#130130=CARTESIAN_POINT ( 'NONE',  ( -14.34966873604972548, 8.224510206698743886, 63.33442372801900433 ) ) ;
#130131=CARTESIAN_POINT ( 'NONE',  ( 10.72451020669871369, 18.67979575497193778, 107.0844237280190043 ) ) ;
#130132=CARTESIAN_POINT ( 'NONE',  ( -19.05341960407611168, -5.049401038298163336, 46.45724293864768129 ) ) ;
#130133=CARTESIAN_POINT ( 'NONE',  ( -16.53943276465976808, 0.05219959533911058130, 46.24890960531435979 ) ) ;
#130134=CARTESIAN_POINT ( 'NONE',  ( 16.52544592524342804, -4.483927247898539470, 78.54057627198103830 ) ) ;
#130135=CARTESIAN_POINT ( 'NONE',  ( -16.46253265017160317, 9.564922557960807481, 80.83224293864769550 ) ) ;
#130136=CARTESIAN_POINT ( 'NONE',  ( 18.67979575497194134, -10.72451020669871369, 40.83442372801901854 ) ) ;
#130137=CARTESIAN_POINT ( 'NONE',  ( -9.474510206698964154, 16.51473224551069663, 95.41557627198102409 ) ) ;
#130138=CARTESIAN_POINT ( 'NONE',  ( 21.52544592524334988, 5.823673210054432836, 101.4594237280190185 ) ) ;
#130139=CARTESIAN_POINT ( 'NONE',  ( -14.34966873604972548, 8.224510206698743886, 63.33442372801900433 ) ) ;
#130140=CARTESIAN_POINT ( 'NONE',  ( 0.05219959533937995610, -21.53943276465977519, 30.00109039468568284 ) ) ;
#130141=CARTESIAN_POINT ( 'NONE',  ( 0.05219959533909260263, 19.03943276465977164, 114.9989096053143669 ) ) ;
#130142=CARTESIAN_POINT ( 'NONE',  ( 18.67979575497178502, 10.72451020669898547, 84.16557627198103830 ) ) ;
#130143=CARTESIAN_POINT ( 'NONE',  ( -8.314922557960811034, -14.29746914071050412, 52.08224293864768839 ) ) ;
#130144=CARTESIAN_POINT ( 'NONE',  ( 9.474510206698971260, -16.51473224551069308, 47.91557627198102409 ) ) ;
#130145=CARTESIAN_POINT ( 'NONE',  ( 14.29746914071049879, -8.314922557960816363, 63.33224293864770260 ) ) ;
#130146=CARTESIAN_POINT ( 'NONE',  ( -21.52544592524343514, 5.823673210054127303, 31.04057627198102409 ) ) ;
#130147=CARTESIAN_POINT ( 'NONE',  ( -9.564922557961040184, 16.46253265017147172, 27.91775706135232582 ) ) ;
#130148=CARTESIAN_POINT ( 'NONE',  ( 16.52544592524342804, -4.483927247898539470, 93.54057627198103830 ) ) ;
#130149=CARTESIAN_POINT ( 'NONE',  ( 9.564922557960805705, 16.46253265017160317, 114.5822429386476955 ) ) ;
#130151=CARTESIAN_POINT ( 'NONE',  ( 4.483927247898790824, -16.52544592524335698, 55.20942372801902565 ) ) ;
#130152=CARTESIAN_POINT ( 'NONE',  ( -9.564922557960796823, -16.46253265017161027, 52.08224293864768839 ) ) ;
#130154=CARTESIAN_POINT ( 'NONE',  ( -4.483927247898782831, 16.52544592524335698, 97.70942372801904696 ) ) ;
#130155=CARTESIAN_POINT ( 'NONE',  ( 16.46253265017146816, 9.564922557961045513, 106.6677570613523471 ) ) ;
#130156=CARTESIAN_POINT ( 'NONE',  ( 21.55341960407619695, -5.719274019375665929, 76.04275706135237556 ) ) ;
#130157=CARTESIAN_POINT ( 'NONE',  ( 19.03943276465977164, -0.05219959533909143690, 68.74890960531436690 ) ) ;
#130158=CARTESIAN_POINT ( 'NONE',  ( 5.823673210054125526, 21.52544592524343514, 109.7905762719810383 ) ) ;
#130159=CARTESIAN_POINT ( 'NONE',  ( 16.52544592524335698, 4.483927247898782831, 41.45942372801901143 ) ) ;
#130160=CARTESIAN_POINT ( 'NONE',  ( 8.314922557960818139, 14.29746914071049879, 114.5822429386477097 ) ) ;
#130161=CARTESIAN_POINT ( 'NONE',  ( -13.97604488694547697, 13.89961937509957934, 113.1260903946856757 ) ) ;
#130162=CARTESIAN_POINT ( 'NONE',  ( -0.05219959533936034679, 19.03943276465977164, 87.50109039468567573 ) ) ;
#130163=CARTESIAN_POINT ( 'NONE',  ( -5.719274019375978568, 21.55341960407610458, 80.20724293864769550 ) ) ;
#130164=CARTESIAN_POINT ( 'NONE',  ( 9.474510206698729675, 16.51473224551082808, 57.08442372801900433 ) ) ;
#130165=CARTESIAN_POINT ( 'NONE',  ( -16.51473224551069308, -9.474510206698971260, 111.6655762719810383 ) ) ;
#130166=CARTESIAN_POINT ( 'NONE',  ( 21.55341960407610458, 5.719274019375980345, 98.95724293864770971 ) ) ;
#130167=CARTESIAN_POINT ( 'NONE',  ( 17.50000000000001421, 3.209263204892573995, 27.73803174393734494 ) ) ;
#130168=CARTESIAN_POINT ( 'NONE',  ( 16.46253265017160672, -9.564922557960803928, 63.33224293864769550 ) ) ;
#130169=LINE ( 'NONE', #24028, #136973 ) ;
#130170=CARTESIAN_POINT ( 'NONE',  ( 0.05219959533936267826, -19.03943276465977164, 110.0010903946856757 ) ) ;
#130172=CARTESIAN_POINT ( 'NONE',  ( 5.823673210054444382, -21.52544592524334988, 55.20942372801902565 ) ) ;
#130173=CARTESIAN_POINT ( 'NONE',  ( 15.72974639402199770, -15.80617190586745480, 103.1239096053143811 ) ) ;
#130174=CARTESIAN_POINT ( 'NONE',  ( -12.14591786802309592, -12.06949235617757132, 61.87390960531436690 ) ) ;
#130175=CARTESIAN_POINT ( 'NONE',  ( 19.05341960407611168, 5.049401038298154454, 73.95724293864768129 ) ) ;
#130176=CARTESIAN_POINT ( 'NONE',  ( -10.81492255796105439, 18.62759615963255655, 67.91775706135234714 ) ) ;
#130177=CARTESIAN_POINT ( 'NONE',  ( -4.483927247898782831, 16.52544592524335698, 22.70942372801901499 ) ) ;
#130178=CARTESIAN_POINT ( 'NONE',  ( -19.05341960407617563, 5.049401038297882671, 28.54275706135232937 ) ) ;
#130180=CARTESIAN_POINT ( 'NONE',  ( -21.52544592524334988, -5.823673210054445271, 58.95942372801902565 ) ) ;
#130181=CARTESIAN_POINT ( 'NONE',  ( 18.62759615963271287, -10.81492255796078972, 108.3322429386477097 ) ) ;
#130182=CARTESIAN_POINT ( 'NONE',  ( -0.05219959533907301413, -21.53943276465977519, 57.49890960531435979 ) ) ;
#130183=CARTESIAN_POINT ( 'NONE',  ( 9.474510206698729675, 16.51473224551082808, 102.0844237280190043 ) ) ;
#130184=CARTESIAN_POINT ( 'NONE',  ( -16.46253265017146816, -9.564922557961047289, 64.16775706135233293 ) ) ;
#130185=CARTESIAN_POINT ( 'NONE',  ( 10.81492255796106328, -18.62759615963255655, 85.41775706135236135 ) ) ;
#130186=CARTESIAN_POINT ( 'NONE',  ( -13.97604488694547697, 13.89961937509957934, 53.12609039468565442 ) ) ;
#130187=CARTESIAN_POINT ( 'NONE',  ( -0.05219959533909027116, -19.03943276465977164, 42.49890960531435269 ) ) ;
#130188=CARTESIAN_POINT ( 'NONE',  ( -21.55341960407610458, -5.719274019375992779, 61.45724293864770260 ) ) ;
#130189=CARTESIAN_POINT ( 'NONE',  ( 14.29746914071049879, -8.314922557960816363, 53.33224293864769550 ) ) ;
#130191=CARTESIAN_POINT ( 'NONE',  ( 13.89961937509957401, 13.97604488694547697, 36.87609039468565442 ) ) ;
#130192=CARTESIAN_POINT ( 'NONE',  ( -16.53943276465976808, -0.05219959533934237506, 88.75109039468567573 ) ) ;
#130193=CARTESIAN_POINT ( 'NONE',  ( 16.52544592524342804, -4.483927247898539470, 53.54057627198103120 ) ) ;
#130194=CARTESIAN_POINT ( 'NONE',  ( 10.72451020669871369, 18.67979575497193778, 77.08442372801901854 ) ) ;
#130195=CARTESIAN_POINT ( 'NONE',  ( 15.72974639402176855, 15.80617190586768217, 76.87609039468567573 ) ) ;
#130196=CARTESIAN_POINT ( 'NONE',  ( -5.719274019375978568, 21.55341960407610458, 75.20724293864769550 ) ) ;
#130198=CARTESIAN_POINT ( 'NONE',  ( 5.153800228976335163, 19.02544592524342804, 39.79057627198100988 ) ) ;
#130199=CARTESIAN_POINT ( 'NONE',  ( 21.55341960407619695, -5.719274019375665929, 51.04275706135234714 ) ) ;
#130200=CARTESIAN_POINT ( 'NONE',  ( -13.97604488694527625, -13.89961937509977652, 31.87390960531435979 ) ) ;
#130201=CARTESIAN_POINT ( 'NONE',  ( 13.89961937509977652, -13.97604488694527269, 58.12390960531436690 ) ) ;
#130202=CARTESIAN_POINT ( 'NONE',  ( -8.224510206698948167, 14.34966873604960824, 100.4155762719810241 ) ) ;
#130203=CARTESIAN_POINT ( 'NONE',  ( 19.05341960407611168, 5.049401038298154454, 103.9572429386476671 ) ) ;
#130204=CARTESIAN_POINT ( 'NONE',  ( -14.34966873604960291, -8.224510206698953496, 46.66557627198102409 ) ) ;
#130205=CARTESIAN_POINT ( 'NONE',  ( 4.379528057220339221, -16.55341960407611168, 112.7072429386476955 ) ) ;
#130206=CARTESIAN_POINT ( 'NONE',  ( -0.05219959533907301413, -21.53943276465977519, 87.49890960531436690 ) ) ;
#130207=CARTESIAN_POINT ( 'NONE',  ( -5.719274019375665041, -21.55341960407619695, 19.79275706135235069 ) ) ;
#130209=CARTESIAN_POINT ( 'NONE',  ( 12.14591786802327356, -12.06949235617739191, 35.62609039468568994 ) ) ;
#130210=ORIENTED_EDGE ( 'NONE', *, *, #108344, .T. ) ;
#130211=CARTESIAN_POINT ( 'NONE',  ( -15.72974639402197994, 15.80617190586746368, 65.62390960531436690 ) ) ;
#130212=CARTESIAN_POINT ( 'NONE',  ( 10.81492255796106328, -18.62759615963255655, 95.41775706135234714 ) ) ;
#130213=CARTESIAN_POINT ( 'NONE',  ( -5.153800228976328057, -19.02544592524343514, 97.29057627198099567 ) ) ;
#130214=CARTESIAN_POINT ( 'NONE',  ( 15.80617190586769283, -15.72974639402175789, 25.62609039468567929 ) ) ;
#130216=CARTESIAN_POINT ( 'NONE',  ( -21.53943276465977519, 0.05219959533907696930, 26.24890960531435624 ) ) ;
#130217=CARTESIAN_POINT ( 'NONE',  ( 4.483927247898790824, -16.52544592524335698, 85.20942372801901854 ) ) ;
#130218=CARTESIAN_POINT ( 'NONE',  ( -5.823673210054431948, 21.52544592524334988, 87.70942372801901854 ) ) ;
#130219=CARTESIAN_POINT ( 'NONE',  ( -10.81492255796105439, 18.62759615963255655, 112.9177570613523329 ) ) ;
#130220=CARTESIAN_POINT ( 'NONE',  ( -8.224510206698735004, -14.34966873604973081, 79.58442372801903275 ) ) ;
#130221=CARTESIAN_POINT ( 'NONE',  ( -15.80617190586768217, 15.72974639402176855, 23.12609039468567573 ) ) ;
#130222=CARTESIAN_POINT ( 'NONE',  ( -13.89961937509977652, 13.97604488694528158, 30.62390960531435269 ) ) ;
#130223=CARTESIAN_POINT ( 'NONE',  ( 10.72451020669871369, 18.67979575497193778, 102.0844237280190185 ) ) ;
#130224=CARTESIAN_POINT ( 'NONE',  ( -13.97604488694527625, -13.89961937509977652, 111.8739096053143243 ) ) ;
#130225=CARTESIAN_POINT ( 'NONE',  ( -15.80617190586745835, -15.72974639402198527, 106.8739096053143811 ) ) ;
#130226=CARTESIAN_POINT ( 'NONE',  ( 19.20446147854523389, 5.500000000000087041, 81.88999695167674986 ) ) ;
#130227=CARTESIAN_POINT ( 'NONE',  ( -21.55341960407610458, -5.719274019375992779, 61.45724293864770260 ) ) ;
#130228=CARTESIAN_POINT ( 'NONE',  ( 12.14591786802327356, -12.06949235617739191, 50.62609039468568994 ) ) ;
#130229=CARTESIAN_POINT ( 'NONE',  ( -14.29746914071049879, 8.314922557960819915, 50.83224293864770971 ) ) ;
#130231=CARTESIAN_POINT ( 'NONE',  ( -13.97604488694547697, 13.89961937509957934, 78.12609039468567573 ) ) ;
#130232=CARTESIAN_POINT ( 'NONE',  ( -17.26172910966780094, 6.454744622555846689, 105.8064690864922426 ) ) ;
#130233=CARTESIAN_POINT ( 'NONE',  ( -8.224510206698735004, -14.34966873604973081, 24.58442372801901499 ) ) ;
#130234=CARTESIAN_POINT ( 'NONE',  ( 15.72974639402199770, -15.80617190586745480, 83.12390960531436690 ) ) ;
#130235=CARTESIAN_POINT ( 'NONE',  ( 16.53943276465976808, -0.05219959533910856209, 63.74890960531435979 ) ) ;
#130236=CARTESIAN_POINT ( 'NONE',  ( 0.05219959533909260263, 19.03943276465977164, 104.9989096053143669 ) ) ;
#130237=CARTESIAN_POINT ( 'NONE',  ( -4.483927247898782831, 16.52544592524335698, 47.70942372801902565 ) ) ;
#130238=CARTESIAN_POINT ( 'NONE',  ( -13.97604488694527625, -13.89961937509977652, 51.87390960531436690 ) ) ;
#130239=CARTESIAN_POINT ( 'NONE',  ( -0.05219959533937732626, 21.53943276465977519, 27.50109039468567929 ) ) ;
#130240=CARTESIAN_POINT ( 'NONE',  ( 16.46253265017146816, 9.564922557961045513, 101.6677570613523329 ) ) ;
#130241=CARTESIAN_POINT ( 'NONE',  ( -19.05341960407611168, -5.049401038298163336, 96.45724293864769550 ) ) ;
#130242=CARTESIAN_POINT ( 'NONE',  ( -13.89961937509977652, 13.97604488694528158, 85.62390960531433848 ) ) ;
#130243=CARTESIAN_POINT ( 'NONE',  ( -5.823673210054116645, -21.52544592524344225, 87.29057627198103830 ) ) ;
#130244=CARTESIAN_POINT ( 'NONE',  ( 13.97604488694527802, 13.89961937509977652, 44.37390960531435269 ) ) ;
#130245=CARTESIAN_POINT ( 'NONE',  ( -17.49999999999999645, -5.624438216177605199, 59.18329655085358354 ) ) ;
#130246=CARTESIAN_POINT ( 'NONE',  ( 0.05219959533910956823, 16.53943276465976808, 69.99890960531435269 ) ) ;
#130247=CARTESIAN_POINT ( 'NONE',  ( 5.049401038298161559, -19.05341960407611168, 107.7072429386476955 ) ) ;
#130249=CARTESIAN_POINT ( 'NONE',  ( 19.02544592524334988, 5.153800228976608722, 76.45942372801897591 ) ) ;
#130250=CARTESIAN_POINT ( 'NONE',  ( -5.719274019375978568, 21.55341960407610458, 85.20724293864770971 ) ) ;
#130251=CARTESIAN_POINT ( 'NONE',  ( -19.02544592524334988, -5.153800228976617603, 43.95942372801899012 ) ) ;
#130252=CARTESIAN_POINT ( 'NONE',  ( -13.89961937509977652, 13.97604488694528158, 100.6239096053143669 ) ) ;
#130253=( NAMED_UNIT ( * ) PLANE_ANGLE_UNIT ( ) SI_UNIT ( $, .RADIAN. ) );
#130254=CARTESIAN_POINT ( 'NONE',  ( -18.62759615963270932, 10.81492255796079327, 45.83224293864769550 ) ) ;
#130255=CARTESIAN_POINT ( 'NONE',  ( 9.564922557960805705, 16.46253265017160317, 89.58224293864769550 ) ) ;
#130256=CARTESIAN_POINT ( 'NONE',  ( 18.62759615963255655, 10.81492255796105972, 71.66775706135234714 ) ) ;
#130257=CARTESIAN_POINT ( 'NONE',  ( 19.03943276465977164, -0.05219959533909143690, 33.74890960531435979 ) ) ;
#130258=CARTESIAN_POINT ( 'NONE',  ( 14.29746914071049879, -8.314922557960816363, 73.33224293864769550 ) ) ;
#130259=CARTESIAN_POINT ( 'NONE',  ( 16.53943276465976808, 0.05219959533934440121, 21.25109039468567218 ) ) ;
#130260=CARTESIAN_POINT ( 'NONE',  ( 15.72974639402176855, 15.80617190586768217, 46.87609039468568994 ) ) ;
#130262=CARTESIAN_POINT ( 'NONE',  ( 5.153800228976335163, 19.02544592524342804, 114.7905762719810241 ) ) ;
#130263=CARTESIAN_POINT ( 'NONE',  ( -9.474510206698720793, -16.51473224551083518, 84.58442372801900433 ) ) ;
#130264=EDGE_CURVE ( 'NONE', #102413, #165180, #13310, .T. ) ;
#130266=CARTESIAN_POINT ( 'NONE',  ( -21.53943276465977519, -0.05219959533937600094, 23.75109039468567929 ) ) ;
#130267=CARTESIAN_POINT ( 'NONE',  ( -19.35543954521082100, -5.499999999999585221, 44.58901960356452321 ) ) ;
#130268=CARTESIAN_POINT ( 'NONE',  ( 15.80617190586769283, -15.72974639402175789, 110.6260903946857042 ) ) ;
#130269=CARTESIAN_POINT ( 'NONE',  ( 13.97604488694527802, 13.89961937509977652, 49.37390960531434558 ) ) ;
#130270=CARTESIAN_POINT ( 'NONE',  ( 9.564922557961047289, -16.46253265017146816, 20.41775706135233293 ) ) ;
#130271=CARTESIAN_POINT ( 'NONE',  ( -4.379528057220086978, -16.55341960407618274, 99.79275706135234714 ) ) ;
#130272=CARTESIAN_POINT ( 'NONE',  ( -16.51473224551069308, -9.474510206698971260, 106.6655762719810383 ) ) ;
#130273=CARTESIAN_POINT ( 'NONE',  ( -10.81492255796105439, 18.62759615963255655, 77.91775706135231871 ) ) ;
#130277=CARTESIAN_POINT ( 'NONE',  ( -18.67979575497193778, 10.72451020669871902, 73.33442372801901854 ) ) ;
#130278=CARTESIAN_POINT ( 'NONE',  ( -5.823673210054431948, 21.52544592524334988, 97.70942372801904696 ) ) ;
#130280=CARTESIAN_POINT ( 'NONE',  ( 17.44270441346513678, -5.991230190323081573, 41.13664920735773478 ) ) ;
#130281=CARTESIAN_POINT ( 'NONE',  ( 9.564922557960805705, 16.46253265017160317, 89.58224293864769550 ) ) ;
#130282=CARTESIAN_POINT ( 'NONE',  ( 19.03943276465977164, -0.05219959533909143690, 108.7489096053143527 ) ) ;
#130284=CARTESIAN_POINT ( 'NONE',  ( -16.51473224551069308, -9.474510206698971260, 41.66557627198103120 ) ) ;
#130285=CARTESIAN_POINT ( 'NONE',  ( 5.823673210054125526, 21.52544592524343514, 54.79057627198104541 ) ) ;
#130286=CARTESIAN_POINT ( 'NONE',  ( 12.14591786802327356, -12.06949235617739191, 100.6260903946857184 ) ) ;
#130287=CARTESIAN_POINT ( 'NONE',  ( 8.224510206698953496, -14.34966873604960469, 97.91557627198103830 ) ) ;
#130288=CARTESIAN_POINT ( 'NONE',  ( 9.474510206698971260, -16.51473224551069308, 87.91557627198102409 ) ) ;
#130289=CARTESIAN_POINT ( 'NONE',  ( -15.72974639402176322, -15.80617190586768395, 104.3760903946856899 ) ) ;
#130290=CARTESIAN_POINT ( 'NONE',  ( 13.89961937509977652, -13.97604488694527269, 38.12390960531436690 ) ) ;
#130291=CARTESIAN_POINT ( 'NONE',  ( 16.55341960407611168, 4.379528057220329451, 93.95724293864770971 ) ) ;
#130292=CARTESIAN_POINT ( 'NONE',  ( -21.53943276465977519, -0.05219959533937600094, 53.75109039468568994 ) ) ;
#130293=CARTESIAN_POINT ( 'NONE',  ( 0.05219959533907565091, 21.53943276465977519, 84.99890960531436690 ) ) ;
#130294=CARTESIAN_POINT ( 'NONE',  ( 19.03943276465977164, 0.05219959533936151252, 46.25109039468566863 ) ) ;
#130296=CARTESIAN_POINT ( 'NONE',  ( -16.51473224551069308, -9.474510206698971260, 91.66557627198103830 ) ) ;
#130297=CARTESIAN_POINT ( 'NONE',  ( -0.05219959533910754901, -16.53943276465976808, 57.49890960531435979 ) ) ;
#130298=CARTESIAN_POINT ( 'NONE',  ( 5.153800228976615827, -19.02544592524334988, 45.20942372801901143 ) ) ;
#130299=CARTESIAN_POINT ( 'NONE',  ( 13.89961937509977652, -13.97604488694527269, 53.12390960531434558 ) ) ;
#130300=CARTESIAN_POINT ( 'NONE',  ( 16.55341960407611168, 4.379528057220329451, 43.95724293864769550 ) ) ;
#130301=CARTESIAN_POINT ( 'NONE',  ( -16.51473224551082808, 9.474510206698731452, 78.33442372801900433 ) ) ;
#130302=CARTESIAN_POINT ( 'NONE',  ( -18.56453257813363678, 5.500000000000055955, 85.99000423690684158 ) ) ;
#130303=CARTESIAN_POINT ( 'NONE',  ( -21.55341960407610458, -5.719274019375992779, 41.45724293864769550 ) ) ;
#130304=CARTESIAN_POINT ( 'NONE',  ( 14.29746914071049879, -8.314922557960816363, 103.3322429386476955 ) ) ;
#130306=CARTESIAN_POINT ( 'NONE',  ( 0.05219959533909260263, 19.03943276465977164, 54.99890960531435979 ) ) ;
#130307=CARTESIAN_POINT ( 'NONE',  ( 21.53943276465977519, -0.05219959533907433946, 43.74890960531435979 ) ) ;
#130308=CARTESIAN_POINT ( 'NONE',  ( 16.51473224551069308, 9.474510206698969483, 29.16557627198103475 ) ) ;
#130309=CARTESIAN_POINT ( 'NONE',  ( 14.29746914071037800, 8.314922557961029526, 76.66775706135234714 ) ) ;
#130310=CARTESIAN_POINT ( 'NONE',  ( -0.05219959533909027116, -19.03943276465977164, 62.49890960531435979 ) ) ;
#130311=CARTESIAN_POINT ( 'NONE',  ( -19.02544592524334988, -5.153800228976617603, 38.95942372801900433 ) ) ;
#130312=CARTESIAN_POINT ( 'NONE',  ( -21.53943276465977519, -0.05219959533937600094, 73.75109039468567573 ) ) ;
#130313=CARTESIAN_POINT ( 'NONE',  ( -21.52544592524343514, 5.823673210054127303, 46.04057627198103830 ) ) ;
#130314=CARTESIAN_POINT ( 'NONE',  ( -16.51473224551069308, -9.474510206698971260, 21.66557627198102765 ) ) ;
#130315=CARTESIAN_POINT ( 'NONE',  ( -16.51473224551082808, 9.474510206698731452, 108.3344237280190043 ) ) ;
#130316=DIRECTION ( 'NONE',  ( -1.734723475976805517E-15, 0.000000000000000000, -1.000000000000000000 ) ) ;
#130318=CARTESIAN_POINT ( 'NONE',  ( -5.823673210054116645, -21.52544592524344225, 42.29057627198103120 ) ) ;
#130319=CARTESIAN_POINT ( 'NONE',  ( 16.18388926212234935, -7.379444403734663815, 67.06046848633847901 ) ) ;
#130320=CARTESIAN_POINT ( 'NONE',  ( 21.52544592524334988, 5.823673210054432836, 86.45942372801901854 ) ) ;
#130321=CARTESIAN_POINT ( 'NONE',  ( -8.314922557960811034, -14.29746914071050412, 52.08224293864768839 ) ) ;
#130322=CARTESIAN_POINT ( 'NONE',  ( 4.483927247898545687, 16.52544592524342804, 59.79057627198103120 ) ) ;
#130323=CARTESIAN_POINT ( 'NONE',  ( 18.62759615963271287, -10.81492255796078972, 83.33224293864769550 ) ) ;
#130324=CARTESIAN_POINT ( 'NONE',  ( -5.823673210054116645, -21.52544592524344225, 72.29057627198102409 ) ) ;
#130326=CARTESIAN_POINT ( 'NONE',  ( -10.72451020669898014, 18.67979575497178502, 35.41557627198102409 ) ) ;
#130327=CARTESIAN_POINT ( 'NONE',  ( 4.483927247898790824, -16.52544592524335698, 60.20942372801902565 ) ) ;
#130328=CARTESIAN_POINT ( 'NONE',  ( 8.314922557960818139, 14.29746914071049879, 79.58224293864769550 ) ) ;
#130329=CARTESIAN_POINT ( 'NONE',  ( 5.049401038298161559, -19.05341960407611168, 57.70724293864769550 ) ) ;
#130330=CARTESIAN_POINT ( 'NONE',  ( -16.51473224551069308, -9.474510206698971260, 26.66557627198103120 ) ) ;
#130333=CARTESIAN_POINT ( 'NONE',  ( -16.53943276465976808, -0.05219959533934237506, 88.75109039468567573 ) ) ;
#130334=CARTESIAN_POINT ( 'NONE',  ( 18.62759615963255655, 10.81492255796105972, 21.66775706135235069 ) ) ;
#130335=CARTESIAN_POINT ( 'NONE',  ( 19.03943276465977164, -0.05219959533909143690, 83.74890960531436690 ) ) ;
#130336=CARTESIAN_POINT ( 'NONE',  ( 15.80617190586769283, -15.72974639402175789, 50.62609039468568994 ) ) ;
#130337=CARTESIAN_POINT ( 'NONE',  ( 16.46253265017160672, -9.564922557960803928, 113.3322429386476955 ) ) ;
#130339=ORIENTED_EDGE ( 'NONE', *, *, #83608, .F. ) ;
#130340=CARTESIAN_POINT ( 'NONE',  ( 21.53943276465977519, 0.05219959533937863772, 46.25109039468567573 ) ) ;
#130341=CARTESIAN_POINT ( 'NONE',  ( -16.46253265017160317, 9.564922557960807481, 40.83224293864769550 ) ) ;
#130342=CARTESIAN_POINT ( 'NONE',  ( 5.049401038298161559, -19.05341960407611168, 102.7072429386476955 ) ) ;
#130343=CARTESIAN_POINT ( 'NONE',  ( 19.02544592524334988, 5.153800228976608722, 51.45942372801900433 ) ) ;
#130344=CARTESIAN_POINT ( 'NONE',  ( -21.55341960407619339, 5.719274019375674811, 28.54275706135234358 ) ) ;
#130345=CARTESIAN_POINT ( 'NONE',  ( -19.02544592524334988, -5.153800228976617603, 43.95942372801899012 ) ) ;
#130346=CARTESIAN_POINT ( 'NONE',  ( 9.564922557960805705, 16.46253265017160317, 29.58224293864769550 ) ) ;
#130347=CARTESIAN_POINT ( 'NONE',  ( 12.14591786802327356, -12.06949235617739191, 95.62609039468568994 ) ) ;
#130348=CARTESIAN_POINT ( 'NONE',  ( -13.97604488694547697, 13.89961937509957934, 63.12609039468566152 ) ) ;
#130349=CARTESIAN_POINT ( 'NONE',  ( -4.483927247898782831, 16.52544592524335698, 107.7094237280190328 ) ) ;
#130351=CARTESIAN_POINT ( 'NONE',  ( -5.049401038298153566, 19.05341960407611168, 85.20724293864766707 ) ) ;
#130352=CARTESIAN_POINT ( 'NONE',  ( 18.62759615963255655, 10.81492255796105972, 96.66775706135234714 ) ) ;
#130353=CARTESIAN_POINT ( 'NONE',  ( -18.62759615963255300, -10.81492255796106328, 109.1677570613523613 ) ) ;
#130355=CARTESIAN_POINT ( 'NONE',  ( 16.46253265017160672, -9.564922557960803928, 103.3322429386476955 ) ) ;
#130356=CARTESIAN_POINT ( 'NONE',  ( -21.52544592524334988, -5.823673210054445271, 73.95942372801901854 ) ) ;
#130357=CARTESIAN_POINT ( 'NONE',  ( -13.97604488694547697, 13.89961937509957934, 113.1260903946856757 ) ) ;
#130359=CARTESIAN_POINT ( 'NONE',  ( -16.46253265017160317, 9.564922557960807481, 85.83224293864769550 ) ) ;
#130360=CARTESIAN_POINT ( 'NONE',  ( 0.05219959533907565091, 21.53943276465977519, 24.99890960531435624 ) ) ;
#130362=CARTESIAN_POINT ( 'NONE',  ( 5.049401038298161559, -19.05341960407611168, 87.70724293864769550 ) ) ;
#130363=CARTESIAN_POINT ( 'NONE',  ( -16.61371651742602396, -7.165104196376147705, 91.14584930007005426 ) ) ;
#130364=CARTESIAN_POINT ( 'NONE',  ( -19.02544592524342804, 5.153800228976336051, 76.04057627198102409 ) ) ;
#130365=CARTESIAN_POINT ( 'NONE',  ( -5.049401038298153566, 19.05341960407611168, 70.20724293864769550 ) ) ;
#130366=CARTESIAN_POINT ( 'NONE',  ( -4.379528057220086978, -16.55341960407618274, 99.79275706135234714 ) ) ;
#130368=CARTESIAN_POINT ( 'NONE',  ( -13.89961937509957401, -13.97604488694547875, 64.37609039468567573 ) ) ;
#130369=CARTESIAN_POINT ( 'NONE',  ( 0.05219959533909260263, 19.03943276465977164, 89.99890960531436690 ) ) ;
#130370=CARTESIAN_POINT ( 'NONE',  ( 16.53943276465976808, -0.05219959533910856209, 83.74890960531435269 ) ) ;
#130371=CARTESIAN_POINT ( 'NONE',  ( 15.72974639402199770, -15.80617190586745480, 28.12390960531435979 ) ) ;
#130372=CARTESIAN_POINT ( 'NONE',  ( 19.05341960407611168, 5.049401038298154454, 113.9572429386477097 ) ) ;
#130373=CARTESIAN_POINT ( 'NONE',  ( 0.05219959533910956823, 16.53943276465976808, 89.99890960531438111 ) ) ;
#130375=CARTESIAN_POINT ( 'NONE',  ( 0.05219959533936267826, -19.03943276465977164, 40.00109039468566152 ) ) ;
#130376=CARTESIAN_POINT ( 'NONE',  ( -8.314922557960811034, -14.29746914071050412, 22.08224293864769194 ) ) ;
#130377=CARTESIAN_POINT ( 'NONE',  ( 19.02544592524343514, -5.153800228976328945, 103.5405762719809957 ) ) ;
#130378=CARTESIAN_POINT ( 'NONE',  ( -5.823673210054431948, 21.52544592524334988, 62.70942372801902565 ) ) ;
#130379=CARTESIAN_POINT ( 'NONE',  ( 18.62759615963271287, -10.81492255796078972, 53.33224293864769550 ) ) ;
#130380=CARTESIAN_POINT ( 'NONE',  ( 15.72974639402176855, 15.80617190586768217, 31.87609039468567929 ) ) ;
#130381=CARTESIAN_POINT ( 'NONE',  ( 5.719274019375991003, -21.55341960407610458, 87.70724293864769550 ) ) ;
#130382=CARTESIAN_POINT ( 'NONE',  ( -18.67979575497193778, 10.72451020669871902, 43.33442372801901143 ) ) ;
#130383=CARTESIAN_POINT ( 'NONE',  ( -4.483927247898539470, -16.52544592524342804, 112.2905762719810241 ) ) ;
#130385=CARTESIAN_POINT ( 'NONE',  ( -13.97604488694547697, 13.89961937509957934, 73.12609039468568994 ) ) ;
#130386=CARTESIAN_POINT ( 'NONE',  ( 19.03943276465977164, -0.05219959533909143690, 48.74890960531435979 ) ) ;
#130387=CARTESIAN_POINT ( 'NONE',  ( -14.29746914071049879, 8.314922557960819915, 85.83224293864768129 ) ) ;
#130388=CARTESIAN_POINT ( 'NONE',  ( -13.97604488694527625, -13.89961937509977652, 91.87390960531432427 ) ) ;
#130389=CARTESIAN_POINT ( 'NONE',  ( -13.89961937509977652, 13.97604488694528158, 90.62390960531432427 ) ) ;
#130390=CARTESIAN_POINT ( 'NONE',  ( 0.05219959533909260263, 19.03943276465977164, 24.99890960531435269 ) ) ;
#130391=CARTESIAN_POINT ( 'NONE',  ( -16.53943276465976808, 0.05219959533911058130, 36.24890960531435979 ) ) ;
#130392=CARTESIAN_POINT ( 'NONE',  ( -16.53943276465976808, -0.05219959533934237506, 93.75109039468567573 ) ) ;
#130393=CARTESIAN_POINT ( 'NONE',  ( 19.05341960407611168, 5.049401038298154454, 58.95724293864768129 ) ) ;
#130394=CARTESIAN_POINT ( 'NONE',  ( -19.05341960407611168, -5.049401038298163336, 21.45724293864768839 ) ) ;
#130395=CARTESIAN_POINT ( 'NONE',  ( -16.46253265017146816, -9.564922557961047289, 29.16775706135232937 ) ) ;
#130396=CARTESIAN_POINT ( 'NONE',  ( -13.89961937509977652, 13.97604488694528158, 110.6239096053143243 ) ) ;
#130397=CARTESIAN_POINT ( 'NONE',  ( 16.53943276465976808, 0.05219959533934440121, 111.2510903946856899 ) ) ;
#130398=CARTESIAN_POINT ( 'NONE',  ( -21.53943276465977519, -0.05219959533937600094, 43.75109039468568284 ) ) ;
#130399=CARTESIAN_POINT ( 'NONE',  ( 0.05219959533909260263, 19.03943276465977164, 99.99890960531436690 ) ) ;
#130400=CARTESIAN_POINT ( 'NONE',  ( 0.05219959533934541429, -16.53943276465976808, 50.00109039468568994 ) ) ;
#130401=CARTESIAN_POINT ( 'NONE',  ( 14.29746914071037800, 8.314922557961029526, 106.6677570613523756 ) ) ;
#130402=CARTESIAN_POINT ( 'NONE',  ( 13.89961937509977652, -13.97604488694527269, 48.12390960531435979 ) ) ;
#130403=CARTESIAN_POINT ( 'NONE',  ( -14.34966873604972548, 8.224510206698743886, 88.33442372801901854 ) ) ;
#130404=CARTESIAN_POINT ( 'NONE',  ( -8.314922557961024197, 14.29746914071037800, 32.91775706135234714 ) ) ;
#130405=CARTESIAN_POINT ( 'NONE',  ( -16.51473224551069308, -9.474510206698971260, 51.66557627198102409 ) ) ;
#130406=CARTESIAN_POINT ( 'NONE',  ( -8.224510206698948167, 14.34966873604960824, 110.4155762719810383 ) ) ;
#130407=CARTESIAN_POINT ( 'NONE',  ( -21.53943276465977519, 0.05219959533907696930, 111.2489096053143669 ) ) ;
#130408=CARTESIAN_POINT ( 'NONE',  ( -13.97604488694527625, -13.89961937509977652, 51.87390960531436690 ) ) ;
#130409=CARTESIAN_POINT ( 'NONE',  ( -16.51473224551069308, -9.474510206698971260, 106.6655762719810383 ) ) ;
#130410=CARTESIAN_POINT ( 'NONE',  ( 13.97604488694527802, 13.89961937509977652, 29.37390960531435979 ) ) ;
#130411=CARTESIAN_POINT ( 'NONE',  ( -19.02544592524342804, 5.153800228976336051, 111.0405762719810099 ) ) ;
#130412=CARTESIAN_POINT ( 'NONE',  ( -17.40861289039006010, -6.110651285853200498, 36.37232470827432707 ) ) ;
#130413=CARTESIAN_POINT ( 'NONE',  ( 9.474510206698971260, -16.51473224551069308, 97.91557627198102409 ) ) ;
#130414=CARTESIAN_POINT ( 'NONE',  ( -10.72451020669870658, -18.67979575497194134, 44.58442372801901854 ) ) ;
#130415=CARTESIAN_POINT ( 'NONE',  ( 4.379528057220339221, -16.55341960407611168, 102.7072429386476955 ) ) ;
#130416=CARTESIAN_POINT ( 'NONE',  ( 19.02544592524343514, -5.153800228976328945, 103.5405762719809957 ) ) ;
#130419=CARTESIAN_POINT ( 'NONE',  ( 8.314922557961029526, -14.29746914071037800, 60.41775706135235424 ) ) ;
#130420=CARTESIAN_POINT ( 'NONE',  ( -5.823673210054431948, 21.52544592524334988, 87.70942372801901854 ) ) ;
#130421=CARTESIAN_POINT ( 'NONE',  ( -16.55341960407617563, 4.379528057220093196, 38.54275706135234714 ) ) ;
#130422=CARTESIAN_POINT ( 'NONE',  ( -16.51473224551069308, -9.474510206698971260, 81.66557627198103830 ) ) ;
#130423=CARTESIAN_POINT ( 'NONE',  ( -16.55341960407617563, 4.379528057220093196, 33.54275706135234714 ) ) ;
#130424=CARTESIAN_POINT ( 'NONE',  ( 0.05219959533934541429, -16.53943276465976808, 20.00109039468568639 ) ) ;
#130425=CARTESIAN_POINT ( 'NONE',  ( 12.06949235617739724, 12.14591786802326823, 76.87609039468567573 ) ) ;
#130426=CARTESIAN_POINT ( 'NONE',  ( -5.153800228976607833, 19.02544592524334988, 92.70942372801901854 ) ) ;
#130427=CARTESIAN_POINT ( 'NONE',  ( -9.564922557960796823, -16.46253265017161027, 82.08224293864768129 ) ) ;
#130428=CARTESIAN_POINT ( 'NONE',  ( -15.72974639402197994, 15.80617190586746368, 95.62390960531436690 ) ) ;
#130429=CARTESIAN_POINT ( 'NONE',  ( 16.55341960407611168, 4.379528057220329451, 88.95724293864769550 ) ) ;
#130430=CARTESIAN_POINT ( 'NONE',  ( 13.97604488694548053, -13.89961937509957401, 90.62609039468567573 ) ) ;
#130431=CARTESIAN_POINT ( 'NONE',  ( 4.483927247898790824, -16.52544592524335698, 70.20942372801904696 ) ) ;
#130433=CARTESIAN_POINT ( 'NONE',  ( -16.51473224551082808, 9.474510206698731452, 73.33442372801900433 ) ) ;
#130434=CARTESIAN_POINT ( 'NONE',  ( -14.29746914071049879, 8.314922557960819915, 30.83224293864770260 ) ) ;
#130435=CARTESIAN_POINT ( 'NONE',  ( 8.224510206698953496, -14.34966873604960469, 97.91557627198103830 ) ) ;
#130436=CARTESIAN_POINT ( 'NONE',  ( -13.89961937509957401, -13.97604488694547875, 34.37609039468566863 ) ) ;
#130437=CARTESIAN_POINT ( 'NONE',  ( -5.049401038297874678, -19.05341960407618274, 44.79275706135232582 ) ) ;
#130438=CARTESIAN_POINT ( 'NONE',  ( -10.72451020669898014, 18.67979575497178502, 115.4155762719810241 ) ) ;
#130439=CARTESIAN_POINT ( 'NONE',  ( 13.97604488694527802, 13.89961937509977652, 109.3739096053143669 ) ) ;
#130440=CARTESIAN_POINT ( 'NONE',  ( -19.02544592524342804, 5.153800228976336051, 96.04057627198103830 ) ) ;
#130441=CARTESIAN_POINT ( 'NONE',  ( 0.05219959533937995610, -21.53943276465977519, 95.00109039468568994 ) ) ;
#130442=CARTESIAN_POINT ( 'NONE',  ( -19.02544592524342804, 5.153800228976336051, 71.04057627198099567 ) ) ;
#130444=CARTESIAN_POINT ( 'NONE',  ( -15.80617190586745835, -15.72974639402198527, 41.87390960531435979 ) ) ;
#130445=CARTESIAN_POINT ( 'NONE',  ( 16.55341960407611168, 4.379528057220329451, 93.95724293864770971 ) ) ;
#130446=CARTESIAN_POINT ( 'NONE',  ( 16.51473224551069308, 9.474510206698969483, 59.16557627198102409 ) ) ;
#130447=CARTESIAN_POINT ( 'NONE',  ( -16.52544592524342804, 4.483927247898546575, 116.0405762719810383 ) ) ;
#130449=CARTESIAN_POINT ( 'NONE',  ( -15.80617190586768217, 15.72974639402176855, 23.12609039468567573 ) ) ;
#130450=CARTESIAN_POINT ( 'NONE',  ( -18.62759615963255300, -10.81492255796106328, 64.16775706135234714 ) ) ;
#130451=CARTESIAN_POINT ( 'NONE',  ( -16.51473224551069308, -9.474510206698971260, 46.66557627198102409 ) ) ;
#130452=CARTESIAN_POINT ( 'NONE',  ( 12.14591786802327356, -12.06949235617739191, 80.62609039468567573 ) ) ;
#130453=B_SPLINE_CURVE_WITH_KNOTS ( 'NONE', 3,
 ( #66823, #128486, #175013, #51657, #191179, #36477, #98134, #99150, #160839, #22328, #83978, #115336, #64842, #177027, #38497, #100153, #150676, #166840, #12174, #39483, #54653, #73839, #193180, #11168, #57671, #70833, #103166, #84972, #72843, #134513, #41502, #165843 ),
 .UNSPECIFIED., .F., .F.,
 ( 4, 2, 2, 2, 2, 2, 2, 2, 2, 2, 2, 2, 2, 2, 2, 4 ),
 ( 1.684111863762029156E-17, 0.0003712461730036760443, 0.0007424923460073351751, 0.001113738519010994523, 0.001484984692014653654, 0.002227477038021980372, 0.002598723211025658585, 0.002969969384029335930, 0.003341215557033014143, 0.003712461730036691488, 0.004083707903040368833, 0.004454954076044045745, 0.004826200249047724392, 0.005197446422051402171, 0.005568692595055079082, 0.005939938768058757729 ),
 .UNSPECIFIED. ) ;
#130454=CARTESIAN_POINT ( 'NONE',  ( -21.52544592524343514, 5.823673210054127303, 111.0405762719810525 ) ) ;
#130456=CARTESIAN_POINT ( 'NONE',  ( -18.62759615963270932, 10.81492255796079327, 105.8322429386476955 ) ) ;
#130457=CARTESIAN_POINT ( 'NONE',  ( 19.05341960407617918, -5.049401038297876454, 56.04275706135234714 ) ) ;
#130458=CARTESIAN_POINT ( 'NONE',  ( 13.89961937509977652, -13.97604488694527269, 63.12390960531435979 ) ) ;
#130459=CARTESIAN_POINT ( 'NONE',  ( 19.05341960407617918, -5.049401038297876454, 31.04275706135232227 ) ) ;
#130460=CARTESIAN_POINT ( 'NONE',  ( 0.05219959533937995610, -21.53943276465977519, 75.00109039468568994 ) ) ;
#130461=CARTESIAN_POINT ( 'NONE',  ( 5.719274019375991003, -21.55341960407610458, 67.70724293864769550 ) ) ;
#130462=CARTESIAN_POINT ( 'NONE',  ( -4.379528057220328563, 16.55341960407611168, 50.20724293864769550 ) ) ;
#130463=CARTESIAN_POINT ( 'NONE',  ( -18.62759615963255300, -10.81492255796106328, 84.16775706135234714 ) ) ;
#130464=CARTESIAN_POINT ( 'NONE',  ( -19.02544592524334988, -5.153800228976617603, 33.95942372801897591 ) ) ;
#130465=CARTESIAN_POINT ( 'NONE',  ( 14.29746914071049879, -8.314922557960816363, 68.33224293864769550 ) ) ;
#130466=CARTESIAN_POINT ( 'NONE',  ( -0.05219959533910754901, -16.53943276465976808, 107.4989096053143669 ) ) ;
#130467=CARTESIAN_POINT ( 'NONE',  ( -19.03943276465977164, -0.05219959533935918106, 63.75109039468566863 ) ) ;
#130468=CARTESIAN_POINT ( 'NONE',  ( -16.53943276465976808, -0.05219959533934237506, 113.7510903946856757 ) ) ;
#130469=CARTESIAN_POINT ( 'NONE',  ( 18.62759615963255655, 10.81492255796105972, 66.66775706135234714 ) ) ;
#130471=CARTESIAN_POINT ( 'NONE',  ( 5.153800228976335163, 19.02544592524342804, 74.79057627198103830 ) ) ;
#130472=CARTESIAN_POINT ( 'NONE',  ( 9.564922557961047289, -16.46253265017146816, 45.41775706135232582 ) ) ;
#130473=CARTESIAN_POINT ( 'NONE',  ( -5.823673210054116645, -21.52544592524344225, 52.29057627198102409 ) ) ;
#130474=CARTESIAN_POINT ( 'NONE',  ( -18.62759615963255300, -10.81492255796106328, 44.16775706135234714 ) ) ;
#130475=CARTESIAN_POINT ( 'NONE',  ( -5.823673210054116645, -21.52544592524344225, 107.2905762719810525 ) ) ;
#130476=CARTESIAN_POINT ( 'NONE',  ( -9.564922557961040184, 16.46253265017147172, 102.9177570613523329 ) ) ;
#130477=CARTESIAN_POINT ( 'NONE',  ( -16.55341960407617563, 4.379528057220093196, 68.54275706135234714 ) ) ;
#130479=CARTESIAN_POINT ( 'NONE',  ( -21.53943276465977519, 0.05219959533907696930, 101.2489096053143669 ) ) ;
#130480=CARTESIAN_POINT ( 'NONE',  ( 4.483927247898545687, 16.52544592524342804, 94.79057627198105251 ) ) ;
#130481=CARTESIAN_POINT ( 'NONE',  ( -17.49999999999999645, -3.209263204892548238, 30.23803174393719573 ) ) ;
#130482=CARTESIAN_POINT ( 'NONE',  ( 16.55341960407618274, -4.379528057220086978, 21.04275706135234714 ) ) ;
#130483=CARTESIAN_POINT ( 'NONE',  ( -18.62759615963270932, 10.81492255796079327, 50.83224293864770971 ) ) ;
#130484=CARTESIAN_POINT ( 'NONE',  ( 14.34966873604972726, -8.224510206698740333, 90.83442372801901854 ) ) ;
#130487=CARTESIAN_POINT ( 'NONE',  ( -16.53943276465976808, -0.05219959533934237506, 68.75109039468568994 ) ) ;
#130488=CARTESIAN_POINT ( 'NONE',  ( -5.719274019375665041, -21.55341960407619695, 34.79275706135235424 ) ) ;
#130489=CARTESIAN_POINT ( 'NONE',  ( 18.62759615963271287, -10.81492255796078972, 58.33224293864768839 ) ) ;
#130490=CARTESIAN_POINT ( 'NONE',  ( 8.224510206698742110, 14.34966873604972548, 82.08442372801901854 ) ) ;
#130491=CARTESIAN_POINT ( 'NONE',  ( 5.049401038298161559, -19.05341960407611168, 92.70724293864769550 ) ) ;
#130492=CARTESIAN_POINT ( 'NONE',  ( -10.72451020669870658, -18.67979575497194134, 69.58442372801900433 ) ) ;
#130493=CARTESIAN_POINT ( 'NONE',  ( 10.72451020669898902, -18.67979575497178502, 42.91557627198103120 ) ) ;
#130494=CARTESIAN_POINT ( 'NONE',  ( -18.62759615963270932, 10.81492255796079327, 30.83224293864770260 ) ) ;
#130496=CARTESIAN_POINT ( 'NONE',  ( -13.97604488694547697, 13.89961937509957934, 58.12609039468566863 ) ) ;
#130497=CARTESIAN_POINT ( 'NONE',  ( 0.05219959533934541429, -16.53943276465976808, 65.00109039468568994 ) ) ;
#130498=CARTESIAN_POINT ( 'NONE',  ( 10.72451020669898902, -18.67979575497178502, 32.91557627198102409 ) ) ;
#130500=CARTESIAN_POINT ( 'NONE',  ( -5.049401038298153566, 19.05341960407611168, 85.20724293864766707 ) ) ;
#130501=CARTESIAN_POINT ( 'NONE',  ( 8.314922557960818139, 14.29746914071049879, 24.58224293864768839 ) ) ;
#130502=CARTESIAN_POINT ( 'NONE',  ( -18.22780087662123805, 5.499999999999981348, 86.01763182126894947 ) ) ;
#130503=CARTESIAN_POINT ( 'NONE',  ( 4.483927247898545687, 16.52544592524342804, 109.7905762719810383 ) ) ;
#130504=CARTESIAN_POINT ( 'NONE',  ( -21.52544592524343514, 5.823673210054127303, 46.04057627198103830 ) ) ;
#130505=CARTESIAN_POINT ( 'NONE',  ( 5.153800228976335163, 19.02544592524342804, 49.79057627198100988 ) ) ;
#130506=CARTESIAN_POINT ( 'NONE',  ( 4.379528057220092307, 16.55341960407617563, 87.29275706135236135 ) ) ;
#130507=CARTESIAN_POINT ( 'NONE',  ( -10.81492255796105439, 18.62759615963255655, 27.91775706135234358 ) ) ;
#130508=CARTESIAN_POINT ( 'NONE',  ( 13.97604488694548053, -13.89961937509957401, 85.62609039468568994 ) ) ;
#130509=CARTESIAN_POINT ( 'NONE',  ( 16.55341960407611168, 4.379528057220329451, 93.95724293864770971 ) ) ;
#130510=CARTESIAN_POINT ( 'NONE',  ( -13.89961937509977652, 13.97604488694528158, 50.62390960531435979 ) ) ;
#130511=CARTESIAN_POINT ( 'NONE',  ( -9.474510206698964154, 16.51473224551069663, 30.41557627198102054 ) ) ;
#130512=CARTESIAN_POINT ( 'NONE',  ( 21.52544592524334988, 5.823673210054432836, 106.4594237280190328 ) ) ;
#130513=CARTESIAN_POINT ( 'NONE',  ( -16.51473224551069308, -9.474510206698971260, 71.66557627198102409 ) ) ;
#130514=CARTESIAN_POINT ( 'NONE',  ( -8.314922557961024197, 14.29746914071037800, 62.91775706135236135 ) ) ;
#130515=CARTESIAN_POINT ( 'NONE',  ( 18.62759615963255655, 10.81492255796105972, 96.66775706135234714 ) ) ;
#130516=CARTESIAN_POINT ( 'NONE',  ( -5.823673210054116645, -21.52544592524344225, 52.29057627198102409 ) ) ;
#130517=CARTESIAN_POINT ( 'NONE',  ( -14.29746914071037622, -8.314922557961029526, 69.16775706135234714 ) ) ;
#130518=CARTESIAN_POINT ( 'NONE',  ( 16.46253265017146816, 9.564922557961045513, 51.66775706135233293 ) ) ;
#130519=CARTESIAN_POINT ( 'NONE',  ( 19.05341960407617918, -5.049401038297876454, 61.04275706135232582 ) ) ;
#130521=CARTESIAN_POINT ( 'NONE',  ( -5.823673210054431948, 21.52544592524334988, 62.70942372801902565 ) ) ;
#130522=CARTESIAN_POINT ( 'NONE',  ( -16.46253265017160317, 9.564922557960807481, 60.83224293864769550 ) ) ;
#130523=CARTESIAN_POINT ( 'NONE',  ( -13.97604488694527625, -13.89961937509977652, 31.87390960531435979 ) ) ;
#130524=CARTESIAN_POINT ( 'NONE',  ( -16.51473224551082808, 9.474510206698731452, 63.33442372801900433 ) ) ;
#130525=CARTESIAN_POINT ( 'NONE',  ( -5.049401038298153566, 19.05341960407611168, 115.2072429386477097 ) ) ;
#130526=CARTESIAN_POINT ( 'NONE',  ( -19.03943276465977164, 0.05219959533909376836, 101.2489096053143669 ) ) ;
#130527=CARTESIAN_POINT ( 'NONE',  ( -14.34966873604960291, -8.224510206698953496, 51.66557627198102409 ) ) ;
#130528=CARTESIAN_POINT ( 'NONE',  ( -21.53943276465977519, 0.05219959533907696930, 51.24890960531436690 ) ) ;
#130529=CARTESIAN_POINT ( 'NONE',  ( 18.22780087662122384, -5.500000000000022204, 91.01540105326107266 ) ) ;
#130530=CARTESIAN_POINT ( 'NONE',  ( 18.62759615963255655, 10.81492255796105972, 111.6677570613523613 ) ) ;
#130531=CARTESIAN_POINT ( 'NONE',  ( -16.21995358207303184, -7.366697692864244473, 80.06448998487843483 ) ) ;
#130532=CARTESIAN_POINT ( 'NONE',  ( 19.05341960407611168, 5.049401038298154454, 53.95724293864770260 ) ) ;
#130535=CARTESIAN_POINT ( 'NONE',  ( 0.05219959533934541429, -16.53943276465976808, 75.00109039468568994 ) ) ;
#130536=CARTESIAN_POINT ( 'NONE',  ( 15.80617190586746368, 15.72974639402197994, 99.37390960531436690 ) ) ;
#130538=CARTESIAN_POINT ( 'NONE',  ( 4.483927247898545687, 16.52544592524342804, 54.79057627198104541 ) ) ;
#130539=CARTESIAN_POINT ( 'NONE',  ( 16.46253265017160672, -9.564922557960803928, 43.33224293864769550 ) ) ;
#130541=CARTESIAN_POINT ( 'NONE',  ( -10.72451020669870658, -18.67979575497194134, 34.58442372801900433 ) ) ;
#130542=CARTESIAN_POINT ( 'NONE',  ( -5.153800228976607833, 19.02544592524334988, 42.70942372801901143 ) ) ;
#130543=CARTESIAN_POINT ( 'NONE',  ( 9.474510206698971260, -16.51473224551069308, 42.91557627198103120 ) ) ;
#130544=CARTESIAN_POINT ( 'NONE',  ( -5.719274019375665041, -21.55341960407619695, 89.79275706135236135 ) ) ;
#130545=CARTESIAN_POINT ( 'NONE',  ( -0.05219959533909027116, -19.03943276465977164, 22.49890960531436690 ) ) ;
#130546=ORIENTED_EDGE ( 'NONE', *, *, #189415, .F. ) ;
#130547=CARTESIAN_POINT ( 'NONE',  ( -14.29746914071049879, 8.314922557960819915, 40.83224293864769550 ) ) ;
#130548=CARTESIAN_POINT ( 'NONE',  ( 18.22780087662126647, 5.499999999999818812, 41.48236817873107185 ) ) ;
#130549=CARTESIAN_POINT ( 'NONE',  ( 21.55341960407610458, 5.719274019375980345, 43.95724293864769550 ) ) ;
#130551=CARTESIAN_POINT ( 'NONE',  ( 9.564922557960805705, 16.46253265017160317, 104.5822429386476955 ) ) ;
#130552=CARTESIAN_POINT ( 'NONE',  ( -16.53943276465976808, 0.05219959533911058130, 86.24890960531436690 ) ) ;
#130553=CARTESIAN_POINT ( 'NONE',  ( -4.379528057220086978, -16.55341960407618274, 19.79275706135235069 ) ) ;
#130554=CARTESIAN_POINT ( 'NONE',  ( -8.224510206698735004, -14.34966873604973081, 109.5844237280190328 ) ) ;
#130556=CARTESIAN_POINT ( 'NONE',  ( 16.46253265017160672, -9.564922557960803928, 93.33224293864769550 ) ) ;
#130557=CARTESIAN_POINT ( 'NONE',  ( -5.823673210054116645, -21.52544592524344225, 102.2905762719810383 ) ) ;
#130558=CARTESIAN_POINT ( 'NONE',  ( 16.52544592524342804, -4.483927247898539470, 28.54057627198103120 ) ) ;
#130559=CARTESIAN_POINT ( 'NONE',  ( 0.05219959533909260263, 19.03943276465977164, 99.99890960531436690 ) ) ;
#130560=CARTESIAN_POINT ( 'NONE',  ( 9.474510206698729675, 16.51473224551082808, 77.08442372801900433 ) ) ;
#130561=CARTESIAN_POINT ( 'NONE',  ( 15.72974639402176855, 15.80617190586768217, 111.8760903946856615 ) ) ;
#130562=CARTESIAN_POINT ( 'NONE',  ( -15.72974639402197994, 15.80617190586746368, 85.62390960531436690 ) ) ;
#130563=CARTESIAN_POINT ( 'NONE',  ( -15.72974639402197994, 15.80617190586746368, 50.62390960531435979 ) ) ;
#130565=CARTESIAN_POINT ( 'NONE',  ( -9.564922557960796823, -16.46253265017161027, 67.08224293864769550 ) ) ;
#130566=CARTESIAN_POINT ( 'NONE',  ( -14.34966873604960291, -8.224510206698953496, 31.66557627198102054 ) ) ;
#130567=CARTESIAN_POINT ( 'NONE',  ( 16.46253265017160672, -9.564922557960803928, 78.33224293864769550 ) ) ;
#130568=ORIENTED_EDGE ( 'NONE', *, *, #63230, .F. ) ;
#130570=CARTESIAN_POINT ( 'NONE',  ( 19.05341960407617918, -5.049401038297876454, 26.04275706135233293 ) ) ;
#130571=CARTESIAN_POINT ( 'NONE',  ( 16.55341960407611168, 4.379528057220329451, 88.95724293864769550 ) ) ;
#130573=( BOUNDED_SURFACE ( )  B_SPLINE_SURFACE ( 3, 2, ( 
 ( #71969, #85122, #147827, #7283, #116476, #129618, #191313, #178165, #39630, #24485, #130631, #68967, #52790, #86136, #54801, #21464, #131645, #176160, #117474, #102309, #175153, #84121, #114458, #192325, #8300, #145800, #69977, #100299, #36620, #37630, #190323, #148822, #98277, #132646, #38642, #99293, #159978, #161977, #9313, #179172, #160979, #23473, #193327, #25495, #163999, #101290, #162980, #70978, #194334, #115481, #22473, #53806, #55802, #40640, #146806, #177169, #87138, #10312, #51800, #113459, #83126, #144802, #6285, #67964, #165987, #166980, #119483, #58783, #15272, #42642, #41648, #56814, #137614, #152779, #184129, #28483, #92088, #59777, #90117, #133643, #73980, #122437, #26486, #72988, #198300, #104304, #164992, #75939, #105292, #88128, #199298, #195334, #181165, #45612, #151801, #27487, #106275, #135649, #149812, #118488, #153777, #136619, #60765, #11318, #44622, #134657, #43629, #13292, #12315, #74957, #121446, #183138, #89130, #180179, #196343, #30442, #150818, #167960, #107264, #29459, #168935, #14270, #91091, #103312, #57811, #197320, #120452, #182145, #46604, #154773, #112248, #156772, #3079, #142581, #169944, #173939, #31435, #17262, #50588, #65738, #62750, #35407, #126417, #34419, #80904, #63762, #97059, #94085, #187131, #158741, #171936, #16270, #78915, #140592, #157767, #2082, #125435, #95084, #48603, #170939, #110255, #49586, #76932, #172940, #123421, #186127, #108265, #33425, #111249, #18266, #188114, #64755, #4060, #79919, #32431, #127406, #138601, #96078, #141592, #19258, #189115, #155764, #93089, #83, #77922, #61753, #47606, #185114, #139589, #1075, #124430, #109260, #81193, #17564, #157068, #95382, #65049, #171246, #138906, #16572, #189406, #140894, #48899, #1379, #142874, #172235, #385, #18564, #32735, #62058, #127706, #79225, #66039, #20530, #33720, #96370, #156066, #126705, #78219, #139890, #188409, #49886, #173237, #2383, #64062, #63058, #34713, #3374, #170249, #80212, #124738, #50883, #112541, #123723, #94387, #186435, #125732, #141883, #187431, #111552, #110554, #185420, #47911, #158058, #109565, #19548, #4354, #174235, #35704, #97351, #159037, #46912, #108572, #31743, #93391, #155077, #36687, #23540, #114527, #115548, #68031, #7347, #164063, #191380, #190393, #5353, #86202, #101356, #132710, #177236, #40704, #8367, #38708, #82178, #22538, #71043, #175222, #21533, #146875, #52856, #113528, #24552, #53874, #98347, #147892, #143873, #129682, #194398, #100365, #176228, #54868, #84185, #160046, #67037, #102374, #85186, #9378, #83194, #128696, #55866, #145865, #117540, #161044, #162044, #70042, #131711, #37697, #51868, #144868, #179238, #69032, #192391, #6351, #99361, #193392, #130697, #116542, #178230, #39694, #163045, #104368, #152842, #107324, #120516, #183202, #42707, #151862, #165055, #26548, #13353, #75017, #59839, #166052, #27552, #88192, #121508, #90179, #56878, #167041, #11381, #14336, #137675, #10378, #119548, #149876, #89192, #43692, #181231, #105354, #135713, #72035, #73051, #25562, #184191, #133708, #168023, #74042, #134723, #195400, #197384, #44684, #76001, #196406, #58849, #28543, #60826, #199361, #136682, #198364, #106337, #29519, #182208, #57876, #118552, #91153, #122500, #45673, #150885, #87206, #148887, #180243, #41712, #103377, #12380, #171997, #172999, #94147, #77982, #32494, #126476, #141650, #125495, #154834, #78978, #157825, #124494, #110315, #4117, #19315, #123484, #33485, #1137, #2144, #16333, #155826, #50643, #139649, #76993, #92152, #34477, #188174, #80963, #63822, #127465, #95143, #187192, #168997, #109322, #142639, #61814, #108326, #156832, #62811, #145, #111310, #140653, #185176, #96136, #30501, #186189, #65796, #48663, #47670, #3140, #171002, #46667, #153838, #189171, #18325, #15335, #170006, #138664, #31497, #17323, #93150, #79982, #64815, #49647, #38465, #144629, #112305, #190151, #162800, #114285, #22297, #174982, #116296 ),
 ( #100121, #130447, #6112, #146624, #175988, #66791, #20287, #160809, #177986, #52623, #23299, #143625, #173995, #24309, #194160, #113291, #83948, #85958, #81933, #131462, #70801, #35464, #53627, #158798, #161804, #9135, #82951, #7108, #147646, #51626, #132469, #37457, #145628, #36446, #39453, #68790, #97115, #192146, #67794, #5110, #101114, #191149, #128455, #98101, #115302, #69795, #129450, #84943, #159799, #21294, #8117, #193149, #54621, #99117, #176995, #195155, #151631, #120282, #86961, #197149, #41470, #182967, #167789, #40460, #149640, #56637, #72812, #73808, #11137, #135480, #165812, #102133, #180002, #55624, #14095, #163817, #198131, #104130, #103134, #25319, #27309, #13125, #44450, #118310, #88957, #58615, #90919, #29288, #181974, #43456, #105125, #59599, #180990, #164815, #119306, #74788, #28311, #12144, #26311, #150647, #106104, #134481, #166811, #152605, #75762, #10135, #89951, #87951, #136450, #196166, #42467, #137440, #57640, #148646, #178992, #121273, #117297, #71796, #133465, #157590, #125262, #93916, #199119, #139419, #187944, #91908, #138432, #63588, #108084, #30264, #141417, #170769, #153601, #2905, #60586, #46426, #111076, #32258, #31262, #171766, #901, #15098, #122262, #19082, #1909, #64583, #76757, #45437, #126248, #62575, #49413, #77753, #17089, #155594, #186960, #92913, #183951, #34246, #172765, #200113, #140418, #154599, #78742, #184941, #124253, #80730, #169769, #107090, #168761, #95906, #18093, #61581, #48431, #123250, #110087, #33255, #16095, #185949, #47433, #109089, #94913, #156598, #79748, #173766, #87481, #116817, #96887, #149168, #3887, #192668, #57159, #178508, #177514, #117827, #147161, #35233, #142409, #103660, #148166, #10658, #158570, #188940, #72321, #85472, #133997, #23822, #163335, #101644, #71323, #38984, #65566, #20059, #195688, #8649, #55146, #7627, #118838, #39974, #127226, #24831, #100640, #50418, #180521, #70323, #41994, #26830, #86481, #102657, #162321, #132986, #81703, #143386, #194677, #56146, #179520, #131990, #193675, #69311, #40989, #9657, #130977, #164342, #54151, #165338, #112077, #115824, #25837, #27834, #105634, #106623, #43972, #168297, #198653, #135006, #12654, #88471, #46945, #196684, #30786, #136964, #135988, #58153, #60119, #184468, #77270, #89475, #121787, #29793, #123756, #419, #14620, #91429, #153116, #92433, #13626, #197659, #152143, #45947, #61105, #44965, #74321, #183481, #138939, #167323, #76277, #73334, #11668, #150168, #104649, #122778, #59125, #28819, #75293, #151166, #119821, #154120, #137955, #90459, #199639, #182491, #107602, #169280, #108605, #185455, #15613, #62093, #181506, #170282, #42984, #166336, #120791, #128731, #158091, #49921, #125764, #66073, #95416, #186470, #139925, #80245, #97385, #172267, #142907, #63093, #31776, #143907, #113562, #32769, #3406, #82216, #1414, #50918, #190427, #93424, #173271, #78252, #19583, #51903, #2416, #126739, #5389, #34745, #174270, #112576, #111586, #96404, #65081, #124772, #35738, #155111, #47947, #109598, #67072, #81226, #4388, #159071, #171281, #16605, #94421, #33757, #156101, #20565, #17599, #79258, #127739, #189441, #140930, #18597, #64096, #48932, #141915, #187464, #188442, #110586, #157101, #177273, #55904, #38744, #100402, #193430, #115585, #69069, #85225, #147927, #195440, #71079, #21568, #84222, #144903, #23577, #9413, #162083, #24589, #101392, #179277, #146916, #130736, #25598, #133745, #194433, #54906, #132745, #116579, #192428, #129719, #8405, #6386, #70080, #145901, #131748, #37735, #53910, #178268, #117577, #98384, #163085, #72072, #86237, #39731, #40742, #102412, #164099, #191416, #83228, #87242, #148925, #10414, #56915, #68065, #175256, #36722, #160081, #176264, #52892, #114567, #99397, #161080, #22575, #7385, #59879, #165092, #106377, #15373, #89230, #13390, #30539, #121545, #60862, #199398, #198401, #183240, #151900, #26586, #137714, #180280, #88229, #196443 ),
 ( #76039, #122537, #105393, #138701, #135750, #28581, #77029, #75054, #57913, #120553, #182246, #184228, #43731, #167079, #136720, #58887, #12417, #90217, #91189, #183, #14373, #149913, #27592, #11420, #44721, #152878, #168059, #29556, #45709, #107360, #169033, #74079, #92191, #118590, #153875, #41750, #103414, #73090, #197421, #134761, #119585, #181268, #42745, #150924, #104407, #166089, #79014, #95183, #46704, #185213, #123520, #78017, #96174, #32530, #140688, #187228, #62847, #61851, #4156, #141687, #2180, #48699, #155861, #126513, #142677, #20326, #97155, #173038, #50687, #108366, #81003, #188211, #3178, #64851, #65835, #110351, #171039, #125531, #19354, #34516, #18365, #47707, #172033, #112344, #17359, #49683, #158838, #174034, #16369, #111348, #94182, #156869, #109357, #33521, #143669, #63860, #170044, #31534, #127505, #189209, #35505, #80018, #81975, #157864, #93187, #154872, #139686, #1172, #124531, #186226, #69834, #114325, #36486, #147687, #177035, #159841, #9174, #66832, #52663, #117337, #38505, #37496, #178024, #7147, #98142, #5150, #163859, #8158, #70841, #21334, #51666, #132509, #145666, #194198, #83987, #23337, #161843, #131501, #99158, #128496, #82992, #55663, #68831, #115345, #67833, #179032, #100161, #190191, #84981, #160847, #113330, #40499, #130490, #102171, #86999, #146663, #162839, #22336, #193188, #144668, #6153, #54661, #116335, #39492, #192186, #53667, #129489, #101152, #24347, #191187, #85998, #176028, #25358, #175023, #133503, #42505, #87990, #165851, #166847, #104169, #28349, #58652, #195195, #72851, #148686, #107126, #56675, #90954, #197188, #196207, #118348, #120318, #44487, #137476, #149678, #182012, #89987, #183987, #60623, #10174, #180042, #26350, #45472, #151668, #74826, #14131, #41511, #168797, #103174, #88993, #122297, #199156, #134521, #30301, #198167, #106143, #152641, #135517, #71834, #27347, #43495, #164854, #105161, #11176, #150684, #12182, #29324, #73846, #13162, #136487, #59637, #121311, #183003, #167825, #57679, #75798, #119347, #181031, #61616, #140452, #64618, #17124, #141453, #18126, #95938, #32294, #185984, #142442, #50449, #111109, #171799, #49446, #110121, #109124, #46460, #1942, #123284, #78776, #62608, #93950, #154634, #170802, #125298, #76794, #15132, #153637, #108120, #126280, #124287, #155628, #63622, #92948, #91944, #34279, #33287, #186994, #48464, #47467, #156631, #172798, #112108, #127260, #2938, #80764, #138465, #157624, #19114, #200146, #79781, #188973, #187977, #94947, #3920, #65600, #173799, #169803, #184975, #31296, #16129, #77784, #139453, #934, #35265, #147438, #117087, #36246, #6902, #85751, #143422, #54424, #193953, #96920, #176786, #81736, #23092, #132262, #5910, #130237, #8926, #38259, #177782, #116094, #115094, #99913, #68581, #4909, #39252, #37251, #128256, #158602, #55416, #161598, #100908, #189954, #66592, #162592, #175777, #24097, #114076, #53417, #191933, #84737, #67587, #20092, #113088, #70594, #98908, #145420, #97899, #51428, #146415, #174780, #7906, #129245, #159590, #21087, #160601, #82744, #144424, #69590, #192945, #52418, #131257, #190941, #22091, #83741, #104916, #12915, #119105, #57432, #118101, #74579, #43248, #9929, #120079, #164607, #105900, #90720, #163606, #72598, #179791, #195959, #196944, #134272, #58412, #88748, #25107, #102922, #178782, #137233, #86751, #121065, #27102, #26101, #148434, #150441, #136247, #167586, #41260, #11937, #181767, #13890, #152403, #166603, #28103, #89742, #182759, #103923, #87744, #42263, #197923, #151428, #135272, #149429, #73600, #29081, #180786, #59391, #75557, #198917, #133254, #44243, #10925, #60386, #165603, #40250, #101924, #71588, #194945, #56421, #126042, #141207, #172552, #16879, #80522, #48218, #78530, #122058, #62365, #110867, #14894, #61377, #186748, #31057, #153396, #64374, #93707, #76555, #187738, #183750, #169560, #34038, #155389, #154393, #94701, #156378, #92705 ),
 ( #45236, #95695, #693, #49209, #3679, #140204, #79537, #139218, #109872, #123048, #184734, #171556, #33046, #17883, #124034, #185733, #46219, #2697, #157383, #138231, #63374, #107872, #18876, #142196, #106890, #15888, #77546, #47222, #1698, #108881, #125051, #32050, #168563, #170560, #30061, #91702, #199913, #7661, #113836, #112851, #35023, #175532, #161360, #54186, #4662, #98667, #6663, #100673, #177549, #191691, #68341, #129991, #69345, #190705, #174542, #129006, #22851, #38020, #21851, #51190, #37006, #115859, #20843, #53173, #162355, #39018, #19855, #114850, #97658, #160361, #36009, #52178, #147195, #159347, #173554, #188725, #131012, #84498, #23856, #83502, #85506, #176544, #145179, #65357, #5669, #127018, #158366, #66354, #99676, #82501, #96678, #192703, #146176, #81495, #50210, #111864, #144183, #143182, #128015, #67345, #189717, #10694, #101679, #8685, #167357, #11703, #151200, #163369, #55181, #12688, #149203, #74354, #87515, #26867, #194711, #136020, #120828, #193712, #102690, #148199, #25871, #88510, #164378, #150205, #118872, #116850, #133021, #70356, #28855, #178541, #197694, #57197, #56180, #40007, #180556, #104685, #59160, #9692, #42030, #73370, #44010, #182528, #135042, #196718, #58187, #105671, #134031, #117863, #72357, #166373, #181539, #165373, #179554, #103694, #90495, #195724, #119855, #132023, #24866, #86515, #43018, #41024, #27869, #89510, #71357, #36517, #63891, #60154, #75328, #158868, #174066, #5181, #49714, #113361, #81030, #111379, #152177, #95213, #143699, #47736, #94213, #19381, #125562, #186258, #97182, #126540, #109389, #20357, #13661, #2210, #66862, #188239, #187259, #127536, #156899, #171069, #136998, #175053, #157892, #82005, #32559, #198687, #128525, #18395, #190219, #33551, #173067, #34544, #142706, #48728, #124561, #155892, #51698, #80046, #64879, #17390, #79046, #96203, #140720, #4185, #110381, #172064, #141715, #3205, #65864, #189238, #50716, #112374, #35534, #24382, #37528, #99191, #86033, #147720, #132542, #38539, #177068, #160879, #194230, #162874, #129518, #39525, #130524, #131538, #84021, #23371, #180074, #7181, #6183, #21365, #102206, #117369, #148718, #193222, #56707, #9207, #54696, #98172, #100195, #87033, #191218, #22370, #70874, #68865, #52692, #40535, #69869, #114356, #163895, #159874, #145699, #10206, #116369, #192221, #55696, #161877, #176061, #83023, #118380, #101185, #25391, #53703, #144697, #71866, #85016, #133534, #146697, #178057, #179066, #195226, #115380, #67863, #8194, #91975, #43526, #151700, #104200, #45503, #74856, #41543, #121341, #135547, #103206, #30334, #120348, #168829, #123315, #136518, #199189, #58681, #167856, #181062, #42537, #29356, #90986, #75830, #182043, #105191, #165881, #137508, #106173, #72883, #183034, #27378, #153669, #15166, #26382, #197219, #89024, #166878, #59669, #28379, #44517, #13193, #88021, #150715, #164888, #200178, #149709, #184021, #90017, #12214, #11208, #198199, #60656, #76825, #73877, #152673, #14162, #138496, #61647, #122329, #107158, #134551, #196240, #57709, #119379, #48498, #142473, #157656, #141486, #170835, #94979, #173830, #140488, #126311, #20122, #35295, #139485, #188007, #19145, #155660, #154666, #143453, #967, #31330, #187027, #156664, #47500, #189003, #18159, #185008, #64649, #78809, #46493, #96951, #63656, #112138, #66622, #79815, #3951, #1976, #111140, #124320, #186018, #172830, #34309, #80795, #125330, #110152, #109156, #65630, #49477, #16162, #95972, #32327, #158631, #81766, #169836, #171830, #93980, #33318, #2969, #127290, #50478, #4938, #92981, #17156, #108154, #77816, #62643, #70628, #176817, #175809, #97930, #38289, #24132, #117120, #67616, #161629, #69622, #163639, #40284, #54455, #131288, #192976, #132295, #53449, #37282, #191963, #85784, #100941, #84768, #114106, #99943, #178814, #83771, #116125, #25141, #101958, #82774, #177814, #160630, #23123, #98939, #115124, #9961 ),
 ( #21118, #129277, #39284, #22121, #159623, #193987, #146446, #144455, #55449, #189984, #145451, #86783, #7939, #6933, #162625, #130268, #5940, #128286, #148468, #147470, #51458, #190972, #174810, #113120, #68612, #36275, #8960, #52449, #179824, #11968, #12950, #88780, #89777, #28137, #182794, #165635, #180817, #167620, #13924, #197957, #181801, #59426, #120111, #42296, #102955, #73633, #41294, #135304, #57465, #27133, #10957, #103956, #196976, #194977, #133287, #56456, #164639, #74615, #119137, #150473, #26134, #118135, #43280, #121100, #104949, #58443, #166635, #151462, #136281, #44277, #75591, #90755, #105935, #29116, #71621, #137270, #152438, #149462, #87777, #72631, #134306, #195992, #146109, #86449, #115792, #6596, #160294, #100607, #117796, #192636, #163301, #83435, #52113, #164311, #133965, #53105, #23789, #102626, #21784, #71292, #10626, #113770, #193643, #98600, #39942, #149136, #22785, #147130, #25804, #55115, #194643, #132955, #131958, #116784, #85439, #145112, #56113, #175466, #68274, #129925, #87450, #178475, #101612, #179489, #191625, #72287, #114783, #54119, #36938, #40953, #37952, #176476, #24800, #9625, #99610, #38951, #161290, #69280, #162290, #84432, #8618, #7593, #177481, #70290, #130946, #148134, #120757, #13591, #135955, #89440, #105599, #168262, #15579, #91393, #41962, #197625, #58119, #12621, #28783, #180490, #118803, #57128, #11635, #29758, #166303, #74285, #26798, #103628, #198617, #137920, #75258, #59091, #182458, #151129, #60084, #76242, #154085, #30751, #106585, #184433, #195657, #14585, #153082, #165304, #183445, #92399, #121752, #136929, #43938, #199604, #167286, #150134, #88439, #90422, #61070, #152107, #122742, #73302, #134973, #107566, #77237, #196649, #44929, #45913, #119788, #169244, #181472, #42950, #104614, #27799, #146694, #52689, #118378, #6180, #40532, #8191, #145696, #67860, #69866, #194227, #87030, #37525, #131535, #39522, #133532, #10203, #24379, #101182, #162871, #102203, #23368, #7178, #161874, #55693, #70871, #54693, #84018, #193219, #148715, #53700, #86030, #195224, #71863, #114353, #147717, #130521, #116366, #68862, #85013, #180072, #192217, #129515, #21362, #163892, #117366, #56705, #178054, #98169, #9205, #132539, #159870, #38536, #83020, #191215, #99188, #179063, #115377, #176057, #25388, #144694, #160876, #22367, #177065, #100192, #153667, #74854, #73875, #14160, #43524, #134549, #41541, #200176, #44515, #88019, #106171, #184019, #121339, #58679, #166876, #135544, #167854, #122327, #61645, #76823, #152671, #30332, #103204, #60654, #199186, #164885, #29354, #138494, #90983, #59667, #197217, #75828, #105189, #196238, #149707, #90015, #107156, #182041, #137506, #72881, #26380, #15163, #123313, #42535, #13190, #91973, #11206, #45501, #57707, #119377, #183032, #181059, #168826, #136516, #104198, #198197, #165879, #27376, #89022, #150713, #12212, #120346, #28377, #151699, #3949, #46490, #154664, #62641, #20120, #64647, #111138, #50476, #77814, #81764, #139483, #125328, #158629, #173828, #170833, #143451, #34307, #142471, #189001, #171829, #4936, #1973, #94977, #66620, #79811, #124317, #187025, #48496, #65628, #110150, #33316, #2967, #156662, #78807, #18157, #157653, #185006, #80793, #31327, #93978, #16160, #141484, #19143, #126309, #95969, #172828, #112136, #188005, #140486, #35292, #108152, #127288, #49475, #96949, #169834, #63654, #965, #92979, #186016, #47497, #155658, #109154, #32325, #17154, #161627, #113117, #51456, #189982, #144453, #162622, #98937, #145449, #159621, #7936, #54452, #193983, #21116, #25137, #82772, #68609, #101953, #117116, #114104, #86779, #177811, #85781, #132291, #115122, #148464, #6931, #38287, #9957, #23121, #5938, #130266, #191961, #8957, #53447, #176815, #146443, #99941, #22119, #84766, #100938, #128284, #24128, #174808, #37280, #97928, #69619, #147467, #131285, #39281, #116122, #55445, #192973, #83769, #178810, #36273 ),
 ( #70625, #67614, #129275, #190969, #52447, #40280, #160628, #163635, #175807, #118131, #74611, #13920, #151458, #88776, #196972, #165631, #136277, #152434, #30093, #106920, #182790, #60416, #71617, #90751, #29112, #194973, #59422, #168593, #197953, #89773, #27129, #105931, #135299, #26130, #179819, #120107, #137266, #11964, #44273, #102951, #133283, #183780, #153428, #72627, #43276, #122089, #41290, #75587, #91732, #56452, #12946, #149458, #167616, #166631, #164635, #28133, #45266, #121096, #198949, #87773, #10953, #134302, #104945, #195988, #57460, #119133, #180813, #42292, #103952, #58439, #150469, #73629, #181797, #114622, #109905, #92738, #16911, #78564, #98445, #140237, #1730, #33077, #155421, #108913, #125083, #190487, #37791, #113619, #61409, #124067, #184766, #63408, #51959, #186781, #67129, #143965, #21627, #48251, #170593, #68121, #176323, #36778, #94733, #175313, #156412, #31090, #123080, #171589, #99455, #17914, #185769, #82273, #77578, #32083, #5445, #199945, #138262, #76586, #154426, #160139, #47256, #93740, #46252, #107906, #128787, #83284, #144958, #6439, #129773, #191469, #52947, #14926, #169592, #15920, #139250, #726, #62398, #180336, #118644, #84278, #148981, #57969, #87297, #179335, #54962, #195497, #24645, #115640, #69124, #9472, #26641, #101450, #72131, #192483, #161135, #73149, #42802, #162137, #132801, #11478, #130791, #41804, #119640, #22631, #102467, #38800, #56971, #55960, #181323, #117636, #134819, #164155, #103471, #165150, #40798, #25652, #194488, #53966, #88284, #145959, #177329, #100457, #196499, #10470, #133805, #149972, #23633, #7440, #85281, #163142, #146973, #8461, #70134, #131806, #193485, #116634, #178323, #39786, #86293, #147983, #71135, #58943, #12474, #152930, #170097, #44777, #15428, #135806, #104464, #16424, #186282, #105451, #76092, #154926, #74135, #123576, #62906, #166147, #45765, #182306, #238, #199451, #1228, #60919, #78071, #107417, #46763, #185271, #184282, #169090, #137767, #197477, #108422, #27650, #120612, #43787, #139739, #30596, #92249, #31591, #167135, #124587, #28635, #106430, #89289, #93241, #90272, #150980, #153934, #61905, #151955, #91240, #13444, #121600, #14427, #75108, #122594, #136775, #168111, #29608, #198461, #77087, #138756, #59933, #183295, #141739, #157915, #20382, #67887, #143725, #94238, #156923, #17414, #96226, #82029, #173092, #97206, #174089, #51721, #188263, #3229, #98196, #6207, #66886, #127562, #5205, #65888, #63915, #155919, #4210, #144721, #34570, #18420, #49738, #110406, #64903, #81054, #32585, #171094, #109415, #125585, #128547, #80069, #126564, #79071, #140745, #50739, #190244, #189264, #111406, #19405, #142730, #112398, #113384, #129540, #83046, #158892, #36540, #47761, #175074, #159899, #2233, #35558, #187282, #21388, #48753, #172088, #33575, #95237, #72909, #132566, #68889, #87058, #86056, #88046, #147745, #103231, #194255, #133561, #71891, #70899, #55722, #24407, #99214, #10231, #52714, #160902, #130549, #26407, #117394, #179093, #56736, #84045, #149734, #145724, #131563, #164913, #180100, #177091, #11235, #40562, #148743, #195251, #178082, #191240, #8219, #101209, #114378, #9232, #192246, #193247, #54720, #118406, #116392, #39550, #102231, #162898, #85041, #163920, #25416, #176082, #41568, #37551, #100219, #22395, #7205, #53727, #115403, #38563, #161900, #23395, #146722, #69895, #185034, #93006, #153694, #14187, #92000, #152698, #150739, #42562, #91012, #31355, #121366, #105216, #136542, #197243, #151724, #167882, #119404, #57734, #196265, #12239, #168853, #166903, #13217, #165906, #181087, #137532, #76849, #75856, #74880, #59695, #28403, #199214, #15190, #154692, #169861, #45528, #123341, #134578, #138520, #14549, #104225, #122356, #16187, #60681, #184045, #90042, #30358, #198223, #89049, #27404, #183059, #61672, #44543, #107182, #73901, #135571, #46521, #58704, #120374, #106198, #182067, #43550, #29381, #108180 ),
 ( #64672, #97957, #95001, #188031, #174837, #172853, #155684, #79839, #141509, #158656, #2994, #126334, #95995, #18182, #171854, #49501, #50502, #159649, #173855, #124346, #187051, #47524, #111164, #112166, #34334, #127317, #3975, #81792, #157680, #33342, #128311, #36302, #96975, #19170, #35321, #80819, #94003, #186041, #142497, #77842, #65655, #48521, #189028, #140511, #156688, #20147, #62666, #992, #139509, #17179, #143479, #110175, #4963, #109180, #170859, #66649, #190011, #51485, #113147, #32350, #78833, #2000, #63679, #125354, #56485, #132325, #9991, #21145, #40312, #178845, #144482, #8991, #118163, #147500, #39313, #115154, #55480, #84797, #175835, #129303, #69651, #86814, #161657, #194017, #52475, #82800, #133318, #102984, #22149, #193007, #71651, #190999, #101989, #179853, #5966, #162657, #98967, #117150, #116154, #41324, #177845, #195007, #24163, #163670, #25172, #100972, #85814, #54484, #114134, #148500, #67644, #37308, #160657, #83799, #70659, #145479, #6960, #68640, #130296, #191990, #53477, #176847, #38318, #99973, #23153, #146476, #7968, #131317, #183811, #26165, #134336, #42325, #199977, #44307, #90784, #30125, #57496, #61442, #119165, #104979, #138296, #153461, #150503, #123114, #13954, #122123, #168625, #151491, #184799, #181832, #74646, #46285, #59457, #103986, #166666, #28167, #45300, #89809, #12982, #182825, #136312, #58474, #197987, #137300, #164669, #60448, #10988, #73663, #196020, #121131, #198981, #105966, #75620, #152468, #91766, #167651, #120141, #14958, #87806, #106952, #29147, #76618, #149492, #180848, #72661, #165665, #27163, #88811, #135335, #12000, #197008, #43311, #141271, #92772, #31124, #169628, #124104, #142260, #78599, #125118, #139284, #154462, #110930, #50273, #187803, #186816, #33111, #1765, #172616, #188790, #66418, #143245, #18941, #96740, #107941, #127082, #65421, #15954, #95761, #4728, #34104, #126107, #63442, #3744, #171623, #62432, #77613, #156449, #173617, #48286, #80586, #761, #185804, #19917, #189782, #108947, #79602, #158429, #47291, #111931, #109941, #94767, #81559, #128079, #35087, #49272, #170628, #157446, #32117, #93774, #64437, #155455, #17949, #140272, #2761, #16945, #68405, #84562, #36074, #174608, #112914, #67411, #85573, #21915, #130057, #82567, #97723, #54250, #193776, #131078, #191757, #176610, #145246, #115922, #132087, #9754, #86577, #162417, #40069, #51254, #70420, #8750, #159413, #39080, #148261, #177612, #69412, #6727, #147260, #114917, #5732, #20908, #99740, #116913, #53240, #23919, #144248, #129066, #163435, #133082, #52242, #22916, #101746, #190767, #55245, #71418, #113899, #192767, #175597, #178606, #146240, #37073, #7726, #24932, #100736, #98733, #160426, #83567, #38084, #161424, #102752, #13723, #56246, #164440, #72420, #29891, #74415, #120891, #60216, #87577, #91529, #149264, #135103, #168396, #183579, #180619, #153216, #44074, #152238, #198751, #181601, #14721, #11766, #104745, #76381, #89574, #134097, #196779, #58247, #75389, #119915, #43078, #12750, #166436, #88573, #27931, #167420, #194772, #90556, #41089, #103757, #25934, #151260, #28916, #136081, #105733, #182590, #197755, #137061, #59222, #121886, #45064, #106722, #150271, #117927, #179617, #10756, #195788, #57260, #165436, #118934, #42092, #26931, #73432, #187566, #64199, #142017, #78355, #31877, #188547, #96502, #157204, #17704, #95518, #156204, #154224, #46046, #94522, #34847, #124875, #108707, #140029, #522, #155216, #171385, #122877, #61205, #199739, #15714, #172368, #170386, #16705, #169380, #184565, #141032, #80345, #79361, #1518, #63195, #93531, #2519, #18698, #158192, #173377, #49033, #126841, #138058, #3506, #65182, #107701, #125866, #19682, #110688, #33858, #186574, #50025, #48047, #92535, #30888, #109703, #111690, #32872, #77374, #139042, #62194, #123858, #185556, #47050, #52993, #131849, #189543, #100502, #39830, #163185, #22677, #159170, #177373 ) ),
 .UNSPECIFIED., .T., .F., .F. ) 
 B_SPLINE_SURFACE_WITH_KNOTS ( ( 4, 3, 4 ),
 ( 3, 2, 2, 2, 2, 2, 2, 2, 2, 2, 2, 2, 2, 2, 2, 2, 2, 2, 2, 2, 2, 2, 2, 2, 2, 2, 2, 2, 2, 2, 2, 2, 2, 2, 2, 2, 2, 2, 2, 2, 2, 2, 2, 2, 2, 2, 2, 2, 2, 2, 2, 2, 2, 2, 2, 2, 2, 2, 2, 2, 2, 2, 2, 2, 2, 2, 2, 2, 2, 2, 2, 2, 2, 2, 2, 2, 2, 2, 2, 2, 2, 2, 2, 2, 2, 2, 2, 2, 2, 2, 2, 2, 2, 2, 2, 2, 2, 2, 2, 2, 2, 2, 2, 2, 2, 2, 2, 2, 2, 2, 2, 2, 2, 2, 2, 2, 2, 2, 2, 2, 2, 2, 2, 2, 2, 2, 2, 2, 2, 2, 2, 2, 2, 2, 2, 2, 2, 2, 2, 2, 2, 2, 2, 2, 2, 2, 2, 2, 2, 2, 2, 2, 2, 2, 2, 2, 2, 2, 2, 2, 2, 2, 2, 2, 2, 2, 2, 2, 2, 2, 2, 2, 2, 2, 2, 2, 2, 2, 2, 2, 2, 2, 2, 2, 2, 2, 2, 2, 2, 2, 2, 2, 2, 2, 2, 2, 2, 2, 2, 2, 2, 2, 2, 2, 2, 2, 2, 2, 2, 2, 2, 2, 2, 2, 2, 2, 2, 2, 2, 2, 2, 2, 2, 2, 2, 2, 2, 2, 3 ),
 ( 0.000000000000000000, 0.5000000000000000000, 1.000000000000000000 ),
 ( 0.000000000000000000, 0.004385964912280701511, 0.008771929824561403022, 0.01315789473684210453, 0.01754385964912280604, 0.02192982456140350755, 0.02631578947368420907, 0.03070175438596491058, 0.03508771929824561209, 0.03947368421052631360, 0.04385964912280701511, 0.04824561403508771662, 0.05263157894736841813, 0.05701754385964911964, 0.06140350877192982115, 0.06578947368421052266, 0.07017543859649122417, 0.07456140350877192569, 0.07894736842105262720, 0.08333333333333332871, 0.08771929824561403022, 0.09210526315789473173, 0.09649122807017543324, 0.1008771929824561348, 0.1052631578947368363, 0.1096491228070175378, 0.1140350877192982393, 0.1184210526315789408, 0.1228070175438596423, 0.1271929824561403577, 0.1315789473684210453, 0.1359649122807017607, 0.1403508771929824483, 0.1447368421052631637, 0.1491228070175438514, 0.1535087719298245668, 0.1578947368421052544, 0.1622807017543859698, 0.1666666666666666574, 0.1710526315789473728, 0.1754385964912280604, 0.1798245614035087758, 0.1842105263157894635, 0.1885964912280701788, 0.1929824561403508665, 0.1973684210526315819, 0.2017543859649122695, 0.2061403508771929849, 0.2105263157894736725, 0.2149122807017543879, 0.2192982456140350755, 0.2236842105263157909, 0.2280701754385964786, 0.2324561403508771940, 0.2368421052631578816, 0.2412280701754385970, 0.2456140350877192846, 0.2500000000000000000, 0.2543859649122807154, 0.2587719298245614308, 0.2631578947368420907, 0.2675438596491228060, 0.2719298245614035214, 0.2763157894736842368, 0.2807017543859648967, 0.2850877192982456121, 0.2894736842105263275, 0.2938596491228070429, 0.2982456140350877027, 0.3026315789473684181, 0.3070175438596491335, 0.3114035087719298489, 0.3157894736842105088, 0.3201754385964912242, 0.3245614035087719396, 0.3289473684210526550, 0.3333333333333333148, 0.3377192982456140302, 0.3421052631578947456, 0.3464912280701754610, 0.3508771929824561209, 0.3552631578947368363, 0.3596491228070175517, 0.3640350877192982670, 0.3684210526315789269, 0.3728070175438596423, 0.3771929824561403577, 0.3815789473684210731, 0.3859649122807017330, 0.3903508771929824483, 0.3947368421052631637, 0.3991228070175438791, 0.4035087719298245390, 0.4078947368421052544, 0.4122807017543859698, 0.4166666666666666852, 0.4210526315789473450, 0.4254385964912280604, 0.4298245614035087758, 0.4342105263157894912, 0.4385964912280701511, 0.4429824561403508665, 0.4473684210526315819, 0.4517543859649122973, 0.4561403508771929571, 0.4605263157894736725, 0.4649122807017543879, 0.4692982456140351033, 0.4736842105263157632, 0.4780701754385964786, 0.4824561403508771940, 0.4868421052631579093, 0.4912280701754385692, 0.4956140350877192846, 0.5000000000000000000, 0.5043859649122807154, 0.5087719298245614308, 0.5131578947368421462, 0.5175438596491228616, 0.5219298245614034659, 0.5263157894736841813, 0.5307017543859648967, 0.5350877192982456121, 0.5394736842105263275, 0.5438596491228070429, 0.5482456140350877583, 0.5526315789473684736, 0.5570175438596490780, 0.5614035087719297934, 0.5657894736842105088, 0.5701754385964912242, 0.5745614035087719396, 0.5789473684210526550, 0.5833333333333333703, 0.5877192982456140857, 0.5921052631578946901, 0.5964912280701754055, 0.6008771929824561209, 0.6052631578947368363, 0.6096491228070175517, 0.6140350877192982670, 0.6184210526315789824, 0.6228070175438596978, 0.6271929824561403022, 0.6315789473684210176, 0.6359649122807017330, 0.6403508771929824483, 0.6447368421052631637, 0.6491228070175438791, 0.6535087719298245945, 0.6578947368421053099, 0.6622807017543859143, 0.6666666666666666297, 0.6710526315789473450, 0.6754385964912280604, 0.6798245614035087758, 0.6842105263157894912, 0.6885964912280702066, 0.6929824561403509220, 0.6973684210526315264, 0.7017543859649122417, 0.7061403508771929571, 0.7105263157894736725, 0.7149122807017543879, 0.7192982456140351033, 0.7236842105263158187, 0.7280701754385965341, 0.7324561403508771384, 0.7368421052631578538, 0.7412280701754385692, 0.7456140350877192846, 0.7500000000000000000, 0.7543859649122807154, 0.7587719298245614308, 0.7631578947368421462, 0.7675438596491228616, 0.7719298245614034659, 0.7763157894736841813, 0.7807017543859648967, 0.7850877192982456121, 0.7894736842105263275, 0.7938596491228070429, 0.7982456140350877583, 0.8026315789473684736, 0.8070175438596490780, 0.8114035087719297934, 0.8157894736842105088, 0.8201754385964912242, 0.8245614035087719396, 0.8289473684210526550, 0.8333333333333333703, 0.8377192982456140857, 0.8421052631578946901, 0.8464912280701754055, 0.8508771929824561209, 0.8552631578947368363, 0.8596491228070175517, 0.8640350877192982670, 0.8684210526315789824, 0.8728070175438596978, 0.8771929824561403022, 0.8815789473684210176, 0.8859649122807017330, 0.8903508771929824483, 0.8947368421052631637, 0.8991228070175438791, 0.9035087719298245945, 0.9078947368421053099, 0.9122807017543859143, 0.9166666666666666297, 0.9210526315789473450, 0.9254385964912280604, 0.9298245614035087758, 0.9342105263157894912, 0.9385964912280702066, 0.9429824561403509220, 0.9473684210526315264, 0.9517543859649122417, 0.9561403508771929571, 0.9605263157894736725, 0.9649122807017543879, 0.9692982456140351033, 0.9736842105263158187, 0.9780701754385965341, 0.9824561403508771384, 0.9868421052631578538, 0.9912280701754385692, 0.9956140350877192846, 1.000000000000000000 ),
 .UNSPECIFIED. ) 
 GEOMETRIC_REPRESENTATION_ITEM ( )  RATIONAL_B_SPLINE_SURFACE ( (
 ( 1.000000000000000000, 0.9659258262890683122, 1.000000000000000000, 0.9659258262890683122, 1.000000000000000000, 0.9659258262890683122, 1.000000000000000000, 0.9659258262890683122, 1.000000000000000000, 0.9659258262890683122, 1.000000000000000000, 0.9659258262890683122, 1.000000000000000000, 0.9659258262890683122, 1.000000000000000000, 0.9659258262890683122, 1.000000000000000000, 0.9659258262890683122, 1.000000000000000000, 0.9659258262890683122, 1.000000000000000000, 0.9659258262890683122, 1.000000000000000000, 0.9659258262890683122, 1.000000000000000000, 0.9659258262890683122, 1.000000000000000000, 0.9659258262890683122, 1.000000000000000000, 0.9659258262890683122, 1.000000000000000000, 0.9659258262890683122, 1.000000000000000000, 0.9659258262890683122, 1.000000000000000000, 0.9659258262890683122, 1.000000000000000000, 0.9659258262890683122, 1.000000000000000000, 0.9659258262890683122, 1.000000000000000000, 0.9659258262890683122, 1.000000000000000000, 0.9659258262890683122, 1.000000000000000000, 0.9659258262890683122, 1.000000000000000000, 0.9659258262890683122, 1.000000000000000000, 0.9659258262890683122, 1.000000000000000000, 0.9659258262890683122, 1.000000000000000000, 0.9659258262890683122, 1.000000000000000000, 0.9659258262890683122, 1.000000000000000000, 0.9659258262890683122, 1.000000000000000000, 0.9659258262890683122, 1.000000000000000000, 0.9659258262890683122, 1.000000000000000000, 0.9659258262890683122, 1.000000000000000000, 0.9659258262890683122, 1.000000000000000000, 0.9659258262890683122, 1.000000000000000000, 0.9659258262890683122, 1.000000000000000000, 0.9659258262890683122, 1.000000000000000000, 0.9659258262890683122, 1.000000000000000000, 0.9659258262890683122, 1.000000000000000000, 0.9659258262890683122, 1.000000000000000000, 0.9659258262890683122, 1.000000000000000000, 0.9659258262890683122, 1.000000000000000000, 0.9659258262890683122, 1.000000000000000000, 0.9659258262890683122, 1.000000000000000000, 0.9659258262890683122, 1.000000000000000000, 0.9659258262890683122, 1.000000000000000000, 0.9659258262890683122, 1.000000000000000000, 0.9659258262890683122, 1.000000000000000000, 0.9659258262890683122, 1.000000000000000000, 0.9659258262890683122, 1.000000000000000000, 0.9659258262890683122, 1.000000000000000000, 0.9659258262890683122, 1.000000000000000000, 0.9659258262890683122, 1.000000000000000000, 0.9659258262890683122, 1.000000000000000000, 0.9659258262890683122, 1.000000000000000000, 0.9659258262890683122, 1.000000000000000000, 0.9659258262890683122, 1.000000000000000000, 0.9659258262890683122, 1.000000000000000000, 0.9659258262890683122, 1.000000000000000000, 0.9659258262890683122, 1.000000000000000000, 0.9659258262890683122, 1.000000000000000000, 0.9659258262890683122, 1.000000000000000000, 0.9659258262890683122, 1.000000000000000000, 0.9659258262890683122, 1.000000000000000000, 0.9659258262890683122, 1.000000000000000000, 0.9659258262890683122, 1.000000000000000000, 0.9659258262890683122, 1.000000000000000000, 0.9659258262890683122, 1.000000000000000000, 0.9659258262890683122, 1.000000000000000000, 0.9659258262890683122, 1.000000000000000000, 0.9659258262890683122, 1.000000000000000000, 0.9659258262890683122, 1.000000000000000000, 0.9659258262890683122, 1.000000000000000000, 0.9659258262890683122, 1.000000000000000000, 0.9659258262890683122, 1.000000000000000000, 0.9659258262890683122, 1.000000000000000000, 0.9659258262890683122, 1.000000000000000000, 0.9659258262890683122, 1.000000000000000000, 0.9659258262890683122, 1.000000000000000000, 0.9659258262890683122, 1.000000000000000000, 0.9659258262890683122, 1.000000000000000000, 0.9659258262890683122, 1.000000000000000000, 0.9659258262890683122, 1.000000000000000000, 0.9659258262890683122, 1.000000000000000000, 0.9659258262890683122, 1.000000000000000000, 0.9659258262890683122, 1.000000000000000000, 0.9659258262890683122, 1.000000000000000000, 0.9659258262890683122, 1.000000000000000000, 0.9659258262890683122, 1.000000000000000000, 0.9659258262890683122, 1.000000000000000000, 0.9659258262890683122, 1.000000000000000000, 0.9659258262890683122, 1.000000000000000000, 0.9659258262890683122, 1.000000000000000000, 0.9659258262890683122, 1.000000000000000000, 0.9659258262890683122, 1.000000000000000000, 0.9659258262890683122, 1.000000000000000000, 0.9659258262890683122, 1.000000000000000000, 0.9659258262890683122, 1.000000000000000000, 0.9659258262890683122, 1.000000000000000000, 0.9659258262890683122, 1.000000000000000000, 0.9659258262890683122, 1.000000000000000000, 0.9659258262890683122, 1.000000000000000000, 0.9659258262890683122, 1.000000000000000000, 0.9659258262890683122, 1.000000000000000000, 0.9659258262890683122, 1.000000000000000000, 0.9659258262890683122, 1.000000000000000000, 0.9659258262890683122, 1.000000000000000000, 0.9659258262890683122, 1.000000000000000000, 0.9659258262890683122, 1.000000000000000000, 0.9659258262890683122, 1.000000000000000000, 0.9659258262890683122, 1.000000000000000000, 0.9659258262890683122, 1.000000000000000000, 0.9659258262890683122, 1.000000000000000000, 0.9659258262890683122, 1.000000000000000000, 0.9659258262890683122, 1.000000000000000000, 0.9659258262890683122, 1.000000000000000000, 0.9659258262890683122, 1.000000000000000000, 0.9659258262890683122, 1.000000000000000000, 0.9659258262890683122, 1.000000000000000000, 0.9659258262890683122, 1.000000000000000000, 0.9659258262890683122, 1.000000000000000000, 0.9659258262890683122, 1.000000000000000000, 0.9659258262890683122, 1.000000000000000000, 0.9659258262890683122, 1.000000000000000000, 0.9659258262890683122, 1.000000000000000000, 0.9659258262890683122, 1.000000000000000000, 0.9659258262890683122, 1.000000000000000000, 0.9659258262890683122, 1.000000000000000000, 0.9659258262890683122, 1.000000000000000000, 0.9659258262890683122, 1.000000000000000000, 0.9659258262890683122, 1.000000000000000000, 0.9659258262890683122, 1.000000000000000000, 0.9659258262890683122, 1.000000000000000000, 0.9659258262890683122, 1.000000000000000000, 0.9659258262890683122, 1.000000000000000000, 0.9659258262890683122, 1.000000000000000000, 0.9659258262890683122, 1.000000000000000000, 0.9659258262890683122, 1.000000000000000000, 0.9659258262890683122, 1.000000000000000000, 0.9659258262890683122, 1.000000000000000000, 0.9659258262890683122, 1.000000000000000000, 0.9659258262890683122, 1.000000000000000000, 0.9659258262890683122, 1.000000000000000000, 0.9659258262890683122, 1.000000000000000000, 0.9659258262890683122, 1.000000000000000000, 0.9659258262890683122, 1.000000000000000000, 0.9659258262890683122, 1.000000000000000000, 0.9659258262890683122, 1.000000000000000000, 0.9659258262890683122, 1.000000000000000000, 0.9659258262890683122, 1.000000000000000000, 0.9659258262890683122, 1.000000000000000000, 0.9659258262890683122, 1.000000000000000000, 0.9659258262890683122, 1.000000000000000000, 0.9659258262890683122, 1.000000000000000000, 0.9659258262890683122, 1.000000000000000000, 0.9659258262890683122, 1.000000000000000000, 0.9659258262890683122, 1.000000000000000000, 0.9659258262890683122, 1.000000000000000000, 0.9659258262890683122, 1.000000000000000000, 0.9659258262890683122, 1.000000000000000000, 0.9659258262890683122, 1.000000000000000000, 0.9659258262890683122, 1.000000000000000000, 0.9659258262890683122, 1.000000000000000000, 0.9659258262890683122, 1.000000000000000000, 0.9659258262890683122, 1.000000000000000000, 0.9659258262890683122, 1.000000000000000000, 0.9659258262890683122, 1.000000000000000000, 0.9659258262890683122, 1.000000000000000000, 0.9659258262890683122, 1.000000000000000000, 0.9659258262890683122, 1.000000000000000000, 0.9659258262890683122, 1.000000000000000000, 0.9659258262890683122, 1.000000000000000000, 0.9659258262890683122, 1.000000000000000000, 0.9659258262890683122, 1.000000000000000000, 0.9659258262890683122, 1.000000000000000000, 0.9659258262890683122, 1.000000000000000000, 0.9659258262890683122, 1.000000000000000000, 0.9659258262890683122, 1.000000000000000000, 0.9659258262890683122, 1.000000000000000000, 0.9659258262890683122, 1.000000000000000000, 0.9659258262890683122, 1.000000000000000000, 0.9659258262890683122, 1.000000000000000000, 0.9659258262890683122, 1.000000000000000000, 0.9659258262890683122, 1.000000000000000000, 0.9659258262890683122, 1.000000000000000000, 0.9659258262890683122, 1.000000000000000000, 0.9659258262890683122, 1.000000000000000000, 0.9659258262890683122, 1.000000000000000000, 0.9659258262890683122, 1.000000000000000000, 0.9659258262890683122, 1.000000000000000000, 0.9659258262890683122, 1.000000000000000000, 0.9659258262890683122, 1.000000000000000000, 0.9659258262890683122, 1.000000000000000000, 0.9659258262890683122, 1.000000000000000000, 0.9659258262890683122, 1.000000000000000000, 0.9659258262890683122, 1.000000000000000000, 0.9659258262890683122, 1.000000000000000000, 0.9659258262890683122, 1.000000000000000000, 0.9659258262890683122, 1.000000000000000000, 0.9659258262890683122, 1.000000000000000000, 0.9659258262890683122, 1.000000000000000000, 0.9659258262890683122, 1.000000000000000000, 0.9659258262890683122, 1.000000000000000000, 0.9659258262890683122, 1.000000000000000000, 0.9659258262890683122, 1.000000000000000000, 0.9659258262890683122, 1.000000000000000000, 0.9659258262890683122, 1.000000000000000000, 0.9659258262890683122, 1.000000000000000000, 0.9659258262890683122, 1.000000000000000000, 0.9659258262890683122, 1.000000000000000000, 0.9659258262890683122, 1.000000000000000000, 0.9659258262890683122, 1.000000000000000000, 0.9659258262890683122, 1.000000000000000000, 0.9659258262890683122, 1.000000000000000000, 0.9659258262890683122, 1.000000000000000000, 0.9659258262890683122, 1.000000000000000000, 0.9659258262890683122, 1.000000000000000000, 0.9659258262890683122, 1.000000000000000000, 0.9659258262890683122, 1.000000000000000000, 0.9659258262890683122, 1.000000000000000000, 0.9659258262890683122, 1.000000000000000000, 0.9659258262890683122, 1.000000000000000000, 0.9659258262890683122, 1.000000000000000000, 0.9659258262890683122, 1.000000000000000000, 0.9659258262890683122, 1.000000000000000000, 0.9659258262890683122, 1.000000000000000000, 0.9659258262890683122, 1.000000000000000000, 0.9659258262890683122, 1.000000000000000000, 0.9659258262890683122, 1.000000000000000000),
 ( 0.3333333333333333703, 0.3219752754296894559, 0.3333333333333333703, 0.3219752754296894559, 0.3333333333333333703, 0.3219752754296894559, 0.3333333333333333703, 0.3219752754296894559, 0.3333333333333333703, 0.3219752754296894559, 0.3333333333333333703, 0.3219752754296894559, 0.3333333333333333703, 0.3219752754296894559, 0.3333333333333333703, 0.3219752754296894559, 0.3333333333333333703, 0.3219752754296894559, 0.3333333333333333703, 0.3219752754296894559, 0.3333333333333333703, 0.3219752754296894559, 0.3333333333333333703, 0.3219752754296894559, 0.3333333333333333703, 0.3219752754296894559, 0.3333333333333333703, 0.3219752754296894559, 0.3333333333333333703, 0.3219752754296894559, 0.3333333333333333703, 0.3219752754296894559, 0.3333333333333333703, 0.3219752754296894559, 0.3333333333333333703, 0.3219752754296894559, 0.3333333333333333703, 0.3219752754296894559, 0.3333333333333333703, 0.3219752754296894559, 0.3333333333333333703, 0.3219752754296894559, 0.3333333333333333703, 0.3219752754296894559, 0.3333333333333333703, 0.3219752754296894559, 0.3333333333333333703, 0.3219752754296894559, 0.3333333333333333703, 0.3219752754296894559, 0.3333333333333333703, 0.3219752754296894559, 0.3333333333333333703, 0.3219752754296894559, 0.3333333333333333703, 0.3219752754296894559, 0.3333333333333333703, 0.3219752754296894559, 0.3333333333333333703, 0.3219752754296894559, 0.3333333333333333703, 0.3219752754296894559, 0.3333333333333333703, 0.3219752754296894559, 0.3333333333333333703, 0.3219752754296894559, 0.3333333333333333703, 0.3219752754296894559, 0.3333333333333333703, 0.3219752754296894559, 0.3333333333333333703, 0.3219752754296894559, 0.3333333333333333703, 0.3219752754296894559, 0.3333333333333333703, 0.3219752754296894559, 0.3333333333333333703, 0.3219752754296894559, 0.3333333333333333703, 0.3219752754296894559, 0.3333333333333333703, 0.3219752754296894559, 0.3333333333333333703, 0.3219752754296894559, 0.3333333333333333703, 0.3219752754296894559, 0.3333333333333333703, 0.3219752754296894559, 0.3333333333333333703, 0.3219752754296894559, 0.3333333333333333703, 0.3219752754296894559, 0.3333333333333333703, 0.3219752754296894559, 0.3333333333333333703, 0.3219752754296894559, 0.3333333333333333703, 0.3219752754296894559, 0.3333333333333333703, 0.3219752754296894559, 0.3333333333333333703, 0.3219752754296894559, 0.3333333333333333703, 0.3219752754296894559, 0.3333333333333333703, 0.3219752754296894559, 0.3333333333333333703, 0.3219752754296894559, 0.3333333333333333703, 0.3219752754296894559, 0.3333333333333333703, 0.3219752754296894559, 0.3333333333333333703, 0.3219752754296894559, 0.3333333333333333703, 0.3219752754296894559, 0.3333333333333333703, 0.3219752754296894559, 0.3333333333333333703, 0.3219752754296894559, 0.3333333333333333703, 0.3219752754296894559, 0.3333333333333333703, 0.3219752754296894559, 0.3333333333333333703, 0.3219752754296894559, 0.3333333333333333703, 0.3219752754296894559, 0.3333333333333333703, 0.3219752754296894559, 0.3333333333333333703, 0.3219752754296894559, 0.3333333333333333703, 0.3219752754296894559, 0.3333333333333333703, 0.3219752754296894559, 0.3333333333333333703, 0.3219752754296894559, 0.3333333333333333703, 0.3219752754296894559, 0.3333333333333333703, 0.3219752754296894559, 0.3333333333333333703, 0.3219752754296894559, 0.3333333333333333703, 0.3219752754296894559, 0.3333333333333333703, 0.3219752754296894559, 0.3333333333333333703, 0.3219752754296894559, 0.3333333333333333703, 0.3219752754296894559, 0.3333333333333333703, 0.3219752754296894559, 0.3333333333333333703, 0.3219752754296894559, 0.3333333333333333703, 0.3219752754296894559, 0.3333333333333333703, 0.3219752754296894559, 0.3333333333333333703, 0.3219752754296894559, 0.3333333333333333703, 0.3219752754296894559, 0.3333333333333333703, 0.3219752754296894559, 0.3333333333333333703, 0.3219752754296894559, 0.3333333333333333703, 0.3219752754296894559, 0.3333333333333333703, 0.3219752754296894559, 0.3333333333333333703, 0.3219752754296894559, 0.3333333333333333703, 0.3219752754296894559, 0.3333333333333333703, 0.3219752754296894559, 0.3333333333333333703, 0.3219752754296894559, 0.3333333333333333703, 0.3219752754296894559, 0.3333333333333333703, 0.3219752754296894559, 0.3333333333333333703, 0.3219752754296894559, 0.3333333333333333703, 0.3219752754296894559, 0.3333333333333333703, 0.3219752754296894559, 0.3333333333333333703, 0.3219752754296894559, 0.3333333333333333703, 0.3219752754296894559, 0.3333333333333333703, 0.3219752754296894559, 0.3333333333333333703, 0.3219752754296894559, 0.3333333333333333703, 0.3219752754296894559, 0.3333333333333333703, 0.3219752754296894559, 0.3333333333333333703, 0.3219752754296894559, 0.3333333333333333703, 0.3219752754296894559, 0.3333333333333333703, 0.3219752754296894559, 0.3333333333333333703, 0.3219752754296894559, 0.3333333333333333703, 0.3219752754296894559, 0.3333333333333333703, 0.3219752754296894559, 0.3333333333333333703, 0.3219752754296894559, 0.3333333333333333703, 0.3219752754296894559, 0.3333333333333333703, 0.3219752754296894559, 0.3333333333333333703, 0.3219752754296894559, 0.3333333333333333703, 0.3219752754296894559, 0.3333333333333333703, 0.3219752754296894559, 0.3333333333333333703, 0.3219752754296894559, 0.3333333333333333703, 0.3219752754296894559, 0.3333333333333333703, 0.3219752754296894559, 0.3333333333333333703, 0.3219752754296894559, 0.3333333333333333703, 0.3219752754296894559, 0.3333333333333333703, 0.3219752754296894559, 0.3333333333333333703, 0.3219752754296894559, 0.3333333333333333703, 0.3219752754296894559, 0.3333333333333333703, 0.3219752754296894559, 0.3333333333333333703, 0.3219752754296894559, 0.3333333333333333703, 0.3219752754296894559, 0.3333333333333333703, 0.3219752754296894559, 0.3333333333333333703, 0.3219752754296894559, 0.3333333333333333703, 0.3219752754296894559, 0.3333333333333333703, 0.3219752754296894559, 0.3333333333333333703, 0.3219752754296894559, 0.3333333333333333703, 0.3219752754296894559, 0.3333333333333333703, 0.3219752754296894559, 0.3333333333333333703, 0.3219752754296894559, 0.3333333333333333703, 0.3219752754296894559, 0.3333333333333333703, 0.3219752754296894559, 0.3333333333333333703, 0.3219752754296894559, 0.3333333333333333703, 0.3219752754296894559, 0.3333333333333333703, 0.3219752754296894559, 0.3333333333333333703, 0.3219752754296894559, 0.3333333333333333703, 0.3219752754296894559, 0.3333333333333333703, 0.3219752754296894559, 0.3333333333333333703, 0.3219752754296894559, 0.3333333333333333703, 0.3219752754296894559, 0.3333333333333333703, 0.3219752754296894559, 0.3333333333333333703, 0.3219752754296894559, 0.3333333333333333703, 0.3219752754296894559, 0.3333333333333333703, 0.3219752754296894559, 0.3333333333333333703, 0.3219752754296894559, 0.3333333333333333703, 0.3219752754296894559, 0.3333333333333333703, 0.3219752754296894559, 0.3333333333333333703, 0.3219752754296894559, 0.3333333333333333703, 0.3219752754296894559, 0.3333333333333333703, 0.3219752754296894559, 0.3333333333333333703, 0.3219752754296894559, 0.3333333333333333703, 0.3219752754296894559, 0.3333333333333333703, 0.3219752754296894559, 0.3333333333333333703, 0.3219752754296894559, 0.3333333333333333703, 0.3219752754296894559, 0.3333333333333333703, 0.3219752754296894559, 0.3333333333333333703, 0.3219752754296894559, 0.3333333333333333703, 0.3219752754296894559, 0.3333333333333333703, 0.3219752754296894559, 0.3333333333333333703, 0.3219752754296894559, 0.3333333333333333703, 0.3219752754296894559, 0.3333333333333333703, 0.3219752754296894559, 0.3333333333333333703, 0.3219752754296894559, 0.3333333333333333703, 0.3219752754296894559, 0.3333333333333333703, 0.3219752754296894559, 0.3333333333333333703, 0.3219752754296894559, 0.3333333333333333703, 0.3219752754296894559, 0.3333333333333333703, 0.3219752754296894559, 0.3333333333333333703, 0.3219752754296894559, 0.3333333333333333703, 0.3219752754296894559, 0.3333333333333333703, 0.3219752754296894559, 0.3333333333333333703, 0.3219752754296894559, 0.3333333333333333703, 0.3219752754296894559, 0.3333333333333333703, 0.3219752754296894559, 0.3333333333333333703, 0.3219752754296894559, 0.3333333333333333703, 0.3219752754296894559, 0.3333333333333333703, 0.3219752754296894559, 0.3333333333333333703, 0.3219752754296894559, 0.3333333333333333703, 0.3219752754296894559, 0.3333333333333333703, 0.3219752754296894559, 0.3333333333333333703, 0.3219752754296894559, 0.3333333333333333703, 0.3219752754296894559, 0.3333333333333333703, 0.3219752754296894559, 0.3333333333333333703, 0.3219752754296894559, 0.3333333333333333703, 0.3219752754296894559, 0.3333333333333333703, 0.3219752754296894559, 0.3333333333333333703, 0.3219752754296894559, 0.3333333333333333703, 0.3219752754296894559, 0.3333333333333333703, 0.3219752754296894559, 0.3333333333333333703, 0.3219752754296894559, 0.3333333333333333703, 0.3219752754296894559, 0.3333333333333333703, 0.3219752754296894559, 0.3333333333333333703, 0.3219752754296894559, 0.3333333333333333703, 0.3219752754296894559, 0.3333333333333333703, 0.3219752754296894559, 0.3333333333333333703, 0.3219752754296894559, 0.3333333333333333703, 0.3219752754296894559, 0.3333333333333333703, 0.3219752754296894559, 0.3333333333333333703, 0.3219752754296894559, 0.3333333333333333703, 0.3219752754296894559, 0.3333333333333333703, 0.3219752754296894559, 0.3333333333333333703, 0.3219752754296894559, 0.3333333333333333703, 0.3219752754296894559, 0.3333333333333333703, 0.3219752754296894559, 0.3333333333333333703, 0.3219752754296894559, 0.3333333333333333703, 0.3219752754296894559, 0.3333333333333333703, 0.3219752754296894559, 0.3333333333333333703, 0.3219752754296894559, 0.3333333333333333703, 0.3219752754296894559, 0.3333333333333333703, 0.3219752754296894559, 0.3333333333333333703, 0.3219752754296894559, 0.3333333333333333703, 0.3219752754296894559, 0.3333333333333333703, 0.3219752754296894559, 0.3333333333333333703, 0.3219752754296894559, 0.3333333333333333703, 0.3219752754296894559, 0.3333333333333333703, 0.3219752754296894559, 0.3333333333333333703, 0.3219752754296894559, 0.3333333333333333703, 0.3219752754296894559, 0.3333333333333333703, 0.3219752754296894559, 0.3333333333333333703, 0.3219752754296894559, 0.3333333333333333703, 0.3219752754296894559, 0.3333333333333333703, 0.3219752754296894559, 0.3333333333333333703, 0.3219752754296894559, 0.3333333333333333703, 0.3219752754296894559, 0.3333333333333333703, 0.3219752754296894559, 0.3333333333333333703, 0.3219752754296894559, 0.3333333333333333703),
 ( 0.3333333333333333703, 0.3219752754296894559, 0.3333333333333333703, 0.3219752754296894559, 0.3333333333333333703, 0.3219752754296894559, 0.3333333333333333703, 0.3219752754296894559, 0.3333333333333333703, 0.3219752754296894559, 0.3333333333333333703, 0.3219752754296894559, 0.3333333333333333703, 0.3219752754296894559, 0.3333333333333333703, 0.3219752754296894559, 0.3333333333333333703, 0.3219752754296894559, 0.3333333333333333703, 0.3219752754296894559, 0.3333333333333333703, 0.3219752754296894559, 0.3333333333333333703, 0.3219752754296894559, 0.3333333333333333703, 0.3219752754296894559, 0.3333333333333333703, 0.3219752754296894559, 0.3333333333333333703, 0.3219752754296894559, 0.3333333333333333703, 0.3219752754296894559, 0.3333333333333333703, 0.3219752754296894559, 0.3333333333333333703, 0.3219752754296894559, 0.3333333333333333703, 0.3219752754296894559, 0.3333333333333333703, 0.3219752754296894559, 0.3333333333333333703, 0.3219752754296894559, 0.3333333333333333703, 0.3219752754296894559, 0.3333333333333333703, 0.3219752754296894559, 0.3333333333333333703, 0.3219752754296894559, 0.3333333333333333703, 0.3219752754296894559, 0.3333333333333333703, 0.3219752754296894559, 0.3333333333333333703, 0.3219752754296894559, 0.3333333333333333703, 0.3219752754296894559, 0.3333333333333333703, 0.3219752754296894559, 0.3333333333333333703, 0.3219752754296894559, 0.3333333333333333703, 0.3219752754296894559, 0.3333333333333333703, 0.3219752754296894559, 0.3333333333333333703, 0.3219752754296894559, 0.3333333333333333703, 0.3219752754296894559, 0.3333333333333333703, 0.3219752754296894559, 0.3333333333333333703, 0.3219752754296894559, 0.3333333333333333703, 0.3219752754296894559, 0.3333333333333333703, 0.3219752754296894559, 0.3333333333333333703, 0.3219752754296894559, 0.3333333333333333703, 0.3219752754296894559, 0.3333333333333333703, 0.3219752754296894559, 0.3333333333333333703, 0.3219752754296894559, 0.3333333333333333703, 0.3219752754296894559, 0.3333333333333333703, 0.3219752754296894559, 0.3333333333333333703, 0.3219752754296894559, 0.3333333333333333703, 0.3219752754296894559, 0.3333333333333333703, 0.3219752754296894559, 0.3333333333333333703, 0.3219752754296894559, 0.3333333333333333703, 0.3219752754296894559, 0.3333333333333333703, 0.3219752754296894559, 0.3333333333333333703, 0.3219752754296894559, 0.3333333333333333703, 0.3219752754296894559, 0.3333333333333333703, 0.3219752754296894559, 0.3333333333333333703, 0.3219752754296894559, 0.3333333333333333703, 0.3219752754296894559, 0.3333333333333333703, 0.3219752754296894559, 0.3333333333333333703, 0.3219752754296894559, 0.3333333333333333703, 0.3219752754296894559, 0.3333333333333333703, 0.3219752754296894559, 0.3333333333333333703, 0.3219752754296894559, 0.3333333333333333703, 0.3219752754296894559, 0.3333333333333333703, 0.3219752754296894559, 0.3333333333333333703, 0.3219752754296894559, 0.3333333333333333703, 0.3219752754296894559, 0.3333333333333333703, 0.3219752754296894559, 0.3333333333333333703, 0.3219752754296894559, 0.3333333333333333703, 0.3219752754296894559, 0.3333333333333333703, 0.3219752754296894559, 0.3333333333333333703, 0.3219752754296894559, 0.3333333333333333703, 0.3219752754296894559, 0.3333333333333333703, 0.3219752754296894559, 0.3333333333333333703, 0.3219752754296894559, 0.3333333333333333703, 0.3219752754296894559, 0.3333333333333333703, 0.3219752754296894559, 0.3333333333333333703, 0.3219752754296894559, 0.3333333333333333703, 0.3219752754296894559, 0.3333333333333333703, 0.3219752754296894559, 0.3333333333333333703, 0.3219752754296894559, 0.3333333333333333703, 0.3219752754296894559, 0.3333333333333333703, 0.3219752754296894559, 0.3333333333333333703, 0.3219752754296894559, 0.3333333333333333703, 0.3219752754296894559, 0.3333333333333333703, 0.3219752754296894559, 0.3333333333333333703, 0.3219752754296894559, 0.3333333333333333703, 0.3219752754296894559, 0.3333333333333333703, 0.3219752754296894559, 0.3333333333333333703, 0.3219752754296894559, 0.3333333333333333703, 0.3219752754296894559, 0.3333333333333333703, 0.3219752754296894559, 0.3333333333333333703, 0.3219752754296894559, 0.3333333333333333703, 0.3219752754296894559, 0.3333333333333333703, 0.3219752754296894559, 0.3333333333333333703, 0.3219752754296894559, 0.3333333333333333703, 0.3219752754296894559, 0.3333333333333333703, 0.3219752754296894559, 0.3333333333333333703, 0.3219752754296894559, 0.3333333333333333703, 0.3219752754296894559, 0.3333333333333333703, 0.3219752754296894559, 0.3333333333333333703, 0.3219752754296894559, 0.3333333333333333703, 0.3219752754296894559, 0.3333333333333333703, 0.3219752754296894559, 0.3333333333333333703, 0.3219752754296894559, 0.3333333333333333703, 0.3219752754296894559, 0.3333333333333333703, 0.3219752754296894559, 0.3333333333333333703, 0.3219752754296894559, 0.3333333333333333703, 0.3219752754296894559, 0.3333333333333333703, 0.3219752754296894559, 0.3333333333333333703, 0.3219752754296894559, 0.3333333333333333703, 0.3219752754296894559, 0.3333333333333333703, 0.3219752754296894559, 0.3333333333333333703, 0.3219752754296894559, 0.3333333333333333703, 0.3219752754296894559, 0.3333333333333333703, 0.3219752754296894559, 0.3333333333333333703, 0.3219752754296894559, 0.3333333333333333703, 0.3219752754296894559, 0.3333333333333333703, 0.3219752754296894559, 0.3333333333333333703, 0.3219752754296894559, 0.3333333333333333703, 0.3219752754296894559, 0.3333333333333333703, 0.3219752754296894559, 0.3333333333333333703, 0.3219752754296894559, 0.3333333333333333703, 0.3219752754296894559, 0.3333333333333333703, 0.3219752754296894559, 0.3333333333333333703, 0.3219752754296894559, 0.3333333333333333703, 0.3219752754296894559, 0.3333333333333333703, 0.3219752754296894559, 0.3333333333333333703, 0.3219752754296894559, 0.3333333333333333703, 0.3219752754296894559, 0.3333333333333333703, 0.3219752754296894559, 0.3333333333333333703, 0.3219752754296894559, 0.3333333333333333703, 0.3219752754296894559, 0.3333333333333333703, 0.3219752754296894559, 0.3333333333333333703, 0.3219752754296894559, 0.3333333333333333703, 0.3219752754296894559, 0.3333333333333333703, 0.3219752754296894559, 0.3333333333333333703, 0.3219752754296894559, 0.3333333333333333703, 0.3219752754296894559, 0.3333333333333333703, 0.3219752754296894559, 0.3333333333333333703, 0.3219752754296894559, 0.3333333333333333703, 0.3219752754296894559, 0.3333333333333333703, 0.3219752754296894559, 0.3333333333333333703, 0.3219752754296894559, 0.3333333333333333703, 0.3219752754296894559, 0.3333333333333333703, 0.3219752754296894559, 0.3333333333333333703, 0.3219752754296894559, 0.3333333333333333703, 0.3219752754296894559, 0.3333333333333333703, 0.3219752754296894559, 0.3333333333333333703, 0.3219752754296894559, 0.3333333333333333703, 0.3219752754296894559, 0.3333333333333333703, 0.3219752754296894559, 0.3333333333333333703, 0.3219752754296894559, 0.3333333333333333703, 0.3219752754296894559, 0.3333333333333333703, 0.3219752754296894559, 0.3333333333333333703, 0.3219752754296894559, 0.3333333333333333703, 0.3219752754296894559, 0.3333333333333333703, 0.3219752754296894559, 0.3333333333333333703, 0.3219752754296894559, 0.3333333333333333703, 0.3219752754296894559, 0.3333333333333333703, 0.3219752754296894559, 0.3333333333333333703, 0.3219752754296894559, 0.3333333333333333703, 0.3219752754296894559, 0.3333333333333333703, 0.3219752754296894559, 0.3333333333333333703, 0.3219752754296894559, 0.3333333333333333703, 0.3219752754296894559, 0.3333333333333333703, 0.3219752754296894559, 0.3333333333333333703, 0.3219752754296894559, 0.3333333333333333703, 0.3219752754296894559, 0.3333333333333333703, 0.3219752754296894559, 0.3333333333333333703, 0.3219752754296894559, 0.3333333333333333703, 0.3219752754296894559, 0.3333333333333333703, 0.3219752754296894559, 0.3333333333333333703, 0.3219752754296894559, 0.3333333333333333703, 0.3219752754296894559, 0.3333333333333333703, 0.3219752754296894559, 0.3333333333333333703, 0.3219752754296894559, 0.3333333333333333703, 0.3219752754296894559, 0.3333333333333333703, 0.3219752754296894559, 0.3333333333333333703, 0.3219752754296894559, 0.3333333333333333703, 0.3219752754296894559, 0.3333333333333333703, 0.3219752754296894559, 0.3333333333333333703, 0.3219752754296894559, 0.3333333333333333703, 0.3219752754296894559, 0.3333333333333333703, 0.3219752754296894559, 0.3333333333333333703, 0.3219752754296894559, 0.3333333333333333703, 0.3219752754296894559, 0.3333333333333333703, 0.3219752754296894559, 0.3333333333333333703, 0.3219752754296894559, 0.3333333333333333703, 0.3219752754296894559, 0.3333333333333333703, 0.3219752754296894559, 0.3333333333333333703, 0.3219752754296894559, 0.3333333333333333703, 0.3219752754296894559, 0.3333333333333333703, 0.3219752754296894559, 0.3333333333333333703, 0.3219752754296894559, 0.3333333333333333703, 0.3219752754296894559, 0.3333333333333333703, 0.3219752754296894559, 0.3333333333333333703, 0.3219752754296894559, 0.3333333333333333703, 0.3219752754296894559, 0.3333333333333333703, 0.3219752754296894559, 0.3333333333333333703, 0.3219752754296894559, 0.3333333333333333703, 0.3219752754296894559, 0.3333333333333333703, 0.3219752754296894559, 0.3333333333333333703, 0.3219752754296894559, 0.3333333333333333703, 0.3219752754296894559, 0.3333333333333333703, 0.3219752754296894559, 0.3333333333333333703, 0.3219752754296894559, 0.3333333333333333703, 0.3219752754296894559, 0.3333333333333333703, 0.3219752754296894559, 0.3333333333333333703, 0.3219752754296894559, 0.3333333333333333703, 0.3219752754296894559, 0.3333333333333333703, 0.3219752754296894559, 0.3333333333333333703, 0.3219752754296894559, 0.3333333333333333703, 0.3219752754296894559, 0.3333333333333333703, 0.3219752754296894559, 0.3333333333333333703, 0.3219752754296894559, 0.3333333333333333703, 0.3219752754296894559, 0.3333333333333333703, 0.3219752754296894559, 0.3333333333333333703, 0.3219752754296894559, 0.3333333333333333703, 0.3219752754296894559, 0.3333333333333333703, 0.3219752754296894559, 0.3333333333333333703, 0.3219752754296894559, 0.3333333333333333703, 0.3219752754296894559, 0.3333333333333333703, 0.3219752754296894559, 0.3333333333333333703, 0.3219752754296894559, 0.3333333333333333703, 0.3219752754296894559, 0.3333333333333333703, 0.3219752754296894559, 0.3333333333333333703, 0.3219752754296894559, 0.3333333333333333703, 0.3219752754296894559, 0.3333333333333333703, 0.3219752754296894559, 0.3333333333333333703, 0.3219752754296894559, 0.3333333333333333703),
 ( 1.000000000000000000, 0.9659258262890683122, 1.000000000000000000, 0.9659258262890683122, 1.000000000000000000, 0.9659258262890683122, 1.000000000000000000, 0.9659258262890683122, 1.000000000000000000, 0.9659258262890683122, 1.000000000000000000, 0.9659258262890683122, 1.000000000000000000, 0.9659258262890683122, 1.000000000000000000, 0.9659258262890683122, 1.000000000000000000, 0.9659258262890683122, 1.000000000000000000, 0.9659258262890683122, 1.000000000000000000, 0.9659258262890683122, 1.000000000000000000, 0.9659258262890683122, 1.000000000000000000, 0.9659258262890683122, 1.000000000000000000, 0.9659258262890683122, 1.000000000000000000, 0.9659258262890683122, 1.000000000000000000, 0.9659258262890683122, 1.000000000000000000, 0.9659258262890683122, 1.000000000000000000, 0.9659258262890683122, 1.000000000000000000, 0.9659258262890683122, 1.000000000000000000, 0.9659258262890683122, 1.000000000000000000, 0.9659258262890683122, 1.000000000000000000, 0.9659258262890683122, 1.000000000000000000, 0.9659258262890683122, 1.000000000000000000, 0.9659258262890683122, 1.000000000000000000, 0.9659258262890683122, 1.000000000000000000, 0.9659258262890683122, 1.000000000000000000, 0.9659258262890683122, 1.000000000000000000, 0.9659258262890683122, 1.000000000000000000, 0.9659258262890683122, 1.000000000000000000, 0.9659258262890683122, 1.000000000000000000, 0.9659258262890683122, 1.000000000000000000, 0.9659258262890683122, 1.000000000000000000, 0.9659258262890683122, 1.000000000000000000, 0.9659258262890683122, 1.000000000000000000, 0.9659258262890683122, 1.000000000000000000, 0.9659258262890683122, 1.000000000000000000, 0.9659258262890683122, 1.000000000000000000, 0.9659258262890683122, 1.000000000000000000, 0.9659258262890683122, 1.000000000000000000, 0.9659258262890683122, 1.000000000000000000, 0.9659258262890683122, 1.000000000000000000, 0.9659258262890683122, 1.000000000000000000, 0.9659258262890683122, 1.000000000000000000, 0.9659258262890683122, 1.000000000000000000, 0.9659258262890683122, 1.000000000000000000, 0.9659258262890683122, 1.000000000000000000, 0.9659258262890683122, 1.000000000000000000, 0.9659258262890683122, 1.000000000000000000, 0.9659258262890683122, 1.000000000000000000, 0.9659258262890683122, 1.000000000000000000, 0.9659258262890683122, 1.000000000000000000, 0.9659258262890683122, 1.000000000000000000, 0.9659258262890683122, 1.000000000000000000, 0.9659258262890683122, 1.000000000000000000, 0.9659258262890683122, 1.000000000000000000, 0.9659258262890683122, 1.000000000000000000, 0.9659258262890683122, 1.000000000000000000, 0.9659258262890683122, 1.000000000000000000, 0.9659258262890683122, 1.000000000000000000, 0.9659258262890683122, 1.000000000000000000, 0.9659258262890683122, 1.000000000000000000, 0.9659258262890683122, 1.000000000000000000, 0.9659258262890683122, 1.000000000000000000, 0.9659258262890683122, 1.000000000000000000, 0.9659258262890683122, 1.000000000000000000, 0.9659258262890683122, 1.000000000000000000, 0.9659258262890683122, 1.000000000000000000, 0.9659258262890683122, 1.000000000000000000, 0.9659258262890683122, 1.000000000000000000, 0.9659258262890683122, 1.000000000000000000, 0.9659258262890683122, 1.000000000000000000, 0.9659258262890683122, 1.000000000000000000, 0.9659258262890683122, 1.000000000000000000, 0.9659258262890683122, 1.000000000000000000, 0.9659258262890683122, 1.000000000000000000, 0.9659258262890683122, 1.000000000000000000, 0.9659258262890683122, 1.000000000000000000, 0.9659258262890683122, 1.000000000000000000, 0.9659258262890683122, 1.000000000000000000, 0.9659258262890683122, 1.000000000000000000, 0.9659258262890683122, 1.000000000000000000, 0.9659258262890683122, 1.000000000000000000, 0.9659258262890683122, 1.000000000000000000, 0.9659258262890683122, 1.000000000000000000, 0.9659258262890683122, 1.000000000000000000, 0.9659258262890683122, 1.000000000000000000, 0.9659258262890683122, 1.000000000000000000, 0.9659258262890683122, 1.000000000000000000, 0.9659258262890683122, 1.000000000000000000, 0.9659258262890683122, 1.000000000000000000, 0.9659258262890683122, 1.000000000000000000, 0.9659258262890683122, 1.000000000000000000, 0.9659258262890683122, 1.000000000000000000, 0.9659258262890683122, 1.000000000000000000, 0.9659258262890683122, 1.000000000000000000, 0.9659258262890683122, 1.000000000000000000, 0.9659258262890683122, 1.000000000000000000, 0.9659258262890683122, 1.000000000000000000, 0.9659258262890683122, 1.000000000000000000, 0.9659258262890683122, 1.000000000000000000, 0.9659258262890683122, 1.000000000000000000, 0.9659258262890683122, 1.000000000000000000, 0.9659258262890683122, 1.000000000000000000, 0.9659258262890683122, 1.000000000000000000, 0.9659258262890683122, 1.000000000000000000, 0.9659258262890683122, 1.000000000000000000, 0.9659258262890683122, 1.000000000000000000, 0.9659258262890683122, 1.000000000000000000, 0.9659258262890683122, 1.000000000000000000, 0.9659258262890683122, 1.000000000000000000, 0.9659258262890683122, 1.000000000000000000, 0.9659258262890683122, 1.000000000000000000, 0.9659258262890683122, 1.000000000000000000, 0.9659258262890683122, 1.000000000000000000, 0.9659258262890683122, 1.000000000000000000, 0.9659258262890683122, 1.000000000000000000, 0.9659258262890683122, 1.000000000000000000, 0.9659258262890683122, 1.000000000000000000, 0.9659258262890683122, 1.000000000000000000, 0.9659258262890683122, 1.000000000000000000, 0.9659258262890683122, 1.000000000000000000, 0.9659258262890683122, 1.000000000000000000, 0.9659258262890683122, 1.000000000000000000, 0.9659258262890683122, 1.000000000000000000, 0.9659258262890683122, 1.000000000000000000, 0.9659258262890683122, 1.000000000000000000, 0.9659258262890683122, 1.000000000000000000, 0.9659258262890683122, 1.000000000000000000, 0.9659258262890683122, 1.000000000000000000, 0.9659258262890683122, 1.000000000000000000, 0.9659258262890683122, 1.000000000000000000, 0.9659258262890683122, 1.000000000000000000, 0.9659258262890683122, 1.000000000000000000, 0.9659258262890683122, 1.000000000000000000, 0.9659258262890683122, 1.000000000000000000, 0.9659258262890683122, 1.000000000000000000, 0.9659258262890683122, 1.000000000000000000, 0.9659258262890683122, 1.000000000000000000, 0.9659258262890683122, 1.000000000000000000, 0.9659258262890683122, 1.000000000000000000, 0.9659258262890683122, 1.000000000000000000, 0.9659258262890683122, 1.000000000000000000, 0.9659258262890683122, 1.000000000000000000, 0.9659258262890683122, 1.000000000000000000, 0.9659258262890683122, 1.000000000000000000, 0.9659258262890683122, 1.000000000000000000, 0.9659258262890683122, 1.000000000000000000, 0.9659258262890683122, 1.000000000000000000, 0.9659258262890683122, 1.000000000000000000, 0.9659258262890683122, 1.000000000000000000, 0.9659258262890683122, 1.000000000000000000, 0.9659258262890683122, 1.000000000000000000, 0.9659258262890683122, 1.000000000000000000, 0.9659258262890683122, 1.000000000000000000, 0.9659258262890683122, 1.000000000000000000, 0.9659258262890683122, 1.000000000000000000, 0.9659258262890683122, 1.000000000000000000, 0.9659258262890683122, 1.000000000000000000, 0.9659258262890683122, 1.000000000000000000, 0.9659258262890683122, 1.000000000000000000, 0.9659258262890683122, 1.000000000000000000, 0.9659258262890683122, 1.000000000000000000, 0.9659258262890683122, 1.000000000000000000, 0.9659258262890683122, 1.000000000000000000, 0.9659258262890683122, 1.000000000000000000, 0.9659258262890683122, 1.000000000000000000, 0.9659258262890683122, 1.000000000000000000, 0.9659258262890683122, 1.000000000000000000, 0.9659258262890683122, 1.000000000000000000, 0.9659258262890683122, 1.000000000000000000, 0.9659258262890683122, 1.000000000000000000, 0.9659258262890683122, 1.000000000000000000, 0.9659258262890683122, 1.000000000000000000, 0.9659258262890683122, 1.000000000000000000, 0.9659258262890683122, 1.000000000000000000, 0.9659258262890683122, 1.000000000000000000, 0.9659258262890683122, 1.000000000000000000, 0.9659258262890683122, 1.000000000000000000, 0.9659258262890683122, 1.000000000000000000, 0.9659258262890683122, 1.000000000000000000, 0.9659258262890683122, 1.000000000000000000, 0.9659258262890683122, 1.000000000000000000, 0.9659258262890683122, 1.000000000000000000, 0.9659258262890683122, 1.000000000000000000, 0.9659258262890683122, 1.000000000000000000, 0.9659258262890683122, 1.000000000000000000, 0.9659258262890683122, 1.000000000000000000, 0.9659258262890683122, 1.000000000000000000, 0.9659258262890683122, 1.000000000000000000, 0.9659258262890683122, 1.000000000000000000, 0.9659258262890683122, 1.000000000000000000, 0.9659258262890683122, 1.000000000000000000, 0.9659258262890683122, 1.000000000000000000, 0.9659258262890683122, 1.000000000000000000, 0.9659258262890683122, 1.000000000000000000, 0.9659258262890683122, 1.000000000000000000, 0.9659258262890683122, 1.000000000000000000, 0.9659258262890683122, 1.000000000000000000, 0.9659258262890683122, 1.000000000000000000, 0.9659258262890683122, 1.000000000000000000, 0.9659258262890683122, 1.000000000000000000, 0.9659258262890683122, 1.000000000000000000, 0.9659258262890683122, 1.000000000000000000, 0.9659258262890683122, 1.000000000000000000, 0.9659258262890683122, 1.000000000000000000, 0.9659258262890683122, 1.000000000000000000, 0.9659258262890683122, 1.000000000000000000, 0.9659258262890683122, 1.000000000000000000, 0.9659258262890683122, 1.000000000000000000, 0.9659258262890683122, 1.000000000000000000, 0.9659258262890683122, 1.000000000000000000, 0.9659258262890683122, 1.000000000000000000, 0.9659258262890683122, 1.000000000000000000, 0.9659258262890683122, 1.000000000000000000, 0.9659258262890683122, 1.000000000000000000, 0.9659258262890683122, 1.000000000000000000, 0.9659258262890683122, 1.000000000000000000, 0.9659258262890683122, 1.000000000000000000, 0.9659258262890683122, 1.000000000000000000, 0.9659258262890683122, 1.000000000000000000, 0.9659258262890683122, 1.000000000000000000, 0.9659258262890683122, 1.000000000000000000, 0.9659258262890683122, 1.000000000000000000, 0.9659258262890683122, 1.000000000000000000, 0.9659258262890683122, 1.000000000000000000, 0.9659258262890683122, 1.000000000000000000, 0.9659258262890683122, 1.000000000000000000, 0.9659258262890683122, 1.000000000000000000),
 ( 0.3333333333333333703, 0.3219752754296894559, 0.3333333333333333703, 0.3219752754296894559, 0.3333333333333333703, 0.3219752754296894559, 0.3333333333333333703, 0.3219752754296894559, 0.3333333333333333703, 0.3219752754296894559, 0.3333333333333333703, 0.3219752754296894559, 0.3333333333333333703, 0.3219752754296894559, 0.3333333333333333703, 0.3219752754296894559, 0.3333333333333333703, 0.3219752754296894559, 0.3333333333333333703, 0.3219752754296894559, 0.3333333333333333703, 0.3219752754296894559, 0.3333333333333333703, 0.3219752754296894559, 0.3333333333333333703, 0.3219752754296894559, 0.3333333333333333703, 0.3219752754296894559, 0.3333333333333333703, 0.3219752754296894559, 0.3333333333333333703, 0.3219752754296894559, 0.3333333333333333703, 0.3219752754296894559, 0.3333333333333333703, 0.3219752754296894559, 0.3333333333333333703, 0.3219752754296894559, 0.3333333333333333703, 0.3219752754296894559, 0.3333333333333333703, 0.3219752754296894559, 0.3333333333333333703, 0.3219752754296894559, 0.3333333333333333703, 0.3219752754296894559, 0.3333333333333333703, 0.3219752754296894559, 0.3333333333333333703, 0.3219752754296894559, 0.3333333333333333703, 0.3219752754296894559, 0.3333333333333333703, 0.3219752754296894559, 0.3333333333333333703, 0.3219752754296894559, 0.3333333333333333703, 0.3219752754296894559, 0.3333333333333333703, 0.3219752754296894559, 0.3333333333333333703, 0.3219752754296894559, 0.3333333333333333703, 0.3219752754296894559, 0.3333333333333333703, 0.3219752754296894559, 0.3333333333333333703, 0.3219752754296894559, 0.3333333333333333703, 0.3219752754296894559, 0.3333333333333333703, 0.3219752754296894559, 0.3333333333333333703, 0.3219752754296894559, 0.3333333333333333703, 0.3219752754296894559, 0.3333333333333333703, 0.3219752754296894559, 0.3333333333333333703, 0.3219752754296894559, 0.3333333333333333703, 0.3219752754296894559, 0.3333333333333333703, 0.3219752754296894559, 0.3333333333333333703, 0.3219752754296894559, 0.3333333333333333703, 0.3219752754296894559, 0.3333333333333333703, 0.3219752754296894559, 0.3333333333333333703, 0.3219752754296894559, 0.3333333333333333703, 0.3219752754296894559, 0.3333333333333333703, 0.3219752754296894559, 0.3333333333333333703, 0.3219752754296894559, 0.3333333333333333703, 0.3219752754296894559, 0.3333333333333333703, 0.3219752754296894559, 0.3333333333333333703, 0.3219752754296894559, 0.3333333333333333703, 0.3219752754296894559, 0.3333333333333333703, 0.3219752754296894559, 0.3333333333333333703, 0.3219752754296894559, 0.3333333333333333703, 0.3219752754296894559, 0.3333333333333333703, 0.3219752754296894559, 0.3333333333333333703, 0.3219752754296894559, 0.3333333333333333703, 0.3219752754296894559, 0.3333333333333333703, 0.3219752754296894559, 0.3333333333333333703, 0.3219752754296894559, 0.3333333333333333703, 0.3219752754296894559, 0.3333333333333333703, 0.3219752754296894559, 0.3333333333333333703, 0.3219752754296894559, 0.3333333333333333703, 0.3219752754296894559, 0.3333333333333333703, 0.3219752754296894559, 0.3333333333333333703, 0.3219752754296894559, 0.3333333333333333703, 0.3219752754296894559, 0.3333333333333333703, 0.3219752754296894559, 0.3333333333333333703, 0.3219752754296894559, 0.3333333333333333703, 0.3219752754296894559, 0.3333333333333333703, 0.3219752754296894559, 0.3333333333333333703, 0.3219752754296894559, 0.3333333333333333703, 0.3219752754296894559, 0.3333333333333333703, 0.3219752754296894559, 0.3333333333333333703, 0.3219752754296894559, 0.3333333333333333703, 0.3219752754296894559, 0.3333333333333333703, 0.3219752754296894559, 0.3333333333333333703, 0.3219752754296894559, 0.3333333333333333703, 0.3219752754296894559, 0.3333333333333333703, 0.3219752754296894559, 0.3333333333333333703, 0.3219752754296894559, 0.3333333333333333703, 0.3219752754296894559, 0.3333333333333333703, 0.3219752754296894559, 0.3333333333333333703, 0.3219752754296894559, 0.3333333333333333703, 0.3219752754296894559, 0.3333333333333333703, 0.3219752754296894559, 0.3333333333333333703, 0.3219752754296894559, 0.3333333333333333703, 0.3219752754296894559, 0.3333333333333333703, 0.3219752754296894559, 0.3333333333333333703, 0.3219752754296894559, 0.3333333333333333703, 0.3219752754296894559, 0.3333333333333333703, 0.3219752754296894559, 0.3333333333333333703, 0.3219752754296894559, 0.3333333333333333703, 0.3219752754296894559, 0.3333333333333333703, 0.3219752754296894559, 0.3333333333333333703, 0.3219752754296894559, 0.3333333333333333703, 0.3219752754296894559, 0.3333333333333333703, 0.3219752754296894559, 0.3333333333333333703, 0.3219752754296894559, 0.3333333333333333703, 0.3219752754296894559, 0.3333333333333333703, 0.3219752754296894559, 0.3333333333333333703, 0.3219752754296894559, 0.3333333333333333703, 0.3219752754296894559, 0.3333333333333333703, 0.3219752754296894559, 0.3333333333333333703, 0.3219752754296894559, 0.3333333333333333703, 0.3219752754296894559, 0.3333333333333333703, 0.3219752754296894559, 0.3333333333333333703, 0.3219752754296894559, 0.3333333333333333703, 0.3219752754296894559, 0.3333333333333333703, 0.3219752754296894559, 0.3333333333333333703, 0.3219752754296894559, 0.3333333333333333703, 0.3219752754296894559, 0.3333333333333333703, 0.3219752754296894559, 0.3333333333333333703, 0.3219752754296894559, 0.3333333333333333703, 0.3219752754296894559, 0.3333333333333333703, 0.3219752754296894559, 0.3333333333333333703, 0.3219752754296894559, 0.3333333333333333703, 0.3219752754296894559, 0.3333333333333333703, 0.3219752754296894559, 0.3333333333333333703, 0.3219752754296894559, 0.3333333333333333703, 0.3219752754296894559, 0.3333333333333333703, 0.3219752754296894559, 0.3333333333333333703, 0.3219752754296894559, 0.3333333333333333703, 0.3219752754296894559, 0.3333333333333333703, 0.3219752754296894559, 0.3333333333333333703, 0.3219752754296894559, 0.3333333333333333703, 0.3219752754296894559, 0.3333333333333333703, 0.3219752754296894559, 0.3333333333333333703, 0.3219752754296894559, 0.3333333333333333703, 0.3219752754296894559, 0.3333333333333333703, 0.3219752754296894559, 0.3333333333333333703, 0.3219752754296894559, 0.3333333333333333703, 0.3219752754296894559, 0.3333333333333333703, 0.3219752754296894559, 0.3333333333333333703, 0.3219752754296894559, 0.3333333333333333703, 0.3219752754296894559, 0.3333333333333333703, 0.3219752754296894559, 0.3333333333333333703, 0.3219752754296894559, 0.3333333333333333703, 0.3219752754296894559, 0.3333333333333333703, 0.3219752754296894559, 0.3333333333333333703, 0.3219752754296894559, 0.3333333333333333703, 0.3219752754296894559, 0.3333333333333333703, 0.3219752754296894559, 0.3333333333333333703, 0.3219752754296894559, 0.3333333333333333703, 0.3219752754296894559, 0.3333333333333333703, 0.3219752754296894559, 0.3333333333333333703, 0.3219752754296894559, 0.3333333333333333703, 0.3219752754296894559, 0.3333333333333333703, 0.3219752754296894559, 0.3333333333333333703, 0.3219752754296894559, 0.3333333333333333703, 0.3219752754296894559, 0.3333333333333333703, 0.3219752754296894559, 0.3333333333333333703, 0.3219752754296894559, 0.3333333333333333703, 0.3219752754296894559, 0.3333333333333333703, 0.3219752754296894559, 0.3333333333333333703, 0.3219752754296894559, 0.3333333333333333703, 0.3219752754296894559, 0.3333333333333333703, 0.3219752754296894559, 0.3333333333333333703, 0.3219752754296894559, 0.3333333333333333703, 0.3219752754296894559, 0.3333333333333333703, 0.3219752754296894559, 0.3333333333333333703, 0.3219752754296894559, 0.3333333333333333703, 0.3219752754296894559, 0.3333333333333333703, 0.3219752754296894559, 0.3333333333333333703, 0.3219752754296894559, 0.3333333333333333703, 0.3219752754296894559, 0.3333333333333333703, 0.3219752754296894559, 0.3333333333333333703, 0.3219752754296894559, 0.3333333333333333703, 0.3219752754296894559, 0.3333333333333333703, 0.3219752754296894559, 0.3333333333333333703, 0.3219752754296894559, 0.3333333333333333703, 0.3219752754296894559, 0.3333333333333333703, 0.3219752754296894559, 0.3333333333333333703, 0.3219752754296894559, 0.3333333333333333703, 0.3219752754296894559, 0.3333333333333333703, 0.3219752754296894559, 0.3333333333333333703, 0.3219752754296894559, 0.3333333333333333703, 0.3219752754296894559, 0.3333333333333333703, 0.3219752754296894559, 0.3333333333333333703, 0.3219752754296894559, 0.3333333333333333703, 0.3219752754296894559, 0.3333333333333333703, 0.3219752754296894559, 0.3333333333333333703, 0.3219752754296894559, 0.3333333333333333703, 0.3219752754296894559, 0.3333333333333333703, 0.3219752754296894559, 0.3333333333333333703, 0.3219752754296894559, 0.3333333333333333703, 0.3219752754296894559, 0.3333333333333333703, 0.3219752754296894559, 0.3333333333333333703, 0.3219752754296894559, 0.3333333333333333703, 0.3219752754296894559, 0.3333333333333333703, 0.3219752754296894559, 0.3333333333333333703, 0.3219752754296894559, 0.3333333333333333703, 0.3219752754296894559, 0.3333333333333333703, 0.3219752754296894559, 0.3333333333333333703, 0.3219752754296894559, 0.3333333333333333703, 0.3219752754296894559, 0.3333333333333333703, 0.3219752754296894559, 0.3333333333333333703, 0.3219752754296894559, 0.3333333333333333703, 0.3219752754296894559, 0.3333333333333333703, 0.3219752754296894559, 0.3333333333333333703, 0.3219752754296894559, 0.3333333333333333703, 0.3219752754296894559, 0.3333333333333333703, 0.3219752754296894559, 0.3333333333333333703, 0.3219752754296894559, 0.3333333333333333703, 0.3219752754296894559, 0.3333333333333333703, 0.3219752754296894559, 0.3333333333333333703, 0.3219752754296894559, 0.3333333333333333703, 0.3219752754296894559, 0.3333333333333333703, 0.3219752754296894559, 0.3333333333333333703, 0.3219752754296894559, 0.3333333333333333703, 0.3219752754296894559, 0.3333333333333333703, 0.3219752754296894559, 0.3333333333333333703, 0.3219752754296894559, 0.3333333333333333703, 0.3219752754296894559, 0.3333333333333333703, 0.3219752754296894559, 0.3333333333333333703, 0.3219752754296894559, 0.3333333333333333703, 0.3219752754296894559, 0.3333333333333333703, 0.3219752754296894559, 0.3333333333333333703, 0.3219752754296894559, 0.3333333333333333703, 0.3219752754296894559, 0.3333333333333333703, 0.3219752754296894559, 0.3333333333333333703, 0.3219752754296894559, 0.3333333333333333703, 0.3219752754296894559, 0.3333333333333333703, 0.3219752754296894559, 0.3333333333333333703, 0.3219752754296894559, 0.3333333333333333703, 0.3219752754296894559, 0.3333333333333333703, 0.3219752754296894559, 0.3333333333333333703),
 ( 0.3333333333333333703, 0.3219752754296894559, 0.3333333333333333703, 0.3219752754296894559, 0.3333333333333333703, 0.3219752754296894559, 0.3333333333333333703, 0.3219752754296894559, 0.3333333333333333703, 0.3219752754296894559, 0.3333333333333333703, 0.3219752754296894559, 0.3333333333333333703, 0.3219752754296894559, 0.3333333333333333703, 0.3219752754296894559, 0.3333333333333333703, 0.3219752754296894559, 0.3333333333333333703, 0.3219752754296894559, 0.3333333333333333703, 0.3219752754296894559, 0.3333333333333333703, 0.3219752754296894559, 0.3333333333333333703, 0.3219752754296894559, 0.3333333333333333703, 0.3219752754296894559, 0.3333333333333333703, 0.3219752754296894559, 0.3333333333333333703, 0.3219752754296894559, 0.3333333333333333703, 0.3219752754296894559, 0.3333333333333333703, 0.3219752754296894559, 0.3333333333333333703, 0.3219752754296894559, 0.3333333333333333703, 0.3219752754296894559, 0.3333333333333333703, 0.3219752754296894559, 0.3333333333333333703, 0.3219752754296894559, 0.3333333333333333703, 0.3219752754296894559, 0.3333333333333333703, 0.3219752754296894559, 0.3333333333333333703, 0.3219752754296894559, 0.3333333333333333703, 0.3219752754296894559, 0.3333333333333333703, 0.3219752754296894559, 0.3333333333333333703, 0.3219752754296894559, 0.3333333333333333703, 0.3219752754296894559, 0.3333333333333333703, 0.3219752754296894559, 0.3333333333333333703, 0.3219752754296894559, 0.3333333333333333703, 0.3219752754296894559, 0.3333333333333333703, 0.3219752754296894559, 0.3333333333333333703, 0.3219752754296894559, 0.3333333333333333703, 0.3219752754296894559, 0.3333333333333333703, 0.3219752754296894559, 0.3333333333333333703, 0.3219752754296894559, 0.3333333333333333703, 0.3219752754296894559, 0.3333333333333333703, 0.3219752754296894559, 0.3333333333333333703, 0.3219752754296894559, 0.3333333333333333703, 0.3219752754296894559, 0.3333333333333333703, 0.3219752754296894559, 0.3333333333333333703, 0.3219752754296894559, 0.3333333333333333703, 0.3219752754296894559, 0.3333333333333333703, 0.3219752754296894559, 0.3333333333333333703, 0.3219752754296894559, 0.3333333333333333703, 0.3219752754296894559, 0.3333333333333333703, 0.3219752754296894559, 0.3333333333333333703, 0.3219752754296894559, 0.3333333333333333703, 0.3219752754296894559, 0.3333333333333333703, 0.3219752754296894559, 0.3333333333333333703, 0.3219752754296894559, 0.3333333333333333703, 0.3219752754296894559, 0.3333333333333333703, 0.3219752754296894559, 0.3333333333333333703, 0.3219752754296894559, 0.3333333333333333703, 0.3219752754296894559, 0.3333333333333333703, 0.3219752754296894559, 0.3333333333333333703, 0.3219752754296894559, 0.3333333333333333703, 0.3219752754296894559, 0.3333333333333333703, 0.3219752754296894559, 0.3333333333333333703, 0.3219752754296894559, 0.3333333333333333703, 0.3219752754296894559, 0.3333333333333333703, 0.3219752754296894559, 0.3333333333333333703, 0.3219752754296894559, 0.3333333333333333703, 0.3219752754296894559, 0.3333333333333333703, 0.3219752754296894559, 0.3333333333333333703, 0.3219752754296894559, 0.3333333333333333703, 0.3219752754296894559, 0.3333333333333333703, 0.3219752754296894559, 0.3333333333333333703, 0.3219752754296894559, 0.3333333333333333703, 0.3219752754296894559, 0.3333333333333333703, 0.3219752754296894559, 0.3333333333333333703, 0.3219752754296894559, 0.3333333333333333703, 0.3219752754296894559, 0.3333333333333333703, 0.3219752754296894559, 0.3333333333333333703, 0.3219752754296894559, 0.3333333333333333703, 0.3219752754296894559, 0.3333333333333333703, 0.3219752754296894559, 0.3333333333333333703, 0.3219752754296894559, 0.3333333333333333703, 0.3219752754296894559, 0.3333333333333333703, 0.3219752754296894559, 0.3333333333333333703, 0.3219752754296894559, 0.3333333333333333703, 0.3219752754296894559, 0.3333333333333333703, 0.3219752754296894559, 0.3333333333333333703, 0.3219752754296894559, 0.3333333333333333703, 0.3219752754296894559, 0.3333333333333333703, 0.3219752754296894559, 0.3333333333333333703, 0.3219752754296894559, 0.3333333333333333703, 0.3219752754296894559, 0.3333333333333333703, 0.3219752754296894559, 0.3333333333333333703, 0.3219752754296894559, 0.3333333333333333703, 0.3219752754296894559, 0.3333333333333333703, 0.3219752754296894559, 0.3333333333333333703, 0.3219752754296894559, 0.3333333333333333703, 0.3219752754296894559, 0.3333333333333333703, 0.3219752754296894559, 0.3333333333333333703, 0.3219752754296894559, 0.3333333333333333703, 0.3219752754296894559, 0.3333333333333333703, 0.3219752754296894559, 0.3333333333333333703, 0.3219752754296894559, 0.3333333333333333703, 0.3219752754296894559, 0.3333333333333333703, 0.3219752754296894559, 0.3333333333333333703, 0.3219752754296894559, 0.3333333333333333703, 0.3219752754296894559, 0.3333333333333333703, 0.3219752754296894559, 0.3333333333333333703, 0.3219752754296894559, 0.3333333333333333703, 0.3219752754296894559, 0.3333333333333333703, 0.3219752754296894559, 0.3333333333333333703, 0.3219752754296894559, 0.3333333333333333703, 0.3219752754296894559, 0.3333333333333333703, 0.3219752754296894559, 0.3333333333333333703, 0.3219752754296894559, 0.3333333333333333703, 0.3219752754296894559, 0.3333333333333333703, 0.3219752754296894559, 0.3333333333333333703, 0.3219752754296894559, 0.3333333333333333703, 0.3219752754296894559, 0.3333333333333333703, 0.3219752754296894559, 0.3333333333333333703, 0.3219752754296894559, 0.3333333333333333703, 0.3219752754296894559, 0.3333333333333333703, 0.3219752754296894559, 0.3333333333333333703, 0.3219752754296894559, 0.3333333333333333703, 0.3219752754296894559, 0.3333333333333333703, 0.3219752754296894559, 0.3333333333333333703, 0.3219752754296894559, 0.3333333333333333703, 0.3219752754296894559, 0.3333333333333333703, 0.3219752754296894559, 0.3333333333333333703, 0.3219752754296894559, 0.3333333333333333703, 0.3219752754296894559, 0.3333333333333333703, 0.3219752754296894559, 0.3333333333333333703, 0.3219752754296894559, 0.3333333333333333703, 0.3219752754296894559, 0.3333333333333333703, 0.3219752754296894559, 0.3333333333333333703, 0.3219752754296894559, 0.3333333333333333703, 0.3219752754296894559, 0.3333333333333333703, 0.3219752754296894559, 0.3333333333333333703, 0.3219752754296894559, 0.3333333333333333703, 0.3219752754296894559, 0.3333333333333333703, 0.3219752754296894559, 0.3333333333333333703, 0.3219752754296894559, 0.3333333333333333703, 0.3219752754296894559, 0.3333333333333333703, 0.3219752754296894559, 0.3333333333333333703, 0.3219752754296894559, 0.3333333333333333703, 0.3219752754296894559, 0.3333333333333333703, 0.3219752754296894559, 0.3333333333333333703, 0.3219752754296894559, 0.3333333333333333703, 0.3219752754296894559, 0.3333333333333333703, 0.3219752754296894559, 0.3333333333333333703, 0.3219752754296894559, 0.3333333333333333703, 0.3219752754296894559, 0.3333333333333333703, 0.3219752754296894559, 0.3333333333333333703, 0.3219752754296894559, 0.3333333333333333703, 0.3219752754296894559, 0.3333333333333333703, 0.3219752754296894559, 0.3333333333333333703, 0.3219752754296894559, 0.3333333333333333703, 0.3219752754296894559, 0.3333333333333333703, 0.3219752754296894559, 0.3333333333333333703, 0.3219752754296894559, 0.3333333333333333703, 0.3219752754296894559, 0.3333333333333333703, 0.3219752754296894559, 0.3333333333333333703, 0.3219752754296894559, 0.3333333333333333703, 0.3219752754296894559, 0.3333333333333333703, 0.3219752754296894559, 0.3333333333333333703, 0.3219752754296894559, 0.3333333333333333703, 0.3219752754296894559, 0.3333333333333333703, 0.3219752754296894559, 0.3333333333333333703, 0.3219752754296894559, 0.3333333333333333703, 0.3219752754296894559, 0.3333333333333333703, 0.3219752754296894559, 0.3333333333333333703, 0.3219752754296894559, 0.3333333333333333703, 0.3219752754296894559, 0.3333333333333333703, 0.3219752754296894559, 0.3333333333333333703, 0.3219752754296894559, 0.3333333333333333703, 0.3219752754296894559, 0.3333333333333333703, 0.3219752754296894559, 0.3333333333333333703, 0.3219752754296894559, 0.3333333333333333703, 0.3219752754296894559, 0.3333333333333333703, 0.3219752754296894559, 0.3333333333333333703, 0.3219752754296894559, 0.3333333333333333703, 0.3219752754296894559, 0.3333333333333333703, 0.3219752754296894559, 0.3333333333333333703, 0.3219752754296894559, 0.3333333333333333703, 0.3219752754296894559, 0.3333333333333333703, 0.3219752754296894559, 0.3333333333333333703, 0.3219752754296894559, 0.3333333333333333703, 0.3219752754296894559, 0.3333333333333333703, 0.3219752754296894559, 0.3333333333333333703, 0.3219752754296894559, 0.3333333333333333703, 0.3219752754296894559, 0.3333333333333333703, 0.3219752754296894559, 0.3333333333333333703, 0.3219752754296894559, 0.3333333333333333703, 0.3219752754296894559, 0.3333333333333333703, 0.3219752754296894559, 0.3333333333333333703, 0.3219752754296894559, 0.3333333333333333703, 0.3219752754296894559, 0.3333333333333333703, 0.3219752754296894559, 0.3333333333333333703, 0.3219752754296894559, 0.3333333333333333703, 0.3219752754296894559, 0.3333333333333333703, 0.3219752754296894559, 0.3333333333333333703, 0.3219752754296894559, 0.3333333333333333703, 0.3219752754296894559, 0.3333333333333333703, 0.3219752754296894559, 0.3333333333333333703, 0.3219752754296894559, 0.3333333333333333703, 0.3219752754296894559, 0.3333333333333333703, 0.3219752754296894559, 0.3333333333333333703, 0.3219752754296894559, 0.3333333333333333703, 0.3219752754296894559, 0.3333333333333333703, 0.3219752754296894559, 0.3333333333333333703, 0.3219752754296894559, 0.3333333333333333703, 0.3219752754296894559, 0.3333333333333333703, 0.3219752754296894559, 0.3333333333333333703, 0.3219752754296894559, 0.3333333333333333703, 0.3219752754296894559, 0.3333333333333333703, 0.3219752754296894559, 0.3333333333333333703, 0.3219752754296894559, 0.3333333333333333703, 0.3219752754296894559, 0.3333333333333333703, 0.3219752754296894559, 0.3333333333333333703, 0.3219752754296894559, 0.3333333333333333703, 0.3219752754296894559, 0.3333333333333333703, 0.3219752754296894559, 0.3333333333333333703, 0.3219752754296894559, 0.3333333333333333703, 0.3219752754296894559, 0.3333333333333333703, 0.3219752754296894559, 0.3333333333333333703, 0.3219752754296894559, 0.3333333333333333703, 0.3219752754296894559, 0.3333333333333333703, 0.3219752754296894559, 0.3333333333333333703, 0.3219752754296894559, 0.3333333333333333703, 0.3219752754296894559, 0.3333333333333333703, 0.3219752754296894559, 0.3333333333333333703),
 ( 1.000000000000000000, 0.9659258262890683122, 1.000000000000000000, 0.9659258262890683122, 1.000000000000000000, 0.9659258262890683122, 1.000000000000000000, 0.9659258262890683122, 1.000000000000000000, 0.9659258262890683122, 1.000000000000000000, 0.9659258262890683122, 1.000000000000000000, 0.9659258262890683122, 1.000000000000000000, 0.9659258262890683122, 1.000000000000000000, 0.9659258262890683122, 1.000000000000000000, 0.9659258262890683122, 1.000000000000000000, 0.9659258262890683122, 1.000000000000000000, 0.9659258262890683122, 1.000000000000000000, 0.9659258262890683122, 1.000000000000000000, 0.9659258262890683122, 1.000000000000000000, 0.9659258262890683122, 1.000000000000000000, 0.9659258262890683122, 1.000000000000000000, 0.9659258262890683122, 1.000000000000000000, 0.9659258262890683122, 1.000000000000000000, 0.9659258262890683122, 1.000000000000000000, 0.9659258262890683122, 1.000000000000000000, 0.9659258262890683122, 1.000000000000000000, 0.9659258262890683122, 1.000000000000000000, 0.9659258262890683122, 1.000000000000000000, 0.9659258262890683122, 1.000000000000000000, 0.9659258262890683122, 1.000000000000000000, 0.9659258262890683122, 1.000000000000000000, 0.9659258262890683122, 1.000000000000000000, 0.9659258262890683122, 1.000000000000000000, 0.9659258262890683122, 1.000000000000000000, 0.9659258262890683122, 1.000000000000000000, 0.9659258262890683122, 1.000000000000000000, 0.9659258262890683122, 1.000000000000000000, 0.9659258262890683122, 1.000000000000000000, 0.9659258262890683122, 1.000000000000000000, 0.9659258262890683122, 1.000000000000000000, 0.9659258262890683122, 1.000000000000000000, 0.9659258262890683122, 1.000000000000000000, 0.9659258262890683122, 1.000000000000000000, 0.9659258262890683122, 1.000000000000000000, 0.9659258262890683122, 1.000000000000000000, 0.9659258262890683122, 1.000000000000000000, 0.9659258262890683122, 1.000000000000000000, 0.9659258262890683122, 1.000000000000000000, 0.9659258262890683122, 1.000000000000000000, 0.9659258262890683122, 1.000000000000000000, 0.9659258262890683122, 1.000000000000000000, 0.9659258262890683122, 1.000000000000000000, 0.9659258262890683122, 1.000000000000000000, 0.9659258262890683122, 1.000000000000000000, 0.9659258262890683122, 1.000000000000000000, 0.9659258262890683122, 1.000000000000000000, 0.9659258262890683122, 1.000000000000000000, 0.9659258262890683122, 1.000000000000000000, 0.9659258262890683122, 1.000000000000000000, 0.9659258262890683122, 1.000000000000000000, 0.9659258262890683122, 1.000000000000000000, 0.9659258262890683122, 1.000000000000000000, 0.9659258262890683122, 1.000000000000000000, 0.9659258262890683122, 1.000000000000000000, 0.9659258262890683122, 1.000000000000000000, 0.9659258262890683122, 1.000000000000000000, 0.9659258262890683122, 1.000000000000000000, 0.9659258262890683122, 1.000000000000000000, 0.9659258262890683122, 1.000000000000000000, 0.9659258262890683122, 1.000000000000000000, 0.9659258262890683122, 1.000000000000000000, 0.9659258262890683122, 1.000000000000000000, 0.9659258262890683122, 1.000000000000000000, 0.9659258262890683122, 1.000000000000000000, 0.9659258262890683122, 1.000000000000000000, 0.9659258262890683122, 1.000000000000000000, 0.9659258262890683122, 1.000000000000000000, 0.9659258262890683122, 1.000000000000000000, 0.9659258262890683122, 1.000000000000000000, 0.9659258262890683122, 1.000000000000000000, 0.9659258262890683122, 1.000000000000000000, 0.9659258262890683122, 1.000000000000000000, 0.9659258262890683122, 1.000000000000000000, 0.9659258262890683122, 1.000000000000000000, 0.9659258262890683122, 1.000000000000000000, 0.9659258262890683122, 1.000000000000000000, 0.9659258262890683122, 1.000000000000000000, 0.9659258262890683122, 1.000000000000000000, 0.9659258262890683122, 1.000000000000000000, 0.9659258262890683122, 1.000000000000000000, 0.9659258262890683122, 1.000000000000000000, 0.9659258262890683122, 1.000000000000000000, 0.9659258262890683122, 1.000000000000000000, 0.9659258262890683122, 1.000000000000000000, 0.9659258262890683122, 1.000000000000000000, 0.9659258262890683122, 1.000000000000000000, 0.9659258262890683122, 1.000000000000000000, 0.9659258262890683122, 1.000000000000000000, 0.9659258262890683122, 1.000000000000000000, 0.9659258262890683122, 1.000000000000000000, 0.9659258262890683122, 1.000000000000000000, 0.9659258262890683122, 1.000000000000000000, 0.9659258262890683122, 1.000000000000000000, 0.9659258262890683122, 1.000000000000000000, 0.9659258262890683122, 1.000000000000000000, 0.9659258262890683122, 1.000000000000000000, 0.9659258262890683122, 1.000000000000000000, 0.9659258262890683122, 1.000000000000000000, 0.9659258262890683122, 1.000000000000000000, 0.9659258262890683122, 1.000000000000000000, 0.9659258262890683122, 1.000000000000000000, 0.9659258262890683122, 1.000000000000000000, 0.9659258262890683122, 1.000000000000000000, 0.9659258262890683122, 1.000000000000000000, 0.9659258262890683122, 1.000000000000000000, 0.9659258262890683122, 1.000000000000000000, 0.9659258262890683122, 1.000000000000000000, 0.9659258262890683122, 1.000000000000000000, 0.9659258262890683122, 1.000000000000000000, 0.9659258262890683122, 1.000000000000000000, 0.9659258262890683122, 1.000000000000000000, 0.9659258262890683122, 1.000000000000000000, 0.9659258262890683122, 1.000000000000000000, 0.9659258262890683122, 1.000000000000000000, 0.9659258262890683122, 1.000000000000000000, 0.9659258262890683122, 1.000000000000000000, 0.9659258262890683122, 1.000000000000000000, 0.9659258262890683122, 1.000000000000000000, 0.9659258262890683122, 1.000000000000000000, 0.9659258262890683122, 1.000000000000000000, 0.9659258262890683122, 1.000000000000000000, 0.9659258262890683122, 1.000000000000000000, 0.9659258262890683122, 1.000000000000000000, 0.9659258262890683122, 1.000000000000000000, 0.9659258262890683122, 1.000000000000000000, 0.9659258262890683122, 1.000000000000000000, 0.9659258262890683122, 1.000000000000000000, 0.9659258262890683122, 1.000000000000000000, 0.9659258262890683122, 1.000000000000000000, 0.9659258262890683122, 1.000000000000000000, 0.9659258262890683122, 1.000000000000000000, 0.9659258262890683122, 1.000000000000000000, 0.9659258262890683122, 1.000000000000000000, 0.9659258262890683122, 1.000000000000000000, 0.9659258262890683122, 1.000000000000000000, 0.9659258262890683122, 1.000000000000000000, 0.9659258262890683122, 1.000000000000000000, 0.9659258262890683122, 1.000000000000000000, 0.9659258262890683122, 1.000000000000000000, 0.9659258262890683122, 1.000000000000000000, 0.9659258262890683122, 1.000000000000000000, 0.9659258262890683122, 1.000000000000000000, 0.9659258262890683122, 1.000000000000000000, 0.9659258262890683122, 1.000000000000000000, 0.9659258262890683122, 1.000000000000000000, 0.9659258262890683122, 1.000000000000000000, 0.9659258262890683122, 1.000000000000000000, 0.9659258262890683122, 1.000000000000000000, 0.9659258262890683122, 1.000000000000000000, 0.9659258262890683122, 1.000000000000000000, 0.9659258262890683122, 1.000000000000000000, 0.9659258262890683122, 1.000000000000000000, 0.9659258262890683122, 1.000000000000000000, 0.9659258262890683122, 1.000000000000000000, 0.9659258262890683122, 1.000000000000000000, 0.9659258262890683122, 1.000000000000000000, 0.9659258262890683122, 1.000000000000000000, 0.9659258262890683122, 1.000000000000000000, 0.9659258262890683122, 1.000000000000000000, 0.9659258262890683122, 1.000000000000000000, 0.9659258262890683122, 1.000000000000000000, 0.9659258262890683122, 1.000000000000000000, 0.9659258262890683122, 1.000000000000000000, 0.9659258262890683122, 1.000000000000000000, 0.9659258262890683122, 1.000000000000000000, 0.9659258262890683122, 1.000000000000000000, 0.9659258262890683122, 1.000000000000000000, 0.9659258262890683122, 1.000000000000000000, 0.9659258262890683122, 1.000000000000000000, 0.9659258262890683122, 1.000000000000000000, 0.9659258262890683122, 1.000000000000000000, 0.9659258262890683122, 1.000000000000000000, 0.9659258262890683122, 1.000000000000000000, 0.9659258262890683122, 1.000000000000000000, 0.9659258262890683122, 1.000000000000000000, 0.9659258262890683122, 1.000000000000000000, 0.9659258262890683122, 1.000000000000000000, 0.9659258262890683122, 1.000000000000000000, 0.9659258262890683122, 1.000000000000000000, 0.9659258262890683122, 1.000000000000000000, 0.9659258262890683122, 1.000000000000000000, 0.9659258262890683122, 1.000000000000000000, 0.9659258262890683122, 1.000000000000000000, 0.9659258262890683122, 1.000000000000000000, 0.9659258262890683122, 1.000000000000000000, 0.9659258262890683122, 1.000000000000000000, 0.9659258262890683122, 1.000000000000000000, 0.9659258262890683122, 1.000000000000000000, 0.9659258262890683122, 1.000000000000000000, 0.9659258262890683122, 1.000000000000000000, 0.9659258262890683122, 1.000000000000000000, 0.9659258262890683122, 1.000000000000000000, 0.9659258262890683122, 1.000000000000000000, 0.9659258262890683122, 1.000000000000000000, 0.9659258262890683122, 1.000000000000000000, 0.9659258262890683122, 1.000000000000000000, 0.9659258262890683122, 1.000000000000000000, 0.9659258262890683122, 1.000000000000000000, 0.9659258262890683122, 1.000000000000000000, 0.9659258262890683122, 1.000000000000000000, 0.9659258262890683122, 1.000000000000000000, 0.9659258262890683122, 1.000000000000000000, 0.9659258262890683122, 1.000000000000000000, 0.9659258262890683122, 1.000000000000000000, 0.9659258262890683122, 1.000000000000000000, 0.9659258262890683122, 1.000000000000000000, 0.9659258262890683122, 1.000000000000000000, 0.9659258262890683122, 1.000000000000000000, 0.9659258262890683122, 1.000000000000000000, 0.9659258262890683122, 1.000000000000000000, 0.9659258262890683122, 1.000000000000000000, 0.9659258262890683122, 1.000000000000000000, 0.9659258262890683122, 1.000000000000000000, 0.9659258262890683122, 1.000000000000000000, 0.9659258262890683122, 1.000000000000000000, 0.9659258262890683122, 1.000000000000000000, 0.9659258262890683122, 1.000000000000000000, 0.9659258262890683122, 1.000000000000000000, 0.9659258262890683122, 1.000000000000000000, 0.9659258262890683122, 1.000000000000000000, 0.9659258262890683122, 1.000000000000000000, 0.9659258262890683122, 1.000000000000000000, 0.9659258262890683122, 1.000000000000000000) ) ) 
 REPRESENTATION_ITEM ( '' )  SURFACE ( )  );
#130574=CARTESIAN_POINT ( 'NONE',  ( 15.72974639402176855, 15.80617190586768217, 26.87609039468567218 ) ) ;
#130576=CARTESIAN_POINT ( 'NONE',  ( 8.224510206698742110, 14.34966873604972548, 107.0844237280190043 ) ) ;
#130577=CARTESIAN_POINT ( 'NONE',  ( 16.55341960407611168, 4.379528057220329451, 113.9572429386477239 ) ) ;
#130578=CARTESIAN_POINT ( 'NONE',  ( -19.02544592524342804, 5.153800228976336051, 76.04057627198102409 ) ) ;
#130579=CARTESIAN_POINT ( 'NONE',  ( 16.20063489777861676, -7.373262058553140541, 22.00000000000000711 ) ) ;
#130581=CARTESIAN_POINT ( 'NONE',  ( -16.52544592524342804, 4.483927247898546575, 31.04057627198102409 ) ) ;
#130582=CARTESIAN_POINT ( 'NONE',  ( 21.53943276465977519, 0.05219959533937863772, 56.25109039468568284 ) ) ;
#130584=CARTESIAN_POINT ( 'NONE',  ( -10.81492255796105439, 18.62759615963255655, 87.91775706135234714 ) ) ;
#130585=CARTESIAN_POINT ( 'NONE',  ( -5.049401038298153566, 19.05341960407611168, 50.20724293864770260 ) ) ;
#130586=CARTESIAN_POINT ( 'NONE',  ( -16.46253265017160317, 9.564922557960807481, 50.83224293864770260 ) ) ;
#130587=ORIENTED_EDGE ( 'NONE', *, *, #181371, .F. ) ;
#130588=CARTESIAN_POINT ( 'NONE',  ( 21.55341960407619695, -5.719274019375665929, 96.04275706135236135 ) ) ;
#130589=CARTESIAN_POINT ( 'NONE',  ( 14.34966873604972726, -8.224510206698740333, 60.83442372801901854 ) ) ;
#130590=CARTESIAN_POINT ( 'NONE',  ( -21.52544592524334988, -5.823673210054445271, 88.95942372801901854 ) ) ;
#130591=CARTESIAN_POINT ( 'NONE',  ( 10.81492255796078972, 18.62759615963270932, 24.58224293864768839 ) ) ;
#130592=CARTESIAN_POINT ( 'NONE',  ( 5.153800228976615827, -19.02544592524334988, 95.20942372801897591 ) ) ;
#130593=CARTESIAN_POINT ( 'NONE',  ( 21.53943276465977519, 0.05219959533937863772, 66.25109039468567573 ) ) ;
#130594=CARTESIAN_POINT ( 'NONE',  ( 4.483927247898790824, -16.52544592524335698, 35.20942372801901854 ) ) ;
#130595=CARTESIAN_POINT ( 'NONE',  ( 21.55341960407610458, 5.719274019375980345, 88.95724293864769550 ) ) ;
#130596=CARTESIAN_POINT ( 'NONE',  ( 13.97604488694548053, -13.89961937509957401, 80.62609039468567573 ) ) ;
#130597=CARTESIAN_POINT ( 'NONE',  ( 13.97604488694527802, 13.89961937509977652, 64.37390960531436690 ) ) ;
#130598=CARTESIAN_POINT ( 'NONE',  ( -9.564922557961040184, 16.46253265017147172, 97.91775706135233293 ) ) ;
#130600=CARTESIAN_POINT ( 'NONE',  ( 5.049401038297881783, 19.05341960407617563, 107.2927570613523187 ) ) ;
#130601=CARTESIAN_POINT ( 'NONE',  ( 14.29746914071049879, -8.314922557960816363, 53.33224293864769550 ) ) ;
#130603=CARTESIAN_POINT ( 'NONE',  ( 16.51473224551083163, -9.474510206698727899, 75.83442372801900433 ) ) ;
#130604=CARTESIAN_POINT ( 'NONE',  ( 4.483927247898790824, -16.52544592524335698, 65.20942372801901854 ) ) ;
#130605=CARTESIAN_POINT ( 'NONE',  ( -13.89961937509977652, 13.97604488694528158, 35.62390960531435269 ) ) ;
#130606=CARTESIAN_POINT ( 'NONE',  ( -0.05219959533909027116, -19.03943276465977164, 57.49890960531435979 ) ) ;
#130607=CARTESIAN_POINT ( 'NONE',  ( 16.55341960407618274, -4.379528057220086978, 56.04275706135235424 ) ) ;
#130609=CARTESIAN_POINT ( 'NONE',  ( -5.049401038298153566, 19.05341960407611168, 110.2072429386476671 ) ) ;
#130610=CARTESIAN_POINT ( 'NONE',  ( 19.05341960407611168, 5.049401038298154454, 23.95724293864769194 ) ) ;
#130612=CARTESIAN_POINT ( 'NONE',  ( 13.89961937509957401, 13.97604488694547697, 106.8760903946856757 ) ) ;
#130613=CARTESIAN_POINT ( 'NONE',  ( -10.81492255796078084, -18.62759615963271287, 42.08224293864769550 ) ) ;
#130614=CARTESIAN_POINT ( 'NONE',  ( 9.564922557961047289, -16.46253265017146816, 35.41775706135233293 ) ) ;
#130615=CARTESIAN_POINT ( 'NONE',  ( -14.34966873604972548, 8.224510206698743886, 28.33442372801902209 ) ) ;
#130616=CARTESIAN_POINT ( 'NONE',  ( 19.03943276465977164, -0.05219959533909143690, 23.74890960531435269 ) ) ;
#130617=CARTESIAN_POINT ( 'NONE',  ( -9.474510206698964154, 16.51473224551069663, 45.41557627198103120 ) ) ;
#130618=CARTESIAN_POINT ( 'NONE',  ( -15.72974639402197994, 15.80617190586746368, 75.62390960531439532 ) ) ;
#130619=CARTESIAN_POINT ( 'NONE',  ( -16.51473224551069308, -9.474510206698971260, 101.6655762719810241 ) ) ;
#130620=CARTESIAN_POINT ( 'NONE',  ( 19.05341960407611168, 5.049401038298154454, 53.95724293864770260 ) ) ;
#130622=CARTESIAN_POINT ( 'NONE',  ( 5.153800228976615827, -19.02544592524334988, 80.20942372801901854 ) ) ;
#130623=CARTESIAN_POINT ( 'NONE',  ( -16.52544592524342804, 4.483927247898546575, 71.04057627198103830 ) ) ;
#130624=CARTESIAN_POINT ( 'NONE',  ( 21.52544592524344225, -5.823673210054117533, 48.54057627198103120 ) ) ;
#130625=CARTESIAN_POINT ( 'NONE',  ( -18.62759615963255300, -10.81492255796106328, 109.1677570613523613 ) ) ;
#130626=CARTESIAN_POINT ( 'NONE',  ( -5.823673210054116645, -21.52544592524344225, 97.29057627198105251 ) ) ;
#130627=CARTESIAN_POINT ( 'NONE',  ( -10.72451020669870658, -18.67979575497194134, 69.58442372801900433 ) ) ;
#130628=B_SPLINE_CURVE_WITH_KNOTS ( 'NONE', 3,
 ( #73957, #130862, #29435, #105270, #91066, #182119, #59753, #122414, #137589, #38870, #90095, #131873, #199272, #12292, #167936, #70206, #152753, #54036, #121423, #14243, #106253, #197296, #75915, #151777, #115710, #74933, #193558, #177398, #58759, #183115, #120428, #136596 ),
 .UNSPECIFIED., .F., .F.,
 ( 4, 2, 2, 2, 2, 2, 2, 2, 2, 2, 2, 2, 2, 2, 2, 4 ),
 ( 2.969368287472575283E-17, 0.0003712461730036904100, 0.0007424923460073511129, 0.001113738519011011653, 0.001484984692014672519, 0.002227477038022000321, 0.002598723211025682003, 0.002969969384029364119, 0.003341215557033045368, 0.003712461730036727917, 0.004083707903040409599, 0.004454954076044090848, 0.004826200249047772964, 0.005197446422051455080, 0.005568692595055137196, 0.005939938768058818444 ),
 .UNSPECIFIED. ) ;
#130629=CARTESIAN_POINT ( 'NONE',  ( -21.52544592524334988, -5.823673210054445271, 78.95942372801901854 ) ) ;
#130631=CARTESIAN_POINT ( 'NONE',  ( 16.51473224551069308, 9.474510206698969483, 114.1655762719810241 ) ) ;
#130632=CARTESIAN_POINT ( 'NONE',  ( -0.05219959533934338120, 16.53943276465976808, 112.5010903946857042 ) ) ;
#130633=CARTESIAN_POINT ( 'NONE',  ( 15.72974639402176855, 15.80617190586768217, 71.87609039468568994 ) ) ;
#130634=CARTESIAN_POINT ( 'NONE',  ( -19.03943276465977164, 0.05219959533909376836, 66.24890960531436690 ) ) ;
#130635=CARTESIAN_POINT ( 'NONE',  ( -21.53943276465977519, -0.05219959533937600094, 28.75109039468567929 ) ) ;
#130636=CARTESIAN_POINT ( 'NONE',  ( -5.049401038298153566, 19.05341960407611168, 65.20724293864765286 ) ) ;
#130637=CARTESIAN_POINT ( 'NONE',  ( 12.14591786802309770, 12.06949235617756955, 74.37390960531436690 ) ) ;
#130638=CARTESIAN_POINT ( 'NONE',  ( 12.06949235617757843, -12.14591786802309237, 43.12390960531435269 ) ) ;
#130639=CARTESIAN_POINT ( 'NONE',  ( 15.72974639402199770, -15.80617190586745480, 53.12390960531436690 ) ) ;
#130641=CARTESIAN_POINT ( 'NONE',  ( -19.05341960407611168, -5.049401038298163336, 61.45724293864769550 ) ) ;
#130642=CARTESIAN_POINT ( 'NONE',  ( 21.55341960407610458, 5.719274019375980345, 68.95724293864769550 ) ) ;
#130643=CARTESIAN_POINT ( 'NONE',  ( 19.05341960407617918, -5.049401038297876454, 66.04275706135233293 ) ) ;
#130644=CARTESIAN_POINT ( 'NONE',  ( -16.46253265017146816, -9.564922557961047289, 19.16775706135233293 ) ) ;
#130645=CARTESIAN_POINT ( 'NONE',  ( 4.483927247898545687, 16.52544592524342804, 64.79057627198103830 ) ) ;
#130646=CARTESIAN_POINT ( 'NONE',  ( 18.62759615963271287, -10.81492255796078972, 43.33224293864769550 ) ) ;
#130648=LINE ( 'NONE', #126654, #133424 ) ;
#130649=CARTESIAN_POINT ( 'NONE',  ( 16.52544592524335698, 4.483927247898782831, 96.45942372801901854 ) ) ;
#130651=CARTESIAN_POINT ( 'NONE',  ( -13.89961937509957401, -13.97604488694547875, 84.37609039468567573 ) ) ;
#130652=CARTESIAN_POINT ( 'NONE',  ( 12.06949235617757843, -12.14591786802309237, 73.12390960531436690 ) ) ;
#130654=CARTESIAN_POINT ( 'NONE',  ( -5.049401038298153566, 19.05341960407611168, 65.20724293864765286 ) ) ;
#130655=CARTESIAN_POINT ( 'NONE',  ( -14.34966873604960291, -8.224510206698953496, 51.66557627198102409 ) ) ;
#130656=CARTESIAN_POINT ( 'NONE',  ( -5.153800228976328057, -19.02544592524343514, 82.29057627198103830 ) ) ;
#130658=CARTESIAN_POINT ( 'NONE',  ( 13.97604488694548053, -13.89961937509957401, 75.62609039468564731 ) ) ;
#130659=CARTESIAN_POINT ( 'NONE',  ( 0.05219959533909260263, 19.03943276465977164, 49.99890960531435979 ) ) ;
#130660=CARTESIAN_POINT ( 'NONE',  ( -9.474510206698964154, 16.51473224551069663, 80.41557627198103830 ) ) ;
#130661=CARTESIAN_POINT ( 'NONE',  ( -16.51473224551069308, -9.474510206698971260, 21.66557627198102765 ) ) ;
#130662=CARTESIAN_POINT ( 'NONE',  ( -19.05341960407611168, -5.049401038298163336, 66.45724293864769550 ) ) ;
#130663=CARTESIAN_POINT ( 'NONE',  ( -21.53943276465977519, 0.05219959533907696930, 56.24890960531436690 ) ) ;
#130664=CARTESIAN_POINT ( 'NONE',  ( -16.46253265017160317, 9.564922557960807481, 45.83224293864769550 ) ) ;
#130665=CARTESIAN_POINT ( 'NONE',  ( 21.52544592524344225, -5.823673210054117533, 53.54057627198103120 ) ) ;
#130666=CARTESIAN_POINT ( 'NONE',  ( 9.564922557961047289, -16.46253265017146816, 80.41775706135234714 ) ) ;
#130667=CARTESIAN_POINT ( 'NONE',  ( -8.314922557961024197, 14.29746914071037800, 102.9177570613523756 ) ) ;
#130668=CARTESIAN_POINT ( 'NONE',  ( 9.474510206698729675, 16.51473224551082808, 42.08442372801900433 ) ) ;
#130669=CARTESIAN_POINT ( 'NONE',  ( -0.05219959533934338120, 16.53943276465976808, 57.50109039468568994 ) ) ;
#130670=CARTESIAN_POINT ( 'NONE',  ( -16.53943276465976808, -0.05219959533934237506, 98.75109039468568994 ) ) ;
#130671=CARTESIAN_POINT ( 'NONE',  ( 18.39443945427631277, -5.499999999999984013, 41.01745347608650860 ) ) ;
#130672=CARTESIAN_POINT ( 'NONE',  ( 14.29746914071037800, 8.314922557961029526, 76.66775706135234714 ) ) ;
#130673=CARTESIAN_POINT ( 'NONE',  ( -5.719274019375978568, 21.55341960407610458, 30.20724293864769550 ) ) ;
#130674=CARTESIAN_POINT ( 'NONE',  ( -19.05341960407611168, -5.049401038298163336, 31.45724293864769550 ) ) ;
#130675=CARTESIAN_POINT ( 'NONE',  ( -16.53943276465976808, -0.05219959533934237506, 33.75109039468568284 ) ) ;
#130676=CARTESIAN_POINT ( 'NONE',  ( 9.564922557960805705, 16.46253265017160317, 44.58224293864769550 ) ) ;
#130677=CARTESIAN_POINT ( 'NONE',  ( -18.67979575497193778, 10.72451020669871902, 43.33442372801901143 ) ) ;
#130678=CARTESIAN_POINT ( 'NONE',  ( -16.52544592524335698, -4.483927247898792601, 43.95942372801902565 ) ) ;
#130679=CARTESIAN_POINT ( 'NONE',  ( -8.314922557960811034, -14.29746914071050412, 22.08224293864769194 ) ) ;
#130680=CARTESIAN_POINT ( 'NONE',  ( 5.153800228976335163, 19.02544592524342804, 24.79057627198102765 ) ) ;
#130681=CARTESIAN_POINT ( 'NONE',  ( 16.46253265017146816, 9.564922557961045513, 21.66775706135233648 ) ) ;
#130682=CARTESIAN_POINT ( 'NONE',  ( 13.97604488694548053, -13.89961937509957401, 110.6260903946856615 ) ) ;
#130683=CARTESIAN_POINT ( 'NONE',  ( -9.564922557961040184, 16.46253265017147172, 67.91775706135233293 ) ) ;
#130684=CARTESIAN_POINT ( 'NONE',  ( 14.34966873604960469, 8.224510206698951720, 69.16557627198102409 ) ) ;
#130685=CARTESIAN_POINT ( 'NONE',  ( 5.049401038298161559, -19.05341960407611168, 42.70724293864767418 ) ) ;
#130686=CARTESIAN_POINT ( 'NONE',  ( 13.97604488694548053, -13.89961937509957401, 80.62609039468567573 ) ) ;
#130688=CARTESIAN_POINT ( 'NONE',  ( 21.53943276465977519, 0.05219959533937863772, 66.25109039468567573 ) ) ;
#130689=CARTESIAN_POINT ( 'NONE',  ( 16.52544592524335698, 4.483927247898782831, 46.45942372801901854 ) ) ;
#130690=CARTESIAN_POINT ( 'NONE',  ( 19.52837319214028255, -5.499999999999890754, 57.10471352585541638 ) ) ;
#130691=CARTESIAN_POINT ( 'NONE',  ( -21.55341960407610458, -5.719274019375992779, 31.45724293864769550 ) ) ;
#130692=CARTESIAN_POINT ( 'NONE',  ( 16.53943276465976808, 0.05219959533934440121, 26.25109039468567573 ) ) ;
#130695=CARTESIAN_POINT ( 'NONE',  ( 19.03943276465977164, -0.05219959533909143690, 43.74890960531435979 ) ) ;
#130696=CARTESIAN_POINT ( 'NONE',  ( -0.05219959533937732626, 21.53943276465977519, 107.5010903946856899 ) ) ;
#130697=CARTESIAN_POINT ( 'NONE',  ( -13.89961937509977652, 13.97604488694528158, 50.62390960531435979 ) ) ;
#130698=CARTESIAN_POINT ( 'NONE',  ( -10.72451020669870658, -18.67979575497194134, 69.58442372801900433 ) ) ;
#130699=CARTESIAN_POINT ( 'NONE',  ( 21.52544592524334988, 5.823673210054432836, 106.4594237280190328 ) ) ;
#130700=CARTESIAN_POINT ( 'NONE',  ( -16.55341960407617563, 4.379528057220093196, 113.5427570613523756 ) ) ;
#130701=CARTESIAN_POINT ( 'NONE',  ( -13.89961937509977652, 13.97604488694528158, 35.62390960531435269 ) ) ;
#130702=CARTESIAN_POINT ( 'NONE',  ( -19.05341960407611168, -5.049401038298163336, 86.45724293864769550 ) ) ;
#130703=CARTESIAN_POINT ( 'NONE',  ( 21.52544592524334988, 5.823673210054432836, 51.45942372801901854 ) ) ;
#130704=CARTESIAN_POINT ( 'NONE',  ( -9.564922557960796823, -16.46253265017161027, 32.08224293864769550 ) ) ;
#130706=CARTESIAN_POINT ( 'NONE',  ( -18.67979575497193778, 10.72451020669871902, 48.33442372801902565 ) ) ;
#130707=CARTESIAN_POINT ( 'NONE',  ( -16.46253265017146816, -9.564922557961047289, 94.16775706135233293 ) ) ;
#130708=CARTESIAN_POINT ( 'NONE',  ( -5.153800228976328057, -19.02544592524343514, 107.2905762719810383 ) ) ;
#130709=CARTESIAN_POINT ( 'NONE',  ( 19.05341960407611168, 5.049401038298154454, 23.95724293864769194 ) ) ;
#130710=CARTESIAN_POINT ( 'NONE',  ( -21.52544592524343514, 5.823673210054127303, 111.0405762719810525 ) ) ;
#130711=CARTESIAN_POINT ( 'NONE',  ( 16.46253265017146816, 9.564922557961045513, 31.66775706135232937 ) ) ;
#130712=CARTESIAN_POINT ( 'NONE',  ( 16.52544592524342804, -4.483927247898539470, 113.5405762719810383 ) ) ;
#130713=CARTESIAN_POINT ( 'NONE',  ( -0.05219959533909027116, -19.03943276465977164, 62.49890960531435979 ) ) ;
#130714=CARTESIAN_POINT ( 'NONE',  ( 13.89961937509957401, 13.97604488694547697, 91.87609039468567573 ) ) ;
#130716=CARTESIAN_POINT ( 'NONE',  ( -4.379528057220328563, 16.55341960407611168, 65.20724293864768129 ) ) ;
#130717=CARTESIAN_POINT ( 'NONE',  ( 5.049401038297881783, 19.05341960407617563, 27.29275706135232937 ) ) ;
#130718=CARTESIAN_POINT ( 'NONE',  ( 5.049401038298161559, -19.05341960407611168, 112.7072429386476813 ) ) ;
#130719=CARTESIAN_POINT ( 'NONE',  ( -9.474510206698720793, -16.51473224551083518, 94.58442372801900433 ) ) ;
#130720=CARTESIAN_POINT ( 'NONE',  ( -21.53943276465977519, 0.05219959533907696930, 91.24890960531436690 ) ) ;
#130722=CARTESIAN_POINT ( 'NONE',  ( 15.80617190586769283, -15.72974639402175789, 45.62609039468567573 ) ) ;
#130723=CARTESIAN_POINT ( 'NONE',  ( -4.483927247898782831, 16.52544592524335698, 42.70942372801901854 ) ) ;
#130724=CARTESIAN_POINT ( 'NONE',  ( -0.05219959533934338120, 16.53943276465976808, 102.5010903946856899 ) ) ;
#130725=CARTESIAN_POINT ( 'NONE',  ( 4.483927247898790824, -16.52544592524335698, 45.20942372801901854 ) ) ;
#130726=CARTESIAN_POINT ( 'NONE',  ( -10.72451020669870658, -18.67979575497194134, 49.58442372801901143 ) ) ;
#130727=CARTESIAN_POINT ( 'NONE',  ( -21.55341960407610458, -5.719274019375992779, 51.45724293864770260 ) ) ;
#130728=CARTESIAN_POINT ( 'NONE',  ( 13.89961937509977652, -13.97604488694527269, 28.12390960531435624 ) ) ;
#130730=CARTESIAN_POINT ( 'NONE',  ( 0.05219959533934541429, -16.53943276465976808, 60.00109039468568284 ) ) ;
#130731=CARTESIAN_POINT ( 'NONE',  ( 10.72451020669898902, -18.67979575497178502, 87.91557627198103830 ) ) ;
#130732=CARTESIAN_POINT ( 'NONE',  ( 4.483927247898545687, 16.52544592524342804, 39.79057627198103830 ) ) ;
#130733=CARTESIAN_POINT ( 'NONE',  ( -8.224510206698735004, -14.34966873604973081, 59.58442372801901854 ) ) ;
#130734=CARTESIAN_POINT ( 'NONE',  ( -19.05341960407617563, 5.049401038297882671, 103.5427570613523329 ) ) ;
#130735=CARTESIAN_POINT ( 'NONE',  ( 5.719274019375991003, -21.55341960407610458, 97.70724293864772392 ) ) ;
#130736=CARTESIAN_POINT ( 'NONE',  ( 16.53943276465976808, -0.05219959533910856209, 33.74890960531436690 ) ) ;
#130738=CARTESIAN_POINT ( 'NONE',  ( -16.53943276465976808, -0.05219959533934237506, 73.75109039468567573 ) ) ;
#130740=CARTESIAN_POINT ( 'NONE',  ( -18.62759615963270932, 10.81492255796079327, 70.83224293864770971 ) ) ;
#130741=CARTESIAN_POINT ( 'NONE',  ( 16.52544592524335698, 4.483927247898782831, 101.4594237280190185 ) ) ;
#130743=CARTESIAN_POINT ( 'NONE',  ( 19.20446147854527297, 5.499999999999894307, 86.88999695167679249 ) ) ;
#130744=CARTESIAN_POINT ( 'NONE',  ( 21.55341960407610458, 5.719274019375980345, 93.95724293864770971 ) ) ;
#130745=CARTESIAN_POINT ( 'NONE',  ( -18.62759615963270932, 10.81492255796079327, 105.8322429386476955 ) ) ;
#130746=CARTESIAN_POINT ( 'NONE',  ( 12.14591786802309770, 12.06949235617756955, 39.37390960531436690 ) ) ;
#130748=CARTESIAN_POINT ( 'NONE',  ( -14.29746914071037622, -8.314922557961029526, 39.16775706135235424 ) ) ;
#130749=CARTESIAN_POINT ( 'NONE',  ( -19.05341960407611168, -5.049401038298163336, 46.45724293864768129 ) ) ;
#130750=CARTESIAN_POINT ( 'NONE',  ( 19.03943276465977164, -0.05219959533909143690, 63.74890960531435979 ) ) ;
#130751=CARTESIAN_POINT ( 'NONE',  ( 13.97604488694527802, 13.89961937509977652, 114.3739096053143669 ) ) ;
#130752=CARTESIAN_POINT ( 'NONE',  ( -9.474510206698964154, 16.51473224551069663, 115.4155762719810241 ) ) ;
#130753=CARTESIAN_POINT ( 'NONE',  ( -9.564922557961040184, 16.46253265017147172, 102.9177570613523329 ) ) ;
#130754=CARTESIAN_POINT ( 'NONE',  ( -19.02544592524334988, -5.153800228976617603, 48.95942372801900433 ) ) ;
#130755=CARTESIAN_POINT ( 'NONE',  ( 18.67979575497178502, 10.72451020669898547, 94.16557627198103830 ) ) ;
#130756=CARTESIAN_POINT ( 'NONE',  ( -12.06949235617756955, 12.14591786802309770, 25.62390960531435624 ) ) ;
#130757=CARTESIAN_POINT ( 'NONE',  ( 10.72451020669898902, -18.67979575497178502, 42.91557627198103120 ) ) ;
#130758=CARTESIAN_POINT ( 'NONE',  ( 18.67979575497178502, 10.72451020669898547, 84.16557627198103830 ) ) ;
#130759=CARTESIAN_POINT ( 'NONE',  ( -5.049401038297874678, -19.05341960407617918, 109.7927570613523187 ) ) ;
#130760=CARTESIAN_POINT ( 'NONE',  ( -5.049401038298153566, 19.05341960407611168, 105.2072429386476671 ) ) ;
#130761=CARTESIAN_POINT ( 'NONE',  ( 5.823673210054444382, -21.52544592524334988, 75.20942372801901854 ) ) ;
#130762=CARTESIAN_POINT ( 'NONE',  ( 13.89961937509977652, -13.97604488694527269, 68.12390960531436690 ) ) ;
#130764=CARTESIAN_POINT ( 'NONE',  ( -5.049401038298153566, 19.05341960407611168, 70.20724293864769550 ) ) ;
#130765=CARTESIAN_POINT ( 'NONE',  ( -8.224510206698948167, 14.34966873604960824, 85.41557627198102409 ) ) ;
#130767=CARTESIAN_POINT ( 'NONE',  ( -9.474510206698720793, -16.51473224551083518, 104.5844237280190043 ) ) ;
#130768=CARTESIAN_POINT ( 'NONE',  ( 16.18388926212238488, -7.379444403734519931, 82.06046848633847901 ) ) ;
#130769=CARTESIAN_POINT ( 'NONE',  ( 19.05341960407611168, 5.049401038298154454, 68.95724293864769550 ) ) ;
#130770=CARTESIAN_POINT ( 'NONE',  ( -5.719274019375665041, -21.55341960407619695, 84.79275706135234714 ) ) ;
#130771=CARTESIAN_POINT ( 'NONE',  ( -9.564922557960796823, -16.46253265017161027, 97.08224293864769550 ) ) ;
#130772=CARTESIAN_POINT ( 'NONE',  ( 8.224510206698742110, 14.34966873604972548, 82.08442372801901854 ) ) ;
#130774=CARTESIAN_POINT ( 'NONE',  ( -5.153800228976607833, 19.02544592524334988, 62.70942372801899722 ) ) ;
#130775=CARTESIAN_POINT ( 'NONE',  ( -15.72974639402176322, -15.80617190586768395, 94.37609039468568994 ) ) ;
#130779=CARTESIAN_POINT ( 'NONE',  ( -4.379528057220086978, -16.55341960407618274, 109.7927570613523613 ) ) ;
#130780=CARTESIAN_POINT ( 'NONE',  ( 0.05219959533936267826, -19.03943276465977164, 75.00109039468566152 ) ) ;
#130781=CARTESIAN_POINT ( 'NONE',  ( 0.05219959533934541429, -16.53943276465976808, 90.00109039468567573 ) ) ;
#130783=CARTESIAN_POINT ( 'NONE',  ( -12.14591786802326823, 12.06949235617739902, 73.12609039468567573 ) ) ;
#130784=CARTESIAN_POINT ( 'NONE',  ( 5.719274019375673035, 21.55341960407619339, 82.29275706135234714 ) ) ;
#130785=CARTESIAN_POINT ( 'NONE',  ( 19.03943276465977164, 0.05219959533936151252, 86.25109039468567573 ) ) ;
#130786=CARTESIAN_POINT ( 'NONE',  ( -19.05341960407617563, 5.049401038297882671, 33.54275706135231871 ) ) ;
#130788=CARTESIAN_POINT ( 'NONE',  ( -19.03943276465977164, 0.05219959533909376836, 66.24890960531436690 ) ) ;
#130789=CARTESIAN_POINT ( 'NONE',  ( -5.049401038298153566, 19.05341960407611168, 55.20724293864769550 ) ) ;
#130790=CARTESIAN_POINT ( 'NONE',  ( -16.51473224551069308, -9.474510206698971260, 86.66557627198102409 ) ) ;
#130791=CARTESIAN_POINT ( 'NONE',  ( 10.72451020669898902, -18.67979575497178502, 82.91557627198103830 ) ) ;
#130792=CARTESIAN_POINT ( 'NONE',  ( -18.62759615963270932, 10.81492255796079327, 50.83224293864770971 ) ) ;
#130793=CARTESIAN_POINT ( 'NONE',  ( 5.049401038298161559, -19.05341960407611168, 27.70724293864769550 ) ) ;
#130794=CARTESIAN_POINT ( 'NONE',  ( 4.483927247898790824, -16.52544592524335698, 70.20942372801904696 ) ) ;
#130797=CARTESIAN_POINT ( 'NONE',  ( 18.67979575497194134, -10.72451020669871369, 45.83442372801901854 ) ) ;
#130798=CONICAL_SURFACE ( 'NONE', #43654, 2.500000000000002220, 1.029744258676656754 ) ;
#130799=CARTESIAN_POINT ( 'NONE',  ( -8.224510206698948167, 14.34966873604960824, 60.41557627198102409 ) ) ;
#130801=CARTESIAN_POINT ( 'NONE',  ( 12.06949235617739724, 12.14591786802326823, 41.87609039468568284 ) ) ;
#130802=CARTESIAN_POINT ( 'NONE',  ( 5.049401038297881783, 19.05341960407617563, 57.29275706135231871 ) ) ;
#130803=CARTESIAN_POINT ( 'NONE',  ( 16.55341960407611168, 4.379528057220329451, 53.95724293864770260 ) ) ;
#130804=CARTESIAN_POINT ( 'NONE',  ( 18.62759615963255655, 10.81492255796105972, 36.66775706135234714 ) ) ;
#130806=CARTESIAN_POINT ( 'NONE',  ( 5.719274019375991003, -21.55341960407610458, 87.70724293864769550 ) ) ;
#130807=CARTESIAN_POINT ( 'NONE',  ( 19.02544592524343514, -5.153800228976328945, 103.5405762719809957 ) ) ;
#130808=CARTESIAN_POINT ( 'NONE',  ( 0.05219959533910956823, 16.53943276465976808, 79.99890960531435269 ) ) ;
#130811=CARTESIAN_POINT ( 'NONE',  ( 16.46253265017146816, 9.564922557961045513, 66.66775706135233293 ) ) ;
#130812=CARTESIAN_POINT ( 'NONE',  ( -21.53943276465977519, -0.05219959533937600094, 18.75109039468568639 ) ) ;
#130813=CARTESIAN_POINT ( 'NONE',  ( -0.05219959533909027116, -19.03943276465977164, 57.49890960531435979 ) ) ;
#130814=CARTESIAN_POINT ( 'NONE',  ( 19.03943276465977164, 0.05219959533936151252, 61.25109039468566863 ) ) ;
#130815=CARTESIAN_POINT ( 'NONE',  ( 9.474510206698971260, -16.51473224551069308, 27.91557627198103120 ) ) ;
#130816=CARTESIAN_POINT ( 'NONE',  ( 5.823673210054444382, -21.52544592524334988, 70.20942372801904696 ) ) ;
#130817=CARTESIAN_POINT ( 'NONE',  ( -16.21995358207302829, -7.366697692864232039, 70.06448998487846325 ) ) ;
#130818=CARTESIAN_POINT ( 'NONE',  ( -12.14591786802309592, -12.06949235617757132, 51.87390960531437401 ) ) ;
#130819=CARTESIAN_POINT ( 'NONE',  ( -5.049401038298153566, 19.05341960407611168, 60.20724293864768129 ) ) ;
#130820=CARTESIAN_POINT ( 'NONE',  ( -21.53943276465977519, 0.05219959533907696930, 91.24890960531436690 ) ) ;
#130821=CARTESIAN_POINT ( 'NONE',  ( 9.474510206698971260, -16.51473224551069308, 52.91557627198102409 ) ) ;
#130822=ORIENTED_EDGE ( 'NONE', *, *, #94296, .T. ) ;
#130823=CARTESIAN_POINT ( 'NONE',  ( 5.823673210054125526, 21.52544592524343514, 79.79057627198102409 ) ) ;
#130825=CARTESIAN_POINT ( 'NONE',  ( -18.67979575497193778, 10.72451020669871902, 103.3344237280190043 ) ) ;
#130826=CARTESIAN_POINT ( 'NONE',  ( 9.474510206698971260, -16.51473224551069308, 22.91557627198102765 ) ) ;
#130827=CARTESIAN_POINT ( 'NONE',  ( -16.52544592524335698, -4.483927247898792601, 93.95942372801903275 ) ) ;
#130828=CARTESIAN_POINT ( 'NONE',  ( 14.34966873604960469, 8.224510206698951720, 94.16557627198103830 ) ) ;
#130829=CARTESIAN_POINT ( 'NONE',  ( -9.564922557961040184, 16.46253265017147172, 97.91775706135233293 ) ) ;
#130831=CARTESIAN_POINT ( 'NONE',  ( 10.72451020669871369, 18.67979575497193778, 22.08442372801901143 ) ) ;
#130832=CARTESIAN_POINT ( 'NONE',  ( -5.153800228976607833, 19.02544592524334988, 37.70942372801899722 ) ) ;
#130833=CARTESIAN_POINT ( 'NONE',  ( -14.34966873604972548, 8.224510206698743886, 103.3344237280190043 ) ) ;
#130834=CARTESIAN_POINT ( 'NONE',  ( -16.46253265017146816, -9.564922557961047289, 29.16775706135232937 ) ) ;
#130835=CARTESIAN_POINT ( 'NONE',  ( -9.564922557960796823, -16.46253265017161027, 92.08224293864769550 ) ) ;
#130836=CARTESIAN_POINT ( 'NONE',  ( -0.05219959533907301413, -21.53943276465977519, 67.49890960531436690 ) ) ;
#130837=CARTESIAN_POINT ( 'NONE',  ( -19.01533133064921088, 5.499999999999432454, 48.76586590595736226 ) ) ;
#130838=CARTESIAN_POINT ( 'NONE',  ( -19.05341960407611168, -5.049401038298163336, 21.45724293864768839 ) ) ;
#130839=CARTESIAN_POINT ( 'NONE',  ( -16.46253265017146816, -9.564922557961047289, 19.16775706135233293 ) ) ;
#130840=CARTESIAN_POINT ( 'NONE',  ( 16.55341960407618274, -4.379528057220086978, 81.04275706135236135 ) ) ;
#130841=CARTESIAN_POINT ( 'NONE',  ( -0.05219959533937732626, 21.53943276465977519, 22.50109039468567573 ) ) ;
#130842=CARTESIAN_POINT ( 'NONE',  ( -14.29746914071037622, -8.314922557961029526, 29.16775706135234003 ) ) ;
#130843=CARTESIAN_POINT ( 'NONE',  ( 5.049401038298161559, -19.05341960407611168, 107.7072429386476955 ) ) ;
#130844=CARTESIAN_POINT ( 'NONE',  ( -13.89961937509977652, 13.97604488694528158, 40.62390960531435979 ) ) ;
#130845=CARTESIAN_POINT ( 'NONE',  ( -5.049401038298153566, 19.05341960407611168, 70.20724293864769550 ) ) ;
#130846=CARTESIAN_POINT ( 'NONE',  ( 8.314922557961029526, -14.29746914071037800, 45.41775706135234003 ) ) ;
#130847=CARTESIAN_POINT ( 'NONE',  ( -8.314922557960811034, -14.29746914071050412, 87.08224293864769550 ) ) ;
#130848=CARTESIAN_POINT ( 'NONE',  ( 16.55341960407618274, -4.379528057220086978, 96.04275706135236135 ) ) ;
#130849=CARTESIAN_POINT ( 'NONE',  ( -15.80617190586768217, 15.72974639402176855, 58.12609039468568994 ) ) ;
#130850=CARTESIAN_POINT ( 'NONE',  ( -19.03943276465977164, 0.05219959533909376836, 76.24890960531435269 ) ) ;
#130851=CARTESIAN_POINT ( 'NONE',  ( -13.89961937509977652, 13.97604488694528158, 70.62390960531432427 ) ) ;
#130852=CARTESIAN_POINT ( 'NONE',  ( -19.02544592524342804, 5.153800228976336051, 101.0405762719810241 ) ) ;
#130853=CARTESIAN_POINT ( 'NONE',  ( -16.55341960407611168, -4.379528057220339221, 46.45724293864769550 ) ) ;
#130854=CARTESIAN_POINT ( 'NONE',  ( -4.379528057220086978, -16.55341960407618274, 94.79275706135234714 ) ) ;
#130856=CARTESIAN_POINT ( 'NONE',  ( 13.89961937509957401, 13.97604488694547697, 46.87609039468565442 ) ) ;
#130857=CARTESIAN_POINT ( 'NONE',  ( 9.564922557960805705, 16.46253265017160317, 114.5822429386476955 ) ) ;
#130859=CARTESIAN_POINT ( 'NONE',  ( -9.564922557960796823, -16.46253265017161027, 62.08224293864769550 ) ) ;
#130860=CARTESIAN_POINT ( 'NONE',  ( 0.05219959533936267826, -19.03943276465977164, 45.00109039468566863 ) ) ;
#130862=CARTESIAN_POINT ( 'NONE',  ( -17.49999999999998934, -5.624438216177606087, 64.18329655085355512 ) ) ;
#130863=CARTESIAN_POINT ( 'NONE',  ( -14.29746914071037622, -8.314922557961029526, 59.16775706135234714 ) ) ;
#130865=CARTESIAN_POINT ( 'NONE',  ( 0.05219959533936267826, -19.03943276465977164, 70.00109039468566152 ) ) ;
#130866=CARTESIAN_POINT ( 'NONE',  ( 12.06949235617739724, 12.14591786802326823, 71.87609039468568994 ) ) ;
#130867=CARTESIAN_POINT ( 'NONE',  ( 17.40805194822030799, 6.112264579159338851, 91.66628727489390371 ) ) ;
#130868=CARTESIAN_POINT ( 'NONE',  ( 16.51473224551069308, 9.474510206698969483, 84.16557627198102409 ) ) ;
#130869=CARTESIAN_POINT ( 'NONE',  ( -5.823673210054431948, 21.52544592524334988, 27.70942372801901854 ) ) ;
#130870=CARTESIAN_POINT ( 'NONE',  ( -0.05219959533936034679, 19.03943276465977164, 77.50109039468566152 ) ) ;
#130871=CARTESIAN_POINT ( 'NONE',  ( -16.51473224551069308, -9.474510206698971260, 106.6655762719810383 ) ) ;
#130872=CARTESIAN_POINT ( 'NONE',  ( 16.51473224551069308, 9.474510206698969483, 39.16557627198103120 ) ) ;
#130873=CARTESIAN_POINT ( 'NONE',  ( 9.564922557960805705, 16.46253265017160317, 94.58224293864769550 ) ) ;
#130874=CARTESIAN_POINT ( 'NONE',  ( 8.224510206698953496, -14.34966873604960469, 47.91557627198102409 ) ) ;
#130875=CARTESIAN_POINT ( 'NONE',  ( -19.02544592524342804, 5.153800228976336051, 41.04057627198103120 ) ) ;
#130876=CARTESIAN_POINT ( 'NONE',  ( 9.564922557961047289, -16.46253265017146816, 45.41775706135232582 ) ) ;
#130877=CARTESIAN_POINT ( 'NONE',  ( 14.34966873604960469, 8.224510206698951720, 94.16557627198103830 ) ) ;
#130878=CARTESIAN_POINT ( 'NONE',  ( 18.67979575497194134, -10.72451020669871369, 110.8344237280190043 ) ) ;
#130879=CARTESIAN_POINT ( 'NONE',  ( 19.05341960407611168, 5.049401038298154454, 53.95724293864770260 ) ) ;
#130881=CARTESIAN_POINT ( 'NONE',  ( 21.53943276465977519, -0.05219959533907433946, 58.74890960531436690 ) ) ;
#130882=CARTESIAN_POINT ( 'NONE',  ( 14.34966873604960469, 8.224510206698951720, 49.16557627198102409 ) ) ;
#130883=CARTESIAN_POINT ( 'NONE',  ( 16.51473224551083163, -9.474510206698727899, 20.83442372801899722 ) ) ;
#130884=CARTESIAN_POINT ( 'NONE',  ( -5.049401038298153566, 19.05341960407611168, 105.2072429386476671 ) ) ;
#130885=CARTESIAN_POINT ( 'NONE',  ( -5.049401038298153566, 19.05341960407611168, 110.2072429386476671 ) ) ;
#130886=CARTESIAN_POINT ( 'NONE',  ( 5.049401038298161559, -19.05341960407611168, 52.70724293864767418 ) ) ;
#130887=CARTESIAN_POINT ( 'NONE',  ( -13.89961937509977652, 13.97604488694528158, 25.62390960531434558 ) ) ;
#130888=CARTESIAN_POINT ( 'NONE',  ( -14.34966873604960291, -8.224510206698953496, 91.66557627198103830 ) ) ;
#130889=CARTESIAN_POINT ( 'NONE',  ( -5.719274019375978568, 21.55341960407610458, 100.2072429386476955 ) ) ;
#130890=CARTESIAN_POINT ( 'NONE',  ( 13.89961937509977652, -13.97604488694527269, 98.12390960531433848 ) ) ;
#130891=CARTESIAN_POINT ( 'NONE',  ( -10.72451020669870658, -18.67979575497194134, 19.58442372801901143 ) ) ;
#130892=CARTESIAN_POINT ( 'NONE',  ( 5.153800228976335163, 19.02544592524342804, 109.7905762719810099 ) ) ;
#130893=CARTESIAN_POINT ( 'NONE',  ( 16.51473224551069308, 9.474510206698969483, 24.16557627198102765 ) ) ;
#130894=CARTESIAN_POINT ( 'NONE',  ( -10.81492255796105439, 18.62759615963255655, 77.91775706135231871 ) ) ;
#130895=CARTESIAN_POINT ( 'NONE',  ( -21.53943276465977519, 0.05219959533907696930, 91.24890960531436690 ) ) ;
#130896=CARTESIAN_POINT ( 'NONE',  ( 17.50000000000000355, -5.624438216177586547, 108.3167034491464591 ) ) ;
#130899=CARTESIAN_POINT ( 'NONE',  ( -14.34966873604972548, 8.224510206698743886, 33.33442372801900433 ) ) ;
#130900=CARTESIAN_POINT ( 'NONE',  ( 14.34966873604960469, 8.224510206698951720, 104.1655762719810241 ) ) ;
#130902=CARTESIAN_POINT ( 'NONE',  ( -9.474510206698964154, 16.51473224551069663, 55.41557627198103120 ) ) ;
#130903=CARTESIAN_POINT ( 'NONE',  ( 12.14591786802309770, 12.06949235617756955, 89.37390960531435269 ) ) ;
#130904=CARTESIAN_POINT ( 'NONE',  ( 21.55341960407610458, 5.719274019375980345, 28.95724293864769905 ) ) ;
#130905=CARTESIAN_POINT ( 'NONE',  ( 0.05219959533910956823, 16.53943276465976808, 59.99890960531436690 ) ) ;
#130906=CARTESIAN_POINT ( 'NONE',  ( 16.51473224551083163, -9.474510206698727899, 110.8344237280190043 ) ) ;
#130907=CARTESIAN_POINT ( 'NONE',  ( 15.72974639402176855, 15.80617190586768217, 66.87609039468568994 ) ) ;
#130908=CARTESIAN_POINT ( 'NONE',  ( 16.29526858892876362, -7.335722546920109721, 76.70329402199793378 ) ) ;
#130909=CARTESIAN_POINT ( 'NONE',  ( 16.46253265017160672, -9.564922557960803928, 108.3322429386476955 ) ) ;
#130910=CARTESIAN_POINT ( 'NONE',  ( 14.29746914071037800, 8.314922557961029526, 96.66775706135234714 ) ) ;
#130911=CARTESIAN_POINT ( 'NONE',  ( -19.03943276465977164, 0.05219959533909376836, 41.24890960531435269 ) ) ;
#130912=CARTESIAN_POINT ( 'NONE',  ( 9.564922557960805705, 16.46253265017160317, 84.58224293864769550 ) ) ;
#130913=CARTESIAN_POINT ( 'NONE',  ( -10.81492255796078084, -18.62759615963271287, 92.08224293864769550 ) ) ;
#130914=CARTESIAN_POINT ( 'NONE',  ( 12.14591786802327356, -12.06949235617739191, 30.62609039468567929 ) ) ;
#130915=CARTESIAN_POINT ( 'NONE',  ( 0.05219959533910956823, 16.53943276465976808, 59.99890960531436690 ) ) ;
#130916=CARTESIAN_POINT ( 'NONE',  ( 5.719274019375673035, 21.55341960407619339, 67.29275706135234714 ) ) ;
#130917=CARTESIAN_POINT ( 'NONE',  ( 16.55341960407618274, -4.379528057220086978, 101.0427570613523756 ) ) ;
#130918=CARTESIAN_POINT ( 'NONE',  ( 16.19135201231369692, 7.376712067591807198, 27.68680854052031393 ) ) ;
#130919=CARTESIAN_POINT ( 'NONE',  ( -17.49999999999999645, 5.624438216177592764, 80.81670344914644488 ) ) ;
#130920=CARTESIAN_POINT ( 'NONE',  ( -16.52544592524342804, 4.483927247898546575, 31.04057627198102409 ) ) ;
#130921=CARTESIAN_POINT ( 'NONE',  ( -4.483927247898782831, 16.52544592524335698, 67.70942372801901854 ) ) ;
#130922=CARTESIAN_POINT ( 'NONE',  ( 5.153800228976335163, 19.02544592524342804, 74.79057627198103830 ) ) ;
#130923=CARTESIAN_POINT ( 'NONE',  ( -16.51473224551069308, -9.474510206698971260, 91.66557627198103830 ) ) ;
#130924=CARTESIAN_POINT ( 'NONE',  ( 15.72974639402176855, 15.80617190586768217, 91.87609039468568994 ) ) ;
#130925=CARTESIAN_POINT ( 'NONE',  ( -16.53943276465976808, -0.05219959533934237506, 83.75109039468568994 ) ) ;
#130926=CARTESIAN_POINT ( 'NONE',  ( 16.53943276465976808, -0.05219959533910856209, 63.74890960531435979 ) ) ;
#130927=CARTESIAN_POINT ( 'NONE',  ( 9.564922557960805705, 16.46253265017160317, 74.58224293864769550 ) ) ;
#130928=ORIENTED_EDGE ( 'NONE', *, *, #183592, .T. ) ;
#130929=CARTESIAN_POINT ( 'NONE',  ( -5.153800228976607833, 19.02544592524334988, 112.7094237280190043 ) ) ;
#130930=CARTESIAN_POINT ( 'NONE',  ( 0.05219959533910956823, 16.53943276465976808, 109.9989096053143527 ) ) ;
#130931=CARTESIAN_POINT ( 'NONE',  ( -0.05219959533909027116, -19.03943276465977164, 77.49890960531435269 ) ) ;
#130932=CARTESIAN_POINT ( 'NONE',  ( -9.564922557961040184, 16.46253265017147172, 107.9177570613523471 ) ) ;
#130934=CARTESIAN_POINT ( 'NONE',  ( 13.97604488694548053, -13.89961937509957401, 20.62609039468567573 ) ) ;
#130935=CARTESIAN_POINT ( 'NONE',  ( -12.06949235617739369, -12.14591786802326823, 79.37609039468567573 ) ) ;
#130936=CARTESIAN_POINT ( 'NONE',  ( 5.049401038297881783, 19.05341960407617563, 87.29275706135234714 ) ) ;
#130937=CARTESIAN_POINT ( 'NONE',  ( 14.34966873604960469, 8.224510206698951720, 109.1655762719810383 ) ) ;
#130938=CARTESIAN_POINT ( 'NONE',  ( -16.55341960407617563, 4.379528057220093196, 68.54275706135234714 ) ) ;
#130940=CARTESIAN_POINT ( 'NONE',  ( 0.05219959533936267826, -19.03943276465977164, 60.00109039468566863 ) ) ;
#130942=CARTESIAN_POINT ( 'NONE',  ( 18.67979575497194134, -10.72451020669871369, 95.83442372801903275 ) ) ;
#130943=CARTESIAN_POINT ( 'NONE',  ( -16.51473224551069308, -9.474510206698971260, 36.66557627198102409 ) ) ;
#130944=CARTESIAN_POINT ( 'NONE',  ( -9.564922557960796823, -16.46253265017161027, 77.08224293864769550 ) ) ;
#130945=CARTESIAN_POINT ( 'NONE',  ( -16.55341960407611168, -4.379528057220339221, 76.45724293864769550 ) ) ;
#130946=CARTESIAN_POINT ( 'NONE',  ( -21.53943276465977519, -0.05219959533937600094, 83.75109039468568994 ) ) ;
#130947=CARTESIAN_POINT ( 'NONE',  ( 16.46253265017146816, 9.564922557961045513, 61.66775706135234003 ) ) ;
#130948=CARTESIAN_POINT ( 'NONE',  ( 19.03943276465977164, 0.05219959533936151252, 46.25109039468566863 ) ) ;
#130949=CARTESIAN_POINT ( 'NONE',  ( -18.62759615963270932, 10.81492255796079327, 35.83224293864768839 ) ) ;
#130950=CARTESIAN_POINT ( 'NONE',  ( 18.67979575497194134, -10.72451020669871369, 95.83442372801903275 ) ) ;
#130951=CARTESIAN_POINT ( 'NONE',  ( -5.153800228976328057, -19.02544592524343514, 82.29057627198103830 ) ) ;
#130952=CARTESIAN_POINT ( 'NONE',  ( 18.62759615963255655, 10.81492255796105972, 106.6677570613523756 ) ) ;
#130953=CARTESIAN_POINT ( 'NONE',  ( -18.62759615963270932, 10.81492255796079327, 45.83224293864769550 ) ) ;
#130954=CARTESIAN_POINT ( 'NONE',  ( -19.02544592524342804, 5.153800228976336051, 101.0405762719810241 ) ) ;
#130955=CARTESIAN_POINT ( 'NONE',  ( -16.46253265017146816, -9.564922557961047289, 69.16775706135233293 ) ) ;
#130956=CARTESIAN_POINT ( 'NONE',  ( -16.46253265017160317, 9.564922557960807481, 100.8322429386477097 ) ) ;
#130957=CARTESIAN_POINT ( 'NONE',  ( -19.02544592524334988, -5.153800228976617603, 93.95942372801900433 ) ) ;
#130958=CARTESIAN_POINT ( 'NONE',  ( 16.52544592524335698, 4.483927247898782831, 46.45942372801901854 ) ) ;
#130959=CARTESIAN_POINT ( 'NONE',  ( -14.34966873604960291, -8.224510206698953496, 96.66557627198102409 ) ) ;
#130960=CARTESIAN_POINT ( 'NONE',  ( 19.03943276465977164, -0.05219959533909143690, 83.74890960531436690 ) ) ;
#130961=CARTESIAN_POINT ( 'NONE',  ( 21.53943276465977519, -0.05219959533907433946, 58.74890960531436690 ) ) ;
#130962=CARTESIAN_POINT ( 'NONE',  ( -8.314922557961024197, 14.29746914071037800, 32.91775706135234714 ) ) ;
#130963=CARTESIAN_POINT ( 'NONE',  ( 15.80617190586769283, -15.72974639402175789, 30.62609039468567929 ) ) ;
#130964=CARTESIAN_POINT ( 'NONE',  ( -21.53943276465977519, -0.05219959533937600094, 88.75109039468567573 ) ) ;
#130965=CARTESIAN_POINT ( 'NONE',  ( 16.55341960407618274, -4.379528057220086978, 81.04275706135236135 ) ) ;
#130966=CARTESIAN_POINT ( 'NONE',  ( 19.03943276465977164, -0.05219959533909143690, 73.74890960531435269 ) ) ;
#130967=CARTESIAN_POINT ( 'NONE',  ( -16.55341960407611168, -4.379528057220339221, 81.45724293864769550 ) ) ;
#130968=CARTESIAN_POINT ( 'NONE',  ( -12.06949235617739369, -12.14591786802326823, 109.3760903946857042 ) ) ;
#130969=CARTESIAN_POINT ( 'NONE',  ( 16.46253265017146816, 9.564922557961045513, 51.66775706135233293 ) ) ;
#130970=CARTESIAN_POINT ( 'NONE',  ( -21.52544592524334988, -5.823673210054445271, 28.95942372801902209 ) ) ;
#130971=CARTESIAN_POINT ( 'NONE',  ( 12.14591786802309770, 12.06949235617756955, 84.37390960531438111 ) ) ;
#130972=CARTESIAN_POINT ( 'NONE',  ( 5.153800228976335163, 19.02544592524342804, 104.7905762719809957 ) ) ;
#130973=CARTESIAN_POINT ( 'NONE',  ( -16.52544592524335698, -4.483927247898792601, 103.9594237280190185 ) ) ;
#130974=CARTESIAN_POINT ( 'NONE',  ( 21.53943276465977519, 0.05219959533937863772, 76.25109039468568994 ) ) ;
#130975=CARTESIAN_POINT ( 'NONE',  ( 8.314922557961029526, -14.29746914071037800, 50.41775706135235424 ) ) ;
#130976=CARTESIAN_POINT ( 'NONE',  ( 10.72451020669871369, 18.67979575497193778, 47.08442372801901854 ) ) ;
#130977=CARTESIAN_POINT ( 'NONE',  ( -16.53943276465976808, 0.05219959533911058130, 66.24890960531436690 ) ) ;
#130979=CARTESIAN_POINT ( 'NONE',  ( 15.80617190586746368, 15.72974639402197994, 114.3739096053143527 ) ) ;
#130980=CARTESIAN_POINT ( 'NONE',  ( -14.34966873604960291, -8.224510206698953496, 91.66557627198103830 ) ) ;
#130981=CARTESIAN_POINT ( 'NONE',  ( 17.50000000000001776, -3.565345528327878100, 26.92494486806473120 ) ) ;
#130982=CARTESIAN_POINT ( 'NONE',  ( 14.34966873604960469, 8.224510206698951720, 59.16557627198103120 ) ) ;
#130983=CARTESIAN_POINT ( 'NONE',  ( -9.474510206698964154, 16.51473224551069663, 25.41557627198103120 ) ) ;
#130984=CARTESIAN_POINT ( 'NONE',  ( -21.53943276465977519, 0.05219959533907696930, 41.24890960531435269 ) ) ;
#130985=CARTESIAN_POINT ( 'NONE',  ( -12.14591786802309592, -12.06949235617757132, 81.87390960531435269 ) ) ;
#130986=CARTESIAN_POINT ( 'NONE',  ( 18.62759615963271287, -10.81492255796078972, 78.33224293864770971 ) ) ;
#130987=CARTESIAN_POINT ( 'NONE',  ( 16.51473224551069308, 9.474510206698969483, 84.16557627198102409 ) ) ;
#130988=CARTESIAN_POINT ( 'NONE',  ( 5.049401038298161559, -19.05341960407611168, 37.70724293864768839 ) ) ;
#130989=CARTESIAN_POINT ( 'NONE',  ( 5.153800228976615827, -19.02544592524334988, 85.20942372801900433 ) ) ;
#130990=CARTESIAN_POINT ( 'NONE',  ( 0.05219959533937995610, -21.53943276465977519, 55.00109039468568284 ) ) ;
#130991=CARTESIAN_POINT ( 'NONE',  ( 5.719274019375991003, -21.55341960407610458, 67.70724293864769550 ) ) ;
#130992=CARTESIAN_POINT ( 'NONE',  ( -9.474510206698964154, 16.51473224551069663, 35.41557627198102409 ) ) ;
#130993=CARTESIAN_POINT ( 'NONE',  ( -0.05219959533909027116, -19.03943276465977164, 77.49890960531435269 ) ) ;
#130995=CARTESIAN_POINT ( 'NONE',  ( 16.55341960407618274, -4.379528057220086978, 46.04275706135234714 ) ) ;
#130996=CARTESIAN_POINT ( 'NONE',  ( 15.72974639402176855, 15.80617190586768217, 31.87609039468567929 ) ) ;
#130997=CARTESIAN_POINT ( 'NONE',  ( 21.52544592524334988, 5.823673210054432836, 76.45942372801901854 ) ) ;
#130998=CARTESIAN_POINT ( 'NONE',  ( 15.80617190586746368, 15.72974639402197994, 24.37390960531435979 ) ) ;
#130999=CARTESIAN_POINT ( 'NONE',  ( -15.72974639402197994, 15.80617190586746368, 90.62390960531436690 ) ) ;
#131000=CARTESIAN_POINT ( 'NONE',  ( -21.53943276465977519, -0.05219959533937600094, 18.75109039468568639 ) ) ;
#131001=CARTESIAN_POINT ( 'NONE',  ( -16.55341960407617563, 4.379528057220093196, 48.54275706135234714 ) ) ;
#131002=CARTESIAN_POINT ( 'NONE',  ( -15.80617190586745835, -15.72974639402198527, 51.87390960531437401 ) ) ;
#131003=CARTESIAN_POINT ( 'NONE',  ( -19.03943276465977164, -0.05219959533935918106, 23.75109039468566152 ) ) ;
#131004=CARTESIAN_POINT ( 'NONE',  ( 19.03943276465977164, -0.05219959533909143690, 58.74890960531435979 ) ) ;
#131005=CARTESIAN_POINT ( 'NONE',  ( -0.05219959533909027116, -19.03943276465977164, 112.4989096053143669 ) ) ;
#131006=CARTESIAN_POINT ( 'NONE',  ( 16.51473224551069308, 9.474510206698969483, 89.16557627198103830 ) ) ;
#131007=CARTESIAN_POINT ( 'NONE',  ( 9.474510206698729675, 16.51473224551082808, 52.08442372801900433 ) ) ;
#131008=EDGE_CURVE ( 'NONE', #165007, #21338, #188507, .T. ) ;
#131009=CARTESIAN_POINT ( 'NONE',  ( -9.564922557961040184, 16.46253265017147172, 62.91775706135233293 ) ) ;
#131010=CARTESIAN_POINT ( 'NONE',  ( -5.823673210054116645, -21.52544592524344225, 42.29057627198103120 ) ) ;
#131011=CARTESIAN_POINT ( 'NONE',  ( 14.34966873604960469, 8.224510206698951720, 29.16557627198103120 ) ) ;
#131012=CARTESIAN_POINT ( 'NONE',  ( -9.564922557961040184, 16.46253265017147172, 97.91775706135233293 ) ) ;
#131013=EDGE_CURVE ( 'NONE', #127046, #164406, #155783, .T. ) ;
#131015=CARTESIAN_POINT ( 'NONE',  ( 19.03943276465977164, 0.05219959533936151252, 21.25109039468565797 ) ) ;
#131016=CARTESIAN_POINT ( 'NONE',  ( 16.51473224551083163, -9.474510206698727899, 100.8344237280190043 ) ) ;
#131017=CARTESIAN_POINT ( 'NONE',  ( -21.55341960407610458, -5.719274019375992779, 86.45724293864770971 ) ) ;
#131018=CARTESIAN_POINT ( 'NONE',  ( -16.51473224551082808, 9.474510206698731452, 53.33442372801900433 ) ) ;
#131021=CARTESIAN_POINT ( 'NONE',  ( -16.51473224551069308, -9.474510206698971260, 56.66557627198103120 ) ) ;
#131022=CARTESIAN_POINT ( 'NONE',  ( -12.14591786802309592, -12.06949235617757132, 66.87390960531436690 ) ) ;
#131023=CARTESIAN_POINT ( 'NONE',  ( -5.153800228976328057, -19.02544592524343514, 37.29057627198102409 ) ) ;
#131024=CARTESIAN_POINT ( 'NONE',  ( -12.14591786802309592, -12.06949235617757132, 36.87390960531435979 ) ) ;
#131025=FACE_OUTER_BOUND ( 'NONE', #7505, .T. ) ;
#131026=CARTESIAN_POINT ( 'NONE',  ( -16.53943276465976808, -0.05219959533934237506, 103.7510903946857042 ) ) ;
#131027=CARTESIAN_POINT ( 'NONE',  ( -13.89961937509977652, 13.97604488694528158, 65.62390960531436690 ) ) ;
#131028=CARTESIAN_POINT ( 'NONE',  ( -13.97604488694547697, 13.89961937509957934, 23.12609039468565442 ) ) ;
#131029=CARTESIAN_POINT ( 'NONE',  ( -4.379528057220086978, -16.55341960407618274, 39.79275706135235424 ) ) ;
#131030=CARTESIAN_POINT ( 'NONE',  ( -5.719274019375978568, 21.55341960407610458, 55.20724293864770260 ) ) ;
#131031=CARTESIAN_POINT ( 'NONE',  ( -15.72974639402176322, -15.80617190586768395, 109.3760903946857042 ) ) ;
#131032=EDGE_LOOP ( 'NONE', ( #123245, #160459, #5632, #18952 ) ) ;
#131033=CARTESIAN_POINT ( 'NONE',  ( -19.02544592524342804, 5.153800228976336051, 61.04057627198103120 ) ) ;
#131034=CARTESIAN_POINT ( 'NONE',  ( 16.51473224551069308, 9.474510206698969483, 114.1655762719810241 ) ) ;
#131035=CARTESIAN_POINT ( 'NONE',  ( -9.564922557960796823, -16.46253265017161027, 97.08224293864769550 ) ) ;
#131037=CARTESIAN_POINT ( 'NONE',  ( 21.55341960407619695, -5.719274019375665929, 21.04275706135234714 ) ) ;
#131039=CARTESIAN_POINT ( 'NONE',  ( 14.34966873604960469, 8.224510206698951720, 94.16557627198103830 ) ) ;
#131040=CARTESIAN_POINT ( 'NONE',  ( 10.81492255796078972, 18.62759615963270932, 94.58224293864769550 ) ) ;
#131041=CARTESIAN_POINT ( 'NONE',  ( 9.564922557960805705, 16.46253265017160317, 64.58224293864769550 ) ) ;
#131042=CARTESIAN_POINT ( 'NONE',  ( 16.46253265017160672, -9.564922557960803928, 68.33224293864770971 ) ) ;
#131043=CARTESIAN_POINT ( 'NONE',  ( 15.80617190586746368, 15.72974639402197994, 104.3739096053143669 ) ) ;
#131045=CARTESIAN_POINT ( 'NONE',  ( -0.05219959533909027116, -19.03943276465977164, 72.49890960531435269 ) ) ;
#131046=CARTESIAN_POINT ( 'NONE',  ( 18.22780087662123805, -5.499999999999976019, 98.51763182126896368 ) ) ;
#131047=CARTESIAN_POINT ( 'NONE',  ( -16.55341960407611168, -4.379528057220339221, 101.4572429386476955 ) ) ;
#131049=CARTESIAN_POINT ( 'NONE',  ( 9.564922557961047289, -16.46253265017146816, 90.41775706135234714 ) ) ;
#131050=CARTESIAN_POINT ( 'NONE',  ( -14.29746914071049879, 8.314922557960819915, 100.8322429386477097 ) ) ;
#131051=CARTESIAN_POINT ( 'NONE',  ( 5.719274019375673035, 21.55341960407619339, 77.29275706135234714 ) ) ;
#131052=CARTESIAN_POINT ( 'NONE',  ( 19.05341960407611168, 5.049401038298154454, 58.95724293864768129 ) ) ;
#131053=CARTESIAN_POINT ( 'NONE',  ( 18.62759615963255655, 10.81492255796105972, 31.66775706135234358 ) ) ;
#131054=CARTESIAN_POINT ( 'NONE',  ( 0.05219959533907565091, 21.53943276465977519, 109.9989096053143527 ) ) ;
#131056=CARTESIAN_POINT ( 'NONE',  ( 5.049401038298161559, -19.05341960407611168, 72.70724293864768129 ) ) ;
#131058=CARTESIAN_POINT ( 'NONE',  ( -16.53943276465976808, -0.05219959533934237506, 23.75109039468567929 ) ) ;
#131059=CARTESIAN_POINT ( 'NONE',  ( 0.05219959533907565091, 21.53943276465977519, 24.99890960531435624 ) ) ;
#131060=CARTESIAN_POINT ( 'NONE',  ( -18.62759615963255300, -10.81492255796106328, 69.16775706135234714 ) ) ;
#131061=CARTESIAN_POINT ( 'NONE',  ( 9.564922557960805705, 16.46253265017160317, 104.5822429386476955 ) ) ;
#131062=CARTESIAN_POINT ( 'NONE',  ( -13.97604488694547697, 13.89961937509957934, 98.12609039468566152 ) ) ;
#131063=CARTESIAN_POINT ( 'NONE',  ( 0.05219959533909260263, 19.03943276465977164, 44.99890960531435979 ) ) ;
#131064=CARTESIAN_POINT ( 'NONE',  ( -19.03943276465977164, 0.05219959533909376836, 76.24890960531435269 ) ) ;
#131065=CARTESIAN_POINT ( 'NONE',  ( 8.314922557960818139, 14.29746914071049879, 94.58224293864769550 ) ) ;
#131066=CARTESIAN_POINT ( 'NONE',  ( -9.474510206698964154, 16.51473224551069663, 100.4155762719810241 ) ) ;
#131067=CARTESIAN_POINT ( 'NONE',  ( 16.53943276465976808, -0.05219959533910856209, 88.74890960531436690 ) ) ;
#131068=CARTESIAN_POINT ( 'NONE',  ( 13.97604488694527802, 13.89961937509977652, 104.3739096053143385 ) ) ;
#131069=CARTESIAN_POINT ( 'NONE',  ( 14.34966873604960469, 8.224510206698951720, 49.16557627198102409 ) ) ;
#131070=CARTESIAN_POINT ( 'NONE',  ( -0.05219959533909027116, -19.03943276465977164, 42.49890960531435269 ) ) ;
#131071=CARTESIAN_POINT ( 'NONE',  ( -21.52544592524334988, -5.823673210054445271, 58.95942372801902565 ) ) ;
#131072=CARTESIAN_POINT ( 'NONE',  ( -0.05219959533936034679, 19.03943276465977164, 92.50109039468566152 ) ) ;
#131073=CARTESIAN_POINT ( 'NONE',  ( 12.14591786802309770, 12.06949235617756955, 49.37390960531436690 ) ) ;
#131074=CARTESIAN_POINT ( 'NONE',  ( -10.81492255796078084, -18.62759615963271287, 102.0822429386476955 ) ) ;
#131075=CARTESIAN_POINT ( 'NONE',  ( 10.72451020669898902, -18.67979575497178502, 42.91557627198103120 ) ) ;
#131076=CARTESIAN_POINT ( 'NONE',  ( 9.474510206698971260, -16.51473224551069308, 107.9155762719810383 ) ) ;
#131077=CARTESIAN_POINT ( 'NONE',  ( 8.224510206698953496, -14.34966873604960469, 82.91557627198103830 ) ) ;
#131078=CARTESIAN_POINT ( 'NONE',  ( -5.049401038298153566, 19.05341960407611168, 60.20724293864768129 ) ) ;
#131079=CARTESIAN_POINT ( 'NONE',  ( 4.483927247898545687, 16.52544592524342804, 29.79057627198102409 ) ) ;
#131080=CARTESIAN_POINT ( 'NONE',  ( -0.05219959533934338120, 16.53943276465976808, 102.5010903946856899 ) ) ;
#131081=CARTESIAN_POINT ( 'NONE',  ( -8.314922557961024197, 14.29746914071037800, 87.91775706135234714 ) ) ;
#131082=CARTESIAN_POINT ( 'NONE',  ( 0.05219959533936267826, -19.03943276465977164, 35.00109039468566863 ) ) ;
#131084=CARTESIAN_POINT ( 'NONE',  ( 19.05341960407611168, 5.049401038298154454, 103.9572429386476671 ) ) ;
#131085=CARTESIAN_POINT ( 'NONE',  ( 16.46253265017160672, -9.564922557960803928, 73.33224293864769550 ) ) ;
#131086=CARTESIAN_POINT ( 'NONE',  ( -5.153800228976328057, -19.02544592524343514, 32.29057627198102409 ) ) ;
#131087=EDGE_CURVE ( 'NONE', #179813, #123998, #60648, .T. ) ;
#131088=CARTESIAN_POINT ( 'NONE',  ( 16.55341960407611168, 4.379528057220329451, 53.95724293864770260 ) ) ;
#131089=CARTESIAN_POINT ( 'NONE',  ( 16.46253265017160672, -9.564922557960803928, 113.3322429386476955 ) ) ;
#131090=CARTESIAN_POINT ( 'NONE',  ( 19.05341960407611168, 5.049401038298154454, 108.9572429386477097 ) ) ;
#131091=CARTESIAN_POINT ( 'NONE',  ( 15.80617190586746368, 15.72974639402197994, 44.37390960531435979 ) ) ;
#131092=CARTESIAN_POINT ( 'NONE',  ( 12.06949235617757843, -12.14591786802309237, 88.12390960531436690 ) ) ;
#131093=CARTESIAN_POINT ( 'NONE',  ( -4.379528057220086978, -16.55341960407618274, 34.79275706135235424 ) ) ;
#131094=CARTESIAN_POINT ( 'NONE',  ( 14.34966873604960469, 8.224510206698951720, 59.16557627198103120 ) ) ;
#131096=CARTESIAN_POINT ( 'NONE',  ( 16.51473224551083163, -9.474510206698727899, 70.83442372801900433 ) ) ;
#131097=CARTESIAN_POINT ( 'NONE',  ( 19.02544592524343514, -5.153800228976328945, 108.5405762719810383 ) ) ;
#131098=CARTESIAN_POINT ( 'NONE',  ( 5.153800228976615827, -19.02544592524334988, 80.20942372801901854 ) ) ;
#131099=ADVANCED_FACE ( 'NONE', ( #93106 ), #185404, .F. ) ;
#131101=CARTESIAN_POINT ( 'NONE',  ( -14.29746914071037622, -8.314922557961029526, 29.16775706135234003 ) ) ;
#131102=CARTESIAN_POINT ( 'NONE',  ( -4.483927247898782831, 16.52544592524335698, 102.7094237280190185 ) ) ;
#131103=CARTESIAN_POINT ( 'NONE',  ( -5.049401038297874678, -19.05341960407617918, 69.79275706135233293 ) ) ;
#131104=CARTESIAN_POINT ( 'NONE',  ( -5.719274019375978568, 21.55341960407610458, 30.20724293864769550 ) ) ;
#131105=CARTESIAN_POINT ( 'NONE',  ( -0.05219959533937732626, 21.53943276465977519, 67.50109039468568994 ) ) ;
#131107=CARTESIAN_POINT ( 'NONE',  ( 16.51473224551083163, -9.474510206698727899, 110.8344237280190043 ) ) ;
#131108=LINE ( 'NONE', #192796, #60450 ) ;
#131109=CARTESIAN_POINT ( 'NONE',  ( -19.02544592524342804, 5.153800228976336051, 71.04057627198099567 ) ) ;
#131110=CARTESIAN_POINT ( 'NONE',  ( -5.049401038298153566, 19.05341960407611168, 25.20724293864768484 ) ) ;
#131111=CARTESIAN_POINT ( 'NONE',  ( -12.14591786802309592, -12.06949235617757132, 81.87390960531435269 ) ) ;
#131112=CARTESIAN_POINT ( 'NONE',  ( -16.51473224551069308, -9.474510206698971260, 71.66557627198102409 ) ) ;
#131113=CARTESIAN_POINT ( 'NONE',  ( 0.05219959533909260263, 19.03943276465977164, 89.99890960531436690 ) ) ;
#131115=CARTESIAN_POINT ( 'NONE',  ( 13.89961937509957401, 13.97604488694547697, 86.87609039468567573 ) ) ;
#131116=CARTESIAN_POINT ( 'NONE',  ( -18.62759615963270932, 10.81492255796079327, 75.83224293864769550 ) ) ;
#131117=CARTESIAN_POINT ( 'NONE',  ( 19.02544592524343514, -5.153800228976328945, 28.54057627198102409 ) ) ;
#131118=CARTESIAN_POINT ( 'NONE',  ( 19.05341960407617918, -5.049401038297876454, 66.04275706135233293 ) ) ;
#131119=CARTESIAN_POINT ( 'NONE',  ( 21.55341960407610458, 5.719274019375980345, 108.9572429386476955 ) ) ;
#131120=CARTESIAN_POINT ( 'NONE',  ( -5.153800228976328057, -19.02544592524343514, 67.29057627198102409 ) ) ;
#131121=CARTESIAN_POINT ( 'NONE',  ( -9.474510206698964154, 16.51473224551069663, 105.4155762719810383 ) ) ;
#131123=CARTESIAN_POINT ( 'NONE',  ( 21.53943276465977519, -0.05219959533907433946, 98.74890960531438111 ) ) ;
#131124=CARTESIAN_POINT ( 'NONE',  ( 16.53943276465976808, -0.05219959533910856209, 98.74890960531438111 ) ) ;
#131125=CARTESIAN_POINT ( 'NONE',  ( 5.153800228976335163, 19.02544592524342804, 84.79057627198099567 ) ) ;
#131126=CARTESIAN_POINT ( 'NONE',  ( 13.89961937509957401, 13.97604488694547697, 66.87609039468567573 ) ) ;
#131127=CARTESIAN_POINT ( 'NONE',  ( 18.62759615963271287, -10.81492255796078972, 83.33224293864769550 ) ) ;
#131128=CARTESIAN_POINT ( 'NONE',  ( 15.80617190586746368, 15.72974639402197994, 69.37390960531436690 ) ) ;
#131129=CARTESIAN_POINT ( 'NONE',  ( -14.29746914071049879, 8.314922557960819915, 40.83224293864769550 ) ) ;
#131130=CARTESIAN_POINT ( 'NONE',  ( 10.72451020669871369, 18.67979575497193778, 107.0844237280190043 ) ) ;
#131131=CARTESIAN_POINT ( 'NONE',  ( 16.53943276465976808, 0.05219959533934440121, 66.25109039468567573 ) ) ;
#131133=CARTESIAN_POINT ( 'NONE',  ( -19.02544592524342804, 5.153800228976336051, 96.04057627198103830 ) ) ;
#131134=CARTESIAN_POINT ( 'NONE',  ( 19.02544592524343514, -5.153800228976328945, 33.54057627198102409 ) ) ;
#131135=CARTESIAN_POINT ( 'NONE',  ( 21.53943276465977519, 0.05219959533937863772, 36.25109039468567573 ) ) ;
#131136=CARTESIAN_POINT ( 'NONE',  ( 18.67979575497194134, -10.72451020669871369, 55.83442372801901854 ) ) ;
#131137=CARTESIAN_POINT ( 'NONE',  ( -19.03943276465977164, 0.05219959533909376836, 61.24890960531436690 ) ) ;
#131138=CARTESIAN_POINT ( 'NONE',  ( -18.67979575497193778, 10.72451020669871902, 33.33442372801900433 ) ) ;
#131139=CARTESIAN_POINT ( 'NONE',  ( -9.474510206698720793, -16.51473224551083518, 79.58442372801899012 ) ) ;
#131140=CARTESIAN_POINT ( 'NONE',  ( -19.02544592524334988, -5.153800228976617603, 73.95942372801900433 ) ) ;
#131141=CARTESIAN_POINT ( 'NONE',  ( 16.46253265017160672, -9.564922557960803928, 43.33224293864769550 ) ) ;
#131142=CARTESIAN_POINT ( 'NONE',  ( 12.14591786802327356, -12.06949235617739191, 90.62609039468567573 ) ) ;
#131143=CARTESIAN_POINT ( 'NONE',  ( -19.05341960407611168, -5.049401038298163336, 51.45724293864770260 ) ) ;
#131144=DIRECTION ( 'NONE',  ( 0.5150380749100522682, 1.049727191138620051E-16, 0.8571673007021134438 ) ) ;
#131145=CARTESIAN_POINT ( 'NONE',  ( -16.46253265017160317, 9.564922557960807481, 95.83224293864769550 ) ) ;
#131146=CARTESIAN_POINT ( 'NONE',  ( 16.51473224551069308, 9.474510206698969483, 44.16557627198103120 ) ) ;
#131147=CARTESIAN_POINT ( 'NONE',  ( -5.719274019375978568, 21.55341960407610458, 70.20724293864769550 ) ) ;
#131148=CARTESIAN_POINT ( 'NONE',  ( 12.14591786802327356, -12.06949235617739191, 60.62609039468567573 ) ) ;
#131149=CARTESIAN_POINT ( 'NONE',  ( -15.80617190586768217, 15.72974639402176855, 113.1260903946856899 ) ) ;
#131150=CARTESIAN_POINT ( 'NONE',  ( -16.51473224551069308, -9.474510206698971260, 56.66557627198103120 ) ) ;
#131151=CARTESIAN_POINT ( 'NONE',  ( -4.379528057220328563, 16.55341960407611168, 40.20724293864769550 ) ) ;
#131152=CARTESIAN_POINT ( 'NONE',  ( -0.05219959533910754901, -16.53943276465976808, 77.49890960531433848 ) ) ;
#131153=CARTESIAN_POINT ( 'NONE',  ( 0.05219959533909260263, 19.03943276465977164, 79.99890960531436690 ) ) ;
#131154=CARTESIAN_POINT ( 'NONE',  ( -5.823673210054431948, 21.52544592524334988, 37.70942372801900433 ) ) ;
#131155=CARTESIAN_POINT ( 'NONE',  ( -9.564922557960796823, -16.46253265017161027, 92.08224293864769550 ) ) ;
#131156=CARTESIAN_POINT ( 'NONE',  ( -18.67979575497193778, 10.72451020669871902, 103.3344237280190043 ) ) ;
#131157=CARTESIAN_POINT ( 'NONE',  ( -4.483927247898782831, 16.52544592524335698, 62.70942372801902565 ) ) ;
#131158=CARTESIAN_POINT ( 'NONE',  ( 5.719274019375673035, 21.55341960407619339, 32.29275706135235424 ) ) ;
#131159=CARTESIAN_POINT ( 'NONE',  ( -5.153800228976328057, -19.02544592524343514, 102.2905762719810383 ) ) ;
#131160=CARTESIAN_POINT ( 'NONE',  ( 21.53943276465977519, -0.05219959533907433946, 83.74890960531435269 ) ) ;
#131161=CARTESIAN_POINT ( 'NONE',  ( -4.483927247898539470, -16.52544592524342804, 52.29057627198102409 ) ) ;
#131162=CARTESIAN_POINT ( 'NONE',  ( -13.89961937509977652, 13.97604488694528158, 45.62390960531433848 ) ) ;
#131163=CARTESIAN_POINT ( 'NONE',  ( 4.379528057220339221, -16.55341960407611168, 62.70724293864769550 ) ) ;
#131164=CARTESIAN_POINT ( 'NONE',  ( 5.719274019375991003, -21.55341960407610458, 32.70724293864770260 ) ) ;
#131165=CARTESIAN_POINT ( 'NONE',  ( 10.72451020669898902, -18.67979575497178502, 27.91557627198103830 ) ) ;
#131166=CARTESIAN_POINT ( 'NONE',  ( 19.03943276465977164, 0.05219959533936151252, 26.25109039468566507 ) ) ;
#131167=CARTESIAN_POINT ( 'NONE',  ( -12.06949235617756955, 12.14591786802309770, 95.62390960531436690 ) ) ;
#131168=CARTESIAN_POINT ( 'NONE',  ( -13.89961937509977652, 13.97604488694528158, 105.6239096053143527 ) ) ;
#131169=ORIENTED_EDGE ( 'NONE', *, *, #137592, .T. ) ;
#131170=CARTESIAN_POINT ( 'NONE',  ( -12.14591786802326823, 12.06949235617739902, 53.12609039468568284 ) ) ;
#131171=CARTESIAN_POINT ( 'NONE',  ( 19.03943276465977164, -0.05219959533909143690, 48.74890960531435979 ) ) ;
#131172=CARTESIAN_POINT ( 'NONE',  ( -16.75229466661211930, -6.775384016297254952, 21.10007927763472679 ) ) ;
#131173=CARTESIAN_POINT ( 'NONE',  ( 13.97604488694548053, -13.89961937509957401, 60.62609039468564731 ) ) ;
#131174=CARTESIAN_POINT ( 'NONE',  ( 4.483927247898790824, -16.52544592524335698, 100.2094237280190043 ) ) ;
#131175=CARTESIAN_POINT ( 'NONE',  ( 0.05219959533936267826, -19.03943276465977164, 95.00109039468567573 ) ) ;
#131176=CARTESIAN_POINT ( 'NONE',  ( 0.05219959533937995610, -21.53943276465977519, 65.00109039468568994 ) ) ;
#131177=CARTESIAN_POINT ( 'NONE',  ( -16.51473224551069308, -9.474510206698971260, 71.66557627198102409 ) ) ;
#131178=CARTESIAN_POINT ( 'NONE',  ( 0.05219959533907565091, 21.53943276465977519, 89.99890960531438111 ) ) ;
#131179=CARTESIAN_POINT ( 'NONE',  ( -4.483927247898782831, 16.52544592524335698, 47.70942372801902565 ) ) ;
#131180=CARTESIAN_POINT ( 'NONE',  ( -8.314922557960811034, -14.29746914071050412, 112.0822429386477097 ) ) ;
#131181=CARTESIAN_POINT ( 'NONE',  ( -13.97604488694547697, 13.89961937509957934, 78.12609039468567573 ) ) ;
#131182=CARTESIAN_POINT ( 'NONE',  ( -5.823673210054116645, -21.52544592524344225, 72.29057627198102409 ) ) ;
#131183=CARTESIAN_POINT ( 'NONE',  ( 5.153800228976615827, -19.02544592524334988, 45.20942372801901143 ) ) ;
#131184=CARTESIAN_POINT ( 'NONE',  ( 13.97604488694527802, 13.89961937509977652, 114.3739096053143669 ) ) ;
#131185=CARTESIAN_POINT ( 'NONE',  ( 21.55341960407610458, 5.719274019375980345, 88.95724293864769550 ) ) ;
#131186=CARTESIAN_POINT ( 'NONE',  ( 17.50000000000001421, 3.189878218039106983, 27.62948562571252964 ) ) ;
#131187=CARTESIAN_POINT ( 'NONE',  ( -13.89961937509977652, 13.97604488694528158, 70.62390960531432427 ) ) ;
#131189=CARTESIAN_POINT ( 'NONE',  ( -19.05341960407617563, 5.049401038297882671, 113.5427570613523471 ) ) ;
#131191=CARTESIAN_POINT ( 'NONE',  ( -9.474510206698964154, 16.51473224551069663, 50.41557627198102409 ) ) ;
#131192=CARTESIAN_POINT ( 'NONE',  ( 5.823673210054125526, 21.52544592524343514, 104.7905762719810241 ) ) ;
#131193=CARTESIAN_POINT ( 'NONE',  ( 12.14591786802309770, 12.06949235617756955, 54.37390960531435979 ) ) ;
#131194=CARTESIAN_POINT ( 'NONE',  ( 5.049401038298161559, -19.05341960407611168, 52.70724293864767418 ) ) ;
#131195=CARTESIAN_POINT ( 'NONE',  ( -10.81492255796105439, 18.62759615963255655, 72.91775706135234714 ) ) ;
#131196=CARTESIAN_POINT ( 'NONE',  ( -16.51473224551082808, 9.474510206698731452, 113.3344237280190043 ) ) ;
#131197=CARTESIAN_POINT ( 'NONE',  ( 0.05219959533936267826, -19.03943276465977164, 25.00109039468566152 ) ) ;
#131198=CARTESIAN_POINT ( 'NONE',  ( -8.224510206698948167, 14.34966873604960824, 25.41557627198103120 ) ) ;
#131199=CARTESIAN_POINT ( 'NONE',  ( -10.72451020669870658, -18.67979575497194134, 44.58442372801901854 ) ) ;
#131200=CARTESIAN_POINT ( 'NONE',  ( -5.823673210054431948, 21.52544592524334988, 22.70942372801901499 ) ) ;
#131201=CARTESIAN_POINT ( 'NONE',  ( 5.823673210054125526, 21.52544592524343514, 59.79057627198103120 ) ) ;
#131202=CARTESIAN_POINT ( 'NONE',  ( -16.46253265017146816, -9.564922557961047289, 94.16775706135233293 ) ) ;
#131203=CARTESIAN_POINT ( 'NONE',  ( 5.049401038297881783, 19.05341960407617563, 62.29275706135234003 ) ) ;
#131204=CARTESIAN_POINT ( 'NONE',  ( 18.62759615963255655, 10.81492255796105972, 66.66775706135234714 ) ) ;
#131205=CARTESIAN_POINT ( 'NONE',  ( -5.153800228976607833, 19.02544592524334988, 52.70942372801900433 ) ) ;
#131206=CARTESIAN_POINT ( 'NONE',  ( -16.52544592524342804, 4.483927247898546575, 116.0405762719810383 ) ) ;
#131207=CARTESIAN_POINT ( 'NONE',  ( -0.05219959533907301413, -21.53943276465977519, 52.49890960531435979 ) ) ;
#131208=CARTESIAN_POINT ( 'NONE',  ( -8.224510206698948167, 14.34966873604960824, 45.41557627198103830 ) ) ;
#131210=CARTESIAN_POINT ( 'NONE',  ( -10.72451020669870658, -18.67979575497194134, 109.5844237280190328 ) ) ;
#131211=CARTESIAN_POINT ( 'NONE',  ( 12.14591786802327356, -12.06949235617739191, 85.62609039468568994 ) ) ;
#131212=CARTESIAN_POINT ( 'NONE',  ( 12.06949235617757843, -12.14591786802309237, 38.12390960531436690 ) ) ;
#131213=CARTESIAN_POINT ( 'NONE',  ( 15.80617190586769283, -15.72974639402175789, 75.62609039468567573 ) ) ;
#131214=CARTESIAN_POINT ( 'NONE',  ( 5.823673210054444382, -21.52544592524334988, 75.20942372801901854 ) ) ;
#131215=CARTESIAN_POINT ( 'NONE',  ( 21.55341960407610458, 5.719274019375980345, 83.95724293864770971 ) ) ;
#131216=CARTESIAN_POINT ( 'NONE',  ( 13.97604488694527802, 13.89961937509977652, 34.37390960531436690 ) ) ;
#131217=CARTESIAN_POINT ( 'NONE',  ( -10.72451020669870658, -18.67979575497194134, 59.58442372801901854 ) ) ;
#131218=CARTESIAN_POINT ( 'NONE',  ( 5.049401038298161559, -19.05341960407611168, 42.70724293864767418 ) ) ;
#131219=CARTESIAN_POINT ( 'NONE',  ( 13.97604488694527802, 13.89961937509977652, 54.37390960531435979 ) ) ;
#131220=CARTESIAN_POINT ( 'NONE',  ( 16.55341960407611168, 4.379528057220329451, 98.95724293864770971 ) ) ;
#131221=CARTESIAN_POINT ( 'NONE',  ( 9.474510206698971260, -16.51473224551069308, 97.91557627198102409 ) ) ;
#131223=CARTESIAN_POINT ( 'NONE',  ( 12.14591786802309770, 12.06949235617756955, 34.37390960531435979 ) ) ;
#131224=CARTESIAN_POINT ( 'NONE',  ( 8.224510206698953496, -14.34966873604960469, 107.9155762719810241 ) ) ;
#131225=CARTESIAN_POINT ( 'NONE',  ( 21.52544592524344225, -5.823673210054117533, 78.54057627198103830 ) ) ;
#131227=CARTESIAN_POINT ( 'NONE',  ( -21.55341960407619339, 5.719274019375674811, 23.54275706135235424 ) ) ;
#131229=CARTESIAN_POINT ( 'NONE',  ( 8.314922557961029526, -14.29746914071037800, 25.41775706135235779 ) ) ;
#131230=CARTESIAN_POINT ( 'NONE',  ( 18.67979575497178502, 10.72451020669898547, 74.16557627198102409 ) ) ;
#131231=CARTESIAN_POINT ( 'NONE',  ( -21.53943276465977519, -0.05219959533937600094, 93.75109039468567573 ) ) ;
#131232=B_SPLINE_CURVE_WITH_KNOTS ( 'NONE', 3,
 ( #54595, #115274, #85930, #129421, #71767, #131435 ),
 .UNSPECIFIED., .F., .F.,
 ( 4, 2, 4 ),
 ( 0.003239945802372248222, 0.003620412082092099547, 0.004000878361811951306 ),
 .UNSPECIFIED. ) ;
#131233=CARTESIAN_POINT ( 'NONE',  ( -9.474510206698964154, 16.51473224551069663, 85.41557627198102409 ) ) ;
#131234=CARTESIAN_POINT ( 'NONE',  ( -18.62759615963255300, -10.81492255796106328, 24.16775706135235424 ) ) ;
#131235=CARTESIAN_POINT ( 'NONE',  ( 5.049401038298161559, -19.05341960407611168, 112.7072429386476813 ) ) ;
#131236=CARTESIAN_POINT ( 'NONE',  ( -8.224510206698735004, -14.34966873604973081, 94.58442372801901854 ) ) ;
#131237=CARTESIAN_POINT ( 'NONE',  ( 18.62759615963255655, 10.81492255796105972, 76.66775706135234714 ) ) ;
#131238=CARTESIAN_POINT ( 'NONE',  ( 19.02544592524334988, 5.153800228976608722, 21.45942372801899012 ) ) ;
#131239=CARTESIAN_POINT ( 'NONE',  ( 4.483927247898790824, -16.52544592524335698, 70.20942372801904696 ) ) ;
#131240=CARTESIAN_POINT ( 'NONE',  ( 15.72974639402176855, 15.80617190586768217, 31.87609039468567929 ) ) ;
#131241=CARTESIAN_POINT ( 'NONE',  ( 16.46253265017160672, -9.564922557960803928, 33.33224293864770260 ) ) ;
#131242=CARTESIAN_POINT ( 'NONE',  ( -21.53943276465977519, -0.05219959533937600094, 88.75109039468567573 ) ) ;
#131243=CARTESIAN_POINT ( 'NONE',  ( -19.05341960407611168, -5.049401038298163336, 91.45724293864766707 ) ) ;
#131244=CARTESIAN_POINT ( 'NONE',  ( 0.05219959533907565091, 21.53943276465977519, 104.9989096053143669 ) ) ;
#131245=CARTESIAN_POINT ( 'NONE',  ( 19.34837522270368027, 5.499999999999741540, 83.36337684832578532 ) ) ;
#131246=CARTESIAN_POINT ( 'NONE',  ( 21.55341960407610458, 5.719274019375980345, 58.95724293864770971 ) ) ;
#131247=CARTESIAN_POINT ( 'NONE',  ( 13.89961937509977652, -13.97604488694527269, 93.12390960531436690 ) ) ;
#131248=CARTESIAN_POINT ( 'NONE',  ( 4.379528057220339221, -16.55341960407611168, 47.70724293864770260 ) ) ;
#131250=CARTESIAN_POINT ( 'NONE',  ( -0.05219959533936034679, 19.03943276465977164, 82.50109039468567573 ) ) ;
#131251=CARTESIAN_POINT ( 'NONE',  ( -16.18388926212237777, 7.379444403734522595, 104.5604684863385216 ) ) ;
#131252=EDGE_CURVE ( 'NONE', #22005, #114833, #18284, .T. ) ;
#131253=CARTESIAN_POINT ( 'NONE',  ( 9.564922557961047289, -16.46253265017146816, 105.4177570613523471 ) ) ;
#131254=CARTESIAN_POINT ( 'NONE',  ( -10.72451020669898014, 18.67979575497178502, 80.41557627198103830 ) ) ;
#131255=CARTESIAN_POINT ( 'NONE',  ( -8.224510206698948167, 14.34966873604960824, 65.41557627198102409 ) ) ;
#131256=CARTESIAN_POINT ( 'NONE',  ( -13.89961937509977652, 13.97604488694528158, 100.6239096053143669 ) ) ;
#131257=CARTESIAN_POINT ( 'NONE',  ( -14.34966873604972548, 8.224510206698743886, 38.33442372801900433 ) ) ;
#131258=CARTESIAN_POINT ( 'NONE',  ( 19.05341960407611168, 5.049401038298154454, 63.95724293864769550 ) ) ;
#131259=CARTESIAN_POINT ( 'NONE',  ( 21.52544592524334988, 5.823673210054432836, 26.45942372801901854 ) ) ;
#131260=CARTESIAN_POINT ( 'NONE',  ( -0.05219959533936034679, 19.03943276465977164, 97.50109039468567573 ) ) ;
#131261=CARTESIAN_POINT ( 'NONE',  ( -19.02544592524342804, 5.153800228976336051, 101.0405762719810241 ) ) ;
#131262=CARTESIAN_POINT ( 'NONE',  ( -19.03943276465977164, 0.05219959533909376836, 86.24890960531436690 ) ) ;
#131263=CARTESIAN_POINT ( 'NONE',  ( -5.719274019375978568, 21.55341960407610458, 90.20724293864770971 ) ) ;
#131264=CARTESIAN_POINT ( 'NONE',  ( -9.474510206698964154, 16.51473224551069663, 40.41557627198103120 ) ) ;
#131265=CARTESIAN_POINT ( 'NONE',  ( -16.29526858892878494, -7.335722546920003140, 60.79670597800208753 ) ) ;
#131266=CARTESIAN_POINT ( 'NONE',  ( -16.52544592524342804, 4.483927247898546575, 71.04057627198103830 ) ) ;
#131267=CARTESIAN_POINT ( 'NONE',  ( 5.049401038298161559, -19.05341960407611168, 102.7072429386476955 ) ) ;
#131268=CARTESIAN_POINT ( 'NONE',  ( -18.09805431107247031, 5.500000000000101252, 61.01606229291886763 ) ) ;
#131269=CARTESIAN_POINT ( 'NONE',  ( -9.474510206698720793, -16.51473224551083518, 59.58442372801900433 ) ) ;
#131270=CARTESIAN_POINT ( 'NONE',  ( 15.72974639402199770, -15.80617190586745480, 93.12390960531436690 ) ) ;
#131271=CARTESIAN_POINT ( 'NONE',  ( 5.049401038297881783, 19.05341960407617563, 52.29275706135234003 ) ) ;
#131272=CARTESIAN_POINT ( 'NONE',  ( -0.05219959533909027116, -19.03943276465977164, 97.49890960531436690 ) ) ;
#131273=CARTESIAN_POINT ( 'NONE',  ( 5.719274019375991003, -21.55341960407610458, 47.70724293864770260 ) ) ;
#131274=CARTESIAN_POINT ( 'NONE',  ( -13.97604488694527625, -13.89961937509977652, 91.87390960531432427 ) ) ;
#131275=CARTESIAN_POINT ( 'NONE',  ( -10.72451020669870658, -18.67979575497194134, 69.58442372801900433 ) ) ;
#131276=CARTESIAN_POINT ( 'NONE',  ( -19.03943276465977164, 0.05219959533909376836, 41.24890960531435269 ) ) ;
#131278=CARTESIAN_POINT ( 'NONE',  ( -8.224510206698948167, 14.34966873604960824, 75.41557627198102409 ) ) ;
#131279=CARTESIAN_POINT ( 'NONE',  ( -8.224510206698735004, -14.34966873604973081, 24.58442372801901499 ) ) ;
#131280=CARTESIAN_POINT ( 'NONE',  ( 5.823673210054444382, -21.52544592524334988, 50.20942372801901854 ) ) ;
#131282=CARTESIAN_POINT ( 'NONE',  ( 19.02544592524343514, -5.153800228976328945, 113.5405762719810241 ) ) ;
#131283=CARTESIAN_POINT ( 'NONE',  ( 9.564922557961047289, -16.46253265017146816, 65.41775706135233293 ) ) ;
#131285=CARTESIAN_POINT ( 'NONE',  ( 5.823673210054444382, -21.52544592524334988, 20.20942372801900788 ) ) ;
#131286=CARTESIAN_POINT ( 'NONE',  ( -19.03943276465977164, 0.05219959533909376836, 56.24890960531435979 ) ) ;
#131288=CARTESIAN_POINT ( 'NONE',  ( -16.51473224551082808, 9.474510206698731452, 23.33442372801900078 ) ) ;
#131289=CARTESIAN_POINT ( 'NONE',  ( -5.049401038298153566, 19.05341960407611168, 55.20724293864769550 ) ) ;
#131290=CARTESIAN_POINT ( 'NONE',  ( -18.67979575497193778, 10.72451020669871902, 108.3344237280190185 ) ) ;
#131291=CARTESIAN_POINT ( 'NONE',  ( 0.05219959533934541429, -16.53943276465976808, 100.0010903946857042 ) ) ;
#131292=CARTESIAN_POINT ( 'NONE',  ( -9.564922557960796823, -16.46253265017161027, 102.0822429386477097 ) ) ;
#131293=CARTESIAN_POINT ( 'NONE',  ( 5.719274019375673035, 21.55341960407619339, 72.29275706135236135 ) ) ;
#131295=CARTESIAN_POINT ( 'NONE',  ( 16.51473224551069308, 9.474510206698969483, 114.1655762719810241 ) ) ;
#131296=CARTESIAN_POINT ( 'NONE',  ( -17.49999999999999645, -5.499999999999992895, 94.20309617465827046 ) ) ;
#131297=CARTESIAN_POINT ( 'NONE',  ( -4.379528057220086978, -16.55341960407618274, 59.79275706135234714 ) ) ;
#131298=CARTESIAN_POINT ( 'NONE',  ( 10.81492255796106328, -18.62759615963255655, 75.41775706135233293 ) ) ;
#131299=CARTESIAN_POINT ( 'NONE',  ( -15.80617190586768217, 15.72974639402176855, 103.1260903946856757 ) ) ;
#131301=CARTESIAN_POINT ( 'NONE',  ( -19.02544592524342804, 5.153800228976336051, 81.04057627198103830 ) ) ;
#131302=CARTESIAN_POINT ( 'NONE',  ( -5.049401038298153566, 19.05341960407611168, 105.2072429386476671 ) ) ;
#131304=CARTESIAN_POINT ( 'NONE',  ( 16.52216118717209170, 7.221426719304526287, 43.57599021046996057 ) ) ;
#131305=CARTESIAN_POINT ( 'NONE',  ( -5.049401038298153566, 19.05341960407611168, 45.20724293864769550 ) ) ;
#131306=CARTESIAN_POINT ( 'NONE',  ( 5.719274019375991003, -21.55341960407610458, 47.70724293864770260 ) ) ;
#131307=CARTESIAN_POINT ( 'NONE',  ( 14.29746914071037800, 8.314922557961029526, 111.6677570613523613 ) ) ;
#131308=CARTESIAN_POINT ( 'NONE',  ( 16.55341960407611168, 4.379528057220329451, 83.95724293864770971 ) ) ;
#131309=CARTESIAN_POINT ( 'NONE',  ( 5.153800228976335163, 19.02544592524342804, 84.79057627198099567 ) ) ;
#131310=CARTESIAN_POINT ( 'NONE',  ( 21.53943276465977519, 0.05219959533937863772, 101.2510903946856757 ) ) ;
#131311=CARTESIAN_POINT ( 'NONE',  ( -5.153800228976328057, -19.02544592524343514, 32.29057627198102409 ) ) ;
#131312=CARTESIAN_POINT ( 'NONE',  ( -16.52544592524342804, 4.483927247898546575, 86.04057627198102409 ) ) ;
#131313=CARTESIAN_POINT ( 'NONE',  ( -21.52544592524334988, -5.823673210054445271, 43.95942372801902565 ) ) ;
#131314=CARTESIAN_POINT ( 'NONE',  ( 18.67979575497178502, 10.72451020669898547, 89.16557627198102409 ) ) ;
#131315=CARTESIAN_POINT ( 'NONE',  ( 0.05219959533936267826, -19.03943276465977164, 45.00109039468566863 ) ) ;
#131317=CARTESIAN_POINT ( 'NONE',  ( 5.153800228976335163, 19.02544592524342804, 89.79057627198102409 ) ) ;
#131318=CARTESIAN_POINT ( 'NONE',  ( 14.34966873604960469, 8.224510206698951720, 64.16557627198102409 ) ) ;
#131320=CARTESIAN_POINT ( 'NONE',  ( -16.53943276465976808, 0.05219959533911058130, 51.24890960531436690 ) ) ;
#131321=CARTESIAN_POINT ( 'NONE',  ( -16.46253265017146816, -9.564922557961047289, 84.16775706135233293 ) ) ;
#131323=CARTESIAN_POINT ( 'NONE',  ( -5.719274019375978568, 21.55341960407610458, 25.20724293864769550 ) ) ;
#131325=CARTESIAN_POINT ( 'NONE',  ( -4.483927247898539470, -16.52544592524342804, 92.29057627198103830 ) ) ;
#131327=CARTESIAN_POINT ( 'NONE',  ( 9.564922557960805705, 16.46253265017160317, 49.58224293864770260 ) ) ;
#131328=CARTESIAN_POINT ( 'NONE',  ( -21.55341960407610458, -5.719274019375992779, 51.45724293864770260 ) ) ;
#131329=CARTESIAN_POINT ( 'NONE',  ( -5.049401038298153566, 19.05341960407611168, 30.20724293864768839 ) ) ;
#131330=CARTESIAN_POINT ( 'NONE',  ( -14.34966873604972548, 8.224510206698743886, 73.33442372801901854 ) ) ;
#131331=CARTESIAN_POINT ( 'NONE',  ( -16.51473224551069308, -9.474510206698971260, 61.66557627198103120 ) ) ;
#131332=CARTESIAN_POINT ( 'NONE',  ( -13.89961937509957401, -13.97604488694547875, 34.37609039468566863 ) ) ;
#131333=CARTESIAN_POINT ( 'NONE',  ( 18.67979575497194134, -10.72451020669871369, 70.83442372801901854 ) ) ;
#131334=CARTESIAN_POINT ( 'NONE',  ( 18.62759615963271287, -10.81492255796078972, 38.33224293864768839 ) ) ;
#131335=CARTESIAN_POINT ( 'NONE',  ( 16.46253265017160672, -9.564922557960803928, 23.33224293864769194 ) ) ;
#131336=CARTESIAN_POINT ( 'NONE',  ( 13.89961937509957401, 13.97604488694547697, 96.87609039468566152 ) ) ;
#131339=CARTESIAN_POINT ( 'NONE',  ( -0.05219959533907301413, -21.53943276465977519, 42.49890960531435979 ) ) ;
#131340=CARTESIAN_POINT ( 'NONE',  ( 16.51473224551069308, 9.474510206698969483, 24.16557627198102765 ) ) ;
#131341=CARTESIAN_POINT ( 'NONE',  ( -15.80617190586768217, 15.72974639402176855, 78.12609039468570415 ) ) ;
#131342=CARTESIAN_POINT ( 'NONE',  ( -14.34966873604960291, -8.224510206698953496, 46.66557627198102409 ) ) ;
#131343=CARTESIAN_POINT ( 'NONE',  ( -4.379528057220086978, -16.55341960407618274, 74.79275706135234714 ) ) ;
#131344=CARTESIAN_POINT ( 'NONE',  ( 16.52544592524342804, -4.483927247898539470, 53.54057627198103120 ) ) ;
#131345=CARTESIAN_POINT ( 'NONE',  ( 21.52544592524344225, -5.823673210054117533, 78.54057627198103830 ) ) ;
#131346=CARTESIAN_POINT ( 'NONE',  ( 0.05219959533907565091, 21.53943276465977519, 74.99890960531435269 ) ) ;
#131348=CARTESIAN_POINT ( 'NONE',  ( -10.81492255796078084, -18.62759615963271287, 37.08224293864768129 ) ) ;
#131349=CARTESIAN_POINT ( 'NONE',  ( -0.05219959533934338120, 16.53943276465976808, 47.50109039468568994 ) ) ;
#131350=CARTESIAN_POINT ( 'NONE',  ( 16.52544592524342804, -4.483927247898539470, 78.54057627198103830 ) ) ;
#131351=CARTESIAN_POINT ( 'NONE',  ( 16.46253265017160672, -9.564922557960803928, 68.33224293864770971 ) ) ;
#131352=CARTESIAN_POINT ( 'NONE',  ( -16.51473224551069308, -9.474510206698971260, 31.66557627198102054 ) ) ;
#131353=CARTESIAN_POINT ( 'NONE',  ( -17.72517630440434289, 5.499999999999977796, 75.92175719257211597 ) ) ;
#131354=CARTESIAN_POINT ( 'NONE',  ( 12.06949235617739724, 12.14591786802326823, 76.87609039468567573 ) ) ;
#131355=CARTESIAN_POINT ( 'NONE',  ( 15.80617190586746368, 15.72974639402197994, 114.3739096053143527 ) ) ;
#131356=CARTESIAN_POINT ( 'NONE',  ( -16.51473224551069308, -9.474510206698971260, 66.66557627198102409 ) ) ;
#131357=CARTESIAN_POINT ( 'NONE',  ( -5.823673210054431948, 21.52544592524334988, 52.70942372801902565 ) ) ;
#131358=CARTESIAN_POINT ( 'NONE',  ( -0.05219959533909027116, -19.03943276465977164, 112.4989096053143669 ) ) ;
#131361=CARTESIAN_POINT ( 'NONE',  ( 0.05219959533937995610, -21.53943276465977519, 50.00109039468568994 ) ) ;
#131362=CARTESIAN_POINT ( 'NONE',  ( -9.474510206698964154, 16.51473224551069663, 115.4155762719810241 ) ) ;
#131363=CARTESIAN_POINT ( 'NONE',  ( 16.46253265017160672, -9.564922557960803928, 103.3322429386476955 ) ) ;
#131364=CARTESIAN_POINT ( 'NONE',  ( 0.05219959533936267826, -19.03943276465977164, 55.00109039468566863 ) ) ;
#131365=CARTESIAN_POINT ( 'NONE',  ( -21.52544592524343514, 5.823673210054127303, 111.0405762719810525 ) ) ;
#131366=CARTESIAN_POINT ( 'NONE',  ( -9.564922557961040184, 16.46253265017147172, 42.91775706135234003 ) ) ;
#131367=CARTESIAN_POINT ( 'NONE',  ( -19.03943276465977164, -0.05219959533935918106, 68.75109039468566152 ) ) ;
#131368=CARTESIAN_POINT ( 'NONE',  ( 12.14591786802327356, -12.06949235617739191, 100.6260903946857184 ) ) ;
#131369=CARTESIAN_POINT ( 'NONE',  ( 30.00000000000000000, -5.510910596163089556E-15, 42.49999999999999289 ) ) ;
#131371=CARTESIAN_POINT ( 'NONE',  ( 16.51473224551069308, 9.474510206698969483, 84.16557627198102409 ) ) ;
#131373=CARTESIAN_POINT ( 'NONE',  ( 18.62759615963255655, 10.81492255796105972, 91.66775706135234714 ) ) ;
#131374=CARTESIAN_POINT ( 'NONE',  ( 10.81492255796106328, -18.62759615963255655, 90.41775706135236135 ) ) ;
#131376=CARTESIAN_POINT ( 'NONE',  ( -5.153800228976328057, -19.02544592524343514, 107.2905762719810383 ) ) ;
#131377=CARTESIAN_POINT ( 'NONE',  ( 5.823673210054444382, -21.52544592524334988, 75.20942372801901854 ) ) ;
#131378=CARTESIAN_POINT ( 'NONE',  ( -19.03943276465977164, -0.05219959533935918106, 108.7510903946856615 ) ) ;
#131379=CARTESIAN_POINT ( 'NONE',  ( -19.05341960407611168, -5.049401038298163336, 81.45724293864769550 ) ) ;
#131380=CARTESIAN_POINT ( 'NONE',  ( -5.823673210054116645, -21.52544592524344225, 27.29057627198103120 ) ) ;
#131381=CARTESIAN_POINT ( 'NONE',  ( 19.02544592524343514, -5.153800228976328945, 98.54057627198100988 ) ) ;
#131382=CARTESIAN_POINT ( 'NONE',  ( -17.05116617787826527, -6.768360034955815507, 91.34324446740806991 ) ) ;
#131383=CARTESIAN_POINT ( 'NONE',  ( 13.97604488694527802, 13.89961937509977652, 79.37390960531435269 ) ) ;
#131384=CARTESIAN_POINT ( 'NONE',  ( -19.05341960407611168, -5.049401038298163336, 66.45724293864769550 ) ) ;
#131385=CARTESIAN_POINT ( 'NONE',  ( 0.05219959533907565091, 21.53943276465977519, 109.9989096053143527 ) ) ;
#131386=CARTESIAN_POINT ( 'NONE',  ( -8.314922557961024197, 14.29746914071037800, 97.91775706135236135 ) ) ;
#131388=CARTESIAN_POINT ( 'NONE',  ( -5.153800228976607833, 19.02544592524334988, 52.70942372801900433 ) ) ;
#131389=CARTESIAN_POINT ( 'NONE',  ( -13.97604488694527625, -13.89961937509977652, 96.87390960531433848 ) ) ;
#131390=CARTESIAN_POINT ( 'NONE',  ( -8.314922557960811034, -14.29746914071050412, 87.08224293864769550 ) ) ;
#131391=B_SPLINE_CURVE_WITH_KNOTS ( 'NONE', 3,
 ( #44873, #27741, #89383, #182402, #169187, #12563, #14526, #74229, #75202, #106529, #168206, #76187, #199546, #61016, #144814, #156010, #17507, #173182, #159991, #79165 ),
 .UNSPECIFIED., .F., .F.,
 ( 4, 2, 2, 2, 2, 2, 2, 2, 2, 4 ),
 ( 0.000000000000000000, 0.0004987090165372591501, 0.0009974180330745183003, 0.001246772541343151670, 0.001496127049611785040, 0.001994836066149047443, 0.002493545082686309412, 0.002742899590954942565, 0.002992254099223575717, 0.003989672132298185958 ),
 .UNSPECIFIED. ) ;
#131392=CARTESIAN_POINT ( 'NONE',  ( 21.53943276465977519, -0.05219959533907433946, 28.74890960531435624 ) ) ;
#131393=CARTESIAN_POINT ( 'NONE',  ( -9.564922557960796823, -16.46253265017161027, 112.0822429386476955 ) ) ;
#131394=CARTESIAN_POINT ( 'NONE',  ( -16.55341960407611168, -4.379528057220339221, 96.45724293864770971 ) ) ;
#131395=CARTESIAN_POINT ( 'NONE',  ( -16.61371651742604172, 7.165104196376022472, 53.85415069992998127 ) ) ;
#131396=CARTESIAN_POINT ( 'NONE',  ( 19.05341960407617918, -5.049401038297876454, 41.04275706135233293 ) ) ;
#131397=CARTESIAN_POINT ( 'NONE',  ( -16.53943276465976808, -0.05219959533934237506, 108.7510903946857042 ) ) ;
#131398=CARTESIAN_POINT ( 'NONE',  ( 9.564922557960805705, 16.46253265017160317, 84.58224293864769550 ) ) ;
#131399=CARTESIAN_POINT ( 'NONE',  ( 21.53943276465977519, 0.05219959533937863772, 71.25109039468568994 ) ) ;
#131400=CARTESIAN_POINT ( 'NONE',  ( -21.53943276465977519, 0.05219959533907696930, 51.24890960531436690 ) ) ;
#131401=CARTESIAN_POINT ( 'NONE',  ( -15.72974639402176322, -15.80617190586768395, 34.37609039468568284 ) ) ;
#131402=CARTESIAN_POINT ( 'NONE',  ( 21.53943276465977519, -0.05219959533907433946, 88.74890960531436690 ) ) ;
#131403=CARTESIAN_POINT ( 'NONE',  ( 8.314922557960818139, 14.29746914071049879, 114.5822429386477097 ) ) ;
#131404=CARTESIAN_POINT ( 'NONE',  ( -19.05341960407617563, 5.049401038297882671, 68.54275706135230450 ) ) ;
#131405=CARTESIAN_POINT ( 'NONE',  ( 13.97604488694527802, 13.89961937509977652, 44.37390960531435269 ) ) ;
#131406=( BOUNDED_SURFACE ( )  B_SPLINE_SURFACE ( 3, 2, ( 
 ( #39061, #142242, #20892, #96724, #173600, #129050, #18922, #53221, #130039, #127065, #191738, #190751, #21898, #6709, #38066, #143229, #189765, #114898, #82550, #83548, #176592, #80567, #36057, #99722, #144232, #37056, #51237, #97706, #5716, #175579, #4712, #65404, #84544, #3727, #174592, #145227, #66401, #67393, #128063, #52225, #35069, #146221, #161406, #22898, #188773, #112898, #50256, #68387, #98715, #111912, #54233, #158412, #7709, #69393, #115904, #160409, #131061, #192750, #177594, #157428, #19901, #81542, #193759, #133066, #102734, #164423, #178588, #59202, #23902, #179599, #89555, #150253, #40052, #120871, #25916, #58228, #57242, #55227, #181582, #182571, #103738, #117910, #104726, #74396, #101729, #88554, #165418, #9738, #27912, #26911, #135085, #163417, #11747, #196761, #119897, #87560, #24913, #132070, #162399, #134079, #10738, #73414, #43060, #194756, #116896, #166418, #149247, #151241, #195768, #86560, #118916, #180600, #12730, #41071, #42074, #136061, #85556, #100719, #147241, #8733, #72402, #197736, #70402, #148244, #71402, #56228, #183559, #155196, #47029, #106703, #125844, #185536, #44054, #105714, #502, #170365, #138039, #121867, #108687, #31857, #141011, #93510, #154204, #167401, #153196, #107682, #123838, #79341, #61186, #28897, #13703, #124854, #60197, #90537, #122858, #16685, #75370, #17683, #186554, #30869, #156184, #152219, #199720, #168376, #184546, #137040, #29872, #91509, #2498, #1497, #109683, #78335, #45045, #171364, #198731, #32852, #62174, #46026, #14700, #140008, #48026, #76362, #169359, #63175, #92515, #94502, #64179, #15694, #77355, #139022, #112655, #67151, #81302, #127816, #174346, #143988, #34826, #95497, #114646, #110668, #4464, #51982, #173355, #97462, #96481, #159148, #65161, #176344, #68143, #21652, #172348, #158169, #18677, #113640, #20644, #80323, #84301, #128809, #188526, #35816, #142986, #50003, #37816, #33837, #157183, #141996, #82297, #83305, #3484, #190508, #126820, #19661, #144982, #111668, #99477, #36802, #66153, #189521, #49013, #6462, #50994, #5469, #175335, #98467, #160161, #129794, #161158, #69146, #191491, #187546, #52969, #22654, #145980, #7462, #8481, #133827, #72151, #27670, #118665, #40818, #53988, #39806, #194508, #10491, #166169, #148003, #192504, #100479, #11499, #146994, #115661, #9493, #195518, #162158, #104485, #73170, #117658, #42822, #12494, #24665, #54984, #86314, #130813, #193507, #116653, #89310, #88305, #196519, #56991, #70156, #57990, #23654, #119661, #87318, #132822, #178344, #177351, #180356, #181343, #151003, #71156, #179355, #149002, #41825, #163162, #38821, #103492, #85302, #134840, #165170, #131826, #101472, #55981, #26663, #102488, #164175, #25673, #149993, #75128, #60941, #168132, #136796, #65667, #120632, #58964, #182329, #122616, #111176, #90292, #77109, #13464, #121621, #172866, #105471, #127329, #126346, #151976, #198482, #135827, #34347, #76113, #92271, #183316, #64684, #96008, #197497, #138779, #260, #184306, #45787, #59954, #44798, #107439, #43808, #152951, #169111, #49513, #3987, #189041, #153955, #50516, #188043, #157692, #167157, #30618, #106453, #19183, #28657, #137790, #29628, #15451, #80832, #142509, #74156, #112179, #35335, #91260, #173867, #96988, #158670, #14450, #199474, #159661, #193017, #145492, #6972, #55492, #161669, #81805, #146487, #117162, #143492, #176859, #84808, #102000, #4977, #22161, #21158, #36315, #192003, #66663, #116166, #54494, #190025, #177856, #53489, #7978, #69662, #100984, #5978, #52487, #39325, #68652, #131329, #162668, #128326, #98979, #24174, #130308, #99984, #114147, #160669, #115166, #38328, #67658, #51499, #147513, #113159, #37321, #85825, #129315, #23165, #191011, #9003, #97969, #83812, #70670, #132337, #175848, #174849, #194029, #82813, #178858, #40324, #20160, #144495, #149504, #73675, #41336, #90796, #44319, #198000, #148513, #72673, #195021, #28180, #135347 ),
 ( #197021, #58487, #59470, #42338, #43324, #13967, #10003, #183823, #122136, #71663, #120154, #12014, #25185, #118175, #136325, #181844, #86827, #11001, #182837, #121143, #45313, #104991, #163682, #133330, #166679, #89822, #57508, #102997, #151503, #12995, #60461, #74658, #105978, #56497, #134350, #27176, #167663, #198993, #180862, #179866, #164683, #29159, #26177, #87818, #103999, #152480, #196032, #137312, #75634, #150516, #119177, #165677, #88823, #31138, #62444, #188803, #169642, #92786, #65433, #64450, #172627, #186830, #123127, #34115, #76630, #95773, #63456, #108961, #154474, #168637, #33123, #157459, #3756, #774, #155467, #125132, #48298, #139296, #106963, #109955, #199989, #124118, #170641, #32129, #184812, #127094, #30137, #185818, #18953, #156461, #46298, #91780, #93787, #94780, #153474, #16958, #15967, #78612, #140286, #171634, #14970, #17960, #138308, #61456, #1777, #79615, #141284, #142274, #107955, #77627, #2774, #126120, #187815, #47305, #49284, #110942, #80598, #85586, #111943, #6739, #114930, #132098, #35100, #52254, #189795, #66430, #21928, #173630, #146253, #22929, #19930, #84575, #83579, #176623, #99753, #131092, #36086, #82579, #7739, #175610, #38098, #69425, #96752, #129078, #192780, #37086, #130070, #144260, #190779, #98745, #68417, #97736, #158442, #177625, #81571, #67423, #161437, #159425, #160438, #20921, #145258, #128091, #39093, #54263, #115935, #143257, #5747, #4741, #100749, #191769, #51266, #147272, #53252, #112926, #162430, #113911, #174621, #23931, #8763, #70432, #50286, #42105, #27945, #9767, #196791, #133095, #41101, #89586, #24944, #182603, #43091, #71431, #194785, #55257, #151272, #195800, #11780, #102766, #181613, #12762, #116925, #58259, #119928, #103769, #165448, #56258, #117941, #180632, #178618, #72435, #26943, #166448, #120904, #44088, #73444, #105747, #104759, #74427, #40081, #88585, #25947, #136093, #75403, #135115, #193788, #101759, #150284, #197768, #87590, #179630, #59234, #167433, #90569, #28929, #152251, #163447, #164453, #57272, #13736, #86592, #10769, #148275, #149276, #134111, #118947, #60230, #15728, #16721, #106735, #110706, #17721, #123872, #49051, #18716, #30902, #61219, #92549, #137075, #199752, #122890, #95536, #94540, #2536, #78370, #153231, #64217, #168409, #125883, #93546, #139057, #184578, #198764, #63212, #187583, #33877, #154238, #185571, #155231, #140044, #169394, #121899, #1534, #29904, #77388, #536, #62208, #14734, #157223, #183593, #47064, #172387, #186591, #76395, #45077, #108724, #156221, #124892, #91542, #79379, #138071, #48063, #170401, #141050, #46059, #107714, #109719, #171402, #31892, #32889, #145021, #114689, #158209, #6502, #176384, #37858, #144027, #4502, #111708, #142036, #113679, #190546, #53010, #161199, #112693, #173394, #99517, #5509, #68182, #175373, #143024, #36841, #98506, #22694, #159187, #160201, #130853, #65200, #100518, #38862, #126859, #52020, #128847, #3524, #34864, #84341, #21691, #188565, #127856, #146020, #69187, #50045, #96519, #19699, #83345, #7503, #81341, #129834, #66193, #189560, #192545, #51032, #54028, #191533, #174385, #35855, #97501, #115701, #82337, #177390, #20682, #162197, #80363, #67190, #57032, #118705, #164214, #25711, #39846, #116693, #87356, #147036, #56019, #149042, #165208, #196556, #119697, #133867, #181380, #41867, #180396, #85343, #102531, #71196, #103533, #8520, #117697, #148041, #10530, #72194, #195558, #23695, #26703, #70198, #163202, #88343, #150035, #11541, #131865, #193549, #132860, #58027, #73209, #134880, #55022, #42858, #101512, #104523, #178382, #86355, #166204, #27706, #24706, #194549, #89348, #9530, #179394, #40857, #65843, #100172, #177046, #174045, #38516, #176037, #68842, #53679, #84993, #190199, #36496, #161854, #129497, #130501, #23348, #127513, #83001, #146674, #191196, #83998, #98150, #144676, #52671, #160857, #51677, #112354, #131513, #189217, #21343, #192197 ),
 ( #35514, #101163, #145677, #5158, #114334, #159850, #66841, #37505, #7159, #4165, #115356, #162851, #97162, #99167, #22347, #8169, #39503, #24358, #143677, #69845, #193199, #54672, #86009, #116346, #50696, #178035, #158847, #20335, #81984, #128504, #113339, #175031, #6161, #67841, #163871, #119358, #9186, #43505, #120327, #117348, #182022, #181042, #12193, #197198, #28359, #133515, #180054, #105171, #72863, #73858, #166857, #70851, #26362, #89997, #134533, #27358, #41523, #88002, #196220, #104180, #195207, #55674, #74835, #132520, #164867, #135527, #56687, #57690, #118361, #42517, #25370, #136497, #151679, #13172, #194209, #103186, #179044, #58661, #165862, #40512, #44497, #89004, #148698, #150695, #149690, #10186, #198177, #102183, #87012, #71846, #59647, #121321, #11188, #183013, #106153, #167835, #29336, #147698, #99803, #7793, #34162, #159475, #97786, #110992, #3804, #21978, #20969, #172677, #96805, #68469, #6790, #131142, #190828, #49331, #95823, #5798, #175660, #143304, #127144, #52304, #113961, #146304, #37134, #82626, #157508, #158491, #112976, #129130, #84626, #66480, #19002, #80648, #130124, #65482, #142324, #67471, #81621, #188851, #98794, #50335, #4790, #51315, #174669, #111992, #69476, #173682, #128142, #38149, #160488, #35149, #19978, #36134, #191821, #83630, #189842, #53301, #144308, #145307, #114980, #176673, #22977, #161489, #180677, #195845, #101808, #119971, #57318, #26989, #70480, #118994, #88634, #150330, #56306, #116975, #23980, #54311, #25991, #102813, #165493, #73490, #24994, #85636, #11825, #117988, #42153, #87634, #55303, #149320, #10814, #135163, #71477, #134157, #133142, #72484, #43136, #151319, #177672, #164498, #41150, #115983, #147323, #196836, #103813, #39140, #40130, #58304, #181657, #74475, #104805, #192830, #100795, #166494, #27992, #86638, #132146, #89631, #12808, #162478, #8811, #193839, #178667, #163496, #179678, #148321, #9816, #194833, #197816, #105793, #16765, #152298, #59281, #14782, #15774, #167479, #109760, #78413, #122937, #48104, #17766, #29953, #60275, #91591, #136140, #198810, #121948, #94586, #93590, #1581, #77433, #13782, #63256, #28974, #124936, #92594, #138119, #183641, #120951, #62250, #186633, #32931, #153281, #184624, #154284, #168456, #123919, #182650, #199800, #45123, #46106, #169445, #139105, #44134, #185618, #156265, #90616, #30947, #579, #47108, #171444, #75449, #137123, #108767, #61267, #107760, #106781, #170445, #76442, #31936, #155276, #140089, #35898, #144071, #161243, #64260, #81382, #18760, #95579, #51074, #141093, #175418, #52065, #49095, #113722, #112735, #5552, #128889, #160246, #65243, #111750, #36886, #4545, #67231, #98552, #2580, #158251, #21735, #66239, #159231, #173438, #19741, #127899, #97544, #126903, #187625, #6546, #125926, #96563, #190589, #188609, #189601, #50090, #174428, #157264, #68225, #83388, #145065, #110752, #34907, #172433, #129878, #20726, #33922, #176429, #82383, #80407, #191577, #143067, #142079, #53055, #3565, #114735, #37903, #99561, #79422, #56063, #57077, #101558, #164260, #163250, #102576, #73251, #181422, #7546, #132904, #71241, #84385, #177433, #195604, #194592, #146062, #70243, #41912, #180440, #104565, #25755, #22737, #69232, #179437, #149086, #116737, #100561, #87401, #10574, #119739, #72237, #117742, #130899, #131911, #86399, #133913, #118751, #178427, #24752, #148084, #40903, #193595, #192589, #150079, #54072, #39891, #103578, #8568, #165253, #55066, #26747, #162241, #11584, #88385, #134921, #115746, #9575, #38904, #196598, #58069, #23741, #42900, #85390, #147084, #153033, #60036, #167238, #155028, #12570, #93343, #75209, #46861, #91342, #182409, #169194, #105552, #13543, #108522, #170201, #16524, #76194, #43888, #28736, #27748, #339, #168213, #184384, #136880, #154037, #123672, #89391, #30701, #92351, #14533, #137873, #90373, #152058, #199553, #151079, #44880, #61023, #138859, #78171 ),
 ( #74236, #106536, #45865, #135905, #139840, #31694, #122695, #1329, #47862, #121703, #198566, #183397, #166247, #29710, #107518, #124688, #185370, #63009, #15532, #77189, #186384, #197576, #59043, #62007, #120709, #172185, #171197, #35654, #36638, #6304, #3326, #158009, #65988, #127658, #141834, #191332, #189358, #2332, #64999, #111502, #173188, #187380, #67982, #32686, #188360, #98295, #158988, #48849, #129636, #110503, #159997, #190342, #143823, #94338, #18515, #140843, #174186, #19500, #64013, #109515, #50835, #33670, #96322, #126657, #95332, #21484, #156017, #83146, #80162, #51818, #34664, #125682, #112492, #157017, #49838, #113478, #175172, #144820, #81145, #142826, #4306, #17514, #5304, #97302, #20480, #82130, #66988, #128647, #79172, #55822, #117495, #101311, #163000, #192345, #68987, #39650, #37650, #131665, #24506, #25515, #180198, #103331, #132666, #165010, #102329, #40660, #114477, #86157, #85142, #164019, #176180, #54822, #161997, #147847, #9333, #194355, #52810, #179192, #11336, #145819, #70999, #87160, #148842, #88146, #73007, #53827, #10332, #178185, #71989, #149832, #133663, #99314, #195353, #134676, #160999, #56833, #118508, #22493, #84140, #116497, #115502, #130651, #41667, #7302, #26504, #177189, #38663, #100318, #23493, #146827, #8321, #69997, #193347, #28500, #153793, #121464, #60783, #15288, #119503, #74974, #76947, #183157, #75957, #90134, #136636, #44641, #152797, #43647, #104323, #123436, #181184, #13308, #122454, #182163, #106293, #105311, #167979, #151819, #120471, #198318, #77937, #58803, #166998, #154788, #138617, #61768, #137631, #12334, #185129, #166007, #46620, #14289, #59795, #29477, #57830, #184147, #108281, #93104, #91108, #199316, #45628, #107280, #168951, #196362, #30457, #89149, #92105, #99, #169959, #73998, #16287, #42661, #31451, #27508, #150838, #135668, #197340, #141607, #97074, #96094, #32448, #20244, #162511, #142596, #156789, #143585, #116013, #17278, #127423, #4076, #48620, #69507, #65753, #173954, #78932, #189131, #35421, #158755, #3094, #63779, #170955, #1090, #172956, #49602, #112262, #81892, #171953, #94102, #5068, #110271, #19273, #155781, #111265, #34434, #157783, #131173, #18282, #80920, #79937, #50603, #192863, #100828, #124447, #54342, #188130, #62766, #140608, #177703, #39170, #186143, #187147, #24012, #139604, #47622, #109276, #2098, #125451, #33441, #95100, #64771, #126433, #88670, #27025, #182685, #73527, #195881, #8843, #194865, #149352, #165529, #120987, #102844, #147355, #55336, #166530, #101838, #70511, #164529, #150366, #117006, #59318, #28027, #72518, #197851, #167516, #87667, #103848, #133175, #135198, #43172, #132179, #11862, #196871, #134193, #57354, #25025, #163525, #119029, #193870, #26022, #180712, #58338, #12844, #136176, #120006, #44170, #181691, #104839, #178701, #42188, #118020, #89668, #40163, #10849, #56338, #151355, #74510, #105829, #85668, #86669, #148352, #9848, #71507, #179709, #41181, #64296, #187661, #168492, #1617, #154320, #15809, #125963, #170482, #90651, #155313, #49132, #152333, #185653, #93628, #110790, #13819, #30981, #29990, #45162, #617, #75485, #124973, #63293, #198847, #186670, #62287, #16802, #78452, #109797, #14818, #61304, #48140, #77470, #140126, #171480, #137158, #107797, #32969, #139140, #108803, #122974, #169481, #123955, #47145, #76479, #60311, #156302, #121987, #46143, #94623, #138156, #31972, #199837, #17803, #106818, #79460, #141129, #2619, #183677, #184661, #91629, #29011, #153317, #92629, #69268, #52101, #173474, #159267, #66276, #34947, #161278, #18798, #99598, #81418, #53092, #97579, #188647, #175454, #111786, #19777, #114770, #176464, #22773, #82418, #50126, #96599, #33958, #6583, #20763, #127935, #158288, #84421, #80443, #146098, #143104, #37937, #144107, #4583, #36925, #189637, #51112, #7582, #130934, #192625, #5587, #112771, #174464, #95616, #68262, #35933, #190626, #67267 ),
 ( #145100, #54107, #172471, #113758, #157301, #21772, #160281, #142116, #128925, #98587, #83423, #3601, #129913, #191613, #65280, #126939, #57117, #115781, #41951, #74275, #8606, #10615, #72276, #133953, #151119, #135945, #55103, #88428, #40942, #102614, #12611, #118791, #177470, #103617, #197615, #38939, #195644, #180480, #100596, #162278, #117783, #116773, #131947, #87439, #23778, #11623, #150122, #85428, #73291, #149124, #165293, #26786, #196639, #101600, #148123, #134961, #164300, #58108, #119778, #147119, #194632, #181462, #25793, #42940, #9614, #56102, #104604, #166292, #163288, #70279, #27788, #193631, #132944, #89430, #24789, #178464, #86437, #39931, #71279, #179477, #139879, #93381, #43926, #168251, #90411, #123713, #169234, #152096, #156056, #138896, #60073, #185410, #153071, #136918, #62048, #376, #17553, #46901, #30740, #182446, #29747, #122732, #108561, #94376, #76231, #120747, #28773, #1368, #75247, #105588, #137911, #170239, #13580, #32724, #63047, #45903, #171235, #140882, #14573, #183433, #199593, #59080, #121741, #44918, #79213, #16562, #124726, #31733, #198605, #186424, #106574, #47900, #15569, #61060, #91382, #167274, #155067, #109554, #184423, #107556, #92388, #77227, #78209, #154075, #84176, #20520, #95372, #34703, #4344, #66029, #80202, #161035, #125722, #81183, #191370, #51858, #141873, #22529, #127696, #160036, #159027, #157057, #83184, #2372, #5343, #19538, #6341, #176218, #3364, #190383, #67027, #111542, #129672, #128686, #36677, #65039, #113518, #98337, #21523, #189396, #126695, #33710, #64052, #35694, #112531, #175212, #144858, #96360, #18554, #68021, #173227, #82168, #188399, #174225, #97341, #143864, #52846, #142865, #114517, #50873, #37687, #99352, #187421, #48889, #110544, #172225, #49877, #158048, #118544, #194390, #7338, #193383, #165046, #103368, #27542, #87197, #145856, #69023, #102365, #10369, #180234, #23531, #72026, #41703, #26539, #9369, #70033, #177227, #130688, #179229, #55857, #88183, #149867, #178221, #38699, #11372, #116533, #25553, #100356, #117531, #40695, #164054, #73042, #24543, #148878, #86193, #133699, #196397, #104358, #192382, #195391, #56869, #53865, #162035, #134714, #57866, #115539, #54859, #119538, #181221, #85177, #42697, #146866, #8358, #166042, #131702, #39685, #101347, #163036, #147883, #71034, #132701, #199351, #12369, #198354, #152832, #168987, #124483, #106327, #150875, #58839, #169996, #105344, #74032, #168013, #30491, #120506, #62801, #31487, #75991, #1127, #170991, #183192, #13343, #44674, #89183, #151852, #75007, #47661, #46657, #154824, #92142, #167031, #16322, #182197, #77972, #45663, #91143, #136672, #135703, #15324, #139639, #186179, #29509, #137664, #107314, #153829, #121498, #197374, #76983, #43682, #14326, #60816, #122490, #28533, #109312, #90169, #184181, #59828, #138654, #135, #61804, #123474, #108316, #185166, #93139, #113282, #52613, #35456, #49639, #36437, #6103, #110307, #20279, #97107, #141642, #159790, #34469, #171989, #48655, #4109, #94137, #128445, #5101, #2134, #66783, #65788, #158790, #81925, #174973, #18317, #64807, #190141, #157817, #143617, #51617, #155816, #111302, #98092, #19307, #112297, #126468, #172991, #80955, #189163, #79974, #140644, #21285, #17314, #96128, #82942, #3132, #142630, #188166, #127457, #33477, #144620, #67784, #129441, #78969, #50635, #63814, #191140, #173987, #125487, #114275, #32484, #95135, #187184, #156824, #176987, #164807, #22288, #103126, #84935, #56628, #101106, #192137, #178984, #115294, #23291, #118302, #179994, #26302, #85949, #53618, #38457, #37447, #10127, #177978, #194152, #146616, #163809, #133457, #99108, #40451, #102125, #24301, #147638, #100112, #161796, #162792, #160800, #54613, #9127, #148637, #87942, #149630, #55616, #11128, #25311, #86953, #83939, #70793, #8108, #71787, #145620, #39446, #69786, #132461, #117290, #195147, #175979, #131454, #41461, #72803, #134473 ),
 ( #7099, #196158, #57631, #68781, #130438, #193141, #116288, #197139, #45428, #15088, #153590, #182958, #43446, #150638, #180981, #152596, #29279, #91899, #200104, #151623, #12134, #76749, #89942, #199110, #73798, #90911, #14087, #75753, #138424, #198123, #60577, #59590, #122253, #169759, #77744, #104121, #137430, #167781, #42457, #135471, #61572, #183943, #165803, #166801, #123241, #184932, #892, #107081, #119298, #27300, #168753, #30256, #13116, #58606, #46417, #108075, #16086, #31254, #92904, #88947, #28302, #44441, #154590, #139410, #136442, #120272, #181964, #105115, #74780, #121264, #106095, #111066, #156588, #110077, #143375, #49403, #174741, #144382, #18083, #186950, #79738, #62567, #125252, #48421, #21045, #20050, #128216, #142399, #78733, #189913, #32248, #51388, #19073, #64574, #171757, #124244, #188930, #113049, #159547, #141407, #172754, #80721, #3878, #94904, #185939, #65557, #155584, #2895, #126239, #187934, #140409, #82698, #47424, #34235, #36204, #112068, #1898, #109080, #95897, #81693, #127216, #17079, #4867, #170759, #50408, #157580, #66552, #97858, #63578, #173756, #35224, #33246, #93906, #96877, #158560, #192906, #38219, #193912, #67545, #7864, #115054, #116055, #39213, #40204, #114034, #99875, #84697, #98866, #100869, #162551, #24055, #41222, #164568, #145380, #178741, #131215, #54383, #102883, #147397, #129203, #132220, #26062, #190901, #85711, #70553, #87705, #52377, #69551, #6862, #22051, #177744, #175731, #101884, #163566, #37210, #25066, #8885, #55376, #117046, #86709, #191892, #161559, #148394, #9888, #71548, #133214, #160561, #146377, #194905, #56379, #118062, #23052, #179752, #5869, #83702, #53376, #68541, #130196, #176746, #166567, #13856, #135237, #59357, #196909, #121026, #27063, #79249, #32760, #186459, #134234, #58376, #180749, #75523, #182723, #42225, #48923, #29049, #150405, #136213, #43211, #11901, #140920, #195919, #2407, #120043, #94411, #74548, #165566, #152371, #88709, #181730, #156092, #17589, #64086, #44208, #73564, #104878, #10886, #47935, #151393, #167554, #28067, #137198, #109589, #72557, #198884, #60351, #197888, #105867, #89707, #12883, #90689, #57394, #122025, #171272, #125755, #187455, #110577, #172258, #33746, #149390, #103886, #119067, #128721, #5379, #68056, #176255, #127730, #126730, #129710, #66063, #175247, #188433, #67063, #190418, #51894, #191406, #174261, #36712, #35729, #98374, #145892, #53901, #80235, #113553, #143898, #157092, #49911, #52883, #160072, #18588, #142897, #114557, #37726, #177263, #21559, #95406, #141906, #83219, #144894, #189432, #173261, #6376, #99388, #192419, #161071, #22566, #3397, #4379, #159062, #84212, #130727, #112566, #65072, #111577, #7375, #34736, #96394, #69060, #115576, #50908, #97376, #158081, #82206, #19572, #81216, #20556, #39719, #147917, #104395, #178258, #101382, #42733, #103402, #149901, #148913, #131738, #11408, #146905, #73077, #25587, #194423, #116569, #38735, #56904, #134749, #100393, #71069, #102401, #10403, #72060, #9403, #162071, #133734, #193420, #132735, #117566, #179266, #163073, #23567, #8395, #40731, #181256, #165080, #24578, #85215, #164088, #196431, #118578, #86227, #57901, #70070, #26574, #87231, #54895, #55893, #119573, #195427, #180268, #41738, #88217, #83862, #53540, #97038, #145544, #115217, #176910, #82868, #143544, #38381, #142560, #98018, #100037, #144546, #99031, #113212, #159713, #6031, #175902, #66715, #127383, #146538, #4038, #36366, #7022, #5030, #129368, #128376, #191064, #158718, #8032, #161723, #23218, #65716, #190072, #50567, #68704, #52537, #112227, #116217, #160721, #20208, #67710, #174901, #81854, #69713, #189094, #131380, #51548, #84861, #114197, #35386, #22213, #21211, #37373, #193068, #54544, #177908, #130360, #192058, #39376, #80883, #101035, #19235, #173917, #10052, #150564, #120202, #85877, #165727, #27223, #11049, #72725, #102051, #178909, #149554, #147565 ),
 ( #24226, #164732, #71712, #134398, #196085, #197069, #70720, #195070, #41385, #55544, #57555, #119225, #180909, #198049, #121192, #163736, #135398, #87866, #42384, #59515, #104047, #9050, #88871, #182885, #132388, #12063, #73725, #44368, #194081, #26226, #25236, #40377, #58536, #117216, #181892, #43370, #86877, #105042, #166726, #28230, #89870, #151552, #148561, #56550, #13042, #74709, #136372, #162720, #133380, #179918, #118227, #103050, #183875, #93833, #109009, #15018, #33172, #170688, #140335, #45360, #32177, #1825, #63507, #169688, #30186, #137359, #167712, #139342, #16016, #78660, #186878, #138355, #199038, #125182, #76679, #185868, #60508, #77673, #821, #62495, #48348, #184862, #47354, #46345, #155513, #156509, #64500, #90842, #124166, #154519, #29208, #122183, #110002, #17008, #152527, #153521, #171683, #94831, #187862, #18010, #106025, #14014, #79664, #141335, #200037, #107012, #2822, #126167, #75680, #168685, #91828, #61505, #123174, #31183, #108002, #92834, #189366, #4314, #20489, #127666, #128655, #51826, #52818, #126665, #50843, #97310, #111510, #113486, #175180, #36646, #53837, #177199, #158017, #191340, #143832, #5312, #115511, #160005, #80171, #144828, #38672, #141843, #98305, #83154, #100327, #3334, #82138, #19508, #34672, #190350, #65008, #114486, #176189, #188369, #37658, #21493, #6312, #67990, #99323, #65997, #112500, #161007, #66996, #129644, #22501, #49846, #158996, #84148, #145827, #7310, #174194, #68995, #130660, #192353, #173196, #18524, #96330, #35662, #81153, #142835, #71997, #147855, #133671, #39658, #89157, #42671, #196371, #146836, #71007, #193355, #26512, #195362, #54831, #58811, #41675, #163008, #148850, #55830, #24515, #150846, #8329, #12342, #132675, #104332, #87169, #178193, #165019, #101319, #9342, #166016, #27516, #74006, #56841, #86165, #194363, #23502, #57839, #164027, #180206, #117503, #149841, #119512, #85150, #88156, #11345, #10341, #118516, #179200, #40668, #103339, #70004, #102337, #73016, #134685, #135676, #197348, #181193, #120480, #182171, #43657, #131674, #162006, #116505, #25523, #91116, #107288, #14298, #15296, #138626, #139612, #13316, #137639, #184155, #198327, #107, #61777, #123445, #140616, #63787, #44649, #77945, #30465, #92113, #2106, #46629, #167006, #31460, #125459, #28508, #185138, #169967, #187156, #90142, #168959, #106301, #121473, #76956, #151827, #1098, #62774, #74982, #124455, #108289, #93112, #154797, #186151, #152806, #199326, #47630, #153802, #16295, #109285, #136644, #45636, #170963, #32457, #94110, #60791, #155789, #17286, #78940, #75966, #105319, #59803, #122462, #183165, #167987, #29485, #160769, #130408, #142604, #172964, #4083, #48628, #111273, #34442, #7069, #6076, #114243, #128419, #64780, #175950, #18290, #37419, #5075, #50610, #96101, #110280, #174946, #99079, #145591, #65761, #97081, #66758, #190115, #80927, #171961, #51590, #141615, #127430, #112269, #173961, #126441, #68751, #33449, #189138, #22259, #98063, #188139, #95108, #35428, #67754, #113255, #3102, #129412, #156797, #36408, #158762, #52584, #83908, #49610, #159762, #21257, #157790, #79945, #82912, #144590, #19280, #191109, #20253, #81899, #143592, #116259, #23263, #53589, #25280, #102094, #164777, #72773, #24271, #84907, #26271, #162762, #71757, #146586, #163779, #86923, #148605, #87913, #70763, #133427, #132431, #195115, #42429, #150609, #176958, #10097, #40423, #115265, #8080, #149600, #56598, #38427, #39418, #11097, #134443, #73768, #118272, #192106, #100083, #179962, #41429, #85920, #69756, #103095, #196128, #88917, #57599, #119268, #161768, #101077, #55586, #147608, #12105, #180951, #131426, #193112, #104091, #54586, #177950, #9096, #194123, #117261, #165774, #27268, #178953, #93877, #137400, #92874, #91869, #28273, #16057, #155555, #138395, #152568, #139381, #109051, #13085, #123213, #200076, #44412, #62538, #61544, #169730, #74750, #184903, #31225 ) ),
 .UNSPECIFIED., .T., .F., .T. ) 
 B_SPLINE_SURFACE_WITH_KNOTS ( ( 4, 3, 4 ),
 ( 3, 2, 2, 2, 2, 2, 2, 2, 2, 2, 2, 2, 2, 2, 2, 2, 2, 2, 2, 2, 2, 2, 2, 2, 2, 2, 2, 2, 2, 2, 2, 2, 2, 2, 2, 2, 2, 2, 2, 2, 2, 2, 2, 2, 2, 2, 2, 2, 2, 2, 2, 2, 2, 2, 2, 2, 2, 2, 2, 2, 2, 2, 2, 2, 2, 2, 2, 2, 2, 2, 2, 2, 2, 2, 2, 2, 2, 2, 2, 2, 2, 2, 2, 2, 2, 2, 2, 2, 2, 2, 2, 2, 2, 2, 2, 2, 2, 2, 2, 2, 2, 2, 2, 2, 2, 2, 2, 2, 2, 2, 2, 2, 2, 2, 2, 2, 2, 2, 2, 2, 2, 2, 2, 2, 2, 2, 2, 2, 2, 2, 2, 2, 2, 2, 2, 2, 2, 2, 2, 2, 2, 2, 2, 2, 2, 2, 2, 2, 2, 2, 2, 2, 2, 2, 2, 2, 2, 2, 2, 2, 2, 2, 2, 2, 2, 2, 2, 2, 2, 2, 2, 2, 2, 2, 2, 2, 2, 2, 2, 2, 2, 2, 2, 2, 2, 2, 2, 2, 2, 2, 2, 2, 2, 2, 2, 2, 2, 2, 2, 2, 2, 2, 2, 2, 2, 2, 2, 2, 2, 2, 2, 2, 2, 2, 2, 2, 2, 2, 2, 2, 2, 2, 2, 2, 2, 2, 2, 2, 3 ),
 ( 0.000000000000000000, 0.5000000000000000000, 1.000000000000000000 ),
 ( 0.000000000000000000, 0.004385964912280701511, 0.008771929824561403022, 0.01315789473684210453, 0.01754385964912280604, 0.02192982456140350755, 0.02631578947368420907, 0.03070175438596491058, 0.03508771929824561209, 0.03947368421052631360, 0.04385964912280701511, 0.04824561403508771662, 0.05263157894736841813, 0.05701754385964911964, 0.06140350877192982115, 0.06578947368421052266, 0.07017543859649122417, 0.07456140350877192569, 0.07894736842105262720, 0.08333333333333332871, 0.08771929824561403022, 0.09210526315789473173, 0.09649122807017543324, 0.1008771929824561348, 0.1052631578947368363, 0.1096491228070175378, 0.1140350877192982393, 0.1184210526315789408, 0.1228070175438596423, 0.1271929824561403577, 0.1315789473684210453, 0.1359649122807017607, 0.1403508771929824483, 0.1447368421052631637, 0.1491228070175438514, 0.1535087719298245668, 0.1578947368421052544, 0.1622807017543859698, 0.1666666666666666574, 0.1710526315789473728, 0.1754385964912280604, 0.1798245614035087758, 0.1842105263157894635, 0.1885964912280701788, 0.1929824561403508665, 0.1973684210526315819, 0.2017543859649122695, 0.2061403508771929849, 0.2105263157894736725, 0.2149122807017543879, 0.2192982456140350755, 0.2236842105263157909, 0.2280701754385964786, 0.2324561403508771940, 0.2368421052631578816, 0.2412280701754385970, 0.2456140350877192846, 0.2500000000000000000, 0.2543859649122807154, 0.2587719298245614308, 0.2631578947368420907, 0.2675438596491228060, 0.2719298245614035214, 0.2763157894736842368, 0.2807017543859648967, 0.2850877192982456121, 0.2894736842105263275, 0.2938596491228070429, 0.2982456140350877027, 0.3026315789473684181, 0.3070175438596491335, 0.3114035087719298489, 0.3157894736842105088, 0.3201754385964912242, 0.3245614035087719396, 0.3289473684210526550, 0.3333333333333333148, 0.3377192982456140302, 0.3421052631578947456, 0.3464912280701754610, 0.3508771929824561209, 0.3552631578947368363, 0.3596491228070175517, 0.3640350877192982670, 0.3684210526315789269, 0.3728070175438596423, 0.3771929824561403577, 0.3815789473684210731, 0.3859649122807017330, 0.3903508771929824483, 0.3947368421052631637, 0.3991228070175438791, 0.4035087719298245390, 0.4078947368421052544, 0.4122807017543859698, 0.4166666666666666852, 0.4210526315789473450, 0.4254385964912280604, 0.4298245614035087758, 0.4342105263157894912, 0.4385964912280701511, 0.4429824561403508665, 0.4473684210526315819, 0.4517543859649122973, 0.4561403508771929571, 0.4605263157894736725, 0.4649122807017543879, 0.4692982456140351033, 0.4736842105263157632, 0.4780701754385964786, 0.4824561403508771940, 0.4868421052631579093, 0.4912280701754385692, 0.4956140350877192846, 0.5000000000000000000, 0.5043859649122807154, 0.5087719298245614308, 0.5131578947368421462, 0.5175438596491228616, 0.5219298245614034659, 0.5263157894736841813, 0.5307017543859648967, 0.5350877192982456121, 0.5394736842105263275, 0.5438596491228070429, 0.5482456140350877583, 0.5526315789473684736, 0.5570175438596490780, 0.5614035087719297934, 0.5657894736842105088, 0.5701754385964912242, 0.5745614035087719396, 0.5789473684210526550, 0.5833333333333333703, 0.5877192982456140857, 0.5921052631578946901, 0.5964912280701754055, 0.6008771929824561209, 0.6052631578947368363, 0.6096491228070175517, 0.6140350877192982670, 0.6184210526315789824, 0.6228070175438596978, 0.6271929824561403022, 0.6315789473684210176, 0.6359649122807017330, 0.6403508771929824483, 0.6447368421052631637, 0.6491228070175438791, 0.6535087719298245945, 0.6578947368421053099, 0.6622807017543859143, 0.6666666666666666297, 0.6710526315789473450, 0.6754385964912280604, 0.6798245614035087758, 0.6842105263157894912, 0.6885964912280702066, 0.6929824561403509220, 0.6973684210526315264, 0.7017543859649122417, 0.7061403508771929571, 0.7105263157894736725, 0.7149122807017543879, 0.7192982456140351033, 0.7236842105263158187, 0.7280701754385965341, 0.7324561403508771384, 0.7368421052631578538, 0.7412280701754385692, 0.7456140350877192846, 0.7500000000000000000, 0.7543859649122807154, 0.7587719298245614308, 0.7631578947368421462, 0.7675438596491228616, 0.7719298245614034659, 0.7763157894736841813, 0.7807017543859648967, 0.7850877192982456121, 0.7894736842105263275, 0.7938596491228070429, 0.7982456140350877583, 0.8026315789473684736, 0.8070175438596490780, 0.8114035087719297934, 0.8157894736842105088, 0.8201754385964912242, 0.8245614035087719396, 0.8289473684210526550, 0.8333333333333333703, 0.8377192982456140857, 0.8421052631578946901, 0.8464912280701754055, 0.8508771929824561209, 0.8552631578947368363, 0.8596491228070175517, 0.8640350877192982670, 0.8684210526315789824, 0.8728070175438596978, 0.8771929824561403022, 0.8815789473684210176, 0.8859649122807017330, 0.8903508771929824483, 0.8947368421052631637, 0.8991228070175438791, 0.9035087719298245945, 0.9078947368421053099, 0.9122807017543859143, 0.9166666666666666297, 0.9210526315789473450, 0.9254385964912280604, 0.9298245614035087758, 0.9342105263157894912, 0.9385964912280702066, 0.9429824561403509220, 0.9473684210526315264, 0.9517543859649122417, 0.9561403508771929571, 0.9605263157894736725, 0.9649122807017543879, 0.9692982456140351033, 0.9736842105263158187, 0.9780701754385965341, 0.9824561403508771384, 0.9868421052631578538, 0.9912280701754385692, 0.9956140350877192846, 1.000000000000000000 ),
 .UNSPECIFIED. ) 
 GEOMETRIC_REPRESENTATION_ITEM ( )  RATIONAL_B_SPLINE_SURFACE ( (
 ( 1.000000000000000000, 0.9659258262890683122, 1.000000000000000000, 0.9659258262890683122, 1.000000000000000000, 0.9659258262890683122, 1.000000000000000000, 0.9659258262890683122, 1.000000000000000000, 0.9659258262890683122, 1.000000000000000000, 0.9659258262890683122, 1.000000000000000000, 0.9659258262890683122, 1.000000000000000000, 0.9659258262890683122, 1.000000000000000000, 0.9659258262890683122, 1.000000000000000000, 0.9659258262890683122, 1.000000000000000000, 0.9659258262890683122, 1.000000000000000000, 0.9659258262890683122, 1.000000000000000000, 0.9659258262890683122, 1.000000000000000000, 0.9659258262890683122, 1.000000000000000000, 0.9659258262890683122, 1.000000000000000000, 0.9659258262890683122, 1.000000000000000000, 0.9659258262890683122, 1.000000000000000000, 0.9659258262890683122, 1.000000000000000000, 0.9659258262890683122, 1.000000000000000000, 0.9659258262890683122, 1.000000000000000000, 0.9659258262890683122, 1.000000000000000000, 0.9659258262890683122, 1.000000000000000000, 0.9659258262890683122, 1.000000000000000000, 0.9659258262890683122, 1.000000000000000000, 0.9659258262890683122, 1.000000000000000000, 0.9659258262890683122, 1.000000000000000000, 0.9659258262890683122, 1.000000000000000000, 0.9659258262890683122, 1.000000000000000000, 0.9659258262890683122, 1.000000000000000000, 0.9659258262890683122, 1.000000000000000000, 0.9659258262890683122, 1.000000000000000000, 0.9659258262890683122, 1.000000000000000000, 0.9659258262890683122, 1.000000000000000000, 0.9659258262890683122, 1.000000000000000000, 0.9659258262890683122, 1.000000000000000000, 0.9659258262890683122, 1.000000000000000000, 0.9659258262890683122, 1.000000000000000000, 0.9659258262890683122, 1.000000000000000000, 0.9659258262890683122, 1.000000000000000000, 0.9659258262890683122, 1.000000000000000000, 0.9659258262890683122, 1.000000000000000000, 0.9659258262890683122, 1.000000000000000000, 0.9659258262890683122, 1.000000000000000000, 0.9659258262890683122, 1.000000000000000000, 0.9659258262890683122, 1.000000000000000000, 0.9659258262890683122, 1.000000000000000000, 0.9659258262890683122, 1.000000000000000000, 0.9659258262890683122, 1.000000000000000000, 0.9659258262890683122, 1.000000000000000000, 0.9659258262890683122, 1.000000000000000000, 0.9659258262890683122, 1.000000000000000000, 0.9659258262890683122, 1.000000000000000000, 0.9659258262890683122, 1.000000000000000000, 0.9659258262890683122, 1.000000000000000000, 0.9659258262890683122, 1.000000000000000000, 0.9659258262890683122, 1.000000000000000000, 0.9659258262890683122, 1.000000000000000000, 0.9659258262890683122, 1.000000000000000000, 0.9659258262890683122, 1.000000000000000000, 0.9659258262890683122, 1.000000000000000000, 0.9659258262890683122, 1.000000000000000000, 0.9659258262890683122, 1.000000000000000000, 0.9659258262890683122, 1.000000000000000000, 0.9659258262890683122, 1.000000000000000000, 0.9659258262890683122, 1.000000000000000000, 0.9659258262890683122, 1.000000000000000000, 0.9659258262890683122, 1.000000000000000000, 0.9659258262890683122, 1.000000000000000000, 0.9659258262890683122, 1.000000000000000000, 0.9659258262890683122, 1.000000000000000000, 0.9659258262890683122, 1.000000000000000000, 0.9659258262890683122, 1.000000000000000000, 0.9659258262890683122, 1.000000000000000000, 0.9659258262890683122, 1.000000000000000000, 0.9659258262890683122, 1.000000000000000000, 0.9659258262890683122, 1.000000000000000000, 0.9659258262890683122, 1.000000000000000000, 0.9659258262890683122, 1.000000000000000000, 0.9659258262890683122, 1.000000000000000000, 0.9659258262890683122, 1.000000000000000000, 0.9659258262890683122, 1.000000000000000000, 0.9659258262890683122, 1.000000000000000000, 0.9659258262890683122, 1.000000000000000000, 0.9659258262890683122, 1.000000000000000000, 0.9659258262890683122, 1.000000000000000000, 0.9659258262890683122, 1.000000000000000000, 0.9659258262890683122, 1.000000000000000000, 0.9659258262890683122, 1.000000000000000000, 0.9659258262890683122, 1.000000000000000000, 0.9659258262890683122, 1.000000000000000000, 0.9659258262890683122, 1.000000000000000000, 0.9659258262890683122, 1.000000000000000000, 0.9659258262890683122, 1.000000000000000000, 0.9659258262890683122, 1.000000000000000000, 0.9659258262890683122, 1.000000000000000000, 0.9659258262890683122, 1.000000000000000000, 0.9659258262890683122, 1.000000000000000000, 0.9659258262890683122, 1.000000000000000000, 0.9659258262890683122, 1.000000000000000000, 0.9659258262890683122, 1.000000000000000000, 0.9659258262890683122, 1.000000000000000000, 0.9659258262890683122, 1.000000000000000000, 0.9659258262890683122, 1.000000000000000000, 0.9659258262890683122, 1.000000000000000000, 0.9659258262890683122, 1.000000000000000000, 0.9659258262890683122, 1.000000000000000000, 0.9659258262890683122, 1.000000000000000000, 0.9659258262890683122, 1.000000000000000000, 0.9659258262890683122, 1.000000000000000000, 0.9659258262890683122, 1.000000000000000000, 0.9659258262890683122, 1.000000000000000000, 0.9659258262890683122, 1.000000000000000000, 0.9659258262890683122, 1.000000000000000000, 0.9659258262890683122, 1.000000000000000000, 0.9659258262890683122, 1.000000000000000000, 0.9659258262890683122, 1.000000000000000000, 0.9659258262890683122, 1.000000000000000000, 0.9659258262890683122, 1.000000000000000000, 0.9659258262890683122, 1.000000000000000000, 0.9659258262890683122, 1.000000000000000000, 0.9659258262890683122, 1.000000000000000000, 0.9659258262890683122, 1.000000000000000000, 0.9659258262890683122, 1.000000000000000000, 0.9659258262890683122, 1.000000000000000000, 0.9659258262890683122, 1.000000000000000000, 0.9659258262890683122, 1.000000000000000000, 0.9659258262890683122, 1.000000000000000000, 0.9659258262890683122, 1.000000000000000000, 0.9659258262890683122, 1.000000000000000000, 0.9659258262890683122, 1.000000000000000000, 0.9659258262890683122, 1.000000000000000000, 0.9659258262890683122, 1.000000000000000000, 0.9659258262890683122, 1.000000000000000000, 0.9659258262890683122, 1.000000000000000000, 0.9659258262890683122, 1.000000000000000000, 0.9659258262890683122, 1.000000000000000000, 0.9659258262890683122, 1.000000000000000000, 0.9659258262890683122, 1.000000000000000000, 0.9659258262890683122, 1.000000000000000000, 0.9659258262890683122, 1.000000000000000000, 0.9659258262890683122, 1.000000000000000000, 0.9659258262890683122, 1.000000000000000000, 0.9659258262890683122, 1.000000000000000000, 0.9659258262890683122, 1.000000000000000000, 0.9659258262890683122, 1.000000000000000000, 0.9659258262890683122, 1.000000000000000000, 0.9659258262890683122, 1.000000000000000000, 0.9659258262890683122, 1.000000000000000000, 0.9659258262890683122, 1.000000000000000000, 0.9659258262890683122, 1.000000000000000000, 0.9659258262890683122, 1.000000000000000000, 0.9659258262890683122, 1.000000000000000000, 0.9659258262890683122, 1.000000000000000000, 0.9659258262890683122, 1.000000000000000000, 0.9659258262890683122, 1.000000000000000000, 0.9659258262890683122, 1.000000000000000000, 0.9659258262890683122, 1.000000000000000000, 0.9659258262890683122, 1.000000000000000000, 0.9659258262890683122, 1.000000000000000000, 0.9659258262890683122, 1.000000000000000000, 0.9659258262890683122, 1.000000000000000000, 0.9659258262890683122, 1.000000000000000000, 0.9659258262890683122, 1.000000000000000000, 0.9659258262890683122, 1.000000000000000000, 0.9659258262890683122, 1.000000000000000000, 0.9659258262890683122, 1.000000000000000000, 0.9659258262890683122, 1.000000000000000000, 0.9659258262890683122, 1.000000000000000000, 0.9659258262890683122, 1.000000000000000000, 0.9659258262890683122, 1.000000000000000000, 0.9659258262890683122, 1.000000000000000000, 0.9659258262890683122, 1.000000000000000000, 0.9659258262890683122, 1.000000000000000000, 0.9659258262890683122, 1.000000000000000000, 0.9659258262890683122, 1.000000000000000000, 0.9659258262890683122, 1.000000000000000000, 0.9659258262890683122, 1.000000000000000000, 0.9659258262890683122, 1.000000000000000000, 0.9659258262890683122, 1.000000000000000000, 0.9659258262890683122, 1.000000000000000000, 0.9659258262890683122, 1.000000000000000000, 0.9659258262890683122, 1.000000000000000000, 0.9659258262890683122, 1.000000000000000000, 0.9659258262890683122, 1.000000000000000000, 0.9659258262890683122, 1.000000000000000000, 0.9659258262890683122, 1.000000000000000000, 0.9659258262890683122, 1.000000000000000000, 0.9659258262890683122, 1.000000000000000000, 0.9659258262890683122, 1.000000000000000000, 0.9659258262890683122, 1.000000000000000000, 0.9659258262890683122, 1.000000000000000000, 0.9659258262890683122, 1.000000000000000000, 0.9659258262890683122, 1.000000000000000000, 0.9659258262890683122, 1.000000000000000000, 0.9659258262890683122, 1.000000000000000000, 0.9659258262890683122, 1.000000000000000000, 0.9659258262890683122, 1.000000000000000000, 0.9659258262890683122, 1.000000000000000000, 0.9659258262890683122, 1.000000000000000000, 0.9659258262890683122, 1.000000000000000000, 0.9659258262890683122, 1.000000000000000000, 0.9659258262890683122, 1.000000000000000000, 0.9659258262890683122, 1.000000000000000000, 0.9659258262890683122, 1.000000000000000000, 0.9659258262890683122, 1.000000000000000000, 0.9659258262890683122, 1.000000000000000000, 0.9659258262890683122, 1.000000000000000000, 0.9659258262890683122, 1.000000000000000000, 0.9659258262890683122, 1.000000000000000000, 0.9659258262890683122, 1.000000000000000000, 0.9659258262890683122, 1.000000000000000000, 0.9659258262890683122, 1.000000000000000000, 0.9659258262890683122, 1.000000000000000000, 0.9659258262890683122, 1.000000000000000000, 0.9659258262890683122, 1.000000000000000000, 0.9659258262890683122, 1.000000000000000000, 0.9659258262890683122, 1.000000000000000000, 0.9659258262890683122, 1.000000000000000000, 0.9659258262890683122, 1.000000000000000000, 0.9659258262890683122, 1.000000000000000000, 0.9659258262890683122, 1.000000000000000000, 0.9659258262890683122, 1.000000000000000000, 0.9659258262890683122, 1.000000000000000000, 0.9659258262890683122, 1.000000000000000000, 0.9659258262890683122, 1.000000000000000000, 0.9659258262890683122, 1.000000000000000000, 0.9659258262890683122, 1.000000000000000000, 0.9659258262890683122, 1.000000000000000000),
 ( 0.3333333333333333703, 0.3219752754296894559, 0.3333333333333333703, 0.3219752754296894559, 0.3333333333333333703, 0.3219752754296894559, 0.3333333333333333703, 0.3219752754296894559, 0.3333333333333333703, 0.3219752754296894559, 0.3333333333333333703, 0.3219752754296894559, 0.3333333333333333703, 0.3219752754296894559, 0.3333333333333333703, 0.3219752754296894559, 0.3333333333333333703, 0.3219752754296894559, 0.3333333333333333703, 0.3219752754296894559, 0.3333333333333333703, 0.3219752754296894559, 0.3333333333333333703, 0.3219752754296894559, 0.3333333333333333703, 0.3219752754296894559, 0.3333333333333333703, 0.3219752754296894559, 0.3333333333333333703, 0.3219752754296894559, 0.3333333333333333703, 0.3219752754296894559, 0.3333333333333333703, 0.3219752754296894559, 0.3333333333333333703, 0.3219752754296894559, 0.3333333333333333703, 0.3219752754296894559, 0.3333333333333333703, 0.3219752754296894559, 0.3333333333333333703, 0.3219752754296894559, 0.3333333333333333703, 0.3219752754296894559, 0.3333333333333333703, 0.3219752754296894559, 0.3333333333333333703, 0.3219752754296894559, 0.3333333333333333703, 0.3219752754296894559, 0.3333333333333333703, 0.3219752754296894559, 0.3333333333333333703, 0.3219752754296894559, 0.3333333333333333703, 0.3219752754296894559, 0.3333333333333333703, 0.3219752754296894559, 0.3333333333333333703, 0.3219752754296894559, 0.3333333333333333703, 0.3219752754296894559, 0.3333333333333333703, 0.3219752754296894559, 0.3333333333333333703, 0.3219752754296894559, 0.3333333333333333703, 0.3219752754296894559, 0.3333333333333333703, 0.3219752754296894559, 0.3333333333333333703, 0.3219752754296894559, 0.3333333333333333703, 0.3219752754296894559, 0.3333333333333333703, 0.3219752754296894559, 0.3333333333333333703, 0.3219752754296894559, 0.3333333333333333703, 0.3219752754296894559, 0.3333333333333333703, 0.3219752754296894559, 0.3333333333333333703, 0.3219752754296894559, 0.3333333333333333703, 0.3219752754296894559, 0.3333333333333333703, 0.3219752754296894559, 0.3333333333333333703, 0.3219752754296894559, 0.3333333333333333703, 0.3219752754296894559, 0.3333333333333333703, 0.3219752754296894559, 0.3333333333333333703, 0.3219752754296894559, 0.3333333333333333703, 0.3219752754296894559, 0.3333333333333333703, 0.3219752754296894559, 0.3333333333333333703, 0.3219752754296894559, 0.3333333333333333703, 0.3219752754296894559, 0.3333333333333333703, 0.3219752754296894559, 0.3333333333333333703, 0.3219752754296894559, 0.3333333333333333703, 0.3219752754296894559, 0.3333333333333333703, 0.3219752754296894559, 0.3333333333333333703, 0.3219752754296894559, 0.3333333333333333703, 0.3219752754296894559, 0.3333333333333333703, 0.3219752754296894559, 0.3333333333333333703, 0.3219752754296894559, 0.3333333333333333703, 0.3219752754296894559, 0.3333333333333333703, 0.3219752754296894559, 0.3333333333333333703, 0.3219752754296894559, 0.3333333333333333703, 0.3219752754296894559, 0.3333333333333333703, 0.3219752754296894559, 0.3333333333333333703, 0.3219752754296894559, 0.3333333333333333703, 0.3219752754296894559, 0.3333333333333333703, 0.3219752754296894559, 0.3333333333333333703, 0.3219752754296894559, 0.3333333333333333703, 0.3219752754296894559, 0.3333333333333333703, 0.3219752754296894559, 0.3333333333333333703, 0.3219752754296894559, 0.3333333333333333703, 0.3219752754296894559, 0.3333333333333333703, 0.3219752754296894559, 0.3333333333333333703, 0.3219752754296894559, 0.3333333333333333703, 0.3219752754296894559, 0.3333333333333333703, 0.3219752754296894559, 0.3333333333333333703, 0.3219752754296894559, 0.3333333333333333703, 0.3219752754296894559, 0.3333333333333333703, 0.3219752754296894559, 0.3333333333333333703, 0.3219752754296894559, 0.3333333333333333703, 0.3219752754296894559, 0.3333333333333333703, 0.3219752754296894559, 0.3333333333333333703, 0.3219752754296894559, 0.3333333333333333703, 0.3219752754296894559, 0.3333333333333333703, 0.3219752754296894559, 0.3333333333333333703, 0.3219752754296894559, 0.3333333333333333703, 0.3219752754296894559, 0.3333333333333333703, 0.3219752754296894559, 0.3333333333333333703, 0.3219752754296894559, 0.3333333333333333703, 0.3219752754296894559, 0.3333333333333333703, 0.3219752754296894559, 0.3333333333333333703, 0.3219752754296894559, 0.3333333333333333703, 0.3219752754296894559, 0.3333333333333333703, 0.3219752754296894559, 0.3333333333333333703, 0.3219752754296894559, 0.3333333333333333703, 0.3219752754296894559, 0.3333333333333333703, 0.3219752754296894559, 0.3333333333333333703, 0.3219752754296894559, 0.3333333333333333703, 0.3219752754296894559, 0.3333333333333333703, 0.3219752754296894559, 0.3333333333333333703, 0.3219752754296894559, 0.3333333333333333703, 0.3219752754296894559, 0.3333333333333333703, 0.3219752754296894559, 0.3333333333333333703, 0.3219752754296894559, 0.3333333333333333703, 0.3219752754296894559, 0.3333333333333333703, 0.3219752754296894559, 0.3333333333333333703, 0.3219752754296894559, 0.3333333333333333703, 0.3219752754296894559, 0.3333333333333333703, 0.3219752754296894559, 0.3333333333333333703, 0.3219752754296894559, 0.3333333333333333703, 0.3219752754296894559, 0.3333333333333333703, 0.3219752754296894559, 0.3333333333333333703, 0.3219752754296894559, 0.3333333333333333703, 0.3219752754296894559, 0.3333333333333333703, 0.3219752754296894559, 0.3333333333333333703, 0.3219752754296894559, 0.3333333333333333703, 0.3219752754296894559, 0.3333333333333333703, 0.3219752754296894559, 0.3333333333333333703, 0.3219752754296894559, 0.3333333333333333703, 0.3219752754296894559, 0.3333333333333333703, 0.3219752754296894559, 0.3333333333333333703, 0.3219752754296894559, 0.3333333333333333703, 0.3219752754296894559, 0.3333333333333333703, 0.3219752754296894559, 0.3333333333333333703, 0.3219752754296894559, 0.3333333333333333703, 0.3219752754296894559, 0.3333333333333333703, 0.3219752754296894559, 0.3333333333333333703, 0.3219752754296894559, 0.3333333333333333703, 0.3219752754296894559, 0.3333333333333333703, 0.3219752754296894559, 0.3333333333333333703, 0.3219752754296894559, 0.3333333333333333703, 0.3219752754296894559, 0.3333333333333333703, 0.3219752754296894559, 0.3333333333333333703, 0.3219752754296894559, 0.3333333333333333703, 0.3219752754296894559, 0.3333333333333333703, 0.3219752754296894559, 0.3333333333333333703, 0.3219752754296894559, 0.3333333333333333703, 0.3219752754296894559, 0.3333333333333333703, 0.3219752754296894559, 0.3333333333333333703, 0.3219752754296894559, 0.3333333333333333703, 0.3219752754296894559, 0.3333333333333333703, 0.3219752754296894559, 0.3333333333333333703, 0.3219752754296894559, 0.3333333333333333703, 0.3219752754296894559, 0.3333333333333333703, 0.3219752754296894559, 0.3333333333333333703, 0.3219752754296894559, 0.3333333333333333703, 0.3219752754296894559, 0.3333333333333333703, 0.3219752754296894559, 0.3333333333333333703, 0.3219752754296894559, 0.3333333333333333703, 0.3219752754296894559, 0.3333333333333333703, 0.3219752754296894559, 0.3333333333333333703, 0.3219752754296894559, 0.3333333333333333703, 0.3219752754296894559, 0.3333333333333333703, 0.3219752754296894559, 0.3333333333333333703, 0.3219752754296894559, 0.3333333333333333703, 0.3219752754296894559, 0.3333333333333333703, 0.3219752754296894559, 0.3333333333333333703, 0.3219752754296894559, 0.3333333333333333703, 0.3219752754296894559, 0.3333333333333333703, 0.3219752754296894559, 0.3333333333333333703, 0.3219752754296894559, 0.3333333333333333703, 0.3219752754296894559, 0.3333333333333333703, 0.3219752754296894559, 0.3333333333333333703, 0.3219752754296894559, 0.3333333333333333703, 0.3219752754296894559, 0.3333333333333333703, 0.3219752754296894559, 0.3333333333333333703, 0.3219752754296894559, 0.3333333333333333703, 0.3219752754296894559, 0.3333333333333333703, 0.3219752754296894559, 0.3333333333333333703, 0.3219752754296894559, 0.3333333333333333703, 0.3219752754296894559, 0.3333333333333333703, 0.3219752754296894559, 0.3333333333333333703, 0.3219752754296894559, 0.3333333333333333703, 0.3219752754296894559, 0.3333333333333333703, 0.3219752754296894559, 0.3333333333333333703, 0.3219752754296894559, 0.3333333333333333703, 0.3219752754296894559, 0.3333333333333333703, 0.3219752754296894559, 0.3333333333333333703, 0.3219752754296894559, 0.3333333333333333703, 0.3219752754296894559, 0.3333333333333333703, 0.3219752754296894559, 0.3333333333333333703, 0.3219752754296894559, 0.3333333333333333703, 0.3219752754296894559, 0.3333333333333333703, 0.3219752754296894559, 0.3333333333333333703, 0.3219752754296894559, 0.3333333333333333703, 0.3219752754296894559, 0.3333333333333333703, 0.3219752754296894559, 0.3333333333333333703, 0.3219752754296894559, 0.3333333333333333703, 0.3219752754296894559, 0.3333333333333333703, 0.3219752754296894559, 0.3333333333333333703, 0.3219752754296894559, 0.3333333333333333703, 0.3219752754296894559, 0.3333333333333333703, 0.3219752754296894559, 0.3333333333333333703, 0.3219752754296894559, 0.3333333333333333703, 0.3219752754296894559, 0.3333333333333333703, 0.3219752754296894559, 0.3333333333333333703, 0.3219752754296894559, 0.3333333333333333703, 0.3219752754296894559, 0.3333333333333333703, 0.3219752754296894559, 0.3333333333333333703, 0.3219752754296894559, 0.3333333333333333703, 0.3219752754296894559, 0.3333333333333333703, 0.3219752754296894559, 0.3333333333333333703, 0.3219752754296894559, 0.3333333333333333703, 0.3219752754296894559, 0.3333333333333333703, 0.3219752754296894559, 0.3333333333333333703, 0.3219752754296894559, 0.3333333333333333703, 0.3219752754296894559, 0.3333333333333333703, 0.3219752754296894559, 0.3333333333333333703, 0.3219752754296894559, 0.3333333333333333703, 0.3219752754296894559, 0.3333333333333333703, 0.3219752754296894559, 0.3333333333333333703, 0.3219752754296894559, 0.3333333333333333703, 0.3219752754296894559, 0.3333333333333333703, 0.3219752754296894559, 0.3333333333333333703, 0.3219752754296894559, 0.3333333333333333703, 0.3219752754296894559, 0.3333333333333333703, 0.3219752754296894559, 0.3333333333333333703, 0.3219752754296894559, 0.3333333333333333703, 0.3219752754296894559, 0.3333333333333333703, 0.3219752754296894559, 0.3333333333333333703, 0.3219752754296894559, 0.3333333333333333703, 0.3219752754296894559, 0.3333333333333333703, 0.3219752754296894559, 0.3333333333333333703, 0.3219752754296894559, 0.3333333333333333703, 0.3219752754296894559, 0.3333333333333333703, 0.3219752754296894559, 0.3333333333333333703, 0.3219752754296894559, 0.3333333333333333703),
 ( 0.3333333333333333703, 0.3219752754296894559, 0.3333333333333333703, 0.3219752754296894559, 0.3333333333333333703, 0.3219752754296894559, 0.3333333333333333703, 0.3219752754296894559, 0.3333333333333333703, 0.3219752754296894559, 0.3333333333333333703, 0.3219752754296894559, 0.3333333333333333703, 0.3219752754296894559, 0.3333333333333333703, 0.3219752754296894559, 0.3333333333333333703, 0.3219752754296894559, 0.3333333333333333703, 0.3219752754296894559, 0.3333333333333333703, 0.3219752754296894559, 0.3333333333333333703, 0.3219752754296894559, 0.3333333333333333703, 0.3219752754296894559, 0.3333333333333333703, 0.3219752754296894559, 0.3333333333333333703, 0.3219752754296894559, 0.3333333333333333703, 0.3219752754296894559, 0.3333333333333333703, 0.3219752754296894559, 0.3333333333333333703, 0.3219752754296894559, 0.3333333333333333703, 0.3219752754296894559, 0.3333333333333333703, 0.3219752754296894559, 0.3333333333333333703, 0.3219752754296894559, 0.3333333333333333703, 0.3219752754296894559, 0.3333333333333333703, 0.3219752754296894559, 0.3333333333333333703, 0.3219752754296894559, 0.3333333333333333703, 0.3219752754296894559, 0.3333333333333333703, 0.3219752754296894559, 0.3333333333333333703, 0.3219752754296894559, 0.3333333333333333703, 0.3219752754296894559, 0.3333333333333333703, 0.3219752754296894559, 0.3333333333333333703, 0.3219752754296894559, 0.3333333333333333703, 0.3219752754296894559, 0.3333333333333333703, 0.3219752754296894559, 0.3333333333333333703, 0.3219752754296894559, 0.3333333333333333703, 0.3219752754296894559, 0.3333333333333333703, 0.3219752754296894559, 0.3333333333333333703, 0.3219752754296894559, 0.3333333333333333703, 0.3219752754296894559, 0.3333333333333333703, 0.3219752754296894559, 0.3333333333333333703, 0.3219752754296894559, 0.3333333333333333703, 0.3219752754296894559, 0.3333333333333333703, 0.3219752754296894559, 0.3333333333333333703, 0.3219752754296894559, 0.3333333333333333703, 0.3219752754296894559, 0.3333333333333333703, 0.3219752754296894559, 0.3333333333333333703, 0.3219752754296894559, 0.3333333333333333703, 0.3219752754296894559, 0.3333333333333333703, 0.3219752754296894559, 0.3333333333333333703, 0.3219752754296894559, 0.3333333333333333703, 0.3219752754296894559, 0.3333333333333333703, 0.3219752754296894559, 0.3333333333333333703, 0.3219752754296894559, 0.3333333333333333703, 0.3219752754296894559, 0.3333333333333333703, 0.3219752754296894559, 0.3333333333333333703, 0.3219752754296894559, 0.3333333333333333703, 0.3219752754296894559, 0.3333333333333333703, 0.3219752754296894559, 0.3333333333333333703, 0.3219752754296894559, 0.3333333333333333703, 0.3219752754296894559, 0.3333333333333333703, 0.3219752754296894559, 0.3333333333333333703, 0.3219752754296894559, 0.3333333333333333703, 0.3219752754296894559, 0.3333333333333333703, 0.3219752754296894559, 0.3333333333333333703, 0.3219752754296894559, 0.3333333333333333703, 0.3219752754296894559, 0.3333333333333333703, 0.3219752754296894559, 0.3333333333333333703, 0.3219752754296894559, 0.3333333333333333703, 0.3219752754296894559, 0.3333333333333333703, 0.3219752754296894559, 0.3333333333333333703, 0.3219752754296894559, 0.3333333333333333703, 0.3219752754296894559, 0.3333333333333333703, 0.3219752754296894559, 0.3333333333333333703, 0.3219752754296894559, 0.3333333333333333703, 0.3219752754296894559, 0.3333333333333333703, 0.3219752754296894559, 0.3333333333333333703, 0.3219752754296894559, 0.3333333333333333703, 0.3219752754296894559, 0.3333333333333333703, 0.3219752754296894559, 0.3333333333333333703, 0.3219752754296894559, 0.3333333333333333703, 0.3219752754296894559, 0.3333333333333333703, 0.3219752754296894559, 0.3333333333333333703, 0.3219752754296894559, 0.3333333333333333703, 0.3219752754296894559, 0.3333333333333333703, 0.3219752754296894559, 0.3333333333333333703, 0.3219752754296894559, 0.3333333333333333703, 0.3219752754296894559, 0.3333333333333333703, 0.3219752754296894559, 0.3333333333333333703, 0.3219752754296894559, 0.3333333333333333703, 0.3219752754296894559, 0.3333333333333333703, 0.3219752754296894559, 0.3333333333333333703, 0.3219752754296894559, 0.3333333333333333703, 0.3219752754296894559, 0.3333333333333333703, 0.3219752754296894559, 0.3333333333333333703, 0.3219752754296894559, 0.3333333333333333703, 0.3219752754296894559, 0.3333333333333333703, 0.3219752754296894559, 0.3333333333333333703, 0.3219752754296894559, 0.3333333333333333703, 0.3219752754296894559, 0.3333333333333333703, 0.3219752754296894559, 0.3333333333333333703, 0.3219752754296894559, 0.3333333333333333703, 0.3219752754296894559, 0.3333333333333333703, 0.3219752754296894559, 0.3333333333333333703, 0.3219752754296894559, 0.3333333333333333703, 0.3219752754296894559, 0.3333333333333333703, 0.3219752754296894559, 0.3333333333333333703, 0.3219752754296894559, 0.3333333333333333703, 0.3219752754296894559, 0.3333333333333333703, 0.3219752754296894559, 0.3333333333333333703, 0.3219752754296894559, 0.3333333333333333703, 0.3219752754296894559, 0.3333333333333333703, 0.3219752754296894559, 0.3333333333333333703, 0.3219752754296894559, 0.3333333333333333703, 0.3219752754296894559, 0.3333333333333333703, 0.3219752754296894559, 0.3333333333333333703, 0.3219752754296894559, 0.3333333333333333703, 0.3219752754296894559, 0.3333333333333333703, 0.3219752754296894559, 0.3333333333333333703, 0.3219752754296894559, 0.3333333333333333703, 0.3219752754296894559, 0.3333333333333333703, 0.3219752754296894559, 0.3333333333333333703, 0.3219752754296894559, 0.3333333333333333703, 0.3219752754296894559, 0.3333333333333333703, 0.3219752754296894559, 0.3333333333333333703, 0.3219752754296894559, 0.3333333333333333703, 0.3219752754296894559, 0.3333333333333333703, 0.3219752754296894559, 0.3333333333333333703, 0.3219752754296894559, 0.3333333333333333703, 0.3219752754296894559, 0.3333333333333333703, 0.3219752754296894559, 0.3333333333333333703, 0.3219752754296894559, 0.3333333333333333703, 0.3219752754296894559, 0.3333333333333333703, 0.3219752754296894559, 0.3333333333333333703, 0.3219752754296894559, 0.3333333333333333703, 0.3219752754296894559, 0.3333333333333333703, 0.3219752754296894559, 0.3333333333333333703, 0.3219752754296894559, 0.3333333333333333703, 0.3219752754296894559, 0.3333333333333333703, 0.3219752754296894559, 0.3333333333333333703, 0.3219752754296894559, 0.3333333333333333703, 0.3219752754296894559, 0.3333333333333333703, 0.3219752754296894559, 0.3333333333333333703, 0.3219752754296894559, 0.3333333333333333703, 0.3219752754296894559, 0.3333333333333333703, 0.3219752754296894559, 0.3333333333333333703, 0.3219752754296894559, 0.3333333333333333703, 0.3219752754296894559, 0.3333333333333333703, 0.3219752754296894559, 0.3333333333333333703, 0.3219752754296894559, 0.3333333333333333703, 0.3219752754296894559, 0.3333333333333333703, 0.3219752754296894559, 0.3333333333333333703, 0.3219752754296894559, 0.3333333333333333703, 0.3219752754296894559, 0.3333333333333333703, 0.3219752754296894559, 0.3333333333333333703, 0.3219752754296894559, 0.3333333333333333703, 0.3219752754296894559, 0.3333333333333333703, 0.3219752754296894559, 0.3333333333333333703, 0.3219752754296894559, 0.3333333333333333703, 0.3219752754296894559, 0.3333333333333333703, 0.3219752754296894559, 0.3333333333333333703, 0.3219752754296894559, 0.3333333333333333703, 0.3219752754296894559, 0.3333333333333333703, 0.3219752754296894559, 0.3333333333333333703, 0.3219752754296894559, 0.3333333333333333703, 0.3219752754296894559, 0.3333333333333333703, 0.3219752754296894559, 0.3333333333333333703, 0.3219752754296894559, 0.3333333333333333703, 0.3219752754296894559, 0.3333333333333333703, 0.3219752754296894559, 0.3333333333333333703, 0.3219752754296894559, 0.3333333333333333703, 0.3219752754296894559, 0.3333333333333333703, 0.3219752754296894559, 0.3333333333333333703, 0.3219752754296894559, 0.3333333333333333703, 0.3219752754296894559, 0.3333333333333333703, 0.3219752754296894559, 0.3333333333333333703, 0.3219752754296894559, 0.3333333333333333703, 0.3219752754296894559, 0.3333333333333333703, 0.3219752754296894559, 0.3333333333333333703, 0.3219752754296894559, 0.3333333333333333703, 0.3219752754296894559, 0.3333333333333333703, 0.3219752754296894559, 0.3333333333333333703, 0.3219752754296894559, 0.3333333333333333703, 0.3219752754296894559, 0.3333333333333333703, 0.3219752754296894559, 0.3333333333333333703, 0.3219752754296894559, 0.3333333333333333703, 0.3219752754296894559, 0.3333333333333333703, 0.3219752754296894559, 0.3333333333333333703, 0.3219752754296894559, 0.3333333333333333703, 0.3219752754296894559, 0.3333333333333333703, 0.3219752754296894559, 0.3333333333333333703, 0.3219752754296894559, 0.3333333333333333703, 0.3219752754296894559, 0.3333333333333333703, 0.3219752754296894559, 0.3333333333333333703, 0.3219752754296894559, 0.3333333333333333703, 0.3219752754296894559, 0.3333333333333333703, 0.3219752754296894559, 0.3333333333333333703, 0.3219752754296894559, 0.3333333333333333703, 0.3219752754296894559, 0.3333333333333333703, 0.3219752754296894559, 0.3333333333333333703, 0.3219752754296894559, 0.3333333333333333703, 0.3219752754296894559, 0.3333333333333333703, 0.3219752754296894559, 0.3333333333333333703, 0.3219752754296894559, 0.3333333333333333703, 0.3219752754296894559, 0.3333333333333333703, 0.3219752754296894559, 0.3333333333333333703, 0.3219752754296894559, 0.3333333333333333703, 0.3219752754296894559, 0.3333333333333333703, 0.3219752754296894559, 0.3333333333333333703, 0.3219752754296894559, 0.3333333333333333703, 0.3219752754296894559, 0.3333333333333333703, 0.3219752754296894559, 0.3333333333333333703, 0.3219752754296894559, 0.3333333333333333703, 0.3219752754296894559, 0.3333333333333333703, 0.3219752754296894559, 0.3333333333333333703, 0.3219752754296894559, 0.3333333333333333703, 0.3219752754296894559, 0.3333333333333333703, 0.3219752754296894559, 0.3333333333333333703, 0.3219752754296894559, 0.3333333333333333703, 0.3219752754296894559, 0.3333333333333333703, 0.3219752754296894559, 0.3333333333333333703, 0.3219752754296894559, 0.3333333333333333703, 0.3219752754296894559, 0.3333333333333333703, 0.3219752754296894559, 0.3333333333333333703, 0.3219752754296894559, 0.3333333333333333703, 0.3219752754296894559, 0.3333333333333333703, 0.3219752754296894559, 0.3333333333333333703, 0.3219752754296894559, 0.3333333333333333703, 0.3219752754296894559, 0.3333333333333333703, 0.3219752754296894559, 0.3333333333333333703, 0.3219752754296894559, 0.3333333333333333703),
 ( 1.000000000000000000, 0.9659258262890683122, 1.000000000000000000, 0.9659258262890683122, 1.000000000000000000, 0.9659258262890683122, 1.000000000000000000, 0.9659258262890683122, 1.000000000000000000, 0.9659258262890683122, 1.000000000000000000, 0.9659258262890683122, 1.000000000000000000, 0.9659258262890683122, 1.000000000000000000, 0.9659258262890683122, 1.000000000000000000, 0.9659258262890683122, 1.000000000000000000, 0.9659258262890683122, 1.000000000000000000, 0.9659258262890683122, 1.000000000000000000, 0.9659258262890683122, 1.000000000000000000, 0.9659258262890683122, 1.000000000000000000, 0.9659258262890683122, 1.000000000000000000, 0.9659258262890683122, 1.000000000000000000, 0.9659258262890683122, 1.000000000000000000, 0.9659258262890683122, 1.000000000000000000, 0.9659258262890683122, 1.000000000000000000, 0.9659258262890683122, 1.000000000000000000, 0.9659258262890683122, 1.000000000000000000, 0.9659258262890683122, 1.000000000000000000, 0.9659258262890683122, 1.000000000000000000, 0.9659258262890683122, 1.000000000000000000, 0.9659258262890683122, 1.000000000000000000, 0.9659258262890683122, 1.000000000000000000, 0.9659258262890683122, 1.000000000000000000, 0.9659258262890683122, 1.000000000000000000, 0.9659258262890683122, 1.000000000000000000, 0.9659258262890683122, 1.000000000000000000, 0.9659258262890683122, 1.000000000000000000, 0.9659258262890683122, 1.000000000000000000, 0.9659258262890683122, 1.000000000000000000, 0.9659258262890683122, 1.000000000000000000, 0.9659258262890683122, 1.000000000000000000, 0.9659258262890683122, 1.000000000000000000, 0.9659258262890683122, 1.000000000000000000, 0.9659258262890683122, 1.000000000000000000, 0.9659258262890683122, 1.000000000000000000, 0.9659258262890683122, 1.000000000000000000, 0.9659258262890683122, 1.000000000000000000, 0.9659258262890683122, 1.000000000000000000, 0.9659258262890683122, 1.000000000000000000, 0.9659258262890683122, 1.000000000000000000, 0.9659258262890683122, 1.000000000000000000, 0.9659258262890683122, 1.000000000000000000, 0.9659258262890683122, 1.000000000000000000, 0.9659258262890683122, 1.000000000000000000, 0.9659258262890683122, 1.000000000000000000, 0.9659258262890683122, 1.000000000000000000, 0.9659258262890683122, 1.000000000000000000, 0.9659258262890683122, 1.000000000000000000, 0.9659258262890683122, 1.000000000000000000, 0.9659258262890683122, 1.000000000000000000, 0.9659258262890683122, 1.000000000000000000, 0.9659258262890683122, 1.000000000000000000, 0.9659258262890683122, 1.000000000000000000, 0.9659258262890683122, 1.000000000000000000, 0.9659258262890683122, 1.000000000000000000, 0.9659258262890683122, 1.000000000000000000, 0.9659258262890683122, 1.000000000000000000, 0.9659258262890683122, 1.000000000000000000, 0.9659258262890683122, 1.000000000000000000, 0.9659258262890683122, 1.000000000000000000, 0.9659258262890683122, 1.000000000000000000, 0.9659258262890683122, 1.000000000000000000, 0.9659258262890683122, 1.000000000000000000, 0.9659258262890683122, 1.000000000000000000, 0.9659258262890683122, 1.000000000000000000, 0.9659258262890683122, 1.000000000000000000, 0.9659258262890683122, 1.000000000000000000, 0.9659258262890683122, 1.000000000000000000, 0.9659258262890683122, 1.000000000000000000, 0.9659258262890683122, 1.000000000000000000, 0.9659258262890683122, 1.000000000000000000, 0.9659258262890683122, 1.000000000000000000, 0.9659258262890683122, 1.000000000000000000, 0.9659258262890683122, 1.000000000000000000, 0.9659258262890683122, 1.000000000000000000, 0.9659258262890683122, 1.000000000000000000, 0.9659258262890683122, 1.000000000000000000, 0.9659258262890683122, 1.000000000000000000, 0.9659258262890683122, 1.000000000000000000, 0.9659258262890683122, 1.000000000000000000, 0.9659258262890683122, 1.000000000000000000, 0.9659258262890683122, 1.000000000000000000, 0.9659258262890683122, 1.000000000000000000, 0.9659258262890683122, 1.000000000000000000, 0.9659258262890683122, 1.000000000000000000, 0.9659258262890683122, 1.000000000000000000, 0.9659258262890683122, 1.000000000000000000, 0.9659258262890683122, 1.000000000000000000, 0.9659258262890683122, 1.000000000000000000, 0.9659258262890683122, 1.000000000000000000, 0.9659258262890683122, 1.000000000000000000, 0.9659258262890683122, 1.000000000000000000, 0.9659258262890683122, 1.000000000000000000, 0.9659258262890683122, 1.000000000000000000, 0.9659258262890683122, 1.000000000000000000, 0.9659258262890683122, 1.000000000000000000, 0.9659258262890683122, 1.000000000000000000, 0.9659258262890683122, 1.000000000000000000, 0.9659258262890683122, 1.000000000000000000, 0.9659258262890683122, 1.000000000000000000, 0.9659258262890683122, 1.000000000000000000, 0.9659258262890683122, 1.000000000000000000, 0.9659258262890683122, 1.000000000000000000, 0.9659258262890683122, 1.000000000000000000, 0.9659258262890683122, 1.000000000000000000, 0.9659258262890683122, 1.000000000000000000, 0.9659258262890683122, 1.000000000000000000, 0.9659258262890683122, 1.000000000000000000, 0.9659258262890683122, 1.000000000000000000, 0.9659258262890683122, 1.000000000000000000, 0.9659258262890683122, 1.000000000000000000, 0.9659258262890683122, 1.000000000000000000, 0.9659258262890683122, 1.000000000000000000, 0.9659258262890683122, 1.000000000000000000, 0.9659258262890683122, 1.000000000000000000, 0.9659258262890683122, 1.000000000000000000, 0.9659258262890683122, 1.000000000000000000, 0.9659258262890683122, 1.000000000000000000, 0.9659258262890683122, 1.000000000000000000, 0.9659258262890683122, 1.000000000000000000, 0.9659258262890683122, 1.000000000000000000, 0.9659258262890683122, 1.000000000000000000, 0.9659258262890683122, 1.000000000000000000, 0.9659258262890683122, 1.000000000000000000, 0.9659258262890683122, 1.000000000000000000, 0.9659258262890683122, 1.000000000000000000, 0.9659258262890683122, 1.000000000000000000, 0.9659258262890683122, 1.000000000000000000, 0.9659258262890683122, 1.000000000000000000, 0.9659258262890683122, 1.000000000000000000, 0.9659258262890683122, 1.000000000000000000, 0.9659258262890683122, 1.000000000000000000, 0.9659258262890683122, 1.000000000000000000, 0.9659258262890683122, 1.000000000000000000, 0.9659258262890683122, 1.000000000000000000, 0.9659258262890683122, 1.000000000000000000, 0.9659258262890683122, 1.000000000000000000, 0.9659258262890683122, 1.000000000000000000, 0.9659258262890683122, 1.000000000000000000, 0.9659258262890683122, 1.000000000000000000, 0.9659258262890683122, 1.000000000000000000, 0.9659258262890683122, 1.000000000000000000, 0.9659258262890683122, 1.000000000000000000, 0.9659258262890683122, 1.000000000000000000, 0.9659258262890683122, 1.000000000000000000, 0.9659258262890683122, 1.000000000000000000, 0.9659258262890683122, 1.000000000000000000, 0.9659258262890683122, 1.000000000000000000, 0.9659258262890683122, 1.000000000000000000, 0.9659258262890683122, 1.000000000000000000, 0.9659258262890683122, 1.000000000000000000, 0.9659258262890683122, 1.000000000000000000, 0.9659258262890683122, 1.000000000000000000, 0.9659258262890683122, 1.000000000000000000, 0.9659258262890683122, 1.000000000000000000, 0.9659258262890683122, 1.000000000000000000, 0.9659258262890683122, 1.000000000000000000, 0.9659258262890683122, 1.000000000000000000, 0.9659258262890683122, 1.000000000000000000, 0.9659258262890683122, 1.000000000000000000, 0.9659258262890683122, 1.000000000000000000, 0.9659258262890683122, 1.000000000000000000, 0.9659258262890683122, 1.000000000000000000, 0.9659258262890683122, 1.000000000000000000, 0.9659258262890683122, 1.000000000000000000, 0.9659258262890683122, 1.000000000000000000, 0.9659258262890683122, 1.000000000000000000, 0.9659258262890683122, 1.000000000000000000, 0.9659258262890683122, 1.000000000000000000, 0.9659258262890683122, 1.000000000000000000, 0.9659258262890683122, 1.000000000000000000, 0.9659258262890683122, 1.000000000000000000, 0.9659258262890683122, 1.000000000000000000, 0.9659258262890683122, 1.000000000000000000, 0.9659258262890683122, 1.000000000000000000, 0.9659258262890683122, 1.000000000000000000, 0.9659258262890683122, 1.000000000000000000, 0.9659258262890683122, 1.000000000000000000, 0.9659258262890683122, 1.000000000000000000, 0.9659258262890683122, 1.000000000000000000, 0.9659258262890683122, 1.000000000000000000, 0.9659258262890683122, 1.000000000000000000, 0.9659258262890683122, 1.000000000000000000, 0.9659258262890683122, 1.000000000000000000, 0.9659258262890683122, 1.000000000000000000, 0.9659258262890683122, 1.000000000000000000, 0.9659258262890683122, 1.000000000000000000, 0.9659258262890683122, 1.000000000000000000, 0.9659258262890683122, 1.000000000000000000, 0.9659258262890683122, 1.000000000000000000, 0.9659258262890683122, 1.000000000000000000, 0.9659258262890683122, 1.000000000000000000, 0.9659258262890683122, 1.000000000000000000, 0.9659258262890683122, 1.000000000000000000, 0.9659258262890683122, 1.000000000000000000, 0.9659258262890683122, 1.000000000000000000, 0.9659258262890683122, 1.000000000000000000, 0.9659258262890683122, 1.000000000000000000, 0.9659258262890683122, 1.000000000000000000, 0.9659258262890683122, 1.000000000000000000, 0.9659258262890683122, 1.000000000000000000, 0.9659258262890683122, 1.000000000000000000, 0.9659258262890683122, 1.000000000000000000, 0.9659258262890683122, 1.000000000000000000, 0.9659258262890683122, 1.000000000000000000, 0.9659258262890683122, 1.000000000000000000, 0.9659258262890683122, 1.000000000000000000, 0.9659258262890683122, 1.000000000000000000, 0.9659258262890683122, 1.000000000000000000, 0.9659258262890683122, 1.000000000000000000, 0.9659258262890683122, 1.000000000000000000, 0.9659258262890683122, 1.000000000000000000, 0.9659258262890683122, 1.000000000000000000, 0.9659258262890683122, 1.000000000000000000, 0.9659258262890683122, 1.000000000000000000, 0.9659258262890683122, 1.000000000000000000, 0.9659258262890683122, 1.000000000000000000, 0.9659258262890683122, 1.000000000000000000, 0.9659258262890683122, 1.000000000000000000, 0.9659258262890683122, 1.000000000000000000, 0.9659258262890683122, 1.000000000000000000, 0.9659258262890683122, 1.000000000000000000, 0.9659258262890683122, 1.000000000000000000, 0.9659258262890683122, 1.000000000000000000, 0.9659258262890683122, 1.000000000000000000),
 ( 0.3333333333333333703, 0.3219752754296894559, 0.3333333333333333703, 0.3219752754296894559, 0.3333333333333333703, 0.3219752754296894559, 0.3333333333333333703, 0.3219752754296894559, 0.3333333333333333703, 0.3219752754296894559, 0.3333333333333333703, 0.3219752754296894559, 0.3333333333333333703, 0.3219752754296894559, 0.3333333333333333703, 0.3219752754296894559, 0.3333333333333333703, 0.3219752754296894559, 0.3333333333333333703, 0.3219752754296894559, 0.3333333333333333703, 0.3219752754296894559, 0.3333333333333333703, 0.3219752754296894559, 0.3333333333333333703, 0.3219752754296894559, 0.3333333333333333703, 0.3219752754296894559, 0.3333333333333333703, 0.3219752754296894559, 0.3333333333333333703, 0.3219752754296894559, 0.3333333333333333703, 0.3219752754296894559, 0.3333333333333333703, 0.3219752754296894559, 0.3333333333333333703, 0.3219752754296894559, 0.3333333333333333703, 0.3219752754296894559, 0.3333333333333333703, 0.3219752754296894559, 0.3333333333333333703, 0.3219752754296894559, 0.3333333333333333703, 0.3219752754296894559, 0.3333333333333333703, 0.3219752754296894559, 0.3333333333333333703, 0.3219752754296894559, 0.3333333333333333703, 0.3219752754296894559, 0.3333333333333333703, 0.3219752754296894559, 0.3333333333333333703, 0.3219752754296894559, 0.3333333333333333703, 0.3219752754296894559, 0.3333333333333333703, 0.3219752754296894559, 0.3333333333333333703, 0.3219752754296894559, 0.3333333333333333703, 0.3219752754296894559, 0.3333333333333333703, 0.3219752754296894559, 0.3333333333333333703, 0.3219752754296894559, 0.3333333333333333703, 0.3219752754296894559, 0.3333333333333333703, 0.3219752754296894559, 0.3333333333333333703, 0.3219752754296894559, 0.3333333333333333703, 0.3219752754296894559, 0.3333333333333333703, 0.3219752754296894559, 0.3333333333333333703, 0.3219752754296894559, 0.3333333333333333703, 0.3219752754296894559, 0.3333333333333333703, 0.3219752754296894559, 0.3333333333333333703, 0.3219752754296894559, 0.3333333333333333703, 0.3219752754296894559, 0.3333333333333333703, 0.3219752754296894559, 0.3333333333333333703, 0.3219752754296894559, 0.3333333333333333703, 0.3219752754296894559, 0.3333333333333333703, 0.3219752754296894559, 0.3333333333333333703, 0.3219752754296894559, 0.3333333333333333703, 0.3219752754296894559, 0.3333333333333333703, 0.3219752754296894559, 0.3333333333333333703, 0.3219752754296894559, 0.3333333333333333703, 0.3219752754296894559, 0.3333333333333333703, 0.3219752754296894559, 0.3333333333333333703, 0.3219752754296894559, 0.3333333333333333703, 0.3219752754296894559, 0.3333333333333333703, 0.3219752754296894559, 0.3333333333333333703, 0.3219752754296894559, 0.3333333333333333703, 0.3219752754296894559, 0.3333333333333333703, 0.3219752754296894559, 0.3333333333333333703, 0.3219752754296894559, 0.3333333333333333703, 0.3219752754296894559, 0.3333333333333333703, 0.3219752754296894559, 0.3333333333333333703, 0.3219752754296894559, 0.3333333333333333703, 0.3219752754296894559, 0.3333333333333333703, 0.3219752754296894559, 0.3333333333333333703, 0.3219752754296894559, 0.3333333333333333703, 0.3219752754296894559, 0.3333333333333333703, 0.3219752754296894559, 0.3333333333333333703, 0.3219752754296894559, 0.3333333333333333703, 0.3219752754296894559, 0.3333333333333333703, 0.3219752754296894559, 0.3333333333333333703, 0.3219752754296894559, 0.3333333333333333703, 0.3219752754296894559, 0.3333333333333333703, 0.3219752754296894559, 0.3333333333333333703, 0.3219752754296894559, 0.3333333333333333703, 0.3219752754296894559, 0.3333333333333333703, 0.3219752754296894559, 0.3333333333333333703, 0.3219752754296894559, 0.3333333333333333703, 0.3219752754296894559, 0.3333333333333333703, 0.3219752754296894559, 0.3333333333333333703, 0.3219752754296894559, 0.3333333333333333703, 0.3219752754296894559, 0.3333333333333333703, 0.3219752754296894559, 0.3333333333333333703, 0.3219752754296894559, 0.3333333333333333703, 0.3219752754296894559, 0.3333333333333333703, 0.3219752754296894559, 0.3333333333333333703, 0.3219752754296894559, 0.3333333333333333703, 0.3219752754296894559, 0.3333333333333333703, 0.3219752754296894559, 0.3333333333333333703, 0.3219752754296894559, 0.3333333333333333703, 0.3219752754296894559, 0.3333333333333333703, 0.3219752754296894559, 0.3333333333333333703, 0.3219752754296894559, 0.3333333333333333703, 0.3219752754296894559, 0.3333333333333333703, 0.3219752754296894559, 0.3333333333333333703, 0.3219752754296894559, 0.3333333333333333703, 0.3219752754296894559, 0.3333333333333333703, 0.3219752754296894559, 0.3333333333333333703, 0.3219752754296894559, 0.3333333333333333703, 0.3219752754296894559, 0.3333333333333333703, 0.3219752754296894559, 0.3333333333333333703, 0.3219752754296894559, 0.3333333333333333703, 0.3219752754296894559, 0.3333333333333333703, 0.3219752754296894559, 0.3333333333333333703, 0.3219752754296894559, 0.3333333333333333703, 0.3219752754296894559, 0.3333333333333333703, 0.3219752754296894559, 0.3333333333333333703, 0.3219752754296894559, 0.3333333333333333703, 0.3219752754296894559, 0.3333333333333333703, 0.3219752754296894559, 0.3333333333333333703, 0.3219752754296894559, 0.3333333333333333703, 0.3219752754296894559, 0.3333333333333333703, 0.3219752754296894559, 0.3333333333333333703, 0.3219752754296894559, 0.3333333333333333703, 0.3219752754296894559, 0.3333333333333333703, 0.3219752754296894559, 0.3333333333333333703, 0.3219752754296894559, 0.3333333333333333703, 0.3219752754296894559, 0.3333333333333333703, 0.3219752754296894559, 0.3333333333333333703, 0.3219752754296894559, 0.3333333333333333703, 0.3219752754296894559, 0.3333333333333333703, 0.3219752754296894559, 0.3333333333333333703, 0.3219752754296894559, 0.3333333333333333703, 0.3219752754296894559, 0.3333333333333333703, 0.3219752754296894559, 0.3333333333333333703, 0.3219752754296894559, 0.3333333333333333703, 0.3219752754296894559, 0.3333333333333333703, 0.3219752754296894559, 0.3333333333333333703, 0.3219752754296894559, 0.3333333333333333703, 0.3219752754296894559, 0.3333333333333333703, 0.3219752754296894559, 0.3333333333333333703, 0.3219752754296894559, 0.3333333333333333703, 0.3219752754296894559, 0.3333333333333333703, 0.3219752754296894559, 0.3333333333333333703, 0.3219752754296894559, 0.3333333333333333703, 0.3219752754296894559, 0.3333333333333333703, 0.3219752754296894559, 0.3333333333333333703, 0.3219752754296894559, 0.3333333333333333703, 0.3219752754296894559, 0.3333333333333333703, 0.3219752754296894559, 0.3333333333333333703, 0.3219752754296894559, 0.3333333333333333703, 0.3219752754296894559, 0.3333333333333333703, 0.3219752754296894559, 0.3333333333333333703, 0.3219752754296894559, 0.3333333333333333703, 0.3219752754296894559, 0.3333333333333333703, 0.3219752754296894559, 0.3333333333333333703, 0.3219752754296894559, 0.3333333333333333703, 0.3219752754296894559, 0.3333333333333333703, 0.3219752754296894559, 0.3333333333333333703, 0.3219752754296894559, 0.3333333333333333703, 0.3219752754296894559, 0.3333333333333333703, 0.3219752754296894559, 0.3333333333333333703, 0.3219752754296894559, 0.3333333333333333703, 0.3219752754296894559, 0.3333333333333333703, 0.3219752754296894559, 0.3333333333333333703, 0.3219752754296894559, 0.3333333333333333703, 0.3219752754296894559, 0.3333333333333333703, 0.3219752754296894559, 0.3333333333333333703, 0.3219752754296894559, 0.3333333333333333703, 0.3219752754296894559, 0.3333333333333333703, 0.3219752754296894559, 0.3333333333333333703, 0.3219752754296894559, 0.3333333333333333703, 0.3219752754296894559, 0.3333333333333333703, 0.3219752754296894559, 0.3333333333333333703, 0.3219752754296894559, 0.3333333333333333703, 0.3219752754296894559, 0.3333333333333333703, 0.3219752754296894559, 0.3333333333333333703, 0.3219752754296894559, 0.3333333333333333703, 0.3219752754296894559, 0.3333333333333333703, 0.3219752754296894559, 0.3333333333333333703, 0.3219752754296894559, 0.3333333333333333703, 0.3219752754296894559, 0.3333333333333333703, 0.3219752754296894559, 0.3333333333333333703, 0.3219752754296894559, 0.3333333333333333703, 0.3219752754296894559, 0.3333333333333333703, 0.3219752754296894559, 0.3333333333333333703, 0.3219752754296894559, 0.3333333333333333703, 0.3219752754296894559, 0.3333333333333333703, 0.3219752754296894559, 0.3333333333333333703, 0.3219752754296894559, 0.3333333333333333703, 0.3219752754296894559, 0.3333333333333333703, 0.3219752754296894559, 0.3333333333333333703, 0.3219752754296894559, 0.3333333333333333703, 0.3219752754296894559, 0.3333333333333333703, 0.3219752754296894559, 0.3333333333333333703, 0.3219752754296894559, 0.3333333333333333703, 0.3219752754296894559, 0.3333333333333333703, 0.3219752754296894559, 0.3333333333333333703, 0.3219752754296894559, 0.3333333333333333703, 0.3219752754296894559, 0.3333333333333333703, 0.3219752754296894559, 0.3333333333333333703, 0.3219752754296894559, 0.3333333333333333703, 0.3219752754296894559, 0.3333333333333333703, 0.3219752754296894559, 0.3333333333333333703, 0.3219752754296894559, 0.3333333333333333703, 0.3219752754296894559, 0.3333333333333333703, 0.3219752754296894559, 0.3333333333333333703, 0.3219752754296894559, 0.3333333333333333703, 0.3219752754296894559, 0.3333333333333333703, 0.3219752754296894559, 0.3333333333333333703, 0.3219752754296894559, 0.3333333333333333703, 0.3219752754296894559, 0.3333333333333333703, 0.3219752754296894559, 0.3333333333333333703, 0.3219752754296894559, 0.3333333333333333703, 0.3219752754296894559, 0.3333333333333333703, 0.3219752754296894559, 0.3333333333333333703, 0.3219752754296894559, 0.3333333333333333703, 0.3219752754296894559, 0.3333333333333333703, 0.3219752754296894559, 0.3333333333333333703, 0.3219752754296894559, 0.3333333333333333703, 0.3219752754296894559, 0.3333333333333333703, 0.3219752754296894559, 0.3333333333333333703, 0.3219752754296894559, 0.3333333333333333703, 0.3219752754296894559, 0.3333333333333333703, 0.3219752754296894559, 0.3333333333333333703, 0.3219752754296894559, 0.3333333333333333703, 0.3219752754296894559, 0.3333333333333333703, 0.3219752754296894559, 0.3333333333333333703, 0.3219752754296894559, 0.3333333333333333703, 0.3219752754296894559, 0.3333333333333333703, 0.3219752754296894559, 0.3333333333333333703, 0.3219752754296894559, 0.3333333333333333703, 0.3219752754296894559, 0.3333333333333333703, 0.3219752754296894559, 0.3333333333333333703, 0.3219752754296894559, 0.3333333333333333703, 0.3219752754296894559, 0.3333333333333333703, 0.3219752754296894559, 0.3333333333333333703),
 ( 0.3333333333333333703, 0.3219752754296894559, 0.3333333333333333703, 0.3219752754296894559, 0.3333333333333333703, 0.3219752754296894559, 0.3333333333333333703, 0.3219752754296894559, 0.3333333333333333703, 0.3219752754296894559, 0.3333333333333333703, 0.3219752754296894559, 0.3333333333333333703, 0.3219752754296894559, 0.3333333333333333703, 0.3219752754296894559, 0.3333333333333333703, 0.3219752754296894559, 0.3333333333333333703, 0.3219752754296894559, 0.3333333333333333703, 0.3219752754296894559, 0.3333333333333333703, 0.3219752754296894559, 0.3333333333333333703, 0.3219752754296894559, 0.3333333333333333703, 0.3219752754296894559, 0.3333333333333333703, 0.3219752754296894559, 0.3333333333333333703, 0.3219752754296894559, 0.3333333333333333703, 0.3219752754296894559, 0.3333333333333333703, 0.3219752754296894559, 0.3333333333333333703, 0.3219752754296894559, 0.3333333333333333703, 0.3219752754296894559, 0.3333333333333333703, 0.3219752754296894559, 0.3333333333333333703, 0.3219752754296894559, 0.3333333333333333703, 0.3219752754296894559, 0.3333333333333333703, 0.3219752754296894559, 0.3333333333333333703, 0.3219752754296894559, 0.3333333333333333703, 0.3219752754296894559, 0.3333333333333333703, 0.3219752754296894559, 0.3333333333333333703, 0.3219752754296894559, 0.3333333333333333703, 0.3219752754296894559, 0.3333333333333333703, 0.3219752754296894559, 0.3333333333333333703, 0.3219752754296894559, 0.3333333333333333703, 0.3219752754296894559, 0.3333333333333333703, 0.3219752754296894559, 0.3333333333333333703, 0.3219752754296894559, 0.3333333333333333703, 0.3219752754296894559, 0.3333333333333333703, 0.3219752754296894559, 0.3333333333333333703, 0.3219752754296894559, 0.3333333333333333703, 0.3219752754296894559, 0.3333333333333333703, 0.3219752754296894559, 0.3333333333333333703, 0.3219752754296894559, 0.3333333333333333703, 0.3219752754296894559, 0.3333333333333333703, 0.3219752754296894559, 0.3333333333333333703, 0.3219752754296894559, 0.3333333333333333703, 0.3219752754296894559, 0.3333333333333333703, 0.3219752754296894559, 0.3333333333333333703, 0.3219752754296894559, 0.3333333333333333703, 0.3219752754296894559, 0.3333333333333333703, 0.3219752754296894559, 0.3333333333333333703, 0.3219752754296894559, 0.3333333333333333703, 0.3219752754296894559, 0.3333333333333333703, 0.3219752754296894559, 0.3333333333333333703, 0.3219752754296894559, 0.3333333333333333703, 0.3219752754296894559, 0.3333333333333333703, 0.3219752754296894559, 0.3333333333333333703, 0.3219752754296894559, 0.3333333333333333703, 0.3219752754296894559, 0.3333333333333333703, 0.3219752754296894559, 0.3333333333333333703, 0.3219752754296894559, 0.3333333333333333703, 0.3219752754296894559, 0.3333333333333333703, 0.3219752754296894559, 0.3333333333333333703, 0.3219752754296894559, 0.3333333333333333703, 0.3219752754296894559, 0.3333333333333333703, 0.3219752754296894559, 0.3333333333333333703, 0.3219752754296894559, 0.3333333333333333703, 0.3219752754296894559, 0.3333333333333333703, 0.3219752754296894559, 0.3333333333333333703, 0.3219752754296894559, 0.3333333333333333703, 0.3219752754296894559, 0.3333333333333333703, 0.3219752754296894559, 0.3333333333333333703, 0.3219752754296894559, 0.3333333333333333703, 0.3219752754296894559, 0.3333333333333333703, 0.3219752754296894559, 0.3333333333333333703, 0.3219752754296894559, 0.3333333333333333703, 0.3219752754296894559, 0.3333333333333333703, 0.3219752754296894559, 0.3333333333333333703, 0.3219752754296894559, 0.3333333333333333703, 0.3219752754296894559, 0.3333333333333333703, 0.3219752754296894559, 0.3333333333333333703, 0.3219752754296894559, 0.3333333333333333703, 0.3219752754296894559, 0.3333333333333333703, 0.3219752754296894559, 0.3333333333333333703, 0.3219752754296894559, 0.3333333333333333703, 0.3219752754296894559, 0.3333333333333333703, 0.3219752754296894559, 0.3333333333333333703, 0.3219752754296894559, 0.3333333333333333703, 0.3219752754296894559, 0.3333333333333333703, 0.3219752754296894559, 0.3333333333333333703, 0.3219752754296894559, 0.3333333333333333703, 0.3219752754296894559, 0.3333333333333333703, 0.3219752754296894559, 0.3333333333333333703, 0.3219752754296894559, 0.3333333333333333703, 0.3219752754296894559, 0.3333333333333333703, 0.3219752754296894559, 0.3333333333333333703, 0.3219752754296894559, 0.3333333333333333703, 0.3219752754296894559, 0.3333333333333333703, 0.3219752754296894559, 0.3333333333333333703, 0.3219752754296894559, 0.3333333333333333703, 0.3219752754296894559, 0.3333333333333333703, 0.3219752754296894559, 0.3333333333333333703, 0.3219752754296894559, 0.3333333333333333703, 0.3219752754296894559, 0.3333333333333333703, 0.3219752754296894559, 0.3333333333333333703, 0.3219752754296894559, 0.3333333333333333703, 0.3219752754296894559, 0.3333333333333333703, 0.3219752754296894559, 0.3333333333333333703, 0.3219752754296894559, 0.3333333333333333703, 0.3219752754296894559, 0.3333333333333333703, 0.3219752754296894559, 0.3333333333333333703, 0.3219752754296894559, 0.3333333333333333703, 0.3219752754296894559, 0.3333333333333333703, 0.3219752754296894559, 0.3333333333333333703, 0.3219752754296894559, 0.3333333333333333703, 0.3219752754296894559, 0.3333333333333333703, 0.3219752754296894559, 0.3333333333333333703, 0.3219752754296894559, 0.3333333333333333703, 0.3219752754296894559, 0.3333333333333333703, 0.3219752754296894559, 0.3333333333333333703, 0.3219752754296894559, 0.3333333333333333703, 0.3219752754296894559, 0.3333333333333333703, 0.3219752754296894559, 0.3333333333333333703, 0.3219752754296894559, 0.3333333333333333703, 0.3219752754296894559, 0.3333333333333333703, 0.3219752754296894559, 0.3333333333333333703, 0.3219752754296894559, 0.3333333333333333703, 0.3219752754296894559, 0.3333333333333333703, 0.3219752754296894559, 0.3333333333333333703, 0.3219752754296894559, 0.3333333333333333703, 0.3219752754296894559, 0.3333333333333333703, 0.3219752754296894559, 0.3333333333333333703, 0.3219752754296894559, 0.3333333333333333703, 0.3219752754296894559, 0.3333333333333333703, 0.3219752754296894559, 0.3333333333333333703, 0.3219752754296894559, 0.3333333333333333703, 0.3219752754296894559, 0.3333333333333333703, 0.3219752754296894559, 0.3333333333333333703, 0.3219752754296894559, 0.3333333333333333703, 0.3219752754296894559, 0.3333333333333333703, 0.3219752754296894559, 0.3333333333333333703, 0.3219752754296894559, 0.3333333333333333703, 0.3219752754296894559, 0.3333333333333333703, 0.3219752754296894559, 0.3333333333333333703, 0.3219752754296894559, 0.3333333333333333703, 0.3219752754296894559, 0.3333333333333333703, 0.3219752754296894559, 0.3333333333333333703, 0.3219752754296894559, 0.3333333333333333703, 0.3219752754296894559, 0.3333333333333333703, 0.3219752754296894559, 0.3333333333333333703, 0.3219752754296894559, 0.3333333333333333703, 0.3219752754296894559, 0.3333333333333333703, 0.3219752754296894559, 0.3333333333333333703, 0.3219752754296894559, 0.3333333333333333703, 0.3219752754296894559, 0.3333333333333333703, 0.3219752754296894559, 0.3333333333333333703, 0.3219752754296894559, 0.3333333333333333703, 0.3219752754296894559, 0.3333333333333333703, 0.3219752754296894559, 0.3333333333333333703, 0.3219752754296894559, 0.3333333333333333703, 0.3219752754296894559, 0.3333333333333333703, 0.3219752754296894559, 0.3333333333333333703, 0.3219752754296894559, 0.3333333333333333703, 0.3219752754296894559, 0.3333333333333333703, 0.3219752754296894559, 0.3333333333333333703, 0.3219752754296894559, 0.3333333333333333703, 0.3219752754296894559, 0.3333333333333333703, 0.3219752754296894559, 0.3333333333333333703, 0.3219752754296894559, 0.3333333333333333703, 0.3219752754296894559, 0.3333333333333333703, 0.3219752754296894559, 0.3333333333333333703, 0.3219752754296894559, 0.3333333333333333703, 0.3219752754296894559, 0.3333333333333333703, 0.3219752754296894559, 0.3333333333333333703, 0.3219752754296894559, 0.3333333333333333703, 0.3219752754296894559, 0.3333333333333333703, 0.3219752754296894559, 0.3333333333333333703, 0.3219752754296894559, 0.3333333333333333703, 0.3219752754296894559, 0.3333333333333333703, 0.3219752754296894559, 0.3333333333333333703, 0.3219752754296894559, 0.3333333333333333703, 0.3219752754296894559, 0.3333333333333333703, 0.3219752754296894559, 0.3333333333333333703, 0.3219752754296894559, 0.3333333333333333703, 0.3219752754296894559, 0.3333333333333333703, 0.3219752754296894559, 0.3333333333333333703, 0.3219752754296894559, 0.3333333333333333703, 0.3219752754296894559, 0.3333333333333333703, 0.3219752754296894559, 0.3333333333333333703, 0.3219752754296894559, 0.3333333333333333703, 0.3219752754296894559, 0.3333333333333333703, 0.3219752754296894559, 0.3333333333333333703, 0.3219752754296894559, 0.3333333333333333703, 0.3219752754296894559, 0.3333333333333333703, 0.3219752754296894559, 0.3333333333333333703, 0.3219752754296894559, 0.3333333333333333703, 0.3219752754296894559, 0.3333333333333333703, 0.3219752754296894559, 0.3333333333333333703, 0.3219752754296894559, 0.3333333333333333703, 0.3219752754296894559, 0.3333333333333333703, 0.3219752754296894559, 0.3333333333333333703, 0.3219752754296894559, 0.3333333333333333703, 0.3219752754296894559, 0.3333333333333333703, 0.3219752754296894559, 0.3333333333333333703, 0.3219752754296894559, 0.3333333333333333703, 0.3219752754296894559, 0.3333333333333333703, 0.3219752754296894559, 0.3333333333333333703, 0.3219752754296894559, 0.3333333333333333703, 0.3219752754296894559, 0.3333333333333333703, 0.3219752754296894559, 0.3333333333333333703, 0.3219752754296894559, 0.3333333333333333703, 0.3219752754296894559, 0.3333333333333333703, 0.3219752754296894559, 0.3333333333333333703, 0.3219752754296894559, 0.3333333333333333703, 0.3219752754296894559, 0.3333333333333333703, 0.3219752754296894559, 0.3333333333333333703, 0.3219752754296894559, 0.3333333333333333703, 0.3219752754296894559, 0.3333333333333333703, 0.3219752754296894559, 0.3333333333333333703, 0.3219752754296894559, 0.3333333333333333703, 0.3219752754296894559, 0.3333333333333333703, 0.3219752754296894559, 0.3333333333333333703, 0.3219752754296894559, 0.3333333333333333703, 0.3219752754296894559, 0.3333333333333333703, 0.3219752754296894559, 0.3333333333333333703, 0.3219752754296894559, 0.3333333333333333703, 0.3219752754296894559, 0.3333333333333333703, 0.3219752754296894559, 0.3333333333333333703, 0.3219752754296894559, 0.3333333333333333703, 0.3219752754296894559, 0.3333333333333333703, 0.3219752754296894559, 0.3333333333333333703),
 ( 1.000000000000000000, 0.9659258262890683122, 1.000000000000000000, 0.9659258262890683122, 1.000000000000000000, 0.9659258262890683122, 1.000000000000000000, 0.9659258262890683122, 1.000000000000000000, 0.9659258262890683122, 1.000000000000000000, 0.9659258262890683122, 1.000000000000000000, 0.9659258262890683122, 1.000000000000000000, 0.9659258262890683122, 1.000000000000000000, 0.9659258262890683122, 1.000000000000000000, 0.9659258262890683122, 1.000000000000000000, 0.9659258262890683122, 1.000000000000000000, 0.9659258262890683122, 1.000000000000000000, 0.9659258262890683122, 1.000000000000000000, 0.9659258262890683122, 1.000000000000000000, 0.9659258262890683122, 1.000000000000000000, 0.9659258262890683122, 1.000000000000000000, 0.9659258262890683122, 1.000000000000000000, 0.9659258262890683122, 1.000000000000000000, 0.9659258262890683122, 1.000000000000000000, 0.9659258262890683122, 1.000000000000000000, 0.9659258262890683122, 1.000000000000000000, 0.9659258262890683122, 1.000000000000000000, 0.9659258262890683122, 1.000000000000000000, 0.9659258262890683122, 1.000000000000000000, 0.9659258262890683122, 1.000000000000000000, 0.9659258262890683122, 1.000000000000000000, 0.9659258262890683122, 1.000000000000000000, 0.9659258262890683122, 1.000000000000000000, 0.9659258262890683122, 1.000000000000000000, 0.9659258262890683122, 1.000000000000000000, 0.9659258262890683122, 1.000000000000000000, 0.9659258262890683122, 1.000000000000000000, 0.9659258262890683122, 1.000000000000000000, 0.9659258262890683122, 1.000000000000000000, 0.9659258262890683122, 1.000000000000000000, 0.9659258262890683122, 1.000000000000000000, 0.9659258262890683122, 1.000000000000000000, 0.9659258262890683122, 1.000000000000000000, 0.9659258262890683122, 1.000000000000000000, 0.9659258262890683122, 1.000000000000000000, 0.9659258262890683122, 1.000000000000000000, 0.9659258262890683122, 1.000000000000000000, 0.9659258262890683122, 1.000000000000000000, 0.9659258262890683122, 1.000000000000000000, 0.9659258262890683122, 1.000000000000000000, 0.9659258262890683122, 1.000000000000000000, 0.9659258262890683122, 1.000000000000000000, 0.9659258262890683122, 1.000000000000000000, 0.9659258262890683122, 1.000000000000000000, 0.9659258262890683122, 1.000000000000000000, 0.9659258262890683122, 1.000000000000000000, 0.9659258262890683122, 1.000000000000000000, 0.9659258262890683122, 1.000000000000000000, 0.9659258262890683122, 1.000000000000000000, 0.9659258262890683122, 1.000000000000000000, 0.9659258262890683122, 1.000000000000000000, 0.9659258262890683122, 1.000000000000000000, 0.9659258262890683122, 1.000000000000000000, 0.9659258262890683122, 1.000000000000000000, 0.9659258262890683122, 1.000000000000000000, 0.9659258262890683122, 1.000000000000000000, 0.9659258262890683122, 1.000000000000000000, 0.9659258262890683122, 1.000000000000000000, 0.9659258262890683122, 1.000000000000000000, 0.9659258262890683122, 1.000000000000000000, 0.9659258262890683122, 1.000000000000000000, 0.9659258262890683122, 1.000000000000000000, 0.9659258262890683122, 1.000000000000000000, 0.9659258262890683122, 1.000000000000000000, 0.9659258262890683122, 1.000000000000000000, 0.9659258262890683122, 1.000000000000000000, 0.9659258262890683122, 1.000000000000000000, 0.9659258262890683122, 1.000000000000000000, 0.9659258262890683122, 1.000000000000000000, 0.9659258262890683122, 1.000000000000000000, 0.9659258262890683122, 1.000000000000000000, 0.9659258262890683122, 1.000000000000000000, 0.9659258262890683122, 1.000000000000000000, 0.9659258262890683122, 1.000000000000000000, 0.9659258262890683122, 1.000000000000000000, 0.9659258262890683122, 1.000000000000000000, 0.9659258262890683122, 1.000000000000000000, 0.9659258262890683122, 1.000000000000000000, 0.9659258262890683122, 1.000000000000000000, 0.9659258262890683122, 1.000000000000000000, 0.9659258262890683122, 1.000000000000000000, 0.9659258262890683122, 1.000000000000000000, 0.9659258262890683122, 1.000000000000000000, 0.9659258262890683122, 1.000000000000000000, 0.9659258262890683122, 1.000000000000000000, 0.9659258262890683122, 1.000000000000000000, 0.9659258262890683122, 1.000000000000000000, 0.9659258262890683122, 1.000000000000000000, 0.9659258262890683122, 1.000000000000000000, 0.9659258262890683122, 1.000000000000000000, 0.9659258262890683122, 1.000000000000000000, 0.9659258262890683122, 1.000000000000000000, 0.9659258262890683122, 1.000000000000000000, 0.9659258262890683122, 1.000000000000000000, 0.9659258262890683122, 1.000000000000000000, 0.9659258262890683122, 1.000000000000000000, 0.9659258262890683122, 1.000000000000000000, 0.9659258262890683122, 1.000000000000000000, 0.9659258262890683122, 1.000000000000000000, 0.9659258262890683122, 1.000000000000000000, 0.9659258262890683122, 1.000000000000000000, 0.9659258262890683122, 1.000000000000000000, 0.9659258262890683122, 1.000000000000000000, 0.9659258262890683122, 1.000000000000000000, 0.9659258262890683122, 1.000000000000000000, 0.9659258262890683122, 1.000000000000000000, 0.9659258262890683122, 1.000000000000000000, 0.9659258262890683122, 1.000000000000000000, 0.9659258262890683122, 1.000000000000000000, 0.9659258262890683122, 1.000000000000000000, 0.9659258262890683122, 1.000000000000000000, 0.9659258262890683122, 1.000000000000000000, 0.9659258262890683122, 1.000000000000000000, 0.9659258262890683122, 1.000000000000000000, 0.9659258262890683122, 1.000000000000000000, 0.9659258262890683122, 1.000000000000000000, 0.9659258262890683122, 1.000000000000000000, 0.9659258262890683122, 1.000000000000000000, 0.9659258262890683122, 1.000000000000000000, 0.9659258262890683122, 1.000000000000000000, 0.9659258262890683122, 1.000000000000000000, 0.9659258262890683122, 1.000000000000000000, 0.9659258262890683122, 1.000000000000000000, 0.9659258262890683122, 1.000000000000000000, 0.9659258262890683122, 1.000000000000000000, 0.9659258262890683122, 1.000000000000000000, 0.9659258262890683122, 1.000000000000000000, 0.9659258262890683122, 1.000000000000000000, 0.9659258262890683122, 1.000000000000000000, 0.9659258262890683122, 1.000000000000000000, 0.9659258262890683122, 1.000000000000000000, 0.9659258262890683122, 1.000000000000000000, 0.9659258262890683122, 1.000000000000000000, 0.9659258262890683122, 1.000000000000000000, 0.9659258262890683122, 1.000000000000000000, 0.9659258262890683122, 1.000000000000000000, 0.9659258262890683122, 1.000000000000000000, 0.9659258262890683122, 1.000000000000000000, 0.9659258262890683122, 1.000000000000000000, 0.9659258262890683122, 1.000000000000000000, 0.9659258262890683122, 1.000000000000000000, 0.9659258262890683122, 1.000000000000000000, 0.9659258262890683122, 1.000000000000000000, 0.9659258262890683122, 1.000000000000000000, 0.9659258262890683122, 1.000000000000000000, 0.9659258262890683122, 1.000000000000000000, 0.9659258262890683122, 1.000000000000000000, 0.9659258262890683122, 1.000000000000000000, 0.9659258262890683122, 1.000000000000000000, 0.9659258262890683122, 1.000000000000000000, 0.9659258262890683122, 1.000000000000000000, 0.9659258262890683122, 1.000000000000000000, 0.9659258262890683122, 1.000000000000000000, 0.9659258262890683122, 1.000000000000000000, 0.9659258262890683122, 1.000000000000000000, 0.9659258262890683122, 1.000000000000000000, 0.9659258262890683122, 1.000000000000000000, 0.9659258262890683122, 1.000000000000000000, 0.9659258262890683122, 1.000000000000000000, 0.9659258262890683122, 1.000000000000000000, 0.9659258262890683122, 1.000000000000000000, 0.9659258262890683122, 1.000000000000000000, 0.9659258262890683122, 1.000000000000000000, 0.9659258262890683122, 1.000000000000000000, 0.9659258262890683122, 1.000000000000000000, 0.9659258262890683122, 1.000000000000000000, 0.9659258262890683122, 1.000000000000000000, 0.9659258262890683122, 1.000000000000000000, 0.9659258262890683122, 1.000000000000000000, 0.9659258262890683122, 1.000000000000000000, 0.9659258262890683122, 1.000000000000000000, 0.9659258262890683122, 1.000000000000000000, 0.9659258262890683122, 1.000000000000000000, 0.9659258262890683122, 1.000000000000000000, 0.9659258262890683122, 1.000000000000000000, 0.9659258262890683122, 1.000000000000000000, 0.9659258262890683122, 1.000000000000000000, 0.9659258262890683122, 1.000000000000000000, 0.9659258262890683122, 1.000000000000000000, 0.9659258262890683122, 1.000000000000000000, 0.9659258262890683122, 1.000000000000000000, 0.9659258262890683122, 1.000000000000000000, 0.9659258262890683122, 1.000000000000000000, 0.9659258262890683122, 1.000000000000000000, 0.9659258262890683122, 1.000000000000000000, 0.9659258262890683122, 1.000000000000000000, 0.9659258262890683122, 1.000000000000000000, 0.9659258262890683122, 1.000000000000000000, 0.9659258262890683122, 1.000000000000000000, 0.9659258262890683122, 1.000000000000000000, 0.9659258262890683122, 1.000000000000000000, 0.9659258262890683122, 1.000000000000000000, 0.9659258262890683122, 1.000000000000000000, 0.9659258262890683122, 1.000000000000000000, 0.9659258262890683122, 1.000000000000000000, 0.9659258262890683122, 1.000000000000000000, 0.9659258262890683122, 1.000000000000000000, 0.9659258262890683122, 1.000000000000000000, 0.9659258262890683122, 1.000000000000000000, 0.9659258262890683122, 1.000000000000000000, 0.9659258262890683122, 1.000000000000000000, 0.9659258262890683122, 1.000000000000000000, 0.9659258262890683122, 1.000000000000000000, 0.9659258262890683122, 1.000000000000000000, 0.9659258262890683122, 1.000000000000000000, 0.9659258262890683122, 1.000000000000000000, 0.9659258262890683122, 1.000000000000000000, 0.9659258262890683122, 1.000000000000000000, 0.9659258262890683122, 1.000000000000000000, 0.9659258262890683122, 1.000000000000000000, 0.9659258262890683122, 1.000000000000000000, 0.9659258262890683122, 1.000000000000000000, 0.9659258262890683122, 1.000000000000000000, 0.9659258262890683122, 1.000000000000000000, 0.9659258262890683122, 1.000000000000000000, 0.9659258262890683122, 1.000000000000000000, 0.9659258262890683122, 1.000000000000000000, 0.9659258262890683122, 1.000000000000000000, 0.9659258262890683122, 1.000000000000000000, 0.9659258262890683122, 1.000000000000000000, 0.9659258262890683122, 1.000000000000000000, 0.9659258262890683122, 1.000000000000000000, 0.9659258262890683122, 1.000000000000000000) ) ) 
 REPRESENTATION_ITEM ( '' )  SURFACE ( )  );
#131407=CARTESIAN_POINT ( 'NONE',  ( -9.474510206698964154, 16.51473224551069663, 100.4155762719810241 ) ) ;
#131408=CARTESIAN_POINT ( 'NONE',  ( -19.03943276465977164, 0.05219959533909376836, 96.24890960531436690 ) ) ;
#131409=CARTESIAN_POINT ( 'NONE',  ( 16.53943276465976808, -0.05219959533910856209, 108.7489096053143669 ) ) ;
#131410=CARTESIAN_POINT ( 'NONE',  ( -12.06949235617756955, 12.14591786802309770, 45.62390960531436690 ) ) ;
#131411=CARTESIAN_POINT ( 'NONE',  ( 14.29746914071037800, 8.314922557961029526, 46.66775706135234714 ) ) ;
#131412=CARTESIAN_POINT ( 'NONE',  ( 5.049401038298161559, -19.05341960407611168, 22.70724293864769194 ) ) ;
#131413=CARTESIAN_POINT ( 'NONE',  ( 5.823673210054444382, -21.52544592524334988, 100.2094237280190043 ) ) ;
#131414=CARTESIAN_POINT ( 'NONE',  ( 19.02544592524343514, -5.153800228976328945, 108.5405762719810383 ) ) ;
#131415=CARTESIAN_POINT ( 'NONE',  ( -8.224510206698735004, -14.34966873604973081, 109.5844237280190328 ) ) ;
#131416=CARTESIAN_POINT ( 'NONE',  ( -0.05219959533937732626, 21.53943276465977519, 32.50109039468568284 ) ) ;
#131417=CARTESIAN_POINT ( 'NONE',  ( -9.564922557960796823, -16.46253265017161027, 107.0822429386476955 ) ) ;
#131418=CARTESIAN_POINT ( 'NONE',  ( 8.314922557961029526, -14.29746914071037800, 40.41775706135234714 ) ) ;
#131419=CARTESIAN_POINT ( 'NONE',  ( 8.314922557961029526, -14.29746914071037800, 110.4177570613523756 ) ) ;
#131420=CARTESIAN_POINT ( 'NONE',  ( 12.06949235617739724, 12.14591786802326823, 86.87609039468568994 ) ) ;
#131421=CARTESIAN_POINT ( 'NONE',  ( 8.314922557961029526, -14.29746914071037800, 30.41775706135234358 ) ) ;
#131423=CARTESIAN_POINT ( 'NONE',  ( 16.46253265017160672, -9.564922557960803928, 53.33224293864768839 ) ) ;
#131424=CARTESIAN_POINT ( 'NONE',  ( 0.05219959533910956823, 16.53943276465976808, 109.9989096053143527 ) ) ;
#131425=CARTESIAN_POINT ( 'NONE',  ( -18.67979575497178146, -10.72451020669898902, 111.6655762719810525 ) ) ;
#131426=CARTESIAN_POINT ( 'NONE',  ( 5.049401038298161559, -19.05341960407611168, 27.70724293864769550 ) ) ;
#131427=CARTESIAN_POINT ( 'NONE',  ( -19.05341960407611168, -5.049401038298163336, 101.4572429386476955 ) ) ;
#131428=CARTESIAN_POINT ( 'NONE',  ( 16.46253265017160672, -9.564922557960803928, 38.33224293864768839 ) ) ;
#131429=CARTESIAN_POINT ( 'NONE',  ( -16.46253265017160317, 9.564922557960807481, 105.8322429386476955 ) ) ;
#131430=CARTESIAN_POINT ( 'NONE',  ( -17.50000000000000711, -5.624438216177558125, 34.18329655085356933 ) ) ;
#131431=CARTESIAN_POINT ( 'NONE',  ( -19.02544592524342804, 5.153800228976336051, 96.04057627198103830 ) ) ;
#131432=CARTESIAN_POINT ( 'NONE',  ( -0.05219959533937732626, 21.53943276465977519, 42.50109039468567573 ) ) ;
#131433=CARTESIAN_POINT ( 'NONE',  ( 12.14591786802309770, 12.06949235617756955, 94.37390960531436690 ) ) ;
#131434=CARTESIAN_POINT ( 'NONE',  ( -16.46253265017160317, 9.564922557960807481, 110.8322429386476955 ) ) ;
#131435=CARTESIAN_POINT ( 'NONE',  ( 18.22780087662122384, -5.500000000000022204, 96.01540105326108687 ) ) ;
#131436=CARTESIAN_POINT ( 'NONE',  ( 14.34966873604972726, -8.224510206698740333, 60.83442372801901854 ) ) ;
#131437=CARTESIAN_POINT ( 'NONE',  ( -0.05219959533937732626, 21.53943276465977519, 72.50109039468568994 ) ) ;
#131438=CARTESIAN_POINT ( 'NONE',  ( 16.55341960407618274, -4.379528057220086978, 41.04275706135236135 ) ) ;
#131439=CARTESIAN_POINT ( 'NONE',  ( -16.46253265017160317, 9.564922557960807481, 75.83224293864769550 ) ) ;
#131440=CARTESIAN_POINT ( 'NONE',  ( -19.02544592524334988, -5.153800228976617603, 108.9594237280189759 ) ) ;
#131441=CARTESIAN_POINT ( 'NONE',  ( -12.06949235617739369, -12.14591786802326823, 89.37609039468568994 ) ) ;
#131442=CARTESIAN_POINT ( 'NONE',  ( -13.89961937509957401, -13.97604488694547875, 89.37609039468563310 ) ) ;
#131443=CARTESIAN_POINT ( 'NONE',  ( 16.46253265017160672, -9.564922557960803928, 58.33224293864769550 ) ) ;
#131444=CARTESIAN_POINT ( 'NONE',  ( 10.81492255796078972, 18.62759615963270932, 94.58224293864769550 ) ) ;
#131445=CARTESIAN_POINT ( 'NONE',  ( 8.314922557960818139, 14.29746914071049879, 94.58224293864769550 ) ) ;
#131446=CARTESIAN_POINT ( 'NONE',  ( 16.46253265017146816, 9.564922557961045513, 91.66775706135234714 ) ) ;
#131447=CARTESIAN_POINT ( 'NONE',  ( 0.05219959533934541429, -16.53943276465976808, 60.00109039468568284 ) ) ;
#131449=CARTESIAN_POINT ( 'NONE',  ( -19.05341960407617563, 5.049401038297882671, 73.54275706135233293 ) ) ;
#131450=CARTESIAN_POINT ( 'NONE',  ( -16.55341960407611168, -4.379528057220339221, 36.45724293864768839 ) ) ;
#131451=CARTESIAN_POINT ( 'NONE',  ( 14.29746914071049879, -8.314922557960816363, 78.33224293864770971 ) ) ;
#131452=CARTESIAN_POINT ( 'NONE',  ( -13.97604488694547697, 13.89961937509957934, 23.12609039468565442 ) ) ;
#131453=CARTESIAN_POINT ( 'NONE',  ( -17.44270441346522560, 5.991230190322816895, 38.63664920735773478 ) ) ;
#131454=CARTESIAN_POINT ( 'NONE',  ( -15.72974639402176322, -15.80617190586768395, 19.37609039468568639 ) ) ;
#131455=CARTESIAN_POINT ( 'NONE',  ( 5.153800228976335163, 19.02544592524342804, 114.7905762719810241 ) ) ;
#131456=CARTESIAN_POINT ( 'NONE',  ( -16.51473224551069308, -9.474510206698971260, 81.66557627198103830 ) ) ;
#131457=CARTESIAN_POINT ( 'NONE',  ( -10.81492255796105439, 18.62759615963255655, 97.91775706135236135 ) ) ;
#131458=CARTESIAN_POINT ( 'NONE',  ( -19.02544592524342804, 5.153800228976336051, 81.04057627198103830 ) ) ;
#131459=CARTESIAN_POINT ( 'NONE',  ( 0.05219959533907565091, 21.53943276465977519, 39.99890960531436690 ) ) ;
#131460=CARTESIAN_POINT ( 'NONE',  ( 14.34966873604960469, 8.224510206698951720, 79.16557627198103830 ) ) ;
#131461=CARTESIAN_POINT ( 'NONE',  ( 0.05219959533909260263, 19.03943276465977164, 54.99890960531435979 ) ) ;
#131462=CARTESIAN_POINT ( 'NONE',  ( -4.483927247898539470, -16.52544592524342804, 112.2905762719810241 ) ) ;
#131464=CARTESIAN_POINT ( 'NONE',  ( -5.823673210054431948, 21.52544592524334988, 27.70942372801901854 ) ) ;
#131465=CARTESIAN_POINT ( 'NONE',  ( -0.05219959533937732626, 21.53943276465977519, 67.50109039468568994 ) ) ;
#131466=CARTESIAN_POINT ( 'NONE',  ( -19.02544592524342804, 5.153800228976336051, 46.04057627198101699 ) ) ;
#131467=CARTESIAN_POINT ( 'NONE',  ( 16.53943276465976808, 0.05219959533934440121, 71.25109039468568994 ) ) ;
#131468=CARTESIAN_POINT ( 'NONE',  ( -18.62759615963270932, 10.81492255796079327, 110.8322429386476955 ) ) ;
#131469=CARTESIAN_POINT ( 'NONE',  ( 5.719274019375991003, -21.55341960407610458, 112.7072429386476955 ) ) ;
#131470=CARTESIAN_POINT ( 'NONE',  ( -16.46253265017146816, -9.564922557961047289, 44.16775706135232582 ) ) ;
#131471=CARTESIAN_POINT ( 'NONE',  ( 0.05219959533909260263, 19.03943276465977164, 59.99890960531436690 ) ) ;
#131472=CARTESIAN_POINT ( 'NONE',  ( 19.03943276465977164, 0.05219959533936151252, 31.25109039468566863 ) ) ;
#131473=CARTESIAN_POINT ( 'NONE',  ( -18.67979575497193778, 10.72451020669871902, 68.33442372801900433 ) ) ;
#131474=CARTESIAN_POINT ( 'NONE',  ( 15.72974639402199770, -15.80617190586745480, 68.12390960531436690 ) ) ;
#131475=CARTESIAN_POINT ( 'NONE',  ( 4.379528057220339221, -16.55341960407611168, 32.70724293864770260 ) ) ;
#131476=CARTESIAN_POINT ( 'NONE',  ( 0.05219959533937995610, -21.53943276465977519, 85.00109039468568994 ) ) ;
#131477=CARTESIAN_POINT ( 'NONE',  ( -10.81492255796105439, 18.62759615963255655, 107.9177570613523471 ) ) ;
#131478=CARTESIAN_POINT ( 'NONE',  ( 4.483927247898545687, 16.52544592524342804, 54.79057627198104541 ) ) ;
#131479=CARTESIAN_POINT ( 'NONE',  ( -0.05219959533910754901, -16.53943276465976808, 102.4989096053143811 ) ) ;
#131480=CARTESIAN_POINT ( 'NONE',  ( -5.049401038297874678, -19.05341960407617918, 54.79275706135234003 ) ) ;
#131481=CARTESIAN_POINT ( 'NONE',  ( 8.224510206698953496, -14.34966873604960469, 22.91557627198102765 ) ) ;
#131482=CARTESIAN_POINT ( 'NONE',  ( -10.81492255796105439, 18.62759615963255655, 62.91775706135236135 ) ) ;
#131483=CARTESIAN_POINT ( 'NONE',  ( 16.46253265017160672, -9.564922557960803928, 73.33224293864769550 ) ) ;
#131484=CARTESIAN_POINT ( 'NONE',  ( -19.03943276465977164, -0.05219959533935918106, 33.75109039468566863 ) ) ;
#131485=CARTESIAN_POINT ( 'NONE',  ( 21.52544592524344225, -5.823673210054117533, 53.54057627198103120 ) ) ;
#131486=CARTESIAN_POINT ( 'NONE',  ( 10.81492255796106328, -18.62759615963255655, 40.41775706135234714 ) ) ;
#131487=CARTESIAN_POINT ( 'NONE',  ( 21.52544592524344225, -5.823673210054117533, 98.54057627198105251 ) ) ;
#131488=CARTESIAN_POINT ( 'NONE',  ( 0.05219959533936267826, -19.03943276465977164, 95.00109039468567573 ) ) ;
#131489=CARTESIAN_POINT ( 'NONE',  ( -14.29746914071037622, -8.314922557961029526, 69.16775706135234714 ) ) ;
#131491=CARTESIAN_POINT ( 'NONE',  ( 5.823673210054125526, 21.52544592524343514, 99.79057627198103830 ) ) ;
#131492=CARTESIAN_POINT ( 'NONE',  ( -14.34966873604960291, -8.224510206698953496, 86.66557627198102409 ) ) ;
#131494=CARTESIAN_POINT ( 'NONE',  ( -16.55341960407617563, 4.379528057220093196, 28.54275706135234358 ) ) ;
#131495=CARTESIAN_POINT ( 'NONE',  ( 18.62759615963271287, -10.81492255796078972, 48.33224293864770260 ) ) ;
#131496=CARTESIAN_POINT ( 'NONE',  ( -14.29746914071037622, -8.314922557961029526, 94.16775706135237556 ) ) ;
#131497=CARTESIAN_POINT ( 'NONE',  ( -16.51473224551069308, -9.474510206698971260, 21.66557627198102765 ) ) ;
#131498=CARTESIAN_POINT ( 'NONE',  ( 12.06949235617739724, 12.14591786802326823, 56.87609039468568994 ) ) ;
#131499=CARTESIAN_POINT ( 'NONE',  ( -15.80617190586768217, 15.72974639402176855, 28.12609039468568284 ) ) ;
#131500=CARTESIAN_POINT ( 'NONE',  ( 5.719274019375991003, -21.55341960407610458, 47.70724293864770260 ) ) ;
#131501=CARTESIAN_POINT ( 'NONE',  ( 4.483927247898790824, -16.52544592524335698, 85.20942372801901854 ) ) ;
#131502=CARTESIAN_POINT ( 'NONE',  ( 13.89961937509977652, -13.97604488694527269, 98.12390960531433848 ) ) ;
#131503=CARTESIAN_POINT ( 'NONE',  ( -10.81492255796105439, 18.62759615963255655, 72.91775706135234714 ) ) ;
#131504=CARTESIAN_POINT ( 'NONE',  ( 5.823673210054125526, 21.52544592524343514, 44.79057627198103120 ) ) ;
#131505=CARTESIAN_POINT ( 'NONE',  ( -15.72974639402197994, 15.80617190586746368, 25.62390960531435624 ) ) ;
#131507=CARTESIAN_POINT ( 'NONE',  ( 13.89961937509957401, 13.97604488694547697, 56.87609039468564731 ) ) ;
#131508=CARTESIAN_POINT ( 'NONE',  ( -16.52544592524335698, -4.483927247898792601, 63.95942372801901854 ) ) ;
#131509=CARTESIAN_POINT ( 'NONE',  ( -5.719274019375978568, 21.55341960407610458, 35.20724293864768839 ) ) ;
#131511=EDGE_CURVE ( 'NONE', #159561, #168063, #106491, .T. ) ;
#131512=CARTESIAN_POINT ( 'NONE',  ( -19.02544592524342804, 5.153800228976336051, 86.04057627198103830 ) ) ;
#131513=CARTESIAN_POINT ( 'NONE',  ( -12.14591786802309592, -12.06949235617757132, 21.87390960531436690 ) ) ;
#131514=CARTESIAN_POINT ( 'NONE',  ( -17.72560187377287022, -5.499999999999976019, 79.07814504131323474 ) ) ;
#131515=CARTESIAN_POINT ( 'NONE',  ( 0.05219959533910956823, 16.53943276465976808, 104.9989096053143669 ) ) ;
#131516=CARTESIAN_POINT ( 'NONE',  ( -10.81492255796078084, -18.62759615963271287, 42.08224293864769550 ) ) ;
#131517=CARTESIAN_POINT ( 'NONE',  ( -13.89961937509977652, 13.97604488694528158, 50.62390960531435979 ) ) ;
#131518=CARTESIAN_POINT ( 'NONE',  ( -12.14591786802326823, 12.06949235617739902, 78.12609039468570415 ) ) ;
#131519=CARTESIAN_POINT ( 'NONE',  ( -0.05219959533937732626, 21.53943276465977519, 27.50109039468567929 ) ) ;
#131520=CARTESIAN_POINT ( 'NONE',  ( 16.46253265017146816, 9.564922557961045513, 86.66775706135233293 ) ) ;
#131521=CARTESIAN_POINT ( 'NONE',  ( 8.224510206698953496, -14.34966873604960469, 87.91557627198103830 ) ) ;
#131522=CARTESIAN_POINT ( 'NONE',  ( 19.03943276465977164, -0.05219959533909143690, 58.74890960531435979 ) ) ;
#131524=CARTESIAN_POINT ( 'NONE',  ( 5.049401038298161559, -19.05341960407611168, 27.70724293864769550 ) ) ;
#131525=CARTESIAN_POINT ( 'NONE',  ( 21.52544592524334988, 5.823673210054432836, 101.4594237280190185 ) ) ;
#131526=CARTESIAN_POINT ( 'NONE',  ( 16.46253265017160672, -9.564922557960803928, 83.33224293864768129 ) ) ;
#131528=CARTESIAN_POINT ( 'NONE',  ( -14.29746914071037622, -8.314922557961029526, 69.16775706135234714 ) ) ;
#131529=CARTESIAN_POINT ( 'NONE',  ( -21.52544592524334988, -5.823673210054445271, 93.95942372801903275 ) ) ;
#131530=CARTESIAN_POINT ( 'NONE',  ( -10.72451020669898014, 18.67979575497178502, 45.41557627198103830 ) ) ;
#131531=CARTESIAN_POINT ( 'NONE',  ( -8.224510206698735004, -14.34966873604973081, 79.58442372801903275 ) ) ;
#131532=CARTESIAN_POINT ( 'NONE',  ( 5.049401038297881783, 19.05341960407617563, 47.29275706135231161 ) ) ;
#131533=CARTESIAN_POINT ( 'NONE',  ( 13.97604488694548053, -13.89961937509957401, 60.62609039468564731 ) ) ;
#131534=ORIENTED_EDGE ( 'NONE', *, *, #27507, .F. ) ;
#131535=CARTESIAN_POINT ( 'NONE',  ( -0.05219959533937732626, 21.53943276465977519, 67.50109039468568994 ) ) ;
#131536=CARTESIAN_POINT ( 'NONE',  ( -9.564922557960796823, -16.46253265017161027, 62.08224293864769550 ) ) ;
#131537=CARTESIAN_POINT ( 'NONE',  ( -18.22780087662123805, 5.499999999999981348, 91.01763182126894947 ) ) ;
#131538=CARTESIAN_POINT ( 'NONE',  ( -13.97604488694547697, 13.89961937509957934, 63.12609039468566152 ) ) ;
#131539=DIRECTION ( 'NONE',  ( 0.000000000000000000, 0.000000000000000000, -1.000000000000000000 ) ) ;
#131540=CARTESIAN_POINT ( 'NONE',  ( -16.46253265017160317, 9.564922557960807481, 90.83224293864769550 ) ) ;
#131541=CARTESIAN_POINT ( 'NONE',  ( -12.14591786802309592, -12.06949235617757132, 46.87390960531435979 ) ) ;
#131542=CARTESIAN_POINT ( 'NONE',  ( 21.55341960407610458, 5.719274019375980345, 48.95724293864770971 ) ) ;
#131544=CARTESIAN_POINT ( 'NONE',  ( 21.53943276465977519, 0.05219959533937863772, 111.2510903946856899 ) ) ;
#131545=CARTESIAN_POINT ( 'NONE',  ( -17.50000000000001421, -5.622605283950846911, 81.31207310596113302 ) ) ;
#131546=CARTESIAN_POINT ( 'NONE',  ( -9.474510206698964154, 16.51473224551069663, 55.41557627198103120 ) ) ;
#131547=CARTESIAN_POINT ( 'NONE',  ( 16.46253265017160672, -9.564922557960803928, 28.33224293864769550 ) ) ;
#131550=CARTESIAN_POINT ( 'NONE',  ( -12.14591786802326823, 12.06949235617739902, 68.12609039468567573 ) ) ;
#131551=CARTESIAN_POINT ( 'NONE',  ( -21.53943276465977519, 0.05219959533907696930, 86.24890960531436690 ) ) ;
#131552=CARTESIAN_POINT ( 'NONE',  ( 4.483927247898545687, 16.52544592524342804, 59.79057627198103120 ) ) ;
#131553=CARTESIAN_POINT ( 'NONE',  ( -13.89961937509977652, 13.97604488694528158, 45.62390960531433848 ) ) ;
#131554=CARTESIAN_POINT ( 'NONE',  ( -19.02544592524342804, 5.153800228976336051, 116.0405762719810383 ) ) ;
#131555=CARTESIAN_POINT ( 'NONE',  ( -5.719274019375665041, -21.55341960407619695, 34.79275706135235424 ) ) ;
#131556=CARTESIAN_POINT ( 'NONE',  ( -9.474510206698720793, -16.51473224551083518, 54.58442372801899722 ) ) ;
#131557=CARTESIAN_POINT ( 'NONE',  ( -0.05219959533909027116, -19.03943276465977164, 37.49890960531436690 ) ) ;
#131558=CARTESIAN_POINT ( 'NONE',  ( -21.55341960407619339, 5.719274019375674811, 93.54275706135234714 ) ) ;
#131561=CARTESIAN_POINT ( 'NONE',  ( 12.14591786802309770, 12.06949235617756955, 44.37390960531435979 ) ) ;
#131563=CARTESIAN_POINT ( 'NONE',  ( -5.823673210054116645, -21.52544592524344225, 42.29057627198103120 ) ) ;
#131565=CARTESIAN_POINT ( 'NONE',  ( -19.02544592524342804, 5.153800228976336051, 91.04057627198100988 ) ) ;
#131566=CARTESIAN_POINT ( 'NONE',  ( -4.379528057220328563, 16.55341960407611168, 85.20724293864770971 ) ) ;
#131567=CARTESIAN_POINT ( 'NONE',  ( 14.29746914071037800, 8.314922557961029526, 21.66775706135235069 ) ) ;
#131568=CARTESIAN_POINT ( 'NONE',  ( 14.29746914071037800, 8.314922557961029526, 111.6677570613523613 ) ) ;
#131570=CARTESIAN_POINT ( 'NONE',  ( 16.51473224551069308, 9.474510206698969483, 44.16557627198103120 ) ) ;
#131571=CARTESIAN_POINT ( 'NONE',  ( -19.03943276465977164, 0.05219959533909376836, 91.24890960531436690 ) ) ;
#131572=CARTESIAN_POINT ( 'NONE',  ( -10.72451020669898014, 18.67979575497178502, 85.41557627198102409 ) ) ;
#131573=CARTESIAN_POINT ( 'NONE',  ( -12.14591786802309592, -12.06949235617757132, 31.87390960531435979 ) ) ;
#131574=CARTESIAN_POINT ( 'NONE',  ( 9.564922557960805705, 16.46253265017160317, 99.58224293864770971 ) ) ;
#131575=CARTESIAN_POINT ( 'NONE',  ( -5.049401038297874678, -19.05341960407617918, 74.79275706135231871 ) ) ;
#131576=CARTESIAN_POINT ( 'NONE',  ( -21.53943276465977519, -0.05219959533937600094, 103.7510903946857042 ) ) ;
#131577=CARTESIAN_POINT ( 'NONE',  ( -15.72974639402197994, 15.80617190586746368, 95.62390960531436690 ) ) ;
#131578=CARTESIAN_POINT ( 'NONE',  ( -0.05219959533907301413, -21.53943276465977519, 37.49890960531436690 ) ) ;
#131579=CARTESIAN_POINT ( 'NONE',  ( -5.153800228976328057, -19.02544592524343514, 67.29057627198102409 ) ) ;
#131580=CARTESIAN_POINT ( 'NONE',  ( -14.29746914071037622, -8.314922557961029526, 109.1677570613523613 ) ) ;
#131581=CARTESIAN_POINT ( 'NONE',  ( -16.51473224551069308, -9.474510206698971260, 71.66557627198102409 ) ) ;
#131584=CARTESIAN_POINT ( 'NONE',  ( -9.564922557961040184, 16.46253265017147172, 22.91775706135233648 ) ) ;
#131585=CARTESIAN_POINT ( 'NONE',  ( -14.29746914071049879, 8.314922557960819915, 85.83224293864768129 ) ) ;
#131586=CARTESIAN_POINT ( 'NONE',  ( 10.72451020669871369, 18.67979575497193778, 22.08442372801901143 ) ) ;
#131588=CARTESIAN_POINT ( 'NONE',  ( 21.53943276465977519, -0.05219959533907433946, 68.74890960531435269 ) ) ;
#131589=CARTESIAN_POINT ( 'NONE',  ( 4.379528057220092307, 16.55341960407617563, 97.29275706135234714 ) ) ;
#131590=CARTESIAN_POINT ( 'NONE',  ( 19.02544592524343514, -5.153800228976328945, 23.54057627198102054 ) ) ;
#131591=CARTESIAN_POINT ( 'NONE',  ( -0.05219959533909027116, -19.03943276465977164, 72.49890960531435269 ) ) ;
#131593=CARTESIAN_POINT ( 'NONE',  ( -16.55341960407611168, -4.379528057220339221, 36.45724293864768839 ) ) ;
#131594=CARTESIAN_POINT ( 'NONE',  ( 18.62759615963255655, 10.81492255796105972, 66.66775706135234714 ) ) ;
#131595=CARTESIAN_POINT ( 'NONE',  ( -13.97604488694527625, -13.89961937509977652, 106.8739096053143669 ) ) ;
#131596=CARTESIAN_POINT ( 'NONE',  ( 10.81492255796106328, -18.62759615963255655, 90.41775706135236135 ) ) ;
#131597=CARTESIAN_POINT ( 'NONE',  ( -19.02544592524342804, 5.153800228976336051, 41.04057627198103120 ) ) ;
#131598=CARTESIAN_POINT ( 'NONE',  ( 16.46253265017160672, -9.564922557960803928, 48.33224293864769550 ) ) ;
#131599=ORIENTED_EDGE ( 'NONE', *, *, #137500, .T. ) ;
#131600=CARTESIAN_POINT ( 'NONE',  ( -21.52544592524334988, -5.823673210054445271, 98.95942372801903275 ) ) ;
#131601=CARTESIAN_POINT ( 'NONE',  ( -0.05219959533934338120, 16.53943276465976808, 62.50109039468568284 ) ) ;
#131602=CARTESIAN_POINT ( 'NONE',  ( -15.80617190586768217, 15.72974639402176855, 88.12609039468570415 ) ) ;
#131603=CARTESIAN_POINT ( 'NONE',  ( -5.049401038298153566, 19.05341960407611168, 115.2072429386477097 ) ) ;
#131604=CARTESIAN_POINT ( 'NONE',  ( 19.03943276465977164, 0.05219959533936151252, 91.25109039468566152 ) ) ;
#131605=CARTESIAN_POINT ( 'NONE',  ( -21.52544592524334988, -5.823673210054445271, 58.95942372801902565 ) ) ;
#131606=CARTESIAN_POINT ( 'NONE',  ( 0.05219959533934541429, -16.53943276465976808, 40.00109039468567573 ) ) ;
#131607=CARTESIAN_POINT ( 'NONE',  ( -21.55341960407610458, -5.719274019375992779, 91.45724293864769550 ) ) ;
#131608=CARTESIAN_POINT ( 'NONE',  ( 19.03943276465977164, 0.05219959533936151252, 86.25109039468567573 ) ) ;
#131609=CARTESIAN_POINT ( 'NONE',  ( 0.05219959533909260263, 19.03943276465977164, 59.99890960531436690 ) ) ;
#131610=CARTESIAN_POINT ( 'NONE',  ( -13.89961937509957401, -13.97604488694547875, 94.37609039468566152 ) ) ;
#131612=CARTESIAN_POINT ( 'NONE',  ( -13.97604488694547697, 13.89961937509957934, 103.1260903946856473 ) ) ;
#131613=CARTESIAN_POINT ( 'NONE',  ( -12.14591786802309592, -12.06949235617757132, 51.87390960531437401 ) ) ;
#131614=CARTESIAN_POINT ( 'NONE',  ( -16.46253265017146816, -9.564922557961047289, 79.16775706135234714 ) ) ;
#131615=CARTESIAN_POINT ( 'NONE',  ( 8.224510206698742110, 14.34966873604972548, 67.08442372801901854 ) ) ;
#131616=CARTESIAN_POINT ( 'NONE',  ( -16.46253265017146816, -9.564922557961047289, 44.16775706135232582 ) ) ;
#131617=CARTESIAN_POINT ( 'NONE',  ( -9.564922557960796823, -16.46253265017161027, 42.08224293864769550 ) ) ;
#131618=CARTESIAN_POINT ( 'NONE',  ( -19.05341960407611168, -5.049401038298163336, 51.45724293864770260 ) ) ;
#131619=CARTESIAN_POINT ( 'NONE',  ( 16.52544592524335698, 4.483927247898782831, 61.45942372801901854 ) ) ;
#131622=CARTESIAN_POINT ( 'NONE',  ( -5.049401038298153566, 19.05341960407611168, 105.2072429386476671 ) ) ;
#131624=CARTESIAN_POINT ( 'NONE',  ( -9.564922557960796823, -16.46253265017161027, 22.08224293864768839 ) ) ;
#131626=CARTESIAN_POINT ( 'NONE',  ( -19.05341960407617563, 5.049401038297882671, 98.54275706135233293 ) ) ;
#131627=CARTESIAN_POINT ( 'NONE',  ( -18.67979575497178146, -10.72451020669898902, 36.66557627198103120 ) ) ;
#131628=CARTESIAN_POINT ( 'NONE',  ( -13.97604488694547697, 13.89961937509957934, 28.12609039468565797 ) ) ;
#131629=CARTESIAN_POINT ( 'NONE',  ( 8.224510206698742110, 14.34966873604972548, 22.08442372801901143 ) ) ;
#131630=CARTESIAN_POINT ( 'NONE',  ( 19.02544592524343514, -5.153800228976328945, 33.54057627198102409 ) ) ;
#131631=CARTESIAN_POINT ( 'NONE',  ( 5.153800228976335163, 19.02544592524342804, 44.79057627198103830 ) ) ;
#131632=CARTESIAN_POINT ( 'NONE',  ( 5.823673210054125526, 21.52544592524343514, 69.79057627198102409 ) ) ;
#131633=CARTESIAN_POINT ( 'NONE',  ( -19.05341960407611168, -5.049401038298163336, 101.4572429386476955 ) ) ;
#131634=CARTESIAN_POINT ( 'NONE',  ( 16.51473224551069308, 9.474510206698969483, 34.16557627198102409 ) ) ;
#131636=CARTESIAN_POINT ( 'NONE',  ( 0.05219959533936267826, -19.03943276465977164, 90.00109039468567573 ) ) ;
#131637=CARTESIAN_POINT ( 'NONE',  ( 4.379528057220339221, -16.55341960407611168, 52.70724293864769550 ) ) ;
#131639=CARTESIAN_POINT ( 'NONE',  ( 10.72451020669898902, -18.67979575497178502, 42.91557627198103120 ) ) ;
#131640=CARTESIAN_POINT ( 'NONE',  ( -5.823673210054431948, 21.52544592524334988, 107.7094237280190328 ) ) ;
#131642=CARTESIAN_POINT ( 'NONE',  ( -18.62759615963270932, 10.81492255796079327, 95.83224293864770971 ) ) ;
#131643=CARTESIAN_POINT ( 'NONE',  ( 21.53943276465977519, 0.05219959533937863772, 66.25109039468567573 ) ) ;
#131644=CARTESIAN_POINT ( 'NONE',  ( -0.05219959533937732626, 21.53943276465977519, 72.50109039468568994 ) ) ;
#131645=CARTESIAN_POINT ( 'NONE',  ( 9.474510206698971260, -16.51473224551069308, 112.9155762719810383 ) ) ;
#131646=CARTESIAN_POINT ( 'NONE',  ( -16.55341960407617563, 4.379528057220093196, 108.5427570613523756 ) ) ;
#131647=CARTESIAN_POINT ( 'NONE',  ( 21.52544592524334988, 5.823673210054432836, 66.45942372801903275 ) ) ;
#131648=CARTESIAN_POINT ( 'NONE',  ( 9.474510206698971260, -16.51473224551069308, 62.91557627198102409 ) ) ;
#131649=CARTESIAN_POINT ( 'NONE',  ( 13.89961937509957401, 13.97604488694547697, 31.87609039468566863 ) ) ;
#131650=CARTESIAN_POINT ( 'NONE',  ( -15.72974639402176322, -15.80617190586768395, 29.37609039468568284 ) ) ;
#131651=CARTESIAN_POINT ( 'NONE',  ( 19.05341960407611168, 5.049401038298154454, 68.95724293864769550 ) ) ;
#131652=CARTESIAN_POINT ( 'NONE',  ( -4.379528057220328563, 16.55341960407611168, 85.20724293864770971 ) ) ;
#131653=CARTESIAN_POINT ( 'NONE',  ( -14.34966873604960291, -8.224510206698953496, 41.66557627198103120 ) ) ;
#131654=CARTESIAN_POINT ( 'NONE',  ( -18.67979575497178146, -10.72451020669898902, 56.66557627198103830 ) ) ;
#131655=CARTESIAN_POINT ( 'NONE',  ( -0.05219959533909027116, -19.03943276465977164, 62.49890960531435979 ) ) ;
#131656=CARTESIAN_POINT ( 'NONE',  ( -5.823673210054116645, -21.52544592524344225, 67.29057627198103830 ) ) ;
#131657=CARTESIAN_POINT ( 'NONE',  ( 19.03943276465977164, 0.05219959533936151252, 66.25109039468567573 ) ) ;
#131658=CARTESIAN_POINT ( 'NONE',  ( 13.89961937509957579, 13.97604488694547520, 26.87609039468566507 ) ) ;
#131659=CARTESIAN_POINT ( 'NONE',  ( -0.05219959533910754901, -16.53943276465976808, 57.49890960531435979 ) ) ;
#131660=CARTESIAN_POINT ( 'NONE',  ( -21.53943276465977519, 0.05219959533907696930, 36.24890960531435979 ) ) ;
#131663=CARTESIAN_POINT ( 'NONE',  ( 12.06949235617739724, 12.14591786802326823, 81.87609039468568994 ) ) ;
#131665=CARTESIAN_POINT ( 'NONE',  ( -19.05341960407617563, 5.049401038297882671, 93.54275706135234714 ) ) ;
#131666=CARTESIAN_POINT ( 'NONE',  ( -16.52544592524342804, 4.483927247898546575, 61.04057627198103120 ) ) ;
#131668=CARTESIAN_POINT ( 'NONE',  ( -5.153800228976328057, -19.02544592524343514, 52.29057627198100988 ) ) ;
#131669=CARTESIAN_POINT ( 'NONE',  ( 16.53943276465976808, -0.05219959533910856209, 43.74890960531435979 ) ) ;
#131671=CARTESIAN_POINT ( 'NONE',  ( -9.564922557960796823, -16.46253265017161027, 87.08224293864769550 ) ) ;
#131672=CARTESIAN_POINT ( 'NONE',  ( -13.97604488694527625, -13.89961937509977652, 46.87390960531435979 ) ) ;
#131673=CARTESIAN_POINT ( 'NONE',  ( 10.72451020669871369, 18.67979575497193778, 62.08442372801901143 ) ) ;
#131674=CARTESIAN_POINT ( 'NONE',  ( -19.03943276465977164, 0.05219959533909376836, 66.24890960531436690 ) ) ;
#131675=CARTESIAN_POINT ( 'NONE',  ( -19.03943276465977164, 0.05219959533909376836, 21.24890960531436335 ) ) ;
#131676=CARTESIAN_POINT ( 'NONE',  ( 19.02544592524343514, -5.153800228976328945, 78.54057627198099567 ) ) ;
#131677=CARTESIAN_POINT ( 'NONE',  ( -5.823673210054116645, -21.52544592524344225, 47.29057627198103120 ) ) ;
#131678=CARTESIAN_POINT ( 'NONE',  ( -13.97604488694527625, -13.89961937509977652, 51.87390960531436690 ) ) ;
#131679=CARTESIAN_POINT ( 'NONE',  ( 21.55341960407610458, 5.719274019375980345, 58.95724293864770971 ) ) ;
#131680=CARTESIAN_POINT ( 'NONE',  ( -19.05341960407617563, 5.049401038297882671, 78.54275706135233293 ) ) ;
#131681=CARTESIAN_POINT ( 'NONE',  ( -16.52544592524335698, -4.483927247898792601, 103.9594237280190185 ) ) ;
#131682=CARTESIAN_POINT ( 'NONE',  ( -5.153800228976607833, 19.02544592524334988, 27.70942372801899722 ) ) ;
#131683=CARTESIAN_POINT ( 'NONE',  ( 4.483927247898790824, -16.52544592524335698, 65.20942372801901854 ) ) ;
#131684=CARTESIAN_POINT ( 'NONE',  ( 14.34966873604972726, -8.224510206698740333, 85.83442372801901854 ) ) ;
#131685=CARTESIAN_POINT ( 'NONE',  ( -17.97182807773871716, 5.500000000000050626, 68.53038844047289047 ) ) ;
#131686=CARTESIAN_POINT ( 'NONE',  ( 0.05219959533934541429, -16.53943276465976808, 65.00109039468568994 ) ) ;
#131687=CARTESIAN_POINT ( 'NONE',  ( -15.72974639402197994, 15.80617190586746368, 30.62390960531436335 ) ) ;
#131688=CARTESIAN_POINT ( 'NONE',  ( 19.02544592524343514, -5.153800228976328945, 38.54057627198103120 ) ) ;
#131689=CARTESIAN_POINT ( 'NONE',  ( -16.55341960407617563, 4.379528057220093196, 38.54275706135234714 ) ) ;
#131690=CARTESIAN_POINT ( 'NONE',  ( 19.03943276465977164, -0.05219959533909143690, 48.74890960531435979 ) ) ;
#131691=CARTESIAN_POINT ( 'NONE',  ( 15.80617190586769283, -15.72974639402175789, 40.62609039468567573 ) ) ;
#131692=CARTESIAN_POINT ( 'NONE',  ( 4.379528057220092307, 16.55341960407617563, 32.29275706135235424 ) ) ;
#131693=CARTESIAN_POINT ( 'NONE',  ( 12.14591786802327356, -12.06949235617739191, 100.6260903946857184 ) ) ;
#131695=CARTESIAN_POINT ( 'NONE',  ( -0.05219959533936034679, 19.03943276465977164, 22.50109039468566152 ) ) ;
#131696=CARTESIAN_POINT ( 'NONE',  ( 19.02544592524334988, 5.153800228976608722, 106.4594237280190185 ) ) ;
#131697=CARTESIAN_POINT ( 'NONE',  ( -9.474510206698720793, -16.51473224551083518, 64.58442372801900433 ) ) ;
#131698=CARTESIAN_POINT ( 'NONE',  ( -4.483927247898539470, -16.52544592524342804, 72.29057627198102409 ) ) ;
#131699=CARTESIAN_POINT ( 'NONE',  ( -9.564922557960796823, -16.46253265017161027, 22.08224293864768839 ) ) ;
#131700=CARTESIAN_POINT ( 'NONE',  ( 16.46253265017146816, 9.564922557961045513, 61.66775706135234003 ) ) ;
#131701=DIRECTION ( 'NONE',  ( 0.000000000000000000, 1.000000000000000000, -4.336808689942013299E-16 ) ) ;
#131702=CARTESIAN_POINT ( 'NONE',  ( -21.55341960407619339, 5.719274019375674811, 58.54275706135235424 ) ) ;
#131703=CARTESIAN_POINT ( 'NONE',  ( 0.05219959533934541429, -16.53943276465976808, 40.00109039468567573 ) ) ;
#131705=CARTESIAN_POINT ( 'NONE',  ( -10.81492255796078084, -18.62759615963271287, 27.08224293864769550 ) ) ;
#131706=CARTESIAN_POINT ( 'NONE',  ( -9.564922557961040184, 16.46253265017147172, 102.9177570613523329 ) ) ;
#131709=CARTESIAN_POINT ( 'NONE',  ( -9.564922557960796823, -16.46253265017161027, 27.08224293864769550 ) ) ;
#131710=CARTESIAN_POINT ( 'NONE',  ( -21.52544592524334988, -5.823673210054445271, 103.9594237280190185 ) ) ;
#131711=CARTESIAN_POINT ( 'NONE',  ( 5.049401038298161559, -19.05341960407611168, 52.70724293864767418 ) ) ;
#131712=CARTESIAN_POINT ( 'NONE',  ( -21.53943276465977519, -0.05219959533937600094, 58.75109039468568994 ) ) ;
#131713=CARTESIAN_POINT ( 'NONE',  ( 21.53943276465977519, 0.05219959533937863772, 96.25109039468568994 ) ) ;
#131714=CARTESIAN_POINT ( 'NONE',  ( 12.06949235617757843, -12.14591786802309237, 23.12390960531436335 ) ) ;
#131715=CARTESIAN_POINT ( 'NONE',  ( -9.474510206698964154, 16.51473224551069663, 35.41557627198102409 ) ) ;
#131716=CARTESIAN_POINT ( 'NONE',  ( -19.02544592524342804, 5.153800228976336051, 76.04057627198102409 ) ) ;
#131717=CARTESIAN_POINT ( 'NONE',  ( -10.81492255796105439, 18.62759615963255655, 57.91775706135234714 ) ) ;
#131718=CARTESIAN_POINT ( 'NONE',  ( 13.89961937509977652, -13.97604488694527269, 43.12390960531434558 ) ) ;
#131719=CARTESIAN_POINT ( 'NONE',  ( 10.72451020669871369, 18.67979575497193778, 57.08442372801901854 ) ) ;
#131720=CARTESIAN_POINT ( 'NONE',  ( -19.05341960407617563, 5.049401038297882671, 78.54275706135233293 ) ) ;
#131721=CARTESIAN_POINT ( 'NONE',  ( 19.02544592524343514, -5.153800228976328945, 108.5405762719810383 ) ) ;
#131722=CARTESIAN_POINT ( 'NONE',  ( -19.02544592524342804, 5.153800228976336051, 26.04057627198103120 ) ) ;
#131723=CARTESIAN_POINT ( 'NONE',  ( -18.67979575497178146, -10.72451020669898902, 111.6655762719810525 ) ) ;
#131724=CARTESIAN_POINT ( 'NONE',  ( 16.51473224551083163, -9.474510206698727899, 40.83442372801900433 ) ) ;
#131725=CARTESIAN_POINT ( 'NONE',  ( -12.14591786802309592, -12.06949235617757132, 96.87390960531436690 ) ) ;
#131726=CARTESIAN_POINT ( 'NONE',  ( 9.564922557960805705, 16.46253265017160317, 54.58224293864769550 ) ) ;
#131727=CARTESIAN_POINT ( 'NONE',  ( 0.05219959533936267826, -19.03943276465977164, 100.0010903946856757 ) ) ;
#131728=CARTESIAN_POINT ( 'NONE',  ( -8.314922557960811034, -14.29746914071050412, 62.08224293864769550 ) ) ;
#131729=CARTESIAN_POINT ( 'NONE',  ( -5.823673210054431948, 21.52544592524334988, 112.7094237280190328 ) ) ;
#131730=CARTESIAN_POINT ( 'NONE',  ( -5.049401038298153566, 19.05341960407611168, 100.2072429386476955 ) ) ;
#131731=CARTESIAN_POINT ( 'NONE',  ( 9.474510206698729675, 16.51473224551082808, 92.08442372801900433 ) ) ;
#131732=CARTESIAN_POINT ( 'NONE',  ( -5.719274019375978568, 21.55341960407610458, 90.20724293864770971 ) ) ;
#131733=CARTESIAN_POINT ( 'NONE',  ( -5.823673210054431948, 21.52544592524334988, 42.70942372801901854 ) ) ;
#131734=CARTESIAN_POINT ( 'NONE',  ( -16.55341960407617563, 4.379528057220093196, 43.54275706135235424 ) ) ;
#131735=CARTESIAN_POINT ( 'NONE',  ( -12.14591786802326823, 12.06949235617739902, 108.1260903946856757 ) ) ;
#131736=CARTESIAN_POINT ( 'NONE',  ( 0.05219959533934541429, -16.53943276465976808, 40.00109039468567573 ) ) ;
#131737=CARTESIAN_POINT ( 'NONE',  ( -5.823673210054431948, 21.52544592524334988, 42.70942372801901854 ) ) ;
#131738=CARTESIAN_POINT ( 'NONE',  ( -21.53943276465977519, 0.05219959533907696930, 46.24890960531435979 ) ) ;
#131739=CARTESIAN_POINT ( 'NONE',  ( -0.05219959533909027116, -19.03943276465977164, 32.49890960531435979 ) ) ;
#131741=CARTESIAN_POINT ( 'NONE',  ( -12.14591786802326823, 12.06949235617739902, 68.12609039468567573 ) ) ;
#131742=CARTESIAN_POINT ( 'NONE',  ( -5.823673210054116645, -21.52544592524344225, 92.29057627198103830 ) ) ;
#131743=CARTESIAN_POINT ( 'NONE',  ( 16.52544592524342804, -4.483927247898539470, 43.54057627198103830 ) ) ;
#131744=CARTESIAN_POINT ( 'NONE',  ( 12.06949235617739724, 12.14591786802326823, 56.87609039468568994 ) ) ;
#131745=CARTESIAN_POINT ( 'NONE',  ( -5.153800228976328057, -19.02544592524343514, 62.29057627198100988 ) ) ;
#131746=CARTESIAN_POINT ( 'NONE',  ( 9.564922557961047289, -16.46253265017146816, 95.41775706135233293 ) ) ;
#131747=CARTESIAN_POINT ( 'NONE',  ( -10.72451020669898014, 18.67979575497178502, 90.41557627198103830 ) ) ;
#131748=CARTESIAN_POINT ( 'NONE',  ( -16.52544592524342804, 4.483927247898546575, 31.04057627198102409 ) ) ;
#131749=ORIENTED_EDGE ( 'NONE', *, *, #6444, .F. ) ;
#131751=CARTESIAN_POINT ( 'NONE',  ( 21.53943276465977519, -0.05219959533907433946, 68.74890960531435269 ) ) ;
#131753=CARTESIAN_POINT ( 'NONE',  ( -16.53943276465976808, -0.05219959533934237506, 108.7510903946857042 ) ) ;
#131755=CARTESIAN_POINT ( 'NONE',  ( 17.50000000000000711, -4.703611302593163401, 103.1505057453771030 ) ) ;
#131756=CARTESIAN_POINT ( 'NONE',  ( 15.80617190586746368, 15.72974639402197994, 89.37390960531435269 ) ) ;
#131757=CARTESIAN_POINT ( 'NONE',  ( 15.80617190586746368, 15.72974639402197994, 114.3739096053143527 ) ) ;
#131758=CARTESIAN_POINT ( 'NONE',  ( 4.483927247898545687, 16.52544592524342804, 24.79057627198103120 ) ) ;
#131759=CARTESIAN_POINT ( 'NONE',  ( -14.34966873604972548, 8.224510206698743886, 28.33442372801902209 ) ) ;
#131760=CARTESIAN_POINT ( 'NONE',  ( 19.03943276465977164, -0.05219959533909143690, 38.74890960531436690 ) ) ;
#131761=CARTESIAN_POINT ( 'NONE',  ( 19.05341960407611168, 5.049401038298154454, 68.95724293864769550 ) ) ;
#131763=CARTESIAN_POINT ( 'NONE',  ( 15.72974639402199770, -15.80617190586745480, 28.12390960531435979 ) ) ;
#131765=CARTESIAN_POINT ( 'NONE',  ( 5.049401038297881783, 19.05341960407617563, 102.2927570613523045 ) ) ;
#131766=CARTESIAN_POINT ( 'NONE',  ( -13.97604488694547697, 13.89961937509957934, 43.12609039468566152 ) ) ;
#131767=CARTESIAN_POINT ( 'NONE',  ( -10.72451020669898014, 18.67979575497178502, 85.41557627198102409 ) ) ;
#131768=CARTESIAN_POINT ( 'NONE',  ( -12.06949235617739369, -12.14591786802326823, 109.3760903946857042 ) ) ;
#131769=CARTESIAN_POINT ( 'NONE',  ( -18.67979575497178146, -10.72451020669898902, 51.66557627198102409 ) ) ;
#131770=CARTESIAN_POINT ( 'NONE',  ( -5.719274019375978568, 21.55341960407610458, 80.20724293864769550 ) ) ;
#131771=CARTESIAN_POINT ( 'NONE',  ( 19.02544592524334988, 5.153800228976608722, 101.4594237280189759 ) ) ;
#131772=CARTESIAN_POINT ( 'NONE',  ( 19.03943276465977164, -0.05219959533909143690, 98.74890960531436690 ) ) ;
#131773=CARTESIAN_POINT ( 'NONE',  ( -18.62759615963255300, -10.81492255796106328, 74.16775706135231871 ) ) ;
#131774=CARTESIAN_POINT ( 'NONE',  ( 5.153800228976335163, 19.02544592524342804, 79.79057627198102409 ) ) ;
#131775=CARTESIAN_POINT ( 'NONE',  ( -0.05219959533910754901, -16.53943276465976808, 97.49890960531436690 ) ) ;
#131777=CARTESIAN_POINT ( 'NONE',  ( 19.03943276465977164, -0.05219959533909143690, 68.74890960531436690 ) ) ;
#131778=CARTESIAN_POINT ( 'NONE',  ( 4.379528057220339221, -16.55341960407611168, 97.70724293864772392 ) ) ;
#131779=ORIENTED_EDGE ( 'NONE', *, *, #27507, .T. ) ;
#131780=CARTESIAN_POINT ( 'NONE',  ( 5.153800228976615827, -19.02544592524334988, 90.20942372801900433 ) ) ;
#131783=CARTESIAN_POINT ( 'NONE',  ( 19.05341960407611168, 5.049401038298154454, 63.95724293864769550 ) ) ;
#131785=CARTESIAN_POINT ( 'NONE',  ( -21.53943276465977519, -0.05219959533937600094, 83.75109039468568994 ) ) ;
#131786=CARTESIAN_POINT ( 'NONE',  ( 16.51473224551069308, 9.474510206698969483, 104.1655762719810241 ) ) ;
#131787=CARTESIAN_POINT ( 'NONE',  ( -12.14591786802326823, 12.06949235617739902, 83.12609039468568994 ) ) ;
#131789=CARTESIAN_POINT ( 'NONE',  ( 19.03943276465977164, 0.05219959533936151252, 56.25109039468566863 ) ) ;
#131790=CARTESIAN_POINT ( 'NONE',  ( -10.72451020669870658, -18.67979575497194134, 99.58442372801900433 ) ) ;
#131793=CARTESIAN_POINT ( 'NONE',  ( 14.34966873604972726, -8.224510206698740333, 105.8344237280190328 ) ) ;
#131794=ADVANCED_FACE ( 'NONE', ( #74639 ), #82738, .T. ) ;
#131796=CARTESIAN_POINT ( 'NONE',  ( -4.379528057220086978, -16.55341960407618274, 94.79275706135234714 ) ) ;
#131798=CARTESIAN_POINT ( 'NONE',  ( -16.52544592524335698, -4.483927247898792601, 73.95942372801901854 ) ) ;
#131800=CARTESIAN_POINT ( 'NONE',  ( 21.55341960407619695, -5.719274019375665929, 81.04275706135236135 ) ) ;
#131801=CARTESIAN_POINT ( 'NONE',  ( 0.05219959533936267826, -19.03943276465977164, 85.00109039468567573 ) ) ;
#131802=CARTESIAN_POINT ( 'NONE',  ( 16.51473224551083163, -9.474510206698727899, 45.83442372801900433 ) ) ;
#131803=CARTESIAN_POINT ( 'NONE',  ( 9.474510206698971260, -16.51473224551069308, 67.91557627198102409 ) ) ;
#131804=CARTESIAN_POINT ( 'NONE',  ( -13.97604488694527625, -13.89961937509977652, 61.87390960531435979 ) ) ;
#131806=CARTESIAN_POINT ( 'NONE',  ( -21.52544592524343514, 5.823673210054127303, 76.04057627198102409 ) ) ;
#131807=CARTESIAN_POINT ( 'NONE',  ( -21.52544592524343514, 5.823673210054127303, 41.04057627198103120 ) ) ;
#131808=CARTESIAN_POINT ( 'NONE',  ( 9.474510206698971260, -16.51473224551069308, 27.91557627198103120 ) ) ;
#131809=CARTESIAN_POINT ( 'NONE',  ( -4.379528057220086978, -16.55341960407618274, 64.79275706135234714 ) ) ;
#131811=CARTESIAN_POINT ( 'NONE',  ( 5.823673210054444382, -21.52544592524334988, 30.20942372801902565 ) ) ;
#131812=CARTESIAN_POINT ( 'NONE',  ( -14.29746914071049879, 8.314922557960819915, 70.83224293864770971 ) ) ;
#131814=CARTESIAN_POINT ( 'NONE',  ( -8.314922557961024197, 14.29746914071037800, 22.91775706135235069 ) ) ;
#131815=CARTESIAN_POINT ( 'NONE',  ( 5.153800228976615827, -19.02544592524334988, 55.20942372801899722 ) ) ;
#131816=CARTESIAN_POINT ( 'NONE',  ( 4.483927247898545687, 16.52544592524342804, 54.79057627198104541 ) ) ;
#131817=CARTESIAN_POINT ( 'NONE',  ( 21.55341960407619695, -5.719274019375665929, 26.04275706135235779 ) ) ;
#131819=CARTESIAN_POINT ( 'NONE',  ( -21.53943276465977519, 0.05219959533907696930, 71.24890960531435269 ) ) ;
#131820=CARTESIAN_POINT ( 'NONE',  ( 5.153800228976335163, 19.02544592524342804, 99.79057627198102409 ) ) ;
#131821=CARTESIAN_POINT ( 'NONE',  ( -16.52544592524342804, 4.483927247898546575, 81.04057627198102409 ) ) ;
#131824=CARTESIAN_POINT ( 'NONE',  ( 16.51473224551083163, -9.474510206698727899, 65.83442372801900433 ) ) ;
#131825=CARTESIAN_POINT ( 'NONE',  ( 10.81492255796106328, -18.62759615963255655, 25.41775706135235779 ) ) ;
#131826=CARTESIAN_POINT ( 'NONE',  ( -16.51473224551069308, -9.474510206698971260, 51.66557627198102409 ) ) ;
#131827=CARTESIAN_POINT ( 'NONE',  ( 19.02544592524334988, 5.153800228976608722, 41.45942372801900433 ) ) ;
#131828=CARTESIAN_POINT ( 'NONE',  ( -16.46253265017160317, 9.564922557960807481, 25.83224293864769194 ) ) ;
#131829=CARTESIAN_POINT ( 'NONE',  ( -15.80617190586768217, 15.72974639402176855, 58.12609039468568994 ) ) ;
#131831=CARTESIAN_POINT ( 'NONE',  ( 16.53943276465976808, -0.05219959533910856209, 43.74890960531435979 ) ) ;
#131832=CARTESIAN_POINT ( 'NONE',  ( 16.51473224551069308, 9.474510206698969483, 64.16557627198102409 ) ) ;
#131833=CARTESIAN_POINT ( 'NONE',  ( 0.05219959533907565091, 21.53943276465977519, 84.99890960531436690 ) ) ;
#131834=CARTESIAN_POINT ( 'NONE',  ( -19.02544592524342804, 5.153800228976336051, 61.04057627198103120 ) ) ;
#131836=CARTESIAN_POINT ( 'NONE',  ( 10.81492255796078972, 18.62759615963270932, 69.58224293864769550 ) ) ;
#131837=CARTESIAN_POINT ( 'NONE',  ( -21.53943276465977519, -0.05219959533937600094, 103.7510903946857042 ) ) ;
#131838=CARTESIAN_POINT ( 'NONE',  ( -9.474510206698964154, 16.51473224551069663, 25.41557627198103120 ) ) ;
#131839=CARTESIAN_POINT ( 'NONE',  ( 16.55341960407618274, -4.379528057220086978, 91.04275706135236135 ) ) ;
#131840=CARTESIAN_POINT ( 'NONE',  ( 14.29746914071049879, -8.314922557960816363, 88.33224293864769550 ) ) ;
#131841=CARTESIAN_POINT ( 'NONE',  ( 16.51473224551083163, -9.474510206698727899, 90.83442372801900433 ) ) ;
#131843=CARTESIAN_POINT ( 'NONE',  ( 15.80617190586746368, 15.72974639402197994, 114.3739096053143527 ) ) ;
#131844=CARTESIAN_POINT ( 'NONE',  ( 5.049401038297881783, 19.05341960407617563, 42.29275706135234003 ) ) ;
#131845=CARTESIAN_POINT ( 'NONE',  ( 16.52544592524335698, 4.483927247898782831, 96.45942372801901854 ) ) ;
#131846=CARTESIAN_POINT ( 'NONE',  ( -13.97604488694547697, 13.89961937509957934, 33.12609039468566863 ) ) ;
#131847=CARTESIAN_POINT ( 'NONE',  ( -0.05219959533909027116, -19.03943276465977164, 87.49890960531436690 ) ) ;
#131848=CARTESIAN_POINT ( 'NONE',  ( -15.80617190586745835, -15.72974639402198527, 61.87390960531436690 ) ) ;
#131849=CARTESIAN_POINT ( 'NONE',  ( 5.049401038298161559, -19.05341960407611168, 22.70724293864769194 ) ) ;
#131850=CARTESIAN_POINT ( 'NONE',  ( -0.05219959533910754901, -16.53943276465976808, 112.4989096053143669 ) ) ;
#131851=CARTESIAN_POINT ( 'NONE',  ( 18.67979575497194134, -10.72451020669871369, 100.8344237280190185 ) ) ;
#131852=CARTESIAN_POINT ( 'NONE',  ( 0.05219959533934541429, -16.53943276465976808, 75.00109039468568994 ) ) ;
#131853=CARTESIAN_POINT ( 'NONE',  ( -10.72451020669870658, -18.67979575497194134, 34.58442372801900433 ) ) ;
#131854=CARTESIAN_POINT ( 'NONE',  ( 8.224510206698742110, 14.34966873604972548, 32.08442372801901854 ) ) ;
#131855=CARTESIAN_POINT ( 'NONE',  ( 9.474510206698971260, -16.51473224551069308, 102.9155762719810241 ) ) ;
#131856=CARTESIAN_POINT ( 'NONE',  ( -13.89961937509977652, 13.97604488694528158, 35.62390960531435269 ) ) ;
#131857=CARTESIAN_POINT ( 'NONE',  ( -19.02544592524342804, 5.153800228976336051, 61.04057627198103120 ) ) ;
#131858=CARTESIAN_POINT ( 'NONE',  ( -4.483927247898782831, 16.52544592524335698, 52.70942372801902565 ) ) ;
#131859=CARTESIAN_POINT ( 'NONE',  ( 4.379528057220339221, -16.55341960407611168, 97.70724293864772392 ) ) ;
#131860=CARTESIAN_POINT ( 'NONE',  ( -4.379528057220086978, -16.55341960407618274, 94.79275706135234714 ) ) ;
#131861=CARTESIAN_POINT ( 'NONE',  ( -18.62759615963255300, -10.81492255796106328, 44.16775706135234714 ) ) ;
#131862=CARTESIAN_POINT ( 'NONE',  ( -5.049401038298153566, 19.05341960407611168, 80.20724293864769550 ) ) ;
#131863=CARTESIAN_POINT ( 'NONE',  ( -16.51473224551069308, -9.474510206698971260, 66.66557627198102409 ) ) ;
#131864=CARTESIAN_POINT ( 'NONE',  ( -16.46253265017160317, 9.564922557960807481, 100.8322429386477097 ) ) ;
#131865=CARTESIAN_POINT ( 'NONE',  ( -16.55341960407611168, -4.379528057220339221, 31.45724293864769550 ) ) ;
#131866=CARTESIAN_POINT ( 'NONE',  ( -0.05219959533934338120, 16.53943276465976808, 97.50109039468567573 ) ) ;
#131867=ORIENTED_EDGE ( 'NONE', *, *, #181095, .T. ) ;
#131868=CARTESIAN_POINT ( 'NONE',  ( -16.51473224551082808, 9.474510206698731452, 43.33442372801900433 ) ) ;
#131869=CARTESIAN_POINT ( 'NONE',  ( 16.46253265017160672, -9.564922557960803928, 108.3322429386476955 ) ) ;
#131870=CARTESIAN_POINT ( 'NONE',  ( 9.474510206698971260, -16.51473224551069308, 62.91557627198102409 ) ) ;
#131871=CARTESIAN_POINT ( 'NONE',  ( -13.89961937509957401, -13.97604488694547875, 44.37609039468566863 ) ) ;
#131873=CARTESIAN_POINT ( 'NONE',  ( -16.38665767535052353, -7.295008042176046814, 64.73599135785458714 ) ) ;
#131874=CARTESIAN_POINT ( 'NONE',  ( -0.05219959533934338120, 16.53943276465976808, 42.50109039468567573 ) ) ;
#131875=CARTESIAN_POINT ( 'NONE',  ( 0.05219959533936267826, -19.03943276465977164, 65.00109039468567573 ) ) ;
#131876=CARTESIAN_POINT ( 'NONE',  ( -8.314922557961024197, 14.29746914071037800, 52.91775706135235424 ) ) ;
#131877=CARTESIAN_POINT ( 'NONE',  ( -5.049401038298153566, 19.05341960407611168, 115.2072429386477097 ) ) ;
#131878=CARTESIAN_POINT ( 'NONE',  ( -19.02544592524342804, 5.153800228976336051, 96.04057627198103830 ) ) ;
#131879=CARTESIAN_POINT ( 'NONE',  ( 15.80617190586746368, 15.72974639402197994, 109.3739096053143811 ) ) ;
#131880=CARTESIAN_POINT ( 'NONE',  ( 13.97604488694548053, -13.89961937509957401, 75.62609039468564731 ) ) ;
#131881=CARTESIAN_POINT ( 'NONE',  ( -5.153800228976328057, -19.02544592524343514, 102.2905762719810383 ) ) ;
#131882=CARTESIAN_POINT ( 'NONE',  ( 19.03943276465977164, -0.05219959533909143690, 28.74890960531435624 ) ) ;
#131883=CARTESIAN_POINT ( 'NONE',  ( 19.02544592524343514, -5.153800228976328945, 78.54057627198099567 ) ) ;
#131884=CARTESIAN_POINT ( 'NONE',  ( -0.05219959533910754901, -16.53943276465976808, 52.49890960531435979 ) ) ;
#131885=CARTESIAN_POINT ( 'NONE',  ( 5.049401038298161559, -19.05341960407611168, 42.70724293864767418 ) ) ;
#131886=CARTESIAN_POINT ( 'NONE',  ( 19.02544592524334988, 5.153800228976608722, 51.45942372801900433 ) ) ;
#131887=B_SPLINE_CURVE_WITH_KNOTS ( 'NONE', 3,
 ( #183120, #88110, #148804, #26468, #11299, #72970, #15253, #139571 ),
 .UNSPECIFIED., .F., .F.,
 ( 4, 2, 2, 4 ),
 ( 0.002324770996991016962, 0.005594641632892926458, 0.007229576950843881640, 0.008864512268794836822 ),
 .UNSPECIFIED. ) ;
#131888=CARTESIAN_POINT ( 'NONE',  ( 8.224510206698953496, -14.34966873604960469, 87.91557627198103830 ) ) ;
#131889=CARTESIAN_POINT ( 'NONE',  ( 15.72974639402176855, 15.80617190586768217, 106.8760903946856899 ) ) ;
#131890=CARTESIAN_POINT ( 'NONE',  ( -5.049401038298153566, 19.05341960407611168, 55.20724293864769550 ) ) ;
#131891=CARTESIAN_POINT ( 'NONE',  ( -10.72451020669898014, 18.67979575497178502, 55.41557627198102409 ) ) ;
#131892=CARTESIAN_POINT ( 'NONE',  ( -4.483927247898539470, -16.52544592524342804, 47.29057627198103120 ) ) ;
#131893=CARTESIAN_POINT ( 'NONE',  ( -13.97604488694547697, 13.89961937509957934, 23.12609039468565442 ) ) ;
#131894=CARTESIAN_POINT ( 'NONE',  ( 9.564922557960805705, 16.46253265017160317, 104.5822429386476955 ) ) ;
#131895=CARTESIAN_POINT ( 'NONE',  ( 16.46253265017160672, -9.564922557960803928, 103.3322429386476955 ) ) ;
#131896=CARTESIAN_POINT ( 'NONE',  ( -9.474510206698964154, 16.51473224551069663, 35.41557627198102409 ) ) ;
#131897=CARTESIAN_POINT ( 'NONE',  ( -13.97604488694527625, -13.89961937509977652, 31.87390960531435979 ) ) ;
#131898=CARTESIAN_POINT ( 'NONE',  ( 8.224510206698953496, -14.34966873604960469, 87.91557627198103830 ) ) ;
#131899=CARTESIAN_POINT ( 'NONE',  ( -18.67979575497178146, -10.72451020669898902, 91.66557627198103830 ) ) ;
#131900=CARTESIAN_POINT ( 'NONE',  ( -16.46253265017160317, 9.564922557960807481, 105.8322429386476955 ) ) ;
#131901=CARTESIAN_POINT ( 'NONE',  ( -18.67979575497178146, -10.72451020669898902, 106.6655762719810383 ) ) ;
#131902=CARTESIAN_POINT ( 'NONE',  ( 13.89961937509977652, -13.97604488694527269, 98.12390960531433848 ) ) ;
#131904=CARTESIAN_POINT ( 'NONE',  ( 4.483927247898545687, 16.52544592524342804, 104.7905762719810241 ) ) ;
#131905=CARTESIAN_POINT ( 'NONE',  ( 13.97604488694527802, 13.89961937509977652, 74.37390960531436690 ) ) ;
#131906=CARTESIAN_POINT ( 'NONE',  ( -21.53943276465977519, 0.05219959533907696930, 86.24890960531436690 ) ) ;
#131907=CARTESIAN_POINT ( 'NONE',  ( 17.50000000000001066, -5.622605283950885990, 106.1879268940388954 ) ) ;
#131909=CARTESIAN_POINT ( 'NONE',  ( -15.72974639402197994, 15.80617190586746368, 25.62390960531435624 ) ) ;
#131910=CARTESIAN_POINT ( 'NONE',  ( 19.49149378614658090, -5.499999999999772626, 66.93757513605362419 ) ) ;
#131911=CARTESIAN_POINT ( 'NONE',  ( -12.14591786802326823, 12.06949235617739902, 33.12609039468569705 ) ) ;
#131912=CARTESIAN_POINT ( 'NONE',  ( -16.53943276465976808, 0.05219959533911058130, 101.2489096053143669 ) ) ;
#131913=CARTESIAN_POINT ( 'NONE',  ( 18.39443945427642291, -5.499999999999867661, 51.01745347608655123 ) ) ;
#131914=CARTESIAN_POINT ( 'NONE',  ( -0.05219959533909027116, -19.03943276465977164, 52.49890960531436690 ) ) ;
#131915=CARTESIAN_POINT ( 'NONE',  ( -4.379528057220328563, 16.55341960407611168, 75.20724293864769550 ) ) ;
#131916=CARTESIAN_POINT ( 'NONE',  ( -18.67979575497178146, -10.72451020669898902, 26.66557627198103475 ) ) ;
#131917=CARTESIAN_POINT ( 'NONE',  ( -16.52544592524342804, 4.483927247898546575, 66.04057627198103830 ) ) ;
#131918=CARTESIAN_POINT ( 'NONE',  ( -16.53943276465976808, -0.05219959533934237506, 23.75109039468567929 ) ) ;
#131919=CARTESIAN_POINT ( 'NONE',  ( -21.55341960407619339, 5.719274019375674811, 78.54275706135236135 ) ) ;
#131920=CARTESIAN_POINT ( 'NONE',  ( 17.26058549869092573, -6.457015423128476428, 76.12254162523932166 ) ) ;
#131921=CARTESIAN_POINT ( 'NONE',  ( 5.719274019375991003, -21.55341960407610458, 22.70724293864769194 ) ) ;
#131922=CARTESIAN_POINT ( 'NONE',  ( 8.314922557961029526, -14.29746914071037800, 80.41775706135234714 ) ) ;
#131923=CARTESIAN_POINT ( 'NONE',  ( 16.46253265017160672, -9.564922557960803928, 43.33224293864769550 ) ) ;
#131924=CARTESIAN_POINT ( 'NONE',  ( -0.05219959533909027116, -19.03943276465977164, 92.49890960531436690 ) ) ;
#131925=CARTESIAN_POINT ( 'NONE',  ( -18.67979575497178146, -10.72451020669898902, 96.66557627198102409 ) ) ;
#131926=CARTESIAN_POINT ( 'NONE',  ( 16.52544592524335698, 4.483927247898782831, 21.45942372801901499 ) ) ;
#131927=CARTESIAN_POINT ( 'NONE',  ( -8.314922557960811034, -14.29746914071050412, 57.08224293864769550 ) ) ;
#131928=CARTESIAN_POINT ( 'NONE',  ( 18.67979575497194134, -10.72451020669871369, 70.83442372801901854 ) ) ;
#131930=CARTESIAN_POINT ( 'NONE',  ( 4.379528057220092307, 16.55341960407617563, 102.2927570613523613 ) ) ;
#131933=CARTESIAN_POINT ( 'NONE',  ( -16.55341960407611168, -4.379528057220339221, 21.45724293864769550 ) ) ;
#131934=CARTESIAN_POINT ( 'NONE',  ( -14.34966873604972548, 8.224510206698743886, 63.33442372801900433 ) ) ;
#131935=CARTESIAN_POINT ( 'NONE',  ( -9.474510206698964154, 16.51473224551069663, 75.41557627198103830 ) ) ;
#131936=CARTESIAN_POINT ( 'NONE',  ( -13.97604488694527625, -13.89961937509977652, 81.87390960531436690 ) ) ;
#131937=CARTESIAN_POINT ( 'NONE',  ( 21.53943276465977519, 0.05219959533937863772, 66.25109039468567573 ) ) ;
#131938=CARTESIAN_POINT ( 'NONE',  ( 16.53943276465976808, 0.05219959533934440121, 71.25109039468568994 ) ) ;
#131939=CARTESIAN_POINT ( 'NONE',  ( -16.55341960407611168, -4.379528057220339221, 56.45724293864768839 ) ) ;
#131940=CARTESIAN_POINT ( 'NONE',  ( 0.05219959533909260263, 19.03943276465977164, 49.99890960531435979 ) ) ;
#131942=CARTESIAN_POINT ( 'NONE',  ( -0.05219959533936034679, 19.03943276465977164, 102.5010903946856757 ) ) ;
#131943=CARTESIAN_POINT ( 'NONE',  ( -16.52544592524342804, 4.483927247898546575, 106.0405762719810525 ) ) ;
#131944=CARTESIAN_POINT ( 'NONE',  ( 9.564922557960805705, 16.46253265017160317, 84.58224293864769550 ) ) ;
#131945=CARTESIAN_POINT ( 'NONE',  ( 8.314922557961029526, -14.29746914071037800, 20.41775706135234714 ) ) ;
#131947=CARTESIAN_POINT ( 'NONE',  ( 0.05219959533937995610, -21.53943276465977519, 105.0010903946856757 ) ) ;
#131948=CARTESIAN_POINT ( 'NONE',  ( 4.483927247898790824, -16.52544592524335698, 75.20942372801901854 ) ) ;
#131949=CARTESIAN_POINT ( 'NONE',  ( -0.05219959533936034679, 19.03943276465977164, 92.50109039468566152 ) ) ;
#131950=CARTESIAN_POINT ( 'NONE',  ( 10.72451020669898902, -18.67979575497178502, 57.91557627198103120 ) ) ;
#131951=CARTESIAN_POINT ( 'NONE',  ( -16.52544592524335698, -4.483927247898792601, 68.95942372801901854 ) ) ;
#131953=CARTESIAN_POINT ( 'NONE',  ( 5.153800228976615827, -19.02544592524334988, 50.20942372801897591 ) ) ;
#131954=CARTESIAN_POINT ( 'NONE',  ( -18.67979575497193778, 10.72451020669871902, 93.33442372801901854 ) ) ;
#131955=CARTESIAN_POINT ( 'NONE',  ( 13.97604488694527802, 13.89961937509977652, 39.37390960531435269 ) ) ;
#131956=CARTESIAN_POINT ( 'NONE',  ( 9.474510206698971260, -16.51473224551069308, 77.91557627198103830 ) ) ;
#131957=CARTESIAN_POINT ( 'NONE',  ( -12.06949235617756955, 12.14591786802309770, 70.62390960531436690 ) ) ;
#131958=CARTESIAN_POINT ( 'NONE',  ( 10.81492255796106328, -18.62759615963255655, 90.41775706135236135 ) ) ;
#131959=CARTESIAN_POINT ( 'NONE',  ( 13.89961937509957401, 13.97604488694547697, 51.87609039468566863 ) ) ;
#131960=CARTESIAN_POINT ( 'NONE',  ( 19.02544592524334988, 5.153800228976608722, 36.45942372801900433 ) ) ;
#131961=CARTESIAN_POINT ( 'NONE',  ( 21.53943276465977519, -0.05219959533907433946, 38.74890960531435979 ) ) ;
#131962=CARTESIAN_POINT ( 'NONE',  ( -18.67979575497193778, 10.72451020669871902, 98.33442372801901854 ) ) ;
#131963=CARTESIAN_POINT ( 'NONE',  ( 19.03943276465977164, -0.05219959533909143690, 78.74890960531436690 ) ) ;
#131964=CARTESIAN_POINT ( 'NONE',  ( 10.72451020669871369, 18.67979575497193778, 97.08442372801904696 ) ) ;
#131965=CARTESIAN_POINT ( 'NONE',  ( -0.05219959533907301413, -21.53943276465977519, 52.49890960531435979 ) ) ;
#131966=CARTESIAN_POINT ( 'NONE',  ( 5.153800228976335163, 19.02544592524342804, 89.79057627198102409 ) ) ;
#131967=B_SPLINE_CURVE_WITH_KNOTS ( 'NONE', 3,
 ( #128697, #51869, #173239, #113529, #66040, #127707, #16573, #172236, #157070, #18565, #34714, #175223, #50884, #174236, #35705, #159038, #196523, #102494, #195522, #101476 ),
 .UNSPECIFIED., .F., .F.,
 ( 4, 2, 2, 2, 2, 2, 2, 2, 2, 4 ),
 ( 0.004000878361811991205, 0.004499404418915995893, 0.004997930476019999714, 0.005496456533124003535, 0.005994982590228008223, 0.006244245618780010568, 0.006493508647332012912, 0.006992034704436012396, 0.007490560761540013615, 0.007989086818644013099 ),
 .UNSPECIFIED. ) ;
#131968=CARTESIAN_POINT ( 'NONE',  ( -9.474510206698720793, -16.51473224551083518, 79.58442372801899012 ) ) ;
#131969=CARTESIAN_POINT ( 'NONE',  ( 16.46253265017160672, -9.564922557960803928, 93.33224293864769550 ) ) ;
#131970=CARTESIAN_POINT ( 'NONE',  ( 13.97604488694548053, -13.89961937509957401, 90.62609039468567573 ) ) ;
#131971=CARTESIAN_POINT ( 'NONE',  ( 16.53943276465976808, 0.05219959533934440121, 36.25109039468567573 ) ) ;
#131972=CARTESIAN_POINT ( 'NONE',  ( -14.29746914071049879, 8.314922557960819915, 95.83224293864770971 ) ) ;
#131973=CARTESIAN_POINT ( 'NONE',  ( 9.564922557960805705, 16.46253265017160317, 69.58224293864770971 ) ) ;
#131974=CARTESIAN_POINT ( 'NONE',  ( -21.52544592524343514, 5.823673210054127303, 66.04057627198103830 ) ) ;
#131975=CARTESIAN_POINT ( 'NONE',  ( 0.05219959533934541429, -16.53943276465976808, 30.00109039468568284 ) ) ;
#131976=CARTESIAN_POINT ( 'NONE',  ( 15.72974639402176855, 15.80617190586768217, 36.87609039468568994 ) ) ;
#131977=CARTESIAN_POINT ( 'NONE',  ( -15.80617190586768217, 15.72974639402176855, 88.12609039468570415 ) ) ;
#131978=CARTESIAN_POINT ( 'NONE',  ( -8.314922557961024197, 14.29746914071037800, 82.91775706135234714 ) ) ;
#131979=CARTESIAN_POINT ( 'NONE',  ( 13.89961937509977652, -13.97604488694527269, 68.12390960531436690 ) ) ;
#131980=CARTESIAN_POINT ( 'NONE',  ( 16.53943276465976808, -0.05219959533910856209, 78.74890960531436690 ) ) ;
#131981=CARTESIAN_POINT ( 'NONE',  ( 16.52544592524335698, 4.483927247898782831, 96.45942372801901854 ) ) ;
#131982=CARTESIAN_POINT ( 'NONE',  ( -5.049401038297874678, -19.05341960407617918, 59.79275706135231871 ) ) ;
#131983=CARTESIAN_POINT ( 'NONE',  ( 21.53943276465977519, 0.05219959533937863772, 26.25109039468567573 ) ) ;
#131984=CARTESIAN_POINT ( 'NONE',  ( 16.55341960407611168, 4.379528057220329451, 78.95724293864769550 ) ) ;
#131985=CARTESIAN_POINT ( 'NONE',  ( -5.049401038298153566, 19.05341960407611168, 95.20724293864770971 ) ) ;
#131986=CARTESIAN_POINT ( 'NONE',  ( 12.14591786802327356, -12.06949235617739191, 100.6260903946857184 ) ) ;
#131987=CARTESIAN_POINT ( 'NONE',  ( 15.80617190586769283, -15.72974639402175789, 75.62609039468567573 ) ) ;
#131988=CARTESIAN_POINT ( 'NONE',  ( 8.314922557961029526, -14.29746914071037800, 45.41775706135234003 ) ) ;
#131989=CARTESIAN_POINT ( 'NONE',  ( -5.823673210054431948, 21.52544592524334988, 27.70942372801901854 ) ) ;
#131990=CARTESIAN_POINT ( 'NONE',  ( -4.483927247898539470, -16.52544592524342804, 67.29057627198103830 ) ) ;
#131992=CARTESIAN_POINT ( 'NONE',  ( 5.719274019375991003, -21.55341960407610458, 112.7072429386476955 ) ) ;
#131994=CARTESIAN_POINT ( 'NONE',  ( -12.06949235617756955, 12.14591786802309770, 55.62390960531436690 ) ) ;
#131995=CARTESIAN_POINT ( 'NONE',  ( -13.97604488694527625, -13.89961937509977652, 21.87390960531435979 ) ) ;
#131996=CARTESIAN_POINT ( 'NONE',  ( -21.52544592524343514, 5.823673210054127303, 36.04057627198102409 ) ) ;
#131997=CARTESIAN_POINT ( 'NONE',  ( 8.224510206698953496, -14.34966873604960469, 77.91557627198102409 ) ) ;
#131998=CARTESIAN_POINT ( 'NONE',  ( 18.67979575497178502, 10.72451020669898547, 79.16557627198103830 ) ) ;
#131999=CARTESIAN_POINT ( 'NONE',  ( 16.46253265017160672, -9.564922557960803928, 73.33224293864769550 ) ) ;
#132000=CARTESIAN_POINT ( 'NONE',  ( -19.02544592524342804, 5.153800228976336051, 36.04057627198100988 ) ) ;
#132001=CARTESIAN_POINT ( 'NONE',  ( 13.89961937509957401, 13.97604488694547697, 81.87609039468564731 ) ) ;
#132002=CARTESIAN_POINT ( 'NONE',  ( -21.55341960407619339, 5.719274019375674811, 53.54275706135234714 ) ) ;
#132003=CARTESIAN_POINT ( 'NONE',  ( 18.67979575497178502, 10.72451020669898547, 59.16557627198103120 ) ) ;
#132004=CARTESIAN_POINT ( 'NONE',  ( 9.564922557960805705, 16.46253265017160317, 44.58224293864769550 ) ) ;
#132005=CARTESIAN_POINT ( 'NONE',  ( 16.46253265017160672, -9.564922557960803928, 78.33224293864769550 ) ) ;
#132007=CARTESIAN_POINT ( 'NONE',  ( -8.224510206698735004, -14.34966873604973081, 49.58442372801901143 ) ) ;
#132008=CARTESIAN_POINT ( 'NONE',  ( 5.823673210054444382, -21.52544592524334988, 25.20942372801901854 ) ) ;
#132009=CARTESIAN_POINT ( 'NONE',  ( -21.53943276465977519, -0.05219959533937600094, 58.75109039468568994 ) ) ;
#132010=CARTESIAN_POINT ( 'NONE',  ( 0.05219959533909260263, 19.03943276465977164, 109.9989096053143669 ) ) ;
#132011=CARTESIAN_POINT ( 'NONE',  ( 10.72451020669898902, -18.67979575497178502, 87.91557627198103830 ) ) ;
#132012=CARTESIAN_POINT ( 'NONE',  ( 18.62759615963255655, 10.81492255796105972, 21.66775706135235069 ) ) ;
#132013=CARTESIAN_POINT ( 'NONE',  ( 8.314922557961029526, -14.29746914071037800, 55.41775706135234714 ) ) ;
#132014=CARTESIAN_POINT ( 'NONE',  ( 21.53943276465977519, -0.05219959533907433946, 48.74890960531435979 ) ) ;
#132015=CARTESIAN_POINT ( 'NONE',  ( -21.55341960407619339, 5.719274019375674811, 113.5427570613523756 ) ) ;
#132016=CARTESIAN_POINT ( 'NONE',  ( 13.97604488694527802, 13.89961937509977652, 59.37390960531434558 ) ) ;
#132017=CARTESIAN_POINT ( 'NONE',  ( 19.05341960407611168, 5.049401038298154454, 108.9572429386477097 ) ) ;
#132018=CARTESIAN_POINT ( 'NONE',  ( -19.05341960407611168, -5.049401038298163336, 86.45724293864769550 ) ) ;
#132019=CARTESIAN_POINT ( 'NONE',  ( 16.46253265017146816, 9.564922557961045513, 51.66775706135233293 ) ) ;
#132020=CARTESIAN_POINT ( 'NONE',  ( -5.049401038297874678, -19.05341960407617918, 69.79275706135233293 ) ) ;
#132021=CARTESIAN_POINT ( 'NONE',  ( -10.72451020669898014, 18.67979575497178502, 45.41557627198103830 ) ) ;
#132022=CARTESIAN_POINT ( 'NONE',  ( -8.224510206698948167, 14.34966873604960824, 30.41557627198101699 ) ) ;
#132023=CARTESIAN_POINT ( 'NONE',  ( 19.05341960407617918, -5.049401038297876454, 81.04275706135231871 ) ) ;
#132025=CARTESIAN_POINT ( 'NONE',  ( 21.55341960407619695, -5.719274019375665929, 111.0427570613523613 ) ) ;
#132026=CARTESIAN_POINT ( 'NONE',  ( 5.153800228976615827, -19.02544592524334988, 95.20942372801897591 ) ) ;
#132027=CARTESIAN_POINT ( 'NONE',  ( -5.153800228976607833, 19.02544592524334988, 47.70942372801900433 ) ) ;
#132029=CARTESIAN_POINT ( 'NONE',  ( -19.05341960407611168, -5.049401038298163336, 51.45724293864770260 ) ) ;
#132030=CARTESIAN_POINT ( 'NONE',  ( 16.53943276465976808, -0.05219959533910856209, 68.74890960531435269 ) ) ;
#132032=CARTESIAN_POINT ( 'NONE',  ( -19.02544592524342804, 5.153800228976336051, 31.04057627198102409 ) ) ;
#132033=CARTESIAN_POINT ( 'NONE',  ( -4.483927247898539470, -16.52544592524342804, 37.29057627198102409 ) ) ;
#132035=CARTESIAN_POINT ( 'NONE',  ( -0.05219959533934338120, 16.53943276465976808, 102.5010903946856899 ) ) ;
#132036=CARTESIAN_POINT ( 'NONE',  ( 0.05219959533909260263, 19.03943276465977164, 64.99890960531436690 ) ) ;
#132037=CARTESIAN_POINT ( 'NONE',  ( 5.153800228976615827, -19.02544592524334988, 20.20942372801899722 ) ) ;
#132038=CARTESIAN_POINT ( 'NONE',  ( -0.05219959533934338120, 16.53943276465976808, 27.50109039468567929 ) ) ;
#132039=CARTESIAN_POINT ( 'NONE',  ( 21.53943276465977519, -0.05219959533907433946, 48.74890960531435979 ) ) ;
#132040=CARTESIAN_POINT ( 'NONE',  ( -21.52544592524334988, -5.823673210054445271, 103.9594237280190185 ) ) ;
#132042=CARTESIAN_POINT ( 'NONE',  ( 5.153800228976335163, 19.02544592524342804, 59.79057627198100988 ) ) ;
#132043=CARTESIAN_POINT ( 'NONE',  ( 0.05219959533909260263, 19.03943276465977164, 109.9989096053143669 ) ) ;
#132044=CARTESIAN_POINT ( 'NONE',  ( 9.564922557960805705, 16.46253265017160317, 99.58224293864770971 ) ) ;
#132046=CARTESIAN_POINT ( 'NONE',  ( 10.81492255796106328, -18.62759615963255655, 20.41775706135234714 ) ) ;
#132047=CARTESIAN_POINT ( 'NONE',  ( -8.224510206698948167, 14.34966873604960824, 90.41557627198103830 ) ) ;
#132048=CARTESIAN_POINT ( 'NONE',  ( 5.719274019375991003, -21.55341960407610458, 82.70724293864770971 ) ) ;
#132049=CARTESIAN_POINT ( 'NONE',  ( -9.564922557960796823, -16.46253265017161027, 62.08224293864769550 ) ) ;
#132050=CARTESIAN_POINT ( 'NONE',  ( -5.153800228976328057, -19.02544592524343514, 67.29057627198102409 ) ) ;
#132051=CARTESIAN_POINT ( 'NONE',  ( -21.52544592524334988, -5.823673210054445271, 18.95942372801901143 ) ) ;
#132053=CARTESIAN_POINT ( 'NONE',  ( 16.46253265017160672, -9.564922557960803928, 68.33224293864770971 ) ) ;
#132055=CARTESIAN_POINT ( 'NONE',  ( -0.05219959533910754901, -16.53943276465976808, 107.4989096053143669 ) ) ;
#132057=CARTESIAN_POINT ( 'NONE',  ( 9.564922557960805705, 16.46253265017160317, 64.58224293864769550 ) ) ;
#132058=CARTESIAN_POINT ( 'NONE',  ( -5.049401038297874678, -19.05341960407617918, 94.79275706135230450 ) ) ;
#132059=CARTESIAN_POINT ( 'NONE',  ( 16.53943276465976808, -0.05219959533910856209, 98.74890960531438111 ) ) ;
#132060=CARTESIAN_POINT ( 'NONE',  ( -18.67979575497193778, 10.72451020669871902, 78.33442372801901854 ) ) ;
#132061=CARTESIAN_POINT ( 'NONE',  ( 16.51473224551069308, 9.474510206698969483, 54.16557627198103120 ) ) ;
#132062=CARTESIAN_POINT ( 'NONE',  ( -10.72451020669870658, -18.67979575497194134, 29.58442372801901854 ) ) ;
#132063=CARTESIAN_POINT ( 'NONE',  ( -5.823673210054116645, -21.52544592524344225, 107.2905762719810525 ) ) ;
#132065=CARTESIAN_POINT ( 'NONE',  ( -16.51473224551069308, -9.474510206698971260, 66.66557627198102409 ) ) ;
#132067=CARTESIAN_POINT ( 'NONE',  ( -19.02544592524334988, -5.153800228976617603, 103.9594237280190043 ) ) ;
#132068=CARTESIAN_POINT ( 'NONE',  ( -21.52544592524343514, 5.823673210054127303, 31.04057627198102409 ) ) ;
#132069=CARTESIAN_POINT ( 'NONE',  ( 5.823673210054444382, -21.52544592524334988, 65.20942372801901854 ) ) ;
#132070=CARTESIAN_POINT ( 'NONE',  ( -19.02544592524342804, 5.153800228976336051, 96.04057627198103830 ) ) ;
#132071=CARTESIAN_POINT ( 'NONE',  ( 19.03943276465977164, 0.05219959533936151252, 86.25109039468567573 ) ) ;
#132072=CARTESIAN_POINT ( 'NONE',  ( 16.46253265017160672, -9.564922557960803928, 48.33224293864769550 ) ) ;
#132073=CARTESIAN_POINT ( 'NONE',  ( 9.474510206698971260, -16.51473224551069308, 77.91557627198103830 ) ) ;
#132074=CARTESIAN_POINT ( 'NONE',  ( 8.224510206698953496, -14.34966873604960469, 82.91557627198103830 ) ) ;
#132075=CARTESIAN_POINT ( 'NONE',  ( 9.564922557960805705, 16.46253265017160317, 99.58224293864770971 ) ) ;
#132076=CARTESIAN_POINT ( 'NONE',  ( 14.29746914071049879, -8.314922557960816363, 93.33224293864769550 ) ) ;
#132077=CARTESIAN_POINT ( 'NONE',  ( -16.46253265017160317, 9.564922557960807481, 95.83224293864769550 ) ) ;
#132078=CARTESIAN_POINT ( 'NONE',  ( -0.05219959533910754901, -16.53943276465976808, 37.49890960531436690 ) ) ;
#132079=CARTESIAN_POINT ( 'NONE',  ( -13.89961937509977652, 13.97604488694528158, 25.62390960531434558 ) ) ;
#132081=CARTESIAN_POINT ( 'NONE',  ( 18.67979575497194134, -10.72451020669871369, 55.83442372801901854 ) ) ;
#132082=CARTESIAN_POINT ( 'NONE',  ( -13.97604488694547697, 13.89961937509957934, 83.12609039468564731 ) ) ;
#132083=CARTESIAN_POINT ( 'NONE',  ( 16.53943276465976808, -0.05219959533910856209, 43.74890960531435979 ) ) ;
#132084=CARTESIAN_POINT ( 'NONE',  ( 5.823673210054125526, 21.52544592524343514, 94.79057627198105251 ) ) ;
#132085=CARTESIAN_POINT ( 'NONE',  ( -0.05219959533907301413, -21.53943276465977519, 32.49890960531435979 ) ) ;
#132086=CARTESIAN_POINT ( 'NONE',  ( 12.14591786802309770, 12.06949235617756955, 89.37390960531435269 ) ) ;
#132087=CARTESIAN_POINT ( 'NONE',  ( 16.51473224551069308, 9.474510206698969483, 59.16557627198102409 ) ) ;
#132088=CARTESIAN_POINT ( 'NONE',  ( -14.29746914071049879, 8.314922557960819915, 25.83224293864769194 ) ) ;
#132089=CARTESIAN_POINT ( 'NONE',  ( -0.05219959533934338120, 16.53943276465976808, 97.50109039468567573 ) ) ;
#132090=CARTESIAN_POINT ( 'NONE',  ( 12.06949235617739724, 12.14591786802326823, 71.87609039468568994 ) ) ;
#132091=CARTESIAN_POINT ( 'NONE',  ( 0.05219959533936267826, -19.03943276465977164, 25.00109039468566152 ) ) ;
#132092=CARTESIAN_POINT ( 'NONE',  ( -13.97604488694527625, -13.89961937509977652, 101.8739096053143811 ) ) ;
#132093=CARTESIAN_POINT ( 'NONE',  ( -13.97604488694527625, -13.89961937509977652, 71.87390960531433848 ) ) ;
#132094=CARTESIAN_POINT ( 'NONE',  ( -19.02544592524342804, 5.153800228976336051, 36.04057627198100988 ) ) ;
#132095=CARTESIAN_POINT ( 'NONE',  ( -4.483927247898539470, -16.52544592524342804, 47.29057627198103120 ) ) ;
#132096=CARTESIAN_POINT ( 'NONE',  ( 16.51473224551069308, 9.474510206698969483, 109.1655762719810383 ) ) ;
#132097=CARTESIAN_POINT ( 'NONE',  ( 15.72974639402199770, -15.80617190586745480, 38.12390960531436690 ) ) ;
#132098=CARTESIAN_POINT ( 'NONE',  ( -16.52544592524342804, 4.483927247898546575, 91.04057627198103830 ) ) ;
#132099=CARTESIAN_POINT ( 'NONE',  ( -8.224510206698735004, -14.34966873604973081, 24.58442372801901499 ) ) ;
#132100=CARTESIAN_POINT ( 'NONE',  ( -16.53943276465976808, 0.05219959533911058130, 66.24890960531436690 ) ) ;
#132102=CARTESIAN_POINT ( 'NONE',  ( 9.474510206698729675, 16.51473224551082808, 67.08442372801900433 ) ) ;
#132103=CARTESIAN_POINT ( 'NONE',  ( 19.03943276465977164, -0.05219959533909143690, 108.7489096053143527 ) ) ;
#132104=CARTESIAN_POINT ( 'NONE',  ( -9.474510206698720793, -16.51473224551083518, 84.58442372801900433 ) ) ;
#132106=CARTESIAN_POINT ( 'NONE',  ( -19.02544592524334988, -5.153800228976617603, 108.9594237280189759 ) ) ;
#132107=CARTESIAN_POINT ( 'NONE',  ( 12.14591786802327356, -12.06949235617739191, 110.6260903946857042 ) ) ;
#132108=CARTESIAN_POINT ( 'NONE',  ( -9.474510206698964154, 16.51473224551069663, 45.41557627198103120 ) ) ;
#132109=CARTESIAN_POINT ( 'NONE',  ( 21.53943276465977519, -0.05219959533907433946, 33.74890960531436690 ) ) ;
#132110=CARTESIAN_POINT ( 'NONE',  ( -21.53943276465977519, -0.05219959533937600094, 53.75109039468568994 ) ) ;
#132111=CARTESIAN_POINT ( 'NONE',  ( 19.15291303114474886, 5.500000000000047962, 38.60837706366875466 ) ) ;
#132112=CARTESIAN_POINT ( 'NONE',  ( 8.314922557961029526, -14.29746914071037800, 25.41775706135235779 ) ) ;
#132113=CARTESIAN_POINT ( 'NONE',  ( 17.50000000000000355, 3.201899417648170321, 22.70706107622752512 ) ) ;
#132114=CARTESIAN_POINT ( 'NONE',  ( 5.153800228976335163, 19.02544592524342804, 69.79057627198103830 ) ) ;
#132116=CARTESIAN_POINT ( 'NONE',  ( 16.55341960407611168, 4.379528057220329451, 83.95724293864770971 ) ) ;
#132117=CARTESIAN_POINT ( 'NONE',  ( -13.97604488694527625, -13.89961937509977652, 76.87390960531433848 ) ) ;
#132118=CARTESIAN_POINT ( 'NONE',  ( 9.474510206698971260, -16.51473224551069308, 87.91557627198102409 ) ) ;
#132119=ORIENTED_EDGE ( 'NONE', *, *, #109656, .F. ) ;
#132120=CARTESIAN_POINT ( 'NONE',  ( -13.89961937509957401, -13.97604488694547875, 94.37609039468566152 ) ) ;
#132121=CARTESIAN_POINT ( 'NONE',  ( 0.05219959533907565091, 21.53943276465977519, 64.99890960531435269 ) ) ;
#132122=CARTESIAN_POINT ( 'NONE',  ( 19.05341960407611168, 5.049401038298154454, 23.95724293864769194 ) ) ;
#132123=CARTESIAN_POINT ( 'NONE',  ( -5.153800228976607833, 19.02544592524334988, 62.70942372801899722 ) ) ;
#132124=CARTESIAN_POINT ( 'NONE',  ( -13.89961937509977652, 13.97604488694528158, 50.62390960531435979 ) ) ;
#132125=CARTESIAN_POINT ( 'NONE',  ( -9.564922557960796823, -16.46253265017161027, 97.08224293864769550 ) ) ;
#132127=CARTESIAN_POINT ( 'NONE',  ( -18.62759615963270932, 10.81492255796079327, 85.83224293864768129 ) ) ;
#132128=CARTESIAN_POINT ( 'NONE',  ( -8.314922557960811034, -14.29746914071050412, 87.08224293864769550 ) ) ;
#132129=CARTESIAN_POINT ( 'NONE',  ( -19.03943276465977164, 0.05219959533909376836, 86.24890960531436690 ) ) ;
#132130=CARTESIAN_POINT ( 'NONE',  ( -16.51473224551082808, 9.474510206698731452, 58.33442372801900433 ) ) ;
#132131=CARTESIAN_POINT ( 'NONE',  ( -18.62759615963270932, 10.81492255796079327, 90.83224293864769550 ) ) ;
#132132=B_SPLINE_CURVE_WITH_KNOTS ( 'NONE', 3,
 ( #140050, #44092, #167436, #12766, #47068, #43095 ),
 .UNSPECIFIED., .F., .F.,
 ( 4, 2, 4 ),
 ( 0.007228050697041446017, 0.007608510107494925040, 0.007988969517948404930 ),
 .UNSPECIFIED. ) ;
#132133=CARTESIAN_POINT ( 'NONE',  ( 10.72451020669898902, -18.67979575497178502, 72.91557627198103830 ) ) ;
#132134=CARTESIAN_POINT ( 'NONE',  ( 16.55341960407611168, 4.379528057220329451, 38.95724293864768839 ) ) ;
#132135=CARTESIAN_POINT ( 'NONE',  ( -10.81492255796105439, 18.62759615963255655, 97.91775706135236135 ) ) ;
#132136=CARTESIAN_POINT ( 'NONE',  ( 0.05219959533934541429, -16.53943276465976808, 70.00109039468568994 ) ) ;
#132137=CARTESIAN_POINT ( 'NONE',  ( -19.05341960407611168, -5.049401038298163336, 76.45724293864769550 ) ) ;
#132138=CARTESIAN_POINT ( 'NONE',  ( 9.474510206698971260, -16.51473224551069308, 27.91557627198103120 ) ) ;
#132139=CARTESIAN_POINT ( 'NONE',  ( -21.55341960407619339, 5.719274019375674811, 33.54275706135234714 ) ) ;
#132140=CARTESIAN_POINT ( 'NONE',  ( -21.55341960407619339, 5.719274019375674811, 58.54275706135235424 ) ) ;
#132141=CARTESIAN_POINT ( 'NONE',  ( 5.153800228976335163, 19.02544592524342804, 44.79057627198103830 ) ) ;
#132142=CARTESIAN_POINT ( 'NONE',  ( -18.62759615963255300, -10.81492255796106328, 24.16775706135235424 ) ) ;
#132143=CARTESIAN_POINT ( 'NONE',  ( -19.02544592524334988, -5.153800228976617603, 73.95942372801900433 ) ) ;
#132144=CARTESIAN_POINT ( 'NONE',  ( 5.049401038297881783, 19.05341960407617563, 72.29275706135234714 ) ) ;
#132145=CARTESIAN_POINT ( 'NONE',  ( -5.049401038298153566, 19.05341960407611168, 25.20724293864768484 ) ) ;
#132146=CARTESIAN_POINT ( 'NONE',  ( -14.29746914071037622, -8.314922557961029526, 69.16775706135234714 ) ) ;
#132147=CARTESIAN_POINT ( 'NONE',  ( -0.05219959533909027116, -19.03943276465977164, 47.49890960531435979 ) ) ;
#132149=CARTESIAN_POINT ( 'NONE',  ( -19.03943276465977164, 0.05219959533909376836, 96.24890960531436690 ) ) ;
#132150=CARTESIAN_POINT ( 'NONE',  ( 16.46253265017160672, -9.564922557960803928, 38.33224293864768839 ) ) ;
#132151=CARTESIAN_POINT ( 'NONE',  ( -10.81492255796078084, -18.62759615963271287, 67.08224293864770971 ) ) ;
#132152=CARTESIAN_POINT ( 'NONE',  ( 16.55341960407618274, -4.379528057220086978, 56.04275706135235424 ) ) ;
#132153=CARTESIAN_POINT ( 'NONE',  ( -21.55341960407619339, 5.719274019375674811, 108.5427570613523756 ) ) ;
#132154=CARTESIAN_POINT ( 'NONE',  ( -19.03943276465977164, 0.05219959533909376836, 51.24890960531436690 ) ) ;
#132155=CARTESIAN_POINT ( 'NONE',  ( -16.52544592524342804, 4.483927247898546575, 26.04057627198103475 ) ) ;
#132156=CARTESIAN_POINT ( 'NONE',  ( -8.224510206698948167, 14.34966873604960824, 70.41557627198102409 ) ) ;
#132158=CARTESIAN_POINT ( 'NONE',  ( -5.049401038298153566, 19.05341960407611168, 75.20724293864769550 ) ) ;
#132159=CARTESIAN_POINT ( 'NONE',  ( -21.53943276465977519, -0.05219959533937600094, 33.75109039468568284 ) ) ;
#132160=CARTESIAN_POINT ( 'NONE',  ( -9.564922557960796823, -16.46253265017161027, 97.08224293864769550 ) ) ;
#132161=CARTESIAN_POINT ( 'NONE',  ( 18.62759615963255655, 10.81492255796105972, 96.66775706135234714 ) ) ;
#132162=CARTESIAN_POINT ( 'NONE',  ( 8.224510206698742110, 14.34966873604972548, 67.08442372801901854 ) ) ;
#132164=CARTESIAN_POINT ( 'NONE',  ( 13.97604488694527802, 13.89961937509977652, 109.3739096053143669 ) ) ;
#132165=CARTESIAN_POINT ( 'NONE',  ( 18.62759615963271287, -10.81492255796078972, 93.33224293864769550 ) ) ;
#132166=CARTESIAN_POINT ( 'NONE',  ( -16.53943276465976808, 0.05219959533911058130, 51.24890960531436690 ) ) ;
#132167=CARTESIAN_POINT ( 'NONE',  ( 5.153800228976335163, 19.02544592524342804, 29.79057627198102409 ) ) ;
#132168=CARTESIAN_POINT ( 'NONE',  ( 4.379528057220092307, 16.55341960407617563, 57.29275706135234714 ) ) ;
#132169=CARTESIAN_POINT ( 'NONE',  ( -12.14591786802309592, -12.06949235617757132, 61.87390960531436690 ) ) ;
#132170=CARTESIAN_POINT ( 'NONE',  ( -16.51473224551069308, -9.474510206698971260, 111.6655762719810383 ) ) ;
#132171=CARTESIAN_POINT ( 'NONE',  ( -5.823673210054116645, -21.52544592524344225, 37.29057627198102409 ) ) ;
#132172=CARTESIAN_POINT ( 'NONE',  ( 19.02544592524334988, 5.153800228976608722, 26.45942372801899722 ) ) ;
#132173=CARTESIAN_POINT ( 'NONE',  ( 16.53943276465976808, -0.05219959533910856209, 98.74890960531438111 ) ) ;
#132174=CARTESIAN_POINT ( 'NONE',  ( 13.89961937509977652, -13.97604488694527269, 108.1239096053143669 ) ) ;
#132175=ORIENTED_EDGE ( 'NONE', *, *, #56209, .F. ) ;
#132176=CARTESIAN_POINT ( 'NONE',  ( -0.05219959533934338120, 16.53943276465976808, 57.50109039468568994 ) ) ;
#132177=CARTESIAN_POINT ( 'NONE',  ( -0.05219959533909027116, -19.03943276465977164, 57.49890960531435979 ) ) ;
#132179=CARTESIAN_POINT ( 'NONE',  ( -16.46253265017146816, -9.564922557961047289, 49.16775706135233293 ) ) ;
#132180=CARTESIAN_POINT ( 'NONE',  ( -16.52544592524335698, -4.483927247898792601, 98.95942372801903275 ) ) ;
#132181=CARTESIAN_POINT ( 'NONE',  ( 16.51473224551083163, -9.474510206698727899, 90.83442372801900433 ) ) ;
#132182=CARTESIAN_POINT ( 'NONE',  ( 18.62759615963255655, 10.81492255796105972, 61.66775706135235424 ) ) ;
#132183=CARTESIAN_POINT ( 'NONE',  ( 5.153800228976335163, 19.02544592524342804, 69.79057627198103830 ) ) ;
#132184=CARTESIAN_POINT ( 'NONE',  ( -10.72451020669898014, 18.67979575497178502, 90.41557627198103830 ) ) ;
#132185=CARTESIAN_POINT ( 'NONE',  ( 8.314922557960818139, 14.29746914071049879, 109.5822429386476955 ) ) ;
#132187=CARTESIAN_POINT ( 'NONE',  ( 16.51473224551083163, -9.474510206698727899, 85.83442372801900433 ) ) ;
#132188=CARTESIAN_POINT ( 'NONE',  ( 18.62759615963271287, -10.81492255796078972, 83.33224293864769550 ) ) ;
#132189=CARTESIAN_POINT ( 'NONE',  ( -9.564922557961040184, 16.46253265017147172, 37.91775706135233293 ) ) ;
#132191=CARTESIAN_POINT ( 'NONE',  ( -18.67979575497178146, -10.72451020669898902, 86.66557627198102409 ) ) ;
#132192=CARTESIAN_POINT ( 'NONE',  ( -19.35633801406906684, 5.499999999999777955, 54.13373818172763663 ) ) ;
#132193=CARTESIAN_POINT ( 'NONE',  ( -16.46253265017160317, 9.564922557960807481, 70.83224293864770971 ) ) ;
#132195=CARTESIAN_POINT ( 'NONE',  ( 16.55341960407618274, -4.379528057220086978, 26.04275706135235779 ) ) ;
#132197=CARTESIAN_POINT ( 'NONE',  ( 13.89961937509977652, -13.97604488694527269, 48.12390960531435979 ) ) ;
#132198=CARTESIAN_POINT ( 'NONE',  ( 5.049401038298161559, -19.05341960407611168, 107.7072429386476955 ) ) ;
#132199=CARTESIAN_POINT ( 'NONE',  ( 21.55341960407610458, 5.719274019375980345, 108.9572429386476955 ) ) ;
#132200=CARTESIAN_POINT ( 'NONE',  ( -12.06949235617756955, 12.14591786802309770, 45.62390960531436690 ) ) ;
#132201=CARTESIAN_POINT ( 'NONE',  ( 10.72451020669871369, 18.67979575497193778, 77.08442372801901854 ) ) ;
#132202=CARTESIAN_POINT ( 'NONE',  ( -12.06949235617739369, -12.14591786802326823, 29.37609039468568284 ) ) ;
#132203=CARTESIAN_POINT ( 'NONE',  ( -19.03943276465977164, -0.05219959533935918106, 23.75109039468566152 ) ) ;
#132204=CARTESIAN_POINT ( 'NONE',  ( 8.224510206698953496, -14.34966873604960469, 32.91557627198102409 ) ) ;
#132205=CARTESIAN_POINT ( 'NONE',  ( -10.81492255796105439, 18.62759615963255655, 32.91775706135234714 ) ) ;
#132206=CARTESIAN_POINT ( 'NONE',  ( -21.53943276465977519, 0.05219959533907696930, 116.2489096053143669 ) ) ;
#132207=CARTESIAN_POINT ( 'NONE',  ( 14.34966873604960469, 8.224510206698951720, 44.16557627198103120 ) ) ;
#132208=CARTESIAN_POINT ( 'NONE',  ( -19.03943276465977164, -0.05219959533935918106, 98.75109039468567573 ) ) ;
#132209=CARTESIAN_POINT ( 'NONE',  ( 13.89961937509957401, 13.97604488694547697, 71.87609039468567573 ) ) ;
#132210=CARTESIAN_POINT ( 'NONE',  ( -18.67979575497193778, 10.72451020669871902, 73.33442372801901854 ) ) ;
#132211=CARTESIAN_POINT ( 'NONE',  ( 9.564922557961047289, -16.46253265017146816, 55.41775706135234003 ) ) ;
#132212=CARTESIAN_POINT ( 'NONE',  ( -19.03943276465977164, 0.05219959533909376836, 26.24890960531435624 ) ) ;
#132213=CARTESIAN_POINT ( 'NONE',  ( 15.72974639402199770, -15.80617190586745480, 48.12390960531436690 ) ) ;
#132214=CARTESIAN_POINT ( 'NONE',  ( 14.29746914071049879, -8.314922557960816363, 48.33224293864770260 ) ) ;
#132215=CARTESIAN_POINT ( 'NONE',  ( 5.049401038297881783, 19.05341960407617563, 22.29275706135233648 ) ) ;
#132216=CARTESIAN_POINT ( 'NONE',  ( 16.53943276465976808, 0.05219959533934440121, 81.25109039468568994 ) ) ;
#132217=CARTESIAN_POINT ( 'NONE',  ( 12.14591786802309770, 12.06949235617756955, 34.37390960531435979 ) ) ;
#132218=CARTESIAN_POINT ( 'NONE',  ( 5.719274019375673035, 21.55341960407619339, 82.29275706135234714 ) ) ;
#132219=CARTESIAN_POINT ( 'NONE',  ( -5.823673210054431948, 21.52544592524334988, 77.70942372801900433 ) ) ;
#132220=CARTESIAN_POINT ( 'NONE',  ( 10.72451020669898902, -18.67979575497178502, 82.91557627198103830 ) ) ;
#132221=CARTESIAN_POINT ( 'NONE',  ( -5.153800228976328057, -19.02544592524343514, 32.29057627198102409 ) ) ;
#132222=CARTESIAN_POINT ( 'NONE',  ( -10.81492255796105439, 18.62759615963255655, 62.91775706135236135 ) ) ;
#132223=CARTESIAN_POINT ( 'NONE',  ( 9.474510206698971260, -16.51473224551069308, 42.91557627198103120 ) ) ;
#132224=CARTESIAN_POINT ( 'NONE',  ( -19.05341960407611168, -5.049401038298163336, 56.45724293864768129 ) ) ;
#132225=CARTESIAN_POINT ( 'NONE',  ( -16.53943276465976808, 0.05219959533911058130, 86.24890960531436690 ) ) ;
#132226=CARTESIAN_POINT ( 'NONE',  ( 16.46253265017160672, -9.564922557960803928, 98.33224293864769550 ) ) ;
#132227=CARTESIAN_POINT ( 'NONE',  ( -8.314922557960811034, -14.29746914071050412, 37.08224293864768129 ) ) ;
#132228=CARTESIAN_POINT ( 'NONE',  ( -16.53943276465976808, 0.05219959533911058130, 111.2489096053143669 ) ) ;
#132229=CARTESIAN_POINT ( 'NONE',  ( -21.55341960407610458, -5.719274019375992779, 76.45724293864769550 ) ) ;
#132230=CARTESIAN_POINT ( 'NONE',  ( -21.53943276465977519, -0.05219959533937600094, 28.75109039468567929 ) ) ;
#132231=DIRECTION ( 'NONE',  ( 0.000000000000000000, 0.000000000000000000, -1.000000000000000000 ) ) ;
#132233=CARTESIAN_POINT ( 'NONE',  ( -13.89961937509977652, 13.97604488694528158, 75.62390960531438111 ) ) ;
#132234=CARTESIAN_POINT ( 'NONE',  ( 16.55341960407618274, -4.379528057220086978, 26.04275706135235779 ) ) ;
#132235=CARTESIAN_POINT ( 'NONE',  ( 10.72451020669898902, -18.67979575497178502, 72.91557627198103830 ) ) ;
#132236=CARTESIAN_POINT ( 'NONE',  ( 21.52544592524334988, 5.823673210054432836, 96.45942372801901854 ) ) ;
#132237=CARTESIAN_POINT ( 'NONE',  ( -9.474510206698964154, 16.51473224551069663, 80.41557627198103830 ) ) ;
#132238=CARTESIAN_POINT ( 'NONE',  ( 5.823673210054444382, -21.52544592524334988, 35.20942372801901854 ) ) ;
#132239=CARTESIAN_POINT ( 'NONE',  ( 15.72974639402199770, -15.80617190586745480, 23.12390960531436335 ) ) ;
#132240=CARTESIAN_POINT ( 'NONE',  ( -12.06949235617739369, -12.14591786802326823, 84.37609039468570415 ) ) ;
#132241=CARTESIAN_POINT ( 'NONE',  ( -10.72451020669870658, -18.67979575497194134, 69.58442372801900433 ) ) ;
#132242=CARTESIAN_POINT ( 'NONE',  ( -21.52544592524334988, -5.823673210054445271, 103.9594237280190185 ) ) ;
#132243=CARTESIAN_POINT ( 'NONE',  ( 4.379528057220092307, 16.55341960407617563, 77.29275706135234714 ) ) ;
#132244=CARTESIAN_POINT ( 'NONE',  ( -10.81492255796105439, 18.62759615963255655, 22.91775706135235069 ) ) ;
#132245=CARTESIAN_POINT ( 'NONE',  ( -13.89961937509977652, 13.97604488694528158, 25.62390960531434558 ) ) ;
#132246=CARTESIAN_POINT ( 'NONE',  ( -21.53943276465977519, -0.05219959533937600094, 93.75109039468567573 ) ) ;
#132247=CARTESIAN_POINT ( 'NONE',  ( -0.05219959533909027116, -19.03943276465977164, 87.49890960531436690 ) ) ;
#132249=CARTESIAN_POINT ( 'NONE',  ( 21.55341960407610458, 5.719274019375980345, 93.95724293864770971 ) ) ;
#132250=CARTESIAN_POINT ( 'NONE',  ( 19.05341960407617918, -5.049401038297876454, 61.04275706135232582 ) ) ;
#132251=CARTESIAN_POINT ( 'NONE',  ( 18.39639308325437028, 5.500000000000035527, 83.98252246182197212 ) ) ;
#132252=CARTESIAN_POINT ( 'NONE',  ( -15.80617190586745835, -15.72974639402198527, 51.87390960531437401 ) ) ;
#132253=CARTESIAN_POINT ( 'NONE',  ( -0.05219959533909027116, -19.03943276465977164, 92.49890960531436690 ) ) ;
#132254=CARTESIAN_POINT ( 'NONE',  ( 8.314922557960818139, 14.29746914071049879, 54.58224293864769550 ) ) ;
#132256=CARTESIAN_POINT ( 'NONE',  ( 19.05341960407617918, -5.049401038297876454, 81.04275706135231871 ) ) ;
#132258=CARTESIAN_POINT ( 'NONE',  ( 13.89961937509957401, 13.97604488694547697, 101.8760903946856331 ) ) ;
#132259=CARTESIAN_POINT ( 'NONE',  ( -21.55341960407610458, -5.719274019375992779, 86.45724293864770971 ) ) ;
#132260=CARTESIAN_POINT ( 'NONE',  ( -16.52544592524342804, 4.483927247898546575, 71.04057627198103830 ) ) ;
#132261=CARTESIAN_POINT ( 'NONE',  ( 16.46253265017160672, -9.564922557960803928, 103.3322429386476955 ) ) ;
#132262=CARTESIAN_POINT ( 'NONE',  ( -12.14591786802326823, 12.06949235617739902, 48.12609039468568284 ) ) ;
#132263=CARTESIAN_POINT ( 'NONE',  ( 5.049401038298161559, -19.05341960407611168, 52.70724293864767418 ) ) ;
#132264=CARTESIAN_POINT ( 'NONE',  ( -5.823673210054431948, 21.52544592524334988, 22.70942372801901499 ) ) ;
#132265=CARTESIAN_POINT ( 'NONE',  ( -13.97604488694547697, 13.89961937509957934, 83.12609039468564731 ) ) ;
#132266=CARTESIAN_POINT ( 'NONE',  ( 16.46253265017160672, -9.564922557960803928, 93.33224293864769550 ) ) ;
#132267=CARTESIAN_POINT ( 'NONE',  ( 9.474510206698971260, -16.51473224551069308, 72.91557627198102409 ) ) ;
#132268=CARTESIAN_POINT ( 'NONE',  ( -15.72974639402197994, 15.80617190586746368, 80.62390960531438111 ) ) ;
#132269=CARTESIAN_POINT ( 'NONE',  ( 19.02544592524343514, -5.153800228976328945, 43.54057627198103120 ) ) ;
#132271=CARTESIAN_POINT ( 'NONE',  ( 16.52544592524342804, -4.483927247898539470, 53.54057627198103120 ) ) ;
#132272=CARTESIAN_POINT ( 'NONE',  ( -19.03943276465977164, 0.05219959533909376836, 106.2489096053143669 ) ) ;
#132274=CARTESIAN_POINT ( 'NONE',  ( 13.97604488694548053, -13.89961937509957401, 70.62609039468567573 ) ) ;
#132275=CARTESIAN_POINT ( 'NONE',  ( 0.05219959533907565091, 21.53943276465977519, 89.99890960531438111 ) ) ;
#132276=CARTESIAN_POINT ( 'NONE',  ( -19.02544592524334988, -5.153800228976617603, 48.95942372801900433 ) ) ;
#132277=CARTESIAN_POINT ( 'NONE',  ( 5.153800228976335163, 19.02544592524342804, 94.79057627198103830 ) ) ;
#132279=CARTESIAN_POINT ( 'NONE',  ( -15.80617190586745835, -15.72974639402198527, 41.87390960531435979 ) ) ;
#132280=CARTESIAN_POINT ( 'NONE',  ( 19.03943276465977164, -0.05219959533909143690, 78.74890960531436690 ) ) ;
#132281=CARTESIAN_POINT ( 'NONE',  ( 21.53943276465977519, 0.05219959533937863772, 71.25109039468568994 ) ) ;
#132282=CARTESIAN_POINT ( 'NONE',  ( 9.564922557960805705, 16.46253265017160317, 39.58224293864768839 ) ) ;
#132283=CARTESIAN_POINT ( 'NONE',  ( 16.52544592524342804, -4.483927247898539470, 73.54057627198102409 ) ) ;
#132285=CARTESIAN_POINT ( 'NONE',  ( 12.06949235617739724, 12.14591786802326823, 26.87609039468567218 ) ) ;
#132286=CARTESIAN_POINT ( 'NONE',  ( -10.81492255796105439, 18.62759615963255655, 57.91775706135234714 ) ) ;
#132287=ORIENTED_EDGE ( 'NONE', *, *, #70955, .F. ) ;
#132289=CARTESIAN_POINT ( 'NONE',  ( 13.97604488694548053, -13.89961937509957401, 70.62609039468567573 ) ) ;
#132291=CARTESIAN_POINT ( 'NONE',  ( 10.81492255796106328, -18.62759615963255655, 25.41775706135235779 ) ) ;
#132292=CARTESIAN_POINT ( 'NONE',  ( 5.153800228976335163, 19.02544592524342804, 59.79057627198100988 ) ) ;
#132293=CARTESIAN_POINT ( 'NONE',  ( -0.05219959533934338120, 16.53943276465976808, 42.50109039468567573 ) ) ;
#132295=CARTESIAN_POINT ( 'NONE',  ( -9.564922557961040184, 16.46253265017147172, 22.91775706135233648 ) ) ;
#132296=CARTESIAN_POINT ( 'NONE',  ( -13.97604488694527625, -13.89961937509977652, 41.87390960531435979 ) ) ;
#132297=CARTESIAN_POINT ( 'NONE',  ( 5.823673210054444382, -21.52544592524334988, 110.2094237280190185 ) ) ;
#132298=CARTESIAN_POINT ( 'NONE',  ( 16.52544592524335698, 4.483927247898782831, 96.45942372801901854 ) ) ;
#132299=CARTESIAN_POINT ( 'NONE',  ( -16.46253265017160317, 9.564922557960807481, 105.8322429386476955 ) ) ;
#132300=CARTESIAN_POINT ( 'NONE',  ( -21.55341960407619339, 5.719274019375674811, 68.54275706135234714 ) ) ;
#132302=CARTESIAN_POINT ( 'NONE',  ( -19.03943276465977164, 0.05219959533909376836, 111.2489096053143669 ) ) ;
#132303=DIRECTION ( 'NONE',  ( 0.000000000000000000, 0.000000000000000000, -1.000000000000000000 ) ) ;
#132304=CARTESIAN_POINT ( 'NONE',  ( -8.224510206698735004, -14.34966873604973081, 54.58442372801901143 ) ) ;
#132305=CARTESIAN_POINT ( 'NONE',  ( 5.823673210054444382, -21.52544592524334988, 70.20942372801904696 ) ) ;
#132306=CARTESIAN_POINT ( 'NONE',  ( -15.72974639402176322, -15.80617190586768395, 99.37609039468568994 ) ) ;
#132308=CARTESIAN_POINT ( 'NONE',  ( 16.52544592524335698, 4.483927247898782831, 31.45942372801901854 ) ) ;
#132309=CARTESIAN_POINT ( 'NONE',  ( 19.03943276465977164, -0.05219959533909143690, 83.74890960531436690 ) ) ;
#132310=CARTESIAN_POINT ( 'NONE',  ( 19.05341960407611168, 5.049401038298154454, 108.9572429386477097 ) ) ;
#132312=CARTESIAN_POINT ( 'NONE',  ( 16.21995358207306026, 7.366697692864113911, 42.56448998487845614 ) ) ;
#132313=CARTESIAN_POINT ( 'NONE',  ( 19.05341960407611168, 5.049401038298154454, 33.95724293864769550 ) ) ;
#132314=CARTESIAN_POINT ( 'NONE',  ( 18.62759615963271287, -10.81492255796078972, 48.33224293864770260 ) ) ;
#132315=CARTESIAN_POINT ( 'NONE',  ( -16.55341960407617563, 4.379528057220093196, 108.5427570613523756 ) ) ;
#132316=CARTESIAN_POINT ( 'NONE',  ( 14.34966873604960469, 8.224510206698951720, 89.16557627198102409 ) ) ;
#132317=CARTESIAN_POINT ( 'NONE',  ( -19.02544592524342804, 5.153800228976336051, 66.04057627198103830 ) ) ;
#132318=CARTESIAN_POINT ( 'NONE',  ( 5.823673210054444382, -21.52544592524334988, 100.2094237280190043 ) ) ;
#132319=CARTESIAN_POINT ( 'NONE',  ( 12.06949235617739724, 12.14591786802326823, 26.87609039468567218 ) ) ;
#132320=CARTESIAN_POINT ( 'NONE',  ( -12.06949235617756955, 12.14591786802309770, 85.62390960531436690 ) ) ;
#132321=CARTESIAN_POINT ( 'NONE',  ( 5.823673210054444382, -21.52544592524334988, 35.20942372801901854 ) ) ;
#132322=CARTESIAN_POINT ( 'NONE',  ( 15.80617190586746368, 15.72974639402197994, 69.37390960531436690 ) ) ;
#132323=CARTESIAN_POINT ( 'NONE',  ( 19.02544592524334988, 5.153800228976608722, 56.45942372801898301 ) ) ;
#132325=CARTESIAN_POINT ( 'NONE',  ( 5.049401038298161559, -19.05341960407611168, 102.7072429386476955 ) ) ;
#132326=CARTESIAN_POINT ( 'NONE',  ( 4.483927247898545687, 16.52544592524342804, 69.79057627198102409 ) ) ;
#132328=CARTESIAN_POINT ( 'NONE',  ( 14.29746914071049879, -8.314922557960816363, 48.33224293864770260 ) ) ;
#132329=CARTESIAN_POINT ( 'NONE',  ( -4.483927247898782831, 16.52544592524335698, 112.7094237280190328 ) ) ;
#132330=CARTESIAN_POINT ( 'NONE',  ( 9.474510206698729675, 16.51473224551082808, 72.08442372801900433 ) ) ;
#132331=CARTESIAN_POINT ( 'NONE',  ( -19.26498983726237313, 5.499999999999802824, 85.55319577422001487 ) ) ;
#132332=CARTESIAN_POINT ( 'NONE',  ( 21.55341960407610458, 5.719274019375980345, 23.95724293864769550 ) ) ;
#132333=CARTESIAN_POINT ( 'NONE',  ( -14.34966873604960291, -8.224510206698953496, 86.66557627198102409 ) ) ;
#132335=CARTESIAN_POINT ( 'NONE',  ( -19.03943276465977164, 0.05219959533909376836, 51.24890960531436690 ) ) ;
#132336=CARTESIAN_POINT ( 'NONE',  ( -15.80617190586745835, -15.72974639402198527, 51.87390960531437401 ) ) ;
#132337=CARTESIAN_POINT ( 'NONE',  ( -5.049401038298153566, 19.05341960407611168, 25.20724293864768484 ) ) ;
#132338=CARTESIAN_POINT ( 'NONE',  ( -0.05219959533934338120, 16.53943276465976808, 67.50109039468568994 ) ) ;
#132339=CARTESIAN_POINT ( 'NONE',  ( 19.05341960407611168, 5.049401038298154454, 58.95724293864768129 ) ) ;
#132340=CARTESIAN_POINT ( 'NONE',  ( 5.153800228976615827, -19.02544592524334988, 35.20942372801899722 ) ) ;
#132341=CARTESIAN_POINT ( 'NONE',  ( -10.72451020669870658, -18.67979575497194134, 49.58442372801901143 ) ) ;
#132342=CARTESIAN_POINT ( 'NONE',  ( 5.719274019375991003, -21.55341960407610458, 42.70724293864770260 ) ) ;
#132343=CARTESIAN_POINT ( 'NONE',  ( 14.34966873604960469, 8.224510206698951720, 99.16557627198100988 ) ) ;
#132344=CARTESIAN_POINT ( 'NONE',  ( -19.02544592524334988, -5.153800228976617603, 93.95942372801900433 ) ) ;
#132347=CARTESIAN_POINT ( 'NONE',  ( -15.80617190586745835, -15.72974639402198527, 46.87390960531435979 ) ) ;
#132348=CARTESIAN_POINT ( 'NONE',  ( -13.89961937509977652, 13.97604488694528158, 25.62390960531434558 ) ) ;
#132349=CARTESIAN_POINT ( 'NONE',  ( -15.80617190586768217, 15.72974639402176855, 88.12609039468570415 ) ) ;
#132350=CARTESIAN_POINT ( 'NONE',  ( 16.52544592524342804, -4.483927247898539470, 48.54057627198103120 ) ) ;
#132351=CARTESIAN_POINT ( 'NONE',  ( -14.29746914071037622, -8.314922557961029526, 59.16775706135234714 ) ) ;
#132352=CARTESIAN_POINT ( 'NONE',  ( 16.55341960407611168, 4.379528057220329451, 53.95724293864770260 ) ) ;
#132353=CARTESIAN_POINT ( 'NONE',  ( 15.72974639402199770, -15.80617190586745480, 83.12390960531436690 ) ) ;
#132354=CARTESIAN_POINT ( 'NONE',  ( -10.72451020669898014, 18.67979575497178502, 70.41557627198102409 ) ) ;
#132356=CARTESIAN_POINT ( 'NONE',  ( 13.89961937509957401, 13.97604488694547697, 86.87609039468567573 ) ) ;
#132357=CARTESIAN_POINT ( 'NONE',  ( -15.80617190586745835, -15.72974639402198527, 21.87390960531436690 ) ) ;
#132359=CARTESIAN_POINT ( 'NONE',  ( 19.02544592524343514, -5.153800228976328945, 63.54057627198103830 ) ) ;
#132360=CARTESIAN_POINT ( 'NONE',  ( 19.05341960407611168, 5.049401038298154454, 28.95724293864769550 ) ) ;
#132361=CARTESIAN_POINT ( 'NONE',  ( 17.49999999999999289, 5.500000000000006217, 48.78230962303565121 ) ) ;
#132362=ORIENTED_EDGE ( 'NONE', *, *, #98398, .T. ) ;
#132363=CARTESIAN_POINT ( 'NONE',  ( -16.55341960407617563, 4.379528057220093196, 88.54275706135236135 ) ) ;
#132364=CARTESIAN_POINT ( 'NONE',  ( -15.80617190586768217, 15.72974639402176855, 23.12609039468567573 ) ) ;
#132365=CARTESIAN_POINT ( 'NONE',  ( 16.46253265017160672, -9.564922557960803928, 63.33224293864769550 ) ) ;
#132366=CARTESIAN_POINT ( 'NONE',  ( 5.823673210054444382, -21.52544592524334988, 50.20942372801901854 ) ) ;
#132367=CARTESIAN_POINT ( 'NONE',  ( -5.153800228976328057, -19.02544592524343514, 102.2905762719810383 ) ) ;
#132370=CARTESIAN_POINT ( 'NONE',  ( -5.823673210054431948, 21.52544592524334988, 42.70942372801901854 ) ) ;
#132371=CARTESIAN_POINT ( 'NONE',  ( -19.05341960407611168, -5.049401038298163336, 21.45724293864768839 ) ) ;
#132372=CARTESIAN_POINT ( 'NONE',  ( 19.02544592524343514, -5.153800228976328945, 108.5405762719810383 ) ) ;
#132373=CARTESIAN_POINT ( 'NONE',  ( -16.46253265017146816, -9.564922557961047289, 54.16775706135234003 ) ) ;
#132374=CARTESIAN_POINT ( 'NONE',  ( 21.55341960407610458, 5.719274019375980345, 113.9572429386477239 ) ) ;
#132375=CARTESIAN_POINT ( 'NONE',  ( -19.03943276465977164, -0.05219959533935918106, 43.75109039468566863 ) ) ;
#132376=CARTESIAN_POINT ( 'NONE',  ( 13.97604488694548053, -13.89961937509957401, 45.62609039468566863 ) ) ;
#132377=CARTESIAN_POINT ( 'NONE',  ( -14.34966873604972548, 8.224510206698743886, 108.3344237280190185 ) ) ;
#132379=VERTEX_POINT ( 'NONE', #161718 ) ;
#132380=CARTESIAN_POINT ( 'NONE',  ( 9.474510206698971260, -16.51473224551069308, 72.91557627198102409 ) ) ;
#132381=CARTESIAN_POINT ( 'NONE',  ( -5.823673210054431948, 21.52544592524334988, 77.70942372801900433 ) ) ;
#132382=CARTESIAN_POINT ( 'NONE',  ( 21.53943276465977519, 0.05219959533937863772, 91.25109039468568994 ) ) ;
#132384=CARTESIAN_POINT ( 'NONE',  ( -5.049401038298153566, 19.05341960407611168, 85.20724293864766707 ) ) ;
#132385=CARTESIAN_POINT ( 'NONE',  ( 10.72451020669871369, 18.67979575497193778, 82.08442372801901854 ) ) ;
#132386=CARTESIAN_POINT ( 'NONE',  ( -0.05219959533936034679, 19.03943276465977164, 112.5010903946856757 ) ) ;
#132387=CARTESIAN_POINT ( 'NONE',  ( 0.05219959533909260263, 19.03943276465977164, 74.99890960531435269 ) ) ;
#132388=CARTESIAN_POINT ( 'NONE',  ( -19.03943276465977164, 0.05219959533909376836, 111.2489096053143669 ) ) ;
#132389=CARTESIAN_POINT ( 'NONE',  ( 16.51473224551069308, 9.474510206698969483, 89.16557627198103830 ) ) ;
#132391=CARTESIAN_POINT ( 'NONE',  ( -5.153800228976328057, -19.02544592524343514, 82.29057627198103830 ) ) ;
#132392=CARTESIAN_POINT ( 'NONE',  ( 19.02544592524343514, -5.153800228976328945, 63.54057627198103830 ) ) ;
#132393=CARTESIAN_POINT ( 'NONE',  ( -15.80617190586745835, -15.72974639402198527, 106.8739096053143811 ) ) ;
#132394=CARTESIAN_POINT ( 'NONE',  ( -14.34966873604972548, 8.224510206698743886, 98.33442372801901854 ) ) ;
#132396=CARTESIAN_POINT ( 'NONE',  ( 19.02544592524334988, 5.153800228976608722, 51.45942372801900433 ) ) ;
#132397=CARTESIAN_POINT ( 'NONE',  ( 19.02544592524343514, -5.153800228976328945, 93.54057627198102409 ) ) ;
#132398=CARTESIAN_POINT ( 'NONE',  ( -8.224510206698948167, 14.34966873604960824, 85.41557627198102409 ) ) ;
#132399=CARTESIAN_POINT ( 'NONE',  ( 13.97604488694527802, 13.89961937509977652, 24.37390960531435624 ) ) ;
#132400=CARTESIAN_POINT ( 'NONE',  ( 5.719274019375991003, -21.55341960407610458, 27.70724293864769905 ) ) ;
#132401=CARTESIAN_POINT ( 'NONE',  ( 18.62759615963271287, -10.81492255796078972, 23.33224293864769194 ) ) ;
#132402=CARTESIAN_POINT ( 'NONE',  ( -4.379528057220328563, 16.55341960407611168, 95.20724293864769550 ) ) ;
#132404=CARTESIAN_POINT ( 'NONE',  ( -19.03943276465977164, -0.05219959533935918106, 48.75109039468566863 ) ) ;
#132405=CARTESIAN_POINT ( 'NONE',  ( 4.379528057220092307, 16.55341960407617563, 102.2927570613523613 ) ) ;
#132406=CARTESIAN_POINT ( 'NONE',  ( -5.153800228976328057, -19.02544592524343514, 82.29057627198103830 ) ) ;
#132408=CARTESIAN_POINT ( 'NONE',  ( -18.67979575497193778, 10.72451020669871902, 63.33442372801900433 ) ) ;
#132409=CARTESIAN_POINT ( 'NONE',  ( 0.05219959533907565091, 21.53943276465977519, 44.99890960531435979 ) ) ;
#132410=CARTESIAN_POINT ( 'NONE',  ( 18.62759615963255655, 10.81492255796105972, 36.66775706135234714 ) ) ;
#132411=CARTESIAN_POINT ( 'NONE',  ( 0.05219959533907565091, 21.53943276465977519, 79.99890960531435269 ) ) ;
#132412=CARTESIAN_POINT ( 'NONE',  ( 16.55341960407611168, 4.379528057220329451, 103.9572429386476813 ) ) ;
#132413=CARTESIAN_POINT ( 'NONE',  ( 13.89961937509957401, 13.97604488694547697, 71.87609039468567573 ) ) ;
#132414=CARTESIAN_POINT ( 'NONE',  ( -13.97604488694527625, -13.89961937509977652, 41.87390960531435979 ) ) ;
#132415=CARTESIAN_POINT ( 'NONE',  ( 5.049401038298161559, -19.05341960407611168, 92.70724293864769550 ) ) ;
#132416=CARTESIAN_POINT ( 'NONE',  ( -19.03943276465977164, 0.05219959533909376836, 101.2489096053143669 ) ) ;
#132417=CARTESIAN_POINT ( 'NONE',  ( -9.564922557960796823, -16.46253265017161027, 22.08224293864768839 ) ) ;
#132418=CARTESIAN_POINT ( 'NONE',  ( 4.379528057220339221, -16.55341960407611168, 42.70724293864770260 ) ) ;
#132419=CARTESIAN_POINT ( 'NONE',  ( 12.06949235617739724, 12.14591786802326823, 36.87609039468568994 ) ) ;
#132420=CARTESIAN_POINT ( 'NONE',  ( -10.81492255796105439, 18.62759615963255655, 112.9177570613523329 ) ) ;
#132421=DIRECTION ( 'NONE',  ( 0.000000000000000000, 1.000000000000000000, 0.000000000000000000 ) ) ;
#132422=CARTESIAN_POINT ( 'NONE',  ( -16.55341960407611168, -4.379528057220339221, 21.45724293864769550 ) ) ;
#132423=CARTESIAN_POINT ( 'NONE',  ( -18.62759615963255300, -10.81492255796106328, 34.16775706135234714 ) ) ;
#132424=CARTESIAN_POINT ( 'NONE',  ( 5.049401038298161559, -19.05341960407611168, 102.7072429386476955 ) ) ;
#132425=CARTESIAN_POINT ( 'NONE',  ( -12.14591786802326823, 12.06949235617739902, 108.1260903946856757 ) ) ;
#132426=CARTESIAN_POINT ( 'NONE',  ( 4.379528057220092307, 16.55341960407617563, 97.29275706135234714 ) ) ;
#132427=CARTESIAN_POINT ( 'NONE',  ( 4.483927247898790824, -16.52544592524335698, 25.20942372801901854 ) ) ;
#132428=CARTESIAN_POINT ( 'NONE',  ( 19.05341960407611168, 5.049401038298154454, 53.95724293864770260 ) ) ;
#132429=CARTESIAN_POINT ( 'NONE',  ( -4.379528057220328563, 16.55341960407611168, 105.2072429386477097 ) ) ;
#132430=CARTESIAN_POINT ( 'NONE',  ( 18.62759615963255655, 10.81492255796105972, 21.66775706135235069 ) ) ;
#132431=CARTESIAN_POINT ( 'NONE',  ( 5.153800228976335163, 19.02544592524342804, 34.79057627198102409 ) ) ;
#132432=CARTESIAN_POINT ( 'NONE',  ( 19.03943276465977164, -0.05219959533909143690, 108.7489096053143527 ) ) ;
#132433=CARTESIAN_POINT ( 'NONE',  ( -18.67979575497193778, 10.72451020669871902, 38.33442372801900433 ) ) ;
#132434=CARTESIAN_POINT ( 'NONE',  ( 19.03943276465977164, -0.05219959533909143690, 28.74890960531435624 ) ) ;
#132435=CARTESIAN_POINT ( 'NONE',  ( -13.97604488694527625, -13.89961937509977652, 106.8739096053143669 ) ) ;
#132436=CARTESIAN_POINT ( 'NONE',  ( -16.36317988757060604, -7.306389748694898323, 35.90210391636776421 ) ) ;
#132438=CARTESIAN_POINT ( 'NONE',  ( -0.05219959533909027116, -19.03943276465977164, 97.49890960531436690 ) ) ;
#132439=CARTESIAN_POINT ( 'NONE',  ( -21.52544592524334988, -5.823673210054445271, 48.95942372801902565 ) ) ;
#132440=CARTESIAN_POINT ( 'NONE',  ( 12.06949235617757843, -12.14591786802309237, 88.12390960531436690 ) ) ;
#132441=CARTESIAN_POINT ( 'NONE',  ( 19.05341960407611168, 5.049401038298154454, 98.95724293864766707 ) ) ;
#132443=CARTESIAN_POINT ( 'NONE',  ( 12.06949235617739724, 12.14591786802326823, 66.87609039468568994 ) ) ;
#132444=CARTESIAN_POINT ( 'NONE',  ( -21.52544592524334988, -5.823673210054445271, 78.95942372801901854 ) ) ;
#132445=CARTESIAN_POINT ( 'NONE',  ( 14.34966873604972726, -8.224510206698740333, 35.83442372801901143 ) ) ;
#132446=CARTESIAN_POINT ( 'NONE',  ( -13.97604488694527625, -13.89961937509977652, 76.87390960531433848 ) ) ;
#132447=CARTESIAN_POINT ( 'NONE',  ( -12.06949235617739369, -12.14591786802326823, 19.37609039468568639 ) ) ;
#132448=CARTESIAN_POINT ( 'NONE',  ( 12.06949235617739724, 12.14591786802326823, 71.87609039468568994 ) ) ;
#132449=CARTESIAN_POINT ( 'NONE',  ( -19.05341960407617563, 5.049401038297882671, 88.54275706135230450 ) ) ;
#132450=CARTESIAN_POINT ( 'NONE',  ( 5.153800228976335163, 19.02544592524342804, 64.79057627198100988 ) ) ;
#132451=CARTESIAN_POINT ( 'NONE',  ( -18.62759615963270932, 10.81492255796079327, 90.83224293864769550 ) ) ;
#132452=CARTESIAN_POINT ( 'NONE',  ( 12.06949235617757843, -12.14591786802309237, 93.12390960531436690 ) ) ;
#132453=CARTESIAN_POINT ( 'NONE',  ( -16.46253265017146816, -9.564922557961047289, 94.16775706135233293 ) ) ;
#132454=CARTESIAN_POINT ( 'NONE',  ( -14.34966873604972548, 8.224510206698743886, 53.33442372801901854 ) ) ;
#132455=CARTESIAN_POINT ( 'NONE',  ( -19.48894818550246200, 5.499999999999919176, 80.10307310435239003 ) ) ;
#132456=CARTESIAN_POINT ( 'NONE',  ( -5.153800228976607833, 19.02544592524334988, 62.70942372801899722 ) ) ;
#132457=CARTESIAN_POINT ( 'NONE',  ( -12.06949235617756955, 12.14591786802309770, 35.62390960531437401 ) ) ;
#132458=CARTESIAN_POINT ( 'NONE',  ( 16.53943276465976808, -0.05219959533910856209, 73.74890960531433848 ) ) ;
#132459=CARTESIAN_POINT ( 'NONE',  ( 19.02544592524334988, 5.153800228976608722, 21.45942372801899012 ) ) ;
#132460=CARTESIAN_POINT ( 'NONE',  ( -17.05116617787847844, 6.768360034955528626, 38.65675553259191588 ) ) ;
#132461=CARTESIAN_POINT ( 'NONE',  ( 5.823673210054444382, -21.52544592524334988, 20.20942372801900788 ) ) ;
#132463=CARTESIAN_POINT ( 'NONE',  ( -19.03943276465977164, 0.05219959533909376836, 76.24890960531435269 ) ) ;
#132464=CARTESIAN_POINT ( 'NONE',  ( 5.823673210054444382, -21.52544592524334988, 100.2094237280190043 ) ) ;
#132465=CARTESIAN_POINT ( 'NONE',  ( -9.474510206698964154, 16.51473224551069663, 80.41557627198103830 ) ) ;
#132466=CARTESIAN_POINT ( 'NONE',  ( 15.72974639402199770, -15.80617190586745480, 43.12390960531435269 ) ) ;
#132467=CARTESIAN_POINT ( 'NONE',  ( -14.34966873604960291, -8.224510206698953496, 76.66557627198103830 ) ) ;
#132468=CARTESIAN_POINT ( 'NONE',  ( 19.02544592524343514, -5.153800228976328945, 53.54057627198102409 ) ) ;
#132469=CARTESIAN_POINT ( 'NONE',  ( 0.05219959533910956823, 16.53943276465976808, 109.9989096053143527 ) ) ;
#132470=CARTESIAN_POINT ( 'NONE',  ( -18.62759615963255300, -10.81492255796106328, 19.16775706135234714 ) ) ;
#132471=AXIS2_PLACEMENT_3D ( 'NONE', #77211, #185393, #78193 ) ;
#132472=CARTESIAN_POINT ( 'NONE',  ( 21.52544592524334988, 5.823673210054432836, 66.45942372801903275 ) ) ;
#132473=CARTESIAN_POINT ( 'NONE',  ( -19.05341960407611168, -5.049401038298163336, 46.45724293864768129 ) ) ;
#132474=EDGE_CURVE ( 'NONE', #106381, #23056, #27032, .T. ) ;
#132475=CARTESIAN_POINT ( 'NONE',  ( -16.55341960407617563, 4.379528057220093196, 63.54275706135234003 ) ) ;
#132476=CARTESIAN_POINT ( 'NONE',  ( -5.823673210054431948, 21.52544592524334988, 22.70942372801901499 ) ) ;
#132477=CARTESIAN_POINT ( 'NONE',  ( -18.62759615963255300, -10.81492255796106328, 19.16775706135234714 ) ) ;
#132478=CARTESIAN_POINT ( 'NONE',  ( -5.049401038297874678, -19.05341960407617918, 44.79275706135232582 ) ) ;
#132479=CARTESIAN_POINT ( 'NONE',  ( 16.51473224551069308, 9.474510206698969483, 69.16557627198102409 ) ) ;
#132480=CARTESIAN_POINT ( 'NONE',  ( -18.22780087662119541, 5.500000000000102141, 41.01763182126894236 ) ) ;
#132481=CARTESIAN_POINT ( 'NONE',  ( 0.05219959533937995610, -21.53943276465977519, 65.00109039468568994 ) ) ;
#132482=CARTESIAN_POINT ( 'NONE',  ( -10.81492255796078084, -18.62759615963271287, 57.08224293864769550 ) ) ;
#132483=CARTESIAN_POINT ( 'NONE',  ( -14.29746914071049879, 8.314922557960819915, 35.83224293864768839 ) ) ;
#132484=CARTESIAN_POINT ( 'NONE',  ( -10.81492255796105439, 18.62759615963255655, 72.91775706135234714 ) ) ;
#132485=CARTESIAN_POINT ( 'NONE',  ( 13.89961937509957401, 13.97604488694547697, 21.87609039468566152 ) ) ;
#132486=CARTESIAN_POINT ( 'NONE',  ( 14.29746914071049879, -8.314922557960816363, 63.33224293864770260 ) ) ;
#132487=CARTESIAN_POINT ( 'NONE',  ( -12.06949235617756955, 12.14591786802309770, 110.6239096053143669 ) ) ;
#132488=CARTESIAN_POINT ( 'NONE',  ( -16.51473224551082808, 9.474510206698731452, 63.33442372801900433 ) ) ;
#132489=CARTESIAN_POINT ( 'NONE',  ( 14.29746914071049879, -8.314922557960816363, 28.33224293864769550 ) ) ;
#132490=CARTESIAN_POINT ( 'NONE',  ( 5.719274019375673035, 21.55341960407619339, 72.29275706135236135 ) ) ;
#132491=CARTESIAN_POINT ( 'NONE',  ( -13.97604488694527625, -13.89961937509977652, 76.87390960531433848 ) ) ;
#132492=CARTESIAN_POINT ( 'NONE',  ( 0.05219959533936267826, -19.03943276465977164, 30.00109039468566863 ) ) ;
#132493=CARTESIAN_POINT ( 'NONE',  ( -18.67979575497178146, -10.72451020669898902, 41.66557627198103120 ) ) ;
#132494=CARTESIAN_POINT ( 'NONE',  ( 18.67979575497194134, -10.72451020669871369, 30.83442372801902209 ) ) ;
#132495=CARTESIAN_POINT ( 'NONE',  ( 15.72974639402199770, -15.80617190586745480, 93.12390960531436690 ) ) ;
#132496=CARTESIAN_POINT ( 'NONE',  ( -5.153800228976607833, 19.02544592524334988, 102.7094237280189759 ) ) ;
#132497=CARTESIAN_POINT ( 'NONE',  ( 16.52544592524335698, 4.483927247898782831, 51.45942372801901854 ) ) ;
#132499=CARTESIAN_POINT ( 'NONE',  ( 15.72974639402199770, -15.80617190586745480, 93.12390960531436690 ) ) ;
#132500=CARTESIAN_POINT ( 'NONE',  ( 14.29746914071049879, -8.314922557960816363, 93.33224293864769550 ) ) ;
#132502=CARTESIAN_POINT ( 'NONE',  ( 16.46253265017146816, 9.564922557961045513, 111.6677570613523329 ) ) ;
#132503=CARTESIAN_POINT ( 'NONE',  ( -10.81492255796078084, -18.62759615963271287, 52.08224293864768839 ) ) ;
#132504=CARTESIAN_POINT ( 'NONE',  ( 16.52544592524335698, 4.483927247898782831, 96.45942372801901854 ) ) ;
#132505=CARTESIAN_POINT ( 'NONE',  ( 13.89961937509977652, -13.97604488694527269, 23.12390960531436335 ) ) ;
#132506=CARTESIAN_POINT ( 'NONE',  ( 4.379528057220092307, 16.55341960407617563, 47.29275706135234003 ) ) ;
#132507=CARTESIAN_POINT ( 'NONE',  ( -0.05219959533937732626, 21.53943276465977519, 27.50109039468567929 ) ) ;
#132508=CARTESIAN_POINT ( 'NONE',  ( 18.62759615963271287, -10.81492255796078972, 48.33224293864770260 ) ) ;
#132509=CARTESIAN_POINT ( 'NONE',  ( 16.52544592524335698, 4.483927247898782831, 86.45942372801901854 ) ) ;
#132510=CARTESIAN_POINT ( 'NONE',  ( -9.564922557960796823, -16.46253265017161027, 97.08224293864769550 ) ) ;
#132511=CARTESIAN_POINT ( 'NONE',  ( -15.80617190586768217, 15.72974639402176855, 68.12609039468567573 ) ) ;
#132512=CARTESIAN_POINT ( 'NONE',  ( 15.72974639402199770, -15.80617190586745480, 43.12390960531435269 ) ) ;
#132513=CARTESIAN_POINT ( 'NONE',  ( 13.89961937509977652, -13.97604488694527269, 113.1239096053143527 ) ) ;
#132514=VERTEX_POINT ( 'NONE', #81850 ) ;
#132515=CARTESIAN_POINT ( 'NONE',  ( -5.153800228976607833, 19.02544592524334988, 52.70942372801900433 ) ) ;
#132516=CARTESIAN_POINT ( 'NONE',  ( -14.29746914071037622, -8.314922557961029526, 69.16775706135234714 ) ) ;
#132517=CARTESIAN_POINT ( 'NONE',  ( -19.02544592524342804, 5.153800228976336051, 116.0405762719810383 ) ) ;
#132519=CARTESIAN_POINT ( 'NONE',  ( 16.51473224551069308, 9.474510206698969483, 89.16557627198103830 ) ) ;
#132520=CARTESIAN_POINT ( 'NONE',  ( 12.14591786802327356, -12.06949235617739191, 100.6260903946857184 ) ) ;
#132522=CARTESIAN_POINT ( 'NONE',  ( 16.52544592524342804, -4.483927247898539470, 98.54057627198105251 ) ) ;
#132523=CARTESIAN_POINT ( 'NONE',  ( -18.62759615963270932, 10.81492255796079327, 50.83224293864770971 ) ) ;
#132524=CARTESIAN_POINT ( 'NONE',  ( 13.97604488694527802, 13.89961937509977652, 34.37390960531436690 ) ) ;
#132525=CARTESIAN_POINT ( 'NONE',  ( 16.53943276465976808, 0.05219959533934440121, 71.25109039468568994 ) ) ;
#132526=CARTESIAN_POINT ( 'NONE',  ( -15.72974639402176322, -15.80617190586768395, 34.37609039468568284 ) ) ;
#132527=CARTESIAN_POINT ( 'NONE',  ( 19.02544592524334988, 5.153800228976608722, 86.45942372801900433 ) ) ;
#132528=CARTESIAN_POINT ( 'NONE',  ( -14.34966873604960291, -8.224510206698953496, 91.66557627198103830 ) ) ;
#132529=CARTESIAN_POINT ( 'NONE',  ( -16.46253265017160317, 9.564922557960807481, 55.83224293864769550 ) ) ;
#132530=CARTESIAN_POINT ( 'NONE',  ( 0.05219959533909260263, 19.03943276465977164, 114.9989096053143669 ) ) ;
#132531=CARTESIAN_POINT ( 'NONE',  ( -21.52544592524334988, -5.823673210054445271, 108.9594237280190185 ) ) ;
#132532=CARTESIAN_POINT ( 'NONE',  ( -0.05219959533909027116, -19.03943276465977164, 77.49890960531435269 ) ) ;
#132533=CARTESIAN_POINT ( 'NONE',  ( -16.53943276465976808, -0.05219959533934237506, 58.75109039468568994 ) ) ;
#132534=CARTESIAN_POINT ( 'NONE',  ( -21.53943276465977519, -0.05219959533937600094, 98.75109039468568994 ) ) ;
#132535=CARTESIAN_POINT ( 'NONE',  ( 8.314922557961029526, -14.29746914071037800, 75.41775706135233293 ) ) ;
#132536=CARTESIAN_POINT ( 'NONE',  ( 0.05219959533936267826, -19.03943276465977164, 55.00109039468566863 ) ) ;
#132537=CARTESIAN_POINT ( 'NONE',  ( -5.153800228976607833, 19.02544592524334988, 72.70942372801900433 ) ) ;
#132539=CARTESIAN_POINT ( 'NONE',  ( -5.719274019375665041, -21.55341960407619695, 59.79275706135234714 ) ) ;
#132540=CARTESIAN_POINT ( 'NONE',  ( 16.46253265017160672, -9.564922557960803928, 68.33224293864770971 ) ) ;
#132542=CARTESIAN_POINT ( 'NONE',  ( 0.05219959533936267826, -19.03943276465977164, 65.00109039468567573 ) ) ;
#132543=CARTESIAN_POINT ( 'NONE',  ( 19.05341960407611168, 5.049401038298154454, 88.95724293864769550 ) ) ;
#132544=CARTESIAN_POINT ( 'NONE',  ( -4.483927247898539470, -16.52544592524342804, 42.29057627198103120 ) ) ;
#132545=CARTESIAN_POINT ( 'NONE',  ( 21.55341960407610458, 5.719274019375980345, 53.95724293864770260 ) ) ;
#132548=CARTESIAN_POINT ( 'NONE',  ( 19.02544592524334988, 5.153800228976608722, 21.45942372801899012 ) ) ;
#132549=CARTESIAN_POINT ( 'NONE',  ( -17.44270441346519007, -5.991230190322953675, 81.36335079264232206 ) ) ;
#132550=CARTESIAN_POINT ( 'NONE',  ( -19.03943276465977164, 0.05219959533909376836, 36.24890960531436690 ) ) ;
#132551=CARTESIAN_POINT ( 'NONE',  ( 13.89961937509977652, -13.97604488694527269, 28.12390960531435624 ) ) ;
#132552=CARTESIAN_POINT ( 'NONE',  ( -18.09805431107249518, 5.499999999999980460, 81.01606229291886052 ) ) ;
#132553=CARTESIAN_POINT ( 'NONE',  ( 21.53943276465977519, 0.05219959533937863772, 66.25109039468567573 ) ) ;
#132555=CARTESIAN_POINT ( 'NONE',  ( -4.483927247898782831, 16.52544592524335698, 62.70942372801902565 ) ) ;
#132556=CARTESIAN_POINT ( 'NONE',  ( 15.80617190586746368, 15.72974639402197994, 84.37390960531438111 ) ) ;
#132557=CARTESIAN_POINT ( 'NONE',  ( -8.314922557960811034, -14.29746914071050412, 57.08224293864769550 ) ) ;
#132558=CARTESIAN_POINT ( 'NONE',  ( 19.02544592524343514, -5.153800228976328945, 33.54057627198102409 ) ) ;
#132559=CARTESIAN_POINT ( 'NONE',  ( -5.719274019375665041, -21.55341960407619695, 44.79275706135234714 ) ) ;
#132560=CARTESIAN_POINT ( 'NONE',  ( -9.474510206698720793, -16.51473224551083518, 44.58442372801900433 ) ) ;
#132561=CARTESIAN_POINT ( 'NONE',  ( 9.474510206698971260, -16.51473224551069308, 27.91557627198103120 ) ) ;
#132562=CARTESIAN_POINT ( 'NONE',  ( 5.823673210054444382, -21.52544592524334988, 85.20942372801901854 ) ) ;
#132563=CARTESIAN_POINT ( 'NONE',  ( 16.18388926212238488, 7.379444403734537694, 97.93953151366152099 ) ) ;
#132564=CARTESIAN_POINT ( 'NONE',  ( -8.314922557960811034, -14.29746914071050412, 37.08224293864768129 ) ) ;
#132565=CARTESIAN_POINT ( 'NONE',  ( 17.50000000000000711, 3.237210098469639696, 112.7876301262046894 ) ) ;
#132566=CARTESIAN_POINT ( 'NONE',  ( -0.05219959533907301413, -21.53943276465977519, 47.49890960531435979 ) ) ;
#132568=CARTESIAN_POINT ( 'NONE',  ( 9.564922557960805705, 16.46253265017160317, 89.58224293864769550 ) ) ;
#132569=CARTESIAN_POINT ( 'NONE',  ( -14.34966873604960291, -8.224510206698953496, 91.66557627198103830 ) ) ;
#132570=CARTESIAN_POINT ( 'NONE',  ( 4.483927247898790824, -16.52544592524335698, 30.20942372801902565 ) ) ;
#132571=CARTESIAN_POINT ( 'NONE',  ( -5.719274019375978568, 21.55341960407610458, 60.20724293864768839 ) ) ;
#132573=CARTESIAN_POINT ( 'NONE',  ( -13.97604488694527625, -13.89961937509977652, 31.87390960531435979 ) ) ;
#132575=CARTESIAN_POINT ( 'NONE',  ( 13.97604488694527802, 13.89961937509977652, 79.37390960531435269 ) ) ;
#132576=CARTESIAN_POINT ( 'NONE',  ( 21.52544592524344225, -5.823673210054117533, 83.54057627198102409 ) ) ;
#132577=CARTESIAN_POINT ( 'NONE',  ( -8.314922557960811034, -14.29746914071050412, 32.08224293864769550 ) ) ;
#132578=CARTESIAN_POINT ( 'NONE',  ( -13.89961937509977652, 13.97604488694528158, 95.62390960531436690 ) ) ;
#132579=CARTESIAN_POINT ( 'NONE',  ( 13.89961937509957401, 13.97604488694547697, 76.87609039468566152 ) ) ;
#132580=CARTESIAN_POINT ( 'NONE',  ( -16.46253265017146816, -9.564922557961047289, 19.16775706135233293 ) ) ;
#132581=CARTESIAN_POINT ( 'NONE',  ( -0.05219959533907301413, -21.53943276465977519, 82.49890960531436690 ) ) ;
#132582=CARTESIAN_POINT ( 'NONE',  ( -0.05219959533907301413, -21.53943276465977519, 42.49890960531435979 ) ) ;
#132583=CARTESIAN_POINT ( 'NONE',  ( -13.97604488694527625, -13.89961937509977652, 51.87390960531436690 ) ) ;
#132584=CARTESIAN_POINT ( 'NONE',  ( -14.34966873604972548, 8.224510206698743886, 113.3344237280190328 ) ) ;
#132585=CARTESIAN_POINT ( 'NONE',  ( 16.51473224551069308, 9.474510206698969483, 79.16557627198103830 ) ) ;
#132587=CARTESIAN_POINT ( 'NONE',  ( -19.02544592524334988, -5.153800228976617603, 28.95942372801900433 ) ) ;
#132588=CARTESIAN_POINT ( 'NONE',  ( 12.06949235617757843, -12.14591786802309237, 83.12390960531436690 ) ) ;
#132589=CARTESIAN_POINT ( 'NONE',  ( 10.81492255796106328, -18.62759615963255655, 30.41775706135234358 ) ) ;
#132591=CARTESIAN_POINT ( 'NONE',  ( 10.81492255796078972, 18.62759615963270932, 64.58224293864769550 ) ) ;
#132592=CARTESIAN_POINT ( 'NONE',  ( 4.379528057220092307, 16.55341960407617563, 87.29275706135236135 ) ) ;
#132593=CARTESIAN_POINT ( 'NONE',  ( 0.05219959533909260263, 19.03943276465977164, 24.99890960531435269 ) ) ;
#132594=CARTESIAN_POINT ( 'NONE',  ( -19.03943276465977164, 0.05219959533909376836, 76.24890960531435269 ) ) ;
#132595=CARTESIAN_POINT ( 'NONE',  ( -19.03943276465977164, 0.05219959533909376836, 21.24890960531436335 ) ) ;
#132596=CARTESIAN_POINT ( 'NONE',  ( 12.06949235617757843, -12.14591786802309237, 28.12390960531435979 ) ) ;
#132597=CARTESIAN_POINT ( 'NONE',  ( 21.53943276465977519, 0.05219959533937863772, 61.25109039468567573 ) ) ;
#132598=CARTESIAN_POINT ( 'NONE',  ( -19.02544592524342804, 5.153800228976336051, 111.0405762719810099 ) ) ;
#132599=CARTESIAN_POINT ( 'NONE',  ( 5.823673210054444382, -21.52544592524334988, 95.20942372801903275 ) ) ;
#132600=CARTESIAN_POINT ( 'NONE',  ( 16.51473224551069308, 9.474510206698969483, 39.16557627198103120 ) ) ;
#132601=CARTESIAN_POINT ( 'NONE',  ( 9.474510206698971260, -16.51473224551069308, 42.91557627198103120 ) ) ;
#132603=VERTEX_POINT ( 'NONE', #20204 ) ;
#132604=CARTESIAN_POINT ( 'NONE',  ( -10.72451020669870658, -18.67979575497194134, 94.58442372801901854 ) ) ;
#132605=CARTESIAN_POINT ( 'NONE',  ( 12.14591786802327356, -12.06949235617739191, 60.62609039468567573 ) ) ;
#132606=CARTESIAN_POINT ( 'NONE',  ( 21.55341960407619695, -5.719274019375665929, 81.04275706135236135 ) ) ;
#132607=CARTESIAN_POINT ( 'NONE',  ( 15.72974639402199770, -15.80617190586745480, 23.12390960531436335 ) ) ;
#132608=CARTESIAN_POINT ( 'NONE',  ( -19.05341960407617563, 5.049401038297882671, 93.54275706135234714 ) ) ;
#132609=CARTESIAN_POINT ( 'NONE',  ( -10.72451020669870658, -18.67979575497194134, 59.58442372801901854 ) ) ;
#132610=CARTESIAN_POINT ( 'NONE',  ( 16.55341960407618274, -4.379528057220086978, 36.04275706135234714 ) ) ;
#132611=CARTESIAN_POINT ( 'NONE',  ( -0.05219959533936034679, 19.03943276465977164, 87.50109039468567573 ) ) ;
#132612=CARTESIAN_POINT ( 'NONE',  ( -19.05341960407611168, -5.049401038298163336, 56.45724293864768129 ) ) ;
#132613=CARTESIAN_POINT ( 'NONE',  ( 19.03943276465977164, 0.05219959533936151252, 96.25109039468567573 ) ) ;
#132616=CARTESIAN_POINT ( 'NONE',  ( -5.153800228976607833, 19.02544592524334988, 87.70942372801897591 ) ) ;
#132617=CARTESIAN_POINT ( 'NONE',  ( 12.14591786802309770, 12.06949235617756955, 54.37390960531435979 ) ) ;
#132618=CARTESIAN_POINT ( 'NONE',  ( -16.51473224551082808, 9.474510206698731452, 73.33442372801900433 ) ) ;
#132619=CARTESIAN_POINT ( 'NONE',  ( -12.06949235617739369, -12.14591786802326823, 54.37609039468568994 ) ) ;
#132620=CARTESIAN_POINT ( 'NONE',  ( 19.05341960407617918, -5.049401038297876454, 21.04275706135232582 ) ) ;
#132621=CARTESIAN_POINT ( 'NONE',  ( 19.05341960407611168, 5.049401038298154454, 33.95724293864769550 ) ) ;
#132622=CARTESIAN_POINT ( 'NONE',  ( 19.05341960407611168, 5.049401038298154454, 43.95724293864769550 ) ) ;
#132623=CARTESIAN_POINT ( 'NONE',  ( 4.379528057220092307, 16.55341960407617563, 57.29275706135234714 ) ) ;
#132626=CARTESIAN_POINT ( 'NONE',  ( -0.05219959533909027116, -19.03943276465977164, 102.4989096053143669 ) ) ;
#132629=CARTESIAN_POINT ( 'NONE',  ( 19.03943276465977164, 0.05219959533936151252, 101.2510903946856757 ) ) ;
#132630=CARTESIAN_POINT ( 'NONE',  ( 5.719274019375991003, -21.55341960407610458, 32.70724293864770260 ) ) ;
#132631=CARTESIAN_POINT ( 'NONE',  ( 19.05341960407617918, -5.049401038297876454, 31.04275706135232227 ) ) ;
#132632=CARTESIAN_POINT ( 'NONE',  ( 16.46253265017146816, 9.564922557961045513, 111.6677570613523329 ) ) ;
#132633=CARTESIAN_POINT ( 'NONE',  ( -19.02544592524342804, 5.153800228976336051, 36.04057627198100988 ) ) ;
#132634=CARTESIAN_POINT ( 'NONE',  ( -0.05219959533909027116, -19.03943276465977164, 37.49890960531436690 ) ) ;
#132635=CARTESIAN_POINT ( 'NONE',  ( -15.80617190586745835, -15.72974639402198527, 71.87390960531438111 ) ) ;
#132636=CARTESIAN_POINT ( 'NONE',  ( -0.05219959533909027116, -19.03943276465977164, 102.4989096053143669 ) ) ;
#132637=CARTESIAN_POINT ( 'NONE',  ( -9.564922557960796823, -16.46253265017161027, 32.08224293864769550 ) ) ;
#132639=CARTESIAN_POINT ( 'NONE',  ( 5.049401038297881783, 19.05341960407617563, 87.29275706135234714 ) ) ;
#132640=CARTESIAN_POINT ( 'NONE',  ( 14.29746914071049879, -8.314922557960816363, 48.33224293864770260 ) ) ;
#132641=CARTESIAN_POINT ( 'NONE',  ( 0.05219959533907565091, 21.53943276465977519, 39.99890960531436690 ) ) ;
#132642=CARTESIAN_POINT ( 'NONE',  ( -10.81492255796105439, 18.62759615963255655, 102.9177570613523756 ) ) ;
#132643=CARTESIAN_POINT ( 'NONE',  ( 18.67979575497178502, 10.72451020669898547, 99.16557627198100988 ) ) ;
#132644=CARTESIAN_POINT ( 'NONE',  ( 15.72974639402176855, 15.80617190586768217, 76.87609039468567573 ) ) ;
#132645=CARTESIAN_POINT ( 'NONE',  ( -5.719274019375665041, -21.55341960407619695, 74.79275706135234714 ) ) ;
#132646=CARTESIAN_POINT ( 'NONE',  ( 13.97604488694527802, 13.89961937509977652, 109.3739096053143669 ) ) ;
#132647=CARTESIAN_POINT ( 'NONE',  ( 16.55341960407618274, -4.379528057220086978, 111.0427570613523613 ) ) ;
#132648=CARTESIAN_POINT ( 'NONE',  ( 5.823673210054444382, -21.52544592524334988, 65.20942372801901854 ) ) ;
#132649=CARTESIAN_POINT ( 'NONE',  ( 19.03943276465977164, -0.05219959533909143690, 58.74890960531435979 ) ) ;
#132650=CARTESIAN_POINT ( 'NONE',  ( 5.049401038297881783, 19.05341960407617563, 37.29275706135232582 ) ) ;
#132651=CARTESIAN_POINT ( 'NONE',  ( -0.05219959533937732626, 21.53943276465977519, 32.50109039468568284 ) ) ;
#132652=CARTESIAN_POINT ( 'NONE',  ( -9.564922557960796823, -16.46253265017161027, 67.08224293864769550 ) ) ;
#132653=CARTESIAN_POINT ( 'NONE',  ( -12.06949235617756955, 12.14591786802309770, 85.62390960531436690 ) ) ;
#132654=CARTESIAN_POINT ( 'NONE',  ( -8.314922557960811034, -14.29746914071050412, 52.08224293864768839 ) ) ;
#132655=CARTESIAN_POINT ( 'NONE',  ( -21.55341960407610458, -5.719274019375992779, 61.45724293864770260 ) ) ;
#132656=CARTESIAN_POINT ( 'NONE',  ( 9.564922557960805705, 16.46253265017160317, 64.58224293864769550 ) ) ;
#132657=CARTESIAN_POINT ( 'NONE',  ( 10.72451020669898902, -18.67979575497178502, 77.91557627198102409 ) ) ;
#132658=CARTESIAN_POINT ( 'NONE',  ( 19.02544592524334988, 5.153800228976608722, 56.45942372801898301 ) ) ;
#132660=CARTESIAN_POINT ( 'NONE',  ( 16.52544592524342804, -4.483927247898539470, 58.54057627198103120 ) ) ;
#132661=CARTESIAN_POINT ( 'NONE',  ( -15.72974639402197994, 15.80617190586746368, 35.62390960531437401 ) ) ;
#132663=CARTESIAN_POINT ( 'NONE',  ( 16.21995358207305316, 7.366697692864181413, 102.5644899848784348 ) ) ;
#132664=CARTESIAN_POINT ( 'NONE',  ( 0.05219959533934541429, -16.53943276465976808, 85.00109039468568994 ) ) ;
#132666=CARTESIAN_POINT ( 'NONE',  ( -0.05219959533936034679, 19.03943276465977164, 92.50109039468566152 ) ) ;
#132668=CARTESIAN_POINT ( 'NONE',  ( -14.34966873604960291, -8.224510206698953496, 56.66557627198103830 ) ) ;
#132670=CARTESIAN_POINT ( 'NONE',  ( 16.51473224551069308, 9.474510206698969483, 44.16557627198103120 ) ) ;
#132671=CARTESIAN_POINT ( 'NONE',  ( 0.05219959533910956823, 16.53943276465976808, 44.99890960531435979 ) ) ;
#132672=CARTESIAN_POINT ( 'NONE',  ( 13.97604488694527802, 13.89961937509977652, 84.37390960531433848 ) ) ;
#132673=CARTESIAN_POINT ( 'NONE',  ( -16.46253265017160317, 9.564922557960807481, 50.83224293864770260 ) ) ;
#132674=CARTESIAN_POINT ( 'NONE',  ( 15.80617190586769283, -15.72974639402175789, 55.62609039468568284 ) ) ;
#132675=CARTESIAN_POINT ( 'NONE',  ( 16.51473224551069308, 9.474510206698969483, 74.16557627198103830 ) ) ;
#132676=CARTESIAN_POINT ( 'NONE',  ( 13.97604488694527802, 13.89961937509977652, 24.37390960531435624 ) ) ;
#132677=CARTESIAN_POINT ( 'NONE',  ( -19.05341960407611168, -5.049401038298163336, 71.45724293864766707 ) ) ;
#132678=CARTESIAN_POINT ( 'NONE',  ( 18.67979575497178502, 10.72451020669898547, 44.16557627198103120 ) ) ;
#132679=CARTESIAN_POINT ( 'NONE',  ( -13.89961937509977652, 13.97604488694528158, 40.62390960531435979 ) ) ;
#132680=CARTESIAN_POINT ( 'NONE',  ( 18.62759615963271287, -10.81492255796078972, 38.33224293864768839 ) ) ;
#132681=CARTESIAN_POINT ( 'NONE',  ( 8.224510206698742110, 14.34966873604972548, 107.0844237280190043 ) ) ;
#132682=CARTESIAN_POINT ( 'NONE',  ( -13.89961937509957401, -13.97604488694547875, 29.37609039468565797 ) ) ;
#132683=CARTESIAN_POINT ( 'NONE',  ( 8.314922557961029526, -14.29746914071037800, 45.41775706135234003 ) ) ;
#132684=CARTESIAN_POINT ( 'NONE',  ( 14.34966873604972726, -8.224510206698740333, 80.83442372801901854 ) ) ;
#132685=CARTESIAN_POINT ( 'NONE',  ( -19.02544592524342804, 5.153800228976336051, 116.0405762719810383 ) ) ;
#132686=CARTESIAN_POINT ( 'NONE',  ( -8.314922557961024197, 14.29746914071037800, 62.91775706135236135 ) ) ;
#132687=CARTESIAN_POINT ( 'NONE',  ( 21.55341960407610458, 5.719274019375980345, 28.95724293864769905 ) ) ;
#132688=CARTESIAN_POINT ( 'NONE',  ( -5.049401038298153566, 19.05341960407611168, 30.20724293864768839 ) ) ;
#132689=CARTESIAN_POINT ( 'NONE',  ( 16.55341960407618274, -4.379528057220086978, 36.04275706135234714 ) ) ;
#132690=CARTESIAN_POINT ( 'NONE',  ( -9.474510206698964154, 16.51473224551069663, 45.41557627198103120 ) ) ;
#132691=CARTESIAN_POINT ( 'NONE',  ( 10.81492255796106328, -18.62759615963255655, 20.41775706135234714 ) ) ;
#132692=CARTESIAN_POINT ( 'NONE',  ( -12.14591786802326823, 12.06949235617739902, 33.12609039468569705 ) ) ;
#132693=CARTESIAN_POINT ( 'NONE',  ( 14.34966873604972726, -8.224510206698740333, 105.8344237280190328 ) ) ;
#132694=CARTESIAN_POINT ( 'NONE',  ( 5.719274019375673035, 21.55341960407619339, 107.2927570613523471 ) ) ;
#132695=CARTESIAN_POINT ( 'NONE',  ( 5.049401038297881783, 19.05341960407617563, 102.2927570613523045 ) ) ;
#132696=CARTESIAN_POINT ( 'NONE',  ( 9.474510206698729675, 16.51473224551082808, 52.08442372801900433 ) ) ;
#132697=CARTESIAN_POINT ( 'NONE',  ( 16.55341960407611168, 4.379528057220329451, 73.95724293864769550 ) ) ;
#132698=CARTESIAN_POINT ( 'NONE',  ( -8.224510206698948167, 14.34966873604960824, 115.4155762719810241 ) ) ;
#132699=CARTESIAN_POINT ( 'NONE',  ( 5.153800228976615827, -19.02544592524334988, 55.20942372801899722 ) ) ;
#132701=CARTESIAN_POINT ( 'NONE',  ( 5.719274019375673035, 21.55341960407619339, 57.29275706135234714 ) ) ;
#132702=CARTESIAN_POINT ( 'NONE',  ( 14.34966873604972726, -8.224510206698740333, 30.83442372801902209 ) ) ;
#132703=CARTESIAN_POINT ( 'NONE',  ( 19.49149378614658090, -5.499999999999769074, 56.93757513605362419 ) ) ;
#132704=CARTESIAN_POINT ( 'NONE',  ( 15.72974639402199770, -15.80617190586745480, 28.12390960531435979 ) ) ;
#132705=CARTESIAN_POINT ( 'NONE',  ( -5.049401038297874678, -19.05341960407617918, 109.7927570613523187 ) ) ;
#132708=CARTESIAN_POINT ( 'NONE',  ( 4.483927247898545687, 16.52544592524342804, 114.7905762719810383 ) ) ;
#132709=CARTESIAN_POINT ( 'NONE',  ( 18.67979575497194134, -10.72451020669871369, 110.8344237280190043 ) ) ;
#132710=CARTESIAN_POINT ( 'NONE',  ( -9.474510206698964154, 16.51473224551069663, 60.41557627198102409 ) ) ;
#132711=CARTESIAN_POINT ( 'NONE',  ( 18.67979575497194134, -10.72451020669871369, 65.83442372801900433 ) ) ;
#132712=CARTESIAN_POINT ( 'NONE',  ( 0.05219959533937995610, -21.53943276465977519, 100.0010903946857042 ) ) ;
#132713=CARTESIAN_POINT ( 'NONE',  ( -14.34966873604972548, 8.224510206698743886, 98.33442372801901854 ) ) ;
#132714=CARTESIAN_POINT ( 'NONE',  ( 19.02544592524343514, -5.153800228976328945, 73.54057627198103830 ) ) ;
#132715=CARTESIAN_POINT ( 'NONE',  ( -5.823673210054431948, 21.52544592524334988, 52.70942372801902565 ) ) ;
#132716=CARTESIAN_POINT ( 'NONE',  ( -18.67979575497193778, 10.72451020669871902, 53.33442372801901854 ) ) ;
#132717=CARTESIAN_POINT ( 'NONE',  ( -13.89961937509957401, -13.97604488694547875, 84.37609039468567573 ) ) ;
#132718=CARTESIAN_POINT ( 'NONE',  ( 16.51473224551069308, 9.474510206698969483, 109.1655762719810383 ) ) ;
#132719=CARTESIAN_POINT ( 'NONE',  ( -19.03943276465977164, 0.05219959533909376836, 21.24890960531436335 ) ) ;
#132720=CARTESIAN_POINT ( 'NONE',  ( 10.81492255796078972, 18.62759615963270932, 99.58224293864770971 ) ) ;
#132721=CARTESIAN_POINT ( 'NONE',  ( -0.05219959533936034679, 19.03943276465977164, 27.50109039468566507 ) ) ;
#132722=CARTESIAN_POINT ( 'NONE',  ( 14.34966873604960469, 8.224510206698951720, 99.16557627198100988 ) ) ;
#132723=CARTESIAN_POINT ( 'NONE',  ( 5.049401038298161559, -19.05341960407611168, 47.70724293864770260 ) ) ;
#132724=CARTESIAN_POINT ( 'NONE',  ( -0.05219959533936034679, 19.03943276465977164, 102.5010903946856757 ) ) ;
#132725=CARTESIAN_POINT ( 'NONE',  ( 16.55341960407611168, 4.379528057220329451, 63.95724293864770260 ) ) ;
#132726=CARTESIAN_POINT ( 'NONE',  ( -21.52544592524334988, -5.823673210054445271, 103.9594237280190185 ) ) ;
#132727=CARTESIAN_POINT ( 'NONE',  ( 19.05341960407611168, 5.049401038298154454, 108.9572429386477097 ) ) ;
#132728=CARTESIAN_POINT ( 'NONE',  ( -19.05341960407617563, 5.049401038297882671, 68.54275706135230450 ) ) ;
#132729=CARTESIAN_POINT ( 'NONE',  ( -5.719274019375978568, 21.55341960407610458, 80.20724293864769550 ) ) ;
#132730=CARTESIAN_POINT ( 'NONE',  ( -15.72974639402176322, -15.80617190586768395, 39.37609039468567573 ) ) ;
#132731=CARTESIAN_POINT ( 'NONE',  ( 8.224510206698742110, 14.34966873604972548, 42.08442372801901854 ) ) ;
#132732=CARTESIAN_POINT ( 'NONE',  ( -12.14591786802326823, 12.06949235617739902, 93.12609039468568994 ) ) ;
#132733=CARTESIAN_POINT ( 'NONE',  ( 4.379528057220092307, 16.55341960407617563, 37.29275706135235424 ) ) ;
#132734=CARTESIAN_POINT ( 'NONE',  ( 18.62759615963255655, 10.81492255796105972, 31.66775706135234358 ) ) ;
#132735=CARTESIAN_POINT ( 'NONE',  ( -5.823673210054116645, -21.52544592524344225, 42.29057627198103120 ) ) ;
#132736=CARTESIAN_POINT ( 'NONE',  ( 5.049401038298161559, -19.05341960407611168, 37.70724293864768839 ) ) ;
#132738=CARTESIAN_POINT ( 'NONE',  ( 14.34966873604972726, -8.224510206698740333, 55.83442372801901854 ) ) ;
#132739=CARTESIAN_POINT ( 'NONE',  ( 21.55341960407610458, 5.719274019375980345, 88.95724293864769550 ) ) ;
#132740=CARTESIAN_POINT ( 'NONE',  ( -16.53943276465976808, 0.05219959533911058130, 36.24890960531435979 ) ) ;
#132741=CARTESIAN_POINT ( 'NONE',  ( -4.379528057220086978, -16.55341960407618274, 44.79275706135234714 ) ) ;
#132742=CARTESIAN_POINT ( 'NONE',  ( 5.153800228976335163, 19.02544592524342804, 59.79057627198100988 ) ) ;
#132743=CARTESIAN_POINT ( 'NONE',  ( -16.46253265017146816, -9.564922557961047289, 89.16775706135234714 ) ) ;
#132744=CARTESIAN_POINT ( 'NONE',  ( -18.62759615963270932, 10.81492255796079327, 80.83224293864769550 ) ) ;
#132745=CARTESIAN_POINT ( 'NONE',  ( 4.379528057220339221, -16.55341960407611168, 32.70724293864770260 ) ) ;
#132748=CARTESIAN_POINT ( 'NONE',  ( -18.67979575497178146, -10.72451020669898902, 56.66557627198103830 ) ) ;
#132750=CARTESIAN_POINT ( 'NONE',  ( 16.55341960407618274, -4.379528057220086978, 106.0427570613523471 ) ) ;
#132752=CARTESIAN_POINT ( 'NONE',  ( 19.49671883438228193, 5.499999999999968026, 87.39279849105679432 ) ) ;
#132753=CARTESIAN_POINT ( 'NONE',  ( -10.72451020669898014, 18.67979575497178502, 85.41557627198102409 ) ) ;
#132754=CARTESIAN_POINT ( 'NONE',  ( 16.52544592524342804, -4.483927247898539470, 28.54057627198103120 ) ) ;
#132755=CARTESIAN_POINT ( 'NONE',  ( -14.34966873604972548, 8.224510206698743886, 38.33442372801900433 ) ) ;
#132756=CARTESIAN_POINT ( 'NONE',  ( 13.97604488694527802, 13.89961937509977652, 39.37390960531435269 ) ) ;
#132757=CARTESIAN_POINT ( 'NONE',  ( 13.97604488694527802, 13.89961937509977652, 64.37390960531436690 ) ) ;
#132759=CARTESIAN_POINT ( 'NONE',  ( -16.46253265017160317, 9.564922557960807481, 115.8322429386477097 ) ) ;
#132761=CARTESIAN_POINT ( 'NONE',  ( -12.06949235617739369, -12.14591786802326823, 99.37609039468568994 ) ) ;
#132762=CARTESIAN_POINT ( 'NONE',  ( 19.02544592524334988, 5.153800228976608722, 106.4594237280190185 ) ) ;
#132763=CARTESIAN_POINT ( 'NONE',  ( 9.474510206698729675, 16.51473224551082808, 32.08442372801900433 ) ) ;
#132764=CARTESIAN_POINT ( 'NONE',  ( 10.72451020669898902, -18.67979575497178502, 82.91557627198103830 ) ) ;
#132765=CARTESIAN_POINT ( 'NONE',  ( 8.224510206698953496, -14.34966873604960469, 22.91557627198102765 ) ) ;
#132766=CARTESIAN_POINT ( 'NONE',  ( 10.81492255796078972, 18.62759615963270932, 44.58224293864769550 ) ) ;
#132767=CARTESIAN_POINT ( 'NONE',  ( 15.80617190586746368, 15.72974639402197994, 69.37390960531436690 ) ) ;
#132768=CARTESIAN_POINT ( 'NONE',  ( 16.51473224551083163, -9.474510206698727899, 110.8344237280190043 ) ) ;
#132769=CARTESIAN_POINT ( 'NONE',  ( -5.049401038298153566, 19.05341960407611168, 110.2072429386476671 ) ) ;
#132770=CARTESIAN_POINT ( 'NONE',  ( -18.67979575497193778, 10.72451020669871902, 63.33442372801900433 ) ) ;
#132771=CARTESIAN_POINT ( 'NONE',  ( 13.97604488694527802, 13.89961937509977652, 54.37390960531435979 ) ) ;
#132772=CARTESIAN_POINT ( 'NONE',  ( -16.53943276465976808, 0.05219959533911058130, 96.24890960531435269 ) ) ;
#132774=CARTESIAN_POINT ( 'NONE',  ( 16.51473224551069308, 9.474510206698969483, 69.16557627198102409 ) ) ;
#132775=CARTESIAN_POINT ( 'NONE',  ( 12.14591786802309770, 12.06949235617756955, 79.37390960531436690 ) ) ;
#132776=ORIENTED_EDGE ( 'NONE', *, *, #118723, .T. ) ;
#132777=CARTESIAN_POINT ( 'NONE',  ( -19.05341960407617563, 5.049401038297882671, 93.54275706135234714 ) ) ;
#132779=CARTESIAN_POINT ( 'NONE',  ( 16.51473224551069308, 9.474510206698969483, 54.16557627198103120 ) ) ;
#132781=CARTESIAN_POINT ( 'NONE',  ( 21.52544592524334988, 5.823673210054432836, 86.45942372801901854 ) ) ;
#132782=CARTESIAN_POINT ( 'NONE',  ( 5.153800228976335163, 19.02544592524342804, 104.7905762719809957 ) ) ;
#132783=CARTESIAN_POINT ( 'NONE',  ( 8.314922557961029526, -14.29746914071037800, 70.41775706135236135 ) ) ;
#132785=CARTESIAN_POINT ( 'NONE',  ( 5.049401038297881783, 19.05341960407617563, 47.29275706135231161 ) ) ;
#132786=CARTESIAN_POINT ( 'NONE',  ( -10.72451020669870658, -18.67979575497194134, 104.5844237280190185 ) ) ;
#132788=CARTESIAN_POINT ( 'NONE',  ( -19.05341960407611168, -5.049401038298163336, 21.45724293864768839 ) ) ;
#132789=CARTESIAN_POINT ( 'NONE',  ( -8.314922557961024197, 14.29746914071037800, 102.9177570613523756 ) ) ;
#132791=CARTESIAN_POINT ( 'NONE',  ( -8.314922557961024197, 14.29746914071037800, 97.91775706135236135 ) ) ;
#132793=CARTESIAN_POINT ( 'NONE',  ( -14.29746914071037622, -8.314922557961029526, 74.16775706135231871 ) ) ;
#132794=CARTESIAN_POINT ( 'NONE',  ( 17.60728821186566506, -5.500000000000022204, 68.36690927743006796 ) ) ;
#132795=CARTESIAN_POINT ( 'NONE',  ( 15.80617190586769283, -15.72974639402175789, 75.62609039468567573 ) ) ;
#132796=CARTESIAN_POINT ( 'NONE',  ( -9.474510206698720793, -16.51473224551083518, 94.58442372801900433 ) ) ;
#132797=CARTESIAN_POINT ( 'NONE',  ( 19.02544592524334988, 5.153800228976608722, 21.45942372801899012 ) ) ;
#132798=CARTESIAN_POINT ( 'NONE',  ( -9.474510206698964154, 16.51473224551069663, 65.41557627198102409 ) ) ;
#132799=CARTESIAN_POINT ( 'NONE',  ( 5.049401038298161559, -19.05341960407611168, 62.70724293864769550 ) ) ;
#132801=CARTESIAN_POINT ( 'NONE',  ( 18.62759615963271287, -10.81492255796078972, 83.33224293864769550 ) ) ;
#132802=CARTESIAN_POINT ( 'NONE',  ( -21.52544592524343514, 5.823673210054127303, 31.04057627198102409 ) ) ;
#132803=CARTESIAN_POINT ( 'NONE',  ( -16.46253265017160317, 9.564922557960807481, 35.83224293864768839 ) ) ;
#132804=CARTESIAN_POINT ( 'NONE',  ( 12.14591786802327356, -12.06949235617739191, 65.62609039468568994 ) ) ;
#132807=CARTESIAN_POINT ( 'NONE',  ( -18.67979575497193778, 10.72451020669871902, 33.33442372801900433 ) ) ;
#132808=CARTESIAN_POINT ( 'NONE',  ( 14.29746914071049879, -8.314922557960816363, 63.33224293864770260 ) ) ;
#132810=CARTESIAN_POINT ( 'NONE',  ( -4.379528057220086978, -16.55341960407618274, 29.79275706135234358 ) ) ;
#132811=CARTESIAN_POINT ( 'NONE',  ( -5.153800228976607833, 19.02544592524334988, 52.70942372801900433 ) ) ;
#132812=CARTESIAN_POINT ( 'NONE',  ( -14.34966873604960291, -8.224510206698953496, 61.66557627198103120 ) ) ;
#132813=CARTESIAN_POINT ( 'NONE',  ( 10.81492255796078972, 18.62759615963270932, 114.5822429386477097 ) ) ;
#132814=CARTESIAN_POINT ( 'NONE',  ( -18.22780087662123805, 5.499999999999981348, 101.0176318212689495 ) ) ;
#132815=CARTESIAN_POINT ( 'NONE',  ( -10.81492255796078084, -18.62759615963271287, 72.08224293864769550 ) ) ;
#132816=CARTESIAN_POINT ( 'NONE',  ( 19.05341960407611168, 5.049401038298154454, 93.95724293864769550 ) ) ;
#132817=CARTESIAN_POINT ( 'NONE',  ( 4.483927247898545687, 16.52544592524342804, 64.79057627198103830 ) ) ;
#132818=CARTESIAN_POINT ( 'NONE',  ( -5.049401038298153566, 19.05341960407611168, 115.2072429386477097 ) ) ;
#132820=CARTESIAN_POINT ( 'NONE',  ( -5.153800228976607833, 19.02544592524334988, 62.70942372801899722 ) ) ;
#132821=CARTESIAN_POINT ( 'NONE',  ( 21.52544592524344225, -5.823673210054117533, 113.5405762719810383 ) ) ;
#132822=CARTESIAN_POINT ( 'NONE',  ( 0.05219959533909260263, 19.03943276465977164, 54.99890960531435979 ) ) ;
#132823=CARTESIAN_POINT ( 'NONE',  ( -16.51473224551082808, 9.474510206698731452, 43.33442372801900433 ) ) ;
#132824=CARTESIAN_POINT ( 'NONE',  ( -5.049401038298153566, 19.05341960407611168, 35.20724293864768839 ) ) ;
#132825=CARTESIAN_POINT ( 'NONE',  ( -21.55341960407619339, 5.719274019375674811, 63.54275706135234003 ) ) ;
#132826=CARTESIAN_POINT ( 'NONE',  ( -17.49999999999999645, -5.499999999999992895, 69.20309617465828467 ) ) ;
#132827=CARTESIAN_POINT ( 'NONE',  ( -14.34966873604960291, -8.224510206698953496, 36.66557627198103120 ) ) ;
#132828=CARTESIAN_POINT ( 'NONE',  ( -9.564922557960796823, -16.46253265017161027, 57.08224293864769550 ) ) ;
#132829=CARTESIAN_POINT ( 'NONE',  ( -15.80617190586745835, -15.72974639402198527, 71.87390960531438111 ) ) ;
#132830=CARTESIAN_POINT ( 'NONE',  ( 9.564922557960805705, 16.46253265017160317, 59.58224293864769550 ) ) ;
#132832=CARTESIAN_POINT ( 'NONE',  ( 10.72451020669898902, -18.67979575497178502, 67.91557627198102409 ) ) ;
#132833=CARTESIAN_POINT ( 'NONE',  ( 15.72974639402176855, 15.80617190586768217, 101.8760903946857042 ) ) ;
#132835=CARTESIAN_POINT ( 'NONE',  ( -4.379528057220086978, -16.55341960407618274, 99.79275706135234714 ) ) ;
#132836=CARTESIAN_POINT ( 'NONE',  ( 12.14591786802309770, 12.06949235617756955, 89.37390960531435269 ) ) ;
#132837=CARTESIAN_POINT ( 'NONE',  ( -9.474510206698720793, -16.51473224551083518, 89.58442372801900433 ) ) ;
#132839=CARTESIAN_POINT ( 'NONE',  ( 9.564922557961047289, -16.46253265017146816, 40.41775706135234003 ) ) ;
#132840=CARTESIAN_POINT ( 'NONE',  ( -4.483927247898782831, 16.52544592524335698, 107.7094237280190328 ) ) ;
#132841=CARTESIAN_POINT ( 'NONE',  ( -19.05341960407617563, 5.049401038297882671, 28.54275706135232937 ) ) ;
#132842=CARTESIAN_POINT ( 'NONE',  ( 9.564922557960805705, 16.46253265017160317, 94.58224293864769550 ) ) ;
#132843=CARTESIAN_POINT ( 'NONE',  ( -5.823673210054116645, -21.52544592524344225, 62.29057627198102409 ) ) ;
#132844=CARTESIAN_POINT ( 'NONE',  ( -18.22780087662119541, 5.500000000000102141, 51.01763182126894947 ) ) ;
#132845=CARTESIAN_POINT ( 'NONE',  ( -19.03943276465977164, 0.05219959533909376836, 21.24890960531436335 ) ) ;
#132846=CARTESIAN_POINT ( 'NONE',  ( 21.53943276465977519, 0.05219959533937863772, 91.25109039468568994 ) ) ;
#132847=CARTESIAN_POINT ( 'NONE',  ( 8.224510206698742110, 14.34966873604972548, 82.08442372801901854 ) ) ;
#132848=CARTESIAN_POINT ( 'NONE',  ( -15.80617190586768217, 15.72974639402176855, 23.12609039468567573 ) ) ;
#132849=CARTESIAN_POINT ( 'NONE',  ( 0.05219959533934541429, -16.53943276465976808, 35.00109039468568284 ) ) ;
#132850=CARTESIAN_POINT ( 'NONE',  ( 9.564922557960805705, 16.46253265017160317, 109.5822429386476955 ) ) ;
#132851=CARTESIAN_POINT ( 'NONE',  ( 16.51473224551069308, 9.474510206698969483, 34.16557627198102409 ) ) ;
#132852=CARTESIAN_POINT ( 'NONE',  ( 19.02544592524343514, -5.153800228976328945, 58.54057627198102409 ) ) ;
#132853=CARTESIAN_POINT ( 'NONE',  ( -16.55341960407617563, 4.379528057220093196, 33.54275706135234714 ) ) ;
#132854=CARTESIAN_POINT ( 'NONE',  ( 14.29746914071049879, -8.314922557960816363, 98.33224293864769550 ) ) ;
#132855=CARTESIAN_POINT ( 'NONE',  ( -12.14591786802326823, 12.06949235617739902, 103.1260903946856757 ) ) ;
#132856=CARTESIAN_POINT ( 'NONE',  ( 0.05219959533937995610, -21.53943276465977519, 45.00109039468568284 ) ) ;
#132857=CARTESIAN_POINT ( 'NONE',  ( -9.564922557960796823, -16.46253265017161027, 82.08224293864768129 ) ) ;
#132858=CARTESIAN_POINT ( 'NONE',  ( 0.05219959533909260263, 19.03943276465977164, 69.99890960531435269 ) ) ;
#132859=CARTESIAN_POINT ( 'NONE',  ( -16.51473224551069308, -9.474510206698971260, 86.66557627198102409 ) ) ;
#132860=CARTESIAN_POINT ( 'NONE',  ( -16.52544592524342804, 4.483927247898546575, 31.04057627198102409 ) ) ;
#132861=CARTESIAN_POINT ( 'NONE',  ( 16.55341960407618274, -4.379528057220086978, 96.04275706135236135 ) ) ;
#132863=CARTESIAN_POINT ( 'NONE',  ( -19.02544592524334988, -5.153800228976617603, 38.95942372801900433 ) ) ;
#132864=CARTESIAN_POINT ( 'NONE',  ( -9.564922557960796823, -16.46253265017161027, 107.0822429386476955 ) ) ;
#132865=CARTESIAN_POINT ( 'NONE',  ( -19.05341960407611168, -5.049401038298163336, 56.45724293864768129 ) ) ;
#132866=CARTESIAN_POINT ( 'NONE',  ( -19.05341960407617563, 5.049401038297882671, 43.54275706135232582 ) ) ;
#132868=CARTESIAN_POINT ( 'NONE',  ( 4.483927247898790824, -16.52544592524335698, 40.20942372801901854 ) ) ;
#132869=CARTESIAN_POINT ( 'NONE',  ( 19.05341960407617918, -5.049401038297876454, 76.04275706135230450 ) ) ;
#132870=CARTESIAN_POINT ( 'NONE',  ( 14.29746914071037800, 8.314922557961029526, 51.66775706135234714 ) ) ;
#132871=CARTESIAN_POINT ( 'NONE',  ( 16.51473224551069308, 9.474510206698969483, 114.1655762719810241 ) ) ;
#132872=CARTESIAN_POINT ( 'NONE',  ( -19.05341960407611168, -5.049401038298163336, 86.45724293864769550 ) ) ;
#132873=CARTESIAN_POINT ( 'NONE',  ( -18.67979575497178146, -10.72451020669898902, 106.6655762719810383 ) ) ;
#132874=CARTESIAN_POINT ( 'NONE',  ( 19.03943276465977164, 0.05219959533936151252, 81.25109039468567573 ) ) ;
#132875=CARTESIAN_POINT ( 'NONE',  ( -19.02544592524342804, 5.153800228976336051, 106.0405762719810241 ) ) ;
#132876=CARTESIAN_POINT ( 'NONE',  ( -5.153800228976328057, -19.02544592524343514, 37.29057627198102409 ) ) ;
#132877=CARTESIAN_POINT ( 'NONE',  ( 19.02544592524343514, -5.153800228976328945, 83.54057627198100988 ) ) ;
#132878=CARTESIAN_POINT ( 'NONE',  ( -12.14591786802309592, -12.06949235617757132, 31.87390960531435979 ) ) ;
#132879=CARTESIAN_POINT ( 'NONE',  ( 13.97604488694527802, 13.89961937509977652, 39.37390960531435269 ) ) ;
#132880=CARTESIAN_POINT ( 'NONE',  ( 16.46253265017146816, 9.564922557961045513, 56.66775706135233293 ) ) ;
#132881=CARTESIAN_POINT ( 'NONE',  ( 16.52544592524342804, -4.483927247898539470, 93.54057627198103830 ) ) ;
#132882=CARTESIAN_POINT ( 'NONE',  ( 10.81492255796106328, -18.62759615963255655, 105.4177570613523613 ) ) ;
#132883=CARTESIAN_POINT ( 'NONE',  ( -13.97604488694527625, -13.89961937509977652, 46.87390960531435979 ) ) ;
#132884=CARTESIAN_POINT ( 'NONE',  ( -5.719274019375978568, 21.55341960407610458, 45.20724293864769550 ) ) ;
#132885=CARTESIAN_POINT ( 'NONE',  ( 16.55341960407611168, 4.379528057220329451, 53.95724293864770260 ) ) ;
#132886=CARTESIAN_POINT ( 'NONE',  ( -18.62759615963255300, -10.81492255796106328, 99.16775706135234714 ) ) ;
#132887=CARTESIAN_POINT ( 'NONE',  ( -13.89961937509977652, 13.97604488694528158, 110.6239096053143243 ) ) ;
#132888=CARTESIAN_POINT ( 'NONE',  ( 16.51473224551069308, 9.474510206698969483, 104.1655762719810241 ) ) ;
#132889=CARTESIAN_POINT ( 'NONE',  ( 16.51473224551069308, 9.474510206698969483, 34.16557627198102409 ) ) ;
#132890=CARTESIAN_POINT ( 'NONE',  ( 9.564922557960805705, 16.46253265017160317, 29.58224293864769550 ) ) ;
#132891=CARTESIAN_POINT ( 'NONE',  ( -14.34966873604960291, -8.224510206698953496, 81.66557627198103830 ) ) ;
#132892=CARTESIAN_POINT ( 'NONE',  ( -21.52544592524343514, 5.823673210054127303, 96.04057627198102409 ) ) ;
#132893=CARTESIAN_POINT ( 'NONE',  ( 9.564922557960805705, 16.46253265017160317, 99.58224293864770971 ) ) ;
#132894=CARTESIAN_POINT ( 'NONE',  ( -5.823673210054116645, -21.52544592524344225, 112.2905762719810241 ) ) ;
#132895=CARTESIAN_POINT ( 'NONE',  ( 5.049401038298161559, -19.05341960407611168, 87.70724293864769550 ) ) ;
#132896=CARTESIAN_POINT ( 'NONE',  ( 17.50000000000000000, 5.499999999999997335, 120.0000000000000142 ) ) ;
#132897=CARTESIAN_POINT ( 'NONE',  ( -4.483927247898539470, -16.52544592524342804, 97.29057627198105251 ) ) ;
#132898=CARTESIAN_POINT ( 'NONE',  ( -9.474510206698964154, 16.51473224551069663, 70.41557627198102409 ) ) ;
#132899=CARTESIAN_POINT ( 'NONE',  ( -10.72451020669898014, 18.67979575497178502, 75.41557627198102409 ) ) ;
#132902=CARTESIAN_POINT ( 'NONE',  ( 21.52544592524344225, -5.823673210054117533, 33.54057627198102409 ) ) ;
#132904=CARTESIAN_POINT ( 'NONE',  ( -12.14591786802326823, 12.06949235617739902, 38.12609039468567573 ) ) ;
#132905=EDGE_CURVE ( 'NONE', #94779, #138821, #159548, .T. ) ;
#132906=CARTESIAN_POINT ( 'NONE',  ( 4.483927247898545687, 16.52544592524342804, 94.79057627198105251 ) ) ;
#132907=CARTESIAN_POINT ( 'NONE',  ( -17.50000000000000355, -3.189878218039142954, 110.1294856257124337 ) ) ;
#132908=CARTESIAN_POINT ( 'NONE',  ( 19.02544592524343514, -5.153800228976328945, 93.54057627198102409 ) ) ;
#132909=CARTESIAN_POINT ( 'NONE',  ( -19.02544592524342804, 5.153800228976336051, 51.04057627198103120 ) ) ;
#132910=CARTESIAN_POINT ( 'NONE',  ( 16.52544592524342804, -4.483927247898539470, 83.54057627198102409 ) ) ;
#132911=CARTESIAN_POINT ( 'NONE',  ( 15.80617190586746368, 15.72974639402197994, 34.37390960531435979 ) ) ;
#132912=CARTESIAN_POINT ( 'NONE',  ( -16.55341960407611168, -4.379528057220339221, 51.45724293864770260 ) ) ;
#132913=CARTESIAN_POINT ( 'NONE',  ( 8.314922557961029526, -14.29746914071037800, 25.41775706135235779 ) ) ;
#132914=CARTESIAN_POINT ( 'NONE',  ( -21.53943276465977519, -0.05219959533937600094, 73.75109039468567573 ) ) ;
#132916=CARTESIAN_POINT ( 'NONE',  ( -0.05219959533909027116, -19.03943276465977164, 112.4989096053143669 ) ) ;
#132917=CARTESIAN_POINT ( 'NONE',  ( -16.55341960407617563, 4.379528057220093196, 83.54275706135234714 ) ) ;
#132918=CARTESIAN_POINT ( 'NONE',  ( -16.46253265017160317, 9.564922557960807481, 25.83224293864769194 ) ) ;
#132919=CARTESIAN_POINT ( 'NONE',  ( 19.05341960407611168, 5.049401038298154454, 78.95724293864769550 ) ) ;
#132920=CARTESIAN_POINT ( 'NONE',  ( -15.80617190586745835, -15.72974639402198527, 81.87390960531435269 ) ) ;
#132921=CARTESIAN_POINT ( 'NONE',  ( 8.224510206698742110, 14.34966873604972548, 32.08442372801901854 ) ) ;
#132922=CARTESIAN_POINT ( 'NONE',  ( -8.224510206698948167, 14.34966873604960824, 55.41557627198102409 ) ) ;
#132923=CARTESIAN_POINT ( 'NONE',  ( -10.81492255796105439, 18.62759615963255655, 72.91775706135234714 ) ) ;
#132924=CARTESIAN_POINT ( 'NONE',  ( -8.314922557961024197, 14.29746914071037800, 92.91775706135236135 ) ) ;
#132925=CARTESIAN_POINT ( 'NONE',  ( 16.46253265017160672, -9.564922557960803928, 113.3322429386476955 ) ) ;
#132926=CARTESIAN_POINT ( 'NONE',  ( 17.05116617787826172, 6.768360034955700044, 28.84324446740803083 ) ) ;
#132928=CARTESIAN_POINT ( 'NONE',  ( 8.224510206698742110, 14.34966873604972548, 102.0844237280190185 ) ) ;
#132929=CARTESIAN_POINT ( 'NONE',  ( -4.379528057220086978, -16.55341960407618274, 59.79275706135234714 ) ) ;
#132930=CARTESIAN_POINT ( 'NONE',  ( -19.03943276465977164, 0.05219959533909376836, 66.24890960531436690 ) ) ;
#132931=CARTESIAN_POINT ( 'NONE',  ( -16.46253265017160317, 9.564922557960807481, 90.83224293864769550 ) ) ;
#132932=CARTESIAN_POINT ( 'NONE',  ( -21.53943276465977519, -0.05219959533937600094, 73.75109039468567573 ) ) ;
#132934=CARTESIAN_POINT ( 'NONE',  ( -14.34966873604972548, 8.224510206698743886, 78.33442372801901854 ) ) ;
#132935=CARTESIAN_POINT ( 'NONE',  ( -16.55341960407611168, -4.379528057220339221, 41.45724293864769550 ) ) ;
#132936=CARTESIAN_POINT ( 'NONE',  ( -16.46253265017160317, 9.564922557960807481, 50.83224293864770260 ) ) ;
#132937=CARTESIAN_POINT ( 'NONE',  ( 16.46253265017160672, -9.564922557960803928, 48.33224293864769550 ) ) ;
#132939=CARTESIAN_POINT ( 'NONE',  ( 5.049401038297881783, 19.05341960407617563, 112.2927570613523471 ) ) ;
#132940=CARTESIAN_POINT ( 'NONE',  ( -16.52544592524342804, 4.483927247898546575, 111.0405762719810525 ) ) ;
#132941=CARTESIAN_POINT ( 'NONE',  ( -16.51473224551069308, -9.474510206698971260, 66.66557627198102409 ) ) ;
#132942=CARTESIAN_POINT ( 'NONE',  ( 9.474510206698729675, 16.51473224551082808, 97.08442372801900433 ) ) ;
#132944=CARTESIAN_POINT ( 'NONE',  ( -21.53943276465977519, -0.05219959533937600094, 98.75109039468568994 ) ) ;
#132945=CARTESIAN_POINT ( 'NONE',  ( 0.05219959533934541429, -16.53943276465976808, 70.00109039468568994 ) ) ;
#132946=CARTESIAN_POINT ( 'NONE',  ( -9.474510206698720793, -16.51473224551083518, 94.58442372801900433 ) ) ;
#132947=CARTESIAN_POINT ( 'NONE',  ( -15.72974639402197994, 15.80617190586746368, 60.62390960531437401 ) ) ;
#132948=CARTESIAN_POINT ( 'NONE',  ( -8.314922557961024197, 14.29746914071037800, 57.91775706135234714 ) ) ;
#132950=CARTESIAN_POINT ( 'NONE',  ( 16.51473224551083163, -9.474510206698727899, 60.83442372801900433 ) ) ;
#132951=CARTESIAN_POINT ( 'NONE',  ( -18.67979575497193778, 10.72451020669871902, 103.3344237280190043 ) ) ;
#132952=CARTESIAN_POINT ( 'NONE',  ( -8.224510206698948167, 14.34966873604960824, 115.4155762719810241 ) ) ;
#132953=CARTESIAN_POINT ( 'NONE',  ( -9.474510206698964154, 16.51473224551069663, 65.41557627198102409 ) ) ;
#132954=CARTESIAN_POINT ( 'NONE',  ( 8.314922557960818139, 14.29746914071049879, 59.58224293864770260 ) ) ;
#132955=CARTESIAN_POINT ( 'NONE',  ( 15.80617190586769283, -15.72974639402175789, 90.62609039468567573 ) ) ;
#132956=CARTESIAN_POINT ( 'NONE',  ( -0.05219959533936034679, 19.03943276465977164, 42.50109039468566152 ) ) ;
#132957=CARTESIAN_POINT ( 'NONE',  ( 16.46253265017146816, 9.564922557961045513, 21.66775706135233648 ) ) ;
#132958=CARTESIAN_POINT ( 'NONE',  ( 18.62759615963271287, -10.81492255796078972, 23.33224293864769194 ) ) ;
#132959=CARTESIAN_POINT ( 'NONE',  ( 10.81492255796106328, -18.62759615963255655, 95.41775706135234714 ) ) ;
#132960=CARTESIAN_POINT ( 'NONE',  ( -9.474510206698964154, 16.51473224551069663, 75.41557627198103830 ) ) ;
#132961=CARTESIAN_POINT ( 'NONE',  ( 0.05219959533937995610, -21.53943276465977519, 90.00109039468567573 ) ) ;
#132962=CARTESIAN_POINT ( 'NONE',  ( -15.72974639402197994, 15.80617190586746368, 50.62390960531435979 ) ) ;
#132963=CARTESIAN_POINT ( 'NONE',  ( 19.02544592524343514, -5.153800228976328945, 83.54057627198100988 ) ) ;
#132964=CARTESIAN_POINT ( 'NONE',  ( 16.46253265017146816, 9.564922557961045513, 76.66775706135234714 ) ) ;
#132965=CARTESIAN_POINT ( 'NONE',  ( 13.97604488694527802, 13.89961937509977652, 39.37390960531435269 ) ) ;
#132966=CARTESIAN_POINT ( 'NONE',  ( 13.97604488694527802, 13.89961937509977652, 94.37390960531436690 ) ) ;
#132967=CARTESIAN_POINT ( 'NONE',  ( 16.46253265017146816, 9.564922557961045513, 86.66775706135233293 ) ) ;
#132968=CARTESIAN_POINT ( 'NONE',  ( -12.14591786802326823, 12.06949235617739902, 43.12609039468568284 ) ) ;
#132969=CARTESIAN_POINT ( 'NONE',  ( 16.53943276465976808, -0.05219959533910856209, 108.7489096053143669 ) ) ;
#132970=CARTESIAN_POINT ( 'NONE',  ( 9.474510206698971260, -16.51473224551069308, 67.91557627198102409 ) ) ;
#132971=CARTESIAN_POINT ( 'NONE',  ( 15.80617190586746368, 15.72974639402197994, 44.37390960531435979 ) ) ;
#132972=CARTESIAN_POINT ( 'NONE',  ( -8.314922557961024197, 14.29746914071037800, 22.91775706135235069 ) ) ;
#132973=CARTESIAN_POINT ( 'NONE',  ( -10.81492255796105439, 18.62759615963255655, 32.91775706135234714 ) ) ;
#132974=CARTESIAN_POINT ( 'NONE',  ( 5.719274019375673035, 21.55341960407619339, 87.29275706135236135 ) ) ;
#132975=CARTESIAN_POINT ( 'NONE',  ( -0.05219959533934338120, 16.53943276465976808, 82.50109039468568994 ) ) ;
#132976=CARTESIAN_POINT ( 'NONE',  ( -5.049401038298153566, 19.05341960407611168, 75.20724293864769550 ) ) ;
#132977=CARTESIAN_POINT ( 'NONE',  ( 16.52544592524335698, 4.483927247898782831, 106.4594237280190328 ) ) ;
#132978=CARTESIAN_POINT ( 'NONE',  ( 13.89961937509957401, 13.97604488694547697, 51.87609039468566863 ) ) ;
#132979=CARTESIAN_POINT ( 'NONE',  ( -18.62759615963255300, -10.81492255796106328, 29.16775706135234003 ) ) ;
#132980=CARTESIAN_POINT ( 'NONE',  ( -0.05219959533910754901, -16.53943276465976808, 77.49890960531433848 ) ) ;
#132981=CARTESIAN_POINT ( 'NONE',  ( 16.51473224551069308, 9.474510206698969483, 94.16557627198103830 ) ) ;
#132982=CARTESIAN_POINT ( 'NONE',  ( -4.379528057220086978, -16.55341960407618274, 104.7927570613523898 ) ) ;
#132983=CARTESIAN_POINT ( 'NONE',  ( 5.719274019375673035, 21.55341960407619339, 77.29275706135234714 ) ) ;
#132984=CARTESIAN_POINT ( 'NONE',  ( 16.55341960407618274, -4.379528057220086978, 36.04275706135234714 ) ) ;
#132985=CARTESIAN_POINT ( 'NONE',  ( -18.67979575497193778, 10.72451020669871902, 28.33442372801902209 ) ) ;
#132986=CARTESIAN_POINT ( 'NONE',  ( 16.52544592524342804, -4.483927247898539470, 68.54057627198103830 ) ) ;
#132988=CARTESIAN_POINT ( 'NONE',  ( 5.719274019375991003, -21.55341960407610458, 102.7072429386476955 ) ) ;
#132989=CARTESIAN_POINT ( 'NONE',  ( 16.53943276465976808, -0.05219959533910856209, 53.74890960531437401 ) ) ;
#132990=CARTESIAN_POINT ( 'NONE',  ( 13.89961937509977652, -13.97604488694527269, 23.12390960531436335 ) ) ;
#132991=CARTESIAN_POINT ( 'NONE',  ( 5.719274019375991003, -21.55341960407610458, 27.70724293864769905 ) ) ;
#132992=CARTESIAN_POINT ( 'NONE',  ( 18.62759615963255655, 10.81492255796105972, 51.66775706135234714 ) ) ;
#132993=CARTESIAN_POINT ( 'NONE',  ( 8.224510206698953496, -14.34966873604960469, 67.91557627198102409 ) ) ;
#132994=CARTESIAN_POINT ( 'NONE',  ( 21.53943276465977519, -0.05219959533907433946, 73.74890960531433848 ) ) ;
#132995=CARTESIAN_POINT ( 'NONE',  ( -5.153800228976328057, -19.02544592524343514, 72.29057627198102409 ) ) ;
#132996=CARTESIAN_POINT ( 'NONE',  ( -19.05341960407611168, -5.049401038298163336, 26.45724293864769550 ) ) ;
#132997=CARTESIAN_POINT ( 'NONE',  ( -5.049401038297874678, -19.05341960407617918, 74.79275706135231871 ) ) ;
#132998=CARTESIAN_POINT ( 'NONE',  ( -5.719274019375665041, -21.55341960407619695, 59.79275706135234714 ) ) ;
#132999=CARTESIAN_POINT ( 'NONE',  ( -0.05219959533907301413, -21.53943276465977519, 62.49890960531436690 ) ) ;
#133000=B_SPLINE_CURVE_WITH_KNOTS ( 'NONE', 3,
 ( #106020, #123169, #158235, #89865, #66222, #167707 ),
 .UNSPECIFIED., .F., .F.,
 ( 4, 2, 4 ),
 ( 0.003989672132298083609, 0.004372778065220518998, 0.004755883998142954386 ),
 .UNSPECIFIED. ) ;
#133001=CARTESIAN_POINT ( 'NONE',  ( -5.049401038298153566, 19.05341960407611168, 40.20724293864768839 ) ) ;
#133002=CARTESIAN_POINT ( 'NONE',  ( -13.89961937509977652, 13.97604488694528158, 70.62390960531432427 ) ) ;
#133003=VERTEX_POINT ( 'NONE', #165722 ) ;
#133004=CARTESIAN_POINT ( 'NONE',  ( 4.483927247898790824, -16.52544592524335698, 45.20942372801901854 ) ) ;
#133005=CARTESIAN_POINT ( 'NONE',  ( -18.62759615963255300, -10.81492255796106328, 34.16775706135234714 ) ) ;
#133006=CARTESIAN_POINT ( 'NONE',  ( -15.72974639402176322, -15.80617190586768395, 59.37609039468568284 ) ) ;
#133007=CARTESIAN_POINT ( 'NONE',  ( 16.51473224551069308, 9.474510206698969483, 99.16557627198102409 ) ) ;
#133008=CARTESIAN_POINT ( 'NONE',  ( -5.823673210054116645, -21.52544592524344225, 82.29057627198103830 ) ) ;
#133009=CARTESIAN_POINT ( 'NONE',  ( -0.05219959533937732626, 21.53943276465977519, 22.50109039468567573 ) ) ;
#133010=CARTESIAN_POINT ( 'NONE',  ( 14.29746914071037800, 8.314922557961029526, 46.66775706135234714 ) ) ;
#133012=CARTESIAN_POINT ( 'NONE',  ( 0.05219959533907565091, 21.53943276465977519, 49.99890960531437401 ) ) ;
#133013=CARTESIAN_POINT ( 'NONE',  ( 18.67979575497194134, -10.72451020669871369, 110.8344237280190043 ) ) ;
#133014=CARTESIAN_POINT ( 'NONE',  ( 13.89961937509977652, -13.97604488694527269, 53.12390960531434558 ) ) ;
#133015=CARTESIAN_POINT ( 'NONE',  ( -9.474510206698964154, 16.51473224551069663, 110.4155762719810383 ) ) ;
#133016=CARTESIAN_POINT ( 'NONE',  ( 16.51473224551069308, 9.474510206698969483, 84.16557627198102409 ) ) ;
#133018=CARTESIAN_POINT ( 'NONE',  ( 16.46253265017146816, 9.564922557961045513, 71.66775706135233293 ) ) ;
#133019=CARTESIAN_POINT ( 'NONE',  ( 10.81492255796078972, 18.62759615963270932, 44.58224293864769550 ) ) ;
#133020=CARTESIAN_POINT ( 'NONE',  ( -12.14591786802309592, -12.06949235617757132, 31.87390960531435979 ) ) ;
#133021=CARTESIAN_POINT ( 'NONE',  ( -0.05219959533936034679, 19.03943276465977164, 87.50109039468567573 ) ) ;
#133022=CARTESIAN_POINT ( 'NONE',  ( -17.44279575226822843, 5.990770900252466724, 60.83557567514318265 ) ) ;
#133023=CARTESIAN_POINT ( 'NONE',  ( 5.719274019375673035, 21.55341960407619339, 112.2927570613523471 ) ) ;
#133024=CARTESIAN_POINT ( 'NONE',  ( 16.46253265017146816, 9.564922557961045513, 81.66775706135233293 ) ) ;
#133025=CARTESIAN_POINT ( 'NONE',  ( -5.049401038297874678, -19.05341960407617918, 49.79275706135231871 ) ) ;
#133027=CARTESIAN_POINT ( 'NONE',  ( 5.049401038298161559, -19.05341960407611168, 57.70724293864769550 ) ) ;
#133028=CARTESIAN_POINT ( 'NONE',  ( 14.29746914071049879, -8.314922557960816363, 48.33224293864770260 ) ) ;
#133029=CARTESIAN_POINT ( 'NONE',  ( 5.153800228976335163, 19.02544592524342804, 34.79057627198102409 ) ) ;
#133030=CARTESIAN_POINT ( 'NONE',  ( -8.314922557960811034, -14.29746914071050412, 42.08224293864769550 ) ) ;
#133032=CARTESIAN_POINT ( 'NONE',  ( 16.52544592524335698, 4.483927247898782831, 111.4594237280190328 ) ) ;
#133033=CARTESIAN_POINT ( 'NONE',  ( 9.564922557960805705, 16.46253265017160317, 44.58224293864769550 ) ) ;
#133034=CARTESIAN_POINT ( 'NONE',  ( -19.03943276465977164, -0.05219959533935918106, 23.75109039468566152 ) ) ;
#133035=CARTESIAN_POINT ( 'NONE',  ( -12.06949235617739369, -12.14591786802326823, 39.37609039468567573 ) ) ;
#133036=CARTESIAN_POINT ( 'NONE',  ( 15.72974639402199770, -15.80617190586745480, 33.12390960531435979 ) ) ;
#133037=CARTESIAN_POINT ( 'NONE',  ( 0.05219959533937995610, -21.53943276465977519, 90.00109039468567573 ) ) ;
#133039=CARTESIAN_POINT ( 'NONE',  ( 0.05219959533909260263, 19.03943276465977164, 59.99890960531436690 ) ) ;
#133040=CARTESIAN_POINT ( 'NONE',  ( -9.564922557960796823, -16.46253265017161027, 107.0822429386476955 ) ) ;
#133041=CARTESIAN_POINT ( 'NONE',  ( 19.02544592524343514, -5.153800228976328945, 98.54057627198100988 ) ) ;
#133043=CARTESIAN_POINT ( 'NONE',  ( 21.53943276465977519, 0.05219959533937863772, 26.25109039468567573 ) ) ;
#133044=CARTESIAN_POINT ( 'NONE',  ( 8.224510206698953496, -14.34966873604960469, 82.91557627198103830 ) ) ;
#133045=CARTESIAN_POINT ( 'NONE',  ( 10.72451020669898902, -18.67979575497178502, 72.91557627198103830 ) ) ;
#133046=CARTESIAN_POINT ( 'NONE',  ( -9.474510206698964154, 16.51473224551069663, 70.41557627198102409 ) ) ;
#133047=CARTESIAN_POINT ( 'NONE',  ( -5.049401038298153566, 19.05341960407611168, 70.20724293864769550 ) ) ;
#133048=CARTESIAN_POINT ( 'NONE',  ( 5.823673210054125526, 21.52544592524343514, 109.7905762719810383 ) ) ;
#133050=CARTESIAN_POINT ( 'NONE',  ( 13.97604488694527802, 13.89961937509977652, 69.37390960531436690 ) ) ;
#133051=CARTESIAN_POINT ( 'NONE',  ( 12.06949235617757843, -12.14591786802309237, 103.1239096053143811 ) ) ;
#133053=CARTESIAN_POINT ( 'NONE',  ( 9.564922557960805705, 16.46253265017160317, 59.58224293864769550 ) ) ;
#133054=CARTESIAN_POINT ( 'NONE',  ( 19.02544592524334988, 5.153800228976608722, 96.45942372801897591 ) ) ;
#133055=CARTESIAN_POINT ( 'NONE',  ( 12.06949235617757843, -12.14591786802309237, 103.1239096053143811 ) ) ;
#133056=CARTESIAN_POINT ( 'NONE',  ( -5.719274019375665041, -21.55341960407619695, 74.79275706135234714 ) ) ;
#133057=CARTESIAN_POINT ( 'NONE',  ( -19.03943276465977164, 0.05219959533909376836, 46.24890960531435979 ) ) ;
#133058=CARTESIAN_POINT ( 'NONE',  ( -15.72974639402176322, -15.80617190586768395, 24.37609039468567573 ) ) ;
#133059=CARTESIAN_POINT ( 'NONE',  ( -16.52544592524342804, 4.483927247898546575, 96.04057627198102409 ) ) ;
#133061=CARTESIAN_POINT ( 'NONE',  ( 16.46253265017160672, -9.564922557960803928, 78.33224293864769550 ) ) ;
#133062=CARTESIAN_POINT ( 'NONE',  ( 16.20579543436677739, 7.371946100355099674, 113.0652083417187441 ) ) ;
#133063=CARTESIAN_POINT ( 'NONE',  ( -12.06949235617739369, -12.14591786802326823, 19.37609039468568639 ) ) ;
#133064=CARTESIAN_POINT ( 'NONE',  ( 21.55341960407610458, 5.719274019375980345, 33.95724293864769550 ) ) ;
#133065=CARTESIAN_POINT ( 'NONE',  ( 15.80617190586769283, -15.72974639402175789, 50.62609039468568994 ) ) ;
#133066=CARTESIAN_POINT ( 'NONE',  ( 13.89961937509977652, -13.97604488694527269, 103.1239096053143527 ) ) ;
#133067=CARTESIAN_POINT ( 'NONE',  ( -13.89961937509957401, -13.97604488694547875, 79.37609039468567573 ) ) ;
#133068=CARTESIAN_POINT ( 'NONE',  ( -16.51473224551069308, -9.474510206698971260, 71.66557627198102409 ) ) ;
#133069=CARTESIAN_POINT ( 'NONE',  ( -4.483927247898539470, -16.52544592524342804, 82.29057627198103830 ) ) ;
#133070=CARTESIAN_POINT ( 'NONE',  ( -16.46253265017160317, 9.564922557960807481, 100.8322429386477097 ) ) ;
#133071=CARTESIAN_POINT ( 'NONE',  ( -16.53943276465976808, 0.05219959533911058130, 91.24890960531436690 ) ) ;
#133072=CARTESIAN_POINT ( 'NONE',  ( 5.049401038298161559, -19.05341960407611168, 92.70724293864769550 ) ) ;
#133073=CARTESIAN_POINT ( 'NONE',  ( 16.52544592524342804, -4.483927247898539470, 43.54057627198103830 ) ) ;
#133074=CARTESIAN_POINT ( 'NONE',  ( -19.05341960407611168, -5.049401038298163336, 31.45724293864769550 ) ) ;
#133076=CARTESIAN_POINT ( 'NONE',  ( -10.81492255796105439, 18.62759615963255655, 57.91775706135234714 ) ) ;
#133077=CARTESIAN_POINT ( 'NONE',  ( -9.564922557961040184, 16.46253265017147172, 82.91775706135233293 ) ) ;
#133078=CARTESIAN_POINT ( 'NONE',  ( 16.52544592524342804, -4.483927247898539470, 43.54057627198103830 ) ) ;
#133079=CARTESIAN_POINT ( 'NONE',  ( 21.52544592524344225, -5.823673210054117533, 98.54057627198105251 ) ) ;
#133080=CARTESIAN_POINT ( 'NONE',  ( 18.62759615963271287, -10.81492255796078972, 33.33224293864769550 ) ) ;
#133081=CARTESIAN_POINT ( 'NONE',  ( -8.314922557960811034, -14.29746914071050412, 87.08224293864769550 ) ) ;
#133082=CARTESIAN_POINT ( 'NONE',  ( 19.05341960407611168, 5.049401038298154454, 53.95724293864770260 ) ) ;
#133083=CARTESIAN_POINT ( 'NONE',  ( -12.14591786802309592, -12.06949235617757132, 21.87390960531436690 ) ) ;
#133084=CARTESIAN_POINT ( 'NONE',  ( -14.34966873604972548, 8.224510206698743886, 88.33442372801901854 ) ) ;
#133085=CARTESIAN_POINT ( 'NONE',  ( -16.52544592524335698, -4.483927247898792601, 73.95942372801901854 ) ) ;
#133086=CARTESIAN_POINT ( 'NONE',  ( -9.474510206698720793, -16.51473224551083518, 19.58442372801899722 ) ) ;
#133087=CARTESIAN_POINT ( 'NONE',  ( 19.02544592524343514, -5.153800228976328945, 88.54057627198102409 ) ) ;
#133088=CARTESIAN_POINT ( 'NONE',  ( -9.564922557960796823, -16.46253265017161027, 82.08224293864768129 ) ) ;
#133089=CARTESIAN_POINT ( 'NONE',  ( 16.52544592524335698, 4.483927247898782831, 91.45942372801901854 ) ) ;
#133090=CARTESIAN_POINT ( 'NONE',  ( -19.03943276465977164, 0.05219959533909376836, 41.24890960531435269 ) ) ;
#133091=CARTESIAN_POINT ( 'NONE',  ( 12.14591786802309770, 12.06949235617756955, 54.37390960531435979 ) ) ;
#133093=CARTESIAN_POINT ( 'NONE',  ( 16.46253265017160672, -9.564922557960803928, 103.3322429386476955 ) ) ;
#133094=CARTESIAN_POINT ( 'NONE',  ( -15.72974639402197994, 15.80617190586746368, 35.62390960531437401 ) ) ;
#133095=CARTESIAN_POINT ( 'NONE',  ( 4.379528057220339221, -16.55341960407611168, 77.70724293864770971 ) ) ;
#133096=CARTESIAN_POINT ( 'NONE',  ( 16.55341960407618274, -4.379528057220086978, 31.04275706135234714 ) ) ;
#133098=CARTESIAN_POINT ( 'NONE',  ( 8.314922557960818139, 14.29746914071049879, 59.58224293864770260 ) ) ;
#133100=CARTESIAN_POINT ( 'NONE',  ( -5.153800228976607833, 19.02544592524334988, 57.70942372801899012 ) ) ;
#133101=CARTESIAN_POINT ( 'NONE',  ( -5.049401038298153566, 19.05341960407611168, 100.2072429386476955 ) ) ;
#133102=CARTESIAN_POINT ( 'NONE',  ( -5.049401038297874678, -19.05341960407617918, 74.79275706135231871 ) ) ;
#133104=CARTESIAN_POINT ( 'NONE',  ( 19.02544592524334988, 5.153800228976608722, 106.4594237280190185 ) ) ;
#133105=CARTESIAN_POINT ( 'NONE',  ( 16.53943276465976808, 0.05219959533934440121, 101.2510903946856757 ) ) ;
#133106=CARTESIAN_POINT ( 'NONE',  ( 9.564922557960805705, 16.46253265017160317, 34.58224293864770260 ) ) ;
#133107=CARTESIAN_POINT ( 'NONE',  ( 18.67979575497178502, 10.72451020669898547, 29.16557627198103120 ) ) ;
#133108=CARTESIAN_POINT ( 'NONE',  ( 21.55341960407619695, -5.719274019375665929, 56.04275706135235424 ) ) ;
#133109=CARTESIAN_POINT ( 'NONE',  ( -19.05341960407617563, 5.049401038297882671, 113.5427570613523471 ) ) ;
#133111=CARTESIAN_POINT ( 'NONE',  ( -16.51473224551069308, -9.474510206698971260, 76.66557627198103830 ) ) ;
#133113=CARTESIAN_POINT ( 'NONE',  ( 16.53943276465976808, -0.05219959533910856209, 68.74890960531435269 ) ) ;
#133114=CARTESIAN_POINT ( 'NONE',  ( -13.97604488694527625, -13.89961937509977652, 71.87390960531433848 ) ) ;
#133115=CARTESIAN_POINT ( 'NONE',  ( -9.564922557960796823, -16.46253265017161027, 92.08224293864769550 ) ) ;
#133116=ORIENTED_EDGE ( 'NONE', *, *, #93518, .F. ) ;
#133117=CARTESIAN_POINT ( 'NONE',  ( 19.05341960407617918, -5.049401038297876454, 96.04275706135231871 ) ) ;
#133118=CARTESIAN_POINT ( 'NONE',  ( 21.55341960407610458, 5.719274019375980345, 63.95724293864770260 ) ) ;
#133119=CARTESIAN_POINT ( 'NONE',  ( -9.474510206698964154, 16.51473224551069663, 35.41557627198102409 ) ) ;
#133120=CARTESIAN_POINT ( 'NONE',  ( -13.97604488694547697, 13.89961937509957934, 63.12609039468566152 ) ) ;
#133121=CARTESIAN_POINT ( 'NONE',  ( -16.46253265017160317, 9.564922557960807481, 60.83224293864769550 ) ) ;
#133122=CARTESIAN_POINT ( 'NONE',  ( 19.03943276465977164, -0.05219959533909143690, 88.74890960531436690 ) ) ;
#133123=VERTEX_POINT ( 'NONE', #73720 ) ;
#133124=CARTESIAN_POINT ( 'NONE',  ( -21.53943276465977519, 0.05219959533907696930, 96.24890960531435269 ) ) ;
#133125=CARTESIAN_POINT ( 'NONE',  ( 16.55341960407611168, 4.379528057220329451, 93.95724293864770971 ) ) ;
#133126=CARTESIAN_POINT ( 'NONE',  ( -19.05341960407617563, 5.049401038297882671, 53.54275706135231871 ) ) ;
#133127=CARTESIAN_POINT ( 'NONE',  ( 0.05219959533907565091, 21.53943276465977519, 94.99890960531436690 ) ) ;
#133128=CARTESIAN_POINT ( 'NONE',  ( -21.53943276465977519, 0.05219959533907696930, 76.24890960531435269 ) ) ;
#133129=CARTESIAN_POINT ( 'NONE',  ( -12.14591786802309592, -12.06949235617757132, 31.87390960531435979 ) ) ;
#133130=CARTESIAN_POINT ( 'NONE',  ( 18.67979575497194134, -10.72451020669871369, 105.8344237280190328 ) ) ;
#133131=CARTESIAN_POINT ( 'NONE',  ( -12.06949235617739369, -12.14591786802326823, 49.37609039468569705 ) ) ;
#133132=CARTESIAN_POINT ( 'NONE',  ( -13.97604488694527625, -13.89961937509977652, 81.87390960531436690 ) ) ;
#133133=CARTESIAN_POINT ( 'NONE',  ( -19.02544592524342804, 5.153800228976336051, 26.04057627198103120 ) ) ;
#133134=CARTESIAN_POINT ( 'NONE',  ( -10.81492255796105439, 18.62759615963255655, 37.91775706135235424 ) ) ;
#133135=CARTESIAN_POINT ( 'NONE',  ( 10.81492255796106328, -18.62759615963255655, 60.41775706135235424 ) ) ;
#133136=CARTESIAN_POINT ( 'NONE',  ( 0.05219959533909260263, 19.03943276465977164, 44.99890960531435979 ) ) ;
#133137=CARTESIAN_POINT ( 'NONE',  ( -18.62759615963255300, -10.81492255796106328, 19.16775706135234714 ) ) ;
#133138=CARTESIAN_POINT ( 'NONE',  ( -5.153800228976607833, 19.02544592524334988, 67.70942372801900433 ) ) ;
#133139=CARTESIAN_POINT ( 'NONE',  ( 5.049401038297881783, 19.05341960407617563, 77.29275706135231871 ) ) ;
#133140=CARTESIAN_POINT ( 'NONE',  ( -14.34966873604972548, 8.224510206698743886, 28.33442372801902209 ) ) ;
#133141=CARTESIAN_POINT ( 'NONE',  ( -5.049401038298153566, 19.05341960407611168, 30.20724293864768839 ) ) ;
#133142=CARTESIAN_POINT ( 'NONE',  ( -16.53943276465976808, -0.05219959533934237506, 73.75109039468567573 ) ) ;
#133143=CARTESIAN_POINT ( 'NONE',  ( 13.97604488694527802, 13.89961937509977652, 44.37390960531435269 ) ) ;
#133145=CARTESIAN_POINT ( 'NONE',  ( 5.153800228976335163, 19.02544592524342804, 104.7905762719809957 ) ) ;
#133146=CARTESIAN_POINT ( 'NONE',  ( -19.05341960407611168, -5.049401038298163336, 31.45724293864769550 ) ) ;
#133147=CARTESIAN_POINT ( 'NONE',  ( -21.52544592524343514, 5.823673210054127303, 71.04057627198103830 ) ) ;
#133148=CARTESIAN_POINT ( 'NONE',  ( -12.06949235617739369, -12.14591786802326823, 59.37609039468568284 ) ) ;
#133149=CARTESIAN_POINT ( 'NONE',  ( -21.53943276465977519, -0.05219959533937600094, 108.7510903946857042 ) ) ;
#133151=CARTESIAN_POINT ( 'NONE',  ( -0.05219959533909027116, -19.03943276465977164, 42.49890960531435269 ) ) ;
#133152=CARTESIAN_POINT ( 'NONE',  ( -12.06949235617756955, 12.14591786802309770, 25.62390960531435624 ) ) ;
#133153=CARTESIAN_POINT ( 'NONE',  ( -8.314922557960811034, -14.29746914071050412, 62.08224293864769550 ) ) ;
#133154=CARTESIAN_POINT ( 'NONE',  ( 19.02544592524343514, -5.153800228976328945, 68.54057627198103830 ) ) ;
#133155=CARTESIAN_POINT ( 'NONE',  ( 18.62759615963255655, 10.81492255796105972, 41.66775706135235424 ) ) ;
#133156=CARTESIAN_POINT ( 'NONE',  ( -13.97604488694527625, -13.89961937509977652, 81.87390960531436690 ) ) ;
#133157=CARTESIAN_POINT ( 'NONE',  ( 15.80617190586769283, -15.72974639402175789, 85.62609039468568994 ) ) ;
#133158=CARTESIAN_POINT ( 'NONE',  ( -14.29746914071037622, -8.314922557961029526, 69.16775706135234714 ) ) ;
#133159=CARTESIAN_POINT ( 'NONE',  ( -5.049401038298153566, 19.05341960407611168, 105.2072429386476671 ) ) ;
#133160=CARTESIAN_POINT ( 'NONE',  ( -16.52544592524342804, 4.483927247898546575, 46.04057627198103830 ) ) ;
#133161=CARTESIAN_POINT ( 'NONE',  ( -16.51473224551069308, -9.474510206698971260, 21.66557627198102765 ) ) ;
#133162=CARTESIAN_POINT ( 'NONE',  ( -14.29746914071037622, -8.314922557961029526, 49.16775706135234003 ) ) ;
#133163=CARTESIAN_POINT ( 'NONE',  ( -8.224510206698948167, 14.34966873604960824, 60.41557627198102409 ) ) ;
#133165=CARTESIAN_POINT ( 'NONE',  ( -5.823673210054116645, -21.52544592524344225, 22.29057627198102765 ) ) ;
#133166=CARTESIAN_POINT ( 'NONE',  ( -10.81492255796078084, -18.62759615963271287, 27.08224293864769550 ) ) ;
#133167=CARTESIAN_POINT ( 'NONE',  ( 21.55341960407619695, -5.719274019375665929, 111.0427570613523613 ) ) ;
#133169=CARTESIAN_POINT ( 'NONE',  ( -14.29746914071049879, 8.314922557960819915, 90.83224293864769550 ) ) ;
#133170=CARTESIAN_POINT ( 'NONE',  ( -19.02544592524342804, 5.153800228976336051, 101.0405762719810241 ) ) ;
#133171=VERTEX_POINT ( 'NONE', #87861 ) ;
#133172=CARTESIAN_POINT ( 'NONE',  ( 4.483927247898790824, -16.52544592524335698, 60.20942372801902565 ) ) ;
#133173=CARTESIAN_POINT ( 'NONE',  ( -5.049401038298153566, 19.05341960407611168, 55.20724293864769550 ) ) ;
#133175=CARTESIAN_POINT ( 'NONE',  ( -5.049401038297874678, -19.05341960407617918, 49.79275706135231871 ) ) ;
#133176=CARTESIAN_POINT ( 'NONE',  ( 14.34966873604972726, -8.224510206698740333, 80.83442372801901854 ) ) ;
#133177=CARTESIAN_POINT ( 'NONE',  ( 5.049401038297881783, 19.05341960407617563, 102.2927570613523045 ) ) ;
#133178=CARTESIAN_POINT ( 'NONE',  ( -21.53943276465977519, -0.05219959533937600094, 63.75109039468568284 ) ) ;
#133179=CARTESIAN_POINT ( 'NONE',  ( 5.049401038298161559, -19.05341960407611168, 72.70724293864768129 ) ) ;
#133180=CARTESIAN_POINT ( 'NONE',  ( 15.80617190586746368, 15.72974639402197994, 89.37390960531435269 ) ) ;
#133181=CARTESIAN_POINT ( 'NONE',  ( 16.52544592524342804, -4.483927247898539470, 103.5405762719810383 ) ) ;
#133182=CARTESIAN_POINT ( 'NONE',  ( -13.97604488694547697, 13.89961937509957934, 73.12609039468568994 ) ) ;
#133183=CARTESIAN_POINT ( 'NONE',  ( 15.80617190586746368, 15.72974639402197994, 69.37390960531436690 ) ) ;
#133184=CARTESIAN_POINT ( 'NONE',  ( 16.51473224551083163, -9.474510206698727899, 35.83442372801899722 ) ) ;
#133185=CARTESIAN_POINT ( 'NONE',  ( -5.823673210054116645, -21.52544592524344225, 92.29057627198103830 ) ) ;
#133186=CARTESIAN_POINT ( 'NONE',  ( 18.22780087662125226, -5.499999999999864997, 51.01540105326108687 ) ) ;
#133187=CARTESIAN_POINT ( 'NONE',  ( -13.89961937509977652, 13.97604488694528158, 60.62390960531436690 ) ) ;
#133188=LINE ( 'NONE', #76243, #195009 ) ;
#133189=CARTESIAN_POINT ( 'NONE',  ( 5.153800228976615827, -19.02544592524334988, 110.2094237280189901 ) ) ;
#133191=CARTESIAN_POINT ( 'NONE',  ( 19.02544592524343514, -5.153800228976328945, 53.54057627198102409 ) ) ;
#133192=CARTESIAN_POINT ( 'NONE',  ( -13.89961937509977652, 13.97604488694528158, 105.6239096053143527 ) ) ;
#133193=CARTESIAN_POINT ( 'NONE',  ( 5.823673210054125526, 21.52544592524343514, 84.79057627198102409 ) ) ;
#133194=CARTESIAN_POINT ( 'NONE',  ( -4.379528057220328563, 16.55341960407611168, 45.20724293864769550 ) ) ;
#133195=CARTESIAN_POINT ( 'NONE',  ( 21.55341960407619695, -5.719274019375665929, 76.04275706135237556 ) ) ;
#133196=CARTESIAN_POINT ( 'NONE',  ( 8.314922557961029526, -14.29746914071037800, 25.41775706135235779 ) ) ;
#133197=CARTESIAN_POINT ( 'NONE',  ( -9.474510206698720793, -16.51473224551083518, 24.58442372801900078 ) ) ;
#133198=CARTESIAN_POINT ( 'NONE',  ( 16.52544592524342804, -4.483927247898539470, 28.54057627198103120 ) ) ;
#133199=CARTESIAN_POINT ( 'NONE',  ( 10.81492255796078972, 18.62759615963270932, 109.5822429386476955 ) ) ;
#133200=CARTESIAN_POINT ( 'NONE',  ( 14.29746914071049879, -8.314922557960816363, 48.33224293864770260 ) ) ;
#133201=CARTESIAN_POINT ( 'NONE',  ( -19.02544592524334988, -5.153800228976617603, 98.95942372801900433 ) ) ;
#133202=CARTESIAN_POINT ( 'NONE',  ( -5.153800228976607833, 19.02544592524334988, 72.70942372801900433 ) ) ;
#133203=CARTESIAN_POINT ( 'NONE',  ( 10.72451020669871369, 18.67979575497193778, 67.08442372801901854 ) ) ;
#133204=CARTESIAN_POINT ( 'NONE',  ( 5.049401038297881783, 19.05341960407617563, 57.29275706135231871 ) ) ;
#133205=CARTESIAN_POINT ( 'NONE',  ( 9.564922557960805705, 16.46253265017160317, 29.58224293864769550 ) ) ;
#133206=CARTESIAN_POINT ( 'NONE',  ( -5.719274019375978568, 21.55341960407610458, 45.20724293864769550 ) ) ;
#133207=CARTESIAN_POINT ( 'NONE',  ( 16.53943276465976808, -0.05219959533910856209, 48.74890960531435979 ) ) ;
#133208=CARTESIAN_POINT ( 'NONE',  ( -18.39635199886970440, 5.499999999999980460, 96.01967076360006104 ) ) ;
#133209=CARTESIAN_POINT ( 'NONE',  ( 0.05219959533936267826, -19.03943276465977164, 20.00109039468567218 ) ) ;
#133210=CARTESIAN_POINT ( 'NONE',  ( 16.55341960407618274, -4.379528057220086978, 86.04275706135236135 ) ) ;
#133211=CARTESIAN_POINT ( 'NONE',  ( 4.483927247898545687, 16.52544592524342804, 44.79057627198103120 ) ) ;
#133212=CARTESIAN_POINT ( 'NONE',  ( -5.719274019375665041, -21.55341960407619695, 74.79275706135234714 ) ) ;
#133213=CARTESIAN_POINT ( 'NONE',  ( -21.55341960407619339, 5.719274019375674811, 73.54275706135234714 ) ) ;
#133214=CARTESIAN_POINT ( 'NONE',  ( 5.719274019375991003, -21.55341960407610458, 77.70724293864770971 ) ) ;
#133215=CARTESIAN_POINT ( 'NONE',  ( -19.03943276465977164, 0.05219959533909376836, 41.24890960531435269 ) ) ;
#133216=CARTESIAN_POINT ( 'NONE',  ( -0.05219959533937732626, 21.53943276465977519, 52.50109039468567573 ) ) ;
#133217=CARTESIAN_POINT ( 'NONE',  ( 16.46253265017160672, -9.564922557960803928, 33.33224293864770260 ) ) ;
#133218=CARTESIAN_POINT ( 'NONE',  ( -9.564922557960796823, -16.46253265017161027, 47.08224293864769550 ) ) ;
#133219=CARTESIAN_POINT ( 'NONE',  ( 14.29746914071049879, -8.314922557960816363, 93.33224293864769550 ) ) ;
#133220=CARTESIAN_POINT ( 'NONE',  ( -19.05341960407611168, -5.049401038298163336, 81.45724293864769550 ) ) ;
#133221=CARTESIAN_POINT ( 'NONE',  ( 0.05219959533910956823, 16.53943276465976808, 39.99890960531436690 ) ) ;
#133222=CARTESIAN_POINT ( 'NONE',  ( 16.52544592524342804, -4.483927247898539470, 98.54057627198105251 ) ) ;
#133223=CARTESIAN_POINT ( 'NONE',  ( -18.62759615963270932, 10.81492255796079327, 70.83224293864770971 ) ) ;
#133224=CARTESIAN_POINT ( 'NONE',  ( -15.72974639402176322, -15.80617190586768395, 24.37609039468567573 ) ) ;
#133226=CARTESIAN_POINT ( 'NONE',  ( 5.049401038298161559, -19.05341960407611168, 82.70724293864770971 ) ) ;
#133227=CARTESIAN_POINT ( 'NONE',  ( 8.314922557961029526, -14.29746914071037800, 30.41775706135234358 ) ) ;
#133228=CARTESIAN_POINT ( 'NONE',  ( -10.72451020669898014, 18.67979575497178502, 75.41557627198102409 ) ) ;
#133229=CARTESIAN_POINT ( 'NONE',  ( -5.823673210054431948, 21.52544592524334988, 92.70942372801901854 ) ) ;
#133230=CARTESIAN_POINT ( 'NONE',  ( 19.02544592524343514, -5.153800228976328945, 83.54057627198100988 ) ) ;
#133231=CARTESIAN_POINT ( 'NONE',  ( -18.62759615963270932, 10.81492255796079327, 110.8322429386476955 ) ) ;
#133232=CARTESIAN_POINT ( 'NONE',  ( 13.97604488694527802, 13.89961937509977652, 109.3739096053143669 ) ) ;
#133233=CARTESIAN_POINT ( 'NONE',  ( -12.06949235617739369, -12.14591786802326823, 94.37609039468568994 ) ) ;
#133234=CARTESIAN_POINT ( 'NONE',  ( 21.55341960407619695, -5.719274019375665929, 76.04275706135237556 ) ) ;
#133235=CARTESIAN_POINT ( 'NONE',  ( -21.53943276465977519, -0.05219959533937600094, 93.75109039468567573 ) ) ;
#133236=CARTESIAN_POINT ( 'NONE',  ( -8.314922557961024197, 14.29746914071037800, 62.91775706135236135 ) ) ;
#133237=CARTESIAN_POINT ( 'NONE',  ( 21.52544592524334988, 5.823673210054432836, 26.45942372801901854 ) ) ;
#133238=CARTESIAN_POINT ( 'NONE',  ( 13.97604488694527802, 13.89961937509977652, 114.3739096053143669 ) ) ;
#133239=CARTESIAN_POINT ( 'NONE',  ( -18.67979575497193778, 10.72451020669871902, 88.33442372801901854 ) ) ;
#133240=CARTESIAN_POINT ( 'NONE',  ( -0.05219959533909027116, -19.03943276465977164, 97.49890960531436690 ) ) ;
#133241=CARTESIAN_POINT ( 'NONE',  ( -15.72974639402197994, 15.80617190586746368, 95.62390960531436690 ) ) ;
#133242=CARTESIAN_POINT ( 'NONE',  ( -19.05341960407617563, 5.049401038297882671, 58.54275706135234003 ) ) ;
#133244=CARTESIAN_POINT ( 'NONE',  ( 21.53943276465977519, -0.05219959533907433946, 58.74890960531436690 ) ) ;
#133245=CARTESIAN_POINT ( 'NONE',  ( 16.46253265017160672, -9.564922557960803928, 88.33224293864769550 ) ) ;
#133246=CARTESIAN_POINT ( 'NONE',  ( 8.314922557960818139, 14.29746914071049879, 34.58224293864770260 ) ) ;
#133248=CARTESIAN_POINT ( 'NONE',  ( 5.049401038297881783, 19.05341960407617563, 77.29275706135231871 ) ) ;
#133250=CARTESIAN_POINT ( 'NONE',  ( -13.97604488694547697, 13.89961937509957934, 113.1260903946856757 ) ) ;
#133251=CARTESIAN_POINT ( 'NONE',  ( -15.80617190586745835, -15.72974639402198527, 86.87390960531438111 ) ) ;
#133252=CARTESIAN_POINT ( 'NONE',  ( 16.55341960407611168, 4.379528057220329451, 63.95724293864770260 ) ) ;
#133253=CARTESIAN_POINT ( 'NONE',  ( -5.049401038298153566, 19.05341960407611168, 95.20724293864770971 ) ) ;
#133254=CARTESIAN_POINT ( 'NONE',  ( 16.53943276465976808, 0.05219959533934440121, 26.25109039468567573 ) ) ;
#133255=CARTESIAN_POINT ( 'NONE',  ( 5.049401038298161559, -19.05341960407611168, 47.70724293864770260 ) ) ;
#133256=CARTESIAN_POINT ( 'NONE',  ( -21.55341960407610458, -5.719274019375992779, 111.4572429386476813 ) ) ;
#133257=CARTESIAN_POINT ( 'NONE',  ( 16.51473224551083163, -9.474510206698727899, 85.83442372801900433 ) ) ;
#133258=CARTESIAN_POINT ( 'NONE',  ( -16.51473224551069308, -9.474510206698971260, 96.66557627198102409 ) ) ;
#133259=CARTESIAN_POINT ( 'NONE',  ( -5.049401038298153566, 19.05341960407611168, 75.20724293864769550 ) ) ;
#133260=CARTESIAN_POINT ( 'NONE',  ( -18.62759615963270932, 10.81492255796079327, 70.83224293864770971 ) ) ;
#133261=CARTESIAN_POINT ( 'NONE',  ( 0.05219959533909260263, 19.03943276465977164, 49.99890960531435979 ) ) ;
#133263=CARTESIAN_POINT ( 'NONE',  ( 4.483927247898545687, 16.52544592524342804, 49.79057627198102409 ) ) ;
#133264=CARTESIAN_POINT ( 'NONE',  ( 19.05341960407611168, 5.049401038298154454, 98.95724293864766707 ) ) ;
#133266=CARTESIAN_POINT ( 'NONE',  ( -16.51473224551082808, 9.474510206698731452, 68.33442372801900433 ) ) ;
#133267=CARTESIAN_POINT ( 'NONE',  ( 21.52544592524344225, -5.823673210054117533, 83.54057627198102409 ) ) ;
#133268=CARTESIAN_POINT ( 'NONE',  ( -16.46253265017146816, -9.564922557961047289, 54.16775706135234003 ) ) ;
#133269=CARTESIAN_POINT ( 'NONE',  ( -0.05219959533909027116, -19.03943276465977164, 102.4989096053143669 ) ) ;
#133271=CARTESIAN_POINT ( 'NONE',  ( 21.52544592524344225, -5.823673210054117533, 43.54057627198103830 ) ) ;
#133272=CARTESIAN_POINT ( 'NONE',  ( -0.05219959533909027116, -19.03943276465977164, 67.49890960531436690 ) ) ;
#133273=CARTESIAN_POINT ( 'NONE',  ( 15.72974639402176855, 15.80617190586768217, 71.87609039468568994 ) ) ;
#133274=CARTESIAN_POINT ( 'NONE',  ( 16.52544592524342804, -4.483927247898539470, 113.5405762719810383 ) ) ;
#133275=CARTESIAN_POINT ( 'NONE',  ( 5.719274019375673035, 21.55341960407619339, 22.29275706135235069 ) ) ;
#133277=CARTESIAN_POINT ( 'NONE',  ( 18.67979575497194134, -10.72451020669871369, 50.83442372801901143 ) ) ;
#133278=ORIENTED_EDGE ( 'NONE', *, *, #11460, .T. ) ;
#133279=CARTESIAN_POINT ( 'NONE',  ( -16.46253265017160317, 9.564922557960807481, 110.8322429386476955 ) ) ;
#133280=CARTESIAN_POINT ( 'NONE',  ( 16.51473224551083163, -9.474510206698727899, 65.83442372801900433 ) ) ;
#133283=CARTESIAN_POINT ( 'NONE',  ( 10.72451020669898902, -18.67979575497178502, 107.9155762719810241 ) ) ;
#133284=CARTESIAN_POINT ( 'NONE',  ( -19.02544592524342804, 5.153800228976336051, 66.04057627198103830 ) ) ;
#133285=CARTESIAN_POINT ( 'NONE',  ( -4.483927247898782831, 16.52544592524335698, 42.70942372801901854 ) ) ;
#133287=CARTESIAN_POINT ( 'NONE',  ( -0.05219959533937732626, 21.53943276465977519, 102.5010903946856899 ) ) ;
#133288=CARTESIAN_POINT ( 'NONE',  ( -9.564922557960796823, -16.46253265017161027, 37.08224293864768839 ) ) ;
#133289=CARTESIAN_POINT ( 'NONE',  ( 13.97604488694548053, -13.89961937509957401, 20.62609039468567573 ) ) ;
#133290=CARTESIAN_POINT ( 'NONE',  ( 4.483927247898790824, -16.52544592524335698, 85.20942372801901854 ) ) ;
#133291=CARTESIAN_POINT ( 'NONE',  ( -5.049401038298153566, 19.05341960407611168, 95.20724293864770971 ) ) ;
#133292=CARTESIAN_POINT ( 'NONE',  ( -21.52544592524334988, -5.823673210054445271, 53.95942372801900433 ) ) ;
#133294=CARTESIAN_POINT ( 'NONE',  ( -16.46253265017160317, 9.564922557960807481, 115.8322429386477097 ) ) ;
#133295=CARTESIAN_POINT ( 'NONE',  ( 17.72560187377285601, 5.500000000000048850, 46.57814504131322053 ) ) ;
#133296=CARTESIAN_POINT ( 'NONE',  ( -16.53943276465976808, -0.05219959533934237506, 48.75109039468568284 ) ) ;
#133297=CARTESIAN_POINT ( 'NONE',  ( 0.05219959533937995610, -21.53943276465977519, 70.00109039468568994 ) ) ;
#133298=CARTESIAN_POINT ( 'NONE',  ( -21.52544592524334988, -5.823673210054445271, 93.95942372801903275 ) ) ;
#133300=CARTESIAN_POINT ( 'NONE',  ( 8.314922557961029526, -14.29746914071037800, 25.41775706135235779 ) ) ;
#133301=CARTESIAN_POINT ( 'NONE',  ( -19.02544592524342804, 5.153800228976336051, 91.04057627198100988 ) ) ;
#133303=CARTESIAN_POINT ( 'NONE',  ( 16.51473224551069308, 9.474510206698969483, 109.1655762719810383 ) ) ;
#133305=CARTESIAN_POINT ( 'NONE',  ( 17.50000000000000355, 5.622605283950885990, 43.81207310596114013 ) ) ;
#133306=CARTESIAN_POINT ( 'NONE',  ( -4.379528057220328563, 16.55341960407611168, 115.2072429386476955 ) ) ;
#133307=CARTESIAN_POINT ( 'NONE',  ( 10.72451020669898902, -18.67979575497178502, 42.91557627198103120 ) ) ;
#133308=CARTESIAN_POINT ( 'NONE',  ( -12.06949235617739369, -12.14591786802326823, 109.3760903946857042 ) ) ;
#133309=CARTESIAN_POINT ( 'NONE',  ( -14.29746914071049879, 8.314922557960819915, 85.83224293864768129 ) ) ;
#133310=CARTESIAN_POINT ( 'NONE',  ( 9.564922557960805705, 16.46253265017160317, 64.58224293864769550 ) ) ;
#133311=CARTESIAN_POINT ( 'NONE',  ( 21.53943276465977519, 0.05219959533937863772, 86.25109039468568994 ) ) ;
#133312=CARTESIAN_POINT ( 'NONE',  ( -4.379528057220086978, -16.55341960407618274, 29.79275706135234358 ) ) ;
#133313=CARTESIAN_POINT ( 'NONE',  ( 12.14591786802309770, 12.06949235617756955, 84.37390960531438111 ) ) ;
#133314=CARTESIAN_POINT ( 'NONE',  ( -21.55341960407619339, 5.719274019375674811, 38.54275706135234714 ) ) ;
#133315=CARTESIAN_POINT ( 'NONE',  ( 21.52544592524344225, -5.823673210054117533, 73.54057627198102409 ) ) ;
#133316=CARTESIAN_POINT ( 'NONE',  ( 13.89961937509957401, 13.97604488694547697, 31.87609039468566863 ) ) ;
#133318=CARTESIAN_POINT ( 'NONE',  ( 16.46253265017160672, -9.564922557960803928, 98.33224293864769550 ) ) ;
#133319=CARTESIAN_POINT ( 'NONE',  ( 12.14591786802309770, 12.06949235617756955, 64.37390960531435269 ) ) ;
#133320=CARTESIAN_POINT ( 'NONE',  ( -4.379528057220328563, 16.55341960407611168, 55.20724293864770260 ) ) ;
#133321=CARTESIAN_POINT ( 'NONE',  ( 16.52544592524335698, 4.483927247898782831, 111.4594237280190328 ) ) ;
#133322=CARTESIAN_POINT ( 'NONE',  ( -19.02544592524334988, -5.153800228976617603, 63.95942372801899012 ) ) ;
#133323=CARTESIAN_POINT ( 'NONE',  ( 18.22780087662126647, 5.499999999999818812, 51.48236817873107896 ) ) ;
#133324=CARTESIAN_POINT ( 'NONE',  ( -5.153800228976328057, -19.02544592524343514, 112.2905762719810099 ) ) ;
#133325=CARTESIAN_POINT ( 'NONE',  ( -0.05219959533910754901, -16.53943276465976808, 82.49890960531436690 ) ) ;
#133326=CARTESIAN_POINT ( 'NONE',  ( 19.48255537605750831, -5.500000000000005329, 37.64712184717532750 ) ) ;
#133327=CARTESIAN_POINT ( 'NONE',  ( 19.03943276465977164, -0.05219959533909143690, 48.74890960531435979 ) ) ;
#133328=CARTESIAN_POINT ( 'NONE',  ( 21.52544592524344225, -5.823673210054117533, 48.54057627198103120 ) ) ;
#133329=CARTESIAN_POINT ( 'NONE',  ( 0.05219959533907565091, 21.53943276465977519, 84.99890960531436690 ) ) ;
#133330=CARTESIAN_POINT ( 'NONE',  ( -16.55341960407611168, -4.379528057220339221, 111.4572429386476813 ) ) ;
#133331=CARTESIAN_POINT ( 'NONE',  ( 16.53943276465976808, 0.05219959533934440121, 71.25109039468568994 ) ) ;
#133332=CARTESIAN_POINT ( 'NONE',  ( -13.97604488694527625, -13.89961937509977652, 51.87390960531436690 ) ) ;
#133333=CARTESIAN_POINT ( 'NONE',  ( -19.05341960407617563, 5.049401038297882671, 38.54275706135233293 ) ) ;
#133334=CARTESIAN_POINT ( 'NONE',  ( 18.67979575497194134, -10.72451020669871369, 55.83442372801901854 ) ) ;
#133335=CARTESIAN_POINT ( 'NONE',  ( -14.29746914071049879, 8.314922557960819915, 105.8322429386476955 ) ) ;
#133336=CARTESIAN_POINT ( 'NONE',  ( 9.474510206698729675, 16.51473224551082808, 97.08442372801900433 ) ) ;
#133338=CARTESIAN_POINT ( 'NONE',  ( -18.22780087662123094, -5.499999999999984901, 91.48459894673894155 ) ) ;
#133339=CARTESIAN_POINT ( 'NONE',  ( -21.52544592524343514, 5.823673210054127303, 46.04057627198103830 ) ) ;
#133340=CARTESIAN_POINT ( 'NONE',  ( 19.05341960407611168, 5.049401038298154454, 23.95724293864769194 ) ) ;
#133341=CARTESIAN_POINT ( 'NONE',  ( -18.67979575497193778, 10.72451020669871902, 83.33442372801903275 ) ) ;
#133342=CARTESIAN_POINT ( 'NONE',  ( -8.314922557960811034, -14.29746914071050412, 37.08224293864768129 ) ) ;
#133343=CARTESIAN_POINT ( 'NONE',  ( 4.379528057220092307, 16.55341960407617563, 52.29275706135236135 ) ) ;
#133344=CARTESIAN_POINT ( 'NONE',  ( -0.05219959533910754901, -16.53943276465976808, 37.49890960531436690 ) ) ;
#133345=CARTESIAN_POINT ( 'NONE',  ( -5.719274019375978568, 21.55341960407610458, 75.20724293864769550 ) ) ;
#133346=CARTESIAN_POINT ( 'NONE',  ( -10.81492255796078084, -18.62759615963271287, 82.08224293864768129 ) ) ;
#133348=CARTESIAN_POINT ( 'NONE',  ( -13.97604488694547697, 13.89961937509957934, 88.12609039468563310 ) ) ;
#133349=CARTESIAN_POINT ( 'NONE',  ( 16.51473224551069308, 9.474510206698969483, 109.1655762719810383 ) ) ;
#133350=CARTESIAN_POINT ( 'NONE',  ( 13.89961937509977652, -13.97604488694527269, 43.12390960531434558 ) ) ;
#133351=CARTESIAN_POINT ( 'NONE',  ( 19.05341960407611168, 5.049401038298154454, 33.95724293864769550 ) ) ;
#133354=ORIENTED_EDGE ( 'NONE', *, *, #112928, .F. ) ;
#133355=CARTESIAN_POINT ( 'NONE',  ( 8.314922557961029526, -14.29746914071037800, 85.41775706135236135 ) ) ;
#133356=CARTESIAN_POINT ( 'NONE',  ( 0.05219959533907565091, 21.53943276465977519, 109.9989096053143527 ) ) ;
#133357=CARTESIAN_POINT ( 'NONE',  ( -13.89961937509977652, 13.97604488694528158, 75.62390960531438111 ) ) ;
#133358=CARTESIAN_POINT ( 'NONE',  ( -10.72451020669870658, -18.67979575497194134, 44.58442372801901854 ) ) ;
#133359=CARTESIAN_POINT ( 'NONE',  ( 13.89961937509977652, -13.97604488694527269, 98.12390960531433848 ) ) ;
#133362=CARTESIAN_POINT ( 'NONE',  ( 18.62759615963255655, 10.81492255796105972, 31.66775706135234358 ) ) ;
#133363=CARTESIAN_POINT ( 'NONE',  ( 19.03943276465977164, -0.05219959533909143690, 113.7489096053143669 ) ) ;
#133364=CARTESIAN_POINT ( 'NONE',  ( -19.03943276465977164, 0.05219959533909376836, 101.2489096053143669 ) ) ;
#133365=CARTESIAN_POINT ( 'NONE',  ( 0.05219959533936267826, -19.03943276465977164, 35.00109039468566863 ) ) ;
#133366=CARTESIAN_POINT ( 'NONE',  ( -21.52544592524334988, -5.823673210054445271, 18.95942372801901143 ) ) ;
#133367=CARTESIAN_POINT ( 'NONE',  ( 19.03943276465977164, 0.05219959533936151252, 41.25109039468566152 ) ) ;
#133368=CARTESIAN_POINT ( 'NONE',  ( 19.05341960407617918, -5.049401038297876454, 46.04275706135233293 ) ) ;
#133369=CARTESIAN_POINT ( 'NONE',  ( 4.379528057220092307, 16.55341960407617563, 97.29275706135234714 ) ) ;
#133372=CARTESIAN_POINT ( 'NONE',  ( -19.03943276465977164, 0.05219959533909376836, 71.24890960531435269 ) ) ;
#133373=CARTESIAN_POINT ( 'NONE',  ( -18.62759615963255300, -10.81492255796106328, 74.16775706135231871 ) ) ;
#133374=CARTESIAN_POINT ( 'NONE',  ( -18.62759615963255300, -10.81492255796106328, 89.16775706135236135 ) ) ;
#133376=CARTESIAN_POINT ( 'NONE',  ( 9.474510206698971260, -16.51473224551069308, 82.91557627198103830 ) ) ;
#133377=CARTESIAN_POINT ( 'NONE',  ( -21.53943276465977519, -0.05219959533937600094, 68.75109039468568994 ) ) ;
#133378=CARTESIAN_POINT ( 'NONE',  ( -13.97604488694547697, 13.89961937509957934, 98.12609039468566152 ) ) ;
#133379=CARTESIAN_POINT ( 'NONE',  ( -19.05341960407611168, -5.049401038298163336, 66.45724293864769550 ) ) ;
#133380=CARTESIAN_POINT ( 'NONE',  ( -19.03943276465977164, 0.05219959533909376836, 106.2489096053143669 ) ) ;
#133381=CARTESIAN_POINT ( 'NONE',  ( 0.05219959533909260263, 19.03943276465977164, 84.99890960531436690 ) ) ;
#133382=CARTESIAN_POINT ( 'NONE',  ( -17.49999999999999645, -5.499999999999992895, 89.20309617465829888 ) ) ;
#133383=CARTESIAN_POINT ( 'NONE',  ( -0.05219959533909027116, -19.03943276465977164, 67.49890960531436690 ) ) ;
#133384=CARTESIAN_POINT ( 'NONE',  ( 19.03943276465977164, -0.05219959533909143690, 53.74890960531436690 ) ) ;
#133385=CARTESIAN_POINT ( 'NONE',  ( -21.52544592524343514, 5.823673210054127303, 116.0405762719810383 ) ) ;
#133386=CARTESIAN_POINT ( 'NONE',  ( -14.29746914071037622, -8.314922557961029526, 99.16775706135234714 ) ) ;
#133389=CARTESIAN_POINT ( 'NONE',  ( 16.46253265017146816, 9.564922557961045513, 56.66775706135233293 ) ) ;
#133390=CARTESIAN_POINT ( 'NONE',  ( -13.89961937509977652, 13.97604488694528158, 85.62390960531433848 ) ) ;
#133391=CARTESIAN_POINT ( 'NONE',  ( -14.34966873604960291, -8.224510206698953496, 66.66557627198102409 ) ) ;
#133392=CARTESIAN_POINT ( 'NONE',  ( -0.05219959533910754901, -16.53943276465976808, 102.4989096053143811 ) ) ;
#133393=CARTESIAN_POINT ( 'NONE',  ( 10.72451020669898902, -18.67979575497178502, 37.91557627198102409 ) ) ;
#133394=CARTESIAN_POINT ( 'NONE',  ( 15.80617190586746368, 15.72974639402197994, 29.37390960531435269 ) ) ;
#133396=CARTESIAN_POINT ( 'NONE',  ( 16.52544592524342804, -4.483927247898539470, 98.54057627198105251 ) ) ;
#133398=CARTESIAN_POINT ( 'NONE',  ( -5.049401038297874678, -19.05341960407617918, 24.79275706135233648 ) ) ;
#133399=CARTESIAN_POINT ( 'NONE',  ( 12.14591786802327356, -12.06949235617739191, 110.6260903946857042 ) ) ;
#133400=CARTESIAN_POINT ( 'NONE',  ( 0.05219959533909260263, 19.03943276465977164, 89.99890960531436690 ) ) ;
#133401=CARTESIAN_POINT ( 'NONE',  ( -18.67979575497193778, 10.72451020669871902, 58.33442372801901143 ) ) ;
#133402=CARTESIAN_POINT ( 'NONE',  ( 5.823673210054125526, 21.52544592524343514, 49.79057627198102409 ) ) ;
#133403=CARTESIAN_POINT ( 'NONE',  ( 5.719274019375673035, 21.55341960407619339, 27.29275706135234358 ) ) ;
#133404=CARTESIAN_POINT ( 'NONE',  ( 18.62759615963271287, -10.81492255796078972, 78.33224293864770971 ) ) ;
#133405=CARTESIAN_POINT ( 'NONE',  ( 8.224510206698953496, -14.34966873604960469, 97.91557627198103830 ) ) ;
#133406=CARTESIAN_POINT ( 'NONE',  ( 9.474510206698729675, 16.51473224551082808, 62.08442372801899722 ) ) ;
#133408=CARTESIAN_POINT ( 'NONE',  ( -9.474510206698964154, 16.51473224551069663, 40.41557627198103120 ) ) ;
#133409=CARTESIAN_POINT ( 'NONE',  ( -0.05219959533909027116, -19.03943276465977164, 92.49890960531436690 ) ) ;
#133410=CARTESIAN_POINT ( 'NONE',  ( -19.05341960407611168, -5.049401038298163336, 101.4572429386476955 ) ) ;
#133411=CARTESIAN_POINT ( 'NONE',  ( -14.34966873604960291, -8.224510206698953496, 111.6655762719810525 ) ) ;
#133412=CARTESIAN_POINT ( 'NONE',  ( -16.53943276465976808, 0.05219959533911058130, 41.24890960531435269 ) ) ;
#133413=CARTESIAN_POINT ( 'NONE',  ( 16.53943276465976808, 0.05219959533934440121, 36.25109039468567573 ) ) ;
#133414=CARTESIAN_POINT ( 'NONE',  ( -18.67979575497193778, 10.72451020669871902, 103.3344237280190043 ) ) ;
#133415=CARTESIAN_POINT ( 'NONE',  ( -19.02544592524342804, 5.153800228976336051, 116.0405762719810383 ) ) ;
#133416=CARTESIAN_POINT ( 'NONE',  ( -8.314922557961024197, 14.29746914071037800, 112.9177570613523329 ) ) ;
#133417=CARTESIAN_POINT ( 'NONE',  ( -15.72974639402176322, -15.80617190586768395, 39.37609039468567573 ) ) ;
#133418=CARTESIAN_POINT ( 'NONE',  ( -13.97604488694527625, -13.89961937509977652, 106.8739096053143669 ) ) ;
#133419=CARTESIAN_POINT ( 'NONE',  ( -14.29746914071037622, -8.314922557961029526, 39.16775706135235424 ) ) ;
#133420=CARTESIAN_POINT ( 'NONE',  ( -16.55341960407617563, 4.379528057220093196, 113.5427570613523756 ) ) ;
#133421=CARTESIAN_POINT ( 'NONE',  ( 14.29746914071037800, 8.314922557961029526, 96.66775706135234714 ) ) ;
#133422=CARTESIAN_POINT ( 'NONE',  ( 4.483927247898790824, -16.52544592524335698, 30.20942372801902565 ) ) ;
#133423=CARTESIAN_POINT ( 'NONE',  ( -13.89961937509977652, 13.97604488694528158, 35.62390960531435269 ) ) ;
#133424=VECTOR ( 'NONE', #114474, 1000.000000000000000 ) ;
#133425=CARTESIAN_POINT ( 'NONE',  ( 4.379528057220339221, -16.55341960407611168, 107.7072429386476955 ) ) ;
#133426=CARTESIAN_POINT ( 'NONE',  ( -0.05219959533907301413, -21.53943276465977519, 112.4989096053143669 ) ) ;
#133427=CARTESIAN_POINT ( 'NONE',  ( 0.05219959533909260263, 19.03943276465977164, 34.99890960531435979 ) ) ;
#133428=CARTESIAN_POINT ( 'NONE',  ( 5.153800228976335163, 19.02544592524342804, 104.7905762719809957 ) ) ;
#133429=CARTESIAN_POINT ( 'NONE',  ( 5.719274019375673035, 21.55341960407619339, 32.29275706135235424 ) ) ;
#133430=CARTESIAN_POINT ( 'NONE',  ( -16.46253265017160317, 9.564922557960807481, 25.83224293864769194 ) ) ;
#133431=CARTESIAN_POINT ( 'NONE',  ( -0.05219959533909027116, -19.03943276465977164, 102.4989096053143669 ) ) ;
#133432=CARTESIAN_POINT ( 'NONE',  ( 17.05587630539789146, -6.762274262135674618, 113.2418030903731534 ) ) ;
#133433=CARTESIAN_POINT ( 'NONE',  ( 19.02544592524343514, -5.153800228976328945, 98.54057627198100988 ) ) ;
#133434=CARTESIAN_POINT ( 'NONE',  ( 10.72451020669871369, 18.67979575497193778, 47.08442372801901854 ) ) ;
#133435=CARTESIAN_POINT ( 'NONE',  ( -0.05219959533910754901, -16.53943276465976808, 92.49890960531436690 ) ) ;
#133436=CARTESIAN_POINT ( 'NONE',  ( 9.474510206698971260, -16.51473224551069308, 102.9155762719810241 ) ) ;
#133438=CARTESIAN_POINT ( 'NONE',  ( 8.224510206698742110, 14.34966873604972548, 62.08442372801901143 ) ) ;
#133439=CARTESIAN_POINT ( 'NONE',  ( -5.719274019375665041, -21.55341960407619695, 84.79275706135234714 ) ) ;
#133440=CARTESIAN_POINT ( 'NONE',  ( 12.06949235617739724, 12.14591786802326823, 46.87609039468568994 ) ) ;
#133441=CARTESIAN_POINT ( 'NONE',  ( 19.03943276465977164, -0.05219959533909143690, 78.74890960531436690 ) ) ;
#133442=CARTESIAN_POINT ( 'NONE',  ( -14.29746914071037622, -8.314922557961029526, 19.16775706135234714 ) ) ;
#133443=CARTESIAN_POINT ( 'NONE',  ( -12.06949235617739369, -12.14591786802326823, 64.37609039468568994 ) ) ;
#133444=CARTESIAN_POINT ( 'NONE',  ( -0.05219959533937732626, 21.53943276465977519, 112.5010903946857042 ) ) ;
#133445=CARTESIAN_POINT ( 'NONE',  ( 5.049401038297881783, 19.05341960407617563, 87.29275706135234714 ) ) ;
#133446=CARTESIAN_POINT ( 'NONE',  ( -5.153800228976328057, -19.02544592524343514, 57.29057627198103120 ) ) ;
#133447=CARTESIAN_POINT ( 'NONE',  ( 5.823673210054125526, 21.52544592524343514, 79.79057627198102409 ) ) ;
#133448=CARTESIAN_POINT ( 'NONE',  ( 12.06949235617757843, -12.14591786802309237, 88.12390960531436690 ) ) ;
#133449=CARTESIAN_POINT ( 'NONE',  ( 5.153800228976615827, -19.02544592524334988, 95.20942372801897591 ) ) ;
#133450=CARTESIAN_POINT ( 'NONE',  ( 12.14591786802327356, -12.06949235617739191, 60.62609039468567573 ) ) ;
#133452=CARTESIAN_POINT ( 'NONE',  ( -16.51473224551082808, 9.474510206698731452, 63.33442372801900433 ) ) ;
#133453=CARTESIAN_POINT ( 'NONE',  ( -16.52544592524342804, 4.483927247898546575, 36.04057627198102409 ) ) ;
#133454=CARTESIAN_POINT ( 'NONE',  ( -16.52544592524342804, 4.483927247898546575, 76.04057627198102409 ) ) ;
#133455=CARTESIAN_POINT ( 'NONE',  ( -13.89961937509957401, -13.97604488694547875, 19.37609039468566507 ) ) ;
#133456=CARTESIAN_POINT ( 'NONE',  ( -17.48853670773248226, 5.747243402302952830, 38.66671299749993551 ) ) ;
#133457=CARTESIAN_POINT ( 'NONE',  ( 15.80617190586769283, -15.72974639402175789, 25.62609039468567929 ) ) ;
#133458=CARTESIAN_POINT ( 'NONE',  ( 9.564922557960805705, 16.46253265017160317, 104.5822429386476955 ) ) ;
#133459=CARTESIAN_POINT ( 'NONE',  ( -19.05341960407611168, -5.049401038298163336, 76.45724293864769550 ) ) ;
#133460=CARTESIAN_POINT ( 'NONE',  ( -5.823673210054431948, 21.52544592524334988, 92.70942372801901854 ) ) ;
#133461=CARTESIAN_POINT ( 'NONE',  ( -16.46253265017160317, 9.564922557960807481, 75.83224293864769550 ) ) ;
#133462=CARTESIAN_POINT ( 'NONE',  ( 10.72451020669898902, -18.67979575497178502, 37.91557627198102409 ) ) ;
#133463=CARTESIAN_POINT ( 'NONE',  ( 8.314922557960818139, 14.29746914071049879, 74.58224293864768129 ) ) ;
#133464=CARTESIAN_POINT ( 'NONE',  ( 19.02544592524343514, -5.153800228976328945, 38.54057627198103120 ) ) ;
#133465=CARTESIAN_POINT ( 'NONE',  ( -14.34966873604960291, -8.224510206698953496, 91.66557627198103830 ) ) ;
#133466=CARTESIAN_POINT ( 'NONE',  ( 18.62759615963271287, -10.81492255796078972, 108.3322429386477097 ) ) ;
#133467=CARTESIAN_POINT ( 'NONE',  ( 15.72974639402176855, 15.80617190586768217, 61.87609039468568284 ) ) ;
#133468=CARTESIAN_POINT ( 'NONE',  ( -0.05219959533909027116, -19.03943276465977164, 27.49890960531435624 ) ) ;
#133469=CARTESIAN_POINT ( 'NONE',  ( 12.14591786802327356, -12.06949235617739191, 65.62609039468568994 ) ) ;
#133470=CARTESIAN_POINT ( 'NONE',  ( 5.823673210054444382, -21.52544592524334988, 20.20942372801900788 ) ) ;
#133471=CARTESIAN_POINT ( 'NONE',  ( -15.80617190586745835, -15.72974639402198527, 106.8739096053143811 ) ) ;
#133472=CARTESIAN_POINT ( 'NONE',  ( -16.46253265017146816, -9.564922557961047289, 39.16775706135234003 ) ) ;
#133473=CARTESIAN_POINT ( 'NONE',  ( 16.46253265017160672, -9.564922557960803928, 48.33224293864769550 ) ) ;
#133474=CARTESIAN_POINT ( 'NONE',  ( -18.62759615963255300, -10.81492255796106328, 74.16775706135231871 ) ) ;
#133475=CARTESIAN_POINT ( 'NONE',  ( -18.62759615963270932, 10.81492255796079327, 60.83224293864769550 ) ) ;
#133476=CARTESIAN_POINT ( 'NONE',  ( -12.14591786802309592, -12.06949235617757132, 31.87390960531435979 ) ) ;
#133477=CARTESIAN_POINT ( 'NONE',  ( 18.62759615963255655, 10.81492255796105972, 81.66775706135236135 ) ) ;
#133478=CARTESIAN_POINT ( 'NONE',  ( 16.46253265017146816, 9.564922557961045513, 21.66775706135233648 ) ) ;
#133479=CARTESIAN_POINT ( 'NONE',  ( 14.29746914071049879, -8.314922557960816363, 53.33224293864769550 ) ) ;
#133480=CARTESIAN_POINT ( 'NONE',  ( -16.53943276465976808, 0.05219959533911058130, 106.2489096053143811 ) ) ;
#133481=CARTESIAN_POINT ( 'NONE',  ( 19.03943276465977164, 0.05219959533936151252, 46.25109039468566863 ) ) ;
#133482=CARTESIAN_POINT ( 'NONE',  ( 14.34966873604972726, -8.224510206698740333, 95.83442372801903275 ) ) ;
#133483=CARTESIAN_POINT ( 'NONE',  ( 15.80617190586769283, -15.72974639402175789, 65.62609039468568994 ) ) ;
#133484=CARTESIAN_POINT ( 'NONE',  ( -13.89961937509977652, 13.97604488694528158, 65.62390960531436690 ) ) ;
#133485=CARTESIAN_POINT ( 'NONE',  ( 9.564922557961047289, -16.46253265017146816, 40.41775706135234003 ) ) ;
#133486=CARTESIAN_POINT ( 'NONE',  ( 15.72974639402199770, -15.80617190586745480, 33.12390960531435979 ) ) ;
#133487=CARTESIAN_POINT ( 'NONE',  ( 10.72451020669871369, 18.67979575497193778, 37.08442372801901143 ) ) ;
#133488=CARTESIAN_POINT ( 'NONE',  ( 18.62759615963271287, -10.81492255796078972, 93.33224293864769550 ) ) ;
#133489=CARTESIAN_POINT ( 'NONE',  ( -5.049401038297874678, -19.05341960407617918, 84.79275706135233293 ) ) ;
#133490=CARTESIAN_POINT ( 'NONE',  ( -12.14591786802326823, 12.06949235617739902, 48.12609039468568284 ) ) ;
#133492=CARTESIAN_POINT ( 'NONE',  ( -15.80617190586745835, -15.72974639402198527, 96.87390960531436690 ) ) ;
#133493=CARTESIAN_POINT ( 'NONE',  ( -8.224510206698948167, 14.34966873604960824, 70.41557627198102409 ) ) ;
#133495=CARTESIAN_POINT ( 'NONE',  ( 4.379528057220092307, 16.55341960407617563, 27.29275706135234358 ) ) ;
#133497=CARTESIAN_POINT ( 'NONE',  ( -0.05219959533907301413, -21.53943276465977519, 47.49890960531435979 ) ) ;
#133498=CARTESIAN_POINT ( 'NONE',  ( 14.29746914071037800, 8.314922557961029526, 76.66775706135234714 ) ) ;
#133500=CARTESIAN_POINT ( 'NONE',  ( -8.314922557961024197, 14.29746914071037800, 57.91775706135234714 ) ) ;
#133501=CARTESIAN_POINT ( 'NONE',  ( 15.72974639402176855, 15.80617190586768217, 26.87609039468567218 ) ) ;
#133502=CARTESIAN_POINT ( 'NONE',  ( 15.80617190586746368, 15.72974639402197994, 44.37390960531435979 ) ) ;
#133503=CARTESIAN_POINT ( 'NONE',  ( -0.05219959533934338120, 16.53943276465976808, 77.50109039468567573 ) ) ;
#133504=CARTESIAN_POINT ( 'NONE',  ( 16.51473224551069308, 9.474510206698969483, 99.16557627198102409 ) ) ;
#133505=CARTESIAN_POINT ( 'NONE',  ( -18.62759615963255300, -10.81492255796106328, 59.16775706135234714 ) ) ;
#133506=CARTESIAN_POINT ( 'NONE',  ( 13.97604488694527802, 13.89961937509977652, 29.37390960531435979 ) ) ;
#133507=CARTESIAN_POINT ( 'NONE',  ( -21.52544592524343514, 5.823673210054127303, 36.04057627198102409 ) ) ;
#133508=CARTESIAN_POINT ( 'NONE',  ( -13.89961937509977652, 13.97604488694528158, 110.6239096053143243 ) ) ;
#133510=CARTESIAN_POINT ( 'NONE',  ( 19.02544592524334988, 5.153800228976608722, 36.45942372801900433 ) ) ;
#133511=CARTESIAN_POINT ( 'NONE',  ( -16.53943276465976808, -0.05219959533934237506, 53.75109039468568994 ) ) ;
#133512=CARTESIAN_POINT ( 'NONE',  ( 0.05219959533909260263, 19.03943276465977164, 109.9989096053143669 ) ) ;
#133513=EDGE_LOOP ( 'NONE', ( #53390, #122661, #36845, #161378 ) ) ;
#133514=CARTESIAN_POINT ( 'NONE',  ( -19.05341960407611168, -5.049401038298163336, 86.45724293864769550 ) ) ;
#133515=CARTESIAN_POINT ( 'NONE',  ( -12.06949235617739369, -12.14591786802326823, 104.3760903946856899 ) ) ;
#133517=CARTESIAN_POINT ( 'NONE',  ( -4.379528057220328563, 16.55341960407611168, 90.20724293864770971 ) ) ;
#133518=CARTESIAN_POINT ( 'NONE',  ( 15.80617190586746368, 15.72974639402197994, 49.37390960531436690 ) ) ;
#133519=CARTESIAN_POINT ( 'NONE',  ( -19.05341960407611168, -5.049401038298163336, 31.45724293864769550 ) ) ;
#133520=CARTESIAN_POINT ( 'NONE',  ( -12.14591786802326823, 12.06949235617739902, 73.12609039468567573 ) ) ;
#133521=CARTESIAN_POINT ( 'NONE',  ( 21.55341960407619695, -5.719274019375665929, 26.04275706135235779 ) ) ;
#133522=CARTESIAN_POINT ( 'NONE',  ( 19.05341960407617918, -5.049401038297876454, 96.04275706135231871 ) ) ;
#133523=CARTESIAN_POINT ( 'NONE',  ( -16.51473224551069308, -9.474510206698971260, 46.66557627198102409 ) ) ;
#133524=CARTESIAN_POINT ( 'NONE',  ( -9.564922557960796823, -16.46253265017161027, 107.0822429386476955 ) ) ;
#133525=CARTESIAN_POINT ( 'NONE',  ( 15.80617190586769283, -15.72974639402175789, 105.6260903946856899 ) ) ;
#133526=CARTESIAN_POINT ( 'NONE',  ( 5.153800228976335163, 19.02544592524342804, 84.79057627198099567 ) ) ;
#133527=CARTESIAN_POINT ( 'NONE',  ( 12.06949235617739724, 12.14591786802326823, 56.87609039468568994 ) ) ;
#133528=CARTESIAN_POINT ( 'NONE',  ( -10.81492255796105439, 18.62759615963255655, 97.91775706135236135 ) ) ;
#133529=CARTESIAN_POINT ( 'NONE',  ( -13.89961937509957401, -13.97604488694547875, 49.37609039468567573 ) ) ;
#133530=CARTESIAN_POINT ( 'NONE',  ( -9.474510206698720793, -16.51473224551083518, 69.58442372801901854 ) ) ;
#133531=ORIENTED_EDGE ( 'NONE', *, *, #160688, .T. ) ;
#133532=CARTESIAN_POINT ( 'NONE',  ( 10.72451020669871369, 18.67979575497193778, 67.08442372801901854 ) ) ;
#133533=DIRECTION ( 'NONE',  ( 0.000000000000000000, 0.000000000000000000, -1.000000000000000000 ) ) ;
#133534=CARTESIAN_POINT ( 'NONE',  ( -13.89961937509957401, -13.97604488694547875, 54.37609039468565442 ) ) ;
#133536=CARTESIAN_POINT ( 'NONE',  ( 19.05341960407611168, 5.049401038298154454, 83.95724293864766707 ) ) ;
#133537=CARTESIAN_POINT ( 'NONE',  ( 16.55341960407611168, 4.379528057220329451, 43.95724293864769550 ) ) ;
#133538=CARTESIAN_POINT ( 'NONE',  ( 21.52544592524344225, -5.823673210054117533, 33.54057627198102409 ) ) ;
#133539=CARTESIAN_POINT ( 'NONE',  ( 17.49999999999999645, 5.624438216177602534, 56.68329655085356933 ) ) ;
#133540=( BOUNDED_CURVE ( )  B_SPLINE_CURVE ( 2, ( #173236, #33719, #159036, #68030, #99360, #7346, #161043, #112540, #176227, #5352, #114526, #81192, #67036 ),
 .UNSPECIFIED., .F., .T. ) 
 B_SPLINE_CURVE_WITH_KNOTS ( ( 3, 2, 2, 2, 2, 2, 3 ),
 ( 0.5814234846701880066, 0.5833333333333333703, 0.5877192982456140857, 0.5921052631578946901, 0.5964912280701754055, 0.6008771929824561209, 0.6028327214676918455 ),
 .UNSPECIFIED. ) 
 CURVE ( )  GEOMETRIC_REPRESENTATION_ITEM ( )  RATIONAL_B_SPLINE_CURVE ( ( 0.9832469066685285419, 0.9851625545550100060, 1.000000000000000000, 0.9659258262890683122, 1.000000000000000000, 0.9659258262890683122, 1.000000000000000000, 0.9659258262890683122, 1.000000000000000000, 0.9659258262890683122, 1.000000000000000000, 0.9848076720550078544, 0.9831626618144001517 ) ) 
 REPRESENTATION_ITEM ( '' )  );
#133541=CARTESIAN_POINT ( 'NONE',  ( -21.53943276465977519, -0.05219959533937600094, 113.7510903946856757 ) ) ;
#133543=CARTESIAN_POINT ( 'NONE',  ( -16.46253265017160317, 9.564922557960807481, 40.83224293864769550 ) ) ;
#133544=CARTESIAN_POINT ( 'NONE',  ( -17.58332526062529411, 7.635886036038502134, 85.92334959558466778 ) ) ;
#133546=CARTESIAN_POINT ( 'NONE',  ( -18.22780087662123805, 5.499999999999981348, 81.01763182126896368 ) ) ;
#133547=CARTESIAN_POINT ( 'NONE',  ( 21.52544592524334988, 5.823673210054432836, 66.45942372801903275 ) ) ;
#133549=CARTESIAN_POINT ( 'NONE',  ( -14.34966873604972548, 8.224510206698743886, 63.33442372801900433 ) ) ;
#133550=CARTESIAN_POINT ( 'NONE',  ( 18.67979575497178502, 10.72451020669898547, 84.16557627198103830 ) ) ;
#133551=CARTESIAN_POINT ( 'NONE',  ( 16.52544592524342804, -4.483927247898539470, 53.54057627198103120 ) ) ;
#133552=CARTESIAN_POINT ( 'NONE',  ( 16.46253265017160672, -9.564922557960803928, 23.33224293864769194 ) ) ;
#133553=CARTESIAN_POINT ( 'NONE',  ( -13.97604488694527625, -13.89961937509977652, 106.8739096053143669 ) ) ;
#133554=CARTESIAN_POINT ( 'NONE',  ( 18.62759615963255655, 10.81492255796105972, 31.66775706135234358 ) ) ;
#133555=CARTESIAN_POINT ( 'NONE',  ( -19.02544592524334988, -5.153800228976617603, 53.95942372801898301 ) ) ;
#133556=CARTESIAN_POINT ( 'NONE',  ( 16.51473224551069308, 9.474510206698969483, 39.16557627198103120 ) ) ;
#133557=CARTESIAN_POINT ( 'NONE',  ( 15.72974639402176855, 15.80617190586768217, 81.87609039468568994 ) ) ;
#133558=CARTESIAN_POINT ( 'NONE',  ( 16.18388926212234580, -7.379444403734662927, 32.06046848633847901 ) ) ;
#133559=CARTESIAN_POINT ( 'NONE',  ( 16.53943276465976808, -0.05219959533910856209, 28.74890960531435624 ) ) ;
#133560=CARTESIAN_POINT ( 'NONE',  ( 17.50000000000148148, 3.254303733634527074, 112.4760410692860830 ) ) ;
#133561=CARTESIAN_POINT ( 'NONE',  ( -18.62759615963270932, 10.81492255796079327, 45.83224293864769550 ) ) ;
#133562=CARTESIAN_POINT ( 'NONE',  ( 16.52544592524342804, -4.483927247898539470, 103.5405762719810383 ) ) ;
#133564=CARTESIAN_POINT ( 'NONE',  ( 9.474510206698971260, -16.51473224551069308, 87.91557627198102409 ) ) ;
#133565=CARTESIAN_POINT ( 'NONE',  ( 0.05219959533910956823, 16.53943276465976808, 94.99890960531436690 ) ) ;
#133566=CARTESIAN_POINT ( 'NONE',  ( 16.51473224551083163, -9.474510206698727899, 105.8344237280190043 ) ) ;
#133567=CARTESIAN_POINT ( 'NONE',  ( -5.719274019375978568, 21.55341960407610458, 65.20724293864768129 ) ) ;
#133569=CARTESIAN_POINT ( 'NONE',  ( 19.03943276465977164, -0.05219959533909143690, 28.74890960531435624 ) ) ;
#133570=CARTESIAN_POINT ( 'NONE',  ( -0.05219959533909027116, -19.03943276465977164, 87.49890960531436690 ) ) ;
#133571=CARTESIAN_POINT ( 'NONE',  ( 21.53943276465977519, -0.05219959533907433946, 93.74890960531436690 ) ) ;
#133573=CARTESIAN_POINT ( 'NONE',  ( 12.06949235617739724, 12.14591786802326823, 106.8760903946856899 ) ) ;
#133574=CARTESIAN_POINT ( 'NONE',  ( 9.474510206698971260, -16.51473224551069308, 102.9155762719810241 ) ) ;
#133575=CARTESIAN_POINT ( 'NONE',  ( 19.05341960407617918, -5.049401038297876454, 76.04275706135230450 ) ) ;
#133576=CARTESIAN_POINT ( 'NONE',  ( -21.53943276465977519, -0.05219959533937600094, 98.75109039468568994 ) ) ;
#133577=CARTESIAN_POINT ( 'NONE',  ( 18.67979575497178502, 10.72451020669898547, 74.16557627198102409 ) ) ;
#133578=CARTESIAN_POINT ( 'NONE',  ( 21.53943276465977519, -0.05219959533907433946, 43.74890960531435979 ) ) ;
#133579=CARTESIAN_POINT ( 'NONE',  ( -19.03943276465977164, 0.05219959533909376836, 56.24890960531435979 ) ) ;
#133580=CARTESIAN_POINT ( 'NONE',  ( -8.224510206698735004, -14.34966873604973081, 109.5844237280190328 ) ) ;
#133581=CARTESIAN_POINT ( 'NONE',  ( -19.05341960407611168, -5.049401038298163336, 66.45724293864769550 ) ) ;
#133584=CARTESIAN_POINT ( 'NONE',  ( 16.51473224551083163, -9.474510206698727899, 25.83442372801900078 ) ) ;
#133585=CARTESIAN_POINT ( 'NONE',  ( 16.52544592524342804, -4.483927247898539470, 78.54057627198103830 ) ) ;
#133586=CARTESIAN_POINT ( 'NONE',  ( -21.52544592524343514, 5.823673210054127303, 116.0405762719810383 ) ) ;
#133588=CARTESIAN_POINT ( 'NONE',  ( -18.67979575497178146, -10.72451020669898902, 56.66557627198103830 ) ) ;
#133589=CARTESIAN_POINT ( 'NONE',  ( -8.224510206698735004, -14.34966873604973081, 94.58442372801901854 ) ) ;
#133590=CARTESIAN_POINT ( 'NONE',  ( 4.483927247898545687, 16.52544592524342804, 109.7905762719810383 ) ) ;
#133591=CARTESIAN_POINT ( 'NONE',  ( 13.89961937509977652, -13.97604488694527269, 73.12390960531436690 ) ) ;
#133592=CARTESIAN_POINT ( 'NONE',  ( -14.34966873604960291, -8.224510206698953496, 31.66557627198102054 ) ) ;
#133593=CARTESIAN_POINT ( 'NONE',  ( -0.05219959533937732626, 21.53943276465977519, 42.50109039468567573 ) ) ;
#133594=CARTESIAN_POINT ( 'NONE',  ( -19.02544592524342804, 5.153800228976336051, 106.0405762719810241 ) ) ;
#133595=CARTESIAN_POINT ( 'NONE',  ( 5.823673210054444382, -21.52544592524334988, 80.20942372801901854 ) ) ;
#133596=CARTESIAN_POINT ( 'NONE',  ( 5.049401038298161559, -19.05341960407611168, 27.70724293864769550 ) ) ;
#133597=CARTESIAN_POINT ( 'NONE',  ( -0.05219959533909027116, -19.03943276465977164, 32.49890960531435979 ) ) ;
#133599=CARTESIAN_POINT ( 'NONE',  ( 18.62759615963255655, 10.81492255796105972, 101.6677570613523613 ) ) ;
#133600=CARTESIAN_POINT ( 'NONE',  ( 14.34966873604972726, -8.224510206698740333, 45.83442372801901854 ) ) ;
#133601=CARTESIAN_POINT ( 'NONE',  ( -15.72974639402176322, -15.80617190586768395, 74.37609039468568994 ) ) ;
#133602=CARTESIAN_POINT ( 'NONE',  ( -16.51473224551069308, -9.474510206698971260, 106.6655762719810383 ) ) ;
#133603=CARTESIAN_POINT ( 'NONE',  ( 19.05341960407617918, -5.049401038297876454, 76.04275706135230450 ) ) ;
#133604=CARTESIAN_POINT ( 'NONE',  ( 10.72451020669871369, 18.67979575497193778, 52.08442372801901854 ) ) ;
#133605=CARTESIAN_POINT ( 'NONE',  ( 4.483927247898790824, -16.52544592524335698, 25.20942372801901854 ) ) ;
#133606=CARTESIAN_POINT ( 'NONE',  ( -9.474510206698720793, -16.51473224551083518, 79.58442372801899012 ) ) ;
#133607=CARTESIAN_POINT ( 'NONE',  ( -13.97604488694527625, -13.89961937509977652, 46.87390960531435979 ) ) ;
#133608=CARTESIAN_POINT ( 'NONE',  ( 9.564922557961047289, -16.46253265017146816, 100.4177570613523329 ) ) ;
#133609=CARTESIAN_POINT ( 'NONE',  ( -16.55341960407617563, 4.379528057220093196, 113.5427570613523756 ) ) ;
#133610=CARTESIAN_POINT ( 'NONE',  ( 16.51473224551083163, -9.474510206698727899, 90.83442372801900433 ) ) ;
#133611=CARTESIAN_POINT ( 'NONE',  ( -4.379528057220328563, 16.55341960407611168, 50.20724293864769550 ) ) ;
#133612=CARTESIAN_POINT ( 'NONE',  ( 13.97604488694548053, -13.89961937509957401, 60.62609039468564731 ) ) ;
#133613=CARTESIAN_POINT ( 'NONE',  ( -14.29746914071037622, -8.314922557961029526, 64.16775706135234714 ) ) ;
#133614=CARTESIAN_POINT ( 'NONE',  ( -18.67979575497193778, 10.72451020669871902, 113.3344237280190328 ) ) ;
#133616=CARTESIAN_POINT ( 'NONE',  ( -19.03943276465977164, 0.05219959533909376836, 21.24890960531436335 ) ) ;
#133617=CARTESIAN_POINT ( 'NONE',  ( -9.564922557960796823, -16.46253265017161027, 47.08224293864769550 ) ) ;
#133618=CARTESIAN_POINT ( 'NONE',  ( 0.05219959533934541429, -16.53943276465976808, 55.00109039468568284 ) ) ;
#133621=CARTESIAN_POINT ( 'NONE',  ( -5.153800228976328057, -19.02544592524343514, 87.29057627198103830 ) ) ;
#133622=CARTESIAN_POINT ( 'NONE',  ( 17.50000000000000000, 5.499999999999997335, 120.0000000000000142 ) ) ;
#133624=ORIENTED_EDGE ( 'NONE', *, *, #56474, .T. ) ;
#133625=CARTESIAN_POINT ( 'NONE',  ( 19.05341960407617918, -5.049401038297876454, 101.0427570613523045 ) ) ;
#133627=CARTESIAN_POINT ( 'NONE',  ( -21.55341960407610458, -5.719274019375992779, 36.45724293864768839 ) ) ;
#133628=CARTESIAN_POINT ( 'NONE',  ( 16.46253265017146816, 9.564922557961045513, 36.66775706135233293 ) ) ;
#133629=CARTESIAN_POINT ( 'NONE',  ( 16.51473224551083163, -9.474510206698727899, 110.8344237280190043 ) ) ;
#133630=CARTESIAN_POINT ( 'NONE',  ( -16.55341960407611168, -4.379528057220339221, 111.4572429386476813 ) ) ;
#133631=CARTESIAN_POINT ( 'NONE',  ( -5.153800228976328057, -19.02544592524343514, 42.29057627198101699 ) ) ;
#133632=CARTESIAN_POINT ( 'NONE',  ( 21.53943276465977519, -0.05219959533907433946, 78.74890960531436690 ) ) ;
#133634=CARTESIAN_POINT ( 'NONE',  ( -9.474510206698964154, 16.51473224551069663, 30.41557627198102054 ) ) ;
#133636=CARTESIAN_POINT ( 'NONE',  ( 19.02544592524334988, 5.153800228976608722, 86.45942372801900433 ) ) ;
#133637=CARTESIAN_POINT ( 'NONE',  ( 12.06949235617757843, -12.14591786802309237, 53.12390960531436690 ) ) ;
#133638=CARTESIAN_POINT ( 'NONE',  ( -15.80617190586745835, -15.72974639402198527, 26.87390960531435979 ) ) ;
#133639=CARTESIAN_POINT ( 'NONE',  ( -15.72974639402176322, -15.80617190586768395, 94.37609039468568994 ) ) ;
#133640=CARTESIAN_POINT ( 'NONE',  ( 10.72451020669898902, -18.67979575497178502, 82.91557627198103830 ) ) ;
#133641=CARTESIAN_POINT ( 'NONE',  ( 10.72451020669871369, 18.67979575497193778, 77.08442372801901854 ) ) ;
#133642=CARTESIAN_POINT ( 'NONE',  ( 0.05219959533937995610, -21.53943276465977519, 60.00109039468568284 ) ) ;
#133643=CARTESIAN_POINT ( 'NONE',  ( 5.153800228976335163, 19.02544592524342804, 99.79057627198102409 ) ) ;
#133644=CARTESIAN_POINT ( 'NONE',  ( -4.483927247898782831, 16.52544592524335698, 112.7094237280190328 ) ) ;
#133645=CARTESIAN_POINT ( 'NONE',  ( -21.52544592524334988, -5.823673210054445271, 63.95942372801901854 ) ) ;
#133646=CARTESIAN_POINT ( 'NONE',  ( 19.05341960407611168, 5.049401038298154454, 53.95724293864770260 ) ) ;
#133647=CARTESIAN_POINT ( 'NONE',  ( -18.67979575497193778, 10.72451020669871902, 33.33442372801900433 ) ) ;
#133648=CARTESIAN_POINT ( 'NONE',  ( 19.05341960407611168, 5.049401038298154454, 63.95724293864769550 ) ) ;
#133649=CARTESIAN_POINT ( 'NONE',  ( 16.52544592524342804, -4.483927247898539470, 83.54057627198102409 ) ) ;
#133650=CARTESIAN_POINT ( 'NONE',  ( -14.29746914071049879, 8.314922557960819915, 45.83224293864769550 ) ) ;
#133651=CARTESIAN_POINT ( 'NONE',  ( 10.72451020669898902, -18.67979575497178502, 62.91557627198102409 ) ) ;
#133652=CARTESIAN_POINT ( 'NONE',  ( 19.05341960407611168, 5.049401038298154454, 43.95724293864769550 ) ) ;
#133653=CARTESIAN_POINT ( 'NONE',  ( -5.719274019375978568, 21.55341960407610458, 65.20724293864768129 ) ) ;
#133654=CARTESIAN_POINT ( 'NONE',  ( -19.05341960407617563, 5.049401038297882671, 48.54275706135233293 ) ) ;
#133656=CARTESIAN_POINT ( 'NONE',  ( 9.564922557961047289, -16.46253265017146816, 20.41775706135233293 ) ) ;
#133657=CARTESIAN_POINT ( 'NONE',  ( -0.05219959533910754901, -16.53943276465976808, 62.49890960531436690 ) ) ;
#133658=CARTESIAN_POINT ( 'NONE',  ( -10.72451020669898014, 18.67979575497178502, 40.41557627198103120 ) ) ;
#133661=CARTESIAN_POINT ( 'NONE',  ( -8.224510206698735004, -14.34966873604973081, 84.58442372801903275 ) ) ;
#133663=CARTESIAN_POINT ( 'NONE',  ( 16.46253265017146816, 9.564922557961045513, 86.66775706135233293 ) ) ;
#133664=CARTESIAN_POINT ( 'NONE',  ( 14.29746914071049879, -8.314922557960816363, 58.33224293864768839 ) ) ;
#133665=CARTESIAN_POINT ( 'NONE',  ( -19.20446147854528718, -5.499999999999910294, 59.38999695167679960 ) ) ;
#133666=CARTESIAN_POINT ( 'NONE',  ( -5.153800228976328057, -19.02544592524343514, 47.29057627198102409 ) ) ;
#133667=CARTESIAN_POINT ( 'NONE',  ( 8.314922557960818139, 14.29746914071049879, 44.58224293864769550 ) ) ;
#133668=CARTESIAN_POINT ( 'NONE',  ( -16.46253265017160317, 9.564922557960807481, 85.83224293864769550 ) ) ;
#133669=CARTESIAN_POINT ( 'NONE',  ( 9.564922557960805705, 16.46253265017160317, 54.58224293864769550 ) ) ;
#133670=CARTESIAN_POINT ( 'NONE',  ( -0.05219959533937732626, 21.53943276465977519, 62.50109039468568284 ) ) ;
#133671=CARTESIAN_POINT ( 'NONE',  ( 16.46253265017160672, -9.564922557960803928, 78.33224293864769550 ) ) ;
#133672=CARTESIAN_POINT ( 'NONE',  ( 16.51473224551069308, 9.474510206698969483, 24.16557627198102765 ) ) ;
#133673=CARTESIAN_POINT ( 'NONE',  ( -13.89961937509977652, 13.97604488694528158, 65.62390960531436690 ) ) ;
#133674=CARTESIAN_POINT ( 'NONE',  ( 15.72974639402199770, -15.80617190586745480, 43.12390960531435269 ) ) ;
#133675=CARTESIAN_POINT ( 'NONE',  ( -5.049401038298153566, 19.05341960407611168, 30.20724293864768839 ) ) ;
#133676=CARTESIAN_POINT ( 'NONE',  ( 5.823673210054125526, 21.52544592524343514, 39.79057627198103830 ) ) ;
#133677=CARTESIAN_POINT ( 'NONE',  ( 4.379528057220092307, 16.55341960407617563, 102.2927570613523613 ) ) ;
#133678=CARTESIAN_POINT ( 'NONE',  ( -13.89961937509957401, -13.97604488694547875, 24.37609039468565442 ) ) ;
#133679=CARTESIAN_POINT ( 'NONE',  ( 16.52544592524335698, 4.483927247898782831, 41.45942372801901143 ) ) ;
#133680=CARTESIAN_POINT ( 'NONE',  ( -12.14591786802326823, 12.06949235617739902, 78.12609039468570415 ) ) ;
#133682=CARTESIAN_POINT ( 'NONE',  ( 8.314922557961029526, -14.29746914071037800, 70.41775706135236135 ) ) ;
#133683=CARTESIAN_POINT ( 'NONE',  ( -16.52544592524335698, -4.483927247898792601, 53.95942372801900433 ) ) ;
#133684=CARTESIAN_POINT ( 'NONE',  ( 19.05341960407611168, 5.049401038298154454, 103.9572429386476671 ) ) ;
#133685=CARTESIAN_POINT ( 'NONE',  ( -16.46253265017160317, 9.564922557960807481, 30.83224293864769550 ) ) ;
#133686=CARTESIAN_POINT ( 'NONE',  ( -0.05219959533934338120, 16.53943276465976808, 32.50109039468568284 ) ) ;
#133687=CARTESIAN_POINT ( 'NONE',  ( 13.97604488694527802, 13.89961937509977652, 49.37390960531434558 ) ) ;
#133688=CARTESIAN_POINT ( 'NONE',  ( 5.719274019375673035, 21.55341960407619339, 27.29275706135234358 ) ) ;
#133689=CARTESIAN_POINT ( 'NONE',  ( -14.34966873604972548, 8.224510206698743886, 38.33442372801900433 ) ) ;
#133690=CARTESIAN_POINT ( 'NONE',  ( -16.53943276465976808, -0.05219959533934237506, 103.7510903946857042 ) ) ;
#133692=CARTESIAN_POINT ( 'NONE',  ( 10.81492255796106328, -18.62759615963255655, 105.4177570613523613 ) ) ;
#133693=CARTESIAN_POINT ( 'NONE',  ( 9.474510206698729675, 16.51473224551082808, 92.08442372801900433 ) ) ;
#133694=CARTESIAN_POINT ( 'NONE',  ( -16.46253265017146816, -9.564922557961047289, 59.16775706135233293 ) ) ;
#133695=CARTESIAN_POINT ( 'NONE',  ( -4.379528057220328563, 16.55341960407611168, 60.20724293864768839 ) ) ;
#133696=CARTESIAN_POINT ( 'NONE',  ( -9.474510206698964154, 16.51473224551069663, 30.41557627198102054 ) ) ;
#133697=CARTESIAN_POINT ( 'NONE',  ( 5.049401038297881783, 19.05341960407617563, 67.29275706135234714 ) ) ;
#133699=CARTESIAN_POINT ( 'NONE',  ( -0.05219959533937732626, 21.53943276465977519, 62.50109039468568284 ) ) ;
#133700=CARTESIAN_POINT ( 'NONE',  ( 16.53943276465976808, 0.05219959533934440121, 31.25109039468568639 ) ) ;
#133701=CARTESIAN_POINT ( 'NONE',  ( 17.50000000000000000, 5.499999999999992895, 81.70309617465829888 ) ) ;
#133702=CARTESIAN_POINT ( 'NONE',  ( -5.049401038298153566, 19.05341960407611168, 115.2072429386477097 ) ) ;
#133703=CARTESIAN_POINT ( 'NONE',  ( 19.05341960407617918, -5.049401038297876454, 111.0427570613523329 ) ) ;
#133706=CARTESIAN_POINT ( 'NONE',  ( 13.97604488694527802, 13.89961937509977652, 24.37390960531435624 ) ) ;
#133707=CARTESIAN_POINT ( 'NONE',  ( 10.72451020669871369, 18.67979575497193778, 107.0844237280190043 ) ) ;
#133708=CARTESIAN_POINT ( 'NONE',  ( -0.05219959533909027116, -19.03943276465977164, 42.49890960531435269 ) ) ;
#133709=CARTESIAN_POINT ( 'NONE',  ( -21.53943276465977519, -0.05219959533937600094, 68.75109039468568994 ) ) ;
#133710=CARTESIAN_POINT ( 'NONE',  ( 21.55341960407619695, -5.719274019375665929, 106.0427570613523471 ) ) ;
#133711=CARTESIAN_POINT ( 'NONE',  ( -16.53943276465976808, -0.05219959533934237506, 103.7510903946857042 ) ) ;
#133712=CARTESIAN_POINT ( 'NONE',  ( 19.05341960407611168, 5.049401038298154454, 78.95724293864769550 ) ) ;
#133713=CARTESIAN_POINT ( 'NONE',  ( -21.55341960407619339, 5.719274019375674811, 53.54275706135234714 ) ) ;
#133715=CARTESIAN_POINT ( 'NONE',  ( -21.52544592524334988, -5.823673210054445271, 53.95942372801900433 ) ) ;
#133716=CARTESIAN_POINT ( 'NONE',  ( 19.02544592524334988, 5.153800228976608722, 76.45942372801897591 ) ) ;
#133717=CARTESIAN_POINT ( 'NONE',  ( 5.049401038298161559, -19.05341960407611168, 107.7072429386476955 ) ) ;
#133718=CARTESIAN_POINT ( 'NONE',  ( 13.89961937509977652, -13.97604488694527269, 28.12390960531435624 ) ) ;
#133719=CARTESIAN_POINT ( 'NONE',  ( -5.719274019375978568, 21.55341960407610458, 95.20724293864769550 ) ) ;
#133720=CARTESIAN_POINT ( 'NONE',  ( -21.53943276465977519, -0.05219959533937600094, 113.7510903946856757 ) ) ;
#133721=CARTESIAN_POINT ( 'NONE',  ( -8.314922557960811034, -14.29746914071050412, 97.08224293864770971 ) ) ;
#133722=CARTESIAN_POINT ( 'NONE',  ( 19.03943276465977164, -0.05219959533909143690, 48.74890960531435979 ) ) ;
#133723=CARTESIAN_POINT ( 'NONE',  ( 9.564922557961047289, -16.46253265017146816, 80.41775706135234714 ) ) ;
#133724=CARTESIAN_POINT ( 'NONE',  ( -8.224510206698948167, 14.34966873604960824, 65.41557627198102409 ) ) ;
#133725=CARTESIAN_POINT ( 'NONE',  ( -19.03943276465977164, -0.05219959533935918106, 18.75109039468567218 ) ) ;
#133726=CARTESIAN_POINT ( 'NONE',  ( -19.05341960407611168, -5.049401038298163336, 106.4572429386476955 ) ) ;
#133727=CARTESIAN_POINT ( 'NONE',  ( 16.46253265017146816, 9.564922557961045513, 76.66775706135234714 ) ) ;
#133728=CARTESIAN_POINT ( 'NONE',  ( 10.81492255796078972, 18.62759615963270932, 74.58224293864768129 ) ) ;
#133729=CARTESIAN_POINT ( 'NONE',  ( -10.81492255796105439, 18.62759615963255655, 32.91775706135234714 ) ) ;
#133730=CARTESIAN_POINT ( 'NONE',  ( 8.314922557961029526, -14.29746914071037800, 30.41775706135234358 ) ) ;
#133731=CARTESIAN_POINT ( 'NONE',  ( 4.379528057220092307, 16.55341960407617563, 87.29275706135236135 ) ) ;
#133732=CARTESIAN_POINT ( 'NONE',  ( -4.379528057220086978, -16.55341960407618274, 44.79275706135234714 ) ) ;
#133733=CARTESIAN_POINT ( 'NONE',  ( -10.72451020669870658, -18.67979575497194134, 34.58442372801900433 ) ) ;
#133734=CARTESIAN_POINT ( 'NONE',  ( 5.719274019375991003, -21.55341960407610458, 42.70724293864770260 ) ) ;
#133735=CARTESIAN_POINT ( 'NONE',  ( -9.474510206698964154, 16.51473224551069663, 30.41557627198102054 ) ) ;
#133737=CARTESIAN_POINT ( 'NONE',  ( -16.53943276465976808, -0.05219959533934237506, 58.75109039468568994 ) ) ;
#133738=CARTESIAN_POINT ( 'NONE',  ( 15.72974639402199770, -15.80617190586745480, 88.12390960531436690 ) ) ;
#133739=CARTESIAN_POINT ( 'NONE',  ( 4.379528057220339221, -16.55341960407611168, 42.70724293864770260 ) ) ;
#133740=CARTESIAN_POINT ( 'NONE',  ( 16.52544592524335698, 4.483927247898782831, 46.45942372801901854 ) ) ;
#133741=CARTESIAN_POINT ( 'NONE',  ( 0.05219959533909260263, 19.03943276465977164, 64.99890960531436690 ) ) ;
#133742=CARTESIAN_POINT ( 'NONE',  ( -16.52544592524335698, -4.483927247898792601, 98.95942372801903275 ) ) ;
#133743=CARTESIAN_POINT ( 'NONE',  ( 9.564922557961047289, -16.46253265017146816, 90.41775706135234714 ) ) ;
#133744=CARTESIAN_POINT ( 'NONE',  ( -5.823673210054116645, -21.52544592524344225, 87.29057627198103830 ) ) ;
#133745=CARTESIAN_POINT ( 'NONE',  ( 14.29746914071049879, -8.314922557960816363, 33.33224293864769550 ) ) ;
#133748=VECTOR ( 'NONE', #92107, 1000.000000000000000 ) ;
#133749=CARTESIAN_POINT ( 'NONE',  ( 18.62759615963271287, -10.81492255796078972, 58.33224293864768839 ) ) ;
#133750=ORIENTED_EDGE ( 'NONE', *, *, #6380, .T. ) ;
#133751=CARTESIAN_POINT ( 'NONE',  ( 4.379528057220092307, 16.55341960407617563, 107.2927570613523471 ) ) ;
#133753=CARTESIAN_POINT ( 'NONE',  ( -5.719274019375978568, 21.55341960407610458, 30.20724293864769550 ) ) ;
#133755=CARTESIAN_POINT ( 'NONE',  ( 5.719274019375991003, -21.55341960407610458, 92.70724293864770971 ) ) ;
#133756=CARTESIAN_POINT ( 'NONE',  ( 12.06949235617739724, 12.14591786802326823, 111.8760903946856615 ) ) ;
#133757=CARTESIAN_POINT ( 'NONE',  ( -16.55341960407617563, 4.379528057220093196, 38.54275706135234714 ) ) ;
#133758=CARTESIAN_POINT ( 'NONE',  ( 19.02544592524343514, -5.153800228976328945, 28.54057627198102409 ) ) ;
#133759=CARTESIAN_POINT ( 'NONE',  ( 16.52544592524335698, 4.483927247898782831, 31.45942372801901854 ) ) ;
#133760=CARTESIAN_POINT ( 'NONE',  ( 19.03943276465977164, -0.05219959533909143690, 53.74890960531436690 ) ) ;
#133762=CARTESIAN_POINT ( 'NONE',  ( 13.97604488694527802, 13.89961937509977652, 109.3739096053143669 ) ) ;
#133763=CARTESIAN_POINT ( 'NONE',  ( 19.03943276465977164, -0.05219959533909143690, 113.7489096053143669 ) ) ;
#133764=CARTESIAN_POINT ( 'NONE',  ( 12.14591786802327356, -12.06949235617739191, 100.6260903946857184 ) ) ;
#133765=CARTESIAN_POINT ( 'NONE',  ( 5.049401038297881783, 19.05341960407617563, 87.29275706135234714 ) ) ;
#133766=CARTESIAN_POINT ( 'NONE',  ( 13.89961937509957401, 13.97604488694547697, 36.87609039468565442 ) ) ;
#133767=CARTESIAN_POINT ( 'NONE',  ( 21.53943276465977519, -0.05219959533907433946, 88.74890960531436690 ) ) ;
#133768=CARTESIAN_POINT ( 'NONE',  ( 0.05219959533934541429, -16.53943276465976808, 100.0010903946857042 ) ) ;
#133769=CARTESIAN_POINT ( 'NONE',  ( -18.67979575497178146, -10.72451020669898902, 31.66557627198102054 ) ) ;
#133770=CARTESIAN_POINT ( 'NONE',  ( -0.05219959533936034679, 19.03943276465977164, 102.5010903946856757 ) ) ;
#133771=CARTESIAN_POINT ( 'NONE',  ( -13.97604488694527625, -13.89961937509977652, 106.8739096053143669 ) ) ;
#133773=CARTESIAN_POINT ( 'NONE',  ( -18.62759615963255300, -10.81492255796106328, 59.16775706135234714 ) ) ;
#133774=CARTESIAN_POINT ( 'NONE',  ( -5.153800228976328057, -19.02544592524343514, 57.29057627198103120 ) ) ;
#133775=CARTESIAN_POINT ( 'NONE',  ( -4.379528057220328563, 16.55341960407611168, 95.20724293864769550 ) ) ;
#133777=CARTESIAN_POINT ( 'NONE',  ( -14.34966873604960291, -8.224510206698953496, 71.66557627198100988 ) ) ;
#133779=CARTESIAN_POINT ( 'NONE',  ( -0.05219959533936034679, 19.03943276465977164, 87.50109039468567573 ) ) ;
#133781=CARTESIAN_POINT ( 'NONE',  ( -5.049401038298153566, 19.05341960407611168, 65.20724293864765286 ) ) ;
#133783=CARTESIAN_POINT ( 'NONE',  ( 16.51473224551069308, 9.474510206698969483, 79.16557627198103830 ) ) ;
#133784=CARTESIAN_POINT ( 'NONE',  ( 19.05341960407611168, 5.049401038298154454, 88.95724293864769550 ) ) ;
#133786=CARTESIAN_POINT ( 'NONE',  ( 8.314922557961029526, -14.29746914071037800, 65.41775706135234714 ) ) ;
#133787=CARTESIAN_POINT ( 'NONE',  ( -16.21995358207306381, -7.366697692864125457, 50.06448998487844904 ) ) ;
#133788=CARTESIAN_POINT ( 'NONE',  ( -9.474510206698720793, -16.51473224551083518, 44.58442372801900433 ) ) ;
#133789=CARTESIAN_POINT ( 'NONE',  ( 21.53943276465977519, 0.05219959533937863772, 101.2510903946856757 ) ) ;
#133791=CARTESIAN_POINT ( 'NONE',  ( -16.46253265017160317, 9.564922557960807481, 115.8322429386477097 ) ) ;
#133792=CARTESIAN_POINT ( 'NONE',  ( 16.55341960407618274, -4.379528057220086978, 96.04275706135236135 ) ) ;
#133794=CARTESIAN_POINT ( 'NONE',  ( 12.06949235617739724, 12.14591786802326823, 91.87609039468568994 ) ) ;
#133795=CARTESIAN_POINT ( 'NONE',  ( -17.44279575226823198, 5.990770900252466724, 30.83557567514319331 ) ) ;
#133796=( BOUNDED_CURVE ( )  B_SPLINE_CURVE ( 2, ( #164806, #134472, #163808, #179993, #100111, #68780, #42456, #130437, #192136, #53617, #176986, #41460, #117289 ),
 .UNSPECIFIED., .F., .T. ) 
 B_SPLINE_CURVE_WITH_KNOTS ( ( 3, 2, 2, 2, 2, 2, 3 ),
 ( 0.7130024320386090242, 0.7149122807017543879, 0.7192982456140351033, 0.7236842105263158187, 0.7280701754385965341, 0.7324561403508771384, 0.7344116688361128631 ),
 .UNSPECIFIED. ) 
 CURVE ( )  GEOMETRIC_REPRESENTATION_ITEM ( )  RATIONAL_B_SPLINE_CURVE ( ( 0.9832469066685285419, 0.9851625545550100060, 1.000000000000000000, 0.9659258262890683122, 1.000000000000000000, 0.9659258262890683122, 1.000000000000000000, 0.9659258262890683122, 1.000000000000000000, 0.9659258262890683122, 1.000000000000000000, 0.9848076720550078544, 0.9831626618144001517 ) ) 
 REPRESENTATION_ITEM ( '' )  );
#133797=CARTESIAN_POINT ( 'NONE',  ( 16.52544592524335698, 4.483927247898782831, 66.45942372801903275 ) ) ;
#133798=CARTESIAN_POINT ( 'NONE',  ( -17.60691670004651499, -5.500000000000069278, 59.13333313366439370 ) ) ;
#133799=CARTESIAN_POINT ( 'NONE',  ( 5.719274019375673035, 21.55341960407619339, 87.29275706135236135 ) ) ;
#133800=CARTESIAN_POINT ( 'NONE',  ( -19.05341960407617563, 5.049401038297882671, 93.54275706135234714 ) ) ;
#133801=CARTESIAN_POINT ( 'NONE',  ( 13.97604488694548053, -13.89961937509957401, 30.62609039468566863 ) ) ;
#133802=CARTESIAN_POINT ( 'NONE',  ( 13.97604488694527802, 13.89961937509977652, 64.37390960531436690 ) ) ;
#133803=CARTESIAN_POINT ( 'NONE',  ( -9.474510206698964154, 16.51473224551069663, 45.41557627198103120 ) ) ;
#133805=CARTESIAN_POINT ( 'NONE',  ( 10.72451020669898902, -18.67979575497178502, 77.91557627198102409 ) ) ;
#133806=AXIS2_PLACEMENT_3D ( 'NONE', #33632, #97261, #191293 ) ;
#133807=CARTESIAN_POINT ( 'NONE',  ( 21.55341960407610458, 5.719274019375980345, 33.95724293864769550 ) ) ;
#133808=CARTESIAN_POINT ( 'NONE',  ( 5.153800228976335163, 19.02544592524342804, 29.79057627198102409 ) ) ;
#133809=CARTESIAN_POINT ( 'NONE',  ( 16.55341960407618274, -4.379528057220086978, 56.04275706135235424 ) ) ;
#133810=EDGE_CURVE ( 'NONE', #46248, #10418, #133000, .T. ) ;
#133811=VERTEX_POINT ( 'NONE', #50074 ) ;
#133812=CARTESIAN_POINT ( 'NONE',  ( 0.05219959533937995610, -21.53943276465977519, 30.00109039468568284 ) ) ;
#133813=CARTESIAN_POINT ( 'NONE',  ( -8.314922557960811034, -14.29746914071050412, 57.08224293864769550 ) ) ;
#133815=CARTESIAN_POINT ( 'NONE',  ( -8.224510206698735004, -14.34966873604973081, 24.58442372801901499 ) ) ;
#133816=CARTESIAN_POINT ( 'NONE',  ( 5.153800228976615827, -19.02544592524334988, 40.20942372801898301 ) ) ;
#133817=CARTESIAN_POINT ( 'NONE',  ( 16.53943276465976808, -0.05219959533910856209, 58.74890960531436690 ) ) ;
#133818=CARTESIAN_POINT ( 'NONE',  ( 21.53943276465977519, -0.05219959533907433946, 113.7489096053143527 ) ) ;
#133820=CARTESIAN_POINT ( 'NONE',  ( -21.53943276465977519, 0.05219959533907696930, 76.24890960531435269 ) ) ;
#133821=CARTESIAN_POINT ( 'NONE',  ( -5.049401038298153566, 19.05341960407611168, 90.20724293864766707 ) ) ;
#133822=CARTESIAN_POINT ( 'NONE',  ( -8.314922557960811034, -14.29746914071050412, 67.08224293864770971 ) ) ;
#133823=CARTESIAN_POINT ( 'NONE',  ( 13.89961937509977652, -13.97604488694527269, 98.12390960531433848 ) ) ;
#133825=CARTESIAN_POINT ( 'NONE',  ( 0.05219959533936267826, -19.03943276465977164, 70.00109039468566152 ) ) ;
#133826=CARTESIAN_POINT ( 'NONE',  ( -0.05219959533907301413, -21.53943276465977519, 107.4989096053143669 ) ) ;
#133827=CARTESIAN_POINT ( 'NONE',  ( 13.89961937509977652, -13.97604488694527269, 63.12390960531435979 ) ) ;
#133828=CARTESIAN_POINT ( 'NONE',  ( -19.02544592524334988, -5.153800228976617603, 48.95942372801900433 ) ) ;
#133829=CARTESIAN_POINT ( 'NONE',  ( 16.52544592524342804, -4.483927247898539470, 108.5405762719810241 ) ) ;
#133830=CARTESIAN_POINT ( 'NONE',  ( 15.80617190586769283, -15.72974639402175789, 65.62609039468568994 ) ) ;
#133831=CARTESIAN_POINT ( 'NONE',  ( -17.05116617787826172, -6.768360034955815507, 71.34324446740799885 ) ) ;
#133832=CARTESIAN_POINT ( 'NONE',  ( 16.55341960407611168, 4.379528057220329451, 43.95724293864769550 ) ) ;
#133833=CARTESIAN_POINT ( 'NONE',  ( -9.564922557960796823, -16.46253265017161027, 62.08224293864769550 ) ) ;
#133834=CARTESIAN_POINT ( 'NONE',  ( -21.55341960407610458, -5.719274019375992779, 76.45724293864769550 ) ) ;
#133836=CARTESIAN_POINT ( 'NONE',  ( -5.049401038298153566, 19.05341960407611168, 55.20724293864769550 ) ) ;
#133838=CARTESIAN_POINT ( 'NONE',  ( -10.81492255796078084, -18.62759615963271287, 67.08224293864770971 ) ) ;
#133840=CARTESIAN_POINT ( 'NONE',  ( -10.81492255796105439, 18.62759615963255655, 102.9177570613523756 ) ) ;
#133841=CARTESIAN_POINT ( 'NONE',  ( 17.60779699588839975, 5.500000000000012434, 53.84981316670104690 ) ) ;
#133842=CARTESIAN_POINT ( 'NONE',  ( 12.14591786802327356, -12.06949235617739191, 95.62609039468568994 ) ) ;
#133843=CARTESIAN_POINT ( 'NONE',  ( 4.379528057220339221, -16.55341960407611168, 87.70724293864769550 ) ) ;
#133844=CARTESIAN_POINT ( 'NONE',  ( 0.05219959533909260263, 19.03943276465977164, 64.99890960531436690 ) ) ;
#133846=CARTESIAN_POINT ( 'NONE',  ( -19.03943276465977164, -0.05219959533935918106, 33.75109039468566863 ) ) ;
#133847=CARTESIAN_POINT ( 'NONE',  ( -8.224510206698735004, -14.34966873604973081, 84.58442372801903275 ) ) ;
#133848=CARTESIAN_POINT ( 'NONE',  ( -16.51473224551082808, 9.474510206698731452, 33.33442372801899722 ) ) ;
#133849=CARTESIAN_POINT ( 'NONE',  ( 16.51473224551069308, 9.474510206698969483, 94.16557627198103830 ) ) ;
#133850=CARTESIAN_POINT ( 'NONE',  ( 18.67979575497178502, 10.72451020669898547, 64.16557627198102409 ) ) ;
#133851=DIRECTION ( 'NONE',  ( -1.000000000000000000, 0.000000000000000000, 0.000000000000000000 ) ) ;
#133852=CARTESIAN_POINT ( 'NONE',  ( -5.153800228976328057, -19.02544592524343514, 22.29057627198102765 ) ) ;
#133853=CARTESIAN_POINT ( 'NONE',  ( 5.823673210054444382, -21.52544592524334988, 100.2094237280190043 ) ) ;
#133854=CARTESIAN_POINT ( 'NONE',  ( 16.52544592524335698, 4.483927247898782831, 61.45942372801901854 ) ) ;
#133855=CARTESIAN_POINT ( 'NONE',  ( -18.67979575497193778, 10.72451020669871902, 28.33442372801902209 ) ) ;
#133856=CARTESIAN_POINT ( 'NONE',  ( -0.05219959533934338120, 16.53943276465976808, 32.50109039468568284 ) ) ;
#133857=CARTESIAN_POINT ( 'NONE',  ( -9.474510206698964154, 16.51473224551069663, 95.41557627198102409 ) ) ;
#133858=CARTESIAN_POINT ( 'NONE',  ( -9.474510206698964154, 16.51473224551069663, 40.41557627198103120 ) ) ;
#133859=CARTESIAN_POINT ( 'NONE',  ( 5.049401038298161559, -19.05341960407611168, 52.70724293864767418 ) ) ;
#133860=CARTESIAN_POINT ( 'NONE',  ( -14.29746914071037622, -8.314922557961029526, 34.16775706135234714 ) ) ;
#133861=CARTESIAN_POINT ( 'NONE',  ( 0.05219959533910956823, 16.53943276465976808, 94.99890960531436690 ) ) ;
#133862=CARTESIAN_POINT ( 'NONE',  ( 4.379528057220092307, 16.55341960407617563, 107.2927570613523471 ) ) ;
#133863=CARTESIAN_POINT ( 'NONE',  ( -5.719274019375665041, -21.55341960407619695, 49.79275706135234714 ) ) ;
#133864=CARTESIAN_POINT ( 'NONE',  ( 13.89961937509977652, -13.97604488694527269, 78.12390960531433848 ) ) ;
#133865=CARTESIAN_POINT ( 'NONE',  ( 13.97604488694527802, 13.89961937509977652, 49.37390960531434558 ) ) ;
#133866=CARTESIAN_POINT ( 'NONE',  ( 5.153800228976335163, 19.02544592524342804, 84.79057627198099567 ) ) ;
#133867=CARTESIAN_POINT ( 'NONE',  ( -14.29746914071049879, 8.314922557960819915, 35.83224293864768839 ) ) ;
#133868=CARTESIAN_POINT ( 'NONE',  ( 8.314922557961029526, -14.29746914071037800, 95.41775706135234714 ) ) ;
#133871=CARTESIAN_POINT ( 'NONE',  ( 16.46253265017146816, 9.564922557961045513, 41.66775706135234003 ) ) ;
#133872=CARTESIAN_POINT ( 'NONE',  ( 19.03943276465977164, -0.05219959533909143690, 113.7489096053143669 ) ) ;
#133873=CARTESIAN_POINT ( 'NONE',  ( -5.049401038298153566, 19.05341960407611168, 50.20724293864770260 ) ) ;
#133874=CARTESIAN_POINT ( 'NONE',  ( -9.474510206698720793, -16.51473224551083518, 19.58442372801899722 ) ) ;
#133876=CARTESIAN_POINT ( 'NONE',  ( 8.224510206698742110, 14.34966873604972548, 37.08442372801901143 ) ) ;
#133877=CARTESIAN_POINT ( 'NONE',  ( -9.564922557961040184, 16.46253265017147172, 72.91775706135233293 ) ) ;
#133878=CARTESIAN_POINT ( 'NONE',  ( 16.55341960407618274, -4.379528057220086978, 61.04275706135234714 ) ) ;
#133879=CARTESIAN_POINT ( 'NONE',  ( 5.153800228976335163, 19.02544592524342804, 114.7905762719810241 ) ) ;
#133880=CARTESIAN_POINT ( 'NONE',  ( -13.97604488694527625, -13.89961937509977652, 76.87390960531433848 ) ) ;
#133881=CARTESIAN_POINT ( 'NONE',  ( 18.67979575497194134, -10.72451020669871369, 20.83442372801901143 ) ) ;
#133882=CARTESIAN_POINT ( 'NONE',  ( 19.05341960407617918, -5.049401038297876454, 81.04275706135231871 ) ) ;
#133883=CARTESIAN_POINT ( 'NONE',  ( 16.51473224551069308, 9.474510206698969483, 109.1655762719810383 ) ) ;
#133884=CARTESIAN_POINT ( 'NONE',  ( 9.564922557960805705, 16.46253265017160317, 29.58224293864769550 ) ) ;
#133885=CARTESIAN_POINT ( 'NONE',  ( 9.564922557960805705, 16.46253265017160317, 74.58224293864769550 ) ) ;
#133886=CARTESIAN_POINT ( 'NONE',  ( 16.52544592524342804, -4.483927247898539470, 28.54057627198103120 ) ) ;
#133887=CARTESIAN_POINT ( 'NONE',  ( 13.89961937509977652, -13.97604488694527269, 33.12390960531434558 ) ) ;
#133888=CARTESIAN_POINT ( 'NONE',  ( -5.153800228976607833, 19.02544592524334988, 52.70942372801900433 ) ) ;
#133889=CARTESIAN_POINT ( 'NONE',  ( 14.29746914071049879, -8.314922557960816363, 78.33224293864770971 ) ) ;
#133890=CARTESIAN_POINT ( 'NONE',  ( -9.474510206698720793, -16.51473224551083518, 19.58442372801899722 ) ) ;
#133891=CARTESIAN_POINT ( 'NONE',  ( -13.97604488694527625, -13.89961937509977652, 56.87390960531434558 ) ) ;
#133893=CARTESIAN_POINT ( 'NONE',  ( -0.05219959533907301413, -21.53943276465977519, 47.49890960531435979 ) ) ;
#133894=CARTESIAN_POINT ( 'NONE',  ( -16.52544592524342804, 4.483927247898546575, 51.04057627198103120 ) ) ;
#133895=CARTESIAN_POINT ( 'NONE',  ( 10.81492255796106328, -18.62759615963255655, 100.4177570613523471 ) ) ;
#133896=CARTESIAN_POINT ( 'NONE',  ( -19.05341960407611168, -5.049401038298163336, 96.45724293864769550 ) ) ;
#133897=CARTESIAN_POINT ( 'NONE',  ( 9.564922557960805705, 16.46253265017160317, 109.5822429386476955 ) ) ;
#133898=CARTESIAN_POINT ( 'NONE',  ( 16.46253265017160672, -9.564922557960803928, 38.33224293864768839 ) ) ;
#133899=CARTESIAN_POINT ( 'NONE',  ( 4.483927247898545687, 16.52544592524342804, 114.7905762719810383 ) ) ;
#133900=CARTESIAN_POINT ( 'NONE',  ( 16.55341960407611168, 4.379528057220329451, 93.95724293864770971 ) ) ;
#133901=CARTESIAN_POINT ( 'NONE',  ( -15.72974639402197994, 15.80617190586746368, 100.6239096053143811 ) ) ;
#133902=CARTESIAN_POINT ( 'NONE',  ( 19.05341960407611168, 5.049401038298154454, 83.95724293864766707 ) ) ;
#133903=CARTESIAN_POINT ( 'NONE',  ( -21.53943276465977519, -0.05219959533937600094, 18.75109039468568639 ) ) ;
#133904=CARTESIAN_POINT ( 'NONE',  ( -19.03943276465977164, 0.05219959533909376836, 91.24890960531436690 ) ) ;
#133906=CARTESIAN_POINT ( 'NONE',  ( 16.55341960407611168, 4.379528057220329451, 103.9572429386476813 ) ) ;
#133907=CARTESIAN_POINT ( 'NONE',  ( 19.03943276465977164, -0.05219959533909143690, 73.74890960531435269 ) ) ;
#133908=CARTESIAN_POINT ( 'NONE',  ( -21.53943276465977519, 0.05219959533907696930, 76.24890960531435269 ) ) ;
#133909=CARTESIAN_POINT ( 'NONE',  ( -13.89961937509977652, 13.97604488694528158, 115.6239096053143669 ) ) ;
#133911=CARTESIAN_POINT ( 'NONE',  ( 18.62759615963271287, -10.81492255796078972, 33.33224293864769550 ) ) ;
#133912=CARTESIAN_POINT ( 'NONE',  ( 18.22780087662119897, -5.500000000000096811, 68.51763182126893525 ) ) ;
#133913=CARTESIAN_POINT ( 'NONE',  ( -4.483927247898782831, 16.52544592524335698, 32.70942372801900433 ) ) ;
#133914=CARTESIAN_POINT ( 'NONE',  ( -12.14591786802309592, -12.06949235617757132, 91.87390960531436690 ) ) ;
#133916=CARTESIAN_POINT ( 'NONE',  ( -17.50000000000001066, -3.471454075611646317, 110.5166741885564505 ) ) ;
#133917=CARTESIAN_POINT ( 'NONE',  ( -0.05219959533909027116, -19.03943276465977164, 82.49890960531436690 ) ) ;
#133918=CARTESIAN_POINT ( 'NONE',  ( 5.049401038298161559, -19.05341960407611168, 42.70724293864767418 ) ) ;
#133919=CARTESIAN_POINT ( 'NONE',  ( 16.52544592524342804, -4.483927247898539470, 78.54057627198103830 ) ) ;
#133920=CARTESIAN_POINT ( 'NONE',  ( -0.05219959533907301413, -21.53943276465977519, 37.49890960531436690 ) ) ;
#133921=CARTESIAN_POINT ( 'NONE',  ( -0.05219959533910754901, -16.53943276465976808, 57.49890960531435979 ) ) ;
#133922=CARTESIAN_POINT ( 'NONE',  ( 13.97604488694548053, -13.89961937509957401, 105.6260903946856757 ) ) ;
#133923=CARTESIAN_POINT ( 'NONE',  ( 15.80617190586769283, -15.72974639402175789, 65.62609039468568994 ) ) ;
#133926=CARTESIAN_POINT ( 'NONE',  ( -5.049401038298153566, 19.05341960407611168, 115.2072429386477097 ) ) ;
#133927=CARTESIAN_POINT ( 'NONE',  ( 12.14591786802327356, -12.06949235617739191, 85.62609039468568994 ) ) ;
#133928=CARTESIAN_POINT ( 'NONE',  ( -17.31728774477212340, 6.344390552233681646, 95.81906651689308774 ) ) ;
#133929=CARTESIAN_POINT ( 'NONE',  ( -0.05219959533909027116, -19.03943276465977164, 72.49890960531435269 ) ) ;
#133930=CARTESIAN_POINT ( 'NONE',  ( 5.719274019375991003, -21.55341960407610458, 77.70724293864770971 ) ) ;
#133931=CARTESIAN_POINT ( 'NONE',  ( -4.483927247898782831, 16.52544592524335698, 22.70942372801901499 ) ) ;
#133932=CARTESIAN_POINT ( 'NONE',  ( -16.53943276465976808, 0.05219959533911058130, 51.24890960531436690 ) ) ;
#133933=CARTESIAN_POINT ( 'NONE',  ( -21.52544592524334988, -5.823673210054445271, 58.95942372801902565 ) ) ;
#133934=CARTESIAN_POINT ( 'NONE',  ( -16.52544592524335698, -4.483927247898792601, 83.95942372801900433 ) ) ;
#133935=CARTESIAN_POINT ( 'NONE',  ( 18.67979575497178502, 10.72451020669898547, 24.16557627198103120 ) ) ;
#133936=CARTESIAN_POINT ( 'NONE',  ( -13.89961937509977830, 13.97604488694528158, 115.6239096053143669 ) ) ;
#133937=CARTESIAN_POINT ( 'NONE',  ( -17.48847506799967633, 5.747544572773789717, 80.82697437843280852 ) ) ;
#133938=CARTESIAN_POINT ( 'NONE',  ( 16.55341960407618274, -4.379528057220086978, 101.0427570613523756 ) ) ;
#133939=CARTESIAN_POINT ( 'NONE',  ( -8.224510206698735004, -14.34966873604973081, 54.58442372801901143 ) ) ;
#133940=CARTESIAN_POINT ( 'NONE',  ( 16.46253265017160672, -9.564922557960803928, 78.33224293864769550 ) ) ;
#133941=CARTESIAN_POINT ( 'NONE',  ( -19.02544592524342804, 5.153800228976336051, 91.04057627198100988 ) ) ;
#133942=CARTESIAN_POINT ( 'NONE',  ( 5.719274019375673035, 21.55341960407619339, 77.29275706135234714 ) ) ;
#133943=CARTESIAN_POINT ( 'NONE',  ( 16.52544592524335698, 4.483927247898782831, 71.45942372801901854 ) ) ;
#133944=CARTESIAN_POINT ( 'NONE',  ( -4.483927247898539470, -16.52544592524342804, 47.29057627198103120 ) ) ;
#133945=CARTESIAN_POINT ( 'NONE',  ( 19.02544592524343514, -5.153800228976328945, 48.54057627198103120 ) ) ;
#133946=CARTESIAN_POINT ( 'NONE',  ( -13.97604488694527625, -13.89961937509977652, 41.87390960531435979 ) ) ;
#133948=CARTESIAN_POINT ( 'NONE',  ( 5.153800228976615827, -19.02544592524334988, 90.20942372801900433 ) ) ;
#133949=CARTESIAN_POINT ( 'NONE',  ( 12.06949235617757843, -12.14591786802309237, 103.1239096053143811 ) ) ;
#133950=CARTESIAN_POINT ( 'NONE',  ( -19.03943276465977164, 0.05219959533909376836, 61.24890960531436690 ) ) ;
#133951=CARTESIAN_POINT ( 'NONE',  ( 5.049401038297881783, 19.05341960407617563, 107.2927570613523187 ) ) ;
#133953=CARTESIAN_POINT ( 'NONE',  ( -21.52544592524334988, -5.823673210054445271, 108.9594237280190185 ) ) ;
#133954=CARTESIAN_POINT ( 'NONE',  ( -4.379528057220086978, -16.55341960407618274, 69.79275706135234714 ) ) ;
#133955=CARTESIAN_POINT ( 'NONE',  ( -19.05341960407617563, 5.049401038297882671, 93.54275706135234714 ) ) ;
#133956=CARTESIAN_POINT ( 'NONE',  ( 15.80617190586746368, 15.72974639402197994, 59.37390960531436690 ) ) ;
#133957=CARTESIAN_POINT ( 'NONE',  ( 16.55341960407618274, -4.379528057220086978, 56.04275706135235424 ) ) ;
#133959=CARTESIAN_POINT ( 'NONE',  ( -5.153800228976607833, 19.02544592524334988, 52.70942372801900433 ) ) ;
#133960=CARTESIAN_POINT ( 'NONE',  ( 0.05219959533909260263, 19.03943276465977164, 84.99890960531436690 ) ) ;
#133961=CARTESIAN_POINT ( 'NONE',  ( -16.52544592524342804, 4.483927247898546575, 111.0405762719810525 ) ) ;
#133962=CARTESIAN_POINT ( 'NONE',  ( -9.564922557960796823, -16.46253265017161027, 62.08224293864769550 ) ) ;
#133963=CARTESIAN_POINT ( 'NONE',  ( -14.34966873604960291, -8.224510206698953496, 56.66557627198103830 ) ) ;
#133965=CARTESIAN_POINT ( 'NONE',  ( -18.62759615963255300, -10.81492255796106328, 94.16775706135237556 ) ) ;
#133966=CARTESIAN_POINT ( 'NONE',  ( -16.51473224551082808, 9.474510206698731452, 48.33442372801900433 ) ) ;
#133967=CARTESIAN_POINT ( 'NONE',  ( -0.05219959533936034679, 19.03943276465977164, 27.50109039468566507 ) ) ;
#133968=CARTESIAN_POINT ( 'NONE',  ( 21.52544592524344225, -5.823673210054117533, 23.54057627198102765 ) ) ;
#133969=CARTESIAN_POINT ( 'NONE',  ( -21.55341960407619339, 5.719274019375674811, 93.54275706135234714 ) ) ;
#133970=CARTESIAN_POINT ( 'NONE',  ( 16.46253265017160672, -9.564922557960803928, 78.33224293864769550 ) ) ;
#133972=CARTESIAN_POINT ( 'NONE',  ( -5.719274019375665041, -21.55341960407619695, 99.79275706135234714 ) ) ;
#133973=CARTESIAN_POINT ( 'NONE',  ( -21.53943276465977519, 0.05219959533907696930, 46.24890960531435979 ) ) ;
#133974=CARTESIAN_POINT ( 'NONE',  ( 5.153800228976335163, 19.02544592524342804, 84.79057627198099567 ) ) ;
#133975=CARTESIAN_POINT ( 'NONE',  ( -0.05219959533936034679, 19.03943276465977164, 67.50109039468566152 ) ) ;
#133976=CARTESIAN_POINT ( 'NONE',  ( -9.564922557960796823, -16.46253265017161027, 37.08224293864768839 ) ) ;
#133977=CARTESIAN_POINT ( 'NONE',  ( 19.03943276465977164, -0.05219959533909143690, 93.74890960531435269 ) ) ;
#133978=CARTESIAN_POINT ( 'NONE',  ( -9.564922557961040184, 16.46253265017147172, 87.91775706135233293 ) ) ;
#133979=CARTESIAN_POINT ( 'NONE',  ( -16.52544592524335698, -4.483927247898792601, 43.95942372801902565 ) ) ;
#133980=CARTESIAN_POINT ( 'NONE',  ( 14.34966873604960469, 8.224510206698951720, 99.16557627198100988 ) ) ;
#133981=CARTESIAN_POINT ( 'NONE',  ( 19.02544592524343514, -5.153800228976328945, 68.54057627198103830 ) ) ;
#133982=CARTESIAN_POINT ( 'NONE',  ( 10.81492255796078972, 18.62759615963270932, 54.58224293864769550 ) ) ;
#133983=CARTESIAN_POINT ( 'NONE',  ( 5.153800228976615827, -19.02544592524334988, 110.2094237280189901 ) ) ;
#133984=CARTESIAN_POINT ( 'NONE',  ( 5.823673210054125526, 21.52544592524343514, 114.7905762719810383 ) ) ;
#133985=CARTESIAN_POINT ( 'NONE',  ( 18.62759615963255655, 10.81492255796105972, 71.66775706135234714 ) ) ;
#133986=CARTESIAN_POINT ( 'NONE',  ( -8.314922557961024197, 14.29746914071037800, 77.91775706135231871 ) ) ;
#133987=CARTESIAN_POINT ( 'NONE',  ( -9.564922557960796823, -16.46253265017161027, 72.08224293864770971 ) ) ;
#133988=CARTESIAN_POINT ( 'NONE',  ( -0.05219959533934338120, 16.53943276465976808, 107.5010903946856899 ) ) ;
#133989=CARTESIAN_POINT ( 'NONE',  ( -13.89961937509957401, -13.97604488694547875, 39.37609039468566152 ) ) ;
#133990=CARTESIAN_POINT ( 'NONE',  ( 18.62759615963255655, 10.81492255796105972, 36.66775706135234714 ) ) ;
#133991=CARTESIAN_POINT ( 'NONE',  ( -0.05219959533910754901, -16.53943276465976808, 82.49890960531436690 ) ) ;
#133992=CARTESIAN_POINT ( 'NONE',  ( -19.03943276465977164, 0.05219959533909376836, 101.2489096053143669 ) ) ;
#133993=CARTESIAN_POINT ( 'NONE',  ( -16.55341960407617563, 4.379528057220093196, 83.54275706135234714 ) ) ;
#133994=CARTESIAN_POINT ( 'NONE',  ( 21.55341960407619695, -5.719274019375665929, 76.04275706135237556 ) ) ;
#133995=CARTESIAN_POINT ( 'NONE',  ( -16.52544592524335698, -4.483927247898792601, 28.95942372801902209 ) ) ;
#133996=CARTESIAN_POINT ( 'NONE',  ( 21.52544592524334988, 5.823673210054432836, 26.45942372801901854 ) ) ;
#133997=CARTESIAN_POINT ( 'NONE',  ( 16.53943276465976808, -0.05219959533910856209, 73.74890960531433848 ) ) ;
#133999=CARTESIAN_POINT ( 'NONE',  ( 5.823673210054125526, 21.52544592524343514, 94.79057627198105251 ) ) ;
#134000=CARTESIAN_POINT ( 'NONE',  ( 0.05219959533910956823, 16.53943276465976808, 54.99890960531435269 ) ) ;
#134001=ORIENTED_EDGE ( 'NONE', *, *, #195051, .T. ) ;
#134002=CARTESIAN_POINT ( 'NONE',  ( -13.97604488694527625, -13.89961937509977652, 31.87390960531435979 ) ) ;
#134003=CARTESIAN_POINT ( 'NONE',  ( 15.80617190586746368, 15.72974639402197994, 24.37390960531435979 ) ) ;
#134004=CARTESIAN_POINT ( 'NONE',  ( 10.81492255796106328, -18.62759615963255655, 40.41775706135234714 ) ) ;
#134005=CARTESIAN_POINT ( 'NONE',  ( 12.14591786802309770, 12.06949235617756955, 69.37390960531436690 ) ) ;
#134006=CARTESIAN_POINT ( 'NONE',  ( -10.81492255796078084, -18.62759615963271287, 72.08224293864769550 ) ) ;
#134007=CARTESIAN_POINT ( 'NONE',  ( 5.049401038298161559, -19.05341960407611168, 77.70724293864765286 ) ) ;
#134008=CARTESIAN_POINT ( 'NONE',  ( 9.564922557960805705, 16.46253265017160317, 24.58224293864769194 ) ) ;
#134009=CARTESIAN_POINT ( 'NONE',  ( 19.03943276465977164, 0.05219959533936151252, 76.25109039468566152 ) ) ;
#134010=CARTESIAN_POINT ( 'NONE',  ( -18.62759615963270932, 10.81492255796079327, 60.83224293864769550 ) ) ;
#134011=CARTESIAN_POINT ( 'NONE',  ( 9.474510206698971260, -16.51473224551069308, 37.91557627198102409 ) ) ;
#134012=CARTESIAN_POINT ( 'NONE',  ( -13.97604488694527625, -13.89961937509977652, 66.87390960531436690 ) ) ;
#134013=ORIENTED_EDGE ( 'NONE', *, *, #193512, .F. ) ;
#134014=CARTESIAN_POINT ( 'NONE',  ( 12.14591786802327356, -12.06949235617739191, 50.62609039468568994 ) ) ;
#134015=CARTESIAN_POINT ( 'NONE',  ( 18.67979575497194134, -10.72451020669871369, 25.83442372801901499 ) ) ;
#134016=CARTESIAN_POINT ( 'NONE',  ( -21.52544592524334988, -5.823673210054445271, 53.95942372801900433 ) ) ;
#134017=CARTESIAN_POINT ( 'NONE',  ( 13.97604488694527802, 13.89961937509977652, 104.3739096053143385 ) ) ;
#134018=CARTESIAN_POINT ( 'NONE',  ( 15.80617190586746368, 15.72974639402197994, 69.37390960531436690 ) ) ;
#134019=CARTESIAN_POINT ( 'NONE',  ( 21.52544592524344225, -5.823673210054117533, 113.5405762719810383 ) ) ;
#134020=CARTESIAN_POINT ( 'NONE',  ( -16.53943276465976808, -0.05219959533934237506, 48.75109039468568284 ) ) ;
#134021=CARTESIAN_POINT ( 'NONE',  ( 15.72974639402199770, -15.80617190586745480, 48.12390960531436690 ) ) ;
#134022=CARTESIAN_POINT ( 'NONE',  ( 18.67979575497194134, -10.72451020669871369, 105.8344237280190328 ) ) ;
#134023=CARTESIAN_POINT ( 'NONE',  ( 9.474510206698971260, -16.51473224551069308, 57.91557627198103120 ) ) ;
#134025=CARTESIAN_POINT ( 'NONE',  ( 13.97604488694527802, 13.89961937509977652, 74.37390960531436690 ) ) ;
#134027=CARTESIAN_POINT ( 'NONE',  ( -5.049401038297874678, -19.05341960407617918, 64.79275706135233293 ) ) ;
#134028=CARTESIAN_POINT ( 'NONE',  ( 16.51473224551083163, -9.474510206698727899, 20.83442372801899722 ) ) ;
#134029=CARTESIAN_POINT ( 'NONE',  ( -5.719274019375978568, 21.55341960407610458, 40.20724293864769550 ) ) ;
#134030=CARTESIAN_POINT ( 'NONE',  ( -14.29746914071037622, -8.314922557961029526, 109.1677570613523613 ) ) ;
#134031=CARTESIAN_POINT ( 'NONE',  ( -16.51473224551082808, 9.474510206698731452, 83.33442372801899012 ) ) ;
#134032=CARTESIAN_POINT ( 'NONE',  ( -17.31728774477273802, 6.344390552232390235, 60.81906651689319432 ) ) ;
#134033=CARTESIAN_POINT ( 'NONE',  ( 19.02544592524334988, 5.153800228976608722, 26.45942372801899722 ) ) ;
#134034=CARTESIAN_POINT ( 'NONE',  ( -19.03943276465977164, -0.05219959533935918106, 78.75109039468567573 ) ) ;
#134035=CARTESIAN_POINT ( 'NONE',  ( 5.049401038297881783, 19.05341960407617563, 47.29275706135231161 ) ) ;
#134036=CARTESIAN_POINT ( 'NONE',  ( -17.44279575226823198, -5.990770900252489817, 44.16442432485681735 ) ) ;
#134037=CARTESIAN_POINT ( 'NONE',  ( 5.153800228976335163, 19.02544592524342804, 39.79057627198100988 ) ) ;
#134038=CARTESIAN_POINT ( 'NONE',  ( -8.314922557960811034, -14.29746914071050412, 52.08224293864768839 ) ) ;
#134039=CARTESIAN_POINT ( 'NONE',  ( -19.02544592524342804, 5.153800228976336051, 36.04057627198100988 ) ) ;
#134040=CARTESIAN_POINT ( 'NONE',  ( 4.483927247898545687, 16.52544592524342804, 44.79057627198103120 ) ) ;
#134042=CARTESIAN_POINT ( 'NONE',  ( -14.34966873604972548, 8.224510206698743886, 108.3344237280190185 ) ) ;
#134043=CARTESIAN_POINT ( 'NONE',  ( 19.02544592524343514, -5.153800228976328945, 48.54057627198103120 ) ) ;
#134044=CARTESIAN_POINT ( 'NONE',  ( -5.153800228976607833, 19.02544592524334988, 27.70942372801899722 ) ) ;
#134045=CARTESIAN_POINT ( 'NONE',  ( 12.14591786802327356, -12.06949235617739191, 30.62609039468567929 ) ) ;
#134046=CARTESIAN_POINT ( 'NONE',  ( 15.80617190586746368, 15.72974639402197994, 39.37390960531436690 ) ) ;
#134047=CARTESIAN_POINT ( 'NONE',  ( -10.72451020669870658, -18.67979575497194134, 94.58442372801901854 ) ) ;
#134048=VERTEX_POINT ( 'NONE', #3549 ) ;
#134049=CARTESIAN_POINT ( 'NONE',  ( -16.46253265017160317, 9.564922557960807481, 110.8322429386476955 ) ) ;
#134050=CARTESIAN_POINT ( 'NONE',  ( 9.564922557960805705, 16.46253265017160317, 94.58224293864769550 ) ) ;
#134052=CARTESIAN_POINT ( 'NONE',  ( 15.72974639402199770, -15.80617190586745480, 103.1239096053143811 ) ) ;
#134054=CARTESIAN_POINT ( 'NONE',  ( 16.52544592524342804, -4.483927247898539470, 73.54057627198102409 ) ) ;
#134055=CARTESIAN_POINT ( 'NONE',  ( 18.62759615963271287, -10.81492255796078972, 78.33224293864770971 ) ) ;
#134056=CARTESIAN_POINT ( 'NONE',  ( -16.46253265017160317, 9.564922557960807481, 65.83224293864769550 ) ) ;
#134057=CARTESIAN_POINT ( 'NONE',  ( -5.153800228976328057, -19.02544592524343514, 72.29057627198102409 ) ) ;
#134058=CARTESIAN_POINT ( 'NONE',  ( 21.55341960407610458, 5.719274019375980345, 98.95724293864770971 ) ) ;
#134061=CARTESIAN_POINT ( 'NONE',  ( -9.564922557960796823, -16.46253265017161027, 62.08224293864769550 ) ) ;
#134062=CARTESIAN_POINT ( 'NONE',  ( -8.314922557960811034, -14.29746914071050412, 112.0822429386477097 ) ) ;
#134063=CARTESIAN_POINT ( 'NONE',  ( -19.05341960407611168, -5.049401038298163336, 26.45724293864769550 ) ) ;
#134064=CARTESIAN_POINT ( 'NONE',  ( 9.474510206698971260, -16.51473224551069308, 57.91557627198103120 ) ) ;
#134065=CARTESIAN_POINT ( 'NONE',  ( 19.03943276465977164, 0.05219959533936151252, 86.25109039468567573 ) ) ;
#134067=CARTESIAN_POINT ( 'NONE',  ( -12.06949235617756955, 12.14591786802309770, 100.6239096053143811 ) ) ;
#134068=CARTESIAN_POINT ( 'NONE',  ( -18.67979575497193778, 10.72451020669871902, 53.33442372801901854 ) ) ;
#134069=CARTESIAN_POINT ( 'NONE',  ( 13.89961937509977652, -13.97604488694527269, 48.12390960531435979 ) ) ;
#134070=CARTESIAN_POINT ( 'NONE',  ( 10.72451020669898902, -18.67979575497178502, 112.9155762719810383 ) ) ;
#134071=CARTESIAN_POINT ( 'NONE',  ( -8.224510206698948167, 14.34966873604960824, 95.41557627198102409 ) ) ;
#134073=CARTESIAN_POINT ( 'NONE',  ( -9.564922557960796823, -16.46253265017161027, 77.08224293864769550 ) ) ;
#134075=CARTESIAN_POINT ( 'NONE',  ( -8.224510206698735004, -14.34966873604973081, 19.58442372801901143 ) ) ;
#134076=CARTESIAN_POINT ( 'NONE',  ( 0.05219959533907565091, 21.53943276465977519, 29.99890960531435979 ) ) ;
#134077=CARTESIAN_POINT ( 'NONE',  ( 10.72451020669871369, 18.67979575497193778, 52.08442372801901854 ) ) ;
#134079=CARTESIAN_POINT ( 'NONE',  ( -13.89961937509977652, 13.97604488694528158, 95.62390960531436690 ) ) ;
#134080=CARTESIAN_POINT ( 'NONE',  ( 13.89961937509957401, 13.97604488694547697, 86.87609039468567573 ) ) ;
#134081=CARTESIAN_POINT ( 'NONE',  ( -16.46253265017160317, 9.564922557960807481, 65.83224293864769550 ) ) ;
#134082=CARTESIAN_POINT ( 'NONE',  ( 0.05219959533910956823, 16.53943276465976808, 84.99890960531436690 ) ) ;
#134083=CARTESIAN_POINT ( 'NONE',  ( 19.03943276465977164, -0.05219959533909143690, 108.7489096053143527 ) ) ;
#134084=CARTESIAN_POINT ( 'NONE',  ( 4.483927247898545687, 16.52544592524342804, 79.79057627198102409 ) ) ;
#134085=CARTESIAN_POINT ( 'NONE',  ( 9.474510206698971260, -16.51473224551069308, 92.91557627198103830 ) ) ;
#134086=CARTESIAN_POINT ( 'NONE',  ( 16.51473224551083163, -9.474510206698727899, 40.83442372801900433 ) ) ;
#134087=CARTESIAN_POINT ( 'NONE',  ( -19.03943276465977164, 0.05219959533909376836, 46.24890960531435979 ) ) ;
#134088=CARTESIAN_POINT ( 'NONE',  ( 12.14591786802309770, 12.06949235617756955, 39.37390960531436690 ) ) ;
#134089=CARTESIAN_POINT ( 'NONE',  ( -19.03943276465977164, 0.05219959533909376836, 31.24890960531435979 ) ) ;
#134091=CARTESIAN_POINT ( 'NONE',  ( -5.719274019375665041, -21.55341960407619695, 39.79275706135235424 ) ) ;
#134092=CARTESIAN_POINT ( 'NONE',  ( 13.97604488694548053, -13.89961937509957401, 85.62609039468568994 ) ) ;
#134093=CARTESIAN_POINT ( 'NONE',  ( 16.53943276465976808, -0.05219959533910856209, 53.74890960531437401 ) ) ;
#134094=CARTESIAN_POINT ( 'NONE',  ( -21.52544592524343514, 5.823673210054127303, 106.0405762719810525 ) ) ;
#134095=CARTESIAN_POINT ( 'NONE',  ( -21.53943276465977519, 0.05219959533907696930, 36.24890960531435979 ) ) ;
#134096=CARTESIAN_POINT ( 'NONE',  ( 4.483927247898545687, 16.52544592524342804, 79.79057627198102409 ) ) ;
#134097=CARTESIAN_POINT ( 'NONE',  ( 16.51473224551069308, 9.474510206698969483, 44.16557627198103120 ) ) ;
#134098=CARTESIAN_POINT ( 'NONE',  ( -12.14591786802326823, 12.06949235617739902, 113.1260903946856899 ) ) ;
#134100=CARTESIAN_POINT ( 'NONE',  ( 12.14591786802327356, -12.06949235617739191, 90.62609039468567573 ) ) ;
#134101=CARTESIAN_POINT ( 'NONE',  ( 16.52544592524335698, 4.483927247898782831, 76.45942372801901854 ) ) ;
#134102=CARTESIAN_POINT ( 'NONE',  ( 5.153800228976615827, -19.02544592524334988, 30.20942372801900433 ) ) ;
#134103=CARTESIAN_POINT ( 'NONE',  ( 19.05341960407611168, 5.049401038298154454, 88.95724293864769550 ) ) ;
#134104=CARTESIAN_POINT ( 'NONE',  ( -13.89961937509977652, 13.97604488694528158, 75.62390960531438111 ) ) ;
#134105=CARTESIAN_POINT ( 'NONE',  ( 8.224510206698742110, 14.34966873604972548, 72.08442372801899012 ) ) ;
#134106=CARTESIAN_POINT ( 'NONE',  ( -0.05219959533909027116, -19.03943276465977164, 37.49890960531436690 ) ) ;
#134107=CARTESIAN_POINT ( 'NONE',  ( 0.05219959533910956823, 16.53943276465976808, 49.99890960531437401 ) ) ;
#134109=CARTESIAN_POINT ( 'NONE',  ( 19.02544592524343514, -5.153800228976328945, 98.54057627198100988 ) ) ;
#134110=CARTESIAN_POINT ( 'NONE',  ( -10.72451020669898014, 18.67979575497178502, 30.41557627198101699 ) ) ;
#134111=CARTESIAN_POINT ( 'NONE',  ( -12.06949235617756955, 12.14591786802309770, 65.62390960531436690 ) ) ;
#134112=ORIENTED_EDGE ( 'NONE', *, *, #66266, .F. ) ;
#134113=CARTESIAN_POINT ( 'NONE',  ( -16.52544592524342804, 4.483927247898546575, 66.04057627198103830 ) ) ;
#134115=CARTESIAN_POINT ( 'NONE',  ( -9.564922557961040184, 16.46253265017147172, 67.91775706135233293 ) ) ;
#134116=CARTESIAN_POINT ( 'NONE',  ( 5.049401038298161559, -19.05341960407611168, 87.70724293864769550 ) ) ;
#134117=CARTESIAN_POINT ( 'NONE',  ( -9.474510206698720793, -16.51473224551083518, 74.58442372801900433 ) ) ;
#134118=CARTESIAN_POINT ( 'NONE',  ( -18.22780087662123805, -5.499999999999968026, 93.98236817873105053 ) ) ;
#134119=CARTESIAN_POINT ( 'NONE',  ( -4.379528057220086978, -16.55341960407618274, 19.79275706135235069 ) ) ;
#134120=CARTESIAN_POINT ( 'NONE',  ( 0.05219959533934541429, -16.53943276465976808, 100.0010903946857042 ) ) ;
#134121=CARTESIAN_POINT ( 'NONE',  ( 9.564922557960805705, 16.46253265017160317, 44.58224293864769550 ) ) ;
#134122=CARTESIAN_POINT ( 'NONE',  ( 21.52544592524344225, -5.823673210054117533, 28.54057627198103120 ) ) ;
#134123=CARTESIAN_POINT ( 'NONE',  ( -18.62759615963255300, -10.81492255796106328, 54.16775706135235424 ) ) ;
#134124=CARTESIAN_POINT ( 'NONE',  ( -4.483927247898782831, 16.52544592524335698, 22.70942372801901499 ) ) ;
#134125=CARTESIAN_POINT ( 'NONE',  ( -18.22780087662126647, -5.499999999999827693, 53.98236817873107185 ) ) ;
#134126=CARTESIAN_POINT ( 'NONE',  ( 0.05219959533909260263, 19.03943276465977164, 74.99890960531435269 ) ) ;
#134127=CARTESIAN_POINT ( 'NONE',  ( -5.153800228976328057, -19.02544592524343514, 112.2905762719810099 ) ) ;
#134128=CARTESIAN_POINT ( 'NONE',  ( -16.53943276465976808, 0.05219959533911058130, 76.24890960531435269 ) ) ;
#134129=CARTESIAN_POINT ( 'NONE',  ( -5.049401038298153566, 19.05341960407611168, 75.20724293864769550 ) ) ;
#134130=CARTESIAN_POINT ( 'NONE',  ( 0.05219959533909260263, 19.03943276465977164, 79.99890960531436690 ) ) ;
#134132=CARTESIAN_POINT ( 'NONE',  ( 13.97604488694548053, -13.89961937509957401, 85.62609039468568994 ) ) ;
#134133=CARTESIAN_POINT ( 'NONE',  ( -10.72451020669898014, 18.67979575497178502, 65.41557627198102409 ) ) ;
#134134=CARTESIAN_POINT ( 'NONE',  ( 5.049401038298161559, -19.05341960407611168, 27.70724293864769550 ) ) ;
#134135=CARTESIAN_POINT ( 'NONE',  ( 16.51473224551083163, -9.474510206698727899, 60.83442372801900433 ) ) ;
#134136=CARTESIAN_POINT ( 'NONE',  ( 9.564922557960805705, 16.46253265017160317, 59.58224293864769550 ) ) ;
#134137=CARTESIAN_POINT ( 'NONE',  ( -16.51473224551069308, -9.474510206698971260, 96.66557627198102409 ) ) ;
#134139=CARTESIAN_POINT ( 'NONE',  ( -15.72974639402197994, 15.80617190586746368, 85.62390960531436690 ) ) ;
#134140=CARTESIAN_POINT ( 'NONE',  ( -8.314922557960811034, -14.29746914071050412, 97.08224293864770971 ) ) ;
#134141=CARTESIAN_POINT ( 'NONE',  ( 16.46253265017146816, 9.564922557961045513, 51.66775706135233293 ) ) ;
#134142=CARTESIAN_POINT ( 'NONE',  ( -5.719274019375978568, 21.55341960407610458, 85.20724293864770971 ) ) ;
#134143=CARTESIAN_POINT ( 'NONE',  ( 18.67979575497178502, 10.72451020669898547, 79.16557627198103830 ) ) ;
#134145=CARTESIAN_POINT ( 'NONE',  ( 16.53943276465976808, -0.05219959533910856209, 38.74890960531435979 ) ) ;
#134146=CARTESIAN_POINT ( 'NONE',  ( -15.80617190586768217, 15.72974639402176855, 108.1260903946856757 ) ) ;
#134147=CARTESIAN_POINT ( 'NONE',  ( 19.05341960407611168, 5.049401038298154454, 73.95724293864768129 ) ) ;
#134148=CARTESIAN_POINT ( 'NONE',  ( -19.02544592524342804, 5.153800228976336051, 36.04057627198100988 ) ) ;
#134149=CARTESIAN_POINT ( 'NONE',  ( 15.80617190586769283, -15.72974639402175789, 45.62609039468567573 ) ) ;
#134150=CARTESIAN_POINT ( 'NONE',  ( 18.67979575497194134, -10.72451020669871369, 50.83442372801901143 ) ) ;
#134151=CARTESIAN_POINT ( 'NONE',  ( 0.05219959533909260263, 19.03943276465977164, 49.99890960531435979 ) ) ;
#134152=CARTESIAN_POINT ( 'NONE',  ( 5.719274019375673035, 21.55341960407619339, 22.29275706135235069 ) ) ;
#134153=CARTESIAN_POINT ( 'NONE',  ( -9.474510206698720793, -16.51473224551083518, 54.58442372801899722 ) ) ;
#134154=CARTESIAN_POINT ( 'NONE',  ( -9.564922557960796823, -16.46253265017161027, 42.08224293864769550 ) ) ;
#134155=CARTESIAN_POINT ( 'NONE',  ( -14.34966873604972548, 8.224510206698743886, 23.33442372801901499 ) ) ;
#134156=CARTESIAN_POINT ( 'NONE',  ( -0.05219959533909027116, -19.03943276465977164, 22.49890960531436690 ) ) ;
#134157=CARTESIAN_POINT ( 'NONE',  ( -16.52544592524335698, -4.483927247898792601, 73.95942372801901854 ) ) ;
#134158=CARTESIAN_POINT ( 'NONE',  ( -13.89961937509977652, 13.97604488694528158, 40.62390960531435979 ) ) ;
#134160=CARTESIAN_POINT ( 'NONE',  ( -5.049401038298153566, 19.05341960407611168, 80.20724293864769550 ) ) ;
#134161=CARTESIAN_POINT ( 'NONE',  ( -13.97604488694527625, -13.89961937509977652, 31.87390960531435979 ) ) ;
#134162=CARTESIAN_POINT ( 'NONE',  ( 10.81492255796078972, 18.62759615963270932, 74.58224293864768129 ) ) ;
#134163=CARTESIAN_POINT ( 'NONE',  ( -12.14591786802326823, 12.06949235617739902, 43.12609039468568284 ) ) ;
#134164=CARTESIAN_POINT ( 'NONE',  ( -21.53943276465977519, -0.05219959533937600094, 113.7510903946856757 ) ) ;
#134166=CARTESIAN_POINT ( 'NONE',  ( 19.02544592524343514, -5.153800228976328945, 33.54057627198102409 ) ) ;
#134167=CARTESIAN_POINT ( 'NONE',  ( -8.224510206698948167, 14.34966873604960824, 25.41557627198103120 ) ) ;
#134168=CARTESIAN_POINT ( 'NONE',  ( 4.483927247898545687, 16.52544592524342804, 69.79057627198102409 ) ) ;
#134169=CARTESIAN_POINT ( 'NONE',  ( 9.564922557960805705, 16.46253265017160317, 69.58224293864770971 ) ) ;
#134170=CARTESIAN_POINT ( 'NONE',  ( -21.55341960407619339, 5.719274019375674811, 108.5427570613523756 ) ) ;
#134171=CARTESIAN_POINT ( 'NONE',  ( -10.81492255796105439, 18.62759615963255655, 27.91775706135234358 ) ) ;
#134172=CARTESIAN_POINT ( 'NONE',  ( -5.049401038298153566, 19.05341960407611168, 75.20724293864769550 ) ) ;
#134173=CARTESIAN_POINT ( 'NONE',  ( -21.52544592524334988, -5.823673210054445271, 88.95942372801901854 ) ) ;
#134174=CARTESIAN_POINT ( 'NONE',  ( 14.29746914071037800, 8.314922557961029526, 66.66775706135234714 ) ) ;
#134175=CARTESIAN_POINT ( 'NONE',  ( 0.05219959533934541429, -16.53943276465976808, 35.00109039468568284 ) ) ;
#134176=CARTESIAN_POINT ( 'NONE',  ( -14.34966873604960291, -8.224510206698953496, 91.66557627198103830 ) ) ;
#134177=CARTESIAN_POINT ( 'NONE',  ( 9.474510206698971260, -16.51473224551069308, 102.9155762719810241 ) ) ;
#134178=ADVANCED_FACE ( 'NONE', ( #90837 ), #47937, .T. ) ;
#134179=CARTESIAN_POINT ( 'NONE',  ( 14.34966873604960469, 8.224510206698951720, 34.16557627198102409 ) ) ;
#134180=CARTESIAN_POINT ( 'NONE',  ( -13.89961937509977652, 13.97604488694528158, 25.62390960531434558 ) ) ;
#134181=CARTESIAN_POINT ( 'NONE',  ( -16.53943276465976808, -0.05219959533934237506, 48.75109039468568284 ) ) ;
#134182=CARTESIAN_POINT ( 'NONE',  ( 0.05219959533910956823, 16.53943276465976808, 49.99890960531437401 ) ) ;
#134183=CARTESIAN_POINT ( 'NONE',  ( -12.14591786802326823, 12.06949235617739902, 98.12609039468570415 ) ) ;
#134184=CARTESIAN_POINT ( 'NONE',  ( -16.46253265017160317, 9.564922557960807481, 115.8322429386477097 ) ) ;
#134185=CARTESIAN_POINT ( 'NONE',  ( -5.719274019375978568, 21.55341960407610458, 30.20724293864769550 ) ) ;
#134186=CARTESIAN_POINT ( 'NONE',  ( 5.823673210054444382, -21.52544592524334988, 110.2094237280190185 ) ) ;
#134187=CARTESIAN_POINT ( 'NONE',  ( -8.314922557960811034, -14.29746914071050412, 82.08224293864768129 ) ) ;
#134188=CARTESIAN_POINT ( 'NONE',  ( 0.05219959533909260263, 19.03943276465977164, 89.99890960531436690 ) ) ;
#134190=CARTESIAN_POINT ( 'NONE',  ( -8.224510206698735004, -14.34966873604973081, 39.58442372801901143 ) ) ;
#134191=CARTESIAN_POINT ( 'NONE',  ( 0.05219959533909260263, 19.03943276465977164, 39.99890960531436690 ) ) ;
#134192=CARTESIAN_POINT ( 'NONE',  ( -17.33423593373957772, -5.611347464745015223, 21.19882084351016971 ) ) ;
#134193=CARTESIAN_POINT ( 'NONE',  ( -19.05341960407617563, 5.049401038297882671, 48.54275706135233293 ) ) ;
#134194=CARTESIAN_POINT ( 'NONE',  ( 5.049401038298161559, -19.05341960407611168, 42.70724293864767418 ) ) ;
#134195=CARTESIAN_POINT ( 'NONE',  ( -14.29746914071037622, -8.314922557961029526, 74.16775706135231871 ) ) ;
#134196=CARTESIAN_POINT ( 'NONE',  ( 16.46253265017146816, 9.564922557961045513, 91.66775706135234714 ) ) ;
#134197=CARTESIAN_POINT ( 'NONE',  ( 9.474510206698971260, -16.51473224551069308, 57.91557627198103120 ) ) ;
#134198=CARTESIAN_POINT ( 'NONE',  ( 10.72451020669898902, -18.67979575497178502, 87.91557627198103830 ) ) ;
#134199=CARTESIAN_POINT ( 'NONE',  ( -16.55341960407611168, -4.379528057220339221, 96.45724293864770971 ) ) ;
#134201=CARTESIAN_POINT ( 'NONE',  ( -9.564922557961040184, 16.46253265017147172, 67.91775706135233293 ) ) ;
#134202=CARTESIAN_POINT ( 'NONE',  ( 0.05219959533907565091, 21.53943276465977519, 59.99890960531436690 ) ) ;
#134203=CARTESIAN_POINT ( 'NONE',  ( 16.46253265017146816, 9.564922557961045513, 46.66775706135233293 ) ) ;
#134204=CARTESIAN_POINT ( 'NONE',  ( 5.049401038298161559, -19.05341960407611168, 112.7072429386476813 ) ) ;
#134206=CARTESIAN_POINT ( 'NONE',  ( -10.81492255796078084, -18.62759615963271287, 92.08224293864769550 ) ) ;
#134207=CARTESIAN_POINT ( 'NONE',  ( -18.56453257813361191, 5.500000000000043521, 55.99000423690686290 ) ) ;
#134208=CARTESIAN_POINT ( 'NONE',  ( -9.474510206698720793, -16.51473224551083518, 104.5844237280190043 ) ) ;
#134209=CARTESIAN_POINT ( 'NONE',  ( -18.39443945427639449, 5.500000000000033751, 58.51745347608655123 ) ) ;
#134210=CARTESIAN_POINT ( 'NONE',  ( -14.29746914071037622, -8.314922557961029526, 29.16775706135234003 ) ) ;
#134211=CARTESIAN_POINT ( 'NONE',  ( -16.46253265017160317, 9.564922557960807481, 45.83224293864769550 ) ) ;
#134212=CARTESIAN_POINT ( 'NONE',  ( 13.89961937509977652, -13.97604488694527269, 113.1239096053143527 ) ) ;
#134213=CARTESIAN_POINT ( 'NONE',  ( 21.53943276465977519, -0.05219959533907433946, 83.74890960531435269 ) ) ;
#134215=CARTESIAN_POINT ( 'NONE',  ( -15.72974639402176322, -15.80617190586768395, 64.37609039468568994 ) ) ;
#134216=CARTESIAN_POINT ( 'NONE',  ( 9.564922557961047289, -16.46253265017146816, 110.4177570613523471 ) ) ;
#134217=CARTESIAN_POINT ( 'NONE',  ( -13.97604488694547697, 13.89961937509957934, 33.12609039468566863 ) ) ;
#134218=CARTESIAN_POINT ( 'NONE',  ( -14.29746914071049879, 8.314922557960819915, 35.83224293864768839 ) ) ;
#134219=CARTESIAN_POINT ( 'NONE',  ( 10.72451020669898902, -18.67979575497178502, 97.91557627198103830 ) ) ;
#134220=CARTESIAN_POINT ( 'NONE',  ( -16.53943276465976808, 0.05219959533911058130, 51.24890960531436690 ) ) ;
#134221=CARTESIAN_POINT ( 'NONE',  ( 0.05219959533936267826, -19.03943276465977164, 100.0010903946856757 ) ) ;
#134222=CARTESIAN_POINT ( 'NONE',  ( 16.51473224551083163, -9.474510206698727899, 55.83442372801899722 ) ) ;
#134224=CARTESIAN_POINT ( 'NONE',  ( -0.05219959533937732626, 21.53943276465977519, 77.50109039468567573 ) ) ;
#134225=CARTESIAN_POINT ( 'NONE',  ( 0.05219959533936267826, -19.03943276465977164, 45.00109039468566863 ) ) ;
#134226=CARTESIAN_POINT ( 'NONE',  ( -19.05341960407611168, -5.049401038298163336, 21.45724293864768839 ) ) ;
#134227=CARTESIAN_POINT ( 'NONE',  ( 21.52544592524344225, -5.823673210054117533, 43.54057627198103830 ) ) ;
#134228=CARTESIAN_POINT ( 'NONE',  ( -12.14591786802309592, -12.06949235617757132, 36.87390960531435979 ) ) ;
#134229=CARTESIAN_POINT ( 'NONE',  ( -21.55341960407619339, 5.719274019375674811, 113.5427570613523756 ) ) ;
#134230=CARTESIAN_POINT ( 'NONE',  ( 8.314922557961029526, -14.29746914071037800, 70.41775706135236135 ) ) ;
#134231=CARTESIAN_POINT ( 'NONE',  ( -14.29746914071049879, 8.314922557960819915, 40.83224293864769550 ) ) ;
#134232=CARTESIAN_POINT ( 'NONE',  ( 21.52544592524334988, 5.823673210054432836, 71.45942372801901854 ) ) ;
#134233=CARTESIAN_POINT ( 'NONE',  ( -18.62759615963255300, -10.81492255796106328, 64.16775706135234714 ) ) ;
#134234=CARTESIAN_POINT ( 'NONE',  ( 5.719274019375991003, -21.55341960407610458, 72.70724293864769550 ) ) ;
#134235=CARTESIAN_POINT ( 'NONE',  ( 13.89961937509977652, -13.97604488694527269, 43.12390960531434558 ) ) ;
#134236=CARTESIAN_POINT ( 'NONE',  ( -0.05219959533937732626, 21.53943276465977519, 47.50109039468568994 ) ) ;
#134237=CARTESIAN_POINT ( 'NONE',  ( -16.52544592524342804, 4.483927247898546575, 116.0405762719810383 ) ) ;
#134238=CARTESIAN_POINT ( 'NONE',  ( -9.474510206698964154, 16.51473224551069663, 40.41557627198103120 ) ) ;
#134239=CARTESIAN_POINT ( 'NONE',  ( 16.55341960407611168, 4.379528057220329451, 88.95724293864769550 ) ) ;
#134240=CARTESIAN_POINT ( 'NONE',  ( 19.03943276465977164, -0.05219959533909143690, 78.74890960531436690 ) ) ;
#134241=CARTESIAN_POINT ( 'NONE',  ( -12.14591786802309592, -12.06949235617757132, 46.87390960531435979 ) ) ;
#134242=CARTESIAN_POINT ( 'NONE',  ( 0.05219959533910956823, 16.53943276465976808, 94.99890960531436690 ) ) ;
#134243=CARTESIAN_POINT ( 'NONE',  ( 21.53943276465977519, -0.05219959533907433946, 63.74890960531435979 ) ) ;
#134244=CARTESIAN_POINT ( 'NONE',  ( -5.719274019375978568, 21.55341960407610458, 110.2072429386477239 ) ) ;
#134245=CARTESIAN_POINT ( 'NONE',  ( -9.564922557960796823, -16.46253265017161027, 112.0822429386476955 ) ) ;
#134246=CARTESIAN_POINT ( 'NONE',  ( 9.564922557960805705, 16.46253265017160317, 59.58224293864769550 ) ) ;
#134247=CARTESIAN_POINT ( 'NONE',  ( -4.379528057220086978, -16.55341960407618274, 24.79275706135235779 ) ) ;
#134248=CARTESIAN_POINT ( 'NONE',  ( -18.67979575497178146, -10.72451020669898902, 61.66557627198103120 ) ) ;
#134249=CARTESIAN_POINT ( 'NONE',  ( -15.80617190586768217, 15.72974639402176855, 98.12609039468570415 ) ) ;
#134250=CARTESIAN_POINT ( 'NONE',  ( 0.05219959533909260263, 19.03943276465977164, 74.99890960531435269 ) ) ;
#134251=CARTESIAN_POINT ( 'NONE',  ( 18.62759615963255655, 10.81492255796105972, 21.66775706135235069 ) ) ;
#134252=CARTESIAN_POINT ( 'NONE',  ( 19.03943276465977164, -0.05219959533909143690, 108.7489096053143527 ) ) ;
#134253=CARTESIAN_POINT ( 'NONE',  ( -8.224510206698735004, -14.34966873604973081, 89.58442372801901854 ) ) ;
#134254=CARTESIAN_POINT ( 'NONE',  ( 18.62759615963255655, 10.81492255796105972, 66.66775706135234714 ) ) ;
#134255=CARTESIAN_POINT ( 'NONE',  ( 5.823673210054444382, -21.52544592524334988, 105.2094237280190328 ) ) ;
#134256=CARTESIAN_POINT ( 'NONE',  ( 12.14591786802327356, -12.06949235617739191, 60.62609039468567573 ) ) ;
#134257=CARTESIAN_POINT ( 'NONE',  ( 18.62759615963255655, 10.81492255796105972, 26.66775706135235424 ) ) ;
#134258=CARTESIAN_POINT ( 'NONE',  ( -19.03943276465977164, 0.05219959533909376836, 111.2489096053143669 ) ) ;
#134259=CARTESIAN_POINT ( 'NONE',  ( 21.55341960407619695, -5.719274019375665929, 86.04275706135236135 ) ) ;
#134260=CARTESIAN_POINT ( 'NONE',  ( 9.474510206698971260, -16.51473224551069308, 92.91557627198103830 ) ) ;
#134261=CARTESIAN_POINT ( 'NONE',  ( 10.72451020669898902, -18.67979575497178502, 87.91557627198103830 ) ) ;
#134262=CARTESIAN_POINT ( 'NONE',  ( -0.05219959533936034679, 19.03943276465977164, 52.50109039468566863 ) ) ;
#134263=CARTESIAN_POINT ( 'NONE',  ( -15.72974639402197994, 15.80617190586746368, 55.62390960531436690 ) ) ;
#134264=CARTESIAN_POINT ( 'NONE',  ( 16.51473224551069308, 9.474510206698969483, 94.16557627198103830 ) ) ;
#134265=CARTESIAN_POINT ( 'NONE',  ( -8.314922557960811034, -14.29746914071050412, 42.08224293864769550 ) ) ;
#134267=CARTESIAN_POINT ( 'NONE',  ( 13.89961937509957401, 13.97604488694547697, 61.87609039468566863 ) ) ;
#134269=CARTESIAN_POINT ( 'NONE',  ( 0.05219959533936267826, -19.03943276465977164, 105.0010903946856615 ) ) ;
#134270=CARTESIAN_POINT ( 'NONE',  ( 18.67979575497178502, 10.72451020669898547, 89.16557627198102409 ) ) ;
#134271=CARTESIAN_POINT ( 'NONE',  ( -16.53943276465976808, 0.05219959533911058130, 56.24890960531436690 ) ) ;
#134272=CARTESIAN_POINT ( 'NONE',  ( -16.52544592524335698, -4.483927247898792601, 33.95942372801901143 ) ) ;
#134273=CARTESIAN_POINT ( 'NONE',  ( 19.02544592524343514, -5.153800228976328945, 48.54057627198103120 ) ) ;
#134274=CARTESIAN_POINT ( 'NONE',  ( -15.72974639402176322, -15.80617190586768395, 19.37609039468568639 ) ) ;
#134275=CARTESIAN_POINT ( 'NONE',  ( 5.153800228976615827, -19.02544592524334988, 90.20942372801900433 ) ) ;
#134276=CARTESIAN_POINT ( 'NONE',  ( -19.02544592524342804, 5.153800228976336051, 91.04057627198100988 ) ) ;
#134277=CARTESIAN_POINT ( 'NONE',  ( -19.02544592524342804, 5.153800228976336051, 81.04057627198103830 ) ) ;
#134278=CARTESIAN_POINT ( 'NONE',  ( 10.72451020669898902, -18.67979575497178502, 82.91557627198103830 ) ) ;
#134279=CARTESIAN_POINT ( 'NONE',  ( -13.97604488694527625, -13.89961937509977652, 46.87390960531435979 ) ) ;
#134281=CARTESIAN_POINT ( 'NONE',  ( 4.483927247898545687, 16.52544592524342804, 59.79057627198103120 ) ) ;
#134282=CARTESIAN_POINT ( 'NONE',  ( 9.474510206698971260, -16.51473224551069308, 92.91557627198103830 ) ) ;
#134284=CARTESIAN_POINT ( 'NONE',  ( -5.153800228976607833, 19.02544592524334988, 62.70942372801899722 ) ) ;
#134286=CARTESIAN_POINT ( 'NONE',  ( -10.81492255796078084, -18.62759615963271287, 72.08224293864769550 ) ) ;
#134287=CARTESIAN_POINT ( 'NONE',  ( -19.03943276465977164, -0.05219959533935918106, 33.75109039468566863 ) ) ;
#134288=CARTESIAN_POINT ( 'NONE',  ( 9.564922557960805705, 16.46253265017160317, 99.58224293864770971 ) ) ;
#134290=CARTESIAN_POINT ( 'NONE',  ( 18.62759615963271287, -10.81492255796078972, 38.33224293864768839 ) ) ;
#134291=CARTESIAN_POINT ( 'NONE',  ( 19.02544592524343514, -5.153800228976328945, 73.54057627198103830 ) ) ;
#134293=CARTESIAN_POINT ( 'NONE',  ( -15.72974639402176322, -15.80617190586768395, 59.37609039468568284 ) ) ;
#134294=CARTESIAN_POINT ( 'NONE',  ( -5.049401038298153566, 19.05341960407611168, 30.20724293864768839 ) ) ;
#134295=CARTESIAN_POINT ( 'NONE',  ( -5.823673210054116645, -21.52544592524344225, 112.2905762719810241 ) ) ;
#134297=CARTESIAN_POINT ( 'NONE',  ( -18.67979575497193778, 10.72451020669871902, 48.33442372801902565 ) ) ;
#134299=CARTESIAN_POINT ( 'NONE',  ( -19.02544592524342804, 5.153800228976336051, 96.04057627198103830 ) ) ;
#134300=CARTESIAN_POINT ( 'NONE',  ( 9.474510206698729675, 16.51473224551082808, 72.08442372801900433 ) ) ;
#134302=CARTESIAN_POINT ( 'NONE',  ( 21.52544592524344225, -5.823673210054117533, 103.5405762719810383 ) ) ;
#134303=CARTESIAN_POINT ( 'NONE',  ( -19.05341960407611168, -5.049401038298163336, 56.45724293864768129 ) ) ;
#134304=CARTESIAN_POINT ( 'NONE',  ( -4.379528057220086978, -16.55341960407618274, 34.79275706135235424 ) ) ;
#134306=CARTESIAN_POINT ( 'NONE',  ( 10.72451020669871369, 18.67979575497193778, 97.08442372801904696 ) ) ;
#134307=CARTESIAN_POINT ( 'NONE',  ( 19.02544592524343514, -5.153800228976328945, 48.54057627198103120 ) ) ;
#134308=CARTESIAN_POINT ( 'NONE',  ( -5.719274019375665041, -21.55341960407619695, 104.7927570613523898 ) ) ;
#134309=CARTESIAN_POINT ( 'NONE',  ( 9.564922557960805705, 16.46253265017160317, 94.58224293864769550 ) ) ;
#134310=CARTESIAN_POINT ( 'NONE',  ( 21.55341960407619695, -5.719274019375665929, 61.04275706135234714 ) ) ;
#134312=CARTESIAN_POINT ( 'NONE',  ( -9.474510206698964154, 16.51473224551069663, 110.4155762719810383 ) ) ;
#134314=CARTESIAN_POINT ( 'NONE',  ( -16.55341960407617563, 4.379528057220093196, 48.54275706135234714 ) ) ;
#134315=CARTESIAN_POINT ( 'NONE',  ( 15.72974639402176855, 15.80617190586768217, 66.87609039468568994 ) ) ;
#134316=CARTESIAN_POINT ( 'NONE',  ( -0.05219959533937732626, 21.53943276465977519, 92.50109039468567573 ) ) ;
#134318=CARTESIAN_POINT ( 'NONE',  ( 16.52544592524335698, 4.483927247898782831, 21.45942372801901499 ) ) ;
#134319=CARTESIAN_POINT ( 'NONE',  ( 9.564922557960805705, 16.46253265017160317, 69.58224293864770971 ) ) ;
#134320=CARTESIAN_POINT ( 'NONE',  ( -13.97604488694527625, -13.89961937509977652, 106.8739096053143669 ) ) ;
#134322=CARTESIAN_POINT ( 'NONE',  ( 5.153800228976335163, 19.02544592524342804, 24.79057627198102765 ) ) ;
#134323=CARTESIAN_POINT ( 'NONE',  ( 21.55341960407610458, 5.719274019375980345, 48.95724293864770971 ) ) ;
#134324=EDGE_CURVE ( 'NONE', #135096, #59793, #169152, .T. ) ;
#134325=CARTESIAN_POINT ( 'NONE',  ( -16.52544592524335698, -4.483927247898792601, 98.95942372801903275 ) ) ;
#134326=CARTESIAN_POINT ( 'NONE',  ( -16.55341960407611168, -4.379528057220339221, 81.45724293864769550 ) ) ;
#134327=CARTESIAN_POINT ( 'NONE',  ( 19.02544592524343514, -5.153800228976328945, 63.54057627198103830 ) ) ;
#134328=CARTESIAN_POINT ( 'NONE',  ( 0.05219959533937995610, -21.53943276465977519, 85.00109039468568994 ) ) ;
#134330=CARTESIAN_POINT ( 'NONE',  ( -16.51473224551082808, 9.474510206698731452, 113.3344237280190043 ) ) ;
#134331=CARTESIAN_POINT ( 'NONE',  ( 14.29746914071049879, -8.314922557960816363, 93.33224293864769550 ) ) ;
#134332=CARTESIAN_POINT ( 'NONE',  ( -15.80617190586768217, 15.72974639402176855, 38.12609039468567573 ) ) ;
#134333=CARTESIAN_POINT ( 'NONE',  ( -5.823673210054116645, -21.52544592524344225, 72.29057627198102409 ) ) ;
#134334=CARTESIAN_POINT ( 'NONE',  ( 13.97604488694548053, -13.89961937509957401, 40.62609039468564731 ) ) ;
#134336=CARTESIAN_POINT ( 'NONE',  ( 16.51473224551069308, 9.474510206698969483, 89.16557627198103830 ) ) ;
#134337=CARTESIAN_POINT ( 'NONE',  ( -16.55341960407611168, -4.379528057220339221, 66.45724293864768129 ) ) ;
#134338=EDGE_CURVE ( 'NONE', #184472, #70081, #144778, .T. ) ;
#134339=CARTESIAN_POINT ( 'NONE',  ( -0.05219959533910754901, -16.53943276465976808, 32.49890960531435979 ) ) ;
#134340=CARTESIAN_POINT ( 'NONE',  ( 14.34966873604972726, -8.224510206698740333, 105.8344237280190328 ) ) ;
#134341=CARTESIAN_POINT ( 'NONE',  ( -5.049401038297874678, -19.05341960407617918, 69.79275706135233293 ) ) ;
#134344=CARTESIAN_POINT ( 'NONE',  ( -18.67979575497178146, -10.72451020669898902, 26.66557627198103475 ) ) ;
#134345=CARTESIAN_POINT ( 'NONE',  ( 4.483927247898545687, 16.52544592524342804, 89.79057627198103830 ) ) ;
#134347=CARTESIAN_POINT ( 'NONE',  ( 5.049401038298161559, -19.05341960407611168, 47.70724293864770260 ) ) ;
#134348=CARTESIAN_POINT ( 'NONE',  ( -15.80617190586745835, -15.72974639402198527, 46.87390960531435979 ) ) ;
#134349=CARTESIAN_POINT ( 'NONE',  ( 0.05219959533907565091, 21.53943276465977519, 69.99890960531435269 ) ) ;
#134350=CARTESIAN_POINT ( 'NONE',  ( 14.34966873604960469, 8.224510206698951720, 109.1655762719810383 ) ) ;
#134351=CARTESIAN_POINT ( 'NONE',  ( -8.224510206698735004, -14.34966873604973081, 59.58442372801901854 ) ) ;
#134352=CARTESIAN_POINT ( 'NONE',  ( -19.05341960407611168, -5.049401038298163336, 41.45724293864769550 ) ) ;
#134353=CARTESIAN_POINT ( 'NONE',  ( -15.80617190586768217, 15.72974639402176855, 53.12609039468568284 ) ) ;
#134354=CARTESIAN_POINT ( 'NONE',  ( -12.06949235617756955, 12.14591786802309770, 105.6239096053143669 ) ) ;
#134355=CARTESIAN_POINT ( 'NONE',  ( 16.46253265017146816, 9.564922557961045513, 91.66775706135234714 ) ) ;
#134358=CARTESIAN_POINT ( 'NONE',  ( 18.67979575497178502, 10.72451020669898547, 49.16557627198102409 ) ) ;
#134359=CARTESIAN_POINT ( 'NONE',  ( 16.19135201231363297, -7.376712067592068323, 67.31319145947966831 ) ) ;
#134360=CARTESIAN_POINT ( 'NONE',  ( 21.53943276465977519, 0.05219959533937863772, 71.25109039468568994 ) ) ;
#134361=CARTESIAN_POINT ( 'NONE',  ( -14.34966873604972548, 8.224510206698743886, 53.33442372801901854 ) ) ;
#134362=CARTESIAN_POINT ( 'NONE',  ( -14.34966873604960291, -8.224510206698953496, 36.66557627198103120 ) ) ;
#134363=CARTESIAN_POINT ( 'NONE',  ( 15.80617190586746368, 15.72974639402197994, 74.37390960531436690 ) ) ;
#134364=CARTESIAN_POINT ( 'NONE',  ( 15.80617190586746368, 15.72974639402197994, 69.37390960531436690 ) ) ;
#134366=CARTESIAN_POINT ( 'NONE',  ( 9.564922557961047289, -16.46253265017146816, 85.41775706135233293 ) ) ;
#134367=CARTESIAN_POINT ( 'NONE',  ( -13.97604488694527625, -13.89961937509977652, 111.8739096053143243 ) ) ;
#134368=CARTESIAN_POINT ( 'NONE',  ( 16.51473224551069308, 9.474510206698969483, 54.16557627198103120 ) ) ;
#134369=CARTESIAN_POINT ( 'NONE',  ( -19.03943276465977164, 0.05219959533909376836, 21.24890960531436335 ) ) ;
#134372=CARTESIAN_POINT ( 'NONE',  ( 14.29746914071037800, 8.314922557961029526, 86.66775706135234714 ) ) ;
#134373=CARTESIAN_POINT ( 'NONE',  ( 15.80617190586746368, 15.72974639402197994, 104.3739096053143669 ) ) ;
#134374=CARTESIAN_POINT ( 'NONE',  ( -9.564922557960796823, -16.46253265017161027, 72.08224293864770971 ) ) ;
#134375=CARTESIAN_POINT ( 'NONE',  ( -5.823673210054431948, 21.52544592524334988, 42.70942372801901854 ) ) ;
#134376=CARTESIAN_POINT ( 'NONE',  ( 9.564922557960805705, 16.46253265017160317, 99.58224293864770971 ) ) ;
#134379=CARTESIAN_POINT ( 'NONE',  ( 18.67979575497194134, -10.72451020669871369, 25.83442372801901499 ) ) ;
#134380=CARTESIAN_POINT ( 'NONE',  ( -16.51473224551069308, -9.474510206698971260, 21.66557627198102765 ) ) ;
#134381=CARTESIAN_POINT ( 'NONE',  ( 13.89961937509957401, 13.97604488694547697, 86.87609039468567573 ) ) ;
#134382=CARTESIAN_POINT ( 'NONE',  ( -9.564922557961040184, 16.46253265017147172, 37.91775706135233293 ) ) ;
#134383=CARTESIAN_POINT ( 'NONE',  ( -21.53943276465977519, 0.05219959533907696930, 116.2489096053143669 ) ) ;
#134384=CARTESIAN_POINT ( 'NONE',  ( 19.02544592524334988, 5.153800228976608722, 36.45942372801900433 ) ) ;
#134385=CARTESIAN_POINT ( 'NONE',  ( -19.02544592524334988, -5.153800228976617603, 43.95942372801899012 ) ) ;
#134386=CARTESIAN_POINT ( 'NONE',  ( 14.34966873604972726, -8.224510206698740333, 95.83442372801903275 ) ) ;
#134387=CARTESIAN_POINT ( 'NONE',  ( 19.05341960407611168, 5.049401038298154454, 113.9572429386477097 ) ) ;
#134389=CARTESIAN_POINT ( 'NONE',  ( 13.89961937509977652, -13.97604488694527269, 68.12390960531436690 ) ) ;
#134391=CARTESIAN_POINT ( 'NONE',  ( 0.05219959533937995610, -21.53943276465977519, 75.00109039468568994 ) ) ;
#134392=CARTESIAN_POINT ( 'NONE',  ( -21.53943276465977519, -0.05219959533937600094, 98.75109039468568994 ) ) ;
#134394=CARTESIAN_POINT ( 'NONE',  ( 16.51473224551069308, 9.474510206698969483, 84.16557627198102409 ) ) ;
#134395=CARTESIAN_POINT ( 'NONE',  ( -18.67979575497193778, 10.72451020669871902, 58.33442372801901143 ) ) ;
#134396=CARTESIAN_POINT ( 'NONE',  ( 0.05219959533936267826, -19.03943276465977164, 95.00109039468567573 ) ) ;
#134397=CARTESIAN_POINT ( 'NONE',  ( 13.97604488694527802, 13.89961937509977652, 64.37390960531436690 ) ) ;
#134398=CARTESIAN_POINT ( 'NONE',  ( -13.89961937509977652, 13.97604488694528158, 115.6239096053143669 ) ) ;
#134399=CARTESIAN_POINT ( 'NONE',  ( 13.97604488694527802, 13.89961937509977652, 74.37390960531436690 ) ) ;
#134401=CARTESIAN_POINT ( 'NONE',  ( 13.89961937509977652, -13.97604488694527269, 68.12390960531436690 ) ) ;
#134402=CARTESIAN_POINT ( 'NONE',  ( -5.049401038298153566, 19.05341960407611168, 55.20724293864769550 ) ) ;
#134403=CARTESIAN_POINT ( 'NONE',  ( 5.823673210054125526, 21.52544592524343514, 114.7905762719810383 ) ) ;
#134404=CARTESIAN_POINT ( 'NONE',  ( -16.53943276465976808, -0.05219959533934237506, 83.75109039468568994 ) ) ;
#134407=CARTESIAN_POINT ( 'NONE',  ( 9.474510206698729675, 16.51473224551082808, 57.08442372801900433 ) ) ;
#134409=CARTESIAN_POINT ( 'NONE',  ( -16.51473224551069308, -9.474510206698971260, 76.66557627198103830 ) ) ;
#134410=CARTESIAN_POINT ( 'NONE',  ( -0.05219959533910754901, -16.53943276465976808, 67.49890960531436690 ) ) ;
#134411=CARTESIAN_POINT ( 'NONE',  ( 14.29746914071049879, -8.314922557960816363, 103.3322429386476955 ) ) ;
#134412=CARTESIAN_POINT ( 'NONE',  ( -21.53943276465977519, 0.05219959533907696930, 31.24890960531435979 ) ) ;
#134413=CARTESIAN_POINT ( 'NONE',  ( -9.564922557960796823, -16.46253265017161027, 107.0822429386476955 ) ) ;
#134414=CARTESIAN_POINT ( 'NONE',  ( 8.314922557960818139, 14.29746914071049879, 94.58224293864769550 ) ) ;
#134416=CARTESIAN_POINT ( 'NONE',  ( 13.89961937509957401, 13.97604488694547697, 36.87609039468565442 ) ) ;
#134417=CARTESIAN_POINT ( 'NONE',  ( -12.14591786802326823, 12.06949235617739902, 103.1260903946856757 ) ) ;
#134418=CARTESIAN_POINT ( 'NONE',  ( 0.05219959533909260263, 19.03943276465977164, 84.99890960531436690 ) ) ;
#134419=CARTESIAN_POINT ( 'NONE',  ( 18.62759615963255655, 10.81492255796105972, 56.66775706135235424 ) ) ;
#134420=CARTESIAN_POINT ( 'NONE',  ( 21.55341960407610458, 5.719274019375980345, 43.95724293864769550 ) ) ;
#134421=CARTESIAN_POINT ( 'NONE',  ( -21.55341960407610458, -5.719274019375992779, 111.4572429386476813 ) ) ;
#134422=CARTESIAN_POINT ( 'NONE',  ( 10.72451020669898902, -18.67979575497178502, 72.91557627198103830 ) ) ;
#134423=CARTESIAN_POINT ( 'NONE',  ( -4.379528057220328563, 16.55341960407611168, 90.20724293864770971 ) ) ;
#134424=CARTESIAN_POINT ( 'NONE',  ( -13.97604488694547697, 13.89961937509957934, 63.12609039468566152 ) ) ;
#134425=CARTESIAN_POINT ( 'NONE',  ( -9.474510206698964154, 16.51473224551069663, 30.41557627198102054 ) ) ;
#134426=CARTESIAN_POINT ( 'NONE',  ( 0.05219959533909260263, 19.03943276465977164, 99.99890960531436690 ) ) ;
#134427=CARTESIAN_POINT ( 'NONE',  ( -19.03943276465977164, 0.05219959533909376836, 91.24890960531436690 ) ) ;
#134428=CARTESIAN_POINT ( 'NONE',  ( 12.06949235617757843, -12.14591786802309237, 108.1239096053143811 ) ) ;
#134429=CARTESIAN_POINT ( 'NONE',  ( 14.34966873604960469, 8.224510206698951720, 24.16557627198103120 ) ) ;
#134430=CARTESIAN_POINT ( 'NONE',  ( 4.483927247898790824, -16.52544592524335698, 40.20942372801901854 ) ) ;
#134431=CARTESIAN_POINT ( 'NONE',  ( -15.80617190586768217, 15.72974639402176855, 113.1260903946856899 ) ) ;
#134432=CARTESIAN_POINT ( 'NONE',  ( 0.05219959533909260263, 19.03943276465977164, 104.9989096053143669 ) ) ;
#134433=CARTESIAN_POINT ( 'NONE',  ( 16.52544592524342804, -4.483927247898539470, 28.54057627198103120 ) ) ;
#134434=CARTESIAN_POINT ( 'NONE',  ( -18.67979575497193778, 10.72451020669871902, 33.33442372801900433 ) ) ;
#134435=CARTESIAN_POINT ( 'NONE',  ( 16.51473224551069308, 9.474510206698969483, 44.16557627198103120 ) ) ;
#134436=CARTESIAN_POINT ( 'NONE',  ( -4.379528057220086978, -16.55341960407618274, 44.79275706135234714 ) ) ;
#134437=CARTESIAN_POINT ( 'NONE',  ( 4.483927247898790824, -16.52544592524335698, 110.2094237280190185 ) ) ;
#134438=CARTESIAN_POINT ( 'NONE',  ( 12.14591786802327356, -12.06949235617739191, 95.62609039468568994 ) ) ;
#134439=CARTESIAN_POINT ( 'NONE',  ( -16.52544592524335698, -4.483927247898792601, 18.95942372801901143 ) ) ;
#134440=CARTESIAN_POINT ( 'NONE',  ( 19.05341960407611168, 5.049401038298154454, 28.95724293864769550 ) ) ;
#134441=CARTESIAN_POINT ( 'NONE',  ( -8.224510206698948167, 14.34966873604960824, 90.41557627198103830 ) ) ;
#134442=CARTESIAN_POINT ( 'NONE',  ( 5.719274019375991003, -21.55341960407610458, 107.7072429386476955 ) ) ;
#134443=CARTESIAN_POINT ( 'NONE',  ( -13.97604488694527625, -13.89961937509977652, 31.87390960531435979 ) ) ;
#134444=CARTESIAN_POINT ( 'NONE',  ( -19.03943276465977164, 0.05219959533909376836, 101.2489096053143669 ) ) ;
#134445=CARTESIAN_POINT ( 'NONE',  ( -5.823673210054431948, 21.52544592524334988, 37.70942372801900433 ) ) ;
#134447=CARTESIAN_POINT ( 'NONE',  ( -13.89961937509977652, 13.97604488694528158, 105.6239096053143527 ) ) ;
#134448=CARTESIAN_POINT ( 'NONE',  ( 16.38665767535056261, -7.295008042176093888, 112.7640086421455123 ) ) ;
#134449=CARTESIAN_POINT ( 'NONE',  ( -16.51473224551069308, -9.474510206698971260, 86.66557627198102409 ) ) ;
#134450=CARTESIAN_POINT ( 'NONE',  ( -21.53943276465977519, -0.05219959533937600094, 28.75109039468567929 ) ) ;
#134451=CARTESIAN_POINT ( 'NONE',  ( 16.55341960407611168, 4.379528057220329451, 93.95724293864770971 ) ) ;
#134452=CARTESIAN_POINT ( 'NONE',  ( -5.153800228976328057, -19.02544592524343514, 92.29057627198099567 ) ) ;
#134453=CARTESIAN_POINT ( 'NONE',  ( -16.51473224551082808, 9.474510206698731452, 28.33442372801900433 ) ) ;
#134454=CARTESIAN_POINT ( 'NONE',  ( -14.29746914071037622, -8.314922557961029526, 59.16775706135234714 ) ) ;
#134455=CARTESIAN_POINT ( 'NONE',  ( -21.55341960407619339, 5.719274019375674811, 73.54275706135234714 ) ) ;
#134456=CARTESIAN_POINT ( 'NONE',  ( -14.34966873604972548, 8.224510206698743886, 38.33442372801900433 ) ) ;
#134457=CARTESIAN_POINT ( 'NONE',  ( -16.51473224551069308, -9.474510206698971260, 76.66557627198103830 ) ) ;
#134458=CARTESIAN_POINT ( 'NONE',  ( 13.97604488694548053, -13.89961937509957401, 100.6260903946856615 ) ) ;
#134459=CARTESIAN_POINT ( 'NONE',  ( -8.314922557961024197, 14.29746914071037800, 62.91775706135236135 ) ) ;
#134460=CARTESIAN_POINT ( 'NONE',  ( 21.53943276465977519, 0.05219959533937863772, 106.2510903946856757 ) ) ;
#134461=CARTESIAN_POINT ( 'NONE',  ( 16.46253265017146816, 9.564922557961045513, 86.66775706135233293 ) ) ;
#134462=CARTESIAN_POINT ( 'NONE',  ( -9.564922557960796823, -16.46253265017161027, 67.08224293864769550 ) ) ;
#134463=CARTESIAN_POINT ( 'NONE',  ( 5.719274019375991003, -21.55341960407610458, 87.70724293864769550 ) ) ;
#134464=CARTESIAN_POINT ( 'NONE',  ( -4.379528057220328563, 16.55341960407611168, 85.20724293864770971 ) ) ;
#134465=CARTESIAN_POINT ( 'NONE',  ( 13.89961937509957401, 13.97604488694547697, 86.87609039468567573 ) ) ;
#134466=CARTESIAN_POINT ( 'NONE',  ( 14.29746914071037800, 8.314922557961029526, 61.66775706135235424 ) ) ;
#134467=CARTESIAN_POINT ( 'NONE',  ( -18.22780087662122028, 5.500000000000031086, 78.51540105326107266 ) ) ;
#134468=CARTESIAN_POINT ( 'NONE',  ( -19.03943276465977164, -0.05219959533935918106, 53.75109039468566863 ) ) ;
#134469=CARTESIAN_POINT ( 'NONE',  ( -16.55341960407611168, -4.379528057220339221, 21.45724293864769550 ) ) ;
#134470=CARTESIAN_POINT ( 'NONE',  ( -0.05219959533910754901, -16.53943276465976808, 82.49890960531436690 ) ) ;
#134471=CARTESIAN_POINT ( 'NONE',  ( 9.564922557961047289, -16.46253265017146816, 20.41775706135233293 ) ) ;
#134472=CARTESIAN_POINT ( 'NONE',  ( 17.59860650958994555, -7.585241751806880650, 45.92337014262493966 ) ) ;
#134473=CARTESIAN_POINT ( 'NONE',  ( -21.53943276465977519, -0.05219959533937600094, 18.75109039468568639 ) ) ;
#134474=CARTESIAN_POINT ( 'NONE',  ( -16.51473224551069308, -9.474510206698971260, 101.6655762719810241 ) ) ;
#134475=CARTESIAN_POINT ( 'NONE',  ( 0.05219959533909260263, 19.03943276465977164, 74.99890960531435269 ) ) ;
#134476=CARTESIAN_POINT ( 'NONE',  ( -21.55341960407619339, 5.719274019375674811, 88.54275706135236135 ) ) ;
#134477=CARTESIAN_POINT ( 'NONE',  ( 19.03943276465977164, -0.05219959533909143690, 58.74890960531435979 ) ) ;
#134478=CARTESIAN_POINT ( 'NONE',  ( 15.80617190586746368, 15.72974639402197994, 29.37390960531435269 ) ) ;
#134479=CARTESIAN_POINT ( 'NONE',  ( -12.06949235617756955, 12.14591786802309770, 80.62390960531438111 ) ) ;
#134480=CARTESIAN_POINT ( 'NONE',  ( 19.05341960407611168, 5.049401038298154454, 38.95724293864767418 ) ) ;
#134481=CARTESIAN_POINT ( 'NONE',  ( -4.379528057220328563, 16.55341960407611168, 95.20724293864769550 ) ) ;
#134482=CARTESIAN_POINT ( 'NONE',  ( 10.81492255796078972, 18.62759615963270932, 104.5822429386477097 ) ) ;
#134483=CARTESIAN_POINT ( 'NONE',  ( 0.05219959533937995610, -21.53943276465977519, 65.00109039468568994 ) ) ;
#134484=CARTESIAN_POINT ( 'NONE',  ( -19.05341960407611168, -5.049401038298163336, 26.45724293864769550 ) ) ;
#134485=CARTESIAN_POINT ( 'NONE',  ( 8.224510206698742110, 14.34966873604972548, 62.08442372801901143 ) ) ;
#134486=CARTESIAN_POINT ( 'NONE',  ( -21.53943276465977519, 0.05219959533907696930, 101.2489096053143669 ) ) ;
#134487=CARTESIAN_POINT ( 'NONE',  ( -18.67979575497178146, -10.72451020669898902, 111.6655762719810525 ) ) ;
#134488=CARTESIAN_POINT ( 'NONE',  ( 9.564922557961047289, -16.46253265017146816, 40.41775706135234003 ) ) ;
#134489=CARTESIAN_POINT ( 'NONE',  ( -0.05219959533909027116, -19.03943276465977164, 47.49890960531435979 ) ) ;
#134491=CARTESIAN_POINT ( 'NONE',  ( -21.52544592524334988, -5.823673210054445271, 53.95942372801900433 ) ) ;
#134492=CARTESIAN_POINT ( 'NONE',  ( -5.719274019375978568, 21.55341960407610458, 60.20724293864768839 ) ) ;
#134493=CARTESIAN_POINT ( 'NONE',  ( 14.29746914071049879, -8.314922557960816363, 38.33224293864768839 ) ) ;
#134494=CARTESIAN_POINT ( 'NONE',  ( 10.72451020669871369, 18.67979575497193778, 72.08442372801899012 ) ) ;
#134495=CARTESIAN_POINT ( 'NONE',  ( 21.52544592524334988, 5.823673210054432836, 111.4594237280190328 ) ) ;
#134496=CARTESIAN_POINT ( 'NONE',  ( 16.52544592524342804, -4.483927247898539470, 63.54057627198103830 ) ) ;
#134497=CARTESIAN_POINT ( 'NONE',  ( 8.314922557960818139, 14.29746914071049879, 104.5822429386477097 ) ) ;
#134498=B_SPLINE_CURVE_WITH_KNOTS ( 'NONE', 3,
 ( #158059, #124740, #189408, #95383, #97352, #17565 ),
 .UNSPECIFIED., .F., .F.,
 ( 4, 2, 4 ),
 ( 3.469446951953614189E-18, 0.0003837532665635036075, 0.0007675065331270037455 ),
 .UNSPECIFIED. ) ;
#134499=CARTESIAN_POINT ( 'NONE',  ( 19.05341960407617918, -5.049401038297876454, 41.04275706135233293 ) ) ;
#134500=CARTESIAN_POINT ( 'NONE',  ( 14.29746914071037800, 8.314922557961029526, 96.66775706135234714 ) ) ;
#134501=CARTESIAN_POINT ( 'NONE',  ( 10.72451020669871369, 18.67979575497193778, 67.08442372801901854 ) ) ;
#134502=CARTESIAN_POINT ( 'NONE',  ( 9.564922557960805705, 16.46253265017160317, 54.58224293864769550 ) ) ;
#134503=CARTESIAN_POINT ( 'NONE',  ( 19.05341960407617918, -5.049401038297876454, 41.04275706135233293 ) ) ;
#134504=CARTESIAN_POINT ( 'NONE',  ( 15.72974639402199770, -15.80617190586745480, 43.12390960531435269 ) ) ;
#134505=CARTESIAN_POINT ( 'NONE',  ( 21.53943276465977519, 0.05219959533937863772, 31.25109039468568639 ) ) ;
#134506=CARTESIAN_POINT ( 'NONE',  ( -15.80617190586745835, -15.72974639402198527, 81.87390960531435269 ) ) ;
#134507=CARTESIAN_POINT ( 'NONE',  ( 9.564922557961047289, -16.46253265017146816, 85.41775706135233293 ) ) ;
#134508=CARTESIAN_POINT ( 'NONE',  ( 16.55341960407618274, -4.379528057220086978, 51.04275706135234714 ) ) ;
#134510=CARTESIAN_POINT ( 'NONE',  ( -21.52544592524343514, 5.823673210054127303, 91.04057627198103830 ) ) ;
#134511=CARTESIAN_POINT ( 'NONE',  ( -12.14591786802326823, 12.06949235617739902, 83.12609039468568994 ) ) ;
#134512=CARTESIAN_POINT ( 'NONE',  ( 12.14591786802309770, 12.06949235617756955, 74.37390960531436690 ) ) ;
#134513=CARTESIAN_POINT ( 'NONE',  ( -17.48853670773243607, -5.747243402303094051, 101.3332870025000574 ) ) ;
#134514=CARTESIAN_POINT ( 'NONE',  ( -0.05219959533934338120, 16.53943276465976808, 22.50109039468567573 ) ) ;
#134515=CARTESIAN_POINT ( 'NONE',  ( 18.62759615963271287, -10.81492255796078972, 33.33224293864769550 ) ) ;
#134516=CARTESIAN_POINT ( 'NONE',  ( 8.224510206698742110, 14.34966873604972548, 82.08442372801901854 ) ) ;
#134518=CARTESIAN_POINT ( 'NONE',  ( 4.379528057220092307, 16.55341960407617563, 52.29275706135236135 ) ) ;
#134519=CARTESIAN_POINT ( 'NONE',  ( -18.67979575497193778, 10.72451020669871902, 33.33442372801900433 ) ) ;
#134520=CARTESIAN_POINT ( 'NONE',  ( 5.719274019375991003, -21.55341960407610458, 42.70724293864770260 ) ) ;
#134521=CARTESIAN_POINT ( 'NONE',  ( -8.224510206698735004, -14.34966873604973081, 69.58442372801900433 ) ) ;
#134522=CARTESIAN_POINT ( 'NONE',  ( 16.51473224551069308, 9.474510206698969483, 89.16557627198103830 ) ) ;
#134523=CARTESIAN_POINT ( 'NONE',  ( -10.72451020669870658, -18.67979575497194134, 54.58442372801901143 ) ) ;
#134524=CARTESIAN_POINT ( 'NONE',  ( 9.564922557960805705, 16.46253265017160317, 29.58224293864769550 ) ) ;
#134525=CARTESIAN_POINT ( 'NONE',  ( -5.719274019375978568, 21.55341960407610458, 35.20724293864768839 ) ) ;
#134526=CARTESIAN_POINT ( 'NONE',  ( -19.03943276465977164, 0.05219959533909376836, 116.2489096053143669 ) ) ;
#134528=CARTESIAN_POINT ( 'NONE',  ( -19.03943276465977164, -0.05219959533935918106, 38.75109039468566152 ) ) ;
#134529=CARTESIAN_POINT ( 'NONE',  ( 8.314922557961029526, -14.29746914071037800, 55.41775706135234714 ) ) ;
#134530=CARTESIAN_POINT ( 'NONE',  ( 9.474510206698971260, -16.51473224551069308, 107.9155762719810383 ) ) ;
#134532=CARTESIAN_POINT ( 'NONE',  ( -9.564922557960796823, -16.46253265017161027, 82.08224293864768129 ) ) ;
#134533=CARTESIAN_POINT ( 'NONE',  ( -0.05219959533934338120, 16.53943276465976808, 102.5010903946856899 ) ) ;
#134534=CARTESIAN_POINT ( 'NONE',  ( -14.29746914071049879, 8.314922557960819915, 95.83224293864770971 ) ) ;
#134535=CARTESIAN_POINT ( 'NONE',  ( 5.719274019375991003, -21.55341960407610458, 32.70724293864770260 ) ) ;
#134536=CARTESIAN_POINT ( 'NONE',  ( 13.89961937509977652, -13.97604488694527269, 33.12390960531434558 ) ) ;
#134537=CARTESIAN_POINT ( 'NONE',  ( -8.224510206698735004, -14.34966873604973081, 79.58442372801903275 ) ) ;
#134538=CARTESIAN_POINT ( 'NONE',  ( 21.52544592524334988, 5.823673210054432836, 21.45942372801901499 ) ) ;
#134539=CARTESIAN_POINT ( 'NONE',  ( 9.564922557961047289, -16.46253265017146816, 80.41775706135234714 ) ) ;
#134540=CARTESIAN_POINT ( 'NONE',  ( 13.97604488694527802, 13.89961937509977652, 34.37390960531436690 ) ) ;
#134542=CARTESIAN_POINT ( 'NONE',  ( 5.823673210054444382, -21.52544592524334988, 105.2094237280190328 ) ) ;
#134543=CARTESIAN_POINT ( 'NONE',  ( -13.97604488694527625, -13.89961937509977652, 61.87390960531435979 ) ) ;
#134544=CARTESIAN_POINT ( 'NONE',  ( 16.52544592524335698, 4.483927247898782831, 51.45942372801901854 ) ) ;
#134545=CARTESIAN_POINT ( 'NONE',  ( 21.53943276465977519, 0.05219959533937863772, 86.25109039468568994 ) ) ;
#134546=CARTESIAN_POINT ( 'NONE',  ( 9.474510206698729675, 16.51473224551082808, 47.08442372801900433 ) ) ;
#134547=CARTESIAN_POINT ( 'NONE',  ( -19.05341960407617563, 5.049401038297882671, 58.54275706135234003 ) ) ;
#134549=CARTESIAN_POINT ( 'NONE',  ( 15.80617190586769283, -15.72974639402175789, 55.62609039468568284 ) ) ;
#134551=CARTESIAN_POINT ( 'NONE',  ( 5.153800228976615827, -19.02544592524334988, 40.20942372801898301 ) ) ;
#134552=B_SPLINE_CURVE_WITH_KNOTS ( 'NONE', 3,
 ( #172578, #54955, #126069, #174570, #132794, #20871 ),
 .UNSPECIFIED., .F., .F.,
 ( 4, 2, 4 ),
 ( 0.000000000000000000, 0.0003837532665635039327, 0.0007675065331270078655 ),
 .UNSPECIFIED. ) ;
#134553=CARTESIAN_POINT ( 'NONE',  ( -13.89961937509977652, 13.97604488694528158, 95.62390960531436690 ) ) ;
#134554=CARTESIAN_POINT ( 'NONE',  ( -0.05219959533909027116, -19.03943276465977164, 77.49890960531435269 ) ) ;
#134555=CARTESIAN_POINT ( 'NONE',  ( -12.14591786802309592, -12.06949235617757132, 31.87390960531435979 ) ) ;
#134556=CARTESIAN_POINT ( 'NONE',  ( 21.53943276465977519, -0.05219959533907433946, 28.74890960531435624 ) ) ;
#134559=CARTESIAN_POINT ( 'NONE',  ( -0.05219959533937732626, 21.53943276465977519, 112.5010903946857042 ) ) ;
#134561=CARTESIAN_POINT ( 'NONE',  ( -19.02544592524342804, 5.153800228976336051, 41.04057627198103120 ) ) ;
#134562=CARTESIAN_POINT ( 'NONE',  ( 19.02544592524343514, -5.153800228976328945, 28.54057627198102409 ) ) ;
#134565=CARTESIAN_POINT ( 'NONE',  ( 12.06949235617739724, 12.14591786802326823, 61.87609039468568284 ) ) ;
#134566=CARTESIAN_POINT ( 'NONE',  ( 18.62759615963271287, -10.81492255796078972, 83.33224293864769550 ) ) ;
#134567=EDGE_CURVE ( 'NONE', #141307, #46822, #120371, .T. ) ;
#134568=CARTESIAN_POINT ( 'NONE',  ( -4.483927247898539470, -16.52544592524342804, 57.29057627198103120 ) ) ;
#134569=CARTESIAN_POINT ( 'NONE',  ( 19.02544592524343514, -5.153800228976328945, 28.54057627198102409 ) ) ;
#134570=CARTESIAN_POINT ( 'NONE',  ( -19.03943276465977164, 0.05219959533909376836, 111.2489096053143669 ) ) ;
#134571=CARTESIAN_POINT ( 'NONE',  ( -15.72974639402176322, -15.80617190586768395, 29.37609039468568284 ) ) ;
#134572=CARTESIAN_POINT ( 'NONE',  ( 13.97604488694548053, -13.89961937509957401, 40.62609039468564731 ) ) ;
#134573=CARTESIAN_POINT ( 'NONE',  ( 9.474510206698971260, -16.51473224551069308, 37.91557627198102409 ) ) ;
#134574=CARTESIAN_POINT ( 'NONE',  ( -10.81492255796105439, 18.62759615963255655, 87.91775706135234714 ) ) ;
#134575=CARTESIAN_POINT ( 'NONE',  ( 16.61371651742598132, -7.165104196376269385, 31.35415069992996706 ) ) ;
#134576=CARTESIAN_POINT ( 'NONE',  ( -4.483927247898539470, -16.52544592524342804, 22.29057627198102765 ) ) ;
#134578=CARTESIAN_POINT ( 'NONE',  ( -18.67979575497178146, -10.72451020669898902, 26.66557627198103475 ) ) ;
#134579=CARTESIAN_POINT ( 'NONE',  ( 12.14591786802309770, 12.06949235617756955, 104.3739096053143669 ) ) ;
#134582=CARTESIAN_POINT ( 'NONE',  ( 19.02544592524343514, -5.153800228976328945, 93.54057627198102409 ) ) ;
#134583=CARTESIAN_POINT ( 'NONE',  ( -16.53943276465976808, 0.05219959533911058130, 81.24890960531436690 ) ) ;
#134584=CARTESIAN_POINT ( 'NONE',  ( 19.05341960407617918, -5.049401038297876454, 101.0427570613523045 ) ) ;
#134585=CARTESIAN_POINT ( 'NONE',  ( 18.62759615963271287, -10.81492255796078972, 68.33224293864769550 ) ) ;
#134587=CARTESIAN_POINT ( 'NONE',  ( -5.153800228976328057, -19.02544592524343514, 27.29057627198103120 ) ) ;
#134588=CARTESIAN_POINT ( 'NONE',  ( -16.46253265017160317, 9.564922557960807481, 90.83224293864769550 ) ) ;
#134589=CARTESIAN_POINT ( 'NONE',  ( 15.72974639402199770, -15.80617190586745480, 93.12390960531436690 ) ) ;
#134590=CARTESIAN_POINT ( 'NONE',  ( 12.06949235617739724, 12.14591786802326823, 111.8760903946856615 ) ) ;
#134591=CARTESIAN_POINT ( 'NONE',  ( -0.05219959533909027116, -19.03943276465977164, 87.49890960531436690 ) ) ;
#134592=CARTESIAN_POINT ( 'NONE',  ( 5.153800228976615827, -19.02544592524334988, 80.20942372801901854 ) ) ;
#134593=CARTESIAN_POINT ( 'NONE',  ( 18.67979575497194134, -10.72451020669871369, 90.83442372801901854 ) ) ;
#134594=CARTESIAN_POINT ( 'NONE',  ( -5.823673210054116645, -21.52544592524344225, 82.29057627198103830 ) ) ;
#134595=CARTESIAN_POINT ( 'NONE',  ( 10.81492255796078972, 18.62759615963270932, 34.58224293864770260 ) ) ;
#134596=CARTESIAN_POINT ( 'NONE',  ( 0.05219959533909260263, 19.03943276465977164, 49.99890960531435979 ) ) ;
#134597=CARTESIAN_POINT ( 'NONE',  ( -16.52544592524342804, 4.483927247898546575, 26.04057627198103475 ) ) ;
#134598=CARTESIAN_POINT ( 'NONE',  ( -19.02544592524342804, 5.153800228976336051, 61.04057627198103120 ) ) ;
#134600=CARTESIAN_POINT ( 'NONE',  ( 5.153800228976615827, -19.02544592524334988, 25.20942372801900433 ) ) ;
#134601=CARTESIAN_POINT ( 'NONE',  ( -4.483927247898539470, -16.52544592524342804, 67.29057627198103830 ) ) ;
#134602=CARTESIAN_POINT ( 'NONE',  ( 21.52544592524344225, -5.823673210054117533, 113.5405762719810383 ) ) ;
#134604=CARTESIAN_POINT ( 'NONE',  ( -5.719274019375978568, 21.55341960407610458, 55.20724293864770260 ) ) ;
#134605=CARTESIAN_POINT ( 'NONE',  ( -12.14591786802326823, 12.06949235617739902, 93.12609039468568994 ) ) ;
#134606=CARTESIAN_POINT ( 'NONE',  ( -12.14591786802309592, -12.06949235617757132, 106.8739096053143811 ) ) ;
#134607=CARTESIAN_POINT ( 'NONE',  ( -16.46253265017160317, 9.564922557960807481, 65.83224293864769550 ) ) ;
#134609=CARTESIAN_POINT ( 'NONE',  ( -4.379528057220328563, 16.55341960407611168, 35.20724293864768839 ) ) ;
#134610=ORIENTED_EDGE ( 'NONE', *, *, #43224, .F. ) ;
#134611=CARTESIAN_POINT ( 'NONE',  ( 21.52544592524334988, 5.823673210054432836, 46.45942372801901854 ) ) ;
#134612=CARTESIAN_POINT ( 'NONE',  ( 5.153800228976335163, 19.02544592524342804, 109.7905762719810099 ) ) ;
#134613=CARTESIAN_POINT ( 'NONE',  ( -5.719274019375665041, -21.55341960407619695, 79.79275706135236135 ) ) ;
#134614=CARTESIAN_POINT ( 'NONE',  ( -0.05219959533909027116, -19.03943276465977164, 27.49890960531435624 ) ) ;
#134615=CARTESIAN_POINT ( 'NONE',  ( 19.03943276465977164, -0.05219959533909143690, 38.74890960531436690 ) ) ;
#134616=ORIENTED_EDGE ( 'NONE', *, *, #145209, .T. ) ;
#134617=CARTESIAN_POINT ( 'NONE',  ( 10.81492255796106328, -18.62759615963255655, 90.41775706135236135 ) ) ;
#134618=CARTESIAN_POINT ( 'NONE',  ( -12.06949235617739369, -12.14591786802326823, 44.37609039468567573 ) ) ;
#134619=CARTESIAN_POINT ( 'NONE',  ( 18.67979575497194134, -10.72451020669871369, 70.83442372801901854 ) ) ;
#134620=CARTESIAN_POINT ( 'NONE',  ( -13.97604488694527625, -13.89961937509977652, 96.87390960531433848 ) ) ;
#134621=CARTESIAN_POINT ( 'NONE',  ( 13.89961937509957401, 13.97604488694547697, 86.87609039468567573 ) ) ;
#134622=CARTESIAN_POINT ( 'NONE',  ( 18.67979575497194134, -10.72451020669871369, 50.83442372801901143 ) ) ;
#134623=CARTESIAN_POINT ( 'NONE',  ( -14.34966873604972548, 8.224510206698743886, 23.33442372801901499 ) ) ;
#134624=CARTESIAN_POINT ( 'NONE',  ( 9.564922557961047289, -16.46253265017146816, 85.41775706135233293 ) ) ;
#134625=CARTESIAN_POINT ( 'NONE',  ( 9.474510206698971260, -16.51473224551069308, 52.91557627198102409 ) ) ;
#134626=CARTESIAN_POINT ( 'NONE',  ( -16.51473224551082808, 9.474510206698731452, 83.33442372801899012 ) ) ;
#134627=CARTESIAN_POINT ( 'NONE',  ( -16.53943276465976808, 0.05219959533911058130, 21.24890960531436690 ) ) ;
#134628=CARTESIAN_POINT ( 'NONE',  ( 0.05219959533936267826, -19.03943276465977164, 90.00109039468567573 ) ) ;
#134629=CARTESIAN_POINT ( 'NONE',  ( -16.53943276465976808, 0.05219959533911058130, 36.24890960531435979 ) ) ;
#134630=CARTESIAN_POINT ( 'NONE',  ( 13.97604488694548053, -13.89961937509957401, 65.62609039468567573 ) ) ;
#134631=CARTESIAN_POINT ( 'NONE',  ( 12.14591786802327356, -12.06949235617739191, 45.62609039468567573 ) ) ;
#134632=CARTESIAN_POINT ( 'NONE',  ( 13.97604488694548053, -13.89961937509957401, 25.62609039468566507 ) ) ;
#134633=CARTESIAN_POINT ( 'NONE',  ( 8.314922557960818139, 14.29746914071049879, 114.5822429386477097 ) ) ;
#134634=CARTESIAN_POINT ( 'NONE',  ( 5.153800228976335163, 19.02544592524342804, 39.79057627198100988 ) ) ;
#134635=CARTESIAN_POINT ( 'NONE',  ( 8.224510206698742110, 14.34966873604972548, 52.08442372801901854 ) ) ;
#134638=CARTESIAN_POINT ( 'NONE',  ( -19.03943276465977164, 0.05219959533909376836, 86.24890960531436690 ) ) ;
#134640=ORIENTED_EDGE ( 'NONE', *, *, #59992, .F. ) ;
#134641=CARTESIAN_POINT ( 'NONE',  ( -13.97604488694547697, 13.89961937509957934, 93.12609039468566152 ) ) ;
#134642=CARTESIAN_POINT ( 'NONE',  ( -15.72974639402197994, 15.80617190586746368, 25.62390960531435624 ) ) ;
#134643=CARTESIAN_POINT ( 'NONE',  ( 19.05341960407617918, -5.049401038297876454, 36.04275706135234003 ) ) ;
#134644=CARTESIAN_POINT ( 'NONE',  ( -9.474510206698720793, -16.51473224551083518, 104.5844237280190043 ) ) ;
#134645=CARTESIAN_POINT ( 'NONE',  ( -12.14591786802309592, -12.06949235617757132, 106.8739096053143811 ) ) ;
#134646=CARTESIAN_POINT ( 'NONE',  ( 19.02544592524343514, -5.153800228976328945, 33.54057627198102409 ) ) ;
#134647=CARTESIAN_POINT ( 'NONE',  ( -15.80617190586745835, -15.72974639402198527, 76.87390960531439532 ) ) ;
#134648=CARTESIAN_POINT ( 'NONE',  ( -19.03943276465977164, 0.05219959533909376836, 36.24890960531436690 ) ) ;
#134649=DIRECTION ( 'NONE',  ( 1.000000000000000000, -0.000000000000000000, -0.000000000000000000 ) ) ;
#134650=CARTESIAN_POINT ( 'NONE',  ( 9.564922557961047289, -16.46253265017146816, 70.41775706135233293 ) ) ;
#134651=CARTESIAN_POINT ( 'NONE',  ( 8.224510206698953496, -14.34966873604960469, 57.91557627198103120 ) ) ;
#134652=CARTESIAN_POINT ( 'NONE',  ( 18.62759615963271287, -10.81492255796078972, 38.33224293864768839 ) ) ;
#134653=CARTESIAN_POINT ( 'NONE',  ( -15.72974639402176322, -15.80617190586768395, 89.37609039468568994 ) ) ;
#134654=CARTESIAN_POINT ( 'NONE',  ( 21.53943276465977519, -0.05219959533907433946, 78.74890960531436690 ) ) ;
#134655=CARTESIAN_POINT ( 'NONE',  ( -18.67979575497193778, 10.72451020669871902, 73.33442372801901854 ) ) ;
#134656=CARTESIAN_POINT ( 'NONE',  ( 18.67979575497194134, -10.72451020669871369, 60.83442372801901854 ) ) ;
#134657=CARTESIAN_POINT ( 'NONE',  ( 13.97604488694527802, 13.89961937509977652, 94.37390960531436690 ) ) ;
#134658=CARTESIAN_POINT ( 'NONE',  ( -12.06949235617739369, -12.14591786802326823, 99.37609039468568994 ) ) ;
#134659=CARTESIAN_POINT ( 'NONE',  ( -18.62759615963255300, -10.81492255796106328, 59.16775706135234714 ) ) ;
#134660=CARTESIAN_POINT ( 'NONE',  ( -13.89961937509977652, 13.97604488694528158, 55.62390960531434558 ) ) ;
#134661=CARTESIAN_POINT ( 'NONE',  ( -21.52544592524334988, -5.823673210054445271, 33.95942372801901143 ) ) ;
#134662=CARTESIAN_POINT ( 'NONE',  ( 13.97604488694527802, 13.89961937509977652, 69.37390960531436690 ) ) ;
#134663=CARTESIAN_POINT ( 'NONE',  ( 0.05219959533910956823, 16.53943276465976808, 69.99890960531435269 ) ) ;
#134664=CARTESIAN_POINT ( 'NONE',  ( -4.379528057220328563, 16.55341960407611168, 40.20724293864769550 ) ) ;
#134665=CARTESIAN_POINT ( 'NONE',  ( 5.823673210054125526, 21.52544592524343514, 49.79057627198102409 ) ) ;
#134666=CARTESIAN_POINT ( 'NONE',  ( -5.049401038298153566, 19.05341960407611168, 45.20724293864769550 ) ) ;
#134667=CARTESIAN_POINT ( 'NONE',  ( 21.55341960407610458, 5.719274019375980345, 63.95724293864770260 ) ) ;
#134668=CARTESIAN_POINT ( 'NONE',  ( 0.05219959533936267826, -19.03943276465977164, 55.00109039468566863 ) ) ;
#134671=CARTESIAN_POINT ( 'NONE',  ( 8.224510206698953496, -14.34966873604960469, 67.91557627198102409 ) ) ;
#134672=CARTESIAN_POINT ( 'NONE',  ( -15.80617190586745835, -15.72974639402198527, 36.87390960531435979 ) ) ;
#134675=CARTESIAN_POINT ( 'NONE',  ( 0.05219959533934541429, -16.53943276465976808, 90.00109039468567573 ) ) ;
#134676=CARTESIAN_POINT ( 'NONE',  ( 19.05341960407617918, -5.049401038297876454, 86.04275706135233293 ) ) ;
#134677=CARTESIAN_POINT ( 'NONE',  ( 8.224510206698953496, -14.34966873604960469, 57.91557627198103120 ) ) ;
#134678=CARTESIAN_POINT ( 'NONE',  ( 17.50000000000002132, -5.624438216177543026, 53.31670344914648041 ) ) ;
#134679=CARTESIAN_POINT ( 'NONE',  ( -19.03943276465977164, 0.05219959533909376836, 51.24890960531436690 ) ) ;
#134680=CARTESIAN_POINT ( 'NONE',  ( -14.29746914071049879, 8.314922557960819915, 35.83224293864768839 ) ) ;
#134681=CARTESIAN_POINT ( 'NONE',  ( -13.89961937509977652, 13.97604488694528158, 50.62390960531435979 ) ) ;
#134682=CARTESIAN_POINT ( 'NONE',  ( -9.474510206698964154, 16.51473224551069663, 70.41557627198102409 ) ) ;
#134683=CARTESIAN_POINT ( 'NONE',  ( 19.03943276465977164, -0.05219959533909143690, 38.74890960531436690 ) ) ;
#134684=CARTESIAN_POINT ( 'NONE',  ( 0.05219959533937995610, -21.53943276465977519, 50.00109039468568994 ) ) ;
#134685=CARTESIAN_POINT ( 'NONE',  ( 5.049401038298161559, -19.05341960407611168, 67.70724293864769550 ) ) ;
#134686=CARTESIAN_POINT ( 'NONE',  ( 5.153800228976335163, 19.02544592524342804, 24.79057627198102765 ) ) ;
#134688=CARTESIAN_POINT ( 'NONE',  ( -19.02544592524342804, 5.153800228976336051, 56.04057627198100988 ) ) ;
#134689=CARTESIAN_POINT ( 'NONE',  ( -15.72974639402197994, 15.80617190586746368, 45.62390960531436690 ) ) ;
#134690=CARTESIAN_POINT ( 'NONE',  ( -19.02544592524342804, 5.153800228976336051, 41.04057627198103120 ) ) ;
#134691=CARTESIAN_POINT ( 'NONE',  ( -15.72974639402197994, 15.80617190586746368, 45.62390960531436690 ) ) ;
#134693=CARTESIAN_POINT ( 'NONE',  ( -8.224510206698735004, -14.34966873604973081, 99.58442372801900433 ) ) ;
#134695=CARTESIAN_POINT ( 'NONE',  ( 19.03943276465977164, 0.05219959533936151252, 21.25109039468565797 ) ) ;
#134696=CARTESIAN_POINT ( 'NONE',  ( -16.55341960407617563, 4.379528057220093196, 43.54275706135235424 ) ) ;
#134697=CARTESIAN_POINT ( 'NONE',  ( -14.29746914071037622, -8.314922557961029526, 79.16775706135234714 ) ) ;
#134699=CARTESIAN_POINT ( 'NONE',  ( -0.05219959533934338120, 16.53943276465976808, 67.50109039468568994 ) ) ;
#134700=CARTESIAN_POINT ( 'NONE',  ( 16.53943276465976808, 0.05219959533934440121, 51.25109039468568994 ) ) ;
#134701=CARTESIAN_POINT ( 'NONE',  ( 0.05219959533909260263, 19.03943276465977164, 104.9989096053143669 ) ) ;
#134702=CARTESIAN_POINT ( 'NONE',  ( 14.29746914071037800, 8.314922557961029526, 41.66775706135235424 ) ) ;
#134703=CARTESIAN_POINT ( 'NONE',  ( -5.049401038298153566, 19.05341960407611168, 35.20724293864768839 ) ) ;
#134704=CARTESIAN_POINT ( 'NONE',  ( 21.52544592524334988, 5.823673210054432836, 31.45942372801901854 ) ) ;
#134705=CARTESIAN_POINT ( 'NONE',  ( -8.224510206698735004, -14.34966873604973081, 34.58442372801900433 ) ) ;
#134706=CARTESIAN_POINT ( 'NONE',  ( 14.29746914071037800, 8.314922557961029526, 101.6677570613523613 ) ) ;
#134707=CARTESIAN_POINT ( 'NONE',  ( -17.97214573761834799, -5.500000000000021316, 71.46970049038654338 ) ) ;
#134708=CARTESIAN_POINT ( 'NONE',  ( 21.52544592524334988, 5.823673210054432836, 106.4594237280190328 ) ) ;
#134709=CARTESIAN_POINT ( 'NONE',  ( 9.564922557961047289, -16.46253265017146816, 100.4177570613523329 ) ) ;
#134710=CARTESIAN_POINT ( 'NONE',  ( 8.224510206698953496, -14.34966873604960469, 62.91557627198102409 ) ) ;
#134711=CARTESIAN_POINT ( 'NONE',  ( 9.474510206698971260, -16.51473224551069308, 22.91557627198102765 ) ) ;
#134712=CARTESIAN_POINT ( 'NONE',  ( 19.03943276465977164, 0.05219959533936151252, 56.25109039468566863 ) ) ;
#134713=CARTESIAN_POINT ( 'NONE',  ( 17.50000000000001066, 5.622605283950888655, 78.81207310596111881 ) ) ;
#134714=CARTESIAN_POINT ( 'NONE',  ( 18.67979575497194134, -10.72451020669871369, 60.83442372801901854 ) ) ;
#134715=CARTESIAN_POINT ( 'NONE',  ( -14.29746914071037622, -8.314922557961029526, 29.16775706135234003 ) ) ;
#134716=CARTESIAN_POINT ( 'NONE',  ( 17.50000000000000000, 5.500000000000013323, 63.78230962303565832 ) ) ;
#134717=CARTESIAN_POINT ( 'NONE',  ( 5.719274019375991003, -21.55341960407610458, 27.70724293864769905 ) ) ;
#134718=CARTESIAN_POINT ( 'NONE',  ( 13.97604488694548053, -13.89961937509957401, 105.6260903946856757 ) ) ;
#134721=CARTESIAN_POINT ( 'NONE',  ( -5.049401038298153566, 19.05341960407611168, 25.20724293864768484 ) ) ;
#134722=CARTESIAN_POINT ( 'NONE',  ( 10.72451020669871369, 18.67979575497193778, 102.0844237280190185 ) ) ;
#134723=CARTESIAN_POINT ( 'NONE',  ( -13.97604488694527625, -13.89961937509977652, 41.87390960531435979 ) ) ;
#134724=CIRCLE ( 'NONE', #166906, 2.000000000000001776 ) ;
#134725=CARTESIAN_POINT ( 'NONE',  ( 15.80617190586769283, -15.72974639402175789, 50.62609039468568994 ) ) ;
#134726=CARTESIAN_POINT ( 'NONE',  ( 5.719274019375673035, 21.55341960407619339, 97.29275706135234714 ) ) ;
#134727=CARTESIAN_POINT ( 'NONE',  ( -14.29746914071037622, -8.314922557961029526, 99.16775706135234714 ) ) ;
#134728=CARTESIAN_POINT ( 'NONE',  ( 19.05341960407611168, 5.049401038298154454, 83.95724293864766707 ) ) ;
#134729=CARTESIAN_POINT ( 'NONE',  ( -15.80617190586768217, 15.72974639402176855, 48.12609039468568284 ) ) ;
#134730=CARTESIAN_POINT ( 'NONE',  ( -18.62759615963255300, -10.81492255796106328, 49.16775706135234003 ) ) ;
#134731=CARTESIAN_POINT ( 'NONE',  ( -9.564922557961040184, 16.46253265017147172, 77.91775706135234714 ) ) ;
#134732=CARTESIAN_POINT ( 'NONE',  ( -13.89961937509977652, 13.97604488694528158, 90.62390960531432427 ) ) ;
#134733=CARTESIAN_POINT ( 'NONE',  ( -12.06949235617756955, 12.14591786802309770, 100.6239096053143811 ) ) ;
#134734=CARTESIAN_POINT ( 'NONE',  ( -5.719274019375978568, 21.55341960407610458, 100.2072429386476955 ) ) ;
#134735=CARTESIAN_POINT ( 'NONE',  ( 19.05341960407617918, -5.049401038297876454, 21.04275706135232582 ) ) ;
#134736=CARTESIAN_POINT ( 'NONE',  ( 14.34966873604960469, 8.224510206698951720, 94.16557627198103830 ) ) ;
#134737=CARTESIAN_POINT ( 'NONE',  ( -9.564922557960796823, -16.46253265017161027, 47.08224293864769550 ) ) ;
#134738=CARTESIAN_POINT ( 'NONE',  ( 0.05219959533936267826, -19.03943276465977164, 80.00109039468567573 ) ) ;
#134739=CARTESIAN_POINT ( 'NONE',  ( 16.52544592524342804, -4.483927247898539470, 43.54057627198103830 ) ) ;
#134740=CARTESIAN_POINT ( 'NONE',  ( -5.049401038297874678, -19.05341960407617918, 19.79275706135233293 ) ) ;
#134741=CARTESIAN_POINT ( 'NONE',  ( 13.89961937509977652, -13.97604488694527269, 108.1239096053143669 ) ) ;
#134742=CARTESIAN_POINT ( 'NONE',  ( -0.05219959533936034679, 19.03943276465977164, 77.50109039468566152 ) ) ;
#134743=CARTESIAN_POINT ( 'NONE',  ( -21.55341960407610458, -5.719274019375992779, 81.45724293864769550 ) ) ;
#134744=CARTESIAN_POINT ( 'NONE',  ( 21.52544592524334988, 5.823673210054432836, 36.45942372801901143 ) ) ;
#134745=CARTESIAN_POINT ( 'NONE',  ( -4.379528057220086978, -16.55341960407618274, 29.79275706135234358 ) ) ;
#134746=CARTESIAN_POINT ( 'NONE',  ( 12.06949235617739724, 12.14591786802326823, 86.87609039468568994 ) ) ;
#134747=CARTESIAN_POINT ( 'NONE',  ( 17.50000000000000000, 5.499999999999992895, 61.70309617465829177 ) ) ;
#134748=CARTESIAN_POINT ( 'NONE',  ( 5.823673210054444382, -21.52544592524334988, 30.20942372801902565 ) ) ;
#134749=CARTESIAN_POINT ( 'NONE',  ( 15.80617190586746368, 15.72974639402197994, 44.37390960531435979 ) ) ;
#134750=CARTESIAN_POINT ( 'NONE',  ( 9.474510206698971260, -16.51473224551069308, 27.91557627198103120 ) ) ;
#134752=CARTESIAN_POINT ( 'NONE',  ( 8.224510206698742110, 14.34966873604972548, 57.08442372801901854 ) ) ;
#134753=CARTESIAN_POINT ( 'NONE',  ( 4.379528057220339221, -16.55341960407611168, 92.70724293864770971 ) ) ;
#134754=CARTESIAN_POINT ( 'NONE',  ( 0.05219959533907565091, 21.53943276465977519, 79.99890960531435269 ) ) ;
#134755=CARTESIAN_POINT ( 'NONE',  ( 14.29746914071037800, 8.314922557961029526, 111.6677570613523613 ) ) ;
#134756=CARTESIAN_POINT ( 'NONE',  ( 0.05219959533934541429, -16.53943276465976808, 45.00109039468568284 ) ) ;
#134757=CARTESIAN_POINT ( 'NONE',  ( -13.89961937509977652, 13.97604488694528158, 55.62390960531434558 ) ) ;
#134758=CARTESIAN_POINT ( 'NONE',  ( 12.06949235617739724, 12.14591786802326823, 86.87609039468568994 ) ) ;
#134759=CARTESIAN_POINT ( 'NONE',  ( -19.02544592524334988, -5.153800228976617603, 83.95942372801901854 ) ) ;
#134760=CARTESIAN_POINT ( 'NONE',  ( 10.81492255796078972, 18.62759615963270932, 84.58224293864769550 ) ) ;
#134761=CARTESIAN_POINT ( 'NONE',  ( 12.14591786802327356, -12.06949235617739191, 105.6260903946856899 ) ) ;
#134764=CARTESIAN_POINT ( 'NONE',  ( 5.823673210054125526, 21.52544592524343514, 59.79057627198103120 ) ) ;
#134765=CARTESIAN_POINT ( 'NONE',  ( 16.53943276465976808, 0.05219959533934440121, 96.25109039468568994 ) ) ;
#134767=CARTESIAN_POINT ( 'NONE',  ( -21.53943276465977519, 0.05219959533907696930, 31.24890960531435979 ) ) ;
#134768=CARTESIAN_POINT ( 'NONE',  ( -19.48894818550246200, 5.499999999999919176, 75.10307310435239003 ) ) ;
#134769=CARTESIAN_POINT ( 'NONE',  ( 21.53943276465977519, -0.05219959533907433946, 83.74890960531435269 ) ) ;
#134770=CARTESIAN_POINT ( 'NONE',  ( -0.05219959533910754901, -16.53943276465976808, 27.49890960531435269 ) ) ;
#134771=CARTESIAN_POINT ( 'NONE',  ( 8.314922557961029526, -14.29746914071037800, 20.41775706135234714 ) ) ;
#134772=CARTESIAN_POINT ( 'NONE',  ( -5.153800228976328057, -19.02544592524343514, 32.29057627198102409 ) ) ;
#134773=CARTESIAN_POINT ( 'NONE',  ( -16.53943276465976808, -0.05219959533934237506, 23.75109039468567929 ) ) ;
#134774=CARTESIAN_POINT ( 'NONE',  ( -13.97604488694527625, -13.89961937509977652, 51.87390960531436690 ) ) ;
#134777=CARTESIAN_POINT ( 'NONE',  ( -5.049401038298153566, 19.05341960407611168, 105.2072429386476671 ) ) ;
#134778=CARTESIAN_POINT ( 'NONE',  ( 9.564922557960805705, 16.46253265017160317, 109.5822429386476955 ) ) ;
#134779=CARTESIAN_POINT ( 'NONE',  ( 16.52544592524335698, 4.483927247898782831, 86.45942372801901854 ) ) ;
#134780=CARTESIAN_POINT ( 'NONE',  ( 9.474510206698729675, 16.51473224551082808, 97.08442372801900433 ) ) ;
#134781=CARTESIAN_POINT ( 'NONE',  ( -19.05341960407617563, 5.049401038297882671, 33.54275706135231871 ) ) ;
#134782=CARTESIAN_POINT ( 'NONE',  ( -15.72974639402197994, 15.80617190586746368, 75.62390960531439532 ) ) ;
#134783=CARTESIAN_POINT ( 'NONE',  ( 16.53943276465976808, 0.05219959533934440121, 106.2510903946856757 ) ) ;
#134784=CARTESIAN_POINT ( 'NONE',  ( -18.67979575497178146, -10.72451020669898902, 36.66557627198103120 ) ) ;
#134785=CARTESIAN_POINT ( 'NONE',  ( -13.97604488694547697, 13.89961937509957934, 93.12609039468566152 ) ) ;
#134786=CARTESIAN_POINT ( 'NONE',  ( 13.89961937509977652, -13.97604488694527269, 53.12390960531434558 ) ) ;
#134787=CARTESIAN_POINT ( 'NONE',  ( -19.05341960407611168, -5.049401038298163336, 101.4572429386476955 ) ) ;
#134788=CARTESIAN_POINT ( 'NONE',  ( 15.80617190586769283, -15.72974639402175789, 65.62609039468568994 ) ) ;
#134789=CARTESIAN_POINT ( 'NONE',  ( -16.51473224551069308, -9.474510206698971260, 66.66557627198102409 ) ) ;
#134790=CARTESIAN_POINT ( 'NONE',  ( 16.55341960407611168, 4.379528057220329451, 93.95724293864770971 ) ) ;
#134792=CARTESIAN_POINT ( 'NONE',  ( -12.06949235617756955, 12.14591786802309770, 75.62390960531439532 ) ) ;
#134793=CARTESIAN_POINT ( 'NONE',  ( -5.719274019375978568, 21.55341960407610458, 80.20724293864769550 ) ) ;
#134795=CARTESIAN_POINT ( 'NONE',  ( 16.51473224551083163, -9.474510206698727899, 85.83442372801900433 ) ) ;
#134796=CARTESIAN_POINT ( 'NONE',  ( 16.52216118717209881, -7.221426719304498754, 81.42400978953010338 ) ) ;
#134797=CARTESIAN_POINT ( 'NONE',  ( 0.05219959533909260263, 19.03943276465977164, 64.99890960531436690 ) ) ;
#134798=CARTESIAN_POINT ( 'NONE',  ( 17.31728774477215183, -6.344390552233685199, 73.31906651689308774 ) ) ;
#134799=CARTESIAN_POINT ( 'NONE',  ( -19.05341960407611168, -5.049401038298163336, 81.45724293864769550 ) ) ;
#134800=CARTESIAN_POINT ( 'NONE',  ( 9.474510206698971260, -16.51473224551069308, 82.91557627198103830 ) ) ;
#134801=CARTESIAN_POINT ( 'NONE',  ( -12.14591786802326823, 12.06949235617739902, 58.12609039468568994 ) ) ;
#134802=EDGE_CURVE ( 'NONE', #38745, #146788, #79610, .T. ) ;
#134803=CARTESIAN_POINT ( 'NONE',  ( -16.18388926212241330, -7.379444403734411573, 50.43953151366153520 ) ) ;
#134804=CARTESIAN_POINT ( 'NONE',  ( -5.049401038297874678, -19.05341960407617918, 39.79275706135232582 ) ) ;
#134805=CARTESIAN_POINT ( 'NONE',  ( 17.31245056299218632, 6.303547735381235917, 21.68954763021610432 ) ) ;
#134806=CARTESIAN_POINT ( 'NONE',  ( 19.03943276465977164, -0.05219959533909143690, 108.7489096053143527 ) ) ;
#134807=CARTESIAN_POINT ( 'NONE',  ( -14.34966873604972548, 8.224510206698743886, 103.3344237280190043 ) ) ;
#134809=CARTESIAN_POINT ( 'NONE',  ( -16.52544592524335698, -4.483927247898792601, 93.95942372801903275 ) ) ;
#134810=CARTESIAN_POINT ( 'NONE',  ( -17.49999999999999645, 5.499999999999992006, 28.71769037696435234 ) ) ;
#134811=CARTESIAN_POINT ( 'NONE',  ( 16.52544592524335698, 4.483927247898782831, 71.45942372801901854 ) ) ;
#134812=CARTESIAN_POINT ( 'NONE',  ( 13.97604488694527802, 13.89961937509977830, 74.37390960531436690 ) ) ;
#134813=CARTESIAN_POINT ( 'NONE',  ( -18.62759615963255300, -10.81492255796106328, 64.16775706135234714 ) ) ;
#134814=CARTESIAN_POINT ( 'NONE',  ( 19.05341960407617918, -5.049401038297876454, 76.04275706135230450 ) ) ;
#134815=CARTESIAN_POINT ( 'NONE',  ( -9.564922557961040184, 16.46253265017147172, 32.91775706135233293 ) ) ;
#134816=CARTESIAN_POINT ( 'NONE',  ( -19.05341960407611168, -5.049401038298163336, 66.45724293864769550 ) ) ;
#134817=CARTESIAN_POINT ( 'NONE',  ( 13.89961937509977652, -13.97604488694527269, 48.12390960531435979 ) ) ;
#134819=CARTESIAN_POINT ( 'NONE',  ( -18.62759615963270932, 10.81492255796079327, 80.83224293864769550 ) ) ;
#134820=AXIS2_PLACEMENT_3D ( 'NONE', #27960, #59252, #182620 ) ;
#134821=CARTESIAN_POINT ( 'NONE',  ( -18.62759615963270932, 10.81492255796079327, 35.83224293864768839 ) ) ;
#134822=CARTESIAN_POINT ( 'NONE',  ( 13.97604488694527802, 13.89961937509977652, 34.37390960531436690 ) ) ;
#134823=CARTESIAN_POINT ( 'NONE',  ( -16.55341960407617563, 4.379528057220093196, 48.54275706135234714 ) ) ;
#134824=VERTEX_POINT ( 'NONE', #117391 ) ;
#134825=CARTESIAN_POINT ( 'NONE',  ( 15.80617190586769283, -15.72974639402175789, 35.62609039468568994 ) ) ;
#134826=CARTESIAN_POINT ( 'NONE',  ( -12.06949235617756955, 12.14591786802309770, 50.62390960531435979 ) ) ;
#134828=CARTESIAN_POINT ( 'NONE',  ( -14.34966873604972548, 8.224510206698743886, 23.33442372801901499 ) ) ;
#134829=CARTESIAN_POINT ( 'NONE',  ( -0.05219959533936034679, 19.03943276465977164, 42.50109039468566152 ) ) ;
#134830=CARTESIAN_POINT ( 'NONE',  ( -16.53943276465976808, 0.05219959533911058130, 61.24890960531435979 ) ) ;
#134831=CARTESIAN_POINT ( 'NONE',  ( -18.67979575497193778, 10.72451020669871902, 23.33442372801901499 ) ) ;
#134833=CARTESIAN_POINT ( 'NONE',  ( 18.62759615963271287, -10.81492255796078972, 73.33224293864769550 ) ) ;
#134834=CARTESIAN_POINT ( 'NONE',  ( -0.05219959533909027116, -19.03943276465977164, 87.49890960531436690 ) ) ;
#134835=CARTESIAN_POINT ( 'NONE',  ( -12.06949235617756955, 12.14591786802309770, 65.62390960531436690 ) ) ;
#134836=CARTESIAN_POINT ( 'NONE',  ( 9.474510206698971260, -16.51473224551069308, 107.9155762719810383 ) ) ;
#134838=CARTESIAN_POINT ( 'NONE',  ( -13.97604488694547697, 13.89961937509957934, 73.12609039468568994 ) ) ;
#134839=CARTESIAN_POINT ( 'NONE',  ( -21.52544592524343514, 5.823673210054127303, 111.0405762719810525 ) ) ;
#134840=CARTESIAN_POINT ( 'NONE',  ( -9.564922557960796823, -16.46253265017161027, 52.08224293864768839 ) ) ;
#134841=CARTESIAN_POINT ( 'NONE',  ( -19.05341960407617563, 5.049401038297882671, 43.54275706135232582 ) ) ;
#134842=CARTESIAN_POINT ( 'NONE',  ( 4.483927247898545687, 16.52544592524342804, 114.7905762719810383 ) ) ;
#134843=CARTESIAN_POINT ( 'NONE',  ( -10.72451020669870658, -18.67979575497194134, 64.58442372801900433 ) ) ;
#134845=CARTESIAN_POINT ( 'NONE',  ( -16.52216118717210591, -7.221426719304506747, 71.07599021046993926 ) ) ;
#134846=CARTESIAN_POINT ( 'NONE',  ( -8.314922557960811034, -14.29746914071050412, 42.08224293864769550 ) ) ;
#134847=CARTESIAN_POINT ( 'NONE',  ( -16.46253265017160317, 9.564922557960807481, 50.83224293864770260 ) ) ;
#134848=CARTESIAN_POINT ( 'NONE',  ( 19.20446147854523389, 5.500000000000086153, 71.88999695167674986 ) ) ;
#134849=CARTESIAN_POINT ( 'NONE',  ( -5.719274019375978568, 21.55341960407610458, 80.20724293864769550 ) ) ;
#134851=CARTESIAN_POINT ( 'NONE',  ( 0.05219959533909260263, 19.03943276465977164, 44.99890960531435979 ) ) ;
#134852=CARTESIAN_POINT ( 'NONE',  ( -0.05219959533907301413, -21.53943276465977519, 62.49890960531436690 ) ) ;
#134854=CARTESIAN_POINT ( 'NONE',  ( 18.67979575497194134, -10.72451020669871369, 80.83442372801901854 ) ) ;
#134856=CARTESIAN_POINT ( 'NONE',  ( 16.53943276465976808, 0.05219959533934440121, 86.25109039468568994 ) ) ;
#134857=CARTESIAN_POINT ( 'NONE',  ( 12.14591786802309770, 12.06949235617756955, 84.37390960531438111 ) ) ;
#134858=CARTESIAN_POINT ( 'NONE',  ( 16.46253265017160672, -9.564922557960803928, 73.33224293864769550 ) ) ;
#134860=CARTESIAN_POINT ( 'NONE',  ( -19.03943276465977164, -0.05219959533935918106, 38.75109039468566152 ) ) ;
#134861=CARTESIAN_POINT ( 'NONE',  ( 12.06949235617739724, 12.14591786802326823, 81.87609039468568994 ) ) ;
#134862=CARTESIAN_POINT ( 'NONE',  ( -13.97604488694547697, 13.89961937509957934, 23.12609039468565442 ) ) ;
#134863=CARTESIAN_POINT ( 'NONE',  ( 9.474510206698971260, -16.51473224551069308, 82.91557627198103830 ) ) ;
#134864=CARTESIAN_POINT ( 'NONE',  ( 21.53943276465977519, -0.05219959533907433946, 43.74890960531435979 ) ) ;
#134865=CARTESIAN_POINT ( 'NONE',  ( 21.53943276465977519, 0.05219959533937863772, 96.25109039468568994 ) ) ;
#134866=CARTESIAN_POINT ( 'NONE',  ( -12.14591786802326823, 12.06949235617739902, 58.12609039468568994 ) ) ;
#134867=CARTESIAN_POINT ( 'NONE',  ( -15.80617190586745835, -15.72974639402198527, 106.8739096053143811 ) ) ;
#134868=CARTESIAN_POINT ( 'NONE',  ( -16.53943276465976808, -0.05219959533934237506, 33.75109039468568284 ) ) ;
#134869=CARTESIAN_POINT ( 'NONE',  ( 19.05341960407611168, 5.049401038298154454, 88.95724293864769550 ) ) ;
#134870=CARTESIAN_POINT ( 'NONE',  ( 16.46253265017160672, -9.564922557960803928, 43.33224293864769550 ) ) ;
#134871=CARTESIAN_POINT ( 'NONE',  ( -19.02544592524342804, 5.153800228976336051, 51.04057627198103120 ) ) ;
#134873=CARTESIAN_POINT ( 'NONE',  ( -14.34966873604972548, 8.224510206698743886, 28.33442372801902209 ) ) ;
#134874=CARTESIAN_POINT ( 'NONE',  ( 8.314922557960818139, 14.29746914071049879, 84.58224293864769550 ) ) ;
#134875=CARTESIAN_POINT ( 'NONE',  ( 0.05219959533934541429, -16.53943276465976808, 90.00109039468567573 ) ) ;
#134876=CARTESIAN_POINT ( 'NONE',  ( -10.81492255796105439, 18.62759615963255655, 47.91775706135234714 ) ) ;
#134877=CARTESIAN_POINT ( 'NONE',  ( -5.049401038298153566, 19.05341960407611168, 70.20724293864769550 ) ) ;
#134878=CARTESIAN_POINT ( 'NONE',  ( -9.474510206698964154, 16.51473224551069663, 55.41557627198103120 ) ) ;
#134879=CARTESIAN_POINT ( 'NONE',  ( -19.03943276465977164, 0.05219959533909376836, 76.24890960531435269 ) ) ;
#134880=CARTESIAN_POINT ( 'NONE',  ( -8.224510206698948167, 14.34966873604960824, 30.41557627198101699 ) ) ;
#134881=CARTESIAN_POINT ( 'NONE',  ( 0.05219959533934541429, -16.53943276465976808, 90.00109039468567573 ) ) ;
#134883=CARTESIAN_POINT ( 'NONE',  ( -5.049401038297874678, -19.05341960407617918, 29.79275706135232227 ) ) ;
#134884=CARTESIAN_POINT ( 'NONE',  ( 13.97604488694527802, 13.89961937509977652, 104.3739096053143385 ) ) ;
#134885=CARTESIAN_POINT ( 'NONE',  ( 19.03943276465977164, -0.05219959533909143690, 43.74890960531435979 ) ) ;
#134887=CARTESIAN_POINT ( 'NONE',  ( 16.55341960407618274, -4.379528057220086978, 41.04275706135236135 ) ) ;
#134888=CARTESIAN_POINT ( 'NONE',  ( 5.049401038297881783, 19.05341960407617563, 72.29275706135234714 ) ) ;
#134889=CARTESIAN_POINT ( 'NONE',  ( -16.52544592524335698, -4.483927247898792601, 58.95942372801902565 ) ) ;
#134891=CARTESIAN_POINT ( 'NONE',  ( 16.46253265017160672, -9.564922557960803928, 83.33224293864768129 ) ) ;
#134892=CARTESIAN_POINT ( 'NONE',  ( -18.62759615963255300, -10.81492255796106328, 19.16775706135234714 ) ) ;
#134893=CARTESIAN_POINT ( 'NONE',  ( -9.564922557961040184, 16.46253265017147172, 62.91775706135233293 ) ) ;
#134894=CARTESIAN_POINT ( 'NONE',  ( -19.05341960407611168, -5.049401038298163336, 111.4572429386476671 ) ) ;
#134895=CARTESIAN_POINT ( 'NONE',  ( -13.97604488694527625, -13.89961937509977652, 36.87390960531436690 ) ) ;
#134896=CARTESIAN_POINT ( 'NONE',  ( -19.02544592524342804, 5.153800228976336051, 81.04057627198103830 ) ) ;
#134897=CARTESIAN_POINT ( 'NONE',  ( -0.05219959533910754901, -16.53943276465976808, 37.49890960531436690 ) ) ;
#134898=CARTESIAN_POINT ( 'NONE',  ( -13.89961937509977830, 13.97604488694528158, 70.62390960531435269 ) ) ;
#134899=CARTESIAN_POINT ( 'NONE',  ( -16.46253265017146816, -9.564922557961047289, 34.16775706135233293 ) ) ;
#134900=CARTESIAN_POINT ( 'NONE',  ( -16.55341960407611168, -4.379528057220339221, 71.45724293864769550 ) ) ;
#134901=CARTESIAN_POINT ( 'NONE',  ( -5.719274019375665041, -21.55341960407619695, 109.7927570613523613 ) ) ;
#134902=CARTESIAN_POINT ( 'NONE',  ( 19.03943276465977164, -0.05219959533909143690, 53.74890960531436690 ) ) ;
#134903=CARTESIAN_POINT ( 'NONE',  ( -12.06949235617756955, 12.14591786802309770, 35.62390960531437401 ) ) ;
#134904=CARTESIAN_POINT ( 'NONE',  ( -10.72451020669870658, -18.67979575497194134, 104.5844237280190185 ) ) ;
#134905=CARTESIAN_POINT ( 'NONE',  ( 13.89961937509977652, -13.97604488694527269, 93.12390960531436690 ) ) ;
#134906=CARTESIAN_POINT ( 'NONE',  ( -13.89961937509977652, 13.97604488694528158, 105.6239096053143527 ) ) ;
#134907=CARTESIAN_POINT ( 'NONE',  ( -9.564922557960796823, -16.46253265017161027, 42.08224293864769550 ) ) ;
#134908=CARTESIAN_POINT ( 'NONE',  ( -12.06949235617756955, 12.14591786802309770, 110.6239096053143669 ) ) ;
#134909=CARTESIAN_POINT ( 'NONE',  ( 8.224510206698953496, -14.34966873604960469, 92.91557627198103830 ) ) ;
#134910=CARTESIAN_POINT ( 'NONE',  ( -21.55341960407610458, -5.719274019375992779, 101.4572429386476955 ) ) ;
#134911=CARTESIAN_POINT ( 'NONE',  ( 19.02544592524343514, -5.153800228976328945, 93.54057627198102409 ) ) ;
#134912=CARTESIAN_POINT ( 'NONE',  ( -18.67979575497178146, -10.72451020669898902, 96.66557627198102409 ) ) ;
#134913=CARTESIAN_POINT ( 'NONE',  ( -13.97604488694527625, -13.89961937509977652, 91.87390960531432427 ) ) ;
#134914=DIRECTION ( 'NONE',  ( 1.000000000000000000, 0.000000000000000000, 0.000000000000000000 ) ) ;
#134915=CARTESIAN_POINT ( 'NONE',  ( 14.34966873604960469, 8.224510206698951720, 104.1655762719810241 ) ) ;
#134916=CARTESIAN_POINT ( 'NONE',  ( -16.51473224551069308, -9.474510206698971260, 66.66557627198102409 ) ) ;
#134917=CARTESIAN_POINT ( 'NONE',  ( 21.55341960407610458, 5.719274019375980345, 83.95724293864770971 ) ) ;
#134919=CARTESIAN_POINT ( 'NONE',  ( 10.72451020669898902, -18.67979575497178502, 32.91557627198102409 ) ) ;
#134920=CARTESIAN_POINT ( 'NONE',  ( 17.50000000000000000, 5.499999999999997335, 120.0000000000000142 ) ) ;
#134921=CARTESIAN_POINT ( 'NONE',  ( -16.53943276465976808, -0.05219959533934237506, 28.75109039468567929 ) ) ;
#134922=CARTESIAN_POINT ( 'NONE',  ( 12.14591786802309770, 12.06949235617756955, 99.37390960531436690 ) ) ;
#134924=CARTESIAN_POINT ( 'NONE',  ( -16.46253265017160317, 9.564922557960807481, 85.83224293864769550 ) ) ;
#134925=CARTESIAN_POINT ( 'NONE',  ( 0.05219959533909260263, 19.03943276465977164, 44.99890960531435979 ) ) ;
#134926=CARTESIAN_POINT ( 'NONE',  ( 16.55341960407611168, 4.379528057220329451, 78.95724293864769550 ) ) ;
#134927=CARTESIAN_POINT ( 'NONE',  ( -5.719274019375978568, 21.55341960407610458, 25.20724293864769550 ) ) ;
#134928=CARTESIAN_POINT ( 'NONE',  ( -16.52544592524342804, 4.483927247898546575, 56.04057627198102409 ) ) ;
#134929=CARTESIAN_POINT ( 'NONE',  ( 9.564922557961047289, -16.46253265017146816, 105.4177570613523471 ) ) ;
#134930=CARTESIAN_POINT ( 'NONE',  ( -0.05219959533937732626, 21.53943276465977519, 57.50109039468568994 ) ) ;
#134932=CARTESIAN_POINT ( 'NONE',  ( 0.05219959533909260263, 19.03943276465977164, 99.99890960531436690 ) ) ;
#134933=CARTESIAN_POINT ( 'NONE',  ( 16.53943276465976808, 0.05219959533934440121, 81.25109039468568994 ) ) ;
#134934=CARTESIAN_POINT ( 'NONE',  ( -17.13100169013222640, 6.664070546374242454, 95.76789835699824494 ) ) ;
#134935=CARTESIAN_POINT ( 'NONE',  ( -16.51473224551069308, -9.474510206698971260, 76.66557627198103830 ) ) ;
#134936=CARTESIAN_POINT ( 'NONE',  ( -5.823673210054116645, -21.52544592524344225, 87.29057627198103830 ) ) ;
#134937=CARTESIAN_POINT ( 'NONE',  ( 16.51473224551083163, -9.474510206698727899, 105.8344237280190043 ) ) ;
#134938=CARTESIAN_POINT ( 'NONE',  ( -12.14591786802309592, -12.06949235617757132, 51.87390960531437401 ) ) ;
#134939=CARTESIAN_POINT ( 'NONE',  ( 21.55341960407619695, -5.719274019375665929, 61.04275706135234714 ) ) ;
#134941=CARTESIAN_POINT ( 'NONE',  ( 8.224510206698742110, 14.34966873604972548, 82.08442372801901854 ) ) ;
#134942=CARTESIAN_POINT ( 'NONE',  ( -9.474510206698964154, 16.51473224551069663, 115.4155762719810241 ) ) ;
#134943=CARTESIAN_POINT ( 'NONE',  ( 16.46253265017160672, -9.564922557960803928, 113.3322429386476955 ) ) ;
#134945=CARTESIAN_POINT ( 'NONE',  ( 12.14591786802327356, -12.06949235617739191, 110.6260903946857042 ) ) ;
#134946=CARTESIAN_POINT ( 'NONE',  ( -8.224510206698735004, -14.34966873604973081, 64.58442372801900433 ) ) ;
#134947=CARTESIAN_POINT ( 'NONE',  ( 19.05341960407611168, 5.049401038298154454, 68.95724293864769550 ) ) ;
#134948=CARTESIAN_POINT ( 'NONE',  ( -13.89961937509977652, 13.97604488694528158, 70.62390960531432427 ) ) ;
#134949=CARTESIAN_POINT ( 'NONE',  ( -5.823673210054431948, 21.52544592524334988, 72.70942372801901854 ) ) ;
#134950=CARTESIAN_POINT ( 'NONE',  ( -8.224510206698735004, -14.34966873604973081, 79.58442372801903275 ) ) ;
#134951=CARTESIAN_POINT ( 'NONE',  ( 4.379528057220339221, -16.55341960407611168, 47.70724293864770260 ) ) ;
#134952=CARTESIAN_POINT ( 'NONE',  ( -9.474510206698964154, 16.51473224551069663, 60.41557627198102409 ) ) ;
#134953=CARTESIAN_POINT ( 'NONE',  ( 0.05219959533909260263, 19.03943276465977164, 49.99890960531435979 ) ) ;
#134954=CARTESIAN_POINT ( 'NONE',  ( -14.34966873604972548, 8.224510206698743886, 48.33442372801902565 ) ) ;
#134956=CARTESIAN_POINT ( 'NONE',  ( -13.89961937509957401, -13.97604488694547875, 99.37609039468567573 ) ) ;
#134957=CARTESIAN_POINT ( 'NONE',  ( -16.52544592524342804, 4.483927247898546575, 101.0405762719810383 ) ) ;
#134958=CARTESIAN_POINT ( 'NONE',  ( -13.89961937509977652, 13.97604488694528158, 70.62390960531432427 ) ) ;
#134959=CARTESIAN_POINT ( 'NONE',  ( -19.03943276465977164, -0.05219959533935918106, 103.7510903946856757 ) ) ;
#134961=CARTESIAN_POINT ( 'NONE',  ( 5.719274019375673035, 21.55341960407619339, 102.2927570613523613 ) ) ;
#134962=CARTESIAN_POINT ( 'NONE',  ( -16.55341960407617563, 4.379528057220093196, 73.54275706135234714 ) ) ;
#134964=CARTESIAN_POINT ( 'NONE',  ( 15.72974639402199770, -15.80617190586745480, 68.12390960531436690 ) ) ;
#134965=CARTESIAN_POINT ( 'NONE',  ( -14.34966873604972548, 8.224510206698743886, 58.33442372801901143 ) ) ;
#134967=CARTESIAN_POINT ( 'NONE',  ( -16.51473224551082808, 9.474510206698731452, 48.33442372801900433 ) ) ;
#134968=CARTESIAN_POINT ( 'NONE',  ( -19.02544592524342804, 5.153800228976336051, 86.04057627198103830 ) ) ;
#134969=CARTESIAN_POINT ( 'NONE',  ( -9.564922557960796823, -16.46253265017161027, 27.08224293864769550 ) ) ;
#134970=CARTESIAN_POINT ( 'NONE',  ( -0.05219959533909027116, -19.03943276465977164, 67.49890960531436690 ) ) ;
#134971=CARTESIAN_POINT ( 'NONE',  ( 0.05219959533910956823, 16.53943276465976808, 59.99890960531436690 ) ) ;
#134973=CARTESIAN_POINT ( 'NONE',  ( -0.05219959533937732626, 21.53943276465977519, 72.50109039468568994 ) ) ;
#134974=CARTESIAN_POINT ( 'NONE',  ( 19.05341960407617918, -5.049401038297876454, 41.04275706135233293 ) ) ;
#134975=CARTESIAN_POINT ( 'NONE',  ( 9.474510206698729675, 16.51473224551082808, 32.08442372801900433 ) ) ;
#134976=CARTESIAN_POINT ( 'NONE',  ( -13.89961937509977652, 13.97604488694528158, 50.62390960531435979 ) ) ;
#134977=CARTESIAN_POINT ( 'NONE',  ( 18.62759615963271287, -10.81492255796078972, 28.33224293864769550 ) ) ;
#134978=CARTESIAN_POINT ( 'NONE',  ( 18.62759615963255655, 10.81492255796105972, 101.6677570613523613 ) ) ;
#134979=CARTESIAN_POINT ( 'NONE',  ( 0.05219959533909260263, 19.03943276465977164, 64.99890960531436690 ) ) ;
#134980=CARTESIAN_POINT ( 'NONE',  ( -18.62759615963255300, -10.81492255796106328, 94.16775706135237556 ) ) ;
#134981=CARTESIAN_POINT ( 'NONE',  ( 15.72974639402199770, -15.80617190586745480, 33.12390960531435979 ) ) ;
#134982=CARTESIAN_POINT ( 'NONE',  ( -9.474510206698964154, 16.51473224551069663, 80.41557627198103830 ) ) ;
#134983=CARTESIAN_POINT ( 'NONE',  ( -5.153800228976607833, 19.02544592524334988, 62.70942372801899722 ) ) ;
#134984=CARTESIAN_POINT ( 'NONE',  ( 19.02544592524343514, -5.153800228976328945, 43.54057627198103120 ) ) ;
#134985=CARTESIAN_POINT ( 'NONE',  ( 0.05219959533909260263, 19.03943276465977164, 89.99890960531436690 ) ) ;
#134986=CARTESIAN_POINT ( 'NONE',  ( 8.314922557961029526, -14.29746914071037800, 30.41775706135234358 ) ) ;
#134987=CARTESIAN_POINT ( 'NONE',  ( -14.34966873604960291, -8.224510206698953496, 91.66557627198103830 ) ) ;
#134988=CARTESIAN_POINT ( 'NONE',  ( -19.05341960407611168, -5.049401038298163336, 76.45724293864769550 ) ) ;
#134989=CARTESIAN_POINT ( 'NONE',  ( -5.719274019375978568, 21.55341960407610458, 50.20724293864769550 ) ) ;
#134990=CARTESIAN_POINT ( 'NONE',  ( -16.51473224551082808, 9.474510206698731452, 108.3344237280190043 ) ) ;
#134991=CARTESIAN_POINT ( 'NONE',  ( 15.72974639402199770, -15.80617190586745480, 113.1239096053143953 ) ) ;
#134992=CARTESIAN_POINT ( 'NONE',  ( -15.72974639402176322, -15.80617190586768395, 64.37609039468568994 ) ) ;
#134993=CARTESIAN_POINT ( 'NONE',  ( -8.224510206698735004, -14.34966873604973081, 69.58442372801900433 ) ) ;
#134994=CARTESIAN_POINT ( 'NONE',  ( 4.483927247898790824, -16.52544592524335698, 65.20942372801901854 ) ) ;
#134995=CARTESIAN_POINT ( 'NONE',  ( -19.02544592524342804, 5.153800228976336051, 56.04057627198100988 ) ) ;
#134996=CARTESIAN_POINT ( 'NONE',  ( -4.483927247898782831, 16.52544592524335698, 97.70942372801904696 ) ) ;
#134997=CARTESIAN_POINT ( 'NONE',  ( -16.46253265017146816, -9.564922557961047289, 44.16775706135232582 ) ) ;
#134999=CARTESIAN_POINT ( 'NONE',  ( -18.67979575497193778, 10.72451020669871902, 28.33442372801902209 ) ) ;
#135000=CARTESIAN_POINT ( 'NONE',  ( -12.14591786802309592, -12.06949235617757132, 61.87390960531436690 ) ) ;
#135001=CARTESIAN_POINT ( 'NONE',  ( 9.564922557960805705, 16.46253265017160317, 104.5822429386476955 ) ) ;
#135002=CARTESIAN_POINT ( 'NONE',  ( -14.29746914071037622, -8.314922557961029526, 89.16775706135236135 ) ) ;
#135003=CARTESIAN_POINT ( 'NONE',  ( -5.823673210054431948, 21.52544592524334988, 72.70942372801901854 ) ) ;
#135004=CARTESIAN_POINT ( 'NONE',  ( 12.14591786802327356, -12.06949235617739191, 30.62609039468567929 ) ) ;
#135005=CARTESIAN_POINT ( 'NONE',  ( -18.62759615963255300, -10.81492255796106328, 29.16775706135234003 ) ) ;
#135006=CARTESIAN_POINT ( 'NONE',  ( 16.52544592524342804, -4.483927247898539470, 63.54057627198103830 ) ) ;
#135009=CARTESIAN_POINT ( 'NONE',  ( -10.72451020669898014, 18.67979575497178502, 105.4155762719810383 ) ) ;
#135010=CARTESIAN_POINT ( 'NONE',  ( -12.14591786802309592, -12.06949235617757132, 41.87390960531435979 ) ) ;
#135012=CARTESIAN_POINT ( 'NONE',  ( 5.049401038298161559, -19.05341960407611168, 22.70724293864769194 ) ) ;
#135013=CARTESIAN_POINT ( 'NONE',  ( 15.72974639402199770, -15.80617190586745480, 33.12390960531435979 ) ) ;
#135014=CARTESIAN_POINT ( 'NONE',  ( -10.72451020669870658, -18.67979575497194134, 39.58442372801901143 ) ) ;
#135015=CARTESIAN_POINT ( 'NONE',  ( -4.379528057220328563, 16.55341960407611168, 65.20724293864768129 ) ) ;
#135016=CARTESIAN_POINT ( 'NONE',  ( 18.62759615963271287, -10.81492255796078972, 68.33224293864769550 ) ) ;
#135017=CARTESIAN_POINT ( 'NONE',  ( 0.05219959533909260263, 19.03943276465977164, 69.99890960531435269 ) ) ;
#135018=CARTESIAN_POINT ( 'NONE',  ( -9.474510206698964154, 16.51473224551069663, 30.41557627198102054 ) ) ;
#135019=CARTESIAN_POINT ( 'NONE',  ( 19.05341960407617918, -5.049401038297876454, 81.04275706135231871 ) ) ;
#135021=CARTESIAN_POINT ( 'NONE',  ( 18.67979575497178502, 10.72451020669898547, 44.16557627198103120 ) ) ;
#135022=CARTESIAN_POINT ( 'NONE',  ( 13.97604488694527802, 13.89961937509977652, 39.37390960531435269 ) ) ;
#135023=CARTESIAN_POINT ( 'NONE',  ( 19.02544592524343514, -5.153800228976328945, 68.54057627198103830 ) ) ;
#135025=CARTESIAN_POINT ( 'NONE',  ( 14.34966873604972726, -8.224510206698740333, 40.83442372801901854 ) ) ;
#135026=CARTESIAN_POINT ( 'NONE',  ( 5.719274019375673035, 21.55341960407619339, 22.29275706135235069 ) ) ;
#135027=CARTESIAN_POINT ( 'NONE',  ( -14.34966873604960291, -8.224510206698953496, 41.66557627198103120 ) ) ;
#135028=CARTESIAN_POINT ( 'NONE',  ( 19.02544592524343514, -5.153800228976328945, 108.5405762719810383 ) ) ;
#135029=CARTESIAN_POINT ( 'NONE',  ( -21.52544592524343514, 5.823673210054127303, 76.04057627198102409 ) ) ;
#135030=CARTESIAN_POINT ( 'NONE',  ( 18.67979575497178502, 10.72451020669898547, 104.1655762719810241 ) ) ;
#135031=CARTESIAN_POINT ( 'NONE',  ( 4.379528057220092307, 16.55341960407617563, 52.29275706135236135 ) ) ;
#135032=CARTESIAN_POINT ( 'NONE',  ( -5.823673210054116645, -21.52544592524344225, 47.29057627198103120 ) ) ;
#135033=CARTESIAN_POINT ( 'NONE',  ( -10.81492255796105439, 18.62759615963255655, 97.91775706135236135 ) ) ;
#135034=CARTESIAN_POINT ( 'NONE',  ( 13.89961937509977652, -13.97604488694527269, 43.12390960531434558 ) ) ;
#135035=CARTESIAN_POINT ( 'NONE',  ( 13.89961937509977652, -13.97604488694527269, 103.1239096053143527 ) ) ;
#135036=CARTESIAN_POINT ( 'NONE',  ( 0.05219959533909260263, 19.03943276465977164, 69.99890960531435269 ) ) ;
#135038=CARTESIAN_POINT ( 'NONE',  ( -5.049401038297874678, -19.05341960407617918, 59.79275706135231871 ) ) ;
#135039=CARTESIAN_POINT ( 'NONE',  ( -15.72974639402176322, -15.80617190586768395, 109.3760903946857042 ) ) ;
#135040=CARTESIAN_POINT ( 'NONE',  ( 21.53943276465977519, -0.05219959533907433946, 33.74890960531436690 ) ) ;
#135041=CARTESIAN_POINT ( 'NONE',  ( -16.52544592524335698, -4.483927247898792601, 98.95942372801903275 ) ) ;
#135042=CARTESIAN_POINT ( 'NONE',  ( -16.46253265017146816, -9.564922557961047289, 84.16775706135233293 ) ) ;
#135044=CARTESIAN_POINT ( 'NONE',  ( 13.89961937509977652, -13.97604488694527269, 103.1239096053143527 ) ) ;
#135045=CARTESIAN_POINT ( 'NONE',  ( -9.564922557961040184, 16.46253265017147172, 82.91775706135233293 ) ) ;
#135046=CARTESIAN_POINT ( 'NONE',  ( -16.46253265017146816, -9.564922557961047289, 49.16775706135233293 ) ) ;
#135047=CARTESIAN_POINT ( 'NONE',  ( -17.13100169013299023, -6.664070546373169535, 44.23210164300152059 ) ) ;
#135048=CARTESIAN_POINT ( 'NONE',  ( 5.049401038298161559, -19.05341960407611168, 47.70724293864770260 ) ) ;
#135049=CARTESIAN_POINT ( 'NONE',  ( -16.55341960407611168, -4.379528057220339221, 51.45724293864770260 ) ) ;
#135050=CARTESIAN_POINT ( 'NONE',  ( 13.97604488694527802, 13.89961937509977652, 39.37390960531435269 ) ) ;
#135051=CARTESIAN_POINT ( 'NONE',  ( -4.379528057220328563, 16.55341960407611168, 45.20724293864769550 ) ) ;
#135053=CARTESIAN_POINT ( 'NONE',  ( 0.05219959533934541429, -16.53943276465976808, 105.0010903946856757 ) ) ;
#135054=CARTESIAN_POINT ( 'NONE',  ( -19.02544592524342804, 5.153800228976336051, 51.04057627198103120 ) ) ;
#135055=CARTESIAN_POINT ( 'NONE',  ( 10.72451020669871369, 18.67979575497193778, 107.0844237280190043 ) ) ;
#135056=CARTESIAN_POINT ( 'NONE',  ( -14.34966873604972548, 8.224510206698743886, 38.33442372801900433 ) ) ;
#135057=CARTESIAN_POINT ( 'NONE',  ( 0.05219959533907565091, 21.53943276465977519, 39.99890960531436690 ) ) ;
#135058=CARTESIAN_POINT ( 'NONE',  ( -5.823673210054431948, 21.52544592524334988, 97.70942372801904696 ) ) ;
#135059=ORIENTED_EDGE ( 'NONE', *, *, #124207, .F. ) ;
#135060=CARTESIAN_POINT ( 'NONE',  ( -19.03943276465977164, 0.05219959533909376836, 111.2489096053143669 ) ) ;
#135061=CARTESIAN_POINT ( 'NONE',  ( 19.05341960407611168, 5.049401038298154454, 83.95724293864766707 ) ) ;
#135063=CARTESIAN_POINT ( 'NONE',  ( 5.719274019375991003, -21.55341960407610458, 107.7072429386476955 ) ) ;
#135064=CARTESIAN_POINT ( 'NONE',  ( 0.05219959533910956823, 16.53943276465976808, 74.99890960531435269 ) ) ;
#135065=CARTESIAN_POINT ( 'NONE',  ( -10.81492255796078084, -18.62759615963271287, 72.08224293864769550 ) ) ;
#135066=CARTESIAN_POINT ( 'NONE',  ( -16.46253265017160317, 9.564922557960807481, 75.83224293864769550 ) ) ;
#135067=CARTESIAN_POINT ( 'NONE',  ( 5.719274019375991003, -21.55341960407610458, 92.70724293864770971 ) ) ;
#135069=CARTESIAN_POINT ( 'NONE',  ( -16.51473224551069308, -9.474510206698971260, 66.66557627198102409 ) ) ;
#135070=CARTESIAN_POINT ( 'NONE',  ( 4.379528057220339221, -16.55341960407611168, 92.70724293864770971 ) ) ;
#135071=CARTESIAN_POINT ( 'NONE',  ( 13.97604488694527802, 13.89961937509977652, 24.37390960531435624 ) ) ;
#135072=CARTESIAN_POINT ( 'NONE',  ( -9.474510206698964154, 16.51473224551069663, 65.41557627198102409 ) ) ;
#135073=CARTESIAN_POINT ( 'NONE',  ( -13.89961937509957401, -13.97604488694547875, 74.37609039468566152 ) ) ;
#135074=CARTESIAN_POINT ( 'NONE',  ( -14.34966873604960291, -8.224510206698953496, 96.66557627198102409 ) ) ;
#135075=CARTESIAN_POINT ( 'NONE',  ( 18.67979575497194134, -10.72451020669871369, 60.83442372801901854 ) ) ;
#135076=CARTESIAN_POINT ( 'NONE',  ( 5.049401038298161559, -19.05341960407611168, 52.70724293864767418 ) ) ;
#135077=CARTESIAN_POINT ( 'NONE',  ( 21.55341960407610458, 5.719274019375980345, 113.9572429386477239 ) ) ;
#135078=CARTESIAN_POINT ( 'NONE',  ( -4.483927247898539470, -16.52544592524342804, 97.29057627198105251 ) ) ;
#135080=CARTESIAN_POINT ( 'NONE',  ( 19.05341960407611168, 5.049401038298154454, 58.95724293864768129 ) ) ;
#135082=CARTESIAN_POINT ( 'NONE',  ( -19.05341960407617563, 5.049401038297882671, 108.5427570613523187 ) ) ;
#135083=CARTESIAN_POINT ( 'NONE',  ( -13.97604488694527625, -13.89961937509977652, 111.8739096053143243 ) ) ;
#135084=CARTESIAN_POINT ( 'NONE',  ( -18.67979575497193778, 10.72451020669871902, 43.33442372801901143 ) ) ;
#135085=CARTESIAN_POINT ( 'NONE',  ( -0.05219959533909027116, -19.03943276465977164, 97.49890960531436690 ) ) ;
#135086=CARTESIAN_POINT ( 'NONE',  ( 5.153800228976615827, -19.02544592524334988, 85.20942372801900433 ) ) ;
#135087=CARTESIAN_POINT ( 'NONE',  ( 16.51473224551069308, 9.474510206698969483, 59.16557627198102409 ) ) ;
#135088=CARTESIAN_POINT ( 'NONE',  ( -4.379528057220328563, 16.55341960407611168, 75.20724293864769550 ) ) ;
#135089=CARTESIAN_POINT ( 'NONE',  ( 5.049401038298161559, -19.05341960407611168, 92.70724293864769550 ) ) ;
#135090=CARTESIAN_POINT ( 'NONE',  ( -0.05219959533910754901, -16.53943276465976808, 72.49890960531435269 ) ) ;
#135091=CARTESIAN_POINT ( 'NONE',  ( 16.46253265017160672, -9.564922557960803928, 78.33224293864769550 ) ) ;
#135092=CARTESIAN_POINT ( 'NONE',  ( 16.46253265017146816, 9.564922557961045513, 31.66775706135232937 ) ) ;
#135093=CARTESIAN_POINT ( 'NONE',  ( -9.474510206698964154, 16.51473224551069663, 55.41557627198103120 ) ) ;
#135094=CARTESIAN_POINT ( 'NONE',  ( -4.483927247898539470, -16.52544592524342804, 42.29057627198103120 ) ) ;
#135095=CARTESIAN_POINT ( 'NONE',  ( 13.89961937509977652, -13.97604488694527269, 23.12390960531436335 ) ) ;
#135096=VERTEX_POINT ( 'NONE', #103228 ) ;
#135097=CARTESIAN_POINT ( 'NONE',  ( 21.52544592524334988, 5.823673210054432836, 41.45942372801901143 ) ) ;
#135098=CARTESIAN_POINT ( 'NONE',  ( 13.97604488694548053, -13.89961937509957401, 75.62609039468564731 ) ) ;
#135099=CARTESIAN_POINT ( 'NONE',  ( 0.05219959533910956823, 16.53943276465976808, 29.99890960531435979 ) ) ;
#135100=CARTESIAN_POINT ( 'NONE',  ( -5.719274019375978568, 21.55341960407610458, 105.2072429386477097 ) ) ;
#135101=CARTESIAN_POINT ( 'NONE',  ( 15.80617190586746368, 15.72974639402197994, 39.37390960531436690 ) ) ;
#135102=CARTESIAN_POINT ( 'NONE',  ( 14.34966873604960469, 8.224510206698951720, 69.16557627198102409 ) ) ;
#135103=CARTESIAN_POINT ( 'NONE',  ( -9.564922557960796823, -16.46253265017161027, 47.08224293864769550 ) ) ;
#135104=CARTESIAN_POINT ( 'NONE',  ( 14.34966873604972726, -8.224510206698740333, 100.8344237280190185 ) ) ;
#135105=CARTESIAN_POINT ( 'NONE',  ( -12.06949235617739369, -12.14591786802326823, 64.37609039468568994 ) ) ;
#135106=CARTESIAN_POINT ( 'NONE',  ( -19.03943276465977164, -0.05219959533935918106, 23.75109039468566152 ) ) ;
#135107=CARTESIAN_POINT ( 'NONE',  ( 19.03943276465977164, -0.05219959533909143690, 98.74890960531436690 ) ) ;
#135108=CARTESIAN_POINT ( 'NONE',  ( -16.51473224551069308, -9.474510206698971260, 81.66557627198103830 ) ) ;
#135109=CARTESIAN_POINT ( 'NONE',  ( -16.55341960407617563, 4.379528057220093196, 68.54275706135234714 ) ) ;
#135110=CARTESIAN_POINT ( 'NONE',  ( 19.03943276465977164, -0.05219959533909143690, 23.74890960531435269 ) ) ;
#135111=CARTESIAN_POINT ( 'NONE',  ( -12.14591786802309592, -12.06949235617757132, 46.87390960531435979 ) ) ;
#135112=CARTESIAN_POINT ( 'NONE',  ( -16.51473224551069308, -9.474510206698971260, 101.6655762719810241 ) ) ;
#135113=CARTESIAN_POINT ( 'NONE',  ( -9.564922557960796823, -16.46253265017161027, 87.08224293864769550 ) ) ;
#135114=CARTESIAN_POINT ( 'NONE',  ( 0.05219959533907565091, 21.53943276465977519, 24.99890960531435624 ) ) ;
#135115=CARTESIAN_POINT ( 'NONE',  ( 4.483927247898545687, 16.52544592524342804, 69.79057627198102409 ) ) ;
#135118=CARTESIAN_POINT ( 'NONE',  ( 14.34966873604960469, 8.224510206698951720, 69.16557627198102409 ) ) ;
#135119=CARTESIAN_POINT ( 'NONE',  ( 16.55341960407618274, -4.379528057220086978, 56.04275706135235424 ) ) ;
#135121=CARTESIAN_POINT ( 'NONE',  ( 16.46253265017146816, 9.564922557961045513, 61.66775706135234003 ) ) ;
#135122=CARTESIAN_POINT ( 'NONE',  ( 19.02544592524343514, -5.153800228976328945, 83.54057627198100988 ) ) ;
#135123=CARTESIAN_POINT ( 'NONE',  ( 0.05219959533936267826, -19.03943276465977164, 60.00109039468566863 ) ) ;
#135125=CARTESIAN_POINT ( 'NONE',  ( 16.46253265017146816, 9.564922557961045513, 111.6677570613523329 ) ) ;
#135126=CARTESIAN_POINT ( 'NONE',  ( -14.29746914071037622, -8.314922557961029526, 94.16775706135237556 ) ) ;
#135127=CARTESIAN_POINT ( 'NONE',  ( 19.02544592524343514, -5.153800228976328945, 38.54057627198103120 ) ) ;
#135128=CARTESIAN_POINT ( 'NONE',  ( 21.55341960407610458, 5.719274019375980345, 23.95724293864769550 ) ) ;
#135129=CARTESIAN_POINT ( 'NONE',  ( -5.719274019375665041, -21.55341960407619695, 49.79275706135234714 ) ) ;
#135130=CARTESIAN_POINT ( 'NONE',  ( -16.46253265017146816, -9.564922557961047289, 109.1677570613523471 ) ) ;
#135132=CARTESIAN_POINT ( 'NONE',  ( -13.89961937509977652, 13.97604488694528158, 80.62390960531436690 ) ) ;
#135135=CARTESIAN_POINT ( 'NONE',  ( 4.483927247898545687, 16.52544592524342804, 74.79057627198105251 ) ) ;
#135136=CARTESIAN_POINT ( 'NONE',  ( 5.049401038298161559, -19.05341960407611168, 77.70724293864765286 ) ) ;
#135137=CARTESIAN_POINT ( 'NONE',  ( 5.049401038298161559, -19.05341960407611168, 72.70724293864768129 ) ) ;
#135138=CARTESIAN_POINT ( 'NONE',  ( -5.049401038297874678, -19.05341960407617918, 74.79275706135231871 ) ) ;
#135139=CARTESIAN_POINT ( 'NONE',  ( 10.72451020669898902, -18.67979575497178502, 62.91557627198102409 ) ) ;
#135140=CARTESIAN_POINT ( 'NONE',  ( -16.55341960407611168, -4.379528057220339221, 111.4572429386476813 ) ) ;
#135141=CARTESIAN_POINT ( 'NONE',  ( -5.049401038297874678, -19.05341960407617918, 54.79275706135234003 ) ) ;
#135142=CARTESIAN_POINT ( 'NONE',  ( -19.03943276465977164, 0.05219959533909376836, 51.24890960531436690 ) ) ;
#135143=CARTESIAN_POINT ( 'NONE',  ( -5.049401038298153566, 19.05341960407611168, 90.20724293864766707 ) ) ;
#135145=CARTESIAN_POINT ( 'NONE',  ( 21.52544592524344225, -5.823673210054117533, 83.54057627198102409 ) ) ;
#135146=CARTESIAN_POINT ( 'NONE',  ( 0.05219959533910956823, 16.53943276465976808, 89.99890960531438111 ) ) ;
#135147=CARTESIAN_POINT ( 'NONE',  ( 13.89961937509957401, 13.97604488694547697, 41.87609039468566152 ) ) ;
#135148=CARTESIAN_POINT ( 'NONE',  ( -5.719274019375978568, 21.55341960407610458, 80.20724293864769550 ) ) ;
#135149=CARTESIAN_POINT ( 'NONE',  ( -10.81492255796078084, -18.62759615963271287, 57.08224293864769550 ) ) ;
#135150=CARTESIAN_POINT ( 'NONE',  ( -12.06949235617756955, 12.14591786802309770, 35.62390960531437401 ) ) ;
#135151=CARTESIAN_POINT ( 'NONE',  ( 21.55341960407619695, -5.719274019375665929, 101.0427570613523756 ) ) ;
#135152=CARTESIAN_POINT ( 'NONE',  ( 9.474510206698971260, -16.51473224551069308, 77.91557627198103830 ) ) ;
#135153=CARTESIAN_POINT ( 'NONE',  ( -0.05219959533909027116, -19.03943276465977164, 37.49890960531436690 ) ) ;
#135154=CARTESIAN_POINT ( 'NONE',  ( 5.719274019375673035, 21.55341960407619339, 42.29275706135235424 ) ) ;
#135155=CARTESIAN_POINT ( 'NONE',  ( 18.67979575497194134, -10.72451020669871369, 35.83442372801901143 ) ) ;
#135156=CARTESIAN_POINT ( 'NONE',  ( -5.049401038298153566, 19.05341960407611168, 50.20724293864770260 ) ) ;
#135157=CARTESIAN_POINT ( 'NONE',  ( -5.823673210054431948, 21.52544592524334988, 22.70942372801901499 ) ) ;
#135158=CARTESIAN_POINT ( 'NONE',  ( 0.05219959533936267826, -19.03943276465977164, 65.00109039468567573 ) ) ;
#135159=B_SPLINE_CURVE_WITH_KNOTS ( 'NONE', 3,
 ( #65593, #4902, #98900, #145413, #50442, #96912, #6895, #68573, #20084, #173791, #158595, #143414 ),
 .UNSPECIFIED., .F., .F.,
 ( 4, 2, 2, 2, 2, 4 ),
 ( 0.002244533994399153676, 0.002800305961463194111, 0.003078191944995206306, 0.003356077928527217633, 0.003911849895591248093, 0.004467621862655278553 ),
 .UNSPECIFIED. ) ;
#135160=CARTESIAN_POINT ( 'NONE',  ( 16.46253265017160672, -9.564922557960803928, 33.33224293864770260 ) ) ;
#135161=CARTESIAN_POINT ( 'NONE',  ( 16.53943276465976808, 0.05219959533934440121, 31.25109039468568639 ) ) ;
#135162=CARTESIAN_POINT ( 'NONE',  ( 19.05341960407611168, 5.049401038298154454, 28.95724293864769550 ) ) ;
#135163=CARTESIAN_POINT ( 'NONE',  ( -12.06949235617739369, -12.14591786802326823, 74.37609039468568994 ) ) ;
#135164=CARTESIAN_POINT ( 'NONE',  ( 0.05219959533909260263, 19.03943276465977164, 39.99890960531436690 ) ) ;
#135166=CARTESIAN_POINT ( 'NONE',  ( -16.46253265017160317, 9.564922557960807481, 90.83224293864769550 ) ) ;
#135167=CARTESIAN_POINT ( 'NONE',  ( -13.89961937509977652, 13.97604488694528158, 30.62390960531435269 ) ) ;
#135168=CARTESIAN_POINT ( 'NONE',  ( -21.55341960407610458, -5.719274019375992779, 71.45724293864769550 ) ) ;
#135169=CARTESIAN_POINT ( 'NONE',  ( -16.53943276465976808, -0.05219959533934237506, 53.75109039468568994 ) ) ;
#135170=CARTESIAN_POINT ( 'NONE',  ( 21.52544592524334988, 5.823673210054432836, 96.45942372801901854 ) ) ;
#135171=CARTESIAN_POINT ( 'NONE',  ( 9.474510206698971260, -16.51473224551069308, 42.91557627198103120 ) ) ;
#135172=CARTESIAN_POINT ( 'NONE',  ( -4.379528057220328563, 16.55341960407611168, 35.20724293864768839 ) ) ;
#135173=CARTESIAN_POINT ( 'NONE',  ( 8.314922557960818139, 14.29746914071049879, 74.58224293864768129 ) ) ;
#135174=CARTESIAN_POINT ( 'NONE',  ( 19.05341960407611168, 5.049401038298154454, 68.95724293864769550 ) ) ;
#135175=CARTESIAN_POINT ( 'NONE',  ( 5.153800228976615827, -19.02544592524334988, 20.20942372801899722 ) ) ;
#135176=CARTESIAN_POINT ( 'NONE',  ( 10.72451020669871369, 18.67979575497193778, 22.08442372801901143 ) ) ;
#135177=CARTESIAN_POINT ( 'NONE',  ( 19.02544592524343514, -5.153800228976328945, 83.54057627198100988 ) ) ;
#135178=CARTESIAN_POINT ( 'NONE',  ( -10.72451020669870658, -18.67979575497194134, 89.58442372801901854 ) ) ;
#135179=CARTESIAN_POINT ( 'NONE',  ( 4.379528057220092307, 16.55341960407617563, 47.29275706135234003 ) ) ;
#135180=CARTESIAN_POINT ( 'NONE',  ( -4.379528057220086978, -16.55341960407618274, 24.79275706135235779 ) ) ;
#135181=CARTESIAN_POINT ( 'NONE',  ( -0.05219959533910754901, -16.53943276465976808, 92.49890960531436690 ) ) ;
#135182=CARTESIAN_POINT ( 'NONE',  ( 10.72451020669871369, 18.67979575497193778, 97.08442372801904696 ) ) ;
#135183=CARTESIAN_POINT ( 'NONE',  ( 4.483927247898545687, 16.52544592524342804, 34.79057627198103120 ) ) ;
#135184=CARTESIAN_POINT ( 'NONE',  ( -16.46253265017160317, 9.564922557960807481, 25.83224293864769194 ) ) ;
#135185=CARTESIAN_POINT ( 'NONE',  ( -8.314922557961024197, 14.29746914071037800, 57.91775706135234714 ) ) ;
#135186=CARTESIAN_POINT ( 'NONE',  ( -4.483927247898539470, -16.52544592524342804, 52.29057627198102409 ) ) ;
#135187=CARTESIAN_POINT ( 'NONE',  ( 16.55341960407618274, -4.379528057220086978, 96.04275706135236135 ) ) ;
#135188=CARTESIAN_POINT ( 'NONE',  ( -10.81492255796078084, -18.62759615963271287, 22.08224293864769194 ) ) ;
#135189=CARTESIAN_POINT ( 'NONE',  ( 5.719274019375991003, -21.55341960407610458, 37.70724293864769550 ) ) ;
#135190=CARTESIAN_POINT ( 'NONE',  ( 15.72974639402176855, 15.80617190586768217, 111.8760903946856615 ) ) ;
#135191=CARTESIAN_POINT ( 'NONE',  ( 8.224510206698953496, -14.34966873604960469, 92.91557627198103830 ) ) ;
#135192=CARTESIAN_POINT ( 'NONE',  ( 5.049401038298161559, -19.05341960407611168, 92.70724293864769550 ) ) ;
#135194=CARTESIAN_POINT ( 'NONE',  ( -8.314922557961024197, 14.29746914071037800, 37.91775706135235424 ) ) ;
#135195=CARTESIAN_POINT ( 'NONE',  ( -16.46253265017160317, 9.564922557960807481, 35.83224293864768839 ) ) ;
#135196=CARTESIAN_POINT ( 'NONE',  ( 16.55341960407618274, -4.379528057220086978, 46.04275706135234714 ) ) ;
#135197=DIRECTION ( 'NONE',  ( -1.000000000000000000, -0.000000000000000000, -0.000000000000000000 ) ) ;
#135198=CARTESIAN_POINT ( 'NONE',  ( -9.474510206698720793, -16.51473224551083518, 49.58442372801899722 ) ) ;
#135200=CARTESIAN_POINT ( 'NONE',  ( -13.89961937509977652, 13.97604488694528158, 40.62390960531435979 ) ) ;
#135201=CARTESIAN_POINT ( 'NONE',  ( 4.483927247898790824, -16.52544592524335698, 85.20942372801901854 ) ) ;
#135202=CARTESIAN_POINT ( 'NONE',  ( 19.05341960407617918, -5.049401038297876454, 96.04275706135231871 ) ) ;
#135203=CARTESIAN_POINT ( 'NONE',  ( 19.02544592524334988, 5.153800228976608722, 31.45942372801900433 ) ) ;
#135204=CARTESIAN_POINT ( 'NONE',  ( 13.97604488694527802, 13.89961937509977652, 59.37390960531434558 ) ) ;
#135205=CARTESIAN_POINT ( 'NONE',  ( 14.29746914071049879, -8.314922557960816363, 93.33224293864769550 ) ) ;
#135207=CARTESIAN_POINT ( 'NONE',  ( -5.049401038297874678, -19.05341960407617918, 64.79275706135233293 ) ) ;
#135208=CARTESIAN_POINT ( 'NONE',  ( 10.81492255796078972, 18.62759615963270932, 64.58224293864769550 ) ) ;
#135209=CARTESIAN_POINT ( 'NONE',  ( -5.049401038297874678, -19.05341960407617918, 34.79275706135233293 ) ) ;
#135210=CARTESIAN_POINT ( 'NONE',  ( -13.89961937509977652, 13.97604488694528158, 100.6239096053143669 ) ) ;
#135211=CARTESIAN_POINT ( 'NONE',  ( -15.80617190586745835, -15.72974639402198527, 86.87390960531438111 ) ) ;
#135212=CARTESIAN_POINT ( 'NONE',  ( -16.18388926212237777, 7.379444403734523483, 84.56046848633847901 ) ) ;
#135213=CARTESIAN_POINT ( 'NONE',  ( -0.05219959533936034679, 19.03943276465977164, 97.50109039468567573 ) ) ;
#135214=CARTESIAN_POINT ( 'NONE',  ( -18.22780087662122028, 5.500000000000031086, 98.51540105326105845 ) ) ;
#135215=CARTESIAN_POINT ( 'NONE',  ( -14.29746914071037622, -8.314922557961029526, 24.16775706135235424 ) ) ;
#135216=CARTESIAN_POINT ( 'NONE',  ( -9.474510206698964154, 16.51473224551069663, 45.41557627198103120 ) ) ;
#135217=CARTESIAN_POINT ( 'NONE',  ( 19.03943276465977164, -0.05219959533909143690, 113.7489096053143669 ) ) ;
#135218=CARTESIAN_POINT ( 'NONE',  ( 21.52544592524344225, -5.823673210054117533, 93.54057627198103830 ) ) ;
#135219=CARTESIAN_POINT ( 'NONE',  ( -15.72974639402176322, -15.80617190586768395, 59.37609039468568284 ) ) ;
#135220=CARTESIAN_POINT ( 'NONE',  ( 16.46253265017146816, 9.564922557961045513, 111.6677570613523329 ) ) ;
#135221=CARTESIAN_POINT ( 'NONE',  ( -10.81492255796105439, 18.62759615963255655, 112.9177570613523329 ) ) ;
#135222=CARTESIAN_POINT ( 'NONE',  ( -4.483927247898539470, -16.52544592524342804, 22.29057627198102765 ) ) ;
#135223=CARTESIAN_POINT ( 'NONE',  ( 21.53943276465977519, -0.05219959533907433946, 103.7489096053143669 ) ) ;
#135224=CARTESIAN_POINT ( 'NONE',  ( 0.05219959533910956823, 16.53943276465976808, 49.99890960531437401 ) ) ;
#135225=CARTESIAN_POINT ( 'NONE',  ( -0.05219959533936034679, 19.03943276465977164, 82.50109039468567573 ) ) ;
#135226=CARTESIAN_POINT ( 'NONE',  ( 19.03943276465977164, 0.05219959533936151252, 51.25109039468567573 ) ) ;
#135227=CARTESIAN_POINT ( 'NONE',  ( 10.72451020669871369, 18.67979575497193778, 72.08442372801899012 ) ) ;
#135228=CARTESIAN_POINT ( 'NONE',  ( -16.51473224551082808, 9.474510206698731452, 33.33442372801899722 ) ) ;
#135229=CARTESIAN_POINT ( 'NONE',  ( 5.153800228976335163, 19.02544592524342804, 24.79057627198102765 ) ) ;
#135230=CARTESIAN_POINT ( 'NONE',  ( -15.72974639402197994, 15.80617190586746368, 40.62390960531435269 ) ) ;
#135231=CARTESIAN_POINT ( 'NONE',  ( 16.55341960407611168, 4.379528057220329451, 38.95724293864768839 ) ) ;
#135232=CARTESIAN_POINT ( 'NONE',  ( 21.53943276465977519, 0.05219959533937863772, 106.2510903946856757 ) ) ;
#135233=CARTESIAN_POINT ( 'NONE',  ( 4.379528057220092307, 16.55341960407617563, 77.29275706135234714 ) ) ;
#135234=CARTESIAN_POINT ( 'NONE',  ( 8.314922557960818139, 14.29746914071049879, 24.58224293864768839 ) ) ;
#135235=CARTESIAN_POINT ( 'NONE',  ( -21.52544592524334988, -5.823673210054445271, 63.95942372801901854 ) ) ;
#135236=CARTESIAN_POINT ( 'NONE',  ( 5.719274019375673035, 21.55341960407619339, 72.29275706135236135 ) ) ;
#135237=CARTESIAN_POINT ( 'NONE',  ( 15.80617190586746368, 15.72974639402197994, 74.37390960531436690 ) ) ;
#135239=CARTESIAN_POINT ( 'NONE',  ( -0.05219959533909027116, -19.03943276465977164, 22.49890960531436690 ) ) ;
#135240=CARTESIAN_POINT ( 'NONE',  ( -10.72451020669870658, -18.67979575497194134, 49.58442372801901143 ) ) ;
#135241=CARTESIAN_POINT ( 'NONE',  ( -0.05219959533909027116, -19.03943276465977164, 27.49890960531435624 ) ) ;
#135242=CARTESIAN_POINT ( 'NONE',  ( 5.049401038298161559, -19.05341960407611168, 42.70724293864767418 ) ) ;
#135243=CARTESIAN_POINT ( 'NONE',  ( -14.29746914071049879, 8.314922557960819915, 90.83224293864769550 ) ) ;
#135244=CARTESIAN_POINT ( 'NONE',  ( 5.049401038298161559, -19.05341960407611168, 87.70724293864769550 ) ) ;
#135245=CARTESIAN_POINT ( 'NONE',  ( 4.483927247898545687, 16.52544592524342804, 29.79057627198102409 ) ) ;
#135246=CARTESIAN_POINT ( 'NONE',  ( -8.224510206698948167, 14.34966873604960824, 100.4155762719810241 ) ) ;
#135247=CARTESIAN_POINT ( 'NONE',  ( -15.72974639402197994, 15.80617190586746368, 70.62390960531436690 ) ) ;
#135248=CARTESIAN_POINT ( 'NONE',  ( -5.823673210054116645, -21.52544592524344225, 102.2905762719810383 ) ) ;
#135249=CARTESIAN_POINT ( 'NONE',  ( -13.97604488694527625, -13.89961937509977652, 111.8739096053143243 ) ) ;
#135250=CARTESIAN_POINT ( 'NONE',  ( 0.05219959533909260263, 19.03943276465977164, 64.99890960531436690 ) ) ;
#135251=CARTESIAN_POINT ( 'NONE',  ( -16.52544592524335698, -4.483927247898792601, 23.95942372801901143 ) ) ;
#135252=CARTESIAN_POINT ( 'NONE',  ( 10.72451020669898902, -18.67979575497178502, 57.91557627198103120 ) ) ;
#135253=CARTESIAN_POINT ( 'NONE',  ( 21.53943276465977519, 0.05219959533937863772, 86.25109039468568994 ) ) ;
#135254=CARTESIAN_POINT ( 'NONE',  ( 5.049401038298161559, -19.05341960407611168, 77.70724293864765286 ) ) ;
#135255=CARTESIAN_POINT ( 'NONE',  ( -5.049401038298153566, 19.05341960407611168, 115.2072429386477097 ) ) ;
#135256=CARTESIAN_POINT ( 'NONE',  ( 14.29746914071037800, 8.314922557961029526, 81.66775706135236135 ) ) ;
#135257=CARTESIAN_POINT ( 'NONE',  ( 5.823673210054444382, -21.52544592524334988, 60.20942372801902565 ) ) ;
#135258=CARTESIAN_POINT ( 'NONE',  ( 10.81492255796106328, -18.62759615963255655, 95.41775706135234714 ) ) ;
#135259=CARTESIAN_POINT ( 'NONE',  ( 14.29746914071037800, 8.314922557961029526, 61.66775706135235424 ) ) ;
#135260=CARTESIAN_POINT ( 'NONE',  ( 21.55341960407610458, 5.719274019375980345, 108.9572429386476955 ) ) ;
#135261=CARTESIAN_POINT ( 'NONE',  ( -0.05219959533909027116, -19.03943276465977164, 22.49890960531436690 ) ) ;
#135263=CARTESIAN_POINT ( 'NONE',  ( 21.53943276465977519, -0.05219959533907433946, 93.74890960531436690 ) ) ;
#135264=CARTESIAN_POINT ( 'NONE',  ( 9.474510206698729675, 16.51473224551082808, 52.08442372801900433 ) ) ;
#135265=CARTESIAN_POINT ( 'NONE',  ( -15.80617190586745835, -15.72974639402198527, 56.87390960531436690 ) ) ;
#135266=CARTESIAN_POINT ( 'NONE',  ( -5.049401038298153566, 19.05341960407611168, 95.20724293864770971 ) ) ;
#135267=CARTESIAN_POINT ( 'NONE',  ( -4.483927247898539470, -16.52544592524342804, 32.29057627198102409 ) ) ;
#135269=CARTESIAN_POINT ( 'NONE',  ( 9.564922557961047289, -16.46253265017146816, 110.4177570613523471 ) ) ;
#135270=CARTESIAN_POINT ( 'NONE',  ( 10.81492255796078972, 18.62759615963270932, 74.58224293864768129 ) ) ;
#135271=CARTESIAN_POINT ( 'NONE',  ( -8.314922557960811034, -14.29746914071050412, 57.08224293864769550 ) ) ;
#135272=CARTESIAN_POINT ( 'NONE',  ( -8.314922557961024197, 14.29746914071037800, 27.91775706135234358 ) ) ;
#135273=CARTESIAN_POINT ( 'NONE',  ( -9.474510206698964154, 16.51473224551069663, 45.41557627198103120 ) ) ;
#135274=CARTESIAN_POINT ( 'NONE',  ( -15.72974639402197994, 15.80617190586746368, 115.6239096053143669 ) ) ;
#135275=CARTESIAN_POINT ( 'NONE',  ( 16.46253265017146816, 9.564922557961045513, 81.66775706135233293 ) ) ;
#135276=CARTESIAN_POINT ( 'NONE',  ( 9.564922557960805705, 16.46253265017160317, 79.58224293864769550 ) ) ;
#135277=CARTESIAN_POINT ( 'NONE',  ( 16.51473224551069308, 9.474510206698969483, 79.16557627198103830 ) ) ;
#135278=CARTESIAN_POINT ( 'NONE',  ( 18.67979575497178502, 10.72451020669898547, 79.16557627198103830 ) ) ;
#135279=CARTESIAN_POINT ( 'NONE',  ( -19.02544592524342804, 5.153800228976336051, 36.04057627198100988 ) ) ;
#135281=CARTESIAN_POINT ( 'NONE',  ( 12.06949235617757843, -12.14591786802309237, 53.12390960531436690 ) ) ;
#135282=CARTESIAN_POINT ( 'NONE',  ( 19.03943276465977164, -0.05219959533909143690, 83.74890960531436690 ) ) ;
#135284=CARTESIAN_POINT ( 'NONE',  ( 19.03943276465977164, 0.05219959533936151252, 71.25109039468566152 ) ) ;
#135285=CARTESIAN_POINT ( 'NONE',  ( -15.80617190586745835, -15.72974639402198527, 76.87390960531439532 ) ) ;
#135286=CARTESIAN_POINT ( 'NONE',  ( 9.564922557961047289, -16.46253265017146816, 40.41775706135234003 ) ) ;
#135287=CARTESIAN_POINT ( 'NONE',  ( 13.97604488694527802, 13.89961937509977652, 84.37390960531433848 ) ) ;
#135289=CARTESIAN_POINT ( 'NONE',  ( 5.719274019375991003, -21.55341960407610458, 32.70724293864770260 ) ) ;
#135290=CARTESIAN_POINT ( 'NONE',  ( 16.46253265017160672, -9.564922557960803928, 78.33224293864769550 ) ) ;
#135291=CARTESIAN_POINT ( 'NONE',  ( 10.81492255796106328, -18.62759615963255655, 50.41775706135235424 ) ) ;
#135292=CARTESIAN_POINT ( 'NONE',  ( -19.05341960407611168, -5.049401038298163336, 26.45724293864769550 ) ) ;
#135293=CARTESIAN_POINT ( 'NONE',  ( 21.52544592524344225, -5.823673210054117533, 113.5405762719810383 ) ) ;
#135294=ORIENTED_EDGE ( 'NONE', *, *, #40745, .T. ) ;
#135295=CARTESIAN_POINT ( 'NONE',  ( -21.52544592524334988, -5.823673210054445271, 43.95942372801902565 ) ) ;
#135296=ORIENTED_EDGE ( 'NONE', *, *, #102991, .T. ) ;
#135297=CARTESIAN_POINT ( 'NONE',  ( -19.02544592524342804, 5.153800228976336051, 106.0405762719810241 ) ) ;
#135299=CARTESIAN_POINT ( 'NONE',  ( 10.81492255796078972, 18.62759615963270932, 109.5822429386476955 ) ) ;
#135300=CARTESIAN_POINT ( 'NONE',  ( -13.97604488694527625, -13.89961937509977652, 61.87390960531435979 ) ) ;
#135301=CARTESIAN_POINT ( 'NONE',  ( -16.52544592524335698, -4.483927247898792601, 18.95942372801901143 ) ) ;
#135302=EDGE_CURVE ( 'NONE', #132379, #88260, #144383, .T. ) ;
#135304=CARTESIAN_POINT ( 'NONE',  ( -21.52544592524334988, -5.823673210054445271, 103.9594237280190185 ) ) ;
#135305=CARTESIAN_POINT ( 'NONE',  ( 9.564922557960805705, 16.46253265017160317, 44.58224293864769550 ) ) ;
#135306=CARTESIAN_POINT ( 'NONE',  ( 10.72451020669871369, 18.67979575497193778, 97.08442372801904696 ) ) ;
#135307=CARTESIAN_POINT ( 'NONE',  ( -5.049401038298153566, 19.05341960407611168, 90.20724293864766707 ) ) ;
#135308=CARTESIAN_POINT ( 'NONE',  ( 10.81492255796106328, -18.62759615963255655, 60.41775706135235424 ) ) ;
#135310=CARTESIAN_POINT ( 'NONE',  ( -5.153800228976328057, -19.02544592524343514, 97.29057627198099567 ) ) ;
#135312=CARTESIAN_POINT ( 'NONE',  ( 16.55341960407618274, -4.379528057220086978, 56.04275706135235424 ) ) ;
#135313=CARTESIAN_POINT ( 'NONE',  ( -16.52544592524335698, -4.483927247898792601, 63.95942372801901854 ) ) ;
#135314=CARTESIAN_POINT ( 'NONE',  ( 21.53943276465977519, 0.05219959533937863772, 61.25109039468567573 ) ) ;
#135315=CARTESIAN_POINT ( 'NONE',  ( -21.53943276465977519, -0.05219959533937600094, 83.75109039468568994 ) ) ;
#135317=CARTESIAN_POINT ( 'NONE',  ( 8.224510206698742110, 14.34966873604972548, 27.08442372801901854 ) ) ;
#135318=CARTESIAN_POINT ( 'NONE',  ( 16.51473224551069308, 9.474510206698969483, 74.16557627198103830 ) ) ;
#135319=CARTESIAN_POINT ( 'NONE',  ( -16.46253265017160317, 9.564922557960807481, 100.8322429386477097 ) ) ;
#135321=CARTESIAN_POINT ( 'NONE',  ( 16.79531203550650176, 7.028104445595485750, 43.75244988220443787 ) ) ;
#135322=CARTESIAN_POINT ( 'NONE',  ( 5.153800228976335163, 19.02544592524342804, 29.79057627198102409 ) ) ;
#135323=CARTESIAN_POINT ( 'NONE',  ( -15.72974639402197994, 15.80617190586746368, 40.62390960531435269 ) ) ;
#135324=CARTESIAN_POINT ( 'NONE',  ( -16.53943276465976808, -0.05219959533934237506, 88.75109039468567573 ) ) ;
#135325=CARTESIAN_POINT ( 'NONE',  ( 8.314922557960818139, 14.29746914071049879, 89.58224293864768129 ) ) ;
#135326=CARTESIAN_POINT ( 'NONE',  ( -16.51473224551069308, -9.474510206698971260, 61.66557627198103120 ) ) ;
#135327=CARTESIAN_POINT ( 'NONE',  ( -15.80617190586768217, 15.72974639402176855, 88.12609039468570415 ) ) ;
#135329=CARTESIAN_POINT ( 'NONE',  ( 8.224510206698742110, 14.34966873604972548, 22.08442372801901143 ) ) ;
#135330=CARTESIAN_POINT ( 'NONE',  ( 12.14591786802309770, 12.06949235617756955, 79.37390960531436690 ) ) ;
#135331=CARTESIAN_POINT ( 'NONE',  ( -10.81492255796105439, 18.62759615963255655, 47.91775706135234714 ) ) ;
#135332=CARTESIAN_POINT ( 'NONE',  ( -15.80617190586745835, -15.72974639402198527, 71.87390960531438111 ) ) ;
#135333=CARTESIAN_POINT ( 'NONE',  ( -13.89961937509957401, -13.97604488694547875, 34.37609039468566863 ) ) ;
#135334=CARTESIAN_POINT ( 'NONE',  ( 18.22780087662121673, 5.500000000000056843, 43.98459894673892734 ) ) ;
#135335=CARTESIAN_POINT ( 'NONE',  ( -9.564922557960796823, -16.46253265017161027, 77.08224293864769550 ) ) ;
#135336=CARTESIAN_POINT ( 'NONE',  ( -8.224510206698948167, 14.34966873604960824, 45.41557627198103830 ) ) ;
#135337=CARTESIAN_POINT ( 'NONE',  ( 16.55341960407611168, 4.379528057220329451, 33.95724293864769550 ) ) ;
#135338=CARTESIAN_POINT ( 'NONE',  ( -16.53943276465976808, 0.05219959533911058130, 21.24890960531436690 ) ) ;
#135339=CARTESIAN_POINT ( 'NONE',  ( 19.02544592524334988, 5.153800228976608722, 66.45942372801899012 ) ) ;
#135340=CARTESIAN_POINT ( 'NONE',  ( 18.87255363501902394, 5.499999999999941380, 53.82513748171829349 ) ) ;
#135341=CARTESIAN_POINT ( 'NONE',  ( 15.80617190586746368, 15.72974639402197994, 29.37390960531435269 ) ) ;
#135342=CARTESIAN_POINT ( 'NONE',  ( 16.55341960407611168, 4.379528057220329451, 93.95724293864770971 ) ) ;
#135344=CARTESIAN_POINT ( 'NONE',  ( 13.97604488694527802, 13.89961937509977652, 39.37390960531435269 ) ) ;
#135345=CARTESIAN_POINT ( 'NONE',  ( -18.62759615963270932, 10.81492255796079327, 30.83224293864770260 ) ) ;
#135346=CARTESIAN_POINT ( 'NONE',  ( 5.719274019375991003, -21.55341960407610458, 62.70724293864769550 ) ) ;
#135347=CARTESIAN_POINT ( 'NONE',  ( -19.03943276465977164, 0.05219959533909376836, 21.24890960531436335 ) ) ;
#135348=CARTESIAN_POINT ( 'NONE',  ( -14.29746914071037622, -8.314922557961029526, 69.16775706135234714 ) ) ;
#135349=CARTESIAN_POINT ( 'NONE',  ( 5.049401038298161559, -19.05341960407611168, 52.70724293864767418 ) ) ;
#135351=CARTESIAN_POINT ( 'NONE',  ( 10.72451020669871369, 18.67979575497193778, 52.08442372801901854 ) ) ;
#135352=VERTEX_POINT ( 'NONE', #184042 ) ;
#135353=CARTESIAN_POINT ( 'NONE',  ( -12.14591786802309592, -12.06949235617757132, 101.8739096053143811 ) ) ;
#135354=CARTESIAN_POINT ( 'NONE',  ( 9.564922557961047289, -16.46253265017146816, 90.41775706135234714 ) ) ;
#135356=LINE ( 'NONE', #124887, #170195 ) ;
#135357=CARTESIAN_POINT ( 'NONE',  ( -15.80617190586745835, -15.72974639402198527, 36.87390960531435979 ) ) ;
#135358=CARTESIAN_POINT ( 'NONE',  ( 17.49999999999998934, -5.500000000000023981, 78.29690382534170112 ) ) ;
#135359=CARTESIAN_POINT ( 'NONE',  ( -21.55341960407619339, 5.719274019375674811, 73.54275706135234714 ) ) ;
#135361=CARTESIAN_POINT ( 'NONE',  ( 4.483927247898790824, -16.52544592524335698, 50.20942372801901854 ) ) ;
#135362=CARTESIAN_POINT ( 'NONE',  ( -0.05219959533910754901, -16.53943276465976808, 42.49890960531435979 ) ) ;
#135363=CARTESIAN_POINT ( 'NONE',  ( 21.53943276465977519, -0.05219959533907433946, 68.74890960531435269 ) ) ;
#135364=CARTESIAN_POINT ( 'NONE',  ( -15.80617190586745835, -15.72974639402198527, 66.87390960531436690 ) ) ;
#135366=CARTESIAN_POINT ( 'NONE',  ( -13.97604488694547697, 13.89961937509957934, 83.12609039468564731 ) ) ;
#135367=CARTESIAN_POINT ( 'NONE',  ( -18.62759615963270932, 10.81492255796079327, 25.83224293864769194 ) ) ;
#135368=CARTESIAN_POINT ( 'NONE',  ( 9.474510206698971260, -16.51473224551069308, 47.91557627198102409 ) ) ;
#135369=CARTESIAN_POINT ( 'NONE',  ( 8.314922557960818139, 14.29746914071049879, 109.5822429386476955 ) ) ;
#135371=CARTESIAN_POINT ( 'NONE',  ( -19.02544592524342804, 5.153800228976336051, 116.0405762719810383 ) ) ;
#135373=CARTESIAN_POINT ( 'NONE',  ( 12.06949235617739724, 12.14591786802326823, 71.87609039468568994 ) ) ;
#135374=CARTESIAN_POINT ( 'NONE',  ( 10.72451020669898902, -18.67979575497178502, 102.9155762719810383 ) ) ;
#135375=CARTESIAN_POINT ( 'NONE',  ( -13.97604488694527625, -13.89961937509977652, 66.87390960531436690 ) ) ;
#135376=CARTESIAN_POINT ( 'NONE',  ( -15.72974639402176322, -15.80617190586768395, 39.37609039468567573 ) ) ;
#135377=CARTESIAN_POINT ( 'NONE',  ( -13.97604488694527625, -13.89961937509977652, 101.8739096053143811 ) ) ;
#135380=CARTESIAN_POINT ( 'NONE',  ( 5.719274019375673035, 21.55341960407619339, 32.29275706135235424 ) ) ;
#135381=CARTESIAN_POINT ( 'NONE',  ( 5.153800228976335163, 19.02544592524342804, 24.79057627198102765 ) ) ;
#135382=CARTESIAN_POINT ( 'NONE',  ( -19.05341960407617563, 5.049401038297882671, 93.54275706135234714 ) ) ;
#135383=CARTESIAN_POINT ( 'NONE',  ( 9.474510206698729675, 16.51473224551082808, 47.08442372801900433 ) ) ;
#135384=CARTESIAN_POINT ( 'NONE',  ( -18.62759615963270932, 10.81492255796079327, 100.8322429386477097 ) ) ;
#135385=CARTESIAN_POINT ( 'NONE',  ( 5.049401038297881783, 19.05341960407617563, 37.29275706135232582 ) ) ;
#135386=CARTESIAN_POINT ( 'NONE',  ( 19.03943276465977164, 0.05219959533936151252, 46.25109039468566863 ) ) ;
#135387=CARTESIAN_POINT ( 'NONE',  ( 4.483927247898790824, -16.52544592524335698, 95.20942372801903275 ) ) ;
#135388=CARTESIAN_POINT ( 'NONE',  ( -16.46253265017160317, 9.564922557960807481, 115.8322429386477097 ) ) ;
#135390=CARTESIAN_POINT ( 'NONE',  ( -5.153800228976328057, -19.02544592524343514, 67.29057627198102409 ) ) ;
#135391=CARTESIAN_POINT ( 'NONE',  ( -0.05219959533937732626, 21.53943276465977519, 82.50109039468568994 ) ) ;
#135392=CARTESIAN_POINT ( 'NONE',  ( 15.80617190586769283, -15.72974639402175789, 90.62609039468567573 ) ) ;
#135394=CARTESIAN_POINT ( 'NONE',  ( 9.564922557960805705, 16.46253265017160317, 89.58224293864769550 ) ) ;
#135395=CARTESIAN_POINT ( 'NONE',  ( 5.823673210054444382, -21.52544592524334988, 60.20942372801902565 ) ) ;
#135396=CARTESIAN_POINT ( 'NONE',  ( 9.474510206698729675, 16.51473224551082808, 107.0844237280190043 ) ) ;
#135397=CARTESIAN_POINT ( 'NONE',  ( -13.97604488694527625, -13.89961937509977652, 61.87390960531435979 ) ) ;
#135398=CARTESIAN_POINT ( 'NONE',  ( 9.474510206698971260, -16.51473224551069308, 112.9155762719810383 ) ) ;
#135399=CARTESIAN_POINT ( 'NONE',  ( 13.97604488694527802, 13.89961937509977652, 84.37390960531433848 ) ) ;
#135400=CARTESIAN_POINT ( 'NONE',  ( -17.44270441346520073, -5.991230190322948346, 91.36335079264229364 ) ) ;
#135401=CARTESIAN_POINT ( 'NONE',  ( 13.97604488694527802, 13.89961937509977652, 64.37390960531436690 ) ) ;
#135402=CARTESIAN_POINT ( 'NONE',  ( -19.02544592524342804, 5.153800228976336051, 46.04057627198101699 ) ) ;
#135403=CARTESIAN_POINT ( 'NONE',  ( -10.72451020669898014, 18.67979575497178502, 110.4155762719810383 ) ) ;
#135404=CARTESIAN_POINT ( 'NONE',  ( -12.14591786802326823, 12.06949235617739902, 88.12609039468570415 ) ) ;
#135406=CARTESIAN_POINT ( 'NONE',  ( -16.46253265017146816, -9.564922557961047289, 49.16775706135233293 ) ) ;
#135407=CARTESIAN_POINT ( 'NONE',  ( 13.89961937509977652, -13.97604488694527269, 73.12390960531436690 ) ) ;
#135408=CARTESIAN_POINT ( 'NONE',  ( -12.06949235617756955, 12.14591786802309770, 65.62390960531436690 ) ) ;
#135409=CARTESIAN_POINT ( 'NONE',  ( -14.34966873604960291, -8.224510206698953496, 106.6655762719810383 ) ) ;
#135410=CARTESIAN_POINT ( 'NONE',  ( -16.46253265017160317, 9.564922557960807481, 110.8322429386476955 ) ) ;
#135411=CARTESIAN_POINT ( 'NONE',  ( -13.97604488694527625, -13.89961937509977652, 111.8739096053143243 ) ) ;
#135412=CARTESIAN_POINT ( 'NONE',  ( -14.29746914071049879, 8.314922557960819915, 75.83224293864769550 ) ) ;
#135414=CARTESIAN_POINT ( 'NONE',  ( -16.46253265017146816, -9.564922557961047289, 29.16775706135232937 ) ) ;
#135415=CARTESIAN_POINT ( 'NONE',  ( 12.14591786802327356, -12.06949235617739191, 100.6260903946857184 ) ) ;
#135416=CARTESIAN_POINT ( 'NONE',  ( -9.474510206698964154, 16.51473224551069663, 85.41557627198102409 ) ) ;
#135417=CARTESIAN_POINT ( 'NONE',  ( 10.81492255796106328, -18.62759615963255655, 55.41775706135234714 ) ) ;
#135418=CARTESIAN_POINT ( 'NONE',  ( -21.55341960407610458, -5.719274019375992779, 46.45724293864769550 ) ) ;
#135419=CARTESIAN_POINT ( 'NONE',  ( -21.53943276465977519, 0.05219959533907696930, 111.2489096053143669 ) ) ;
#135420=CARTESIAN_POINT ( 'NONE',  ( 21.52544592524344225, -5.823673210054117533, 63.54057627198103830 ) ) ;
#135421=CARTESIAN_POINT ( 'NONE',  ( 8.314922557960818139, 14.29746914071049879, 94.58224293864769550 ) ) ;
#135422=CARTESIAN_POINT ( 'NONE',  ( -16.51473224551082808, 9.474510206698731452, 58.33442372801900433 ) ) ;
#135423=CARTESIAN_POINT ( 'NONE',  ( -9.474510206698964154, 16.51473224551069663, 25.41557627198103120 ) ) ;
#135424=CARTESIAN_POINT ( 'NONE',  ( 9.564922557960805705, 16.46253265017160317, 84.58224293864769550 ) ) ;
#135425=CARTESIAN_POINT ( 'NONE',  ( 19.03943276465977164, -0.05219959533909143690, 83.74890960531436690 ) ) ;
#135426=CARTESIAN_POINT ( 'NONE',  ( -8.314922557960811034, -14.29746914071050412, 107.0822429386476955 ) ) ;
#135427=ORIENTED_EDGE ( 'NONE', *, *, #172537, .F. ) ;
#135428=CARTESIAN_POINT ( 'NONE',  ( -8.224510206698948167, 14.34966873604960824, 30.41557627198101699 ) ) ;
#135429=CARTESIAN_POINT ( 'NONE',  ( -16.52544592524335698, -4.483927247898792601, 38.95942372801901854 ) ) ;
#135430=CARTESIAN_POINT ( 'NONE',  ( 0.05219959533937995610, -21.53943276465977519, 105.0010903946856757 ) ) ;
#135431=CARTESIAN_POINT ( 'NONE',  ( -16.46253265017160317, 9.564922557960807481, 95.83224293864769550 ) ) ;
#135432=CARTESIAN_POINT ( 'NONE',  ( -5.719274019375665041, -21.55341960407619695, 34.79275706135235424 ) ) ;
#135433=CARTESIAN_POINT ( 'NONE',  ( 9.564922557960805705, 16.46253265017160317, 49.58224293864770260 ) ) ;
#135434=CARTESIAN_POINT ( 'NONE',  ( 8.314922557961029526, -14.29746914071037800, 45.41775706135234003 ) ) ;
#135436=CARTESIAN_POINT ( 'NONE',  ( -13.97604488694547697, 13.89961937509957934, 108.1260903946856331 ) ) ;
#135437=CARTESIAN_POINT ( 'NONE',  ( 0.05219959533909260263, 19.03943276465977164, 39.99890960531436690 ) ) ;
#135438=CARTESIAN_POINT ( 'NONE',  ( 4.379528057220339221, -16.55341960407611168, 97.70724293864772392 ) ) ;
#135439=CARTESIAN_POINT ( 'NONE',  ( 18.67979575497178502, 10.72451020669898547, 99.16557627198100988 ) ) ;
#135440=CARTESIAN_POINT ( 'NONE',  ( -5.153800228976607833, 19.02544592524334988, 77.70942372801900433 ) ) ;
#135442=CARTESIAN_POINT ( 'NONE',  ( 16.51473224551069308, 9.474510206698969483, 89.16557627198103830 ) ) ;
#135443=CARTESIAN_POINT ( 'NONE',  ( 18.67979575497194134, -10.72451020669871369, 35.83442372801901143 ) ) ;
#135444=CARTESIAN_POINT ( 'NONE',  ( -19.03943276465977164, 0.05219959533909376836, 21.24890960531436335 ) ) ;
#135445=CARTESIAN_POINT ( 'NONE',  ( -16.51473224551069308, -9.474510206698971260, 91.66557627198103830 ) ) ;
#135446=CARTESIAN_POINT ( 'NONE',  ( 17.31728774477275223, -6.344390552232368030, 113.3190665168932014 ) ) ;
#135447=CARTESIAN_POINT ( 'NONE',  ( -13.89961937509977652, 13.97604488694528158, 85.62390960531433848 ) ) ;
#135448=CARTESIAN_POINT ( 'NONE',  ( -18.62759615963255300, -10.81492255796106328, 34.16775706135234714 ) ) ;
#135449=CARTESIAN_POINT ( 'NONE',  ( -4.379528057220328563, 16.55341960407611168, 85.20724293864770971 ) ) ;
#135450=CARTESIAN_POINT ( 'NONE',  ( -13.97604488694527625, -13.89961937509977652, 96.87390960531433848 ) ) ;
#135451=CARTESIAN_POINT ( 'NONE',  ( -21.55341960407619339, 5.719274019375674811, 113.5427570613523756 ) ) ;
#135452=CARTESIAN_POINT ( 'NONE',  ( 12.06949235617739724, 12.14591786802326823, 51.87609039468568284 ) ) ;
#135453=CARTESIAN_POINT ( 'NONE',  ( -18.62759615963255300, -10.81492255796106328, 74.16775706135231871 ) ) ;
#135454=CARTESIAN_POINT ( 'NONE',  ( -16.55341960407617563, 4.379528057220093196, 28.54275706135234358 ) ) ;
#135455=CARTESIAN_POINT ( 'NONE',  ( -19.03943276465977164, 0.05219959533909376836, 66.24890960531436690 ) ) ;
#135456=CARTESIAN_POINT ( 'NONE',  ( 13.97604488694548053, -13.89961937509957401, 90.62609039468567573 ) ) ;
#135457=CARTESIAN_POINT ( 'NONE',  ( -16.52544592524335698, -4.483927247898792601, 68.95942372801901854 ) ) ;
#135458=CARTESIAN_POINT ( 'NONE',  ( 16.46253265017146816, 9.564922557961045513, 21.66775706135233648 ) ) ;
#135459=CARTESIAN_POINT ( 'NONE',  ( 9.474510206698729675, 16.51473224551082808, 82.08442372801899012 ) ) ;
#135460=CARTESIAN_POINT ( 'NONE',  ( 19.05341960407611168, 5.049401038298154454, 58.95724293864768129 ) ) ;
#135461=CARTESIAN_POINT ( 'NONE',  ( 15.80617190586746368, 15.72974639402197994, 89.37390960531435269 ) ) ;
#135462=CARTESIAN_POINT ( 'NONE',  ( -8.224510206698948167, 14.34966873604960824, 75.41557627198102409 ) ) ;
#135463=CARTESIAN_POINT ( 'NONE',  ( -19.03943276465977164, -0.05219959533935918106, 78.75109039468567573 ) ) ;
#135464=CARTESIAN_POINT ( 'NONE',  ( -17.49999999999999645, -5.499999999999992895, 74.20309617465828467 ) ) ;
#135465=CARTESIAN_POINT ( 'NONE',  ( 19.03943276465977164, 0.05219959533936151252, 51.25109039468567573 ) ) ;
#135466=ADVANCED_FACE ( 'NONE', ( #16183 ), #28473, .T. ) ;
#135467=CARTESIAN_POINT ( 'NONE',  ( 8.314922557960818139, 14.29746914071049879, 24.58224293864768839 ) ) ;
#135468=CARTESIAN_POINT ( 'NONE',  ( -14.34966873604960291, -8.224510206698953496, 81.66557627198103830 ) ) ;
#135469=CARTESIAN_POINT ( 'NONE',  ( -15.80617190586768217, 15.72974639402176855, 113.1260903946856899 ) ) ;
#135471=CARTESIAN_POINT ( 'NONE',  ( 15.72974639402199770, -15.80617190586745480, 108.1239096053143811 ) ) ;
#135472=CARTESIAN_POINT ( 'NONE',  ( -9.474510206698964154, 16.51473224551069663, 100.4155762719810241 ) ) ;
#135473=CARTESIAN_POINT ( 'NONE',  ( 13.89961937509977652, -13.97604488694527269, 68.12390960531436690 ) ) ;
#135474=CARTESIAN_POINT ( 'NONE',  ( -15.72974639402176322, -15.80617190586768395, 79.37609039468567573 ) ) ;
#135475=CARTESIAN_POINT ( 'NONE',  ( -19.05341960407611168, -5.049401038298163336, 66.45724293864769550 ) ) ;
#135476=CARTESIAN_POINT ( 'NONE',  ( -16.46253265017160317, 9.564922557960807481, 35.83224293864768839 ) ) ;
#135477=CARTESIAN_POINT ( 'NONE',  ( -5.719274019375978568, 21.55341960407610458, 25.20724293864769550 ) ) ;
#135478=CARTESIAN_POINT ( 'NONE',  ( -14.29746914071049879, 8.314922557960819915, 85.83224293864768129 ) ) ;
#135479=CARTESIAN_POINT ( 'NONE',  ( 5.153800228976335163, 19.02544592524342804, 44.79057627198103830 ) ) ;
#135480=CARTESIAN_POINT ( 'NONE',  ( -12.14591786802309592, -12.06949235617757132, 101.8739096053143811 ) ) ;
#135481=CARTESIAN_POINT ( 'NONE',  ( 18.67979575497178502, 10.72451020669898547, 109.1655762719810383 ) ) ;
#135482=CARTESIAN_POINT ( 'NONE',  ( -10.72451020669870658, -18.67979575497194134, 44.58442372801901854 ) ) ;
#135483=CARTESIAN_POINT ( 'NONE',  ( 16.51473224551069308, 9.474510206698969483, 34.16557627198102409 ) ) ;
#135484=CARTESIAN_POINT ( 'NONE',  ( 4.483927247898790824, -16.52544592524335698, 70.20942372801904696 ) ) ;
#135485=CARTESIAN_POINT ( 'NONE',  ( -15.80617190586745835, -15.72974639402198527, 96.87390960531436690 ) ) ;
#135486=CARTESIAN_POINT ( 'NONE',  ( -21.52544592524343514, 5.823673210054127303, 96.04057627198102409 ) ) ;
#135487=CARTESIAN_POINT ( 'NONE',  ( -19.02544592524334988, -5.153800228976617603, 23.95942372801900078 ) ) ;
#135488=CARTESIAN_POINT ( 'NONE',  ( 19.02544592524343514, -5.153800228976328945, 58.54057627198102409 ) ) ;
#135489=CARTESIAN_POINT ( 'NONE',  ( -17.97161686094258215, 5.499999999999976019, 40.99637206859248550 ) ) ;
#135490=CARTESIAN_POINT ( 'NONE',  ( -10.72451020669870658, -18.67979575497194134, 59.58442372801901854 ) ) ;
#135491=CARTESIAN_POINT ( 'NONE',  ( -15.72974639402197994, 15.80617190586746368, 60.62390960531437401 ) ) ;
#135492=CARTESIAN_POINT ( 'NONE',  ( 0.05219959533910956823, 16.53943276465976808, 24.99890960531435624 ) ) ;
#135493=CARTESIAN_POINT ( 'NONE',  ( -21.55341960407619339, 5.719274019375674811, 73.54275706135234714 ) ) ;
#135494=CARTESIAN_POINT ( 'NONE',  ( 9.474510206698729675, 16.51473224551082808, 22.08442372801899722 ) ) ;
#135495=CARTESIAN_POINT ( 'NONE',  ( 5.049401038297881783, 19.05341960407617563, 47.29275706135231161 ) ) ;
#135496=CARTESIAN_POINT ( 'NONE',  ( 16.53943276465976808, 0.05219959533934440121, 96.25109039468568994 ) ) ;
#135497=CARTESIAN_POINT ( 'NONE',  ( -10.81492255796105439, 18.62759615963255655, 52.91775706135235424 ) ) ;
#135498=CARTESIAN_POINT ( 'NONE',  ( 9.474510206698971260, -16.51473224551069308, 52.91557627198102409 ) ) ;
#135499=CARTESIAN_POINT ( 'NONE',  ( 5.153800228976615827, -19.02544592524334988, 40.20942372801898301 ) ) ;
#135500=CARTESIAN_POINT ( 'NONE',  ( -5.719274019375978568, 21.55341960407610458, 35.20724293864768839 ) ) ;
#135501=CARTESIAN_POINT ( 'NONE',  ( -21.53943276465977519, -0.05219959533937600094, 33.75109039468568284 ) ) ;
#135503=CARTESIAN_POINT ( 'NONE',  ( -21.52544592524343514, 5.823673210054127303, 86.04057627198102409 ) ) ;
#135504=CARTESIAN_POINT ( 'NONE',  ( -5.153800228976607833, 19.02544592524334988, 82.70942372801897591 ) ) ;
#135505=CARTESIAN_POINT ( 'NONE',  ( 14.34966873604972726, -8.224510206698740333, 50.83442372801901143 ) ) ;
#135507=CARTESIAN_POINT ( 'NONE',  ( 0.05219959533907565091, 21.53943276465977519, 94.99890960531436690 ) ) ;
#135508=CARTESIAN_POINT ( 'NONE',  ( 12.06949235617739724, 12.14591786802326823, 81.87609039468568994 ) ) ;
#135509=CARTESIAN_POINT ( 'NONE',  ( -8.224510206698948167, 14.34966873604960824, 80.41557627198103830 ) ) ;
#135511=CARTESIAN_POINT ( 'NONE',  ( 13.89961937509957401, 13.97604488694547697, 101.8760903946856331 ) ) ;
#135512=CARTESIAN_POINT ( 'NONE',  ( 15.80617190586746368, 15.72974639402197994, 34.37390960531435979 ) ) ;
#135513=CARTESIAN_POINT ( 'NONE',  ( -18.22780087662123805, 5.499999999999981348, 96.01763182126897789 ) ) ;
#135514=CARTESIAN_POINT ( 'NONE',  ( -8.224510206698735004, -14.34966873604973081, 49.58442372801901143 ) ) ;
#135515=CARTESIAN_POINT ( 'NONE',  ( -15.80617190586768217, 15.72974639402176855, 33.12609039468569705 ) ) ;
#135516=CARTESIAN_POINT ( 'NONE',  ( 21.52544592524344225, -5.823673210054117533, 33.54057627198102409 ) ) ;
#135517=CARTESIAN_POINT ( 'NONE',  ( -16.55341960407617563, 4.379528057220093196, 68.54275706135234714 ) ) ;
#135518=CARTESIAN_POINT ( 'NONE',  ( -0.05219959533909027116, -19.03943276465977164, 87.49890960531436690 ) ) ;
#135519=CARTESIAN_POINT ( 'NONE',  ( -15.80617190586768217, 15.72974639402176855, 58.12609039468568994 ) ) ;
#135520=CARTESIAN_POINT ( 'NONE',  ( 13.89961937509977652, -13.97604488694527269, 28.12390960531435624 ) ) ;
#135521=CARTESIAN_POINT ( 'NONE',  ( 5.719274019375991003, -21.55341960407610458, 27.70724293864769905 ) ) ;
#135523=CARTESIAN_POINT ( 'NONE',  ( 13.89961937509957401, 13.97604488694547697, 36.87609039468565442 ) ) ;
#135524=CARTESIAN_POINT ( 'NONE',  ( 8.224510206698742110, 14.34966873604972548, 57.08442372801901854 ) ) ;
#135525=CARTESIAN_POINT ( 'NONE',  ( 5.823673210054125526, 21.52544592524343514, 24.79057627198103120 ) ) ;
#135526=CARTESIAN_POINT ( 'NONE',  ( 19.05341960407611168, 5.049401038298154454, 68.95724293864769550 ) ) ;
#135527=CARTESIAN_POINT ( 'NONE',  ( 4.483927247898790824, -16.52544592524335698, 100.2094237280190043 ) ) ;
#135529=CARTESIAN_POINT ( 'NONE',  ( -14.34966873604960291, -8.224510206698953496, 96.66557627198102409 ) ) ;
#135530=CARTESIAN_POINT ( 'NONE',  ( 0.05219959533907565091, 21.53943276465977519, 34.99890960531435979 ) ) ;
#135531=CARTESIAN_POINT ( 'NONE',  ( -13.97604488694527625, -13.89961937509977652, 36.87390960531436690 ) ) ;
#135532=CARTESIAN_POINT ( 'NONE',  ( -8.224510206698735004, -14.34966873604973081, 74.58442372801901854 ) ) ;
#135533=CARTESIAN_POINT ( 'NONE',  ( -5.719274019375665041, -21.55341960407619695, 19.79275706135235069 ) ) ;
#135534=CARTESIAN_POINT ( 'NONE',  ( -16.46253265017146816, -9.564922557961047289, 74.16775706135234714 ) ) ;
#135535=CARTESIAN_POINT ( 'NONE',  ( 13.89961937509977652, -13.97604488694527269, 43.12390960531434558 ) ) ;
#135536=VECTOR ( 'NONE', #65589, 1000.000000000000000 ) ;
#135537=CARTESIAN_POINT ( 'NONE',  ( -13.89961937509977652, 13.97604488694528158, 110.6239096053143243 ) ) ;
#135538=CARTESIAN_POINT ( 'NONE',  ( 5.719274019375673035, 21.55341960407619339, 97.29275706135234714 ) ) ;
#135539=CARTESIAN_POINT ( 'NONE',  ( 19.02544592524343514, -5.153800228976328945, 58.54057627198102409 ) ) ;
#135540=CARTESIAN_POINT ( 'NONE',  ( -12.14591786802326823, 12.06949235617739902, 53.12609039468568284 ) ) ;
#135541=CARTESIAN_POINT ( 'NONE',  ( -21.52544592524334988, -5.823673210054445271, 83.95942372801900433 ) ) ;
#135542=CARTESIAN_POINT ( 'NONE',  ( 19.05341960407617918, -5.049401038297876454, 36.04275706135234003 ) ) ;
#135543=CARTESIAN_POINT ( 'NONE',  ( 0.05219959533936267826, -19.03943276465977164, 55.00109039468566863 ) ) ;
#135544=CARTESIAN_POINT ( 'NONE',  ( -21.55341960407619339, 5.719274019375674811, 53.54275706135234714 ) ) ;
#135545=EDGE_CURVE ( 'NONE', #91305, #199831, #49110, .T. ) ;
#135546=CARTESIAN_POINT ( 'NONE',  ( -5.049401038298153566, 19.05341960407611168, 25.20724293864768484 ) ) ;
#135547=CARTESIAN_POINT ( 'NONE',  ( 19.05341960407617918, -5.049401038297876454, 51.04275706135231871 ) ) ;
#135548=CARTESIAN_POINT ( 'NONE',  ( 13.89961937509977652, -13.97604488694527269, 98.12390960531433848 ) ) ;
#135549=CARTESIAN_POINT ( 'NONE',  ( 16.51473224551069308, 9.474510206698969483, 79.16557627198103830 ) ) ;
#135550=CARTESIAN_POINT ( 'NONE',  ( 14.29746914071049879, -8.314922557960816363, 38.33224293864768839 ) ) ;
#135551=CARTESIAN_POINT ( 'NONE',  ( -21.55341960407610458, -5.719274019375992779, 36.45724293864768839 ) ) ;
#135554=CARTESIAN_POINT ( 'NONE',  ( 10.81492255796106328, -18.62759615963255655, 95.41775706135234714 ) ) ;
#135556=CARTESIAN_POINT ( 'NONE',  ( 19.03943276465977164, -0.05219959533909143690, 38.74890960531436690 ) ) ;
#135558=CARTESIAN_POINT ( 'NONE',  ( 0.05219959533934541429, -16.53943276465976808, 65.00109039468568994 ) ) ;
#135560=CARTESIAN_POINT ( 'NONE',  ( -5.823673210054116645, -21.52544592524344225, 77.29057627198102409 ) ) ;
#135561=CARTESIAN_POINT ( 'NONE',  ( 12.06949235617757843, -12.14591786802309237, 38.12390960531436690 ) ) ;
#135562=CARTESIAN_POINT ( 'NONE',  ( -9.474510206698964154, 16.51473224551069663, 30.41557627198102054 ) ) ;
#135563=CARTESIAN_POINT ( 'NONE',  ( 13.89961937509977652, -13.97604488694527269, 108.1239096053143669 ) ) ;
#135564=CARTESIAN_POINT ( 'NONE',  ( -21.53943276465977519, -0.05219959533937600094, 23.75109039468567929 ) ) ;
#135565=CARTESIAN_POINT ( 'NONE',  ( -9.474510206698720793, -16.51473224551083518, 29.58442372801900433 ) ) ;
#135566=CARTESIAN_POINT ( 'NONE',  ( -19.03943276465977164, 0.05219959533909376836, 21.24890960531436335 ) ) ;
#135567=CARTESIAN_POINT ( 'NONE',  ( 21.53943276465977519, 0.05219959533937863772, 81.25109039468568994 ) ) ;
#135569=CARTESIAN_POINT ( 'NONE',  ( -14.34966873604960291, -8.224510206698953496, 21.66557627198102409 ) ) ;
#135571=CARTESIAN_POINT ( 'NONE',  ( 10.72451020669898902, -18.67979575497178502, 22.91557627198102765 ) ) ;
#135572=CARTESIAN_POINT ( 'NONE',  ( -0.05219959533910754901, -16.53943276465976808, 102.4989096053143811 ) ) ;
#135574=CARTESIAN_POINT ( 'NONE',  ( 0.05219959533909260263, 19.03943276465977164, 84.99890960531436690 ) ) ;
#135575=CARTESIAN_POINT ( 'NONE',  ( -12.06949235617756955, 12.14591786802309770, 70.62390960531436690 ) ) ;
#135576=CARTESIAN_POINT ( 'NONE',  ( -9.474510206698720793, -16.51473224551083518, 99.58442372801900433 ) ) ;
#135577=CARTESIAN_POINT ( 'NONE',  ( -5.823673210054116645, -21.52544592524344225, 62.29057627198102409 ) ) ;
#135579=CARTESIAN_POINT ( 'NONE',  ( 19.02544592524343514, -5.153800228976328945, 33.54057627198102409 ) ) ;
#135580=CARTESIAN_POINT ( 'NONE',  ( -16.51473224551069308, -9.474510206698971260, 91.66557627198103830 ) ) ;
#135581=CARTESIAN_POINT ( 'NONE',  ( -18.67979575497178146, -10.72451020669898902, 86.66557627198102409 ) ) ;
#135582=CARTESIAN_POINT ( 'NONE',  ( -16.52544592524335698, -4.483927247898792601, 98.95942372801903275 ) ) ;
#135583=CARTESIAN_POINT ( 'NONE',  ( -19.02544592524342804, 5.153800228976336051, 81.04057627198103830 ) ) ;
#135584=CARTESIAN_POINT ( 'NONE',  ( -5.153800228976607833, 19.02544592524334988, 67.70942372801900433 ) ) ;
#135585=CARTESIAN_POINT ( 'NONE',  ( 10.72451020669871369, 18.67979575497193778, 92.08442372801901854 ) ) ;
#135586=CARTESIAN_POINT ( 'NONE',  ( -18.62759615963270932, 10.81492255796079327, 70.83224293864770971 ) ) ;
#135587=CARTESIAN_POINT ( 'NONE',  ( 21.55341960407610458, 5.719274019375980345, 38.95724293864768839 ) ) ;
#135588=CARTESIAN_POINT ( 'NONE',  ( -16.51473224551069308, -9.474510206698971260, 56.66557627198103120 ) ) ;
#135589=CARTESIAN_POINT ( 'NONE',  ( -14.34966873604960291, -8.224510206698953496, 21.66557627198102409 ) ) ;
#135590=CARTESIAN_POINT ( 'NONE',  ( 9.474510206698971260, -16.51473224551069308, 62.91557627198102409 ) ) ;
#135591=CARTESIAN_POINT ( 'NONE',  ( 17.50000000000000000, 5.624438216177601646, 51.68329655085358354 ) ) ;
#135592=CARTESIAN_POINT ( 'NONE',  ( 18.67979575497194134, -10.72451020669871369, 105.8344237280190328 ) ) ;
#135593=CARTESIAN_POINT ( 'NONE',  ( -14.29746914071049879, 8.314922557960819915, 75.83224293864769550 ) ) ;
#135594=CARTESIAN_POINT ( 'NONE',  ( 15.72974639402199770, -15.80617190586745480, 108.1239096053143811 ) ) ;
#135595=CARTESIAN_POINT ( 'NONE',  ( -15.72974639402197994, 15.80617190586746368, 105.6239096053143669 ) ) ;
#135597=CARTESIAN_POINT ( 'NONE',  ( 15.80617190586746368, 15.72974639402197994, 64.37390960531435269 ) ) ;
#135598=CARTESIAN_POINT ( 'NONE',  ( 8.314922557961029526, -14.29746914071037800, 85.41775706135236135 ) ) ;
#135599=CARTESIAN_POINT ( 'NONE',  ( -16.52544592524342804, 4.483927247898546575, 106.0405762719810525 ) ) ;
#135600=CARTESIAN_POINT ( 'NONE',  ( -9.474510206698964154, 16.51473224551069663, 65.41557627198102409 ) ) ;
#135602=CARTESIAN_POINT ( 'NONE',  ( -4.379528057220086978, -16.55341960407618274, 104.7927570613523898 ) ) ;
#135603=CARTESIAN_POINT ( 'NONE',  ( -21.53943276465977519, -0.05219959533937600094, 48.75109039468568284 ) ) ;
#135604=CARTESIAN_POINT ( 'NONE',  ( 16.46253265017160672, -9.564922557960803928, 103.3322429386476955 ) ) ;
#135605=CARTESIAN_POINT ( 'NONE',  ( 18.67979575497194134, -10.72451020669871369, 85.83442372801901854 ) ) ;
#135606=CARTESIAN_POINT ( 'NONE',  ( -9.474510206698964154, 16.51473224551069663, 25.41557627198103120 ) ) ;
#135607=CARTESIAN_POINT ( 'NONE',  ( -13.97604488694527625, -13.89961937509977652, 36.87390960531436690 ) ) ;
#135609=CARTESIAN_POINT ( 'NONE',  ( 10.81492255796106328, -18.62759615963255655, 80.41775706135234714 ) ) ;
#135610=CARTESIAN_POINT ( 'NONE',  ( -15.80617190586768217, 15.72974639402176855, 73.12609039468567573 ) ) ;
#135611=CARTESIAN_POINT ( 'NONE',  ( 9.564922557960805705, 16.46253265017160317, 104.5822429386476955 ) ) ;
#135612=CARTESIAN_POINT ( 'NONE',  ( 9.474510206698729675, 16.51473224551082808, 77.08442372801900433 ) ) ;
#135613=CARTESIAN_POINT ( 'NONE',  ( 5.823673210054444382, -21.52544592524334988, 50.20942372801901854 ) ) ;
#135614=CARTESIAN_POINT ( 'NONE',  ( -12.06949235617739369, -12.14591786802326823, 24.37609039468567573 ) ) ;
#135615=CARTESIAN_POINT ( 'NONE',  ( -13.89961937509957401, -13.97604488694547875, 74.37609039468566152 ) ) ;
#135616=CARTESIAN_POINT ( 'NONE',  ( 16.46253265017160672, -9.564922557960803928, 48.33224293864769550 ) ) ;
#135617=CARTESIAN_POINT ( 'NONE',  ( -0.05219959533936034679, 19.03943276465977164, 77.50109039468566152 ) ) ;
#135618=CARTESIAN_POINT ( 'NONE',  ( 0.05219959533910956823, 16.53943276465976808, 24.99890960531435624 ) ) ;
#135619=CARTESIAN_POINT ( 'NONE',  ( 0.05219959533936267826, -19.03943276465977164, 95.00109039468567573 ) ) ;
#135620=CARTESIAN_POINT ( 'NONE',  ( 0.05219959533910956823, 16.53943276465976808, 39.99890960531436690 ) ) ;
#135621=CARTESIAN_POINT ( 'NONE',  ( -13.89961937509957401, -13.97604488694547875, 64.37609039468567573 ) ) ;
#135622=CARTESIAN_POINT ( 'NONE',  ( -8.314922557961024197, 14.29746914071037800, 42.91775706135235424 ) ) ;
#135623=CARTESIAN_POINT ( 'NONE',  ( 5.049401038297881783, 19.05341960407617563, 27.29275706135232937 ) ) ;
#135624=CARTESIAN_POINT ( 'NONE',  ( -9.564922557960796823, -16.46253265017161027, 37.08224293864768839 ) ) ;
#135625=CARTESIAN_POINT ( 'NONE',  ( -17.59860650958989936, -7.585241751807033417, 66.57662985737508166 ) ) ;
#135626=CARTESIAN_POINT ( 'NONE',  ( 16.55341960407618274, -4.379528057220086978, 46.04275706135234714 ) ) ;
#135629=CARTESIAN_POINT ( 'NONE',  ( -16.46253265017160317, 9.564922557960807481, 95.83224293864769550 ) ) ;
#135630=CARTESIAN_POINT ( 'NONE',  ( -17.58332526062526213, -7.635886036038624702, 84.07665040441537485 ) ) ;
#135632=CARTESIAN_POINT ( 'NONE',  ( 0.05219959533936267826, -19.03943276465977164, 95.00109039468567573 ) ) ;
#135634=CARTESIAN_POINT ( 'NONE',  ( -15.80617190586745835, -15.72974639402198527, 21.87390960531436690 ) ) ;
#135635=CARTESIAN_POINT ( 'NONE',  ( 21.53943276465977519, 0.05219959533937863772, 111.2510903946856899 ) ) ;
#135636=CARTESIAN_POINT ( 'NONE',  ( 13.89961937509957401, 13.97604488694547697, 106.8760903946856757 ) ) ;
#135637=CARTESIAN_POINT ( 'NONE',  ( -16.51473224551069308, -9.474510206698971260, 21.66557627198102765 ) ) ;
#135638=CARTESIAN_POINT ( 'NONE',  ( -5.153800228976328057, -19.02544592524343514, 37.29057627198102409 ) ) ;
#135639=CARTESIAN_POINT ( 'NONE',  ( -21.52544592524343514, 5.823673210054127303, 56.04057627198102409 ) ) ;
#135640=CARTESIAN_POINT ( 'NONE',  ( -13.89961937509977652, 13.97604488694528158, 35.62390960531435269 ) ) ;
#135642=CARTESIAN_POINT ( 'NONE',  ( -19.05341960407617563, 5.049401038297882671, 68.54275706135230450 ) ) ;
#135643=CARTESIAN_POINT ( 'NONE',  ( -16.53943276465976808, 0.05219959533911058130, 56.24890960531436690 ) ) ;
#135644=CARTESIAN_POINT ( 'NONE',  ( 21.52544592524344225, -5.823673210054117533, 28.54057627198103120 ) ) ;
#135645=CARTESIAN_POINT ( 'NONE',  ( -21.55341960407619339, 5.719274019375674811, 93.54275706135234714 ) ) ;
#135646=CARTESIAN_POINT ( 'NONE',  ( 21.53943276465977519, -0.05219959533907433946, 83.74890960531435269 ) ) ;
#135647=CARTESIAN_POINT ( 'NONE',  ( 21.55341960407619695, -5.719274019375665929, 61.04275706135234714 ) ) ;
#135648=CARTESIAN_POINT ( 'NONE',  ( 0.05219959533937995610, -21.53943276465977519, 70.00109039468568994 ) ) ;
#135649=CARTESIAN_POINT ( 'NONE',  ( -19.02544592524342804, 5.153800228976336051, 96.04057627198103830 ) ) ;
#135650=CARTESIAN_POINT ( 'NONE',  ( -16.52544592524335698, -4.483927247898792601, 88.95942372801901854 ) ) ;
#135651=CARTESIAN_POINT ( 'NONE',  ( -10.72451020669870658, -18.67979575497194134, 64.58442372801900433 ) ) ;
#135652=CARTESIAN_POINT ( 'NONE',  ( 19.03943276465977164, -0.05219959533909143690, 53.74890960531436690 ) ) ;
#135653=CARTESIAN_POINT ( 'NONE',  ( -9.564922557960796823, -16.46253265017161027, 22.08224293864768839 ) ) ;
#135654=CARTESIAN_POINT ( 'NONE',  ( 16.51473224551069308, 9.474510206698969483, 49.16557627198102409 ) ) ;
#135655=CARTESIAN_POINT ( 'NONE',  ( 16.52544592524342804, -4.483927247898539470, 68.54057627198103830 ) ) ;
#135656=CARTESIAN_POINT ( 'NONE',  ( 16.53943276465976808, -0.05219959533910856209, 33.74890960531436690 ) ) ;
#135657=CARTESIAN_POINT ( 'NONE',  ( 21.53943276465977519, -0.05219959533907433946, 48.74890960531435979 ) ) ;
#135658=CARTESIAN_POINT ( 'NONE',  ( 19.05341960407611168, 5.049401038298154454, 53.95724293864770260 ) ) ;
#135659=CARTESIAN_POINT ( 'NONE',  ( 10.81492255796078972, 18.62759615963270932, 59.58224293864770260 ) ) ;
#135660=CARTESIAN_POINT ( 'NONE',  ( -9.564922557961040184, 16.46253265017147172, 47.91775706135233293 ) ) ;
#135662=CARTESIAN_POINT ( 'NONE',  ( 16.55341960407611168, 4.379528057220329451, 53.95724293864770260 ) ) ;
#135663=CARTESIAN_POINT ( 'NONE',  ( -0.05219959533907301413, -21.53943276465977519, 27.49890960531435269 ) ) ;
#135666=CARTESIAN_POINT ( 'NONE',  ( 17.26058549869091152, 6.457015423128542153, 103.8774583747606783 ) ) ;
#135667=CARTESIAN_POINT ( 'NONE',  ( 12.14591786802327356, -12.06949235617739191, 65.62609039468568994 ) ) ;
#135668=CARTESIAN_POINT ( 'NONE',  ( -19.02544592524334988, -5.153800228976617603, 68.95942372801896170 ) ) ;
#135669=CARTESIAN_POINT ( 'NONE',  ( -8.224510206698948167, 14.34966873604960824, 55.41557627198102409 ) ) ;
#135671=CARTESIAN_POINT ( 'NONE',  ( -14.29746914071049879, 8.314922557960819915, 40.83224293864769550 ) ) ;
#135672=CARTESIAN_POINT ( 'NONE',  ( 5.049401038298161559, -19.05341960407611168, 47.70724293864770260 ) ) ;
#135673=CARTESIAN_POINT ( 'NONE',  ( 9.564922557960805705, 16.46253265017160317, 69.58224293864770971 ) ) ;
#135674=CARTESIAN_POINT ( 'NONE',  ( -19.02544592524342804, 5.153800228976336051, 41.04057627198103120 ) ) ;
#135675=CARTESIAN_POINT ( 'NONE',  ( 15.72974639402176855, 15.80617190586768217, 41.87609039468568284 ) ) ;
#135676=CARTESIAN_POINT ( 'NONE',  ( -0.05219959533909027116, -19.03943276465977164, 67.49890960531436690 ) ) ;
#135677=CARTESIAN_POINT ( 'NONE',  ( 17.97182807773871005, -5.500000000000040856, 81.03038844047284783 ) ) ;
#135678=CARTESIAN_POINT ( 'NONE',  ( -5.153800228976328057, -19.02544592524343514, 57.29057627198103120 ) ) ;
#135679=CARTESIAN_POINT ( 'NONE',  ( 15.80617190586746368, 15.72974639402197994, 39.37390960531436690 ) ) ;
#135680=CARTESIAN_POINT ( 'NONE',  ( 16.46253265017160672, -9.564922557960803928, 33.33224293864770260 ) ) ;
#135681=CARTESIAN_POINT ( 'NONE',  ( 15.72974639402199770, -15.80617190586745480, 43.12390960531435269 ) ) ;
#135682=CARTESIAN_POINT ( 'NONE',  ( 12.14591786802327356, -12.06949235617739191, 95.62609039468568994 ) ) ;
#135683=CARTESIAN_POINT ( 'NONE',  ( 19.05341960407617918, -5.049401038297876454, 21.04275706135232582 ) ) ;
#135684=CARTESIAN_POINT ( 'NONE',  ( -0.05219959533934338120, 16.53943276465976808, 52.50109039468567573 ) ) ;
#135685=CARTESIAN_POINT ( 'NONE',  ( 12.14591786802327356, -12.06949235617739191, 75.62609039468567573 ) ) ;
#135686=CARTESIAN_POINT ( 'NONE',  ( 5.153800228976335163, 19.02544592524342804, 104.7905762719809957 ) ) ;
#135687=CARTESIAN_POINT ( 'NONE',  ( -12.14591786802326823, 12.06949235617739902, 68.12609039468567573 ) ) ;
#135688=CARTESIAN_POINT ( 'NONE',  ( -4.379528057220086978, -16.55341960407618274, 44.79275706135234714 ) ) ;
#135689=CARTESIAN_POINT ( 'NONE',  ( 5.153800228976335163, 19.02544592524342804, 109.7905762719810099 ) ) ;
#135690=CARTESIAN_POINT ( 'NONE',  ( 12.14591786802327356, -12.06949235617739191, 20.62609039468568639 ) ) ;
#135691=CARTESIAN_POINT ( 'NONE',  ( 5.153800228976335163, 19.02544592524342804, 34.79057627198102409 ) ) ;
#135692=CARTESIAN_POINT ( 'NONE',  ( 15.80617190586769283, -15.72974639402175789, 30.62609039468567929 ) ) ;
#135693=CARTESIAN_POINT ( 'NONE',  ( -8.314922557961024197, 14.29746914071037800, 32.91775706135234714 ) ) ;
#135694=CARTESIAN_POINT ( 'NONE',  ( 12.06949235617739724, 12.14591786802326823, 101.8760903946857042 ) ) ;
#135696=CARTESIAN_POINT ( 'NONE',  ( -10.81492255796105439, 18.62759615963255655, 97.91775706135236135 ) ) ;
#135697=CARTESIAN_POINT ( 'NONE',  ( -9.474510206698720793, -16.51473224551083518, 94.58442372801900433 ) ) ;
#135699=CARTESIAN_POINT ( 'NONE',  ( 4.379528057220339221, -16.55341960407611168, 62.70724293864769550 ) ) ;
#135700=CARTESIAN_POINT ( 'NONE',  ( -16.46253265017160317, 9.564922557960807481, 30.83224293864769550 ) ) ;
#135701=CARTESIAN_POINT ( 'NONE',  ( 9.564922557961047289, -16.46253265017146816, 55.41775706135234003 ) ) ;
#135702=CARTESIAN_POINT ( 'NONE',  ( 17.50000000001358202, -5.500000000000038192, 58.29690382535058291 ) ) ;
#135703=CARTESIAN_POINT ( 'NONE',  ( -15.72974639402176322, -15.80617190586768395, 49.37609039468569705 ) ) ;
#135704=CARTESIAN_POINT ( 'NONE',  ( 14.29746914071037800, 8.314922557961029526, 31.66775706135234358 ) ) ;
#135705=CARTESIAN_POINT ( 'NONE',  ( 17.13100169013299734, 6.664070546373167758, 81.73210164300149927 ) ) ;
#135706=CARTESIAN_POINT ( 'NONE',  ( 13.89961937509977652, -13.97604488694527269, 113.1239096053143527 ) ) ;
#135707=CARTESIAN_POINT ( 'NONE',  ( -15.72974639402197994, 15.80617190586746368, 75.62390960531439532 ) ) ;
#135708=CARTESIAN_POINT ( 'NONE',  ( -13.97604488694547697, 13.89961937509957934, 113.1260903946856757 ) ) ;
#135709=CARTESIAN_POINT ( 'NONE',  ( -19.05341960407611168, -5.049401038298163336, 106.4572429386476955 ) ) ;
#135711=CARTESIAN_POINT ( 'NONE',  ( 9.474510206698971260, -16.51473224551069308, 22.91557627198102765 ) ) ;
#135712=CARTESIAN_POINT ( 'NONE',  ( -10.81492255796105439, 18.62759615963255655, 87.91775706135234714 ) ) ;
#135713=CARTESIAN_POINT ( 'NONE',  ( 19.02544592524343514, -5.153800228976328945, 43.54057627198103120 ) ) ;
#135714=CARTESIAN_POINT ( 'NONE',  ( -21.55341960407619339, 5.719274019375674811, 48.54275706135234714 ) ) ;
#135715=CARTESIAN_POINT ( 'NONE',  ( -18.67979575497193778, 10.72451020669871902, 88.33442372801901854 ) ) ;
#135716=CARTESIAN_POINT ( 'NONE',  ( 8.314922557961029526, -14.29746914071037800, 100.4177570613523471 ) ) ;
#135717=CARTESIAN_POINT ( 'NONE',  ( -19.03943276465977164, 0.05219959533909376836, 81.24890960531436690 ) ) ;
#135718=CARTESIAN_POINT ( 'NONE',  ( 21.53943276465977519, 0.05219959533937863772, 46.25109039468567573 ) ) ;
#135719=CARTESIAN_POINT ( 'NONE',  ( 10.72451020669871369, 18.67979575497193778, 37.08442372801901143 ) ) ;
#135720=CARTESIAN_POINT ( 'NONE',  ( -19.02544592524334988, -5.153800228976617603, 73.95942372801900433 ) ) ;
#135721=CARTESIAN_POINT ( 'NONE',  ( -5.049401038298153566, 19.05341960407611168, 90.20724293864766707 ) ) ;
#135722=CARTESIAN_POINT ( 'NONE',  ( -8.224510206698948167, 14.34966873604960824, 110.4155762719810383 ) ) ;
#135723=CARTESIAN_POINT ( 'NONE',  ( 18.62759615963271287, -10.81492255796078972, 93.33224293864769550 ) ) ;
#135724=CARTESIAN_POINT ( 'NONE',  ( 12.14591786802309770, 12.06949235617756955, 79.37390960531436690 ) ) ;
#135725=CARTESIAN_POINT ( 'NONE',  ( 5.049401038297881783, 19.05341960407617563, 22.29275706135233648 ) ) ;
#135726=CARTESIAN_POINT ( 'NONE',  ( -14.29746914071049879, 8.314922557960819915, 95.83224293864770971 ) ) ;
#135727=CARTESIAN_POINT ( 'NONE',  ( -9.564922557960796823, -16.46253265017161027, 52.08224293864768839 ) ) ;
#135728=CARTESIAN_POINT ( 'NONE',  ( 19.03943276465977164, 0.05219959533936151252, 86.25109039468567573 ) ) ;
#135729=CARTESIAN_POINT ( 'NONE',  ( -16.52544592524342804, 4.483927247898546575, 46.04057627198103830 ) ) ;
#135730=CARTESIAN_POINT ( 'NONE',  ( 5.719274019375673035, 21.55341960407619339, 112.2927570613523471 ) ) ;
#135731=CARTESIAN_POINT ( 'NONE',  ( 19.02544592524343514, -5.153800228976328945, 108.5405762719810383 ) ) ;
#135732=CARTESIAN_POINT ( 'NONE',  ( -19.02544592524334988, -5.153800228976617603, 73.95942372801900433 ) ) ;
#135733=CARTESIAN_POINT ( 'NONE',  ( -0.05219959533907301413, -21.53943276465977519, 77.49890960531433848 ) ) ;
#135734=CARTESIAN_POINT ( 'NONE',  ( 5.823673210054444382, -21.52544592524334988, 35.20942372801901854 ) ) ;
#135735=CARTESIAN_POINT ( 'NONE',  ( -16.55341960407617563, 4.379528057220093196, 33.54275706135234714 ) ) ;
#135736=CARTESIAN_POINT ( 'NONE',  ( -8.314922557961024197, 14.29746914071037800, 97.91775706135236135 ) ) ;
#135737=CARTESIAN_POINT ( 'NONE',  ( -9.564922557960796823, -16.46253265017161027, 22.08224293864768839 ) ) ;
#135738=CARTESIAN_POINT ( 'NONE',  ( -21.53943276465977519, -0.05219959533937600094, 38.75109039468567573 ) ) ;
#135739=CARTESIAN_POINT ( 'NONE',  ( -19.02544592524342804, 5.153800228976336051, 26.04057627198103120 ) ) ;
#135741=CARTESIAN_POINT ( 'NONE',  ( 0.05219959533934541429, -16.53943276465976808, 50.00109039468568994 ) ) ;
#135742=CARTESIAN_POINT ( 'NONE',  ( 16.55341960407611168, 4.379528057220329451, 83.95724293864770971 ) ) ;
#135743=CARTESIAN_POINT ( 'NONE',  ( 21.55341960407610458, 5.719274019375980345, 78.95724293864769550 ) ) ;
#135744=CARTESIAN_POINT ( 'NONE',  ( -4.483927247898539470, -16.52544592524342804, 22.29057627198102765 ) ) ;
#135745=CARTESIAN_POINT ( 'NONE',  ( -4.483927247898782831, 16.52544592524335698, 52.70942372801902565 ) ) ;
#135746=CARTESIAN_POINT ( 'NONE',  ( 16.51473224551069308, 9.474510206698969483, 44.16557627198103120 ) ) ;
#135747=CARTESIAN_POINT ( 'NONE',  ( -14.34966873604972548, 8.224510206698743886, 93.33442372801901854 ) ) ;
#135748=CARTESIAN_POINT ( 'NONE',  ( 13.89961937509957401, 13.97604488694547697, 86.87609039468567573 ) ) ;
#135749=CARTESIAN_POINT ( 'NONE',  ( -21.55341960407610458, -5.719274019375992779, 81.45724293864769550 ) ) ;
#135750=CARTESIAN_POINT ( 'NONE',  ( -8.314922557961024197, 14.29746914071037800, 112.9177570613523329 ) ) ;
#135752=CARTESIAN_POINT ( 'NONE',  ( 9.474510206698971260, -16.51473224551069308, 112.9155762719810383 ) ) ;
#135753=CARTESIAN_POINT ( 'NONE',  ( -5.823673210054116645, -21.52544592524344225, 67.29057627198103830 ) ) ;
#135755=CARTESIAN_POINT ( 'NONE',  ( 8.314922557961029526, -14.29746914071037800, 95.41775706135234714 ) ) ;
#135756=ORIENTED_EDGE ( 'NONE', *, *, #109880, .T. ) ;
#135757=CARTESIAN_POINT ( 'NONE',  ( 21.53943276465977519, -0.05219959533907433946, 33.74890960531436690 ) ) ;
#135758=CARTESIAN_POINT ( 'NONE',  ( 17.50000000000014566, 3.417042746626903771, 107.3261960376752455 ) ) ;
#135759=CARTESIAN_POINT ( 'NONE',  ( 21.55341960407610458, 5.719274019375980345, 78.95724293864769550 ) ) ;
#135760=CARTESIAN_POINT ( 'NONE',  ( 8.224510206698953496, -14.34966873604960469, 22.91557627198102765 ) ) ;
#135761=CARTESIAN_POINT ( 'NONE',  ( 9.474510206698729675, 16.51473224551082808, 112.0844237280190043 ) ) ;
#135762=CARTESIAN_POINT ( 'NONE',  ( -19.02544592524342804, 5.153800228976336051, 31.04057627198102409 ) ) ;
#135763=CARTESIAN_POINT ( 'NONE',  ( -4.379528057220086978, -16.55341960407618274, 29.79275706135234358 ) ) ;
#135764=CARTESIAN_POINT ( 'NONE',  ( -9.564922557960796823, -16.46253265017161027, 52.08224293864768839 ) ) ;
#135766=CARTESIAN_POINT ( 'NONE',  ( -13.97604488694527625, -13.89961937509977652, 106.8739096053143669 ) ) ;
#135767=CARTESIAN_POINT ( 'NONE',  ( -16.51473224551069308, -9.474510206698971260, 101.6655762719810241 ) ) ;
#135768=CARTESIAN_POINT ( 'NONE',  ( 4.379528057220092307, 16.55341960407617563, 87.29275706135236135 ) ) ;
#135769=CARTESIAN_POINT ( 'NONE',  ( 19.03943276465977164, 0.05219959533936151252, 86.25109039468567573 ) ) ;
#135770=CARTESIAN_POINT ( 'NONE',  ( 19.05341960407617918, -5.049401038297876454, 31.04275706135232227 ) ) ;
#135771=CARTESIAN_POINT ( 'NONE',  ( -18.62759615963270932, 10.81492255796079327, 80.83224293864769550 ) ) ;
#135772=CARTESIAN_POINT ( 'NONE',  ( 14.29746914071037800, 8.314922557961029526, 96.66775706135234714 ) ) ;
#135773=CARTESIAN_POINT ( 'NONE',  ( -10.81492255796078084, -18.62759615963271287, 32.08224293864769550 ) ) ;
#135774=CARTESIAN_POINT ( 'NONE',  ( -19.02544592524334988, -5.153800228976617603, 98.95942372801900433 ) ) ;
#135775=CARTESIAN_POINT ( 'NONE',  ( -5.049401038298153566, 19.05341960407611168, 45.20724293864769550 ) ) ;
#135776=CARTESIAN_POINT ( 'NONE',  ( 13.89961937509977652, -13.97604488694527269, 93.12390960531436690 ) ) ;
#135777=CARTESIAN_POINT ( 'NONE',  ( 21.55341960407619695, -5.719274019375665929, 66.04275706135236135 ) ) ;
#135778=CARTESIAN_POINT ( 'NONE',  ( 9.564922557960805705, 16.46253265017160317, 54.58224293864769550 ) ) ;
#135779=CARTESIAN_POINT ( 'NONE',  ( -16.52544592524342804, 4.483927247898546575, 106.0405762719810525 ) ) ;
#135781=CARTESIAN_POINT ( 'NONE',  ( 4.379528057220339221, -16.55341960407611168, 82.70724293864770971 ) ) ;
#135782=CARTESIAN_POINT ( 'NONE',  ( 0.05219959533907565091, 21.53943276465977519, 79.99890960531435269 ) ) ;
#135783=CARTESIAN_POINT ( 'NONE',  ( 13.97604488694548053, -13.89961937509957401, 90.62609039468567573 ) ) ;
#135784=CARTESIAN_POINT ( 'NONE',  ( 16.36317988757059894, -7.306389748694929409, 81.59789608363225000 ) ) ;
#135785=CARTESIAN_POINT ( 'NONE',  ( 13.97604488694548053, -13.89961937509957401, 40.62609039468564731 ) ) ;
#135786=CARTESIAN_POINT ( 'NONE',  ( 17.48847506799950224, -5.747544572775296068, 73.32697437843290800 ) ) ;
#135787=CARTESIAN_POINT ( 'NONE',  ( -19.05341960407611168, -5.049401038298163336, 76.45724293864769550 ) ) ;
#135788=CARTESIAN_POINT ( 'NONE',  ( -13.89961937509977652, 13.97604488694528158, 85.62390960531433848 ) ) ;
#135789=CARTESIAN_POINT ( 'NONE',  ( -14.34966873604972548, 8.224510206698743886, 68.33442372801900433 ) ) ;
#135791=CARTESIAN_POINT ( 'NONE',  ( 13.89961937509957401, 13.97604488694547697, 46.87609039468565442 ) ) ;
#135793=CARTESIAN_POINT ( 'NONE',  ( 13.97604488694527802, 13.89961937509977652, 109.3739096053143669 ) ) ;
#135794=CARTESIAN_POINT ( 'NONE',  ( -12.06949235617739369, -12.14591786802326823, 99.37609039468568994 ) ) ;
#135796=CARTESIAN_POINT ( 'NONE',  ( 16.55341960407618274, -4.379528057220086978, 76.04275706135237556 ) ) ;
#135798=CARTESIAN_POINT ( 'NONE',  ( -4.379528057220086978, -16.55341960407618274, 59.79275706135234714 ) ) ;
#135799=CARTESIAN_POINT ( 'NONE',  ( -18.22780087662124160, -5.499999999999927169, 78.98236817873106475 ) ) ;
#135800=CARTESIAN_POINT ( 'NONE',  ( -21.53943276465977519, -0.05219959533937600094, 68.75109039468568994 ) ) ;
#135801=CARTESIAN_POINT ( 'NONE',  ( 9.564922557961047289, -16.46253265017146816, 70.41775706135233293 ) ) ;
#135802=CARTESIAN_POINT ( 'NONE',  ( 5.049401038297881783, 19.05341960407617563, 22.29275706135233648 ) ) ;
#135803=CARTESIAN_POINT ( 'NONE',  ( 19.02544592524343514, -5.153800228976328945, 53.54057627198102409 ) ) ;
#135804=CARTESIAN_POINT ( 'NONE',  ( -9.474510206698964154, 16.51473224551069663, 40.41557627198103120 ) ) ;
#135806=CARTESIAN_POINT ( 'NONE',  ( 15.72974639402199770, -15.80617190586745480, 73.12390960531436690 ) ) ;
#135808=CARTESIAN_POINT ( 'NONE',  ( -15.80617190586745835, -15.72974639402198527, 36.87390960531435979 ) ) ;
#135809=CARTESIAN_POINT ( 'NONE',  ( -16.52544592524342804, 4.483927247898546575, 116.0405762719810383 ) ) ;
#135810=CARTESIAN_POINT ( 'NONE',  ( -16.53943276465976808, -0.05219959533934237506, 48.75109039468568284 ) ) ;
#135811=VERTEX_POINT ( 'NONE', #111338 ) ;
#135812=CARTESIAN_POINT ( 'NONE',  ( -5.823673210054431948, 21.52544592524334988, 32.70942372801900433 ) ) ;
#135813=CARTESIAN_POINT ( 'NONE',  ( 12.06949235617757843, -12.14591786802309237, 48.12390960531436690 ) ) ;
#135815=CARTESIAN_POINT ( 'NONE',  ( 8.314922557961029526, -14.29746914071037800, 30.41775706135234358 ) ) ;
#135816=CARTESIAN_POINT ( 'NONE',  ( 9.474510206698729675, 16.51473224551082808, 42.08442372801900433 ) ) ;
#135817=CARTESIAN_POINT ( 'NONE',  ( 16.55341960407611168, 4.379528057220329451, 43.95724293864769550 ) ) ;
#135818=CARTESIAN_POINT ( 'NONE',  ( -21.52544592524334988, -5.823673210054445271, 18.95942372801901143 ) ) ;
#135819=CARTESIAN_POINT ( 'NONE',  ( -9.474510206698964154, 16.51473224551069663, 100.4155762719810241 ) ) ;
#135820=CARTESIAN_POINT ( 'NONE',  ( 21.53943276465977519, -0.05219959533907433946, 73.74890960531433848 ) ) ;
#135821=CARTESIAN_POINT ( 'NONE',  ( 0.05219959533909260263, 19.03943276465977164, 89.99890960531436690 ) ) ;
#135822=CARTESIAN_POINT ( 'NONE',  ( -16.52544592524342804, 4.483927247898546575, 66.04057627198103830 ) ) ;
#135823=CARTESIAN_POINT ( 'NONE',  ( 19.02544592524343514, -5.153800228976328945, 103.5405762719809957 ) ) ;
#135825=CARTESIAN_POINT ( 'NONE',  ( -9.564922557961040184, 16.46253265017147172, 57.91775706135233293 ) ) ;
#135826=CARTESIAN_POINT ( 'NONE',  ( -18.62759615963270932, 10.81492255796079327, 100.8322429386477097 ) ) ;
#135827=CARTESIAN_POINT ( 'NONE',  ( -16.46253265017160317, 9.564922557960807481, 45.83224293864769550 ) ) ;
#135828=CARTESIAN_POINT ( 'NONE',  ( -0.05219959533909027116, -19.03943276465977164, 22.49890960531436690 ) ) ;
#135830=CARTESIAN_POINT ( 'NONE',  ( 15.72974639402176855, 15.80617190586768217, 51.87609039468568284 ) ) ;
#135832=CARTESIAN_POINT ( 'NONE',  ( -8.224510206698948167, 14.34966873604960824, 35.41557627198102409 ) ) ;
#135833=CARTESIAN_POINT ( 'NONE',  ( 9.564922557960805705, 16.46253265017160317, 44.58224293864769550 ) ) ;
#135834=CARTESIAN_POINT ( 'NONE',  ( 9.474510206698971260, -16.51473224551069308, 97.91557627198102409 ) ) ;
#135835=CARTESIAN_POINT ( 'NONE',  ( -15.72974639402197994, 15.80617190586746368, 75.62390960531439532 ) ) ;
#135837=CARTESIAN_POINT ( 'NONE',  ( 19.03943276465977164, -0.05219959533909143690, 48.74890960531435979 ) ) ;
#135838=CARTESIAN_POINT ( 'NONE',  ( 5.719274019375991003, -21.55341960407610458, 72.70724293864769550 ) ) ;
#135839=CARTESIAN_POINT ( 'NONE',  ( 10.81492255796106328, -18.62759615963255655, 90.41775706135236135 ) ) ;
#135841=CARTESIAN_POINT ( 'NONE',  ( 12.14591786802327356, -12.06949235617739191, 80.62609039468567573 ) ) ;
#135842=CARTESIAN_POINT ( 'NONE',  ( -0.05219959533910754901, -16.53943276465976808, 67.49890960531436690 ) ) ;
#135843=CARTESIAN_POINT ( 'NONE',  ( -9.564922557960796823, -16.46253265017161027, 67.08224293864769550 ) ) ;
#135845=CARTESIAN_POINT ( 'NONE',  ( 13.89961937509957401, 13.97604488694547697, 31.87609039468566863 ) ) ;
#135846=CARTESIAN_POINT ( 'NONE',  ( 14.34966873604972726, -8.224510206698740333, 90.83442372801901854 ) ) ;
#135847=CARTESIAN_POINT ( 'NONE',  ( -10.72451020669870658, -18.67979575497194134, 109.5844237280190328 ) ) ;
#135848=CARTESIAN_POINT ( 'NONE',  ( -9.564922557960796823, -16.46253265017161027, 82.08224293864768129 ) ) ;
#135849=CARTESIAN_POINT ( 'NONE',  ( 5.823673210054125526, 21.52544592524343514, 44.79057627198103120 ) ) ;
#135850=CARTESIAN_POINT ( 'NONE',  ( -10.72451020669870658, -18.67979575497194134, 99.58442372801900433 ) ) ;
#135851=CARTESIAN_POINT ( 'NONE',  ( 0.05219959533934541429, -16.53943276465976808, 65.00109039468568994 ) ) ;
#135852=CARTESIAN_POINT ( 'NONE',  ( 18.62759615963271287, -10.81492255796078972, 108.3322429386477097 ) ) ;
#135853=CARTESIAN_POINT ( 'NONE',  ( 13.97604488694548053, -13.89961937509957401, 110.6260903946856615 ) ) ;
#135854=CARTESIAN_POINT ( 'NONE',  ( 19.03943276465977164, -0.05219959533909143690, 88.74890960531436690 ) ) ;
#135855=CARTESIAN_POINT ( 'NONE',  ( 16.52544592524335698, 4.483927247898782831, 31.45942372801901854 ) ) ;
#135856=CARTESIAN_POINT ( 'NONE',  ( -16.46253265017160317, 9.564922557960807481, 50.83224293864770260 ) ) ;
#135857=CARTESIAN_POINT ( 'NONE',  ( 16.55341960407618274, -4.379528057220086978, 36.04275706135234714 ) ) ;
#135858=CARTESIAN_POINT ( 'NONE',  ( -12.14591786802309592, -12.06949235617757132, 81.87390960531435269 ) ) ;
#135859=CARTESIAN_POINT ( 'NONE',  ( -14.29746914071037622, -8.314922557961029526, 89.16775706135236135 ) ) ;
#135860=CARTESIAN_POINT ( 'NONE',  ( -10.72451020669870658, -18.67979575497194134, 39.58442372801901143 ) ) ;
#135861=CARTESIAN_POINT ( 'NONE',  ( 16.51473224551069308, 9.474510206698969483, 59.16557627198102409 ) ) ;
#135862=CARTESIAN_POINT ( 'NONE',  ( 19.05341960407611168, 5.049401038298154454, 78.95724293864769550 ) ) ;
#135863=CARTESIAN_POINT ( 'NONE',  ( -16.55341960407617563, 4.379528057220093196, 88.54275706135236135 ) ) ;
#135866=CARTESIAN_POINT ( 'NONE',  ( 5.049401038297881783, 19.05341960407617563, 37.29275706135232582 ) ) ;
#135867=CARTESIAN_POINT ( 'NONE',  ( -19.05341960407611168, -5.049401038298163336, 101.4572429386476955 ) ) ;
#135868=CARTESIAN_POINT ( 'NONE',  ( -19.03943276465977164, 0.05219959533909376836, 51.24890960531436690 ) ) ;
#135869=CARTESIAN_POINT ( 'NONE',  ( 5.153800228976335163, 19.02544592524342804, 109.7905762719810099 ) ) ;
#135870=CARTESIAN_POINT ( 'NONE',  ( -16.53943276465976808, -0.05219959533934237506, 48.75109039468568284 ) ) ;
#135871=CARTESIAN_POINT ( 'NONE',  ( -9.474510206698720793, -16.51473224551083518, 59.58442372801900433 ) ) ;
#135872=CARTESIAN_POINT ( 'NONE',  ( -12.06949235617739369, -12.14591786802326823, 59.37609039468568284 ) ) ;
#135874=CARTESIAN_POINT ( 'NONE',  ( -16.46253265017160317, 9.564922557960807481, 80.83224293864769550 ) ) ;
#135875=CARTESIAN_POINT ( 'NONE',  ( -5.719274019375665041, -21.55341960407619695, 19.79275706135235069 ) ) ;
#135876=CARTESIAN_POINT ( 'NONE',  ( -19.02544592524334988, -5.153800228976617603, 68.95942372801896170 ) ) ;
#135877=CARTESIAN_POINT ( 'NONE',  ( 13.97604488694527802, 13.89961937509977652, 89.37390960531436690 ) ) ;
#135878=CARTESIAN_POINT ( 'NONE',  ( -13.97604488694527625, -13.89961937509977652, 26.87390960531434558 ) ) ;
#135879=CARTESIAN_POINT ( 'NONE',  ( 9.474510206698971260, -16.51473224551069308, 72.91557627198102409 ) ) ;
#135880=CARTESIAN_POINT ( 'NONE',  ( -14.29746914071049879, 8.314922557960819915, 30.83224293864770260 ) ) ;
#135881=CARTESIAN_POINT ( 'NONE',  ( 19.03943276465977164, -0.05219959533909143690, 28.74890960531435624 ) ) ;
#135882=CARTESIAN_POINT ( 'NONE',  ( 16.51473224551083163, -9.474510206698727899, 40.83442372801900433 ) ) ;
#135883=CARTESIAN_POINT ( 'NONE',  ( 12.14591786802309770, 12.06949235617756955, 69.37390960531436690 ) ) ;
#135884=CARTESIAN_POINT ( 'NONE',  ( -15.72974639402176322, -15.80617190586768395, 99.37609039468568994 ) ) ;
#135885=CARTESIAN_POINT ( 'NONE',  ( 13.97604488694527802, 13.89961937509977652, 39.37390960531435269 ) ) ;
#135886=CARTESIAN_POINT ( 'NONE',  ( 4.483927247898545687, 16.52544592524342804, 44.79057627198103120 ) ) ;
#135887=CARTESIAN_POINT ( 'NONE',  ( -21.55341960407619339, 5.719274019375674811, 98.54275706135234714 ) ) ;
#135888=CARTESIAN_POINT ( 'NONE',  ( -9.564922557960796823, -16.46253265017161027, 97.08224293864769550 ) ) ;
#135889=CARTESIAN_POINT ( 'NONE',  ( -5.049401038298153566, 19.05341960407611168, 90.20724293864766707 ) ) ;
#135890=CARTESIAN_POINT ( 'NONE',  ( 5.153800228976335163, 19.02544592524342804, 39.79057627198100988 ) ) ;
#135891=CARTESIAN_POINT ( 'NONE',  ( -16.52544592524342804, 4.483927247898546575, 106.0405762719810525 ) ) ;
#135892=CARTESIAN_POINT ( 'NONE',  ( -8.314922557960811034, -14.29746914071050412, 72.08224293864769550 ) ) ;
#135893=CARTESIAN_POINT ( 'NONE',  ( 21.55341960407610458, 5.719274019375980345, 83.95724293864770971 ) ) ;
#135894=CARTESIAN_POINT ( 'NONE',  ( 13.97604488694527802, 13.89961937509977652, 84.37390960531433848 ) ) ;
#135895=CARTESIAN_POINT ( 'NONE',  ( 18.62759615963271287, -10.81492255796078972, 93.33224293864769550 ) ) ;
#135896=CARTESIAN_POINT ( 'NONE',  ( 13.97604488694527802, 13.89961937509977652, 89.37390960531436690 ) ) ;
#135897=CARTESIAN_POINT ( 'NONE',  ( 17.50000000001358202, -5.500000000000038192, 88.29690382535061133 ) ) ;
#135898=CARTESIAN_POINT ( 'NONE',  ( 4.483927247898545687, 16.52544592524342804, 89.79057627198103830 ) ) ;
#135899=CARTESIAN_POINT ( 'NONE',  ( 9.564922557960805705, 16.46253265017160317, 69.58224293864770971 ) ) ;
#135900=CARTESIAN_POINT ( 'NONE',  ( 18.67979575497178502, 10.72451020669898547, 79.16557627198103830 ) ) ;
#135901=EDGE_CURVE ( 'NONE', #167324, #197337, #26645, .T. ) ;
#135903=CARTESIAN_POINT ( 'NONE',  ( 21.53943276465977519, -0.05219959533907433946, 33.74890960531436690 ) ) ;
#135904=CARTESIAN_POINT ( 'NONE',  ( 19.35633801406907750, -5.499999999999773515, 66.63373818172765084 ) ) ;
#135905=CARTESIAN_POINT ( 'NONE',  ( -13.97604488694547697, 13.89961937509957934, 113.1260903946856757 ) ) ;
#135906=CARTESIAN_POINT ( 'NONE',  ( 16.55341960407611168, 4.379528057220329451, 93.95724293864770971 ) ) ;
#135907=CARTESIAN_POINT ( 'NONE',  ( -17.05116617787827238, -6.768360034955764881, 96.34324446740805570 ) ) ;
#135908=CARTESIAN_POINT ( 'NONE',  ( 16.51473224551069308, 9.474510206698969483, 89.16557627198103830 ) ) ;
#135909=CARTESIAN_POINT ( 'NONE',  ( -5.153800228976328057, -19.02544592524343514, 52.29057627198100988 ) ) ;
#135910=CARTESIAN_POINT ( 'NONE',  ( -12.14591786802309592, -12.06949235617757132, 81.87390960531435269 ) ) ;
#135911=CARTESIAN_POINT ( 'NONE',  ( -19.02544592524342804, 5.153800228976336051, 111.0405762719810099 ) ) ;
#135912=CARTESIAN_POINT ( 'NONE',  ( -8.224510206698948167, 14.34966873604960824, 55.41557627198102409 ) ) ;
#135913=CARTESIAN_POINT ( 'NONE',  ( -13.97604488694547697, 13.89961937509957934, 108.1260903946856331 ) ) ;
#135914=CARTESIAN_POINT ( 'NONE',  ( 0.05219959533937995610, -21.53943276465977519, 55.00109039468568284 ) ) ;
#135916=CARTESIAN_POINT ( 'NONE',  ( 19.03943276465977164, -0.05219959533909143690, 93.74890960531435269 ) ) ;
#135917=CARTESIAN_POINT ( 'NONE',  ( -0.05219959533907301413, -21.53943276465977519, 92.49890960531436690 ) ) ;
#135918=CARTESIAN_POINT ( 'NONE',  ( -16.52544592524335698, -4.483927247898792601, 83.95942372801900433 ) ) ;
#135919=CARTESIAN_POINT ( 'NONE',  ( 9.564922557960805705, 16.46253265017160317, 24.58224293864769194 ) ) ;
#135920=CARTESIAN_POINT ( 'NONE',  ( -13.89961937509977652, 13.97604488694528158, 80.62390960531436690 ) ) ;
#135921=CARTESIAN_POINT ( 'NONE',  ( 5.823673210054125526, 21.52544592524343514, 84.79057627198102409 ) ) ;
#135923=CARTESIAN_POINT ( 'NONE',  ( -19.02544592524334988, -5.153800228976617603, 103.9594237280190043 ) ) ;
#135924=CARTESIAN_POINT ( 'NONE',  ( -4.483927247898539470, -16.52544592524342804, 47.29057627198103120 ) ) ;
#135925=CARTESIAN_POINT ( 'NONE',  ( 10.81492255796106328, -18.62759615963255655, 65.41775706135234714 ) ) ;
#135926=CARTESIAN_POINT ( 'NONE',  ( 4.379528057220092307, 16.55341960407617563, 92.29275706135236135 ) ) ;
#135927=CARTESIAN_POINT ( 'NONE',  ( 19.05341960407611168, 5.049401038298154454, 113.9572429386477097 ) ) ;
#135928=CARTESIAN_POINT ( 'NONE',  ( 16.51473224551069308, 9.474510206698969483, 109.1655762719810383 ) ) ;
#135929=CARTESIAN_POINT ( 'NONE',  ( -16.29526858892876717, 7.335722546920118603, 79.20329402199793378 ) ) ;
#135930=CARTESIAN_POINT ( 'NONE',  ( -4.483927247898782831, 16.52544592524335698, 102.7094237280190185 ) ) ;
#135931=CARTESIAN_POINT ( 'NONE',  ( -14.34966873604972548, 8.224510206698743886, 53.33442372801901854 ) ) ;
#135932=CARTESIAN_POINT ( 'NONE',  ( -19.03943276465977164, 0.05219959533909376836, 61.24890960531436690 ) ) ;
#135933=CARTESIAN_POINT ( 'NONE',  ( 19.02544592524343514, -5.153800228976328945, 73.54057627198103830 ) ) ;
#135934=CARTESIAN_POINT ( 'NONE',  ( 0.05219959533934541429, -16.53943276465976808, 80.00109039468568994 ) ) ;
#135935=CARTESIAN_POINT ( 'NONE',  ( 16.52544592524342804, -4.483927247898539470, 43.54057627198103830 ) ) ;
#135936=CARTESIAN_POINT ( 'NONE',  ( 13.97604488694527802, 13.89961937509977652, 54.37390960531435979 ) ) ;
#135937=CARTESIAN_POINT ( 'NONE',  ( -9.564922557960796823, -16.46253265017161027, 47.08224293864769550 ) ) ;
#135938=CARTESIAN_POINT ( 'NONE',  ( -8.314922557961024197, 14.29746914071037800, 47.91775706135234714 ) ) ;
#135940=CARTESIAN_POINT ( 'NONE',  ( 19.02544592524334988, 5.153800228976608722, 91.45942372801900433 ) ) ;
#135941=CARTESIAN_POINT ( 'NONE',  ( 14.29746914071049879, -8.314922557960816363, 93.33224293864769550 ) ) ;
#135942=CARTESIAN_POINT ( 'NONE',  ( 9.474510206698971260, -16.51473224551069308, 67.91557627198102409 ) ) ;
#135943=CARTESIAN_POINT ( 'NONE',  ( -9.474510206698720793, -16.51473224551083518, 104.5844237280190043 ) ) ;
#135945=CARTESIAN_POINT ( 'NONE',  ( -21.55341960407619339, 5.719274019375674811, 108.5427570613523756 ) ) ;
#135946=CARTESIAN_POINT ( 'NONE',  ( 16.55341960407618274, -4.379528057220086978, 71.04275706135234714 ) ) ;
#135947=CARTESIAN_POINT ( 'NONE',  ( 30.00000000000000000, -5.499999999999992895, 102.5000000000000142 ) ) ;
#135948=CARTESIAN_POINT ( 'NONE',  ( 0.05219959533907565091, 21.53943276465977519, 59.99890960531436690 ) ) ;
#135949=CARTESIAN_POINT ( 'NONE',  ( -16.55341960407617563, 4.379528057220093196, 58.54275706135235424 ) ) ;
#135950=CARTESIAN_POINT ( 'NONE',  ( -19.05341960407611168, -5.049401038298164224, 31.45724293864769905 ) ) ;
#135951=CARTESIAN_POINT ( 'NONE',  ( -5.153800228976607833, 19.02544592524334988, 37.70942372801899722 ) ) ;
#135952=CARTESIAN_POINT ( 'NONE',  ( -0.05219959533909027116, -19.03943276465977164, 92.49890960531436690 ) ) ;
#135953=CARTESIAN_POINT ( 'NONE',  ( 16.52544592524342804, -4.483927247898539470, 113.5405762719810383 ) ) ;
#135954=CARTESIAN_POINT ( 'NONE',  ( -16.51473224551069308, -9.474510206698971260, 61.66557627198103120 ) ) ;
#135955=CARTESIAN_POINT ( 'NONE',  ( -10.81492255796105439, 18.62759615963255655, 82.91775706135234714 ) ) ;
#135956=CARTESIAN_POINT ( 'NONE',  ( -16.51473224551082808, 9.474510206698731452, 38.33442372801899722 ) ) ;
#135957=CARTESIAN_POINT ( 'NONE',  ( -0.05219959533936034679, 19.03943276465977164, 32.50109039468566863 ) ) ;
#135958=CARTESIAN_POINT ( 'NONE',  ( -16.46253265017160317, 9.564922557960807481, 55.83224293864769550 ) ) ;
#135959=CARTESIAN_POINT ( 'NONE',  ( 5.823673210054125526, 21.52544592524343514, 29.79057627198102409 ) ) ;
#135960=CARTESIAN_POINT ( 'NONE',  ( 10.72451020669871369, 18.67979575497193778, 82.08442372801901854 ) ) ;
#135961=CARTESIAN_POINT ( 'NONE',  ( -13.89961937509977652, 13.97604488694528158, 60.62390960531436690 ) ) ;
#135962=CARTESIAN_POINT ( 'NONE',  ( -5.823673210054431948, 21.52544592524334988, 92.70942372801901854 ) ) ;
#135963=CARTESIAN_POINT ( 'NONE',  ( -15.80617190586745835, -15.72974639402198527, 41.87390960531435979 ) ) ;
#135964=CARTESIAN_POINT ( 'NONE',  ( -13.97604488694527625, -13.89961937509977652, 81.87390960531436690 ) ) ;
#135965=CARTESIAN_POINT ( 'NONE',  ( 0.05219959533937995610, -21.53943276465977519, 40.00109039468567573 ) ) ;
#135966=CARTESIAN_POINT ( 'NONE',  ( 16.51473224551083163, -9.474510206698727899, 55.83442372801899722 ) ) ;
#135967=CARTESIAN_POINT ( 'NONE',  ( -16.46253265017160317, 9.564922557960807481, 35.83224293864768839 ) ) ;
#135968=CARTESIAN_POINT ( 'NONE',  ( -16.46253265017160317, 9.564922557960807481, 85.83224293864769550 ) ) ;
#135969=CARTESIAN_POINT ( 'NONE',  ( -12.14591786802326823, 12.06949235617739902, 23.12609039468567573 ) ) ;
#135970=CARTESIAN_POINT ( 'NONE',  ( 14.34966873604960469, 8.224510206698951720, 94.16557627198103830 ) ) ;
#135971=CARTESIAN_POINT ( 'NONE',  ( -19.02544592524342804, 5.153800228976336051, 71.04057627198099567 ) ) ;
#135972=CARTESIAN_POINT ( 'NONE',  ( -5.823673210054116645, -21.52544592524344225, 47.29057627198103120 ) ) ;
#135973=CARTESIAN_POINT ( 'NONE',  ( 14.34966873604972726, -8.224510206698740333, 25.83442372801901499 ) ) ;
#135974=CARTESIAN_POINT ( 'NONE',  ( 5.719274019375991003, -21.55341960407610458, 112.7072429386476955 ) ) ;
#135975=CARTESIAN_POINT ( 'NONE',  ( 21.55341960407619695, -5.719274019375665929, 76.04275706135237556 ) ) ;
#135976=CARTESIAN_POINT ( 'NONE',  ( -8.314922557961024197, 14.29746914071037800, 72.91775706135234714 ) ) ;
#135977=CARTESIAN_POINT ( 'NONE',  ( 4.379528057220092307, 16.55341960407617563, 62.29275706135236845 ) ) ;
#135978=CARTESIAN_POINT ( 'NONE',  ( -19.05341960407611168, -5.049401038298163336, 66.45724293864769550 ) ) ;
#135979=CARTESIAN_POINT ( 'NONE',  ( -12.06949235617739369, -12.14591786802326823, 99.37609039468568994 ) ) ;
#135980=CARTESIAN_POINT ( 'NONE',  ( 5.049401038297881783, 19.05341960407617563, 47.29275706135231161 ) ) ;
#135981=CARTESIAN_POINT ( 'NONE',  ( 15.72974639402199770, -15.80617190586745480, 113.1239096053143953 ) ) ;
#135982=CARTESIAN_POINT ( 'NONE',  ( -4.379528057220328563, 16.55341960407611168, 60.20724293864768839 ) ) ;
#135983=CARTESIAN_POINT ( 'NONE',  ( 5.049401038298161559, -19.05341960407611168, 92.70724293864769550 ) ) ;
#135984=CARTESIAN_POINT ( 'NONE',  ( -12.06949235617739369, -12.14591786802326823, 94.37609039468568994 ) ) ;
#135985=CARTESIAN_POINT ( 'NONE',  ( 21.52544592524334988, 5.823673210054432836, 56.45942372801902565 ) ) ;
#135986=CARTESIAN_POINT ( 'NONE',  ( -4.379528057220086978, -16.55341960407618274, 29.79275706135234358 ) ) ;
#135987=CARTESIAN_POINT ( 'NONE',  ( -21.55341960407619339, 5.719274019375674811, 33.54275706135234714 ) ) ;
#135988=CARTESIAN_POINT ( 'NONE',  ( -8.314922557960811034, -14.29746914071050412, 62.08224293864769550 ) ) ;
#135989=VERTEX_POINT ( 'NONE', #50675 ) ;
#135990=CARTESIAN_POINT ( 'NONE',  ( -21.52544592524343514, 5.823673210054127303, 101.0405762719810383 ) ) ;
#135991=CARTESIAN_POINT ( 'NONE',  ( -12.14591786802309592, -12.06949235617757132, 36.87390960531435979 ) ) ;
#135994=CARTESIAN_POINT ( 'NONE',  ( 0.05219959533907565091, 21.53943276465977519, 34.99890960531435979 ) ) ;
#135995=CARTESIAN_POINT ( 'NONE',  ( -10.81492255796105439, 18.62759615963255655, 37.91775706135235424 ) ) ;
#135996=CARTESIAN_POINT ( 'NONE',  ( -16.52544592524342804, 4.483927247898546575, 61.04057627198103120 ) ) ;
#135997=CARTESIAN_POINT ( 'NONE',  ( -5.823673210054116645, -21.52544592524344225, 67.29057627198103830 ) ) ;
#135998=CARTESIAN_POINT ( 'NONE',  ( -9.474510206698964154, 16.51473224551069663, 70.41557627198102409 ) ) ;
#135999=CARTESIAN_POINT ( 'NONE',  ( -5.049401038298153566, 19.05341960407611168, 30.20724293864768839 ) ) ;
#136000=CARTESIAN_POINT ( 'NONE',  ( -16.46253265017146816, -9.564922557961047289, 69.16775706135233293 ) ) ;
#136001=CARTESIAN_POINT ( 'NONE',  ( -18.67979575497178146, -10.72451020669898902, 46.66557627198102409 ) ) ;
#136002=CARTESIAN_POINT ( 'NONE',  ( 5.153800228976335163, 19.02544592524342804, 59.79057627198100988 ) ) ;
#136003=CARTESIAN_POINT ( 'NONE',  ( 12.06949235617739724, 12.14591786802326823, 41.87609039468568284 ) ) ;
#136004=CARTESIAN_POINT ( 'NONE',  ( 18.67979575497194134, -10.72451020669871369, 20.83442372801901143 ) ) ;
#136005=CARTESIAN_POINT ( 'NONE',  ( 16.55341960407611168, 4.379528057220329451, 53.95724293864770260 ) ) ;
#136006=CARTESIAN_POINT ( 'NONE',  ( -16.46253265017160317, 9.564922557960807481, 85.83224293864769550 ) ) ;
#136007=CARTESIAN_POINT ( 'NONE',  ( -10.81492255796078084, -18.62759615963271287, 77.08224293864769550 ) ) ;
#136008=CARTESIAN_POINT ( 'NONE',  ( -18.62759615963270932, 10.81492255796079327, 110.8322429386476955 ) ) ;
#136009=CARTESIAN_POINT ( 'NONE',  ( -12.14591786802326823, 12.06949235617739902, 38.12609039468567573 ) ) ;
#136010=CARTESIAN_POINT ( 'NONE',  ( -10.81492255796078084, -18.62759615963271287, 37.08224293864768129 ) ) ;
#136011=CARTESIAN_POINT ( 'NONE',  ( -18.67979575497193778, 10.72451020669871902, 98.33442372801901854 ) ) ;
#136012=CARTESIAN_POINT ( 'NONE',  ( 13.89961937509977652, -13.97604488694527269, 48.12390960531435979 ) ) ;
#136013=CARTESIAN_POINT ( 'NONE',  ( -9.564922557960796823, -16.46253265017161027, 102.0822429386477097 ) ) ;
#136014=CARTESIAN_POINT ( 'NONE',  ( -19.02544592524342804, 5.153800228976336051, 76.04057627198102409 ) ) ;
#136016=CARTESIAN_POINT ( 'NONE',  ( 19.02544592524334988, 5.153800228976608722, 51.45942372801900433 ) ) ;
#136017=CARTESIAN_POINT ( 'NONE',  ( 21.53943276465977519, 0.05219959533937863772, 106.2510903946856757 ) ) ;
#136018=CARTESIAN_POINT ( 'NONE',  ( 10.81492255796078972, 18.62759615963270932, 29.58224293864769905 ) ) ;
#136019=CARTESIAN_POINT ( 'NONE',  ( 8.224510206698742110, 14.34966873604972548, 102.0844237280190185 ) ) ;
#136020=CARTESIAN_POINT ( 'NONE',  ( -5.049401038297874678, -19.05341960407617918, 89.79275706135230450 ) ) ;
#136021=CARTESIAN_POINT ( 'NONE',  ( -16.81555441253552274, 7.025013491695479395, 60.63685445334257906 ) ) ;
#136022=CARTESIAN_POINT ( 'NONE',  ( 5.153800228976615827, -19.02544592524334988, 90.20942372801900433 ) ) ;
#136023=CARTESIAN_POINT ( 'NONE',  ( 0.05219959533936267826, -19.03943276465977164, 50.00109039468566863 ) ) ;
#136024=CARTESIAN_POINT ( 'NONE',  ( -16.21995358207306026, -7.366697692864121016, 45.06448998487843483 ) ) ;
#136025=CARTESIAN_POINT ( 'NONE',  ( 19.03943276465977164, -0.05219959533909143690, 38.74890960531436690 ) ) ;
#136026=CARTESIAN_POINT ( 'NONE',  ( 0.05219959533910956823, 16.53943276465976808, 54.99890960531435269 ) ) ;
#136027=CARTESIAN_POINT ( 'NONE',  ( 5.153800228976335163, 19.02544592524342804, 24.79057627198102765 ) ) ;
#136028=CARTESIAN_POINT ( 'NONE',  ( 14.29746914071049879, -8.314922557960816363, 23.33224293864769194 ) ) ;
#136029=DIRECTION ( 'NONE',  ( -1.000000000000000000, -0.000000000000000000, -0.000000000000000000 ) ) ;
#136030=CARTESIAN_POINT ( 'NONE',  ( 8.314922557961029526, -14.29746914071037800, 90.41775706135236135 ) ) ;
#136031=CARTESIAN_POINT ( 'NONE',  ( -13.89961937509977652, 13.97604488694528158, 50.62390960531435979 ) ) ;
#136032=CARTESIAN_POINT ( 'NONE',  ( -10.81492255796105439, 18.62759615963255655, 102.9177570613523756 ) ) ;
#136033=CARTESIAN_POINT ( 'NONE',  ( 14.29746914071037800, 8.314922557961029526, 21.66775706135235069 ) ) ;
#136034=CARTESIAN_POINT ( 'NONE',  ( 15.80617190586746368, 15.72974639402197994, 34.37390960531435979 ) ) ;
#136035=CARTESIAN_POINT ( 'NONE',  ( -21.53943276465977519, -0.05219959533937600094, 93.75109039468567573 ) ) ;
#136036=CARTESIAN_POINT ( 'NONE',  ( 16.46253265017160672, -9.564922557960803928, 103.3322429386476955 ) ) ;
#136037=CARTESIAN_POINT ( 'NONE',  ( 19.05341960407611168, 5.049401038298154454, 88.95724293864769550 ) ) ;
#136039=CARTESIAN_POINT ( 'NONE',  ( 21.53943276465977519, -0.05219959533907433946, 103.7489096053143669 ) ) ;
#136040=CARTESIAN_POINT ( 'NONE',  ( 16.53943276465976808, -0.05219959533910856209, 78.74890960531436690 ) ) ;
#136041=CARTESIAN_POINT ( 'NONE',  ( 5.823673210054125526, 21.52544592524343514, 79.79057627198102409 ) ) ;
#136042=CARTESIAN_POINT ( 'NONE',  ( -19.05341960407611168, -5.049401038298163336, 66.45724293864769550 ) ) ;
#136043=CARTESIAN_POINT ( 'NONE',  ( 21.52544592524344225, -5.823673210054117533, 103.5405762719810383 ) ) ;
#136045=CARTESIAN_POINT ( 'NONE',  ( 19.03943276465977164, -0.05219959533909143690, 63.74890960531435979 ) ) ;
#136046=CARTESIAN_POINT ( 'NONE',  ( 16.55341960407611168, 4.379528057220329451, 88.95724293864769550 ) ) ;
#136048=CARTESIAN_POINT ( 'NONE',  ( 16.51473224551069308, 9.474510206698969483, 64.16557627198102409 ) ) ;
#136049=CARTESIAN_POINT ( 'NONE',  ( 19.03943276465977164, 0.05219959533936151252, 81.25109039468567573 ) ) ;
#136050=CARTESIAN_POINT ( 'NONE',  ( -8.224510206698948167, 14.34966873604960824, 90.41557627198103830 ) ) ;
#136051=CARTESIAN_POINT ( 'NONE',  ( -18.67979575497193778, 10.72451020669871902, 58.33442372801901143 ) ) ;
#136052=CARTESIAN_POINT ( 'NONE',  ( -19.05341960407611168, -5.049401038298163336, 51.45724293864770260 ) ) ;
#136053=CARTESIAN_POINT ( 'NONE',  ( 5.823673210054444382, -21.52544592524334988, 25.20942372801901854 ) ) ;
#136054=CARTESIAN_POINT ( 'NONE',  ( 14.34966873604960469, 8.224510206698951720, 99.16557627198100988 ) ) ;
#136055=CARTESIAN_POINT ( 'NONE',  ( 0.000000000000000000, -5.500000000000000888, 118.0000000000000142 ) ) ;
#136056=CARTESIAN_POINT ( 'NONE',  ( -16.51473224551069308, -9.474510206698971260, 61.66557627198103120 ) ) ;
#136058=CARTESIAN_POINT ( 'NONE',  ( 13.97604488694548053, -13.89961937509957401, 110.6260903946856615 ) ) ;
#136059=CARTESIAN_POINT ( 'NONE',  ( 19.05341960407611168, 5.049401038298154454, 113.9572429386477097 ) ) ;
#136060=CARTESIAN_POINT ( 'NONE',  ( -21.55341960407619339, 5.719274019375674811, 53.54275706135234714 ) ) ;
#136061=CARTESIAN_POINT ( 'NONE',  ( -5.153800228976328057, -19.02544592524343514, 92.29057627198099567 ) ) ;
#136062=CARTESIAN_POINT ( 'NONE',  ( 5.049401038297881783, 19.05341960407617563, 82.29275706135229029 ) ) ;
#136063=CARTESIAN_POINT ( 'NONE',  ( 9.474510206698971260, -16.51473224551069308, 62.91557627198102409 ) ) ;
#136064=EDGE_CURVE ( 'NONE', #129907, #115190, #6143, .T. ) ;
#136065=CARTESIAN_POINT ( 'NONE',  ( -16.55341960407611168, -4.379528057220339221, 76.45724293864769550 ) ) ;
#136066=CARTESIAN_POINT ( 'NONE',  ( -16.53943276465976808, 0.05219959533911058130, 86.24890960531436690 ) ) ;
#136067=CARTESIAN_POINT ( 'NONE',  ( -13.97604488694527625, -13.89961937509977652, 86.87390960531436690 ) ) ;
#136068=CARTESIAN_POINT ( 'NONE',  ( 4.379528057220339221, -16.55341960407611168, 82.70724293864770971 ) ) ;
#136069=CARTESIAN_POINT ( 'NONE',  ( 5.049401038298161559, -19.05341960407611168, 82.70724293864770971 ) ) ;
#136070=CARTESIAN_POINT ( 'NONE',  ( 13.97604488694548053, -13.89961937509957401, 25.62609039468566507 ) ) ;
#136071=CARTESIAN_POINT ( 'NONE',  ( -0.05219959533909027116, -19.03943276465977164, 52.49890960531436690 ) ) ;
#136072=CARTESIAN_POINT ( 'NONE',  ( 12.14591786802309770, 12.06949235617756955, 24.37390960531435979 ) ) ;
#136073=CARTESIAN_POINT ( 'NONE',  ( -16.51473224551069308, -9.474510206698971260, 31.66557627198102054 ) ) ;
#136075=CARTESIAN_POINT ( 'NONE',  ( 21.53943276465977519, 0.05219959533937863772, 46.25109039468567573 ) ) ;
#136076=CARTESIAN_POINT ( 'NONE',  ( 5.153800228976615827, -19.02544592524334988, 60.20942372801899012 ) ) ;
#136077=CARTESIAN_POINT ( 'NONE',  ( 16.53943276465976808, -0.05219959533910856209, 38.74890960531435979 ) ) ;
#136078=CARTESIAN_POINT ( 'NONE',  ( -15.72974639402197994, 15.80617190586746368, 90.62390960531436690 ) ) ;
#136079=CARTESIAN_POINT ( 'NONE',  ( -18.62759615963270932, 10.81492255796079327, 30.83224293864770260 ) ) ;
#136080=CARTESIAN_POINT ( 'NONE',  ( -14.29746914071049879, 8.314922557960819915, 70.83224293864770971 ) ) ;
#136081=CARTESIAN_POINT ( 'NONE',  ( -9.474510206698964154, 16.51473224551069663, 40.41557627198103120 ) ) ;
#136082=CARTESIAN_POINT ( 'NONE',  ( 16.53943276465976808, 0.05219959533934440121, 96.25109039468568994 ) ) ;
#136083=CARTESIAN_POINT ( 'NONE',  ( -12.14591786802326823, 12.06949235617739902, 73.12609039468567573 ) ) ;
#136084=CARTESIAN_POINT ( 'NONE',  ( -15.80617190586745835, -15.72974639402198527, 31.87390960531435979 ) ) ;
#136085=CARTESIAN_POINT ( 'NONE',  ( -0.05219959533936034679, 19.03943276465977164, 32.50109039468566863 ) ) ;
#136086=CARTESIAN_POINT ( 'NONE',  ( -19.03943276465977164, 0.05219959533909376836, 91.24890960531436690 ) ) ;
#136087=CARTESIAN_POINT ( 'NONE',  ( -12.06949235617739369, -12.14591786802326823, 74.37609039468568994 ) ) ;
#136088=CARTESIAN_POINT ( 'NONE',  ( -14.29746914071049879, 8.314922557960819915, 115.8322429386477097 ) ) ;
#136089=CARTESIAN_POINT ( 'NONE',  ( 16.55341960407611168, 4.379528057220329451, 33.95724293864769550 ) ) ;
#136090=CARTESIAN_POINT ( 'NONE',  ( -9.474510206698964154, 16.51473224551069663, 100.4155762719810241 ) ) ;
#136091=CARTESIAN_POINT ( 'NONE',  ( -16.51473224551069308, -9.474510206698971260, 86.66557627198102409 ) ) ;
#136092=CARTESIAN_POINT ( 'NONE',  ( -15.80617190586745835, -15.72974639402198527, 26.87390960531435979 ) ) ;
#136093=CARTESIAN_POINT ( 'NONE',  ( -4.379528057220328563, 16.55341960407611168, 70.20724293864769550 ) ) ;
#136094=EDGE_LOOP ( 'NONE', ( #109478, #49470, #157584, #175686, #35349, #184558, #114952, #23873, #3836, #65623, #93046, #19137, #160113, #130210, #136780, #23823, #94303, #188215, #12940, #28354, #168177, #186232, #165856, #181507, #68982, #185332, #103476, #25898, #60413, #157197, #25599, #71922, #41540, #108371, #181180, #804, #132287, #143522, #134112, #197042, #14921, #126620, #119677, #193519, #199020, #151527, #132175, #113184, #147059, #185460, #147486, #176387, #175513, #194967, #166096, #5581 ) ) ;
#136095=CARTESIAN_POINT ( 'NONE',  ( 16.53943276465976808, -0.05219959533910856209, 53.74890960531437401 ) ) ;
#136096=CARTESIAN_POINT ( 'NONE',  ( -8.314922557961024197, 14.29746914071037800, 52.91775706135235424 ) ) ;
#136098=CARTESIAN_POINT ( 'NONE',  ( 5.153800228976615827, -19.02544592524334988, 50.20942372801897591 ) ) ;
#136099=CARTESIAN_POINT ( 'NONE',  ( -19.02544592524342804, 5.153800228976336051, 86.04057627198103830 ) ) ;
#136100=CARTESIAN_POINT ( 'NONE',  ( -16.51473224551082808, 9.474510206698731452, 68.33442372801900433 ) ) ;
#136102=CARTESIAN_POINT ( 'NONE',  ( 5.153800228976615827, -19.02544592524334988, 60.20942372801899012 ) ) ;
#136103=CARTESIAN_POINT ( 'NONE',  ( 5.049401038297881783, 19.05341960407617563, 112.2927570613523471 ) ) ;
#136104=CARTESIAN_POINT ( 'NONE',  ( -4.379528057220086978, -16.55341960407618274, 89.79275706135236135 ) ) ;
#136106=CARTESIAN_POINT ( 'NONE',  ( -9.564922557960796823, -16.46253265017161027, 37.08224293864768839 ) ) ;
#136107=CARTESIAN_POINT ( 'NONE',  ( -15.80617190586745835, -15.72974639402198527, 21.87390960531436690 ) ) ;
#136108=CARTESIAN_POINT ( 'NONE',  ( -21.53943276465977519, -0.05219959533937600094, 58.75109039468568994 ) ) ;
#136109=CARTESIAN_POINT ( 'NONE',  ( -5.153800228976607833, 19.02544592524334988, 97.70942372801900433 ) ) ;
#136111=CARTESIAN_POINT ( 'NONE',  ( 19.02544592524343514, -5.153800228976328945, 63.54057627198103830 ) ) ;
#136112=CARTESIAN_POINT ( 'NONE',  ( 5.153800228976335163, 19.02544592524342804, 114.7905762719810241 ) ) ;
#136113=CARTESIAN_POINT ( 'NONE',  ( -16.52544592524342804, 4.483927247898546575, 76.04057627198102409 ) ) ;
#136114=CARTESIAN_POINT ( 'NONE',  ( 9.564922557960805705, 16.46253265017160317, 69.58224293864770971 ) ) ;
#136115=CARTESIAN_POINT ( 'NONE',  ( -19.03943276465977164, 0.05219959533909376836, 71.24890960531435269 ) ) ;
#136116=CARTESIAN_POINT ( 'NONE',  ( -13.97604488694547697, 13.89961937509957934, 78.12609039468567573 ) ) ;
#136117=CARTESIAN_POINT ( 'NONE',  ( -10.72451020669898014, 18.67979575497178502, 70.41557627198102409 ) ) ;
#136118=CARTESIAN_POINT ( 'NONE',  ( 8.314922557960818139, 14.29746914071049879, 109.5822429386476955 ) ) ;
#136119=CARTESIAN_POINT ( 'NONE',  ( 13.97604488694548053, -13.89961937509957401, 60.62609039468564731 ) ) ;
#136120=CARTESIAN_POINT ( 'NONE',  ( -19.02544592524342804, 5.153800228976336051, 51.04057627198103120 ) ) ;
#136121=CARTESIAN_POINT ( 'NONE',  ( -13.97604488694527625, -13.89961937509977652, 81.87390960531436690 ) ) ;
#136122=CARTESIAN_POINT ( 'NONE',  ( -10.81492255796078084, -18.62759615963271287, 92.08224293864769550 ) ) ;
#136123=CARTESIAN_POINT ( 'NONE',  ( 14.29746914071049879, -8.314922557960816363, 83.33224293864769550 ) ) ;
#136124=CARTESIAN_POINT ( 'NONE',  ( 13.89961937509957401, 13.97604488694547697, 46.87609039468565442 ) ) ;
#136125=CARTESIAN_POINT ( 'NONE',  ( -5.823673210054116645, -21.52544592524344225, 82.29057627198103830 ) ) ;
#136126=CARTESIAN_POINT ( 'NONE',  ( -10.72451020669898014, 18.67979575497178502, 55.41557627198102409 ) ) ;
#136127=CARTESIAN_POINT ( 'NONE',  ( -12.14591786802309592, -12.06949235617757132, 36.87390960531435979 ) ) ;
#136128=CARTESIAN_POINT ( 'NONE',  ( 5.823673210054444382, -21.52544592524334988, 90.20942372801903275 ) ) ;
#136129=CARTESIAN_POINT ( 'NONE',  ( 9.564922557960805705, 16.46253265017160317, 84.58224293864769550 ) ) ;
#136130=CARTESIAN_POINT ( 'NONE',  ( 12.06949235617757843, -12.14591786802309237, 113.1239096053143953 ) ) ;
#136131=CARTESIAN_POINT ( 'NONE',  ( 15.72974639402176855, 15.80617190586768217, 26.87609039468567218 ) ) ;
#136132=CARTESIAN_POINT ( 'NONE',  ( 21.55341960407619695, -5.719274019375665929, 41.04275706135236135 ) ) ;
#136133=CARTESIAN_POINT ( 'NONE',  ( -16.46253265017160317, 9.564922557960807481, 45.83224293864769550 ) ) ;
#136134=CARTESIAN_POINT ( 'NONE',  ( 21.55341960407619695, -5.719274019375665929, 26.04275706135235779 ) ) ;
#136135=EDGE_CURVE ( 'NONE', #99274, #91848, #130453, .T. ) ;
#136136=CARTESIAN_POINT ( 'NONE',  ( 16.51473224551083163, -9.474510206698727899, 60.83442372801900433 ) ) ;
#136137=CARTESIAN_POINT ( 'NONE',  ( -13.97604488694527625, -13.89961937509977652, 41.87390960531435979 ) ) ;
#136138=CARTESIAN_POINT ( 'NONE',  ( 4.379528057220092307, 16.55341960407617563, 32.29275706135235424 ) ) ;
#136139=CARTESIAN_POINT ( 'NONE',  ( -13.89961937509977652, 13.97604488694528158, 30.62390960531435269 ) ) ;
#136140=CARTESIAN_POINT ( 'NONE',  ( -14.34966873604972548, 8.224510206698743886, 63.33442372801900433 ) ) ;
#136141=CARTESIAN_POINT ( 'NONE',  ( 19.05341960407611168, 5.049401038298154454, 38.95724293864767418 ) ) ;
#136143=CARTESIAN_POINT ( 'NONE',  ( -5.049401038298153566, 19.05341960407611168, 85.20724293864766707 ) ) ;
#136144=CARTESIAN_POINT ( 'NONE',  ( -9.564922557960796823, -16.46253265017161027, 27.08224293864769550 ) ) ;
#136145=CARTESIAN_POINT ( 'NONE',  ( 18.62759615963271287, -10.81492255796078972, 58.33224293864768839 ) ) ;
#136146=CARTESIAN_POINT ( 'NONE',  ( 14.34966873604972726, -8.224510206698740333, 45.83442372801901854 ) ) ;
#136147=CARTESIAN_POINT ( 'NONE',  ( 18.67979575497194134, -10.72451020669871369, 95.83442372801903275 ) ) ;
#136148=CARTESIAN_POINT ( 'NONE',  ( 13.89961937509977652, -13.97604488694527269, 43.12390960531434558 ) ) ;
#136149=EDGE_CURVE ( 'NONE', #13391, #20566, #19460, .T. ) ;
#136150=CARTESIAN_POINT ( 'NONE',  ( 0.05219959533910956823, 16.53943276465976808, 29.99890960531435979 ) ) ;
#136151=CARTESIAN_POINT ( 'NONE',  ( -12.06949235617756955, 12.14591786802309770, 65.62390960531436690 ) ) ;
#136152=CARTESIAN_POINT ( 'NONE',  ( 5.049401038298161559, -19.05341960407611168, 62.70724293864769550 ) ) ;
#136153=CARTESIAN_POINT ( 'NONE',  ( 13.97604488694548053, -13.89961937509957401, 20.62609039468567573 ) ) ;
#136154=CARTESIAN_POINT ( 'NONE',  ( -15.72974639402176322, -15.80617190586768395, 24.37609039468567573 ) ) ;
#136155=CARTESIAN_POINT ( 'NONE',  ( 19.02544592524343514, -5.153800228976328945, 78.54057627198099567 ) ) ;
#136156=CARTESIAN_POINT ( 'NONE',  ( 18.62759615963255655, 10.81492255796105972, 86.66775706135234714 ) ) ;
#136157=CARTESIAN_POINT ( 'NONE',  ( -12.06949235617739369, -12.14591786802326823, 49.37609039468569705 ) ) ;
#136158=CARTESIAN_POINT ( 'NONE',  ( 0.05219959533934541429, -16.53943276465976808, 25.00109039468567218 ) ) ;
#136159=CARTESIAN_POINT ( 'NONE',  ( 12.06949235617757843, -12.14591786802309237, 98.12390960531436690 ) ) ;
#136160=CARTESIAN_POINT ( 'NONE',  ( 15.80617190586769283, -15.72974639402175789, 95.62609039468568994 ) ) ;
#136161=CARTESIAN_POINT ( 'NONE',  ( -0.05219959533910754901, -16.53943276465976808, 32.49890960531435979 ) ) ;
#136162=CARTESIAN_POINT ( 'NONE',  ( 16.46253265017160672, -9.564922557960803928, 33.33224293864770260 ) ) ;
#136163=CARTESIAN_POINT ( 'NONE',  ( -8.314922557961024197, 14.29746914071037800, 47.91775706135234714 ) ) ;
#136164=CARTESIAN_POINT ( 'NONE',  ( -8.314922557960811034, -14.29746914071050412, 57.08224293864769550 ) ) ;
#136165=CARTESIAN_POINT ( 'NONE',  ( 12.14591786802327356, -12.06949235617739191, 100.6260903946857184 ) ) ;
#136166=CARTESIAN_POINT ( 'NONE',  ( -19.02544592524342804, 5.153800228976336051, 111.0405762719810099 ) ) ;
#136167=CARTESIAN_POINT ( 'NONE',  ( 9.474510206698971260, -16.51473224551069308, 107.9155762719810383 ) ) ;
#136168=CARTESIAN_POINT ( 'NONE',  ( -19.03943276465977164, -0.05219959533935918106, 23.75109039468566152 ) ) ;
#136169=CARTESIAN_POINT ( 'NONE',  ( -14.34966873604960291, -8.224510206698953496, 86.66557627198102409 ) ) ;
#136170=CARTESIAN_POINT ( 'NONE',  ( -16.51473224551069308, -9.474510206698971260, 101.6655762719810241 ) ) ;
#136171=ORIENTED_EDGE ( 'NONE', *, *, #63061, .F. ) ;
#136172=CARTESIAN_POINT ( 'NONE',  ( -14.29746914071037622, -8.314922557961029526, 39.16775706135235424 ) ) ;
#136173=CARTESIAN_POINT ( 'NONE',  ( -9.474510206698964154, 16.51473224551069663, 35.41557627198102409 ) ) ;
#136174=CARTESIAN_POINT ( 'NONE',  ( -16.55341960407617563, 4.379528057220093196, 48.54275706135234714 ) ) ;
#136176=CARTESIAN_POINT ( 'NONE',  ( 19.02544592524334988, 5.153800228976608722, 46.45942372801899012 ) ) ;
#136177=CARTESIAN_POINT ( 'NONE',  ( -13.89961937509977652, 13.97604488694528158, 50.62390960531435979 ) ) ;
#136178=CARTESIAN_POINT ( 'NONE',  ( 16.55341960407618274, -4.379528057220086978, 81.04275706135236135 ) ) ;
#136179=CARTESIAN_POINT ( 'NONE',  ( 13.89961937509957401, 13.97604488694547697, 81.87609039468564731 ) ) ;
#136180=CARTESIAN_POINT ( 'NONE',  ( -9.474510206698720793, -16.51473224551083518, 29.58442372801900433 ) ) ;
#136181=CARTESIAN_POINT ( 'NONE',  ( -13.97604488694527625, -13.89961937509977652, 61.87390960531435979 ) ) ;
#136182=CARTESIAN_POINT ( 'NONE',  ( -12.14591786802309592, -12.06949235617757132, 101.8739096053143811 ) ) ;
#136183=CARTESIAN_POINT ( 'NONE',  ( 19.03943276465977164, 0.05219959533936151252, 66.25109039468567573 ) ) ;
#136184=CARTESIAN_POINT ( 'NONE',  ( 21.52544592524344225, -5.823673210054117533, 63.54057627198103830 ) ) ;
#136185=CARTESIAN_POINT ( 'NONE',  ( -9.474510206698720793, -16.51473224551083518, 24.58442372801900078 ) ) ;
#136186=CARTESIAN_POINT ( 'NONE',  ( -16.46253265017160317, 9.564922557960807481, 105.8322429386476955 ) ) ;
#136187=CARTESIAN_POINT ( 'NONE',  ( -18.67979575497178146, -10.72451020669898902, 81.66557627198103830 ) ) ;
#136188=CARTESIAN_POINT ( 'NONE',  ( -17.05587630539787014, 6.762274262135701264, 85.74180309037315340 ) ) ;
#136189=CARTESIAN_POINT ( 'NONE',  ( -5.049401038297874678, -19.05341960407617918, 99.79275706135234714 ) ) ;
#136190=CARTESIAN_POINT ( 'NONE',  ( -17.59860650958993844, 7.585241751806885979, 98.42337014262494677 ) ) ;
#136191=CARTESIAN_POINT ( 'NONE',  ( 4.379528057220092307, 16.55341960407617563, 32.29275706135235424 ) ) ;
#136192=CARTESIAN_POINT ( 'NONE',  ( 5.049401038298161559, -19.05341960407611168, 32.70724293864768129 ) ) ;
#136193=CARTESIAN_POINT ( 'NONE',  ( -5.153800228976328057, -19.02544592524343514, 107.2905762719810383 ) ) ;
#136194=CARTESIAN_POINT ( 'NONE',  ( -21.53943276465977519, 0.05219959533907696930, 96.24890960531435269 ) ) ;
#136195=CARTESIAN_POINT ( 'NONE',  ( -0.05219959533937732626, 21.53943276465977519, 62.50109039468568284 ) ) ;
#136196=CARTESIAN_POINT ( 'NONE',  ( 5.049401038297881783, 19.05341960407617563, 107.2927570613523187 ) ) ;
#136197=CARTESIAN_POINT ( 'NONE',  ( -15.80617190586768217, 15.72974639402176855, 113.1260903946856899 ) ) ;
#136198=CARTESIAN_POINT ( 'NONE',  ( -14.34966873604972548, 8.224510206698743886, 103.3344237280190043 ) ) ;
#136199=CARTESIAN_POINT ( 'NONE',  ( -21.55341960407610458, -5.719274019375992779, 106.4572429386477097 ) ) ;
#136200=CARTESIAN_POINT ( 'NONE',  ( 4.379528057220339221, -16.55341960407611168, 47.70724293864770260 ) ) ;
#136201=CARTESIAN_POINT ( 'NONE',  ( 5.049401038297881783, 19.05341960407617563, 87.29275706135234714 ) ) ;
#136202=CARTESIAN_POINT ( 'NONE',  ( -9.474510206698720793, -16.51473224551083518, 54.58442372801899722 ) ) ;
#136203=CARTESIAN_POINT ( 'NONE',  ( -18.67979575497193778, 10.72451020669871902, 53.33442372801901854 ) ) ;
#136204=CARTESIAN_POINT ( 'NONE',  ( 19.03943276465977164, 0.05219959533936151252, 46.25109039468566863 ) ) ;
#136205=CARTESIAN_POINT ( 'NONE',  ( 8.314922557960818139, 14.29746914071049879, 104.5822429386477097 ) ) ;
#136206=CARTESIAN_POINT ( 'NONE',  ( 10.81492255796078972, 18.62759615963270932, 24.58224293864768839 ) ) ;
#136207=CARTESIAN_POINT ( 'NONE',  ( -14.34966873604960291, -8.224510206698953496, 36.66557627198103120 ) ) ;
#136208=CARTESIAN_POINT ( 'NONE',  ( 21.52544592524334988, 5.823673210054432836, 101.4594237280190185 ) ) ;
#136209=CARTESIAN_POINT ( 'NONE',  ( 8.314922557961029526, -14.29746914071037800, 75.41775706135233293 ) ) ;
#136210=CARTESIAN_POINT ( 'NONE',  ( -0.05219959533910754901, -16.53943276465976808, 22.49890960531436335 ) ) ;
#136211=CARTESIAN_POINT ( 'NONE',  ( 18.62759615963255655, 10.81492255796105972, 56.66775706135235424 ) ) ;
#136212=CARTESIAN_POINT ( 'NONE',  ( -5.823673210054431948, 21.52544592524334988, 62.70942372801902565 ) ) ;
#136213=CARTESIAN_POINT ( 'NONE',  ( -18.62759615963270932, 10.81492255796079327, 70.83224293864770971 ) ) ;
#136215=CARTESIAN_POINT ( 'NONE',  ( 5.153800228976335163, 19.02544592524342804, 29.79057627198102409 ) ) ;
#136216=CARTESIAN_POINT ( 'NONE',  ( -18.62759615963255300, -10.81492255796106328, 44.16775706135234714 ) ) ;
#136217=CARTESIAN_POINT ( 'NONE',  ( -8.224510206698948167, 14.34966873604960824, 115.4155762719810241 ) ) ;
#136218=CARTESIAN_POINT ( 'NONE',  ( -5.049401038298153566, 19.05341960407611168, 45.20724293864769550 ) ) ;
#136219=CARTESIAN_POINT ( 'NONE',  ( 16.53943276465976808, -0.05219959533910856209, 78.74890960531436690 ) ) ;
#136220=CARTESIAN_POINT ( 'NONE',  ( -19.02544592524342804, 5.153800228976336051, 86.04057627198103830 ) ) ;
#136221=CARTESIAN_POINT ( 'NONE',  ( -14.34966873604972548, 8.224510206698743886, 113.3344237280190328 ) ) ;
#136222=CARTESIAN_POINT ( 'NONE',  ( -12.14591786802309592, -12.06949235617757132, 96.87390960531436690 ) ) ;
#136223=CARTESIAN_POINT ( 'NONE',  ( -21.53943276465977519, 0.05219959533907696930, 71.24890960531435269 ) ) ;
#136224=CARTESIAN_POINT ( 'NONE',  ( -15.80617190586745835, -15.72974639402198527, 111.8739096053143669 ) ) ;
#136225=CARTESIAN_POINT ( 'NONE',  ( 9.474510206698971260, -16.51473224551069308, 112.9155762719810383 ) ) ;
#136226=CARTESIAN_POINT ( 'NONE',  ( -19.02544592524342804, 5.153800228976336051, 66.04057627198103830 ) ) ;
#136227=CARTESIAN_POINT ( 'NONE',  ( 19.05341960407617918, -5.049401038297876454, 101.0427570613523045 ) ) ;
#136228=CARTESIAN_POINT ( 'NONE',  ( -21.52544592524343514, 5.823673210054127303, 61.04057627198103120 ) ) ;
#136229=CARTESIAN_POINT ( 'NONE',  ( -21.52544592524334988, -5.823673210054445271, 83.95942372801900433 ) ) ;
#136230=CARTESIAN_POINT ( 'NONE',  ( 5.049401038298161559, -19.05341960407611168, 62.70724293864769550 ) ) ;
#136232=CARTESIAN_POINT ( 'NONE',  ( -19.05341960407611168, -5.049401038298163336, 96.45724293864769550 ) ) ;
#136233=CARTESIAN_POINT ( 'NONE',  ( 4.483927247898790824, -16.52544592524335698, 80.20942372801901854 ) ) ;
#136234=CARTESIAN_POINT ( 'NONE',  ( -10.81492255796105439, 18.62759615963255655, 57.91775706135234714 ) ) ;
#136235=CARTESIAN_POINT ( 'NONE',  ( -10.81492255796105439, 18.62759615963255655, 102.9177570613523756 ) ) ;
#136236=CARTESIAN_POINT ( 'NONE',  ( 18.62759615963271287, -10.81492255796078972, 113.3322429386476955 ) ) ;
#136237=CARTESIAN_POINT ( 'NONE',  ( -21.53943276465977519, 0.05219959533907696930, 86.24890960531436690 ) ) ;
#136238=CARTESIAN_POINT ( 'NONE',  ( 16.46253265017146816, 9.564922557961045513, 51.66775706135233293 ) ) ;
#136239=CARTESIAN_POINT ( 'NONE',  ( -21.55341960407610458, -5.719274019375992779, 46.45724293864769550 ) ) ;
#136240=CARTESIAN_POINT ( 'NONE',  ( -5.049401038298153566, 19.05341960407611168, 80.20724293864769550 ) ) ;
#136241=CARTESIAN_POINT ( 'NONE',  ( -16.52544592524342804, 4.483927247898546575, 31.04057627198102409 ) ) ;
#136243=CARTESIAN_POINT ( 'NONE',  ( -18.56101223717333326, -5.500000000000065725, 81.44978406935680937 ) ) ;
#136244=CARTESIAN_POINT ( 'NONE',  ( 16.51473224551083163, -9.474510206698727899, 95.83442372801900433 ) ) ;
#136245=CARTESIAN_POINT ( 'NONE',  ( -21.52544592524343514, 5.823673210054127303, 66.04057627198103830 ) ) ;
#136246=CARTESIAN_POINT ( 'NONE',  ( 4.483927247898545687, 16.52544592524342804, 49.79057627198102409 ) ) ;
#136247=CARTESIAN_POINT ( 'NONE',  ( 16.53943276465976808, 0.05219959533934440121, 31.25109039468568639 ) ) ;
#136248=CARTESIAN_POINT ( 'NONE',  ( -16.51473224551069308, -9.474510206698971260, 46.66557627198102409 ) ) ;
#136249=CARTESIAN_POINT ( 'NONE',  ( 10.72451020669898902, -18.67979575497178502, 107.9155762719810241 ) ) ;
#136250=CARTESIAN_POINT ( 'NONE',  ( 0.05219959533936267826, -19.03943276465977164, 85.00109039468567573 ) ) ;
#136251=CARTESIAN_POINT ( 'NONE',  ( -9.474510206698964154, 16.51473224551069663, 75.41557627198103830 ) ) ;
#136252=CARTESIAN_POINT ( 'NONE',  ( -16.52544592524342804, 4.483927247898546575, 86.04057627198102409 ) ) ;
#136253=CARTESIAN_POINT ( 'NONE',  ( -13.89961937509977652, 13.97604488694528158, 80.62390960531436690 ) ) ;
#136254=CARTESIAN_POINT ( 'NONE',  ( -0.05219959533907301413, -21.53943276465977519, 77.49890960531433848 ) ) ;
#136255=CARTESIAN_POINT ( 'NONE',  ( 9.474510206698971260, -16.51473224551069308, 27.91557627198103120 ) ) ;
#136257=CARTESIAN_POINT ( 'NONE',  ( 14.34966873604960469, 8.224510206698951720, 54.16557627198103120 ) ) ;
#136258=CARTESIAN_POINT ( 'NONE',  ( -13.97604488694527625, -13.89961937509977652, 91.87390960531432427 ) ) ;
#136260=CARTESIAN_POINT ( 'NONE',  ( -16.46253265017146816, -9.564922557961047289, 49.16775706135233293 ) ) ;
#136261=CARTESIAN_POINT ( 'NONE',  ( -8.224510206698735004, -14.34966873604973081, 54.58442372801901143 ) ) ;
#136262=CARTESIAN_POINT ( 'NONE',  ( -18.67979575497178146, -10.72451020669898902, 76.66557627198103830 ) ) ;
#136263=CARTESIAN_POINT ( 'NONE',  ( -9.564922557961040184, 16.46253265017147172, 37.91775706135233293 ) ) ;
#136264=CARTESIAN_POINT ( 'NONE',  ( 9.564922557960805705, 16.46253265017160317, 84.58224293864769550 ) ) ;
#136265=CARTESIAN_POINT ( 'NONE',  ( -17.49999999999999645, 3.209263204892610410, 114.7619682560627297 ) ) ;
#136266=CARTESIAN_POINT ( 'NONE',  ( 21.52544592524344225, -5.823673210054117533, 23.54057627198102765 ) ) ;
#136267=CARTESIAN_POINT ( 'NONE',  ( -9.564922557960796823, -16.46253265017161027, 72.08224293864770971 ) ) ;
#136268=CARTESIAN_POINT ( 'NONE',  ( -18.62759615963255300, -10.81492255796106328, 49.16775706135234003 ) ) ;
#136269=CARTESIAN_POINT ( 'NONE',  ( 16.51473224551069308, 9.474510206698969483, 24.16557627198102765 ) ) ;
#136270=CARTESIAN_POINT ( 'NONE',  ( -18.62759615963270932, 10.81492255796079327, 110.8322429386476955 ) ) ;
#136271=CARTESIAN_POINT ( 'NONE',  ( 16.46253265017160672, -9.564922557960803928, 93.33224293864769550 ) ) ;
#136273=CARTESIAN_POINT ( 'NONE',  ( -5.823673210054431948, 21.52544592524334988, 42.70942372801901854 ) ) ;
#136275=CARTESIAN_POINT ( 'NONE',  ( 13.97604488694527802, 13.89961937509977652, 99.37390960531436690 ) ) ;
#136276=CARTESIAN_POINT ( 'NONE',  ( 16.51473224551069308, 9.474510206698969483, 89.16557627198103830 ) ) ;
#136277=CARTESIAN_POINT ( 'NONE',  ( 10.72451020669898902, -18.67979575497178502, 112.9155762719810383 ) ) ;
#136278=CARTESIAN_POINT ( 'NONE',  ( 13.89961937509977652, -13.97604488694527269, 48.12390960531435979 ) ) ;
#136279=CARTESIAN_POINT ( 'NONE',  ( -16.53943276465976808, -0.05219959533934237506, 28.75109039468567929 ) ) ;
#136281=CARTESIAN_POINT ( 'NONE',  ( -10.72451020669870658, -18.67979575497194134, 99.58442372801900433 ) ) ;
#136282=CARTESIAN_POINT ( 'NONE',  ( -9.564922557960796823, -16.46253265017161027, 32.08224293864769550 ) ) ;
#136283=CARTESIAN_POINT ( 'NONE',  ( -5.823673210054431948, 21.52544592524334988, 92.70942372801901854 ) ) ;
#136284=CARTESIAN_POINT ( 'NONE',  ( 16.51473224551069308, 9.474510206698969483, 89.16557627198103830 ) ) ;
#136285=CARTESIAN_POINT ( 'NONE',  ( 10.72451020669871369, 18.67979575497193778, 62.08442372801901143 ) ) ;
#136287=CARTESIAN_POINT ( 'NONE',  ( -9.474510206698964154, 16.51473224551069663, 105.4155762719810383 ) ) ;
#136288=CARTESIAN_POINT ( 'NONE',  ( 15.50000000000000178, -5.500000000000000888, 22.00000000000000711 ) ) ;
#136289=CARTESIAN_POINT ( 'NONE',  ( 14.29746914071037800, 8.314922557961029526, 51.66775706135234714 ) ) ;
#136290=CARTESIAN_POINT ( 'NONE',  ( 16.52544592524335698, 4.483927247898782831, 71.45942372801901854 ) ) ;
#136291=CARTESIAN_POINT ( 'NONE',  ( 21.55341960407619695, -5.719274019375665929, 56.04275706135235424 ) ) ;
#136292=CARTESIAN_POINT ( 'NONE',  ( 5.719274019375673035, 21.55341960407619339, 92.29275706135236135 ) ) ;
#136293=CARTESIAN_POINT ( 'NONE',  ( -18.22780087662124160, -5.499999999999927169, 68.98236817873106475 ) ) ;
#136294=CARTESIAN_POINT ( 'NONE',  ( -16.53943276465976808, -0.05219959533934237506, 28.75109039468567929 ) ) ;
#136295=CARTESIAN_POINT ( 'NONE',  ( 5.049401038298161559, -19.05341960407611168, 72.70724293864768129 ) ) ;
#136296=CARTESIAN_POINT ( 'NONE',  ( -19.02544592524342804, 5.153800228976336051, 96.04057627198103830 ) ) ;
#136299=CARTESIAN_POINT ( 'NONE',  ( -9.564922557960796823, -16.46253265017161027, 22.08224293864768839 ) ) ;
#136300=CARTESIAN_POINT ( 'NONE',  ( 15.80617190586746368, 15.72974639402197994, 24.37390960531435979 ) ) ;
#136301=CARTESIAN_POINT ( 'NONE',  ( -12.06949235617739369, -12.14591786802326823, 89.37609039468568994 ) ) ;
#136302=CARTESIAN_POINT ( 'NONE',  ( -14.34966873604960291, -8.224510206698953496, 76.66557627198103830 ) ) ;
#136303=CARTESIAN_POINT ( 'NONE',  ( 16.46253265017160672, -9.564922557960803928, 68.33224293864770971 ) ) ;
#136304=CARTESIAN_POINT ( 'NONE',  ( 5.719274019375673035, 21.55341960407619339, 97.29275706135234714 ) ) ;
#136306=CARTESIAN_POINT ( 'NONE',  ( 14.34966873604972726, -8.224510206698740333, 25.83442372801901499 ) ) ;
#136307=CARTESIAN_POINT ( 'NONE',  ( 12.14591786802309770, 12.06949235617756955, 69.37390960531436690 ) ) ;
#136308=CARTESIAN_POINT ( 'NONE',  ( 0.05219959533937995610, -21.53943276465977519, 25.00109039468567218 ) ) ;
#136309=CARTESIAN_POINT ( 'NONE',  ( 0.05219959533907565091, 21.53943276465977519, 79.99890960531435269 ) ) ;
#136310=CARTESIAN_POINT ( 'NONE',  ( -19.05341960407617563, 5.049401038297882671, 38.54275706135233293 ) ) ;
#136312=CARTESIAN_POINT ( 'NONE',  ( 9.474510206698971260, -16.51473224551069308, 82.91557627198103830 ) ) ;
#136313=CARTESIAN_POINT ( 'NONE',  ( -16.53943276465976808, 0.05219959533911058130, 46.24890960531435979 ) ) ;
#136314=CARTESIAN_POINT ( 'NONE',  ( 14.29746914071049879, -8.314922557960816363, 33.33224293864769550 ) ) ;
#136315=CARTESIAN_POINT ( 'NONE',  ( -12.14591786802326823, 12.06949235617739902, 113.1260903946856899 ) ) ;
#136316=CARTESIAN_POINT ( 'NONE',  ( 16.51473224551083163, -9.474510206698727899, 60.83442372801900433 ) ) ;
#136317=CARTESIAN_POINT ( 'NONE',  ( 19.35543954521082455, 5.499999999999579892, 52.08901960356453742 ) ) ;
#136318=CARTESIAN_POINT ( 'NONE',  ( -13.89961937509977652, 13.97604488694528158, 110.6239096053143243 ) ) ;
#136320=CARTESIAN_POINT ( 'NONE',  ( -4.379528057220328563, 16.55341960407611168, 75.20724293864769550 ) ) ;
#136322=CARTESIAN_POINT ( 'NONE',  ( -19.03943276465977164, 0.05219959533909376836, 31.24890960531435979 ) ) ;
#136323=CARTESIAN_POINT ( 'NONE',  ( -21.55341960407610458, -5.719274019375992779, 41.45724293864769550 ) ) ;
#136324=CARTESIAN_POINT ( 'NONE',  ( -0.05219959533907301413, -21.53943276465977519, 67.49890960531436690 ) ) ;
#136325=CARTESIAN_POINT ( 'NONE',  ( 14.29746914071049879, -8.314922557960816363, 113.3322429386476955 ) ) ;
#136326=CARTESIAN_POINT ( 'NONE',  ( 14.29746914071037800, 8.314922557961029526, 61.66775706135235424 ) ) ;
#136327=CARTESIAN_POINT ( 'NONE',  ( 19.02544592524343514, -5.153800228976328945, 53.54057627198102409 ) ) ;
#136328=CARTESIAN_POINT ( 'NONE',  ( 15.80617190586769283, -15.72974639402175789, 50.62609039468568994 ) ) ;
#136329=ORIENTED_EDGE ( 'NONE', *, *, #70955, .T. ) ;
#136330=CARTESIAN_POINT ( 'NONE',  ( -8.224510206698948167, 14.34966873604960824, 95.41557627198102409 ) ) ;
#136331=CARTESIAN_POINT ( 'NONE',  ( -17.50000000001356781, 5.500000000000039968, 40.79690382535057580 ) ) ;
#136332=CARTESIAN_POINT ( 'NONE',  ( -17.49999999999999645, 5.624438216177593652, 50.81670344914645909 ) ) ;
#136333=CARTESIAN_POINT ( 'NONE',  ( 21.55341960407610458, 5.719274019375980345, 38.95724293864768839 ) ) ;
#136335=CARTESIAN_POINT ( 'NONE',  ( -21.52544592524334988, -5.823673210054445271, 73.95942372801901854 ) ) ;
#136336=DIRECTION ( 'NONE',  ( 0.000000000000000000, 0.000000000000000000, -1.000000000000000000 ) ) ;
#136337=CARTESIAN_POINT ( 'NONE',  ( 14.29746914071037800, 8.314922557961029526, 61.66775706135235424 ) ) ;
#136338=CARTESIAN_POINT ( 'NONE',  ( 8.224510206698953496, -14.34966873604960469, 37.91557627198102409 ) ) ;
#136339=CARTESIAN_POINT ( 'NONE',  ( 5.823673210054125526, 21.52544592524343514, 74.79057627198105251 ) ) ;
#136340=CARTESIAN_POINT ( 'NONE',  ( 15.72974639402199770, -15.80617190586745480, 58.12390960531435979 ) ) ;
#136342=CARTESIAN_POINT ( 'NONE',  ( -19.02544592524334988, -5.153800228976617603, 78.95942372801900433 ) ) ;
#136343=CARTESIAN_POINT ( 'NONE',  ( 19.02544592524343514, -5.153800228976328945, 113.5405762719810241 ) ) ;
#136344=CARTESIAN_POINT ( 'NONE',  ( 9.564922557960805705, 16.46253265017160317, 54.58224293864769550 ) ) ;
#136345=CARTESIAN_POINT ( 'NONE',  ( -9.564922557960796823, -16.46253265017161027, 22.08224293864768839 ) ) ;
#136348=CARTESIAN_POINT ( 'NONE',  ( -16.53943276465976808, -0.05219959533934237506, 63.75109039468568284 ) ) ;
#136349=CARTESIAN_POINT ( 'NONE',  ( -15.80617190586745835, -15.72974639402198527, 101.8739096053143811 ) ) ;
#136350=CARTESIAN_POINT ( 'NONE',  ( -19.02544592524342804, 5.153800228976336051, 51.04057627198103120 ) ) ;
#136351=CARTESIAN_POINT ( 'NONE',  ( 21.55341960407619695, -5.719274019375665929, 41.04275706135236135 ) ) ;
#136352=CARTESIAN_POINT ( 'NONE',  ( -16.46253265017160317, 9.564922557960807481, 95.83224293864769550 ) ) ;
#136354=ORIENTED_EDGE ( 'NONE', *, *, #26797, .F. ) ;
#136355=CARTESIAN_POINT ( 'NONE',  ( -10.72451020669870658, -18.67979575497194134, 29.58442372801901854 ) ) ;
#136356=CARTESIAN_POINT ( 'NONE',  ( -19.03943276465977164, 0.05219959533909376836, 106.2489096053143669 ) ) ;
#136357=CARTESIAN_POINT ( 'NONE',  ( -16.46253265017146816, -9.564922557961047289, 84.16775706135233293 ) ) ;
#136358=CARTESIAN_POINT ( 'NONE',  ( 16.46253265017146816, 9.564922557961045513, 41.66775706135234003 ) ) ;
#136359=CARTESIAN_POINT ( 'NONE',  ( 15.80617190586746368, 15.72974639402197994, 104.3739096053143669 ) ) ;
#136360=CARTESIAN_POINT ( 'NONE',  ( 16.51473224551083163, -9.474510206698727899, 35.83442372801899722 ) ) ;
#136361=CARTESIAN_POINT ( 'NONE',  ( 5.153800228976615827, -19.02544592524334988, 40.20942372801898301 ) ) ;
#136362=CARTESIAN_POINT ( 'NONE',  ( -16.52544592524335698, -4.483927247898792601, 88.95942372801901854 ) ) ;
#136363=FACE_OUTER_BOUND ( 'NONE', #102840, .T. ) ;
#136364=CARTESIAN_POINT ( 'NONE',  ( -19.03943276465977164, 0.05219959533909376836, 66.24890960531436690 ) ) ;
#136365=CARTESIAN_POINT ( 'NONE',  ( -18.67979575497193778, 10.72451020669871902, 78.33442372801901854 ) ) ;
#136366=CARTESIAN_POINT ( 'NONE',  ( 5.823673210054444382, -21.52544592524334988, 75.20942372801901854 ) ) ;
#136368=CARTESIAN_POINT ( 'NONE',  ( 5.049401038298161559, -19.05341960407611168, 87.70724293864769550 ) ) ;
#136369=CARTESIAN_POINT ( 'NONE',  ( 18.67979575497194134, -10.72451020669871369, 65.83442372801900433 ) ) ;
#136370=CARTESIAN_POINT ( 'NONE',  ( -19.05341960407617563, 5.049401038297882671, 98.54275706135233293 ) ) ;
#136371=CARTESIAN_POINT ( 'NONE',  ( -9.564922557960796823, -16.46253265017161027, 67.08224293864769550 ) ) ;
#136372=CARTESIAN_POINT ( 'NONE',  ( -16.51473224551069308, -9.474510206698971260, 106.6655762719810383 ) ) ;
#136373=CARTESIAN_POINT ( 'NONE',  ( -16.46253265017160317, 9.564922557960807481, 75.83224293864769550 ) ) ;
#136375=CARTESIAN_POINT ( 'NONE',  ( -13.97604488694527625, -13.89961937509977652, 71.87390960531433848 ) ) ;
#136376=CARTESIAN_POINT ( 'NONE',  ( -19.05341960407611168, -5.049401038298163336, 51.45724293864770260 ) ) ;
#136377=CARTESIAN_POINT ( 'NONE',  ( -21.52544592524343514, 5.823673210054127303, 101.0405762719810383 ) ) ;
#136378=CARTESIAN_POINT ( 'NONE',  ( 14.34966873604972726, -8.224510206698740333, 80.83442372801901854 ) ) ;
#136379=CARTESIAN_POINT ( 'NONE',  ( -15.49999999999999822, 5.499999999999998224, 22.00000000000000000 ) ) ;
#136380=CARTESIAN_POINT ( 'NONE',  ( 19.02544592524334988, 5.153800228976608722, 41.45942372801900433 ) ) ;
#136381=CARTESIAN_POINT ( 'NONE',  ( 16.51473224551069308, 9.474510206698969483, 79.16557627198103830 ) ) ;
#136382=CARTESIAN_POINT ( 'NONE',  ( 0.05219959533910956823, 16.53943276465976808, 74.99890960531435269 ) ) ;
#136383=CARTESIAN_POINT ( 'NONE',  ( 12.14591786802309770, 12.06949235617756955, 114.3739096053143527 ) ) ;
#136384=CARTESIAN_POINT ( 'NONE',  ( 5.823673210054125526, 21.52544592524343514, 24.79057627198103120 ) ) ;
#136385=CARTESIAN_POINT ( 'NONE',  ( -19.02544592524342804, 5.153800228976336051, 101.0405762719810241 ) ) ;
#136386=CARTESIAN_POINT ( 'NONE',  ( -14.29746914071049879, 8.314922557960819915, 80.83224293864769550 ) ) ;
#136388=CARTESIAN_POINT ( 'NONE',  ( 13.97604488694548053, -13.89961937509957401, 25.62609039468566507 ) ) ;
#136389=CARTESIAN_POINT ( 'NONE',  ( -8.314922557961024197, 14.29746914071037800, 97.91775706135236135 ) ) ;
#136390=CARTESIAN_POINT ( 'NONE',  ( 16.46253265017160672, -9.564922557960803928, 78.33224293864769550 ) ) ;
#136391=CARTESIAN_POINT ( 'NONE',  ( 15.80617190586769283, -15.72974639402175789, 50.62609039468568994 ) ) ;
#136392=CARTESIAN_POINT ( 'NONE',  ( 15.80617190586746368, 15.72974639402197994, 39.37390960531436690 ) ) ;
#136393=CARTESIAN_POINT ( 'NONE',  ( 18.62759615963271287, -10.81492255796078972, 113.3322429386476955 ) ) ;
#136394=CARTESIAN_POINT ( 'NONE',  ( 18.62759615963271287, -10.81492255796078972, 73.33224293864769550 ) ) ;
#136395=CARTESIAN_POINT ( 'NONE',  ( 16.52544592524342804, -4.483927247898539470, 93.54057627198103830 ) ) ;
#136396=CARTESIAN_POINT ( 'NONE',  ( 13.89961937509957401, 13.97604488694547697, 61.87609039468566863 ) ) ;
#136397=CARTESIAN_POINT ( 'NONE',  ( -9.474510206698964154, 16.51473224551069663, 35.41557627198102409 ) ) ;
#136398=CARTESIAN_POINT ( 'NONE',  ( 13.97604488694527802, 13.89961937509977652, 79.37390960531435269 ) ) ;
#136399=CARTESIAN_POINT ( 'NONE',  ( 5.049401038298161559, -19.05341960407611168, 82.70724293864770971 ) ) ;
#136400=CARTESIAN_POINT ( 'NONE',  ( 14.29746914071049879, -8.314922557960816363, 98.33224293864769550 ) ) ;
#136401=CARTESIAN_POINT ( 'NONE',  ( 8.224510206698953496, -14.34966873604960469, 27.91557627198103830 ) ) ;
#136402=CARTESIAN_POINT ( 'NONE',  ( 16.52544592524335698, 4.483927247898782831, 21.45942372801901499 ) ) ;
#136403=CARTESIAN_POINT ( 'NONE',  ( -10.81492255796105439, 18.62759615963255655, 97.91775706135236135 ) ) ;
#136404=CARTESIAN_POINT ( 'NONE',  ( -19.02544592524342804, 5.153800228976336051, 101.0405762719810241 ) ) ;
#136405=CARTESIAN_POINT ( 'NONE',  ( 21.52544592524344225, -5.823673210054117533, 113.5405762719810383 ) ) ;
#136406=CARTESIAN_POINT ( 'NONE',  ( -16.51473224551069308, -9.474510206698971260, 41.66557627198103120 ) ) ;
#136407=CARTESIAN_POINT ( 'NONE',  ( -16.52544592524335698, -4.483927247898792601, 43.95942372801902565 ) ) ;
#136408=CARTESIAN_POINT ( 'NONE',  ( -19.05341960407617563, 5.049401038297882671, 103.5427570613523329 ) ) ;
#136409=CARTESIAN_POINT ( 'NONE',  ( -5.153800228976328057, -19.02544592524343514, 37.29057627198102409 ) ) ;
#136410=CARTESIAN_POINT ( 'NONE',  ( 16.53943276465976808, -0.05219959533910856209, 98.74890960531438111 ) ) ;
#136411=CARTESIAN_POINT ( 'NONE',  ( 15.72974639402199770, -15.80617190586745480, 103.1239096053143811 ) ) ;
#136412=CARTESIAN_POINT ( 'NONE',  ( 19.02544592524334988, 5.153800228976608722, 66.45942372801899012 ) ) ;
#136413=CARTESIAN_POINT ( 'NONE',  ( -17.60691670004651499, -5.500000000000069278, 64.13333313366436528 ) ) ;
#136414=CARTESIAN_POINT ( 'NONE',  ( 5.153800228976335163, 19.02544592524342804, 94.79057627198103830 ) ) ;
#136415=CARTESIAN_POINT ( 'NONE',  ( 18.62759615963255655, 10.81492255796105972, 21.66775706135235069 ) ) ;
#136417=CARTESIAN_POINT ( 'NONE',  ( -19.05341960407611168, -5.049401038298163336, 86.45724293864769550 ) ) ;
#136418=CARTESIAN_POINT ( 'NONE',  ( 17.05116617787824396, -6.768360034955819060, 111.1567555325920011 ) ) ;
#136419=CARTESIAN_POINT ( 'NONE',  ( 13.89961937509977652, -13.97604488694527269, 83.12390960531436690 ) ) ;
#136420=CARTESIAN_POINT ( 'NONE',  ( -15.80617190586768217, 15.72974639402176855, 38.12609039468567573 ) ) ;
#136421=CARTESIAN_POINT ( 'NONE',  ( 16.53943276465976808, -0.05219959533910856209, 78.74890960531436690 ) ) ;
#136422=CARTESIAN_POINT ( 'NONE',  ( -19.02544592524342804, 5.153800228976336051, 86.04057627198103830 ) ) ;
#136423=CARTESIAN_POINT ( 'NONE',  ( 9.564922557961047289, -16.46253265017146816, 25.41775706135234003 ) ) ;
#136424=CARTESIAN_POINT ( 'NONE',  ( 14.34966873604972726, -8.224510206698740333, 55.83442372801901854 ) ) ;
#136425=CARTESIAN_POINT ( 'NONE',  ( 21.53943276465977519, 0.05219959533937863772, 71.25109039468568994 ) ) ;
#136426=CARTESIAN_POINT ( 'NONE',  ( 16.52544592524335698, 4.483927247898782831, 21.45942372801901499 ) ) ;
#136427=CARTESIAN_POINT ( 'NONE',  ( 9.564922557960805705, 16.46253265017160317, 64.58224293864769550 ) ) ;
#136428=CARTESIAN_POINT ( 'NONE',  ( -5.049401038297874678, -19.05341960407617918, 94.79275706135230450 ) ) ;
#136429=CARTESIAN_POINT ( 'NONE',  ( 14.34966873604972726, -8.224510206698740333, 65.83442372801900433 ) ) ;
#136430=CARTESIAN_POINT ( 'NONE',  ( -10.81492255796105439, 18.62759615963255655, 107.9177570613523471 ) ) ;
#136431=CARTESIAN_POINT ( 'NONE',  ( -19.03943276465977164, -0.05219959533935918106, 73.75109039468566152 ) ) ;
#136432=CARTESIAN_POINT ( 'NONE',  ( 13.89961937509977652, -13.97604488694527269, 53.12390960531434558 ) ) ;
#136433=CARTESIAN_POINT ( 'NONE',  ( 0.05219959533907565091, 21.53943276465977519, 79.99890960531435269 ) ) ;
#136434=CARTESIAN_POINT ( 'NONE',  ( 16.53943276465976808, -0.05219959533910856209, 73.74890960531433848 ) ) ;
#136435=CARTESIAN_POINT ( 'NONE',  ( 13.89961937509957401, 13.97604488694547697, 81.87609039468564731 ) ) ;
#136437=CARTESIAN_POINT ( 'NONE',  ( -9.474510206698720793, -16.51473224551083518, 44.58442372801900433 ) ) ;
#136438=CARTESIAN_POINT ( 'NONE',  ( 16.53943276465976808, 0.05219959533934440121, 106.2510903946856757 ) ) ;
#136439=CARTESIAN_POINT ( 'NONE',  ( 14.29746914071049879, -8.314922557960816363, 63.33224293864770260 ) ) ;
#136440=CARTESIAN_POINT ( 'NONE',  ( -0.05219959533937732626, 21.53943276465977519, 97.50109039468567573 ) ) ;
#136442=CARTESIAN_POINT ( 'NONE',  ( 10.72451020669898902, -18.67979575497178502, 102.9155762719810383 ) ) ;
#136443=CARTESIAN_POINT ( 'NONE',  ( -13.89961937509977652, 13.97604488694528158, 60.62390960531436690 ) ) ;
#136444=CARTESIAN_POINT ( 'NONE',  ( -10.81492255796105439, 18.62759615963255655, 77.91775706135231871 ) ) ;
#136445=CARTESIAN_POINT ( 'NONE',  ( -0.05219959533909027116, -19.03943276465977164, 67.49890960531436690 ) ) ;
#136446=CARTESIAN_POINT ( 'NONE',  ( -5.049401038298153566, 19.05341960407611168, 25.20724293864768484 ) ) ;
#136447=CARTESIAN_POINT ( 'NONE',  ( -15.72974639402197994, 15.80617190586746368, 25.62390960531435624 ) ) ;
#136448=CARTESIAN_POINT ( 'NONE',  ( 4.483927247898545687, 16.52544592524342804, 64.79057627198103830 ) ) ;
#136449=CARTESIAN_POINT ( 'NONE',  ( 19.03943276465977164, -0.05219959533909143690, 38.74890960531436690 ) ) ;
#136450=CARTESIAN_POINT ( 'NONE',  ( 16.53943276465976808, -0.05219959533910856209, 93.74890960531436690 ) ) ;
#136451=CARTESIAN_POINT ( 'NONE',  ( 15.72974639402199770, -15.80617190586745480, 108.1239096053143811 ) ) ;
#136452=CARTESIAN_POINT ( 'NONE',  ( -18.67979575497193778, 10.72451020669871902, 53.33442372801901854 ) ) ;
#136453=CARTESIAN_POINT ( 'NONE',  ( 16.46253265017160672, -9.564922557960803928, 28.33224293864769550 ) ) ;
#136454=CARTESIAN_POINT ( 'NONE',  ( -14.29746914071037622, -8.314922557961029526, 69.16775706135234714 ) ) ;
#136455=CARTESIAN_POINT ( 'NONE',  ( -21.53943276465977519, 0.05219959533907696930, 106.2489096053143811 ) ) ;
#136456=CARTESIAN_POINT ( 'NONE',  ( -18.67979575497178146, -10.72451020669898902, 101.6655762719810383 ) ) ;
#136457=CARTESIAN_POINT ( 'NONE',  ( -9.474510206698720793, -16.51473224551083518, 24.58442372801900078 ) ) ;
#136458=CARTESIAN_POINT ( 'NONE',  ( -13.89961937509977652, 13.97604488694528158, 55.62390960531434558 ) ) ;
#136459=CARTESIAN_POINT ( 'NONE',  ( -18.10062525802553424, 5.500000000000031086, 83.51383468041922242 ) ) ;
#136460=CARTESIAN_POINT ( 'NONE',  ( -15.72974639402176322, -15.80617190586768395, 54.37609039468568994 ) ) ;
#136462=CARTESIAN_POINT ( 'NONE',  ( -15.72974639402197994, 15.80617190586746368, 50.62390960531435979 ) ) ;
#136463=CARTESIAN_POINT ( 'NONE',  ( 4.379528057220339221, -16.55341960407611168, 22.70724293864769194 ) ) ;
#136464=CARTESIAN_POINT ( 'NONE',  ( 21.53943276465977519, 0.05219959533937863772, 76.25109039468568994 ) ) ;
#136465=CARTESIAN_POINT ( 'NONE',  ( 18.62759615963255655, 10.81492255796105972, 101.6677570613523613 ) ) ;
#136466=CARTESIAN_POINT ( 'NONE',  ( 16.46253265017146816, 9.564922557961045513, 46.66775706135233293 ) ) ;
#136467=CARTESIAN_POINT ( 'NONE',  ( 0.05219959533934541429, -16.53943276465976808, 105.0010903946856757 ) ) ;
#136468=CARTESIAN_POINT ( 'NONE',  ( -5.719274019375665041, -21.55341960407619695, 59.79275706135234714 ) ) ;
#136469=CARTESIAN_POINT ( 'NONE',  ( 0.05219959533909260263, 19.03943276465977164, 64.99890960531436690 ) ) ;
#136470=CARTESIAN_POINT ( 'NONE',  ( 19.03943276465977164, 0.05219959533936151252, 26.25109039468566507 ) ) ;
#136471=CARTESIAN_POINT ( 'NONE',  ( -10.72451020669898014, 18.67979575497178502, 40.41557627198103120 ) ) ;
#136472=CARTESIAN_POINT ( 'NONE',  ( 15.72974639402176855, 15.80617190586768217, 26.87609039468567218 ) ) ;
#136473=CARTESIAN_POINT ( 'NONE',  ( 21.52544592524344225, -5.823673210054117533, 83.54057627198102409 ) ) ;
#136474=CARTESIAN_POINT ( 'NONE',  ( -19.02544592524334988, -5.153800228976617603, 88.95942372801897591 ) ) ;
#136475=CARTESIAN_POINT ( 'NONE',  ( -16.52544592524335698, -4.483927247898792601, 53.95942372801900433 ) ) ;
#136476=CARTESIAN_POINT ( 'NONE',  ( 18.22780087662121673, 5.500000000000056843, 63.98459894673894155 ) ) ;
#136477=CARTESIAN_POINT ( 'NONE',  ( 5.719274019375991003, -21.55341960407610458, 82.70724293864770971 ) ) ;
#136478=CARTESIAN_POINT ( 'NONE',  ( 8.314922557961029526, -14.29746914071037800, 70.41775706135236135 ) ) ;
#136479=CARTESIAN_POINT ( 'NONE',  ( 4.379528057220339221, -16.55341960407611168, 77.70724293864770971 ) ) ;
#136481=CARTESIAN_POINT ( 'NONE',  ( -13.97604488694547697, 13.89961937509957934, 98.12609039468566152 ) ) ;
#136482=CARTESIAN_POINT ( 'NONE',  ( 5.719274019375991003, -21.55341960407610458, 37.70724293864769550 ) ) ;
#136483=CARTESIAN_POINT ( 'NONE',  ( -17.58332526062529411, 7.635886036038502134, 95.92334959558468199 ) ) ;
#136484=CARTESIAN_POINT ( 'NONE',  ( 14.29746914071037800, 8.314922557961029526, 41.66775706135235424 ) ) ;
#136485=CARTESIAN_POINT ( 'NONE',  ( 5.719274019375991003, -21.55341960407610458, 107.7072429386476955 ) ) ;
#136486=CARTESIAN_POINT ( 'NONE',  ( 21.52544592524344225, -5.823673210054117533, 38.54057627198103120 ) ) ;
#136487=CARTESIAN_POINT ( 'NONE',  ( 16.55341960407618274, -4.379528057220086978, 66.04275706135236135 ) ) ;
#136488=CARTESIAN_POINT ( 'NONE',  ( 19.03943276465977164, -0.05219959533909143690, 83.74890960531436690 ) ) ;
#136489=CARTESIAN_POINT ( 'NONE',  ( 15.80617190586769283, -15.72974639402175789, 50.62609039468568994 ) ) ;
#136490=CARTESIAN_POINT ( 'NONE',  ( -16.51473224551069308, -9.474510206698971260, 31.66557627198102054 ) ) ;
#136491=CARTESIAN_POINT ( 'NONE',  ( -18.67979575497178146, -10.72451020669898902, 21.66557627198102409 ) ) ;
#136493=CARTESIAN_POINT ( 'NONE',  ( 5.153800228976615827, -19.02544592524334988, 40.20942372801898301 ) ) ;
#136494=CARTESIAN_POINT ( 'NONE',  ( 4.379528057220092307, 16.55341960407617563, 47.29275706135234003 ) ) ;
#136495=CARTESIAN_POINT ( 'NONE',  ( -16.46253265017160317, 9.564922557960807481, 110.8322429386476955 ) ) ;
#136496=CARTESIAN_POINT ( 'NONE',  ( 9.474510206698971260, -16.51473224551069308, 72.91557627198102409 ) ) ;
#136497=CARTESIAN_POINT ( 'NONE',  ( -16.52544592524335698, -4.483927247898792601, 98.95942372801903275 ) ) ;
#136499=CARTESIAN_POINT ( 'NONE',  ( 4.483927247898545687, 16.52544592524342804, 99.79057627198103830 ) ) ;
#136500=CARTESIAN_POINT ( 'NONE',  ( 18.67979575497178502, 10.72451020669898547, 29.16557627198103120 ) ) ;
#136501=CARTESIAN_POINT ( 'NONE',  ( 5.153800228976335163, 19.02544592524342804, 29.79057627198102409 ) ) ;
#136502=CARTESIAN_POINT ( 'NONE',  ( -16.55341960407617563, 4.379528057220093196, 63.54275706135234003 ) ) ;
#136503=CARTESIAN_POINT ( 'NONE',  ( 10.81492255796078972, 18.62759615963270932, 114.5822429386477097 ) ) ;
#136504=CARTESIAN_POINT ( 'NONE',  ( 13.89961937509957401, 13.97604488694547697, 81.87609039468564731 ) ) ;
#136505=CARTESIAN_POINT ( 'NONE',  ( -5.049401038298153566, 19.05341960407611168, 45.20724293864769550 ) ) ;
#136506=CARTESIAN_POINT ( 'NONE',  ( -0.05219959533907301413, -21.53943276465977519, 67.49890960531436690 ) ) ;
#136507=CARTESIAN_POINT ( 'NONE',  ( 19.05341960407611168, 5.049401038298154454, 108.9572429386477097 ) ) ;
#136508=CARTESIAN_POINT ( 'NONE',  ( 5.719274019375673035, 21.55341960407619339, 87.29275706135236135 ) ) ;
#136509=CARTESIAN_POINT ( 'NONE',  ( 0.05219959533909260263, 19.03943276465977164, 69.99890960531435269 ) ) ;
#136510=CARTESIAN_POINT ( 'NONE',  ( 8.314922557961029526, -14.29746914071037800, 50.41775706135235424 ) ) ;
#136511=CARTESIAN_POINT ( 'NONE',  ( -19.03943276465977164, 0.05219959533909376836, 66.24890960531436690 ) ) ;
#136512=CARTESIAN_POINT ( 'NONE',  ( 21.52544592524334988, 5.823673210054432836, 81.45942372801900433 ) ) ;
#136513=CARTESIAN_POINT ( 'NONE',  ( 0.05219959533936267826, -19.03943276465977164, 35.00109039468566863 ) ) ;
#136514=CARTESIAN_POINT ( 'NONE',  ( -19.03943276465977164, -0.05219959533935918106, 53.75109039468566863 ) ) ;
#136516=CARTESIAN_POINT ( 'NONE',  ( 15.80617190586769283, -15.72974639402175789, 45.62609039468567573 ) ) ;
#136518=CARTESIAN_POINT ( 'NONE',  ( -5.049401038297874678, -19.05341960407617918, 49.79275706135231871 ) ) ;
#136519=CARTESIAN_POINT ( 'NONE',  ( 5.153800228976335163, 19.02544592524342804, 99.79057627198102409 ) ) ;
#136520=CARTESIAN_POINT ( 'NONE',  ( 16.46253265017160672, -9.564922557960803928, 83.33224293864768129 ) ) ;
#136521=CARTESIAN_POINT ( 'NONE',  ( 12.14591786802309770, 12.06949235617756955, 34.37390960531435979 ) ) ;
#136522=CARTESIAN_POINT ( 'NONE',  ( -10.81492255796078084, -18.62759615963271287, 32.08224293864769550 ) ) ;
#136525=CARTESIAN_POINT ( 'NONE',  ( -10.72451020669870658, -18.67979575497194134, 94.58442372801901854 ) ) ;
#136527=CARTESIAN_POINT ( 'NONE',  ( 5.049401038298161559, -19.05341960407611168, 32.70724293864768129 ) ) ;
#136528=CARTESIAN_POINT ( 'NONE',  ( 0.05219959533909260263, 19.03943276465977164, 109.9989096053143669 ) ) ;
#136529=DIRECTION ( 'NONE',  ( 1.000000000000000000, -0.000000000000000000, -0.000000000000000000 ) ) ;
#136530=CARTESIAN_POINT ( 'NONE',  ( -14.34966873604972548, 8.224510206698743886, 48.33442372801902565 ) ) ;
#136531=CARTESIAN_POINT ( 'NONE',  ( -18.62759615963270932, 10.81492255796079327, 75.83224293864769550 ) ) ;
#136532=CARTESIAN_POINT ( 'NONE',  ( 16.53943276465976808, -0.05219959533910856209, 33.74890960531436690 ) ) ;
#136533=CARTESIAN_POINT ( 'NONE',  ( -19.02544592524342804, 5.153800228976336051, 26.04057627198103120 ) ) ;
#136534=CARTESIAN_POINT ( 'NONE',  ( 5.049401038298161559, -19.05341960407611168, 107.7072429386476955 ) ) ;
#136535=CARTESIAN_POINT ( 'NONE',  ( 15.72974639402176855, 15.80617190586768217, 26.87609039468567218 ) ) ;
#136536=CARTESIAN_POINT ( 'NONE',  ( 19.05341960407617918, -5.049401038297876454, 41.04275706135233293 ) ) ;
#136537=CARTESIAN_POINT ( 'NONE',  ( -8.224510206698948167, 14.34966873604960824, 110.4155762719810383 ) ) ;
#136538=CARTESIAN_POINT ( 'NONE',  ( -0.05219959533937732626, 21.53943276465977519, 87.50109039468568994 ) ) ;
#136539=CARTESIAN_POINT ( 'NONE',  ( 17.31747979337950483, -6.344076630960993946, 31.12055131934817354 ) ) ;
#136540=CARTESIAN_POINT ( 'NONE',  ( -12.14591786802309592, -12.06949235617757132, 26.87390960531435979 ) ) ;
#136542=CARTESIAN_POINT ( 'NONE',  ( -15.80617190586745835, -15.72974639402198527, 31.87390960531435979 ) ) ;
#136543=CARTESIAN_POINT ( 'NONE',  ( -16.53943276465976808, 0.05219959533911058130, 91.24890960531436690 ) ) ;
#136545=CARTESIAN_POINT ( 'NONE',  ( -19.02544592524342804, 5.153800228976336051, 76.04057627198102409 ) ) ;
#136546=CARTESIAN_POINT ( 'NONE',  ( -12.06949235617756955, 12.14591786802309770, 80.62390960531438111 ) ) ;
#136547=CARTESIAN_POINT ( 'NONE',  ( 5.049401038297881783, 19.05341960407617563, 112.2927570613523471 ) ) ;
#136548=CARTESIAN_POINT ( 'NONE',  ( -10.72451020669898014, 18.67979575497178502, 60.41557627198102409 ) ) ;
#136549=ORIENTED_EDGE ( 'NONE', *, *, #181095, .F. ) ;
#136551=CARTESIAN_POINT ( 'NONE',  ( -5.049401038298153566, 19.05341960407611168, 35.20724293864768839 ) ) ;
#136552=CARTESIAN_POINT ( 'NONE',  ( -5.049401038298153566, 19.05341960407611168, 70.20724293864769550 ) ) ;
#136553=CARTESIAN_POINT ( 'NONE',  ( 10.81492255796078972, 18.62759615963270932, 69.58224293864769550 ) ) ;
#136554=CARTESIAN_POINT ( 'NONE',  ( 14.34966873604972726, -8.224510206698740333, 105.8344237280190328 ) ) ;
#136555=CARTESIAN_POINT ( 'NONE',  ( 5.049401038298161559, -19.05341960407611168, 82.70724293864770971 ) ) ;
#136556=CARTESIAN_POINT ( 'NONE',  ( -13.89961937509957401, -13.97604488694547875, 64.37609039468567573 ) ) ;
#136557=CARTESIAN_POINT ( 'NONE',  ( -15.72974639402176322, -15.80617190586768395, 99.37609039468568994 ) ) ;
#136558=CARTESIAN_POINT ( 'NONE',  ( -10.81492255796078084, -18.62759615963271287, 77.08224293864769550 ) ) ;
#136559=CARTESIAN_POINT ( 'NONE',  ( -15.80617190586745835, -15.72974639402198527, 21.87390960531436690 ) ) ;
#136560=CARTESIAN_POINT ( 'NONE',  ( 9.564922557960805705, 16.46253265017160317, 49.58224293864770260 ) ) ;
#136561=CARTESIAN_POINT ( 'NONE',  ( 8.224510206698742110, 14.34966873604972548, 97.08442372801904696 ) ) ;
#136562=CARTESIAN_POINT ( 'NONE',  ( 13.97604488694527802, 13.89961937509977652, 64.37390960531436690 ) ) ;
#136564=CARTESIAN_POINT ( 'NONE',  ( -21.55341960407619339, 5.719274019375674811, 103.5427570613523613 ) ) ;
#136565=CARTESIAN_POINT ( 'NONE',  ( -12.14591786802309592, -12.06949235617757132, 66.87390960531436690 ) ) ;
#136567=CARTESIAN_POINT ( 'NONE',  ( -21.55341960407610458, -5.719274019375992779, 111.4572429386476813 ) ) ;
#136568=CARTESIAN_POINT ( 'NONE',  ( 15.72974639402199770, -15.80617190586745480, 98.12390960531436690 ) ) ;
#136569=LINE ( 'NONE', #150766, #62630 ) ;
#136570=CARTESIAN_POINT ( 'NONE',  ( -15.80617190586745835, -15.72974639402198527, 61.87390960531436690 ) ) ;
#136571=CARTESIAN_POINT ( 'NONE',  ( -4.379528057220086978, -16.55341960407618274, 79.79275706135236135 ) ) ;
#136572=CARTESIAN_POINT ( 'NONE',  ( -4.379528057220328563, 16.55341960407611168, 100.2072429386476955 ) ) ;
#136573=CARTESIAN_POINT ( 'NONE',  ( 13.89961937509977652, -13.97604488694527269, 58.12390960531436690 ) ) ;
#136574=CARTESIAN_POINT ( 'NONE',  ( 16.52544592524335698, 4.483927247898782831, 111.4594237280190328 ) ) ;
#136575=CARTESIAN_POINT ( 'NONE',  ( 5.719274019375673035, 21.55341960407619339, 47.29275706135234003 ) ) ;
#136576=CARTESIAN_POINT ( 'NONE',  ( -19.05341960407611168, -5.049401038298163336, 96.45724293864769550 ) ) ;
#136577=CARTESIAN_POINT ( 'NONE',  ( -0.05219959533937732626, 21.53943276465977519, 77.50109039468567573 ) ) ;
#136578=CARTESIAN_POINT ( 'NONE',  ( 13.97604488694527802, 13.89961937509977652, 24.37390960531435624 ) ) ;
#136579=CARTESIAN_POINT ( 'NONE',  ( 13.97604488694527802, 13.89961937509977652, 34.37390960531436690 ) ) ;
#136580=ORIENTED_EDGE ( 'NONE', *, *, #117330, .T. ) ;
#136581=CARTESIAN_POINT ( 'NONE',  ( -10.81492255796105439, 18.62759615963255655, 77.91775706135231871 ) ) ;
#136582=CARTESIAN_POINT ( 'NONE',  ( -16.46253265017160317, 9.564922557960807481, 105.8322429386476955 ) ) ;
#136583=CARTESIAN_POINT ( 'NONE',  ( 13.97604488694548053, -13.89961937509957401, 85.62609039468568994 ) ) ;
#136584=CARTESIAN_POINT ( 'NONE',  ( 10.81492255796106328, -18.62759615963255655, 40.41775706135234714 ) ) ;
#136585=CARTESIAN_POINT ( 'NONE',  ( 0.05219959533934541429, -16.53943276465976808, 20.00109039468568639 ) ) ;
#136586=CARTESIAN_POINT ( 'NONE',  ( -16.51473224551082808, 9.474510206698731452, 68.33442372801900433 ) ) ;
#136587=CARTESIAN_POINT ( 'NONE',  ( 16.46253265017160672, -9.564922557960803928, 53.33224293864768839 ) ) ;
#136588=CARTESIAN_POINT ( 'NONE',  ( -19.05341960407617563, 5.049401038297882671, 83.54275706135233293 ) ) ;
#136589=CARTESIAN_POINT ( 'NONE',  ( 0.05219959533910956823, 16.53943276465976808, 29.99890960531435979 ) ) ;
#136590=CARTESIAN_POINT ( 'NONE',  ( 9.564922557961047289, -16.46253265017146816, 85.41775706135233293 ) ) ;
#136591=CARTESIAN_POINT ( 'NONE',  ( 8.314922557960818139, 14.29746914071049879, 39.58224293864769550 ) ) ;
#136592=CARTESIAN_POINT ( 'NONE',  ( 0.05219959533936267826, -19.03943276465977164, 60.00109039468566863 ) ) ;
#136593=CARTESIAN_POINT ( 'NONE',  ( 12.06949235617739724, 12.14591786802326823, 46.87609039468568994 ) ) ;
#136594=CARTESIAN_POINT ( 'NONE',  ( 9.474510206698729675, 16.51473224551082808, 27.08442372801900433 ) ) ;
#136595=CARTESIAN_POINT ( 'NONE',  ( 19.03943276465977164, -0.05219959533909143690, 38.74890960531436690 ) ) ;
#136596=CARTESIAN_POINT ( 'NONE',  ( -17.50000000000000355, -5.500000000000022204, 66.28230962303567253 ) ) ;
#136597=CARTESIAN_POINT ( 'NONE',  ( 4.379528057220092307, 16.55341960407617563, 47.29275706135234003 ) ) ;
#136600=CARTESIAN_POINT ( 'NONE',  ( 13.89961937509977652, -13.97604488694527269, 93.12390960531436690 ) ) ;
#136601=CARTESIAN_POINT ( 'NONE',  ( -18.22780087662124160, -5.499999999999927169, 68.98236817873106475 ) ) ;
#136602=ORIENTED_EDGE ( 'NONE', *, *, #85875, .F. ) ;
#136603=CARTESIAN_POINT ( 'NONE',  ( -16.51473224551082808, 9.474510206698731452, 88.33442372801900433 ) ) ;
#136604=CARTESIAN_POINT ( 'NONE',  ( 18.62759615963271287, -10.81492255796078972, 23.33224293864769194 ) ) ;
#136605=CARTESIAN_POINT ( 'NONE',  ( -13.97604488694547697, 13.89961937509957934, 23.12609039468565442 ) ) ;
#136606=CARTESIAN_POINT ( 'NONE',  ( -5.153800228976607833, 19.02544592524334988, 102.7094237280189759 ) ) ;
#136607=CARTESIAN_POINT ( 'NONE',  ( -19.05341960407611168, -5.049401038298163336, 21.45724293864768839 ) ) ;
#136608=CARTESIAN_POINT ( 'NONE',  ( -19.05341960407611168, -5.049401038298163336, 36.45724293864766707 ) ) ;
#136609=CARTESIAN_POINT ( 'NONE',  ( 18.62759615963271287, -10.81492255796078972, 58.33224293864768839 ) ) ;
#136610=CARTESIAN_POINT ( 'NONE',  ( -5.153800228976328057, -19.02544592524343514, 22.29057627198102765 ) ) ;
#136611=CARTESIAN_POINT ( 'NONE',  ( 18.22780087662121673, 5.500000000000056843, 78.98459894673892734 ) ) ;
#136612=CARTESIAN_POINT ( 'NONE',  ( 5.049401038297881783, 19.05341960407617563, 72.29275706135234714 ) ) ;
#136613=CARTESIAN_POINT ( 'NONE',  ( 0.05219959533910956823, 16.53943276465976808, 34.99890960531435979 ) ) ;
#136614=CARTESIAN_POINT ( 'NONE',  ( 18.62759615963271287, -10.81492255796078972, 28.33224293864769550 ) ) ;
#136615=CARTESIAN_POINT ( 'NONE',  ( -18.67979575497193778, 10.72451020669871902, 98.33442372801901854 ) ) ;
#136616=CARTESIAN_POINT ( 'NONE',  ( -10.81492255796078084, -18.62759615963271287, 87.08224293864769550 ) ) ;
#136617=CARTESIAN_POINT ( 'NONE',  ( 5.719274019375673035, 21.55341960407619339, 52.29275706135236135 ) ) ;
#136618=CARTESIAN_POINT ( 'NONE',  ( 10.72451020669871369, 18.67979575497193778, 67.08442372801901854 ) ) ;
#136619=CARTESIAN_POINT ( 'NONE',  ( -5.049401038298153566, 19.05341960407611168, 95.20724293864770971 ) ) ;
#136620=CARTESIAN_POINT ( 'NONE',  ( 16.52544592524335698, 4.483927247898782831, 91.45942372801901854 ) ) ;
#136621=CARTESIAN_POINT ( 'NONE',  ( 5.823673210054444382, -21.52544592524334988, 55.20942372801902565 ) ) ;
#136622=CARTESIAN_POINT ( 'NONE',  ( 16.55341960407611168, 4.379528057220329451, 113.9572429386477239 ) ) ;
#136623=CARTESIAN_POINT ( 'NONE',  ( -16.53943276465976808, 0.05219959533911058130, 61.24890960531435979 ) ) ;
#136624=CARTESIAN_POINT ( 'NONE',  ( -16.55341960407611168, -4.379528057220339221, 36.45724293864768839 ) ) ;
#136625=CARTESIAN_POINT ( 'NONE',  ( 5.719274019375991003, -21.55341960407610458, 37.70724293864769550 ) ) ;
#136626=CARTESIAN_POINT ( 'NONE',  ( 19.05341960407611168, 5.049401038298154454, 48.95724293864768129 ) ) ;
#136627=CARTESIAN_POINT ( 'NONE',  ( 21.53943276465977519, -0.05219959533907433946, 53.74890960531437401 ) ) ;
#136628=CARTESIAN_POINT ( 'NONE',  ( 5.153800228976615827, -19.02544592524334988, 45.20942372801901143 ) ) ;
#136630=CARTESIAN_POINT ( 'NONE',  ( -16.53943276465976808, 0.05219959533911058130, 51.24890960531436690 ) ) ;
#136631=CARTESIAN_POINT ( 'NONE',  ( 15.72974639402199770, -15.80617190586745480, 33.12390960531435979 ) ) ;
#136633=ORIENTED_EDGE ( 'NONE', *, *, #185965, .F. ) ;
#136634=CARTESIAN_POINT ( 'NONE',  ( -22.00000000000000000, -5.510910596163089556E-15, 45.00000000000000000 ) ) ;
#136635=CARTESIAN_POINT ( 'NONE',  ( 4.379528057220092307, 16.55341960407617563, 72.29275706135236135 ) ) ;
#136636=CARTESIAN_POINT ( 'NONE',  ( -9.474510206698720793, -16.51473224551083518, 79.58442372801899012 ) ) ;
#136637=CARTESIAN_POINT ( 'NONE',  ( 12.14591786802309770, 12.06949235617756955, 44.37390960531435979 ) ) ;
#136639=CARTESIAN_POINT ( 'NONE',  ( -0.05219959533910754901, -16.53943276465976808, 32.49890960531435979 ) ) ;
#136640=CARTESIAN_POINT ( 'NONE',  ( 13.89961937509977652, -13.97604488694527269, 53.12390960531434558 ) ) ;
#136641=CARTESIAN_POINT ( 'NONE',  ( 13.97604488694527802, 13.89961937509977652, 79.37390960531435269 ) ) ;
#136642=CARTESIAN_POINT ( 'NONE',  ( -0.05219959533909027116, -19.03943276465977164, 42.49890960531435269 ) ) ;
#136643=CARTESIAN_POINT ( 'NONE',  ( 18.62759615963255655, 10.81492255796105972, 46.66775706135234714 ) ) ;
#136644=CARTESIAN_POINT ( 'NONE',  ( -9.474510206698964154, 16.51473224551069663, 55.41557627198103120 ) ) ;
#136646=CARTESIAN_POINT ( 'NONE',  ( 19.03943276465977164, -0.05219959533909143690, 58.74890960531435979 ) ) ;
#136648=CARTESIAN_POINT ( 'NONE',  ( 15.80617190586746368, 15.72974639402197994, 34.37390960531435979 ) ) ;
#136649=CARTESIAN_POINT ( 'NONE',  ( -9.564922557960796823, -16.46253265017161027, 42.08224293864769550 ) ) ;
#136650=CARTESIAN_POINT ( 'NONE',  ( -21.53943276465977519, 0.05219959533907696930, 46.24890960531435979 ) ) ;
#136652=CARTESIAN_POINT ( 'NONE',  ( 8.224510206698742110, 14.34966873604972548, 87.08442372801901854 ) ) ;
#136653=CARTESIAN_POINT ( 'NONE',  ( 10.72451020669871369, 18.67979575497193778, 112.0844237280190185 ) ) ;
#136654=CARTESIAN_POINT ( 'NONE',  ( -4.483927247898782831, 16.52544592524335698, 62.70942372801902565 ) ) ;
#136655=CARTESIAN_POINT ( 'NONE',  ( -5.153800228976328057, -19.02544592524343514, 102.2905762719810383 ) ) ;
#136657=CARTESIAN_POINT ( 'NONE',  ( 0.05219959533934541429, -16.53943276465976808, 55.00109039468568284 ) ) ;
#136658=CARTESIAN_POINT ( 'NONE',  ( -12.14591786802326823, 12.06949235617739902, 43.12609039468568284 ) ) ;
#136659=CARTESIAN_POINT ( 'NONE',  ( 19.03943276465977164, -0.05219959533909143690, 113.7489096053143669 ) ) ;
#136660=CARTESIAN_POINT ( 'NONE',  ( -14.29746914071037622, -8.314922557961029526, 29.16775706135234003 ) ) ;
#136661=CARTESIAN_POINT ( 'NONE',  ( -5.049401038298153566, 19.05341960407611168, 40.20724293864768839 ) ) ;
#136662=CARTESIAN_POINT ( 'NONE',  ( 15.72974639402176855, 15.80617190586768217, 26.87609039468567218 ) ) ;
#136663=CARTESIAN_POINT ( 'NONE',  ( 19.03943276465977164, 0.05219959533936151252, 111.2510903946856757 ) ) ;
#136664=CARTESIAN_POINT ( 'NONE',  ( -8.224510206698735004, -14.34966873604973081, 89.58442372801901854 ) ) ;
#136666=CARTESIAN_POINT ( 'NONE',  ( -15.80617190586768217, 15.72974639402176855, 98.12609039468570415 ) ) ;
#136667=CARTESIAN_POINT ( 'NONE',  ( -13.89961937509957401, -13.97604488694547875, 94.37609039468566152 ) ) ;
#136668=CARTESIAN_POINT ( 'NONE',  ( -16.53943276465976808, 0.05219959533911058130, 51.24890960531436690 ) ) ;
#136669=CARTESIAN_POINT ( 'NONE',  ( 4.379528057220339221, -16.55341960407611168, 102.7072429386476955 ) ) ;
#136670=CARTESIAN_POINT ( 'NONE',  ( 5.153800228976615827, -19.02544592524334988, 45.20942372801901143 ) ) ;
#136672=CARTESIAN_POINT ( 'NONE',  ( -10.72451020669870658, -18.67979575497194134, 49.58442372801901143 ) ) ;
#136673=CARTESIAN_POINT ( 'NONE',  ( -0.05219959533936034679, 19.03943276465977164, 107.5010903946856615 ) ) ;
#136674=CARTESIAN_POINT ( 'NONE',  ( -17.49999999999999645, 5.499999999999992895, 63.71769037696435589 ) ) ;
#136675=CARTESIAN_POINT ( 'NONE',  ( 16.51473224551069308, 9.474510206698969483, 104.1655762719810241 ) ) ;
#136676=CARTESIAN_POINT ( 'NONE',  ( -15.80617190586745835, -15.72974639402198527, 71.87390960531438111 ) ) ;
#136677=CARTESIAN_POINT ( 'NONE',  ( 9.564922557961047289, -16.46253265017146816, 95.41775706135233293 ) ) ;
#136678=CARTESIAN_POINT ( 'NONE',  ( 9.564922557960805705, 16.46253265017160317, 109.5822429386476955 ) ) ;
#136680=CARTESIAN_POINT ( 'NONE',  ( 4.379528057220339221, -16.55341960407611168, 102.7072429386476955 ) ) ;
#136681=CARTESIAN_POINT ( 'NONE',  ( -18.62759615963255300, -10.81492255796106328, 94.16775706135237556 ) ) ;
#136682=CARTESIAN_POINT ( 'NONE',  ( 5.153800228976335163, 19.02544592524342804, 39.79057627198100988 ) ) ;
#136683=CARTESIAN_POINT ( 'NONE',  ( -21.53943276465977519, -0.05219959533937600094, 53.75109039468568994 ) ) ;
#136684=CARTESIAN_POINT ( 'NONE',  ( 10.72451020669871369, 18.67979575497193778, 92.08442372801901854 ) ) ;
#136685=CARTESIAN_POINT ( 'NONE',  ( -8.224510206698735004, -14.34966873604973081, 109.5844237280190328 ) ) ;
#136686=CARTESIAN_POINT ( 'NONE',  ( -16.51473224551069308, -9.474510206698971260, 61.66557627198103120 ) ) ;
#136687=CARTESIAN_POINT ( 'NONE',  ( -10.81492255796105439, 18.62759615963255655, 37.91775706135235424 ) ) ;
#136688=CARTESIAN_POINT ( 'NONE',  ( -10.72451020669870658, -18.67979575497194134, 44.58442372801901854 ) ) ;
#136689=CARTESIAN_POINT ( 'NONE',  ( 0.05219959533936267826, -19.03943276465977164, 70.00109039468566152 ) ) ;
#136690=CARTESIAN_POINT ( 'NONE',  ( 5.153800228976335163, 19.02544592524342804, 94.79057627198103830 ) ) ;
#136691=CARTESIAN_POINT ( 'NONE',  ( 0.05219959533910956823, 16.53943276465976808, 104.9989096053143669 ) ) ;
#136693=CARTESIAN_POINT ( 'NONE',  ( 10.81492255796078972, 18.62759615963270932, 94.58224293864769550 ) ) ;
#136694=CARTESIAN_POINT ( 'NONE',  ( 14.34966873604960469, 8.224510206698951720, 69.16557627198102409 ) ) ;
#136695=CARTESIAN_POINT ( 'NONE',  ( -16.51473224551082808, 9.474510206698731452, 23.33442372801900078 ) ) ;
#136696=CARTESIAN_POINT ( 'NONE',  ( -12.14591786802309592, -12.06949235617757132, 86.87390960531438111 ) ) ;
#136697=CARTESIAN_POINT ( 'NONE',  ( 19.03943276465977164, -0.05219959533909143690, 38.74890960531436690 ) ) ;
#136698=CARTESIAN_POINT ( 'NONE',  ( 0.05219959533936267826, -19.03943276465977164, 90.00109039468567573 ) ) ;
#136699=CARTESIAN_POINT ( 'NONE',  ( -12.14591786802309592, -12.06949235617757132, 51.87390960531437401 ) ) ;
#136700=CARTESIAN_POINT ( 'NONE',  ( -18.67979575497193778, 10.72451020669871902, 93.33442372801901854 ) ) ;
#136701=CARTESIAN_POINT ( 'NONE',  ( 5.049401038298161559, -19.05341960407611168, 87.70724293864769550 ) ) ;
#136702=CARTESIAN_POINT ( 'NONE',  ( -19.02544592524334988, -5.153800228976617603, 78.95942372801900433 ) ) ;
#136703=CARTESIAN_POINT ( 'NONE',  ( -5.719274019375978568, 21.55341960407610458, 75.20724293864769550 ) ) ;
#136704=CARTESIAN_POINT ( 'NONE',  ( 21.53943276465977519, 0.05219959533937863772, 26.25109039468567573 ) ) ;
#136705=CARTESIAN_POINT ( 'NONE',  ( -4.379528057220086978, -16.55341960407618274, 34.79275706135235424 ) ) ;
#136706=CARTESIAN_POINT ( 'NONE',  ( -16.52544592524335698, -4.483927247898792601, 88.95942372801901854 ) ) ;
#136707=CARTESIAN_POINT ( 'NONE',  ( -16.51473224551069308, -9.474510206698971260, 26.66557627198103120 ) ) ;
#136708=CARTESIAN_POINT ( 'NONE',  ( -21.52544592524334988, -5.823673210054445271, 38.95942372801901854 ) ) ;
#136709=CARTESIAN_POINT ( 'NONE',  ( 19.03943276465977164, -0.05219959533909143690, 23.74890960531435269 ) ) ;
#136711=CARTESIAN_POINT ( 'NONE',  ( 0.05219959533934541429, -16.53943276465976808, 55.00109039468568284 ) ) ;
#136712=CARTESIAN_POINT ( 'NONE',  ( 8.314922557960818139, 14.29746914071049879, 74.58224293864768129 ) ) ;
#136713=CARTESIAN_POINT ( 'NONE',  ( -10.72451020669898014, 18.67979575497178502, 80.41557627198103830 ) ) ;
#136714=CARTESIAN_POINT ( 'NONE',  ( 12.06949235617757843, -12.14591786802309237, 28.12390960531435979 ) ) ;
#136715=CARTESIAN_POINT ( 'NONE',  ( -0.05219959533934338120, 16.53943276465976808, 52.50109039468567573 ) ) ;
#136716=CARTESIAN_POINT ( 'NONE',  ( -13.97604488694527625, -13.89961937509977652, 41.87390960531435979 ) ) ;
#136717=CARTESIAN_POINT ( 'NONE',  ( -14.34966873604972548, 8.224510206698743886, 98.33442372801901854 ) ) ;
#136718=CARTESIAN_POINT ( 'NONE',  ( 13.97604488694548053, -13.89961937509957401, 80.62609039468567573 ) ) ;
#136719=CARTESIAN_POINT ( 'NONE',  ( 18.62759615963271287, -10.81492255796078972, 78.33224293864770971 ) ) ;
#136720=CARTESIAN_POINT ( 'NONE',  ( 14.34966873604972726, -8.224510206698740333, 110.8344237280190043 ) ) ;
#136723=CARTESIAN_POINT ( 'NONE',  ( 18.67979575497178502, 10.72451020669898547, 59.16557627198103120 ) ) ;
#136725=CARTESIAN_POINT ( 'NONE',  ( 16.53943276465976808, 0.05219959533934440121, 86.25109039468568994 ) ) ;
#136727=CARTESIAN_POINT ( 'NONE',  ( -5.153800228976328057, -19.02544592524343514, 107.2905762719810383 ) ) ;
#136728=CARTESIAN_POINT ( 'NONE',  ( 17.49999999999999289, 4.640572885337564735, 106.8621183545116082 ) ) ;
#136729=CARTESIAN_POINT ( 'NONE',  ( 18.67979575497178502, 10.72451020669898547, 79.16557627198103830 ) ) ;
#136730=CARTESIAN_POINT ( 'NONE',  ( -8.224510206698735004, -14.34966873604973081, 109.5844237280190328 ) ) ;
#136731=CARTESIAN_POINT ( 'NONE',  ( -19.05341960407617563, 5.049401038297882671, 113.5427570613523471 ) ) ;
#136732=CARTESIAN_POINT ( 'NONE',  ( 0.05219959533909260263, 19.03943276465977164, 24.99890960531435269 ) ) ;
#136733=CARTESIAN_POINT ( 'NONE',  ( 16.53943276465976808, 0.05219959533934440121, 26.25109039468567573 ) ) ;
#136734=CARTESIAN_POINT ( 'NONE',  ( -13.97604488694527625, -13.89961937509977652, 56.87390960531434558 ) ) ;
#136736=CARTESIAN_POINT ( 'NONE',  ( 19.02544592524343514, -5.153800228976328945, 103.5405762719809957 ) ) ;
#136737=CARTESIAN_POINT ( 'NONE',  ( -14.34966873604972548, 8.224510206698743886, 93.33442372801901854 ) ) ;
#136738=CARTESIAN_POINT ( 'NONE',  ( 13.89961937509957401, 13.97604488694547697, 96.87609039468566152 ) ) ;
#136739=CARTESIAN_POINT ( 'NONE',  ( -16.51473224551082808, 9.474510206698731452, 23.33442372801900078 ) ) ;
#136740=CARTESIAN_POINT ( 'NONE',  ( 15.80617190586746368, 15.72974639402197994, 79.37390960531436690 ) ) ;
#136741=CARTESIAN_POINT ( 'NONE',  ( 16.52544592524335698, 4.483927247898782831, 106.4594237280190328 ) ) ;
#136743=CARTESIAN_POINT ( 'NONE',  ( -19.02544592524334988, -5.153800228976617603, 93.95942372801900433 ) ) ;
#136744=CARTESIAN_POINT ( 'NONE',  ( -9.474510206698964154, 16.51473224551069663, 55.41557627198103120 ) ) ;
#136745=CARTESIAN_POINT ( 'NONE',  ( -0.05219959533909027116, -19.03943276465977164, 92.49890960531436690 ) ) ;
#136746=CARTESIAN_POINT ( 'NONE',  ( 21.52544592524334988, 5.823673210054432836, 56.45942372801902565 ) ) ;
#136747=CARTESIAN_POINT ( 'NONE',  ( 19.05341960407611168, 5.049401038298154454, 63.95724293864769550 ) ) ;
#136748=CARTESIAN_POINT ( 'NONE',  ( -0.05219959533910754901, -16.53943276465976808, 92.49890960531436690 ) ) ;
#136750=CARTESIAN_POINT ( 'NONE',  ( -16.55341960407611168, -4.379528057220339221, 76.45724293864769550 ) ) ;
#136751=CARTESIAN_POINT ( 'NONE',  ( -15.72974639402197994, 15.80617190586746368, 80.62390960531438111 ) ) ;
#136753=CARTESIAN_POINT ( 'NONE',  ( 16.61371651742602396, -7.165104196376141488, 81.35415069992998838 ) ) ;
#136754=CARTESIAN_POINT ( 'NONE',  ( 19.05341960407617918, -5.049401038297876454, 46.04275706135233293 ) ) ;
#136755=CARTESIAN_POINT ( 'NONE',  ( 17.26172910966714724, -6.454744622557085698, 73.30646908649207205 ) ) ;
#136756=CARTESIAN_POINT ( 'NONE',  ( 16.51473224551069308, 9.474510206698969483, 74.16557627198103830 ) ) ;
#136757=CARTESIAN_POINT ( 'NONE',  ( -19.02544592524342804, 5.153800228976336051, 86.04057627198103830 ) ) ;
#136758=CARTESIAN_POINT ( 'NONE',  ( 8.224510206698742110, 14.34966873604972548, 62.08442372801901143 ) ) ;
#136760=CARTESIAN_POINT ( 'NONE',  ( -16.46253265017146816, -9.564922557961047289, 49.16775706135233293 ) ) ;
#136762=CARTESIAN_POINT ( 'NONE',  ( 19.02544592524343514, -5.153800228976328945, 108.5405762719810383 ) ) ;
#136763=CARTESIAN_POINT ( 'NONE',  ( 14.29746914071037800, 8.314922557961029526, 86.66775706135234714 ) ) ;
#136765=CARTESIAN_POINT ( 'NONE',  ( -14.29746914071037622, -8.314922557961029526, 74.16775706135231871 ) ) ;
#136766=DIRECTION ( 'NONE',  ( 0.000000000000000000, -1.000000000000000000, 0.000000000000000000 ) ) ;
#136767=CARTESIAN_POINT ( 'NONE',  ( 12.14591786802327356, -12.06949235617739191, 55.62609039468568284 ) ) ;
#136768=CARTESIAN_POINT ( 'NONE',  ( -16.46253265017160317, 9.564922557960807481, 75.83224293864769550 ) ) ;
#136769=CARTESIAN_POINT ( 'NONE',  ( 21.53943276465977519, 0.05219959533937863772, 61.25109039468567573 ) ) ;
#136770=CARTESIAN_POINT ( 'NONE',  ( -9.474510206698720793, -16.51473224551083518, 79.58442372801899012 ) ) ;
#136771=CARTESIAN_POINT ( 'NONE',  ( 5.153800228976615827, -19.02544592524334988, 20.20942372801899722 ) ) ;
#136772=CARTESIAN_POINT ( 'NONE',  ( -5.049401038298153566, 19.05341960407611168, 50.20724293864770260 ) ) ;
#136773=CARTESIAN_POINT ( 'NONE',  ( 5.153800228976335163, 19.02544592524342804, 44.79057627198103830 ) ) ;
#136774=CARTESIAN_POINT ( 'NONE',  ( 16.62544781628812274, 7.153289815129877383, 22.00000000000000000 ) ) ;
#136775=CARTESIAN_POINT ( 'NONE',  ( 5.719274019375991003, -21.55341960407610458, 62.70724293864769550 ) ) ;
#136777=CARTESIAN_POINT ( 'NONE',  ( 19.05341960407611168, 5.049401038298154454, 113.9572429386477097 ) ) ;
#136778=CARTESIAN_POINT ( 'NONE',  ( 4.379528057220339221, -16.55341960407611168, 112.7072429386476955 ) ) ;
#136779=CARTESIAN_POINT ( 'NONE',  ( -14.29746914071037622, -8.314922557961029526, 54.16775706135235424 ) ) ;
#136780=ORIENTED_EDGE ( 'NONE', *, *, #87285, .F. ) ;
#136781=CARTESIAN_POINT ( 'NONE',  ( -21.53943276465977519, -0.05219959533937600094, 23.75109039468567929 ) ) ;
#136782=CARTESIAN_POINT ( 'NONE',  ( -16.53943276465976808, 0.05219959533911058130, 51.24890960531436690 ) ) ;
#136784=CARTESIAN_POINT ( 'NONE',  ( -0.05219959533936034679, 19.03943276465977164, 107.5010903946856615 ) ) ;
#136785=CARTESIAN_POINT ( 'NONE',  ( 5.049401038297881783, 19.05341960407617563, 37.29275706135232582 ) ) ;
#136786=CARTESIAN_POINT ( 'NONE',  ( 12.14591786802309770, 12.06949235617756955, 39.37390960531436690 ) ) ;
#136787=CARTESIAN_POINT ( 'NONE',  ( -10.81492255796105439, 18.62759615963255655, 22.91775706135235069 ) ) ;
#136788=CARTESIAN_POINT ( 'NONE',  ( 17.12812012977024878, 6.668231424566067211, 33.85948759323144941 ) ) ;
#136789=CARTESIAN_POINT ( 'NONE',  ( 10.72451020669898902, -18.67979575497178502, 57.91557627198103120 ) ) ;
#136790=CARTESIAN_POINT ( 'NONE',  ( 19.02544592524343514, -5.153800228976328945, 93.54057627198102409 ) ) ;
#136791=CARTESIAN_POINT ( 'NONE',  ( -16.53943276465976808, 0.05219959533911058130, 56.24890960531436690 ) ) ;
#136792=CARTESIAN_POINT ( 'NONE',  ( 5.049401038298161559, -19.05341960407611168, 107.7072429386476955 ) ) ;
#136794=CARTESIAN_POINT ( 'NONE',  ( -19.03943276465977164, -0.05219959533935918106, 48.75109039468566863 ) ) ;
#136795=CARTESIAN_POINT ( 'NONE',  ( -18.67979575497178146, -10.72451020669898902, 91.66557627198103830 ) ) ;
#136796=CARTESIAN_POINT ( 'NONE',  ( 13.97604488694527802, 13.89961937509977652, 49.37390960531434558 ) ) ;
#136797=B_SPLINE_CURVE_WITH_KNOTS ( 'NONE', 3,
 ( #81462, #92675, #32019, #66319, #187706, #49178, #46188, #154363 ),
 .UNSPECIFIED., .F., .F.,
 ( 4, 2, 2, 4 ),
 ( 2.110382192020081086E-17, 0.002784256700436093385, 0.005568513400872164218, 0.01113702680174430762 ),
 .UNSPECIFIED. ) ;
#136798=CARTESIAN_POINT ( 'NONE',  ( -4.379528057220328563, 16.55341960407611168, 110.2072429386477239 ) ) ;
#136800=CARTESIAN_POINT ( 'NONE',  ( 5.823673210054444382, -21.52544592524334988, 45.20942372801901854 ) ) ;
#136802=CARTESIAN_POINT ( 'NONE',  ( 14.34966873604960469, 8.224510206698951720, 24.16557627198103120 ) ) ;
#136803=CARTESIAN_POINT ( 'NONE',  ( -16.46253265017160317, 9.564922557960807481, 55.83224293864769550 ) ) ;
#136804=CARTESIAN_POINT ( 'NONE',  ( 19.05341960407611168, 5.049401038298154454, 93.95724293864769550 ) ) ;
#136805=CARTESIAN_POINT ( 'NONE',  ( 5.719274019375991003, -21.55341960407610458, 72.70724293864769550 ) ) ;
#136807=CARTESIAN_POINT ( 'NONE',  ( 5.153800228976335163, 19.02544592524342804, 49.79057627198100988 ) ) ;
#136808=CARTESIAN_POINT ( 'NONE',  ( 21.52544592524344225, -5.823673210054117533, 48.54057627198103120 ) ) ;
#136811=CARTESIAN_POINT ( 'NONE',  ( -15.72974639402176322, -15.80617190586768395, 89.37609039468568994 ) ) ;
#136813=CARTESIAN_POINT ( 'NONE',  ( 14.29746914071037800, 8.314922557961029526, 76.66775706135234714 ) ) ;
#136814=CARTESIAN_POINT ( 'NONE',  ( 12.14591786802309770, 12.06949235617756955, 64.37390960531435269 ) ) ;
#136815=CARTESIAN_POINT ( 'NONE',  ( 9.564922557960805705, 16.46253265017160317, 74.58224293864769550 ) ) ;
#136817=CARTESIAN_POINT ( 'NONE',  ( -13.89961937509957401, -13.97604488694547875, 29.37609039468565797 ) ) ;
#136818=CARTESIAN_POINT ( 'NONE',  ( -14.29746914071037622, -8.314922557961029526, 89.16775706135236135 ) ) ;
#136819=CARTESIAN_POINT ( 'NONE',  ( 10.81492255796106328, -18.62759615963255655, 110.4177570613523756 ) ) ;
#136820=CARTESIAN_POINT ( 'NONE',  ( -5.049401038298153566, 19.05341960407611168, 75.20724293864769550 ) ) ;
#136821=CARTESIAN_POINT ( 'NONE',  ( -5.823673210054116645, -21.52544592524344225, 47.29057627198103120 ) ) ;
#136822=CARTESIAN_POINT ( 'NONE',  ( -16.55341960407617563, 4.379528057220093196, 28.54275706135234358 ) ) ;
#136823=CARTESIAN_POINT ( 'NONE',  ( -21.53943276465977519, -0.05219959533937600094, 88.75109039468567573 ) ) ;
#136824=CARTESIAN_POINT ( 'NONE',  ( -16.55341960407617563, 4.379528057220093196, 68.54275706135234714 ) ) ;
#136825=CARTESIAN_POINT ( 'NONE',  ( -18.62759615963270932, 10.81492255796079327, 110.8322429386476955 ) ) ;
#136826=CARTESIAN_POINT ( 'NONE',  ( 19.03943276465977164, 0.05219959533936151252, 111.2510903946856757 ) ) ;
#136827=CARTESIAN_POINT ( 'NONE',  ( -9.474510206698964154, 16.51473224551069663, 85.41557627198102409 ) ) ;
#136829=CARTESIAN_POINT ( 'NONE',  ( -14.34966873604972548, 8.224510206698743886, 33.33442372801900433 ) ) ;
#136830=CARTESIAN_POINT ( 'NONE',  ( 16.51473224551069308, 9.474510206698969483, 59.16557627198102409 ) ) ;
#136831=CARTESIAN_POINT ( 'NONE',  ( 12.14591786802327356, -12.06949235617739191, 30.62609039468567929 ) ) ;
#136832=CARTESIAN_POINT ( 'NONE',  ( -12.06949235617756955, 12.14591786802309770, 85.62390960531436690 ) ) ;
#136833=CARTESIAN_POINT ( 'NONE',  ( -8.224510206698735004, -14.34966873604973081, 89.58442372801901854 ) ) ;
#136834=CARTESIAN_POINT ( 'NONE',  ( -5.719274019375665041, -21.55341960407619695, 24.79275706135235779 ) ) ;
#136835=CARTESIAN_POINT ( 'NONE',  ( 13.97604488694527802, 13.89961937509977652, 69.37390960531436690 ) ) ;
#136836=CARTESIAN_POINT ( 'NONE',  ( 19.03943276465977164, -0.05219959533909143690, 78.74890960531436690 ) ) ;
#136837=CARTESIAN_POINT ( 'NONE',  ( -0.05219959533934338120, 16.53943276465976808, 87.50109039468568994 ) ) ;
#136839=ORIENTED_EDGE ( 'NONE', *, *, #95776, .F. ) ;
#136841=CARTESIAN_POINT ( 'NONE',  ( 5.153800228976615827, -19.02544592524334988, 30.20942372801900433 ) ) ;
#136842=CARTESIAN_POINT ( 'NONE',  ( 9.564922557960805705, 16.46253265017160317, 104.5822429386476955 ) ) ;
#136843=CARTESIAN_POINT ( 'NONE',  ( -19.03943276465977164, 0.05219959533909376836, 46.24890960531435979 ) ) ;
#136844=CARTESIAN_POINT ( 'NONE',  ( 16.51473224551069308, 9.474510206698969483, 114.1655762719810241 ) ) ;
#136845=CARTESIAN_POINT ( 'NONE',  ( 12.06949235617739724, 12.14591786802326823, 31.87609039468567929 ) ) ;
#136846=CARTESIAN_POINT ( 'NONE',  ( -16.46253265017146816, -9.564922557961047289, 54.16775706135234003 ) ) ;
#136847=CARTESIAN_POINT ( 'NONE',  ( -14.29746914071037622, -8.314922557961029526, 39.16775706135235424 ) ) ;
#136848=CARTESIAN_POINT ( 'NONE',  ( -16.51473224551069308, -9.474510206698971260, 111.6655762719810383 ) ) ;
#136849=CARTESIAN_POINT ( 'NONE',  ( 19.02544592524343514, -5.153800228976328945, 78.54057627198099567 ) ) ;
#136850=CARTESIAN_POINT ( 'NONE',  ( 18.67979575497178502, 10.72451020669898547, 99.16557627198100988 ) ) ;
#136851=CARTESIAN_POINT ( 'NONE',  ( -5.049401038297874678, -19.05341960407617918, 69.79275706135233293 ) ) ;
#136852=CARTESIAN_POINT ( 'NONE',  ( -19.05341960407611168, -5.049401038298163336, 86.45724293864769550 ) ) ;
#136853=CARTESIAN_POINT ( 'NONE',  ( 17.49809244619821413, -3.610541912967066835, 21.90429107297349987 ) ) ;
#136854=CARTESIAN_POINT ( 'NONE',  ( 5.049401038298161559, -19.05341960407611168, 67.70724293864769550 ) ) ;
#136855=CARTESIAN_POINT ( 'NONE',  ( -8.224510206698948167, 14.34966873604960824, 35.41557627198102409 ) ) ;
#136856=CARTESIAN_POINT ( 'NONE',  ( 0.05219959533909260263, 19.03943276465977164, 24.99890960531435269 ) ) ;
#136857=CARTESIAN_POINT ( 'NONE',  ( -0.05219959533936034679, 19.03943276465977164, 37.50109039468567573 ) ) ;
#136858=CARTESIAN_POINT ( 'NONE',  ( 12.06949235617757843, -12.14591786802309237, 78.12390960531436690 ) ) ;
#136859=CARTESIAN_POINT ( 'NONE',  ( 15.80617190586769283, -15.72974639402175789, 95.62609039468568994 ) ) ;
#136860=CARTESIAN_POINT ( 'NONE',  ( 19.02544592524343514, -5.153800228976328945, 33.54057627198102409 ) ) ;
#136861=CARTESIAN_POINT ( 'NONE',  ( -0.05219959533934338120, 16.53943276465976808, 57.50109039468568994 ) ) ;
#136862=CARTESIAN_POINT ( 'NONE',  ( -4.483927247898539470, -16.52544592524342804, 42.29057627198103120 ) ) ;
#136863=CARTESIAN_POINT ( 'NONE',  ( 18.67979575497194134, -10.72451020669871369, 100.8344237280190185 ) ) ;
#136864=CARTESIAN_POINT ( 'NONE',  ( -19.05341960407611168, -5.049401038298163336, 91.45724293864766707 ) ) ;
#136865=CARTESIAN_POINT ( 'NONE',  ( -19.02544592524342804, 5.153800228976336051, 96.04057627198103830 ) ) ;
#136866=CARTESIAN_POINT ( 'NONE',  ( 0.05219959533909260263, 19.03943276465977164, 24.99890960531435269 ) ) ;
#136867=CARTESIAN_POINT ( 'NONE',  ( 14.29746914071049879, -8.314922557960816363, 103.3322429386476955 ) ) ;
#136868=CARTESIAN_POINT ( 'NONE',  ( 0.05219959533910956823, 16.53943276465976808, 79.99890960531435269 ) ) ;
#136869=CARTESIAN_POINT ( 'NONE',  ( 21.55341960407610458, 5.719274019375980345, 78.95724293864769550 ) ) ;
#136870=CARTESIAN_POINT ( 'NONE',  ( -16.46253265017160317, 9.564922557960807481, 85.83224293864769550 ) ) ;
#136871=CARTESIAN_POINT ( 'NONE',  ( 5.823673210054125526, 21.52544592524343514, 99.79057627198103830 ) ) ;
#136872=CARTESIAN_POINT ( 'NONE',  ( -13.97604488694527625, -13.89961937509977652, 86.87390960531436690 ) ) ;
#136874=CARTESIAN_POINT ( 'NONE',  ( -12.14591786802309592, -12.06949235617757132, 86.87390960531438111 ) ) ;
#136875=CARTESIAN_POINT ( 'NONE',  ( -5.153800228976328057, -19.02544592524343514, 57.29057627198103120 ) ) ;
#136876=CARTESIAN_POINT ( 'NONE',  ( -21.55341960407610458, -5.719274019375992779, 71.45724293864769550 ) ) ;
#136878=CARTESIAN_POINT ( 'NONE',  ( 8.314922557960818139, 14.29746914071049879, 24.58224293864768839 ) ) ;
#136880=CARTESIAN_POINT ( 'NONE',  ( 12.06949235617739724, 12.14591786802326823, 21.87609039468567573 ) ) ;
#136881=CARTESIAN_POINT ( 'NONE',  ( 4.379528057220339221, -16.55341960407611168, 77.70724293864770971 ) ) ;
#136882=CARTESIAN_POINT ( 'NONE',  ( -17.44270441346516165, -5.991230190323025617, 96.36335079264230785 ) ) ;
#136883=CARTESIAN_POINT ( 'NONE',  ( -16.46253265017160317, 9.564922557960807481, 80.83224293864769550 ) ) ;
#136884=CARTESIAN_POINT ( 'NONE',  ( 0.05219959533909260263, 19.03943276465977164, 49.99890960531435979 ) ) ;
#136885=CARTESIAN_POINT ( 'NONE',  ( -16.55341960407611168, -4.379528057220339221, 66.45724293864768129 ) ) ;
#136887=CARTESIAN_POINT ( 'NONE',  ( -19.03943276465977164, 0.05219959533909376836, 111.2489096053143669 ) ) ;
#136888=CARTESIAN_POINT ( 'NONE',  ( -19.03943276465977164, -0.05219959533935918106, 98.75109039468567573 ) ) ;
#136889=CARTESIAN_POINT ( 'NONE',  ( 5.719274019375673035, 21.55341960407619339, 57.29275706135234714 ) ) ;
#136890=CARTESIAN_POINT ( 'NONE',  ( -5.049401038298153566, 19.05341960407611168, 105.2072429386476671 ) ) ;
#136891=CARTESIAN_POINT ( 'NONE',  ( 21.55341960407610458, 5.719274019375980345, 78.95724293864769550 ) ) ;
#136892=CARTESIAN_POINT ( 'NONE',  ( 8.224510206698742110, 14.34966873604972548, 67.08442372801901854 ) ) ;
#136893=CARTESIAN_POINT ( 'NONE',  ( 5.153800228976335163, 19.02544592524342804, 29.79057627198102409 ) ) ;
#136894=CARTESIAN_POINT ( 'NONE',  ( -16.46253265017160317, 9.564922557960807481, 75.83224293864769550 ) ) ;
#136895=CARTESIAN_POINT ( 'NONE',  ( 21.53943276465977519, -0.05219959533907433946, 83.74890960531435269 ) ) ;
#136896=CARTESIAN_POINT ( 'NONE',  ( -13.97604488694547697, 13.89961937509957934, 113.1260903946856757 ) ) ;
#136897=CARTESIAN_POINT ( 'NONE',  ( -16.53943276465976808, 0.05219959533911058130, 41.24890960531435269 ) ) ;
#136898=CARTESIAN_POINT ( 'NONE',  ( 0.05219959533937995610, -21.53943276465977519, 60.00109039468568284 ) ) ;
#136899=CARTESIAN_POINT ( 'NONE',  ( 16.52544592524335698, 4.483927247898782831, 91.45942372801901854 ) ) ;
#136900=CARTESIAN_POINT ( 'NONE',  ( -9.564922557960796823, -16.46253265017161027, 102.0822429386477097 ) ) ;
#136901=CARTESIAN_POINT ( 'NONE',  ( -16.51473224551069308, -9.474510206698971260, 106.6655762719810383 ) ) ;
#136903=CARTESIAN_POINT ( 'NONE',  ( 16.52544592524335698, 4.483927247898782831, 91.45942372801901854 ) ) ;
#136904=CARTESIAN_POINT ( 'NONE',  ( -14.29746914071037622, -8.314922557961029526, 49.16775706135234003 ) ) ;
#136905=CARTESIAN_POINT ( 'NONE',  ( -13.89961937509977652, 13.97604488694528158, 55.62390960531434558 ) ) ;
#136906=CARTESIAN_POINT ( 'NONE',  ( 16.46253265017160672, -9.564922557960803928, 68.33224293864770971 ) ) ;
#136907=CARTESIAN_POINT ( 'NONE',  ( 10.81492255796106328, -18.62759615963255655, 65.41775706135234714 ) ) ;
#136908=CARTESIAN_POINT ( 'NONE',  ( 8.314922557961029526, -14.29746914071037800, 65.41775706135234714 ) ) ;
#136909=CARTESIAN_POINT ( 'NONE',  ( -16.52544592524342804, 4.483927247898546575, 51.04057627198103120 ) ) ;
#136910=CARTESIAN_POINT ( 'NONE',  ( -9.474510206698964154, 16.51473224551069663, 45.41557627198103120 ) ) ;
#136911=CARTESIAN_POINT ( 'NONE',  ( -9.564922557960796823, -16.46253265017161027, 52.08224293864768839 ) ) ;
#136912=CARTESIAN_POINT ( 'NONE',  ( 12.06949235617739724, 12.14591786802326823, 46.87609039468568994 ) ) ;
#136913=CARTESIAN_POINT ( 'NONE',  ( -16.51473224551082808, 9.474510206698731452, 93.33442372801900433 ) ) ;
#136914=CARTESIAN_POINT ( 'NONE',  ( -14.29746914071049879, 8.314922557960819915, 90.83224293864769550 ) ) ;
#136915=CARTESIAN_POINT ( 'NONE',  ( -19.02544592524342804, 5.153800228976336051, 66.04057627198103830 ) ) ;
#136916=CARTESIAN_POINT ( 'NONE',  ( -19.02544592524334988, -5.153800228976617603, 103.9594237280190043 ) ) ;
#136917=CARTESIAN_POINT ( 'NONE',  ( 30.00000000000000000, 5.499999999999992895, 102.5000000000000142 ) ) ;
#136918=CARTESIAN_POINT ( 'NONE',  ( -15.72974639402176322, -15.80617190586768395, 94.37609039468568994 ) ) ;
#136919=CARTESIAN_POINT ( 'NONE',  ( 8.224510206698742110, 14.34966873604972548, 67.08442372801901854 ) ) ;
#136921=CARTESIAN_POINT ( 'NONE',  ( 5.719274019375991003, -21.55341960407610458, 52.70724293864769550 ) ) ;
#136922=CARTESIAN_POINT ( 'NONE',  ( -16.53943276465976808, -0.05219959533934237506, 48.75109039468568284 ) ) ;
#136923=CARTESIAN_POINT ( 'NONE',  ( -19.53037848336980886, 5.499999999999899636, 69.85532783611442653 ) ) ;
#136924=CARTESIAN_POINT ( 'NONE',  ( 0.05219959533936267826, -19.03943276465977164, 45.00109039468566863 ) ) ;
#136925=CARTESIAN_POINT ( 'NONE',  ( -19.03943276465977164, 0.05219959533909376836, 96.24890960531436690 ) ) ;
#136926=CARTESIAN_POINT ( 'NONE',  ( 5.153800228976335163, 19.02544592524342804, 24.79057627198102765 ) ) ;
#136927=CARTESIAN_POINT ( 'NONE',  ( -19.02544592524342804, 5.153800228976336051, 46.04057627198101699 ) ) ;
#136928=DIRECTION ( 'NONE',  ( 1.000000000000000000, -0.000000000000000000, -0.000000000000000000 ) ) ;
#136929=CARTESIAN_POINT ( 'NONE',  ( -5.719274019375665041, -21.55341960407619695, 74.79275706135234714 ) ) ;
#136931=CARTESIAN_POINT ( 'NONE',  ( -19.02544592524334988, -5.153800228976617603, 28.95942372801900433 ) ) ;
#136932=CARTESIAN_POINT ( 'NONE',  ( -0.05219959533936034679, 19.03943276465977164, 22.50109039468566152 ) ) ;
#136933=CARTESIAN_POINT ( 'NONE',  ( 0.05219959533910956823, 16.53943276465976808, 54.99890960531435269 ) ) ;
#136934=CARTESIAN_POINT ( 'NONE',  ( -13.89961937509977652, 13.97604488694528158, 55.62390960531434558 ) ) ;
#136935=CARTESIAN_POINT ( 'NONE',  ( 10.72451020669898902, -18.67979575497178502, 22.91557627198102765 ) ) ;
#136936=CARTESIAN_POINT ( 'NONE',  ( 18.67979575497194134, -10.72451020669871369, 80.83442372801901854 ) ) ;
#136937=CARTESIAN_POINT ( 'NONE',  ( -5.153800228976328057, -19.02544592524343514, 62.29057627198100988 ) ) ;
#136938=CARTESIAN_POINT ( 'NONE',  ( 10.81492255796106328, -18.62759615963255655, 75.41775706135233293 ) ) ;
#136939=CARTESIAN_POINT ( 'NONE',  ( -18.62759615963270932, 10.81492255796079327, 30.83224293864770260 ) ) ;
#136940=CARTESIAN_POINT ( 'NONE',  ( 18.62759615963255655, 10.81492255796105972, 36.66775706135234714 ) ) ;
#136941=CARTESIAN_POINT ( 'NONE',  ( -5.153800228976607833, 19.02544592524334988, 67.70942372801900433 ) ) ;
#136942=CARTESIAN_POINT ( 'NONE',  ( 13.97604488694527802, 13.89961937509977652, 44.37390960531435269 ) ) ;
#136943=CARTESIAN_POINT ( 'NONE',  ( -9.564922557960796823, -16.46253265017161027, 82.08224293864768129 ) ) ;
#136944=CARTESIAN_POINT ( 'NONE',  ( -12.06949235617739369, -12.14591786802326823, 34.37609039468568284 ) ) ;
#136945=CARTESIAN_POINT ( 'NONE',  ( 16.53943276465976808, -0.05219959533910856209, 88.74890960531436690 ) ) ;
#136946=CARTESIAN_POINT ( 'NONE',  ( 13.97604488694527802, 13.89961937509977652, 54.37390960531435979 ) ) ;
#136947=CARTESIAN_POINT ( 'NONE',  ( -10.72451020669898014, 18.67979575497178502, 45.41557627198103830 ) ) ;
#136948=CARTESIAN_POINT ( 'NONE',  ( -8.224510206698735004, -14.34966873604973081, 19.58442372801901143 ) ) ;
#136949=CARTESIAN_POINT ( 'NONE',  ( 5.719274019375673035, 21.55341960407619339, 22.29275706135235069 ) ) ;
#136950=CARTESIAN_POINT ( 'NONE',  ( 10.72451020669871369, 18.67979575497193778, 72.08442372801899012 ) ) ;
#136951=CARTESIAN_POINT ( 'NONE',  ( -12.14591786802326823, 12.06949235617739902, 73.12609039468567573 ) ) ;
#136952=CARTESIAN_POINT ( 'NONE',  ( -8.224510206698735004, -14.34966873604973081, 74.58442372801901854 ) ) ;
#136954=CARTESIAN_POINT ( 'NONE',  ( 0.05219959533909260263, 19.03943276465977164, 54.99890960531435979 ) ) ;
#136955=CARTESIAN_POINT ( 'NONE',  ( -12.14591786802326823, 12.06949235617739902, 88.12609039468570415 ) ) ;
#136956=CARTESIAN_POINT ( 'NONE',  ( 16.51473224551083163, -9.474510206698727899, 40.83442372801900433 ) ) ;
#136957=CARTESIAN_POINT ( 'NONE',  ( -5.719274019375665041, -21.55341960407619695, 19.79275706135235069 ) ) ;
#136958=CARTESIAN_POINT ( 'NONE',  ( 14.34966873604960469, 8.224510206698951720, 59.16557627198103120 ) ) ;
#136959=CARTESIAN_POINT ( 'NONE',  ( -16.51473224551069308, -9.474510206698971260, 81.66557627198103830 ) ) ;
#136960=CARTESIAN_POINT ( 'NONE',  ( -16.55341960407617563, 4.379528057220093196, 93.54275706135234714 ) ) ;
#136961=CARTESIAN_POINT ( 'NONE',  ( 18.62759615963255655, 10.81492255796105972, 61.66775706135235424 ) ) ;
#136962=CARTESIAN_POINT ( 'NONE',  ( -12.14591786802326823, 12.06949235617739902, 38.12609039468567573 ) ) ;
#136963=CARTESIAN_POINT ( 'NONE',  ( -10.72451020669898014, 18.67979575497178502, 105.4155762719810383 ) ) ;
#136964=CARTESIAN_POINT ( 'NONE',  ( -4.483927247898539470, -16.52544592524342804, 62.29057627198102409 ) ) ;
#136966=CARTESIAN_POINT ( 'NONE',  ( 21.53943276465977519, -0.05219959533907433946, 103.7489096053143669 ) ) ;
#136967=CARTESIAN_POINT ( 'NONE',  ( 12.06949235617757843, -12.14591786802309237, 38.12390960531436690 ) ) ;
#136970=CARTESIAN_POINT ( 'NONE',  ( 16.46253265017160672, -9.564922557960803928, 108.3322429386476955 ) ) ;
#136971=CARTESIAN_POINT ( 'NONE',  ( -21.53943276465977519, -0.05219959533937600094, 38.75109039468567573 ) ) ;
#136972=CARTESIAN_POINT ( 'NONE',  ( -16.55341960407611168, -4.379528057220339221, 71.45724293864769550 ) ) ;
#136973=VECTOR ( 'NONE', #191866, 1000.000000000000000 ) ;
#136974=CARTESIAN_POINT ( 'NONE',  ( 19.02544592524343514, -5.153800228976328945, 63.54057627198103830 ) ) ;
#136975=CARTESIAN_POINT ( 'NONE',  ( 16.46253265017146816, 9.564922557961045513, 61.66775706135234003 ) ) ;
#136976=CARTESIAN_POINT ( 'NONE',  ( 21.52544592524344225, -5.823673210054117533, 53.54057627198103120 ) ) ;
#136978=CARTESIAN_POINT ( 'NONE',  ( -0.05219959533909027116, -19.03943276465977164, 57.49890960531435979 ) ) ;
#136979=CARTESIAN_POINT ( 'NONE',  ( 4.483927247898790824, -16.52544592524335698, 40.20942372801901854 ) ) ;
#136980=CARTESIAN_POINT ( 'NONE',  ( -18.67979575497193778, 10.72451020669871902, 23.33442372801901499 ) ) ;
#136981=CARTESIAN_POINT ( 'NONE',  ( -16.55341960407611168, -4.379528057220339221, 51.45724293864770260 ) ) ;
#136983=CARTESIAN_POINT ( 'NONE',  ( -13.97604488694527625, -13.89961937509977652, 86.87390960531436690 ) ) ;
#136984=CARTESIAN_POINT ( 'NONE',  ( 21.53943276465977519, -0.05219959533907433946, 68.74890960531435269 ) ) ;
#136985=CARTESIAN_POINT ( 'NONE',  ( -21.53943276465977519, 0.05219959533907696930, 111.2489096053143669 ) ) ;
#136986=CARTESIAN_POINT ( 'NONE',  ( -16.53943276465976808, -0.05219959533934237506, 38.75109039468567573 ) ) ;
#136987=CARTESIAN_POINT ( 'NONE',  ( -10.81492255796078084, -18.62759615963271287, 32.08224293864769550 ) ) ;
#136988=CARTESIAN_POINT ( 'NONE',  ( -21.53943276465977519, -0.05219959533937600094, 103.7510903946857042 ) ) ;
#136989=CARTESIAN_POINT ( 'NONE',  ( -5.153800228976328057, -19.02544592524343514, 102.2905762719810383 ) ) ;
#136990=CARTESIAN_POINT ( 'NONE',  ( -19.05341960407611168, -5.049401038298163336, 46.45724293864768129 ) ) ;
#136991=CARTESIAN_POINT ( 'NONE',  ( 5.049401038298161559, -19.05341960407611168, 92.70724293864769550 ) ) ;
#136992=CARTESIAN_POINT ( 'NONE',  ( -9.474510206698964154, 16.51473224551069663, 75.41557627198103830 ) ) ;
#136994=CARTESIAN_POINT ( 'NONE',  ( -19.02544592524334988, -5.153800228976617603, 53.95942372801898301 ) ) ;
#136995=CARTESIAN_POINT ( 'NONE',  ( -21.55341960407619339, 5.719274019375674811, 108.5427570613523756 ) ) ;
#136996=CARTESIAN_POINT ( 'NONE',  ( 18.67979575497178502, 10.72451020669898547, 29.16557627198103120 ) ) ;
#136997=CARTESIAN_POINT ( 'NONE',  ( 12.06949235617739724, 12.14591786802326823, 101.8760903946857042 ) ) ;
#136998=CARTESIAN_POINT ( 'NONE',  ( -9.564922557961040184, 16.46253265017147172, 72.91775706135233293 ) ) ;
#137000=CARTESIAN_POINT ( 'NONE',  ( 17.59860650958989936, 7.585241751807028088, 39.07662985737508166 ) ) ;
#137001=CARTESIAN_POINT ( 'NONE',  ( -0.05219959533936034679, 19.03943276465977164, 82.50109039468567573 ) ) ;
#137002=CARTESIAN_POINT ( 'NONE',  ( -13.89961937509957401, -13.97604488694547875, 34.37609039468566863 ) ) ;
#137003=CARTESIAN_POINT ( 'NONE',  ( 13.97604488694527802, 13.89961937509977652, 39.37390960531435269 ) ) ;
#137004=CARTESIAN_POINT ( 'NONE',  ( 12.14591786802309770, 12.06949235617756955, 44.37390960531435979 ) ) ;
#137005=CARTESIAN_POINT ( 'NONE',  ( -17.44279575226825685, -5.990770900252416098, 109.1644243248568387 ) ) ;
#137006=CARTESIAN_POINT ( 'NONE',  ( 8.314922557960818139, 14.29746914071049879, 29.58224293864769905 ) ) ;
#137008=CARTESIAN_POINT ( 'NONE',  ( -14.34966873604972548, 8.224510206698743886, 88.33442372801901854 ) ) ;
#137009=CARTESIAN_POINT ( 'NONE',  ( 5.153800228976335163, 19.02544592524342804, 54.79057627198103120 ) ) ;
#137010=CARTESIAN_POINT ( 'NONE',  ( 15.72974639402176855, 15.80617190586768217, 106.8760903946856899 ) ) ;
#137011=CARTESIAN_POINT ( 'NONE',  ( -8.314922557961024197, 14.29746914071037800, 22.91775706135235069 ) ) ;
#137012=CARTESIAN_POINT ( 'NONE',  ( 18.67979575497194134, -10.72451020669871369, 90.83442372801901854 ) ) ;
#137013=CARTESIAN_POINT ( 'NONE',  ( -19.02544592524342804, 5.153800228976336051, 91.04057627198100988 ) ) ;
#137014=CARTESIAN_POINT ( 'NONE',  ( -19.05341960407611168, -5.049401038298163336, 86.45724293864769550 ) ) ;
#137016=CARTESIAN_POINT ( 'NONE',  ( -10.72451020669898014, 18.67979575497178502, 105.4155762719810383 ) ) ;
#137017=CARTESIAN_POINT ( 'NONE',  ( -16.55341960407611168, -4.379528057220339221, 81.45724293864769550 ) ) ;
#137019=CARTESIAN_POINT ( 'NONE',  ( -0.05219959533907301413, -21.53943276465977519, 72.49890960531435269 ) ) ;
#137020=CARTESIAN_POINT ( 'NONE',  ( 5.049401038298161559, -19.05341960407611168, 62.70724293864769550 ) ) ;
#137021=CARTESIAN_POINT ( 'NONE',  ( -10.81492255796078084, -18.62759615963271287, 97.08224293864770971 ) ) ;
#137022=CARTESIAN_POINT ( 'NONE',  ( 12.14591786802327356, -12.06949235617739191, 85.62609039468568994 ) ) ;
#137024=CARTESIAN_POINT ( 'NONE',  ( 16.46253265017160672, -9.564922557960803928, 58.33224293864769550 ) ) ;
#137025=CARTESIAN_POINT ( 'NONE',  ( -16.52544592524342804, 4.483927247898546575, 86.04057627198102409 ) ) ;
#137027=CARTESIAN_POINT ( 'NONE',  ( 5.049401038298161559, -19.05341960407611168, 47.70724293864770260 ) ) ;
#137028=CARTESIAN_POINT ( 'NONE',  ( 0.05219959533936267826, -19.03943276465977164, 85.00109039468567573 ) ) ;
#137029=CARTESIAN_POINT ( 'NONE',  ( -16.53943276465976808, 0.05219959533911058130, 86.24890960531436690 ) ) ;
#137030=CARTESIAN_POINT ( 'NONE',  ( 15.72974639402176855, 15.80617190586768217, 61.87609039468568284 ) ) ;
#137031=CARTESIAN_POINT ( 'NONE',  ( -0.05219959533909027116, -19.03943276465977164, 32.49890960531435979 ) ) ;
#137032=CARTESIAN_POINT ( 'NONE',  ( 18.67979575497178502, 10.72451020669898547, 99.16557627198100988 ) ) ;
#137033=CARTESIAN_POINT ( 'NONE',  ( -4.483927247898539470, -16.52544592524342804, 102.2905762719810383 ) ) ;
#137035=CARTESIAN_POINT ( 'NONE',  ( 19.03943276465977164, -0.05219959533909143690, 63.74890960531435979 ) ) ;
#137036=CARTESIAN_POINT ( 'NONE',  ( 17.40861289039003879, 6.110651285853319514, 113.8723247082744052 ) ) ;
#137037=CARTESIAN_POINT ( 'NONE',  ( 19.02544592524334988, 5.153800228976608722, 101.4594237280189759 ) ) ;
#137038=CARTESIAN_POINT ( 'NONE',  ( -13.97604488694527625, -13.89961937509977652, 106.8739096053143669 ) ) ;
#137039=CARTESIAN_POINT ( 'NONE',  ( -21.52544592524334988, -5.823673210054445271, 43.95942372801902565 ) ) ;
#137040=CARTESIAN_POINT ( 'NONE',  ( -13.97604488694527625, -13.89961937509977652, 81.87390960531436690 ) ) ;
#137041=CARTESIAN_POINT ( 'NONE',  ( -0.05219959533936034679, 19.03943276465977164, 72.50109039468566152 ) ) ;
#137042=CARTESIAN_POINT ( 'NONE',  ( 19.02544592524343514, -5.153800228976328945, 63.54057627198103830 ) ) ;
#137043=CARTESIAN_POINT ( 'NONE',  ( 14.29746914071049879, -8.314922557960816363, 73.33224293864769550 ) ) ;
#137044=CARTESIAN_POINT ( 'NONE',  ( -8.314922557960811034, -14.29746914071050412, 67.08224293864770971 ) ) ;
#137045=CARTESIAN_POINT ( 'NONE',  ( 13.97604488694527802, 13.89961937509977652, 84.37390960531433848 ) ) ;
#137046=CARTESIAN_POINT ( 'NONE',  ( -8.224510206698948167, 14.34966873604960824, 80.41557627198103830 ) ) ;
#137047=CARTESIAN_POINT ( 'NONE',  ( -16.51473224551069308, -9.474510206698971260, 86.66557627198102409 ) ) ;
#137050=CARTESIAN_POINT ( 'NONE',  ( -13.89961937509957401, -13.97604488694547875, 29.37609039468565797 ) ) ;
#137051=CARTESIAN_POINT ( 'NONE',  ( -16.51473224551069308, -9.474510206698971260, 46.66557627198102409 ) ) ;
#137052=CARTESIAN_POINT ( 'NONE',  ( -14.34966873604960291, -8.224510206698953496, 26.66557627198103475 ) ) ;
#137053=CARTESIAN_POINT ( 'NONE',  ( 8.224510206698953496, -14.34966873604960469, 112.9155762719810383 ) ) ;
#137055=CARTESIAN_POINT ( 'NONE',  ( -15.72974639402176322, -15.80617190586768395, 39.37609039468567573 ) ) ;
#137056=CARTESIAN_POINT ( 'NONE',  ( 19.05341960407617918, -5.049401038297876454, 71.04275706135234714 ) ) ;
#137057=CARTESIAN_POINT ( 'NONE',  ( 14.29746914071049879, -8.314922557960816363, 38.33224293864768839 ) ) ;
#137058=CARTESIAN_POINT ( 'NONE',  ( 0.05219959533907565091, 21.53943276465977519, 79.99890960531435269 ) ) ;
#137059=CARTESIAN_POINT ( 'NONE',  ( -5.823673210054116645, -21.52544592524344225, 22.29057627198102765 ) ) ;
#137060=CARTESIAN_POINT ( 'NONE',  ( 8.314922557960818139, 14.29746914071049879, 74.58224293864768129 ) ) ;
#137061=CARTESIAN_POINT ( 'NONE',  ( 9.564922557960805705, 16.46253265017160317, 39.58224293864768839 ) ) ;
#137062=CARTESIAN_POINT ( 'NONE',  ( -0.05219959533936034679, 19.03943276465977164, 37.50109039468567573 ) ) ;
#137063=CARTESIAN_POINT ( 'NONE',  ( 14.29746914071037800, 8.314922557961029526, 101.6677570613523613 ) ) ;
#137064=CARTESIAN_POINT ( 'NONE',  ( 14.34966873604972726, -8.224510206698740333, 60.83442372801901854 ) ) ;
#137065=CARTESIAN_POINT ( 'NONE',  ( -10.72451020669898014, 18.67979575497178502, 35.41557627198102409 ) ) ;
#137066=CARTESIAN_POINT ( 'NONE',  ( 5.719274019375673035, 21.55341960407619339, 102.2927570613523613 ) ) ;
#137067=CARTESIAN_POINT ( 'NONE',  ( -19.05341960407611168, -5.049401038298163336, 91.45724293864766707 ) ) ;
#137068=CARTESIAN_POINT ( 'NONE',  ( 16.55341960407618274, -4.379528057220086978, 76.04275706135237556 ) ) ;
#137069=CARTESIAN_POINT ( 'NONE',  ( 12.06949235617757843, -12.14591786802309237, 113.1239096053143953 ) ) ;
#137070=CARTESIAN_POINT ( 'NONE',  ( 14.34966873604960469, 8.224510206698951720, 29.16557627198103120 ) ) ;
#137071=CARTESIAN_POINT ( 'NONE',  ( -16.46253265017160317, 9.564922557960807481, 110.8322429386476955 ) ) ;
#137072=CARTESIAN_POINT ( 'NONE',  ( -16.46253265017160317, 9.564922557960807481, 85.83224293864769550 ) ) ;
#137073=CARTESIAN_POINT ( 'NONE',  ( -19.02544592524342804, 5.153800228976336051, 116.0405762719810383 ) ) ;
#137075=CARTESIAN_POINT ( 'NONE',  ( 4.379528057220339221, -16.55341960407611168, 62.70724293864769550 ) ) ;
#137076=CARTESIAN_POINT ( 'NONE',  ( -16.53943276465976808, 0.05219959533911058130, 36.24890960531435979 ) ) ;
#137077=CARTESIAN_POINT ( 'NONE',  ( 4.483927247898545687, 16.52544592524342804, 54.79057627198104541 ) ) ;
#137078=CARTESIAN_POINT ( 'NONE',  ( -12.14591786802326823, 12.06949235617739902, 53.12609039468568284 ) ) ;
#137079=CARTESIAN_POINT ( 'NONE',  ( -13.89961937509957401, -13.97604488694547697, 59.37609039468566863 ) ) ;
#137081=CARTESIAN_POINT ( 'NONE',  ( 9.564922557961047289, -16.46253265017146816, 50.41775706135233293 ) ) ;
#137082=CARTESIAN_POINT ( 'NONE',  ( 9.564922557960805705, 16.46253265017160317, 94.58224293864769550 ) ) ;
#137083=CARTESIAN_POINT ( 'NONE',  ( 16.46253265017146816, 9.564922557961045513, 71.66775706135233293 ) ) ;
#137085=CARTESIAN_POINT ( 'NONE',  ( 13.97604488694548053, -13.89961937509957401, 50.62609039468566152 ) ) ;
#137086=CARTESIAN_POINT ( 'NONE',  ( -19.02544592524334988, -5.153800228976617603, 93.95942372801900433 ) ) ;
#137087=CARTESIAN_POINT ( 'NONE',  ( -0.05219959533934338120, 16.53943276465976808, 97.50109039468567573 ) ) ;
#137090=CARTESIAN_POINT ( 'NONE',  ( -16.51473224551069308, -9.474510206698971260, 21.66557627198102765 ) ) ;
#137092=CARTESIAN_POINT ( 'NONE',  ( 13.89961937509977652, -13.97604488694527269, 113.1239096053143527 ) ) ;
#137093=CARTESIAN_POINT ( 'NONE',  ( 10.81492255796106328, -18.62759615963255655, 40.41775706135234714 ) ) ;
#137094=CARTESIAN_POINT ( 'NONE',  ( 13.97604488694548053, -13.89961937509957401, 105.6260903946856757 ) ) ;
#137095=CARTESIAN_POINT ( 'NONE',  ( 17.50000000000147793, -3.254303733634592799, 107.5239589307140591 ) ) ;
#137096=CARTESIAN_POINT ( 'NONE',  ( 0.05219959533909260263, 19.03943276465977164, 54.99890960531435979 ) ) ;
#137097=CARTESIAN_POINT ( 'NONE',  ( 0.05219959533909260263, 19.03943276465977164, 99.99890960531436690 ) ) ;
#137098=CARTESIAN_POINT ( 'NONE',  ( -4.379528057220328563, 16.55341960407611168, 75.20724293864769550 ) ) ;
#137099=CARTESIAN_POINT ( 'NONE',  ( 5.153800228976335163, 19.02544592524342804, 59.79057627198100988 ) ) ;
#137100=CARTESIAN_POINT ( 'NONE',  ( -16.46253265017160317, 9.564922557960807481, 75.83224293864769550 ) ) ;
#137101=CARTESIAN_POINT ( 'NONE',  ( 5.153800228976615827, -19.02544592524334988, 80.20942372801901854 ) ) ;
#137102=CARTESIAN_POINT ( 'NONE',  ( -21.52544592524343514, 5.823673210054127303, 51.04057627198103120 ) ) ;
#137103=CARTESIAN_POINT ( 'NONE',  ( 12.06949235617757843, -12.14591786802309237, 108.1239096053143811 ) ) ;
#137104=CARTESIAN_POINT ( 'NONE',  ( -13.89961937509957401, -13.97604488694547875, 49.37609039468567573 ) ) ;
#137105=CARTESIAN_POINT ( 'NONE',  ( 13.89961937509977652, -13.97604488694527269, 73.12390960531436690 ) ) ;
#137106=CARTESIAN_POINT ( 'NONE',  ( -10.81492255796078084, -18.62759615963271287, 72.08224293864769550 ) ) ;
#137107=CARTESIAN_POINT ( 'NONE',  ( -8.224510206698948167, 14.34966873604960824, 80.41557627198103830 ) ) ;
#137108=CARTESIAN_POINT ( 'NONE',  ( -5.049401038297874678, -19.05341960407617918, 54.79275706135234003 ) ) ;
#137109=CARTESIAN_POINT ( 'NONE',  ( 15.80617190586746368, 15.72974639402197994, 74.37390960531436690 ) ) ;
#137110=CARTESIAN_POINT ( 'NONE',  ( 15.72974639402199770, -15.80617190586745480, 58.12390960531435979 ) ) ;
#137111=CARTESIAN_POINT ( 'NONE',  ( -21.52544592524343514, 5.823673210054127303, 46.04057627198103830 ) ) ;
#137112=CARTESIAN_POINT ( 'NONE',  ( 10.81492255796106328, -18.62759615963255655, 90.41775706135236135 ) ) ;
#137113=CARTESIAN_POINT ( 'NONE',  ( 16.51473224551069308, 9.474510206698969483, 69.16557627198102409 ) ) ;
#137114=CARTESIAN_POINT ( 'NONE',  ( 16.51473224551069308, 9.474510206698969483, 24.16557627198102765 ) ) ;
#137116=CARTESIAN_POINT ( 'NONE',  ( 21.55341960407619695, -5.719274019375665929, 21.04275706135234714 ) ) ;
#137117=CARTESIAN_POINT ( 'NONE',  ( -21.53943276465977519, -0.05219959533937600094, 38.75109039468567573 ) ) ;
#137118=CARTESIAN_POINT ( 'NONE',  ( 9.564922557960805705, 16.46253265017160317, 29.58224293864769550 ) ) ;
#137119=CARTESIAN_POINT ( 'NONE',  ( -15.80617190586745835, -15.72974639402198527, 106.8739096053143811 ) ) ;
#137120=CARTESIAN_POINT ( 'NONE',  ( 16.51473224551083163, -9.474510206698727899, 55.83442372801899722 ) ) ;
#137121=CARTESIAN_POINT ( 'NONE',  ( 9.564922557960805705, 16.46253265017160317, 34.58224293864770260 ) ) ;
#137122=CARTESIAN_POINT ( 'NONE',  ( 14.34966873604972726, -8.224510206698740333, 25.83442372801901499 ) ) ;
#137123=CARTESIAN_POINT ( 'NONE',  ( 8.314922557961029526, -14.29746914071037800, 55.41775706135234714 ) ) ;
#137124=CARTESIAN_POINT ( 'NONE',  ( 16.51473224551069308, 9.474510206698969483, 34.16557627198102409 ) ) ;
#137126=CARTESIAN_POINT ( 'NONE',  ( 16.51473224551069308, 9.474510206698969483, 89.16557627198103830 ) ) ;
#137127=CARTESIAN_POINT ( 'NONE',  ( 12.14591786802309770, 12.06949235617756955, 104.3739096053143669 ) ) ;
#137128=CARTESIAN_POINT ( 'NONE',  ( -18.62759615963270932, 10.81492255796079327, 60.83224293864769550 ) ) ;
#137129=CARTESIAN_POINT ( 'NONE',  ( 16.55341960407618274, -4.379528057220086978, 46.04275706135234714 ) ) ;
#137130=CARTESIAN_POINT ( 'NONE',  ( -15.72974639402176322, -15.80617190586768395, 99.37609039468568994 ) ) ;
#137131=CARTESIAN_POINT ( 'NONE',  ( -16.51473224551069308, -9.474510206698971260, 41.66557627198103120 ) ) ;
#137132=CARTESIAN_POINT ( 'NONE',  ( 4.483927247898790824, -16.52544592524335698, 105.2094237280190328 ) ) ;
#137133=CARTESIAN_POINT ( 'NONE',  ( 8.224510206698953496, -14.34966873604960469, 57.91557627198103120 ) ) ;
#137134=CARTESIAN_POINT ( 'NONE',  ( 0.05219959533909260263, 19.03943276465977164, 64.99890960531436690 ) ) ;
#137135=CARTESIAN_POINT ( 'NONE',  ( 15.72974639402176855, 15.80617190586768217, 106.8760903946856899 ) ) ;
#137136=CARTESIAN_POINT ( 'NONE',  ( 18.62759615963255655, 10.81492255796105972, 21.66775706135235069 ) ) ;
#137137=CARTESIAN_POINT ( 'NONE',  ( 5.823673210054444382, -21.52544592524334988, 80.20942372801901854 ) ) ;
#137138=CARTESIAN_POINT ( 'NONE',  ( 16.53943276465976808, 0.05219959533934440121, 46.25109039468567573 ) ) ;
#137139=CARTESIAN_POINT ( 'NONE',  ( -16.53943276465976808, -0.05219959533934237506, 33.75109039468568284 ) ) ;
#137140=CARTESIAN_POINT ( 'NONE',  ( 14.34966873604960469, 8.224510206698951720, 74.16557627198102409 ) ) ;
#137141=CARTESIAN_POINT ( 'NONE',  ( 21.55341960407619695, -5.719274019375665929, 106.0427570613523471 ) ) ;
#137142=CARTESIAN_POINT ( 'NONE',  ( -8.224510206698948167, 14.34966873604960824, 30.41557627198101699 ) ) ;
#137143=CARTESIAN_POINT ( 'NONE',  ( -16.18388926212238133, 7.379444403734517266, 114.5604684863385359 ) ) ;
#137144=CARTESIAN_POINT ( 'NONE',  ( 14.34966873604972726, -8.224510206698740333, 40.83442372801901854 ) ) ;
#137145=CARTESIAN_POINT ( 'NONE',  ( 8.224510206698953496, -14.34966873604960469, 52.91557627198103830 ) ) ;
#137146=CARTESIAN_POINT ( 'NONE',  ( 12.06949235617739724, 12.14591786802326823, 91.87609039468568994 ) ) ;
#137147=CARTESIAN_POINT ( 'NONE',  ( -0.05219959533909027116, -19.03943276465977164, 97.49890960531436690 ) ) ;
#137148=CARTESIAN_POINT ( 'NONE',  ( 0.05219959533907565091, 21.53943276465977519, 24.99890960531435624 ) ) ;
#137149=CARTESIAN_POINT ( 'NONE',  ( -21.52544592524334988, -5.823673210054445271, 98.95942372801903275 ) ) ;
#137150=CARTESIAN_POINT ( 'NONE',  ( -4.483927247898539470, -16.52544592524342804, 82.29057627198103830 ) ) ;
#137151=CARTESIAN_POINT ( 'NONE',  ( 19.02544592524343514, -5.153800228976328945, 98.54057627198100988 ) ) ;
#137153=CARTESIAN_POINT ( 'NONE',  ( 8.314922557961029526, -14.29746914071037800, 35.41775706135234003 ) ) ;
#137154=CARTESIAN_POINT ( 'NONE',  ( 19.03943276465977164, -0.05219959533909143690, 38.74890960531436690 ) ) ;
#137155=CARTESIAN_POINT ( 'NONE',  ( -19.05341960407611168, -5.049401038298163336, 106.4572429386476955 ) ) ;
#137156=CARTESIAN_POINT ( 'NONE',  ( 12.14591786802327356, -12.06949235617739191, 40.62609039468567573 ) ) ;
#137157=CARTESIAN_POINT ( 'NONE',  ( 18.09873248133752810, 5.499999999999960032, 101.4839295033382882 ) ) ;
#137158=CARTESIAN_POINT ( 'NONE',  ( -9.474510206698720793, -16.51473224551083518, 34.58442372801899722 ) ) ;
#137159=CARTESIAN_POINT ( 'NONE',  ( -5.049401038298153566, 19.05341960407611168, 45.20724293864769550 ) ) ;
#137160=CARTESIAN_POINT ( 'NONE',  ( -16.55341960407617563, 4.379528057220093196, 78.54275706135236135 ) ) ;
#137161=CARTESIAN_POINT ( 'NONE',  ( -5.153800228976607833, 19.02544592524334988, 77.70942372801900433 ) ) ;
#137162=CARTESIAN_POINT ( 'NONE',  ( 9.564922557961047289, -16.46253265017146816, 25.41775706135234003 ) ) ;
#137163=CARTESIAN_POINT ( 'NONE',  ( -13.97604488694527625, -13.89961937509977652, 66.87390960531436690 ) ) ;
#137164=CARTESIAN_POINT ( 'NONE',  ( -4.483927247898539470, -16.52544592524342804, 102.2905762719810383 ) ) ;
#137165=CARTESIAN_POINT ( 'NONE',  ( 0.05219959533936267826, -19.03943276465977164, 65.00109039468567573 ) ) ;
#137166=CARTESIAN_POINT ( 'NONE',  ( 21.52544592524344225, -5.823673210054117533, 58.54057627198103120 ) ) ;
#137167=CARTESIAN_POINT ( 'NONE',  ( -0.05219959533936034679, 19.03943276465977164, 32.50109039468566863 ) ) ;
#137168=CARTESIAN_POINT ( 'NONE',  ( 13.89961937509977652, -13.97604488694527269, 108.1239096053143669 ) ) ;
#137169=CONICAL_SURFACE ( 'NONE', #20826, 2.500000000000002220, 1.029744260000000189 ) ;
#137170=CARTESIAN_POINT ( 'NONE',  ( -10.81492255796078084, -18.62759615963271287, 72.08224293864769550 ) ) ;
#137171=CARTESIAN_POINT ( 'NONE',  ( -16.51473224551069308, -9.474510206698971260, 106.6655762719810383 ) ) ;
#137172=CARTESIAN_POINT ( 'NONE',  ( 16.51473224551083163, -9.474510206698727899, 95.83442372801900433 ) ) ;
#137173=CARTESIAN_POINT ( 'NONE',  ( -9.474510206698964154, 16.51473224551069663, 110.4155762719810383 ) ) ;
#137174=CARTESIAN_POINT ( 'NONE',  ( 16.52544592524335698, 4.483927247898782831, 21.45942372801901499 ) ) ;
#137175=CARTESIAN_POINT ( 'NONE',  ( 19.02544592524343514, -5.153800228976328945, 33.54057627198102409 ) ) ;
#137176=CARTESIAN_POINT ( 'NONE',  ( 16.46253265017160672, -9.564922557960803928, 93.33224293864769550 ) ) ;
#137177=CARTESIAN_POINT ( 'NONE',  ( -5.719274019375978568, 21.55341960407610458, 95.20724293864769550 ) ) ;
#137178=CARTESIAN_POINT ( 'NONE',  ( 10.81492255796106328, -18.62759615963255655, 60.41775706135235424 ) ) ;
#137179=CARTESIAN_POINT ( 'NONE',  ( -0.05219959533936034679, 19.03943276465977164, 102.5010903946856757 ) ) ;
#137180=CARTESIAN_POINT ( 'NONE',  ( -5.823673210054431948, 21.52544592524334988, 112.7094237280190328 ) ) ;
#137181=CARTESIAN_POINT ( 'NONE',  ( 12.06949235617739724, 12.14591786802326823, 111.8760903946856615 ) ) ;
#137182=CARTESIAN_POINT ( 'NONE',  ( -10.72451020669898014, 18.67979575497178502, 100.4155762719810241 ) ) ;
#137183=CARTESIAN_POINT ( 'NONE',  ( -16.52544592524342804, 4.483927247898546575, 36.04057627198102409 ) ) ;
#137184=CARTESIAN_POINT ( 'NONE',  ( 19.03943276465977164, 0.05219959533936151252, 86.25109039468567573 ) ) ;
#137186=CARTESIAN_POINT ( 'NONE',  ( 5.049401038297881783, 19.05341960407617563, 57.29275706135231871 ) ) ;
#137187=CARTESIAN_POINT ( 'NONE',  ( 21.53943276465977519, 0.05219959533937863772, 56.25109039468568284 ) ) ;
#137188=CARTESIAN_POINT ( 'NONE',  ( 9.564922557961047289, -16.46253265017146816, 40.41775706135234003 ) ) ;
#137189=CARTESIAN_POINT ( 'NONE',  ( 16.55341960407611168, 4.379528057220329451, 103.9572429386476813 ) ) ;
#137190=CARTESIAN_POINT ( 'NONE',  ( 18.62759615963271287, -10.81492255796078972, 33.33224293864769550 ) ) ;
#137191=CARTESIAN_POINT ( 'NONE',  ( 8.224510206698953496, -14.34966873604960469, 37.91557627198102409 ) ) ;
#137193=CARTESIAN_POINT ( 'NONE',  ( 15.72974639402176855, 15.80617190586768217, 96.87609039468568994 ) ) ;
#137194=CARTESIAN_POINT ( 'NONE',  ( -16.52544592524335698, -4.483927247898792601, 68.95942372801901854 ) ) ;
#137195=CARTESIAN_POINT ( 'NONE',  ( 16.52544592524342804, -4.483927247898539470, 28.54057627198103120 ) ) ;
#137196=CARTESIAN_POINT ( 'NONE',  ( 15.72974639402176855, 15.80617190586768217, 61.87609039468568284 ) ) ;
#137197=CARTESIAN_POINT ( 'NONE',  ( -21.53943276465977519, -0.05219959533937600094, 68.75109039468568994 ) ) ;
#137198=CARTESIAN_POINT ( 'NONE',  ( -18.62759615963270932, 10.81492255796079327, 65.83224293864769550 ) ) ;
#137200=CARTESIAN_POINT ( 'NONE',  ( 5.049401038298161559, -19.05341960407611168, 22.70724293864769194 ) ) ;
#137201=CARTESIAN_POINT ( 'NONE',  ( -15.80617190586768217, 15.72974639402176855, 43.12609039468568284 ) ) ;
#137202=CARTESIAN_POINT ( 'NONE',  ( 4.483927247898545687, 16.52544592524342804, 114.7905762719810383 ) ) ;
#137203=CARTESIAN_POINT ( 'NONE',  ( 16.46253265017160672, -9.564922557960803928, 33.33224293864770260 ) ) ;
#137204=CARTESIAN_POINT ( 'NONE',  ( -8.224510206698948167, 14.34966873604960824, 85.41557627198102409 ) ) ;
#137205=CARTESIAN_POINT ( 'NONE',  ( -19.02544592524342804, 5.153800228976336051, 81.04057627198103830 ) ) ;
#137206=CARTESIAN_POINT ( 'NONE',  ( 16.53943276465976808, -0.05219959533910856209, 28.74890960531435624 ) ) ;
#137207=CARTESIAN_POINT ( 'NONE',  ( -21.52544592524343514, 5.823673210054127303, 71.04057627198103830 ) ) ;
#137208=CARTESIAN_POINT ( 'NONE',  ( -0.05219959533907301413, -21.53943276465977519, 107.4989096053143669 ) ) ;
#137209=CARTESIAN_POINT ( 'NONE',  ( -5.153800228976328057, -19.02544592524343514, 112.2905762719810099 ) ) ;
#137210=CARTESIAN_POINT ( 'NONE',  ( -19.05341960407611168, -5.049401038298163336, 71.45724293864766707 ) ) ;
#137211=CARTESIAN_POINT ( 'NONE',  ( 5.153800228976615827, -19.02544592524334988, 105.2094237280190185 ) ) ;
#137212=CARTESIAN_POINT ( 'NONE',  ( 21.55341960407610458, 5.719274019375980345, 63.95724293864770260 ) ) ;
#137213=CARTESIAN_POINT ( 'NONE',  ( 21.55341960407619695, -5.719274019375665929, 76.04275706135237556 ) ) ;
#137214=CARTESIAN_POINT ( 'NONE',  ( -13.89961937509977652, 13.97604488694528158, 60.62390960531436690 ) ) ;
#137215=CARTESIAN_POINT ( 'NONE',  ( -9.474510206698964154, 16.51473224551069663, 100.4155762719810241 ) ) ;
#137216=CARTESIAN_POINT ( 'NONE',  ( 8.224510206698742110, 14.34966873604972548, 77.08442372801901854 ) ) ;
#137217=CARTESIAN_POINT ( 'NONE',  ( 15.72974639402176855, 15.80617190586768217, 51.87609039468568284 ) ) ;
#137218=CARTESIAN_POINT ( 'NONE',  ( -0.05219959533937732626, 21.53943276465977519, 82.50109039468568994 ) ) ;
#137219=CARTESIAN_POINT ( 'NONE',  ( -5.719274019375978568, 21.55341960407610458, 115.2072429386476955 ) ) ;
#137221=CARTESIAN_POINT ( 'NONE',  ( -5.823673210054116645, -21.52544592524344225, 72.29057627198102409 ) ) ;
#137222=CARTESIAN_POINT ( 'NONE',  ( -13.89961937509957401, -13.97604488694547875, 49.37609039468567573 ) ) ;
#137223=CARTESIAN_POINT ( 'NONE',  ( -18.62759615963270932, 10.81492255796079327, 35.83224293864768839 ) ) ;
#137224=VECTOR ( 'NONE', #111630, 1000.000000000000000 ) ;
#137225=CARTESIAN_POINT ( 'NONE',  ( 5.153800228976335163, 19.02544592524342804, 84.79057627198099567 ) ) ;
#137226=CARTESIAN_POINT ( 'NONE',  ( -0.05219959533910754901, -16.53943276465976808, 32.49890960531435979 ) ) ;
#137230=CARTESIAN_POINT ( 'NONE',  ( 19.05341960407617918, -5.049401038297876454, 91.04275706135234714 ) ) ;
#137231=CARTESIAN_POINT ( 'NONE',  ( -5.719274019375978568, 21.55341960407610458, 65.20724293864768129 ) ) ;
#137232=CARTESIAN_POINT ( 'NONE',  ( -12.14591786802309592, -12.06949235617757132, 56.87390960531436690 ) ) ;
#137233=CARTESIAN_POINT ( 'NONE',  ( -4.483927247898782831, 16.52544592524335698, 32.70942372801900433 ) ) ;
#137234=CARTESIAN_POINT ( 'NONE',  ( 5.153800228976335163, 19.02544592524342804, 44.79057627198103830 ) ) ;
#137235=CARTESIAN_POINT ( 'NONE',  ( -18.62759615963270932, 10.81492255796079327, 100.8322429386477097 ) ) ;
#137236=CARTESIAN_POINT ( 'NONE',  ( -16.51473224551082808, 9.474510206698731452, 68.33442372801900433 ) ) ;
#137237=CARTESIAN_POINT ( 'NONE',  ( -9.564922557960796823, -16.46253265017161027, 87.08224293864769550 ) ) ;
#137238=CARTESIAN_POINT ( 'NONE',  ( 4.483927247898545687, 16.52544592524342804, 89.79057627198103830 ) ) ;
#137239=CARTESIAN_POINT ( 'NONE',  ( -19.03943276465977164, 0.05219959533909376836, 61.24890960531436690 ) ) ;
#137240=CARTESIAN_POINT ( 'NONE',  ( -8.224510206698948167, 14.34966873604960824, 70.41557627198102409 ) ) ;
#137241=CARTESIAN_POINT ( 'NONE',  ( 19.05341960407611168, 5.049401038298154454, 38.95724293864767418 ) ) ;
#137242=CARTESIAN_POINT ( 'NONE',  ( -17.10208260729133301, -5.355177916403385474, 20.80190055885774569 ) ) ;
#137243=CARTESIAN_POINT ( 'NONE',  ( 14.34966873604960469, 8.224510206698951720, 44.16557627198103120 ) ) ;
#137244=CARTESIAN_POINT ( 'NONE',  ( -19.03943276465977164, 0.05219959533909376836, 86.24890960531436690 ) ) ;
#137246=CARTESIAN_POINT ( 'NONE',  ( -16.51473224551082808, 9.474510206698731452, 53.33442372801900433 ) ) ;
#137247=CARTESIAN_POINT ( 'NONE',  ( -12.06949235617739369, -12.14591786802326823, 59.37609039468568284 ) ) ;
#137248=CARTESIAN_POINT ( 'NONE',  ( -21.55341960407610458, -5.719274019375992779, 81.45724293864769550 ) ) ;
#137249=CARTESIAN_POINT ( 'NONE',  ( 19.05341960407617918, -5.049401038297876454, 41.04275706135233293 ) ) ;
#137250=CARTESIAN_POINT ( 'NONE',  ( -19.05341960407611168, -5.049401038298163336, 91.45724293864766707 ) ) ;
#137252=CARTESIAN_POINT ( 'NONE',  ( 15.72974639402199770, -15.80617190586745480, 33.12390960531435979 ) ) ;
#137254=CARTESIAN_POINT ( 'NONE',  ( 19.05341960407611168, 5.049401038298154454, 58.95724293864768129 ) ) ;
#137255=CARTESIAN_POINT ( 'NONE',  ( 15.72974639402176855, 15.80617190586768217, 51.87609039468568284 ) ) ;
#137257=CARTESIAN_POINT ( 'NONE',  ( 12.14591786802309770, 12.06949235617756955, 114.3739096053143527 ) ) ;
#137259=CARTESIAN_POINT ( 'NONE',  ( -21.55341960407610458, -5.719274019375992779, 111.4572429386476813 ) ) ;
#137260=CARTESIAN_POINT ( 'NONE',  ( -13.97604488694527625, -13.89961937509977652, 96.87390960531433848 ) ) ;
#137262=CARTESIAN_POINT ( 'NONE',  ( -21.55341960407619339, 5.719274019375674811, 43.54275706135235424 ) ) ;
#137264=CARTESIAN_POINT ( 'NONE',  ( -5.153800228976328057, -19.02544592524343514, 102.2905762719810383 ) ) ;
#137266=CARTESIAN_POINT ( 'NONE',  ( 21.53943276465977519, -0.05219959533907433946, 108.7489096053143669 ) ) ;
#137267=CARTESIAN_POINT ( 'NONE',  ( -9.474510206698964154, 16.51473224551069663, 50.41557627198102409 ) ) ;
#137268=CARTESIAN_POINT ( 'NONE',  ( -8.314922557961024197, 14.29746914071037800, 22.91775706135235069 ) ) ;
#137270=CARTESIAN_POINT ( 'NONE',  ( -15.80617190586768217, 15.72974639402176855, 98.12609039468570415 ) ) ;
#137271=CARTESIAN_POINT ( 'NONE',  ( -13.89961937509977652, 13.97604488694528158, 30.62390960531435269 ) ) ;
#137272=CARTESIAN_POINT ( 'NONE',  ( -15.72974639402176322, -15.80617190586768395, 94.37609039468568994 ) ) ;
#137273=CARTESIAN_POINT ( 'NONE',  ( 19.05341960407611168, 5.049401038298154454, 93.95724293864769550 ) ) ;
#137274=CARTESIAN_POINT ( 'NONE',  ( 18.67979575497194134, -10.72451020669871369, 65.83442372801900433 ) ) ;
#137276=CARTESIAN_POINT ( 'NONE',  ( 19.05341960407611168, 5.049401038298154454, 93.95724293864769550 ) ) ;
#137277=CARTESIAN_POINT ( 'NONE',  ( 18.87255363501903105, 5.499999999999943157, 63.82513748171827928 ) ) ;
#137278=CARTESIAN_POINT ( 'NONE',  ( 14.34966873604972726, -8.224510206698740333, 40.83442372801901854 ) ) ;
#137279=CARTESIAN_POINT ( 'NONE',  ( 16.53943276465976808, 0.05219959533934440121, 66.25109039468567573 ) ) ;
#137280=CARTESIAN_POINT ( 'NONE',  ( -15.80617190586768217, 15.72974639402176855, 53.12609039468568284 ) ) ;
#137281=CARTESIAN_POINT ( 'NONE',  ( -18.67979575497193778, 10.72451020669871902, 93.33442372801901854 ) ) ;
#137282=CARTESIAN_POINT ( 'NONE',  ( -17.49999999999999645, -5.500000000000000888, 39.20309617465829177 ) ) ;
#137283=CARTESIAN_POINT ( 'NONE',  ( -0.05219959533936034679, 19.03943276465977164, 112.5010903946856757 ) ) ;
#137284=CARTESIAN_POINT ( 'NONE',  ( 9.564922557960805705, 16.46253265017160317, 74.58224293864769550 ) ) ;
#137285=CARTESIAN_POINT ( 'NONE',  ( -19.05341960407611168, -5.049401038298163336, 101.4572429386476955 ) ) ;
#137286=CARTESIAN_POINT ( 'NONE',  ( 13.97604488694527802, 13.89961937509977652, 24.37390960531435624 ) ) ;
#137287=CARTESIAN_POINT ( 'NONE',  ( 21.52544592524344225, -5.823673210054117533, 23.54057627198102765 ) ) ;
#137288=CARTESIAN_POINT ( 'NONE',  ( -0.05219959533934338120, 16.53943276465976808, 92.50109039468567573 ) ) ;
#137289=CARTESIAN_POINT ( 'NONE',  ( 14.34966873604960469, 8.224510206698951720, 64.16557627198102409 ) ) ;
#137290=CARTESIAN_POINT ( 'NONE',  ( 5.153800228976335163, 19.02544592524342804, 54.79057627198103120 ) ) ;
#137291=CARTESIAN_POINT ( 'NONE',  ( -15.72974639402176322, -15.80617190586768395, 89.37609039468568994 ) ) ;
#137292=CARTESIAN_POINT ( 'NONE',  ( 17.50000000000000000, 4.189786006557876696, 22.00000000000000711 ) ) ;
#137293=CARTESIAN_POINT ( 'NONE',  ( -16.46253265017146816, -9.564922557961047289, 104.1677570613523329 ) ) ;
#137294=CARTESIAN_POINT ( 'NONE',  ( 14.34966873604960469, 8.224510206698951720, 79.16557627198103830 ) ) ;
#137295=CARTESIAN_POINT ( 'NONE',  ( -10.72451020669870658, -18.67979575497194134, 29.58442372801901854 ) ) ;
#137296=CARTESIAN_POINT ( 'NONE',  ( -15.72974639402197994, 15.80617190586746368, 65.62390960531436690 ) ) ;
#137298=CARTESIAN_POINT ( 'NONE',  ( 5.153800228976615827, -19.02544592524334988, 40.20942372801898301 ) ) ;
#137300=CARTESIAN_POINT ( 'NONE',  ( -5.153800228976328057, -19.02544592524343514, 82.29057627198103830 ) ) ;
#137301=CARTESIAN_POINT ( 'NONE',  ( -16.55341960407611168, -4.379528057220339221, 51.45724293864770260 ) ) ;
#137302=CARTESIAN_POINT ( 'NONE',  ( -12.14591786802309592, -12.06949235617757132, 41.87390960531435979 ) ) ;
#137303=CARTESIAN_POINT ( 'NONE',  ( -16.55341960407617563, 4.379528057220093196, 98.54275706135234714 ) ) ;
#137304=CARTESIAN_POINT ( 'NONE',  ( -19.03943276465977164, -0.05219959533935918106, 48.75109039468566863 ) ) ;
#137305=CARTESIAN_POINT ( 'NONE',  ( 18.56399227203345959, 5.499999999999819700, 51.47830131249905605 ) ) ;
#137306=CARTESIAN_POINT ( 'NONE',  ( 13.97604488694527802, 13.89961937509977652, 99.37390960531436690 ) ) ;
#137307=CARTESIAN_POINT ( 'NONE',  ( 4.483927247898545687, 16.52544592524342804, 74.79057627198105251 ) ) ;
#137308=CARTESIAN_POINT ( 'NONE',  ( 16.51473224551083163, -9.474510206698727899, 45.83442372801900433 ) ) ;
#137309=CARTESIAN_POINT ( 'NONE',  ( -9.474510206698964154, 16.51473224551069663, 30.41557627198102054 ) ) ;
#137310=CARTESIAN_POINT ( 'NONE',  ( -18.62759615963270932, 10.81492255796079327, 35.83224293864768839 ) ) ;
#137311=CARTESIAN_POINT ( 'NONE',  ( 15.80617190586746368, 15.72974639402197994, 69.37390960531436690 ) ) ;
#137312=CARTESIAN_POINT ( 'NONE',  ( -16.55341960407611168, -4.379528057220339221, 106.4572429386477097 ) ) ;
#137313=CARTESIAN_POINT ( 'NONE',  ( -16.53943276465976808, -0.05219959533934237506, 53.75109039468568994 ) ) ;
#137314=CARTESIAN_POINT ( 'NONE',  ( 19.03943276465977164, -0.05219959533909143690, 53.74890960531436690 ) ) ;
#137315=CARTESIAN_POINT ( 'NONE',  ( 21.53943276465977519, 0.05219959533937863772, 41.25109039468568284 ) ) ;
#137316=CARTESIAN_POINT ( 'NONE',  ( 16.55341960407611168, 4.379528057220329451, 93.95724293864770971 ) ) ;
#137319=CARTESIAN_POINT ( 'NONE',  ( 21.52544592524344225, -5.823673210054117533, 28.54057627198103120 ) ) ;
#137320=CARTESIAN_POINT ( 'NONE',  ( 17.40861289039004944, -6.110651285853255565, 66.12767529172569425 ) ) ;
#137322=CARTESIAN_POINT ( 'NONE',  ( 14.29746914071037800, 8.314922557961029526, 46.66775706135234714 ) ) ;
#137323=CARTESIAN_POINT ( 'NONE',  ( -14.29746914071049879, 8.314922557960819915, 45.83224293864769550 ) ) ;
#137324=CARTESIAN_POINT ( 'NONE',  ( -10.81492255796078084, -18.62759615963271287, 67.08224293864770971 ) ) ;
#137325=CARTESIAN_POINT ( 'NONE',  ( -21.52544592524343514, 5.823673210054127303, 56.04057627198102409 ) ) ;
#137327=CARTESIAN_POINT ( 'NONE',  ( 16.46253265017160672, -9.564922557960803928, 38.33224293864768839 ) ) ;
#137328=CARTESIAN_POINT ( 'NONE',  ( -5.049401038298153566, 19.05341960407611168, 105.2072429386476671 ) ) ;
#137329=CARTESIAN_POINT ( 'NONE',  ( -5.049401038298153566, 19.05341960407611168, 50.20724293864770260 ) ) ;
#137330=CARTESIAN_POINT ( 'NONE',  ( -19.05341960407611168, -5.049401038298163336, 21.45724293864768839 ) ) ;
#137332=CARTESIAN_POINT ( 'NONE',  ( 16.51473224551069308, 9.474510206698969483, 114.1655762719810241 ) ) ;
#137334=CARTESIAN_POINT ( 'NONE',  ( -12.14591786802326823, 12.06949235617739902, 68.12609039468567573 ) ) ;
#137335=CARTESIAN_POINT ( 'NONE',  ( 5.823673210054125526, 21.52544592524343514, 99.79057627198103830 ) ) ;
#137336=CARTESIAN_POINT ( 'NONE',  ( -5.153800228976328057, -19.02544592524343514, 57.29057627198103120 ) ) ;
#137337=CARTESIAN_POINT ( 'NONE',  ( 18.67979575497194134, -10.72451020669871369, 45.83442372801901854 ) ) ;
#137338=CARTESIAN_POINT ( 'NONE',  ( -5.153800228976328057, -19.02544592524343514, 87.29057627198103830 ) ) ;
#137339=CARTESIAN_POINT ( 'NONE',  ( 13.97604488694527802, 13.89961937509977652, 114.3739096053143669 ) ) ;
#137341=CARTESIAN_POINT ( 'NONE',  ( -21.53943276465977519, -0.05219959533937600094, 28.75109039468567929 ) ) ;
#137342=CARTESIAN_POINT ( 'NONE',  ( -19.05341960407611168, -5.049401038298163336, 111.4572429386476671 ) ) ;
#137343=CARTESIAN_POINT ( 'NONE',  ( 19.03943276465977164, 0.05219959533936151252, 86.25109039468567573 ) ) ;
#137344=CARTESIAN_POINT ( 'NONE',  ( 16.51473224551083163, -9.474510206698727899, 40.83442372801900433 ) ) ;
#137345=CARTESIAN_POINT ( 'NONE',  ( 21.52544592524344225, -5.823673210054117533, 103.5405762719810383 ) ) ;
#137346=CARTESIAN_POINT ( 'NONE',  ( -13.97604488694547697, 13.89961937509957934, 38.12609039468566152 ) ) ;
#137347=CARTESIAN_POINT ( 'NONE',  ( 0.05219959533936267826, -19.03943276465977164, 35.00109039468566863 ) ) ;
#137348=CARTESIAN_POINT ( 'NONE',  ( 0.05219959533934541429, -16.53943276465976808, 90.00109039468567573 ) ) ;
#137350=CARTESIAN_POINT ( 'NONE',  ( 0.05219959533909260263, 19.03943276465977164, 54.99890960531435979 ) ) ;
#137352=CARTESIAN_POINT ( 'NONE',  ( -15.80617190586768217, 15.72974639402176855, 63.12609039468568994 ) ) ;
#137353=CARTESIAN_POINT ( 'NONE',  ( 18.62759615963255655, 10.81492255796105972, 81.66775706135236135 ) ) ;
#137355=CARTESIAN_POINT ( 'NONE',  ( -0.05219959533909027116, -19.03943276465977164, 72.49890960531435269 ) ) ;
#137356=CARTESIAN_POINT ( 'NONE',  ( 5.823673210054444382, -21.52544592524334988, 65.20942372801901854 ) ) ;
#137357=CARTESIAN_POINT ( 'NONE',  ( 0.05219959533936267826, -19.03943276465977164, 105.0010903946856615 ) ) ;
#137358=CARTESIAN_POINT ( 'NONE',  ( 19.02544592524343514, -5.153800228976328945, 58.54057627198102409 ) ) ;
#137359=CARTESIAN_POINT ( 'NONE',  ( 5.049401038298161559, -19.05341960407611168, 102.7072429386476955 ) ) ;
#137360=CARTESIAN_POINT ( 'NONE',  ( -0.05219959533909027116, -19.03943276465977164, 77.49890960531435269 ) ) ;
#137362=CARTESIAN_POINT ( 'NONE',  ( -9.474510206698964154, 16.51473224551069663, 60.41557627198102409 ) ) ;
#137363=CARTESIAN_POINT ( 'NONE',  ( 21.53943276465977519, -0.05219959533907433946, 93.74890960531436690 ) ) ;
#137364=CARTESIAN_POINT ( 'NONE',  ( -8.314922557961024197, 14.29746914071037800, 92.91775706135236135 ) ) ;
#137366=CARTESIAN_POINT ( 'NONE',  ( 13.89961937509957401, 13.97604488694547697, 41.87609039468566152 ) ) ;
#137367=CARTESIAN_POINT ( 'NONE',  ( 16.51473224551069308, 9.474510206698969483, 84.16557627198102409 ) ) ;
#137368=CARTESIAN_POINT ( 'NONE',  ( 12.14591786802309770, 12.06949235617756955, 69.37390960531436690 ) ) ;
#137369=CARTESIAN_POINT ( 'NONE',  ( 8.224510206698953496, -14.34966873604960469, 107.9155762719810241 ) ) ;
#137371=CARTESIAN_POINT ( 'NONE',  ( 5.719274019375991003, -21.55341960407610458, 22.70724293864769194 ) ) ;
#137372=CARTESIAN_POINT ( 'NONE',  ( -0.05219959533909027116, -19.03943276465977164, 102.4989096053143669 ) ) ;
#137374=CARTESIAN_POINT ( 'NONE',  ( 0.05219959533936267826, -19.03943276465977164, 25.00109039468566152 ) ) ;
#137375=CARTESIAN_POINT ( 'NONE',  ( 8.224510206698742110, 14.34966873604972548, 92.08442372801901854 ) ) ;
#137376=CARTESIAN_POINT ( 'NONE',  ( -19.05341960407611168, -5.049401038298163336, 81.45724293864769550 ) ) ;
#137377=CARTESIAN_POINT ( 'NONE',  ( 15.72974639402176855, 15.80617190586768217, 51.87609039468568284 ) ) ;
#137378=CARTESIAN_POINT ( 'NONE',  ( 18.62759615963271287, -10.81492255796078972, 33.33224293864769550 ) ) ;
#137379=CARTESIAN_POINT ( 'NONE',  ( 5.823673210054444382, -21.52544592524334988, 25.20942372801901854 ) ) ;
#137380=CARTESIAN_POINT ( 'NONE',  ( -18.67979575497178146, -10.72451020669898902, 66.66557627198102409 ) ) ;
#137381=CARTESIAN_POINT ( 'NONE',  ( -4.379528057220328563, 16.55341960407611168, 100.2072429386476955 ) ) ;
#137382=CARTESIAN_POINT ( 'NONE',  ( -5.153800228976607833, 19.02544592524334988, 52.70942372801900433 ) ) ;
#137383=CARTESIAN_POINT ( 'NONE',  ( 16.46253265017160672, -9.564922557960803928, 28.33224293864769550 ) ) ;
#137384=CARTESIAN_POINT ( 'NONE',  ( -13.97604488694527625, -13.89961937509977652, 86.87390960531436690 ) ) ;
#137385=CARTESIAN_POINT ( 'NONE',  ( -0.05219959533909027116, -19.03943276465977164, 82.49890960531436690 ) ) ;
#137386=CARTESIAN_POINT ( 'NONE',  ( 16.53943276465976808, -0.05219959533910856209, 98.74890960531438111 ) ) ;
#137387=ORIENTED_EDGE ( 'NONE', *, *, #21229, .T. ) ;
#137388=CARTESIAN_POINT ( 'NONE',  ( -12.14591786802309592, -12.06949235617757132, 31.87390960531435979 ) ) ;
#137389=CARTESIAN_POINT ( 'NONE',  ( -4.483927247898782831, 16.52544592524335698, 22.70942372801901499 ) ) ;
#137390=CARTESIAN_POINT ( 'NONE',  ( -21.53943276465977519, -0.05219959533937600094, 88.75109039468567573 ) ) ;
#137391=CARTESIAN_POINT ( 'NONE',  ( 9.564922557960805705, 16.46253265017160317, 99.58224293864770971 ) ) ;
#137392=CARTESIAN_POINT ( 'NONE',  ( -18.62759615963255300, -10.81492255796106328, 24.16775706135235424 ) ) ;
#137393=CARTESIAN_POINT ( 'NONE',  ( 13.89961937509977652, -13.97604488694527269, 48.12390960531435979 ) ) ;
#137394=CARTESIAN_POINT ( 'NONE',  ( -16.53943276465976808, -0.05219959533934237506, 38.75109039468567573 ) ) ;
#137395=CARTESIAN_POINT ( 'NONE',  ( -19.02544592524334988, -5.153800228976617603, 103.9594237280190043 ) ) ;
#137396=CARTESIAN_POINT ( 'NONE',  ( -19.02544592524342804, 5.153800228976336051, 31.04057627198102409 ) ) ;
#137397=CARTESIAN_POINT ( 'NONE',  ( 0.05219959533910956823, 16.53943276465976808, 99.99890960531436690 ) ) ;
#137398=CARTESIAN_POINT ( 'NONE',  ( 18.62759615963271287, -10.81492255796078972, 108.3322429386477097 ) ) ;
#137399=CARTESIAN_POINT ( 'NONE',  ( 9.474510206698729675, 16.51473224551082808, 62.08442372801899722 ) ) ;
#137400=CARTESIAN_POINT ( 'NONE',  ( -5.049401038298153566, 19.05341960407611168, 25.20724293864768484 ) ) ;
#137401=CARTESIAN_POINT ( 'NONE',  ( 5.823673210054444382, -21.52544592524334988, 20.20942372801900788 ) ) ;
#137403=CARTESIAN_POINT ( 'NONE',  ( -13.89961937509977652, 13.97604488694528158, 85.62390960531433848 ) ) ;
#137404=CARTESIAN_POINT ( 'NONE',  ( 16.88567814943161594, -6.947325034625701612, 111.2099887734741799 ) ) ;
#137405=B_SPLINE_CURVE_WITH_KNOTS ( 'NONE', 3,
 ( #198691, #105675, #9697, #183521, #41029, #73375 ),
 .UNSPECIFIED., .F., .F.,
 ( 4, 2, 4 ),
 ( 0.003989672132298154733, 0.004372778065220565835, 0.004755883998142976937 ),
 .UNSPECIFIED. ) ;
#137406=CARTESIAN_POINT ( 'NONE',  ( 5.153800228976335163, 19.02544592524342804, 79.79057627198102409 ) ) ;
#137407=CARTESIAN_POINT ( 'NONE',  ( 10.81492255796106328, -18.62759615963255655, 35.41775706135234003 ) ) ;
#137408=CARTESIAN_POINT ( 'NONE',  ( -16.52544592524342804, 4.483927247898546575, 76.04057627198102409 ) ) ;
#137409=CARTESIAN_POINT ( 'NONE',  ( 13.97604488694527802, 13.89961937509977652, 89.37390960531436690 ) ) ;
#137410=CARTESIAN_POINT ( 'NONE',  ( 16.55341960407618274, -4.379528057220086978, 51.04275706135234714 ) ) ;
#137411=CARTESIAN_POINT ( 'NONE',  ( 13.97604488694548053, -13.89961937509957401, 50.62609039468566152 ) ) ;
#137412=CARTESIAN_POINT ( 'NONE',  ( 0.05219959533937995610, -21.53943276465977519, 70.00109039468568994 ) ) ;
#137413=CARTESIAN_POINT ( 'NONE',  ( 16.53943276465976808, 0.05219959533934440121, 26.25109039468567573 ) ) ;
#137414=CARTESIAN_POINT ( 'NONE',  ( -16.46253265017160317, 9.564922557960807481, 70.83224293864770971 ) ) ;
#137416=CARTESIAN_POINT ( 'NONE',  ( -9.564922557961040184, 16.46253265017147172, 92.91775706135233293 ) ) ;
#137417=CARTESIAN_POINT ( 'NONE',  ( 0.05219959533934541429, -16.53943276465976808, 55.00109039468568284 ) ) ;
#137418=CARTESIAN_POINT ( 'NONE',  ( -21.53943276465977519, -0.05219959533937600094, 98.75109039468568994 ) ) ;
#137419=CARTESIAN_POINT ( 'NONE',  ( 19.02544592524334988, 5.153800228976608722, 86.45942372801900433 ) ) ;
#137420=CARTESIAN_POINT ( 'NONE',  ( 16.51473224551069308, 9.474510206698969483, 49.16557627198102409 ) ) ;
#137421=CARTESIAN_POINT ( 'NONE',  ( 18.62759615963271287, -10.81492255796078972, 73.33224293864769550 ) ) ;
#137422=CARTESIAN_POINT ( 'NONE',  ( -8.314922557960811034, -14.29746914071050412, 72.08224293864769550 ) ) ;
#137423=CARTESIAN_POINT ( 'NONE',  ( 19.02544592524334988, 5.153800228976608722, 71.45942372801900433 ) ) ;
#137424=CARTESIAN_POINT ( 'NONE',  ( 17.48853670773246805, -5.747243402303059412, 61.16671299749989288 ) ) ;
#137425=CARTESIAN_POINT ( 'NONE',  ( -16.46253265017146816, -9.564922557961047289, 44.16775706135232582 ) ) ;
#137426=CARTESIAN_POINT ( 'NONE',  ( 16.55341960407611168, 4.379528057220329451, 23.95724293864769550 ) ) ;
#137427=CARTESIAN_POINT ( 'NONE',  ( -8.224510206698948167, 14.34966873604960824, 70.41557627198102409 ) ) ;
#137428=CARTESIAN_POINT ( 'NONE',  ( 21.52544592524334988, 5.823673210054432836, 96.45942372801901854 ) ) ;
#137430=CARTESIAN_POINT ( 'NONE',  ( 21.53943276465977519, -0.05219959533907433946, 108.7489096053143669 ) ) ;
#137431=CARTESIAN_POINT ( 'NONE',  ( -19.03943276465977164, 0.05219959533909376836, 71.24890960531435269 ) ) ;
#137432=CARTESIAN_POINT ( 'NONE',  ( 10.81492255796106328, -18.62759615963255655, 85.41775706135236135 ) ) ;
#137433=CARTESIAN_POINT ( 'NONE',  ( 13.89961937509977652, -13.97604488694527269, 63.12390960531435979 ) ) ;
#137435=CARTESIAN_POINT ( 'NONE',  ( -19.02544592524342804, 5.153800228976336051, 26.04057627198103120 ) ) ;
#137436=CARTESIAN_POINT ( 'NONE',  ( -21.55341960407610458, -5.719274019375992779, 36.45724293864768839 ) ) ;
#137437=VECTOR ( 'NONE', #137, 1000.000000000000000 ) ;
#137438=CARTESIAN_POINT ( 'NONE',  ( -0.05219959533910754901, -16.53943276465976808, 72.49890960531435269 ) ) ;
#137439=CARTESIAN_POINT ( 'NONE',  ( 5.049401038298161559, -19.05341960407611168, 42.70724293864767418 ) ) ;
#137440=CARTESIAN_POINT ( 'NONE',  ( 12.06949235617757843, -12.14591786802309237, 93.12390960531436690 ) ) ;
#137441=CARTESIAN_POINT ( 'NONE',  ( 5.823673210054125526, 21.52544592524343514, 114.7905762719810383 ) ) ;
#137442=CARTESIAN_POINT ( 'NONE',  ( -10.81492255796105439, 18.62759615963255655, 52.91775706135235424 ) ) ;
#137443=CARTESIAN_POINT ( 'NONE',  ( -5.049401038298153566, 19.05341960407611168, 35.20724293864768839 ) ) ;
#137444=CARTESIAN_POINT ( 'NONE',  ( -4.483927247898782831, 16.52544592524335698, 47.70942372801902565 ) ) ;
#137446=CARTESIAN_POINT ( 'NONE',  ( 15.72974639402199770, -15.80617190586745480, 98.12390960531436690 ) ) ;
#137447=CARTESIAN_POINT ( 'NONE',  ( 21.55341960407610458, 5.719274019375980345, 103.9572429386476813 ) ) ;
#137448=CARTESIAN_POINT ( 'NONE',  ( 19.02544592524334988, 5.153800228976608722, 26.45942372801899722 ) ) ;
#137449=CARTESIAN_POINT ( 'NONE',  ( 5.153800228976335163, 19.02544592524342804, 49.79057627198100988 ) ) ;
#137450=CARTESIAN_POINT ( 'NONE',  ( 0.05219959533909260263, 19.03943276465977164, 104.9989096053143669 ) ) ;
#137451=CARTESIAN_POINT ( 'NONE',  ( 21.55341960407619695, -5.719274019375665929, 56.04275706135235424 ) ) ;
#137452=CARTESIAN_POINT ( 'NONE',  ( 0.05219959533907565091, 21.53943276465977519, 49.99890960531437401 ) ) ;
#137453=CARTESIAN_POINT ( 'NONE',  ( 16.53943276465976808, 0.05219959533934440121, 111.2510903946856899 ) ) ;
#137454=CARTESIAN_POINT ( 'NONE',  ( 15.80617190586769283, -15.72974639402175789, 65.62609039468568994 ) ) ;
#137455=CARTESIAN_POINT ( 'NONE',  ( 10.81492255796106328, -18.62759615963255655, 95.41775706135234714 ) ) ;
#137456=CARTESIAN_POINT ( 'NONE',  ( 5.153800228976615827, -19.02544592524334988, 50.20942372801897591 ) ) ;
#137457=CARTESIAN_POINT ( 'NONE',  ( 14.29746914071037800, 8.314922557961029526, 106.6677570613523756 ) ) ;
#137458=CARTESIAN_POINT ( 'NONE',  ( 18.62759615963255655, 10.81492255796105972, 61.66775706135235424 ) ) ;
#137459=CARTESIAN_POINT ( 'NONE',  ( -19.02544592524342804, 5.153800228976336051, 56.04057627198100988 ) ) ;
#137460=CARTESIAN_POINT ( 'NONE',  ( -16.51473224551082808, 9.474510206698731452, 23.33442372801900078 ) ) ;
#137461=CARTESIAN_POINT ( 'NONE',  ( 5.719274019375991003, -21.55341960407610458, 22.70724293864769194 ) ) ;
#137462=CARTESIAN_POINT ( 'NONE',  ( 15.80617190586769283, -15.72974639402175789, 20.62609039468568639 ) ) ;
#137463=CARTESIAN_POINT ( 'NONE',  ( -0.05219959533907301413, -21.53943276465977519, 72.49890960531435269 ) ) ;
#137464=CARTESIAN_POINT ( 'NONE',  ( 16.53943276465976808, 0.05219959533934440121, 46.25109039468567573 ) ) ;
#137466=CARTESIAN_POINT ( 'NONE',  ( 21.55341960407610458, 5.719274019375980345, 83.95724293864770971 ) ) ;
#137467=CARTESIAN_POINT ( 'NONE',  ( 14.29746914071037800, 8.314922557961029526, 71.66775706135234714 ) ) ;
#137468=CARTESIAN_POINT ( 'NONE',  ( 16.55341960407611168, 4.379528057220329451, 73.95724293864769550 ) ) ;
#137470=CARTESIAN_POINT ( 'NONE',  ( -9.564922557961040184, 16.46253265017147172, 102.9177570613523329 ) ) ;
#137471=CARTESIAN_POINT ( 'NONE',  ( -15.80617190586745835, -15.72974639402198527, 36.87390960531435979 ) ) ;
#137472=CARTESIAN_POINT ( 'NONE',  ( 16.51473224551069308, 9.474510206698969483, 94.16557627198103830 ) ) ;
#137473=CARTESIAN_POINT ( 'NONE',  ( -4.379528057220086978, -16.55341960407618274, 34.79275706135235424 ) ) ;
#137474=CARTESIAN_POINT ( 'NONE',  ( -5.719274019375978568, 21.55341960407610458, 105.2072429386477097 ) ) ;
#137475=CARTESIAN_POINT ( 'NONE',  ( 10.72451020669898902, -18.67979575497178502, 37.91557627198102409 ) ) ;
#137476=CARTESIAN_POINT ( 'NONE',  ( -16.55341960407617563, 4.379528057220093196, 73.54275706135234714 ) ) ;
#137477=CARTESIAN_POINT ( 'NONE',  ( -9.564922557960796823, -16.46253265017161027, 87.08224293864769550 ) ) ;
#137478=CARTESIAN_POINT ( 'NONE',  ( -0.05219959533937732626, 21.53943276465977519, 37.50109039468568284 ) ) ;
#137479=CARTESIAN_POINT ( 'NONE',  ( 9.474510206698971260, -16.51473224551069308, 22.91557627198102765 ) ) ;
#137480=CARTESIAN_POINT ( 'NONE',  ( 0.05219959533907565091, 21.53943276465977519, 24.99890960531435624 ) ) ;
#137482=CARTESIAN_POINT ( 'NONE',  ( 16.51473224551083163, -9.474510206698727899, 25.83442372801900078 ) ) ;
#137483=CARTESIAN_POINT ( 'NONE',  ( -14.29746914071037622, -8.314922557961029526, 54.16775706135235424 ) ) ;
#137484=CARTESIAN_POINT ( 'NONE',  ( -19.02544592524342804, 5.153800228976336051, 106.0405762719810241 ) ) ;
#137485=CARTESIAN_POINT ( 'NONE',  ( -5.823673210054116645, -21.52544592524344225, 97.29057627198105251 ) ) ;
#137486=CARTESIAN_POINT ( 'NONE',  ( 19.02544592524343514, -5.153800228976328945, 73.54057627198103830 ) ) ;
#137489=CARTESIAN_POINT ( 'NONE',  ( 8.224510206698953496, -14.34966873604960469, 87.91557627198103830 ) ) ;
#137490=CARTESIAN_POINT ( 'NONE',  ( -15.72974639402197994, 15.80617190586746368, 30.62390960531436335 ) ) ;
#137491=CARTESIAN_POINT ( 'NONE',  ( -17.31747979337949417, 6.344076630960994834, 33.62055131934815932 ) ) ;
#137492=CARTESIAN_POINT ( 'NONE',  ( 14.34966873604972726, -8.224510206698740333, 65.83442372801900433 ) ) ;
#137493=CARTESIAN_POINT ( 'NONE',  ( 15.72974639402199770, -15.80617190586745480, 113.1239096053143953 ) ) ;
#137494=CARTESIAN_POINT ( 'NONE',  ( -9.564922557961040184, 16.46253265017147172, 72.91775706135233293 ) ) ;
#137495=CARTESIAN_POINT ( 'NONE',  ( 16.51473224551069308, 9.474510206698969483, 44.16557627198103120 ) ) ;
#137496=CARTESIAN_POINT ( 'NONE',  ( 21.53943276465977519, -0.05219959533907433946, 63.74890960531435979 ) ) ;
#137497=CARTESIAN_POINT ( 'NONE',  ( 5.153800228976335163, 19.02544592524342804, 99.79057627198102409 ) ) ;
#137498=CARTESIAN_POINT ( 'NONE',  ( 21.55341960407619695, -5.719274019375665929, 91.04275706135236135 ) ) ;
#137499=CARTESIAN_POINT ( 'NONE',  ( 9.564922557960805705, 16.46253265017160317, 69.58224293864770971 ) ) ;
#137500=EDGE_CURVE ( 'NONE', #62281, #123348, #135159, .T. ) ;
#137501=CARTESIAN_POINT ( 'NONE',  ( -16.52544592524335698, -4.483927247898792601, 43.95942372801902565 ) ) ;
#137502=CARTESIAN_POINT ( 'NONE',  ( -19.02544592524342804, 5.153800228976336051, 61.04057627198103120 ) ) ;
#137503=CARTESIAN_POINT ( 'NONE',  ( -15.72974639402176322, -15.80617190586768395, 74.37609039468568994 ) ) ;
#137504=CARTESIAN_POINT ( 'NONE',  ( 19.03943276465977164, 0.05219959533936151252, 41.25109039468566152 ) ) ;
#137505=CARTESIAN_POINT ( 'NONE',  ( -16.51473224551082808, 9.474510206698731452, 48.33442372801900433 ) ) ;
#137506=CARTESIAN_POINT ( 'NONE',  ( -21.53943276465977519, -0.05219959533937600094, 48.75109039468568284 ) ) ;
#137507=CARTESIAN_POINT ( 'NONE',  ( -18.56101223717332971, -5.499999999999953815, 46.44978406935678805 ) ) ;
#137508=CARTESIAN_POINT ( 'NONE',  ( 5.049401038297881783, 19.05341960407617563, 47.29275706135231161 ) ) ;
#137509=CARTESIAN_POINT ( 'NONE',  ( 19.02544592524343514, -5.153800228976328945, 103.5405762719809957 ) ) ;
#137510=CARTESIAN_POINT ( 'NONE',  ( 16.51473224551069308, 9.474510206698969483, 69.16557627198102409 ) ) ;
#137511=CARTESIAN_POINT ( 'NONE',  ( -16.53943276465976808, -0.05219959533934237506, 113.7510903946856757 ) ) ;
#137512=CARTESIAN_POINT ( 'NONE',  ( 21.52544592524344225, -5.823673210054117533, 28.54057627198103120 ) ) ;
#137513=CARTESIAN_POINT ( 'NONE',  ( 18.67979575497194134, -10.72451020669871369, 100.8344237280190185 ) ) ;
#137515=CARTESIAN_POINT ( 'NONE',  ( 16.21995358207306026, 7.366697692864117464, 57.56448998487844904 ) ) ;
#137516=CARTESIAN_POINT ( 'NONE',  ( -18.62759615963255300, -10.81492255796106328, 99.16775706135234714 ) ) ;
#137518=CARTESIAN_POINT ( 'NONE',  ( 5.153800228976335163, 19.02544592524342804, 24.79057627198102765 ) ) ;
#137519=CARTESIAN_POINT ( 'NONE',  ( 19.05341960407611168, 5.049401038298154454, 108.9572429386477097 ) ) ;
#137521=CARTESIAN_POINT ( 'NONE',  ( 4.379528057220092307, 16.55341960407617563, 52.29275706135236135 ) ) ;
#137522=CARTESIAN_POINT ( 'NONE',  ( 21.53943276465977519, -0.05219959533907433946, 73.74890960531433848 ) ) ;
#137523=CARTESIAN_POINT ( 'NONE',  ( 14.29746914071049879, -8.314922557960816363, 43.33224293864769550 ) ) ;
#137524=CARTESIAN_POINT ( 'NONE',  ( -16.52544592524342804, 4.483927247898546575, 111.0405762719810525 ) ) ;
#137525=CARTESIAN_POINT ( 'NONE',  ( 5.153800228976335163, 19.02544592524342804, 104.7905762719809957 ) ) ;
#137526=CARTESIAN_POINT ( 'NONE',  ( 9.474510206698729675, 16.51473224551082808, 37.08442372801899722 ) ) ;
#137527=CARTESIAN_POINT ( 'NONE',  ( -16.53943276465976808, 0.05219959533911058130, 111.2489096053143669 ) ) ;
#137528=CARTESIAN_POINT ( 'NONE',  ( -18.62759615963255300, -10.81492255796106328, 74.16775706135231871 ) ) ;
#137530=CARTESIAN_POINT ( 'NONE',  ( -16.55341960407611168, -4.379528057220339221, 31.45724293864769550 ) ) ;
#137531=CARTESIAN_POINT ( 'NONE',  ( -17.59860650958993844, 7.585241751806885979, 68.42337014262493256 ) ) ;
#137532=CARTESIAN_POINT ( 'NONE',  ( 18.67979575497178502, 10.72451020669898547, 29.16557627198103120 ) ) ;
#137533=CARTESIAN_POINT ( 'NONE',  ( 16.53943276465976808, -0.05219959533910856209, 83.74890960531435269 ) ) ;
#137536=CARTESIAN_POINT ( 'NONE',  ( 16.51473224551069308, 9.474510206698969483, 74.16557627198103830 ) ) ;
#137537=CARTESIAN_POINT ( 'NONE',  ( 0.05219959533910956823, 16.53943276465976808, 79.99890960531435269 ) ) ;
#137538=CARTESIAN_POINT ( 'NONE',  ( 5.153800228976615827, -19.02544592524334988, 110.2094237280189901 ) ) ;
#137539=CARTESIAN_POINT ( 'NONE',  ( -18.62759615963270932, 10.81492255796079327, 50.83224293864770971 ) ) ;
#137540=ORIENTED_EDGE ( 'NONE', *, *, #103145, .F. ) ;
#137541=CARTESIAN_POINT ( 'NONE',  ( -9.474510206698964154, 16.51473224551069663, 25.41557627198103120 ) ) ;
#137542=CARTESIAN_POINT ( 'NONE',  ( -9.474510206698964154, 16.51473224551069663, 75.41557627198103830 ) ) ;
#137543=CARTESIAN_POINT ( 'NONE',  ( -18.67979575497178146, -10.72451020669898902, 71.66557627198100988 ) ) ;
#137544=CARTESIAN_POINT ( 'NONE',  ( 8.314922557961029526, -14.29746914071037800, 100.4177570613523471 ) ) ;
#137545=CARTESIAN_POINT ( 'NONE',  ( -19.02544592524342804, 5.153800228976336051, 91.04057627198100988 ) ) ;
#137546=CARTESIAN_POINT ( 'NONE',  ( -5.049401038297874678, -19.05341960407617918, 64.79275706135233293 ) ) ;
#137547=CARTESIAN_POINT ( 'NONE',  ( -18.67979575497193778, 10.72451020669871902, 83.33442372801903275 ) ) ;
#137548=CARTESIAN_POINT ( 'NONE',  ( 5.719274019375991003, -21.55341960407610458, 62.70724293864769550 ) ) ;
#137549=CARTESIAN_POINT ( 'NONE',  ( -10.72451020669898014, 18.67979575497178502, 25.41557627198103120 ) ) ;
#137550=CARTESIAN_POINT ( 'NONE',  ( 16.46253265017160672, -9.564922557960803928, 43.33224293864769550 ) ) ;
#137551=CARTESIAN_POINT ( 'NONE',  ( 14.29746914071037800, 8.314922557961029526, 96.66775706135234714 ) ) ;
#137552=CARTESIAN_POINT ( 'NONE',  ( 19.02544592524343514, -5.153800228976328945, 58.54057627198102409 ) ) ;
#137553=CARTESIAN_POINT ( 'NONE',  ( -16.53943276465976808, -0.05219959533934237506, 28.75109039468567929 ) ) ;
#137554=CARTESIAN_POINT ( 'NONE',  ( 18.22780087662122739, 5.500000000000000888, 81.48236817873103632 ) ) ;
#137555=CARTESIAN_POINT ( 'NONE',  ( 16.51473224551083163, -9.474510206698727899, 20.83442372801899722 ) ) ;
#137556=CARTESIAN_POINT ( 'NONE',  ( 16.53943276465976808, -0.05219959533910856209, 68.74890960531435269 ) ) ;
#137557=CARTESIAN_POINT ( 'NONE',  ( 21.55341960407610458, 5.719274019375980345, 108.9572429386476955 ) ) ;
#137558=CARTESIAN_POINT ( 'NONE',  ( -18.67979575497178146, -10.72451020669898902, 101.6655762719810383 ) ) ;
#137560=CARTESIAN_POINT ( 'NONE',  ( 10.81492255796078972, 18.62759615963270932, 39.58224293864769550 ) ) ;
#137561=CARTESIAN_POINT ( 'NONE',  ( 8.224510206698742110, 14.34966873604972548, 82.08442372801901854 ) ) ;
#137562=CARTESIAN_POINT ( 'NONE',  ( 12.14591786802309770, 12.06949235617756955, 99.37390960531436690 ) ) ;
#137563=CARTESIAN_POINT ( 'NONE',  ( -19.03943276465977164, 0.05219959533909376836, 56.24890960531435979 ) ) ;
#137565=CARTESIAN_POINT ( 'NONE',  ( 12.06949235617739724, 12.14591786802326823, 111.8760903946856615 ) ) ;
#137567=CARTESIAN_POINT ( 'NONE',  ( 21.52544592524334988, 5.823673210054432836, 41.45942372801901143 ) ) ;
#137568=CARTESIAN_POINT ( 'NONE',  ( 16.51473224551069308, 9.474510206698969483, 94.16557627198103830 ) ) ;
#137569=CARTESIAN_POINT ( 'NONE',  ( -21.53943276465977519, -0.05219959533937600094, 83.75109039468568994 ) ) ;
#137570=CARTESIAN_POINT ( 'NONE',  ( -9.564922557960796823, -16.46253265017161027, 32.08224293864769550 ) ) ;
#137571=CARTESIAN_POINT ( 'NONE',  ( 13.89961937509977652, -13.97604488694527269, 23.12390960531436335 ) ) ;
#137573=CARTESIAN_POINT ( 'NONE',  ( 5.823673210054444382, -21.52544592524334988, 75.20942372801901854 ) ) ;
#137574=CARTESIAN_POINT ( 'NONE',  ( -9.474510206698964154, 16.51473224551069663, 100.4155762719810241 ) ) ;
#137575=CARTESIAN_POINT ( 'NONE',  ( 16.46253265017146816, 9.564922557961045513, 86.66775706135233293 ) ) ;
#137576=CARTESIAN_POINT ( 'NONE',  ( 15.72974639402176855, 15.80617190586768217, 36.87609039468568994 ) ) ;
#137577=CARTESIAN_POINT ( 'NONE',  ( -16.51473224551082808, 9.474510206698731452, 113.3344237280190043 ) ) ;
#137579=CARTESIAN_POINT ( 'NONE',  ( -19.03943276465977164, -0.05219959533935918106, 73.75109039468566152 ) ) ;
#137580=CARTESIAN_POINT ( 'NONE',  ( -5.153800228976328057, -19.02544592524343514, 42.29057627198101699 ) ) ;
#137581=CARTESIAN_POINT ( 'NONE',  ( 5.049401038297881783, 19.05341960407617563, 77.29275706135231871 ) ) ;
#137582=CARTESIAN_POINT ( 'NONE',  ( 8.224510206698953496, -14.34966873604960469, 22.91557627198102765 ) ) ;
#137583=CARTESIAN_POINT ( 'NONE',  ( -16.46253265017146816, -9.564922557961047289, 79.16775706135234714 ) ) ;
#137584=CARTESIAN_POINT ( 'NONE',  ( 16.53943276465976808, -0.05219959533910856209, 33.74890960531436690 ) ) ;
#137585=CARTESIAN_POINT ( 'NONE',  ( 0.05219959533936267826, -19.03943276465977164, 65.00109039468567573 ) ) ;
#137586=CARTESIAN_POINT ( 'NONE',  ( -21.55341960407619339, 5.719274019375674811, 108.5427570613523756 ) ) ;
#137587=CARTESIAN_POINT ( 'NONE',  ( -5.049401038297874678, -19.05341960407617918, 29.79275706135232227 ) ) ;
#137588=CARTESIAN_POINT ( 'NONE',  ( 13.89961937509977652, -13.97604488694527269, 28.12390960531435624 ) ) ;
#137589=CARTESIAN_POINT ( 'NONE',  ( -17.05587630539784527, -6.762274262135712810, 64.25819690962687503 ) ) ;
#137590=CARTESIAN_POINT ( 'NONE',  ( -14.34966873604972548, 8.224510206698743886, 48.33442372801902565 ) ) ;
#137591=CARTESIAN_POINT ( 'NONE',  ( -17.49999999999999645, 5.499999999999992895, 120.0000000000000142 ) ) ;
#137592=EDGE_CURVE ( 'NONE', #92102, #170830, #191925, .T. ) ;
#137594=CARTESIAN_POINT ( 'NONE',  ( 5.049401038298161559, -19.05341960407611168, 87.70724293864769550 ) ) ;
#137597=CARTESIAN_POINT ( 'NONE',  ( 16.51473224551083163, -9.474510206698727899, 90.83442372801900433 ) ) ;
#137598=CARTESIAN_POINT ( 'NONE',  ( -13.89961937509977652, 13.97604488694528158, 115.6239096053143669 ) ) ;
#137599=CARTESIAN_POINT ( 'NONE',  ( 5.153800228976615827, -19.02544592524334988, 20.20942372801899722 ) ) ;
#137600=CARTESIAN_POINT ( 'NONE',  ( 9.474510206698729675, 16.51473224551082808, 97.08442372801900433 ) ) ;
#137601=CARTESIAN_POINT ( 'NONE',  ( -8.314922557960811034, -14.29746914071050412, 107.0822429386476955 ) ) ;
#137602=CARTESIAN_POINT ( 'NONE',  ( 16.46253265017160672, -9.564922557960803928, 28.33224293864769550 ) ) ;
#137603=CARTESIAN_POINT ( 'NONE',  ( -21.55341960407610458, -5.719274019375992779, 56.45724293864768839 ) ) ;
#137604=CARTESIAN_POINT ( 'NONE',  ( 18.67979575497178502, 10.72451020669898547, 49.16557627198102409 ) ) ;
#137605=CARTESIAN_POINT ( 'NONE',  ( -9.474510206698964154, 16.51473224551069663, 25.41557627198103120 ) ) ;
#137607=CARTESIAN_POINT ( 'NONE',  ( -19.05341960407617563, 5.049401038297882671, 73.54275706135233293 ) ) ;
#137608=CARTESIAN_POINT ( 'NONE',  ( 12.14591786802309770, 12.06949235617756955, 34.37390960531435979 ) ) ;
#137609=CARTESIAN_POINT ( 'NONE',  ( -21.55341960407610458, -5.719274019375992779, 26.45724293864768839 ) ) ;
#137610=CARTESIAN_POINT ( 'NONE',  ( -5.823673210054431948, 21.52544592524334988, 87.70942372801901854 ) ) ;
#137611=CARTESIAN_POINT ( 'NONE',  ( -5.823673210054116645, -21.52544592524344225, 82.29057627198103830 ) ) ;
#137612=CARTESIAN_POINT ( 'NONE',  ( -10.72451020669870658, -18.67979575497194134, 54.58442372801901143 ) ) ;
#137613=CARTESIAN_POINT ( 'NONE',  ( -10.72451020669870658, -18.67979575497194134, 69.58442372801900433 ) ) ;
#137614=CARTESIAN_POINT ( 'NONE',  ( -19.03943276465977164, 0.05219959533909376836, 101.2489096053143669 ) ) ;
#137615=CARTESIAN_POINT ( 'NONE',  ( -4.483927247898782831, 16.52544592524335698, 92.70942372801901854 ) ) ;
#137616=CARTESIAN_POINT ( 'NONE',  ( -18.67979575497193778, 10.72451020669871902, 53.33442372801901854 ) ) ;
#137617=CARTESIAN_POINT ( 'NONE',  ( 4.483927247898545687, 16.52544592524342804, 114.7905762719810383 ) ) ;
#137619=CARTESIAN_POINT ( 'NONE',  ( -0.05219959533910754901, -16.53943276465976808, 72.49890960531435269 ) ) ;
#137620=CARTESIAN_POINT ( 'NONE',  ( 16.53943276465976808, -0.05219959533910856209, 38.74890960531435979 ) ) ;
#137621=CARTESIAN_POINT ( 'NONE',  ( 9.564922557960805705, 16.46253265017160317, 64.58224293864769550 ) ) ;
#137622=CARTESIAN_POINT ( 'NONE',  ( -0.05219959533909027116, -19.03943276465977164, 52.49890960531436690 ) ) ;
#137623=CARTESIAN_POINT ( 'NONE',  ( 18.62759615963271287, -10.81492255796078972, 63.33224293864770260 ) ) ;
#137624=CARTESIAN_POINT ( 'NONE',  ( -5.049401038297874678, -19.05341960407617918, 39.79275706135232582 ) ) ;
#137626=CARTESIAN_POINT ( 'NONE',  ( -8.224510206698948167, 14.34966873604960824, 55.41557627198102409 ) ) ;
#137627=CARTESIAN_POINT ( 'NONE',  ( 21.55341960407610458, 5.719274019375980345, 23.95724293864769550 ) ) ;
#137630=CARTESIAN_POINT ( 'NONE',  ( -16.55341960407617563, 4.379528057220093196, 68.54275706135234714 ) ) ;
#137631=CARTESIAN_POINT ( 'NONE',  ( 0.05219959533936267826, -19.03943276465977164, 75.00109039468566152 ) ) ;
#137632=CARTESIAN_POINT ( 'NONE',  ( -14.34966873604960291, -8.224510206698953496, 46.66557627198102409 ) ) ;
#137634=CARTESIAN_POINT ( 'NONE',  ( -14.34966873604960291, -8.224510206698953496, 26.66557627198103475 ) ) ;
#137635=CARTESIAN_POINT ( 'NONE',  ( 19.03943276465977164, -0.05219959533909143690, 53.74890960531436690 ) ) ;
#137636=CARTESIAN_POINT ( 'NONE',  ( -5.153800228976328057, -19.02544592524343514, 77.29057627198099567 ) ) ;
#137637=CARTESIAN_POINT ( 'NONE',  ( -13.89961937509977652, 13.97604488694528158, 45.62390960531433848 ) ) ;
#137638=CARTESIAN_POINT ( 'NONE',  ( -18.62759615963255300, -10.81492255796106328, 44.16775706135234714 ) ) ;
#137639=CARTESIAN_POINT ( 'NONE',  ( 19.05341960407611168, 5.049401038298154454, 63.95724293864769550 ) ) ;
#137641=CARTESIAN_POINT ( 'NONE',  ( 13.97604488694527802, 13.89961937509977652, 64.37390960531436690 ) ) ;
#137642=CARTESIAN_POINT ( 'NONE',  ( -5.823673210054116645, -21.52544592524344225, 42.29057627198103120 ) ) ;
#137643=CARTESIAN_POINT ( 'NONE',  ( 16.51473224551069308, 9.474510206698969483, 24.16557627198102765 ) ) ;
#137644=CARTESIAN_POINT ( 'NONE',  ( -10.81492255796078084, -18.62759615963271287, 32.08224293864769550 ) ) ;
#137645=CARTESIAN_POINT ( 'NONE',  ( -16.55341960407617563, 4.379528057220093196, 93.54275706135234714 ) ) ;
#137646=CARTESIAN_POINT ( 'NONE',  ( -5.719274019375665041, -21.55341960407619695, 109.7927570613523613 ) ) ;
#137647=CARTESIAN_POINT ( 'NONE',  ( 12.06949235617739724, 12.14591786802326823, 71.87609039468568994 ) ) ;
#137648=CARTESIAN_POINT ( 'NONE',  ( -5.153800228976328057, -19.02544592524343514, 112.2905762719810099 ) ) ;
#137649=CARTESIAN_POINT ( 'NONE',  ( -4.379528057220086978, -16.55341960407618274, 59.79275706135234714 ) ) ;
#137650=CARTESIAN_POINT ( 'NONE',  ( 8.314922557961029526, -14.29746914071037800, 45.41775706135234003 ) ) ;
#137651=CARTESIAN_POINT ( 'NONE',  ( -5.153800228976328057, -19.02544592524343514, 107.2905762719810383 ) ) ;
#137652=CARTESIAN_POINT ( 'NONE',  ( -12.14591786802326823, 12.06949235617739902, 23.12609039468567573 ) ) ;
#137653=CARTESIAN_POINT ( 'NONE',  ( 5.153800228976335163, 19.02544592524342804, 39.79057627198100988 ) ) ;
#137654=CARTESIAN_POINT ( 'NONE',  ( 18.67979575497178502, 10.72451020669898547, 109.1655762719810383 ) ) ;
#137655=CARTESIAN_POINT ( 'NONE',  ( -16.53943276465976808, -0.05219959533934237506, 18.75109039468568639 ) ) ;
#137656=CARTESIAN_POINT ( 'NONE',  ( 8.314922557961029526, -14.29746914071037800, 85.41775706135236135 ) ) ;
#137657=CARTESIAN_POINT ( 'NONE',  ( -17.31728774477213051, 6.344390552233684311, 45.81906651689308063 ) ) ;
#137658=CARTESIAN_POINT ( 'NONE',  ( 10.81492255796106328, -18.62759615963255655, 85.41775706135236135 ) ) ;
#137659=CARTESIAN_POINT ( 'NONE',  ( -13.97604488694547697, 13.89961937509957934, 88.12609039468563310 ) ) ;
#137660=CARTESIAN_POINT ( 'NONE',  ( 16.53943276465976808, -0.05219959533910856209, 48.74890960531435979 ) ) ;
#137661=CARTESIAN_POINT ( 'NONE',  ( 12.14591786802309770, 12.06949235617756955, 104.3739096053143669 ) ) ;
#137662=CARTESIAN_POINT ( 'NONE',  ( -9.564922557961040184, 16.46253265017147172, 42.91775706135234003 ) ) ;
#137664=CARTESIAN_POINT ( 'NONE',  ( -18.67979575497193778, 10.72451020669871902, 48.33442372801902565 ) ) ;
#137665=CARTESIAN_POINT ( 'NONE',  ( -19.02544592524334988, -5.153800228976617603, 103.9594237280190043 ) ) ;
#137666=CARTESIAN_POINT ( 'NONE',  ( 16.19135201231366494, 7.376712067591956412, 82.68680854052030327 ) ) ;
#137667=CARTESIAN_POINT ( 'NONE',  ( -19.03943276465977164, 0.05219959533909376836, 101.2489096053143669 ) ) ;
#137668=CARTESIAN_POINT ( 'NONE',  ( 10.81492255796078972, 18.62759615963270932, 74.58224293864768129 ) ) ;
#137669=CARTESIAN_POINT ( 'NONE',  ( 19.02544592524334988, 5.153800228976608722, 101.4594237280189759 ) ) ;
#137671=CARTESIAN_POINT ( 'NONE',  ( 13.97604488694527802, 13.89961937509977652, 104.3739096053143385 ) ) ;
#137672=CARTESIAN_POINT ( 'NONE',  ( 9.564922557961047289, -16.46253265017146816, 50.41775706135233293 ) ) ;
#137673=CARTESIAN_POINT ( 'NONE',  ( -14.29746914071049879, 8.314922557960819915, 100.8322429386477097 ) ) ;
#137674=CARTESIAN_POINT ( 'NONE',  ( -21.53943276465977519, -0.05219959533937600094, 88.75109039468567573 ) ) ;
#137675=CARTESIAN_POINT ( 'NONE',  ( -5.049401038298153566, 19.05341960407611168, 45.20724293864769550 ) ) ;
#137677=CARTESIAN_POINT ( 'NONE',  ( 18.67979575497194134, -10.72451020669871369, 50.83442372801901143 ) ) ;
#137678=CARTESIAN_POINT ( 'NONE',  ( -18.62759615963255300, -10.81492255796106328, 89.16775706135236135 ) ) ;
#137679=CARTESIAN_POINT ( 'NONE',  ( 0.05219959533934541429, -16.53943276465976808, 85.00109039468568994 ) ) ;
#137681=CARTESIAN_POINT ( 'NONE',  ( 5.823673210054444382, -21.52544592524334988, 40.20942372801901854 ) ) ;
#137682=CARTESIAN_POINT ( 'NONE',  ( -0.05219959533937732626, 21.53943276465977519, 42.50109039468567573 ) ) ;
#137683=CARTESIAN_POINT ( 'NONE',  ( -19.05341960407617563, 5.049401038297882671, 63.54275706135234003 ) ) ;
#137684=CARTESIAN_POINT ( 'NONE',  ( -16.51473224551069308, -9.474510206698971260, 96.66557627198102409 ) ) ;
#137685=CARTESIAN_POINT ( 'NONE',  ( 16.52544592524342804, -4.483927247898539470, 103.5405762719810383 ) ) ;
#137686=CARTESIAN_POINT ( 'NONE',  ( -15.80617190586745835, -15.72974639402198527, 81.87390960531435269 ) ) ;
#137687=CARTESIAN_POINT ( 'NONE',  ( 14.29746914071049879, -8.314922557960816363, 68.33224293864769550 ) ) ;
#137688=CARTESIAN_POINT ( 'NONE',  ( -10.72451020669870658, -18.67979575497194134, 109.5844237280190328 ) ) ;
#137689=CARTESIAN_POINT ( 'NONE',  ( 14.29746914071049879, -8.314922557960816363, 78.33224293864770971 ) ) ;
#137690=CARTESIAN_POINT ( 'NONE',  ( -16.51473224551069308, -9.474510206698971260, 36.66557627198102409 ) ) ;
#137691=CARTESIAN_POINT ( 'NONE',  ( 19.05341960407617918, -5.049401038297876454, 91.04275706135234714 ) ) ;
#137692=CARTESIAN_POINT ( 'NONE',  ( 14.34966873604960469, 8.224510206698951720, 49.16557627198102409 ) ) ;
#137693=CARTESIAN_POINT ( 'NONE',  ( -15.72974639402176322, -15.80617190586768395, 89.37609039468568994 ) ) ;
#137694=CARTESIAN_POINT ( 'NONE',  ( -13.89961937509977652, 13.97604488694528158, 85.62390960531433848 ) ) ;
#137695=CARTESIAN_POINT ( 'NONE',  ( 16.51473224551083163, -9.474510206698727899, 65.83442372801900433 ) ) ;
#137696=CARTESIAN_POINT ( 'NONE',  ( -5.719274019375978568, 21.55341960407610458, 60.20724293864768839 ) ) ;
#137697=CARTESIAN_POINT ( 'NONE',  ( -15.80617190586768217, 15.72974639402176855, 28.12609039468568284 ) ) ;
#137698=CARTESIAN_POINT ( 'NONE',  ( 12.06949235617739724, 12.14591786802326823, 26.87609039468567218 ) ) ;
#137699=CARTESIAN_POINT ( 'NONE',  ( 16.53943276465976808, 0.05219959533934440121, 81.25109039468568994 ) ) ;
#137700=CARTESIAN_POINT ( 'NONE',  ( 16.51473224551069308, 9.474510206698969483, 29.16557627198103475 ) ) ;
#137701=CARTESIAN_POINT ( 'NONE',  ( -21.52544592524334988, -5.823673210054445271, 18.95942372801901143 ) ) ;
#137702=CARTESIAN_POINT ( 'NONE',  ( -16.55341960407611168, -4.379528057220339221, 111.4572429386476813 ) ) ;
#137704=CARTESIAN_POINT ( 'NONE',  ( -14.29746914071037622, -8.314922557961029526, 54.16775706135235424 ) ) ;
#137705=B_SPLINE_CURVE_WITH_KNOTS ( 'NONE', 3,
 ( #162881, #51705, #129525, #160886, #145706, #36525, #55703, #143708, #68872, #147727, #146704, #98179, #117376, #130531, #9214, #115387, #113368, #70881, #179073, #100202, #192229, #177075, #23378, #83030, #38546, #144704, #85024, #159883, #132549, #194237, #131545, #5188 ),
 .UNSPECIFIED., .F., .F.,
 ( 4, 2, 2, 2, 2, 2, 2, 2, 2, 2, 2, 2, 2, 2, 2, 4 ),
 ( 4.336808689942017736E-18, 0.0003712461730036830374, 0.0007424923460073617381, 0.001113738519011040493, 0.001484984692014719139, 0.002227477038022076649, 0.002598723211025741418, 0.002969969384029406186, 0.003341215557033070955, 0.003712461730036735724, 0.004083707903040400058, 0.004454954076044064827, 0.004826200249047730463, 0.005197446422051395232, 0.005568692595055060000, 0.005939938768058724769 ),
 .UNSPECIFIED. ) ;
#137706=CARTESIAN_POINT ( 'NONE',  ( 12.14591786802309770, 12.06949235617756955, 79.37390960531436690 ) ) ;
#137707=CARTESIAN_POINT ( 'NONE',  ( 15.72974639402199770, -15.80617190586745480, 78.12390960531436690 ) ) ;
#137708=CARTESIAN_POINT ( 'NONE',  ( 16.53943276465976808, -0.05219959533910856209, 23.74890960531435269 ) ) ;
#137709=CARTESIAN_POINT ( 'NONE',  ( 0.05219959533934541429, -16.53943276465976808, 35.00109039468568284 ) ) ;
#137710=CARTESIAN_POINT ( 'NONE',  ( -13.89961937509977652, 13.97604488694528158, 40.62390960531435979 ) ) ;
#137711=CARTESIAN_POINT ( 'NONE',  ( -16.55341960407617563, 4.379528057220093196, 78.54275706135236135 ) ) ;
#137712=CARTESIAN_POINT ( 'NONE',  ( 16.46253265017146816, 9.564922557961045513, 71.66775706135233293 ) ) ;
#137713=CARTESIAN_POINT ( 'NONE',  ( -18.62759615963270932, 10.81492255796079327, 65.83224293864769550 ) ) ;
#137714=CARTESIAN_POINT ( 'NONE',  ( -12.14591786802309592, -12.06949235617757132, 21.87390960531436690 ) ) ;
#137717=CARTESIAN_POINT ( 'NONE',  ( 21.52544592524344225, -5.823673210054117533, 43.54057627198103830 ) ) ;
#137719=ORIENTED_EDGE ( 'NONE', *, *, #55537, .F. ) ;
#137720=CARTESIAN_POINT ( 'NONE',  ( -14.29746914071037622, -8.314922557961029526, 89.16775706135236135 ) ) ;
#137722=CARTESIAN_POINT ( 'NONE',  ( 16.46253265017160672, -9.564922557960803928, 113.3322429386476955 ) ) ;
#137724=CARTESIAN_POINT ( 'NONE',  ( 21.53943276465977519, -0.05219959533907433946, 78.74890960531436690 ) ) ;
#137725=CARTESIAN_POINT ( 'NONE',  ( -16.53943276465976808, -0.05219959533934237506, 108.7510903946857042 ) ) ;
#137726=CARTESIAN_POINT ( 'NONE',  ( 18.67979575497194134, -10.72451020669871369, 65.83442372801900433 ) ) ;
#137727=CARTESIAN_POINT ( 'NONE',  ( -4.379528057220086978, -16.55341960407618274, 24.79275706135235779 ) ) ;
#137728=CARTESIAN_POINT ( 'NONE',  ( -12.06949235617756955, 12.14591786802309770, 110.6239096053143669 ) ) ;
#137729=CARTESIAN_POINT ( 'NONE',  ( -12.14591786802326823, 12.06949235617739902, 23.12609039468567573 ) ) ;
#137730=CARTESIAN_POINT ( 'NONE',  ( 16.51473224551069308, 9.474510206698969483, 59.16557627198102409 ) ) ;
#137732=CARTESIAN_POINT ( 'NONE',  ( 16.46253265017160672, -9.564922557960803928, 108.3322429386476955 ) ) ;
#137733=CARTESIAN_POINT ( 'NONE',  ( -14.29746914071037622, -8.314922557961029526, 94.16775706135237556 ) ) ;
#137734=CARTESIAN_POINT ( 'NONE',  ( 0.05219959533936267826, -19.03943276465977164, 90.00109039468567573 ) ) ;
#137735=CARTESIAN_POINT ( 'NONE',  ( -21.55341960407619339, 5.719274019375674811, 113.5427570613523756 ) ) ;
#137736=CARTESIAN_POINT ( 'NONE',  ( 18.67979575497178502, 10.72451020669898547, 69.16557627198102409 ) ) ;
#137737=CARTESIAN_POINT ( 'NONE',  ( 8.314922557961029526, -14.29746914071037800, 105.4177570613523613 ) ) ;
#137738=CARTESIAN_POINT ( 'NONE',  ( -9.474510206698720793, -16.51473224551083518, 94.58442372801900433 ) ) ;
#137739=CARTESIAN_POINT ( 'NONE',  ( -0.05219959533909027116, -19.03943276465977164, 52.49890960531436690 ) ) ;
#137740=CARTESIAN_POINT ( 'NONE',  ( -0.05219959533909027116, -19.03943276465977164, 97.49890960531436690 ) ) ;
#137741=CARTESIAN_POINT ( 'NONE',  ( 18.62759615963255655, 10.81492255796105972, 46.66775706135234714 ) ) ;
#137742=CARTESIAN_POINT ( 'NONE',  ( 0.05219959533909260263, 19.03943276465977164, 44.99890960531435979 ) ) ;
#137744=CARTESIAN_POINT ( 'NONE',  ( 16.52544592524342804, -4.483927247898539470, 58.54057627198103120 ) ) ;
#137745=CARTESIAN_POINT ( 'NONE',  ( 10.72451020669898902, -18.67979575497178502, 72.91557627198103830 ) ) ;
#137747=CARTESIAN_POINT ( 'NONE',  ( 5.049401038297881783, 19.05341960407617563, 37.29275706135232582 ) ) ;
#137749=CARTESIAN_POINT ( 'NONE',  ( 19.02544592524343514, -5.153800228976328945, 73.54057627198103830 ) ) ;
#137750=CARTESIAN_POINT ( 'NONE',  ( 16.46253265017160672, -9.564922557960803928, 88.33224293864769550 ) ) ;
#137751=CARTESIAN_POINT ( 'NONE',  ( 16.55341960407618274, -4.379528057220086978, 56.04275706135235424 ) ) ;
#137753=CARTESIAN_POINT ( 'NONE',  ( 19.02544592524334988, 5.153800228976608722, 31.45942372801900433 ) ) ;
#137755=CARTESIAN_POINT ( 'NONE',  ( 16.53943276465976808, 0.05219959533934440121, 91.25109039468568994 ) ) ;
#137757=CARTESIAN_POINT ( 'NONE',  ( 16.53943276465976808, 0.05219959533934440121, 86.25109039468568994 ) ) ;
#137758=CARTESIAN_POINT ( 'NONE',  ( -12.06949235617739369, -12.14591786802326823, 54.37609039468568994 ) ) ;
#137759=CARTESIAN_POINT ( 'NONE',  ( -19.05341960407611168, -5.049401038298163336, 61.45724293864769550 ) ) ;
#137761=CARTESIAN_POINT ( 'NONE',  ( -5.823673210054431948, 21.52544592524334988, 62.70942372801902565 ) ) ;
#137762=CARTESIAN_POINT ( 'NONE',  ( 16.51473224551083163, -9.474510206698727899, 75.83442372801900433 ) ) ;
#137763=CARTESIAN_POINT ( 'NONE',  ( -16.46253265017146816, -9.564922557961047289, 19.16775706135233293 ) ) ;
#137764=CARTESIAN_POINT ( 'NONE',  ( 0.05219959533909260263, 19.03943276465977164, 49.99890960531435979 ) ) ;
#137765=CARTESIAN_POINT ( 'NONE',  ( -5.153800228976328057, -19.02544592524343514, 37.29057627198102409 ) ) ;
#137767=CARTESIAN_POINT ( 'NONE',  ( 18.62759615963271287, -10.81492255796078972, 68.33224293864769550 ) ) ;
#137768=CARTESIAN_POINT ( 'NONE',  ( -9.474510206698964154, 16.51473224551069663, 110.4155762719810383 ) ) ;
#137769=CARTESIAN_POINT ( 'NONE',  ( -14.29746914071049879, 8.314922557960819915, 110.8322429386476955 ) ) ;
#137770=CARTESIAN_POINT ( 'NONE',  ( -4.379528057220086978, -16.55341960407618274, 44.79275706135234714 ) ) ;
#137771=CARTESIAN_POINT ( 'NONE',  ( -12.06949235617756955, 12.14591786802309770, 30.62390960531436335 ) ) ;
#137773=CARTESIAN_POINT ( 'NONE',  ( 15.80617190586746368, 15.72974639402197994, 109.3739096053143811 ) ) ;
#137774=CARTESIAN_POINT ( 'NONE',  ( 16.55341960407611168, 4.379528057220329451, 58.95724293864770971 ) ) ;
#137776=CARTESIAN_POINT ( 'NONE',  ( -19.02544592524334988, -5.153800228976617603, 103.9594237280190043 ) ) ;
#137777=CARTESIAN_POINT ( 'NONE',  ( -5.049401038297874678, -19.05341960407617918, 39.79275706135232582 ) ) ;
#137778=CARTESIAN_POINT ( 'NONE',  ( -12.06949235617756955, 12.14591786802309770, 50.62390960531435979 ) ) ;
#137779=CARTESIAN_POINT ( 'NONE',  ( -5.719274019375978568, 21.55341960407610458, 105.2072429386477097 ) ) ;
#137781=CARTESIAN_POINT ( 'NONE',  ( 17.40861289039003879, 6.110651285853275994, 33.87232470827431996 ) ) ;
#137782=CARTESIAN_POINT ( 'NONE',  ( 18.67979575497178502, 10.72451020669898547, 59.16557627198103120 ) ) ;
#137783=CARTESIAN_POINT ( 'NONE',  ( 9.474510206698971260, -16.51473224551069308, 72.91557627198102409 ) ) ;
#137784=CARTESIAN_POINT ( 'NONE',  ( 14.29746914071049879, -8.314922557960816363, 48.33224293864770260 ) ) ;
#137785=CARTESIAN_POINT ( 'NONE',  ( -5.153800228976328057, -19.02544592524343514, 107.2905762719810383 ) ) ;
#137788=CARTESIAN_POINT ( 'NONE',  ( 5.153800228976615827, -19.02544592524334988, 55.20942372801899722 ) ) ;
#137789=CARTESIAN_POINT ( 'NONE',  ( 5.719274019375991003, -21.55341960407610458, 92.70724293864770971 ) ) ;
#137790=CARTESIAN_POINT ( 'NONE',  ( 9.564922557960805705, 16.46253265017160317, 39.58224293864768839 ) ) ;
#137791=CARTESIAN_POINT ( 'NONE',  ( -16.52544592524342804, 4.483927247898546575, 116.0405762719810383 ) ) ;
#137792=CARTESIAN_POINT ( 'NONE',  ( 10.81492255796106328, -18.62759615963255655, 50.41775706135235424 ) ) ;
#137795=CARTESIAN_POINT ( 'NONE',  ( 14.29746914071049879, -8.314922557960816363, 33.33224293864769550 ) ) ;
#137796=CARTESIAN_POINT ( 'NONE',  ( 9.474510206698971260, -16.51473224551069308, 47.91557627198102409 ) ) ;
#137797=CARTESIAN_POINT ( 'NONE',  ( 5.153800228976335163, 19.02544592524342804, 104.7905762719809957 ) ) ;
#137798=CARTESIAN_POINT ( 'NONE',  ( -15.72974639402197994, 15.80617190586746368, 65.62390960531436690 ) ) ;
#137800=CARTESIAN_POINT ( 'NONE',  ( -19.03943276465977164, 0.05219959533909376836, 46.24890960531435979 ) ) ;
#137801=CARTESIAN_POINT ( 'NONE',  ( -10.72451020669898014, 18.67979575497178502, 50.41557627198103120 ) ) ;
#137802=CARTESIAN_POINT ( 'NONE',  ( 18.62759615963255655, 10.81492255796105972, 81.66775706135236135 ) ) ;
#137804=CARTESIAN_POINT ( 'NONE',  ( -14.29746914071037622, -8.314922557961029526, 84.16775706135234714 ) ) ;
#137805=CARTESIAN_POINT ( 'NONE',  ( -14.29746914071049879, 8.314922557960819915, 70.83224293864770971 ) ) ;
#137806=CARTESIAN_POINT ( 'NONE',  ( 12.14591786802327356, -12.06949235617739191, 85.62609039468568994 ) ) ;
#137807=CARTESIAN_POINT ( 'NONE',  ( 0.05219959533909260263, 19.03943276465977164, 74.99890960531435269 ) ) ;
#137808=VERTEX_POINT ( 'NONE', #73595 ) ;
#137809=CARTESIAN_POINT ( 'NONE',  ( 13.97604488694548053, -13.89961937509957401, 25.62609039468566507 ) ) ;
#137810=CARTESIAN_POINT ( 'NONE',  ( -0.05219959533934338120, 16.53943276465976808, 92.50109039468567573 ) ) ;
#137811=CARTESIAN_POINT ( 'NONE',  ( -21.53943276465977519, -0.05219959533937600094, 113.7510903946856757 ) ) ;
#137812=CARTESIAN_POINT ( 'NONE',  ( 16.46253265017160672, -9.564922557960803928, 78.33224293864769550 ) ) ;
#137813=CARTESIAN_POINT ( 'NONE',  ( 21.52544592524344225, -5.823673210054117533, 53.54057627198103120 ) ) ;
#137814=CARTESIAN_POINT ( 'NONE',  ( 16.53943276465976808, 0.05219959533934440121, 26.25109039468567573 ) ) ;
#137815=CARTESIAN_POINT ( 'NONE',  ( 5.719274019375673035, 21.55341960407619339, 77.29275706135234714 ) ) ;
#137816=CARTESIAN_POINT ( 'NONE',  ( 4.379528057220092307, 16.55341960407617563, 67.29275706135234714 ) ) ;
#137817=CARTESIAN_POINT ( 'NONE',  ( -15.72974639402176322, -15.80617190586768395, 19.37609039468568639 ) ) ;
#137818=CARTESIAN_POINT ( 'NONE',  ( 16.46253265017146816, 9.564922557961045513, 111.6677570613523329 ) ) ;
#137819=CARTESIAN_POINT ( 'NONE',  ( -19.05341960407611168, -5.049401038298163336, 96.45724293864769550 ) ) ;
#137820=CARTESIAN_POINT ( 'NONE',  ( 14.29746914071037800, 8.314922557961029526, 26.66775706135235424 ) ) ;
#137821=CARTESIAN_POINT ( 'NONE',  ( -0.05219959533909027116, -19.03943276465977164, 37.49890960531436690 ) ) ;
#137823=CARTESIAN_POINT ( 'NONE',  ( 16.52544592524335698, 4.483927247898782831, 21.45942372801901499 ) ) ;
#137824=CARTESIAN_POINT ( 'NONE',  ( -14.29746914071049879, 8.314922557960819915, 85.83224293864768129 ) ) ;
#137825=CARTESIAN_POINT ( 'NONE',  ( 16.53943276465976808, 0.05219959533934440121, 91.25109039468568994 ) ) ;
#137826=CARTESIAN_POINT ( 'NONE',  ( 5.719274019375673035, 21.55341960407619339, 27.29275706135234358 ) ) ;
#137827=CARTESIAN_POINT ( 'NONE',  ( 16.46253265017160672, -9.564922557960803928, 68.33224293864770971 ) ) ;
#137828=CARTESIAN_POINT ( 'NONE',  ( -13.97604488694527625, -13.89961937509977652, 71.87390960531433848 ) ) ;
#137829=CARTESIAN_POINT ( 'NONE',  ( -4.379528057220086978, -16.55341960407618274, 84.79275706135234714 ) ) ;
#137834=CARTESIAN_POINT ( 'NONE',  ( 9.564922557961047289, -16.46253265017146816, 30.41775706135232937 ) ) ;
#137836=CARTESIAN_POINT ( 'NONE',  ( 13.89961937509977652, -13.97604488694527269, 48.12390960531435979 ) ) ;
#137837=CARTESIAN_POINT ( 'NONE',  ( -5.049401038298153566, 19.05341960407611168, 110.2072429386476671 ) ) ;
#137838=ORIENTED_EDGE ( 'NONE', *, *, #143824, .F. ) ;
#137839=CARTESIAN_POINT ( 'NONE',  ( -8.224510206698735004, -14.34966873604973081, 24.58442372801901499 ) ) ;
#137840=CARTESIAN_POINT ( 'NONE',  ( 13.89961937509957401, 13.97604488694547697, 56.87609039468564731 ) ) ;
#137841=CARTESIAN_POINT ( 'NONE',  ( -8.224510206698735004, -14.34966873604973081, 44.58442372801901854 ) ) ;
#137842=CARTESIAN_POINT ( 'NONE',  ( 5.153800228976335163, 19.02544592524342804, 99.79057627198102409 ) ) ;
#137843=CARTESIAN_POINT ( 'NONE',  ( 19.03943276465977164, -0.05219959533909143690, 78.74890960531436690 ) ) ;
#137844=CARTESIAN_POINT ( 'NONE',  ( 18.67979575497178502, 10.72451020669898547, 104.1655762719810241 ) ) ;
#137845=CARTESIAN_POINT ( 'NONE',  ( 9.474510206698729675, 16.51473224551082808, 67.08442372801900433 ) ) ;
#137846=CARTESIAN_POINT ( 'NONE',  ( 9.474510206698971260, -16.51473224551069308, 92.91557627198103830 ) ) ;
#137847=CARTESIAN_POINT ( 'NONE',  ( -9.564922557960796823, -16.46253265017161027, 22.08224293864768839 ) ) ;
#137848=CARTESIAN_POINT ( 'NONE',  ( 0.05219959533909260263, 19.03943276465977164, 64.99890960531436690 ) ) ;
#137849=CARTESIAN_POINT ( 'NONE',  ( 4.379528057220339221, -16.55341960407611168, 22.70724293864769194 ) ) ;
#137850=CARTESIAN_POINT ( 'NONE',  ( -0.05219959533909027116, -19.03943276465977164, 22.49890960531436690 ) ) ;
#137851=CARTESIAN_POINT ( 'NONE',  ( -13.97604488694547697, 13.89961937509957934, 43.12609039468566152 ) ) ;
#137852=CARTESIAN_POINT ( 'NONE',  ( 12.14591786802309770, 12.06949235617756955, 74.37390960531436690 ) ) ;
#137853=CARTESIAN_POINT ( 'NONE',  ( -10.81492255796105439, 18.62759615963255655, 92.91775706135236135 ) ) ;
#137854=CARTESIAN_POINT ( 'NONE',  ( -13.89961937509977652, 13.97604488694528158, 40.62390960531435979 ) ) ;
#137855=CARTESIAN_POINT ( 'NONE',  ( 16.55341960407618274, -4.379528057220086978, 56.04275706135235424 ) ) ;
#137856=CARTESIAN_POINT ( 'NONE',  ( 8.314922557960818139, 14.29746914071049879, 44.58224293864769550 ) ) ;
#137857=CARTESIAN_POINT ( 'NONE',  ( -0.05219959533937732626, 21.53943276465977519, 87.50109039468568994 ) ) ;
#137858=CARTESIAN_POINT ( 'NONE',  ( -5.153800228976328057, -19.02544592524343514, 97.29057627198099567 ) ) ;
#137859=CARTESIAN_POINT ( 'NONE',  ( 16.46253265017160672, -9.564922557960803928, 93.33224293864769550 ) ) ;
#137860=CARTESIAN_POINT ( 'NONE',  ( -4.483927247898539470, -16.52544592524342804, 107.2905762719810525 ) ) ;
#137861=CARTESIAN_POINT ( 'NONE',  ( 12.06949235617757843, -12.14591786802309237, 68.12390960531436690 ) ) ;
#137862=CARTESIAN_POINT ( 'NONE',  ( 5.823673210054125526, 21.52544592524343514, 89.79057627198103830 ) ) ;
#137863=CARTESIAN_POINT ( 'NONE',  ( -16.51473224551069308, -9.474510206698971260, 91.66557627198103830 ) ) ;
#137864=CARTESIAN_POINT ( 'NONE',  ( -15.80617190586745835, -15.72974639402198527, 96.87390960531436690 ) ) ;
#137865=CARTESIAN_POINT ( 'NONE',  ( -16.51473224551082808, 9.474510206698731452, 73.33442372801900433 ) ) ;
#137867=CARTESIAN_POINT ( 'NONE',  ( 0.05219959533910956823, 16.53943276465976808, 84.99890960531436690 ) ) ;
#137869=CARTESIAN_POINT ( 'NONE',  ( 16.46253265017160672, -9.564922557960803928, 53.33224293864768839 ) ) ;
#137870=CARTESIAN_POINT ( 'NONE',  ( 0.05219959533907565091, 21.53943276465977519, 69.99890960531435269 ) ) ;
#137871=CARTESIAN_POINT ( 'NONE',  ( 17.31728774477274158, -6.344390552232384906, 28.31906651689320142 ) ) ;
#137872=CARTESIAN_POINT ( 'NONE',  ( 4.483927247898545687, 16.52544592524342804, 24.79057627198103120 ) ) ;
#137873=CARTESIAN_POINT ( 'NONE',  ( 8.314922557961029526, -14.29746914071037800, 20.41775706135234714 ) ) ;
#137874=CARTESIAN_POINT ( 'NONE',  ( -4.483927247898539470, -16.52544592524342804, 87.29057627198103830 ) ) ;
#137875=CARTESIAN_POINT ( 'NONE',  ( -17.31747979337947285, -6.344076630961057006, 96.37944868065184778 ) ) ;
#137876=CARTESIAN_POINT ( 'NONE',  ( 5.153800228976335163, 19.02544592524342804, 69.79057627198103830 ) ) ;
#137877=CARTESIAN_POINT ( 'NONE',  ( -19.02544592524342804, 5.153800228976336051, 36.04057627198100988 ) ) ;
#137878=CARTESIAN_POINT ( 'NONE',  ( -12.06949235617756955, 12.14591786802309770, 65.62390960531436690 ) ) ;
#137879=CARTESIAN_POINT ( 'NONE',  ( -18.62759615963270932, 10.81492255796079327, 25.83224293864769194 ) ) ;
#137880=CARTESIAN_POINT ( 'NONE',  ( 5.153800228976615827, -19.02544592524334988, 90.20942372801900433 ) ) ;
#137881=CARTESIAN_POINT ( 'NONE',  ( 5.049401038298161559, -19.05341960407611168, 102.7072429386476955 ) ) ;
#137882=CARTESIAN_POINT ( 'NONE',  ( -15.80617190586745835, -15.72974639402198527, 71.87390960531438111 ) ) ;
#137883=CARTESIAN_POINT ( 'NONE',  ( -14.34966873604972548, 8.224510206698743886, 68.33442372801900433 ) ) ;
#137884=CARTESIAN_POINT ( 'NONE',  ( 13.89961937509957579, 13.97604488694547520, 106.8760903946856615 ) ) ;
#137885=CARTESIAN_POINT ( 'NONE',  ( -9.474510206698964154, 16.51473224551069663, 65.41557627198102409 ) ) ;
#137886=CARTESIAN_POINT ( 'NONE',  ( -15.80617190586745835, -15.72974639402198527, 71.87390960531438111 ) ) ;
#137887=CARTESIAN_POINT ( 'NONE',  ( -5.153800228976607833, 19.02544592524334988, 107.7094237280189759 ) ) ;
#137888=CARTESIAN_POINT ( 'NONE',  ( 8.314922557960818139, 14.29746914071049879, 39.58224293864769550 ) ) ;
#137889=CARTESIAN_POINT ( 'NONE',  ( -21.55341960407619339, 5.719274019375674811, 58.54275706135235424 ) ) ;
#137891=CARTESIAN_POINT ( 'NONE',  ( -14.34966873604972548, 8.224510206698743886, 78.33442372801901854 ) ) ;
#137892=CARTESIAN_POINT ( 'NONE',  ( -13.89961937509977652, 13.97604488694528158, 100.6239096053143669 ) ) ;
#137893=CARTESIAN_POINT ( 'NONE',  ( -13.89961937509977830, 13.97604488694528158, 105.6239096053143527 ) ) ;
#137894=CARTESIAN_POINT ( 'NONE',  ( -16.61371651742601685, 7.165104196376145040, 78.85415069992998838 ) ) ;
#137895=CARTESIAN_POINT ( 'NONE',  ( -12.14591786802326823, 12.06949235617739902, 98.12609039468570415 ) ) ;
#137896=CARTESIAN_POINT ( 'NONE',  ( 12.14591786802327356, -12.06949235617739191, 40.62609039468567573 ) ) ;
#137897=CARTESIAN_POINT ( 'NONE',  ( 0.05219959533909260263, 19.03943276465977164, 59.99890960531436690 ) ) ;
#137898=CARTESIAN_POINT ( 'NONE',  ( -5.153800228976328057, -19.02544592524343514, 72.29057627198102409 ) ) ;
#137899=CARTESIAN_POINT ( 'NONE',  ( 21.53943276465977519, 0.05219959533937863772, 66.25109039468567573 ) ) ;
#137900=CARTESIAN_POINT ( 'NONE',  ( -4.379528057220086978, -16.55341960407618274, 59.79275706135234714 ) ) ;
#137901=CARTESIAN_POINT ( 'NONE',  ( 12.06949235617757843, -12.14591786802309237, 33.12390960531435979 ) ) ;
#137902=CARTESIAN_POINT ( 'NONE',  ( 19.03943276465977164, -0.05219959533909143690, 38.74890960531436690 ) ) ;
#137903=CARTESIAN_POINT ( 'NONE',  ( -16.46253265017160317, 9.564922557960807481, 35.83224293864768839 ) ) ;
#137904=CARTESIAN_POINT ( 'NONE',  ( 12.06949235617739724, 12.14591786802326823, 31.87609039468567929 ) ) ;
#137906=CARTESIAN_POINT ( 'NONE',  ( -16.46253265017146816, -9.564922557961047289, 99.16775706135233293 ) ) ;
#137907=CARTESIAN_POINT ( 'NONE',  ( -16.53943276465976808, 0.05219959533911058130, 96.24890960531435269 ) ) ;
#137908=CARTESIAN_POINT ( 'NONE',  ( 13.97604488694527802, 13.89961937509977652, 54.37390960531435979 ) ) ;
#137909=CARTESIAN_POINT ( 'NONE',  ( -19.03943276465977164, -0.05219959533935918106, 83.75109039468567573 ) ) ;
#137911=CARTESIAN_POINT ( 'NONE',  ( 18.67979575497194134, -10.72451020669871369, 90.83442372801901854 ) ) ;
#137912=CARTESIAN_POINT ( 'NONE',  ( 0.05219959533934541429, -16.53943276465976808, 60.00109039468568284 ) ) ;
#137914=CARTESIAN_POINT ( 'NONE',  ( -5.719274019375978568, 21.55341960407610458, 45.20724293864769550 ) ) ;
#137915=CARTESIAN_POINT ( 'NONE',  ( -4.379528057220086978, -16.55341960407618274, 34.79275706135235424 ) ) ;
#137916=CARTESIAN_POINT ( 'NONE',  ( -19.02544592524334988, -5.153800228976617603, 38.95942372801900433 ) ) ;
#137917=CARTESIAN_POINT ( 'NONE',  ( -13.89961937509977652, 13.97604488694528158, 95.62390960531436690 ) ) ;
#137918=CARTESIAN_POINT ( 'NONE',  ( -13.89961937509977652, 13.97604488694528158, 50.62390960531435979 ) ) ;
#137920=CARTESIAN_POINT ( 'NONE',  ( -21.55341960407619339, 5.719274019375674811, 78.54275706135236135 ) ) ;
#137922=CARTESIAN_POINT ( 'NONE',  ( 5.049401038297881783, 19.05341960407617563, 27.29275706135232937 ) ) ;
#137923=CARTESIAN_POINT ( 'NONE',  ( -15.80617190586768217, 15.72974639402176855, 108.1260903946856757 ) ) ;
#137924=CARTESIAN_POINT ( 'NONE',  ( -4.483927247898539470, -16.52544592524342804, 47.29057627198103120 ) ) ;
#137925=CARTESIAN_POINT ( 'NONE',  ( -19.02544592524342804, 5.153800228976336051, 61.04057627198103120 ) ) ;
#137926=CARTESIAN_POINT ( 'NONE',  ( -5.049401038298153566, 19.05341960407611168, 110.2072429386476671 ) ) ;
#137927=CARTESIAN_POINT ( 'NONE',  ( -18.67979575497193778, 10.72451020669871902, 78.33442372801901854 ) ) ;
#137928=CARTESIAN_POINT ( 'NONE',  ( 5.153800228976335163, 19.02544592524342804, 69.79057627198103830 ) ) ;
#137929=CARTESIAN_POINT ( 'NONE',  ( -18.67979575497193778, 10.72451020669871902, 73.33442372801901854 ) ) ;
#137930=CARTESIAN_POINT ( 'NONE',  ( 21.52544592524344225, -5.823673210054117533, 43.54057627198103830 ) ) ;
#137931=CARTESIAN_POINT ( 'NONE',  ( -18.62759615963255300, -10.81492255796106328, 24.16775706135235424 ) ) ;
#137932=CARTESIAN_POINT ( 'NONE',  ( -9.564922557961040184, 16.46253265017147172, 62.91775706135233293 ) ) ;
#137933=CARTESIAN_POINT ( 'NONE',  ( 16.46253265017160672, -9.564922557960803928, 33.33224293864770260 ) ) ;
#137934=CARTESIAN_POINT ( 'NONE',  ( -0.05219959533909027116, -19.03943276465977164, 72.49890960531435269 ) ) ;
#137935=CARTESIAN_POINT ( 'NONE',  ( -4.379528057220086978, -16.55341960407618274, 24.79275706135235779 ) ) ;
#137936=CARTESIAN_POINT ( 'NONE',  ( 12.06949235617757843, -12.14591786802309237, 88.12390960531436690 ) ) ;
#137937=CARTESIAN_POINT ( 'NONE',  ( 9.564922557960805705, 16.46253265017160317, 54.58224293864769550 ) ) ;
#137938=CARTESIAN_POINT ( 'NONE',  ( 15.80617190586746368, 15.72974639402197994, 39.37390960531436690 ) ) ;
#137939=CARTESIAN_POINT ( 'NONE',  ( -13.89961937509957401, -13.97604488694547875, 99.37609039468567573 ) ) ;
#137940=CARTESIAN_POINT ( 'NONE',  ( -15.80617190586768217, 15.72974639402176855, 23.12609039468567573 ) ) ;
#137941=CARTESIAN_POINT ( 'NONE',  ( -18.62759615963255300, -10.81492255796106328, 74.16775706135231871 ) ) ;
#137942=CARTESIAN_POINT ( 'NONE',  ( -8.224510206698735004, -14.34966873604973081, 74.58442372801901854 ) ) ;
#137943=CARTESIAN_POINT ( 'NONE',  ( 4.379528057220092307, 16.55341960407617563, 67.29275706135234714 ) ) ;
#137945=CARTESIAN_POINT ( 'NONE',  ( 5.049401038298161559, -19.05341960407611168, 62.70724293864769550 ) ) ;
#137946=CARTESIAN_POINT ( 'NONE',  ( -12.06949235617739369, -12.14591786802326823, 84.37609039468570415 ) ) ;
#137947=CARTESIAN_POINT ( 'NONE',  ( -16.51473224551082808, 9.474510206698731452, 43.33442372801900433 ) ) ;
#137948=CARTESIAN_POINT ( 'NONE',  ( -21.55341960407610458, -5.719274019375992779, 111.4572429386476813 ) ) ;
#137949=CARTESIAN_POINT ( 'NONE',  ( 8.314922557960818139, 14.29746914071049879, 69.58224293864769550 ) ) ;
#137950=CARTESIAN_POINT ( 'NONE',  ( 9.564922557960805705, 16.46253265017160317, 89.58224293864769550 ) ) ;
#137951=CARTESIAN_POINT ( 'NONE',  ( 0.05219959533934541429, -16.53943276465976808, 85.00109039468568994 ) ) ;
#137952=CARTESIAN_POINT ( 'NONE',  ( -18.62759615963255300, -10.81492255796106328, 59.16775706135234714 ) ) ;
#137953=CARTESIAN_POINT ( 'NONE',  ( 5.049401038297881783, 19.05341960407617563, 112.2927570613523471 ) ) ;
#137954=CARTESIAN_POINT ( 'NONE',  ( -5.719274019375978568, 21.55341960407610458, 115.2072429386476955 ) ) ;
#137955=CARTESIAN_POINT ( 'NONE',  ( 8.314922557960818139, 14.29746914071049879, 54.58224293864769550 ) ) ;
#137958=CARTESIAN_POINT ( 'NONE',  ( -5.823673210054116645, -21.52544592524344225, 92.29057627198103830 ) ) ;
#137959=CARTESIAN_POINT ( 'NONE',  ( -8.224510206698948167, 14.34966873604960824, 40.41557627198103120 ) ) ;
#137960=VERTEX_POINT ( 'NONE', #195953 ) ;
#137962=CARTESIAN_POINT ( 'NONE',  ( -21.53943276465977519, -0.05219959533937600094, 23.75109039468567929 ) ) ;
#137963=CARTESIAN_POINT ( 'NONE',  ( 19.03943276465977164, -0.05219959533909143690, 108.7489096053143527 ) ) ;
#137964=CARTESIAN_POINT ( 'NONE',  ( 15.80617190586769283, -15.72974639402175789, 30.62609039468567929 ) ) ;
#137965=CARTESIAN_POINT ( 'NONE',  ( 12.06949235617757843, -12.14591786802309237, 58.12390960531435979 ) ) ;
#137967=CARTESIAN_POINT ( 'NONE',  ( -19.03943276465977164, 0.05219959533909376836, 56.24890960531435979 ) ) ;
#137968=CARTESIAN_POINT ( 'NONE',  ( -9.564922557961040184, 16.46253265017147172, 62.91775706135233293 ) ) ;
#137969=CARTESIAN_POINT ( 'NONE',  ( 13.97604488694527802, 13.89961937509977652, 89.37390960531436690 ) ) ;
#137970=CARTESIAN_POINT ( 'NONE',  ( 0.05219959533907565091, 21.53943276465977519, 44.99890960531435979 ) ) ;
#137972=CARTESIAN_POINT ( 'NONE',  ( -5.049401038298153566, 19.05341960407611168, 65.20724293864765286 ) ) ;
#137973=CARTESIAN_POINT ( 'NONE',  ( -12.14591786802326823, 12.06949235617739902, 43.12609039468568284 ) ) ;
#137974=CARTESIAN_POINT ( 'NONE',  ( 19.05341960407617918, -5.049401038297876454, 66.04275706135233293 ) ) ;
#137975=CARTESIAN_POINT ( 'NONE',  ( -5.719274019375978568, 21.55341960407610458, 110.2072429386477239 ) ) ;
#137976=CARTESIAN_POINT ( 'NONE',  ( 16.55341960407611168, 4.379528057220329451, 48.95724293864770971 ) ) ;
#137978=CARTESIAN_POINT ( 'NONE',  ( -5.153800228976328057, -19.02544592524343514, 97.29057627198099567 ) ) ;
#137979=CARTESIAN_POINT ( 'NONE',  ( 21.53943276465977519, -0.05219959533907433946, 73.74890960531433848 ) ) ;
#137980=CARTESIAN_POINT ( 'NONE',  ( 21.53943276465977519, -0.05219959533907433946, 103.7489096053143669 ) ) ;
#137981=CARTESIAN_POINT ( 'NONE',  ( 12.14591786802327356, -12.06949235617739191, 35.62609039468568994 ) ) ;
#137982=CARTESIAN_POINT ( 'NONE',  ( -21.55341960407610458, -5.719274019375992779, 31.45724293864769550 ) ) ;
#137983=CARTESIAN_POINT ( 'NONE',  ( -21.55341960407619339, 5.719274019375674811, 98.54275706135234714 ) ) ;
#137984=CARTESIAN_POINT ( 'NONE',  ( -16.51473224551069308, -9.474510206698971260, 91.66557627198103830 ) ) ;
#137985=CARTESIAN_POINT ( 'NONE',  ( -13.89961937509977652, 13.97604488694528158, 40.62390960531435979 ) ) ;
#137986=CARTESIAN_POINT ( 'NONE',  ( 13.97604488694527802, 13.89961937509977652, 99.37390960531436690 ) ) ;
#137987=CARTESIAN_POINT ( 'NONE',  ( -16.51473224551069308, -9.474510206698971260, 71.66557627198102409 ) ) ;
#137988=CARTESIAN_POINT ( 'NONE',  ( 4.483927247898790824, -16.52544592524335698, 20.20942372801900788 ) ) ;
#137989=CARTESIAN_POINT ( 'NONE',  ( 0.05219959533936267826, -19.03943276465977164, 55.00109039468566863 ) ) ;
#137991=CARTESIAN_POINT ( 'NONE',  ( -21.52544592524334988, -5.823673210054445271, 108.9594237280190185 ) ) ;
#137992=CARTESIAN_POINT ( 'NONE',  ( -21.53943276465977519, 0.05219959533907696930, 31.24890960531435979 ) ) ;
#137993=CARTESIAN_POINT ( 'NONE',  ( -16.55341960407617563, 4.379528057220093196, 103.5427570613523613 ) ) ;
#137995=CARTESIAN_POINT ( 'NONE',  ( -19.02544592524334988, -5.153800228976617603, 73.95942372801900433 ) ) ;
#137996=CARTESIAN_POINT ( 'NONE',  ( 9.564922557961047289, -16.46253265017146816, 35.41775706135233293 ) ) ;
#137998=CARTESIAN_POINT ( 'NONE',  ( -9.474510206698964154, 16.51473224551069663, 45.41557627198103120 ) ) ;
#137999=CARTESIAN_POINT ( 'NONE',  ( -16.53943276465976808, 0.05219959533911058130, 41.24890960531435269 ) ) ;
#138000=CARTESIAN_POINT ( 'NONE',  ( -0.05219959533909027116, -19.03943276465977164, 22.49890960531436690 ) ) ;
#138001=CARTESIAN_POINT ( 'NONE',  ( -0.05219959533910754901, -16.53943276465976808, 32.49890960531435979 ) ) ;
#138002=LINE ( 'NONE', #153163, #145266 ) ;
#138003=CARTESIAN_POINT ( 'NONE',  ( 0.05219959533934541429, -16.53943276465976808, 100.0010903946857042 ) ) ;
#138004=CARTESIAN_POINT ( 'NONE',  ( -19.05341960407611168, -5.049401038298163336, 36.45724293864766707 ) ) ;
#138005=CARTESIAN_POINT ( 'NONE',  ( 5.719274019375673035, 21.55341960407619339, 107.2927570613523471 ) ) ;
#138006=CARTESIAN_POINT ( 'NONE',  ( -19.03943276465977164, -0.05219959533935918106, 113.7510903946856757 ) ) ;
#138007=CARTESIAN_POINT ( 'NONE',  ( -21.53943276465977519, -0.05219959533937600094, 83.75109039468568994 ) ) ;
#138009=CARTESIAN_POINT ( 'NONE',  ( 19.02544592524334988, 5.153800228976608722, 56.45942372801898301 ) ) ;
#138010=CARTESIAN_POINT ( 'NONE',  ( 13.97604488694527802, 13.89961937509977652, 94.37390960531436690 ) ) ;
#138011=CARTESIAN_POINT ( 'NONE',  ( -0.05219959533909027116, -19.03943276465977164, 82.49890960531436690 ) ) ;
#138013=CARTESIAN_POINT ( 'NONE',  ( 21.53943276465977519, -0.05219959533907433946, 108.7489096053143669 ) ) ;
#138015=CARTESIAN_POINT ( 'NONE',  ( -16.52544592524342804, 4.483927247898546575, 66.04057627198103830 ) ) ;
#138016=CARTESIAN_POINT ( 'NONE',  ( -0.05219959533907301413, -21.53943276465977519, 67.49890960531436690 ) ) ;
#138017=CARTESIAN_POINT ( 'NONE',  ( -9.474510206698964154, 16.51473224551069663, 65.41557627198102409 ) ) ;
#138018=CARTESIAN_POINT ( 'NONE',  ( -5.823673210054116645, -21.52544592524344225, 92.29057627198103830 ) ) ;
#138019=CARTESIAN_POINT ( 'NONE',  ( 16.53943276465976808, 0.05219959533934440121, 96.25109039468568994 ) ) ;
#138020=B_SPLINE_CURVE_WITH_KNOTS ( 'NONE', 3,
 ( #86159, #40662, #37652, #22495, #145821, #53829, #38665, #100320, #161999, #89151, #195355, #44643, #56835, #90136, #10335, #150840, #133665, #183159, #165012, #12336 ),
 .UNSPECIFIED., .F., .F.,
 ( 4, 2, 2, 2, 2, 2, 2, 2, 2, 4 ),
 ( 0.000000000000000000, 0.0004987090165372568733, 0.0009974180330745137466, 0.001246772541343134973, 0.001496127049611756417, 0.001994836066149022289, 0.002493545082686287728, 0.002742899590954930421, 0.002992254099223572682, 0.003989672132298142590 ),
 .UNSPECIFIED. ) ;
#138021=VERTEX_POINT ( 'NONE', #165598 ) ;
#138022=CARTESIAN_POINT ( 'NONE',  ( -16.51473224551069308, -9.474510206698971260, 56.66557627198103120 ) ) ;
#138023=CARTESIAN_POINT ( 'NONE',  ( 8.224510206698953496, -14.34966873604960469, 97.91557627198103830 ) ) ;
#138025=CARTESIAN_POINT ( 'NONE',  ( 13.97604488694527802, 13.89961937509977652, 44.37390960531435269 ) ) ;
#138026=CARTESIAN_POINT ( 'NONE',  ( -16.51473224551082808, 9.474510206698731452, 83.33442372801899012 ) ) ;
#138027=CARTESIAN_POINT ( 'NONE',  ( 14.29746914071049879, -8.314922557960816363, 78.33224293864770971 ) ) ;
#138028=CARTESIAN_POINT ( 'NONE',  ( -0.05219959533937732626, 21.53943276465977519, 62.50109039468568284 ) ) ;
#138029=CARTESIAN_POINT ( 'NONE',  ( -9.474510206698964154, 16.51473224551069663, 30.41557627198102054 ) ) ;
#138030=CARTESIAN_POINT ( 'NONE',  ( 10.81492255796078972, 18.62759615963270932, 104.5822429386477097 ) ) ;
#138031=CARTESIAN_POINT ( 'NONE',  ( -14.34966873604960291, -8.224510206698953496, 86.66557627198102409 ) ) ;
#138034=CARTESIAN_POINT ( 'NONE',  ( 13.97604488694527802, 13.89961937509977652, 59.37390960531434558 ) ) ;
#138035=CARTESIAN_POINT ( 'NONE',  ( 19.52851543214741881, 5.500000000000026645, 47.89357721762581122 ) ) ;
#138036=CARTESIAN_POINT ( 'NONE',  ( 5.153800228976615827, -19.02544592524334988, 95.20942372801897591 ) ) ;
#138037=CARTESIAN_POINT ( 'NONE',  ( -19.03943276465977164, 0.05219959533909376836, 111.2489096053143669 ) ) ;
#138038=CARTESIAN_POINT ( 'NONE',  ( -15.72974639402176322, -15.80617190586768395, 34.37609039468568284 ) ) ;
#138039=CARTESIAN_POINT ( 'NONE',  ( 9.474510206698971260, -16.51473224551069308, 87.91557627198102409 ) ) ;
#138040=CARTESIAN_POINT ( 'NONE',  ( -13.97604488694547697, 13.89961937509957934, 73.12609039468568994 ) ) ;
#138041=CARTESIAN_POINT ( 'NONE',  ( 16.46253265017160672, -9.564922557960803928, 63.33224293864769550 ) ) ;
#138042=CARTESIAN_POINT ( 'NONE',  ( -16.53943276465976808, 0.05219959533911058130, 76.24890960531435269 ) ) ;
#138043=CARTESIAN_POINT ( 'NONE',  ( 16.52544592524342804, -4.483927247898539470, 63.54057627198103830 ) ) ;
#138044=CARTESIAN_POINT ( 'NONE',  ( -0.05219959533909027116, -19.03943276465977164, 92.49890960531436690 ) ) ;
#138045=CARTESIAN_POINT ( 'NONE',  ( 10.72451020669898902, -18.67979575497178502, 102.9155762719810383 ) ) ;
#138046=CARTESIAN_POINT ( 'NONE',  ( 16.46253265017160672, -9.564922557960803928, 88.33224293864769550 ) ) ;
#138047=CARTESIAN_POINT ( 'NONE',  ( -19.05341960407617563, 5.049401038297882671, 33.54275706135231871 ) ) ;
#138048=CARTESIAN_POINT ( 'NONE',  ( -16.46253265017160317, 9.564922557960807481, 30.83224293864769550 ) ) ;
#138049=CARTESIAN_POINT ( 'NONE',  ( 4.483927247898545687, 16.52544592524342804, 34.79057627198103120 ) ) ;
#138050=CARTESIAN_POINT ( 'NONE',  ( 12.14591786802309770, 12.06949235617756955, 104.3739096053143669 ) ) ;
#138052=CARTESIAN_POINT ( 'NONE',  ( -10.81492255796105439, 18.62759615963255655, 37.91775706135235424 ) ) ;
#138053=CARTESIAN_POINT ( 'NONE',  ( 19.02544592524334988, 5.153800228976608722, 66.45942372801899012 ) ) ;
#138054=CARTESIAN_POINT ( 'NONE',  ( 4.483927247898545687, 16.52544592524342804, 34.79057627198103120 ) ) ;
#138055=CARTESIAN_POINT ( 'NONE',  ( 21.55341960407610458, 5.719274019375980345, 88.95724293864769550 ) ) ;
#138056=CARTESIAN_POINT ( 'NONE',  ( -9.474510206698964154, 16.51473224551069663, 110.4155762719810383 ) ) ;
#138057=CARTESIAN_POINT ( 'NONE',  ( 0.05219959533910956823, 16.53943276465976808, 69.99890960531435269 ) ) ;
#138058=CARTESIAN_POINT ( 'NONE',  ( -0.05219959533909027116, -19.03943276465977164, 27.49890960531435624 ) ) ;
#138059=CARTESIAN_POINT ( 'NONE',  ( -13.97604488694547697, 13.89961937509957934, 23.12609039468565442 ) ) ;
#138060=CARTESIAN_POINT ( 'NONE',  ( 12.06949235617739724, 12.14591786802326823, 96.87609039468568994 ) ) ;
#138061=CARTESIAN_POINT ( 'NONE',  ( -16.53943276465976808, -0.05219959533934237506, 58.75109039468568994 ) ) ;
#138062=CARTESIAN_POINT ( 'NONE',  ( 10.72451020669898902, -18.67979575497178502, 37.91557627198102409 ) ) ;
#138063=CARTESIAN_POINT ( 'NONE',  ( 21.52544592524334988, 5.823673210054432836, 101.4594237280190185 ) ) ;
#138064=CARTESIAN_POINT ( 'NONE',  ( 13.89961937509977652, -13.97604488694527269, 78.12390960531433848 ) ) ;
#138065=CARTESIAN_POINT ( 'NONE',  ( -12.06949235617739369, -12.14591786802326823, 79.37609039468567573 ) ) ;
#138066=CARTESIAN_POINT ( 'NONE',  ( 16.51473224551069308, 9.474510206698969483, 24.16557627198102765 ) ) ;
#138067=CARTESIAN_POINT ( 'NONE',  ( 14.34966873604960469, 8.224510206698951720, 34.16557627198102409 ) ) ;
#138068=CARTESIAN_POINT ( 'NONE',  ( 19.03943276465977164, -0.05219959533909143690, 103.7489096053143669 ) ) ;
#138069=CARTESIAN_POINT ( 'NONE',  ( -13.89961937509977652, 13.97604488694528158, 90.62390960531432427 ) ) ;
#138070=CARTESIAN_POINT ( 'NONE',  ( 21.53943276465977519, -0.05219959533907433946, 28.74890960531435624 ) ) ;
#138071=CARTESIAN_POINT ( 'NONE',  ( 16.55341960407611168, 4.379528057220329451, 53.95724293864770260 ) ) ;
#138072=CARTESIAN_POINT ( 'NONE',  ( -4.379528057220328563, 16.55341960407611168, 35.20724293864768839 ) ) ;
#138074=CARTESIAN_POINT ( 'NONE',  ( -4.379528057220328563, 16.55341960407611168, 50.20724293864769550 ) ) ;
#138075=CARTESIAN_POINT ( 'NONE',  ( -16.52544592524335698, -4.483927247898792601, 43.95942372801902565 ) ) ;
#138077=CARTESIAN_POINT ( 'NONE',  ( -9.474510206698720793, -16.51473224551083518, 54.58442372801899722 ) ) ;
#138078=CARTESIAN_POINT ( 'NONE',  ( 19.05341960407611168, 5.049401038298154454, 88.95724293864769550 ) ) ;
#138079=CARTESIAN_POINT ( 'NONE',  ( 13.97604488694548053, -13.89961937509957401, 60.62609039468564731 ) ) ;
#138081=CARTESIAN_POINT ( 'NONE',  ( 19.02544592524334988, 5.153800228976608722, 61.45942372801900433 ) ) ;
#138082=CARTESIAN_POINT ( 'NONE',  ( 5.153800228976615827, -19.02544592524334988, 95.20942372801897591 ) ) ;
#138083=CARTESIAN_POINT ( 'NONE',  ( -14.29746914071037622, -8.314922557961029526, 84.16775706135234714 ) ) ;
#138085=CARTESIAN_POINT ( 'NONE',  ( 9.474510206698971260, -16.51473224551069308, 27.91557627198103120 ) ) ;
#138086=CARTESIAN_POINT ( 'NONE',  ( 18.62759615963271287, -10.81492255796078972, 23.33224293864769194 ) ) ;
#138087=CARTESIAN_POINT ( 'NONE',  ( 5.719274019375673035, 21.55341960407619339, 37.29275706135235424 ) ) ;
#138088=CARTESIAN_POINT ( 'NONE',  ( 5.153800228976615827, -19.02544592524334988, 110.2094237280189901 ) ) ;
#138089=CARTESIAN_POINT ( 'NONE',  ( 17.50000000000001066, 3.604700896430133472, 23.09746379124990767 ) ) ;
#138090=CARTESIAN_POINT ( 'NONE',  ( 16.46253265017160672, -9.564922557960803928, 63.33224293864769550 ) ) ;
#138091=CARTESIAN_POINT ( 'NONE',  ( -13.97604488694527625, -13.89961937509977652, 106.8739096053143669 ) ) ;
#138092=CARTESIAN_POINT ( 'NONE',  ( -14.29746914071049879, 8.314922557960819915, 55.83224293864770260 ) ) ;
#138093=CARTESIAN_POINT ( 'NONE',  ( 9.564922557960805705, 16.46253265017160317, 59.58224293864769550 ) ) ;
#138094=CARTESIAN_POINT ( 'NONE',  ( 19.02544592524343514, -5.153800228976328945, 73.54057627198103830 ) ) ;
#138095=CARTESIAN_POINT ( 'NONE',  ( -0.05219959533936034679, 19.03943276465977164, 77.50109039468566152 ) ) ;
#138096=CARTESIAN_POINT ( 'NONE',  ( 10.81492255796078972, 18.62759615963270932, 54.58224293864769550 ) ) ;
#138097=CARTESIAN_POINT ( 'NONE',  ( -14.29746914071049879, 8.314922557960819915, 110.8322429386476955 ) ) ;
#138098=CARTESIAN_POINT ( 'NONE',  ( -16.51473224551082808, 9.474510206698731452, 48.33442372801900433 ) ) ;
#138099=CARTESIAN_POINT ( 'NONE',  ( -5.049401038298153566, 19.05341960407611168, 85.20724293864766707 ) ) ;
#138100=CARTESIAN_POINT ( 'NONE',  ( -21.52544592524343514, 5.823673210054127303, 71.04057627198103830 ) ) ;
#138101=CARTESIAN_POINT ( 'NONE',  ( 14.34966873604960469, 8.224510206698951720, 79.16557627198103830 ) ) ;
#138102=CARTESIAN_POINT ( 'NONE',  ( 5.153800228976615827, -19.02544592524334988, 30.20942372801900433 ) ) ;
#138103=CARTESIAN_POINT ( 'NONE',  ( -15.80617190586745835, -15.72974639402198527, 71.87390960531438111 ) ) ;
#138104=CARTESIAN_POINT ( 'NONE',  ( 21.55341960407610458, 5.719274019375980345, 58.95724293864770971 ) ) ;
#138105=CARTESIAN_POINT ( 'NONE',  ( 5.719274019375991003, -21.55341960407610458, 42.70724293864770260 ) ) ;
#138106=CARTESIAN_POINT ( 'NONE',  ( 5.823673210054444382, -21.52544592524334988, 85.20942372801901854 ) ) ;
#138107=CARTESIAN_POINT ( 'NONE',  ( -9.564922557960796823, -16.46253265017161027, 62.08224293864769550 ) ) ;
#138108=CARTESIAN_POINT ( 'NONE',  ( 0.05219959533910956823, 16.53943276465976808, 114.9989096053143669 ) ) ;
#138110=CARTESIAN_POINT ( 'NONE',  ( -10.81492255796105439, 18.62759615963255655, 27.91775706135234358 ) ) ;
#138112=CARTESIAN_POINT ( 'NONE',  ( 15.72974639402176855, 15.80617190586768217, 36.87609039468568994 ) ) ;
#138113=CARTESIAN_POINT ( 'NONE',  ( 5.153800228976335163, 19.02544592524342804, 34.79057627198102409 ) ) ;
#138114=CARTESIAN_POINT ( 'NONE',  ( 15.72974639402199770, -15.80617190586745480, 103.1239096053143811 ) ) ;
#138115=CARTESIAN_POINT ( 'NONE',  ( -13.89961937509957401, -13.97604488694547875, 44.37609039468566863 ) ) ;
#138116=CARTESIAN_POINT ( 'NONE',  ( 0.05219959533909260263, 19.03943276465977164, 39.99890960531436690 ) ) ;
#138117=CARTESIAN_POINT ( 'NONE',  ( -9.474510206698964154, 16.51473224551069663, 25.41557627198103120 ) ) ;
#138119=CARTESIAN_POINT ( 'NONE',  ( 14.34966873604972726, -8.224510206698740333, 60.83442372801901854 ) ) ;
#138120=CARTESIAN_POINT ( 'NONE',  ( -5.153800228976328057, -19.02544592524343514, 27.29057627198103120 ) ) ;
#138122=CARTESIAN_POINT ( 'NONE',  ( -19.02544592524342804, 5.153800228976336051, 91.04057627198100988 ) ) ;
#138123=CARTESIAN_POINT ( 'NONE',  ( 14.34966873604960469, 8.224510206698951720, 104.1655762719810241 ) ) ;
#138124=CARTESIAN_POINT ( 'NONE',  ( 21.52544592524344225, -5.823673210054117533, 58.54057627198103120 ) ) ;
#138125=CARTESIAN_POINT ( 'NONE',  ( 12.14591786802327356, -12.06949235617739191, 45.62609039468567573 ) ) ;
#138126=CARTESIAN_POINT ( 'NONE',  ( 0.05219959533937995610, -21.53943276465977519, 95.00109039468568994 ) ) ;
#138127=CARTESIAN_POINT ( 'NONE',  ( -9.564922557960796823, -16.46253265017161027, 27.08224293864769550 ) ) ;
#138128=CARTESIAN_POINT ( 'NONE',  ( 12.06949235617757843, -12.14591786802309237, 23.12390960531436335 ) ) ;
#138129=CARTESIAN_POINT ( 'NONE',  ( 14.34966873604960469, 8.224510206698951720, 59.16557627198103120 ) ) ;
#138130=CARTESIAN_POINT ( 'NONE',  ( -9.474510206698964154, 16.51473224551069663, 55.41557627198103120 ) ) ;
#138131=CARTESIAN_POINT ( 'NONE',  ( -19.02544592524334988, -5.153800228976617603, 18.95942372801899722 ) ) ;
#138132=CARTESIAN_POINT ( 'NONE',  ( 10.72451020669871369, 18.67979575497193778, 27.08442372801901854 ) ) ;
#138133=CARTESIAN_POINT ( 'NONE',  ( 0.05219959533937995610, -21.53943276465977519, 75.00109039468568994 ) ) ;
#138134=CARTESIAN_POINT ( 'NONE',  ( -0.05219959533934338120, 16.53943276465976808, 57.50109039468568994 ) ) ;
#138135=CARTESIAN_POINT ( 'NONE',  ( -14.34966873604972548, 8.224510206698743886, 28.33442372801902209 ) ) ;
#138136=CARTESIAN_POINT ( 'NONE',  ( 4.379528057220339221, -16.55341960407611168, 82.70724293864770971 ) ) ;
#138137=CARTESIAN_POINT ( 'NONE',  ( -15.80617190586768217, 15.72974639402176855, 93.12609039468568994 ) ) ;
#138139=CARTESIAN_POINT ( 'NONE',  ( -8.224510206698948167, 14.34966873604960824, 25.41557627198103120 ) ) ;
#138140=CARTESIAN_POINT ( 'NONE',  ( -17.49999999999999645, 5.499999999999996447, 113.7176903769643417 ) ) ;
#138141=CARTESIAN_POINT ( 'NONE',  ( 12.06949235617739724, 12.14591786802326823, 36.87609039468568994 ) ) ;
#138142=CARTESIAN_POINT ( 'NONE',  ( 16.52544592524342804, -4.483927247898539470, 38.54057627198103120 ) ) ;
#138143=CARTESIAN_POINT ( 'NONE',  ( -12.14591786802326823, 12.06949235617739902, 88.12609039468570415 ) ) ;
#138144=CARTESIAN_POINT ( 'NONE',  ( 5.049401038298161559, -19.05341960407611168, 97.70724293864766707 ) ) ;
#138145=CARTESIAN_POINT ( 'NONE',  ( 13.97604488694527802, 13.89961937509977652, 114.3739096053143669 ) ) ;
#138146=CARTESIAN_POINT ( 'NONE',  ( 18.67979575497194134, -10.72451020669871369, 95.83442372801903275 ) ) ;
#138147=CARTESIAN_POINT ( 'NONE',  ( -4.483927247898782831, 16.52544592524335698, 97.70942372801904696 ) ) ;
#138148=CARTESIAN_POINT ( 'NONE',  ( -16.53943276465976808, 0.05219959533911058130, 71.24890960531435269 ) ) ;
#138149=CARTESIAN_POINT ( 'NONE',  ( -16.46253265017160317, 9.564922557960807481, 85.83224293864769550 ) ) ;
#138150=ORIENTED_EDGE ( 'NONE', *, *, #85603, .F. ) ;
#138151=CARTESIAN_POINT ( 'NONE',  ( 4.483927247898790824, -16.52544592524335698, 40.20942372801901854 ) ) ;
#138152=CARTESIAN_POINT ( 'NONE',  ( 16.51473224551069308, 9.474510206698969483, 44.16557627198103120 ) ) ;
#138153=CARTESIAN_POINT ( 'NONE',  ( -0.05219959533909027116, -19.03943276465977164, 97.49890960531436690 ) ) ;
#138154=CARTESIAN_POINT ( 'NONE',  ( -14.29746914071037622, -8.314922557961029526, 34.16775706135234714 ) ) ;
#138156=CARTESIAN_POINT ( 'NONE',  ( 19.02544592524334988, 5.153800228976608722, 31.45942372801900433 ) ) ;
#138157=CARTESIAN_POINT ( 'NONE',  ( -0.05219959533934338120, 16.53943276465976808, 92.50109039468567573 ) ) ;
#138158=CARTESIAN_POINT ( 'NONE',  ( 13.89961937509977652, -13.97604488694527269, 38.12390960531436690 ) ) ;
#138159=CARTESIAN_POINT ( 'NONE',  ( 8.314922557961029526, -14.29746914071037800, 85.41775706135236135 ) ) ;
#138160=CARTESIAN_POINT ( 'NONE',  ( 16.55341960407618274, -4.379528057220086978, 66.04275706135236135 ) ) ;
#138161=CARTESIAN_POINT ( 'NONE',  ( -13.97604488694547697, 13.89961937509957934, 88.12609039468563310 ) ) ;
#138162=CARTESIAN_POINT ( 'NONE',  ( -16.46253265017146816, -9.564922557961047289, 29.16775706135232937 ) ) ;
#138163=CARTESIAN_POINT ( 'NONE',  ( 13.89961937509977652, -13.97604488694527269, 63.12390960531435979 ) ) ;
#138164=CARTESIAN_POINT ( 'NONE',  ( -14.34966873604960291, -8.224510206698953496, 86.66557627198102409 ) ) ;
#138165=EDGE_CURVE ( 'NONE', #115190, #22576, #103994, .T. ) ;
#138166=CARTESIAN_POINT ( 'NONE',  ( 19.03943276465977164, 0.05219959533936151252, 56.25109039468566863 ) ) ;
#138167=CARTESIAN_POINT ( 'NONE',  ( -21.55341960407610458, -5.719274019375992779, 56.45724293864768839 ) ) ;
#138168=CARTESIAN_POINT ( 'NONE',  ( 16.46253265017146816, 9.564922557961045513, 21.66775706135233648 ) ) ;
#138169=CARTESIAN_POINT ( 'NONE',  ( 9.474510206698971260, -16.51473224551069308, 107.9155762719810383 ) ) ;
#138170=CARTESIAN_POINT ( 'NONE',  ( 21.52544592524344225, -5.823673210054117533, 83.54057627198102409 ) ) ;
#138171=CARTESIAN_POINT ( 'NONE',  ( 19.05341960407611168, 5.049401038298154454, 103.9572429386476671 ) ) ;
#138172=CARTESIAN_POINT ( 'NONE',  ( 9.474510206698729675, 16.51473224551082808, 97.08442372801900433 ) ) ;
#138173=CARTESIAN_POINT ( 'NONE',  ( -9.564922557960796823, -16.46253265017161027, 112.0822429386476955 ) ) ;
#138174=CARTESIAN_POINT ( 'NONE',  ( -13.97604488694547697, 13.89961937509957934, 108.1260903946856331 ) ) ;
#138175=CARTESIAN_POINT ( 'NONE',  ( 19.03943276465977164, -0.05219959533909143690, 33.74890960531435979 ) ) ;
#138176=CARTESIAN_POINT ( 'NONE',  ( -5.153800228976328057, -19.02544592524343514, 102.2905762719810383 ) ) ;
#138177=CARTESIAN_POINT ( 'NONE',  ( -0.05219959533907301413, -21.53943276465977519, 82.49890960531436690 ) ) ;
#138178=CARTESIAN_POINT ( 'NONE',  ( -16.52544592524335698, -4.483927247898792601, 63.95942372801901854 ) ) ;
#138179=CARTESIAN_POINT ( 'NONE',  ( 21.53943276465977519, 0.05219959533937863772, 66.25109039468567573 ) ) ;
#138180=CARTESIAN_POINT ( 'NONE',  ( 0.05219959533936267826, -19.03943276465977164, 100.0010903946856757 ) ) ;
#138181=CARTESIAN_POINT ( 'NONE',  ( 10.72451020669871369, 18.67979575497193778, 112.0844237280190185 ) ) ;
#138182=CARTESIAN_POINT ( 'NONE',  ( -12.14591786802309592, -12.06949235617757132, 21.87390960531436690 ) ) ;
#138183=CARTESIAN_POINT ( 'NONE',  ( 10.72451020669898902, -18.67979575497178502, 102.9155762719810383 ) ) ;
#138184=CARTESIAN_POINT ( 'NONE',  ( -12.06949235617756955, 12.14591786802309770, 35.62390960531437401 ) ) ;
#138185=CARTESIAN_POINT ( 'NONE',  ( 13.89961937509957401, 13.97604488694547697, 76.87609039468566152 ) ) ;
#138186=CARTESIAN_POINT ( 'NONE',  ( -21.52544592524334988, -5.823673210054445271, 58.95942372801902565 ) ) ;
#138187=CARTESIAN_POINT ( 'NONE',  ( 5.153800228976615827, -19.02544592524334988, 35.20942372801899722 ) ) ;
#138188=CARTESIAN_POINT ( 'NONE',  ( -16.55341960407611168, -4.379528057220339221, 101.4572429386476955 ) ) ;
#138189=CARTESIAN_POINT ( 'NONE',  ( -21.52544592524343514, 5.823673210054127303, 26.04057627198103475 ) ) ;
#138190=CARTESIAN_POINT ( 'NONE',  ( 12.06949235617757843, -12.14591786802309237, 38.12390960531436690 ) ) ;
#138191=CARTESIAN_POINT ( 'NONE',  ( 5.719274019375673035, 21.55341960407619339, 97.29275706135234714 ) ) ;
#138192=CARTESIAN_POINT ( 'NONE',  ( -0.05219959533934338120, 16.53943276465976808, 72.50109039468568994 ) ) ;
#138193=CARTESIAN_POINT ( 'NONE',  ( 4.379528057220339221, -16.55341960407611168, 32.70724293864770260 ) ) ;
#138194=CARTESIAN_POINT ( 'NONE',  ( -18.67979575497193778, 10.72451020669871902, 58.33442372801901143 ) ) ;
#138195=CARTESIAN_POINT ( 'NONE',  ( 10.72451020669871369, 18.67979575497193778, 52.08442372801901854 ) ) ;
#138198=CARTESIAN_POINT ( 'NONE',  ( 19.05341960407611168, 5.049401038298154454, 23.95724293864769194 ) ) ;
#138199=CARTESIAN_POINT ( 'NONE',  ( -18.62759615963255300, -10.81492255796106328, 49.16775706135234003 ) ) ;
#138200=CARTESIAN_POINT ( 'NONE',  ( 19.03943276465977164, -0.05219959533909143690, 23.74890960531435269 ) ) ;
#138201=CARTESIAN_POINT ( 'NONE',  ( 16.46253265017160672, -9.564922557960803928, 38.33224293864768839 ) ) ;
#138202=CARTESIAN_POINT ( 'NONE',  ( 4.483927247898545687, 16.52544592524342804, 84.79057627198102409 ) ) ;
#138203=CARTESIAN_POINT ( 'NONE',  ( 5.153800228976335163, 19.02544592524342804, 74.79057627198103830 ) ) ;
#138204=CARTESIAN_POINT ( 'NONE',  ( 8.224510206698953496, -14.34966873604960469, 27.91557627198103830 ) ) ;
#138205=CARTESIAN_POINT ( 'NONE',  ( -21.55341960407610458, -5.719274019375992779, 61.45724293864770260 ) ) ;
#138206=CARTESIAN_POINT ( 'NONE',  ( 16.52544592524342804, -4.483927247898539470, 93.54057627198103830 ) ) ;
#138207=CARTESIAN_POINT ( 'NONE',  ( -18.62759615963270932, 10.81492255796079327, 105.8322429386476955 ) ) ;
#138208=CARTESIAN_POINT ( 'NONE',  ( 16.46253265017160672, -9.564922557960803928, 103.3322429386476955 ) ) ;
#138209=CARTESIAN_POINT ( 'NONE',  ( -13.97604488694527625, -13.89961937509977652, 71.87390960531433848 ) ) ;
#138210=CARTESIAN_POINT ( 'NONE',  ( -9.474510206698720793, -16.51473224551083518, 99.58442372801900433 ) ) ;
#138211=CARTESIAN_POINT ( 'NONE',  ( -10.72451020669898014, 18.67979575497178502, 55.41557627198102409 ) ) ;
#138212=CARTESIAN_POINT ( 'NONE',  ( -0.05219959533937732626, 21.53943276465977519, 77.50109039468567573 ) ) ;
#138213=CARTESIAN_POINT ( 'NONE',  ( 0.05219959533909260263, 19.03943276465977164, 69.99890960531435269 ) ) ;
#138214=CARTESIAN_POINT ( 'NONE',  ( 9.564922557960805705, 16.46253265017160317, 104.5822429386476955 ) ) ;
#138215=CARTESIAN_POINT ( 'NONE',  ( -0.05219959533934338120, 16.53943276465976808, 72.50109039468568994 ) ) ;
#138216=CARTESIAN_POINT ( 'NONE',  ( -5.719274019375665041, -21.55341960407619695, 54.79275706135235424 ) ) ;
#138217=CARTESIAN_POINT ( 'NONE',  ( 21.52544592524334988, 5.823673210054432836, 81.45942372801900433 ) ) ;
#138218=CARTESIAN_POINT ( 'NONE',  ( 5.719274019375991003, -21.55341960407610458, 107.7072429386476955 ) ) ;
#138219=CARTESIAN_POINT ( 'NONE',  ( -4.483927247898782831, 16.52544592524335698, 72.70942372801901854 ) ) ;
#138220=CARTESIAN_POINT ( 'NONE',  ( 0.05219959533907565091, 21.53943276465977519, 69.99890960531435269 ) ) ;
#138221=CARTESIAN_POINT ( 'NONE',  ( -5.049401038297874678, -19.05341960407617918, 44.79275706135232582 ) ) ;
#138222=CARTESIAN_POINT ( 'NONE',  ( 10.72451020669898902, -18.67979575497178502, 37.91557627198102409 ) ) ;
#138223=CARTESIAN_POINT ( 'NONE',  ( -19.02544592524342804, 5.153800228976336051, 86.04057627198103830 ) ) ;
#138224=CARTESIAN_POINT ( 'NONE',  ( -14.34966873604972548, 8.224510206698743886, 113.3344237280190328 ) ) ;
#138225=CARTESIAN_POINT ( 'NONE',  ( -17.40861289039003168, 6.110651285853254677, 63.62767529172569425 ) ) ;
#138226=CARTESIAN_POINT ( 'NONE',  ( 19.02544592524343514, -5.153800228976328945, 113.5405762719810241 ) ) ;
#138228=CARTESIAN_POINT ( 'NONE',  ( -16.46253265017146816, -9.564922557961047289, 89.16775706135234714 ) ) ;
#138229=CARTESIAN_POINT ( 'NONE',  ( -15.80617190586745835, -15.72974639402198527, 71.87390960531438111 ) ) ;
#138230=CARTESIAN_POINT ( 'NONE',  ( -16.52544592524342804, 4.483927247898546575, 56.04057627198102409 ) ) ;
#138231=CARTESIAN_POINT ( 'NONE',  ( -5.049401038297874678, -19.05341960407617918, 109.7927570613523187 ) ) ;
#138232=CARTESIAN_POINT ( 'NONE',  ( 5.049401038298161559, -19.05341960407611168, 32.70724293864768129 ) ) ;
#138233=CARTESIAN_POINT ( 'NONE',  ( -21.52544592524343514, 5.823673210054127303, 96.04057627198102409 ) ) ;
#138234=CARTESIAN_POINT ( 'NONE',  ( -19.03943276465977164, -0.05219959533935918106, 73.75109039468566152 ) ) ;
#138235=CARTESIAN_POINT ( 'NONE',  ( 9.474510206698971260, -16.51473224551069308, 77.91557627198103830 ) ) ;
#138236=CARTESIAN_POINT ( 'NONE',  ( -16.55341960407611168, -4.379528057220339221, 81.45724293864769550 ) ) ;
#138237=CARTESIAN_POINT ( 'NONE',  ( -0.05219959533909027116, -19.03943276465977164, 57.49890960531435979 ) ) ;
#138238=CARTESIAN_POINT ( 'NONE',  ( -12.06949235617756955, 12.14591786802309770, 60.62390960531437401 ) ) ;
#138239=CARTESIAN_POINT ( 'NONE',  ( 5.049401038298161559, -19.05341960407611168, 27.70724293864769550 ) ) ;
#138241=CARTESIAN_POINT ( 'NONE',  ( 4.483927247898545687, 16.52544592524342804, 44.79057627198103120 ) ) ;
#138242=CARTESIAN_POINT ( 'NONE',  ( 16.51473224551069308, 9.474510206698969483, 89.16557627198103830 ) ) ;
#138244=CARTESIAN_POINT ( 'NONE',  ( -5.153800228976607833, 19.02544592524334988, 47.70942372801900433 ) ) ;
#138245=CARTESIAN_POINT ( 'NONE',  ( -4.483927247898782831, 16.52544592524335698, 57.70942372801901143 ) ) ;
#138246=CARTESIAN_POINT ( 'NONE',  ( -10.72451020669898014, 18.67979575497178502, 60.41557627198102409 ) ) ;
#138247=CARTESIAN_POINT ( 'NONE',  ( -0.05219959533937732626, 21.53943276465977519, 112.5010903946857042 ) ) ;
#138248=CARTESIAN_POINT ( 'NONE',  ( -13.89961937509977652, 13.97604488694528158, 90.62390960531432427 ) ) ;
#138250=CARTESIAN_POINT ( 'NONE',  ( -0.05219959533907301413, -21.53943276465977519, 27.49890960531435269 ) ) ;
#138252=CARTESIAN_POINT ( 'NONE',  ( -16.46253265017160317, 9.564922557960807481, 55.83224293864769550 ) ) ;
#138253=CARTESIAN_POINT ( 'NONE',  ( 10.81492255796106328, -18.62759615963255655, 45.41775706135234003 ) ) ;
#138254=CARTESIAN_POINT ( 'NONE',  ( 0.05219959533910956823, 16.53943276465976808, 104.9989096053143669 ) ) ;
#138255=CARTESIAN_POINT ( 'NONE',  ( 15.72974639402199770, -15.80617190586745480, 98.12390960531436690 ) ) ;
#138256=CARTESIAN_POINT ( 'NONE',  ( -5.049401038298153566, 19.05341960407611168, 100.2072429386476955 ) ) ;
#138258=CARTESIAN_POINT ( 'NONE',  ( -10.72451020669870658, -18.67979575497194134, 44.58442372801901854 ) ) ;
#138260=CARTESIAN_POINT ( 'NONE',  ( -16.46253265017160317, 9.564922557960807481, 95.83224293864769550 ) ) ;
#138262=CARTESIAN_POINT ( 'NONE',  ( -10.81492255796078084, -18.62759615963271287, 92.08224293864769550 ) ) ;
#138263=CARTESIAN_POINT ( 'NONE',  ( 16.51473224551069308, 9.474510206698969483, 44.16557627198103120 ) ) ;
#138264=CARTESIAN_POINT ( 'NONE',  ( 14.34966873604972726, -8.224510206698740333, 20.83442372801901143 ) ) ;
#138266=CARTESIAN_POINT ( 'NONE',  ( 9.474510206698971260, -16.51473224551069308, 22.91557627198102765 ) ) ;
#138267=CARTESIAN_POINT ( 'NONE',  ( -21.55341960407619339, 5.719274019375674811, 103.5427570613523613 ) ) ;
#138268=CARTESIAN_POINT ( 'NONE',  ( -13.89961937509977652, 13.97604488694528158, 75.62390960531438111 ) ) ;
#138269=CARTESIAN_POINT ( 'NONE',  ( 18.67979575497194134, -10.72451020669871369, 50.83442372801901143 ) ) ;
#138271=CARTESIAN_POINT ( 'NONE',  ( 13.89961937509977652, -13.97604488694527269, 93.12390960531436690 ) ) ;
#138272=CARTESIAN_POINT ( 'NONE',  ( 19.35543954521082455, 5.499999999999579892, 62.08901960356454452 ) ) ;
#138273=CARTESIAN_POINT ( 'NONE',  ( 14.34966873604972726, -8.224510206698740333, 35.83442372801901143 ) ) ;
#138274=CARTESIAN_POINT ( 'NONE',  ( -4.483927247898782831, 16.52544592524335698, 67.70942372801901854 ) ) ;
#138275=CARTESIAN_POINT ( 'NONE',  ( -18.67979575497193778, 10.72451020669871902, 63.33442372801900433 ) ) ;
#138276=CARTESIAN_POINT ( 'NONE',  ( 21.53943276465977519, 0.05219959533937863772, 81.25109039468568994 ) ) ;
#138278=( BOUNDED_SURFACE ( )  B_SPLINE_SURFACE ( 3, 2, ( 
 ( #41765, #22591, #115601, #69085, #130752, #99414, #25612, #24605, #148941, #177290, #10431, #72089, #133763, #161096, #56933, #103430, #165109, #149930, #84239, #129734, #192444, #53926, #100418, #45729, #201, #123540, #152894, #183257, #92211, #170064, #184247, #14390, #134778, #30559, #196460, #31554, #90234, #107381, #137732, #93206, #154891, #27609, #76056, #181284, #199416, #60880, #150941, #42761, #169053, #122557, #15392, #138720, #121562, #104424, #153896, #57930, #77049, #108387, #119601, #166107, #43748, #136736, #73108, #61870, #89249, #12435, #105411, #74097, #185233, #46724, #135767, #197438, #44738, #58904, #120570, #182264, #167095, #28596, #151917, #13406, #106394, #75070, #198418, #59895, #168076, #29573, #91204, #140709, #109376, #126531, #187247, #63880, #124550, #143688, #139705, #17378, #66853, #175043, #33539, #142696, #172052, #173058, #36508, #1192, #188230, #64869, #78036, #171058, #189229, #49703, #34535, #157883, #158858, #62868, #186247, #97173, #3196, #18385, #96194, #4176, #110370, #94201, #19372, #81021, #113351, #65854, #98162, #5170, #47725, #111369, #127525, #32548, #80036, #155881, #50707, #112365, #79034, #2199, #174056, #48717, #190210, #35525, #20346, #81995, #125551, #128515, #51689, #16389, #95202, #156889, #141705, #133526, #146686, #10197, #25381, #39515, #176050, #87023, #131526, #70864, #38528, #177058, #193211, #101175, #53691, #148709, #56699, #115369, #8182, #116358, #178047, #192209, #41534, #162863, #69858, #195218, #6173, #67853, #23360, #71857, #129508, #147711, #118372, #9198, #37518, #180066, #132532, #159863, #21356, #54685, #40525, #83013, #24371, #100184, #85005, #84011, #144688, #191208, #52683, #99180, #161866, #194221, #55686, #160869, #86022, #117360, #179056, #102196, #145689, #114346, #68854, #22359, #163884, #7171, #130513, #103198, #26373, #58673, #120339, #88013, #57701, #153659, #136509, #198189, #137499, #182034, #90009, #14154, #199180, #60646, #59659, #149701, #107149, #43517, #122320, #105183, #119370, #151693, #11199, #166870, #13183, #75821, #30324, #15155, #183026, #74846, #184012, #200169, #45494, #44509, #164878, #168819, #72875, #61638, #28371, #91966, #167848, #123306, #184999, #181053, #106165, #134543, #29348, #90977, #42528, #196232, #76816, #152664, #138487, #104191, #121333, #165873, #27369, #89016, #150707, #12206, #73869, #135539, #197210, #110141, #66612, #19133, #46483, #128276, #78798, #108143, #142461, #80784, #16153, #3939, #18148, #111129, #95960, #139476, #20111, #77807, #169827, #157644, #79802, #172818, #109145, #125319, #127279, #171820, #126299, #170824, #957, #156652, #17145, #93970, #154657, #173819, #31319, #47489, #96940, #4929, #63644, #34298, #1964, #143443, #140476, #188992, #65619, #92971, #155650, #62633, #50468, #141474, #124309, #186007, #35284, #48486, #112128, #2958, #187015, #64637, #158621, #33308, #32317, #94968, #187996, #49466, #81755, #129267, #37271, #162613, #40272, #82764, #175798, #67606, #190961, #51448, #24118, #191953, #7927, #98929, #177803, #9949, #71608, #144445, #131276, #97919, #192964, #39272, #52438, #159612, #85771, #54444, #132282, #55436, #38279, #21109, #147458, #113109, #116114, #25129, #174799, #5930, #160620, #53438, #189973, #8947, #36265, #114096, #22111, #83761, #70615, #193974, #145441, #117107, #161619, #100929, #178802, #6923, #163626, #68601, #130257, #101945, #23113, #86771, #115113, #176807, #148454, #99933, #69611, #84758, #146436, #43268, #103943, #180806, #41281, #60408, #56444, #134294, #183772, #91724, #150462, #59413, #88769, #30083, #165623, #13913, #167608, #118123, #42285, #164627, #197944, #104937, #26121, #102943, #122081, #135292, #152425, #89765, #27122, #151450, #90742, #196964, #87764, #11957, #73622, #149449, #136269, #72619, #58432, #105923, #45258, #10945, #119125, #195980, #57453, #194965, #29104, #120099, #12937, #181787, #121088 ),
 ( #106912, #168585, #74602, #166623, #75579, #153420, #44265, #182782, #179811, #137257, #28125, #14917, #198941, #133274, #141229, #48242, #2720, #126065, #169584, #50233, #46243, #158389, #187762, #109897, #64397, #139242, #155413, #157406, #1722, #156402, #717, #31082, #186772, #47248, #124059, #184758, #3702, #199937, #77570, #127041, #35046, #93732, #49232, #32075, #173577, #110890, #154418, #172575, #34061, #95720, #140229, #62389, #107897, #185760, #138254, #18899, #16903, #17906, #76578, #61401, #78554, #63398, #123072, #92729, #188748, #171581, #33069, #80545, #125075, #94724, #142219, #65381, #79562, #96700, #15912, #111888, #108905, #170584, #174567, #192728, #68365, #38044, #161384, #162377, #81518, #189740, #100696, #6687, #21876, #176570, #146199, #113860, #97682, #22875, #84522, #116873, #7685, #178564, #8710, #128039, #130016, #69369, #4686, #83526, #51213, #191715, #131039, #159371, #112874, #53199, #190729, #193736, #115882, #54211, #177572, #66378, #99700, #114875, #39039, #36033, #37031, #70379, #55204, #23879, #132047, #85531, #147219, #20868, #40029, #101703, #19878, #98693, #160387, #143205, #82526, #175556, #144208, #5693, #145204, #67369, #129028, #52202, #195746, #104705, #57220, #28875, #60175, #118893, #11725, #119876, #181561, #180578, #45022, #43039, #150229, #198708, #9716, #71380, #26889, #13681, #133044, #151220, #152197, #12709, #41048, #121844, #74375, #137017, #183537, #196740, #44031, #163393, #166395, #42052, #88532, #87538, #24890, #86538, #75348, #105692, #136040, #167378, #197715, #102712, #89533, #59180, #120849, #73393, #149225, #194734, #72379, #148222, #182549, #103716, #27891, #56204, #117887, #165396, #135064, #179577, #164401, #25893, #58207, #90515, #10716, #134054, #93485, #17657, #140987, #63151, #65139, #91487, #16662, #155171, #168354, #61164, #79317, #78310, #124830, #48003, #48989, #29850, #76339, #187524, #139983, #108664, #186530, #32827, #477, #184524, #109659, #171339, #3462, #94478, #126796, #95474, #14677, #1472, #156159, #153174, #170342, #138015, #2475, #64156, #46004, #199698, #125820, #77331, #80301, #110644, #172325, #33814, #122835, #157161, #18655, #141974, #107659, #123815, #188502, #106681, #169336, #30845, #92492, #154181, #15671, #138998, #62151, #185513, #47005, #31834, #24397, #131552, #69883, #86046, #194245, #146712, #118396, #149724, #8208, #101198, #9222, #70889, #85031, #134568, #132557, #39539, #88036, #99204, #160892, #116382, #103221, #22384, #40552, #41558, #102221, #130538, #11225, #163910, #26397, #72899, #147735, #133551, #49981, #55712, #193237, #178072, #177081, #111645, #173331, #164903, #195242, #25406, #56726, #87048, #192236, #179083, #148733, #10221, #162888, #38552, #84034, #161889, #37540, #71881, #54710, #117384, #145713, #7194, #180090, #68878, #53716, #115393, #100209, #23385, #29371, #30349, #74870, #183049, #107173, #91991, #152688, #154682, #181077, #106188, #44533, #57724, #150729, #168844, #167872, #14177, #137523, #138511, #119394, #165896, #76840, #91002, #198213, #75847, #122347, #90032, #73891, #199205, #60672, #92996, #184036, #16177, #185024, #104215, #45519, #153685, #42552, #59685, #27394, #15181, #153389, #135561, #89039, #61662, #166893, #169851, #123331, #46511, #108170, #12229, #31345, #77832, #196255, #197233, #13207, #58694, #120364, #182057, #43540, #105206, #28393, #151714, #136532, #121356, #50492, #187041, #157671, #96965, #2983, #109170, #33332, #18172, #155674, #142487, #78823, #48511, #112156, #190001, #32340, #125343, #17169, #140501, #982, #173845, #141499, #19160, #110165, #127307, #35311, #34325, #62657, #143469, #79829, #158645, #156678, #93993, #126324, #124336, #64662, #49493, #20137, #66638, #51475, #80808, #111155, #81782, #36291, #4953, #3965, #186032, #128301, #47514, #97947, #188021, #113137, #65645, #159639, #21135, #1990, #189018, #170849, #174827, #139499 ),
 ( #172844, #63669, #95986, #171844, #94992, #24153, #176837, #148490, #179843, #38308, #131307, #39303, #100962, #115144, #164659, #162647, #69641, #118153, #129293, #190989, #146466, #133308, #52465, #70649, #71641, #132315, #160647, #41314, #194007, #56475, #102974, #116144, #163659, #82790, #85804, #99963, #7958, #6950, #144472, #5956, #194997, #25162, #55470, #86804, #117140, #22139, #8981, #178835, #40303, #192997, #68630, #114123, #191980, #67634, #101979, #23143, #147490, #175825, #9981, #37298, #98957, #83789, #145469, #130286, #161647, #53467, #84787, #54474, #177835, #180837, #167640, #134325, #29136, #13943, #103975, #196010, #60437, #90773, #168614, #91755, #74635, #57485, #198970, #87796, #152457, #61431, #149481, #119155, #196996, #89798, #46274, #122112, #26154, #107930, #58463, #10977, #183801, #45289, #42314, #106941, #197976, #75609, #137288, #165654, #199966, #27152, #72650, #30114, #59446, #153449, #88799, #104968, #14947, #151480, #105955, #150492, #11989, #136301, #120130, #73652, #135324, #76607, #181821, #43300, #138285, #184788, #166655, #123103, #28156, #12971, #121119, #182813, #44296, #154450, #93763, #77602, #64426, #171612, #139273, #15943, #142249, #63431, #95750, #156438, #32106, #17937, #34092, #125107, #750, #16934, #1753, #62421, #141260, #185792, #155444, #110919, #65411, #124093, #170617, #47280, #108936, #31113, #172605, #186805, #79591, #78588, #126095, #157435, #94756, #92761, #18930, #48275, #80575, #140261, #109930, #33100, #2750, #187792, #49261, #3734, #127072, #188780, #50263, #111920, #173607, #35077, #169616, #106610, #136952, #198641, #58142, #167311, #409, #123746, #60107, #62081, #15602, #29782, #166325, #77260, #121775, #61094, #28807, #90447, #183468, #91418, #43961, #138929, #46935, #105623, #44954, #168285, #153105, #182480, #31765, #14609, #76265, #185445, #196673, #119810, #13615, #108594, #181495, #137943, #170271, #199627, #27822, #150156, #122767, #11657, #73323, #184456, #30775, #134994, #45936, #152132, #75282, #74310, #42973, #104636, #89464, #92422, #107591, #154108, #169269, #151153, #12643, #135977, #197648, #59114, #120779, #124762, #2406, #155100, #81215, #33745, #34735, #93414, #16594, #48922, #110576, #78242, #47934, #143896, #126729, #188432, #127729, #172257, #80234, #4378, #189431, #49910, #51892, #139913, #3396, #141905, #1404, #109588, #66062, #65071, #111576, #96393, #35727, #63083, #186458, #174259, #173260, #95405, #158080, #19571, #187454, #171271, #142896, #50906, #190416, #112564, #113551, #82204, #32759, #97374, #159060, #94410, #157091, #156091, #20554, #5377, #17588, #79248, #67061, #64085, #128719, #175245, #140919, #125754, #18587, #87229, #10401, #23565, #148911, #102399, #116567, #52881, #164086, #8393, #147915, #115574, #53899, #70068, #178256, #130725, #25585, #133732, #192417, #85213, #193418, #54893, #69058, #118576, #39717, #146903, #72058, #83217, #144892, #100391, #195425, #6374, #24576, #56902, #86225, #114555, #36710, #9401, #98372, #160070, #131736, #117564, #21557, #101380, #177261, #162069, #161069, #68054, #129708, #191404, #179264, #71067, #40729, #132733, #176253, #163071, #194421, #55891, #37724, #22564, #99386, #145890, #84210, #7373, #38733, #199504, #27697, #60970, #46811, #121650, #89338, #152006, #136829, #74185, #122644, #197525, #105500, #30648, #108470, #151030, #43836, #135855, #58994, #119688, #92302, #59983, #76142, #167186, #45816, #153985, #152981, #181372, #61958, #198512, #15482, #75157, #12521, #44827, #42850, #183345, #168161, #77139, #185320, #170148, #137820, #29658, #138808, #154976, #169143, #184334, #104515, #289, #166196, #16472, #106482, #123625, #107467, #78121, #139790, #120660, #31642, #182358, #93291, #58018, #28685, #90320, #13492, #91290, #14480, #111455, #20429, #98243, #112446, #142778, #62955, #158940, #124636, #159946, #18466, #174135, #65938, #21433, #83093 ),
 ( #35606, #186330, #127610, #36588, #47813, #171145, #172137, #64951, #1278, #97252, #109462, #32634, #33623, #94288, #82079, #143772, #155966, #5253, #173141, #189309, #50786, #17463, #175120, #79120, #140793, #66934, #34616, #128597, #63964, #80117, #190291, #126610, #81100, #125634, #2281, #96275, #95286, #48802, #187331, #51767, #110456, #156970, #113428, #141785, #3279, #188312, #49789, #157961, #19452, #4259, #179140, #129587, #53774, #176129, #9280, #54769, #37599, #52758, #71938, #146773, #163967, #86103, #114427, #147794, #133608, #8267, #99261, #38610, #23442, #160948, #70945, #84090, #192295, #117442, #195301, #22441, #130598, #145769, #7251, #6254, #40609, #69946, #162947, #115448, #132613, #102279, #39599, #67933, #148790, #85089, #25465, #161947, #68936, #131610, #191283, #193295, #116443, #87105, #56783, #118455, #180146, #178132, #10279, #164960, #194302, #101258, #24454, #177139, #26453, #41615, #103280, #144769, #55768, #100266, #122405, #165955, #14235, #184095, #45578, #151769, #12283, #119450, #197288, #149781, #75906, #28451, #61722, #138569, #104273, #182111, #43596, #11283, #42609, #47, #121414, #183107, #107231, #166948, #74925, #199264, #168902, #44588, #46571, #72957, #198268, #136588, #134626, #27455, #196310, #123390, #30408, #106245, #57780, #92054, #90087, #153744, #105262, #89097, #59744, #181135, #13262, #167927, #60731, #15239, #185082, #29427, #91058, #76898, #110969, #172653, #152745, #150788, #88095, #73948, #135617, #137581, #58751, #120420, #54289, #115961, #188828, #175636, #142302, #37110, #21954, #111968, #3782, #68445, #98769, #176649, #99779, #82603, #65459, #6766, #95800, #160463, #69451, #157486, #127122, #4768, #97763, #34141, #130099, #18979, #80625, #66455, #50312, #191796, #53277, #173660, #114956, #5773, #83604, #145283, #35127, #7768, #96779, #158468, #38125, #67448, #161464, #19956, #112953, #22954, #159450, #113937, #84602, #146281, #81598, #131118, #192807, #143282, #20946, #128117, #189820, #51292, #174646, #36111, #144284, #129106, #190805, #52279, #71455, #133120, #100773, #132123, #27970, #10793, #72461, #11804, #56283, #164476, #88611, #73468, #134135, #136119, #162456, #87613, #25970, #40107, #42131, #194809, #43116, #195824, #118972, #119951, #39117, #147299, #58282, #149299, #179656, #57295, #103792, #117965, #55281, #180655, #165472, #74453, #26968, #197795, #166472, #85612, #150307, #135141, #23957, #41126, #8788, #196815, #181636, #116952, #70458, #104784, #148299, #151299, #89610, #12788, #59261, #193816, #177649, #178644, #101785, #163473, #102790, #24970, #86616, #9793, #171425, #186613, #561, #137104, #48085, #92576, #31917, #199779, #138098, #154264, #62232, #14761, #109741, #17747, #76422, #169423, #77414, #139084, #153259, #2559, #123900, #107742, #156245, #167459, #28955, #184606, #32912, #90596, #108749, #94566, #170425, #198790, #79403, #93571, #141074, #120930, #15755, #1561, #182629, #185599, #61246, #46087, #45104, #44114, #105772, #152278, #63236, #155256, #122918, #13762, #75430, #30928, #60256, #121927, #47088, #183621, #106761, #16745, #78394, #140070, #124915, #168436, #29932, #91571, #129858, #161223, #158230, #112715, #20705, #82361, #96542, #146042, #144050, #51053, #99541, #110731, #172413, #127877, #114715, #33901, #52045, #53033, #113701, #142058, #22717, #175397, #37883, #84365, #97523, #145045, #64241, #67211, #81362, #189581, #188588, #125908, #187606, #176407, #6526, #36865, #68205, #98531, #3544, #190569, #160224, #21715, #174408, #50069, #95558, #173417, #49075, #83368, #4524, #157245, #18739, #80386, #19720, #143046, #65222, #126882, #111730, #159211, #5532, #191556, #66217, #35877, #34887, #128869, #164237, #166226, #192568, #117719, #56041, #70221, #72216, #24728, #73230, #25733, #149064, #150058, #69210, #177413, #88365, #194571, #9553, #87379, #133890, #101535, #85367, #10552, #195582 ),
 ( #180417, #57054, #27727, #89370, #162220, #118729, #115726, #41889, #103556, #147061, #38884, #165231, #26726, #196578, #130878, #42880, #11564, #102553, #54051, #134901, #86377, #58048, #148062, #23719, #179415, #100541, #71219, #40880, #119718, #181402, #104545, #7526, #8543, #131889, #193573, #55045, #116716, #178405, #39869, #163228, #132882, #168193, #123653, #15512, #171178, #32666, #105532, #92331, #59023, #154017, #138839, #28715, #120690, #185351, #77169, #93324, #16505, #199533, #182389, #46842, #12550, #319, #186363, #74216, #43867, #121682, #14512, #151059, #108501, #135884, #197555, #183378, #167218, #170181, #31675, #90352, #155008, #122675, #61987, #78153, #152037, #124667, #13522, #75187, #139821, #184364, #1310, #136859, #29690, #62989, #76173, #30679, #198545, #60015, #61003, #44860, #106515, #91321, #47843, #153012, #137853, #109496, #45845, #107498, #169174, #3306, #63992, #21462, #175149, #128627, #79151, #64979, #125663, #158968, #4286, #187361, #2311, #83124, #96302, #113456, #35635, #48830, #97280, #144800, #157988, #110483, #188339, #173167, #172166, #20460, #33651, #141813, #66967, #6283, #95312, #80143, #156997, #18495, #155997, #190320, #142806, #51797, #140822, #126637, #49818, #82110, #65967, #111482, #34643, #67961, #19479, #36617, #143801, #81125, #5284, #129616, #127637, #189337, #50815, #112472, #174165, #98274, #159975, #191311, #52787, #114456, #176158, #94319, #17493, #115479, #99291, #71967, #86133, #26484, #160977, #72986, #133641, #132644, #22471, #41645, #116474, #195332, #54799, #192323, #24483, #84119, #178163, #147825, #10310, #164990, #88126, #117472, #9311, #56812, #134655, #148820, #179170, #145798, #118486, #7281, #196341, #39628, #180177, #102307, #57809, #119480, #53804, #40638, #68965, #163996, #25493, #177167, #130627, #103310, #87136, #149810, #11316, #70976, #38640, #37628, #100297, #161975, #23471, #85120, #146804, #8297, #101288, #69975, #131643, #193325, #162978, #194332, #55800, #76930, #153775, #150816, #15270, #152776, #45610, #30439, #73978, #154771, #12313, #62746, #92086, #14268, #107262, #43627, #59775, #61751, #106273, #60763, #105290, #135647, #91089, #151799, #28481, #89128, #108262, #104302, #182143, #31433, #139586, #198298, #16268, #90115, #197317, #169942, #123419, #29457, #93087, #165985, #77919, #138599, #75937, #27485, #185112, #121444, #81, #183136, #58781, #167958, #120450, #44620, #137612, #46602, #1071, #181163, #122435, #199296, #42640, #166978, #13290, #184127, #74954, #136617, #168933, #82887, #141587, #97054, #189111, #144565, #6051, #78911, #65734, #32427, #127402, #112244, #2078, #94081, #158737, #50584, #66734, #190091, #172936, #155760, #20226, #186122, #173935, #159735, #47602, #17258, #95080, #188110, #124426, #81874, #109256, #170935, #156768, #140588, #143566, #5048, #63757, #128394, #96074, #35403, #51566, #125431, #98038, #187127, #48599, #113230, #157763, #174920, #110251, #3075, #36384, #49582, #4056, #171932, #33421, #34415, #18262, #79915, #64751, #21232, #126413, #111245, #19253, #80900, #142577, #41407, #176930, #37393, #195092, #148583, #102072, #52556, #38400, #99051, #132410, #177928, #160740, #175922, #56575, #69733, #86899, #9072, #22232, #70742, #118249, #131401, #83881, #161742, #146559, #145563, #194102, #7041, #115238, #40401, #179940, #68723, #53560, #130380, #192078, #129387, #163757, #191083, #100056, #103072, #101056, #162741, #25257, #8054, #54565, #178931, #10074, #24249, #26249, #114217, #39396, #116237, #23237, #55564, #84881, #133403, #85898, #117238, #71733, #193089, #147586, #164754, #87889, #149576, #67729, #137379, #105064, #88893, #14034, #152546, #108022, #199058, #169709, #200055, #119247, #121215, #75699, #196107, #74729, #180931, #182905, #60527, #150585, #42406, #59536, #181913, #184882, #107032, #122202, #168704, #57577, #167730, #198070, #44389, #104069, #28251, #61524 ),
 ( #166748, #76699, #31202, #89891, #106044, #29228, #90861, #43393, #92853, #183894, #45379, #46364, #165751, #27244, #136393, #123193, #12084, #30206, #11072, #91847, #73747, #72750, #153541, #134421, #135419, #15038, #138375, #197090, #58557, #151574, #120223, #13063, #36153, #128161, #4810, #96825, #3823, #35170, #188871, #32197, #80667, #50354, #112013, #18030, #78679, #185888, #63525, #16035, #142343, #94850, #189861, #66498, #170707, #48367, #110023, #65502, #126186, #19021, #17026, #33191, #158509, #79684, #34182, #140355, #47373, #64519, #125200, #1843, #62515, #81640, #77693, #155531, #51335, #112995, #171702, #174689, #186896, #124187, #143323, #19996, #173702, #139361, #156531, #109028, #127163, #187882, #93854, #141354, #154539, #2841, #842, #95843, #49349, #157527, #111011, #172697, #67492, #191839, #176693, #113980, #100814, #37152, #145327, #70497, #151092, #190846, #83649, #175678, #98812, #159494, #132165, #146322, #89403, #20989, #135917, #193856, #192850, #82644, #101825, #38167, #55321, #114999, #52323, #84645, #144327, #99822, #7811, #116992, #27760, #12583, #177689, #69495, #178687, #197588, #8829, #39157, #5816, #40148, #129149, #59054, #161507, #166261, #162497, #120721, #182420, #160506, #23997, #21996, #85654, #147341, #6809, #68487, #74248, #97805, #130142, #53320, #131160, #22999, #54329, #116000, #170211, #79183, #105562, #13553, #14543, #107527, #64023, #16534, #43899, #125693, #76203, #167248, #139850, #78181, #75219, #1339, #15541, #108532, #93353, #136891, #17524, #198577, #28747, #155039, #140853, #2342, #77199, #124698, #90383, #46872, #61032, #169204, #168222, #152068, #60046, #94348, #186395, #63019, #47872, #109525, #121713, #31704, #171207, #32697, #30711, #29719, #183406, #153043, #44889, #156027, #184394, #106546, #91351, #137882, #199563, #122704, #45874, #92360, #154046, #138868, #348, #62018, #123682, #185381, #98307, #21495, #143834, #145829, #172196, #97312, #35664, #49848, #51829, #4316, #52820, #5314, #128657, #129646, #48860, #157028, #67993, #174196, #189368, #66998, #113488, #81155, #65010, #190352, #175182, #84150, #36649, #37660, #160007, #80173, #50845, #83156, #110515, #144830, #33681, #7312, #65999, #6314, #191342, #68997, #187392, #141845, #114489, #95343, #176191, #99325, #126667, #18526, #161009, #22503, #3336, #188371, #158998, #111512, #173198, #34674, #96332, #158019, #19510, #142837, #127668, #112502, #20491, #82140, #130663, #150850, #163011, #192357, #26515, #103343, #100330, #165022, #102341, #195365, #180209, #23505, #104335, #162009, #12345, #41678, #164030, #56844, #193358, #9345, #11348, #55833, #88159, #85153, #166019, #146839, #53840, #149844, #25527, #118520, #54834, #71010, #73019, #117506, #10344, #116508, #8332, #40671, #101322, #178196, #38675, #57842, #115514, #131677, #181197, #89160, #147859, #27519, #39661, #70008, #119515, #134689, #196374, #177202, #24518, #86169, #42674, #87172, #132678, #194366, #179203, #148853, #72000, #133674, #43660, #15299, #62777, #137642, #105322, #167990, #152809, #90145, #76959, #13319, #121476, #46632, #124458, #167010, #59806, #151830, #74985, #135679, #108292, #122465, #186154, #197351, #109288, #169971, #168962, #58815, #77948, #14302, #31463, #91120, #28511, #60794, #120483, #75969, #184158, #93115, #1101, #47634, #153805, #170966, #61780, #136648, #199329, #138629, #182174, #154800, #198330, #32460, #45639, #16298, #110, #94113, #155792, #183169, #123448, #44652, #185141, #139615, #106304, #29487, #74008, #107291, #30468, #92117, #65764, #187159, #190118, #78943, #143595, #52587, #140619, #48631, #188142, #80931, #37422, #51593, #17289, #99082, #49613, #2109, #113258, #174950, #110283, #36412, #189140, #81902, #97084, #141618, #171964, #127433, #111276, #64783, #125463, #144593, #63790, #18293, #67757, #175953, #34445, #191113, #126444, #33452, #6079, #98066, #159765 ),
 ( #172967, #96104, #95111, #156800, #129415, #50613, #112272, #21260, #157793, #4086, #128422, #82915, #173964, #79948, #3106, #35431, #158767, #19283, #5078, #142607, #114247, #20256, #66761, #103100, #22262, #130411, #41433, #147613, #162765, #117265, #86927, #54589, #38430, #163783, #102098, #57603, #148609, #164781, #24275, #85924, #83911, #25284, #145594, #9100, #68754, #132435, #10101, #100086, #192110, #70767, #131429, #134447, #56602, #71761, #118276, #7073, #178957, #194127, #55590, #53592, #177953, #11101, #196132, #40427, #72777, #26275, #133431, #176961, #87917, #195119, #179967, #39421, #101080, #149604, #119272, #116262, #180955, #42432, #160772, #115268, #161771, #23266, #193115, #84910, #146589, #8083, #69760, #150613, #12109, #167755, #154564, #73772, #91872, #92877, #153565, #181938, #62541, #27272, #108048, #182932, #138398, #121238, #58581, #90885, #88921, #44415, #14060, #76722, #31228, #16060, #183918, #77718, #15062, #197114, #29253, #45403, #165778, #61547, #135445, #124215, #106069, #200079, #168727, #185913, #104095, #120247, #107056, #43420, #30231, #123216, #105090, #166776, #184906, #46390, #169733, #139384, #152571, #28277, #866, #89916, #151598, #13089, #74754, #136417, #198097, #75727, #59562, #137403, #199084, #60552, #122227, #109054, #143351, #20026, #17052, #81668, #19048, #112042, #96852, #140383, #21016, #78707, #129176, #158536, #80695, #173730, #110051, #126213, #128189, #172727, #127190, #171731, #1871, #157555, #18058, #94879, #155558, #174715, #170731, #48394, #97832, #5843, #64548, #82672, #156559, #63552, #36179, #189887, #4839, #32222, #79713, #125226, #35199, #142372, #186924, #33219, #159520, #49378, #66526, #188901, #141382, #50382, #144356, #111041, #2870, #187909, #34209, #95872, #51362, #3851, #65530, #113023, #67519, #47398, #93880, #145353, #6835, #52350, #132193, #131187, #86682, #114006, #71520, #55349, #116027, #194878, #38192, #175704, #193884, #117019, #98839, #178714, #54355, #24027, #8857, #22023, #9861, #160534, #56352, #70524, #177716, #85681, #68514, #23025, #40176, #69522, #100842, #191865, #83675, #192877, #176719, #53347, #37180, #163539, #130168, #115026, #148366, #190874, #101855, #99848, #147368, #39184, #161532, #84670, #146349, #162524, #25039, #133187, #7836, #81331, #2525, #79367, #98497, #173384, #190536, #112683, #141038, #174375, #160190, #34854, #64205, #65189, #50032, #187572, #35845, #110695, #18705, #144016, #21680, #125872, #157211, #49040, #172375, #32878, #5497, #19689, #83334, #94528, #6492, #67180, #66182, #156210, #175363, #111697, #128837, #188554, #33865, #158199, #17710, #96509, #143014, #52010, #145011, #68172, #51022, #129824, #159177, #95525, #4492, #97491, #80352, #113669, #142024, #191523, #127844, #36831, #20672, #53000, #171391, #3513, #82326, #126848, #189550, #102521, #192535, #84331, #149033, #179385, #57022, #180387, #163192, #146010, #87347, #176374, #40847, #150025, #37847, #7493, #85334, #178373, #134870, #10521, #114678, #11530, #99507, #69178, #147026, #39837, #196548, #72184, #161188, #22684, #8510, #130844, #133858, #195548, #54018, #118695, #86345, #164204, #25702, #115692, #88334, #177380, #38852, #41857, #148032, #103524, #100509, #193539, #165199, #101503, #194539, #162188, #23686, #24696, #70188, #131856, #55013, #26694, #116683, #9521, #73200, #71187, #132851, #56010, #117688, #25524, #165020, #8330, #56842, #26513, #88157, #194364, #54832, #162007, #39659, #192354, #118517, #71008, #104333, #181194, #146837, #24516, #86166, #53838, #85151, #42672, #164028, #87170, #149842, #9343, #117504, #41676, #11346, #148851, #89158, #115512, #40669, #179201, #193356, #195363, #147856, #196372, #10342, #71998, #73017, #177200, #100328, #134686, #102338, #132676, #133672, #180207, #55831, #70005, #103340, #57840, #27517, #119513, #166017, #150847, #12343, #38673, #130661, #23503, #131675 ) ),
 .UNSPECIFIED., .T., .F., .F. ) 
 B_SPLINE_SURFACE_WITH_KNOTS ( ( 4, 3, 4 ),
 ( 3, 2, 2, 2, 2, 2, 2, 2, 2, 2, 2, 2, 2, 2, 2, 2, 2, 2, 2, 2, 2, 2, 2, 2, 2, 2, 2, 2, 2, 2, 2, 2, 2, 2, 2, 2, 2, 2, 2, 2, 2, 2, 2, 2, 2, 2, 2, 2, 2, 2, 2, 2, 2, 2, 2, 2, 2, 2, 2, 2, 2, 2, 2, 2, 2, 2, 2, 2, 2, 2, 2, 2, 2, 2, 2, 2, 2, 2, 2, 2, 2, 2, 2, 2, 2, 2, 2, 2, 2, 2, 2, 2, 2, 2, 2, 2, 2, 2, 2, 2, 2, 2, 2, 2, 2, 2, 2, 2, 2, 2, 2, 2, 2, 2, 2, 2, 2, 2, 2, 2, 2, 2, 2, 2, 2, 2, 2, 2, 2, 2, 2, 2, 2, 2, 2, 2, 2, 2, 2, 2, 2, 2, 2, 2, 2, 2, 2, 2, 2, 2, 2, 2, 2, 2, 2, 2, 2, 2, 2, 2, 2, 2, 2, 2, 2, 2, 2, 2, 2, 2, 2, 2, 2, 2, 2, 2, 2, 2, 2, 2, 2, 2, 2, 2, 2, 2, 2, 2, 2, 2, 2, 2, 2, 2, 2, 2, 2, 2, 2, 2, 2, 2, 2, 2, 2, 2, 2, 2, 2, 2, 2, 2, 2, 2, 2, 2, 2, 2, 2, 2, 2, 2, 2, 2, 2, 2, 2, 2, 3 ),
 ( 0.000000000000000000, 0.5000000000000000000, 1.000000000000000000 ),
 ( 0.000000000000000000, 0.004385964912280701511, 0.008771929824561403022, 0.01315789473684210453, 0.01754385964912280604, 0.02192982456140350755, 0.02631578947368420907, 0.03070175438596491058, 0.03508771929824561209, 0.03947368421052631360, 0.04385964912280701511, 0.04824561403508771662, 0.05263157894736841813, 0.05701754385964911964, 0.06140350877192982115, 0.06578947368421052266, 0.07017543859649122417, 0.07456140350877192569, 0.07894736842105262720, 0.08333333333333332871, 0.08771929824561403022, 0.09210526315789473173, 0.09649122807017543324, 0.1008771929824561348, 0.1052631578947368363, 0.1096491228070175378, 0.1140350877192982393, 0.1184210526315789408, 0.1228070175438596423, 0.1271929824561403577, 0.1315789473684210453, 0.1359649122807017607, 0.1403508771929824483, 0.1447368421052631637, 0.1491228070175438514, 0.1535087719298245668, 0.1578947368421052544, 0.1622807017543859698, 0.1666666666666666574, 0.1710526315789473728, 0.1754385964912280604, 0.1798245614035087758, 0.1842105263157894635, 0.1885964912280701788, 0.1929824561403508665, 0.1973684210526315819, 0.2017543859649122695, 0.2061403508771929849, 0.2105263157894736725, 0.2149122807017543879, 0.2192982456140350755, 0.2236842105263157909, 0.2280701754385964786, 0.2324561403508771940, 0.2368421052631578816, 0.2412280701754385970, 0.2456140350877192846, 0.2500000000000000000, 0.2543859649122807154, 0.2587719298245614308, 0.2631578947368420907, 0.2675438596491228060, 0.2719298245614035214, 0.2763157894736842368, 0.2807017543859648967, 0.2850877192982456121, 0.2894736842105263275, 0.2938596491228070429, 0.2982456140350877027, 0.3026315789473684181, 0.3070175438596491335, 0.3114035087719298489, 0.3157894736842105088, 0.3201754385964912242, 0.3245614035087719396, 0.3289473684210526550, 0.3333333333333333148, 0.3377192982456140302, 0.3421052631578947456, 0.3464912280701754610, 0.3508771929824561209, 0.3552631578947368363, 0.3596491228070175517, 0.3640350877192982670, 0.3684210526315789269, 0.3728070175438596423, 0.3771929824561403577, 0.3815789473684210731, 0.3859649122807017330, 0.3903508771929824483, 0.3947368421052631637, 0.3991228070175438791, 0.4035087719298245390, 0.4078947368421052544, 0.4122807017543859698, 0.4166666666666666852, 0.4210526315789473450, 0.4254385964912280604, 0.4298245614035087758, 0.4342105263157894912, 0.4385964912280701511, 0.4429824561403508665, 0.4473684210526315819, 0.4517543859649122973, 0.4561403508771929571, 0.4605263157894736725, 0.4649122807017543879, 0.4692982456140351033, 0.4736842105263157632, 0.4780701754385964786, 0.4824561403508771940, 0.4868421052631579093, 0.4912280701754385692, 0.4956140350877192846, 0.5000000000000000000, 0.5043859649122807154, 0.5087719298245614308, 0.5131578947368421462, 0.5175438596491228616, 0.5219298245614034659, 0.5263157894736841813, 0.5307017543859648967, 0.5350877192982456121, 0.5394736842105263275, 0.5438596491228070429, 0.5482456140350877583, 0.5526315789473684736, 0.5570175438596490780, 0.5614035087719297934, 0.5657894736842105088, 0.5701754385964912242, 0.5745614035087719396, 0.5789473684210526550, 0.5833333333333333703, 0.5877192982456140857, 0.5921052631578946901, 0.5964912280701754055, 0.6008771929824561209, 0.6052631578947368363, 0.6096491228070175517, 0.6140350877192982670, 0.6184210526315789824, 0.6228070175438596978, 0.6271929824561403022, 0.6315789473684210176, 0.6359649122807017330, 0.6403508771929824483, 0.6447368421052631637, 0.6491228070175438791, 0.6535087719298245945, 0.6578947368421053099, 0.6622807017543859143, 0.6666666666666666297, 0.6710526315789473450, 0.6754385964912280604, 0.6798245614035087758, 0.6842105263157894912, 0.6885964912280702066, 0.6929824561403509220, 0.6973684210526315264, 0.7017543859649122417, 0.7061403508771929571, 0.7105263157894736725, 0.7149122807017543879, 0.7192982456140351033, 0.7236842105263158187, 0.7280701754385965341, 0.7324561403508771384, 0.7368421052631578538, 0.7412280701754385692, 0.7456140350877192846, 0.7500000000000000000, 0.7543859649122807154, 0.7587719298245614308, 0.7631578947368421462, 0.7675438596491228616, 0.7719298245614034659, 0.7763157894736841813, 0.7807017543859648967, 0.7850877192982456121, 0.7894736842105263275, 0.7938596491228070429, 0.7982456140350877583, 0.8026315789473684736, 0.8070175438596490780, 0.8114035087719297934, 0.8157894736842105088, 0.8201754385964912242, 0.8245614035087719396, 0.8289473684210526550, 0.8333333333333333703, 0.8377192982456140857, 0.8421052631578946901, 0.8464912280701754055, 0.8508771929824561209, 0.8552631578947368363, 0.8596491228070175517, 0.8640350877192982670, 0.8684210526315789824, 0.8728070175438596978, 0.8771929824561403022, 0.8815789473684210176, 0.8859649122807017330, 0.8903508771929824483, 0.8947368421052631637, 0.8991228070175438791, 0.9035087719298245945, 0.9078947368421053099, 0.9122807017543859143, 0.9166666666666666297, 0.9210526315789473450, 0.9254385964912280604, 0.9298245614035087758, 0.9342105263157894912, 0.9385964912280702066, 0.9429824561403509220, 0.9473684210526315264, 0.9517543859649122417, 0.9561403508771929571, 0.9605263157894736725, 0.9649122807017543879, 0.9692982456140351033, 0.9736842105263158187, 0.9780701754385965341, 0.9824561403508771384, 0.9868421052631578538, 0.9912280701754385692, 0.9956140350877192846, 1.000000000000000000 ),
 .UNSPECIFIED. ) 
 GEOMETRIC_REPRESENTATION_ITEM ( )  RATIONAL_B_SPLINE_SURFACE ( (
 ( 1.000000000000000000, 0.9659258262890683122, 1.000000000000000000, 0.9659258262890683122, 1.000000000000000000, 0.9659258262890683122, 1.000000000000000000, 0.9659258262890683122, 1.000000000000000000, 0.9659258262890683122, 1.000000000000000000, 0.9659258262890683122, 1.000000000000000000, 0.9659258262890683122, 1.000000000000000000, 0.9659258262890683122, 1.000000000000000000, 0.9659258262890683122, 1.000000000000000000, 0.9659258262890683122, 1.000000000000000000, 0.9659258262890683122, 1.000000000000000000, 0.9659258262890683122, 1.000000000000000000, 0.9659258262890683122, 1.000000000000000000, 0.9659258262890683122, 1.000000000000000000, 0.9659258262890683122, 1.000000000000000000, 0.9659258262890683122, 1.000000000000000000, 0.9659258262890683122, 1.000000000000000000, 0.9659258262890683122, 1.000000000000000000, 0.9659258262890683122, 1.000000000000000000, 0.9659258262890683122, 1.000000000000000000, 0.9659258262890683122, 1.000000000000000000, 0.9659258262890683122, 1.000000000000000000, 0.9659258262890683122, 1.000000000000000000, 0.9659258262890683122, 1.000000000000000000, 0.9659258262890683122, 1.000000000000000000, 0.9659258262890683122, 1.000000000000000000, 0.9659258262890683122, 1.000000000000000000, 0.9659258262890683122, 1.000000000000000000, 0.9659258262890683122, 1.000000000000000000, 0.9659258262890683122, 1.000000000000000000, 0.9659258262890683122, 1.000000000000000000, 0.9659258262890683122, 1.000000000000000000, 0.9659258262890683122, 1.000000000000000000, 0.9659258262890683122, 1.000000000000000000, 0.9659258262890683122, 1.000000000000000000, 0.9659258262890683122, 1.000000000000000000, 0.9659258262890683122, 1.000000000000000000, 0.9659258262890683122, 1.000000000000000000, 0.9659258262890683122, 1.000000000000000000, 0.9659258262890683122, 1.000000000000000000, 0.9659258262890683122, 1.000000000000000000, 0.9659258262890683122, 1.000000000000000000, 0.9659258262890683122, 1.000000000000000000, 0.9659258262890683122, 1.000000000000000000, 0.9659258262890683122, 1.000000000000000000, 0.9659258262890683122, 1.000000000000000000, 0.9659258262890683122, 1.000000000000000000, 0.9659258262890683122, 1.000000000000000000, 0.9659258262890683122, 1.000000000000000000, 0.9659258262890683122, 1.000000000000000000, 0.9659258262890683122, 1.000000000000000000, 0.9659258262890683122, 1.000000000000000000, 0.9659258262890683122, 1.000000000000000000, 0.9659258262890683122, 1.000000000000000000, 0.9659258262890683122, 1.000000000000000000, 0.9659258262890683122, 1.000000000000000000, 0.9659258262890683122, 1.000000000000000000, 0.9659258262890683122, 1.000000000000000000, 0.9659258262890683122, 1.000000000000000000, 0.9659258262890683122, 1.000000000000000000, 0.9659258262890683122, 1.000000000000000000, 0.9659258262890683122, 1.000000000000000000, 0.9659258262890683122, 1.000000000000000000, 0.9659258262890683122, 1.000000000000000000, 0.9659258262890683122, 1.000000000000000000, 0.9659258262890683122, 1.000000000000000000, 0.9659258262890683122, 1.000000000000000000, 0.9659258262890683122, 1.000000000000000000, 0.9659258262890683122, 1.000000000000000000, 0.9659258262890683122, 1.000000000000000000, 0.9659258262890683122, 1.000000000000000000, 0.9659258262890683122, 1.000000000000000000, 0.9659258262890683122, 1.000000000000000000, 0.9659258262890683122, 1.000000000000000000, 0.9659258262890683122, 1.000000000000000000, 0.9659258262890683122, 1.000000000000000000, 0.9659258262890683122, 1.000000000000000000, 0.9659258262890683122, 1.000000000000000000, 0.9659258262890683122, 1.000000000000000000, 0.9659258262890683122, 1.000000000000000000, 0.9659258262890683122, 1.000000000000000000, 0.9659258262890683122, 1.000000000000000000, 0.9659258262890683122, 1.000000000000000000, 0.9659258262890683122, 1.000000000000000000, 0.9659258262890683122, 1.000000000000000000, 0.9659258262890683122, 1.000000000000000000, 0.9659258262890683122, 1.000000000000000000, 0.9659258262890683122, 1.000000000000000000, 0.9659258262890683122, 1.000000000000000000, 0.9659258262890683122, 1.000000000000000000, 0.9659258262890683122, 1.000000000000000000, 0.9659258262890683122, 1.000000000000000000, 0.9659258262890683122, 1.000000000000000000, 0.9659258262890683122, 1.000000000000000000, 0.9659258262890683122, 1.000000000000000000, 0.9659258262890683122, 1.000000000000000000, 0.9659258262890683122, 1.000000000000000000, 0.9659258262890683122, 1.000000000000000000, 0.9659258262890683122, 1.000000000000000000, 0.9659258262890683122, 1.000000000000000000, 0.9659258262890683122, 1.000000000000000000, 0.9659258262890683122, 1.000000000000000000, 0.9659258262890683122, 1.000000000000000000, 0.9659258262890683122, 1.000000000000000000, 0.9659258262890683122, 1.000000000000000000, 0.9659258262890683122, 1.000000000000000000, 0.9659258262890683122, 1.000000000000000000, 0.9659258262890683122, 1.000000000000000000, 0.9659258262890683122, 1.000000000000000000, 0.9659258262890683122, 1.000000000000000000, 0.9659258262890683122, 1.000000000000000000, 0.9659258262890683122, 1.000000000000000000, 0.9659258262890683122, 1.000000000000000000, 0.9659258262890683122, 1.000000000000000000, 0.9659258262890683122, 1.000000000000000000, 0.9659258262890683122, 1.000000000000000000, 0.9659258262890683122, 1.000000000000000000, 0.9659258262890683122, 1.000000000000000000, 0.9659258262890683122, 1.000000000000000000, 0.9659258262890683122, 1.000000000000000000, 0.9659258262890683122, 1.000000000000000000, 0.9659258262890683122, 1.000000000000000000, 0.9659258262890683122, 1.000000000000000000, 0.9659258262890683122, 1.000000000000000000, 0.9659258262890683122, 1.000000000000000000, 0.9659258262890683122, 1.000000000000000000, 0.9659258262890683122, 1.000000000000000000, 0.9659258262890683122, 1.000000000000000000, 0.9659258262890683122, 1.000000000000000000, 0.9659258262890683122, 1.000000000000000000, 0.9659258262890683122, 1.000000000000000000, 0.9659258262890683122, 1.000000000000000000, 0.9659258262890683122, 1.000000000000000000, 0.9659258262890683122, 1.000000000000000000, 0.9659258262890683122, 1.000000000000000000, 0.9659258262890683122, 1.000000000000000000, 0.9659258262890683122, 1.000000000000000000, 0.9659258262890683122, 1.000000000000000000, 0.9659258262890683122, 1.000000000000000000, 0.9659258262890683122, 1.000000000000000000, 0.9659258262890683122, 1.000000000000000000, 0.9659258262890683122, 1.000000000000000000, 0.9659258262890683122, 1.000000000000000000, 0.9659258262890683122, 1.000000000000000000, 0.9659258262890683122, 1.000000000000000000, 0.9659258262890683122, 1.000000000000000000, 0.9659258262890683122, 1.000000000000000000, 0.9659258262890683122, 1.000000000000000000, 0.9659258262890683122, 1.000000000000000000, 0.9659258262890683122, 1.000000000000000000, 0.9659258262890683122, 1.000000000000000000, 0.9659258262890683122, 1.000000000000000000, 0.9659258262890683122, 1.000000000000000000, 0.9659258262890683122, 1.000000000000000000, 0.9659258262890683122, 1.000000000000000000, 0.9659258262890683122, 1.000000000000000000, 0.9659258262890683122, 1.000000000000000000, 0.9659258262890683122, 1.000000000000000000, 0.9659258262890683122, 1.000000000000000000, 0.9659258262890683122, 1.000000000000000000, 0.9659258262890683122, 1.000000000000000000, 0.9659258262890683122, 1.000000000000000000, 0.9659258262890683122, 1.000000000000000000, 0.9659258262890683122, 1.000000000000000000, 0.9659258262890683122, 1.000000000000000000, 0.9659258262890683122, 1.000000000000000000, 0.9659258262890683122, 1.000000000000000000, 0.9659258262890683122, 1.000000000000000000, 0.9659258262890683122, 1.000000000000000000, 0.9659258262890683122, 1.000000000000000000, 0.9659258262890683122, 1.000000000000000000, 0.9659258262890683122, 1.000000000000000000, 0.9659258262890683122, 1.000000000000000000, 0.9659258262890683122, 1.000000000000000000, 0.9659258262890683122, 1.000000000000000000, 0.9659258262890683122, 1.000000000000000000, 0.9659258262890683122, 1.000000000000000000, 0.9659258262890683122, 1.000000000000000000, 0.9659258262890683122, 1.000000000000000000, 0.9659258262890683122, 1.000000000000000000, 0.9659258262890683122, 1.000000000000000000, 0.9659258262890683122, 1.000000000000000000, 0.9659258262890683122, 1.000000000000000000, 0.9659258262890683122, 1.000000000000000000, 0.9659258262890683122, 1.000000000000000000, 0.9659258262890683122, 1.000000000000000000, 0.9659258262890683122, 1.000000000000000000, 0.9659258262890683122, 1.000000000000000000, 0.9659258262890683122, 1.000000000000000000, 0.9659258262890683122, 1.000000000000000000, 0.9659258262890683122, 1.000000000000000000, 0.9659258262890683122, 1.000000000000000000, 0.9659258262890683122, 1.000000000000000000, 0.9659258262890683122, 1.000000000000000000, 0.9659258262890683122, 1.000000000000000000, 0.9659258262890683122, 1.000000000000000000, 0.9659258262890683122, 1.000000000000000000, 0.9659258262890683122, 1.000000000000000000, 0.9659258262890683122, 1.000000000000000000, 0.9659258262890683122, 1.000000000000000000, 0.9659258262890683122, 1.000000000000000000, 0.9659258262890683122, 1.000000000000000000, 0.9659258262890683122, 1.000000000000000000, 0.9659258262890683122, 1.000000000000000000, 0.9659258262890683122, 1.000000000000000000, 0.9659258262890683122, 1.000000000000000000, 0.9659258262890683122, 1.000000000000000000, 0.9659258262890683122, 1.000000000000000000, 0.9659258262890683122, 1.000000000000000000, 0.9659258262890683122, 1.000000000000000000, 0.9659258262890683122, 1.000000000000000000, 0.9659258262890683122, 1.000000000000000000, 0.9659258262890683122, 1.000000000000000000, 0.9659258262890683122, 1.000000000000000000, 0.9659258262890683122, 1.000000000000000000, 0.9659258262890683122, 1.000000000000000000, 0.9659258262890683122, 1.000000000000000000, 0.9659258262890683122, 1.000000000000000000, 0.9659258262890683122, 1.000000000000000000, 0.9659258262890683122, 1.000000000000000000, 0.9659258262890683122, 1.000000000000000000, 0.9659258262890683122, 1.000000000000000000, 0.9659258262890683122, 1.000000000000000000, 0.9659258262890683122, 1.000000000000000000, 0.9659258262890683122, 1.000000000000000000, 0.9659258262890683122, 1.000000000000000000, 0.9659258262890683122, 1.000000000000000000, 0.9659258262890683122, 1.000000000000000000),
 ( 0.3333333333333333703, 0.3219752754296894559, 0.3333333333333333703, 0.3219752754296894559, 0.3333333333333333703, 0.3219752754296894559, 0.3333333333333333703, 0.3219752754296894559, 0.3333333333333333703, 0.3219752754296894559, 0.3333333333333333703, 0.3219752754296894559, 0.3333333333333333703, 0.3219752754296894559, 0.3333333333333333703, 0.3219752754296894559, 0.3333333333333333703, 0.3219752754296894559, 0.3333333333333333703, 0.3219752754296894559, 0.3333333333333333703, 0.3219752754296894559, 0.3333333333333333703, 0.3219752754296894559, 0.3333333333333333703, 0.3219752754296894559, 0.3333333333333333703, 0.3219752754296894559, 0.3333333333333333703, 0.3219752754296894559, 0.3333333333333333703, 0.3219752754296894559, 0.3333333333333333703, 0.3219752754296894559, 0.3333333333333333703, 0.3219752754296894559, 0.3333333333333333703, 0.3219752754296894559, 0.3333333333333333703, 0.3219752754296894559, 0.3333333333333333703, 0.3219752754296894559, 0.3333333333333333703, 0.3219752754296894559, 0.3333333333333333703, 0.3219752754296894559, 0.3333333333333333703, 0.3219752754296894559, 0.3333333333333333703, 0.3219752754296894559, 0.3333333333333333703, 0.3219752754296894559, 0.3333333333333333703, 0.3219752754296894559, 0.3333333333333333703, 0.3219752754296894559, 0.3333333333333333703, 0.3219752754296894559, 0.3333333333333333703, 0.3219752754296894559, 0.3333333333333333703, 0.3219752754296894559, 0.3333333333333333703, 0.3219752754296894559, 0.3333333333333333703, 0.3219752754296894559, 0.3333333333333333703, 0.3219752754296894559, 0.3333333333333333703, 0.3219752754296894559, 0.3333333333333333703, 0.3219752754296894559, 0.3333333333333333703, 0.3219752754296894559, 0.3333333333333333703, 0.3219752754296894559, 0.3333333333333333703, 0.3219752754296894559, 0.3333333333333333703, 0.3219752754296894559, 0.3333333333333333703, 0.3219752754296894559, 0.3333333333333333703, 0.3219752754296894559, 0.3333333333333333703, 0.3219752754296894559, 0.3333333333333333703, 0.3219752754296894559, 0.3333333333333333703, 0.3219752754296894559, 0.3333333333333333703, 0.3219752754296894559, 0.3333333333333333703, 0.3219752754296894559, 0.3333333333333333703, 0.3219752754296894559, 0.3333333333333333703, 0.3219752754296894559, 0.3333333333333333703, 0.3219752754296894559, 0.3333333333333333703, 0.3219752754296894559, 0.3333333333333333703, 0.3219752754296894559, 0.3333333333333333703, 0.3219752754296894559, 0.3333333333333333703, 0.3219752754296894559, 0.3333333333333333703, 0.3219752754296894559, 0.3333333333333333703, 0.3219752754296894559, 0.3333333333333333703, 0.3219752754296894559, 0.3333333333333333703, 0.3219752754296894559, 0.3333333333333333703, 0.3219752754296894559, 0.3333333333333333703, 0.3219752754296894559, 0.3333333333333333703, 0.3219752754296894559, 0.3333333333333333703, 0.3219752754296894559, 0.3333333333333333703, 0.3219752754296894559, 0.3333333333333333703, 0.3219752754296894559, 0.3333333333333333703, 0.3219752754296894559, 0.3333333333333333703, 0.3219752754296894559, 0.3333333333333333703, 0.3219752754296894559, 0.3333333333333333703, 0.3219752754296894559, 0.3333333333333333703, 0.3219752754296894559, 0.3333333333333333703, 0.3219752754296894559, 0.3333333333333333703, 0.3219752754296894559, 0.3333333333333333703, 0.3219752754296894559, 0.3333333333333333703, 0.3219752754296894559, 0.3333333333333333703, 0.3219752754296894559, 0.3333333333333333703, 0.3219752754296894559, 0.3333333333333333703, 0.3219752754296894559, 0.3333333333333333703, 0.3219752754296894559, 0.3333333333333333703, 0.3219752754296894559, 0.3333333333333333703, 0.3219752754296894559, 0.3333333333333333703, 0.3219752754296894559, 0.3333333333333333703, 0.3219752754296894559, 0.3333333333333333703, 0.3219752754296894559, 0.3333333333333333703, 0.3219752754296894559, 0.3333333333333333703, 0.3219752754296894559, 0.3333333333333333703, 0.3219752754296894559, 0.3333333333333333703, 0.3219752754296894559, 0.3333333333333333703, 0.3219752754296894559, 0.3333333333333333703, 0.3219752754296894559, 0.3333333333333333703, 0.3219752754296894559, 0.3333333333333333703, 0.3219752754296894559, 0.3333333333333333703, 0.3219752754296894559, 0.3333333333333333703, 0.3219752754296894559, 0.3333333333333333703, 0.3219752754296894559, 0.3333333333333333703, 0.3219752754296894559, 0.3333333333333333703, 0.3219752754296894559, 0.3333333333333333703, 0.3219752754296894559, 0.3333333333333333703, 0.3219752754296894559, 0.3333333333333333703, 0.3219752754296894559, 0.3333333333333333703, 0.3219752754296894559, 0.3333333333333333703, 0.3219752754296894559, 0.3333333333333333703, 0.3219752754296894559, 0.3333333333333333703, 0.3219752754296894559, 0.3333333333333333703, 0.3219752754296894559, 0.3333333333333333703, 0.3219752754296894559, 0.3333333333333333703, 0.3219752754296894559, 0.3333333333333333703, 0.3219752754296894559, 0.3333333333333333703, 0.3219752754296894559, 0.3333333333333333703, 0.3219752754296894559, 0.3333333333333333703, 0.3219752754296894559, 0.3333333333333333703, 0.3219752754296894559, 0.3333333333333333703, 0.3219752754296894559, 0.3333333333333333703, 0.3219752754296894559, 0.3333333333333333703, 0.3219752754296894559, 0.3333333333333333703, 0.3219752754296894559, 0.3333333333333333703, 0.3219752754296894559, 0.3333333333333333703, 0.3219752754296894559, 0.3333333333333333703, 0.3219752754296894559, 0.3333333333333333703, 0.3219752754296894559, 0.3333333333333333703, 0.3219752754296894559, 0.3333333333333333703, 0.3219752754296894559, 0.3333333333333333703, 0.3219752754296894559, 0.3333333333333333703, 0.3219752754296894559, 0.3333333333333333703, 0.3219752754296894559, 0.3333333333333333703, 0.3219752754296894559, 0.3333333333333333703, 0.3219752754296894559, 0.3333333333333333703, 0.3219752754296894559, 0.3333333333333333703, 0.3219752754296894559, 0.3333333333333333703, 0.3219752754296894559, 0.3333333333333333703, 0.3219752754296894559, 0.3333333333333333703, 0.3219752754296894559, 0.3333333333333333703, 0.3219752754296894559, 0.3333333333333333703, 0.3219752754296894559, 0.3333333333333333703, 0.3219752754296894559, 0.3333333333333333703, 0.3219752754296894559, 0.3333333333333333703, 0.3219752754296894559, 0.3333333333333333703, 0.3219752754296894559, 0.3333333333333333703, 0.3219752754296894559, 0.3333333333333333703, 0.3219752754296894559, 0.3333333333333333703, 0.3219752754296894559, 0.3333333333333333703, 0.3219752754296894559, 0.3333333333333333703, 0.3219752754296894559, 0.3333333333333333703, 0.3219752754296894559, 0.3333333333333333703, 0.3219752754296894559, 0.3333333333333333703, 0.3219752754296894559, 0.3333333333333333703, 0.3219752754296894559, 0.3333333333333333703, 0.3219752754296894559, 0.3333333333333333703, 0.3219752754296894559, 0.3333333333333333703, 0.3219752754296894559, 0.3333333333333333703, 0.3219752754296894559, 0.3333333333333333703, 0.3219752754296894559, 0.3333333333333333703, 0.3219752754296894559, 0.3333333333333333703, 0.3219752754296894559, 0.3333333333333333703, 0.3219752754296894559, 0.3333333333333333703, 0.3219752754296894559, 0.3333333333333333703, 0.3219752754296894559, 0.3333333333333333703, 0.3219752754296894559, 0.3333333333333333703, 0.3219752754296894559, 0.3333333333333333703, 0.3219752754296894559, 0.3333333333333333703, 0.3219752754296894559, 0.3333333333333333703, 0.3219752754296894559, 0.3333333333333333703, 0.3219752754296894559, 0.3333333333333333703, 0.3219752754296894559, 0.3333333333333333703, 0.3219752754296894559, 0.3333333333333333703, 0.3219752754296894559, 0.3333333333333333703, 0.3219752754296894559, 0.3333333333333333703, 0.3219752754296894559, 0.3333333333333333703, 0.3219752754296894559, 0.3333333333333333703, 0.3219752754296894559, 0.3333333333333333703, 0.3219752754296894559, 0.3333333333333333703, 0.3219752754296894559, 0.3333333333333333703, 0.3219752754296894559, 0.3333333333333333703, 0.3219752754296894559, 0.3333333333333333703, 0.3219752754296894559, 0.3333333333333333703, 0.3219752754296894559, 0.3333333333333333703, 0.3219752754296894559, 0.3333333333333333703, 0.3219752754296894559, 0.3333333333333333703, 0.3219752754296894559, 0.3333333333333333703, 0.3219752754296894559, 0.3333333333333333703, 0.3219752754296894559, 0.3333333333333333703, 0.3219752754296894559, 0.3333333333333333703, 0.3219752754296894559, 0.3333333333333333703, 0.3219752754296894559, 0.3333333333333333703, 0.3219752754296894559, 0.3333333333333333703, 0.3219752754296894559, 0.3333333333333333703, 0.3219752754296894559, 0.3333333333333333703, 0.3219752754296894559, 0.3333333333333333703, 0.3219752754296894559, 0.3333333333333333703, 0.3219752754296894559, 0.3333333333333333703, 0.3219752754296894559, 0.3333333333333333703, 0.3219752754296894559, 0.3333333333333333703, 0.3219752754296894559, 0.3333333333333333703, 0.3219752754296894559, 0.3333333333333333703, 0.3219752754296894559, 0.3333333333333333703, 0.3219752754296894559, 0.3333333333333333703, 0.3219752754296894559, 0.3333333333333333703, 0.3219752754296894559, 0.3333333333333333703, 0.3219752754296894559, 0.3333333333333333703, 0.3219752754296894559, 0.3333333333333333703, 0.3219752754296894559, 0.3333333333333333703, 0.3219752754296894559, 0.3333333333333333703, 0.3219752754296894559, 0.3333333333333333703, 0.3219752754296894559, 0.3333333333333333703, 0.3219752754296894559, 0.3333333333333333703, 0.3219752754296894559, 0.3333333333333333703, 0.3219752754296894559, 0.3333333333333333703, 0.3219752754296894559, 0.3333333333333333703, 0.3219752754296894559, 0.3333333333333333703, 0.3219752754296894559, 0.3333333333333333703, 0.3219752754296894559, 0.3333333333333333703, 0.3219752754296894559, 0.3333333333333333703, 0.3219752754296894559, 0.3333333333333333703, 0.3219752754296894559, 0.3333333333333333703, 0.3219752754296894559, 0.3333333333333333703, 0.3219752754296894559, 0.3333333333333333703, 0.3219752754296894559, 0.3333333333333333703, 0.3219752754296894559, 0.3333333333333333703, 0.3219752754296894559, 0.3333333333333333703, 0.3219752754296894559, 0.3333333333333333703, 0.3219752754296894559, 0.3333333333333333703, 0.3219752754296894559, 0.3333333333333333703, 0.3219752754296894559, 0.3333333333333333703, 0.3219752754296894559, 0.3333333333333333703, 0.3219752754296894559, 0.3333333333333333703, 0.3219752754296894559, 0.3333333333333333703, 0.3219752754296894559, 0.3333333333333333703, 0.3219752754296894559, 0.3333333333333333703, 0.3219752754296894559, 0.3333333333333333703, 0.3219752754296894559, 0.3333333333333333703),
 ( 0.3333333333333333703, 0.3219752754296894559, 0.3333333333333333703, 0.3219752754296894559, 0.3333333333333333703, 0.3219752754296894559, 0.3333333333333333703, 0.3219752754296894559, 0.3333333333333333703, 0.3219752754296894559, 0.3333333333333333703, 0.3219752754296894559, 0.3333333333333333703, 0.3219752754296894559, 0.3333333333333333703, 0.3219752754296894559, 0.3333333333333333703, 0.3219752754296894559, 0.3333333333333333703, 0.3219752754296894559, 0.3333333333333333703, 0.3219752754296894559, 0.3333333333333333703, 0.3219752754296894559, 0.3333333333333333703, 0.3219752754296894559, 0.3333333333333333703, 0.3219752754296894559, 0.3333333333333333703, 0.3219752754296894559, 0.3333333333333333703, 0.3219752754296894559, 0.3333333333333333703, 0.3219752754296894559, 0.3333333333333333703, 0.3219752754296894559, 0.3333333333333333703, 0.3219752754296894559, 0.3333333333333333703, 0.3219752754296894559, 0.3333333333333333703, 0.3219752754296894559, 0.3333333333333333703, 0.3219752754296894559, 0.3333333333333333703, 0.3219752754296894559, 0.3333333333333333703, 0.3219752754296894559, 0.3333333333333333703, 0.3219752754296894559, 0.3333333333333333703, 0.3219752754296894559, 0.3333333333333333703, 0.3219752754296894559, 0.3333333333333333703, 0.3219752754296894559, 0.3333333333333333703, 0.3219752754296894559, 0.3333333333333333703, 0.3219752754296894559, 0.3333333333333333703, 0.3219752754296894559, 0.3333333333333333703, 0.3219752754296894559, 0.3333333333333333703, 0.3219752754296894559, 0.3333333333333333703, 0.3219752754296894559, 0.3333333333333333703, 0.3219752754296894559, 0.3333333333333333703, 0.3219752754296894559, 0.3333333333333333703, 0.3219752754296894559, 0.3333333333333333703, 0.3219752754296894559, 0.3333333333333333703, 0.3219752754296894559, 0.3333333333333333703, 0.3219752754296894559, 0.3333333333333333703, 0.3219752754296894559, 0.3333333333333333703, 0.3219752754296894559, 0.3333333333333333703, 0.3219752754296894559, 0.3333333333333333703, 0.3219752754296894559, 0.3333333333333333703, 0.3219752754296894559, 0.3333333333333333703, 0.3219752754296894559, 0.3333333333333333703, 0.3219752754296894559, 0.3333333333333333703, 0.3219752754296894559, 0.3333333333333333703, 0.3219752754296894559, 0.3333333333333333703, 0.3219752754296894559, 0.3333333333333333703, 0.3219752754296894559, 0.3333333333333333703, 0.3219752754296894559, 0.3333333333333333703, 0.3219752754296894559, 0.3333333333333333703, 0.3219752754296894559, 0.3333333333333333703, 0.3219752754296894559, 0.3333333333333333703, 0.3219752754296894559, 0.3333333333333333703, 0.3219752754296894559, 0.3333333333333333703, 0.3219752754296894559, 0.3333333333333333703, 0.3219752754296894559, 0.3333333333333333703, 0.3219752754296894559, 0.3333333333333333703, 0.3219752754296894559, 0.3333333333333333703, 0.3219752754296894559, 0.3333333333333333703, 0.3219752754296894559, 0.3333333333333333703, 0.3219752754296894559, 0.3333333333333333703, 0.3219752754296894559, 0.3333333333333333703, 0.3219752754296894559, 0.3333333333333333703, 0.3219752754296894559, 0.3333333333333333703, 0.3219752754296894559, 0.3333333333333333703, 0.3219752754296894559, 0.3333333333333333703, 0.3219752754296894559, 0.3333333333333333703, 0.3219752754296894559, 0.3333333333333333703, 0.3219752754296894559, 0.3333333333333333703, 0.3219752754296894559, 0.3333333333333333703, 0.3219752754296894559, 0.3333333333333333703, 0.3219752754296894559, 0.3333333333333333703, 0.3219752754296894559, 0.3333333333333333703, 0.3219752754296894559, 0.3333333333333333703, 0.3219752754296894559, 0.3333333333333333703, 0.3219752754296894559, 0.3333333333333333703, 0.3219752754296894559, 0.3333333333333333703, 0.3219752754296894559, 0.3333333333333333703, 0.3219752754296894559, 0.3333333333333333703, 0.3219752754296894559, 0.3333333333333333703, 0.3219752754296894559, 0.3333333333333333703, 0.3219752754296894559, 0.3333333333333333703, 0.3219752754296894559, 0.3333333333333333703, 0.3219752754296894559, 0.3333333333333333703, 0.3219752754296894559, 0.3333333333333333703, 0.3219752754296894559, 0.3333333333333333703, 0.3219752754296894559, 0.3333333333333333703, 0.3219752754296894559, 0.3333333333333333703, 0.3219752754296894559, 0.3333333333333333703, 0.3219752754296894559, 0.3333333333333333703, 0.3219752754296894559, 0.3333333333333333703, 0.3219752754296894559, 0.3333333333333333703, 0.3219752754296894559, 0.3333333333333333703, 0.3219752754296894559, 0.3333333333333333703, 0.3219752754296894559, 0.3333333333333333703, 0.3219752754296894559, 0.3333333333333333703, 0.3219752754296894559, 0.3333333333333333703, 0.3219752754296894559, 0.3333333333333333703, 0.3219752754296894559, 0.3333333333333333703, 0.3219752754296894559, 0.3333333333333333703, 0.3219752754296894559, 0.3333333333333333703, 0.3219752754296894559, 0.3333333333333333703, 0.3219752754296894559, 0.3333333333333333703, 0.3219752754296894559, 0.3333333333333333703, 0.3219752754296894559, 0.3333333333333333703, 0.3219752754296894559, 0.3333333333333333703, 0.3219752754296894559, 0.3333333333333333703, 0.3219752754296894559, 0.3333333333333333703, 0.3219752754296894559, 0.3333333333333333703, 0.3219752754296894559, 0.3333333333333333703, 0.3219752754296894559, 0.3333333333333333703, 0.3219752754296894559, 0.3333333333333333703, 0.3219752754296894559, 0.3333333333333333703, 0.3219752754296894559, 0.3333333333333333703, 0.3219752754296894559, 0.3333333333333333703, 0.3219752754296894559, 0.3333333333333333703, 0.3219752754296894559, 0.3333333333333333703, 0.3219752754296894559, 0.3333333333333333703, 0.3219752754296894559, 0.3333333333333333703, 0.3219752754296894559, 0.3333333333333333703, 0.3219752754296894559, 0.3333333333333333703, 0.3219752754296894559, 0.3333333333333333703, 0.3219752754296894559, 0.3333333333333333703, 0.3219752754296894559, 0.3333333333333333703, 0.3219752754296894559, 0.3333333333333333703, 0.3219752754296894559, 0.3333333333333333703, 0.3219752754296894559, 0.3333333333333333703, 0.3219752754296894559, 0.3333333333333333703, 0.3219752754296894559, 0.3333333333333333703, 0.3219752754296894559, 0.3333333333333333703, 0.3219752754296894559, 0.3333333333333333703, 0.3219752754296894559, 0.3333333333333333703, 0.3219752754296894559, 0.3333333333333333703, 0.3219752754296894559, 0.3333333333333333703, 0.3219752754296894559, 0.3333333333333333703, 0.3219752754296894559, 0.3333333333333333703, 0.3219752754296894559, 0.3333333333333333703, 0.3219752754296894559, 0.3333333333333333703, 0.3219752754296894559, 0.3333333333333333703, 0.3219752754296894559, 0.3333333333333333703, 0.3219752754296894559, 0.3333333333333333703, 0.3219752754296894559, 0.3333333333333333703, 0.3219752754296894559, 0.3333333333333333703, 0.3219752754296894559, 0.3333333333333333703, 0.3219752754296894559, 0.3333333333333333703, 0.3219752754296894559, 0.3333333333333333703, 0.3219752754296894559, 0.3333333333333333703, 0.3219752754296894559, 0.3333333333333333703, 0.3219752754296894559, 0.3333333333333333703, 0.3219752754296894559, 0.3333333333333333703, 0.3219752754296894559, 0.3333333333333333703, 0.3219752754296894559, 0.3333333333333333703, 0.3219752754296894559, 0.3333333333333333703, 0.3219752754296894559, 0.3333333333333333703, 0.3219752754296894559, 0.3333333333333333703, 0.3219752754296894559, 0.3333333333333333703, 0.3219752754296894559, 0.3333333333333333703, 0.3219752754296894559, 0.3333333333333333703, 0.3219752754296894559, 0.3333333333333333703, 0.3219752754296894559, 0.3333333333333333703, 0.3219752754296894559, 0.3333333333333333703, 0.3219752754296894559, 0.3333333333333333703, 0.3219752754296894559, 0.3333333333333333703, 0.3219752754296894559, 0.3333333333333333703, 0.3219752754296894559, 0.3333333333333333703, 0.3219752754296894559, 0.3333333333333333703, 0.3219752754296894559, 0.3333333333333333703, 0.3219752754296894559, 0.3333333333333333703, 0.3219752754296894559, 0.3333333333333333703, 0.3219752754296894559, 0.3333333333333333703, 0.3219752754296894559, 0.3333333333333333703, 0.3219752754296894559, 0.3333333333333333703, 0.3219752754296894559, 0.3333333333333333703, 0.3219752754296894559, 0.3333333333333333703, 0.3219752754296894559, 0.3333333333333333703, 0.3219752754296894559, 0.3333333333333333703, 0.3219752754296894559, 0.3333333333333333703, 0.3219752754296894559, 0.3333333333333333703, 0.3219752754296894559, 0.3333333333333333703, 0.3219752754296894559, 0.3333333333333333703, 0.3219752754296894559, 0.3333333333333333703, 0.3219752754296894559, 0.3333333333333333703, 0.3219752754296894559, 0.3333333333333333703, 0.3219752754296894559, 0.3333333333333333703, 0.3219752754296894559, 0.3333333333333333703, 0.3219752754296894559, 0.3333333333333333703, 0.3219752754296894559, 0.3333333333333333703, 0.3219752754296894559, 0.3333333333333333703, 0.3219752754296894559, 0.3333333333333333703, 0.3219752754296894559, 0.3333333333333333703, 0.3219752754296894559, 0.3333333333333333703, 0.3219752754296894559, 0.3333333333333333703, 0.3219752754296894559, 0.3333333333333333703, 0.3219752754296894559, 0.3333333333333333703, 0.3219752754296894559, 0.3333333333333333703, 0.3219752754296894559, 0.3333333333333333703, 0.3219752754296894559, 0.3333333333333333703, 0.3219752754296894559, 0.3333333333333333703, 0.3219752754296894559, 0.3333333333333333703, 0.3219752754296894559, 0.3333333333333333703, 0.3219752754296894559, 0.3333333333333333703, 0.3219752754296894559, 0.3333333333333333703, 0.3219752754296894559, 0.3333333333333333703, 0.3219752754296894559, 0.3333333333333333703, 0.3219752754296894559, 0.3333333333333333703, 0.3219752754296894559, 0.3333333333333333703, 0.3219752754296894559, 0.3333333333333333703, 0.3219752754296894559, 0.3333333333333333703, 0.3219752754296894559, 0.3333333333333333703, 0.3219752754296894559, 0.3333333333333333703, 0.3219752754296894559, 0.3333333333333333703, 0.3219752754296894559, 0.3333333333333333703, 0.3219752754296894559, 0.3333333333333333703, 0.3219752754296894559, 0.3333333333333333703, 0.3219752754296894559, 0.3333333333333333703, 0.3219752754296894559, 0.3333333333333333703, 0.3219752754296894559, 0.3333333333333333703, 0.3219752754296894559, 0.3333333333333333703, 0.3219752754296894559, 0.3333333333333333703, 0.3219752754296894559, 0.3333333333333333703, 0.3219752754296894559, 0.3333333333333333703, 0.3219752754296894559, 0.3333333333333333703, 0.3219752754296894559, 0.3333333333333333703, 0.3219752754296894559, 0.3333333333333333703, 0.3219752754296894559, 0.3333333333333333703),
 ( 1.000000000000000000, 0.9659258262890683122, 1.000000000000000000, 0.9659258262890683122, 1.000000000000000000, 0.9659258262890683122, 1.000000000000000000, 0.9659258262890683122, 1.000000000000000000, 0.9659258262890683122, 1.000000000000000000, 0.9659258262890683122, 1.000000000000000000, 0.9659258262890683122, 1.000000000000000000, 0.9659258262890683122, 1.000000000000000000, 0.9659258262890683122, 1.000000000000000000, 0.9659258262890683122, 1.000000000000000000, 0.9659258262890683122, 1.000000000000000000, 0.9659258262890683122, 1.000000000000000000, 0.9659258262890683122, 1.000000000000000000, 0.9659258262890683122, 1.000000000000000000, 0.9659258262890683122, 1.000000000000000000, 0.9659258262890683122, 1.000000000000000000, 0.9659258262890683122, 1.000000000000000000, 0.9659258262890683122, 1.000000000000000000, 0.9659258262890683122, 1.000000000000000000, 0.9659258262890683122, 1.000000000000000000, 0.9659258262890683122, 1.000000000000000000, 0.9659258262890683122, 1.000000000000000000, 0.9659258262890683122, 1.000000000000000000, 0.9659258262890683122, 1.000000000000000000, 0.9659258262890683122, 1.000000000000000000, 0.9659258262890683122, 1.000000000000000000, 0.9659258262890683122, 1.000000000000000000, 0.9659258262890683122, 1.000000000000000000, 0.9659258262890683122, 1.000000000000000000, 0.9659258262890683122, 1.000000000000000000, 0.9659258262890683122, 1.000000000000000000, 0.9659258262890683122, 1.000000000000000000, 0.9659258262890683122, 1.000000000000000000, 0.9659258262890683122, 1.000000000000000000, 0.9659258262890683122, 1.000000000000000000, 0.9659258262890683122, 1.000000000000000000, 0.9659258262890683122, 1.000000000000000000, 0.9659258262890683122, 1.000000000000000000, 0.9659258262890683122, 1.000000000000000000, 0.9659258262890683122, 1.000000000000000000, 0.9659258262890683122, 1.000000000000000000, 0.9659258262890683122, 1.000000000000000000, 0.9659258262890683122, 1.000000000000000000, 0.9659258262890683122, 1.000000000000000000, 0.9659258262890683122, 1.000000000000000000, 0.9659258262890683122, 1.000000000000000000, 0.9659258262890683122, 1.000000000000000000, 0.9659258262890683122, 1.000000000000000000, 0.9659258262890683122, 1.000000000000000000, 0.9659258262890683122, 1.000000000000000000, 0.9659258262890683122, 1.000000000000000000, 0.9659258262890683122, 1.000000000000000000, 0.9659258262890683122, 1.000000000000000000, 0.9659258262890683122, 1.000000000000000000, 0.9659258262890683122, 1.000000000000000000, 0.9659258262890683122, 1.000000000000000000, 0.9659258262890683122, 1.000000000000000000, 0.9659258262890683122, 1.000000000000000000, 0.9659258262890683122, 1.000000000000000000, 0.9659258262890683122, 1.000000000000000000, 0.9659258262890683122, 1.000000000000000000, 0.9659258262890683122, 1.000000000000000000, 0.9659258262890683122, 1.000000000000000000, 0.9659258262890683122, 1.000000000000000000, 0.9659258262890683122, 1.000000000000000000, 0.9659258262890683122, 1.000000000000000000, 0.9659258262890683122, 1.000000000000000000, 0.9659258262890683122, 1.000000000000000000, 0.9659258262890683122, 1.000000000000000000, 0.9659258262890683122, 1.000000000000000000, 0.9659258262890683122, 1.000000000000000000, 0.9659258262890683122, 1.000000000000000000, 0.9659258262890683122, 1.000000000000000000, 0.9659258262890683122, 1.000000000000000000, 0.9659258262890683122, 1.000000000000000000, 0.9659258262890683122, 1.000000000000000000, 0.9659258262890683122, 1.000000000000000000, 0.9659258262890683122, 1.000000000000000000, 0.9659258262890683122, 1.000000000000000000, 0.9659258262890683122, 1.000000000000000000, 0.9659258262890683122, 1.000000000000000000, 0.9659258262890683122, 1.000000000000000000, 0.9659258262890683122, 1.000000000000000000, 0.9659258262890683122, 1.000000000000000000, 0.9659258262890683122, 1.000000000000000000, 0.9659258262890683122, 1.000000000000000000, 0.9659258262890683122, 1.000000000000000000, 0.9659258262890683122, 1.000000000000000000, 0.9659258262890683122, 1.000000000000000000, 0.9659258262890683122, 1.000000000000000000, 0.9659258262890683122, 1.000000000000000000, 0.9659258262890683122, 1.000000000000000000, 0.9659258262890683122, 1.000000000000000000, 0.9659258262890683122, 1.000000000000000000, 0.9659258262890683122, 1.000000000000000000, 0.9659258262890683122, 1.000000000000000000, 0.9659258262890683122, 1.000000000000000000, 0.9659258262890683122, 1.000000000000000000, 0.9659258262890683122, 1.000000000000000000, 0.9659258262890683122, 1.000000000000000000, 0.9659258262890683122, 1.000000000000000000, 0.9659258262890683122, 1.000000000000000000, 0.9659258262890683122, 1.000000000000000000, 0.9659258262890683122, 1.000000000000000000, 0.9659258262890683122, 1.000000000000000000, 0.9659258262890683122, 1.000000000000000000, 0.9659258262890683122, 1.000000000000000000, 0.9659258262890683122, 1.000000000000000000, 0.9659258262890683122, 1.000000000000000000, 0.9659258262890683122, 1.000000000000000000, 0.9659258262890683122, 1.000000000000000000, 0.9659258262890683122, 1.000000000000000000, 0.9659258262890683122, 1.000000000000000000, 0.9659258262890683122, 1.000000000000000000, 0.9659258262890683122, 1.000000000000000000, 0.9659258262890683122, 1.000000000000000000, 0.9659258262890683122, 1.000000000000000000, 0.9659258262890683122, 1.000000000000000000, 0.9659258262890683122, 1.000000000000000000, 0.9659258262890683122, 1.000000000000000000, 0.9659258262890683122, 1.000000000000000000, 0.9659258262890683122, 1.000000000000000000, 0.9659258262890683122, 1.000000000000000000, 0.9659258262890683122, 1.000000000000000000, 0.9659258262890683122, 1.000000000000000000, 0.9659258262890683122, 1.000000000000000000, 0.9659258262890683122, 1.000000000000000000, 0.9659258262890683122, 1.000000000000000000, 0.9659258262890683122, 1.000000000000000000, 0.9659258262890683122, 1.000000000000000000, 0.9659258262890683122, 1.000000000000000000, 0.9659258262890683122, 1.000000000000000000, 0.9659258262890683122, 1.000000000000000000, 0.9659258262890683122, 1.000000000000000000, 0.9659258262890683122, 1.000000000000000000, 0.9659258262890683122, 1.000000000000000000, 0.9659258262890683122, 1.000000000000000000, 0.9659258262890683122, 1.000000000000000000, 0.9659258262890683122, 1.000000000000000000, 0.9659258262890683122, 1.000000000000000000, 0.9659258262890683122, 1.000000000000000000, 0.9659258262890683122, 1.000000000000000000, 0.9659258262890683122, 1.000000000000000000, 0.9659258262890683122, 1.000000000000000000, 0.9659258262890683122, 1.000000000000000000, 0.9659258262890683122, 1.000000000000000000, 0.9659258262890683122, 1.000000000000000000, 0.9659258262890683122, 1.000000000000000000, 0.9659258262890683122, 1.000000000000000000, 0.9659258262890683122, 1.000000000000000000, 0.9659258262890683122, 1.000000000000000000, 0.9659258262890683122, 1.000000000000000000, 0.9659258262890683122, 1.000000000000000000, 0.9659258262890683122, 1.000000000000000000, 0.9659258262890683122, 1.000000000000000000, 0.9659258262890683122, 1.000000000000000000, 0.9659258262890683122, 1.000000000000000000, 0.9659258262890683122, 1.000000000000000000, 0.9659258262890683122, 1.000000000000000000, 0.9659258262890683122, 1.000000000000000000, 0.9659258262890683122, 1.000000000000000000, 0.9659258262890683122, 1.000000000000000000, 0.9659258262890683122, 1.000000000000000000, 0.9659258262890683122, 1.000000000000000000, 0.9659258262890683122, 1.000000000000000000, 0.9659258262890683122, 1.000000000000000000, 0.9659258262890683122, 1.000000000000000000, 0.9659258262890683122, 1.000000000000000000, 0.9659258262890683122, 1.000000000000000000, 0.9659258262890683122, 1.000000000000000000, 0.9659258262890683122, 1.000000000000000000, 0.9659258262890683122, 1.000000000000000000, 0.9659258262890683122, 1.000000000000000000, 0.9659258262890683122, 1.000000000000000000, 0.9659258262890683122, 1.000000000000000000, 0.9659258262890683122, 1.000000000000000000, 0.9659258262890683122, 1.000000000000000000, 0.9659258262890683122, 1.000000000000000000, 0.9659258262890683122, 1.000000000000000000, 0.9659258262890683122, 1.000000000000000000, 0.9659258262890683122, 1.000000000000000000, 0.9659258262890683122, 1.000000000000000000, 0.9659258262890683122, 1.000000000000000000, 0.9659258262890683122, 1.000000000000000000, 0.9659258262890683122, 1.000000000000000000, 0.9659258262890683122, 1.000000000000000000, 0.9659258262890683122, 1.000000000000000000, 0.9659258262890683122, 1.000000000000000000, 0.9659258262890683122, 1.000000000000000000, 0.9659258262890683122, 1.000000000000000000, 0.9659258262890683122, 1.000000000000000000, 0.9659258262890683122, 1.000000000000000000, 0.9659258262890683122, 1.000000000000000000, 0.9659258262890683122, 1.000000000000000000, 0.9659258262890683122, 1.000000000000000000, 0.9659258262890683122, 1.000000000000000000, 0.9659258262890683122, 1.000000000000000000, 0.9659258262890683122, 1.000000000000000000, 0.9659258262890683122, 1.000000000000000000, 0.9659258262890683122, 1.000000000000000000, 0.9659258262890683122, 1.000000000000000000, 0.9659258262890683122, 1.000000000000000000, 0.9659258262890683122, 1.000000000000000000, 0.9659258262890683122, 1.000000000000000000, 0.9659258262890683122, 1.000000000000000000, 0.9659258262890683122, 1.000000000000000000, 0.9659258262890683122, 1.000000000000000000, 0.9659258262890683122, 1.000000000000000000, 0.9659258262890683122, 1.000000000000000000, 0.9659258262890683122, 1.000000000000000000, 0.9659258262890683122, 1.000000000000000000, 0.9659258262890683122, 1.000000000000000000, 0.9659258262890683122, 1.000000000000000000, 0.9659258262890683122, 1.000000000000000000, 0.9659258262890683122, 1.000000000000000000, 0.9659258262890683122, 1.000000000000000000, 0.9659258262890683122, 1.000000000000000000, 0.9659258262890683122, 1.000000000000000000, 0.9659258262890683122, 1.000000000000000000, 0.9659258262890683122, 1.000000000000000000, 0.9659258262890683122, 1.000000000000000000, 0.9659258262890683122, 1.000000000000000000, 0.9659258262890683122, 1.000000000000000000, 0.9659258262890683122, 1.000000000000000000, 0.9659258262890683122, 1.000000000000000000, 0.9659258262890683122, 1.000000000000000000, 0.9659258262890683122, 1.000000000000000000, 0.9659258262890683122, 1.000000000000000000),
 ( 0.3333333333333333703, 0.3219752754296894559, 0.3333333333333333703, 0.3219752754296894559, 0.3333333333333333703, 0.3219752754296894559, 0.3333333333333333703, 0.3219752754296894559, 0.3333333333333333703, 0.3219752754296894559, 0.3333333333333333703, 0.3219752754296894559, 0.3333333333333333703, 0.3219752754296894559, 0.3333333333333333703, 0.3219752754296894559, 0.3333333333333333703, 0.3219752754296894559, 0.3333333333333333703, 0.3219752754296894559, 0.3333333333333333703, 0.3219752754296894559, 0.3333333333333333703, 0.3219752754296894559, 0.3333333333333333703, 0.3219752754296894559, 0.3333333333333333703, 0.3219752754296894559, 0.3333333333333333703, 0.3219752754296894559, 0.3333333333333333703, 0.3219752754296894559, 0.3333333333333333703, 0.3219752754296894559, 0.3333333333333333703, 0.3219752754296894559, 0.3333333333333333703, 0.3219752754296894559, 0.3333333333333333703, 0.3219752754296894559, 0.3333333333333333703, 0.3219752754296894559, 0.3333333333333333703, 0.3219752754296894559, 0.3333333333333333703, 0.3219752754296894559, 0.3333333333333333703, 0.3219752754296894559, 0.3333333333333333703, 0.3219752754296894559, 0.3333333333333333703, 0.3219752754296894559, 0.3333333333333333703, 0.3219752754296894559, 0.3333333333333333703, 0.3219752754296894559, 0.3333333333333333703, 0.3219752754296894559, 0.3333333333333333703, 0.3219752754296894559, 0.3333333333333333703, 0.3219752754296894559, 0.3333333333333333703, 0.3219752754296894559, 0.3333333333333333703, 0.3219752754296894559, 0.3333333333333333703, 0.3219752754296894559, 0.3333333333333333703, 0.3219752754296894559, 0.3333333333333333703, 0.3219752754296894559, 0.3333333333333333703, 0.3219752754296894559, 0.3333333333333333703, 0.3219752754296894559, 0.3333333333333333703, 0.3219752754296894559, 0.3333333333333333703, 0.3219752754296894559, 0.3333333333333333703, 0.3219752754296894559, 0.3333333333333333703, 0.3219752754296894559, 0.3333333333333333703, 0.3219752754296894559, 0.3333333333333333703, 0.3219752754296894559, 0.3333333333333333703, 0.3219752754296894559, 0.3333333333333333703, 0.3219752754296894559, 0.3333333333333333703, 0.3219752754296894559, 0.3333333333333333703, 0.3219752754296894559, 0.3333333333333333703, 0.3219752754296894559, 0.3333333333333333703, 0.3219752754296894559, 0.3333333333333333703, 0.3219752754296894559, 0.3333333333333333703, 0.3219752754296894559, 0.3333333333333333703, 0.3219752754296894559, 0.3333333333333333703, 0.3219752754296894559, 0.3333333333333333703, 0.3219752754296894559, 0.3333333333333333703, 0.3219752754296894559, 0.3333333333333333703, 0.3219752754296894559, 0.3333333333333333703, 0.3219752754296894559, 0.3333333333333333703, 0.3219752754296894559, 0.3333333333333333703, 0.3219752754296894559, 0.3333333333333333703, 0.3219752754296894559, 0.3333333333333333703, 0.3219752754296894559, 0.3333333333333333703, 0.3219752754296894559, 0.3333333333333333703, 0.3219752754296894559, 0.3333333333333333703, 0.3219752754296894559, 0.3333333333333333703, 0.3219752754296894559, 0.3333333333333333703, 0.3219752754296894559, 0.3333333333333333703, 0.3219752754296894559, 0.3333333333333333703, 0.3219752754296894559, 0.3333333333333333703, 0.3219752754296894559, 0.3333333333333333703, 0.3219752754296894559, 0.3333333333333333703, 0.3219752754296894559, 0.3333333333333333703, 0.3219752754296894559, 0.3333333333333333703, 0.3219752754296894559, 0.3333333333333333703, 0.3219752754296894559, 0.3333333333333333703, 0.3219752754296894559, 0.3333333333333333703, 0.3219752754296894559, 0.3333333333333333703, 0.3219752754296894559, 0.3333333333333333703, 0.3219752754296894559, 0.3333333333333333703, 0.3219752754296894559, 0.3333333333333333703, 0.3219752754296894559, 0.3333333333333333703, 0.3219752754296894559, 0.3333333333333333703, 0.3219752754296894559, 0.3333333333333333703, 0.3219752754296894559, 0.3333333333333333703, 0.3219752754296894559, 0.3333333333333333703, 0.3219752754296894559, 0.3333333333333333703, 0.3219752754296894559, 0.3333333333333333703, 0.3219752754296894559, 0.3333333333333333703, 0.3219752754296894559, 0.3333333333333333703, 0.3219752754296894559, 0.3333333333333333703, 0.3219752754296894559, 0.3333333333333333703, 0.3219752754296894559, 0.3333333333333333703, 0.3219752754296894559, 0.3333333333333333703, 0.3219752754296894559, 0.3333333333333333703, 0.3219752754296894559, 0.3333333333333333703, 0.3219752754296894559, 0.3333333333333333703, 0.3219752754296894559, 0.3333333333333333703, 0.3219752754296894559, 0.3333333333333333703, 0.3219752754296894559, 0.3333333333333333703, 0.3219752754296894559, 0.3333333333333333703, 0.3219752754296894559, 0.3333333333333333703, 0.3219752754296894559, 0.3333333333333333703, 0.3219752754296894559, 0.3333333333333333703, 0.3219752754296894559, 0.3333333333333333703, 0.3219752754296894559, 0.3333333333333333703, 0.3219752754296894559, 0.3333333333333333703, 0.3219752754296894559, 0.3333333333333333703, 0.3219752754296894559, 0.3333333333333333703, 0.3219752754296894559, 0.3333333333333333703, 0.3219752754296894559, 0.3333333333333333703, 0.3219752754296894559, 0.3333333333333333703, 0.3219752754296894559, 0.3333333333333333703, 0.3219752754296894559, 0.3333333333333333703, 0.3219752754296894559, 0.3333333333333333703, 0.3219752754296894559, 0.3333333333333333703, 0.3219752754296894559, 0.3333333333333333703, 0.3219752754296894559, 0.3333333333333333703, 0.3219752754296894559, 0.3333333333333333703, 0.3219752754296894559, 0.3333333333333333703, 0.3219752754296894559, 0.3333333333333333703, 0.3219752754296894559, 0.3333333333333333703, 0.3219752754296894559, 0.3333333333333333703, 0.3219752754296894559, 0.3333333333333333703, 0.3219752754296894559, 0.3333333333333333703, 0.3219752754296894559, 0.3333333333333333703, 0.3219752754296894559, 0.3333333333333333703, 0.3219752754296894559, 0.3333333333333333703, 0.3219752754296894559, 0.3333333333333333703, 0.3219752754296894559, 0.3333333333333333703, 0.3219752754296894559, 0.3333333333333333703, 0.3219752754296894559, 0.3333333333333333703, 0.3219752754296894559, 0.3333333333333333703, 0.3219752754296894559, 0.3333333333333333703, 0.3219752754296894559, 0.3333333333333333703, 0.3219752754296894559, 0.3333333333333333703, 0.3219752754296894559, 0.3333333333333333703, 0.3219752754296894559, 0.3333333333333333703, 0.3219752754296894559, 0.3333333333333333703, 0.3219752754296894559, 0.3333333333333333703, 0.3219752754296894559, 0.3333333333333333703, 0.3219752754296894559, 0.3333333333333333703, 0.3219752754296894559, 0.3333333333333333703, 0.3219752754296894559, 0.3333333333333333703, 0.3219752754296894559, 0.3333333333333333703, 0.3219752754296894559, 0.3333333333333333703, 0.3219752754296894559, 0.3333333333333333703, 0.3219752754296894559, 0.3333333333333333703, 0.3219752754296894559, 0.3333333333333333703, 0.3219752754296894559, 0.3333333333333333703, 0.3219752754296894559, 0.3333333333333333703, 0.3219752754296894559, 0.3333333333333333703, 0.3219752754296894559, 0.3333333333333333703, 0.3219752754296894559, 0.3333333333333333703, 0.3219752754296894559, 0.3333333333333333703, 0.3219752754296894559, 0.3333333333333333703, 0.3219752754296894559, 0.3333333333333333703, 0.3219752754296894559, 0.3333333333333333703, 0.3219752754296894559, 0.3333333333333333703, 0.3219752754296894559, 0.3333333333333333703, 0.3219752754296894559, 0.3333333333333333703, 0.3219752754296894559, 0.3333333333333333703, 0.3219752754296894559, 0.3333333333333333703, 0.3219752754296894559, 0.3333333333333333703, 0.3219752754296894559, 0.3333333333333333703, 0.3219752754296894559, 0.3333333333333333703, 0.3219752754296894559, 0.3333333333333333703, 0.3219752754296894559, 0.3333333333333333703, 0.3219752754296894559, 0.3333333333333333703, 0.3219752754296894559, 0.3333333333333333703, 0.3219752754296894559, 0.3333333333333333703, 0.3219752754296894559, 0.3333333333333333703, 0.3219752754296894559, 0.3333333333333333703, 0.3219752754296894559, 0.3333333333333333703, 0.3219752754296894559, 0.3333333333333333703, 0.3219752754296894559, 0.3333333333333333703, 0.3219752754296894559, 0.3333333333333333703, 0.3219752754296894559, 0.3333333333333333703, 0.3219752754296894559, 0.3333333333333333703, 0.3219752754296894559, 0.3333333333333333703, 0.3219752754296894559, 0.3333333333333333703, 0.3219752754296894559, 0.3333333333333333703, 0.3219752754296894559, 0.3333333333333333703, 0.3219752754296894559, 0.3333333333333333703, 0.3219752754296894559, 0.3333333333333333703, 0.3219752754296894559, 0.3333333333333333703, 0.3219752754296894559, 0.3333333333333333703, 0.3219752754296894559, 0.3333333333333333703, 0.3219752754296894559, 0.3333333333333333703, 0.3219752754296894559, 0.3333333333333333703, 0.3219752754296894559, 0.3333333333333333703, 0.3219752754296894559, 0.3333333333333333703, 0.3219752754296894559, 0.3333333333333333703, 0.3219752754296894559, 0.3333333333333333703, 0.3219752754296894559, 0.3333333333333333703, 0.3219752754296894559, 0.3333333333333333703, 0.3219752754296894559, 0.3333333333333333703, 0.3219752754296894559, 0.3333333333333333703, 0.3219752754296894559, 0.3333333333333333703, 0.3219752754296894559, 0.3333333333333333703, 0.3219752754296894559, 0.3333333333333333703, 0.3219752754296894559, 0.3333333333333333703, 0.3219752754296894559, 0.3333333333333333703, 0.3219752754296894559, 0.3333333333333333703, 0.3219752754296894559, 0.3333333333333333703, 0.3219752754296894559, 0.3333333333333333703, 0.3219752754296894559, 0.3333333333333333703, 0.3219752754296894559, 0.3333333333333333703, 0.3219752754296894559, 0.3333333333333333703, 0.3219752754296894559, 0.3333333333333333703, 0.3219752754296894559, 0.3333333333333333703, 0.3219752754296894559, 0.3333333333333333703, 0.3219752754296894559, 0.3333333333333333703, 0.3219752754296894559, 0.3333333333333333703, 0.3219752754296894559, 0.3333333333333333703, 0.3219752754296894559, 0.3333333333333333703, 0.3219752754296894559, 0.3333333333333333703, 0.3219752754296894559, 0.3333333333333333703, 0.3219752754296894559, 0.3333333333333333703, 0.3219752754296894559, 0.3333333333333333703, 0.3219752754296894559, 0.3333333333333333703, 0.3219752754296894559, 0.3333333333333333703, 0.3219752754296894559, 0.3333333333333333703, 0.3219752754296894559, 0.3333333333333333703, 0.3219752754296894559, 0.3333333333333333703, 0.3219752754296894559, 0.3333333333333333703, 0.3219752754296894559, 0.3333333333333333703, 0.3219752754296894559, 0.3333333333333333703, 0.3219752754296894559, 0.3333333333333333703),
 ( 0.3333333333333333703, 0.3219752754296894559, 0.3333333333333333703, 0.3219752754296894559, 0.3333333333333333703, 0.3219752754296894559, 0.3333333333333333703, 0.3219752754296894559, 0.3333333333333333703, 0.3219752754296894559, 0.3333333333333333703, 0.3219752754296894559, 0.3333333333333333703, 0.3219752754296894559, 0.3333333333333333703, 0.3219752754296894559, 0.3333333333333333703, 0.3219752754296894559, 0.3333333333333333703, 0.3219752754296894559, 0.3333333333333333703, 0.3219752754296894559, 0.3333333333333333703, 0.3219752754296894559, 0.3333333333333333703, 0.3219752754296894559, 0.3333333333333333703, 0.3219752754296894559, 0.3333333333333333703, 0.3219752754296894559, 0.3333333333333333703, 0.3219752754296894559, 0.3333333333333333703, 0.3219752754296894559, 0.3333333333333333703, 0.3219752754296894559, 0.3333333333333333703, 0.3219752754296894559, 0.3333333333333333703, 0.3219752754296894559, 0.3333333333333333703, 0.3219752754296894559, 0.3333333333333333703, 0.3219752754296894559, 0.3333333333333333703, 0.3219752754296894559, 0.3333333333333333703, 0.3219752754296894559, 0.3333333333333333703, 0.3219752754296894559, 0.3333333333333333703, 0.3219752754296894559, 0.3333333333333333703, 0.3219752754296894559, 0.3333333333333333703, 0.3219752754296894559, 0.3333333333333333703, 0.3219752754296894559, 0.3333333333333333703, 0.3219752754296894559, 0.3333333333333333703, 0.3219752754296894559, 0.3333333333333333703, 0.3219752754296894559, 0.3333333333333333703, 0.3219752754296894559, 0.3333333333333333703, 0.3219752754296894559, 0.3333333333333333703, 0.3219752754296894559, 0.3333333333333333703, 0.3219752754296894559, 0.3333333333333333703, 0.3219752754296894559, 0.3333333333333333703, 0.3219752754296894559, 0.3333333333333333703, 0.3219752754296894559, 0.3333333333333333703, 0.3219752754296894559, 0.3333333333333333703, 0.3219752754296894559, 0.3333333333333333703, 0.3219752754296894559, 0.3333333333333333703, 0.3219752754296894559, 0.3333333333333333703, 0.3219752754296894559, 0.3333333333333333703, 0.3219752754296894559, 0.3333333333333333703, 0.3219752754296894559, 0.3333333333333333703, 0.3219752754296894559, 0.3333333333333333703, 0.3219752754296894559, 0.3333333333333333703, 0.3219752754296894559, 0.3333333333333333703, 0.3219752754296894559, 0.3333333333333333703, 0.3219752754296894559, 0.3333333333333333703, 0.3219752754296894559, 0.3333333333333333703, 0.3219752754296894559, 0.3333333333333333703, 0.3219752754296894559, 0.3333333333333333703, 0.3219752754296894559, 0.3333333333333333703, 0.3219752754296894559, 0.3333333333333333703, 0.3219752754296894559, 0.3333333333333333703, 0.3219752754296894559, 0.3333333333333333703, 0.3219752754296894559, 0.3333333333333333703, 0.3219752754296894559, 0.3333333333333333703, 0.3219752754296894559, 0.3333333333333333703, 0.3219752754296894559, 0.3333333333333333703, 0.3219752754296894559, 0.3333333333333333703, 0.3219752754296894559, 0.3333333333333333703, 0.3219752754296894559, 0.3333333333333333703, 0.3219752754296894559, 0.3333333333333333703, 0.3219752754296894559, 0.3333333333333333703, 0.3219752754296894559, 0.3333333333333333703, 0.3219752754296894559, 0.3333333333333333703, 0.3219752754296894559, 0.3333333333333333703, 0.3219752754296894559, 0.3333333333333333703, 0.3219752754296894559, 0.3333333333333333703, 0.3219752754296894559, 0.3333333333333333703, 0.3219752754296894559, 0.3333333333333333703, 0.3219752754296894559, 0.3333333333333333703, 0.3219752754296894559, 0.3333333333333333703, 0.3219752754296894559, 0.3333333333333333703, 0.3219752754296894559, 0.3333333333333333703, 0.3219752754296894559, 0.3333333333333333703, 0.3219752754296894559, 0.3333333333333333703, 0.3219752754296894559, 0.3333333333333333703, 0.3219752754296894559, 0.3333333333333333703, 0.3219752754296894559, 0.3333333333333333703, 0.3219752754296894559, 0.3333333333333333703, 0.3219752754296894559, 0.3333333333333333703, 0.3219752754296894559, 0.3333333333333333703, 0.3219752754296894559, 0.3333333333333333703, 0.3219752754296894559, 0.3333333333333333703, 0.3219752754296894559, 0.3333333333333333703, 0.3219752754296894559, 0.3333333333333333703, 0.3219752754296894559, 0.3333333333333333703, 0.3219752754296894559, 0.3333333333333333703, 0.3219752754296894559, 0.3333333333333333703, 0.3219752754296894559, 0.3333333333333333703, 0.3219752754296894559, 0.3333333333333333703, 0.3219752754296894559, 0.3333333333333333703, 0.3219752754296894559, 0.3333333333333333703, 0.3219752754296894559, 0.3333333333333333703, 0.3219752754296894559, 0.3333333333333333703, 0.3219752754296894559, 0.3333333333333333703, 0.3219752754296894559, 0.3333333333333333703, 0.3219752754296894559, 0.3333333333333333703, 0.3219752754296894559, 0.3333333333333333703, 0.3219752754296894559, 0.3333333333333333703, 0.3219752754296894559, 0.3333333333333333703, 0.3219752754296894559, 0.3333333333333333703, 0.3219752754296894559, 0.3333333333333333703, 0.3219752754296894559, 0.3333333333333333703, 0.3219752754296894559, 0.3333333333333333703, 0.3219752754296894559, 0.3333333333333333703, 0.3219752754296894559, 0.3333333333333333703, 0.3219752754296894559, 0.3333333333333333703, 0.3219752754296894559, 0.3333333333333333703, 0.3219752754296894559, 0.3333333333333333703, 0.3219752754296894559, 0.3333333333333333703, 0.3219752754296894559, 0.3333333333333333703, 0.3219752754296894559, 0.3333333333333333703, 0.3219752754296894559, 0.3333333333333333703, 0.3219752754296894559, 0.3333333333333333703, 0.3219752754296894559, 0.3333333333333333703, 0.3219752754296894559, 0.3333333333333333703, 0.3219752754296894559, 0.3333333333333333703, 0.3219752754296894559, 0.3333333333333333703, 0.3219752754296894559, 0.3333333333333333703, 0.3219752754296894559, 0.3333333333333333703, 0.3219752754296894559, 0.3333333333333333703, 0.3219752754296894559, 0.3333333333333333703, 0.3219752754296894559, 0.3333333333333333703, 0.3219752754296894559, 0.3333333333333333703, 0.3219752754296894559, 0.3333333333333333703, 0.3219752754296894559, 0.3333333333333333703, 0.3219752754296894559, 0.3333333333333333703, 0.3219752754296894559, 0.3333333333333333703, 0.3219752754296894559, 0.3333333333333333703, 0.3219752754296894559, 0.3333333333333333703, 0.3219752754296894559, 0.3333333333333333703, 0.3219752754296894559, 0.3333333333333333703, 0.3219752754296894559, 0.3333333333333333703, 0.3219752754296894559, 0.3333333333333333703, 0.3219752754296894559, 0.3333333333333333703, 0.3219752754296894559, 0.3333333333333333703, 0.3219752754296894559, 0.3333333333333333703, 0.3219752754296894559, 0.3333333333333333703, 0.3219752754296894559, 0.3333333333333333703, 0.3219752754296894559, 0.3333333333333333703, 0.3219752754296894559, 0.3333333333333333703, 0.3219752754296894559, 0.3333333333333333703, 0.3219752754296894559, 0.3333333333333333703, 0.3219752754296894559, 0.3333333333333333703, 0.3219752754296894559, 0.3333333333333333703, 0.3219752754296894559, 0.3333333333333333703, 0.3219752754296894559, 0.3333333333333333703, 0.3219752754296894559, 0.3333333333333333703, 0.3219752754296894559, 0.3333333333333333703, 0.3219752754296894559, 0.3333333333333333703, 0.3219752754296894559, 0.3333333333333333703, 0.3219752754296894559, 0.3333333333333333703, 0.3219752754296894559, 0.3333333333333333703, 0.3219752754296894559, 0.3333333333333333703, 0.3219752754296894559, 0.3333333333333333703, 0.3219752754296894559, 0.3333333333333333703, 0.3219752754296894559, 0.3333333333333333703, 0.3219752754296894559, 0.3333333333333333703, 0.3219752754296894559, 0.3333333333333333703, 0.3219752754296894559, 0.3333333333333333703, 0.3219752754296894559, 0.3333333333333333703, 0.3219752754296894559, 0.3333333333333333703, 0.3219752754296894559, 0.3333333333333333703, 0.3219752754296894559, 0.3333333333333333703, 0.3219752754296894559, 0.3333333333333333703, 0.3219752754296894559, 0.3333333333333333703, 0.3219752754296894559, 0.3333333333333333703, 0.3219752754296894559, 0.3333333333333333703, 0.3219752754296894559, 0.3333333333333333703, 0.3219752754296894559, 0.3333333333333333703, 0.3219752754296894559, 0.3333333333333333703, 0.3219752754296894559, 0.3333333333333333703, 0.3219752754296894559, 0.3333333333333333703, 0.3219752754296894559, 0.3333333333333333703, 0.3219752754296894559, 0.3333333333333333703, 0.3219752754296894559, 0.3333333333333333703, 0.3219752754296894559, 0.3333333333333333703, 0.3219752754296894559, 0.3333333333333333703, 0.3219752754296894559, 0.3333333333333333703, 0.3219752754296894559, 0.3333333333333333703, 0.3219752754296894559, 0.3333333333333333703, 0.3219752754296894559, 0.3333333333333333703, 0.3219752754296894559, 0.3333333333333333703, 0.3219752754296894559, 0.3333333333333333703, 0.3219752754296894559, 0.3333333333333333703, 0.3219752754296894559, 0.3333333333333333703, 0.3219752754296894559, 0.3333333333333333703, 0.3219752754296894559, 0.3333333333333333703, 0.3219752754296894559, 0.3333333333333333703, 0.3219752754296894559, 0.3333333333333333703, 0.3219752754296894559, 0.3333333333333333703, 0.3219752754296894559, 0.3333333333333333703, 0.3219752754296894559, 0.3333333333333333703, 0.3219752754296894559, 0.3333333333333333703, 0.3219752754296894559, 0.3333333333333333703, 0.3219752754296894559, 0.3333333333333333703, 0.3219752754296894559, 0.3333333333333333703, 0.3219752754296894559, 0.3333333333333333703, 0.3219752754296894559, 0.3333333333333333703, 0.3219752754296894559, 0.3333333333333333703, 0.3219752754296894559, 0.3333333333333333703, 0.3219752754296894559, 0.3333333333333333703, 0.3219752754296894559, 0.3333333333333333703, 0.3219752754296894559, 0.3333333333333333703, 0.3219752754296894559, 0.3333333333333333703, 0.3219752754296894559, 0.3333333333333333703, 0.3219752754296894559, 0.3333333333333333703, 0.3219752754296894559, 0.3333333333333333703, 0.3219752754296894559, 0.3333333333333333703, 0.3219752754296894559, 0.3333333333333333703, 0.3219752754296894559, 0.3333333333333333703, 0.3219752754296894559, 0.3333333333333333703, 0.3219752754296894559, 0.3333333333333333703, 0.3219752754296894559, 0.3333333333333333703, 0.3219752754296894559, 0.3333333333333333703, 0.3219752754296894559, 0.3333333333333333703, 0.3219752754296894559, 0.3333333333333333703, 0.3219752754296894559, 0.3333333333333333703, 0.3219752754296894559, 0.3333333333333333703, 0.3219752754296894559, 0.3333333333333333703, 0.3219752754296894559, 0.3333333333333333703, 0.3219752754296894559, 0.3333333333333333703, 0.3219752754296894559, 0.3333333333333333703),
 ( 1.000000000000000000, 0.9659258262890683122, 1.000000000000000000, 0.9659258262890683122, 1.000000000000000000, 0.9659258262890683122, 1.000000000000000000, 0.9659258262890683122, 1.000000000000000000, 0.9659258262890683122, 1.000000000000000000, 0.9659258262890683122, 1.000000000000000000, 0.9659258262890683122, 1.000000000000000000, 0.9659258262890683122, 1.000000000000000000, 0.9659258262890683122, 1.000000000000000000, 0.9659258262890683122, 1.000000000000000000, 0.9659258262890683122, 1.000000000000000000, 0.9659258262890683122, 1.000000000000000000, 0.9659258262890683122, 1.000000000000000000, 0.9659258262890683122, 1.000000000000000000, 0.9659258262890683122, 1.000000000000000000, 0.9659258262890683122, 1.000000000000000000, 0.9659258262890683122, 1.000000000000000000, 0.9659258262890683122, 1.000000000000000000, 0.9659258262890683122, 1.000000000000000000, 0.9659258262890683122, 1.000000000000000000, 0.9659258262890683122, 1.000000000000000000, 0.9659258262890683122, 1.000000000000000000, 0.9659258262890683122, 1.000000000000000000, 0.9659258262890683122, 1.000000000000000000, 0.9659258262890683122, 1.000000000000000000, 0.9659258262890683122, 1.000000000000000000, 0.9659258262890683122, 1.000000000000000000, 0.9659258262890683122, 1.000000000000000000, 0.9659258262890683122, 1.000000000000000000, 0.9659258262890683122, 1.000000000000000000, 0.9659258262890683122, 1.000000000000000000, 0.9659258262890683122, 1.000000000000000000, 0.9659258262890683122, 1.000000000000000000, 0.9659258262890683122, 1.000000000000000000, 0.9659258262890683122, 1.000000000000000000, 0.9659258262890683122, 1.000000000000000000, 0.9659258262890683122, 1.000000000000000000, 0.9659258262890683122, 1.000000000000000000, 0.9659258262890683122, 1.000000000000000000, 0.9659258262890683122, 1.000000000000000000, 0.9659258262890683122, 1.000000000000000000, 0.9659258262890683122, 1.000000000000000000, 0.9659258262890683122, 1.000000000000000000, 0.9659258262890683122, 1.000000000000000000, 0.9659258262890683122, 1.000000000000000000, 0.9659258262890683122, 1.000000000000000000, 0.9659258262890683122, 1.000000000000000000, 0.9659258262890683122, 1.000000000000000000, 0.9659258262890683122, 1.000000000000000000, 0.9659258262890683122, 1.000000000000000000, 0.9659258262890683122, 1.000000000000000000, 0.9659258262890683122, 1.000000000000000000, 0.9659258262890683122, 1.000000000000000000, 0.9659258262890683122, 1.000000000000000000, 0.9659258262890683122, 1.000000000000000000, 0.9659258262890683122, 1.000000000000000000, 0.9659258262890683122, 1.000000000000000000, 0.9659258262890683122, 1.000000000000000000, 0.9659258262890683122, 1.000000000000000000, 0.9659258262890683122, 1.000000000000000000, 0.9659258262890683122, 1.000000000000000000, 0.9659258262890683122, 1.000000000000000000, 0.9659258262890683122, 1.000000000000000000, 0.9659258262890683122, 1.000000000000000000, 0.9659258262890683122, 1.000000000000000000, 0.9659258262890683122, 1.000000000000000000, 0.9659258262890683122, 1.000000000000000000, 0.9659258262890683122, 1.000000000000000000, 0.9659258262890683122, 1.000000000000000000, 0.9659258262890683122, 1.000000000000000000, 0.9659258262890683122, 1.000000000000000000, 0.9659258262890683122, 1.000000000000000000, 0.9659258262890683122, 1.000000000000000000, 0.9659258262890683122, 1.000000000000000000, 0.9659258262890683122, 1.000000000000000000, 0.9659258262890683122, 1.000000000000000000, 0.9659258262890683122, 1.000000000000000000, 0.9659258262890683122, 1.000000000000000000, 0.9659258262890683122, 1.000000000000000000, 0.9659258262890683122, 1.000000000000000000, 0.9659258262890683122, 1.000000000000000000, 0.9659258262890683122, 1.000000000000000000, 0.9659258262890683122, 1.000000000000000000, 0.9659258262890683122, 1.000000000000000000, 0.9659258262890683122, 1.000000000000000000, 0.9659258262890683122, 1.000000000000000000, 0.9659258262890683122, 1.000000000000000000, 0.9659258262890683122, 1.000000000000000000, 0.9659258262890683122, 1.000000000000000000, 0.9659258262890683122, 1.000000000000000000, 0.9659258262890683122, 1.000000000000000000, 0.9659258262890683122, 1.000000000000000000, 0.9659258262890683122, 1.000000000000000000, 0.9659258262890683122, 1.000000000000000000, 0.9659258262890683122, 1.000000000000000000, 0.9659258262890683122, 1.000000000000000000, 0.9659258262890683122, 1.000000000000000000, 0.9659258262890683122, 1.000000000000000000, 0.9659258262890683122, 1.000000000000000000, 0.9659258262890683122, 1.000000000000000000, 0.9659258262890683122, 1.000000000000000000, 0.9659258262890683122, 1.000000000000000000, 0.9659258262890683122, 1.000000000000000000, 0.9659258262890683122, 1.000000000000000000, 0.9659258262890683122, 1.000000000000000000, 0.9659258262890683122, 1.000000000000000000, 0.9659258262890683122, 1.000000000000000000, 0.9659258262890683122, 1.000000000000000000, 0.9659258262890683122, 1.000000000000000000, 0.9659258262890683122, 1.000000000000000000, 0.9659258262890683122, 1.000000000000000000, 0.9659258262890683122, 1.000000000000000000, 0.9659258262890683122, 1.000000000000000000, 0.9659258262890683122, 1.000000000000000000, 0.9659258262890683122, 1.000000000000000000, 0.9659258262890683122, 1.000000000000000000, 0.9659258262890683122, 1.000000000000000000, 0.9659258262890683122, 1.000000000000000000, 0.9659258262890683122, 1.000000000000000000, 0.9659258262890683122, 1.000000000000000000, 0.9659258262890683122, 1.000000000000000000, 0.9659258262890683122, 1.000000000000000000, 0.9659258262890683122, 1.000000000000000000, 0.9659258262890683122, 1.000000000000000000, 0.9659258262890683122, 1.000000000000000000, 0.9659258262890683122, 1.000000000000000000, 0.9659258262890683122, 1.000000000000000000, 0.9659258262890683122, 1.000000000000000000, 0.9659258262890683122, 1.000000000000000000, 0.9659258262890683122, 1.000000000000000000, 0.9659258262890683122, 1.000000000000000000, 0.9659258262890683122, 1.000000000000000000, 0.9659258262890683122, 1.000000000000000000, 0.9659258262890683122, 1.000000000000000000, 0.9659258262890683122, 1.000000000000000000, 0.9659258262890683122, 1.000000000000000000, 0.9659258262890683122, 1.000000000000000000, 0.9659258262890683122, 1.000000000000000000, 0.9659258262890683122, 1.000000000000000000, 0.9659258262890683122, 1.000000000000000000, 0.9659258262890683122, 1.000000000000000000, 0.9659258262890683122, 1.000000000000000000, 0.9659258262890683122, 1.000000000000000000, 0.9659258262890683122, 1.000000000000000000, 0.9659258262890683122, 1.000000000000000000, 0.9659258262890683122, 1.000000000000000000, 0.9659258262890683122, 1.000000000000000000, 0.9659258262890683122, 1.000000000000000000, 0.9659258262890683122, 1.000000000000000000, 0.9659258262890683122, 1.000000000000000000, 0.9659258262890683122, 1.000000000000000000, 0.9659258262890683122, 1.000000000000000000, 0.9659258262890683122, 1.000000000000000000, 0.9659258262890683122, 1.000000000000000000, 0.9659258262890683122, 1.000000000000000000, 0.9659258262890683122, 1.000000000000000000, 0.9659258262890683122, 1.000000000000000000, 0.9659258262890683122, 1.000000000000000000, 0.9659258262890683122, 1.000000000000000000, 0.9659258262890683122, 1.000000000000000000, 0.9659258262890683122, 1.000000000000000000, 0.9659258262890683122, 1.000000000000000000, 0.9659258262890683122, 1.000000000000000000, 0.9659258262890683122, 1.000000000000000000, 0.9659258262890683122, 1.000000000000000000, 0.9659258262890683122, 1.000000000000000000, 0.9659258262890683122, 1.000000000000000000, 0.9659258262890683122, 1.000000000000000000, 0.9659258262890683122, 1.000000000000000000, 0.9659258262890683122, 1.000000000000000000, 0.9659258262890683122, 1.000000000000000000, 0.9659258262890683122, 1.000000000000000000, 0.9659258262890683122, 1.000000000000000000, 0.9659258262890683122, 1.000000000000000000, 0.9659258262890683122, 1.000000000000000000, 0.9659258262890683122, 1.000000000000000000, 0.9659258262890683122, 1.000000000000000000, 0.9659258262890683122, 1.000000000000000000, 0.9659258262890683122, 1.000000000000000000, 0.9659258262890683122, 1.000000000000000000, 0.9659258262890683122, 1.000000000000000000, 0.9659258262890683122, 1.000000000000000000, 0.9659258262890683122, 1.000000000000000000, 0.9659258262890683122, 1.000000000000000000, 0.9659258262890683122, 1.000000000000000000, 0.9659258262890683122, 1.000000000000000000, 0.9659258262890683122, 1.000000000000000000, 0.9659258262890683122, 1.000000000000000000, 0.9659258262890683122, 1.000000000000000000, 0.9659258262890683122, 1.000000000000000000, 0.9659258262890683122, 1.000000000000000000, 0.9659258262890683122, 1.000000000000000000, 0.9659258262890683122, 1.000000000000000000, 0.9659258262890683122, 1.000000000000000000, 0.9659258262890683122, 1.000000000000000000, 0.9659258262890683122, 1.000000000000000000, 0.9659258262890683122, 1.000000000000000000, 0.9659258262890683122, 1.000000000000000000, 0.9659258262890683122, 1.000000000000000000, 0.9659258262890683122, 1.000000000000000000, 0.9659258262890683122, 1.000000000000000000, 0.9659258262890683122, 1.000000000000000000, 0.9659258262890683122, 1.000000000000000000, 0.9659258262890683122, 1.000000000000000000, 0.9659258262890683122, 1.000000000000000000, 0.9659258262890683122, 1.000000000000000000, 0.9659258262890683122, 1.000000000000000000, 0.9659258262890683122, 1.000000000000000000, 0.9659258262890683122, 1.000000000000000000, 0.9659258262890683122, 1.000000000000000000, 0.9659258262890683122, 1.000000000000000000, 0.9659258262890683122, 1.000000000000000000, 0.9659258262890683122, 1.000000000000000000, 0.9659258262890683122, 1.000000000000000000, 0.9659258262890683122, 1.000000000000000000, 0.9659258262890683122, 1.000000000000000000, 0.9659258262890683122, 1.000000000000000000, 0.9659258262890683122, 1.000000000000000000, 0.9659258262890683122, 1.000000000000000000, 0.9659258262890683122, 1.000000000000000000, 0.9659258262890683122, 1.000000000000000000, 0.9659258262890683122, 1.000000000000000000, 0.9659258262890683122, 1.000000000000000000, 0.9659258262890683122, 1.000000000000000000, 0.9659258262890683122, 1.000000000000000000, 0.9659258262890683122, 1.000000000000000000, 0.9659258262890683122, 1.000000000000000000, 0.9659258262890683122, 1.000000000000000000) ) ) 
 REPRESENTATION_ITEM ( '' )  SURFACE ( )  );
#138279=CARTESIAN_POINT ( 'NONE',  ( -16.46253265017146816, -9.564922557961047289, 104.1677570613523329 ) ) ;
#138280=CARTESIAN_POINT ( 'NONE',  ( 5.153800228976335163, 19.02544592524342804, 69.79057627198103830 ) ) ;
#138281=CARTESIAN_POINT ( 'NONE',  ( -9.564922557960796823, -16.46253265017161027, 97.08224293864769550 ) ) ;
#138283=CARTESIAN_POINT ( 'NONE',  ( -14.34966873604960291, -8.224510206698953496, 106.6655762719810383 ) ) ;
#138284=CARTESIAN_POINT ( 'NONE',  ( -21.53943276465977519, 0.05219959533907696930, 36.24890960531435979 ) ) ;
#138285=CARTESIAN_POINT ( 'NONE',  ( -8.314922557961024197, 14.29746914071037800, 87.91775706135234714 ) ) ;
#138286=CARTESIAN_POINT ( 'NONE',  ( 16.53943276465976808, -0.05219959533910856209, 73.74890960531433848 ) ) ;
#138287=CARTESIAN_POINT ( 'NONE',  ( -9.474510206698964154, 16.51473224551069663, 55.41557627198103120 ) ) ;
#138288=CARTESIAN_POINT ( 'NONE',  ( -0.05219959533937732626, 21.53943276465977519, 77.50109039468567573 ) ) ;
#138290=CARTESIAN_POINT ( 'NONE',  ( 9.564922557961047289, -16.46253265017146816, 100.4177570613523329 ) ) ;
#138291=CARTESIAN_POINT ( 'NONE',  ( 16.55341960407611168, 4.379528057220329451, 78.95724293864769550 ) ) ;
#138292=CARTESIAN_POINT ( 'NONE',  ( 15.80617190586769283, -15.72974639402175789, 30.62609039468567929 ) ) ;
#138293=CARTESIAN_POINT ( 'NONE',  ( -15.72974639402197994, 15.80617190586746368, 55.62390960531436690 ) ) ;
#138294=CARTESIAN_POINT ( 'NONE',  ( -17.26172910966779739, -6.454744622555836919, 104.1935309135077574 ) ) ;
#138296=CARTESIAN_POINT ( 'NONE',  ( -9.564922557960796823, -16.46253265017161027, 87.08224293864769550 ) ) ;
#138297=CARTESIAN_POINT ( 'NONE',  ( 14.34966873604960469, 8.224510206698951720, 49.16557627198102409 ) ) ;
#138298=CARTESIAN_POINT ( 'NONE',  ( -16.55341960407611168, -4.379528057220339221, 36.45724293864768839 ) ) ;
#138299=CARTESIAN_POINT ( 'NONE',  ( -14.29746914071037622, -8.314922557961029526, 99.16775706135234714 ) ) ;
#138300=CARTESIAN_POINT ( 'NONE',  ( 13.89961937509957401, 13.97604488694547697, 46.87609039468565442 ) ) ;
#138301=CARTESIAN_POINT ( 'NONE',  ( 16.20579543436682002, 7.371946100354975329, 48.06520834171878676 ) ) ;
#138302=CARTESIAN_POINT ( 'NONE',  ( 19.02544592524343514, -5.153800228976328945, 108.5405762719810383 ) ) ;
#138303=CARTESIAN_POINT ( 'NONE',  ( -0.05219959533910754901, -16.53943276465976808, 77.49890960531433848 ) ) ;
#138304=CARTESIAN_POINT ( 'NONE',  ( -9.564922557961040184, 16.46253265017147172, 37.91775706135233293 ) ) ;
#138305=CARTESIAN_POINT ( 'NONE',  ( 19.05341960407611168, 5.049401038298154454, 33.95724293864769550 ) ) ;
#138306=CARTESIAN_POINT ( 'NONE',  ( 21.53943276465977519, -0.05219959533907433946, 33.74890960531436690 ) ) ;
#138307=CARTESIAN_POINT ( 'NONE',  ( -18.62759615963270932, 10.81492255796079327, 60.83224293864769550 ) ) ;
#138308=CARTESIAN_POINT ( 'NONE',  ( 0.05219959533910956823, 16.53943276465976808, 94.99890960531436690 ) ) ;
#138309=CARTESIAN_POINT ( 'NONE',  ( 16.55341960407618274, -4.379528057220086978, 56.04275706135235424 ) ) ;
#138310=CARTESIAN_POINT ( 'NONE',  ( -15.80617190586768217, 15.72974639402176855, 48.12609039468568284 ) ) ;
#138311=CARTESIAN_POINT ( 'NONE',  ( 4.483927247898545687, 16.52544592524342804, 89.79057627198103830 ) ) ;
#138312=CARTESIAN_POINT ( 'NONE',  ( 17.40861289039004944, -6.110651285853252901, 36.12767529172568715 ) ) ;
#138313=CARTESIAN_POINT ( 'NONE',  ( -17.40861289039003523, 6.110651285853255565, 48.62767529172570136 ) ) ;
#138314=CARTESIAN_POINT ( 'NONE',  ( 0.05219959533907565091, 21.53943276465977519, 29.99890960531435979 ) ) ;
#138315=CARTESIAN_POINT ( 'NONE',  ( -17.49999999999999645, 5.499999999999992895, 63.71769037696435589 ) ) ;
#138317=CARTESIAN_POINT ( 'NONE',  ( -4.379528057220086978, -16.55341960407618274, 39.79275706135235424 ) ) ;
#138318=CARTESIAN_POINT ( 'NONE',  ( -12.14591786802309592, -12.06949235617757132, 31.87390960531435979 ) ) ;
#138319=CARTESIAN_POINT ( 'NONE',  ( -21.55341960407610458, -5.719274019375992779, 66.45724293864768129 ) ) ;
#138320=CARTESIAN_POINT ( 'NONE',  ( -16.51473224551082808, 9.474510206698731452, 83.33442372801899012 ) ) ;
#138321=CARTESIAN_POINT ( 'NONE',  ( 5.719274019375991003, -21.55341960407610458, 62.70724293864769550 ) ) ;
#138323=CARTESIAN_POINT ( 'NONE',  ( -14.34966873604972548, 8.224510206698743886, 53.33442372801901854 ) ) ;
#138324=CARTESIAN_POINT ( 'NONE',  ( 9.474510206698971260, -16.51473224551069308, 32.91557627198102409 ) ) ;
#138325=CARTESIAN_POINT ( 'NONE',  ( -19.02544592524342804, 5.153800228976336051, 106.0405762719810241 ) ) ;
#138327=CARTESIAN_POINT ( 'NONE',  ( -5.153800228976328057, -19.02544592524343514, 42.29057627198101699 ) ) ;
#138328=CARTESIAN_POINT ( 'NONE',  ( -16.46253265017160317, 9.564922557960807481, 25.83224293864769194 ) ) ;
#138330=CARTESIAN_POINT ( 'NONE',  ( 13.97604488694527802, 13.89961937509977652, 114.3739096053143669 ) ) ;
#138332=CARTESIAN_POINT ( 'NONE',  ( 16.55341960407618274, -4.379528057220086978, 76.04275706135237556 ) ) ;
#138333=CARTESIAN_POINT ( 'NONE',  ( 21.55341960407610458, 5.719274019375980345, 88.95724293864769550 ) ) ;
#138334=CARTESIAN_POINT ( 'NONE',  ( 16.51473224551069308, 9.474510206698969483, 59.16557627198102409 ) ) ;
#138335=CARTESIAN_POINT ( 'NONE',  ( 5.823673210054444382, -21.52544592524334988, 30.20942372801902565 ) ) ;
#138336=CARTESIAN_POINT ( 'NONE',  ( -19.02544592524342804, 5.153800228976336051, 86.04057627198103830 ) ) ;
#138337=CARTESIAN_POINT ( 'NONE',  ( 13.89961937509977652, -13.97604488694527269, 113.1239096053143527 ) ) ;
#138339=CARTESIAN_POINT ( 'NONE',  ( -21.53943276465977519, -0.05219959533937600094, 18.75109039468568639 ) ) ;
#138340=CARTESIAN_POINT ( 'NONE',  ( -8.224510206698948167, 14.34966873604960824, 115.4155762719810241 ) ) ;
#138341=CARTESIAN_POINT ( 'NONE',  ( 0.05219959533909260263, 19.03943276465977164, 104.9989096053143669 ) ) ;
#138342=CARTESIAN_POINT ( 'NONE',  ( 16.46253265017146816, 9.564922557961045513, 91.66775706135234714 ) ) ;
#138343=CARTESIAN_POINT ( 'NONE',  ( 5.049401038297881783, 19.05341960407617563, 27.29275706135232937 ) ) ;
#138344=CARTESIAN_POINT ( 'NONE',  ( -10.72451020669898014, 18.67979575497178502, 100.4155762719810241 ) ) ;
#138345=CARTESIAN_POINT ( 'NONE',  ( 9.564922557961047289, -16.46253265017146816, 30.41775706135232937 ) ) ;
#138346=CARTESIAN_POINT ( 'NONE',  ( 16.53943276465976808, 0.05219959533934440121, 81.25109039468568994 ) ) ;
#138347=CARTESIAN_POINT ( 'NONE',  ( -0.05219959533909027116, -19.03943276465977164, 112.4989096053143669 ) ) ;
#138348=CARTESIAN_POINT ( 'NONE',  ( 19.05341960407611168, 5.049401038298154454, 53.95724293864770260 ) ) ;
#138349=CARTESIAN_POINT ( 'NONE',  ( 18.67979575497194134, -10.72451020669871369, 70.83442372801901854 ) ) ;
#138350=CARTESIAN_POINT ( 'NONE',  ( 21.55341960407619695, -5.719274019375665929, 86.04275706135236135 ) ) ;
#138351=CARTESIAN_POINT ( 'NONE',  ( 5.049401038298161559, -19.05341960407611168, 72.70724293864768129 ) ) ;
#138352=CARTESIAN_POINT ( 'NONE',  ( 15.72974639402176855, 15.80617190586768217, 46.87609039468568994 ) ) ;
#138353=CARTESIAN_POINT ( 'NONE',  ( 5.153800228976615827, -19.02544592524334988, 90.20942372801900433 ) ) ;
#138354=CARTESIAN_POINT ( 'NONE',  ( -19.03943276465977164, 0.05219959533909376836, 46.24890960531435979 ) ) ;
#138355=CARTESIAN_POINT ( 'NONE',  ( -19.05341960407611168, -5.049401038298163336, 101.4572429386476955 ) ) ;
#138356=CARTESIAN_POINT ( 'NONE',  ( -13.97604488694527625, -13.89961937509977652, 71.87390960531433848 ) ) ;
#138358=CARTESIAN_POINT ( 'NONE',  ( 13.97604488694527802, 13.89961937509977652, 49.37390960531434558 ) ) ;
#138359=CARTESIAN_POINT ( 'NONE',  ( 21.55341960407610458, 5.719274019375980345, 98.95724293864770971 ) ) ;
#138360=CARTESIAN_POINT ( 'NONE',  ( -16.55341960407617563, 4.379528057220093196, 93.54275706135234714 ) ) ;
#138362=CARTESIAN_POINT ( 'NONE',  ( 19.03943276465977164, 0.05219959533936151252, 51.25109039468567573 ) ) ;
#138363=CARTESIAN_POINT ( 'NONE',  ( -19.03943276465977164, 0.05219959533909376836, 66.24890960531436690 ) ) ;
#138364=CARTESIAN_POINT ( 'NONE',  ( -12.06949235617756955, 12.14591786802309770, 60.62390960531437401 ) ) ;
#138365=CARTESIAN_POINT ( 'NONE',  ( 8.224510206698953496, -14.34966873604960469, 92.91557627198103830 ) ) ;
#138366=CARTESIAN_POINT ( 'NONE',  ( 16.51473224551069308, 9.474510206698969483, 114.1655762719810241 ) ) ;
#138367=CARTESIAN_POINT ( 'NONE',  ( -0.05219959533909027116, -19.03943276465977164, 87.49890960531436690 ) ) ;
#138368=CARTESIAN_POINT ( 'NONE',  ( 5.049401038298161559, -19.05341960407611168, 112.7072429386476813 ) ) ;
#138370=CARTESIAN_POINT ( 'NONE',  ( -5.823673210054431948, 21.52544592524334988, 112.7094237280190328 ) ) ;
#138371=CARTESIAN_POINT ( 'NONE',  ( 16.52544592524335698, 4.483927247898782831, 86.45942372801901854 ) ) ;
#138372=CARTESIAN_POINT ( 'NONE',  ( -13.89961937509977652, 13.97604488694528158, 80.62390960531436690 ) ) ;
#138373=CARTESIAN_POINT ( 'NONE',  ( 21.53943276465977519, 0.05219959533937863772, 46.25109039468567573 ) ) ;
#138374=CARTESIAN_POINT ( 'NONE',  ( -15.80617190586745835, -15.72974639402198527, 26.87390960531435979 ) ) ;
#138375=CARTESIAN_POINT ( 'NONE',  ( -18.62759615963270932, 10.81492255796079327, 110.8322429386476955 ) ) ;
#138376=CARTESIAN_POINT ( 'NONE',  ( 5.823673210054125526, 21.52544592524343514, 64.79057627198103830 ) ) ;
#138377=CARTESIAN_POINT ( 'NONE',  ( -12.06949235617756955, 12.14591786802309770, 85.62390960531436690 ) ) ;
#138378=CARTESIAN_POINT ( 'NONE',  ( 13.89961937509957401, 13.97604488694547697, 46.87609039468565442 ) ) ;
#138379=CARTESIAN_POINT ( 'NONE',  ( -0.05219959533909027116, -19.03943276465977164, 27.49890960531435624 ) ) ;
#138380=CARTESIAN_POINT ( 'NONE',  ( 13.97604488694527802, 13.89961937509977652, 84.37390960531433848 ) ) ;
#138381=CARTESIAN_POINT ( 'NONE',  ( -19.03943276465977164, 0.05219959533909376836, 76.24890960531435269 ) ) ;
#138383=CARTESIAN_POINT ( 'NONE',  ( -4.379528057220328563, 16.55341960407611168, 100.2072429386476955 ) ) ;
#138384=CARTESIAN_POINT ( 'NONE',  ( -8.314922557961024197, 14.29746914071037800, 107.9177570613523471 ) ) ;
#138385=CARTESIAN_POINT ( 'NONE',  ( -16.52544592524335698, -4.483927247898792601, 33.95942372801901143 ) ) ;
#138386=CARTESIAN_POINT ( 'NONE',  ( 5.719274019375673035, 21.55341960407619339, 87.29275706135236135 ) ) ;
#138387=CARTESIAN_POINT ( 'NONE',  ( -16.46253265017160317, 9.564922557960807481, 100.8322429386477097 ) ) ;
#138388=CARTESIAN_POINT ( 'NONE',  ( -18.67979575497193778, 10.72451020669871902, 23.33442372801901499 ) ) ;
#138389=CARTESIAN_POINT ( 'NONE',  ( -9.564922557960796823, -16.46253265017161027, 47.08224293864769550 ) ) ;
#138391=CARTESIAN_POINT ( 'NONE',  ( -0.05219959533934338120, 16.53943276465976808, 27.50109039468567929 ) ) ;
#138392=CARTESIAN_POINT ( 'NONE',  ( -16.51473224551082808, 9.474510206698731452, 108.3344237280190043 ) ) ;
#138393=CARTESIAN_POINT ( 'NONE',  ( 18.62759615963271287, -10.81492255796078972, 98.33224293864769550 ) ) ;
#138394=CARTESIAN_POINT ( 'NONE',  ( -0.05219959533936034679, 19.03943276465977164, 67.50109039468566152 ) ) ;
#138395=CARTESIAN_POINT ( 'NONE',  ( 19.05341960407611168, 5.049401038298154454, 23.95724293864769194 ) ) ;
#138396=CARTESIAN_POINT ( 'NONE',  ( -21.52544592524343514, 5.823673210054127303, 111.0405762719810525 ) ) ;
#138398=CARTESIAN_POINT ( 'NONE',  ( -9.474510206698964154, 16.51473224551069663, 95.41557627198102409 ) ) ;
#138399=CARTESIAN_POINT ( 'NONE',  ( -17.50000000001358202, 5.499999999999951150, 100.7969038253505687 ) ) ;
#138400=CARTESIAN_POINT ( 'NONE',  ( 16.46253265017160672, -9.564922557960803928, 78.33224293864769550 ) ) ;
#138401=CARTESIAN_POINT ( 'NONE',  ( 15.72974639402176855, 15.80617190586768217, 26.87609039468567218 ) ) ;
#138402=CARTESIAN_POINT ( 'NONE',  ( 14.34966873604960469, 8.224510206698951720, 84.16557627198103830 ) ) ;
#138403=CARTESIAN_POINT ( 'NONE',  ( -9.474510206698964154, 16.51473224551069663, 80.41557627198103830 ) ) ;
#138404=CARTESIAN_POINT ( 'NONE',  ( 16.53943276465976808, 0.05219959533934440121, 51.25109039468568994 ) ) ;
#138405=CARTESIAN_POINT ( 'NONE',  ( 9.564922557961047289, -16.46253265017146816, 60.41775706135233293 ) ) ;
#138406=CARTESIAN_POINT ( 'NONE',  ( 18.67979575497194134, -10.72451020669871369, 70.83442372801901854 ) ) ;
#138407=VECTOR ( 'NONE', #79385, 1000.000000000000000 ) ;
#138408=CARTESIAN_POINT ( 'NONE',  ( -8.314922557961024197, 14.29746914071037800, 22.91775706135235069 ) ) ;
#138409=CARTESIAN_POINT ( 'NONE',  ( 9.474510206698971260, -16.51473224551069308, 62.91557627198102409 ) ) ;
#138410=CARTESIAN_POINT ( 'NONE',  ( 0.05219959533936267826, -19.03943276465977164, 90.00109039468567573 ) ) ;
#138411=CARTESIAN_POINT ( 'NONE',  ( 16.55341960407618274, -4.379528057220086978, 51.04275706135234714 ) ) ;
#138412=CARTESIAN_POINT ( 'NONE',  ( -0.05219959533937732626, 21.53943276465977519, 92.50109039468567573 ) ) ;
#138413=CARTESIAN_POINT ( 'NONE',  ( -9.564922557961040184, 16.46253265017147172, 77.91775706135234714 ) ) ;
#138414=CARTESIAN_POINT ( 'NONE',  ( 5.153800228976335163, 19.02544592524342804, 54.79057627198103120 ) ) ;
#138415=CARTESIAN_POINT ( 'NONE',  ( 5.823673210054125526, 21.52544592524343514, 69.79057627198102409 ) ) ;
#138416=CARTESIAN_POINT ( 'NONE',  ( 0.05219959533910956823, 16.53943276465976808, 79.99890960531435269 ) ) ;
#138417=CARTESIAN_POINT ( 'NONE',  ( -16.46253265017146816, -9.564922557961047289, 84.16775706135233293 ) ) ;
#138418=CARTESIAN_POINT ( 'NONE',  ( 16.38665767535056617, -7.295008042175987306, 62.76400864214551234 ) ) ;
#138419=CARTESIAN_POINT ( 'NONE',  ( -16.46253265017146816, -9.564922557961047289, 49.16775706135233293 ) ) ;
#138420=CARTESIAN_POINT ( 'NONE',  ( -12.14591786802326823, 12.06949235617739902, 113.1260903946856899 ) ) ;
#138421=CARTESIAN_POINT ( 'NONE',  ( -14.34966873604960291, -8.224510206698953496, 61.66557627198103120 ) ) ;
#138422=CARTESIAN_POINT ( 'NONE',  ( -21.53943276465977519, -0.05219959533937600094, 108.7510903946857042 ) ) ;
#138424=CARTESIAN_POINT ( 'NONE',  ( -10.72451020669898014, 18.67979575497178502, 110.4155762719810383 ) ) ;
#138425=CARTESIAN_POINT ( 'NONE',  ( -16.51473224551069308, -9.474510206698971260, 66.66557627198102409 ) ) ;
#138426=CARTESIAN_POINT ( 'NONE',  ( -0.05219959533937732626, 21.53943276465977519, 82.50109039468568994 ) ) ;
#138427=CARTESIAN_POINT ( 'NONE',  ( 19.03943276465977164, -0.05219959533909143690, 68.74890960531436690 ) ) ;
#138428=CARTESIAN_POINT ( 'NONE',  ( -5.049401038298153566, 19.05341960407611168, 30.20724293864768839 ) ) ;
#138429=CARTESIAN_POINT ( 'NONE',  ( -21.53943276465977519, 0.05219959533907696930, 31.24890960531435979 ) ) ;
#138430=CARTESIAN_POINT ( 'NONE',  ( -8.224510206698948167, 14.34966873604960824, 70.41557627198102409 ) ) ;
#138431=CARTESIAN_POINT ( 'NONE',  ( -13.89961937509977652, 13.97604488694528158, 25.62390960531434558 ) ) ;
#138432=CARTESIAN_POINT ( 'NONE',  ( 0.05219959533910956823, 16.53943276465976808, 89.99890960531438111 ) ) ;
#138433=CARTESIAN_POINT ( 'NONE',  ( -0.05219959533907301413, -21.53943276465977519, 102.4989096053143811 ) ) ;
#138434=CARTESIAN_POINT ( 'NONE',  ( -15.72974639402176322, -15.80617190586768395, 54.37609039468568994 ) ) ;
#138436=CARTESIAN_POINT ( 'NONE',  ( 12.14591786802327356, -12.06949235617739191, 55.62609039468568284 ) ) ;
#138437=CARTESIAN_POINT ( 'NONE',  ( -10.81492255796078084, -18.62759615963271287, 102.0822429386476955 ) ) ;
#138438=CARTESIAN_POINT ( 'NONE',  ( -16.51473224551082808, 9.474510206698731452, 23.33442372801900078 ) ) ;
#138439=CARTESIAN_POINT ( 'NONE',  ( -19.05341960407611168, -5.049401038298163336, 101.4572429386476955 ) ) ;
#138440=CARTESIAN_POINT ( 'NONE',  ( -18.62759615963255300, -10.81492255796106328, 59.16775706135234714 ) ) ;
#138441=CARTESIAN_POINT ( 'NONE',  ( 5.823673210054125526, 21.52544592524343514, 39.79057627198103830 ) ) ;
#138442=CARTESIAN_POINT ( 'NONE',  ( 16.55341960407618274, -4.379528057220086978, 111.0427570613523613 ) ) ;
#138443=CARTESIAN_POINT ( 'NONE',  ( -21.52544592524334988, -5.823673210054445271, 63.95942372801901854 ) ) ;
#138444=CARTESIAN_POINT ( 'NONE',  ( 15.72974639402176855, 15.80617190586768217, 91.87609039468568994 ) ) ;
#138445=CARTESIAN_POINT ( 'NONE',  ( -19.05341960407617563, 5.049401038297882671, 28.54275706135232937 ) ) ;
#138446=CARTESIAN_POINT ( 'NONE',  ( 14.34966873604972726, -8.224510206698740333, 90.83442372801901854 ) ) ;
#138447=CARTESIAN_POINT ( 'NONE',  ( -21.55341960407619339, 5.719274019375674811, 53.54275706135234714 ) ) ;
#138448=CARTESIAN_POINT ( 'NONE',  ( 13.89961937509977652, -13.97604488694527269, 43.12390960531434558 ) ) ;
#138449=CARTESIAN_POINT ( 'NONE',  ( -21.53943276465977519, -0.05219959533937600094, 113.7510903946856757 ) ) ;
#138450=CARTESIAN_POINT ( 'NONE',  ( 15.80617190586746368, 15.72974639402197994, 29.37390960531435269 ) ) ;
#138451=CARTESIAN_POINT ( 'NONE',  ( 0.05219959533907565091, 21.53943276465977519, 109.9989096053143527 ) ) ;
#138452=CARTESIAN_POINT ( 'NONE',  ( 21.53943276465977519, -0.05219959533907433946, 68.74890960531435269 ) ) ;
#138453=CARTESIAN_POINT ( 'NONE',  ( -12.06949235617739369, -12.14591786802326823, 39.37609039468567573 ) ) ;
#138454=CARTESIAN_POINT ( 'NONE',  ( -18.09918380851992836, -5.500000000000039968, 61.48618307335612343 ) ) ;
#138455=CARTESIAN_POINT ( 'NONE',  ( -10.72451020669898014, 18.67979575497178502, 85.41557627198102409 ) ) ;
#138456=CARTESIAN_POINT ( 'NONE',  ( 16.52544592524335698, 4.483927247898782831, 66.45942372801903275 ) ) ;
#138457=CARTESIAN_POINT ( 'NONE',  ( 16.52544592524342804, -4.483927247898539470, 68.54057627198103830 ) ) ;
#138459=CARTESIAN_POINT ( 'NONE',  ( -9.564922557961040184, 16.46253265017147172, 107.9177570613523471 ) ) ;
#138460=CARTESIAN_POINT ( 'NONE',  ( 21.55341960407610458, 5.719274019375980345, 38.95724293864768839 ) ) ;
#138461=CARTESIAN_POINT ( 'NONE',  ( -5.049401038298153566, 19.05341960407611168, 95.20724293864769550 ) ) ;
#138462=CARTESIAN_POINT ( 'NONE',  ( -14.34966873604972548, 8.224510206698743886, 43.33442372801901143 ) ) ;
#138463=CARTESIAN_POINT ( 'NONE',  ( 10.81492255796078972, 18.62759615963270932, 109.5822429386476955 ) ) ;
#138464=CARTESIAN_POINT ( 'NONE',  ( 10.81492255796078972, 18.62759615963270932, 34.58224293864770260 ) ) ;
#138465=CARTESIAN_POINT ( 'NONE',  ( -8.224510206698735004, -14.34966873604973081, 54.58442372801901143 ) ) ;
#138466=CARTESIAN_POINT ( 'NONE',  ( 19.05341960407611168, 5.049401038298154454, 88.95724293864769550 ) ) ;
#138467=CARTESIAN_POINT ( 'NONE',  ( -10.81492255796105439, 18.62759615963255655, 47.91775706135234714 ) ) ;
#138468=CARTESIAN_POINT ( 'NONE',  ( 14.34966873604972726, -8.224510206698740333, 20.83442372801901143 ) ) ;
#138469=CARTESIAN_POINT ( 'NONE',  ( -5.719274019375978568, 21.55341960407610458, 25.20724293864769550 ) ) ;
#138471=CARTESIAN_POINT ( 'NONE',  ( 16.46253265017146816, 9.564922557961045513, 26.66775706135234003 ) ) ;
#138472=CARTESIAN_POINT ( 'NONE',  ( 12.14591786802327356, -12.06949235617739191, 40.62609039468567573 ) ) ;
#138473=CARTESIAN_POINT ( 'NONE',  ( 13.89961937509977652, -13.97604488694527269, 103.1239096053143527 ) ) ;
#138474=CARTESIAN_POINT ( 'NONE',  ( -10.81492255796078084, -18.62759615963271287, 107.0822429386476955 ) ) ;
#138475=CARTESIAN_POINT ( 'NONE',  ( 5.049401038298161559, -19.05341960407611168, 77.70724293864765286 ) ) ;
#138477=CARTESIAN_POINT ( 'NONE',  ( -12.06949235617756955, 12.14591786802309770, 80.62390960531438111 ) ) ;
#138478=CARTESIAN_POINT ( 'NONE',  ( -0.05219959533907301413, -21.53943276465977519, 37.49890960531436690 ) ) ;
#138479=CARTESIAN_POINT ( 'NONE',  ( -16.20579543436675252, 7.371946100355235565, 34.43479165828124877 ) ) ;
#138480=CARTESIAN_POINT ( 'NONE',  ( -8.224510206698735004, -14.34966873604973081, 64.58442372801900433 ) ) ;
#138481=CARTESIAN_POINT ( 'NONE',  ( 10.81492255796078972, 18.62759615963270932, 99.58224293864770971 ) ) ;
#138482=CARTESIAN_POINT ( 'NONE',  ( 9.474510206698729675, 16.51473224551082808, 77.08442372801900433 ) ) ;
#138483=CARTESIAN_POINT ( 'NONE',  ( -5.153800228976328057, -19.02544592524343514, 27.29057627198103120 ) ) ;
#138484=CARTESIAN_POINT ( 'NONE',  ( 18.67979575497178502, 10.72451020669898547, 64.16557627198102409 ) ) ;
#138485=CARTESIAN_POINT ( 'NONE',  ( -16.46253265017160317, 9.564922557960807481, 95.83224293864769550 ) ) ;
#138486=CARTESIAN_POINT ( 'NONE',  ( 10.81492255796106328, -18.62759615963255655, 95.41775706135234714 ) ) ;
#138487=CARTESIAN_POINT ( 'NONE',  ( -9.474510206698964154, 16.51473224551069663, 60.41557627198102409 ) ) ;
#138488=CARTESIAN_POINT ( 'NONE',  ( 16.53943276465976808, 0.05219959533934440121, 51.25109039468568994 ) ) ;
#138489=CARTESIAN_POINT ( 'NONE',  ( 19.02544592524343514, -5.153800228976328945, 53.54057627198102409 ) ) ;
#138490=CARTESIAN_POINT ( 'NONE',  ( 18.62759615963255655, 10.81492255796105972, 76.66775706135234714 ) ) ;
#138491=ORIENTED_EDGE ( 'NONE', *, *, #13540, .F. ) ;
#138492=CARTESIAN_POINT ( 'NONE',  ( -9.564922557961040184, 16.46253265017147172, 32.91775706135233293 ) ) ;
#138493=CARTESIAN_POINT ( 'NONE',  ( 13.89961937509957401, 13.97604488694547697, 56.87609039468564731 ) ) ;
#138494=CARTESIAN_POINT ( 'NONE',  ( 21.55341960407619695, -5.719274019375665929, 51.04275706135234714 ) ) ;
#138496=CARTESIAN_POINT ( 'NONE',  ( 19.05341960407617918, -5.049401038297876454, 41.04275706135233293 ) ) ;
#138497=CARTESIAN_POINT ( 'NONE',  ( 0.05219959533909260263, 19.03943276465977164, 84.99890960531436690 ) ) ;
#138498=CARTESIAN_POINT ( 'NONE',  ( -9.564922557960796823, -16.46253265017161027, 72.08224293864770971 ) ) ;
#138499=CARTESIAN_POINT ( 'NONE',  ( 12.06949235617757843, -12.14591786802309237, 28.12390960531435979 ) ) ;
#138500=CARTESIAN_POINT ( 'NONE',  ( 5.823673210054125526, 21.52544592524343514, 24.79057627198103120 ) ) ;
#138501=CARTESIAN_POINT ( 'NONE',  ( -0.05219959533937732626, 21.53943276465977519, 92.50109039468567573 ) ) ;
#138502=VECTOR ( 'NONE', #101087, 1000.000000000000000 ) ;
#138505=CARTESIAN_POINT ( 'NONE',  ( 15.72974639402176855, 15.80617190586768217, 96.87609039468568994 ) ) ;
#138506=CARTESIAN_POINT ( 'NONE',  ( 19.05341960407611168, 5.049401038298154454, 23.95724293864769194 ) ) ;
#138507=CARTESIAN_POINT ( 'NONE',  ( 19.05341960407611168, 5.049401038298154454, 113.9572429386477097 ) ) ;
#138509=CARTESIAN_POINT ( 'NONE',  ( -12.06949235617739369, -12.14591786802326823, 49.37609039468569705 ) ) ;
#138510=CARTESIAN_POINT ( 'NONE',  ( -10.72451020669898014, 18.67979575497178502, 75.41557627198102409 ) ) ;
#138511=CARTESIAN_POINT ( 'NONE',  ( 12.06949235617757843, -12.14591786802309237, 43.12390960531435269 ) ) ;
#138512=CARTESIAN_POINT ( 'NONE',  ( 14.34966873604960469, 8.224510206698951720, 114.1655762719810383 ) ) ;
#138513=CARTESIAN_POINT ( 'NONE',  ( -5.153800228976328057, -19.02544592524343514, 92.29057627198099567 ) ) ;
#138514=CARTESIAN_POINT ( 'NONE',  ( -5.049401038297874678, -19.05341960407617918, 34.79275706135233293 ) ) ;
#138515=CARTESIAN_POINT ( 'NONE',  ( 4.379528057220339221, -16.55341960407611168, 112.7072429386476955 ) ) ;
#138516=CARTESIAN_POINT ( 'NONE',  ( 0.05219959533937995610, -21.53943276465977519, 75.00109039468568994 ) ) ;
#138517=CARTESIAN_POINT ( 'NONE',  ( -19.03943276465977164, 0.05219959533909376836, 116.2489096053143669 ) ) ;
#138518=CARTESIAN_POINT ( 'NONE',  ( 8.314922557961029526, -14.29746914071037800, 110.4177570613523756 ) ) ;
#138520=CARTESIAN_POINT ( 'NONE',  ( -21.55341960407610458, -5.719274019375992779, 26.45724293864768839 ) ) ;
#138521=CARTESIAN_POINT ( 'NONE',  ( -12.14591786802309592, -12.06949235617757132, 91.87390960531436690 ) ) ;
#138522=CARTESIAN_POINT ( 'NONE',  ( -5.049401038297874678, -19.05341960407617918, 59.79275706135231871 ) ) ;
#138523=CARTESIAN_POINT ( 'NONE',  ( 13.97604488694527802, 13.89961937509977652, 74.37390960531436690 ) ) ;
#138524=CARTESIAN_POINT ( 'NONE',  ( -16.53943276465976808, 0.05219959533911058130, 71.24890960531435269 ) ) ;
#138525=CARTESIAN_POINT ( 'NONE',  ( -19.05341960407617563, 5.049401038297882671, 88.54275706135230450 ) ) ;
#138526=CARTESIAN_POINT ( 'NONE',  ( 0.05219959533907565091, 21.53943276465977519, 54.99890960531435269 ) ) ;
#138528=CARTESIAN_POINT ( 'NONE',  ( 0.05219959533910956823, 16.53943276465976808, 114.9989096053143669 ) ) ;
#138530=CARTESIAN_POINT ( 'NONE',  ( -19.02544592524342804, 5.153800228976336051, 66.04057627198103830 ) ) ;
#138531=CARTESIAN_POINT ( 'NONE',  ( -5.719274019375978568, 21.55341960407610458, 75.20724293864769550 ) ) ;
#138532=CARTESIAN_POINT ( 'NONE',  ( 0.05219959533934541429, -16.53943276465976808, 90.00109039468567573 ) ) ;
#138533=CARTESIAN_POINT ( 'NONE',  ( 19.05341960407611168, 5.049401038298154454, 88.95724293864769550 ) ) ;
#138534=CARTESIAN_POINT ( 'NONE',  ( 9.564922557961047289, -16.46253265017146816, 70.41775706135233293 ) ) ;
#138535=CARTESIAN_POINT ( 'NONE',  ( -18.67979575497193778, 10.72451020669871902, 78.33442372801901854 ) ) ;
#138536=CARTESIAN_POINT ( 'NONE',  ( -10.81492255796078084, -18.62759615963271287, 57.08224293864769550 ) ) ;
#138537=CARTESIAN_POINT ( 'NONE',  ( -18.67979575497178146, -10.72451020669898902, 26.66557627198103475 ) ) ;
#138538=CARTESIAN_POINT ( 'NONE',  ( 9.564922557960805705, 16.46253265017160317, 34.58224293864770260 ) ) ;
#138539=CARTESIAN_POINT ( 'NONE',  ( -12.14591786802326823, 12.06949235617739902, 98.12609039468570415 ) ) ;
#138540=CARTESIAN_POINT ( 'NONE',  ( 16.51473224551069308, 9.474510206698969483, 49.16557627198102409 ) ) ;
#138541=CARTESIAN_POINT ( 'NONE',  ( -14.29746914071037622, -8.314922557961029526, 24.16775706135235424 ) ) ;
#138542=CARTESIAN_POINT ( 'NONE',  ( 17.50000000000000000, 5.499999999999992895, 51.70309617465830598 ) ) ;
#138543=CARTESIAN_POINT ( 'NONE',  ( -19.03943276465977164, -0.05219959533935918106, 18.75109039468567218 ) ) ;
#138544=CARTESIAN_POINT ( 'NONE',  ( -16.55341960407611168, -4.379528057220339221, 56.45724293864768839 ) ) ;
#138545=CARTESIAN_POINT ( 'NONE',  ( -21.55341960407610458, -5.719274019375992779, 106.4572429386477097 ) ) ;
#138546=CARTESIAN_POINT ( 'NONE',  ( 10.72451020669898902, -18.67979575497178502, 97.91557627198103830 ) ) ;
#138548=CARTESIAN_POINT ( 'NONE',  ( 18.62759615963271287, -10.81492255796078972, 43.33224293864769550 ) ) ;
#138549=EDGE_CURVE ( 'NONE', #17000, #88586, #13884, .T. ) ;
#138550=CARTESIAN_POINT ( 'NONE',  ( -4.379528057220086978, -16.55341960407618274, 74.79275706135234714 ) ) ;
#138551=CARTESIAN_POINT ( 'NONE',  ( 4.483927247898545687, 16.52544592524342804, 89.79057627198103830 ) ) ;
#138552=CARTESIAN_POINT ( 'NONE',  ( -19.05341960407611168, -5.049401038298163336, 61.45724293864769550 ) ) ;
#138554=CARTESIAN_POINT ( 'NONE',  ( -0.05219959533934338120, 16.53943276465976808, 107.5010903946856899 ) ) ;
#138555=CARTESIAN_POINT ( 'NONE',  ( 18.67979575497194134, -10.72451020669871369, 35.83442372801901143 ) ) ;
#138556=CARTESIAN_POINT ( 'NONE',  ( -9.564922557960796823, -16.46253265017161027, 92.08224293864769550 ) ) ;
#138557=CARTESIAN_POINT ( 'NONE',  ( 21.53943276465977519, 0.05219959533937863772, 71.25109039468568994 ) ) ;
#138558=FACE_OUTER_BOUND ( 'NONE', #81593, .T. ) ;
#138561=CARTESIAN_POINT ( 'NONE',  ( -15.72974639402176322, -15.80617190586768395, 59.37609039468568284 ) ) ;
#138562=CARTESIAN_POINT ( 'NONE',  ( -16.46253265017160317, 9.564922557960807481, 55.83224293864769550 ) ) ;
#138563=CARTESIAN_POINT ( 'NONE',  ( -19.03943276465977164, 0.05219959533909376836, 91.24890960531436690 ) ) ;
#138564=CARTESIAN_POINT ( 'NONE',  ( -19.03943276465977164, -0.05219959533935918106, 63.75109039468566863 ) ) ;
#138565=CARTESIAN_POINT ( 'NONE',  ( 18.67979575497194134, -10.72451020669871369, 45.83442372801901854 ) ) ;
#138566=CARTESIAN_POINT ( 'NONE',  ( -9.474510206698720793, -16.51473224551083518, 104.5844237280190043 ) ) ;
#138567=CARTESIAN_POINT ( 'NONE',  ( 9.564922557961047289, -16.46253265017146816, 70.41775706135233293 ) ) ;
#138568=CARTESIAN_POINT ( 'NONE',  ( 16.51473224551069308, 9.474510206698969483, 39.16557627198103120 ) ) ;
#138569=CARTESIAN_POINT ( 'NONE',  ( 5.049401038297881783, 19.05341960407617563, 87.29275706135234714 ) ) ;
#138570=CARTESIAN_POINT ( 'NONE',  ( -14.29746914071037622, -8.314922557961029526, 99.16775706135234714 ) ) ;
#138571=CARTESIAN_POINT ( 'NONE',  ( 9.474510206698729675, 16.51473224551082808, 72.08442372801900433 ) ) ;
#138572=CARTESIAN_POINT ( 'NONE',  ( -8.314922557960811034, -14.29746914071050412, 27.08224293864769550 ) ) ;
#138573=CARTESIAN_POINT ( 'NONE',  ( -13.97604488694547697, 13.89961937509957934, 48.12609039468566863 ) ) ;
#138574=CARTESIAN_POINT ( 'NONE',  ( -18.62759615963255300, -10.81492255796106328, 109.1677570613523613 ) ) ;
#138575=CARTESIAN_POINT ( 'NONE',  ( -9.474510206698720793, -16.51473224551083518, 24.58442372801900078 ) ) ;
#138576=CARTESIAN_POINT ( 'NONE',  ( 0.05219959533909260263, 19.03943276465977164, 34.99890960531435979 ) ) ;
#138577=CARTESIAN_POINT ( 'NONE',  ( 15.80617190586769283, -15.72974639402175789, 85.62609039468568994 ) ) ;
#138578=CARTESIAN_POINT ( 'NONE',  ( -0.05219959533934338120, 16.53943276465976808, 42.50109039468567573 ) ) ;
#138579=CARTESIAN_POINT ( 'NONE',  ( 13.97604488694527802, 13.89961937509977652, 99.37390960531436690 ) ) ;
#138581=CARTESIAN_POINT ( 'NONE',  ( -5.049401038298153566, 19.05341960407611168, 80.20724293864769550 ) ) ;
#138582=CARTESIAN_POINT ( 'NONE',  ( -17.60728821187772297, 5.500000000000019540, 95.86690927743606494 ) ) ;
#138584=CARTESIAN_POINT ( 'NONE',  ( -19.03943276465977164, -0.05219959533935918106, 88.75109039468567573 ) ) ;
#138585=CARTESIAN_POINT ( 'NONE',  ( -19.03943276465977164, 0.05219959533909376836, 116.2489096053143669 ) ) ;
#138586=CARTESIAN_POINT ( 'NONE',  ( -5.719274019375665041, -21.55341960407619695, 109.7927570613523613 ) ) ;
#138587=CARTESIAN_POINT ( 'NONE',  ( -16.51473224551082808, 9.474510206698731452, 103.3344237280190043 ) ) ;
#138588=CARTESIAN_POINT ( 'NONE',  ( 8.224510206698953496, -14.34966873604960469, 97.91557627198103830 ) ) ;
#138589=CARTESIAN_POINT ( 'NONE',  ( 19.03943276465977164, -0.05219959533909143690, 28.74890960531435624 ) ) ;
#138590=CARTESIAN_POINT ( 'NONE',  ( -5.719274019375978568, 21.55341960407610458, 55.20724293864770260 ) ) ;
#138591=CARTESIAN_POINT ( 'NONE',  ( 18.62759615963271287, -10.81492255796078972, 48.33224293864770260 ) ) ;
#138592=CARTESIAN_POINT ( 'NONE',  ( 0.05219959533910956823, 16.53943276465976808, 114.9989096053143669 ) ) ;
#138594=CARTESIAN_POINT ( 'NONE',  ( -0.05219959533936034679, 19.03943276465977164, 72.50109039468566152 ) ) ;
#138595=CARTESIAN_POINT ( 'NONE',  ( -12.06949235617756955, 12.14591786802309770, 45.62390960531436690 ) ) ;
#138596=CARTESIAN_POINT ( 'NONE',  ( -9.474510206698964154, 16.51473224551069663, 115.4155762719810241 ) ) ;
#138597=CARTESIAN_POINT ( 'NONE',  ( 21.55341960407619695, -5.719274019375665929, 76.04275706135237556 ) ) ;
#138598=CARTESIAN_POINT ( 'NONE',  ( -21.53943276465977519, 0.05219959533907696930, 66.24890960531436690 ) ) ;
#138599=CARTESIAN_POINT ( 'NONE',  ( 15.72974639402176855, 15.80617190586768217, 56.87609039468568994 ) ) ;
#138600=CARTESIAN_POINT ( 'NONE',  ( 21.55341960407619695, -5.719274019375665929, 46.04275706135234714 ) ) ;
#138601=CARTESIAN_POINT ( 'NONE',  ( 9.564922557960805705, 16.46253265017160317, 79.58224293864769550 ) ) ;
#138602=CARTESIAN_POINT ( 'NONE',  ( 4.483927247898790824, -16.52544592524335698, 90.20942372801903275 ) ) ;
#138603=CARTESIAN_POINT ( 'NONE',  ( 5.049401038298161559, -19.05341960407611168, 27.70724293864769550 ) ) ;
#138605=CARTESIAN_POINT ( 'NONE',  ( 0.05219959533910956823, 16.53943276465976808, 64.99890960531435269 ) ) ;
#138606=CARTESIAN_POINT ( 'NONE',  ( 4.483927247898545687, 16.52544592524342804, 29.79057627198102409 ) ) ;
#138607=CARTESIAN_POINT ( 'NONE',  ( -5.049401038298153566, 19.05341960407611168, 65.20724293864765286 ) ) ;
#138608=CARTESIAN_POINT ( 'NONE',  ( -13.97604488694527625, -13.89961937509977652, 36.87390960531436690 ) ) ;
#138609=CARTESIAN_POINT ( 'NONE',  ( 18.62759615963271287, -10.81492255796078972, 48.33224293864770260 ) ) ;
#138610=CARTESIAN_POINT ( 'NONE',  ( -0.05219959533936034679, 19.03943276465977164, 32.50109039468566863 ) ) ;
#138612=CARTESIAN_POINT ( 'NONE',  ( 14.29746914071049879, -8.314922557960816363, 48.33224293864770260 ) ) ;
#138613=CARTESIAN_POINT ( 'NONE',  ( -0.05219959533907301413, -21.53943276465977519, 32.49890960531435979 ) ) ;
#138615=CARTESIAN_POINT ( 'NONE',  ( -14.29746914071037622, -8.314922557961029526, 74.16775706135231871 ) ) ;
#138617=CARTESIAN_POINT ( 'NONE',  ( 9.564922557961047289, -16.46253265017146816, 75.41775706135234714 ) ) ;
#138618=CARTESIAN_POINT ( 'NONE',  ( -8.224510206698948167, 14.34966873604960824, 45.41557627198103830 ) ) ;
#138620=CARTESIAN_POINT ( 'NONE',  ( 17.50000000000006040, -5.622605283950772304, 51.18792689403892382 ) ) ;
#138621=CARTESIAN_POINT ( 'NONE',  ( -8.314922557960811034, -14.29746914071050412, 32.08224293864769550 ) ) ;
#138622=CARTESIAN_POINT ( 'NONE',  ( 19.02544592524343514, -5.153800228976328945, 48.54057627198103120 ) ) ;
#138623=CARTESIAN_POINT ( 'NONE',  ( 13.97604488694527802, 13.89961937509977652, 74.37390960531436690 ) ) ;
#138624=CARTESIAN_POINT ( 'NONE',  ( -9.474510206698964154, 16.51473224551069663, 40.41557627198103120 ) ) ;
#138625=CARTESIAN_POINT ( 'NONE',  ( 21.53943276465977519, 0.05219959533937863772, 41.25109039468568284 ) ) ;
#138626=CARTESIAN_POINT ( 'NONE',  ( 9.564922557960805705, 16.46253265017160317, 64.58224293864769550 ) ) ;
#138628=CARTESIAN_POINT ( 'NONE',  ( 9.474510206698971260, -16.51473224551069308, 47.91557627198102409 ) ) ;
#138629=CARTESIAN_POINT ( 'NONE',  ( 21.55341960407610458, 5.719274019375980345, 33.95724293864769550 ) ) ;
#138630=AXIS2_PLACEMENT_3D ( 'NONE', #77192, #122697, #150082 ) ;
#138631=CARTESIAN_POINT ( 'NONE',  ( 21.55341960407619695, -5.719274019375665929, 76.04275706135237556 ) ) ;
#138632=CARTESIAN_POINT ( 'NONE',  ( 19.03943276465977164, -0.05219959533909143690, 28.74890960531435624 ) ) ;
#138633=CARTESIAN_POINT ( 'NONE',  ( 18.62759615963271287, -10.81492255796078972, 33.33224293864769550 ) ) ;
#138634=CARTESIAN_POINT ( 'NONE',  ( 0.05219959533934541429, -16.53943276465976808, 95.00109039468568994 ) ) ;
#138635=CARTESIAN_POINT ( 'NONE',  ( -18.62759615963255300, -10.81492255796106328, 99.16775706135234714 ) ) ;
#138636=CARTESIAN_POINT ( 'NONE',  ( -14.29746914071037622, -8.314922557961029526, 64.16775706135234714 ) ) ;
#138637=CARTESIAN_POINT ( 'NONE',  ( 5.049401038298161559, -19.05341960407611168, 107.7072429386476955 ) ) ;
#138638=CARTESIAN_POINT ( 'NONE',  ( -4.483927247898782831, 16.52544592524335698, 52.70942372801902565 ) ) ;
#138639=CARTESIAN_POINT ( 'NONE',  ( 8.314922557961029526, -14.29746914071037800, 40.41775706135234714 ) ) ;
#138640=CARTESIAN_POINT ( 'NONE',  ( -16.53943276465976808, -0.05219959533934237506, 93.75109039468567573 ) ) ;
#138641=CARTESIAN_POINT ( 'NONE',  ( 21.52544592524334988, 5.823673210054432836, 56.45942372801902565 ) ) ;
#138642=CARTESIAN_POINT ( 'NONE',  ( -14.34966873604972548, 8.224510206698743886, 23.33442372801901499 ) ) ;
#138643=CARTESIAN_POINT ( 'NONE',  ( 21.53943276465977519, -0.05219959533907433946, 113.7489096053143527 ) ) ;
#138644=CARTESIAN_POINT ( 'NONE',  ( -0.05219959533934338120, 16.53943276465976808, 27.50109039468567929 ) ) ;
#138645=CARTESIAN_POINT ( 'NONE',  ( 8.224510206698742110, 14.34966873604972548, 87.08442372801901854 ) ) ;
#138646=CARTESIAN_POINT ( 'NONE',  ( -16.81555441253465943, 7.025013491696272538, 45.63685445334211011 ) ) ;
#138647=CARTESIAN_POINT ( 'NONE',  ( 21.53943276465977519, 0.05219959533937863772, 81.25109039468568994 ) ) ;
#138648=CARTESIAN_POINT ( 'NONE',  ( -5.049401038297874678, -19.05341960407617918, 79.79275706135233293 ) ) ;
#138649=CARTESIAN_POINT ( 'NONE',  ( 12.06949235617757843, -12.14591786802309237, 58.12390960531435979 ) ) ;
#138650=CARTESIAN_POINT ( 'NONE',  ( 16.52544592524342804, -4.483927247898539470, 43.54057627198103830 ) ) ;
#138651=CARTESIAN_POINT ( 'NONE',  ( 12.06949235617757843, -12.14591786802309237, 113.1239096053143953 ) ) ;
#138652=CARTESIAN_POINT ( 'NONE',  ( -19.02544592524334988, -5.153800228976617603, 53.95942372801898301 ) ) ;
#138653=CARTESIAN_POINT ( 'NONE',  ( -19.03943276465977164, 0.05219959533909376836, 21.24890960531436335 ) ) ;
#138654=CARTESIAN_POINT ( 'NONE',  ( 5.823673210054444382, -21.52544592524334988, 45.20942372801901854 ) ) ;
#138655=CARTESIAN_POINT ( 'NONE',  ( 13.89961937509957401, 13.97604488694547697, 106.8760903946856757 ) ) ;
#138656=LINE ( 'NONE', #32486, #137437 ) ;
#138657=CARTESIAN_POINT ( 'NONE',  ( -16.51473224551069308, -9.474510206698971260, 106.6655762719810383 ) ) ;
#138658=CARTESIAN_POINT ( 'NONE',  ( 21.52544592524344225, -5.823673210054117533, 73.54057627198102409 ) ) ;
#138659=CARTESIAN_POINT ( 'NONE',  ( -16.51473224551082808, 9.474510206698731452, 98.33442372801900433 ) ) ;
#138660=CARTESIAN_POINT ( 'NONE',  ( -19.03943276465977164, 0.05219959533909376836, 106.2489096053143669 ) ) ;
#138662=CARTESIAN_POINT ( 'NONE',  ( -0.05219959533910754901, -16.53943276465976808, 102.4989096053143811 ) ) ;
#138663=CARTESIAN_POINT ( 'NONE',  ( -18.62759615963255300, -10.81492255796106328, 99.16775706135234714 ) ) ;
#138664=CARTESIAN_POINT ( 'NONE',  ( 13.97604488694527802, 13.89961937509977652, 24.37390960531435624 ) ) ;
#138665=CARTESIAN_POINT ( 'NONE',  ( 21.53943276465977519, 0.05219959533937863772, 46.25109039468567573 ) ) ;
#138667=CARTESIAN_POINT ( 'NONE',  ( -5.823673210054431948, 21.52544592524334988, 87.70942372801901854 ) ) ;
#138668=CARTESIAN_POINT ( 'NONE',  ( -0.05219959533934338120, 16.53943276465976808, 87.50109039468568994 ) ) ;
#138669=CARTESIAN_POINT ( 'NONE',  ( 10.72451020669871369, 18.67979575497193778, 42.08442372801901854 ) ) ;
#138670=CARTESIAN_POINT ( 'NONE',  ( -0.05219959533937732626, 21.53943276465977519, 37.50109039468568284 ) ) ;
#138671=CARTESIAN_POINT ( 'NONE',  ( -5.153800228976607833, 19.02544592524334988, 72.70942372801900433 ) ) ;
#138672=CARTESIAN_POINT ( 'NONE',  ( -5.153800228976328057, -19.02544592524343514, 97.29057627198099567 ) ) ;
#138673=CARTESIAN_POINT ( 'NONE',  ( 4.379528057220339221, -16.55341960407611168, 107.7072429386476955 ) ) ;
#138674=CARTESIAN_POINT ( 'NONE',  ( 21.53943276465977519, -0.05219959533907433946, 88.74890960531436690 ) ) ;
#138675=CARTESIAN_POINT ( 'NONE',  ( -16.55341960407611168, -4.379528057220339221, 66.45724293864768129 ) ) ;
#138676=CARTESIAN_POINT ( 'NONE',  ( -0.05219959533937732626, 21.53943276465977519, 97.50109039468567573 ) ) ;
#138677=CARTESIAN_POINT ( 'NONE',  ( 0.05219959533910956823, 16.53943276465976808, 79.99890960531435269 ) ) ;
#138678=CARTESIAN_POINT ( 'NONE',  ( -0.05219959533909027116, -19.03943276465977164, 32.49890960531435979 ) ) ;
#138679=CARTESIAN_POINT ( 'NONE',  ( 19.05341960407617918, -5.049401038297876454, 66.04275706135233293 ) ) ;
#138680=CARTESIAN_POINT ( 'NONE',  ( 14.29746914071049879, -8.314922557960816363, 53.33224293864769550 ) ) ;
#138681=CARTESIAN_POINT ( 'NONE',  ( 5.823673210054444382, -21.52544592524334988, 90.20942372801903275 ) ) ;
#138682=CARTESIAN_POINT ( 'NONE',  ( 5.153800228976335163, 19.02544592524342804, 89.79057627198102409 ) ) ;
#138683=CARTESIAN_POINT ( 'NONE',  ( 9.564922557961047289, -16.46253265017146816, 55.41775706135234003 ) ) ;
#138684=CARTESIAN_POINT ( 'NONE',  ( 21.55341960407610458, 5.719274019375980345, 58.95724293864770971 ) ) ;
#138685=CARTESIAN_POINT ( 'NONE',  ( 15.80617190586746368, 15.72974639402197994, 109.3739096053143811 ) ) ;
#138686=CARTESIAN_POINT ( 'NONE',  ( 16.46253265017146816, 9.564922557961045513, 111.6677570613523329 ) ) ;
#138687=CARTESIAN_POINT ( 'NONE',  ( -14.29746914071037622, -8.314922557961029526, 84.16775706135234714 ) ) ;
#138688=CARTESIAN_POINT ( 'NONE',  ( 19.03943276465977164, -0.05219959533909143690, 28.74890960531435624 ) ) ;
#138689=CARTESIAN_POINT ( 'NONE',  ( 5.823673210054444382, -21.52544592524334988, 20.20942372801900788 ) ) ;
#138690=CARTESIAN_POINT ( 'NONE',  ( -16.53943276465976808, 0.05219959533911058130, 111.2489096053143669 ) ) ;
#138692=CARTESIAN_POINT ( 'NONE',  ( 12.06949235617739724, 12.14591786802326823, 46.87609039468568994 ) ) ;
#138693=CARTESIAN_POINT ( 'NONE',  ( 0.05219959533910956823, 16.53943276465976808, 79.99890960531435269 ) ) ;
#138694=CARTESIAN_POINT ( 'NONE',  ( -21.52544592524343514, 5.823673210054127303, 76.04057627198102409 ) ) ;
#138695=CARTESIAN_POINT ( 'NONE',  ( -12.14591786802326823, 12.06949235617739902, 113.1260903946856899 ) ) ;
#138696=CARTESIAN_POINT ( 'NONE',  ( -8.314922557961024197, 14.29746914071037800, 32.91775706135234714 ) ) ;
#138697=CARTESIAN_POINT ( 'NONE',  ( 19.05341960407611168, 5.049401038298154454, 38.95724293864767418 ) ) ;
#138698=CARTESIAN_POINT ( 'NONE',  ( 0.05219959533934541429, -16.53943276465976808, 85.00109039468568994 ) ) ;
#138699=CARTESIAN_POINT ( 'NONE',  ( -16.46253265017146816, -9.564922557961047289, 74.16775706135234714 ) ) ;
#138700=CARTESIAN_POINT ( 'NONE',  ( -10.72451020669898014, 18.67979575497178502, 65.41557627198102409 ) ) ;
#138701=CARTESIAN_POINT ( 'NONE',  ( -12.14591786802326823, 12.06949235617739902, 113.1260903946856899 ) ) ;
#138702=ORIENTED_EDGE ( 'NONE', *, *, #148381, .F. ) ;
#138703=CARTESIAN_POINT ( 'NONE',  ( 5.823673210054444382, -21.52544592524334988, 85.20942372801901854 ) ) ;
#138704=CARTESIAN_POINT ( 'NONE',  ( 21.52544592524344225, -5.823673210054117533, 48.54057627198103120 ) ) ;
#138706=CARTESIAN_POINT ( 'NONE',  ( 8.224510206698742110, 14.34966873604972548, 87.08442372801901854 ) ) ;
#138707=CARTESIAN_POINT ( 'NONE',  ( 5.719274019375991003, -21.55341960407610458, 47.70724293864770260 ) ) ;
#138709=CARTESIAN_POINT ( 'NONE',  ( -5.049401038298153566, 19.05341960407611168, 115.2072429386477097 ) ) ;
#138710=CARTESIAN_POINT ( 'NONE',  ( -18.56197773271726703, 5.500000000000080824, 73.55066217314454491 ) ) ;
#138711=CARTESIAN_POINT ( 'NONE',  ( 16.46253265017160672, -9.564922557960803928, 28.33224293864769550 ) ) ;
#138712=CARTESIAN_POINT ( 'NONE',  ( 18.62759615963271287, -10.81492255796078972, 78.33224293864770971 ) ) ;
#138713=CARTESIAN_POINT ( 'NONE',  ( 14.34966873604972726, -8.224510206698740333, 100.8344237280190185 ) ) ;
#138714=CARTESIAN_POINT ( 'NONE',  ( -10.81492255796105439, 18.62759615963255655, 62.91775706135236135 ) ) ;
#138715=CARTESIAN_POINT ( 'NONE',  ( -4.483927247898782831, 16.52544592524335698, 22.70942372801901499 ) ) ;
#138716=CARTESIAN_POINT ( 'NONE',  ( 8.314922557960818139, 14.29746914071049879, 114.5822429386477097 ) ) ;
#138717=CARTESIAN_POINT ( 'NONE',  ( 13.97604488694548053, -13.89961937509957401, 105.6260903946856757 ) ) ;
#138718=CARTESIAN_POINT ( 'NONE',  ( -9.474510206698964154, 16.51473224551069663, 35.41557627198102409 ) ) ;
#138720=CARTESIAN_POINT ( 'NONE',  ( -13.89961937509977652, 13.97604488694528158, 105.6239096053143527 ) ) ;
#138721=CARTESIAN_POINT ( 'NONE',  ( -16.52544592524335698, -4.483927247898792601, 88.95942372801901854 ) ) ;
#138722=CARTESIAN_POINT ( 'NONE',  ( 0.05219959533936267826, -19.03943276465977164, 80.00109039468567573 ) ) ;
#138723=CARTESIAN_POINT ( 'NONE',  ( -13.97604488694547697, 13.89961937509957934, 23.12609039468565442 ) ) ;
#138724=CARTESIAN_POINT ( 'NONE',  ( -21.53943276465977519, 0.05219959533907696930, 66.24890960531436690 ) ) ;
#138726=CARTESIAN_POINT ( 'NONE',  ( -16.55341960407617563, 4.379528057220093196, 83.54275706135234714 ) ) ;
#138727=CARTESIAN_POINT ( 'NONE',  ( -19.02544592524334988, -5.153800228976617603, 88.95942372801897591 ) ) ;
#138728=CARTESIAN_POINT ( 'NONE',  ( -19.03943276465977164, 0.05219959533909376836, 46.24890960531435979 ) ) ;
#138729=CARTESIAN_POINT ( 'NONE',  ( -19.02544592524342804, 5.153800228976336051, 86.04057627198103830 ) ) ;
#138730=CARTESIAN_POINT ( 'NONE',  ( -18.67979575497193778, 10.72451020669871902, 48.33442372801902565 ) ) ;
#138731=CARTESIAN_POINT ( 'NONE',  ( -9.564922557960796823, -16.46253265017161027, 42.08224293864769550 ) ) ;
#138732=CARTESIAN_POINT ( 'NONE',  ( -17.50000000000001421, -5.622605283950843358, 86.31207310596114723 ) ) ;
#138733=CARTESIAN_POINT ( 'NONE',  ( 0.05219959533909260263, 19.03943276465977164, 114.9989096053143669 ) ) ;
#138734=CARTESIAN_POINT ( 'NONE',  ( 12.14591786802309770, 12.06949235617756955, 59.37390960531436690 ) ) ;
#138735=CARTESIAN_POINT ( 'NONE',  ( -18.67979575497178146, -10.72451020669898902, 76.66557627198103830 ) ) ;
#138736=CARTESIAN_POINT ( 'NONE',  ( -13.89961937509957401, -13.97604488694547875, 49.37609039468567573 ) ) ;
#138738=CARTESIAN_POINT ( 'NONE',  ( 19.05341960407611168, 5.049401038298154454, 63.95724293864769550 ) ) ;
#138739=CARTESIAN_POINT ( 'NONE',  ( 16.51473224551069308, 9.474510206698969483, 69.16557627198102409 ) ) ;
#138740=CARTESIAN_POINT ( 'NONE',  ( -12.06949235617739369, -12.14591786802326823, 49.37609039468569705 ) ) ;
#138742=CARTESIAN_POINT ( 'NONE',  ( -9.564922557961040184, 16.46253265017147172, 32.91775706135233293 ) ) ;
#138743=CARTESIAN_POINT ( 'NONE',  ( -17.49999999999999645, 5.624438216177580330, 110.8167034491464449 ) ) ;
#138744=CARTESIAN_POINT ( 'NONE',  ( 0.05219959533934541429, -16.53943276465976808, 85.00109039468568994 ) ) ;
#138746=CARTESIAN_POINT ( 'NONE',  ( -14.34966873604972548, 8.224510206698743886, 83.33442372801903275 ) ) ;
#138747=CARTESIAN_POINT ( 'NONE',  ( 4.379528057220092307, 16.55341960407617563, 52.29275706135236135 ) ) ;
#138748=CARTESIAN_POINT ( 'NONE',  ( -10.81492255796105439, 18.62759615963255655, 112.9177570613523329 ) ) ;
#138749=CARTESIAN_POINT ( 'NONE',  ( 5.049401038298161559, -19.05341960407611168, 57.70724293864769550 ) ) ;
#138751=CARTESIAN_POINT ( 'NONE',  ( 15.80617190586769283, -15.72974639402175789, 70.62609039468567573 ) ) ;
#138752=CARTESIAN_POINT ( 'NONE',  ( 19.03943276465977164, 0.05219959533936151252, 76.25109039468566152 ) ) ;
#138753=CARTESIAN_POINT ( 'NONE',  ( -21.53943276465977519, -0.05219959533937600094, 113.7510903946856757 ) ) ;
#138754=CARTESIAN_POINT ( 'NONE',  ( 9.564922557960805705, 16.46253265017160317, 29.58224293864769550 ) ) ;
#138756=CARTESIAN_POINT ( 'NONE',  ( -18.67979575497178146, -10.72451020669898902, 61.66557627198103120 ) ) ;
#138757=CARTESIAN_POINT ( 'NONE',  ( 21.53943276465977519, -0.05219959533907433946, 23.74890960531435269 ) ) ;
#138758=CARTESIAN_POINT ( 'NONE',  ( 8.224510206698953496, -14.34966873604960469, 112.9155762719810383 ) ) ;
#138759=CARTESIAN_POINT ( 'NONE',  ( 8.314922557961029526, -14.29746914071037800, 35.41775706135234003 ) ) ;
#138760=CARTESIAN_POINT ( 'NONE',  ( 4.483927247898545687, 16.52544592524342804, 24.79057627198103120 ) ) ;
#138762=B_SPLINE_CURVE_WITH_KNOTS ( 'NONE', 3,
 ( #98292, #128644, #97299, #20477, #82127, #190339, #51815, #191329, #87157, #27505, #161994, #73996, #117492, #132663, #8318, #42659, #196360, #40657, #10329, #54819, #25512, #194351, #116493, #41665, #180195, #135666, #26502, #104321, #102326, #164016, #23490, #103329 ),
 .UNSPECIFIED., .F., .F.,
 ( 4, 2, 2, 2, 2, 2, 2, 2, 2, 2, 2, 2, 2, 2, 2, 4 ),
 ( 1.430489624538199204E-17, 0.0003712461730036792969, 0.0007424923460073442824, 0.001113738519011009268, 0.001484984692014674253, 0.002227477038022005959, 0.002598723211025686340, 0.002969969384029366288, 0.003341215557033046235, 0.003712461730036726616, 0.004083707903040406130, 0.004454954076044086511, 0.004826200249047766025, 0.005197446422051446406, 0.005568692595055126787, 0.005939938768058806301 ),
 .UNSPECIFIED. ) ;
#138763=CARTESIAN_POINT ( 'NONE',  ( 10.72451020669898902, -18.67979575497178502, 112.9155762719810383 ) ) ;
#138764=CARTESIAN_POINT ( 'NONE',  ( 12.06949235617757843, -12.14591786802309237, 38.12390960531436690 ) ) ;
#138766=CARTESIAN_POINT ( 'NONE',  ( -16.46253265017146816, -9.564922557961047289, 104.1677570613523329 ) ) ;
#138767=CARTESIAN_POINT ( 'NONE',  ( -19.02544592524334988, -5.153800228976617603, 23.95942372801900078 ) ) ;
#138768=CARTESIAN_POINT ( 'NONE',  ( -14.34966873604960291, -8.224510206698953496, 46.66557627198102409 ) ) ;
#138769=CARTESIAN_POINT ( 'NONE',  ( 15.80617190586746368, 15.72974639402197994, 99.37390960531436690 ) ) ;
#138771=CARTESIAN_POINT ( 'NONE',  ( 5.823673210054125526, 21.52544592524343514, 59.79057627198103120 ) ) ;
#138772=CARTESIAN_POINT ( 'NONE',  ( -13.97604488694527625, -13.89961937509977652, 71.87390960531433848 ) ) ;
#138773=CARTESIAN_POINT ( 'NONE',  ( -8.224510206698948167, 14.34966873604960824, 50.41557627198103120 ) ) ;
#138774=CARTESIAN_POINT ( 'NONE',  ( 9.474510206698971260, -16.51473224551069308, 87.91557627198102409 ) ) ;
#138775=AXIS2_PLACEMENT_3D ( 'NONE', #136634, #106291, #76945 ) ;
#138777=CARTESIAN_POINT ( 'NONE',  ( -16.51473224551082808, 9.474510206698731452, 53.33442372801900433 ) ) ;
#138778=CARTESIAN_POINT ( 'NONE',  ( 21.52544592524344225, -5.823673210054117533, 88.54057627198103830 ) ) ;
#138779=CARTESIAN_POINT ( 'NONE',  ( 16.51473224551069308, 9.474510206698969483, 44.16557627198103120 ) ) ;
#138780=CARTESIAN_POINT ( 'NONE',  ( -8.224510206698948167, 14.34966873604960824, 105.4155762719810383 ) ) ;
#138781=CARTESIAN_POINT ( 'NONE',  ( 5.719274019375673035, 21.55341960407619339, 57.29275706135234714 ) ) ;
#138783=CARTESIAN_POINT ( 'NONE',  ( -4.483927247898539470, -16.52544592524342804, 27.29057627198103120 ) ) ;
#138784=CARTESIAN_POINT ( 'NONE',  ( -5.153800228976328057, -19.02544592524343514, 52.29057627198100988 ) ) ;
#138785=CARTESIAN_POINT ( 'NONE',  ( -13.97604488694527625, -13.89961937509977652, 101.8739096053143811 ) ) ;
#138786=CARTESIAN_POINT ( 'NONE',  ( -21.55341960407610458, -5.719274019375992779, 66.45724293864768129 ) ) ;
#138787=CARTESIAN_POINT ( 'NONE',  ( -0.05219959533936034679, 19.03943276465977164, 92.50109039468566152 ) ) ;
#138788=CARTESIAN_POINT ( 'NONE',  ( -16.51473224551069308, -9.474510206698971260, 46.66557627198102409 ) ) ;
#138789=CARTESIAN_POINT ( 'NONE',  ( -0.05219959533907301413, -21.53943276465977519, 52.49890960531435979 ) ) ;
#138790=CARTESIAN_POINT ( 'NONE',  ( 5.719274019375673035, 21.55341960407619339, 82.29275706135234714 ) ) ;
#138792=CARTESIAN_POINT ( 'NONE',  ( 14.34966873604972726, -8.224510206698740333, 85.83442372801901854 ) ) ;
#138793=CARTESIAN_POINT ( 'NONE',  ( -12.14591786802326823, 12.06949235617739902, 93.12609039468568994 ) ) ;
#138794=CARTESIAN_POINT ( 'NONE',  ( -19.05341960407611168, -5.049401038298163336, 56.45724293864768129 ) ) ;
#138795=CARTESIAN_POINT ( 'NONE',  ( 9.474510206698971260, -16.51473224551069308, 67.91557627198102409 ) ) ;
#138797=CARTESIAN_POINT ( 'NONE',  ( 13.97604488694548053, -13.89961937509957401, 30.62609039468566863 ) ) ;
#138798=CARTESIAN_POINT ( 'NONE',  ( -16.53943276465976808, -0.05219959533934237506, 78.75109039468568994 ) ) ;
#138799=CARTESIAN_POINT ( 'NONE',  ( -21.53943276465977519, -0.05219959533937600094, 108.7510903946857042 ) ) ;
#138800=CARTESIAN_POINT ( 'NONE',  ( -13.97604488694527625, -13.89961937509977652, 71.87390960531433848 ) ) ;
#138801=CARTESIAN_POINT ( 'NONE',  ( -21.53943276465977519, 0.05219959533907696930, 46.24890960531435979 ) ) ;
#138802=CARTESIAN_POINT ( 'NONE',  ( 16.52544592524335698, 4.483927247898782831, 26.45942372801901854 ) ) ;
#138803=CARTESIAN_POINT ( 'NONE',  ( 5.719274019375673035, 21.55341960407619339, 82.29275706135234714 ) ) ;
#138804=CARTESIAN_POINT ( 'NONE',  ( -16.52544592524335698, -4.483927247898792601, 43.95942372801902565 ) ) ;
#138805=CARTESIAN_POINT ( 'NONE',  ( -10.81492255796078084, -18.62759615963271287, 107.0822429386476955 ) ) ;
#138806=CARTESIAN_POINT ( 'NONE',  ( 16.55341960407618274, -4.379528057220086978, 21.04275706135234714 ) ) ;
#138807=CARTESIAN_POINT ( 'NONE',  ( 9.474510206698971260, -16.51473224551069308, 82.91557627198103830 ) ) ;
#138808=CARTESIAN_POINT ( 'NONE',  ( 16.53943276465976808, 0.05219959533934440121, 26.25109039468567573 ) ) ;
#138809=CARTESIAN_POINT ( 'NONE',  ( 16.51473224551069308, 9.474510206698969483, 39.16557627198103120 ) ) ;
#138811=CARTESIAN_POINT ( 'NONE',  ( -12.06949235617739369, -12.14591786802326823, 19.37609039468568639 ) ) ;
#138812=CARTESIAN_POINT ( 'NONE',  ( 4.483927247898545687, 16.52544592524342804, 84.79057627198102409 ) ) ;
#138813=CARTESIAN_POINT ( 'NONE',  ( -16.53943276465976808, -0.05219959533934237506, 88.75109039468567573 ) ) ;
#138814=CARTESIAN_POINT ( 'NONE',  ( -18.67979575497193778, 10.72451020669871902, 28.33442372801902209 ) ) ;
#138815=CARTESIAN_POINT ( 'NONE',  ( 9.564922557960805705, 16.46253265017160317, 59.58224293864769550 ) ) ;
#138816=CARTESIAN_POINT ( 'NONE',  ( 16.46253265017160672, -9.564922557960803928, 63.33224293864769550 ) ) ;
#138818=CARTESIAN_POINT ( 'NONE',  ( -8.314922557961024197, 14.29746914071037800, 87.91775706135234714 ) ) ;
#138821=VERTEX_POINT ( 'NONE', #66347 ) ;
#138822=CARTESIAN_POINT ( 'NONE',  ( -13.89961937509957401, -13.97604488694547875, 29.37609039468565797 ) ) ;
#138823=CARTESIAN_POINT ( 'NONE',  ( -19.02544592524342804, 5.153800228976336051, 31.04057627198102409 ) ) ;
#138824=CARTESIAN_POINT ( 'NONE',  ( -13.89961937509977652, 13.97604488694528158, 110.6239096053143243 ) ) ;
#138826=CARTESIAN_POINT ( 'NONE',  ( -14.34966873604972548, 8.224510206698743886, 33.33442372801900433 ) ) ;
#138827=CARTESIAN_POINT ( 'NONE',  ( 13.89961937509957401, 13.97604488694547697, 61.87609039468566863 ) ) ;
#138828=CARTESIAN_POINT ( 'NONE',  ( 4.483927247898790824, -16.52544592524335698, 45.20942372801901854 ) ) ;
#138829=CARTESIAN_POINT ( 'NONE',  ( 19.05341960407611168, 5.049401038298154454, 103.9572429386476671 ) ) ;
#138830=CARTESIAN_POINT ( 'NONE',  ( 16.46253265017160672, -9.564922557960803928, 68.33224293864770971 ) ) ;
#138831=CARTESIAN_POINT ( 'NONE',  ( -15.72974639402197994, 15.80617190586746368, 95.62390960531436690 ) ) ;
#138832=CARTESIAN_POINT ( 'NONE',  ( -19.03943276465977164, 0.05219959533909376836, 91.24890960531436690 ) ) ;
#138834=CARTESIAN_POINT ( 'NONE',  ( 16.51473224551069308, 9.474510206698969483, 69.16557627198102409 ) ) ;
#138835=CARTESIAN_POINT ( 'NONE',  ( 12.06949235617739724, 12.14591786802326823, 111.8760903946856615 ) ) ;
#138836=CARTESIAN_POINT ( 'NONE',  ( -16.51473224551069308, -9.474510206698971260, 21.66557627198102765 ) ) ;
#138837=CARTESIAN_POINT ( 'NONE',  ( 19.03943276465977164, 0.05219959533936151252, 36.25109039468567573 ) ) ;
#138838=CARTESIAN_POINT ( 'NONE',  ( -12.06949235617756955, 12.14591786802309770, 60.62390960531437401 ) ) ;
#138839=CARTESIAN_POINT ( 'NONE',  ( -18.67979575497193778, 10.72451020669871902, 103.3344237280190043 ) ) ;
#138840=CARTESIAN_POINT ( 'NONE',  ( -9.474510206698964154, 16.51473224551069663, 40.41557627198103120 ) ) ;
#138841=CARTESIAN_POINT ( 'NONE',  ( -4.483927247898782831, 16.52544592524335698, 57.70942372801901143 ) ) ;
#138842=CARTESIAN_POINT ( 'NONE',  ( -16.52544592524342804, 4.483927247898546575, 36.04057627198102409 ) ) ;
#138843=CARTESIAN_POINT ( 'NONE',  ( 0.05219959533937995610, -21.53943276465977519, 90.00109039468567573 ) ) ;
#138844=CARTESIAN_POINT ( 'NONE',  ( 9.564922557960805705, 16.46253265017160317, 84.58224293864769550 ) ) ;
#138845=CARTESIAN_POINT ( 'NONE',  ( 0.05219959533909260263, 19.03943276465977164, 99.99890960531436690 ) ) ;
#138846=CARTESIAN_POINT ( 'NONE',  ( 8.224510206698953496, -14.34966873604960469, 107.9155762719810241 ) ) ;
#138847=CARTESIAN_POINT ( 'NONE',  ( 12.06949235617757843, -12.14591786802309237, 78.12390960531436690 ) ) ;
#138848=CARTESIAN_POINT ( 'NONE',  ( 5.823673210054125526, 21.52544592524343514, 84.79057627198102409 ) ) ;
#138849=CARTESIAN_POINT ( 'NONE',  ( -16.51473224551069308, -9.474510206698971260, 71.66557627198102409 ) ) ;
#138850=CARTESIAN_POINT ( 'NONE',  ( 18.67979575497178502, 10.72451020669898547, 99.16557627198100988 ) ) ;
#138851=CARTESIAN_POINT ( 'NONE',  ( 13.89961937509957401, 13.97604488694547697, 71.87609039468567573 ) ) ;
#138852=CARTESIAN_POINT ( 'NONE',  ( 19.26498983726237668, -5.499999999999590550, 48.05319577422005040 ) ) ;
#138853=CARTESIAN_POINT ( 'NONE',  ( 14.34966873604960469, 8.224510206698951720, 94.16557627198103830 ) ) ;
#138854=CARTESIAN_POINT ( 'NONE',  ( -5.049401038298153566, 19.05341960407611168, 60.20724293864768129 ) ) ;
#138855=CARTESIAN_POINT ( 'NONE',  ( 10.72451020669898902, -18.67979575497178502, 67.91557627198102409 ) ) ;
#138856=CARTESIAN_POINT ( 'NONE',  ( -18.22780087662124160, -5.499999999999927169, 83.98236817873107896 ) ) ;
#138857=CARTESIAN_POINT ( 'NONE',  ( -14.34966873604960291, -8.224510206698953496, 21.66557627198102409 ) ) ;
#138859=CARTESIAN_POINT ( 'NONE',  ( -16.52544592524335698, -4.483927247898792601, 18.95942372801901143 ) ) ;
#138860=CARTESIAN_POINT ( 'NONE',  ( 8.224510206698953496, -14.34966873604960469, 77.91557627198102409 ) ) ;
#138861=CARTESIAN_POINT ( 'NONE',  ( -19.49190055781012276, -5.500000000000019540, 95.56116087098779133 ) ) ;
#138862=CARTESIAN_POINT ( 'NONE',  ( -19.02544592524342804, 5.153800228976336051, 81.04057627198103830 ) ) ;
#138863=CARTESIAN_POINT ( 'NONE',  ( 5.049401038298161559, -19.05341960407611168, 32.70724293864768129 ) ) ;
#138864=CARTESIAN_POINT ( 'NONE',  ( -16.53943276465976808, 0.05219959533911058130, 66.24890960531436690 ) ) ;
#138865=CARTESIAN_POINT ( 'NONE',  ( 21.55341960407610458, 5.719274019375980345, 23.95724293864769550 ) ) ;
#138866=CARTESIAN_POINT ( 'NONE',  ( 16.46253265017146816, 9.564922557961045513, 86.66775706135233293 ) ) ;
#138867=CARTESIAN_POINT ( 'NONE',  ( -19.05341960407611168, -5.049401038298163336, 96.45724293864769550 ) ) ;
#138868=CARTESIAN_POINT ( 'NONE',  ( -15.72974639402197994, 15.80617190586746368, 70.62390960531436690 ) ) ;
#138869=CARTESIAN_POINT ( 'NONE',  ( -8.314922557961024197, 14.29746914071037800, 72.91775706135234714 ) ) ;
#138870=CARTESIAN_POINT ( 'NONE',  ( -0.05219959533936034679, 19.03943276465977164, 112.5010903946856757 ) ) ;
#138871=CARTESIAN_POINT ( 'NONE',  ( -5.153800228976328057, -19.02544592524343514, 57.29057627198103120 ) ) ;
#138872=CARTESIAN_POINT ( 'NONE',  ( 15.80617190586746368, 15.72974639402197994, 74.37390960531436690 ) ) ;
#138873=CARTESIAN_POINT ( 'NONE',  ( 19.05341960407617918, -5.049401038297876454, 111.0427570613523329 ) ) ;
#138874=CARTESIAN_POINT ( 'NONE',  ( -12.14591786802309592, -12.06949235617757132, 36.87390960531435979 ) ) ;
#138875=CARTESIAN_POINT ( 'NONE',  ( 5.719274019375673035, 21.55341960407619339, 47.29275706135234003 ) ) ;
#138877=CARTESIAN_POINT ( 'NONE',  ( -14.29746914071037622, -8.314922557961029526, 74.16775706135231871 ) ) ;
#138878=CARTESIAN_POINT ( 'NONE',  ( 19.03943276465977164, -0.05219959533909143690, 103.7489096053143669 ) ) ;
#138880=CARTESIAN_POINT ( 'NONE',  ( -16.88567814943162659, 6.947325034625691842, 78.70998877347415146 ) ) ;
#138881=CARTESIAN_POINT ( 'NONE',  ( 16.55341960407618274, -4.379528057220086978, 91.04275706135236135 ) ) ;
#138882=CARTESIAN_POINT ( 'NONE',  ( 8.224510206698742110, 14.34966873604972548, 52.08442372801901854 ) ) ;
#138883=CARTESIAN_POINT ( 'NONE',  ( 13.89961937509977652, -13.97604488694527269, 63.12390960531435979 ) ) ;
#138884=CARTESIAN_POINT ( 'NONE',  ( 16.46253265017160672, -9.564922557960803928, 78.33224293864769550 ) ) ;
#138885=CARTESIAN_POINT ( 'NONE',  ( 5.823673210054444382, -21.52544592524334988, 55.20942372801902565 ) ) ;
#138886=CARTESIAN_POINT ( 'NONE',  ( 12.14591786802327356, -12.06949235617739191, 65.62609039468568994 ) ) ;
#138887=CARTESIAN_POINT ( 'NONE',  ( -0.05219959533910754901, -16.53943276465976808, 27.49890960531435269 ) ) ;
#138888=CARTESIAN_POINT ( 'NONE',  ( 13.89961937509977652, -13.97604488694527269, 43.12390960531434558 ) ) ;
#138889=CARTESIAN_POINT ( 'NONE',  ( -9.564922557960796823, -16.46253265017161027, 37.08224293864768839 ) ) ;
#138890=CARTESIAN_POINT ( 'NONE',  ( -0.05219959533934338120, 16.53943276465976808, 27.50109039468567929 ) ) ;
#138891=CARTESIAN_POINT ( 'NONE',  ( -16.51473224551082808, 9.474510206698731452, 78.33442372801900433 ) ) ;
#138892=CARTESIAN_POINT ( 'NONE',  ( 16.55341960407611168, 4.379528057220329451, 83.95724293864770971 ) ) ;
#138893=CARTESIAN_POINT ( 'NONE',  ( 5.049401038298161559, -19.05341960407611168, 57.70724293864769550 ) ) ;
#138894=CARTESIAN_POINT ( 'NONE',  ( 9.564922557961047289, -16.46253265017146816, 90.41775706135234714 ) ) ;
#138896=CARTESIAN_POINT ( 'NONE',  ( 5.823673210054444382, -21.52544592524334988, 95.20942372801903275 ) ) ;
#138897=CARTESIAN_POINT ( 'NONE',  ( -16.55341960407617563, 4.379528057220093196, 48.54275706135234714 ) ) ;
#138899=CARTESIAN_POINT ( 'NONE',  ( 15.72974639402199770, -15.80617190586745480, 53.12390960531436690 ) ) ;
#138900=CARTESIAN_POINT ( 'NONE',  ( -16.55341960407617563, 4.379528057220093196, 33.54275706135234714 ) ) ;
#138901=CARTESIAN_POINT ( 'NONE',  ( 16.46253265017160672, -9.564922557960803928, 33.33224293864770260 ) ) ;
#138902=CARTESIAN_POINT ( 'NONE',  ( 19.05341960407617918, -5.049401038297876454, 36.04275706135234003 ) ) ;
#138903=CARTESIAN_POINT ( 'NONE',  ( -13.97604488694527625, -13.89961937509977652, 76.87390960531433848 ) ) ;
#138904=CARTESIAN_POINT ( 'NONE',  ( -13.97604488694527625, -13.89961937509977652, 46.87390960531435979 ) ) ;
#138905=CARTESIAN_POINT ( 'NONE',  ( -18.22780087662123805, 5.499999999999981348, 81.01763182126896368 ) ) ;
#138906=CARTESIAN_POINT ( 'NONE',  ( 0.05219959533909260263, 19.03943276465977164, 74.99890960531435269 ) ) ;
#138907=CARTESIAN_POINT ( 'NONE',  ( 5.153800228976615827, -19.02544592524334988, 30.20942372801900433 ) ) ;
#138908=CARTESIAN_POINT ( 'NONE',  ( 19.03943276465977164, 0.05219959533936151252, 21.25109039468565797 ) ) ;
#138909=CARTESIAN_POINT ( 'NONE',  ( -12.14591786802309592, -12.06949235617757132, 41.87390960531435979 ) ) ;
#138910=CARTESIAN_POINT ( 'NONE',  ( 16.46253265017160672, -9.564922557960803928, 38.33224293864768839 ) ) ;
#138911=CARTESIAN_POINT ( 'NONE',  ( 13.97604488694527802, 13.89961937509977652, 109.3739096053143669 ) ) ;
#138912=CARTESIAN_POINT ( 'NONE',  ( -10.72451020669870658, -18.67979575497194134, 84.58442372801903275 ) ) ;
#138913=CARTESIAN_POINT ( 'NONE',  ( -9.564922557960796823, -16.46253265017161027, 57.08224293864769550 ) ) ;
#138914=CARTESIAN_POINT ( 'NONE',  ( -10.81492255796105439, 18.62759615963255655, 77.91775706135231871 ) ) ;
#138915=CARTESIAN_POINT ( 'NONE',  ( -10.72451020669898014, 18.67979575497178502, 40.41557627198103120 ) ) ;
#138916=CARTESIAN_POINT ( 'NONE',  ( 15.80617190586769283, -15.72974639402175789, 25.62609039468567929 ) ) ;
#138917=CARTESIAN_POINT ( 'NONE',  ( -19.02544592524334988, -5.153800228976617603, 48.95942372801900433 ) ) ;
#138918=CARTESIAN_POINT ( 'NONE',  ( 5.049401038298161559, -19.05341960407611168, 22.70724293864769194 ) ) ;
#138919=CARTESIAN_POINT ( 'NONE',  ( 5.049401038298161559, -19.05341960407611168, 82.70724293864770971 ) ) ;
#138920=CARTESIAN_POINT ( 'NONE',  ( 14.34966873604972726, -8.224510206698740333, 35.83442372801901143 ) ) ;
#138921=CARTESIAN_POINT ( 'NONE',  ( -16.52544592524342804, 4.483927247898546575, 91.04057627198103830 ) ) ;
#138922=CARTESIAN_POINT ( 'NONE',  ( -19.05341960407611168, -5.049401038298163336, 61.45724293864769550 ) ) ;
#138923=CARTESIAN_POINT ( 'NONE',  ( 21.53943276465977519, -0.05219959533907433946, 38.74890960531435979 ) ) ;
#138925=CARTESIAN_POINT ( 'NONE',  ( -9.564922557961040184, 16.46253265017147172, 97.91775706135233293 ) ) ;
#138926=CARTESIAN_POINT ( 'NONE',  ( 18.67979575497178502, 10.72451020669898547, 104.1655762719810241 ) ) ;
#138927=CARTESIAN_POINT ( 'NONE',  ( -10.72451020669870658, -18.67979575497194134, 54.58442372801901143 ) ) ;
#138928=CARTESIAN_POINT ( 'NONE',  ( 8.314922557961029526, -14.29746914071037800, 70.41775706135236135 ) ) ;
#138929=CARTESIAN_POINT ( 'NONE',  ( 12.14591786802327356, -12.06949235617739191, 70.62609039468567573 ) ) ;
#138930=CARTESIAN_POINT ( 'NONE',  ( 16.51473224551069308, 9.474510206698969483, 59.16557627198102409 ) ) ;
#138931=CARTESIAN_POINT ( 'NONE',  ( 8.224510206698742110, 14.34966873604972548, 87.08442372801901854 ) ) ;
#138932=CARTESIAN_POINT ( 'NONE',  ( -10.81492255796078084, -18.62759615963271287, 112.0822429386477097 ) ) ;
#138933=CARTESIAN_POINT ( 'NONE',  ( 8.224510206698953496, -14.34966873604960469, 67.91557627198102409 ) ) ;
#138934=CARTESIAN_POINT ( 'NONE',  ( -19.03943276465977164, 0.05219959533909376836, 91.24890960531436690 ) ) ;
#138935=CARTESIAN_POINT ( 'NONE',  ( 8.224510206698742110, 14.34966873604972548, 77.08442372801901854 ) ) ;
#138936=CARTESIAN_POINT ( 'NONE',  ( -15.80617190586768217, 15.72974639402176855, 63.12609039468568994 ) ) ;
#138937=CARTESIAN_POINT ( 'NONE',  ( -14.29746914071037622, -8.314922557961029526, 24.16775706135235424 ) ) ;
#138938=CARTESIAN_POINT ( 'NONE',  ( 21.52544592524344225, -5.823673210054117533, 108.5405762719810241 ) ) ;
#138939=CARTESIAN_POINT ( 'NONE',  ( -0.05219959533910754901, -16.53943276465976808, 57.49890960531435979 ) ) ;
#138941=CARTESIAN_POINT ( 'NONE',  ( -16.18388926212238133, 7.379444403734531477, 74.56046848633853585 ) ) ;
#138942=CARTESIAN_POINT ( 'NONE',  ( 0.05219959533907565091, 21.53943276465977519, 84.99890960531436690 ) ) ;
#138943=CARTESIAN_POINT ( 'NONE',  ( 8.314922557960818139, 14.29746914071049879, 34.58224293864770260 ) ) ;
#138946=CARTESIAN_POINT ( 'NONE',  ( -21.52544592524334988, -5.823673210054445271, 18.95942372801901143 ) ) ;
#138947=CARTESIAN_POINT ( 'NONE',  ( -19.02544592524342804, 5.153800228976336051, 116.0405762719810383 ) ) ;
#138948=CARTESIAN_POINT ( 'NONE',  ( 21.53943276465977519, 0.05219959533937863772, 21.25109039468567218 ) ) ;
#138949=CARTESIAN_POINT ( 'NONE',  ( 16.52544592524342804, -4.483927247898539470, 53.54057627198103120 ) ) ;
#138950=CARTESIAN_POINT ( 'NONE',  ( 4.379528057220092307, 16.55341960407617563, 57.29275706135234714 ) ) ;
#138951=CIRCLE ( 'NONE', #184143, 2.000000000000001776 ) ;
#138952=CARTESIAN_POINT ( 'NONE',  ( 0.05219959533909260263, 19.03943276465977164, 59.99890960531436690 ) ) ;
#138953=CARTESIAN_POINT ( 'NONE',  ( -0.05219959533936034679, 19.03943276465977164, 67.50109039468566152 ) ) ;
#138954=CARTESIAN_POINT ( 'NONE',  ( -19.05341960407611168, -5.049401038298163336, 76.45724293864769550 ) ) ;
#138955=CARTESIAN_POINT ( 'NONE',  ( -15.80617190586745835, -15.72974639402198527, 41.87390960531435979 ) ) ;
#138957=CARTESIAN_POINT ( 'NONE',  ( 16.51473224551069308, 9.474510206698969483, 64.16557627198102409 ) ) ;
#138958=CARTESIAN_POINT ( 'NONE',  ( -12.06949235617739369, -12.14591786802326823, 24.37609039468567573 ) ) ;
#138959=CARTESIAN_POINT ( 'NONE',  ( -9.474510206698720793, -16.51473224551083518, 69.58442372801901854 ) ) ;
#138960=CARTESIAN_POINT ( 'NONE',  ( -21.52544592524343514, 5.823673210054127303, 116.0405762719810383 ) ) ;
#138961=EDGE_CURVE ( 'NONE', #141234, #61486, #173822, .T. ) ;
#138962=CARTESIAN_POINT ( 'NONE',  ( -4.483927247898539470, -16.52544592524342804, 52.29057627198102409 ) ) ;
#138963=CARTESIAN_POINT ( 'NONE',  ( 19.05341960407611168, 5.049401038298154454, 93.95724293864769550 ) ) ;
#138964=CARTESIAN_POINT ( 'NONE',  ( 18.67979575497178502, 10.72451020669898547, 59.16557627198103120 ) ) ;
#138965=CARTESIAN_POINT ( 'NONE',  ( 15.72974639402199770, -15.80617190586745480, 93.12390960531436690 ) ) ;
#138966=CARTESIAN_POINT ( 'NONE',  ( -4.379528057220086978, -16.55341960407618274, 34.79275706135235424 ) ) ;
#138967=CARTESIAN_POINT ( 'NONE',  ( -10.72451020669898014, 18.67979575497178502, 30.41557627198101699 ) ) ;
#138968=CARTESIAN_POINT ( 'NONE',  ( 5.823673210054444382, -21.52544592524334988, 90.20942372801903275 ) ) ;
#138969=CARTESIAN_POINT ( 'NONE',  ( 9.474510206698971260, -16.51473224551069308, 82.91557627198103830 ) ) ;
#138970=CARTESIAN_POINT ( 'NONE',  ( 13.97604488694527802, 13.89961937509977652, 39.37390960531435269 ) ) ;
#138971=CARTESIAN_POINT ( 'NONE',  ( 16.46253265017160672, -9.564922557960803928, 98.33224293864769550 ) ) ;
#138972=CARTESIAN_POINT ( 'NONE',  ( 16.55341960407611168, 4.379528057220329451, 103.9572429386476813 ) ) ;
#138973=CARTESIAN_POINT ( 'NONE',  ( -9.474510206698964154, 16.51473224551069663, 60.41557627198102409 ) ) ;
#138974=CARTESIAN_POINT ( 'NONE',  ( 12.14591786802327356, -12.06949235617739191, 25.62609039468567929 ) ) ;
#138975=CARTESIAN_POINT ( 'NONE',  ( 17.50000000000003197, 4.049696124445839374, 33.31960329334057747 ) ) ;
#138976=CARTESIAN_POINT ( 'NONE',  ( 15.80617190586769283, -15.72974639402175789, 100.6260903946857184 ) ) ;
#138977=CARTESIAN_POINT ( 'NONE',  ( 15.72974639402199770, -15.80617190586745480, 28.12390960531435979 ) ) ;
#138978=CARTESIAN_POINT ( 'NONE',  ( -12.14591786802326823, 12.06949235617739902, 88.12609039468570415 ) ) ;
#138980=CARTESIAN_POINT ( 'NONE',  ( -19.02544592524334988, -5.153800228976617603, 63.95942372801899012 ) ) ;
#138981=CARTESIAN_POINT ( 'NONE',  ( -16.46253265017146816, -9.564922557961047289, 34.16775706135233293 ) ) ;
#138983=CARTESIAN_POINT ( 'NONE',  ( 19.03943276465977164, -0.05219959533909143690, 28.74890960531435624 ) ) ;
#138984=CARTESIAN_POINT ( 'NONE',  ( -12.14591786802309592, -12.06949235617757132, 41.87390960531435979 ) ) ;
#138985=CARTESIAN_POINT ( 'NONE',  ( -16.20579543436677383, -7.371946100355105003, 110.5652083417187157 ) ) ;
#138986=CARTESIAN_POINT ( 'NONE',  ( -4.483927247898539470, -16.52544592524342804, 27.29057627198103120 ) ) ;
#138987=CARTESIAN_POINT ( 'NONE',  ( 17.50000000000000000, 5.499999999999992895, 66.70309617465828467 ) ) ;
#138988=CARTESIAN_POINT ( 'NONE',  ( 4.379528057220092307, 16.55341960407617563, 97.29275706135234714 ) ) ;
#138989=CARTESIAN_POINT ( 'NONE',  ( -9.564922557960796823, -16.46253265017161027, 32.08224293864769550 ) ) ;
#138990=CARTESIAN_POINT ( 'NONE',  ( 5.823673210054444382, -21.52544592524334988, 105.2094237280190328 ) ) ;
#138991=CARTESIAN_POINT ( 'NONE',  ( 16.53943276465976808, 0.05219959533934440121, 26.25109039468567573 ) ) ;
#138992=CARTESIAN_POINT ( 'NONE',  ( -15.72974639402176322, -15.80617190586768395, 74.37609039468568994 ) ) ;
#138993=CARTESIAN_POINT ( 'NONE',  ( 16.51473224551083163, -9.474510206698727899, 55.83442372801899722 ) ) ;
#138994=CARTESIAN_POINT ( 'NONE',  ( 0.05219959533909260263, 19.03943276465977164, 94.99890960531436690 ) ) ;
#138995=CARTESIAN_POINT ( 'NONE',  ( -16.51473224551069308, -9.474510206698971260, 71.66557627198102409 ) ) ;
#138996=CARTESIAN_POINT ( 'NONE',  ( -19.25663599770061296, 5.499999999999452882, 38.99419308057201050 ) ) ;
#138997=CARTESIAN_POINT ( 'NONE',  ( 15.72974639402199770, -15.80617190586745480, 93.12390960531436690 ) ) ;
#138998=CARTESIAN_POINT ( 'NONE',  ( -16.52544592524342804, 4.483927247898546575, 61.04057627198103120 ) ) ;
#138999=CARTESIAN_POINT ( 'NONE',  ( -15.72974639402197994, 15.80617190586746368, 55.62390960531436690 ) ) ;
#139000=CARTESIAN_POINT ( 'NONE',  ( 13.97604488694527802, 13.89961937509977652, 54.37390960531435979 ) ) ;
#139001=CARTESIAN_POINT ( 'NONE',  ( 18.67979575497178502, 10.72451020669898547, 89.16557627198102409 ) ) ;
#139002=CARTESIAN_POINT ( 'NONE',  ( 8.224510206698742110, 14.34966873604972548, 77.08442372801901854 ) ) ;
#139004=CARTESIAN_POINT ( 'NONE',  ( -0.05219959533909027116, -19.03943276465977164, 42.49890960531435269 ) ) ;
#139005=CARTESIAN_POINT ( 'NONE',  ( 8.224510206698953496, -14.34966873604960469, 87.91557627198103830 ) ) ;
#139007=CARTESIAN_POINT ( 'NONE',  ( 9.564922557960805705, 16.46253265017160317, 44.58224293864769550 ) ) ;
#139008=CARTESIAN_POINT ( 'NONE',  ( -4.379528057220328563, 16.55341960407611168, 115.2072429386476955 ) ) ;
#139009=CARTESIAN_POINT ( 'NONE',  ( 16.46253265017146816, 9.564922557961045513, 66.66775706135233293 ) ) ;
#139010=CARTESIAN_POINT ( 'NONE',  ( -4.379528057220328563, 16.55341960407611168, 90.20724293864770971 ) ) ;
#139011=CARTESIAN_POINT ( 'NONE',  ( 18.67979575497194134, -10.72451020669871369, 50.83442372801901143 ) ) ;
#139012=CARTESIAN_POINT ( 'NONE',  ( -9.474510206698964154, 16.51473224551069663, 35.41557627198102409 ) ) ;
#139013=CARTESIAN_POINT ( 'NONE',  ( 10.81492255796078972, 18.62759615963270932, 109.5822429386476955 ) ) ;
#139014=B_SPLINE_CURVE_WITH_KNOTS ( 'NONE', 3,
 ( #144720, #7204, #53726, #19404, #66885, #146721, #190243, #161899, #158891, #68888, #176081, #20381, #96225, #82028, #67886, #37550, #54719, #51720, #6206, #130548 ),
 .UNSPECIFIED., .F., .F.,
 ( 4, 2, 2, 2, 2, 2, 2, 2, 2, 4 ),
 ( 0.000000000000000000, 0.0004987090165372665227, 0.0009974180330745330454, 0.001246772541343162946, 0.001496127049611792846, 0.001994836066149056984, 0.002493545082686320687, 0.002742899590954941264, 0.002992254099223561406, 0.003989672132298042843 ),
 .UNSPECIFIED. ) ;
#139015=CARTESIAN_POINT ( 'NONE',  ( 16.55341960407611168, 4.379528057220329451, 83.95724293864770971 ) ) ;
#139016=CARTESIAN_POINT ( 'NONE',  ( 17.72662750342728444, 5.499999999999958256, 93.90179492283741070 ) ) ;
#139017=CARTESIAN_POINT ( 'NONE',  ( -5.049401038298153566, 19.05341960407611168, 65.20724293864765286 ) ) ;
#139019=CARTESIAN_POINT ( 'NONE',  ( -19.05341960407617563, 5.049401038297882671, 93.54275706135234714 ) ) ;
#139020=CARTESIAN_POINT ( 'NONE',  ( -0.05219959533909027116, -19.03943276465977164, 97.49890960531436690 ) ) ;
#139021=CARTESIAN_POINT ( 'NONE',  ( 18.67979575497194134, -10.72451020669871369, 40.83442372801901854 ) ) ;
#139022=CARTESIAN_POINT ( 'NONE',  ( -13.97604488694527625, -13.89961937509977652, 76.87390960531433848 ) ) ;
#139023=CARTESIAN_POINT ( 'NONE',  ( 13.97604488694548053, -13.89961937509957401, 65.62609039468567573 ) ) ;
#139024=CARTESIAN_POINT ( 'NONE',  ( -9.474510206698964154, 16.51473224551069663, 60.41557627198102409 ) ) ;
#139025=CARTESIAN_POINT ( 'NONE',  ( 8.224510206698953496, -14.34966873604960469, 77.91557627198102409 ) ) ;
#139026=B_SPLINE_CURVE_WITH_KNOTS ( 'NONE', 3,
 ( #154304, #186654, #48124, #171464, #15793, #2602 ),
 .UNSPECIFIED., .F., .F.,
 ( 4, 2, 4 ),
 ( 0.003239945802372271207, 0.003620412082092145951, 0.004000878361812020695 ),
 .UNSPECIFIED. ) ;
#139027=CARTESIAN_POINT ( 'NONE',  ( -14.34966873604960291, -8.224510206698953496, 66.66557627198102409 ) ) ;
#139028=CARTESIAN_POINT ( 'NONE',  ( -19.05341960407611168, -5.049401038298163336, 91.45724293864766707 ) ) ;
#139029=CARTESIAN_POINT ( 'NONE',  ( 0.05219959533907565091, 21.53943276465977519, 94.99890960531436690 ) ) ;
#139030=CARTESIAN_POINT ( 'NONE',  ( -19.03943276465977164, 0.05219959533909376836, 81.24890960531436690 ) ) ;
#139031=CARTESIAN_POINT ( 'NONE',  ( 19.02544592524334988, 5.153800228976608722, 36.45942372801900433 ) ) ;
#139032=CARTESIAN_POINT ( 'NONE',  ( -13.89961937509977652, 13.97604488694528158, 30.62390960531435269 ) ) ;
#139033=CARTESIAN_POINT ( 'NONE',  ( 16.52544592524342804, -4.483927247898539470, 33.54057627198102409 ) ) ;
#139034=CARTESIAN_POINT ( 'NONE',  ( 8.314922557960818139, 14.29746914071049879, 104.5822429386477097 ) ) ;
#139036=CARTESIAN_POINT ( 'NONE',  ( -5.823673210054431948, 21.52544592524334988, 32.70942372801900433 ) ) ;
#139037=CARTESIAN_POINT ( 'NONE',  ( -5.153800228976607833, 19.02544592524334988, 72.70942372801900433 ) ) ;
#139038=CARTESIAN_POINT ( 'NONE',  ( 4.379528057220339221, -16.55341960407611168, 27.70724293864769905 ) ) ;
#139039=CARTESIAN_POINT ( 'NONE',  ( 15.72974639402199770, -15.80617190586745480, 83.12390960531436690 ) ) ;
#139040=CARTESIAN_POINT ( 'NONE',  ( -21.53943276465977519, 0.05219959533907696930, 21.24890960531436690 ) ) ;
#139041=CARTESIAN_POINT ( 'NONE',  ( -12.06949235617756955, 12.14591786802309770, 65.62390960531436690 ) ) ;
#139042=CARTESIAN_POINT ( 'NONE',  ( 19.05341960407611168, 5.049401038298154454, 23.95724293864769194 ) ) ;
#139043=CARTESIAN_POINT ( 'NONE',  ( 16.51473224551083163, -9.474510206698727899, 30.83442372801900433 ) ) ;
#139044=CARTESIAN_POINT ( 'NONE',  ( -4.379528057220086978, -16.55341960407618274, 99.79275706135234714 ) ) ;
#139045=CARTESIAN_POINT ( 'NONE',  ( 4.379528057220092307, 16.55341960407617563, 52.29275706135236135 ) ) ;
#139046=CARTESIAN_POINT ( 'NONE',  ( 0.05219959533907565091, 21.53943276465977519, 24.99890960531435624 ) ) ;
#139047=CARTESIAN_POINT ( 'NONE',  ( 21.55341960407619695, -5.719274019375665929, 106.0427570613523471 ) ) ;
#139048=CARTESIAN_POINT ( 'NONE',  ( 19.05341960407611168, 5.049401038298154454, 78.95724293864769550 ) ) ;
#139049=CARTESIAN_POINT ( 'NONE',  ( -8.224510206698735004, -14.34966873604973081, 64.58442372801900433 ) ) ;
#139050=CARTESIAN_POINT ( 'NONE',  ( 4.379528057220339221, -16.55341960407611168, 112.7072429386476955 ) ) ;
#139051=CARTESIAN_POINT ( 'NONE',  ( -12.06949235617756955, 12.14591786802309770, 35.62390960531437401 ) ) ;
#139052=CARTESIAN_POINT ( 'NONE',  ( -18.09805431107249873, 5.499999999999980460, 71.01606229291884631 ) ) ;
#139053=CARTESIAN_POINT ( 'NONE',  ( -5.049401038298153566, 19.05341960407611168, 110.2072429386476671 ) ) ;
#139054=CARTESIAN_POINT ( 'NONE',  ( 19.02544592524343514, -5.153800228976328945, 93.54057627198102409 ) ) ;
#139055=CARTESIAN_POINT ( 'NONE',  ( -19.03943276465977164, 0.05219959533909376836, 111.2489096053143669 ) ) ;
#139057=CARTESIAN_POINT ( 'NONE',  ( -4.379528057220328563, 16.55341960407611168, 60.20724293864768839 ) ) ;
#139058=CARTESIAN_POINT ( 'NONE',  ( 12.14591786802309770, 12.06949235617756955, 34.37390960531435979 ) ) ;
#139059=CARTESIAN_POINT ( 'NONE',  ( -4.379528057220328563, 16.55341960407611168, 55.20724293864770260 ) ) ;
#139061=CARTESIAN_POINT ( 'NONE',  ( 0.05219959533934541429, -16.53943276465976808, 45.00109039468568284 ) ) ;
#139062=CARTESIAN_POINT ( 'NONE',  ( 17.59860650958997397, -7.585241751806833577, 60.92337014262493966 ) ) ;
#139063=CARTESIAN_POINT ( 'NONE',  ( 0.05219959533936267826, -19.03943276465977164, 55.00109039468566863 ) ) ;
#139064=CARTESIAN_POINT ( 'NONE',  ( -13.97604488694527625, -13.89961937509977652, 81.87390960531436690 ) ) ;
#139065=CARTESIAN_POINT ( 'NONE',  ( 19.03943276465977164, 0.05219959533936151252, 71.25109039468566152 ) ) ;
#139067=CARTESIAN_POINT ( 'NONE',  ( 16.51473224551083163, -9.474510206698727899, 60.83442372801900433 ) ) ;
#139068=CARTESIAN_POINT ( 'NONE',  ( -5.049401038297874678, -19.05341960407617918, 104.7927570613523471 ) ) ;
#139069=CARTESIAN_POINT ( 'NONE',  ( 4.483927247898790824, -16.52544592524335698, 85.20942372801901854 ) ) ;
#139071=CARTESIAN_POINT ( 'NONE',  ( -19.03943276465977164, 0.05219959533909376836, 31.24890960531435979 ) ) ;
#139072=CARTESIAN_POINT ( 'NONE',  ( 13.89961937509977652, -13.97604488694527269, 98.12390960531433848 ) ) ;
#139073=CARTESIAN_POINT ( 'NONE',  ( -15.72974639402176322, -15.80617190586768395, 39.37609039468567573 ) ) ;
#139074=CARTESIAN_POINT ( 'NONE',  ( 13.89961937509957401, 13.97604488694547697, 101.8760903946856331 ) ) ;
#139075=CARTESIAN_POINT ( 'NONE',  ( 17.50000000000000711, 4.873317850230757031, 23.61681730595545758 ) ) ;
#139076=CARTESIAN_POINT ( 'NONE',  ( 13.89961937509977652, -13.97604488694527269, 58.12390960531436690 ) ) ;
#139077=CARTESIAN_POINT ( 'NONE',  ( -9.474510206698964154, 16.51473224551069663, 105.4155762719810383 ) ) ;
#139078=CARTESIAN_POINT ( 'NONE',  ( -16.53943276465976808, 0.05219959533911058130, 61.24890960531435979 ) ) ;
#139079=CARTESIAN_POINT ( 'NONE',  ( -9.564922557960796823, -16.46253265017161027, 57.08224293864769550 ) ) ;
#139080=CARTESIAN_POINT ( 'NONE',  ( 16.46253265017160672, -9.564922557960803928, 63.33224293864769550 ) ) ;
#139081=CARTESIAN_POINT ( 'NONE',  ( 5.049401038297881783, 19.05341960407617563, 82.29275706135229029 ) ) ;
#139082=CARTESIAN_POINT ( 'NONE',  ( -18.62759615963270932, 10.81492255796079327, 45.83224293864769550 ) ) ;
#139083=CARTESIAN_POINT ( 'NONE',  ( -0.05219959533909027116, -19.03943276465977164, 22.49890960531436690 ) ) ;
#139084=CARTESIAN_POINT ( 'NONE',  ( 19.02544592524334988, 5.153800228976608722, 46.45942372801899012 ) ) ;
#139085=CARTESIAN_POINT ( 'NONE',  ( 13.97604488694527802, 13.89961937509977652, 79.37390960531435269 ) ) ;
#139088=CARTESIAN_POINT ( 'NONE',  ( -21.52544592524343514, 5.823673210054127303, 81.04057627198102409 ) ) ;
#139089=CARTESIAN_POINT ( 'NONE',  ( 16.52544592524342804, -4.483927247898539470, 78.54057627198103830 ) ) ;
#139090=CARTESIAN_POINT ( 'NONE',  ( -0.05219959533936034679, 19.03943276465977164, 32.50109039468566863 ) ) ;
#139091=CARTESIAN_POINT ( 'NONE',  ( -15.72974639402197994, 15.80617190586746368, 55.62390960531436690 ) ) ;
#139092=CARTESIAN_POINT ( 'NONE',  ( 21.52544592524344225, -5.823673210054117533, 43.54057627198103830 ) ) ;
#139093=CARTESIAN_POINT ( 'NONE',  ( 21.53943276465977519, 0.05219959533937863772, 91.25109039468568994 ) ) ;
#139094=CARTESIAN_POINT ( 'NONE',  ( -9.474510206698964154, 16.51473224551069663, 70.41557627198102409 ) ) ;
#139095=CARTESIAN_POINT ( 'NONE',  ( -4.379528057220328563, 16.55341960407611168, 110.2072429386477239 ) ) ;
#139096=CARTESIAN_POINT ( 'NONE',  ( 18.67979575497194134, -10.72451020669871369, 30.83442372801902209 ) ) ;
#139097=CARTESIAN_POINT ( 'NONE',  ( -19.25918095147780917, -5.499999999999586997, 39.45284276293936188 ) ) ;
#139098=CARTESIAN_POINT ( 'NONE',  ( -5.719274019375665041, -21.55341960407619695, 39.79275706135235424 ) ) ;
#139099=CARTESIAN_POINT ( 'NONE',  ( 16.46253265017160672, -9.564922557960803928, 33.33224293864770260 ) ) ;
#139100=CARTESIAN_POINT ( 'NONE',  ( -18.67979575497178146, -10.72451020669898902, 101.6655762719810383 ) ) ;
#139101=CARTESIAN_POINT ( 'NONE',  ( -13.89961937509957401, -13.97604488694547875, 49.37609039468567573 ) ) ;
#139103=CARTESIAN_POINT ( 'NONE',  ( 18.39443945427639449, -5.500000000000023093, 76.01745347608652992 ) ) ;
#139105=CARTESIAN_POINT ( 'NONE',  ( -0.05219959533934338120, 16.53943276465976808, 57.50109039468568994 ) ) ;
#139106=CARTESIAN_POINT ( 'NONE',  ( -0.05219959533909027116, -19.03943276465977164, 22.49890960531436690 ) ) ;
#139108=CARTESIAN_POINT ( 'NONE',  ( -5.153800228976328057, -19.02544592524343514, 72.29057627198102409 ) ) ;
#139109=CARTESIAN_POINT ( 'NONE',  ( 8.314922557960818139, 14.29746914071049879, 104.5822429386477097 ) ) ;
#139110=CARTESIAN_POINT ( 'NONE',  ( -10.72451020669898014, 18.67979575497178502, 60.41557627198102409 ) ) ;
#139111=CARTESIAN_POINT ( 'NONE',  ( -16.55341960407617563, 4.379528057220093196, 33.54275706135234714 ) ) ;
#139112=CARTESIAN_POINT ( 'NONE',  ( 10.72451020669871369, 18.67979575497193778, 97.08442372801904696 ) ) ;
#139114=CARTESIAN_POINT ( 'NONE',  ( 8.224510206698742110, 14.34966873604972548, 107.0844237280190043 ) ) ;
#139115=CARTESIAN_POINT ( 'NONE',  ( 16.55341960407611168, 4.379528057220329451, 48.95724293864770971 ) ) ;
#139116=CARTESIAN_POINT ( 'NONE',  ( 0.05219959533909260263, 19.03943276465977164, 54.99890960531435979 ) ) ;
#139117=CARTESIAN_POINT ( 'NONE',  ( 0.05219959533937995610, -21.53943276465977519, 95.00109039468568994 ) ) ;
#139118=CARTESIAN_POINT ( 'NONE',  ( -0.05219959533907301413, -21.53943276465977519, 112.4989096053143669 ) ) ;
#139119=CARTESIAN_POINT ( 'NONE',  ( 21.53943276465977519, 0.05219959533937863772, 66.25109039468567573 ) ) ;
#139120=CARTESIAN_POINT ( 'NONE',  ( -12.06949235617739369, -12.14591786802326823, 54.37609039468568994 ) ) ;
#139121=CARTESIAN_POINT ( 'NONE',  ( -4.379528057220328563, 16.55341960407611168, 80.20724293864769550 ) ) ;
#139122=CARTESIAN_POINT ( 'NONE',  ( 15.80617190586769283, -15.72974639402175789, 105.6260903946856899 ) ) ;
#139123=CARTESIAN_POINT ( 'NONE',  ( 4.483927247898545687, 16.52544592524342804, 24.79057627198103120 ) ) ;
#139125=CARTESIAN_POINT ( 'NONE',  ( -16.55341960407617563, 4.379528057220093196, 33.54275706135234714 ) ) ;
#139126=CARTESIAN_POINT ( 'NONE',  ( -16.52544592524342804, 4.483927247898546575, 41.04057627198103120 ) ) ;
#139127=CARTESIAN_POINT ( 'NONE',  ( 16.52544592524335698, 4.483927247898782831, 81.45942372801900433 ) ) ;
#139128=CARTESIAN_POINT ( 'NONE',  ( -19.02544592524342804, 5.153800228976336051, 96.04057627198103830 ) ) ;
#139129=CARTESIAN_POINT ( 'NONE',  ( -19.05341960407611168, -5.049401038298163336, 111.4572429386476671 ) ) ;
#139130=CARTESIAN_POINT ( 'NONE',  ( 18.62759615963255655, 10.81492255796105972, 96.66775706135234714 ) ) ;
#139131=CARTESIAN_POINT ( 'NONE',  ( -12.06949235617739369, -12.14591786802326823, 104.3760903946856899 ) ) ;
#139132=CARTESIAN_POINT ( 'NONE',  ( -0.05219959533910754901, -16.53943276465976808, 77.49890960531433848 ) ) ;
#139133=CARTESIAN_POINT ( 'NONE',  ( -16.51473224551069308, -9.474510206698971260, 76.66557627198103830 ) ) ;
#139135=CARTESIAN_POINT ( 'NONE',  ( 0.05219959533934541429, -16.53943276465976808, 30.00109039468568284 ) ) ;
#139136=CARTESIAN_POINT ( 'NONE',  ( -19.02544592524342804, 5.153800228976336051, 26.04057627198103120 ) ) ;
#139137=CARTESIAN_POINT ( 'NONE',  ( 16.46253265017160672, -9.564922557960803928, 88.33224293864769550 ) ) ;
#139138=CARTESIAN_POINT ( 'NONE',  ( -16.55341960407617563, 4.379528057220093196, 38.54275706135234714 ) ) ;
#139139=CARTESIAN_POINT ( 'NONE',  ( 18.09918380851992481, 5.500000000000035527, 68.98618307335613054 ) ) ;
#139140=CARTESIAN_POINT ( 'NONE',  ( -19.02544592524334988, -5.153800228976617603, 33.95942372801897591 ) ) ;
#139141=CARTESIAN_POINT ( 'NONE',  ( -4.483927247898782831, 16.52544592524335698, 97.70942372801904696 ) ) ;
#139142=CARTESIAN_POINT ( 'NONE',  ( -19.05341960407611168, -5.049401038298163336, 31.45724293864769550 ) ) ;
#139143=CARTESIAN_POINT ( 'NONE',  ( -12.06949235617739369, -12.14591786802326823, 74.37609039468568994 ) ) ;
#139144=CARTESIAN_POINT ( 'NONE',  ( 8.224510206698742110, 14.34966873604972548, 62.08442372801901143 ) ) ;
#139145=CARTESIAN_POINT ( 'NONE',  ( -19.02544592524334988, -5.153800228976617603, 83.95942372801901854 ) ) ;
#139146=CARTESIAN_POINT ( 'NONE',  ( -5.049401038297874678, -19.05341960407617918, 29.79275706135232227 ) ) ;
#139147=CARTESIAN_POINT ( 'NONE',  ( 19.02544592524343514, -5.153800228976328945, 43.54057627198103120 ) ) ;
#139148=CARTESIAN_POINT ( 'NONE',  ( -4.379528057220328563, 16.55341960407611168, 85.20724293864770971 ) ) ;
#139149=CARTESIAN_POINT ( 'NONE',  ( 9.564922557961047289, -16.46253265017146816, 50.41775706135233293 ) ) ;
#139150=CARTESIAN_POINT ( 'NONE',  ( 18.62759615963271287, -10.81492255796078972, 48.33224293864770260 ) ) ;
#139151=CARTESIAN_POINT ( 'NONE',  ( -19.02544592524334988, -5.153800228976617603, 33.95942372801897591 ) ) ;
#139152=CARTESIAN_POINT ( 'NONE',  ( 19.05341960407611168, 5.049401038298154454, 98.95724293864766707 ) ) ;
#139153=CARTESIAN_POINT ( 'NONE',  ( -18.67979575497178146, -10.72451020669898902, 76.66557627198103830 ) ) ;
#139154=FACE_OUTER_BOUND ( 'NONE', #89946, .T. ) ;
#139155=CARTESIAN_POINT ( 'NONE',  ( -16.51473224551082808, 9.474510206698731452, 93.33442372801900433 ) ) ;
#139157=EDGE_CURVE ( 'NONE', #91492, #147765, #24122, .T. ) ;
#139158=CARTESIAN_POINT ( 'NONE',  ( 16.46253265017146816, 9.564922557961045513, 111.6677570613523329 ) ) ;
#139159=CARTESIAN_POINT ( 'NONE',  ( 5.153800228976335163, 19.02544592524342804, 39.79057627198100988 ) ) ;
#139160=CARTESIAN_POINT ( 'NONE',  ( -9.564922557960796823, -16.46253265017161027, 102.0822429386477097 ) ) ;
#139161=CARTESIAN_POINT ( 'NONE',  ( -15.80617190586745835, -15.72974639402198527, 71.87390960531438111 ) ) ;
#139162=CARTESIAN_POINT ( 'NONE',  ( 14.34966873604972726, -8.224510206698740333, 50.83442372801901143 ) ) ;
#139163=CARTESIAN_POINT ( 'NONE',  ( -21.55341960407619339, 5.719274019375674811, 43.54275706135235424 ) ) ;
#139164=CARTESIAN_POINT ( 'NONE',  ( -5.049401038297874678, -19.05341960407617918, 94.79275706135230450 ) ) ;
#139165=CARTESIAN_POINT ( 'NONE',  ( -15.80617190586768217, 15.72974639402176855, 108.1260903946856757 ) ) ;
#139166=CARTESIAN_POINT ( 'NONE',  ( 16.55341960407618274, -4.379528057220086978, 106.0427570613523471 ) ) ;
#139167=CARTESIAN_POINT ( 'NONE',  ( 5.153800228976335163, 19.02544592524342804, 99.79057627198102409 ) ) ;
#139168=CARTESIAN_POINT ( 'NONE',  ( 8.224510206698953496, -14.34966873604960469, 92.91557627198103830 ) ) ;
#139169=CARTESIAN_POINT ( 'NONE',  ( 14.34966873604960469, 8.224510206698951720, 39.16557627198102409 ) ) ;
#139170=CARTESIAN_POINT ( 'NONE',  ( 16.46253265017146816, 9.564922557961045513, 86.66775706135233293 ) ) ;
#139171=CARTESIAN_POINT ( 'NONE',  ( -15.80617190586768217, 15.72974639402176855, 58.12609039468568994 ) ) ;
#139172=CARTESIAN_POINT ( 'NONE',  ( 9.474510206698729675, 16.51473224551082808, 32.08442372801900433 ) ) ;
#139174=CARTESIAN_POINT ( 'NONE',  ( -16.55341960407611168, -4.379528057220339221, 111.4572429386476813 ) ) ;
#139175=CARTESIAN_POINT ( 'NONE',  ( -5.719274019375978568, 21.55341960407610458, 25.20724293864769550 ) ) ;
#139176=CARTESIAN_POINT ( 'NONE',  ( 12.06949235617757843, -12.14591786802309237, 28.12390960531435979 ) ) ;
#139177=CARTESIAN_POINT ( 'NONE',  ( 0.05219959533937995610, -21.53943276465977519, 105.0010903946856757 ) ) ;
#139178=CARTESIAN_POINT ( 'NONE',  ( 12.06949235617739724, 12.14591786802326823, 56.87609039468568994 ) ) ;
#139179=CARTESIAN_POINT ( 'NONE',  ( 16.55341960407611168, 4.379528057220329451, 28.95724293864769905 ) ) ;
#139180=CARTESIAN_POINT ( 'NONE',  ( -0.05219959533937732626, 21.53943276465977519, 57.50109039468568994 ) ) ;
#139181=CARTESIAN_POINT ( 'NONE',  ( 15.72974639402176855, 15.80617190586768217, 51.87609039468568284 ) ) ;
#139183=EDGE_LOOP ( 'NONE', ( #135294, #41309, #121667, #68605, #164343, #116610, #56975, #110468 ) ) ;
#139184=CARTESIAN_POINT ( 'NONE',  ( -17.59860650958989936, -7.585241751807033417, 61.57662985737508876 ) ) ;
#139185=CARTESIAN_POINT ( 'NONE',  ( 21.52544592524334988, 5.823673210054432836, 26.45942372801901854 ) ) ;
#139186=CARTESIAN_POINT ( 'NONE',  ( -4.483927247898539470, -16.52544592524342804, 102.2905762719810383 ) ) ;
#139187=CARTESIAN_POINT ( 'NONE',  ( 19.03943276465977164, -0.05219959533909143690, 23.74890960531435269 ) ) ;
#139188=CARTESIAN_POINT ( 'NONE',  ( -12.06949235617756955, 12.14591786802309770, 85.62390960531436690 ) ) ;
#139189=CARTESIAN_POINT ( 'NONE',  ( 13.89961937509977652, -13.97604488694527269, 68.12390960531436690 ) ) ;
#139190=CARTESIAN_POINT ( 'NONE',  ( -12.06949235617756955, 12.14591786802309770, 25.62390960531435624 ) ) ;
#139191=CARTESIAN_POINT ( 'NONE',  ( -0.05219959533907301413, -21.53943276465977519, 52.49890960531435979 ) ) ;
#139192=CARTESIAN_POINT ( 'NONE',  ( -16.53943276465976808, 0.05219959533911058130, 91.24890960531436690 ) ) ;
#139193=CARTESIAN_POINT ( 'NONE',  ( -5.823673210054116645, -21.52544592524344225, 92.29057627198103830 ) ) ;
#139194=CARTESIAN_POINT ( 'NONE',  ( 0.05219959533909260263, 19.03943276465977164, 104.9989096053143669 ) ) ;
#139195=CARTESIAN_POINT ( 'NONE',  ( -5.153800228976328057, -19.02544592524343514, 47.29057627198102409 ) ) ;
#139196=CARTESIAN_POINT ( 'NONE',  ( 9.474510206698729675, 16.51473224551082808, 112.0844237280190043 ) ) ;
#139197=CARTESIAN_POINT ( 'NONE',  ( -5.823673210054116645, -21.52544592524344225, 42.29057627198103120 ) ) ;
#139198=CARTESIAN_POINT ( 'NONE',  ( 18.62759615963255655, 10.81492255796105972, 76.66775706135234714 ) ) ;
#139199=CARTESIAN_POINT ( 'NONE',  ( 19.05341960407611168, 5.049401038298154454, 63.95724293864769550 ) ) ;
#139200=CARTESIAN_POINT ( 'NONE',  ( -19.02544592524342804, 5.153800228976336051, 101.0405762719810241 ) ) ;
#139201=CARTESIAN_POINT ( 'NONE',  ( 16.55341960407618274, -4.379528057220086978, 81.04275706135236135 ) ) ;
#139202=CARTESIAN_POINT ( 'NONE',  ( -0.05219959533937732626, 21.53943276465977519, 62.50109039468568284 ) ) ;
#139203=CARTESIAN_POINT ( 'NONE',  ( 15.80617190586769283, -15.72974639402175789, 90.62609039468567573 ) ) ;
#139204=CARTESIAN_POINT ( 'NONE',  ( -5.719274019375978568, 21.55341960407610458, 110.2072429386477239 ) ) ;
#139205=CARTESIAN_POINT ( 'NONE',  ( -18.62759615963255300, -10.81492255796106328, 39.16775706135235424 ) ) ;
#139206=CARTESIAN_POINT ( 'NONE',  ( -12.06949235617739369, -12.14591786802326823, 84.37609039468570415 ) ) ;
#139207=CARTESIAN_POINT ( 'NONE',  ( -10.72451020669898014, 18.67979575497178502, 80.41557627198103830 ) ) ;
#139208=CARTESIAN_POINT ( 'NONE',  ( -13.89961937509957401, -13.97604488694547875, 34.37609039468566863 ) ) ;
#139209=CARTESIAN_POINT ( 'NONE',  ( 21.53943276465977519, -0.05219959533907433946, 43.74890960531435979 ) ) ;
#139210=CARTESIAN_POINT ( 'NONE',  ( 16.46253265017160672, -9.564922557960803928, 83.33224293864768129 ) ) ;
#139211=CARTESIAN_POINT ( 'NONE',  ( -14.29746914071049879, 8.314922557960819915, 25.83224293864769194 ) ) ;
#139212=CARTESIAN_POINT ( 'NONE',  ( -17.48847506799968343, 5.747544572773785276, 65.82697437843285115 ) ) ;
#139213=CARTESIAN_POINT ( 'NONE',  ( -0.05219959533909027116, -19.03943276465977164, 107.4989096053143527 ) ) ;
#139215=CARTESIAN_POINT ( 'NONE',  ( 9.474510206698729675, 16.51473224551082808, 97.08442372801900433 ) ) ;
#139216=CARTESIAN_POINT ( 'NONE',  ( 0.05219959533907565091, 21.53943276465977519, 69.99890960531435269 ) ) ;
#139217=CARTESIAN_POINT ( 'NONE',  ( -14.29746914071049879, 8.314922557960819915, 40.83224293864769550 ) ) ;
#139218=CARTESIAN_POINT ( 'NONE',  ( 5.049401038297881783, 19.05341960407617563, 112.2927570613523471 ) ) ;
#139219=CARTESIAN_POINT ( 'NONE',  ( 9.474510206698971260, -16.51473224551069308, 32.91557627198102409 ) ) ;
#139220=CARTESIAN_POINT ( 'NONE',  ( 5.049401038297881783, 19.05341960407617563, 107.2927570613523187 ) ) ;
#139221=CARTESIAN_POINT ( 'NONE',  ( -21.52544592524343514, 5.823673210054127303, 101.0405762719810383 ) ) ;
#139222=CARTESIAN_POINT ( 'NONE',  ( 0.05219959533936267826, -19.03943276465977164, 65.00109039468567573 ) ) ;
#139223=CARTESIAN_POINT ( 'NONE',  ( 14.29746914071037800, 8.314922557961029526, 76.66775706135234714 ) ) ;
#139224=CARTESIAN_POINT ( 'NONE',  ( -19.03943276465977164, 0.05219959533909376836, 81.24890960531436690 ) ) ;
#139225=CARTESIAN_POINT ( 'NONE',  ( 16.53943276465976808, -0.05219959533910856209, 78.74890960531436690 ) ) ;
#139226=CARTESIAN_POINT ( 'NONE',  ( -5.153800228976328057, -19.02544592524343514, 67.29057627198102409 ) ) ;
#139227=CARTESIAN_POINT ( 'NONE',  ( 8.314922557960818139, 14.29746914071049879, 69.58224293864769550 ) ) ;
#139228=CARTESIAN_POINT ( 'NONE',  ( -19.05341960407611168, -5.049401038298163336, 31.45724293864769550 ) ) ;
#139230=CARTESIAN_POINT ( 'NONE',  ( -14.29746914071049879, 8.314922557960819915, 40.83224293864769550 ) ) ;
#139231=CARTESIAN_POINT ( 'NONE',  ( 13.89961937509977652, -13.97604488694527269, 78.12390960531433848 ) ) ;
#139233=CARTESIAN_POINT ( 'NONE',  ( 19.05341960407617918, -5.049401038297876454, 46.04275706135233293 ) ) ;
#139234=CARTESIAN_POINT ( 'NONE',  ( 14.34966873604972726, -8.224510206698740333, 60.83442372801901854 ) ) ;
#139235=CARTESIAN_POINT ( 'NONE',  ( 5.719274019375991003, -21.55341960407610458, 57.70724293864770260 ) ) ;
#139236=CARTESIAN_POINT ( 'NONE',  ( -16.51473224551082808, 9.474510206698731452, 23.33442372801900078 ) ) ;
#139237=CARTESIAN_POINT ( 'NONE',  ( -5.049401038298153566, 19.05341960407611168, 90.20724293864766707 ) ) ;
#139239=CARTESIAN_POINT ( 'NONE',  ( -21.55341960407610458, -5.719274019375992779, 26.45724293864768839 ) ) ;
#139240=CARTESIAN_POINT ( 'NONE',  ( -16.46253265017160317, 9.564922557960807481, 60.83224293864769550 ) ) ;
#139241=CARTESIAN_POINT ( 'NONE',  ( 18.62759615963255655, 10.81492255796105972, 56.66775706135235424 ) ) ;
#139242=CARTESIAN_POINT ( 'NONE',  ( -16.52544592524342804, 4.483927247898546575, 111.0405762719810525 ) ) ;
#139243=CARTESIAN_POINT ( 'NONE',  ( 21.55341960407610458, 5.719274019375980345, 103.9572429386476813 ) ) ;
#139244=CARTESIAN_POINT ( 'NONE',  ( 9.474510206698971260, -16.51473224551069308, 92.91557627198103830 ) ) ;
#139245=VERTEX_POINT ( 'NONE', #187732 ) ;
#139246=CARTESIAN_POINT ( 'NONE',  ( 0.05219959533937995610, -21.53943276465977519, 40.00109039468567573 ) ) ;
#139248=CARTESIAN_POINT ( 'NONE',  ( -13.89961937509977652, 13.97604488694528158, 90.62390960531432427 ) ) ;
#139249=CARTESIAN_POINT ( 'NONE',  ( 18.56197773271728479, -5.500000000000079048, 81.05066217314454491 ) ) ;
#139250=CARTESIAN_POINT ( 'NONE',  ( 18.62759615963271287, -10.81492255796078972, 88.33224293864769550 ) ) ;
#139251=CARTESIAN_POINT ( 'NONE',  ( -19.02544592524342804, 5.153800228976336051, 51.04057627198103120 ) ) ;
#139252=CARTESIAN_POINT ( 'NONE',  ( 0.05219959533934541429, -16.53943276465976808, 20.00109039468568639 ) ) ;
#139254=CARTESIAN_POINT ( 'NONE',  ( -9.474510206698964154, 16.51473224551069663, 30.41557627198102054 ) ) ;
#139255=CARTESIAN_POINT ( 'NONE',  ( -21.53943276465977519, -0.05219959533937600094, 83.75109039468568994 ) ) ;
#139256=CARTESIAN_POINT ( 'NONE',  ( -5.153800228976328057, -19.02544592524343514, 72.29057627198102409 ) ) ;
#139257=CARTESIAN_POINT ( 'NONE',  ( -15.80617190586768217, 15.72974639402176855, 48.12609039468568284 ) ) ;
#139258=CARTESIAN_POINT ( 'NONE',  ( 0.05219959533937995610, -21.53943276465977519, 25.00109039468567218 ) ) ;
#139260=CARTESIAN_POINT ( 'NONE',  ( 9.474510206698971260, -16.51473224551069308, 92.91557627198103830 ) ) ;
#139261=CARTESIAN_POINT ( 'NONE',  ( 18.22780087662121673, 5.500000000000056843, 63.98459894673894155 ) ) ;
#139262=CARTESIAN_POINT ( 'NONE',  ( -12.14591786802326823, 12.06949235617739902, 33.12609039468569705 ) ) ;
#139263=CARTESIAN_POINT ( 'NONE',  ( 14.29746914071037800, 8.314922557961029526, 66.66775706135234714 ) ) ;
#139264=CARTESIAN_POINT ( 'NONE',  ( 0.05219959533937995610, -21.53943276465977519, 45.00109039468568284 ) ) ;
#139265=CARTESIAN_POINT ( 'NONE',  ( 18.67979575497194134, -10.72451020669871369, 80.83442372801901854 ) ) ;
#139267=CARTESIAN_POINT ( 'NONE',  ( 9.564922557961047289, -16.46253265017146816, 110.4177570613523471 ) ) ;
#139268=CARTESIAN_POINT ( 'NONE',  ( -5.049401038298153566, 19.05341960407611168, 60.20724293864768129 ) ) ;
#139269=CARTESIAN_POINT ( 'NONE',  ( 19.05341960407611168, 5.049401038298154454, 98.95724293864766707 ) ) ;
#139270=CARTESIAN_POINT ( 'NONE',  ( 4.379528057220339221, -16.55341960407611168, 112.7072429386476955 ) ) ;
#139271=CARTESIAN_POINT ( 'NONE',  ( 0.05219959533910956823, 16.53943276465976808, 99.99890960531436690 ) ) ;
#139272=CARTESIAN_POINT ( 'NONE',  ( 15.72974639402199770, -15.80617190586745480, 33.12390960531435979 ) ) ;
#139273=CARTESIAN_POINT ( 'NONE',  ( 0.05219959533934541429, -16.53943276465976808, 85.00109039468568994 ) ) ;
#139274=CARTESIAN_POINT ( 'NONE',  ( 14.34966873604960469, 8.224510206698951720, 69.16557627198102409 ) ) ;
#139275=CARTESIAN_POINT ( 'NONE',  ( 9.564922557960805705, 16.46253265017160317, 59.58224293864769550 ) ) ;
#139276=CARTESIAN_POINT ( 'NONE',  ( -5.823673210054431948, 21.52544592524334988, 72.70942372801901854 ) ) ;
#139277=CARTESIAN_POINT ( 'NONE',  ( 21.53943276465977519, 0.05219959533937863772, 71.25109039468568994 ) ) ;
#139278=CARTESIAN_POINT ( 'NONE',  ( -13.89961937509957401, -13.97604488694547875, 109.3760903946856331 ) ) ;
#139279=CARTESIAN_POINT ( 'NONE',  ( -12.14591786802309592, -12.06949235617757132, 71.87390960531438111 ) ) ;
#139280=CARTESIAN_POINT ( 'NONE',  ( -18.67979575497193778, 10.72451020669871902, 23.33442372801901499 ) ) ;
#139281=CARTESIAN_POINT ( 'NONE',  ( -21.52544592524343514, 5.823673210054127303, 56.04057627198102409 ) ) ;
#139282=CARTESIAN_POINT ( 'NONE',  ( -17.40861289039000326, -6.110651285853326620, 106.3723247082743057 ) ) ;
#139284=CARTESIAN_POINT ( 'NONE',  ( 9.564922557960805705, 16.46253265017160317, 74.58224293864769550 ) ) ;
#139285=CARTESIAN_POINT ( 'NONE',  ( 4.379528057220339221, -16.55341960407611168, 52.70724293864769550 ) ) ;
#139286=CARTESIAN_POINT ( 'NONE',  ( -12.14591786802309592, -12.06949235617757132, 26.87390960531435979 ) ) ;
#139287=CARTESIAN_POINT ( 'NONE',  ( 16.55341960407618274, -4.379528057220086978, 91.04275706135236135 ) ) ;
#139288=CARTESIAN_POINT ( 'NONE',  ( -19.05341960407617563, 5.049401038297882671, 53.54275706135231871 ) ) ;
#139290=CARTESIAN_POINT ( 'NONE',  ( -19.05341960407611168, -5.049401038298163336, 106.4572429386476955 ) ) ;
#139291=CARTESIAN_POINT ( 'NONE',  ( 8.314922557960818139, 14.29746914071049879, 79.58224293864769550 ) ) ;
#139292=CARTESIAN_POINT ( 'NONE',  ( -13.89961937509957401, -13.97604488694547875, 44.37609039468566863 ) ) ;
#139293=CARTESIAN_POINT ( 'NONE',  ( -5.049401038298153566, 19.05341960407611168, 35.20724293864768839 ) ) ;
#139294=CARTESIAN_POINT ( 'NONE',  ( 21.52544592524344225, -5.823673210054117533, 33.54057627198102409 ) ) ;
#139295=CARTESIAN_POINT ( 'NONE',  ( 0.05219959533907565091, 21.53943276465977519, 54.99890960531435269 ) ) ;
#139296=CARTESIAN_POINT ( 'NONE',  ( -4.379528057220328563, 16.55341960407611168, 100.2072429386476955 ) ) ;
#139297=CARTESIAN_POINT ( 'NONE',  ( 8.224510206698742110, 14.34966873604972548, 57.08442372801901854 ) ) ;
#139298=CARTESIAN_POINT ( 'NONE',  ( 16.52544592524342804, -4.483927247898539470, 93.54057627198103830 ) ) ;
#139300=CARTESIAN_POINT ( 'NONE',  ( -17.05587630539785948, 6.762274262135695047, 50.74180309037313208 ) ) ;
#139301=CARTESIAN_POINT ( 'NONE',  ( -15.80617190586745835, -15.72974639402198527, 31.87390960531435979 ) ) ;
#139304=CARTESIAN_POINT ( 'NONE',  ( 16.52544592524335698, 4.483927247898782831, 41.45942372801901143 ) ) ;
#139305=CARTESIAN_POINT ( 'NONE',  ( -14.29746914071049879, 8.314922557960819915, 25.83224293864769194 ) ) ;
#139306=CARTESIAN_POINT ( 'NONE',  ( 10.72451020669898902, -18.67979575497178502, 52.91557627198103830 ) ) ;
#139307=CARTESIAN_POINT ( 'NONE',  ( 13.89961937509957401, 13.97604488694547697, 86.87609039468567573 ) ) ;
#139308=CARTESIAN_POINT ( 'NONE',  ( 21.53943276465977519, -0.05219959533907433946, 58.74890960531436690 ) ) ;
#139309=CARTESIAN_POINT ( 'NONE',  ( -15.80617190586768217, 15.72974639402176855, 83.12609039468568994 ) ) ;
#139311=CARTESIAN_POINT ( 'NONE',  ( 8.224510206698742110, 14.34966873604972548, 42.08442372801901854 ) ) ;
#139312=CARTESIAN_POINT ( 'NONE',  ( -19.02544592524342804, 5.153800228976336051, 31.04057627198102409 ) ) ;
#139313=CARTESIAN_POINT ( 'NONE',  ( 19.02544592524343514, -5.153800228976328945, 103.5405762719809957 ) ) ;
#139314=CARTESIAN_POINT ( 'NONE',  ( -9.474510206698964154, 16.51473224551069663, 30.41557627198102054 ) ) ;
#139315=CARTESIAN_POINT ( 'NONE',  ( -8.224510206698948167, 14.34966873604960824, 95.41557627198102409 ) ) ;
#139318=CARTESIAN_POINT ( 'NONE',  ( 12.14591786802327356, -12.06949235617739191, 75.62609039468567573 ) ) ;
#139319=CARTESIAN_POINT ( 'NONE',  ( 5.823673210054125526, 21.52544592524343514, 89.79057627198103830 ) ) ;
#139320=CARTESIAN_POINT ( 'NONE',  ( -19.05341960407611168, -5.049401038298163336, 56.45724293864768129 ) ) ;
#139321=CARTESIAN_POINT ( 'NONE',  ( 5.719274019375673035, 21.55341960407619339, 22.29275706135235069 ) ) ;
#139322=CARTESIAN_POINT ( 'NONE',  ( -9.564922557960796823, -16.46253265017161027, 87.08224293864769550 ) ) ;
#139326=CARTESIAN_POINT ( 'NONE',  ( 10.81492255796106328, -18.62759615963255655, 25.41775706135235779 ) ) ;
#139327=CARTESIAN_POINT ( 'NONE',  ( -13.89961937509977652, 13.97604488694528158, 30.62390960531435269 ) ) ;
#139328=CARTESIAN_POINT ( 'NONE',  ( -5.153800228976328057, -19.02544592524343514, 107.2905762719810383 ) ) ;
#139329=CARTESIAN_POINT ( 'NONE',  ( 13.97604488694548053, -13.89961937509957401, 75.62609039468564731 ) ) ;
#139330=CARTESIAN_POINT ( 'NONE',  ( -5.153800228976607833, 19.02544592524334988, 32.70942372801899722 ) ) ;
#139331=CARTESIAN_POINT ( 'NONE',  ( -18.67979575497178146, -10.72451020669898902, 106.6655762719810383 ) ) ;
#139332=CARTESIAN_POINT ( 'NONE',  ( 5.153800228976615827, -19.02544592524334988, 35.20942372801899722 ) ) ;
#139333=CARTESIAN_POINT ( 'NONE',  ( -16.53943276465976808, -0.05219959533934237506, 78.75109039468568994 ) ) ;
#139334=CARTESIAN_POINT ( 'NONE',  ( 19.05341960407611168, 5.049401038298154454, 103.9572429386476671 ) ) ;
#139335=CARTESIAN_POINT ( 'NONE',  ( 9.474510206698971260, -16.51473224551069308, 52.91557627198102409 ) ) ;
#139336=CARTESIAN_POINT ( 'NONE',  ( -5.719274019375665041, -21.55341960407619695, 59.79275706135234714 ) ) ;
#139337=CARTESIAN_POINT ( 'NONE',  ( 21.53943276465977519, 0.05219959533937863772, 76.25109039468568994 ) ) ;
#139338=CARTESIAN_POINT ( 'NONE',  ( 19.05341960407611168, 5.049401038298154454, 68.95724293864769550 ) ) ;
#139339=CARTESIAN_POINT ( 'NONE',  ( 18.67979575497194134, -10.72451020669871369, 50.83442372801901143 ) ) ;
#139340=CARTESIAN_POINT ( 'NONE',  ( -16.51473224551082808, 9.474510206698731452, 88.33442372801900433 ) ) ;
#139341=CARTESIAN_POINT ( 'NONE',  ( 9.474510206698971260, -16.51473224551069308, 47.91557627198102409 ) ) ;
#139342=CARTESIAN_POINT ( 'NONE',  ( -5.153800228976328057, -19.02544592524343514, 102.2905762719810383 ) ) ;
#139343=CARTESIAN_POINT ( 'NONE',  ( -5.153800228976328057, -19.02544592524343514, 62.29057627198100988 ) ) ;
#139344=CARTESIAN_POINT ( 'NONE',  ( 5.153800228976335163, 19.02544592524342804, 109.7905762719810099 ) ) ;
#139345=CARTESIAN_POINT ( 'NONE',  ( -5.049401038298153566, 19.05341960407611168, 55.20724293864769550 ) ) ;
#139346=CARTESIAN_POINT ( 'NONE',  ( -10.72451020669898014, 18.67979575497178502, 100.4155762719810241 ) ) ;
#139347=CARTESIAN_POINT ( 'NONE',  ( 4.379528057220092307, 16.55341960407617563, 77.29275706135234714 ) ) ;
#139349=CARTESIAN_POINT ( 'NONE',  ( 9.564922557961047289, -16.46253265017146816, 40.41775706135234003 ) ) ;
#139350=CARTESIAN_POINT ( 'NONE',  ( 13.97604488694527802, 13.89961937509977652, 64.37390960531436690 ) ) ;
#139351=CARTESIAN_POINT ( 'NONE',  ( -14.29746914071049879, 8.314922557960819915, 60.83224293864769550 ) ) ;
#139352=CARTESIAN_POINT ( 'NONE',  ( 8.314922557960818139, 14.29746914071049879, 89.58224293864768129 ) ) ;
#139353=CARTESIAN_POINT ( 'NONE',  ( 5.153800228976335163, 19.02544592524342804, 114.7905762719810241 ) ) ;
#139354=CARTESIAN_POINT ( 'NONE',  ( -9.564922557960796823, -16.46253265017161027, 87.08224293864769550 ) ) ;
#139355=CARTESIAN_POINT ( 'NONE',  ( 9.564922557960805705, 16.46253265017160317, 109.5822429386476955 ) ) ;
#139356=CARTESIAN_POINT ( 'NONE',  ( 10.72451020669871369, 18.67979575497193778, 107.0844237280190043 ) ) ;
#139357=CARTESIAN_POINT ( 'NONE',  ( 12.06949235617739724, 12.14591786802326823, 91.87609039468568994 ) ) ;
#139358=CARTESIAN_POINT ( 'NONE',  ( -13.97604488694527625, -13.89961937509977652, 81.87390960531436690 ) ) ;
#139359=CARTESIAN_POINT ( 'NONE',  ( -21.53943276465977519, -0.05219959533937600094, 33.75109039468568284 ) ) ;
#139360=CARTESIAN_POINT ( 'NONE',  ( -15.72974639402197994, 15.80617190586746368, 35.62390960531437401 ) ) ;
#139361=CARTESIAN_POINT ( 'NONE',  ( 15.80617190586746368, 15.72974639402197994, 99.37390960531436690 ) ) ;
#139362=CARTESIAN_POINT ( 'NONE',  ( 0.05219959533910956823, 16.53943276465976808, 59.99890960531436690 ) ) ;
#139363=CARTESIAN_POINT ( 'NONE',  ( 5.049401038298161559, -19.05341960407611168, 52.70724293864767418 ) ) ;
#139364=CARTESIAN_POINT ( 'NONE',  ( 0.05219959533910956823, 16.53943276465976808, 84.99890960531436690 ) ) ;
#139365=CARTESIAN_POINT ( 'NONE',  ( -9.474510206698720793, -16.51473224551083518, 39.58442372801899722 ) ) ;
#139366=CARTESIAN_POINT ( 'NONE',  ( 13.97604488694527802, 13.89961937509977652, 24.37390960531435624 ) ) ;
#139367=CARTESIAN_POINT ( 'NONE',  ( 4.379528057220092307, 16.55341960407617563, 67.29275706135234714 ) ) ;
#139368=CARTESIAN_POINT ( 'NONE',  ( -5.049401038298153566, 19.05341960407611168, 75.20724293864769550 ) ) ;
#139370=CARTESIAN_POINT ( 'NONE',  ( 4.379528057220339221, -16.55341960407611168, 102.7072429386476955 ) ) ;
#139371=CARTESIAN_POINT ( 'NONE',  ( 16.55341960407618274, -4.379528057220086978, 101.0427570613523756 ) ) ;
#139372=CARTESIAN_POINT ( 'NONE',  ( -12.14591786802326823, 12.06949235617739902, 28.12609039468568284 ) ) ;
#139373=CARTESIAN_POINT ( 'NONE',  ( -5.719274019375665041, -21.55341960407619695, 89.79275706135236135 ) ) ;
#139374=CARTESIAN_POINT ( 'NONE',  ( 9.564922557960805705, 16.46253265017160317, 84.58224293864769550 ) ) ;
#139375=CARTESIAN_POINT ( 'NONE',  ( -18.62759615963255300, -10.81492255796106328, 19.16775706135234714 ) ) ;
#139376=CARTESIAN_POINT ( 'NONE',  ( -13.97604488694527625, -13.89961937509977652, 36.87390960531436690 ) ) ;
#139377=CARTESIAN_POINT ( 'NONE',  ( 4.483927247898790824, -16.52544592524335698, 25.20942372801901854 ) ) ;
#139378=CARTESIAN_POINT ( 'NONE',  ( 13.97604488694548053, -13.89961937509957401, 95.62609039468563310 ) ) ;
#139379=CARTESIAN_POINT ( 'NONE',  ( 15.80617190586746368, 15.72974639402197994, 94.37390960531436690 ) ) ;
#139380=CARTESIAN_POINT ( 'NONE',  ( 16.46253265017146816, 9.564922557961045513, 66.66775706135233293 ) ) ;
#139381=CARTESIAN_POINT ( 'NONE',  ( 19.02544592524343514, -5.153800228976328945, 23.54057627198102054 ) ) ;
#139382=CARTESIAN_POINT ( 'NONE',  ( 21.55341960407619695, -5.719274019375665929, 26.04275706135235779 ) ) ;
#139384=CARTESIAN_POINT ( 'NONE',  ( 13.89961937509977652, -13.97604488694527269, 88.12390960531438111 ) ) ;
#139385=CARTESIAN_POINT ( 'NONE',  ( 4.379528057220092307, 16.55341960407617563, 47.29275706135234003 ) ) ;
#139387=CARTESIAN_POINT ( 'NONE',  ( -19.02544592524334988, -5.153800228976617603, 53.95942372801898301 ) ) ;
#139388=CARTESIAN_POINT ( 'NONE',  ( -10.72451020669870658, -18.67979575497194134, 19.58442372801901143 ) ) ;
#139389=CARTESIAN_POINT ( 'NONE',  ( 8.314922557960818139, 14.29746914071049879, 74.58224293864768129 ) ) ;
#139390=CARTESIAN_POINT ( 'NONE',  ( 5.153800228976335163, 19.02544592524342804, 89.79057627198102409 ) ) ;
#139391=CARTESIAN_POINT ( 'NONE',  ( 16.52544592524335698, 4.483927247898782831, 56.45942372801902565 ) ) ;
#139392=CARTESIAN_POINT ( 'NONE',  ( 16.51473224551083163, -9.474510206698727899, 60.83442372801900433 ) ) ;
#139393=CARTESIAN_POINT ( 'NONE',  ( 15.72974639402176855, 15.80617190586768217, 71.87609039468568994 ) ) ;
#139394=CARTESIAN_POINT ( 'NONE',  ( -12.14591786802326823, 12.06949235617739902, 28.12609039468568284 ) ) ;
#139395=CARTESIAN_POINT ( 'NONE',  ( 9.564922557960805705, 16.46253265017160317, 69.58224293864770971 ) ) ;
#139396=CARTESIAN_POINT ( 'NONE',  ( -19.03943276465977164, -0.05219959533935918106, 78.75109039468567573 ) ) ;
#139397=CARTESIAN_POINT ( 'NONE',  ( -4.379528057220086978, -16.55341960407618274, 59.79275706135234714 ) ) ;
#139398=CARTESIAN_POINT ( 'NONE',  ( -5.823673210054431948, 21.52544592524334988, 92.70942372801901854 ) ) ;
#139399=CARTESIAN_POINT ( 'NONE',  ( -19.02544592524334988, -5.153800228976617603, 68.95942372801896170 ) ) ;
#139400=CARTESIAN_POINT ( 'NONE',  ( 9.564922557960805705, 16.46253265017160317, 54.58224293864769550 ) ) ;
#139401=CARTESIAN_POINT ( 'NONE',  ( -10.81492255796078084, -18.62759615963271287, 72.08224293864769550 ) ) ;
#139402=CARTESIAN_POINT ( 'NONE',  ( -8.314922557960811034, -14.29746914071050412, 82.08224293864768129 ) ) ;
#139403=CARTESIAN_POINT ( 'NONE',  ( 9.564922557961047289, -16.46253265017146816, 80.41775706135234714 ) ) ;
#139404=CARTESIAN_POINT ( 'NONE',  ( -19.49671883438224640, -5.500000000000076383, 69.89279849105676590 ) ) ;
#139405=CARTESIAN_POINT ( 'NONE',  ( -13.89961937509957401, -13.97604488694547875, 44.37609039468566863 ) ) ;
#139406=CARTESIAN_POINT ( 'NONE',  ( -12.14591786802326823, 12.06949235617739902, 103.1260903946856757 ) ) ;
#139407=CARTESIAN_POINT ( 'NONE',  ( 8.224510206698953496, -14.34966873604960469, 67.91557627198102409 ) ) ;
#139408=CARTESIAN_POINT ( 'NONE',  ( -15.72974639402176322, -15.80617190586768395, 104.3760903946856899 ) ) ;
#139410=CARTESIAN_POINT ( 'NONE',  ( 15.72974639402199770, -15.80617190586745480, 103.1239096053143811 ) ) ;
#139411=CARTESIAN_POINT ( 'NONE',  ( 16.51473224551069308, 9.474510206698969483, 64.16557627198102409 ) ) ;
#139412=CARTESIAN_POINT ( 'NONE',  ( -21.53943276465977519, -0.05219959533937600094, 73.75109039468567573 ) ) ;
#139413=CARTESIAN_POINT ( 'NONE',  ( 0.05219959533909260263, 19.03943276465977164, 54.99890960531435979 ) ) ;
#139415=CARTESIAN_POINT ( 'NONE',  ( -5.153800228976328057, -19.02544592524343514, 22.29057627198102765 ) ) ;
#139416=CARTESIAN_POINT ( 'NONE',  ( 9.474510206698971260, -16.51473224551069308, 112.9155762719810383 ) ) ;
#139417=CARTESIAN_POINT ( 'NONE',  ( -16.55341960407611168, -4.379528057220339221, 66.45724293864768129 ) ) ;
#139418=CARTESIAN_POINT ( 'NONE',  ( 16.51473224551069308, 9.474510206698969483, 24.16557627198102765 ) ) ;
#139419=CARTESIAN_POINT ( 'NONE',  ( -12.06949235617756955, 12.14591786802309770, 90.62390960531436690 ) ) ;
#139420=CARTESIAN_POINT ( 'NONE',  ( -0.05219959533907301413, -21.53943276465977519, 92.49890960531436690 ) ) ;
#139421=CARTESIAN_POINT ( 'NONE',  ( 21.55341960407619695, -5.719274019375665929, 36.04275706135234714 ) ) ;
#139423=CARTESIAN_POINT ( 'NONE',  ( 0.05219959533934541429, -16.53943276465976808, 50.00109039468568994 ) ) ;
#139424=CARTESIAN_POINT ( 'NONE',  ( -15.72974639402197994, 15.80617190586746368, 100.6239096053143811 ) ) ;
#139425=CARTESIAN_POINT ( 'NONE',  ( -13.89961937509957401, -13.97604488694547875, 29.37609039468565797 ) ) ;
#139426=CARTESIAN_POINT ( 'NONE',  ( 5.153800228976335163, 19.02544592524342804, 109.7905762719810099 ) ) ;
#139427=CARTESIAN_POINT ( 'NONE',  ( -0.05219959533937732626, 21.53943276465977519, 47.50109039468568994 ) ) ;
#139428=CARTESIAN_POINT ( 'NONE',  ( -10.72451020669898014, 18.67979575497178502, 45.41557627198103830 ) ) ;
#139429=CARTESIAN_POINT ( 'NONE',  ( -4.483927247898539470, -16.52544592524342804, 27.29057627198103120 ) ) ;
#139431=CARTESIAN_POINT ( 'NONE',  ( 15.80617190586769283, -15.72974639402175789, 60.62609039468567573 ) ) ;
#139432=CARTESIAN_POINT ( 'NONE',  ( -10.81492255796105439, 18.62759615963255655, 102.9177570613523756 ) ) ;
#139433=CARTESIAN_POINT ( 'NONE',  ( 13.97604488694548053, -13.89961937509957401, 30.62609039468566863 ) ) ;
#139434=CARTESIAN_POINT ( 'NONE',  ( -8.314922557961024197, 14.29746914071037800, 92.91775706135236135 ) ) ;
#139435=CARTESIAN_POINT ( 'NONE',  ( 18.67979575497194134, -10.72451020669871369, 50.83442372801901143 ) ) ;
#139436=CARTESIAN_POINT ( 'NONE',  ( 16.51473224551069308, 9.474510206698969483, 49.16557627198102409 ) ) ;
#139437=CARTESIAN_POINT ( 'NONE',  ( -0.05219959533936034679, 19.03943276465977164, 27.50109039468566507 ) ) ;
#139438=CARTESIAN_POINT ( 'NONE',  ( 0.05219959533907565091, 21.53943276465977519, 24.99890960531435624 ) ) ;
#139439=CARTESIAN_POINT ( 'NONE',  ( -18.62759615963255300, -10.81492255796106328, 24.16775706135235424 ) ) ;
#139440=CARTESIAN_POINT ( 'NONE',  ( 15.80617190586746368, 15.72974639402197994, 74.37390960531436690 ) ) ;
#139441=CARTESIAN_POINT ( 'NONE',  ( 8.314922557961029526, -14.29746914071037800, 40.41775706135234714 ) ) ;
#139443=CARTESIAN_POINT ( 'NONE',  ( -15.72974639402197994, 15.80617190586746368, 75.62390960531439532 ) ) ;
#139444=CARTESIAN_POINT ( 'NONE',  ( -14.29746914071037622, -8.314922557961029526, 64.16775706135234714 ) ) ;
#139445=CARTESIAN_POINT ( 'NONE',  ( 14.34966873604960469, 8.224510206698951720, 59.16557627198103120 ) ) ;
#139447=CARTESIAN_POINT ( 'NONE',  ( -13.89961937509957401, -13.97604488694547875, 109.3760903946856331 ) ) ;
#139448=( BOUNDED_CURVE ( )  B_SPLINE_CURVE ( 2, ( #34657, #143817, #65982, #128641, #66981, #64993, #140836, #96316, #6297, #2324, #64006, #158002, #21478, #125676, #97296, #67976, #50829, #187374, #112486, #20474, #83138, #19494, #80156, #142820, #48843, #174179, #110497, #81139, #171190, #172179, #109508, #32679, #18508, #111496, #141827, #190335, #51812, #94332, #3320, #82124, #36632, #33664, #113471, #189352, #175166, #127652, #129630, #191325, #95326, #126651, #157011, #4300, #158982, #98289, #188354, #49832, #87152, #131658, #146819, #52803, #145812, #115494, #176173, #39643, #177182, #161990, #101304, #41661, #37643, #88140, #193340, #8314, #22485, #56826, #10325, #54814, #24498, #68979, #162993, #99306, #116489, #147840, #160991, #149825, #178178, #148835, #9326, #71981, #133656, #69990, #84133, #86150, #11330, #7295, #130644, #70991, #103324 ),
 .UNSPECIFIED., .F., .F. ) 
 B_SPLINE_CURVE_WITH_KNOTS ( ( 3, 2, 2, 2, 2, 2, 2, 2, 2, 2, 2, 2, 2, 2, 2, 2, 2, 2, 2, 2, 2, 2, 2, 2, 2, 2, 2, 2, 2, 2, 2, 2, 2, 2, 2, 2, 2, 2, 2, 2, 2, 2, 2, 2, 2, 2, 2, 2, 3 ),
 ( 0.7919498004596616791, 0.7938596491228070429, 0.7982456140350877583, 0.8026315789473684736, 0.8070175438596490780, 0.8114035087719297934, 0.8157894736842105088, 0.8201754385964912242, 0.8245614035087719396, 0.8289473684210526550, 0.8333333333333333703, 0.8377192982456140857, 0.8421052631578946901, 0.8464912280701754055, 0.8508771929824561209, 0.8552631578947368363, 0.8596491228070175517, 0.8640350877192982670, 0.8684210526315789824, 0.8728070175438596978, 0.8771929824561403022, 0.8815789473684210176, 0.8859649122807017330, 0.8903508771929824483, 0.8947368421052631637, 0.8991228070175438791, 0.9035087719298245945, 0.9078947368421053099, 0.9122807017543859143, 0.9166666666666666297, 0.9210526315789473450, 0.9254385964912280604, 0.9298245614035087758, 0.9342105263157894912, 0.9385964912280702066, 0.9429824561403509220, 0.9473684210526315264, 0.9517543859649122417, 0.9561403508771929571, 0.9605263157894736725, 0.9649122807017543879, 0.9692982456140351033, 0.9736842105263158187, 0.9780701754385965341, 0.9824561403508771384, 0.9868421052631578538, 0.9912280701754385692, 0.9956140350877192846, 1.000000000000000000 ),
 .UNSPECIFIED. ) 
 CURVE ( )  GEOMETRIC_REPRESENTATION_ITEM ( )  RATIONAL_B_SPLINE_CURVE ( ( 0.9832469066685285419, 0.9851625545550100060, 1.000000000000000000, 0.9659258262890683122, 1.000000000000000000, 0.9659258262890683122, 1.000000000000000000, 0.9659258262890683122, 1.000000000000000000, 0.9659258262890683122, 1.000000000000000000, 0.9659258262890683122, 1.000000000000000000, 0.9659258262890683122, 1.000000000000000000, 0.9659258262890683122, 1.000000000000000000, 0.9659258262890683122, 1.000000000000000000, 0.9659258262890683122, 1.000000000000000000, 0.9659258262890683122, 1.000000000000000000, 0.9659258262890683122, 1.000000000000000000, 0.9659258262890683122, 1.000000000000000000, 0.9659258262890683122, 1.000000000000000000, 0.9659258262890683122, 1.000000000000000000, 0.9659258262890683122, 1.000000000000000000, 0.9659258262890683122, 1.000000000000000000, 0.9659258262890683122, 1.000000000000000000, 0.9659258262890683122, 1.000000000000000000, 0.9659258262890683122, 1.000000000000000000, 0.9659258262890683122, 1.000000000000000000, 0.9659258262890683122, 1.000000000000000000, 0.9659258262890683122, 1.000000000000000000, 0.9659258262890683122, 1.000000000000000000, 0.9659258262890683122, 1.000000000000000000, 0.9659258262890683122, 1.000000000000000000, 0.9659258262890683122, 1.000000000000000000, 0.9659258262890683122, 1.000000000000000000, 0.9659258262890683122, 1.000000000000000000, 0.9659258262890683122, 1.000000000000000000, 0.9659258262890683122, 1.000000000000000000, 0.9659258262890683122, 1.000000000000000000, 0.9659258262890683122, 1.000000000000000000, 0.9659258262890683122, 1.000000000000000000, 0.9659258262890683122, 1.000000000000000000, 0.9659258262890683122, 1.000000000000000000, 0.9659258262890683122, 1.000000000000000000, 0.9659258262890683122, 1.000000000000000000, 0.9659258262890683122, 1.000000000000000000, 0.9659258262890683122, 1.000000000000000000, 0.9659258262890683122, 1.000000000000000000, 0.9659258262890683122, 1.000000000000000000, 0.9659258262890683122, 1.000000000000000000, 0.9659258262890683122, 1.000000000000000000, 0.9659258262890683122, 1.000000000000000000, 0.9659258262890683122, 1.000000000000000000, 0.9659258262890683122, 1.000000000000000000, 0.9659258262890683122, 1.000000000000000000 ) ) 
 REPRESENTATION_ITEM ( '' )  );
#139450=CARTESIAN_POINT ( 'NONE',  ( -14.34966873604972548, 8.224510206698743886, 38.33442372801900433 ) ) ;
#139451=CARTESIAN_POINT ( 'NONE',  ( -5.823673210054116645, -21.52544592524344225, 112.2905762719810241 ) ) ;
#139452=CARTESIAN_POINT ( 'NONE',  ( 5.719274019375991003, -21.55341960407610458, 32.70724293864770260 ) ) ;
#139453=CARTESIAN_POINT ( 'NONE',  ( 16.53943276465976808, 0.05219959533934440121, 51.25109039468568994 ) ) ;
#139454=CARTESIAN_POINT ( 'NONE',  ( -19.05341960407611168, -5.049401038298163336, 71.45724293864766707 ) ) ;
#139455=CARTESIAN_POINT ( 'NONE',  ( -10.81492255796105439, 18.62759615963255655, 42.91775706135235424 ) ) ;
#139456=CARTESIAN_POINT ( 'NONE',  ( 8.224510206698742110, 14.34966873604972548, 22.08442372801901143 ) ) ;
#139457=CARTESIAN_POINT ( 'NONE',  ( 21.53943276465977519, -0.05219959533907433946, 23.74890960531435269 ) ) ;
#139458=ORIENTED_EDGE ( 'NONE', *, *, #176553, .F. ) ;
#139459=CARTESIAN_POINT ( 'NONE',  ( -5.153800228976607833, 19.02544592524334988, 27.70942372801899722 ) ) ;
#139460=CARTESIAN_POINT ( 'NONE',  ( -8.224510206698735004, -14.34966873604973081, 44.58442372801901854 ) ) ;
#139461=CARTESIAN_POINT ( 'NONE',  ( -19.03943276465977164, 0.05219959533909376836, 106.2489096053143669 ) ) ;
#139462=CARTESIAN_POINT ( 'NONE',  ( -10.81492255796078084, -18.62759615963271287, 97.08224293864770971 ) ) ;
#139463=CARTESIAN_POINT ( 'NONE',  ( 16.51473224551069308, 9.474510206698969483, 69.16557627198102409 ) ) ;
#139465=CARTESIAN_POINT ( 'NONE',  ( 12.14591786802309770, 12.06949235617756955, 79.37390960531436690 ) ) ;
#139466=CARTESIAN_POINT ( 'NONE',  ( -13.97604488694527625, -13.89961937509977652, 111.8739096053143243 ) ) ;
#139467=CARTESIAN_POINT ( 'NONE',  ( -17.49999999999999645, 5.499999999999997335, 35.79690382534171533 ) ) ;
#139468=CARTESIAN_POINT ( 'NONE',  ( 0.05219959533934541429, -16.53943276465976808, 60.00109039468568284 ) ) ;
#139469=CARTESIAN_POINT ( 'NONE',  ( -15.80617190586745835, -15.72974639402198527, 101.8739096053143811 ) ) ;
#139470=CARTESIAN_POINT ( 'NONE',  ( -9.564922557961040184, 16.46253265017147172, 57.91775706135233293 ) ) ;
#139471=CARTESIAN_POINT ( 'NONE',  ( -10.81492255796078084, -18.62759615963271287, 27.08224293864769550 ) ) ;
#139472=CARTESIAN_POINT ( 'NONE',  ( 5.153800228976335163, 19.02544592524342804, 29.79057627198102409 ) ) ;
#139473=CARTESIAN_POINT ( 'NONE',  ( 5.719274019375991003, -21.55341960407610458, 72.70724293864769550 ) ) ;
#139474=CARTESIAN_POINT ( 'NONE',  ( -13.89961937509977652, 13.97604488694528158, 105.6239096053143527 ) ) ;
#139475=CARTESIAN_POINT ( 'NONE',  ( 15.72974639402176855, 15.80617190586768217, 91.87609039468568994 ) ) ;
#139476=CARTESIAN_POINT ( 'NONE',  ( -5.049401038298153566, 19.05341960407611168, 55.20724293864769550 ) ) ;
#139477=CARTESIAN_POINT ( 'NONE',  ( 14.29746914071037800, 8.314922557961029526, 31.66775706135234358 ) ) ;
#139478=CARTESIAN_POINT ( 'NONE',  ( -5.049401038298153566, 19.05341960407611168, 55.20724293864769550 ) ) ;
#139479=CARTESIAN_POINT ( 'NONE',  ( -10.72451020669870658, -18.67979575497194134, 74.58442372801901854 ) ) ;
#139481=CARTESIAN_POINT ( 'NONE',  ( 9.564922557961047289, -16.46253265017146816, 40.41775706135234003 ) ) ;
#139482=CARTESIAN_POINT ( 'NONE',  ( -5.049401038297874678, -19.05341960407617918, 44.79275706135232582 ) ) ;
#139483=CARTESIAN_POINT ( 'NONE',  ( 21.53943276465977519, 0.05219959533937863772, 41.25109039468568284 ) ) ;
#139485=CARTESIAN_POINT ( 'NONE',  ( 9.474510206698729675, 16.51473224551082808, 37.08442372801899722 ) ) ;
#139486=CARTESIAN_POINT ( 'NONE',  ( -5.153800228976328057, -19.02544592524343514, 82.29057627198103830 ) ) ;
#139487=CARTESIAN_POINT ( 'NONE',  ( -9.474510206698964154, 16.51473224551069663, 75.41557627198103830 ) ) ;
#139488=CARTESIAN_POINT ( 'NONE',  ( 12.14591786802309770, 12.06949235617756955, 24.37390960531435979 ) ) ;
#139489=CARTESIAN_POINT ( 'NONE',  ( -19.05341960407611168, -5.049401038298163336, 111.4572429386476671 ) ) ;
#139490=CARTESIAN_POINT ( 'NONE',  ( -18.67979575497193778, 10.72451020669871902, 83.33442372801903275 ) ) ;
#139492=CARTESIAN_POINT ( 'NONE',  ( 17.48847506799968343, 5.747544572773806593, 56.67302562156723411 ) ) ;
#139493=CARTESIAN_POINT ( 'NONE',  ( -15.80617190586768217, 15.72974639402176855, 98.12609039468570415 ) ) ;
#139495=CARTESIAN_POINT ( 'NONE',  ( -5.049401038298153566, 19.05341960407611168, 115.2072429386477097 ) ) ;
#139496=DIRECTION ( 'NONE',  ( -0.5150380737757255245, 1.049727191973305394E-16, -0.8571673013836856869 ) ) ;
#139497=CARTESIAN_POINT ( 'NONE',  ( -16.52544592524335698, -4.483927247898792601, 53.95942372801900433 ) ) ;
#139498=CARTESIAN_POINT ( 'NONE',  ( -21.52544592524343514, 5.823673210054127303, 76.04057627198102409 ) ) ;
#139499=CARTESIAN_POINT ( 'NONE',  ( -16.53943276465976808, 0.05219959533911058130, 21.24890960531436690 ) ) ;
#139500=CARTESIAN_POINT ( 'NONE',  ( 0.05219959533910956823, 16.53943276465976808, 114.9989096053143669 ) ) ;
#139501=CARTESIAN_POINT ( 'NONE',  ( 19.03943276465977164, -0.05219959533909143690, 88.74890960531436690 ) ) ;
#139502=CARTESIAN_POINT ( 'NONE',  ( -5.153800228976607833, 19.02544592524334988, 22.70942372801899012 ) ) ;
#139503=CARTESIAN_POINT ( 'NONE',  ( 19.02544592524343514, -5.153800228976328945, 23.54057627198102054 ) ) ;
#139504=CARTESIAN_POINT ( 'NONE',  ( 18.67979575497194134, -10.72451020669871369, 65.83442372801900433 ) ) ;
#139506=CARTESIAN_POINT ( 'NONE',  ( -8.224510206698735004, -14.34966873604973081, 109.5844237280190328 ) ) ;
#139507=CARTESIAN_POINT ( 'NONE',  ( 19.03943276465977164, 0.05219959533936151252, 66.25109039468567573 ) ) ;
#139509=CARTESIAN_POINT ( 'NONE',  ( -19.03943276465977164, 0.05219959533909376836, 106.2489096053143669 ) ) ;
#139510=CARTESIAN_POINT ( 'NONE',  ( 12.06949235617757843, -12.14591786802309237, 88.12390960531436690 ) ) ;
#139511=CARTESIAN_POINT ( 'NONE',  ( 16.46253265017146816, 9.564922557961045513, 51.66775706135233293 ) ) ;
#139512=CARTESIAN_POINT ( 'NONE',  ( 19.03943276465977164, -0.05219959533909143690, 78.74890960531436690 ) ) ;
#139513=CARTESIAN_POINT ( 'NONE',  ( 12.06949235617757843, -12.14591786802309237, 68.12390960531436690 ) ) ;
#139514=CARTESIAN_POINT ( 'NONE',  ( -16.51473224551082808, 9.474510206698731452, 88.33442372801900433 ) ) ;
#139515=CARTESIAN_POINT ( 'NONE',  ( 15.72974639402199770, -15.80617190586745480, 53.12390960531436690 ) ) ;
#139517=CARTESIAN_POINT ( 'NONE',  ( 12.14591786802309770, 12.06949235617756955, 109.3739096053143811 ) ) ;
#139518=CARTESIAN_POINT ( 'NONE',  ( 0.05219959533936267826, -19.03943276465977164, 100.0010903946856757 ) ) ;
#139519=CARTESIAN_POINT ( 'NONE',  ( -19.03943276465977164, 0.05219959533909376836, 76.24890960531435269 ) ) ;
#139520=CARTESIAN_POINT ( 'NONE',  ( -10.72451020669898014, 18.67979575497178502, 70.41557627198102409 ) ) ;
#139521=CARTESIAN_POINT ( 'NONE',  ( -0.05219959533934338120, 16.53943276465976808, 92.50109039468567573 ) ) ;
#139522=CARTESIAN_POINT ( 'NONE',  ( -9.564922557960796823, -16.46253265017161027, 72.08224293864770971 ) ) ;
#139523=CARTESIAN_POINT ( 'NONE',  ( 9.474510206698729675, 16.51473224551082808, 67.08442372801900433 ) ) ;
#139524=CARTESIAN_POINT ( 'NONE',  ( -15.80617190586768217, 15.72974639402176855, 78.12609039468570415 ) ) ;
#139525=CARTESIAN_POINT ( 'NONE',  ( -0.05219959533907301413, -21.53943276465977519, 67.49890960531436690 ) ) ;
#139526=CARTESIAN_POINT ( 'NONE',  ( 21.53943276465977519, -0.05219959533907433946, 23.74890960531435269 ) ) ;
#139527=CARTESIAN_POINT ( 'NONE',  ( -9.564922557960796823, -16.46253265017161027, 32.08224293864769550 ) ) ;
#139528=CARTESIAN_POINT ( 'NONE',  ( -0.05219959533934338120, 16.53943276465976808, 97.50109039468567573 ) ) ;
#139529=CARTESIAN_POINT ( 'NONE',  ( -13.89961937509977652, 13.97604488694528158, 45.62390960531433848 ) ) ;
#139530=CARTESIAN_POINT ( 'NONE',  ( -4.379528057220086978, -16.55341960407618274, 19.79275706135235069 ) ) ;
#139532=CARTESIAN_POINT ( 'NONE',  ( 15.72974639402176855, 15.80617190586768217, 111.8760903946856615 ) ) ;
#139533=CARTESIAN_POINT ( 'NONE',  ( 0.05219959533910956823, 16.53943276465976808, 64.99890960531435269 ) ) ;
#139534=CARTESIAN_POINT ( 'NONE',  ( 10.81492255796078972, 18.62759615963270932, 99.58224293864770971 ) ) ;
#139535=CARTESIAN_POINT ( 'NONE',  ( 15.80617190586746368, 15.72974639402197994, 104.3739096053143669 ) ) ;
#139536=CARTESIAN_POINT ( 'NONE',  ( 16.19135201231366494, -7.376712067591922661, 97.31319145947975358 ) ) ;
#139537=CARTESIAN_POINT ( 'NONE',  ( -21.55341960407610458, -5.719274019375992779, 51.45724293864770260 ) ) ;
#139538=CARTESIAN_POINT ( 'NONE',  ( -14.34966873604972548, 8.224510206698743886, 83.33442372801903275 ) ) ;
#139539=CARTESIAN_POINT ( 'NONE',  ( 16.55341960407611168, 4.379528057220329451, 88.95724293864769550 ) ) ;
#139540=CARTESIAN_POINT ( 'NONE',  ( 19.03943276465977164, -0.05219959533909143690, 48.74890960531435979 ) ) ;
#139542=CARTESIAN_POINT ( 'NONE',  ( -16.55341960407617563, 4.379528057220093196, 103.5427570613523613 ) ) ;
#139543=CARTESIAN_POINT ( 'NONE',  ( -5.823673210054431948, 21.52544592524334988, 27.70942372801901854 ) ) ;
#139544=CARTESIAN_POINT ( 'NONE',  ( 16.46253265017160672, -9.564922557960803928, 98.33224293864769550 ) ) ;
#139545=CARTESIAN_POINT ( 'NONE',  ( -21.52544592524334988, -5.823673210054445271, 68.95942372801901854 ) ) ;
#139547=CARTESIAN_POINT ( 'NONE',  ( 16.51473224551069308, 9.474510206698969483, 29.16557627198103475 ) ) ;
#139550=CARTESIAN_POINT ( 'NONE',  ( -0.05219959533937732626, 21.53943276465977519, 57.50109039468568994 ) ) ;
#139551=CARTESIAN_POINT ( 'NONE',  ( -5.049401038298153566, 19.05341960407611168, 45.20724293864769550 ) ) ;
#139552=CARTESIAN_POINT ( 'NONE',  ( 0.05219959533909260263, 19.03943276465977164, 24.99890960531435269 ) ) ;
#139553=CARTESIAN_POINT ( 'NONE',  ( 5.153800228976335163, 19.02544592524342804, 89.79057627198102409 ) ) ;
#139554=CARTESIAN_POINT ( 'NONE',  ( 5.153800228976615827, -19.02544592524334988, 70.20942372801899012 ) ) ;
#139555=CARTESIAN_POINT ( 'NONE',  ( 5.823673210054444382, -21.52544592524334988, 40.20942372801901854 ) ) ;
#139556=CARTESIAN_POINT ( 'NONE',  ( -0.05219959533936034679, 19.03943276465977164, 107.5010903946856615 ) ) ;
#139557=CARTESIAN_POINT ( 'NONE',  ( 13.97604488694548053, -13.89961937509957401, 75.62609039468564731 ) ) ;
#139558=CARTESIAN_POINT ( 'NONE',  ( -9.564922557960796823, -16.46253265017161027, 32.08224293864769550 ) ) ;
#139559=CARTESIAN_POINT ( 'NONE',  ( -8.314922557961024197, 14.29746914071037800, 102.9177570613523756 ) ) ;
#139560=CARTESIAN_POINT ( 'NONE',  ( 5.153800228976615827, -19.02544592524334988, 75.20942372801896170 ) ) ;
#139561=CARTESIAN_POINT ( 'NONE',  ( -16.53943276465976808, 0.05219959533911058130, 21.24890960531436690 ) ) ;
#139562=CARTESIAN_POINT ( 'NONE',  ( 16.46253265017146816, 9.564922557961045513, 56.66775706135233293 ) ) ;
#139563=CARTESIAN_POINT ( 'NONE',  ( 15.72974639402176855, 15.80617190586768217, 106.8760903946856899 ) ) ;
#139564=CARTESIAN_POINT ( 'NONE',  ( 19.05341960407617918, -5.049401038297876454, 31.04275706135232227 ) ) ;
#139565=CARTESIAN_POINT ( 'NONE',  ( -13.97604488694527625, -13.89961937509977652, 31.87390960531435979 ) ) ;
#139566=CARTESIAN_POINT ( 'NONE',  ( 10.81492255796106328, -18.62759615963255655, 95.41775706135234714 ) ) ;
#139567=CARTESIAN_POINT ( 'NONE',  ( 8.224510206698742110, 14.34966873604972548, 27.08442372801901854 ) ) ;
#139568=CARTESIAN_POINT ( 'NONE',  ( -16.46253265017160317, 9.564922557960807481, 90.83224293864769550 ) ) ;
#139570=CARTESIAN_POINT ( 'NONE',  ( 5.153800228976335163, 19.02544592524342804, 74.79057627198103830 ) ) ;
#139571=CARTESIAN_POINT ( 'NONE',  ( 17.50000000000001066, -3.242565516153302241, 102.5000000000090807 ) ) ;
#139572=CARTESIAN_POINT ( 'NONE',  ( -9.474510206698720793, -16.51473224551083518, 89.58442372801900433 ) ) ;
#139573=CARTESIAN_POINT ( 'NONE',  ( -16.51473224551069308, -9.474510206698971260, 111.6655762719810383 ) ) ;
#139574=CARTESIAN_POINT ( 'NONE',  ( 9.564922557961047289, -16.46253265017146816, 20.41775706135233293 ) ) ;
#139575=CARTESIAN_POINT ( 'NONE',  ( -12.14591786802309592, -12.06949235617757132, 91.87390960531436690 ) ) ;
#139577=CARTESIAN_POINT ( 'NONE',  ( -21.52544592524343514, 5.823673210054127303, 61.04057627198103120 ) ) ;
#139578=CARTESIAN_POINT ( 'NONE',  ( -0.05219959533907301413, -21.53943276465977519, 32.49890960531435979 ) ) ;
#139579=CARTESIAN_POINT ( 'NONE',  ( 16.51473224551069308, 9.474510206698969483, 29.16557627198103475 ) ) ;
#139581=CARTESIAN_POINT ( 'NONE',  ( -5.049401038297874678, -19.05341960407617918, 59.79275706135231871 ) ) ;
#139582=CARTESIAN_POINT ( 'NONE',  ( -4.483927247898539470, -16.52544592524342804, 42.29057627198103120 ) ) ;
#139583=CARTESIAN_POINT ( 'NONE',  ( -5.153800228976328057, -19.02544592524343514, 112.2905762719810099 ) ) ;
#139584=CARTESIAN_POINT ( 'NONE',  ( -5.719274019375665041, -21.55341960407619695, 74.79275706135234714 ) ) ;
#139585=CARTESIAN_POINT ( 'NONE',  ( -10.81492255796078084, -18.62759615963271287, 77.08224293864769550 ) ) ;
#139586=CARTESIAN_POINT ( 'NONE',  ( -18.62759615963255300, -10.81492255796106328, 59.16775706135234714 ) ) ;
#139587=CARTESIAN_POINT ( 'NONE',  ( 10.72451020669898902, -18.67979575497178502, 97.91557627198103830 ) ) ;
#139588=CARTESIAN_POINT ( 'NONE',  ( 0.05219959533937995610, -21.53943276465977519, 55.00109039468568284 ) ) ;
#139589=CARTESIAN_POINT ( 'NONE',  ( -9.564922557960796823, -16.46253265017161027, 77.08224293864769550 ) ) ;
#139590=CARTESIAN_POINT ( 'NONE',  ( 8.314922557961029526, -14.29746914071037800, 85.41775706135236135 ) ) ;
#139591=CARTESIAN_POINT ( 'NONE',  ( -5.153800228976328057, -19.02544592524343514, 22.29057627198102765 ) ) ;
#139593=CARTESIAN_POINT ( 'NONE',  ( -4.379528057220328563, 16.55341960407611168, 60.20724293864768839 ) ) ;
#139594=CARTESIAN_POINT ( 'NONE',  ( -4.483927247898539470, -16.52544592524342804, 22.29057627198102765 ) ) ;
#139595=CARTESIAN_POINT ( 'NONE',  ( 19.02544592524343514, -5.153800228976328945, 68.54057627198103830 ) ) ;
#139596=CARTESIAN_POINT ( 'NONE',  ( -19.05341960407611168, -5.049401038298163336, 31.45724293864769550 ) ) ;
#139597=CARTESIAN_POINT ( 'NONE',  ( 21.53943276465977519, -0.05219959533907433946, 43.74890960531435979 ) ) ;
#139598=CARTESIAN_POINT ( 'NONE',  ( 5.153800228976615827, -19.02544592524334988, 40.20942372801898301 ) ) ;
#139599=CARTESIAN_POINT ( 'NONE',  ( -18.22780087662123094, -5.499999999999984901, 86.48459894673892734 ) ) ;
#139600=CARTESIAN_POINT ( 'NONE',  ( -14.34966873604960291, -8.224510206698953496, 51.66557627198102409 ) ) ;
#139601=CARTESIAN_POINT ( 'NONE',  ( -5.823673210054116645, -21.52544592524344225, 32.29057627198102409 ) ) ;
#139603=CARTESIAN_POINT ( 'NONE',  ( -8.314922557961024197, 14.29746914071037800, 77.91775706135231871 ) ) ;
#139604=CARTESIAN_POINT ( 'NONE',  ( 9.474510206698729675, 16.51473224551082808, 57.08442372801900433 ) ) ;
#139605=CARTESIAN_POINT ( 'NONE',  ( 12.06949235617757843, -12.14591786802309237, 38.12390960531436690 ) ) ;
#139606=CARTESIAN_POINT ( 'NONE',  ( -19.25918095147780562, -5.499999999999489297, 74.45284276293934056 ) ) ;
#139607=CARTESIAN_POINT ( 'NONE',  ( 8.224510206698953496, -14.34966873604960469, 22.91557627198102765 ) ) ;
#139608=CARTESIAN_POINT ( 'NONE',  ( 5.153800228976335163, 19.02544592524342804, 44.79057627198103830 ) ) ;
#139609=CARTESIAN_POINT ( 'NONE',  ( -13.89961937509977652, 13.97604488694528158, 65.62390960531436690 ) ) ;
#139610=CARTESIAN_POINT ( 'NONE',  ( 19.02544592524343514, -5.153800228976328945, 23.54057627198102054 ) ) ;
#139611=CARTESIAN_POINT ( 'NONE',  ( 15.72974639402176855, 15.80617190586768217, 26.87609039468567218 ) ) ;
#139612=CARTESIAN_POINT ( 'NONE',  ( 13.97604488694527802, 13.89961937509977652, 64.37390960531436690 ) ) ;
#139613=FACE_OUTER_BOUND ( 'NONE', #154876, .T. ) ;
#139614=CARTESIAN_POINT ( 'NONE',  ( -19.03943276465977164, 0.05219959533909376836, 41.24890960531435269 ) ) ;
#139615=CARTESIAN_POINT ( 'NONE',  ( -21.52544592524343514, 5.823673210054127303, 31.04057627198102409 ) ) ;
#139616=CARTESIAN_POINT ( 'NONE',  ( -21.52544592524334988, -5.823673210054445271, 58.95942372801902565 ) ) ;
#139617=CARTESIAN_POINT ( 'NONE',  ( -14.29746914071049879, 8.314922557960819915, 115.8322429386477097 ) ) ;
#139618=CARTESIAN_POINT ( 'NONE',  ( 21.53943276465977519, -0.05219959533907433946, 33.74890960531436690 ) ) ;
#139619=CARTESIAN_POINT ( 'NONE',  ( -0.05219959533934338120, 16.53943276465976808, 87.50109039468568994 ) ) ;
#139620=CARTESIAN_POINT ( 'NONE',  ( 5.823673210054444382, -21.52544592524334988, 110.2094237280190185 ) ) ;
#139621=CARTESIAN_POINT ( 'NONE',  ( 16.53943276465976808, 0.05219959533934440121, 66.25109039468567573 ) ) ;
#139622=CARTESIAN_POINT ( 'NONE',  ( -16.46253265017160317, 9.564922557960807481, 110.8322429386476955 ) ) ;
#139623=CARTESIAN_POINT ( 'NONE',  ( -0.05219959533934338120, 16.53943276465976808, 52.50109039468567573 ) ) ;
#139624=CARTESIAN_POINT ( 'NONE',  ( 16.55341960407618274, -4.379528057220086978, 41.04275706135236135 ) ) ;
#139625=CARTESIAN_POINT ( 'NONE',  ( 12.14591786802327356, -12.06949235617739191, 90.62609039468567573 ) ) ;
#139626=CARTESIAN_POINT ( 'NONE',  ( 0.05219959533937995610, -21.53943276465977519, 50.00109039468568994 ) ) ;
#139627=CARTESIAN_POINT ( 'NONE',  ( -16.51473224551082808, 9.474510206698731452, 113.3344237280190043 ) ) ;
#139628=CARTESIAN_POINT ( 'NONE',  ( -5.719274019375978568, 21.55341960407610458, 105.2072429386477097 ) ) ;
#139629=CARTESIAN_POINT ( 'NONE',  ( 12.14591786802327356, -12.06949235617739191, 20.62609039468568639 ) ) ;
#139630=CARTESIAN_POINT ( 'NONE',  ( 14.34966873604972726, -8.224510206698740333, 90.83442372801901854 ) ) ;
#139632=CARTESIAN_POINT ( 'NONE',  ( 18.67979575497194134, -10.72451020669871369, 90.83442372801901854 ) ) ;
#139633=CARTESIAN_POINT ( 'NONE',  ( -19.03943276465977164, -0.05219959533935918106, 88.75109039468567573 ) ) ;
#139634=CARTESIAN_POINT ( 'NONE',  ( 14.29746914071049879, -8.314922557960816363, 63.33224293864770260 ) ) ;
#139635=CARTESIAN_POINT ( 'NONE',  ( -0.05219959533910754901, -16.53943276465976808, 37.49890960531436690 ) ) ;
#139636=CARTESIAN_POINT ( 'NONE',  ( 16.52544592524342804, -4.483927247898539470, 113.5405762719810383 ) ) ;
#139637=CARTESIAN_POINT ( 'NONE',  ( 13.97604488694548053, -13.89961937509957401, 50.62609039468566152 ) ) ;
#139639=CARTESIAN_POINT ( 'NONE',  ( -21.52544592524334988, -5.823673210054445271, 48.95942372801902565 ) ) ;
#139640=CARTESIAN_POINT ( 'NONE',  ( 9.474510206698729675, 16.51473224551082808, 107.0844237280190043 ) ) ;
#139642=CARTESIAN_POINT ( 'NONE',  ( -13.97604488694527625, -13.89961937509977652, 106.8739096053143669 ) ) ;
#139643=CARTESIAN_POINT ( 'NONE',  ( 10.81492255796078972, 18.62759615963270932, 69.58224293864769550 ) ) ;
#139644=CARTESIAN_POINT ( 'NONE',  ( -0.05219959533936034679, 19.03943276465977164, 92.50109039468566152 ) ) ;
#139645=CARTESIAN_POINT ( 'NONE',  ( -19.05341960407611168, -5.049401038298163336, 86.45724293864769550 ) ) ;
#139646=CARTESIAN_POINT ( 'NONE',  ( -15.72974639402197994, 15.80617190586746368, 60.62390960531437401 ) ) ;
#139647=CARTESIAN_POINT ( 'NONE',  ( -16.55341960407611168, -4.379528057220339221, 101.4572429386476955 ) ) ;
#139648=CARTESIAN_POINT ( 'NONE',  ( -5.153800228976328057, -19.02544592524343514, 67.29057627198102409 ) ) ;
#139649=CARTESIAN_POINT ( 'NONE',  ( -16.51473224551069308, -9.474510206698971260, 31.66557627198102054 ) ) ;
#139650=CARTESIAN_POINT ( 'NONE',  ( -15.80617190586768217, 15.72974639402176855, 43.12609039468568284 ) ) ;
#139651=CARTESIAN_POINT ( 'NONE',  ( -21.52544592524334988, -5.823673210054445271, 83.95942372801900433 ) ) ;
#139652=CARTESIAN_POINT ( 'NONE',  ( 16.55341960407618274, -4.379528057220086978, 96.04275706135236135 ) ) ;
#139653=CARTESIAN_POINT ( 'NONE',  ( 5.823673210054444382, -21.52544592524334988, 35.20942372801901854 ) ) ;
#139654=CARTESIAN_POINT ( 'NONE',  ( 10.72451020669871369, 18.67979575497193778, 42.08442372801901854 ) ) ;
#139655=CARTESIAN_POINT ( 'NONE',  ( -19.03943276465977164, -0.05219959533935918106, 63.75109039468566863 ) ) ;
#139656=CARTESIAN_POINT ( 'NONE',  ( 19.02544592524343514, -5.153800228976328945, 78.54057627198099567 ) ) ;
#139657=CARTESIAN_POINT ( 'NONE',  ( -21.52544592524334988, -5.823673210054445271, 83.95942372801900433 ) ) ;
#139658=CARTESIAN_POINT ( 'NONE',  ( 10.81492255796078972, 18.62759615963270932, 84.58224293864769550 ) ) ;
#139659=CARTESIAN_POINT ( 'NONE',  ( 0.05219959533910956823, 16.53943276465976808, 69.99890960531435269 ) ) ;
#139660=CARTESIAN_POINT ( 'NONE',  ( 21.55341960407619695, -5.719274019375665929, 106.0427570613523471 ) ) ;
#139661=CARTESIAN_POINT ( 'NONE',  ( -12.06949235617756955, 12.14591786802309770, 90.62390960531436690 ) ) ;
#139662=CARTESIAN_POINT ( 'NONE',  ( 19.02544592524343514, -5.153800228976328945, 33.54057627198102409 ) ) ;
#139663=CARTESIAN_POINT ( 'NONE',  ( -19.03943276465977164, -0.05219959533935918106, 68.75109039468566152 ) ) ;
#139664=CARTESIAN_POINT ( 'NONE',  ( -14.34966873604960291, -8.224510206698953496, 36.66557627198103120 ) ) ;
#139665=CARTESIAN_POINT ( 'NONE',  ( 15.80617190586769283, -15.72974639402175789, 100.6260903946857184 ) ) ;
#139666=CARTESIAN_POINT ( 'NONE',  ( -9.474510206698964154, 16.51473224551069663, 90.41557627198103830 ) ) ;
#139667=CARTESIAN_POINT ( 'NONE',  ( 13.97604488694548053, -13.89961937509957401, 65.62609039468567573 ) ) ;
#139668=CARTESIAN_POINT ( 'NONE',  ( -15.80617190586745835, -15.72974639402198527, 61.87390960531436690 ) ) ;
#139669=CARTESIAN_POINT ( 'NONE',  ( 15.80617190586769283, -15.72974639402175789, 20.62609039468568639 ) ) ;
#139670=CARTESIAN_POINT ( 'NONE',  ( 19.03943276465977164, 0.05219959533936151252, 106.2510903946856615 ) ) ;
#139671=CARTESIAN_POINT ( 'NONE',  ( -16.53943276465976808, -0.05219959533934237506, 78.75109039468568994 ) ) ;
#139672=CARTESIAN_POINT ( 'NONE',  ( 16.88567814943165146, 6.947325034625595030, 63.79001122652589117 ) ) ;
#139673=CARTESIAN_POINT ( 'NONE',  ( 18.62759615963255655, 10.81492255796105972, 26.66775706135235424 ) ) ;
#139674=CARTESIAN_POINT ( 'NONE',  ( -4.483927247898539470, -16.52544592524342804, 102.2905762719810383 ) ) ;
#139676=CARTESIAN_POINT ( 'NONE',  ( -16.55341960407617563, 4.379528057220093196, 43.54275706135235424 ) ) ;
#139677=ADVANCED_FACE ( 'NONE', ( #178534 ), #128198, .T. ) ;
#139678=CARTESIAN_POINT ( 'NONE',  ( 0.05219959533907565091, 21.53943276465977519, 64.99890960531435269 ) ) ;
#139679=CARTESIAN_POINT ( 'NONE',  ( -16.52544592524335698, -4.483927247898792601, 98.95942372801903275 ) ) ;
#139680=CARTESIAN_POINT ( 'NONE',  ( -16.53943276465976808, -0.05219959533934237506, 38.75109039468567573 ) ) ;
#139681=CARTESIAN_POINT ( 'NONE',  ( 19.02544592524343514, -5.153800228976328945, 48.54057627198103120 ) ) ;
#139682=CARTESIAN_POINT ( 'NONE',  ( -4.483927247898782831, 16.52544592524335698, 82.70942372801900433 ) ) ;
#139683=CARTESIAN_POINT ( 'NONE',  ( -13.97604488694547697, 13.89961937509957934, 78.12609039468567573 ) ) ;
#139685=CARTESIAN_POINT ( 'NONE',  ( -21.53943276465977519, 0.05219959533907696930, 66.24890960531436690 ) ) ;
#139686=CARTESIAN_POINT ( 'NONE',  ( 14.29746914071037800, 8.314922557961029526, 91.66775706135234714 ) ) ;
#139687=CARTESIAN_POINT ( 'NONE',  ( -21.55341960407619339, 5.719274019375674811, 83.54275706135234714 ) ) ;
#139688=CARTESIAN_POINT ( 'NONE',  ( 0.05219959533907565091, 21.53943276465977519, 69.99890960531435269 ) ) ;
#139689=CARTESIAN_POINT ( 'NONE',  ( 21.53943276465977519, -0.05219959533907433946, 53.74890960531437401 ) ) ;
#139691=CARTESIAN_POINT ( 'NONE',  ( 14.29746914071037800, 8.314922557961029526, 76.66775706135234714 ) ) ;
#139692=CARTESIAN_POINT ( 'NONE',  ( 0.05219959533907565091, 21.53943276465977519, 44.99890960531435979 ) ) ;
#139694=CARTESIAN_POINT ( 'NONE',  ( -5.049401038298153566, 19.05341960407611168, 110.2072429386476671 ) ) ;
#139696=CARTESIAN_POINT ( 'NONE',  ( 9.474510206698971260, -16.51473224551069308, 22.91557627198102765 ) ) ;
#139697=CARTESIAN_POINT ( 'NONE',  ( -10.81492255796078084, -18.62759615963271287, 72.08224293864769550 ) ) ;
#139698=CARTESIAN_POINT ( 'NONE',  ( -14.29746914071037622, -8.314922557961029526, 99.16775706135234714 ) ) ;
#139699=CARTESIAN_POINT ( 'NONE',  ( 15.72974639402176855, 15.80617190586768217, 51.87609039468568284 ) ) ;
#139700=CARTESIAN_POINT ( 'NONE',  ( 19.05341960407617918, -5.049401038297876454, 106.0427570613523471 ) ) ;
#139701=CARTESIAN_POINT ( 'NONE',  ( 14.29746914071049879, -8.314922557960816363, 113.3322429386476955 ) ) ;
#139702=CARTESIAN_POINT ( 'NONE',  ( 5.153800228976615827, -19.02544592524334988, 105.2094237280190185 ) ) ;
#139703=CARTESIAN_POINT ( 'NONE',  ( -19.02544592524342804, 5.153800228976336051, 46.04057627198101699 ) ) ;
#139705=CARTESIAN_POINT ( 'NONE',  ( -16.51473224551069308, -9.474510206698971260, 96.66557627198102409 ) ) ;
#139706=CARTESIAN_POINT ( 'NONE',  ( 12.14591786802327356, -12.06949235617739191, 80.62609039468567573 ) ) ;
#139707=CARTESIAN_POINT ( 'NONE',  ( 19.05341960407617918, -5.049401038297876454, 76.04275706135230450 ) ) ;
#139708=CARTESIAN_POINT ( 'NONE',  ( 13.97604488694548053, -13.89961937509957401, 20.62609039468567573 ) ) ;
#139709=CARTESIAN_POINT ( 'NONE',  ( 21.55341960407610458, 5.719274019375980345, 63.95724293864770260 ) ) ;
#139710=CARTESIAN_POINT ( 'NONE',  ( 4.379528057220092307, 16.55341960407617563, 82.29275706135234714 ) ) ;
#139711=CARTESIAN_POINT ( 'NONE',  ( 16.46253265017146816, 9.564922557961045513, 81.66775706135233293 ) ) ;
#139712=CARTESIAN_POINT ( 'NONE',  ( 16.46253265017160672, -9.564922557960803928, 33.33224293864770260 ) ) ;
#139713=CARTESIAN_POINT ( 'NONE',  ( -5.049401038298153566, 19.05341960407611168, 90.20724293864766707 ) ) ;
#139714=CARTESIAN_POINT ( 'NONE',  ( 5.823673210054444382, -21.52544592524334988, 45.20942372801901854 ) ) ;
#139715=CARTESIAN_POINT ( 'NONE',  ( 16.51473224551069308, 9.474510206698969483, 49.16557627198102409 ) ) ;
#139717=CARTESIAN_POINT ( 'NONE',  ( 19.03943276465977164, -0.05219959533909143690, 113.7489096053143669 ) ) ;
#139718=CARTESIAN_POINT ( 'NONE',  ( 12.06949235617757843, -12.14591786802309237, 58.12390960531435979 ) ) ;
#139719=CARTESIAN_POINT ( 'NONE',  ( 0.05219959533907565091, 21.53943276465977519, 59.99890960531436690 ) ) ;
#139721=CARTESIAN_POINT ( 'NONE',  ( -5.153800228976607833, 19.02544592524334988, 47.70942372801900433 ) ) ;
#139722=CARTESIAN_POINT ( 'NONE',  ( 13.97604488694527802, 13.89961937509977652, 59.37390960531434558 ) ) ;
#139723=CARTESIAN_POINT ( 'NONE',  ( 9.474510206698971260, -16.51473224551069308, 77.91557627198103830 ) ) ;
#139724=CARTESIAN_POINT ( 'NONE',  ( 12.14591786802327356, -12.06949235617739191, 55.62609039468568284 ) ) ;
#139727=CARTESIAN_POINT ( 'NONE',  ( -8.314922557961024197, 14.29746914071037800, 87.91775706135234714 ) ) ;
#139729=CARTESIAN_POINT ( 'NONE',  ( 16.52544592524335698, 4.483927247898782831, 76.45942372801901854 ) ) ;
#139730=CARTESIAN_POINT ( 'NONE',  ( 14.34966873604972726, -8.224510206698740333, 50.83442372801901143 ) ) ;
#139731=CARTESIAN_POINT ( 'NONE',  ( 13.89961937509957401, 13.97604488694547697, 26.87609039468566507 ) ) ;
#139732=CARTESIAN_POINT ( 'NONE',  ( 19.02544592524343514, -5.153800228976328945, 58.54057627198102409 ) ) ;
#139734=CARTESIAN_POINT ( 'NONE',  ( 10.72451020669871369, 18.67979575497193778, 52.08442372801901854 ) ) ;
#139735=CARTESIAN_POINT ( 'NONE',  ( -0.05219959533936034679, 19.03943276465977164, 67.50109039468566152 ) ) ;
#139736=CARTESIAN_POINT ( 'NONE',  ( 5.719274019375673035, 21.55341960407619339, 112.2927570613523471 ) ) ;
#139737=CARTESIAN_POINT ( 'NONE',  ( 16.51473224551069308, 9.474510206698969483, 24.16557627198102765 ) ) ;
#139739=CARTESIAN_POINT ( 'NONE',  ( -10.81492255796078084, -18.62759615963271287, 67.08224293864770971 ) ) ;
#139740=CARTESIAN_POINT ( 'NONE',  ( -10.81492255796078084, -18.62759615963271287, 22.08224293864769194 ) ) ;
#139741=CARTESIAN_POINT ( 'NONE',  ( 4.483927247898545687, 16.52544592524342804, 114.7905762719810383 ) ) ;
#139742=CARTESIAN_POINT ( 'NONE',  ( -14.34966873604972548, 8.224510206698743886, 38.33442372801900433 ) ) ;
#139744=CARTESIAN_POINT ( 'NONE',  ( -14.34966873604960291, -8.224510206698953496, 36.66557627198103120 ) ) ;
#139745=ORIENTED_EDGE ( 'NONE', *, *, #166522, .T. ) ;
#139746=CARTESIAN_POINT ( 'NONE',  ( 10.81492255796078972, 18.62759615963270932, 114.5822429386477097 ) ) ;
#139748=CARTESIAN_POINT ( 'NONE',  ( 16.55341960407611168, 4.379528057220329451, 43.95724293864769550 ) ) ;
#139749=CARTESIAN_POINT ( 'NONE',  ( -19.03943276465977164, 0.05219959533909376836, 116.2489096053143669 ) ) ;
#139750=CARTESIAN_POINT ( 'NONE',  ( -9.474510206698720793, -16.51473224551083518, 109.5844237280190043 ) ) ;
#139751=CARTESIAN_POINT ( 'NONE',  ( 9.564922557961047289, -16.46253265017146816, 20.41775706135233293 ) ) ;
#139752=CARTESIAN_POINT ( 'NONE',  ( -0.05219959533910754901, -16.53943276465976808, 27.49890960531435269 ) ) ;
#139753=CARTESIAN_POINT ( 'NONE',  ( -15.80617190586745835, -15.72974639402198527, 96.87390960531436690 ) ) ;
#139754=CARTESIAN_POINT ( 'NONE',  ( 17.05587630539785593, 6.762274262135710146, 31.75819690962688924 ) ) ;
#139755=CARTESIAN_POINT ( 'NONE',  ( -5.719274019375978568, 21.55341960407610458, 60.20724293864768839 ) ) ;
#139756=CARTESIAN_POINT ( 'NONE',  ( -13.89961937509977652, 13.97604488694528158, 80.62390960531436690 ) ) ;
#139757=CARTESIAN_POINT ( 'NONE',  ( 12.14591786802309770, 12.06949235617756955, 54.37390960531435979 ) ) ;
#139758=CARTESIAN_POINT ( 'NONE',  ( 0.05219959533909260263, 19.03943276465977164, 84.99890960531436690 ) ) ;
#139760=LINE ( 'NONE', #61926, #160386 ) ;
#139761=CARTESIAN_POINT ( 'NONE',  ( 16.51473224551083163, -9.474510206698727899, 50.83442372801899722 ) ) ;
#139762=CARTESIAN_POINT ( 'NONE',  ( 0.05219959533907565091, 21.53943276465977519, 94.99890960531436690 ) ) ;
#139763=CARTESIAN_POINT ( 'NONE',  ( 16.52544592524342804, -4.483927247898539470, 98.54057627198105251 ) ) ;
#139764=CARTESIAN_POINT ( 'NONE',  ( 21.52544592524334988, 5.823673210054432836, 56.45942372801902565 ) ) ;
#139766=CARTESIAN_POINT ( 'NONE',  ( 8.314922557960818139, 14.29746914071049879, 29.58224293864769905 ) ) ;
#139767=CARTESIAN_POINT ( 'NONE',  ( -16.46253265017160317, 9.564922557960807481, 35.83224293864768839 ) ) ;
#139768=CARTESIAN_POINT ( 'NONE',  ( -0.05219959533909027116, -19.03943276465977164, 97.49890960531436690 ) ) ;
#139769=CARTESIAN_POINT ( 'NONE',  ( -15.72974639402197994, 15.80617190586746368, 60.62390960531437401 ) ) ;
#139770=CARTESIAN_POINT ( 'NONE',  ( -18.39443945427639449, 5.500000000000030198, 43.51745347608652281 ) ) ;
#139771=CARTESIAN_POINT ( 'NONE',  ( 5.049401038298161559, -19.05341960407611168, 32.70724293864768129 ) ) ;
#139772=CARTESIAN_POINT ( 'NONE',  ( -10.81492255796078084, -18.62759615963271287, 47.08224293864770260 ) ) ;
#139773=CARTESIAN_POINT ( 'NONE',  ( -15.72974639402176322, -15.80617190586768395, 79.37609039468567573 ) ) ;
#139775=CARTESIAN_POINT ( 'NONE',  ( 8.314922557961029526, -14.29746914071037800, 70.41775706135236135 ) ) ;
#139776=CARTESIAN_POINT ( 'NONE',  ( 5.153800228976335163, 19.02544592524342804, 59.79057627198100988 ) ) ;
#139777=CARTESIAN_POINT ( 'NONE',  ( 5.153800228976335163, 19.02544592524342804, 59.79057627198100988 ) ) ;
#139779=CARTESIAN_POINT ( 'NONE',  ( 16.46253265017146816, 9.564922557961045513, 26.66775706135234003 ) ) ;
#139780=CARTESIAN_POINT ( 'NONE',  ( 12.06949235617739724, 12.14591786802326823, 76.87609039468567573 ) ) ;
#139781=CARTESIAN_POINT ( 'NONE',  ( -18.62759615963255300, -10.81492255796106328, 94.16775706135237556 ) ) ;
#139782=CARTESIAN_POINT ( 'NONE',  ( 13.97604488694527802, 13.89961937509977652, 74.37390960531436690 ) ) ;
#139783=CARTESIAN_POINT ( 'NONE',  ( 15.80617190586746368, 15.72974639402197994, 39.37390960531436690 ) ) ;
#139784=CARTESIAN_POINT ( 'NONE',  ( -9.474510206698720793, -16.51473224551083518, 109.5844237280190043 ) ) ;
#139785=CARTESIAN_POINT ( 'NONE',  ( -5.823673210054431948, 21.52544592524334988, 77.70942372801900433 ) ) ;
#139786=CARTESIAN_POINT ( 'NONE',  ( -12.06949235617739369, -12.14591786802326823, 49.37609039468569705 ) ) ;
#139787=CARTESIAN_POINT ( 'NONE',  ( 10.81492255796078972, 18.62759615963270932, 94.58224293864769550 ) ) ;
#139788=CARTESIAN_POINT ( 'NONE',  ( -4.379528057220086978, -16.55341960407618274, 19.79275706135235069 ) ) ;
#139789=CARTESIAN_POINT ( 'NONE',  ( -5.153800228976328057, -19.02544592524343514, 82.29057627198103830 ) ) ;
#139790=CARTESIAN_POINT ( 'NONE',  ( -16.53943276465976808, -0.05219959533934237506, 23.75109039468567929 ) ) ;
#139791=CARTESIAN_POINT ( 'NONE',  ( -16.46253265017160317, 9.564922557960807481, 45.83224293864769550 ) ) ;
#139792=CARTESIAN_POINT ( 'NONE',  ( -9.474510206698720793, -16.51473224551083518, 109.5844237280190043 ) ) ;
#139793=CARTESIAN_POINT ( 'NONE',  ( -4.483927247898539470, -16.52544592524342804, 72.29057627198102409 ) ) ;
#139794=CARTESIAN_POINT ( 'NONE',  ( 16.53943276465976808, 0.05219959533934440121, 71.25109039468568994 ) ) ;
#139795=CARTESIAN_POINT ( 'NONE',  ( 10.72451020669871369, 18.67979575497193778, 27.08442372801901854 ) ) ;
#139796=CARTESIAN_POINT ( 'NONE',  ( 19.02544592524343514, -5.153800228976328945, 53.54057627198102409 ) ) ;
#139797=CARTESIAN_POINT ( 'NONE',  ( 19.05341960407611168, 5.049401038298154454, 68.95724293864769550 ) ) ;
#139798=CARTESIAN_POINT ( 'NONE',  ( -0.05219959533934338120, 16.53943276465976808, 77.50109039468567573 ) ) ;
#139799=CARTESIAN_POINT ( 'NONE',  ( -18.09918380851993902, -5.499999999999988454, 81.48618307335611632 ) ) ;
#139802=CARTESIAN_POINT ( 'NONE',  ( 21.53943276465977519, 0.05219959533937863772, 111.2510903946856899 ) ) ;
#139803=CARTESIAN_POINT ( 'NONE',  ( 5.049401038298161559, -19.05341960407611168, 42.70724293864767418 ) ) ;
#139806=CARTESIAN_POINT ( 'NONE',  ( 4.379528057220092307, 16.55341960407617563, 32.29275706135235424 ) ) ;
#139807=CARTESIAN_POINT ( 'NONE',  ( -16.46253265017146816, -9.564922557961047289, 64.16775706135233293 ) ) ;
#139808=CARTESIAN_POINT ( 'NONE',  ( -12.14591786802326823, 12.06949235617739902, 38.12609039468567573 ) ) ;
#139809=CARTESIAN_POINT ( 'NONE',  ( 16.51473224551069308, 9.474510206698969483, 39.16557627198103120 ) ) ;
#139810=CARTESIAN_POINT ( 'NONE',  ( -5.153800228976328057, -19.02544592524343514, 112.2905762719810099 ) ) ;
#139811=CARTESIAN_POINT ( 'NONE',  ( 9.564922557960805705, 16.46253265017160317, 59.58224293864769550 ) ) ;
#139812=CARTESIAN_POINT ( 'NONE',  ( 5.823673210054125526, 21.52544592524343514, 94.79057627198105251 ) ) ;
#139813=CARTESIAN_POINT ( 'NONE',  ( 19.05341960407611168, 5.049401038298154454, 88.95724293864769550 ) ) ;
#139814=CARTESIAN_POINT ( 'NONE',  ( -19.03943276465977164, 0.05219959533909376836, 21.24890960531436335 ) ) ;
#139816=CARTESIAN_POINT ( 'NONE',  ( 16.51473224551069308, 9.474510206698969483, 59.16557627198102409 ) ) ;
#139817=CARTESIAN_POINT ( 'NONE',  ( -16.53943276465976808, 0.05219959533911058130, 21.24890960531436690 ) ) ;
#139818=CARTESIAN_POINT ( 'NONE',  ( 19.03943276465977164, 0.05219959533936151252, 101.2510903946856757 ) ) ;
#139819=CARTESIAN_POINT ( 'NONE',  ( -9.564922557961040184, 16.46253265017147172, 22.91775706135233648 ) ) ;
#139820=CARTESIAN_POINT ( 'NONE',  ( -12.06949235617756955, 12.14591786802309770, 55.62390960531436690 ) ) ;
#139821=CARTESIAN_POINT ( 'NONE',  ( 21.53943276465977519, 0.05219959533937863772, 96.25109039468568994 ) ) ;
#139822=CARTESIAN_POINT ( 'NONE',  ( -5.049401038298153566, 19.05341960407611168, 45.20724293864769550 ) ) ;
#139823=CARTESIAN_POINT ( 'NONE',  ( -8.224510206698948167, 14.34966873604960824, 30.41557627198101699 ) ) ;
#139824=CARTESIAN_POINT ( 'NONE',  ( -10.72451020669870658, -18.67979575497194134, 84.58442372801903275 ) ) ;
#139825=CARTESIAN_POINT ( 'NONE',  ( -5.049401038298153566, 19.05341960407611168, 80.20724293864769550 ) ) ;
#139826=CARTESIAN_POINT ( 'NONE',  ( 13.97604488694527802, 13.89961937509977652, 94.37390960531436690 ) ) ;
#139827=CARTESIAN_POINT ( 'NONE',  ( -8.224510206698948167, 14.34966873604960824, 95.41557627198102409 ) ) ;
#139828=CARTESIAN_POINT ( 'NONE',  ( -0.05219959533910754901, -16.53943276465976808, 72.49890960531435269 ) ) ;
#139829=CARTESIAN_POINT ( 'NONE',  ( -21.52544592524343514, 5.823673210054127303, 81.04057627198102409 ) ) ;
#139830=CARTESIAN_POINT ( 'NONE',  ( -19.02544592524342804, 5.153800228976336051, 76.04057627198102409 ) ) ;
#139831=CARTESIAN_POINT ( 'NONE',  ( 15.80617190586746368, 15.72974639402197994, 79.37390960531436690 ) ) ;
#139832=CARTESIAN_POINT ( 'NONE',  ( -13.89961937509957401, -13.97604488694547875, 74.37609039468566152 ) ) ;
#139834=CARTESIAN_POINT ( 'NONE',  ( -8.314922557960811034, -14.29746914071050412, 92.08224293864769550 ) ) ;
#139835=CARTESIAN_POINT ( 'NONE',  ( 13.97604488694527802, 13.89961937509977652, 64.37390960531436690 ) ) ;
#139836=CARTESIAN_POINT ( 'NONE',  ( 21.53943276465977519, -0.05219959533907433946, 68.74890960531435269 ) ) ;
#139838=CARTESIAN_POINT ( 'NONE',  ( 12.14591786802309770, 12.06949235617756955, 24.37390960531435979 ) ) ;
#139840=CARTESIAN_POINT ( 'NONE',  ( -9.564922557961040184, 16.46253265017147172, 112.9177570613523329 ) ) ;
#139841=CARTESIAN_POINT ( 'NONE',  ( 12.06949235617757843, -12.14591786802309237, 83.12390960531436690 ) ) ;
#139843=CARTESIAN_POINT ( 'NONE',  ( 16.51473224551069308, 9.474510206698969483, 79.16557627198103830 ) ) ;
#139844=CARTESIAN_POINT ( 'NONE',  ( -9.564922557960796823, -16.46253265017161027, 27.08224293864769550 ) ) ;
#139845=CARTESIAN_POINT ( 'NONE',  ( 8.224510206698953496, -14.34966873604960469, 62.91557627198102409 ) ) ;
#139846=CARTESIAN_POINT ( 'NONE',  ( -0.05219959533909027116, -19.03943276465977164, 102.4989096053143669 ) ) ;
#139847=CARTESIAN_POINT ( 'NONE',  ( 16.46253265017146816, 9.564922557961045513, 91.66775706135234714 ) ) ;
#139848=CARTESIAN_POINT ( 'NONE',  ( 0.05219959533909260263, 19.03943276465977164, 84.99890960531436690 ) ) ;
#139849=CARTESIAN_POINT ( 'NONE',  ( 16.46253265017160672, -9.564922557960803928, 88.33224293864769550 ) ) ;
#139850=CARTESIAN_POINT ( 'NONE',  ( -10.72451020669898014, 18.67979575497178502, 80.41557627198103830 ) ) ;
#139851=CARTESIAN_POINT ( 'NONE',  ( -16.55341960407617563, 4.379528057220093196, 68.54275706135234714 ) ) ;
#139852=CARTESIAN_POINT ( 'NONE',  ( -16.52216118717250737, 7.221426719304233188, 93.92400978952976232 ) ) ;
#139853=CARTESIAN_POINT ( 'NONE',  ( -5.153800228976328057, -19.02544592524343514, 67.29057627198102409 ) ) ;
#139854=CARTESIAN_POINT ( 'NONE',  ( -5.823673210054116645, -21.52544592524344225, 67.29057627198103830 ) ) ;
#139855=CARTESIAN_POINT ( 'NONE',  ( 19.03943276465977164, 0.05219959533936151252, 96.25109039468567573 ) ) ;
#139857=CARTESIAN_POINT ( 'NONE',  ( -8.314922557960811034, -14.29746914071050412, 32.08224293864769550 ) ) ;
#139858=CARTESIAN_POINT ( 'NONE',  ( -5.719274019375665041, -21.55341960407619695, 49.79275706135234714 ) ) ;
#139859=CARTESIAN_POINT ( 'NONE',  ( 18.09918380851992126, 5.500000000000036415, 83.98618307335611632 ) ) ;
#139860=CARTESIAN_POINT ( 'NONE',  ( -12.14591786802326823, 12.06949235617739902, 78.12609039468570415 ) ) ;
#139861=CARTESIAN_POINT ( 'NONE',  ( -16.51473224551069308, -9.474510206698971260, 101.6655762719810241 ) ) ;
#139862=CARTESIAN_POINT ( 'NONE',  ( -0.05219959533909027116, -19.03943276465977164, 107.4989096053143527 ) ) ;
#139864=CARTESIAN_POINT ( 'NONE',  ( -8.224510206698735004, -14.34966873604973081, 94.58442372801901854 ) ) ;
#139865=CARTESIAN_POINT ( 'NONE',  ( 4.379528057220092307, 16.55341960407617563, 42.29275706135235424 ) ) ;
#139866=CARTESIAN_POINT ( 'NONE',  ( -9.564922557960796823, -16.46253265017161027, 62.08224293864769550 ) ) ;
#139867=CARTESIAN_POINT ( 'NONE',  ( -19.03943276465977164, 0.05219959533909376836, 66.24890960531436690 ) ) ;
#139868=CARTESIAN_POINT ( 'NONE',  ( -21.52544592524334988, -5.823673210054445271, 48.95942372801902565 ) ) ;
#139869=CARTESIAN_POINT ( 'NONE',  ( -14.29746914071037622, -8.314922557961029526, 69.16775706135234714 ) ) ;
#139870=CARTESIAN_POINT ( 'NONE',  ( 4.483927247898545687, 16.52544592524342804, 29.79057627198102409 ) ) ;
#139871=CARTESIAN_POINT ( 'NONE',  ( 0.05219959533909260263, 19.03943276465977164, 44.99890960531435979 ) ) ;
#139872=CARTESIAN_POINT ( 'NONE',  ( 19.03943276465977164, -0.05219959533909143690, 28.74890960531435624 ) ) ;
#139873=CARTESIAN_POINT ( 'NONE',  ( 8.224510206698742110, 14.34966873604972548, 22.08442372801901143 ) ) ;
#139874=CARTESIAN_POINT ( 'NONE',  ( 13.89961937509957401, 13.97604488694547697, 76.87609039468566152 ) ) ;
#139875=CARTESIAN_POINT ( 'NONE',  ( 16.55341960407611168, 4.379528057220329451, 88.95724293864769550 ) ) ;
#139876=CARTESIAN_POINT ( 'NONE',  ( -19.05341960407611168, -5.049401038298163336, 56.45724293864768129 ) ) ;
#139877=CARTESIAN_POINT ( 'NONE',  ( 19.05341960407617918, -5.049401038297876454, 86.04275706135233293 ) ) ;
#139878=DIRECTION ( 'NONE',  ( 0.000000000000000000, 1.000000000000000000, 0.000000000000000000 ) ) ;
#139879=CARTESIAN_POINT ( 'NONE',  ( 10.72451020669871369, 18.67979575497193778, 97.08442372801904696 ) ) ;
#139880=CARTESIAN_POINT ( 'NONE',  ( -4.483927247898782831, 16.52544592524335698, 52.70942372801902565 ) ) ;
#139881=CARTESIAN_POINT ( 'NONE',  ( 17.50000000000000000, -5.499999999999992895, 81.21769037696435589 ) ) ;
#139882=CARTESIAN_POINT ( 'NONE',  ( -5.719274019375978568, 21.55341960407610458, 50.20724293864769550 ) ) ;
#139883=CARTESIAN_POINT ( 'NONE',  ( 16.53943276465976808, 0.05219959533934440121, 46.25109039468567573 ) ) ;
#139884=CARTESIAN_POINT ( 'NONE',  ( -13.97604488694527625, -13.89961937509977830, 36.87390960531436690 ) ) ;
#139885=CARTESIAN_POINT ( 'NONE',  ( -0.05219959533936034679, 19.03943276465977164, 32.50109039468566863 ) ) ;
#139886=CARTESIAN_POINT ( 'NONE',  ( 19.05341960407611168, 5.049401038298154454, 73.95724293864768129 ) ) ;
#139888=CARTESIAN_POINT ( 'NONE',  ( -19.05341960407611168, -5.049401038298163336, 46.45724293864768129 ) ) ;
#139890=CARTESIAN_POINT ( 'NONE',  ( -13.89961937509977652, 13.97604488694528158, 70.62390960531432427 ) ) ;
#139891=CARTESIAN_POINT ( 'NONE',  ( 17.50000000000001066, -4.658240926743199672, 111.4447041781679957 ) ) ;
#139892=CARTESIAN_POINT ( 'NONE',  ( 9.474510206698729675, 16.51473224551082808, 32.08442372801900433 ) ) ;
#139893=CARTESIAN_POINT ( 'NONE',  ( -21.55341960407619339, 5.719274019375674811, 103.5427570613523613 ) ) ;
#139894=CARTESIAN_POINT ( 'NONE',  ( 16.55341960407611168, 4.379528057220329451, 33.95724293864769550 ) ) ;
#139895=CARTESIAN_POINT ( 'NONE',  ( 16.51473224551069308, 9.474510206698969483, 44.16557627198103120 ) ) ;
#139896=CARTESIAN_POINT ( 'NONE',  ( 13.89961937509977652, -13.97604488694527269, 108.1239096053143669 ) ) ;
#139897=CARTESIAN_POINT ( 'NONE',  ( 5.719274019375673035, 21.55341960407619339, 67.29275706135234714 ) ) ;
#139898=CARTESIAN_POINT ( 'NONE',  ( -16.51473224551069308, -9.474510206698971260, 46.66557627198102409 ) ) ;
#139900=CARTESIAN_POINT ( 'NONE',  ( 0.05219959533937995610, -21.53943276465977519, 75.00109039468568994 ) ) ;
#139901=CARTESIAN_POINT ( 'NONE',  ( 21.55341960407610458, 5.719274019375980345, 28.95724293864769905 ) ) ;
#139902=CARTESIAN_POINT ( 'NONE',  ( 5.719274019375673035, 21.55341960407619339, 32.29275706135235424 ) ) ;
#139903=CARTESIAN_POINT ( 'NONE',  ( -0.05219959533936034679, 19.03943276465977164, 52.50109039468566863 ) ) ;
#139904=CARTESIAN_POINT ( 'NONE',  ( -16.51473224551069308, -9.474510206698971260, 31.66557627198102054 ) ) ;
#139905=CARTESIAN_POINT ( 'NONE',  ( 16.51473224551069308, 9.474510206698969483, 79.16557627198103830 ) ) ;
#139906=CARTESIAN_POINT ( 'NONE',  ( 0.05219959533936267826, -19.03943276465977164, 110.0010903946856757 ) ) ;
#139907=CARTESIAN_POINT ( 'NONE',  ( -8.314922557960811034, -14.29746914071050412, 77.08224293864769550 ) ) ;
#139908=CARTESIAN_POINT ( 'NONE',  ( 18.62759615963271287, -10.81492255796078972, 38.33224293864768839 ) ) ;
#139909=CARTESIAN_POINT ( 'NONE',  ( -5.049401038297874678, -19.05341960407617918, 94.79275706135230450 ) ) ;
#139910=CARTESIAN_POINT ( 'NONE',  ( 5.719274019375991003, -21.55341960407610458, 102.7072429386476955 ) ) ;
#139911=CARTESIAN_POINT ( 'NONE',  ( 15.80617190586769283, -15.72974639402175789, 60.62609039468567573 ) ) ;
#139912=CARTESIAN_POINT ( 'NONE',  ( -4.379528057220086978, -16.55341960407618274, 59.79275706135234714 ) ) ;
#139913=CARTESIAN_POINT ( 'NONE',  ( 12.06949235617739724, 12.14591786802326823, 56.87609039468568994 ) ) ;
#139915=CARTESIAN_POINT ( 'NONE',  ( 19.03943276465977164, -0.05219959533909143690, 43.74890960531435979 ) ) ;
#139916=CARTESIAN_POINT ( 'NONE',  ( -16.55341960407617563, 4.379528057220093196, 83.54275706135234714 ) ) ;
#139918=CARTESIAN_POINT ( 'NONE',  ( -21.52544592524334988, -5.823673210054445271, 18.95942372801901143 ) ) ;
#139919=CARTESIAN_POINT ( 'NONE',  ( -4.483927247898539470, -16.52544592524342804, 47.29057627198103120 ) ) ;
#139920=CARTESIAN_POINT ( 'NONE',  ( -13.97604488694527625, -13.89961937509977652, 81.87390960531436690 ) ) ;
#139921=CARTESIAN_POINT ( 'NONE',  ( -8.224510206698735004, -14.34966873604973081, 69.58442372801900433 ) ) ;
#139922=CARTESIAN_POINT ( 'NONE',  ( -21.52544592524334988, -5.823673210054445271, 48.95942372801902565 ) ) ;
#139923=CARTESIAN_POINT ( 'NONE',  ( -14.34966873604972548, 8.224510206698743886, 23.33442372801901499 ) ) ;
#139924=CARTESIAN_POINT ( 'NONE',  ( -21.55341960407610458, -5.719274019375992779, 111.4572429386476813 ) ) ;
#139925=CARTESIAN_POINT ( 'NONE',  ( 0.05219959533910956823, 16.53943276465976808, 49.99890960531437401 ) ) ;
#139927=CARTESIAN_POINT ( 'NONE',  ( -17.44270441346519362, 5.991230190322974103, 73.63664920735772057 ) ) ;
#139928=CARTESIAN_POINT ( 'NONE',  ( -21.53943276465977519, 0.05219959533907696930, 81.24890960531436690 ) ) ;
#139929=CARTESIAN_POINT ( 'NONE',  ( -4.483927247898782831, 16.52544592524335698, 112.7094237280190328 ) ) ;
#139932=CARTESIAN_POINT ( 'NONE',  ( -15.80617190586768217, 15.72974639402176855, 23.12609039468567573 ) ) ;
#139933=CARTESIAN_POINT ( 'NONE',  ( -5.049401038298153566, 19.05341960407611168, 110.2072429386476671 ) ) ;
#139934=CARTESIAN_POINT ( 'NONE',  ( 5.823673210054444382, -21.52544592524334988, 20.20942372801900788 ) ) ;
#139935=CARTESIAN_POINT ( 'NONE',  ( -14.29746914071049879, 8.314922557960819915, 50.83224293864770971 ) ) ;
#139936=CARTESIAN_POINT ( 'NONE',  ( -14.34966873604972548, 8.224510206698743886, 63.33442372801900433 ) ) ;
#139937=CARTESIAN_POINT ( 'NONE',  ( -5.049401038298153566, 19.05341960407611168, 65.20724293864765286 ) ) ;
#139938=CARTESIAN_POINT ( 'NONE',  ( 13.89961937509957401, 13.97604488694547697, 71.87609039468567573 ) ) ;
#139939=CARTESIAN_POINT ( 'NONE',  ( 13.97604488694527802, 13.89961937509977652, 74.37390960531436690 ) ) ;
#139941=CARTESIAN_POINT ( 'NONE',  ( -21.53943276465977519, 0.05219959533907696930, 41.24890960531435269 ) ) ;
#139943=CARTESIAN_POINT ( 'NONE',  ( 13.89961937509977652, -13.97604488694527269, 63.12390960531435979 ) ) ;
#139944=CARTESIAN_POINT ( 'NONE',  ( 16.52544592524335698, 4.483927247898782831, 21.45942372801901499 ) ) ;
#139945=CARTESIAN_POINT ( 'NONE',  ( -19.03943276465977164, -0.05219959533935918106, 63.75109039468566863 ) ) ;
#139946=CARTESIAN_POINT ( 'NONE',  ( 5.719274019375991003, -21.55341960407610458, 107.7072429386476955 ) ) ;
#139947=CARTESIAN_POINT ( 'NONE',  ( 16.53943276465976808, -0.05219959533910856209, 38.74890960531435979 ) ) ;
#139948=CARTESIAN_POINT ( 'NONE',  ( 13.89961937509977652, -13.97604488694527269, 93.12390960531436690 ) ) ;
#139949=CARTESIAN_POINT ( 'NONE',  ( -18.62759615963270932, 10.81492255796079327, 60.83224293864769550 ) ) ;
#139950=CARTESIAN_POINT ( 'NONE',  ( -5.719274019375978568, 21.55341960407610458, 90.20724293864770971 ) ) ;
#139951=CARTESIAN_POINT ( 'NONE',  ( -8.224510206698735004, -14.34966873604973081, 39.58442372801901143 ) ) ;
#139952=CARTESIAN_POINT ( 'NONE',  ( -18.62759615963270932, 10.81492255796079327, 30.83224293864770260 ) ) ;
#139953=CARTESIAN_POINT ( 'NONE',  ( 15.80617190586769283, -15.72974639402175789, 85.62609039468568994 ) ) ;
#139954=CARTESIAN_POINT ( 'NONE',  ( -9.564922557960796823, -16.46253265017161027, 82.08224293864768129 ) ) ;
#139955=CARTESIAN_POINT ( 'NONE',  ( -19.02544592524342804, 5.153800228976336051, 26.04057627198103120 ) ) ;
#139956=CARTESIAN_POINT ( 'NONE',  ( -19.05341960407611168, -5.049401038298163336, 86.45724293864769550 ) ) ;
#139957=CARTESIAN_POINT ( 'NONE',  ( 16.53943276465976808, -0.05219959533910856209, 108.7489096053143669 ) ) ;
#139958=CARTESIAN_POINT ( 'NONE',  ( 9.564922557960805705, 16.46253265017160317, 64.58224293864769550 ) ) ;
#139959=CARTESIAN_POINT ( 'NONE',  ( 19.02544592524334988, 5.153800228976608722, 111.4594237280190043 ) ) ;
#139961=CARTESIAN_POINT ( 'NONE',  ( 17.58332526062528345, 7.635886036038587399, 41.57665040441534643 ) ) ;
#139962=CARTESIAN_POINT ( 'NONE',  ( -15.72974639402176322, -15.80617190586768395, 94.37609039468568994 ) ) ;
#139963=CARTESIAN_POINT ( 'NONE',  ( 10.81492255796078972, 18.62759615963270932, 24.58224293864768839 ) ) ;
#139964=CARTESIAN_POINT ( 'NONE',  ( 14.34966873604972726, -8.224510206698740333, 85.83442372801901854 ) ) ;
#139965=DIRECTION ( 'NONE',  ( 1.000000000000000000, 0.000000000000000000, 0.000000000000000000 ) ) ;
#139966=CARTESIAN_POINT ( 'NONE',  ( 5.049401038297881783, 19.05341960407617563, 67.29275706135234714 ) ) ;
#139967=CARTESIAN_POINT ( 'NONE',  ( -16.46253265017146816, -9.564922557961047289, 29.16775706135232937 ) ) ;
#139969=CARTESIAN_POINT ( 'NONE',  ( 13.97604488694527802, 13.89961937509977652, 24.37390960531435624 ) ) ;
#139970=CARTESIAN_POINT ( 'NONE',  ( -8.224510206698948167, 14.34966873604960824, 30.41557627198101699 ) ) ;
#139972=CARTESIAN_POINT ( 'NONE',  ( -16.55341960407611168, -4.379528057220339221, 26.45724293864768839 ) ) ;
#139974=CARTESIAN_POINT ( 'NONE',  ( 16.53943276465976808, 0.05219959533934440121, 96.25109039468568994 ) ) ;
#139975=CARTESIAN_POINT ( 'NONE',  ( -19.03943276465977164, 0.05219959533909376836, 41.24890960531435269 ) ) ;
#139976=CARTESIAN_POINT ( 'NONE',  ( 10.72451020669871369, 18.67979575497193778, 97.08442372801904696 ) ) ;
#139977=CARTESIAN_POINT ( 'NONE',  ( -9.564922557961040184, 16.46253265017147172, 102.9177570613523329 ) ) ;
#139978=CARTESIAN_POINT ( 'NONE',  ( -5.719274019375665041, -21.55341960407619695, 84.79275706135234714 ) ) ;
#139979=CARTESIAN_POINT ( 'NONE',  ( -19.05341960407617563, 5.049401038297882671, 58.54275706135234003 ) ) ;
#139980=CARTESIAN_POINT ( 'NONE',  ( -9.564922557960796823, -16.46253265017161027, 87.08224293864769550 ) ) ;
#139981=CARTESIAN_POINT ( 'NONE',  ( 13.89961937509977652, -13.97604488694527269, 68.12390960531436690 ) ) ;
#139983=CARTESIAN_POINT ( 'NONE',  ( 8.314922557960818139, 14.29746914071049879, 69.58224293864769550 ) ) ;
#139984=CARTESIAN_POINT ( 'NONE',  ( 5.719274019375991003, -21.55341960407610458, 57.70724293864770260 ) ) ;
#139985=CARTESIAN_POINT ( 'NONE',  ( -9.474510206698964154, 16.51473224551069663, 60.41557627198102409 ) ) ;
#139986=CARTESIAN_POINT ( 'NONE',  ( 5.823673210054125526, 21.52544592524343514, 84.79057627198102409 ) ) ;
#139987=CARTESIAN_POINT ( 'NONE',  ( -0.05219959533934338120, 16.53943276465976808, 72.50109039468568994 ) ) ;
#139990=CARTESIAN_POINT ( 'NONE',  ( -19.05341960407611168, -5.049401038298163336, 51.45724293864770260 ) ) ;
#139991=CARTESIAN_POINT ( 'NONE',  ( -12.06949235617756955, 12.14591786802309770, 80.62390960531438111 ) ) ;
#139993=CARTESIAN_POINT ( 'NONE',  ( 9.474510206698971260, -16.51473224551069308, 52.91557627198102409 ) ) ;
#139994=CARTESIAN_POINT ( 'NONE',  ( 5.153800228976335163, 19.02544592524342804, 24.79057627198102765 ) ) ;
#139995=CARTESIAN_POINT ( 'NONE',  ( 5.153800228976615827, -19.02544592524334988, 70.20942372801899012 ) ) ;
#139996=CARTESIAN_POINT ( 'NONE',  ( 14.29746914071049879, -8.314922557960816363, 83.33224293864769550 ) ) ;
#139997=CARTESIAN_POINT ( 'NONE',  ( 21.53943276465977519, 0.05219959533937863772, 41.25109039468568284 ) ) ;
#139998=CARTESIAN_POINT ( 'NONE',  ( 13.89961937509977652, -13.97604488694527269, 33.12390960531434558 ) ) ;
#139999=CARTESIAN_POINT ( 'NONE',  ( -21.53943276465977519, 0.05219959533907696930, 106.2489096053143811 ) ) ;
#140000=CARTESIAN_POINT ( 'NONE',  ( 13.89961937509977652, -13.97604488694527269, 113.1239096053143527 ) ) ;
#140001=CARTESIAN_POINT ( 'NONE',  ( 14.29746914071049879, -8.314922557960816363, 88.33224293864769550 ) ) ;
#140003=CARTESIAN_POINT ( 'NONE',  ( 5.153800228976335163, 19.02544592524342804, 44.79057627198103830 ) ) ;
#140005=CARTESIAN_POINT ( 'NONE',  ( -9.474510206698720793, -16.51473224551083518, 89.58442372801900433 ) ) ;
#140006=CARTESIAN_POINT ( 'NONE',  ( 13.97604488694527802, 13.89961937509977652, 94.37390960531436690 ) ) ;
#140007=CARTESIAN_POINT ( 'NONE',  ( -18.67979575497193778, 10.72451020669871902, 38.33442372801900433 ) ) ;
#140008=CARTESIAN_POINT ( 'NONE',  ( 19.05341960407611168, 5.049401038298154454, 78.95724293864769550 ) ) ;
#140010=CARTESIAN_POINT ( 'NONE',  ( -16.46253265017146816, -9.564922557961047289, 74.16775706135234714 ) ) ;
#140011=CARTESIAN_POINT ( 'NONE',  ( 19.02544592524343514, -5.153800228976328945, 48.54057627198103120 ) ) ;
#140012=CARTESIAN_POINT ( 'NONE',  ( -14.29746914071049879, 8.314922557960819915, 70.83224293864770971 ) ) ;
#140013=CARTESIAN_POINT ( 'NONE',  ( 16.53943276465976808, -0.05219959533910856209, 73.74890960531433848 ) ) ;
#140014=CARTESIAN_POINT ( 'NONE',  ( 9.564922557960805705, 16.46253265017160317, 79.58224293864769550 ) ) ;
#140015=CARTESIAN_POINT ( 'NONE',  ( -15.72974639402197994, 15.80617190586746368, 100.6239096053143811 ) ) ;
#140016=CARTESIAN_POINT ( 'NONE',  ( 19.03943276465977164, -0.05219959533909143690, 73.74890960531435269 ) ) ;
#140017=CARTESIAN_POINT ( 'NONE',  ( -9.564922557961040184, 16.46253265017147172, 22.91775706135233648 ) ) ;
#140018=CARTESIAN_POINT ( 'NONE',  ( 19.03943276465977164, -0.05219959533909143690, 38.74890960531436690 ) ) ;
#140019=CARTESIAN_POINT ( 'NONE',  ( -4.379528057220328563, 16.55341960407611168, 30.20724293864769550 ) ) ;
#140020=CARTESIAN_POINT ( 'NONE',  ( -8.314922557960811034, -14.29746914071050412, 107.0822429386476955 ) ) ;
#140021=CARTESIAN_POINT ( 'NONE',  ( -13.97604488694547697, 13.89961937509957934, 108.1260903946856331 ) ) ;
#140023=CARTESIAN_POINT ( 'NONE',  ( 21.53943276465977519, 0.05219959533937863772, 26.25109039468567573 ) ) ;
#140024=CARTESIAN_POINT ( 'NONE',  ( -5.049401038297874678, -19.05341960407617918, 64.79275706135233293 ) ) ;
#140025=CARTESIAN_POINT ( 'NONE',  ( -8.314922557960811034, -14.29746914071050412, 27.08224293864769550 ) ) ;
#140026=CARTESIAN_POINT ( 'NONE',  ( -18.67979575497178146, -10.72451020669898902, 91.66557627198103830 ) ) ;
#140027=CARTESIAN_POINT ( 'NONE',  ( -10.81492255796078084, -18.62759615963271287, 27.08224293864769550 ) ) ;
#140028=CARTESIAN_POINT ( 'NONE',  ( -4.379528057220328563, 16.55341960407611168, 55.20724293864770260 ) ) ;
#140029=CARTESIAN_POINT ( 'NONE',  ( 5.049401038298161559, -19.05341960407611168, 32.70724293864768129 ) ) ;
#140030=CARTESIAN_POINT ( 'NONE',  ( 16.51473224551083163, -9.474510206698727899, 20.83442372801899722 ) ) ;
#140031=CARTESIAN_POINT ( 'NONE',  ( -16.52544592524335698, -4.483927247898792601, 83.95942372801900433 ) ) ;
#140032=CARTESIAN_POINT ( 'NONE',  ( 12.14591786802327356, -12.06949235617739191, 50.62609039468568994 ) ) ;
#140033=CARTESIAN_POINT ( 'NONE',  ( 10.81492255796078972, 18.62759615963270932, 29.58224293864769905 ) ) ;
#140034=CARTESIAN_POINT ( 'NONE',  ( -18.62759615963255300, -10.81492255796106328, 104.1677570613523471 ) ) ;
#140035=CARTESIAN_POINT ( 'NONE',  ( 13.89961937509977652, -13.97604488694527269, 83.12390960531436690 ) ) ;
#140036=CARTESIAN_POINT ( 'NONE',  ( 12.14591786802327356, -12.06949235617739191, 65.62609039468568994 ) ) ;
#140037=CARTESIAN_POINT ( 'NONE',  ( -4.483927247898539470, -16.52544592524342804, 107.2905762719810525 ) ) ;
#140038=CARTESIAN_POINT ( 'NONE',  ( 12.14591786802309770, 12.06949235617756955, 39.37390960531436690 ) ) ;
#140040=CARTESIAN_POINT ( 'NONE',  ( -15.72974639402176322, -15.80617190586768395, 69.37609039468567573 ) ) ;
#140041=CARTESIAN_POINT ( 'NONE',  ( 5.049401038298161559, -19.05341960407611168, 92.70724293864769550 ) ) ;
#140042=CARTESIAN_POINT ( 'NONE',  ( 5.049401038298161559, -19.05341960407611168, 72.70724293864768129 ) ) ;
#140043=CARTESIAN_POINT ( 'NONE',  ( -16.51473224551069308, -9.474510206698971260, 111.6655762719810383 ) ) ;
#140044=CARTESIAN_POINT ( 'NONE',  ( 14.29746914071049879, -8.314922557960816363, 58.33224293864768839 ) ) ;
#140045=CARTESIAN_POINT ( 'NONE',  ( -14.34966873604960291, -8.224510206698953496, 21.66557627198102409 ) ) ;
#140048=CARTESIAN_POINT ( 'NONE',  ( -14.29746914071049879, 8.314922557960819915, 50.83224293864770971 ) ) ;
#140049=CARTESIAN_POINT ( 'NONE',  ( 12.14591786802327356, -12.06949235617739191, 40.62609039468567573 ) ) ;
#140050=CARTESIAN_POINT ( 'NONE',  ( -17.49999999999998934, -5.500000000000015987, 56.28230962303566542 ) ) ;
#140051=CARTESIAN_POINT ( 'NONE',  ( -9.474510206698720793, -16.51473224551083518, 44.58442372801900433 ) ) ;
#140052=CARTESIAN_POINT ( 'NONE',  ( -0.05219959533909027116, -19.03943276465977164, 72.49890960531435269 ) ) ;
#140053=CARTESIAN_POINT ( 'NONE',  ( 19.05341960407617918, -5.049401038297876454, 46.04275706135233293 ) ) ;
#140054=CARTESIAN_POINT ( 'NONE',  ( 0.05219959533936267826, -19.03943276465977164, 60.00109039468566863 ) ) ;
#140055=CARTESIAN_POINT ( 'NONE',  ( -16.46253265017146816, -9.564922557961047289, 104.1677570613523329 ) ) ;
#140056=CARTESIAN_POINT ( 'NONE',  ( -16.55341960407617563, 4.379528057220093196, 83.54275706135234714 ) ) ;
#140058=CARTESIAN_POINT ( 'NONE',  ( -9.474510206698964154, 16.51473224551069663, 30.41557627198102054 ) ) ;
#140059=CARTESIAN_POINT ( 'NONE',  ( -9.564922557960796823, -16.46253265017161027, 107.0822429386476955 ) ) ;
#140060=CARTESIAN_POINT ( 'NONE',  ( -18.67979575497193778, 10.72451020669871902, 43.33442372801901143 ) ) ;
#140061=CARTESIAN_POINT ( 'NONE',  ( -16.46253265017146816, -9.564922557961047289, 89.16775706135234714 ) ) ;
#140062=CARTESIAN_POINT ( 'NONE',  ( 17.49999999999999645, -3.305555262949659401, 107.1251715215659317 ) ) ;
#140063=CARTESIAN_POINT ( 'NONE',  ( 13.89961937509977652, -13.97604488694527269, 63.12390960531435979 ) ) ;
#140064=CARTESIAN_POINT ( 'NONE',  ( -19.05341960407611168, -5.049401038298163336, 106.4572429386476955 ) ) ;
#140065=CARTESIAN_POINT ( 'NONE',  ( -12.14591786802309592, -12.06949235617757132, 66.87390960531436690 ) ) ;
#140066=CARTESIAN_POINT ( 'NONE',  ( 19.05341960407611168, 5.049401038298154454, 68.95724293864769550 ) ) ;
#140067=CARTESIAN_POINT ( 'NONE',  ( 5.153800228976335163, 19.02544592524342804, 64.79057627198100988 ) ) ;
#140068=CARTESIAN_POINT ( 'NONE',  ( -13.89961937509957401, -13.97604488694547875, 59.37609039468566863 ) ) ;
#140069=CARTESIAN_POINT ( 'NONE',  ( -5.823673210054116645, -21.52544592524344225, 52.29057627198102409 ) ) ;
#140070=CARTESIAN_POINT ( 'NONE',  ( -5.153800228976607833, 19.02544592524334988, 37.70942372801899722 ) ) ;
#140071=CARTESIAN_POINT ( 'NONE',  ( 13.89961937509977652, -13.97604488694527269, 78.12390960531433848 ) ) ;
#140072=CARTESIAN_POINT ( 'NONE',  ( -10.72451020669898014, 18.67979575497178502, 80.41557627198103830 ) ) ;
#140073=CARTESIAN_POINT ( 'NONE',  ( -14.34966873604960291, -8.224510206698953496, 76.66557627198103830 ) ) ;
#140074=CARTESIAN_POINT ( 'NONE',  ( -19.02544592524334988, -5.153800228976617603, 38.95942372801900433 ) ) ;
#140075=CARTESIAN_POINT ( 'NONE',  ( -18.62759615963270932, 10.81492255796079327, 45.83224293864769550 ) ) ;
#140076=CARTESIAN_POINT ( 'NONE',  ( 0.05219959533907565091, 21.53943276465977519, 34.99890960531435979 ) ) ;
#140077=CARTESIAN_POINT ( 'NONE',  ( -0.05219959533909027116, -19.03943276465977164, 67.49890960531436690 ) ) ;
#140078=CARTESIAN_POINT ( 'NONE',  ( 9.474510206698971260, -16.51473224551069308, 57.91557627198103120 ) ) ;
#140079=CARTESIAN_POINT ( 'NONE',  ( 9.474510206698971260, -16.51473224551069308, 22.91557627198102765 ) ) ;
#140080=CARTESIAN_POINT ( 'NONE',  ( 21.52544592524334988, 5.823673210054432836, 21.45942372801901499 ) ) ;
#140082=CARTESIAN_POINT ( 'NONE',  ( -21.52544592524334988, -5.823673210054445271, 33.95942372801901143 ) ) ;
#140083=CARTESIAN_POINT ( 'NONE',  ( -13.97604488694527625, -13.89961937509977652, 36.87390960531436690 ) ) ;
#140084=CARTESIAN_POINT ( 'NONE',  ( 5.823673210054125526, 21.52544592524343514, 104.7905762719810241 ) ) ;
#140085=CARTESIAN_POINT ( 'NONE',  ( -19.03943276465977164, -0.05219959533935918106, 48.75109039468566863 ) ) ;
#140086=CARTESIAN_POINT ( 'NONE',  ( 19.03943276465977164, -0.05219959533909143690, 28.74890960531435624 ) ) ;
#140088=CARTESIAN_POINT ( 'NONE',  ( 16.65483384399521682, -7.017357588706441440, 21.38698616505659444 ) ) ;
#140089=CARTESIAN_POINT ( 'NONE',  ( -16.55341960407617563, 4.379528057220093196, 53.54275706135234714 ) ) ;
#140090=CARTESIAN_POINT ( 'NONE',  ( -9.474510206698964154, 16.51473224551069663, 25.41557627198103120 ) ) ;
#140092=CARTESIAN_POINT ( 'NONE',  ( 19.05341960407611168, 5.049401038298154454, 78.95724293864769550 ) ) ;
#140093=CARTESIAN_POINT ( 'NONE',  ( -14.29746914071049879, 8.314922557960819915, 110.8322429386476955 ) ) ;
#140095=CARTESIAN_POINT ( 'NONE',  ( -5.823673210054116645, -21.52544592524344225, 57.29057627198103120 ) ) ;
#140096=CARTESIAN_POINT ( 'NONE',  ( 12.06949235617757843, -12.14591786802309237, 73.12390960531436690 ) ) ;
#140097=CARTESIAN_POINT ( 'NONE',  ( -12.06949235617739369, -12.14591786802326823, 29.37609039468568284 ) ) ;
#140098=CARTESIAN_POINT ( 'NONE',  ( -10.81492255796105439, 18.62759615963255655, 87.91775706135234714 ) ) ;
#140099=CARTESIAN_POINT ( 'NONE',  ( 19.05341960407611168, 5.049401038298154454, 28.95724293864769550 ) ) ;
#140100=CARTESIAN_POINT ( 'NONE',  ( 0.05219959533910956823, 16.53943276465976808, 24.99890960531435624 ) ) ;
#140101=CARTESIAN_POINT ( 'NONE',  ( -14.29746914071049879, 8.314922557960819915, 60.83224293864769550 ) ) ;
#140102=CARTESIAN_POINT ( 'NONE',  ( -19.02544592524342804, 5.153800228976336051, 56.04057627198100988 ) ) ;
#140103=CARTESIAN_POINT ( 'NONE',  ( -0.05219959533937732626, 21.53943276465977519, 102.5010903946856899 ) ) ;
#140104=CARTESIAN_POINT ( 'NONE',  ( -18.67979575497178146, -10.72451020669898902, 101.6655762719810383 ) ) ;
#140105=CARTESIAN_POINT ( 'NONE',  ( 21.55341960407619695, -5.719274019375665929, 76.04275706135237556 ) ) ;
#140106=CARTESIAN_POINT ( 'NONE',  ( -14.29746914071037622, -8.314922557961029526, 44.16775706135234714 ) ) ;
#140107=CARTESIAN_POINT ( 'NONE',  ( -16.52544592524342804, 4.483927247898546575, 81.04057627198102409 ) ) ;
#140108=CARTESIAN_POINT ( 'NONE',  ( -10.72451020669870658, -18.67979575497194134, 89.58442372801901854 ) ) ;
#140109=CARTESIAN_POINT ( 'NONE',  ( -16.53943276465976808, 0.05219959533911058130, 21.24890960531436690 ) ) ;
#140111=CARTESIAN_POINT ( 'NONE',  ( 14.29746914071037800, 8.314922557961029526, 41.66775706135235424 ) ) ;
#140112=CARTESIAN_POINT ( 'NONE',  ( -12.14591786802309592, -12.06949235617757132, 46.87390960531435979 ) ) ;
#140113=CARTESIAN_POINT ( 'NONE',  ( 12.14591786802327356, -12.06949235617739191, 90.62609039468567573 ) ) ;
#140114=CARTESIAN_POINT ( 'NONE',  ( 5.153800228976335163, 19.02544592524342804, 99.79057627198102409 ) ) ;
#140115=CARTESIAN_POINT ( 'NONE',  ( -19.02544592524342804, 5.153800228976336051, 116.0405762719810383 ) ) ;
#140116=CARTESIAN_POINT ( 'NONE',  ( -21.55341960407619339, 5.719274019375674811, 103.5427570613523613 ) ) ;
#140117=CARTESIAN_POINT ( 'NONE',  ( 12.06949235617739724, 12.14591786802326823, 101.8760903946857042 ) ) ;
#140118=CARTESIAN_POINT ( 'NONE',  ( -16.55341960407611168, -4.379528057220339221, 76.45724293864769550 ) ) ;
#140119=CARTESIAN_POINT ( 'NONE',  ( 0.05219959533909260263, 19.03943276465977164, 84.99890960531436690 ) ) ;
#140121=CARTESIAN_POINT ( 'NONE',  ( -16.52544592524335698, -4.483927247898792601, 23.95942372801901143 ) ) ;
#140122=CARTESIAN_POINT ( 'NONE',  ( 5.153800228976335163, 19.02544592524342804, 34.79057627198102409 ) ) ;
#140123=CARTESIAN_POINT ( 'NONE',  ( -9.564922557960796823, -16.46253265017161027, 92.08224293864769550 ) ) ;
#140124=CARTESIAN_POINT ( 'NONE',  ( 12.06949235617739724, 12.14591786802326823, 31.87609039468567929 ) ) ;
#140126=CARTESIAN_POINT ( 'NONE',  ( 0.05219959533936267826, -19.03943276465977164, 35.00109039468566863 ) ) ;
#140127=CARTESIAN_POINT ( 'NONE',  ( -4.379528057220086978, -16.55341960407618274, 99.79275706135234714 ) ) ;
#140128=CARTESIAN_POINT ( 'NONE',  ( 0.05219959533936267826, -19.03943276465977164, 110.0010903946856757 ) ) ;
#140129=CARTESIAN_POINT ( 'NONE',  ( 13.89961937509977652, -13.97604488694527269, 28.12390960531435624 ) ) ;
#140130=CARTESIAN_POINT ( 'NONE',  ( -8.224510206698735004, -14.34966873604973081, 74.58442372801901854 ) ) ;
#140131=CARTESIAN_POINT ( 'NONE',  ( -4.379528057220086978, -16.55341960407618274, 69.79275706135234714 ) ) ;
#140132=CARTESIAN_POINT ( 'NONE',  ( 19.03943276465977164, 0.05219959533936151252, 86.25109039468567573 ) ) ;
#140133=CARTESIAN_POINT ( 'NONE',  ( -15.80617190586768217, 15.72974639402176855, 113.1260903946856899 ) ) ;
#140134=CARTESIAN_POINT ( 'NONE',  ( 13.89961937509977652, -13.97604488694527269, 43.12390960531434558 ) ) ;
#140135=CARTESIAN_POINT ( 'NONE',  ( -16.51473224551069308, -9.474510206698971260, 96.66557627198102409 ) ) ;
#140136=CARTESIAN_POINT ( 'NONE',  ( 16.55341960407611168, 4.379528057220329451, 88.95724293864769550 ) ) ;
#140138=CARTESIAN_POINT ( 'NONE',  ( -0.05219959533936034679, 19.03943276465977164, 57.50109039468566863 ) ) ;
#140139=CARTESIAN_POINT ( 'NONE',  ( 21.55341960407610458, 5.719274019375980345, 48.95724293864770971 ) ) ;
#140140=CARTESIAN_POINT ( 'NONE',  ( -13.89961937509957401, -13.97604488694547875, 24.37609039468565442 ) ) ;
#140141=CARTESIAN_POINT ( 'NONE',  ( -9.474510206698964154, 16.51473224551069663, 90.41557627198103830 ) ) ;
#140142=CARTESIAN_POINT ( 'NONE',  ( 5.153800228976615827, -19.02544592524334988, 25.20942372801900433 ) ) ;
#140143=CARTESIAN_POINT ( 'NONE',  ( 15.80617190586746368, 15.72974639402197994, 69.37390960531436690 ) ) ;
#140144=CARTESIAN_POINT ( 'NONE',  ( 9.474510206698971260, -16.51473224551069308, 107.9155762719810383 ) ) ;
#140145=CARTESIAN_POINT ( 'NONE',  ( 13.97604488694548053, -13.89961937509957401, 85.62609039468568994 ) ) ;
#140146=CARTESIAN_POINT ( 'NONE',  ( 19.05341960407611168, 5.049401038298154454, 113.9572429386477097 ) ) ;
#140147=CARTESIAN_POINT ( 'NONE',  ( 9.564922557961047289, -16.46253265017146816, 105.4177570613523471 ) ) ;
#140148=CARTESIAN_POINT ( 'NONE',  ( -0.05219959533909027116, -19.03943276465977164, 32.49890960531435979 ) ) ;
#140149=CARTESIAN_POINT ( 'NONE',  ( -16.51473224551069308, -9.474510206698971260, 101.6655762719810241 ) ) ;
#140150=CARTESIAN_POINT ( 'NONE',  ( 18.67979575497178502, 10.72451020669898547, 74.16557627198102409 ) ) ;
#140151=CARTESIAN_POINT ( 'NONE',  ( 12.06949235617739724, 12.14591786802326823, 46.87609039468568994 ) ) ;
#140152=CARTESIAN_POINT ( 'NONE',  ( 5.823673210054444382, -21.52544592524334988, 50.20942372801901854 ) ) ;
#140153=CARTESIAN_POINT ( 'NONE',  ( 16.46253265017146816, 9.564922557961045513, 86.66775706135233293 ) ) ;
#140154=CARTESIAN_POINT ( 'NONE',  ( -5.823673210054431948, 21.52544592524334988, 92.70942372801901854 ) ) ;
#140155=CARTESIAN_POINT ( 'NONE',  ( -12.14591786802326823, 12.06949235617739902, 98.12609039468570415 ) ) ;
#140156=CARTESIAN_POINT ( 'NONE',  ( 0.05219959533909260263, 19.03943276465977164, 94.99890960531436690 ) ) ;
#140157=CARTESIAN_POINT ( 'NONE',  ( -8.224510206698948167, 14.34966873604960824, 85.41557627198102409 ) ) ;
#140158=CARTESIAN_POINT ( 'NONE',  ( -16.55341960407611168, -4.379528057220339221, 36.45724293864768839 ) ) ;
#140159=CARTESIAN_POINT ( 'NONE',  ( -19.05341960407617563, 5.049401038297882671, 73.54275706135233293 ) ) ;
#140160=CARTESIAN_POINT ( 'NONE',  ( 21.55341960407619695, -5.719274019375665929, 56.04275706135235424 ) ) ;
#140161=CARTESIAN_POINT ( 'NONE',  ( -0.05219959533936034679, 19.03943276465977164, 32.50109039468566863 ) ) ;
#140162=CARTESIAN_POINT ( 'NONE',  ( 12.14591786802309770, 12.06949235617756955, 94.37390960531436690 ) ) ;
#140163=CARTESIAN_POINT ( 'NONE',  ( -0.05219959533907301413, -21.53943276465977519, 27.49890960531435269 ) ) ;
#140164=CARTESIAN_POINT ( 'NONE',  ( 16.53943276465976808, -0.05219959533910856209, 23.74890960531435269 ) ) ;
#140165=CARTESIAN_POINT ( 'NONE',  ( 10.81492255796106328, -18.62759615963255655, 95.41775706135234714 ) ) ;
#140166=CARTESIAN_POINT ( 'NONE',  ( 14.34966873604972726, -8.224510206698740333, 60.83442372801901854 ) ) ;
#140167=CARTESIAN_POINT ( 'NONE',  ( -12.14591786802326823, 12.06949235617739902, 103.1260903946856757 ) ) ;
#140168=CARTESIAN_POINT ( 'NONE',  ( -5.823673210054431948, 21.52544592524334988, 47.70942372801902565 ) ) ;
#140169=CARTESIAN_POINT ( 'NONE',  ( -15.80617190586768217, 15.72974639402176855, 58.12609039468568994 ) ) ;
#140171=CARTESIAN_POINT ( 'NONE',  ( -18.62759615963255300, -10.81492255796106328, 29.16775706135234003 ) ) ;
#140172=CARTESIAN_POINT ( 'NONE',  ( 12.14591786802309770, 12.06949235617756955, 99.37390960531436690 ) ) ;
#140173=CARTESIAN_POINT ( 'NONE',  ( 13.97604488694527802, 13.89961937509977652, 24.37390960531435624 ) ) ;
#140174=CARTESIAN_POINT ( 'NONE',  ( 14.34966873604960469, 8.224510206698951720, 74.16557627198102409 ) ) ;
#140175=CARTESIAN_POINT ( 'NONE',  ( -19.02544592524342804, 5.153800228976336051, 66.04057627198103830 ) ) ;
#140176=CARTESIAN_POINT ( 'NONE',  ( -16.52544592524335698, -4.483927247898792601, 108.9594237280190185 ) ) ;
#140177=CARTESIAN_POINT ( 'NONE',  ( -21.52544592524343514, 5.823673210054127303, 56.04057627198102409 ) ) ;
#140178=CARTESIAN_POINT ( 'NONE',  ( 14.34966873604960469, 8.224510206698951720, 89.16557627198102409 ) ) ;
#140179=CARTESIAN_POINT ( 'NONE',  ( -0.05219959533907301413, -21.53943276465977519, 87.49890960531436690 ) ) ;
#140180=CARTESIAN_POINT ( 'NONE',  ( -5.153800228976328057, -19.02544592524343514, 102.2905762719810383 ) ) ;
#140181=CARTESIAN_POINT ( 'NONE',  ( -16.51473224551069308, -9.474510206698971260, 46.66557627198102409 ) ) ;
#140182=CARTESIAN_POINT ( 'NONE',  ( 5.049401038297881783, 19.05341960407617563, 112.2927570613523471 ) ) ;
#140184=CARTESIAN_POINT ( 'NONE',  ( 5.823673210054125526, 21.52544592524343514, 49.79057627198102409 ) ) ;
#140185=CARTESIAN_POINT ( 'NONE',  ( -10.72451020669870658, -18.67979575497194134, 69.58442372801900433 ) ) ;
#140186=CARTESIAN_POINT ( 'NONE',  ( 13.89961937509977652, -13.97604488694527269, 68.12390960531436690 ) ) ;
#140187=CARTESIAN_POINT ( 'NONE',  ( -5.153800228976328057, -19.02544592524343514, 102.2905762719810383 ) ) ;
#140188=CARTESIAN_POINT ( 'NONE',  ( -16.52544592524335698, -4.483927247898792601, 58.95942372801902565 ) ) ;
#140189=CARTESIAN_POINT ( 'NONE',  ( -10.81492255796105439, 18.62759615963255655, 47.91775706135234714 ) ) ;
#140190=CARTESIAN_POINT ( 'NONE',  ( -5.719274019375665041, -21.55341960407619695, 84.79275706135234714 ) ) ;
#140191=CARTESIAN_POINT ( 'NONE',  ( 18.62759615963271287, -10.81492255796078972, 93.33224293864769550 ) ) ;
#140192=CARTESIAN_POINT ( 'NONE',  ( -5.719274019375665041, -21.55341960407619695, 34.79275706135235424 ) ) ;
#140193=CARTESIAN_POINT ( 'NONE',  ( -16.55341960407617563, 4.379528057220093196, 78.54275706135236135 ) ) ;
#140194=CARTESIAN_POINT ( 'NONE',  ( -10.72451020669898014, 18.67979575497178502, 75.41557627198102409 ) ) ;
#140195=CARTESIAN_POINT ( 'NONE',  ( 5.153800228976615827, -19.02544592524334988, 40.20942372801898301 ) ) ;
#140196=CARTESIAN_POINT ( 'NONE',  ( -13.89961937509977652, 13.97604488694528158, 85.62390960531433848 ) ) ;
#140197=CARTESIAN_POINT ( 'NONE',  ( 16.52544592524342804, -4.483927247898539470, 23.54057627198102765 ) ) ;
#140198=CARTESIAN_POINT ( 'NONE',  ( -17.13100169013298668, 6.664070546373142889, 65.76789835699850073 ) ) ;
#140199=CARTESIAN_POINT ( 'NONE',  ( 19.03943276465977164, -0.05219959533909143690, 98.74890960531436690 ) ) ;
#140201=CARTESIAN_POINT ( 'NONE',  ( -19.05341960407617563, 5.049401038297882671, 98.54275706135233293 ) ) ;
#140202=CARTESIAN_POINT ( 'NONE',  ( 10.72451020669898902, -18.67979575497178502, 52.91557627198103830 ) ) ;
#140203=CARTESIAN_POINT ( 'NONE',  ( -16.52544592524342804, 4.483927247898546575, 41.04057627198103120 ) ) ;
#140204=CARTESIAN_POINT ( 'NONE',  ( -5.153800228976607833, 19.02544592524334988, 112.7094237280190043 ) ) ;
#140205=CARTESIAN_POINT ( 'NONE',  ( -5.049401038298153566, 19.05341960407611168, 25.20724293864768484 ) ) ;
#140206=CARTESIAN_POINT ( 'NONE',  ( 8.314922557961029526, -14.29746914071037800, 20.41775706135234714 ) ) ;
#140207=CARTESIAN_POINT ( 'NONE',  ( -10.81492255796078084, -18.62759615963271287, 107.0822429386476955 ) ) ;
#140208=CARTESIAN_POINT ( 'NONE',  ( -9.474510206698720793, -16.51473224551083518, 74.58442372801900433 ) ) ;
#140209=CARTESIAN_POINT ( 'NONE',  ( -12.14591786802326823, 12.06949235617739902, 78.12609039468570415 ) ) ;
#140210=CARTESIAN_POINT ( 'NONE',  ( -5.049401038298153566, 19.05341960407611168, 65.20724293864765286 ) ) ;
#140211=CARTESIAN_POINT ( 'NONE',  ( -16.53943276465976808, 0.05219959533911058130, 81.24890960531436690 ) ) ;
#140213=CARTESIAN_POINT ( 'NONE',  ( 5.049401038298161559, -19.05341960407611168, 62.70724293864769550 ) ) ;
#140214=CARTESIAN_POINT ( 'NONE',  ( 8.314922557960818139, 14.29746914071049879, 64.58224293864769550 ) ) ;
#140217=CARTESIAN_POINT ( 'NONE',  ( -8.314922557960811034, -14.29746914071050412, 42.08224293864769550 ) ) ;
#140218=CARTESIAN_POINT ( 'NONE',  ( -5.153800228976328057, -19.02544592524343514, 77.29057627198099567 ) ) ;
#140220=CARTESIAN_POINT ( 'NONE',  ( 13.89961937509957401, 13.97604488694547697, 51.87609039468566863 ) ) ;
#140221=CARTESIAN_POINT ( 'NONE',  ( -12.06949235617739369, -12.14591786802326823, 64.37609039468568994 ) ) ;
#140222=CARTESIAN_POINT ( 'NONE',  ( -15.72974639402197994, 15.80617190586746368, 70.62390960531436690 ) ) ;
#140223=CARTESIAN_POINT ( 'NONE',  ( -19.02544592524334988, -5.153800228976617603, 18.95942372801899722 ) ) ;
#140224=CARTESIAN_POINT ( 'NONE',  ( -0.05219959533909027116, -19.03943276465977164, 77.49890960531435269 ) ) ;
#140226=CARTESIAN_POINT ( 'NONE',  ( -16.46253265017160317, 9.564922557960807481, 110.8322429386476955 ) ) ;
#140227=CARTESIAN_POINT ( 'NONE',  ( -19.05341960407611168, -5.049401038298163336, 61.45724293864769550 ) ) ;
#140228=CARTESIAN_POINT ( 'NONE',  ( -5.719274019375665041, -21.55341960407619695, 39.79275706135235424 ) ) ;
#140229=CARTESIAN_POINT ( 'NONE',  ( -14.29746914071049879, 8.314922557960819915, 105.8322429386476955 ) ) ;
#140230=CARTESIAN_POINT ( 'NONE',  ( 10.72451020669898902, -18.67979575497178502, 107.9155762719810241 ) ) ;
#140231=CARTESIAN_POINT ( 'NONE',  ( 5.153800228976335163, 19.02544592524342804, 94.79057627198103830 ) ) ;
#140233=CARTESIAN_POINT ( 'NONE',  ( 15.72974639402176855, 15.80617190586768217, 31.87609039468567929 ) ) ;
#140235=CARTESIAN_POINT ( 'NONE',  ( 13.89961937509977652, -13.97604488694527269, 83.12390960531436690 ) ) ;
#140237=CARTESIAN_POINT ( 'NONE',  ( 5.823673210054125526, 21.52544592524343514, 99.79057627198103830 ) ) ;
#140238=CARTESIAN_POINT ( 'NONE',  ( 13.97604488694527802, 13.89961937509977652, 44.37390960531435269 ) ) ;
#140239=CARTESIAN_POINT ( 'NONE',  ( 5.049401038297881783, 19.05341960407617563, 102.2927570613523045 ) ) ;
#140242=CARTESIAN_POINT ( 'NONE',  ( -19.05341960407611168, -5.049401038298163336, 31.45724293864769550 ) ) ;
#140243=CARTESIAN_POINT ( 'NONE',  ( 15.80617190586769283, -15.72974639402175789, 80.62609039468567573 ) ) ;
#140244=CARTESIAN_POINT ( 'NONE',  ( 9.474510206698971260, -16.51473224551069308, 72.91557627198102409 ) ) ;
#140245=CARTESIAN_POINT ( 'NONE',  ( -0.05219959533937732626, 21.53943276465977519, 42.50109039468567573 ) ) ;
#140246=CARTESIAN_POINT ( 'NONE',  ( 10.81492255796106328, -18.62759615963255655, 20.41775706135234714 ) ) ;
#140248=CARTESIAN_POINT ( 'NONE',  ( -16.51473224551069308, -9.474510206698971260, 91.66557627198103830 ) ) ;
#140250=CARTESIAN_POINT ( 'NONE',  ( -14.34966873604972548, 8.224510206698743886, 38.33442372801900433 ) ) ;
#140251=CARTESIAN_POINT ( 'NONE',  ( 18.67979575497178502, 10.72451020669898547, 44.16557627198103120 ) ) ;
#140252=CARTESIAN_POINT ( 'NONE',  ( 5.719274019375673035, 21.55341960407619339, 42.29275706135235424 ) ) ;
#140253=CARTESIAN_POINT ( 'NONE',  ( 10.81492255796106328, -18.62759615963255655, 80.41775706135234714 ) ) ;
#140255=CARTESIAN_POINT ( 'NONE',  ( -19.03943276465977164, -0.05219959533935918106, 108.7510903946856615 ) ) ;
#140256=CARTESIAN_POINT ( 'NONE',  ( 19.02544592524343514, -5.153800228976328945, 58.54057627198102409 ) ) ;
#140257=CARTESIAN_POINT ( 'NONE',  ( -9.474510206698964154, 16.51473224551069663, 90.41557627198103830 ) ) ;
#140258=CARTESIAN_POINT ( 'NONE',  ( -4.483927247898539470, -16.52544592524342804, 102.2905762719810383 ) ) ;
#140259=CARTESIAN_POINT ( 'NONE',  ( -4.379528057220328563, 16.55341960407611168, 105.2072429386477097 ) ) ;
#140260=CARTESIAN_POINT ( 'NONE',  ( -10.81492255796078084, -18.62759615963271287, 22.08224293864769194 ) ) ;
#140261=CARTESIAN_POINT ( 'NONE',  ( -4.483927247898782831, 16.52544592524335698, 77.70942372801900433 ) ) ;
#140262=CARTESIAN_POINT ( 'NONE',  ( 12.14591786802309770, 12.06949235617756955, 64.37390960531435269 ) ) ;
#140263=CARTESIAN_POINT ( 'NONE',  ( 5.049401038298161559, -19.05341960407611168, 57.70724293864769550 ) ) ;
#140264=CARTESIAN_POINT ( 'NONE',  ( 21.55341960407619695, -5.719274019375665929, 81.04275706135236135 ) ) ;
#140265=CARTESIAN_POINT ( 'NONE',  ( -18.67979575497193778, 10.72451020669871902, 73.33442372801901854 ) ) ;
#140266=CARTESIAN_POINT ( 'NONE',  ( 16.46253265017146816, 9.564922557961045513, 106.6677570613523471 ) ) ;
#140267=CARTESIAN_POINT ( 'NONE',  ( 12.06949235617757843, -12.14591786802309237, 68.12390960531436690 ) ) ;
#140268=CARTESIAN_POINT ( 'NONE',  ( 5.719274019375673035, 21.55341960407619339, 22.29275706135235069 ) ) ;
#140269=CARTESIAN_POINT ( 'NONE',  ( 5.719274019375991003, -21.55341960407610458, 62.70724293864769550 ) ) ;
#140270=CARTESIAN_POINT ( 'NONE',  ( 19.19724070472095789, 5.499999999999971578, 73.56193348274379673 ) ) ;
#140272=CARTESIAN_POINT ( 'NONE',  ( 19.02544592524343514, -5.153800228976328945, 63.54057627198103830 ) ) ;
#140273=CARTESIAN_POINT ( 'NONE',  ( -8.314922557960811034, -14.29746914071050412, 42.08224293864769550 ) ) ;
#140275=CARTESIAN_POINT ( 'NONE',  ( 16.52544592524342804, -4.483927247898539470, 23.54057627198102765 ) ) ;
#140276=CARTESIAN_POINT ( 'NONE',  ( -8.314922557961024197, 14.29746914071037800, 97.91775706135236135 ) ) ;
#140277=CARTESIAN_POINT ( 'NONE',  ( -19.05341960407617563, 5.049401038297882671, 58.54275706135234003 ) ) ;
#140279=CARTESIAN_POINT ( 'NONE',  ( -19.05341960407611168, -5.049401038298163336, 111.4572429386476671 ) ) ;
#140280=CARTESIAN_POINT ( 'NONE',  ( -4.379528057220328563, 16.55341960407611168, 80.20724293864769550 ) ) ;
#140281=CARTESIAN_POINT ( 'NONE',  ( 5.049401038297881783, 19.05341960407617563, 47.29275706135231161 ) ) ;
#140282=CARTESIAN_POINT ( 'NONE',  ( -16.46253265017160317, 9.564922557960807481, 35.83224293864768839 ) ) ;
#140283=CARTESIAN_POINT ( 'NONE',  ( 0.05219959533909260263, 19.03943276465977164, 114.9989096053143669 ) ) ;
#140284=CARTESIAN_POINT ( 'NONE',  ( 18.67979575497178502, 10.72451020669898547, 49.16557627198102409 ) ) ;
#140286=CARTESIAN_POINT ( 'NONE',  ( -14.29746914071049879, 8.314922557960819915, 95.83224293864770971 ) ) ;
#140287=CARTESIAN_POINT ( 'NONE',  ( -8.224510206698735004, -14.34966873604973081, 54.58442372801901143 ) ) ;
#140288=CARTESIAN_POINT ( 'NONE',  ( -16.55341960407611168, -4.379528057220339221, 86.45724293864770971 ) ) ;
#140292=CARTESIAN_POINT ( 'NONE',  ( -18.67979575497178146, -10.72451020669898902, 26.66557627198103475 ) ) ;
#140296=CARTESIAN_POINT ( 'NONE',  ( 12.14591786802327356, -12.06949235617739191, 45.62609039468567573 ) ) ;
#140297=CARTESIAN_POINT ( 'NONE',  ( -8.224510206698948167, 14.34966873604960824, 30.41557627198101699 ) ) ;
#140298=CARTESIAN_POINT ( 'NONE',  ( -15.72974639402197994, 15.80617190586746368, 55.62390960531436690 ) ) ;
#140299=CARTESIAN_POINT ( 'NONE',  ( -16.46253265017146816, -9.564922557961047289, 79.16775706135234714 ) ) ;
#140300=CARTESIAN_POINT ( 'NONE',  ( -10.72451020669898014, 18.67979575497178502, 45.41557627198103830 ) ) ;
#140301=CARTESIAN_POINT ( 'NONE',  ( -10.72451020669870658, -18.67979575497194134, 84.58442372801903275 ) ) ;
#140303=CARTESIAN_POINT ( 'NONE',  ( -4.379528057220086978, -16.55341960407618274, 54.79275706135235424 ) ) ;
#140304=CARTESIAN_POINT ( 'NONE',  ( 5.049401038298161559, -19.05341960407611168, 37.70724293864768839 ) ) ;
#140305=CARTESIAN_POINT ( 'NONE',  ( -0.05219959533909027116, -19.03943276465977164, 102.4989096053143669 ) ) ;
#140306=CARTESIAN_POINT ( 'NONE',  ( 9.564922557960805705, 16.46253265017160317, 34.58224293864770260 ) ) ;
#140307=CARTESIAN_POINT ( 'NONE',  ( 12.06949235617757843, -12.14591786802309237, 103.1239096053143811 ) ) ;
#140308=EDGE_CURVE ( 'NONE', #112403, #152017, #18401, .T. ) ;
#140309=CARTESIAN_POINT ( 'NONE',  ( -13.89961937509977652, 13.97604488694528158, 95.62390960531436690 ) ) ;
#140311=CARTESIAN_POINT ( 'NONE',  ( 4.379528057220092307, 16.55341960407617563, 52.29275706135236135 ) ) ;
#140312=CARTESIAN_POINT ( 'NONE',  ( -10.72451020669898014, 18.67979575497178502, 90.41557627198103830 ) ) ;
#140313=CARTESIAN_POINT ( 'NONE',  ( 13.97604488694527802, 13.89961937509977652, 59.37390960531434558 ) ) ;
#140314=CARTESIAN_POINT ( 'NONE',  ( 21.52544592524334988, 5.823673210054432836, 26.45942372801901854 ) ) ;
#140315=CARTESIAN_POINT ( 'NONE',  ( 19.03943276465977164, -0.05219959533909143690, 88.74890960531436690 ) ) ;
#140316=CARTESIAN_POINT ( 'NONE',  ( -17.49999999999999645, -5.499999999999992895, 84.20309617465829888 ) ) ;
#140318=CARTESIAN_POINT ( 'NONE',  ( 16.52544592524335698, 4.483927247898782831, 51.45942372801901854 ) ) ;
#140319=CARTESIAN_POINT ( 'NONE',  ( -10.81492255796078084, -18.62759615963271287, 112.0822429386477097 ) ) ;
#140320=CARTESIAN_POINT ( 'NONE',  ( -16.46253265017160317, 9.564922557960807481, 25.83224293864769194 ) ) ;
#140321=CARTESIAN_POINT ( 'NONE',  ( 13.89961937509977652, -13.97604488694527269, 103.1239096053143527 ) ) ;
#140322=CARTESIAN_POINT ( 'NONE',  ( 5.153800228976615827, -19.02544592524334988, 70.20942372801899012 ) ) ;
#140323=CARTESIAN_POINT ( 'NONE',  ( 19.02544592524334988, 5.153800228976608722, 26.45942372801899722 ) ) ;
#140324=CARTESIAN_POINT ( 'NONE',  ( -5.719274019375978568, 21.55341960407610458, 90.20724293864770971 ) ) ;
#140325=CARTESIAN_POINT ( 'NONE',  ( -16.46253265017146816, -9.564922557961047289, 34.16775706135233293 ) ) ;
#140326=CARTESIAN_POINT ( 'NONE',  ( 16.53943276465976808, 0.05219959533934440121, 76.25109039468568994 ) ) ;
#140327=CARTESIAN_POINT ( 'NONE',  ( 5.153800228976335163, 19.02544592524342804, 109.7905762719810099 ) ) ;
#140328=CARTESIAN_POINT ( 'NONE',  ( -0.05219959533909027116, -19.03943276465977164, 62.49890960531435979 ) ) ;
#140329=CARTESIAN_POINT ( 'NONE',  ( 15.80617190586769283, -15.72974639402175789, 70.62609039468567573 ) ) ;
#140330=CARTESIAN_POINT ( 'NONE',  ( 21.52544592524334988, 5.823673210054432836, 76.45942372801901854 ) ) ;
#140331=CARTESIAN_POINT ( 'NONE',  ( 9.474510206698971260, -16.51473224551069308, 77.91557627198103830 ) ) ;
#140332=CARTESIAN_POINT ( 'NONE',  ( -21.52544592524334988, -5.823673210054445271, 53.95942372801900433 ) ) ;
#140333=CARTESIAN_POINT ( 'NONE',  ( -13.97604488694547697, 13.89961937509957934, 88.12609039468563310 ) ) ;
#140334=CARTESIAN_POINT ( 'NONE',  ( -19.03943276465977164, 0.05219959533909376836, 51.24890960531436690 ) ) ;
#140335=CARTESIAN_POINT ( 'NONE',  ( 16.51473224551069308, 9.474510206698969483, 104.1655762719810241 ) ) ;
#140336=CARTESIAN_POINT ( 'NONE',  ( 19.03943276465977164, -0.05219959533909143690, 68.74890960531436690 ) ) ;
#140337=CARTESIAN_POINT ( 'NONE',  ( -9.474510206698964154, 16.51473224551069663, 115.4155762719810241 ) ) ;
#140338=CARTESIAN_POINT ( 'NONE',  ( -19.05341960407611168, -5.049401038298163336, 56.45724293864768129 ) ) ;
#140341=CARTESIAN_POINT ( 'NONE',  ( -10.72451020669898014, 18.67979575497178502, 105.4155762719810383 ) ) ;
#140342=CARTESIAN_POINT ( 'NONE',  ( -14.29746914071037622, -8.314922557961029526, 74.16775706135231871 ) ) ;
#140344=CARTESIAN_POINT ( 'NONE',  ( -5.153800228976607833, 19.02544592524334988, 32.70942372801899722 ) ) ;
#140345=CARTESIAN_POINT ( 'NONE',  ( -5.153800228976328057, -19.02544592524343514, 72.29057627198102409 ) ) ;
#140346=CARTESIAN_POINT ( 'NONE',  ( -16.53943276465976808, 0.05219959533911058130, 61.24890960531435979 ) ) ;
#140347=CARTESIAN_POINT ( 'NONE',  ( 12.14591786802309770, 12.06949235617756955, 94.37390960531436690 ) ) ;
#140348=CARTESIAN_POINT ( 'NONE',  ( 13.89961937509977652, -13.97604488694527269, 98.12390960531433848 ) ) ;
#140349=CARTESIAN_POINT ( 'NONE',  ( -16.46253265017160317, 9.564922557960807481, 85.83224293864769550 ) ) ;
#140350=CARTESIAN_POINT ( 'NONE',  ( -19.02544592524342804, 5.153800228976336051, 111.0405762719810099 ) ) ;
#140351=CARTESIAN_POINT ( 'NONE',  ( 9.564922557961047289, -16.46253265017146816, 20.41775706135233293 ) ) ;
#140352=CARTESIAN_POINT ( 'NONE',  ( 16.53943276465976808, 0.05219959533934440121, 86.25109039468568994 ) ) ;
#140353=CARTESIAN_POINT ( 'NONE',  ( -15.72974639402176322, -15.80617190586768395, 39.37609039468567573 ) ) ;
#140354=CARTESIAN_POINT ( 'NONE',  ( 15.72974639402199770, -15.80617190586745480, 33.12390960531435979 ) ) ;
#140355=CARTESIAN_POINT ( 'NONE',  ( 15.72974639402199770, -15.80617190586745480, 103.1239096053143811 ) ) ;
#140356=CARTESIAN_POINT ( 'NONE',  ( 8.314922557960818139, 14.29746914071049879, 54.58224293864769550 ) ) ;
#140357=CARTESIAN_POINT ( 'NONE',  ( -13.97604488694527625, -13.89961937509977652, 51.87390960531436690 ) ) ;
#140358=CARTESIAN_POINT ( 'NONE',  ( -14.34966873604960291, -8.224510206698953496, 86.66557627198102409 ) ) ;
#140359=CARTESIAN_POINT ( 'NONE',  ( -15.80617190586745835, -15.72974639402198527, 46.87390960531435979 ) ) ;
#140360=CARTESIAN_POINT ( 'NONE',  ( 19.02544592524334988, 5.153800228976608722, 41.45942372801900433 ) ) ;
#140362=CARTESIAN_POINT ( 'NONE',  ( 12.06949235617757843, -12.14591786802309237, 108.1239096053143811 ) ) ;
#140364=CARTESIAN_POINT ( 'NONE',  ( -14.29746914071037622, -8.314922557961029526, 64.16775706135234714 ) ) ;
#140365=CARTESIAN_POINT ( 'NONE',  ( 19.02544592524343514, -5.153800228976328945, 68.54057627198103830 ) ) ;
#140367=CARTESIAN_POINT ( 'NONE',  ( -4.483927247898539470, -16.52544592524342804, 87.29057627198103830 ) ) ;
#140368=CARTESIAN_POINT ( 'NONE',  ( 10.81492255796078972, 18.62759615963270932, 34.58224293864770260 ) ) ;
#140370=CARTESIAN_POINT ( 'NONE',  ( 16.53943276465976808, 0.05219959533934440121, 106.2510903946856757 ) ) ;
#140371=CARTESIAN_POINT ( 'NONE',  ( 14.29746914071037800, 8.314922557961029526, 31.66775706135234358 ) ) ;
#140372=CARTESIAN_POINT ( 'NONE',  ( 18.62759615963255655, 10.81492255796105972, 96.66775706135234714 ) ) ;
#140373=CARTESIAN_POINT ( 'NONE',  ( -16.51473224551069308, -9.474510206698971260, 86.66557627198102409 ) ) ;
#140374=CARTESIAN_POINT ( 'NONE',  ( 10.81492255796078972, 18.62759615963270932, 114.5822429386477097 ) ) ;
#140375=CARTESIAN_POINT ( 'NONE',  ( -16.46253265017160317, 9.564922557960807481, 35.83224293864768839 ) ) ;
#140376=CARTESIAN_POINT ( 'NONE',  ( -4.379528057220086978, -16.55341960407618274, 24.79275706135235779 ) ) ;
#140378=CARTESIAN_POINT ( 'NONE',  ( 16.51473224551083163, -9.474510206698727899, 100.8344237280190043 ) ) ;
#140379=CARTESIAN_POINT ( 'NONE',  ( -10.81492255796078084, -18.62759615963271287, 97.08224293864770971 ) ) ;
#140380=CARTESIAN_POINT ( 'NONE',  ( 16.51473224551083163, -9.474510206698727899, 65.83442372801900433 ) ) ;
#140382=CARTESIAN_POINT ( 'NONE',  ( -15.80617190586768217, 15.72974639402176855, 23.12609039468567573 ) ) ;
#140383=CARTESIAN_POINT ( 'NONE',  ( 13.89961937509977652, -13.97604488694527269, 83.12390960531436690 ) ) ;
#140385=CARTESIAN_POINT ( 'NONE',  ( -0.05219959533934338120, 16.53943276465976808, 37.50109039468568284 ) ) ;
#140386=CARTESIAN_POINT ( 'NONE',  ( 13.89961937509957401, 13.97604488694547697, 66.87609039468567573 ) ) ;
#140387=CARTESIAN_POINT ( 'NONE',  ( 0.05219959533907565091, 21.53943276465977519, 114.9989096053143669 ) ) ;
#140388=CARTESIAN_POINT ( 'NONE',  ( -14.34966873604960291, -8.224510206698953496, 71.66557627198100988 ) ) ;
#140389=CARTESIAN_POINT ( 'NONE',  ( -5.049401038298153566, 19.05341960407611168, 80.20724293864769550 ) ) ;
#140390=CARTESIAN_POINT ( 'NONE',  ( -12.06949235617739369, -12.14591786802326823, 34.37609039468568284 ) ) ;
#140391=CARTESIAN_POINT ( 'NONE',  ( -9.474510206698720793, -16.51473224551083518, 39.58442372801899722 ) ) ;
#140392=CARTESIAN_POINT ( 'NONE',  ( 5.719274019375673035, 21.55341960407619339, 67.29275706135234714 ) ) ;
#140393=CARTESIAN_POINT ( 'NONE',  ( 4.483927247898790824, -16.52544592524335698, 20.20942372801900788 ) ) ;
#140394=CARTESIAN_POINT ( 'NONE',  ( -5.153800228976328057, -19.02544592524343514, 57.29057627198103120 ) ) ;
#140395=CARTESIAN_POINT ( 'NONE',  ( -16.46253265017146816, -9.564922557961047289, 84.16775706135233293 ) ) ;
#140396=CARTESIAN_POINT ( 'NONE',  ( -14.29746914071037622, -8.314922557961029526, 59.16775706135234714 ) ) ;
#140397=CARTESIAN_POINT ( 'NONE',  ( -21.53943276465977519, -0.05219959533937600094, 103.7510903946857042 ) ) ;
#140398=CARTESIAN_POINT ( 'NONE',  ( 5.153800228976615827, -19.02544592524334988, 65.20942372801900433 ) ) ;
#140399=CARTESIAN_POINT ( 'NONE',  ( 0.05219959533909260263, 19.03943276465977164, 49.99890960531435979 ) ) ;
#140400=CARTESIAN_POINT ( 'NONE',  ( -5.823673210054116645, -21.52544592524344225, 67.29057627198103830 ) ) ;
#140401=CARTESIAN_POINT ( 'NONE',  ( 8.314922557960818139, 14.29746914071049879, 64.58224293864769550 ) ) ;
#140402=CARTESIAN_POINT ( 'NONE',  ( -13.89961937509957401, -13.97604488694547875, 69.37609039468564731 ) ) ;
#140404=CARTESIAN_POINT ( 'NONE',  ( -16.51473224551082808, 9.474510206698731452, 43.33442372801900433 ) ) ;
#140405=CARTESIAN_POINT ( 'NONE',  ( 12.14591786802327356, -12.06949235617739191, 95.62609039468568994 ) ) ;
#140406=CARTESIAN_POINT ( 'NONE',  ( -12.06949235617756955, 12.14591786802309770, 70.62390960531436690 ) ) ;
#140407=CARTESIAN_POINT ( 'NONE',  ( 18.62759615963255655, 10.81492255796105972, 101.6677570613523613 ) ) ;
#140409=CARTESIAN_POINT ( 'NONE',  ( 18.62759615963271287, -10.81492255796078972, 93.33224293864769550 ) ) ;
#140410=CARTESIAN_POINT ( 'NONE',  ( 13.89961937509977652, -13.97604488694527269, 58.12390960531436690 ) ) ;
#140411=CARTESIAN_POINT ( 'NONE',  ( -5.719274019375665041, -21.55341960407619695, 69.79275706135234714 ) ) ;
#140412=CARTESIAN_POINT ( 'NONE',  ( 16.46253265017160672, -9.564922557960803928, 48.33224293864769550 ) ) ;
#140413=CARTESIAN_POINT ( 'NONE',  ( 0.05219959533909260263, 19.03943276465977164, 64.99890960531436690 ) ) ;
#140414=CARTESIAN_POINT ( 'NONE',  ( 9.474510206698971260, -16.51473224551069308, 27.91557627198103120 ) ) ;
#140415=CARTESIAN_POINT ( 'NONE',  ( -16.51473224551069308, -9.474510206698971260, 106.6655762719810383 ) ) ;
#140416=CARTESIAN_POINT ( 'NONE',  ( 4.379528057220339221, -16.55341960407611168, 47.70724293864770260 ) ) ;
#140417=CARTESIAN_POINT ( 'NONE',  ( 19.05341960407611168, 5.049401038298154454, 28.95724293864769550 ) ) ;
#140418=CARTESIAN_POINT ( 'NONE',  ( 8.224510206698953496, -14.34966873604960469, 82.91557627198103830 ) ) ;
#140420=CARTESIAN_POINT ( 'NONE',  ( -10.72451020669898014, 18.67979575497178502, 100.4155762719810241 ) ) ;
#140421=CARTESIAN_POINT ( 'NONE',  ( 21.52544592524334988, 5.823673210054432836, 31.45942372801901854 ) ) ;
#140423=CARTESIAN_POINT ( 'NONE',  ( 4.483927247898790824, -16.52544592524335698, 45.20942372801901854 ) ) ;
#140424=CARTESIAN_POINT ( 'NONE',  ( 5.823673210054125526, 21.52544592524343514, 84.79057627198102409 ) ) ;
#140425=CARTESIAN_POINT ( 'NONE',  ( -5.719274019375665041, -21.55341960407619695, 109.7927570613523613 ) ) ;
#140426=CARTESIAN_POINT ( 'NONE',  ( -0.05219959533909027116, -19.03943276465977164, 107.4989096053143527 ) ) ;
#140427=CARTESIAN_POINT ( 'NONE',  ( -10.81492255796105439, 18.62759615963255655, 42.91775706135235424 ) ) ;
#140428=CARTESIAN_POINT ( 'NONE',  ( -5.823673210054116645, -21.52544592524344225, 47.29057627198103120 ) ) ;
#140429=CARTESIAN_POINT ( 'NONE',  ( 0.05219959533934541429, -16.53943276465976808, 110.0010903946856757 ) ) ;
#140430=CARTESIAN_POINT ( 'NONE',  ( -10.72451020669870658, -18.67979575497194134, 59.58442372801901854 ) ) ;
#140431=CARTESIAN_POINT ( 'NONE',  ( -18.67979575497193778, 10.72451020669871902, 98.33442372801901854 ) ) ;
#140432=CARTESIAN_POINT ( 'NONE',  ( -19.03943276465977164, -0.05219959533935918106, 28.75109039468566507 ) ) ;
#140433=CARTESIAN_POINT ( 'NONE',  ( 0.05219959533934541429, -16.53943276465976808, 90.00109039468567573 ) ) ;
#140434=CARTESIAN_POINT ( 'NONE',  ( 21.55341960407619695, -5.719274019375665929, 46.04275706135234714 ) ) ;
#140435=CARTESIAN_POINT ( 'NONE',  ( 5.153800228976335163, 19.02544592524342804, 44.79057627198103830 ) ) ;
#140436=CARTESIAN_POINT ( 'NONE',  ( 9.564922557961047289, -16.46253265017146816, 20.41775706135233293 ) ) ;
#140437=CARTESIAN_POINT ( 'NONE',  ( -18.67979575497178146, -10.72451020669898902, 31.66557627198102054 ) ) ;
#140438=CARTESIAN_POINT ( 'NONE',  ( 10.81492255796106328, -18.62759615963255655, 20.41775706135234714 ) ) ;
#140439=CARTESIAN_POINT ( 'NONE',  ( -10.72451020669898014, 18.67979575497178502, 70.41557627198102409 ) ) ;
#140440=CARTESIAN_POINT ( 'NONE',  ( -0.05219959533934338120, 16.53943276465976808, 42.50109039468567573 ) ) ;
#140442=CARTESIAN_POINT ( 'NONE',  ( -5.823673210054116645, -21.52544592524344225, 77.29057627198102409 ) ) ;
#140443=CARTESIAN_POINT ( 'NONE',  ( 16.53943276465976808, 0.05219959533934440121, 61.25109039468567573 ) ) ;
#140444=CARTESIAN_POINT ( 'NONE',  ( -16.53943276465976808, 0.05219959533911058130, 66.24890960531436690 ) ) ;
#140446=CARTESIAN_POINT ( 'NONE',  ( -13.89961937509957401, -13.97604488694547875, 94.37609039468566152 ) ) ;
#140448=CARTESIAN_POINT ( 'NONE',  ( 16.52544592524335698, 4.483927247898782831, 46.45942372801901854 ) ) ;
#140449=CARTESIAN_POINT ( 'NONE',  ( 0.05219959533937995610, -21.53943276465977519, 20.00109039468568639 ) ) ;
#140450=CARTESIAN_POINT ( 'NONE',  ( -10.72451020669898014, 18.67979575497178502, 70.41557627198102409 ) ) ;
#140451=CARTESIAN_POINT ( 'NONE',  ( 16.51473224551069308, 9.474510206698969483, 114.1655762719810241 ) ) ;
#140452=CARTESIAN_POINT ( 'NONE',  ( -16.52544592524335698, -4.483927247898792601, 63.95942372801901854 ) ) ;
#140453=CARTESIAN_POINT ( 'NONE',  ( 5.153800228976335163, 19.02544592524342804, 69.79057627198103830 ) ) ;
#140454=CARTESIAN_POINT ( 'NONE',  ( -18.67979575497193778, 10.72451020669871902, 43.33442372801901143 ) ) ;
#140455=CARTESIAN_POINT ( 'NONE',  ( -5.153800228976607833, 19.02544592524334988, 107.7094237280189759 ) ) ;
#140457=CARTESIAN_POINT ( 'NONE',  ( 0.05219959533909260263, 19.03943276465977164, 109.9989096053143669 ) ) ;
#140458=CARTESIAN_POINT ( 'NONE',  ( -9.564922557961040184, 16.46253265017147172, 27.91775706135232582 ) ) ;
#140459=CARTESIAN_POINT ( 'NONE',  ( -12.14591786802326823, 12.06949235617739902, 43.12609039468568284 ) ) ;
#140460=CARTESIAN_POINT ( 'NONE',  ( 16.51473224551069308, 9.474510206698969483, 104.1655762719810241 ) ) ;
#140461=CARTESIAN_POINT ( 'NONE',  ( 18.62759615963271287, -10.81492255796078972, 103.3322429386476955 ) ) ;
#140462=CARTESIAN_POINT ( 'NONE',  ( 5.049401038298161559, -19.05341960407611168, 57.70724293864769550 ) ) ;
#140463=CARTESIAN_POINT ( 'NONE',  ( -16.18388926212242751, 7.379444403734384039, 24.56046848633850033 ) ) ;
#140464=CARTESIAN_POINT ( 'NONE',  ( 14.29746914071049879, -8.314922557960816363, 78.33224293864770971 ) ) ;
#140465=CARTESIAN_POINT ( 'NONE',  ( -5.153800228976328057, -19.02544592524343514, 112.2905762719810099 ) ) ;
#140466=CARTESIAN_POINT ( 'NONE',  ( 5.153800228976335163, 19.02544592524342804, 24.79057627198102765 ) ) ;
#140468=CARTESIAN_POINT ( 'NONE',  ( 15.72974639402199770, -15.80617190586745480, 98.12390960531436690 ) ) ;
#140469=CARTESIAN_POINT ( 'NONE',  ( -19.02544592524334988, -5.153800228976617603, 63.95942372801899012 ) ) ;
#140470=CARTESIAN_POINT ( 'NONE',  ( 5.719274019375991003, -21.55341960407610458, 32.70724293864770260 ) ) ;
#140471=ADVANCED_FACE ( 'NONE', ( #32221 ), #170730, .F. ) ;
#140472=CARTESIAN_POINT ( 'NONE',  ( -9.474510206698964154, 16.51473224551069663, 30.41557627198102054 ) ) ;
#140473=CARTESIAN_POINT ( 'NONE',  ( 0.05219959533907565091, 21.53943276465977519, 49.99890960531437401 ) ) ;
#140474=CARTESIAN_POINT ( 'NONE',  ( 9.474510206698971260, -16.51473224551069308, 102.9155762719810241 ) ) ;
#140475=CARTESIAN_POINT ( 'NONE',  ( -21.53943276465977519, -0.05219959533937600094, 83.75109039468568994 ) ) ;
#140476=CARTESIAN_POINT ( 'NONE',  ( 9.564922557960805705, 16.46253265017160317, 49.58224293864770260 ) ) ;
#140477=CARTESIAN_POINT ( 'NONE',  ( -16.55341960407611168, -4.379528057220339221, 91.45724293864769550 ) ) ;
#140478=CARTESIAN_POINT ( 'NONE',  ( -4.379528057220086978, -16.55341960407618274, 39.79275706135235424 ) ) ;
#140479=CARTESIAN_POINT ( 'NONE',  ( -19.03943276465977164, 0.05219959533909376836, 56.24890960531435979 ) ) ;
#140480=CARTESIAN_POINT ( 'NONE',  ( -21.53943276465977519, -0.05219959533937600094, 68.75109039468568994 ) ) ;
#140481=ORIENTED_EDGE ( 'NONE', *, *, #163492, .F. ) ;
#140482=CARTESIAN_POINT ( 'NONE',  ( -0.05219959533936034679, 19.03943276465977164, 27.50109039468566507 ) ) ;
#140484=CARTESIAN_POINT ( 'NONE',  ( -16.51473224551082808, 9.474510206698731452, 43.33442372801900433 ) ) ;
#140486=CARTESIAN_POINT ( 'NONE',  ( -18.67979575497193778, 10.72451020669871902, 33.33442372801900433 ) ) ;
#140488=CARTESIAN_POINT ( 'NONE',  ( -9.564922557961040184, 16.46253265017147172, 37.91775706135233293 ) ) ;
#140489=CARTESIAN_POINT ( 'NONE',  ( -9.564922557960796823, -16.46253265017161027, 87.08224293864769550 ) ) ;
#140490=CARTESIAN_POINT ( 'NONE',  ( -13.97604488694527625, -13.89961937509977652, 66.87390960531436690 ) ) ;
#140491=CARTESIAN_POINT ( 'NONE',  ( -16.53943276465976808, 0.05219959533911058130, 31.24890960531435979 ) ) ;
#140492=CARTESIAN_POINT ( 'NONE',  ( -19.03943276465977164, 0.05219959533909376836, 116.2489096053143669 ) ) ;
#140493=CARTESIAN_POINT ( 'NONE',  ( -5.823673210054431948, 21.52544592524334988, 87.70942372801901854 ) ) ;
#140495=CARTESIAN_POINT ( 'NONE',  ( 17.40805194822031510, 6.112264579159357503, 56.66628727489389661 ) ) ;
#140496=CARTESIAN_POINT ( 'NONE',  ( -10.81492255796105439, 18.62759615963255655, 82.91775706135234714 ) ) ;
#140498=CARTESIAN_POINT ( 'NONE',  ( 16.46253265017160672, -9.564922557960803928, 98.33224293864769550 ) ) ;
#140500=CARTESIAN_POINT ( 'NONE',  ( 10.81492255796078972, 18.62759615963270932, 64.58224293864769550 ) ) ;
#140501=CARTESIAN_POINT ( 'NONE',  ( 4.483927247898545687, 16.52544592524342804, 29.79057627198102409 ) ) ;
#140502=CARTESIAN_POINT ( 'NONE',  ( 8.314922557960818139, 14.29746914071049879, 109.5822429386476955 ) ) ;
#140503=CARTESIAN_POINT ( 'NONE',  ( -19.03943276465977164, 0.05219959533909376836, 101.2489096053143669 ) ) ;
#140504=CARTESIAN_POINT ( 'NONE',  ( -19.02544592524334988, -5.153800228976617603, 23.95942372801900078 ) ) ;
#140505=CARTESIAN_POINT ( 'NONE',  ( -12.14591786802309592, -12.06949235617757132, 96.87390960531436690 ) ) ;
#140506=CARTESIAN_POINT ( 'NONE',  ( 15.72974639402176855, 15.80617190586768217, 66.87609039468568994 ) ) ;
#140507=CARTESIAN_POINT ( 'NONE',  ( 19.05341960407611168, 5.049401038298154454, 113.9572429386477097 ) ) ;
#140508=CARTESIAN_POINT ( 'NONE',  ( 12.14591786802327356, -12.06949235617739191, 105.6260903946856899 ) ) ;
#140509=CARTESIAN_POINT ( 'NONE',  ( -16.46253265017146816, -9.564922557961047289, 69.16775706135233293 ) ) ;
#140511=CARTESIAN_POINT ( 'NONE',  ( -5.153800228976328057, -19.02544592524343514, 107.2905762719810383 ) ) ;
#140512=CARTESIAN_POINT ( 'NONE',  ( 12.06949235617757843, -12.14591786802309237, 83.12390960531436690 ) ) ;
#140513=CARTESIAN_POINT ( 'NONE',  ( 16.51473224551083163, -9.474510206698727899, 55.83442372801899722 ) ) ;
#140514=CARTESIAN_POINT ( 'NONE',  ( 9.564922557960805705, 16.46253265017160317, 74.58224293864769550 ) ) ;
#140515=CARTESIAN_POINT ( 'NONE',  ( -14.29746914071049879, 8.314922557960819915, 55.83224293864770260 ) ) ;
#140516=CARTESIAN_POINT ( 'NONE',  ( -19.02544592524334988, -5.153800228976617603, 88.95942372801897591 ) ) ;
#140517=CARTESIAN_POINT ( 'NONE',  ( 15.80617190586746368, 15.72974639402197994, 49.37390960531436690 ) ) ;
#140519=CARTESIAN_POINT ( 'NONE',  ( -4.379528057220328563, 16.55341960407611168, 110.2072429386477239 ) ) ;
#140520=CARTESIAN_POINT ( 'NONE',  ( 13.97604488694548053, -13.89961937509957401, 100.6260903946856757 ) ) ;
#140521=CARTESIAN_POINT ( 'NONE',  ( -19.02544592524342804, 5.153800228976336051, 71.04057627198099567 ) ) ;
#140522=CARTESIAN_POINT ( 'NONE',  ( -5.823673210054116645, -21.52544592524344225, 82.29057627198103830 ) ) ;
#140523=CARTESIAN_POINT ( 'NONE',  ( 16.52544592524335698, 4.483927247898782831, 96.45942372801901854 ) ) ;
#140524=CARTESIAN_POINT ( 'NONE',  ( 16.46253265017160672, -9.564922557960803928, 68.33224293864770971 ) ) ;
#140525=CARTESIAN_POINT ( 'NONE',  ( 9.564922557961047289, -16.46253265017146816, 50.41775706135233293 ) ) ;
#140526=CARTESIAN_POINT ( 'NONE',  ( 21.55341960407619695, -5.719274019375665929, 86.04275706135236135 ) ) ;
#140527=CARTESIAN_POINT ( 'NONE',  ( 21.52544592524344225, -5.823673210054117533, 68.54057627198103830 ) ) ;
#140528=CARTESIAN_POINT ( 'NONE',  ( -5.049401038298153566, 19.05341960407611168, 105.2072429386476671 ) ) ;
#140529=VECTOR ( 'NONE', #161034, 1000.000000000000000 ) ;
#140530=CARTESIAN_POINT ( 'NONE',  ( 16.51473224551069308, 9.474510206698969483, 34.16557627198102409 ) ) ;
#140531=CARTESIAN_POINT ( 'NONE',  ( -12.06949235617739369, -12.14591786802326823, 104.3760903946856899 ) ) ;
#140532=CARTESIAN_POINT ( 'NONE',  ( 16.52544592524335698, 4.483927247898782831, 26.45942372801901854 ) ) ;
#140533=CARTESIAN_POINT ( 'NONE',  ( 17.72517630440429670, -5.500000000000135891, 43.42175719257209465 ) ) ;
#140534=CARTESIAN_POINT ( 'NONE',  ( -15.80617190586768217, 15.72974639402176855, 103.1260903946856757 ) ) ;
#140536=CARTESIAN_POINT ( 'NONE',  ( -8.224510206698948167, 14.34966873604960824, 55.41557627198102409 ) ) ;
#140537=CARTESIAN_POINT ( 'NONE',  ( 0.05219959533907565091, 21.53943276465977519, 89.99890960531438111 ) ) ;
#140538=CARTESIAN_POINT ( 'NONE',  ( 10.72451020669898902, -18.67979575497178502, 87.91557627198103830 ) ) ;
#140539=CARTESIAN_POINT ( 'NONE',  ( 17.05116617787824396, -6.768360034955806626, 96.15675553259195851 ) ) ;
#140540=CARTESIAN_POINT ( 'NONE',  ( -5.719274019375978568, 21.55341960407610458, 40.20724293864769550 ) ) ;
#140541=CARTESIAN_POINT ( 'NONE',  ( 12.06949235617739724, 12.14591786802326823, 61.87609039468568284 ) ) ;
#140542=CARTESIAN_POINT ( 'NONE',  ( -16.52544592524342804, 4.483927247898546575, 91.04057627198103830 ) ) ;
#140543=CARTESIAN_POINT ( 'NONE',  ( 5.049401038298161559, -19.05341960407611168, 52.70724293864767418 ) ) ;
#140544=CARTESIAN_POINT ( 'NONE',  ( 15.50000000000000178, -5.500000000000000888, 120.0000000000000142 ) ) ;
#140545=CARTESIAN_POINT ( 'NONE',  ( -4.483927247898782831, 16.52544592524335698, 102.7094237280190185 ) ) ;
#140546=CARTESIAN_POINT ( 'NONE',  ( -21.55341960407619339, 5.719274019375674811, 33.54275706135234714 ) ) ;
#140547=CARTESIAN_POINT ( 'NONE',  ( -0.05219959533909027116, -19.03943276465977164, 97.49890960531436690 ) ) ;
#140548=CARTESIAN_POINT ( 'NONE',  ( -18.67979575497193778, 10.72451020669871902, 68.33442372801900433 ) ) ;
#140550=CARTESIAN_POINT ( 'NONE',  ( 9.474510206698971260, -16.51473224551069308, 27.91557627198103120 ) ) ;
#140552=CARTESIAN_POINT ( 'NONE',  ( 15.72974639402176855, 15.80617190586768217, 56.87609039468568994 ) ) ;
#140553=CARTESIAN_POINT ( 'NONE',  ( 16.46253265017160672, -9.564922557960803928, 53.33224293864768839 ) ) ;
#140554=CARTESIAN_POINT ( 'NONE',  ( -16.46253265017160317, 9.564922557960807481, 115.8322429386477097 ) ) ;
#140555=CARTESIAN_POINT ( 'NONE',  ( -19.05341960407611168, -5.049401038298163336, 91.45724293864766707 ) ) ;
#140556=CARTESIAN_POINT ( 'NONE',  ( 13.89961937509957401, 13.97604488694547697, 61.87609039468566863 ) ) ;
#140557=CARTESIAN_POINT ( 'NONE',  ( 10.72451020669871369, 18.67979575497193778, 42.08442372801901854 ) ) ;
#140558=CARTESIAN_POINT ( 'NONE',  ( -5.153800228976607833, 19.02544592524334988, 57.70942372801899012 ) ) ;
#140559=CARTESIAN_POINT ( 'NONE',  ( 16.51473224551069308, 9.474510206698969483, 44.16557627198103120 ) ) ;
#140560=CARTESIAN_POINT ( 'NONE',  ( -14.29746914071037622, -8.314922557961029526, 109.1677570613523613 ) ) ;
#140561=CARTESIAN_POINT ( 'NONE',  ( -5.049401038297874678, -19.05341960407617918, 79.79275706135233293 ) ) ;
#140562=CARTESIAN_POINT ( 'NONE',  ( -16.55341960407617563, 4.379528057220093196, 113.5427570613523756 ) ) ;
#140563=CARTESIAN_POINT ( 'NONE',  ( -19.02544592524334988, -5.153800228976617603, 53.95942372801898301 ) ) ;
#140564=CARTESIAN_POINT ( 'NONE',  ( 16.51473224551069308, 9.474510206698969483, 99.16557627198102409 ) ) ;
#140565=CARTESIAN_POINT ( 'NONE',  ( 0.05219959533937995610, -21.53943276465977519, 110.0010903946856757 ) ) ;
#140566=CARTESIAN_POINT ( 'NONE',  ( -0.05219959533936034679, 19.03943276465977164, 27.50109039468566507 ) ) ;
#140567=CARTESIAN_POINT ( 'NONE',  ( -5.153800228976328057, -19.02544592524343514, 27.29057627198103120 ) ) ;
#140568=CARTESIAN_POINT ( 'NONE',  ( 10.81492255796106328, -18.62759615963255655, 90.41775706135236135 ) ) ;
#140569=CARTESIAN_POINT ( 'NONE',  ( -4.483927247898782831, 16.52544592524335698, 32.70942372801900433 ) ) ;
#140570=CARTESIAN_POINT ( 'NONE',  ( 16.51473224551069308, 9.474510206698969483, 99.16557627198102409 ) ) ;
#140572=CARTESIAN_POINT ( 'NONE',  ( -0.05219959533909027116, -19.03943276465977164, 82.49890960531436690 ) ) ;
#140574=CARTESIAN_POINT ( 'NONE',  ( -16.46253265017146816, -9.564922557961047289, 84.16775706135233293 ) ) ;
#140575=CARTESIAN_POINT ( 'NONE',  ( 9.474510206698971260, -16.51473224551069308, 107.9155762719810383 ) ) ;
#140576=CARTESIAN_POINT ( 'NONE',  ( 5.719274019375673035, 21.55341960407619339, 97.29275706135234714 ) ) ;
#140577=CARTESIAN_POINT ( 'NONE',  ( -14.34966873604960291, -8.224510206698953496, 101.6655762719810383 ) ) ;
#140578=CARTESIAN_POINT ( 'NONE',  ( 9.474510206698971260, -16.51473224551069308, 27.91557627198103120 ) ) ;
#140579=CARTESIAN_POINT ( 'NONE',  ( -21.53943276465977519, 0.05219959533907696930, 51.24890960531436690 ) ) ;
#140580=CARTESIAN_POINT ( 'NONE',  ( -18.62759615963270932, 10.81492255796079327, 30.83224293864770260 ) ) ;
#140581=CARTESIAN_POINT ( 'NONE',  ( 0.05219959533910956823, 16.53943276465976808, 109.9989096053143527 ) ) ;
#140583=CARTESIAN_POINT ( 'NONE',  ( -16.46253265017146816, -9.564922557961047289, 64.16775706135233293 ) ) ;
#140584=CARTESIAN_POINT ( 'NONE',  ( 8.224510206698953496, -14.34966873604960469, 37.91557627198102409 ) ) ;
#140585=CARTESIAN_POINT ( 'NONE',  ( -15.72974639402197994, 15.80617190586746368, 25.62390960531435624 ) ) ;
#140586=CARTESIAN_POINT ( 'NONE',  ( -18.67979575497193778, 10.72451020669871902, 73.33442372801901854 ) ) ;
#140587=CARTESIAN_POINT ( 'NONE',  ( 10.81492255796078972, 18.62759615963270932, 74.58224293864768129 ) ) ;
#140588=CARTESIAN_POINT ( 'NONE',  ( 5.823673210054444382, -21.52544592524334988, 45.20942372801901854 ) ) ;
#140589=CARTESIAN_POINT ( 'NONE',  ( -5.719274019375978568, 21.55341960407610458, 95.20724293864769550 ) ) ;
#140590=CARTESIAN_POINT ( 'NONE',  ( -21.52544592524334988, -5.823673210054445271, 53.95942372801900433 ) ) ;
#140591=CARTESIAN_POINT ( 'NONE',  ( -16.51473224551069308, -9.474510206698971260, 26.66557627198103120 ) ) ;
#140592=CARTESIAN_POINT ( 'NONE',  ( 13.97604488694527802, 13.89961937509977652, 84.37390960531433848 ) ) ;
#140593=CARTESIAN_POINT ( 'NONE',  ( -12.06949235617739369, -12.14591786802326823, 79.37609039468567573 ) ) ;
#140594=CARTESIAN_POINT ( 'NONE',  ( 4.483927247898545687, 16.52544592524342804, 104.7905762719810241 ) ) ;
#140595=CARTESIAN_POINT ( 'NONE',  ( 0.05219959533909260263, 19.03943276465977164, 114.9989096053143669 ) ) ;
#140596=CARTESIAN_POINT ( 'NONE',  ( 14.29746914071049879, -8.314922557960816363, 53.33224293864769550 ) ) ;
#140597=CARTESIAN_POINT ( 'NONE',  ( -16.55341960407611168, -4.379528057220339221, 26.45724293864768839 ) ) ;
#140598=CARTESIAN_POINT ( 'NONE',  ( -13.89961937509977652, 13.97604488694528158, 60.62390960531436690 ) ) ;
#140599=CARTESIAN_POINT ( 'NONE',  ( 16.46253265017160672, -9.564922557960803928, 33.33224293864770260 ) ) ;
#140600=CARTESIAN_POINT ( 'NONE',  ( -15.80617190586745835, -15.72974639402198527, 41.87390960531435979 ) ) ;
#140601=CARTESIAN_POINT ( 'NONE',  ( 19.03943276465977164, 0.05219959533936151252, 41.25109039468566152 ) ) ;
#140603=CARTESIAN_POINT ( 'NONE',  ( 14.29746914071049879, -8.314922557960816363, 33.33224293864769550 ) ) ;
#140604=CARTESIAN_POINT ( 'NONE',  ( -5.153800228976328057, -19.02544592524343514, 107.2905762719810383 ) ) ;
#140605=CARTESIAN_POINT ( 'NONE',  ( 21.55341960407619695, -5.719274019375665929, 61.04275706135234714 ) ) ;
#140607=CARTESIAN_POINT ( 'NONE',  ( -16.52544592524335698, -4.483927247898792601, 63.95942372801901854 ) ) ;
#140608=CARTESIAN_POINT ( 'NONE',  ( -16.51473224551082808, 9.474510206698731452, 58.33442372801900433 ) ) ;
#140609=CARTESIAN_POINT ( 'NONE',  ( 12.14591786802309770, 12.06949235617756955, 39.37390960531436690 ) ) ;
#140610=CARTESIAN_POINT ( 'NONE',  ( 17.40861289039001036, -6.110651285853410108, 51.12767529172567293 ) ) ;
#140611=CARTESIAN_POINT ( 'NONE',  ( -14.34966873604972548, 8.224510206698743886, 108.3344237280190185 ) ) ;
#140612=CARTESIAN_POINT ( 'NONE',  ( -13.97604488694527625, -13.89961937509977652, 41.87390960531435979 ) ) ;
#140613=CARTESIAN_POINT ( 'NONE',  ( -13.89961937509977652, 13.97604488694528158, 55.62390960531434558 ) ) ;
#140614=CARTESIAN_POINT ( 'NONE',  ( 13.97604488694527802, 13.89961937509977652, 29.37390960531435979 ) ) ;
#140615=CARTESIAN_POINT ( 'NONE',  ( 21.52544592524334988, 5.823673210054432836, 26.45942372801901854 ) ) ;
#140616=CARTESIAN_POINT ( 'NONE',  ( 5.049401038298161559, -19.05341960407611168, 62.70724293864769550 ) ) ;
#140617=CARTESIAN_POINT ( 'NONE',  ( -16.46253265017160317, 9.564922557960807481, 115.8322429386477097 ) ) ;
#140618=CARTESIAN_POINT ( 'NONE',  ( 16.46253265017160672, -9.564922557960803928, 43.33224293864769550 ) ) ;
#140619=CARTESIAN_POINT ( 'NONE',  ( 18.62759615963271287, -10.81492255796078972, 28.33224293864769550 ) ) ;
#140620=CARTESIAN_POINT ( 'NONE',  ( 5.719274019375673035, 21.55341960407619339, 57.29275706135234714 ) ) ;
#140621=CARTESIAN_POINT ( 'NONE',  ( 13.89961937509977652, -13.97604488694527269, 28.12390960531435624 ) ) ;
#140622=CARTESIAN_POINT ( 'NONE',  ( -21.53943276465977519, 0.05219959533907696930, 26.24890960531435624 ) ) ;
#140623=CARTESIAN_POINT ( 'NONE',  ( -8.314922557961024197, 14.29746914071037800, 72.91775706135234714 ) ) ;
#140624=CARTESIAN_POINT ( 'NONE',  ( -15.72974639402176322, -15.80617190586768395, 104.3760903946856899 ) ) ;
#140625=CARTESIAN_POINT ( 'NONE',  ( -16.53943276465976808, -0.05219959533934237506, 63.75109039468568284 ) ) ;
#140626=CARTESIAN_POINT ( 'NONE',  ( -19.05341960407611168, -5.049401038298163336, 101.4572429386476955 ) ) ;
#140627=CARTESIAN_POINT ( 'NONE',  ( -4.379528057220086978, -16.55341960407618274, 54.79275706135235424 ) ) ;
#140628=CARTESIAN_POINT ( 'NONE',  ( 12.06949235617739724, 12.14591786802326823, 21.87609039468567573 ) ) ;
#140629=CARTESIAN_POINT ( 'NONE',  ( 4.483927247898790824, -16.52544592524335698, 95.20942372801903275 ) ) ;
#140630=CARTESIAN_POINT ( 'NONE',  ( -10.72451020669870658, -18.67979575497194134, 49.58442372801901143 ) ) ;
#140631=CARTESIAN_POINT ( 'NONE',  ( -5.049401038297874678, -19.05341960407617918, 104.7927570613523471 ) ) ;
#140632=CARTESIAN_POINT ( 'NONE',  ( 21.55341960407610458, 5.719274019375980345, 113.9572429386477239 ) ) ;
#140633=CARTESIAN_POINT ( 'NONE',  ( -4.379528057220328563, 16.55341960407611168, 105.2072429386477097 ) ) ;
#140634=CARTESIAN_POINT ( 'NONE',  ( -16.51473224551082808, 9.474510206698731452, 113.3344237280190043 ) ) ;
#140635=CARTESIAN_POINT ( 'NONE',  ( -14.29746914071037622, -8.314922557961029526, 84.16775706135234714 ) ) ;
#140637=CARTESIAN_POINT ( 'NONE',  ( -21.55341960407619339, 5.719274019375674811, 88.54275706135236135 ) ) ;
#140638=CARTESIAN_POINT ( 'NONE',  ( -19.05341960407617563, 5.049401038297882671, 78.54275706135233293 ) ) ;
#140639=CARTESIAN_POINT ( 'NONE',  ( -16.55341960407611168, -4.379528057220339221, 41.45724293864769550 ) ) ;
#140640=CARTESIAN_POINT ( 'NONE',  ( -0.05219959533910754901, -16.53943276465976808, 47.49890960531435979 ) ) ;
#140641=CARTESIAN_POINT ( 'NONE',  ( -8.314922557960811034, -14.29746914071050412, 112.0822429386477097 ) ) ;
#140642=CARTESIAN_POINT ( 'NONE',  ( 19.02544592524334988, 5.153800228976608722, 41.45942372801900433 ) ) ;
#140644=CARTESIAN_POINT ( 'NONE',  ( 10.81492255796106328, -18.62759615963255655, 35.41775706135234003 ) ) ;
#140645=CARTESIAN_POINT ( 'NONE',  ( 13.97604488694548053, -13.89961937509957401, 110.6260903946856615 ) ) ;
#140647=CARTESIAN_POINT ( 'NONE',  ( -5.049401038298153566, 19.05341960407611168, 110.2072429386476671 ) ) ;
#140648=CARTESIAN_POINT ( 'NONE',  ( 10.81492255796078972, 18.62759615963270932, 64.58224293864769550 ) ) ;
#140649=CARTESIAN_POINT ( 'NONE',  ( 13.97604488694527802, 13.89961937509977652, 84.37390960531433848 ) ) ;
#140650=CARTESIAN_POINT ( 'NONE',  ( -21.55341960407610458, -5.719274019375992779, 51.45724293864770260 ) ) ;
#140651=CARTESIAN_POINT ( 'NONE',  ( 16.53943276465976808, -0.05219959533910856209, 113.7489096053143527 ) ) ;
#140652=CARTESIAN_POINT ( 'NONE',  ( 16.46253265017160672, -9.564922557960803928, 73.33224293864769550 ) ) ;
#140653=CARTESIAN_POINT ( 'NONE',  ( 5.049401038298161559, -19.05341960407611168, 27.70724293864769550 ) ) ;
#140654=CARTESIAN_POINT ( 'NONE',  ( 5.719274019375673035, 21.55341960407619339, 32.29275706135235424 ) ) ;
#140655=CARTESIAN_POINT ( 'NONE',  ( -15.72974639402176322, -15.80617190586768395, 79.37609039468567573 ) ) ;
#140656=CARTESIAN_POINT ( 'NONE',  ( -16.53943276465976808, -0.05219959533934237506, 93.75109039468567573 ) ) ;
#140657=CARTESIAN_POINT ( 'NONE',  ( 15.72974639402176855, 15.80617190586768217, 31.87609039468567929 ) ) ;
#140658=CARTESIAN_POINT ( 'NONE',  ( 21.53943276465977519, 0.05219959533937863772, 31.25109039468568639 ) ) ;
#140659=CARTESIAN_POINT ( 'NONE',  ( 19.02544592524334988, 5.153800228976608722, 71.45942372801900433 ) ) ;
#140660=CARTESIAN_POINT ( 'NONE',  ( -5.049401038298153566, 19.05341960407611168, 80.20724293864769550 ) ) ;
#140661=CARTESIAN_POINT ( 'NONE',  ( -21.52544592524334988, -5.823673210054445271, 88.95942372801901854 ) ) ;
#140662=CARTESIAN_POINT ( 'NONE',  ( 5.823673210054125526, 21.52544592524343514, 89.79057627198103830 ) ) ;
#140663=CARTESIAN_POINT ( 'NONE',  ( 4.379528057220339221, -16.55341960407611168, 62.70724293864769550 ) ) ;
#140664=CARTESIAN_POINT ( 'NONE',  ( -21.52544592524334988, -5.823673210054445271, 108.9594237280190185 ) ) ;
#140665=CARTESIAN_POINT ( 'NONE',  ( 4.483927247898545687, 16.52544592524342804, 79.79057627198102409 ) ) ;
#140666=CARTESIAN_POINT ( 'NONE',  ( 16.52544592524342804, -4.483927247898539470, 113.5405762719810383 ) ) ;
#140667=CARTESIAN_POINT ( 'NONE',  ( -5.153800228976607833, 19.02544592524334988, 67.70942372801900433 ) ) ;
#140668=CARTESIAN_POINT ( 'NONE',  ( 8.314922557960818139, 14.29746914071049879, 34.58224293864770260 ) ) ;
#140669=CARTESIAN_POINT ( 'NONE',  ( 21.55341960407619695, -5.719274019375665929, 91.04275706135236135 ) ) ;
#140670=CARTESIAN_POINT ( 'NONE',  ( -19.05341960407611168, -5.049401038298163336, 91.45724293864766707 ) ) ;
#140671=CARTESIAN_POINT ( 'NONE',  ( -9.474510206698720793, -16.51473224551083518, 64.58442372801900433 ) ) ;
#140672=CARTESIAN_POINT ( 'NONE',  ( -21.52544592524343514, 5.823673210054127303, 66.04057627198103830 ) ) ;
#140673=CARTESIAN_POINT ( 'NONE',  ( -5.823673210054116645, -21.52544592524344225, 112.2905762719810241 ) ) ;
#140674=CARTESIAN_POINT ( 'NONE',  ( 13.97604488694548053, -13.89961937509957401, 110.6260903946856615 ) ) ;
#140675=CARTESIAN_POINT ( 'NONE',  ( -14.29746914071037622, -8.314922557961029526, 74.16775706135231871 ) ) ;
#140676=CARTESIAN_POINT ( 'NONE',  ( 17.40861289039003523, 6.110651285853275994, 63.87232470827430575 ) ) ;
#140677=CARTESIAN_POINT ( 'NONE',  ( -21.52544592524334988, -5.823673210054445271, 23.95942372801901143 ) ) ;
#140678=CARTESIAN_POINT ( 'NONE',  ( 16.53943276465976808, -0.05219959533910856209, 108.7489096053143669 ) ) ;
#140680=CARTESIAN_POINT ( 'NONE',  ( -16.52544592524335698, -4.483927247898792601, 33.95942372801901143 ) ) ;
#140681=CARTESIAN_POINT ( 'NONE',  ( -5.823673210054116645, -21.52544592524344225, 62.29057627198102409 ) ) ;
#140682=CARTESIAN_POINT ( 'NONE',  ( 8.224510206698742110, 14.34966873604972548, 102.0844237280190185 ) ) ;
#140683=CARTESIAN_POINT ( 'NONE',  ( 16.53943276465976808, 0.05219959533934440121, 36.25109039468567573 ) ) ;
#140684=CARTESIAN_POINT ( 'NONE',  ( 5.049401038298161559, -19.05341960407611168, 37.70724293864768839 ) ) ;
#140685=CARTESIAN_POINT ( 'NONE',  ( -12.14591786802326823, 12.06949235617739902, 78.12609039468570415 ) ) ;
#140686=CARTESIAN_POINT ( 'NONE',  ( 5.153800228976615827, -19.02544592524334988, 70.20942372801899012 ) ) ;
#140687=CARTESIAN_POINT ( 'NONE',  ( -21.52544592524343514, 5.823673210054127303, 66.04057627198103830 ) ) ;
#140688=CARTESIAN_POINT ( 'NONE',  ( -0.05219959533934338120, 16.53943276465976808, 102.5010903946856899 ) ) ;
#140690=CARTESIAN_POINT ( 'NONE',  ( -0.05219959533937732626, 21.53943276465977519, 87.50109039468568994 ) ) ;
#140692=CARTESIAN_POINT ( 'NONE',  ( -18.62759615963270932, 10.81492255796079327, 65.83224293864769550 ) ) ;
#140693=CARTESIAN_POINT ( 'NONE',  ( 5.719274019375991003, -21.55341960407610458, 52.70724293864769550 ) ) ;
#140694=CARTESIAN_POINT ( 'NONE',  ( -16.53943276465976808, -0.05219959533934237506, 73.75109039468567573 ) ) ;
#140695=CARTESIAN_POINT ( 'NONE',  ( -18.67979575497178146, -10.72451020669898902, 41.66557627198103120 ) ) ;
#140697=CARTESIAN_POINT ( 'NONE',  ( -21.55341960407610458, -5.719274019375992779, 21.45724293864769550 ) ) ;
#140699=CARTESIAN_POINT ( 'NONE',  ( 13.89961937509977652, -13.97604488694527269, 33.12390960531434558 ) ) ;
#140700=CARTESIAN_POINT ( 'NONE',  ( -5.823673210054116645, -21.52544592524344225, 62.29057627198102409 ) ) ;
#140701=CARTESIAN_POINT ( 'NONE',  ( -4.483927247898782831, 16.52544592524335698, 107.7094237280190328 ) ) ;
#140702=CARTESIAN_POINT ( 'NONE',  ( -15.72974639402176322, -15.80617190586768395, 44.37609039468567573 ) ) ;
#140703=CARTESIAN_POINT ( 'NONE',  ( -19.05341960407617563, 5.049401038297882671, 98.54275706135233293 ) ) ;
#140704=CARTESIAN_POINT ( 'NONE',  ( 13.97604488694527802, 13.89961937509977652, 24.37390960531435624 ) ) ;
#140705=CARTESIAN_POINT ( 'NONE',  ( 5.153800228976615827, -19.02544592524334988, 110.2094237280189901 ) ) ;
#140707=CARTESIAN_POINT ( 'NONE',  ( 5.153800228976335163, 19.02544592524342804, 44.79057627198103830 ) ) ;
#140709=CARTESIAN_POINT ( 'NONE',  ( 13.89961937509977652, -13.97604488694527269, 98.12390960531433848 ) ) ;
#140710=CARTESIAN_POINT ( 'NONE',  ( 0.05219959533934541429, -16.53943276465976808, 75.00109039468568994 ) ) ;
#140711=CARTESIAN_POINT ( 'NONE',  ( 16.46253265017146816, 9.564922557961045513, 81.66775706135233293 ) ) ;
#140712=CARTESIAN_POINT ( 'NONE',  ( 19.03943276465977164, 0.05219959533936151252, 21.25109039468565797 ) ) ;
#140713=CARTESIAN_POINT ( 'NONE',  ( -10.81492255796078084, -18.62759615963271287, 57.08224293864769550 ) ) ;
#140714=CARTESIAN_POINT ( 'NONE',  ( 8.314922557961029526, -14.29746914071037800, 80.41775706135234714 ) ) ;
#140715=CARTESIAN_POINT ( 'NONE',  ( 0.05219959533936267826, -19.03943276465977164, 80.00109039468567573 ) ) ;
#140716=CARTESIAN_POINT ( 'NONE',  ( -0.05219959533909027116, -19.03943276465977164, 32.49890960531435979 ) ) ;
#140717=CARTESIAN_POINT ( 'NONE',  ( -13.97604488694527625, -13.89961937509977652, 76.87390960531433848 ) ) ;
#140718=CARTESIAN_POINT ( 'NONE',  ( 0.05219959533937995610, -21.53943276465977519, 55.00109039468568284 ) ) ;
#140719=CARTESIAN_POINT ( 'NONE',  ( -5.153800228976328057, -19.02544592524343514, 47.29057627198102409 ) ) ;
#140720=CARTESIAN_POINT ( 'NONE',  ( -16.51473224551082808, 9.474510206698731452, 68.33442372801900433 ) ) ;
#140722=CARTESIAN_POINT ( 'NONE',  ( 9.474510206698971260, -16.51473224551069308, 112.9155762719810383 ) ) ;
#140723=CARTESIAN_POINT ( 'NONE',  ( 4.379528057220339221, -16.55341960407611168, 67.70724293864769550 ) ) ;
#140724=CARTESIAN_POINT ( 'NONE',  ( -5.719274019375978568, 21.55341960407610458, 65.20724293864768129 ) ) ;
#140726=CARTESIAN_POINT ( 'NONE',  ( -9.564922557961040184, 16.46253265017147172, 27.91775706135232582 ) ) ;
#140727=CARTESIAN_POINT ( 'NONE',  ( -18.10062525802553424, 5.500000000000031974, 88.51383468041920821 ) ) ;
#140728=CARTESIAN_POINT ( 'NONE',  ( 16.46253265017160672, -9.564922557960803928, 58.33224293864769550 ) ) ;
#140729=CARTESIAN_POINT ( 'NONE',  ( -13.89961937509977652, 13.97604488694528158, 70.62390960531432427 ) ) ;
#140730=CARTESIAN_POINT ( 'NONE',  ( 14.29746914071037800, 8.314922557961029526, 51.66775706135234714 ) ) ;
#140731=CARTESIAN_POINT ( 'NONE',  ( -18.22780087662124160, -5.499999999999927169, 78.98236817873106475 ) ) ;
#140733=CARTESIAN_POINT ( 'NONE',  ( -8.224510206698735004, -14.34966873604973081, 89.58442372801901854 ) ) ;
#140735=CARTESIAN_POINT ( 'NONE',  ( -12.06949235617739369, -12.14591786802326823, 69.37609039468567573 ) ) ;
#140736=CARTESIAN_POINT ( 'NONE',  ( 4.483927247898790824, -16.52544592524335698, 45.20942372801901854 ) ) ;
#140737=CARTESIAN_POINT ( 'NONE',  ( 13.89961937509977652, -13.97604488694527269, 58.12390960531436690 ) ) ;
#140739=CARTESIAN_POINT ( 'NONE',  ( 0.05219959533937995610, -21.53943276465977519, 60.00109039468568284 ) ) ;
#140740=CARTESIAN_POINT ( 'NONE',  ( -13.89961937509957401, -13.97604488694547875, 59.37609039468566863 ) ) ;
#140741=CARTESIAN_POINT ( 'NONE',  ( 10.72451020669871369, 18.67979575497193778, 107.0844237280190043 ) ) ;
#140743=CARTESIAN_POINT ( 'NONE',  ( -19.05341960407611168, -5.049401038298163336, 26.45724293864769550 ) ) ;
#140745=CARTESIAN_POINT ( 'NONE',  ( 5.719274019375991003, -21.55341960407610458, 52.70724293864769550 ) ) ;
#140746=CARTESIAN_POINT ( 'NONE',  ( -16.51473224551069308, -9.474510206698971260, 111.6655762719810383 ) ) ;
#140747=CARTESIAN_POINT ( 'NONE',  ( -8.224510206698948167, 14.34966873604960824, 105.4155762719810383 ) ) ;
#140748=CARTESIAN_POINT ( 'NONE',  ( -14.29746914071037622, -8.314922557961029526, 39.16775706135235424 ) ) ;
#140749=CARTESIAN_POINT ( 'NONE',  ( 4.379528057220339221, -16.55341960407611168, 27.70724293864769905 ) ) ;
#140751=CARTESIAN_POINT ( 'NONE',  ( 21.53943276465977519, -0.05219959533907433946, 113.7489096053143527 ) ) ;
#140752=CARTESIAN_POINT ( 'NONE',  ( 8.224510206698953496, -14.34966873604960469, 42.91557627198103120 ) ) ;
#140754=CARTESIAN_POINT ( 'NONE',  ( 19.03943276465977164, 0.05219959533936151252, 101.2510903946856757 ) ) ;
#140755=CARTESIAN_POINT ( 'NONE',  ( -5.049401038297874678, -19.05341960407617918, 24.79275706135233648 ) ) ;
#140756=CARTESIAN_POINT ( 'NONE',  ( 4.379528057220339221, -16.55341960407611168, 37.70724293864769550 ) ) ;
#140757=CARTESIAN_POINT ( 'NONE',  ( -21.55341960407610458, -5.719274019375992779, 106.4572429386477097 ) ) ;
#140758=CARTESIAN_POINT ( 'NONE',  ( 21.55341960407610458, 5.719274019375980345, 63.95724293864770260 ) ) ;
#140759=CARTESIAN_POINT ( 'NONE',  ( -9.564922557960796823, -16.46253265017161027, 72.08224293864770971 ) ) ;
#140760=CARTESIAN_POINT ( 'NONE',  ( 16.53943276465976808, -0.05219959533910856209, 43.74890960531435979 ) ) ;
#140761=CARTESIAN_POINT ( 'NONE',  ( 9.474510206698971260, -16.51473224551069308, 92.91557627198103830 ) ) ;
#140762=CARTESIAN_POINT ( 'NONE',  ( 19.49190055781009789, 5.500000000000041744, 58.06116087098783396 ) ) ;
#140763=CARTESIAN_POINT ( 'NONE',  ( 5.049401038297881783, 19.05341960407617563, 47.29275706135231161 ) ) ;
#140764=CARTESIAN_POINT ( 'NONE',  ( -21.52544592524343514, 5.823673210054127303, 91.04057627198103830 ) ) ;
#140765=CARTESIAN_POINT ( 'NONE',  ( 16.52544592524342804, -4.483927247898539470, 93.54057627198103830 ) ) ;
#140766=CARTESIAN_POINT ( 'NONE',  ( -15.80617190586768217, 15.72974639402176855, 33.12609039468569705 ) ) ;
#140768=CARTESIAN_POINT ( 'NONE',  ( -12.14591786802309592, -12.06949235617757132, 31.87390960531435979 ) ) ;
#140769=CARTESIAN_POINT ( 'NONE',  ( -16.51473224551069308, -9.474510206698971260, 31.66557627198102054 ) ) ;
#140770=CARTESIAN_POINT ( 'NONE',  ( 16.51473224551069308, 9.474510206698969483, 89.16557627198103830 ) ) ;
#140771=CARTESIAN_POINT ( 'NONE',  ( 21.52544592524344225, -5.823673210054117533, 58.54057627198103120 ) ) ;
#140773=CARTESIAN_POINT ( 'NONE',  ( -13.89961937509977652, 13.97604488694528158, 25.62390960531434558 ) ) ;
#140774=CARTESIAN_POINT ( 'NONE',  ( 15.80617190586746368, 15.72974639402197994, 49.37390960531436690 ) ) ;
#140775=CARTESIAN_POINT ( 'NONE',  ( 21.53943276465977519, 0.05219959533937863772, 76.25109039468568994 ) ) ;
#140777=CARTESIAN_POINT ( 'NONE',  ( -8.314922557961024197, 14.29746914071037800, 72.91775706135234714 ) ) ;
#140778=CARTESIAN_POINT ( 'NONE',  ( 5.049401038298161559, -19.05341960407611168, 52.70724293864767418 ) ) ;
#140779=CARTESIAN_POINT ( 'NONE',  ( 19.05341960407611168, 5.049401038298154454, 63.95724293864769550 ) ) ;
#140781=CARTESIAN_POINT ( 'NONE',  ( 10.81492255796106328, -18.62759615963255655, 105.4177570613523613 ) ) ;
#140782=CARTESIAN_POINT ( 'NONE',  ( 16.52544592524335698, 4.483927247898782831, 71.45942372801901854 ) ) ;
#140783=CARTESIAN_POINT ( 'NONE',  ( -5.719274019375665041, -21.55341960407619695, 99.79275706135234714 ) ) ;
#140784=CARTESIAN_POINT ( 'NONE',  ( -13.89961937509977652, 13.97604488694528158, 60.62390960531436690 ) ) ;
#140785=CARTESIAN_POINT ( 'NONE',  ( 18.62759615963271287, -10.81492255796078972, 28.33224293864769550 ) ) ;
#140786=CARTESIAN_POINT ( 'NONE',  ( -13.97604488694547697, 13.89961937509957934, 103.1260903946856473 ) ) ;
#140787=CARTESIAN_POINT ( 'NONE',  ( -0.05219959533937732626, 21.53943276465977519, 87.50109039468568994 ) ) ;
#140788=CARTESIAN_POINT ( 'NONE',  ( 0.05219959533934541429, -16.53943276465976808, 45.00109039468568284 ) ) ;
#140789=CARTESIAN_POINT ( 'NONE',  ( 10.72451020669898902, -18.67979575497178502, 92.91557627198103830 ) ) ;
#140790=CARTESIAN_POINT ( 'NONE',  ( -16.46253265017146816, -9.564922557961047289, 104.1677570613523329 ) ) ;
#140792=CARTESIAN_POINT ( 'NONE',  ( -0.05219959533909027116, -19.03943276465977164, 72.49890960531435269 ) ) ;
#140793=CARTESIAN_POINT ( 'NONE',  ( -19.03943276465977164, -0.05219959533935918106, 108.7510903946856615 ) ) ;
#140794=CARTESIAN_POINT ( 'NONE',  ( -5.049401038298153566, 19.05341960407611168, 35.20724293864768839 ) ) ;
#140795=CARTESIAN_POINT ( 'NONE',  ( 14.29746914071037800, 8.314922557961029526, 26.66775706135235424 ) ) ;
#140796=CARTESIAN_POINT ( 'NONE',  ( 8.224510206698953496, -14.34966873604960469, 62.91557627198102409 ) ) ;
#140797=CARTESIAN_POINT ( 'NONE',  ( -14.29746914071037622, -8.314922557961029526, 69.16775706135234714 ) ) ;
#140798=CARTESIAN_POINT ( 'NONE',  ( 10.72451020669871369, 18.67979575497193778, 32.08442372801901854 ) ) ;
#140799=CARTESIAN_POINT ( 'NONE',  ( -19.05341960407611168, -5.049401038298163336, 51.45724293864770260 ) ) ;
#140800=CARTESIAN_POINT ( 'NONE',  ( 19.03943276465977164, -0.05219959533909143690, 68.74890960531436690 ) ) ;
#140801=CARTESIAN_POINT ( 'NONE',  ( 4.379528057220092307, 16.55341960407617563, 77.29275706135234714 ) ) ;
#140804=CARTESIAN_POINT ( 'NONE',  ( -10.72451020669870658, -18.67979575497194134, 109.5844237280190328 ) ) ;
#140805=CARTESIAN_POINT ( 'NONE',  ( 13.89961937509977652, -13.97604488694527269, 38.12390960531436690 ) ) ;
#140806=EDGE_LOOP ( 'NONE', ( #192152, #147931, #192488, #62853, #39274, #38, #183572, #121223, #77154, #113113, #146949, #29109, #12658, #25838, #32209, #29797 ) ) ;
#140807=CARTESIAN_POINT ( 'NONE',  ( 16.52544592524335698, 4.483927247898782831, 26.45942372801901854 ) ) ;
#140808=CARTESIAN_POINT ( 'NONE',  ( 19.05341960407617918, -5.049401038297876454, 51.04275706135231871 ) ) ;
#140809=CARTESIAN_POINT ( 'NONE',  ( 8.314922557961029526, -14.29746914071037800, 45.41775706135234003 ) ) ;
#140810=CARTESIAN_POINT ( 'NONE',  ( 5.153800228976335163, 19.02544592524342804, 39.79057627198100988 ) ) ;
#140811=CARTESIAN_POINT ( 'NONE',  ( -0.05219959533909027116, -19.03943276465977164, 102.4989096053143669 ) ) ;
#140812=CARTESIAN_POINT ( 'NONE',  ( 5.049401038298161559, -19.05341960407611168, 57.70724293864769550 ) ) ;
#140813=CARTESIAN_POINT ( 'NONE',  ( 5.823673210054125526, 21.52544592524343514, 104.7905762719810241 ) ) ;
#140814=CARTESIAN_POINT ( 'NONE',  ( -0.05219959533909027116, -19.03943276465977164, 77.49890960531435269 ) ) ;
#140817=CARTESIAN_POINT ( 'NONE',  ( -9.474510206698964154, 16.51473224551069663, 65.41557627198102409 ) ) ;
#140819=CARTESIAN_POINT ( 'NONE',  ( -13.97604488694547697, 13.89961937509957934, 93.12609039468566152 ) ) ;
#140820=CARTESIAN_POINT ( 'NONE',  ( -13.89961937509957401, -13.97604488694547875, 19.37609039468566507 ) ) ;
#140821=CARTESIAN_POINT ( 'NONE',  ( -14.29746914071049879, 8.314922557960819915, 65.83224293864769550 ) ) ;
#140822=CARTESIAN_POINT ( 'NONE',  ( -18.62759615963255300, -10.81492255796106328, 84.16775706135234714 ) ) ;
#140823=CARTESIAN_POINT ( 'NONE',  ( -16.51473224551069308, -9.474510206698971260, 21.66557627198102765 ) ) ;
#140824=CARTESIAN_POINT ( 'NONE',  ( -0.05219959533910754901, -16.53943276465976808, 27.49890960531435269 ) ) ;
#140825=CARTESIAN_POINT ( 'NONE',  ( -15.72974639402176322, -15.80617190586768395, 94.37609039468568994 ) ) ;
#140826=CARTESIAN_POINT ( 'NONE',  ( -16.46253265017160317, 9.564922557960807481, 80.83224293864769550 ) ) ;
#140827=CARTESIAN_POINT ( 'NONE',  ( -15.80617190586768217, 15.72974639402176855, 48.12609039468568284 ) ) ;
#140828=CARTESIAN_POINT ( 'NONE',  ( -5.049401038298153566, 19.05341960407611168, 80.20724293864769550 ) ) ;
#140829=CARTESIAN_POINT ( 'NONE',  ( 0.05219959533910956823, 16.53943276465976808, 89.99890960531438111 ) ) ;
#140830=CARTESIAN_POINT ( 'NONE',  ( -16.53943276465976808, 0.05219959533911058130, 61.24890960531435979 ) ) ;
#140831=CARTESIAN_POINT ( 'NONE',  ( 10.72451020669898902, -18.67979575497178502, 72.91557627198103830 ) ) ;
#140832=CARTESIAN_POINT ( 'NONE',  ( 5.153800228976335163, 19.02544592524342804, 74.79057627198103830 ) ) ;
#140833=CARTESIAN_POINT ( 'NONE',  ( 0.05219959533907565091, 21.53943276465977519, 84.99890960531436690 ) ) ;
#140834=CARTESIAN_POINT ( 'NONE',  ( -13.97604488694547697, 13.89961937509957934, 83.12609039468564731 ) ) ;
#140836=CARTESIAN_POINT ( 'NONE',  ( -0.05219959533936034679, 19.03943276465977164, 37.50109039468567573 ) ) ;
#140837=CARTESIAN_POINT ( 'NONE',  ( 4.379528057220339221, -16.55341960407611168, 82.70724293864770971 ) ) ;
#140838=CARTESIAN_POINT ( 'NONE',  ( 19.03943276465977164, -0.05219959533909143690, 63.74890960531435979 ) ) ;
#140839=CARTESIAN_POINT ( 'NONE',  ( -5.719274019375978568, 21.55341960407610458, 70.20724293864769550 ) ) ;
#140841=CARTESIAN_POINT ( 'NONE',  ( -8.314922557960811034, -14.29746914071050412, 22.08224293864769194 ) ) ;
#140843=CARTESIAN_POINT ( 'NONE',  ( 5.049401038297881783, 19.05341960407617563, 102.2927570613523045 ) ) ;
#140844=CARTESIAN_POINT ( 'NONE',  ( -12.14591786802309592, -12.06949235617757132, 81.87390960531435269 ) ) ;
#140846=CARTESIAN_POINT ( 'NONE',  ( -5.153800228976328057, -19.02544592524343514, 77.29057627198099567 ) ) ;
#140847=CARTESIAN_POINT ( 'NONE',  ( 13.89961937509977652, -13.97604488694527269, 33.12390960531434558 ) ) ;
#140848=CARTESIAN_POINT ( 'NONE',  ( -4.483927247898539470, -16.52544592524342804, 62.29057627198102409 ) ) ;
#140849=CARTESIAN_POINT ( 'NONE',  ( -19.05341960407611168, -5.049401038298163336, 96.45724293864769550 ) ) ;
#140850=CARTESIAN_POINT ( 'NONE',  ( 19.02544592524334988, 5.153800228976608722, 86.45942372801900433 ) ) ;
#140851=CARTESIAN_POINT ( 'NONE',  ( -13.97604488694527625, -13.89961937509977652, 61.87390960531435979 ) ) ;
#140852=CARTESIAN_POINT ( 'NONE',  ( -16.46253265017160317, 9.564922557960807481, 90.83224293864769550 ) ) ;
#140853=CARTESIAN_POINT ( 'NONE',  ( 10.72451020669898902, -18.67979575497178502, 77.91557627198102409 ) ) ;
#140854=CARTESIAN_POINT ( 'NONE',  ( 0.05219959533934541429, -16.53943276465976808, 75.00109039468568994 ) ) ;
#140855=CARTESIAN_POINT ( 'NONE',  ( -19.03943276465977164, -0.05219959533935918106, 108.7510903946856615 ) ) ;
#140856=CARTESIAN_POINT ( 'NONE',  ( -19.05341960407611168, -5.049401038298163336, 66.45724293864769550 ) ) ;
#140857=CARTESIAN_POINT ( 'NONE',  ( -21.55341960407610458, -5.719274019375992779, 71.45724293864769550 ) ) ;
#140858=CARTESIAN_POINT ( 'NONE',  ( 5.049401038297881783, 19.05341960407617563, 97.29275706135233293 ) ) ;
#140859=CARTESIAN_POINT ( 'NONE',  ( 16.52544592524342804, -4.483927247898539470, 43.54057627198103830 ) ) ;
#140860=CARTESIAN_POINT ( 'NONE',  ( 21.53943276465977519, 0.05219959533937863772, 46.25109039468567573 ) ) ;
#140862=CARTESIAN_POINT ( 'NONE',  ( -8.314922557961024197, 14.29746914071037800, 77.91775706135231871 ) ) ;
#140863=CARTESIAN_POINT ( 'NONE',  ( 19.05341960407611168, 5.049401038298154454, 103.9572429386476671 ) ) ;
#140864=CARTESIAN_POINT ( 'NONE',  ( -16.46253265017160317, 9.564922557960807481, 105.8322429386476955 ) ) ;
#140865=CARTESIAN_POINT ( 'NONE',  ( -17.13100169013302221, -6.664070546373105586, 34.23210164300150637 ) ) ;
#140866=CARTESIAN_POINT ( 'NONE',  ( 16.55341960407618274, -4.379528057220086978, 96.04275706135236135 ) ) ;
#140867=CARTESIAN_POINT ( 'NONE',  ( 12.06949235617739724, 12.14591786802326823, 36.87609039468568994 ) ) ;
#140868=CARTESIAN_POINT ( 'NONE',  ( 0.05219959533909260263, 19.03943276465977164, 44.99890960531435979 ) ) ;
#140869=CARTESIAN_POINT ( 'NONE',  ( -16.46253265017160317, 9.564922557960807481, 55.83224293864769550 ) ) ;
#140870=CARTESIAN_POINT ( 'NONE',  ( -13.89961937509977652, 13.97604488694528158, 60.62390960531436690 ) ) ;
#140871=CARTESIAN_POINT ( 'NONE',  ( 21.55341960407619695, -5.719274019375665929, 56.04275706135235424 ) ) ;
#140872=CARTESIAN_POINT ( 'NONE',  ( -12.14591786802326823, 12.06949235617739902, 68.12609039468567573 ) ) ;
#140873=CARTESIAN_POINT ( 'NONE',  ( 12.14591786802309770, 12.06949235617756955, 34.37390960531435979 ) ) ;
#140874=CARTESIAN_POINT ( 'NONE',  ( 0.05219959533909260263, 19.03943276465977164, 39.99890960531436690 ) ) ;
#140875=CARTESIAN_POINT ( 'NONE',  ( 19.03943276465977164, -0.05219959533909143690, 38.74890960531436690 ) ) ;
#140876=CARTESIAN_POINT ( 'NONE',  ( -14.34966873604972548, 8.224510206698743886, 28.33442372801902209 ) ) ;
#140877=CARTESIAN_POINT ( 'NONE',  ( 16.51473224551083163, -9.474510206698727899, 85.83442372801900433 ) ) ;
#140878=CARTESIAN_POINT ( 'NONE',  ( -8.224510206698948167, 14.34966873604960824, 80.41557627198103830 ) ) ;
#140879=CARTESIAN_POINT ( 'NONE',  ( -16.51473224551069308, -9.474510206698971260, 46.66557627198102409 ) ) ;
#140880=CARTESIAN_POINT ( 'NONE',  ( -9.564922557961040184, 16.46253265017147172, 82.91775706135233293 ) ) ;
#140882=CARTESIAN_POINT ( 'NONE',  ( -15.72974639402176322, -15.80617190586768395, 89.37609039468568994 ) ) ;
#140883=CARTESIAN_POINT ( 'NONE',  ( 12.14591786802327356, -12.06949235617739191, 60.62609039468567573 ) ) ;
#140884=CARTESIAN_POINT ( 'NONE',  ( 17.31747979337949772, 6.344076630961017038, 38.87944868065184778 ) ) ;
#140885=CARTESIAN_POINT ( 'NONE',  ( -21.53943276465977519, 0.05219959533907696930, 56.24890960531436690 ) ) ;
#140886=CARTESIAN_POINT ( 'NONE',  ( 16.52544592524335698, 4.483927247898782831, 46.45942372801901854 ) ) ;
#140887=CARTESIAN_POINT ( 'NONE',  ( 5.153800228976335163, 19.02544592524342804, 24.79057627198102765 ) ) ;
#140888=CARTESIAN_POINT ( 'NONE',  ( -16.51473224551082808, 9.474510206698731452, 23.33442372801900078 ) ) ;
#140890=CARTESIAN_POINT ( 'NONE',  ( -13.89961937509977652, 13.97604488694528158, 80.62390960531436690 ) ) ;
#140892=CARTESIAN_POINT ( 'NONE',  ( 19.03943276465977164, -0.05219959533909143690, 48.74890960531435979 ) ) ;
#140894=CARTESIAN_POINT ( 'NONE',  ( 13.97604488694527802, 13.89961937509977652, 74.37390960531436690 ) ) ;
#140896=CARTESIAN_POINT ( 'NONE',  ( 17.49999999999999645, -3.305555262949672279, 112.1251715215659743 ) ) ;
#140898=CARTESIAN_POINT ( 'NONE',  ( -21.53943276465977519, -0.05219959533937600094, 113.7510903946856757 ) ) ;
#140899=CARTESIAN_POINT ( 'NONE',  ( -5.823673210054431948, 21.52544592524334988, 112.7094237280190328 ) ) ;
#140900=CARTESIAN_POINT ( 'NONE',  ( 8.224510206698953496, -14.34966873604960469, 37.91557627198102409 ) ) ;
#140901=CARTESIAN_POINT ( 'NONE',  ( 5.049401038298161559, -19.05341960407611168, 47.70724293864770260 ) ) ;
#140902=CARTESIAN_POINT ( 'NONE',  ( -0.05219959533909027116, -19.03943276465977164, 107.4989096053143527 ) ) ;
#140903=CARTESIAN_POINT ( 'NONE',  ( -21.52544592524334988, -5.823673210054445271, 68.95942372801901854 ) ) ;
#140904=CARTESIAN_POINT ( 'NONE',  ( 5.049401038298161559, -19.05341960407611168, 47.70724293864770260 ) ) ;
#140905=CARTESIAN_POINT ( 'NONE',  ( -21.53943276465977519, -0.05219959533937600094, 78.75109039468568994 ) ) ;
#140906=CARTESIAN_POINT ( 'NONE',  ( -10.72451020669898014, 18.67979575497178502, 25.41557627198103120 ) ) ;
#140907=CARTESIAN_POINT ( 'NONE',  ( 19.02544592524343514, -5.153800228976328945, 33.54057627198102409 ) ) ;
#140908=CARTESIAN_POINT ( 'NONE',  ( -21.52544592524334988, -5.823673210054445271, 23.95942372801901143 ) ) ;
#140909=CARTESIAN_POINT ( 'NONE',  ( -16.51473224551082808, 9.474510206698731452, 53.33442372801900433 ) ) ;
#140910=CARTESIAN_POINT ( 'NONE',  ( -9.564922557960796823, -16.46253265017161027, 27.08224293864769550 ) ) ;
#140911=CARTESIAN_POINT ( 'NONE',  ( -13.97604488694527625, -13.89961937509977652, 71.87390960531433848 ) ) ;
#140912=CARTESIAN_POINT ( 'NONE',  ( 13.97604488694548053, -13.89961937509957401, 105.6260903946856757 ) ) ;
#140913=CARTESIAN_POINT ( 'NONE',  ( -4.483927247898539470, -16.52544592524342804, 72.29057627198102409 ) ) ;
#140914=CARTESIAN_POINT ( 'NONE',  ( -15.80617190586745835, -15.72974639402198527, 31.87390960531435979 ) ) ;
#140915=CARTESIAN_POINT ( 'NONE',  ( 19.02544592524334988, 5.153800228976608722, 96.45942372801897591 ) ) ;
#140916=CARTESIAN_POINT ( 'NONE',  ( -21.55341960407610458, -5.719274019375992779, 106.4572429386477097 ) ) ;
#140917=CARTESIAN_POINT ( 'NONE',  ( -15.80617190586768217, 15.72974639402176855, 58.12609039468568994 ) ) ;
#140918=CARTESIAN_POINT ( 'NONE',  ( 0.05219959533934541429, -16.53943276465976808, 50.00109039468568994 ) ) ;
#140919=CARTESIAN_POINT ( 'NONE',  ( -16.53943276465976808, -0.05219959533934237506, 48.75109039468568284 ) ) ;
#140920=CARTESIAN_POINT ( 'NONE',  ( -5.719274019375978568, 21.55341960407610458, 70.20724293864769550 ) ) ;
#140922=CARTESIAN_POINT ( 'NONE',  ( 16.51473224551069308, 9.474510206698969483, 44.16557627198103120 ) ) ;
#140923=CARTESIAN_POINT ( 'NONE',  ( -8.314922557961024197, 14.29746914071037800, 87.91775706135234714 ) ) ;
#140924=CARTESIAN_POINT ( 'NONE',  ( -5.823673210054116645, -21.52544592524344225, 97.29057627198105251 ) ) ;
#140925=CARTESIAN_POINT ( 'NONE',  ( -16.52544592524342804, 4.483927247898546575, 56.04057627198102409 ) ) ;
#140926=CARTESIAN_POINT ( 'NONE',  ( 0.05219959533909260263, 19.03943276465977164, 69.99890960531435269 ) ) ;
#140927=CARTESIAN_POINT ( 'NONE',  ( 8.314922557961029526, -14.29746914071037800, 80.41775706135234714 ) ) ;
#140928=CARTESIAN_POINT ( 'NONE',  ( -16.51473224551082808, 9.474510206698731452, 113.3344237280190043 ) ) ;
#140929=CARTESIAN_POINT ( 'NONE',  ( -21.53943276465977519, 0.05219959533907696930, 106.2489096053143811 ) ) ;
#140930=CARTESIAN_POINT ( 'NONE',  ( 0.05219959533910956823, 16.53943276465976808, 39.99890960531436690 ) ) ;
#140932=CARTESIAN_POINT ( 'NONE',  ( -17.31747979337945154, 6.344076630961109409, 73.62055131934816643 ) ) ;
#140933=CARTESIAN_POINT ( 'NONE',  ( 15.72974639402199770, -15.80617190586745480, 88.12390960531436690 ) ) ;
#140934=CARTESIAN_POINT ( 'NONE',  ( -14.29746914071049879, 8.314922557960819915, 30.83224293864770260 ) ) ;
#140936=CARTESIAN_POINT ( 'NONE',  ( -17.05587630539787014, -6.762274262135727021, 54.25819690962693187 ) ) ;
#140937=CARTESIAN_POINT ( 'NONE',  ( 18.62759615963271287, -10.81492255796078972, 103.3322429386476955 ) ) ;
#140938=CARTESIAN_POINT ( 'NONE',  ( 16.51473224551069308, 9.474510206698969483, 114.1655762719810241 ) ) ;
#140939=CARTESIAN_POINT ( 'NONE',  ( -18.62759615963270932, 10.81492255796079327, 115.8322429386477097 ) ) ;
#140940=CARTESIAN_POINT ( 'NONE',  ( 4.483927247898545687, 16.52544592524342804, 49.79057627198102409 ) ) ;
#140941=CARTESIAN_POINT ( 'NONE',  ( -14.29746914071037622, -8.314922557961029526, 54.16775706135235424 ) ) ;
#140942=CARTESIAN_POINT ( 'NONE',  ( -16.46253265017160317, 9.564922557960807481, 60.83224293864769550 ) ) ;
#140943=CARTESIAN_POINT ( 'NONE',  ( -16.51473224551082808, 9.474510206698731452, 53.33442372801900433 ) ) ;
#140944=CARTESIAN_POINT ( 'NONE',  ( 0.05219959533909260263, 19.03943276465977164, 79.99890960531436690 ) ) ;
#140945=CARTESIAN_POINT ( 'NONE',  ( 5.719274019375991003, -21.55341960407610458, 37.70724293864769550 ) ) ;
#140947=CARTESIAN_POINT ( 'NONE',  ( 0.05219959533909260263, 19.03943276465977164, 49.99890960531435979 ) ) ;
#140948=CARTESIAN_POINT ( 'NONE',  ( -16.52544592524335698, -4.483927247898792601, 18.95942372801901143 ) ) ;
#140949=CARTESIAN_POINT ( 'NONE',  ( -5.153800228976607833, 19.02544592524334988, 67.70942372801900433 ) ) ;
#140950=CARTESIAN_POINT ( 'NONE',  ( -18.62759615963270932, 10.81492255796079327, 105.8322429386476955 ) ) ;
#140951=CARTESIAN_POINT ( 'NONE',  ( -16.55341960407611168, -4.379528057220339221, 36.45724293864768839 ) ) ;
#140952=CARTESIAN_POINT ( 'NONE',  ( 19.03943276465977164, -0.05219959533909143690, 78.74890960531436690 ) ) ;
#140953=CARTESIAN_POINT ( 'NONE',  ( 21.52544592524344225, -5.823673210054117533, 63.54057627198103830 ) ) ;
#140954=CARTESIAN_POINT ( 'NONE',  ( -5.823673210054116645, -21.52544592524344225, 97.29057627198105251 ) ) ;
#140955=CARTESIAN_POINT ( 'NONE',  ( 14.29746914071037800, 8.314922557961029526, 26.66775706135235424 ) ) ;
#140956=CARTESIAN_POINT ( 'NONE',  ( 13.89961937509977652, -13.97604488694527269, 113.1239096053143527 ) ) ;
#140957=CARTESIAN_POINT ( 'NONE',  ( -21.53943276465977519, -0.05219959533937600094, 88.75109039468567573 ) ) ;
#140958=CARTESIAN_POINT ( 'NONE',  ( -19.03943276465977164, 0.05219959533909376836, 81.24890960531436690 ) ) ;
#140959=CARTESIAN_POINT ( 'NONE',  ( 0.05219959533909260263, 19.03943276465977164, 29.99890960531435979 ) ) ;
#140960=CARTESIAN_POINT ( 'NONE',  ( -19.05341960407611168, -5.049401038298163336, 81.45724293864769550 ) ) ;
#140961=CARTESIAN_POINT ( 'NONE',  ( 12.14591786802309770, 12.06949235617756955, 99.37390960531436690 ) ) ;
#140962=CARTESIAN_POINT ( 'NONE',  ( 5.049401038298161559, -19.05341960407611168, 62.70724293864769550 ) ) ;
#140963=CARTESIAN_POINT ( 'NONE',  ( -5.153800228976607833, 19.02544592524334988, 112.7094237280190043 ) ) ;
#140964=CARTESIAN_POINT ( 'NONE',  ( -0.05219959533936034679, 19.03943276465977164, 42.50109039468566152 ) ) ;
#140965=CARTESIAN_POINT ( 'NONE',  ( 21.52544592524334988, 5.823673210054432836, 91.45942372801901854 ) ) ;
#140966=CARTESIAN_POINT ( 'NONE',  ( 21.55341960407610458, 5.719274019375980345, 23.95724293864769550 ) ) ;
#140967=CARTESIAN_POINT ( 'NONE',  ( 16.55341960407618274, -4.379528057220086978, 86.04275706135236135 ) ) ;
#140969=CARTESIAN_POINT ( 'NONE',  ( -19.03943276465977164, -0.05219959533935918106, 73.75109039468566152 ) ) ;
#140970=CARTESIAN_POINT ( 'NONE',  ( 19.02544592524334988, 5.153800228976608722, 31.45942372801900433 ) ) ;
#140972=CARTESIAN_POINT ( 'NONE',  ( 0.05219959533909260263, 19.03943276465977164, 29.99890960531435979 ) ) ;
#140973=CARTESIAN_POINT ( 'NONE',  ( 4.483927247898545687, 16.52544592524342804, 34.79057627198103120 ) ) ;
#140975=CARTESIAN_POINT ( 'NONE',  ( -16.55341960407617563, 4.379528057220093196, 108.5427570613523756 ) ) ;
#140976=CARTESIAN_POINT ( 'NONE',  ( 16.81555441253552274, 7.025013491695498047, 66.86314554665746357 ) ) ;
#140977=CARTESIAN_POINT ( 'NONE',  ( -8.224510206698735004, -14.34966873604973081, 84.58442372801903275 ) ) ;
#140978=CARTESIAN_POINT ( 'NONE',  ( 16.51473224551069308, 9.474510206698969483, 39.16557627198103120 ) ) ;
#140979=CARTESIAN_POINT ( 'NONE',  ( -0.05219959533937732626, 21.53943276465977519, 87.50109039468568994 ) ) ;
#140980=CARTESIAN_POINT ( 'NONE',  ( -5.153800228976607833, 19.02544592524334988, 97.70942372801900433 ) ) ;
#140981=CARTESIAN_POINT ( 'NONE',  ( -5.823673210054431948, 21.52544592524334988, 77.70942372801900433 ) ) ;
#140982=CARTESIAN_POINT ( 'NONE',  ( -19.03943276465977164, -0.05219959533935918106, 48.75109039468566863 ) ) ;
#140983=CARTESIAN_POINT ( 'NONE',  ( 16.46253265017160672, -9.564922557960803928, 88.33224293864769550 ) ) ;
#140984=CARTESIAN_POINT ( 'NONE',  ( 19.05341960407611168, 5.049401038298154454, 73.95724293864768129 ) ) ;
#140987=CARTESIAN_POINT ( 'NONE',  ( 8.224510206698953496, -14.34966873604960469, 72.91557627198103830 ) ) ;
#140988=CARTESIAN_POINT ( 'NONE',  ( -0.05219959533907301413, -21.53943276465977519, 62.49890960531436690 ) ) ;
#140989=CARTESIAN_POINT ( 'NONE',  ( 9.474510206698971260, -16.51473224551069308, 52.91557627198102409 ) ) ;
#140990=CARTESIAN_POINT ( 'NONE',  ( -15.80617190586745835, -15.72974639402198527, 86.87390960531438111 ) ) ;
#140991=CARTESIAN_POINT ( 'NONE',  ( 12.06949235617739724, 12.14591786802326823, 76.87609039468567573 ) ) ;
#140993=CARTESIAN_POINT ( 'NONE',  ( -9.474510206698964154, 16.51473224551069663, 45.41557627198103120 ) ) ;
#140994=CARTESIAN_POINT ( 'NONE',  ( 16.52544592524342804, -4.483927247898539470, 73.54057627198102409 ) ) ;
#140996=CARTESIAN_POINT ( 'NONE',  ( -0.05219959533909027116, -19.03943276465977164, 47.49890960531435979 ) ) ;
#140997=CARTESIAN_POINT ( 'NONE',  ( 9.564922557960805705, 16.46253265017160317, 24.58224293864769194 ) ) ;
#140998=CARTESIAN_POINT ( 'NONE',  ( 13.89961937509957401, 13.97604488694547697, 71.87609039468567573 ) ) ;
#140999=CARTESIAN_POINT ( 'NONE',  ( -16.52544592524342804, 4.483927247898546575, 76.04057627198102409 ) ) ;
#141000=CARTESIAN_POINT ( 'NONE',  ( 10.72451020669871369, 18.67979575497193778, 52.08442372801901854 ) ) ;
#141001=CARTESIAN_POINT ( 'NONE',  ( 0.05219959533909260263, 19.03943276465977164, 29.99890960531435979 ) ) ;
#141002=CARTESIAN_POINT ( 'NONE',  ( -18.62759615963270932, 10.81492255796079327, 105.8322429386476955 ) ) ;
#141003=CARTESIAN_POINT ( 'NONE',  ( -19.02544592524342804, 5.153800228976336051, 116.0405762719810383 ) ) ;
#141004=CARTESIAN_POINT ( 'NONE',  ( 4.379528057220339221, -16.55341960407611168, 87.70724293864769550 ) ) ;
#141006=CARTESIAN_POINT ( 'NONE',  ( -19.05341960407611168, -5.049401038298163336, 41.45724293864769550 ) ) ;
#141007=CARTESIAN_POINT ( 'NONE',  ( 16.79531203550646623, 7.028104445595634076, 113.7524498822045302 ) ) ;
#141008=CARTESIAN_POINT ( 'NONE',  ( 9.474510206698729675, 16.51473224551082808, 92.08442372801900433 ) ) ;
#141009=CARTESIAN_POINT ( 'NONE',  ( 19.05341960407611168, 5.049401038298154454, 103.9572429386476671 ) ) ;
#141010=CARTESIAN_POINT ( 'NONE',  ( -10.81492255796105439, 18.62759615963255655, 32.91775706135234714 ) ) ;
#141011=CARTESIAN_POINT ( 'NONE',  ( -9.564922557960796823, -16.46253265017161027, 87.08224293864769550 ) ) ;
#141012=CARTESIAN_POINT ( 'NONE',  ( -19.05341960407617563, 5.049401038297882671, 68.54275706135230450 ) ) ;
#141013=CARTESIAN_POINT ( 'NONE',  ( -0.05219959533909027116, -19.03943276465977164, 47.49890960531435979 ) ) ;
#141015=CARTESIAN_POINT ( 'NONE',  ( -16.52544592524342804, 4.483927247898546575, 61.04057627198103120 ) ) ;
#141016=CARTESIAN_POINT ( 'NONE',  ( 16.55341960407611168, 4.379528057220329451, 73.95724293864769550 ) ) ;
#141017=CARTESIAN_POINT ( 'NONE',  ( -16.51473224551069308, -9.474510206698971260, 71.66557627198102409 ) ) ;
#141018=CARTESIAN_POINT ( 'NONE',  ( 21.53943276465977519, -0.05219959533907433946, 103.7489096053143669 ) ) ;
#141019=CARTESIAN_POINT ( 'NONE',  ( -16.51473224551069308, -9.474510206698971260, 76.66557627198103830 ) ) ;
#141020=CARTESIAN_POINT ( 'NONE',  ( -5.719274019375665041, -21.55341960407619695, 109.7927570613523613 ) ) ;
#141021=CARTESIAN_POINT ( 'NONE',  ( 16.46253265017160672, -9.564922557960803928, 33.33224293864770260 ) ) ;
#141022=CARTESIAN_POINT ( 'NONE',  ( 16.55341960407618274, -4.379528057220086978, 111.0427570613523613 ) ) ;
#141023=CARTESIAN_POINT ( 'NONE',  ( 0.05219959533910956823, 16.53943276465976808, 109.9989096053143527 ) ) ;
#141024=CARTESIAN_POINT ( 'NONE',  ( 19.05341960407617918, -5.049401038297876454, 106.0427570613523471 ) ) ;
#141026=CARTESIAN_POINT ( 'NONE',  ( 21.52544592524334988, 5.823673210054432836, 36.45942372801901143 ) ) ;
#141027=CARTESIAN_POINT ( 'NONE',  ( -16.46253265017146816, -9.564922557961047289, 49.16775706135233293 ) ) ;
#141028=CARTESIAN_POINT ( 'NONE',  ( -14.34966873604972548, 8.224510206698743886, 113.3344237280190328 ) ) ;
#141029=CARTESIAN_POINT ( 'NONE',  ( 18.62759615963271287, -10.81492255796078972, 78.33224293864770971 ) ) ;
#141030=CARTESIAN_POINT ( 'NONE',  ( -0.05219959533909027116, -19.03943276465977164, 112.4989096053143669 ) ) ;
#141031=CARTESIAN_POINT ( 'NONE',  ( 12.06949235617757843, -12.14591786802309237, 58.12390960531435979 ) ) ;
#141032=CARTESIAN_POINT ( 'NONE',  ( 0.05219959533909260263, 19.03943276465977164, 29.99890960531435979 ) ) ;
#141033=CARTESIAN_POINT ( 'NONE',  ( 19.02544592524343514, -5.153800228976328945, 38.54057627198103120 ) ) ;
#141034=CARTESIAN_POINT ( 'NONE',  ( -0.05219959533936034679, 19.03943276465977164, 27.50109039468566507 ) ) ;
#141035=CARTESIAN_POINT ( 'NONE',  ( 14.29746914071037800, 8.314922557961029526, 91.66775706135234714 ) ) ;
#141036=CARTESIAN_POINT ( 'NONE',  ( -16.53943276465976808, -0.05219959533934237506, 63.75109039468568284 ) ) ;
#141037=CARTESIAN_POINT ( 'NONE',  ( -13.97604488694527625, -13.89961937509977652, 111.8739096053143243 ) ) ;
#141038=CARTESIAN_POINT ( 'NONE',  ( 19.03943276465977164, -0.05219959533909143690, 58.74890960531435979 ) ) ;
#141039=CARTESIAN_POINT ( 'NONE',  ( -15.80617190586768217, 15.72974639402176855, 103.1260903946856757 ) ) ;
#141040=CARTESIAN_POINT ( 'NONE',  ( -9.474510206698964154, 16.51473224551069663, 80.41557627198103830 ) ) ;
#141042=CARTESIAN_POINT ( 'NONE',  ( 16.52544592524335698, 4.483927247898782831, 61.45942372801901854 ) ) ;
#141043=CARTESIAN_POINT ( 'NONE',  ( 0.05219959533910956823, 16.53943276465976808, 109.9989096053143527 ) ) ;
#141044=CARTESIAN_POINT ( 'NONE',  ( -16.53943276465976808, -0.05219959533934237506, 113.7510903946856757 ) ) ;
#141046=CARTESIAN_POINT ( 'NONE',  ( 21.55341960407619695, -5.719274019375665929, 76.04275706135237556 ) ) ;
#141047=CARTESIAN_POINT ( 'NONE',  ( -19.05341960407611168, -5.049401038298163336, 86.45724293864769550 ) ) ;
#141048=CARTESIAN_POINT ( 'NONE',  ( -19.05341960407611168, -5.049401038298163336, 81.45724293864769550 ) ) ;
#141049=CARTESIAN_POINT ( 'NONE',  ( 5.153800228976335163, 19.02544592524342804, 104.7905762719809957 ) ) ;
#141050=CARTESIAN_POINT ( 'NONE',  ( 14.29746914071049879, -8.314922557960816363, 53.33224293864769550 ) ) ;
#141051=CARTESIAN_POINT ( 'NONE',  ( -0.05219959533934338120, 16.53943276465976808, 112.5010903946857042 ) ) ;
#141052=CARTESIAN_POINT ( 'NONE',  ( -12.14591786802309592, -12.06949235617757132, 41.87390960531435979 ) ) ;
#141053=CARTESIAN_POINT ( 'NONE',  ( 16.52544592524335698, 4.483927247898782831, 46.45942372801901854 ) ) ;
#141055=CARTESIAN_POINT ( 'NONE',  ( -13.89961937509957401, -13.97604488694547875, 34.37609039468566863 ) ) ;
#141056=CARTESIAN_POINT ( 'NONE',  ( -19.03943276465977164, 0.05219959533909376836, 76.24890960531435269 ) ) ;
#141057=CARTESIAN_POINT ( 'NONE',  ( 19.02544592524334988, 5.153800228976608722, 51.45942372801900433 ) ) ;
#141060=CARTESIAN_POINT ( 'NONE',  ( 13.97604488694548053, -13.89961937509957401, 80.62609039468567573 ) ) ;
#141061=CARTESIAN_POINT ( 'NONE',  ( 16.52544592524335698, 4.483927247898782831, 86.45942372801901854 ) ) ;
#141062=CARTESIAN_POINT ( 'NONE',  ( 5.049401038298161559, -19.05341960407611168, 22.70724293864769194 ) ) ;
#141063=CARTESIAN_POINT ( 'NONE',  ( 5.049401038298161559, -19.05341960407611168, 107.7072429386476955 ) ) ;
#141064=CARTESIAN_POINT ( 'NONE',  ( 5.823673210054444382, -21.52544592524334988, 45.20942372801901854 ) ) ;
#141065=CARTESIAN_POINT ( 'NONE',  ( -19.03943276465977164, -0.05219959533935918106, 83.75109039468567573 ) ) ;
#141066=CARTESIAN_POINT ( 'NONE',  ( 17.50000000000001066, -3.189878218039145175, 107.3705143742875947 ) ) ;
#141067=CARTESIAN_POINT ( 'NONE',  ( -16.51473224551069308, -9.474510206698971260, 41.66557627198103120 ) ) ;
#141069=CARTESIAN_POINT ( 'NONE',  ( 5.049401038298161559, -19.05341960407611168, 107.7072429386476955 ) ) ;
#141070=CARTESIAN_POINT ( 'NONE',  ( -16.52544592524342804, 4.483927247898546575, 66.04057627198103830 ) ) ;
#141071=CARTESIAN_POINT ( 'NONE',  ( 0.05219959533909260263, 19.03943276465977164, 44.99890960531435979 ) ) ;
#141072=CARTESIAN_POINT ( 'NONE',  ( 13.89961937509977652, -13.97604488694527269, 63.12390960531435979 ) ) ;
#141073=CARTESIAN_POINT ( 'NONE',  ( 0.05219959533936267826, -19.03943276465977164, 70.00109039468566152 ) ) ;
#141074=CARTESIAN_POINT ( 'NONE',  ( -9.564922557961040184, 16.46253265017147172, 42.91775706135234003 ) ) ;
#141075=CARTESIAN_POINT ( 'NONE',  ( 9.564922557960805705, 16.46253265017160317, 64.58224293864769550 ) ) ;
#141076=CARTESIAN_POINT ( 'NONE',  ( -10.72451020669898014, 18.67979575497178502, 75.41557627198102409 ) ) ;
#141077=CARTESIAN_POINT ( 'NONE',  ( 8.224510206698953496, -14.34966873604960469, 62.91557627198102409 ) ) ;
#141078=CARTESIAN_POINT ( 'NONE',  ( -9.564922557961040184, 16.46253265017147172, 32.91775706135233293 ) ) ;
#141079=CARTESIAN_POINT ( 'NONE',  ( -10.72451020669898014, 18.67979575497178502, 50.41557627198103120 ) ) ;
#141080=CARTESIAN_POINT ( 'NONE',  ( 0.05219959533907565091, 21.53943276465977519, 44.99890960531435979 ) ) ;
#141081=CARTESIAN_POINT ( 'NONE',  ( -16.51473224551069308, -9.474510206698971260, 71.66557627198102409 ) ) ;
#141082=CARTESIAN_POINT ( 'NONE',  ( -0.05219959533909027116, -19.03943276465977164, 42.49890960531435269 ) ) ;
#141083=CARTESIAN_POINT ( 'NONE',  ( 4.483927247898545687, 16.52544592524342804, 99.79057627198103830 ) ) ;
#141084=CARTESIAN_POINT ( 'NONE',  ( -21.55341960407610458, -5.719274019375992779, 106.4572429386477097 ) ) ;
#141086=CARTESIAN_POINT ( 'NONE',  ( -5.823673210054431948, 21.52544592524334988, 27.70942372801901854 ) ) ;
#141087=CARTESIAN_POINT ( 'NONE',  ( -5.153800228976328057, -19.02544592524343514, 32.29057627198102409 ) ) ;
#141088=CARTESIAN_POINT ( 'NONE',  ( -5.823673210054116645, -21.52544592524344225, 112.2905762719810241 ) ) ;
#141089=CARTESIAN_POINT ( 'NONE',  ( 19.05341960407617918, -5.049401038297876454, 51.04275706135231871 ) ) ;
#141090=CARTESIAN_POINT ( 'NONE',  ( 16.46253265017160672, -9.564922557960803928, 23.33224293864769194 ) ) ;
#141091=CARTESIAN_POINT ( 'NONE',  ( 9.474510206698971260, -16.51473224551069308, 27.91557627198103120 ) ) ;
#141092=CARTESIAN_POINT ( 'NONE',  ( 17.05217265608910537, -6.523264755457947928, 21.23078202051969399 ) ) ;
#141093=CARTESIAN_POINT ( 'NONE',  ( 14.29746914071037800, 8.314922557961029526, 51.66775706135234714 ) ) ;
#141094=CARTESIAN_POINT ( 'NONE',  ( -13.97604488694527625, -13.89961937509977652, 26.87390960531434558 ) ) ;
#141096=CARTESIAN_POINT ( 'NONE',  ( -9.564922557960796823, -16.46253265017161027, 77.08224293864769550 ) ) ;
#141097=CARTESIAN_POINT ( 'NONE',  ( 12.06949235617757843, -12.14591786802309237, 113.1239096053143953 ) ) ;
#141098=CARTESIAN_POINT ( 'NONE',  ( -5.719274019375978568, 21.55341960407610458, 50.20724293864769550 ) ) ;
#141099=CARTESIAN_POINT ( 'NONE',  ( 0.05219959533910956823, 16.53943276465976808, 84.99890960531436690 ) ) ;
#141100=CARTESIAN_POINT ( 'NONE',  ( 12.14591786802327356, -12.06949235617739191, 35.62609039468568994 ) ) ;
#141101=CARTESIAN_POINT ( 'NONE',  ( -18.67979575497193778, 10.72451020669871902, 83.33442372801903275 ) ) ;
#141102=CARTESIAN_POINT ( 'NONE',  ( -5.153800228976328057, -19.02544592524343514, 27.29057627198103120 ) ) ;
#141103=CARTESIAN_POINT ( 'NONE',  ( -12.14591786802326823, 12.06949235617739902, 108.1260903946856757 ) ) ;
#141104=CARTESIAN_POINT ( 'NONE',  ( 4.379528057220339221, -16.55341960407611168, 57.70724293864770260 ) ) ;
#141105=CARTESIAN_POINT ( 'NONE',  ( -5.153800228976328057, -19.02544592524343514, 57.29057627198103120 ) ) ;
#141106=CARTESIAN_POINT ( 'NONE',  ( 15.80617190586769283, -15.72974639402175789, 95.62609039468568994 ) ) ;
#141107=CARTESIAN_POINT ( 'NONE',  ( -15.80617190586745835, -15.72974639402198527, 111.8739096053143669 ) ) ;
#141108=CARTESIAN_POINT ( 'NONE',  ( 21.52544592524334988, 5.823673210054432836, 71.45942372801901854 ) ) ;
#141109=CARTESIAN_POINT ( 'NONE',  ( 0.05219959533934541429, -16.53943276465976808, 35.00109039468568284 ) ) ;
#141110=CARTESIAN_POINT ( 'NONE',  ( -4.483927247898539470, -16.52544592524342804, 82.29057627198103830 ) ) ;
#141111=CARTESIAN_POINT ( 'NONE',  ( -5.823673210054431948, 21.52544592524334988, 87.70942372801901854 ) ) ;
#141112=CARTESIAN_POINT ( 'NONE',  ( -16.52544592524342804, 4.483927247898546575, 26.04057627198103475 ) ) ;
#141114=CARTESIAN_POINT ( 'NONE',  ( 16.52544592524335698, 4.483927247898782831, 36.45942372801901143 ) ) ;
#141115=CARTESIAN_POINT ( 'NONE',  ( 8.314922557960818139, 14.29746914071049879, 39.58224293864769550 ) ) ;
#141116=CARTESIAN_POINT ( 'NONE',  ( 4.379528057220092307, 16.55341960407617563, 92.29275706135236135 ) ) ;
#141117=CARTESIAN_POINT ( 'NONE',  ( 0.05219959533909260263, 19.03943276465977164, 94.99890960531436690 ) ) ;
#141118=CARTESIAN_POINT ( 'NONE',  ( -13.89961937509977652, 13.97604488694528158, 95.62390960531436690 ) ) ;
#141119=CARTESIAN_POINT ( 'NONE',  ( 10.72451020669871369, 18.67979575497193778, 102.0844237280190185 ) ) ;
#141120=CARTESIAN_POINT ( 'NONE',  ( -4.379528057220086978, -16.55341960407618274, 99.79275706135234714 ) ) ;
#141121=CARTESIAN_POINT ( 'NONE',  ( -4.379528057220328563, 16.55341960407611168, 70.20724293864769550 ) ) ;
#141122=CARTESIAN_POINT ( 'NONE',  ( 13.89961937509977652, -13.97604488694527269, 78.12390960531433848 ) ) ;
#141124=CARTESIAN_POINT ( 'NONE',  ( -12.14591786802326823, 12.06949235617739902, 28.12609039468568284 ) ) ;
#141125=CARTESIAN_POINT ( 'NONE',  ( -9.474510206698964154, 16.51473224551069663, 30.41557627198102054 ) ) ;
#141126=CARTESIAN_POINT ( 'NONE',  ( 5.153800228976335163, 19.02544592524342804, 89.79057627198102409 ) ) ;
#141127=CARTESIAN_POINT ( 'NONE',  ( -8.224510206698735004, -14.34966873604973081, 29.58442372801901854 ) ) ;
#141129=CARTESIAN_POINT ( 'NONE',  ( 5.153800228976615827, -19.02544592524334988, 30.20942372801900433 ) ) ;
#141130=CARTESIAN_POINT ( 'NONE',  ( -8.224510206698735004, -14.34966873604973081, 94.58442372801901854 ) ) ;
#141131=CARTESIAN_POINT ( 'NONE',  ( 16.51473224551083163, -9.474510206698727899, 100.8344237280190043 ) ) ;
#141132=CARTESIAN_POINT ( 'NONE',  ( -19.05341960407611168, -5.049401038298163336, 36.45724293864766707 ) ) ;
#141133=CARTESIAN_POINT ( 'NONE',  ( -8.224510206698735004, -14.34966873604973081, 84.58442372801903275 ) ) ;
#141134=CARTESIAN_POINT ( 'NONE',  ( -4.483927247898782831, 16.52544592524335698, 67.70942372801901854 ) ) ;
#141136=CARTESIAN_POINT ( 'NONE',  ( 0.05219959533936267826, -19.03943276465977164, 75.00109039468566152 ) ) ;
#141137=CARTESIAN_POINT ( 'NONE',  ( 18.62759615963255655, 10.81492255796105972, 106.6677570613523756 ) ) ;
#141138=CARTESIAN_POINT ( 'NONE',  ( 9.474510206698971260, -16.51473224551069308, 47.91557627198102409 ) ) ;
#141139=CARTESIAN_POINT ( 'NONE',  ( 19.02544592524343514, -5.153800228976328945, 88.54057627198102409 ) ) ;
#141140=CARTESIAN_POINT ( 'NONE',  ( -16.55341960407611168, -4.379528057220339221, 86.45724293864770971 ) ) ;
#141141=EDGE_CURVE ( 'NONE', #146788, #82599, #184905, .T. ) ;
#141142=CARTESIAN_POINT ( 'NONE',  ( 16.46253265017146816, 9.564922557961045513, 56.66775706135233293 ) ) ;
#141143=CARTESIAN_POINT ( 'NONE',  ( -18.62759615963270932, 10.81492255796079327, 55.83224293864770260 ) ) ;
#141144=CARTESIAN_POINT ( 'NONE',  ( -10.72451020669870658, -18.67979575497194134, 109.5844237280190328 ) ) ;
#141145=CARTESIAN_POINT ( 'NONE',  ( -16.51473224551069308, -9.474510206698971260, 96.66557627198102409 ) ) ;
#141146=CARTESIAN_POINT ( 'NONE',  ( -19.05341960407617563, 5.049401038297882671, 23.54275706135233648 ) ) ;
#141147=CARTESIAN_POINT ( 'NONE',  ( 5.823673210054125526, 21.52544592524343514, 64.79057627198103830 ) ) ;
#141148=CARTESIAN_POINT ( 'NONE',  ( -18.22780087662119541, 5.500000000000102141, 56.01763182126894947 ) ) ;
#141150=CARTESIAN_POINT ( 'NONE',  ( -19.05341960407617563, 5.049401038297882671, 88.54275706135230450 ) ) ;
#141151=CARTESIAN_POINT ( 'NONE',  ( 13.97604488694527802, 13.89961937509977652, 114.3739096053143669 ) ) ;
#141152=CARTESIAN_POINT ( 'NONE',  ( -16.51473224551082808, 9.474510206698731452, 113.3344237280190043 ) ) ;
#141153=CARTESIAN_POINT ( 'NONE',  ( -12.06949235617756955, 12.14591786802309770, 110.6239096053143669 ) ) ;
#141154=CARTESIAN_POINT ( 'NONE',  ( -0.05219959533909027116, -19.03943276465977164, 102.4989096053143669 ) ) ;
#141155=CARTESIAN_POINT ( 'NONE',  ( -10.72451020669898014, 18.67979575497178502, 75.41557627198102409 ) ) ;
#141156=CARTESIAN_POINT ( 'NONE',  ( 8.314922557961029526, -14.29746914071037800, 45.41775706135234003 ) ) ;
#141157=CARTESIAN_POINT ( 'NONE',  ( -5.719274019375665041, -21.55341960407619695, 44.79275706135234714 ) ) ;
#141158=CARTESIAN_POINT ( 'NONE',  ( -15.80617190586768217, 15.72974639402176855, 103.1260903946856757 ) ) ;
#141159=CARTESIAN_POINT ( 'NONE',  ( 16.55341960407618274, -4.379528057220086978, 96.04275706135236135 ) ) ;
#141160=CARTESIAN_POINT ( 'NONE',  ( -13.97604488694527625, -13.89961937509977652, 86.87390960531436690 ) ) ;
#141161=CARTESIAN_POINT ( 'NONE',  ( -12.06949235617756955, 12.14591786802309770, 90.62390960531436690 ) ) ;
#141162=CARTESIAN_POINT ( 'NONE',  ( -8.314922557960811034, -14.29746914071050412, 37.08224293864768129 ) ) ;
#141163=CARTESIAN_POINT ( 'NONE',  ( 19.02544592524334988, 5.153800228976608722, 71.45942372801900433 ) ) ;
#141164=CARTESIAN_POINT ( 'NONE',  ( -18.62759615963255300, -10.81492255796106328, 49.16775706135234003 ) ) ;
#141165=CARTESIAN_POINT ( 'NONE',  ( -5.049401038297874678, -19.05341960407617918, 24.79275706135233648 ) ) ;
#141166=CARTESIAN_POINT ( 'NONE',  ( 8.314922557960818139, 14.29746914071049879, 89.58224293864768129 ) ) ;
#141167=CARTESIAN_POINT ( 'NONE',  ( -5.153800228976328057, -19.02544592524343514, 112.2905762719810099 ) ) ;
#141168=CARTESIAN_POINT ( 'NONE',  ( 8.224510206698953496, -14.34966873604960469, 22.91557627198102765 ) ) ;
#141169=CARTESIAN_POINT ( 'NONE',  ( -10.81492255796105439, 18.62759615963255655, 87.91775706135234714 ) ) ;
#141170=CARTESIAN_POINT ( 'NONE',  ( -14.34966873604972548, 8.224510206698743886, 63.33442372801900433 ) ) ;
#141171=CARTESIAN_POINT ( 'NONE',  ( -4.379528057220086978, -16.55341960407618274, 104.7927570613523898 ) ) ;
#141172=CARTESIAN_POINT ( 'NONE',  ( -18.67979575497193778, 10.72451020669871902, 48.33442372801902565 ) ) ;
#141173=CARTESIAN_POINT ( 'NONE',  ( -21.53943276465977519, -0.05219959533937600094, 33.75109039468568284 ) ) ;
#141174=CARTESIAN_POINT ( 'NONE',  ( -8.224510206698948167, 14.34966873604960824, 105.4155762719810383 ) ) ;
#141175=CARTESIAN_POINT ( 'NONE',  ( -19.05341960407611168, -5.049401038298163336, 21.45724293864768839 ) ) ;
#141176=CARTESIAN_POINT ( 'NONE',  ( 14.34966873604960469, 8.224510206698951720, 69.16557627198102409 ) ) ;
#141177=CARTESIAN_POINT ( 'NONE',  ( 5.049401038298161559, -19.05341960407611168, 77.70724293864765286 ) ) ;
#141178=CARTESIAN_POINT ( 'NONE',  ( 4.379528057220092307, 16.55341960407617563, 102.2927570613523613 ) ) ;
#141179=CARTESIAN_POINT ( 'NONE',  ( 13.89961937509977652, -13.97604488694527269, 43.12390960531434558 ) ) ;
#141180=CARTESIAN_POINT ( 'NONE',  ( 10.72451020669898902, -18.67979575497178502, 62.91557627198102409 ) ) ;
#141181=CARTESIAN_POINT ( 'NONE',  ( -8.224510206698948167, 14.34966873604960824, 95.41557627198102409 ) ) ;
#141183=CARTESIAN_POINT ( 'NONE',  ( 5.719274019375991003, -21.55341960407610458, 97.70724293864772392 ) ) ;
#141184=CARTESIAN_POINT ( 'NONE',  ( -16.46253265017160317, 9.564922557960807481, 95.83224293864769550 ) ) ;
#141185=CARTESIAN_POINT ( 'NONE',  ( 19.03943276465977164, -0.05219959533909143690, 48.74890960531435979 ) ) ;
#141186=CARTESIAN_POINT ( 'NONE',  ( 5.049401038297881783, 19.05341960407617563, 87.29275706135234714 ) ) ;
#141187=CARTESIAN_POINT ( 'NONE',  ( 5.719274019375991003, -21.55341960407610458, 47.70724293864770260 ) ) ;
#141188=CARTESIAN_POINT ( 'NONE',  ( 18.62759615963255655, 10.81492255796105972, 61.66775706135235424 ) ) ;
#141189=CARTESIAN_POINT ( 'NONE',  ( -13.97604488694527625, -13.89961937509977652, 46.87390960531435979 ) ) ;
#141190=CARTESIAN_POINT ( 'NONE',  ( -9.474510206698964154, 16.51473224551069663, 80.41557627198103830 ) ) ;
#141191=CARTESIAN_POINT ( 'NONE',  ( -16.52544592524335698, -4.483927247898792601, 68.95942372801901854 ) ) ;
#141192=CARTESIAN_POINT ( 'NONE',  ( -21.52544592524334988, -5.823673210054445271, 38.95942372801901854 ) ) ;
#141193=CARTESIAN_POINT ( 'NONE',  ( 21.52544592524334988, 5.823673210054432836, 86.45942372801901854 ) ) ;
#141194=CARTESIAN_POINT ( 'NONE',  ( 21.52544592524344225, -5.823673210054117533, 103.5405762719810383 ) ) ;
#141195=CARTESIAN_POINT ( 'NONE',  ( 10.72451020669871369, 18.67979575497193778, 32.08442372801901854 ) ) ;
#141196=CARTESIAN_POINT ( 'NONE',  ( -16.52544592524335698, -4.483927247898792601, 58.95942372801902565 ) ) ;
#141197=CARTESIAN_POINT ( 'NONE',  ( -15.80617190586745835, -15.72974639402198527, 81.87390960531435269 ) ) ;
#141198=CARTESIAN_POINT ( 'NONE',  ( -0.05219959533936034679, 19.03943276465977164, 32.50109039468566863 ) ) ;
#141199=CARTESIAN_POINT ( 'NONE',  ( -5.153800228976328057, -19.02544592524343514, 62.29057627198100988 ) ) ;
#141200=CARTESIAN_POINT ( 'NONE',  ( 14.29746914071037800, 8.314922557961029526, 111.6677570613523613 ) ) ;
#141202=CARTESIAN_POINT ( 'NONE',  ( -9.564922557960796823, -16.46253265017161027, 102.0822429386477097 ) ) ;
#141204=CARTESIAN_POINT ( 'NONE',  ( -16.46253265017146816, -9.564922557961047289, 84.16775706135233293 ) ) ;
#141205=CARTESIAN_POINT ( 'NONE',  ( -0.05219959533907301413, -21.53943276465977519, 57.49890960531435979 ) ) ;
#141206=CARTESIAN_POINT ( 'NONE',  ( 12.14591786802309770, 12.06949235617756955, 39.37390960531436690 ) ) ;
#141207=CARTESIAN_POINT ( 'NONE',  ( -16.52544592524335698, -4.483927247898792601, 23.95942372801901143 ) ) ;
#141208=CARTESIAN_POINT ( 'NONE',  ( 16.46253265017160672, -9.564922557960803928, 28.33224293864769550 ) ) ;
#141209=CARTESIAN_POINT ( 'NONE',  ( 19.03943276465977164, 0.05219959533936151252, 106.2510903946856615 ) ) ;
#141210=CARTESIAN_POINT ( 'NONE',  ( 0.05219959533907565091, 21.53943276465977519, 94.99890960531436690 ) ) ;
#141211=CARTESIAN_POINT ( 'NONE',  ( -9.564922557961040184, 16.46253265017147172, 67.91775706135233293 ) ) ;
#141212=CARTESIAN_POINT ( 'NONE',  ( 12.14591786802327356, -12.06949235617739191, 75.62609039468567573 ) ) ;
#141213=CARTESIAN_POINT ( 'NONE',  ( 19.05341960407611168, 5.049401038298154454, 63.95724293864769550 ) ) ;
#141214=CARTESIAN_POINT ( 'NONE',  ( -0.05219959533910754901, -16.53943276465976808, 72.49890960531435269 ) ) ;
#141215=CARTESIAN_POINT ( 'NONE',  ( 16.51473224551069308, 9.474510206698969483, 64.16557627198102409 ) ) ;
#141216=CARTESIAN_POINT ( 'NONE',  ( 4.379528057220339221, -16.55341960407611168, 67.70724293864769550 ) ) ;
#141218=CARTESIAN_POINT ( 'NONE',  ( -14.34966873604960291, -8.224510206698953496, 36.66557627198103120 ) ) ;
#141219=CARTESIAN_POINT ( 'NONE',  ( -16.46253265017160317, 9.564922557960807481, 70.83224293864770971 ) ) ;
#141221=CARTESIAN_POINT ( 'NONE',  ( 5.153800228976615827, -19.02544592524334988, 45.20942372801901143 ) ) ;
#141222=CARTESIAN_POINT ( 'NONE',  ( 16.55341960407618274, -4.379528057220086978, 51.04275706135234714 ) ) ;
#141223=CARTESIAN_POINT ( 'NONE',  ( -5.719274019375978568, 21.55341960407610458, 65.20724293864768129 ) ) ;
#141224=CARTESIAN_POINT ( 'NONE',  ( 13.89961937509957401, 13.97604488694547697, 21.87609039468566152 ) ) ;
#141225=CARTESIAN_POINT ( 'NONE',  ( 5.153800228976335163, 19.02544592524342804, 69.79057627198103830 ) ) ;
#141227=CARTESIAN_POINT ( 'NONE',  ( -5.049401038298153566, 19.05341960407611168, 105.2072429386476671 ) ) ;
#141228=CARTESIAN_POINT ( 'NONE',  ( -5.719274019375665041, -21.55341960407619695, 34.79275706135235424 ) ) ;
#141229=CARTESIAN_POINT ( 'NONE',  ( 14.29746914071049879, -8.314922557960816363, 113.3322429386476955 ) ) ;
#141230=CARTESIAN_POINT ( 'NONE',  ( -21.53943276465977519, 0.05219959533907696930, 101.2489096053143669 ) ) ;
#141231=CARTESIAN_POINT ( 'NONE',  ( -5.153800228976328057, -19.02544592524343514, 82.29057627198103830 ) ) ;
#141233=CARTESIAN_POINT ( 'NONE',  ( 10.81492255796106328, -18.62759615963255655, 30.41775706135234358 ) ) ;
#141234=VERTEX_POINT ( 'NONE', #147367 ) ;
#141235=CARTESIAN_POINT ( 'NONE',  ( -9.474510206698964154, 16.51473224551069663, 90.41557627198103830 ) ) ;
#141236=EDGE_CURVE ( 'NONE', #106384, #76130, #173356, .T. ) ;
#141239=CARTESIAN_POINT ( 'NONE',  ( 16.51473224551069308, 9.474510206698969483, 29.16557627198103475 ) ) ;
#141240=CARTESIAN_POINT ( 'NONE',  ( -9.474510206698720793, -16.51473224551083518, 104.5844237280190043 ) ) ;
#141242=CARTESIAN_POINT ( 'NONE',  ( -8.314922557960811034, -14.29746914071050412, 112.0822429386477097 ) ) ;
#141243=CARTESIAN_POINT ( 'NONE',  ( 0.05219959533937995610, -21.53943276465977519, 85.00109039468568994 ) ) ;
#141244=CARTESIAN_POINT ( 'NONE',  ( 5.153800228976335163, 19.02544592524342804, 74.79057627198103830 ) ) ;
#141245=CARTESIAN_POINT ( 'NONE',  ( 21.52544592524334988, 5.823673210054432836, 51.45942372801901854 ) ) ;
#141246=CARTESIAN_POINT ( 'NONE',  ( 21.52544592524334988, 5.823673210054432836, 31.45942372801901854 ) ) ;
#141248=CARTESIAN_POINT ( 'NONE',  ( -19.03943276465977164, 0.05219959533909376836, 91.24890960531436690 ) ) ;
#141250=CARTESIAN_POINT ( 'NONE',  ( 8.314922557961029526, -14.29746914071037800, 40.41775706135234714 ) ) ;
#141251=CARTESIAN_POINT ( 'NONE',  ( 18.67979575497178502, 10.72451020669898547, 39.16557627198102409 ) ) ;
#141252=CARTESIAN_POINT ( 'NONE',  ( -15.80617190586768217, 15.72974639402176855, 78.12609039468570415 ) ) ;
#141254=CARTESIAN_POINT ( 'NONE',  ( 16.51473224551083163, -9.474510206698727899, 105.8344237280190043 ) ) ;
#141255=CARTESIAN_POINT ( 'NONE',  ( -19.05341960407611168, -5.049401038298163336, 66.45724293864769550 ) ) ;
#141256=CARTESIAN_POINT ( 'NONE',  ( 19.02544592524343514, -5.153800228976328945, 78.54057627198099567 ) ) ;
#141257=CARTESIAN_POINT ( 'NONE',  ( -4.483927247898539470, -16.52544592524342804, 107.2905762719810525 ) ) ;
#141258=CARTESIAN_POINT ( 'NONE',  ( 16.55341960407611168, 4.379528057220329451, 103.9572429386476813 ) ) ;
#141259=CARTESIAN_POINT ( 'NONE',  ( -16.46253265017160317, 9.564922557960807481, 105.8322429386476955 ) ) ;
#141260=CARTESIAN_POINT ( 'NONE',  ( 8.224510206698742110, 14.34966873604972548, 82.08442372801901854 ) ) ;
#141261=CARTESIAN_POINT ( 'NONE',  ( -12.14591786802309592, -12.06949235617757132, 56.87390960531436690 ) ) ;
#141262=CARTESIAN_POINT ( 'NONE',  ( 5.049401038298161559, -19.05341960407611168, 52.70724293864767418 ) ) ;
#141263=CARTESIAN_POINT ( 'NONE',  ( 5.719274019375673035, 21.55341960407619339, 77.29275706135234714 ) ) ;
#141264=CARTESIAN_POINT ( 'NONE',  ( -5.719274019375665041, -21.55341960407619695, 64.79275706135234714 ) ) ;
#141265=CARTESIAN_POINT ( 'NONE',  ( 13.97604488694548053, -13.89961937509957401, 110.6260903946856615 ) ) ;
#141266=CARTESIAN_POINT ( 'NONE',  ( 16.53943276465976808, -0.05219959533910856209, 63.74890960531435979 ) ) ;
#141267=CARTESIAN_POINT ( 'NONE',  ( 5.719274019375991003, -21.55341960407610458, 107.7072429386476955 ) ) ;
#141268=CARTESIAN_POINT ( 'NONE',  ( 21.55341960407610458, 5.719274019375980345, 53.95724293864770260 ) ) ;
#141269=CARTESIAN_POINT ( 'NONE',  ( 18.56101223717333326, 5.499999999999950262, 73.94978406935678095 ) ) ;
#141271=CARTESIAN_POINT ( 'NONE',  ( -19.03943276465977164, 0.05219959533909376836, 76.24890960531435269 ) ) ;
#141272=CARTESIAN_POINT ( 'NONE',  ( 8.224510206698953496, -14.34966873604960469, 37.91557627198102409 ) ) ;
#141274=CARTESIAN_POINT ( 'NONE',  ( -0.05219959533910754901, -16.53943276465976808, 27.49890960531435269 ) ) ;
#141275=CARTESIAN_POINT ( 'NONE',  ( 14.34966873604972726, -8.224510206698740333, 90.83442372801901854 ) ) ;
#141276=CARTESIAN_POINT ( 'NONE',  ( -16.46253265017146816, -9.564922557961047289, 49.16775706135233293 ) ) ;
#141278=CARTESIAN_POINT ( 'NONE',  ( -13.97604488694527625, -13.89961937509977652, 86.87390960531436690 ) ) ;
#141279=CARTESIAN_POINT ( 'NONE',  ( -14.34966873604960291, -8.224510206698953496, 66.66557627198102409 ) ) ;
#141280=CARTESIAN_POINT ( 'NONE',  ( 17.44270441346516520, -5.991230190323024729, 101.1366492073577206 ) ) ;
#141281=CARTESIAN_POINT ( 'NONE',  ( -18.67979575497178146, -10.72451020669898902, 26.66557627198103475 ) ) ;
#141282=CARTESIAN_POINT ( 'NONE',  ( -15.80617190586745835, -15.72974639402198527, 51.87390960531437401 ) ) ;
#141283=ORIENTED_EDGE ( 'NONE', *, *, #130264, .T. ) ;
#141284=CARTESIAN_POINT ( 'NONE',  ( 14.34966873604960469, 8.224510206698951720, 94.16557627198103830 ) ) ;
#141285=CARTESIAN_POINT ( 'NONE',  ( -0.05219959533934338120, 16.53943276465976808, 52.50109039468567573 ) ) ;
#141286=CARTESIAN_POINT ( 'NONE',  ( -4.483927247898539470, -16.52544592524342804, 72.29057627198102409 ) ) ;
#141288=CARTESIAN_POINT ( 'NONE',  ( 9.474510206698729675, 16.51473224551082808, 82.08442372801899012 ) ) ;
#141289=CARTESIAN_POINT ( 'NONE',  ( -21.55341960407610458, -5.719274019375992779, 26.45724293864768839 ) ) ;
#141292=CARTESIAN_POINT ( 'NONE',  ( -4.483927247898782831, 16.52544592524335698, 42.70942372801901854 ) ) ;
#141293=CARTESIAN_POINT ( 'NONE',  ( 16.53943276465976808, -0.05219959533910856209, 28.74890960531435624 ) ) ;
#141294=CARTESIAN_POINT ( 'NONE',  ( 0.05219959533907565091, 21.53943276465977519, 54.99890960531435269 ) ) ;
#141295=CARTESIAN_POINT ( 'NONE',  ( 19.02544592524334988, 5.153800228976608722, 81.45942372801897591 ) ) ;
#141296=CARTESIAN_POINT ( 'NONE',  ( 21.53943276465977519, -0.05219959533907433946, 43.74890960531435979 ) ) ;
#141297=CARTESIAN_POINT ( 'NONE',  ( -21.52544592524334988, -5.823673210054445271, 78.95942372801901854 ) ) ;
#141299=CARTESIAN_POINT ( 'NONE',  ( 16.55341960407618274, -4.379528057220086978, 31.04275706135234714 ) ) ;
#141300=CARTESIAN_POINT ( 'NONE',  ( 9.474510206698971260, -16.51473224551069308, 37.91557627198102409 ) ) ;
#141301=CARTESIAN_POINT ( 'NONE',  ( -19.05341960407611168, -5.049401038298163336, 96.45724293864769550 ) ) ;
#141303=CARTESIAN_POINT ( 'NONE',  ( 16.51473224551069308, 9.474510206698969483, 39.16557627198103120 ) ) ;
#141304=CARTESIAN_POINT ( 'NONE',  ( -14.34966873604960291, -8.224510206698953496, 101.6655762719810383 ) ) ;
#141306=CARTESIAN_POINT ( 'NONE',  ( -16.51473224551069308, -9.474510206698971260, 106.6655762719810383 ) ) ;
#141307=VERTEX_POINT ( 'NONE', #65529 ) ;
#141308=CARTESIAN_POINT ( 'NONE',  ( 0.05219959533934541429, -16.53943276465976808, 50.00109039468568994 ) ) ;
#141309=CARTESIAN_POINT ( 'NONE',  ( -18.62759615963270932, 10.81492255796079327, 95.83224293864770971 ) ) ;
#141310=CARTESIAN_POINT ( 'NONE',  ( 19.05341960407611168, 5.049401038298154454, 43.95724293864769550 ) ) ;
#141311=CARTESIAN_POINT ( 'NONE',  ( -18.62759615963255300, -10.81492255796106328, 24.16775706135235424 ) ) ;
#141312=CARTESIAN_POINT ( 'NONE',  ( 9.474510206698971260, -16.51473224551069308, 87.91557627198102409 ) ) ;
#141315=CARTESIAN_POINT ( 'NONE',  ( -16.52544592524335698, -4.483927247898792601, 48.95942372801902565 ) ) ;
#141316=CARTESIAN_POINT ( 'NONE',  ( -15.72974639402176322, -15.80617190586768395, 19.37609039468568639 ) ) ;
#141317=CARTESIAN_POINT ( 'NONE',  ( -4.483927247898539470, -16.52544592524342804, 107.2905762719810525 ) ) ;
#141318=CARTESIAN_POINT ( 'NONE',  ( 9.564922557960805705, 16.46253265017160317, 94.58224293864769550 ) ) ;
#141319=CARTESIAN_POINT ( 'NONE',  ( -19.02544592524334988, -5.153800228976617603, 68.95942372801896170 ) ) ;
#141320=CARTESIAN_POINT ( 'NONE',  ( 19.03943276465977164, 0.05219959533936151252, 31.25109039468566863 ) ) ;
#141321=CARTESIAN_POINT ( 'NONE',  ( -21.53943276465977519, 0.05219959533907696930, 91.24890960531436690 ) ) ;
#141322=CARTESIAN_POINT ( 'NONE',  ( -16.46253265017146816, -9.564922557961047289, 19.16775706135233293 ) ) ;
#141323=CARTESIAN_POINT ( 'NONE',  ( 0.05219959533934541429, -16.53943276465976808, 80.00109039468568994 ) ) ;
#141324=CARTESIAN_POINT ( 'NONE',  ( 13.89961937509977652, -13.97604488694527269, 108.1239096053143669 ) ) ;
#141325=CARTESIAN_POINT ( 'NONE',  ( -19.03943276465977164, 0.05219959533909376836, 61.24890960531436690 ) ) ;
#141327=CARTESIAN_POINT ( 'NONE',  ( 10.81492255796106328, -18.62759615963255655, 65.41775706135234714 ) ) ;
#141328=CARTESIAN_POINT ( 'NONE',  ( -18.62759615963255300, -10.81492255796106328, 64.16775706135234714 ) ) ;
#141329=CARTESIAN_POINT ( 'NONE',  ( -9.474510206698964154, 16.51473224551069663, 70.41557627198102409 ) ) ;
#141330=CARTESIAN_POINT ( 'NONE',  ( 10.81492255796106328, -18.62759615963255655, 55.41775706135234714 ) ) ;
#141331=ORIENTED_EDGE ( 'NONE', *, *, #53585, .T. ) ;
#141332=CARTESIAN_POINT ( 'NONE',  ( -0.05219959533936034679, 19.03943276465977164, 87.50109039468567573 ) ) ;
#141334=CARTESIAN_POINT ( 'NONE',  ( -9.474510206698964154, 16.51473224551069663, 55.41557627198103120 ) ) ;
#141335=CARTESIAN_POINT ( 'NONE',  ( 5.153800228976335163, 19.02544592524342804, 94.79057627198103830 ) ) ;
#141336=CARTESIAN_POINT ( 'NONE',  ( 9.474510206698971260, -16.51473224551069308, 62.91557627198102409 ) ) ;
#141337=CARTESIAN_POINT ( 'NONE',  ( 19.03943276465977164, -0.05219959533909143690, 113.7489096053143669 ) ) ;
#141338=CARTESIAN_POINT ( 'NONE',  ( -9.474510206698964154, 16.51473224551069663, 55.41557627198103120 ) ) ;
#141339=CARTESIAN_POINT ( 'NONE',  ( -5.823673210054116645, -21.52544592524344225, 82.29057627198103830 ) ) ;
#141340=CARTESIAN_POINT ( 'NONE',  ( -4.379528057220086978, -16.55341960407618274, 69.79275706135234714 ) ) ;
#141342=CARTESIAN_POINT ( 'NONE',  ( 19.02544592524334988, 5.153800228976608722, 26.45942372801899722 ) ) ;
#141343=CARTESIAN_POINT ( 'NONE',  ( 0.05219959533909260263, 19.03943276465977164, 64.99890960531436690 ) ) ;
#141344=CARTESIAN_POINT ( 'NONE',  ( 0.05219959533910956823, 16.53943276465976808, 59.99890960531436690 ) ) ;
#141345=CARTESIAN_POINT ( 'NONE',  ( 0.05219959533910956823, 16.53943276465976808, 94.99890960531436690 ) ) ;
#141346=CARTESIAN_POINT ( 'NONE',  ( -13.97604488694527625, -13.89961937509977652, 96.87390960531433848 ) ) ;
#141347=CARTESIAN_POINT ( 'NONE',  ( -19.05341960407611168, -5.049401038298163336, 91.45724293864766707 ) ) ;
#141348=CARTESIAN_POINT ( 'NONE',  ( 5.823673210054444382, -21.52544592524334988, 45.20942372801901854 ) ) ;
#141349=CARTESIAN_POINT ( 'NONE',  ( 5.049401038298161559, -19.05341960407611168, 107.7072429386476955 ) ) ;
#141350=CARTESIAN_POINT ( 'NONE',  ( -0.05219959533937732626, 21.53943276465977519, 112.5010903946857042 ) ) ;
#141351=CARTESIAN_POINT ( 'NONE',  ( 14.29746914071037800, 8.314922557961029526, 81.66775706135236135 ) ) ;
#141352=CARTESIAN_POINT ( 'NONE',  ( 15.80617190586769283, -15.72974639402175789, 35.62609039468568994 ) ) ;
#141353=CARTESIAN_POINT ( 'NONE',  ( -15.72974639402197994, 15.80617190586746368, 30.62390960531436335 ) ) ;
#141354=CARTESIAN_POINT ( 'NONE',  ( 15.72974639402199770, -15.80617190586745480, 98.12390960531436690 ) ) ;
#141355=CARTESIAN_POINT ( 'NONE',  ( -16.53943276465976808, 0.05219959533911058130, 66.24890960531436690 ) ) ;
#141356=CARTESIAN_POINT ( 'NONE',  ( -19.05341960407611168, -5.049401038298163336, 61.45724293864769550 ) ) ;
#141357=CARTESIAN_POINT ( 'NONE',  ( 8.314922557960818139, 14.29746914071049879, 79.58224293864769550 ) ) ;
#141358=CARTESIAN_POINT ( 'NONE',  ( 0.05219959533907565091, 21.53943276465977519, 49.99890960531437401 ) ) ;
#141359=CARTESIAN_POINT ( 'NONE',  ( -13.97604488694547697, 13.89961937509957934, 48.12609039468566863 ) ) ;
#141360=CARTESIAN_POINT ( 'NONE',  ( -16.52544592524342804, 4.483927247898546575, 111.0405762719810525 ) ) ;
#141362=CARTESIAN_POINT ( 'NONE',  ( 12.14591786802327356, -12.06949235617739191, 70.62609039468567573 ) ) ;
#141363=CARTESIAN_POINT ( 'NONE',  ( -5.153800228976328057, -19.02544592524343514, 72.29057627198102409 ) ) ;
#141365=CARTESIAN_POINT ( 'NONE',  ( 16.55341960407611168, 4.379528057220329451, 93.95724293864770971 ) ) ;
#141366=CARTESIAN_POINT ( 'NONE',  ( 18.67979575497178502, 10.72451020669898547, 39.16557627198102409 ) ) ;
#141368=CARTESIAN_POINT ( 'NONE',  ( -16.53943276465976808, -0.05219959533934237506, 103.7510903946857042 ) ) ;
#141369=CARTESIAN_POINT ( 'NONE',  ( 5.153800228976615827, -19.02544592524334988, 105.2094237280190185 ) ) ;
#141370=CARTESIAN_POINT ( 'NONE',  ( -18.62759615963255300, -10.81492255796106328, 84.16775706135234714 ) ) ;
#141371=CARTESIAN_POINT ( 'NONE',  ( -0.05219959533909027116, -19.03943276465977164, 92.49890960531436690 ) ) ;
#141372=CARTESIAN_POINT ( 'NONE',  ( -10.72451020669898014, 18.67979575497178502, 100.4155762719810241 ) ) ;
#141373=CARTESIAN_POINT ( 'NONE',  ( 16.52544592524335698, 4.483927247898782831, 56.45942372801902565 ) ) ;
#141374=CARTESIAN_POINT ( 'NONE',  ( 13.97604488694527802, 13.89961937509977652, 29.37390960531435979 ) ) ;
#141375=CARTESIAN_POINT ( 'NONE',  ( 14.29746914071037800, 8.314922557961029526, 36.66775706135234714 ) ) ;
#141376=CARTESIAN_POINT ( 'NONE',  ( -5.049401038297874678, -19.05341960407617918, 99.79275706135234714 ) ) ;
#141377=CARTESIAN_POINT ( 'NONE',  ( -0.05219959533907301413, -21.53943276465977519, 92.49890960531436690 ) ) ;
#141378=CARTESIAN_POINT ( 'NONE',  ( -13.97604488694547697, 13.89961937509957934, 48.12609039468566863 ) ) ;
#141379=LINE ( 'NONE', #3848, #109118 ) ;
#141380=CARTESIAN_POINT ( 'NONE',  ( 18.62759615963271287, -10.81492255796078972, 108.3322429386477097 ) ) ;
#141381=CARTESIAN_POINT ( 'NONE',  ( -18.22780087662123094, -5.499999999999984901, 71.48459894673891313 ) ) ;
#141382=CARTESIAN_POINT ( 'NONE',  ( 9.564922557960805705, 16.46253265017160317, 74.58224293864769550 ) ) ;
#141383=CARTESIAN_POINT ( 'NONE',  ( -12.14591786802326823, 12.06949235617739902, 38.12609039468567573 ) ) ;
#141385=CARTESIAN_POINT ( 'NONE',  ( 13.97604488694548053, -13.89961937509957401, 55.62609039468566863 ) ) ;
#141386=CARTESIAN_POINT ( 'NONE',  ( 21.53943276465977519, -0.05219959533907433946, 113.7489096053143527 ) ) ;
#141387=CARTESIAN_POINT ( 'NONE',  ( 0.05219959533910956823, 16.53943276465976808, 64.99890960531435269 ) ) ;
#141388=CARTESIAN_POINT ( 'NONE',  ( -19.02544592524342804, 5.153800228976336051, 71.04057627198099567 ) ) ;
#141389=CARTESIAN_POINT ( 'NONE',  ( 0.05219959533934541429, -16.53943276465976808, 35.00109039468568284 ) ) ;
#141390=CARTESIAN_POINT ( 'NONE',  ( -0.05219959533936034679, 19.03943276465977164, 42.50109039468566152 ) ) ;
#141391=CARTESIAN_POINT ( 'NONE',  ( -18.62759615963255300, -10.81492255796106328, 49.16775706135234003 ) ) ;
#141392=CARTESIAN_POINT ( 'NONE',  ( 19.02544592524334988, 5.153800228976608722, 111.4594237280190043 ) ) ;
#141393=CARTESIAN_POINT ( 'NONE',  ( 19.02544592524343514, -5.153800228976328945, 58.54057627198102409 ) ) ;
#141394=CARTESIAN_POINT ( 'NONE',  ( 19.05341960407617918, -5.049401038297876454, 76.04275706135230450 ) ) ;
#141395=CARTESIAN_POINT ( 'NONE',  ( -10.81492255796105439, 18.62759615963255655, 92.91775706135236135 ) ) ;
#141396=CARTESIAN_POINT ( 'NONE',  ( 16.51473224551083163, -9.474510206698727899, 70.83442372801900433 ) ) ;
#141397=CARTESIAN_POINT ( 'NONE',  ( 19.05341960407611168, 5.049401038298154454, 38.95724293864767418 ) ) ;
#141398=CARTESIAN_POINT ( 'NONE',  ( 0.05219959533907565091, 21.53943276465977519, 74.99890960531435269 ) ) ;
#141399=CARTESIAN_POINT ( 'NONE',  ( -16.52544592524342804, 4.483927247898546575, 66.04057627198103830 ) ) ;
#141400=CARTESIAN_POINT ( 'NONE',  ( 5.049401038297881783, 19.05341960407617563, 67.29275706135234714 ) ) ;
#141401=CARTESIAN_POINT ( 'NONE',  ( -16.62475595723697097, -7.163666690055194408, 24.47286648189534830 ) ) ;
#141402=CARTESIAN_POINT ( 'NONE',  ( 19.05341960407617918, -5.049401038297876454, 36.04275706135234003 ) ) ;
#141403=CARTESIAN_POINT ( 'NONE',  ( -12.06949235617739369, -12.14591786802326823, 94.37609039468568994 ) ) ;
#141404=CARTESIAN_POINT ( 'NONE',  ( -16.53943276465976808, 0.05219959533911058130, 51.24890960531436690 ) ) ;
#141405=CARTESIAN_POINT ( 'NONE',  ( -21.53943276465977519, -0.05219959533937600094, 83.75109039468568994 ) ) ;
#141407=CARTESIAN_POINT ( 'NONE',  ( -15.72974639402197994, 15.80617190586746368, 95.62390960531436690 ) ) ;
#141408=CARTESIAN_POINT ( 'NONE',  ( 5.049401038298161559, -19.05341960407611168, 47.70724293864770260 ) ) ;
#141409=CARTESIAN_POINT ( 'NONE',  ( 5.719274019375673035, 21.55341960407619339, 67.29275706135234714 ) ) ;
#141410=CARTESIAN_POINT ( 'NONE',  ( 16.46253265017160672, -9.564922557960803928, 43.33224293864769550 ) ) ;
#141412=CARTESIAN_POINT ( 'NONE',  ( 19.02544592524343514, -5.153800228976328945, 63.54057627198103830 ) ) ;
#141413=CARTESIAN_POINT ( 'NONE',  ( 8.314922557960818139, 14.29746914071049879, 99.58224293864770971 ) ) ;
#141414=CARTESIAN_POINT ( 'NONE',  ( 13.89961937509977652, -13.97604488694527269, 113.1239096053143527 ) ) ;
#141415=CARTESIAN_POINT ( 'NONE',  ( -8.314922557960811034, -14.29746914071050412, 57.08224293864769550 ) ) ;
#141416=CARTESIAN_POINT ( 'NONE',  ( 19.02544592524343514, -5.153800228976328945, 33.54057627198102409 ) ) ;
#141417=CARTESIAN_POINT ( 'NONE',  ( 14.34966873604960469, 8.224510206698951720, 89.16557627198102409 ) ) ;
#141419=CARTESIAN_POINT ( 'NONE',  ( 10.72451020669898902, -18.67979575497178502, 97.91557627198103830 ) ) ;
#141420=CARTESIAN_POINT ( 'NONE',  ( -21.53943276465977519, -0.05219959533937600094, 33.75109039468568284 ) ) ;
#141422=CARTESIAN_POINT ( 'NONE',  ( -4.379528057220086978, -16.55341960407618274, 49.79275706135234714 ) ) ;
#141423=CARTESIAN_POINT ( 'NONE',  ( 10.72451020669898902, -18.67979575497178502, 87.91557627198103830 ) ) ;
#141425=CARTESIAN_POINT ( 'NONE',  ( -19.02544592524334988, -5.153800228976617603, 18.95942372801899722 ) ) ;
#141426=CARTESIAN_POINT ( 'NONE',  ( -13.89961937509977652, 13.97604488694528158, 105.6239096053143527 ) ) ;
#141427=CARTESIAN_POINT ( 'NONE',  ( 21.53943276465977519, 0.05219959533937863772, 46.25109039468567573 ) ) ;
#141428=CARTESIAN_POINT ( 'NONE',  ( 21.55341960407610458, 5.719274019375980345, 33.95724293864769550 ) ) ;
#141429=CARTESIAN_POINT ( 'NONE',  ( -16.53943276465976808, -0.05219959533934237506, 108.7510903946857042 ) ) ;
#141430=CARTESIAN_POINT ( 'NONE',  ( 0.05219959533937995610, -21.53943276465977519, 65.00109039468568994 ) ) ;
#141431=CARTESIAN_POINT ( 'NONE',  ( -18.62759615963255300, -10.81492255796106328, 89.16775706135236135 ) ) ;
#141432=CARTESIAN_POINT ( 'NONE',  ( 13.89961937509957401, 13.97604488694547697, 36.87609039468565442 ) ) ;
#141433=CARTESIAN_POINT ( 'NONE',  ( -12.14591786802326823, 12.06949235617739902, 88.12609039468570415 ) ) ;
#141434=CARTESIAN_POINT ( 'NONE',  ( 5.823673210054444382, -21.52544592524334988, 35.20942372801901854 ) ) ;
#141435=CARTESIAN_POINT ( 'NONE',  ( 9.564922557960805705, 16.46253265017160317, 44.58224293864769550 ) ) ;
#141436=CARTESIAN_POINT ( 'NONE',  ( -18.67979575497193778, 10.72451020669871902, 103.3344237280190043 ) ) ;
#141437=CARTESIAN_POINT ( 'NONE',  ( -5.823673210054116645, -21.52544592524344225, 22.29057627198102765 ) ) ;
#141438=CARTESIAN_POINT ( 'NONE',  ( 18.67979575497194134, -10.72451020669871369, 20.83442372801901143 ) ) ;
#141439=CARTESIAN_POINT ( 'NONE',  ( 5.823673210054125526, 21.52544592524343514, 79.79057627198102409 ) ) ;
#141441=CARTESIAN_POINT ( 'NONE',  ( 10.72451020669898902, -18.67979575497178502, 72.91557627198103830 ) ) ;
#141442=CARTESIAN_POINT ( 'NONE',  ( -8.224510206698735004, -14.34966873604973081, 54.58442372801901143 ) ) ;
#141443=CARTESIAN_POINT ( 'NONE',  ( 16.52544592524342804, -4.483927247898539470, 58.54057627198103120 ) ) ;
#141445=CARTESIAN_POINT ( 'NONE',  ( 16.46253265017146816, 9.564922557961045513, 91.66775706135234714 ) ) ;
#141448=EDGE_CURVE ( 'NONE', #133123, #126008, #120355, .T. ) ;
#141449=CARTESIAN_POINT ( 'NONE',  ( -12.14591786802326823, 12.06949235617739902, 23.12609039468567573 ) ) ;
#141450=CARTESIAN_POINT ( 'NONE',  ( 21.53943276465977519, -0.05219959533907433946, 98.74890960531438111 ) ) ;
#141451=CARTESIAN_POINT ( 'NONE',  ( 21.52544592524344225, -5.823673210054117533, 73.54057627198102409 ) ) ;
#141452=CARTESIAN_POINT ( 'NONE',  ( 15.72974639402199770, -15.80617190586745480, 23.12390960531436335 ) ) ;
#141453=CARTESIAN_POINT ( 'NONE',  ( -14.34966873604972548, 8.224510206698743886, 63.33442372801900433 ) ) ;
#141454=CARTESIAN_POINT ( 'NONE',  ( 19.03943276465977164, -0.05219959533909143690, 68.74890960531436690 ) ) ;
#141455=CARTESIAN_POINT ( 'NONE',  ( -21.55341960407619339, 5.719274019375674811, 38.54275706135234714 ) ) ;
#141456=CARTESIAN_POINT ( 'NONE',  ( -8.224510206698735004, -14.34966873604973081, 19.58442372801901143 ) ) ;
#141457=CARTESIAN_POINT ( 'NONE',  ( 9.474510206698971260, -16.51473224551069308, 102.9155762719810241 ) ) ;
#141458=CARTESIAN_POINT ( 'NONE',  ( 0.05219959533936267826, -19.03943276465977164, 25.00109039468566152 ) ) ;
#141460=CARTESIAN_POINT ( 'NONE',  ( -16.46253265017160317, 9.564922557960807481, 95.83224293864769550 ) ) ;
#141461=CARTESIAN_POINT ( 'NONE',  ( 15.72974639402199770, -15.80617190586745480, 108.1239096053143811 ) ) ;
#141462=CARTESIAN_POINT ( 'NONE',  ( 5.153800228976335163, 19.02544592524342804, 54.79057627198103120 ) ) ;
#141463=CARTESIAN_POINT ( 'NONE',  ( -16.31925111598458855, 7.325300261831456439, 25.16424538967252644 ) ) ;
#141464=CARTESIAN_POINT ( 'NONE',  ( -14.34966873604960291, -8.224510206698953496, 81.66557627198103830 ) ) ;
#141465=CARTESIAN_POINT ( 'NONE',  ( -5.823673210054116645, -21.52544592524344225, 22.29057627198102765 ) ) ;
#141466=CARTESIAN_POINT ( 'NONE',  ( -16.19135201231370047, 7.376712067591781441, 34.81319145947970384 ) ) ;
#141467=CARTESIAN_POINT ( 'NONE',  ( -15.72974639402197994, 15.80617190586746368, 105.6239096053143669 ) ) ;
#141468=CARTESIAN_POINT ( 'NONE',  ( 5.153800228976615827, -19.02544592524334988, 65.20942372801900433 ) ) ;
#141469=CARTESIAN_POINT ( 'NONE',  ( -21.55341960407610458, -5.719274019375992779, 21.45724293864769550 ) ) ;
#141470=CARTESIAN_POINT ( 'NONE',  ( -16.51473224551069308, -9.474510206698971260, 26.66557627198103120 ) ) ;
#141471=CARTESIAN_POINT ( 'NONE',  ( 5.719274019375991003, -21.55341960407610458, 52.70724293864769550 ) ) ;
#141472=CARTESIAN_POINT ( 'NONE',  ( -13.89961937509977652, 13.97604488694528158, 95.62390960531436690 ) ) ;
#141473=CARTESIAN_POINT ( 'NONE',  ( -0.05219959533937732626, 21.53943276465977519, 72.50109039468568994 ) ) ;
#141474=CARTESIAN_POINT ( 'NONE',  ( 13.89961937509977652, -13.97604488694527269, 48.12390960531435979 ) ) ;
#141475=CARTESIAN_POINT ( 'NONE',  ( -4.379528057220328563, 16.55341960407611168, 90.20724293864770971 ) ) ;
#141476=CARTESIAN_POINT ( 'NONE',  ( 16.52544592524335698, 4.483927247898782831, 41.45942372801901143 ) ) ;
#141477=CARTESIAN_POINT ( 'NONE',  ( 21.52544592524334988, 5.823673210054432836, 61.45942372801901854 ) ) ;
#141479=CARTESIAN_POINT ( 'NONE',  ( -19.05341960407617563, 5.049401038297882671, 28.54275706135232937 ) ) ;
#141480=CARTESIAN_POINT ( 'NONE',  ( 5.153800228976615827, -19.02544592524334988, 85.20942372801900433 ) ) ;
#141482=CARTESIAN_POINT ( 'NONE',  ( -16.51473224551082808, 9.474510206698731452, 38.33442372801899722 ) ) ;
#141483=CARTESIAN_POINT ( 'NONE',  ( -17.97214573761834799, -5.500000000000021316, 91.46970049038660022 ) ) ;
#141484=CARTESIAN_POINT ( 'NONE',  ( -5.719274019375665041, -21.55341960407619695, 34.79275706135235424 ) ) ;
#141486=CARTESIAN_POINT ( 'NONE',  ( -19.03943276465977164, -0.05219959533935918106, 38.75109039468566152 ) ) ;
#141487=CARTESIAN_POINT ( 'NONE',  ( -5.049401038298153566, 19.05341960407611168, 75.20724293864769550 ) ) ;
#141488=CARTESIAN_POINT ( 'NONE',  ( 8.314922557960818139, 14.29746914071049879, 24.58224293864768839 ) ) ;
#141489=CARTESIAN_POINT ( 'NONE',  ( 16.51473224551069308, 9.474510206698969483, 114.1655762719810241 ) ) ;
#141490=CARTESIAN_POINT ( 'NONE',  ( -21.52544592524334988, -5.823673210054445271, 88.95942372801901854 ) ) ;
#141492=DIRECTION ( 'NONE',  ( 1.000000000000000000, -0.000000000000000000, -0.000000000000000000 ) ) ;
#141493=CARTESIAN_POINT ( 'NONE',  ( -18.62759615963255300, -10.81492255796106328, 84.16775706135234714 ) ) ;
#141495=CARTESIAN_POINT ( 'NONE',  ( 5.049401038298161559, -19.05341960407611168, 97.70724293864766707 ) ) ;
#141497=CARTESIAN_POINT ( 'NONE',  ( 19.05341960407611168, 5.049401038298154454, 48.95724293864768129 ) ) ;
#141498=CARTESIAN_POINT ( 'NONE',  ( 18.67979575497178502, 10.72451020669898547, 54.16557627198103120 ) ) ;
#141499=CARTESIAN_POINT ( 'NONE',  ( 14.34966873604960469, 8.224510206698951720, 29.16557627198103120 ) ) ;
#141500=CARTESIAN_POINT ( 'NONE',  ( 8.314922557960818139, 14.29746914071049879, 114.5822429386477097 ) ) ;
#141501=CARTESIAN_POINT ( 'NONE',  ( 19.05341960407611168, 5.049401038298154454, 88.95724293864769550 ) ) ;
#141502=CARTESIAN_POINT ( 'NONE',  ( -5.049401038297874678, -19.05341960407617918, 19.79275706135233293 ) ) ;
#141503=CARTESIAN_POINT ( 'NONE',  ( -16.55341960407611168, -4.379528057220339221, 101.4572429386476955 ) ) ;
#141504=CARTESIAN_POINT ( 'NONE',  ( 21.52544592524334988, 5.823673210054432836, 51.45942372801901854 ) ) ;
#141505=CARTESIAN_POINT ( 'NONE',  ( -16.46253265017160317, 9.564922557960807481, 115.8322429386477097 ) ) ;
#141506=CARTESIAN_POINT ( 'NONE',  ( 14.29746914071037800, 8.314922557961029526, 101.6677570613523613 ) ) ;
#141507=CARTESIAN_POINT ( 'NONE',  ( 5.153800228976615827, -19.02544592524334988, 60.20942372801899012 ) ) ;
#141509=CARTESIAN_POINT ( 'NONE',  ( 9.564922557960805705, 16.46253265017160317, 114.5822429386476955 ) ) ;
#141510=CARTESIAN_POINT ( 'NONE',  ( 14.29746914071049879, -8.314922557960816363, 78.33224293864770971 ) ) ;
#141511=CARTESIAN_POINT ( 'NONE',  ( -19.03943276465977164, -0.05219959533935918106, 63.75109039468566863 ) ) ;
#141512=CARTESIAN_POINT ( 'NONE',  ( -19.05341960407611168, -5.049401038298163336, 66.45724293864769550 ) ) ;
#141513=CARTESIAN_POINT ( 'NONE',  ( -16.55341960407611168, -4.379528057220339221, 66.45724293864768129 ) ) ;
#141514=CARTESIAN_POINT ( 'NONE',  ( -19.05341960407617563, 5.049401038297882671, 98.54275706135233293 ) ) ;
#141515=CARTESIAN_POINT ( 'NONE',  ( -21.52544592524343514, 5.823673210054127303, 56.04057627198102409 ) ) ;
#141517=CARTESIAN_POINT ( 'NONE',  ( -14.34966873604960291, -8.224510206698953496, 101.6655762719810383 ) ) ;
#141518=CARTESIAN_POINT ( 'NONE',  ( -16.29526858892880625, -7.335722546920006693, 30.79670597800208398 ) ) ;
#141519=CARTESIAN_POINT ( 'NONE',  ( -19.02544592524342804, 5.153800228976336051, 56.04057627198100988 ) ) ;
#141520=CARTESIAN_POINT ( 'NONE',  ( 18.62759615963271287, -10.81492255796078972, 63.33224293864770260 ) ) ;
#141521=CARTESIAN_POINT ( 'NONE',  ( -12.14591786802326823, 12.06949235617739902, 98.12609039468570415 ) ) ;
#141522=CARTESIAN_POINT ( 'NONE',  ( -0.05219959533909027116, -19.03943276465977164, 72.49890960531435269 ) ) ;
#141523=CARTESIAN_POINT ( 'NONE',  ( 9.564922557961047289, -16.46253265017146816, 55.41775706135234003 ) ) ;
#141524=CARTESIAN_POINT ( 'NONE',  ( 21.55341960407619695, -5.719274019375665929, 81.04275706135236135 ) ) ;
#141525=CARTESIAN_POINT ( 'NONE',  ( 15.72974639402199770, -15.80617190586745480, 58.12390960531435979 ) ) ;
#141526=CARTESIAN_POINT ( 'NONE',  ( -19.05341960407611168, -5.049401038298163336, 101.4572429386476955 ) ) ;
#141527=CARTESIAN_POINT ( 'NONE',  ( 13.97604488694527802, 13.89961937509977652, 34.37390960531436690 ) ) ;
#141528=CARTESIAN_POINT ( 'NONE',  ( 12.06949235617739724, 12.14591786802326823, 91.87609039468568994 ) ) ;
#141529=CARTESIAN_POINT ( 'NONE',  ( 12.14591786802327356, -12.06949235617739191, 20.62609039468568639 ) ) ;
#141531=CARTESIAN_POINT ( 'NONE',  ( 18.22780087662119897, -5.500000000000096811, 43.51763182126894236 ) ) ;
#141532=CARTESIAN_POINT ( 'NONE',  ( 5.719274019375673035, 21.55341960407619339, 92.29275706135236135 ) ) ;
#141533=CARTESIAN_POINT ( 'NONE',  ( 12.14591786802309770, 12.06949235617756955, 64.37390960531435269 ) ) ;
#141534=CARTESIAN_POINT ( 'NONE',  ( 8.314922557960818139, 14.29746914071049879, 74.58224293864768129 ) ) ;
#141535=CARTESIAN_POINT ( 'NONE',  ( -15.72974639402197994, 15.80617190586746368, 95.62390960531436690 ) ) ;
#141536=CARTESIAN_POINT ( 'NONE',  ( 21.53943276465977519, -0.05219959533907433946, 93.74890960531436690 ) ) ;
#141538=CARTESIAN_POINT ( 'NONE',  ( -18.62759615963270932, 10.81492255796079327, 50.83224293864770971 ) ) ;
#141539=CARTESIAN_POINT ( 'NONE',  ( 16.52544592524335698, 4.483927247898782831, 61.45942372801901854 ) ) ;
#141540=CARTESIAN_POINT ( 'NONE',  ( 16.55341960407611168, 4.379528057220329451, 93.95724293864770971 ) ) ;
#141541=CARTESIAN_POINT ( 'NONE',  ( 13.89961937509977652, -13.97604488694527269, 48.12390960531435979 ) ) ;
#141543=CARTESIAN_POINT ( 'NONE',  ( -12.14591786802326823, 12.06949235617739902, 93.12609039468568994 ) ) ;
#141544=CARTESIAN_POINT ( 'NONE',  ( 10.72451020669871369, 18.67979575497193778, 37.08442372801901143 ) ) ;
#141545=CARTESIAN_POINT ( 'NONE',  ( -13.89961937509977652, 13.97604488694528158, 80.62390960531436690 ) ) ;
#141546=CARTESIAN_POINT ( 'NONE',  ( -15.80617190586768217, 15.72974639402176855, 73.12609039468567573 ) ) ;
#141548=CARTESIAN_POINT ( 'NONE',  ( -13.97604488694527625, -13.89961937509977652, 21.87390960531435979 ) ) ;
#141550=CARTESIAN_POINT ( 'NONE',  ( 10.72451020669871369, 18.67979575497193778, 62.08442372801901143 ) ) ;
#141551=CARTESIAN_POINT ( 'NONE',  ( -5.153800228976328057, -19.02544592524343514, 32.29057627198102409 ) ) ;
#141552=CARTESIAN_POINT ( 'NONE',  ( 13.89961937509977652, -13.97604488694527269, 113.1239096053143527 ) ) ;
#141553=CARTESIAN_POINT ( 'NONE',  ( -13.89961937509977652, 13.97604488694528158, 90.62390960531432427 ) ) ;
#141554=CARTESIAN_POINT ( 'NONE',  ( -19.05341960407617563, 5.049401038297882671, 63.54275706135234003 ) ) ;
#141555=CARTESIAN_POINT ( 'NONE',  ( 21.55341960407619695, -5.719274019375665929, 31.04275706135234714 ) ) ;
#141556=CARTESIAN_POINT ( 'NONE',  ( -13.89961937509957401, -13.97604488694547875, 54.37609039468565442 ) ) ;
#141557=CARTESIAN_POINT ( 'NONE',  ( -13.97604488694527625, -13.89961937509977652, 41.87390960531435979 ) ) ;
#141558=CARTESIAN_POINT ( 'NONE',  ( 8.314922557961029526, -14.29746914071037800, 105.4177570613523613 ) ) ;
#141559=CARTESIAN_POINT ( 'NONE',  ( -9.474510206698720793, -16.51473224551083518, 69.58442372801901854 ) ) ;
#141560=CARTESIAN_POINT ( 'NONE',  ( -12.14591786802326823, 12.06949235617739902, 113.1260903946856899 ) ) ;
#141561=CARTESIAN_POINT ( 'NONE',  ( 19.03943276465977164, 0.05219959533936151252, 51.25109039468567573 ) ) ;
#141562=CARTESIAN_POINT ( 'NONE',  ( 13.89961937509977652, -13.97604488694527269, 98.12390960531433848 ) ) ;
#141563=CARTESIAN_POINT ( 'NONE',  ( 0.05219959533937995610, -21.53943276465977519, 105.0010903946856757 ) ) ;
#141564=CARTESIAN_POINT ( 'NONE',  ( -19.02544592524334988, -5.153800228976617603, 18.95942372801899722 ) ) ;
#141565=CARTESIAN_POINT ( 'NONE',  ( -19.02544592524342804, 5.153800228976336051, 31.04057627198102409 ) ) ;
#141566=CARTESIAN_POINT ( 'NONE',  ( 5.719274019375673035, 21.55341960407619339, 87.29275706135236135 ) ) ;
#141567=CARTESIAN_POINT ( 'NONE',  ( 4.483927247898790824, -16.52544592524335698, 30.20942372801902565 ) ) ;
#141568=EDGE_CURVE ( 'NONE', #40349, #179309, #52349, .T. ) ;
#141569=CARTESIAN_POINT ( 'NONE',  ( -16.46253265017160317, 9.564922557960807481, 95.83224293864769550 ) ) ;
#141571=CARTESIAN_POINT ( 'NONE',  ( 19.02544592524343514, -5.153800228976328945, 73.54057627198103830 ) ) ;
#141572=CARTESIAN_POINT ( 'NONE',  ( -30.00000000000000000, -1.132798289211302014E-14, 92.50000000000000000 ) ) ;
#141573=CARTESIAN_POINT ( 'NONE',  ( 0.05219959533936267826, -19.03943276465977164, 65.00109039468567573 ) ) ;
#141574=CARTESIAN_POINT ( 'NONE',  ( 16.46253265017160672, -9.564922557960803928, 103.3322429386476955 ) ) ;
#141575=CARTESIAN_POINT ( 'NONE',  ( 15.80617190586769283, -15.72974639402175789, 105.6260903946856899 ) ) ;
#141576=CARTESIAN_POINT ( 'NONE',  ( 4.379528057220339221, -16.55341960407611168, 97.70724293864772392 ) ) ;
#141577=CARTESIAN_POINT ( 'NONE',  ( 5.719274019375991003, -21.55341960407610458, 47.70724293864770260 ) ) ;
#141578=CARTESIAN_POINT ( 'NONE',  ( 15.72974639402199770, -15.80617190586745480, 33.12390960531435979 ) ) ;
#141579=CARTESIAN_POINT ( 'NONE',  ( 4.379528057220339221, -16.55341960407611168, 107.7072429386476955 ) ) ;
#141581=CARTESIAN_POINT ( 'NONE',  ( -19.03943276465977164, -0.05219959533935918106, 58.75109039468566863 ) ) ;
#141582=CARTESIAN_POINT ( 'NONE',  ( 12.06949235617757843, -12.14591786802309237, 33.12390960531435979 ) ) ;
#141583=VECTOR ( 'NONE', #156468, 1000.000000000000000 ) ;
#141584=CARTESIAN_POINT ( 'NONE',  ( -19.05341960407611168, -5.049401038298163336, 101.4572429386476955 ) ) ;
#141585=CARTESIAN_POINT ( 'NONE',  ( -15.80617190586768217, 15.72974639402176855, 78.12609039468570415 ) ) ;
#141586=CARTESIAN_POINT ( 'NONE',  ( 15.80617190586746368, 15.72974639402197994, 69.37390960531436690 ) ) ;
#141587=CARTESIAN_POINT ( 'NONE',  ( 18.62759615963255655, 10.81492255796105972, 51.66775706135234714 ) ) ;
#141588=CARTESIAN_POINT ( 'NONE',  ( 5.823673210054125526, 21.52544592524343514, 99.79057627198103830 ) ) ;
#141589=CARTESIAN_POINT ( 'NONE',  ( 18.62759615963255655, 10.81492255796105972, 51.66775706135234714 ) ) ;
#141590=CARTESIAN_POINT ( 'NONE',  ( 16.51473224551069308, 9.474510206698969483, 24.16557627198102765 ) ) ;
#141592=CARTESIAN_POINT ( 'NONE',  ( 16.51473224551069308, 9.474510206698969483, 79.16557627198103830 ) ) ;
#141593=CARTESIAN_POINT ( 'NONE',  ( 16.55341960407618274, -4.379528057220086978, 81.04275706135236135 ) ) ;
#141594=CARTESIAN_POINT ( 'NONE',  ( -16.52544592524342804, 4.483927247898546575, 106.0405762719810525 ) ) ;
#141595=CARTESIAN_POINT ( 'NONE',  ( 9.564922557960805705, 16.46253265017160317, 104.5822429386476955 ) ) ;
#141596=CARTESIAN_POINT ( 'NONE',  ( -14.34966873604960291, -8.224510206698953496, 56.66557627198103830 ) ) ;
#141597=CARTESIAN_POINT ( 'NONE',  ( 14.34966873604972726, -8.224510206698740333, 110.8344237280190043 ) ) ;
#141598=CARTESIAN_POINT ( 'NONE',  ( 9.564922557960805705, 16.46253265017160317, 59.58224293864769550 ) ) ;
#141599=CARTESIAN_POINT ( 'NONE',  ( 16.51473224551069308, 9.474510206698969483, 34.16557627198102409 ) ) ;
#141600=CARTESIAN_POINT ( 'NONE',  ( 15.80617190586746368, 15.72974639402197994, 44.37390960531435979 ) ) ;
#141601=CARTESIAN_POINT ( 'NONE',  ( 5.153800228976615827, -19.02544592524334988, 35.20942372801899722 ) ) ;
#141603=CARTESIAN_POINT ( 'NONE',  ( -4.379528057220328563, 16.55341960407611168, 30.20724293864769550 ) ) ;
#141604=CARTESIAN_POINT ( 'NONE',  ( -5.823673210054431948, 21.52544592524334988, 42.70942372801901854 ) ) ;
#141605=CARTESIAN_POINT ( 'NONE',  ( -13.97604488694527625, -13.89961937509977652, 111.8739096053143243 ) ) ;
#141606=CARTESIAN_POINT ( 'NONE',  ( -12.06949235617739369, -12.14591786802326823, 54.37609039468568994 ) ) ;
#141607=CARTESIAN_POINT ( 'NONE',  ( -19.05341960407617563, 5.049401038297882671, 68.54275706135230450 ) ) ;
#141608=CARTESIAN_POINT ( 'NONE',  ( -12.14591786802309592, -12.06949235617757132, 26.87390960531435979 ) ) ;
#141609=CARTESIAN_POINT ( 'NONE',  ( 16.18388926212236356, -7.379444403734617630, 52.06046848633854296 ) ) ;
#141610=CARTESIAN_POINT ( 'NONE',  ( -14.34966873604972548, 8.224510206698743886, 103.3344237280190043 ) ) ;
#141611=CARTESIAN_POINT ( 'NONE',  ( -19.03943276465977164, 0.05219959533909376836, 41.24890960531435269 ) ) ;
#141612=CARTESIAN_POINT ( 'NONE',  ( -19.02544592524342804, 5.153800228976336051, 61.04057627198103120 ) ) ;
#141613=CARTESIAN_POINT ( 'NONE',  ( -16.51473224551069308, -9.474510206698971260, 26.66557627198103120 ) ) ;
#141614=CARTESIAN_POINT ( 'NONE',  ( -15.72974639402176322, -15.80617190586768395, 39.37609039468567573 ) ) ;
#141615=CARTESIAN_POINT ( 'NONE',  ( -16.46253265017160317, 9.564922557960807481, 45.83224293864769550 ) ) ;
#141617=CARTESIAN_POINT ( 'NONE',  ( -0.05219959533909027116, -19.03943276465977164, 47.49890960531435979 ) ) ;
#141618=CARTESIAN_POINT ( 'NONE',  ( 5.823673210054125526, 21.52544592524343514, 24.79057627198103120 ) ) ;
#141619=CARTESIAN_POINT ( 'NONE',  ( -15.72974639402176322, -15.80617190586768395, 59.37609039468568284 ) ) ;
#141620=CARTESIAN_POINT ( 'NONE',  ( -5.153800228976328057, -19.02544592524343514, 27.29057627198103120 ) ) ;
#141621=CARTESIAN_POINT ( 'NONE',  ( -0.05219959533907301413, -21.53943276465977519, 32.49890960531435979 ) ) ;
#141622=CARTESIAN_POINT ( 'NONE',  ( 12.06949235617739724, 12.14591786802326823, 71.87609039468568994 ) ) ;
#141623=CARTESIAN_POINT ( 'NONE',  ( -18.67979575497193778, 10.72451020669871902, 98.33442372801901854 ) ) ;
#141624=CARTESIAN_POINT ( 'NONE',  ( 14.34966873604972726, -8.224510206698740333, 50.83442372801901143 ) ) ;
#141625=CARTESIAN_POINT ( 'NONE',  ( 19.05341960407611168, 5.049401038298154454, 93.95724293864769550 ) ) ;
#141626=CARTESIAN_POINT ( 'NONE',  ( -12.06949235617739369, -12.14591786802326823, 39.37609039468567573 ) ) ;
#141627=CARTESIAN_POINT ( 'NONE',  ( -4.379528057220086978, -16.55341960407618274, 29.79275706135234358 ) ) ;
#141628=CARTESIAN_POINT ( 'NONE',  ( -16.52544592524335698, -4.483927247898792601, 98.95942372801903275 ) ) ;
#141629=CARTESIAN_POINT ( 'NONE',  ( 5.719274019375673035, 21.55341960407619339, 57.29275706135234714 ) ) ;
#141630=CARTESIAN_POINT ( 'NONE',  ( 19.02544592524334988, 5.153800228976608722, 101.4594237280189759 ) ) ;
#141631=CARTESIAN_POINT ( 'NONE',  ( -21.53943276465977519, -0.05219959533937600094, 18.75109039468568639 ) ) ;
#141632=CARTESIAN_POINT ( 'NONE',  ( 4.379528057220339221, -16.55341960407611168, 97.70724293864772392 ) ) ;
#141633=CARTESIAN_POINT ( 'NONE',  ( 13.89961937509957401, 13.97604488694547697, 106.8760903946856757 ) ) ;
#141634=CARTESIAN_POINT ( 'NONE',  ( -0.05219959533934338120, 16.53943276465976808, 77.50109039468567573 ) ) ;
#141635=CARTESIAN_POINT ( 'NONE',  ( -16.61371651742640410, 7.165104196375925660, 43.85415069992968995 ) ) ;
#141636=CARTESIAN_POINT ( 'NONE',  ( -5.049401038297874678, -19.05341960407617918, 84.79275706135233293 ) ) ;
#141637=CARTESIAN_POINT ( 'NONE',  ( -14.34966873604960291, -8.224510206698953496, 51.66557627198102409 ) ) ;
#141638=CARTESIAN_POINT ( 'NONE',  ( 0.05219959533910956823, 16.53943276465976808, 49.99890960531437401 ) ) ;
#141639=CARTESIAN_POINT ( 'NONE',  ( 14.29746914071049879, -8.314922557960816363, 98.33224293864769550 ) ) ;
#141640=CARTESIAN_POINT ( 'NONE',  ( 16.46253265017146816, 9.564922557961045513, 31.66775706135232937 ) ) ;
#141641=CARTESIAN_POINT ( 'NONE',  ( -18.56197773271727769, 5.500000000000086153, 88.55066217314450228 ) ) ;
#141642=CARTESIAN_POINT ( 'NONE',  ( 15.72974639402176855, 15.80617190586768217, 41.87609039468568284 ) ) ;
#141643=CARTESIAN_POINT ( 'NONE',  ( 9.564922557961047289, -16.46253265017146816, 95.41775706135233293 ) ) ;
#141645=CARTESIAN_POINT ( 'NONE',  ( -16.51473224551069308, -9.474510206698971260, 91.66557627198103830 ) ) ;
#141646=CARTESIAN_POINT ( 'NONE',  ( 0.05219959533909260263, 19.03943276465977164, 94.99890960531436690 ) ) ;
#141647=CARTESIAN_POINT ( 'NONE',  ( -10.81492255796078084, -18.62759615963271287, 52.08224293864768839 ) ) ;
#141648=CARTESIAN_POINT ( 'NONE',  ( -16.52544592524342804, 4.483927247898546575, 91.04057627198103830 ) ) ;
#141649=CARTESIAN_POINT ( 'NONE',  ( -19.05341960407611168, -5.049401038298163336, 71.45724293864766707 ) ) ;
#141650=CARTESIAN_POINT ( 'NONE',  ( 0.05219959533909260263, 19.03943276465977164, 34.99890960531435979 ) ) ;
#141651=CARTESIAN_POINT ( 'NONE',  ( -21.53943276465977519, -0.05219959533937600094, 43.75109039468568284 ) ) ;
#141652=CARTESIAN_POINT ( 'NONE',  ( 0.05219959533937995610, -21.53943276465977519, 70.00109039468568994 ) ) ;
#141653=CARTESIAN_POINT ( 'NONE',  ( 12.06949235617739724, 12.14591786802326823, 91.87609039468568994 ) ) ;
#141654=CARTESIAN_POINT ( 'NONE',  ( 18.62759615963255655, 10.81492255796105972, 31.66775706135234358 ) ) ;
#141655=CARTESIAN_POINT ( 'NONE',  ( 18.67979575497194134, -10.72451020669871369, 20.83442372801901143 ) ) ;
#141656=CARTESIAN_POINT ( 'NONE',  ( 16.46253265017146816, 9.564922557961045513, 51.66775706135233293 ) ) ;
#141657=CARTESIAN_POINT ( 'NONE',  ( 19.02544592524343514, -5.153800228976328945, 73.54057627198103830 ) ) ;
#141658=CARTESIAN_POINT ( 'NONE',  ( 15.80617190586769283, -15.72974639402175789, 80.62609039468567573 ) ) ;
#141659=CARTESIAN_POINT ( 'NONE',  ( 21.52544592524344225, -5.823673210054117533, 83.54057627198102409 ) ) ;
#141660=CARTESIAN_POINT ( 'NONE',  ( 16.52544592524342804, -4.483927247898539470, 53.54057627198103120 ) ) ;
#141661=CARTESIAN_POINT ( 'NONE',  ( -10.81492255796105439, 18.62759615963255655, 102.9177570613523756 ) ) ;
#141662=CARTESIAN_POINT ( 'NONE',  ( -19.03943276465977164, -0.05219959533935918106, 33.75109039468566863 ) ) ;
#141663=CARTESIAN_POINT ( 'NONE',  ( 12.06949235617757843, -12.14591786802309237, 73.12390960531436690 ) ) ;
#141664=CARTESIAN_POINT ( 'NONE',  ( 4.379528057220339221, -16.55341960407611168, 112.7072429386476955 ) ) ;
#141665=CARTESIAN_POINT ( 'NONE',  ( 19.02544592524334988, 5.153800228976608722, 71.45942372801900433 ) ) ;
#141666=CARTESIAN_POINT ( 'NONE',  ( 4.483927247898545687, 16.52544592524342804, 39.79057627198103830 ) ) ;
#141667=CARTESIAN_POINT ( 'NONE',  ( -18.67979575497193778, 10.72451020669871902, 78.33442372801901854 ) ) ;
#141668=EDGE_CURVE ( 'NONE', #50018, #116638, #55175, .T. ) ;
#141669=CARTESIAN_POINT ( 'NONE',  ( -19.03943276465977164, 0.05219959533909376836, 81.24890960531436690 ) ) ;
#141670=CARTESIAN_POINT ( 'NONE',  ( -19.03943276465977164, -0.05219959533935918106, 63.75109039468566863 ) ) ;
#141671=CARTESIAN_POINT ( 'NONE',  ( 15.72974639402199770, -15.80617190586745480, 63.12390960531435979 ) ) ;
#141672=CARTESIAN_POINT ( 'NONE',  ( 5.823673210054125526, 21.52544592524343514, 109.7905762719810383 ) ) ;
#141673=CARTESIAN_POINT ( 'NONE',  ( 16.51473224551083163, -9.474510206698727899, 110.8344237280190043 ) ) ;
#141674=CARTESIAN_POINT ( 'NONE',  ( 12.14591786802327356, -12.06949235617739191, 80.62609039468567573 ) ) ;
#141676=CARTESIAN_POINT ( 'NONE',  ( -5.719274019375665041, -21.55341960407619695, 19.79275706135235069 ) ) ;
#141677=CARTESIAN_POINT ( 'NONE',  ( -8.314922557960811034, -14.29746914071050412, 102.0822429386476955 ) ) ;
#141679=CARTESIAN_POINT ( 'NONE',  ( -12.06949235617739369, -12.14591786802326823, 34.37609039468568284 ) ) ;
#141680=CARTESIAN_POINT ( 'NONE',  ( -15.72974639402197994, 15.80617190586746368, 55.62390960531436690 ) ) ;
#141681=CARTESIAN_POINT ( 'NONE',  ( 8.314922557961029526, -14.29746914071037800, 105.4177570613523613 ) ) ;
#141682=CARTESIAN_POINT ( 'NONE',  ( 19.02544592524343514, -5.153800228976328945, 38.54057627198103120 ) ) ;
#141683=CARTESIAN_POINT ( 'NONE',  ( -4.379528057220086978, -16.55341960407618274, 79.79275706135236135 ) ) ;
#141684=CARTESIAN_POINT ( 'NONE',  ( 19.05341960407617918, -5.049401038297876454, 76.04275706135230450 ) ) ;
#141685=CARTESIAN_POINT ( 'NONE',  ( -21.53943276465977519, -0.05219959533937600094, 43.75109039468568284 ) ) ;
#141686=CARTESIAN_POINT ( 'NONE',  ( -21.53943276465977519, 0.05219959533907696930, 61.24890960531435979 ) ) ;
#141687=CARTESIAN_POINT ( 'NONE',  ( 16.52544592524335698, 4.483927247898782831, 101.4594237280190185 ) ) ;
#141688=CARTESIAN_POINT ( 'NONE',  ( 15.80617190586769283, -15.72974639402175789, 85.62609039468568994 ) ) ;
#141689=CARTESIAN_POINT ( 'NONE',  ( 21.55341960407610458, 5.719274019375980345, 48.95724293864770971 ) ) ;
#141690=CARTESIAN_POINT ( 'NONE',  ( 5.719274019375991003, -21.55341960407610458, 47.70724293864770260 ) ) ;
#141691=CARTESIAN_POINT ( 'NONE',  ( 12.14591786802327356, -12.06949235617739191, 80.62609039468567573 ) ) ;
#141692=CARTESIAN_POINT ( 'NONE',  ( 21.55341960407610458, 5.719274019375980345, 48.95724293864770971 ) ) ;
#141693=ORIENTED_EDGE ( 'NONE', *, *, #148381, .T. ) ;
#141694=CARTESIAN_POINT ( 'NONE',  ( 16.51473224551069308, 9.474510206698969483, 94.16557627198103830 ) ) ;
#141696=CARTESIAN_POINT ( 'NONE',  ( 9.564922557960805705, 16.46253265017160317, 29.58224293864769550 ) ) ;
#141697=CARTESIAN_POINT ( 'NONE',  ( 18.67979575497178502, 10.72451020669898547, 64.16557627198102409 ) ) ;
#141698=CARTESIAN_POINT ( 'NONE',  ( 8.224510206698742110, 14.34966873604972548, 92.08442372801901854 ) ) ;
#141699=CARTESIAN_POINT ( 'NONE',  ( -10.81492255796105439, 18.62759615963255655, 52.91775706135235424 ) ) ;
#141700=CARTESIAN_POINT ( 'NONE',  ( 13.89961937509957401, 13.97604488694547697, 96.87609039468566152 ) ) ;
#141701=CARTESIAN_POINT ( 'NONE',  ( -8.314922557960811034, -14.29746914071050412, 102.0822429386476955 ) ) ;
#141702=CARTESIAN_POINT ( 'NONE',  ( 13.89961937509957401, 13.97604488694547697, 111.8760903946856757 ) ) ;
#141703=CARTESIAN_POINT ( 'NONE',  ( 9.474510206698971260, -16.51473224551069308, 37.91557627198102409 ) ) ;
#141705=CARTESIAN_POINT ( 'NONE',  ( 0.05219959533909260263, 19.03943276465977164, 84.99890960531436690 ) ) ;
#141706=CARTESIAN_POINT ( 'NONE',  ( 12.06949235617739724, 12.14591786802326823, 76.87609039468567573 ) ) ;
#141707=CARTESIAN_POINT ( 'NONE',  ( 21.53943276465977519, 0.05219959533937863772, 101.2510903946856757 ) ) ;
#141708=CARTESIAN_POINT ( 'NONE',  ( 21.55341960407610458, 5.719274019375980345, 58.95724293864770971 ) ) ;
#141709=CARTESIAN_POINT ( 'NONE',  ( -16.55341960407617563, 4.379528057220093196, 88.54275706135236135 ) ) ;
#141710=CARTESIAN_POINT ( 'NONE',  ( -19.03943276465977164, -0.05219959533935918106, 73.75109039468566152 ) ) ;
#141711=CARTESIAN_POINT ( 'NONE',  ( 9.474510206698971260, -16.51473224551069308, 32.91557627198102409 ) ) ;
#141712=CARTESIAN_POINT ( 'NONE',  ( 19.02544592524343514, -5.153800228976328945, 78.54057627198099567 ) ) ;
#141713=CARTESIAN_POINT ( 'NONE',  ( -5.719274019375665041, -21.55341960407619695, 49.79275706135234714 ) ) ;
#141714=CARTESIAN_POINT ( 'NONE',  ( 5.153800228976335163, 19.02544592524342804, 29.79057627198102409 ) ) ;
#141715=CARTESIAN_POINT ( 'NONE',  ( -0.05219959533936034679, 19.03943276465977164, 67.50109039468566152 ) ) ;
#141717=CARTESIAN_POINT ( 'NONE',  ( -5.049401038298153566, 19.05341960407611168, 115.2072429386477097 ) ) ;
#141718=CARTESIAN_POINT ( 'NONE',  ( 12.14591786802309770, 12.06949235617756955, 69.37390960531436690 ) ) ;
#141719=CARTESIAN_POINT ( 'NONE',  ( -10.72451020669898014, 18.67979575497178502, 60.41557627198102409 ) ) ;
#141721=CARTESIAN_POINT ( 'NONE',  ( -19.03943276465977164, -0.05219959533935918106, 33.75109039468566863 ) ) ;
#141722=CARTESIAN_POINT ( 'NONE',  ( -17.60769864724391809, 5.499999999999989342, 88.65024842019164453 ) ) ;
#141723=CARTESIAN_POINT ( 'NONE',  ( -16.51473224551069308, -9.474510206698971260, 61.66557627198103120 ) ) ;
#141724=CARTESIAN_POINT ( 'NONE',  ( 16.46253265017160672, -9.564922557960803928, 78.33224293864769550 ) ) ;
#141725=CARTESIAN_POINT ( 'NONE',  ( 0.05219959533934541429, -16.53943276465976808, 55.00109039468568284 ) ) ;
#141726=LINE ( 'NONE', #97193, #104660 ) ;
#141727=CARTESIAN_POINT ( 'NONE',  ( -17.44279575226824619, 5.990770900252421427, 110.8355756751432040 ) ) ;
#141728=CARTESIAN_POINT ( 'NONE',  ( -16.52544592524335698, -4.483927247898792601, 73.95942372801901854 ) ) ;
#141730=CARTESIAN_POINT ( 'NONE',  ( 16.53943276465976808, 0.05219959533934440121, 61.25109039468567573 ) ) ;
#141731=CARTESIAN_POINT ( 'NONE',  ( 16.55341960407618274, -4.379528057220086978, 36.04275706135234714 ) ) ;
#141732=CARTESIAN_POINT ( 'NONE',  ( 5.049401038298161559, -19.05341960407611168, 52.70724293864767418 ) ) ;
#141734=CARTESIAN_POINT ( 'NONE',  ( -18.62759615963255300, -10.81492255796106328, 54.16775706135235424 ) ) ;
#141735=CARTESIAN_POINT ( 'NONE',  ( 13.97604488694548053, -13.89961937509957401, 65.62609039468567573 ) ) ;
#141736=CARTESIAN_POINT ( 'NONE',  ( -19.02544592524334988, -5.153800228976617603, 18.95942372801899722 ) ) ;
#141737=CARTESIAN_POINT ( 'NONE',  ( 0.05219959533909260263, 19.03943276465977164, 29.99890960531435979 ) ) ;
#141738=CARTESIAN_POINT ( 'NONE',  ( 16.18414358144004694, 7.379350812367110102, 22.98974271850655526 ) ) ;
#141739=CARTESIAN_POINT ( 'NONE',  ( -21.52544592524343514, 5.823673210054127303, 61.04057627198103120 ) ) ;
#141740=CARTESIAN_POINT ( 'NONE',  ( 19.03943276465977164, -0.05219959533909143690, 108.7489096053143527 ) ) ;
#141741=CARTESIAN_POINT ( 'NONE',  ( 12.14591786802309770, 12.06949235617756955, 104.3739096053143669 ) ) ;
#141742=CARTESIAN_POINT ( 'NONE',  ( 16.53943276465976808, 0.05219959533934440121, 41.25109039468568284 ) ) ;
#141743=CARTESIAN_POINT ( 'NONE',  ( -12.06949235617756955, 12.14591786802309770, 25.62390960531435624 ) ) ;
#141745=CARTESIAN_POINT ( 'NONE',  ( 10.81492255796078972, 18.62759615963270932, 99.58224293864770971 ) ) ;
#141746=CARTESIAN_POINT ( 'NONE',  ( -0.05219959533910754901, -16.53943276465976808, 42.49890960531435979 ) ) ;
#141747=CARTESIAN_POINT ( 'NONE',  ( -9.474510206698964154, 16.51473224551069663, 115.4155762719810241 ) ) ;
#141748=CARTESIAN_POINT ( 'NONE',  ( -19.03943276465977164, -0.05219959533935918106, 93.75109039468566152 ) ) ;
#141749=CARTESIAN_POINT ( 'NONE',  ( 0.05219959533936267826, -19.03943276465977164, 25.00109039468566152 ) ) ;
#141750=CARTESIAN_POINT ( 'NONE',  ( 8.224510206698953496, -14.34966873604960469, 27.91557627198103830 ) ) ;
#141751=CARTESIAN_POINT ( 'NONE',  ( 15.72974639402199770, -15.80617190586745480, 103.1239096053143811 ) ) ;
#141752=CARTESIAN_POINT ( 'NONE',  ( 0.05219959533907565091, 21.53943276465977519, 49.99890960531437401 ) ) ;
#141753=CARTESIAN_POINT ( 'NONE',  ( -16.51473224551069308, -9.474510206698971260, 81.66557627198103830 ) ) ;
#141754=CARTESIAN_POINT ( 'NONE',  ( -4.483927247898539470, -16.52544592524342804, 52.29057627198102409 ) ) ;
#141755=CARTESIAN_POINT ( 'NONE',  ( -5.049401038298153566, 19.05341960407611168, 90.20724293864766707 ) ) ;
#141757=CARTESIAN_POINT ( 'NONE',  ( 5.153800228976615827, -19.02544592524334988, 35.20942372801899722 ) ) ;
#141758=CARTESIAN_POINT ( 'NONE',  ( 10.72451020669898902, -18.67979575497178502, 77.91557627198102409 ) ) ;
#141759=CARTESIAN_POINT ( 'NONE',  ( 14.34966873604960469, 8.224510206698951720, 104.1655762719810241 ) ) ;
#141760=CARTESIAN_POINT ( 'NONE',  ( 21.53943276465977519, 0.05219959533937863772, 31.25109039468568639 ) ) ;
#141762=CARTESIAN_POINT ( 'NONE',  ( -12.06949235617739369, -12.14591786802326823, 109.3760903946857042 ) ) ;
#141763=CARTESIAN_POINT ( 'NONE',  ( -16.51473224551069308, -9.474510206698971260, 36.66557627198102409 ) ) ;
#141764=CARTESIAN_POINT ( 'NONE',  ( -19.05341960407611168, -5.049401038298163336, 91.45724293864766707 ) ) ;
#141766=CARTESIAN_POINT ( 'NONE',  ( -5.049401038298153566, 19.05341960407611168, 35.20724293864768839 ) ) ;
#141767=CARTESIAN_POINT ( 'NONE',  ( 16.52544592524342804, -4.483927247898539470, 43.54057627198103830 ) ) ;
#141768=CARTESIAN_POINT ( 'NONE',  ( 15.80617190586769283, -15.72974639402175789, 75.62609039468567573 ) ) ;
#141770=CARTESIAN_POINT ( 'NONE',  ( -12.06949235617739369, -12.14591786802326823, 69.37609039468567573 ) ) ;
#141771=CARTESIAN_POINT ( 'NONE',  ( 19.03943276465977164, -0.05219959533909143690, 58.74890960531435979 ) ) ;
#141772=CARTESIAN_POINT ( 'NONE',  ( -19.05341960407611168, -5.049401038298163336, 61.45724293864769550 ) ) ;
#141774=CARTESIAN_POINT ( 'NONE',  ( -18.62759615963255300, -10.81492255796106328, 104.1677570613523471 ) ) ;
#141775=CARTESIAN_POINT ( 'NONE',  ( -8.224510206698735004, -14.34966873604973081, 69.58442372801900433 ) ) ;
#141776=CARTESIAN_POINT ( 'NONE',  ( -15.72974639402176322, -15.80617190586768395, 104.3760903946856899 ) ) ;
#141777=CARTESIAN_POINT ( 'NONE',  ( 9.474510206698971260, -16.51473224551069308, 62.91557627198102409 ) ) ;
#141778=CARTESIAN_POINT ( 'NONE',  ( 21.53943276465977519, -0.05219959533907433946, 38.74890960531435979 ) ) ;
#141779=CARTESIAN_POINT ( 'NONE',  ( 16.51473224551083163, -9.474510206698727899, 100.8344237280190043 ) ) ;
#141780=CARTESIAN_POINT ( 'NONE',  ( 5.719274019375673035, 21.55341960407619339, 67.29275706135234714 ) ) ;
#141781=CARTESIAN_POINT ( 'NONE',  ( 14.34966873604972726, -8.224510206698740333, 55.83442372801901854 ) ) ;
#141782=CARTESIAN_POINT ( 'NONE',  ( -15.72974639402197994, 15.80617190586746368, 100.6239096053143811 ) ) ;
#141783=CARTESIAN_POINT ( 'NONE',  ( -0.05219959533936034679, 19.03943276465977164, 102.5010903946856757 ) ) ;
#141784=CARTESIAN_POINT ( 'NONE',  ( 13.89961937509977652, -13.97604488694527269, 78.12390960531433848 ) ) ;
#141785=CARTESIAN_POINT ( 'NONE',  ( -5.049401038297874678, -19.05341960407617918, 104.7927570613523471 ) ) ;
#141786=CARTESIAN_POINT ( 'NONE',  ( 12.06949235617739724, 12.14591786802326823, 26.87609039468567218 ) ) ;
#141787=CARTESIAN_POINT ( 'NONE',  ( -0.05219959533910754901, -16.53943276465976808, 72.49890960531435269 ) ) ;
#141789=CARTESIAN_POINT ( 'NONE',  ( -4.483927247898782831, 16.52544592524335698, 67.70942372801901854 ) ) ;
#141790=CARTESIAN_POINT ( 'NONE',  ( 10.81492255796106328, -18.62759615963255655, 20.41775706135234714 ) ) ;
#141791=CARTESIAN_POINT ( 'NONE',  ( 9.564922557960805705, 16.46253265017160317, 49.58224293864770260 ) ) ;
#141792=CARTESIAN_POINT ( 'NONE',  ( 16.51473224551069308, 9.474510206698969483, 69.16557627198102409 ) ) ;
#141793=CARTESIAN_POINT ( 'NONE',  ( 16.55341960407618274, -4.379528057220086978, 76.04275706135237556 ) ) ;
#141795=ORIENTED_EDGE ( 'NONE', *, *, #169539, .F. ) ;
#141796=CARTESIAN_POINT ( 'NONE',  ( 18.62759615963255655, 10.81492255796105972, 111.6677570613523613 ) ) ;
#141797=CARTESIAN_POINT ( 'NONE',  ( 0.05219959533909260263, 19.03943276465977164, 39.99890960531436690 ) ) ;
#141798=ORIENTED_EDGE ( 'NONE', *, *, #115652, .T. ) ;
#141799=CARTESIAN_POINT ( 'NONE',  ( -19.03943276465977164, -0.05219959533935918106, 108.7510903946856615 ) ) ;
#141800=VECTOR ( 'NONE', #131144, 1000.000000000000000 ) ;
#141801=CARTESIAN_POINT ( 'NONE',  ( -5.049401038297874678, -19.05341960407617918, 44.79275706135232582 ) ) ;
#141802=CARTESIAN_POINT ( 'NONE',  ( -16.55341960407617563, 4.379528057220093196, 28.54275706135234358 ) ) ;
#141803=CARTESIAN_POINT ( 'NONE',  ( -16.51473224551069308, -9.474510206698971260, 46.66557627198102409 ) ) ;
#141804=CARTESIAN_POINT ( 'NONE',  ( 16.51473224551069308, 9.474510206698969483, 64.16557627198102409 ) ) ;
#141805=CARTESIAN_POINT ( 'NONE',  ( -15.80617190586745835, -15.72974639402198527, 86.87390960531438111 ) ) ;
#141806=CARTESIAN_POINT ( 'NONE',  ( 19.02544592524343514, -5.153800228976328945, 108.5405762719810383 ) ) ;
#141807=CARTESIAN_POINT ( 'NONE',  ( -16.46253265017160317, 9.564922557960807481, 45.83224293864769550 ) ) ;
#141809=CARTESIAN_POINT ( 'NONE',  ( 5.049401038297881783, 19.05341960407617563, 97.29275706135233293 ) ) ;
#141810=CARTESIAN_POINT ( 'NONE',  ( -15.72974639402197994, 15.80617190586746368, 70.62390960531436690 ) ) ;
#141811=CARTESIAN_POINT ( 'NONE',  ( -19.02544592524334988, -5.153800228976617603, 23.95942372801900078 ) ) ;
#141812=CARTESIAN_POINT ( 'NONE',  ( 14.34966873604960469, 8.224510206698951720, 64.16557627198102409 ) ) ;
#141813=CARTESIAN_POINT ( 'NONE',  ( 21.52544592524334988, 5.823673210054432836, 86.45942372801901854 ) ) ;
#141814=CARTESIAN_POINT ( 'NONE',  ( -16.51473224551069308, -9.474510206698971260, 31.66557627198102054 ) ) ;
#141816=CARTESIAN_POINT ( 'NONE',  ( 16.53943276465976808, -0.05219959533910856209, 28.74890960531435624 ) ) ;
#141817=CARTESIAN_POINT ( 'NONE',  ( 18.67979575497194134, -10.72451020669871369, 90.83442372801901854 ) ) ;
#141818=CARTESIAN_POINT ( 'NONE',  ( 13.89961937509977652, -13.97604488694527269, 78.12390960531433848 ) ) ;
#141819=CARTESIAN_POINT ( 'NONE',  ( -10.72451020669870658, -18.67979575497194134, 39.58442372801901143 ) ) ;
#141820=CARTESIAN_POINT ( 'NONE',  ( -19.05341960407611168, -5.049401038298163336, 76.45724293864769550 ) ) ;
#141821=CARTESIAN_POINT ( 'NONE',  ( 16.53943276465976808, -0.05219959533910856209, 88.74890960531436690 ) ) ;
#141822=CARTESIAN_POINT ( 'NONE',  ( 14.34966873604960469, 8.224510206698951720, 59.16557627198103120 ) ) ;
#141823=CARTESIAN_POINT ( 'NONE',  ( 18.67979575497178502, 10.72451020669898547, 69.16557627198102409 ) ) ;
#141824=CARTESIAN_POINT ( 'NONE',  ( -19.03943276465977164, 0.05219959533909376836, 76.24890960531435269 ) ) ;
#141825=CARTESIAN_POINT ( 'NONE',  ( 15.80617190586746368, 15.72974639402197994, 89.37390960531435269 ) ) ;
#141826=CARTESIAN_POINT ( 'NONE',  ( -9.474510206698720793, -16.51473224551083518, 74.58442372801900433 ) ) ;
#141827=CARTESIAN_POINT ( 'NONE',  ( 16.46253265017146816, 9.564922557961045513, 31.66775706135232937 ) ) ;
#141828=CARTESIAN_POINT ( 'NONE',  ( 12.06949235617757843, -12.14591786802309237, 78.12390960531436690 ) ) ;
#141829=CARTESIAN_POINT ( 'NONE',  ( -10.81492255796078084, -18.62759615963271287, 52.08224293864768839 ) ) ;
#141831=CARTESIAN_POINT ( 'NONE',  ( -17.49999999999999645, 5.499999999999997335, 115.7969038253417438 ) ) ;
#141832=CARTESIAN_POINT ( 'NONE',  ( -8.314922557961024197, 14.29746914071037800, 97.91775706135236135 ) ) ;
#141834=CARTESIAN_POINT ( 'NONE',  ( 16.46253265017146816, 9.564922557961045513, 106.6677570613523471 ) ) ;
#141835=CARTESIAN_POINT ( 'NONE',  ( 16.53943276465976808, -0.05219959533910856209, 73.74890960531433848 ) ) ;
#141836=CARTESIAN_POINT ( 'NONE',  ( -18.56399227203342051, -5.499999999999968026, 93.97830131249902763 ) ) ;
#141837=CARTESIAN_POINT ( 'NONE',  ( -5.153800228976328057, -19.02544592524343514, 67.29057627198102409 ) ) ;
#141838=CARTESIAN_POINT ( 'NONE',  ( -16.51473224551069308, -9.474510206698971260, 26.66557627198103120 ) ) ;
#141839=CARTESIAN_POINT ( 'NONE',  ( -16.52544592524342804, 4.483927247898546575, 56.04057627198102409 ) ) ;
#141840=CARTESIAN_POINT ( 'NONE',  ( 16.46253265017160672, -9.564922557960803928, 98.33224293864769550 ) ) ;
#141841=CARTESIAN_POINT ( 'NONE',  ( 5.049401038297881783, 19.05341960407617563, 92.29275706135234714 ) ) ;
#141842=CARTESIAN_POINT ( 'NONE',  ( 5.049401038298161559, -19.05341960407611168, 62.70724293864769550 ) ) ;
#141843=CARTESIAN_POINT ( 'NONE',  ( -13.97604488694527625, -13.89961937509977652, 86.87390960531436690 ) ) ;
#141844=CARTESIAN_POINT ( 'NONE',  ( 9.474510206698971260, -16.51473224551069308, 87.91557627198102409 ) ) ;
#141845=CARTESIAN_POINT ( 'NONE',  ( -21.52544592524343514, 5.823673210054127303, 61.04057627198103120 ) ) ;
#141846=CARTESIAN_POINT ( 'NONE',  ( -14.34966873604972548, 8.224510206698743886, 63.33442372801900433 ) ) ;
#141848=CARTESIAN_POINT ( 'NONE',  ( -19.05341960407611168, -5.049401038298163336, 61.45724293864769550 ) ) ;
#141849=CARTESIAN_POINT ( 'NONE',  ( -10.72451020669898014, 18.67979575497178502, 65.41557627198102409 ) ) ;
#141850=CARTESIAN_POINT ( 'NONE',  ( -19.03943276465977164, -0.05219959533935918106, 88.75109039468567573 ) ) ;
#141851=CARTESIAN_POINT ( 'NONE',  ( 16.52544592524342804, -4.483927247898539470, 23.54057627198102765 ) ) ;
#141852=CARTESIAN_POINT ( 'NONE',  ( -15.72974639402176322, -15.80617190586768395, 44.37609039468567573 ) ) ;
#141854=CARTESIAN_POINT ( 'NONE',  ( 12.06949235617739724, 12.14591786802326823, 66.87609039468568994 ) ) ;
#141855=CARTESIAN_POINT ( 'NONE',  ( -12.14591786802326823, 12.06949235617739902, 98.12609039468570415 ) ) ;
#141857=CARTESIAN_POINT ( 'NONE',  ( 12.14591786802327356, -12.06949235617739191, 80.62609039468567573 ) ) ;
#141858=CARTESIAN_POINT ( 'NONE',  ( 0.05219959533934541429, -16.53943276465976808, 30.00109039468568284 ) ) ;
#141859=CARTESIAN_POINT ( 'NONE',  ( -9.564922557960796823, -16.46253265017161027, 52.08224293864768839 ) ) ;
#141860=CARTESIAN_POINT ( 'NONE',  ( -5.153800228976328057, -19.02544592524343514, 52.29057627198100988 ) ) ;
#141861=CARTESIAN_POINT ( 'NONE',  ( 16.46253265017160672, -9.564922557960803928, 63.33224293864769550 ) ) ;
#141862=CARTESIAN_POINT ( 'NONE',  ( 10.81492255796106328, -18.62759615963255655, 55.41775706135234714 ) ) ;
#141863=CARTESIAN_POINT ( 'NONE',  ( -14.34966873604972548, 8.224510206698743886, 48.33442372801902565 ) ) ;
#141864=CARTESIAN_POINT ( 'NONE',  ( 0.05219959533910956823, 16.53943276465976808, 34.99890960531435979 ) ) ;
#141865=CARTESIAN_POINT ( 'NONE',  ( 9.474510206698971260, -16.51473224551069308, 22.91557627198102765 ) ) ;
#141866=CARTESIAN_POINT ( 'NONE',  ( -13.89961937509977652, 13.97604488694528158, 35.62390960531435269 ) ) ;
#141867=CARTESIAN_POINT ( 'NONE',  ( 16.53943276465976808, 0.05219959533934440121, 26.25109039468567573 ) ) ;
#141868=CARTESIAN_POINT ( 'NONE',  ( 19.05341960407617918, -5.049401038297876454, 86.04275706135233293 ) ) ;
#141869=CARTESIAN_POINT ( 'NONE',  ( -4.483927247898539470, -16.52544592524342804, 77.29057627198102409 ) ) ;
#141870=CARTESIAN_POINT ( 'NONE',  ( 9.474510206698971260, -16.51473224551069308, 52.91557627198102409 ) ) ;
#141871=CARTESIAN_POINT ( 'NONE',  ( 5.049401038297881783, 19.05341960407617563, 72.29275706135234714 ) ) ;
#141872=CARTESIAN_POINT ( 'NONE',  ( -17.49999999999999645, -5.499999999999992895, 54.20309617465830598 ) ) ;
#141873=CARTESIAN_POINT ( 'NONE',  ( 21.53943276465977519, 0.05219959533937863772, 81.25109039468568994 ) ) ;
#141874=CARTESIAN_POINT ( 'NONE',  ( -16.52544592524335698, -4.483927247898792601, 53.95942372801900433 ) ) ;
#141876=CARTESIAN_POINT ( 'NONE',  ( 5.719274019375991003, -21.55341960407610458, 37.70724293864769550 ) ) ;
#141877=CARTESIAN_POINT ( 'NONE',  ( 16.52544592524335698, 4.483927247898782831, 36.45942372801901143 ) ) ;
#141878=CARTESIAN_POINT ( 'NONE',  ( -13.89961937509977830, 13.97604488694528158, 25.62390960531435269 ) ) ;
#141879=CARTESIAN_POINT ( 'NONE',  ( -5.153800228976607833, 19.02544592524334988, 27.70942372801899722 ) ) ;
#141881=CARTESIAN_POINT ( 'NONE',  ( 5.049401038298161559, -19.05341960407611168, 42.70724293864767418 ) ) ;
#141883=CARTESIAN_POINT ( 'NONE',  ( -13.97604488694527625, -13.89961937509977652, 66.87390960531436690 ) ) ;
#141884=CARTESIAN_POINT ( 'NONE',  ( 17.50000000000000711, -3.512728167236853771, 112.7280999518112310 ) ) ;
#141885=CARTESIAN_POINT ( 'NONE',  ( -9.474510206698720793, -16.51473224551083518, 19.58442372801899722 ) ) ;
#141886=CARTESIAN_POINT ( 'NONE',  ( 4.483927247898545687, 16.52544592524342804, 39.79057627198103830 ) ) ;
#141887=CARTESIAN_POINT ( 'NONE',  ( -19.02544592524342804, 5.153800228976336051, 41.04057627198103120 ) ) ;
#141888=CARTESIAN_POINT ( 'NONE',  ( -13.89961937509977652, 13.97604488694528158, 105.6239096053143527 ) ) ;
#141889=CARTESIAN_POINT ( 'NONE',  ( 21.52544592524334988, 5.823673210054432836, 66.45942372801903275 ) ) ;
#141890=CARTESIAN_POINT ( 'NONE',  ( -16.46253265017160317, 9.564922557960807481, 55.83224293864769550 ) ) ;
#141891=CARTESIAN_POINT ( 'NONE',  ( -15.80617190586768217, 15.72974639402176855, 63.12609039468568994 ) ) ;
#141892=CARTESIAN_POINT ( 'NONE',  ( 5.153800228976335163, 19.02544592524342804, 114.7905762719810241 ) ) ;
#141893=CARTESIAN_POINT ( 'NONE',  ( -5.153800228976328057, -19.02544592524343514, 37.29057627198102409 ) ) ;
#141894=CARTESIAN_POINT ( 'NONE',  ( 10.72451020669871369, 18.67979575497193778, 27.08442372801901854 ) ) ;
#141895=CARTESIAN_POINT ( 'NONE',  ( -0.05219959533936034679, 19.03943276465977164, 42.50109039468566152 ) ) ;
#141896=CARTESIAN_POINT ( 'NONE',  ( -4.379528057220328563, 16.55341960407611168, 115.2072429386476955 ) ) ;
#141897=CARTESIAN_POINT ( 'NONE',  ( -5.153800228976328057, -19.02544592524343514, 67.29057627198102409 ) ) ;
#141898=CARTESIAN_POINT ( 'NONE',  ( 16.53943276465976808, 0.05219959533934440121, 21.25109039468567218 ) ) ;
#141899=CARTESIAN_POINT ( 'NONE',  ( 8.314922557960818139, 14.29746914071049879, 79.58224293864769550 ) ) ;
#141900=CARTESIAN_POINT ( 'NONE',  ( 10.81492255796078972, 18.62759615963270932, 34.58224293864770260 ) ) ;
#141901=CARTESIAN_POINT ( 'NONE',  ( 13.97604488694548053, -13.89961937509957401, 100.6260903946856615 ) ) ;
#141902=CARTESIAN_POINT ( 'NONE',  ( -21.52544592524343514, 5.823673210054127303, 111.0405762719810525 ) ) ;
#141903=CARTESIAN_POINT ( 'NONE',  ( -10.81492255796105439, 18.62759615963255655, 57.91775706135234714 ) ) ;
#141904=CARTESIAN_POINT ( 'NONE',  ( -8.314922557961024197, 14.29746914071037800, 57.91775706135234714 ) ) ;
#141905=CARTESIAN_POINT ( 'NONE',  ( 16.52544592524335698, 4.483927247898782831, 56.45942372801902565 ) ) ;
#141906=CARTESIAN_POINT ( 'NONE',  ( 15.80617190586746368, 15.72974639402197994, 54.37390960531435979 ) ) ;
#141907=CARTESIAN_POINT ( 'NONE',  ( 19.05341960407611168, 5.049401038298154454, 53.95724293864770260 ) ) ;
#141908=CARTESIAN_POINT ( 'NONE',  ( -12.14591786802326823, 12.06949235617739902, 78.12609039468570415 ) ) ;
#141909=CARTESIAN_POINT ( 'NONE',  ( -21.53943276465977519, 0.05219959533907696930, 96.24890960531435269 ) ) ;
#141910=CARTESIAN_POINT ( 'NONE',  ( 8.224510206698953496, -14.34966873604960469, 52.91557627198103830 ) ) ;
#141911=CARTESIAN_POINT ( 'NONE',  ( 19.05341960407611168, 5.049401038298154454, 68.95724293864769550 ) ) ;
#141912=CARTESIAN_POINT ( 'NONE',  ( -8.314922557961024197, 14.29746914071037800, 77.91775706135231871 ) ) ;
#141913=CARTESIAN_POINT ( 'NONE',  ( -13.97604488694547697, 13.89961937509957934, 113.1260903946856757 ) ) ;
#141914=CARTESIAN_POINT ( 'NONE',  ( -21.53943276465977519, 0.05219959533907696930, 101.2489096053143669 ) ) ;
#141915=CARTESIAN_POINT ( 'NONE',  ( 14.34966873604960469, 8.224510206698951720, 39.16557627198102409 ) ) ;
#141917=CARTESIAN_POINT ( 'NONE',  ( -17.13100169013299734, 6.664070546373147330, 75.76789835699851494 ) ) ;
#141918=CARTESIAN_POINT ( 'NONE',  ( -21.52544592524343514, 5.823673210054127303, 86.04057627198102409 ) ) ;
#141919=CARTESIAN_POINT ( 'NONE',  ( 16.53943276465976808, -0.05219959533910856209, 28.74890960531435624 ) ) ;
#141920=VERTEX_POINT ( 'NONE', #133186 ) ;
#141922=CARTESIAN_POINT ( 'NONE',  ( -18.67979575497178146, -10.72451020669898902, 96.66557627198102409 ) ) ;
#141923=CARTESIAN_POINT ( 'NONE',  ( 19.03943276465977164, -0.05219959533909143690, 98.74890960531436690 ) ) ;
#141924=CARTESIAN_POINT ( 'NONE',  ( 15.80617190586769283, -15.72974639402175789, 25.62609039468567929 ) ) ;
#141925=CARTESIAN_POINT ( 'NONE',  ( -14.34966873604960291, -8.224510206698953496, 46.66557627198102409 ) ) ;
#141926=CARTESIAN_POINT ( 'NONE',  ( 0.05219959533934541429, -16.53943276465976808, 45.00109039468568284 ) ) ;
#141927=CARTESIAN_POINT ( 'NONE',  ( 13.97604488694527802, 13.89961937509977652, 54.37390960531435979 ) ) ;
#141928=CARTESIAN_POINT ( 'NONE',  ( -5.153800228976607833, 19.02544592524334988, 57.70942372801899012 ) ) ;
#141929=CARTESIAN_POINT ( 'NONE',  ( 5.153800228976335163, 19.02544592524342804, 84.79057627198099567 ) ) ;
#141930=CARTESIAN_POINT ( 'NONE',  ( -21.55341960407610458, -5.719274019375992779, 36.45724293864768839 ) ) ;
#141932=CARTESIAN_POINT ( 'NONE',  ( -12.06949235617739369, -12.14591786802326823, 19.37609039468568639 ) ) ;
#141933=CARTESIAN_POINT ( 'NONE',  ( 9.474510206698729675, 16.51473224551082808, 52.08442372801900433 ) ) ;
#141934=CARTESIAN_POINT ( 'NONE',  ( -18.67979575497178146, -10.72451020669898902, 101.6655762719810383 ) ) ;
#141935=CARTESIAN_POINT ( 'NONE',  ( -4.379528057220328563, 16.55341960407611168, 40.20724293864769550 ) ) ;
#141936=CARTESIAN_POINT ( 'NONE',  ( -9.474510206698964154, 16.51473224551069663, 75.41557627198103830 ) ) ;
#141937=CARTESIAN_POINT ( 'NONE',  ( -15.80617190586745835, -15.72974639402198527, 56.87390960531436690 ) ) ;
#141938=CARTESIAN_POINT ( 'NONE',  ( -18.62759615963270932, 10.81492255796079327, 90.83224293864769550 ) ) ;
#141939=CARTESIAN_POINT ( 'NONE',  ( -12.06949235617739369, -12.14591786802326823, 19.37609039468568639 ) ) ;
#141940=CARTESIAN_POINT ( 'NONE',  ( -13.97604488694527625, -13.89961937509977652, 111.8739096053143243 ) ) ;
#141941=CARTESIAN_POINT ( 'NONE',  ( -10.81492255796105439, 18.62759615963255655, 92.91775706135236135 ) ) ;
#141942=CARTESIAN_POINT ( 'NONE',  ( 16.46253265017160672, -9.564922557960803928, 83.33224293864768129 ) ) ;
#141944=CARTESIAN_POINT ( 'NONE',  ( -9.564922557960796823, -16.46253265017161027, 27.08224293864769550 ) ) ;
#141945=CARTESIAN_POINT ( 'NONE',  ( 5.049401038298161559, -19.05341960407611168, 87.70724293864769550 ) ) ;
#141946=CARTESIAN_POINT ( 'NONE',  ( -16.53943276465976808, 0.05219959533911058130, 106.2489096053143811 ) ) ;
#141947=CARTESIAN_POINT ( 'NONE',  ( 19.02544592524343514, -5.153800228976328945, 63.54057627198103830 ) ) ;
#141948=CARTESIAN_POINT ( 'NONE',  ( 14.34966873604972726, -8.224510206698740333, 20.83442372801901143 ) ) ;
#141950=EDGE_CURVE ( 'NONE', #56021, #184472, #149365, .T. ) ;
#141951=CARTESIAN_POINT ( 'NONE',  ( 5.153800228976335163, 19.02544592524342804, 79.79057627198102409 ) ) ;
#141952=CARTESIAN_POINT ( 'NONE',  ( -10.81492255796105439, 18.62759615963255655, 97.91775706135236135 ) ) ;
#141953=CARTESIAN_POINT ( 'NONE',  ( 19.03943276465977164, -0.05219959533909143690, 113.7489096053143669 ) ) ;
#141954=CARTESIAN_POINT ( 'NONE',  ( -14.29746914071037622, -8.314922557961029526, 94.16775706135237556 ) ) ;
#141956=CARTESIAN_POINT ( 'NONE',  ( -0.05219959533936034679, 19.03943276465977164, 67.50109039468566152 ) ) ;
#141957=CARTESIAN_POINT ( 'NONE',  ( 10.81492255796106328, -18.62759615963255655, 110.4177570613523756 ) ) ;
#141959=CARTESIAN_POINT ( 'NONE',  ( 13.97604488694527802, 13.89961937509977652, 29.37390960531435979 ) ) ;
#141960=CARTESIAN_POINT ( 'NONE',  ( 16.52544592524342804, -4.483927247898539470, 33.54057627198102409 ) ) ;
#141962=CARTESIAN_POINT ( 'NONE',  ( 16.53943276465976808, 0.05219959533934440121, 101.2510903946856757 ) ) ;
#141964=CARTESIAN_POINT ( 'NONE',  ( -8.224510206698735004, -14.34966873604973081, 79.58442372801903275 ) ) ;
#141965=CARTESIAN_POINT ( 'NONE',  ( -19.05341960407611168, -5.049401038298163336, 41.45724293864769550 ) ) ;
#141966=CARTESIAN_POINT ( 'NONE',  ( -15.80617190586768217, 15.72974639402176855, 93.12609039468568994 ) ) ;
#141967=CARTESIAN_POINT ( 'NONE',  ( -9.564922557961040184, 16.46253265017147172, 107.9177570613523471 ) ) ;
#141968=CARTESIAN_POINT ( 'NONE',  ( 0.05219959533937995610, -21.53943276465977519, 75.00109039468568994 ) ) ;
#141969=CARTESIAN_POINT ( 'NONE',  ( -5.049401038297874678, -19.05341960407617918, 49.79275706135231871 ) ) ;
#141970=CARTESIAN_POINT ( 'NONE',  ( 13.97604488694527802, 13.89961937509977652, 84.37390960531433848 ) ) ;
#141971=CARTESIAN_POINT ( 'NONE',  ( 13.97604488694527802, 13.89961937509977652, 74.37390960531436690 ) ) ;
#141974=CARTESIAN_POINT ( 'NONE',  ( 12.06949235617757843, -12.14591786802309237, 63.12390960531435979 ) ) ;
#141975=CARTESIAN_POINT ( 'NONE',  ( 10.72451020669898902, -18.67979575497178502, 67.91557627198102409 ) ) ;
#141976=CARTESIAN_POINT ( 'NONE',  ( -16.46253265017160317, 9.564922557960807481, 40.83224293864769550 ) ) ;
#141977=CARTESIAN_POINT ( 'NONE',  ( -21.52544592524343514, 5.823673210054127303, 86.04057627198102409 ) ) ;
#141978=CARTESIAN_POINT ( 'NONE',  ( 4.379528057220092307, 16.55341960407617563, 77.29275706135234714 ) ) ;
#141980=CARTESIAN_POINT ( 'NONE',  ( -4.379528057220328563, 16.55341960407611168, 80.20724293864769550 ) ) ;
#141982=CARTESIAN_POINT ( 'NONE',  ( -4.483927247898782831, 16.52544592524335698, 32.70942372801900433 ) ) ;
#141983=CARTESIAN_POINT ( 'NONE',  ( 16.46253265017160672, -9.564922557960803928, 23.33224293864769194 ) ) ;
#141984=CARTESIAN_POINT ( 'NONE',  ( 16.46253265017146816, 9.564922557961045513, 71.66775706135233293 ) ) ;
#141985=CARTESIAN_POINT ( 'NONE',  ( 12.06949235617757843, -12.14591786802309237, 73.12390960531436690 ) ) ;
#141986=CARTESIAN_POINT ( 'NONE',  ( 18.67979575497194134, -10.72451020669871369, 45.83442372801901854 ) ) ;
#141987=CARTESIAN_POINT ( 'NONE',  ( 19.03943276465977164, -0.05219959533909143690, 23.74890960531435269 ) ) ;
#141988=CARTESIAN_POINT ( 'NONE',  ( -0.05219959533907301413, -21.53943276465977519, 97.49890960531436690 ) ) ;
#141989=CARTESIAN_POINT ( 'NONE',  ( 19.03943276465977164, -0.05219959533909143690, 113.7489096053143669 ) ) ;
#141990=CARTESIAN_POINT ( 'NONE',  ( -12.06949235617756955, 12.14591786802309770, 90.62390960531436690 ) ) ;
#141992=CARTESIAN_POINT ( 'NONE',  ( 19.02544592524343514, -5.153800228976328945, 43.54057627198103120 ) ) ;
#141994=CARTESIAN_POINT ( 'NONE',  ( -0.05219959533936034679, 19.03943276465977164, 82.50109039468567573 ) ) ;
#141995=CARTESIAN_POINT ( 'NONE',  ( 21.53943276465977519, 0.05219959533937863772, 36.25109039468567573 ) ) ;
#141996=CARTESIAN_POINT ( 'NONE',  ( 13.97604488694527802, 13.89961937509977652, 69.37390960531436690 ) ) ;
#141997=CARTESIAN_POINT ( 'NONE',  ( 13.89961937509957401, 13.97604488694547697, 61.87609039468566863 ) ) ;
#141998=CARTESIAN_POINT ( 'NONE',  ( 5.049401038298161559, -19.05341960407611168, 42.70724293864767418 ) ) ;
#141999=CARTESIAN_POINT ( 'NONE',  ( -4.483927247898539470, -16.52544592524342804, 67.29057627198103830 ) ) ;
#142000=CARTESIAN_POINT ( 'NONE',  ( -12.06949235617756955, 12.14591786802309770, 50.62390960531435979 ) ) ;
#142001=CARTESIAN_POINT ( 'NONE',  ( -16.46253265017160317, 9.564922557960807481, 70.83224293864770971 ) ) ;
#142002=CARTESIAN_POINT ( 'NONE',  ( -18.67979575497178146, -10.72451020669898902, 96.66557627198102409 ) ) ;
#142003=CARTESIAN_POINT ( 'NONE',  ( -0.05219959533909027116, -19.03943276465977164, 67.49890960531436690 ) ) ;
#142004=CARTESIAN_POINT ( 'NONE',  ( -18.62759615963270932, 10.81492255796079327, 80.83224293864769550 ) ) ;
#142005=CARTESIAN_POINT ( 'NONE',  ( -21.53943276465977519, -0.05219959533937600094, 108.7510903946857042 ) ) ;
#142006=CARTESIAN_POINT ( 'NONE',  ( 13.89961937509977652, -13.97604488694527269, 33.12390960531434558 ) ) ;
#142007=CARTESIAN_POINT ( 'NONE',  ( -8.224510206698735004, -14.34966873604973081, 104.5844237280190185 ) ) ;
#142008=CARTESIAN_POINT ( 'NONE',  ( -16.52544592524342804, 4.483927247898546575, 91.04057627198103830 ) ) ;
#142009=CARTESIAN_POINT ( 'NONE',  ( 13.89961937509957401, 13.97604488694547697, 106.8760903946856757 ) ) ;
#142011=CARTESIAN_POINT ( 'NONE',  ( 15.72974639402176855, 15.80617190586768217, 31.87609039468567929 ) ) ;
#142012=CARTESIAN_POINT ( 'NONE',  ( 9.564922557961047289, -16.46253265017146816, 55.41775706135234003 ) ) ;
#142013=CARTESIAN_POINT ( 'NONE',  ( -12.06949235617756955, 12.14591786802309770, 25.62390960531435624 ) ) ;
#142014=CARTESIAN_POINT ( 'NONE',  ( 21.55341960407610458, 5.719274019375980345, 78.95724293864769550 ) ) ;
#142015=CARTESIAN_POINT ( 'NONE',  ( -9.564922557960796823, -16.46253265017161027, 102.0822429386477097 ) ) ;
#142016=CARTESIAN_POINT ( 'NONE',  ( -0.05219959533910754901, -16.53943276465976808, 57.49890960531435979 ) ) ;
#142017=CARTESIAN_POINT ( 'NONE',  ( -16.46253265017160317, 9.564922557960807481, 35.83224293864768839 ) ) ;
#142018=CARTESIAN_POINT ( 'NONE',  ( -13.97604488694527625, -13.89961937509977652, 31.87390960531435979 ) ) ;
#142019=CARTESIAN_POINT ( 'NONE',  ( -16.51473224551082808, 9.474510206698731452, 28.33442372801900433 ) ) ;
#142020=CARTESIAN_POINT ( 'NONE',  ( -12.06949235617739369, -12.14591786802326823, 94.37609039468568994 ) ) ;
#142021=CARTESIAN_POINT ( 'NONE',  ( 10.81492255796106328, -18.62759615963255655, 35.41775706135234003 ) ) ;
#142022=CARTESIAN_POINT ( 'NONE',  ( 8.224510206698742110, 14.34966873604972548, 42.08442372801901854 ) ) ;
#142023=CARTESIAN_POINT ( 'NONE',  ( -9.474510206698964154, 16.51473224551069663, 115.4155762719810241 ) ) ;
#142024=CARTESIAN_POINT ( 'NONE',  ( 16.51473224551069308, 9.474510206698969483, 49.16557627198102409 ) ) ;
#142025=CARTESIAN_POINT ( 'NONE',  ( -10.72451020669870658, -18.67979575497194134, 99.58442372801900433 ) ) ;
#142026=CARTESIAN_POINT ( 'NONE',  ( -16.46253265017160317, 9.564922557960807481, 80.83224293864769550 ) ) ;
#142027=CARTESIAN_POINT ( 'NONE',  ( -16.52544592524335698, -4.483927247898792601, 58.95942372801902565 ) ) ;
#142028=CARTESIAN_POINT ( 'NONE',  ( 16.53943276465976808, -0.05219959533910856209, 103.7489096053143669 ) ) ;
#142030=CARTESIAN_POINT ( 'NONE',  ( 12.14591786802327356, -12.06949235617739191, 110.6260903946857042 ) ) ;
#142031=CARTESIAN_POINT ( 'NONE',  ( -17.58332526062525858, 7.635886036038558977, 50.92334959558467489 ) ) ;
#142032=CARTESIAN_POINT ( 'NONE',  ( 15.72974639402176855, 15.80617190586768217, 56.87609039468568994 ) ) ;
#142033=CARTESIAN_POINT ( 'NONE',  ( -9.564922557960796823, -16.46253265017161027, 97.08224293864769550 ) ) ;
#142034=CARTESIAN_POINT ( 'NONE',  ( -5.049401038298153566, 19.05341960407611168, 75.20724293864769550 ) ) ;
#142035=CARTESIAN_POINT ( 'NONE',  ( 16.51473224551069308, 9.474510206698969483, 104.1655762719810241 ) ) ;
#142036=CARTESIAN_POINT ( 'NONE',  ( 0.05219959533910956823, 16.53943276465976808, 49.99890960531437401 ) ) ;
#142037=CARTESIAN_POINT ( 'NONE',  ( 4.483927247898545687, 16.52544592524342804, 24.79057627198103120 ) ) ;
#142038=CARTESIAN_POINT ( 'NONE',  ( -16.53943276465976808, 0.05219959533911058130, 36.24890960531435979 ) ) ;
#142040=CARTESIAN_POINT ( 'NONE',  ( -9.564922557961040184, 16.46253265017147172, 32.91775706135233293 ) ) ;
#142041=CARTESIAN_POINT ( 'NONE',  ( -19.03943276465977164, 0.05219959533909376836, 81.24890960531436690 ) ) ;
#142042=CARTESIAN_POINT ( 'NONE',  ( -19.03943276465977164, -0.05219959533935918106, 48.75109039468566863 ) ) ;
#142045=CARTESIAN_POINT ( 'NONE',  ( -19.02544592524334988, -5.153800228976617603, 83.95942372801901854 ) ) ;
#142046=CARTESIAN_POINT ( 'NONE',  ( -14.34966873604972548, 8.224510206698743886, 68.33442372801900433 ) ) ;
#142047=CARTESIAN_POINT ( 'NONE',  ( 16.29526858892874941, 7.335722546920129261, 93.29670597800205201 ) ) ;
#142048=CARTESIAN_POINT ( 'NONE',  ( 19.03943276465977164, -0.05219959533909143690, 103.7489096053143669 ) ) ;
#142049=CARTESIAN_POINT ( 'NONE',  ( 15.72974639402176855, 15.80617190586768217, 31.87609039468567929 ) ) ;
#142050=CARTESIAN_POINT ( 'NONE',  ( 5.153800228976615827, -19.02544592524334988, 90.20942372801900433 ) ) ;
#142051=CARTESIAN_POINT ( 'NONE',  ( 16.79531203550646978, 7.028104445595628746, 88.75244988220444498 ) ) ;
#142052=CARTESIAN_POINT ( 'NONE',  ( -9.474510206698964154, 16.51473224551069663, 45.41557627198103120 ) ) ;
#142053=CARTESIAN_POINT ( 'NONE',  ( 0.05219959533909260263, 19.03943276465977164, 89.99890960531436690 ) ) ;
#142054=CARTESIAN_POINT ( 'NONE',  ( -16.55341960407611168, -4.379528057220339221, 66.45724293864768129 ) ) ;
#142055=CARTESIAN_POINT ( 'NONE',  ( 19.02544592524343514, -5.153800228976328945, 43.54057627198103120 ) ) ;
#142056=CARTESIAN_POINT ( 'NONE',  ( -9.564922557960796823, -16.46253265017161027, 62.08224293864769550 ) ) ;
#142057=CARTESIAN_POINT ( 'NONE',  ( -9.474510206698720793, -16.51473224551083518, 64.58442372801900433 ) ) ;
#142058=CARTESIAN_POINT ( 'NONE',  ( -5.153800228976607833, 19.02544592524334988, 32.70942372801899722 ) ) ;
#142059=CARTESIAN_POINT ( 'NONE',  ( -13.97604488694527625, -13.89961937509977652, 66.87390960531436690 ) ) ;
#142060=CARTESIAN_POINT ( 'NONE',  ( 21.52544592524344225, -5.823673210054117533, 63.54057627198103830 ) ) ;
#142061=CARTESIAN_POINT ( 'NONE',  ( -4.483927247898539470, -16.52544592524342804, 67.29057627198103830 ) ) ;
#142062=CARTESIAN_POINT ( 'NONE',  ( -19.02544592524334988, -5.153800228976617603, 33.95942372801897591 ) ) ;
#142064=CARTESIAN_POINT ( 'NONE',  ( -5.719274019375978568, 21.55341960407610458, 50.20724293864769550 ) ) ;
#142065=CARTESIAN_POINT ( 'NONE',  ( -21.55341960407610458, -5.719274019375992779, 26.45724293864768839 ) ) ;
#142066=CARTESIAN_POINT ( 'NONE',  ( -0.05219959533909027116, -19.03943276465977164, 47.49890960531435979 ) ) ;
#142067=CARTESIAN_POINT ( 'NONE',  ( -5.049401038298153566, 19.05341960407611168, 35.20724293864768839 ) ) ;
#142068=CARTESIAN_POINT ( 'NONE',  ( 16.52544592524342804, -4.483927247898539470, 103.5405762719810383 ) ) ;
#142069=CARTESIAN_POINT ( 'NONE',  ( -5.719274019375978568, 21.55341960407610458, 115.2072429386476955 ) ) ;
#142070=CARTESIAN_POINT ( 'NONE',  ( 19.05341960407611168, 5.049401038298154454, 108.9572429386477097 ) ) ;
#142071=CARTESIAN_POINT ( 'NONE',  ( -15.72974639402176322, -15.80617190586768395, 29.37609039468568284 ) ) ;
#142072=CARTESIAN_POINT ( 'NONE',  ( 14.34966873604960469, 8.224510206698951720, 114.1655762719810383 ) ) ;
#142073=CARTESIAN_POINT ( 'NONE',  ( 5.719274019375673035, 21.55341960407619339, 82.29275706135234714 ) ) ;
#142074=CARTESIAN_POINT ( 'NONE',  ( 18.62759615963271287, -10.81492255796078972, 88.33224293864769550 ) ) ;
#142075=CARTESIAN_POINT ( 'NONE',  ( -5.049401038297874678, -19.05341960407617918, 49.79275706135231871 ) ) ;
#142076=CARTESIAN_POINT ( 'NONE',  ( 16.51473224551069308, 9.474510206698969483, 24.16557627198102765 ) ) ;
#142077=CARTESIAN_POINT ( 'NONE',  ( 5.153800228976335163, 19.02544592524342804, 24.79057627198102765 ) ) ;
#142079=CARTESIAN_POINT ( 'NONE',  ( 16.52544592524335698, 4.483927247898782831, 41.45942372801901143 ) ) ;
#142080=CARTESIAN_POINT ( 'NONE',  ( 4.483927247898545687, 16.52544592524342804, 114.7905762719810383 ) ) ;
#142082=CARTESIAN_POINT ( 'NONE',  ( 16.46253265017160672, -9.564922557960803928, 73.33224293864769550 ) ) ;
#142083=CARTESIAN_POINT ( 'NONE',  ( 8.224510206698953496, -14.34966873604960469, 87.91557627198103830 ) ) ;
#142084=CARTESIAN_POINT ( 'NONE',  ( 5.823673210054125526, 21.52544592524343514, 44.79057627198103120 ) ) ;
#142085=CARTESIAN_POINT ( 'NONE',  ( 16.55341960407611168, 4.379528057220329451, 73.95724293864769550 ) ) ;
#142086=CARTESIAN_POINT ( 'NONE',  ( 4.483927247898790824, -16.52544592524335698, 30.20942372801902565 ) ) ;
#142087=CARTESIAN_POINT ( 'NONE',  ( 18.62759615963255655, 10.81492255796105972, 86.66775706135234714 ) ) ;
#142088=CARTESIAN_POINT ( 'NONE',  ( -5.049401038298153566, 19.05341960407611168, 30.20724293864768839 ) ) ;
#142089=CARTESIAN_POINT ( 'NONE',  ( -16.55341960407617563, 4.379528057220093196, 103.5427570613523613 ) ) ;
#142090=CARTESIAN_POINT ( 'NONE',  ( -14.29746914071049879, 8.314922557960819915, 45.83224293864769550 ) ) ;
#142092=CARTESIAN_POINT ( 'NONE',  ( 5.153800228976335163, 19.02544592524342804, 54.79057627198103120 ) ) ;
#142093=CARTESIAN_POINT ( 'NONE',  ( -15.80617190586768217, 15.72974639402176855, 98.12609039468570415 ) ) ;
#142094=CARTESIAN_POINT ( 'NONE',  ( 15.72974639402199770, -15.80617190586745480, 103.1239096053143811 ) ) ;
#142095=CARTESIAN_POINT ( 'NONE',  ( -0.05219959533937732626, 21.53943276465977519, 77.50109039468567573 ) ) ;
#142096=CARTESIAN_POINT ( 'NONE',  ( -14.29746914071037622, -8.314922557961029526, 34.16775706135234714 ) ) ;
#142097=CARTESIAN_POINT ( 'NONE',  ( -4.379528057220328563, 16.55341960407611168, 70.20724293864769550 ) ) ;
#142098=CARTESIAN_POINT ( 'NONE',  ( 10.81492255796106328, -18.62759615963255655, 90.41775706135236135 ) ) ;
#142099=CARTESIAN_POINT ( 'NONE',  ( 16.52544592524342804, -4.483927247898539470, 23.54057627198102765 ) ) ;
#142100=CARTESIAN_POINT ( 'NONE',  ( 16.38665767534995865, -7.295008042176399421, 47.76400864214470232 ) ) ;
#142102=CARTESIAN_POINT ( 'NONE',  ( 14.34966873604960469, 8.224510206698951720, 44.16557627198103120 ) ) ;
#142103=CARTESIAN_POINT ( 'NONE',  ( 4.379528057220092307, 16.55341960407617563, 77.29275706135234714 ) ) ;
#142104=CARTESIAN_POINT ( 'NONE',  ( 9.564922557960805705, 16.46253265017160317, 84.58224293864769550 ) ) ;
#142105=CARTESIAN_POINT ( 'NONE',  ( -19.03943276465977164, 0.05219959533909376836, 96.24890960531436690 ) ) ;
#142106=CARTESIAN_POINT ( 'NONE',  ( -15.80617190586768217, 15.72974639402176855, 88.12609039468570415 ) ) ;
#142107=CARTESIAN_POINT ( 'NONE',  ( 12.06949235617739724, 12.14591786802326823, 86.87609039468568994 ) ) ;
#142108=CARTESIAN_POINT ( 'NONE',  ( 4.483927247898545687, 16.52544592524342804, 69.79057627198102409 ) ) ;
#142109=CARTESIAN_POINT ( 'NONE',  ( 5.049401038298161559, -19.05341960407611168, 82.70724293864770971 ) ) ;
#142111=CARTESIAN_POINT ( 'NONE',  ( -12.14591786802326823, 12.06949235617739902, 33.12609039468569705 ) ) ;
#142112=CARTESIAN_POINT ( 'NONE',  ( -5.153800228976328057, -19.02544592524343514, 27.29057627198103120 ) ) ;
#142113=CARTESIAN_POINT ( 'NONE',  ( -19.03943276465977164, 0.05219959533909376836, 96.24890960531436690 ) ) ;
#142114=CARTESIAN_POINT ( 'NONE',  ( 16.52544592524335698, 4.483927247898782831, 26.45942372801901854 ) ) ;
#142116=CARTESIAN_POINT ( 'NONE',  ( 5.719274019375673035, 21.55341960407619339, 112.2927570613523471 ) ) ;
#142117=CARTESIAN_POINT ( 'NONE',  ( 4.483927247898790824, -16.52544592524335698, 100.2094237280190043 ) ) ;
#142118=CARTESIAN_POINT ( 'NONE',  ( 19.05341960407617918, -5.049401038297876454, 106.0427570613523471 ) ) ;
#142119=CARTESIAN_POINT ( 'NONE',  ( -19.03943276465977164, 0.05219959533909376836, 26.24890960531435624 ) ) ;
#142120=CARTESIAN_POINT ( 'NONE',  ( -16.52544592524335698, -4.483927247898792601, 83.95942372801900433 ) ) ;
#142121=CARTESIAN_POINT ( 'NONE',  ( -0.05219959533934338120, 16.53943276465976808, 67.50109039468568994 ) ) ;
#142123=CARTESIAN_POINT ( 'NONE',  ( 13.89961937509957401, 13.97604488694547697, 66.87609039468567573 ) ) ;
#142124=CARTESIAN_POINT ( 'NONE',  ( -5.719274019375665041, -21.55341960407619695, 104.7927570613523898 ) ) ;
#142125=CARTESIAN_POINT ( 'NONE',  ( -13.97604488694527625, -13.89961937509977652, 51.87390960531436690 ) ) ;
#142126=CARTESIAN_POINT ( 'NONE',  ( 19.05341960407611168, 5.049401038298154454, 93.95724293864769550 ) ) ;
#142127=CARTESIAN_POINT ( 'NONE',  ( -0.05219959533910754901, -16.53943276465976808, 82.49890960531436690 ) ) ;
#142128=CIRCLE ( 'NONE', #132471, 1.250000000000006439 ) ;
#142129=CARTESIAN_POINT ( 'NONE',  ( -9.564922557961040184, 16.46253265017147172, 52.91775706135233293 ) ) ;
#142130=CARTESIAN_POINT ( 'NONE',  ( -15.72974639402197994, 15.80617190586746368, 55.62390960531436690 ) ) ;
#142131=CARTESIAN_POINT ( 'NONE',  ( 19.03943276465977164, 0.05219959533936151252, 21.25109039468565797 ) ) ;
#142132=CARTESIAN_POINT ( 'NONE',  ( 5.049401038298161559, -19.05341960407611168, 87.70724293864769550 ) ) ;
#142133=CARTESIAN_POINT ( 'NONE',  ( 10.81492255796106328, -18.62759615963255655, 110.4177570613523756 ) ) ;
#142134=CARTESIAN_POINT ( 'NONE',  ( -15.80617190586745835, -15.72974639402198527, 61.87390960531436690 ) ) ;
#142135=CARTESIAN_POINT ( 'NONE',  ( -13.89961937509977652, 13.97604488694528158, 95.62390960531436690 ) ) ;
#142136=CARTESIAN_POINT ( 'NONE',  ( -9.474510206698720793, -16.51473224551083518, 84.58442372801900433 ) ) ;
#142137=CARTESIAN_POINT ( 'NONE',  ( 0.05219959533909260263, 19.03943276465977164, 104.9989096053143669 ) ) ;
#142138=CARTESIAN_POINT ( 'NONE',  ( -16.51473224551082808, 9.474510206698731452, 103.3344237280190043 ) ) ;
#142139=CARTESIAN_POINT ( 'NONE',  ( 4.483927247898545687, 16.52544592524342804, 114.7905762719810383 ) ) ;
#142140=CARTESIAN_POINT ( 'NONE',  ( -19.03943276465977164, 0.05219959533909376836, 86.24890960531436690 ) ) ;
#142141=CARTESIAN_POINT ( 'NONE',  ( -10.72451020669898014, 18.67979575497178502, 80.41557627198103830 ) ) ;
#142142=CARTESIAN_POINT ( 'NONE',  ( -16.53943276465976808, -0.05219959533934237506, 43.75109039468568284 ) ) ;
#142143=CARTESIAN_POINT ( 'NONE',  ( 18.67979575497194134, -10.72451020669871369, 45.83442372801901854 ) ) ;
#142144=CARTESIAN_POINT ( 'NONE',  ( 10.72451020669871369, 18.67979575497193778, 92.08442372801901854 ) ) ;
#142145=CARTESIAN_POINT ( 'NONE',  ( 0.05219959533934541429, -16.53943276465976808, 90.00109039468567573 ) ) ;
#142146=CARTESIAN_POINT ( 'NONE',  ( -5.049401038298153566, 19.05341960407611168, 90.20724293864766707 ) ) ;
#142147=CARTESIAN_POINT ( 'NONE',  ( -4.483927247898539470, -16.52544592524342804, 87.29057627198103830 ) ) ;
#142148=CARTESIAN_POINT ( 'NONE',  ( -4.379528057220328563, 16.55341960407611168, 25.20724293864769550 ) ) ;
#142149=CARTESIAN_POINT ( 'NONE',  ( -13.89961937509957401, -13.97604488694547875, 64.37609039468567573 ) ) ;
#142150=EDGE_CURVE ( 'NONE', #23884, #10184, #93846, .T. ) ;
#142151=CARTESIAN_POINT ( 'NONE',  ( -0.05219959533937732626, 21.53943276465977519, 42.50109039468567573 ) ) ;
#142152=CARTESIAN_POINT ( 'NONE',  ( 16.46253265017146816, 9.564922557961045513, 26.66775706135234003 ) ) ;
#142153=CARTESIAN_POINT ( 'NONE',  ( -16.55341960407611168, -4.379528057220339221, 86.45724293864770971 ) ) ;
#142154=CARTESIAN_POINT ( 'NONE',  ( 19.03943276465977164, -0.05219959533909143690, 113.7489096053143669 ) ) ;
#142155=CARTESIAN_POINT ( 'NONE',  ( -8.314922557961024197, 14.29746914071037800, 112.9177570613523329 ) ) ;
#142156=CARTESIAN_POINT ( 'NONE',  ( 10.81492255796106328, -18.62759615963255655, 90.41775706135236135 ) ) ;
#142157=CARTESIAN_POINT ( 'NONE',  ( -14.34966873604972548, 8.224510206698743886, 58.33442372801901143 ) ) ;
#142158=CARTESIAN_POINT ( 'NONE',  ( -16.52544592524335698, -4.483927247898792601, 103.9594237280190185 ) ) ;
#142159=CARTESIAN_POINT ( 'NONE',  ( 5.719274019375673035, 21.55341960407619339, 57.29275706135234714 ) ) ;
#142161=CARTESIAN_POINT ( 'NONE',  ( -18.62759615963255300, -10.81492255796106328, 34.16775706135234714 ) ) ;
#142162=CARTESIAN_POINT ( 'NONE',  ( -0.05219959533910754901, -16.53943276465976808, 102.4989096053143811 ) ) ;
#142163=CARTESIAN_POINT ( 'NONE',  ( 13.97604488694527802, 13.89961937509977652, 29.37390960531435979 ) ) ;
#142164=CARTESIAN_POINT ( 'NONE',  ( -8.314922557960811034, -14.29746914071050412, 62.08224293864769550 ) ) ;
#142165=CARTESIAN_POINT ( 'NONE',  ( 16.46253265017160672, -9.564922557960803928, 73.33224293864769550 ) ) ;
#142166=CARTESIAN_POINT ( 'NONE',  ( -16.55341960407617563, 4.379528057220093196, 103.5427570613523613 ) ) ;
#142167=CARTESIAN_POINT ( 'NONE',  ( 5.153800228976335163, 19.02544592524342804, 34.79057627198102409 ) ) ;
#142168=CARTESIAN_POINT ( 'NONE',  ( 0.05219959533907565091, 21.53943276465977519, 49.99890960531437401 ) ) ;
#142169=CARTESIAN_POINT ( 'NONE',  ( 16.52544592524342804, -4.483927247898539470, 88.54057627198103830 ) ) ;
#142170=CARTESIAN_POINT ( 'NONE',  ( 10.81492255796078972, 18.62759615963270932, 89.58224293864768129 ) ) ;
#142171=CARTESIAN_POINT ( 'NONE',  ( -19.05341960407611168, -5.049401038298163336, 101.4572429386476955 ) ) ;
#142172=CARTESIAN_POINT ( 'NONE',  ( 16.51473224551069308, 9.474510206698969483, 49.16557627198102409 ) ) ;
#142173=CARTESIAN_POINT ( 'NONE',  ( 16.46253265017146816, 9.564922557961045513, 86.66775706135233293 ) ) ;
#142174=CARTESIAN_POINT ( 'NONE',  ( 10.81492255796078972, 18.62759615963270932, 39.58224293864769550 ) ) ;
#142175=CARTESIAN_POINT ( 'NONE',  ( 5.719274019375673035, 21.55341960407619339, 72.29275706135236135 ) ) ;
#142176=CARTESIAN_POINT ( 'NONE',  ( -19.03943276465977164, 0.05219959533909376836, 56.24890960531435979 ) ) ;
#142177=CARTESIAN_POINT ( 'NONE',  ( 0.05219959533909260263, 19.03943276465977164, 79.99890960531436690 ) ) ;
#142178=CARTESIAN_POINT ( 'NONE',  ( 16.52544592524335698, 4.483927247898782831, 61.45942372801901854 ) ) ;
#142179=CARTESIAN_POINT ( 'NONE',  ( -15.80617190586768217, 15.72974639402176855, 38.12609039468567573 ) ) ;
#142180=CARTESIAN_POINT ( 'NONE',  ( 5.823673210054444382, -21.52544592524334988, 70.20942372801904696 ) ) ;
#142181=CARTESIAN_POINT ( 'NONE',  ( -0.05219959533907301413, -21.53943276465977519, 22.49890960531436335 ) ) ;
#142182=CARTESIAN_POINT ( 'NONE',  ( 0.05219959533907565091, 21.53943276465977519, 99.99890960531436690 ) ) ;
#142183=CARTESIAN_POINT ( 'NONE',  ( -21.53943276465977519, -0.05219959533937600094, 33.75109039468568284 ) ) ;
#142184=CARTESIAN_POINT ( 'NONE',  ( -14.34966873604972548, 8.224510206698743886, 58.33442372801901143 ) ) ;
#142185=CARTESIAN_POINT ( 'NONE',  ( 21.55341960407610458, 5.719274019375980345, 58.95724293864770971 ) ) ;
#142186=CARTESIAN_POINT ( 'NONE',  ( 13.89961937509957401, 13.97604488694547697, 36.87609039468565442 ) ) ;
#142187=CARTESIAN_POINT ( 'NONE',  ( -0.05219959533909027116, -19.03943276465977164, 72.49890960531435269 ) ) ;
#142188=CARTESIAN_POINT ( 'NONE',  ( 12.14591786802309770, 12.06949235617756955, 29.37390960531435269 ) ) ;
#142189=CARTESIAN_POINT ( 'NONE',  ( -17.49999999999998934, -4.640572885337569176, 104.3621183545115940 ) ) ;
#142190=CARTESIAN_POINT ( 'NONE',  ( 16.51473224551069308, 9.474510206698969483, 104.1655762719810241 ) ) ;
#142192=ADVANCED_FACE ( 'NONE', ( #139154 ), #142380, .T. ) ;
#142193=CARTESIAN_POINT ( 'NONE',  ( 19.05341960407617918, -5.049401038297876454, 86.04275706135233293 ) ) ;
#142194=CARTESIAN_POINT ( 'NONE',  ( 21.53943276465977519, -0.05219959533907433946, 63.74890960531435979 ) ) ;
#142195=CARTESIAN_POINT ( 'NONE',  ( 16.53943276465976808, -0.05219959533910856209, 33.74890960531436690 ) ) ;
#142196=CARTESIAN_POINT ( 'NONE',  ( -19.02544592524334988, -5.153800228976617603, 108.9594237280189759 ) ) ;
#142197=CARTESIAN_POINT ( 'NONE',  ( 5.049401038298161559, -19.05341960407611168, 27.70724293864769550 ) ) ;
#142198=CARTESIAN_POINT ( 'NONE',  ( -0.05219959533936034679, 19.03943276465977164, 107.5010903946856615 ) ) ;
#142199=CARTESIAN_POINT ( 'NONE',  ( 15.80617190586746368, 15.72974639402197994, 84.37390960531438111 ) ) ;
#142200=CARTESIAN_POINT ( 'NONE',  ( 13.89961937509957401, 13.97604488694547697, 61.87609039468566863 ) ) ;
#142201=CARTESIAN_POINT ( 'NONE',  ( 8.314922557961029526, -14.29746914071037800, 80.41775706135234714 ) ) ;
#142202=CARTESIAN_POINT ( 'NONE',  ( -16.46253265017160317, 9.564922557960807481, 65.83224293864769550 ) ) ;
#142203=CARTESIAN_POINT ( 'NONE',  ( 4.379528057220339221, -16.55341960407611168, 72.70724293864769550 ) ) ;
#142204=CARTESIAN_POINT ( 'NONE',  ( -13.97604488694527625, -13.89961937509977652, 41.87390960531435979 ) ) ;
#142205=CARTESIAN_POINT ( 'NONE',  ( -14.34966873604960291, -8.224510206698953496, 51.66557627198102409 ) ) ;
#142208=CARTESIAN_POINT ( 'NONE',  ( 16.52544592524342804, -4.483927247898539470, 23.54057627198102765 ) ) ;
#142209=CARTESIAN_POINT ( 'NONE',  ( 19.05341960407611168, 5.049401038298154454, 73.95724293864768129 ) ) ;
#142210=CARTESIAN_POINT ( 'NONE',  ( -18.22780087662119541, 5.500000000000102141, 51.01763182126894947 ) ) ;
#142211=CARTESIAN_POINT ( 'NONE',  ( -19.03943276465977164, -0.05219959533935918106, 33.75109039468566863 ) ) ;
#142212=CARTESIAN_POINT ( 'NONE',  ( 4.379528057220092307, 16.55341960407617563, 47.29275706135234003 ) ) ;
#142213=CARTESIAN_POINT ( 'NONE',  ( -5.823673210054116645, -21.52544592524344225, 67.29057627198103830 ) ) ;
#142214=CARTESIAN_POINT ( 'NONE',  ( 5.049401038297881783, 19.05341960407617563, 27.29275706135232937 ) ) ;
#142215=CARTESIAN_POINT ( 'NONE',  ( -19.02544592524342804, 5.153800228976336051, 76.04057627198102409 ) ) ;
#142216=CARTESIAN_POINT ( 'NONE',  ( -19.03943276465977164, 0.05219959533909376836, 116.2489096053143669 ) ) ;
#142217=CARTESIAN_POINT ( 'NONE',  ( 16.51473224551069308, 9.474510206698969483, 104.1655762719810241 ) ) ;
#142218=CARTESIAN_POINT ( 'NONE',  ( -21.55341960407619339, 5.719274019375674811, 38.54275706135234714 ) ) ;
#142219=CARTESIAN_POINT ( 'NONE',  ( -14.34966873604960291, -8.224510206698953496, 101.6655762719810383 ) ) ;
#142220=CARTESIAN_POINT ( 'NONE',  ( 5.823673210054125526, 21.52544592524343514, 104.7905762719810241 ) ) ;
#142221=CARTESIAN_POINT ( 'NONE',  ( -16.46253265017160317, 9.564922557960807481, 80.83224293864769550 ) ) ;
#142223=CARTESIAN_POINT ( 'NONE',  ( -10.81492255796105439, 18.62759615963255655, 22.91775706135235069 ) ) ;
#142224=VERTEX_POINT ( 'NONE', #81568 ) ;
#142225=CARTESIAN_POINT ( 'NONE',  ( 19.03943276465977164, -0.05219959533909143690, 83.74890960531436690 ) ) ;
#142227=CARTESIAN_POINT ( 'NONE',  ( 13.97604488694527802, 13.89961937509977652, 24.37390960531435624 ) ) ;
#142228=CARTESIAN_POINT ( 'NONE',  ( -16.46253265017160317, 9.564922557960807481, 30.83224293864769550 ) ) ;
#142229=CARTESIAN_POINT ( 'NONE',  ( -5.049401038297874678, -19.05341960407617918, 104.7927570613523471 ) ) ;
#142231=CARTESIAN_POINT ( 'NONE',  ( 8.224510206698953496, -14.34966873604960469, 112.9155762719810383 ) ) ;
#142232=CARTESIAN_POINT ( 'NONE',  ( -10.81492255796105439, 18.62759615963255655, 87.91775706135234714 ) ) ;
#142233=CARTESIAN_POINT ( 'NONE',  ( -19.02544592524342804, 5.153800228976336051, 71.04057627198099567 ) ) ;
#142234=CARTESIAN_POINT ( 'NONE',  ( 15.80617190586769283, -15.72974639402175789, 40.62609039468567573 ) ) ;
#142235=CARTESIAN_POINT ( 'NONE',  ( 21.53943276465977519, 0.05219959533937863772, 21.25109039468567218 ) ) ;
#142237=CARTESIAN_POINT ( 'NONE',  ( -16.46253265017160317, 9.564922557960807481, 90.83224293864769550 ) ) ;
#142239=CARTESIAN_POINT ( 'NONE',  ( 12.06949235617739724, 12.14591786802326823, 31.87609039468567929 ) ) ;
#142240=CARTESIAN_POINT ( 'NONE',  ( -5.823673210054116645, -21.52544592524344225, 42.29057627198103120 ) ) ;
#142241=CARTESIAN_POINT ( 'NONE',  ( -21.55341960407619339, 5.719274019375674811, 73.54275706135234714 ) ) ;
#142242=CARTESIAN_POINT ( 'NONE',  ( -19.02544592524342804, 5.153800228976336051, 116.0405762719810383 ) ) ;
#142243=CARTESIAN_POINT ( 'NONE',  ( 16.46253265017146816, 9.564922557961045513, 91.66775706135234714 ) ) ;
#142244=CARTESIAN_POINT ( 'NONE',  ( 9.564922557960805705, 16.46253265017160317, 64.58224293864769550 ) ) ;
#142245=CARTESIAN_POINT ( 'NONE',  ( -5.153800228976328057, -19.02544592524343514, 82.29057627198103830 ) ) ;
#142246=CARTESIAN_POINT ( 'NONE',  ( -16.53943276465976808, 0.05219959533911058130, 101.2489096053143669 ) ) ;
#142247=CARTESIAN_POINT ( 'NONE',  ( -8.224510206698948167, 14.34966873604960824, 105.4155762719810383 ) ) ;
#142248=CARTESIAN_POINT ( 'NONE',  ( -19.02544592524342804, 5.153800228976336051, 116.0405762719810383 ) ) ;
#142249=CARTESIAN_POINT ( 'NONE',  ( -8.224510206698735004, -14.34966873604973081, 84.58442372801903275 ) ) ;
#142250=CARTESIAN_POINT ( 'NONE',  ( 4.379528057220339221, -16.55341960407611168, 52.70724293864769550 ) ) ;
#142251=CARTESIAN_POINT ( 'NONE',  ( 9.474510206698971260, -16.51473224551069308, 42.91557627198103120 ) ) ;
#142252=CARTESIAN_POINT ( 'NONE',  ( -5.823673210054431948, 21.52544592524334988, 77.70942372801900433 ) ) ;
#142253=CARTESIAN_POINT ( 'NONE',  ( 5.719274019375673035, 21.55341960407619339, 67.29275706135234714 ) ) ;
#142254=CARTESIAN_POINT ( 'NONE',  ( 9.564922557961047289, -16.46253265017146816, 90.41775706135234714 ) ) ;
#142255=CARTESIAN_POINT ( 'NONE',  ( -4.379528057220328563, 16.55341960407611168, 65.20724293864768129 ) ) ;
#142256=CARTESIAN_POINT ( 'NONE',  ( -10.72451020669870658, -18.67979575497194134, 19.58442372801901143 ) ) ;
#142257=CARTESIAN_POINT ( 'NONE',  ( 0.05219959533907565091, 21.53943276465977519, 49.99890960531437401 ) ) ;
#142258=CARTESIAN_POINT ( 'NONE',  ( -16.20579543436677739, -7.371946100355105891, 105.5652083417187299 ) ) ;
#142260=CARTESIAN_POINT ( 'NONE',  ( -5.049401038298153566, 19.05341960407611168, 75.20724293864769550 ) ) ;
#142261=CARTESIAN_POINT ( 'NONE',  ( -4.379528057220328563, 16.55341960407611168, 30.20724293864769550 ) ) ;
#142262=AXIS2_PLACEMENT_3D ( 'NONE', #35918, #97564, #126924 ) ;
#142263=CARTESIAN_POINT ( 'NONE',  ( 4.483927247898545687, 16.52544592524342804, 24.79057627198103120 ) ) ;
#142264=CARTESIAN_POINT ( 'NONE',  ( 0.05219959533934541429, -16.53943276465976808, 90.00109039468567573 ) ) ;
#142265=CARTESIAN_POINT ( 'NONE',  ( -9.564922557961040184, 16.46253265017147172, 42.91775706135234003 ) ) ;
#142267=CARTESIAN_POINT ( 'NONE',  ( -9.564922557960796823, -16.46253265017161027, 87.08224293864769550 ) ) ;
#142268=EDGE_CURVE ( 'NONE', #154217, #190522, #163698, .T. ) ;
#142269=CARTESIAN_POINT ( 'NONE',  ( -12.06949235617756955, 12.14591786802309770, 60.62390960531437401 ) ) ;
#142270=CARTESIAN_POINT ( 'NONE',  ( 9.564922557960805705, 16.46253265017160317, 24.58224293864769194 ) ) ;
#142271=CARTESIAN_POINT ( 'NONE',  ( 5.719274019375991003, -21.55341960407610458, 27.70724293864769905 ) ) ;
#142272=CARTESIAN_POINT ( 'NONE',  ( -0.05219959533907301413, -21.53943276465977519, 52.49890960531435979 ) ) ;
#142274=CARTESIAN_POINT ( 'NONE',  ( 16.55341960407611168, 4.379528057220329451, 93.95724293864770971 ) ) ;
#142275=CARTESIAN_POINT ( 'NONE',  ( 8.224510206698742110, 14.34966873604972548, 42.08442372801901854 ) ) ;
#142276=ORIENTED_EDGE ( 'NONE', *, *, #155303, .T. ) ;
#142277=CARTESIAN_POINT ( 'NONE',  ( -4.379528057220328563, 16.55341960407611168, 75.20724293864769550 ) ) ;
#142278=CARTESIAN_POINT ( 'NONE',  ( -19.36337904590691750, 5.499999999999950262, 65.41494137495624273 ) ) ;
#142279=CARTESIAN_POINT ( 'NONE',  ( -16.46253265017146816, -9.564922557961047289, 79.16775706135234714 ) ) ;
#142280=CARTESIAN_POINT ( 'NONE',  ( -10.81492255796078084, -18.62759615963271287, 27.08224293864769550 ) ) ;
#142282=EDGE_CURVE ( 'NONE', #12092, #198282, #156523, .T. ) ;
#142284=CARTESIAN_POINT ( 'NONE',  ( -8.314922557961024197, 14.29746914071037800, 32.91775706135234714 ) ) ;
#142285=CARTESIAN_POINT ( 'NONE',  ( -4.379528057220328563, 16.55341960407611168, 30.20724293864769550 ) ) ;
#142286=CARTESIAN_POINT ( 'NONE',  ( -10.81492255796078084, -18.62759615963271287, 52.08224293864768839 ) ) ;
#142287=CARTESIAN_POINT ( 'NONE',  ( -0.05219959533936034679, 19.03943276465977164, 87.50109039468567573 ) ) ;
#142288=CARTESIAN_POINT ( 'NONE',  ( 21.52544592524344225, -5.823673210054117533, 53.54057627198103120 ) ) ;
#142289=CARTESIAN_POINT ( 'NONE',  ( -18.67979575497193778, 10.72451020669871902, 63.33442372801900433 ) ) ;
#142291=CARTESIAN_POINT ( 'NONE',  ( 14.34966873604972726, -8.224510206698740333, 40.83442372801901854 ) ) ;
#142292=CARTESIAN_POINT ( 'NONE',  ( 16.51473224551083163, -9.474510206698727899, 55.83442372801899722 ) ) ;
#142293=CARTESIAN_POINT ( 'NONE',  ( 9.564922557960805705, 16.46253265017160317, 84.58224293864769550 ) ) ;
#142294=CARTESIAN_POINT ( 'NONE',  ( -5.049401038298153566, 19.05341960407611168, 40.20724293864768839 ) ) ;
#142295=CARTESIAN_POINT ( 'NONE',  ( -4.379528057220328563, 16.55341960407611168, 105.2072429386477097 ) ) ;
#142297=CARTESIAN_POINT ( 'NONE',  ( -9.564922557960796823, -16.46253265017161027, 102.0822429386477097 ) ) ;
#142299=CARTESIAN_POINT ( 'NONE',  ( 0.05219959533934541429, -16.53943276465976808, 60.00109039468568284 ) ) ;
#142300=CARTESIAN_POINT ( 'NONE',  ( -15.80617190586745835, -15.72974639402198527, 91.87390960531436690 ) ) ;
#142301=CARTESIAN_POINT ( 'NONE',  ( 5.153800228976335163, 19.02544592524342804, 49.79057627198100988 ) ) ;
#142302=CARTESIAN_POINT ( 'NONE',  ( 16.51473224551083163, -9.474510206698727899, 75.83442372801900433 ) ) ;
#142303=CARTESIAN_POINT ( 'NONE',  ( -21.55341960407619339, 5.719274019375674811, 28.54275706135234358 ) ) ;
#142304=CARTESIAN_POINT ( 'NONE',  ( 9.564922557960805705, 16.46253265017160317, 74.58224293864769550 ) ) ;
#142305=CARTESIAN_POINT ( 'NONE',  ( -13.89961937509977652, 13.97604488694528158, 110.6239096053143243 ) ) ;
#142306=VERTEX_POINT ( 'NONE', #98742 ) ;
#142307=CARTESIAN_POINT ( 'NONE',  ( 12.14591786802327356, -12.06949235617739191, 40.62609039468567573 ) ) ;
#142308=CARTESIAN_POINT ( 'NONE',  ( 15.80617190586769283, -15.72974639402175789, 25.62609039468567929 ) ) ;
#142309=CARTESIAN_POINT ( 'NONE',  ( -8.224510206698948167, 14.34966873604960824, 100.4155762719810241 ) ) ;
#142310=CARTESIAN_POINT ( 'NONE',  ( 16.51473224551069308, 9.474510206698969483, 99.16557627198102409 ) ) ;
#142311=CARTESIAN_POINT ( 'NONE',  ( -13.89961937509957401, -13.97604488694547875, 74.37609039468566152 ) ) ;
#142312=CARTESIAN_POINT ( 'NONE',  ( 18.67979575497178502, 10.72451020669898547, 84.16557627198103830 ) ) ;
#142313=CARTESIAN_POINT ( 'NONE',  ( -14.34966873604960291, -8.224510206698953496, 51.66557627198102409 ) ) ;
#142314=CARTESIAN_POINT ( 'NONE',  ( 16.46253265017146816, 9.564922557961045513, 26.66775706135234003 ) ) ;
#142315=CARTESIAN_POINT ( 'NONE',  ( 8.314922557961029526, -14.29746914071037800, 75.41775706135233293 ) ) ;
#142316=CARTESIAN_POINT ( 'NONE',  ( 19.02544592524343514, -5.153800228976328945, 108.5405762719810383 ) ) ;
#142317=CARTESIAN_POINT ( 'NONE',  ( -13.89961937509977652, 13.97604488694528158, 45.62390960531433848 ) ) ;
#142318=CARTESIAN_POINT ( 'NONE',  ( 21.52544592524334988, 5.823673210054432836, 51.45942372801901854 ) ) ;
#142319=CARTESIAN_POINT ( 'NONE',  ( 18.62759615963255655, 10.81492255796105972, 61.66775706135235424 ) ) ;
#142320=CARTESIAN_POINT ( 'NONE',  ( -13.89961937509977652, 13.97604488694528158, 55.62390960531434558 ) ) ;
#142321=CARTESIAN_POINT ( 'NONE',  ( 21.55341960407619695, -5.719274019375665929, 51.04275706135234714 ) ) ;
#142322=CARTESIAN_POINT ( 'NONE',  ( -16.46253265017146816, -9.564922557961047289, 84.16775706135233293 ) ) ;
#142323=CARTESIAN_POINT ( 'NONE',  ( -5.153800228976328057, -19.02544592524343514, 37.29057627198102409 ) ) ;
#142324=CARTESIAN_POINT ( 'NONE',  ( 14.34966873604972726, -8.224510206698740333, 85.83442372801901854 ) ) ;
#142325=CARTESIAN_POINT ( 'NONE',  ( -19.02544592524342804, 5.153800228976336051, 61.04057627198103120 ) ) ;
#142326=CARTESIAN_POINT ( 'NONE',  ( -19.02544592524342804, 5.153800228976336051, 111.0405762719810099 ) ) ;
#142327=CARTESIAN_POINT ( 'NONE',  ( -0.05219959533909027116, -19.03943276465977164, 52.49890960531436690 ) ) ;
#142328=CARTESIAN_POINT ( 'NONE',  ( -18.67979575497178146, -10.72451020669898902, 81.66557627198103830 ) ) ;
#142329=CARTESIAN_POINT ( 'NONE',  ( -14.29746914071037622, -8.314922557961029526, 79.16775706135234714 ) ) ;
#142331=CARTESIAN_POINT ( 'NONE',  ( -5.049401038297874678, -19.05341960407617918, 29.79275706135232227 ) ) ;
#142332=CARTESIAN_POINT ( 'NONE',  ( 19.05341960407611168, 5.049401038298154454, 63.95724293864769550 ) ) ;
#142333=CARTESIAN_POINT ( 'NONE',  ( 4.379528057220339221, -16.55341960407611168, 52.70724293864769550 ) ) ;
#142334=CARTESIAN_POINT ( 'NONE',  ( -12.06949235617756955, 12.14591786802309770, 75.62390960531439532 ) ) ;
#142335=CARTESIAN_POINT ( 'NONE',  ( -19.05341960407611168, -5.049401038298163336, 101.4572429386476955 ) ) ;
#142336=CARTESIAN_POINT ( 'NONE',  ( -13.97604488694527625, -13.89961937509977652, 86.87390960531436690 ) ) ;
#142337=CARTESIAN_POINT ( 'NONE',  ( -21.53943276465977519, -0.05219959533937600094, 43.75109039468568284 ) ) ;
#142338=CARTESIAN_POINT ( 'NONE',  ( -0.05219959533909027116, -19.03943276465977164, 102.4989096053143669 ) ) ;
#142339=CARTESIAN_POINT ( 'NONE',  ( 10.81492255796106328, -18.62759615963255655, 110.4177570613523756 ) ) ;
#142340=CARTESIAN_POINT ( 'NONE',  ( 12.14591786802327356, -12.06949235617739191, 80.62609039468567573 ) ) ;
#142341=CARTESIAN_POINT ( 'NONE',  ( -5.719274019375665041, -21.55341960407619695, 39.79275706135235424 ) ) ;
#142342=CARTESIAN_POINT ( 'NONE',  ( 19.03943276465977164, -0.05219959533909143690, 108.7489096053143527 ) ) ;
#142343=CARTESIAN_POINT ( 'NONE',  ( -21.53943276465977519, 0.05219959533907696930, 106.2489096053143811 ) ) ;
#142344=CARTESIAN_POINT ( 'NONE',  ( -4.483927247898539470, -16.52544592524342804, 57.29057627198103120 ) ) ;
#142345=CARTESIAN_POINT ( 'NONE',  ( -5.153800228976328057, -19.02544592524343514, 57.29057627198103120 ) ) ;
#142346=CARTESIAN_POINT ( 'NONE',  ( 16.55341960407611168, 4.379528057220329451, 83.95724293864770971 ) ) ;
#142347=CARTESIAN_POINT ( 'NONE',  ( -15.72974639402197994, 15.80617190586746368, 25.62390960531435624 ) ) ;
#142348=CARTESIAN_POINT ( 'NONE',  ( 19.05341960407617918, -5.049401038297876454, 41.04275706135233293 ) ) ;
#142349=CARTESIAN_POINT ( 'NONE',  ( -4.379528057220328563, 16.55341960407611168, 110.2072429386477239 ) ) ;
#142351=CARTESIAN_POINT ( 'NONE',  ( 16.55341960407618274, -4.379528057220086978, 71.04275706135234714 ) ) ;
#142352=CARTESIAN_POINT ( 'NONE',  ( 19.05341960407611168, 5.049401038298154454, 68.95724293864769550 ) ) ;
#142354=CARTESIAN_POINT ( 'NONE',  ( 16.53943276465976808, -0.05219959533910856209, 93.74890960531436690 ) ) ;
#142355=CARTESIAN_POINT ( 'NONE',  ( -18.67979575497178146, -10.72451020669898902, 31.66557627198102054 ) ) ;
#142357=CARTESIAN_POINT ( 'NONE',  ( -4.379528057220086978, -16.55341960407618274, 109.7927570613523613 ) ) ;
#142358=CARTESIAN_POINT ( 'NONE',  ( 9.564922557961047289, -16.46253265017146816, 110.4177570613523471 ) ) ;
#142359=CARTESIAN_POINT ( 'NONE',  ( -15.72974639402176322, -15.80617190586768395, 79.37609039468567573 ) ) ;
#142360=CARTESIAN_POINT ( 'NONE',  ( -16.51473224551069308, -9.474510206698971260, 91.66557627198103830 ) ) ;
#142361=CARTESIAN_POINT ( 'NONE',  ( 10.72451020669898902, -18.67979575497178502, 102.9155762719810383 ) ) ;
#142362=CARTESIAN_POINT ( 'NONE',  ( -12.06949235617739369, -12.14591786802326823, 59.37609039468568284 ) ) ;
#142363=CARTESIAN_POINT ( 'NONE',  ( 19.05341960407611168, 5.049401038298154454, 23.95724293864769194 ) ) ;
#142364=CARTESIAN_POINT ( 'NONE',  ( 16.52544592524335698, 4.483927247898782831, 31.45942372801901854 ) ) ;
#142365=CARTESIAN_POINT ( 'NONE',  ( -0.05219959533936034679, 19.03943276465977164, 97.50109039468567573 ) ) ;
#142367=CARTESIAN_POINT ( 'NONE',  ( 0.05219959533907565091, 21.53943276465977519, 94.99890960531436690 ) ) ;
#142368=CARTESIAN_POINT ( 'NONE',  ( -5.153800228976607833, 19.02544592524334988, 57.70942372801899012 ) ) ;
#142370=CARTESIAN_POINT ( 'NONE',  ( 5.823673210054125526, 21.52544592524343514, 109.7905762719810383 ) ) ;
#142371=CARTESIAN_POINT ( 'NONE',  ( -16.51473224551069308, -9.474510206698971260, 71.66557627198102409 ) ) ;
#142372=CARTESIAN_POINT ( 'NONE',  ( -19.02544592524342804, 5.153800228976336051, 76.04057627198102409 ) ) ;
#142373=CARTESIAN_POINT ( 'NONE',  ( -16.53943276465976808, -0.05219959533934237506, 33.75109039468568284 ) ) ;
#142375=CARTESIAN_POINT ( 'NONE',  ( -13.97604488694547697, 13.89961937509957934, 63.12609039468566152 ) ) ;
#142376=CARTESIAN_POINT ( 'NONE',  ( 5.823673210054444382, -21.52544592524334988, 25.20942372801901854 ) ) ;
#142377=CARTESIAN_POINT ( 'NONE',  ( 8.224510206698953496, -14.34966873604960469, 57.91557627198103120 ) ) ;
#142378=CARTESIAN_POINT ( 'NONE',  ( 16.51473224551069308, 9.474510206698969483, 69.16557627198102409 ) ) ;
#142379=CARTESIAN_POINT ( 'NONE',  ( -4.483927247898782831, 16.52544592524335698, 42.70942372801901854 ) ) ;
#142380=( BOUNDED_SURFACE ( )  B_SPLINE_SURFACE ( 3, 2, ( 
 ( #33978, #45177, #16819, #15824, #187680, #108819, #92644, #77485, #632, #122989, #184675, #2638, #62302, #107813, #153331, #185669, #46158, #48158, #183690, #47160, #64314, #75497, #109816, #106831, #170498, #17822, #152346, #30995, #123972, #198859, #168506, #110808, #31988, #169496, #49150, #93646, #155331, #91642, #78470, #61318, #140144, #1636, #13831, #63313, #172490, #94641, #137171, #124992, #186688, #171499, #32988, #60325, #30004, #156322, #79480, #125982, #122000, #14832, #76494, #138171, #199852, #50145, #69288, #143122, #6604, #54127, #128944, #175473, #4602, #177490, #188666, #160301, #159285, #130954, #52121, #35951, #20782, #115800, #129934, #68283, #36945, #176484, #113777, #157321, #111805, #191633, #66294, #97597, #95634, #114791, #53113, #37960, #21791, #190645, #82437, #98607, #83442, #146118, #51130, #142135, #189657, #145120, #99618, #161298, #192644, #173493, #22794, #84440, #34966, #18817, #127953, #7602, #112790, #80461, #3619, #65298, #126957, #96618, #144125, #174484, #158307, #19795, #5606, #67286, #81436, #58128, #70298, #131966, #8626, #72295, #88448, #119797, #150143, #181482, #27809, #11645, #149145, #85448, #55123, #197635, #179497, #194652, #74295, #118812, #41970, #178484, #40962, #148142, #102634, #57136, #100616, #133974, #59101, #42960, #23798, #180498, #164319, #132963, #10635, #162298, #116792, #104623, #25812, #73311, #12630, #135964, #195665, #147138, #24808, #193651, #120766, #86457, #134982, #38959, #103637, #165315, #9633, #39950, #101621, #26808, #87458, #163310, #196659, #166312, #89450, #71300, #151139, #56122, #117804, #65795, #3139, #43948, #1136, #19314, #155825, #187191, #66790, #4116, #80962, #127464, #49646, #18324, #125494, #64814, #188173, #35463, #140652, #28794, #78977, #34476, #172998, #189170, #81932, #77981, #126475, #141649, #62810, #20286, #17322, #96135, #2142, #111309, #112304, #157824, #158797, #142638, #48662, #63821, #79981, #50642, #95142, #110314, #152119, #173994, #16331, #139648, #124492, #97114, #143624, #5109, #182467, #105610, #167298, #90433, #33484, #171996, #156831, #186188, #47669, #109321, #171001, #32493, #94146, #24308, #159798, #23298, #117296, #51625, #85957, #21293, #161803, #194159, #10134, #7107, #148645, #70800, #113290, #146623, #68788, #22296, #38464, #174981, #6111, #9134, #130446, #39452, #102132, #163816, #84942, #36445, #114284, #82950, #25318, #175987, #101113, #86960, #8116, #69793, #37455, #128454, #144628, #193148, #192145, #190150, #131461, #53625, #115301, #98100, #162799, #147645, #54620, #132468, #116295, #67793, #129449, #55623, #99116, #176994, #191148, #178991, #40459, #52622, #177985, #160808, #100120, #83947, #145627, #122261, #27308, #118309, #165811, #121272, #59598, #90918, #168760, #164814, #151630, #28310, #149639, #107089, #104129, #182966, #88956, #89950, #199118, #44449, #45436, #106103, #12143, #42466, #166810, #167788, #181973, #135479, #41469, #152604, #103133, #26310, #87950, #105124, #29287, #14094, #75761, #137439, #60585, #183950, #120281, #150646, #73807, #30263, #197148, #58614, #72811, #13124, #43455, #91907, #11136, #74787, #153600, #195154, #71795, #134480, #136449, #133464, #56636, #198130, #180001, #196165, #57639, #119305, #180989, #170768, #50417, #94912, #18092, #154598, #155593, #124252, #17088, #33254, #76756, #110086, #34245, #79747, #48430, #78741, #156597, #141416, #65565, #32257, #61580, #109088, #64582, #2904, #95905, #112076, #108083, #126247, #171765, #92912, #173765, #47432, #187943, #93915, #49412, #142408, #111075, #188939, #172764, #140417, #185948, #157589, #19081, #125261, #1908, #184940, #80729, #46425, #169768, #31261, #3886, #127225, #35232, #96886, #15097, #138431, #200112, #63587, #186959, #123249, #16094, #77752, #139418, #900, #62574, #129211, #54391, #189922, #53385, #147405, #81702, #116064, #51397, #191900, #24064, #40213, #37218 ),
 ( #39221, #85719, #23061, #177752, #115063, #8893, #6870, #162559, #100877, #70561, #176755, #68549, #178749, #190909, #38228, #82709, #113057, #130205, #52386, #158569, #161568, #159556, #143385, #174749, #132228, #193921, #84706, #55384, #66560, #69559, #144392, #146385, #98874, #36213, #97866, #4877, #7873, #21053, #5877, #117054, #131224, #20058, #192914, #160570, #99883, #128225, #67554, #114043, #175741, #22059, #83710, #145388, #164576, #11909, #59366, #120052, #197897, #150414, #167563, #194913, #165574, #56388, #28076, #166576, #103894, #181739, #71557, #73573, #43220, #101892, #9896, #121035, #119075, #163574, #104888, #72567, #135246, #27073, #196918, #148402, #118070, #179760, #105876, #58385, #89717, #133222, #151402, #42233, #88719, #41230, #74555, #102891, #12892, #136222, #26070, #182733, #25074, #44217, #86717, #87713, #149399, #10894, #134242, #195927, #57403, #180757, #130877, #86376, #101534, #132881, #177412, #192567, #102552, #53032, #115725, #6525, #175396, #54050, #114714, #164236, #85366, #83367, #67210, #36864, #178404, #148061, #147060, #71218, #190568, #193572, #68204, #8542, #22716, #160223, #98530, #128868, #131888, #21714, #145044, #9552, #70220, #194570, #116715, #161222, #100540, #38883, #55044, #56040, #39868, #117718, #52044, #82360, #162219, #113700, #129857, #40879, #146041, #163227, #24727, #5531, #69209, #191555, #176406, #37882, #99540, #84364, #179414, #7525, #23718, #144049, #29689, #10551, #152036, #42879, #180416, #26725, #11563, #73229, #121681, #91320, #90351, #14511, #133889, #136858, #150057, #28714, #166225, #103555, #41888, #72215, #75186, #118728, #165230, #153011, #13521, #76172, #60014, #104544, #43866, #182388, #198544, #137852, #183377, #199532, #195581, #107497, #197554, #57053, #88364, #184363, #89369, #44859, #106514, #149063, #12549, #134900, #196577, #58047, #181401, #119717, #168192, #27726, #151058, #74215, #61002, #135883, #122674, #59022, #120689, #105531, #167217, #45844, #25732, #87378, #16504, #48829, #81124, #156996, #157987, #187360, #50814, #185350, #140821, #123652, #188338, #64978, #79150, #18494, #61986, #172165, #141812, #169173, #77168, #96301, #171177, #127636, #3305, #1309, #110482, #17492, #125662, #154016, #46841, #108500, #4285, #33650, #80142, #138838, #95311, #94318, #155996, #15511, #111481, #318, #126636, #49817, #155007, #173166, #30678, #34642, #19478, #142805, #65966, #189336, #92330, #170180, #2310, #31674, #63991, #93323, #78152, #139820, #62988, #124666, #186362, #47842, #109495, #32665, #105652, #136005, #150188, #89494, #58172, #77291, #151184, #14639, #119839, #138962, #12672, #76298, #62115, #136981, #183500, #74339, #185477, #196702, #168316, #167340, #440, #60137, #43990, #28837, #123778, #137976, #199658, #44983, #184488, #121805, #165357, #181524, #61125, #197676, #90478, #103678, #122798, #45967, #107621, #29812, #198670, #152160, #106643, #91448, #154142, #59141, #11688, #120811, #153136, #169299, #30805, #26851, #43003, #92454, #15634, #104670, #88492, #182510, #73354, #13643, #135027, #166355, #27854, #75310, #19603, #187487, #17622, #141935, #81245, #157122, #110606, #16627, #66093, #78274, #139947, #1437, #80265, #96425, #127760, #158111, #189460, #35758, #142926, #95438, #79281, #140951, #97403, #48953, #2438, #47968, #3426, #64120, #4408, #63115, #65102, #159090, #170304, #50938, #124793, #126760, #112596, #128751, #125785, #18618, #93446, #186492, #5409, #172289, #33778, #82237, #188463, #49945, #109620, #111609, #156123, #173294, #34768, #108626, #174288, #67092, #20585, #31797, #143927, #46967, #155133, #171304, #32790, #94443, #71098, #192448, #191435, #102432, #53930, #22595, #36742, #176285, #163105, #130756, #161101, #85246, #24609, #100422, #115605, #160102, #9433, #21589, #83248, #144923, #23599, #39750, #132765, #101413, #194453, #179299, #86257, #38765, #72095, #129738, #117598 ),
 ( #98406, #54926, #177294, #162103, #6405, #55923, #68086, #116599, #147947, #37757, #8427, #190448, #178287, #40763, #146937, #164119, #25617, #87261, #148946, #70099, #10436, #131768, #51923, #113582, #175276, #193450, #52912, #114588, #84243, #99418, #145922, #7405, #69089, #105417, #15397, #136741, #134783, #118612, #88250, #29578, #137737, #198425, #122562, #41770, #44743, #57935, #59900, #74102, #11442, #149936, #180302, #183263, #26607, #73113, #60886, #121568, #184252, #168081, #12440, #151922, #90239, #106399, #199421, #91209, #45734, #103435, #133768, #167100, #165115, #196465, #92216, #197443, #152899, #14396, #56938, #120576, #119606, #42767, #181289, #89254, #27615, #76062, #135772, #150946, #104429, #107386, #166112, #169058, #58909, #182270, #43753, #30565, #13411, #195463, #28601, #75075, #153902, #96198, #173062, #187253, #126535, #170069, #110375, #34539, #158862, #16395, #4180, #79039, #35529, #49708, #109383, #156893, #125556, #33544, #61875, #31560, #93211, #112369, #95206, #188234, #185238, #141709, #2204, #63885, #123545, #19376, #46730, #3200, #111373, #62874, #18389, #77054, #64874, #157887, #80040, #81025, #142701, #65858, #127530, #172058, #189233, #48722, #50711, #174060, #97177, #138726, #206, #108392, #47730, #154896, #78041, #139710, #171063, #1197, #124555, #186252, #32553, #94207, #155886, #17383, #140714, #85010, #9202, #128519, #131531, #144692, #23364, #160873, #98167, #36512, #5175, #69862, #113355, #159867, #147714, #8186, #70867, #54689, #99184, #38532, #177062, #146690, #24375, #193215, #132535, #66857, #102199, #192213, #190214, #51693, #179059, #84015, #39519, #116362, #143692, #7175, #83018, #129512, #6177, #176055, #114350, #178051, #22363, #37522, #175047, #86025, #21360, #101179, #145693, #67857, #191212, #52687, #68858, #53696, #130517, #115373, #100188, #194224, #162867, #40528, #55689, #161870, #117363, #20351, #81999, #76570, #89756, #44257, #47238, #168577, #167600, #78546, #30075, #198932, #12929, #152417, #121079, #140221, #13905, #77562, #125067, #199929, #46235, #75571, #48234, #59405, #31073, #91716, #1714, #123064, #106904, #153410, #186764, #709, #139234, #107889, #108897, #184750, #25384, #182773, #62381, #137247, #14908, #163887, #185750, #124051, #170576, #92721, #61392, #138245, #169576, #154410, #16895, #122072, #74593, #60400, #15904, #32067, #93723, #63390, #105914, #155405, #151442, #29095, #136261, #183764, #197936, #45250, #90734, #37023, #82517, #83518, #144199, #50226, #80538, #4679, #5685, #19871, #173570, #79553, #129020, #141222, #2713, #64390, #143198, #159363, #190721, #20860, #52194, #98684, #174558, #191706, #128031, #158382, #160377, #111880, #65374, #110883, #66371, #142212, #67361, #126058, #189733, #21868, #33062, #113852, #187755, #51206, #175548, #109889, #188741, #81511, #156395, #49225, #68356, #35039, #127034, #145195, #112867, #36025, #172568, #96693, #18892, #97674, #6678, #171573, #130007, #94717, #17899, #34054, #95711, #157399, #3695, #100687, #24880, #131029, #162369, #133035, #165388, #41038, #42044, #71371, #135056, #69360, #86529, #7676, #72371, #149217, #163383, #102704, #146191, #148213, #10708, #53190, #192718, #180570, #55195, #11717, #25885, #85521, #194725, #101694, #9707, #38035, #54202, #115874, #88524, #56195, #164392, #161375, #117878, #178555, #40021, #99691, #195738, #22866, #179568, #87530, #39032, #134045, #114865, #57211, #118886, #103708, #26881, #150220, #73384, #176560, #84513, #177563, #23870, #147209, #8700, #70370, #132038, #193727, #116864, #167371, #29842, #91479, #138991, #90508, #168346, #78304, #199690, #197707, #181553, #151213, #92484, #470, #61155, #185506, #104698, #107652, #120842, #122828, #137011, #74367, #12701, #43032, #45997, #89524, #136033, #123808, #184517, #46997, #30836, #75341, #14668, #153167, #169329, #62144, #154173, #108656, #166386, #196732, #76329 ),
 ( #138006, #15664, #59173, #31827, #28868, #77323, #170334, #182541, #44023, #93477, #155164, #16656, #58200, #119868, #27882, #105684, #152190, #13674, #198701, #60167, #106673, #121836, #183530, #45014, #97436, #21621, #79311, #67123, #141967, #98438, #112627, #172319, #19633, #188496, #96454, #124823, #94472, #32821, #175307, #158141, #189490, #47997, #4437, #65133, #126790, #186523, #82267, #109651, #66125, #174319, #125814, #81275, #139977, #127790, #50968, #142957, #20617, #5439, #35789, #159121, #173324, #128781, #49975, #143959, #190481, #51953, #34799, #111639, #160133, #110638, #113613, #36773, #1466, #33808, #63144, #171333, #156153, #140980, #17651, #2468, #64150, #187517, #48983, #95468, #157154, #18649, #80295, #3456, #23628, #161130, #99450, #68116, #132796, #176316, #22626, #10465, #71130, #133800, #117631, #162132, #101445, #39781, #9467, #87292, #194483, #195491, #129768, #165145, #54957, #191464, #52942, #41799, #146967, #102462, #86288, #6434, #70129, #145954, #192477, #7435, #38795, #177324, #179329, #85276, #100452, #114616, #148976, #37786, #55955, #8456, #84273, #69119, #130785, #53960, #115635, #118639, #163136, #40793, #131801, #147978, #193480, #116629, #178318, #25647, #24640, #164150, #72126, #56966, #180331, #83278, #103466, #144953, #183290, #107413, #92244, #91235, #122590, #59927, #15424, #75103, #30592, #45761, #77083, #121595, #136770, #46759, #197472, #44772, #106425, #169086, #120607, #198456, #108417, #29603, #27644, #11473, #181318, #184278, #153930, #152925, #138752, #134814, #137762, #150975, #14422, #167130, #104459, #42797, #73144, #76086, #119635, #166142, #234, #199446, #61901, #60914, #105446, #168106, #123572, #185267, #26636, #88279, #149967, #196494, #57964, #89284, #12469, #74130, #135801, #90267, #58938, #182301, #43781, #13439, #28630, #151950, #94234, #125581, #63911, #4206, #48749, #187279, #139735, #174085, #154922, #96222, #110402, #124582, #171090, #155915, #17410, #141735, #47757, #79067, #49734, #82024, #157911, #158887, #188260, #51716, #186278, #3225, #109411, #189259, #65884, #80065, #19401, #62902, #64899, #127558, #170093, #32581, #97201, #172084, #128542, #142726, #2229, #111402, #18416, #126560, #16420, #140740, #173087, #20377, #93237, #50735, #33571, #34566, #35554, #31587, #95233, #81050, #78067, #156919, #190239, #112394, #143720, #5199, #66881, #1224, #52708, #53720, #22388, #115397, #131556, #175069, #8212, #133555, #55716, #98190, #193241, #177085, #7198, #23389, #36534, #191234, #194249, #38556, #114372, #25410, #100213, #145717, #159893, #99208, #67881, #87052, #160896, #24401, #71885, #146716, #54714, #84038, #195246, #6201, #178076, #161893, #148737, #69887, #85035, #116386, #113379, #147739, #86050, #39543, #117388, #101202, #21381, #129534, #9226, #68882, #162892, #83040, #132560, #70893, #179087, #40556, #102225, #163914, #10225, #144715, #176076, #130542, #37544, #192240, #106192, #44537, #75850, #153688, #149728, #136536, #13211, #134572, #91994, #89043, #167876, #150733, #74874, #184039, #29375, #30352, #91006, #197237, #27398, #151718, #152692, #166897, #120368, #26401, #137526, #88040, #11229, #72903, #90036, #14181, #199208, #60675, #122350, #45522, #121360, #138514, #198217, #105210, #107176, #58698, #12233, #57728, #59689, #73895, #168847, #196259, #164907, #183053, #15184, #42556, #76843, #56730, #118400, #180094, #41562, #103225, #119398, #181081, #104219, #165900, #135565, #28397, #182061, #43544, #50495, #94995, #48514, #20140, #170852, #33335, #156681, #142490, #93996, #171847, #81785, #2986, #985, #185027, #154685, #95989, #3968, #64665, #189021, #108173, #111158, #124339, #126327, #140504, #77835, #16180, #46514, #49496, #92999, #139502, #127310, #188024, #112159, #34328, #78826, #18175, #79832, #172847, #65648, #157674, #173848, #169854, #66205, #141502, #31348, #62660, #158648, #63672, #19163 ),
 ( #186035, #80811, #17172, #47517, #109173, #32343, #155677, #35314, #1993, #125346, #96968, #61665, #123334, #187044, #110168, #25165, #159642, #115147, #97950, #162650, #39306, #53470, #193000, #36294, #176840, #100965, #143472, #82793, #70652, #145472, #101982, #116147, #175828, #23146, #191983, #99966, #128304, #21138, #144475, #178838, #161650, #54477, #51478, #7961, #68633, #130289, #190004, #85807, #5959, #69644, #6953, #40306, #84790, #83792, #38311, #163662, #177838, #24156, #146469, #147493, #131310, #4956, #67637, #8984, #114126, #132318, #66641, #194010, #55473, #117143, #113140, #174830, #129296, #190992, #52468, #37301, #98960, #160650, #22142, #136304, #74638, #105958, #183804, #179846, #166658, #43303, #164662, #122115, #119158, #197979, #180840, #104971, #13946, #59449, #60440, #121122, #27155, #57488, #181824, #182817, #168617, #44299, #75612, #28159, #86807, #102977, #58466, #41317, #167643, #29139, #197000, #90776, #26157, #120133, #152460, #148493, #87799, #137291, #88802, #45292, #198973, #42317, #89801, #135327, #151483, #71644, #149484, #10980, #106944, #12974, #9984, #195000, #133311, #11992, #73655, #56478, #118156, #72653, #134328, #196013, #103978, #165657, #150495, #17940, #156441, #186808, #110922, #95753, #94759, #126099, #63434, #18933, #78591, #34095, #49264, #80578, #125110, #140264, #52972, #753, #48278, #109933, #172608, #124096, #1756, #114649, #33103, #31116, #14950, #184791, #187795, #157438, #79594, #142252, #138288, #141263, #6465, #64429, #108939, #171615, #2753, #68146, #129797, #191496, #30117, #76610, #91758, #153452, #199969, #61434, #123106, #93766, #46277, #107933, #169619, #16937, #92764, #139276, #154454, #185795, #47283, #15946, #170620, #32109, #77605, #62424, #155447, #102492, #193510, #130816, #177354, #162161, #23658, #148006, #7465, #161161, #192507, #57993, #164178, #165173, #194511, #176347, #53991, #9496, #115664, #195521, #72155, #86318, #25676, #69150, #71159, #133830, #37819, #38824, #103495, #178347, #134843, #149005, #8484, #55985, #24669, #132825, #22657, #100482, #85305, #11502, #117661, #87321, #84304, #40821, #101475, #163165, #145983, #118668, #146998, #10494, #56994, #70159, #179358, #99480, #180360, #41828, #26666, #88308, #149996, #73173, #196522, #131829, #54987, #116656, #39810, #138781, #170120, #14452, #168134, #139764, #90294, #152954, #76115, #61930, #13467, #91263, #1252, #122618, #120635, #104488, #74158, #15453, #123599, #184308, #108444, #27672, #30620, #43810, #45789, #59956, #197499, #135830, #166171, #169115, #12496, #58966, #46785, #167159, #137792, #151005, #89312, #182331, #119663, #107441, #31614, #199476, #181345, #105473, #60943, #28659, #262, #77111, #29630, #92273, #151978, #153957, #185294, #42824, #75130, #93264, #121623, #78095, #154950, #136800, #16446, #198484, #183318, #44800, #106455, #155941, #98220, #81074, #112420, #171118, #127585, #188287, #49763, #109436, #5228, #32608, #189285, #35582, #48775, #142753, #62929, #50763, #174112, #19427, #143749, #128573, #97228, #158916, #96248, #51745, #111429, #66910, #82055, #113406, #157936, #173116, #83069, #33598, #4233, #65913, #190268, #156944, #34591, #144745, #20406, #63937, #47784, #17437, #175097, #36565, #159923, #21412, #94261, #124609, #187305, #186304, #3252, #140766, #79093, #2255, #125606, #110430, #172111, #95261, #18441, #80092, #141760, #64925, #126585, #162922, #132589, #10255, #117419, #118431, #191261, #88072, #178106, #114403, #176104, #164938, #69920, #25440, #9255, #129563, #193270, #68912, #115425, #130574, #161923, #100241, #40585, #85065, #23417, #37574, #71914, #52736, #194278, #146747, #160924, #7227, #192269, #177114, #8242, #24430, #67910, #101233, #26431, #148766, #99237, #86078, #131586, #54744, #116417, #22417, #84067, #87081, #39574, #53751, #180124, #147769, #38585, #145746, #70922, #55745, #41592, #179117, #102256 ),
 ( #163943, #133586, #195277, #56759, #103256, #6231, #28428, #167906, #106222, #75882, #153720, #60705, #61697, #134602, #31382, #121392, #57757, #119427, #108209, #13240, #168878, #152723, #72933, #136567, #12261, #58728, #73925, #105239, #43575, #184070, #90065, #166927, #181111, #15216, #196288, #137557, #151747, #104248, #150764, #135594, #197266, #183084, #42585, #165931, #27429, #149757, #199240, #138545, #29406, #11261, #89073, #44567, #120398, #30383, #45554, #59722, #122381, #182091, #91036, #107208, #74903, #198247, #76875, #14213, #169888, #92030, #23, #123366, #185059, #46547, #77867, #47551, #186068, #128340, #111191, #142525, #1018, #157709, #18208, #79866, #139534, #35352, #62691, #19199, #65682, #78857, #172882, #93031, #80848, #4003, #127345, #189059, #49528, #173882, #158685, #50531, #112193, #126362, #81820, #141535, #97003, #20174, #143507, #188058, #3024, #113175, #63705, #34362, #96023, #4993, #187077, #64700, #174865, #66678, #94028, #124373, #109204, #190039, #51513, #154719, #16212, #170884, #32375, #17204, #155708, #33368, #140537, #2025, #125380, #48546, #110200, #171879, #95026, #156716, #86843, #70687, #115181, #54510, #193033, #162685, #40341, #147531, #148528, #21174, #118191, #7994, #144510, #5995, #195036, #99999, #55509, #39341, #159678, #23181, #98995, #145507, #160684, #192020, #130323, #132353, #176874, #53504, #67674, #102016, #82829, #24191, #38343, #191027, #37337, #22176, #83826, #69678, #129332, #52502, #114162, #36331, #85841, #25200, #116182, #97984, #175864, #131345, #6988, #117179, #194045, #146504, #9019, #68668, #177873, #178874, #161684, #84824, #163699, #101000, #56513, #10019, #71678, #133345, #28194, #136339, #164697, #134363, #72688, #14981, #198013, #29173, #87832, #44333, #105005, #166691, #26192, #122147, #149518, #105990, #152492, #165691, #59483, #179882, #61467, #199005, #13979, #60471, #167676, #13008, #120167, #121157, #182850, #30148, #135363, #11015, #73691, #90809, #75646, #183836, #76641, #196047, #137324, #45325, #57522, #138319, #12028, #106975, #197034, #168649, #91791, #153485, #200001, #41350, #181858, #43337, #119191, #103013, #180875, #89836, #42351, #104013, #27189, #88836, #150529, #74672, #58501, #151517, #2784, #110952, #18963, #17972, #188812, #171644, #63467, #157470, #16969, #32140, #785, #48310, #108971, #187825, #92796, #109965, #80609, #184824, #126130, #154484, #33134, #34125, #123138, #78622, #94791, #31148, #62456, #46309, #1789, #140298, #127104, #79626, #141294, #124130, #125142, #93797, #186841, #156471, #169652, #64463, #107965, #65443, #139306, #49294, #172637, #95784, #142286, #185829, #170652, #3766, #15978, #155477, #77637, #47316, #110910, #190749, #111910, #109919, #93753, #63421, #4709, #112896, #173598, #97704, #16924, #19899, #33090, #35067, #49252, #186794, #125096, #155434, #158410, #1743, #48265, #36055, #96722, #159395, #143227, #187782, #127063, #65402, #81540, #80565, #140251, #78577, #171602, #108926, #66399, #20890, #188770, #170606, #94746, #142240, #156426, #128061, #189763, #18920, #51235, #17927, #3725, #174590, #32096, #79582, #82548, #172596, #67391, #144230, #141251, #50254, #157426, #5714, #2740, #64417, #126086, #129048, #34082, #95740, #160407, #116894, #177592, #39059, #98713, #194754, #21896, #178586, #24911, #38064, #70400, #52223, #40050, #101726, #8731, #133064, #117908, #163415, #148242, #85553, #41069, #100717, #56226, #71400, #102732, #147239, #162397, #72400, #22896, #132068, #9736, #84542, #192748, #54231, #134076, #55225, #53218, #37054, #6707, #179597, #164421, #86558, #25914, #83546, #87558, #176590, #149245, #115902, #130037, #68385, #145225, #10736, #191736, #114896, #113880, #175577, #99720, #161404, #131059, #193757, #146219, #7707, #69390, #23900, #107680, #180598, #77353, #167399, #103736, #165416, #154202, #59200, #14698, #198729, #118914, #182569, #58226 ),
 ( #196759, #181580, #43058, #27910, #183557, #89553, #13701, #122856, #168374, #169357, #29870, #136059, #197734, #26909, #15692, #88552, #120869, #150251, #76360, #11745, #73412, #135083, #28895, #45043, #138037, #106701, #199718, #184544, #60195, #195766, #75368, #44052, #46024, #105712, #151239, #119895, #90535, #166416, #91507, #104724, #152217, #30867, #42072, #153194, #12728, #137038, #61184, #57240, #74394, #121865, #92513, #155194, #100226, #79339, #94500, #177099, #21396, #144728, #78333, #141009, #48024, #5212, #159907, #500, #36548, #161908, #84053, #123836, #83054, #66893, #32850, #51728, #62172, #16683, #22402, #128555, #17681, #67894, #113391, #171362, #185534, #124852, #93508, #115410, #186552, #52721, #23402, #175081, #6215, #109681, #139020, #31855, #129547, #190251, #38570, #98203, #191247, #114387, #47027, #176089, #37559, #99222, #145731, #160909, #108685, #140006, #7212, #156182, #68896, #170363, #130556, #192254, #53735, #1495, #63173, #25425, #164923, #88056, #135580, #40570, #131571, #179101, #134588, #72919, #104234, #182076, #178090, #26416, #41577, #162907, #120383, #165916, #196274, #27413, #73910, #149743, #166913, #103241, #133570, #197252, #87066, #102240, #86064, #118416, #55730, #181097, #116401, #180109, #58714, #8227, #42571, #39560, #11245, #150750, #85049, #163928, #195261, #193255, #101217, #43560, #148751, #10240, #105225, #57743, #119413, #24415, #71899, #194263, #56745, #89059, #146731, #12248, #69905, #54729, #147754, #9240, #70907, #132575, #117403, #151733, #106207, #109190, #30368, #107192, #154703, #8, #60690, #74889, #14197, #183069, #2011, #75866, #139519, #187061, #61682, #108191, #137542, #110185, #121377, #93016, #92012, #63690, #185044, #167891, #186052, #125365, #123351, #155694, #16197, #78843, #62676, #168863, #46531, #169873, #77852, #32360, #1002, #140521, #13226, #28414, #31366, #136552, #198232, #48531, #153705, #47536, #124357, #59704, #15201, #91021, #199225, #152707, #184055, #122366, #170869, #76860, #45538, #44552, #94013, #29390, #17189, #138530, #90051, #172864, #157690, #19181, #143490, #3006, #156699, #126344, #53487, #159659, #160667, #190023, #171863, #188041, #4975, #49511, #191009, #174847, #34345, #18193, #111174, #67656, #175846, #36313, #22159, #79850, #82811, #96006, #97967, #112177, #80830, #142507, #3985, #129313, #6970, #66661, #98977, #21156, #83810, #5976, #50514, #51497, #128324, #144493, #37319, #52485, #145490, #141519, #33352, #113157, #64682, #65665, #130306, #35333, #114145, #68650, #95011, #158668, #127327, #189039, #173865, #96986, #20158, #192001, #81803, #9001, #84806, #119174, #99982, #41333, #132335, #69660, #116164, #100982, #162666, #86824, #146485, #161667, #131327, #197018, #102994, #103996, #133327, #115164, #193015, #148510, #54492, #134347, #10998, #25182, #164680, #7976, #10000, #72670, #176857, #177854, #42335, #117159, #73672, #87815, #147511, #195018, #163679, #71660, #23163, #39323, #24172, #150513, #56494, #26174, #85823, #179863, #40321, #101997, #70668, #57505, #194026, #149501, #196029, #55489, #118172, #38326, #180859, #165674, #27173, #88820, #12011, #135344, #178855, #91777, #47301, #106960, #62440, #77623, #108958, #153471, #168634, #78608, #29156, #14967, #154471, #90793, #198990, #60458, #140282, #122133, #58484, #139293, #92782, #770, #123123, #76627, #183820, #138305, #61453, #170637, #13964, #104988, #152477, #107951, #46294, #124114, #155464, #151500, #199986, #184808, #136322, #93783, #75631, #169638, #137309, #31134, #185814, #15963, #32126, #16954, #45310, #30134, #166676, #120151, #28177, #181841, #89819, #43321, #12992, #74655, #197997, #59467, #121140, #182834, #44316, #105975, #167660, #66427, #83576, #19927, #50282, #190776, #142270, #157455, #2770, #35097, #172624, #97733, #33119, #96749, #52251, #125129, #159422, #94776, #158439, #67420, #1774, #80595, #111940 ) ),
 .UNSPECIFIED., .T., .F., .T. ) 
 B_SPLINE_SURFACE_WITH_KNOTS ( ( 4, 3, 4 ),
 ( 3, 2, 2, 2, 2, 2, 2, 2, 2, 2, 2, 2, 2, 2, 2, 2, 2, 2, 2, 2, 2, 2, 2, 2, 2, 2, 2, 2, 2, 2, 2, 2, 2, 2, 2, 2, 2, 2, 2, 2, 2, 2, 2, 2, 2, 2, 2, 2, 2, 2, 2, 2, 2, 2, 2, 2, 2, 2, 2, 2, 2, 2, 2, 2, 2, 2, 2, 2, 2, 2, 2, 2, 2, 2, 2, 2, 2, 2, 2, 2, 2, 2, 2, 2, 2, 2, 2, 2, 2, 2, 2, 2, 2, 2, 2, 2, 2, 2, 2, 2, 2, 2, 2, 2, 2, 2, 2, 2, 2, 2, 2, 2, 2, 2, 2, 2, 2, 2, 2, 2, 2, 2, 2, 2, 2, 2, 2, 2, 2, 2, 2, 2, 2, 2, 2, 2, 2, 2, 2, 2, 2, 2, 2, 2, 2, 2, 2, 2, 2, 2, 2, 2, 2, 2, 2, 2, 2, 2, 2, 2, 2, 2, 2, 2, 2, 2, 2, 2, 2, 2, 2, 2, 2, 2, 2, 2, 2, 2, 2, 2, 2, 2, 2, 2, 2, 2, 2, 2, 2, 2, 2, 2, 2, 2, 2, 2, 2, 2, 2, 2, 2, 2, 2, 2, 2, 2, 2, 2, 2, 2, 2, 2, 2, 2, 2, 2, 2, 2, 2, 2, 2, 2, 2, 2, 2, 2, 2, 2, 3 ),
 ( 0.000000000000000000, 0.5000000000000000000, 1.000000000000000000 ),
 ( 0.000000000000000000, 0.004385964912280701511, 0.008771929824561403022, 0.01315789473684210453, 0.01754385964912280604, 0.02192982456140350755, 0.02631578947368420907, 0.03070175438596491058, 0.03508771929824561209, 0.03947368421052631360, 0.04385964912280701511, 0.04824561403508771662, 0.05263157894736841813, 0.05701754385964911964, 0.06140350877192982115, 0.06578947368421052266, 0.07017543859649122417, 0.07456140350877192569, 0.07894736842105262720, 0.08333333333333332871, 0.08771929824561403022, 0.09210526315789473173, 0.09649122807017543324, 0.1008771929824561348, 0.1052631578947368363, 0.1096491228070175378, 0.1140350877192982393, 0.1184210526315789408, 0.1228070175438596423, 0.1271929824561403577, 0.1315789473684210453, 0.1359649122807017607, 0.1403508771929824483, 0.1447368421052631637, 0.1491228070175438514, 0.1535087719298245668, 0.1578947368421052544, 0.1622807017543859698, 0.1666666666666666574, 0.1710526315789473728, 0.1754385964912280604, 0.1798245614035087758, 0.1842105263157894635, 0.1885964912280701788, 0.1929824561403508665, 0.1973684210526315819, 0.2017543859649122695, 0.2061403508771929849, 0.2105263157894736725, 0.2149122807017543879, 0.2192982456140350755, 0.2236842105263157909, 0.2280701754385964786, 0.2324561403508771940, 0.2368421052631578816, 0.2412280701754385970, 0.2456140350877192846, 0.2500000000000000000, 0.2543859649122807154, 0.2587719298245614308, 0.2631578947368420907, 0.2675438596491228060, 0.2719298245614035214, 0.2763157894736842368, 0.2807017543859648967, 0.2850877192982456121, 0.2894736842105263275, 0.2938596491228070429, 0.2982456140350877027, 0.3026315789473684181, 0.3070175438596491335, 0.3114035087719298489, 0.3157894736842105088, 0.3201754385964912242, 0.3245614035087719396, 0.3289473684210526550, 0.3333333333333333148, 0.3377192982456140302, 0.3421052631578947456, 0.3464912280701754610, 0.3508771929824561209, 0.3552631578947368363, 0.3596491228070175517, 0.3640350877192982670, 0.3684210526315789269, 0.3728070175438596423, 0.3771929824561403577, 0.3815789473684210731, 0.3859649122807017330, 0.3903508771929824483, 0.3947368421052631637, 0.3991228070175438791, 0.4035087719298245390, 0.4078947368421052544, 0.4122807017543859698, 0.4166666666666666852, 0.4210526315789473450, 0.4254385964912280604, 0.4298245614035087758, 0.4342105263157894912, 0.4385964912280701511, 0.4429824561403508665, 0.4473684210526315819, 0.4517543859649122973, 0.4561403508771929571, 0.4605263157894736725, 0.4649122807017543879, 0.4692982456140351033, 0.4736842105263157632, 0.4780701754385964786, 0.4824561403508771940, 0.4868421052631579093, 0.4912280701754385692, 0.4956140350877192846, 0.5000000000000000000, 0.5043859649122807154, 0.5087719298245614308, 0.5131578947368421462, 0.5175438596491228616, 0.5219298245614034659, 0.5263157894736841813, 0.5307017543859648967, 0.5350877192982456121, 0.5394736842105263275, 0.5438596491228070429, 0.5482456140350877583, 0.5526315789473684736, 0.5570175438596490780, 0.5614035087719297934, 0.5657894736842105088, 0.5701754385964912242, 0.5745614035087719396, 0.5789473684210526550, 0.5833333333333333703, 0.5877192982456140857, 0.5921052631578946901, 0.5964912280701754055, 0.6008771929824561209, 0.6052631578947368363, 0.6096491228070175517, 0.6140350877192982670, 0.6184210526315789824, 0.6228070175438596978, 0.6271929824561403022, 0.6315789473684210176, 0.6359649122807017330, 0.6403508771929824483, 0.6447368421052631637, 0.6491228070175438791, 0.6535087719298245945, 0.6578947368421053099, 0.6622807017543859143, 0.6666666666666666297, 0.6710526315789473450, 0.6754385964912280604, 0.6798245614035087758, 0.6842105263157894912, 0.6885964912280702066, 0.6929824561403509220, 0.6973684210526315264, 0.7017543859649122417, 0.7061403508771929571, 0.7105263157894736725, 0.7149122807017543879, 0.7192982456140351033, 0.7236842105263158187, 0.7280701754385965341, 0.7324561403508771384, 0.7368421052631578538, 0.7412280701754385692, 0.7456140350877192846, 0.7500000000000000000, 0.7543859649122807154, 0.7587719298245614308, 0.7631578947368421462, 0.7675438596491228616, 0.7719298245614034659, 0.7763157894736841813, 0.7807017543859648967, 0.7850877192982456121, 0.7894736842105263275, 0.7938596491228070429, 0.7982456140350877583, 0.8026315789473684736, 0.8070175438596490780, 0.8114035087719297934, 0.8157894736842105088, 0.8201754385964912242, 0.8245614035087719396, 0.8289473684210526550, 0.8333333333333333703, 0.8377192982456140857, 0.8421052631578946901, 0.8464912280701754055, 0.8508771929824561209, 0.8552631578947368363, 0.8596491228070175517, 0.8640350877192982670, 0.8684210526315789824, 0.8728070175438596978, 0.8771929824561403022, 0.8815789473684210176, 0.8859649122807017330, 0.8903508771929824483, 0.8947368421052631637, 0.8991228070175438791, 0.9035087719298245945, 0.9078947368421053099, 0.9122807017543859143, 0.9166666666666666297, 0.9210526315789473450, 0.9254385964912280604, 0.9298245614035087758, 0.9342105263157894912, 0.9385964912280702066, 0.9429824561403509220, 0.9473684210526315264, 0.9517543859649122417, 0.9561403508771929571, 0.9605263157894736725, 0.9649122807017543879, 0.9692982456140351033, 0.9736842105263158187, 0.9780701754385965341, 0.9824561403508771384, 0.9868421052631578538, 0.9912280701754385692, 0.9956140350877192846, 1.000000000000000000 ),
 .UNSPECIFIED. ) 
 GEOMETRIC_REPRESENTATION_ITEM ( )  RATIONAL_B_SPLINE_SURFACE ( (
 ( 1.000000000000000000, 0.9659258262890683122, 1.000000000000000000, 0.9659258262890683122, 1.000000000000000000, 0.9659258262890683122, 1.000000000000000000, 0.9659258262890683122, 1.000000000000000000, 0.9659258262890683122, 1.000000000000000000, 0.9659258262890683122, 1.000000000000000000, 0.9659258262890683122, 1.000000000000000000, 0.9659258262890683122, 1.000000000000000000, 0.9659258262890683122, 1.000000000000000000, 0.9659258262890683122, 1.000000000000000000, 0.9659258262890683122, 1.000000000000000000, 0.9659258262890683122, 1.000000000000000000, 0.9659258262890683122, 1.000000000000000000, 0.9659258262890683122, 1.000000000000000000, 0.9659258262890683122, 1.000000000000000000, 0.9659258262890683122, 1.000000000000000000, 0.9659258262890683122, 1.000000000000000000, 0.9659258262890683122, 1.000000000000000000, 0.9659258262890683122, 1.000000000000000000, 0.9659258262890683122, 1.000000000000000000, 0.9659258262890683122, 1.000000000000000000, 0.9659258262890683122, 1.000000000000000000, 0.9659258262890683122, 1.000000000000000000, 0.9659258262890683122, 1.000000000000000000, 0.9659258262890683122, 1.000000000000000000, 0.9659258262890683122, 1.000000000000000000, 0.9659258262890683122, 1.000000000000000000, 0.9659258262890683122, 1.000000000000000000, 0.9659258262890683122, 1.000000000000000000, 0.9659258262890683122, 1.000000000000000000, 0.9659258262890683122, 1.000000000000000000, 0.9659258262890683122, 1.000000000000000000, 0.9659258262890683122, 1.000000000000000000, 0.9659258262890683122, 1.000000000000000000, 0.9659258262890683122, 1.000000000000000000, 0.9659258262890683122, 1.000000000000000000, 0.9659258262890683122, 1.000000000000000000, 0.9659258262890683122, 1.000000000000000000, 0.9659258262890683122, 1.000000000000000000, 0.9659258262890683122, 1.000000000000000000, 0.9659258262890683122, 1.000000000000000000, 0.9659258262890683122, 1.000000000000000000, 0.9659258262890683122, 1.000000000000000000, 0.9659258262890683122, 1.000000000000000000, 0.9659258262890683122, 1.000000000000000000, 0.9659258262890683122, 1.000000000000000000, 0.9659258262890683122, 1.000000000000000000, 0.9659258262890683122, 1.000000000000000000, 0.9659258262890683122, 1.000000000000000000, 0.9659258262890683122, 1.000000000000000000, 0.9659258262890683122, 1.000000000000000000, 0.9659258262890683122, 1.000000000000000000, 0.9659258262890683122, 1.000000000000000000, 0.9659258262890683122, 1.000000000000000000, 0.9659258262890683122, 1.000000000000000000, 0.9659258262890683122, 1.000000000000000000, 0.9659258262890683122, 1.000000000000000000, 0.9659258262890683122, 1.000000000000000000, 0.9659258262890683122, 1.000000000000000000, 0.9659258262890683122, 1.000000000000000000, 0.9659258262890683122, 1.000000000000000000, 0.9659258262890683122, 1.000000000000000000, 0.9659258262890683122, 1.000000000000000000, 0.9659258262890683122, 1.000000000000000000, 0.9659258262890683122, 1.000000000000000000, 0.9659258262890683122, 1.000000000000000000, 0.9659258262890683122, 1.000000000000000000, 0.9659258262890683122, 1.000000000000000000, 0.9659258262890683122, 1.000000000000000000, 0.9659258262890683122, 1.000000000000000000, 0.9659258262890683122, 1.000000000000000000, 0.9659258262890683122, 1.000000000000000000, 0.9659258262890683122, 1.000000000000000000, 0.9659258262890683122, 1.000000000000000000, 0.9659258262890683122, 1.000000000000000000, 0.9659258262890683122, 1.000000000000000000, 0.9659258262890683122, 1.000000000000000000, 0.9659258262890683122, 1.000000000000000000, 0.9659258262890683122, 1.000000000000000000, 0.9659258262890683122, 1.000000000000000000, 0.9659258262890683122, 1.000000000000000000, 0.9659258262890683122, 1.000000000000000000, 0.9659258262890683122, 1.000000000000000000, 0.9659258262890683122, 1.000000000000000000, 0.9659258262890683122, 1.000000000000000000, 0.9659258262890683122, 1.000000000000000000, 0.9659258262890683122, 1.000000000000000000, 0.9659258262890683122, 1.000000000000000000, 0.9659258262890683122, 1.000000000000000000, 0.9659258262890683122, 1.000000000000000000, 0.9659258262890683122, 1.000000000000000000, 0.9659258262890683122, 1.000000000000000000, 0.9659258262890683122, 1.000000000000000000, 0.9659258262890683122, 1.000000000000000000, 0.9659258262890683122, 1.000000000000000000, 0.9659258262890683122, 1.000000000000000000, 0.9659258262890683122, 1.000000000000000000, 0.9659258262890683122, 1.000000000000000000, 0.9659258262890683122, 1.000000000000000000, 0.9659258262890683122, 1.000000000000000000, 0.9659258262890683122, 1.000000000000000000, 0.9659258262890683122, 1.000000000000000000, 0.9659258262890683122, 1.000000000000000000, 0.9659258262890683122, 1.000000000000000000, 0.9659258262890683122, 1.000000000000000000, 0.9659258262890683122, 1.000000000000000000, 0.9659258262890683122, 1.000000000000000000, 0.9659258262890683122, 1.000000000000000000, 0.9659258262890683122, 1.000000000000000000, 0.9659258262890683122, 1.000000000000000000, 0.9659258262890683122, 1.000000000000000000, 0.9659258262890683122, 1.000000000000000000, 0.9659258262890683122, 1.000000000000000000, 0.9659258262890683122, 1.000000000000000000, 0.9659258262890683122, 1.000000000000000000, 0.9659258262890683122, 1.000000000000000000, 0.9659258262890683122, 1.000000000000000000, 0.9659258262890683122, 1.000000000000000000, 0.9659258262890683122, 1.000000000000000000, 0.9659258262890683122, 1.000000000000000000, 0.9659258262890683122, 1.000000000000000000, 0.9659258262890683122, 1.000000000000000000, 0.9659258262890683122, 1.000000000000000000, 0.9659258262890683122, 1.000000000000000000, 0.9659258262890683122, 1.000000000000000000, 0.9659258262890683122, 1.000000000000000000, 0.9659258262890683122, 1.000000000000000000, 0.9659258262890683122, 1.000000000000000000, 0.9659258262890683122, 1.000000000000000000, 0.9659258262890683122, 1.000000000000000000, 0.9659258262890683122, 1.000000000000000000, 0.9659258262890683122, 1.000000000000000000, 0.9659258262890683122, 1.000000000000000000, 0.9659258262890683122, 1.000000000000000000, 0.9659258262890683122, 1.000000000000000000, 0.9659258262890683122, 1.000000000000000000, 0.9659258262890683122, 1.000000000000000000, 0.9659258262890683122, 1.000000000000000000, 0.9659258262890683122, 1.000000000000000000, 0.9659258262890683122, 1.000000000000000000, 0.9659258262890683122, 1.000000000000000000, 0.9659258262890683122, 1.000000000000000000, 0.9659258262890683122, 1.000000000000000000, 0.9659258262890683122, 1.000000000000000000, 0.9659258262890683122, 1.000000000000000000, 0.9659258262890683122, 1.000000000000000000, 0.9659258262890683122, 1.000000000000000000, 0.9659258262890683122, 1.000000000000000000, 0.9659258262890683122, 1.000000000000000000, 0.9659258262890683122, 1.000000000000000000, 0.9659258262890683122, 1.000000000000000000, 0.9659258262890683122, 1.000000000000000000, 0.9659258262890683122, 1.000000000000000000, 0.9659258262890683122, 1.000000000000000000, 0.9659258262890683122, 1.000000000000000000, 0.9659258262890683122, 1.000000000000000000, 0.9659258262890683122, 1.000000000000000000, 0.9659258262890683122, 1.000000000000000000, 0.9659258262890683122, 1.000000000000000000, 0.9659258262890683122, 1.000000000000000000, 0.9659258262890683122, 1.000000000000000000, 0.9659258262890683122, 1.000000000000000000, 0.9659258262890683122, 1.000000000000000000, 0.9659258262890683122, 1.000000000000000000, 0.9659258262890683122, 1.000000000000000000, 0.9659258262890683122, 1.000000000000000000, 0.9659258262890683122, 1.000000000000000000, 0.9659258262890683122, 1.000000000000000000, 0.9659258262890683122, 1.000000000000000000, 0.9659258262890683122, 1.000000000000000000, 0.9659258262890683122, 1.000000000000000000, 0.9659258262890683122, 1.000000000000000000, 0.9659258262890683122, 1.000000000000000000, 0.9659258262890683122, 1.000000000000000000, 0.9659258262890683122, 1.000000000000000000, 0.9659258262890683122, 1.000000000000000000, 0.9659258262890683122, 1.000000000000000000, 0.9659258262890683122, 1.000000000000000000, 0.9659258262890683122, 1.000000000000000000, 0.9659258262890683122, 1.000000000000000000, 0.9659258262890683122, 1.000000000000000000, 0.9659258262890683122, 1.000000000000000000, 0.9659258262890683122, 1.000000000000000000, 0.9659258262890683122, 1.000000000000000000, 0.9659258262890683122, 1.000000000000000000, 0.9659258262890683122, 1.000000000000000000, 0.9659258262890683122, 1.000000000000000000, 0.9659258262890683122, 1.000000000000000000, 0.9659258262890683122, 1.000000000000000000, 0.9659258262890683122, 1.000000000000000000, 0.9659258262890683122, 1.000000000000000000, 0.9659258262890683122, 1.000000000000000000, 0.9659258262890683122, 1.000000000000000000, 0.9659258262890683122, 1.000000000000000000, 0.9659258262890683122, 1.000000000000000000, 0.9659258262890683122, 1.000000000000000000, 0.9659258262890683122, 1.000000000000000000, 0.9659258262890683122, 1.000000000000000000, 0.9659258262890683122, 1.000000000000000000, 0.9659258262890683122, 1.000000000000000000, 0.9659258262890683122, 1.000000000000000000, 0.9659258262890683122, 1.000000000000000000, 0.9659258262890683122, 1.000000000000000000, 0.9659258262890683122, 1.000000000000000000, 0.9659258262890683122, 1.000000000000000000, 0.9659258262890683122, 1.000000000000000000, 0.9659258262890683122, 1.000000000000000000, 0.9659258262890683122, 1.000000000000000000, 0.9659258262890683122, 1.000000000000000000, 0.9659258262890683122, 1.000000000000000000, 0.9659258262890683122, 1.000000000000000000, 0.9659258262890683122, 1.000000000000000000, 0.9659258262890683122, 1.000000000000000000, 0.9659258262890683122, 1.000000000000000000, 0.9659258262890683122, 1.000000000000000000, 0.9659258262890683122, 1.000000000000000000, 0.9659258262890683122, 1.000000000000000000, 0.9659258262890683122, 1.000000000000000000, 0.9659258262890683122, 1.000000000000000000, 0.9659258262890683122, 1.000000000000000000, 0.9659258262890683122, 1.000000000000000000, 0.9659258262890683122, 1.000000000000000000, 0.9659258262890683122, 1.000000000000000000, 0.9659258262890683122, 1.000000000000000000, 0.9659258262890683122, 1.000000000000000000, 0.9659258262890683122, 1.000000000000000000, 0.9659258262890683122, 1.000000000000000000, 0.9659258262890683122, 1.000000000000000000),
 ( 0.3333333333333333703, 0.3219752754296894559, 0.3333333333333333703, 0.3219752754296894559, 0.3333333333333333703, 0.3219752754296894559, 0.3333333333333333703, 0.3219752754296894559, 0.3333333333333333703, 0.3219752754296894559, 0.3333333333333333703, 0.3219752754296894559, 0.3333333333333333703, 0.3219752754296894559, 0.3333333333333333703, 0.3219752754296894559, 0.3333333333333333703, 0.3219752754296894559, 0.3333333333333333703, 0.3219752754296894559, 0.3333333333333333703, 0.3219752754296894559, 0.3333333333333333703, 0.3219752754296894559, 0.3333333333333333703, 0.3219752754296894559, 0.3333333333333333703, 0.3219752754296894559, 0.3333333333333333703, 0.3219752754296894559, 0.3333333333333333703, 0.3219752754296894559, 0.3333333333333333703, 0.3219752754296894559, 0.3333333333333333703, 0.3219752754296894559, 0.3333333333333333703, 0.3219752754296894559, 0.3333333333333333703, 0.3219752754296894559, 0.3333333333333333703, 0.3219752754296894559, 0.3333333333333333703, 0.3219752754296894559, 0.3333333333333333703, 0.3219752754296894559, 0.3333333333333333703, 0.3219752754296894559, 0.3333333333333333703, 0.3219752754296894559, 0.3333333333333333703, 0.3219752754296894559, 0.3333333333333333703, 0.3219752754296894559, 0.3333333333333333703, 0.3219752754296894559, 0.3333333333333333703, 0.3219752754296894559, 0.3333333333333333703, 0.3219752754296894559, 0.3333333333333333703, 0.3219752754296894559, 0.3333333333333333703, 0.3219752754296894559, 0.3333333333333333703, 0.3219752754296894559, 0.3333333333333333703, 0.3219752754296894559, 0.3333333333333333703, 0.3219752754296894559, 0.3333333333333333703, 0.3219752754296894559, 0.3333333333333333703, 0.3219752754296894559, 0.3333333333333333703, 0.3219752754296894559, 0.3333333333333333703, 0.3219752754296894559, 0.3333333333333333703, 0.3219752754296894559, 0.3333333333333333703, 0.3219752754296894559, 0.3333333333333333703, 0.3219752754296894559, 0.3333333333333333703, 0.3219752754296894559, 0.3333333333333333703, 0.3219752754296894559, 0.3333333333333333703, 0.3219752754296894559, 0.3333333333333333703, 0.3219752754296894559, 0.3333333333333333703, 0.3219752754296894559, 0.3333333333333333703, 0.3219752754296894559, 0.3333333333333333703, 0.3219752754296894559, 0.3333333333333333703, 0.3219752754296894559, 0.3333333333333333703, 0.3219752754296894559, 0.3333333333333333703, 0.3219752754296894559, 0.3333333333333333703, 0.3219752754296894559, 0.3333333333333333703, 0.3219752754296894559, 0.3333333333333333703, 0.3219752754296894559, 0.3333333333333333703, 0.3219752754296894559, 0.3333333333333333703, 0.3219752754296894559, 0.3333333333333333703, 0.3219752754296894559, 0.3333333333333333703, 0.3219752754296894559, 0.3333333333333333703, 0.3219752754296894559, 0.3333333333333333703, 0.3219752754296894559, 0.3333333333333333703, 0.3219752754296894559, 0.3333333333333333703, 0.3219752754296894559, 0.3333333333333333703, 0.3219752754296894559, 0.3333333333333333703, 0.3219752754296894559, 0.3333333333333333703, 0.3219752754296894559, 0.3333333333333333703, 0.3219752754296894559, 0.3333333333333333703, 0.3219752754296894559, 0.3333333333333333703, 0.3219752754296894559, 0.3333333333333333703, 0.3219752754296894559, 0.3333333333333333703, 0.3219752754296894559, 0.3333333333333333703, 0.3219752754296894559, 0.3333333333333333703, 0.3219752754296894559, 0.3333333333333333703, 0.3219752754296894559, 0.3333333333333333703, 0.3219752754296894559, 0.3333333333333333703, 0.3219752754296894559, 0.3333333333333333703, 0.3219752754296894559, 0.3333333333333333703, 0.3219752754296894559, 0.3333333333333333703, 0.3219752754296894559, 0.3333333333333333703, 0.3219752754296894559, 0.3333333333333333703, 0.3219752754296894559, 0.3333333333333333703, 0.3219752754296894559, 0.3333333333333333703, 0.3219752754296894559, 0.3333333333333333703, 0.3219752754296894559, 0.3333333333333333703, 0.3219752754296894559, 0.3333333333333333703, 0.3219752754296894559, 0.3333333333333333703, 0.3219752754296894559, 0.3333333333333333703, 0.3219752754296894559, 0.3333333333333333703, 0.3219752754296894559, 0.3333333333333333703, 0.3219752754296894559, 0.3333333333333333703, 0.3219752754296894559, 0.3333333333333333703, 0.3219752754296894559, 0.3333333333333333703, 0.3219752754296894559, 0.3333333333333333703, 0.3219752754296894559, 0.3333333333333333703, 0.3219752754296894559, 0.3333333333333333703, 0.3219752754296894559, 0.3333333333333333703, 0.3219752754296894559, 0.3333333333333333703, 0.3219752754296894559, 0.3333333333333333703, 0.3219752754296894559, 0.3333333333333333703, 0.3219752754296894559, 0.3333333333333333703, 0.3219752754296894559, 0.3333333333333333703, 0.3219752754296894559, 0.3333333333333333703, 0.3219752754296894559, 0.3333333333333333703, 0.3219752754296894559, 0.3333333333333333703, 0.3219752754296894559, 0.3333333333333333703, 0.3219752754296894559, 0.3333333333333333703, 0.3219752754296894559, 0.3333333333333333703, 0.3219752754296894559, 0.3333333333333333703, 0.3219752754296894559, 0.3333333333333333703, 0.3219752754296894559, 0.3333333333333333703, 0.3219752754296894559, 0.3333333333333333703, 0.3219752754296894559, 0.3333333333333333703, 0.3219752754296894559, 0.3333333333333333703, 0.3219752754296894559, 0.3333333333333333703, 0.3219752754296894559, 0.3333333333333333703, 0.3219752754296894559, 0.3333333333333333703, 0.3219752754296894559, 0.3333333333333333703, 0.3219752754296894559, 0.3333333333333333703, 0.3219752754296894559, 0.3333333333333333703, 0.3219752754296894559, 0.3333333333333333703, 0.3219752754296894559, 0.3333333333333333703, 0.3219752754296894559, 0.3333333333333333703, 0.3219752754296894559, 0.3333333333333333703, 0.3219752754296894559, 0.3333333333333333703, 0.3219752754296894559, 0.3333333333333333703, 0.3219752754296894559, 0.3333333333333333703, 0.3219752754296894559, 0.3333333333333333703, 0.3219752754296894559, 0.3333333333333333703, 0.3219752754296894559, 0.3333333333333333703, 0.3219752754296894559, 0.3333333333333333703, 0.3219752754296894559, 0.3333333333333333703, 0.3219752754296894559, 0.3333333333333333703, 0.3219752754296894559, 0.3333333333333333703, 0.3219752754296894559, 0.3333333333333333703, 0.3219752754296894559, 0.3333333333333333703, 0.3219752754296894559, 0.3333333333333333703, 0.3219752754296894559, 0.3333333333333333703, 0.3219752754296894559, 0.3333333333333333703, 0.3219752754296894559, 0.3333333333333333703, 0.3219752754296894559, 0.3333333333333333703, 0.3219752754296894559, 0.3333333333333333703, 0.3219752754296894559, 0.3333333333333333703, 0.3219752754296894559, 0.3333333333333333703, 0.3219752754296894559, 0.3333333333333333703, 0.3219752754296894559, 0.3333333333333333703, 0.3219752754296894559, 0.3333333333333333703, 0.3219752754296894559, 0.3333333333333333703, 0.3219752754296894559, 0.3333333333333333703, 0.3219752754296894559, 0.3333333333333333703, 0.3219752754296894559, 0.3333333333333333703, 0.3219752754296894559, 0.3333333333333333703, 0.3219752754296894559, 0.3333333333333333703, 0.3219752754296894559, 0.3333333333333333703, 0.3219752754296894559, 0.3333333333333333703, 0.3219752754296894559, 0.3333333333333333703, 0.3219752754296894559, 0.3333333333333333703, 0.3219752754296894559, 0.3333333333333333703, 0.3219752754296894559, 0.3333333333333333703, 0.3219752754296894559, 0.3333333333333333703, 0.3219752754296894559, 0.3333333333333333703, 0.3219752754296894559, 0.3333333333333333703, 0.3219752754296894559, 0.3333333333333333703, 0.3219752754296894559, 0.3333333333333333703, 0.3219752754296894559, 0.3333333333333333703, 0.3219752754296894559, 0.3333333333333333703, 0.3219752754296894559, 0.3333333333333333703, 0.3219752754296894559, 0.3333333333333333703, 0.3219752754296894559, 0.3333333333333333703, 0.3219752754296894559, 0.3333333333333333703, 0.3219752754296894559, 0.3333333333333333703, 0.3219752754296894559, 0.3333333333333333703, 0.3219752754296894559, 0.3333333333333333703, 0.3219752754296894559, 0.3333333333333333703, 0.3219752754296894559, 0.3333333333333333703, 0.3219752754296894559, 0.3333333333333333703, 0.3219752754296894559, 0.3333333333333333703, 0.3219752754296894559, 0.3333333333333333703, 0.3219752754296894559, 0.3333333333333333703, 0.3219752754296894559, 0.3333333333333333703, 0.3219752754296894559, 0.3333333333333333703, 0.3219752754296894559, 0.3333333333333333703, 0.3219752754296894559, 0.3333333333333333703, 0.3219752754296894559, 0.3333333333333333703, 0.3219752754296894559, 0.3333333333333333703, 0.3219752754296894559, 0.3333333333333333703, 0.3219752754296894559, 0.3333333333333333703, 0.3219752754296894559, 0.3333333333333333703, 0.3219752754296894559, 0.3333333333333333703, 0.3219752754296894559, 0.3333333333333333703, 0.3219752754296894559, 0.3333333333333333703, 0.3219752754296894559, 0.3333333333333333703, 0.3219752754296894559, 0.3333333333333333703, 0.3219752754296894559, 0.3333333333333333703, 0.3219752754296894559, 0.3333333333333333703, 0.3219752754296894559, 0.3333333333333333703, 0.3219752754296894559, 0.3333333333333333703, 0.3219752754296894559, 0.3333333333333333703, 0.3219752754296894559, 0.3333333333333333703, 0.3219752754296894559, 0.3333333333333333703, 0.3219752754296894559, 0.3333333333333333703, 0.3219752754296894559, 0.3333333333333333703, 0.3219752754296894559, 0.3333333333333333703, 0.3219752754296894559, 0.3333333333333333703, 0.3219752754296894559, 0.3333333333333333703, 0.3219752754296894559, 0.3333333333333333703, 0.3219752754296894559, 0.3333333333333333703, 0.3219752754296894559, 0.3333333333333333703, 0.3219752754296894559, 0.3333333333333333703, 0.3219752754296894559, 0.3333333333333333703, 0.3219752754296894559, 0.3333333333333333703, 0.3219752754296894559, 0.3333333333333333703, 0.3219752754296894559, 0.3333333333333333703, 0.3219752754296894559, 0.3333333333333333703, 0.3219752754296894559, 0.3333333333333333703, 0.3219752754296894559, 0.3333333333333333703, 0.3219752754296894559, 0.3333333333333333703, 0.3219752754296894559, 0.3333333333333333703, 0.3219752754296894559, 0.3333333333333333703, 0.3219752754296894559, 0.3333333333333333703, 0.3219752754296894559, 0.3333333333333333703, 0.3219752754296894559, 0.3333333333333333703, 0.3219752754296894559, 0.3333333333333333703, 0.3219752754296894559, 0.3333333333333333703, 0.3219752754296894559, 0.3333333333333333703, 0.3219752754296894559, 0.3333333333333333703, 0.3219752754296894559, 0.3333333333333333703, 0.3219752754296894559, 0.3333333333333333703, 0.3219752754296894559, 0.3333333333333333703),
 ( 0.3333333333333333703, 0.3219752754296894559, 0.3333333333333333703, 0.3219752754296894559, 0.3333333333333333703, 0.3219752754296894559, 0.3333333333333333703, 0.3219752754296894559, 0.3333333333333333703, 0.3219752754296894559, 0.3333333333333333703, 0.3219752754296894559, 0.3333333333333333703, 0.3219752754296894559, 0.3333333333333333703, 0.3219752754296894559, 0.3333333333333333703, 0.3219752754296894559, 0.3333333333333333703, 0.3219752754296894559, 0.3333333333333333703, 0.3219752754296894559, 0.3333333333333333703, 0.3219752754296894559, 0.3333333333333333703, 0.3219752754296894559, 0.3333333333333333703, 0.3219752754296894559, 0.3333333333333333703, 0.3219752754296894559, 0.3333333333333333703, 0.3219752754296894559, 0.3333333333333333703, 0.3219752754296894559, 0.3333333333333333703, 0.3219752754296894559, 0.3333333333333333703, 0.3219752754296894559, 0.3333333333333333703, 0.3219752754296894559, 0.3333333333333333703, 0.3219752754296894559, 0.3333333333333333703, 0.3219752754296894559, 0.3333333333333333703, 0.3219752754296894559, 0.3333333333333333703, 0.3219752754296894559, 0.3333333333333333703, 0.3219752754296894559, 0.3333333333333333703, 0.3219752754296894559, 0.3333333333333333703, 0.3219752754296894559, 0.3333333333333333703, 0.3219752754296894559, 0.3333333333333333703, 0.3219752754296894559, 0.3333333333333333703, 0.3219752754296894559, 0.3333333333333333703, 0.3219752754296894559, 0.3333333333333333703, 0.3219752754296894559, 0.3333333333333333703, 0.3219752754296894559, 0.3333333333333333703, 0.3219752754296894559, 0.3333333333333333703, 0.3219752754296894559, 0.3333333333333333703, 0.3219752754296894559, 0.3333333333333333703, 0.3219752754296894559, 0.3333333333333333703, 0.3219752754296894559, 0.3333333333333333703, 0.3219752754296894559, 0.3333333333333333703, 0.3219752754296894559, 0.3333333333333333703, 0.3219752754296894559, 0.3333333333333333703, 0.3219752754296894559, 0.3333333333333333703, 0.3219752754296894559, 0.3333333333333333703, 0.3219752754296894559, 0.3333333333333333703, 0.3219752754296894559, 0.3333333333333333703, 0.3219752754296894559, 0.3333333333333333703, 0.3219752754296894559, 0.3333333333333333703, 0.3219752754296894559, 0.3333333333333333703, 0.3219752754296894559, 0.3333333333333333703, 0.3219752754296894559, 0.3333333333333333703, 0.3219752754296894559, 0.3333333333333333703, 0.3219752754296894559, 0.3333333333333333703, 0.3219752754296894559, 0.3333333333333333703, 0.3219752754296894559, 0.3333333333333333703, 0.3219752754296894559, 0.3333333333333333703, 0.3219752754296894559, 0.3333333333333333703, 0.3219752754296894559, 0.3333333333333333703, 0.3219752754296894559, 0.3333333333333333703, 0.3219752754296894559, 0.3333333333333333703, 0.3219752754296894559, 0.3333333333333333703, 0.3219752754296894559, 0.3333333333333333703, 0.3219752754296894559, 0.3333333333333333703, 0.3219752754296894559, 0.3333333333333333703, 0.3219752754296894559, 0.3333333333333333703, 0.3219752754296894559, 0.3333333333333333703, 0.3219752754296894559, 0.3333333333333333703, 0.3219752754296894559, 0.3333333333333333703, 0.3219752754296894559, 0.3333333333333333703, 0.3219752754296894559, 0.3333333333333333703, 0.3219752754296894559, 0.3333333333333333703, 0.3219752754296894559, 0.3333333333333333703, 0.3219752754296894559, 0.3333333333333333703, 0.3219752754296894559, 0.3333333333333333703, 0.3219752754296894559, 0.3333333333333333703, 0.3219752754296894559, 0.3333333333333333703, 0.3219752754296894559, 0.3333333333333333703, 0.3219752754296894559, 0.3333333333333333703, 0.3219752754296894559, 0.3333333333333333703, 0.3219752754296894559, 0.3333333333333333703, 0.3219752754296894559, 0.3333333333333333703, 0.3219752754296894559, 0.3333333333333333703, 0.3219752754296894559, 0.3333333333333333703, 0.3219752754296894559, 0.3333333333333333703, 0.3219752754296894559, 0.3333333333333333703, 0.3219752754296894559, 0.3333333333333333703, 0.3219752754296894559, 0.3333333333333333703, 0.3219752754296894559, 0.3333333333333333703, 0.3219752754296894559, 0.3333333333333333703, 0.3219752754296894559, 0.3333333333333333703, 0.3219752754296894559, 0.3333333333333333703, 0.3219752754296894559, 0.3333333333333333703, 0.3219752754296894559, 0.3333333333333333703, 0.3219752754296894559, 0.3333333333333333703, 0.3219752754296894559, 0.3333333333333333703, 0.3219752754296894559, 0.3333333333333333703, 0.3219752754296894559, 0.3333333333333333703, 0.3219752754296894559, 0.3333333333333333703, 0.3219752754296894559, 0.3333333333333333703, 0.3219752754296894559, 0.3333333333333333703, 0.3219752754296894559, 0.3333333333333333703, 0.3219752754296894559, 0.3333333333333333703, 0.3219752754296894559, 0.3333333333333333703, 0.3219752754296894559, 0.3333333333333333703, 0.3219752754296894559, 0.3333333333333333703, 0.3219752754296894559, 0.3333333333333333703, 0.3219752754296894559, 0.3333333333333333703, 0.3219752754296894559, 0.3333333333333333703, 0.3219752754296894559, 0.3333333333333333703, 0.3219752754296894559, 0.3333333333333333703, 0.3219752754296894559, 0.3333333333333333703, 0.3219752754296894559, 0.3333333333333333703, 0.3219752754296894559, 0.3333333333333333703, 0.3219752754296894559, 0.3333333333333333703, 0.3219752754296894559, 0.3333333333333333703, 0.3219752754296894559, 0.3333333333333333703, 0.3219752754296894559, 0.3333333333333333703, 0.3219752754296894559, 0.3333333333333333703, 0.3219752754296894559, 0.3333333333333333703, 0.3219752754296894559, 0.3333333333333333703, 0.3219752754296894559, 0.3333333333333333703, 0.3219752754296894559, 0.3333333333333333703, 0.3219752754296894559, 0.3333333333333333703, 0.3219752754296894559, 0.3333333333333333703, 0.3219752754296894559, 0.3333333333333333703, 0.3219752754296894559, 0.3333333333333333703, 0.3219752754296894559, 0.3333333333333333703, 0.3219752754296894559, 0.3333333333333333703, 0.3219752754296894559, 0.3333333333333333703, 0.3219752754296894559, 0.3333333333333333703, 0.3219752754296894559, 0.3333333333333333703, 0.3219752754296894559, 0.3333333333333333703, 0.3219752754296894559, 0.3333333333333333703, 0.3219752754296894559, 0.3333333333333333703, 0.3219752754296894559, 0.3333333333333333703, 0.3219752754296894559, 0.3333333333333333703, 0.3219752754296894559, 0.3333333333333333703, 0.3219752754296894559, 0.3333333333333333703, 0.3219752754296894559, 0.3333333333333333703, 0.3219752754296894559, 0.3333333333333333703, 0.3219752754296894559, 0.3333333333333333703, 0.3219752754296894559, 0.3333333333333333703, 0.3219752754296894559, 0.3333333333333333703, 0.3219752754296894559, 0.3333333333333333703, 0.3219752754296894559, 0.3333333333333333703, 0.3219752754296894559, 0.3333333333333333703, 0.3219752754296894559, 0.3333333333333333703, 0.3219752754296894559, 0.3333333333333333703, 0.3219752754296894559, 0.3333333333333333703, 0.3219752754296894559, 0.3333333333333333703, 0.3219752754296894559, 0.3333333333333333703, 0.3219752754296894559, 0.3333333333333333703, 0.3219752754296894559, 0.3333333333333333703, 0.3219752754296894559, 0.3333333333333333703, 0.3219752754296894559, 0.3333333333333333703, 0.3219752754296894559, 0.3333333333333333703, 0.3219752754296894559, 0.3333333333333333703, 0.3219752754296894559, 0.3333333333333333703, 0.3219752754296894559, 0.3333333333333333703, 0.3219752754296894559, 0.3333333333333333703, 0.3219752754296894559, 0.3333333333333333703, 0.3219752754296894559, 0.3333333333333333703, 0.3219752754296894559, 0.3333333333333333703, 0.3219752754296894559, 0.3333333333333333703, 0.3219752754296894559, 0.3333333333333333703, 0.3219752754296894559, 0.3333333333333333703, 0.3219752754296894559, 0.3333333333333333703, 0.3219752754296894559, 0.3333333333333333703, 0.3219752754296894559, 0.3333333333333333703, 0.3219752754296894559, 0.3333333333333333703, 0.3219752754296894559, 0.3333333333333333703, 0.3219752754296894559, 0.3333333333333333703, 0.3219752754296894559, 0.3333333333333333703, 0.3219752754296894559, 0.3333333333333333703, 0.3219752754296894559, 0.3333333333333333703, 0.3219752754296894559, 0.3333333333333333703, 0.3219752754296894559, 0.3333333333333333703, 0.3219752754296894559, 0.3333333333333333703, 0.3219752754296894559, 0.3333333333333333703, 0.3219752754296894559, 0.3333333333333333703, 0.3219752754296894559, 0.3333333333333333703, 0.3219752754296894559, 0.3333333333333333703, 0.3219752754296894559, 0.3333333333333333703, 0.3219752754296894559, 0.3333333333333333703, 0.3219752754296894559, 0.3333333333333333703, 0.3219752754296894559, 0.3333333333333333703, 0.3219752754296894559, 0.3333333333333333703, 0.3219752754296894559, 0.3333333333333333703, 0.3219752754296894559, 0.3333333333333333703, 0.3219752754296894559, 0.3333333333333333703, 0.3219752754296894559, 0.3333333333333333703, 0.3219752754296894559, 0.3333333333333333703, 0.3219752754296894559, 0.3333333333333333703, 0.3219752754296894559, 0.3333333333333333703, 0.3219752754296894559, 0.3333333333333333703, 0.3219752754296894559, 0.3333333333333333703, 0.3219752754296894559, 0.3333333333333333703, 0.3219752754296894559, 0.3333333333333333703, 0.3219752754296894559, 0.3333333333333333703, 0.3219752754296894559, 0.3333333333333333703, 0.3219752754296894559, 0.3333333333333333703, 0.3219752754296894559, 0.3333333333333333703, 0.3219752754296894559, 0.3333333333333333703, 0.3219752754296894559, 0.3333333333333333703, 0.3219752754296894559, 0.3333333333333333703, 0.3219752754296894559, 0.3333333333333333703, 0.3219752754296894559, 0.3333333333333333703, 0.3219752754296894559, 0.3333333333333333703, 0.3219752754296894559, 0.3333333333333333703, 0.3219752754296894559, 0.3333333333333333703, 0.3219752754296894559, 0.3333333333333333703, 0.3219752754296894559, 0.3333333333333333703, 0.3219752754296894559, 0.3333333333333333703, 0.3219752754296894559, 0.3333333333333333703, 0.3219752754296894559, 0.3333333333333333703, 0.3219752754296894559, 0.3333333333333333703, 0.3219752754296894559, 0.3333333333333333703, 0.3219752754296894559, 0.3333333333333333703, 0.3219752754296894559, 0.3333333333333333703, 0.3219752754296894559, 0.3333333333333333703, 0.3219752754296894559, 0.3333333333333333703, 0.3219752754296894559, 0.3333333333333333703, 0.3219752754296894559, 0.3333333333333333703, 0.3219752754296894559, 0.3333333333333333703, 0.3219752754296894559, 0.3333333333333333703, 0.3219752754296894559, 0.3333333333333333703, 0.3219752754296894559, 0.3333333333333333703, 0.3219752754296894559, 0.3333333333333333703, 0.3219752754296894559, 0.3333333333333333703),
 ( 1.000000000000000000, 0.9659258262890683122, 1.000000000000000000, 0.9659258262890683122, 1.000000000000000000, 0.9659258262890683122, 1.000000000000000000, 0.9659258262890683122, 1.000000000000000000, 0.9659258262890683122, 1.000000000000000000, 0.9659258262890683122, 1.000000000000000000, 0.9659258262890683122, 1.000000000000000000, 0.9659258262890683122, 1.000000000000000000, 0.9659258262890683122, 1.000000000000000000, 0.9659258262890683122, 1.000000000000000000, 0.9659258262890683122, 1.000000000000000000, 0.9659258262890683122, 1.000000000000000000, 0.9659258262890683122, 1.000000000000000000, 0.9659258262890683122, 1.000000000000000000, 0.9659258262890683122, 1.000000000000000000, 0.9659258262890683122, 1.000000000000000000, 0.9659258262890683122, 1.000000000000000000, 0.9659258262890683122, 1.000000000000000000, 0.9659258262890683122, 1.000000000000000000, 0.9659258262890683122, 1.000000000000000000, 0.9659258262890683122, 1.000000000000000000, 0.9659258262890683122, 1.000000000000000000, 0.9659258262890683122, 1.000000000000000000, 0.9659258262890683122, 1.000000000000000000, 0.9659258262890683122, 1.000000000000000000, 0.9659258262890683122, 1.000000000000000000, 0.9659258262890683122, 1.000000000000000000, 0.9659258262890683122, 1.000000000000000000, 0.9659258262890683122, 1.000000000000000000, 0.9659258262890683122, 1.000000000000000000, 0.9659258262890683122, 1.000000000000000000, 0.9659258262890683122, 1.000000000000000000, 0.9659258262890683122, 1.000000000000000000, 0.9659258262890683122, 1.000000000000000000, 0.9659258262890683122, 1.000000000000000000, 0.9659258262890683122, 1.000000000000000000, 0.9659258262890683122, 1.000000000000000000, 0.9659258262890683122, 1.000000000000000000, 0.9659258262890683122, 1.000000000000000000, 0.9659258262890683122, 1.000000000000000000, 0.9659258262890683122, 1.000000000000000000, 0.9659258262890683122, 1.000000000000000000, 0.9659258262890683122, 1.000000000000000000, 0.9659258262890683122, 1.000000000000000000, 0.9659258262890683122, 1.000000000000000000, 0.9659258262890683122, 1.000000000000000000, 0.9659258262890683122, 1.000000000000000000, 0.9659258262890683122, 1.000000000000000000, 0.9659258262890683122, 1.000000000000000000, 0.9659258262890683122, 1.000000000000000000, 0.9659258262890683122, 1.000000000000000000, 0.9659258262890683122, 1.000000000000000000, 0.9659258262890683122, 1.000000000000000000, 0.9659258262890683122, 1.000000000000000000, 0.9659258262890683122, 1.000000000000000000, 0.9659258262890683122, 1.000000000000000000, 0.9659258262890683122, 1.000000000000000000, 0.9659258262890683122, 1.000000000000000000, 0.9659258262890683122, 1.000000000000000000, 0.9659258262890683122, 1.000000000000000000, 0.9659258262890683122, 1.000000000000000000, 0.9659258262890683122, 1.000000000000000000, 0.9659258262890683122, 1.000000000000000000, 0.9659258262890683122, 1.000000000000000000, 0.9659258262890683122, 1.000000000000000000, 0.9659258262890683122, 1.000000000000000000, 0.9659258262890683122, 1.000000000000000000, 0.9659258262890683122, 1.000000000000000000, 0.9659258262890683122, 1.000000000000000000, 0.9659258262890683122, 1.000000000000000000, 0.9659258262890683122, 1.000000000000000000, 0.9659258262890683122, 1.000000000000000000, 0.9659258262890683122, 1.000000000000000000, 0.9659258262890683122, 1.000000000000000000, 0.9659258262890683122, 1.000000000000000000, 0.9659258262890683122, 1.000000000000000000, 0.9659258262890683122, 1.000000000000000000, 0.9659258262890683122, 1.000000000000000000, 0.9659258262890683122, 1.000000000000000000, 0.9659258262890683122, 1.000000000000000000, 0.9659258262890683122, 1.000000000000000000, 0.9659258262890683122, 1.000000000000000000, 0.9659258262890683122, 1.000000000000000000, 0.9659258262890683122, 1.000000000000000000, 0.9659258262890683122, 1.000000000000000000, 0.9659258262890683122, 1.000000000000000000, 0.9659258262890683122, 1.000000000000000000, 0.9659258262890683122, 1.000000000000000000, 0.9659258262890683122, 1.000000000000000000, 0.9659258262890683122, 1.000000000000000000, 0.9659258262890683122, 1.000000000000000000, 0.9659258262890683122, 1.000000000000000000, 0.9659258262890683122, 1.000000000000000000, 0.9659258262890683122, 1.000000000000000000, 0.9659258262890683122, 1.000000000000000000, 0.9659258262890683122, 1.000000000000000000, 0.9659258262890683122, 1.000000000000000000, 0.9659258262890683122, 1.000000000000000000, 0.9659258262890683122, 1.000000000000000000, 0.9659258262890683122, 1.000000000000000000, 0.9659258262890683122, 1.000000000000000000, 0.9659258262890683122, 1.000000000000000000, 0.9659258262890683122, 1.000000000000000000, 0.9659258262890683122, 1.000000000000000000, 0.9659258262890683122, 1.000000000000000000, 0.9659258262890683122, 1.000000000000000000, 0.9659258262890683122, 1.000000000000000000, 0.9659258262890683122, 1.000000000000000000, 0.9659258262890683122, 1.000000000000000000, 0.9659258262890683122, 1.000000000000000000, 0.9659258262890683122, 1.000000000000000000, 0.9659258262890683122, 1.000000000000000000, 0.9659258262890683122, 1.000000000000000000, 0.9659258262890683122, 1.000000000000000000, 0.9659258262890683122, 1.000000000000000000, 0.9659258262890683122, 1.000000000000000000, 0.9659258262890683122, 1.000000000000000000, 0.9659258262890683122, 1.000000000000000000, 0.9659258262890683122, 1.000000000000000000, 0.9659258262890683122, 1.000000000000000000, 0.9659258262890683122, 1.000000000000000000, 0.9659258262890683122, 1.000000000000000000, 0.9659258262890683122, 1.000000000000000000, 0.9659258262890683122, 1.000000000000000000, 0.9659258262890683122, 1.000000000000000000, 0.9659258262890683122, 1.000000000000000000, 0.9659258262890683122, 1.000000000000000000, 0.9659258262890683122, 1.000000000000000000, 0.9659258262890683122, 1.000000000000000000, 0.9659258262890683122, 1.000000000000000000, 0.9659258262890683122, 1.000000000000000000, 0.9659258262890683122, 1.000000000000000000, 0.9659258262890683122, 1.000000000000000000, 0.9659258262890683122, 1.000000000000000000, 0.9659258262890683122, 1.000000000000000000, 0.9659258262890683122, 1.000000000000000000, 0.9659258262890683122, 1.000000000000000000, 0.9659258262890683122, 1.000000000000000000, 0.9659258262890683122, 1.000000000000000000, 0.9659258262890683122, 1.000000000000000000, 0.9659258262890683122, 1.000000000000000000, 0.9659258262890683122, 1.000000000000000000, 0.9659258262890683122, 1.000000000000000000, 0.9659258262890683122, 1.000000000000000000, 0.9659258262890683122, 1.000000000000000000, 0.9659258262890683122, 1.000000000000000000, 0.9659258262890683122, 1.000000000000000000, 0.9659258262890683122, 1.000000000000000000, 0.9659258262890683122, 1.000000000000000000, 0.9659258262890683122, 1.000000000000000000, 0.9659258262890683122, 1.000000000000000000, 0.9659258262890683122, 1.000000000000000000, 0.9659258262890683122, 1.000000000000000000, 0.9659258262890683122, 1.000000000000000000, 0.9659258262890683122, 1.000000000000000000, 0.9659258262890683122, 1.000000000000000000, 0.9659258262890683122, 1.000000000000000000, 0.9659258262890683122, 1.000000000000000000, 0.9659258262890683122, 1.000000000000000000, 0.9659258262890683122, 1.000000000000000000, 0.9659258262890683122, 1.000000000000000000, 0.9659258262890683122, 1.000000000000000000, 0.9659258262890683122, 1.000000000000000000, 0.9659258262890683122, 1.000000000000000000, 0.9659258262890683122, 1.000000000000000000, 0.9659258262890683122, 1.000000000000000000, 0.9659258262890683122, 1.000000000000000000, 0.9659258262890683122, 1.000000000000000000, 0.9659258262890683122, 1.000000000000000000, 0.9659258262890683122, 1.000000000000000000, 0.9659258262890683122, 1.000000000000000000, 0.9659258262890683122, 1.000000000000000000, 0.9659258262890683122, 1.000000000000000000, 0.9659258262890683122, 1.000000000000000000, 0.9659258262890683122, 1.000000000000000000, 0.9659258262890683122, 1.000000000000000000, 0.9659258262890683122, 1.000000000000000000, 0.9659258262890683122, 1.000000000000000000, 0.9659258262890683122, 1.000000000000000000, 0.9659258262890683122, 1.000000000000000000, 0.9659258262890683122, 1.000000000000000000, 0.9659258262890683122, 1.000000000000000000, 0.9659258262890683122, 1.000000000000000000, 0.9659258262890683122, 1.000000000000000000, 0.9659258262890683122, 1.000000000000000000, 0.9659258262890683122, 1.000000000000000000, 0.9659258262890683122, 1.000000000000000000, 0.9659258262890683122, 1.000000000000000000, 0.9659258262890683122, 1.000000000000000000, 0.9659258262890683122, 1.000000000000000000, 0.9659258262890683122, 1.000000000000000000, 0.9659258262890683122, 1.000000000000000000, 0.9659258262890683122, 1.000000000000000000, 0.9659258262890683122, 1.000000000000000000, 0.9659258262890683122, 1.000000000000000000, 0.9659258262890683122, 1.000000000000000000, 0.9659258262890683122, 1.000000000000000000, 0.9659258262890683122, 1.000000000000000000, 0.9659258262890683122, 1.000000000000000000, 0.9659258262890683122, 1.000000000000000000, 0.9659258262890683122, 1.000000000000000000, 0.9659258262890683122, 1.000000000000000000, 0.9659258262890683122, 1.000000000000000000, 0.9659258262890683122, 1.000000000000000000, 0.9659258262890683122, 1.000000000000000000, 0.9659258262890683122, 1.000000000000000000, 0.9659258262890683122, 1.000000000000000000, 0.9659258262890683122, 1.000000000000000000, 0.9659258262890683122, 1.000000000000000000, 0.9659258262890683122, 1.000000000000000000, 0.9659258262890683122, 1.000000000000000000, 0.9659258262890683122, 1.000000000000000000, 0.9659258262890683122, 1.000000000000000000, 0.9659258262890683122, 1.000000000000000000, 0.9659258262890683122, 1.000000000000000000, 0.9659258262890683122, 1.000000000000000000, 0.9659258262890683122, 1.000000000000000000, 0.9659258262890683122, 1.000000000000000000, 0.9659258262890683122, 1.000000000000000000, 0.9659258262890683122, 1.000000000000000000, 0.9659258262890683122, 1.000000000000000000, 0.9659258262890683122, 1.000000000000000000, 0.9659258262890683122, 1.000000000000000000, 0.9659258262890683122, 1.000000000000000000, 0.9659258262890683122, 1.000000000000000000, 0.9659258262890683122, 1.000000000000000000, 0.9659258262890683122, 1.000000000000000000, 0.9659258262890683122, 1.000000000000000000),
 ( 0.3333333333333333703, 0.3219752754296894559, 0.3333333333333333703, 0.3219752754296894559, 0.3333333333333333703, 0.3219752754296894559, 0.3333333333333333703, 0.3219752754296894559, 0.3333333333333333703, 0.3219752754296894559, 0.3333333333333333703, 0.3219752754296894559, 0.3333333333333333703, 0.3219752754296894559, 0.3333333333333333703, 0.3219752754296894559, 0.3333333333333333703, 0.3219752754296894559, 0.3333333333333333703, 0.3219752754296894559, 0.3333333333333333703, 0.3219752754296894559, 0.3333333333333333703, 0.3219752754296894559, 0.3333333333333333703, 0.3219752754296894559, 0.3333333333333333703, 0.3219752754296894559, 0.3333333333333333703, 0.3219752754296894559, 0.3333333333333333703, 0.3219752754296894559, 0.3333333333333333703, 0.3219752754296894559, 0.3333333333333333703, 0.3219752754296894559, 0.3333333333333333703, 0.3219752754296894559, 0.3333333333333333703, 0.3219752754296894559, 0.3333333333333333703, 0.3219752754296894559, 0.3333333333333333703, 0.3219752754296894559, 0.3333333333333333703, 0.3219752754296894559, 0.3333333333333333703, 0.3219752754296894559, 0.3333333333333333703, 0.3219752754296894559, 0.3333333333333333703, 0.3219752754296894559, 0.3333333333333333703, 0.3219752754296894559, 0.3333333333333333703, 0.3219752754296894559, 0.3333333333333333703, 0.3219752754296894559, 0.3333333333333333703, 0.3219752754296894559, 0.3333333333333333703, 0.3219752754296894559, 0.3333333333333333703, 0.3219752754296894559, 0.3333333333333333703, 0.3219752754296894559, 0.3333333333333333703, 0.3219752754296894559, 0.3333333333333333703, 0.3219752754296894559, 0.3333333333333333703, 0.3219752754296894559, 0.3333333333333333703, 0.3219752754296894559, 0.3333333333333333703, 0.3219752754296894559, 0.3333333333333333703, 0.3219752754296894559, 0.3333333333333333703, 0.3219752754296894559, 0.3333333333333333703, 0.3219752754296894559, 0.3333333333333333703, 0.3219752754296894559, 0.3333333333333333703, 0.3219752754296894559, 0.3333333333333333703, 0.3219752754296894559, 0.3333333333333333703, 0.3219752754296894559, 0.3333333333333333703, 0.3219752754296894559, 0.3333333333333333703, 0.3219752754296894559, 0.3333333333333333703, 0.3219752754296894559, 0.3333333333333333703, 0.3219752754296894559, 0.3333333333333333703, 0.3219752754296894559, 0.3333333333333333703, 0.3219752754296894559, 0.3333333333333333703, 0.3219752754296894559, 0.3333333333333333703, 0.3219752754296894559, 0.3333333333333333703, 0.3219752754296894559, 0.3333333333333333703, 0.3219752754296894559, 0.3333333333333333703, 0.3219752754296894559, 0.3333333333333333703, 0.3219752754296894559, 0.3333333333333333703, 0.3219752754296894559, 0.3333333333333333703, 0.3219752754296894559, 0.3333333333333333703, 0.3219752754296894559, 0.3333333333333333703, 0.3219752754296894559, 0.3333333333333333703, 0.3219752754296894559, 0.3333333333333333703, 0.3219752754296894559, 0.3333333333333333703, 0.3219752754296894559, 0.3333333333333333703, 0.3219752754296894559, 0.3333333333333333703, 0.3219752754296894559, 0.3333333333333333703, 0.3219752754296894559, 0.3333333333333333703, 0.3219752754296894559, 0.3333333333333333703, 0.3219752754296894559, 0.3333333333333333703, 0.3219752754296894559, 0.3333333333333333703, 0.3219752754296894559, 0.3333333333333333703, 0.3219752754296894559, 0.3333333333333333703, 0.3219752754296894559, 0.3333333333333333703, 0.3219752754296894559, 0.3333333333333333703, 0.3219752754296894559, 0.3333333333333333703, 0.3219752754296894559, 0.3333333333333333703, 0.3219752754296894559, 0.3333333333333333703, 0.3219752754296894559, 0.3333333333333333703, 0.3219752754296894559, 0.3333333333333333703, 0.3219752754296894559, 0.3333333333333333703, 0.3219752754296894559, 0.3333333333333333703, 0.3219752754296894559, 0.3333333333333333703, 0.3219752754296894559, 0.3333333333333333703, 0.3219752754296894559, 0.3333333333333333703, 0.3219752754296894559, 0.3333333333333333703, 0.3219752754296894559, 0.3333333333333333703, 0.3219752754296894559, 0.3333333333333333703, 0.3219752754296894559, 0.3333333333333333703, 0.3219752754296894559, 0.3333333333333333703, 0.3219752754296894559, 0.3333333333333333703, 0.3219752754296894559, 0.3333333333333333703, 0.3219752754296894559, 0.3333333333333333703, 0.3219752754296894559, 0.3333333333333333703, 0.3219752754296894559, 0.3333333333333333703, 0.3219752754296894559, 0.3333333333333333703, 0.3219752754296894559, 0.3333333333333333703, 0.3219752754296894559, 0.3333333333333333703, 0.3219752754296894559, 0.3333333333333333703, 0.3219752754296894559, 0.3333333333333333703, 0.3219752754296894559, 0.3333333333333333703, 0.3219752754296894559, 0.3333333333333333703, 0.3219752754296894559, 0.3333333333333333703, 0.3219752754296894559, 0.3333333333333333703, 0.3219752754296894559, 0.3333333333333333703, 0.3219752754296894559, 0.3333333333333333703, 0.3219752754296894559, 0.3333333333333333703, 0.3219752754296894559, 0.3333333333333333703, 0.3219752754296894559, 0.3333333333333333703, 0.3219752754296894559, 0.3333333333333333703, 0.3219752754296894559, 0.3333333333333333703, 0.3219752754296894559, 0.3333333333333333703, 0.3219752754296894559, 0.3333333333333333703, 0.3219752754296894559, 0.3333333333333333703, 0.3219752754296894559, 0.3333333333333333703, 0.3219752754296894559, 0.3333333333333333703, 0.3219752754296894559, 0.3333333333333333703, 0.3219752754296894559, 0.3333333333333333703, 0.3219752754296894559, 0.3333333333333333703, 0.3219752754296894559, 0.3333333333333333703, 0.3219752754296894559, 0.3333333333333333703, 0.3219752754296894559, 0.3333333333333333703, 0.3219752754296894559, 0.3333333333333333703, 0.3219752754296894559, 0.3333333333333333703, 0.3219752754296894559, 0.3333333333333333703, 0.3219752754296894559, 0.3333333333333333703, 0.3219752754296894559, 0.3333333333333333703, 0.3219752754296894559, 0.3333333333333333703, 0.3219752754296894559, 0.3333333333333333703, 0.3219752754296894559, 0.3333333333333333703, 0.3219752754296894559, 0.3333333333333333703, 0.3219752754296894559, 0.3333333333333333703, 0.3219752754296894559, 0.3333333333333333703, 0.3219752754296894559, 0.3333333333333333703, 0.3219752754296894559, 0.3333333333333333703, 0.3219752754296894559, 0.3333333333333333703, 0.3219752754296894559, 0.3333333333333333703, 0.3219752754296894559, 0.3333333333333333703, 0.3219752754296894559, 0.3333333333333333703, 0.3219752754296894559, 0.3333333333333333703, 0.3219752754296894559, 0.3333333333333333703, 0.3219752754296894559, 0.3333333333333333703, 0.3219752754296894559, 0.3333333333333333703, 0.3219752754296894559, 0.3333333333333333703, 0.3219752754296894559, 0.3333333333333333703, 0.3219752754296894559, 0.3333333333333333703, 0.3219752754296894559, 0.3333333333333333703, 0.3219752754296894559, 0.3333333333333333703, 0.3219752754296894559, 0.3333333333333333703, 0.3219752754296894559, 0.3333333333333333703, 0.3219752754296894559, 0.3333333333333333703, 0.3219752754296894559, 0.3333333333333333703, 0.3219752754296894559, 0.3333333333333333703, 0.3219752754296894559, 0.3333333333333333703, 0.3219752754296894559, 0.3333333333333333703, 0.3219752754296894559, 0.3333333333333333703, 0.3219752754296894559, 0.3333333333333333703, 0.3219752754296894559, 0.3333333333333333703, 0.3219752754296894559, 0.3333333333333333703, 0.3219752754296894559, 0.3333333333333333703, 0.3219752754296894559, 0.3333333333333333703, 0.3219752754296894559, 0.3333333333333333703, 0.3219752754296894559, 0.3333333333333333703, 0.3219752754296894559, 0.3333333333333333703, 0.3219752754296894559, 0.3333333333333333703, 0.3219752754296894559, 0.3333333333333333703, 0.3219752754296894559, 0.3333333333333333703, 0.3219752754296894559, 0.3333333333333333703, 0.3219752754296894559, 0.3333333333333333703, 0.3219752754296894559, 0.3333333333333333703, 0.3219752754296894559, 0.3333333333333333703, 0.3219752754296894559, 0.3333333333333333703, 0.3219752754296894559, 0.3333333333333333703, 0.3219752754296894559, 0.3333333333333333703, 0.3219752754296894559, 0.3333333333333333703, 0.3219752754296894559, 0.3333333333333333703, 0.3219752754296894559, 0.3333333333333333703, 0.3219752754296894559, 0.3333333333333333703, 0.3219752754296894559, 0.3333333333333333703, 0.3219752754296894559, 0.3333333333333333703, 0.3219752754296894559, 0.3333333333333333703, 0.3219752754296894559, 0.3333333333333333703, 0.3219752754296894559, 0.3333333333333333703, 0.3219752754296894559, 0.3333333333333333703, 0.3219752754296894559, 0.3333333333333333703, 0.3219752754296894559, 0.3333333333333333703, 0.3219752754296894559, 0.3333333333333333703, 0.3219752754296894559, 0.3333333333333333703, 0.3219752754296894559, 0.3333333333333333703, 0.3219752754296894559, 0.3333333333333333703, 0.3219752754296894559, 0.3333333333333333703, 0.3219752754296894559, 0.3333333333333333703, 0.3219752754296894559, 0.3333333333333333703, 0.3219752754296894559, 0.3333333333333333703, 0.3219752754296894559, 0.3333333333333333703, 0.3219752754296894559, 0.3333333333333333703, 0.3219752754296894559, 0.3333333333333333703, 0.3219752754296894559, 0.3333333333333333703, 0.3219752754296894559, 0.3333333333333333703, 0.3219752754296894559, 0.3333333333333333703, 0.3219752754296894559, 0.3333333333333333703, 0.3219752754296894559, 0.3333333333333333703, 0.3219752754296894559, 0.3333333333333333703, 0.3219752754296894559, 0.3333333333333333703, 0.3219752754296894559, 0.3333333333333333703, 0.3219752754296894559, 0.3333333333333333703, 0.3219752754296894559, 0.3333333333333333703, 0.3219752754296894559, 0.3333333333333333703, 0.3219752754296894559, 0.3333333333333333703, 0.3219752754296894559, 0.3333333333333333703, 0.3219752754296894559, 0.3333333333333333703, 0.3219752754296894559, 0.3333333333333333703, 0.3219752754296894559, 0.3333333333333333703, 0.3219752754296894559, 0.3333333333333333703, 0.3219752754296894559, 0.3333333333333333703, 0.3219752754296894559, 0.3333333333333333703, 0.3219752754296894559, 0.3333333333333333703, 0.3219752754296894559, 0.3333333333333333703, 0.3219752754296894559, 0.3333333333333333703, 0.3219752754296894559, 0.3333333333333333703, 0.3219752754296894559, 0.3333333333333333703, 0.3219752754296894559, 0.3333333333333333703, 0.3219752754296894559, 0.3333333333333333703, 0.3219752754296894559, 0.3333333333333333703, 0.3219752754296894559, 0.3333333333333333703, 0.3219752754296894559, 0.3333333333333333703, 0.3219752754296894559, 0.3333333333333333703, 0.3219752754296894559, 0.3333333333333333703, 0.3219752754296894559, 0.3333333333333333703),
 ( 0.3333333333333333703, 0.3219752754296894559, 0.3333333333333333703, 0.3219752754296894559, 0.3333333333333333703, 0.3219752754296894559, 0.3333333333333333703, 0.3219752754296894559, 0.3333333333333333703, 0.3219752754296894559, 0.3333333333333333703, 0.3219752754296894559, 0.3333333333333333703, 0.3219752754296894559, 0.3333333333333333703, 0.3219752754296894559, 0.3333333333333333703, 0.3219752754296894559, 0.3333333333333333703, 0.3219752754296894559, 0.3333333333333333703, 0.3219752754296894559, 0.3333333333333333703, 0.3219752754296894559, 0.3333333333333333703, 0.3219752754296894559, 0.3333333333333333703, 0.3219752754296894559, 0.3333333333333333703, 0.3219752754296894559, 0.3333333333333333703, 0.3219752754296894559, 0.3333333333333333703, 0.3219752754296894559, 0.3333333333333333703, 0.3219752754296894559, 0.3333333333333333703, 0.3219752754296894559, 0.3333333333333333703, 0.3219752754296894559, 0.3333333333333333703, 0.3219752754296894559, 0.3333333333333333703, 0.3219752754296894559, 0.3333333333333333703, 0.3219752754296894559, 0.3333333333333333703, 0.3219752754296894559, 0.3333333333333333703, 0.3219752754296894559, 0.3333333333333333703, 0.3219752754296894559, 0.3333333333333333703, 0.3219752754296894559, 0.3333333333333333703, 0.3219752754296894559, 0.3333333333333333703, 0.3219752754296894559, 0.3333333333333333703, 0.3219752754296894559, 0.3333333333333333703, 0.3219752754296894559, 0.3333333333333333703, 0.3219752754296894559, 0.3333333333333333703, 0.3219752754296894559, 0.3333333333333333703, 0.3219752754296894559, 0.3333333333333333703, 0.3219752754296894559, 0.3333333333333333703, 0.3219752754296894559, 0.3333333333333333703, 0.3219752754296894559, 0.3333333333333333703, 0.3219752754296894559, 0.3333333333333333703, 0.3219752754296894559, 0.3333333333333333703, 0.3219752754296894559, 0.3333333333333333703, 0.3219752754296894559, 0.3333333333333333703, 0.3219752754296894559, 0.3333333333333333703, 0.3219752754296894559, 0.3333333333333333703, 0.3219752754296894559, 0.3333333333333333703, 0.3219752754296894559, 0.3333333333333333703, 0.3219752754296894559, 0.3333333333333333703, 0.3219752754296894559, 0.3333333333333333703, 0.3219752754296894559, 0.3333333333333333703, 0.3219752754296894559, 0.3333333333333333703, 0.3219752754296894559, 0.3333333333333333703, 0.3219752754296894559, 0.3333333333333333703, 0.3219752754296894559, 0.3333333333333333703, 0.3219752754296894559, 0.3333333333333333703, 0.3219752754296894559, 0.3333333333333333703, 0.3219752754296894559, 0.3333333333333333703, 0.3219752754296894559, 0.3333333333333333703, 0.3219752754296894559, 0.3333333333333333703, 0.3219752754296894559, 0.3333333333333333703, 0.3219752754296894559, 0.3333333333333333703, 0.3219752754296894559, 0.3333333333333333703, 0.3219752754296894559, 0.3333333333333333703, 0.3219752754296894559, 0.3333333333333333703, 0.3219752754296894559, 0.3333333333333333703, 0.3219752754296894559, 0.3333333333333333703, 0.3219752754296894559, 0.3333333333333333703, 0.3219752754296894559, 0.3333333333333333703, 0.3219752754296894559, 0.3333333333333333703, 0.3219752754296894559, 0.3333333333333333703, 0.3219752754296894559, 0.3333333333333333703, 0.3219752754296894559, 0.3333333333333333703, 0.3219752754296894559, 0.3333333333333333703, 0.3219752754296894559, 0.3333333333333333703, 0.3219752754296894559, 0.3333333333333333703, 0.3219752754296894559, 0.3333333333333333703, 0.3219752754296894559, 0.3333333333333333703, 0.3219752754296894559, 0.3333333333333333703, 0.3219752754296894559, 0.3333333333333333703, 0.3219752754296894559, 0.3333333333333333703, 0.3219752754296894559, 0.3333333333333333703, 0.3219752754296894559, 0.3333333333333333703, 0.3219752754296894559, 0.3333333333333333703, 0.3219752754296894559, 0.3333333333333333703, 0.3219752754296894559, 0.3333333333333333703, 0.3219752754296894559, 0.3333333333333333703, 0.3219752754296894559, 0.3333333333333333703, 0.3219752754296894559, 0.3333333333333333703, 0.3219752754296894559, 0.3333333333333333703, 0.3219752754296894559, 0.3333333333333333703, 0.3219752754296894559, 0.3333333333333333703, 0.3219752754296894559, 0.3333333333333333703, 0.3219752754296894559, 0.3333333333333333703, 0.3219752754296894559, 0.3333333333333333703, 0.3219752754296894559, 0.3333333333333333703, 0.3219752754296894559, 0.3333333333333333703, 0.3219752754296894559, 0.3333333333333333703, 0.3219752754296894559, 0.3333333333333333703, 0.3219752754296894559, 0.3333333333333333703, 0.3219752754296894559, 0.3333333333333333703, 0.3219752754296894559, 0.3333333333333333703, 0.3219752754296894559, 0.3333333333333333703, 0.3219752754296894559, 0.3333333333333333703, 0.3219752754296894559, 0.3333333333333333703, 0.3219752754296894559, 0.3333333333333333703, 0.3219752754296894559, 0.3333333333333333703, 0.3219752754296894559, 0.3333333333333333703, 0.3219752754296894559, 0.3333333333333333703, 0.3219752754296894559, 0.3333333333333333703, 0.3219752754296894559, 0.3333333333333333703, 0.3219752754296894559, 0.3333333333333333703, 0.3219752754296894559, 0.3333333333333333703, 0.3219752754296894559, 0.3333333333333333703, 0.3219752754296894559, 0.3333333333333333703, 0.3219752754296894559, 0.3333333333333333703, 0.3219752754296894559, 0.3333333333333333703, 0.3219752754296894559, 0.3333333333333333703, 0.3219752754296894559, 0.3333333333333333703, 0.3219752754296894559, 0.3333333333333333703, 0.3219752754296894559, 0.3333333333333333703, 0.3219752754296894559, 0.3333333333333333703, 0.3219752754296894559, 0.3333333333333333703, 0.3219752754296894559, 0.3333333333333333703, 0.3219752754296894559, 0.3333333333333333703, 0.3219752754296894559, 0.3333333333333333703, 0.3219752754296894559, 0.3333333333333333703, 0.3219752754296894559, 0.3333333333333333703, 0.3219752754296894559, 0.3333333333333333703, 0.3219752754296894559, 0.3333333333333333703, 0.3219752754296894559, 0.3333333333333333703, 0.3219752754296894559, 0.3333333333333333703, 0.3219752754296894559, 0.3333333333333333703, 0.3219752754296894559, 0.3333333333333333703, 0.3219752754296894559, 0.3333333333333333703, 0.3219752754296894559, 0.3333333333333333703, 0.3219752754296894559, 0.3333333333333333703, 0.3219752754296894559, 0.3333333333333333703, 0.3219752754296894559, 0.3333333333333333703, 0.3219752754296894559, 0.3333333333333333703, 0.3219752754296894559, 0.3333333333333333703, 0.3219752754296894559, 0.3333333333333333703, 0.3219752754296894559, 0.3333333333333333703, 0.3219752754296894559, 0.3333333333333333703, 0.3219752754296894559, 0.3333333333333333703, 0.3219752754296894559, 0.3333333333333333703, 0.3219752754296894559, 0.3333333333333333703, 0.3219752754296894559, 0.3333333333333333703, 0.3219752754296894559, 0.3333333333333333703, 0.3219752754296894559, 0.3333333333333333703, 0.3219752754296894559, 0.3333333333333333703, 0.3219752754296894559, 0.3333333333333333703, 0.3219752754296894559, 0.3333333333333333703, 0.3219752754296894559, 0.3333333333333333703, 0.3219752754296894559, 0.3333333333333333703, 0.3219752754296894559, 0.3333333333333333703, 0.3219752754296894559, 0.3333333333333333703, 0.3219752754296894559, 0.3333333333333333703, 0.3219752754296894559, 0.3333333333333333703, 0.3219752754296894559, 0.3333333333333333703, 0.3219752754296894559, 0.3333333333333333703, 0.3219752754296894559, 0.3333333333333333703, 0.3219752754296894559, 0.3333333333333333703, 0.3219752754296894559, 0.3333333333333333703, 0.3219752754296894559, 0.3333333333333333703, 0.3219752754296894559, 0.3333333333333333703, 0.3219752754296894559, 0.3333333333333333703, 0.3219752754296894559, 0.3333333333333333703, 0.3219752754296894559, 0.3333333333333333703, 0.3219752754296894559, 0.3333333333333333703, 0.3219752754296894559, 0.3333333333333333703, 0.3219752754296894559, 0.3333333333333333703, 0.3219752754296894559, 0.3333333333333333703, 0.3219752754296894559, 0.3333333333333333703, 0.3219752754296894559, 0.3333333333333333703, 0.3219752754296894559, 0.3333333333333333703, 0.3219752754296894559, 0.3333333333333333703, 0.3219752754296894559, 0.3333333333333333703, 0.3219752754296894559, 0.3333333333333333703, 0.3219752754296894559, 0.3333333333333333703, 0.3219752754296894559, 0.3333333333333333703, 0.3219752754296894559, 0.3333333333333333703, 0.3219752754296894559, 0.3333333333333333703, 0.3219752754296894559, 0.3333333333333333703, 0.3219752754296894559, 0.3333333333333333703, 0.3219752754296894559, 0.3333333333333333703, 0.3219752754296894559, 0.3333333333333333703, 0.3219752754296894559, 0.3333333333333333703, 0.3219752754296894559, 0.3333333333333333703, 0.3219752754296894559, 0.3333333333333333703, 0.3219752754296894559, 0.3333333333333333703, 0.3219752754296894559, 0.3333333333333333703, 0.3219752754296894559, 0.3333333333333333703, 0.3219752754296894559, 0.3333333333333333703, 0.3219752754296894559, 0.3333333333333333703, 0.3219752754296894559, 0.3333333333333333703, 0.3219752754296894559, 0.3333333333333333703, 0.3219752754296894559, 0.3333333333333333703, 0.3219752754296894559, 0.3333333333333333703, 0.3219752754296894559, 0.3333333333333333703, 0.3219752754296894559, 0.3333333333333333703, 0.3219752754296894559, 0.3333333333333333703, 0.3219752754296894559, 0.3333333333333333703, 0.3219752754296894559, 0.3333333333333333703, 0.3219752754296894559, 0.3333333333333333703, 0.3219752754296894559, 0.3333333333333333703, 0.3219752754296894559, 0.3333333333333333703, 0.3219752754296894559, 0.3333333333333333703, 0.3219752754296894559, 0.3333333333333333703, 0.3219752754296894559, 0.3333333333333333703, 0.3219752754296894559, 0.3333333333333333703, 0.3219752754296894559, 0.3333333333333333703, 0.3219752754296894559, 0.3333333333333333703, 0.3219752754296894559, 0.3333333333333333703, 0.3219752754296894559, 0.3333333333333333703, 0.3219752754296894559, 0.3333333333333333703, 0.3219752754296894559, 0.3333333333333333703, 0.3219752754296894559, 0.3333333333333333703, 0.3219752754296894559, 0.3333333333333333703, 0.3219752754296894559, 0.3333333333333333703, 0.3219752754296894559, 0.3333333333333333703, 0.3219752754296894559, 0.3333333333333333703, 0.3219752754296894559, 0.3333333333333333703, 0.3219752754296894559, 0.3333333333333333703, 0.3219752754296894559, 0.3333333333333333703, 0.3219752754296894559, 0.3333333333333333703, 0.3219752754296894559, 0.3333333333333333703, 0.3219752754296894559, 0.3333333333333333703, 0.3219752754296894559, 0.3333333333333333703, 0.3219752754296894559, 0.3333333333333333703, 0.3219752754296894559, 0.3333333333333333703),
 ( 1.000000000000000000, 0.9659258262890683122, 1.000000000000000000, 0.9659258262890683122, 1.000000000000000000, 0.9659258262890683122, 1.000000000000000000, 0.9659258262890683122, 1.000000000000000000, 0.9659258262890683122, 1.000000000000000000, 0.9659258262890683122, 1.000000000000000000, 0.9659258262890683122, 1.000000000000000000, 0.9659258262890683122, 1.000000000000000000, 0.9659258262890683122, 1.000000000000000000, 0.9659258262890683122, 1.000000000000000000, 0.9659258262890683122, 1.000000000000000000, 0.9659258262890683122, 1.000000000000000000, 0.9659258262890683122, 1.000000000000000000, 0.9659258262890683122, 1.000000000000000000, 0.9659258262890683122, 1.000000000000000000, 0.9659258262890683122, 1.000000000000000000, 0.9659258262890683122, 1.000000000000000000, 0.9659258262890683122, 1.000000000000000000, 0.9659258262890683122, 1.000000000000000000, 0.9659258262890683122, 1.000000000000000000, 0.9659258262890683122, 1.000000000000000000, 0.9659258262890683122, 1.000000000000000000, 0.9659258262890683122, 1.000000000000000000, 0.9659258262890683122, 1.000000000000000000, 0.9659258262890683122, 1.000000000000000000, 0.9659258262890683122, 1.000000000000000000, 0.9659258262890683122, 1.000000000000000000, 0.9659258262890683122, 1.000000000000000000, 0.9659258262890683122, 1.000000000000000000, 0.9659258262890683122, 1.000000000000000000, 0.9659258262890683122, 1.000000000000000000, 0.9659258262890683122, 1.000000000000000000, 0.9659258262890683122, 1.000000000000000000, 0.9659258262890683122, 1.000000000000000000, 0.9659258262890683122, 1.000000000000000000, 0.9659258262890683122, 1.000000000000000000, 0.9659258262890683122, 1.000000000000000000, 0.9659258262890683122, 1.000000000000000000, 0.9659258262890683122, 1.000000000000000000, 0.9659258262890683122, 1.000000000000000000, 0.9659258262890683122, 1.000000000000000000, 0.9659258262890683122, 1.000000000000000000, 0.9659258262890683122, 1.000000000000000000, 0.9659258262890683122, 1.000000000000000000, 0.9659258262890683122, 1.000000000000000000, 0.9659258262890683122, 1.000000000000000000, 0.9659258262890683122, 1.000000000000000000, 0.9659258262890683122, 1.000000000000000000, 0.9659258262890683122, 1.000000000000000000, 0.9659258262890683122, 1.000000000000000000, 0.9659258262890683122, 1.000000000000000000, 0.9659258262890683122, 1.000000000000000000, 0.9659258262890683122, 1.000000000000000000, 0.9659258262890683122, 1.000000000000000000, 0.9659258262890683122, 1.000000000000000000, 0.9659258262890683122, 1.000000000000000000, 0.9659258262890683122, 1.000000000000000000, 0.9659258262890683122, 1.000000000000000000, 0.9659258262890683122, 1.000000000000000000, 0.9659258262890683122, 1.000000000000000000, 0.9659258262890683122, 1.000000000000000000, 0.9659258262890683122, 1.000000000000000000, 0.9659258262890683122, 1.000000000000000000, 0.9659258262890683122, 1.000000000000000000, 0.9659258262890683122, 1.000000000000000000, 0.9659258262890683122, 1.000000000000000000, 0.9659258262890683122, 1.000000000000000000, 0.9659258262890683122, 1.000000000000000000, 0.9659258262890683122, 1.000000000000000000, 0.9659258262890683122, 1.000000000000000000, 0.9659258262890683122, 1.000000000000000000, 0.9659258262890683122, 1.000000000000000000, 0.9659258262890683122, 1.000000000000000000, 0.9659258262890683122, 1.000000000000000000, 0.9659258262890683122, 1.000000000000000000, 0.9659258262890683122, 1.000000000000000000, 0.9659258262890683122, 1.000000000000000000, 0.9659258262890683122, 1.000000000000000000, 0.9659258262890683122, 1.000000000000000000, 0.9659258262890683122, 1.000000000000000000, 0.9659258262890683122, 1.000000000000000000, 0.9659258262890683122, 1.000000000000000000, 0.9659258262890683122, 1.000000000000000000, 0.9659258262890683122, 1.000000000000000000, 0.9659258262890683122, 1.000000000000000000, 0.9659258262890683122, 1.000000000000000000, 0.9659258262890683122, 1.000000000000000000, 0.9659258262890683122, 1.000000000000000000, 0.9659258262890683122, 1.000000000000000000, 0.9659258262890683122, 1.000000000000000000, 0.9659258262890683122, 1.000000000000000000, 0.9659258262890683122, 1.000000000000000000, 0.9659258262890683122, 1.000000000000000000, 0.9659258262890683122, 1.000000000000000000, 0.9659258262890683122, 1.000000000000000000, 0.9659258262890683122, 1.000000000000000000, 0.9659258262890683122, 1.000000000000000000, 0.9659258262890683122, 1.000000000000000000, 0.9659258262890683122, 1.000000000000000000, 0.9659258262890683122, 1.000000000000000000, 0.9659258262890683122, 1.000000000000000000, 0.9659258262890683122, 1.000000000000000000, 0.9659258262890683122, 1.000000000000000000, 0.9659258262890683122, 1.000000000000000000, 0.9659258262890683122, 1.000000000000000000, 0.9659258262890683122, 1.000000000000000000, 0.9659258262890683122, 1.000000000000000000, 0.9659258262890683122, 1.000000000000000000, 0.9659258262890683122, 1.000000000000000000, 0.9659258262890683122, 1.000000000000000000, 0.9659258262890683122, 1.000000000000000000, 0.9659258262890683122, 1.000000000000000000, 0.9659258262890683122, 1.000000000000000000, 0.9659258262890683122, 1.000000000000000000, 0.9659258262890683122, 1.000000000000000000, 0.9659258262890683122, 1.000000000000000000, 0.9659258262890683122, 1.000000000000000000, 0.9659258262890683122, 1.000000000000000000, 0.9659258262890683122, 1.000000000000000000, 0.9659258262890683122, 1.000000000000000000, 0.9659258262890683122, 1.000000000000000000, 0.9659258262890683122, 1.000000000000000000, 0.9659258262890683122, 1.000000000000000000, 0.9659258262890683122, 1.000000000000000000, 0.9659258262890683122, 1.000000000000000000, 0.9659258262890683122, 1.000000000000000000, 0.9659258262890683122, 1.000000000000000000, 0.9659258262890683122, 1.000000000000000000, 0.9659258262890683122, 1.000000000000000000, 0.9659258262890683122, 1.000000000000000000, 0.9659258262890683122, 1.000000000000000000, 0.9659258262890683122, 1.000000000000000000, 0.9659258262890683122, 1.000000000000000000, 0.9659258262890683122, 1.000000000000000000, 0.9659258262890683122, 1.000000000000000000, 0.9659258262890683122, 1.000000000000000000, 0.9659258262890683122, 1.000000000000000000, 0.9659258262890683122, 1.000000000000000000, 0.9659258262890683122, 1.000000000000000000, 0.9659258262890683122, 1.000000000000000000, 0.9659258262890683122, 1.000000000000000000, 0.9659258262890683122, 1.000000000000000000, 0.9659258262890683122, 1.000000000000000000, 0.9659258262890683122, 1.000000000000000000, 0.9659258262890683122, 1.000000000000000000, 0.9659258262890683122, 1.000000000000000000, 0.9659258262890683122, 1.000000000000000000, 0.9659258262890683122, 1.000000000000000000, 0.9659258262890683122, 1.000000000000000000, 0.9659258262890683122, 1.000000000000000000, 0.9659258262890683122, 1.000000000000000000, 0.9659258262890683122, 1.000000000000000000, 0.9659258262890683122, 1.000000000000000000, 0.9659258262890683122, 1.000000000000000000, 0.9659258262890683122, 1.000000000000000000, 0.9659258262890683122, 1.000000000000000000, 0.9659258262890683122, 1.000000000000000000, 0.9659258262890683122, 1.000000000000000000, 0.9659258262890683122, 1.000000000000000000, 0.9659258262890683122, 1.000000000000000000, 0.9659258262890683122, 1.000000000000000000, 0.9659258262890683122, 1.000000000000000000, 0.9659258262890683122, 1.000000000000000000, 0.9659258262890683122, 1.000000000000000000, 0.9659258262890683122, 1.000000000000000000, 0.9659258262890683122, 1.000000000000000000, 0.9659258262890683122, 1.000000000000000000, 0.9659258262890683122, 1.000000000000000000, 0.9659258262890683122, 1.000000000000000000, 0.9659258262890683122, 1.000000000000000000, 0.9659258262890683122, 1.000000000000000000, 0.9659258262890683122, 1.000000000000000000, 0.9659258262890683122, 1.000000000000000000, 0.9659258262890683122, 1.000000000000000000, 0.9659258262890683122, 1.000000000000000000, 0.9659258262890683122, 1.000000000000000000, 0.9659258262890683122, 1.000000000000000000, 0.9659258262890683122, 1.000000000000000000, 0.9659258262890683122, 1.000000000000000000, 0.9659258262890683122, 1.000000000000000000, 0.9659258262890683122, 1.000000000000000000, 0.9659258262890683122, 1.000000000000000000, 0.9659258262890683122, 1.000000000000000000, 0.9659258262890683122, 1.000000000000000000, 0.9659258262890683122, 1.000000000000000000, 0.9659258262890683122, 1.000000000000000000, 0.9659258262890683122, 1.000000000000000000, 0.9659258262890683122, 1.000000000000000000, 0.9659258262890683122, 1.000000000000000000, 0.9659258262890683122, 1.000000000000000000, 0.9659258262890683122, 1.000000000000000000, 0.9659258262890683122, 1.000000000000000000, 0.9659258262890683122, 1.000000000000000000, 0.9659258262890683122, 1.000000000000000000, 0.9659258262890683122, 1.000000000000000000, 0.9659258262890683122, 1.000000000000000000, 0.9659258262890683122, 1.000000000000000000, 0.9659258262890683122, 1.000000000000000000, 0.9659258262890683122, 1.000000000000000000, 0.9659258262890683122, 1.000000000000000000, 0.9659258262890683122, 1.000000000000000000, 0.9659258262890683122, 1.000000000000000000, 0.9659258262890683122, 1.000000000000000000, 0.9659258262890683122, 1.000000000000000000, 0.9659258262890683122, 1.000000000000000000, 0.9659258262890683122, 1.000000000000000000, 0.9659258262890683122, 1.000000000000000000, 0.9659258262890683122, 1.000000000000000000, 0.9659258262890683122, 1.000000000000000000, 0.9659258262890683122, 1.000000000000000000, 0.9659258262890683122, 1.000000000000000000, 0.9659258262890683122, 1.000000000000000000, 0.9659258262890683122, 1.000000000000000000, 0.9659258262890683122, 1.000000000000000000, 0.9659258262890683122, 1.000000000000000000, 0.9659258262890683122, 1.000000000000000000, 0.9659258262890683122, 1.000000000000000000, 0.9659258262890683122, 1.000000000000000000, 0.9659258262890683122, 1.000000000000000000, 0.9659258262890683122, 1.000000000000000000, 0.9659258262890683122, 1.000000000000000000, 0.9659258262890683122, 1.000000000000000000, 0.9659258262890683122, 1.000000000000000000, 0.9659258262890683122, 1.000000000000000000, 0.9659258262890683122, 1.000000000000000000, 0.9659258262890683122, 1.000000000000000000, 0.9659258262890683122, 1.000000000000000000, 0.9659258262890683122, 1.000000000000000000) ) ) 
 REPRESENTATION_ITEM ( '' )  SURFACE ( )  );
#142381=CARTESIAN_POINT ( 'NONE',  ( 19.02544592524334988, 5.153800228976608722, 46.45942372801899012 ) ) ;
#142382=CARTESIAN_POINT ( 'NONE',  ( -5.823673210054431948, 21.52544592524334988, 57.70942372801901143 ) ) ;
#142383=CARTESIAN_POINT ( 'NONE',  ( 13.89961937509957401, 13.97604488694547697, 111.8760903946856757 ) ) ;
#142384=CARTESIAN_POINT ( 'NONE',  ( 0.05219959533909260263, 19.03943276465977164, 59.99890960531436690 ) ) ;
#142385=CARTESIAN_POINT ( 'NONE',  ( 16.51473224551083163, -9.474510206698727899, 85.83442372801900433 ) ) ;
#142386=CARTESIAN_POINT ( 'NONE',  ( 21.52544592524334988, 5.823673210054432836, 86.45942372801901854 ) ) ;
#142387=CARTESIAN_POINT ( 'NONE',  ( 5.153800228976615827, -19.02544592524334988, 70.20942372801899012 ) ) ;
#142388=CARTESIAN_POINT ( 'NONE',  ( -19.03943276465977164, 0.05219959533909376836, 41.24890960531435269 ) ) ;
#142389=CARTESIAN_POINT ( 'NONE',  ( -0.05219959533907301413, -21.53943276465977519, 57.49890960531435979 ) ) ;
#142390=CARTESIAN_POINT ( 'NONE',  ( 16.52544592524342804, -4.483927247898539470, 68.54057627198103830 ) ) ;
#142391=CARTESIAN_POINT ( 'NONE',  ( 5.153800228976615827, -19.02544592524334988, 65.20942372801900433 ) ) ;
#142392=CARTESIAN_POINT ( 'NONE',  ( -16.19135201231362942, -7.376712067592052335, 25.18680854052033169 ) ) ;
#142393=CARTESIAN_POINT ( 'NONE',  ( 16.46253265017146816, 9.564922557961045513, 26.66775706135234003 ) ) ;
#142394=CARTESIAN_POINT ( 'NONE',  ( 16.52544592524335698, 4.483927247898782831, 101.4594237280190185 ) ) ;
#142395=CARTESIAN_POINT ( 'NONE',  ( 16.53943276465976808, -0.05219959533910856209, 48.74890960531435979 ) ) ;
#142396=CARTESIAN_POINT ( 'NONE',  ( 0.05219959533937995610, -21.53943276465977519, 90.00109039468567573 ) ) ;
#142398=CARTESIAN_POINT ( 'NONE',  ( -10.81492255796105439, 18.62759615963255655, 92.91775706135236135 ) ) ;
#142399=CARTESIAN_POINT ( 'NONE',  ( 15.72974639402199770, -15.80617190586745480, 98.12390960531436690 ) ) ;
#142400=CARTESIAN_POINT ( 'NONE',  ( -13.89961937509977652, 13.97604488694528158, 45.62390960531433848 ) ) ;
#142401=CARTESIAN_POINT ( 'NONE',  ( -10.81492255796105439, 18.62759615963255655, 67.91775706135234714 ) ) ;
#142402=CARTESIAN_POINT ( 'NONE',  ( -16.51473224551069308, -9.474510206698971260, 51.66557627198102409 ) ) ;
#142404=CARTESIAN_POINT ( 'NONE',  ( -19.03943276465977164, 0.05219959533909376836, 71.24890960531435269 ) ) ;
#142405=CARTESIAN_POINT ( 'NONE',  ( 12.14591786802309770, 12.06949235617756955, 104.3739096053143669 ) ) ;
#142406=CARTESIAN_POINT ( 'NONE',  ( -13.97604488694527625, -13.89961937509977652, 111.8739096053143243 ) ) ;
#142407=CARTESIAN_POINT ( 'NONE',  ( 14.29746914071049879, -8.314922557960816363, 53.33224293864769550 ) ) ;
#142408=CARTESIAN_POINT ( 'NONE',  ( 5.153800228976335163, 19.02544592524342804, 29.79057627198102409 ) ) ;
#142409=CARTESIAN_POINT ( 'NONE',  ( -8.224510206698948167, 14.34966873604960824, 75.41557627198102409 ) ) ;
#142410=CARTESIAN_POINT ( 'NONE',  ( -15.80617190586745835, -15.72974639402198527, 91.87390960531436690 ) ) ;
#142411=CARTESIAN_POINT ( 'NONE',  ( 21.52544592524334988, 5.823673210054432836, 36.45942372801901143 ) ) ;
#142412=CARTESIAN_POINT ( 'NONE',  ( 13.89961937509977652, -13.97604488694527269, 23.12390960531436335 ) ) ;
#142413=CARTESIAN_POINT ( 'NONE',  ( 14.34966873604972726, -8.224510206698740333, 35.83442372801901143 ) ) ;
#142414=CARTESIAN_POINT ( 'NONE',  ( -10.72451020669898014, 18.67979575497178502, 90.41557627198103830 ) ) ;
#142415=CARTESIAN_POINT ( 'NONE',  ( 21.53943276465977519, 0.05219959533937863772, 106.2510903946856757 ) ) ;
#142416=CARTESIAN_POINT ( 'NONE',  ( 9.474510206698971260, -16.51473224551069308, 87.91557627198102409 ) ) ;
#142417=CARTESIAN_POINT ( 'NONE',  ( -21.55341960407619339, 5.719274019375674811, 38.54275706135234714 ) ) ;
#142418=CARTESIAN_POINT ( 'NONE',  ( 21.53943276465977519, -0.05219959533907433946, 28.74890960531435624 ) ) ;
#142419=CARTESIAN_POINT ( 'NONE',  ( -12.06949235617739369, -12.14591786802326823, 104.3760903946856899 ) ) ;
#142420=CARTESIAN_POINT ( 'NONE',  ( -15.80617190586768217, 15.72974639402176855, 53.12609039468568284 ) ) ;
#142421=CARTESIAN_POINT ( 'NONE',  ( -18.62759615963255300, -10.81492255796106328, 84.16775706135234714 ) ) ;
#142422=CARTESIAN_POINT ( 'NONE',  ( 16.46253265017146816, 9.564922557961045513, 31.66775706135232937 ) ) ;
#142423=CARTESIAN_POINT ( 'NONE',  ( 4.483927247898790824, -16.52544592524335698, 90.20942372801903275 ) ) ;
#142424=CARTESIAN_POINT ( 'NONE',  ( -10.72451020669870658, -18.67979575497194134, 39.58442372801901143 ) ) ;
#142425=CARTESIAN_POINT ( 'NONE',  ( 19.02544592524343514, -5.153800228976328945, 28.54057627198102409 ) ) ;
#142426=CARTESIAN_POINT ( 'NONE',  ( -15.72974639402176322, -15.80617190586768395, 109.3760903946857042 ) ) ;
#142427=CARTESIAN_POINT ( 'NONE',  ( -13.89961937509977652, 13.97604488694528158, 105.6239096053143527 ) ) ;
#142428=CARTESIAN_POINT ( 'NONE',  ( 18.67979575497178502, 10.72451020669898547, 99.16557627198100988 ) ) ;
#142429=CARTESIAN_POINT ( 'NONE',  ( 15.80617190586746368, 15.72974639402197994, 64.37390960531435269 ) ) ;
#142431=CARTESIAN_POINT ( 'NONE',  ( 15.72974639402199770, -15.80617190586745480, 63.12390960531435979 ) ) ;
#142432=CARTESIAN_POINT ( 'NONE',  ( 8.224510206698742110, 14.34966873604972548, 47.08442372801901854 ) ) ;
#142433=CARTESIAN_POINT ( 'NONE',  ( 4.379528057220339221, -16.55341960407611168, 57.70724293864770260 ) ) ;
#142435=CARTESIAN_POINT ( 'NONE',  ( -5.049401038297874678, -19.05341960407617918, 89.79275706135230450 ) ) ;
#142438=CARTESIAN_POINT ( 'NONE',  ( 4.483927247898790824, -16.52544592524335698, 20.20942372801900788 ) ) ;
#142439=CARTESIAN_POINT ( 'NONE',  ( 0.05219959533907565091, 21.53943276465977519, 104.9989096053143669 ) ) ;
#142440=CARTESIAN_POINT ( 'NONE',  ( -0.05219959533907301413, -21.53943276465977519, 77.49890960531433848 ) ) ;
#142441=CARTESIAN_POINT ( 'NONE',  ( 10.81492255796078972, 18.62759615963270932, 24.58224293864768839 ) ) ;
#142442=CARTESIAN_POINT ( 'NONE',  ( 4.379528057220092307, 16.55341960407617563, 62.29275706135236845 ) ) ;
#142443=CARTESIAN_POINT ( 'NONE',  ( -13.97604488694527625, -13.89961937509977652, 76.87390960531433848 ) ) ;
#142444=CARTESIAN_POINT ( 'NONE',  ( -21.55341960407619339, 5.719274019375674811, 33.54275706135234714 ) ) ;
#142445=CARTESIAN_POINT ( 'NONE',  ( 12.06949235617739724, 12.14591786802326823, 21.87609039468567573 ) ) ;
#142446=CARTESIAN_POINT ( 'NONE',  ( -16.51473224551069308, -9.474510206698971260, 111.6655762719810383 ) ) ;
#142447=CARTESIAN_POINT ( 'NONE',  ( -0.05219959533909027116, -19.03943276465977164, 82.49890960531436690 ) ) ;
#142448=CARTESIAN_POINT ( 'NONE',  ( -18.62759615963270932, 10.81492255796079327, 85.83224293864768129 ) ) ;
#142449=CARTESIAN_POINT ( 'NONE',  ( 19.02544592524343514, -5.153800228976328945, 63.54057627198103830 ) ) ;
#142450=CARTESIAN_POINT ( 'NONE',  ( -16.61371651742604527, -7.165104196376050893, 61.14584930007005426 ) ) ;
#142451=CARTESIAN_POINT ( 'NONE',  ( 8.314922557960818139, 14.29746914071049879, 64.58224293864769550 ) ) ;
#142452=CARTESIAN_POINT ( 'NONE',  ( -15.72974639402197994, 15.80617190586746368, 25.62390960531435624 ) ) ;
#142454=CARTESIAN_POINT ( 'NONE',  ( -18.62759615963270932, 10.81492255796079327, 110.8322429386476955 ) ) ;
#142455=CARTESIAN_POINT ( 'NONE',  ( 9.474510206698729675, 16.51473224551082808, 62.08442372801899722 ) ) ;
#142456=CARTESIAN_POINT ( 'NONE',  ( 19.05341960407611168, 5.049401038298154454, 108.9572429386477097 ) ) ;
#142458=CARTESIAN_POINT ( 'NONE',  ( -18.62759615963270932, 10.81492255796079327, 50.83224293864770971 ) ) ;
#142459=CARTESIAN_POINT ( 'NONE',  ( -5.049401038298153566, 19.05341960407611168, 90.20724293864766707 ) ) ;
#142460=CARTESIAN_POINT ( 'NONE',  ( -21.53943276465977519, -0.05219959533937600094, 78.75109039468568994 ) ) ;
#142461=CARTESIAN_POINT ( 'NONE',  ( -16.51473224551069308, -9.474510206698971260, 56.66557627198103120 ) ) ;
#142463=CARTESIAN_POINT ( 'NONE',  ( -12.14591786802309592, -12.06949235617757132, 81.87390960531435269 ) ) ;
#142464=CARTESIAN_POINT ( 'NONE',  ( -4.379528057220086978, -16.55341960407618274, 34.79275706135235424 ) ) ;
#142465=CARTESIAN_POINT ( 'NONE',  ( 18.62759615963255655, 10.81492255796105972, 66.66775706135234714 ) ) ;
#142467=CARTESIAN_POINT ( 'NONE',  ( 19.03943276465977164, 0.05219959533936151252, 26.25109039468566507 ) ) ;
#142468=CARTESIAN_POINT ( 'NONE',  ( -19.05341960407617563, 5.049401038297882671, 78.54275706135233293 ) ) ;
#142469=CARTESIAN_POINT ( 'NONE',  ( 16.51473224551083163, -9.474510206698727899, 40.83442372801900433 ) ) ;
#142471=CARTESIAN_POINT ( 'NONE',  ( -5.719274019375665041, -21.55341960407619695, 39.79275706135235424 ) ) ;
#142473=CARTESIAN_POINT ( 'NONE',  ( -16.46253265017146816, -9.564922557961047289, 39.16775706135234003 ) ) ;
#142474=CARTESIAN_POINT ( 'NONE',  ( -13.97604488694527625, -13.89961937509977652, 51.87390960531436690 ) ) ;
#142475=CARTESIAN_POINT ( 'NONE',  ( 9.564922557961047289, -16.46253265017146816, 35.41775706135233293 ) ) ;
#142476=CARTESIAN_POINT ( 'NONE',  ( -14.29746914071037622, -8.314922557961029526, 99.16775706135234714 ) ) ;
#142477=CARTESIAN_POINT ( 'NONE',  ( 9.564922557960805705, 16.46253265017160317, 109.5822429386476955 ) ) ;
#142478=CARTESIAN_POINT ( 'NONE',  ( -5.823673210054431948, 21.52544592524334988, 82.70942372801900433 ) ) ;
#142481=CARTESIAN_POINT ( 'NONE',  ( 18.62759615963255655, 10.81492255796105972, 81.66775706135236135 ) ) ;
#142483=CARTESIAN_POINT ( 'NONE',  ( 16.51473224551069308, 9.474510206698969483, 104.1655762719810241 ) ) ;
#142484=FACE_OUTER_BOUND ( 'NONE', #98933, .T. ) ;
#142485=CARTESIAN_POINT ( 'NONE',  ( -13.97604488694527625, -13.89961937509977652, 46.87390960531435979 ) ) ;
#142486=CARTESIAN_POINT ( 'NONE',  ( 10.72451020669898902, -18.67979575497178502, 52.91557627198103830 ) ) ;
#142487=CARTESIAN_POINT ( 'NONE',  ( -16.55341960407611168, -4.379528057220339221, 31.45724293864769550 ) ) ;
#142488=CARTESIAN_POINT ( 'NONE',  ( 16.52544592524342804, -4.483927247898539470, 98.54057627198105251 ) ) ;
#142489=CARTESIAN_POINT ( 'NONE',  ( 5.153800228976335163, 19.02544592524342804, 94.79057627198103830 ) ) ;
#142490=CARTESIAN_POINT ( 'NONE',  ( 5.049401038297881783, 19.05341960407617563, 27.29275706135232937 ) ) ;
#142491=CARTESIAN_POINT ( 'NONE',  ( -16.51473224551069308, -9.474510206698971260, 36.66557627198102409 ) ) ;
#142492=CARTESIAN_POINT ( 'NONE',  ( 16.55341960407611168, 4.379528057220329451, 103.9572429386476813 ) ) ;
#142493=CARTESIAN_POINT ( 'NONE',  ( -21.52544592524334988, -5.823673210054445271, 53.95942372801900433 ) ) ;
#142494=CARTESIAN_POINT ( 'NONE',  ( -4.379528057220086978, -16.55341960407618274, 109.7927570613523613 ) ) ;
#142495=CARTESIAN_POINT ( 'NONE',  ( 13.97604488694548053, -13.89961937509957401, 65.62609039468567573 ) ) ;
#142497=CARTESIAN_POINT ( 'NONE',  ( 16.46253265017160672, -9.564922557960803928, 108.3322429386476955 ) ) ;
#142498=CARTESIAN_POINT ( 'NONE',  ( -16.52544592524342804, 4.483927247898546575, 81.04057627198102409 ) ) ;
#142499=CARTESIAN_POINT ( 'NONE',  ( 16.46253265017146816, 9.564922557961045513, 61.66775706135234003 ) ) ;
#142500=CARTESIAN_POINT ( 'NONE',  ( -16.51473224551069308, -9.474510206698971260, 61.66557627198103120 ) ) ;
#142501=CARTESIAN_POINT ( 'NONE',  ( -16.52544592524342804, 4.483927247898546575, 61.04057627198103120 ) ) ;
#142502=CARTESIAN_POINT ( 'NONE',  ( -19.03943276465977164, -0.05219959533935918106, 83.75109039468567573 ) ) ;
#142503=CARTESIAN_POINT ( 'NONE',  ( 18.62759615963271287, -10.81492255796078972, 38.33224293864768839 ) ) ;
#142505=CARTESIAN_POINT ( 'NONE',  ( -12.06949235617756955, 12.14591786802309770, 95.62390960531436690 ) ) ;
#142506=CARTESIAN_POINT ( 'NONE',  ( -17.13100169013300089, -6.664070546373174864, 29.23210164300154190 ) ) ;
#142507=CARTESIAN_POINT ( 'NONE',  ( 13.97604488694527802, 13.89961937509977652, 59.37390960531434558 ) ) ;
#142508=CARTESIAN_POINT ( 'NONE',  ( -5.823673210054116645, -21.52544592524344225, 67.29057627198103830 ) ) ;
#142509=CARTESIAN_POINT ( 'NONE',  ( 19.03943276465977164, -0.05219959533909143690, 38.74890960531436690 ) ) ;
#142510=CARTESIAN_POINT ( 'NONE',  ( 8.224510206698742110, 14.34966873604972548, 92.08442372801901854 ) ) ;
#142511=CARTESIAN_POINT ( 'NONE',  ( 13.89961937509977652, -13.97604488694527269, 73.12390960531436690 ) ) ;
#142512=CARTESIAN_POINT ( 'NONE',  ( 16.46253265017146816, 9.564922557961045513, 56.66775706135233293 ) ) ;
#142513=CARTESIAN_POINT ( 'NONE',  ( 0.05219959533937995610, -21.53943276465977519, 75.00109039468568994 ) ) ;
#142514=CARTESIAN_POINT ( 'NONE',  ( 18.62759615963271287, -10.81492255796078972, 48.33224293864770260 ) ) ;
#142515=CARTESIAN_POINT ( 'NONE',  ( -16.46253265017160317, 9.564922557960807481, 100.8322429386477097 ) ) ;
#142516=CARTESIAN_POINT ( 'NONE',  ( 13.89961937509977652, -13.97604488694527269, 23.12390960531436335 ) ) ;
#142517=CARTESIAN_POINT ( 'NONE',  ( -16.52544592524335698, -4.483927247898792601, 88.95942372801901854 ) ) ;
#142518=CARTESIAN_POINT ( 'NONE',  ( 9.474510206698729675, 16.51473224551082808, 102.0844237280190043 ) ) ;
#142521=CARTESIAN_POINT ( 'NONE',  ( 10.72451020669871369, 18.67979575497193778, 97.08442372801904696 ) ) ;
#142522=ORIENTED_EDGE ( 'NONE', *, *, #34865, .F. ) ;
#142523=CARTESIAN_POINT ( 'NONE',  ( -4.379528057220328563, 16.55341960407611168, 65.20724293864768129 ) ) ;
#142524=CARTESIAN_POINT ( 'NONE',  ( 16.55341960407611168, 4.379528057220329451, 73.95724293864769550 ) ) ;
#142525=CARTESIAN_POINT ( 'NONE',  ( -15.72974639402197994, 15.80617190586746368, 100.6239096053143811 ) ) ;
#142526=CARTESIAN_POINT ( 'NONE',  ( 18.67979575497178502, 10.72451020669898547, 89.16557627198102409 ) ) ;
#142527=CARTESIAN_POINT ( 'NONE',  ( 16.20579543436678449, -7.371946100355080134, 96.93479165828125588 ) ) ;
#142528=CARTESIAN_POINT ( 'NONE',  ( 18.62759615963271287, -10.81492255796078972, 28.33224293864769550 ) ) ;
#142529=CARTESIAN_POINT ( 'NONE',  ( 4.483927247898790824, -16.52544592524335698, 65.20942372801901854 ) ) ;
#142530=CARTESIAN_POINT ( 'NONE',  ( -8.224510206698948167, 14.34966873604960824, 95.41557627198102409 ) ) ;
#142531=CARTESIAN_POINT ( 'NONE',  ( -16.51473224551069308, -9.474510206698971260, 41.66557627198103120 ) ) ;
#142533=CARTESIAN_POINT ( 'NONE',  ( -14.29746914071037622, -8.314922557961029526, 99.16775706135234714 ) ) ;
#142534=CARTESIAN_POINT ( 'NONE',  ( 15.80617190586769283, -15.72974639402175789, 30.62609039468567929 ) ) ;
#142535=CARTESIAN_POINT ( 'NONE',  ( -13.97604488694527625, -13.89961937509977652, 86.87390960531436690 ) ) ;
#142536=CARTESIAN_POINT ( 'NONE',  ( 21.53943276465977519, 0.05219959533937863772, 66.25109039468567573 ) ) ;
#142540=CARTESIAN_POINT ( 'NONE',  ( -10.72451020669870658, -18.67979575497194134, 64.58442372801900433 ) ) ;
#142541=CARTESIAN_POINT ( 'NONE',  ( -0.05219959533909027116, -19.03943276465977164, 42.49890960531435269 ) ) ;
#142542=CARTESIAN_POINT ( 'NONE',  ( -19.02544592524342804, 5.153800228976336051, 116.0405762719810383 ) ) ;
#142543=CARTESIAN_POINT ( 'NONE',  ( -16.51473224551069308, -9.474510206698971260, 86.66557627198102409 ) ) ;
#142544=CARTESIAN_POINT ( 'NONE',  ( 13.97604488694548053, -13.89961937509957401, 65.62609039468567573 ) ) ;
#142545=CARTESIAN_POINT ( 'NONE',  ( 18.67979575497194134, -10.72451020669871369, 25.83442372801901499 ) ) ;
#142546=CARTESIAN_POINT ( 'NONE',  ( 19.02544592524334988, 5.153800228976608722, 56.45942372801898301 ) ) ;
#142547=CARTESIAN_POINT ( 'NONE',  ( -0.05219959533909027116, -19.03943276465977164, 22.49890960531436690 ) ) ;
#142548=CARTESIAN_POINT ( 'NONE',  ( 14.34966873604972726, -8.224510206698740333, 90.83442372801901854 ) ) ;
#142549=CARTESIAN_POINT ( 'NONE',  ( -5.049401038297874678, -19.05341960407617918, 59.79275706135231871 ) ) ;
#142550=CARTESIAN_POINT ( 'NONE',  ( 12.06949235617757843, -12.14591786802309237, 23.12390960531436335 ) ) ;
#142551=CARTESIAN_POINT ( 'NONE',  ( -19.05341960407617563, 5.049401038297882671, 48.54275706135233293 ) ) ;
#142553=CARTESIAN_POINT ( 'NONE',  ( -9.474510206698964154, 16.51473224551069663, 90.41557627198103830 ) ) ;
#142554=CARTESIAN_POINT ( 'NONE',  ( -15.80617190586768217, 15.72974639402176855, 93.12609039468568994 ) ) ;
#142555=CARTESIAN_POINT ( 'NONE',  ( 21.53943276465977519, 0.05219959533937863772, 101.2510903946856757 ) ) ;
#142556=CARTESIAN_POINT ( 'NONE',  ( 18.09867054820431065, 5.500000000000001776, 66.48393025253587041 ) ) ;
#142557=CARTESIAN_POINT ( 'NONE',  ( 10.72451020669871369, 18.67979575497193778, 92.08442372801901854 ) ) ;
#142558=CARTESIAN_POINT ( 'NONE',  ( -0.05219959533934338120, 16.53943276465976808, 37.50109039468568284 ) ) ;
#142559=CARTESIAN_POINT ( 'NONE',  ( 13.89961937509977652, -13.97604488694527269, 88.12390960531438111 ) ) ;
#142560=CARTESIAN_POINT ( 'NONE',  ( 0.05219959533907565091, 21.53943276465977519, 34.99890960531435979 ) ) ;
#142562=CARTESIAN_POINT ( 'NONE',  ( 13.97604488694527802, 13.89961937509977652, 84.37390960531433848 ) ) ;
#142564=CARTESIAN_POINT ( 'NONE',  ( -9.474510206698720793, -16.51473224551083518, 74.58442372801900433 ) ) ;
#142565=CARTESIAN_POINT ( 'NONE',  ( -19.03943276465977164, 0.05219959533909376836, 106.2489096053143669 ) ) ;
#142566=CARTESIAN_POINT ( 'NONE',  ( 10.81492255796106328, -18.62759615963255655, 105.4177570613523613 ) ) ;
#142567=CARTESIAN_POINT ( 'NONE',  ( 4.483927247898545687, 16.52544592524342804, 99.79057627198103830 ) ) ;
#142568=CARTESIAN_POINT ( 'NONE',  ( -15.80617190586745835, -15.72974639402198527, 46.87390960531435979 ) ) ;
#142569=CARTESIAN_POINT ( 'NONE',  ( 10.72451020669898902, -18.67979575497178502, 37.91557627198102409 ) ) ;
#142570=CARTESIAN_POINT ( 'NONE',  ( -16.55341960407611168, -4.379528057220339221, 106.4572429386477097 ) ) ;
#142572=CARTESIAN_POINT ( 'NONE',  ( 9.564922557961047289, -16.46253265017146816, 55.41775706135234003 ) ) ;
#142573=CARTESIAN_POINT ( 'NONE',  ( -14.34966873604960291, -8.224510206698953496, 21.66557627198102409 ) ) ;
#142574=CARTESIAN_POINT ( 'NONE',  ( -16.51473224551069308, -9.474510206698971260, 96.66557627198102409 ) ) ;
#142575=CARTESIAN_POINT ( 'NONE',  ( 18.62759615963255655, 10.81492255796105972, 76.66775706135234714 ) ) ;
#142576=CARTESIAN_POINT ( 'NONE',  ( -21.55341960407610458, -5.719274019375992779, 56.45724293864768839 ) ) ;
#142577=CARTESIAN_POINT ( 'NONE',  ( -21.53943276465977519, -0.05219959533937600094, 38.75109039468567573 ) ) ;
#142578=CARTESIAN_POINT ( 'NONE',  ( -18.67979575497178146, -10.72451020669898902, 96.66557627198102409 ) ) ;
#142579=CARTESIAN_POINT ( 'NONE',  ( -21.53943276465977519, -0.05219959533937600094, 33.75109039468568284 ) ) ;
#142580=CARTESIAN_POINT ( 'NONE',  ( -14.29746914071049879, 8.314922557960819915, 115.8322429386477097 ) ) ;
#142581=CARTESIAN_POINT ( 'NONE',  ( 19.02544592524343514, -5.153800228976328945, 88.54057627198102409 ) ) ;
#142582=CARTESIAN_POINT ( 'NONE',  ( 8.224510206698742110, 14.34966873604972548, 82.08442372801901854 ) ) ;
#142583=CARTESIAN_POINT ( 'NONE',  ( 12.06949235617757843, -12.14591786802309237, 103.1239096053143811 ) ) ;
#142584=CARTESIAN_POINT ( 'NONE',  ( -9.474510206698964154, 16.51473224551069663, 110.4155762719810383 ) ) ;
#142585=CARTESIAN_POINT ( 'NONE',  ( -4.379528057220328563, 16.55341960407611168, 50.20724293864769550 ) ) ;
#142586=CARTESIAN_POINT ( 'NONE',  ( -0.05219959533934338120, 16.53943276465976808, 112.5010903946857042 ) ) ;
#142587=CARTESIAN_POINT ( 'NONE',  ( -19.02544592524342804, 5.153800228976336051, 56.04057627198100988 ) ) ;
#142588=CARTESIAN_POINT ( 'NONE',  ( -19.03943276465977164, 0.05219959533909376836, 31.24890960531435979 ) ) ;
#142589=CARTESIAN_POINT ( 'NONE',  ( -10.81492255796078084, -18.62759615963271287, 42.08224293864769550 ) ) ;
#142590=CARTESIAN_POINT ( 'NONE',  ( -16.51473224551082808, 9.474510206698731452, 28.33442372801900433 ) ) ;
#142592=CARTESIAN_POINT ( 'NONE',  ( 12.06949235617757843, -12.14591786802309237, 33.12390960531435979 ) ) ;
#142593=CARTESIAN_POINT ( 'NONE',  ( 21.52544592524334988, 5.823673210054432836, 51.45942372801901854 ) ) ;
#142595=CARTESIAN_POINT ( 'NONE',  ( 12.14591786802327356, -12.06949235617739191, 55.62609039468568284 ) ) ;
#142596=CARTESIAN_POINT ( 'NONE',  ( 5.049401038297881783, 19.05341960407617563, 67.29275706135234714 ) ) ;
#142597=CARTESIAN_POINT ( 'NONE',  ( 16.55341960407611168, 4.379528057220329451, 23.95724293864769550 ) ) ;
#142598=CARTESIAN_POINT ( 'NONE',  ( -8.224510206698735004, -14.34966873604973081, 104.5844237280190185 ) ) ;
#142599=CARTESIAN_POINT ( 'NONE',  ( 9.474510206698971260, -16.51473224551069308, 32.91557627198102409 ) ) ;
#142601=CARTESIAN_POINT ( 'NONE',  ( -19.03943276465977164, 0.05219959533909376836, 66.24890960531436690 ) ) ;
#142602=CARTESIAN_POINT ( 'NONE',  ( -13.89961937509977652, 13.97604488694528158, 25.62390960531434558 ) ) ;
#142603=CARTESIAN_POINT ( 'NONE',  ( 10.72451020669871369, 18.67979575497193778, 27.08442372801901854 ) ) ;
#142604=CARTESIAN_POINT ( 'NONE',  ( -16.51473224551069308, -9.474510206698971260, 51.66557627198102409 ) ) ;
#142606=CARTESIAN_POINT ( 'NONE',  ( 16.46253265017160672, -9.564922557960803928, 48.33224293864769550 ) ) ;
#142607=CARTESIAN_POINT ( 'NONE',  ( -5.153800228976328057, -19.02544592524343514, 112.2905762719810099 ) ) ;
#142608=CARTESIAN_POINT ( 'NONE',  ( 15.80617190586769283, -15.72974639402175789, 60.62609039468567573 ) ) ;
#142609=CARTESIAN_POINT ( 'NONE',  ( 14.34966873604960469, 8.224510206698951720, 104.1655762719810241 ) ) ;
#142610=CARTESIAN_POINT ( 'NONE',  ( -19.03943276465977164, 0.05219959533909376836, 111.2489096053143669 ) ) ;
#142611=CARTESIAN_POINT ( 'NONE',  ( -16.55341960407617563, 4.379528057220093196, 83.54275706135234714 ) ) ;
#142612=CARTESIAN_POINT ( 'NONE',  ( -21.55341960407619339, 5.719274019375674811, 88.54275706135236135 ) ) ;
#142613=CARTESIAN_POINT ( 'NONE',  ( -16.55341960407617563, 4.379528057220093196, 48.54275706135234714 ) ) ;
#142614=CARTESIAN_POINT ( 'NONE',  ( 19.05341960407611168, 5.049401038298154454, 88.95724293864769550 ) ) ;
#142615=CARTESIAN_POINT ( 'NONE',  ( -4.379528057220086978, -16.55341960407618274, 34.79275706135235424 ) ) ;
#142616=CARTESIAN_POINT ( 'NONE',  ( 4.379528057220092307, 16.55341960407617563, 27.29275706135234358 ) ) ;
#142617=CARTESIAN_POINT ( 'NONE',  ( -16.52544592524335698, -4.483927247898792601, 93.95942372801903275 ) ) ;
#142618=CARTESIAN_POINT ( 'NONE',  ( -13.97604488694547697, 13.89961937509957934, 108.1260903946856331 ) ) ;
#142619=CARTESIAN_POINT ( 'NONE',  ( -21.53943276465977519, 0.05219959533907696930, 96.24890960531435269 ) ) ;
#142620=CARTESIAN_POINT ( 'NONE',  ( -14.34966873604960291, -8.224510206698953496, 96.66557627198102409 ) ) ;
#142621=CARTESIAN_POINT ( 'NONE',  ( -5.049401038297874678, -19.05341960407617918, 99.79275706135234714 ) ) ;
#142622=CARTESIAN_POINT ( 'NONE',  ( -14.34966873604972548, 8.224510206698743886, 68.33442372801900433 ) ) ;
#142624=CARTESIAN_POINT ( 'NONE',  ( 9.564922557961047289, -16.46253265017146816, 65.41775706135233293 ) ) ;
#142625=CARTESIAN_POINT ( 'NONE',  ( 16.52544592524342804, -4.483927247898539470, 43.54057627198103830 ) ) ;
#142626=CARTESIAN_POINT ( 'NONE',  ( 8.314922557960818139, 14.29746914071049879, 29.58224293864769905 ) ) ;
#142627=CARTESIAN_POINT ( 'NONE',  ( -16.53943276465976808, 0.05219959533911058130, 91.24890960531436690 ) ) ;
#142628=CARTESIAN_POINT ( 'NONE',  ( -9.564922557961040184, 16.46253265017147172, 27.91775706135232582 ) ) ;
#142629=CARTESIAN_POINT ( 'NONE',  ( -17.40805194822031154, 6.112264579159341515, 90.83371272510612471 ) ) ;
#142630=CARTESIAN_POINT ( 'NONE',  ( -18.62759615963255300, -10.81492255796106328, 34.16775706135234714 ) ) ;
#142631=CARTESIAN_POINT ( 'NONE',  ( -13.97604488694547697, 13.89961937509957934, 93.12609039468566152 ) ) ;
#142634=CARTESIAN_POINT ( 'NONE',  ( -9.474510206698964154, 16.51473224551069663, 85.41557627198102409 ) ) ;
#142635=CARTESIAN_POINT ( 'NONE',  ( -5.049401038298153566, 19.05341960407611168, 90.20724293864766707 ) ) ;
#142636=CARTESIAN_POINT ( 'NONE',  ( -21.53943276465977519, 0.05219959533907696930, 51.24890960531436690 ) ) ;
#142637=CARTESIAN_POINT ( 'NONE',  ( 16.52544592524342804, -4.483927247898539470, 88.54057627198103830 ) ) ;
#142638=CARTESIAN_POINT ( 'NONE',  ( 13.97604488694527802, 13.89961937509977652, 69.37390960531436690 ) ) ;
#142639=CARTESIAN_POINT ( 'NONE',  ( 16.51473224551069308, 9.474510206698969483, 29.16557627198103475 ) ) ;
#142640=CARTESIAN_POINT ( 'NONE',  ( 21.52544592524334988, 5.823673210054432836, 36.45942372801901143 ) ) ;
#142641=CARTESIAN_POINT ( 'NONE',  ( -15.80617190586768217, 15.72974639402176855, 73.12609039468567573 ) ) ;
#142642=CARTESIAN_POINT ( 'NONE',  ( 16.46253265017160672, -9.564922557960803928, 63.33224293864769550 ) ) ;
#142643=CARTESIAN_POINT ( 'NONE',  ( -8.314922557961024197, 14.29746914071037800, 82.91775706135234714 ) ) ;
#142644=CARTESIAN_POINT ( 'NONE',  ( -21.52544592524334988, -5.823673210054445271, 33.95942372801901143 ) ) ;
#142645=CARTESIAN_POINT ( 'NONE',  ( 5.823673210054444382, -21.52544592524334988, 20.20942372801900788 ) ) ;
#142646=CARTESIAN_POINT ( 'NONE',  ( -19.05341960407617563, 5.049401038297882671, 58.54275706135234003 ) ) ;
#142647=CARTESIAN_POINT ( 'NONE',  ( -13.97604488694527625, -13.89961937509977652, 76.87390960531433848 ) ) ;
#142648=CARTESIAN_POINT ( 'NONE',  ( 13.97604488694548053, -13.89961937509957401, 30.62609039468566863 ) ) ;
#142649=CARTESIAN_POINT ( 'NONE',  ( 21.52544592524334988, 5.823673210054432836, 86.45942372801901854 ) ) ;
#142650=CARTESIAN_POINT ( 'NONE',  ( 10.81492255796078972, 18.62759615963270932, 69.58224293864769550 ) ) ;
#142651=CARTESIAN_POINT ( 'NONE',  ( 12.14591786802309770, 12.06949235617756955, 44.37390960531435979 ) ) ;
#142652=CARTESIAN_POINT ( 'NONE',  ( -15.72974639402176322, -15.80617190586768395, 94.37609039468568994 ) ) ;
#142653=CARTESIAN_POINT ( 'NONE',  ( 19.05341960407617918, -5.049401038297876454, 26.04275706135233293 ) ) ;
#142654=CARTESIAN_POINT ( 'NONE',  ( 16.52544592524342804, -4.483927247898539470, 73.54057627198102409 ) ) ;
#142655=CARTESIAN_POINT ( 'NONE',  ( -19.03943276465977164, 0.05219959533909376836, 26.24890960531435624 ) ) ;
#142656=CARTESIAN_POINT ( 'NONE',  ( -9.564922557961040184, 16.46253265017147172, 72.91775706135233293 ) ) ;
#142657=CARTESIAN_POINT ( 'NONE',  ( 4.379528057220339221, -16.55341960407611168, 37.70724293864769550 ) ) ;
#142658=CARTESIAN_POINT ( 'NONE',  ( -10.81492255796105439, 18.62759615963255655, 87.91775706135234714 ) ) ;
#142659=CARTESIAN_POINT ( 'NONE',  ( 19.03943276465977164, -0.05219959533909143690, 73.74890960531435269 ) ) ;
#142660=CARTESIAN_POINT ( 'NONE',  ( -9.564922557961040184, 16.46253265017147172, 47.91775706135233293 ) ) ;
#142661=CARTESIAN_POINT ( 'NONE',  ( -21.53943276465977519, 0.05219959533907696930, 51.24890960531436690 ) ) ;
#142662=CARTESIAN_POINT ( 'NONE',  ( 5.823673210054444382, -21.52544592524334988, 20.20942372801900788 ) ) ;
#142663=CARTESIAN_POINT ( 'NONE',  ( -0.05219959533936034679, 19.03943276465977164, 112.5010903946856757 ) ) ;
#142664=CARTESIAN_POINT ( 'NONE',  ( 12.06949235617739724, 12.14591786802326823, 66.87609039468568994 ) ) ;
#142666=CARTESIAN_POINT ( 'NONE',  ( -0.05219959533907301413, -21.53943276465977519, 112.4989096053143669 ) ) ;
#142667=CARTESIAN_POINT ( 'NONE',  ( -16.55341960407611168, -4.379528057220339221, 101.4572429386476955 ) ) ;
#142669=CARTESIAN_POINT ( 'NONE',  ( 0.05219959533934541429, -16.53943276465976808, 40.00109039468567573 ) ) ;
#142670=CARTESIAN_POINT ( 'NONE',  ( 18.67979575497178502, 10.72451020669898547, 64.16557627198102409 ) ) ;
#142671=CARTESIAN_POINT ( 'NONE',  ( -4.379528057220086978, -16.55341960407618274, 109.7927570613523613 ) ) ;
#142672=CARTESIAN_POINT ( 'NONE',  ( -13.89961937509977652, 13.97604488694528158, 30.62390960531435269 ) ) ;
#142673=CARTESIAN_POINT ( 'NONE',  ( 0.05219959533934541429, -16.53943276465976808, 65.00109039468568994 ) ) ;
#142674=CARTESIAN_POINT ( 'NONE',  ( -19.03943276465977164, -0.05219959533935918106, 58.75109039468566863 ) ) ;
#142675=CARTESIAN_POINT ( 'NONE',  ( -21.52544592524334988, -5.823673210054445271, 43.95942372801902565 ) ) ;
#142676=CARTESIAN_POINT ( 'NONE',  ( -5.719274019375978568, 21.55341960407610458, 65.20724293864768129 ) ) ;
#142677=CARTESIAN_POINT ( 'NONE',  ( 8.314922557961029526, -14.29746914071037800, 100.4177570613523471 ) ) ;
#142678=CARTESIAN_POINT ( 'NONE',  ( -5.823673210054431948, 21.52544592524334988, 82.70942372801900433 ) ) ;
#142679=CARTESIAN_POINT ( 'NONE',  ( -5.719274019375978568, 21.55341960407610458, 55.20724293864770260 ) ) ;
#142680=CARTESIAN_POINT ( 'NONE',  ( 18.67979575497178502, 10.72451020669898547, 29.16557627198103120 ) ) ;
#142682=CARTESIAN_POINT ( 'NONE',  ( -0.05219959533934338120, 16.53943276465976808, 82.50109039468568994 ) ) ;
#142683=CARTESIAN_POINT ( 'NONE',  ( -5.719274019375978568, 21.55341960407610458, 40.20724293864769550 ) ) ;
#142685=CARTESIAN_POINT ( 'NONE',  ( -19.03943276465977164, 0.05219959533909376836, 101.2489096053143669 ) ) ;
#142687=CARTESIAN_POINT ( 'NONE',  ( 19.05341960407611168, 5.049401038298154454, 28.95724293864769550 ) ) ;
#142688=CARTESIAN_POINT ( 'NONE',  ( 15.72974639402199770, -15.80617190586745480, 68.12390960531436690 ) ) ;
#142689=CARTESIAN_POINT ( 'NONE',  ( 16.52544592524335698, 4.483927247898782831, 86.45942372801901854 ) ) ;
#142690=CARTESIAN_POINT ( 'NONE',  ( 5.719274019375673035, 21.55341960407619339, 52.29275706135236135 ) ) ;
#142691=CARTESIAN_POINT ( 'NONE',  ( 16.51473224551083163, -9.474510206698727899, 105.8344237280190043 ) ) ;
#142692=CARTESIAN_POINT ( 'NONE',  ( 16.55341960407611168, 4.379528057220329451, 98.95724293864770971 ) ) ;
#142693=CARTESIAN_POINT ( 'NONE',  ( 16.52544592524335698, 4.483927247898782831, 21.45942372801901499 ) ) ;
#142694=CARTESIAN_POINT ( 'NONE',  ( -13.89961937509977652, 13.97604488694528158, 40.62390960531435979 ) ) ;
#142695=DIRECTION ( 'NONE',  ( 1.000000000000000000, 0.000000000000000000, 0.000000000000000000 ) ) ;
#142696=CARTESIAN_POINT ( 'NONE',  ( -13.89961937509977652, 13.97604488694528158, 95.62390960531436690 ) ) ;
#142697=EDGE_CURVE ( 'NONE', #88111, #43212, #24941, .T. ) ;
#142698=CARTESIAN_POINT ( 'NONE',  ( -16.55341960407617563, 4.379528057220093196, 73.54275706135234714 ) ) ;
#142699=CARTESIAN_POINT ( 'NONE',  ( -21.53943276465977519, -0.05219959533937600094, 108.7510903946857042 ) ) ;
#142700=CARTESIAN_POINT ( 'NONE',  ( 15.72974639402199770, -15.80617190586745480, 63.12390960531435979 ) ) ;
#142701=CARTESIAN_POINT ( 'NONE',  ( 8.314922557961029526, -14.29746914071037800, 85.41775706135236135 ) ) ;
#142702=CARTESIAN_POINT ( 'NONE',  ( -5.049401038297874678, -19.05341960407617918, 84.79275706135233293 ) ) ;
#142703=CARTESIAN_POINT ( 'NONE',  ( -16.51473224551069308, -9.474510206698971260, 31.66557627198102054 ) ) ;
#142704=CARTESIAN_POINT ( 'NONE',  ( 9.564922557960805705, 16.46253265017160317, 84.58224293864769550 ) ) ;
#142705=CARTESIAN_POINT ( 'NONE',  ( -19.05341960407611168, -5.049401038298163336, 31.45724293864769550 ) ) ;
#142706=CARTESIAN_POINT ( 'NONE',  ( 9.564922557961047289, -16.46253265017146816, 70.41775706135233293 ) ) ;
#142708=CARTESIAN_POINT ( 'NONE',  ( -13.89961937509977652, 13.97604488694528158, 90.62390960531432427 ) ) ;
#142709=CARTESIAN_POINT ( 'NONE',  ( 8.224510206698953496, -14.34966873604960469, 47.91557627198102409 ) ) ;
#142710=CARTESIAN_POINT ( 'NONE',  ( -18.67979575497178146, -10.72451020669898902, 66.66557627198102409 ) ) ;
#142711=CARTESIAN_POINT ( 'NONE',  ( -17.50000000000147438, 3.202012800152229666, 104.9282241602725634 ) ) ;
#142712=CARTESIAN_POINT ( 'NONE',  ( 0.05219959533936267826, -19.03943276465977164, 25.00109039468566152 ) ) ;
#142714=CARTESIAN_POINT ( 'NONE',  ( -16.46253265017160317, 9.564922557960807481, 65.83224293864769550 ) ) ;
#142715=CARTESIAN_POINT ( 'NONE',  ( -9.564922557960796823, -16.46253265017161027, 72.08224293864770971 ) ) ;
#142716=CARTESIAN_POINT ( 'NONE',  ( 4.379528057220092307, 16.55341960407617563, 37.29275706135235424 ) ) ;
#142719=CARTESIAN_POINT ( 'NONE',  ( -0.05219959533934338120, 16.53943276465976808, 72.50109039468568994 ) ) ;
#142720=CARTESIAN_POINT ( 'NONE',  ( 8.224510206698742110, 14.34966873604972548, 67.08442372801901854 ) ) ;
#142721=CARTESIAN_POINT ( 'NONE',  ( -10.72451020669898014, 18.67979575497178502, 90.41557627198103830 ) ) ;
#142722=CARTESIAN_POINT ( 'NONE',  ( -0.05219959533934338120, 16.53943276465976808, 47.50109039468568994 ) ) ;
#142723=CARTESIAN_POINT ( 'NONE',  ( -5.153800228976328057, -19.02544592524343514, 42.29057627198101699 ) ) ;
#142725=CARTESIAN_POINT ( 'NONE',  ( 10.81492255796106328, -18.62759615963255655, 55.41775706135234714 ) ) ;
#142726=CARTESIAN_POINT ( 'NONE',  ( 13.97604488694548053, -13.89961937509957401, 60.62609039468564731 ) ) ;
#142727=CARTESIAN_POINT ( 'NONE',  ( -21.52544592524334988, -5.823673210054445271, 98.95942372801903275 ) ) ;
#142728=CARTESIAN_POINT ( 'NONE',  ( -19.02544592524342804, 5.153800228976336051, 26.04057627198103120 ) ) ;
#142730=CARTESIAN_POINT ( 'NONE',  ( -21.55341960407610458, -5.719274019375992779, 51.45724293864770260 ) ) ;
#142732=CARTESIAN_POINT ( 'NONE',  ( -5.049401038298153566, 19.05341960407611168, 100.2072429386476955 ) ) ;
#142733=CARTESIAN_POINT ( 'NONE',  ( 16.53943276465976808, -0.05219959533910856209, 103.7489096053143669 ) ) ;
#142734=CARTESIAN_POINT ( 'NONE',  ( -16.53943276465976808, -0.05219959533934237506, 33.75109039468568284 ) ) ;
#142735=CARTESIAN_POINT ( 'NONE',  ( 4.379528057220092307, 16.55341960407617563, 107.2927570613523471 ) ) ;
#142736=VERTEX_POINT ( 'NONE', #165445 ) ;
#142737=CARTESIAN_POINT ( 'NONE',  ( -18.62759615963270932, 10.81492255796079327, 100.8322429386477097 ) ) ;
#142738=CARTESIAN_POINT ( 'NONE',  ( -8.314922557960811034, -14.29746914071050412, 37.08224293864768129 ) ) ;
#142740=CARTESIAN_POINT ( 'NONE',  ( 9.564922557961047289, -16.46253265017146816, 100.4177570613523329 ) ) ;
#142741=CARTESIAN_POINT ( 'NONE',  ( 19.02544592524334988, 5.153800228976608722, 26.45942372801899722 ) ) ;
#142742=CARTESIAN_POINT ( 'NONE',  ( -12.06949235617756955, 12.14591786802309770, 35.62390960531437401 ) ) ;
#142743=CARTESIAN_POINT ( 'NONE',  ( -21.55341960407610458, -5.719274019375992779, 96.45724293864770971 ) ) ;
#142744=CARTESIAN_POINT ( 'NONE',  ( 21.52544592524344225, -5.823673210054117533, 48.54057627198103120 ) ) ;
#142745=CARTESIAN_POINT ( 'NONE',  ( 19.03943276465977164, -0.05219959533909143690, 68.74890960531436690 ) ) ;
#142746=CARTESIAN_POINT ( 'NONE',  ( -12.06949235617756955, 12.14591786802309770, 35.62390960531437401 ) ) ;
#142747=CARTESIAN_POINT ( 'NONE',  ( 13.97604488694527802, 13.89961937509977652, 89.37390960531436690 ) ) ;
#142749=CARTESIAN_POINT ( 'NONE',  ( 9.564922557960805705, 16.46253265017160317, 79.58224293864769550 ) ) ;
#142750=CARTESIAN_POINT ( 'NONE',  ( -9.474510206698720793, -16.51473224551083518, 39.58442372801899722 ) ) ;
#142751=CARTESIAN_POINT ( 'NONE',  ( -10.72451020669898014, 18.67979575497178502, 75.41557627198102409 ) ) ;
#142752=CARTESIAN_POINT ( 'NONE',  ( 8.224510206698953496, -14.34966873604960469, 97.91557627198103830 ) ) ;
#142753=CARTESIAN_POINT ( 'NONE',  ( 21.55341960407619695, -5.719274019375665929, 41.04275706135236135 ) ) ;
#142755=CARTESIAN_POINT ( 'NONE',  ( -14.29746914071037622, -8.314922557961029526, 104.1677570613523471 ) ) ;
#142756=CARTESIAN_POINT ( 'NONE',  ( 9.564922557960805705, 16.46253265017160317, 34.58224293864770260 ) ) ;
#142757=CARTESIAN_POINT ( 'NONE',  ( -16.51473224551069308, -9.474510206698971260, 86.66557627198102409 ) ) ;
#142759=CARTESIAN_POINT ( 'NONE',  ( -9.474510206698964154, 16.51473224551069663, 30.41557627198102054 ) ) ;
#142760=CARTESIAN_POINT ( 'NONE',  ( -4.483927247898539470, -16.52544592524342804, 37.29057627198102409 ) ) ;
#142761=CARTESIAN_POINT ( 'NONE',  ( -18.62759615963255300, -10.81492255796106328, 74.16775706135231871 ) ) ;
#142763=CARTESIAN_POINT ( 'NONE',  ( -14.34966873604972548, 8.224510206698743886, 73.33442372801901854 ) ) ;
#142764=CARTESIAN_POINT ( 'NONE',  ( 16.46253265017160672, -9.564922557960803928, 63.33224293864769550 ) ) ;
#142765=CARTESIAN_POINT ( 'NONE',  ( 5.049401038298161559, -19.05341960407611168, 67.70724293864769550 ) ) ;
#142766=ORIENTED_EDGE ( 'NONE', *, *, #176553, .T. ) ;
#142767=CARTESIAN_POINT ( 'NONE',  ( -21.55341960407619339, 5.719274019375674811, 113.5427570613523756 ) ) ;
#142768=CARTESIAN_POINT ( 'NONE',  ( -4.379528057220086978, -16.55341960407618274, 69.79275706135234714 ) ) ;
#142769=CARTESIAN_POINT ( 'NONE',  ( -5.719274019375665041, -21.55341960407619695, 104.7927570613523898 ) ) ;
#142770=CARTESIAN_POINT ( 'NONE',  ( -5.153800228976328057, -19.02544592524343514, 57.29057627198103120 ) ) ;
#142771=CARTESIAN_POINT ( 'NONE',  ( 21.55341960407610458, 5.719274019375980345, 33.95724293864769550 ) ) ;
#142772=CARTESIAN_POINT ( 'NONE',  ( -19.05341960407617563, 5.049401038297882671, 108.5427570613523187 ) ) ;
#142773=CARTESIAN_POINT ( 'NONE',  ( -10.81492255796105439, 18.62759615963255655, 62.91775706135236135 ) ) ;
#142774=CARTESIAN_POINT ( 'NONE',  ( 14.29746914071037800, 8.314922557961029526, 51.66775706135234714 ) ) ;
#142775=CARTESIAN_POINT ( 'NONE',  ( 10.72451020669898902, -18.67979575497178502, 102.9155762719810383 ) ) ;
#142776=CARTESIAN_POINT ( 'NONE',  ( 19.05341960407617918, -5.049401038297876454, 96.04275706135231871 ) ) ;
#142777=CARTESIAN_POINT ( 'NONE',  ( 9.474510206698971260, -16.51473224551069308, 77.91557627198103830 ) ) ;
#142778=CARTESIAN_POINT ( 'NONE',  ( 12.14591786802327356, -12.06949235617739191, 20.62609039468568639 ) ) ;
#142779=CARTESIAN_POINT ( 'NONE',  ( 19.05341960407617918, -5.049401038297876454, 101.0427570613523045 ) ) ;
#142780=CARTESIAN_POINT ( 'NONE',  ( 4.483927247898545687, 16.52544592524342804, 69.79057627198102409 ) ) ;
#142781=CARTESIAN_POINT ( 'NONE',  ( 14.29746914071037800, 8.314922557961029526, 76.66775706135234714 ) ) ;
#142782=CARTESIAN_POINT ( 'NONE',  ( -5.719274019375978568, 21.55341960407610458, 110.2072429386477239 ) ) ;
#142783=CARTESIAN_POINT ( 'NONE',  ( 19.02544592524343514, -5.153800228976328945, 48.54057627198103120 ) ) ;
#142784=CARTESIAN_POINT ( 'NONE',  ( -16.51473224551069308, -9.474510206698971260, 61.66557627198103120 ) ) ;
#142785=CARTESIAN_POINT ( 'NONE',  ( 8.314922557961029526, -14.29746914071037800, 75.41775706135233293 ) ) ;
#142788=CARTESIAN_POINT ( 'NONE',  ( -19.02544592524334988, -5.153800228976617603, 18.95942372801899722 ) ) ;
#142790=CARTESIAN_POINT ( 'NONE',  ( -9.474510206698964154, 16.51473224551069663, 30.41557627198102054 ) ) ;
#142791=EDGE_LOOP ( 'NONE', ( #21301, #114598, #69074, #17797 ) ) ;
#142792=CARTESIAN_POINT ( 'NONE',  ( 19.02544592524334988, 5.153800228976608722, 106.4594237280190185 ) ) ;
#142793=CARTESIAN_POINT ( 'NONE',  ( -13.89961937509957401, -13.97604488694547875, 44.37609039468566863 ) ) ;
#142794=CARTESIAN_POINT ( 'NONE',  ( -14.29746914071037622, -8.314922557961029526, 24.16775706135235424 ) ) ;
#142795=CARTESIAN_POINT ( 'NONE',  ( 9.474510206698971260, -16.51473224551069308, 37.91557627198102409 ) ) ;
#142796=CARTESIAN_POINT ( 'NONE',  ( -5.049401038298153566, 19.05341960407611168, 60.20724293864768129 ) ) ;
#142797=CARTESIAN_POINT ( 'NONE',  ( 18.62759615963271287, -10.81492255796078972, 88.33224293864769550 ) ) ;
#142798=CARTESIAN_POINT ( 'NONE',  ( 19.05341960407611168, 5.049401038298154454, 113.9572429386477097 ) ) ;
#142799=CARTESIAN_POINT ( 'NONE',  ( 5.049401038298161559, -19.05341960407611168, 47.70724293864770260 ) ) ;
#142800=DIRECTION ( 'NONE',  ( -1.000000000000000000, -0.000000000000000000, -0.000000000000000000 ) ) ;
#142801=CARTESIAN_POINT ( 'NONE',  ( 19.03943276465977164, 0.05219959533936151252, 96.25109039468567573 ) ) ;
#142802=CARTESIAN_POINT ( 'NONE',  ( 4.379528057220339221, -16.55341960407611168, 67.70724293864769550 ) ) ;
#142803=CARTESIAN_POINT ( 'NONE',  ( -16.51473224551082808, 9.474510206698731452, 28.33442372801900433 ) ) ;
#142805=CARTESIAN_POINT ( 'NONE',  ( 4.379528057220339221, -16.55341960407611168, 57.70724293864770260 ) ) ;
#142806=CARTESIAN_POINT ( 'NONE',  ( -10.72451020669870658, -18.67979575497194134, 84.58442372801903275 ) ) ;
#142807=CARTESIAN_POINT ( 'NONE',  ( 0.05219959533909260263, 19.03943276465977164, 29.99890960531435979 ) ) ;
#142808=CARTESIAN_POINT ( 'NONE',  ( -10.72451020669870658, -18.67979575497194134, 94.58442372801901854 ) ) ;
#142809=CARTESIAN_POINT ( 'NONE',  ( -4.379528057220328563, 16.55341960407611168, 25.20724293864769550 ) ) ;
#142810=CARTESIAN_POINT ( 'NONE',  ( 15.80617190586769283, -15.72974639402175789, 70.62609039468567573 ) ) ;
#142811=CARTESIAN_POINT ( 'NONE',  ( 5.153800228976335163, 19.02544592524342804, 79.79057627198102409 ) ) ;
#142812=CARTESIAN_POINT ( 'NONE',  ( -5.719274019375665041, -21.55341960407619695, 39.79275706135235424 ) ) ;
#142813=CARTESIAN_POINT ( 'NONE',  ( -5.049401038298153566, 19.05341960407611168, 85.20724293864766707 ) ) ;
#142814=CARTESIAN_POINT ( 'NONE',  ( -14.34966873604960291, -8.224510206698953496, 96.66557627198102409 ) ) ;
#142815=CARTESIAN_POINT ( 'NONE',  ( -14.34966873604960291, -8.224510206698953496, 56.66557627198103830 ) ) ;
#142816=CARTESIAN_POINT ( 'NONE',  ( 5.719274019375991003, -21.55341960407610458, 67.70724293864769550 ) ) ;
#142817=CARTESIAN_POINT ( 'NONE',  ( 0.05219959533909260263, 19.03943276465977164, 74.99890960531435269 ) ) ;
#142818=CARTESIAN_POINT ( 'NONE',  ( -10.72451020669898014, 18.67979575497178502, 80.41557627198103830 ) ) ;
#142819=CARTESIAN_POINT ( 'NONE',  ( 13.97604488694548053, -13.89961937509957401, 65.62609039468567573 ) ) ;
#142820=CARTESIAN_POINT ( 'NONE',  ( -19.02544592524335343, -5.153800228976618492, 33.95942372801899012 ) ) ;
#142821=CARTESIAN_POINT ( 'NONE',  ( 4.379528057220339221, -16.55341960407611168, 72.70724293864769550 ) ) ;
#142822=CARTESIAN_POINT ( 'NONE',  ( 18.62759615963271287, -10.81492255796078972, 48.33224293864770260 ) ) ;
#142824=CARTESIAN_POINT ( 'NONE',  ( 16.52544592524335698, 4.483927247898782831, 101.4594237280190185 ) ) ;
#142826=CARTESIAN_POINT ( 'NONE',  ( 5.049401038297881783, 19.05341960407617563, 97.29275706135233293 ) ) ;
#142827=CARTESIAN_POINT ( 'NONE',  ( -4.483927247898539470, -16.52544592524342804, 62.29057627198102409 ) ) ;
#142829=CARTESIAN_POINT ( 'NONE',  ( -19.05341960407611168, -5.049401038298163336, 56.45724293864768129 ) ) ;
#142830=CARTESIAN_POINT ( 'NONE',  ( 14.34966873604960469, 8.224510206698951720, 54.16557627198103120 ) ) ;
#142831=ADVANCED_FACE ( 'NONE', ( #10766 ), #13097, .T. ) ;
#142832=CARTESIAN_POINT ( 'NONE',  ( 16.46253265017160672, -9.564922557960803928, 103.3322429386476955 ) ) ;
#142833=CARTESIAN_POINT ( 'NONE',  ( -16.51473224551082808, 9.474510206698731452, 78.33442372801900433 ) ) ;
#142834=CARTESIAN_POINT ( 'NONE',  ( -16.46253265017160317, 9.564922557960807481, 70.83224293864770971 ) ) ;
#142835=CARTESIAN_POINT ( 'NONE',  ( 19.05341960407611168, 5.049401038298154454, 78.95724293864769550 ) ) ;
#142836=CARTESIAN_POINT ( 'NONE',  ( -19.02544592524342804, 5.153800228976336051, 81.04057627198103830 ) ) ;
#142837=CARTESIAN_POINT ( 'NONE',  ( -5.823673210054116645, -21.52544592524344225, 57.29057627198103120 ) ) ;
#142838=CARTESIAN_POINT ( 'NONE',  ( -16.55341960407617563, 4.379528057220093196, 63.54275706135234003 ) ) ;
#142840=CARTESIAN_POINT ( 'NONE',  ( -5.153800228976328057, -19.02544592524343514, 52.29057627198100988 ) ) ;
#142841=CARTESIAN_POINT ( 'NONE',  ( -21.52544592524343514, 5.823673210054127303, 61.04057627198103120 ) ) ;
#142842=CARTESIAN_POINT ( 'NONE',  ( -19.03943276465977164, -0.05219959533935918106, 93.75109039468566152 ) ) ;
#142843=CARTESIAN_POINT ( 'NONE',  ( 14.34966873604960469, 8.224510206698951720, 29.16557627198103120 ) ) ;
#142844=CARTESIAN_POINT ( 'NONE',  ( -18.67979575497193778, 10.72451020669871902, 48.33442372801902565 ) ) ;
#142845=CARTESIAN_POINT ( 'NONE',  ( 16.46253265017146816, 9.564922557961045513, 36.66775706135233293 ) ) ;
#142846=CARTESIAN_POINT ( 'NONE',  ( -8.224510206698735004, -14.34966873604973081, 59.58442372801901854 ) ) ;
#142847=CARTESIAN_POINT ( 'NONE',  ( 8.314922557961029526, -14.29746914071037800, 90.41775706135236135 ) ) ;
#142849=CARTESIAN_POINT ( 'NONE',  ( 14.29746914071037800, 8.314922557961029526, 81.66775706135236135 ) ) ;
#142850=CARTESIAN_POINT ( 'NONE',  ( -12.14591786802326823, 12.06949235617739902, 38.12609039468567573 ) ) ;
#142851=CARTESIAN_POINT ( 'NONE',  ( 9.564922557960805705, 16.46253265017160317, 44.58224293864769550 ) ) ;
#142852=CARTESIAN_POINT ( 'NONE',  ( 5.153800228976335163, 19.02544592524342804, 44.79057627198103830 ) ) ;
#142853=CARTESIAN_POINT ( 'NONE',  ( -5.049401038298153566, 19.05341960407611168, 65.20724293864765286 ) ) ;
#142854=CARTESIAN_POINT ( 'NONE',  ( -18.67979575497193778, 10.72451020669871902, 58.33442372801901143 ) ) ;
#142855=CARTESIAN_POINT ( 'NONE',  ( -4.483927247898782831, 16.52544592524335698, 52.70942372801902565 ) ) ;
#142856=CARTESIAN_POINT ( 'NONE',  ( -16.55341960407617563, 4.379528057220093196, 113.5427570613523756 ) ) ;
#142857=CARTESIAN_POINT ( 'NONE',  ( 16.46253265017160672, -9.564922557960803928, 23.33224293864769194 ) ) ;
#142858=CARTESIAN_POINT ( 'NONE',  ( -13.89961937509957401, -13.97604488694547875, 24.37609039468565442 ) ) ;
#142859=CARTESIAN_POINT ( 'NONE',  ( -9.474510206698720793, -16.51473224551083518, 104.5844237280190043 ) ) ;
#142860=CARTESIAN_POINT ( 'NONE',  ( -19.05341960407617563, 5.049401038297882671, 68.54275706135230450 ) ) ;
#142861=CARTESIAN_POINT ( 'NONE',  ( 16.55341960407611168, 4.379528057220329451, 78.95724293864769550 ) ) ;
#142862=CARTESIAN_POINT ( 'NONE',  ( -16.46253265017160317, 9.564922557960807481, 40.83224293864769550 ) ) ;
#142863=CARTESIAN_POINT ( 'NONE',  ( -19.05341960407617563, 5.049401038297882671, 68.54275706135230450 ) ) ;
#142865=CARTESIAN_POINT ( 'NONE',  ( -5.823673210054431948, 21.52544592524334988, 72.70942372801901854 ) ) ;
#142866=CARTESIAN_POINT ( 'NONE',  ( -8.314922557961024197, 14.29746914071037800, 37.91775706135235424 ) ) ;
#142867=CARTESIAN_POINT ( 'NONE',  ( -17.49999999999999289, 3.565345528327877211, 24.42494486806482712 ) ) ;
#142868=CARTESIAN_POINT ( 'NONE',  ( -18.62759615963270932, 10.81492255796079327, 30.83224293864770260 ) ) ;
#142869=CARTESIAN_POINT ( 'NONE',  ( 0.05219959533934541429, -16.53943276465976808, 25.00109039468567218 ) ) ;
#142870=CARTESIAN_POINT ( 'NONE',  ( 16.46253265017160672, -9.564922557960803928, 23.33224293864769194 ) ) ;
#142871=CARTESIAN_POINT ( 'NONE',  ( -5.049401038297874678, -19.05341960407617918, 24.79275706135233648 ) ) ;
#142872=CARTESIAN_POINT ( 'NONE',  ( 5.049401038298161559, -19.05341960407611168, 37.70724293864768839 ) ) ;
#142874=CARTESIAN_POINT ( 'NONE',  ( 19.03943276465977164, -0.05219959533909143690, 73.74890960531435269 ) ) ;
#142875=CARTESIAN_POINT ( 'NONE',  ( 17.50000000000147793, -3.202012800152233218, 112.4282241602725634 ) ) ;
#142876=CARTESIAN_POINT ( 'NONE',  ( -18.62759615963255300, -10.81492255796106328, 109.1677570613523613 ) ) ;
#142877=CARTESIAN_POINT ( 'NONE',  ( -16.55341960407611168, -4.379528057220339221, 31.45724293864769550 ) ) ;
#142878=CARTESIAN_POINT ( 'NONE',  ( 16.46253265017160672, -9.564922557960803928, 48.33224293864769550 ) ) ;
#142879=CARTESIAN_POINT ( 'NONE',  ( 9.564922557960805705, 16.46253265017160317, 94.58224293864769550 ) ) ;
#142880=CARTESIAN_POINT ( 'NONE',  ( 10.81492255796106328, -18.62759615963255655, 75.41775706135233293 ) ) ;
#142881=CARTESIAN_POINT ( 'NONE',  ( -16.51473224551069308, -9.474510206698971260, 51.66557627198102409 ) ) ;
#142882=CARTESIAN_POINT ( 'NONE',  ( 15.72974639402176855, 15.80617190586768217, 71.87609039468568994 ) ) ;
#142883=CARTESIAN_POINT ( 'NONE',  ( 5.823673210054125526, 21.52544592524343514, 24.79057627198103120 ) ) ;
#142884=CARTESIAN_POINT ( 'NONE',  ( -13.89961937509977652, 13.97604488694528158, 40.62390960531435979 ) ) ;
#142885=CARTESIAN_POINT ( 'NONE',  ( -18.62759615963270932, 10.81492255796079327, 115.8322429386477097 ) ) ;
#142886=CARTESIAN_POINT ( 'NONE',  ( 9.474510206698729675, 16.51473224551082808, 52.08442372801900433 ) ) ;
#142887=CARTESIAN_POINT ( 'NONE',  ( -12.06949235617756955, 12.14591786802309770, 110.6239096053143669 ) ) ;
#142888=CARTESIAN_POINT ( 'NONE',  ( -19.02544592524342804, 5.153800228976336051, 66.04057627198103830 ) ) ;
#142889=CARTESIAN_POINT ( 'NONE',  ( 12.06949235617739724, 12.14591786802326823, 21.87609039468567573 ) ) ;
#142890=CARTESIAN_POINT ( 'NONE',  ( -14.34966873604960291, -8.224510206698953496, 76.66557627198103830 ) ) ;
#142891=CARTESIAN_POINT ( 'NONE',  ( 0.05219959533907565091, 21.53943276465977519, 29.99890960531435979 ) ) ;
#142892=CARTESIAN_POINT ( 'NONE',  ( 5.049401038297881783, 19.05341960407617563, 87.29275706135234714 ) ) ;
#142893=CARTESIAN_POINT ( 'NONE',  ( 10.72451020669898902, -18.67979575497178502, 102.9155762719810383 ) ) ;
#142894=CARTESIAN_POINT ( 'NONE',  ( -5.719274019375665041, -21.55341960407619695, 59.79275706135234714 ) ) ;
#142895=CARTESIAN_POINT ( 'NONE',  ( -4.379528057220086978, -16.55341960407618274, 54.79275706135235424 ) ) ;
#142896=CARTESIAN_POINT ( 'NONE',  ( -8.314922557961024197, 14.29746914071037800, 52.91775706135235424 ) ) ;
#142897=CARTESIAN_POINT ( 'NONE',  ( -15.72974639402197994, 15.80617190586746368, 55.62390960531436690 ) ) ;
#142898=CARTESIAN_POINT ( 'NONE',  ( -9.564922557960796823, -16.46253265017161027, 52.08224293864768839 ) ) ;
#142900=CARTESIAN_POINT ( 'NONE',  ( -4.379528057220086978, -16.55341960407618274, 79.79275706135236135 ) ) ;
#142901=CARTESIAN_POINT ( 'NONE',  ( 18.62759615963271287, -10.81492255796078972, 103.3322429386476955 ) ) ;
#142902=CARTESIAN_POINT ( 'NONE',  ( 12.14591786802309770, 12.06949235617756955, 54.37390960531435979 ) ) ;
#142903=CARTESIAN_POINT ( 'NONE',  ( 9.474510206698971260, -16.51473224551069308, 72.91557627198102409 ) ) ;
#142904=CARTESIAN_POINT ( 'NONE',  ( -14.29746914071037622, -8.314922557961029526, 74.16775706135231871 ) ) ;
#142905=CARTESIAN_POINT ( 'NONE',  ( -13.89961937509957401, -13.97604488694547875, 99.37609039468567573 ) ) ;
#142906=CARTESIAN_POINT ( 'NONE',  ( -21.53943276465977519, 0.05219959533907696930, 96.24890960531435269 ) ) ;
#142907=CARTESIAN_POINT ( 'NONE',  ( 14.34966873604960469, 8.224510206698951720, 49.16557627198102409 ) ) ;
#142908=ORIENTED_EDGE ( 'NONE', *, *, #177312, .T. ) ;
#142909=CARTESIAN_POINT ( 'NONE',  ( -16.18388926212238843, 7.379444403734526148, 69.56046848633849322 ) ) ;
#142910=CARTESIAN_POINT ( 'NONE',  ( -10.72451020669898014, 18.67979575497178502, 75.41557627198102409 ) ) ;
#142911=CARTESIAN_POINT ( 'NONE',  ( -16.55341960407617563, 4.379528057220093196, 113.5427570613523756 ) ) ;
#142913=CARTESIAN_POINT ( 'NONE',  ( -17.40861289039003523, -6.110651285853283099, 56.37232470827432707 ) ) ;
#142914=CARTESIAN_POINT ( 'NONE',  ( -5.823673210054116645, -21.52544592524344225, 97.29057627198105251 ) ) ;
#142915=CARTESIAN_POINT ( 'NONE',  ( 0.05219959533937995610, -21.53943276465977519, 25.00109039468567218 ) ) ;
#142916=CARTESIAN_POINT ( 'NONE',  ( 16.52544592524342804, -4.483927247898539470, 43.54057627198103830 ) ) ;
#142917=CARTESIAN_POINT ( 'NONE',  ( -14.29746914071037622, -8.314922557961029526, 49.16775706135234003 ) ) ;
#142918=CARTESIAN_POINT ( 'NONE',  ( 16.51473224551069308, 9.474510206698969483, 49.16557627198102409 ) ) ;
#142919=CARTESIAN_POINT ( 'NONE',  ( 19.03943276465977164, -0.05219959533909143690, 83.74890960531436690 ) ) ;
#142921=CARTESIAN_POINT ( 'NONE',  ( 18.67979575497178502, 10.72451020669898547, 29.16557627198103120 ) ) ;
#142923=CARTESIAN_POINT ( 'NONE',  ( 14.29746914071037800, 8.314922557961029526, 26.66775706135235424 ) ) ;
#142924=CARTESIAN_POINT ( 'NONE',  ( -19.02544592524334988, -5.153800228976617603, 53.95942372801898301 ) ) ;
#142925=CARTESIAN_POINT ( 'NONE',  ( -21.53943276465977519, 0.05219959533907696930, 101.2489096053143669 ) ) ;
#142926=CARTESIAN_POINT ( 'NONE',  ( -8.314922557960811034, -14.29746914071050412, 37.08224293864768129 ) ) ;
#142928=CARTESIAN_POINT ( 'NONE',  ( -5.049401038298153566, 19.05341960407611168, 75.20724293864769550 ) ) ;
#142929=CARTESIAN_POINT ( 'NONE',  ( 10.81492255796078972, 18.62759615963270932, 64.58224293864769550 ) ) ;
#142930=CARTESIAN_POINT ( 'NONE',  ( 10.81492255796078972, 18.62759615963270932, 94.58224293864769550 ) ) ;
#142931=CARTESIAN_POINT ( 'NONE',  ( -14.29746914071037622, -8.314922557961029526, 19.16775706135234714 ) ) ;
#142932=CARTESIAN_POINT ( 'NONE',  ( -21.55341960407610458, -5.719274019375992779, 26.45724293864768839 ) ) ;
#142933=CARTESIAN_POINT ( 'NONE',  ( -21.55341960407619339, 5.719274019375674811, 83.54275706135234714 ) ) ;
#142934=CARTESIAN_POINT ( 'NONE',  ( -9.474510206698964154, 16.51473224551069663, 75.41557627198103830 ) ) ;
#142935=CARTESIAN_POINT ( 'NONE',  ( 19.03943276465977164, -0.05219959533909143690, 33.74890960531435979 ) ) ;
#142936=CARTESIAN_POINT ( 'NONE',  ( 19.02544592524343514, -5.153800228976328945, 83.54057627198100988 ) ) ;
#142937=CARTESIAN_POINT ( 'NONE',  ( -14.29746914071049879, 8.314922557960819915, 100.8322429386477097 ) ) ;
#142938=CARTESIAN_POINT ( 'NONE',  ( -9.474510206698720793, -16.51473224551083518, 99.58442372801900433 ) ) ;
#142939=CARTESIAN_POINT ( 'NONE',  ( 17.50000000000000355, 5.076555817581247076, 33.67951492049776618 ) ) ;
#142940=CARTESIAN_POINT ( 'NONE',  ( -0.05219959533909027116, -19.03943276465977164, 77.49890960531435269 ) ) ;
#142941=CARTESIAN_POINT ( 'NONE',  ( 15.72974639402176855, 15.80617190586768217, 96.87609039468568994 ) ) ;
#142942=CARTESIAN_POINT ( 'NONE',  ( 21.52544592524344225, -5.823673210054117533, 23.54057627198102765 ) ) ;
#142943=CARTESIAN_POINT ( 'NONE',  ( -12.14591786802326823, 12.06949235617739902, 93.12609039468568994 ) ) ;
#142944=CARTESIAN_POINT ( 'NONE',  ( -16.36317988757059894, -7.306389748694932962, 75.90210391636779264 ) ) ;
#142945=CARTESIAN_POINT ( 'NONE',  ( -9.474510206698720793, -16.51473224551083518, 59.58442372801900433 ) ) ;
#142946=CARTESIAN_POINT ( 'NONE',  ( -0.05219959533937732626, 21.53943276465977519, 107.5010903946856899 ) ) ;
#142948=CARTESIAN_POINT ( 'NONE',  ( -19.03943276465977164, 0.05219959533909376836, 31.24890960531435979 ) ) ;
#142949=CARTESIAN_POINT ( 'NONE',  ( 16.55341960407618274, -4.379528057220086978, 111.0427570613523613 ) ) ;
#142951=CARTESIAN_POINT ( 'NONE',  ( 18.22780087662121673, 5.500000000000056843, 83.98459894673892734 ) ) ;
#142952=CARTESIAN_POINT ( 'NONE',  ( -4.483927247898782831, 16.52544592524335698, 102.7094237280190185 ) ) ;
#142954=CARTESIAN_POINT ( 'NONE',  ( -4.483927247898782831, 16.52544592524335698, 82.70942372801900433 ) ) ;
#142955=CARTESIAN_POINT ( 'NONE',  ( 17.59860650958989936, 7.585241751807028088, 84.07662985737508166 ) ) ;
#142956=CARTESIAN_POINT ( 'NONE',  ( -5.823673210054431948, 21.52544592524334988, 97.70942372801904696 ) ) ;
#142957=CARTESIAN_POINT ( 'NONE',  ( 5.049401038297881783, 19.05341960407617563, 102.2927570613523045 ) ) ;
#142958=CARTESIAN_POINT ( 'NONE',  ( 0.05219959533937995610, -21.53943276465977519, 65.00109039468568994 ) ) ;
#142959=CARTESIAN_POINT ( 'NONE',  ( 19.03943276465977164, 0.05219959533936151252, 36.25109039468567573 ) ) ;
#142960=CARTESIAN_POINT ( 'NONE',  ( -16.46253265017160317, 9.564922557960807481, 80.83224293864769550 ) ) ;
#142961=CARTESIAN_POINT ( 'NONE',  ( 9.564922557960805705, 16.46253265017160317, 64.58224293864769550 ) ) ;
#142963=CARTESIAN_POINT ( 'NONE',  ( 17.05587630539786304, 6.762274262135722580, 71.75819690962690345 ) ) ;
#142964=CARTESIAN_POINT ( 'NONE',  ( -5.823673210054116645, -21.52544592524344225, 47.29057627198103120 ) ) ;
#142965=CARTESIAN_POINT ( 'NONE',  ( 13.89961937509977652, -13.97604488694527269, 43.12390960531434558 ) ) ;
#142966=CARTESIAN_POINT ( 'NONE',  ( -5.719274019375978568, 21.55341960407610458, 90.20724293864770971 ) ) ;
#142967=CARTESIAN_POINT ( 'NONE',  ( -16.53943276465976808, -0.05219959533934237506, 83.75109039468568994 ) ) ;
#142970=CARTESIAN_POINT ( 'NONE',  ( -4.483927247898539470, -16.52544592524342804, 77.29057627198102409 ) ) ;
#142972=CARTESIAN_POINT ( 'NONE',  ( 12.14591786802327356, -12.06949235617739191, 40.62609039468567573 ) ) ;
#142973=CARTESIAN_POINT ( 'NONE',  ( -13.89961937509977652, 13.97604488694528158, 25.62390960531434558 ) ) ;
#142974=CARTESIAN_POINT ( 'NONE',  ( 19.02544592524334988, 5.153800228976608722, 66.45942372801899012 ) ) ;
#142975=CARTESIAN_POINT ( 'NONE',  ( -12.06949235617756955, 12.14591786802309770, 70.62390960531436690 ) ) ;
#142976=CARTESIAN_POINT ( 'NONE',  ( 18.67979575497194134, -10.72451020669871369, 40.83442372801901854 ) ) ;
#142978=CARTESIAN_POINT ( 'NONE',  ( 18.67979575497178502, 10.72451020669898547, 89.16557627198102409 ) ) ;
#142979=CARTESIAN_POINT ( 'NONE',  ( 9.564922557960805705, 16.46253265017160317, 114.5822429386476955 ) ) ;
#142980=CARTESIAN_POINT ( 'NONE',  ( -12.06949235617756955, 12.14591786802309770, 75.62390960531439532 ) ) ;
#142982=CARTESIAN_POINT ( 'NONE',  ( -5.049401038298153566, 19.05341960407611168, 45.20724293864769550 ) ) ;
#142984=CARTESIAN_POINT ( 'NONE',  ( 16.46253265017146816, 9.564922557961045513, 86.66775706135233293 ) ) ;
#142985=CARTESIAN_POINT ( 'NONE',  ( 15.72974639402176855, 15.80617190586768217, 21.87609039468567573 ) ) ;
#142986=CARTESIAN_POINT ( 'NONE',  ( -9.474510206698964154, 16.51473224551069663, 70.41557627198102409 ) ) ;
#142987=CARTESIAN_POINT ( 'NONE',  ( 19.02544592524334988, 5.153800228976608722, 56.45942372801898301 ) ) ;
#142988=CARTESIAN_POINT ( 'NONE',  ( -5.153800228976328057, -19.02544592524343514, 42.29057627198101699 ) ) ;
#142989=CARTESIAN_POINT ( 'NONE',  ( 16.53943276465976808, -0.05219959533910856209, 58.74890960531436690 ) ) ;
#142990=CARTESIAN_POINT ( 'NONE',  ( 16.53943276465976808, -0.05219959533910856209, 48.74890960531435979 ) ) ;
#142991=CARTESIAN_POINT ( 'NONE',  ( -19.02544592524342804, 5.153800228976336051, 81.04057627198103830 ) ) ;
#142992=CARTESIAN_POINT ( 'NONE',  ( 21.53943276465977519, -0.05219959533907433946, 88.74890960531436690 ) ) ;
#142993=CARTESIAN_POINT ( 'NONE',  ( 5.049401038298161559, -19.05341960407611168, 77.70724293864765286 ) ) ;
#142994=CARTESIAN_POINT ( 'NONE',  ( 21.52544592524344225, -5.823673210054117533, 83.54057627198102409 ) ) ;
#142995=CARTESIAN_POINT ( 'NONE',  ( -5.823673210054431948, 21.52544592524334988, 112.7094237280190328 ) ) ;
#142996=CARTESIAN_POINT ( 'NONE',  ( -0.05219959533909027116, -19.03943276465977164, 27.49890960531435624 ) ) ;
#142997=CARTESIAN_POINT ( 'NONE',  ( 16.55341960407618274, -4.379528057220086978, 106.0427570613523471 ) ) ;
#142998=CARTESIAN_POINT ( 'NONE',  ( 8.314922557960818139, 14.29746914071049879, 94.58224293864769550 ) ) ;
#142999=CARTESIAN_POINT ( 'NONE',  ( -19.03943276465977164, -0.05219959533935918106, 108.7510903946856615 ) ) ;
#143001=CARTESIAN_POINT ( 'NONE',  ( 18.67979575497194134, -10.72451020669871369, 30.83442372801902209 ) ) ;
#143002=CARTESIAN_POINT ( 'NONE',  ( -9.474510206698720793, -16.51473224551083518, 49.58442372801899722 ) ) ;
#143003=CARTESIAN_POINT ( 'NONE',  ( 8.314922557960818139, 14.29746914071049879, 24.58224293864768839 ) ) ;
#143004=CARTESIAN_POINT ( 'NONE',  ( -21.52544592524343514, 5.823673210054127303, 71.04057627198103830 ) ) ;
#143005=CARTESIAN_POINT ( 'NONE',  ( -19.05341960407611168, -5.049401038298163336, 106.4572429386476955 ) ) ;
#143006=CARTESIAN_POINT ( 'NONE',  ( 16.55341960407611168, 4.379528057220329451, 53.95724293864770260 ) ) ;
#143008=CARTESIAN_POINT ( 'NONE',  ( -19.05341960407611168, -5.049401038298163336, 36.45724293864766707 ) ) ;
#143009=CARTESIAN_POINT ( 'NONE',  ( -21.53943276465977519, -0.05219959533937600094, 103.7510903946857042 ) ) ;
#143010=CARTESIAN_POINT ( 'NONE',  ( 16.55341960407618274, -4.379528057220086978, 86.04275706135236135 ) ) ;
#143011=CARTESIAN_POINT ( 'NONE',  ( -18.62759615963255300, -10.81492255796106328, 44.16775706135234714 ) ) ;
#143012=CARTESIAN_POINT ( 'NONE',  ( 14.34966873604972726, -8.224510206698740333, 40.83442372801901854 ) ) ;
#143013=CARTESIAN_POINT ( 'NONE',  ( 5.823673210054125526, 21.52544592524343514, 29.79057627198102409 ) ) ;
#143014=CARTESIAN_POINT ( 'NONE',  ( -16.51473224551069308, -9.474510206698971260, 51.66557627198102409 ) ) ;
#143015=CARTESIAN_POINT ( 'NONE',  ( -13.97604488694527625, -13.89961937509977652, 71.87390960531433848 ) ) ;
#143016=CARTESIAN_POINT ( 'NONE',  ( -4.379528057220086978, -16.55341960407618274, 64.79275706135234714 ) ) ;
#143017=CARTESIAN_POINT ( 'NONE',  ( 4.483927247898545687, 16.52544592524342804, 104.7905762719810241 ) ) ;
#143018=CARTESIAN_POINT ( 'NONE',  ( -4.483927247898782831, 16.52544592524335698, 112.7094237280190328 ) ) ;
#143020=CARTESIAN_POINT ( 'NONE',  ( 15.80617190586769283, -15.72974639402175789, 50.62609039468568994 ) ) ;
#143021=CARTESIAN_POINT ( 'NONE',  ( 9.474510206698971260, -16.51473224551069308, 92.91557627198103830 ) ) ;
#143022=CARTESIAN_POINT ( 'NONE',  ( -16.51473224551069308, -9.474510206698971260, 76.66557627198103830 ) ) ;
#143023=CARTESIAN_POINT ( 'NONE',  ( 19.02544592524343514, -5.153800228976328945, 93.54057627198102409 ) ) ;
#143024=CARTESIAN_POINT ( 'NONE',  ( 4.379528057220339221, -16.55341960407611168, 47.70724293864770260 ) ) ;
#143026=CARTESIAN_POINT ( 'NONE',  ( -16.55341960407611168, -4.379528057220339221, 21.45724293864769550 ) ) ;
#143027=CARTESIAN_POINT ( 'NONE',  ( 16.53943276465976808, -0.05219959533910856209, 33.74890960531436690 ) ) ;
#143029=CARTESIAN_POINT ( 'NONE',  ( 19.05341960407617918, -5.049401038297876454, 31.04275706135232227 ) ) ;
#143030=CARTESIAN_POINT ( 'NONE',  ( -5.153800228976328057, -19.02544592524343514, 72.29057627198102409 ) ) ;
#143031=CARTESIAN_POINT ( 'NONE',  ( 16.46253265017146816, 9.564922557961045513, 46.66775706135233293 ) ) ;
#143033=CARTESIAN_POINT ( 'NONE',  ( 16.46253265017160672, -9.564922557960803928, 68.33224293864770971 ) ) ;
#143034=CARTESIAN_POINT ( 'NONE',  ( 9.564922557961047289, -16.46253265017146816, 85.41775706135233293 ) ) ;
#143035=CARTESIAN_POINT ( 'NONE',  ( -12.06949235617739369, -12.14591786802326823, 64.37609039468568994 ) ) ;
#143036=CARTESIAN_POINT ( 'NONE',  ( -19.03943276465977164, -0.05219959533935918106, 113.7510903946856757 ) ) ;
#143037=CARTESIAN_POINT ( 'NONE',  ( -9.564922557960796823, -16.46253265017161027, 102.0822429386477097 ) ) ;
#143038=CARTESIAN_POINT ( 'NONE',  ( -21.52544592524334988, -5.823673210054445271, 33.95942372801901143 ) ) ;
#143039=CARTESIAN_POINT ( 'NONE',  ( -16.51473224551082808, 9.474510206698731452, 93.33442372801900433 ) ) ;
#143040=CARTESIAN_POINT ( 'NONE',  ( -0.05219959533909027116, -19.03943276465977164, 112.4989096053143669 ) ) ;
#143041=CARTESIAN_POINT ( 'NONE',  ( 19.02544592524343514, -5.153800228976328945, 53.54057627198102409 ) ) ;
#143042=CARTESIAN_POINT ( 'NONE',  ( -0.05219959533909027116, -19.03943276465977164, 92.49890960531436690 ) ) ;
#143043=CARTESIAN_POINT ( 'NONE',  ( 16.52544592524342804, -4.483927247898539470, 48.54057627198103120 ) ) ;
#143044=CARTESIAN_POINT ( 'NONE',  ( -16.46253265017160317, 9.564922557960807481, 55.83224293864769550 ) ) ;
#143045=CARTESIAN_POINT ( 'NONE',  ( 5.153800228976615827, -19.02544592524334988, 70.20942372801899012 ) ) ;
#143046=CARTESIAN_POINT ( 'NONE',  ( 13.97604488694548053, -13.89961937509957401, 25.62609039468566507 ) ) ;
#143047=CARTESIAN_POINT ( 'NONE',  ( -13.97604488694527625, -13.89961937509977652, 61.87390960531435979 ) ) ;
#143048=CARTESIAN_POINT ( 'NONE',  ( 0.05219959533907565091, 21.53943276465977519, 59.99890960531436690 ) ) ;
#143049=CARTESIAN_POINT ( 'NONE',  ( 14.29746914071049879, -8.314922557960816363, 73.33224293864769550 ) ) ;
#143050=CARTESIAN_POINT ( 'NONE',  ( -0.05219959533937732626, 21.53943276465977519, 112.5010903946857042 ) ) ;
#143052=CARTESIAN_POINT ( 'NONE',  ( -19.02544592524342804, 5.153800228976336051, 116.0405762719810383 ) ) ;
#143053=CARTESIAN_POINT ( 'NONE',  ( -16.46253265017160317, 9.564922557960807481, 55.83224293864769550 ) ) ;
#143054=CARTESIAN_POINT ( 'NONE',  ( 19.05341960407611168, 5.049401038298154454, 43.95724293864769550 ) ) ;
#143055=CARTESIAN_POINT ( 'NONE',  ( 0.05219959533910956823, 16.53943276465976808, 99.99890960531436690 ) ) ;
#143056=MANIFOLD_SOLID_BREP ( 'AdvancedHole2', #20735 ) ;
#143057=CARTESIAN_POINT ( 'NONE',  ( -18.67979575497178146, -10.72451020669898902, 111.6655762719810525 ) ) ;
#143058=CARTESIAN_POINT ( 'NONE',  ( 5.153800228976335163, 19.02544592524342804, 114.7905762719810241 ) ) ;
#143059=CARTESIAN_POINT ( 'NONE',  ( -5.719274019375665041, -21.55341960407619695, 24.79275706135235779 ) ) ;
#143060=CARTESIAN_POINT ( 'NONE',  ( 0.05219959533910956823, 16.53943276465976808, 109.9989096053143527 ) ) ;
#143061=CARTESIAN_POINT ( 'NONE',  ( 21.53943276465977519, 0.05219959533937863772, 76.25109039468568994 ) ) ;
#143062=CARTESIAN_POINT ( 'NONE',  ( 0.05219959533907565091, 21.53943276465977519, 94.99890960531436690 ) ) ;
#143063=CARTESIAN_POINT ( 'NONE',  ( -13.97604488694547697, 13.89961937509957934, 38.12609039468566152 ) ) ;
#143064=CARTESIAN_POINT ( 'NONE',  ( -9.564922557960796823, -16.46253265017161027, 27.08224293864769550 ) ) ;
#143065=CARTESIAN_POINT ( 'NONE',  ( -18.22780087662126647, -5.499999999999827693, 58.98236817873108606 ) ) ;
#143067=CARTESIAN_POINT ( 'NONE',  ( 14.29746914071037800, 8.314922557961029526, 41.66775706135235424 ) ) ;
#143068=CARTESIAN_POINT ( 'NONE',  ( -14.29746914071049879, 8.314922557960819915, 110.8322429386476955 ) ) ;
#143070=CARTESIAN_POINT ( 'NONE',  ( 13.89961937509977652, -13.97604488694527269, 73.12390960531436690 ) ) ;
#143071=CARTESIAN_POINT ( 'NONE',  ( 16.53943276465976808, -0.05219959533910856209, 98.74890960531438111 ) ) ;
#143073=CARTESIAN_POINT ( 'NONE',  ( -15.80617190586745835, -15.72974639402198527, 51.87390960531437401 ) ) ;
#143074=CARTESIAN_POINT ( 'NONE',  ( 12.14591786802309770, 12.06949235617756955, 69.37390960531436690 ) ) ;
#143075=CARTESIAN_POINT ( 'NONE',  ( -8.224510206698735004, -14.34966873604973081, 34.58442372801900433 ) ) ;
#143076=CARTESIAN_POINT ( 'NONE',  ( 5.823673210054444382, -21.52544592524334988, 90.20942372801903275 ) ) ;
#143078=CARTESIAN_POINT ( 'NONE',  ( 16.55341960407618274, -4.379528057220086978, 96.04275706135236135 ) ) ;
#143079=CARTESIAN_POINT ( 'NONE',  ( -8.224510206698948167, 14.34966873604960824, 40.41557627198103120 ) ) ;
#143080=CARTESIAN_POINT ( 'NONE',  ( -9.474510206698964154, 16.51473224551069663, 40.41557627198103120 ) ) ;
#143081=CARTESIAN_POINT ( 'NONE',  ( -18.67979575497193778, 10.72451020669871902, 93.33442372801901854 ) ) ;
#143082=CARTESIAN_POINT ( 'NONE',  ( 21.53943276465977519, -0.05219959533907433946, 108.7489096053143669 ) ) ;
#143083=CARTESIAN_POINT ( 'NONE',  ( -10.72451020669870658, -18.67979575497194134, 59.58442372801901854 ) ) ;
#143084=CARTESIAN_POINT ( 'NONE',  ( 16.55341960407618274, -4.379528057220086978, 41.04275706135236135 ) ) ;
#143085=CARTESIAN_POINT ( 'NONE',  ( -14.34966873604960291, -8.224510206698953496, 61.66557627198103120 ) ) ;
#143086=CARTESIAN_POINT ( 'NONE',  ( -5.719274019375665041, -21.55341960407619695, 89.79275706135236135 ) ) ;
#143087=CARTESIAN_POINT ( 'NONE',  ( 4.379528057220092307, 16.55341960407617563, 97.29275706135234714 ) ) ;
#143088=CARTESIAN_POINT ( 'NONE',  ( 16.61371651742603461, 7.165104196376042012, 28.64584930007005781 ) ) ;
#143089=CARTESIAN_POINT ( 'NONE',  ( -15.49999999999999822, 5.499999999999998224, 118.0000000000000142 ) ) ;
#143090=CARTESIAN_POINT ( 'NONE',  ( -0.05219959533910754901, -16.53943276465976808, 27.49890960531435269 ) ) ;
#143091=CARTESIAN_POINT ( 'NONE',  ( 4.483927247898790824, -16.52544592524335698, 80.20942372801901854 ) ) ;
#143092=CARTESIAN_POINT ( 'NONE',  ( -13.89961937509977652, 13.97604488694528158, 85.62390960531433848 ) ) ;
#143093=CARTESIAN_POINT ( 'NONE',  ( -5.049401038298153566, 19.05341960407611168, 95.20724293864770971 ) ) ;
#143094=CARTESIAN_POINT ( 'NONE',  ( -18.62759615963255300, -10.81492255796106328, 89.16775706135236135 ) ) ;
#143095=CARTESIAN_POINT ( 'NONE',  ( -14.34966873604972548, 8.224510206698743886, 88.33442372801901854 ) ) ;
#143096=CARTESIAN_POINT ( 'NONE',  ( 16.53943276465976808, -0.05219959533910856209, 58.74890960531436690 ) ) ;
#143097=CARTESIAN_POINT ( 'NONE',  ( 13.89961937509977652, -13.97604488694527269, 68.12390960531436690 ) ) ;
#143099=CARTESIAN_POINT ( 'NONE',  ( -4.483927247898782831, 16.52544592524335698, 27.70942372801901854 ) ) ;
#143100=CARTESIAN_POINT ( 'NONE',  ( -9.564922557960796823, -16.46253265017161027, 32.08224293864769550 ) ) ;
#143101=CARTESIAN_POINT ( 'NONE',  ( -13.89961937509977652, 13.97604488694528158, 75.62390960531438111 ) ) ;
#143102=CARTESIAN_POINT ( 'NONE',  ( 12.06949235617739724, 12.14591786802326823, 21.87609039468567573 ) ) ;
#143104=CARTESIAN_POINT ( 'NONE',  ( 5.049401038297881783, 19.05341960407617563, 22.29275706135233648 ) ) ;
#143105=CARTESIAN_POINT ( 'NONE',  ( -8.224510206698735004, -14.34966873604973081, 79.58442372801903275 ) ) ;
#143106=CARTESIAN_POINT ( 'NONE',  ( -9.474510206698720793, -16.51473224551083518, 104.5844237280190043 ) ) ;
#143107=CARTESIAN_POINT ( 'NONE',  ( -19.02544592524342804, 5.153800228976336051, 26.04057627198103120 ) ) ;
#143108=CARTESIAN_POINT ( 'NONE',  ( 14.34966873604972726, -8.224510206698740333, 70.83442372801901854 ) ) ;
#143109=CARTESIAN_POINT ( 'NONE',  ( -4.379528057220086978, -16.55341960407618274, 49.79275706135234714 ) ) ;
#143110=CARTESIAN_POINT ( 'NONE',  ( -19.03943276465977164, 0.05219959533909376836, 26.24890960531435624 ) ) ;
#143111=CARTESIAN_POINT ( 'NONE',  ( 0.05219959533936267826, -19.03943276465977164, 70.00109039468566152 ) ) ;
#143112=CARTESIAN_POINT ( 'NONE',  ( 9.474510206698729675, 16.51473224551082808, 22.08442372801899722 ) ) ;
#143113=CARTESIAN_POINT ( 'NONE',  ( -9.474510206698964154, 16.51473224551069663, 35.41557627198102409 ) ) ;
#143114=CARTESIAN_POINT ( 'NONE',  ( 16.51473224551069308, 9.474510206698969483, 79.16557627198103830 ) ) ;
#143115=CARTESIAN_POINT ( 'NONE',  ( 8.224510206698953496, -14.34966873604960469, 77.91557627198102409 ) ) ;
#143116=CARTESIAN_POINT ( 'NONE',  ( 5.153800228976615827, -19.02544592524334988, 40.20942372801898301 ) ) ;
#143117=CARTESIAN_POINT ( 'NONE',  ( 5.719274019375991003, -21.55341960407610458, 32.70724293864770260 ) ) ;
#143118=CARTESIAN_POINT ( 'NONE',  ( -19.03943276465977164, -0.05219959533935918106, 18.75109039468567218 ) ) ;
#143119=CARTESIAN_POINT ( 'NONE',  ( -19.02544592524342804, 5.153800228976336051, 91.04057627198100988 ) ) ;
#143120=CARTESIAN_POINT ( 'NONE',  ( -21.52544592524334988, -5.823673210054445271, 103.9594237280190185 ) ) ;
#143121=CARTESIAN_POINT ( 'NONE',  ( -10.72451020669898014, 18.67979575497178502, 60.41557627198102409 ) ) ;
#143122=CARTESIAN_POINT ( 'NONE',  ( 13.89961937509977652, -13.97604488694527269, 103.1239096053143527 ) ) ;
#143123=CARTESIAN_POINT ( 'NONE',  ( -19.05341960407617563, 5.049401038297882671, 83.54275706135233293 ) ) ;
#143124=CARTESIAN_POINT ( 'NONE',  ( -0.05219959533909027116, -19.03943276465977164, 102.4989096053143669 ) ) ;
#143125=CARTESIAN_POINT ( 'NONE',  ( 13.97604488694548053, -13.89961937509957401, 100.6260903946856615 ) ) ;
#143126=CARTESIAN_POINT ( 'NONE',  ( 19.05341960407611168, 5.049401038298154454, 23.95724293864769194 ) ) ;
#143127=CARTESIAN_POINT ( 'NONE',  ( 5.153800228976335163, 19.02544592524342804, 84.79057627198099567 ) ) ;
#143128=CARTESIAN_POINT ( 'NONE',  ( -5.823673210054116645, -21.52544592524344225, 67.29057627198103830 ) ) ;
#143129=CARTESIAN_POINT ( 'NONE',  ( 12.14591786802327356, -12.06949235617739191, 40.62609039468567573 ) ) ;
#143130=CARTESIAN_POINT ( 'NONE',  ( -21.52544592524334988, -5.823673210054445271, 53.95942372801900433 ) ) ;
#143131=CARTESIAN_POINT ( 'NONE',  ( 21.53943276465977519, 0.05219959533937863772, 91.25109039468568994 ) ) ;
#143132=CARTESIAN_POINT ( 'NONE',  ( 8.314922557961029526, -14.29746914071037800, 100.4177570613523471 ) ) ;
#143134=CARTESIAN_POINT ( 'NONE',  ( 9.564922557960805705, 16.46253265017160317, 94.58224293864769550 ) ) ;
#143135=CARTESIAN_POINT ( 'NONE',  ( -0.05219959533910754901, -16.53943276465976808, 92.49890960531436690 ) ) ;
#143136=CARTESIAN_POINT ( 'NONE',  ( 16.53943276465976808, 0.05219959533934440121, 111.2510903946856899 ) ) ;
#143137=CARTESIAN_POINT ( 'NONE',  ( -16.51473224551082808, 9.474510206698731452, 63.33442372801900433 ) ) ;
#143138=CARTESIAN_POINT ( 'NONE',  ( 15.72974639402176855, 15.80617190586768217, 46.87609039468568994 ) ) ;
#143139=CARTESIAN_POINT ( 'NONE',  ( -8.224510206698948167, 14.34966873604960824, 95.41557627198102409 ) ) ;
#143140=CARTESIAN_POINT ( 'NONE',  ( -19.05341960407611168, -5.049401038298163336, 111.4572429386476671 ) ) ;
#143141=CARTESIAN_POINT ( 'NONE',  ( -12.14591786802309592, -12.06949235617757132, 26.87390960531435979 ) ) ;
#143142=CARTESIAN_POINT ( 'NONE',  ( 15.72974639402176855, 15.80617190586768217, 86.87609039468568994 ) ) ;
#143143=CARTESIAN_POINT ( 'NONE',  ( 8.314922557961029526, -14.29746914071037800, 60.41775706135235424 ) ) ;
#143144=CARTESIAN_POINT ( 'NONE',  ( -10.72451020669870658, -18.67979575497194134, 44.58442372801901854 ) ) ;
#143146=CARTESIAN_POINT ( 'NONE',  ( -5.823673210054431948, 21.52544592524334988, 27.70942372801901854 ) ) ;
#143147=CARTESIAN_POINT ( 'NONE',  ( 0.05219959533910956823, 16.53943276465976808, 94.99890960531436690 ) ) ;
#143148=CARTESIAN_POINT ( 'NONE',  ( -16.51473224551069308, -9.474510206698971260, 31.66557627198102054 ) ) ;
#143149=CARTESIAN_POINT ( 'NONE',  ( 12.06949235617757843, -12.14591786802309237, 68.12390960531436690 ) ) ;
#143150=CARTESIAN_POINT ( 'NONE',  ( -19.02544592524342804, 5.153800228976336051, 56.04057627198100988 ) ) ;
#143151=CARTESIAN_POINT ( 'NONE',  ( 14.29746914071037800, 8.314922557961029526, 106.6677570613523756 ) ) ;
#143152=CARTESIAN_POINT ( 'NONE',  ( -9.474510206698964154, 16.51473224551069663, 40.41557627198103120 ) ) ;
#143153=CARTESIAN_POINT ( 'NONE',  ( -21.52544592524343514, 5.823673210054127303, 46.04057627198103830 ) ) ;
#143154=CARTESIAN_POINT ( 'NONE',  ( -12.14591786802309592, -12.06949235617757132, 76.87390960531439532 ) ) ;
#143155=CARTESIAN_POINT ( 'NONE',  ( 21.55341960407610458, 5.719274019375980345, 88.95724293864769550 ) ) ;
#143156=CARTESIAN_POINT ( 'NONE',  ( 19.02544592524343514, -5.153800228976328945, 83.54057627198100988 ) ) ;
#143157=EDGE_CURVE ( 'NONE', #73939, #106381, #199864, .T. ) ;
#143158=CARTESIAN_POINT ( 'NONE',  ( 19.05341960407611168, 5.049401038298154454, 48.95724293864768129 ) ) ;
#143159=CARTESIAN_POINT ( 'NONE',  ( -13.97604488694547697, 13.89961937509957934, 98.12609039468566152 ) ) ;
#143160=CARTESIAN_POINT ( 'NONE',  ( -5.823673210054116645, -21.52544592524344225, 47.29057627198103120 ) ) ;
#143161=CARTESIAN_POINT ( 'NONE',  ( -18.67979575497193778, 10.72451020669871902, 63.33442372801900433 ) ) ;
#143162=CARTESIAN_POINT ( 'NONE',  ( -13.97604488694527625, -13.89961937509977652, 51.87390960531436690 ) ) ;
#143163=CARTESIAN_POINT ( 'NONE',  ( 16.51473224551069308, 9.474510206698969483, 84.16557627198102409 ) ) ;
#143165=CARTESIAN_POINT ( 'NONE',  ( -12.06949235617739369, -12.14591786802326823, 64.37609039468568994 ) ) ;
#143166=CARTESIAN_POINT ( 'NONE',  ( -10.72451020669870658, -18.67979575497194134, 44.58442372801901854 ) ) ;
#143167=CARTESIAN_POINT ( 'NONE',  ( -18.67979575497193778, 10.72451020669871902, 68.33442372801900433 ) ) ;
#143168=CARTESIAN_POINT ( 'NONE',  ( 5.823673210054125526, 21.52544592524343514, 24.79057627198103120 ) ) ;
#143169=CARTESIAN_POINT ( 'NONE',  ( 21.53943276465977519, -0.05219959533907433946, 103.7489096053143669 ) ) ;
#143170=CARTESIAN_POINT ( 'NONE',  ( -10.81492255796105439, 18.62759615963255655, 32.91775706135234714 ) ) ;
#143171=CARTESIAN_POINT ( 'NONE',  ( -4.483927247898782831, 16.52544592524335698, 62.70942372801902565 ) ) ;
#143172=CARTESIAN_POINT ( 'NONE',  ( -21.55341960407610458, -5.719274019375992779, 61.45724293864770260 ) ) ;
#143173=CARTESIAN_POINT ( 'NONE',  ( -16.51473224551082808, 9.474510206698731452, 38.33442372801899722 ) ) ;
#143174=CARTESIAN_POINT ( 'NONE',  ( -19.03943276465977164, 0.05219959533909376836, 71.24890960531435269 ) ) ;
#143175=CARTESIAN_POINT ( 'NONE',  ( 8.224510206698742110, 14.34966873604972548, 102.0844237280190185 ) ) ;
#143176=CARTESIAN_POINT ( 'NONE',  ( -17.49999999999999645, -3.850315288878843223, 105.7337086939655535 ) ) ;
#143177=CARTESIAN_POINT ( 'NONE',  ( 9.564922557960805705, 16.46253265017160317, 109.5822429386476955 ) ) ;
#143179=CARTESIAN_POINT ( 'NONE',  ( 19.05341960407617918, -5.049401038297876454, 76.04275706135230450 ) ) ;
#143180=CARTESIAN_POINT ( 'NONE',  ( 5.823673210054125526, 21.52544592524343514, 59.79057627198103120 ) ) ;
#143181=CARTESIAN_POINT ( 'NONE',  ( 4.483927247898545687, 16.52544592524342804, 44.79057627198103120 ) ) ;
#143182=CARTESIAN_POINT ( 'NONE',  ( -19.05341960407617563, 5.049401038297882671, 93.54275706135234714 ) ) ;
#143183=CARTESIAN_POINT ( 'NONE',  ( -16.51473224551069308, -9.474510206698971260, 21.66557627198102765 ) ) ;
#143184=CARTESIAN_POINT ( 'NONE',  ( 9.474510206698729675, 16.51473224551082808, 97.08442372801900433 ) ) ;
#143185=CARTESIAN_POINT ( 'NONE',  ( -5.823673210054116645, -21.52544592524344225, 82.29057627198103830 ) ) ;
#143186=CARTESIAN_POINT ( 'NONE',  ( -0.05219959533936034679, 19.03943276465977164, 57.50109039468566863 ) ) ;
#143187=CARTESIAN_POINT ( 'NONE',  ( 16.55341960407618274, -4.379528057220086978, 81.04275706135236135 ) ) ;
#143188=CARTESIAN_POINT ( 'NONE',  ( -0.05219959533909027116, -19.03943276465977164, 72.49890960531435269 ) ) ;
#143189=CARTESIAN_POINT ( 'NONE',  ( 12.06949235617757843, -12.14591786802309237, 63.12390960531435979 ) ) ;
#143191=CARTESIAN_POINT ( 'NONE',  ( -9.564922557960796823, -16.46253265017161027, 52.08224293864768839 ) ) ;
#143192=CARTESIAN_POINT ( 'NONE',  ( 16.52544592524342804, -4.483927247898539470, 48.54057627198103120 ) ) ;
#143193=CARTESIAN_POINT ( 'NONE',  ( -9.564922557960796823, -16.46253265017161027, 22.08224293864768839 ) ) ;
#143195=CARTESIAN_POINT ( 'NONE',  ( -4.379528057220328563, 16.55341960407611168, 35.20724293864768839 ) ) ;
#143196=CARTESIAN_POINT ( 'NONE',  ( 5.049401038298161559, -19.05341960407611168, 82.70724293864770971 ) ) ;
#143197=CARTESIAN_POINT ( 'NONE',  ( -0.05219959533936034679, 19.03943276465977164, 37.50109039468567573 ) ) ;
#143198=CARTESIAN_POINT ( 'NONE',  ( 8.314922557961029526, -14.29746914071037800, 50.41775706135235424 ) ) ;
#143199=CARTESIAN_POINT ( 'NONE',  ( -0.05219959533907301413, -21.53943276465977519, 57.49890960531435979 ) ) ;
#143200=CARTESIAN_POINT ( 'NONE',  ( 5.823673210054444382, -21.52544592524334988, 100.2094237280190043 ) ) ;
#143201=CARTESIAN_POINT ( 'NONE',  ( 19.05341960407611168, 5.049401038298154454, 73.95724293864768129 ) ) ;
#143202=CARTESIAN_POINT ( 'NONE',  ( 19.02544592524343514, -5.153800228976328945, 113.5405762719810241 ) ) ;
#143203=CARTESIAN_POINT ( 'NONE',  ( -19.05341960407611168, -5.049401038298163336, 111.4572429386476671 ) ) ;
#143204=CARTESIAN_POINT ( 'NONE',  ( 10.72451020669871369, 18.67979575497193778, 42.08442372801901854 ) ) ;
#143205=CARTESIAN_POINT ( 'NONE',  ( 16.52544592524342804, -4.483927247898539470, 88.54057627198103830 ) ) ;
#143206=CARTESIAN_POINT ( 'NONE',  ( -0.05219959533907301413, -21.53943276465977519, 87.49890960531436690 ) ) ;
#143207=CARTESIAN_POINT ( 'NONE',  ( 9.564922557960805705, 16.46253265017160317, 84.58224293864769550 ) ) ;
#143209=CARTESIAN_POINT ( 'NONE',  ( -15.72974639402176322, -15.80617190586768395, 24.37609039468567573 ) ) ;
#143211=CARTESIAN_POINT ( 'NONE',  ( 19.02544592524343514, -5.153800228976328945, 88.54057627198102409 ) ) ;
#143213=CARTESIAN_POINT ( 'NONE',  ( 18.39443945427639093, -5.500000000000021316, 81.01745347608652992 ) ) ;
#143214=CARTESIAN_POINT ( 'NONE',  ( -19.02544592524342804, 5.153800228976336051, 26.04057627198103120 ) ) ;
#143215=CARTESIAN_POINT ( 'NONE',  ( 0.05219959533909260263, 19.03943276465977164, 29.99890960531435979 ) ) ;
#143216=CARTESIAN_POINT ( 'NONE',  ( -16.51473224551082808, 9.474510206698731452, 108.3344237280190043 ) ) ;
#143218=CARTESIAN_POINT ( 'NONE',  ( -16.55341960407611168, -4.379528057220339221, 106.4572429386477097 ) ) ;
#143219=CARTESIAN_POINT ( 'NONE',  ( -0.05219959533937732626, 21.53943276465977519, 82.50109039468568994 ) ) ;
#143220=CARTESIAN_POINT ( 'NONE',  ( -5.049401038298153566, 19.05341960407611168, 65.20724293864765286 ) ) ;
#143221=CARTESIAN_POINT ( 'NONE',  ( -0.05219959533937732626, 21.53943276465977519, 37.50109039468568284 ) ) ;
#143222=CARTESIAN_POINT ( 'NONE',  ( -21.55341960407619339, 5.719274019375674811, 28.54275706135234358 ) ) ;
#143224=CARTESIAN_POINT ( 'NONE',  ( 19.02544592524343514, -5.153800228976328945, 88.54057627198102409 ) ) ;
#143226=CARTESIAN_POINT ( 'NONE',  ( 8.314922557961029526, -14.29746914071037800, 25.41775706135235779 ) ) ;
#143227=CARTESIAN_POINT ( 'NONE',  ( -10.72451020669898014, 18.67979575497178502, 45.41557627198103830 ) ) ;
#143228=CARTESIAN_POINT ( 'NONE',  ( -10.81492255796105439, 18.62759615963255655, 62.91775706135236135 ) ) ;
#143229=CARTESIAN_POINT ( 'NONE',  ( 13.89961937509977652, -13.97604488694527269, 113.1239096053143527 ) ) ;
#143230=CARTESIAN_POINT ( 'NONE',  ( -5.153800228976607833, 19.02544592524334988, 92.70942372801901854 ) ) ;
#143231=CARTESIAN_POINT ( 'NONE',  ( -16.46253265017160317, 9.564922557960807481, 55.83224293864769550 ) ) ;
#143232=CARTESIAN_POINT ( 'NONE',  ( 16.46253265017160672, -9.564922557960803928, 83.33224293864768129 ) ) ;
#143233=CARTESIAN_POINT ( 'NONE',  ( -16.52544592524342804, 4.483927247898546575, 96.04057627198102409 ) ) ;
#143234=CARTESIAN_POINT ( 'NONE',  ( -16.52544592524342804, 4.483927247898546575, 101.0405762719810383 ) ) ;
#143235=CARTESIAN_POINT ( 'NONE',  ( -9.564922557960796823, -16.46253265017161027, 112.0822429386476955 ) ) ;
#143236=CARTESIAN_POINT ( 'NONE',  ( -8.314922557960811034, -14.29746914071050412, 62.08224293864769550 ) ) ;
#143237=CARTESIAN_POINT ( 'NONE',  ( -19.05341960407611168, -5.049401038298163336, 36.45724293864766707 ) ) ;
#143238=CARTESIAN_POINT ( 'NONE',  ( 21.55341960407619695, -5.719274019375665929, 76.04275706135237556 ) ) ;
#143239=CARTESIAN_POINT ( 'NONE',  ( -5.153800228976607833, 19.02544592524334988, 92.70942372801901854 ) ) ;
#143240=CARTESIAN_POINT ( 'NONE',  ( -16.52544592524342804, 4.483927247898546575, 66.04057627198103830 ) ) ;
#143241=CARTESIAN_POINT ( 'NONE',  ( -21.52544592524343514, 5.823673210054127303, 116.0405762719810383 ) ) ;
#143242=CARTESIAN_POINT ( 'NONE',  ( -18.67979575497178146, -10.72451020669898902, 41.66557627198103120 ) ) ;
#143243=CARTESIAN_POINT ( 'NONE',  ( -19.03943276465977164, 0.05219959533909376836, 116.2489096053143669 ) ) ;
#143245=CARTESIAN_POINT ( 'NONE',  ( -5.153800228976328057, -19.02544592524343514, 72.29057627198102409 ) ) ;
#143246=CARTESIAN_POINT ( 'NONE',  ( -12.14591786802309592, -12.06949235617757132, 41.87390960531435979 ) ) ;
#143247=CARTESIAN_POINT ( 'NONE',  ( -14.34966873604972548, 8.224510206698743886, 108.3344237280190185 ) ) ;
#143248=CARTESIAN_POINT ( 'NONE',  ( -16.52544592524335698, -4.483927247898792601, 78.95942372801901854 ) ) ;
#143249=CARTESIAN_POINT ( 'NONE',  ( 16.51473224551083163, -9.474510206698727899, 45.83442372801900433 ) ) ;
#143251=CARTESIAN_POINT ( 'NONE',  ( 13.97604488694527802, 13.89961937509977652, 89.37390960531436690 ) ) ;
#143252=CARTESIAN_POINT ( 'NONE',  ( 9.474510206698971260, -16.51473224551069308, 47.91557627198102409 ) ) ;
#143253=CARTESIAN_POINT ( 'NONE',  ( -14.29746914071049879, 8.314922557960819915, 65.83224293864769550 ) ) ;
#143254=CARTESIAN_POINT ( 'NONE',  ( 17.50000000000000000, -5.624438216177590988, 103.3167034491464733 ) ) ;
#143255=CARTESIAN_POINT ( 'NONE',  ( 18.62759615963271287, -10.81492255796078972, 23.33224293864769194 ) ) ;
#143256=CARTESIAN_POINT ( 'NONE',  ( -21.52544592524343514, 5.823673210054127303, 51.04057627198103120 ) ) ;
#143257=CARTESIAN_POINT ( 'NONE',  ( -12.14591786802309592, -12.06949235617757132, 81.87390960531435269 ) ) ;
#143258=CARTESIAN_POINT ( 'NONE',  ( 14.29746914071037800, 8.314922557961029526, 36.66775706135234714 ) ) ;
#143259=CARTESIAN_POINT ( 'NONE',  ( 12.06949235617757843, -12.14591786802309237, 73.12390960531436690 ) ) ;
#143261=CARTESIAN_POINT ( 'NONE',  ( -19.05341960407617563, 5.049401038297882671, 78.54275706135233293 ) ) ;
#143262=CARTESIAN_POINT ( 'NONE',  ( 18.67979575497178502, 10.72451020669898547, 24.16557627198103120 ) ) ;
#143265=CARTESIAN_POINT ( 'NONE',  ( -12.06949235617739369, -12.14591786802326823, 34.37609039468568284 ) ) ;
#143266=CARTESIAN_POINT ( 'NONE',  ( -16.55341960407617563, 4.379528057220093196, 108.5427570613523756 ) ) ;
#143268=CARTESIAN_POINT ( 'NONE',  ( -9.474510206698720793, -16.51473224551083518, 69.58442372801901854 ) ) ;
#143269=CARTESIAN_POINT ( 'NONE',  ( 21.55341960407610458, 5.719274019375980345, 53.95724293864770260 ) ) ;
#143270=CARTESIAN_POINT ( 'NONE',  ( 15.72974639402176855, 15.80617190586768217, 71.87609039468568994 ) ) ;
#143272=CARTESIAN_POINT ( 'NONE',  ( 4.379528057220092307, 16.55341960407617563, 37.29275706135235424 ) ) ;
#143274=CARTESIAN_POINT ( 'NONE',  ( -9.564922557960796823, -16.46253265017161027, 82.08224293864768129 ) ) ;
#143276=CARTESIAN_POINT ( 'NONE',  ( -14.29746914071049879, 8.314922557960819915, 105.8322429386476955 ) ) ;
#143277=CARTESIAN_POINT ( 'NONE',  ( 19.05341960407611168, 5.049401038298154454, 98.95724293864766707 ) ) ;
#143278=CARTESIAN_POINT ( 'NONE',  ( -4.483927247898782831, 16.52544592524335698, 52.70942372801902565 ) ) ;
#143279=CARTESIAN_POINT ( 'NONE',  ( -16.51473224551082808, 9.474510206698731452, 103.3344237280190043 ) ) ;
#143280=CARTESIAN_POINT ( 'NONE',  ( -15.72974639402197994, 15.80617190586746368, 80.62390960531438111 ) ) ;
#143281=CARTESIAN_POINT ( 'NONE',  ( -16.51473224551069308, -9.474510206698971260, 36.66557627198102409 ) ) ;
#143282=CARTESIAN_POINT ( 'NONE',  ( 13.97604488694548053, -13.89961937509957401, 65.62609039468567573 ) ) ;
#143283=CARTESIAN_POINT ( 'NONE',  ( -5.719274019375665041, -21.55341960407619695, 19.79275706135235069 ) ) ;
#143284=CARTESIAN_POINT ( 'NONE',  ( 0.05219959533909260263, 19.03943276465977164, 74.99890960531435269 ) ) ;
#143285=CARTESIAN_POINT ( 'NONE',  ( -16.51473224551069308, -9.474510206698971260, 111.6655762719810383 ) ) ;
#143287=CARTESIAN_POINT ( 'NONE',  ( 4.379528057220092307, 16.55341960407617563, 37.29275706135235424 ) ) ;
#143288=CARTESIAN_POINT ( 'NONE',  ( 10.81492255796078972, 18.62759615963270932, 99.58224293864770971 ) ) ;
#143289=CARTESIAN_POINT ( 'NONE',  ( -16.53943276465976808, 0.05219959533911058130, 111.2489096053143669 ) ) ;
#143290=CARTESIAN_POINT ( 'NONE',  ( 19.02544592524343514, -5.153800228976328945, 93.54057627198102409 ) ) ;
#143291=CARTESIAN_POINT ( 'NONE',  ( -5.049401038297874678, -19.05341960407617918, 74.79275706135231871 ) ) ;
#143292=CARTESIAN_POINT ( 'NONE',  ( -0.05219959533907301413, -21.53943276465977519, 87.49890960531436690 ) ) ;
#143293=CARTESIAN_POINT ( 'NONE',  ( 16.52544592524342804, -4.483927247898539470, 43.54057627198103830 ) ) ;
#143294=CARTESIAN_POINT ( 'NONE',  ( -5.153800228976607833, 19.02544592524334988, 27.70942372801899722 ) ) ;
#143295=CARTESIAN_POINT ( 'NONE',  ( 14.29746914071037800, 8.314922557961029526, 71.66775706135234714 ) ) ;
#143296=CARTESIAN_POINT ( 'NONE',  ( -13.97604488694527625, -13.89961937509977652, 96.87390960531433848 ) ) ;
#143297=CARTESIAN_POINT ( 'NONE',  ( -16.46253265017160317, 9.564922557960807481, 50.83224293864770260 ) ) ;
#143298=CARTESIAN_POINT ( 'NONE',  ( -10.81492255796105439, 18.62759615963255655, 52.91775706135235424 ) ) ;
#143299=CARTESIAN_POINT ( 'NONE',  ( -15.80617190586768217, 15.72974639402176855, 73.12609039468567573 ) ) ;
#143300=CARTESIAN_POINT ( 'NONE',  ( -9.474510206698964154, 16.51473224551069663, 60.41557627198102409 ) ) ;
#143301=CARTESIAN_POINT ( 'NONE',  ( 18.62759615963255655, 10.81492255796105972, 31.66775706135234358 ) ) ;
#143302=CARTESIAN_POINT ( 'NONE',  ( 9.474510206698729675, 16.51473224551082808, 72.08442372801900433 ) ) ;
#143303=CARTESIAN_POINT ( 'NONE',  ( 5.153800228976335163, 19.02544592524342804, 34.79057627198102409 ) ) ;
#143304=CARTESIAN_POINT ( 'NONE',  ( -12.06949235617739369, -12.14591786802326823, 89.37609039468568994 ) ) ;
#143305=CARTESIAN_POINT ( 'NONE',  ( 13.89961937509977652, -13.97604488694527269, 53.12390960531434558 ) ) ;
#143306=CARTESIAN_POINT ( 'NONE',  ( -16.51473224551069308, -9.474510206698971260, 106.6655762719810383 ) ) ;
#143307=CARTESIAN_POINT ( 'NONE',  ( -19.05341960407611168, -5.049401038298163336, 41.45724293864769550 ) ) ;
#143308=CARTESIAN_POINT ( 'NONE',  ( 15.80617190586746368, 15.72974639402197994, 84.37390960531438111 ) ) ;
#143309=CARTESIAN_POINT ( 'NONE',  ( 12.06949235617739724, 12.14591786802326823, 76.87609039468567573 ) ) ;
#143311=CARTESIAN_POINT ( 'NONE',  ( -16.51473224551082808, 9.474510206698731452, 33.33442372801899722 ) ) ;
#143312=CARTESIAN_POINT ( 'NONE',  ( 16.46253265017160672, -9.564922557960803928, 58.33224293864769550 ) ) ;
#143313=CARTESIAN_POINT ( 'NONE',  ( 16.55341960407611168, 4.379528057220329451, 43.95724293864769550 ) ) ;
#143314=CARTESIAN_POINT ( 'NONE',  ( 0.05219959533910956823, 16.53943276465976808, 79.99890960531435269 ) ) ;
#143315=CARTESIAN_POINT ( 'NONE',  ( 9.474510206698971260, -16.51473224551069308, 102.9155762719810241 ) ) ;
#143316=CARTESIAN_POINT ( 'NONE',  ( -5.049401038298153566, 19.05341960407611168, 80.20724293864769550 ) ) ;
#143317=CARTESIAN_POINT ( 'NONE',  ( 21.52544592524334988, 5.823673210054432836, 56.45942372801902565 ) ) ;
#143318=CARTESIAN_POINT ( 'NONE',  ( -16.46253265017160317, 9.564922557960807481, 95.83224293864769550 ) ) ;
#143319=CARTESIAN_POINT ( 'NONE',  ( -21.53943276465977519, -0.05219959533937600094, 103.7510903946857042 ) ) ;
#143320=CARTESIAN_POINT ( 'NONE',  ( -16.55341960407617563, 4.379528057220093196, 78.54275706135236135 ) ) ;
#143322=CARTESIAN_POINT ( 'NONE',  ( 0.05219959533937995610, -21.53943276465977519, 25.00109039468567218 ) ) ;
#143323=CARTESIAN_POINT ( 'NONE',  ( 0.05219959533907565091, 21.53943276465977519, 99.99890960531436690 ) ) ;
#143325=CARTESIAN_POINT ( 'NONE',  ( 12.06949235617757843, -12.14591786802309237, 63.12390960531435979 ) ) ;
#143326=CARTESIAN_POINT ( 'NONE',  ( 5.153800228976335163, 19.02544592524342804, 44.79057627198103830 ) ) ;
#143327=CARTESIAN_POINT ( 'NONE',  ( -14.29746914071049879, 8.314922557960819915, 65.83224293864769550 ) ) ;
#143328=CARTESIAN_POINT ( 'NONE',  ( 15.80617190586746368, 15.72974639402197994, 24.37390960531435979 ) ) ;
#143329=CARTESIAN_POINT ( 'NONE',  ( -5.049401038297874678, -19.05341960407617918, 24.79275706135233648 ) ) ;
#143330=CARTESIAN_POINT ( 'NONE',  ( -0.05219959533910754901, -16.53943276465976808, 107.4989096053143669 ) ) ;
#143332=CARTESIAN_POINT ( 'NONE',  ( 8.224510206698742110, 14.34966873604972548, 72.08442372801899012 ) ) ;
#143333=CARTESIAN_POINT ( 'NONE',  ( -0.05219959533909027116, -19.03943276465977164, 67.49890960531436690 ) ) ;
#143334=CARTESIAN_POINT ( 'NONE',  ( -16.63122886436918435, -6.465204090714604668, 20.66090433330151654 ) ) ;
#143335=CARTESIAN_POINT ( 'NONE',  ( -8.314922557960811034, -14.29746914071050412, 87.08224293864769550 ) ) ;
#143336=CARTESIAN_POINT ( 'NONE',  ( -15.80617190586745835, -15.72974639402198527, 31.87390960531435979 ) ) ;
#143337=CARTESIAN_POINT ( 'NONE',  ( -8.224510206698735004, -14.34966873604973081, 94.58442372801901854 ) ) ;
#143338=CARTESIAN_POINT ( 'NONE',  ( 0.05219959533936267826, -19.03943276465977164, 105.0010903946856615 ) ) ;
#143339=CARTESIAN_POINT ( 'NONE',  ( -21.55341960407619339, 5.719274019375674811, 73.54275706135234714 ) ) ;
#143340=CARTESIAN_POINT ( 'NONE',  ( 19.05341960407611168, 5.049401038298154454, 93.95724293864769550 ) ) ;
#143341=CARTESIAN_POINT ( 'NONE',  ( -21.52544592524343514, 5.823673210054127303, 101.0405762719810383 ) ) ;
#143342=CARTESIAN_POINT ( 'NONE',  ( 8.314922557961029526, -14.29746914071037800, 60.41775706135235424 ) ) ;
#143343=CARTESIAN_POINT ( 'NONE',  ( 14.34966873604960469, 8.224510206698951720, 109.1655762719810383 ) ) ;
#143344=CARTESIAN_POINT ( 'NONE',  ( 4.483927247898790824, -16.52544592524335698, 20.20942372801900788 ) ) ;
#143345=CARTESIAN_POINT ( 'NONE',  ( 16.46253265017146816, 9.564922557961045513, 91.66775706135234714 ) ) ;
#143346=CARTESIAN_POINT ( 'NONE',  ( -18.62759615963270932, 10.81492255796079327, 95.83224293864770971 ) ) ;
#143347=CARTESIAN_POINT ( 'NONE',  ( -19.02544592524334988, -5.153800228976617603, 53.95942372801898301 ) ) ;
#143348=CARTESIAN_POINT ( 'NONE',  ( 18.87075004821566537, -5.500000000000075495, 86.17408112101047379 ) ) ;
#143349=CARTESIAN_POINT ( 'NONE',  ( -21.55341960407610458, -5.719274019375992779, 101.4572429386476955 ) ) ;
#143351=CARTESIAN_POINT ( 'NONE',  ( 9.564922557960805705, 16.46253265017160317, 84.58224293864769550 ) ) ;
#143353=CARTESIAN_POINT ( 'NONE',  ( -12.06949235617739369, -12.14591786802326823, 29.37609039468568284 ) ) ;
#143355=CARTESIAN_POINT ( 'NONE',  ( -15.72974639402197994, 15.80617190586746368, 100.6239096053143811 ) ) ;
#143356=CARTESIAN_POINT ( 'NONE',  ( 8.314922557960818139, 14.29746914071049879, 59.58224293864770260 ) ) ;
#143357=CARTESIAN_POINT ( 'NONE',  ( -19.03943276465977164, 0.05219959533909376836, 76.24890960531435269 ) ) ;
#143358=CARTESIAN_POINT ( 'NONE',  ( -16.55341960407617563, 4.379528057220093196, 43.54275706135235424 ) ) ;
#143359=CARTESIAN_POINT ( 'NONE',  ( -13.97604488694547697, 13.89961937509957934, 43.12609039468566152 ) ) ;
#143360=CARTESIAN_POINT ( 'NONE',  ( -18.67979575497193778, 10.72451020669871902, 48.33442372801902565 ) ) ;
#143361=CARTESIAN_POINT ( 'NONE',  ( -14.29746914071037622, -8.314922557961029526, 19.16775706135234714 ) ) ;
#143362=CARTESIAN_POINT ( 'NONE',  ( -19.02544592524342804, 5.153800228976336051, 61.04057627198103120 ) ) ;
#143363=CARTESIAN_POINT ( 'NONE',  ( -5.153800228976607833, 19.02544592524334988, 82.70942372801897591 ) ) ;
#143364=CARTESIAN_POINT ( 'NONE',  ( 10.81492255796106328, -18.62759615963255655, 80.41775706135234714 ) ) ;
#143365=CARTESIAN_POINT ( 'NONE',  ( 0.05219959533936267826, -19.03943276465977164, 60.00109039468566863 ) ) ;
#143366=CARTESIAN_POINT ( 'NONE',  ( -19.03943276465977164, 0.05219959533909376836, 36.24890960531436690 ) ) ;
#143367=CARTESIAN_POINT ( 'NONE',  ( -5.719274019375978568, 21.55341960407610458, 60.20724293864768839 ) ) ;
#143368=CARTESIAN_POINT ( 'NONE',  ( 16.55341960407611168, 4.379528057220329451, 58.95724293864770971 ) ) ;
#143369=CARTESIAN_POINT ( 'NONE',  ( -17.31728774477276289, -6.344390552232334279, 24.18093348310682700 ) ) ;
#143370=CARTESIAN_POINT ( 'NONE',  ( 19.02544592524334988, 5.153800228976608722, 31.45942372801900433 ) ) ;
#143371=CARTESIAN_POINT ( 'NONE',  ( 12.06949235617739724, 12.14591786802326823, 101.8760903946857042 ) ) ;
#143372=CARTESIAN_POINT ( 'NONE',  ( -4.483927247898539470, -16.52544592524342804, 57.29057627198103120 ) ) ;
#143373=CARTESIAN_POINT ( 'NONE',  ( -10.72451020669870658, -18.67979575497194134, 89.58442372801901854 ) ) ;
#143374=CARTESIAN_POINT ( 'NONE',  ( -0.05219959533937732626, 21.53943276465977519, 77.50109039468567573 ) ) ;
#143375=CARTESIAN_POINT ( 'NONE',  ( -18.62759615963270932, 10.81492255796079327, 100.8322429386477097 ) ) ;
#143377=CARTESIAN_POINT ( 'NONE',  ( 0.05219959533909260263, 19.03943276465977164, 54.99890960531435979 ) ) ;
#143378=CARTESIAN_POINT ( 'NONE',  ( 5.719274019375673035, 21.55341960407619339, 72.29275706135236135 ) ) ;
#143379=CARTESIAN_POINT ( 'NONE',  ( 5.049401038298161559, -19.05341960407611168, 52.70724293864767418 ) ) ;
#143380=ORIENTED_EDGE ( 'NONE', *, *, #122956, .F. ) ;
#143381=CARTESIAN_POINT ( 'NONE',  ( -13.97604488694527625, -13.89961937509977652, 66.87390960531436690 ) ) ;
#143382=CARTESIAN_POINT ( 'NONE',  ( -14.34966873604960291, -8.224510206698953496, 106.6655762719810383 ) ) ;
#143383=CARTESIAN_POINT ( 'NONE',  ( 13.89961937509977652, -13.97604488694527269, 93.12390960531436690 ) ) ;
#143384=CARTESIAN_POINT ( 'NONE',  ( -0.05219959533910754901, -16.53943276465976808, 52.49890960531435979 ) ) ;
#143385=CARTESIAN_POINT ( 'NONE',  ( -14.34966873604960291, -8.224510206698953496, 111.6655762719810525 ) ) ;
#143386=CARTESIAN_POINT ( 'NONE',  ( 12.06949235617757843, -12.14591786802309237, 68.12390960531436690 ) ) ;
#143387=CARTESIAN_POINT ( 'NONE',  ( 21.52544592524344225, -5.823673210054117533, 83.54057627198102409 ) ) ;
#143388=CARTESIAN_POINT ( 'NONE',  ( -21.55341960407619339, 5.719274019375674811, 38.54275706135234714 ) ) ;
#143390=EDGE_CURVE ( 'NONE', #61770, #82999, #117856, .T. ) ;
#143391=CARTESIAN_POINT ( 'NONE',  ( -8.314922557961024197, 14.29746914071037800, 37.91775706135235424 ) ) ;
#143392=CARTESIAN_POINT ( 'NONE',  ( 18.67979575497178502, 10.72451020669898547, 84.16557627198103830 ) ) ;
#143395=CARTESIAN_POINT ( 'NONE',  ( -15.80617190586768217, 15.72974639402176855, 113.1260903946856899 ) ) ;
#143396=CARTESIAN_POINT ( 'NONE',  ( -5.049401038298153566, 19.05341960407611168, 95.20724293864770971 ) ) ;
#143397=CARTESIAN_POINT ( 'NONE',  ( -15.72974639402176322, -15.80617190586768395, 44.37609039468567573 ) ) ;
#143398=CARTESIAN_POINT ( 'NONE',  ( 5.823673210054125526, 21.52544592524343514, 34.79057627198103120 ) ) ;
#143399=CARTESIAN_POINT ( 'NONE',  ( 12.14591786802327356, -12.06949235617739191, 100.6260903946857184 ) ) ;
#143400=CARTESIAN_POINT ( 'NONE',  ( -18.62759615963255300, -10.81492255796106328, 44.16775706135234714 ) ) ;
#143401=CARTESIAN_POINT ( 'NONE',  ( 21.52544592524334988, 5.823673210054432836, 81.45942372801900433 ) ) ;
#143402=CARTESIAN_POINT ( 'NONE',  ( 21.55341960407619695, -5.719274019375665929, 111.0427570613523613 ) ) ;
#143403=CARTESIAN_POINT ( 'NONE',  ( -4.379528057220086978, -16.55341960407618274, 79.79275706135236135 ) ) ;
#143404=CARTESIAN_POINT ( 'NONE',  ( 15.80617190586769283, -15.72974639402175789, 45.62609039468567573 ) ) ;
#143406=CARTESIAN_POINT ( 'NONE',  ( -0.05219959533909027116, -19.03943276465977164, 32.49890960531435979 ) ) ;
#143407=CARTESIAN_POINT ( 'NONE',  ( 10.72451020669871369, 18.67979575497193778, 97.08442372801904696 ) ) ;
#143408=CARTESIAN_POINT ( 'NONE',  ( -0.05219959533909027116, -19.03943276465977164, 102.4989096053143669 ) ) ;
#143409=CARTESIAN_POINT ( 'NONE',  ( 15.72974639402199770, -15.80617190586745480, 108.1239096053143811 ) ) ;
#143411=CARTESIAN_POINT ( 'NONE',  ( 15.80617190586746368, 15.72974639402197994, 69.37390960531436690 ) ) ;
#143412=CARTESIAN_POINT ( 'NONE',  ( -0.05219959533934338120, 16.53943276465976808, 57.50109039468568994 ) ) ;
#143413=CARTESIAN_POINT ( 'NONE',  ( 16.55341960407611168, 4.379528057220329451, 43.95724293864769550 ) ) ;
#143414=CARTESIAN_POINT ( 'NONE',  ( 19.50973618000807264, -5.499999999999992895, 102.5000000000000142 ) ) ;
#143415=CARTESIAN_POINT ( 'NONE',  ( 13.97604488694548053, -13.89961937509957401, 95.62609039468563310 ) ) ;
#143418=CARTESIAN_POINT ( 'NONE',  ( -16.53943276465976808, -0.05219959533934237506, 28.75109039468567929 ) ) ;
#143419=CARTESIAN_POINT ( 'NONE',  ( 10.81492255796078972, 18.62759615963270932, 104.5822429386477097 ) ) ;
#143420=CARTESIAN_POINT ( 'NONE',  ( 10.72451020669898902, -18.67979575497178502, 77.91557627198102409 ) ) ;
#143421=CARTESIAN_POINT ( 'NONE',  ( 9.564922557960805705, 16.46253265017160317, 114.5822429386476955 ) ) ;
#143422=CARTESIAN_POINT ( 'NONE',  ( -8.224510206698735004, -14.34966873604973081, 49.58442372801901143 ) ) ;
#143423=CARTESIAN_POINT ( 'NONE',  ( 9.564922557960805705, 16.46253265017160317, 74.58224293864769550 ) ) ;
#143424=CARTESIAN_POINT ( 'NONE',  ( 5.823673210054444382, -21.52544592524334988, 35.20942372801901854 ) ) ;
#143425=CARTESIAN_POINT ( 'NONE',  ( -19.03943276465977164, -0.05219959533935918106, 98.75109039468567573 ) ) ;
#143426=CARTESIAN_POINT ( 'NONE',  ( 5.049401038298161559, -19.05341960407611168, 107.7072429386476955 ) ) ;
#143428=CARTESIAN_POINT ( 'NONE',  ( -9.564922557960796823, -16.46253265017161027, 92.08224293864769550 ) ) ;
#143429=CARTESIAN_POINT ( 'NONE',  ( 21.55341960407610458, 5.719274019375980345, 83.95724293864770971 ) ) ;
#143430=CARTESIAN_POINT ( 'NONE',  ( 19.02544592524343514, -5.153800228976328945, 58.54057627198102409 ) ) ;
#143432=CARTESIAN_POINT ( 'NONE',  ( -0.05219959533910754901, -16.53943276465976808, 62.49890960531436690 ) ) ;
#143433=CARTESIAN_POINT ( 'NONE',  ( 15.80617190586746368, 15.72974639402197994, 24.37390960531435979 ) ) ;
#143435=CARTESIAN_POINT ( 'NONE',  ( 5.719274019375991003, -21.55341960407610458, 92.70724293864770971 ) ) ;
#143436=CARTESIAN_POINT ( 'NONE',  ( 9.564922557961047289, -16.46253265017146816, 65.41775706135233293 ) ) ;
#143437=CARTESIAN_POINT ( 'NONE',  ( -10.72451020669898014, 18.67979575497178502, 25.41557627198103120 ) ) ;
#143438=CARTESIAN_POINT ( 'NONE',  ( 19.52851543214744012, 5.500000000000030198, 67.89357721762580411 ) ) ;
#143439=CARTESIAN_POINT ( 'NONE',  ( -5.719274019375978568, 21.55341960407610458, 60.20724293864768839 ) ) ;
#143441=CARTESIAN_POINT ( 'NONE',  ( -13.97604488694527625, -13.89961937509977652, 81.87390960531436690 ) ) ;
#143442=CARTESIAN_POINT ( 'NONE',  ( -21.55341960407619339, 5.719274019375674811, 78.54275706135236135 ) ) ;
#143443=CARTESIAN_POINT ( 'NONE',  ( 5.153800228976335163, 19.02544592524342804, 49.79057627198100988 ) ) ;
#143444=CARTESIAN_POINT ( 'NONE',  ( 16.53943276465976808, -0.05219959533910856209, 78.74890960531436690 ) ) ;
#143445=CARTESIAN_POINT ( 'NONE',  ( -14.34966873604972548, 8.224510206698743886, 38.33442372801900433 ) ) ;
#143446=CARTESIAN_POINT ( 'NONE',  ( 15.80617190586769283, -15.72974639402175789, 65.62609039468568994 ) ) ;
#143447=ORIENTED_EDGE ( 'NONE', *, *, #190013, .T. ) ;
#143448=CARTESIAN_POINT ( 'NONE',  ( 13.89961937509957401, 13.97604488694547697, 21.87609039468566152 ) ) ;
#143449=CARTESIAN_POINT ( 'NONE',  ( 19.02544592524334988, 5.153800228976608722, 76.45942372801897591 ) ) ;
#143451=CARTESIAN_POINT ( 'NONE',  ( 5.823673210054444382, -21.52544592524334988, 40.20942372801901854 ) ) ;
#143453=CARTESIAN_POINT ( 'NONE',  ( 19.05341960407617918, -5.049401038297876454, 36.04275706135234003 ) ) ;
#143454=CARTESIAN_POINT ( 'NONE',  ( 13.89961937509977652, -13.97604488694527269, 53.12390960531434558 ) ) ;
#143455=CARTESIAN_POINT ( 'NONE',  ( 9.474510206698729675, 16.51473224551082808, 32.08442372801900433 ) ) ;
#143456=CARTESIAN_POINT ( 'NONE',  ( 8.314922557961029526, -14.29746914071037800, 100.4177570613523471 ) ) ;
#143457=CARTESIAN_POINT ( 'NONE',  ( 5.049401038298161559, -19.05341960407611168, 97.70724293864766707 ) ) ;
#143458=CARTESIAN_POINT ( 'NONE',  ( -21.55341960407619339, 5.719274019375674811, 73.54275706135234714 ) ) ;
#143461=CARTESIAN_POINT ( 'NONE',  ( 21.52544592524334988, 5.823673210054432836, 81.45942372801900433 ) ) ;
#143462=CARTESIAN_POINT ( 'NONE',  ( 17.40861289039005300, -6.110651285853256454, 41.12767529172569425 ) ) ;
#143463=CARTESIAN_POINT ( 'NONE',  ( -19.02544592524342804, 5.153800228976336051, 101.0405762719810241 ) ) ;
#143464=CARTESIAN_POINT ( 'NONE',  ( -13.97604488694547697, 13.89961937509957934, 28.12609039468565797 ) ) ;
#143467=CARTESIAN_POINT ( 'NONE',  ( 16.51473224551069308, 9.474510206698969483, 39.16557627198103120 ) ) ;
#143468=CARTESIAN_POINT ( 'NONE',  ( -15.72974639402197994, 15.80617190586746368, 55.62390960531436690 ) ) ;
#143469=CARTESIAN_POINT ( 'NONE',  ( 4.379528057220339221, -16.55341960407611168, 27.70724293864769905 ) ) ;
#143470=CARTESIAN_POINT ( 'NONE',  ( -4.483927247898539470, -16.52544592524342804, 92.29057627198103830 ) ) ;
#143471=CARTESIAN_POINT ( 'NONE',  ( -13.89961937509977652, 13.97604488694528158, 75.62390960531438111 ) ) ;
#143472=CARTESIAN_POINT ( 'NONE',  ( -18.67979575497193778, 10.72451020669871902, 108.3344237280190185 ) ) ;
#143473=CARTESIAN_POINT ( 'NONE',  ( 16.46253265017160672, -9.564922557960803928, 38.33224293864768839 ) ) ;
#143474=CARTESIAN_POINT ( 'NONE',  ( -4.483927247898539470, -16.52544592524342804, 107.2905762719810525 ) ) ;
#143475=CARTESIAN_POINT ( 'NONE',  ( -18.62759615963255300, -10.81492255796106328, 59.16775706135234714 ) ) ;
#143476=CARTESIAN_POINT ( 'NONE',  ( -18.62759615963270932, 10.81492255796079327, 80.83224293864769550 ) ) ;
#143477=CARTESIAN_POINT ( 'NONE',  ( -13.89961937509957401, -13.97604488694547875, 59.37609039468566863 ) ) ;
#143479=CARTESIAN_POINT ( 'NONE',  ( -16.46253265017160317, 9.564922557960807481, 105.8322429386476955 ) ) ;
#143480=CARTESIAN_POINT ( 'NONE',  ( -14.34966873604960291, -8.224510206698953496, 76.66557627198103830 ) ) ;
#143481=CARTESIAN_POINT ( 'NONE',  ( 0.05219959533936267826, -19.03943276465977164, 40.00109039468566152 ) ) ;
#143482=CARTESIAN_POINT ( 'NONE',  ( 5.049401038298161559, -19.05341960407611168, 62.70724293864769550 ) ) ;
#143483=CARTESIAN_POINT ( 'NONE',  ( -14.34966873604960291, -8.224510206698953496, 56.66557627198103830 ) ) ;
#143484=CARTESIAN_POINT ( 'NONE',  ( -19.02544592524334988, -5.153800228976617603, 73.95942372801900433 ) ) ;
#143485=CARTESIAN_POINT ( 'NONE',  ( 16.31925111598457079, 7.325300261831479531, 32.33575461032751974 ) ) ;
#143486=CARTESIAN_POINT ( 'NONE',  ( 10.81492255796078972, 18.62759615963270932, 34.58224293864770260 ) ) ;
#143488=CARTESIAN_POINT ( 'NONE',  ( 14.34966873604960469, 8.224510206698951720, 99.16557627198100988 ) ) ;
#143490=CARTESIAN_POINT ( 'NONE',  ( 0.05219959533909260263, 19.03943276465977164, 64.99890960531436690 ) ) ;
#143491=CARTESIAN_POINT ( 'NONE',  ( 21.55341960407610458, 5.719274019375980345, 68.95724293864769550 ) ) ;
#143492=CARTESIAN_POINT ( 'NONE',  ( 5.153800228976335163, 19.02544592524342804, 34.79057627198102409 ) ) ;
#143493=CARTESIAN_POINT ( 'NONE',  ( -14.29746914071037622, -8.314922557961029526, 79.16775706135234714 ) ) ;
#143494=CARTESIAN_POINT ( 'NONE',  ( -5.153800228976328057, -19.02544592524343514, 67.29057627198102409 ) ) ;
#143495=CARTESIAN_POINT ( 'NONE',  ( -5.153800228976607833, 19.02544592524334988, 52.70942372801900433 ) ) ;
#143496=CARTESIAN_POINT ( 'NONE',  ( -0.05219959533937732626, 21.53943276465977519, 67.50109039468568994 ) ) ;
#143498=CARTESIAN_POINT ( 'NONE',  ( 15.80617190586746368, 15.72974639402197994, 44.37390960531435979 ) ) ;
#143499=CARTESIAN_POINT ( 'NONE',  ( 16.55341960407611168, 4.379528057220329451, 113.9572429386477239 ) ) ;
#143500=CARTESIAN_POINT ( 'NONE',  ( 14.34966873604972726, -8.224510206698740333, 85.83442372801901854 ) ) ;
#143501=CARTESIAN_POINT ( 'NONE',  ( 5.049401038297881783, 19.05341960407617563, 102.2927570613523045 ) ) ;
#143503=CARTESIAN_POINT ( 'NONE',  ( -15.49999999999999822, 5.499999999999998224, 22.00000000000000711 ) ) ;
#143504=CARTESIAN_POINT ( 'NONE',  ( 18.62759615963255655, 10.81492255796105972, 91.66775706135234714 ) ) ;
#143505=CARTESIAN_POINT ( 'NONE',  ( 12.06949235617757843, -12.14591786802309237, 48.12390960531436690 ) ) ;
#143506=CARTESIAN_POINT ( 'NONE',  ( 0.05219959533910956823, 16.53943276465976808, 59.99890960531436690 ) ) ;
#143507=CARTESIAN_POINT ( 'NONE',  ( 0.05219959533907565091, 21.53943276465977519, 94.99890960531436690 ) ) ;
#143508=CARTESIAN_POINT ( 'NONE',  ( 21.55341960407610458, 5.719274019375980345, 93.95724293864770971 ) ) ;
#143510=CARTESIAN_POINT ( 'NONE',  ( -18.62759615963270932, 10.81492255796079327, 30.83224293864770260 ) ) ;
#143511=CARTESIAN_POINT ( 'NONE',  ( 14.34966873604972726, -8.224510206698740333, 70.83442372801901854 ) ) ;
#143512=CARTESIAN_POINT ( 'NONE',  ( 12.06949235617757843, -12.14591786802309237, 78.12390960531436690 ) ) ;
#143513=CARTESIAN_POINT ( 'NONE',  ( -0.05219959533909027116, -19.03943276465977164, 47.49890960531435979 ) ) ;
#143515=CARTESIAN_POINT ( 'NONE',  ( 12.06949235617739724, 12.14591786802326823, 96.87609039468568994 ) ) ;
#143516=CARTESIAN_POINT ( 'NONE',  ( -21.52544592524343514, 5.823673210054127303, 116.0405762719810383 ) ) ;
#143517=CARTESIAN_POINT ( 'NONE',  ( 13.89961937509977652, -13.97604488694527269, 78.12390960531433848 ) ) ;
#143518=CARTESIAN_POINT ( 'NONE',  ( -18.62759615963255300, -10.81492255796106328, 49.16775706135234003 ) ) ;
#143519=CARTESIAN_POINT ( 'NONE',  ( 19.03943276465977164, -0.05219959533909143690, 103.7489096053143669 ) ) ;
#143522=ORIENTED_EDGE ( 'NONE', *, *, #6444, .T. ) ;
#143523=CARTESIAN_POINT ( 'NONE',  ( 5.719274019375673035, 21.55341960407619339, 47.29275706135234003 ) ) ;
#143524=CARTESIAN_POINT ( 'NONE',  ( -13.89961937509977652, 13.97604488694528158, 40.62390960531435979 ) ) ;
#143525=CARTESIAN_POINT ( 'NONE',  ( -5.049401038298153566, 19.05341960407611168, 115.2072429386477097 ) ) ;
#143526=CARTESIAN_POINT ( 'NONE',  ( 19.05341960407617918, -5.049401038297876454, 51.04275706135231871 ) ) ;
#143527=CARTESIAN_POINT ( 'NONE',  ( -10.72451020669870658, -18.67979575497194134, 34.58442372801900433 ) ) ;
#143528=CARTESIAN_POINT ( 'NONE',  ( -19.03943276465977164, -0.05219959533935918106, 53.75109039468566863 ) ) ;
#143529=CARTESIAN_POINT ( 'NONE',  ( -9.564922557960796823, -16.46253265017161027, 22.08224293864768839 ) ) ;
#143530=CARTESIAN_POINT ( 'NONE',  ( -0.05219959533934338120, 16.53943276465976808, 87.50109039468568994 ) ) ;
#143531=CARTESIAN_POINT ( 'NONE',  ( 16.51473224551083163, -9.474510206698727899, 65.83442372801900433 ) ) ;
#143532=CARTESIAN_POINT ( 'NONE',  ( -0.05219959533934338120, 16.53943276465976808, 102.5010903946856899 ) ) ;
#143535=CARTESIAN_POINT ( 'NONE',  ( 9.564922557960805705, 16.46253265017160317, 89.58224293864769550 ) ) ;
#143536=CARTESIAN_POINT ( 'NONE',  ( -10.81492255796105439, 18.62759615963255655, 87.91775706135234714 ) ) ;
#143537=CARTESIAN_POINT ( 'NONE',  ( -19.03943276465977164, -0.05219959533935918106, 18.75109039468567218 ) ) ;
#143539=CARTESIAN_POINT ( 'NONE',  ( -5.049401038298153566, 19.05341960407611168, 95.20724293864770971 ) ) ;
#143540=CARTESIAN_POINT ( 'NONE',  ( -10.72451020669870658, -18.67979575497194134, 79.58442372801903275 ) ) ;
#143541=CARTESIAN_POINT ( 'NONE',  ( -9.564922557961040184, 16.46253265017147172, 107.9177570613523471 ) ) ;
#143543=CARTESIAN_POINT ( 'NONE',  ( 16.46253265017160672, -9.564922557960803928, 73.33224293864769550 ) ) ;
#143544=CARTESIAN_POINT ( 'NONE',  ( -10.72451020669898014, 18.67979575497178502, 35.41557627198102409 ) ) ;
#143546=CARTESIAN_POINT ( 'NONE',  ( 9.564922557960805705, 16.46253265017160317, 59.58224293864769550 ) ) ;
#143547=CARTESIAN_POINT ( 'NONE',  ( 8.224510206698742110, 14.34966873604972548, 112.0844237280190185 ) ) ;
#143550=CARTESIAN_POINT ( 'NONE',  ( 5.153800228976615827, -19.02544592524334988, 70.20942372801899012 ) ) ;
#143551=CARTESIAN_POINT ( 'NONE',  ( -16.51473224551069308, -9.474510206698971260, 101.6655762719810241 ) ) ;
#143552=CARTESIAN_POINT ( 'NONE',  ( -21.52544592524334988, -5.823673210054445271, 103.9594237280190185 ) ) ;
#143553=CARTESIAN_POINT ( 'NONE',  ( 16.55341960407611168, 4.379528057220329451, 88.95724293864769550 ) ) ;
#143554=B_SPLINE_CURVE_WITH_KNOTS ( 'NONE', 3,
 ( #28729, #13536, #186376, #62000, #91334, #29703, #166240, #121695, #184377, #332, #90366, #154030, #123666, #151072, #138852, #155021, #152051, #185363, #45858, #108515 ),
 .UNSPECIFIED., .F., .F.,
 ( 4, 2, 2, 2, 2, 2, 2, 2, 2, 4 ),
 ( 0.004000878361811896662, 0.004499404418915904820, 0.004997930476019913845, 0.005496456533123922003, 0.005994982590227930161, 0.006244245618779934240, 0.006493508647331939186, 0.006992034704435923925, 0.007490560761539909532, 0.007989086818643895138 ),
 .UNSPECIFIED. ) ;
#143555=CARTESIAN_POINT ( 'NONE',  ( -18.67979575497178146, -10.72451020669898902, 46.66557627198102409 ) ) ;
#143556=( BOUNDED_CURVE ( )  B_SPLINE_CURVE ( 2, ( #135513, #136483, #181027, #57675, #14127, #138461, #75794, #59633, #121307, #182999, #137472, #30296, #108115 ),
 .UNSPECIFIED., .F., .T. ) 
 B_SPLINE_CURVE_WITH_KNOTS ( ( 3, 2, 2, 2, 2, 2, 3 ),
 ( 0.2129567522165188298, 0.2149122807017543879, 0.2192982456140350755, 0.2236842105263157909, 0.2280701754385964786, 0.2324561403508771940, 0.2343659890140226687 ),
 .UNSPECIFIED. ) 
 CURVE ( )  GEOMETRIC_REPRESENTATION_ITEM ( )  RATIONAL_B_SPLINE_CURVE ( ( 0.9831626618144004848, 0.9848076720550091867, 1.000000000000000000, 0.9659258262890683122, 1.000000000000000000, 0.9659258262890683122, 1.000000000000000000, 0.9659258262890683122, 1.000000000000000000, 0.9659258262890683122, 1.000000000000000000, 0.9851625545550090068, 0.9832469066685280978 ) ) 
 REPRESENTATION_ITEM ( '' )  );
#143557=CARTESIAN_POINT ( 'NONE',  ( -18.67979575497178146, -10.72451020669898902, 36.66557627198103120 ) ) ;
#143558=CARTESIAN_POINT ( 'NONE',  ( -16.52544592524342804, 4.483927247898546575, 111.0405762719810525 ) ) ;
#143560=CARTESIAN_POINT ( 'NONE',  ( -9.474510206698720793, -16.51473224551083518, 44.58442372801900433 ) ) ;
#143561=CARTESIAN_POINT ( 'NONE',  ( 16.52544592524342804, -4.483927247898539470, 23.54057627198102765 ) ) ;
#143562=CARTESIAN_POINT ( 'NONE',  ( -16.46253265017160317, 9.564922557960807481, 100.8322429386477097 ) ) ;
#143564=CARTESIAN_POINT ( 'NONE',  ( -0.05219959533937732626, 21.53943276465977519, 67.50109039468568994 ) ) ;
#143565=CARTESIAN_POINT ( 'NONE',  ( 10.81492255796078972, 18.62759615963270932, 54.58224293864769550 ) ) ;
#143566=CARTESIAN_POINT ( 'NONE',  ( 0.05219959533937995610, -21.53943276465977519, 45.00109039468568284 ) ) ;
#143567=CARTESIAN_POINT ( 'NONE',  ( -18.67979575497178146, -10.72451020669898902, 101.6655762719810383 ) ) ;
#143568=CARTESIAN_POINT ( 'NONE',  ( -21.52544592524334988, -5.823673210054445271, 33.95942372801901143 ) ) ;
#143569=CARTESIAN_POINT ( 'NONE',  ( -16.46253265017160317, 9.564922557960807481, 25.83224293864769194 ) ) ;
#143570=CARTESIAN_POINT ( 'NONE',  ( 16.46253265017146816, 9.564922557961045513, 71.66775706135233293 ) ) ;
#143571=CARTESIAN_POINT ( 'NONE',  ( 16.52544592524342804, -4.483927247898539470, 98.54057627198105251 ) ) ;
#143572=CARTESIAN_POINT ( 'NONE',  ( 13.97604488694527802, 13.89961937509977652, 109.3739096053143669 ) ) ;
#143573=CARTESIAN_POINT ( 'NONE',  ( 14.34966873604960469, 8.224510206698951720, 49.16557627198102409 ) ) ;
#143574=CARTESIAN_POINT ( 'NONE',  ( 4.483927247898790824, -16.52544592524335698, 110.2094237280190185 ) ) ;
#143575=CARTESIAN_POINT ( 'NONE',  ( -19.02544592524342804, 5.153800228976336051, 51.04057627198103120 ) ) ;
#143576=CARTESIAN_POINT ( 'NONE',  ( 5.049401038298161559, -19.05341960407611168, 27.70724293864769550 ) ) ;
#143577=CARTESIAN_POINT ( 'NONE',  ( 18.67979575497178502, 10.72451020669898547, 34.16557627198102409 ) ) ;
#143578=CARTESIAN_POINT ( 'NONE',  ( -16.46253265017146816, -9.564922557961047289, 19.16775706135233293 ) ) ;
#143580=DIRECTION ( 'NONE',  ( -0.000000000000000000, -0.000000000000000000, 1.000000000000000000 ) ) ;
#143581=CARTESIAN_POINT ( 'NONE',  ( 4.379528057220339221, -16.55341960407611168, 37.70724293864769550 ) ) ;
#143582=CARTESIAN_POINT ( 'NONE',  ( 15.72974639402176855, 15.80617190586768217, 51.87609039468568284 ) ) ;
#143584=CARTESIAN_POINT ( 'NONE',  ( -4.483927247898782831, 16.52544592524335698, 57.70942372801901143 ) ) ;
#143585=CARTESIAN_POINT ( 'NONE',  ( 13.89961937509957401, 13.97604488694547697, 66.87609039468567573 ) ) ;
#143586=CARTESIAN_POINT ( 'NONE',  ( 0.05219959533910956823, 16.53943276465976808, 29.99890960531435979 ) ) ;
#143587=CARTESIAN_POINT ( 'NONE',  ( 14.29746914071037800, 8.314922557961029526, 111.6677570613523613 ) ) ;
#143588=CARTESIAN_POINT ( 'NONE',  ( -5.153800228976328057, -19.02544592524343514, 37.29057627198102409 ) ) ;
#143589=CARTESIAN_POINT ( 'NONE',  ( -5.153800228976328057, -19.02544592524343514, 62.29057627198100988 ) ) ;
#143590=CARTESIAN_POINT ( 'NONE',  ( 5.049401038298161559, -19.05341960407611168, 27.70724293864769550 ) ) ;
#143591=CARTESIAN_POINT ( 'NONE',  ( -21.53943276465977519, -0.05219959533937600094, 38.75109039468567573 ) ) ;
#143592=CARTESIAN_POINT ( 'NONE',  ( 19.05341960407611168, 5.049401038298154454, 38.95724293864767418 ) ) ;
#143594=CARTESIAN_POINT ( 'NONE',  ( -13.97604488694527625, -13.89961937509977652, 36.87390960531436690 ) ) ;
#143595=CARTESIAN_POINT ( 'NONE',  ( 21.53943276465977519, -0.05219959533907433946, 28.74890960531435624 ) ) ;
#143596=CARTESIAN_POINT ( 'NONE',  ( 15.72974639402176855, 15.80617190586768217, 56.87609039468568994 ) ) ;
#143597=CARTESIAN_POINT ( 'NONE',  ( 8.314922557960818139, 14.29746914071049879, 109.5822429386476955 ) ) ;
#143598=CARTESIAN_POINT ( 'NONE',  ( 9.474510206698971260, -16.51473224551069308, 107.9155762719810383 ) ) ;
#143599=CARTESIAN_POINT ( 'NONE',  ( 16.55341960407618274, -4.379528057220086978, 76.04275706135237556 ) ) ;
#143600=CARTESIAN_POINT ( 'NONE',  ( 0.05219959533937995610, -21.53943276465977519, 95.00109039468568994 ) ) ;
#143601=CARTESIAN_POINT ( 'NONE',  ( -14.29746914071037622, -8.314922557961029526, 49.16775706135234003 ) ) ;
#143602=CARTESIAN_POINT ( 'NONE',  ( -16.46253265017160317, 9.564922557960807481, 100.8322429386477097 ) ) ;
#143603=CARTESIAN_POINT ( 'NONE',  ( 4.483927247898790824, -16.52544592524335698, 45.20942372801901854 ) ) ;
#143604=CARTESIAN_POINT ( 'NONE',  ( -8.314922557961024197, 14.29746914071037800, 32.91775706135234714 ) ) ;
#143605=CARTESIAN_POINT ( 'NONE',  ( 14.29746914071037800, 8.314922557961029526, 81.66775706135236135 ) ) ;
#143606=CARTESIAN_POINT ( 'NONE',  ( -9.474510206698720793, -16.51473224551083518, 109.5844237280190043 ) ) ;
#143607=CARTESIAN_POINT ( 'NONE',  ( 18.67979575497178502, 10.72451020669898547, 94.16557627198103830 ) ) ;
#143608=CARTESIAN_POINT ( 'NONE',  ( 8.314922557960818139, 14.29746914071049879, 109.5822429386476955 ) ) ;
#143609=CARTESIAN_POINT ( 'NONE',  ( -9.474510206698720793, -16.51473224551083518, 99.58442372801900433 ) ) ;
#143610=CARTESIAN_POINT ( 'NONE',  ( -16.53943276465976808, -0.05219959533934237506, 78.75109039468568994 ) ) ;
#143612=CARTESIAN_POINT ( 'NONE',  ( 16.46253265017146816, 9.564922557961045513, 66.66775706135233293 ) ) ;
#143613=CARTESIAN_POINT ( 'NONE',  ( -14.34966873604960291, -8.224510206698953496, 41.66557627198103120 ) ) ;
#143614=CARTESIAN_POINT ( 'NONE',  ( -8.314922557960811034, -14.29746914071050412, 97.08224293864770971 ) ) ;
#143615=CARTESIAN_POINT ( 'NONE',  ( -9.564922557961040184, 16.46253265017147172, 37.91775706135233293 ) ) ;
#143616=CARTESIAN_POINT ( 'NONE',  ( -19.35633801406908461, 5.499999999999578115, 89.13373818172762242 ) ) ;
#143617=CARTESIAN_POINT ( 'NONE',  ( -10.81492255796105439, 18.62759615963255655, 37.91775706135235424 ) ) ;
#143618=CARTESIAN_POINT ( 'NONE',  ( -9.564922557961040184, 16.46253265017147172, 97.91775706135233293 ) ) ;
#143620=CARTESIAN_POINT ( 'NONE',  ( -13.89961937509977652, 13.97604488694528158, 95.62390960531436690 ) ) ;
#143621=CARTESIAN_POINT ( 'NONE',  ( -16.46253265017160317, 9.564922557960807481, 85.83224293864769550 ) ) ;
#143622=CARTESIAN_POINT ( 'NONE',  ( 21.52544592524344225, -5.823673210054117533, 53.54057627198103120 ) ) ;
#143623=CARTESIAN_POINT ( 'NONE',  ( 8.224510206698953496, -14.34966873604960469, 87.91557627198103830 ) ) ;
#143624=CARTESIAN_POINT ( 'NONE',  ( -16.51473224551069308, -9.474510206698971260, 66.66557627198102409 ) ) ;
#143625=CARTESIAN_POINT ( 'NONE',  ( 16.55341960407611168, 4.379528057220329451, 113.9572429386477239 ) ) ;
#143626=CARTESIAN_POINT ( 'NONE',  ( -21.52544592524334988, -5.823673210054445271, 38.95942372801901854 ) ) ;
#143627=CARTESIAN_POINT ( 'NONE',  ( -18.67979575497193778, 10.72451020669871902, 73.33442372801901854 ) ) ;
#143628=CARTESIAN_POINT ( 'NONE',  ( 13.89961937509977652, -13.97604488694527269, 48.12390960531435979 ) ) ;
#143630=CARTESIAN_POINT ( 'NONE',  ( -16.53943276465976808, -0.05219959533934237506, 73.75109039468567573 ) ) ;
#143631=CARTESIAN_POINT ( 'NONE',  ( 10.81492255796106328, -18.62759615963255655, 25.41775706135235779 ) ) ;
#143632=CARTESIAN_POINT ( 'NONE',  ( 0.05219959533937995610, -21.53943276465977519, 30.00109039468568284 ) ) ;
#143633=CARTESIAN_POINT ( 'NONE',  ( -19.03943276465977164, -0.05219959533935918106, 53.75109039468566863 ) ) ;
#143634=CARTESIAN_POINT ( 'NONE',  ( -9.564922557960796823, -16.46253265017161027, 72.08224293864770971 ) ) ;
#143635=CARTESIAN_POINT ( 'NONE',  ( 13.89961937509957401, 13.97604488694547697, 26.87609039468566507 ) ) ;
#143636=CARTESIAN_POINT ( 'NONE',  ( -15.72974639402176322, -15.80617190586768395, 89.37609039468568994 ) ) ;
#143638=CARTESIAN_POINT ( 'NONE',  ( -5.719274019375978568, 21.55341960407610458, 65.20724293864768129 ) ) ;
#143639=CARTESIAN_POINT ( 'NONE',  ( -0.05219959533910754901, -16.53943276465976808, 52.49890960531435979 ) ) ;
#143640=CARTESIAN_POINT ( 'NONE',  ( 18.67979575497194134, -10.72451020669871369, 85.83442372801901854 ) ) ;
#143641=CARTESIAN_POINT ( 'NONE',  ( 0.05219959533936267826, -19.03943276465977164, 35.00109039468566863 ) ) ;
#143642=CARTESIAN_POINT ( 'NONE',  ( -14.29746914071049879, 8.314922557960819915, 70.83224293864770971 ) ) ;
#143643=CARTESIAN_POINT ( 'NONE',  ( 19.05341960407611168, 5.049401038298154454, 28.95724293864769550 ) ) ;
#143644=CARTESIAN_POINT ( 'NONE',  ( 13.97604488694548053, -13.89961937509957401, 55.62609039468566863 ) ) ;
#143645=CARTESIAN_POINT ( 'NONE',  ( -8.314922557960811034, -14.29746914071050412, 32.08224293864769550 ) ) ;
#143646=CARTESIAN_POINT ( 'NONE',  ( -0.05219959533937732626, 21.53943276465977519, 87.50109039468568994 ) ) ;
#143647=CARTESIAN_POINT ( 'NONE',  ( -5.153800228976328057, -19.02544592524343514, 72.29057627198102409 ) ) ;
#143648=CARTESIAN_POINT ( 'NONE',  ( -0.05219959533936034679, 19.03943276465977164, 52.50109039468566863 ) ) ;
#143649=CARTESIAN_POINT ( 'NONE',  ( 18.67979575497178502, 10.72451020669898547, 49.16557627198102409 ) ) ;
#143650=CARTESIAN_POINT ( 'NONE',  ( -18.62759615963255300, -10.81492255796106328, 39.16775706135235424 ) ) ;
#143651=CARTESIAN_POINT ( 'NONE',  ( -18.67979575497178146, -10.72451020669898902, 96.66557627198102409 ) ) ;
#143652=CARTESIAN_POINT ( 'NONE',  ( -9.474510206698720793, -16.51473224551083518, 94.58442372801900433 ) ) ;
#143653=CARTESIAN_POINT ( 'NONE',  ( -0.05219959533934338120, 16.53943276465976808, 62.50109039468568284 ) ) ;
#143655=CARTESIAN_POINT ( 'NONE',  ( -21.52544592524343514, 5.823673210054127303, 101.0405762719810383 ) ) ;
#143656=CARTESIAN_POINT ( 'NONE',  ( -14.34966873604960291, -8.224510206698953496, 96.66557627198102409 ) ) ;
#143658=CARTESIAN_POINT ( 'NONE',  ( 12.06949235617739724, 12.14591786802326823, 36.87609039468568994 ) ) ;
#143660=CARTESIAN_POINT ( 'NONE',  ( -15.80617190586745835, -15.72974639402198527, 66.87390960531436690 ) ) ;
#143661=CARTESIAN_POINT ( 'NONE',  ( -4.483927247898782831, 16.52544592524335698, 92.70942372801901854 ) ) ;
#143662=CARTESIAN_POINT ( 'NONE',  ( -19.05341960407611168, -5.049401038298163336, 36.45724293864766707 ) ) ;
#143663=B_SPLINE_CURVE_WITH_KNOTS ( 'NONE', 3,
 ( #112755, #83407, #66259, #191597, #159251, #84405, #20747, #129897, #114754, #176448, #82402, #69252, #100580, #67251, #130918, #34930, #96583, #158272, #81402, #19761, #143088, #127919, #41933, #132926, #148106, #86420, #24773, #9597, #120731, #119760, #27770, #103599 ),
 .UNSPECIFIED., .F., .F.,
 ( 4, 2, 2, 2, 2, 2, 2, 2, 2, 2, 2, 2, 2, 2, 2, 4 ),
 ( 2.281672496420497865E-17, 0.0003712461730036942047, 0.0007424923460073655328, 0.001113738519011037023, 0.001484984692014708297, 0.002227477038022051496, 0.002598723211025726239, 0.002969969384029401416, 0.003341215557033076159, 0.003712461730036750469, 0.004083707903040425212, 0.004454954076044099522, 0.004826200249047774699, 0.005197446422051449008, 0.005568692595055124185, 0.005939938768058799362 ),
 .UNSPECIFIED. ) ;
#143664=CARTESIAN_POINT ( 'NONE',  ( 16.53943276465976808, 0.05219959533934440121, 61.25109039468567573 ) ) ;
#143665=CARTESIAN_POINT ( 'NONE',  ( -19.02544592524334988, -5.153800228976617603, 58.95942372801900433 ) ) ;
#143666=CARTESIAN_POINT ( 'NONE',  ( -10.81492255796105439, 18.62759615963255655, 37.91775706135235424 ) ) ;
#143668=CARTESIAN_POINT ( 'NONE',  ( -5.823673210054116645, -21.52544592524344225, 57.29057627198103120 ) ) ;
#143669=CARTESIAN_POINT ( 'NONE',  ( -14.29746914071037622, -8.314922557961029526, 94.16775706135237556 ) ) ;
#143670=CARTESIAN_POINT ( 'NONE',  ( -21.52544592524334988, -5.823673210054445271, 73.95942372801901854 ) ) ;
#143671=CARTESIAN_POINT ( 'NONE',  ( 5.823673210054125526, 21.52544592524343514, 54.79057627198104541 ) ) ;
#143672=CARTESIAN_POINT ( 'NONE',  ( 21.53943276465977519, -0.05219959533907433946, 38.74890960531435979 ) ) ;
#143673=CARTESIAN_POINT ( 'NONE',  ( -0.05219959533934338120, 16.53943276465976808, 72.50109039468568994 ) ) ;
#143674=CARTESIAN_POINT ( 'NONE',  ( -10.81492255796078084, -18.62759615963271287, 37.08224293864768129 ) ) ;
#143676=CARTESIAN_POINT ( 'NONE',  ( -9.564922557960796823, -16.46253265017161027, 97.08224293864769550 ) ) ;
#143677=CARTESIAN_POINT ( 'NONE',  ( 0.05219959533934541429, -16.53943276465976808, 110.0010903946856757 ) ) ;
#143679=CARTESIAN_POINT ( 'NONE',  ( 14.29746914071049879, -8.314922557960816363, 103.3322429386476955 ) ) ;
#143680=CARTESIAN_POINT ( 'NONE',  ( 21.53943276465977519, -0.05219959533907433946, 58.74890960531436690 ) ) ;
#143681=CARTESIAN_POINT ( 'NONE',  ( 16.52544592524335698, 4.483927247898782831, 96.45942372801901854 ) ) ;
#143682=CARTESIAN_POINT ( 'NONE',  ( 18.62759615963255655, 10.81492255796105972, 51.66775706135234714 ) ) ;
#143683=CARTESIAN_POINT ( 'NONE',  ( 16.46253265017146816, 9.564922557961045513, 101.6677570613523329 ) ) ;
#143684=CARTESIAN_POINT ( 'NONE',  ( 8.224510206698953496, -14.34966873604960469, 97.91557627198103830 ) ) ;
#143685=CARTESIAN_POINT ( 'NONE',  ( -0.05219959533909027116, -19.03943276465977164, 52.49890960531436690 ) ) ;
#143686=CARTESIAN_POINT ( 'NONE',  ( 5.153800228976335163, 19.02544592524342804, 29.79057627198102409 ) ) ;
#143688=CARTESIAN_POINT ( 'NONE',  ( -13.97604488694527625, -13.89961937509977652, 96.87390960531433848 ) ) ;
#143689=CARTESIAN_POINT ( 'NONE',  ( 0.05219959533934541429, -16.53943276465976808, 70.00109039468568994 ) ) ;
#143690=CARTESIAN_POINT ( 'NONE',  ( 0.05219959533937995610, -21.53943276465977519, 105.0010903946856757 ) ) ;
#143691=CARTESIAN_POINT ( 'NONE',  ( 18.67979575497178502, 10.72451020669898547, 49.16557627198102409 ) ) ;
#143692=CARTESIAN_POINT ( 'NONE',  ( -14.34966873604972548, 8.224510206698743886, 73.33442372801901854 ) ) ;
#143693=CARTESIAN_POINT ( 'NONE',  ( 5.153800228976615827, -19.02544592524334988, 85.20942372801900433 ) ) ;
#143695=CARTESIAN_POINT ( 'NONE',  ( -5.153800228976328057, -19.02544592524343514, 42.29057627198101699 ) ) ;
#143696=CARTESIAN_POINT ( 'NONE',  ( -16.46253265017160317, 9.564922557960807481, 80.83224293864769550 ) ) ;
#143697=AXIS2_PLACEMENT_3D ( 'NONE', #178700, #135197, #166529 ) ;
#143698=CARTESIAN_POINT ( 'NONE',  ( 16.46253265017160672, -9.564922557960803928, 38.33224293864768839 ) ) ;
#143699=CARTESIAN_POINT ( 'NONE',  ( 16.46253265017146816, 9.564922557961045513, 76.66775706135234714 ) ) ;
#143701=CARTESIAN_POINT ( 'NONE',  ( 9.474510206698971260, -16.51473224551069308, 92.91557627198103830 ) ) ;
#143702=CARTESIAN_POINT ( 'NONE',  ( 8.224510206698953496, -14.34966873604960469, 57.91557627198103120 ) ) ;
#143703=CARTESIAN_POINT ( 'NONE',  ( 18.67979575497178502, 10.72451020669898547, 49.16557627198102409 ) ) ;
#143707=CARTESIAN_POINT ( 'NONE',  ( 19.05341960407617918, -5.049401038297876454, 36.04275706135234003 ) ) ;
#143708=CARTESIAN_POINT ( 'NONE',  ( -17.13100169013301866, -6.664070546373139337, 79.23210164300157032 ) ) ;
#143709=CARTESIAN_POINT ( 'NONE',  ( -0.05219959533909027116, -19.03943276465977164, 52.49890960531436690 ) ) ;
#143710=CARTESIAN_POINT ( 'NONE',  ( -9.474510206698964154, 16.51473224551069663, 60.41557627198102409 ) ) ;
#143711=CARTESIAN_POINT ( 'NONE',  ( -16.52544592524335698, -4.483927247898792601, 43.95942372801902565 ) ) ;
#143713=CARTESIAN_POINT ( 'NONE',  ( -16.20579543436678094, 7.371946100355097897, 109.4347916582812985 ) ) ;
#143714=CARTESIAN_POINT ( 'NONE',  ( 16.52544592524335698, 4.483927247898782831, 81.45942372801900433 ) ) ;
#143715=CARTESIAN_POINT ( 'NONE',  ( -10.81492255796078084, -18.62759615963271287, 97.08224293864770971 ) ) ;
#143716=CARTESIAN_POINT ( 'NONE',  ( 8.224510206698742110, 14.34966873604972548, 42.08442372801901854 ) ) ;
#143717=CARTESIAN_POINT ( 'NONE',  ( 19.05341960407611168, 5.049401038298154454, 38.95724293864767418 ) ) ;
#143719=CARTESIAN_POINT ( 'NONE',  ( 21.55341960407619695, -5.719274019375665929, 51.04275706135234714 ) ) ;
#143720=CARTESIAN_POINT ( 'NONE',  ( 19.03943276465977164, 0.05219959533936151252, 56.25109039468566863 ) ) ;
#143721=CARTESIAN_POINT ( 'NONE',  ( 21.53943276465977519, 0.05219959533937863772, 96.25109039468568994 ) ) ;
#143723=CARTESIAN_POINT ( 'NONE',  ( 14.29746914071049879, -8.314922557960816363, 43.33224293864769550 ) ) ;
#143725=CARTESIAN_POINT ( 'NONE',  ( -5.719274019375978568, 21.55341960407610458, 60.20724293864768839 ) ) ;
#143728=CARTESIAN_POINT ( 'NONE',  ( 9.474510206698971260, -16.51473224551069308, 97.91557627198102409 ) ) ;
#143729=CARTESIAN_POINT ( 'NONE',  ( 14.29746914071049879, -8.314922557960816363, 98.33224293864769550 ) ) ;
#143730=CARTESIAN_POINT ( 'NONE',  ( -8.224510206698735004, -14.34966873604973081, 19.58442372801901143 ) ) ;
#143731=CARTESIAN_POINT ( 'NONE',  ( 8.224510206698953496, -14.34966873604960469, 22.91557627198102765 ) ) ;
#143734=CARTESIAN_POINT ( 'NONE',  ( 21.55341960407610458, 5.719274019375980345, 103.9572429386476813 ) ) ;
#143735=CARTESIAN_POINT ( 'NONE',  ( 16.55341960407611168, 4.379528057220329451, 28.95724293864769905 ) ) ;
#143736=CARTESIAN_POINT ( 'NONE',  ( -9.564922557960796823, -16.46253265017161027, 112.0822429386476955 ) ) ;
#143737=CARTESIAN_POINT ( 'NONE',  ( 9.474510206698729675, 16.51473224551082808, 97.08442372801900433 ) ) ;
#143738=CARTESIAN_POINT ( 'NONE',  ( -0.05219959533937732626, 21.53943276465977519, 102.5010903946856899 ) ) ;
#143739=CARTESIAN_POINT ( 'NONE',  ( -8.314922557960811034, -14.29746914071050412, 37.08224293864768129 ) ) ;
#143740=CARTESIAN_POINT ( 'NONE',  ( -5.823673210054116645, -21.52544592524344225, 87.29057627198103830 ) ) ;
#143741=CARTESIAN_POINT ( 'NONE',  ( -18.67979575497178146, -10.72451020669898902, 51.66557627198102409 ) ) ;
#143742=CARTESIAN_POINT ( 'NONE',  ( 19.05341960407611168, 5.049401038298154454, 68.95724293864769550 ) ) ;
#143743=CARTESIAN_POINT ( 'NONE',  ( 16.53943276465976808, -0.05219959533910856209, 28.74890960531435624 ) ) ;
#143744=CARTESIAN_POINT ( 'NONE',  ( 19.03943276465977164, -0.05219959533909143690, 83.74890960531436690 ) ) ;
#143746=CARTESIAN_POINT ( 'NONE',  ( -16.46253265017146816, -9.564922557961047289, 44.16775706135232582 ) ) ;
#143747=CARTESIAN_POINT ( 'NONE',  ( 15.80617190586746368, 15.72974639402197994, 74.37390960531436690 ) ) ;
#143748=CARTESIAN_POINT ( 'NONE',  ( 4.379528057220339221, -16.55341960407611168, 92.70724293864770971 ) ) ;
#143749=CARTESIAN_POINT ( 'NONE',  ( 0.05219959533937995610, -21.53943276465977519, 40.00109039468567573 ) ) ;
#143751=CARTESIAN_POINT ( 'NONE',  ( 12.06949235617739724, 12.14591786802326823, 101.8760903946857042 ) ) ;
#143752=CARTESIAN_POINT ( 'NONE',  ( -13.97604488694527625, -13.89961937509977652, 41.87390960531435979 ) ) ;
#143753=CARTESIAN_POINT ( 'NONE',  ( 19.02544592524343514, -5.153800228976328945, 83.54057627198100988 ) ) ;
#143755=CARTESIAN_POINT ( 'NONE',  ( 12.06949235617757843, -12.14591786802309237, 43.12390960531435269 ) ) ;
#143756=CARTESIAN_POINT ( 'NONE',  ( 15.72974639402176855, 15.80617190586768217, 66.87609039468568994 ) ) ;
#143758=CARTESIAN_POINT ( 'NONE',  ( 16.52544592524335698, 4.483927247898782831, 71.45942372801901854 ) ) ;
#143759=CARTESIAN_POINT ( 'NONE',  ( 19.05341960407611168, 5.049401038298154454, 43.95724293864769550 ) ) ;
#143760=CARTESIAN_POINT ( 'NONE',  ( 13.97604488694527802, 13.89961937509977652, 49.37390960531434558 ) ) ;
#143762=CARTESIAN_POINT ( 'NONE',  ( 18.67979575497194134, -10.72451020669871369, 110.8344237280190043 ) ) ;
#143763=CARTESIAN_POINT ( 'NONE',  ( -12.14591786802326823, 12.06949235617739902, 68.12609039468567573 ) ) ;
#143764=CARTESIAN_POINT ( 'NONE',  ( 18.62759615963255655, 10.81492255796105972, 96.66775706135234714 ) ) ;
#143765=CARTESIAN_POINT ( 'NONE',  ( 10.72451020669898902, -18.67979575497178502, 22.91557627198102765 ) ) ;
#143766=CARTESIAN_POINT ( 'NONE',  ( -16.46253265017146816, -9.564922557961047289, 104.1677570613523329 ) ) ;
#143767=CARTESIAN_POINT ( 'NONE',  ( -21.52544592524334988, -5.823673210054445271, 73.95942372801901854 ) ) ;
#143768=CARTESIAN_POINT ( 'NONE',  ( 14.29746914071037800, 8.314922557961029526, 31.66775706135234358 ) ) ;
#143769=CARTESIAN_POINT ( 'NONE',  ( 5.823673210054125526, 21.52544592524343514, 84.79057627198102409 ) ) ;
#143770=CARTESIAN_POINT ( 'NONE',  ( -19.05341960407617563, 5.049401038297882671, 103.5427570613523329 ) ) ;
#143771=CARTESIAN_POINT ( 'NONE',  ( -13.89961937509977652, 13.97604488694528158, 70.62390960531432427 ) ) ;
#143772=CARTESIAN_POINT ( 'NONE',  ( 13.97604488694548053, -13.89961937509957401, 110.6260903946856615 ) ) ;
#143773=CARTESIAN_POINT ( 'NONE',  ( 9.474510206698729675, 16.51473224551082808, 107.0844237280190043 ) ) ;
#143774=CARTESIAN_POINT ( 'NONE',  ( 4.379528057220339221, -16.55341960407611168, 62.70724293864769550 ) ) ;
#143775=CARTESIAN_POINT ( 'NONE',  ( 5.153800228976615827, -19.02544592524334988, 75.20942372801896170 ) ) ;
#143776=CARTESIAN_POINT ( 'NONE',  ( -8.314922557961024197, 14.29746914071037800, 72.91775706135234714 ) ) ;
#143777=CARTESIAN_POINT ( 'NONE',  ( -10.72451020669898014, 18.67979575497178502, 115.4155762719810241 ) ) ;
#143778=CARTESIAN_POINT ( 'NONE',  ( -19.05341960407611168, -5.049401038298163336, 56.45724293864768129 ) ) ;
#143779=CARTESIAN_POINT ( 'NONE',  ( -13.89961937509977652, 13.97604488694528158, 55.62390960531434558 ) ) ;
#143780=CARTESIAN_POINT ( 'NONE',  ( 16.55341960407618274, -4.379528057220086978, 66.04275706135236135 ) ) ;
#143784=CARTESIAN_POINT ( 'NONE',  ( 18.67979575497194134, -10.72451020669871369, 110.8344237280190043 ) ) ;
#143787=CARTESIAN_POINT ( 'NONE',  ( 16.46253265017146816, 9.564922557961045513, 111.6677570613523329 ) ) ;
#143788=CARTESIAN_POINT ( 'NONE',  ( 21.52544592524344225, -5.823673210054117533, 48.54057627198103120 ) ) ;
#143789=CARTESIAN_POINT ( 'NONE',  ( 13.97604488694548053, -13.89961937509957401, 50.62609039468566152 ) ) ;
#143790=CARTESIAN_POINT ( 'NONE',  ( 14.34966873604972726, -8.224510206698740333, 35.83442372801901143 ) ) ;
#143791=CARTESIAN_POINT ( 'NONE',  ( -19.03943276465977164, 0.05219959533909376836, 46.24890960531435979 ) ) ;
#143792=CARTESIAN_POINT ( 'NONE',  ( 9.564922557960805705, 16.46253265017160317, 44.58224293864769550 ) ) ;
#143793=CARTESIAN_POINT ( 'NONE',  ( -5.719274019375978568, 21.55341960407610458, 85.20724293864770971 ) ) ;
#143794=CARTESIAN_POINT ( 'NONE',  ( -13.89961937509977652, 13.97604488694528158, 115.6239096053143669 ) ) ;
#143795=CARTESIAN_POINT ( 'NONE',  ( 9.564922557960805705, 16.46253265017160317, 49.58224293864770260 ) ) ;
#143797=CARTESIAN_POINT ( 'NONE',  ( 19.02544592524334988, 5.153800228976608722, 91.45942372801900433 ) ) ;
#143798=CARTESIAN_POINT ( 'NONE',  ( -16.55341960407611168, -4.379528057220339221, 61.45724293864770260 ) ) ;
#143799=CARTESIAN_POINT ( 'NONE',  ( 0.05219959533936267826, -19.03943276465977164, 20.00109039468567218 ) ) ;
#143800=CARTESIAN_POINT ( 'NONE',  ( -5.823673210054116645, -21.52544592524344225, 92.29057627198103830 ) ) ;
#143801=CARTESIAN_POINT ( 'NONE',  ( 10.72451020669871369, 18.67979575497193778, 82.08442372801901854 ) ) ;
#143802=CARTESIAN_POINT ( 'NONE',  ( -19.05341960407611168, -5.049401038298163336, 26.45724293864769550 ) ) ;
#143803=CARTESIAN_POINT ( 'NONE',  ( -15.72974639402176322, -15.80617190586768395, 84.37609039468570415 ) ) ;
#143804=CARTESIAN_POINT ( 'NONE',  ( -16.53943276465976808, 0.05219959533911058130, 21.24890960531436690 ) ) ;
#143805=CARTESIAN_POINT ( 'NONE',  ( 15.80617190586769283, -15.72974639402175789, 80.62609039468567573 ) ) ;
#143806=CARTESIAN_POINT ( 'NONE',  ( -5.153800228976328057, -19.02544592524343514, 67.29057627198102409 ) ) ;
#143807=EDGE_CURVE ( 'NONE', #96182, #11730, #114680, .T. ) ;
#143808=CARTESIAN_POINT ( 'NONE',  ( 0.05219959533937995610, -21.53943276465977519, 50.00109039468568994 ) ) ;
#143809=CARTESIAN_POINT ( 'NONE',  ( 9.564922557960805705, 16.46253265017160317, 84.58224293864769550 ) ) ;
#143810=CARTESIAN_POINT ( 'NONE',  ( 14.29746914071049879, -8.314922557960816363, 93.33224293864769550 ) ) ;
#143811=CARTESIAN_POINT ( 'NONE',  ( -8.224510206698948167, 14.34966873604960824, 55.41557627198102409 ) ) ;
#143812=CARTESIAN_POINT ( 'NONE',  ( 5.823673210054125526, 21.52544592524343514, 74.79057627198105251 ) ) ;
#143813=CARTESIAN_POINT ( 'NONE',  ( 19.03943276465977164, -0.05219959533909143690, 58.74890960531435979 ) ) ;
#143814=CARTESIAN_POINT ( 'NONE',  ( 10.81492255796078972, 18.62759615963270932, 79.58224293864769550 ) ) ;
#143816=CARTESIAN_POINT ( 'NONE',  ( -9.474510206698720793, -16.51473224551083518, 69.58442372801901854 ) ) ;
#143817=CARTESIAN_POINT ( 'NONE',  ( -17.59860650958993844, 7.585241751806885979, 38.42337014262493256 ) ) ;
#143818=CARTESIAN_POINT ( 'NONE',  ( 16.55341960407611168, 4.379528057220329451, 78.95724293864769550 ) ) ;
#143819=CARTESIAN_POINT ( 'NONE',  ( -10.81492255796078084, -18.62759615963271287, 47.08224293864770260 ) ) ;
#143821=CARTESIAN_POINT ( 'NONE',  ( 4.379528057220092307, 16.55341960407617563, 102.2927570613523613 ) ) ;
#143823=CARTESIAN_POINT ( 'NONE',  ( -9.564922557961040184, 16.46253265017147172, 102.9177570613523329 ) ) ;
#143824=EDGE_CURVE ( 'NONE', #115197, #33312, #72003, .T. ) ;
#143825=CARTESIAN_POINT ( 'NONE',  ( 8.224510206698953496, -14.34966873604960469, 72.91557627198103830 ) ) ;
#143827=CARTESIAN_POINT ( 'NONE',  ( 9.564922557960805705, 16.46253265017160317, 59.58224293864769550 ) ) ;
#143828=CARTESIAN_POINT ( 'NONE',  ( -8.224510206698948167, 14.34966873604960824, 60.41557627198102409 ) ) ;
#143829=CARTESIAN_POINT ( 'NONE',  ( -0.05219959533909027116, -19.03943276465977164, 107.4989096053143527 ) ) ;
#143830=CARTESIAN_POINT ( 'NONE',  ( 19.03943276465977164, 0.05219959533936151252, 76.25109039468566152 ) ) ;
#143831=CARTESIAN_POINT ( 'NONE',  ( -0.05219959533909027116, -19.03943276465977164, 72.49890960531435269 ) ) ;
#143832=CARTESIAN_POINT ( 'NONE',  ( 16.46253265017160672, -9.564922557960803928, 88.33224293864769550 ) ) ;
#143833=CARTESIAN_POINT ( 'NONE',  ( -13.97604488694527625, -13.89961937509977652, 86.87390960531436690 ) ) ;
#143834=CARTESIAN_POINT ( 'NONE',  ( 18.67979575497178502, 10.72451020669898547, 69.16557627198102409 ) ) ;
#143835=CARTESIAN_POINT ( 'NONE',  ( -16.52544592524335698, -4.483927247898792601, 63.95942372801901854 ) ) ;
#143836=CONICAL_SURFACE ( 'NONE', #163212, 2.500000000000002220, 1.029744260000000189 ) ;
#143837=CARTESIAN_POINT ( 'NONE',  ( -15.49999999999999822, -5.500000000000000888, 22.00000000000000000 ) ) ;
#143838=CARTESIAN_POINT ( 'NONE',  ( 0.05219959533909260263, 19.03943276465977164, 44.99890960531435979 ) ) ;
#143839=CARTESIAN_POINT ( 'NONE',  ( -5.719274019375978568, 21.55341960407610458, 50.20724293864769550 ) ) ;
#143840=CARTESIAN_POINT ( 'NONE',  ( 19.02544592524334988, 5.153800228976608722, 96.45942372801897591 ) ) ;
#143841=CARTESIAN_POINT ( 'NONE',  ( 4.483927247898545687, 16.52544592524342804, 24.79057627198103120 ) ) ;
#143842=CARTESIAN_POINT ( 'NONE',  ( -21.53943276465977519, -0.05219959533937600094, 33.75109039468568284 ) ) ;
#143843=CARTESIAN_POINT ( 'NONE',  ( 9.474510206698729675, 16.51473224551082808, 32.08442372801900433 ) ) ;
#143844=CARTESIAN_POINT ( 'NONE',  ( -16.52544592524335698, -4.483927247898792601, 58.95942372801902565 ) ) ;
#143845=CARTESIAN_POINT ( 'NONE',  ( -12.14591786802326823, 12.06949235617739902, 88.12609039468570415 ) ) ;
#143847=CARTESIAN_POINT ( 'NONE',  ( -16.55341960407617563, 4.379528057220093196, 78.54275706135236135 ) ) ;
#143848=CARTESIAN_POINT ( 'NONE',  ( -15.80617190586745835, -15.72974639402198527, 26.87390960531435979 ) ) ;
#143849=CARTESIAN_POINT ( 'NONE',  ( -16.55341960407617563, 4.379528057220093196, 33.54275706135234714 ) ) ;
#143850=CARTESIAN_POINT ( 'NONE',  ( -19.05341960407611168, -5.049401038298163336, 41.45724293864769550 ) ) ;
#143851=CARTESIAN_POINT ( 'NONE',  ( 5.049401038298161559, -19.05341960407611168, 52.70724293864767418 ) ) ;
#143852=CARTESIAN_POINT ( 'NONE',  ( -19.05341960407611168, -5.049401038298163336, 56.45724293864768129 ) ) ;
#143853=CARTESIAN_POINT ( 'NONE',  ( -10.72451020669870658, -18.67979575497194134, 34.58442372801900433 ) ) ;
#143854=CARTESIAN_POINT ( 'NONE',  ( 16.52544592524335698, 4.483927247898782831, 46.45942372801901854 ) ) ;
#143855=CARTESIAN_POINT ( 'NONE',  ( 16.52544592524335698, 4.483927247898782831, 106.4594237280190328 ) ) ;
#143856=CARTESIAN_POINT ( 'NONE',  ( -0.05219959533909027116, -19.03943276465977164, 32.49890960531435979 ) ) ;
#143857=CARTESIAN_POINT ( 'NONE',  ( -5.719274019375665041, -21.55341960407619695, 109.7927570613523613 ) ) ;
#143858=CARTESIAN_POINT ( 'NONE',  ( 9.564922557961047289, -16.46253265017146816, 110.4177570613523471 ) ) ;
#143859=CARTESIAN_POINT ( 'NONE',  ( 0.05219959533936267826, -19.03943276465977164, 70.00109039468566152 ) ) ;
#143860=CARTESIAN_POINT ( 'NONE',  ( -14.34966873604960291, -8.224510206698953496, 66.66557627198102409 ) ) ;
#143861=CARTESIAN_POINT ( 'NONE',  ( 16.51473224551069308, 9.474510206698969483, 34.16557627198102409 ) ) ;
#143862=CARTESIAN_POINT ( 'NONE',  ( -16.46253265017146816, -9.564922557961047289, 69.16775706135233293 ) ) ;
#143864=CARTESIAN_POINT ( 'NONE',  ( -15.80617190586768217, 15.72974639402176855, 73.12609039468567573 ) ) ;
#143865=CARTESIAN_POINT ( 'NONE',  ( 16.53943276465976808, 0.05219959533934440121, 36.25109039468567573 ) ) ;
#143867=CARTESIAN_POINT ( 'NONE',  ( -10.81492255796078084, -18.62759615963271287, 37.08224293864768129 ) ) ;
#143868=CARTESIAN_POINT ( 'NONE',  ( 16.52544592524335698, 4.483927247898782831, 26.45942372801901854 ) ) ;
#143869=CARTESIAN_POINT ( 'NONE',  ( 9.474510206698971260, -16.51473224551069308, 27.91557627198103120 ) ) ;
#143870=CARTESIAN_POINT ( 'NONE',  ( 19.03943276465977164, 0.05219959533936151252, 31.25109039468566863 ) ) ;
#143872=CARTESIAN_POINT ( 'NONE',  ( -0.05219959533909027116, -19.03943276465977164, 37.49890960531436690 ) ) ;
#143873=CARTESIAN_POINT ( 'NONE',  ( -13.97604488694527625, -13.89961937509977652, 56.87390960531434558 ) ) ;
#143874=CARTESIAN_POINT ( 'NONE',  ( -19.34837522270365895, -5.499999999999741540, 55.86337684832579953 ) ) ;
#143875=CARTESIAN_POINT ( 'NONE',  ( 0.05219959533936267826, -19.03943276465977164, 25.00109039468566152 ) ) ;
#143876=CARTESIAN_POINT ( 'NONE',  ( 12.14591786802309770, 12.06949235617756955, 24.37390960531435979 ) ) ;
#143877=CARTESIAN_POINT ( 'NONE',  ( 13.97604488694527802, 13.89961937509977652, 29.37390960531435979 ) ) ;
#143878=CARTESIAN_POINT ( 'NONE',  ( 9.474510206698971260, -16.51473224551069308, 97.91557627198102409 ) ) ;
#143879=CARTESIAN_POINT ( 'NONE',  ( -10.81492255796105439, 18.62759615963255655, 72.91775706135234714 ) ) ;
#143880=CARTESIAN_POINT ( 'NONE',  ( -0.05219959533909027116, -19.03943276465977164, 37.49890960531436690 ) ) ;
#143881=CARTESIAN_POINT ( 'NONE',  ( 10.81492255796106328, -18.62759615963255655, 65.41775706135234714 ) ) ;
#143882=CARTESIAN_POINT ( 'NONE',  ( -13.89961937509957401, -13.97604488694547875, 99.37609039468567573 ) ) ;
#143883=CARTESIAN_POINT ( 'NONE',  ( -18.67979575497178146, -10.72451020669898902, 26.66557627198103475 ) ) ;
#143884=CARTESIAN_POINT ( 'NONE',  ( -9.474510206698964154, 16.51473224551069663, 40.41557627198103120 ) ) ;
#143885=CARTESIAN_POINT ( 'NONE',  ( 18.62759615963271287, -10.81492255796078972, 113.3322429386476955 ) ) ;
#143886=CARTESIAN_POINT ( 'NONE',  ( -5.049401038297874678, -19.05341960407617918, 34.79275706135233293 ) ) ;
#143887=CARTESIAN_POINT ( 'NONE',  ( -13.97604488694527625, -13.89961937509977652, 21.87390960531435979 ) ) ;
#143888=CARTESIAN_POINT ( 'NONE',  ( -19.05341960407611168, -5.049401038298163336, 61.45724293864769550 ) ) ;
#143889=CARTESIAN_POINT ( 'NONE',  ( 19.05341960407617918, -5.049401038297876454, 111.0427570613523329 ) ) ;
#143890=CARTESIAN_POINT ( 'NONE',  ( 12.14591786802309770, 12.06949235617756955, 74.37390960531436690 ) ) ;
#143891=CARTESIAN_POINT ( 'NONE',  ( -13.89961937509977652, 13.97604488694528158, 115.6239096053143669 ) ) ;
#143892=CARTESIAN_POINT ( 'NONE',  ( 13.89961937509957401, 13.97604488694547697, 91.87609039468567573 ) ) ;
#143893=CARTESIAN_POINT ( 'NONE',  ( -0.05219959533907301413, -21.53943276465977519, 97.49890960531436690 ) ) ;
#143894=CARTESIAN_POINT ( 'NONE',  ( -18.62759615963255300, -10.81492255796106328, 44.16775706135234714 ) ) ;
#143895=CARTESIAN_POINT ( 'NONE',  ( 4.483927247898790824, -16.52544592524335698, 45.20942372801901854 ) ) ;
#143896=CARTESIAN_POINT ( 'NONE',  ( -16.52544592524335698, -4.483927247898792601, 58.95942372801902565 ) ) ;
#143897=CARTESIAN_POINT ( 'NONE',  ( -18.67979575497193778, 10.72451020669871902, 43.33442372801901143 ) ) ;
#143898=CARTESIAN_POINT ( 'NONE',  ( -15.80617190586745835, -15.72974639402198527, 56.87390960531436690 ) ) ;
#143899=CARTESIAN_POINT ( 'NONE',  ( -9.474510206698964154, 16.51473224551069663, 50.41557627198102409 ) ) ;
#143901=CARTESIAN_POINT ( 'NONE',  ( 12.14591786802327356, -12.06949235617739191, 75.62609039468567573 ) ) ;
#143902=CARTESIAN_POINT ( 'NONE',  ( -0.05219959533907301413, -21.53943276465977519, 102.4989096053143811 ) ) ;
#143903=CARTESIAN_POINT ( 'NONE',  ( -4.483927247898539470, -16.52544592524342804, 57.29057627198103120 ) ) ;
#143904=CARTESIAN_POINT ( 'NONE',  ( 8.224510206698742110, 14.34966873604972548, 67.08442372801901854 ) ) ;
#143905=CARTESIAN_POINT ( 'NONE',  ( -5.153800228976607833, 19.02544592524334988, 97.70942372801900433 ) ) ;
#143906=CARTESIAN_POINT ( 'NONE',  ( 10.81492255796078972, 18.62759615963270932, 99.58224293864770971 ) ) ;
#143907=CARTESIAN_POINT ( 'NONE',  ( 16.52544592524342804, -4.483927247898539470, 48.54057627198103120 ) ) ;
#143909=CARTESIAN_POINT ( 'NONE',  ( -18.67979575497178146, -10.72451020669898902, 76.66557627198103830 ) ) ;
#143911=CARTESIAN_POINT ( 'NONE',  ( -14.34966873604960291, -8.224510206698953496, 26.66557627198103475 ) ) ;
#143912=ORIENTED_EDGE ( 'NONE', *, *, #74692, .F. ) ;
#143913=CARTESIAN_POINT ( 'NONE',  ( -17.49999999999999289, -5.622605283950892208, 56.31207310596111171 ) ) ;
#143914=CARTESIAN_POINT ( 'NONE',  ( 21.53943276465977519, -0.05219959533907433946, 103.7489096053143669 ) ) ;
#143916=CARTESIAN_POINT ( 'NONE',  ( -18.62759615963270932, 10.81492255796079327, 110.8322429386476955 ) ) ;
#143917=CARTESIAN_POINT ( 'NONE',  ( 0.05219959533910956823, 16.53943276465976808, 39.99890960531436690 ) ) ;
#143918=CARTESIAN_POINT ( 'NONE',  ( 0.05219959533934541429, -16.53943276465976808, 50.00109039468568994 ) ) ;
#143919=CARTESIAN_POINT ( 'NONE',  ( -19.03943276465977164, 0.05219959533909376836, 46.24890960531435979 ) ) ;
#143920=CARTESIAN_POINT ( 'NONE',  ( -9.564922557960796823, -16.46253265017161027, 72.08224293864770971 ) ) ;
#143922=CARTESIAN_POINT ( 'NONE',  ( 21.52544592524344225, -5.823673210054117533, 28.54057627198103120 ) ) ;
#143924=CARTESIAN_POINT ( 'NONE',  ( -5.153800228976607833, 19.02544592524334988, 102.7094237280189759 ) ) ;
#143925=CARTESIAN_POINT ( 'NONE',  ( 16.46253265017146816, 9.564922557961045513, 56.66775706135233293 ) ) ;
#143926=CARTESIAN_POINT ( 'NONE',  ( -15.72974639402197994, 15.80617190586746368, 105.6239096053143669 ) ) ;
#143927=CARTESIAN_POINT ( 'NONE',  ( 16.53943276465976808, -0.05219959533910856209, 28.74890960531435624 ) ) ;
#143928=CARTESIAN_POINT ( 'NONE',  ( 9.564922557960805705, 16.46253265017160317, 79.58224293864769550 ) ) ;
#143929=CARTESIAN_POINT ( 'NONE',  ( 15.80617190586746368, 15.72974639402197994, 49.37390960531436690 ) ) ;
#143930=CARTESIAN_POINT ( 'NONE',  ( 10.81492255796078972, 18.62759615963270932, 79.58224293864769550 ) ) ;
#143931=CARTESIAN_POINT ( 'NONE',  ( -12.14591786802326823, 12.06949235617739902, 28.12609039468568284 ) ) ;
#143933=CARTESIAN_POINT ( 'NONE',  ( 0.05219959533909260263, 19.03943276465977164, 114.9989096053143669 ) ) ;
#143934=CARTESIAN_POINT ( 'NONE',  ( 10.72451020669871369, 18.67979575497193778, 72.08442372801899012 ) ) ;
#143935=CARTESIAN_POINT ( 'NONE',  ( 16.46253265017160672, -9.564922557960803928, 68.33224293864770971 ) ) ;
#143936=CARTESIAN_POINT ( 'NONE',  ( -19.05341960407611168, -5.049401038298163336, 26.45724293864769550 ) ) ;
#143937=CARTESIAN_POINT ( 'NONE',  ( 5.153800228976335163, 19.02544592524342804, 89.79057627198102409 ) ) ;
#143938=CARTESIAN_POINT ( 'NONE',  ( 8.224510206698953496, -14.34966873604960469, 97.91557627198103830 ) ) ;
#143940=CARTESIAN_POINT ( 'NONE',  ( -5.049401038297874678, -19.05341960407617918, 104.7927570613523471 ) ) ;
#143941=CARTESIAN_POINT ( 'NONE',  ( 17.48847506799968698, -5.747544572773781724, 83.32697437843280852 ) ) ;
#143942=CARTESIAN_POINT ( 'NONE',  ( 16.46253265017160672, -9.564922557960803928, 68.33224293864770971 ) ) ;
#143943=CARTESIAN_POINT ( 'NONE',  ( -21.52544592524334988, -5.823673210054445271, 83.95942372801900433 ) ) ;
#143944=CARTESIAN_POINT ( 'NONE',  ( 18.67979575497178502, 10.72451020669898547, 24.16557627198103120 ) ) ;
#143945=CARTESIAN_POINT ( 'NONE',  ( 12.06949235617739724, 12.14591786802326823, 76.87609039468567573 ) ) ;
#143947=CARTESIAN_POINT ( 'NONE',  ( -17.12812012977029497, -6.668231424565920662, 76.35948759323146362 ) ) ;
#143948=CARTESIAN_POINT ( 'NONE',  ( -9.564922557961040184, 16.46253265017147172, 52.91775706135233293 ) ) ;
#143949=CARTESIAN_POINT ( 'NONE',  ( -9.474510206698720793, -16.51473224551083518, 24.58442372801900078 ) ) ;
#143951=CARTESIAN_POINT ( 'NONE',  ( -16.51473224551069308, -9.474510206698971260, 21.66557627198102765 ) ) ;
#143953=CARTESIAN_POINT ( 'NONE',  ( 12.14591786802327356, -12.06949235617739191, 110.6260903946857042 ) ) ;
#143954=DIRECTION ( 'NONE',  ( 0.000000000000000000, 0.000000000000000000, 1.000000000000000000 ) ) ;
#143955=CARTESIAN_POINT ( 'NONE',  ( 8.224510206698742110, 14.34966873604972548, 102.0844237280190185 ) ) ;
#143957=CARTESIAN_POINT ( 'NONE',  ( 12.14591786802327356, -12.06949235617739191, 80.62609039468567573 ) ) ;
#143958=CARTESIAN_POINT ( 'NONE',  ( 21.52544592524334988, 5.823673210054432836, 91.45942372801901854 ) ) ;
#143959=CARTESIAN_POINT ( 'NONE',  ( 13.97604488694548053, -13.89961937509957401, 100.6260903946856615 ) ) ;
#143960=CARTESIAN_POINT ( 'NONE',  ( 21.53943276465977519, 0.05219959533937863772, 61.25109039468567573 ) ) ;
#143961=CARTESIAN_POINT ( 'NONE',  ( 9.564922557961047289, -16.46253265017146816, 40.41775706135234003 ) ) ;
#143962=CARTESIAN_POINT ( 'NONE',  ( -9.564922557960796823, -16.46253265017161027, 82.08224293864768129 ) ) ;
#143963=CARTESIAN_POINT ( 'NONE',  ( -19.02544592524342804, 5.153800228976336051, 51.04057627198103120 ) ) ;
#143964=CARTESIAN_POINT ( 'NONE',  ( -19.26498983726237313, 5.499999999999599432, 40.55319577422005040 ) ) ;
#143965=CARTESIAN_POINT ( 'NONE',  ( -21.55341960407610458, -5.719274019375992779, 96.45724293864770971 ) ) ;
#143966=B_SPLINE_CURVE_WITH_KNOTS ( 'NONE', 3,
 ( #193995, #165642, #42303, #104956, #12958, #164647, #163647, #166642, #57472, #196984, #27140, #194985, #29124, #148478, #74622, #120118, #56463, #182801, #167627, #28144, #90762, #9969 ),
 .UNSPECIFIED., .F., .F.,
 ( 4, 2, 2, 2, 2, 2, 2, 2, 2, 2, 4 ),
 ( 1.262897753262583006E-17, 0.001309639967555230192, 0.001964459951332838891, 0.002291869943221642916, 0.002455574939166047747, 0.002619279935110452578, 0.002782984931054856975, 0.002946689926999261806, 0.003274099918888071035, 0.003928919902665695130, 0.005238559870220941585 ),
 .UNSPECIFIED. ) ;
#143967=CARTESIAN_POINT ( 'NONE',  ( 10.72451020669898902, -18.67979575497178502, 47.91557627198102409 ) ) ;
#143968=CARTESIAN_POINT ( 'NONE',  ( 5.049401038298161559, -19.05341960407611168, 52.70724293864767418 ) ) ;
#143969=CARTESIAN_POINT ( 'NONE',  ( 0.05219959533934541429, -16.53943276465976808, 65.00109039468568994 ) ) ;
#143971=EDGE_CURVE ( 'NONE', #123998, #163715, #52653, .T. ) ;
#143972=CARTESIAN_POINT ( 'NONE',  ( 21.52544592524334988, 5.823673210054432836, 41.45942372801901143 ) ) ;
#143973=CARTESIAN_POINT ( 'NONE',  ( 4.379528057220339221, -16.55341960407611168, 77.70724293864770971 ) ) ;
#143975=CARTESIAN_POINT ( 'NONE',  ( 8.314922557961029526, -14.29746914071037800, 40.41775706135234714 ) ) ;
#143976=CARTESIAN_POINT ( 'NONE',  ( 14.29746914071049879, -8.314922557960816363, 108.3322429386477097 ) ) ;
#143977=CARTESIAN_POINT ( 'NONE',  ( 0.05219959533936267826, -19.03943276465977164, 55.00109039468566863 ) ) ;
#143978=CARTESIAN_POINT ( 'NONE',  ( 14.29746914071049879, -8.314922557960816363, 68.33224293864769550 ) ) ;
#143979=CARTESIAN_POINT ( 'NONE',  ( 10.72451020669871369, 18.67979575497193778, 32.08442372801901854 ) ) ;
#143980=CARTESIAN_POINT ( 'NONE',  ( 13.89961937509977652, -13.97604488694527269, 28.12390960531435624 ) ) ;
#143981=CARTESIAN_POINT ( 'NONE',  ( 21.52544592524344225, -5.823673210054117533, 93.54057627198103830 ) ) ;
#143982=CARTESIAN_POINT ( 'NONE',  ( -5.049401038298153566, 19.05341960407611168, 100.2072429386476955 ) ) ;
#143983=CARTESIAN_POINT ( 'NONE',  ( 16.52544592524342804, -4.483927247898539470, 68.54057627198103830 ) ) ;
#143986=CARTESIAN_POINT ( 'NONE',  ( -5.049401038297874678, -19.05341960407617918, 84.79275706135233293 ) ) ;
#143987=CARTESIAN_POINT ( 'NONE',  ( -5.719274019375978568, 21.55341960407610458, 115.2072429386476955 ) ) ;
#143988=CARTESIAN_POINT ( 'NONE',  ( -13.89961937509977652, 13.97604488694528158, 75.62390960531438111 ) ) ;
#143989=CARTESIAN_POINT ( 'NONE',  ( -5.153800228976607833, 19.02544592524334988, 62.70942372801899722 ) ) ;
#143990=CARTESIAN_POINT ( 'NONE',  ( 16.46253265017160672, -9.564922557960803928, 48.33224293864769550 ) ) ;
#143991=CARTESIAN_POINT ( 'NONE',  ( 12.14591786802309770, 12.06949235617756955, 64.37390960531435269 ) ) ;
#143992=CARTESIAN_POINT ( 'NONE',  ( -12.06949235617756955, 12.14591786802309770, 55.62390960531436690 ) ) ;
#143993=CARTESIAN_POINT ( 'NONE',  ( 16.46253265017160672, -9.564922557960803928, 73.33224293864769550 ) ) ;
#143994=CARTESIAN_POINT ( 'NONE',  ( -0.05219959533907301413, -21.53943276465977519, 87.49890960531436690 ) ) ;
#143995=CARTESIAN_POINT ( 'NONE',  ( 9.474510206698971260, -16.51473224551069308, 77.91557627198103830 ) ) ;
#143996=CARTESIAN_POINT ( 'NONE',  ( 10.81492255796078972, 18.62759615963270932, 84.58224293864769550 ) ) ;
#143997=CARTESIAN_POINT ( 'NONE',  ( 16.46253265017146816, 9.564922557961045513, 21.66775706135233648 ) ) ;
#143999=CARTESIAN_POINT ( 'NONE',  ( -16.53943276465976808, -0.05219959533934237506, 108.7510903946857042 ) ) ;
#144000=CARTESIAN_POINT ( 'NONE',  ( -16.53943276465976808, 0.05219959533911058130, 91.24890960531436690 ) ) ;
#144001=CARTESIAN_POINT ( 'NONE',  ( 16.46253265017146816, 9.564922557961045513, 86.66775706135233293 ) ) ;
#144002=ORIENTED_EDGE ( 'NONE', *, *, #44938, .T. ) ;
#144003=CARTESIAN_POINT ( 'NONE',  ( 18.62759615963255655, 10.81492255796105972, 21.66775706135235069 ) ) ;
#144004=CARTESIAN_POINT ( 'NONE',  ( 16.46253265017146816, 9.564922557961045513, 56.66775706135233293 ) ) ;
#144005=CARTESIAN_POINT ( 'NONE',  ( 12.14591786802327356, -12.06949235617739191, 100.6260903946857184 ) ) ;
#144006=CARTESIAN_POINT ( 'NONE',  ( 16.51473224551083163, -9.474510206698727899, 40.83442372801900433 ) ) ;
#144007=CARTESIAN_POINT ( 'NONE',  ( 19.05341960407611168, 5.049401038298154454, 103.9572429386476671 ) ) ;
#144008=CARTESIAN_POINT ( 'NONE',  ( -8.224510206698948167, 14.34966873604960824, 60.41557627198102409 ) ) ;
#144009=CARTESIAN_POINT ( 'NONE',  ( -19.52837319214026834, 5.499999999999896971, 49.60471352585536664 ) ) ;
#144010=CARTESIAN_POINT ( 'NONE',  ( 0.05219959533909260263, 19.03943276465977164, 39.99890960531436690 ) ) ;
#144011=CARTESIAN_POINT ( 'NONE',  ( -21.52544592524334988, -5.823673210054445271, 103.9594237280190185 ) ) ;
#144012=CARTESIAN_POINT ( 'NONE',  ( -0.05219959533934338120, 16.53943276465976808, 72.50109039468568994 ) ) ;
#144013=CARTESIAN_POINT ( 'NONE',  ( -21.53943276465977519, -0.05219959533937600094, 38.75109039468567573 ) ) ;
#144014=CARTESIAN_POINT ( 'NONE',  ( -8.224510206698735004, -14.34966873604973081, 49.58442372801901143 ) ) ;
#144015=CARTESIAN_POINT ( 'NONE',  ( 19.02544592524343514, -5.153800228976328945, 103.5405762719809957 ) ) ;
#144016=CARTESIAN_POINT ( 'NONE',  ( -19.05341960407611168, -5.049401038298163336, 56.45724293864768129 ) ) ;
#144017=CARTESIAN_POINT ( 'NONE',  ( 5.153800228976335163, 19.02544592524342804, 69.79057627198103830 ) ) ;
#144018=VECTOR ( 'NONE', #188004, 1000.000000000000000 ) ;
#144019=CARTESIAN_POINT ( 'NONE',  ( -16.52544592524335698, -4.483927247898792601, 53.95942372801900433 ) ) ;
#144020=CARTESIAN_POINT ( 'NONE',  ( 16.53943276465976808, -0.05219959533910856209, 108.7489096053143669 ) ) ;
#144021=CARTESIAN_POINT ( 'NONE',  ( -4.483927247898782831, 16.52544592524335698, 107.7094237280190328 ) ) ;
#144023=CARTESIAN_POINT ( 'NONE',  ( 18.67979575497194134, -10.72451020669871369, 55.83442372801901854 ) ) ;
#144024=CARTESIAN_POINT ( 'NONE',  ( 19.02544592524343514, -5.153800228976328945, 88.54057627198102409 ) ) ;
#144025=CARTESIAN_POINT ( 'NONE',  ( -5.153800228976328057, -19.02544592524343514, 77.29057627198099567 ) ) ;
#144026=CARTESIAN_POINT ( 'NONE',  ( 19.02544592524343514, -5.153800228976328945, 98.54057627198100988 ) ) ;
#144027=CARTESIAN_POINT ( 'NONE',  ( -12.06949235617756955, 12.14591786802309770, 50.62390960531435979 ) ) ;
#144028=CARTESIAN_POINT ( 'NONE',  ( 14.34966873604972726, -8.224510206698740333, 110.8344237280190043 ) ) ;
#144029=CARTESIAN_POINT ( 'NONE',  ( -14.29746914071049879, 8.314922557960819915, 35.83224293864768839 ) ) ;
#144032=CARTESIAN_POINT ( 'NONE',  ( -16.51473224551069308, -9.474510206698971260, 66.66557627198102409 ) ) ;
#144033=CARTESIAN_POINT ( 'NONE',  ( 19.03943276465977164, 0.05219959533936151252, 51.25109039468567573 ) ) ;
#144036=CARTESIAN_POINT ( 'NONE',  ( -13.97604488694547697, 13.89961937509957934, 83.12609039468564731 ) ) ;
#144037=CARTESIAN_POINT ( 'NONE',  ( -12.14591786802326823, 12.06949235617739902, 63.12609039468568994 ) ) ;
#144039=CARTESIAN_POINT ( 'NONE',  ( 13.97604488694527802, 13.89961937509977652, 94.37390960531436690 ) ) ;
#144040=CARTESIAN_POINT ( 'NONE',  ( -15.72974639402176322, -15.80617190586768395, 29.37609039468568284 ) ) ;
#144041=CARTESIAN_POINT ( 'NONE',  ( -5.049401038297874678, -19.05341960407617918, 89.79275706135230450 ) ) ;
#144042=CARTESIAN_POINT ( 'NONE',  ( 9.564922557960805705, 16.46253265017160317, 114.5822429386476955 ) ) ;
#144043=CARTESIAN_POINT ( 'NONE',  ( -5.153800228976328057, -19.02544592524343514, 42.29057627198101699 ) ) ;
#144044=CARTESIAN_POINT ( 'NONE',  ( -16.51473224551069308, -9.474510206698971260, 96.66557627198102409 ) ) ;
#144045=CARTESIAN_POINT ( 'NONE',  ( -8.314922557960811034, -14.29746914071050412, 42.08224293864769550 ) ) ;
#144046=CARTESIAN_POINT ( 'NONE',  ( -16.51473224551069308, -9.474510206698971260, 46.66557627198102409 ) ) ;
#144047=CARTESIAN_POINT ( 'NONE',  ( -5.153800228976607833, 19.02544592524334988, 62.70942372801899722 ) ) ;
#144049=CARTESIAN_POINT ( 'NONE',  ( -16.52544592524342804, 4.483927247898546575, 81.04057627198102409 ) ) ;
#144050=CARTESIAN_POINT ( 'NONE',  ( 0.05219959533936267826, -19.03943276465977164, 35.00109039468566863 ) ) ;
#144051=CARTESIAN_POINT ( 'NONE',  ( -13.89961937509977652, 13.97604488694528158, 70.62390960531432427 ) ) ;
#144052=CARTESIAN_POINT ( 'NONE',  ( -21.55341960407610458, -5.719274019375992779, 66.45724293864768129 ) ) ;
#144053=CARTESIAN_POINT ( 'NONE',  ( -14.29746914071049879, 8.314922557960819915, 65.83224293864769550 ) ) ;
#144054=CARTESIAN_POINT ( 'NONE',  ( 16.51473224551083163, -9.474510206698727899, 25.83442372801900078 ) ) ;
#144055=CARTESIAN_POINT ( 'NONE',  ( 19.03943276465977164, -0.05219959533909143690, 108.7489096053143527 ) ) ;
#144057=CARTESIAN_POINT ( 'NONE',  ( 21.52544592524344225, -5.823673210054117533, 28.54057627198103120 ) ) ;
#144058=CARTESIAN_POINT ( 'NONE',  ( 19.05341960407611168, 5.049401038298154454, 48.95724293864768129 ) ) ;
#144059=CARTESIAN_POINT ( 'NONE',  ( 5.049401038298161559, -19.05341960407611168, 32.70724293864768129 ) ) ;
#144060=CARTESIAN_POINT ( 'NONE',  ( -12.14591786802309592, -12.06949235617757132, 101.8739096053143811 ) ) ;
#144061=CARTESIAN_POINT ( 'NONE',  ( -15.72974639402197994, 15.80617190586746368, 105.6239096053143669 ) ) ;
#144062=CARTESIAN_POINT ( 'NONE',  ( -16.51473224551069308, -9.474510206698971260, 111.6655762719810383 ) ) ;
#144063=CARTESIAN_POINT ( 'NONE',  ( -18.67979575497193778, 10.72451020669871902, 23.33442372801901499 ) ) ;
#144064=CARTESIAN_POINT ( 'NONE',  ( -19.03943276465977164, 0.05219959533909376836, 106.2489096053143669 ) ) ;
#144065=CARTESIAN_POINT ( 'NONE',  ( 4.483927247898545687, 16.52544592524342804, 114.7905762719810383 ) ) ;
#144066=CARTESIAN_POINT ( 'NONE',  ( -15.80617190586768217, 15.72974639402176855, 78.12609039468570415 ) ) ;
#144067=CARTESIAN_POINT ( 'NONE',  ( 10.72451020669898902, -18.67979575497178502, 92.91557627198103830 ) ) ;
#144069=CARTESIAN_POINT ( 'NONE',  ( 18.56453257813364743, -5.500000000000051514, 78.49000423690682737 ) ) ;
#144071=CARTESIAN_POINT ( 'NONE',  ( -12.14591786802326823, 12.06949235617739902, 53.12609039468568284 ) ) ;
#144072=CARTESIAN_POINT ( 'NONE',  ( -12.14591786802309592, -12.06949235617757132, 101.8739096053143811 ) ) ;
#144074=CARTESIAN_POINT ( 'NONE',  ( -13.97604488694527625, -13.89961937509977652, 61.87390960531435979 ) ) ;
#144075=CARTESIAN_POINT ( 'NONE',  ( -12.06949235617756955, 12.14591786802309770, 90.62390960531436690 ) ) ;
#144076=CARTESIAN_POINT ( 'NONE',  ( -10.81492255796078084, -18.62759615963271287, 47.08224293864770260 ) ) ;
#144077=CARTESIAN_POINT ( 'NONE',  ( 8.224510206698953496, -14.34966873604960469, 67.91557627198102409 ) ) ;
#144078=CARTESIAN_POINT ( 'NONE',  ( -14.34966873604972548, 8.224510206698743886, 23.33442372801901499 ) ) ;
#144079=CARTESIAN_POINT ( 'NONE',  ( 10.72451020669871369, 18.67979575497193778, 82.08442372801901854 ) ) ;
#144081=CARTESIAN_POINT ( 'NONE',  ( -14.29746914071037622, -8.314922557961029526, 99.16775706135234714 ) ) ;
#144082=CARTESIAN_POINT ( 'NONE',  ( -4.483927247898539470, -16.52544592524342804, 37.29057627198102409 ) ) ;
#144083=CARTESIAN_POINT ( 'NONE',  ( -9.564922557960796823, -16.46253265017161027, 32.08224293864769550 ) ) ;
#144084=CARTESIAN_POINT ( 'NONE',  ( 9.564922557960805705, 16.46253265017160317, 89.58224293864769550 ) ) ;
#144085=CARTESIAN_POINT ( 'NONE',  ( -10.81492255796078084, -18.62759615963271287, 97.08224293864770971 ) ) ;
#144086=CARTESIAN_POINT ( 'NONE',  ( -8.314922557961024197, 14.29746914071037800, 42.91775706135235424 ) ) ;
#144087=CARTESIAN_POINT ( 'NONE',  ( 4.379528057220339221, -16.55341960407611168, 62.70724293864769550 ) ) ;
#144088=CARTESIAN_POINT ( 'NONE',  ( -0.05219959533937732626, 21.53943276465977519, 92.50109039468567573 ) ) ;
#144089=CARTESIAN_POINT ( 'NONE',  ( -4.379528057220086978, -16.55341960407618274, 94.79275706135234714 ) ) ;
#144090=CARTESIAN_POINT ( 'NONE',  ( 17.40805194821983903, -6.112264579160780364, 48.33371272510606786 ) ) ;
#144092=CARTESIAN_POINT ( 'NONE',  ( -16.53943276465976808, 0.05219959533911058130, 31.24890960531435979 ) ) ;
#144093=CARTESIAN_POINT ( 'NONE',  ( 0.05219959533934541429, -16.53943276465976808, 75.00109039468568994 ) ) ;
#144094=CARTESIAN_POINT ( 'NONE',  ( -19.03943276465977164, 0.05219959533909376836, 91.24890960531436690 ) ) ;
#144095=CARTESIAN_POINT ( 'NONE',  ( -13.89961937509977652, 13.97604488694528158, 105.6239096053143527 ) ) ;
#144096=CARTESIAN_POINT ( 'NONE',  ( 21.55341960407619695, -5.719274019375665929, 86.04275706135236135 ) ) ;
#144098=CARTESIAN_POINT ( 'NONE',  ( -4.379528057220086978, -16.55341960407618274, 94.79275706135234714 ) ) ;
#144099=CARTESIAN_POINT ( 'NONE',  ( -0.05219959533910754901, -16.53943276465976808, 57.49890960531435979 ) ) ;
#144100=CARTESIAN_POINT ( 'NONE',  ( 0.05219959533909260263, 19.03943276465977164, 74.99890960531435269 ) ) ;
#144102=CARTESIAN_POINT ( 'NONE',  ( -19.03943276465977164, -0.05219959533935918106, 108.7510903946856615 ) ) ;
#144103=CARTESIAN_POINT ( 'NONE',  ( -0.05219959533910754901, -16.53943276465976808, 107.4989096053143669 ) ) ;
#144104=CARTESIAN_POINT ( 'NONE',  ( 5.153800228976335163, 19.02544592524342804, 74.79057627198103830 ) ) ;
#144105=CARTESIAN_POINT ( 'NONE',  ( 14.34966873604972726, -8.224510206698740333, 20.83442372801901143 ) ) ;
#144107=CARTESIAN_POINT ( 'NONE',  ( 13.89961937509957401, 13.97604488694547697, 21.87609039468566152 ) ) ;
#144108=CARTESIAN_POINT ( 'NONE',  ( 12.14591786802327356, -12.06949235617739191, 75.62609039468567573 ) ) ;
#144109=CARTESIAN_POINT ( 'NONE',  ( -5.049401038297874678, -19.05341960407617918, 104.7927570613523471 ) ) ;
#144110=CARTESIAN_POINT ( 'NONE',  ( -12.06949235617756955, 12.14591786802309770, 110.6239096053143669 ) ) ;
#144111=CARTESIAN_POINT ( 'NONE',  ( -16.52544592524335698, -4.483927247898792601, 63.95942372801901854 ) ) ;
#144112=CARTESIAN_POINT ( 'NONE',  ( 4.379528057220092307, 16.55341960407617563, 57.29275706135234714 ) ) ;
#144113=CARTESIAN_POINT ( 'NONE',  ( -0.05219959533909027116, -19.03943276465977164, 22.49890960531436690 ) ) ;
#144114=CARTESIAN_POINT ( 'NONE',  ( -5.049401038297874678, -19.05341960407617918, 64.79275706135233293 ) ) ;
#144115=CARTESIAN_POINT ( 'NONE',  ( 21.52544592524334988, 5.823673210054432836, 111.4594237280190328 ) ) ;
#144116=CARTESIAN_POINT ( 'NONE',  ( 9.474510206698971260, -16.51473224551069308, 32.91557627198102409 ) ) ;
#144117=CARTESIAN_POINT ( 'NONE',  ( -5.049401038298153566, 19.05341960407611168, 85.20724293864766707 ) ) ;
#144118=CARTESIAN_POINT ( 'NONE',  ( 4.379528057220339221, -16.55341960407611168, 67.70724293864769550 ) ) ;
#144119=CARTESIAN_POINT ( 'NONE',  ( 5.153800228976615827, -19.02544592524334988, 45.20942372801901143 ) ) ;
#144120=CARTESIAN_POINT ( 'NONE',  ( 21.52544592524344225, -5.823673210054117533, 33.54057627198102409 ) ) ;
#144121=CARTESIAN_POINT ( 'NONE',  ( 10.72451020669871369, 18.67979575497193778, 107.0844237280190043 ) ) ;
#144122=CARTESIAN_POINT ( 'NONE',  ( -19.05341960407611168, -5.049401038298163336, 86.45724293864769550 ) ) ;
#144123=CARTESIAN_POINT ( 'NONE',  ( 21.55341960407619695, -5.719274019375665929, 106.0427570613523471 ) ) ;
#144124=CARTESIAN_POINT ( 'NONE',  ( 15.80617190586746368, 15.72974639402197994, 64.37390960531435269 ) ) ;
#144125=CARTESIAN_POINT ( 'NONE',  ( -16.51473224551069308, -9.474510206698971260, 91.66557627198103830 ) ) ;
#144126=CARTESIAN_POINT ( 'NONE',  ( -16.51473224551082808, 9.474510206698731452, 73.33442372801900433 ) ) ;
#144127=CARTESIAN_POINT ( 'NONE',  ( 19.03943276465977164, -0.05219959533909143690, 103.7489096053143669 ) ) ;
#144128=CARTESIAN_POINT ( 'NONE',  ( 0.05219959533936267826, -19.03943276465977164, 90.00109039468567573 ) ) ;
#144129=CARTESIAN_POINT ( 'NONE',  ( 4.483927247898790824, -16.52544592524335698, 60.20942372801902565 ) ) ;
#144130=CARTESIAN_POINT ( 'NONE',  ( 8.224510206698953496, -14.34966873604960469, 112.9155762719810383 ) ) ;
#144131=CARTESIAN_POINT ( 'NONE',  ( 9.564922557960805705, 16.46253265017160317, 84.58224293864769550 ) ) ;
#144132=CARTESIAN_POINT ( 'NONE',  ( 5.719274019375991003, -21.55341960407610458, 62.70724293864769550 ) ) ;
#144133=CARTESIAN_POINT ( 'NONE',  ( -16.53943276465976808, -0.05219959533934237506, 38.75109039468567573 ) ) ;
#144134=CARTESIAN_POINT ( 'NONE',  ( 5.719274019375673035, 21.55341960407619339, 32.29275706135235424 ) ) ;
#144135=CARTESIAN_POINT ( 'NONE',  ( 21.53943276465977519, 0.05219959533937863772, 96.25109039468568994 ) ) ;
#144136=CARTESIAN_POINT ( 'NONE',  ( 14.29746914071037800, 8.314922557961029526, 96.66775706135234714 ) ) ;
#144137=CARTESIAN_POINT ( 'NONE',  ( 9.474510206698971260, -16.51473224551069308, 87.91557627198102409 ) ) ;
#144138=CARTESIAN_POINT ( 'NONE',  ( -4.483927247898539470, -16.52544592524342804, 82.29057627198103830 ) ) ;
#144139=CARTESIAN_POINT ( 'NONE',  ( 16.55341960407611168, 4.379528057220329451, 28.95724293864769905 ) ) ;
#144140=CARTESIAN_POINT ( 'NONE',  ( 13.89961937509957401, 13.97604488694547697, 66.87609039468567573 ) ) ;
#144141=CARTESIAN_POINT ( 'NONE',  ( -18.62759615963255300, -10.81492255796106328, 44.16775706135234714 ) ) ;
#144142=CARTESIAN_POINT ( 'NONE',  ( 16.52544592524342804, -4.483927247898539470, 98.54057627198105251 ) ) ;
#144143=CARTESIAN_POINT ( 'NONE',  ( 16.51473224551069308, 9.474510206698969483, 114.1655762719810241 ) ) ;
#144144=CARTESIAN_POINT ( 'NONE',  ( 4.483927247898790824, -16.52544592524335698, 100.2094237280190043 ) ) ;
#144145=CARTESIAN_POINT ( 'NONE',  ( -15.72974639402176322, -15.80617190586768395, 89.37609039468568994 ) ) ;
#144146=CARTESIAN_POINT ( 'NONE',  ( 8.224510206698742110, 14.34966873604972548, 47.08442372801901854 ) ) ;
#144147=CARTESIAN_POINT ( 'NONE',  ( -21.53943276465977519, -0.05219959533937600094, 43.75109039468568284 ) ) ;
#144148=CARTESIAN_POINT ( 'NONE',  ( 0.05219959533907565091, 21.53943276465977519, 109.9989096053143527 ) ) ;
#144149=CARTESIAN_POINT ( 'NONE',  ( -4.379528057220328563, 16.55341960407611168, 95.20724293864769550 ) ) ;
#144151=CARTESIAN_POINT ( 'NONE',  ( 16.53943276465976808, -0.05219959533910856209, 63.74890960531435979 ) ) ;
#144152=CARTESIAN_POINT ( 'NONE',  ( 16.52544592524335698, 4.483927247898782831, 106.4594237280190328 ) ) ;
#144153=CARTESIAN_POINT ( 'NONE',  ( -9.474510206698964154, 16.51473224551069663, 45.41557627198103120 ) ) ;
#144154=CARTESIAN_POINT ( 'NONE',  ( -15.80617190586745835, -15.72974639402198527, 36.87390960531435979 ) ) ;
#144155=CARTESIAN_POINT ( 'NONE',  ( 8.224510206698953496, -14.34966873604960469, 72.91557627198103830 ) ) ;
#144156=CARTESIAN_POINT ( 'NONE',  ( -21.53943276465977519, 0.05219959533907696930, 86.24890960531436690 ) ) ;
#144157=CARTESIAN_POINT ( 'NONE',  ( -9.474510206698964154, 16.51473224551069663, 85.41557627198102409 ) ) ;
#144158=CARTESIAN_POINT ( 'NONE',  ( -13.89961937509977652, 13.97604488694528158, 40.62390960531435979 ) ) ;
#144159=CARTESIAN_POINT ( 'NONE',  ( -0.05219959533936034679, 19.03943276465977164, 97.50109039468567573 ) ) ;
#144160=CARTESIAN_POINT ( 'NONE',  ( -0.05219959533907301413, -21.53943276465977519, 37.49890960531436690 ) ) ;
#144161=CARTESIAN_POINT ( 'NONE',  ( 21.55341960407619695, -5.719274019375665929, 71.04275706135234714 ) ) ;
#144162=CARTESIAN_POINT ( 'NONE',  ( -5.153800228976328057, -19.02544592524343514, 52.29057627198100988 ) ) ;
#144163=CARTESIAN_POINT ( 'NONE',  ( 13.89961937509977652, -13.97604488694527269, 88.12390960531438111 ) ) ;
#144164=ORIENTED_EDGE ( 'NONE', *, *, #91586, .T. ) ;
#144165=CARTESIAN_POINT ( 'NONE',  ( -16.53943276465976808, -0.05219959533934237506, 68.75109039468568994 ) ) ;
#144166=CARTESIAN_POINT ( 'NONE',  ( -15.72974639402176322, -15.80617190586768395, 39.37609039468567573 ) ) ;
#144167=CARTESIAN_POINT ( 'NONE',  ( 18.62759615963255655, 10.81492255796105972, 66.66775706135234714 ) ) ;
#144168=CARTESIAN_POINT ( 'NONE',  ( 21.52544592524344225, -5.823673210054117533, 23.54057627198102765 ) ) ;
#144169=CARTESIAN_POINT ( 'NONE',  ( -5.719274019375978568, 21.55341960407610458, 100.2072429386476955 ) ) ;
#144170=CARTESIAN_POINT ( 'NONE',  ( -5.719274019375665041, -21.55341960407619695, 19.79275706135235069 ) ) ;
#144171=CARTESIAN_POINT ( 'NONE',  ( -8.224510206698735004, -14.34966873604973081, 59.58442372801901854 ) ) ;
#144172=CARTESIAN_POINT ( 'NONE',  ( 18.67979575497178502, 10.72451020669898547, 59.16557627198103120 ) ) ;
#144173=CARTESIAN_POINT ( 'NONE',  ( -21.53943276465977519, -0.05219959533937600094, 113.7510903946856757 ) ) ;
#144174=CARTESIAN_POINT ( 'NONE',  ( 9.564922557960805705, 16.46253265017160317, 64.58224293864769550 ) ) ;
#144175=CARTESIAN_POINT ( 'NONE',  ( 8.314922557961029526, -14.29746914071037800, 105.4177570613523613 ) ) ;
#144176=CARTESIAN_POINT ( 'NONE',  ( -17.49999999999999645, -3.237210098469652131, 105.2876301262046468 ) ) ;
#144177=CARTESIAN_POINT ( 'NONE',  ( 19.03943276465977164, -0.05219959533909143690, 88.74890960531436690 ) ) ;
#144178=CARTESIAN_POINT ( 'NONE',  ( -4.483927247898782831, 16.52544592524335698, 37.70942372801900433 ) ) ;
#144180=CARTESIAN_POINT ( 'NONE',  ( 9.564922557961047289, -16.46253265017146816, 80.41775706135234714 ) ) ;
#144181=CARTESIAN_POINT ( 'NONE',  ( 5.823673210054125526, 21.52544592524343514, 64.79057627198103830 ) ) ;
#144182=CARTESIAN_POINT ( 'NONE',  ( -4.483927247898539470, -16.52544592524342804, 22.29057627198102765 ) ) ;
#144183=CARTESIAN_POINT ( 'NONE',  ( -19.03943276465977164, -0.05219959533935918106, 93.75109039468566152 ) ) ;
#144184=CARTESIAN_POINT ( 'NONE',  ( -18.22780087662119897, 5.500000000000102141, 41.01763182126894236 ) ) ;
#144185=CARTESIAN_POINT ( 'NONE',  ( -16.51473224551082808, 9.474510206698731452, 98.33442372801900433 ) ) ;
#144186=CARTESIAN_POINT ( 'NONE',  ( -21.52544592524343514, 5.823673210054127303, 86.04057627198102409 ) ) ;
#144187=CARTESIAN_POINT ( 'NONE',  ( 16.51473224551083163, -9.474510206698727899, 60.83442372801900433 ) ) ;
#144189=CARTESIAN_POINT ( 'NONE',  ( 16.51473224551069308, 9.474510206698969483, 69.16557627198102409 ) ) ;
#144190=CARTESIAN_POINT ( 'NONE',  ( 12.06949235617757843, -12.14591786802309237, 58.12390960531435979 ) ) ;
#144191=CARTESIAN_POINT ( 'NONE',  ( 13.97604488694527802, 13.89961937509977652, 44.37390960531435269 ) ) ;
#144192=CARTESIAN_POINT ( 'NONE',  ( 8.224510206698953496, -14.34966873604960469, 47.91557627198102409 ) ) ;
#144193=CARTESIAN_POINT ( 'NONE',  ( 5.049401038298161559, -19.05341960407611168, 22.70724293864769194 ) ) ;
#144195=CARTESIAN_POINT ( 'NONE',  ( -12.14591786802309592, -12.06949235617757132, 31.87390960531435979 ) ) ;
#144196=CARTESIAN_POINT ( 'NONE',  ( -13.89961937509977652, 13.97604488694528158, 60.62390960531436690 ) ) ;
#144197=CARTESIAN_POINT ( 'NONE',  ( -16.51473224551082808, 9.474510206698731452, 73.33442372801900433 ) ) ;
#144198=CARTESIAN_POINT ( 'NONE',  ( -13.97604488694547697, 13.89961937509957934, 43.12609039468566152 ) ) ;
#144199=CARTESIAN_POINT ( 'NONE',  ( -8.314922557961024197, 14.29746914071037800, 52.91775706135235424 ) ) ;
#144200=CARTESIAN_POINT ( 'NONE',  ( 15.80617190586746368, 15.72974639402197994, 49.37390960531436690 ) ) ;
#144201=CARTESIAN_POINT ( 'NONE',  ( -10.72451020669870658, -18.67979575497194134, 99.58442372801900433 ) ) ;
#144202=CARTESIAN_POINT ( 'NONE',  ( -19.03943276465977164, 0.05219959533909376836, 71.24890960531435269 ) ) ;
#144203=CARTESIAN_POINT ( 'NONE',  ( 5.049401038298161559, -19.05341960407611168, 112.7072429386476813 ) ) ;
#144204=CARTESIAN_POINT ( 'NONE',  ( 5.049401038298161559, -19.05341960407611168, 107.7072429386476955 ) ) ;
#144206=CARTESIAN_POINT ( 'NONE',  ( -21.52544592524334988, -5.823673210054445271, 33.95942372801901143 ) ) ;
#144208=CARTESIAN_POINT ( 'NONE',  ( 8.224510206698953496, -14.34966873604960469, 87.91557627198103830 ) ) ;
#144209=CARTESIAN_POINT ( 'NONE',  ( 10.81492255796078972, 18.62759615963270932, 84.58224293864769550 ) ) ;
#144210=CARTESIAN_POINT ( 'NONE',  ( -5.049401038298153566, 19.05341960407611168, 85.20724293864766707 ) ) ;
#144212=CARTESIAN_POINT ( 'NONE',  ( -9.474510206698964154, 16.51473224551069663, 80.41557627198103830 ) ) ;
#144213=CARTESIAN_POINT ( 'NONE',  ( 21.53943276465977519, 0.05219959533937863772, 26.25109039468567573 ) ) ;
#144215=CARTESIAN_POINT ( 'NONE',  ( -19.03943276465977164, 0.05219959533909376836, 76.24890960531435269 ) ) ;
#144216=CARTESIAN_POINT ( 'NONE',  ( 18.39635199886969730, -5.499999999999974243, 98.51967076360000419 ) ) ;
#144217=CARTESIAN_POINT ( 'NONE',  ( 9.564922557960805705, 16.46253265017160317, 24.58224293864769194 ) ) ;
#144218=CARTESIAN_POINT ( 'NONE',  ( -16.46253265017160317, 9.564922557960807481, 35.83224293864768839 ) ) ;
#144219=CARTESIAN_POINT ( 'NONE',  ( -9.474510206698720793, -16.51473224551083518, 109.5844237280190043 ) ) ;
#144221=CARTESIAN_POINT ( 'NONE',  ( 8.314922557960818139, 14.29746914071049879, 109.5822429386476955 ) ) ;
#144222=CARTESIAN_POINT ( 'NONE',  ( -21.53943276465977519, -0.05219959533937600094, 78.75109039468568994 ) ) ;
#144223=CARTESIAN_POINT ( 'NONE',  ( -16.46253265017160317, 9.564922557960807481, 65.83224293864769550 ) ) ;
#144224=CARTESIAN_POINT ( 'NONE',  ( -21.52544592524334988, -5.823673210054445271, 33.95942372801901143 ) ) ;
#144225=CARTESIAN_POINT ( 'NONE',  ( -15.72974639402197994, 15.80617190586746368, 115.6239096053143669 ) ) ;
#144227=CARTESIAN_POINT ( 'NONE',  ( -19.03943276465977164, 0.05219959533909376836, 86.24890960531436690 ) ) ;
#144229=CARTESIAN_POINT ( 'NONE',  ( -16.52544592524335698, -4.483927247898792601, 28.95942372801902209 ) ) ;
#144230=CARTESIAN_POINT ( 'NONE',  ( 15.80617190586746368, 15.72974639402197994, 39.37390960531436690 ) ) ;
#144231=CARTESIAN_POINT ( 'NONE',  ( -21.52544592524334988, -5.823673210054445271, 68.95942372801901854 ) ) ;
#144232=CARTESIAN_POINT ( 'NONE',  ( -19.03943276465977164, 0.05219959533909376836, 111.2489096053143669 ) ) ;
#144233=CARTESIAN_POINT ( 'NONE',  ( 16.51473224551083163, -9.474510206698727899, 100.8344237280190043 ) ) ;
#144234=CARTESIAN_POINT ( 'NONE',  ( -13.97604488694527625, -13.89961937509977652, 51.87390960531436690 ) ) ;
#144235=CARTESIAN_POINT ( 'NONE',  ( 9.474510206698971260, -16.51473224551069308, 87.91557627198102409 ) ) ;
#144236=CARTESIAN_POINT ( 'NONE',  ( 4.379528057220339221, -16.55341960407611168, 87.70724293864769550 ) ) ;
#144237=CARTESIAN_POINT ( 'NONE',  ( -4.483927247898539470, -16.52544592524342804, 92.29057627198103830 ) ) ;
#144238=CARTESIAN_POINT ( 'NONE',  ( 16.51473224551069308, 9.474510206698969483, 109.1655762719810383 ) ) ;
#144239=CARTESIAN_POINT ( 'NONE',  ( -14.29746914071049879, 8.314922557960819915, 55.83224293864770260 ) ) ;
#144240=CARTESIAN_POINT ( 'NONE',  ( -13.89961937509977652, 13.97604488694528158, 40.62390960531435979 ) ) ;
#144241=CARTESIAN_POINT ( 'NONE',  ( 21.55341960407619695, -5.719274019375665929, 61.04275706135234714 ) ) ;
#144242=CARTESIAN_POINT ( 'NONE',  ( 19.02544592524334988, 5.153800228976608722, 91.45942372801900433 ) ) ;
#144243=CARTESIAN_POINT ( 'NONE',  ( -14.29746914071049879, 8.314922557960819915, 60.83224293864769550 ) ) ;
#144244=CARTESIAN_POINT ( 'NONE',  ( 15.72974639402199770, -15.80617190586745480, 113.1239096053143953 ) ) ;
#144245=CARTESIAN_POINT ( 'NONE',  ( 18.62759615963271287, -10.81492255796078972, 53.33224293864769550 ) ) ;
#144246=CARTESIAN_POINT ( 'NONE',  ( -16.51473224551069308, -9.474510206698971260, 106.6655762719810383 ) ) ;
#144248=CARTESIAN_POINT ( 'NONE',  ( 9.564922557960805705, 16.46253265017160317, 54.58224293864769550 ) ) ;
#144249=CARTESIAN_POINT ( 'NONE',  ( 4.379528057220339221, -16.55341960407611168, 32.70724293864770260 ) ) ;
#144250=CARTESIAN_POINT ( 'NONE',  ( -4.483927247898782831, 16.52544592524335698, 97.70942372801904696 ) ) ;
#144251=CARTESIAN_POINT ( 'NONE',  ( 8.314922557961029526, -14.29746914071037800, 80.41775706135234714 ) ) ;
#144252=CARTESIAN_POINT ( 'NONE',  ( -19.02544592524334988, -5.153800228976617603, 33.95942372801897591 ) ) ;
#144254=CARTESIAN_POINT ( 'NONE',  ( -16.51473224551069308, -9.474510206698971260, 96.66557627198102409 ) ) ;
#144255=CARTESIAN_POINT ( 'NONE',  ( -16.46253265017160317, 9.564922557960807481, 45.83224293864769550 ) ) ;
#144256=CARTESIAN_POINT ( 'NONE',  ( 8.314922557960818139, 14.29746914071049879, 64.58224293864769550 ) ) ;
#144257=CARTESIAN_POINT ( 'NONE',  ( 17.26058549869091507, -6.457015423128539489, 101.1225416252393217 ) ) ;
#144258=CARTESIAN_POINT ( 'NONE',  ( 21.53943276465977519, -0.05219959533907433946, 28.74890960531435624 ) ) ;
#144259=CARTESIAN_POINT ( 'NONE',  ( -18.62759615963270932, 10.81492255796079327, 45.83224293864769550 ) ) ;
#144260=CARTESIAN_POINT ( 'NONE',  ( -12.06949235617756955, 12.14591786802309770, 85.62390960531436690 ) ) ;
#144261=CARTESIAN_POINT ( 'NONE',  ( -4.483927247898782831, 16.52544592524335698, 32.70942372801900433 ) ) ;
#144262=CARTESIAN_POINT ( 'NONE',  ( -4.379528057220328563, 16.55341960407611168, 80.20724293864769550 ) ) ;
#144264=CARTESIAN_POINT ( 'NONE',  ( -5.049401038297874678, -19.05341960407617918, 74.79275706135231871 ) ) ;
#144265=CARTESIAN_POINT ( 'NONE',  ( -19.03943276465977164, 0.05219959533909376836, 101.2489096053143669 ) ) ;
#144268=CARTESIAN_POINT ( 'NONE',  ( -14.34966873604972548, 8.224510206698743886, 28.33442372801902209 ) ) ;
#144269=CARTESIAN_POINT ( 'NONE',  ( 4.379528057220339221, -16.55341960407611168, 22.70724293864769194 ) ) ;
#144270=CARTESIAN_POINT ( 'NONE',  ( 0.05219959533936267826, -19.03943276465977164, 70.00109039468566152 ) ) ;
#144271=CARTESIAN_POINT ( 'NONE',  ( -5.823673210054116645, -21.52544592524344225, 47.29057627198103120 ) ) ;
#144272=CARTESIAN_POINT ( 'NONE',  ( -10.72451020669870658, -18.67979575497194134, 69.58442372801900433 ) ) ;
#144274=CARTESIAN_POINT ( 'NONE',  ( 14.29746914071037800, 8.314922557961029526, 41.66775706135235424 ) ) ;
#144275=CARTESIAN_POINT ( 'NONE',  ( 0.05219959533909260263, 19.03943276465977164, 24.99890960531435269 ) ) ;
#144276=CARTESIAN_POINT ( 'NONE',  ( -5.153800228976328057, -19.02544592524343514, 82.29057627198103830 ) ) ;
#144278=CARTESIAN_POINT ( 'NONE',  ( -4.379528057220328563, 16.55341960407611168, 85.20724293864770971 ) ) ;
#144279=CARTESIAN_POINT ( 'NONE',  ( -0.05219959533909027116, -19.03943276465977164, 87.49890960531436690 ) ) ;
#144281=CARTESIAN_POINT ( 'NONE',  ( -16.46253265017146816, -9.564922557961047289, 104.1677570613523329 ) ) ;
#144282=CARTESIAN_POINT ( 'NONE',  ( 5.719274019375991003, -21.55341960407610458, 77.70724293864770971 ) ) ;
#144283=CARTESIAN_POINT ( 'NONE',  ( -16.46253265017160317, 9.564922557960807481, 45.83224293864769550 ) ) ;
#144284=CARTESIAN_POINT ( 'NONE',  ( -16.46253265017146816, -9.564922557961047289, 64.16775706135233293 ) ) ;
#144285=CARTESIAN_POINT ( 'NONE',  ( 18.62759615963271287, -10.81492255796078972, 113.3322429386476955 ) ) ;
#144286=CARTESIAN_POINT ( 'NONE',  ( 9.564922557960805705, 16.46253265017160317, 64.58224293864769550 ) ) ;
#144287=CARTESIAN_POINT ( 'NONE',  ( -9.564922557960796823, -16.46253265017161027, 107.0822429386476955 ) ) ;
#144289=CARTESIAN_POINT ( 'NONE',  ( -14.34966873604972548, 8.224510206698743886, 38.33442372801900433 ) ) ;
#144290=CARTESIAN_POINT ( 'NONE',  ( -18.67979575497178146, -10.72451020669898902, 101.6655762719810383 ) ) ;
#144291=CARTESIAN_POINT ( 'NONE',  ( 8.224510206698953496, -14.34966873604960469, 112.9155762719810383 ) ) ;
#144292=CARTESIAN_POINT ( 'NONE',  ( -19.05341960407611168, -5.049401038298163336, 91.45724293864766707 ) ) ;
#144293=CARTESIAN_POINT ( 'NONE',  ( 9.564922557961047289, -16.46253265017146816, 55.41775706135234003 ) ) ;
#144294=CARTESIAN_POINT ( 'NONE',  ( -21.52544592524343514, 5.823673210054127303, 86.04057627198102409 ) ) ;
#144295=CARTESIAN_POINT ( 'NONE',  ( 12.14591786802309770, 12.06949235617756955, 49.37390960531436690 ) ) ;
#144296=CARTESIAN_POINT ( 'NONE',  ( -9.474510206698720793, -16.51473224551083518, 19.58442372801899722 ) ) ;
#144297=CARTESIAN_POINT ( 'NONE',  ( -8.314922557961024197, 14.29746914071037800, 67.91775706135234714 ) ) ;
#144298=CARTESIAN_POINT ( 'NONE',  ( -0.05219959533909027116, -19.03943276465977164, 87.49890960531436690 ) ) ;
#144299=CARTESIAN_POINT ( 'NONE',  ( -5.153800228976328057, -19.02544592524343514, 42.29057627198101699 ) ) ;
#144301=CARTESIAN_POINT ( 'NONE',  ( 10.72451020669871369, 18.67979575497193778, 57.08442372801901854 ) ) ;
#144302=CARTESIAN_POINT ( 'NONE',  ( 21.55341960407619695, -5.719274019375665929, 61.04275706135234714 ) ) ;
#144303=CARTESIAN_POINT ( 'NONE',  ( 13.89961937509977652, -13.97604488694527269, 58.12390960531436690 ) ) ;
#144304=CARTESIAN_POINT ( 'NONE',  ( 21.53943276465977519, 0.05219959533937863772, 31.25109039468568639 ) ) ;
#144305=CARTESIAN_POINT ( 'NONE',  ( 0.05219959533936267826, -19.03943276465977164, 75.00109039468566152 ) ) ;
#144306=CARTESIAN_POINT ( 'NONE',  ( 19.05341960407617918, -5.049401038297876454, 76.04275706135230450 ) ) ;
#144307=CARTESIAN_POINT ( 'NONE',  ( -0.05219959533909027116, -19.03943276465977164, 42.49890960531435269 ) ) ;
#144308=CARTESIAN_POINT ( 'NONE',  ( 16.53943276465976808, 0.05219959533934440121, 81.25109039468568994 ) ) ;
#144309=CARTESIAN_POINT ( 'NONE',  ( 16.46253265017160672, -9.564922557960803928, 53.33224293864768839 ) ) ;
#144310=CARTESIAN_POINT ( 'NONE',  ( -9.474510206698964154, 16.51473224551069663, 25.41557627198103120 ) ) ;
#144311=CARTESIAN_POINT ( 'NONE',  ( -0.05219959533909027116, -19.03943276465977164, 102.4989096053143669 ) ) ;
#144312=CARTESIAN_POINT ( 'NONE',  ( 0.05219959533909260263, 19.03943276465977164, 34.99890960531435979 ) ) ;
#144313=CARTESIAN_POINT ( 'NONE',  ( -15.72974639402197994, 15.80617190586746368, 85.62390960531436690 ) ) ;
#144314=CARTESIAN_POINT ( 'NONE',  ( -16.52544592524335698, -4.483927247898792601, 63.95942372801901854 ) ) ;
#144316=CARTESIAN_POINT ( 'NONE',  ( 13.89961937509957401, 13.97604488694547697, 36.87609039468565442 ) ) ;
#144317=CARTESIAN_POINT ( 'NONE',  ( 9.474510206698971260, -16.51473224551069308, 47.91557627198102409 ) ) ;
#144318=CARTESIAN_POINT ( 'NONE',  ( 12.14591786802309770, 12.06949235617756955, 44.37390960531435979 ) ) ;
#144319=CARTESIAN_POINT ( 'NONE',  ( -16.52544592524342804, 4.483927247898546575, 86.04057627198102409 ) ) ;
#144320=CARTESIAN_POINT ( 'NONE',  ( -19.02544592524342804, 5.153800228976336051, 96.04057627198103830 ) ) ;
#144321=CARTESIAN_POINT ( 'NONE',  ( 5.049401038298161559, -19.05341960407611168, 77.70724293864765286 ) ) ;
#144322=CARTESIAN_POINT ( 'NONE',  ( -21.55341960407619339, 5.719274019375674811, 33.54275706135234714 ) ) ;
#144323=CARTESIAN_POINT ( 'NONE',  ( -5.153800228976328057, -19.02544592524343514, 87.29057627198103830 ) ) ;
#144324=CARTESIAN_POINT ( 'NONE',  ( 0.05219959533937995610, -21.53943276465977519, 95.00109039468568994 ) ) ;
#144325=CARTESIAN_POINT ( 'NONE',  ( -4.379528057220086978, -16.55341960407618274, 74.79275706135234714 ) ) ;
#144326=CARTESIAN_POINT ( 'NONE',  ( -0.05219959533937732626, 21.53943276465977519, 22.50109039468567573 ) ) ;
#144327=CARTESIAN_POINT ( 'NONE',  ( -10.72451020669898014, 18.67979575497178502, 90.41557627198103830 ) ) ;
#144328=CARTESIAN_POINT ( 'NONE',  ( -14.34966873604960291, -8.224510206698953496, 46.66557627198102409 ) ) ;
#144329=CARTESIAN_POINT ( 'NONE',  ( -16.51473224551069308, -9.474510206698971260, 41.66557627198103120 ) ) ;
#144330=CARTESIAN_POINT ( 'NONE',  ( -8.314922557960811034, -14.29746914071050412, 72.08224293864769550 ) ) ;
#144331=CARTESIAN_POINT ( 'NONE',  ( 21.53943276465977519, -0.05219959533907433946, 33.74890960531436690 ) ) ;
#144332=CARTESIAN_POINT ( 'NONE',  ( 9.564922557961047289, -16.46253265017146816, 30.41775706135232937 ) ) ;
#144334=CARTESIAN_POINT ( 'NONE',  ( 8.224510206698953496, -14.34966873604960469, 102.9155762719810383 ) ) ;
#144335=CARTESIAN_POINT ( 'NONE',  ( 0.05219959533909260263, 19.03943276465977164, 114.9989096053143669 ) ) ;
#144336=ORIENTED_EDGE ( 'NONE', *, *, #87651, .T. ) ;
#144337=CARTESIAN_POINT ( 'NONE',  ( 12.06949235617739724, 12.14591786802326823, 56.87609039468568994 ) ) ;
#144338=CARTESIAN_POINT ( 'NONE',  ( -0.05219959533909027116, -19.03943276465977164, 62.49890960531435979 ) ) ;
#144340=CARTESIAN_POINT ( 'NONE',  ( 21.53943276465977519, -0.05219959533907433946, 38.74890960531435979 ) ) ;
#144341=CARTESIAN_POINT ( 'NONE',  ( 0.05219959533934541429, -16.53943276465976808, 90.00109039468567573 ) ) ;
#144342=CARTESIAN_POINT ( 'NONE',  ( 8.314922557961029526, -14.29746914071037800, 20.41775706135234714 ) ) ;
#144343=CARTESIAN_POINT ( 'NONE',  ( 5.719274019375673035, 21.55341960407619339, 77.29275706135234714 ) ) ;
#144344=CARTESIAN_POINT ( 'NONE',  ( 5.153800228976335163, 19.02544592524342804, 79.79057627198102409 ) ) ;
#144345=CARTESIAN_POINT ( 'NONE',  ( 18.62759615963271287, -10.81492255796078972, 98.33224293864769550 ) ) ;
#144346=CARTESIAN_POINT ( 'NONE',  ( -4.483927247898782831, 16.52544592524335698, 52.70942372801902565 ) ) ;
#144347=CARTESIAN_POINT ( 'NONE',  ( -14.29746914071049879, 8.314922557960819915, 110.8322429386476955 ) ) ;
#144349=CARTESIAN_POINT ( 'NONE',  ( -12.14591786802326823, 12.06949235617739902, 23.12609039468567573 ) ) ;
#144350=CARTESIAN_POINT ( 'NONE',  ( 13.89961937509957401, 13.97604488694547697, 76.87609039468566152 ) ) ;
#144351=CARTESIAN_POINT ( 'NONE',  ( 15.72974639402199770, -15.80617190586745480, 78.12390960531436690 ) ) ;
#144352=CARTESIAN_POINT ( 'NONE',  ( -19.05341960407617563, 5.049401038297882671, 53.54275706135231871 ) ) ;
#144354=CARTESIAN_POINT ( 'NONE',  ( -15.72974639402197994, 15.80617190586746368, 105.6239096053143669 ) ) ;
#144356=CARTESIAN_POINT ( 'NONE',  ( 16.51473224551069308, 9.474510206698969483, 74.16557627198103830 ) ) ;
#144358=CARTESIAN_POINT ( 'NONE',  ( -12.14591786802326823, 12.06949235617739902, 23.12609039468567573 ) ) ;
#144360=CARTESIAN_POINT ( 'NONE',  ( 18.67979575497178502, 10.72451020669898547, 99.16557627198100988 ) ) ;
#144361=CARTESIAN_POINT ( 'NONE',  ( -12.06949235617756955, 12.14591786802309770, 70.62390960531436690 ) ) ;
#144362=CARTESIAN_POINT ( 'NONE',  ( 19.05341960407611168, 5.049401038298154454, 68.95724293864769550 ) ) ;
#144363=CARTESIAN_POINT ( 'NONE',  ( -15.72974639402176322, -15.80617190586768395, 84.37609039468570415 ) ) ;
#144364=CARTESIAN_POINT ( 'NONE',  ( -14.29746914071037622, -8.314922557961029526, 44.16775706135234714 ) ) ;
#144365=CARTESIAN_POINT ( 'NONE',  ( -5.049401038297874678, -19.05341960407617918, 39.79275706135232582 ) ) ;
#144366=CARTESIAN_POINT ( 'NONE',  ( 18.62759615963255655, 10.81492255796105972, 46.66775706135234714 ) ) ;
#144367=CARTESIAN_POINT ( 'NONE',  ( -21.52544592524343514, 5.823673210054127303, 61.04057627198103120 ) ) ;
#144368=CARTESIAN_POINT ( 'NONE',  ( 13.89961937509957401, 13.97604488694547697, 106.8760903946856757 ) ) ;
#144369=CARTESIAN_POINT ( 'NONE',  ( 5.049401038298161559, -19.05341960407611168, 52.70724293864767418 ) ) ;
#144370=CARTESIAN_POINT ( 'NONE',  ( 5.153800228976615827, -19.02544592524334988, 75.20942372801896170 ) ) ;
#144371=CARTESIAN_POINT ( 'NONE',  ( -21.53943276465977519, -0.05219959533937600094, 78.75109039468568994 ) ) ;
#144372=CARTESIAN_POINT ( 'NONE',  ( -19.05341960407617563, 5.049401038297882671, 53.54275706135231871 ) ) ;
#144373=CARTESIAN_POINT ( 'NONE',  ( 5.153800228976335163, 19.02544592524342804, 39.79057627198100988 ) ) ;
#144374=CARTESIAN_POINT ( 'NONE',  ( 21.55341960407610458, 5.719274019375980345, 53.95724293864770260 ) ) ;
#144375=CARTESIAN_POINT ( 'NONE',  ( 4.483927247898545687, 16.52544592524342804, 69.79057627198102409 ) ) ;
#144377=CARTESIAN_POINT ( 'NONE',  ( -19.02544592524334988, -5.153800228976617603, 28.95942372801900433 ) ) ;
#144378=CARTESIAN_POINT ( 'NONE',  ( 12.06949235617739724, 12.14591786802326823, 86.87609039468568994 ) ) ;
#144379=CARTESIAN_POINT ( 'NONE',  ( 14.29746914071049879, -8.314922557960816363, 58.33224293864768839 ) ) ;
#144380=CARTESIAN_POINT ( 'NONE',  ( 0.05219959533937995610, -21.53943276465977519, 95.00109039468568994 ) ) ;
#144381=CARTESIAN_POINT ( 'NONE',  ( 21.53943276465977519, 0.05219959533937863772, 86.25109039468568994 ) ) ;
#144382=CARTESIAN_POINT ( 'NONE',  ( -5.719274019375978568, 21.55341960407610458, 100.2072429386476955 ) ) ;
#144383=( BOUNDED_CURVE ( )  B_SPLINE_CURVE ( 2, ( #45525, #93002, #48517, #187047, #18178, #98720, #91997, #78829, #155680, #76846, #37061, #31351, #199211 ),
 .UNSPECIFIED., .F., .T. ) 
 B_SPLINE_CURVE_WITH_KNOTS ( ( 3, 2, 2, 2, 2, 2, 3 ),
 ( 0.1866409627428346207, 0.1885964912280701788, 0.1929824561403508665, 0.1973684210526315819, 0.2017543859649122695, 0.2061403508771929849, 0.2080501995403384596 ),
 .UNSPECIFIED. ) 
 CURVE ( )  GEOMETRIC_REPRESENTATION_ITEM ( )  RATIONAL_B_SPLINE_CURVE ( ( 0.9831626618144004848, 0.9848076720550091867, 1.000000000000000000, 0.9659258262890683122, 1.000000000000000000, 0.9659258262890683122, 1.000000000000000000, 0.9659258262890683122, 1.000000000000000000, 0.9659258262890683122, 1.000000000000000000, 0.9851625545550090068, 0.9832469066685280978 ) ) 
 REPRESENTATION_ITEM ( '' )  );
#144384=CARTESIAN_POINT ( 'NONE',  ( -13.97604488694527625, -13.89961937509977652, 51.87390960531436690 ) ) ;
#144385=CARTESIAN_POINT ( 'NONE',  ( 21.52544592524334988, 5.823673210054432836, 56.45942372801902565 ) ) ;
#144386=CARTESIAN_POINT ( 'NONE',  ( 0.05219959533909260263, 19.03943276465977164, 34.99890960531435979 ) ) ;
#144387=VERTEX_POINT ( 'NONE', #124055 ) ;
#144388=CARTESIAN_POINT ( 'NONE',  ( -19.02544592524342804, 5.153800228976336051, 56.04057627198100988 ) ) ;
#144389=CARTESIAN_POINT ( 'NONE',  ( 4.379528057220339221, -16.55341960407611168, 107.7072429386476955 ) ) ;
#144390=CARTESIAN_POINT ( 'NONE',  ( -0.05219959533909027116, -19.03943276465977164, 92.49890960531436690 ) ) ;
#144391=CARTESIAN_POINT ( 'NONE',  ( 8.224510206698953496, -14.34966873604960469, 47.91557627198102409 ) ) ;
#144392=CARTESIAN_POINT ( 'NONE',  ( 0.05219959533910956823, 16.53943276465976808, 109.9989096053143527 ) ) ;
#144393=CARTESIAN_POINT ( 'NONE',  ( 5.719274019375991003, -21.55341960407610458, 87.70724293864769550 ) ) ;
#144394=CARTESIAN_POINT ( 'NONE',  ( 21.55341960407619695, -5.719274019375665929, 21.04275706135234714 ) ) ;
#144395=FACE_OUTER_BOUND ( 'NONE', #144909, .T. ) ;
#144396=CARTESIAN_POINT ( 'NONE',  ( 12.06949235617739724, 12.14591786802326823, 41.87609039468568284 ) ) ;
#144398=CARTESIAN_POINT ( 'NONE',  ( -18.67979575497178146, -10.72451020669898902, 86.66557627198102409 ) ) ;
#144399=CARTESIAN_POINT ( 'NONE',  ( -0.05219959533937732626, 21.53943276465977519, 107.5010903946856899 ) ) ;
#144400=CARTESIAN_POINT ( 'NONE',  ( 9.474510206698971260, -16.51473224551069308, 97.91557627198102409 ) ) ;
#144401=CARTESIAN_POINT ( 'NONE',  ( -0.05219959533937732626, 21.53943276465977519, 27.50109039468567929 ) ) ;
#144402=CARTESIAN_POINT ( 'NONE',  ( -18.62759615963270932, 10.81492255796079327, 30.83224293864770260 ) ) ;
#144403=CARTESIAN_POINT ( 'NONE',  ( -12.14591786802326823, 12.06949235617739902, 108.1260903946856757 ) ) ;
#144404=CARTESIAN_POINT ( 'NONE',  ( 10.72451020669871369, 18.67979575497193778, 47.08442372801901854 ) ) ;
#144405=CARTESIAN_POINT ( 'NONE',  ( -0.05219959533937732626, 21.53943276465977519, 82.50109039468568994 ) ) ;
#144406=CARTESIAN_POINT ( 'NONE',  ( -0.05219959533937732626, 21.53943276465977519, 107.5010903946856899 ) ) ;
#144407=CARTESIAN_POINT ( 'NONE',  ( 14.29746914071037800, 8.314922557961029526, 76.66775706135234714 ) ) ;
#144408=CARTESIAN_POINT ( 'NONE',  ( 10.72451020669871369, 18.67979575497193778, 37.08442372801901143 ) ) ;
#144409=CARTESIAN_POINT ( 'NONE',  ( 16.51473224551069308, 9.474510206698969483, 29.16557627198103475 ) ) ;
#144410=CARTESIAN_POINT ( 'NONE',  ( 0.05219959533937995610, -21.53943276465977519, 105.0010903946856757 ) ) ;
#144411=CARTESIAN_POINT ( 'NONE',  ( 19.05341960407611168, 5.049401038298154454, 103.9572429386476671 ) ) ;
#144412=CARTESIAN_POINT ( 'NONE',  ( -21.52544592524343514, 5.823673210054127303, 101.0405762719810383 ) ) ;
#144414=CARTESIAN_POINT ( 'NONE',  ( -21.52544592524343514, 5.823673210054127303, 66.04057627198103830 ) ) ;
#144415=CARTESIAN_POINT ( 'NONE',  ( -14.34966873604972548, 8.224510206698743886, 53.33442372801901854 ) ) ;
#144416=CARTESIAN_POINT ( 'NONE',  ( 4.483927247898545687, 16.52544592524342804, 44.79057627198103120 ) ) ;
#144418=CARTESIAN_POINT ( 'NONE',  ( 19.03943276465977164, 0.05219959533936151252, 86.25109039468567573 ) ) ;
#144419=CARTESIAN_POINT ( 'NONE',  ( -17.05116617787824040, 6.768360034955803073, 103.6567555325919585 ) ) ;
#144420=CARTESIAN_POINT ( 'NONE',  ( -4.379528057220086978, -16.55341960407618274, 29.79275706135234358 ) ) ;
#144421=CARTESIAN_POINT ( 'NONE',  ( 21.55341960407610458, 5.719274019375980345, 93.95724293864770971 ) ) ;
#144422=CARTESIAN_POINT ( 'NONE',  ( 5.823673210054125526, 21.52544592524343514, 79.79057627198102409 ) ) ;
#144423=CARTESIAN_POINT ( 'NONE',  ( -5.153800228976328057, -19.02544592524343514, 112.2905762719810099 ) ) ;
#144424=CARTESIAN_POINT ( 'NONE',  ( -14.29746914071037622, -8.314922557961029526, 39.16775706135235424 ) ) ;
#144425=CARTESIAN_POINT ( 'NONE',  ( 16.46253265017160672, -9.564922557960803928, 53.33224293864768839 ) ) ;
#144426=CARTESIAN_POINT ( 'NONE',  ( 15.80617190586769283, -15.72974639402175789, 30.62609039468567929 ) ) ;
#144427=CARTESIAN_POINT ( 'NONE',  ( 19.05341960407617918, -5.049401038297876454, 96.04275706135231871 ) ) ;
#144428=CARTESIAN_POINT ( 'NONE',  ( 19.02544592524343514, -5.153800228976328945, 103.5405762719809957 ) ) ;
#144429=CARTESIAN_POINT ( 'NONE',  ( -13.97604488694527625, -13.89961937509977652, 91.87390960531432427 ) ) ;
#144430=CARTESIAN_POINT ( 'NONE',  ( -21.53943276465977519, 0.05219959533907696930, 91.24890960531436690 ) ) ;
#144431=CARTESIAN_POINT ( 'NONE',  ( -16.51473224551069308, -9.474510206698971260, 56.66557627198103120 ) ) ;
#144433=CARTESIAN_POINT ( 'NONE',  ( 16.55341960407611168, 4.379528057220329451, 73.95724293864769550 ) ) ;
#144434=CARTESIAN_POINT ( 'NONE',  ( -5.049401038298153566, 19.05341960407611168, 105.2072429386476671 ) ) ;
#144436=CARTESIAN_POINT ( 'NONE',  ( 19.02544592524334988, 5.153800228976608722, 81.45942372801897591 ) ) ;
#144437=CARTESIAN_POINT ( 'NONE',  ( -10.81492255796078084, -18.62759615963271287, 87.08224293864769550 ) ) ;
#144438=CARTESIAN_POINT ( 'NONE',  ( 19.02544592524334988, 5.153800228976608722, 46.45942372801899012 ) ) ;
#144439=CARTESIAN_POINT ( 'NONE',  ( 13.97604488694527802, 13.89961937509977652, 114.3739096053143669 ) ) ;
#144440=CARTESIAN_POINT ( 'NONE',  ( 18.22780087662121673, 5.500000000000056843, 68.98459894673892734 ) ) ;
#144441=CARTESIAN_POINT ( 'NONE',  ( -10.72451020669898014, 18.67979575497178502, 60.41557627198102409 ) ) ;
#144443=CARTESIAN_POINT ( 'NONE',  ( 9.564922557960805705, 16.46253265017160317, 79.58224293864769550 ) ) ;
#144444=CARTESIAN_POINT ( 'NONE',  ( 21.53943276465977519, 0.05219959533937863772, 81.25109039468568994 ) ) ;
#144445=CARTESIAN_POINT ( 'NONE',  ( -19.05341960407611168, -5.049401038298163336, 41.45724293864769550 ) ) ;
#144446=CARTESIAN_POINT ( 'NONE',  ( -14.34966873604960291, -8.224510206698953496, 76.66557627198103830 ) ) ;
#144447=CARTESIAN_POINT ( 'NONE',  ( -16.52544592524335698, -4.483927247898792601, 18.95942372801901143 ) ) ;
#144448=CARTESIAN_POINT ( 'NONE',  ( 5.719274019375673035, 21.55341960407619339, 72.29275706135236135 ) ) ;
#144450=CARTESIAN_POINT ( 'NONE',  ( 13.97604488694548053, -13.89961937509957401, 30.62609039468566863 ) ) ;
#144451=CARTESIAN_POINT ( 'NONE',  ( -19.05341960407617563, 5.049401038297882671, 83.54275706135233293 ) ) ;
#144452=CARTESIAN_POINT ( 'NONE',  ( -17.49999999999999645, 5.499999999999997335, 120.0000000000000142 ) ) ;
#144453=CARTESIAN_POINT ( 'NONE',  ( -18.62759615963255300, -10.81492255796106328, 29.16775706135234003 ) ) ;
#144454=CARTESIAN_POINT ( 'NONE',  ( -15.49999999999999822, 5.499999999999998224, 22.00000000000000000 ) ) ;
#144455=CARTESIAN_POINT ( 'NONE',  ( 5.719274019375673035, 21.55341960407619339, 112.2927570613523471 ) ) ;
#144456=CARTESIAN_POINT ( 'NONE',  ( -19.05341960407611168, -5.049401038298163336, 61.45724293864769550 ) ) ;
#144457=CARTESIAN_POINT ( 'NONE',  ( 13.89961937509957401, 13.97604488694547697, 26.87609039468566507 ) ) ;
#144458=CARTESIAN_POINT ( 'NONE',  ( 16.52544592524335698, 4.483927247898782831, 101.4594237280190185 ) ) ;
#144459=CARTESIAN_POINT ( 'NONE',  ( 5.153800228976335163, 19.02544592524342804, 99.79057627198102409 ) ) ;
#144460=CARTESIAN_POINT ( 'NONE',  ( 15.72974639402176855, 15.80617190586768217, 66.87609039468568994 ) ) ;
#144462=CARTESIAN_POINT ( 'NONE',  ( -17.50000000000002132, -5.076555817581204444, 36.17951492049775197 ) ) ;
#144463=CARTESIAN_POINT ( 'NONE',  ( 0.05219959533937995610, -21.53943276465977519, 90.00109039468567573 ) ) ;
#144464=CARTESIAN_POINT ( 'NONE',  ( -15.72974639402176322, -15.80617190586768395, 104.3760903946856899 ) ) ;
#144466=CARTESIAN_POINT ( 'NONE',  ( -19.03943276465977164, 0.05219959533909376836, 106.2489096053143669 ) ) ;
#144468=CARTESIAN_POINT ( 'NONE',  ( 16.51473224551083163, -9.474510206698727899, 25.83442372801900078 ) ) ;
#144470=CARTESIAN_POINT ( 'NONE',  ( 9.474510206698971260, -16.51473224551069308, 37.91557627198102409 ) ) ;
#144471=CARTESIAN_POINT ( 'NONE',  ( -0.05219959533907301413, -21.53943276465977519, 62.49890960531436690 ) ) ;
#144472=CARTESIAN_POINT ( 'NONE',  ( 14.34966873604972726, -8.224510206698740333, 105.8344237280190328 ) ) ;
#144473=CARTESIAN_POINT ( 'NONE',  ( 0.05219959533910956823, 16.53943276465976808, 99.99890960531436690 ) ) ;
#144474=CARTESIAN_POINT ( 'NONE',  ( 16.51473224551069308, 9.474510206698969483, 84.16557627198102409 ) ) ;
#144475=CARTESIAN_POINT ( 'NONE',  ( 18.67979575497194134, -10.72451020669871369, 105.8344237280190328 ) ) ;
#144476=CARTESIAN_POINT ( 'NONE',  ( -19.02544592524342804, 5.153800228976336051, 36.04057627198100988 ) ) ;
#144477=CARTESIAN_POINT ( 'NONE',  ( 16.53943276465976808, -0.05219959533910856209, 98.74890960531438111 ) ) ;
#144478=CARTESIAN_POINT ( 'NONE',  ( 0.05219959533937995610, -21.53943276465977519, 60.00109039468568284 ) ) ;
#144479=CARTESIAN_POINT ( 'NONE',  ( -5.823673210054116645, -21.52544592524344225, 87.29057627198103830 ) ) ;
#144480=CARTESIAN_POINT ( 'NONE',  ( -9.564922557961040184, 16.46253265017147172, 47.91775706135233293 ) ) ;
#144481=CARTESIAN_POINT ( 'NONE',  ( 18.22780087662119897, -5.500000000000096811, 48.51763182126894236 ) ) ;
#144482=CARTESIAN_POINT ( 'NONE',  ( -16.51473224551069308, -9.474510206698971260, 101.6655762719810241 ) ) ;
#144483=CARTESIAN_POINT ( 'NONE',  ( -14.34966873604960291, -8.224510206698953496, 71.66557627198100988 ) ) ;
#144484=CARTESIAN_POINT ( 'NONE',  ( 9.564922557961047289, -16.46253265017146816, 45.41775706135232582 ) ) ;
#144486=CARTESIAN_POINT ( 'NONE',  ( -16.46253265017160317, 9.564922557960807481, 65.83224293864769550 ) ) ;
#144487=CARTESIAN_POINT ( 'NONE',  ( -16.55341960407611168, -4.379528057220339221, 51.45724293864770260 ) ) ;
#144488=CARTESIAN_POINT ( 'NONE',  ( -19.03943276465977164, -0.05219959533935918106, 78.75109039468567573 ) ) ;
#144489=CARTESIAN_POINT ( 'NONE',  ( 16.51473224551083163, -9.474510206698727899, 90.83442372801900433 ) ) ;
#144490=CARTESIAN_POINT ( 'NONE',  ( -0.05219959533907301413, -21.53943276465977519, 37.49890960531436690 ) ) ;
#144491=CARTESIAN_POINT ( 'NONE',  ( -4.483927247898539470, -16.52544592524342804, 102.2905762719810383 ) ) ;
#144493=CARTESIAN_POINT ( 'NONE',  ( -13.97604488694527625, -13.89961937509977652, 56.87390960531434558 ) ) ;
#144494=CARTESIAN_POINT ( 'NONE',  ( 10.72451020669898902, -18.67979575497178502, 67.91557627198102409 ) ) ;
#144495=CARTESIAN_POINT ( 'NONE',  ( 19.02544592524343514, -5.153800228976328945, 23.54057627198102054 ) ) ;
#144496=CARTESIAN_POINT ( 'NONE',  ( -8.314922557961024197, 14.29746914071037800, 72.91775706135234714 ) ) ;
#144497=CARTESIAN_POINT ( 'NONE',  ( -13.89961937509977652, 13.97604488694528158, 55.62390960531434558 ) ) ;
#144498=CARTESIAN_POINT ( 'NONE',  ( -19.03943276465977164, -0.05219959533935918106, 58.75109039468566863 ) ) ;
#144499=CARTESIAN_POINT ( 'NONE',  ( 15.72974639402176855, 15.80617190586768217, 61.87609039468568284 ) ) ;
#144500=CARTESIAN_POINT ( 'NONE',  ( -21.52544592524343514, 5.823673210054127303, 51.04057627198103120 ) ) ;
#144501=CARTESIAN_POINT ( 'NONE',  ( 12.14591786802309770, 12.06949235617756955, 114.3739096053143527 ) ) ;
#144502=CARTESIAN_POINT ( 'NONE',  ( -12.06949235617739369, -12.14591786802326823, 84.37609039468570415 ) ) ;
#144503=CARTESIAN_POINT ( 'NONE',  ( 19.02544592524334988, 5.153800228976608722, 106.4594237280190185 ) ) ;
#144504=CARTESIAN_POINT ( 'NONE',  ( -19.05341960407611168, -5.049401038298163336, 26.45724293864769550 ) ) ;
#144506=CARTESIAN_POINT ( 'NONE',  ( 21.52544592524344225, -5.823673210054117533, 63.54057627198103830 ) ) ;
#144507=CARTESIAN_POINT ( 'NONE',  ( 5.823673210054444382, -21.52544592524334988, 100.2094237280190043 ) ) ;
#144508=CARTESIAN_POINT ( 'NONE',  ( 8.314922557960818139, 14.29746914071049879, 49.58224293864769550 ) ) ;
#144509=CARTESIAN_POINT ( 'NONE',  ( -14.34966873604960291, -8.224510206698953496, 51.66557627198102409 ) ) ;
#144510=CARTESIAN_POINT ( 'NONE',  ( -18.62759615963270932, 10.81492255796079327, 85.83224293864768129 ) ) ;
#144511=CARTESIAN_POINT ( 'NONE',  ( -21.53943276465977519, 0.05219959533907696930, 91.24890960531436690 ) ) ;
#144513=CARTESIAN_POINT ( 'NONE',  ( 15.72974639402199770, -15.80617190586745480, 33.12390960531435979 ) ) ;
#144514=CARTESIAN_POINT ( 'NONE',  ( 16.55341960407618274, -4.379528057220086978, 71.04275706135234714 ) ) ;
#144515=CARTESIAN_POINT ( 'NONE',  ( 14.29746914071049879, -8.314922557960816363, 78.33224293864770971 ) ) ;
#144516=CARTESIAN_POINT ( 'NONE',  ( -0.05219959533909027116, -19.03943276465977164, 32.49890960531435979 ) ) ;
#144519=CARTESIAN_POINT ( 'NONE',  ( 16.53943276465976808, 0.05219959533934440121, 91.25109039468568994 ) ) ;
#144520=CARTESIAN_POINT ( 'NONE',  ( 15.80617190586769283, -15.72974639402175789, 25.62609039468567929 ) ) ;
#144521=CARTESIAN_POINT ( 'NONE',  ( 9.564922557960805705, 16.46253265017160317, 79.58224293864769550 ) ) ;
#144522=CARTESIAN_POINT ( 'NONE',  ( -21.55341960407619339, 5.719274019375674811, 58.54275706135235424 ) ) ;
#144523=CARTESIAN_POINT ( 'NONE',  ( -19.03943276465977164, 0.05219959533909376836, 111.2489096053143669 ) ) ;
#144526=CARTESIAN_POINT ( 'NONE',  ( 15.72974639402176855, 15.80617190586768217, 41.87609039468568284 ) ) ;
#144527=CARTESIAN_POINT ( 'NONE',  ( 19.03943276465977164, -0.05219959533909143690, 43.74890960531435979 ) ) ;
#144528=CARTESIAN_POINT ( 'NONE',  ( 13.89961937509977652, -13.97604488694527269, 98.12390960531433848 ) ) ;
#144529=CARTESIAN_POINT ( 'NONE',  ( 13.89961937509957401, 13.97604488694547697, 51.87609039468566863 ) ) ;
#144530=CARTESIAN_POINT ( 'NONE',  ( 0.05219959533937995610, -21.53943276465977519, 25.00109039468567218 ) ) ;
#144531=CARTESIAN_POINT ( 'NONE',  ( -19.03943276465977164, -0.05219959533935918106, 58.75109039468566863 ) ) ;
#144532=CARTESIAN_POINT ( 'NONE',  ( -9.564922557960796823, -16.46253265017161027, 27.08224293864769550 ) ) ;
#144533=CARTESIAN_POINT ( 'NONE',  ( -12.06949235617739369, -12.14591786802326823, 94.37609039468568994 ) ) ;
#144534=CARTESIAN_POINT ( 'NONE',  ( 19.05341960407617918, -5.049401038297876454, 61.04275706135232582 ) ) ;
#144535=CARTESIAN_POINT ( 'NONE',  ( -14.29746914071037622, -8.314922557961029526, 109.1677570613523613 ) ) ;
#144536=CARTESIAN_POINT ( 'NONE',  ( 17.97058386085786807, 5.500000000000046185, 86.50390968646220813 ) ) ;
#144537=CARTESIAN_POINT ( 'NONE',  ( 13.97604488694527802, 13.89961937509977652, 84.37390960531433848 ) ) ;
#144538=CARTESIAN_POINT ( 'NONE',  ( 18.67979575497194134, -10.72451020669871369, 95.83442372801903275 ) ) ;
#144539=CARTESIAN_POINT ( 'NONE',  ( 18.67979575497194134, -10.72451020669871369, 110.8344237280190043 ) ) ;
#144542=CARTESIAN_POINT ( 'NONE',  ( -0.05219959533909027116, -19.03943276465977164, 107.4989096053143527 ) ) ;
#144543=CARTESIAN_POINT ( 'NONE',  ( -21.55341960407619339, 5.719274019375674811, 78.54275706135236135 ) ) ;
#144544=CARTESIAN_POINT ( 'NONE',  ( -16.51473224551082808, 9.474510206698731452, 113.3344237280190043 ) ) ;
#144545=CARTESIAN_POINT ( 'NONE',  ( 19.03943276465977164, -0.05219959533909143690, 73.74890960531435269 ) ) ;
#144546=CARTESIAN_POINT ( 'NONE',  ( 15.80617190586746368, 15.72974639402197994, 34.37390960531435979 ) ) ;
#144547=CARTESIAN_POINT ( 'NONE',  ( 13.89961937509977652, -13.97604488694527269, 93.12390960531436690 ) ) ;
#144549=CARTESIAN_POINT ( 'NONE',  ( 9.564922557960805705, 16.46253265017160317, 74.58224293864769550 ) ) ;
#144550=CARTESIAN_POINT ( 'NONE',  ( -9.474510206698964154, 16.51473224551069663, 70.41557627198102409 ) ) ;
#144551=CARTESIAN_POINT ( 'NONE',  ( -8.224510206698948167, 14.34966873604960824, 25.41557627198103120 ) ) ;
#144553=CARTESIAN_POINT ( 'NONE',  ( -13.97604488694547697, 13.89961937509957934, 68.12609039468563310 ) ) ;
#144554=CARTESIAN_POINT ( 'NONE',  ( 5.049401038298161559, -19.05341960407611168, 87.70724293864769550 ) ) ;
#144555=CARTESIAN_POINT ( 'NONE',  ( -14.34966873604960291, -8.224510206698953496, 81.66557627198103830 ) ) ;
#144556=CARTESIAN_POINT ( 'NONE',  ( -21.55341960407610458, -5.719274019375992779, 41.45724293864769550 ) ) ;
#144557=CARTESIAN_POINT ( 'NONE',  ( -10.72451020669898014, 18.67979575497178502, 25.41557627198103120 ) ) ;
#144558=CARTESIAN_POINT ( 'NONE',  ( 4.483927247898545687, 16.52544592524342804, 99.79057627198103830 ) ) ;
#144559=CARTESIAN_POINT ( 'NONE',  ( -17.31747979337950127, 6.344076630960999275, 53.62055131934816643 ) ) ;
#144560=CARTESIAN_POINT ( 'NONE',  ( 9.474510206698729675, 16.51473224551082808, 47.08442372801900433 ) ) ;
#144561=CARTESIAN_POINT ( 'NONE',  ( 0.05219959533910956823, 16.53943276465976808, 29.99890960531435979 ) ) ;
#144562=CARTESIAN_POINT ( 'NONE',  ( 5.049401038298161559, -19.05341960407611168, 107.7072429386476955 ) ) ;
#144563=CARTESIAN_POINT ( 'NONE',  ( -15.80617190586768217, 15.72974639402176855, 63.12609039468568994 ) ) ;
#144564=CARTESIAN_POINT ( 'NONE',  ( -10.81492255796078084, -18.62759615963271287, 62.08224293864769550 ) ) ;
#144565=CARTESIAN_POINT ( 'NONE',  ( 21.55341960407619695, -5.719274019375665929, 51.04275706135234714 ) ) ;
#144566=CARTESIAN_POINT ( 'NONE',  ( -10.81492255796078084, -18.62759615963271287, 82.08224293864768129 ) ) ;
#144567=CARTESIAN_POINT ( 'NONE',  ( -15.72974639402176322, -15.80617190586768395, 34.37609039468568284 ) ) ;
#144568=CARTESIAN_POINT ( 'NONE',  ( 16.52544592524342804, -4.483927247898539470, 113.5405762719810383 ) ) ;
#144569=CARTESIAN_POINT ( 'NONE',  ( -9.474510206698720793, -16.51473224551083518, 64.58442372801900433 ) ) ;
#144570=CARTESIAN_POINT ( 'NONE',  ( 19.02544592524343514, -5.153800228976328945, 43.54057627198103120 ) ) ;
#144571=CARTESIAN_POINT ( 'NONE',  ( -12.14591786802309592, -12.06949235617757132, 101.8739096053143811 ) ) ;
#144572=CARTESIAN_POINT ( 'NONE',  ( 5.153800228976335163, 19.02544592524342804, 104.7905762719809957 ) ) ;
#144573=CARTESIAN_POINT ( 'NONE',  ( -16.55341960407611168, -4.379528057220339221, 46.45724293864769550 ) ) ;
#144574=CARTESIAN_POINT ( 'NONE',  ( 4.379528057220092307, 16.55341960407617563, 97.29275706135234714 ) ) ;
#144575=CARTESIAN_POINT ( 'NONE',  ( 13.89961937509977652, -13.97604488694527269, 58.12390960531436690 ) ) ;
#144576=CARTESIAN_POINT ( 'NONE',  ( -4.483927247898539470, -16.52544592524342804, 112.2905762719810241 ) ) ;
#144577=CARTESIAN_POINT ( 'NONE',  ( 19.05341960407617918, -5.049401038297876454, 26.04275706135233293 ) ) ;
#144578=VECTOR ( 'NONE', #115189, 1000.000000000000000 ) ;
#144579=CARTESIAN_POINT ( 'NONE',  ( -9.474510206698964154, 16.51473224551069663, 110.4155762719810383 ) ) ;
#144580=CARTESIAN_POINT ( 'NONE',  ( 14.29746914071049879, -8.314922557960816363, 38.33224293864768839 ) ) ;
#144581=CARTESIAN_POINT ( 'NONE',  ( -10.81492255796105439, 18.62759615963255655, 52.91775706135235424 ) ) ;
#144583=CARTESIAN_POINT ( 'NONE',  ( -4.483927247898782831, 16.52544592524335698, 62.70942372801902565 ) ) ;
#144584=CARTESIAN_POINT ( 'NONE',  ( 16.52544592524342804, -4.483927247898539470, 23.54057627198102765 ) ) ;
#144585=CARTESIAN_POINT ( 'NONE',  ( 8.314922557961029526, -14.29746914071037800, 110.4177570613523756 ) ) ;
#144586=CARTESIAN_POINT ( 'NONE',  ( -4.483927247898782831, 16.52544592524335698, 27.70942372801901854 ) ) ;
#144587=CARTESIAN_POINT ( 'NONE',  ( -13.89961937509977652, 13.97604488694528158, 50.62390960531435979 ) ) ;
#144588=CARTESIAN_POINT ( 'NONE',  ( -4.379528057220328563, 16.55341960407611168, 110.2072429386477239 ) ) ;
#144589=CARTESIAN_POINT ( 'NONE',  ( -15.72974639402197994, 15.80617190586746368, 115.6239096053143669 ) ) ;
#144590=CARTESIAN_POINT ( 'NONE',  ( 0.05219959533909260263, 19.03943276465977164, 39.99890960531436690 ) ) ;
#144592=CARTESIAN_POINT ( 'NONE',  ( 13.89961937509977652, -13.97604488694527269, 28.12390960531435624 ) ) ;
#144593=CARTESIAN_POINT ( 'NONE',  ( 21.52544592524344225, -5.823673210054117533, 23.54057627198102765 ) ) ;
#144594=CARTESIAN_POINT ( 'NONE',  ( -17.31747979337952614, -6.344076630960945984, 36.37944868065184068 ) ) ;
#144595=CARTESIAN_POINT ( 'NONE',  ( -19.03943276465977164, 0.05219959533909376836, 101.2489096053143669 ) ) ;
#144596=CARTESIAN_POINT ( 'NONE',  ( -15.80617190586768217, 15.72974639402176855, 43.12609039468568284 ) ) ;
#144597=CARTESIAN_POINT ( 'NONE',  ( 14.29746914071049879, -8.314922557960816363, 108.3322429386477097 ) ) ;
#144598=CARTESIAN_POINT ( 'NONE',  ( -13.97604488694527625, -13.89961937509977652, 106.8739096053143669 ) ) ;
#144599=CARTESIAN_POINT ( 'NONE',  ( -30.00000000000000000, -5.499999999999992895, 102.5000000000000142 ) ) ;
#144600=CARTESIAN_POINT ( 'NONE',  ( -12.06949235617739369, -12.14591786802326823, 74.37609039468568994 ) ) ;
#144601=CARTESIAN_POINT ( 'NONE',  ( -21.52544592524334988, -5.823673210054445271, 93.95942372801903275 ) ) ;
#144603=CARTESIAN_POINT ( 'NONE',  ( 0.05219959533934541429, -16.53943276465976808, 55.00109039468568284 ) ) ;
#144604=CARTESIAN_POINT ( 'NONE',  ( 16.46253265017160672, -9.564922557960803928, 93.33224293864769550 ) ) ;
#144605=CARTESIAN_POINT ( 'NONE',  ( 16.52544592524335698, 4.483927247898782831, 41.45942372801901143 ) ) ;
#144606=CARTESIAN_POINT ( 'NONE',  ( 16.51473224551083163, -9.474510206698727899, 110.8344237280190043 ) ) ;
#144607=CARTESIAN_POINT ( 'NONE',  ( -14.29746914071037622, -8.314922557961029526, 89.16775706135236135 ) ) ;
#144608=CARTESIAN_POINT ( 'NONE',  ( 19.02544592524334988, 5.153800228976608722, 111.4594237280190043 ) ) ;
#144609=CARTESIAN_POINT ( 'NONE',  ( 5.049401038298161559, -19.05341960407611168, 77.70724293864765286 ) ) ;
#144610=CARTESIAN_POINT ( 'NONE',  ( -18.67979575497178146, -10.72451020669898902, 91.66557627198103830 ) ) ;
#144611=CARTESIAN_POINT ( 'NONE',  ( 16.55341960407611168, 4.379528057220329451, 108.9572429386476955 ) ) ;
#144612=CARTESIAN_POINT ( 'NONE',  ( -19.02544592524334988, -5.153800228976617603, 108.9594237280189759 ) ) ;
#144613=CARTESIAN_POINT ( 'NONE',  ( 0.05219959533934541429, -16.53943276465976808, 70.00109039468568994 ) ) ;
#144614=CARTESIAN_POINT ( 'NONE',  ( -17.44270441346521849, 5.991230190322816007, 43.63664920735774899 ) ) ;
#144615=CARTESIAN_POINT ( 'NONE',  ( -9.564922557961040184, 16.46253265017147172, 67.91775706135233293 ) ) ;
#144616=CARTESIAN_POINT ( 'NONE',  ( 0.05219959533910956823, 16.53943276465976808, 49.99890960531437401 ) ) ;
#144617=CARTESIAN_POINT ( 'NONE',  ( -14.34966873604960291, -8.224510206698953496, 91.66557627198103830 ) ) ;
#144618=CARTESIAN_POINT ( 'NONE',  ( -13.97604488694547697, 13.89961937509957934, 38.12609039468566152 ) ) ;
#144619=CARTESIAN_POINT ( 'NONE',  ( -16.79531203550646978, 7.028104445595602989, 88.74755011779558345 ) ) ;
#144620=CARTESIAN_POINT ( 'NONE',  ( -18.67979575497193778, 10.72451020669871902, 33.33442372801900433 ) ) ;
#144621=CARTESIAN_POINT ( 'NONE',  ( -16.51473224551082808, 9.474510206698731452, 98.33442372801900433 ) ) ;
#144622=CARTESIAN_POINT ( 'NONE',  ( -13.89961937509977652, 13.97604488694528158, 110.6239096053143243 ) ) ;
#144623=CARTESIAN_POINT ( 'NONE',  ( 0.05219959533909260263, 19.03943276465977164, 89.99890960531436690 ) ) ;
#144624=CARTESIAN_POINT ( 'NONE',  ( -5.719274019375665041, -21.55341960407619695, 109.7927570613523613 ) ) ;
#144625=CARTESIAN_POINT ( 'NONE',  ( -19.02544592524342804, 5.153800228976336051, 76.04057627198102409 ) ) ;
#144626=CARTESIAN_POINT ( 'NONE',  ( 0.05219959533907565091, 21.53943276465977519, 49.99890960531437401 ) ) ;
#144627=CARTESIAN_POINT ( 'NONE',  ( 16.53943276465976808, -0.05219959533910856209, 98.74890960531438111 ) ) ;
#144628=CARTESIAN_POINT ( 'NONE',  ( -16.46253265017160317, 9.564922557960807481, 55.83224293864769550 ) ) ;
#144629=CARTESIAN_POINT ( 'NONE',  ( 5.049401038298161559, -19.05341960407611168, 22.70724293864769194 ) ) ;
#144630=CARTESIAN_POINT ( 'NONE',  ( -5.719274019375665041, -21.55341960407619695, 29.79275706135234358 ) ) ;
#144631=CARTESIAN_POINT ( 'NONE',  ( 21.52544592524334988, 5.823673210054432836, 81.45942372801900433 ) ) ;
#144632=CARTESIAN_POINT ( 'NONE',  ( 9.564922557960805705, 16.46253265017160317, 39.58224293864768839 ) ) ;
#144633=CARTESIAN_POINT ( 'NONE',  ( -4.483927247898782831, 16.52544592524335698, 82.70942372801900433 ) ) ;
#144634=CARTESIAN_POINT ( 'NONE',  ( 21.53943276465977519, -0.05219959533907433946, 113.7489096053143527 ) ) ;
#144636=CARTESIAN_POINT ( 'NONE',  ( 10.72451020669871369, 18.67979575497193778, 27.08442372801901854 ) ) ;
#144637=CARTESIAN_POINT ( 'NONE',  ( -19.02544592524334988, -5.153800228976617603, 53.95942372801898301 ) ) ;
#144638=CARTESIAN_POINT ( 'NONE',  ( -0.05219959533909027116, -19.03943276465977164, 67.49890960531436690 ) ) ;
#144639=CARTESIAN_POINT ( 'NONE',  ( 0.05219959533936267826, -19.03943276465977164, 35.00109039468566863 ) ) ;
#144640=CARTESIAN_POINT ( 'NONE',  ( -15.80617190586768217, 15.72974639402176855, 73.12609039468567573 ) ) ;
#144641=CARTESIAN_POINT ( 'NONE',  ( -5.719274019375978568, 21.55341960407610458, 70.20724293864769550 ) ) ;
#144642=CARTESIAN_POINT ( 'NONE',  ( -12.14591786802309592, -12.06949235617757132, 46.87390960531435979 ) ) ;
#144643=CARTESIAN_POINT ( 'NONE',  ( -21.52544592524334988, -5.823673210054445271, 93.95942372801903275 ) ) ;
#144644=CARTESIAN_POINT ( 'NONE',  ( 5.153800228976615827, -19.02544592524334988, 30.20942372801900433 ) ) ;
#144645=CARTESIAN_POINT ( 'NONE',  ( 16.52544592524342804, -4.483927247898539470, 68.54057627198103830 ) ) ;
#144646=CARTESIAN_POINT ( 'NONE',  ( -8.224510206698948167, 14.34966873604960824, 115.4155762719810241 ) ) ;
#144647=CARTESIAN_POINT ( 'NONE',  ( -19.05341960407617563, 5.049401038297882671, 58.54275706135234003 ) ) ;
#144648=CARTESIAN_POINT ( 'NONE',  ( -8.314922557961024197, 14.29746914071037800, 112.9177570613523329 ) ) ;
#144649=CARTESIAN_POINT ( 'NONE',  ( 10.72451020669871369, 18.67979575497193778, 77.08442372801901854 ) ) ;
#144650=CARTESIAN_POINT ( 'NONE',  ( 16.51473224551069308, 9.474510206698969483, 84.16557627198102409 ) ) ;
#144651=CARTESIAN_POINT ( 'NONE',  ( 0.05219959533936267826, -19.03943276465977164, 45.00109039468566863 ) ) ;
#144652=CARTESIAN_POINT ( 'NONE',  ( 21.53943276465977519, -0.05219959533907433946, 48.74890960531435979 ) ) ;
#144653=CARTESIAN_POINT ( 'NONE',  ( 21.55341960407619695, -5.719274019375665929, 46.04275706135234714 ) ) ;
#144654=CARTESIAN_POINT ( 'NONE',  ( 15.72974639402199770, -15.80617190586745480, 108.1239096053143811 ) ) ;
#144655=CARTESIAN_POINT ( 'NONE',  ( 19.03943276465977164, 0.05219959533936151252, 96.25109039468567573 ) ) ;
#144656=CARTESIAN_POINT ( 'NONE',  ( -4.379528057220086978, -16.55341960407618274, 59.79275706135234714 ) ) ;
#144658=CARTESIAN_POINT ( 'NONE',  ( -5.823673210054116645, -21.52544592524344225, 112.2905762719810241 ) ) ;
#144659=CARTESIAN_POINT ( 'NONE',  ( 14.34966873604960469, 8.224510206698951720, 89.16557627198102409 ) ) ;
#144661=CARTESIAN_POINT ( 'NONE',  ( 14.29746914071037800, 8.314922557961029526, 41.66775706135235424 ) ) ;
#144662=CARTESIAN_POINT ( 'NONE',  ( 21.53943276465977519, -0.05219959533907433946, 43.74890960531435979 ) ) ;
#144663=CARTESIAN_POINT ( 'NONE',  ( 8.314922557961029526, -14.29746914071037800, 90.41775706135236135 ) ) ;
#144664=CARTESIAN_POINT ( 'NONE',  ( -19.02544592524342804, 5.153800228976336051, 26.04057627198103120 ) ) ;
#144665=CARTESIAN_POINT ( 'NONE',  ( -14.29746914071037622, -8.314922557961029526, 64.16775706135234714 ) ) ;
#144666=CARTESIAN_POINT ( 'NONE',  ( 18.62759615963255655, 10.81492255796105972, 36.66775706135234714 ) ) ;
#144667=CARTESIAN_POINT ( 'NONE',  ( -0.05219959533907301413, -21.53943276465977519, 57.49890960531435979 ) ) ;
#144668=CARTESIAN_POINT ( 'NONE',  ( 12.14591786802327356, -12.06949235617739191, 80.62609039468567573 ) ) ;
#144669=CARTESIAN_POINT ( 'NONE',  ( 15.72974639402176855, 15.80617190586768217, 66.87609039468568994 ) ) ;
#144670=CARTESIAN_POINT ( 'NONE',  ( -21.53943276465977519, 0.05219959533907696930, 56.24890960531436690 ) ) ;
#144671=CARTESIAN_POINT ( 'NONE',  ( 18.62759615963271287, -10.81492255796078972, 38.33224293864768839 ) ) ;
#144672=CARTESIAN_POINT ( 'NONE',  ( 4.379528057220092307, 16.55341960407617563, 62.29275706135236845 ) ) ;
#144673=CARTESIAN_POINT ( 'NONE',  ( 21.53943276465977519, -0.05219959533907433946, 38.74890960531435979 ) ) ;
#144675=CARTESIAN_POINT ( 'NONE',  ( 16.51473224551069308, 9.474510206698969483, 104.1655762719810241 ) ) ;
#144676=CARTESIAN_POINT ( 'NONE',  ( 8.224510206698953496, -14.34966873604960469, 22.91557627198102765 ) ) ;
#144677=CARTESIAN_POINT ( 'NONE',  ( -17.49999999999999645, -5.499999999999992895, 79.20309617465829888 ) ) ;
#144678=CARTESIAN_POINT ( 'NONE',  ( 16.53943276465976808, -0.05219959533910856209, 113.7489096053143527 ) ) ;
#144679=CARTESIAN_POINT ( 'NONE',  ( -10.81492255796078084, -18.62759615963271287, 62.08224293864769550 ) ) ;
#144680=CARTESIAN_POINT ( 'NONE',  ( 13.89961937509977652, -13.97604488694527269, 43.12390960531434558 ) ) ;
#144681=CARTESIAN_POINT ( 'NONE',  ( -8.314922557961024197, 14.29746914071037800, 92.91775706135236135 ) ) ;
#144682=CARTESIAN_POINT ( 'NONE',  ( 21.55341960407619695, -5.719274019375665929, 31.04275706135234714 ) ) ;
#144683=CARTESIAN_POINT ( 'NONE',  ( 19.03943276465977164, 0.05219959533936151252, 86.25109039468567573 ) ) ;
#144684=CARTESIAN_POINT ( 'NONE',  ( 4.379528057220339221, -16.55341960407611168, 97.70724293864772392 ) ) ;
#144685=CARTESIAN_POINT ( 'NONE',  ( -5.153800228976328057, -19.02544592524343514, 47.29057627198102409 ) ) ;
#144686=CARTESIAN_POINT ( 'NONE',  ( -17.49999999999999645, -5.500000000000000888, 29.20309617465828467 ) ) ;
#144687=CARTESIAN_POINT ( 'NONE',  ( 18.09805431107249518, -5.499999999999988454, 63.51606229291888184 ) ) ;
#144688=CARTESIAN_POINT ( 'NONE',  ( -9.474510206698964154, 16.51473224551069663, 75.41557627198103830 ) ) ;
#144689=CARTESIAN_POINT ( 'NONE',  ( 14.29746914071037800, 8.314922557961029526, 66.66775706135234714 ) ) ;
#144690=CARTESIAN_POINT ( 'NONE',  ( -15.80617190586768217, 15.72974639402176855, 103.1260903946856757 ) ) ;
#144691=CARTESIAN_POINT ( 'NONE',  ( 15.80617190586746368, 15.72974639402197994, 54.37390960531435979 ) ) ;
#144692=CARTESIAN_POINT ( 'NONE',  ( -12.06949235617739369, -12.14591786802326823, 79.37609039468567573 ) ) ;
#144693=CARTESIAN_POINT ( 'NONE',  ( -5.049401038297874678, -19.05341960407617918, 64.79275706135233293 ) ) ;
#144694=CARTESIAN_POINT ( 'NONE',  ( -5.823673210054431948, 21.52544592524334988, 57.70942372801901143 ) ) ;
#144695=CARTESIAN_POINT ( 'NONE',  ( 0.05219959533909260263, 19.03943276465977164, 84.99890960531436690 ) ) ;
#144696=CARTESIAN_POINT ( 'NONE',  ( 5.049401038298161559, -19.05341960407611168, 32.70724293864768129 ) ) ;
#144697=CARTESIAN_POINT ( 'NONE',  ( 0.05219959533936267826, -19.03943276465977164, 55.00109039468566863 ) ) ;
#144698=CARTESIAN_POINT ( 'NONE',  ( 9.564922557960805705, 16.46253265017160317, 109.5822429386476955 ) ) ;
#144699=CARTESIAN_POINT ( 'NONE',  ( 9.564922557960805705, 16.46253265017160317, 89.58224293864769550 ) ) ;
#144700=CARTESIAN_POINT ( 'NONE',  ( 12.14591786802309770, 12.06949235617756955, 49.37390960531436690 ) ) ;
#144701=CARTESIAN_POINT ( 'NONE',  ( 5.823673210054125526, 21.52544592524343514, 44.79057627198103120 ) ) ;
#144702=CARTESIAN_POINT ( 'NONE',  ( -30.00000000000000000, -5.510910596163089556E-15, 45.00000000000000000 ) ) ;
#144703=CARTESIAN_POINT ( 'NONE',  ( -9.564922557961040184, 16.46253265017147172, 32.91775706135233293 ) ) ;
#144704=CARTESIAN_POINT ( 'NONE',  ( -17.26058549869093994, -6.457015423128468434, 81.37745837476070676 ) ) ;
#144705=CARTESIAN_POINT ( 'NONE',  ( -19.05341960407611168, -5.049401038298163336, 56.45724293864768129 ) ) ;
#144707=CARTESIAN_POINT ( 'NONE',  ( 8.224510206698742110, 14.34966873604972548, 42.08442372801901854 ) ) ;
#144709=CARTESIAN_POINT ( 'NONE',  ( -16.88567814943162304, 6.947325034625684737, 108.7099887734741799 ) ) ;
#144710=CARTESIAN_POINT ( 'NONE',  ( -8.224510206698735004, -14.34966873604973081, 74.58442372801901854 ) ) ;
#144711=CARTESIAN_POINT ( 'NONE',  ( -18.67979575497178146, -10.72451020669898902, 101.6655762719810383 ) ) ;
#144712=CARTESIAN_POINT ( 'NONE',  ( 9.474510206698971260, -16.51473224551069308, 37.91557627198102409 ) ) ;
#144714=CARTESIAN_POINT ( 'NONE',  ( 5.823673210054444382, -21.52544592524334988, 40.20942372801901854 ) ) ;
#144715=CARTESIAN_POINT ( 'NONE',  ( -13.97604488694547697, 13.89961937509957934, 43.12609039468566152 ) ) ;
#144716=CARTESIAN_POINT ( 'NONE',  ( -19.03943276465977164, 0.05219959533909376836, 46.24890960531435979 ) ) ;
#144717=CARTESIAN_POINT ( 'NONE',  ( -10.72451020669870658, -18.67979575497194134, 99.58442372801900433 ) ) ;
#144718=CARTESIAN_POINT ( 'NONE',  ( 16.88567814943163015, 6.947325034625698947, 98.79001122652587696 ) ) ;
#144719=CARTESIAN_POINT ( 'NONE',  ( 4.483927247898545687, 16.52544592524342804, 34.79057627198103120 ) ) ;
#144720=CARTESIAN_POINT ( 'NONE',  ( 18.22780087662121673, 5.500000000000056843, 43.98459894673892734 ) ) ;
#144721=CARTESIAN_POINT ( 'NONE',  ( -18.62759615963270932, 10.81492255796079327, 55.83224293864770260 ) ) ;
#144723=CARTESIAN_POINT ( 'NONE',  ( 13.89961937509977652, -13.97604488694527269, 108.1239096053143669 ) ) ;
#144724=CARTESIAN_POINT ( 'NONE',  ( 14.34966873604960469, 8.224510206698951720, 94.16557627198103830 ) ) ;
#144725=CARTESIAN_POINT ( 'NONE',  ( -16.53943276465976808, -0.05219959533934237506, 18.75109039468568639 ) ) ;
#144726=CARTESIAN_POINT ( 'NONE',  ( -16.52544592524335698, -4.483927247898792601, 103.9594237280190185 ) ) ;
#144727=VERTEX_POINT ( 'NONE', #14913 ) ;
#144728=CARTESIAN_POINT ( 'NONE',  ( 13.97604488694527802, 13.89961937509977652, 104.3739096053143385 ) ) ;
#144729=CARTESIAN_POINT ( 'NONE',  ( -21.55341960407610458, -5.719274019375992779, 101.4572429386476955 ) ) ;
#144730=CARTESIAN_POINT ( 'NONE',  ( 0.05219959533910956823, 16.53943276465976808, 24.99890960531435624 ) ) ;
#144731=CARTESIAN_POINT ( 'NONE',  ( 19.02544592524343514, -5.153800228976328945, 98.54057627198100988 ) ) ;
#144732=CARTESIAN_POINT ( 'NONE',  ( -16.51473224551082808, 9.474510206698731452, 98.33442372801900433 ) ) ;
#144733=CARTESIAN_POINT ( 'NONE',  ( 10.72451020669871369, 18.67979575497193778, 112.0844237280190185 ) ) ;
#144734=CARTESIAN_POINT ( 'NONE',  ( 10.81492255796078972, 18.62759615963270932, 84.58224293864769550 ) ) ;
#144735=CARTESIAN_POINT ( 'NONE',  ( -15.72974639402197994, 15.80617190586746368, 45.62390960531436690 ) ) ;
#144736=CARTESIAN_POINT ( 'NONE',  ( -19.02544592524342804, 5.153800228976336051, 61.04057627198103120 ) ) ;
#144737=CARTESIAN_POINT ( 'NONE',  ( -12.06949235617756955, 12.14591786802309770, 40.62390960531435269 ) ) ;
#144738=CARTESIAN_POINT ( 'NONE',  ( -19.03943276465977164, 0.05219959533909376836, 76.24890960531435269 ) ) ;
#144740=CARTESIAN_POINT ( 'NONE',  ( 18.87580814761077619, -5.499999999999873879, 63.37172394265759579 ) ) ;
#144741=CARTESIAN_POINT ( 'NONE',  ( -13.97604488694547697, 13.89961937509957934, 43.12609039468566152 ) ) ;
#144742=CARTESIAN_POINT ( 'NONE',  ( 10.81492255796078972, 18.62759615963270932, 84.58224293864769550 ) ) ;
#144743=CARTESIAN_POINT ( 'NONE',  ( 4.483927247898545687, 16.52544592524342804, 89.79057627198103830 ) ) ;
#144745=CARTESIAN_POINT ( 'NONE',  ( 21.55341960407619695, -5.719274019375665929, 36.04275706135234714 ) ) ;
#144748=CARTESIAN_POINT ( 'NONE',  ( -16.55341960407617563, 4.379528057220093196, 113.5427570613523756 ) ) ;
#144749=CARTESIAN_POINT ( 'NONE',  ( -19.02544592524342804, 5.153800228976336051, 26.04057627198103120 ) ) ;
#144750=CARTESIAN_POINT ( 'NONE',  ( -13.97604488694527625, -13.89961937509977652, 81.87390960531436690 ) ) ;
#144753=CARTESIAN_POINT ( 'NONE',  ( 14.29746914071049879, -8.314922557960816363, 38.33224293864768839 ) ) ;
#144754=CARTESIAN_POINT ( 'NONE',  ( -21.53943276465977519, -0.05219959533937600094, 58.75109039468568994 ) ) ;
#144756=CARTESIAN_POINT ( 'NONE',  ( -13.97604488694527625, -13.89961937509977652, 46.87390960531435979 ) ) ;
#144757=CARTESIAN_POINT ( 'NONE',  ( 16.51473224551069308, 9.474510206698969483, 54.16557627198103120 ) ) ;
#144759=CARTESIAN_POINT ( 'NONE',  ( -21.55341960407619339, 5.719274019375674811, 108.5427570613523756 ) ) ;
#144760=CARTESIAN_POINT ( 'NONE',  ( -16.53943276465976808, -0.05219959533934237506, 58.75109039468568994 ) ) ;
#144761=CARTESIAN_POINT ( 'NONE',  ( -0.05219959533937732626, 21.53943276465977519, 87.50109039468568994 ) ) ;
#144762=CARTESIAN_POINT ( 'NONE',  ( -16.46253265017160317, 9.564922557960807481, 115.8322429386477097 ) ) ;
#144763=CARTESIAN_POINT ( 'NONE',  ( -5.049401038297874678, -19.05341960407617918, 89.79275706135230450 ) ) ;
#144764=CARTESIAN_POINT ( 'NONE',  ( 15.80617190586769283, -15.72974639402175789, 65.62609039468568994 ) ) ;
#144765=CARTESIAN_POINT ( 'NONE',  ( -8.314922557961024197, 14.29746914071037800, 37.91775706135235424 ) ) ;
#144766=CARTESIAN_POINT ( 'NONE',  ( -0.05219959533907301413, -21.53943276465977519, 82.49890960531436690 ) ) ;
#144767=CARTESIAN_POINT ( 'NONE',  ( -0.05219959533936034679, 19.03943276465977164, 92.50109039468566152 ) ) ;
#144768=CARTESIAN_POINT ( 'NONE',  ( 9.474510206698971260, -16.51473224551069308, 67.91557627198102409 ) ) ;
#144769=CARTESIAN_POINT ( 'NONE',  ( 13.97604488694548053, -13.89961937509957401, 90.62609039468567573 ) ) ;
#144770=CARTESIAN_POINT ( 'NONE',  ( -13.97604488694547697, 13.89961937509957934, 98.12609039468566152 ) ) ;
#144771=CARTESIAN_POINT ( 'NONE',  ( 16.53943276465976808, -0.05219959533910856209, 58.74890960531436690 ) ) ;
#144772=CARTESIAN_POINT ( 'NONE',  ( 5.049401038297881783, 19.05341960407617563, 72.29275706135234714 ) ) ;
#144773=CARTESIAN_POINT ( 'NONE',  ( -16.55341960407617563, 4.379528057220093196, 63.54275706135234003 ) ) ;
#144775=CARTESIAN_POINT ( 'NONE',  ( -10.81492255796105439, 18.62759615963255655, 22.91775706135235069 ) ) ;
#144776=CARTESIAN_POINT ( 'NONE',  ( -5.153800228976328057, -19.02544592524343514, 32.29057627198102409 ) ) ;
#144777=CARTESIAN_POINT ( 'NONE',  ( 5.153800228976335163, 19.02544592524342804, 49.79057627198100988 ) ) ;
#144778=B_SPLINE_CURVE_WITH_KNOTS ( 'NONE', 3,
 ( #54717, #146719, #174087, #113381, #8215, #83043, #175071, #36537, #116389, #98193, #101205, #162895, #7201, #114375, #24404, #132563, #112396, #129537, #159896, #6204, #35556, #21385, #144718, #191237, #99211, #160899, #22391, #84041, #68885, #59692, #148740, #43547 ),
 .UNSPECIFIED., .F., .F.,
 ( 4, 2, 2, 2, 2, 2, 2, 2, 2, 2, 2, 2, 2, 2, 2, 4 ),
 ( 1.430489624538199204E-17, 0.0003712461730036907895, 0.0007424923460073672675, 0.001113738519011043746, 0.001484984692014720224, 0.002227477038022073180, 0.002598723211025749658, 0.002969969384029426136, 0.003341215557033102614, 0.003712461730036779092, 0.004083707903040455570, 0.004454954076044131614, 0.004826200249047807658, 0.005197446422051484570, 0.005568692595055161482, 0.005939938768058837526 ),
 .UNSPECIFIED. ) ;
#144779=CARTESIAN_POINT ( 'NONE',  ( -4.483927247898782831, 16.52544592524335698, 52.70942372801902565 ) ) ;
#144780=CARTESIAN_POINT ( 'NONE',  ( -17.50000000001357847, 5.500000000000046185, 45.79690382535059001 ) ) ;
#144782=CARTESIAN_POINT ( 'NONE',  ( 19.02544592524343514, -5.153800228976328945, 103.5405762719809957 ) ) ;
#144783=CARTESIAN_POINT ( 'NONE',  ( 5.049401038298161559, -19.05341960407611168, 27.70724293864769550 ) ) ;
#144784=EDGE_LOOP ( 'NONE', ( #138491, #67103, #114416, #1477, #2186, #86003, #182962, #26360, #29331, #126193, #39072, #189680, #8784, #15493, #92423, #10659, #122396, #197748, #140481, #137719, #72325, #98450, #153642, #53328, #59545, #154992, #152705, #29473, #48934, #185276, #168065, #197059, #169131, #41365, #40531, #154988, #177097, #192265, #68370, #160961, #62394, #101393, #178360, #59491, #101398, #117629, #195529, #72078, #54101, #72880, #82340, #81846, #80246, #142276, #51996, #152507 ) ) ;
#144785=CARTESIAN_POINT ( 'NONE',  ( -16.52544592524335698, -4.483927247898792601, 18.95942372801901143 ) ) ;
#144786=B_SPLINE_CURVE_WITH_KNOTS ( 'NONE', 3,
 ( #119673, #133841, #101486, #28669, #118678, #167170 ),
 .UNSPECIFIED., .F., .F.,
 ( 4, 2, 4 ),
 ( 0.007228050697041362750, 0.007608510107494831365, 0.007988969517948299112 ),
 .UNSPECIFIED. ) ;
#144787=CARTESIAN_POINT ( 'NONE',  ( -21.55341960407610458, -5.719274019375992779, 41.45724293864769550 ) ) ;
#144788=CARTESIAN_POINT ( 'NONE',  ( -5.153800228976607833, 19.02544592524334988, 47.70942372801900433 ) ) ;
#144789=CARTESIAN_POINT ( 'NONE',  ( 16.53943276465976808, 0.05219959533934440121, 26.25109039468567573 ) ) ;
#144790=CARTESIAN_POINT ( 'NONE',  ( 16.51473224551069308, 9.474510206698969483, 24.16557627198102765 ) ) ;
#144791=CARTESIAN_POINT ( 'NONE',  ( 13.89961937509977652, -13.97604488694527269, 48.12390960531435979 ) ) ;
#144792=CARTESIAN_POINT ( 'NONE',  ( 10.72451020669898902, -18.67979575497178502, 82.91557627198103830 ) ) ;
#144793=CARTESIAN_POINT ( 'NONE',  ( 19.03943276465977164, -0.05219959533909143690, 108.7489096053143527 ) ) ;
#144794=CARTESIAN_POINT ( 'NONE',  ( 5.049401038298161559, -19.05341960407611168, 52.70724293864767418 ) ) ;
#144796=CARTESIAN_POINT ( 'NONE',  ( -13.89961937509957401, -13.97604488694547875, 84.37609039468567573 ) ) ;
#144797=CARTESIAN_POINT ( 'NONE',  ( 4.379528057220339221, -16.55341960407611168, 72.70724293864769550 ) ) ;
#144798=CARTESIAN_POINT ( 'NONE',  ( 21.52544592524334988, 5.823673210054432836, 101.4594237280190185 ) ) ;
#144799=CARTESIAN_POINT ( 'NONE',  ( -21.55341960407610458, -5.719274019375992779, 91.45724293864769550 ) ) ;
#144800=CARTESIAN_POINT ( 'NONE',  ( -15.80617190586768217, 15.72974639402176855, 88.12609039468570415 ) ) ;
#144801=CARTESIAN_POINT ( 'NONE',  ( 15.72974639402176855, 15.80617190586768217, 81.87609039468568994 ) ) ;
#144802=CARTESIAN_POINT ( 'NONE',  ( 19.02544592524343514, -5.153800228976328945, 103.5405762719809957 ) ) ;
#144803=CARTESIAN_POINT ( 'NONE',  ( -14.29746914071037622, -8.314922557961029526, 104.1677570613523471 ) ) ;
#144804=CARTESIAN_POINT ( 'NONE',  ( 18.67979575497194134, -10.72451020669871369, 75.83442372801900433 ) ) ;
#144805=CARTESIAN_POINT ( 'NONE',  ( 19.02544592524343514, -5.153800228976328945, 63.54057627198103830 ) ) ;
#144806=CARTESIAN_POINT ( 'NONE',  ( -18.62759615963255300, -10.81492255796106328, 49.16775706135234003 ) ) ;
#144807=CARTESIAN_POINT ( 'NONE',  ( 0.05219959533909260263, 19.03943276465977164, 84.99890960531436690 ) ) ;
#144808=CARTESIAN_POINT ( 'NONE',  ( -4.483927247898539470, -16.52544592524342804, 87.29057627198103830 ) ) ;
#144809=CARTESIAN_POINT ( 'NONE',  ( -14.29746914071049879, 8.314922557960819915, 65.83224293864769550 ) ) ;
#144810=CARTESIAN_POINT ( 'NONE',  ( 15.80617190586746368, 15.72974639402197994, 64.37390960531435269 ) ) ;
#144811=CARTESIAN_POINT ( 'NONE',  ( -13.97604488694527625, -13.89961937509977652, 56.87390960531434558 ) ) ;
#144812=CARTESIAN_POINT ( 'NONE',  ( 15.80617190586746368, 15.72974639402197994, 69.37390960531436690 ) ) ;
#144813=CARTESIAN_POINT ( 'NONE',  ( 0.05219959533936267826, -19.03943276465977164, 70.00109039468566152 ) ) ;
#144814=CARTESIAN_POINT ( 'NONE',  ( -19.35543954521082455, -5.499999999999490186, 89.58901960356449479 ) ) ;
#144815=CARTESIAN_POINT ( 'NONE',  ( 16.55341960407611168, 4.379528057220329451, 73.95724293864769550 ) ) ;
#144816=CARTESIAN_POINT ( 'NONE',  ( -0.05219959533907301413, -21.53943276465977519, 57.49890960531435979 ) ) ;
#144818=CARTESIAN_POINT ( 'NONE',  ( 4.379528057220092307, 16.55341960407617563, 97.29275706135234714 ) ) ;
#144820=CARTESIAN_POINT ( 'NONE',  ( -5.153800228976607833, 19.02544592524334988, 97.70942372801900433 ) ) ;
#144821=CARTESIAN_POINT ( 'NONE',  ( -12.14591786802309592, -12.06949235617757132, 66.87390960531436690 ) ) ;
#144823=CARTESIAN_POINT ( 'NONE',  ( -13.97604488694527625, -13.89961937509977652, 66.87390960531436690 ) ) ;
#144824=CARTESIAN_POINT ( 'NONE',  ( 4.379528057220339221, -16.55341960407611168, 52.70724293864769550 ) ) ;
#144825=CARTESIAN_POINT ( 'NONE',  ( -13.97604488694527625, -13.89961937509977652, 86.87390960531436690 ) ) ;
#144826=CARTESIAN_POINT ( 'NONE',  ( 9.474510206698729675, 16.51473224551082808, 82.08442372801899012 ) ) ;
#144827=CARTESIAN_POINT ( 'NONE',  ( 16.46253265017160672, -9.564922557960803928, 68.33224293864770971 ) ) ;
#144828=CARTESIAN_POINT ( 'NONE',  ( -5.153800228976328057, -19.02544592524343514, 87.29057627198103830 ) ) ;
#144829=CARTESIAN_POINT ( 'NONE',  ( 19.02544592524343514, -5.153800228976328945, 68.54057627198103830 ) ) ;
#144830=CARTESIAN_POINT ( 'NONE',  ( 5.719274019375991003, -21.55341960407610458, 62.70724293864769550 ) ) ;
#144831=CARTESIAN_POINT ( 'NONE',  ( -4.483927247898782831, 16.52544592524335698, 62.70942372801902565 ) ) ;
#144832=CARTESIAN_POINT ( 'NONE',  ( 5.153800228976617603, -19.02544592524335343, 105.2094237280189901 ) ) ;
#144833=CARTESIAN_POINT ( 'NONE',  ( 9.564922557960805705, 16.46253265017160317, 54.58224293864769550 ) ) ;
#144834=CARTESIAN_POINT ( 'NONE',  ( 21.53943276465977519, -0.05219959533907433946, 58.74890960531436690 ) ) ;
#144835=CARTESIAN_POINT ( 'NONE',  ( 9.474510206698729675, 16.51473224551082808, 87.08442372801900433 ) ) ;
#144836=CARTESIAN_POINT ( 'NONE',  ( -14.34966873604972548, 8.224510206698743886, 113.3344237280190328 ) ) ;
#144837=CARTESIAN_POINT ( 'NONE',  ( 19.02544592524334988, 5.153800228976608722, 41.45942372801900433 ) ) ;
#144838=CARTESIAN_POINT ( 'NONE',  ( 12.06949235617739724, 12.14591786802326823, 61.87609039468568284 ) ) ;
#144839=CARTESIAN_POINT ( 'NONE',  ( 12.14591786802327356, -12.06949235617739191, 95.62609039468568994 ) ) ;
#144841=CARTESIAN_POINT ( 'NONE',  ( -12.14591786802326823, 12.06949235617739902, 83.12609039468568994 ) ) ;
#144842=CARTESIAN_POINT ( 'NONE',  ( -5.823673210054116645, -21.52544592524344225, 27.29057627198103120 ) ) ;
#144843=CARTESIAN_POINT ( 'NONE',  ( 4.483927247898790824, -16.52544592524335698, 35.20942372801901854 ) ) ;
#144844=CARTESIAN_POINT ( 'NONE',  ( 13.97604488694527802, 13.89961937509977652, 49.37390960531434558 ) ) ;
#144845=CARTESIAN_POINT ( 'NONE',  ( 19.03943276465977164, -0.05219959533909143690, 48.74890960531435979 ) ) ;
#144846=CARTESIAN_POINT ( 'NONE',  ( -0.05219959533909027116, -19.03943276465977164, 52.49890960531436690 ) ) ;
#144847=CARTESIAN_POINT ( 'NONE',  ( 10.72451020669871369, 18.67979575497193778, 37.08442372801901143 ) ) ;
#144848=CARTESIAN_POINT ( 'NONE',  ( -12.14591786802326823, 12.06949235617739902, 53.12609039468568284 ) ) ;
#144849=CARTESIAN_POINT ( 'NONE',  ( -14.34966873604972548, 8.224510206698743886, 113.3344237280190328 ) ) ;
#144850=CARTESIAN_POINT ( 'NONE',  ( 19.02544592524343514, -5.153800228976328945, 28.54057627198102409 ) ) ;
#144851=CARTESIAN_POINT ( 'NONE',  ( -15.72974639402176322, -15.80617190586768395, 109.3760903946857042 ) ) ;
#144852=CARTESIAN_POINT ( 'NONE',  ( -13.97604488694547697, 13.89961937509957934, 113.1260903946856757 ) ) ;
#144853=CARTESIAN_POINT ( 'NONE',  ( -16.51473224551082808, 9.474510206698731452, 63.33442372801900433 ) ) ;
#144854=CARTESIAN_POINT ( 'NONE',  ( 12.06949235617757843, -12.14591786802309237, 68.12390960531436690 ) ) ;
#144855=CARTESIAN_POINT ( 'NONE',  ( -0.05219959533909027116, -19.03943276465977164, 42.49890960531435269 ) ) ;
#144856=CARTESIAN_POINT ( 'NONE',  ( 5.153800228976615827, -19.02544592524334988, 70.20942372801899012 ) ) ;
#144858=CARTESIAN_POINT ( 'NONE',  ( 0.05219959533937995610, -21.53943276465977519, 75.00109039468568994 ) ) ;
#144859=CARTESIAN_POINT ( 'NONE',  ( 4.483927247898790824, -16.52544592524335698, 35.20942372801901854 ) ) ;
#144860=CARTESIAN_POINT ( 'NONE',  ( 19.02130022317638236, -5.499999999999594102, 58.28188669246577547 ) ) ;
#144861=CARTESIAN_POINT ( 'NONE',  ( 21.53943276465977519, -0.05219959533907433946, 33.74890960531436690 ) ) ;
#144862=CARTESIAN_POINT ( 'NONE',  ( 4.379528057220092307, 16.55341960407617563, 27.29275706135234358 ) ) ;
#144863=CARTESIAN_POINT ( 'NONE',  ( -13.89961937509977830, 13.97604488694528158, 30.62390960531435624 ) ) ;
#144864=CARTESIAN_POINT ( 'NONE',  ( 21.55341960407619695, -5.719274019375665929, 106.0427570613523471 ) ) ;
#144866=CARTESIAN_POINT ( 'NONE',  ( -16.46253265017160317, 9.564922557960807481, 35.83224293864768839 ) ) ;
#144868=CARTESIAN_POINT ( 'NONE',  ( -9.564922557960796823, -16.46253265017161027, 52.08224293864768839 ) ) ;
#144869=CARTESIAN_POINT ( 'NONE',  ( 5.719274019375673035, 21.55341960407619339, 67.29275706135234714 ) ) ;
#144870=CARTESIAN_POINT ( 'NONE',  ( 18.62759615963255655, 10.81492255796105972, 111.6677570613523613 ) ) ;
#144871=CARTESIAN_POINT ( 'NONE',  ( -12.14591786802309592, -12.06949235617757132, 26.87390960531435979 ) ) ;
#144872=CARTESIAN_POINT ( 'NONE',  ( -19.03943276465977164, 0.05219959533909376836, 31.24890960531435979 ) ) ;
#144873=CARTESIAN_POINT ( 'NONE',  ( 19.02544592524343514, -5.153800228976328945, 88.54057627198102409 ) ) ;
#144874=CARTESIAN_POINT ( 'NONE',  ( 15.80617190586769283, -15.72974639402175789, 60.62609039468567573 ) ) ;
#144875=CARTESIAN_POINT ( 'NONE',  ( 19.05341960407611168, 5.049401038298154454, 38.95724293864767418 ) ) ;
#144877=CARTESIAN_POINT ( 'NONE',  ( 21.55341960407619695, -5.719274019375665929, 66.04275706135236135 ) ) ;
#144878=CARTESIAN_POINT ( 'NONE',  ( 19.02544592524334988, 5.153800228976608722, 91.45942372801900433 ) ) ;
#144879=CARTESIAN_POINT ( 'NONE',  ( -19.05341960407611168, -5.049401038298163336, 111.4572429386476671 ) ) ;
#144880=CARTESIAN_POINT ( 'NONE',  ( 9.474510206698971260, -16.51473224551069308, 27.91557627198103120 ) ) ;
#144881=CARTESIAN_POINT ( 'NONE',  ( 21.52544592524344225, -5.823673210054117533, 103.5405762719810383 ) ) ;
#144882=CARTESIAN_POINT ( 'NONE',  ( 9.564922557961047289, -16.46253265017146816, 35.41775706135233293 ) ) ;
#144883=CARTESIAN_POINT ( 'NONE',  ( 0.05219959533910956823, 16.53943276465976808, 114.9989096053143669 ) ) ;
#144884=CARTESIAN_POINT ( 'NONE',  ( 9.474510206698971260, -16.51473224551069308, 67.91557627198102409 ) ) ;
#144885=CARTESIAN_POINT ( 'NONE',  ( 13.97604488694548053, -13.89961937509957401, 95.62609039468563310 ) ) ;
#144886=CARTESIAN_POINT ( 'NONE',  ( 12.14591786802309770, 12.06949235617756955, 64.37390960531435269 ) ) ;
#144887=CARTESIAN_POINT ( 'NONE',  ( -18.62759615963270932, 10.81492255796079327, 25.83224293864769194 ) ) ;
#144888=CARTESIAN_POINT ( 'NONE',  ( 19.02544592524334988, 5.153800228976608722, 91.45942372801900433 ) ) ;
#144889=CARTESIAN_POINT ( 'NONE',  ( -18.62759615963270932, 10.81492255796079327, 85.83224293864768129 ) ) ;
#144890=CARTESIAN_POINT ( 'NONE',  ( -5.719274019375665041, -21.55341960407619695, 44.79275706135234714 ) ) ;
#144891=CARTESIAN_POINT ( 'NONE',  ( -14.29746914071037622, -8.314922557961029526, 39.16775706135235424 ) ) ;
#144892=CARTESIAN_POINT ( 'NONE',  ( -0.05219959533934338120, 16.53943276465976808, 42.50109039468567573 ) ) ;
#144893=CARTESIAN_POINT ( 'NONE',  ( 0.05219959533937995610, -21.53943276465977519, 45.00109039468568284 ) ) ;
#144894=CARTESIAN_POINT ( 'NONE',  ( 21.55341960407610458, 5.719274019375980345, 53.95724293864770260 ) ) ;
#144895=CARTESIAN_POINT ( 'NONE',  ( -16.51473224551069308, -9.474510206698971260, 36.66557627198102409 ) ) ;
#144897=CARTESIAN_POINT ( 'NONE',  ( 12.14591786802327356, -12.06949235617739191, 70.62609039468567573 ) ) ;
#144898=CARTESIAN_POINT ( 'NONE',  ( -21.52544592524343514, 5.823673210054127303, 106.0405762719810525 ) ) ;
#144899=CARTESIAN_POINT ( 'NONE',  ( 8.224510206698953496, -14.34966873604960469, 37.91557627198102409 ) ) ;
#144900=CARTESIAN_POINT ( 'NONE',  ( -16.53943276465976808, -0.05219959533934237506, 63.75109039468568284 ) ) ;
#144901=CARTESIAN_POINT ( 'NONE',  ( -5.153800228976607833, 19.02544592524334988, 102.7094237280189759 ) ) ;
#144902=CARTESIAN_POINT ( 'NONE',  ( 15.80617190586746368, 15.72974639402197994, 94.37390960531436690 ) ) ;
#144903=CARTESIAN_POINT ( 'NONE',  ( -8.224510206698948167, 14.34966873604960824, 35.41557627198102409 ) ) ;
#144905=CARTESIAN_POINT ( 'NONE',  ( -4.379528057220086978, -16.55341960407618274, 74.79275706135234714 ) ) ;
#144907=CARTESIAN_POINT ( 'NONE',  ( -10.72451020669898014, 18.67979575497178502, 70.41557627198102409 ) ) ;
#144908=CARTESIAN_POINT ( 'NONE',  ( 8.224510206698742110, 14.34966873604972548, 102.0844237280190185 ) ) ;
#144909=EDGE_LOOP ( 'NONE', ( #102507, #72971 ) ) ;
#144911=CARTESIAN_POINT ( 'NONE',  ( 15.72974639402199770, -15.80617190586745480, 103.1239096053143811 ) ) ;
#144912=CARTESIAN_POINT ( 'NONE',  ( -15.80617190586745835, -15.72974639402198527, 106.8739096053143811 ) ) ;
#144913=CARTESIAN_POINT ( 'NONE',  ( 8.224510206698953496, -14.34966873604960469, 37.91557627198102409 ) ) ;
#144914=CARTESIAN_POINT ( 'NONE',  ( -14.29746914071037622, -8.314922557961029526, 44.16775706135234714 ) ) ;
#144915=CARTESIAN_POINT ( 'NONE',  ( -13.97604488694527625, -13.89961937509977652, 46.87390960531435979 ) ) ;
#144916=CARTESIAN_POINT ( 'NONE',  ( -9.564922557960796823, -16.46253265017161027, 67.08224293864769550 ) ) ;
#144918=CARTESIAN_POINT ( 'NONE',  ( -19.03943276465977164, 0.05219959533909376836, 111.2489096053143669 ) ) ;
#144920=CARTESIAN_POINT ( 'NONE',  ( -0.05219959533936034679, 19.03943276465977164, 102.5010903946856757 ) ) ;
#144921=CARTESIAN_POINT ( 'NONE',  ( 5.153800228976615827, -19.02544592524334988, 50.20942372801897591 ) ) ;
#144922=CARTESIAN_POINT ( 'NONE',  ( -5.719274019375978568, 21.55341960407610458, 90.20724293864770971 ) ) ;
#144923=CARTESIAN_POINT ( 'NONE',  ( 16.52544592524342804, -4.483927247898539470, 23.54057627198102765 ) ) ;
#144924=CARTESIAN_POINT ( 'NONE',  ( -19.05341960407611168, -5.049401038298163336, 81.45724293864769550 ) ) ;
#144925=CARTESIAN_POINT ( 'NONE',  ( -15.80617190586745835, -15.72974639402198527, 41.87390960531435979 ) ) ;
#144926=CARTESIAN_POINT ( 'NONE',  ( -18.62759615963270932, 10.81492255796079327, 85.83224293864768129 ) ) ;
#144927=CARTESIAN_POINT ( 'NONE',  ( 14.34966873604972726, -8.224510206698740333, 20.83442372801901143 ) ) ;
#144928=CARTESIAN_POINT ( 'NONE',  ( -19.02544592524342804, 5.153800228976336051, 116.0405762719810383 ) ) ;
#144929=CARTESIAN_POINT ( 'NONE',  ( 5.823673210054444382, -21.52544592524334988, 80.20942372801901854 ) ) ;
#144930=CARTESIAN_POINT ( 'NONE',  ( 16.51473224551069308, 9.474510206698969483, 79.16557627198103830 ) ) ;
#144932=CARTESIAN_POINT ( 'NONE',  ( 5.049401038298161559, -19.05341960407611168, 72.70724293864768129 ) ) ;
#144933=CARTESIAN_POINT ( 'NONE',  ( -4.483927247898539470, -16.52544592524342804, 92.29057627198103830 ) ) ;
#144935=CARTESIAN_POINT ( 'NONE',  ( -0.05219959533936034679, 19.03943276465977164, 107.5010903946856615 ) ) ;
#144937=CARTESIAN_POINT ( 'NONE',  ( 0.05219959533909260263, 19.03943276465977164, 74.99890960531435269 ) ) ;
#144938=CARTESIAN_POINT ( 'NONE',  ( 15.72974639402176855, 15.80617190586768217, 81.87609039468568994 ) ) ;
#144939=CARTESIAN_POINT ( 'NONE',  ( -19.03943276465977164, 0.05219959533909376836, 96.24890960531436690 ) ) ;
#144940=CARTESIAN_POINT ( 'NONE',  ( -14.29746914071037622, -8.314922557961029526, 79.16775706135234714 ) ) ;
#144941=CARTESIAN_POINT ( 'NONE',  ( -16.52216118717209170, -7.221426719304500530, 76.07599021046995347 ) ) ;
#144942=CARTESIAN_POINT ( 'NONE',  ( -13.97604488694547697, 13.89961937509957934, 53.12609039468565442 ) ) ;
#144943=CARTESIAN_POINT ( 'NONE',  ( 5.719274019375673035, 21.55341960407619339, 112.2927570613523471 ) ) ;
#144947=CARTESIAN_POINT ( 'NONE',  ( 4.379528057220092307, 16.55341960407617563, 112.2927570613523471 ) ) ;
#144948=DIRECTION ( 'NONE',  ( 0.000000000000000000, -1.000000000000000000, 0.000000000000000000 ) ) ;
#144949=CARTESIAN_POINT ( 'NONE',  ( 8.314922557961029526, -14.29746914071037800, 110.4177570613523756 ) ) ;
#144951=CARTESIAN_POINT ( 'NONE',  ( 16.52544592524335698, 4.483927247898782831, 86.45942372801901854 ) ) ;
#144952=CARTESIAN_POINT ( 'NONE',  ( 21.53943276465977519, 0.05219959533937863772, 86.25109039468568994 ) ) ;
#144953=CARTESIAN_POINT ( 'NONE',  ( 5.049401038297881783, 19.05341960407617563, 82.29275706135229029 ) ) ;
#144954=CARTESIAN_POINT ( 'NONE',  ( -5.049401038297874678, -19.05341960407617918, 34.79275706135233293 ) ) ;
#144955=CARTESIAN_POINT ( 'NONE',  ( 0.05219959533909260263, 19.03943276465977164, 74.99890960531435269 ) ) ;
#144956=CARTESIAN_POINT ( 'NONE',  ( 19.02544592524343514, -5.153800228976328945, 58.54057627198102409 ) ) ;
#144957=CARTESIAN_POINT ( 'NONE',  ( 17.97182807773870294, -5.499999999999849010, 41.03038844047290468 ) ) ;
#144958=CARTESIAN_POINT ( 'NONE',  ( 0.05219959533907565091, 21.53943276465977519, 89.99890960531438111 ) ) ;
#144959=CARTESIAN_POINT ( 'NONE',  ( -15.72974639402197994, 15.80617190586746368, 45.62390960531436690 ) ) ;
#144960=CARTESIAN_POINT ( 'NONE',  ( -19.03943276465977164, 0.05219959533909376836, 46.24890960531435979 ) ) ;
#144961=CARTESIAN_POINT ( 'NONE',  ( -12.14591786802326823, 12.06949235617739902, 58.12609039468568994 ) ) ;
#144963=UNCERTAINTY_MEASURE_WITH_UNIT (LENGTH_MEASURE( 1.000000000000000082E-05 ), #183092, 'distance_accuracy_value', 'NONE');
#144965=CARTESIAN_POINT ( 'NONE',  ( 21.52544592524334988, 5.823673210054432836, 51.45942372801901854 ) ) ;
#144966=CARTESIAN_POINT ( 'NONE',  ( -16.52544592524342804, 4.483927247898546575, 71.04057627198103830 ) ) ;
#144968=CARTESIAN_POINT ( 'NONE',  ( -16.55341960407617563, 4.379528057220093196, 33.54275706135234714 ) ) ;
#144969=CARTESIAN_POINT ( 'NONE',  ( 12.06949235617757843, -12.14591786802309237, 103.1239096053143811 ) ) ;
#144970=CARTESIAN_POINT ( 'NONE',  ( 16.51473224551083163, -9.474510206698727899, 55.83442372801899722 ) ) ;
#144971=CARTESIAN_POINT ( 'NONE',  ( 16.52544592524342804, -4.483927247898539470, 68.54057627198103830 ) ) ;
#144972=CARTESIAN_POINT ( 'NONE',  ( -21.55341960407619339, 5.719274019375674811, 33.54275706135234714 ) ) ;
#144973=CARTESIAN_POINT ( 'NONE',  ( 19.05341960407611168, 5.049401038298154454, 23.95724293864769194 ) ) ;
#144974=CARTESIAN_POINT ( 'NONE',  ( 5.823673210054125526, 21.52544592524343514, 94.79057627198105251 ) ) ;
#144975=CARTESIAN_POINT ( 'NONE',  ( 5.153800228976335163, 19.02544592524342804, 109.7905762719810099 ) ) ;
#144976=CARTESIAN_POINT ( 'NONE',  ( -12.06949235617756955, 12.14591786802309770, 70.62390960531436690 ) ) ;
#144980=CARTESIAN_POINT ( 'NONE',  ( -9.564922557961040184, 16.46253265017147172, 77.91775706135234714 ) ) ;
#144981=CARTESIAN_POINT ( 'NONE',  ( 21.53943276465977519, 0.05219959533937863772, 26.25109039468567573 ) ) ;
#144982=CARTESIAN_POINT ( 'NONE',  ( 9.474510206698971260, -16.51473224551069308, 67.91557627198102409 ) ) ;
#144983=CARTESIAN_POINT ( 'NONE',  ( 9.474510206698729675, 16.51473224551082808, 62.08442372801899722 ) ) ;
#144984=CARTESIAN_POINT ( 'NONE',  ( 9.564922557960805705, 16.46253265017160317, 29.58224293864769550 ) ) ;
#144985=CARTESIAN_POINT ( 'NONE',  ( -0.05219959533910754901, -16.53943276465976808, 67.49890960531436690 ) ) ;
#144986=CARTESIAN_POINT ( 'NONE',  ( 8.314922557960818139, 14.29746914071049879, 54.58224293864769550 ) ) ;
#144987=CARTESIAN_POINT ( 'NONE',  ( -0.05219959533909027116, -19.03943276465977164, 62.49890960531435979 ) ) ;
#144988=CARTESIAN_POINT ( 'NONE',  ( 15.72974639402199770, -15.80617190586745480, 83.12390960531436690 ) ) ;
#144989=CARTESIAN_POINT ( 'NONE',  ( 19.03943276465977164, -0.05219959533909143690, 63.74890960531435979 ) ) ;
#144990=ORIENTED_EDGE ( 'NONE', *, *, #174403, .F. ) ;
#144991=CARTESIAN_POINT ( 'NONE',  ( -5.719274019375978568, 21.55341960407610458, 80.20724293864769550 ) ) ;
#144992=CARTESIAN_POINT ( 'NONE',  ( 18.67979575497194134, -10.72451020669871369, 100.8344237280190185 ) ) ;
#144994=CARTESIAN_POINT ( 'NONE',  ( 14.29746914071037800, 8.314922557961029526, 106.6677570613523756 ) ) ;
#144995=CARTESIAN_POINT ( 'NONE',  ( 12.14591786802309770, 12.06949235617756955, 94.37390960531436690 ) ) ;
#144996=CARTESIAN_POINT ( 'NONE',  ( -16.51473224551082808, 9.474510206698731452, 98.33442372801900433 ) ) ;
#144998=CARTESIAN_POINT ( 'NONE',  ( -10.72451020669870658, -18.67979575497194134, 19.58442372801901143 ) ) ;
#144999=CARTESIAN_POINT ( 'NONE',  ( 9.474510206698729675, 16.51473224551082808, 47.08442372801900433 ) ) ;
#145000=CARTESIAN_POINT ( 'NONE',  ( -14.29746914071037622, -8.314922557961029526, 99.16775706135234714 ) ) ;
#145001=CARTESIAN_POINT ( 'NONE',  ( -5.049401038297874678, -19.05341960407617918, 34.79275706135233293 ) ) ;
#145002=CARTESIAN_POINT ( 'NONE',  ( 19.02544592524343514, -5.153800228976328945, 98.54057627198100988 ) ) ;
#145003=CARTESIAN_POINT ( 'NONE',  ( 10.72451020669898902, -18.67979575497178502, 67.91557627198102409 ) ) ;
#145005=CARTESIAN_POINT ( 'NONE',  ( 9.564922557960805705, 16.46253265017160317, 29.58224293864769550 ) ) ;
#145006=CARTESIAN_POINT ( 'NONE',  ( 18.67979575497194134, -10.72451020669871369, 110.8344237280190043 ) ) ;
#145007=CARTESIAN_POINT ( 'NONE',  ( 14.29746914071037800, 8.314922557961029526, 71.66775706135234714 ) ) ;
#145008=CARTESIAN_POINT ( 'NONE',  ( 15.80617190586769283, -15.72974639402175789, 25.62609039468567929 ) ) ;
#145009=CARTESIAN_POINT ( 'NONE',  ( -14.29746914071037622, -8.314922557961029526, 39.16775706135235424 ) ) ;
#145010=CARTESIAN_POINT ( 'NONE',  ( -9.474510206698964154, 16.51473224551069663, 100.4155762719810241 ) ) ;
#145011=CARTESIAN_POINT ( 'NONE',  ( -19.03943276465977164, 0.05219959533909376836, 51.24890960531436690 ) ) ;
#145012=CARTESIAN_POINT ( 'NONE',  ( 5.049401038298161559, -19.05341960407611168, 72.70724293864768129 ) ) ;
#145013=CARTESIAN_POINT ( 'NONE',  ( 14.29746914071037800, 8.314922557961029526, 41.66775706135235424 ) ) ;
#145014=CARTESIAN_POINT ( 'NONE',  ( 16.53943276465976808, -0.05219959533910856209, 98.74890960531438111 ) ) ;
#145015=CARTESIAN_POINT ( 'NONE',  ( 14.34966873604972726, -8.224510206698740333, 105.8344237280190328 ) ) ;
#145017=CARTESIAN_POINT ( 'NONE',  ( 5.823673210054444382, -21.52544592524334988, 55.20942372801902565 ) ) ;
#145018=CARTESIAN_POINT ( 'NONE',  ( 19.02544592524343514, -5.153800228976328945, 78.54057627198099567 ) ) ;
#145019=CARTESIAN_POINT ( 'NONE',  ( -5.153800228976328057, -19.02544592524343514, 67.29057627198102409 ) ) ;
#145020=CARTESIAN_POINT ( 'NONE',  ( 0.05219959533909260263, 19.03943276465977164, 89.99890960531436690 ) ) ;
#145021=CARTESIAN_POINT ( 'NONE',  ( -12.14591786802309592, -12.06949235617757132, 51.87390960531437401 ) ) ;
#145022=CARTESIAN_POINT ( 'NONE',  ( 14.34966873604972726, -8.224510206698740333, 100.8344237280190185 ) ) ;
#145023=CARTESIAN_POINT ( 'NONE',  ( -16.52544592524342804, 4.483927247898546575, 36.04057627198102409 ) ) ;
#145025=CARTESIAN_POINT ( 'NONE',  ( -9.564922557961040184, 16.46253265017147172, 42.91775706135234003 ) ) ;
#145027=CARTESIAN_POINT ( 'NONE',  ( 19.05341960407611168, 5.049401038298154454, 68.95724293864769550 ) ) ;
#145028=CARTESIAN_POINT ( 'NONE',  ( -13.89961937509957401, -13.97604488694547875, 39.37609039468566152 ) ) ;
#145030=CARTESIAN_POINT ( 'NONE',  ( 17.49999999999999645, 5.500000000000007994, 73.78230962303568674 ) ) ;
#145031=CARTESIAN_POINT ( 'NONE',  ( 19.02544592524334988, 5.153800228976608722, 91.45942372801900433 ) ) ;
#145032=CARTESIAN_POINT ( 'NONE',  ( -16.53943276465976808, -0.05219959533934237506, 63.75109039468568284 ) ) ;
#145033=FACE_OUTER_BOUND ( 'NONE', #120792, .T. ) ;
#145034=CARTESIAN_POINT ( 'NONE',  ( 13.89961937509977652, -13.97604488694527269, 88.12390960531438111 ) ) ;
#145035=CARTESIAN_POINT ( 'NONE',  ( -10.72451020669870658, -18.67979575497194134, 24.58442372801901499 ) ) ;
#145036=CARTESIAN_POINT ( 'NONE',  ( 13.97604488694548053, -13.89961937509957401, 80.62609039468567573 ) ) ;
#145037=CARTESIAN_POINT ( 'NONE',  ( 16.19135201231366139, 7.376712067591958188, 87.68680854052034590 ) ) ;
#145038=CARTESIAN_POINT ( 'NONE',  ( 5.049401038298161559, -19.05341960407611168, 42.70724293864767418 ) ) ;
#145039=CARTESIAN_POINT ( 'NONE',  ( 0.05219959533909260263, 19.03943276465977164, 94.99890960531436690 ) ) ;
#145040=CARTESIAN_POINT ( 'NONE',  ( -12.14591786802309592, -12.06949235617757132, 51.87390960531437401 ) ) ;
#145041=CARTESIAN_POINT ( 'NONE',  ( 9.474510206698971260, -16.51473224551069308, 47.91557627198102409 ) ) ;
#145042=CARTESIAN_POINT ( 'NONE',  ( 13.89961937509957401, 13.97604488694547697, 46.87609039468565442 ) ) ;
#145043=EDGE_LOOP ( 'NONE', ( #147976, #57706, #55909, #39925, #51105, #34750, #174524, #23672, #57001, #86332, #144990, #131749, #178088, #103664, #66451, #29855, #1800, #190492, #176563, #40773, #178523, #74379, #37114, #109151, #159918, #198172, #124354, #127118, #122656, #134013, #138702, #48008, #96179, #195201, #55532, #137540, #26884, #19360, #163469, #194203, #47304 ) ) ;
#145044=CARTESIAN_POINT ( 'NONE',  ( -0.05219959533910754901, -16.53943276465976808, 87.49890960531436690 ) ) ;
#145045=CARTESIAN_POINT ( 'NONE',  ( 19.02544592524334988, 5.153800228976608722, 31.45942372801900433 ) ) ;
#145046=CARTESIAN_POINT ( 'NONE',  ( 0.05219959533909260263, 19.03943276465977164, 59.99890960531436690 ) ) ;
#145047=CARTESIAN_POINT ( 'NONE',  ( -10.72451020669898014, 18.67979575497178502, 65.41557627198102409 ) ) ;
#145048=CARTESIAN_POINT ( 'NONE',  ( -14.29746914071049879, 8.314922557960819915, 60.83224293864769550 ) ) ;
#145049=CARTESIAN_POINT ( 'NONE',  ( -9.564922557961040184, 16.46253265017147172, 22.91775706135233648 ) ) ;
#145050=CARTESIAN_POINT ( 'NONE',  ( -5.049401038298153566, 19.05341960407611168, 100.2072429386476955 ) ) ;
#145051=CARTESIAN_POINT ( 'NONE',  ( 0.05219959533907565091, 21.53943276465977519, 24.99890960531435624 ) ) ;
#145052=CARTESIAN_POINT ( 'NONE',  ( 19.02544592524343514, -5.153800228976328945, 58.54057627198102409 ) ) ;
#145053=CARTESIAN_POINT ( 'NONE',  ( -16.46253265017160317, 9.564922557960807481, 35.83224293864768839 ) ) ;
#145054=CARTESIAN_POINT ( 'NONE',  ( -0.05219959533910754901, -16.53943276465976808, 97.49890960531436690 ) ) ;
#145055=CARTESIAN_POINT ( 'NONE',  ( 5.823673210054125526, 21.52544592524343514, 114.7905762719810383 ) ) ;
#145056=CARTESIAN_POINT ( 'NONE',  ( 0.05219959533909260263, 19.03943276465977164, 99.99890960531436690 ) ) ;
#145057=CARTESIAN_POINT ( 'NONE',  ( 0.05219959533907565091, 21.53943276465977519, 109.9989096053143527 ) ) ;
#145058=CARTESIAN_POINT ( 'NONE',  ( 5.049401038298161559, -19.05341960407611168, 102.7072429386476955 ) ) ;
#145059=CARTESIAN_POINT ( 'NONE',  ( -12.06949235617756955, 12.14591786802309770, 115.6239096053143669 ) ) ;
#145060=CARTESIAN_POINT ( 'NONE',  ( -15.72974639402176322, -15.80617190586768395, 84.37609039468570415 ) ) ;
#145061=CARTESIAN_POINT ( 'NONE',  ( -15.72974639402197994, 15.80617190586746368, 90.62390960531436690 ) ) ;
#145062=CARTESIAN_POINT ( 'NONE',  ( 16.36317988757058117, -7.306389748694945396, 106.5978960836322642 ) ) ;
#145065=CARTESIAN_POINT ( 'NONE',  ( -16.52544592524335698, -4.483927247898792601, 43.95942372801902565 ) ) ;
#145066=CARTESIAN_POINT ( 'NONE',  ( -12.14591786802309592, -12.06949235617757132, 106.8739096053143811 ) ) ;
#145068=CARTESIAN_POINT ( 'NONE',  ( 16.46253265017160672, -9.564922557960803928, 58.33224293864769550 ) ) ;
#145069=CARTESIAN_POINT ( 'NONE',  ( 14.29746914071049879, -8.314922557960816363, 98.33224293864769550 ) ) ;
#145070=CARTESIAN_POINT ( 'NONE',  ( 21.52544592524344225, -5.823673210054117533, 43.54057627198103830 ) ) ;
#145071=CARTESIAN_POINT ( 'NONE',  ( -8.224510206698948167, 14.34966873604960824, 70.41557627198102409 ) ) ;
#145072=CARTESIAN_POINT ( 'NONE',  ( -16.52544592524335698, -4.483927247898792601, 18.95942372801901143 ) ) ;
#145073=CARTESIAN_POINT ( 'NONE',  ( 0.05219959533937995610, -21.53943276465977519, 70.00109039468568994 ) ) ;
#145075=CARTESIAN_POINT ( 'NONE',  ( 14.29746914071037800, 8.314922557961029526, 101.6677570613523613 ) ) ;
#145076=CARTESIAN_POINT ( 'NONE',  ( 12.06949235617757843, -12.14591786802309237, 43.12390960531435269 ) ) ;
#145077=CARTESIAN_POINT ( 'NONE',  ( 9.564922557960805705, 16.46253265017160317, 44.58224293864769550 ) ) ;
#145078=CARTESIAN_POINT ( 'NONE',  ( 0.05219959533909260263, 19.03943276465977164, 94.99890960531436690 ) ) ;
#145079=CARTESIAN_POINT ( 'NONE',  ( 10.81492255796078972, 18.62759615963270932, 94.58224293864769550 ) ) ;
#145080=CARTESIAN_POINT ( 'NONE',  ( 8.314922557961029526, -14.29746914071037800, 30.41775706135234358 ) ) ;
#145081=CARTESIAN_POINT ( 'NONE',  ( -16.52544592524342804, 4.483927247898546575, 66.04057627198103830 ) ) ;
#145082=CARTESIAN_POINT ( 'NONE',  ( 21.52544592524334988, 5.823673210054432836, 71.45942372801901854 ) ) ;
#145083=CARTESIAN_POINT ( 'NONE',  ( -16.53943276465976808, -0.05219959533934237506, 93.75109039468567573 ) ) ;
#145084=CARTESIAN_POINT ( 'NONE',  ( 16.81555441253467365, -7.025013491696276091, 48.13685445334212432 ) ) ;
#145085=CARTESIAN_POINT ( 'NONE',  ( -18.89770734986050016, -5.499999999999905853, 64.10214472496640781 ) ) ;
#145086=CARTESIAN_POINT ( 'NONE',  ( -14.29746914071049879, 8.314922557960819915, 25.83224293864769194 ) ) ;
#145087=CARTESIAN_POINT ( 'NONE',  ( 4.483927247898790824, -16.52544592524335698, 75.20942372801901854 ) ) ;
#145088=CARTESIAN_POINT ( 'NONE',  ( 5.049401038298161559, -19.05341960407611168, 87.70724293864769550 ) ) ;
#145089=CARTESIAN_POINT ( 'NONE',  ( 19.05341960407611168, 5.049401038298154454, 98.95724293864766707 ) ) ;
#145090=CARTESIAN_POINT ( 'NONE',  ( 10.81492255796106328, -18.62759615963255655, 85.41775706135236135 ) ) ;
#145091=CARTESIAN_POINT ( 'NONE',  ( 4.483927247898790824, -16.52544592524335698, 95.20942372801903275 ) ) ;
#145092=CARTESIAN_POINT ( 'NONE',  ( 12.06949235617757843, -12.14591786802309237, 63.12390960531435979 ) ) ;
#145093=CARTESIAN_POINT ( 'NONE',  ( 9.474510206698971260, -16.51473224551069308, 72.91557627198102409 ) ) ;
#145094=ORIENTED_EDGE ( 'NONE', *, *, #38977, .F. ) ;
#145095=CARTESIAN_POINT ( 'NONE',  ( 19.03943276465977164, 0.05219959533936151252, 111.2510903946856757 ) ) ;
#145096=CARTESIAN_POINT ( 'NONE',  ( 4.483927247898545687, 16.52544592524342804, 114.7905762719810383 ) ) ;
#145097=CARTESIAN_POINT ( 'NONE',  ( 9.564922557960805705, 16.46253265017160317, 74.58224293864769550 ) ) ;
#145098=CARTESIAN_POINT ( 'NONE',  ( 4.483927247898790824, -16.52544592524335698, 25.20942372801901854 ) ) ;
#145100=CARTESIAN_POINT ( 'NONE',  ( -21.53943276465977519, -0.05219959533937600094, 113.7510903946856757 ) ) ;
#145101=CARTESIAN_POINT ( 'NONE',  ( -16.52544592524335698, -4.483927247898792601, 78.95942372801901854 ) ) ;
#145102=CARTESIAN_POINT ( 'NONE',  ( 19.05341960407617918, -5.049401038297876454, 91.04275706135234714 ) ) ;
#145103=CARTESIAN_POINT ( 'NONE',  ( 16.55341960407611168, 4.379528057220329451, 113.9572429386477239 ) ) ;
#145104=CARTESIAN_POINT ( 'NONE',  ( -0.05219959533934338120, 16.53943276465976808, 67.50109039468568994 ) ) ;
#145105=CARTESIAN_POINT ( 'NONE',  ( 4.379528057220092307, 16.55341960407617563, 47.29275706135234003 ) ) ;
#145107=CARTESIAN_POINT ( 'NONE',  ( -0.05219959533936034679, 19.03943276465977164, 67.50109039468566152 ) ) ;
#145108=CARTESIAN_POINT ( 'NONE',  ( -21.53943276465977519, -0.05219959533937600094, 103.7510903946857042 ) ) ;
#145109=CARTESIAN_POINT ( 'NONE',  ( -0.05219959533909027116, -19.03943276465977164, 32.49890960531435979 ) ) ;
#145110=CARTESIAN_POINT ( 'NONE',  ( 19.05341960407611168, 5.049401038298154454, 83.95724293864766707 ) ) ;
#145111=CARTESIAN_POINT ( 'NONE',  ( 4.483927247898545687, 16.52544592524342804, 74.79057627198105251 ) ) ;
#145112=CARTESIAN_POINT ( 'NONE',  ( -5.719274019375665041, -21.55341960407619695, 89.79275706135236135 ) ) ;
#145113=CARTESIAN_POINT ( 'NONE',  ( 5.049401038297881783, 19.05341960407617563, 47.29275706135231161 ) ) ;
#145114=CARTESIAN_POINT ( 'NONE',  ( -5.719274019375978568, 21.55341960407610458, 35.20724293864768839 ) ) ;
#145115=CARTESIAN_POINT ( 'NONE',  ( 18.62759615963255655, 10.81492255796105972, 106.6677570613523756 ) ) ;
#145116=CARTESIAN_POINT ( 'NONE',  ( -9.564922557960796823, -16.46253265017161027, 82.08224293864768129 ) ) ;
#145118=CARTESIAN_POINT ( 'NONE',  ( -18.62759615963255300, -10.81492255796106328, 109.1677570613523613 ) ) ;
#145119=CARTESIAN_POINT ( 'NONE',  ( -10.81492255796078084, -18.62759615963271287, 47.08224293864770260 ) ) ;
#145120=CARTESIAN_POINT ( 'NONE',  ( -5.049401038298153566, 19.05341960407611168, 95.20724293864770971 ) ) ;
#145121=CARTESIAN_POINT ( 'NONE',  ( 19.03943276465977164, 0.05219959533936151252, 81.25109039468567573 ) ) ;
#145122=CARTESIAN_POINT ( 'NONE',  ( 13.97604488694527802, 13.89961937509977652, 109.3739096053143669 ) ) ;
#145123=CARTESIAN_POINT ( 'NONE',  ( -19.05341960407617563, 5.049401038297882671, 98.54275706135233293 ) ) ;
#145124=CARTESIAN_POINT ( 'NONE',  ( -0.05219959533934338120, 16.53943276465976808, 42.50109039468567573 ) ) ;
#145125=CARTESIAN_POINT ( 'NONE',  ( 14.34966873604960469, 8.224510206698951720, 114.1655762719810383 ) ) ;
#145126=CARTESIAN_POINT ( 'NONE',  ( 16.46253265017160672, -9.564922557960803928, 78.33224293864769550 ) ) ;
#145127=CARTESIAN_POINT ( 'NONE',  ( 21.52544592524344225, -5.823673210054117533, 63.54057627198103830 ) ) ;
#145129=CARTESIAN_POINT ( 'NONE',  ( 16.52544592524335698, 4.483927247898782831, 26.45942372801901854 ) ) ;
#145130=CARTESIAN_POINT ( 'NONE',  ( -21.55341960407619339, 5.719274019375674811, 28.54275706135234358 ) ) ;
#145131=CARTESIAN_POINT ( 'NONE',  ( -15.80617190586768217, 15.72974639402176855, 78.12609039468570415 ) ) ;
#145132=CARTESIAN_POINT ( 'NONE',  ( 4.379528057220092307, 16.55341960407617563, 82.29275706135234714 ) ) ;
#145133=CARTESIAN_POINT ( 'NONE',  ( -5.153800228976328057, -19.02544592524343514, 92.29057627198099567 ) ) ;
#145134=CARTESIAN_POINT ( 'NONE',  ( 4.483927247898545687, 16.52544592524342804, 74.79057627198105251 ) ) ;
#145135=CARTESIAN_POINT ( 'NONE',  ( -16.55341960407611168, -4.379528057220339221, 21.45724293864769550 ) ) ;
#145136=CARTESIAN_POINT ( 'NONE',  ( -16.46253265017146816, -9.564922557961047289, 54.16775706135234003 ) ) ;
#145137=CARTESIAN_POINT ( 'NONE',  ( 10.72451020669871369, 18.67979575497193778, 42.08442372801901854 ) ) ;
#145138=CARTESIAN_POINT ( 'NONE',  ( 16.53943276465976808, -0.05219959533910856209, 78.74890960531436690 ) ) ;
#145139=CARTESIAN_POINT ( 'NONE',  ( 21.52544592524344225, -5.823673210054117533, 23.54057627198102765 ) ) ;
#145140=CARTESIAN_POINT ( 'NONE',  ( 8.224510206698742110, 14.34966873604972548, 97.08442372801904696 ) ) ;
#145141=CARTESIAN_POINT ( 'NONE',  ( 15.72974639402176855, 15.80617190586768217, 91.87609039468568994 ) ) ;
#145142=CARTESIAN_POINT ( 'NONE',  ( 16.55341960407618274, -4.379528057220086978, 46.04275706135234714 ) ) ;
#145143=CARTESIAN_POINT ( 'NONE',  ( 21.52544592524334988, 5.823673210054432836, 46.45942372801901854 ) ) ;
#145145=CARTESIAN_POINT ( 'NONE',  ( -21.55341960407610458, -5.719274019375992779, 111.4572429386476813 ) ) ;
#145146=CARTESIAN_POINT ( 'NONE',  ( -8.314922557960811034, -14.29746914071050412, 97.08224293864770971 ) ) ;
#145147=CARTESIAN_POINT ( 'NONE',  ( 17.50000000000000711, -3.305555262949588791, 27.12517152156594591 ) ) ;
#145148=CARTESIAN_POINT ( 'NONE',  ( 4.379528057220339221, -16.55341960407611168, 47.70724293864770260 ) ) ;
#145149=CARTESIAN_POINT ( 'NONE',  ( 8.314922557961029526, -14.29746914071037800, 95.41775706135234714 ) ) ;
#145150=CARTESIAN_POINT ( 'NONE',  ( 19.05341960407611168, 5.049401038298154454, 43.95724293864769550 ) ) ;
#145151=CARTESIAN_POINT ( 'NONE',  ( 5.719274019375991003, -21.55341960407610458, 42.70724293864770260 ) ) ;
#145152=CARTESIAN_POINT ( 'NONE',  ( -0.05219959533910754901, -16.53943276465976808, 72.49890960531435269 ) ) ;
#145154=CARTESIAN_POINT ( 'NONE',  ( -18.67979575497178146, -10.72451020669898902, 76.66557627198103830 ) ) ;
#145155=CARTESIAN_POINT ( 'NONE',  ( 5.153800228976335163, 19.02544592524342804, 89.79057627198102409 ) ) ;
#145156=CARTESIAN_POINT ( 'NONE',  ( -13.97604488694527625, -13.89961937509977652, 41.87390960531435979 ) ) ;
#145157=CARTESIAN_POINT ( 'NONE',  ( -0.05219959533936034679, 19.03943276465977164, 92.50109039468566152 ) ) ;
#145158=CARTESIAN_POINT ( 'NONE',  ( 21.55341960407610458, 5.719274019375980345, 33.95724293864769550 ) ) ;
#145159=CARTESIAN_POINT ( 'NONE',  ( 10.81492255796106328, -18.62759615963255655, 60.41775706135235424 ) ) ;
#145160=CARTESIAN_POINT ( 'NONE',  ( 9.564922557960805705, 16.46253265017160317, 54.58224293864769550 ) ) ;
#145161=CARTESIAN_POINT ( 'NONE',  ( -13.97604488694527625, -13.89961937509977652, 91.87390960531432427 ) ) ;
#145162=ORIENTED_EDGE ( 'NONE', *, *, #22998, .T. ) ;
#145163=CARTESIAN_POINT ( 'NONE',  ( -16.52544592524335698, -4.483927247898792601, 53.95942372801900433 ) ) ;
#145164=CARTESIAN_POINT ( 'NONE',  ( 15.80617190586769283, -15.72974639402175789, 35.62609039468568994 ) ) ;
#145165=CARTESIAN_POINT ( 'NONE',  ( 18.67979575497194134, -10.72451020669871369, 70.83442372801901854 ) ) ;
#145166=CARTESIAN_POINT ( 'NONE',  ( -5.823673210054116645, -21.52544592524344225, 27.29057627198103120 ) ) ;
#145167=CARTESIAN_POINT ( 'NONE',  ( -10.72451020669898014, 18.67979575497178502, 90.41557627198103830 ) ) ;
#145168=CARTESIAN_POINT ( 'NONE',  ( 15.72974639402176855, 15.80617190586768217, 21.87609039468567573 ) ) ;
#145169=CARTESIAN_POINT ( 'NONE',  ( 14.29746914071037800, 8.314922557961029526, 66.66775706135234714 ) ) ;
#145170=CARTESIAN_POINT ( 'NONE',  ( -5.823673210054116645, -21.52544592524344225, 57.29057627198103120 ) ) ;
#145171=CARTESIAN_POINT ( 'NONE',  ( 16.46253265017146816, 9.564922557961045513, 26.66775706135234003 ) ) ;
#145172=CARTESIAN_POINT ( 'NONE',  ( 16.46253265017160672, -9.564922557960803928, 63.33224293864769550 ) ) ;
#145173=CARTESIAN_POINT ( 'NONE',  ( 13.89961937509977652, -13.97604488694527269, 108.1239096053143669 ) ) ;
#145174=CARTESIAN_POINT ( 'NONE',  ( 13.89961937509977652, -13.97604488694527269, 93.12390960531436690 ) ) ;
#145176=CARTESIAN_POINT ( 'NONE',  ( 13.97604488694548053, -13.89961937509957401, 75.62609039468564731 ) ) ;
#145177=CARTESIAN_POINT ( 'NONE',  ( -10.72451020669898014, 18.67979575497178502, 40.41557627198103120 ) ) ;
#145178=CARTESIAN_POINT ( 'NONE',  ( 14.29746914071037800, 8.314922557961029526, 111.6677570613523613 ) ) ;
#145179=CARTESIAN_POINT ( 'NONE',  ( 16.46253265017146816, 9.564922557961045513, 96.66775706135233293 ) ) ;
#145180=CARTESIAN_POINT ( 'NONE',  ( 13.89961937509977652, -13.97604488694527269, 23.12390960531436335 ) ) ;
#145181=CARTESIAN_POINT ( 'NONE',  ( 19.05341960407617918, -5.049401038297876454, 96.04275706135231871 ) ) ;
#145182=CARTESIAN_POINT ( 'NONE',  ( 18.67979575497178502, 10.72451020669898547, 84.16557627198103830 ) ) ;
#145183=CARTESIAN_POINT ( 'NONE',  ( -13.89961937509957401, -13.97604488694547875, 64.37609039468567573 ) ) ;
#145185=CARTESIAN_POINT ( 'NONE',  ( -19.03943276465977164, 0.05219959533909376836, 56.24890960531435979 ) ) ;
#145186=CARTESIAN_POINT ( 'NONE',  ( -8.314922557960811034, -14.29746914071050412, 67.08224293864770971 ) ) ;
#145187=CARTESIAN_POINT ( 'NONE',  ( 13.89961937509977652, -13.97604488694527269, 43.12390960531434558 ) ) ;
#145188=CARTESIAN_POINT ( 'NONE',  ( 14.29746914071049879, -8.314922557960816363, 58.33224293864768839 ) ) ;
#145191=CARTESIAN_POINT ( 'NONE',  ( -4.483927247898539470, -16.52544592524342804, 27.29057627198103120 ) ) ;
#145192=CARTESIAN_POINT ( 'NONE',  ( 9.564922557960805705, 16.46253265017160317, 69.58224293864770971 ) ) ;
#145194=CARTESIAN_POINT ( 'NONE',  ( -19.02544592524334988, -5.153800228976617603, 23.95942372801900078 ) ) ;
#145195=CARTESIAN_POINT ( 'NONE',  ( -16.55341960407617563, 4.379528057220093196, 43.54275706135235424 ) ) ;
#145196=CARTESIAN_POINT ( 'NONE',  ( 21.52544592524344225, -5.823673210054117533, 53.54057627198103120 ) ) ;
#145197=CARTESIAN_POINT ( 'NONE',  ( 10.81492255796106328, -18.62759615963255655, 100.4177570613523471 ) ) ;
#145199=CARTESIAN_POINT ( 'NONE',  ( 5.049401038298161559, -19.05341960407611168, 57.70724293864769550 ) ) ;
#145201=CARTESIAN_POINT ( 'NONE',  ( -0.05219959533909027116, -19.03943276465977164, 102.4989096053143669 ) ) ;
#145203=CARTESIAN_POINT ( 'NONE',  ( -10.72451020669870658, -18.67979575497194134, 24.58442372801901499 ) ) ;
#145204=CARTESIAN_POINT ( 'NONE',  ( -0.05219959533910754901, -16.53943276465976808, 87.49890960531436690 ) ) ;
#145205=CARTESIAN_POINT ( 'NONE',  ( 10.72451020669898902, -18.67979575497178502, 87.91557627198103830 ) ) ;
#145206=CARTESIAN_POINT ( 'NONE',  ( -19.02544592524342804, 5.153800228976336051, 81.04057627198103830 ) ) ;
#145207=CARTESIAN_POINT ( 'NONE',  ( 19.03943276465977164, -0.05219959533909143690, 88.74890960531436690 ) ) ;
#145208=CARTESIAN_POINT ( 'NONE',  ( -10.72451020669898014, 18.67979575497178502, 105.4155762719810383 ) ) ;
#145209=EDGE_CURVE ( 'NONE', #20330, #29984, #4683, .T. ) ;
#145211=CARTESIAN_POINT ( 'NONE',  ( 16.51473224551069308, 9.474510206698969483, 69.16557627198102409 ) ) ;
#145212=CARTESIAN_POINT ( 'NONE',  ( 19.25663599770060586, -5.499999999999437783, 96.49419308057204603 ) ) ;
#145213=CARTESIAN_POINT ( 'NONE',  ( -12.14591786802309592, -12.06949235617757132, 106.8739096053143811 ) ) ;
#145214=CARTESIAN_POINT ( 'NONE',  ( 5.049401038298161559, -19.05341960407611168, 37.70724293864768839 ) ) ;
#145215=CARTESIAN_POINT ( 'NONE',  ( 19.03943276465977164, 0.05219959533936151252, 96.25109039468567573 ) ) ;
#145216=CARTESIAN_POINT ( 'NONE',  ( -4.483927247898539470, -16.52544592524342804, 107.2905762719810525 ) ) ;
#145217=CARTESIAN_POINT ( 'NONE',  ( 21.52544592524334988, 5.823673210054432836, 66.45942372801903275 ) ) ;
#145218=CARTESIAN_POINT ( 'NONE',  ( 16.46253265017160672, -9.564922557960803928, 58.33224293864769550 ) ) ;
#145219=CARTESIAN_POINT ( 'NONE',  ( 5.719274019375673035, 21.55341960407619339, 37.29275706135235424 ) ) ;
#145220=CARTESIAN_POINT ( 'NONE',  ( -10.72451020669898014, 18.67979575497178502, 105.4155762719810383 ) ) ;
#145222=CARTESIAN_POINT ( 'NONE',  ( 16.46253265017160672, -9.564922557960803928, 73.33224293864769550 ) ) ;
#145224=CARTESIAN_POINT ( 'NONE',  ( 12.06949235617739724, 12.14591786802326823, 26.87609039468567218 ) ) ;
#145225=CARTESIAN_POINT ( 'NONE',  ( -18.67979575497178146, -10.72451020669898902, 26.66557627198103475 ) ) ;
#145226=CARTESIAN_POINT ( 'NONE',  ( -15.72974639402176322, -15.80617190586768395, 64.37609039468568994 ) ) ;
#145227=CARTESIAN_POINT ( 'NONE',  ( 19.05341960407611168, 5.049401038298154454, 108.9572429386477097 ) ) ;
#145228=CARTESIAN_POINT ( 'NONE',  ( -16.46253265017146816, -9.564922557961047289, 94.16775706135233293 ) ) ;
#145229=CARTESIAN_POINT ( 'NONE',  ( -0.05219959533909027116, -19.03943276465977164, 42.49890960531435269 ) ) ;
#145230=CARTESIAN_POINT ( 'NONE',  ( 19.05341960407611168, 5.049401038298154454, 68.95724293864769550 ) ) ;
#145231=CARTESIAN_POINT ( 'NONE',  ( -16.55341960407611168, -4.379528057220339221, 91.45724293864769550 ) ) ;
#145232=CARTESIAN_POINT ( 'NONE',  ( 5.049401038298161559, -19.05341960407611168, 102.7072429386476955 ) ) ;
#145233=CARTESIAN_POINT ( 'NONE',  ( 4.483927247898545687, 16.52544592524342804, 94.79057627198105251 ) ) ;
#145234=CARTESIAN_POINT ( 'NONE',  ( -16.51473224551069308, -9.474510206698971260, 96.66557627198102409 ) ) ;
#145236=CARTESIAN_POINT ( 'NONE',  ( 12.14591786802309770, 12.06949235617756955, 54.37390960531435979 ) ) ;
#145237=CARTESIAN_POINT ( 'NONE',  ( 16.51473224551069308, 9.474510206698969483, 39.16557627198103120 ) ) ;
#145238=CARTESIAN_POINT ( 'NONE',  ( 10.81492255796106328, -18.62759615963255655, 55.41775706135234714 ) ) ;
#145239=CARTESIAN_POINT ( 'NONE',  ( -19.02544592524334988, -5.153800228976617603, 98.95942372801900433 ) ) ;
#145240=CARTESIAN_POINT ( 'NONE',  ( -14.29746914071049879, 8.314922557960819915, 50.83224293864770971 ) ) ;
#145241=CARTESIAN_POINT ( 'NONE',  ( 21.53943276465977519, -0.05219959533907433946, 113.7489096053143527 ) ) ;
#145242=CARTESIAN_POINT ( 'NONE',  ( 15.72974639402199770, -15.80617190586745480, 43.12390960531435269 ) ) ;
#145243=CARTESIAN_POINT ( 'NONE',  ( -5.153800228976328057, -19.02544592524343514, 107.2905762719810383 ) ) ;
#145244=CARTESIAN_POINT ( 'NONE',  ( -16.55341960407611168, -4.379528057220339221, 86.45724293864770971 ) ) ;
#145246=CARTESIAN_POINT ( 'NONE',  ( 9.564922557960805705, 16.46253265017160317, 59.58224293864769550 ) ) ;
#145247=CARTESIAN_POINT ( 'NONE',  ( 14.34966873604972726, -8.224510206698740333, 110.8344237280190043 ) ) ;
#145248=CARTESIAN_POINT ( 'NONE',  ( 12.14591786802327356, -12.06949235617739191, 100.6260903946857184 ) ) ;
#145249=CARTESIAN_POINT ( 'NONE',  ( -8.314922557961024197, 14.29746914071037800, 82.91775706135234714 ) ) ;
#145250=CARTESIAN_POINT ( 'NONE',  ( 13.97604488694548053, -13.89961937509957401, 40.62609039468564731 ) ) ;
#145252=CARTESIAN_POINT ( 'NONE',  ( -19.03943276465977164, 0.05219959533909376836, 91.24890960531436690 ) ) ;
#145253=CARTESIAN_POINT ( 'NONE',  ( 5.049401038298161559, -19.05341960407611168, 52.70724293864767418 ) ) ;
#145254=CARTESIAN_POINT ( 'NONE',  ( -12.14591786802309592, -12.06949235617757132, 61.87390960531436690 ) ) ;
#145256=CARTESIAN_POINT ( 'NONE',  ( -19.05341960407611168, -5.049401038298163336, 106.4572429386476955 ) ) ;
#145257=CARTESIAN_POINT ( 'NONE',  ( -5.823673210054116645, -21.52544592524344225, 37.29057627198102409 ) ) ;
#145258=CARTESIAN_POINT ( 'NONE',  ( 8.224510206698953496, -14.34966873604960469, 82.91557627198103830 ) ) ;
#145259=CARTESIAN_POINT ( 'NONE',  ( 4.483927247898790824, -16.52544592524335698, 40.20942372801901854 ) ) ;
#145260=CARTESIAN_POINT ( 'NONE',  ( -4.483927247898539470, -16.52544592524342804, 77.29057627198102409 ) ) ;
#145262=CARTESIAN_POINT ( 'NONE',  ( 9.474510206698729675, 16.51473224551082808, 72.08442372801900433 ) ) ;
#145263=CARTESIAN_POINT ( 'NONE',  ( -9.564922557960796823, -16.46253265017161027, 97.08224293864769550 ) ) ;
#145264=CARTESIAN_POINT ( 'NONE',  ( -16.51473224551082808, 9.474510206698731452, 78.33442372801900433 ) ) ;
#145266=VECTOR ( 'NONE', #136029, 1000.000000000000000 ) ;
#145267=CARTESIAN_POINT ( 'NONE',  ( 16.55341960407618274, -4.379528057220086978, 26.04275706135235779 ) ) ;
#145268=CARTESIAN_POINT ( 'NONE',  ( 0.05219959533934541429, -16.53943276465976808, 105.0010903946856757 ) ) ;
#145269=CARTESIAN_POINT ( 'NONE',  ( 13.89961937509957401, 13.97604488694547697, 71.87609039468567573 ) ) ;
#145270=CARTESIAN_POINT ( 'NONE',  ( 0.05219959533907565091, 21.53943276465977519, 34.99890960531435979 ) ) ;
#145271=CARTESIAN_POINT ( 'NONE',  ( 0.05219959533937995610, -21.53943276465977519, 75.00109039468568994 ) ) ;
#145273=CARTESIAN_POINT ( 'NONE',  ( 4.379528057220092307, 16.55341960407617563, 22.29275706135235069 ) ) ;
#145275=CARTESIAN_POINT ( 'NONE',  ( 9.564922557960805705, 16.46253265017160317, 94.58224293864769550 ) ) ;
#145276=CARTESIAN_POINT ( 'NONE',  ( -19.05341960407611168, -5.049401038298163336, 21.45724293864768839 ) ) ;
#145277=CARTESIAN_POINT ( 'NONE',  ( -4.483927247898539470, -16.52544592524342804, 92.29057627198103830 ) ) ;
#145278=CARTESIAN_POINT ( 'NONE',  ( 16.46253265017160672, -9.564922557960803928, 83.33224293864768129 ) ) ;
#145280=CARTESIAN_POINT ( 'NONE',  ( 0.05219959533936267826, -19.03943276465977164, 105.0010903946856615 ) ) ;
#145281=CARTESIAN_POINT ( 'NONE',  ( -21.53943276465977519, 0.05219959533907696930, 81.24890960531436690 ) ) ;
#145282=CARTESIAN_POINT ( 'NONE',  ( -9.564922557960796823, -16.46253265017161027, 47.08224293864769550 ) ) ;
#145283=CARTESIAN_POINT ( 'NONE',  ( -13.89961937509957401, -13.97604488694547875, 69.37609039468564731 ) ) ;
#145284=CARTESIAN_POINT ( 'NONE',  ( 5.823673210054125526, 21.52544592524343514, 114.7905762719810383 ) ) ;
#145285=CARTESIAN_POINT ( 'NONE',  ( -16.46253265017160317, 9.564922557960807481, 75.83224293864769550 ) ) ;
#145286=CARTESIAN_POINT ( 'NONE',  ( 13.89961937509977652, -13.97604488694527269, 103.1239096053143527 ) ) ;
#145287=ORIENTED_EDGE ( 'NONE', *, *, #34066, .T. ) ;
#145288=CARTESIAN_POINT ( 'NONE',  ( -14.29746914071037622, -8.314922557961029526, 39.16775706135235424 ) ) ;
#145289=CARTESIAN_POINT ( 'NONE',  ( -21.53943276465977519, 0.05219959533907696930, 106.2489096053143811 ) ) ;
#145290=CARTESIAN_POINT ( 'NONE',  ( -16.52544592524342804, 4.483927247898546575, 111.0405762719810525 ) ) ;
#145291=CARTESIAN_POINT ( 'NONE',  ( -0.05219959533909027116, -19.03943276465977164, 87.49890960531436690 ) ) ;
#145292=CARTESIAN_POINT ( 'NONE',  ( -16.51473224551082808, 9.474510206698731452, 68.33442372801900433 ) ) ;
#145293=CARTESIAN_POINT ( 'NONE',  ( 5.823673210054125526, 21.52544592524343514, 89.79057627198103830 ) ) ;
#145294=CARTESIAN_POINT ( 'NONE',  ( -21.55341960407610458, -5.719274019375992779, 71.45724293864769550 ) ) ;
#145295=CARTESIAN_POINT ( 'NONE',  ( -16.52544592524342804, 4.483927247898546575, 46.04057627198103830 ) ) ;
#145296=CARTESIAN_POINT ( 'NONE',  ( -21.55341960407619339, 5.719274019375674811, 113.5427570613523756 ) ) ;
#145297=CARTESIAN_POINT ( 'NONE',  ( -12.06949235617739369, -12.14591786802326823, 69.37609039468567573 ) ) ;
#145298=CARTESIAN_POINT ( 'NONE',  ( -16.51473224551069308, -9.474510206698971260, 86.66557627198102409 ) ) ;
#145299=CARTESIAN_POINT ( 'NONE',  ( -13.97604488694527625, -13.89961937509977652, 46.87390960531435979 ) ) ;
#145300=CARTESIAN_POINT ( 'NONE',  ( -0.05219959533937732626, 21.53943276465977519, 57.50109039468568994 ) ) ;
#145301=CARTESIAN_POINT ( 'NONE',  ( -5.823673210054431948, 21.52544592524334988, 72.70942372801901854 ) ) ;
#145302=CARTESIAN_POINT ( 'NONE',  ( -19.03943276465977164, 0.05219959533909376836, 56.24890960531435979 ) ) ;
#145303=CARTESIAN_POINT ( 'NONE',  ( -15.72974639402176322, -15.80617190586768395, 39.37609039468567573 ) ) ;
#145304=CARTESIAN_POINT ( 'NONE',  ( 5.049401038297881783, 19.05341960407617563, 77.29275706135231871 ) ) ;
#145305=CARTESIAN_POINT ( 'NONE',  ( -19.02544592524334988, -5.153800228976617603, 68.95942372801896170 ) ) ;
#145306=CARTESIAN_POINT ( 'NONE',  ( -9.474510206698964154, 16.51473224551069663, 35.41557627198102409 ) ) ;
#145307=CARTESIAN_POINT ( 'NONE',  ( 16.55341960407618274, -4.379528057220086978, 81.04275706135236135 ) ) ;
#145308=CARTESIAN_POINT ( 'NONE',  ( -9.474510206698964154, 16.51473224551069663, 55.41557627198103120 ) ) ;
#145310=CARTESIAN_POINT ( 'NONE',  ( 9.474510206698971260, -16.51473224551069308, 97.91557627198102409 ) ) ;
#145311=CARTESIAN_POINT ( 'NONE',  ( 0.05219959533909260263, 19.03943276465977164, 44.99890960531435979 ) ) ;
#145312=CARTESIAN_POINT ( 'NONE',  ( -5.823673210054116645, -21.52544592524344225, 92.29057627198103830 ) ) ;
#145313=CARTESIAN_POINT ( 'NONE',  ( -16.55341960407617563, 4.379528057220093196, 63.54275706135234003 ) ) ;
#145314=CARTESIAN_POINT ( 'NONE',  ( 18.67979575497194134, -10.72451020669871369, 110.8344237280190043 ) ) ;
#145316=CARTESIAN_POINT ( 'NONE',  ( 13.89961937509977652, -13.97604488694527269, 48.12390960531435979 ) ) ;
#145317=CARTESIAN_POINT ( 'NONE',  ( 4.483927247898545687, 16.52544592524342804, 49.79057627198102409 ) ) ;
#145318=CARTESIAN_POINT ( 'NONE',  ( 4.379528057220339221, -16.55341960407611168, 77.70724293864770971 ) ) ;
#145319=CARTESIAN_POINT ( 'NONE',  ( 19.05341960407611168, 5.049401038298154454, 78.95724293864769550 ) ) ;
#145320=CARTESIAN_POINT ( 'NONE',  ( 21.52544592524334988, 5.823673210054432836, 36.45942372801901143 ) ) ;
#145321=CARTESIAN_POINT ( 'NONE',  ( -5.153800228976328057, -19.02544592524343514, 92.29057627198099567 ) ) ;
#145322=CARTESIAN_POINT ( 'NONE',  ( -10.81492255796105439, 18.62759615963255655, 102.9177570613523756 ) ) ;
#145323=CARTESIAN_POINT ( 'NONE',  ( 16.55341960407618274, -4.379528057220086978, 81.04275706135236135 ) ) ;
#145324=CARTESIAN_POINT ( 'NONE',  ( -10.81492255796105439, 18.62759615963255655, 32.91775706135234714 ) ) ;
#145325=CARTESIAN_POINT ( 'NONE',  ( 9.474510206698971260, -16.51473224551069308, 107.9155762719810383 ) ) ;
#145327=CARTESIAN_POINT ( 'NONE',  ( 0.05219959533907565091, 21.53943276465977519, 94.99890960531436690 ) ) ;
#145328=CARTESIAN_POINT ( 'NONE',  ( -14.34966873604960291, -8.224510206698953496, 51.66557627198102409 ) ) ;
#145329=CARTESIAN_POINT ( 'NONE',  ( -5.153800228976328057, -19.02544592524343514, 42.29057627198101699 ) ) ;
#145330=CARTESIAN_POINT ( 'NONE',  ( 4.483927247898545687, 16.52544592524342804, 64.79057627198103830 ) ) ;
#145331=CARTESIAN_POINT ( 'NONE',  ( -10.72451020669898014, 18.67979575497178502, 35.41557627198102409 ) ) ;
#145332=CARTESIAN_POINT ( 'NONE',  ( -16.51473224551082808, 9.474510206698731452, 33.33442372801899722 ) ) ;
#145333=CARTESIAN_POINT ( 'NONE',  ( 14.34966873604960469, 8.224510206698951720, 94.16557627198103830 ) ) ;
#145334=CARTESIAN_POINT ( 'NONE',  ( -9.474510206698964154, 16.51473224551069663, 105.4155762719810383 ) ) ;
#145336=CARTESIAN_POINT ( 'NONE',  ( 16.53943276465976808, 0.05219959533934440121, 51.25109039468568994 ) ) ;
#145337=CARTESIAN_POINT ( 'NONE',  ( 13.97604488694527802, 13.89961937509977652, 54.37390960531435979 ) ) ;
#145339=CARTESIAN_POINT ( 'NONE',  ( -8.314922557961024197, 14.29746914071037800, 87.91775706135234714 ) ) ;
#145340=CARTESIAN_POINT ( 'NONE',  ( 9.564922557961047289, -16.46253265017146816, 105.4177570613523471 ) ) ;
#145341=CARTESIAN_POINT ( 'NONE',  ( 0.05219959533937995610, -21.53943276465977519, 80.00109039468568994 ) ) ;
#145342=CARTESIAN_POINT ( 'NONE',  ( -5.049401038298153566, 19.05341960407611168, 70.20724293864769550 ) ) ;
#145343=CARTESIAN_POINT ( 'NONE',  ( 18.62759615963271287, -10.81492255796078972, 103.3322429386476955 ) ) ;
#145344=CARTESIAN_POINT ( 'NONE',  ( 12.06949235617739724, 12.14591786802326823, 51.87609039468568284 ) ) ;
#145345=CARTESIAN_POINT ( 'NONE',  ( -16.55341960407611168, -4.379528057220339221, 106.4572429386477097 ) ) ;
#145346=CARTESIAN_POINT ( 'NONE',  ( -12.06949235617739369, -12.14591786802326823, 19.37609039468568639 ) ) ;
#145347=CARTESIAN_POINT ( 'NONE',  ( -5.049401038297874678, -19.05341960407617918, 79.79275706135233293 ) ) ;
#145348=CARTESIAN_POINT ( 'NONE',  ( 10.81492255796078972, 18.62759615963270932, 79.58224293864769550 ) ) ;
#145349=CARTESIAN_POINT ( 'NONE',  ( 19.05341960407617918, -5.049401038297876454, 51.04275706135231871 ) ) ;
#145350=CARTESIAN_POINT ( 'NONE',  ( -19.03943276465977164, 0.05219959533909376836, 116.2489096053143669 ) ) ;
#145351=CARTESIAN_POINT ( 'NONE',  ( 18.67979575497178502, 10.72451020669898547, 104.1655762719810241 ) ) ;
#145352=CARTESIAN_POINT ( 'NONE',  ( 17.50000000000003553, 4.658240926743142829, 28.55529582183200077 ) ) ;
#145353=CARTESIAN_POINT ( 'NONE',  ( -19.05341960407611168, -5.049401038298163336, 71.45724293864766707 ) ) ;
#145354=CARTESIAN_POINT ( 'NONE',  ( -17.49999999999999645, -5.500000000000020428, 61.28230962303567964 ) ) ;
#145355=CARTESIAN_POINT ( 'NONE',  ( -0.05219959533934338120, 16.53943276465976808, 22.50109039468567573 ) ) ;
#145357=CARTESIAN_POINT ( 'NONE',  ( -0.05219959533937732626, 21.53943276465977519, 52.50109039468567573 ) ) ;
#145358=CARTESIAN_POINT ( 'NONE',  ( 0.05219959533907565091, 21.53943276465977519, 99.99890960531436690 ) ) ;
#145359=CARTESIAN_POINT ( 'NONE',  ( 16.55341960407611168, 4.379528057220329451, 68.95724293864769550 ) ) ;
#145360=CARTESIAN_POINT ( 'NONE',  ( -9.474510206698964154, 16.51473224551069663, 75.41557627198103830 ) ) ;
#145361=CARTESIAN_POINT ( 'NONE',  ( -21.52544592524334988, -5.823673210054445271, 78.95942372801901854 ) ) ;
#145362=CARTESIAN_POINT ( 'NONE',  ( 14.29746914071037800, 8.314922557961029526, 21.66775706135235069 ) ) ;
#145363=CARTESIAN_POINT ( 'NONE',  ( -16.51473224551082808, 9.474510206698731452, 28.33442372801900433 ) ) ;
#145364=CARTESIAN_POINT ( 'NONE',  ( -21.52544592524334988, -5.823673210054445271, 48.95942372801902565 ) ) ;
#145365=CARTESIAN_POINT ( 'NONE',  ( 21.52544592524344225, -5.823673210054117533, 113.5405762719810383 ) ) ;
#145366=CARTESIAN_POINT ( 'NONE',  ( 15.80617190586746368, 15.72974639402197994, 59.37390960531436690 ) ) ;
#145367=CARTESIAN_POINT ( 'NONE',  ( -13.89961937509957401, -13.97604488694547875, 99.37609039468567573 ) ) ;
#145368=CARTESIAN_POINT ( 'NONE',  ( -19.03943276465977164, -0.05219959533935918106, 73.75109039468566152 ) ) ;
#145369=CARTESIAN_POINT ( 'NONE',  ( 15.80617190586769283, -15.72974639402175789, 80.62609039468567573 ) ) ;
#145370=CARTESIAN_POINT ( 'NONE',  ( -19.05341960407617563, 5.049401038297882671, 58.54275706135234003 ) ) ;
#145371=CARTESIAN_POINT ( 'NONE',  ( -0.05219959533909027116, -19.03943276465977164, 32.49890960531435979 ) ) ;
#145372=CARTESIAN_POINT ( 'NONE',  ( 18.62759615963271287, -10.81492255796078972, 53.33224293864769550 ) ) ;
#145373=CARTESIAN_POINT ( 'NONE',  ( 12.14591786802309770, 12.06949235617756955, 54.37390960531435979 ) ) ;
#145374=CARTESIAN_POINT ( 'NONE',  ( -17.44270441346514389, -5.991230190323014071, 26.36335079264227588 ) ) ;
#145375=CARTESIAN_POINT ( 'NONE',  ( 5.153800228976615827, -19.02544592524334988, 25.20942372801900433 ) ) ;
#145376=CARTESIAN_POINT ( 'NONE',  ( 4.483927247898790824, -16.52544592524335698, 80.20942372801901854 ) ) ;
#145377=CARTESIAN_POINT ( 'NONE',  ( -8.314922557960811034, -14.29746914071050412, 57.08224293864769550 ) ) ;
#145378=CARTESIAN_POINT ( 'NONE',  ( 18.67979575497194134, -10.72451020669871369, 70.83442372801901854 ) ) ;
#145379=CARTESIAN_POINT ( 'NONE',  ( 0.05219959533937995610, -21.53943276465977519, 80.00109039468568994 ) ) ;
#145380=CARTESIAN_POINT ( 'NONE',  ( 15.80617190586746368, 15.72974639402197994, 84.37390960531438111 ) ) ;
#145381=CARTESIAN_POINT ( 'NONE',  ( 19.05341960407611168, 5.049401038298154454, 38.95724293864767418 ) ) ;
#145382=CARTESIAN_POINT ( 'NONE',  ( 21.52544592524334988, 5.823673210054432836, 51.45942372801901854 ) ) ;
#145383=CARTESIAN_POINT ( 'NONE',  ( -13.89961937509977652, 13.97604488694528158, 35.62390960531435269 ) ) ;
#145384=CARTESIAN_POINT ( 'NONE',  ( 9.474510206698971260, -16.51473224551069308, 47.91557627198102409 ) ) ;
#145385=CARTESIAN_POINT ( 'NONE',  ( -16.55341960407611168, -4.379528057220339221, 111.4572429386476813 ) ) ;
#145386=CARTESIAN_POINT ( 'NONE',  ( 5.153800228976335163, 19.02544592524342804, 104.7905762719809957 ) ) ;
#145387=CARTESIAN_POINT ( 'NONE',  ( -0.05219959533910754901, -16.53943276465976808, 42.49890960531435979 ) ) ;
#145388=CARTESIAN_POINT ( 'NONE',  ( -12.06949235617756955, 12.14591786802309770, 105.6239096053143669 ) ) ;
#145389=CARTESIAN_POINT ( 'NONE',  ( 21.55341960407610458, 5.719274019375980345, 88.95724293864769550 ) ) ;
#145390=CARTESIAN_POINT ( 'NONE',  ( 18.62759615963255655, 10.81492255796105972, 26.66775706135235424 ) ) ;
#145391=PLANE ( 'NONE',  #56523 ) ;
#145392=CARTESIAN_POINT ( 'NONE',  ( -16.53943276465976808, -0.05219959533934237506, 43.75109039468568284 ) ) ;
#145394=CARTESIAN_POINT ( 'NONE',  ( -0.05219959533907301413, -21.53943276465977519, 77.49890960531433848 ) ) ;
#145395=CARTESIAN_POINT ( 'NONE',  ( -21.55341960407619339, 5.719274019375674811, 88.54275706135236135 ) ) ;
#145396=CARTESIAN_POINT ( 'NONE',  ( 0.05219959533909260263, 19.03943276465977164, 89.99890960531436690 ) ) ;
#145397=CARTESIAN_POINT ( 'NONE',  ( 0.05219959533937995610, -21.53943276465977519, 35.00109039468568284 ) ) ;
#145398=B_SPLINE_CURVE_WITH_KNOTS ( 'NONE', 3,
 ( #13151, #149667, #57667, #182992, #60611, #103163, #196195, #11165, #72839, #71823, #106130, #12170, #28337, #119334 ),
 .UNSPECIFIED., .F., .F.,
 ( 4, 2, 2, 2, 2, 2, 4 ),
 ( 0.002427643230453598207, 0.002603325520439036134, 0.002779007810424474062, 0.003130372390395366397, 0.003833101550337150200, 0.004535830710278934003, 0.005238559870220718673 ),
 .UNSPECIFIED. ) ;
#145399=CARTESIAN_POINT ( 'NONE',  ( -21.55341960407610458, -5.719274019375992779, 26.45724293864768839 ) ) ;
#145400=CARTESIAN_POINT ( 'NONE',  ( -0.05219959533934338120, 16.53943276465976808, 87.50109039468568994 ) ) ;
#145401=CARTESIAN_POINT ( 'NONE',  ( 15.80617190586769283, -15.72974639402175789, 90.62609039468567573 ) ) ;
#145402=CARTESIAN_POINT ( 'NONE',  ( 5.153800228976615827, -19.02544592524334988, 20.20942372801899722 ) ) ;
#145403=CARTESIAN_POINT ( 'NONE',  ( -12.14591786802326823, 12.06949235617739902, 78.12609039468570415 ) ) ;
#145404=CARTESIAN_POINT ( 'NONE',  ( -5.719274019375665041, -21.55341960407619695, 24.79275706135235779 ) ) ;
#145405=CARTESIAN_POINT ( 'NONE',  ( 5.153800228976335163, 19.02544592524342804, 29.79057627198102409 ) ) ;
#145406=CARTESIAN_POINT ( 'NONE',  ( 15.72974639402176855, 15.80617190586768217, 106.8760903946856899 ) ) ;
#145407=CARTESIAN_POINT ( 'NONE',  ( -19.02544592524342804, 5.153800228976336051, 111.0405762719810099 ) ) ;
#145408=CARTESIAN_POINT ( 'NONE',  ( 10.81492255796078972, 18.62759615963270932, 99.58224293864770971 ) ) ;
#145410=CARTESIAN_POINT ( 'NONE',  ( -18.67979575497178146, -10.72451020669898902, 61.66557627198103120 ) ) ;
#145411=CARTESIAN_POINT ( 'NONE',  ( 4.379528057220092307, 16.55341960407617563, 47.29275706135234003 ) ) ;
#145412=CARTESIAN_POINT ( 'NONE',  ( -16.52544592524342804, 4.483927247898546575, 51.04057627198103120 ) ) ;
#145413=CARTESIAN_POINT ( 'NONE',  ( 18.85284094683698086, -5.499999999999990230, 101.1723727239295414 ) ) ;
#145414=CARTESIAN_POINT ( 'NONE',  ( -16.46253265017146816, -9.564922557961047289, 84.16775706135233293 ) ) ;
#145416=CARTESIAN_POINT ( 'NONE',  ( 16.55341960407618274, -4.379528057220086978, 31.04275706135234714 ) ) ;
#145417=CARTESIAN_POINT ( 'NONE',  ( -18.67979575497178146, -10.72451020669898902, 96.66557627198102409 ) ) ;
#145418=CARTESIAN_POINT ( 'NONE',  ( 8.314922557960818139, 14.29746914071049879, 59.58224293864770260 ) ) ;
#145419=CARTESIAN_POINT ( 'NONE',  ( -5.049401038298153566, 19.05341960407611168, 100.2072429386476955 ) ) ;
#145420=CARTESIAN_POINT ( 'NONE',  ( 16.52544592524335698, 4.483927247898782831, 41.45942372801901143 ) ) ;
#145421=CARTESIAN_POINT ( 'NONE',  ( -9.564922557960796823, -16.46253265017161027, 57.08224293864769550 ) ) ;
#145422=CARTESIAN_POINT ( 'NONE',  ( 15.72974639402176855, 15.80617190586768217, 31.87609039468567929 ) ) ;
#145423=CARTESIAN_POINT ( 'NONE',  ( -19.03943276465977164, -0.05219959533935918106, 93.75109039468566152 ) ) ;
#145424=CARTESIAN_POINT ( 'NONE',  ( -0.05219959533909027116, -19.03943276465977164, 92.49890960531436690 ) ) ;
#145425=CARTESIAN_POINT ( 'NONE',  ( -5.153800228976328057, -19.02544592524343514, 87.29057627198103830 ) ) ;
#145426=CARTESIAN_POINT ( 'NONE',  ( 5.823673210054125526, 21.52544592524343514, 89.79057627198103830 ) ) ;
#145427=CARTESIAN_POINT ( 'NONE',  ( -9.564922557960796823, -16.46253265017161027, 42.08224293864769550 ) ) ;
#145428=CARTESIAN_POINT ( 'NONE',  ( -17.40805194822029378, -6.112264579159359279, 59.16628727489389661 ) ) ;
#145429=CARTESIAN_POINT ( 'NONE',  ( -14.34966873604960291, -8.224510206698953496, 66.66557627198102409 ) ) ;
#145430=CARTESIAN_POINT ( 'NONE',  ( 5.049401038298161559, -19.05341960407611168, 97.70724293864766707 ) ) ;
#145432=CARTESIAN_POINT ( 'NONE',  ( 13.89961937509957401, 13.97604488694547697, 76.87609039468566152 ) ) ;
#145433=CARTESIAN_POINT ( 'NONE',  ( -15.72974639402197994, 15.80617190586746368, 95.62390960531436690 ) ) ;
#145434=CARTESIAN_POINT ( 'NONE',  ( -16.46253265017146816, -9.564922557961047289, 44.16775706135232582 ) ) ;
#145435=CARTESIAN_POINT ( 'NONE',  ( -16.46253265017160317, 9.564922557960807481, 115.8322429386477097 ) ) ;
#145436=CARTESIAN_POINT ( 'NONE',  ( 18.56399227203340985, 5.500000000000002665, 66.47830131249901342 ) ) ;
#145437=CARTESIAN_POINT ( 'NONE',  ( 18.62759615963271287, -10.81492255796078972, 48.33224293864770260 ) ) ;
#145439=CARTESIAN_POINT ( 'NONE',  ( 19.03943276465977164, -0.05219959533909143690, 83.74890960531436690 ) ) ;
#145440=CARTESIAN_POINT ( 'NONE',  ( -15.72974639402176322, -15.80617190586768395, 64.37609039468568994 ) ) ;
#145441=CARTESIAN_POINT ( 'NONE',  ( -9.474510206698964154, 16.51473224551069663, 35.41557627198102409 ) ) ;
#145442=CARTESIAN_POINT ( 'NONE',  ( -12.14591786802309592, -12.06949235617757132, 71.87390960531438111 ) ) ;
#145443=CARTESIAN_POINT ( 'NONE',  ( -16.55341960407617563, 4.379528057220093196, 28.54275706135234358 ) ) ;
#145444=CARTESIAN_POINT ( 'NONE',  ( -0.05219959533937732626, 21.53943276465977519, 52.50109039468567573 ) ) ;
#145446=CARTESIAN_POINT ( 'NONE',  ( -13.89961937509977652, 13.97604488694528158, 110.6239096053143243 ) ) ;
#145447=CARTESIAN_POINT ( 'NONE',  ( 16.51473224551083163, -9.474510206698727899, 85.83442372801900433 ) ) ;
#145449=CARTESIAN_POINT ( 'NONE',  ( -21.55341960407619339, 5.719274019375674811, 28.54275706135234358 ) ) ;
#145451=CARTESIAN_POINT ( 'NONE',  ( 18.62759615963255655, 10.81492255796105972, 111.6677570613523613 ) ) ;
#145452=CARTESIAN_POINT ( 'NONE',  ( -16.51473224551069308, -9.474510206698971260, 51.66557627198102409 ) ) ;
#145453=CARTESIAN_POINT ( 'NONE',  ( 15.72974639402176855, 15.80617190586768217, 111.8760903946856615 ) ) ;
#145454=CARTESIAN_POINT ( 'NONE',  ( 16.53943276465976808, 0.05219959533934440121, 101.2510903946856757 ) ) ;
#145455=CARTESIAN_POINT ( 'NONE',  ( 19.02544592524343514, -5.153800228976328945, 108.5405762719810383 ) ) ;
#145456=CARTESIAN_POINT ( 'NONE',  ( 0.05219959533937995610, -21.53943276465977519, 75.00109039468568994 ) ) ;
#145459=DIRECTION ( 'NONE',  ( 0.000000000000000000, -1.000000000000000000, 0.000000000000000000 ) ) ;
#145460=CARTESIAN_POINT ( 'NONE',  ( -18.62759615963255300, -10.81492255796106328, 74.16775706135231871 ) ) ;
#145461=CARTESIAN_POINT ( 'NONE',  ( 21.55341960407619695, -5.719274019375665929, 101.0427570613523756 ) ) ;
#145463=CARTESIAN_POINT ( 'NONE',  ( -9.564922557960796823, -16.46253265017161027, 92.08224293864769550 ) ) ;
#145464=CARTESIAN_POINT ( 'NONE',  ( -5.049401038297874678, -19.05341960407617918, 24.79275706135233648 ) ) ;
#145466=CARTESIAN_POINT ( 'NONE',  ( -16.51473224551069308, -9.474510206698971260, 36.66557627198102409 ) ) ;
#145467=CARTESIAN_POINT ( 'NONE',  ( -21.53943276465977519, 0.05219959533907696930, 51.24890960531436690 ) ) ;
#145469=CARTESIAN_POINT ( 'NONE',  ( 14.34966873604972726, -8.224510206698740333, 100.8344237280190185 ) ) ;
#145470=CARTESIAN_POINT ( 'NONE',  ( 4.379528057220339221, -16.55341960407611168, 92.70724293864770971 ) ) ;
#145471=CARTESIAN_POINT ( 'NONE',  ( 16.46253265017160672, -9.564922557960803928, 83.33224293864768129 ) ) ;
#145472=CARTESIAN_POINT ( 'NONE',  ( -5.823673210054431948, 21.52544592524334988, 107.7094237280190328 ) ) ;
#145473=CARTESIAN_POINT ( 'NONE',  ( 19.03943276465977164, -0.05219959533909143690, 38.74890960531436690 ) ) ;
#145474=CARTESIAN_POINT ( 'NONE',  ( -14.29746914071049879, 8.314922557960819915, 90.83224293864769550 ) ) ;
#145475=CARTESIAN_POINT ( 'NONE',  ( -5.719274019375665041, -21.55341960407619695, 54.79275706135235424 ) ) ;
#145476=CARTESIAN_POINT ( 'NONE',  ( -21.53943276465977519, 0.05219959533907696930, 91.24890960531436690 ) ) ;
#145477=CARTESIAN_POINT ( 'NONE',  ( 9.564922557961047289, -16.46253265017146816, 55.41775706135234003 ) ) ;
#145479=CARTESIAN_POINT ( 'NONE',  ( -5.153800228976328057, -19.02544592524343514, 92.29057627198099567 ) ) ;
#145480=CARTESIAN_POINT ( 'NONE',  ( 12.06949235617757843, -12.14591786802309237, 58.12390960531435979 ) ) ;
#145482=CARTESIAN_POINT ( 'NONE',  ( 19.05341960407617918, -5.049401038297876454, 51.04275706135231871 ) ) ;
#145483=CARTESIAN_POINT ( 'NONE',  ( -13.97604488694527625, -13.89961937509977652, 66.87390960531436690 ) ) ;
#145484=CARTESIAN_POINT ( 'NONE',  ( 16.55341960407611168, 4.379528057220329451, 53.95724293864770260 ) ) ;
#145485=CARTESIAN_POINT ( 'NONE',  ( -0.05219959533936034679, 19.03943276465977164, 82.50109039468567573 ) ) ;
#145486=CARTESIAN_POINT ( 'NONE',  ( -19.49149378614661643, 5.499999999999580780, 84.43757513605359577 ) ) ;
#145487=CARTESIAN_POINT ( 'NONE',  ( 21.52544592524344225, -5.823673210054117533, 33.54057627198102409 ) ) ;
#145488=CARTESIAN_POINT ( 'NONE',  ( 16.52544592524342804, -4.483927247898539470, 98.54057627198105251 ) ) ;
#145489=CARTESIAN_POINT ( 'NONE',  ( -17.50000000000003908, -5.076555817581120067, 26.17951492049773776 ) ) ;
#145490=CARTESIAN_POINT ( 'NONE',  ( -19.03943276465977164, 0.05219959533909376836, 56.24890960531435979 ) ) ;
#145491=CARTESIAN_POINT ( 'NONE',  ( 10.72451020669898902, -18.67979575497178502, 47.91557627198102409 ) ) ;
#145492=CARTESIAN_POINT ( 'NONE',  ( -19.03943276465977164, 0.05219959533909376836, 36.24890960531436690 ) ) ;
#145493=CARTESIAN_POINT ( 'NONE',  ( -16.53943276465976808, -0.05219959533934237506, 83.75109039468568994 ) ) ;
#145494=CARTESIAN_POINT ( 'NONE',  ( -5.153800228976328057, -19.02544592524343514, 62.29057627198100988 ) ) ;
#145495=CARTESIAN_POINT ( 'NONE',  ( -13.89961937509957401, -13.97604488694547875, 39.37609039468566152 ) ) ;
#145496=CARTESIAN_POINT ( 'NONE',  ( 10.72451020669871369, 18.67979575497193778, 72.08442372801899012 ) ) ;
#145497=CARTESIAN_POINT ( 'NONE',  ( 0.05219959533907565091, 21.53943276465977519, 54.99890960531435269 ) ) ;
#145498=CARTESIAN_POINT ( 'NONE',  ( -5.049401038298153566, 19.05341960407611168, 25.20724293864768484 ) ) ;
#145499=CARTESIAN_POINT ( 'NONE',  ( 5.153800228976615827, -19.02544592524334988, 110.2094237280189901 ) ) ;
#145500=DIRECTION ( 'NONE',  ( 0.000000000000000000, 1.000000000000000000, 0.000000000000000000 ) ) ;
#145502=CARTESIAN_POINT ( 'NONE',  ( -10.81492255796078084, -18.62759615963271287, 47.08224293864770260 ) ) ;
#145503=CARTESIAN_POINT ( 'NONE',  ( 16.29526858892872099, -7.335722546920259823, 66.70329402199793378 ) ) ;
#145504=CARTESIAN_POINT ( 'NONE',  ( 10.81492255796106328, -18.62759615963255655, 85.41775706135236135 ) ) ;
#145505=CARTESIAN_POINT ( 'NONE',  ( -16.53943276465976808, 0.05219959533911058130, 41.24890960531435269 ) ) ;
#145506=CARTESIAN_POINT ( 'NONE',  ( 8.224510206698953496, -14.34966873604960469, 57.91557627198103120 ) ) ;
#145507=CARTESIAN_POINT ( 'NONE',  ( 21.55341960407610458, 5.719274019375980345, 83.95724293864770971 ) ) ;
#145508=CARTESIAN_POINT ( 'NONE',  ( -18.62759615963270932, 10.81492255796079327, 80.83224293864769550 ) ) ;
#145510=CARTESIAN_POINT ( 'NONE',  ( 15.72974639402199770, -15.80617190586745480, 38.12390960531436690 ) ) ;
#145511=CARTESIAN_POINT ( 'NONE',  ( -16.55341960407617563, 4.379528057220093196, 48.54275706135234714 ) ) ;
#145512=CARTESIAN_POINT ( 'NONE',  ( -8.314922557960811034, -14.29746914071050412, 82.08224293864768129 ) ) ;
#145513=CARTESIAN_POINT ( 'NONE',  ( -0.05219959533909027116, -19.03943276465977164, 27.49890960531435624 ) ) ;
#145514=CARTESIAN_POINT ( 'NONE',  ( -22.00000000000000000, -5.204748896376250896E-15, 42.49999999999999289 ) ) ;
#145516=CARTESIAN_POINT ( 'NONE',  ( -4.379528057220086978, -16.55341960407618274, 79.79275706135236135 ) ) ;
#145517=CARTESIAN_POINT ( 'NONE',  ( -21.53943276465977519, -0.05219959533937600094, 23.75109039468567929 ) ) ;
#145518=CARTESIAN_POINT ( 'NONE',  ( 19.03943276465977164, -0.05219959533909143690, 88.74890960531436690 ) ) ;
#145519=CARTESIAN_POINT ( 'NONE',  ( -10.72451020669870658, -18.67979575497194134, 59.58442372801901854 ) ) ;
#145520=CARTESIAN_POINT ( 'NONE',  ( 9.474510206698971260, -16.51473224551069308, 112.9155762719810383 ) ) ;
#145524=CARTESIAN_POINT ( 'NONE',  ( 0.05219959533937995610, -21.53943276465977519, 40.00109039468567573 ) ) ;
#145525=CARTESIAN_POINT ( 'NONE',  ( 9.474510206698971260, -16.51473224551069308, 37.91557627198102409 ) ) ;
#145526=CARTESIAN_POINT ( 'NONE',  ( -0.05219959533909027116, -19.03943276465977164, 107.4989096053143527 ) ) ;
#145527=CARTESIAN_POINT ( 'NONE',  ( -0.05219959533936034679, 19.03943276465977164, 57.50109039468566863 ) ) ;
#145528=CARTESIAN_POINT ( 'NONE',  ( 0.05219959533937995610, -21.53943276465977519, 35.00109039468568284 ) ) ;
#145529=CARTESIAN_POINT ( 'NONE',  ( 19.02544592524334988, 5.153800228976608722, 46.45942372801899012 ) ) ;
#145530=CARTESIAN_POINT ( 'NONE',  ( 16.46253265017160672, -9.564922557960803928, 28.33224293864769550 ) ) ;
#145531=CARTESIAN_POINT ( 'NONE',  ( -14.34966873604972548, 8.224510206698743886, 88.33442372801901854 ) ) ;
#145532=CARTESIAN_POINT ( 'NONE',  ( 9.564922557961047289, -16.46253265017146816, 60.41775706135233293 ) ) ;
#145533=CARTESIAN_POINT ( 'NONE',  ( -8.314922557961024197, 14.29746914071037800, 102.9177570613523756 ) ) ;
#145535=CARTESIAN_POINT ( 'NONE',  ( -16.46253265017160317, 9.564922557960807481, 85.83224293864769550 ) ) ;
#145536=CARTESIAN_POINT ( 'NONE',  ( 15.72974639402176855, 15.80617190586768217, 96.87609039468568994 ) ) ;
#145537=CARTESIAN_POINT ( 'NONE',  ( -21.53943276465977519, -0.05219959533937600094, 113.7510903946856757 ) ) ;
#145539=CARTESIAN_POINT ( 'NONE',  ( -16.46253265017160317, 9.564922557960807481, 100.8322429386477097 ) ) ;
#145540=CARTESIAN_POINT ( 'NONE',  ( 0.05219959533937995610, -21.53943276465977519, 75.00109039468568994 ) ) ;
#145541=CARTESIAN_POINT ( 'NONE',  ( 14.34966873604972726, -8.224510206698740333, 25.83442372801901499 ) ) ;
#145543=CARTESIAN_POINT ( 'NONE',  ( -13.97604488694527625, -13.89961937509977652, 81.87390960531436690 ) ) ;
#145544=CARTESIAN_POINT ( 'NONE',  ( -21.53943276465977519, 0.05219959533907696930, 36.24890960531435979 ) ) ;
#145545=CARTESIAN_POINT ( 'NONE',  ( 9.474510206698971260, -16.51473224551069308, 87.91557627198102409 ) ) ;
#145546=CARTESIAN_POINT ( 'NONE',  ( 0.000000000000000000, -5.500000000000000888, 120.0000000000000142 ) ) ;
#145547=CARTESIAN_POINT ( 'NONE',  ( -5.153800228976328057, -19.02544592524343514, 72.29057627198102409 ) ) ;
#145548=CARTESIAN_POINT ( 'NONE',  ( -19.03943276465977164, 0.05219959533909376836, 71.24890960531435269 ) ) ;
#145549=CARTESIAN_POINT ( 'NONE',  ( 0.05219959533934541429, -16.53943276465976808, 95.00109039468568994 ) ) ;
#145550=CARTESIAN_POINT ( 'NONE',  ( -16.88567814943197831, 6.947325034625352558, 98.70998877347405198 ) ) ;
#145551=CARTESIAN_POINT ( 'NONE',  ( -19.05341960407617563, 5.049401038297882671, 73.54275706135233293 ) ) ;
#145552=CARTESIAN_POINT ( 'NONE',  ( -19.05341960407611168, -5.049401038298163336, 86.45724293864769550 ) ) ;
#145553=CARTESIAN_POINT ( 'NONE',  ( -16.52544592524342804, 4.483927247898546575, 81.04057627198102409 ) ) ;
#145554=CARTESIAN_POINT ( 'NONE',  ( 21.55341960407610458, 5.719274019375980345, 38.95724293864768839 ) ) ;
#145555=CARTESIAN_POINT ( 'NONE',  ( -13.89961937509977652, 13.97604488694528158, 115.6239096053143669 ) ) ;
#145556=CARTESIAN_POINT ( 'NONE',  ( -14.29746914071049879, 8.314922557960819915, 90.83224293864769550 ) ) ;
#145558=CARTESIAN_POINT ( 'NONE',  ( -16.51473224551082808, 9.474510206698731452, 43.33442372801900433 ) ) ;
#145559=CARTESIAN_POINT ( 'NONE',  ( 14.29746914071049879, -8.314922557960816363, 23.33224293864769194 ) ) ;
#145560=CARTESIAN_POINT ( 'NONE',  ( -13.89961937509977652, 13.97604488694528158, 105.6239096053143527 ) ) ;
#145561=CARTESIAN_POINT ( 'NONE',  ( 21.52544592524334988, 5.823673210054432836, 61.45942372801901854 ) ) ;
#145562=CARTESIAN_POINT ( 'NONE',  ( -0.05219959533907301413, -21.53943276465977519, 62.49890960531436690 ) ) ;
#145563=CARTESIAN_POINT ( 'NONE',  ( -21.55341960407619339, 5.719274019375674811, 33.54275706135234714 ) ) ;
#145564=CARTESIAN_POINT ( 'NONE',  ( -21.53943276465977519, 0.05219959533907696930, 81.24890960531436690 ) ) ;
#145565=CARTESIAN_POINT ( 'NONE',  ( -15.72974639402176322, -15.80617190586768395, 39.37609039468567573 ) ) ;
#145566=CARTESIAN_POINT ( 'NONE',  ( 4.483927247898545687, 16.52544592524342804, 104.7905762719810241 ) ) ;
#145567=CARTESIAN_POINT ( 'NONE',  ( -19.03943276465977164, -0.05219959533935918106, 68.75109039468566152 ) ) ;
#145568=CARTESIAN_POINT ( 'NONE',  ( 19.02544592524343514, -5.153800228976328945, 48.54057627198103120 ) ) ;
#145570=CARTESIAN_POINT ( 'NONE',  ( -4.483927247898539470, -16.52544592524342804, 97.29057627198105251 ) ) ;
#145571=CARTESIAN_POINT ( 'NONE',  ( 16.46253265017160672, -9.564922557960803928, 93.33224293864769550 ) ) ;
#145572=CARTESIAN_POINT ( 'NONE',  ( -0.05219959533909027116, -19.03943276465977164, 97.49890960531436690 ) ) ;
#145573=CARTESIAN_POINT ( 'NONE',  ( 8.224510206698953496, -14.34966873604960469, 107.9155762719810241 ) ) ;
#145574=CARTESIAN_POINT ( 'NONE',  ( 4.483927247898545687, 16.52544592524342804, 39.79057627198103830 ) ) ;
#145575=CARTESIAN_POINT ( 'NONE',  ( -14.29746914071037622, -8.314922557961029526, 94.16775706135237556 ) ) ;
#145576=CARTESIAN_POINT ( 'NONE',  ( -5.153800228976328057, -19.02544592524343514, 57.29057627198103120 ) ) ;
#145577=CARTESIAN_POINT ( 'NONE',  ( -16.51473224551069308, -9.474510206698971260, 26.66557627198103120 ) ) ;
#145578=CARTESIAN_POINT ( 'NONE',  ( 5.153800228976615827, -19.02544592524334988, 30.20942372801900433 ) ) ;
#145580=CARTESIAN_POINT ( 'NONE',  ( 8.314922557960818139, 14.29746914071049879, 29.58224293864769905 ) ) ;
#145581=CARTESIAN_POINT ( 'NONE',  ( -21.53943276465977519, -0.05219959533937600094, 48.75109039468568284 ) ) ;
#145583=CARTESIAN_POINT ( 'NONE',  ( 14.34966873604972726, -8.224510206698740333, 50.83442372801901143 ) ) ;
#145584=CARTESIAN_POINT ( 'NONE',  ( -12.14591786802309592, -12.06949235617757132, 21.87390960531436690 ) ) ;
#145585=CARTESIAN_POINT ( 'NONE',  ( 19.03943276465977164, -0.05219959533909143690, 48.74890960531435979 ) ) ;
#145586=CARTESIAN_POINT ( 'NONE',  ( -16.52544592524335698, -4.483927247898792601, 98.95942372801903275 ) ) ;
#145587=CARTESIAN_POINT ( 'NONE',  ( 4.379528057220092307, 16.55341960407617563, 22.29275706135235069 ) ) ;
#145588=CARTESIAN_POINT ( 'NONE',  ( 13.89961937509977652, -13.97604488694527269, 43.12390960531434558 ) ) ;
#145589=CARTESIAN_POINT ( 'NONE',  ( -8.314922557960811034, -14.29746914071050412, 107.0822429386476955 ) ) ;
#145590=CARTESIAN_POINT ( 'NONE',  ( -15.80617190586745835, -15.72974639402198527, 111.8739096053143669 ) ) ;
#145591=CARTESIAN_POINT ( 'NONE',  ( -0.05219959533909027116, -19.03943276465977164, 47.49890960531435979 ) ) ;
#145592=CARTESIAN_POINT ( 'NONE',  ( -16.51473224551069308, -9.474510206698971260, 111.6655762719810383 ) ) ;
#145593=CARTESIAN_POINT ( 'NONE',  ( 13.89961937509977652, -13.97604488694527269, 38.12390960531436690 ) ) ;
#145594=CARTESIAN_POINT ( 'NONE',  ( -0.05219959533909027116, -19.03943276465977164, 107.4989096053143527 ) ) ;
#145596=CARTESIAN_POINT ( 'NONE',  ( -5.153800228976328057, -19.02544592524343514, 92.29057627198099567 ) ) ;
#145597=CARTESIAN_POINT ( 'NONE',  ( -10.72451020669870658, -18.67979575497194134, 39.58442372801901143 ) ) ;
#145598=CARTESIAN_POINT ( 'NONE',  ( 8.224510206698953496, -14.34966873604960469, 107.9155762719810241 ) ) ;
#145599=CARTESIAN_POINT ( 'NONE',  ( 13.89961937509977652, -13.97604488694527269, 108.1239096053143669 ) ) ;
#145600=CARTESIAN_POINT ( 'NONE',  ( -16.46253265017146816, -9.564922557961047289, 69.16775706135233293 ) ) ;
#145601=CARTESIAN_POINT ( 'NONE',  ( 4.483927247898790824, -16.52544592524335698, 60.20942372801902565 ) ) ;
#145602=CARTESIAN_POINT ( 'NONE',  ( 5.823673210054444382, -21.52544592524334988, 90.20942372801903275 ) ) ;
#145603=CARTESIAN_POINT ( 'NONE',  ( -16.53943276465976808, -0.05219959533934237506, 53.75109039468568994 ) ) ;
#145604=CARTESIAN_POINT ( 'NONE',  ( -5.153800228976328057, -19.02544592524343514, 82.29057627198103830 ) ) ;
#145605=CARTESIAN_POINT ( 'NONE',  ( -4.483927247898782831, 16.52544592524335698, 37.70942372801900433 ) ) ;
#145606=CARTESIAN_POINT ( 'NONE',  ( -16.51473224551082808, 9.474510206698731452, 113.3344237280190043 ) ) ;
#145607=CARTESIAN_POINT ( 'NONE',  ( -4.379528057220086978, -16.55341960407618274, 84.79275706135234714 ) ) ;
#145608=CARTESIAN_POINT ( 'NONE',  ( -9.564922557961040184, 16.46253265017147172, 97.91775706135233293 ) ) ;
#145609=CARTESIAN_POINT ( 'NONE',  ( -5.153800228976328057, -19.02544592524343514, 72.29057627198102409 ) ) ;
#145610=CARTESIAN_POINT ( 'NONE',  ( -15.80617190586745835, -15.72974639402198527, 101.8739096053143811 ) ) ;
#145611=CARTESIAN_POINT ( 'NONE',  ( -8.224510206698948167, 14.34966873604960824, 85.41557627198102409 ) ) ;
#145612=CARTESIAN_POINT ( 'NONE',  ( -19.02544592524334988, -5.153800228976617603, 88.95942372801897591 ) ) ;
#145613=CARTESIAN_POINT ( 'NONE',  ( 12.14591786802327356, -12.06949235617739191, 70.62609039468567573 ) ) ;
#145615=CARTESIAN_POINT ( 'NONE',  ( 13.97604488694548053, -13.89961937509957401, 75.62609039468564731 ) ) ;
#145616=CARTESIAN_POINT ( 'NONE',  ( 12.14591786802309770, 12.06949235617756955, 29.37390960531435269 ) ) ;
#145617=CARTESIAN_POINT ( 'NONE',  ( -0.05219959533910754901, -16.53943276465976808, 92.49890960531436690 ) ) ;
#145618=CARTESIAN_POINT ( 'NONE',  ( -0.05219959533936034679, 19.03943276465977164, 32.50109039468566863 ) ) ;
#145620=CARTESIAN_POINT ( 'NONE',  ( 18.67979575497194134, -10.72451020669871369, 20.83442372801901143 ) ) ;
#145621=CARTESIAN_POINT ( 'NONE',  ( -16.51473224551069308, -9.474510206698971260, 111.6655762719810383 ) ) ;
#145622=CARTESIAN_POINT ( 'NONE',  ( 13.97604488694527802, 13.89961937509977652, 94.37390960531436690 ) ) ;
#145623=CARTESIAN_POINT ( 'NONE',  ( 10.81492255796106328, -18.62759615963255655, 95.41775706135234714 ) ) ;
#145624=CARTESIAN_POINT ( 'NONE',  ( -16.51473224551069308, -9.474510206698971260, 71.66557627198102409 ) ) ;
#145625=CARTESIAN_POINT ( 'NONE',  ( -18.67979575497178146, -10.72451020669898902, 46.66557627198102409 ) ) ;
#145626=CARTESIAN_POINT ( 'NONE',  ( 0.05219959533910956823, 16.53943276465976808, 99.99890960531436690 ) ) ;
#145627=CARTESIAN_POINT ( 'NONE',  ( -9.474510206698964154, 16.51473224551069663, 50.41557627198102409 ) ) ;
#145628=CARTESIAN_POINT ( 'NONE',  ( 8.314922557960818139, 14.29746914071049879, 109.5822429386476955 ) ) ;
#145629=CARTESIAN_POINT ( 'NONE',  ( 21.52544592524334988, 5.823673210054432836, 31.45942372801901854 ) ) ;
#145630=CARTESIAN_POINT ( 'NONE',  ( -10.81492255796105439, 18.62759615963255655, 62.91775706135236135 ) ) ;
#145631=CARTESIAN_POINT ( 'NONE',  ( 16.46253265017160672, -9.564922557960803928, 38.33224293864768839 ) ) ;
#145632=CARTESIAN_POINT ( 'NONE',  ( -14.34966873604972548, 8.224510206698743886, 78.33442372801901854 ) ) ;
#145633=CARTESIAN_POINT ( 'NONE',  ( -21.55341960407610458, -5.719274019375992779, 111.4572429386476813 ) ) ;
#145635=CARTESIAN_POINT ( 'NONE',  ( -5.719274019375978568, 21.55341960407610458, 110.2072429386477239 ) ) ;
#145636=CARTESIAN_POINT ( 'NONE',  ( -16.46253265017146816, -9.564922557961047289, 59.16775706135233293 ) ) ;
#145637=CARTESIAN_POINT ( 'NONE',  ( 5.049401038298161559, -19.05341960407611168, 62.70724293864769550 ) ) ;
#145638=CARTESIAN_POINT ( 'NONE',  ( 5.049401038297881783, 19.05341960407617563, 32.29275706135233293 ) ) ;
#145639=CARTESIAN_POINT ( 'NONE',  ( 21.55341960407619695, -5.719274019375665929, 76.04275706135237556 ) ) ;
#145640=CARTESIAN_POINT ( 'NONE',  ( 21.53943276465977519, -0.05219959533907433946, 68.74890960531435269 ) ) ;
#145641=CARTESIAN_POINT ( 'NONE',  ( 4.483927247898545687, 16.52544592524342804, 49.79057627198102409 ) ) ;
#145642=CARTESIAN_POINT ( 'NONE',  ( 0.05219959533937995610, -21.53943276465977519, 90.00109039468567573 ) ) ;
#145643=CARTESIAN_POINT ( 'NONE',  ( 5.153800228976615827, -19.02544592524334988, 35.20942372801899722 ) ) ;
#145644=CARTESIAN_POINT ( 'NONE',  ( -8.224510206698948167, 14.34966873604960824, 65.41557627198102409 ) ) ;
#145645=CARTESIAN_POINT ( 'NONE',  ( 0.05219959533910956823, 16.53943276465976808, 109.9989096053143527 ) ) ;
#145646=CARTESIAN_POINT ( 'NONE',  ( -9.474510206698720793, -16.51473224551083518, 64.58442372801900433 ) ) ;
#145647=CARTESIAN_POINT ( 'NONE',  ( -16.55341960407611168, -4.379528057220339221, 26.45724293864768839 ) ) ;
#145648=CARTESIAN_POINT ( 'NONE',  ( 15.72974639402176855, 15.80617190586768217, 71.87609039468568994 ) ) ;
#145649=CARTESIAN_POINT ( 'NONE',  ( -13.97604488694547697, 13.89961937509957934, 48.12609039468566863 ) ) ;
#145650=CARTESIAN_POINT ( 'NONE',  ( -21.53943276465977519, 0.05219959533907696930, 56.24890960531436690 ) ) ;
#145651=CARTESIAN_POINT ( 'NONE',  ( -21.53943276465977519, -0.05219959533937600094, 48.75109039468568284 ) ) ;
#145652=CARTESIAN_POINT ( 'NONE',  ( 18.67979575497178502, 10.72451020669898547, 99.16557627198100988 ) ) ;
#145653=CARTESIAN_POINT ( 'NONE',  ( 19.03943276465977164, 0.05219959533936151252, 101.2510903946856757 ) ) ;
#145654=CARTESIAN_POINT ( 'NONE',  ( 12.14591786802327356, -12.06949235617739191, 60.62609039468567573 ) ) ;
#145655=DIRECTION ( 'NONE',  ( -1.000000000000000000, -0.000000000000000000, -0.000000000000000000 ) ) ;
#145656=CARTESIAN_POINT ( 'NONE',  ( -5.823673210054116645, -21.52544592524344225, 107.2905762719810525 ) ) ;
#145657=CARTESIAN_POINT ( 'NONE',  ( -12.14591786802309592, -12.06949235617757132, 91.87390960531436690 ) ) ;
#145659=CARTESIAN_POINT ( 'NONE',  ( 0.05219959533934541429, -16.53943276465976808, 25.00109039468567218 ) ) ;
#145660=CARTESIAN_POINT ( 'NONE',  ( -5.823673210054116645, -21.52544592524344225, 47.29057627198103120 ) ) ;
#145661=CARTESIAN_POINT ( 'NONE',  ( 12.14591786802327356, -12.06949235617739191, 85.62609039468568994 ) ) ;
#145663=CARTESIAN_POINT ( 'NONE',  ( 8.314922557961029526, -14.29746914071037800, 70.41775706135236135 ) ) ;
#145664=CARTESIAN_POINT ( 'NONE',  ( 15.80617190586769283, -15.72974639402175789, 35.62609039468568994 ) ) ;
#145665=CARTESIAN_POINT ( 'NONE',  ( 5.719274019375991003, -21.55341960407610458, 62.70724293864769550 ) ) ;
#145666=CARTESIAN_POINT ( 'NONE',  ( 16.53943276465976808, 0.05219959533934440121, 86.25109039468568994 ) ) ;
#145667=CARTESIAN_POINT ( 'NONE',  ( 16.46253265017160672, -9.564922557960803928, 93.33224293864769550 ) ) ;
#145668=CARTESIAN_POINT ( 'NONE',  ( 10.72451020669871369, 18.67979575497193778, 72.08442372801899012 ) ) ;
#145669=CARTESIAN_POINT ( 'NONE',  ( -18.62759615963270932, 10.81492255796079327, 35.83224293864768839 ) ) ;
#145670=CARTESIAN_POINT ( 'NONE',  ( -5.823673210054116645, -21.52544592524344225, 32.29057627198102409 ) ) ;
#145671=EDGE_LOOP ( 'NONE', ( #69363, #186318, #65841, #141798, #20658, #55024, #57349, #102947, #26646, #17969, #95243, #44966, #100270, #173287 ) ) ;
#145672=CARTESIAN_POINT ( 'NONE',  ( 13.97604488694548053, -13.89961937509957401, 55.62609039468566863 ) ) ;
#145673=CARTESIAN_POINT ( 'NONE',  ( -16.52544592524335698, -4.483927247898792601, 58.95942372801902565 ) ) ;
#145674=CARTESIAN_POINT ( 'NONE',  ( 10.81492255796078972, 18.62759615963270932, 34.58224293864770260 ) ) ;
#145676=CARTESIAN_POINT ( 'NONE',  ( -13.97604488694527625, -13.89961937509977652, 96.87390960531433848 ) ) ;
#145677=CARTESIAN_POINT ( 'NONE',  ( -14.34966873604972548, 8.224510206698743886, 113.3344237280190328 ) ) ;
#145678=CARTESIAN_POINT ( 'NONE',  ( 18.09918380851992836, 5.500000000000035527, 73.98618307335611632 ) ) ;
#145679=CARTESIAN_POINT ( 'NONE',  ( -16.52544592524342804, 4.483927247898546575, 111.0405762719810525 ) ) ;
#145680=CARTESIAN_POINT ( 'NONE',  ( 5.719274019375991003, -21.55341960407610458, 42.70724293864770260 ) ) ;
#145681=CARTESIAN_POINT ( 'NONE',  ( -16.51473224551069308, -9.474510206698971260, 41.66557627198103120 ) ) ;
#145682=CARTESIAN_POINT ( 'NONE',  ( -4.483927247898782831, 16.52544592524335698, 87.70942372801901854 ) ) ;
#145683=CARTESIAN_POINT ( 'NONE',  ( 18.62759615963255655, 10.81492255796105972, 31.66775706135234358 ) ) ;
#145684=CARTESIAN_POINT ( 'NONE',  ( -5.153800228976607833, 19.02544592524334988, 87.70942372801897591 ) ) ;
#145685=CARTESIAN_POINT ( 'NONE',  ( -16.53943276465976808, 0.05219959533911058130, 101.2489096053143669 ) ) ;
#145686=CARTESIAN_POINT ( 'NONE',  ( -13.97604488694527625, -13.89961937509977652, 56.87390960531434558 ) ) ;
#145687=CARTESIAN_POINT ( 'NONE',  ( -9.564922557960796823, -16.46253265017161027, 32.08224293864769550 ) ) ;
#145689=CARTESIAN_POINT ( 'NONE',  ( 9.474510206698971260, -16.51473224551069308, 72.91557627198102409 ) ) ;
#145690=CARTESIAN_POINT ( 'NONE',  ( 14.29746914071037800, 8.314922557961029526, 56.66775706135235424 ) ) ;
#145691=CARTESIAN_POINT ( 'NONE',  ( 5.719274019375673035, 21.55341960407619339, 112.2927570613523471 ) ) ;
#145692=CARTESIAN_POINT ( 'NONE',  ( -15.80617190586745835, -15.72974639402198527, 51.87390960531437401 ) ) ;
#145693=CARTESIAN_POINT ( 'NONE',  ( 8.314922557961029526, -14.29746914071037800, 70.41775706135236135 ) ) ;
#145694=CARTESIAN_POINT ( 'NONE',  ( -16.46253265017146816, -9.564922557961047289, 54.16775706135234003 ) ) ;
#145695=CARTESIAN_POINT ( 'NONE',  ( -16.51473224551082808, 9.474510206698731452, 63.33442372801900433 ) ) ;
#145696=CARTESIAN_POINT ( 'NONE',  ( -21.53943276465977519, -0.05219959533937600094, 68.75109039468568994 ) ) ;
#145697=CARTESIAN_POINT ( 'NONE',  ( -13.97604488694527625, -13.89961937509977652, 61.87390960531435979 ) ) ;
#145698=CARTESIAN_POINT ( 'NONE',  ( 0.05219959533909260263, 19.03943276465977164, 39.99890960531436690 ) ) ;
#145699=CARTESIAN_POINT ( 'NONE',  ( -0.05219959533936034679, 19.03943276465977164, 57.50109039468566863 ) ) ;
#145700=CARTESIAN_POINT ( 'NONE',  ( 19.02544592524343514, -5.153800228976328945, 113.5405762719810241 ) ) ;
#145701=CARTESIAN_POINT ( 'NONE',  ( -5.153800228976328057, -19.02544592524343514, 92.29057627198099567 ) ) ;
#145702=CARTESIAN_POINT ( 'NONE',  ( 14.34966873604960469, 8.224510206698951720, 49.16557627198102409 ) ) ;
#145703=CARTESIAN_POINT ( 'NONE',  ( 10.81492255796078972, 18.62759615963270932, 49.58224293864769550 ) ) ;
#145705=CARTESIAN_POINT ( 'NONE',  ( 0.05219959533937995610, -21.53943276465977519, 105.0010903946856757 ) ) ;
#145706=CARTESIAN_POINT ( 'NONE',  ( -17.40805194822031510, -6.112264579159320199, 79.16628727489391792 ) ) ;
#145707=CARTESIAN_POINT ( 'NONE',  ( -19.05341960407611168, -5.049401038298163336, 51.45724293864770260 ) ) ;
#145710=CARTESIAN_POINT ( 'NONE',  ( 12.06949235617739724, 12.14591786802326823, 71.87609039468568994 ) ) ;
#145711=CARTESIAN_POINT ( 'NONE',  ( 15.72974639402199770, -15.80617190586745480, 98.12390960531436690 ) ) ;
#145713=CARTESIAN_POINT ( 'NONE',  ( 14.29746914071049879, -8.314922557960816363, 48.33224293864770260 ) ) ;
#145714=CARTESIAN_POINT ( 'NONE',  ( 5.049401038298161559, -19.05341960407611168, 47.70724293864770260 ) ) ;
#145716=CARTESIAN_POINT ( 'NONE',  ( -18.67979575497193778, 10.72451020669871902, 38.33442372801900433 ) ) ;
#145717=CARTESIAN_POINT ( 'NONE',  ( 19.05341960407617918, -5.049401038297876454, 51.04275706135231871 ) ) ;
#145718=CARTESIAN_POINT ( 'NONE',  ( 19.05341960407611168, 5.049401038298154454, 43.95724293864769550 ) ) ;
#145719=CARTESIAN_POINT ( 'NONE',  ( 10.81492255796106328, -18.62759615963255655, 90.41775706135236135 ) ) ;
#145720=CARTESIAN_POINT ( 'NONE',  ( 19.03943276465977164, -0.05219959533909143690, 23.74890960531435269 ) ) ;
#145722=CARTESIAN_POINT ( 'NONE',  ( -8.224510206698948167, 14.34966873604960824, 45.41557627198103830 ) ) ;
#145724=CARTESIAN_POINT ( 'NONE',  ( -0.05219959533907301413, -21.53943276465977519, 42.49890960531435979 ) ) ;
#145726=CARTESIAN_POINT ( 'NONE',  ( -5.153800228976328057, -19.02544592524343514, 107.2905762719810383 ) ) ;
#145727=CARTESIAN_POINT ( 'NONE',  ( -16.52544592524342804, 4.483927247898546575, 86.04057627198102409 ) ) ;
#145728=CARTESIAN_POINT ( 'NONE',  ( 14.34966873604972726, -8.224510206698740333, 25.83442372801901499 ) ) ;
#145729=CARTESIAN_POINT ( 'NONE',  ( 4.483927247898790824, -16.52544592524335698, 110.2094237280190185 ) ) ;
#145731=CARTESIAN_POINT ( 'NONE',  ( 0.05219959533909260263, 19.03943276465977164, 94.99890960531436690 ) ) ;
#145732=CARTESIAN_POINT ( 'NONE',  ( 10.72451020669898902, -18.67979575497178502, 102.9155762719810383 ) ) ;
#145733=CARTESIAN_POINT ( 'NONE',  ( -16.55341960407617563, 4.379528057220093196, 113.5427570613523756 ) ) ;
#145734=CARTESIAN_POINT ( 'NONE',  ( 13.97604488694527802, 13.89961937509977652, 94.37390960531436690 ) ) ;
#145735=CARTESIAN_POINT ( 'NONE',  ( 16.51473224551083163, -9.474510206698727899, 95.83442372801900433 ) ) ;
#145736=CARTESIAN_POINT ( 'NONE',  ( 18.67979575497194134, -10.72451020669871369, 105.8344237280190328 ) ) ;
#145737=CARTESIAN_POINT ( 'NONE',  ( -10.72451020669898014, 18.67979575497178502, 90.41557627198103830 ) ) ;
#145738=CARTESIAN_POINT ( 'NONE',  ( 15.80617190586746368, 15.72974639402197994, 44.37390960531435979 ) ) ;
#145739=CARTESIAN_POINT ( 'NONE',  ( -9.564922557960796823, -16.46253265017161027, 57.08224293864769550 ) ) ;
#145740=CARTESIAN_POINT ( 'NONE',  ( -0.05219959533910754901, -16.53943276465976808, 32.49890960531435979 ) ) ;
#145741=CARTESIAN_POINT ( 'NONE',  ( 9.474510206698971260, -16.51473224551069308, 72.91557627198102409 ) ) ;
#145744=CARTESIAN_POINT ( 'NONE',  ( 19.02544592524334988, 5.153800228976608722, 31.45942372801900433 ) ) ;
#145745=CARTESIAN_POINT ( 'NONE',  ( 0.05219959533910956823, 16.53943276465976808, 89.99890960531438111 ) ) ;
#145746=CARTESIAN_POINT ( 'NONE',  ( -5.719274019375665041, -21.55341960407619695, 19.79275706135235069 ) ) ;
#145748=CARTESIAN_POINT ( 'NONE',  ( 16.52544592524335698, 4.483927247898782831, 101.4594237280190185 ) ) ;
#145749=CARTESIAN_POINT ( 'NONE',  ( -19.05341960407611168, -5.049401038298163336, 26.45724293864769550 ) ) ;
#145750=CARTESIAN_POINT ( 'NONE',  ( 19.02544592524343514, -5.153800228976328945, 73.54057627198103830 ) ) ;
#145751=CARTESIAN_POINT ( 'NONE',  ( -0.05219959533909027116, -19.03943276465977164, 22.49890960531436690 ) ) ;
#145752=CARTESIAN_POINT ( 'NONE',  ( -12.14591786802309592, -12.06949235617757132, 46.87390960531435979 ) ) ;
#145753=CARTESIAN_POINT ( 'NONE',  ( -15.80617190586768217, 15.72974639402176855, 58.12609039468568994 ) ) ;
#145755=CARTESIAN_POINT ( 'NONE',  ( 18.62759615963255655, 10.81492255796105972, 91.66775706135234714 ) ) ;
#145756=CARTESIAN_POINT ( 'NONE',  ( 13.97604488694527802, 13.89961937509977652, 49.37390960531434558 ) ) ;
#145757=CARTESIAN_POINT ( 'NONE',  ( -5.049401038298153566, 19.05341960407611168, 55.20724293864769550 ) ) ;
#145759=CARTESIAN_POINT ( 'NONE',  ( -18.67979575497193778, 10.72451020669871902, 98.33442372801901854 ) ) ;
#145760=CARTESIAN_POINT ( 'NONE',  ( 4.483927247898790824, -16.52544592524335698, 60.20942372801902565 ) ) ;
#145761=CARTESIAN_POINT ( 'NONE',  ( 5.719274019375673035, 21.55341960407619339, 82.29275706135234714 ) ) ;
#145762=CARTESIAN_POINT ( 'NONE',  ( 16.51473224551069308, 9.474510206698969483, 114.1655762719810241 ) ) ;
#145763=CARTESIAN_POINT ( 'NONE',  ( -19.05341960407617563, 5.049401038297882671, 88.54275706135230450 ) ) ;
#145764=CARTESIAN_POINT ( 'NONE',  ( 21.52544592524334988, 5.823673210054432836, 66.45942372801903275 ) ) ;
#145765=CARTESIAN_POINT ( 'NONE',  ( 4.379528057220092307, 16.55341960407617563, 37.29275706135235424 ) ) ;
#145766=CARTESIAN_POINT ( 'NONE',  ( -0.05219959533907301413, -21.53943276465977519, 92.49890960531436690 ) ) ;
#145767=CARTESIAN_POINT ( 'NONE',  ( -0.05219959533936034679, 19.03943276465977164, 82.50109039468567573 ) ) ;
#145768=CARTESIAN_POINT ( 'NONE',  ( 13.97604488694527802, 13.89961937509977652, 69.37390960531436690 ) ) ;
#145769=CARTESIAN_POINT ( 'NONE',  ( -5.153800228976607833, 19.02544592524334988, 97.70942372801900433 ) ) ;
#145770=CARTESIAN_POINT ( 'NONE',  ( 13.89961937509957401, 13.97604488694547697, 106.8760903946856757 ) ) ;
#145771=CARTESIAN_POINT ( 'NONE',  ( 16.52544592524342804, -4.483927247898539470, 48.54057627198103120 ) ) ;
#145772=CARTESIAN_POINT ( 'NONE',  ( 13.97604488694548053, -13.89961937509957401, 70.62609039468567573 ) ) ;
#145773=VERTEX_POINT ( 'NONE', #115878 ) ;
#145774=CARTESIAN_POINT ( 'NONE',  ( 0.05219959533934541429, -16.53943276465976808, 55.00109039468568284 ) ) ;
#145775=CARTESIAN_POINT ( 'NONE',  ( 19.03943276465977164, -0.05219959533909143690, 43.74890960531435979 ) ) ;
#145776=CARTESIAN_POINT ( 'NONE',  ( 9.564922557960805705, 16.46253265017160317, 59.58224293864769550 ) ) ;
#145777=CARTESIAN_POINT ( 'NONE',  ( -12.06949235617739369, -12.14591786802326823, 59.37609039468568284 ) ) ;
#145780=CARTESIAN_POINT ( 'NONE',  ( -13.97604488694527625, -13.89961937509977652, 111.8739096053143243 ) ) ;
#145781=CARTESIAN_POINT ( 'NONE',  ( 19.02544592524343514, -5.153800228976328945, 28.54057627198102409 ) ) ;
#145783=CARTESIAN_POINT ( 'NONE',  ( 19.02544592524334988, 5.153800228976608722, 111.4594237280190043 ) ) ;
#145784=CARTESIAN_POINT ( 'NONE',  ( -15.72974639402197994, 15.80617190586746368, 35.62390960531437401 ) ) ;
#145785=CARTESIAN_POINT ( 'NONE',  ( -19.02544592524334988, -5.153800228976617603, 33.95942372801897591 ) ) ;
#145786=CARTESIAN_POINT ( 'NONE',  ( -14.29746914071037622, -8.314922557961029526, 34.16775706135234714 ) ) ;
#145787=CARTESIAN_POINT ( 'NONE',  ( -19.05341960407611168, -5.049401038298163336, 26.45724293864769550 ) ) ;
#145788=CARTESIAN_POINT ( 'NONE',  ( -19.05341960407611168, -5.049401038298163336, 51.45724293864770260 ) ) ;
#145789=CARTESIAN_POINT ( 'NONE',  ( -5.823673210054116645, -21.52544592524344225, 77.29057627198102409 ) ) ;
#145790=CARTESIAN_POINT ( 'NONE',  ( 5.049401038298161559, -19.05341960407611168, 97.70724293864766707 ) ) ;
#145791=CARTESIAN_POINT ( 'NONE',  ( 5.153800228976335163, 19.02544592524342804, 44.79057627198103830 ) ) ;
#145793=CARTESIAN_POINT ( 'NONE',  ( 13.97604488694548053, -13.89961937509957401, 85.62609039468568994 ) ) ;
#145794=CARTESIAN_POINT ( 'NONE',  ( -4.379528057220328563, 16.55341960407611168, 65.20724293864768129 ) ) ;
#145795=CARTESIAN_POINT ( 'NONE',  ( 21.55341960407610458, 5.719274019375980345, 48.95724293864770971 ) ) ;
#145796=CARTESIAN_POINT ( 'NONE',  ( 10.72451020669871369, 18.67979575497193778, 112.0844237280190185 ) ) ;
#145797=CARTESIAN_POINT ( 'NONE',  ( -5.823673210054116645, -21.52544592524344225, 102.2905762719810383 ) ) ;
#145798=CARTESIAN_POINT ( 'NONE',  ( -5.823673210054431948, 21.52544592524334988, 72.70942372801901854 ) ) ;
#145799=CARTESIAN_POINT ( 'NONE',  ( -21.53943276465977519, -0.05219959533937600094, 83.75109039468568994 ) ) ;
#145800=CARTESIAN_POINT ( 'NONE',  ( -19.02544592524342804, 5.153800228976336051, 111.0405762719810099 ) ) ;
#145801=CARTESIAN_POINT ( 'NONE',  ( -14.34966873604972548, 8.224510206698743886, 103.3344237280190043 ) ) ;
#145802=CARTESIAN_POINT ( 'NONE',  ( -5.823673210054431948, 21.52544592524334988, 77.70942372801900433 ) ) ;
#145803=CARTESIAN_POINT ( 'NONE',  ( 9.474510206698971260, -16.51473224551069308, 72.91557627198102409 ) ) ;
#145804=CARTESIAN_POINT ( 'NONE',  ( 21.55341960407619695, -5.719274019375665929, 36.04275706135234714 ) ) ;
#145805=CARTESIAN_POINT ( 'NONE',  ( -19.05341960407611168, -5.049401038298163336, 66.45724293864769550 ) ) ;
#145806=CARTESIAN_POINT ( 'NONE',  ( -12.06949235617756955, 12.14591786802309770, 80.62390960531438111 ) ) ;
#145807=CARTESIAN_POINT ( 'NONE',  ( 16.55341960407611168, 4.379528057220329451, 53.95724293864770260 ) ) ;
#145808=CARTESIAN_POINT ( 'NONE',  ( 5.823673210054125526, 21.52544592524343514, 59.79057627198103120 ) ) ;
#145809=CARTESIAN_POINT ( 'NONE',  ( -16.51473224551069308, -9.474510206698971260, 61.66557627198103120 ) ) ;
#145810=CARTESIAN_POINT ( 'NONE',  ( -18.62759615963270932, 10.81492255796079327, 70.83224293864770971 ) ) ;
#145811=CARTESIAN_POINT ( 'NONE',  ( -13.97604488694547697, 13.89961937509957934, 63.12609039468566152 ) ) ;
#145812=CARTESIAN_POINT ( 'NONE',  ( 19.03943276465977164, 0.05219959533936151252, 26.25109039468566507 ) ) ;
#145813=CARTESIAN_POINT ( 'NONE',  ( 4.483927247898545687, 16.52544592524342804, 59.79057627198103120 ) ) ;
#145814=CARTESIAN_POINT ( 'NONE',  ( 15.72974639402199770, -15.80617190586745480, 58.12390960531435979 ) ) ;
#145815=ORIENTED_EDGE ( 'NONE', *, *, #180229, .F. ) ;
#145816=CARTESIAN_POINT ( 'NONE',  ( -17.97214573761831247, -5.500000000000087930, 41.46970049038657180 ) ) ;
#145817=CARTESIAN_POINT ( 'NONE',  ( -8.314922557961024197, 14.29746914071037800, 102.9177570613523756 ) ) ;
#145819=CARTESIAN_POINT ( 'NONE',  ( -19.02544592524334988, -5.153800228976617603, 88.95942372801897591 ) ) ;
#145820=CARTESIAN_POINT ( 'NONE',  ( -8.314922557960811034, -14.29746914071050412, 62.08224293864769550 ) ) ;
#145821=CARTESIAN_POINT ( 'NONE',  ( -19.01529144963332385, -5.500000000000167866, 61.23431955728440812 ) ) ;
#145822=CARTESIAN_POINT ( 'NONE',  ( 16.51473224551069308, 9.474510206698969483, 59.16557627198102409 ) ) ;
#145823=CARTESIAN_POINT ( 'NONE',  ( 0.05219959533910956823, 16.53943276465976808, 54.99890960531435269 ) ) ;
#145824=CARTESIAN_POINT ( 'NONE',  ( 9.474510206698971260, -16.51473224551069308, 82.91557627198103830 ) ) ;
#145825=CARTESIAN_POINT ( 'NONE',  ( -19.02544592524334988, -5.153800228976617603, 73.95942372801900433 ) ) ;
#145826=CARTESIAN_POINT ( 'NONE',  ( 16.46253265017160672, -9.564922557960803928, 53.33224293864768839 ) ) ;
#145827=CARTESIAN_POINT ( 'NONE',  ( -19.03943276465977164, 0.05219959533909376836, 81.24890960531436690 ) ) ;
#145828=CARTESIAN_POINT ( 'NONE',  ( -13.89961937509977652, 13.97604488694528158, 70.62390960531432427 ) ) ;
#145829=CARTESIAN_POINT ( 'NONE',  ( 21.55341960407610458, 5.719274019375980345, 68.95724293864769550 ) ) ;
#145830=FACE_OUTER_BOUND ( 'NONE', #114664, .T. ) ;
#145831=CARTESIAN_POINT ( 'NONE',  ( 13.89961937509977652, -13.97604488694527269, 53.12390960531434558 ) ) ;
#145832=CARTESIAN_POINT ( 'NONE',  ( 15.72974639402199770, -15.80617190586745480, 53.12390960531436690 ) ) ;
#145833=CARTESIAN_POINT ( 'NONE',  ( 5.153800228976615827, -19.02544592524334988, 80.20942372801901854 ) ) ;
#145834=CARTESIAN_POINT ( 'NONE',  ( 14.29746914071049879, -8.314922557960816363, 23.33224293864769194 ) ) ;
#145836=CARTESIAN_POINT ( 'NONE',  ( -13.97604488694547697, 13.89961937509957934, 33.12609039468566863 ) ) ;
#145837=CARTESIAN_POINT ( 'NONE',  ( -14.29746914071037622, -8.314922557961029526, 59.16775706135234714 ) ) ;
#145838=CARTESIAN_POINT ( 'NONE',  ( 0.05219959533934541429, -16.53943276465976808, 95.00109039468568994 ) ) ;
#145839=CARTESIAN_POINT ( 'NONE',  ( -18.09867054820431420, -5.499999999999968026, 93.98393025253582778 ) ) ;
#145840=CARTESIAN_POINT ( 'NONE',  ( -14.29746914071037622, -8.314922557961029526, 79.16775706135234714 ) ) ;
#145841=CARTESIAN_POINT ( 'NONE',  ( -5.049401038298153566, 19.05341960407611168, 115.2072429386477097 ) ) ;
#145842=CARTESIAN_POINT ( 'NONE',  ( 9.474510206698971260, -16.51473224551069308, 32.91557627198102409 ) ) ;
#145843=CARTESIAN_POINT ( 'NONE',  ( -12.06949235617739369, -12.14591786802326823, 34.37609039468568284 ) ) ;
#145844=CARTESIAN_POINT ( 'NONE',  ( 9.474510206698971260, -16.51473224551069308, 47.91557627198102409 ) ) ;
#145845=CARTESIAN_POINT ( 'NONE',  ( -5.719274019375665041, -21.55341960407619695, 39.79275706135235424 ) ) ;
#145846=CARTESIAN_POINT ( 'NONE',  ( -16.53943276465976808, -0.05219959533934237506, 48.75109039468568284 ) ) ;
#145847=CARTESIAN_POINT ( 'NONE',  ( -16.55341960407617563, 4.379528057220093196, 108.5427570613523756 ) ) ;
#145848=CARTESIAN_POINT ( 'NONE',  ( 16.51473224551069308, 9.474510206698969483, 29.16557627198103475 ) ) ;
#145849=CARTESIAN_POINT ( 'NONE',  ( 9.564922557961047289, -16.46253265017146816, 25.41775706135234003 ) ) ;
#145850=CARTESIAN_POINT ( 'NONE',  ( 19.03943276465977164, 0.05219959533936151252, 111.2510903946856757 ) ) ;
#145851=CARTESIAN_POINT ( 'NONE',  ( -5.049401038297874678, -19.05341960407617918, 69.79275706135233293 ) ) ;
#145852=CARTESIAN_POINT ( 'NONE',  ( -14.29746914071049879, 8.314922557960819915, 65.83224293864769550 ) ) ;
#145853=CARTESIAN_POINT ( 'NONE',  ( 19.03943276465977164, -0.05219959533909143690, 38.74890960531436690 ) ) ;
#145854=CARTESIAN_POINT ( 'NONE',  ( 19.05341960407617918, -5.049401038297876454, 76.04275706135230450 ) ) ;
#145855=CARTESIAN_POINT ( 'NONE',  ( 16.20579543436678804, -7.371946100355086351, 91.93479165828122746 ) ) ;
#145856=CARTESIAN_POINT ( 'NONE',  ( -21.53943276465977519, -0.05219959533937600094, 68.75109039468568994 ) ) ;
#145857=CARTESIAN_POINT ( 'NONE',  ( 12.14591786802327356, -12.06949235617739191, 40.62609039468567573 ) ) ;
#145859=CARTESIAN_POINT ( 'NONE',  ( -15.80617190586745835, -15.72974639402198527, 31.87390960531435979 ) ) ;
#145860=CARTESIAN_POINT ( 'NONE',  ( 16.52544592524335698, 4.483927247898782831, 31.45942372801901854 ) ) ;
#145861=CARTESIAN_POINT ( 'NONE',  ( 9.564922557960805705, 16.46253265017160317, 114.5822429386476955 ) ) ;
#145863=CARTESIAN_POINT ( 'NONE',  ( 19.03943276465977164, -0.05219959533909143690, 33.74890960531435979 ) ) ;
#145865=CARTESIAN_POINT ( 'NONE',  ( 19.03943276465977164, -0.05219959533909143690, 53.74890960531436690 ) ) ;
#145866=CARTESIAN_POINT ( 'NONE',  ( -10.81492255796105439, 18.62759615963255655, 67.91775706135234714 ) ) ;
#145867=CARTESIAN_POINT ( 'NONE',  ( -15.80617190586768217, 15.72974639402176855, 108.1260903946856757 ) ) ;
#145868=CARTESIAN_POINT ( 'NONE',  ( -4.483927247898539470, -16.52544592524342804, 27.29057627198103120 ) ) ;
#145869=CARTESIAN_POINT ( 'NONE',  ( 5.049401038298161559, -19.05341960407611168, 32.70724293864768129 ) ) ;
#145870=CARTESIAN_POINT ( 'NONE',  ( 19.02544592524343514, -5.153800228976328945, 93.54057627198102409 ) ) ;
#145871=CARTESIAN_POINT ( 'NONE',  ( 10.72451020669871369, 18.67979575497193778, 52.08442372801901854 ) ) ;
#145872=CARTESIAN_POINT ( 'NONE',  ( 13.89961937509977652, -13.97604488694527269, 38.12390960531436690 ) ) ;
#145873=CARTESIAN_POINT ( 'NONE',  ( -5.719274019375665041, -21.55341960407619695, 49.79275706135234714 ) ) ;
#145874=CARTESIAN_POINT ( 'NONE',  ( -16.51473224551082808, 9.474510206698731452, 98.33442372801900433 ) ) ;
#145875=CARTESIAN_POINT ( 'NONE',  ( -9.474510206698964154, 16.51473224551069663, 105.4155762719810383 ) ) ;
#145876=CARTESIAN_POINT ( 'NONE',  ( -13.89961937509977652, 13.97604488694528158, 25.62390960531434558 ) ) ;
#145877=CARTESIAN_POINT ( 'NONE',  ( -0.05219959533907301413, -21.53943276465977519, 107.4989096053143669 ) ) ;
#145878=CARTESIAN_POINT ( 'NONE',  ( -5.049401038297874678, -19.05341960407617918, 39.79275706135232582 ) ) ;
#145879=CARTESIAN_POINT ( 'NONE',  ( 14.34966873604960469, 8.224510206698951720, 109.1655762719810383 ) ) ;
#145880=CARTESIAN_POINT ( 'NONE',  ( 19.02544592524343514, -5.153800228976328945, 58.54057627198102409 ) ) ;
#145881=CARTESIAN_POINT ( 'NONE',  ( 0.05219959533936267826, -19.03943276465977164, 95.00109039468567573 ) ) ;
#145882=CARTESIAN_POINT ( 'NONE',  ( 8.224510206698953496, -14.34966873604960469, 57.91557627198103120 ) ) ;
#145883=CARTESIAN_POINT ( 'NONE',  ( 13.89961937509957401, 13.97604488694547697, 21.87609039468566152 ) ) ;
#145884=CARTESIAN_POINT ( 'NONE',  ( 5.719274019375991003, -21.55341960407610458, 27.70724293864769905 ) ) ;
#145885=CARTESIAN_POINT ( 'NONE',  ( -16.51473224551082808, 9.474510206698731452, 93.33442372801900433 ) ) ;
#145886=CARTESIAN_POINT ( 'NONE',  ( 10.72451020669898902, -18.67979575497178502, 92.91557627198103830 ) ) ;
#145887=CARTESIAN_POINT ( 'NONE',  ( -5.823673210054431948, 21.52544592524334988, 37.70942372801900433 ) ) ;
#145888=CARTESIAN_POINT ( 'NONE',  ( -14.34966873604972548, 8.224510206698743886, 48.33442372801902565 ) ) ;
#145889=CARTESIAN_POINT ( 'NONE',  ( 4.379528057220092307, 16.55341960407617563, 112.2927570613523471 ) ) ;
#145890=CARTESIAN_POINT ( 'NONE',  ( 12.14591786802327356, -12.06949235617739191, 35.62609039468568994 ) ) ;
#145891=CARTESIAN_POINT ( 'NONE',  ( -18.62759615963255300, -10.81492255796106328, 54.16775706135235424 ) ) ;
#145892=CARTESIAN_POINT ( 'NONE',  ( 5.719274019375991003, -21.55341960407610458, 57.70724293864770260 ) ) ;
#145893=CARTESIAN_POINT ( 'NONE',  ( 19.02544592524343514, -5.153800228976328945, 28.54057627198102409 ) ) ;
#145895=CARTESIAN_POINT ( 'NONE',  ( 0.05219959533934541429, -16.53943276465976808, 75.00109039468568994 ) ) ;
#145896=CARTESIAN_POINT ( 'NONE',  ( -21.52544592524343514, 5.823673210054127303, 91.04057627198103830 ) ) ;
#145897=CARTESIAN_POINT ( 'NONE',  ( 16.52544592524342804, -4.483927247898539470, 33.54057627198102409 ) ) ;
#145898=CARTESIAN_POINT ( 'NONE',  ( 16.53943276465976808, 0.05219959533934440121, 66.25109039468567573 ) ) ;
#145899=CARTESIAN_POINT ( 'NONE',  ( -13.89961937509957401, -13.97604488694547875, 104.3760903946856757 ) ) ;
#145900=CARTESIAN_POINT ( 'NONE',  ( 0.05219959533907565091, 21.53943276465977519, 99.99890960531436690 ) ) ;
#145901=CARTESIAN_POINT ( 'NONE',  ( -16.53943276465976808, 0.05219959533911058130, 31.24890960531435979 ) ) ;
#145902=ORIENTED_EDGE ( 'NONE', *, *, #122956, .T. ) ;
#145903=CARTESIAN_POINT ( 'NONE',  ( 16.52544592524335698, 4.483927247898782831, 76.45942372801901854 ) ) ;
#145905=CARTESIAN_POINT ( 'NONE',  ( 10.81492255796078972, 18.62759615963270932, 69.58224293864769550 ) ) ;
#145906=CARTESIAN_POINT ( 'NONE',  ( -4.379528057220086978, -16.55341960407618274, 109.7927570613523613 ) ) ;
#145909=CARTESIAN_POINT ( 'NONE',  ( -5.823673210054116645, -21.52544592524344225, 82.29057627198103830 ) ) ;
#145910=CARTESIAN_POINT ( 'NONE',  ( -15.72974639402197994, 15.80617190586746368, 105.6239096053143669 ) ) ;
#145911=CARTESIAN_POINT ( 'NONE',  ( 14.29746914071049879, -8.314922557960816363, 38.33224293864768839 ) ) ;
#145912=CARTESIAN_POINT ( 'NONE',  ( 0.05219959533934541429, -16.53943276465976808, 35.00109039468568284 ) ) ;
#145913=CARTESIAN_POINT ( 'NONE',  ( -9.474510206698964154, 16.51473224551069663, 45.41557627198103120 ) ) ;
#145914=CARTESIAN_POINT ( 'NONE',  ( -5.049401038298153566, 19.05341960407611168, 70.20724293864769550 ) ) ;
#145917=CARTESIAN_POINT ( 'NONE',  ( 15.72974639402199770, -15.80617190586745480, 23.12390960531436335 ) ) ;
#145919=CARTESIAN_POINT ( 'NONE',  ( -16.46253265017146816, -9.564922557961047289, 99.16775706135233293 ) ) ;
#145920=CARTESIAN_POINT ( 'NONE',  ( 16.51473224551083163, -9.474510206698727899, 45.83442372801900433 ) ) ;
#145921=CARTESIAN_POINT ( 'NONE',  ( 0.05219959533907565091, 21.53943276465977519, 94.99890960531436690 ) ) ;
#145922=CARTESIAN_POINT ( 'NONE',  ( -0.05219959533934338120, 16.53943276465976808, 107.5010903946856899 ) ) ;
#145924=CARTESIAN_POINT ( 'NONE',  ( -21.52544592524343514, 5.823673210054127303, 51.04057627198103120 ) ) ;
#145925=CARTESIAN_POINT ( 'NONE',  ( 21.55341960407610458, 5.719274019375980345, 83.95724293864770971 ) ) ;
#145926=CARTESIAN_POINT ( 'NONE',  ( 5.049401038297881783, 19.05341960407617563, 107.2927570613523187 ) ) ;
#145927=CARTESIAN_POINT ( 'NONE',  ( 9.474510206698971260, -16.51473224551069308, 102.9155762719810241 ) ) ;
#145928=CARTESIAN_POINT ( 'NONE',  ( -10.81492255796105439, 18.62759615963255655, 77.91775706135231871 ) ) ;
#145929=CARTESIAN_POINT ( 'NONE',  ( 16.51473224551069308, 9.474510206698969483, 69.16557627198102409 ) ) ;
#145932=CARTESIAN_POINT ( 'NONE',  ( -19.05341960407611168, -5.049401038298163336, 76.45724293864769550 ) ) ;
#145933=CARTESIAN_POINT ( 'NONE',  ( 4.483927247898545687, 16.52544592524342804, 89.79057627198103830 ) ) ;
#145935=CARTESIAN_POINT ( 'NONE',  ( -19.02544592524334988, -5.153800228976617603, 108.9594237280189759 ) ) ;
#145936=( BOUNDED_CURVE ( )  B_SPLINE_CURVE ( 2, ( #64025, #78183, #14546, #187394, #170213, #171209, #138870, #15543, #155041, #1341, #123684, #110517, #95346, #16536, #156029, #124700, #186397, #30714, #80175, #47874, #79185, #172198, #76205, #198580, #140855, #2344, #33683, #61034, #157030, #44891, #18528, #60048, #122706, #137884, #199565, #169206, #184396, #45876, #175185, #111515, #20493, #144832, #159000, #188373, #6316, #3338, #67000, #83158, #96334, #36651, #67995, #129648, #97314, #81157, #173200, #66001, #65012, #98309, #174198, #99327, #176193 ),
 .UNSPECIFIED., .F., .F. ) 
 B_SPLINE_CURVE_WITH_KNOTS ( ( 3, 2, 2, 2, 2, 2, 2, 2, 2, 2, 2, 2, 2, 2, 2, 2, 2, 2, 2, 2, 2, 2, 2, 2, 2, 2, 2, 2, 2, 2, 3 ),
 ( 0.000000000000000000, 0.004385964912280701511, 0.008771929824561403022, 0.01315789473684210453, 0.01754385964912280604, 0.02192982456140350755, 0.02631578947368420907, 0.03070175438596491058, 0.03508771929824561209, 0.03947368421052631360, 0.04385964912280701511, 0.04824561403508771662, 0.05263157894736841813, 0.05701754385964911964, 0.06140350877192982115, 0.06578947368421052266, 0.07017543859649122417, 0.07456140350877192569, 0.07894736842105262720, 0.08333333333333332871, 0.08771929824561403022, 0.09210526315789473173, 0.09649122807017543324, 0.1008771929824561348, 0.1052631578947368363, 0.1096491228070175378, 0.1140350877192982393, 0.1184210526315789408, 0.1228070175438596423, 0.1271929824561403577, 0.1291485109413760268 ),
 .UNSPECIFIED. ) 
 CURVE ( )  GEOMETRIC_REPRESENTATION_ITEM ( )  RATIONAL_B_SPLINE_CURVE ( ( 1.000000000000000000, 0.9659258262890683122, 1.000000000000000000, 0.9659258262890683122, 1.000000000000000000, 0.9659258262890683122, 1.000000000000000000, 0.9659258262890683122, 1.000000000000000000, 0.9659258262890683122, 1.000000000000000000, 0.9659258262890683122, 1.000000000000000000, 0.9659258262890683122, 1.000000000000000000, 0.9659258262890683122, 1.000000000000000000, 0.9659258262890683122, 1.000000000000000000, 0.9659258262890683122, 1.000000000000000000, 0.9659258262890683122, 1.000000000000000000, 0.9659258262890683122, 1.000000000000000000, 0.9659258262890683122, 1.000000000000000000, 0.9659258262890683122, 1.000000000000000000, 0.9659258262890683122, 1.000000000000000000, 0.9659258262890683122, 1.000000000000000000, 0.9659258262890683122, 1.000000000000000000, 0.9659258262890683122, 1.000000000000000000, 0.9659258262890683122, 1.000000000000000000, 0.9659258262890683122, 1.000000000000000000, 0.9659258262890683122, 1.000000000000000000, 0.9659258262890683122, 1.000000000000000000, 0.9659258262890683122, 1.000000000000000000, 0.9659258262890683122, 1.000000000000000000, 0.9659258262890683122, 1.000000000000000000, 0.9659258262890683122, 1.000000000000000000, 0.9659258262890683122, 1.000000000000000000, 0.9659258262890683122, 1.000000000000000000, 0.9659258262890683122, 1.000000000000000000, 0.9848076720550082985, 0.9831626618144004848 ) ) 
 REPRESENTATION_ITEM ( '' )  );
#145937=CARTESIAN_POINT ( 'NONE',  ( 16.31925111598454947, -7.325300261831590554, 82.66424538967253000 ) ) ;
#145938=CARTESIAN_POINT ( 'NONE',  ( -13.89961937509977652, 13.97604488694528158, 70.62390960531432427 ) ) ;
#145939=CARTESIAN_POINT ( 'NONE',  ( 0.05219959533937995610, -21.53943276465977519, 90.00109039468567573 ) ) ;
#145940=CARTESIAN_POINT ( 'NONE',  ( 0.05219959533909260263, 19.03943276465977164, 104.9989096053143669 ) ) ;
#145941=CARTESIAN_POINT ( 'NONE',  ( -16.55341960407617563, 4.379528057220093196, 73.54275706135234714 ) ) ;
#145942=CARTESIAN_POINT ( 'NONE',  ( -17.44270441346519718, -5.991230190322950122, 76.36335079264230785 ) ) ;
#145943=CARTESIAN_POINT ( 'NONE',  ( 19.02544592524334988, 5.153800228976608722, 56.45942372801898301 ) ) ;
#145944=CARTESIAN_POINT ( 'NONE',  ( -21.55341960407619339, 5.719274019375674811, 108.5427570613523756 ) ) ;
#145948=CARTESIAN_POINT ( 'NONE',  ( 16.52544592524342804, -4.483927247898539470, 28.54057627198103120 ) ) ;
#145950=CARTESIAN_POINT ( 'NONE',  ( 14.34966873604972726, -8.224510206698740333, 90.83442372801901854 ) ) ;
#145951=CARTESIAN_POINT ( 'NONE',  ( 16.36317988757057051, 7.306389748694940067, 68.40210391636775000 ) ) ;
#145952=CARTESIAN_POINT ( 'NONE',  ( 0.05219959533934541429, -16.53943276465976808, 70.00109039468568994 ) ) ;
#145953=CARTESIAN_POINT ( 'NONE',  ( -18.67979575497193778, 10.72451020669871902, 83.33442372801903275 ) ) ;
#145954=CARTESIAN_POINT ( 'NONE',  ( -13.89961937509957401, -13.97604488694547875, 89.37609039468563310 ) ) ;
#145955=CARTESIAN_POINT ( 'NONE',  ( 19.05341960407617918, -5.049401038297876454, 36.04275706135234003 ) ) ;
#145956=CARTESIAN_POINT ( 'NONE',  ( -9.564922557960796823, -16.46253265017161027, 77.08224293864769550 ) ) ;
#145957=CARTESIAN_POINT ( 'NONE',  ( 9.564922557960805705, 16.46253265017160317, 59.58224293864769550 ) ) ;
#145958=CARTESIAN_POINT ( 'NONE',  ( -0.05219959533909027116, -19.03943276465977164, 87.49890960531436690 ) ) ;
#145959=CARTESIAN_POINT ( 'NONE',  ( 21.55341960407610458, 5.719274019375980345, 78.95724293864769550 ) ) ;
#145960=CARTESIAN_POINT ( 'NONE',  ( 21.52544592524344225, -5.823673210054117533, 43.54057627198103830 ) ) ;
#145961=CARTESIAN_POINT ( 'NONE',  ( 19.02544592524343514, -5.153800228976328945, 28.54057627198102409 ) ) ;
#145962=CARTESIAN_POINT ( 'NONE',  ( -0.05219959533934338120, 16.53943276465976808, 57.50109039468568994 ) ) ;
#145964=CARTESIAN_POINT ( 'NONE',  ( 5.719274019375673035, 21.55341960407619339, 47.29275706135234003 ) ) ;
#145965=CARTESIAN_POINT ( 'NONE',  ( -12.14591786802309592, -12.06949235617757132, 66.87390960531436690 ) ) ;
#145967=CARTESIAN_POINT ( 'NONE',  ( 14.29746914071037800, 8.314922557961029526, 41.66775706135235424 ) ) ;
#145968=CARTESIAN_POINT ( 'NONE',  ( 12.14591786802309770, 12.06949235617756955, 109.3739096053143811 ) ) ;
#145969=CARTESIAN_POINT ( 'NONE',  ( -0.05219959533936034679, 19.03943276465977164, 52.50109039468566863 ) ) ;
#145970=CARTESIAN_POINT ( 'NONE',  ( -16.52544592524342804, 4.483927247898546575, 61.04057627198103120 ) ) ;
#145971=CARTESIAN_POINT ( 'NONE',  ( 21.55341960407619695, -5.719274019375665929, 36.04275706135234714 ) ) ;
#145973=CARTESIAN_POINT ( 'NONE',  ( 21.52544592524344225, -5.823673210054117533, 88.54057627198103830 ) ) ;
#145974=CARTESIAN_POINT ( 'NONE',  ( 13.97604488694527802, 13.89961937509977652, 109.3739096053143669 ) ) ;
#145975=CARTESIAN_POINT ( 'NONE',  ( -4.379528057220328563, 16.55341960407611168, 75.20724293864769550 ) ) ;
#145978=CARTESIAN_POINT ( 'NONE',  ( -5.153800228976607833, 19.02544592524334988, 87.70942372801897591 ) ) ;
#145979=CARTESIAN_POINT ( 'NONE',  ( -18.62759615963255300, -10.81492255796106328, 19.16775706135234714 ) ) ;
#145980=CARTESIAN_POINT ( 'NONE',  ( 19.03943276465977164, -0.05219959533909143690, 63.74890960531435979 ) ) ;
#145981=CARTESIAN_POINT ( 'NONE',  ( 16.46253265017146816, 9.564922557961045513, 51.66775706135233293 ) ) ;
#145982=CARTESIAN_POINT ( 'NONE',  ( 13.97604488694527802, 13.89961937509977652, 29.37390960531435979 ) ) ;
#145983=CARTESIAN_POINT ( 'NONE',  ( 21.53943276465977519, 0.05219959533937863772, 61.25109039468567573 ) ) ;
#145984=CARTESIAN_POINT ( 'NONE',  ( -18.22780087662123805, 5.499999999999981348, 76.01763182126894947 ) ) ;
#145985=CARTESIAN_POINT ( 'NONE',  ( 16.55341960407611168, 4.379528057220329451, 58.95724293864770971 ) ) ;
#145986=CARTESIAN_POINT ( 'NONE',  ( 19.03943276465977164, -0.05219959533909143690, 58.74890960531435979 ) ) ;
#145987=CARTESIAN_POINT ( 'NONE',  ( -15.80617190586745835, -15.72974639402198527, 91.87390960531436690 ) ) ;
#145988=CARTESIAN_POINT ( 'NONE',  ( 19.05341960407611168, 5.049401038298154454, 63.95724293864769550 ) ) ;
#145990=CARTESIAN_POINT ( 'NONE',  ( 15.72974639402199770, -15.80617190586745480, 83.12390960531436690 ) ) ;
#145991=CARTESIAN_POINT ( 'NONE',  ( -21.52544592524334988, -5.823673210054445271, 93.95942372801903275 ) ) ;
#145993=CARTESIAN_POINT ( 'NONE',  ( 0.05219959533934541429, -16.53943276465976808, 100.0010903946857042 ) ) ;
#145994=CARTESIAN_POINT ( 'NONE',  ( -8.224510206698948167, 14.34966873604960824, 95.41557627198102409 ) ) ;
#145995=CARTESIAN_POINT ( 'NONE',  ( -5.153800228976607833, 19.02544592524334988, 87.70942372801897591 ) ) ;
#145997=CARTESIAN_POINT ( 'NONE',  ( 21.53943276465977519, -0.05219959533907433946, 113.7489096053143527 ) ) ;
#145998=CARTESIAN_POINT ( 'NONE',  ( 19.03943276465977164, 0.05219959533936151252, 41.25109039468566152 ) ) ;
#145999=CARTESIAN_POINT ( 'NONE',  ( -12.06949235617739369, -12.14591786802326823, 104.3760903946856899 ) ) ;
#146000=CARTESIAN_POINT ( 'NONE',  ( -5.049401038297874678, -19.05341960407617918, 24.79275706135233648 ) ) ;
#146001=CARTESIAN_POINT ( 'NONE',  ( -5.049401038298153566, 19.05341960407611168, 100.2072429386476955 ) ) ;
#146002=CARTESIAN_POINT ( 'NONE',  ( 15.72974639402199770, -15.80617190586745480, 63.12390960531435979 ) ) ;
#146004=CARTESIAN_POINT ( 'NONE',  ( 14.29746914071049879, -8.314922557960816363, 113.3322429386476955 ) ) ;
#146005=CARTESIAN_POINT ( 'NONE',  ( 5.719274019375673035, 21.55341960407619339, 112.2927570613523471 ) ) ;
#146006=CARTESIAN_POINT ( 'NONE',  ( -8.224510206698735004, -14.34966873604973081, 74.58442372801901854 ) ) ;
#146007=CARTESIAN_POINT ( 'NONE',  ( -10.81492255796105439, 18.62759615963255655, 22.91775706135235069 ) ) ;
#146008=CARTESIAN_POINT ( 'NONE',  ( -8.224510206698735004, -14.34966873604973081, 24.58442372801901499 ) ) ;
#146009=CARTESIAN_POINT ( 'NONE',  ( -13.97604488694527625, -13.89961937509977652, 106.8739096053143669 ) ) ;
#146010=CARTESIAN_POINT ( 'NONE',  ( -5.049401038298153566, 19.05341960407611168, 45.20724293864769550 ) ) ;
#146011=CARTESIAN_POINT ( 'NONE',  ( -9.564922557960796823, -16.46253265017161027, 72.08224293864770971 ) ) ;
#146012=CARTESIAN_POINT ( 'NONE',  ( 14.29746914071037800, 8.314922557961029526, 46.66775706135234714 ) ) ;
#146013=CARTESIAN_POINT ( 'NONE',  ( 4.379528057220339221, -16.55341960407611168, 92.70724293864770971 ) ) ;
#146014=CARTESIAN_POINT ( 'NONE',  ( 0.05219959533934541429, -16.53943276465976808, 105.0010903946856757 ) ) ;
#146016=CARTESIAN_POINT ( 'NONE',  ( 10.72451020669871369, 18.67979575497193778, 52.08442372801901854 ) ) ;
#146017=CARTESIAN_POINT ( 'NONE',  ( -13.97604488694527625, -13.89961937509977652, 76.87390960531433848 ) ) ;
#146018=CARTESIAN_POINT ( 'NONE',  ( -13.89961937509977652, 13.97604488694528158, 60.62390960531436690 ) ) ;
#146019=CARTESIAN_POINT ( 'NONE',  ( -5.049401038298153566, 19.05341960407611168, 95.20724293864770971 ) ) ;
#146020=CARTESIAN_POINT ( 'NONE',  ( 16.53943276465976808, -0.05219959533910856209, 43.74890960531435979 ) ) ;
#146021=CARTESIAN_POINT ( 'NONE',  ( -16.53943276465976808, -0.05219959533934237506, 93.75109039468567573 ) ) ;
#146023=CARTESIAN_POINT ( 'NONE',  ( -19.03943276465977164, -0.05219959533935918106, 43.75109039468566863 ) ) ;
#146024=CARTESIAN_POINT ( 'NONE',  ( 9.564922557960805705, 16.46253265017160317, 109.5822429386476955 ) ) ;
#146025=CARTESIAN_POINT ( 'NONE',  ( 19.05341960407611168, 5.049401038298154454, 58.95724293864768129 ) ) ;
#146026=CARTESIAN_POINT ( 'NONE',  ( -9.564922557961040184, 16.46253265017147172, 42.91775706135234003 ) ) ;
#146028=CARTESIAN_POINT ( 'NONE',  ( 18.39443945427639093, -5.500000000000021316, 71.01745347608650150 ) ) ;
#146029=CARTESIAN_POINT ( 'NONE',  ( 16.51473224551083163, -9.474510206698727899, 65.83442372801900433 ) ) ;
#146030=CARTESIAN_POINT ( 'NONE',  ( 0.05219959533934541429, -16.53943276465976808, 70.00109039468568994 ) ) ;
#146032=CARTESIAN_POINT ( 'NONE',  ( 5.153800228976335163, 19.02544592524342804, 84.79057627198099567 ) ) ;
#146033=CARTESIAN_POINT ( 'NONE',  ( 21.53943276465977519, 0.05219959533937863772, 31.25109039468568639 ) ) ;
#146034=CARTESIAN_POINT ( 'NONE',  ( 19.02544592524334988, 5.153800228976608722, 76.45942372801897591 ) ) ;
#146035=CARTESIAN_POINT ( 'NONE',  ( 5.153800228976335163, 19.02544592524342804, 114.7905762719810241 ) ) ;
#146036=CARTESIAN_POINT ( 'NONE',  ( -9.474510206698964154, 16.51473224551069663, 40.41557627198103120 ) ) ;
#146037=CARTESIAN_POINT ( 'NONE',  ( -19.03943276465977164, 0.05219959533909376836, 86.24890960531436690 ) ) ;
#146038=CARTESIAN_POINT ( 'NONE',  ( -12.14591786802309592, -12.06949235617757132, 46.87390960531435979 ) ) ;
#146039=CARTESIAN_POINT ( 'NONE',  ( -19.03943276465977164, 0.05219959533909376836, 36.24890960531436690 ) ) ;
#146040=CARTESIAN_POINT ( 'NONE',  ( 9.474510206698729675, 16.51473224551082808, 52.08442372801900433 ) ) ;
#146041=CARTESIAN_POINT ( 'NONE',  ( 16.53943276465976808, -0.05219959533910856209, 83.74890960531435269 ) ) ;
#146042=CARTESIAN_POINT ( 'NONE',  ( 5.153800228976615827, -19.02544592524334988, 35.20942372801899722 ) ) ;
#146043=CARTESIAN_POINT ( 'NONE',  ( -16.46253265017160317, 9.564922557960807481, 55.83224293864769550 ) ) ;
#146044=CARTESIAN_POINT ( 'NONE',  ( -10.72451020669898014, 18.67979575497178502, 60.41557627198102409 ) ) ;
#146045=CARTESIAN_POINT ( 'NONE',  ( -4.379528057220328563, 16.55341960407611168, 55.20724293864770260 ) ) ;
#146046=CARTESIAN_POINT ( 'NONE',  ( -13.97604488694547697, 13.89961937509957934, 28.12609039468565797 ) ) ;
#146047=CARTESIAN_POINT ( 'NONE',  ( -16.46253265017160317, 9.564922557960807481, 105.8322429386476955 ) ) ;
#146048=CARTESIAN_POINT ( 'NONE',  ( -18.62759615963270932, 10.81492255796079327, 30.83224293864770260 ) ) ;
#146049=CARTESIAN_POINT ( 'NONE',  ( -5.153800228976328057, -19.02544592524343514, 57.29057627198103120 ) ) ;
#146050=CARTESIAN_POINT ( 'NONE',  ( -13.89961937509977652, 13.97604488694528158, 30.62390960531435269 ) ) ;
#146051=CARTESIAN_POINT ( 'NONE',  ( -14.29746914071049879, 8.314922557960819915, 85.83224293864768129 ) ) ;
#146052=CARTESIAN_POINT ( 'NONE',  ( 15.80617190586746368, 15.72974639402197994, 94.37390960531436690 ) ) ;
#146053=CARTESIAN_POINT ( 'NONE',  ( 5.153800228976335163, 19.02544592524342804, 94.79057627198103830 ) ) ;
#146054=CARTESIAN_POINT ( 'NONE',  ( -21.52544592524343514, 5.823673210054127303, 111.0405762719810525 ) ) ;
#146055=CARTESIAN_POINT ( 'NONE',  ( 5.153800228976335163, 19.02544592524342804, 104.7905762719809957 ) ) ;
#146056=CARTESIAN_POINT ( 'NONE',  ( -9.564922557960796823, -16.46253265017161027, 22.08224293864768839 ) ) ;
#146057=CARTESIAN_POINT ( 'NONE',  ( -5.719274019375665041, -21.55341960407619695, 84.79275706135234714 ) ) ;
#146058=CARTESIAN_POINT ( 'NONE',  ( 15.72974639402199770, -15.80617190586745480, 98.12390960531436690 ) ) ;
#146059=CARTESIAN_POINT ( 'NONE',  ( 16.38665767535054485, -7.295008042176105434, 107.7640086421454839 ) ) ;
#146062=CARTESIAN_POINT ( 'NONE',  ( 12.06949235617739724, 12.14591786802326823, 36.87609039468568994 ) ) ;
#146063=CARTESIAN_POINT ( 'NONE',  ( -16.55341960407611168, -4.379528057220339221, 111.4572429386476813 ) ) ;
#146064=CARTESIAN_POINT ( 'NONE',  ( 18.56197773271729545, -5.500000000000105693, 51.05066217314452359 ) ) ;
#146065=CARTESIAN_POINT ( 'NONE',  ( -19.05341960407611168, -5.049401038298163336, 56.45724293864768129 ) ) ;
#146066=CARTESIAN_POINT ( 'NONE',  ( 14.34966873604960469, 8.224510206698951720, 89.16557627198102409 ) ) ;
#146067=CARTESIAN_POINT ( 'NONE',  ( 10.81492255796078972, 18.62759615963270932, 34.58224293864770260 ) ) ;
#146068=CARTESIAN_POINT ( 'NONE',  ( -4.379528057220328563, 16.55341960407611168, 60.20724293864768839 ) ) ;
#146069=CARTESIAN_POINT ( 'NONE',  ( 12.06949235617739724, 12.14591786802326823, 21.87609039468567573 ) ) ;
#146070=CARTESIAN_POINT ( 'NONE',  ( -15.80617190586768217, 15.72974639402176855, 78.12609039468570415 ) ) ;
#146072=CARTESIAN_POINT ( 'NONE',  ( 9.564922557960805705, 16.46253265017160317, 114.5822429386476955 ) ) ;
#146073=CARTESIAN_POINT ( 'NONE',  ( 16.53943276465976808, 0.05219959533934440121, 91.25109039468568994 ) ) ;
#146074=CARTESIAN_POINT ( 'NONE',  ( -13.97604488694527625, -13.89961937509977652, 41.87390960531435979 ) ) ;
#146075=CARTESIAN_POINT ( 'NONE',  ( 5.049401038298161559, -19.05341960407611168, 92.70724293864769550 ) ) ;
#146076=CARTESIAN_POINT ( 'NONE',  ( -0.05219959533907301413, -21.53943276465977519, 92.49890960531436690 ) ) ;
#146077=CARTESIAN_POINT ( 'NONE',  ( 4.379528057220092307, 16.55341960407617563, 22.29275706135235069 ) ) ;
#146078=CARTESIAN_POINT ( 'NONE',  ( 16.53943276465976808, -0.05219959533910856209, 63.74890960531435979 ) ) ;
#146079=CARTESIAN_POINT ( 'NONE',  ( 5.823673210054444382, -21.52544592524334988, 70.20942372801904696 ) ) ;
#146080=ADVANCED_FACE ( 'NONE', ( #54207 ), #169554, .T. ) ;
#146081=CARTESIAN_POINT ( 'NONE',  ( -12.06949235617739369, -12.14591786802326823, 104.3760903946856899 ) ) ;
#146082=CARTESIAN_POINT ( 'NONE',  ( 17.50000000000000000, -5.499999999999992895, 46.21769037696434168 ) ) ;
#146084=CARTESIAN_POINT ( 'NONE',  ( 4.379528057220339221, -16.55341960407611168, 27.70724293864769905 ) ) ;
#146085=CARTESIAN_POINT ( 'NONE',  ( -4.379528057220086978, -16.55341960407618274, 69.79275706135234714 ) ) ;
#146086=CARTESIAN_POINT ( 'NONE',  ( -0.05219959533909027116, -19.03943276465977164, 82.49890960531436690 ) ) ;
#146087=CARTESIAN_POINT ( 'NONE',  ( -13.97604488694527625, -13.89961937509977652, 86.87390960531436690 ) ) ;
#146088=CARTESIAN_POINT ( 'NONE',  ( -21.52544592524334988, -5.823673210054445271, 83.95942372801900433 ) ) ;
#146089=CARTESIAN_POINT ( 'NONE',  ( -16.52544592524335698, -4.483927247898792601, 83.95942372801900433 ) ) ;
#146090=CARTESIAN_POINT ( 'NONE',  ( 12.06949235617757843, -12.14591786802309237, 58.12390960531435979 ) ) ;
#146091=CARTESIAN_POINT ( 'NONE',  ( 19.03943276465977164, -0.05219959533909143690, 73.74890960531435269 ) ) ;
#146093=CARTESIAN_POINT ( 'NONE',  ( -9.564922557961040184, 16.46253265017147172, 102.9177570613523329 ) ) ;
#146094=CARTESIAN_POINT ( 'NONE',  ( 8.224510206698953496, -14.34966873604960469, 112.9155762719810383 ) ) ;
#146095=CARTESIAN_POINT ( 'NONE',  ( -19.02544592524342804, 5.153800228976336051, 81.04057627198103830 ) ) ;
#146096=CARTESIAN_POINT ( 'NONE',  ( -4.483927247898782831, 16.52544592524335698, 22.70942372801901499 ) ) ;
#146098=CARTESIAN_POINT ( 'NONE',  ( -0.05219959533936034679, 19.03943276465977164, 22.50109039468566152 ) ) ;
#146099=CARTESIAN_POINT ( 'NONE',  ( 14.29746914071037800, 8.314922557961029526, 81.66775706135236135 ) ) ;
#146100=CARTESIAN_POINT ( 'NONE',  ( -16.46253265017146816, -9.564922557961047289, 89.16775706135234714 ) ) ;
#146101=CARTESIAN_POINT ( 'NONE',  ( -0.05219959533910754901, -16.53943276465976808, 112.4989096053143669 ) ) ;
#146102=CARTESIAN_POINT ( 'NONE',  ( 12.06949235617739724, 12.14591786802326823, 71.87609039468568994 ) ) ;
#146104=CARTESIAN_POINT ( 'NONE',  ( 19.02544592524334988, 5.153800228976608722, 51.45942372801900433 ) ) ;
#146105=CARTESIAN_POINT ( 'NONE',  ( 5.823673210054444382, -21.52544592524334988, 100.2094237280190043 ) ) ;
#146106=CARTESIAN_POINT ( 'NONE',  ( -19.03943276465977164, 0.05219959533909376836, 36.24890960531436690 ) ) ;
#146107=CARTESIAN_POINT ( 'NONE',  ( -19.05341960407611168, -5.049401038298163336, 81.45724293864769550 ) ) ;
#146108=CARTESIAN_POINT ( 'NONE',  ( 8.314922557960818139, 14.29746914071049879, 69.58224293864769550 ) ) ;
#146109=CARTESIAN_POINT ( 'NONE',  ( 18.62759615963255655, 10.81492255796105972, 96.66775706135234714 ) ) ;
#146110=EDGE_CURVE ( 'NONE', #43212, #22958, #136797, .T. ) ;
#146111=CARTESIAN_POINT ( 'NONE',  ( 19.05341960407617918, -5.049401038297876454, 66.04275706135233293 ) ) ;
#146112=CARTESIAN_POINT ( 'NONE',  ( 16.46253265017146816, 9.564922557961045513, 41.66775706135234003 ) ) ;
#146113=CARTESIAN_POINT ( 'NONE',  ( 5.719274019375991003, -21.55341960407610458, 37.70724293864769550 ) ) ;
#146114=CARTESIAN_POINT ( 'NONE',  ( 21.52544592524334988, 5.823673210054432836, 96.45942372801901854 ) ) ;
#146115=CARTESIAN_POINT ( 'NONE',  ( 0.05219959533909260263, 19.03943276465977164, 74.99890960531435269 ) ) ;
#146116=CARTESIAN_POINT ( 'NONE',  ( -0.05219959533937732626, 21.53943276465977519, 107.5010903946856899 ) ) ;
#146117=CARTESIAN_POINT ( 'NONE',  ( 21.53943276465977519, -0.05219959533907433946, 48.74890960531435979 ) ) ;
#146118=CARTESIAN_POINT ( 'NONE',  ( -19.02544592524342804, 5.153800228976336051, 96.04057627198103830 ) ) ;
#146119=CARTESIAN_POINT ( 'NONE',  ( 19.03943276465977164, 0.05219959533936151252, 71.25109039468566152 ) ) ;
#146120=CARTESIAN_POINT ( 'NONE',  ( -16.46253265017160317, 9.564922557960807481, 105.8322429386476955 ) ) ;
#146121=CARTESIAN_POINT ( 'NONE',  ( -0.05219959533936034679, 19.03943276465977164, 97.50109039468567573 ) ) ;
#146122=CARTESIAN_POINT ( 'NONE',  ( -0.05219959533934338120, 16.53943276465976808, 37.50109039468568284 ) ) ;
#146123=CARTESIAN_POINT ( 'NONE',  ( -0.05219959533910754901, -16.53943276465976808, 107.4989096053143669 ) ) ;
#146124=CARTESIAN_POINT ( 'NONE',  ( 19.05341960407611168, 5.049401038298154454, 78.95724293864769550 ) ) ;
#146125=CARTESIAN_POINT ( 'NONE',  ( -10.81492255796078084, -18.62759615963271287, 67.08224293864770971 ) ) ;
#146126=CARTESIAN_POINT ( 'NONE',  ( 8.314922557961029526, -14.29746914071037800, 35.41775706135234003 ) ) ;
#146127=CARTESIAN_POINT ( 'NONE',  ( 10.72451020669871369, 18.67979575497193778, 37.08442372801901143 ) ) ;
#146128=CARTESIAN_POINT ( 'NONE',  ( 21.55341960407619695, -5.719274019375665929, 86.04275706135236135 ) ) ;
#146129=CARTESIAN_POINT ( 'NONE',  ( 16.53943276465976808, 0.05219959533934440121, 81.25109039468568994 ) ) ;
#146130=CARTESIAN_POINT ( 'NONE',  ( -19.05341960407611168, -5.049401038298163336, 76.45724293864769550 ) ) ;
#146131=CARTESIAN_POINT ( 'NONE',  ( -16.53943276465976808, 0.05219959533911058130, 76.24890960531435269 ) ) ;
#146132=CARTESIAN_POINT ( 'NONE',  ( 4.483927247898790824, -16.52544592524335698, 110.2094237280190185 ) ) ;
#146133=CARTESIAN_POINT ( 'NONE',  ( 9.564922557961047289, -16.46253265017146816, 55.41775706135234003 ) ) ;
#146134=CARTESIAN_POINT ( 'NONE',  ( 21.55341960407619695, -5.719274019375665929, 26.04275706135235779 ) ) ;
#146135=CARTESIAN_POINT ( 'NONE',  ( 16.52544592524342804, -4.483927247898539470, 78.54057627198103830 ) ) ;
#146136=CARTESIAN_POINT ( 'NONE',  ( -13.89961937509977652, 13.97604488694528158, 95.62390960531436690 ) ) ;
#146137=CARTESIAN_POINT ( 'NONE',  ( -0.05219959533934338120, 16.53943276465976808, 107.5010903946856899 ) ) ;
#146138=CARTESIAN_POINT ( 'NONE',  ( -0.05219959533937732626, 21.53943276465977519, 72.50109039468568994 ) ) ;
#146139=CARTESIAN_POINT ( 'NONE',  ( -4.379528057220086978, -16.55341960407618274, 49.79275706135234714 ) ) ;
#146140=CARTESIAN_POINT ( 'NONE',  ( -5.719274019375665041, -21.55341960407619695, 34.79275706135235424 ) ) ;
#146142=CARTESIAN_POINT ( 'NONE',  ( 21.53943276465977519, -0.05219959533907433946, 108.7489096053143669 ) ) ;
#146143=CARTESIAN_POINT ( 'NONE',  ( 0.05219959533910956823, 16.53943276465976808, 84.99890960531436690 ) ) ;
#146144=CARTESIAN_POINT ( 'NONE',  ( -19.49190055781009789, -5.500000000000052403, 50.56116087098784107 ) ) ;
#146145=CARTESIAN_POINT ( 'NONE',  ( -14.29746914071049879, 8.314922557960819915, 55.83224293864770260 ) ) ;
#146146=CARTESIAN_POINT ( 'NONE',  ( 5.153800228976335163, 19.02544592524342804, 29.79057627198102409 ) ) ;
#146147=CARTESIAN_POINT ( 'NONE',  ( -5.823673210054116645, -21.52544592524344225, 47.29057627198103120 ) ) ;
#146148=CARTESIAN_POINT ( 'NONE',  ( -8.224510206698948167, 14.34966873604960824, 80.41557627198103830 ) ) ;
#146149=CARTESIAN_POINT ( 'NONE',  ( -0.05219959533907301413, -21.53943276465977519, 77.49890960531433848 ) ) ;
#146150=CARTESIAN_POINT ( 'NONE',  ( 19.02544592524343514, -5.153800228976328945, 88.54057627198102409 ) ) ;
#146151=CARTESIAN_POINT ( 'NONE',  ( -19.05341960407611168, -5.049401038298163336, 41.45724293864769550 ) ) ;
#146152=CARTESIAN_POINT ( 'NONE',  ( 16.51473224551083163, -9.474510206698727899, 75.83442372801900433 ) ) ;
#146153=EDGE_CURVE ( 'NONE', #82599, #9179, #21126, .T. ) ;
#146154=CARTESIAN_POINT ( 'NONE',  ( 21.53943276465977519, 0.05219959533937863772, 56.25109039468568284 ) ) ;
#146155=CARTESIAN_POINT ( 'NONE',  ( 21.55341960407610458, 5.719274019375980345, 58.95724293864770971 ) ) ;
#146156=CARTESIAN_POINT ( 'NONE',  ( -5.153800228976328057, -19.02544592524343514, 37.29057627198102409 ) ) ;
#146157=CARTESIAN_POINT ( 'NONE',  ( 9.474510206698971260, -16.51473224551069308, 72.91557627198102409 ) ) ;
#146159=CARTESIAN_POINT ( 'NONE',  ( -16.53943276465976808, -0.05219959533934237506, 43.75109039468568284 ) ) ;
#146160=CARTESIAN_POINT ( 'NONE',  ( -5.719274019375665041, -21.55341960407619695, 34.79275706135235424 ) ) ;
#146161=CARTESIAN_POINT ( 'NONE',  ( -21.52544592524334988, -5.823673210054445271, 68.95942372801901854 ) ) ;
#146162=CARTESIAN_POINT ( 'NONE',  ( -16.46253265017160317, 9.564922557960807481, 115.8322429386477097 ) ) ;
#146163=CARTESIAN_POINT ( 'NONE',  ( -21.53943276465977519, 0.05219959533907696930, 81.24890960531436690 ) ) ;
#146164=CARTESIAN_POINT ( 'NONE',  ( -15.80617190586768217, 15.72974639402176855, 23.12609039468567573 ) ) ;
#146165=CARTESIAN_POINT ( 'NONE',  ( -16.52544592524335698, -4.483927247898792601, 48.95942372801902565 ) ) ;
#146166=ADVANCED_BREP_SHAPE_REPRESENTATION ( '', ( #143056, #82054 ), #78902 ) ;
#146167=CARTESIAN_POINT ( 'NONE',  ( 21.55341960407610458, 5.719274019375980345, 53.95724293864770260 ) ) ;
#146168=CARTESIAN_POINT ( 'NONE',  ( 9.474510206698729675, 16.51473224551082808, 22.08442372801899722 ) ) ;
#146169=CARTESIAN_POINT ( 'NONE',  ( 9.564922557960805705, 16.46253265017160317, 54.58224293864769550 ) ) ;
#146170=CARTESIAN_POINT ( 'NONE',  ( 13.97604488694527802, 13.89961937509977652, 114.3739096053143669 ) ) ;
#146171=CARTESIAN_POINT ( 'NONE',  ( 13.97604488694527802, 13.89961937509977652, 89.37390960531436690 ) ) ;
#146172=CARTESIAN_POINT ( 'NONE',  ( 17.50000000000000355, 3.242565516147348337, 102.5000000000000142 ) ) ;
#146173=CARTESIAN_POINT ( 'NONE',  ( -13.97604488694547697, 13.89961937509957934, 68.12609039468563310 ) ) ;
#146174=CARTESIAN_POINT ( 'NONE',  ( 21.52544592524344225, -5.823673210054117533, 48.54057627198103120 ) ) ;
#146175=CARTESIAN_POINT ( 'NONE',  ( -14.29746914071049879, 8.314922557960819915, 30.83224293864770260 ) ) ;
#146176=CARTESIAN_POINT ( 'NONE',  ( -9.474510206698720793, -16.51473224551083518, 94.58442372801900433 ) ) ;
#146177=CARTESIAN_POINT ( 'NONE',  ( -9.564922557960796823, -16.46253265017161027, 22.08224293864768839 ) ) ;
#146178=CARTESIAN_POINT ( 'NONE',  ( 19.05341960407617918, -5.049401038297876454, 21.04275706135232582 ) ) ;
#146179=CARTESIAN_POINT ( 'NONE',  ( 5.049401038297881783, 19.05341960407617563, 92.29275706135234714 ) ) ;
#146180=CARTESIAN_POINT ( 'NONE',  ( 5.719274019375991003, -21.55341960407610458, 92.70724293864770971 ) ) ;
#146181=CARTESIAN_POINT ( 'NONE',  ( -9.564922557961040184, 16.46253265017147172, 62.91775706135233293 ) ) ;
#146183=CARTESIAN_POINT ( 'NONE',  ( 16.46253265017160672, -9.564922557960803928, 53.33224293864768839 ) ) ;
#146184=CARTESIAN_POINT ( 'NONE',  ( 14.34966873604960469, 8.224510206698951720, 59.16557627198103120 ) ) ;
#146185=CARTESIAN_POINT ( 'NONE',  ( 5.153800228976335163, 19.02544592524342804, 49.79057627198100988 ) ) ;
#146186=CARTESIAN_POINT ( 'NONE',  ( 12.14591786802309770, 12.06949235617756955, 59.37390960531436690 ) ) ;
#146188=CARTESIAN_POINT ( 'NONE',  ( 0.05219959533910956823, 16.53943276465976808, 24.99890960531435624 ) ) ;
#146189=CARTESIAN_POINT ( 'NONE',  ( 19.05341960407611168, 5.049401038298154454, 58.95724293864768129 ) ) ;
#146190=CARTESIAN_POINT ( 'NONE',  ( -5.153800228976607833, 19.02544592524334988, 22.70942372801899012 ) ) ;
#146191=CARTESIAN_POINT ( 'NONE',  ( 14.29746914071037800, 8.314922557961029526, 36.66775706135234714 ) ) ;
#146192=CARTESIAN_POINT ( 'NONE',  ( 5.823673210054125526, 21.52544592524343514, 44.79057627198103120 ) ) ;
#146193=CARTESIAN_POINT ( 'NONE',  ( 18.67979575497194134, -10.72451020669871369, 105.8344237280190328 ) ) ;
#146195=CARTESIAN_POINT ( 'NONE',  ( -9.564922557960796823, -16.46253265017161027, 57.08224293864769550 ) ) ;
#146196=CARTESIAN_POINT ( 'NONE',  ( -19.02544592524342804, 5.153800228976336051, 91.04057627198100988 ) ) ;
#146197=CARTESIAN_POINT ( 'NONE',  ( -18.22780087662126647, -5.499999999999827693, 43.98236817873107185 ) ) ;
#146198=CARTESIAN_POINT ( 'NONE',  ( -10.81492255796105439, 18.62759615963255655, 22.91775706135235069 ) ) ;
#146199=CARTESIAN_POINT ( 'NONE',  ( -0.05219959533910754901, -16.53943276465976808, 97.49890960531436690 ) ) ;
#146200=CARTESIAN_POINT ( 'NONE',  ( -5.719274019375978568, 21.55341960407610458, 85.20724293864770971 ) ) ;
#146201=CARTESIAN_POINT ( 'NONE',  ( 0.05219959533909260263, 19.03943276465977164, 69.99890960531435269 ) ) ;
#146202=CARTESIAN_POINT ( 'NONE',  ( 9.564922557960805705, 16.46253265017160317, 74.58224293864769550 ) ) ;
#146203=CARTESIAN_POINT ( 'NONE',  ( -15.72974639402197994, 15.80617190586746368, 115.6239096053143669 ) ) ;
#146205=CARTESIAN_POINT ( 'NONE',  ( -19.02544592524342804, 5.153800228976336051, 76.04057627198102409 ) ) ;
#146207=CARTESIAN_POINT ( 'NONE',  ( -4.379528057220328563, 16.55341960407611168, 105.2072429386477097 ) ) ;
#146208=CARTESIAN_POINT ( 'NONE',  ( -9.474510206698964154, 16.51473224551069663, 25.41557627198103120 ) ) ;
#146209=CARTESIAN_POINT ( 'NONE',  ( -16.51473224551082808, 9.474510206698731452, 93.33442372801900433 ) ) ;
#146210=CARTESIAN_POINT ( 'NONE',  ( 0.05219959533910956823, 16.53943276465976808, 94.99890960531436690 ) ) ;
#146211=CARTESIAN_POINT ( 'NONE',  ( 18.62759615963255655, 10.81492255796105972, 71.66775706135234714 ) ) ;
#146212=CARTESIAN_POINT ( 'NONE',  ( 5.049401038298161559, -19.05341960407611168, 62.70724293864769550 ) ) ;
#146213=CARTESIAN_POINT ( 'NONE',  ( -18.67979575497193778, 10.72451020669871902, 38.33442372801900433 ) ) ;
#146214=CARTESIAN_POINT ( 'NONE',  ( -21.52544592524343514, 5.823673210054127303, 116.0405762719810383 ) ) ;
#146216=CARTESIAN_POINT ( 'NONE',  ( 13.97604488694527802, 13.89961937509977652, 79.37390960531435269 ) ) ;
#146218=CARTESIAN_POINT ( 'NONE',  ( -4.379528057220086978, -16.55341960407618274, 24.79275706135235779 ) ) ;
#146219=CARTESIAN_POINT ( 'NONE',  ( 10.81492255796078972, 18.62759615963270932, 24.58224293864768839 ) ) ;
#146220=CARTESIAN_POINT ( 'NONE',  ( 15.80617190586769283, -15.72974639402175789, 65.62609039468568994 ) ) ;
#146221=CARTESIAN_POINT ( 'NONE',  ( 5.049401038298161559, -19.05341960407611168, 107.7072429386476955 ) ) ;
#146222=CARTESIAN_POINT ( 'NONE',  ( 16.46253265017146816, 9.564922557961045513, 96.66775706135233293 ) ) ;
#146224=CARTESIAN_POINT ( 'NONE',  ( 19.05341960407611168, 5.049401038298154454, 48.95724293864768129 ) ) ;
#146225=CARTESIAN_POINT ( 'NONE',  ( -9.564922557960796823, -16.46253265017161027, 77.08224293864769550 ) ) ;
#146226=CARTESIAN_POINT ( 'NONE',  ( -14.34966873604960291, -8.224510206698953496, 96.66557627198102409 ) ) ;
#146227=CARTESIAN_POINT ( 'NONE',  ( 5.153800228976335163, 19.02544592524342804, 99.79057627198102409 ) ) ;
#146228=CARTESIAN_POINT ( 'NONE',  ( -8.224510206698948167, 14.34966873604960824, 95.41557627198102409 ) ) ;
#146229=CARTESIAN_POINT ( 'NONE',  ( 9.564922557960805705, 16.46253265017160317, 99.58224293864770971 ) ) ;
#146230=CARTESIAN_POINT ( 'NONE',  ( -8.314922557960811034, -14.29746914071050412, 42.08224293864769550 ) ) ;
#146231=CARTESIAN_POINT ( 'NONE',  ( 5.049401038298161559, -19.05341960407611168, 47.70724293864770260 ) ) ;
#146232=CARTESIAN_POINT ( 'NONE',  ( -15.72974639402176322, -15.80617190586768395, 54.37609039468568994 ) ) ;
#146233=CARTESIAN_POINT ( 'NONE',  ( 19.03943276465977164, 0.05219959533936151252, 91.25109039468566152 ) ) ;
#146234=CARTESIAN_POINT ( 'NONE',  ( -16.55341960407611168, -4.379528057220339221, 51.45724293864770260 ) ) ;
#146235=CARTESIAN_POINT ( 'NONE',  ( -0.05219959533907301413, -21.53943276465977519, 102.4989096053143811 ) ) ;
#146236=CARTESIAN_POINT ( 'NONE',  ( -5.719274019375978568, 21.55341960407610458, 45.20724293864769550 ) ) ;
#146237=CARTESIAN_POINT ( 'NONE',  ( -13.89961937509977652, 13.97604488694528158, 115.6239096053143669 ) ) ;
#146238=CARTESIAN_POINT ( 'NONE',  ( -12.14591786802309592, -12.06949235617757132, 81.87390960531435269 ) ) ;
#146240=CARTESIAN_POINT ( 'NONE',  ( -16.51473224551069308, -9.474510206698971260, 51.66557627198102409 ) ) ;
#146241=CARTESIAN_POINT ( 'NONE',  ( -0.05219959533934338120, 16.53943276465976808, 112.5010903946857042 ) ) ;
#146242=CARTESIAN_POINT ( 'NONE',  ( 4.379528057220092307, 16.55341960407617563, 102.2927570613523613 ) ) ;
#146243=CARTESIAN_POINT ( 'NONE',  ( -8.224510206698735004, -14.34966873604973081, 79.58442372801903275 ) ) ;
#146244=CARTESIAN_POINT ( 'NONE',  ( 16.46253265017146816, 9.564922557961045513, 36.66775706135233293 ) ) ;
#146246=CARTESIAN_POINT ( 'NONE',  ( -9.474510206698964154, 16.51473224551069663, 105.4155762719810383 ) ) ;
#146247=CARTESIAN_POINT ( 'NONE',  ( 5.153800228976335163, 19.02544592524342804, 84.79057627198099567 ) ) ;
#146248=CARTESIAN_POINT ( 'NONE',  ( -13.97604488694527625, -13.89961937509977652, 36.87390960531436690 ) ) ;
#146249=CARTESIAN_POINT ( 'NONE',  ( -4.379528057220328563, 16.55341960407611168, 45.20724293864769550 ) ) ;
#146250=CARTESIAN_POINT ( 'NONE',  ( -19.02544592524342804, 5.153800228976336051, 116.0405762719810383 ) ) ;
#146251=CARTESIAN_POINT ( 'NONE',  ( -19.03943276465977164, 0.05219959533909376836, 106.2489096053143669 ) ) ;
#146252=CARTESIAN_POINT ( 'NONE',  ( -15.80617190586745835, -15.72974639402198527, 41.87390960531435979 ) ) ;
#146253=CARTESIAN_POINT ( 'NONE',  ( 8.314922557960818139, 14.29746914071049879, 89.58224293864768129 ) ) ;
#146254=CARTESIAN_POINT ( 'NONE',  ( -16.55341960407617563, 4.379528057220093196, 38.54275706135234714 ) ) ;
#146257=CARTESIAN_POINT ( 'NONE',  ( 4.379528057220339221, -16.55341960407611168, 67.70724293864769550 ) ) ;
#146259=CARTESIAN_POINT ( 'NONE',  ( -19.05341960407617563, 5.049401038297882671, 63.54275706135234003 ) ) ;
#146260=CARTESIAN_POINT ( 'NONE',  ( 19.05341960407611168, 5.049401038298154454, 98.95724293864766707 ) ) ;
#146261=CARTESIAN_POINT ( 'NONE',  ( 19.03943276465977164, 0.05219959533936151252, 81.25109039468567573 ) ) ;
#146263=CARTESIAN_POINT ( 'NONE',  ( -4.483927247898782831, 16.52544592524335698, 27.70942372801901854 ) ) ;
#146264=CARTESIAN_POINT ( 'NONE',  ( -16.55341960407617563, 4.379528057220093196, 103.5427570613523613 ) ) ;
#146265=CARTESIAN_POINT ( 'NONE',  ( 13.97604488694548053, -13.89961937509957401, 70.62609039468567573 ) ) ;
#146266=CARTESIAN_POINT ( 'NONE',  ( -21.53943276465977519, 0.05219959533907696930, 31.24890960531435979 ) ) ;
#146267=CARTESIAN_POINT ( 'NONE',  ( 18.62759615963255655, 10.81492255796105972, 71.66775706135234714 ) ) ;
#146269=CARTESIAN_POINT ( 'NONE',  ( -14.29746914071037622, -8.314922557961029526, 19.16775706135234714 ) ) ;
#146271=CARTESIAN_POINT ( 'NONE',  ( 16.46253265017160672, -9.564922557960803928, 88.33224293864769550 ) ) ;
#146273=CARTESIAN_POINT ( 'NONE',  ( 8.314922557960818139, 14.29746914071049879, 94.58224293864769550 ) ) ;
#146274=CARTESIAN_POINT ( 'NONE',  ( 9.474510206698971260, -16.51473224551069308, 72.91557627198102409 ) ) ;
#146276=CARTESIAN_POINT ( 'NONE',  ( 19.03943276465977164, -0.05219959533909143690, 83.74890960531436690 ) ) ;
#146278=CARTESIAN_POINT ( 'NONE',  ( 19.05341960407617918, -5.049401038297876454, 91.04275706135234714 ) ) ;
#146279=CARTESIAN_POINT ( 'NONE',  ( 21.55341960407610458, 5.719274019375980345, 78.95724293864769550 ) ) ;
#146280=CARTESIAN_POINT ( 'NONE',  ( 9.474510206698971260, -16.51473224551069308, 27.91557627198103120 ) ) ;
#146281=CARTESIAN_POINT ( 'NONE',  ( 19.02544592524334988, 5.153800228976608722, 66.45942372801899012 ) ) ;
#146282=CARTESIAN_POINT ( 'NONE',  ( -15.72974639402197994, 15.80617190586746368, 110.6239096053143669 ) ) ;
#146283=CARTESIAN_POINT ( 'NONE',  ( 9.474510206698971260, -16.51473224551069308, 72.91557627198102409 ) ) ;
#146284=CARTESIAN_POINT ( 'NONE',  ( -13.89961937509977652, 13.97604488694528158, 105.6239096053143527 ) ) ;
#146286=CARTESIAN_POINT ( 'NONE',  ( -18.67979575497178146, -10.72451020669898902, 106.6655762719810383 ) ) ;
#146287=CARTESIAN_POINT ( 'NONE',  ( 16.53943276465976808, -0.05219959533910856209, 88.74890960531436690 ) ) ;
#146288=CARTESIAN_POINT ( 'NONE',  ( 5.049401038298161559, -19.05341960407611168, 82.70724293864770971 ) ) ;
#146289=CARTESIAN_POINT ( 'NONE',  ( -13.97604488694547697, 13.89961937509957934, 63.12609039468566152 ) ) ;
#146290=CARTESIAN_POINT ( 'NONE',  ( 15.80617190586746368, 15.72974639402197994, 84.37390960531438111 ) ) ;
#146291=CARTESIAN_POINT ( 'NONE',  ( 5.719274019375991003, -21.55341960407610458, 67.70724293864769550 ) ) ;
#146292=CARTESIAN_POINT ( 'NONE',  ( -12.06949235617756955, 12.14591786802309770, 40.62390960531435269 ) ) ;
#146293=CARTESIAN_POINT ( 'NONE',  ( 5.823673210054444382, -21.52544592524334988, 100.2094237280190043 ) ) ;
#146294=CARTESIAN_POINT ( 'NONE',  ( -8.224510206698735004, -14.34966873604973081, 69.58442372801900433 ) ) ;
#146295=CARTESIAN_POINT ( 'NONE',  ( 13.89961937509977652, -13.97604488694527269, 93.12390960531436690 ) ) ;
#146296=CARTESIAN_POINT ( 'NONE',  ( 9.564922557960805705, 16.46253265017160317, 39.58224293864768839 ) ) ;
#146297=CARTESIAN_POINT ( 'NONE',  ( -5.823673210054431948, 21.52544592524334988, 47.70942372801902565 ) ) ;
#146298=CARTESIAN_POINT ( 'NONE',  ( -5.823673210054431948, 21.52544592524334988, 47.70942372801902565 ) ) ;
#146299=CARTESIAN_POINT ( 'NONE',  ( 9.564922557960805705, 16.46253265017160317, 64.58224293864769550 ) ) ;
#146300=CARTESIAN_POINT ( 'NONE',  ( -15.72974639402176322, -15.80617190586768395, 34.37609039468568284 ) ) ;
#146301=CARTESIAN_POINT ( 'NONE',  ( 9.474510206698729675, 16.51473224551082808, 77.08442372801900433 ) ) ;
#146302=CARTESIAN_POINT ( 'NONE',  ( -0.05219959533936034679, 19.03943276465977164, 72.50109039468566152 ) ) ;
#146303=CARTESIAN_POINT ( 'NONE',  ( 19.02544592524343514, -5.153800228976328945, 43.54057627198103120 ) ) ;
#146304=CARTESIAN_POINT ( 'NONE',  ( -16.55341960407617563, 4.379528057220093196, 88.54275706135236135 ) ) ;
#146305=CARTESIAN_POINT ( 'NONE',  ( 19.05341960407611168, 5.049401038298154454, 53.95724293864770260 ) ) ;
#146307=CARTESIAN_POINT ( 'NONE',  ( 19.03943276465977164, -0.05219959533909143690, 103.7489096053143669 ) ) ;
#146308=CARTESIAN_POINT ( 'NONE',  ( -0.05219959533909027116, -19.03943276465977164, 32.49890960531435979 ) ) ;
#146309=CARTESIAN_POINT ( 'NONE',  ( -10.72451020669898014, 18.67979575497178502, 75.41557627198102409 ) ) ;
#146310=CARTESIAN_POINT ( 'NONE',  ( -14.34966873604972548, 8.224510206698743886, 58.33442372801901143 ) ) ;
#146311=CARTESIAN_POINT ( 'NONE',  ( -16.46253265017146816, -9.564922557961047289, 19.16775706135233293 ) ) ;
#146312=CARTESIAN_POINT ( 'NONE',  ( -16.46253265017160317, 9.564922557960807481, 50.83224293864770260 ) ) ;
#146313=CARTESIAN_POINT ( 'NONE',  ( -16.55341960407611168, -4.379528057220339221, 41.45724293864769550 ) ) ;
#146314=CARTESIAN_POINT ( 'NONE',  ( -12.14591786802309592, -12.06949235617757132, 81.87390960531435269 ) ) ;
#146315=CARTESIAN_POINT ( 'NONE',  ( 19.03943276465977164, -0.05219959533909143690, 83.74890960531436690 ) ) ;
#146316=CARTESIAN_POINT ( 'NONE',  ( -21.55341960407619339, 5.719274019375674811, 38.54275706135234714 ) ) ;
#146317=CARTESIAN_POINT ( 'NONE',  ( -0.05219959533909027116, -19.03943276465977164, 97.49890960531436690 ) ) ;
#146318=CARTESIAN_POINT ( 'NONE',  ( -15.80617190586768217, 15.72974639402176855, 98.12609039468570415 ) ) ;
#146319=CARTESIAN_POINT ( 'NONE',  ( 0.05219959533934541429, -16.53943276465976808, 65.00109039468568994 ) ) ;
#146320=CARTESIAN_POINT ( 'NONE',  ( -5.823673210054431948, 21.52544592524334988, 32.70942372801900433 ) ) ;
#146321=CARTESIAN_POINT ( 'NONE',  ( 19.05341960407611168, 5.049401038298154454, 103.9572429386476671 ) ) ;
#146322=CARTESIAN_POINT ( 'NONE',  ( 15.72974639402199770, -15.80617190586745480, 93.12390960531436690 ) ) ;
#146323=CARTESIAN_POINT ( 'NONE',  ( 16.53943276465976808, -0.05219959533910856209, 43.74890960531435979 ) ) ;
#146324=CARTESIAN_POINT ( 'NONE',  ( 5.049401038298161559, -19.05341960407611168, 37.70724293864768839 ) ) ;
#146325=CARTESIAN_POINT ( 'NONE',  ( -8.224510206698948167, 14.34966873604960824, 70.41557627198102409 ) ) ;
#146326=CARTESIAN_POINT ( 'NONE',  ( -18.67979575497178146, -10.72451020669898902, 36.66557627198103120 ) ) ;
#146327=CARTESIAN_POINT ( 'NONE',  ( -19.02544592524334988, -5.153800228976617603, 33.95942372801897591 ) ) ;
#146328=CARTESIAN_POINT ( 'NONE',  ( 8.314922557960818139, 14.29746914071049879, 104.5822429386477097 ) ) ;
#146329=CARTESIAN_POINT ( 'NONE',  ( 19.03943276465977164, -0.05219959533909143690, 108.7489096053143527 ) ) ;
#146331=CARTESIAN_POINT ( 'NONE',  ( -16.52544592524335698, -4.483927247898792601, 58.95942372801902565 ) ) ;
#146332=CARTESIAN_POINT ( 'NONE',  ( 16.51473224551069308, 9.474510206698969483, 49.16557627198102409 ) ) ;
#146335=CARTESIAN_POINT ( 'NONE',  ( 14.34966873604972726, -8.224510206698740333, 95.83442372801903275 ) ) ;
#146336=CARTESIAN_POINT ( 'NONE',  ( 13.89961937509957401, 13.97604488694547697, 101.8760903946856331 ) ) ;
#146337=CARTESIAN_POINT ( 'NONE',  ( 15.72974639402176855, 15.80617190586768217, 66.87609039468568994 ) ) ;
#146338=CARTESIAN_POINT ( 'NONE',  ( 9.564922557960805705, 16.46253265017160317, 74.58224293864769550 ) ) ;
#146339=CARTESIAN_POINT ( 'NONE',  ( -18.67979575497178146, -10.72451020669898902, 91.66557627198103830 ) ) ;
#146340=CARTESIAN_POINT ( 'NONE',  ( 0.05219959533934541429, -16.53943276465976808, 45.00109039468568284 ) ) ;
#146341=CARTESIAN_POINT ( 'NONE',  ( 0.05219959533910956823, 16.53943276465976808, 114.9989096053143669 ) ) ;
#146343=CARTESIAN_POINT ( 'NONE',  ( -19.02544592524334988, -5.153800228976617603, 83.95942372801901854 ) ) ;
#146344=CARTESIAN_POINT ( 'NONE',  ( 18.62759615963271287, -10.81492255796078972, 78.33224293864770971 ) ) ;
#146345=CARTESIAN_POINT ( 'NONE',  ( 19.03943276465977164, 0.05219959533936151252, 41.25109039468566152 ) ) ;
#146346=CARTESIAN_POINT ( 'NONE',  ( -5.049401038298153566, 19.05341960407611168, 115.2072429386477097 ) ) ;
#146347=CARTESIAN_POINT ( 'NONE',  ( 15.72974639402199770, -15.80617190586745480, 93.12390960531436690 ) ) ;
#146348=CARTESIAN_POINT ( 'NONE',  ( 17.72560187377285956, 5.500000000000053291, 61.57814504131322764 ) ) ;
#146349=CARTESIAN_POINT ( 'NONE',  ( -19.03943276465977164, 0.05219959533909376836, 61.24890960531436690 ) ) ;
#146351=CARTESIAN_POINT ( 'NONE',  ( -19.03943276465977164, -0.05219959533935918106, 113.7510903946856757 ) ) ;
#146353=CARTESIAN_POINT ( 'NONE',  ( 16.51473224551069308, 9.474510206698969483, 44.16557627198103120 ) ) ;
#146354=CARTESIAN_POINT ( 'NONE',  ( -0.05219959533907301413, -21.53943276465977519, 107.4989096053143669 ) ) ;
#146355=CARTESIAN_POINT ( 'NONE',  ( -8.224510206698948167, 14.34966873604960824, 50.41557627198103120 ) ) ;
#146356=CARTESIAN_POINT ( 'NONE',  ( 16.51473224551069308, 9.474510206698969483, 54.16557627198103120 ) ) ;
#146357=CARTESIAN_POINT ( 'NONE',  ( -5.719274019375665041, -21.55341960407619695, 79.79275706135236135 ) ) ;
#146358=CARTESIAN_POINT ( 'NONE',  ( -16.55341960407617563, 4.379528057220093196, 23.54275706135235424 ) ) ;
#146359=CARTESIAN_POINT ( 'NONE',  ( 13.97604488694548053, -13.89961937509957401, 30.62609039468566863 ) ) ;
#146360=CARTESIAN_POINT ( 'NONE',  ( -14.29746914071049879, 8.314922557960819915, 25.83224293864769194 ) ) ;
#146361=CARTESIAN_POINT ( 'NONE',  ( 21.52544592524334988, 5.823673210054432836, 36.45942372801901143 ) ) ;
#146362=CARTESIAN_POINT ( 'NONE',  ( 18.62759615963255655, 10.81492255796105972, 21.66775706135235069 ) ) ;
#146363=CARTESIAN_POINT ( 'NONE',  ( 18.67979575497178502, 10.72451020669898547, 54.16557627198103120 ) ) ;
#146364=CARTESIAN_POINT ( 'NONE',  ( 19.02544592524334988, 5.153800228976608722, 101.4594237280189759 ) ) ;
#146365=CARTESIAN_POINT ( 'NONE',  ( -5.153800228976607833, 19.02544592524334988, 62.70942372801899722 ) ) ;
#146366=CARTESIAN_POINT ( 'NONE',  ( -21.55341960407619339, 5.719274019375674811, 78.54275706135236135 ) ) ;
#146367=CARTESIAN_POINT ( 'NONE',  ( 16.46253265017146816, 9.564922557961045513, 46.66775706135233293 ) ) ;
#146368=CARTESIAN_POINT ( 'NONE',  ( 16.51473224551069308, 9.474510206698969483, 24.16557627198102765 ) ) ;
#146369=CARTESIAN_POINT ( 'NONE',  ( 0.05219959533907565091, 21.53943276465977519, 59.99890960531436690 ) ) ;
#146370=CARTESIAN_POINT ( 'NONE',  ( 12.14591786802309770, 12.06949235617756955, 49.37390960531436690 ) ) ;
#146372=CARTESIAN_POINT ( 'NONE',  ( -5.049401038297874678, -19.05341960407617918, 19.79275706135233293 ) ) ;
#146373=CARTESIAN_POINT ( 'NONE',  ( 14.29746914071037800, 8.314922557961029526, 81.66775706135236135 ) ) ;
#146374=CARTESIAN_POINT ( 'NONE',  ( 12.14591786802309770, 12.06949235617756955, 39.37390960531436690 ) ) ;
#146375=CARTESIAN_POINT ( 'NONE',  ( -15.80617190586768217, 15.72974639402176855, 73.12609039468567573 ) ) ;
#146376=CARTESIAN_POINT ( 'NONE',  ( 18.67979575497194134, -10.72451020669871369, 75.83442372801900433 ) ) ;
#146377=CARTESIAN_POINT ( 'NONE',  ( -5.823673210054116645, -21.52544592524344225, 77.29057627198102409 ) ) ;
#146378=CARTESIAN_POINT ( 'NONE',  ( -9.474510206698964154, 16.51473224551069663, 35.41557627198102409 ) ) ;
#146379=CARTESIAN_POINT ( 'NONE',  ( 15.72974639402176855, 15.80617190586768217, 61.87609039468568284 ) ) ;
#146380=CARTESIAN_POINT ( 'NONE',  ( 5.153800228976335163, 19.02544592524342804, 29.79057627198102409 ) ) ;
#146381=CARTESIAN_POINT ( 'NONE',  ( 19.02544592524343514, -5.153800228976328945, 48.54057627198103120 ) ) ;
#146382=CARTESIAN_POINT ( 'NONE',  ( 16.53943276465976808, -0.05219959533910856209, 88.74890960531436690 ) ) ;
#146383=CARTESIAN_POINT ( 'NONE',  ( 19.05341960407611168, 5.049401038298154454, 98.95724293864766707 ) ) ;
#146384=CARTESIAN_POINT ( 'NONE',  ( -8.224510206698948167, 14.34966873604960824, 35.41557627198102409 ) ) ;
#146385=CARTESIAN_POINT ( 'NONE',  ( 4.483927247898545687, 16.52544592524342804, 109.7905762719810383 ) ) ;
#146386=CARTESIAN_POINT ( 'NONE',  ( -10.81492255796078084, -18.62759615963271287, 82.08224293864768129 ) ) ;
#146387=CARTESIAN_POINT ( 'NONE',  ( -10.72451020669898014, 18.67979575497178502, 115.4155762719810241 ) ) ;
#146389=CARTESIAN_POINT ( 'NONE',  ( 16.52544592524335698, 4.483927247898782831, 31.45942372801901854 ) ) ;
#146390=CARTESIAN_POINT ( 'NONE',  ( 18.62759615963271287, -10.81492255796078972, 73.33224293864769550 ) ) ;
#146391=CARTESIAN_POINT ( 'NONE',  ( 21.53943276465977519, 0.05219959533937863772, 96.25109039468568994 ) ) ;
#146392=CARTESIAN_POINT ( 'NONE',  ( 19.03943276465977164, -0.05219959533909143690, 78.74890960531436690 ) ) ;
#146393=CARTESIAN_POINT ( 'NONE',  ( 10.72451020669871369, 18.67979575497193778, 32.08442372801901854 ) ) ;
#146394=CARTESIAN_POINT ( 'NONE',  ( -13.97604488694527625, -13.89961937509977652, 106.8739096053143669 ) ) ;
#146395=CARTESIAN_POINT ( 'NONE',  ( 16.52544592524335698, 4.483927247898782831, 96.45942372801901854 ) ) ;
#146396=CARTESIAN_POINT ( 'NONE',  ( -21.52544592524334988, -5.823673210054445271, 73.95942372801901854 ) ) ;
#146397=CARTESIAN_POINT ( 'NONE',  ( -16.46253265017146816, -9.564922557961047289, 24.16775706135233648 ) ) ;
#146398=CARTESIAN_POINT ( 'NONE',  ( -4.379528057220086978, -16.55341960407618274, 74.79275706135234714 ) ) ;
#146399=CARTESIAN_POINT ( 'NONE',  ( -5.823673210054431948, 21.52544592524334988, 32.70942372801900433 ) ) ;
#146400=CARTESIAN_POINT ( 'NONE',  ( 19.05341960407611168, 5.049401038298154454, 33.95724293864769550 ) ) ;
#146401=CARTESIAN_POINT ( 'NONE',  ( 18.67979575497194134, -10.72451020669871369, 90.83442372801901854 ) ) ;
#146402=CARTESIAN_POINT ( 'NONE',  ( -9.564922557960796823, -16.46253265017161027, 102.0822429386477097 ) ) ;
#146403=CARTESIAN_POINT ( 'NONE',  ( 21.52544592524344225, -5.823673210054117533, 98.54057627198105251 ) ) ;
#146404=CARTESIAN_POINT ( 'NONE',  ( 18.56399227203341340, 5.500000000000001776, 81.47830131249899921 ) ) ;
#146405=CARTESIAN_POINT ( 'NONE',  ( -0.05219959533907301413, -21.53943276465977519, 52.49890960531435979 ) ) ;
#146406=CARTESIAN_POINT ( 'NONE',  ( -9.474510206698964154, 16.51473224551069663, 95.41557627198102409 ) ) ;
#146407=CARTESIAN_POINT ( 'NONE',  ( -16.52544592524342804, 4.483927247898546575, 56.04057627198102409 ) ) ;
#146409=CARTESIAN_POINT ( 'NONE',  ( -9.474510206698720793, -16.51473224551083518, 74.58442372801900433 ) ) ;
#146410=CARTESIAN_POINT ( 'NONE',  ( -17.44270441346517586, 5.991230190323018512, 103.6366492073577490 ) ) ;
#146411=CARTESIAN_POINT ( 'NONE',  ( 19.02544592524334988, 5.153800228976608722, 111.4594237280190043 ) ) ;
#146412=CARTESIAN_POINT ( 'NONE',  ( 18.62759615963271287, -10.81492255796078972, 88.33224293864769550 ) ) ;
#146413=CARTESIAN_POINT ( 'NONE',  ( -12.14591786802309592, -12.06949235617757132, 61.87390960531436690 ) ) ;
#146414=CARTESIAN_POINT ( 'NONE',  ( -9.564922557960796823, -16.46253265017161027, 97.08224293864769550 ) ) ;
#146415=CARTESIAN_POINT ( 'NONE',  ( 14.34966873604972726, -8.224510206698740333, 40.83442372801901854 ) ) ;
#146416=CARTESIAN_POINT ( 'NONE',  ( 16.46253265017160672, -9.564922557960803928, 63.33224293864769550 ) ) ;
#146417=CARTESIAN_POINT ( 'NONE',  ( -5.823673210054431948, 21.52544592524334988, 27.70942372801901854 ) ) ;
#146418=CARTESIAN_POINT ( 'NONE',  ( -19.03943276465977164, -0.05219959533935918106, 103.7510903946856757 ) ) ;
#146419=CARTESIAN_POINT ( 'NONE',  ( -16.46253265017160317, 9.564922557960807481, 100.8322429386477097 ) ) ;
#146420=CARTESIAN_POINT ( 'NONE',  ( 19.05341960407611168, 5.049401038298154454, 83.95724293864766707 ) ) ;
#146421=CARTESIAN_POINT ( 'NONE',  ( -21.52544592524343514, 5.823673210054127303, 96.04057627198102409 ) ) ;
#146422=CARTESIAN_POINT ( 'NONE',  ( -0.05219959533909027116, -19.03943276465977164, 47.49890960531435979 ) ) ;
#146423=CARTESIAN_POINT ( 'NONE',  ( -17.40861289039003879, -6.110651285853285763, 61.37232470827434838 ) ) ;
#146424=CARTESIAN_POINT ( 'NONE',  ( -8.314922557960811034, -14.29746914071050412, 72.08224293864769550 ) ) ;
#146425=B_SPLINE_CURVE_WITH_KNOTS ( 'NONE', 3,
 ( #126127, #128098, #189802, #51274, #2781, #67430, #97745, #175618 ),
 .UNSPECIFIED., .F., .F.,
 ( 4, 2, 2, 4 ),
 ( 0.000000000000000000, 0.0004423531491111584095, 0.0008847062982223168190, 0.001769412596444650985 ),
 .UNSPECIFIED. ) ;
#146426=CARTESIAN_POINT ( 'NONE',  ( -5.153800228976328057, -19.02544592524343514, 107.2905762719810383 ) ) ;
#146428=CARTESIAN_POINT ( 'NONE',  ( 13.89961937509957401, 13.97604488694547697, 61.87609039468566863 ) ) ;
#146429=CARTESIAN_POINT ( 'NONE',  ( -21.55341960407610458, -5.719274019375992779, 91.45724293864769550 ) ) ;
#146430=CARTESIAN_POINT ( 'NONE',  ( -5.049401038297874678, -19.05341960407617918, 49.79275706135231871 ) ) ;
#146431=CARTESIAN_POINT ( 'NONE',  ( 9.474510206698971260, -16.51473224551069308, 107.9155762719810383 ) ) ;
#146433=CARTESIAN_POINT ( 'NONE',  ( -0.05219959533907301413, -21.53943276465977519, 47.49890960531435979 ) ) ;
#146434=CARTESIAN_POINT ( 'NONE',  ( -5.049401038298153566, 19.05341960407611168, 85.20724293864766707 ) ) ;
#146435=CARTESIAN_POINT ( 'NONE',  ( 10.81492255796106328, -18.62759615963255655, 70.41775706135236135 ) ) ;
#146436=CARTESIAN_POINT ( 'NONE',  ( -16.51473224551069308, -9.474510206698971260, 31.66557627198102054 ) ) ;
#146437=CARTESIAN_POINT ( 'NONE',  ( -16.53943276465976808, 0.05219959533911058130, 76.24890960531435269 ) ) ;
#146438=CARTESIAN_POINT ( 'NONE',  ( 0.05219959533934541429, -16.53943276465976808, 25.00109039468567218 ) ) ;
#146439=CARTESIAN_POINT ( 'NONE',  ( 10.72451020669871369, 18.67979575497193778, 57.08442372801901854 ) ) ;
#146441=CARTESIAN_POINT ( 'NONE',  ( 19.05341960407617918, -5.049401038297876454, 66.04275706135233293 ) ) ;
#146442=CARTESIAN_POINT ( 'NONE',  ( 17.50000000000000000, -5.499999999999992895, 46.21769037696434168 ) ) ;
#146443=CARTESIAN_POINT ( 'NONE',  ( -5.823673210054431948, 21.52544592524334988, 22.70942372801901499 ) ) ;
#146446=CARTESIAN_POINT ( 'NONE',  ( -0.05219959533937732626, 21.53943276465977519, 112.5010903946857042 ) ) ;
#146447=CARTESIAN_POINT ( 'NONE',  ( -13.89961937509977652, 13.97604488694528158, 50.62390960531435979 ) ) ;
#146448=CARTESIAN_POINT ( 'NONE',  ( 18.62759615963255655, 10.81492255796105972, 106.6677570613523756 ) ) ;
#146449=CARTESIAN_POINT ( 'NONE',  ( 4.483927247898790824, -16.52544592524335698, 100.2094237280190043 ) ) ;
#146450=CARTESIAN_POINT ( 'NONE',  ( -13.89961937509977652, 13.97604488694528158, 105.6239096053143527 ) ) ;
#146451=CARTESIAN_POINT ( 'NONE',  ( -21.52544592524334988, -5.823673210054445271, 73.95942372801901854 ) ) ;
#146454=CARTESIAN_POINT ( 'NONE',  ( 18.22780087662123805, 5.499999999999960032, 96.48236817873105053 ) ) ;
#146455=CARTESIAN_POINT ( 'NONE',  ( -16.52544592524335698, -4.483927247898792601, 68.95942372801901854 ) ) ;
#146456=CARTESIAN_POINT ( 'NONE',  ( -15.80617190586768217, 15.72974639402176855, 68.12609039468567573 ) ) ;
#146457=CARTESIAN_POINT ( 'NONE',  ( 0.05219959533937995610, -21.53943276465977519, 105.0010903946856757 ) ) ;
#146459=CARTESIAN_POINT ( 'NONE',  ( -5.153800228976328057, -19.02544592524343514, 92.29057627198099567 ) ) ;
#146460=CARTESIAN_POINT ( 'NONE',  ( -19.03943276465977164, 0.05219959533909376836, 116.2489096053143669 ) ) ;
#146462=EDGE_CURVE ( 'NONE', #85061, #170763, #105664, .T. ) ;
#146464=CARTESIAN_POINT ( 'NONE',  ( 13.89961937509977652, -13.97604488694527269, 38.12390960531436690 ) ) ;
#146465=CARTESIAN_POINT ( 'NONE',  ( 21.52544592524344225, -5.823673210054117533, 43.54057627198103830 ) ) ;
#146466=CARTESIAN_POINT ( 'NONE',  ( -8.224510206698735004, -14.34966873604973081, 109.5844237280190328 ) ) ;
#146467=CARTESIAN_POINT ( 'NONE',  ( 4.379528057220339221, -16.55341960407611168, 97.70724293864772392 ) ) ;
#146468=CARTESIAN_POINT ( 'NONE',  ( 19.03943276465977164, -0.05219959533909143690, 78.74890960531436690 ) ) ;
#146469=CARTESIAN_POINT ( 'NONE',  ( 18.62759615963255655, 10.81492255796105972, 101.6677570613523613 ) ) ;
#146470=CARTESIAN_POINT ( 'NONE',  ( -5.153800228976328057, -19.02544592524343514, 37.29057627198102409 ) ) ;
#146471=CARTESIAN_POINT ( 'NONE',  ( -12.14591786802309592, -12.06949235617757132, 86.87390960531438111 ) ) ;
#146472=CARTESIAN_POINT ( 'NONE',  ( 21.53943276465977519, 0.05219959533937863772, 41.25109039468568284 ) ) ;
#146473=CARTESIAN_POINT ( 'NONE',  ( 18.62759615963271287, -10.81492255796078972, 83.33224293864769550 ) ) ;
#146474=CARTESIAN_POINT ( 'NONE',  ( 9.564922557961047289, -16.46253265017146816, 45.41775706135232582 ) ) ;
#146476=CARTESIAN_POINT ( 'NONE',  ( -5.049401038298153566, 19.05341960407611168, 90.20724293864766707 ) ) ;
#146477=CARTESIAN_POINT ( 'NONE',  ( 0.05219959533910956823, 16.53943276465976808, 59.99890960531436690 ) ) ;
#146478=CARTESIAN_POINT ( 'NONE',  ( 5.049401038297881783, 19.05341960407617563, 42.29275706135234003 ) ) ;
#146479=CARTESIAN_POINT ( 'NONE',  ( -8.314922557960811034, -14.29746914071050412, 42.08224293864769550 ) ) ;
#146480=CARTESIAN_POINT ( 'NONE',  ( 16.51473224551083163, -9.474510206698727899, 80.83442372801899012 ) ) ;
#146482=CARTESIAN_POINT ( 'NONE',  ( -18.67979575497178146, -10.72451020669898902, 31.66557627198102054 ) ) ;
#146483=CARTESIAN_POINT ( 'NONE',  ( -0.05219959533910754901, -16.53943276465976808, 92.49890960531436690 ) ) ;
#146485=CARTESIAN_POINT ( 'NONE',  ( 0.05219959533909260263, 19.03943276465977164, 49.99890960531435979 ) ) ;
#146486=CARTESIAN_POINT ( 'NONE',  ( 0.05219959533907565091, 21.53943276465977519, 44.99890960531435979 ) ) ;
#146487=CARTESIAN_POINT ( 'NONE',  ( -5.049401038298153566, 19.05341960407611168, 35.20724293864768839 ) ) ;
#146488=CARTESIAN_POINT ( 'NONE',  ( -16.53943276465976808, -0.05219959533934237506, 78.75109039468568994 ) ) ;
#146489=CARTESIAN_POINT ( 'NONE',  ( -19.02544592524342804, 5.153800228976336051, 66.04057627198103830 ) ) ;
#146490=CARTESIAN_POINT ( 'NONE',  ( 9.564922557961047289, -16.46253265017146816, 35.41775706135233293 ) ) ;
#146492=CARTESIAN_POINT ( 'NONE',  ( 15.72974639402176855, 15.80617190586768217, 66.87609039468568994 ) ) ;
#146493=CARTESIAN_POINT ( 'NONE',  ( 0.05219959533907565091, 21.53943276465977519, 49.99890960531437401 ) ) ;
#146494=CARTESIAN_POINT ( 'NONE',  ( 0.05219959533910956823, 16.53943276465976808, 114.9989096053143669 ) ) ;
#146495=CARTESIAN_POINT ( 'NONE',  ( -0.05219959533936034679, 19.03943276465977164, 87.50109039468567573 ) ) ;
#146498=CARTESIAN_POINT ( 'NONE',  ( -21.53943276465977519, 0.05219959533907696930, 46.24890960531435979 ) ) ;
#146499=CARTESIAN_POINT ( 'NONE',  ( 17.40805194822030799, -6.112264579159333522, 68.33371272510613892 ) ) ;
#146500=CARTESIAN_POINT ( 'NONE',  ( -10.72451020669870658, -18.67979575497194134, 89.58442372801901854 ) ) ;
#146501=CARTESIAN_POINT ( 'NONE',  ( -14.34966873604960291, -8.224510206698953496, 41.66557627198103120 ) ) ;
#146503=CARTESIAN_POINT ( 'NONE',  ( -16.53943276465976808, 0.05219959533911058130, 56.24890960531436690 ) ) ;
#146504=CARTESIAN_POINT ( 'NONE',  ( 5.719274019375991003, -21.55341960407610458, 77.70724293864770971 ) ) ;
#146505=CARTESIAN_POINT ( 'NONE',  ( 15.72974639402199770, -15.80617190586745480, 78.12390960531436690 ) ) ;
#146507=CARTESIAN_POINT ( 'NONE',  ( -18.67979575497178146, -10.72451020669898902, 36.66557627198103120 ) ) ;
#146508=CARTESIAN_POINT ( 'NONE',  ( -0.05219959533934338120, 16.53943276465976808, 52.50109039468567573 ) ) ;
#146509=CARTESIAN_POINT ( 'NONE',  ( -4.483927247898539470, -16.52544592524342804, 77.29057627198102409 ) ) ;
#146510=CARTESIAN_POINT ( 'NONE',  ( -16.46253265017160317, 9.564922557960807481, 55.83224293864769550 ) ) ;
#146511=CARTESIAN_POINT ( 'NONE',  ( 5.049401038298161559, -19.05341960407611168, 32.70724293864768129 ) ) ;
#146514=CARTESIAN_POINT ( 'NONE',  ( -14.29746914071037622, -8.314922557961029526, 79.16775706135234714 ) ) ;
#146515=CARTESIAN_POINT ( 'NONE',  ( 21.55341960407610458, 5.719274019375980345, 113.9572429386477239 ) ) ;
#146516=CARTESIAN_POINT ( 'NONE',  ( 19.03943276465977164, -0.05219959533909143690, 63.74890960531435979 ) ) ;
#146517=CARTESIAN_POINT ( 'NONE',  ( 5.823673210054444382, -21.52544592524334988, 55.20942372801902565 ) ) ;
#146518=CARTESIAN_POINT ( 'NONE',  ( -9.474510206698964154, 16.51473224551069663, 115.4155762719810241 ) ) ;
#146521=CARTESIAN_POINT ( 'NONE',  ( 15.72974639402176855, 15.80617190586768217, 51.87609039468568284 ) ) ;
#146522=CARTESIAN_POINT ( 'NONE',  ( 0.05219959533909260263, 19.03943276465977164, 109.9989096053143669 ) ) ;
#146523=CARTESIAN_POINT ( 'NONE',  ( 16.46253265017146816, 9.564922557961045513, 56.66775706135233293 ) ) ;
#146524=CARTESIAN_POINT ( 'NONE',  ( 18.67979575497178502, 10.72451020669898547, 114.1655762719810383 ) ) ;
#146525=CARTESIAN_POINT ( 'NONE',  ( 19.05341960407617918, -5.049401038297876454, 41.04275706135233293 ) ) ;
#146526=CARTESIAN_POINT ( 'NONE',  ( 14.34966873604972726, -8.224510206698740333, 95.83442372801903275 ) ) ;
#146527=CARTESIAN_POINT ( 'NONE',  ( 19.05341960407617918, -5.049401038297876454, 56.04275706135234714 ) ) ;
#146528=CARTESIAN_POINT ( 'NONE',  ( 0.05219959533934541429, -16.53943276465976808, 110.0010903946856757 ) ) ;
#146530=CARTESIAN_POINT ( 'NONE',  ( -16.46253265017160317, 9.564922557960807481, 80.83224293864769550 ) ) ;
#146531=CARTESIAN_POINT ( 'NONE',  ( -15.80617190586768217, 15.72974639402176855, 88.12609039468570415 ) ) ;
#146532=CARTESIAN_POINT ( 'NONE',  ( 5.719274019375673035, 21.55341960407619339, 92.29275706135236135 ) ) ;
#146534=CARTESIAN_POINT ( 'NONE',  ( -13.97604488694527625, -13.89961937509977652, 106.8739096053143669 ) ) ;
#146535=CARTESIAN_POINT ( 'NONE',  ( -5.719274019375665041, -21.55341960407619695, 79.79275706135236135 ) ) ;
#146536=CARTESIAN_POINT ( 'NONE',  ( 19.05341960407617918, -5.049401038297876454, 111.0427570613523329 ) ) ;
#146537=CARTESIAN_POINT ( 'NONE',  ( -13.97604488694527625, -13.89961937509977652, 76.87390960531433848 ) ) ;
#146538=CARTESIAN_POINT ( 'NONE',  ( 5.719274019375991003, -21.55341960407610458, 32.70724293864770260 ) ) ;
#146539=VECTOR ( 'NONE', #29155, 1000.000000000000000 ) ;
#146540=CARTESIAN_POINT ( 'NONE',  ( -5.049401038298153566, 19.05341960407611168, 90.20724293864766707 ) ) ;
#146541=CARTESIAN_POINT ( 'NONE',  ( -9.564922557961040184, 16.46253265017147172, 87.91775706135233293 ) ) ;
#146542=CARTESIAN_POINT ( 'NONE',  ( 5.153800228976335163, 19.02544592524342804, 79.79057627198102409 ) ) ;
#146543=CARTESIAN_POINT ( 'NONE',  ( -5.153800228976328057, -19.02544592524343514, 67.29057627198102409 ) ) ;
#146544=CARTESIAN_POINT ( 'NONE',  ( 16.52544592524335698, 4.483927247898782831, 101.4594237280190185 ) ) ;
#146546=CARTESIAN_POINT ( 'NONE',  ( -19.03943276465977164, -0.05219959533935918106, 53.75109039468566863 ) ) ;
#146547=CARTESIAN_POINT ( 'NONE',  ( 5.153800228976335163, 19.02544592524342804, 94.79057627198103830 ) ) ;
#146548=CARTESIAN_POINT ( 'NONE',  ( 4.483927247898545687, 16.52544592524342804, 89.79057627198103830 ) ) ;
#146549=CARTESIAN_POINT ( 'NONE',  ( 5.719274019375991003, -21.55341960407610458, 37.70724293864769550 ) ) ;
#146550=CARTESIAN_POINT ( 'NONE',  ( 13.97604488694527802, 13.89961937509977652, 114.3739096053143669 ) ) ;
#146551=CARTESIAN_POINT ( 'NONE',  ( -12.06949235617756955, 12.14591786802309770, 90.62390960531436690 ) ) ;
#146552=CARTESIAN_POINT ( 'NONE',  ( -16.29526858892873165, 7.335722546920266041, 54.20329402199794089 ) ) ;
#146553=CARTESIAN_POINT ( 'NONE',  ( -0.05219959533936034679, 19.03943276465977164, 42.50109039468566152 ) ) ;
#146554=CARTESIAN_POINT ( 'NONE',  ( 12.06949235617739724, 12.14591786802326823, 106.8760903946856899 ) ) ;
#146555=CARTESIAN_POINT ( 'NONE',  ( -5.153800228976328057, -19.02544592524343514, 92.29057627198099567 ) ) ;
#146556=CARTESIAN_POINT ( 'NONE',  ( -21.55341960407619339, 5.719274019375674811, 63.54275706135234003 ) ) ;
#146557=CARTESIAN_POINT ( 'NONE',  ( -21.52544592524343514, 5.823673210054127303, 56.04057627198102409 ) ) ;
#146558=B_SPLINE_CURVE_WITH_KNOTS ( 'NONE', 3,
 ( #154755, #199278, #60745, #77904, #107245, #168916, #30421, #92069, #1056, #62729, #124412, #99037, #127386, #83868, #5034, #19238, #6037, #116224, #193076, #52543, #161729, #174907, #145550, #21217, #115224, #158721, #173920, #96059, #81860, #175908, #191070, #190077 ),
 .UNSPECIFIED., .F., .F.,
 ( 4, 2, 2, 2, 2, 2, 2, 2, 2, 2, 2, 2, 2, 2, 2, 4 ),
 ( 1.734980196055371455E-15, 0.0003712461730053016971, 0.0007424923460088683454, 0.001113738519012435211, 0.001484984692016001750, 0.002227477038023130494, 0.002598723211026691612, 0.002969969384030252298, 0.003341215557033814284, 0.003712461730037374535, 0.004083707903040936088, 0.004454954076044496773, 0.004826200249048058326, 0.005197446422051619878, 0.005568692595055181431, 0.005939938768058742984 ),
 .UNSPECIFIED. ) ;
#146559=CARTESIAN_POINT ( 'NONE',  ( -21.53943276465977519, -0.05219959533937600094, 33.75109039468568284 ) ) ;
#146561=CARTESIAN_POINT ( 'NONE',  ( 10.81492255796078972, 18.62759615963270932, 89.58224293864768129 ) ) ;
#146562=CARTESIAN_POINT ( 'NONE',  ( -18.62759615963255300, -10.81492255796106328, 34.16775706135234714 ) ) ;
#146563=CARTESIAN_POINT ( 'NONE',  ( 16.52544592524342804, -4.483927247898539470, 108.5405762719810241 ) ) ;
#146564=CARTESIAN_POINT ( 'NONE',  ( 19.02544592524334988, 5.153800228976608722, 76.45942372801897591 ) ) ;
#146565=CARTESIAN_POINT ( 'NONE',  ( 16.51473224551069308, 9.474510206698969483, 49.16557627198102409 ) ) ;
#146566=CARTESIAN_POINT ( 'NONE',  ( 12.06949235617757843, -12.14591786802309237, 88.12390960531436690 ) ) ;
#146567=CARTESIAN_POINT ( 'NONE',  ( 9.474510206698971260, -16.51473224551069308, 92.91557627198103830 ) ) ;
#146568=CARTESIAN_POINT ( 'NONE',  ( 9.564922557960805705, 16.46253265017160317, 89.58224293864769550 ) ) ;
#146569=CARTESIAN_POINT ( 'NONE',  ( 4.483927247898545687, 16.52544592524342804, 109.7905762719810383 ) ) ;
#146570=CARTESIAN_POINT ( 'NONE',  ( 12.14591786802309770, 12.06949235617756955, 34.37390960531435979 ) ) ;
#146571=CARTESIAN_POINT ( 'NONE',  ( -4.379528057220086978, -16.55341960407618274, 34.79275706135235424 ) ) ;
#146572=CARTESIAN_POINT ( 'NONE',  ( -16.52544592524342804, 4.483927247898546575, 116.0405762719810383 ) ) ;
#146573=CARTESIAN_POINT ( 'NONE',  ( -0.05219959533936034679, 19.03943276465977164, 22.50109039468566152 ) ) ;
#146574=CARTESIAN_POINT ( 'NONE',  ( -5.049401038298153566, 19.05341960407611168, 110.2072429386476671 ) ) ;
#146575=CARTESIAN_POINT ( 'NONE',  ( 16.52544592524342804, -4.483927247898539470, 23.54057627198102765 ) ) ;
#146576=CARTESIAN_POINT ( 'NONE',  ( 18.62759615963255655, 10.81492255796105972, 31.66775706135234358 ) ) ;
#146577=CARTESIAN_POINT ( 'NONE',  ( -19.02544592524342804, 5.153800228976336051, 106.0405762719810241 ) ) ;
#146578=CARTESIAN_POINT ( 'NONE',  ( 16.53943276465976808, 0.05219959533934440121, 41.25109039468568284 ) ) ;
#146579=CARTESIAN_POINT ( 'NONE',  ( -14.29746914071037622, -8.314922557961029526, 104.1677570613523471 ) ) ;
#146580=B_SPLINE_CURVE_WITH_KNOTS ( 'NONE', 3,
 ( #82403, #110774, #53077, #20748, #5572, #188631, #3586, #174449, #172456, #66260, #128910, #21756, #114755, #99582, #190611, #161263, #83408, #145085, #6568, #176449 ),
 .UNSPECIFIED., .F., .F.,
 ( 4, 2, 2, 2, 2, 2, 2, 2, 2, 4 ),
 ( 0.000000000000000000, 0.0004987090165372665227, 0.0009974180330745330454, 0.001246772541343162512, 0.001496127049611791979, 0.001994836066149054815, 0.002493545082686318519, 0.002742899590954949503, 0.002992254099223581355, 0.003989672132298100089 ),
 .UNSPECIFIED. ) ;
#146581=CARTESIAN_POINT ( 'NONE',  ( -8.314922557961024197, 14.29746914071037800, 92.91775706135236135 ) ) ;
#146582=CARTESIAN_POINT ( 'NONE',  ( -16.53943276465976808, -0.05219959533934237506, 28.75109039468567929 ) ) ;
#146583=CARTESIAN_POINT ( 'NONE',  ( 5.153800228976335163, 19.02544592524342804, 49.79057627198100988 ) ) ;
#146584=CARTESIAN_POINT ( 'NONE',  ( 16.52544592524342804, -4.483927247898539470, 108.5405762719810241 ) ) ;
#146585=CARTESIAN_POINT ( 'NONE',  ( 21.52544592524334988, 5.823673210054432836, 21.45942372801901499 ) ) ;
#146586=CARTESIAN_POINT ( 'NONE',  ( -19.03943276465977164, 0.05219959533909376836, 36.24890960531436690 ) ) ;
#146587=CARTESIAN_POINT ( 'NONE',  ( 5.153800228976335163, 19.02544592524342804, 99.79057627198102409 ) ) ;
#146588=CARTESIAN_POINT ( 'NONE',  ( 19.05341960407611168, 5.049401038298154454, 33.95724293864769550 ) ) ;
#146589=CARTESIAN_POINT ( 'NONE',  ( 19.03943276465977164, -0.05219959533909143690, 98.74890960531436690 ) ) ;
#146591=CARTESIAN_POINT ( 'NONE',  ( 19.03943276465977164, -0.05219959533909143690, 98.74890960531436690 ) ) ;
#146592=CARTESIAN_POINT ( 'NONE',  ( -15.72974639402176322, -15.80617190586768395, 49.37609039468569705 ) ) ;
#146593=CARTESIAN_POINT ( 'NONE',  ( 4.379528057220339221, -16.55341960407611168, 107.7072429386476955 ) ) ;
#146594=CARTESIAN_POINT ( 'NONE',  ( 19.05341960407611168, 5.049401038298154454, 113.9572429386477097 ) ) ;
#146597=CARTESIAN_POINT ( 'NONE',  ( -8.314922557961024197, 14.29746914071037800, 57.91775706135234714 ) ) ;
#146598=CARTESIAN_POINT ( 'NONE',  ( -21.53943276465977519, -0.05219959533937600094, 83.75109039468568994 ) ) ;
#146599=CARTESIAN_POINT ( 'NONE',  ( 8.224510206698742110, 14.34966873604972548, 37.08442372801901143 ) ) ;
#146600=CARTESIAN_POINT ( 'NONE',  ( -19.03943276465977164, 0.05219959533909376836, 86.24890960531436690 ) ) ;
#146601=CARTESIAN_POINT ( 'NONE',  ( 5.049401038297881783, 19.05341960407617563, 107.2927570613523187 ) ) ;
#146602=CARTESIAN_POINT ( 'NONE',  ( 12.06949235617739724, 12.14591786802326823, 81.87609039468568994 ) ) ;
#146603=CARTESIAN_POINT ( 'NONE',  ( -9.474510206698720793, -16.51473224551083518, 94.58442372801900433 ) ) ;
#146604=CARTESIAN_POINT ( 'NONE',  ( 19.02544592524343514, -5.153800228976328945, 68.54057627198103830 ) ) ;
#146605=CARTESIAN_POINT ( 'NONE',  ( 21.52544592524344225, -5.823673210054117533, 93.54057627198103830 ) ) ;
#146606=CARTESIAN_POINT ( 'NONE',  ( 16.52544592524342804, -4.483927247898539470, 83.54057627198102409 ) ) ;
#146607=CARTESIAN_POINT ( 'NONE',  ( 16.51473224551083163, -9.474510206698727899, 90.83442372801900433 ) ) ;
#146608=CARTESIAN_POINT ( 'NONE',  ( 12.06949235617739724, 12.14591786802326823, 61.87609039468568284 ) ) ;
#146609=CARTESIAN_POINT ( 'NONE',  ( -19.46398650005390962, 5.499999999999953815, 80.18269651486369298 ) ) ;
#146610=CARTESIAN_POINT ( 'NONE',  ( -19.05341960407617563, 5.049401038297882671, 68.54275706135230450 ) ) ;
#146612=CARTESIAN_POINT ( 'NONE',  ( -4.483927247898539470, -16.52544592524342804, 27.29057627198103120 ) ) ;
#146613=CARTESIAN_POINT ( 'NONE',  ( -16.53943276465976808, 0.05219959533911058130, 86.24890960531436690 ) ) ;
#146614=CARTESIAN_POINT ( 'NONE',  ( -21.55341960407619339, 5.719274019375674811, 113.5427570613523756 ) ) ;
#146615=CARTESIAN_POINT ( 'NONE',  ( -16.88567814943193568, 6.947325034625406737, 38.70998877347406619 ) ) ;
#146616=CARTESIAN_POINT ( 'NONE',  ( 21.55341960407619695, -5.719274019375665929, 26.04275706135235779 ) ) ;
#146617=CARTESIAN_POINT ( 'NONE',  ( 13.89961937509977652, -13.97604488694527269, 108.1239096053143669 ) ) ;
#146618=CARTESIAN_POINT ( 'NONE',  ( 5.153800228976335163, 19.02544592524342804, 79.79057627198102409 ) ) ;
#146619=CARTESIAN_POINT ( 'NONE',  ( 15.72974639402176855, 15.80617190586768217, 96.87609039468568994 ) ) ;
#146620=CARTESIAN_POINT ( 'NONE',  ( 5.153800228976335163, 19.02544592524342804, 69.79057627198103830 ) ) ;
#146621=CARTESIAN_POINT ( 'NONE',  ( 21.53943276465977519, -0.05219959533907433946, 48.74890960531435979 ) ) ;
#146622=CARTESIAN_POINT ( 'NONE',  ( -16.55341960407611168, -4.379528057220339221, 86.45724293864770971 ) ) ;
#146623=CARTESIAN_POINT ( 'NONE',  ( -13.89961937509977652, 13.97604488694528158, 60.62390960531436690 ) ) ;
#146624=CARTESIAN_POINT ( 'NONE',  ( -12.06949235617756955, 12.14591786802309770, 115.6239096053143669 ) ) ;
#146626=CARTESIAN_POINT ( 'NONE',  ( 5.719274019375673035, 21.55341960407619339, 27.29275706135234358 ) ) ;
#146627=CARTESIAN_POINT ( 'NONE',  ( 21.52544592524334988, 5.823673210054432836, 56.45942372801902565 ) ) ;
#146628=CARTESIAN_POINT ( 'NONE',  ( -13.89961937509977652, 13.97604488694528158, 40.62390960531435979 ) ) ;
#146629=CARTESIAN_POINT ( 'NONE',  ( 14.34966873604972726, -8.224510206698740333, 75.83442372801900433 ) ) ;
#146630=CARTESIAN_POINT ( 'NONE',  ( 15.72974639402176855, 15.80617190586768217, 21.87609039468567573 ) ) ;
#146631=CARTESIAN_POINT ( 'NONE',  ( 10.81492255796078972, 18.62759615963270932, 104.5822429386477097 ) ) ;
#146632=CARTESIAN_POINT ( 'NONE',  ( -16.51473224551082808, 9.474510206698731452, 38.33442372801899722 ) ) ;
#146633=CARTESIAN_POINT ( 'NONE',  ( -19.03943276465977164, 0.05219959533909376836, 61.24890960531436690 ) ) ;
#146634=CARTESIAN_POINT ( 'NONE',  ( -16.46253265017146816, -9.564922557961047289, 29.16775706135232937 ) ) ;
#146635=CARTESIAN_POINT ( 'NONE',  ( -10.72451020669870658, -18.67979575497194134, 74.58442372801901854 ) ) ;
#146636=CARTESIAN_POINT ( 'NONE',  ( -21.55341960407610458, -5.719274019375992779, 71.45724293864769550 ) ) ;
#146637=CARTESIAN_POINT ( 'NONE',  ( 16.53943276465976808, -0.05219959533910856209, 38.74890960531435979 ) ) ;
#146638=CARTESIAN_POINT ( 'NONE',  ( -10.81492255796105439, 18.62759615963255655, 87.91775706135234714 ) ) ;
#146639=CARTESIAN_POINT ( 'NONE',  ( -21.55341960407619339, 5.719274019375674811, 108.5427570613523756 ) ) ;
#146640=CARTESIAN_POINT ( 'NONE',  ( -12.14591786802309592, -12.06949235617757132, 56.87390960531436690 ) ) ;
#146641=CARTESIAN_POINT ( 'NONE',  ( 12.14591786802309770, 12.06949235617756955, 104.3739096053143669 ) ) ;
#146642=CARTESIAN_POINT ( 'NONE',  ( -19.05341960407617563, 5.049401038297882671, 53.54275706135231871 ) ) ;
#146643=CARTESIAN_POINT ( 'NONE',  ( 16.55341960407611168, 4.379528057220329451, 23.95724293864769550 ) ) ;
#146644=CARTESIAN_POINT ( 'NONE',  ( -21.52544592524334988, -5.823673210054445271, 73.95942372801901854 ) ) ;
#146645=CARTESIAN_POINT ( 'NONE',  ( -9.474510206698964154, 16.51473224551069663, 75.41557627198103830 ) ) ;
#146646=CARTESIAN_POINT ( 'NONE',  ( 19.03943276465977164, 0.05219959533936151252, 46.25109039468566863 ) ) ;
#146647=CARTESIAN_POINT ( 'NONE',  ( -5.719274019375978568, 21.55341960407610458, 55.20724293864770260 ) ) ;
#146648=CARTESIAN_POINT ( 'NONE',  ( 5.823673210054444382, -21.52544592524334988, 45.20942372801901854 ) ) ;
#146649=CARTESIAN_POINT ( 'NONE',  ( 18.67979575497178502, 10.72451020669898547, 104.1655762719810241 ) ) ;
#146650=CARTESIAN_POINT ( 'NONE',  ( 19.02544592524334988, 5.153800228976608722, 101.4594237280189759 ) ) ;
#146651=CARTESIAN_POINT ( 'NONE',  ( -0.05219959533934338120, 16.53943276465976808, 67.50109039468568994 ) ) ;
#146653=CARTESIAN_POINT ( 'NONE',  ( 10.72451020669898902, -18.67979575497178502, 112.9155762719810383 ) ) ;
#146654=CARTESIAN_POINT ( 'NONE',  ( -16.53943276465976808, 0.05219959533911058130, 96.24890960531435269 ) ) ;
#146655=CARTESIAN_POINT ( 'NONE',  ( 17.49999999999999289, 5.500000000000063061, 41.70309617465829177 ) ) ;
#146656=CARTESIAN_POINT ( 'NONE',  ( 14.29746914071037800, 8.314922557961029526, 21.66775706135235069 ) ) ;
#146657=CARTESIAN_POINT ( 'NONE',  ( -18.62759615963270932, 10.81492255796079327, 45.83224293864769550 ) ) ;
#146658=CARTESIAN_POINT ( 'NONE',  ( 8.314922557961029526, -14.29746914071037800, 85.41775706135236135 ) ) ;
#146660=CARTESIAN_POINT ( 'NONE',  ( -12.14591786802326823, 12.06949235617739902, 48.12609039468568284 ) ) ;
#146661=CARTESIAN_POINT ( 'NONE',  ( 5.823673210054444382, -21.52544592524334988, 30.20942372801902565 ) ) ;
#146662=CARTESIAN_POINT ( 'NONE',  ( 10.72451020669898902, -18.67979575497178502, 42.91557627198103120 ) ) ;
#146663=CARTESIAN_POINT ( 'NONE',  ( 16.52544592524335698, 4.483927247898782831, 81.45942372801900433 ) ) ;
#146664=CARTESIAN_POINT ( 'NONE',  ( 13.97604488694527802, 13.89961937509977652, 99.37390960531436690 ) ) ;
#146665=CARTESIAN_POINT ( 'NONE',  ( 0.05219959533937995610, -21.53943276465977519, 70.00109039468568994 ) ) ;
#146666=CARTESIAN_POINT ( 'NONE',  ( 21.52544592524344225, -5.823673210054117533, 43.54057627198103830 ) ) ;
#146667=CARTESIAN_POINT ( 'NONE',  ( -18.62759615963270932, 10.81492255796079327, 35.83224293864768839 ) ) ;
#146668=ORIENTED_EDGE ( 'NONE', *, *, #200190, .F. ) ;
#146669=CARTESIAN_POINT ( 'NONE',  ( 16.46253265017146816, 9.564922557961045513, 51.66775706135233293 ) ) ;
#146670=CARTESIAN_POINT ( 'NONE',  ( -12.06949235617739369, -12.14591786802326823, 64.37609039468568994 ) ) ;
#146671=CARTESIAN_POINT ( 'NONE',  ( 10.81492255796078972, 18.62759615963270932, 29.58224293864769905 ) ) ;
#146672=EDGE_LOOP ( 'NONE', ( #182583, #141331 ) ) ;
#146673=CARTESIAN_POINT ( 'NONE',  ( 5.049401038298161559, -19.05341960407611168, 82.70724293864770971 ) ) ;
#146674=CARTESIAN_POINT ( 'NONE',  ( 16.53943276465976808, -0.05219959533910856209, 23.74890960531435269 ) ) ;
#146676=CARTESIAN_POINT ( 'NONE',  ( -12.06949235617756955, 12.14591786802309770, 105.6239096053143669 ) ) ;
#146677=CARTESIAN_POINT ( 'NONE',  ( -5.823673210054116645, -21.52544592524344225, 52.29057627198102409 ) ) ;
#146678=CARTESIAN_POINT ( 'NONE',  ( -13.89961937509977652, 13.97604488694528158, 45.62390960531433848 ) ) ;
#146679=CARTESIAN_POINT ( 'NONE',  ( -16.55341960407617563, 4.379528057220093196, 83.54275706135234714 ) ) ;
#146680=CARTESIAN_POINT ( 'NONE',  ( 5.823673210054444382, -21.52544592524334988, 30.20942372801902565 ) ) ;
#146681=CARTESIAN_POINT ( 'NONE',  ( -19.05341960407617563, 5.049401038297882671, 83.54275706135233293 ) ) ;
#146682=CARTESIAN_POINT ( 'NONE',  ( -8.314922557960811034, -14.29746914071050412, 92.08224293864769550 ) ) ;
#146683=CARTESIAN_POINT ( 'NONE',  ( 0.05219959533909260263, 19.03943276465977164, 49.99890960531435979 ) ) ;
#146684=CARTESIAN_POINT ( 'NONE',  ( 13.97604488694527802, 13.89961937509977652, 24.37390960531435624 ) ) ;
#146685=CARTESIAN_POINT ( 'NONE',  ( 10.72451020669871369, 18.67979575497193778, 102.0844237280190185 ) ) ;
#146686=CARTESIAN_POINT ( 'NONE',  ( 9.564922557960805705, 16.46253265017160317, 84.58224293864769550 ) ) ;
#146687=CARTESIAN_POINT ( 'NONE',  ( 16.55341960407618274, -4.379528057220086978, 61.04275706135234714 ) ) ;
#146688=CARTESIAN_POINT ( 'NONE',  ( 18.62759615963255655, 10.81492255796105972, 86.66775706135234714 ) ) ;
#146689=CARTESIAN_POINT ( 'NONE',  ( 18.62759615963271287, -10.81492255796078972, 48.33224293864770260 ) ) ;
#146690=CARTESIAN_POINT ( 'NONE',  ( 16.55341960407618274, -4.379528057220086978, 76.04275706135237556 ) ) ;
#146691=CARTESIAN_POINT ( 'NONE',  ( 19.03943276465977164, 0.05219959533936151252, 46.25109039468566863 ) ) ;
#146692=CARTESIAN_POINT ( 'NONE',  ( 16.51473224551083163, -9.474510206698727899, 60.83442372801900433 ) ) ;
#146694=CARTESIAN_POINT ( 'NONE',  ( 0.05219959533937995610, -21.53943276465977519, 70.00109039468568994 ) ) ;
#146695=CARTESIAN_POINT ( 'NONE',  ( -5.049401038298153566, 19.05341960407611168, 65.20724293864765286 ) ) ;
#146696=CARTESIAN_POINT ( 'NONE',  ( 9.474510206698971260, -16.51473224551069308, 57.91557627198103120 ) ) ;
#146697=CARTESIAN_POINT ( 'NONE',  ( -16.46253265017146816, -9.564922557961047289, 54.16775706135234003 ) ) ;
#146699=CARTESIAN_POINT ( 'NONE',  ( 5.153800228976335163, 19.02544592524342804, 89.79057627198102409 ) ) ;
#146700=CARTESIAN_POINT ( 'NONE',  ( 4.379528057220339221, -16.55341960407611168, 47.70724293864770260 ) ) ;
#146701=CARTESIAN_POINT ( 'NONE',  ( -21.55341960407610458, -5.719274019375992779, 41.45724293864769550 ) ) ;
#146703=CARTESIAN_POINT ( 'NONE',  ( 13.89961937509957401, 13.97604488694547697, 21.87609039468566152 ) ) ;
#146704=CARTESIAN_POINT ( 'NONE',  ( -16.62475595723700650, -7.163666690055230823, 79.47286648189529501 ) ) ;
#146705=CARTESIAN_POINT ( 'NONE',  ( -9.474510206698964154, 16.51473224551069663, 45.41557627198103120 ) ) ;
#146706=CARTESIAN_POINT ( 'NONE',  ( 9.474510206698971260, -16.51473224551069308, 27.91557627198103120 ) ) ;
#146708=CARTESIAN_POINT ( 'NONE',  ( -16.36317988757058828, 7.306389748694926745, 109.0978960836322358 ) ) ;
#146709=CARTESIAN_POINT ( 'NONE',  ( -16.53943276465976808, -0.05219959533934237506, 63.75109039468568284 ) ) ;
#146710=CARTESIAN_POINT ( 'NONE',  ( 0.05219959533907565091, 21.53943276465977519, 84.99890960531436690 ) ) ;
#146712=CARTESIAN_POINT ( 'NONE',  ( 16.55341960407611168, 4.379528057220329451, 58.95724293864770971 ) ) ;
#146713=CARTESIAN_POINT ( 'NONE',  ( -19.02544592524342804, 5.153800228976336051, 41.04057627198103120 ) ) ;
#146715=CARTESIAN_POINT ( 'NONE',  ( 0.05219959533937995610, -21.53943276465977519, 45.00109039468568284 ) ) ;
#146716=CARTESIAN_POINT ( 'NONE',  ( -13.89961937509957401, -13.97604488694547875, 49.37609039468567573 ) ) ;
#146717=CARTESIAN_POINT ( 'NONE',  ( 13.89961937509977652, -13.97604488694527269, 33.12390960531434558 ) ) ;
#146718=CARTESIAN_POINT ( 'NONE',  ( 5.823673210054444382, -21.52544592524334988, 90.20942372801903275 ) ) ;
#146719=CARTESIAN_POINT ( 'NONE',  ( 17.49999999999999289, 5.624438216177591876, 96.68329655085355512 ) ) ;
#146720=CARTESIAN_POINT ( 'NONE',  ( -12.14591786802309592, -12.06949235617757132, 36.87390960531435979 ) ) ;
#146721=CARTESIAN_POINT ( 'NONE',  ( 19.19724070472090816, 5.500000000000156319, 43.56193348274383226 ) ) ;
#146722=CARTESIAN_POINT ( 'NONE',  ( 5.823673210054125526, 21.52544592524343514, 34.79057627198103120 ) ) ;
#146724=CARTESIAN_POINT ( 'NONE',  ( -19.05341960407611168, -5.049401038298163336, 86.45724293864769550 ) ) ;
#146725=CARTESIAN_POINT ( 'NONE',  ( 16.53943276465976808, -0.05219959533910856209, 83.74890960531435269 ) ) ;
#146726=CARTESIAN_POINT ( 'NONE',  ( 16.55341960407618274, -4.379528057220086978, 21.04275706135234714 ) ) ;
#146727=CARTESIAN_POINT ( 'NONE',  ( 14.29746914071037800, 8.314922557961029526, 106.6677570613523756 ) ) ;
#146729=CARTESIAN_POINT ( 'NONE',  ( -19.02544592524342804, 5.153800228976336051, 46.04057627198101699 ) ) ;
#146731=CARTESIAN_POINT ( 'NONE',  ( -16.46253265017160317, 9.564922557960807481, 80.83224293864769550 ) ) ;
#146732=CARTESIAN_POINT ( 'NONE',  ( 10.81492255796078972, 18.62759615963270932, 84.58224293864769550 ) ) ;
#146733=CARTESIAN_POINT ( 'NONE',  ( 8.224510206698953496, -14.34966873604960469, 22.91557627198102765 ) ) ;
#146734=CARTESIAN_POINT ( 'NONE',  ( -0.05219959533909027116, -19.03943276465977164, 102.4989096053143669 ) ) ;
#146735=CARTESIAN_POINT ( 'NONE',  ( -9.474510206698720793, -16.51473224551083518, 84.58442372801900433 ) ) ;
#146736=CARTESIAN_POINT ( 'NONE',  ( 18.62759615963255655, 10.81492255796105972, 111.6677570613523613 ) ) ;
#146737=CARTESIAN_POINT ( 'NONE',  ( -5.719274019375978568, 21.55341960407610458, 95.20724293864769550 ) ) ;
#146738=CARTESIAN_POINT ( 'NONE',  ( 5.823673210054125526, 21.52544592524343514, 34.79057627198103120 ) ) ;
#146740=CARTESIAN_POINT ( 'NONE',  ( -9.564922557960796823, -16.46253265017161027, 62.08224293864769550 ) ) ;
#146741=CARTESIAN_POINT ( 'NONE',  ( 12.14591786802309770, 12.06949235617756955, 39.37390960531436690 ) ) ;
#146742=CARTESIAN_POINT ( 'NONE',  ( 9.564922557960805705, 16.46253265017160317, 79.58224293864769550 ) ) ;
#146745=CARTESIAN_POINT ( 'NONE',  ( 13.89961937509957401, 13.97604488694547697, 26.87609039468566507 ) ) ;
#146746=CARTESIAN_POINT ( 'NONE',  ( -12.14591786802309592, -12.06949235617757132, 81.87390960531435269 ) ) ;
#146747=CARTESIAN_POINT ( 'NONE',  ( -5.719274019375665041, -21.55341960407619695, 24.79275706135235779 ) ) ;
#146749=CARTESIAN_POINT ( 'NONE',  ( -18.62759615963270932, 10.81492255796079327, 75.83224293864769550 ) ) ;
#146750=CARTESIAN_POINT ( 'NONE',  ( -14.29746914071037622, -8.314922557961029526, 99.16775706135234714 ) ) ;
#146751=CARTESIAN_POINT ( 'NONE',  ( 8.314922557960818139, 14.29746914071049879, 114.5822429386477097 ) ) ;
#146752=CARTESIAN_POINT ( 'NONE',  ( 5.049401038298161559, -19.05341960407611168, 77.70724293864765286 ) ) ;
#146753=CARTESIAN_POINT ( 'NONE',  ( 17.50000000000000000, -5.499999999999992895, 71.21769037696435589 ) ) ;
#146755=CARTESIAN_POINT ( 'NONE',  ( 16.53943276465976808, -0.05219959533910856209, 33.74890960531436690 ) ) ;
#146756=CARTESIAN_POINT ( 'NONE',  ( -5.823673210054431948, 21.52544592524334988, 62.70942372801902565 ) ) ;
#146758=CARTESIAN_POINT ( 'NONE',  ( -21.55341960407619339, 5.719274019375674811, 93.54275706135234714 ) ) ;
#146759=CARTESIAN_POINT ( 'NONE',  ( -5.153800228976328057, -19.02544592524343514, 47.29057627198102409 ) ) ;
#146760=CARTESIAN_POINT ( 'NONE',  ( -19.05341960407611168, -5.049401038298163336, 56.45724293864768129 ) ) ;
#146763=CARTESIAN_POINT ( 'NONE',  ( 15.80617190586769283, -15.72974639402175789, 100.6260903946857184 ) ) ;
#146764=CARTESIAN_POINT ( 'NONE',  ( 16.53943276465976808, 0.05219959533934440121, 61.25109039468567573 ) ) ;
#146765=CARTESIAN_POINT ( 'NONE',  ( -18.62759615963255300, -10.81492255796106328, 79.16775706135234714 ) ) ;
#146766=CARTESIAN_POINT ( 'NONE',  ( -5.823673210054116645, -21.52544592524344225, 27.29057627198103120 ) ) ;
#146767=CARTESIAN_POINT ( 'NONE',  ( 19.02544592524334988, 5.153800228976608722, 91.45942372801900433 ) ) ;
#146768=CARTESIAN_POINT ( 'NONE',  ( -21.55341960407619339, 5.719274019375674811, 53.54275706135234714 ) ) ;
#146769=CARTESIAN_POINT ( 'NONE',  ( -14.29746914071037622, -8.314922557961029526, 34.16775706135234714 ) ) ;
#146770=CARTESIAN_POINT ( 'NONE',  ( -18.67979575497178146, -10.72451020669898902, 91.66557627198103830 ) ) ;
#146771=CARTESIAN_POINT ( 'NONE',  ( -16.51473224551082808, 9.474510206698731452, 83.33442372801899012 ) ) ;
#146772=CARTESIAN_POINT ( 'NONE',  ( -5.153800228976328057, -19.02544592524343514, 67.29057627198102409 ) ) ;
#146773=CARTESIAN_POINT ( 'NONE',  ( 19.02544592524334988, 5.153800228976608722, 101.4594237280189759 ) ) ;
#146775=CARTESIAN_POINT ( 'NONE',  ( 5.153800228976615827, -19.02544592524334988, 105.2094237280190185 ) ) ;
#146776=CARTESIAN_POINT ( 'NONE',  ( 16.53943276465976808, -0.05219959533910856209, 53.74890960531437401 ) ) ;
#146777=CARTESIAN_POINT ( 'NONE',  ( -19.02544592524334988, -5.153800228976617603, 73.95942372801900433 ) ) ;
#146778=CARTESIAN_POINT ( 'NONE',  ( 8.314922557961029526, -14.29746914071037800, 60.41775706135235424 ) ) ;
#146779=CARTESIAN_POINT ( 'NONE',  ( -19.03943276465977164, -0.05219959533935918106, 38.75109039468566152 ) ) ;
#146781=CARTESIAN_POINT ( 'NONE',  ( -9.564922557960796823, -16.46253265017161027, 37.08224293864768839 ) ) ;
#146782=CARTESIAN_POINT ( 'NONE',  ( 19.05341960407611168, 5.049401038298154454, 53.95724293864770260 ) ) ;
#146783=CARTESIAN_POINT ( 'NONE',  ( 12.14591786802327356, -12.06949235617739191, 55.62609039468568284 ) ) ;
#146786=CARTESIAN_POINT ( 'NONE',  ( 19.02544592524343514, -5.153800228976328945, 108.5405762719810383 ) ) ;
#146787=CARTESIAN_POINT ( 'NONE',  ( 13.97604488694527802, 13.89961937509977652, 24.37390960531435624 ) ) ;
#146788=VERTEX_POINT ( 'NONE', #152098 ) ;
#146789=CARTESIAN_POINT ( 'NONE',  ( 9.564922557961047289, -16.46253265017146816, 100.4177570613523329 ) ) ;
#146790=CARTESIAN_POINT ( 'NONE',  ( 21.52544592524344225, -5.823673210054117533, 43.54057627198103830 ) ) ;
#146791=CARTESIAN_POINT ( 'NONE',  ( 9.474510206698729675, 16.51473224551082808, 32.08442372801900433 ) ) ;
#146792=CARTESIAN_POINT ( 'NONE',  ( 4.379528057220092307, 16.55341960407617563, 22.29275706135235069 ) ) ;
#146793=CARTESIAN_POINT ( 'NONE',  ( 9.564922557960805705, 16.46253265017160317, 24.58224293864769194 ) ) ;
#146794=CARTESIAN_POINT ( 'NONE',  ( -5.153800228976328057, -19.02544592524343514, 47.29057627198102409 ) ) ;
#146795=CARTESIAN_POINT ( 'NONE',  ( -5.719274019375978568, 21.55341960407610458, 75.20724293864769550 ) ) ;
#146796=CARTESIAN_POINT ( 'NONE',  ( -19.02544592524342804, 5.153800228976336051, 101.0405762719810241 ) ) ;
#146797=CARTESIAN_POINT ( 'NONE',  ( -5.153800228976328057, -19.02544592524343514, 37.29057627198102409 ) ) ;
#146799=CARTESIAN_POINT ( 'NONE',  ( -13.97604488694547697, 13.89961937509957934, 88.12609039468563310 ) ) ;
#146800=CARTESIAN_POINT ( 'NONE',  ( 14.34966873604960469, 8.224510206698951720, 69.16557627198102409 ) ) ;
#146801=CARTESIAN_POINT ( 'NONE',  ( -21.53943276465977519, 0.05219959533907696930, 51.24890960531436690 ) ) ;
#146802=CARTESIAN_POINT ( 'NONE',  ( -15.72974639402176322, -15.80617190586768395, 109.3760903946857042 ) ) ;
#146803=CARTESIAN_POINT ( 'NONE',  ( 15.72974639402199770, -15.80617190586745480, 98.12390960531436690 ) ) ;
#146804=CARTESIAN_POINT ( 'NONE',  ( 10.72451020669871369, 18.67979575497193778, 67.08442372801901854 ) ) ;
#146805=CARTESIAN_POINT ( 'NONE',  ( -21.55341960407619339, 5.719274019375674811, 73.54275706135234714 ) ) ;
#146806=CARTESIAN_POINT ( 'NONE',  ( 0.05219959533909260263, 19.03943276465977164, 104.9989096053143669 ) ) ;
#146807=CARTESIAN_POINT ( 'NONE',  ( -16.53943276465976808, -0.05219959533934237506, 103.7510903946857042 ) ) ;
#146808=CARTESIAN_POINT ( 'NONE',  ( 21.53943276465977519, 0.05219959533937863772, 81.25109039468568994 ) ) ;
#146809=CARTESIAN_POINT ( 'NONE',  ( 19.03943276465977164, -0.05219959533909143690, 63.74890960531435979 ) ) ;
#146810=CARTESIAN_POINT ( 'NONE',  ( 13.97604488694548053, -13.89961937509957401, 40.62609039468564731 ) ) ;
#146811=CARTESIAN_POINT ( 'NONE',  ( 15.72974639402176855, 15.80617190586768217, 31.87609039468567929 ) ) ;
#146812=CARTESIAN_POINT ( 'NONE',  ( -9.564922557960796823, -16.46253265017161027, 62.08224293864769550 ) ) ;
#146813=CARTESIAN_POINT ( 'NONE',  ( 8.314922557960818139, 14.29746914071049879, 79.58224293864769550 ) ) ;
#146814=CARTESIAN_POINT ( 'NONE',  ( -12.14591786802309592, -12.06949235617757132, 41.87390960531435979 ) ) ;
#146815=CARTESIAN_POINT ( 'NONE',  ( -0.05219959533907301413, -21.53943276465977519, 52.49890960531435979 ) ) ;
#146816=CARTESIAN_POINT ( 'NONE',  ( 9.474510206698971260, -16.51473224551069308, 62.91557627198102409 ) ) ;
#146817=CARTESIAN_POINT ( 'NONE',  ( 18.67979575497178502, 10.72451020669898547, 69.16557627198102409 ) ) ;
#146818=CARTESIAN_POINT ( 'NONE',  ( -16.46253265017146816, -9.564922557961047289, 69.16775706135233293 ) ) ;
#146819=CARTESIAN_POINT ( 'NONE',  ( 16.46253265017146816, 9.564922557961045513, 26.66775706135234003 ) ) ;
#146820=CARTESIAN_POINT ( 'NONE',  ( 8.314922557960818139, 14.29746914071049879, 59.58224293864770260 ) ) ;
#146821=CARTESIAN_POINT ( 'NONE',  ( -21.52544592524343514, 5.823673210054127303, 46.04057627198103830 ) ) ;
#146825=CARTESIAN_POINT ( 'NONE',  ( -14.29746914071037622, -8.314922557961029526, 89.16775706135236135 ) ) ;
#146827=CARTESIAN_POINT ( 'NONE',  ( -5.153800228976607833, 19.02544592524334988, 82.70942372801897591 ) ) ;
#146828=CARTESIAN_POINT ( 'NONE',  ( -4.379528057220328563, 16.55341960407611168, 55.20724293864770260 ) ) ;
#146830=CARTESIAN_POINT ( 'NONE',  ( -19.02544592524342804, 5.153800228976336051, 51.04057627198103120 ) ) ;
#146831=CARTESIAN_POINT ( 'NONE',  ( -8.314922557960811034, -14.29746914071050412, 47.08224293864770260 ) ) ;
#146832=CARTESIAN_POINT ( 'NONE',  ( 5.049401038298161559, -19.05341960407611168, 92.70724293864769550 ) ) ;
#146833=CARTESIAN_POINT ( 'NONE',  ( -16.51473224551082808, 9.474510206698731452, 73.33442372801900433 ) ) ;
#146834=CARTESIAN_POINT ( 'NONE',  ( -0.05219959533909027116, -19.03943276465977164, 57.49890960531435979 ) ) ;
#146835=CARTESIAN_POINT ( 'NONE',  ( 10.72451020669871369, 18.67979575497193778, 57.08442372801901854 ) ) ;
#146836=CARTESIAN_POINT ( 'NONE',  ( -5.153800228976328057, -19.02544592524343514, 77.29057627198099567 ) ) ;
#146837=CARTESIAN_POINT ( 'NONE',  ( -9.474510206698964154, 16.51473224551069663, 30.41557627198102054 ) ) ;
#146838=CARTESIAN_POINT ( 'NONE',  ( 13.89961937509977652, -13.97604488694527269, 73.12390960531436690 ) ) ;
#146839=CARTESIAN_POINT ( 'NONE',  ( -21.52544592524343514, 5.823673210054127303, 51.04057627198103120 ) ) ;
#146840=CARTESIAN_POINT ( 'NONE',  ( 9.474510206698971260, -16.51473224551069308, 52.91557627198102409 ) ) ;
#146841=CARTESIAN_POINT ( 'NONE',  ( -5.719274019375978568, 21.55341960407610458, 55.20724293864770260 ) ) ;
#146842=CARTESIAN_POINT ( 'NONE',  ( 9.474510206698729675, 16.51473224551082808, 82.08442372801899012 ) ) ;
#146843=CARTESIAN_POINT ( 'NONE',  ( -8.224510206698735004, -14.34966873604973081, 109.5844237280190328 ) ) ;
#146844=CARTESIAN_POINT ( 'NONE',  ( 16.51473224551083163, -9.474510206698727899, 40.83442372801900433 ) ) ;
#146845=CARTESIAN_POINT ( 'NONE',  ( -16.52544592524335698, -4.483927247898792601, 53.95942372801900433 ) ) ;
#146846=CARTESIAN_POINT ( 'NONE',  ( -4.483927247898782831, 16.52544592524335698, 77.70942372801900433 ) ) ;
#146848=CARTESIAN_POINT ( 'NONE',  ( 16.52544592524335698, 4.483927247898782831, 66.45942372801903275 ) ) ;
#146849=CARTESIAN_POINT ( 'NONE',  ( -10.72451020669898014, 18.67979575497178502, 30.41557627198101699 ) ) ;
#146851=CARTESIAN_POINT ( 'NONE',  ( 19.03943276465977164, -0.05219959533909143690, 33.74890960531435979 ) ) ;
#146852=CARTESIAN_POINT ( 'NONE',  ( -14.34966873604972548, 8.224510206698743886, 38.33442372801900433 ) ) ;
#146853=CARTESIAN_POINT ( 'NONE',  ( 19.05341960407611168, 5.049401038298154454, 43.95724293864769550 ) ) ;
#146854=CARTESIAN_POINT ( 'NONE',  ( 5.719274019375673035, 21.55341960407619339, 42.29275706135235424 ) ) ;
#146855=CARTESIAN_POINT ( 'NONE',  ( -4.379528057220086978, -16.55341960407618274, 29.79275706135234358 ) ) ;
#146856=CARTESIAN_POINT ( 'NONE',  ( 14.34966873604960469, 8.224510206698951720, 24.16557627198103120 ) ) ;
#146858=CARTESIAN_POINT ( 'NONE',  ( 19.05341960407617918, -5.049401038297876454, 21.04275706135232582 ) ) ;
#146859=CARTESIAN_POINT ( 'NONE',  ( 16.51473224551083163, -9.474510206698727899, 105.8344237280190043 ) ) ;
#146861=CARTESIAN_POINT ( 'NONE',  ( -16.51473224551082808, 9.474510206698731452, 73.33442372801900433 ) ) ;
#146862=CARTESIAN_POINT ( 'NONE',  ( -14.29746914071049879, 8.314922557960819915, 70.83224293864770971 ) ) ;
#146863=CARTESIAN_POINT ( 'NONE',  ( -13.89961937509977652, 13.97604488694528158, 35.62390960531435269 ) ) ;
#146864=CARTESIAN_POINT ( 'NONE',  ( -19.02544592524334988, -5.153800228976617603, 63.95942372801899012 ) ) ;
#146865=CARTESIAN_POINT ( 'NONE',  ( 16.18388926212244883, -7.379444403734566116, 57.06046848633770452 ) ) ;
#146866=CARTESIAN_POINT ( 'NONE',  ( -18.62759615963255300, -10.81492255796106328, 59.16775706135234714 ) ) ;
#146867=CARTESIAN_POINT ( 'NONE',  ( 4.379528057220092307, 16.55341960407617563, 42.29275706135235424 ) ) ;
#146868=CARTESIAN_POINT ( 'NONE',  ( -17.97161686093726729, 5.499999999999973355, 90.99637206859165417 ) ) ;
#146869=CARTESIAN_POINT ( 'NONE',  ( 10.72451020669898902, -18.67979575497178502, 22.91557627198102765 ) ) ;
#146870=CARTESIAN_POINT ( 'NONE',  ( -4.379528057220086978, -16.55341960407618274, 19.79275706135235069 ) ) ;
#146872=CARTESIAN_POINT ( 'NONE',  ( -17.49999999999999645, -7.500000000000000888, 120.0000000000000142 ) ) ;
#146873=CARTESIAN_POINT ( 'NONE',  ( 5.153800228976335163, 19.02544592524342804, 29.79057627198102409 ) ) ;
#146874=CARTESIAN_POINT ( 'NONE',  ( -18.62759615963255300, -10.81492255796106328, 104.1677570613523471 ) ) ;
#146875=CARTESIAN_POINT ( 'NONE',  ( 16.46253265017160672, -9.564922557960803928, 58.33224293864769550 ) ) ;
#146877=CARTESIAN_POINT ( 'NONE',  ( -18.67979575497193778, 10.72451020669871902, 68.33442372801900433 ) ) ;
#146878=CARTESIAN_POINT ( 'NONE',  ( -0.05219959533937732626, 21.53943276465977519, 97.50109039468567573 ) ) ;
#146879=CARTESIAN_POINT ( 'NONE',  ( 12.14591786802309770, 12.06949235617756955, 29.37390960531435269 ) ) ;
#146880=CARTESIAN_POINT ( 'NONE',  ( -9.474510206698964154, 16.51473224551069663, 25.41557627198103120 ) ) ;
#146881=CARTESIAN_POINT ( 'NONE',  ( -9.474510206698964154, 16.51473224551069663, 90.41557627198103830 ) ) ;
#146882=CARTESIAN_POINT ( 'NONE',  ( 21.55341960407619695, -5.719274019375665929, 61.04275706135234714 ) ) ;
#146883=CARTESIAN_POINT ( 'NONE',  ( 13.97604488694527802, 13.89961937509977652, 34.37390960531436690 ) ) ;
#146884=CARTESIAN_POINT ( 'NONE',  ( 18.62759615963255655, 10.81492255796105972, 56.66775706135235424 ) ) ;
#146885=CARTESIAN_POINT ( 'NONE',  ( 9.564922557961047289, -16.46253265017146816, 85.41775706135233293 ) ) ;
#146886=CARTESIAN_POINT ( 'NONE',  ( -5.049401038298153566, 19.05341960407611168, 100.2072429386476955 ) ) ;
#146887=CARTESIAN_POINT ( 'NONE',  ( 14.34966873604960469, 8.224510206698951720, 114.1655762719810383 ) ) ;
#146888=CARTESIAN_POINT ( 'NONE',  ( -21.55341960407610458, -5.719274019375992779, 106.4572429386477097 ) ) ;
#146889=CARTESIAN_POINT ( 'NONE',  ( -5.049401038297874678, -19.05341960407617918, 29.79275706135232227 ) ) ;
#146890=CARTESIAN_POINT ( 'NONE',  ( 8.224510206698953496, -14.34966873604960469, 92.91557627198103830 ) ) ;
#146891=CARTESIAN_POINT ( 'NONE',  ( -16.51473224551069308, -9.474510206698971260, 46.66557627198102409 ) ) ;
#146892=CARTESIAN_POINT ( 'NONE',  ( 5.153800228976615827, -19.02544592524334988, 95.20942372801897591 ) ) ;
#146893=VECTOR ( 'NONE', #182408, 1000.000000000000000 ) ;
#146894=CARTESIAN_POINT ( 'NONE',  ( -12.06949235617756955, 12.14591786802309770, 60.62390960531437401 ) ) ;
#146895=CARTESIAN_POINT ( 'NONE',  ( 0.05219959533937995610, -21.53943276465977519, 110.0010903946856757 ) ) ;
#146896=CARTESIAN_POINT ( 'NONE',  ( -19.02544592524342804, 5.153800228976336051, 101.0405762719810241 ) ) ;
#146897=CARTESIAN_POINT ( 'NONE',  ( -16.46253265017146816, -9.564922557961047289, 84.16775706135233293 ) ) ;
#146898=CARTESIAN_POINT ( 'NONE',  ( 15.72974639402199770, -15.80617190586745480, 93.12390960531436690 ) ) ;
#146900=CARTESIAN_POINT ( 'NONE',  ( -15.72974639402176322, -15.80617190586768395, 44.37609039468567573 ) ) ;
#146901=CARTESIAN_POINT ( 'NONE',  ( 4.379528057220092307, 16.55341960407617563, 47.29275706135234003 ) ) ;
#146902=CARTESIAN_POINT ( 'NONE',  ( -0.05219959533934338120, 16.53943276465976808, 112.5010903946857042 ) ) ;
#146903=CARTESIAN_POINT ( 'NONE',  ( -12.14591786802326823, 12.06949235617739902, 43.12609039468568284 ) ) ;
#146904=CARTESIAN_POINT ( 'NONE',  ( -10.81492255796105439, 18.62759615963255655, 42.91775706135235424 ) ) ;
#146905=CARTESIAN_POINT ( 'NONE',  ( -18.62759615963270932, 10.81492255796079327, 45.83224293864769550 ) ) ;
#146907=CARTESIAN_POINT ( 'NONE',  ( 9.564922557960805705, 16.46253265017160317, 34.58224293864770260 ) ) ;
#146909=CARTESIAN_POINT ( 'NONE',  ( 16.52544592524335698, 4.483927247898782831, 61.45942372801901854 ) ) ;
#146910=CARTESIAN_POINT ( 'NONE',  ( -15.72974639402197994, 15.80617190586746368, 85.62390960531436690 ) ) ;
#146911=CARTESIAN_POINT ( 'NONE',  ( -4.483927247898539470, -16.52544592524342804, 42.29057627198103120 ) ) ;
#146912=CARTESIAN_POINT ( 'NONE',  ( -14.29746914071037622, -8.314922557961029526, 69.16775706135234714 ) ) ;
#146913=CARTESIAN_POINT ( 'NONE',  ( -13.89961937509977652, 13.97604488694528158, 60.62390960531436690 ) ) ;
#146914=CARTESIAN_POINT ( 'NONE',  ( -16.51473224551082808, 9.474510206698731452, 98.33442372801900433 ) ) ;
#146915=CARTESIAN_POINT ( 'NONE',  ( -15.72974639402197994, 15.80617190586746368, 80.62390960531438111 ) ) ;
#146916=CARTESIAN_POINT ( 'NONE',  ( 16.55341960407611168, 4.379528057220329451, 33.95724293864769550 ) ) ;
#146918=CARTESIAN_POINT ( 'NONE',  ( 0.05219959533934541429, -16.53943276465976808, 80.00109039468568994 ) ) ;
#146920=CARTESIAN_POINT ( 'NONE',  ( 21.55341960407610458, 5.719274019375980345, 73.95724293864769550 ) ) ;
#146921=CARTESIAN_POINT ( 'NONE',  ( -14.29746914071037622, -8.314922557961029526, 109.1677570613523613 ) ) ;
#146924=CARTESIAN_POINT ( 'NONE',  ( -0.05219959533907301413, -21.53943276465977519, 82.49890960531436690 ) ) ;
#146925=CARTESIAN_POINT ( 'NONE',  ( 10.81492255796078972, 18.62759615963270932, 109.5822429386476955 ) ) ;
#146926=CARTESIAN_POINT ( 'NONE',  ( -0.05219959533934338120, 16.53943276465976808, 112.5010903946857042 ) ) ;
#146928=CARTESIAN_POINT ( 'NONE',  ( 14.34966873604972726, -8.224510206698740333, 35.83442372801901143 ) ) ;
#146929=CARTESIAN_POINT ( 'NONE',  ( 9.564922557960805705, 16.46253265017160317, 39.58224293864768839 ) ) ;
#146930=CARTESIAN_POINT ( 'NONE',  ( 9.564922557960805705, 16.46253265017160317, 64.58224293864769550 ) ) ;
#146932=CARTESIAN_POINT ( 'NONE',  ( -0.05219959533909027116, -19.03943276465977164, 112.4989096053143669 ) ) ;
#146934=CARTESIAN_POINT ( 'NONE',  ( 5.049401038297881783, 19.05341960407617563, 107.2927570613523187 ) ) ;
#146935=CARTESIAN_POINT ( 'NONE',  ( 5.049401038297881783, 19.05341960407617563, 42.29275706135234003 ) ) ;
#146936=CARTESIAN_POINT ( 'NONE',  ( 21.55341960407610458, 5.719274019375980345, 93.95724293864770971 ) ) ;
#146937=CARTESIAN_POINT ( 'NONE',  ( 14.34966873604972726, -8.224510206698740333, 110.8344237280190043 ) ) ;
#146938=CARTESIAN_POINT ( 'NONE',  ( 5.823673210054125526, 21.52544592524343514, 39.79057627198103830 ) ) ;
#146939=CARTESIAN_POINT ( 'NONE',  ( 5.719274019375991003, -21.55341960407610458, 87.70724293864769550 ) ) ;
#146940=CARTESIAN_POINT ( 'NONE',  ( -16.51473224551082808, 9.474510206698731452, 108.3344237280190043 ) ) ;
#146941=CARTESIAN_POINT ( 'NONE',  ( -5.153800228976328057, -19.02544592524343514, 107.2905762719810383 ) ) ;
#146942=CARTESIAN_POINT ( 'NONE',  ( -10.81492255796105439, 18.62759615963255655, 72.91775706135234714 ) ) ;
#146943=CARTESIAN_POINT ( 'NONE',  ( -5.153800228976328057, -19.02544592524343514, 67.29057627198102409 ) ) ;
#146945=CARTESIAN_POINT ( 'NONE',  ( 12.06949235617757843, -12.14591786802309237, 103.1239096053143811 ) ) ;
#146947=CARTESIAN_POINT ( 'NONE',  ( -9.474510206698964154, 16.51473224551069663, 70.41557627198102409 ) ) ;
#146948=CARTESIAN_POINT ( 'NONE',  ( 16.52544592524342804, -4.483927247898539470, 88.54057627198103830 ) ) ;
#146949=ORIENTED_EDGE ( 'NONE', *, *, #101761, .T. ) ;
#146950=CARTESIAN_POINT ( 'NONE',  ( -9.474510206698720793, -16.51473224551083518, 109.5844237280190043 ) ) ;
#146952=CARTESIAN_POINT ( 'NONE',  ( -9.564922557960796823, -16.46253265017161027, 62.08224293864769550 ) ) ;
#146953=CARTESIAN_POINT ( 'NONE',  ( 18.67979575497194134, -10.72451020669871369, 80.83442372801901854 ) ) ;
#146954=CARTESIAN_POINT ( 'NONE',  ( 9.564922557960805705, 16.46253265017160317, 99.58224293864770971 ) ) ;
#146955=CARTESIAN_POINT ( 'NONE',  ( -16.55341960407617563, 4.379528057220093196, 83.54275706135234714 ) ) ;
#146956=CARTESIAN_POINT ( 'NONE',  ( -16.79531203550648399, -7.028104445595611871, 76.25244988220444498 ) ) ;
#146957=CARTESIAN_POINT ( 'NONE',  ( -13.89961937509957401, -13.97604488694547875, 54.37609039468565442 ) ) ;
#146958=CARTESIAN_POINT ( 'NONE',  ( 21.53943276465977519, 0.05219959533937863772, 96.25109039468568994 ) ) ;
#146961=CARTESIAN_POINT ( 'NONE',  ( 14.29746914071049879, -8.314922557960816363, 23.33224293864769194 ) ) ;
#146963=CARTESIAN_POINT ( 'NONE',  ( 8.224510206698742110, 14.34966873604972548, 92.08442372801901854 ) ) ;
#146965=CARTESIAN_POINT ( 'NONE',  ( -8.224510206698735004, -14.34966873604973081, 74.58442372801901854 ) ) ;
#146966=CARTESIAN_POINT ( 'NONE',  ( 5.823673210054444382, -21.52544592524334988, 80.20942372801901854 ) ) ;
#146967=CARTESIAN_POINT ( 'NONE',  ( 9.564922557961047289, -16.46253265017146816, 90.41775706135234714 ) ) ;
#146968=CARTESIAN_POINT ( 'NONE',  ( -9.564922557961040184, 16.46253265017147172, 37.91775706135233293 ) ) ;
#146970=CARTESIAN_POINT ( 'NONE',  ( -19.02544592524342804, 5.153800228976336051, 66.04057627198103830 ) ) ;
#146971=CARTESIAN_POINT ( 'NONE',  ( 19.03943276465977164, -0.05219959533909143690, 63.74890960531435979 ) ) ;
#146972=CARTESIAN_POINT ( 'NONE',  ( -18.22780087662119541, 5.500000000000102141, 41.01763182126894236 ) ) ;
#146973=CARTESIAN_POINT ( 'NONE',  ( -18.67979575497178146, -10.72451020669898902, 76.66557627198103830 ) ) ;
#146974=CARTESIAN_POINT ( 'NONE',  ( -18.67979575497178146, -10.72451020669898902, 36.66557627198103120 ) ) ;
#146975=CARTESIAN_POINT ( 'NONE',  ( 13.97604488694527802, 13.89961937509977652, 29.37390960531435979 ) ) ;
#146976=CARTESIAN_POINT ( 'NONE',  ( -16.55341960407617563, 4.379528057220093196, 68.54275706135234714 ) ) ;
#146979=CARTESIAN_POINT ( 'NONE',  ( 0.05219959533937995610, -21.53943276465977519, 35.00109039468568284 ) ) ;
#146980=CARTESIAN_POINT ( 'NONE',  ( -0.05219959533910754901, -16.53943276465976808, 72.49890960531435269 ) ) ;
#146982=CARTESIAN_POINT ( 'NONE',  ( -16.52544592524335698, -4.483927247898792601, 28.95942372801902209 ) ) ;
#146983=CARTESIAN_POINT ( 'NONE',  ( 13.89961937509957401, 13.97604488694547697, 56.87609039468564731 ) ) ;
#146984=CARTESIAN_POINT ( 'NONE',  ( 8.314922557960818139, 14.29746914071049879, 54.58224293864769550 ) ) ;
#146985=CARTESIAN_POINT ( 'NONE',  ( -5.823673210054431948, 21.52544592524334988, 32.70942372801900433 ) ) ;
#146987=CARTESIAN_POINT ( 'NONE',  ( 18.62759615963271287, -10.81492255796078972, 83.33224293864769550 ) ) ;
#146988=CARTESIAN_POINT ( 'NONE',  ( -16.46253265017160317, 9.564922557960807481, 100.8322429386477097 ) ) ;
#146989=CARTESIAN_POINT ( 'NONE',  ( -16.52544592524342804, 4.483927247898546575, 76.04057627198102409 ) ) ;
#146990=CARTESIAN_POINT ( 'NONE',  ( -16.46253265017160317, 9.564922557960807481, 110.8322429386476955 ) ) ;
#146992=CARTESIAN_POINT ( 'NONE',  ( 5.153800228976615827, -19.02544592524334988, 70.20942372801899012 ) ) ;
#146993=CARTESIAN_POINT ( 'NONE',  ( 21.55341960407619695, -5.719274019375665929, 26.04275706135235779 ) ) ;
#146994=CARTESIAN_POINT ( 'NONE',  ( -5.049401038298153566, 19.05341960407611168, 60.20724293864768129 ) ) ;
#146995=CARTESIAN_POINT ( 'NONE',  ( -13.97604488694547697, 13.89961937509957934, 48.12609039468566863 ) ) ;
#146996=CARTESIAN_POINT ( 'NONE',  ( -13.89961937509977652, 13.97604488694528158, 35.62390960531435269 ) ) ;
#146998=CARTESIAN_POINT ( 'NONE',  ( 18.67979575497194134, -10.72451020669871369, 60.83442372801901854 ) ) ;
#147000=CARTESIAN_POINT ( 'NONE',  ( 12.14591786802309770, 12.06949235617756955, 44.37390960531435979 ) ) ;
#147001=CARTESIAN_POINT ( 'NONE',  ( 5.049401038298161559, -19.05341960407611168, 62.70724293864769550 ) ) ;
#147002=CARTESIAN_POINT ( 'NONE',  ( 21.52544592524344225, -5.823673210054117533, 93.54057627198103830 ) ) ;
#147003=CARTESIAN_POINT ( 'NONE',  ( 5.153800228976335163, 19.02544592524342804, 64.79057627198100988 ) ) ;
#147005=CARTESIAN_POINT ( 'NONE',  ( 5.719274019375991003, -21.55341960407610458, 62.70724293864769550 ) ) ;
#147007=CARTESIAN_POINT ( 'NONE',  ( 21.52544592524334988, 5.823673210054432836, 96.45942372801901854 ) ) ;
#147009=CARTESIAN_POINT ( 'NONE',  ( 12.06949235617739724, 12.14591786802326823, 91.87609039468568994 ) ) ;
#147010=CARTESIAN_POINT ( 'NONE',  ( 4.379528057220339221, -16.55341960407611168, 77.70724293864770971 ) ) ;
#147011=CARTESIAN_POINT ( 'NONE',  ( -19.05341960407617563, 5.049401038297882671, 93.54275706135234714 ) ) ;
#147013=CARTESIAN_POINT ( 'NONE',  ( -18.62759615963270932, 10.81492255796079327, 110.8322429386476955 ) ) ;
#147014=CARTESIAN_POINT ( 'NONE',  ( 16.51473224551083163, -9.474510206698727899, 40.83442372801900433 ) ) ;
#147015=CARTESIAN_POINT ( 'NONE',  ( 12.14591786802327356, -12.06949235617739191, 105.6260903946856899 ) ) ;
#147016=CARTESIAN_POINT ( 'NONE',  ( 19.05341960407617918, -5.049401038297876454, 36.04275706135234003 ) ) ;
#147017=CARTESIAN_POINT ( 'NONE',  ( -19.03943276465977164, 0.05219959533909376836, 86.24890960531436690 ) ) ;
#147018=CARTESIAN_POINT ( 'NONE',  ( -21.55341960407610458, -5.719274019375992779, 66.45724293864768129 ) ) ;
#147020=CARTESIAN_POINT ( 'NONE',  ( 8.224510206698953496, -14.34966873604960469, 112.9155762719810383 ) ) ;
#147021=CARTESIAN_POINT ( 'NONE',  ( -5.823673210054431948, 21.52544592524334988, 112.7094237280190328 ) ) ;
#147022=CARTESIAN_POINT ( 'NONE',  ( 12.14591786802327356, -12.06949235617739191, 80.62609039468567573 ) ) ;
#147023=CARTESIAN_POINT ( 'NONE',  ( -5.823673210054431948, 21.52544592524334988, 27.70942372801901854 ) ) ;
#147024=CARTESIAN_POINT ( 'NONE',  ( -4.483927247898782831, 16.52544592524335698, 27.70942372801901854 ) ) ;
#147025=CARTESIAN_POINT ( 'NONE',  ( -13.97604488694527625, -13.89961937509977652, 101.8739096053143811 ) ) ;
#147026=CARTESIAN_POINT ( 'NONE',  ( -9.564922557960796823, -16.46253265017161027, 42.08224293864769550 ) ) ;
#147027=CARTESIAN_POINT ( 'NONE',  ( -9.564922557960796823, -16.46253265017161027, 62.08224293864769550 ) ) ;
#147029=CARTESIAN_POINT ( 'NONE',  ( 12.14591786802327356, -12.06949235617739191, 45.62609039468567573 ) ) ;
#147030=CARTESIAN_POINT ( 'NONE',  ( 8.224510206698953496, -14.34966873604960469, 87.91557627198103830 ) ) ;
#147031=CARTESIAN_POINT ( 'NONE',  ( 4.483927247898790824, -16.52544592524335698, 95.20942372801903275 ) ) ;
#147032=CARTESIAN_POINT ( 'NONE',  ( 5.719274019375673035, 21.55341960407619339, 47.29275706135234003 ) ) ;
#147033=CARTESIAN_POINT ( 'NONE',  ( -16.51473224551069308, -9.474510206698971260, 81.66557627198103830 ) ) ;
#147034=CARTESIAN_POINT ( 'NONE',  ( 0.05219959533909260263, 19.03943276465977164, 59.99890960531436690 ) ) ;
#147035=CARTESIAN_POINT ( 'NONE',  ( 19.05341960407611168, 5.049401038298154454, 98.95724293864766707 ) ) ;
#147036=CARTESIAN_POINT ( 'NONE',  ( -8.314922557960811034, -14.29746914071050412, 37.08224293864768129 ) ) ;
#147037=CARTESIAN_POINT ( 'NONE',  ( 16.52544592524335698, 4.483927247898782831, 101.4594237280190185 ) ) ;
#147038=ORIENTED_EDGE ( 'NONE', *, *, #163855, .F. ) ;
#147039=CARTESIAN_POINT ( 'NONE',  ( -16.46253265017146816, -9.564922557961047289, 39.16775706135234003 ) ) ;
#147040=CARTESIAN_POINT ( 'NONE',  ( 19.05341960407611168, 5.049401038298154454, 108.9572429386477097 ) ) ;
#147041=CARTESIAN_POINT ( 'NONE',  ( 5.049401038298161559, -19.05341960407611168, 67.70724293864769550 ) ) ;
#147042=CARTESIAN_POINT ( 'NONE',  ( -19.02544592524334988, -5.153800228976617603, 43.95942372801899012 ) ) ;
#147044=CARTESIAN_POINT ( 'NONE',  ( 19.52837319214027900, -5.499999999999891642, 72.10471352585544480 ) ) ;
#147045=CARTESIAN_POINT ( 'NONE',  ( -0.05219959533934338120, 16.53943276465976808, 57.50109039468568994 ) ) ;
#147046=CARTESIAN_POINT ( 'NONE',  ( 9.564922557961047289, -16.46253265017146816, 65.41775706135233293 ) ) ;
#147047=CARTESIAN_POINT ( 'NONE',  ( -14.34966873604972548, 8.224510206698743886, 53.33442372801901854 ) ) ;
#147048=FACE_OUTER_BOUND ( 'NONE', #149947, .T. ) ;
#147049=CARTESIAN_POINT ( 'NONE',  ( -0.05219959533909027116, -19.03943276465977164, 92.49890960531436690 ) ) ;
#147050=CARTESIAN_POINT ( 'NONE',  ( -15.72974639402197994, 15.80617190586746368, 110.6239096053143669 ) ) ;
#147051=CARTESIAN_POINT ( 'NONE',  ( 9.564922557961047289, -16.46253265017146816, 80.41775706135234714 ) ) ;
#147052=CARTESIAN_POINT ( 'NONE',  ( 16.46253265017160672, -9.564922557960803928, 108.3322429386476955 ) ) ;
#147053=CARTESIAN_POINT ( 'NONE',  ( 16.51473224551069308, 9.474510206698969483, 29.16557627198103475 ) ) ;
#147054=CARTESIAN_POINT ( 'NONE',  ( -19.02544592524342804, 5.153800228976336051, 76.04057627198102409 ) ) ;
#147055=CARTESIAN_POINT ( 'NONE',  ( 4.379528057220339221, -16.55341960407611168, 47.70724293864770260 ) ) ;
#147056=CARTESIAN_POINT ( 'NONE',  ( 13.89961937509977652, -13.97604488694527269, 43.12390960531434558 ) ) ;
#147058=CARTESIAN_POINT ( 'NONE',  ( 13.89961937509957401, 13.97604488694547697, 56.87609039468564731 ) ) ;
#147059=ORIENTED_EDGE ( 'NONE', *, *, #100803, .F. ) ;
#147060=CARTESIAN_POINT ( 'NONE',  ( 0.05219959533910956823, 16.53943276465976808, 89.99890960531438111 ) ) ;
#147061=CARTESIAN_POINT ( 'NONE',  ( 15.72974639402176855, 15.80617190586768217, 111.8760903946856615 ) ) ;
#147062=CARTESIAN_POINT ( 'NONE',  ( 13.97604488694527802, 13.89961937509977652, 49.37390960531434558 ) ) ;
#147063=CARTESIAN_POINT ( 'NONE',  ( 21.53943276465977519, -0.05219959533907433946, 53.74890960531437401 ) ) ;
#147064=CARTESIAN_POINT ( 'NONE',  ( -8.314922557960811034, -14.29746914071050412, 47.08224293864770260 ) ) ;
#147065=CARTESIAN_POINT ( 'NONE',  ( 19.03943276465977164, 0.05219959533936151252, 21.25109039468565797 ) ) ;
#147066=CARTESIAN_POINT ( 'NONE',  ( -13.89961937509977652, 13.97604488694528158, 105.6239096053143527 ) ) ;
#147067=CARTESIAN_POINT ( 'NONE',  ( 13.97604488694527802, 13.89961937509977652, 109.3739096053143669 ) ) ;
#147068=CARTESIAN_POINT ( 'NONE',  ( -5.049401038298153566, 19.05341960407611168, 35.20724293864768839 ) ) ;
#147069=CARTESIAN_POINT ( 'NONE',  ( -5.049401038298153566, 19.05341960407611168, 30.20724293864768839 ) ) ;
#147070=CARTESIAN_POINT ( 'NONE',  ( 12.06949235617757843, -12.14591786802309237, 88.12390960531436690 ) ) ;
#147071=CARTESIAN_POINT ( 'NONE',  ( -18.67979575497178146, -10.72451020669898902, 96.66557627198102409 ) ) ;
#147072=CARTESIAN_POINT ( 'NONE',  ( 19.05341960407611168, 5.049401038298154454, 98.95724293864766707 ) ) ;
#147073=CARTESIAN_POINT ( 'NONE',  ( 21.55341960407610458, 5.719274019375980345, 108.9572429386476955 ) ) ;
#147074=CARTESIAN_POINT ( 'NONE',  ( 19.03943276465977164, -0.05219959533909143690, 108.7489096053143527 ) ) ;
#147076=CARTESIAN_POINT ( 'NONE',  ( -4.379528057220328563, 16.55341960407611168, 100.2072429386476955 ) ) ;
#147077=CARTESIAN_POINT ( 'NONE',  ( -19.03943276465977164, 0.05219959533909376836, 71.24890960531435269 ) ) ;
#147078=CARTESIAN_POINT ( 'NONE',  ( -21.52544592524343514, 5.823673210054127303, 81.04057627198102409 ) ) ;
#147082=CARTESIAN_POINT ( 'NONE',  ( 21.55341960407610458, 5.719274019375980345, 28.95724293864769905 ) ) ;
#147084=CARTESIAN_POINT ( 'NONE',  ( 12.06949235617739724, 12.14591786802326823, 26.87609039468567218 ) ) ;
#147085=CARTESIAN_POINT ( 'NONE',  ( 16.55341960407611168, 4.379528057220329451, 108.9572429386476955 ) ) ;
#147086=CARTESIAN_POINT ( 'NONE',  ( -17.49999999999999289, -5.068104630630392293, 109.2718159465996877 ) ) ;
#147087=CARTESIAN_POINT ( 'NONE',  ( 13.89961937509977652, -13.97604488694527269, 53.12390960531434558 ) ) ;
#147088=CARTESIAN_POINT ( 'NONE',  ( 0.05219959533910956823, 16.53943276465976808, 79.99890960531435269 ) ) ;
#147089=CARTESIAN_POINT ( 'NONE',  ( 5.719274019375991003, -21.55341960407610458, 27.70724293864769905 ) ) ;
#147090=CARTESIAN_POINT ( 'NONE',  ( 16.53943276465976808, -0.05219959533910856209, 63.74890960531435979 ) ) ;
#147091=CARTESIAN_POINT ( 'NONE',  ( -16.53943276465976808, -0.05219959533934237506, 18.75109039468568639 ) ) ;
#147092=CARTESIAN_POINT ( 'NONE',  ( -18.67979575497193778, 10.72451020669871902, 78.33442372801901854 ) ) ;
#147093=CARTESIAN_POINT ( 'NONE',  ( 5.049401038297881783, 19.05341960407617918, 62.29275706135234003 ) ) ;
#147094=CARTESIAN_POINT ( 'NONE',  ( -19.03943276465977164, 0.05219959533909376836, 106.2489096053143669 ) ) ;
#147095=CARTESIAN_POINT ( 'NONE',  ( 4.483927247898790824, -16.52544592524335698, 85.20942372801901854 ) ) ;
#147096=CARTESIAN_POINT ( 'NONE',  ( 5.153800228976335163, 19.02544592524342804, 44.79057627198103830 ) ) ;
#147097=CARTESIAN_POINT ( 'NONE',  ( 19.05341960407611168, 5.049401038298154454, 88.95724293864769550 ) ) ;
#147098=CARTESIAN_POINT ( 'NONE',  ( 18.67979575497178502, 10.72451020669898547, 89.16557627198102409 ) ) ;
#147099=CARTESIAN_POINT ( 'NONE',  ( 16.53943276465976808, 0.05219959533934440121, 21.25109039468567218 ) ) ;
#147100=CARTESIAN_POINT ( 'NONE',  ( 12.06949235617757843, -12.14591786802309237, 53.12390960531436690 ) ) ;
#147101=CARTESIAN_POINT ( 'NONE',  ( 0.05219959533937995610, -21.53943276465977519, 70.00109039468568994 ) ) ;
#147102=CARTESIAN_POINT ( 'NONE',  ( -8.224510206698735004, -14.34966873604973081, 94.58442372801901854 ) ) ;
#147103=CARTESIAN_POINT ( 'NONE',  ( 5.153800228976335163, 19.02544592524342804, 114.7905762719810241 ) ) ;
#147105=CARTESIAN_POINT ( 'NONE',  ( 8.224510206698953496, -14.34966873604960469, 32.91557627198102409 ) ) ;
#147106=CARTESIAN_POINT ( 'NONE',  ( -14.34966873604972548, 8.224510206698743886, 58.33442372801901143 ) ) ;
#147107=CARTESIAN_POINT ( 'NONE',  ( -19.03943276465977164, 0.05219959533909376836, 71.24890960531435269 ) ) ;
#147108=CARTESIAN_POINT ( 'NONE',  ( -5.049401038298153566, 19.05341960407611168, 85.20724293864766707 ) ) ;
#147109=CARTESIAN_POINT ( 'NONE',  ( 18.67979575497194134, -10.72451020669871369, 75.83442372801900433 ) ) ;
#147110=CARTESIAN_POINT ( 'NONE',  ( -8.224510206698735004, -14.34966873604973081, 69.58442372801900433 ) ) ;
#147111=CARTESIAN_POINT ( 'NONE',  ( -16.52544592524342804, 4.483927247898546575, 61.04057627198103120 ) ) ;
#147112=CARTESIAN_POINT ( 'NONE',  ( -9.474510206698964154, 16.51473224551069663, 65.41557627198102409 ) ) ;
#147113=ORIENTED_EDGE ( 'NONE', *, *, #160526, .T. ) ;
#147114=CARTESIAN_POINT ( 'NONE',  ( 19.02544592524334988, 5.153800228976608722, 106.4594237280190185 ) ) ;
#147115=CARTESIAN_POINT ( 'NONE',  ( 8.314922557960818139, 14.29746914071049879, 109.5822429386476955 ) ) ;
#147116=CARTESIAN_POINT ( 'NONE',  ( -16.51473224551069308, -9.474510206698971260, 76.66557627198103830 ) ) ;
#147117=CARTESIAN_POINT ( 'NONE',  ( -16.52544592524335698, -4.483927247898792601, 23.95942372801901143 ) ) ;
#147119=CARTESIAN_POINT ( 'NONE',  ( 21.52544592524334988, 5.823673210054432836, 101.4594237280190185 ) ) ;
#147120=CARTESIAN_POINT ( 'NONE',  ( 4.483927247898790824, -16.52544592524335698, 80.20942372801901854 ) ) ;
#147121=CARTESIAN_POINT ( 'NONE',  ( 19.03943276465977164, 0.05219959533936151252, 96.25109039468567573 ) ) ;
#147122=CARTESIAN_POINT ( 'NONE',  ( 14.29746914071049879, -8.314922557960816363, 108.3322429386477097 ) ) ;
#147123=CARTESIAN_POINT ( 'NONE',  ( -8.224510206698735004, -14.34966873604973081, 69.58442372801900433 ) ) ;
#147125=CARTESIAN_POINT ( 'NONE',  ( -13.97604488694547697, 13.89961937509957934, 53.12609039468565442 ) ) ;
#147126=CARTESIAN_POINT ( 'NONE',  ( -21.52544592524334988, -5.823673210054445271, 98.95942372801903275 ) ) ;
#147127=CARTESIAN_POINT ( 'NONE',  ( 13.89961937509977652, -13.97604488694527269, 33.12390960531434558 ) ) ;
#147128=CARTESIAN_POINT ( 'NONE',  ( 16.51473224551069308, 9.474510206698969483, 74.16557627198103830 ) ) ;
#147129=CARTESIAN_POINT ( 'NONE',  ( -8.314922557960811034, -14.29746914071050412, 67.08224293864770971 ) ) ;
#147130=CARTESIAN_POINT ( 'NONE',  ( 21.52544592524334988, 5.823673210054432836, 91.45942372801901854 ) ) ;
#147131=CARTESIAN_POINT ( 'NONE',  ( 9.564922557961047289, -16.46253265017146816, 40.41775706135234003 ) ) ;
#147132=CARTESIAN_POINT ( 'NONE',  ( 16.46253265017146816, 9.564922557961045513, 36.66775706135233293 ) ) ;
#147133=CARTESIAN_POINT ( 'NONE',  ( -10.81492255796078084, -18.62759615963271287, 37.08224293864768129 ) ) ;
#147134=CARTESIAN_POINT ( 'NONE',  ( -21.53943276465977519, -0.05219959533937600094, 98.75109039468568994 ) ) ;
#147135=CARTESIAN_POINT ( 'NONE',  ( -13.97604488694527625, -13.89961937509977652, 81.87390960531436690 ) ) ;
#147136=CARTESIAN_POINT ( 'NONE',  ( 15.72974639402176855, 15.80617190586768217, 86.87609039468568994 ) ) ;
#147137=CARTESIAN_POINT ( 'NONE',  ( 18.67979575497178502, 10.72451020669898547, 44.16557627198103120 ) ) ;
#147138=CARTESIAN_POINT ( 'NONE',  ( -19.05341960407611168, -5.049401038298163336, 81.45724293864769550 ) ) ;
#147139=CARTESIAN_POINT ( 'NONE',  ( -5.153800228976607833, 19.02544592524334988, 72.70942372801900433 ) ) ;
#147140=CARTESIAN_POINT ( 'NONE',  ( -16.51473224551069308, -9.474510206698971260, 91.66557627198103830 ) ) ;
#147141=CARTESIAN_POINT ( 'NONE',  ( -19.03943276465977164, -0.05219959533935918106, 93.75109039468566152 ) ) ;
#147142=CARTESIAN_POINT ( 'NONE',  ( 12.06949235617739724, 12.14591786802326823, 36.87609039468568994 ) ) ;
#147143=CARTESIAN_POINT ( 'NONE',  ( -16.52544592524342804, 4.483927247898546575, 96.04057627198102409 ) ) ;
#147144=CARTESIAN_POINT ( 'NONE',  ( -0.05219959533909027116, -19.03943276465977164, 72.49890960531435269 ) ) ;
#147145=CARTESIAN_POINT ( 'NONE',  ( 0.05219959533907565091, 21.53943276465977519, 64.99890960531435269 ) ) ;
#147146=CARTESIAN_POINT ( 'NONE',  ( 16.53943276465976808, 0.05219959533934440121, 31.25109039468568639 ) ) ;
#147147=CARTESIAN_POINT ( 'NONE',  ( 5.823673210054444382, -21.52544592524334988, 35.20942372801901854 ) ) ;
#147148=CARTESIAN_POINT ( 'NONE',  ( -5.823673210054431948, 21.52544592524334988, 87.70942372801901854 ) ) ;
#147149=CARTESIAN_POINT ( 'NONE',  ( -8.224510206698735004, -14.34966873604973081, 84.58442372801903275 ) ) ;
#147150=CARTESIAN_POINT ( 'NONE',  ( 19.02544592524343514, -5.153800228976328945, 68.54057627198103830 ) ) ;
#147151=CARTESIAN_POINT ( 'NONE',  ( 4.483927247898545687, 16.52544592524342804, 79.79057627198102409 ) ) ;
#147152=CARTESIAN_POINT ( 'NONE',  ( -8.314922557961024197, 14.29746914071037800, 97.91775706135236135 ) ) ;
#147153=CARTESIAN_POINT ( 'NONE',  ( -9.474510206698720793, -16.51473224551083518, 49.58442372801899722 ) ) ;
#147154=CARTESIAN_POINT ( 'NONE',  ( 18.67979575497194134, -10.72451020669871369, 25.83442372801901499 ) ) ;
#147155=CARTESIAN_POINT ( 'NONE',  ( 16.53943276465976808, -0.05219959533910856209, 73.74890960531433848 ) ) ;
#147156=CARTESIAN_POINT ( 'NONE',  ( 16.51473224551069308, 9.474510206698969483, 99.16557627198102409 ) ) ;
#147157=CARTESIAN_POINT ( 'NONE',  ( -12.14591786802326823, 12.06949235617739902, 103.1260903946856757 ) ) ;
#147158=CARTESIAN_POINT ( 'NONE',  ( 15.72974639402176855, 15.80617190586768217, 76.87609039468567573 ) ) ;
#147159=CARTESIAN_POINT ( 'NONE',  ( -12.14591786802326823, 12.06949235617739902, 48.12609039468568284 ) ) ;
#147160=CARTESIAN_POINT ( 'NONE',  ( -0.05219959533937732626, 21.53943276465977519, 47.50109039468568994 ) ) ;
#147161=CARTESIAN_POINT ( 'NONE',  ( -14.29746914071049879, 8.314922557960819915, 75.83224293864769550 ) ) ;
#147162=EDGE_LOOP ( 'NONE', ( #98232, #150406, #79847, #78611 ) ) ;
#147163=CARTESIAN_POINT ( 'NONE',  ( -18.62759615963270932, 10.81492255796079327, 115.8322429386477097 ) ) ;
#147164=CARTESIAN_POINT ( 'NONE',  ( -19.34837522270365895, -5.499999999999739764, 50.86337684832579953 ) ) ;
#147165=CARTESIAN_POINT ( 'NONE',  ( 16.52544592524342804, -4.483927247898539470, 48.54057627198103120 ) ) ;
#147166=CARTESIAN_POINT ( 'NONE',  ( 16.46253265017160672, -9.564922557960803928, 28.33224293864769550 ) ) ;
#147167=CARTESIAN_POINT ( 'NONE',  ( 21.53943276465977519, -0.05219959533907433946, 38.74890960531435979 ) ) ;
#147168=CARTESIAN_POINT ( 'NONE',  ( 8.314922557960818139, 14.29746914071049879, 79.58224293864769550 ) ) ;
#147169=CARTESIAN_POINT ( 'NONE',  ( 10.72451020669898902, -18.67979575497178502, 77.91557627198102409 ) ) ;
#147170=CARTESIAN_POINT ( 'NONE',  ( -5.153800228976328057, -19.02544592524343514, 77.29057627198099567 ) ) ;
#147171=CARTESIAN_POINT ( 'NONE',  ( 13.97604488694527802, 13.89961937509977652, 34.37390960531436690 ) ) ;
#147172=CARTESIAN_POINT ( 'NONE',  ( -19.05341960407617563, 5.049401038297882671, 73.54275706135233293 ) ) ;
#147173=CARTESIAN_POINT ( 'NONE',  ( -15.72974639402176322, -15.80617190586768395, 54.37609039468568994 ) ) ;
#147174=CARTESIAN_POINT ( 'NONE',  ( -10.72451020669898014, 18.67979575497178502, 60.41557627198102409 ) ) ;
#147175=CARTESIAN_POINT ( 'NONE',  ( 5.153800228976335163, 19.02544592524342804, 44.79057627198103830 ) ) ;
#147176=CARTESIAN_POINT ( 'NONE',  ( 16.46253265017160672, -9.564922557960803928, 68.33224293864770971 ) ) ;
#147178=CARTESIAN_POINT ( 'NONE',  ( -8.314922557961024197, 14.29746914071037800, 52.91775706135235424 ) ) ;
#147179=CARTESIAN_POINT ( 'NONE',  ( 21.52544592524334988, 5.823673210054432836, 26.45942372801901854 ) ) ;
#147180=CARTESIAN_POINT ( 'NONE',  ( -21.52544592524334988, -5.823673210054445271, 58.95942372801902565 ) ) ;
#147181=CARTESIAN_POINT ( 'NONE',  ( -19.05341960407611168, -5.049401038298163336, 106.4572429386476955 ) ) ;
#147182=CARTESIAN_POINT ( 'NONE',  ( -18.62759615963270932, 10.81492255796079327, 90.83224293864769550 ) ) ;
#147183=CARTESIAN_POINT ( 'NONE',  ( -0.05219959533937732626, 21.53943276465977519, 27.50109039468567929 ) ) ;
#147184=CARTESIAN_POINT ( 'NONE',  ( 14.34966873604972726, -8.224510206698740333, 45.83442372801901854 ) ) ;
#147185=CARTESIAN_POINT ( 'NONE',  ( -21.55341960407610458, -5.719274019375992779, 51.45724293864770260 ) ) ;
#147186=CARTESIAN_POINT ( 'NONE',  ( 13.89961937509957401, 13.97604488694547697, 26.87609039468566507 ) ) ;
#147187=CARTESIAN_POINT ( 'NONE',  ( 5.049401038298161559, -19.05341960407611168, 52.70724293864767418 ) ) ;
#147188=CARTESIAN_POINT ( 'NONE',  ( -9.564922557960796823, -16.46253265017161027, 112.0822429386476955 ) ) ;
#147189=CARTESIAN_POINT ( 'NONE',  ( -9.564922557960796823, -16.46253265017161027, 87.08224293864769550 ) ) ;
#147192=CARTESIAN_POINT ( 'NONE',  ( -9.564922557961040184, 16.46253265017147172, 72.91775706135233293 ) ) ;
#147193=CARTESIAN_POINT ( 'NONE',  ( 21.55341960407610458, 5.719274019375980345, 48.95724293864770971 ) ) ;
#147194=CARTESIAN_POINT ( 'NONE',  ( -16.52544592524342804, 4.483927247898546575, 26.04057627198103475 ) ) ;
#147195=CARTESIAN_POINT ( 'NONE',  ( -19.03943276465977164, -0.05219959533935918106, 98.75109039468567573 ) ) ;
#147197=CARTESIAN_POINT ( 'NONE',  ( 15.72974639402176855, 15.80617190586768217, 111.8760903946856615 ) ) ;
#147198=CARTESIAN_POINT ( 'NONE',  ( -0.05219959533936034679, 19.03943276465977164, 92.50109039468566152 ) ) ;
#147199=CARTESIAN_POINT ( 'NONE',  ( 16.46253265017146816, 9.564922557961045513, 41.66775706135234003 ) ) ;
#147200=CARTESIAN_POINT ( 'NONE',  ( 16.36317988757056341, 7.306389748694959607, 108.4021039163677358 ) ) ;
#147201=CARTESIAN_POINT ( 'NONE',  ( 13.89961937509977652, -13.97604488694527269, 58.12390960531436690 ) ) ;
#147202=CARTESIAN_POINT ( 'NONE',  ( 16.53943276465976808, -0.05219959533910856209, 58.74890960531436690 ) ) ;
#147203=CARTESIAN_POINT ( 'NONE',  ( -19.05341960407611168, -5.049401038298163336, 36.45724293864766707 ) ) ;
#147204=CARTESIAN_POINT ( 'NONE',  ( 0.05219959533910956823, 16.53943276465976808, 34.99890960531435979 ) ) ;
#147206=CARTESIAN_POINT ( 'NONE',  ( -14.29746914071037622, -8.314922557961029526, 104.1677570613523471 ) ) ;
#147207=CARTESIAN_POINT ( 'NONE',  ( 13.97604488694527802, 13.89961937509977652, 59.37390960531434558 ) ) ;
#147208=CARTESIAN_POINT ( 'NONE',  ( 19.02544592524334988, 5.153800228976608722, 26.45942372801899722 ) ) ;
#147209=CARTESIAN_POINT ( 'NONE',  ( -12.14591786802326823, 12.06949235617739902, 28.12609039468568284 ) ) ;
#147210=CARTESIAN_POINT ( 'NONE',  ( 10.81492255796078972, 18.62759615963270932, 54.58224293864769550 ) ) ;
#147211=CARTESIAN_POINT ( 'NONE',  ( 5.823673210054444382, -21.52544592524334988, 105.2094237280190328 ) ) ;
#147213=CARTESIAN_POINT ( 'NONE',  ( -5.153800228976328057, -19.02544592524343514, 67.29057627198102409 ) ) ;
#147214=CARTESIAN_POINT ( 'NONE',  ( -16.51473224551069308, -9.474510206698971260, 106.6655762719810383 ) ) ;
#147215=CARTESIAN_POINT ( 'NONE',  ( 5.049401038298161559, -19.05341960407611168, 97.70724293864766707 ) ) ;
#147217=CARTESIAN_POINT ( 'NONE',  ( 18.67979575497194134, -10.72451020669871369, 20.83442372801901143 ) ) ;
#147219=CARTESIAN_POINT ( 'NONE',  ( 0.05219959533910956823, 16.53943276465976808, 89.99890960531438111 ) ) ;
#147220=CARTESIAN_POINT ( 'NONE',  ( -18.62759615963270932, 10.81492255796079327, 85.83224293864768129 ) ) ;
#147221=CARTESIAN_POINT ( 'NONE',  ( -5.049401038298153566, 19.05341960407611168, 65.20724293864765286 ) ) ;
#147222=CARTESIAN_POINT ( 'NONE',  ( -5.049401038298153566, 19.05341960407611168, 75.20724293864769550 ) ) ;
#147223=CARTESIAN_POINT ( 'NONE',  ( 18.67979575497178502, 10.72451020669898547, 109.1655762719810383 ) ) ;
#147225=CARTESIAN_POINT ( 'NONE',  ( 9.564922557960805705, 16.46253265017160317, 69.58224293864770971 ) ) ;
#147227=CARTESIAN_POINT ( 'NONE',  ( 14.34966873604960469, 8.224510206698951720, 109.1655762719810383 ) ) ;
#147228=CARTESIAN_POINT ( 'NONE',  ( -18.22780087662122028, 5.500000000000031086, 53.51540105326106556 ) ) ;
#147229=CARTESIAN_POINT ( 'NONE',  ( -19.05341960407617563, 5.049401038297882671, 88.54275706135230450 ) ) ;
#147230=CARTESIAN_POINT ( 'NONE',  ( 16.52544592524342804, -4.483927247898539470, 103.5405762719810383 ) ) ;
#147231=CARTESIAN_POINT ( 'NONE',  ( 5.823673210054444382, -21.52544592524334988, 75.20942372801901854 ) ) ;
#147232=CARTESIAN_POINT ( 'NONE',  ( -19.02544592524342804, 5.153800228976336051, 51.04057627198103120 ) ) ;
#147233=CARTESIAN_POINT ( 'NONE',  ( -10.72451020669870658, -18.67979575497194134, 34.58442372801900433 ) ) ;
#147234=CARTESIAN_POINT ( 'NONE',  ( -21.53943276465977519, -0.05219959533937600094, 18.75109039468568639 ) ) ;
#147236=CARTESIAN_POINT ( 'NONE',  ( -13.97604488694527625, -13.89961937509977652, 66.87390960531436690 ) ) ;
#147238=CARTESIAN_POINT ( 'NONE',  ( 19.03943276465977164, 0.05219959533936151252, 106.2510903946856615 ) ) ;
#147239=CARTESIAN_POINT ( 'NONE',  ( -15.80617190586745835, -15.72974639402198527, 31.87390960531435979 ) ) ;
#147240=CARTESIAN_POINT ( 'NONE',  ( 10.72451020669871369, 18.67979575497193778, 67.08442372801901854 ) ) ;
#147241=CARTESIAN_POINT ( 'NONE',  ( -16.51473224551069308, -9.474510206698971260, 91.66557627198103830 ) ) ;
#147242=CARTESIAN_POINT ( 'NONE',  ( -19.05341960407617563, 5.049401038297882671, 78.54275706135233293 ) ) ;
#147243=CARTESIAN_POINT ( 'NONE',  ( 13.89961937509977652, -13.97604488694527269, 48.12390960531435979 ) ) ;
#147244=CARTESIAN_POINT ( 'NONE',  ( -0.05219959533909027116, -19.03943276465977164, 67.49890960531436690 ) ) ;
#147246=CARTESIAN_POINT ( 'NONE',  ( 16.55341960407611168, 4.379528057220329451, 88.95724293864769550 ) ) ;
#147247=CARTESIAN_POINT ( 'NONE',  ( 0.05219959533909260263, 19.03943276465977164, 104.9989096053143669 ) ) ;
#147248=CARTESIAN_POINT ( 'NONE',  ( 16.52544592524342804, -4.483927247898539470, 93.54057627198103830 ) ) ;
#147249=CARTESIAN_POINT ( 'NONE',  ( 5.049401038298161559, -19.05341960407611168, 102.7072429386476955 ) ) ;
#147250=CARTESIAN_POINT ( 'NONE',  ( 12.06949235617757843, -12.14591786802309237, 38.12390960531436690 ) ) ;
#147251=CARTESIAN_POINT ( 'NONE',  ( 19.03943276465977164, -0.05219959533909143690, 23.74890960531435269 ) ) ;
#147253=CARTESIAN_POINT ( 'NONE',  ( -18.62759615963255300, -10.81492255796106328, 59.16775706135234714 ) ) ;
#147254=CARTESIAN_POINT ( 'NONE',  ( -5.049401038297874678, -19.05341960407617918, 74.79275706135231871 ) ) ;
#147255=CARTESIAN_POINT ( 'NONE',  ( -4.483927247898539470, -16.52544592524342804, 52.29057627198102409 ) ) ;
#147256=CARTESIAN_POINT ( 'NONE',  ( -18.62759615963270932, 10.81492255796079327, 100.8322429386477097 ) ) ;
#147257=CARTESIAN_POINT ( 'NONE',  ( 18.62759615963271287, -10.81492255796078972, 28.33224293864769550 ) ) ;
#147259=CARTESIAN_POINT ( 'NONE',  ( -12.14591786802309592, -12.06949235617757132, 76.87390960531439532 ) ) ;
#147260=CARTESIAN_POINT ( 'NONE',  ( -19.03943276465977164, 0.05219959533909376836, 56.24890960531435979 ) ) ;
#147261=CARTESIAN_POINT ( 'NONE',  ( 12.14591786802309770, 12.06949235617756955, 24.37390960531435979 ) ) ;
#147262=CARTESIAN_POINT ( 'NONE',  ( 16.55341960407618274, -4.379528057220086978, 106.0427570613523471 ) ) ;
#147263=CARTESIAN_POINT ( 'NONE',  ( 14.34966873604972726, -8.224510206698740333, 70.83442372801901854 ) ) ;
#147264=CARTESIAN_POINT ( 'NONE',  ( 9.564922557961047289, -16.46253265017146816, 20.41775706135233293 ) ) ;
#147265=CARTESIAN_POINT ( 'NONE',  ( 16.46253265017160672, -9.564922557960803928, 103.3322429386476955 ) ) ;
#147266=CARTESIAN_POINT ( 'NONE',  ( 19.05341960407611168, 5.049401038298154454, 73.95724293864768129 ) ) ;
#147267=CARTESIAN_POINT ( 'NONE',  ( 9.564922557960805705, 16.46253265017160317, 34.58224293864770260 ) ) ;
#147268=CARTESIAN_POINT ( 'NONE',  ( 4.483927247898545687, 16.52544592524342804, 49.79057627198102409 ) ) ;
#147270=CARTESIAN_POINT ( 'NONE',  ( -0.05219959533909027116, -19.03943276465977164, 102.4989096053143669 ) ) ;
#147271=CARTESIAN_POINT ( 'NONE',  ( 21.53943276465977519, -0.05219959533907433946, 43.74890960531435979 ) ) ;
#147272=CARTESIAN_POINT ( 'NONE',  ( -12.06949235617756955, 12.14591786802309770, 80.62390960531438111 ) ) ;
#147273=CARTESIAN_POINT ( 'NONE',  ( 16.55341960407618274, -4.379528057220086978, 21.04275706135234714 ) ) ;
#147275=CARTESIAN_POINT ( 'NONE',  ( -8.224510206698948167, 14.34966873604960824, 70.41557627198102409 ) ) ;
#147276=CARTESIAN_POINT ( 'NONE',  ( 17.50000000000000000, -5.500000000000000888, 33.29690382534174375 ) ) ;
#147277=CARTESIAN_POINT ( 'NONE',  ( 9.474510206698729675, 16.51473224551082808, 62.08442372801899722 ) ) ;
#147278=CARTESIAN_POINT ( 'NONE',  ( -19.05341960407611168, -5.049401038298163336, 106.4572429386476955 ) ) ;
#147279=CARTESIAN_POINT ( 'NONE',  ( -19.03943276465977164, -0.05219959533935918106, 83.75109039468567573 ) ) ;
#147280=CARTESIAN_POINT ( 'NONE',  ( -18.22780087662126647, -5.499999999999827693, 38.98236817873107185 ) ) ;
#147281=CARTESIAN_POINT ( 'NONE',  ( 12.14591786802327356, -12.06949235617739191, 20.62609039468568639 ) ) ;
#147282=CARTESIAN_POINT ( 'NONE',  ( 8.224510206698742110, 14.34966873604972548, 107.0844237280190043 ) ) ;
#147283=CARTESIAN_POINT ( 'NONE',  ( -9.474510206698964154, 16.51473224551069663, 40.41557627198103120 ) ) ;
#147284=CARTESIAN_POINT ( 'NONE',  ( 10.81492255796078972, 18.62759615963270932, 39.58224293864769550 ) ) ;
#147285=CARTESIAN_POINT ( 'NONE',  ( 18.62759615963255655, 10.81492255796105972, 61.66775706135235424 ) ) ;
#147287=CARTESIAN_POINT ( 'NONE',  ( 16.55341960407618274, -4.379528057220086978, 21.04275706135234714 ) ) ;
#147288=CARTESIAN_POINT ( 'NONE',  ( 17.49999999999984368, 3.200006130778718205, 22.58407523517191962 ) ) ;
#147289=CARTESIAN_POINT ( 'NONE',  ( -9.474510206698964154, 16.51473224551069663, 70.41557627198102409 ) ) ;
#147290=CARTESIAN_POINT ( 'NONE',  ( 19.02544592524343514, -5.153800228976328945, 23.54057627198102054 ) ) ;
#147291=CARTESIAN_POINT ( 'NONE',  ( 4.379528057220339221, -16.55341960407611168, 92.70724293864770971 ) ) ;
#147292=CARTESIAN_POINT ( 'NONE',  ( 16.46253265017160672, -9.564922557960803928, 78.33224293864769550 ) ) ;
#147294=CARTESIAN_POINT ( 'NONE',  ( 16.51473224551069308, 9.474510206698969483, 94.16557627198103830 ) ) ;
#147295=ORIENTED_EDGE ( 'NONE', *, *, #97920, .T. ) ;
#147296=CARTESIAN_POINT ( 'NONE',  ( 16.46253265017146816, 9.564922557961045513, 91.66775706135234714 ) ) ;
#147297=CARTESIAN_POINT ( 'NONE',  ( 18.67979575497178502, 10.72451020669898547, 84.16557627198103830 ) ) ;
#147298=CARTESIAN_POINT ( 'NONE',  ( -19.02544592524342804, 5.153800228976336051, 36.04057627198100988 ) ) ;
#147299=CARTESIAN_POINT ( 'NONE',  ( -13.97604488694547697, 13.89961937509957934, 58.12609039468566863 ) ) ;
#147300=CARTESIAN_POINT ( 'NONE',  ( 16.46253265017160672, -9.564922557960803928, 53.33224293864768839 ) ) ;
#147301=CARTESIAN_POINT ( 'NONE',  ( -19.02544592524342804, 5.153800228976336051, 96.04057627198103830 ) ) ;
#147303=CARTESIAN_POINT ( 'NONE',  ( 0.05219959533907565091, 21.53943276465977519, 99.99890960531436690 ) ) ;
#147304=CARTESIAN_POINT ( 'NONE',  ( 14.34966873604960469, 8.224510206698951720, 99.16557627198100988 ) ) ;
#147305=CARTESIAN_POINT ( 'NONE',  ( -9.474510206698964154, 16.51473224551069663, 85.41557627198102409 ) ) ;
#147306=CARTESIAN_POINT ( 'NONE',  ( -19.03943276465977164, -0.05219959533935918106, 58.75109039468566863 ) ) ;
#147307=CARTESIAN_POINT ( 'NONE',  ( -10.81492255796078084, -18.62759615963271287, 92.08224293864769550 ) ) ;
#147308=CARTESIAN_POINT ( 'NONE',  ( 21.52544592524344225, -5.823673210054117533, 68.54057627198103830 ) ) ;
#147309=CARTESIAN_POINT ( 'NONE',  ( -14.29746914071049879, 8.314922557960819915, 30.83224293864770260 ) ) ;
#147310=CARTESIAN_POINT ( 'NONE',  ( -21.55341960407619339, 5.719274019375674811, 98.54275706135234714 ) ) ;
#147311=CARTESIAN_POINT ( 'NONE',  ( -8.224510206698735004, -14.34966873604973081, 59.58442372801901854 ) ) ;
#147312=CARTESIAN_POINT ( 'NONE',  ( -16.51473224551069308, -9.474510206698971260, 76.66557627198103830 ) ) ;
#147313=CARTESIAN_POINT ( 'NONE',  ( -9.474510206698964154, 16.51473224551069663, 30.41557627198102054 ) ) ;
#147314=CARTESIAN_POINT ( 'NONE',  ( -15.72974639402176322, -15.80617190586768395, 34.37609039468568284 ) ) ;
#147315=CARTESIAN_POINT ( 'NONE',  ( -0.05219959533937732626, 21.53943276465977519, 57.50109039468568994 ) ) ;
#147316=CARTESIAN_POINT ( 'NONE',  ( 5.049401038298161559, -19.05341960407611168, 52.70724293864767418 ) ) ;
#147317=CARTESIAN_POINT ( 'NONE',  ( -5.719274019375665041, -21.55341960407619695, 19.79275706135235069 ) ) ;
#147319=CARTESIAN_POINT ( 'NONE',  ( 19.03943276465977164, 0.05219959533936151252, 76.25109039468566152 ) ) ;
#147321=CARTESIAN_POINT ( 'NONE',  ( -5.153800228976607833, 19.02544592524334988, 77.70942372801900433 ) ) ;
#147322=CARTESIAN_POINT ( 'NONE',  ( 16.46253265017160672, -9.564922557960803928, 23.33224293864769194 ) ) ;
#147323=CARTESIAN_POINT ( 'NONE',  ( 8.224510206698742110, 14.34966873604972548, 72.08442372801899012 ) ) ;
#147324=CARTESIAN_POINT ( 'NONE',  ( -0.05219959533909027116, -19.03943276465977164, 57.49890960531435979 ) ) ;
#147326=CARTESIAN_POINT ( 'NONE',  ( 9.564922557960805705, 16.46253265017160317, 99.58224293864770971 ) ) ;
#147327=CARTESIAN_POINT ( 'NONE',  ( -19.03943276465977164, 0.05219959533909376836, 41.24890960531435269 ) ) ;
#147328=CARTESIAN_POINT ( 'NONE',  ( -5.823673210054116645, -21.52544592524344225, 67.29057627198103830 ) ) ;
#147329=CARTESIAN_POINT ( 'NONE',  ( 14.29746914071037800, 8.314922557961029526, 66.66775706135234714 ) ) ;
#147330=CARTESIAN_POINT ( 'NONE',  ( -5.719274019375665041, -21.55341960407619695, 109.7927570613523613 ) ) ;
#147331=CARTESIAN_POINT ( 'NONE',  ( 13.97604488694527802, 13.89961937509977652, 49.37390960531434558 ) ) ;
#147332=CARTESIAN_POINT ( 'NONE',  ( 16.53943276465976808, -0.05219959533910856209, 43.74890960531435979 ) ) ;
#147333=B_SPLINE_CURVE_WITH_KNOTS ( 'NONE', 3,
 ( #189575, #97517, #50062, #191549, #20698, #187599, #67204, #81356, #49068, #176400, #66211, #114707, #69203, #82354, #145037, #4518, #113693, #126875, #188581, #175389, #36857, #142051, #157238, #35871, #53026, #127871, #98524, #18731, #110724, #99533, #172405, #37875 ),
 .UNSPECIFIED., .F., .F.,
 ( 4, 2, 2, 2, 2, 2, 2, 2, 2, 2, 2, 2, 2, 2, 2, 4 ),
 ( 2.625112965618923682E-17, 0.0003712461730036965900, 0.0007424923460073669422, 0.001113738519011037240, 0.001484984692014707647, 0.002227477038022048460, 0.002598723211025719300, 0.002969969384029389706, 0.003341215557033060547, 0.003712461730036731820, 0.004083707903040401793, 0.004454954076044073501, 0.004826200249047744341, 0.005197446422051415181, 0.005568692595055086021, 0.005939938768058756861 ),
 .UNSPECIFIED. ) ;
#147334=CARTESIAN_POINT ( 'NONE',  ( 12.14591786802309770, 12.06949235617756955, 64.37390960531435269 ) ) ;
#147335=CARTESIAN_POINT ( 'NONE',  ( -19.02544592524342804, 5.153800228976336051, 81.04057627198103830 ) ) ;
#147336=CARTESIAN_POINT ( 'NONE',  ( 15.72974639402176855, 15.80617190586768217, 41.87609039468568284 ) ) ;
#147337=CARTESIAN_POINT ( 'NONE',  ( -5.049401038298153566, 19.05341960407611168, 90.20724293864766707 ) ) ;
#147338=CARTESIAN_POINT ( 'NONE',  ( 10.72451020669871369, 18.67979575497193778, 97.08442372801904696 ) ) ;
#147339=CARTESIAN_POINT ( 'NONE',  ( 16.52544592524335698, 4.483927247898782831, 71.45942372801901854 ) ) ;
#147340=CARTESIAN_POINT ( 'NONE',  ( 0.05219959533909260263, 19.03943276465977164, 109.9989096053143669 ) ) ;
#147341=CARTESIAN_POINT ( 'NONE',  ( -5.719274019375978568, 21.55341960407610458, 85.20724293864770971 ) ) ;
#147342=CARTESIAN_POINT ( 'NONE',  ( 16.55341960407611168, 4.379528057220329451, 43.95724293864769550 ) ) ;
#147343=CARTESIAN_POINT ( 'NONE',  ( -5.049401038298153566, 19.05341960407611168, 45.20724293864769550 ) ) ;
#147344=CARTESIAN_POINT ( 'NONE',  ( 4.483927247898790824, -16.52544592524335698, 50.20942372801901854 ) ) ;
#147345=CARTESIAN_POINT ( 'NONE',  ( -8.224510206698948167, 14.34966873604960824, 65.41557627198102409 ) ) ;
#147346=CARTESIAN_POINT ( 'NONE',  ( 5.153800228976335163, 19.02544592524342804, 114.7905762719810241 ) ) ;
#147347=CARTESIAN_POINT ( 'NONE',  ( -10.72451020669898014, 18.67979575497178502, 25.41557627198103120 ) ) ;
#147348=CARTESIAN_POINT ( 'NONE',  ( -13.89961937509957401, -13.97604488694547875, 29.37609039468565797 ) ) ;
#147349=CARTESIAN_POINT ( 'NONE',  ( -8.224510206698948167, 14.34966873604960824, 95.41557627198102409 ) ) ;
#147350=CARTESIAN_POINT ( 'NONE',  ( 5.049401038298161559, -19.05341960407611168, 112.7072429386476813 ) ) ;
#147352=CARTESIAN_POINT ( 'NONE',  ( 16.55341960407618274, -4.379528057220086978, 56.04275706135235424 ) ) ;
#147353=CARTESIAN_POINT ( 'NONE',  ( 13.97604488694527802, 13.89961937509977652, 59.37390960531434558 ) ) ;
#147355=CARTESIAN_POINT ( 'NONE',  ( -9.564922557961040184, 16.46253265017147172, 52.91775706135233293 ) ) ;
#147356=CARTESIAN_POINT ( 'NONE',  ( -0.05219959533934338120, 16.53943276465976808, 92.50109039468567573 ) ) ;
#147357=CARTESIAN_POINT ( 'NONE',  ( -9.474510206698720793, -16.51473224551083518, 89.58442372801900433 ) ) ;
#147358=CARTESIAN_POINT ( 'NONE',  ( 10.72451020669871369, 18.67979575497193778, 62.08442372801901143 ) ) ;
#147359=CARTESIAN_POINT ( 'NONE',  ( -19.02544592524342804, 5.153800228976336051, 81.04057627198103830 ) ) ;
#147360=CARTESIAN_POINT ( 'NONE',  ( 21.55341960407610458, 5.719274019375980345, 88.95724293864769550 ) ) ;
#147361=CARTESIAN_POINT ( 'NONE',  ( -0.05219959533910754901, -16.53943276465976808, 112.4989096053143669 ) ) ;
#147362=CARTESIAN_POINT ( 'NONE',  ( -13.89961937509957401, -13.97604488694547875, 84.37609039468567573 ) ) ;
#147363=CARTESIAN_POINT ( 'NONE',  ( 21.55341960407610458, 5.719274019375980345, 78.95724293864769550 ) ) ;
#147364=CARTESIAN_POINT ( 'NONE',  ( 5.153800228976615827, -19.02544592524334988, 40.20942372801898301 ) ) ;
#147365=FACE_OUTER_BOUND ( 'NONE', #145671, .T. ) ;
#147366=CARTESIAN_POINT ( 'NONE',  ( -21.53943276465977519, 0.05219959533907696930, 96.24890960531435269 ) ) ;
#147367=CARTESIAN_POINT ( 'NONE',  ( 18.22780087662123805, -5.499999999999976019, 83.51763182126894947 ) ) ;
#147368=CARTESIAN_POINT ( 'NONE',  ( -9.564922557960796823, -16.46253265017161027, 62.08224293864769550 ) ) ;
#147369=CARTESIAN_POINT ( 'NONE',  ( -18.09867054820431775, -5.499999999999928058, 88.98393025253589883 ) ) ;
#147370=CARTESIAN_POINT ( 'NONE',  ( -16.46253265017146816, -9.564922557961047289, 109.1677570613523471 ) ) ;
#147372=CARTESIAN_POINT ( 'NONE',  ( 19.03943276465977164, -0.05219959533909143690, 48.74890960531435979 ) ) ;
#147373=CARTESIAN_POINT ( 'NONE',  ( -21.55341960407610458, -5.719274019375992779, 21.45724293864769550 ) ) ;
#147374=CARTESIAN_POINT ( 'NONE',  ( -10.81492255796078084, -18.62759615963271287, 107.0822429386476955 ) ) ;
#147375=CARTESIAN_POINT ( 'NONE',  ( -16.55341960407611168, -4.379528057220339221, 46.45724293864769550 ) ) ;
#147376=CARTESIAN_POINT ( 'NONE',  ( 5.719274019375673035, 21.55341960407619339, 77.29275706135234714 ) ) ;
#147377=CARTESIAN_POINT ( 'NONE',  ( -8.314922557961024197, 14.29746914071037800, 22.91775706135235069 ) ) ;
#147378=CARTESIAN_POINT ( 'NONE',  ( -19.02544592524334988, -5.153800228976617603, 28.95942372801900433 ) ) ;
#147379=CARTESIAN_POINT ( 'NONE',  ( 16.53943276465976808, -0.05219959533910856209, 23.74890960531435269 ) ) ;
#147380=CARTESIAN_POINT ( 'NONE',  ( -0.05219959533937732626, 21.53943276465977519, 42.50109039468567573 ) ) ;
#147381=CARTESIAN_POINT ( 'NONE',  ( 10.81492255796078972, 18.62759615963270932, 114.5822429386477097 ) ) ;
#147382=CARTESIAN_POINT ( 'NONE',  ( 12.14591786802309770, 12.06949235617756955, 49.37390960531436690 ) ) ;
#147384=CARTESIAN_POINT ( 'NONE',  ( -9.564922557961040184, 16.46253265017147172, 92.91775706135233293 ) ) ;
#147385=CARTESIAN_POINT ( 'NONE',  ( -16.46253265017146816, -9.564922557961047289, 74.16775706135234714 ) ) ;
#147386=CARTESIAN_POINT ( 'NONE',  ( -10.72451020669870658, -18.67979575497194134, 69.58442372801900433 ) ) ;
#147387=CARTESIAN_POINT ( 'NONE',  ( -19.02544592524334988, -5.153800228976617603, 58.95942372801900433 ) ) ;
#147388=CARTESIAN_POINT ( 'NONE',  ( 0.05219959533910956823, 16.53943276465976808, 114.9989096053143669 ) ) ;
#147389=CARTESIAN_POINT ( 'NONE',  ( -21.53943276465977519, 0.05219959533907696930, 41.24890960531435269 ) ) ;
#147390=CARTESIAN_POINT ( 'NONE',  ( -16.55341960407611168, -4.379528057220339221, 56.45724293864768839 ) ) ;
#147391=CARTESIAN_POINT ( 'NONE',  ( -19.53037848336979110, 5.499999999999998224, 94.85532783611444074 ) ) ;
#147392=CARTESIAN_POINT ( 'NONE',  ( -15.80617190586768217, 15.72974639402176855, 113.1260903946856899 ) ) ;
#147393=CARTESIAN_POINT ( 'NONE',  ( 16.53943276465976808, 0.05219959533934440121, 86.25109039468568994 ) ) ;
#147394=CARTESIAN_POINT ( 'NONE',  ( -8.314922557960811034, -14.29746914071050412, 37.08224293864768129 ) ) ;
#147395=CARTESIAN_POINT ( 'NONE',  ( -5.719274019375665041, -21.55341960407619695, 69.79275706135234714 ) ) ;
#147396=CARTESIAN_POINT ( 'NONE',  ( -15.80617190586768217, 15.72974639402176855, 83.12609039468568994 ) ) ;
#147397=CARTESIAN_POINT ( 'NONE',  ( 18.62759615963271287, -10.81492255796078972, 83.33224293864769550 ) ) ;
#147398=CARTESIAN_POINT ( 'NONE',  ( -19.02544592524342804, 5.153800228976336051, 36.04057627198100988 ) ) ;
#147399=CARTESIAN_POINT ( 'NONE',  ( -0.05219959533937732626, 21.53943276465977519, 57.50109039468568994 ) ) ;
#147400=CARTESIAN_POINT ( 'NONE',  ( -9.564922557960796823, -16.46253265017161027, 42.08224293864769550 ) ) ;
#147401=CARTESIAN_POINT ( 'NONE',  ( -9.474510206698964154, 16.51473224551069663, 55.41557627198103120 ) ) ;
#147402=CARTESIAN_POINT ( 'NONE',  ( 14.34966873604960469, 8.224510206698951720, 94.16557627198103830 ) ) ;
#147403=CARTESIAN_POINT ( 'NONE',  ( -13.89961937509977652, 13.97604488694528158, 100.6239096053143669 ) ) ;
#147404=CARTESIAN_POINT ( 'NONE',  ( -8.314922557960811034, -14.29746914071050412, 47.08224293864770260 ) ) ;
#147405=CARTESIAN_POINT ( 'NONE',  ( 5.049401038298161559, -19.05341960407611168, 22.70724293864769194 ) ) ;
#147406=CARTESIAN_POINT ( 'NONE',  ( -15.80617190586745835, -15.72974639402198527, 76.87390960531439532 ) ) ;
#147408=CARTESIAN_POINT ( 'NONE',  ( -21.53943276465977519, 0.05219959533907696930, 116.2489096053143669 ) ) ;
#147410=CARTESIAN_POINT ( 'NONE',  ( 14.34966873604972726, -8.224510206698740333, 25.83442372801901499 ) ) ;
#147411=CARTESIAN_POINT ( 'NONE',  ( -21.52544592524343514, 5.823673210054127303, 76.04057627198102409 ) ) ;
#147412=CARTESIAN_POINT ( 'NONE',  ( 15.72974639402176855, 15.80617190586768217, 91.87609039468568994 ) ) ;
#147413=CARTESIAN_POINT ( 'NONE',  ( -0.05219959533909027116, -19.03943276465977164, 77.49890960531435269 ) ) ;
#147414=CARTESIAN_POINT ( 'NONE',  ( -21.55341960407619339, 5.719274019375674811, 28.54275706135234358 ) ) ;
#147415=ADVANCED_FACE ( 'NONE', ( #91384 ), #77229, .F. ) ;
#147416=CARTESIAN_POINT ( 'NONE',  ( -9.474510206698964154, 16.51473224551069663, 110.4155762719810383 ) ) ;
#147417=CARTESIAN_POINT ( 'NONE',  ( -4.379528057220086978, -16.55341960407618274, 84.79275706135234714 ) ) ;
#147418=CARTESIAN_POINT ( 'NONE',  ( 15.80617190586769283, -15.72974639402175789, 75.62609039468567573 ) ) ;
#147419=CARTESIAN_POINT ( 'NONE',  ( -10.72451020669870658, -18.67979575497194134, 109.5844237280190328 ) ) ;
#147420=CARTESIAN_POINT ( 'NONE',  ( 14.29746914071037800, 8.314922557961029526, 71.66775706135234714 ) ) ;
#147421=CARTESIAN_POINT ( 'NONE',  ( -0.05219959533937732626, 21.53943276465977519, 32.50109039468568284 ) ) ;
#147422=CARTESIAN_POINT ( 'NONE',  ( 13.89961937509977652, -13.97604488694527269, 23.12390960531436335 ) ) ;
#147423=CARTESIAN_POINT ( 'NONE',  ( -5.719274019375665041, -21.55341960407619695, 89.79275706135236135 ) ) ;
#147424=CARTESIAN_POINT ( 'NONE',  ( 9.474510206698971260, -16.51473224551069308, 87.91557627198102409 ) ) ;
#147425=CARTESIAN_POINT ( 'NONE',  ( -10.72451020669898014, 18.67979575497178502, 95.41557627198102409 ) ) ;
#147426=CARTESIAN_POINT ( 'NONE',  ( -13.89961937509957401, -13.97604488694547875, 64.37609039468567573 ) ) ;
#147428=CARTESIAN_POINT ( 'NONE',  ( -10.72451020669898014, 18.67979575497178502, 50.41557627198103120 ) ) ;
#147429=CARTESIAN_POINT ( 'NONE',  ( -5.049401038298153566, 19.05341960407611168, 90.20724293864766707 ) ) ;
#147430=CARTESIAN_POINT ( 'NONE',  ( -16.55341960407611168, -4.379528057220339221, 51.45724293864770260 ) ) ;
#147432=CARTESIAN_POINT ( 'NONE',  ( 9.474510206698729675, 16.51473224551082808, 77.08442372801900433 ) ) ;
#147434=CARTESIAN_POINT ( 'NONE',  ( -0.05219959533936034679, 19.03943276465977164, 102.5010903946856757 ) ) ;
#147435=CARTESIAN_POINT ( 'NONE',  ( 18.67979575497178502, 10.72451020669898547, 79.16557627198103830 ) ) ;
#147436=CARTESIAN_POINT ( 'NONE',  ( 8.314922557960818139, 14.29746914071049879, 64.58224293864769550 ) ) ;
#147437=CARTESIAN_POINT ( 'NONE',  ( 19.03943276465977164, -0.05219959533909143690, 103.7489096053143669 ) ) ;
#147438=CARTESIAN_POINT ( 'NONE',  ( 12.14591786802327356, -12.06949235617739191, 50.62609039468568994 ) ) ;
#147439=CARTESIAN_POINT ( 'NONE',  ( -19.02544592524342804, 5.153800228976336051, 56.04057627198100988 ) ) ;
#147440=CARTESIAN_POINT ( 'NONE',  ( -10.72451020669898014, 18.67979575497178502, 110.4155762719810383 ) ) ;
#147441=CARTESIAN_POINT ( 'NONE',  ( -5.049401038297874678, -19.05341960407617918, 99.79275706135234714 ) ) ;
#147442=CARTESIAN_POINT ( 'NONE',  ( -19.05341960407611168, -5.049401038298163336, 101.4572429386476955 ) ) ;
#147443=CARTESIAN_POINT ( 'NONE',  ( -13.97604488694527625, -13.89961937509977652, 76.87390960531433848 ) ) ;
#147444=CARTESIAN_POINT ( 'NONE',  ( -10.72451020669898014, 18.67979575497178502, 75.41557627198102409 ) ) ;
#147445=CARTESIAN_POINT ( 'NONE',  ( -9.474510206698964154, 16.51473224551069663, 45.41557627198103120 ) ) ;
#147447=CARTESIAN_POINT ( 'NONE',  ( -16.55341960407611168, -4.379528057220339221, 61.45724293864770260 ) ) ;
#147448=CARTESIAN_POINT ( 'NONE',  ( 16.51473224551069308, 9.474510206698969483, 99.16557627198102409 ) ) ;
#147450=CARTESIAN_POINT ( 'NONE',  ( -16.46253265017146816, -9.564922557961047289, 59.16775706135233293 ) ) ;
#147451=CARTESIAN_POINT ( 'NONE',  ( -18.67979575497178146, -10.72451020669898902, 96.66557627198102409 ) ) ;
#147452=CARTESIAN_POINT ( 'NONE',  ( 9.564922557961047289, -16.46253265017146816, 55.41775706135234003 ) ) ;
#147453=CARTESIAN_POINT ( 'NONE',  ( -5.049401038298153566, 19.05341960407611168, 95.20724293864770971 ) ) ;
#147454=CARTESIAN_POINT ( 'NONE',  ( 19.25918095147778786, 5.499999999999573674, 66.95284276293935477 ) ) ;
#147455=CARTESIAN_POINT ( 'NONE',  ( -21.55341960407610458, -5.719274019375992779, 46.45724293864769550 ) ) ;
#147456=CARTESIAN_POINT ( 'NONE',  ( -9.474510206698964154, 16.51473224551069663, 70.41557627198102409 ) ) ;
#147457=CARTESIAN_POINT ( 'NONE',  ( -0.05219959533937732626, 21.53943276465977519, 62.50109039468568284 ) ) ;
#147458=CARTESIAN_POINT ( 'NONE',  ( 19.03943276465977164, -0.05219959533909143690, 38.74890960531436690 ) ) ;
#147459=CARTESIAN_POINT ( 'NONE',  ( 14.34966873604960469, 8.224510206698951720, 79.16557627198103830 ) ) ;
#147460=ORIENTED_EDGE ( 'NONE', *, *, #64457, .T. ) ;
#147461=CARTESIAN_POINT ( 'NONE',  ( -14.34966873604972548, 8.224510206698743886, 23.33442372801901499 ) ) ;
#147462=CARTESIAN_POINT ( 'NONE',  ( -21.55341960407619339, 5.719274019375674811, 53.54275706135234714 ) ) ;
#147463=ORIENTED_EDGE ( 'NONE', *, *, #121212, .T. ) ;
#147464=CARTESIAN_POINT ( 'NONE',  ( 0.05219959533909260263, 19.03943276465977164, 109.9989096053143669 ) ) ;
#147465=CARTESIAN_POINT ( 'NONE',  ( 9.564922557961047289, -16.46253265017146816, 70.41775706135233293 ) ) ;
#147466=CARTESIAN_POINT ( 'NONE',  ( -17.50000000000001066, -5.500000000000021316, 46.28230962303566542 ) ) ;
#147467=CARTESIAN_POINT ( 'NONE',  ( 10.81492255796106328, -18.62759615963255655, 20.41775706135234714 ) ) ;
#147468=CARTESIAN_POINT ( 'NONE',  ( -0.05219959533909027116, -19.03943276465977164, 57.49890960531435979 ) ) ;
#147470=CARTESIAN_POINT ( 'NONE',  ( -5.719274019375665041, -21.55341960407619695, 109.7927570613523613 ) ) ;
#147471=CARTESIAN_POINT ( 'NONE',  ( -16.51473224551069308, -9.474510206698971260, 46.66557627198102409 ) ) ;
#147472=CARTESIAN_POINT ( 'NONE',  ( -16.46253265017146816, -9.564922557961047289, 19.16775706135233293 ) ) ;
#147473=CARTESIAN_POINT ( 'NONE',  ( 8.314922557961029526, -14.29746914071037800, 95.41775706135234714 ) ) ;
#147474=CARTESIAN_POINT ( 'NONE',  ( 13.97604488694527802, 13.89961937509977652, 99.37390960531436690 ) ) ;
#147475=CARTESIAN_POINT ( 'NONE',  ( 10.72451020669871369, 18.67979575497193778, 72.08442372801899012 ) ) ;
#147477=CARTESIAN_POINT ( 'NONE',  ( -13.97604488694527625, -13.89961937509977652, 106.8739096053143669 ) ) ;
#147479=CARTESIAN_POINT ( 'NONE',  ( 12.06949235617739724, 12.14591786802326823, 66.87609039468568994 ) ) ;
#147480=CARTESIAN_POINT ( 'NONE',  ( 5.719274019375673035, 21.55341960407619339, 67.29275706135234714 ) ) ;
#147481=CARTESIAN_POINT ( 'NONE',  ( -10.81492255796105439, 18.62759615963255655, 107.9177570613523471 ) ) ;
#147483=CARTESIAN_POINT ( 'NONE',  ( -8.314922557961024197, 14.29746914071037800, 42.91775706135235424 ) ) ;
#147484=CARTESIAN_POINT ( 'NONE',  ( -13.97604488694527625, -13.89961937509977652, 91.87390960531432427 ) ) ;
#147485=CARTESIAN_POINT ( 'NONE',  ( 19.02544592524343514, -5.153800228976328945, 113.5405762719810241 ) ) ;
#147486=ORIENTED_EDGE ( 'NONE', *, *, #9309, .F. ) ;
#147487=CARTESIAN_POINT ( 'NONE',  ( 17.40805194822029378, 6.112264579159354838, 41.66628727489390371 ) ) ;
#147488=CARTESIAN_POINT ( 'NONE',  ( -16.46253265017160317, 9.564922557960807481, 35.83224293864768839 ) ) ;
#147489=CARTESIAN_POINT ( 'NONE',  ( -15.80617190586745835, -15.72974639402198527, 36.87390960531435979 ) ) ;
#147490=CARTESIAN_POINT ( 'NONE',  ( 8.224510206698742110, 14.34966873604972548, 102.0844237280190185 ) ) ;
#147491=CARTESIAN_POINT ( 'NONE',  ( -16.52544592524342804, 4.483927247898546575, 86.04057627198102409 ) ) ;
#147492=CARTESIAN_POINT ( 'NONE',  ( 13.97604488694527802, 13.89961937509977652, 79.37390960531435269 ) ) ;
#147493=CARTESIAN_POINT ( 'NONE',  ( 21.52544592524334988, 5.823673210054432836, 101.4594237280190185 ) ) ;
#147494=CARTESIAN_POINT ( 'NONE',  ( -14.29746914071037622, -8.314922557961029526, 29.16775706135234003 ) ) ;
#147495=CARTESIAN_POINT ( 'NONE',  ( -8.314922557960811034, -14.29746914071050412, 87.08224293864769550 ) ) ;
#147496=CARTESIAN_POINT ( 'NONE',  ( 21.52544592524334988, 5.823673210054432836, 36.45942372801901143 ) ) ;
#147497=CARTESIAN_POINT ( 'NONE',  ( -21.55341960407610458, -5.719274019375992779, 91.45724293864769550 ) ) ;
#147498=CARTESIAN_POINT ( 'NONE',  ( 16.51473224551083163, -9.474510206698727899, 50.83442372801899722 ) ) ;
#147499=CARTESIAN_POINT ( 'NONE',  ( 13.97604488694527802, 13.89961937509977830, 44.37390960531435979 ) ) ;
#147500=CARTESIAN_POINT ( 'NONE',  ( -19.02544592524342804, 5.153800228976336051, 101.0405762719810241 ) ) ;
#147501=CARTESIAN_POINT ( 'NONE',  ( 4.483927247898545687, 16.52544592524342804, 64.79057627198103830 ) ) ;
#147503=CARTESIAN_POINT ( 'NONE',  ( -12.06949235617756955, 12.14591786802309770, 45.62390960531436690 ) ) ;
#147504=CARTESIAN_POINT ( 'NONE',  ( -14.29746914071037622, -8.314922557961029526, 104.1677570613523471 ) ) ;
#147505=CARTESIAN_POINT ( 'NONE',  ( 13.89961937509957401, 13.97604488694547697, 66.87609039468567573 ) ) ;
#147507=CARTESIAN_POINT ( 'NONE',  ( 5.719274019375991003, -21.55341960407610458, 27.70724293864769905 ) ) ;
#147509=CARTESIAN_POINT ( 'NONE',  ( -8.314922557960811034, -14.29746914071050412, 92.08224293864769550 ) ) ;
#147511=CARTESIAN_POINT ( 'NONE',  ( 0.05219959533909260263, 19.03943276465977164, 44.99890960531435979 ) ) ;
#147512=CARTESIAN_POINT ( 'NONE',  ( -15.72974639402197994, 15.80617190586746368, 45.62390960531436690 ) ) ;
#147513=CARTESIAN_POINT ( 'NONE',  ( -0.05219959533909027116, -19.03943276465977164, 27.49890960531435624 ) ) ;
#147514=CARTESIAN_POINT ( 'NONE',  ( 16.53943276465976808, 0.05219959533934440121, 81.25109039468568994 ) ) ;
#147515=CARTESIAN_POINT ( 'NONE',  ( 13.97604488694527802, 13.89961937509977652, 64.37390960531436690 ) ) ;
#147516=CARTESIAN_POINT ( 'NONE',  ( -19.03943276465977164, -0.05219959533935918106, 38.75109039468566152 ) ) ;
#147517=CARTESIAN_POINT ( 'NONE',  ( -5.719274019375665041, -21.55341960407619695, 49.79275706135234714 ) ) ;
#147519=CARTESIAN_POINT ( 'NONE',  ( 5.719274019375991003, -21.55341960407610458, 37.70724293864769550 ) ) ;
#147521=CARTESIAN_POINT ( 'NONE',  ( -4.483927247898539470, -16.52544592524342804, 102.2905762719810383 ) ) ;
#147522=CARTESIAN_POINT ( 'NONE',  ( 13.89961937509957401, 13.97604488694547697, 86.87609039468567573 ) ) ;
#147524=CARTESIAN_POINT ( 'NONE',  ( -17.50000000001354294, 5.500000000000027534, 95.79690382535056870 ) ) ;
#147525=CARTESIAN_POINT ( 'NONE',  ( 18.62759615963271287, -10.81492255796078972, 48.33224293864770260 ) ) ;
#147526=CARTESIAN_POINT ( 'NONE',  ( 19.02544592524343514, -5.153800228976328945, 23.54057627198102054 ) ) ;
#147527=CARTESIAN_POINT ( 'NONE',  ( -5.823673210054431948, 21.52544592524334988, 87.70942372801901854 ) ) ;
#147528=CARTESIAN_POINT ( 'NONE',  ( 4.483927247898545687, 16.52544592524342804, 49.79057627198102409 ) ) ;
#147529=CARTESIAN_POINT ( 'NONE',  ( -16.53943276465976808, -0.05219959533934237506, 53.75109039468568994 ) ) ;
#147530=CARTESIAN_POINT ( 'NONE',  ( -8.314922557960811034, -14.29746914071050412, 57.08224293864769550 ) ) ;
#147531=CARTESIAN_POINT ( 'NONE',  ( -15.80617190586745835, -15.72974639402198527, 86.87390960531438111 ) ) ;
#147532=CARTESIAN_POINT ( 'NONE',  ( -21.52544592524343514, 5.823673210054127303, 71.04057627198103830 ) ) ;
#147534=CARTESIAN_POINT ( 'NONE',  ( -13.89961937509977652, 13.97604488694528158, 115.6239096053143669 ) ) ;
#147535=CARTESIAN_POINT ( 'NONE',  ( -9.474510206698964154, 16.51473224551069663, 65.41557627198102409 ) ) ;
#147536=CARTESIAN_POINT ( 'NONE',  ( -19.05341960407611168, -5.049401038298163336, 31.45724293864769550 ) ) ;
#147538=CARTESIAN_POINT ( 'NONE',  ( -12.06949235617739369, -12.14591786802326823, 84.37609039468570415 ) ) ;
#147539=CARTESIAN_POINT ( 'NONE',  ( -15.72974639402176322, -15.80617190586768395, 24.37609039468567573 ) ) ;
#147540=CARTESIAN_POINT ( 'NONE',  ( 13.89961937509977652, -13.97604488694527269, 68.12390960531436690 ) ) ;
#147541=CARTESIAN_POINT ( 'NONE',  ( 21.52544592524334988, 5.823673210054432836, 56.45942372801902565 ) ) ;
#147542=CARTESIAN_POINT ( 'NONE',  ( -19.03943276465977164, 0.05219959533909376836, 91.24890960531436690 ) ) ;
#147545=CARTESIAN_POINT ( 'NONE',  ( -15.72974639402176322, -15.80617190586768395, 44.37609039468567573 ) ) ;
#147546=CARTESIAN_POINT ( 'NONE',  ( -9.474510206698964154, 16.51473224551069663, 30.41557627198102054 ) ) ;
#147547=CARTESIAN_POINT ( 'NONE',  ( 19.03943276465977164, -0.05219959533909143690, 103.7489096053143669 ) ) ;
#147548=CARTESIAN_POINT ( 'NONE',  ( 9.474510206698729675, 16.51473224551082808, 57.08442372801900433 ) ) ;
#147549=CARTESIAN_POINT ( 'NONE',  ( -10.81492255796078084, -18.62759615963271287, 107.0822429386476955 ) ) ;
#147550=CARTESIAN_POINT ( 'NONE',  ( -13.89961937509957401, -13.97604488694547875, 49.37609039468567573 ) ) ;
#147551=CARTESIAN_POINT ( 'NONE',  ( -9.564922557961040184, 16.46253265017147172, 47.91775706135233293 ) ) ;
#147552=CARTESIAN_POINT ( 'NONE',  ( -8.314922557961024197, 14.29746914071037800, 107.9177570613523471 ) ) ;
#147553=ORIENTED_EDGE ( 'NONE', *, *, #111017, .F. ) ;
#147556=CARTESIAN_POINT ( 'NONE',  ( -13.97604488694527625, -13.89961937509977652, 76.87390960531433848 ) ) ;
#147558=CARTESIAN_POINT ( 'NONE',  ( 18.67979575497194134, -10.72451020669871369, 85.83442372801901854 ) ) ;
#147559=CARTESIAN_POINT ( 'NONE',  ( 18.67979575497194134, -10.72451020669871369, 95.83442372801903275 ) ) ;
#147561=CARTESIAN_POINT ( 'NONE',  ( -9.564922557960796823, -16.46253265017161027, 97.08224293864769550 ) ) ;
#147562=CARTESIAN_POINT ( 'NONE',  ( -18.62759615963255300, -10.81492255796106328, 74.16775706135231871 ) ) ;
#147563=CARTESIAN_POINT ( 'NONE',  ( 16.52544592524335698, 4.483927247898782831, 21.45942372801901499 ) ) ;
#147564=CARTESIAN_POINT ( 'NONE',  ( 5.153800228976335163, 19.02544592524342804, 79.79057627198102409 ) ) ;
#147565=CARTESIAN_POINT ( 'NONE',  ( -21.53943276465977519, 0.05219959533907696930, 21.24890960531436690 ) ) ;
#147566=CARTESIAN_POINT ( 'NONE',  ( 19.05341960407611168, 5.049401038298154454, 93.95724293864769550 ) ) ;
#147568=CARTESIAN_POINT ( 'NONE',  ( 16.51473224551069308, 9.474510206698969483, 79.16557627198103830 ) ) ;
#147569=CARTESIAN_POINT ( 'NONE',  ( 9.474510206698971260, -16.51473224551069308, 67.91557627198102409 ) ) ;
#147570=CARTESIAN_POINT ( 'NONE',  ( -0.05219959533907301413, -21.53943276465977519, 107.4989096053143669 ) ) ;
#147571=CARTESIAN_POINT ( 'NONE',  ( 0.05219959533934541429, -16.53943276465976808, 100.0010903946857042 ) ) ;
#147572=DIRECTION ( 'NONE',  ( -0.000000000000000000, -0.000000000000000000, 1.000000000000000000 ) ) ;
#147573=CARTESIAN_POINT ( 'NONE',  ( 16.46253265017146816, 9.564922557961045513, 51.66775706135233293 ) ) ;
#147574=CARTESIAN_POINT ( 'NONE',  ( -19.05341960407611168, -5.049401038298163336, 96.45724293864769550 ) ) ;
#147575=CARTESIAN_POINT ( 'NONE',  ( 4.379528057220339221, -16.55341960407611168, 82.70724293864770971 ) ) ;
#147576=CARTESIAN_POINT ( 'NONE',  ( 19.02544592524343514, -5.153800228976328945, 28.54057627198102409 ) ) ;
#147577=CARTESIAN_POINT ( 'NONE',  ( -21.55341960407610458, -5.719274019375992779, 36.45724293864768839 ) ) ;
#147578=CARTESIAN_POINT ( 'NONE',  ( -21.55341960407610458, -5.719274019375992779, 26.45724293864768839 ) ) ;
#147579=CARTESIAN_POINT ( 'NONE',  ( -8.314922557960811034, -14.29746914071050412, 87.08224293864769550 ) ) ;
#147581=CARTESIAN_POINT ( 'NONE',  ( 13.97604488694548053, -13.89961937509957401, 40.62609039468564731 ) ) ;
#147582=CARTESIAN_POINT ( 'NONE',  ( 4.483927247898790824, -16.52544592524335698, 105.2094237280190328 ) ) ;
#147583=CARTESIAN_POINT ( 'NONE',  ( 16.46253265017160672, -9.564922557960803928, 93.33224293864769550 ) ) ;
#147584=CARTESIAN_POINT ( 'NONE',  ( 15.80617190586769283, -15.72974639402175789, 65.62609039468568994 ) ) ;
#147585=CARTESIAN_POINT ( 'NONE',  ( -5.719274019375978568, 21.55341960407610458, 45.20724293864769550 ) ) ;
#147586=CARTESIAN_POINT ( 'NONE',  ( 21.53943276465977519, 0.05219959533937863772, 26.25109039468567573 ) ) ;
#147588=CARTESIAN_POINT ( 'NONE',  ( -21.55341960407610458, -5.719274019375992779, 86.45724293864770971 ) ) ;
#147589=CARTESIAN_POINT ( 'NONE',  ( -14.29746914071049879, 8.314922557960819915, 110.8322429386476955 ) ) ;
#147590=CARTESIAN_POINT ( 'NONE',  ( -13.97604488694547697, 13.89961937509957934, 68.12609039468563310 ) ) ;
#147591=CARTESIAN_POINT ( 'NONE',  ( 9.474510206698971260, -16.51473224551069308, 42.91557627198103120 ) ) ;
#147592=CARTESIAN_POINT ( 'NONE',  ( -19.02544592524342804, 5.153800228976336051, 91.04057627198100988 ) ) ;
#147593=CARTESIAN_POINT ( 'NONE',  ( -9.474510206698964154, 16.51473224551069663, 95.41557627198102409 ) ) ;
#147594=CARTESIAN_POINT ( 'NONE',  ( 4.379528057220339221, -16.55341960407611168, 112.7072429386476955 ) ) ;
#147595=CARTESIAN_POINT ( 'NONE',  ( 14.29746914071049879, -8.314922557960816363, 43.33224293864769550 ) ) ;
#147596=CARTESIAN_POINT ( 'NONE',  ( -12.14591786802326823, 12.06949235617739902, 38.12609039468567573 ) ) ;
#147597=CARTESIAN_POINT ( 'NONE',  ( 21.52544592524334988, 5.823673210054432836, 106.4594237280190328 ) ) ;
#147599=CARTESIAN_POINT ( 'NONE',  ( -16.52544592524342804, 4.483927247898546575, 26.04057627198103475 ) ) ;
#147600=CARTESIAN_POINT ( 'NONE',  ( 15.72974639402176855, 15.80617190586768217, 26.87609039468567218 ) ) ;
#147601=CARTESIAN_POINT ( 'NONE',  ( 19.05341960407611168, 5.049401038298154454, 108.9572429386477097 ) ) ;
#147602=CARTESIAN_POINT ( 'NONE',  ( 8.224510206698742110, 14.34966873604972548, 112.0844237280190185 ) ) ;
#147603=CARTESIAN_POINT ( 'NONE',  ( -12.14591786802326823, 12.06949235617739902, 93.12609039468568994 ) ) ;
#147604=CARTESIAN_POINT ( 'NONE',  ( -16.52544592524335698, -4.483927247898792601, 28.95942372801902209 ) ) ;
#147605=CARTESIAN_POINT ( 'NONE',  ( -19.02544592524342804, 5.153800228976336051, 51.04057627198103120 ) ) ;
#147606=CARTESIAN_POINT ( 'NONE',  ( -16.52544592524342804, 4.483927247898546575, 106.0405762719810525 ) ) ;
#147607=CARTESIAN_POINT ( 'NONE',  ( 21.53943276465977519, 0.05219959533937863772, 21.25109039468567218 ) ) ;
#147608=CARTESIAN_POINT ( 'NONE',  ( 16.46253265017160672, -9.564922557960803928, 28.33224293864769550 ) ) ;
#147609=CARTESIAN_POINT ( 'NONE',  ( -19.03943276465977164, 0.05219959533909376836, 106.2489096053143669 ) ) ;
#147610=CARTESIAN_POINT ( 'NONE',  ( 21.52544592524334988, 5.823673210054432836, 26.45942372801901854 ) ) ;
#147611=CARTESIAN_POINT ( 'NONE',  ( 16.51473224551069308, 9.474510206698969483, 29.16557627198103475 ) ) ;
#147613=CARTESIAN_POINT ( 'NONE',  ( -13.89961937509977652, 13.97604488694528158, 110.6239096053143243 ) ) ;
#147614=CARTESIAN_POINT ( 'NONE',  ( -16.29526858892874586, -7.335722546920246501, 35.79670597800209464 ) ) ;
#147615=CARTESIAN_POINT ( 'NONE',  ( -0.05219959533909027116, -19.03943276465977164, 102.4989096053143669 ) ) ;
#147616=CARTESIAN_POINT ( 'NONE',  ( 5.823673210054444382, -21.52544592524334988, 40.20942372801901854 ) ) ;
#147617=CARTESIAN_POINT ( 'NONE',  ( -16.52544592524342804, 4.483927247898546575, 96.04057627198102409 ) ) ;
#147618=CARTESIAN_POINT ( 'NONE',  ( 13.97604488694527802, 13.89961937509977652, 94.37390960531436690 ) ) ;
#147620=CARTESIAN_POINT ( 'NONE',  ( -8.314922557961024197, 14.29746914071037800, 67.91775706135234714 ) ) ;
#147621=CARTESIAN_POINT ( 'NONE',  ( 10.81492255796106328, -18.62759615963255655, 85.41775706135236135 ) ) ;
#147622=CARTESIAN_POINT ( 'NONE',  ( -8.314922557961024197, 14.29746914071037800, 42.91775706135235424 ) ) ;
#147623=CARTESIAN_POINT ( 'NONE',  ( 9.474510206698971260, -16.51473224551069308, 87.91557627198102409 ) ) ;
#147624=CARTESIAN_POINT ( 'NONE',  ( 9.474510206698729675, 16.51473224551082808, 107.0844237280190043 ) ) ;
#147625=CARTESIAN_POINT ( 'NONE',  ( -8.224510206698735004, -14.34966873604973081, 64.58442372801900433 ) ) ;
#147626=CARTESIAN_POINT ( 'NONE',  ( 9.474510206698729675, 16.51473224551082808, 97.08442372801900433 ) ) ;
#147627=CARTESIAN_POINT ( 'NONE',  ( 5.049401038298161559, -19.05341960407611168, 67.70724293864769550 ) ) ;
#147628=CARTESIAN_POINT ( 'NONE',  ( 0.05219959533907565091, 21.53943276465977519, 89.99890960531438111 ) ) ;
#147629=CARTESIAN_POINT ( 'NONE',  ( 14.34966873604960469, 8.224510206698951720, 84.16557627198103830 ) ) ;
#147630=CARTESIAN_POINT ( 'NONE',  ( 5.049401038297881783, 19.05341960407617563, 97.29275706135233293 ) ) ;
#147631=CARTESIAN_POINT ( 'NONE',  ( -14.29746914071037622, -8.314922557961029526, 54.16775706135235424 ) ) ;
#147633=CARTESIAN_POINT ( 'NONE',  ( -9.474510206698720793, -16.51473224551083518, 54.58442372801899722 ) ) ;
#147634=CARTESIAN_POINT ( 'NONE',  ( 16.53943276465976808, -0.05219959533910856209, 28.74890960531435624 ) ) ;
#147635=CARTESIAN_POINT ( 'NONE',  ( -12.06949235617756955, 12.14591786802309770, 75.62390960531439532 ) ) ;
#147636=CARTESIAN_POINT ( 'NONE',  ( 5.049401038297881783, 19.05341960407617563, 22.29275706135233648 ) ) ;
#147637=CARTESIAN_POINT ( 'NONE',  ( -17.31728774477213406, 6.344390552233685199, 40.81906651689308063 ) ) ;
#147638=CARTESIAN_POINT ( 'NONE',  ( -10.72451020669870658, -18.67979575497194134, 24.58442372801901499 ) ) ;
#147639=CARTESIAN_POINT ( 'NONE',  ( 16.46253265017160672, -9.564922557960803928, 108.3322429386476955 ) ) ;
#147640=CARTESIAN_POINT ( 'NONE',  ( 5.049401038298161559, -19.05341960407611168, 77.70724293864765286 ) ) ;
#147641=CARTESIAN_POINT ( 'NONE',  ( 21.52544592524334988, 5.823673210054432836, 101.4594237280190185 ) ) ;
#147642=CARTESIAN_POINT ( 'NONE',  ( 0.05219959533909260263, 19.03943276465977164, 74.99890960531435269 ) ) ;
#147643=CARTESIAN_POINT ( 'NONE',  ( 5.823673210054125526, 21.52544592524343514, 49.79057627198102409 ) ) ;
#147644=CARTESIAN_POINT ( 'NONE',  ( -12.14591786802309592, -12.06949235617757132, 76.87390960531439532 ) ) ;
#147645=CARTESIAN_POINT ( 'NONE',  ( 19.05341960407611168, 5.049401038298154454, 53.95724293864770260 ) ) ;
#147646=CARTESIAN_POINT ( 'NONE',  ( -8.224510206698948167, 14.34966873604960824, 110.4155762719810383 ) ) ;
#147648=CARTESIAN_POINT ( 'NONE',  ( 5.719274019375673035, 21.55341960407619339, 22.29275706135235069 ) ) ;
#147649=CARTESIAN_POINT ( 'NONE',  ( -21.53943276465977519, -0.05219959533937600094, 63.75109039468568284 ) ) ;
#147650=CARTESIAN_POINT ( 'NONE',  ( -13.97604488694527625, -13.89961937509977652, 41.87390960531435979 ) ) ;
#147651=CARTESIAN_POINT ( 'NONE',  ( -4.483927247898782831, 16.52544592524335698, 57.70942372801901143 ) ) ;
#147652=CARTESIAN_POINT ( 'NONE',  ( -21.53943276465977519, 0.05219959533907696930, 111.2489096053143669 ) ) ;
#147653=CARTESIAN_POINT ( 'NONE',  ( 0.05219959533907565091, 21.53943276465977519, 109.9989096053143527 ) ) ;
#147654=CARTESIAN_POINT ( 'NONE',  ( 19.02544592524334988, 5.153800228976608722, 41.45942372801900433 ) ) ;
#147655=CARTESIAN_POINT ( 'NONE',  ( -9.564922557960796823, -16.46253265017161027, 67.08224293864769550 ) ) ;
#147657=CARTESIAN_POINT ( 'NONE',  ( 21.53943276465977519, 0.05219959533937863772, 66.25109039468567573 ) ) ;
#147658=EDGE_CURVE ( 'NONE', #3830, #142224, #27790, .T. ) ;
#147659=CARTESIAN_POINT ( 'NONE',  ( -5.719274019375978568, 21.55341960407610458, 55.20724293864770260 ) ) ;
#147660=CARTESIAN_POINT ( 'NONE',  ( 8.224510206698953496, -14.34966873604960469, 37.91557627198102409 ) ) ;
#147661=CARTESIAN_POINT ( 'NONE',  ( 5.823673210054444382, -21.52544592524334988, 80.20942372801901854 ) ) ;
#147662=CARTESIAN_POINT ( 'NONE',  ( 19.02544592524334988, 5.153800228976608722, 21.45942372801899012 ) ) ;
#147663=CARTESIAN_POINT ( 'NONE',  ( 16.55341960407611168, 4.379528057220329451, 53.95724293864770260 ) ) ;
#147664=CARTESIAN_POINT ( 'NONE',  ( 16.53943276465976808, -0.05219959533910856209, 108.7489096053143669 ) ) ;
#147665=CARTESIAN_POINT ( 'NONE',  ( -9.474510206698720793, -16.51473224551083518, 59.58442372801900433 ) ) ;
#147666=CARTESIAN_POINT ( 'NONE',  ( -12.14591786802309592, -12.06949235617757132, 21.87390960531436690 ) ) ;
#147667=CARTESIAN_POINT ( 'NONE',  ( 10.72451020669871369, 18.67979575497193778, 62.08442372801901143 ) ) ;
#147668=CARTESIAN_POINT ( 'NONE',  ( 19.03943276465977164, -0.05219959533909143690, 78.74890960531436690 ) ) ;
#147669=CARTESIAN_POINT ( 'NONE',  ( 13.89961937509957401, 13.97604488694547697, 36.87609039468565442 ) ) ;
#147670=CARTESIAN_POINT ( 'NONE',  ( -5.823673210054116645, -21.52544592524344225, 32.29057627198102409 ) ) ;
#147671=CARTESIAN_POINT ( 'NONE',  ( -10.81492255796105439, 18.62759615963255655, 32.91775706135234714 ) ) ;
#147672=CARTESIAN_POINT ( 'NONE',  ( 5.719274019375991003, -21.55341960407610458, 107.7072429386476955 ) ) ;
#147673=CARTESIAN_POINT ( 'NONE',  ( -13.89961937509957401, -13.97604488694547875, 94.37609039468566152 ) ) ;
#147674=CARTESIAN_POINT ( 'NONE',  ( 8.224510206698742110, 14.34966873604972548, 52.08442372801901854 ) ) ;
#147676=CARTESIAN_POINT ( 'NONE',  ( -5.823673210054116645, -21.52544592524344225, 97.29057627198105251 ) ) ;
#147677=CARTESIAN_POINT ( 'NONE',  ( -0.05219959533910754901, -16.53943276465976808, 87.49890960531436690 ) ) ;
#147679=CARTESIAN_POINT ( 'NONE',  ( 14.29746914071037800, 8.314922557961029526, 26.66775706135235424 ) ) ;
#147680=CARTESIAN_POINT ( 'NONE',  ( 21.55341960407610458, 5.719274019375980345, 53.95724293864770260 ) ) ;
#147682=CARTESIAN_POINT ( 'NONE',  ( 0.05219959533934541429, -16.53943276465976808, 95.00109039468568994 ) ) ;
#147683=CARTESIAN_POINT ( 'NONE',  ( -18.22780087662123094, -5.499999999999984901, 76.48459894673894155 ) ) ;
#147684=CARTESIAN_POINT ( 'NONE',  ( -4.483927247898782831, 16.52544592524335698, 47.70942372801902565 ) ) ;
#147685=CARTESIAN_POINT ( 'NONE',  ( -5.823673210054431948, 21.52544592524334988, 27.70942372801901854 ) ) ;
#147686=CARTESIAN_POINT ( 'NONE',  ( 21.52544592524344225, -5.823673210054117533, 43.54057627198103830 ) ) ;
#147687=CARTESIAN_POINT ( 'NONE',  ( 4.483927247898790824, -16.52544592524335698, 90.20942372801903275 ) ) ;
#147688=CARTESIAN_POINT ( 'NONE',  ( 13.89961937509977652, -13.97604488694527269, 103.1239096053143527 ) ) ;
#147689=CARTESIAN_POINT ( 'NONE',  ( 18.62759615963255655, 10.81492255796105972, 71.66775706135234714 ) ) ;
#147690=CARTESIAN_POINT ( 'NONE',  ( 21.52544592524344225, -5.823673210054117533, 33.54057627198102409 ) ) ;
#147691=CARTESIAN_POINT ( 'NONE',  ( -21.55341960407610458, -5.719274019375992779, 21.45724293864769550 ) ) ;
#147693=CARTESIAN_POINT ( 'NONE',  ( 9.564922557961047289, -16.46253265017146816, 55.41775706135234003 ) ) ;
#147694=CARTESIAN_POINT ( 'NONE',  ( 4.483927247898790824, -16.52544592524335698, 65.20942372801901854 ) ) ;
#147695=CARTESIAN_POINT ( 'NONE',  ( 21.55341960407610458, 5.719274019375980345, 33.95724293864769550 ) ) ;
#147697=CARTESIAN_POINT ( 'NONE',  ( -5.049401038298153566, 19.05341960407611168, 80.20724293864769550 ) ) ;
#147698=CARTESIAN_POINT ( 'NONE',  ( -16.55341960407617563, 4.379528057220093196, 93.54275706135234714 ) ) ;
#147700=CARTESIAN_POINT ( 'NONE',  ( -16.53943276465976808, 0.05219959533911058130, 111.2489096053143669 ) ) ;
#147701=CARTESIAN_POINT ( 'NONE',  ( -10.81492255796078084, -18.62759615963271287, 47.08224293864770260 ) ) ;
#147702=CARTESIAN_POINT ( 'NONE',  ( 19.02544592524343514, -5.153800228976328945, 38.54057627198103120 ) ) ;
#147703=CARTESIAN_POINT ( 'NONE',  ( -14.34966873604972548, 8.224510206698743886, 73.33442372801901854 ) ) ;
#147704=CARTESIAN_POINT ( 'NONE',  ( -10.81492255796105439, 18.62759615963255655, 32.91775706135234714 ) ) ;
#147705=CARTESIAN_POINT ( 'NONE',  ( 13.97604488694548053, -13.89961937509957401, 90.62609039468567573 ) ) ;
#147706=CARTESIAN_POINT ( 'NONE',  ( 4.483927247898545687, 16.52544592524342804, 94.79057627198105251 ) ) ;
#147707=CARTESIAN_POINT ( 'NONE',  ( 5.153800228976335163, 19.02544592524342804, 49.79057627198100988 ) ) ;
#147709=CARTESIAN_POINT ( 'NONE',  ( -16.51473224551069308, -9.474510206698971260, 26.66557627198103120 ) ) ;
#147710=CARTESIAN_POINT ( 'NONE',  ( -18.67979575497193778, 10.72451020669871902, 108.3344237280190185 ) ) ;
#147711=CARTESIAN_POINT ( 'NONE',  ( 19.02544592524343514, -5.153800228976328945, 78.54057627198099567 ) ) ;
#147712=CARTESIAN_POINT ( 'NONE',  ( 16.53943276465976808, 0.05219959533934440121, 61.25109039468567573 ) ) ;
#147713=CARTESIAN_POINT ( 'NONE',  ( 21.55341960407619695, -5.719274019375665929, 96.04275706135236135 ) ) ;
#147714=CARTESIAN_POINT ( 'NONE',  ( -0.05219959533934338120, 16.53943276465976808, 77.50109039468567573 ) ) ;
#147715=CARTESIAN_POINT ( 'NONE',  ( 19.05341960407617918, -5.049401038297876454, 56.04275706135234714 ) ) ;
#147716=CARTESIAN_POINT ( 'NONE',  ( -16.46253265017146816, -9.564922557961047289, 69.16775706135233293 ) ) ;
#147717=CARTESIAN_POINT ( 'NONE',  ( -10.81492255796105439, 18.62759615963255655, 62.91775706135236135 ) ) ;
#147718=CARTESIAN_POINT ( 'NONE',  ( -9.474510206698964154, 16.51473224551069663, 70.41557627198102409 ) ) ;
#147720=CARTESIAN_POINT ( 'NONE',  ( 5.153800228976615827, -19.02544592524334988, 65.20942372801900433 ) ) ;
#147721=CARTESIAN_POINT ( 'NONE',  ( -0.05219959533909027116, -19.03943276465977164, 112.4989096053143669 ) ) ;
#147722=CARTESIAN_POINT ( 'NONE',  ( -13.89961937509977652, 13.97604488694528158, 80.62390960531436690 ) ) ;
#147723=CARTESIAN_POINT ( 'NONE',  ( 12.06949235617757843, -12.14591786802309237, 33.12390960531435979 ) ) ;
#147724=CARTESIAN_POINT ( 'NONE',  ( -21.52544592524343514, 5.823673210054127303, 51.04057627198103120 ) ) ;
#147725=CARTESIAN_POINT ( 'NONE',  ( 22.00000000000000000, -5.510910596163089556E-15, 45.00000000000000000 ) ) ;
#147726=CARTESIAN_POINT ( 'NONE',  ( -9.474510206698720793, -16.51473224551083518, 19.58442372801899722 ) ) ;
#147727=CARTESIAN_POINT ( 'NONE',  ( -16.81555441253555117, -7.025013491695478507, 79.36314554665743515 ) ) ;
#147728=CARTESIAN_POINT ( 'NONE',  ( 19.05341960407611168, 5.049401038298154454, 33.95724293864769550 ) ) ;
#147729=CARTESIAN_POINT ( 'NONE',  ( 13.97604488694527802, 13.89961937509977652, 29.37390960531435979 ) ) ;
#147731=CARTESIAN_POINT ( 'NONE',  ( 5.719274019375673035, 21.55341960407619339, 67.29275706135234714 ) ) ;
#147733=CARTESIAN_POINT ( 'NONE',  ( 8.224510206698742110, 14.34966873604972548, 57.08442372801901854 ) ) ;
#147734=CARTESIAN_POINT ( 'NONE',  ( -18.62759615963270932, 10.81492255796079327, 85.83224293864768129 ) ) ;
#147735=CARTESIAN_POINT ( 'NONE',  ( 16.53943276465976808, -0.05219959533910856209, 53.74890960531437401 ) ) ;
#147736=CARTESIAN_POINT ( 'NONE',  ( 9.564922557960805705, 16.46253265017160317, 24.58224293864769194 ) ) ;
#147738=CARTESIAN_POINT ( 'NONE',  ( 21.55341960407619695, -5.719274019375665929, 41.04275706135236135 ) ) ;
#147739=CARTESIAN_POINT ( 'NONE',  ( 13.89961937509957401, 13.97604488694547697, 46.87609039468565442 ) ) ;
#147740=CARTESIAN_POINT ( 'NONE',  ( 19.03943276465977164, -0.05219959533909143690, 28.74890960531435624 ) ) ;
#147741=CARTESIAN_POINT ( 'NONE',  ( -15.80617190586768217, 15.72974639402176855, 88.12609039468570415 ) ) ;
#147742=CARTESIAN_POINT ( 'NONE',  ( -16.51473224551069308, -9.474510206698971260, 21.66557627198102765 ) ) ;
#147743=CARTESIAN_POINT ( 'NONE',  ( 8.314922557960818139, 14.29746914071049879, 44.58224293864769550 ) ) ;
#147745=CARTESIAN_POINT ( 'NONE',  ( -21.55341960407610458, -5.719274019375992779, 46.45724293864769550 ) ) ;
#147747=CARTESIAN_POINT ( 'NONE',  ( -9.564922557960796823, -16.46253265017161027, 87.08224293864769550 ) ) ;
#147748=CARTESIAN_POINT ( 'NONE',  ( -8.314922557960811034, -14.29746914071050412, 92.08224293864769550 ) ) ;
#147749=CARTESIAN_POINT ( 'NONE',  ( 8.224510206698742110, 14.34966873604972548, 22.08442372801901143 ) ) ;
#147750=CARTESIAN_POINT ( 'NONE',  ( -21.53943276465977519, 0.05219959533907696930, 61.24890960531435979 ) ) ;
#147753=CARTESIAN_POINT ( 'NONE',  ( 13.89961937509977652, -13.97604488694527269, 33.12390960531434558 ) ) ;
#147754=CARTESIAN_POINT ( 'NONE',  ( 0.05219959533909260263, 19.03943276465977164, 79.99890960531436690 ) ) ;
#147755=CARTESIAN_POINT ( 'NONE',  ( -18.62759615963270932, 10.81492255796079327, 90.83224293864769550 ) ) ;
#147756=CARTESIAN_POINT ( 'NONE',  ( 14.34966873604960469, 8.224510206698951720, 29.16557627198103120 ) ) ;
#147757=CARTESIAN_POINT ( 'NONE',  ( -0.05219959533909027116, -19.03943276465977164, 97.49890960531436690 ) ) ;
#147758=CARTESIAN_POINT ( 'NONE',  ( -16.46253265017146816, -9.564922557961047289, 74.16775706135234714 ) ) ;
#147759=CARTESIAN_POINT ( 'NONE',  ( 5.719274019375673035, 21.55341960407619339, 112.2927570613523471 ) ) ;
#147760=CARTESIAN_POINT ( 'NONE',  ( -5.719274019375978568, 21.55341960407610458, 70.20724293864769550 ) ) ;
#147761=CARTESIAN_POINT ( 'NONE',  ( 5.719274019375991003, -21.55341960407610458, 37.70724293864769550 ) ) ;
#147762=CARTESIAN_POINT ( 'NONE',  ( -9.564922557960796823, -16.46253265017161027, 52.08224293864768839 ) ) ;
#147763=CARTESIAN_POINT ( 'NONE',  ( 8.314922557960818139, 14.29746914071049879, 24.58224293864768839 ) ) ;
#147764=CARTESIAN_POINT ( 'NONE',  ( -5.049401038298153566, 19.05341960407611168, 75.20724293864769550 ) ) ;
#147765=VERTEX_POINT ( 'NONE', #167276 ) ;
#147766=CARTESIAN_POINT ( 'NONE',  ( 17.49999999999999645, -5.500000000000031086, 83.29690382534172954 ) ) ;
#147767=CARTESIAN_POINT ( 'NONE',  ( 0.05219959533936267826, -19.03943276465977164, 30.00109039468566863 ) ) ;
#147768=CARTESIAN_POINT ( 'NONE',  ( -12.06949235617756955, 12.14591786802309770, 85.62390960531436690 ) ) ;
#147769=CARTESIAN_POINT ( 'NONE',  ( 5.823673210054444382, -21.52544592524334988, 20.20942372801900788 ) ) ;
#147771=CARTESIAN_POINT ( 'NONE',  ( -21.55341960407610458, -5.719274019375992779, 61.45724293864770260 ) ) ;
#147772=CARTESIAN_POINT ( 'NONE',  ( -8.314922557961024197, 14.29746914071037800, 87.91775706135234714 ) ) ;
#147773=CARTESIAN_POINT ( 'NONE',  ( -12.14591786802309592, -12.06949235617757132, 111.8739096053143669 ) ) ;
#147774=CARTESIAN_POINT ( 'NONE',  ( 9.474510206698971260, -16.51473224551069308, 72.91557627198102409 ) ) ;
#147776=CARTESIAN_POINT ( 'NONE',  ( 14.34966873604960469, 8.224510206698951720, 24.16557627198103120 ) ) ;
#147777=EDGE_CURVE ( 'NONE', #88586, #4577, #64462, .T. ) ;
#147778=CARTESIAN_POINT ( 'NONE',  ( 21.55341960407619695, -5.719274019375665929, 56.04275706135235424 ) ) ;
#147779=CARTESIAN_POINT ( 'NONE',  ( -19.03943276465977164, 0.05219959533909376836, 116.2489096053143669 ) ) ;
#147780=CARTESIAN_POINT ( 'NONE',  ( -15.72974639402176322, -15.80617190586768395, 99.37609039468568994 ) ) ;
#147781=CARTESIAN_POINT ( 'NONE',  ( 13.89961937509977652, -13.97604488694527269, 48.12390960531435979 ) ) ;
#147782=CARTESIAN_POINT ( 'NONE',  ( -13.89961937509977652, 13.97604488694528158, 50.62390960531435979 ) ) ;
#147783=VERTEX_POINT ( 'NONE', #139881 ) ;
#147784=CARTESIAN_POINT ( 'NONE',  ( -15.72974639402176322, -15.80617190586768395, 99.37609039468568994 ) ) ;
#147785=CARTESIAN_POINT ( 'NONE',  ( -16.55341960407617563, 4.379528057220093196, 63.54275706135234003 ) ) ;
#147786=CARTESIAN_POINT ( 'NONE',  ( -21.53943276465977519, -0.05219959533937600094, 88.75109039468567573 ) ) ;
#147787=CARTESIAN_POINT ( 'NONE',  ( -5.719274019375978568, 21.55341960407610458, 25.20724293864769550 ) ) ;
#147788=CARTESIAN_POINT ( 'NONE',  ( -5.153800228976607833, 19.02544592524334988, 92.70942372801901854 ) ) ;
#147789=CARTESIAN_POINT ( 'NONE',  ( -5.719274019375665041, -21.55341960407619695, 49.79275706135234714 ) ) ;
#147790=CARTESIAN_POINT ( 'NONE',  ( -4.483927247898782831, 16.52544592524335698, 42.70942372801901854 ) ) ;
#147791=CARTESIAN_POINT ( 'NONE',  ( 21.55341960407610458, 5.719274019375980345, 83.95724293864770971 ) ) ;
#147792=CARTESIAN_POINT ( 'NONE',  ( -19.03943276465977164, -0.05219959533935918106, 83.75109039468567573 ) ) ;
#147793=CARTESIAN_POINT ( 'NONE',  ( 5.153800228976335163, 19.02544592524342804, 64.79057627198100988 ) ) ;
#147794=CARTESIAN_POINT ( 'NONE',  ( 13.97604488694548053, -13.89961937509957401, 100.6260903946856615 ) ) ;
#147796=CARTESIAN_POINT ( 'NONE',  ( 16.46253265017146816, 9.564922557961045513, 91.66775706135234714 ) ) ;
#147797=CARTESIAN_POINT ( 'NONE',  ( 16.53943276465976808, -0.05219959533910856209, 48.74890960531435979 ) ) ;
#147798=CARTESIAN_POINT ( 'NONE',  ( 19.02544592524334988, 5.153800228976608722, 76.45942372801897591 ) ) ;
#147799=CARTESIAN_POINT ( 'NONE',  ( 8.224510206698742110, 14.34966873604972548, 62.08442372801901143 ) ) ;
#147800=CARTESIAN_POINT ( 'NONE',  ( 5.153800228976615827, -19.02544592524334988, 25.20942372801900433 ) ) ;
#147801=CARTESIAN_POINT ( 'NONE',  ( 13.97604488694527802, 13.89961937509977652, 44.37390960531435269 ) ) ;
#147802=CARTESIAN_POINT ( 'NONE',  ( -16.51473224551069308, -9.474510206698971260, 46.66557627198102409 ) ) ;
#147803=CARTESIAN_POINT ( 'NONE',  ( 12.06949235617739724, 12.14591786802326823, 61.87609039468568284 ) ) ;
#147806=CARTESIAN_POINT ( 'NONE',  ( 13.97604488694527802, 13.89961937509977652, 104.3739096053143385 ) ) ;
#147809=CARTESIAN_POINT ( 'NONE',  ( -16.46253265017146816, -9.564922557961047289, 94.16775706135233293 ) ) ;
#147810=CARTESIAN_POINT ( 'NONE',  ( 0.05219959533907565091, 21.53943276465977519, 39.99890960531436690 ) ) ;
#147811=CARTESIAN_POINT ( 'NONE',  ( 5.049401038297881783, 19.05341960407617563, 32.29275706135233293 ) ) ;
#147812=CARTESIAN_POINT ( 'NONE',  ( 16.51473224551083163, -9.474510206698727899, 105.8344237280190043 ) ) ;
#147813=CARTESIAN_POINT ( 'NONE',  ( -13.97604488694527625, -13.89961937509977652, 31.87390960531435979 ) ) ;
#147814=CARTESIAN_POINT ( 'NONE',  ( 16.51473224551069308, 9.474510206698969483, 44.16557627198103120 ) ) ;
#147815=CARTESIAN_POINT ( 'NONE',  ( -21.53943276465977519, 0.05219959533907696930, 66.24890960531436690 ) ) ;
#147816=CARTESIAN_POINT ( 'NONE',  ( -0.05219959533909027116, -19.03943276465977164, 97.49890960531436690 ) ) ;
#147817=CARTESIAN_POINT ( 'NONE',  ( 16.46253265017160672, -9.564922557960803928, 38.33224293864768839 ) ) ;
#147819=CARTESIAN_POINT ( 'NONE',  ( -9.474510206698720793, -16.51473224551083518, 84.58442372801900433 ) ) ;
#147820=CARTESIAN_POINT ( 'NONE',  ( 16.53943276465976808, -0.05219959533910856209, 48.74890960531435979 ) ) ;
#147822=CARTESIAN_POINT ( 'NONE',  ( 18.67979575497178502, 10.72451020669898547, 29.16557627198103120 ) ) ;
#147823=CARTESIAN_POINT ( 'NONE',  ( -21.55341960407619339, 5.719274019375674811, 103.5427570613523613 ) ) ;
#147824=CARTESIAN_POINT ( 'NONE',  ( -0.05219959533907301413, -21.53943276465977519, 102.4989096053143811 ) ) ;
#147825=CARTESIAN_POINT ( 'NONE',  ( -5.719274019375665041, -21.55341960407619695, 74.79275706135234714 ) ) ;
#147826=CARTESIAN_POINT ( 'NONE',  ( 15.72974639402176855, 15.80617190586768217, 76.87609039468567573 ) ) ;
#147827=CARTESIAN_POINT ( 'NONE',  ( -16.46253265017160317, 9.564922557960807481, 115.8322429386477097 ) ) ;
#147828=CARTESIAN_POINT ( 'NONE',  ( -14.34966873604972548, 8.224510206698743886, 108.3344237280190185 ) ) ;
#147829=CARTESIAN_POINT ( 'NONE',  ( 5.719274019375673035, 21.55341960407619339, 57.29275706135234714 ) ) ;
#147830=CARTESIAN_POINT ( 'NONE',  ( -9.564922557960796823, -16.46253265017161027, 72.08224293864770971 ) ) ;
#147831=CARTESIAN_POINT ( 'NONE',  ( -19.05341960407617563, 5.049401038297882671, 38.54275706135233293 ) ) ;
#147832=CARTESIAN_POINT ( 'NONE',  ( -0.05219959533937732626, 21.53943276465977519, 27.50109039468567929 ) ) ;
#147833=CARTESIAN_POINT ( 'NONE',  ( -0.05219959533909027116, -19.03943276465977164, 62.49890960531435979 ) ) ;
#147834=CARTESIAN_POINT ( 'NONE',  ( 14.34966873604960469, 8.224510206698951720, 84.16557627198103830 ) ) ;
#147835=CARTESIAN_POINT ( 'NONE',  ( -16.52544592524342804, 4.483927247898546575, 41.04057627198103120 ) ) ;
#147836=CARTESIAN_POINT ( 'NONE',  ( -21.55341960407610458, -5.719274019375992779, 51.45724293864770260 ) ) ;
#147837=CARTESIAN_POINT ( 'NONE',  ( 5.153800228976335163, 19.02544592524342804, 64.79057627198100988 ) ) ;
#147838=CARTESIAN_POINT ( 'NONE',  ( 18.62759615963271287, -10.81492255796078972, 78.33224293864770971 ) ) ;
#147839=CARTESIAN_POINT ( 'NONE',  ( -19.02544592524334988, -5.153800228976617603, 53.95942372801898301 ) ) ;
#147840=CARTESIAN_POINT ( 'NONE',  ( 13.89961937509957579, 13.97604488694547520, 21.87609039468566152 ) ) ;
#147841=CARTESIAN_POINT ( 'NONE',  ( -14.34966873604960291, -8.224510206698953496, 56.66557627198103830 ) ) ;
#147842=CARTESIAN_POINT ( 'NONE',  ( 10.72451020669898902, -18.67979575497178502, 42.91557627198103120 ) ) ;
#147844=DIRECTION ( 'NONE',  ( 0.000000000000000000, -1.000000000000000000, 0.000000000000000000 ) ) ;
#147845=CARTESIAN_POINT ( 'NONE',  ( 14.34966873604972726, -8.224510206698740333, 85.83442372801901854 ) ) ;
#147847=CARTESIAN_POINT ( 'NONE',  ( 5.153800228976615827, -19.02544592524334988, 90.20942372801900433 ) ) ;
#147848=CARTESIAN_POINT ( 'NONE',  ( 16.53943276465976808, -0.05219959533910856209, 58.74890960531436690 ) ) ;
#147850=CARTESIAN_POINT ( 'NONE',  ( 13.97604488694527802, 13.89961937509977652, 44.37390960531435269 ) ) ;
#147851=CARTESIAN_POINT ( 'NONE',  ( -12.14591786802309592, -12.06949235617757132, 41.87390960531435979 ) ) ;
#147852=CARTESIAN_POINT ( 'NONE',  ( 9.474510206698971260, -16.51473224551069308, 87.91557627198102409 ) ) ;
#147853=CARTESIAN_POINT ( 'NONE',  ( -13.97604488694527625, -13.89961937509977652, 51.87390960531436690 ) ) ;
#147854=CARTESIAN_POINT ( 'NONE',  ( -5.823673210054431948, 21.52544592524334988, 57.70942372801901143 ) ) ;
#147855=CARTESIAN_POINT ( 'NONE',  ( 19.02544592524343514, -5.153800228976328945, 78.54057627198099567 ) ) ;
#147856=CARTESIAN_POINT ( 'NONE',  ( -19.03943276465977164, 0.05219959533909376836, 26.24890960531435624 ) ) ;
#147857=CARTESIAN_POINT ( 'NONE',  ( 19.03943276465977164, -0.05219959533909143690, 73.74890960531435269 ) ) ;
#147859=CARTESIAN_POINT ( 'NONE',  ( -18.67979575497178146, -10.72451020669898902, 46.66557627198102409 ) ) ;
#147860=CARTESIAN_POINT ( 'NONE',  ( 9.474510206698971260, -16.51473224551069308, 32.91557627198102409 ) ) ;
#147861=CARTESIAN_POINT ( 'NONE',  ( -10.81492255796078084, -18.62759615963271287, 47.08224293864770260 ) ) ;
#147862=CARTESIAN_POINT ( 'NONE',  ( 16.55341960407618274, -4.379528057220086978, 101.0427570613523756 ) ) ;
#147863=CARTESIAN_POINT ( 'NONE',  ( 9.564922557961047289, -16.46253265017146816, 25.41775706135234003 ) ) ;
#147864=CARTESIAN_POINT ( 'NONE',  ( 14.34966873604972726, -8.224510206698740333, 45.83442372801901854 ) ) ;
#147865=CARTESIAN_POINT ( 'NONE',  ( -16.52544592524335698, -4.483927247898792601, 73.95942372801901854 ) ) ;
#147867=CARTESIAN_POINT ( 'NONE',  ( 16.53943276465976808, 0.05219959533934440121, 71.25109039468568994 ) ) ;
#147868=CARTESIAN_POINT ( 'NONE',  ( 10.81492255796078972, 18.62759615963270932, 24.58224293864768839 ) ) ;
#147869=CARTESIAN_POINT ( 'NONE',  ( -5.153800228976328057, -19.02544592524343514, 37.29057627198102409 ) ) ;
#147870=CARTESIAN_POINT ( 'NONE',  ( 8.314922557961029526, -14.29746914071037800, 35.41775706135234003 ) ) ;
#147871=CARTESIAN_POINT ( 'NONE',  ( 19.02544592524343514, -5.153800228976328945, 48.54057627198103120 ) ) ;
#147872=CARTESIAN_POINT ( 'NONE',  ( 21.53943276465977519, 0.05219959533937863772, 46.25109039468567573 ) ) ;
#147873=CARTESIAN_POINT ( 'NONE',  ( -14.29746914071037622, -8.314922557961029526, 34.16775706135234714 ) ) ;
#147874=CARTESIAN_POINT ( 'NONE',  ( -16.55341960407617563, 4.379528057220093196, 103.5427570613523613 ) ) ;
#147876=CARTESIAN_POINT ( 'NONE',  ( 15.80617190586769283, -15.72974639402175789, 95.62609039468568994 ) ) ;
#147877=CARTESIAN_POINT ( 'NONE',  ( 13.89961937509957401, 13.97604488694547697, 101.8760903946856331 ) ) ;
#147878=CARTESIAN_POINT ( 'NONE',  ( -5.049401038297874678, -19.05341960407617918, 49.79275706135231871 ) ) ;
#147879=CARTESIAN_POINT ( 'NONE',  ( -12.06949235617756955, 12.14591786802309770, 75.62390960531439532 ) ) ;
#147880=CARTESIAN_POINT ( 'NONE',  ( 0.05219959533909260263, 19.03943276465977164, 29.99890960531435979 ) ) ;
#147881=CARTESIAN_POINT ( 'NONE',  ( 19.02544592524334988, 5.153800228976608722, 56.45942372801898301 ) ) ;
#147883=CARTESIAN_POINT ( 'NONE',  ( -5.823673210054431948, 21.52544592524334988, 57.70942372801901143 ) ) ;
#147884=CARTESIAN_POINT ( 'NONE',  ( -16.52544592524335698, -4.483927247898792601, 23.95942372801901143 ) ) ;
#147886=CARTESIAN_POINT ( 'NONE',  ( 10.81492255796078972, 18.62759615963270932, 24.58224293864768839 ) ) ;
#147887=CARTESIAN_POINT ( 'NONE',  ( -19.02544592524334988, -5.153800228976617603, 103.9594237280190043 ) ) ;
#147888=CARTESIAN_POINT ( 'NONE',  ( -13.89961937509977652, 13.97604488694528158, 115.6239096053143669 ) ) ;
#147890=CARTESIAN_POINT ( 'NONE',  ( -14.29746914071049879, 8.314922557960819915, 115.8322429386477097 ) ) ;
#147891=CARTESIAN_POINT ( 'NONE',  ( -19.02544592524334988, -5.153800228976617603, 18.95942372801899722 ) ) ;
#147892=CARTESIAN_POINT ( 'NONE',  ( -9.564922557960796823, -16.46253265017161027, 57.08224293864769550 ) ) ;
#147893=CARTESIAN_POINT ( 'NONE',  ( 21.53943276465977519, 0.05219959533937863772, 66.25109039468567573 ) ) ;
#147894=CARTESIAN_POINT ( 'NONE',  ( -21.53943276465977519, -0.05219959533937600094, 108.7510903946857042 ) ) ;
#147895=CARTESIAN_POINT ( 'NONE',  ( -12.06949235617756955, 12.14591786802309770, 25.62390960531435624 ) ) ;
#147896=CARTESIAN_POINT ( 'NONE',  ( -5.049401038298153566, 19.05341960407611168, 80.20724293864769550 ) ) ;
#147897=CARTESIAN_POINT ( 'NONE',  ( 0.05219959533937995610, -21.53943276465977519, 55.00109039468568284 ) ) ;
#147898=CARTESIAN_POINT ( 'NONE',  ( 5.823673210054444382, -21.52544592524334988, 50.20942372801901854 ) ) ;
#147899=CARTESIAN_POINT ( 'NONE',  ( 19.05341960407617918, -5.049401038297876454, 76.04275706135230450 ) ) ;
#147900=CARTESIAN_POINT ( 'NONE',  ( -16.46253265017160317, 9.564922557960807481, 110.8322429386476955 ) ) ;
#147901=CARTESIAN_POINT ( 'NONE',  ( 0.05219959533910956823, 16.53943276465976808, 114.9989096053143669 ) ) ;
#147902=CARTESIAN_POINT ( 'NONE',  ( 21.53943276465977519, -0.05219959533907433946, 98.74890960531438111 ) ) ;
#147903=CARTESIAN_POINT ( 'NONE',  ( -13.97604488694547697, 13.89961937509957934, 23.12609039468565442 ) ) ;
#147904=CARTESIAN_POINT ( 'NONE',  ( -16.52544592524342804, 4.483927247898546575, 101.0405762719810383 ) ) ;
#147905=CARTESIAN_POINT ( 'NONE',  ( -19.03943276465977164, 0.05219959533909376836, 46.24890960531435979 ) ) ;
#147906=CARTESIAN_POINT ( 'NONE',  ( 5.049401038297881783, 19.05341960407617563, 97.29275706135233293 ) ) ;
#147907=CARTESIAN_POINT ( 'NONE',  ( -16.53943276465976808, 0.05219959533911058130, 66.24890960531436690 ) ) ;
#147908=CARTESIAN_POINT ( 'NONE',  ( 18.62759615963255655, 10.81492255796105972, 106.6677570613523756 ) ) ;
#147909=CARTESIAN_POINT ( 'NONE',  ( 19.05341960407611168, 5.049401038298154454, 98.95724293864766707 ) ) ;
#147910=CARTESIAN_POINT ( 'NONE',  ( -5.049401038297874678, -19.05341960407617918, 74.79275706135231871 ) ) ;
#147911=CARTESIAN_POINT ( 'NONE',  ( -18.67979575497178146, -10.72451020669898902, 91.66557627198103830 ) ) ;
#147912=CARTESIAN_POINT ( 'NONE',  ( -18.67979575497193778, 10.72451020669871902, 48.33442372801902565 ) ) ;
#147913=CARTESIAN_POINT ( 'NONE',  ( -4.483927247898782831, 16.52544592524335698, 47.70942372801902565 ) ) ;
#147914=CARTESIAN_POINT ( 'NONE',  ( -0.05219959533934338120, 16.53943276465976808, 87.50109039468568994 ) ) ;
#147915=CARTESIAN_POINT ( 'NONE',  ( 16.53943276465976808, 0.05219959533934440121, 46.25109039468567573 ) ) ;
#147916=CARTESIAN_POINT ( 'NONE',  ( 10.72451020669871369, 18.67979575497193778, 32.08442372801901854 ) ) ;
#147917=CARTESIAN_POINT ( 'NONE',  ( 10.72451020669898902, -18.67979575497178502, 47.91557627198102409 ) ) ;
#147918=CARTESIAN_POINT ( 'NONE',  ( -5.153800228976328057, -19.02544592524343514, 32.29057627198102409 ) ) ;
#147920=CARTESIAN_POINT ( 'NONE',  ( -14.34966873604972548, 8.224510206698743886, 58.33442372801901143 ) ) ;
#147921=CARTESIAN_POINT ( 'NONE',  ( -5.719274019375978568, 21.55341960407610458, 85.20724293864770971 ) ) ;
#147922=CARTESIAN_POINT ( 'NONE',  ( 16.53943276465976808, -0.05219959533910856209, 43.74890960531435979 ) ) ;
#147923=CARTESIAN_POINT ( 'NONE',  ( 8.314922557961029526, -14.29746914071037800, 60.41775706135235424 ) ) ;
#147924=CARTESIAN_POINT ( 'NONE',  ( -13.97604488694527625, -13.89961937509977652, 61.87390960531435979 ) ) ;
#147925=CARTESIAN_POINT ( 'NONE',  ( -9.564922557961040184, 16.46253265017147172, 92.91775706135233293 ) ) ;
#147926=CARTESIAN_POINT ( 'NONE',  ( 21.55341960407610458, 5.719274019375980345, 78.95724293864769550 ) ) ;
#147927=CARTESIAN_POINT ( 'NONE',  ( -16.55341960407611168, -4.379528057220339221, 36.45724293864768839 ) ) ;
#147930=CARTESIAN_POINT ( 'NONE',  ( 18.62759615963271287, -10.81492255796078972, 63.33224293864770260 ) ) ;
#147931=ORIENTED_EDGE ( 'NONE', *, *, #59992, .T. ) ;
#147932=CARTESIAN_POINT ( 'NONE',  ( 14.34966873604972726, -8.224510206698740333, 110.8344237280190043 ) ) ;
#147934=CARTESIAN_POINT ( 'NONE',  ( 19.34837522270367671, 5.499999999999739764, 88.36337684832572847 ) ) ;
#147935=CARTESIAN_POINT ( 'NONE',  ( -21.53943276465977519, 0.05219959533907696930, 86.24890960531436690 ) ) ;
#147936=CARTESIAN_POINT ( 'NONE',  ( 8.314922557960818139, 14.29746914071049879, 24.58224293864768839 ) ) ;
#147937=CARTESIAN_POINT ( 'NONE',  ( 16.55341960407618274, -4.379528057220086978, 36.04275706135234714 ) ) ;
#147938=CARTESIAN_POINT ( 'NONE',  ( 16.46253265017160672, -9.564922557960803928, 38.33224293864768839 ) ) ;
#147939=CARTESIAN_POINT ( 'NONE',  ( 5.153800228976335163, 19.02544592524342804, 64.79057627198100988 ) ) ;
#147941=CARTESIAN_POINT ( 'NONE',  ( -9.564922557960796823, -16.46253265017161027, 112.0822429386476955 ) ) ;
#147943=CARTESIAN_POINT ( 'NONE',  ( -16.53943276465976808, -0.05219959533934237506, 98.75109039468568994 ) ) ;
#147944=CARTESIAN_POINT ( 'NONE',  ( 16.51473224551083163, -9.474510206698727899, 105.8344237280190043 ) ) ;
#147945=CARTESIAN_POINT ( 'NONE',  ( -13.97604488694547697, 13.89961937509957934, 38.12609039468566152 ) ) ;
#147946=CARTESIAN_POINT ( 'NONE',  ( 21.52544592524344225, -5.823673210054117533, 83.54057627198102409 ) ) ;
#147947=CARTESIAN_POINT ( 'NONE',  ( 8.224510206698742110, 14.34966873604972548, 112.0844237280190185 ) ) ;
#147948=CARTESIAN_POINT ( 'NONE',  ( 0.05219959533907565091, 21.53943276465977519, 44.99890960531435979 ) ) ;
#147949=CARTESIAN_POINT ( 'NONE',  ( -21.52544592524343514, 5.823673210054127303, 81.04057627198102409 ) ) ;
#147950=CARTESIAN_POINT ( 'NONE',  ( -5.153800228976607833, 19.02544592524334988, 112.7094237280190043 ) ) ;
#147951=CARTESIAN_POINT ( 'NONE',  ( -16.51473224551069308, -9.474510206698971260, 101.6655762719810241 ) ) ;
#147952=CARTESIAN_POINT ( 'NONE',  ( 10.72451020669871369, 18.67979575497193778, 82.08442372801901854 ) ) ;
#147953=CARTESIAN_POINT ( 'NONE',  ( -9.474510206698964154, 16.51473224551069663, 55.41557627198103120 ) ) ;
#147954=CARTESIAN_POINT ( 'NONE',  ( 16.53943276465976808, -0.05219959533910856209, 103.7489096053143669 ) ) ;
#147956=CARTESIAN_POINT ( 'NONE',  ( -13.97604488694527625, -13.89961937509977652, 71.87390960531433848 ) ) ;
#147957=CARTESIAN_POINT ( 'NONE',  ( -14.29746914071049879, 8.314922557960819915, 95.83224293864770971 ) ) ;
#147959=CARTESIAN_POINT ( 'NONE',  ( 16.51473224551083163, -9.474510206698727899, 90.83442372801900433 ) ) ;
#147961=CARTESIAN_POINT ( 'NONE',  ( 9.474510206698971260, -16.51473224551069308, 62.91557627198102409 ) ) ;
#147963=CARTESIAN_POINT ( 'NONE',  ( -10.81492255796105439, 18.62759615963255655, 82.91775706135234714 ) ) ;
#147964=CARTESIAN_POINT ( 'NONE',  ( 16.46253265017160672, -9.564922557960803928, 98.33224293864769550 ) ) ;
#147965=CARTESIAN_POINT ( 'NONE',  ( 14.34966873604972726, -8.224510206698740333, 75.83442372801900433 ) ) ;
#147966=CARTESIAN_POINT ( 'NONE',  ( -16.31925111598457789, -7.325300261831486637, 49.83575461032751264 ) ) ;
#147967=CARTESIAN_POINT ( 'NONE',  ( -16.51473224551082808, 9.474510206698731452, 48.33442372801900433 ) ) ;
#147968=CARTESIAN_POINT ( 'NONE',  ( -21.52544592524334988, -5.823673210054445271, 103.9594237280190185 ) ) ;
#147971=CARTESIAN_POINT ( 'NONE',  ( -12.14591786802326823, 12.06949235617739902, 98.12609039468570415 ) ) ;
#147973=CARTESIAN_POINT ( 'NONE',  ( 8.224510206698742110, 14.34966873604972548, 87.08442372801901854 ) ) ;
#147975=CARTESIAN_POINT ( 'NONE',  ( -0.05219959533934338120, 16.53943276465976808, 67.50109039468568994 ) ) ;
#147976=ORIENTED_EDGE ( 'NONE', *, *, #58944, .F. ) ;
#147977=CARTESIAN_POINT ( 'NONE',  ( -10.72451020669870658, -18.67979575497194134, 74.58442372801901854 ) ) ;
#147978=CARTESIAN_POINT ( 'NONE',  ( -5.049401038297874678, -19.05341960407617918, 84.79275706135233293 ) ) ;
#147979=CARTESIAN_POINT ( 'NONE',  ( -13.97604488694547697, 13.89961937509957934, 28.12609039468565797 ) ) ;
#147980=CARTESIAN_POINT ( 'NONE',  ( -9.564922557960796823, -16.46253265017161027, 72.08224293864770971 ) ) ;
#147981=CARTESIAN_POINT ( 'NONE',  ( 19.03943276465977164, -0.05219959533909143690, 58.74890960531435979 ) ) ;
#147982=CARTESIAN_POINT ( 'NONE',  ( 17.23220907382109957, -6.508304012115882387, 23.29902788568567473 ) ) ;
#147983=CARTESIAN_POINT ( 'NONE',  ( 5.823673210054125526, 21.52544592524343514, 74.79057627198105251 ) ) ;
#147984=CARTESIAN_POINT ( 'NONE',  ( -5.823673210054116645, -21.52544592524344225, 32.29057627198102409 ) ) ;
#147985=CARTESIAN_POINT ( 'NONE',  ( -5.153800228976328057, -19.02544592524343514, 32.29057627198102409 ) ) ;
#147986=CARTESIAN_POINT ( 'NONE',  ( 8.314922557961029526, -14.29746914071037800, 70.41775706135236135 ) ) ;
#147988=CARTESIAN_POINT ( 'NONE',  ( -15.72974639402176322, -15.80617190586768395, 29.37609039468568284 ) ) ;
#147989=CARTESIAN_POINT ( 'NONE',  ( 8.314922557960818139, 14.29746914071049879, 69.58224293864769550 ) ) ;
#147991=CARTESIAN_POINT ( 'NONE',  ( 14.34966873604972726, -8.224510206698740333, 20.83442372801901143 ) ) ;
#147992=CARTESIAN_POINT ( 'NONE',  ( -19.03943276465977164, -0.05219959533935918106, 58.75109039468566863 ) ) ;
#147993=CARTESIAN_POINT ( 'NONE',  ( -12.06949235617756955, 12.14591786802309770, 55.62390960531436690 ) ) ;
#147994=CARTESIAN_POINT ( 'NONE',  ( -18.67979575497193778, 10.72451020669871902, 28.33442372801902209 ) ) ;
#147996=CARTESIAN_POINT ( 'NONE',  ( -10.81492255796078084, -18.62759615963271287, 77.08224293864769550 ) ) ;
#147997=CARTESIAN_POINT ( 'NONE',  ( 5.153800228976335163, 19.02544592524342804, 104.7905762719809957 ) ) ;
#147998=CARTESIAN_POINT ( 'NONE',  ( 14.34966873604960469, 8.224510206698951720, 59.16557627198103120 ) ) ;
#148001=CARTESIAN_POINT ( 'NONE',  ( -0.05219959533936034679, 19.03943276465977164, 62.50109039468566863 ) ) ;
#148002=CARTESIAN_POINT ( 'NONE',  ( 10.81492255796078972, 18.62759615963270932, 104.5822429386477097 ) ) ;
#148003=CARTESIAN_POINT ( 'NONE',  ( -19.02544592524342804, 5.153800228976336051, 61.04057627198103120 ) ) ;
#148004=CARTESIAN_POINT ( 'NONE',  ( 0.05219959533936267826, -19.03943276465977164, 40.00109039468566152 ) ) ;
#148005=CARTESIAN_POINT ( 'NONE',  ( -0.05219959533909027116, -19.03943276465977164, 27.49890960531435624 ) ) ;
#148006=CARTESIAN_POINT ( 'NONE',  ( -15.72974639402176322, -15.80617190586768395, 69.37609039468567573 ) ) ;
#148007=CARTESIAN_POINT ( 'NONE',  ( -17.05587630539786659, -6.762274262135686165, 69.25819690962687503 ) ) ;
#148008=CARTESIAN_POINT ( 'NONE',  ( -14.34966873604960291, -8.224510206698953496, 41.66557627198103120 ) ) ;
#148009=CARTESIAN_POINT ( 'NONE',  ( 19.02544592524343514, -5.153800228976328945, 58.54057627198102409 ) ) ;
#148010=CARTESIAN_POINT ( 'NONE',  ( 15.72974639402199770, -15.80617190586745480, 78.12390960531436690 ) ) ;
#148011=CARTESIAN_POINT ( 'NONE',  ( 19.02544592524343514, -5.153800228976328945, 63.54057627198103830 ) ) ;
#148012=CARTESIAN_POINT ( 'NONE',  ( -18.67979575497178146, -10.72451020669898902, 71.66557627198100988 ) ) ;
#148014=CARTESIAN_POINT ( 'NONE',  ( -15.72974639402176322, -15.80617190586768395, 104.3760903946856899 ) ) ;
#148016=CARTESIAN_POINT ( 'NONE',  ( 16.52544592524335698, 4.483927247898782831, 91.45942372801901854 ) ) ;
#148017=CARTESIAN_POINT ( 'NONE',  ( -4.483927247898539470, -16.52544592524342804, 87.29057627198103830 ) ) ;
#148018=CARTESIAN_POINT ( 'NONE',  ( 16.51473224551083163, -9.474510206698727899, 95.83442372801900433 ) ) ;
#148019=ORIENTED_EDGE ( 'NONE', *, *, #200190, .T. ) ;
#148020=CARTESIAN_POINT ( 'NONE',  ( -19.05341960407617563, 5.049401038297882671, 33.54275706135231871 ) ) ;
#148021=CARTESIAN_POINT ( 'NONE',  ( 12.06949235617739724, 12.14591786802326823, 101.8760903946857042 ) ) ;
#148022=CARTESIAN_POINT ( 'NONE',  ( -19.03943276465977164, -0.05219959533935918106, 28.75109039468566507 ) ) ;
#148023=CARTESIAN_POINT ( 'NONE',  ( -5.049401038298153566, 19.05341960407611168, 90.20724293864766707 ) ) ;
#148024=CARTESIAN_POINT ( 'NONE',  ( 5.823673210054125526, 21.52544592524343514, 64.79057627198103830 ) ) ;
#148026=CARTESIAN_POINT ( 'NONE',  ( -14.34966873604960291, -8.224510206698953496, 111.6655762719810525 ) ) ;
#148027=CARTESIAN_POINT ( 'NONE',  ( -10.81492255796105439, 18.62759615963255655, 92.91775706135236135 ) ) ;
#148028=CARTESIAN_POINT ( 'NONE',  ( 16.53943276465976808, 0.05219959533934440121, 71.25109039468568994 ) ) ;
#148029=CARTESIAN_POINT ( 'NONE',  ( -21.52544592524334988, -5.823673210054445271, 28.95942372801902209 ) ) ;
#148030=CARTESIAN_POINT ( 'NONE',  ( 0.05219959533934541429, -16.53943276465976808, 25.00109039468567218 ) ) ;
#148031=CARTESIAN_POINT ( 'NONE',  ( -5.049401038298153566, 19.05341960407611168, 110.2072429386476671 ) ) ;
#148032=CARTESIAN_POINT ( 'NONE',  ( 9.474510206698971260, -16.51473224551069308, 37.91557627198102409 ) ) ;
#148033=CARTESIAN_POINT ( 'NONE',  ( -13.89961937509977652, 13.97604488694528158, 55.62390960531434558 ) ) ;
#148034=CARTESIAN_POINT ( 'NONE',  ( -14.34966873604972548, 8.224510206698743886, 53.33442372801901854 ) ) ;
#148035=CARTESIAN_POINT ( 'NONE',  ( 16.52544592524342804, -4.483927247898539470, 88.54057627198103830 ) ) ;
#148036=CARTESIAN_POINT ( 'NONE',  ( 8.314922557961029526, -14.29746914071037800, 100.4177570613523471 ) ) ;
#148037=CARTESIAN_POINT ( 'NONE',  ( -15.72974639402176322, -15.80617190586768395, 49.37609039468569705 ) ) ;
#148038=CARTESIAN_POINT ( 'NONE',  ( 9.564922557960805705, 16.46253265017160317, 79.58224293864769550 ) ) ;
#148039=CARTESIAN_POINT ( 'NONE',  ( 9.474510206698971260, -16.51473224551069308, 67.91557627198102409 ) ) ;
#148040=CARTESIAN_POINT ( 'NONE',  ( 9.564922557960805705, 16.46253265017160317, 84.58224293864769550 ) ) ;
#148041=CARTESIAN_POINT ( 'NONE',  ( 16.53943276465976808, -0.05219959533910856209, 33.74890960531436690 ) ) ;
#148042=CARTESIAN_POINT ( 'NONE',  ( 16.53943276465976808, 0.05219959533934440121, 96.25109039468568994 ) ) ;
#148043=CARTESIAN_POINT ( 'NONE',  ( -5.049401038297874678, -19.05341960407617918, 39.79275706135232582 ) ) ;
#148044=CARTESIAN_POINT ( 'NONE',  ( 5.049401038298161559, -19.05341960407611168, 107.7072429386476955 ) ) ;
#148045=CARTESIAN_POINT ( 'NONE',  ( 9.564922557960805705, 16.46253265017160317, 59.58224293864769550 ) ) ;
#148046=CARTESIAN_POINT ( 'NONE',  ( 9.564922557961047289, -16.46253265017146816, 40.41775706135234003 ) ) ;
#148048=CARTESIAN_POINT ( 'NONE',  ( 4.379528057220092307, 16.55341960407617563, 47.29275706135234003 ) ) ;
#148049=CARTESIAN_POINT ( 'NONE',  ( -19.02544592524334988, -5.153800228976617603, 73.95942372801900433 ) ) ;
#148050=CARTESIAN_POINT ( 'NONE',  ( 12.06949235617739724, 12.14591786802326823, 51.87609039468568284 ) ) ;
#148052=CARTESIAN_POINT ( 'NONE',  ( -16.46253265017160317, 9.564922557960807481, 90.83224293864769550 ) ) ;
#148053=CARTESIAN_POINT ( 'NONE',  ( -21.52544592524343514, 5.823673210054127303, 111.0405762719810525 ) ) ;
#148054=CARTESIAN_POINT ( 'NONE',  ( 5.153800228976615827, -19.02544592524334988, 80.20942372801901854 ) ) ;
#148055=CARTESIAN_POINT ( 'NONE',  ( 9.564922557960805705, 16.46253265017160317, 104.5822429386476955 ) ) ;
#148056=CARTESIAN_POINT ( 'NONE',  ( -19.02544592524342804, 5.153800228976336051, 41.04057627198103120 ) ) ;
#148057=CARTESIAN_POINT ( 'NONE',  ( 16.46253265017160672, -9.564922557960803928, 73.33224293864769550 ) ) ;
#148058=CARTESIAN_POINT ( 'NONE',  ( 16.55341960407611168, 4.379528057220329451, 33.95724293864769550 ) ) ;
#148059=CARTESIAN_POINT ( 'NONE',  ( -19.05341960407611168, -5.049401038298163336, 31.45724293864769550 ) ) ;
#148060=CARTESIAN_POINT ( 'NONE',  ( 0.05219959533936267826, -19.03943276465977164, 55.00109039468566863 ) ) ;
#148061=CARTESIAN_POINT ( 'NONE',  ( -4.379528057220328563, 16.55341960407611168, 90.20724293864770971 ) ) ;
#148062=CARTESIAN_POINT ( 'NONE',  ( -18.62759615963255300, -10.81492255796106328, 109.1677570613523613 ) ) ;
#148063=CARTESIAN_POINT ( 'NONE',  ( 13.97604488694527802, 13.89961937509977652, 59.37390960531434558 ) ) ;
#148064=CARTESIAN_POINT ( 'NONE',  ( 21.52544592524344225, -5.823673210054117533, 48.54057627198103120 ) ) ;
#148065=CARTESIAN_POINT ( 'NONE',  ( -16.52544592524342804, 4.483927247898546575, 56.04057627198102409 ) ) ;
#148066=CARTESIAN_POINT ( 'NONE',  ( 5.719274019375673035, 21.55341960407619339, 97.29275706135234714 ) ) ;
#148067=CARTESIAN_POINT ( 'NONE',  ( -19.02544592524342804, 5.153800228976336051, 106.0405762719810241 ) ) ;
#148068=CARTESIAN_POINT ( 'NONE',  ( 16.46253265017160672, -9.564922557960803928, 113.3322429386476955 ) ) ;
#148069=CARTESIAN_POINT ( 'NONE',  ( -9.564922557960796823, -16.46253265017161027, 37.08224293864768839 ) ) ;
#148070=CARTESIAN_POINT ( 'NONE',  ( -19.05341960407611168, -5.049401038298163336, 21.45724293864768839 ) ) ;
#148071=CARTESIAN_POINT ( 'NONE',  ( -16.53943276465976808, 0.05219959533911058130, 86.24890960531436690 ) ) ;
#148072=CARTESIAN_POINT ( 'NONE',  ( -5.719274019375978568, 21.55341960407610458, 95.20724293864769550 ) ) ;
#148073=CARTESIAN_POINT ( 'NONE',  ( 19.02544592524343514, -5.153800228976328945, 103.5405762719809957 ) ) ;
#148074=CARTESIAN_POINT ( 'NONE',  ( -21.52544592524334988, -5.823673210054445271, 18.95942372801901143 ) ) ;
#148075=CARTESIAN_POINT ( 'NONE',  ( -9.474510206698964154, 16.51473224551069663, 110.4155762719810383 ) ) ;
#148077=CARTESIAN_POINT ( 'NONE',  ( 16.52544592524342804, -4.483927247898539470, 98.54057627198105251 ) ) ;
#148078=CARTESIAN_POINT ( 'NONE',  ( -13.97604488694527625, -13.89961937509977652, 76.87390960531433848 ) ) ;
#148079=CARTESIAN_POINT ( 'NONE',  ( 10.81492255796078972, 18.62759615963270932, 79.58224293864769550 ) ) ;
#148082=CARTESIAN_POINT ( 'NONE',  ( 15.72974639402199770, -15.80617190586745480, 33.12390960531435979 ) ) ;
#148083=CARTESIAN_POINT ( 'NONE',  ( -17.49999999999999645, 5.499999999999992895, 73.71769037696435589 ) ) ;
#148084=CARTESIAN_POINT ( 'NONE',  ( 12.06949235617739724, 12.14591786802326823, 31.87609039468567929 ) ) ;
#148085=CARTESIAN_POINT ( 'NONE',  ( -16.55341960407611168, -4.379528057220339221, 91.45724293864769550 ) ) ;
#148086=CARTESIAN_POINT ( 'NONE',  ( 19.52217212775660471, -5.499999999999920064, 52.43993709005258808 ) ) ;
#148087=CARTESIAN_POINT ( 'NONE',  ( -13.89961937509977652, 13.97604488694528158, 85.62390960531433848 ) ) ;
#148088=CARTESIAN_POINT ( 'NONE',  ( 0.05219959533909260263, 19.03943276465977164, 54.99890960531435979 ) ) ;
#148089=CARTESIAN_POINT ( 'NONE',  ( -12.14591786802309592, -12.06949235617757132, 76.87390960531439532 ) ) ;
#148090=CARTESIAN_POINT ( 'NONE',  ( -15.80617190586745835, -15.72974639402198527, 31.87390960531435979 ) ) ;
#148091=CARTESIAN_POINT ( 'NONE',  ( -12.14591786802309592, -12.06949235617757132, 51.87390960531437401 ) ) ;
#148092=CARTESIAN_POINT ( 'NONE',  ( 16.55341960407618274, -4.379528057220086978, 26.04275706135235779 ) ) ;
#148093=CARTESIAN_POINT ( 'NONE',  ( 21.55341960407619695, -5.719274019375665929, 76.04275706135237556 ) ) ;
#148095=CARTESIAN_POINT ( 'NONE',  ( 21.55341960407610458, 5.719274019375980345, 23.95724293864769550 ) ) ;
#148096=CARTESIAN_POINT ( 'NONE',  ( 4.379528057220092307, 16.55341960407617563, 87.29275706135236135 ) ) ;
#148097=CARTESIAN_POINT ( 'NONE',  ( -9.474510206698964154, 16.51473224551069663, 30.41557627198102054 ) ) ;
#148098=CARTESIAN_POINT ( 'NONE',  ( -19.03943276465977164, 0.05219959533909376836, 71.24890960531435269 ) ) ;
#148099=CARTESIAN_POINT ( 'NONE',  ( -5.719274019375978568, 21.55341960407610458, 100.2072429386476955 ) ) ;
#148100=CARTESIAN_POINT ( 'NONE',  ( 4.379528057220092307, 16.55341960407617563, 27.29275706135234358 ) ) ;
#148101=CARTESIAN_POINT ( 'NONE',  ( 12.14591786802309770, 12.06949235617756955, 49.37390960531436690 ) ) ;
#148102=CARTESIAN_POINT ( 'NONE',  ( 5.823673210054444382, -21.52544592524334988, 75.20942372801901854 ) ) ;
#148104=CARTESIAN_POINT ( 'NONE',  ( -12.14591786802326823, 12.06949235617739902, 88.12609039468570415 ) ) ;
#148105=CARTESIAN_POINT ( 'NONE',  ( 0.05219959533909260263, 19.03943276465977164, 114.9989096053143669 ) ) ;
#148106=CARTESIAN_POINT ( 'NONE',  ( 17.12812012977025233, 6.668231424566067211, 28.85948759323144941 ) ) ;
#148108=CARTESIAN_POINT ( 'NONE',  ( -16.55341960407617563, 4.379528057220093196, 103.5427570613523613 ) ) ;
#148109=CARTESIAN_POINT ( 'NONE',  ( -12.06949235617739369, -12.14591786802326823, 59.37609039468568284 ) ) ;
#148110=CARTESIAN_POINT ( 'NONE',  ( 5.049401038298161559, -19.05341960407611168, 72.70724293864768129 ) ) ;
#148111=CARTESIAN_POINT ( 'NONE',  ( -13.89961937509977652, 13.97604488694528158, 85.62390960531433848 ) ) ;
#148112=CARTESIAN_POINT ( 'NONE',  ( 21.55341960407619695, -5.719274019375665929, 66.04275706135236135 ) ) ;
#148113=CARTESIAN_POINT ( 'NONE',  ( 4.483927247898790824, -16.52544592524335698, 70.20942372801904696 ) ) ;
#148114=CARTESIAN_POINT ( 'NONE',  ( 0.05219959533910956823, 16.53943276465976808, 44.99890960531435979 ) ) ;
#148115=CARTESIAN_POINT ( 'NONE',  ( 5.049401038298161559, -19.05341960407611168, 57.70724293864769550 ) ) ;
#148116=CARTESIAN_POINT ( 'NONE',  ( 19.03943276465977164, -0.05219959533909143690, 53.74890960531436690 ) ) ;
#148117=ORIENTED_EDGE ( 'NONE', *, *, #114637, .F. ) ;
#148118=CARTESIAN_POINT ( 'NONE',  ( -19.02544592524334988, -5.153800228976617603, 108.9594237280189759 ) ) ;
#148119=CARTESIAN_POINT ( 'NONE',  ( -8.314922557960811034, -14.29746914071050412, 107.0822429386476955 ) ) ;
#148120=CARTESIAN_POINT ( 'NONE',  ( -13.97604488694527625, -13.89961937509977652, 66.87390960531436690 ) ) ;
#148121=CARTESIAN_POINT ( 'NONE',  ( 9.564922557961047289, -16.46253265017146816, 95.41775706135233293 ) ) ;
#148123=CARTESIAN_POINT ( 'NONE',  ( -0.05219959533937732626, 21.53943276465977519, 102.5010903946856899 ) ) ;
#148124=CARTESIAN_POINT ( 'NONE',  ( -4.379528057220086978, -16.55341960407618274, 64.79275706135234714 ) ) ;
#148125=CARTESIAN_POINT ( 'NONE',  ( -16.51473224551082808, 9.474510206698731452, 93.33442372801900433 ) ) ;
#148126=CARTESIAN_POINT ( 'NONE',  ( -21.55341960407610458, -5.719274019375992779, 61.45724293864770260 ) ) ;
#148127=CARTESIAN_POINT ( 'NONE',  ( 12.14591786802327356, -12.06949235617739191, 50.62609039468568994 ) ) ;
#148128=CARTESIAN_POINT ( 'NONE',  ( -18.22780087662122028, 5.500000000000031086, 68.51540105326107266 ) ) ;
#148129=CARTESIAN_POINT ( 'NONE',  ( 9.474510206698729675, 16.51473224551082808, 62.08442372801899722 ) ) ;
#148130=CARTESIAN_POINT ( 'NONE',  ( -21.55341960407619339, 5.719274019375674811, 93.54275706135234714 ) ) ;
#148131=CARTESIAN_POINT ( 'NONE',  ( 14.29746914071049879, -8.314922557960816363, 113.3322429386476955 ) ) ;
#148132=CARTESIAN_POINT ( 'NONE',  ( -19.05341960407611168, -5.049401038298163336, 66.45724293864769550 ) ) ;
#148133=CARTESIAN_POINT ( 'NONE',  ( -16.55341960407611168, -4.379528057220339221, 61.45724293864770260 ) ) ;
#148134=CARTESIAN_POINT ( 'NONE',  ( -21.55341960407619339, 5.719274019375674811, 83.54275706135234714 ) ) ;
#148135=CARTESIAN_POINT ( 'NONE',  ( -19.02544592524334988, -5.153800228976617603, 43.95942372801899012 ) ) ;
#148136=CARTESIAN_POINT ( 'NONE',  ( -19.03943276465977164, -0.05219959533935918106, 33.75109039468566863 ) ) ;
#148137=CARTESIAN_POINT ( 'NONE',  ( -18.62759615963270932, 10.81492255796079327, 25.83224293864769194 ) ) ;
#148138=CARTESIAN_POINT ( 'NONE',  ( 18.67979575497194134, -10.72451020669871369, 90.83442372801901854 ) ) ;
#148139=CARTESIAN_POINT ( 'NONE',  ( -13.97604488694527625, -13.89961937509977652, 76.87390960531433848 ) ) ;
#148140=CARTESIAN_POINT ( 'NONE',  ( -10.81492255796105439, 18.62759615963255655, 92.91775706135236135 ) ) ;
#148141=CARTESIAN_POINT ( 'NONE',  ( -21.55341960407610458, -5.719274019375992779, 51.45724293864770260 ) ) ;
#148142=CARTESIAN_POINT ( 'NONE',  ( -13.89961937509977652, 13.97604488694528158, 85.62390960531433848 ) ) ;
#148143=CARTESIAN_POINT ( 'NONE',  ( -19.03943276465977164, -0.05219959533935918106, 68.75109039468566152 ) ) ;
#148144=CARTESIAN_POINT ( 'NONE',  ( -5.049401038298153566, 19.05341960407611168, 40.20724293864768839 ) ) ;
#148145=CARTESIAN_POINT ( 'NONE',  ( -16.46253265017160317, 9.564922557960807481, 95.83224293864769550 ) ) ;
#148146=CARTESIAN_POINT ( 'NONE',  ( 9.564922557961047289, -16.46253265017146816, 85.41775706135233293 ) ) ;
#148147=CARTESIAN_POINT ( 'NONE',  ( 8.314922557961029526, -14.29746914071037800, 45.41775706135234003 ) ) ;
#148148=CARTESIAN_POINT ( 'NONE',  ( -14.34966873604960291, -8.224510206698953496, 106.6655762719810383 ) ) ;
#148149=CARTESIAN_POINT ( 'NONE',  ( 9.564922557960805705, 16.46253265017160317, 74.58224293864769550 ) ) ;
#148150=CARTESIAN_POINT ( 'NONE',  ( -10.81492255796078084, -18.62759615963271287, 52.08224293864768839 ) ) ;
#148151=CARTESIAN_POINT ( 'NONE',  ( 16.52544592524335698, 4.483927247898782831, 31.45942372801901854 ) ) ;
#148152=CARTESIAN_POINT ( 'NONE',  ( -21.53943276465977519, -0.05219959533937600094, 38.75109039468567573 ) ) ;
#148153=CARTESIAN_POINT ( 'NONE',  ( 5.823673210054444382, -21.52544592524334988, 90.20942372801903275 ) ) ;
#148154=CARTESIAN_POINT ( 'NONE',  ( -16.52544592524335698, -4.483927247898792601, 83.95942372801900433 ) ) ;
#148155=CARTESIAN_POINT ( 'NONE',  ( -5.153800228976328057, -19.02544592524343514, 77.29057627198099567 ) ) ;
#148156=CARTESIAN_POINT ( 'NONE',  ( -16.52544592524335698, -4.483927247898792601, 108.9594237280190185 ) ) ;
#148157=CARTESIAN_POINT ( 'NONE',  ( -16.51473224551082808, 9.474510206698731452, 53.33442372801900433 ) ) ;
#148159=CARTESIAN_POINT ( 'NONE',  ( 10.72451020669871369, 18.67979575497193778, 37.08442372801901143 ) ) ;
#148160=CARTESIAN_POINT ( 'NONE',  ( 14.29746914071049879, -8.314922557960816363, 83.33224293864769550 ) ) ;
#148161=CARTESIAN_POINT ( 'NONE',  ( 5.153800228976335163, 19.02544592524342804, 99.79057627198102409 ) ) ;
#148162=CARTESIAN_POINT ( 'NONE',  ( 16.52544592524335698, 4.483927247898782831, 106.4594237280190328 ) ) ;
#148163=CARTESIAN_POINT ( 'NONE',  ( -15.80617190586768217, 15.72974639402176855, 78.12609039468570415 ) ) ;
#148164=CARTESIAN_POINT ( 'NONE',  ( -16.53943276465976808, -0.05219959533934237506, 38.75109039468567573 ) ) ;
#148165=CARTESIAN_POINT ( 'NONE',  ( 10.72451020669871369, 18.67979575497193778, 27.08442372801901854 ) ) ;
#148166=CARTESIAN_POINT ( 'NONE',  ( 0.05219959533910956823, 16.53943276465976808, 74.99890960531435269 ) ) ;
#148167=ORIENTED_EDGE ( 'NONE', *, *, #154166, .T. ) ;
#148168=CARTESIAN_POINT ( 'NONE',  ( -15.72974639402197994, 15.80617190586746368, 115.6239096053143669 ) ) ;
#148169=CARTESIAN_POINT ( 'NONE',  ( 12.06949235617757843, -12.14591786802309237, 53.12390960531436690 ) ) ;
#148171=CARTESIAN_POINT ( 'NONE',  ( 21.53943276465977519, -0.05219959533907433946, 28.74890960531435624 ) ) ;
#148172=CARTESIAN_POINT ( 'NONE',  ( -18.67979575497193778, 10.72451020669871902, 48.33442372801902565 ) ) ;
#148173=CARTESIAN_POINT ( 'NONE',  ( -16.52544592524342804, 4.483927247898546575, 66.04057627198103830 ) ) ;
#148174=CARTESIAN_POINT ( 'NONE',  ( 21.55341960407610458, 5.719274019375980345, 78.95724293864769550 ) ) ;
#148175=CARTESIAN_POINT ( 'NONE',  ( 13.97604488694527802, 13.89961937509977652, 79.37390960531435269 ) ) ;
#148176=CARTESIAN_POINT ( 'NONE',  ( -0.05219959533909027116, -19.03943276465977164, 32.49890960531435979 ) ) ;
#148177=CARTESIAN_POINT ( 'NONE',  ( -19.02544592524334988, -5.153800228976617603, 73.95942372801900433 ) ) ;
#148178=CARTESIAN_POINT ( 'NONE',  ( -5.823673210054431948, 21.52544592524334988, 52.70942372801902565 ) ) ;
#148179=CARTESIAN_POINT ( 'NONE',  ( -15.80617190586745835, -15.72974639402198527, 66.87390960531436690 ) ) ;
#148180=CARTESIAN_POINT ( 'NONE',  ( -16.51473224551069308, -9.474510206698971260, 41.66557627198103120 ) ) ;
#148181=CARTESIAN_POINT ( 'NONE',  ( -19.05341960407611168, -5.049401038298163336, 66.45724293864769550 ) ) ;
#148182=CARTESIAN_POINT ( 'NONE',  ( 12.06949235617739724, 12.14591786802326823, 46.87609039468568994 ) ) ;
#148183=CARTESIAN_POINT ( 'NONE',  ( 18.67979575497194134, -10.72451020669871369, 35.83442372801901143 ) ) ;
#148184=CARTESIAN_POINT ( 'NONE',  ( 5.823673210054444382, -21.52544592524334988, 55.20942372801902565 ) ) ;
#148185=CARTESIAN_POINT ( 'NONE',  ( -5.049401038298153566, 19.05341960407611168, 100.2072429386476955 ) ) ;
#148186=CARTESIAN_POINT ( 'NONE',  ( -5.719274019375978568, 21.55341960407610458, 80.20724293864769550 ) ) ;
#148187=CARTESIAN_POINT ( 'NONE',  ( 5.719274019375673035, 21.55341960407619339, 22.29275706135235069 ) ) ;
#148188=CARTESIAN_POINT ( 'NONE',  ( 8.224510206698742110, 14.34966873604972548, 52.08442372801901854 ) ) ;
#148189=CARTESIAN_POINT ( 'NONE',  ( 18.62759615963271287, -10.81492255796078972, 53.33224293864769550 ) ) ;
#148190=CARTESIAN_POINT ( 'NONE',  ( -16.46253265017146816, -9.564922557961047289, 24.16775706135233648 ) ) ;
#148191=AXIS2_PLACEMENT_3D ( 'NONE', #144702, #49719, #51703 ) ;
#148192=CARTESIAN_POINT ( 'NONE',  ( 5.153800228976335163, 19.02544592524342804, 59.79057627198100988 ) ) ;
#148193=CARTESIAN_POINT ( 'NONE',  ( 9.564922557960805705, 16.46253265017160317, 114.5822429386476955 ) ) ;
#148194=CARTESIAN_POINT ( 'NONE',  ( -16.46253265017160317, 9.564922557960807481, 90.83224293864769550 ) ) ;
#148196=CARTESIAN_POINT ( 'NONE',  ( 16.51473224551083163, -9.474510206698727899, 70.83442372801900433 ) ) ;
#148197=CARTESIAN_POINT ( 'NONE',  ( -18.67979575497178146, -10.72451020669898902, 41.66557627198103120 ) ) ;
#148198=CARTESIAN_POINT ( 'NONE',  ( 12.14591786802309770, 12.06949235617756955, 29.37390960531435269 ) ) ;
#148199=CARTESIAN_POINT ( 'NONE',  ( -19.02544592524334988, -5.153800228976617603, 88.95942372801897591 ) ) ;
#148200=FACE_OUTER_BOUND ( 'NONE', #162870, .T. ) ;
#148201=CARTESIAN_POINT ( 'NONE',  ( -16.51473224551082808, 9.474510206698731452, 23.33442372801900078 ) ) ;
#148202=CARTESIAN_POINT ( 'NONE',  ( -5.153800228976607833, 19.02544592524334988, 77.70942372801900433 ) ) ;
#148203=CARTESIAN_POINT ( 'NONE',  ( 19.02544592524334988, 5.153800228976608722, 41.45942372801900433 ) ) ;
#148205=CARTESIAN_POINT ( 'NONE',  ( 5.153800228976335163, 19.02544592524342804, 49.79057627198100988 ) ) ;
#148206=CARTESIAN_POINT ( 'NONE',  ( -16.55341960407611168, -4.379528057220339221, 56.45724293864768839 ) ) ;
#148207=CARTESIAN_POINT ( 'NONE',  ( 16.46253265017160672, -9.564922557960803928, 28.33224293864769550 ) ) ;
#148208=CARTESIAN_POINT ( 'NONE',  ( 4.379528057220339221, -16.55341960407611168, 42.70724293864770260 ) ) ;
#148209=DIRECTION ( 'NONE',  ( 0.000000000000000000, 0.04175967627138096189, 0.9991276842514722478 ) ) ;
#148210=CARTESIAN_POINT ( 'NONE',  ( -0.05219959533934338120, 16.53943276465976808, 112.5010903946857042 ) ) ;
#148211=CARTESIAN_POINT ( 'NONE',  ( 16.46253265017160672, -9.564922557960803928, 68.33224293864770971 ) ) ;
#148212=CARTESIAN_POINT ( 'NONE',  ( 9.474510206698729675, 16.51473224551082808, 22.08442372801899722 ) ) ;
#148213=CARTESIAN_POINT ( 'NONE',  ( 16.52544592524335698, 4.483927247898782831, 36.45942372801901143 ) ) ;
#148214=CARTESIAN_POINT ( 'NONE',  ( 21.52544592524344225, -5.823673210054117533, 33.54057627198102409 ) ) ;
#148215=CARTESIAN_POINT ( 'NONE',  ( 15.80617190586769283, -15.72974639402175789, 85.62609039468568994 ) ) ;
#148217=CARTESIAN_POINT ( 'NONE',  ( -9.564922557960796823, -16.46253265017161027, 62.08224293864769550 ) ) ;
#148218=CARTESIAN_POINT ( 'NONE',  ( -16.46253265017160317, 9.564922557960807481, 100.8322429386477097 ) ) ;
#148219=CARTESIAN_POINT ( 'NONE',  ( 13.89961937509977652, -13.97604488694527269, 98.12390960531433848 ) ) ;
#148221=CARTESIAN_POINT ( 'NONE',  ( -0.05219959533937732626, 21.53943276465977519, 22.50109039468567573 ) ) ;
#148222=CARTESIAN_POINT ( 'NONE',  ( -16.55341960407611168, -4.379528057220339221, 76.45724293864769550 ) ) ;
#148223=CARTESIAN_POINT ( 'NONE',  ( -21.55341960407610458, -5.719274019375992779, 76.45724293864769550 ) ) ;
#148224=CARTESIAN_POINT ( 'NONE',  ( 13.97604488694527802, 13.89961937509977652, 74.37390960531436690 ) ) ;
#148225=CARTESIAN_POINT ( 'NONE',  ( -0.05219959533909027116, -19.03943276465977164, 72.49890960531435269 ) ) ;
#148226=CARTESIAN_POINT ( 'NONE',  ( -21.53943276465977519, 0.05219959533907696930, 106.2489096053143811 ) ) ;
#148228=CARTESIAN_POINT ( 'NONE',  ( 19.02544592524343514, -5.153800228976328945, 73.54057627198103830 ) ) ;
#148229=CARTESIAN_POINT ( 'NONE',  ( -16.53943276465976808, 0.05219959533911058130, 111.2489096053143669 ) ) ;
#148230=CARTESIAN_POINT ( 'NONE',  ( -13.97604488694527625, -13.89961937509977652, 21.87390960531435979 ) ) ;
#148231=CARTESIAN_POINT ( 'NONE',  ( -19.02544592524342804, 5.153800228976336051, 61.04057627198103120 ) ) ;
#148232=CARTESIAN_POINT ( 'NONE',  ( -19.02544592524334988, -5.153800228976617603, 93.95942372801900433 ) ) ;
#148233=CARTESIAN_POINT ( 'NONE',  ( 14.34966873604960469, 8.224510206698951720, 104.1655762719810241 ) ) ;
#148234=CARTESIAN_POINT ( 'NONE',  ( 15.80617190586769283, -15.72974639402175789, 70.62609039468567573 ) ) ;
#148235=CARTESIAN_POINT ( 'NONE',  ( -9.474510206698964154, 16.51473224551069663, 50.41557627198102409 ) ) ;
#148236=CARTESIAN_POINT ( 'NONE',  ( -18.67979575497178146, -10.72451020669898902, 111.6655762719810525 ) ) ;
#148237=CARTESIAN_POINT ( 'NONE',  ( -15.72974639402176322, -15.80617190586768395, 19.37609039468568639 ) ) ;
#148239=CARTESIAN_POINT ( 'NONE',  ( -19.02544592524342804, 5.153800228976336051, 76.04057627198102409 ) ) ;
#148241=CARTESIAN_POINT ( 'NONE',  ( 13.89961937509957401, 13.97604488694547697, 101.8760903946856331 ) ) ;
#148242=CARTESIAN_POINT ( 'NONE',  ( 18.62759615963271287, -10.81492255796078972, 33.33224293864769550 ) ) ;
#148243=CARTESIAN_POINT ( 'NONE',  ( 15.72974639402176855, 15.80617190586768217, 51.87609039468568284 ) ) ;
#148244=CARTESIAN_POINT ( 'NONE',  ( -13.89961937509977652, 13.97604488694528158, 90.62390960531432427 ) ) ;
#148245=CARTESIAN_POINT ( 'NONE',  ( -9.564922557961040184, 16.46253265017147172, 77.91775706135234714 ) ) ;
#148246=CARTESIAN_POINT ( 'NONE',  ( 13.97604488694527802, 13.89961937509977652, 69.37390960531436690 ) ) ;
#148247=CARTESIAN_POINT ( 'NONE',  ( 4.483927247898545687, 16.52544592524342804, 84.79057627198102409 ) ) ;
#148248=CARTESIAN_POINT ( 'NONE',  ( -9.474510206698964154, 16.51473224551069663, 105.4155762719810383 ) ) ;
#148249=CARTESIAN_POINT ( 'NONE',  ( 12.14591786802309770, 12.06949235617756955, 89.37390960531435269 ) ) ;
#148250=CARTESIAN_POINT ( 'NONE',  ( 16.46253265017160672, -9.564922557960803928, 103.3322429386476955 ) ) ;
#148252=CARTESIAN_POINT ( 'NONE',  ( 14.34966873604960469, 8.224510206698951720, 44.16557627198103120 ) ) ;
#148253=CARTESIAN_POINT ( 'NONE',  ( -19.02544592524342804, 5.153800228976336051, 31.04057627198102409 ) ) ;
#148255=CARTESIAN_POINT ( 'NONE',  ( -18.67979575497193778, 10.72451020669871902, 53.33442372801901854 ) ) ;
#148256=CARTESIAN_POINT ( 'NONE',  ( 9.564922557961047289, -16.46253265017146816, 75.41775706135234714 ) ) ;
#148257=CARTESIAN_POINT ( 'NONE',  ( -14.34966873604960291, -8.224510206698953496, 46.66557627198102409 ) ) ;
#148258=CARTESIAN_POINT ( 'NONE',  ( 5.823673210054125526, 21.52544592524343514, 104.7905762719810241 ) ) ;
#148259=CARTESIAN_POINT ( 'NONE',  ( 5.823673210054125526, 21.52544592524343514, 39.79057627198103830 ) ) ;
#148260=CARTESIAN_POINT ( 'NONE',  ( 8.314922557960818139, 14.29746914071049879, 84.58224293864769550 ) ) ;
#148261=CARTESIAN_POINT ( 'NONE',  ( -9.564922557960796823, -16.46253265017161027, 57.08224293864769550 ) ) ;
#148262=CARTESIAN_POINT ( 'NONE',  ( 16.52544592524342804, -4.483927247898539470, 28.54057627198103120 ) ) ;
#148263=CARTESIAN_POINT ( 'NONE',  ( 4.483927247898790824, -16.52544592524335698, 90.20942372801903275 ) ) ;
#148264=CARTESIAN_POINT ( 'NONE',  ( 8.224510206698742110, 14.34966873604972548, 67.08442372801901854 ) ) ;
#148265=CARTESIAN_POINT ( 'NONE',  ( -19.03943276465977164, -0.05219959533935918106, 28.75109039468566507 ) ) ;
#148267=CARTESIAN_POINT ( 'NONE',  ( -9.474510206698964154, 16.51473224551069663, 95.41557627198102409 ) ) ;
#148268=CARTESIAN_POINT ( 'NONE',  ( -19.02544592524342804, 5.153800228976336051, 76.04057627198102409 ) ) ;
#148269=CARTESIAN_POINT ( 'NONE',  ( -0.05219959533934338120, 16.53943276465976808, 82.50109039468568994 ) ) ;
#148270=CARTESIAN_POINT ( 'NONE',  ( -5.153800228976328057, -19.02544592524343514, 37.29057627198102409 ) ) ;
#148271=CARTESIAN_POINT ( 'NONE',  ( -0.05219959533910754901, -16.53943276465976808, 52.49890960531435979 ) ) ;
#148272=CARTESIAN_POINT ( 'NONE',  ( -13.89961937509977652, 13.97604488694528158, 115.6239096053143669 ) ) ;
#148273=CARTESIAN_POINT ( 'NONE',  ( -0.05219959533909027116, -19.03943276465977164, 107.4989096053143527 ) ) ;
#148274=CARTESIAN_POINT ( 'NONE',  ( -21.53943276465977519, 0.05219959533907696930, 46.24890960531435979 ) ) ;
#148275=CARTESIAN_POINT ( 'NONE',  ( -16.52544592524342804, 4.483927247898546575, 66.04057627198103830 ) ) ;
#148276=CARTESIAN_POINT ( 'NONE',  ( -4.379528057220086978, -16.55341960407618274, 29.79275706135234358 ) ) ;
#148277=CARTESIAN_POINT ( 'NONE',  ( -8.314922557960811034, -14.29746914071050412, 62.08224293864769550 ) ) ;
#148279=CARTESIAN_POINT ( 'NONE',  ( -19.05341960407617563, 5.049401038297882671, 58.54275706135234003 ) ) ;
#148280=CARTESIAN_POINT ( 'NONE',  ( 16.51473224551069308, 9.474510206698969483, 99.16557627198102409 ) ) ;
#148281=CARTESIAN_POINT ( 'NONE',  ( 16.46253265017146816, 9.564922557961045513, 81.66775706135233293 ) ) ;
#148283=CARTESIAN_POINT ( 'NONE',  ( 9.474510206698729675, 16.51473224551082808, 112.0844237280190043 ) ) ;
#148284=CARTESIAN_POINT ( 'NONE',  ( 0.05219959533934541429, -16.53943276465976808, 90.00109039468567573 ) ) ;
#148285=CARTESIAN_POINT ( 'NONE',  ( -19.02544592524342804, 5.153800228976336051, 36.04057627198100988 ) ) ;
#148286=CARTESIAN_POINT ( 'NONE',  ( 10.81492255796078972, 18.62759615963270932, 34.58224293864770260 ) ) ;
#148287=CARTESIAN_POINT ( 'NONE',  ( 5.823673210054444382, -21.52544592524334988, 55.20942372801902565 ) ) ;
#148288=CARTESIAN_POINT ( 'NONE',  ( -16.52544592524335698, -4.483927247898792601, 18.95942372801901143 ) ) ;
#148289=CARTESIAN_POINT ( 'NONE',  ( 17.50000000000122213, 3.338341100222780966, 22.91083448979819082 ) ) ;
#148290=CARTESIAN_POINT ( 'NONE',  ( -16.46253265017160317, 9.564922557960807481, 70.83224293864770971 ) ) ;
#148292=CARTESIAN_POINT ( 'NONE',  ( -16.53943276465976808, 0.05219959533911058130, 91.24890960531436690 ) ) ;
#148293=CARTESIAN_POINT ( 'NONE',  ( 13.97604488694527802, 13.89961937509977652, 79.37390960531435269 ) ) ;
#148294=CARTESIAN_POINT ( 'NONE',  ( 19.05341960407611168, 5.049401038298154454, 93.95724293864769550 ) ) ;
#148296=CARTESIAN_POINT ( 'NONE',  ( 5.153800228976615827, -19.02544592524334988, 95.20942372801897591 ) ) ;
#148297=CARTESIAN_POINT ( 'NONE',  ( 5.823673210054125526, 21.52544592524343514, 59.79057627198103120 ) ) ;
#148298=CARTESIAN_POINT ( 'NONE',  ( -19.05341960407611168, -5.049401038298163336, 31.45724293864769550 ) ) ;
#148299=CARTESIAN_POINT ( 'NONE',  ( -9.564922557961040184, 16.46253265017147172, 52.91775706135233293 ) ) ;
#148300=CARTESIAN_POINT ( 'NONE',  ( -13.97604488694527625, -13.89961937509977652, 61.87390960531435979 ) ) ;
#148301=CARTESIAN_POINT ( 'NONE',  ( -9.564922557960796823, -16.46253265017161027, 87.08224293864769550 ) ) ;
#148302=ORIENTED_EDGE ( 'NONE', *, *, #56349, .F. ) ;
#148303=CARTESIAN_POINT ( 'NONE',  ( 18.67979575497178502, 10.72451020669898547, 89.16557627198102409 ) ) ;
#148304=CARTESIAN_POINT ( 'NONE',  ( 14.34966873604960469, 8.224510206698951720, 89.16557627198102409 ) ) ;
#148305=CARTESIAN_POINT ( 'NONE',  ( -16.46253265017146816, -9.564922557961047289, 64.16775706135233293 ) ) ;
#148306=CARTESIAN_POINT ( 'NONE',  ( 10.81492255796078972, 18.62759615963270932, 89.58224293864768129 ) ) ;
#148307=CARTESIAN_POINT ( 'NONE',  ( -21.55341960407610458, -5.719274019375992779, 76.45724293864769550 ) ) ;
#148308=CARTESIAN_POINT ( 'NONE',  ( -8.224510206698948167, 14.34966873604960824, 30.41557627198101699 ) ) ;
#148309=CARTESIAN_POINT ( 'NONE',  ( 10.72451020669871369, 18.67979575497193778, 102.0844237280190185 ) ) ;
#148310=CARTESIAN_POINT ( 'NONE',  ( 14.29746914071037800, 8.314922557961029526, 51.66775706135234714 ) ) ;
#148311=CARTESIAN_POINT ( 'NONE',  ( -9.564922557960796823, -16.46253265017161027, 82.08224293864768129 ) ) ;
#148312=CARTESIAN_POINT ( 'NONE',  ( -9.564922557960796823, -16.46253265017161027, 27.08224293864769550 ) ) ;
#148313=CARTESIAN_POINT ( 'NONE',  ( 21.52544592524334988, 5.823673210054432836, 41.45942372801901143 ) ) ;
#148314=CARTESIAN_POINT ( 'NONE',  ( -5.719274019375665041, -21.55341960407619695, 54.79275706135235424 ) ) ;
#148315=CARTESIAN_POINT ( 'NONE',  ( -5.153800228976328057, -19.02544592524343514, 42.29057627198101699 ) ) ;
#148316=CARTESIAN_POINT ( 'NONE',  ( 21.53943276465977519, 0.05219959533937863772, 21.25109039468567218 ) ) ;
#148317=CARTESIAN_POINT ( 'NONE',  ( 0.05219959533936267826, -19.03943276465977164, 55.00109039468566863 ) ) ;
#148318=CARTESIAN_POINT ( 'NONE',  ( -16.51473224551082808, 9.474510206698731452, 73.33442372801900433 ) ) ;
#148319=CARTESIAN_POINT ( 'NONE',  ( -14.29746914071037622, -8.314922557961029526, 29.16775706135234003 ) ) ;
#148321=CARTESIAN_POINT ( 'NONE',  ( 4.379528057220092307, 16.55341960407617563, 67.29275706135234714 ) ) ;
#148322=CARTESIAN_POINT ( 'NONE',  ( -16.51473224551069308, -9.474510206698971260, 36.66557627198102409 ) ) ;
#148324=CARTESIAN_POINT ( 'NONE',  ( 0.05219959533909260263, 19.03943276465977164, 104.9989096053143669 ) ) ;
#148325=CARTESIAN_POINT ( 'NONE',  ( 4.483927247898545687, 16.52544592524342804, 114.7905762719810383 ) ) ;
#148326=CARTESIAN_POINT ( 'NONE',  ( 5.823673210054125526, 21.52544592524343514, 74.79057627198105251 ) ) ;
#148327=CARTESIAN_POINT ( 'NONE',  ( 16.52544592524335698, 4.483927247898782831, 66.45942372801903275 ) ) ;
#148328=CARTESIAN_POINT ( 'NONE',  ( -15.72974639402176322, -15.80617190586768395, 109.3760903946857042 ) ) ;
#148329=CARTESIAN_POINT ( 'NONE',  ( -16.46253265017160317, 9.564922557960807481, 45.83224293864769550 ) ) ;
#148330=CARTESIAN_POINT ( 'NONE',  ( -12.14591786802309592, -12.06949235617757132, 26.87390960531435979 ) ) ;
#148331=CARTESIAN_POINT ( 'NONE',  ( -16.55341960407611168, -4.379528057220339221, 66.45724293864768129 ) ) ;
#148333=CARTESIAN_POINT ( 'NONE',  ( 13.89961937509977652, -13.97604488694527269, 63.12390960531435979 ) ) ;
#148334=CARTESIAN_POINT ( 'NONE',  ( 15.80617190586769283, -15.72974639402175789, 40.62609039468567573 ) ) ;
#148335=CARTESIAN_POINT ( 'NONE',  ( 19.05341960407611168, 5.049401038298154454, 83.95724293864766707 ) ) ;
#148336=CARTESIAN_POINT ( 'NONE',  ( -15.72974639402176322, -15.80617190586768395, 89.37609039468568994 ) ) ;
#148337=CARTESIAN_POINT ( 'NONE',  ( 8.224510206698742110, 14.34966873604972548, 72.08442372801899012 ) ) ;
#148338=CARTESIAN_POINT ( 'NONE',  ( -19.02544592524342804, 5.153800228976336051, 106.0405762719810241 ) ) ;
#148339=CARTESIAN_POINT ( 'NONE',  ( 14.34966873604960469, 8.224510206698951720, 49.16557627198102409 ) ) ;
#148340=CARTESIAN_POINT ( 'NONE',  ( 19.03943276465977164, -0.05219959533909143690, 33.74890960531435979 ) ) ;
#148341=CARTESIAN_POINT ( 'NONE',  ( -14.34966873604972548, 8.224510206698743886, 53.33442372801901854 ) ) ;
#148342=CARTESIAN_POINT ( 'NONE',  ( -12.06949235617756955, 12.14591786802309770, 50.62390960531435979 ) ) ;
#148343=CARTESIAN_POINT ( 'NONE',  ( -16.51473224551069308, -9.474510206698971260, 106.6655762719810383 ) ) ;
#148344=CARTESIAN_POINT ( 'NONE',  ( 21.52544592524344225, -5.823673210054117533, 38.54057627198103120 ) ) ;
#148345=CARTESIAN_POINT ( 'NONE',  ( -16.51473224551082808, 9.474510206698731452, 23.33442372801900078 ) ) ;
#148346=CARTESIAN_POINT ( 'NONE',  ( 4.379528057220339221, -16.55341960407611168, 87.70724293864769550 ) ) ;
#148347=CARTESIAN_POINT ( 'NONE',  ( -19.03943276465977164, 0.05219959533909376836, 91.24890960531436690 ) ) ;
#148349=CARTESIAN_POINT ( 'NONE',  ( 4.379528057220092307, 16.55341960407617563, 47.29275706135234003 ) ) ;
#148350=CARTESIAN_POINT ( 'NONE',  ( -16.51473224551069308, -9.474510206698971260, 51.66557627198102409 ) ) ;
#148351=CARTESIAN_POINT ( 'NONE',  ( 17.50000000000000000, 5.499999999999992895, 101.7030961746583131 ) ) ;
#148352=CARTESIAN_POINT ( 'NONE',  ( -9.564922557961040184, 16.46253265017147172, 42.91775706135234003 ) ) ;
#148353=CARTESIAN_POINT ( 'NONE',  ( 16.52544592524335698, 4.483927247898782831, 86.45942372801901854 ) ) ;
#148354=CARTESIAN_POINT ( 'NONE',  ( -9.474510206698720793, -16.51473224551083518, 99.58442372801900433 ) ) ;
#148355=CARTESIAN_POINT ( 'NONE',  ( 5.719274019375673035, 21.55341960407619339, 72.29275706135236135 ) ) ;
#148356=CARTESIAN_POINT ( 'NONE',  ( -19.05341960407611168, -5.049401038298163336, 76.45724293864769550 ) ) ;
#148357=CARTESIAN_POINT ( 'NONE',  ( -21.53943276465977519, 0.05219959533907696930, 96.24890960531435269 ) ) ;
#148358=CARTESIAN_POINT ( 'NONE',  ( -14.29746914071049879, 8.314922557960819915, 100.8322429386477097 ) ) ;
#148360=CARTESIAN_POINT ( 'NONE',  ( 9.474510206698729675, 16.51473224551082808, 62.08442372801899722 ) ) ;
#148361=CARTESIAN_POINT ( 'NONE',  ( -10.81492255796078084, -18.62759615963271287, 82.08224293864768129 ) ) ;
#148362=CARTESIAN_POINT ( 'NONE',  ( 19.02544592524334988, 5.153800228976608722, 41.45942372801900433 ) ) ;
#148363=CARTESIAN_POINT ( 'NONE',  ( 18.22780087662122384, 5.500000000000018652, 98.98459894673892734 ) ) ;
#148364=CARTESIAN_POINT ( 'NONE',  ( -21.55341960407610458, -5.719274019375992779, 86.45724293864770971 ) ) ;
#148365=CARTESIAN_POINT ( 'NONE',  ( 17.50000000000000000, 5.499999999999997335, 120.0000000000000142 ) ) ;
#148366=CARTESIAN_POINT ( 'NONE',  ( 9.474510206698971260, -16.51473224551069308, 62.91557627198102409 ) ) ;
#148367=CARTESIAN_POINT ( 'NONE',  ( -13.97604488694527625, -13.89961937509977830, 91.87390960531433848 ) ) ;
#148368=CARTESIAN_POINT ( 'NONE',  ( 0.05219959533934541429, -16.53943276465976808, 20.00109039468568639 ) ) ;
#148369=CARTESIAN_POINT ( 'NONE',  ( -19.48894818550242292, 5.500000000000115463, 60.10307310435243267 ) ) ;
#148370=CARTESIAN_POINT ( 'NONE',  ( -13.97604488694527625, -13.89961937509977652, 51.87390960531436690 ) ) ;
#148371=CARTESIAN_POINT ( 'NONE',  ( -19.02544592524342804, 5.153800228976336051, 111.0405762719810099 ) ) ;
#148372=CARTESIAN_POINT ( 'NONE',  ( -21.55341960407610458, -5.719274019375992779, 91.45724293864769550 ) ) ;
#148373=CARTESIAN_POINT ( 'NONE',  ( 4.483927247898545687, 16.52544592524342804, 54.79057627198104541 ) ) ;
#148374=CARTESIAN_POINT ( 'NONE',  ( 15.80617190586769283, -15.72974639402175789, 70.62609039468567573 ) ) ;
#148375=CARTESIAN_POINT ( 'NONE',  ( -8.314922557961024197, 14.29746914071037800, 27.91775706135234358 ) ) ;
#148376=CARTESIAN_POINT ( 'NONE',  ( 19.03943276465977164, 0.05219959533936151252, 31.25109039468566863 ) ) ;
#148377=CARTESIAN_POINT ( 'NONE',  ( 4.483927247898545687, 16.52544592524342804, 29.79057627198102409 ) ) ;
#148378=CARTESIAN_POINT ( 'NONE',  ( -5.719274019375978568, 21.55341960407610458, 110.2072429386477239 ) ) ;
#148379=CARTESIAN_POINT ( 'NONE',  ( 8.224510206698953496, -14.34966873604960469, 47.91557627198102409 ) ) ;
#148380=CARTESIAN_POINT ( 'NONE',  ( 19.03943276465977164, 0.05219959533936151252, 96.25109039468567573 ) ) ;
#148381=EDGE_CURVE ( 'NONE', #109664, #68126, #100627, .T. ) ;
#148382=CARTESIAN_POINT ( 'NONE',  ( 19.03943276465977164, 0.05219959533936151252, 71.25109039468566152 ) ) ;
#148383=CARTESIAN_POINT ( 'NONE',  ( 5.823673210054444382, -21.52544592524334988, 70.20942372801904696 ) ) ;
#148384=CARTESIAN_POINT ( 'NONE',  ( 0.05219959533936267826, -19.03943276465977164, 55.00109039468566863 ) ) ;
#148385=CARTESIAN_POINT ( 'NONE',  ( 8.224510206698953496, -14.34966873604960469, 112.9155762719810383 ) ) ;
#148386=CARTESIAN_POINT ( 'NONE',  ( 21.55341960407610458, 5.719274019375980345, 38.95724293864768839 ) ) ;
#148387=CARTESIAN_POINT ( 'NONE',  ( 16.55341960407611168, 4.379528057220329451, 43.95724293864769550 ) ) ;
#148388=CARTESIAN_POINT ( 'NONE',  ( -17.40861289039006010, -6.110651285853202275, 26.37232470827433062 ) ) ;
#148389=CARTESIAN_POINT ( 'NONE',  ( -18.67979575497193778, 10.72451020669871902, 113.3344237280190328 ) ) ;
#148390=CARTESIAN_POINT ( 'NONE',  ( -16.55341960407617563, 4.379528057220093196, 78.54275706135236135 ) ) ;
#148391=CARTESIAN_POINT ( 'NONE',  ( -12.06949235617756955, 12.14591786802309770, 40.62390960531435269 ) ) ;
#148392=CARTESIAN_POINT ( 'NONE',  ( 21.55341960407619695, -5.719274019375665929, 76.04275706135237556 ) ) ;
#148393=CARTESIAN_POINT ( 'NONE',  ( 21.55341960407619695, -5.719274019375665929, 71.04275706135234714 ) ) ;
#148394=CARTESIAN_POINT ( 'NONE',  ( 18.62759615963271287, -10.81492255796078972, 78.33224293864770971 ) ) ;
#148395=CARTESIAN_POINT ( 'NONE',  ( -9.564922557960796823, -16.46253265017161027, 37.08224293864768839 ) ) ;
#148396=CARTESIAN_POINT ( 'NONE',  ( -21.55341960407619339, 5.719274019375674811, 53.54275706135234714 ) ) ;
#148397=CARTESIAN_POINT ( 'NONE',  ( 16.51473224551069308, 9.474510206698969483, 39.16557627198103120 ) ) ;
#148398=CARTESIAN_POINT ( 'NONE',  ( -5.049401038298153566, 19.05341960407611168, 55.20724293864769550 ) ) ;
#148399=CARTESIAN_POINT ( 'NONE',  ( 0.05219959533910956823, 16.53943276465976808, 94.99890960531436690 ) ) ;
#148400=CARTESIAN_POINT ( 'NONE',  ( 13.97604488694527802, 13.89961937509977652, 79.37390960531435269 ) ) ;
#148401=CARTESIAN_POINT ( 'NONE',  ( 14.34966873604960469, 8.224510206698951720, 44.16557627198103120 ) ) ;
#148402=CARTESIAN_POINT ( 'NONE',  ( 4.483927247898545687, 16.52544592524342804, 99.79057627198103830 ) ) ;
#148403=CARTESIAN_POINT ( 'NONE',  ( -10.81492255796078084, -18.62759615963271287, 67.08224293864770971 ) ) ;
#148404=CARTESIAN_POINT ( 'NONE',  ( -10.81492255796105439, 18.62759615963255655, 27.91775706135234358 ) ) ;
#148406=CARTESIAN_POINT ( 'NONE',  ( 5.153800228976335163, 19.02544592524342804, 79.79057627198102409 ) ) ;
#148407=CARTESIAN_POINT ( 'NONE',  ( -16.55341960407617563, 4.379528057220093196, 23.54275706135235424 ) ) ;
#148408=CARTESIAN_POINT ( 'NONE',  ( 10.81492255796078972, 18.62759615963270932, 64.58224293864769550 ) ) ;
#148409=CARTESIAN_POINT ( 'NONE',  ( 21.53943276465977519, 0.05219959533937863772, 101.2510903946856757 ) ) ;
#148410=CARTESIAN_POINT ( 'NONE',  ( 9.564922557960805705, 16.46253265017160317, 74.58224293864769550 ) ) ;
#148411=CARTESIAN_POINT ( 'NONE',  ( -15.72974639402176322, -15.80617190586768395, 19.37609039468568639 ) ) ;
#148412=CARTESIAN_POINT ( 'NONE',  ( -0.05219959533909027116, -19.03943276465977164, 107.4989096053143527 ) ) ;
#148413=CARTESIAN_POINT ( 'NONE',  ( -16.53943276465976808, -0.05219959533934237506, 83.75109039468568994 ) ) ;
#148414=CARTESIAN_POINT ( 'NONE',  ( 18.67979575497194134, -10.72451020669871369, 75.83442372801900433 ) ) ;
#148415=CARTESIAN_POINT ( 'NONE',  ( -18.62759615963255300, -10.81492255796106328, 94.16775706135237556 ) ) ;
#148416=CARTESIAN_POINT ( 'NONE',  ( 12.06949235617739724, 12.14591786802326823, 56.87609039468568994 ) ) ;
#148417=CARTESIAN_POINT ( 'NONE',  ( 10.72451020669871369, 18.67979575497193778, 32.08442372801901854 ) ) ;
#148418=CARTESIAN_POINT ( 'NONE',  ( 5.153800228976335163, 19.02544592524342804, 114.7905762719810241 ) ) ;
#148419=CARTESIAN_POINT ( 'NONE',  ( 21.52544592524334988, 5.823673210054432836, 96.45942372801901854 ) ) ;
#148420=CARTESIAN_POINT ( 'NONE',  ( 0.05219959533909260263, 19.03943276465977164, 99.99890960531436690 ) ) ;
#148421=CARTESIAN_POINT ( 'NONE',  ( 21.52544592524344225, -5.823673210054117533, 88.54057627198103830 ) ) ;
#148422=CARTESIAN_POINT ( 'NONE',  ( 19.03943276465977164, 0.05219959533936151252, 61.25109039468566863 ) ) ;
#148424=CARTESIAN_POINT ( 'NONE',  ( 10.81492255796078972, 18.62759615963270932, 54.58224293864769550 ) ) ;
#148425=CARTESIAN_POINT ( 'NONE',  ( 19.05341960407611168, 5.049401038298154454, 88.95724293864769550 ) ) ;
#148426=CARTESIAN_POINT ( 'NONE',  ( -0.05219959533910754901, -16.53943276465976808, 42.49890960531435979 ) ) ;
#148428=CARTESIAN_POINT ( 'NONE',  ( -5.049401038297874678, -19.05341960407617918, 79.79275706135233293 ) ) ;
#148430=CARTESIAN_POINT ( 'NONE',  ( 9.474510206698729675, 16.51473224551082808, 112.0844237280190043 ) ) ;
#148431=CARTESIAN_POINT ( 'NONE',  ( 10.81492255796078972, 18.62759615963270932, 84.58224293864769550 ) ) ;
#148432=CARTESIAN_POINT ( 'NONE',  ( 12.14591786802309770, 12.06949235617756955, 59.37390960531436690 ) ) ;
#148433=CARTESIAN_POINT ( 'NONE',  ( -0.05219959533909027116, -19.03943276465977164, 97.49890960531436690 ) ) ;
#148434=CARTESIAN_POINT ( 'NONE',  ( 14.29746914071037800, 8.314922557961029526, 31.66775706135234358 ) ) ;
#148435=CARTESIAN_POINT ( 'NONE',  ( -13.97604488694527625, -13.89961937509977652, 56.87390960531434558 ) ) ;
#148436=CARTESIAN_POINT ( 'NONE',  ( 10.72451020669871369, 18.67979575497193778, 22.08442372801901143 ) ) ;
#148437=CARTESIAN_POINT ( 'NONE',  ( -19.03943276465977164, -0.05219959533935918106, 88.75109039468567573 ) ) ;
#148438=CARTESIAN_POINT ( 'NONE',  ( -13.97604488694527625, -13.89961937509977652, 91.87390960531432427 ) ) ;
#148439=CARTESIAN_POINT ( 'NONE',  ( 19.02544592524343514, -5.153800228976328945, 73.54057627198103830 ) ) ;
#148440=CARTESIAN_POINT ( 'NONE',  ( -18.62759615963270932, 10.81492255796079327, 75.83224293864769550 ) ) ;
#148441=CARTESIAN_POINT ( 'NONE',  ( 5.049401038298161559, -19.05341960407611168, 52.70724293864767418 ) ) ;
#148443=CARTESIAN_POINT ( 'NONE',  ( -8.224510206698948167, 14.34966873604960824, 50.41557627198103120 ) ) ;
#148444=CARTESIAN_POINT ( 'NONE',  ( -5.049401038298153566, 19.05341960407611168, 110.2072429386476671 ) ) ;
#148446=CARTESIAN_POINT ( 'NONE',  ( 13.89961937509957401, 13.97604488694547697, 66.87609039468567573 ) ) ;
#148447=CARTESIAN_POINT ( 'NONE',  ( 10.72451020669898902, -18.67979575497178502, 77.91557627198102409 ) ) ;
#148448=CARTESIAN_POINT ( 'NONE',  ( 16.46253265017146816, 9.564922557961045513, 56.66775706135233293 ) ) ;
#148449=CARTESIAN_POINT ( 'NONE',  ( 9.474510206698971260, -16.51473224551069308, 102.9155762719810241 ) ) ;
#148450=CARTESIAN_POINT ( 'NONE',  ( -17.49999999999999289, 3.512728167236932375, 115.2280999518112310 ) ) ;
#148451=CARTESIAN_POINT ( 'NONE',  ( -15.72974639402197994, 15.80617190586746368, 45.62390960531436690 ) ) ;
#148452=CARTESIAN_POINT ( 'NONE',  ( 9.474510206698971260, -16.51473224551069308, 67.91557627198102409 ) ) ;
#148453=CARTESIAN_POINT ( 'NONE',  ( -21.53943276465977519, -0.05219959533937600094, 63.75109039468568284 ) ) ;
#148454=CARTESIAN_POINT ( 'NONE',  ( -0.05219959533909027116, -19.03943276465977164, 32.49890960531435979 ) ) ;
#148456=CARTESIAN_POINT ( 'NONE',  ( 10.81492255796078972, 18.62759615963270932, 109.5822429386476955 ) ) ;
#148458=CARTESIAN_POINT ( 'NONE',  ( -21.52544592524334988, -5.823673210054445271, 53.95942372801900433 ) ) ;
#148459=B_SPLINE_CURVE_WITH_KNOTS ( 'NONE', 3,
 ( #121700, #124685, #186381, #199550, #15529, #137871, #61020, #171194, #125679, #122692, #172182, #64010, #187377, #33667, #47859, #123670, #109512, #184381, #32683, #183395, #94336, #2329, #152055, #75206, #44877, #106533, #91339, #153030, #107515, #30698, #92349, #154035 ),
 .UNSPECIFIED., .F., .F.,
 ( 4, 2, 2, 2, 2, 2, 2, 2, 2, 2, 2, 2, 2, 2, 2, 4 ),
 ( 7.806255641895631925E-18, 0.0003712461730036849890, 0.0007424923460073621717, 0.001113738519011039192, 0.001484984692014716537, 0.002227477038022070577, 0.002598723211025750959, 0.002969969384029430906, 0.003341215557033111287, 0.003712461730036792102, 0.004083707903040472049, 0.004454954076044152431, 0.004826200249047833679, 0.005197446422051514060, 0.005568692595055194441, 0.005939938768058873955 ),
 .UNSPECIFIED. ) ;
#148460=ORIENTED_EDGE ( 'NONE', *, *, #84216, .F. ) ;
#148461=CARTESIAN_POINT ( 'NONE',  ( 13.89961937509977652, -13.97604488694527269, 108.1239096053143669 ) ) ;
#148462=CARTESIAN_POINT ( 'NONE',  ( -16.46253265017146816, -9.564922557961047289, 69.16775706135233293 ) ) ;
#148463=LINE ( 'NONE', #23120, #79370 ) ;
#148464=CARTESIAN_POINT ( 'NONE',  ( 0.05219959533937995610, -21.53943276465977519, 25.00109039468567218 ) ) ;
#148465=CARTESIAN_POINT ( 'NONE',  ( -16.51473224551069308, -9.474510206698971260, 61.66557627198103120 ) ) ;
#148466=CARTESIAN_POINT ( 'NONE',  ( 14.34966873604972726, -8.224510206698740333, 35.83442372801901143 ) ) ;
#148468=CARTESIAN_POINT ( 'NONE',  ( 0.05219959533937995610, -21.53943276465977519, 110.0010903946856757 ) ) ;
#148469=CARTESIAN_POINT ( 'NONE',  ( 16.51473224551069308, 9.474510206698969483, 39.16557627198103120 ) ) ;
#148470=CARTESIAN_POINT ( 'NONE',  ( -15.72974639402176322, -15.80617190586768395, 109.3760903946857042 ) ) ;
#148471=CARTESIAN_POINT ( 'NONE',  ( -12.14591786802326823, 12.06949235617739902, 93.12609039468568994 ) ) ;
#148473=CARTESIAN_POINT ( 'NONE',  ( -19.05341960407611168, -5.049401038298163336, 91.45724293864766707 ) ) ;
#148474=CARTESIAN_POINT ( 'NONE',  ( -18.67979575497193778, 10.72451020669871902, 58.33442372801901143 ) ) ;
#148478=CARTESIAN_POINT ( 'NONE',  ( -17.49999999999999645, 3.305555262949589235, 29.62517152156600986 ) ) ;
#148479=CARTESIAN_POINT ( 'NONE',  ( -14.29746914071037622, -8.314922557961029526, 59.16775706135234714 ) ) ;
#148480=CARTESIAN_POINT ( 'NONE',  ( 21.52544592524334988, 5.823673210054432836, 76.45942372801901854 ) ) ;
#148481=CARTESIAN_POINT ( 'NONE',  ( 5.823673210054444382, -21.52544592524334988, 105.2094237280190328 ) ) ;
#148483=CARTESIAN_POINT ( 'NONE',  ( 4.483927247898790824, -16.52544592524335698, 30.20942372801902565 ) ) ;
#148484=CARTESIAN_POINT ( 'NONE',  ( -19.05341960407611168, -5.049401038298163336, 91.45724293864766707 ) ) ;
#148485=CARTESIAN_POINT ( 'NONE',  ( 9.564922557960805705, 16.46253265017160317, 109.5822429386476955 ) ) ;
#148486=ORIENTED_EDGE ( 'NONE', *, *, #7273, .F. ) ;
#148487=CARTESIAN_POINT ( 'NONE',  ( 16.62475595723695676, 7.163666690055255692, 41.97286648189537317 ) ) ;
#148488=CARTESIAN_POINT ( 'NONE',  ( -16.51473224551069308, -9.474510206698971260, 21.66557627198102765 ) ) ;
#148489=CARTESIAN_POINT ( 'NONE',  ( -5.823673210054116645, -21.52544592524344225, 42.29057627198103120 ) ) ;
#148490=CARTESIAN_POINT ( 'NONE',  ( 4.379528057220092307, 16.55341960407617563, 112.2927570613523471 ) ) ;
#148491=CARTESIAN_POINT ( 'NONE',  ( 0.05219959533910956823, 16.53943276465976808, 89.99890960531438111 ) ) ;
#148492=CARTESIAN_POINT ( 'NONE',  ( 13.89961937509977652, -13.97604488694527269, 73.12390960531436690 ) ) ;
#148493=CARTESIAN_POINT ( 'NONE',  ( -5.719274019375665041, -21.55341960407619695, 89.79275706135236135 ) ) ;
#148494=CARTESIAN_POINT ( 'NONE',  ( -8.224510206698735004, -14.34966873604973081, 19.58442372801901143 ) ) ;
#148495=CARTESIAN_POINT ( 'NONE',  ( -4.379528057220328563, 16.55341960407611168, 95.20724293864769550 ) ) ;
#148496=CARTESIAN_POINT ( 'NONE',  ( 18.62759615963255655, 10.81492255796105972, 41.66775706135235424 ) ) ;
#148497=CARTESIAN_POINT ( 'NONE',  ( 21.55341960407610458, 5.719274019375980345, 73.95724293864769550 ) ) ;
#148498=CARTESIAN_POINT ( 'NONE',  ( -5.049401038297874678, -19.05341960407617918, 39.79275706135232582 ) ) ;
#148500=CARTESIAN_POINT ( 'NONE',  ( 19.02544592524343514, -5.153800228976328945, 93.54057627198102409 ) ) ;
#148501=CARTESIAN_POINT ( 'NONE',  ( -14.29746914071049879, 8.314922557960819915, 65.83224293864769550 ) ) ;
#148503=CARTESIAN_POINT ( 'NONE',  ( 12.14591786802309770, 12.06949235617756955, 49.37390960531436690 ) ) ;
#148504=CARTESIAN_POINT ( 'NONE',  ( -4.483927247898539470, -16.52544592524342804, 22.29057627198102765 ) ) ;
#148505=CARTESIAN_POINT ( 'NONE',  ( 5.049401038297881783, 19.05341960407617563, 62.29275706135234003 ) ) ;
#148506=CARTESIAN_POINT ( 'NONE',  ( 5.153800228976617603, -19.02544592524335343, 90.20942372801900433 ) ) ;
#148507=CARTESIAN_POINT ( 'NONE',  ( 15.80617190586746368, 15.72974639402197994, 24.37390960531435979 ) ) ;
#148508=CARTESIAN_POINT ( 'NONE',  ( -14.34966873604960291, -8.224510206698953496, 91.66557627198103830 ) ) ;
#148510=CARTESIAN_POINT ( 'NONE',  ( 13.89961937509977652, -13.97604488694527269, 48.12390960531435979 ) ) ;
#148511=CARTESIAN_POINT ( 'NONE',  ( 15.72974639402199770, -15.80617190586745480, 53.12390960531436690 ) ) ;
#148512=CARTESIAN_POINT ( 'NONE',  ( 10.72451020669898902, -18.67979575497178502, 82.91557627198103830 ) ) ;
#148513=CARTESIAN_POINT ( 'NONE',  ( -9.564922557960796823, -16.46253265017161027, 22.08224293864768839 ) ) ;
#148514=CARTESIAN_POINT ( 'NONE',  ( -12.06949235617739369, -12.14591786802326823, 69.37609039468567573 ) ) ;
#148515=CARTESIAN_POINT ( 'NONE',  ( -19.05341960407611168, -5.049401038298163336, 51.45724293864770260 ) ) ;
#148516=CARTESIAN_POINT ( 'NONE',  ( -19.02544592524334988, -5.153800228976617603, 43.95942372801899012 ) ) ;
#148517=CARTESIAN_POINT ( 'NONE',  ( 18.62759615963255655, 10.81492255796105972, 56.66775706135235424 ) ) ;
#148518=CARTESIAN_POINT ( 'NONE',  ( -12.14591786802309592, -12.06949235617757132, 111.8739096053143669 ) ) ;
#148519=CARTESIAN_POINT ( 'NONE',  ( 13.97604488694548053, -13.89961937509957401, 85.62609039468568994 ) ) ;
#148522=CARTESIAN_POINT ( 'NONE',  ( -18.67979575497178146, -10.72451020669898902, 51.66557627198102409 ) ) ;
#148523=CARTESIAN_POINT ( 'NONE',  ( -16.51473224551069308, -9.474510206698971260, 26.66557627198103120 ) ) ;
#148524=CARTESIAN_POINT ( 'NONE',  ( 0.05219959533937995610, -21.53943276465977519, 80.00109039468568994 ) ) ;
#148525=CARTESIAN_POINT ( 'NONE',  ( -12.14591786802309592, -12.06949235617757132, 26.87390960531435979 ) ) ;
#148526=CARTESIAN_POINT ( 'NONE',  ( -0.05219959533934338120, 16.53943276465976808, 52.50109039468567573 ) ) ;
#148527=CARTESIAN_POINT ( 'NONE',  ( 16.55341960407611168, 4.379528057220329451, 48.95724293864770971 ) ) ;
#148528=CARTESIAN_POINT ( 'NONE',  ( -18.67979575497178146, -10.72451020669898902, 86.66557627198102409 ) ) ;
#148529=CARTESIAN_POINT ( 'NONE',  ( 5.719274019375991003, -21.55341960407610458, 77.70724293864770971 ) ) ;
#148531=CARTESIAN_POINT ( 'NONE',  ( 5.049401038297881783, 19.05341960407617563, 77.29275706135231871 ) ) ;
#148532=CARTESIAN_POINT ( 'NONE',  ( 19.05341960407611168, 5.049401038298154454, 113.9572429386477097 ) ) ;
#148533=CARTESIAN_POINT ( 'NONE',  ( -13.97604488694527625, -13.89961937509977652, 46.87390960531435979 ) ) ;
#148534=CARTESIAN_POINT ( 'NONE',  ( 13.97604488694527802, 13.89961937509977652, 39.37390960531435269 ) ) ;
#148537=CARTESIAN_POINT ( 'NONE',  ( -12.06949235617739369, -12.14591786802326823, 89.37609039468568994 ) ) ;
#148538=CARTESIAN_POINT ( 'NONE',  ( 21.53943276465977519, -0.05219959533907433946, 98.74890960531438111 ) ) ;
#148539=CARTESIAN_POINT ( 'NONE',  ( 19.03943276465977164, -0.05219959533909143690, 68.74890960531436690 ) ) ;
#148540=CARTESIAN_POINT ( 'NONE',  ( -21.55341960407619339, 5.719274019375674811, 38.54275706135234714 ) ) ;
#148541=CARTESIAN_POINT ( 'NONE',  ( 0.05219959533909260263, 19.03943276465977164, 99.99890960531436690 ) ) ;
#148544=CARTESIAN_POINT ( 'NONE',  ( -10.81492255796105439, 18.62759615963255655, 32.91775706135234714 ) ) ;
#148545=CARTESIAN_POINT ( 'NONE',  ( -13.89961937509977652, 13.97604488694528158, 115.6239096053143669 ) ) ;
#148546=CARTESIAN_POINT ( 'NONE',  ( 16.51473224551069308, 9.474510206698969483, 109.1655762719810383 ) ) ;
#148547=CARTESIAN_POINT ( 'NONE',  ( -5.153800228976607833, 19.02544592524334988, 37.70942372801899722 ) ) ;
#148548=CARTESIAN_POINT ( 'NONE',  ( 18.67979575497178502, 10.72451020669898547, 109.1655762719810383 ) ) ;
#148549=CARTESIAN_POINT ( 'NONE',  ( 9.474510206698729675, 16.51473224551082808, 42.08442372801900433 ) ) ;
#148550=CARTESIAN_POINT ( 'NONE',  ( -19.03943276465977164, -0.05219959533935918106, 43.75109039468566863 ) ) ;
#148551=CARTESIAN_POINT ( 'NONE',  ( -8.314922557961024197, 14.29746914071037800, 92.91775706135236135 ) ) ;
#148552=CARTESIAN_POINT ( 'NONE',  ( -13.89961937509977652, 13.97604488694528158, 115.6239096053143669 ) ) ;
#148553=CARTESIAN_POINT ( 'NONE',  ( 9.564922557960805705, 16.46253265017160317, 74.58224293864769550 ) ) ;
#148554=CARTESIAN_POINT ( 'NONE',  ( -15.72974639402176322, -15.80617190586768395, 84.37609039468570415 ) ) ;
#148555=CARTESIAN_POINT ( 'NONE',  ( 15.72974639402176855, 15.80617190586768217, 96.87609039468568994 ) ) ;
#148557=CARTESIAN_POINT ( 'NONE',  ( 19.03943276465977164, -0.05219959533909143690, 88.74890960531436690 ) ) ;
#148558=CARTESIAN_POINT ( 'NONE',  ( -15.80617190586768217, 15.72974639402176855, 63.12609039468568994 ) ) ;
#148559=CARTESIAN_POINT ( 'NONE',  ( -19.03943276465977164, -0.05219959533935918106, 98.75109039468567573 ) ) ;
#148560=CARTESIAN_POINT ( 'NONE',  ( 13.89961937509977652, -13.97604488694527269, 68.12390960531436690 ) ) ;
#148561=CARTESIAN_POINT ( 'NONE',  ( -0.05219959533909027116, -19.03943276465977164, 107.4989096053143527 ) ) ;
#148562=EDGE_CURVE ( 'NONE', #66839, #90870, #168326, .T. ) ;
#148563=CARTESIAN_POINT ( 'NONE',  ( 16.51473224551069308, 9.474510206698969483, 99.16557627198102409 ) ) ;
#148565=CARTESIAN_POINT ( 'NONE',  ( 9.564922557960805705, 16.46253265017160317, 59.58224293864769550 ) ) ;
#148566=CARTESIAN_POINT ( 'NONE',  ( -16.51473224551069308, -9.474510206698971260, 51.66557627198102409 ) ) ;
#148567=CARTESIAN_POINT ( 'NONE',  ( 18.62759615963255655, 10.81492255796105972, 21.66775706135235069 ) ) ;
#148568=CARTESIAN_POINT ( 'NONE',  ( -16.55341960407617563, 4.379528057220093196, 103.5427570613523613 ) ) ;
#148570=CARTESIAN_POINT ( 'NONE',  ( 19.05341960407617918, -5.049401038297876454, 56.04275706135234714 ) ) ;
#148571=CARTESIAN_POINT ( 'NONE',  ( -9.474510206698964154, 16.51473224551069663, 90.41557627198103830 ) ) ;
#148572=CARTESIAN_POINT ( 'NONE',  ( 16.52544592524342804, -4.483927247898539470, 68.54057627198103830 ) ) ;
#148573=CARTESIAN_POINT ( 'NONE',  ( 14.34966873604960469, 8.224510206698951720, 109.1655762719810383 ) ) ;
#148574=CARTESIAN_POINT ( 'NONE',  ( -18.67979575497178146, -10.72451020669898902, 31.66557627198102054 ) ) ;
#148575=CARTESIAN_POINT ( 'NONE',  ( 16.51473224551069308, 9.474510206698969483, 114.1655762719810241 ) ) ;
#148576=CARTESIAN_POINT ( 'NONE',  ( -8.224510206698948167, 14.34966873604960824, 95.41557627198102409 ) ) ;
#148577=CARTESIAN_POINT ( 'NONE',  ( -17.26172910966779028, 6.454744622555849354, 55.80646908649224969 ) ) ;
#148578=CARTESIAN_POINT ( 'NONE',  ( -5.153800228976607833, 19.02544592524334988, 32.70942372801899722 ) ) ;
#148579=CARTESIAN_POINT ( 'NONE',  ( 4.483927247898790824, -16.52544592524335698, 110.2094237280190185 ) ) ;
#148580=CARTESIAN_POINT ( 'NONE',  ( -19.03943276465977164, 0.05219959533909376836, 86.24890960531436690 ) ) ;
#148581=CARTESIAN_POINT ( 'NONE',  ( -21.53943276465977519, -0.05219959533937600094, 48.75109039468568284 ) ) ;
#148582=CARTESIAN_POINT ( 'NONE',  ( 5.823673210054125526, 21.52544592524343514, 44.79057627198103120 ) ) ;
#148583=CARTESIAN_POINT ( 'NONE',  ( -5.823673210054431948, 21.52544592524334988, 37.70942372801900433 ) ) ;
#148584=CARTESIAN_POINT ( 'NONE',  ( 15.80617190586746368, 15.72974639402197994, 79.37390960531436690 ) ) ;
#148585=CARTESIAN_POINT ( 'NONE',  ( -12.14591786802309592, -12.06949235617757132, 101.8739096053143811 ) ) ;
#148586=CARTESIAN_POINT ( 'NONE',  ( -5.153800228976607833, 19.02544592524334988, 57.70942372801899012 ) ) ;
#148587=CARTESIAN_POINT ( 'NONE',  ( -9.564922557960796823, -16.46253265017161027, 42.08224293864769550 ) ) ;
#148588=CARTESIAN_POINT ( 'NONE',  ( 16.51473224551069308, 9.474510206698969483, 94.16557627198103830 ) ) ;
#148589=CARTESIAN_POINT ( 'NONE',  ( 16.46253265017160672, -9.564922557960803928, 93.33224293864769550 ) ) ;
#148590=CARTESIAN_POINT ( 'NONE',  ( 16.55341960407611168, 4.379528057220329451, 113.9572429386477239 ) ) ;
#148591=CARTESIAN_POINT ( 'NONE',  ( 12.06949235617757843, -12.14591786802309237, 38.12390960531436690 ) ) ;
#148592=CARTESIAN_POINT ( 'NONE',  ( -0.05219959533934338120, 16.53943276465976808, 42.50109039468567573 ) ) ;
#148593=CARTESIAN_POINT ( 'NONE',  ( -15.72974639402176322, -15.80617190586768395, 109.3760903946857042 ) ) ;
#148594=CARTESIAN_POINT ( 'NONE',  ( 9.474510206698971260, -16.51473224551069308, 112.9155762719810383 ) ) ;
#148595=CARTESIAN_POINT ( 'NONE',  ( -16.55341960407617563, 4.379528057220093196, 113.5427570613523756 ) ) ;
#148596=CARTESIAN_POINT ( 'NONE',  ( 10.81492255796106328, -18.62759615963255655, 35.41775706135234003 ) ) ;
#148597=CARTESIAN_POINT ( 'NONE',  ( 9.564922557960805705, 16.46253265017160317, 104.5822429386476955 ) ) ;
#148598=CARTESIAN_POINT ( 'NONE',  ( 4.379528057220092307, 16.55341960407617563, 52.29275706135236135 ) ) ;
#148599=CARTESIAN_POINT ( 'NONE',  ( 0.05219959533934541429, -16.53943276465976808, 110.0010903946856757 ) ) ;
#148600=CARTESIAN_POINT ( 'NONE',  ( 14.34966873604972726, -8.224510206698740333, 90.83442372801901854 ) ) ;
#148601=CARTESIAN_POINT ( 'NONE',  ( 12.06949235617739724, 12.14591786802326823, 21.87609039468567573 ) ) ;
#148602=CARTESIAN_POINT ( 'NONE',  ( 0.05219959533909260263, 19.03943276465977164, 44.99890960531435979 ) ) ;
#148603=CARTESIAN_POINT ( 'NONE',  ( -16.55341960407611168, -4.379528057220339221, 101.4572429386476955 ) ) ;
#148604=CARTESIAN_POINT ( 'NONE',  ( 15.72974639402199770, -15.80617190586745480, 113.1239096053143953 ) ) ;
#148605=CARTESIAN_POINT ( 'NONE',  ( -13.89961937509977652, 13.97604488694528158, 35.62390960531435269 ) ) ;
#148606=CARTESIAN_POINT ( 'NONE',  ( -16.46253265017160317, 9.564922557960807481, 105.8322429386476955 ) ) ;
#148607=CARTESIAN_POINT ( 'NONE',  ( -15.80617190586768217, 15.72974639402176855, 28.12609039468568284 ) ) ;
#148609=CARTESIAN_POINT ( 'NONE',  ( 19.03943276465977164, -0.05219959533909143690, 108.7489096053143527 ) ) ;
#148612=CARTESIAN_POINT ( 'NONE',  ( 5.153800228976335163, 19.02544592524342804, 94.79057627198103830 ) ) ;
#148613=CARTESIAN_POINT ( 'NONE',  ( -15.80617190586768217, 15.72974639402176855, 48.12609039468568284 ) ) ;
#148614=CARTESIAN_POINT ( 'NONE',  ( -14.29746914071049879, 8.314922557960819915, 95.83224293864770971 ) ) ;
#148615=CARTESIAN_POINT ( 'NONE',  ( 13.89961937509977652, -13.97604488694527269, 98.12390960531433848 ) ) ;
#148617=CARTESIAN_POINT ( 'NONE',  ( 16.53943276465976808, 0.05219959533934440121, 66.25109039468567573 ) ) ;
#148618=CARTESIAN_POINT ( 'NONE',  ( 15.72974639402176855, 15.80617190586768217, 81.87609039468568994 ) ) ;
#148619=CARTESIAN_POINT ( 'NONE',  ( -12.14591786802326823, 12.06949235617739902, 43.12609039468568284 ) ) ;
#148620=CARTESIAN_POINT ( 'NONE',  ( 9.564922557960805705, 16.46253265017160317, 84.58224293864769550 ) ) ;
#148621=EDGE_CURVE ( 'NONE', #192521, #11672, #122469, .T. ) ;
#148622=CARTESIAN_POINT ( 'NONE',  ( -19.03943276465977164, -0.05219959533935918106, 103.7510903946856757 ) ) ;
#148623=CARTESIAN_POINT ( 'NONE',  ( 0.05219959533934541429, -16.53943276465976808, 70.00109039468568994 ) ) ;
#148624=CARTESIAN_POINT ( 'NONE',  ( 15.80617190586769283, -15.72974639402175789, 105.6260903946856899 ) ) ;
#148625=CARTESIAN_POINT ( 'NONE',  ( 9.474510206698729675, 16.51473224551082808, 92.08442372801900433 ) ) ;
#148626=CARTESIAN_POINT ( 'NONE',  ( 13.89961937509977652, -13.97604488694527269, 58.12390960531436690 ) ) ;
#148627=CARTESIAN_POINT ( 'NONE',  ( -21.53943276465977519, 0.05219959533907696930, 81.24890960531436690 ) ) ;
#148628=CARTESIAN_POINT ( 'NONE',  ( -4.379528057220328563, 16.55341960407611168, 90.20724293864770971 ) ) ;
#148629=CARTESIAN_POINT ( 'NONE',  ( -5.153800228976607833, 19.02544592524334988, 97.70942372801900433 ) ) ;
#148630=CARTESIAN_POINT ( 'NONE',  ( -0.05219959533934338120, 16.53943276465976808, 62.50109039468568284 ) ) ;
#148632=CARTESIAN_POINT ( 'NONE',  ( 16.46253265017146816, 9.564922557961045513, 56.66775706135233293 ) ) ;
#148633=CARTESIAN_POINT ( 'NONE',  ( 16.52544592524342804, -4.483927247898539470, 38.54057627198103120 ) ) ;
#148634=CARTESIAN_POINT ( 'NONE',  ( -12.06949235617756955, 12.14591786802309770, 85.62390960531436690 ) ) ;
#148635=CARTESIAN_POINT ( 'NONE',  ( -5.049401038297874678, -19.05341960407617918, 24.79275706135233648 ) ) ;
#148636=CARTESIAN_POINT ( 'NONE',  ( -17.40861289039010629, 6.110651285853060166, 38.62767529172569425 ) ) ;
#148637=CARTESIAN_POINT ( 'NONE',  ( -15.80617190586768217, 15.72974639402176855, 23.12609039468567573 ) ) ;
#148638=CARTESIAN_POINT ( 'NONE',  ( -13.89961937509977652, 13.97604488694528158, 105.6239096053143527 ) ) ;
#148639=CARTESIAN_POINT ( 'NONE',  ( 19.05341960407611168, 5.049401038298154454, 83.95724293864766707 ) ) ;
#148640=CARTESIAN_POINT ( 'NONE',  ( 15.72974639402176855, 15.80617190586768217, 101.8760903946857042 ) ) ;
#148641=CARTESIAN_POINT ( 'NONE',  ( 13.89961937509977652, -13.97604488694527269, 78.12390960531433848 ) ) ;
#148643=CARTESIAN_POINT ( 'NONE',  ( 18.62759615963271287, -10.81492255796078972, 48.33224293864770260 ) ) ;
#148644=CARTESIAN_POINT ( 'NONE',  ( 12.14591786802309770, 12.06949235617756955, 79.37390960531436690 ) ) ;
#148645=CARTESIAN_POINT ( 'NONE',  ( -19.03943276465977164, 0.05219959533909376836, 61.24890960531436690 ) ) ;
#148646=CARTESIAN_POINT ( 'NONE',  ( 4.379528057220339221, -16.55341960407611168, 92.70724293864770971 ) ) ;
#148647=CARTESIAN_POINT ( 'NONE',  ( -10.81492255796105439, 18.62759615963255655, 27.91775706135234358 ) ) ;
#148649=CARTESIAN_POINT ( 'NONE',  ( -21.55341960407619339, 5.719274019375674811, 63.54275706135234003 ) ) ;
#148650=CARTESIAN_POINT ( 'NONE',  ( 13.97604488694527802, 13.89961937509977652, 34.37390960531436690 ) ) ;
#148651=CARTESIAN_POINT ( 'NONE',  ( 4.379528057220092307, 16.55341960407617563, 57.29275706135234714 ) ) ;
#148653=CARTESIAN_POINT ( 'NONE',  ( 10.72451020669871369, 18.67979575497193778, 22.08442372801901143 ) ) ;
#148654=CARTESIAN_POINT ( 'NONE',  ( 10.81492255796078972, 18.62759615963270932, 114.5822429386477097 ) ) ;
#148655=CARTESIAN_POINT ( 'NONE',  ( -19.05341960407617563, 5.049401038297882671, 38.54275706135233293 ) ) ;
#148656=CARTESIAN_POINT ( 'NONE',  ( 13.97604488694527802, 13.89961937509977652, 49.37390960531434558 ) ) ;
#148658=CARTESIAN_POINT ( 'NONE',  ( 18.67979575497194134, -10.72451020669871369, 70.83442372801901854 ) ) ;
#148659=CARTESIAN_POINT ( 'NONE',  ( 0.05219959533907565091, 21.53943276465977519, 59.99890960531436690 ) ) ;
#148660=CARTESIAN_POINT ( 'NONE',  ( 12.14591786802309770, 12.06949235617756955, 34.37390960531435979 ) ) ;
#148661=CARTESIAN_POINT ( 'NONE',  ( 0.05219959533937995610, -21.53943276465977519, 75.00109039468568994 ) ) ;
#148662=CARTESIAN_POINT ( 'NONE',  ( -19.02544592524334988, -5.153800228976617603, 18.95942372801899722 ) ) ;
#148663=CARTESIAN_POINT ( 'NONE',  ( -8.224510206698948167, 14.34966873604960824, 55.41557627198102409 ) ) ;
#148664=CARTESIAN_POINT ( 'NONE',  ( -16.53943276465976808, 0.05219959533911058130, 111.2489096053143669 ) ) ;
#148665=CARTESIAN_POINT ( 'NONE',  ( -13.97604488694547697, 13.89961937509957934, 48.12609039468566863 ) ) ;
#148666=CARTESIAN_POINT ( 'NONE',  ( 0.05219959533934541429, -16.53943276465976808, 110.0010903946856757 ) ) ;
#148667=CARTESIAN_POINT ( 'NONE',  ( 10.81492255796106328, -18.62759615963255655, 70.41775706135236135 ) ) ;
#148668=CARTESIAN_POINT ( 'NONE',  ( 0.05219959533909260263, 19.03943276465977164, 59.99890960531436690 ) ) ;
#148669=CARTESIAN_POINT ( 'NONE',  ( -16.51473224551082808, 9.474510206698731452, 33.33442372801899722 ) ) ;
#148670=CARTESIAN_POINT ( 'NONE',  ( -21.52544592524343514, 5.823673210054127303, 41.04057627198103120 ) ) ;
#148671=CARTESIAN_POINT ( 'NONE',  ( -21.55341960407619339, 5.719274019375674811, 33.54275706135234714 ) ) ;
#148672=CARTESIAN_POINT ( 'NONE',  ( 18.67979575497178502, 10.72451020669898547, 84.16557627198103830 ) ) ;
#148673=CARTESIAN_POINT ( 'NONE',  ( 13.97604488694548053, -13.89961937509957401, 80.62609039468567573 ) ) ;
#148674=CARTESIAN_POINT ( 'NONE',  ( -4.379528057220086978, -16.55341960407618274, 49.79275706135234714 ) ) ;
#148676=CARTESIAN_POINT ( 'NONE',  ( 10.72451020669898902, -18.67979575497178502, 92.91557627198103830 ) ) ;
#148677=CARTESIAN_POINT ( 'NONE',  ( 16.55341960407611168, 4.379528057220329451, 93.95724293864770971 ) ) ;
#148679=CARTESIAN_POINT ( 'NONE',  ( 0.05219959533934541429, -16.53943276465976808, 20.00109039468568639 ) ) ;
#148680=CARTESIAN_POINT ( 'NONE',  ( -21.55341960407610458, -5.719274019375992779, 46.45724293864769550 ) ) ;
#148681=CARTESIAN_POINT ( 'NONE',  ( 4.379528057220092307, 16.55341960407617563, 82.29275706135234714 ) ) ;
#148682=LINE ( 'NONE', #118344, #122078 ) ;
#148683=CARTESIAN_POINT ( 'NONE',  ( -16.52544592524335698, -4.483927247898792601, 53.95942372801900433 ) ) ;
#148684=CARTESIAN_POINT ( 'NONE',  ( -21.53943276465977519, -0.05219959533937600094, 33.75109039468568284 ) ) ;
#148685=CARTESIAN_POINT ( 'NONE',  ( -21.55341960407610458, -5.719274019375992779, 46.45724293864769550 ) ) ;
#148686=CARTESIAN_POINT ( 'NONE',  ( 8.314922557961029526, -14.29746914071037800, 75.41775706135233293 ) ) ;
#148687=CARTESIAN_POINT ( 'NONE',  ( 9.564922557960805705, 16.46253265017160317, 94.58224293864769550 ) ) ;
#148688=CARTESIAN_POINT ( 'NONE',  ( 21.52544592524334988, 5.823673210054432836, 56.45942372801902565 ) ) ;
#148689=CARTESIAN_POINT ( 'NONE',  ( 16.46253265017160672, -9.564922557960803928, 23.33224293864769194 ) ) ;
#148690=CARTESIAN_POINT ( 'NONE',  ( 5.719274019375991003, -21.55341960407610458, 37.70724293864769550 ) ) ;
#148691=CARTESIAN_POINT ( 'NONE',  ( 0.05219959533907565091, 21.53943276465977519, 24.99890960531435624 ) ) ;
#148693=CARTESIAN_POINT ( 'NONE',  ( 19.02544592524334988, 5.153800228976608722, 41.45942372801900433 ) ) ;
#148694=CARTESIAN_POINT ( 'NONE',  ( 14.34966873604972726, -8.224510206698740333, 45.83442372801901854 ) ) ;
#148695=CARTESIAN_POINT ( 'NONE',  ( -13.97604488694527625, -13.89961937509977652, 111.8739096053143243 ) ) ;
#148697=CARTESIAN_POINT ( 'NONE',  ( 0.05219959533909260263, 19.03943276465977164, 84.99890960531436690 ) ) ;
#148698=CARTESIAN_POINT ( 'NONE',  ( 14.29746914071037800, 8.314922557961029526, 96.66775706135234714 ) ) ;
#148700=CARTESIAN_POINT ( 'NONE',  ( 14.29746914071049879, -8.314922557960816363, 98.33224293864769550 ) ) ;
#148701=CARTESIAN_POINT ( 'NONE',  ( 21.52544592524344225, -5.823673210054117533, 43.54057627198103830 ) ) ;
#148702=CARTESIAN_POINT ( 'NONE',  ( -0.05219959533909027116, -19.03943276465977164, 27.49890960531435624 ) ) ;
#148703=CARTESIAN_POINT ( 'NONE',  ( -12.06949235617739369, -12.14591786802326823, 74.37609039468568994 ) ) ;
#148704=CARTESIAN_POINT ( 'NONE',  ( -18.62759615963255300, -10.81492255796106328, 34.16775706135234714 ) ) ;
#148705=CARTESIAN_POINT ( 'NONE',  ( -19.03943276465977164, -0.05219959533935918106, 88.75109039468567573 ) ) ;
#148706=CARTESIAN_POINT ( 'NONE',  ( -9.474510206698964154, 16.51473224551069663, 40.41557627198103120 ) ) ;
#148708=CARTESIAN_POINT ( 'NONE',  ( 5.823673210054444382, -21.52544592524334988, 110.2094237280190185 ) ) ;
#148709=CARTESIAN_POINT ( 'NONE',  ( -13.97604488694527625, -13.89961937509977652, 81.87390960531436690 ) ) ;
#148710=CARTESIAN_POINT ( 'NONE',  ( 4.379528057220092307, 16.55341960407617563, 57.29275706135234714 ) ) ;
#148711=CARTESIAN_POINT ( 'NONE',  ( 10.72451020669871369, 18.67979575497193778, 97.08442372801904696 ) ) ;
#148712=CARTESIAN_POINT ( 'NONE',  ( -19.02544592524334988, -5.153800228976617603, 58.95942372801900433 ) ) ;
#148713=CARTESIAN_POINT ( 'NONE',  ( -16.51473224551082808, 9.474510206698731452, 73.33442372801900433 ) ) ;
#148715=CARTESIAN_POINT ( 'NONE',  ( -18.62759615963255300, -10.81492255796106328, 64.16775706135234714 ) ) ;
#148716=CARTESIAN_POINT ( 'NONE',  ( 19.03943276465977164, -0.05219959533909143690, 63.74890960531435979 ) ) ;
#148717=CARTESIAN_POINT ( 'NONE',  ( -13.97604488694527625, -13.89961937509977652, 21.87390960531435979 ) ) ;
#148718=CARTESIAN_POINT ( 'NONE',  ( 19.03943276465977164, 0.05219959533936151252, 61.25109039468566863 ) ) ;
#148720=CARTESIAN_POINT ( 'NONE',  ( -5.049401038298153566, 19.05341960407611168, 85.20724293864766707 ) ) ;
#148721=CARTESIAN_POINT ( 'NONE',  ( -14.29746914071049879, 8.314922557960819915, 35.83224293864768839 ) ) ;
#148722=CARTESIAN_POINT ( 'NONE',  ( -15.80617190586745835, -15.72974639402198527, 36.87390960531435979 ) ) ;
#148724=CARTESIAN_POINT ( 'NONE',  ( 10.81492255796106328, -18.62759615963255655, 105.4177570613523613 ) ) ;
#148726=CARTESIAN_POINT ( 'NONE',  ( -13.89961937509977652, 13.97604488694528158, 35.62390960531435269 ) ) ;
#148727=CARTESIAN_POINT ( 'NONE',  ( -15.49999999999999822, 7.499999999999998224, 22.00000000000000711 ) ) ;
#148729=CARTESIAN_POINT ( 'NONE',  ( 15.72974639402176855, 15.80617190586768217, 66.87609039468568994 ) ) ;
#148731=CARTESIAN_POINT ( 'NONE',  ( 4.483927247898790824, -16.52544592524335698, 60.20942372801902565 ) ) ;
#148732=CARTESIAN_POINT ( 'NONE',  ( -15.80617190586745835, -15.72974639402198527, 86.87390960531438111 ) ) ;
#148733=CARTESIAN_POINT ( 'NONE',  ( -8.224510206698948167, 14.34966873604960824, 50.41557627198103120 ) ) ;
#148734=CARTESIAN_POINT ( 'NONE',  ( 19.02544592524343514, -5.153800228976328945, 23.54057627198102054 ) ) ;
#148735=CARTESIAN_POINT ( 'NONE',  ( -16.51473224551069308, -9.474510206698971260, 106.6655762719810383 ) ) ;
#148736=CARTESIAN_POINT ( 'NONE',  ( 5.719274019375673035, 21.55341960407619339, 32.29275706135235424 ) ) ;
#148737=CARTESIAN_POINT ( 'NONE',  ( -9.564922557961040184, 16.46253265017147172, 47.91775706135233293 ) ) ;
#148738=CARTESIAN_POINT ( 'NONE',  ( -5.049401038298153566, 19.05341960407611168, 40.20724293864768839 ) ) ;
#148739=CARTESIAN_POINT ( 'NONE',  ( 21.52544592524334988, 5.823673210054432836, 81.45942372801900433 ) ) ;
#148740=CARTESIAN_POINT ( 'NONE',  ( 17.50000000000002132, 5.622605283950869115, 98.81207310596117566 ) ) ;
#148741=CARTESIAN_POINT ( 'NONE',  ( 8.224510206698953496, -14.34966873604960469, 27.91557627198103830 ) ) ;
#148743=CARTESIAN_POINT ( 'NONE',  ( -21.52544592524343514, 5.823673210054127303, 41.04057627198103120 ) ) ;
#148745=CARTESIAN_POINT ( 'NONE',  ( 16.46253265017160672, -9.564922557960803928, 88.33224293864769550 ) ) ;
#148746=CARTESIAN_POINT ( 'NONE',  ( 14.34966873604960469, 8.224510206698951720, 89.16557627198102409 ) ) ;
#148747=CARTESIAN_POINT ( 'NONE',  ( 19.03943276465977164, 0.05219959533936151252, 111.2510903946856757 ) ) ;
#148748=CARTESIAN_POINT ( 'NONE',  ( -0.05219959533907301413, -21.53943276465977519, 62.49890960531436690 ) ) ;
#148749=ORIENTED_EDGE ( 'NONE', *, *, #174036, .F. ) ;
#148750=CARTESIAN_POINT ( 'NONE',  ( -5.049401038298153566, 19.05341960407611168, 30.20724293864768839 ) ) ;
#148751=CARTESIAN_POINT ( 'NONE',  ( 9.474510206698971260, -16.51473224551069308, 82.91557627198103830 ) ) ;
#148752=CARTESIAN_POINT ( 'NONE',  ( 5.719274019375991003, -21.55341960407610458, 82.70724293864770971 ) ) ;
#148753=CARTESIAN_POINT ( 'NONE',  ( 8.314922557961029526, -14.29746914071037800, 105.4177570613523613 ) ) ;
#148754=CARTESIAN_POINT ( 'NONE',  ( 5.153800228976335163, 19.02544592524342804, 99.79057627198102409 ) ) ;
#148755=CARTESIAN_POINT ( 'NONE',  ( -9.564922557961040184, 16.46253265017147172, 77.91775706135234714 ) ) ;
#148756=CARTESIAN_POINT ( 'NONE',  ( -21.55341960407619339, 5.719274019375674811, 93.54275706135234714 ) ) ;
#148757=CARTESIAN_POINT ( 'NONE',  ( -21.53943276465977519, 0.05219959533907696930, 81.24890960531436690 ) ) ;
#148758=CARTESIAN_POINT ( 'NONE',  ( 10.72451020669898902, -18.67979575497178502, 42.91557627198103120 ) ) ;
#148759=CARTESIAN_POINT ( 'NONE',  ( -19.03943276465977164, 0.05219959533909376836, 51.24890960531436690 ) ) ;
#148760=CARTESIAN_POINT ( 'NONE',  ( -0.05219959533910754901, -16.53943276465976808, 22.49890960531436335 ) ) ;
#148761=CARTESIAN_POINT ( 'NONE',  ( -19.05341960407611168, -5.049401038298163336, 61.45724293864769550 ) ) ;
#148764=CARTESIAN_POINT ( 'NONE',  ( 16.46253265017146816, 9.564922557961045513, 26.66775706135234003 ) ) ;
#148765=CARTESIAN_POINT ( 'NONE',  ( -12.06949235617756955, 12.14591786802309770, 70.62390960531436690 ) ) ;
#148766=CARTESIAN_POINT ( 'NONE',  ( -5.823673210054431948, 21.52544592524334988, 22.70942372801901499 ) ) ;
#148768=CARTESIAN_POINT ( 'NONE',  ( -21.53943276465977519, 0.05219959533907696930, 61.24890960531435979 ) ) ;
#148769=CARTESIAN_POINT ( 'NONE',  ( 12.14591786802327356, -12.06949235617739191, 95.62609039468568994 ) ) ;
#148770=CARTESIAN_POINT ( 'NONE',  ( -16.53943276465976808, 0.05219959533911058130, 106.2489096053143811 ) ) ;
#148771=CARTESIAN_POINT ( 'NONE',  ( -5.049401038298153566, 19.05341960407611168, 75.20724293864769550 ) ) ;
#148774=CARTESIAN_POINT ( 'NONE',  ( 12.06949235617757843, -12.14591786802309237, 33.12390960531435979 ) ) ;
#148775=CARTESIAN_POINT ( 'NONE',  ( 5.719274019375673035, 21.55341960407619339, 57.29275706135234714 ) ) ;
#148776=CARTESIAN_POINT ( 'NONE',  ( 13.97604488694527802, 13.89961937509977652, 109.3739096053143669 ) ) ;
#148777=CARTESIAN_POINT ( 'NONE',  ( -5.719274019375665041, -21.55341960407619695, 84.79275706135234714 ) ) ;
#148778=CARTESIAN_POINT ( 'NONE',  ( -9.474510206698964154, 16.51473224551069663, 35.41557627198102409 ) ) ;
#148779=CARTESIAN_POINT ( 'NONE',  ( 9.564922557960805705, 16.46253265017160317, 44.58224293864769550 ) ) ;
#148781=CARTESIAN_POINT ( 'NONE',  ( -15.80617190586768217, 15.72974639402176855, 93.12609039468568994 ) ) ;
#148782=CARTESIAN_POINT ( 'NONE',  ( 14.29746914071037800, 8.314922557961029526, 46.66775706135234714 ) ) ;
#148783=CARTESIAN_POINT ( 'NONE',  ( 21.53943276465977519, 0.05219959533937863772, 91.25109039468568994 ) ) ;
#148784=CARTESIAN_POINT ( 'NONE',  ( 19.05341960407611168, 5.049401038298154454, 108.9572429386477097 ) ) ;
#148785=CARTESIAN_POINT ( 'NONE',  ( 9.564922557961047289, -16.46253265017146816, 95.41775706135233293 ) ) ;
#148786=CARTESIAN_POINT ( 'NONE',  ( -5.719274019375665041, -21.55341960407619695, 59.79275706135234714 ) ) ;
#148787=CARTESIAN_POINT ( 'NONE',  ( 16.52544592524335698, 4.483927247898782831, 26.45942372801901854 ) ) ;
#148788=CARTESIAN_POINT ( 'NONE',  ( 13.89961937509957401, 13.97604488694547697, 81.87609039468564731 ) ) ;
#148789=CARTESIAN_POINT ( 'NONE',  ( -0.05219959533909027116, -19.03943276465977164, 52.49890960531436690 ) ) ;
#148790=CARTESIAN_POINT ( 'NONE',  ( 9.564922557961047289, -16.46253265017146816, 95.41775706135233293 ) ) ;
#148791=CARTESIAN_POINT ( 'NONE',  ( -14.29746914071049879, 8.314922557960819915, 25.83224293864769194 ) ) ;
#148792=CARTESIAN_POINT ( 'NONE',  ( -5.049401038297874678, -19.05341960407617918, 94.79275706135230450 ) ) ;
#148793=CARTESIAN_POINT ( 'NONE',  ( 12.06949235617757843, -12.14591786802309237, 48.12390960531436690 ) ) ;
#148794=CARTESIAN_POINT ( 'NONE',  ( -16.51473224551082808, 9.474510206698731452, 68.33442372801900433 ) ) ;
#148795=CARTESIAN_POINT ( 'NONE',  ( -0.05219959533934338120, 16.53943276465976808, 57.50109039468568994 ) ) ;
#148796=CARTESIAN_POINT ( 'NONE',  ( -5.153800228976607833, 19.02544592524334988, 22.70942372801899012 ) ) ;
#148797=CARTESIAN_POINT ( 'NONE',  ( -16.51473224551069308, -9.474510206698971260, 21.66557627198102765 ) ) ;
#148798=CARTESIAN_POINT ( 'NONE',  ( -19.02544592524342804, 5.153800228976336051, 41.04057627198103120 ) ) ;
#148799=CARTESIAN_POINT ( 'NONE',  ( -0.05219959533934338120, 16.53943276465976808, 57.50109039468568994 ) ) ;
#148803=CARTESIAN_POINT ( 'NONE',  ( -16.51473224551069308, -9.474510206698971260, 101.6655762719810241 ) ) ;
#148804=CARTESIAN_POINT ( 'NONE',  ( 17.78921395495471103, 1.086248361264983142, 102.5000000000000142 ) ) ;
#148805=ORIENTED_EDGE ( 'NONE', *, *, #101326, .F. ) ;
#148806=CARTESIAN_POINT ( 'NONE',  ( 0.05219959533936267826, -19.03943276465977164, 100.0010903946856757 ) ) ;
#148807=CARTESIAN_POINT ( 'NONE',  ( 21.53943276465977519, -0.05219959533907433946, 38.74890960531435979 ) ) ;
#148808=CARTESIAN_POINT ( 'NONE',  ( 13.89961937509957401, 13.97604488694547697, 26.87609039468566507 ) ) ;
#148809=CARTESIAN_POINT ( 'NONE',  ( -0.05219959533936034679, 19.03943276465977164, 112.5010903946856757 ) ) ;
#148810=CARTESIAN_POINT ( 'NONE',  ( -19.02544592524342804, 5.153800228976336051, 31.04057627198102409 ) ) ;
#148811=CARTESIAN_POINT ( 'NONE',  ( -13.97604488694527625, -13.89961937509977652, 41.87390960531435979 ) ) ;
#148812=CARTESIAN_POINT ( 'NONE',  ( 15.72974639402199770, -15.80617190586745480, 73.12390960531436690 ) ) ;
#148813=CARTESIAN_POINT ( 'NONE',  ( 0.05219959533909260263, 19.03943276465977164, 34.99890960531435979 ) ) ;
#148815=CARTESIAN_POINT ( 'NONE',  ( -0.05219959533936034679, 19.03943276465977164, 82.50109039468567573 ) ) ;
#148816=CARTESIAN_POINT ( 'NONE',  ( -14.34966873604960291, -8.224510206698953496, 51.66557627198102409 ) ) ;
#148817=CARTESIAN_POINT ( 'NONE',  ( 10.81492255796078972, 18.62759615963270932, 29.58224293864769905 ) ) ;
#148818=CARTESIAN_POINT ( 'NONE',  ( -10.72451020669870658, -18.67979575497194134, 109.5844237280190328 ) ) ;
#148819=CARTESIAN_POINT ( 'NONE',  ( 10.72451020669898902, -18.67979575497178502, 87.91557627198103830 ) ) ;
#148820=CARTESIAN_POINT ( 'NONE',  ( -15.80617190586768217, 15.72974639402176855, 73.12609039468567573 ) ) ;
#148821=CARTESIAN_POINT ( 'NONE',  ( -15.72974639402176322, -15.80617190586768395, 69.37609039468567573 ) ) ;
#148822=CARTESIAN_POINT ( 'NONE',  ( 5.153800228976335163, 19.02544592524342804, 109.7905762719810099 ) ) ;
#148823=CARTESIAN_POINT ( 'NONE',  ( 12.14591786802327356, -12.06949235617739191, 100.6260903946857184 ) ) ;
#148824=CARTESIAN_POINT ( 'NONE',  ( -18.62759615963255300, -10.81492255796106328, 64.16775706135234714 ) ) ;
#148825=CARTESIAN_POINT ( 'NONE',  ( -19.05341960407611168, -5.049401038298163336, 56.45724293864768129 ) ) ;
#148826=CARTESIAN_POINT ( 'NONE',  ( 16.51473224551083163, -9.474510206698727899, 35.83442372801899722 ) ) ;
#148827=CARTESIAN_POINT ( 'NONE',  ( 15.80617190586769283, -15.72974639402175789, 35.62609039468568994 ) ) ;
#148828=CARTESIAN_POINT ( 'NONE',  ( 5.049401038298161559, -19.05341960407611168, 67.70724293864769550 ) ) ;
#148829=CARTESIAN_POINT ( 'NONE',  ( -14.29746914071049879, 8.314922557960819915, 80.83224293864769550 ) ) ;
#148830=CARTESIAN_POINT ( 'NONE',  ( -12.14591786802309592, -12.06949235617757132, 46.87390960531435979 ) ) ;
#148831=CARTESIAN_POINT ( 'NONE',  ( 15.80617190586746368, 15.72974639402197994, 59.37390960531436690 ) ) ;
#148832=CARTESIAN_POINT ( 'NONE',  ( 13.97604488694527802, 13.89961937509977652, 54.37390960531435979 ) ) ;
#148833=CARTESIAN_POINT ( 'NONE',  ( -21.55341960407610458, -5.719274019375992779, 66.45724293864768129 ) ) ;
#148834=CARTESIAN_POINT ( 'NONE',  ( -19.03943276465977164, -0.05219959533935918106, 48.75109039468566863 ) ) ;
#148835=CARTESIAN_POINT ( 'NONE',  ( 19.05341960407618274, -5.049401038297876454, 21.04275706135233293 ) ) ;
#148836=CARTESIAN_POINT ( 'NONE',  ( 12.14591786802309770, 12.06949235617756955, 69.37390960531436690 ) ) ;
#148837=CARTESIAN_POINT ( 'NONE',  ( -5.823673210054116645, -21.52544592524344225, 42.29057627198103120 ) ) ;
#148840=CARTESIAN_POINT ( 'NONE',  ( 12.14591786802327356, -12.06949235617739191, 80.62609039468567573 ) ) ;
#148842=CARTESIAN_POINT ( 'NONE',  ( -16.51473224551082808, 9.474510206698731452, 88.33442372801900433 ) ) ;
#148843=CARTESIAN_POINT ( 'NONE',  ( -12.06949235617756955, 12.14591786802309770, 50.62390960531435979 ) ) ;
#148845=CARTESIAN_POINT ( 'NONE',  ( 16.51473224551069308, 9.474510206698969483, 49.16557627198102409 ) ) ;
#148846=CARTESIAN_POINT ( 'NONE',  ( -12.06949235617756955, 12.14591786802309770, 40.62390960531435269 ) ) ;
#148847=CARTESIAN_POINT ( 'NONE',  ( 19.03943276465977164, -0.05219959533909143690, 93.74890960531435269 ) ) ;
#148848=CARTESIAN_POINT ( 'NONE',  ( 9.564922557960805705, 16.46253265017160317, 49.58224293864770260 ) ) ;
#148849=CARTESIAN_POINT ( 'NONE',  ( -21.52544592524334988, -5.823673210054445271, 58.95942372801902565 ) ) ;
#148850=CARTESIAN_POINT ( 'NONE',  ( -9.474510206698964154, 16.51473224551069663, 75.41557627198103830 ) ) ;
#148851=CARTESIAN_POINT ( 'NONE',  ( 5.049401038298161559, -19.05341960407611168, 27.70724293864769550 ) ) ;
#148852=CARTESIAN_POINT ( 'NONE',  ( -13.89961937509977652, 13.97604488694528158, 55.62390960531434558 ) ) ;
#148853=CARTESIAN_POINT ( 'NONE',  ( 21.52544592524344225, -5.823673210054117533, 43.54057627198103830 ) ) ;
#148854=CARTESIAN_POINT ( 'NONE',  ( -9.474510206698964154, 16.51473224551069663, 30.41557627198102054 ) ) ;
#148855=CARTESIAN_POINT ( 'NONE',  ( -21.55341960407610458, -5.719274019375992779, 41.45724293864769550 ) ) ;
#148856=CARTESIAN_POINT ( 'NONE',  ( 16.55341960407618274, -4.379528057220086978, 106.0427570613523471 ) ) ;
#148857=CARTESIAN_POINT ( 'NONE',  ( 9.564922557961047289, -16.46253265017146816, 30.41775706135232937 ) ) ;
#148858=CARTESIAN_POINT ( 'NONE',  ( -8.314922557961024197, 14.29746914071037800, 52.91775706135235424 ) ) ;
#148859=CARTESIAN_POINT ( 'NONE',  ( -4.379528057220086978, -16.55341960407618274, 79.79275706135236135 ) ) ;
#148860=DIRECTION ( 'NONE',  ( 0.000000000000000000, 0.000000000000000000, -1.000000000000000000 ) ) ;
#148861=CARTESIAN_POINT ( 'NONE',  ( 8.224510206698742110, 14.34966873604972548, 67.08442372801901854 ) ) ;
#148862=CARTESIAN_POINT ( 'NONE',  ( 12.06949235617739724, 12.14591786802326823, 51.87609039468568284 ) ) ;
#148863=CARTESIAN_POINT ( 'NONE',  ( -0.05219959533909027116, -19.03943276465977164, 107.4989096053143527 ) ) ;
#148864=CARTESIAN_POINT ( 'NONE',  ( 16.46253265017160672, -9.564922557960803928, 33.33224293864770260 ) ) ;
#148865=CARTESIAN_POINT ( 'NONE',  ( 0.05219959533934541429, -16.53943276465976808, 35.00109039468568284 ) ) ;
#148866=CARTESIAN_POINT ( 'NONE',  ( -19.03943276465977164, 0.05219959533909376836, 46.24890960531435979 ) ) ;
#148867=CARTESIAN_POINT ( 'NONE',  ( -0.05219959533937732626, 21.53943276465977519, 22.50109039468567573 ) ) ;
#148868=CARTESIAN_POINT ( 'NONE',  ( 16.53943276465976808, 0.05219959533934440121, 31.25109039468568639 ) ) ;
#148869=CARTESIAN_POINT ( 'NONE',  ( -4.379528057220086978, -16.55341960407618274, 99.79275706135234714 ) ) ;
#148870=CARTESIAN_POINT ( 'NONE',  ( -19.05341960407611168, -5.049401038298163336, 21.45724293864768839 ) ) ;
#148871=CARTESIAN_POINT ( 'NONE',  ( -18.62759615963255300, -10.81492255796106328, 94.16775706135237556 ) ) ;
#148872=CARTESIAN_POINT ( 'NONE',  ( 16.51473224551083163, -9.474510206698727899, 100.8344237280190043 ) ) ;
#148873=CARTESIAN_POINT ( 'NONE',  ( -9.474510206698720793, -16.51473224551083518, 49.58442372801899722 ) ) ;
#148874=CARTESIAN_POINT ( 'NONE',  ( -14.34966873604960291, -8.224510206698953496, 51.66557627198102409 ) ) ;
#148875=CARTESIAN_POINT ( 'NONE',  ( -5.153800228976328057, -19.02544592524343514, 22.29057627198102765 ) ) ;
#148876=CARTESIAN_POINT ( 'NONE',  ( -16.46253265017146816, -9.564922557961047289, 54.16775706135234003 ) ) ;
#148877=CARTESIAN_POINT ( 'NONE',  ( 17.13100169013227259, -6.664070546374125215, 58.26789835699826625 ) ) ;
#148878=CARTESIAN_POINT ( 'NONE',  ( -10.81492255796105439, 18.62759615963255655, 62.91775706135236135 ) ) ;
#148879=CARTESIAN_POINT ( 'NONE',  ( 14.34966873604972726, -8.224510206698740333, 20.83442372801901143 ) ) ;
#148880=CARTESIAN_POINT ( 'NONE',  ( 16.62475595723701716, 7.163666690055268127, 81.97286648189530922 ) ) ;
#148881=CARTESIAN_POINT ( 'NONE',  ( -5.719274019375978568, 21.55341960407610458, 25.20724293864769550 ) ) ;
#148882=CARTESIAN_POINT ( 'NONE',  ( 13.89961937509957401, 13.97604488694547697, 101.8760903946856331 ) ) ;
#148883=CARTESIAN_POINT ( 'NONE',  ( 0.05219959533909260263, 19.03943276465977164, 114.9989096053143669 ) ) ;
#148885=CARTESIAN_POINT ( 'NONE',  ( 13.89961937509977652, -13.97604488694527269, 28.12390960531435624 ) ) ;
#148886=CARTESIAN_POINT ( 'NONE',  ( 15.80617190586769283, -15.72974639402175789, 110.6260903946857042 ) ) ;
#148887=CARTESIAN_POINT ( 'NONE',  ( -5.153800228976328057, -19.02544592524343514, 37.29057627198102409 ) ) ;
#148888=CARTESIAN_POINT ( 'NONE',  ( 15.72974639402176855, 15.80617190586768217, 66.87609039468568994 ) ) ;
#148889=CARTESIAN_POINT ( 'NONE',  ( -0.05219959533937732626, 21.53943276465977519, 107.5010903946856899 ) ) ;
#148890=CARTESIAN_POINT ( 'NONE',  ( -16.52544592524335698, -4.483927247898792601, 103.9594237280190185 ) ) ;
#148892=CARTESIAN_POINT ( 'NONE',  ( 19.02544592524343514, -5.153800228976328945, 78.54057627198099567 ) ) ;
#148893=CARTESIAN_POINT ( 'NONE',  ( -0.05219959533937732626, 21.53943276465977519, 57.50109039468568994 ) ) ;
#148894=CARTESIAN_POINT ( 'NONE',  ( 18.62759615963255655, 10.81492255796105972, 46.66775706135234714 ) ) ;
#148895=CARTESIAN_POINT ( 'NONE',  ( -16.51473224551082808, 9.474510206698731452, 78.33442372801900433 ) ) ;
#148896=CARTESIAN_POINT ( 'NONE',  ( -0.05219959533909027116, -19.03943276465977164, 102.4989096053143669 ) ) ;
#148897=CARTESIAN_POINT ( 'NONE',  ( 5.153800228976335163, 19.02544592524342804, 24.79057627198102765 ) ) ;
#148898=CARTESIAN_POINT ( 'NONE',  ( -21.53943276465977519, 0.05219959533907696930, 91.24890960531436690 ) ) ;
#148899=CARTESIAN_POINT ( 'NONE',  ( -19.03943276465977164, -0.05219959533935918106, 18.75109039468567218 ) ) ;
#148900=CARTESIAN_POINT ( 'NONE',  ( -16.55341960407611168, -4.379528057220339221, 101.4572429386476955 ) ) ;
#148901=CARTESIAN_POINT ( 'NONE',  ( -5.049401038298153566, 19.05341960407611168, 55.20724293864769550 ) ) ;
#148902=CARTESIAN_POINT ( 'NONE',  ( -16.46253265017146816, -9.564922557961047289, 99.16775706135233293 ) ) ;
#148903=CARTESIAN_POINT ( 'NONE',  ( -14.34966873604960291, -8.224510206698953496, 61.66557627198103120 ) ) ;
#148904=CARTESIAN_POINT ( 'NONE',  ( -21.53943276465977519, -0.05219959533937600094, 108.7510903946857042 ) ) ;
#148905=CARTESIAN_POINT ( 'NONE',  ( -5.153800228976328057, -19.02544592524343514, 102.2905762719810383 ) ) ;
#148906=CARTESIAN_POINT ( 'NONE',  ( 13.89961937509957401, 13.97604488694547697, 71.87609039468567573 ) ) ;
#148907=CARTESIAN_POINT ( 'NONE',  ( -18.67979575497178146, -10.72451020669898902, 76.66557627198103830 ) ) ;
#148908=CARTESIAN_POINT ( 'NONE',  ( -5.719274019375665041, -21.55341960407619695, 29.79275706135234358 ) ) ;
#148909=CARTESIAN_POINT ( 'NONE',  ( 12.14591786802327356, -12.06949235617739191, 35.62609039468568994 ) ) ;
#148910=CARTESIAN_POINT ( 'NONE',  ( 4.483927247898790824, -16.52544592524335698, 90.20942372801903275 ) ) ;
#148911=CARTESIAN_POINT ( 'NONE',  ( -0.05219959533934338120, 16.53943276465976808, 47.50109039468568994 ) ) ;
#148912=CARTESIAN_POINT ( 'NONE',  ( 0.05219959533937995610, -21.53943276465977519, 40.00109039468567573 ) ) ;
#148913=CARTESIAN_POINT ( 'NONE',  ( -21.55341960407610458, -5.719274019375992779, 46.45724293864769550 ) ) ;
#148915=CARTESIAN_POINT ( 'NONE',  ( -5.049401038298153566, 19.05341960407611168, 40.20724293864768839 ) ) ;
#148917=CARTESIAN_POINT ( 'NONE',  ( -8.314922557961024197, 14.29746914071037800, 62.91775706135236135 ) ) ;
#148918=CARTESIAN_POINT ( 'NONE',  ( 18.62759615963271287, -10.81492255796078972, 83.33224293864769550 ) ) ;
#148919=CARTESIAN_POINT ( 'NONE',  ( 16.53943276465976808, -0.05219959533910856209, 38.74890960531435979 ) ) ;
#148920=CARTESIAN_POINT ( 'NONE',  ( -4.483927247898782831, 16.52544592524335698, 47.70942372801902565 ) ) ;
#148921=CARTESIAN_POINT ( 'NONE',  ( -9.564922557960796823, -16.46253265017161027, 57.08224293864769550 ) ) ;
#148922=CARTESIAN_POINT ( 'NONE',  ( -4.483927247898782831, 16.52544592524335698, 92.70942372801901854 ) ) ;
#148923=CARTESIAN_POINT ( 'NONE',  ( 19.05341960407617918, -5.049401038297876454, 91.04275706135234714 ) ) ;
#148924=CARTESIAN_POINT ( 'NONE',  ( -21.53943276465977519, 0.05219959533907696930, 91.24890960531436690 ) ) ;
#148925=CARTESIAN_POINT ( 'NONE',  ( 4.379528057220339221, -16.55341960407611168, 27.70724293864769905 ) ) ;
#148926=VERTEX_POINT ( 'NONE', #175214 ) ;
#148928=CARTESIAN_POINT ( 'NONE',  ( -15.80617190586745835, -15.72974639402198527, 56.87390960531436690 ) ) ;
#148929=CARTESIAN_POINT ( 'NONE',  ( -4.379528057220086978, -16.55341960407618274, 99.79275706135234714 ) ) ;
#148931=CARTESIAN_POINT ( 'NONE',  ( -10.72451020669898014, 18.67979575497178502, 25.41557627198103120 ) ) ;
#148932=CARTESIAN_POINT ( 'NONE',  ( 17.50000000000001421, -3.307050604923627457, 102.5791036533545793 ) ) ;
#148933=CARTESIAN_POINT ( 'NONE',  ( 18.62759615963271287, -10.81492255796078972, 83.33224293864769550 ) ) ;
#148934=CARTESIAN_POINT ( 'NONE',  ( 4.379528057220092307, 16.55341960407617563, 112.2927570613523471 ) ) ;
#148935=CARTESIAN_POINT ( 'NONE',  ( -16.53943276465976808, -0.05219959533934237506, 33.75109039468568284 ) ) ;
#148936=CARTESIAN_POINT ( 'NONE',  ( 5.153800228976335163, 19.02544592524342804, 39.79057627198100988 ) ) ;
#148937=CARTESIAN_POINT ( 'NONE',  ( -0.05219959533934338120, 16.53943276465976808, 27.50109039468567929 ) ) ;
#148938=CARTESIAN_POINT ( 'NONE',  ( 19.02544592524343514, -5.153800228976328945, 48.54057627198103120 ) ) ;
#148940=CARTESIAN_POINT ( 'NONE',  ( 16.51473224551069308, 9.474510206698969483, 114.1655762719810241 ) ) ;
#148941=CARTESIAN_POINT ( 'NONE',  ( 9.564922557960805705, 16.46253265017160317, 114.5822429386476955 ) ) ;
#148942=CARTESIAN_POINT ( 'NONE',  ( 4.379528057220092307, 16.55341960407617563, 97.29275706135234714 ) ) ;
#148943=CARTESIAN_POINT ( 'NONE',  ( 13.89961937509957401, 13.97604488694547697, 91.87609039468567573 ) ) ;
#148944=CARTESIAN_POINT ( 'NONE',  ( -9.564922557961040184, 16.46253265017147172, 37.91775706135233293 ) ) ;
#148945=CARTESIAN_POINT ( 'NONE',  ( 15.80617190586746368, 15.72974639402197994, 94.37390960531436690 ) ) ;
#148946=CARTESIAN_POINT ( 'NONE',  ( 0.05219959533934541429, -16.53943276465976808, 110.0010903946856757 ) ) ;
#148947=CARTESIAN_POINT ( 'NONE',  ( -15.72974639402197994, 15.80617190586746368, 30.62390960531436335 ) ) ;
#148948=CARTESIAN_POINT ( 'NONE',  ( -9.474510206698720793, -16.51473224551083518, 109.5844237280190043 ) ) ;
#148949=CARTESIAN_POINT ( 'NONE',  ( -19.05341960407611168, -5.049401038298163336, 111.4572429386476671 ) ) ;
#148950=CARTESIAN_POINT ( 'NONE',  ( 18.67979575497194134, -10.72451020669871369, 60.83442372801901854 ) ) ;
#148951=CARTESIAN_POINT ( 'NONE',  ( 9.474510206698971260, -16.51473224551069308, 57.91557627198103120 ) ) ;
#148952=CARTESIAN_POINT ( 'NONE',  ( 8.314922557960818139, 14.29746914071049879, 104.5822429386477097 ) ) ;
#148954=CARTESIAN_POINT ( 'NONE',  ( -9.564922557960796823, -16.46253265017161027, 67.08224293864769550 ) ) ;
#148955=CARTESIAN_POINT ( 'NONE',  ( 12.06949235617757843, -12.14591786802309237, 73.12390960531436690 ) ) ;
#148957=CARTESIAN_POINT ( 'NONE',  ( -0.05219959533936034679, 19.03943276465977164, 92.50109039468566152 ) ) ;
#148959=CARTESIAN_POINT ( 'NONE',  ( 13.89961937509977652, -13.97604488694527269, 63.12390960531435979 ) ) ;
#148961=CARTESIAN_POINT ( 'NONE',  ( -19.02544592524342804, 5.153800228976336051, 81.04057627198103830 ) ) ;
#148962=CARTESIAN_POINT ( 'NONE',  ( -13.97604488694527625, -13.89961937509977652, 106.8739096053143669 ) ) ;
#148963=CARTESIAN_POINT ( 'NONE',  ( -16.52544592524335698, -4.483927247898792601, 58.95942372801902565 ) ) ;
#148964=CARTESIAN_POINT ( 'NONE',  ( -17.31747979337947996, -6.344076630961017926, 51.37944868065184778 ) ) ;
#148965=CARTESIAN_POINT ( 'NONE',  ( 19.05341960407617918, -5.049401038297876454, 41.04275706135233293 ) ) ;
#148966=CARTESIAN_POINT ( 'NONE',  ( 5.823673210054444382, -21.52544592524334988, 105.2094237280190328 ) ) ;
#148968=CARTESIAN_POINT ( 'NONE',  ( -0.05219959533909027116, -19.03943276465977164, 112.4989096053143669 ) ) ;
#148969=CARTESIAN_POINT ( 'NONE',  ( 16.52544592524335698, 4.483927247898782831, 96.45942372801901854 ) ) ;
#148971=CARTESIAN_POINT ( 'NONE',  ( -16.53943276465976808, -0.05219959533934237506, 93.75109039468567573 ) ) ;
#148972=CARTESIAN_POINT ( 'NONE',  ( -17.49999999999999289, 5.624438216177594541, 30.81670344914645199 ) ) ;
#148973=CARTESIAN_POINT ( 'NONE',  ( 16.55341960407618274, -4.379528057220086978, 71.04275706135234714 ) ) ;
#148975=CARTESIAN_POINT ( 'NONE',  ( -21.53943276465977519, -0.05219959533937600094, 83.75109039468568994 ) ) ;
#148976=CARTESIAN_POINT ( 'NONE',  ( -0.05219959533936034679, 19.03943276465977164, 87.50109039468567573 ) ) ;
#148977=CARTESIAN_POINT ( 'NONE',  ( -13.97604488694547697, 13.89961937509957934, 23.12609039468565442 ) ) ;
#148978=CARTESIAN_POINT ( 'NONE',  ( 19.03943276465977164, -0.05219959533909143690, 68.74890960531436690 ) ) ;
#148979=CARTESIAN_POINT ( 'NONE',  ( 16.46253265017160672, -9.564922557960803928, 43.33224293864769550 ) ) ;
#148981=CARTESIAN_POINT ( 'NONE',  ( -10.81492255796078084, -18.62759615963271287, 87.08224293864769550 ) ) ;
#148982=CARTESIAN_POINT ( 'NONE',  ( 21.55341960407610458, 5.719274019375980345, 28.95724293864769905 ) ) ;
#148983=CARTESIAN_POINT ( 'NONE',  ( 19.05341960407611168, 5.049401038298154454, 38.95724293864767418 ) ) ;
#148984=CARTESIAN_POINT ( 'NONE',  ( 16.53943276465976808, 0.05219959533934440121, 46.25109039468567573 ) ) ;
#148986=CARTESIAN_POINT ( 'NONE',  ( 5.823673210054444382, -21.52544592524334988, 25.20942372801901854 ) ) ;
#148987=CARTESIAN_POINT ( 'NONE',  ( -8.314922557960811034, -14.29746914071050412, 72.08224293864769550 ) ) ;
#148989=CARTESIAN_POINT ( 'NONE',  ( -14.29746914071037622, -8.314922557961029526, 19.16775706135234714 ) ) ;
#148990=CARTESIAN_POINT ( 'NONE',  ( 5.049401038297881783, 19.05341960407617563, 42.29275706135234003 ) ) ;
#148991=CARTESIAN_POINT ( 'NONE',  ( -4.483927247898539470, -16.52544592524342804, 52.29057627198102409 ) ) ;
#148992=CARTESIAN_POINT ( 'NONE',  ( 18.67979575497178502, 10.72451020669898547, 114.1655762719810383 ) ) ;
#148993=EDGE_CURVE ( 'NONE', #112403, #197846, #66956, .T. ) ;
#148995=CARTESIAN_POINT ( 'NONE',  ( -18.67979575497178146, -10.72451020669898902, 81.66557627198103830 ) ) ;
#148996=CARTESIAN_POINT ( 'NONE',  ( 19.05341960407611168, 5.049401038298154454, 83.95724293864766707 ) ) ;
#148997=CARTESIAN_POINT ( 'NONE',  ( -14.29746914071049879, 8.314922557960819915, 55.83224293864770260 ) ) ;
#148998=CARTESIAN_POINT ( 'NONE',  ( -19.02544592524342804, 5.153800228976336051, 116.0405762719810383 ) ) ;
#149000=CARTESIAN_POINT ( 'NONE',  ( 13.89961937509957401, 13.97604488694547697, 66.87609039468567573 ) ) ;
#149001=CARTESIAN_POINT ( 'NONE',  ( -15.80617190586745835, -15.72974639402198527, 101.8739096053143811 ) ) ;
#149002=CARTESIAN_POINT ( 'NONE',  ( 16.46253265017160672, -9.564922557960803928, 53.33224293864768839 ) ) ;
#149003=CARTESIAN_POINT ( 'NONE',  ( -13.89961937509957401, -13.97604488694547875, 44.37609039468566863 ) ) ;
#149004=CARTESIAN_POINT ( 'NONE',  ( 9.474510206698971260, -16.51473224551069308, 37.91557627198102409 ) ) ;
#149005=CARTESIAN_POINT ( 'NONE',  ( -15.72974639402176322, -15.80617190586768395, 64.37609039468568994 ) ) ;
#149006=CARTESIAN_POINT ( 'NONE',  ( -16.20579543436678449, -7.371946100355100562, 70.56520834171880097 ) ) ;
#149008=CARTESIAN_POINT ( 'NONE',  ( -12.14591786802309592, -12.06949235617757132, 41.87390960531435979 ) ) ;
#149009=CARTESIAN_POINT ( 'NONE',  ( 13.89961937509977652, -13.97604488694527269, 63.12390960531435979 ) ) ;
#149010=CARTESIAN_POINT ( 'NONE',  ( -21.55341960407610458, -5.719274019375992779, 71.45724293864769550 ) ) ;
#149011=CARTESIAN_POINT ( 'NONE',  ( 19.05341960407611168, 5.049401038298154454, 53.95724293864770260 ) ) ;
#149013=CARTESIAN_POINT ( 'NONE',  ( -21.53943276465977519, 0.05219959533907696930, 71.24890960531435269 ) ) ;
#149014=ORIENTED_EDGE ( 'NONE', *, *, #93499, .F. ) ;
#149015=CARTESIAN_POINT ( 'NONE',  ( 15.80617190586769283, -15.72974639402175789, 105.6260903946856899 ) ) ;
#149017=CARTESIAN_POINT ( 'NONE',  ( 16.52544592524335698, 4.483927247898782831, 101.4594237280190185 ) ) ;
#149018=CARTESIAN_POINT ( 'NONE',  ( -0.05219959533910754901, -16.53943276465976808, 87.49890960531436690 ) ) ;
#149019=CARTESIAN_POINT ( 'NONE',  ( -19.02544592524342804, 5.153800228976336051, 66.04057627198103830 ) ) ;
#149021=CARTESIAN_POINT ( 'NONE',  ( 9.564922557961047289, -16.46253265017146816, 35.41775706135233293 ) ) ;
#149022=CARTESIAN_POINT ( 'NONE',  ( -12.14591786802326823, 12.06949235617739902, 83.12609039468568994 ) ) ;
#149023=CARTESIAN_POINT ( 'NONE',  ( -19.05341960407617563, 5.049401038297882671, 33.54275706135231871 ) ) ;
#149024=CARTESIAN_POINT ( 'NONE',  ( 13.89961937509977652, -13.97604488694527269, 83.12390960531436690 ) ) ;
#149025=CARTESIAN_POINT ( 'NONE',  ( -21.55341960407610458, -5.719274019375992779, 56.45724293864768839 ) ) ;
#149027=CARTESIAN_POINT ( 'NONE',  ( -16.52544592524342804, 4.483927247898546575, 116.0405762719810383 ) ) ;
#149028=CARTESIAN_POINT ( 'NONE',  ( -10.72451020669870658, -18.67979575497194134, 94.58442372801901854 ) ) ;
#149029=CARTESIAN_POINT ( 'NONE',  ( 16.55341960407618274, -4.379528057220086978, 66.04275706135236135 ) ) ;
#149030=CARTESIAN_POINT ( 'NONE',  ( 10.81492255796106328, -18.62759615963255655, 30.41775706135234358 ) ) ;
#149031=CARTESIAN_POINT ( 'NONE',  ( 8.314922557961029526, -14.29746914071037800, 35.41775706135234003 ) ) ;
#149032=CARTESIAN_POINT ( 'NONE',  ( -16.51473224551069308, -9.474510206698971260, 86.66557627198102409 ) ) ;
#149033=CARTESIAN_POINT ( 'NONE',  ( -19.03943276465977164, 0.05219959533909376836, 46.24890960531435979 ) ) ;
#149034=CARTESIAN_POINT ( 'NONE',  ( -19.02544592524342804, 5.153800228976336051, 56.04057627198100988 ) ) ;
#149035=CARTESIAN_POINT ( 'NONE',  ( 12.14591786802327356, -12.06949235617739191, 35.62609039468568994 ) ) ;
#149036=CARTESIAN_POINT ( 'NONE',  ( -12.06949235617756955, 12.14591786802309770, 95.62390960531436690 ) ) ;
#149037=CARTESIAN_POINT ( 'NONE',  ( -12.14591786802326823, 12.06949235617739902, 98.12609039468570415 ) ) ;
#149038=CARTESIAN_POINT ( 'NONE',  ( 5.823673210054444382, -21.52544592524334988, 45.20942372801901854 ) ) ;
#149039=CARTESIAN_POINT ( 'NONE',  ( -16.46253265017160317, 9.564922557960807481, 75.83224293864769550 ) ) ;
#149040=CARTESIAN_POINT ( 'NONE',  ( 13.89961937509977652, -13.97604488694527269, 53.12390960531434558 ) ) ;
#149041=CARTESIAN_POINT ( 'NONE',  ( -9.474510206698964154, 16.51473224551069663, 85.41557627198102409 ) ) ;
#149042=CARTESIAN_POINT ( 'NONE',  ( -14.34966873604960291, -8.224510206698953496, 36.66557627198103120 ) ) ;
#149043=CARTESIAN_POINT ( 'NONE',  ( 14.34966873604972726, -8.224510206698740333, 105.8344237280190328 ) ) ;
#149044=EDGE_CURVE ( 'NONE', #1850, #40791, #4276, .T. ) ;
#149045=CARTESIAN_POINT ( 'NONE',  ( 5.153800228976615827, -19.02544592524334988, 50.20942372801897591 ) ) ;
#149046=FACE_OUTER_BOUND ( 'NONE', #156875, .T. ) ;
#149047=CARTESIAN_POINT ( 'NONE',  ( 16.51473224551069308, 9.474510206698969483, 44.16557627198103120 ) ) ;
#149048=CARTESIAN_POINT ( 'NONE',  ( -9.564922557961040184, 16.46253265017147172, 22.91775706135233648 ) ) ;
#149050=CARTESIAN_POINT ( 'NONE',  ( -8.314922557961024197, 14.29746914071037800, 37.91775706135235424 ) ) ;
#149051=CARTESIAN_POINT ( 'NONE',  ( -0.05219959533936034679, 19.03943276465977164, 72.50109039468566152 ) ) ;
#149052=CARTESIAN_POINT ( 'NONE',  ( 14.29746914071037800, 8.314922557961029526, 61.66775706135235424 ) ) ;
#149054=CARTESIAN_POINT ( 'NONE',  ( -13.89961937509977652, 13.97604488694528158, 75.62390960531438111 ) ) ;
#149055=CARTESIAN_POINT ( 'NONE',  ( -21.53943276465977519, 0.05219959533907696930, 111.2489096053143669 ) ) ;
#149056=CARTESIAN_POINT ( 'NONE',  ( 5.049401038297881783, 19.05341960407617563, 72.29275706135234714 ) ) ;
#149057=CARTESIAN_POINT ( 'NONE',  ( -0.05219959533909027116, -19.03943276465977164, 107.4989096053143527 ) ) ;
#149058=CARTESIAN_POINT ( 'NONE',  ( 9.474510206698971260, -16.51473224551069308, 37.91557627198102409 ) ) ;
#149059=CARTESIAN_POINT ( 'NONE',  ( -5.049401038298153566, 19.05341960407611168, 75.20724293864769550 ) ) ;
#149060=CARTESIAN_POINT ( 'NONE',  ( 16.55341960407611168, 4.379528057220329451, 28.95724293864769905 ) ) ;
#149061=CARTESIAN_POINT ( 'NONE',  ( 5.153800228976335163, 19.02544592524342804, 39.79057627198100988 ) ) ;
#149062=CARTESIAN_POINT ( 'NONE',  ( -13.97604488694547697, 13.89961937509957934, 48.12609039468566863 ) ) ;
#149063=CARTESIAN_POINT ( 'NONE',  ( -12.14591786802309592, -12.06949235617757132, 71.87390960531438111 ) ) ;
#149064=CARTESIAN_POINT ( 'NONE',  ( 19.03943276465977164, 0.05219959533936151252, 21.25109039468565797 ) ) ;
#149065=CARTESIAN_POINT ( 'NONE',  ( -9.474510206698964154, 16.51473224551069663, 55.41557627198103120 ) ) ;
#149066=CARTESIAN_POINT ( 'NONE',  ( -18.62759615963270932, 10.81492255796079327, 55.83224293864770260 ) ) ;
#149067=CARTESIAN_POINT ( 'NONE',  ( -16.55341960407611168, -4.379528057220339221, 51.45724293864770260 ) ) ;
#149068=CARTESIAN_POINT ( 'NONE',  ( 18.62759615963255655, 10.81492255796105972, 101.6677570613523613 ) ) ;
#149069=CARTESIAN_POINT ( 'NONE',  ( 9.474510206698971260, -16.51473224551069308, 92.91557627198103830 ) ) ;
#149070=CARTESIAN_POINT ( 'NONE',  ( 16.51473224551069308, 9.474510206698969483, 109.1655762719810383 ) ) ;
#149071=CARTESIAN_POINT ( 'NONE',  ( 19.05341960407611168, 5.049401038298154454, 38.95724293864767418 ) ) ;
#149072=CARTESIAN_POINT ( 'NONE',  ( 9.474510206698971260, -16.51473224551069308, 27.91557627198103120 ) ) ;
#149073=CARTESIAN_POINT ( 'NONE',  ( 16.52544592524342804, -4.483927247898539470, 88.54057627198103830 ) ) ;
#149074=CARTESIAN_POINT ( 'NONE',  ( -21.52544592524343514, 5.823673210054127303, 101.0405762719810383 ) ) ;
#149075=CARTESIAN_POINT ( 'NONE',  ( -19.05341960407611168, -5.049401038298163336, 101.4572429386476955 ) ) ;
#149076=CARTESIAN_POINT ( 'NONE',  ( -15.72974639402176322, -15.80617190586768395, 19.37609039468568639 ) ) ;
#149077=CARTESIAN_POINT ( 'NONE',  ( -5.153800228976328057, -19.02544592524343514, 97.29057627198099567 ) ) ;
#149079=CARTESIAN_POINT ( 'NONE',  ( 16.53943276465976808, -0.05219959533910856209, 98.74890960531438111 ) ) ;
#149080=CARTESIAN_POINT ( 'NONE',  ( 19.05341960407611168, 5.049401038298154454, 68.95724293864769550 ) ) ;
#149081=CARTESIAN_POINT ( 'NONE',  ( 21.55341960407610458, 5.719274019375980345, 73.95724293864769550 ) ) ;
#149084=CARTESIAN_POINT ( 'NONE',  ( 10.81492255796078972, 18.62759615963270932, 34.58224293864770260 ) ) ;
#149085=CARTESIAN_POINT ( 'NONE',  ( 19.01533133064924996, -5.499999999999441336, 66.26586590595739779 ) ) ;
#149086=CARTESIAN_POINT ( 'NONE',  ( 0.05219959533934541429, -16.53943276465976808, 35.00109039468568284 ) ) ;
#149087=CARTESIAN_POINT ( 'NONE',  ( -14.29746914071049879, 8.314922557960819915, 90.83224293864769550 ) ) ;
#149089=CARTESIAN_POINT ( 'NONE',  ( 19.03943276465977164, -0.05219959533909143690, 83.74890960531436690 ) ) ;
#149090=CARTESIAN_POINT ( 'NONE',  ( 16.51473224551069308, 9.474510206698969483, 49.16557627198102409 ) ) ;
#149091=CARTESIAN_POINT ( 'NONE',  ( 12.14591786802309770, 12.06949235617756955, 74.37390960531436690 ) ) ;
#149092=CARTESIAN_POINT ( 'NONE',  ( -10.72451020669898014, 18.67979575497178502, 35.41557627198102409 ) ) ;
#149093=CARTESIAN_POINT ( 'NONE',  ( -16.55341960407611168, -4.379528057220339221, 56.45724293864768839 ) ) ;
#149094=CARTESIAN_POINT ( 'NONE',  ( 19.02544592524334988, 5.153800228976608722, 101.4594237280189759 ) ) ;
#149095=CARTESIAN_POINT ( 'NONE',  ( 0.05219959533937995610, -21.53943276465977519, 75.00109039468568994 ) ) ;
#149097=CARTESIAN_POINT ( 'NONE',  ( -16.46253265017160317, 9.564922557960807481, 115.8322429386477097 ) ) ;
#149098=CARTESIAN_POINT ( 'NONE',  ( -4.483927247898782831, 16.52544592524335698, 82.70942372801900433 ) ) ;
#149099=CARTESIAN_POINT ( 'NONE',  ( -17.49999999999999645, 5.624438216177559902, 95.81670344914641646 ) ) ;
#149100=CARTESIAN_POINT ( 'NONE',  ( -5.049401038298153566, 19.05341960407611168, 75.20724293864769550 ) ) ;
#149101=CARTESIAN_POINT ( 'NONE',  ( -15.72974639402197994, 15.80617190586746368, 85.62390960531436690 ) ) ;
#149102=CARTESIAN_POINT ( 'NONE',  ( -14.34966873604972548, 8.224510206698743886, 23.33442372801901499 ) ) ;
#149103=CARTESIAN_POINT ( 'NONE',  ( 14.34966873604960469, 8.224510206698951720, 54.16557627198103120 ) ) ;
#149104=CARTESIAN_POINT ( 'NONE',  ( -21.52544592524334988, -5.823673210054445271, 73.95942372801901854 ) ) ;
#149105=CARTESIAN_POINT ( 'NONE',  ( 16.55341960407618274, -4.379528057220086978, 86.04275706135236135 ) ) ;
#149106=CARTESIAN_POINT ( 'NONE',  ( 5.823673210054125526, 21.52544592524343514, 24.79057627198103120 ) ) ;
#149109=CARTESIAN_POINT ( 'NONE',  ( 14.34966873604972726, -8.224510206698740333, 105.8344237280190328 ) ) ;
#149110=CARTESIAN_POINT ( 'NONE',  ( 16.52544592524335698, 4.483927247898782831, 56.45942372801902565 ) ) ;
#149111=CARTESIAN_POINT ( 'NONE',  ( -19.05341960407611168, -5.049401038298163336, 66.45724293864769550 ) ) ;
#149112=CARTESIAN_POINT ( 'NONE',  ( 9.474510206698971260, -16.51473224551069308, 87.91557627198102409 ) ) ;
#149113=CARTESIAN_POINT ( 'NONE',  ( -10.81492255796105439, 18.62759615963255655, 72.91775706135234714 ) ) ;
#149114=CARTESIAN_POINT ( 'NONE',  ( 4.379528057220092307, 16.55341960407617563, 82.29275706135234714 ) ) ;
#149115=CARTESIAN_POINT ( 'NONE',  ( -14.34966873604960291, -8.224510206698953496, 41.66557627198103120 ) ) ;
#149116=CARTESIAN_POINT ( 'NONE',  ( -16.51473224551069308, -9.474510206698971260, 61.66557627198103120 ) ) ;
#149117=CARTESIAN_POINT ( 'NONE',  ( -5.153800228976328057, -19.02544592524343514, 42.29057627198101699 ) ) ;
#149119=CARTESIAN_POINT ( 'NONE',  ( 13.97604488694548053, -13.89961937509957401, 100.6260903946856615 ) ) ;
#149120=CARTESIAN_POINT ( 'NONE',  ( -8.224510206698948167, 14.34966873604960824, 95.41557627198102409 ) ) ;
#149121=CARTESIAN_POINT ( 'NONE',  ( 0.05219959533909260263, 19.03943276465977164, 59.99890960531436690 ) ) ;
#149122=CARTESIAN_POINT ( 'NONE',  ( 16.51473224551083163, -9.474510206698727899, 105.8344237280190043 ) ) ;
#149124=CARTESIAN_POINT ( 'NONE',  ( -21.55341960407619339, 5.719274019375674811, 103.5427570613523613 ) ) ;
#149125=CARTESIAN_POINT ( 'NONE',  ( -0.05219959533934338120, 16.53943276465976808, 67.50109039468568994 ) ) ;
#149126=CARTESIAN_POINT ( 'NONE',  ( -9.564922557961040184, 16.46253265017147172, 87.91775706135233293 ) ) ;
#149127=CARTESIAN_POINT ( 'NONE',  ( 5.823673210054125526, 21.52544592524343514, 64.79057627198103830 ) ) ;
#149128=CARTESIAN_POINT ( 'NONE',  ( -0.05219959533934338120, 16.53943276465976808, 57.50109039468568994 ) ) ;
#149129=CARTESIAN_POINT ( 'NONE',  ( 17.47980958864297918, 5.499999999999998224, 21.71653220162190934 ) ) ;
#149130=CARTESIAN_POINT ( 'NONE',  ( -19.03943276465977164, -0.05219959533935918106, 53.75109039468566863 ) ) ;
#149131=CARTESIAN_POINT ( 'NONE',  ( -21.53943276465977519, -0.05219959533937600094, 93.75109039468567573 ) ) ;
#149132=CARTESIAN_POINT ( 'NONE',  ( -14.34966873604960291, -8.224510206698953496, 111.6655762719810525 ) ) ;
#149133=CARTESIAN_POINT ( 'NONE',  ( -13.89961937509977652, 13.97604488694528158, 60.62390960531436690 ) ) ;
#149134=CARTESIAN_POINT ( 'NONE',  ( 16.53943276465976808, -0.05219959533910856209, 53.74890960531437401 ) ) ;
#149136=CARTESIAN_POINT ( 'NONE',  ( 15.72974639402176855, 15.80617190586768217, 91.87609039468568994 ) ) ;
#149137=CARTESIAN_POINT ( 'NONE',  ( 9.564922557961047289, -16.46253265017146816, 45.41775706135232582 ) ) ;
#149138=CARTESIAN_POINT ( 'NONE',  ( -13.97604488694547697, 13.89961937509957934, 33.12609039468566863 ) ) ;
#149139=CARTESIAN_POINT ( 'NONE',  ( -19.03943276465977164, 0.05219959533909376836, 116.2489096053143669 ) ) ;
#149140=CARTESIAN_POINT ( 'NONE',  ( -5.823673210054431948, 21.52544592524334988, 92.70942372801901854 ) ) ;
#149141=CARTESIAN_POINT ( 'NONE',  ( 0.05219959533909260263, 19.03943276465977164, 79.99890960531436690 ) ) ;
#149142=CARTESIAN_POINT ( 'NONE',  ( 15.72974639402176855, 15.80617190586768217, 91.87609039468568994 ) ) ;
#149143=CARTESIAN_POINT ( 'NONE',  ( -5.823673210054116645, -21.52544592524344225, 47.29057627198103120 ) ) ;
#149145=CARTESIAN_POINT ( 'NONE',  ( 9.474510206698971260, -16.51473224551069308, 87.91557627198102409 ) ) ;
#149146=CARTESIAN_POINT ( 'NONE',  ( -5.049401038297874678, -19.05341960407617918, 64.79275706135233293 ) ) ;
#149147=CARTESIAN_POINT ( 'NONE',  ( 19.03943276465977164, -0.05219959533909143690, 43.74890960531435979 ) ) ;
#149148=CARTESIAN_POINT ( 'NONE',  ( 13.89961937509977652, -13.97604488694527269, 83.12390960531436690 ) ) ;
#149149=CARTESIAN_POINT ( 'NONE',  ( -13.89961937509957401, -13.97604488694547875, 89.37609039468563310 ) ) ;
#149150=CARTESIAN_POINT ( 'NONE',  ( 4.379528057220092307, 16.55341960407617563, 42.29275706135235424 ) ) ;
#149151=CARTESIAN_POINT ( 'NONE',  ( 4.483927247898545687, 16.52544592524342804, 99.79057627198103830 ) ) ;
#149152=CARTESIAN_POINT ( 'NONE',  ( -5.049401038298153566, 19.05341960407611168, 75.20724293864769550 ) ) ;
#149153=CARTESIAN_POINT ( 'NONE',  ( 21.53943276465977519, -0.05219959533907433946, 43.74890960531435979 ) ) ;
#149154=CARTESIAN_POINT ( 'NONE',  ( 19.03943276465977164, 0.05219959533936151252, 111.2510903946856757 ) ) ;
#149155=CARTESIAN_POINT ( 'NONE',  ( 0.05219959533937995610, -21.53943276465977519, 25.00109039468567218 ) ) ;
#149156=CARTESIAN_POINT ( 'NONE',  ( -18.67979575497193778, 10.72451020669871902, 73.33442372801901854 ) ) ;
#149157=CARTESIAN_POINT ( 'NONE',  ( -16.55341960407617563, 4.379528057220093196, 83.54275706135234714 ) ) ;
#149158=CARTESIAN_POINT ( 'NONE',  ( 16.51473224551069308, 9.474510206698969483, 74.16557627198103830 ) ) ;
#149159=CARTESIAN_POINT ( 'NONE',  ( -4.379528057220086978, -16.55341960407618274, 104.7927570613523898 ) ) ;
#149160=CARTESIAN_POINT ( 'NONE',  ( -13.97604488694547697, 13.89961937509957934, 58.12609039468566863 ) ) ;
#149161=CARTESIAN_POINT ( 'NONE',  ( 21.53943276465977519, 0.05219959533937863772, 31.25109039468568639 ) ) ;
#149162=CARTESIAN_POINT ( 'NONE',  ( 16.55341960407611168, 4.379528057220329451, 73.95724293864769550 ) ) ;
#149163=CARTESIAN_POINT ( 'NONE',  ( -5.153800228976328057, -19.02544592524343514, 97.29057627198099567 ) ) ;
#149164=CARTESIAN_POINT ( 'NONE',  ( -16.52544592524335698, -4.483927247898792601, 83.95942372801900433 ) ) ;
#149165=CARTESIAN_POINT ( 'NONE',  ( 18.67979575497194134, -10.72451020669871369, 70.83442372801901854 ) ) ;
#149166=CARTESIAN_POINT ( 'NONE',  ( 0.05219959533934541429, -16.53943276465976808, 30.00109039468568284 ) ) ;
#149167=CARTESIAN_POINT ( 'NONE',  ( -10.81492255796105439, 18.62759615963255655, 22.91775706135235069 ) ) ;
#149168=CARTESIAN_POINT ( 'NONE',  ( -4.483927247898539470, -16.52544592524342804, 77.29057627198102409 ) ) ;
#149169=EDGE_CURVE ( 'NONE', #22576, #190052, #194844, .T. ) ;
#149171=CARTESIAN_POINT ( 'NONE',  ( 18.67979575497178502, 10.72451020669898547, 104.1655762719810241 ) ) ;
#149172=CARTESIAN_POINT ( 'NONE',  ( 4.483927247898545687, 16.52544592524342804, 49.79057627198102409 ) ) ;
#149174=CARTESIAN_POINT ( 'NONE',  ( 19.03943276465977164, -0.05219959533909143690, 23.74890960531435269 ) ) ;
#149175=CARTESIAN_POINT ( 'NONE',  ( 15.72974639402199770, -15.80617190586745480, 23.12390960531436335 ) ) ;
#149176=CARTESIAN_POINT ( 'NONE',  ( 0.05219959533937995610, -21.53943276465977519, 55.00109039468568284 ) ) ;
#149177=CARTESIAN_POINT ( 'NONE',  ( 4.483927247898545687, 16.52544592524342804, 64.79057627198103830 ) ) ;
#149179=CARTESIAN_POINT ( 'NONE',  ( -0.05219959533907301413, -21.53943276465977519, 72.49890960531435269 ) ) ;
#149180=CARTESIAN_POINT ( 'NONE',  ( 0.05219959533909260263, 19.03943276465977164, 79.99890960531436690 ) ) ;
#149181=CARTESIAN_POINT ( 'NONE',  ( 13.89961937509977652, -13.97604488694527269, 28.12390960531435624 ) ) ;
#149182=CARTESIAN_POINT ( 'NONE',  ( 16.46253265017146816, 9.564922557961045513, 76.66775706135234714 ) ) ;
#149183=CARTESIAN_POINT ( 'NONE',  ( -10.72451020669898014, 18.67979575497178502, 65.41557627198102409 ) ) ;
#149184=CARTESIAN_POINT ( 'NONE',  ( 13.89961937509977652, -13.97604488694527269, 38.12390960531436690 ) ) ;
#149185=CARTESIAN_POINT ( 'NONE',  ( -13.89961937509977652, 13.97604488694528158, 65.62390960531436690 ) ) ;
#149186=CARTESIAN_POINT ( 'NONE',  ( 4.483927247898790824, -16.52544592524335698, 50.20942372801901854 ) ) ;
#149187=CARTESIAN_POINT ( 'NONE',  ( -0.05219959533937732626, 21.53943276465977519, 27.50109039468567929 ) ) ;
#149188=CARTESIAN_POINT ( 'NONE',  ( -18.62759615963255300, -10.81492255796106328, 54.16775706135235424 ) ) ;
#149189=CARTESIAN_POINT ( 'NONE',  ( -9.474510206698964154, 16.51473224551069663, 100.4155762719810241 ) ) ;
#149190=CARTESIAN_POINT ( 'NONE',  ( -15.80617190586745835, -15.72974639402198527, 71.87390960531438111 ) ) ;
#149191=CARTESIAN_POINT ( 'NONE',  ( -10.81492255796078084, -18.62759615963271287, 107.0822429386476955 ) ) ;
#149192=CARTESIAN_POINT ( 'NONE',  ( 12.06949235617739724, 12.14591786802326823, 51.87609039468568284 ) ) ;
#149193=CARTESIAN_POINT ( 'NONE',  ( 21.52544592524344225, -5.823673210054117533, 48.54057627198103120 ) ) ;
#149194=CARTESIAN_POINT ( 'NONE',  ( -10.72451020669870658, -18.67979575497194134, 104.5844237280190185 ) ) ;
#149195=CARTESIAN_POINT ( 'NONE',  ( 0.05219959533909260263, 19.03943276465977164, 54.99890960531435979 ) ) ;
#149196=CARTESIAN_POINT ( 'NONE',  ( 19.02544592524343514, -5.153800228976328945, 113.5405762719810241 ) ) ;
#149197=CARTESIAN_POINT ( 'NONE',  ( 19.05341960407611168, 5.049401038298154454, 78.95724293864769550 ) ) ;
#149199=CARTESIAN_POINT ( 'NONE',  ( -16.51473224551082808, 9.474510206698731452, 73.33442372801900433 ) ) ;
#149200=CARTESIAN_POINT ( 'NONE',  ( 19.05341960407617918, -5.049401038297876454, 21.04275706135232582 ) ) ;
#149201=CARTESIAN_POINT ( 'NONE',  ( 21.55341960407610458, 5.719274019375980345, 43.95724293864769550 ) ) ;
#149202=CARTESIAN_POINT ( 'NONE',  ( 12.06949235617739724, 12.14591786802326823, 106.8760903946856899 ) ) ;
#149203=CARTESIAN_POINT ( 'NONE',  ( 16.51473224551083163, -9.474510206698727899, 90.83442372801900433 ) ) ;
#149205=CARTESIAN_POINT ( 'NONE',  ( -13.89961937509957401, -13.97604488694547875, 19.37609039468566507 ) ) ;
#149206=CARTESIAN_POINT ( 'NONE',  ( -5.049401038297874678, -19.05341960407617918, 89.79275706135230450 ) ) ;
#149207=CARTESIAN_POINT ( 'NONE',  ( -5.153800228976607833, 19.02544592524334988, 42.70942372801901143 ) ) ;
#149208=CARTESIAN_POINT ( 'NONE',  ( 17.31747979337948351, 6.344076630961065888, 108.8794486806518762 ) ) ;
#149209=CARTESIAN_POINT ( 'NONE',  ( 9.474510206698971260, -16.51473224551069308, 42.91557627198103120 ) ) ;
#149210=CARTESIAN_POINT ( 'NONE',  ( 14.29746914071049879, -8.314922557960816363, 43.33224293864769550 ) ) ;
#149211=CARTESIAN_POINT ( 'NONE',  ( 13.97604488694527802, 13.89961937509977652, 34.37390960531436690 ) ) ;
#149212=CARTESIAN_POINT ( 'NONE',  ( 0.05219959533910956823, 16.53943276465976808, 39.99890960531436690 ) ) ;
#149214=CARTESIAN_POINT ( 'NONE',  ( -16.53943276465976808, -0.05219959533934237506, 108.7510903946857042 ) ) ;
#149215=CARTESIAN_POINT ( 'NONE',  ( 19.03943276465977164, -0.05219959533909143690, 48.74890960531435979 ) ) ;
#149216=CARTESIAN_POINT ( 'NONE',  ( -19.02544592524334988, -5.153800228976617603, 18.95942372801899722 ) ) ;
#149217=CARTESIAN_POINT ( 'NONE',  ( 4.379528057220092307, 16.55341960407617563, 37.29275706135235424 ) ) ;
#149218=CARTESIAN_POINT ( 'NONE',  ( -15.80617190586745835, -15.72974639402198527, 41.87390960531435979 ) ) ;
#149219=CARTESIAN_POINT ( 'NONE',  ( -15.80617190586768217, 15.72974639402176855, 98.12609039468570415 ) ) ;
#149220=ORIENTED_EDGE ( 'NONE', *, *, #172537, .T. ) ;
#149221=CARTESIAN_POINT ( 'NONE',  ( 19.05341960407611168, 5.049401038298154454, 108.9572429386477097 ) ) ;
#149222=CARTESIAN_POINT ( 'NONE',  ( -0.05219959533909027116, -19.03943276465977164, 92.49890960531436690 ) ) ;
#149224=CARTESIAN_POINT ( 'NONE',  ( -15.72974639402176322, -15.80617190586768395, 19.37609039468568639 ) ) ;
#149225=CARTESIAN_POINT ( 'NONE',  ( -8.314922557960811034, -14.29746914071050412, 77.08224293864769550 ) ) ;
#149226=CARTESIAN_POINT ( 'NONE',  ( 15.80617190586746368, 15.72974639402197994, 69.37390960531436690 ) ) ;
#149227=CARTESIAN_POINT ( 'NONE',  ( -16.51473224551069308, -9.474510206698971260, 71.66557627198102409 ) ) ;
#149228=CARTESIAN_POINT ( 'NONE',  ( 5.153800228976335163, 19.02544592524342804, 79.79057627198102409 ) ) ;
#149229=CARTESIAN_POINT ( 'NONE',  ( 21.52544592524344225, -5.823673210054117533, 108.5405762719810241 ) ) ;
#149230=ORIENTED_EDGE ( 'NONE', *, *, #185592, .T. ) ;
#149231=CARTESIAN_POINT ( 'NONE',  ( -13.97604488694527625, -13.89961937509977652, 61.87390960531435979 ) ) ;
#149232=CARTESIAN_POINT ( 'NONE',  ( -12.14591786802309592, -12.06949235617757132, 111.8739096053143669 ) ) ;
#149234=CARTESIAN_POINT ( 'NONE',  ( -0.05219959533909027116, -19.03943276465977164, 62.49890960531435979 ) ) ;
#149235=CARTESIAN_POINT ( 'NONE',  ( 13.89961937509957401, 13.97604488694547697, 86.87609039468567573 ) ) ;
#149236=CARTESIAN_POINT ( 'NONE',  ( -8.314922557960811034, -14.29746914071050412, 97.08224293864770971 ) ) ;
#149237=CARTESIAN_POINT ( 'NONE',  ( -21.52544592524334988, -5.823673210054445271, 53.95942372801900433 ) ) ;
#149238=CARTESIAN_POINT ( 'NONE',  ( 13.89961937509977652, -13.97604488694527269, 53.12390960531434558 ) ) ;
#149239=CARTESIAN_POINT ( 'NONE',  ( -21.53943276465977519, 0.05219959533907696930, 111.2489096053143669 ) ) ;
#149240=CARTESIAN_POINT ( 'NONE',  ( -16.55341960407611168, -4.379528057220339221, 101.4572429386476955 ) ) ;
#149242=CARTESIAN_POINT ( 'NONE',  ( 13.89961937509977652, -13.97604488694527269, 78.12390960531433848 ) ) ;
#149244=CARTESIAN_POINT ( 'NONE',  ( -0.05219959533936034679, 19.03943276465977164, 112.5010903946856757 ) ) ;
#149245=CARTESIAN_POINT ( 'NONE',  ( -0.05219959533907301413, -21.53943276465977519, 27.49890960531435269 ) ) ;
#149246=CARTESIAN_POINT ( 'NONE',  ( 10.81492255796106328, -18.62759615963255655, 45.41775706135234003 ) ) ;
#149247=CARTESIAN_POINT ( 'NONE',  ( 16.51473224551069308, 9.474510206698969483, 94.16557627198103830 ) ) ;
#149248=CARTESIAN_POINT ( 'NONE',  ( -19.05341960407617563, 5.049401038297882671, 88.54275706135230450 ) ) ;
#149249=CARTESIAN_POINT ( 'NONE',  ( -19.05341960407611168, -5.049401038298163336, 66.45724293864769550 ) ) ;
#149250=CARTESIAN_POINT ( 'NONE',  ( -14.34966873604960291, -8.224510206698953496, 86.66557627198102409 ) ) ;
#149251=CARTESIAN_POINT ( 'NONE',  ( -16.51473224551069308, -9.474510206698971260, 96.66557627198102409 ) ) ;
#149252=CARTESIAN_POINT ( 'NONE',  ( -16.55341960407611168, -4.379528057220339221, 76.45724293864769550 ) ) ;
#149253=CARTESIAN_POINT ( 'NONE',  ( 19.03943276465977164, -0.05219959533909143690, 98.74890960531436690 ) ) ;
#149254=CARTESIAN_POINT ( 'NONE',  ( -9.564922557960796823, -16.46253265017161027, 47.08224293864769550 ) ) ;
#149255=CARTESIAN_POINT ( 'NONE',  ( -12.06949235617756955, 12.14591786802309770, 40.62390960531435269 ) ) ;
#149256=CARTESIAN_POINT ( 'NONE',  ( -0.05219959533909027116, -19.03943276465977164, 32.49890960531435979 ) ) ;
#149258=CARTESIAN_POINT ( 'NONE',  ( 18.67979575497194134, -10.72451020669871369, 40.83442372801901854 ) ) ;
#149259=CARTESIAN_POINT ( 'NONE',  ( 13.89961937509957401, 13.97604488694547697, 76.87609039468566152 ) ) ;
#149260=CARTESIAN_POINT ( 'NONE',  ( -12.14591786802309592, -12.06949235617757132, 51.87390960531437401 ) ) ;
#149261=CARTESIAN_POINT ( 'NONE',  ( 10.72451020669898902, -18.67979575497178502, 102.9155762719810383 ) ) ;
#149262=CARTESIAN_POINT ( 'NONE',  ( 21.55341960407610458, 5.719274019375980345, 38.95724293864768839 ) ) ;
#149263=CARTESIAN_POINT ( 'NONE',  ( -4.483927247898539470, -16.52544592524342804, 87.29057627198103830 ) ) ;
#149264=CARTESIAN_POINT ( 'NONE',  ( -5.153800228976328057, -19.02544592524343514, 47.29057627198102409 ) ) ;
#149265=CARTESIAN_POINT ( 'NONE',  ( 12.06949235617757843, -12.14591786802309237, 23.12390960531436335 ) ) ;
#149266=CARTESIAN_POINT ( 'NONE',  ( 16.52544592524335698, 4.483927247898782831, 86.45942372801901854 ) ) ;
#149267=CARTESIAN_POINT ( 'NONE',  ( -0.05219959533934338120, 16.53943276465976808, 72.50109039468568994 ) ) ;
#149268=CARTESIAN_POINT ( 'NONE',  ( 9.474510206698729675, 16.51473224551082808, 32.08442372801900433 ) ) ;
#149269=CARTESIAN_POINT ( 'NONE',  ( 13.89961937509977652, -13.97604488694527269, 98.12390960531433848 ) ) ;
#149270=CARTESIAN_POINT ( 'NONE',  ( 9.564922557960805705, 16.46253265017160317, 74.58224293864769550 ) ) ;
#149271=CARTESIAN_POINT ( 'NONE',  ( -14.29746914071037622, -8.314922557961029526, 74.16775706135231871 ) ) ;
#149272=CARTESIAN_POINT ( 'NONE',  ( 19.03943276465977164, -0.05219959533909143690, 38.74890960531436690 ) ) ;
#149273=CARTESIAN_POINT ( 'NONE',  ( 16.53943276465976808, -0.05219959533910856209, 53.74890960531437401 ) ) ;
#149274=CARTESIAN_POINT ( 'NONE',  ( 19.03943276465977164, -0.05219959533909143690, 98.74890960531436690 ) ) ;
#149275=CARTESIAN_POINT ( 'NONE',  ( 21.55341960407610458, 5.719274019375980345, 33.95724293864769550 ) ) ;
#149276=CARTESIAN_POINT ( 'NONE',  ( -14.29746914071049879, 8.314922557960819915, 65.83224293864769550 ) ) ;
#149277=CARTESIAN_POINT ( 'NONE',  ( 14.34966873604960469, 8.224510206698951720, 64.16557627198102409 ) ) ;
#149279=CARTESIAN_POINT ( 'NONE',  ( -19.03943276465977164, -0.05219959533935918106, 68.75109039468566152 ) ) ;
#149280=CARTESIAN_POINT ( 'NONE',  ( -9.474510206698964154, 16.51473224551069663, 95.41557627198102409 ) ) ;
#149281=CARTESIAN_POINT ( 'NONE',  ( -0.05219959533936034679, 19.03943276465977164, 82.50109039468567573 ) ) ;
#149282=CARTESIAN_POINT ( 'NONE',  ( 18.22780087662122384, -5.500000000000022204, 96.01540105326108687 ) ) ;
#149283=CARTESIAN_POINT ( 'NONE',  ( 0.05219959533936267826, -19.03943276465977164, 105.0010903946856615 ) ) ;
#149284=CARTESIAN_POINT ( 'NONE',  ( 14.34966873604972726, -8.224510206698740333, 100.8344237280190185 ) ) ;
#149285=CARTESIAN_POINT ( 'NONE',  ( 9.474510206698971260, -16.51473224551069308, 32.91557627198102409 ) ) ;
#149286=CARTESIAN_POINT ( 'NONE',  ( -10.81492255796078084, -18.62759615963271287, 37.08224293864768129 ) ) ;
#149287=CARTESIAN_POINT ( 'NONE',  ( 5.719274019375673035, 21.55341960407619339, 52.29275706135236135 ) ) ;
#149288=CARTESIAN_POINT ( 'NONE',  ( -14.34966873604972548, 8.224510206698743886, 28.33442372801902209 ) ) ;
#149289=CARTESIAN_POINT ( 'NONE',  ( 17.50000000000000355, 3.656949067071755710, 22.19957421800376451 ) ) ;
#149290=CARTESIAN_POINT ( 'NONE',  ( 19.02544592524343514, -5.153800228976328945, 78.54057627198099567 ) ) ;
#149291=CARTESIAN_POINT ( 'NONE',  ( -0.05219959533909027116, -19.03943276465977164, 112.4989096053143669 ) ) ;
#149292=CARTESIAN_POINT ( 'NONE',  ( 14.29746914071049879, -8.314922557960816363, 78.33224293864770971 ) ) ;
#149293=CARTESIAN_POINT ( 'NONE',  ( -19.02544592524342804, 5.153800228976336051, 76.04057627198102409 ) ) ;
#149294=CARTESIAN_POINT ( 'NONE',  ( 13.89961937509977652, -13.97604488694527269, 78.12390960531433848 ) ) ;
#149295=ORIENTED_EDGE ( 'NONE', *, *, #25866, .F. ) ;
#149296=CARTESIAN_POINT ( 'NONE',  ( 5.153800228976615827, -19.02544592524334988, 90.20942372801900433 ) ) ;
#149297=CARTESIAN_POINT ( 'NONE',  ( -5.823673210054116645, -21.52544592524344225, 67.29057627198103830 ) ) ;
#149298=CARTESIAN_POINT ( 'NONE',  ( 5.049401038298161559, -19.05341960407611168, 32.70724293864768129 ) ) ;
#149299=CARTESIAN_POINT ( 'NONE',  ( -5.153800228976607833, 19.02544592524334988, 57.70942372801899012 ) ) ;
#149300=CARTESIAN_POINT ( 'NONE',  ( 19.03943276465977164, -0.05219959533909143690, 58.74890960531435979 ) ) ;
#149301=CARTESIAN_POINT ( 'NONE',  ( 5.049401038298161559, -19.05341960407611168, 97.70724293864766707 ) ) ;
#149303=CARTESIAN_POINT ( 'NONE',  ( 0.05219959533907565091, 21.53943276465977519, 84.99890960531436690 ) ) ;
#149304=CARTESIAN_POINT ( 'NONE',  ( 0.05219959533910956823, 16.53943276465976808, 99.99890960531436690 ) ) ;
#149305=CARTESIAN_POINT ( 'NONE',  ( -9.474510206698720793, -16.51473224551083518, 49.58442372801899722 ) ) ;
#149306=CARTESIAN_POINT ( 'NONE',  ( -0.05219959533907301413, -21.53943276465977519, 87.49890960531436690 ) ) ;
#149307=CARTESIAN_POINT ( 'NONE',  ( 21.53943276465977519, -0.05219959533907433946, 73.74890960531433848 ) ) ;
#149308=CARTESIAN_POINT ( 'NONE',  ( 8.314922557960818139, 14.29746914071049879, 34.58224293864770260 ) ) ;
#149309=CARTESIAN_POINT ( 'NONE',  ( -10.72451020669870658, -18.67979575497194134, 99.58442372801900433 ) ) ;
#149310=CARTESIAN_POINT ( 'NONE',  ( -9.474510206698964154, 16.51473224551069663, 85.41557627198102409 ) ) ;
#149311=CARTESIAN_POINT ( 'NONE',  ( 19.02544592524343514, -5.153800228976328945, 38.54057627198103120 ) ) ;
#149312=CARTESIAN_POINT ( 'NONE',  ( -10.72451020669870658, -18.67979575497194134, 39.58442372801901143 ) ) ;
#149313=CARTESIAN_POINT ( 'NONE',  ( 21.53943276465977519, 0.05219959533937863772, 51.25109039468568994 ) ) ;
#149314=CARTESIAN_POINT ( 'NONE',  ( 9.564922557960805705, 16.46253265017160317, 54.58224293864769550 ) ) ;
#149315=CARTESIAN_POINT ( 'NONE',  ( 21.53943276465977519, -0.05219959533907433946, 113.7489096053143527 ) ) ;
#149316=CARTESIAN_POINT ( 'NONE',  ( -9.474510206698720793, -16.51473224551083518, 59.58442372801900433 ) ) ;
#149317=CARTESIAN_POINT ( 'NONE',  ( -19.05341960407611168, -5.049401038298163336, 36.45724293864766707 ) ) ;
#149318=CARTESIAN_POINT ( 'NONE',  ( -16.52544592524335698, -4.483927247898792601, 23.95942372801901143 ) ) ;
#149319=CARTESIAN_POINT ( 'NONE',  ( 9.474510206698971260, -16.51473224551069308, 22.91557627198102765 ) ) ;
#149320=CARTESIAN_POINT ( 'NONE',  ( -4.379528057220086978, -16.55341960407618274, 74.79275706135234714 ) ) ;
#149321=CARTESIAN_POINT ( 'NONE',  ( -13.97604488694527625, -13.89961937509977652, 41.87390960531435979 ) ) ;
#149323=CARTESIAN_POINT ( 'NONE',  ( -0.05219959533909027116, -19.03943276465977164, 82.49890960531436690 ) ) ;
#149324=CARTESIAN_POINT ( 'NONE',  ( 19.03943276465977164, -0.05219959533909143690, 28.74890960531435624 ) ) ;
#149325=CARTESIAN_POINT ( 'NONE',  ( 18.67979575497178502, 10.72451020669898547, 74.16557627198102409 ) ) ;
#149326=CARTESIAN_POINT ( 'NONE',  ( 14.29746914071037800, 8.314922557961029526, 41.66775706135235424 ) ) ;
#149327=CARTESIAN_POINT ( 'NONE',  ( 15.80617190586769283, -15.72974639402175789, 110.6260903946857042 ) ) ;
#149328=CARTESIAN_POINT ( 'NONE',  ( 19.05341960407611168, 5.049401038298154454, 33.95724293864769550 ) ) ;
#149329=CARTESIAN_POINT ( 'NONE',  ( 14.34966873604960469, 8.224510206698951720, 34.16557627198102409 ) ) ;
#149330=CARTESIAN_POINT ( 'NONE',  ( -16.55341960407611168, -4.379528057220339221, 61.45724293864770260 ) ) ;
#149331=CARTESIAN_POINT ( 'NONE',  ( -16.46253265017160317, 9.564922557960807481, 60.83224293864769550 ) ) ;
#149332=CARTESIAN_POINT ( 'NONE',  ( 0.05219959533937995610, -21.53943276465977519, 110.0010903946856757 ) ) ;
#149333=CARTESIAN_POINT ( 'NONE',  ( -18.62759615963270932, 10.81492255796079327, 115.8322429386477097 ) ) ;
#149334=CARTESIAN_POINT ( 'NONE',  ( 9.564922557960805705, 16.46253265017160317, 84.58224293864769550 ) ) ;
#149335=CARTESIAN_POINT ( 'NONE',  ( 18.67979575497194134, -10.72451020669871369, 90.83442372801901854 ) ) ;
#149336=CARTESIAN_POINT ( 'NONE',  ( -12.06949235617739369, -12.14591786802326823, 69.37609039468567573 ) ) ;
#149337=CARTESIAN_POINT ( 'NONE',  ( 13.89961937509977652, -13.97604488694527269, 113.1239096053143527 ) ) ;
#149338=CARTESIAN_POINT ( 'NONE',  ( 12.06949235617757843, -12.14591786802309237, 28.12390960531435979 ) ) ;
#149339=CARTESIAN_POINT ( 'NONE',  ( -13.97604488694527625, -13.89961937509977652, 26.87390960531434558 ) ) ;
#149340=CARTESIAN_POINT ( 'NONE',  ( -12.06949235617739369, -12.14591786802326823, 49.37609039468569705 ) ) ;
#149341=CARTESIAN_POINT ( 'NONE',  ( 14.29746914071049879, -8.314922557960816363, 58.33224293864768839 ) ) ;
#149342=CARTESIAN_POINT ( 'NONE',  ( 12.06949235617739724, 12.14591786802326823, 101.8760903946857042 ) ) ;
#149343=CARTESIAN_POINT ( 'NONE',  ( -13.97604488694527625, -13.89961937509977652, 111.8739096053143243 ) ) ;
#149344=CARTESIAN_POINT ( 'NONE',  ( -18.62759615963270932, 10.81492255796079327, 30.83224293864770260 ) ) ;
#149345=CARTESIAN_POINT ( 'NONE',  ( 21.52544592524334988, 5.823673210054432836, 106.4594237280190328 ) ) ;
#149346=CARTESIAN_POINT ( 'NONE',  ( 0.05219959533910956823, 16.53943276465976808, 84.99890960531436690 ) ) ;
#149347=CARTESIAN_POINT ( 'NONE',  ( -5.049401038298153566, 19.05341960407611168, 90.20724293864766707 ) ) ;
#149349=CARTESIAN_POINT ( 'NONE',  ( -8.314922557961024197, 14.29746914071037800, 42.91775706135235424 ) ) ;
#149350=CARTESIAN_POINT ( 'NONE',  ( -13.97604488694527625, -13.89961937509977652, 56.87390960531434558 ) ) ;
#149351=CARTESIAN_POINT ( 'NONE',  ( 17.50000000000000000, -5.500000000000000888, 120.0000000000000142 ) ) ;
#149352=CARTESIAN_POINT ( 'NONE',  ( -19.03943276465977164, -0.05219959533935918106, 53.75109039468566863 ) ) ;
#149353=CARTESIAN_POINT ( 'NONE',  ( 5.049401038298161559, -19.05341960407611168, 47.70724293864770260 ) ) ;
#149354=CARTESIAN_POINT ( 'NONE',  ( -4.379528057220086978, -16.55341960407618274, 74.79275706135234714 ) ) ;
#149355=CARTESIAN_POINT ( 'NONE',  ( -19.03943276465977164, -0.05219959533935918106, 93.75109039468566152 ) ) ;
#149356=CARTESIAN_POINT ( 'NONE',  ( 19.05341960407611168, 5.049401038298154454, 58.95724293864768129 ) ) ;
#149357=CARTESIAN_POINT ( 'NONE',  ( -21.52544592524343514, 5.823673210054127303, 91.04057627198103830 ) ) ;
#149358=CARTESIAN_POINT ( 'NONE',  ( 12.06949235617757843, -12.14591786802309237, 98.12390960531436690 ) ) ;
#149359=EDGE_CURVE ( 'NONE', #113576, #53672, #88185, .T. ) ;
#149360=CARTESIAN_POINT ( 'NONE',  ( -0.05219959533936034679, 19.03943276465977164, 67.50109039468566152 ) ) ;
#149361=CARTESIAN_POINT ( 'NONE',  ( -21.52544592524343514, 5.823673210054127303, 66.04057627198103830 ) ) ;
#149362=CARTESIAN_POINT ( 'NONE',  ( 13.97604488694548053, -13.89961937509957401, 35.62609039468567573 ) ) ;
#149363=CARTESIAN_POINT ( 'NONE',  ( 18.39639308325437739, 5.500000000000011546, 98.98252246182197212 ) ) ;
#149364=CARTESIAN_POINT ( 'NONE',  ( -10.81492255796078084, -18.62759615963271287, 97.08224293864770971 ) ) ;
#149365=LINE ( 'NONE', #148365, #1505 ) ;
#149366=CARTESIAN_POINT ( 'NONE',  ( -13.97604488694547697, 13.89961937509957934, 98.12609039468566152 ) ) ;
#149367=DIRECTION ( 'NONE',  ( -0.000000000000000000, -0.000000000000000000, 1.000000000000000000 ) ) ;
#149368=CARTESIAN_POINT ( 'NONE',  ( 4.483927247898790824, -16.52544592524335698, 25.20942372801901854 ) ) ;
#149369=CARTESIAN_POINT ( 'NONE',  ( 9.474510206698971260, -16.51473224551069308, 47.91557627198102409 ) ) ;
#149370=CARTESIAN_POINT ( 'NONE',  ( -10.81492255796078084, -18.62759615963271287, 22.08224293864769194 ) ) ;
#149371=CARTESIAN_POINT ( 'NONE',  ( -0.05219959533907301413, -21.53943276465977519, 92.49890960531436690 ) ) ;
#149372=CARTESIAN_POINT ( 'NONE',  ( -0.05219959533937732626, 21.53943276465977519, 57.50109039468568994 ) ) ;
#149373=CARTESIAN_POINT ( 'NONE',  ( -4.379528057220086978, -16.55341960407618274, 24.79275706135235779 ) ) ;
#149374=CARTESIAN_POINT ( 'NONE',  ( -9.564922557961040184, 16.46253265017147172, 27.91775706135232582 ) ) ;
#149375=CARTESIAN_POINT ( 'NONE',  ( -8.314922557960811034, -14.29746914071050412, 27.08224293864769550 ) ) ;
#149376=CARTESIAN_POINT ( 'NONE',  ( 21.53943276465977519, 0.05219959533937863772, 21.25109039468567218 ) ) ;
#149377=CARTESIAN_POINT ( 'NONE',  ( 14.34966873604960469, 8.224510206698951720, 49.16557627198102409 ) ) ;
#149378=CARTESIAN_POINT ( 'NONE',  ( -5.153800228976607833, 19.02544592524334988, 92.70942372801901854 ) ) ;
#149379=CARTESIAN_POINT ( 'NONE',  ( 9.474510206698729675, 16.51473224551082808, 52.08442372801900433 ) ) ;
#149380=CARTESIAN_POINT ( 'NONE',  ( -10.81492255796105439, 18.62759615963255655, 67.91775706135234714 ) ) ;
#149381=CARTESIAN_POINT ( 'NONE',  ( -19.03943276465977164, -0.05219959533935918106, 43.75109039468566863 ) ) ;
#149382=CARTESIAN_POINT ( 'NONE',  ( 9.474510206698971260, -16.51473224551069308, 22.91557627198102765 ) ) ;
#149383=CARTESIAN_POINT ( 'NONE',  ( 5.823673210054125526, 21.52544592524343514, 49.79057627198102409 ) ) ;
#149384=CARTESIAN_POINT ( 'NONE',  ( -16.55341960407611168, -4.379528057220339221, 31.45724293864769550 ) ) ;
#149385=CARTESIAN_POINT ( 'NONE',  ( -19.03943276465977164, -0.05219959533935918106, 18.75109039468567218 ) ) ;
#149386=CARTESIAN_POINT ( 'NONE',  ( 12.06949235617739724, 12.14591786802326823, 71.87609039468568994 ) ) ;
#149387=CARTESIAN_POINT ( 'NONE',  ( -12.14591786802309592, -12.06949235617757132, 36.87390960531435979 ) ) ;
#149388=CARTESIAN_POINT ( 'NONE',  ( -21.53943276465977519, -0.05219959533937600094, 78.75109039468568994 ) ) ;
#149389=CARTESIAN_POINT ( 'NONE',  ( -0.05219959533937732626, 21.53943276465977519, 62.50109039468568284 ) ) ;
#149390=CARTESIAN_POINT ( 'NONE',  ( -10.81492255796078084, -18.62759615963271287, 62.08224293864769550 ) ) ;
#149392=CARTESIAN_POINT ( 'NONE',  ( -13.89961937509977652, 13.97604488694528158, 35.62390960531435269 ) ) ;
#149393=CARTESIAN_POINT ( 'NONE',  ( -5.719274019375665041, -21.55341960407619695, 44.79275706135234714 ) ) ;
#149394=CARTESIAN_POINT ( 'NONE',  ( 13.89961937509977652, -13.97604488694527269, 28.12390960531435624 ) ) ;
#149395=CARTESIAN_POINT ( 'NONE',  ( 19.03943276465977164, -0.05219959533909143690, 33.74890960531435979 ) ) ;
#149396=CARTESIAN_POINT ( 'NONE',  ( -16.52544592524342804, 4.483927247898546575, 96.04057627198102409 ) ) ;
#149397=CARTESIAN_POINT ( 'NONE',  ( -5.153800228976328057, -19.02544592524343514, 82.29057627198103830 ) ) ;
#149398=CARTESIAN_POINT ( 'NONE',  ( -4.379528057220328563, 16.55341960407611168, 35.20724293864768839 ) ) ;
#149399=CARTESIAN_POINT ( 'NONE',  ( -8.224510206698948167, 14.34966873604960824, 95.41557627198102409 ) ) ;
#149400=CARTESIAN_POINT ( 'NONE',  ( 15.80617190586746368, 15.72974639402197994, 64.37390960531435269 ) ) ;
#149401=CARTESIAN_POINT ( 'NONE',  ( -21.53943276465977519, 0.05219959533907696930, 106.2489096053143811 ) ) ;
#149402=CARTESIAN_POINT ( 'NONE',  ( 5.153800228976335163, 19.02544592524342804, 109.7905762719810099 ) ) ;
#149403=CARTESIAN_POINT ( 'NONE',  ( -16.51473224551069308, -9.474510206698971260, 66.66557627198102409 ) ) ;
#149404=CARTESIAN_POINT ( 'NONE',  ( -12.14591786802326823, 12.06949235617739902, 28.12609039468568284 ) ) ;
#149405=CARTESIAN_POINT ( 'NONE',  ( 21.55341960407610458, 5.719274019375980345, 53.95724293864770260 ) ) ;
#149406=CARTESIAN_POINT ( 'NONE',  ( -18.67979575497193778, 10.72451020669871902, 98.33442372801901854 ) ) ;
#149407=CARTESIAN_POINT ( 'NONE',  ( -19.05341960407611168, -5.049401038298163336, 81.45724293864769550 ) ) ;
#149408=CARTESIAN_POINT ( 'NONE',  ( -18.67979575497193778, 10.72451020669871902, 23.33442372801901499 ) ) ;
#149409=CARTESIAN_POINT ( 'NONE',  ( -10.81492255796078084, -18.62759615963271287, 22.08224293864769194 ) ) ;
#149410=CARTESIAN_POINT ( 'NONE',  ( 16.52544592524335698, 4.483927247898782831, 91.45942372801901854 ) ) ;
#149411=CARTESIAN_POINT ( 'NONE',  ( -21.52544592524334988, -5.823673210054445271, 68.95942372801901854 ) ) ;
#149412=CARTESIAN_POINT ( 'NONE',  ( 21.53943276465977519, 0.05219959533937863772, 101.2510903946856757 ) ) ;
#149413=CARTESIAN_POINT ( 'NONE',  ( -8.314922557961024197, 14.29746914071037800, 67.91775706135234714 ) ) ;
#149414=CARTESIAN_POINT ( 'NONE',  ( -10.81492255796105439, 18.62759615963255655, 32.91775706135234714 ) ) ;
#149415=CARTESIAN_POINT ( 'NONE',  ( -16.51473224551069308, -9.474510206698971260, 111.6655762719810383 ) ) ;
#149416=CARTESIAN_POINT ( 'NONE',  ( -10.81492255796105439, 18.62759615963255655, 87.91775706135234714 ) ) ;
#149417=CARTESIAN_POINT ( 'NONE',  ( 9.564922557960805705, 16.46253265017160317, 94.58224293864769550 ) ) ;
#149418=CARTESIAN_POINT ( 'NONE',  ( -10.81492255796078084, -18.62759615963271287, 92.08224293864769550 ) ) ;
#149419=CARTESIAN_POINT ( 'NONE',  ( 19.03943276465977164, 0.05219959533936151252, 66.25109039468567573 ) ) ;
#149420=CARTESIAN_POINT ( 'NONE',  ( 10.81492255796078972, 18.62759615963270932, 59.58224293864770260 ) ) ;
#149421=CARTESIAN_POINT ( 'NONE',  ( 16.46253265017160672, -9.564922557960803928, 98.33224293864769550 ) ) ;
#149422=CARTESIAN_POINT ( 'NONE',  ( 12.06949235617757843, -12.14591786802309237, 33.12390960531435979 ) ) ;
#149424=CARTESIAN_POINT ( 'NONE',  ( 5.153800228976615827, -19.02544592524334988, 80.20942372801901854 ) ) ;
#149426=CARTESIAN_POINT ( 'NONE',  ( 16.46253265017146816, 9.564922557961045513, 106.6677570613523471 ) ) ;
#149427=CARTESIAN_POINT ( 'NONE',  ( 21.53943276465977519, -0.05219959533907433946, 78.74890960531436690 ) ) ;
#149428=CARTESIAN_POINT ( 'NONE',  ( 4.483927247898545687, 16.52544592524342804, 69.79057627198102409 ) ) ;
#149429=CARTESIAN_POINT ( 'NONE',  ( -4.483927247898782831, 16.52544592524335698, 27.70942372801901854 ) ) ;
#149430=CARTESIAN_POINT ( 'NONE',  ( -16.51473224551069308, -9.474510206698971260, 41.66557627198103120 ) ) ;
#149431=CARTESIAN_POINT ( 'NONE',  ( 21.55341960407610458, 5.719274019375980345, 113.9572429386477239 ) ) ;
#149432=CARTESIAN_POINT ( 'NONE',  ( 19.02544592524334988, 5.153800228976608722, 81.45942372801897591 ) ) ;
#149433=CARTESIAN_POINT ( 'NONE',  ( 19.05341960407611168, 5.049401038298154454, 88.95724293864769550 ) ) ;
#149434=CARTESIAN_POINT ( 'NONE',  ( 19.02544592524343514, -5.153800228976328945, 78.54057627198099567 ) ) ;
#149435=CARTESIAN_POINT ( 'NONE',  ( 0.05219959533907565091, 21.53943276465977519, 69.99890960531435269 ) ) ;
#149436=CARTESIAN_POINT ( 'NONE',  ( -13.89961937509977652, 13.97604488694528158, 50.62390960531435979 ) ) ;
#149438=CARTESIAN_POINT ( 'NONE',  ( -4.483927247898539470, -16.52544592524342804, 52.29057627198102409 ) ) ;
#149439=CARTESIAN_POINT ( 'NONE',  ( -9.474510206698964154, 16.51473224551069663, 85.41557627198102409 ) ) ;
#149440=CARTESIAN_POINT ( 'NONE',  ( 18.22780087662119897, -5.500000000000096811, 43.51763182126894236 ) ) ;
#149441=CARTESIAN_POINT ( 'NONE',  ( 0.05219959533936267826, -19.03943276465977164, 70.00109039468566152 ) ) ;
#149442=CARTESIAN_POINT ( 'NONE',  ( -21.52544592524343514, 5.823673210054127303, 81.04057627198102409 ) ) ;
#149443=CARTESIAN_POINT ( 'NONE',  ( 19.05341960407617918, -5.049401038297876454, 36.04275706135234003 ) ) ;
#149444=CARTESIAN_POINT ( 'NONE',  ( -9.564922557960796823, -16.46253265017161027, 102.0822429386477097 ) ) ;
#149446=CARTESIAN_POINT ( 'NONE',  ( -21.52544592524343514, 5.823673210054127303, 46.04057627198103830 ) ) ;
#149447=CARTESIAN_POINT ( 'NONE',  ( 19.03943276465977164, -0.05219959533909143690, 68.74890960531436690 ) ) ;
#149448=CARTESIAN_POINT ( 'NONE',  ( 21.53943276465977519, 0.05219959533937863772, 61.25109039468567573 ) ) ;
#149449=CARTESIAN_POINT ( 'NONE',  ( 13.97604488694527802, 13.89961937509977652, 24.37390960531435624 ) ) ;
#149450=CARTESIAN_POINT ( 'NONE',  ( -21.53943276465977519, 0.05219959533907696930, 111.2489096053143669 ) ) ;
#149451=VERTEX_POINT ( 'NONE', #134716 ) ;
#149452=CARTESIAN_POINT ( 'NONE',  ( -10.81492255796105439, 18.62759615963255655, 52.91775706135235424 ) ) ;
#149454=CARTESIAN_POINT ( 'NONE',  ( -19.02544592524342804, 5.153800228976336051, 116.0405762719810383 ) ) ;
#149455=CARTESIAN_POINT ( 'NONE',  ( -19.05341960407617563, 5.049401038297882671, 68.54275706135230450 ) ) ;
#149458=CARTESIAN_POINT ( 'NONE',  ( -15.72974639402197994, 15.80617190586746368, 105.6239096053143669 ) ) ;
#149459=CARTESIAN_POINT ( 'NONE',  ( -19.02544592524342804, 5.153800228976336051, 61.04057627198103120 ) ) ;
#149460=CARTESIAN_POINT ( 'NONE',  ( 4.379528057220092307, 16.55341960407617563, 32.29275706135235424 ) ) ;
#149462=CARTESIAN_POINT ( 'NONE',  ( -5.823673210054431948, 21.52544592524334988, 97.70942372801904696 ) ) ;
#149463=CARTESIAN_POINT ( 'NONE',  ( 5.153800228976335163, 19.02544592524342804, 39.79057627198100988 ) ) ;
#149464=CARTESIAN_POINT ( 'NONE',  ( 21.55341960407619695, -5.719274019375665929, 96.04275706135236135 ) ) ;
#149465=CARTESIAN_POINT ( 'NONE',  ( -19.05341960407611168, -5.049401038298163336, 86.45724293864769550 ) ) ;
#149466=CARTESIAN_POINT ( 'NONE',  ( -21.52544592524334988, -5.823673210054445271, 58.95942372801902565 ) ) ;
#149470=CARTESIAN_POINT ( 'NONE',  ( -16.53943276465976808, -0.05219959533934237506, 53.75109039468568994 ) ) ;
#149471=CARTESIAN_POINT ( 'NONE',  ( 10.81492255796106328, -18.62759615963255655, 70.41775706135236135 ) ) ;
#149472=CARTESIAN_POINT ( 'NONE',  ( 15.80617190586769283, -15.72974639402175789, 85.62609039468568994 ) ) ;
#149474=CARTESIAN_POINT ( 'NONE',  ( 8.224510206698742110, 14.34966873604972548, 22.08442372801901143 ) ) ;
#149475=CARTESIAN_POINT ( 'NONE',  ( 9.474510206698971260, -16.51473224551069308, 82.91557627198103830 ) ) ;
#149476=CARTESIAN_POINT ( 'NONE',  ( -9.564922557960796823, -16.46253265017161027, 107.0822429386476955 ) ) ;
#149479=CARTESIAN_POINT ( 'NONE',  ( 19.03943276465977164, -0.05219959533909143690, 23.74890960531435269 ) ) ;
#149480=CARTESIAN_POINT ( 'NONE',  ( -18.62759615963270932, 10.81492255796079327, 45.83224293864769550 ) ) ;
#149481=CARTESIAN_POINT ( 'NONE',  ( 14.34966873604972726, -8.224510206698740333, 95.83442372801903275 ) ) ;
#149482=CARTESIAN_POINT ( 'NONE',  ( 8.224510206698953496, -14.34966873604960469, 87.91557627198103830 ) ) ;
#149483=CARTESIAN_POINT ( 'NONE',  ( -19.05341960407611168, -5.049401038298163336, 66.45724293864769550 ) ) ;
#149484=CARTESIAN_POINT ( 'NONE',  ( -0.05219959533937732626, 21.53943276465977519, 87.50109039468568994 ) ) ;
#149486=CARTESIAN_POINT ( 'NONE',  ( -16.53943276465976808, -0.05219959533934237506, 18.75109039468568639 ) ) ;
#149487=CARTESIAN_POINT ( 'NONE',  ( -16.53943276465976808, 0.05219959533911058130, 86.24890960531436690 ) ) ;
#149488=CARTESIAN_POINT ( 'NONE',  ( -15.80617190586768217, 15.72974639402176855, 43.12609039468568284 ) ) ;
#149489=CARTESIAN_POINT ( 'NONE',  ( -10.81492255796078084, -18.62759615963271287, 77.08224293864769550 ) ) ;
#149490=CARTESIAN_POINT ( 'NONE',  ( 19.03943276465977164, 0.05219959533936151252, 36.25109039468567573 ) ) ;
#149491=CARTESIAN_POINT ( 'NONE',  ( -17.58332526062525858, 7.635886036038558977, 45.92334959558467489 ) ) ;
#149492=CARTESIAN_POINT ( 'NONE',  ( 16.46253265017160672, -9.564922557960803928, 78.33224293864769550 ) ) ;
#149493=CARTESIAN_POINT ( 'NONE',  ( 16.53943276465976808, -0.05219959533910856209, 58.74890960531436690 ) ) ;
#149494=CARTESIAN_POINT ( 'NONE',  ( 16.52544592524342804, -4.483927247898539470, 33.54057627198102409 ) ) ;
#149495=CARTESIAN_POINT ( 'NONE',  ( 0.05219959533934541429, -16.53943276465976808, 110.0010903946856757 ) ) ;
#149496=CARTESIAN_POINT ( 'NONE',  ( -9.474510206698720793, -16.51473224551083518, 59.58442372801900433 ) ) ;
#149497=CARTESIAN_POINT ( 'NONE',  ( 17.44279575226823553, 5.990770900252484488, 46.66442432485681024 ) ) ;
#149498=CARTESIAN_POINT ( 'NONE',  ( 18.62759615963271287, -10.81492255796078972, 28.33224293864769550 ) ) ;
#149499=CARTESIAN_POINT ( 'NONE',  ( 12.14591786802309770, 12.06949235617756955, 89.37390960531435269 ) ) ;
#149501=CARTESIAN_POINT ( 'NONE',  ( -19.05341960407611168, -5.049401038298163336, 41.45724293864769550 ) ) ;
#149502=CARTESIAN_POINT ( 'NONE',  ( -21.52544592524343514, 5.823673210054127303, 46.04057627198103830 ) ) ;
#149503=CARTESIAN_POINT ( 'NONE',  ( 5.719274019375991003, -21.55341960407610458, 67.70724293864769550 ) ) ;
#149504=CARTESIAN_POINT ( 'NONE',  ( 16.46253265017160672, -9.564922557960803928, 23.33224293864769194 ) ) ;
#149505=CARTESIAN_POINT ( 'NONE',  ( 4.483927247898790824, -16.52544592524335698, 65.20942372801901854 ) ) ;
#149506=CARTESIAN_POINT ( 'NONE',  ( -19.02544592524342804, 5.153800228976336051, 41.04057627198103120 ) ) ;
#149507=CARTESIAN_POINT ( 'NONE',  ( -10.81492255796105439, 18.62759615963255655, 57.91775706135234714 ) ) ;
#149508=CARTESIAN_POINT ( 'NONE',  ( -16.55341960407611168, -4.379528057220339221, 111.4572429386476813 ) ) ;
#149509=CARTESIAN_POINT ( 'NONE',  ( -0.05219959533936034679, 19.03943276465977164, 92.50109039468566152 ) ) ;
#149512=CARTESIAN_POINT ( 'NONE',  ( 21.52544592524344225, -5.823673210054117533, 53.54057627198103120 ) ) ;
#149513=CARTESIAN_POINT ( 'NONE',  ( -19.03943276465977164, 0.05219959533909376836, 26.24890960531435624 ) ) ;
#149514=CARTESIAN_POINT ( 'NONE',  ( -18.67979575497193778, 10.72451020669871902, 88.33442372801901854 ) ) ;
#149515=CARTESIAN_POINT ( 'NONE',  ( -4.483927247898539470, -16.52544592524342804, 32.29057627198102409 ) ) ;
#149516=CARTESIAN_POINT ( 'NONE',  ( -16.53943276465976808, -0.05219959533934237506, 58.75109039468568994 ) ) ;
#149517=CARTESIAN_POINT ( 'NONE',  ( -4.483927247898539470, -16.52544592524342804, 37.29057627198102409 ) ) ;
#149518=CARTESIAN_POINT ( 'NONE',  ( -10.81492255796078084, -18.62759615963271287, 72.08224293864769550 ) ) ;
#149519=CARTESIAN_POINT ( 'NONE',  ( -0.05219959533907301413, -21.53943276465977519, 77.49890960531433848 ) ) ;
#149521=CARTESIAN_POINT ( 'NONE',  ( 9.474510206698729675, 16.51473224551082808, 87.08442372801900433 ) ) ;
#149522=CARTESIAN_POINT ( 'NONE',  ( 16.46253265017160672, -9.564922557960803928, 113.3322429386476955 ) ) ;
#149524=CARTESIAN_POINT ( 'NONE',  ( 5.153800228976335163, 19.02544592524342804, 49.79057627198100988 ) ) ;
#149525=CARTESIAN_POINT ( 'NONE',  ( -16.52544592524342804, 4.483927247898546575, 116.0405762719810383 ) ) ;
#149527=CARTESIAN_POINT ( 'NONE',  ( 17.97214573761829470, 5.500000000000074607, 48.96970049038657180 ) ) ;
#149529=CARTESIAN_POINT ( 'NONE',  ( -8.224510206698735004, -14.34966873604973081, 79.58442372801903275 ) ) ;
#149530=CARTESIAN_POINT ( 'NONE',  ( -0.05219959533907301413, -21.53943276465977519, 107.4989096053143669 ) ) ;
#149531=CARTESIAN_POINT ( 'NONE',  ( -5.153800228976328057, -19.02544592524343514, 72.29057627198102409 ) ) ;
#149532=CARTESIAN_POINT ( 'NONE',  ( 18.62759615963255655, 10.81492255796105972, 46.66775706135234714 ) ) ;
#149533=CARTESIAN_POINT ( 'NONE',  ( -5.153800228976328057, -19.02544592524343514, 92.29057627198099567 ) ) ;
#149536=CARTESIAN_POINT ( 'NONE',  ( 21.52544592524334988, 5.823673210054432836, 26.45942372801901854 ) ) ;
#149537=CARTESIAN_POINT ( 'NONE',  ( 16.51473224551069308, 9.474510206698969483, 24.16557627198102765 ) ) ;
#149538=CARTESIAN_POINT ( 'NONE',  ( 16.51473224551083163, -9.474510206698727899, 90.83442372801900433 ) ) ;
#149539=CARTESIAN_POINT ( 'NONE',  ( 19.03943276465977164, 0.05219959533936151252, 36.25109039468567573 ) ) ;
#149540=CARTESIAN_POINT ( 'NONE',  ( 18.62759615963255655, 10.81492255796105972, 21.66775706135235069 ) ) ;
#149541=CARTESIAN_POINT ( 'NONE',  ( -9.474510206698720793, -16.51473224551083518, 29.58442372801900433 ) ) ;
#149542=CARTESIAN_POINT ( 'NONE',  ( -9.564922557961040184, 16.46253265017147172, 52.91775706135233293 ) ) ;
#149543=CARTESIAN_POINT ( 'NONE',  ( 16.53943276465976808, 0.05219959533934440121, 91.25109039468568994 ) ) ;
#149546=CARTESIAN_POINT ( 'NONE',  ( 5.153800228976335163, 19.02544592524342804, 74.79057627198103830 ) ) ;
#149547=CARTESIAN_POINT ( 'NONE',  ( 15.72974639402176855, 15.80617190586768217, 81.87609039468568994 ) ) ;
#149548=CARTESIAN_POINT ( 'NONE',  ( 10.72451020669871369, 18.67979575497193778, 92.08442372801901854 ) ) ;
#149550=CARTESIAN_POINT ( 'NONE',  ( -13.89961937509977652, 13.97604488694528158, 85.62390960531433848 ) ) ;
#149551=CARTESIAN_POINT ( 'NONE',  ( 15.72974639402176855, 15.80617190586768217, 61.87609039468568284 ) ) ;
#149552=CARTESIAN_POINT ( 'NONE',  ( 9.564922557961047289, -16.46253265017146816, 95.41775706135233293 ) ) ;
#149553=CARTESIAN_POINT ( 'NONE',  ( 16.46253265017160672, -9.564922557960803928, 68.33224293864770971 ) ) ;
#149554=CARTESIAN_POINT ( 'NONE',  ( -21.55341960407610458, -5.719274019375992779, 21.45724293864769550 ) ) ;
#149555=CARTESIAN_POINT ( 'NONE',  ( -5.049401038298153566, 19.05341960407611168, 75.20724293864769550 ) ) ;
#149556=CARTESIAN_POINT ( 'NONE',  ( -17.05587630539787725, -6.762274262135687053, 89.25819690962691766 ) ) ;
#149557=CARTESIAN_POINT ( 'NONE',  ( 19.05341960407611168, 5.049401038298154454, 58.95724293864768129 ) ) ;
#149558=CARTESIAN_POINT ( 'NONE',  ( -5.153800228976328057, -19.02544592524343514, 47.29057627198102409 ) ) ;
#149559=CARTESIAN_POINT ( 'NONE',  ( 18.67979575497194134, -10.72451020669871369, 20.83442372801901143 ) ) ;
#149560=CARTESIAN_POINT ( 'NONE',  ( -14.29746914071037622, -8.314922557961029526, 104.1677570613523471 ) ) ;
#149563=CARTESIAN_POINT ( 'NONE',  ( -16.46253265017146816, -9.564922557961047289, 54.16775706135234003 ) ) ;
#149564=CARTESIAN_POINT ( 'NONE',  ( 13.89961937509977652, -13.97604488694527269, 83.12390960531436690 ) ) ;
#149565=CARTESIAN_POINT ( 'NONE',  ( -8.314922557960811034, -14.29746914071050412, 72.08224293864769550 ) ) ;
#149566=CARTESIAN_POINT ( 'NONE',  ( -16.55341960407611168, -4.379528057220339221, 106.4572429386477097 ) ) ;
#149567=CARTESIAN_POINT ( 'NONE',  ( -21.53943276465977519, 0.05219959533907696930, 36.24890960531435979 ) ) ;
#149568=CARTESIAN_POINT ( 'NONE',  ( -19.03943276465977164, 0.05219959533909376836, 106.2489096053143669 ) ) ;
#149569=CARTESIAN_POINT ( 'NONE',  ( 4.379528057220339221, -16.55341960407611168, 87.70724293864769550 ) ) ;
#149571=CARTESIAN_POINT ( 'NONE',  ( -13.89961937509957401, -13.97604488694547875, 34.37609039468566863 ) ) ;
#149572=CARTESIAN_POINT ( 'NONE',  ( 0.05219959533934541429, -16.53943276465976808, 105.0010903946856757 ) ) ;
#149573=CARTESIAN_POINT ( 'NONE',  ( 9.564922557960805705, 16.46253265017160317, 89.58224293864769550 ) ) ;
#149574=CARTESIAN_POINT ( 'NONE',  ( 15.72974639402176855, 15.80617190586768217, 46.87609039468568994 ) ) ;
#149575=CARTESIAN_POINT ( 'NONE',  ( 10.72451020669898902, -18.67979575497178502, 37.91557627198102409 ) ) ;
#149576=CARTESIAN_POINT ( 'NONE',  ( 15.80617190586769283, -15.72974639402175789, 25.62609039468567929 ) ) ;
#149577=CARTESIAN_POINT ( 'NONE',  ( 0.05219959533907565091, 21.53943276465977519, 74.99890960531435269 ) ) ;
#149578=CARTESIAN_POINT ( 'NONE',  ( 0.05219959533910956823, 16.53943276465976808, 94.99890960531436690 ) ) ;
#149579=CARTESIAN_POINT ( 'NONE',  ( -9.564922557961040184, 16.46253265017147172, 52.91775706135233293 ) ) ;
#149580=CARTESIAN_POINT ( 'NONE',  ( 9.564922557960805705, 16.46253265017160317, 34.58224293864770260 ) ) ;
#149581=CARTESIAN_POINT ( 'NONE',  ( -0.05219959533909027116, -19.03943276465977164, 97.49890960531436690 ) ) ;
#149582=CARTESIAN_POINT ( 'NONE',  ( 19.05341960407611168, 5.049401038298154454, 93.95724293864769550 ) ) ;
#149583=CARTESIAN_POINT ( 'NONE',  ( 14.34966873604960469, 8.224510206698951720, 114.1655762719810383 ) ) ;
#149584=CARTESIAN_POINT ( 'NONE',  ( 12.06949235617757843, -12.14591786802309237, 28.12390960531435979 ) ) ;
#149585=CARTESIAN_POINT ( 'NONE',  ( -14.29746914071037622, -8.314922557961029526, 39.16775706135235424 ) ) ;
#149586=CARTESIAN_POINT ( 'NONE',  ( 18.62759615963255655, 10.81492255796105972, 106.6677570613523756 ) ) ;
#149587=CARTESIAN_POINT ( 'NONE',  ( -16.46253265017160317, 9.564922557960807481, 105.8322429386476955 ) ) ;
#149588=CARTESIAN_POINT ( 'NONE',  ( -8.224510206698948167, 14.34966873604960824, 25.41557627198103120 ) ) ;
#149589=CARTESIAN_POINT ( 'NONE',  ( -5.719274019375665041, -21.55341960407619695, 29.79275706135234358 ) ) ;
#149590=CARTESIAN_POINT ( 'NONE',  ( 5.049401038298161559, -19.05341960407611168, 47.70724293864770260 ) ) ;
#149592=CARTESIAN_POINT ( 'NONE',  ( -12.14591786802326823, 12.06949235617739902, 48.12609039468568284 ) ) ;
#149593=CARTESIAN_POINT ( 'NONE',  ( 14.29746914071037800, 8.314922557961029526, 111.6677570613523613 ) ) ;
#149594=CARTESIAN_POINT ( 'NONE',  ( 4.483927247898790824, -16.52544592524335698, 90.20942372801903275 ) ) ;
#149595=CARTESIAN_POINT ( 'NONE',  ( 19.03943276465977164, 0.05219959533936151252, 106.2510903946856615 ) ) ;
#149596=CARTESIAN_POINT ( 'NONE',  ( 19.05341960407611168, 5.049401038298154454, 38.95724293864767418 ) ) ;
#149598=CARTESIAN_POINT ( 'NONE',  ( 8.314922557960818139, 14.29746914071049879, 99.58224293864770971 ) ) ;
#149599=CARTESIAN_POINT ( 'NONE',  ( 21.52544592524344225, -5.823673210054117533, 108.5405762719810241 ) ) ;
#149600=CARTESIAN_POINT ( 'NONE',  ( 9.474510206698971260, -16.51473224551069308, 32.91557627198102409 ) ) ;
#149601=CARTESIAN_POINT ( 'NONE',  ( 16.51473224551069308, 9.474510206698969483, 104.1655762719810241 ) ) ;
#149602=CARTESIAN_POINT ( 'NONE',  ( -18.67979575497193778, 10.72451020669871902, 28.33442372801902209 ) ) ;
#149604=CARTESIAN_POINT ( 'NONE',  ( -19.02544592524342804, 5.153800228976336051, 101.0405762719810241 ) ) ;
#149605=CARTESIAN_POINT ( 'NONE',  ( 17.48853670773245028, -5.747243402303102044, 111.1667129974999000 ) ) ;
#149606=CARTESIAN_POINT ( 'NONE',  ( -13.89961937509977652, 13.97604488694528158, 80.62390960531436690 ) ) ;
#149607=CARTESIAN_POINT ( 'NONE',  ( -0.05219959533937732626, 21.53943276465977519, 27.50109039468567929 ) ) ;
#149608=CARTESIAN_POINT ( 'NONE',  ( 14.34966873604960469, 8.224510206698951720, 94.16557627198103830 ) ) ;
#149609=CARTESIAN_POINT ( 'NONE',  ( -19.05341960407611168, -5.049401038298163336, 101.4572429386476955 ) ) ;
#149610=CARTESIAN_POINT ( 'NONE',  ( -16.46253265017146816, -9.564922557961047289, 29.16775706135232937 ) ) ;
#149611=CARTESIAN_POINT ( 'NONE',  ( 4.483927247898790824, -16.52544592524335698, 65.20942372801901854 ) ) ;
#149612=CARTESIAN_POINT ( 'NONE',  ( 15.80617190586769283, -15.72974639402175789, 80.62609039468567573 ) ) ;
#149613=CARTESIAN_POINT ( 'NONE',  ( -14.29746914071037622, -8.314922557961029526, 34.16775706135234714 ) ) ;
#149614=CARTESIAN_POINT ( 'NONE',  ( -0.05219959533909027116, -19.03943276465977164, 77.49890960531435269 ) ) ;
#149615=CARTESIAN_POINT ( 'NONE',  ( 19.03943276465977164, 0.05219959533936151252, 91.25109039468566152 ) ) ;
#149616=CARTESIAN_POINT ( 'NONE',  ( -14.34966873604972548, 8.224510206698743886, 63.33442372801900433 ) ) ;
#149617=CARTESIAN_POINT ( 'NONE',  ( -10.72451020669870658, -18.67979575497194134, 109.5844237280190328 ) ) ;
#149618=CARTESIAN_POINT ( 'NONE',  ( 13.89961937509957401, 13.97604488694547697, 86.87609039468567573 ) ) ;
#149619=CARTESIAN_POINT ( 'NONE',  ( 19.03943276465977164, -0.05219959533909143690, 68.74890960531436690 ) ) ;
#149620=CARTESIAN_POINT ( 'NONE',  ( -5.719274019375978568, 21.55341960407610458, 80.20724293864769550 ) ) ;
#149621=CARTESIAN_POINT ( 'NONE',  ( -0.05219959533910754901, -16.53943276465976808, 87.49890960531436690 ) ) ;
#149622=CARTESIAN_POINT ( 'NONE',  ( 19.03943276465977164, 0.05219959533936151252, 86.25109039468567573 ) ) ;
#149623=CARTESIAN_POINT ( 'NONE',  ( 12.06949235617739724, 12.14591786802326823, 56.87609039468568994 ) ) ;
#149625=CARTESIAN_POINT ( 'NONE',  ( 13.97604488694548053, -13.89961937509957401, 60.62609039468564731 ) ) ;
#149626=CARTESIAN_POINT ( 'NONE',  ( 14.34966873604960469, 8.224510206698951720, 24.16557627198103120 ) ) ;
#149627=CARTESIAN_POINT ( 'NONE',  ( 4.379528057220339221, -16.55341960407611168, 77.70724293864770971 ) ) ;
#149628=CARTESIAN_POINT ( 'NONE',  ( -5.823673210054431948, 21.52544592524334988, 112.7094237280190328 ) ) ;
#149629=CARTESIAN_POINT ( 'NONE',  ( -18.87580814761075487, 5.500000000000055067, 90.87172394265756736 ) ) ;
#149630=CARTESIAN_POINT ( 'NONE',  ( -5.823673210054431948, 21.52544592524334988, 22.70942372801901499 ) ) ;
#149631=CARTESIAN_POINT ( 'NONE',  ( -19.02544592524342804, 5.153800228976336051, 101.0405762719810241 ) ) ;
#149632=CARTESIAN_POINT ( 'NONE',  ( 19.05341960407611168, 5.049401038298154454, 78.95724293864769550 ) ) ;
#149633=CARTESIAN_POINT ( 'NONE',  ( 10.81492255796106328, -18.62759615963255655, 90.41775706135236135 ) ) ;
#149634=CARTESIAN_POINT ( 'NONE',  ( 19.02544592524343514, -5.153800228976328945, 68.54057627198103830 ) ) ;
#149636=CARTESIAN_POINT ( 'NONE',  ( 5.823673210054125526, 21.52544592524343514, 29.79057627198102409 ) ) ;
#149637=CARTESIAN_POINT ( 'NONE',  ( -8.224510206698948167, 14.34966873604960824, 80.41557627198103830 ) ) ;
#149639=CARTESIAN_POINT ( 'NONE',  ( 9.474510206698971260, -16.51473224551069308, 47.91557627198102409 ) ) ;
#149640=CARTESIAN_POINT ( 'NONE',  ( 8.224510206698953496, -14.34966873604960469, 102.9155762719810383 ) ) ;
#149641=CARTESIAN_POINT ( 'NONE',  ( -21.53943276465977519, 0.05219959533907696930, 116.2489096053143669 ) ) ;
#149642=CARTESIAN_POINT ( 'NONE',  ( -15.80617190586768217, 15.72974639402176855, 63.12609039468568994 ) ) ;
#149643=CARTESIAN_POINT ( 'NONE',  ( -19.05341960407611168, -5.049401038298163336, 31.45724293864769550 ) ) ;
#149644=CARTESIAN_POINT ( 'NONE',  ( -4.379528057220086978, -16.55341960407618274, 59.79275706135234714 ) ) ;
#149645=CARTESIAN_POINT ( 'NONE',  ( 18.67979575497178502, 10.72451020669898547, 104.1655762719810241 ) ) ;
#149646=CARTESIAN_POINT ( 'NONE',  ( 21.55341960407610458, 5.719274019375980345, 108.9572429386476955 ) ) ;
#149647=CARTESIAN_POINT ( 'NONE',  ( 5.153800228976615827, -19.02544592524334988, 40.20942372801898301 ) ) ;
#149648=CARTESIAN_POINT ( 'NONE',  ( 5.153800228976335163, 19.02544592524342804, 54.79057627198103120 ) ) ;
#149650=CARTESIAN_POINT ( 'NONE',  ( 15.80617190586769283, -15.72974639402175789, 55.62609039468568284 ) ) ;
#149651=CARTESIAN_POINT ( 'NONE',  ( -10.72451020669898014, 18.67979575497178502, 55.41557627198102409 ) ) ;
#149652=CARTESIAN_POINT ( 'NONE',  ( 12.06949235617757843, -12.14591786802309237, 33.12390960531435979 ) ) ;
#149653=CARTESIAN_POINT ( 'NONE',  ( 15.80617190586769283, -15.72974639402175789, 80.62609039468567573 ) ) ;
#149654=CARTESIAN_POINT ( 'NONE',  ( -19.03943276465977164, -0.05219959533935918106, 18.75109039468567218 ) ) ;
#149655=CARTESIAN_POINT ( 'NONE',  ( -8.314922557960811034, -14.29746914071050412, 57.08224293864769550 ) ) ;
#149656=CARTESIAN_POINT ( 'NONE',  ( -14.29746914071049879, 8.314922557960819915, 110.8322429386476955 ) ) ;
#149657=CARTESIAN_POINT ( 'NONE',  ( -5.049401038297874678, -19.05341960407617918, 39.79275706135232582 ) ) ;
#149658=CARTESIAN_POINT ( 'NONE',  ( 12.14591786802327356, -12.06949235617739191, 100.6260903946857184 ) ) ;
#149659=CARTESIAN_POINT ( 'NONE',  ( -10.72451020669870658, -18.67979575497194134, 69.58442372801900433 ) ) ;
#149660=CARTESIAN_POINT ( 'NONE',  ( 19.03943276465977164, -0.05219959533909143690, 63.74890960531435979 ) ) ;
#149661=CARTESIAN_POINT ( 'NONE',  ( 19.03943276465977164, 0.05219959533936151252, 41.25109039468566152 ) ) ;
#149662=CARTESIAN_POINT ( 'NONE',  ( -18.67979575497178146, -10.72451020669898902, 36.66557627198103120 ) ) ;
#149663=CARTESIAN_POINT ( 'NONE',  ( -21.55341960407619339, 5.719274019375674811, 38.54275706135234714 ) ) ;
#149664=CARTESIAN_POINT ( 'NONE',  ( 15.72974639402199770, -15.80617190586745480, 83.12390960531436690 ) ) ;
#149665=CARTESIAN_POINT ( 'NONE',  ( -16.46253265017146816, -9.564922557961047289, 84.16775706135233293 ) ) ;
#149666=CARTESIAN_POINT ( 'NONE',  ( -14.34966873604972548, 8.224510206698743886, 58.33442372801901143 ) ) ;
#149667=CARTESIAN_POINT ( 'NONE',  ( 17.50000000000001776, -3.210308386893660604, 37.45106242668933305 ) ) ;
#149668=CARTESIAN_POINT ( 'NONE',  ( -18.62759615963270932, 10.81492255796079327, 90.83224293864769550 ) ) ;
#149669=CARTESIAN_POINT ( 'NONE',  ( 14.34966873604960469, 8.224510206698951720, 79.16557627198103830 ) ) ;
#149671=CARTESIAN_POINT ( 'NONE',  ( -13.97604488694547697, 13.89961937509957934, 113.1260903946856757 ) ) ;
#149672=CARTESIAN_POINT ( 'NONE',  ( 0.05219959533907565091, 21.53943276465977519, 39.99890960531436690 ) ) ;
#149673=CARTESIAN_POINT ( 'NONE',  ( 16.52544592524335698, 4.483927247898782831, 76.45942372801901854 ) ) ;
#149675=CARTESIAN_POINT ( 'NONE',  ( -8.314922557961024197, 14.29746914071037800, 52.91775706135235424 ) ) ;
#149676=CARTESIAN_POINT ( 'NONE',  ( 15.72974639402176855, 15.80617190586768217, 31.87609039468567929 ) ) ;
#149677=CARTESIAN_POINT ( 'NONE',  ( -21.55341960407610458, -5.719274019375992779, 51.45724293864770260 ) ) ;
#149678=CARTESIAN_POINT ( 'NONE',  ( -14.34966873604972548, 8.224510206698743886, 73.33442372801901854 ) ) ;
#149679=CARTESIAN_POINT ( 'NONE',  ( -0.05219959533909027116, -19.03943276465977164, 82.49890960531436690 ) ) ;
#149680=CARTESIAN_POINT ( 'NONE',  ( 21.55341960407619695, -5.719274019375665929, 51.04275706135234714 ) ) ;
#149681=CARTESIAN_POINT ( 'NONE',  ( -9.564922557960796823, -16.46253265017161027, 22.08224293864768839 ) ) ;
#149682=CARTESIAN_POINT ( 'NONE',  ( -10.81492255796078084, -18.62759615963271287, 37.08224293864768129 ) ) ;
#149683=CARTESIAN_POINT ( 'NONE',  ( -19.05341960407611168, -5.049401038298163336, 111.4572429386476671 ) ) ;
#149685=CARTESIAN_POINT ( 'NONE',  ( -19.05341960407617563, 5.049401038297882671, 38.54275706135233293 ) ) ;
#149686=CARTESIAN_POINT ( 'NONE',  ( 8.224510206698742110, 14.34966873604972548, 52.08442372801901854 ) ) ;
#149687=CARTESIAN_POINT ( 'NONE',  ( 0.05219959533907565091, 21.53943276465977519, 24.99890960531435624 ) ) ;
#149688=ORIENTED_EDGE ( 'NONE', *, *, #134338, .T. ) ;
#149689=CARTESIAN_POINT ( 'NONE',  ( 5.049401038298161559, -19.05341960407611168, 87.70724293864769550 ) ) ;
#149690=CARTESIAN_POINT ( 'NONE',  ( 16.53943276465976808, 0.05219959533934440121, 96.25109039468568994 ) ) ;
#149692=CARTESIAN_POINT ( 'NONE',  ( 0.05219959533910956823, 16.53943276465976808, 89.99890960531438111 ) ) ;
#149693=CARTESIAN_POINT ( 'NONE',  ( 15.72974639402199770, -15.80617190586745480, 48.12390960531436690 ) ) ;
#149694=CARTESIAN_POINT ( 'NONE',  ( 13.97604488694527802, 13.89961937509977652, 29.37390960531435979 ) ) ;
#149695=CARTESIAN_POINT ( 'NONE',  ( 8.224510206698742110, 14.34966873604972548, 82.08442372801901854 ) ) ;
#149696=CARTESIAN_POINT ( 'NONE',  ( 21.55341960407610458, 5.719274019375980345, 113.9572429386477239 ) ) ;
#149697=CARTESIAN_POINT ( 'NONE',  ( 16.51473224551083163, -9.474510206698727899, 75.83442372801900433 ) ) ;
#149698=CARTESIAN_POINT ( 'NONE',  ( -16.46253265017160317, 9.564922557960807481, 35.83224293864768839 ) ) ;
#149699=CARTESIAN_POINT ( 'NONE',  ( 9.474510206698971260, -16.51473224551069308, 112.9155762719810383 ) ) ;
#149700=CARTESIAN_POINT ( 'NONE',  ( -18.62759615963255300, -10.81492255796106328, 99.16775706135234714 ) ) ;
#149701=CARTESIAN_POINT ( 'NONE',  ( 13.89961937509977652, -13.97604488694527269, 68.12390960531436690 ) ) ;
#149702=CARTESIAN_POINT ( 'NONE',  ( -8.314922557961024197, 14.29746914071037800, 42.91775706135235424 ) ) ;
#149703=CARTESIAN_POINT ( 'NONE',  ( -5.823673210054431948, 21.52544592524334988, 87.70942372801901854 ) ) ;
#149704=CARTESIAN_POINT ( 'NONE',  ( 9.474510206698729675, 16.51473224551082808, 52.08442372801900433 ) ) ;
#149705=CARTESIAN_POINT ( 'NONE',  ( 13.89961937509957401, 13.97604488694547697, 51.87609039468566863 ) ) ;
#149707=CARTESIAN_POINT ( 'NONE',  ( -10.72451020669870658, -18.67979575497194134, 49.58442372801901143 ) ) ;
#149708=CARTESIAN_POINT ( 'NONE',  ( 13.89961937509977652, -13.97604488694527269, 23.12390960531436335 ) ) ;
#149709=CARTESIAN_POINT ( 'NONE',  ( -16.51473224551082808, 9.474510206698731452, 43.33442372801900433 ) ) ;
#149710=CARTESIAN_POINT ( 'NONE',  ( 19.05341960407611168, 5.049401038298154454, 98.95724293864766707 ) ) ;
#149711=CARTESIAN_POINT ( 'NONE',  ( -19.05341960407611168, -5.049401038298163336, 86.45724293864769550 ) ) ;
#149712=CARTESIAN_POINT ( 'NONE',  ( 16.52544592524342804, -4.483927247898539470, 38.54057627198103120 ) ) ;
#149713=CARTESIAN_POINT ( 'NONE',  ( -5.719274019375978568, 21.55341960407610458, 30.20724293864769550 ) ) ;
#149716=CARTESIAN_POINT ( 'NONE',  ( 13.97604488694548053, -13.89961937509957401, 20.62609039468567573 ) ) ;
#149718=CARTESIAN_POINT ( 'NONE',  ( -19.05341960407611168, -5.049401038298163336, 31.45724293864769550 ) ) ;
#149719=CARTESIAN_POINT ( 'NONE',  ( 0.05219959533909260263, 19.03943276465977164, 84.99890960531436690 ) ) ;
#149722=CARTESIAN_POINT ( 'NONE',  ( 8.314922557961029526, -14.29746914071037800, 65.41775706135234714 ) ) ;
#149723=CARTESIAN_POINT ( 'NONE',  ( 10.81492255796078972, 18.62759615963270932, 84.58224293864769550 ) ) ;
#149724=CARTESIAN_POINT ( 'NONE',  ( 16.52544592524342804, -4.483927247898539470, 58.54057627198103120 ) ) ;
#149725=CARTESIAN_POINT ( 'NONE',  ( 16.46253265017160672, -9.564922557960803928, 33.33224293864770260 ) ) ;
#149726=CARTESIAN_POINT ( 'NONE',  ( -16.51473224551069308, -9.474510206698971260, 101.6655762719810241 ) ) ;
#149727=CARTESIAN_POINT ( 'NONE',  ( -21.52544592524334988, -5.823673210054445271, 33.95942372801901143 ) ) ;
#149728=CARTESIAN_POINT ( 'NONE',  ( 19.03943276465977164, 0.05219959533936151252, 41.25109039468566152 ) ) ;
#149729=CARTESIAN_POINT ( 'NONE',  ( 19.02544592524343514, -5.153800228976328945, 33.54057627198102409 ) ) ;
#149730=CARTESIAN_POINT ( 'NONE',  ( -21.55341960407619339, 5.719274019375674811, 78.54275706135236135 ) ) ;
#149731=CARTESIAN_POINT ( 'NONE',  ( 17.13100169013300089, -6.664070546373146442, 33.26789835699850073 ) ) ;
#149732=CARTESIAN_POINT ( 'NONE',  ( 16.52544592524342804, -4.483927247898539470, 28.54057627198103120 ) ) ;
#149733=CARTESIAN_POINT ( 'NONE',  ( 17.50000000000014566, 3.417042746626842931, 112.3261960376753024 ) ) ;
#149734=CARTESIAN_POINT ( 'NONE',  ( 5.719274019375991003, -21.55341960407610458, 42.70724293864770260 ) ) ;
#149735=CARTESIAN_POINT ( 'NONE',  ( 16.53943276465976808, -0.05219959533910856209, 108.7489096053143669 ) ) ;
#149737=CARTESIAN_POINT ( 'NONE',  ( -5.049401038298153566, 19.05341960407611168, 85.20724293864766707 ) ) ;
#149738=CARTESIAN_POINT ( 'NONE',  ( -4.379528057220328563, 16.55341960407611168, 75.20724293864769550 ) ) ;
#149739=CARTESIAN_POINT ( 'NONE',  ( 5.153800228976615827, -19.02544592524334988, 105.2094237280190185 ) ) ;
#149740=CARTESIAN_POINT ( 'NONE',  ( 10.81492255796078972, 18.62759615963270932, 69.58224293864769550 ) ) ;
#149742=CARTESIAN_POINT ( 'NONE',  ( -16.51473224551069308, -9.474510206698971260, 31.66557627198102054 ) ) ;
#149743=CARTESIAN_POINT ( 'NONE',  ( 13.89961937509977652, -13.97604488694527269, 88.12390960531438111 ) ) ;
#149744=CARTESIAN_POINT ( 'NONE',  ( 18.62759615963271287, -10.81492255796078972, 88.33224293864769550 ) ) ;
#149745=CARTESIAN_POINT ( 'NONE',  ( 8.224510206698742110, 14.34966873604972548, 102.0844237280190185 ) ) ;
#149746=CARTESIAN_POINT ( 'NONE',  ( 0.05219959533909260263, 19.03943276465977164, 89.99890960531436690 ) ) ;
#149747=CARTESIAN_POINT ( 'NONE',  ( -19.03943276465977164, -0.05219959533935918106, 78.75109039468567573 ) ) ;
#149748=CARTESIAN_POINT ( 'NONE',  ( -5.719274019375665041, -21.55341960407619695, 94.79275706135234714 ) ) ;
#149749=CARTESIAN_POINT ( 'NONE',  ( -21.55341960407610458, -5.719274019375992779, 71.45724293864769550 ) ) ;
#149750=CARTESIAN_POINT ( 'NONE',  ( -5.719274019375978568, 21.55341960407610458, 40.20724293864769550 ) ) ;
#149751=CARTESIAN_POINT ( 'NONE',  ( 19.05341960407611168, 5.049401038298154454, 53.95724293864770260 ) ) ;
#149752=CARTESIAN_POINT ( 'NONE',  ( -12.14591786802326823, 12.06949235617739902, 113.1260903946856899 ) ) ;
#149753=CARTESIAN_POINT ( 'NONE',  ( -5.153800228976328057, -19.02544592524343514, 62.29057627198100988 ) ) ;
#149754=CARTESIAN_POINT ( 'NONE',  ( 17.97394159160245408, 5.500000000000056843, 38.98772563323827001 ) ) ;
#149755=CARTESIAN_POINT ( 'NONE',  ( -16.51473224551082808, 9.474510206698731452, 33.33442372801899722 ) ) ;
#149756=CARTESIAN_POINT ( 'NONE',  ( 4.379528057220339221, -16.55341960407611168, 72.70724293864769550 ) ) ;
#149757=CARTESIAN_POINT ( 'NONE',  ( -15.80617190586745835, -15.72974639402198527, 106.8739096053143811 ) ) ;
#149759=CARTESIAN_POINT ( 'NONE',  ( 21.52544592524344225, -5.823673210054117533, 63.54057627198103830 ) ) ;
#149761=CARTESIAN_POINT ( 'NONE',  ( -4.483927247898782831, 16.52544592524335698, 97.70942372801904696 ) ) ;
#149762=CARTESIAN_POINT ( 'NONE',  ( -16.53943276465976808, 0.05219959533911058130, 101.2489096053143669 ) ) ;
#149763=CARTESIAN_POINT ( 'NONE',  ( -13.97604488694527625, -13.89961937509977652, 76.87390960531433848 ) ) ;
#149765=CARTESIAN_POINT ( 'NONE',  ( -4.379528057220328563, 16.55341960407611168, 30.20724293864769550 ) ) ;
#149766=CARTESIAN_POINT ( 'NONE',  ( -5.719274019375665041, -21.55341960407619695, 44.79275706135234714 ) ) ;
#149767=CARTESIAN_POINT ( 'NONE',  ( 19.05341960407611168, 5.049401038298154454, 113.9572429386477097 ) ) ;
#149768=CARTESIAN_POINT ( 'NONE',  ( -10.72451020669870658, -18.67979575497194134, 74.58442372801901854 ) ) ;
#149769=CARTESIAN_POINT ( 'NONE',  ( 9.564922557960805705, 16.46253265017160317, 29.58224293864769550 ) ) ;
#149770=CARTESIAN_POINT ( 'NONE',  ( 16.51473224551069308, 9.474510206698969483, 39.16557627198103120 ) ) ;
#149772=CARTESIAN_POINT ( 'NONE',  ( -18.67979575497193778, 10.72451020669871902, 93.33442372801901854 ) ) ;
#149773=CARTESIAN_POINT ( 'NONE',  ( 16.52544592524335698, 4.483927247898782831, 46.45942372801901854 ) ) ;
#149774=CARTESIAN_POINT ( 'NONE',  ( 21.53943276465977519, 0.05219959533937863772, 76.25109039468568994 ) ) ;
#149775=CARTESIAN_POINT ( 'NONE',  ( -5.153800228976328057, -19.02544592524343514, 97.29057627198099567 ) ) ;
#149776=CARTESIAN_POINT ( 'NONE',  ( -9.564922557961040184, 16.46253265017147172, 77.91775706135234714 ) ) ;
#149777=CARTESIAN_POINT ( 'NONE',  ( -18.67979575497193778, 10.72451020669871902, 53.33442372801901854 ) ) ;
#149778=CARTESIAN_POINT ( 'NONE',  ( 4.379528057220092307, 16.55341960407617563, 27.29275706135234358 ) ) ;
#149779=CARTESIAN_POINT ( 'NONE',  ( 19.02544592524334988, 5.153800228976608722, 86.45942372801900433 ) ) ;
#149780=CARTESIAN_POINT ( 'NONE',  ( -5.049401038298153566, 19.05341960407611168, 45.20724293864769550 ) ) ;
#149781=CARTESIAN_POINT ( 'NONE',  ( -13.97604488694547697, 13.89961937509957934, 88.12609039468563310 ) ) ;
#149782=CARTESIAN_POINT ( 'NONE',  ( -4.379528057220328563, 16.55341960407611168, 30.20724293864769550 ) ) ;
#149783=CARTESIAN_POINT ( 'NONE',  ( -5.153800228976607833, 19.02544592524334988, 82.70942372801897591 ) ) ;
#149784=CARTESIAN_POINT ( 'NONE',  ( -12.14591786802309592, -12.06949235617757132, 36.87390960531435979 ) ) ;
#149785=CARTESIAN_POINT ( 'NONE',  ( -13.97604488694547697, 13.89961937509957934, 68.12609039468563310 ) ) ;
#149786=CARTESIAN_POINT ( 'NONE',  ( 12.06949235617739724, 12.14591786802326823, 51.87609039468568284 ) ) ;
#149787=CARTESIAN_POINT ( 'NONE',  ( -16.51473224551082808, 9.474510206698731452, 28.33442372801900433 ) ) ;
#149788=CARTESIAN_POINT ( 'NONE',  ( 16.51473224551069308, 9.474510206698969483, 24.16557627198102765 ) ) ;
#149789=CARTESIAN_POINT ( 'NONE',  ( 9.564922557960805705, 16.46253265017160317, 44.58224293864769550 ) ) ;
#149790=CARTESIAN_POINT ( 'NONE',  ( -8.314922557961024197, 14.29746914071037800, 47.91775706135234714 ) ) ;
#149793=CARTESIAN_POINT ( 'NONE',  ( 16.51473224551069308, 9.474510206698969483, 89.16557627198103830 ) ) ;
#149794=CARTESIAN_POINT ( 'NONE',  ( -5.049401038297874678, -19.05341960407618274, 84.79275706135233293 ) ) ;
#149795=ORIENTED_EDGE ( 'NONE', *, *, #41507, .F. ) ;
#149796=CARTESIAN_POINT ( 'NONE',  ( -13.89961937509957401, -13.97604488694547875, 104.3760903946856757 ) ) ;
#149797=CARTESIAN_POINT ( 'NONE',  ( -10.81492255796078084, -18.62759615963271287, 27.08224293864769550 ) ) ;
#149798=CARTESIAN_POINT ( 'NONE',  ( 9.564922557961047289, -16.46253265017146816, 30.41775706135232937 ) ) ;
#149799=CARTESIAN_POINT ( 'NONE',  ( 0.05219959533936267826, -19.03943276465977164, 105.0010903946856615 ) ) ;
#149800=CARTESIAN_POINT ( 'NONE',  ( -4.379528057220328563, 16.55341960407611168, 115.2072429386476955 ) ) ;
#149801=CARTESIAN_POINT ( 'NONE',  ( 16.51473224551069308, 9.474510206698969483, 39.16557627198103120 ) ) ;
#149802=CARTESIAN_POINT ( 'NONE',  ( 10.81492255796078972, 18.62759615963270932, 69.58224293864769550 ) ) ;
#149804=CARTESIAN_POINT ( 'NONE',  ( -16.51473224551069308, -9.474510206698971260, 41.66557627198103120 ) ) ;
#149805=CARTESIAN_POINT ( 'NONE',  ( -9.474510206698720793, -16.51473224551083518, 74.58442372801900433 ) ) ;
#149806=CARTESIAN_POINT ( 'NONE',  ( 14.34966873604960469, 8.224510206698951720, 54.16557627198103120 ) ) ;
#149807=CARTESIAN_POINT ( 'NONE',  ( -21.52544592524343514, 5.823673210054127303, 36.04057627198102409 ) ) ;
#149808=CARTESIAN_POINT ( 'NONE',  ( 10.72451020669871369, 18.67979575497193778, 97.08442372801904696 ) ) ;
#149809=CARTESIAN_POINT ( 'NONE',  ( -15.72974639402197994, 15.80617190586746368, 85.62390960531436690 ) ) ;
#149810=CARTESIAN_POINT ( 'NONE',  ( -21.52544592524334988, -5.823673210054445271, 68.95942372801901854 ) ) ;
#149811=CARTESIAN_POINT ( 'NONE',  ( -15.80617190586768217, 15.72974639402176855, 63.12609039468568994 ) ) ;
#149812=CARTESIAN_POINT ( 'NONE',  ( -16.46253265017160317, 9.564922557960807481, 95.83224293864769550 ) ) ;
#149813=CARTESIAN_POINT ( 'NONE',  ( 8.314922557961029526, -14.29746914071037800, 95.41775706135234714 ) ) ;
#149814=CARTESIAN_POINT ( 'NONE',  ( -10.72451020669870658, -18.67979575497194134, 59.58442372801901854 ) ) ;
#149815=CARTESIAN_POINT ( 'NONE',  ( 5.153800228976335163, 19.02544592524342804, 59.79057627198100988 ) ) ;
#149816=CARTESIAN_POINT ( 'NONE',  ( 21.52544592524334988, 5.823673210054432836, 26.45942372801901854 ) ) ;
#149817=CARTESIAN_POINT ( 'NONE',  ( 9.564922557960805705, 16.46253265017160317, 74.58224293864769550 ) ) ;
#149818=CARTESIAN_POINT ( 'NONE',  ( -16.55341960407611168, -4.379528057220339221, 71.45724293864769550 ) ) ;
#149819=CARTESIAN_POINT ( 'NONE',  ( 14.29746914071049879, -8.314922557960816363, 48.33224293864770260 ) ) ;
#149820=CARTESIAN_POINT ( 'NONE',  ( 0.05219959533907565091, 21.53943276465977519, 54.99890960531435269 ) ) ;
#149821=CARTESIAN_POINT ( 'NONE',  ( 16.51473224551069308, 9.474510206698969483, 44.16557627198103120 ) ) ;
#149822=CARTESIAN_POINT ( 'NONE',  ( -15.80617190586745835, -15.72974639402198527, 61.87390960531436690 ) ) ;
#149823=CARTESIAN_POINT ( 'NONE',  ( 19.03943276465977164, 0.05219959533936151252, 56.25109039468566863 ) ) ;
#149825=CARTESIAN_POINT ( 'NONE',  ( 19.02544592524335343, 5.153800228976608722, 21.45942372801899367 ) ) ;
#149826=CARTESIAN_POINT ( 'NONE',  ( 16.53943276465976808, -0.05219959533910856209, 58.74890960531436690 ) ) ;
#149827=CARTESIAN_POINT ( 'NONE',  ( -5.719274019375978568, 21.55341960407610458, 45.20724293864769550 ) ) ;
#149828=ORIENTED_EDGE ( 'NONE', *, *, #134802, .T. ) ;
#149830=CARTESIAN_POINT ( 'NONE',  ( 14.29746914071037800, 8.314922557961029526, 86.66775706135234714 ) ) ;
#149832=CARTESIAN_POINT ( 'NONE',  ( 13.89961937509957401, 13.97604488694547697, 86.87609039468567573 ) ) ;
#149833=CARTESIAN_POINT ( 'NONE',  ( -0.05219959533910754901, -16.53943276465976808, 52.49890960531435979 ) ) ;
#149835=CARTESIAN_POINT ( 'NONE',  ( 13.97604488694527802, 13.89961937509977652, 54.37390960531435979 ) ) ;
#149836=CARTESIAN_POINT ( 'NONE',  ( 12.06949235617757843, -12.14591786802309237, 38.12390960531436690 ) ) ;
#149837=CARTESIAN_POINT ( 'NONE',  ( -0.05219959533909027116, -19.03943276465977164, 52.49890960531436690 ) ) ;
#149838=CARTESIAN_POINT ( 'NONE',  ( -16.51473224551069308, -9.474510206698971260, 71.66557627198102409 ) ) ;
#149839=CARTESIAN_POINT ( 'NONE',  ( -16.46253265017160317, 9.564922557960807481, 55.83224293864769550 ) ) ;
#149840=CARTESIAN_POINT ( 'NONE',  ( -15.72974639402176322, -15.80617190586768395, 44.37609039468567573 ) ) ;
#149841=CARTESIAN_POINT ( 'NONE',  ( -9.474510206698964154, 16.51473224551069663, 70.41557627198102409 ) ) ;
#149842=CARTESIAN_POINT ( 'NONE',  ( 19.03943276465977164, -0.05219959533909143690, 28.74890960531435624 ) ) ;
#149843=CARTESIAN_POINT ( 'NONE',  ( -16.46253265017160317, 9.564922557960807481, 55.83224293864769550 ) ) ;
#149844=CARTESIAN_POINT ( 'NONE',  ( -15.72974639402197994, 15.80617190586746368, 50.62390960531435979 ) ) ;
#149845=CARTESIAN_POINT ( 'NONE',  ( 13.89961937509977652, -13.97604488694527269, 38.12390960531436690 ) ) ;
#149846=CARTESIAN_POINT ( 'NONE',  ( -15.80617190586745835, -15.72974639402198527, 41.87390960531435979 ) ) ;
#149847=CARTESIAN_POINT ( 'NONE',  ( 16.55341960407618274, -4.379528057220086978, 111.0427570613523613 ) ) ;
#149848=CARTESIAN_POINT ( 'NONE',  ( -5.153800228976607833, 19.02544592524334988, 22.70942372801899012 ) ) ;
#149849=CARTESIAN_POINT ( 'NONE',  ( 0.05219959533934541429, -16.53943276465976808, 45.00109039468568284 ) ) ;
#149850=CARTESIAN_POINT ( 'NONE',  ( 4.483927247898790824, -16.52544592524335698, 75.20942372801901854 ) ) ;
#149851=CARTESIAN_POINT ( 'NONE',  ( -17.60691670004652565, -5.500000000000036415, 94.13333313366442212 ) ) ;
#149852=CARTESIAN_POINT ( 'NONE',  ( 12.06949235617739724, 12.14591786802326823, 71.87609039468568994 ) ) ;
#149853=CARTESIAN_POINT ( 'NONE',  ( 14.34966873604972726, -8.224510206698740333, 55.83442372801901854 ) ) ;
#149854=CARTESIAN_POINT ( 'NONE',  ( -9.564922557960796823, -16.46253265017161027, 112.0822429386476955 ) ) ;
#149855=CARTESIAN_POINT ( 'NONE',  ( 4.379528057220092307, 16.55341960407617563, 37.29275706135235424 ) ) ;
#149856=CARTESIAN_POINT ( 'NONE',  ( -19.05341960407611168, -5.049401038298163336, 36.45724293864766707 ) ) ;
#149857=CARTESIAN_POINT ( 'NONE',  ( -5.823673210054431948, 21.52544592524334988, 27.70942372801901854 ) ) ;
#149858=CARTESIAN_POINT ( 'NONE',  ( 16.52544592524335698, 4.483927247898782831, 31.45942372801901854 ) ) ;
#149859=CARTESIAN_POINT ( 'NONE',  ( 0.05219959533934541429, -16.53943276465976808, 95.00109039468568994 ) ) ;
#149861=CARTESIAN_POINT ( 'NONE',  ( -18.62759615963255300, -10.81492255796106328, 104.1677570613523471 ) ) ;
#149862=CARTESIAN_POINT ( 'NONE',  ( 5.049401038297881783, 19.05341960407617563, 97.29275706135233293 ) ) ;
#149863=CARTESIAN_POINT ( 'NONE',  ( 16.52544592524342804, -4.483927247898539470, 63.54057627198103830 ) ) ;
#149864=CARTESIAN_POINT ( 'NONE',  ( 0.05219959533909260263, 19.03943276465977164, 24.99890960531435269 ) ) ;
#149865=CARTESIAN_POINT ( 'NONE',  ( -5.153800228976607833, 19.02544592524334988, 57.70942372801899012 ) ) ;
#149867=CARTESIAN_POINT ( 'NONE',  ( 10.81492255796106328, -18.62759615963255655, 65.41775706135234714 ) ) ;
#149868=CARTESIAN_POINT ( 'NONE',  ( -14.34966873604972548, 8.224510206698743886, 33.33442372801900433 ) ) ;
#149869=CARTESIAN_POINT ( 'NONE',  ( 17.49999999999999289, 5.500000000000007994, 83.78230962303564411 ) ) ;
#149870=CARTESIAN_POINT ( 'NONE',  ( 16.51473224551069308, 9.474510206698969483, 114.1655762719810241 ) ) ;
#149871=CARTESIAN_POINT ( 'NONE',  ( -19.02544592524334988, -5.153800228976617603, 108.9594237280189759 ) ) ;
#149873=CARTESIAN_POINT ( 'NONE',  ( -13.89961937509957401, -13.97604488694547697, 49.37609039468566863 ) ) ;
#149874=CARTESIAN_POINT ( 'NONE',  ( -16.51473224551069308, -9.474510206698971260, 26.66557627198103120 ) ) ;
#149875=CARTESIAN_POINT ( 'NONE',  ( 21.55341960407619695, -5.719274019375665929, 101.0427570613523756 ) ) ;
#149876=CARTESIAN_POINT ( 'NONE',  ( 9.564922557960805705, 16.46253265017160317, 44.58224293864769550 ) ) ;
#149877=CARTESIAN_POINT ( 'NONE',  ( 18.62759615963255655, 10.81492255796105972, 46.66775706135234714 ) ) ;
#149878=CARTESIAN_POINT ( 'NONE',  ( -18.67979575497193778, 10.72451020669871902, 103.3344237280190043 ) ) ;
#149879=CARTESIAN_POINT ( 'NONE',  ( 8.224510206698742110, 14.34966873604972548, 102.0844237280190185 ) ) ;
#149880=CARTESIAN_POINT ( 'NONE',  ( 13.97604488694527802, 13.89961937509977652, 79.37390960531435269 ) ) ;
#149881=CARTESIAN_POINT ( 'NONE',  ( 15.72974639402176855, 15.80617190586768217, 46.87609039468568994 ) ) ;
#149882=CARTESIAN_POINT ( 'NONE',  ( 18.67979575497194134, -10.72451020669871369, 50.83442372801901143 ) ) ;
#149883=CARTESIAN_POINT ( 'NONE',  ( 5.153800228976615827, -19.02544592524334988, 80.20942372801901854 ) ) ;
#149884=CARTESIAN_POINT ( 'NONE',  ( 0.05219959533909260263, 19.03943276465977164, 94.99890960531436690 ) ) ;
#149885=CARTESIAN_POINT ( 'NONE',  ( 16.55341960407611168, 4.379528057220329451, 103.9572429386476813 ) ) ;
#149886=CARTESIAN_POINT ( 'NONE',  ( 15.80617190586746368, 15.72974639402197994, 99.37390960531436690 ) ) ;
#149887=CARTESIAN_POINT ( 'NONE',  ( -16.51473224551082808, 9.474510206698731452, 28.33442372801900433 ) ) ;
#149888=CARTESIAN_POINT ( 'NONE',  ( -0.05219959533910754901, -16.53943276465976808, 102.4989096053143811 ) ) ;
#149889=CARTESIAN_POINT ( 'NONE',  ( 13.97604488694527802, 13.89961937509977652, 54.37390960531435979 ) ) ;
#149890=CARTESIAN_POINT ( 'NONE',  ( -5.049401038297874678, -19.05341960407617918, 89.79275706135230450 ) ) ;
#149891=CARTESIAN_POINT ( 'NONE',  ( 14.34966873604960469, 8.224510206698951720, 44.16557627198103120 ) ) ;
#149892=CARTESIAN_POINT ( 'NONE',  ( -0.05219959533937732626, 21.53943276465977519, 102.5010903946856899 ) ) ;
#149893=CARTESIAN_POINT ( 'NONE',  ( -16.46253265017160317, 9.564922557960807481, 110.8322429386476955 ) ) ;
#149894=CARTESIAN_POINT ( 'NONE',  ( -16.46253265017146816, -9.564922557961047289, 74.16775706135234714 ) ) ;
#149895=CARTESIAN_POINT ( 'NONE',  ( 21.55341960407610458, 5.719274019375980345, 73.95724293864769550 ) ) ;
#149896=CARTESIAN_POINT ( 'NONE',  ( 15.72974639402176855, 15.80617190586768217, 31.87609039468567929 ) ) ;
#149897=CARTESIAN_POINT ( 'NONE',  ( 16.55341960407618274, -4.379528057220086978, 31.04275706135234714 ) ) ;
#149898=CARTESIAN_POINT ( 'NONE',  ( -16.52544592524335698, -4.483927247898792601, 98.95942372801903275 ) ) ;
#149899=CARTESIAN_POINT ( 'NONE',  ( -9.474510206698964154, 16.51473224551069663, 30.41557627198102054 ) ) ;
#149900=CARTESIAN_POINT ( 'NONE',  ( -5.719274019375665041, -21.55341960407619695, 34.79275706135235424 ) ) ;
#149901=CARTESIAN_POINT ( 'NONE',  ( -18.67979575497178146, -10.72451020669898902, 46.66557627198102409 ) ) ;
#149902=CARTESIAN_POINT ( 'NONE',  ( 0.05219959533910956823, 16.53943276465976808, 114.9989096053143669 ) ) ;
#149904=CARTESIAN_POINT ( 'NONE',  ( -12.06949235617739369, -12.14591786802326823, 59.37609039468568284 ) ) ;
#149905=CARTESIAN_POINT ( 'NONE',  ( 12.14591786802309770, 12.06949235617756955, 94.37390960531436690 ) ) ;
#149906=CARTESIAN_POINT ( 'NONE',  ( 5.719274019375991003, -21.55341960407610458, 82.70724293864770971 ) ) ;
#149907=CARTESIAN_POINT ( 'NONE',  ( -12.06949235617756955, 12.14591786802309770, 30.62390960531436335 ) ) ;
#149908=CARTESIAN_POINT ( 'NONE',  ( 14.29746914071037800, 8.314922557961029526, 46.66775706135234714 ) ) ;
#149909=CARTESIAN_POINT ( 'NONE',  ( 16.46253265017160672, -9.564922557960803928, 58.33224293864769550 ) ) ;
#149910=CARTESIAN_POINT ( 'NONE',  ( -4.379528057220086978, -16.55341960407618274, 89.79275706135236135 ) ) ;
#149911=CARTESIAN_POINT ( 'NONE',  ( 0.05219959533936267826, -19.03943276465977164, 85.00109039468567573 ) ) ;
#149912=CARTESIAN_POINT ( 'NONE',  ( -0.05219959533907301413, -21.53943276465977519, 82.49890960531436690 ) ) ;
#149913=CARTESIAN_POINT ( 'NONE',  ( -12.06949235617739369, -12.14591786802326823, 109.3760903946857042 ) ) ;
#149914=ORIENTED_EDGE ( 'NONE', *, *, #139157, .F. ) ;
#149915=CARTESIAN_POINT ( 'NONE',  ( 0.05219959533909260263, 19.03943276465977164, 114.9989096053143669 ) ) ;
#149917=CARTESIAN_POINT ( 'NONE',  ( -18.62759615963270932, 10.81492255796079327, 60.83224293864769550 ) ) ;
#149918=CARTESIAN_POINT ( 'NONE',  ( 16.55341960407618274, -4.379528057220086978, 91.04275706135236135 ) ) ;
#149919=ORIENTED_EDGE ( 'NONE', *, *, #133810, .F. ) ;
#149920=CARTESIAN_POINT ( 'NONE',  ( 15.72974639402199770, -15.80617190586745480, 28.12390960531435979 ) ) ;
#149921=CARTESIAN_POINT ( 'NONE',  ( -19.49149378614660932, 5.499999999999579892, 74.43757513605362419 ) ) ;
#149922=CARTESIAN_POINT ( 'NONE',  ( -21.53943276465977519, 0.05219959533907696930, 91.24890960531436690 ) ) ;
#149923=CARTESIAN_POINT ( 'NONE',  ( 16.55341960407618274, -4.379528057220086978, 111.0427570613523613 ) ) ;
#149924=CARTESIAN_POINT ( 'NONE',  ( 14.34966873604972726, -8.224510206698740333, 40.83442372801901854 ) ) ;
#149925=CARTESIAN_POINT ( 'NONE',  ( 5.153800228976335163, 19.02544592524342804, 34.79057627198102409 ) ) ;
#149926=CARTESIAN_POINT ( 'NONE',  ( 14.29746914071037800, 8.314922557961029526, 26.66775706135235424 ) ) ;
#149927=CARTESIAN_POINT ( 'NONE',  ( 16.46253265017160672, -9.564922557960803928, 58.33224293864769550 ) ) ;
#149929=CARTESIAN_POINT ( 'NONE',  ( 13.89961937509977652, -13.97604488694527269, 108.1239096053143669 ) ) ;
#149930=CARTESIAN_POINT ( 'NONE',  ( 5.049401038298161559, -19.05341960407611168, 112.7072429386476813 ) ) ;
#149931=CARTESIAN_POINT ( 'NONE',  ( 8.224510206698742110, 14.34966873604972548, 97.08442372801904696 ) ) ;
#149932=CARTESIAN_POINT ( 'NONE',  ( 5.049401038297881783, 19.05341960407617563, 92.29275706135234714 ) ) ;
#149933=CARTESIAN_POINT ( 'NONE',  ( -19.03943276465977164, -0.05219959533935918106, 33.75109039468566863 ) ) ;
#149934=CARTESIAN_POINT ( 'NONE',  ( -21.53943276465977519, 0.05219959533907696930, 81.24890960531436690 ) ) ;
#149936=CARTESIAN_POINT ( 'NONE',  ( -16.55341960407617563, 4.379528057220093196, 103.5427570613523613 ) ) ;
#149937=CARTESIAN_POINT ( 'NONE',  ( -21.53943276465977519, 0.05219959533907696930, 31.24890960531435979 ) ) ;
#149938=CARTESIAN_POINT ( 'NONE',  ( 5.049401038297881783, 19.05341960407617563, 97.29275706135233293 ) ) ;
#149939=CARTESIAN_POINT ( 'NONE',  ( 19.02544592524343514, -5.153800228976328945, 103.5405762719809957 ) ) ;
#149941=CARTESIAN_POINT ( 'NONE',  ( -5.719274019375665041, -21.55341960407619695, 64.79275706135234714 ) ) ;
#149942=CARTESIAN_POINT ( 'NONE',  ( -13.97604488694527625, -13.89961937509977652, 61.87390960531435979 ) ) ;
#149943=CARTESIAN_POINT ( 'NONE',  ( 12.14591786802309770, 12.06949235617756955, 94.37390960531436690 ) ) ;
#149944=CARTESIAN_POINT ( 'NONE',  ( -16.19135201231366850, -7.376712067591933319, 85.18680854052034590 ) ) ;
#149945=CARTESIAN_POINT ( 'NONE',  ( -0.05219959533910754901, -16.53943276465976808, 77.49890960531433848 ) ) ;
#149946=CARTESIAN_POINT ( 'NONE',  ( -0.05219959533907301413, -21.53943276465977519, 72.49890960531435269 ) ) ;
#149947=EDGE_LOOP ( 'NONE', ( #75479, #102202, #87064, #53917, #133531, #4478, #112880, #99486 ) ) ;
#149948=CARTESIAN_POINT ( 'NONE',  ( -5.049401038297874678, -19.05341960407617918, 94.79275706135230450 ) ) ;
#149949=STYLED_ITEM ( 'NONE', ( #94036 ), #146166 ) ;
#149950=CARTESIAN_POINT ( 'NONE',  ( 19.25176906914650843, 5.499999999999797495, 93.49927264242278113 ) ) ;
#149951=CARTESIAN_POINT ( 'NONE',  ( -16.46253265017160317, 9.564922557960807481, 60.83224293864769550 ) ) ;
#149952=CARTESIAN_POINT ( 'NONE',  ( 17.44270441346517231, -5.991230190322924365, 71.13664920735772057 ) ) ;
#149953=CARTESIAN_POINT ( 'NONE',  ( -19.02544592524342804, 5.153800228976336051, 76.04057627198102409 ) ) ;
#149954=CARTESIAN_POINT ( 'NONE',  ( -9.564922557960796823, -16.46253265017161027, 92.08224293864769550 ) ) ;
#149955=CARTESIAN_POINT ( 'NONE',  ( -16.55341960407617563, 4.379528057220093196, 58.54275706135235424 ) ) ;
#149957=CARTESIAN_POINT ( 'NONE',  ( -9.564922557961040184, 16.46253265017147172, 42.91775706135234003 ) ) ;
#149959=CARTESIAN_POINT ( 'NONE',  ( 13.89961937509977652, -13.97604488694527269, 113.1239096053143527 ) ) ;
#149960=CARTESIAN_POINT ( 'NONE',  ( 16.55341960407618274, -4.379528057220086978, 101.0427570613523756 ) ) ;
#149961=CARTESIAN_POINT ( 'NONE',  ( -13.89961937509957401, -13.97604488694547697, 74.37609039468564731 ) ) ;
#149962=CARTESIAN_POINT ( 'NONE',  ( -12.06949235617739369, -12.14591786802326823, 99.37609039468568994 ) ) ;
#149963=CARTESIAN_POINT ( 'NONE',  ( -17.31747979337949417, 6.344076630960995722, 28.62055131934817354 ) ) ;
#149964=CARTESIAN_POINT ( 'NONE',  ( -16.55341960407617563, 4.379528057220093196, 68.54275706135234714 ) ) ;
#149966=CARTESIAN_POINT ( 'NONE',  ( -21.55341960407619339, 5.719274019375674811, 68.54275706135234714 ) ) ;
#149967=CARTESIAN_POINT ( 'NONE',  ( 16.46253265017146816, 9.564922557961045513, 71.66775706135233293 ) ) ;
#149968=CARTESIAN_POINT ( 'NONE',  ( -0.05219959533936034679, 19.03943276465977164, 27.50109039468566507 ) ) ;
#149969=CARTESIAN_POINT ( 'NONE',  ( 5.153800228976335163, 19.02544592524342804, 64.79057627198100988 ) ) ;
#149970=CARTESIAN_POINT ( 'NONE',  ( -19.02544592524342804, 5.153800228976336051, 41.04057627198103120 ) ) ;
#149972=CARTESIAN_POINT ( 'NONE',  ( 5.719274019375991003, -21.55341960407610458, 77.70724293864770971 ) ) ;
#149974=CARTESIAN_POINT ( 'NONE',  ( 18.67979575497178502, 10.72451020669898547, 39.16557627198102409 ) ) ;
#149975=CARTESIAN_POINT ( 'NONE',  ( -13.97604488694527625, -13.89961937509977652, 31.87390960531435979 ) ) ;
#149976=CARTESIAN_POINT ( 'NONE',  ( 12.14591786802327356, -12.06949235617739191, 55.62609039468568284 ) ) ;
#149978=CARTESIAN_POINT ( 'NONE',  ( -18.62759615963255300, -10.81492255796106328, 34.16775706135234714 ) ) ;
#149979=CARTESIAN_POINT ( 'NONE',  ( 14.29746914071049879, -8.314922557960816363, 58.33224293864768839 ) ) ;
#149981=CARTESIAN_POINT ( 'NONE',  ( 12.06949235617739724, 12.14591786802326823, 31.87609039468567929 ) ) ;
#149982=CARTESIAN_POINT ( 'NONE',  ( 19.05341960407617918, -5.049401038297876454, 41.04275706135233293 ) ) ;
#149983=CARTESIAN_POINT ( 'NONE',  ( 4.379528057220339221, -16.55341960407611168, 62.70724293864769550 ) ) ;
#149984=CARTESIAN_POINT ( 'NONE',  ( -21.53943276465977519, 0.05219959533907696930, 111.2489096053143669 ) ) ;
#149986=CARTESIAN_POINT ( 'NONE',  ( 10.72451020669898902, -18.67979575497178502, 77.91557627198102409 ) ) ;
#149987=CARTESIAN_POINT ( 'NONE',  ( -16.46253265017160317, 9.564922557960807481, 95.83224293864769550 ) ) ;
#149988=CARTESIAN_POINT ( 'NONE',  ( -0.05219959533910754901, -16.53943276465976808, 62.49890960531436690 ) ) ;
#149989=CARTESIAN_POINT ( 'NONE',  ( 5.153800228976335163, 19.02544592524342804, 104.7905762719809957 ) ) ;
#149991=CARTESIAN_POINT ( 'NONE',  ( 19.05341960407617918, -5.049401038297876454, 71.04275706135234714 ) ) ;
#149992=CARTESIAN_POINT ( 'NONE',  ( 21.53943276465977519, -0.05219959533907433946, 113.7489096053143527 ) ) ;
#149993=CARTESIAN_POINT ( 'NONE',  ( -5.049401038298153566, 19.05341960407611168, 50.20724293864770260 ) ) ;
#149994=CARTESIAN_POINT ( 'NONE',  ( 9.474510206698729675, 16.51473224551082808, 47.08442372801900433 ) ) ;
#149995=CARTESIAN_POINT ( 'NONE',  ( -0.05219959533910754901, -16.53943276465976808, 107.4989096053143669 ) ) ;
#149996=CARTESIAN_POINT ( 'NONE',  ( -21.53943276465977519, -0.05219959533937600094, 58.75109039468568994 ) ) ;
#149998=CARTESIAN_POINT ( 'NONE',  ( 14.29746914071049879, -8.314922557960816363, 43.33224293864769550 ) ) ;
#149999=CARTESIAN_POINT ( 'NONE',  ( 0.05219959533909260263, 19.03943276465977164, 49.99890960531435979 ) ) ;
#150000=CARTESIAN_POINT ( 'NONE',  ( -19.02544592524342804, 5.153800228976336051, 111.0405762719810099 ) ) ;
#150001=CARTESIAN_POINT ( 'NONE',  ( 5.719274019375991003, -21.55341960407610458, 77.70724293864770971 ) ) ;
#150003=CARTESIAN_POINT ( 'NONE',  ( -5.153800228976328057, -19.02544592524343514, 42.29057627198101699 ) ) ;
#150004=ORIENTED_EDGE ( 'NONE', *, *, #161905, .F. ) ;
#150005=CARTESIAN_POINT ( 'NONE',  ( 15.72974639402199770, -15.80617190586745480, 68.12390960531436690 ) ) ;
#150006=ORIENTED_EDGE ( 'NONE', *, *, #33328, .T. ) ;
#150007=CARTESIAN_POINT ( 'NONE',  ( -0.05219959533937732626, 21.53943276465977519, 82.50109039468568994 ) ) ;
#150009=CARTESIAN_POINT ( 'NONE',  ( 4.379528057220092307, 16.55341960407617563, 102.2927570613523613 ) ) ;
#150010=CARTESIAN_POINT ( 'NONE',  ( -12.06949235617756955, 12.14591786802309770, 80.62390960531438111 ) ) ;
#150011=CARTESIAN_POINT ( 'NONE',  ( 19.05341960407611168, 5.049401038298154454, 63.95724293864769550 ) ) ;
#150012=ORIENTED_EDGE ( 'NONE', *, *, #79855, .F. ) ;
#150013=CARTESIAN_POINT ( 'NONE',  ( -19.03943276465977164, -0.05219959533935918106, 43.75109039468566863 ) ) ;
#150014=CARTESIAN_POINT ( 'NONE',  ( 4.379528057220092307, 16.55341960407617563, 82.29275706135234714 ) ) ;
#150016=CARTESIAN_POINT ( 'NONE',  ( -9.474510206698720793, -16.51473224551083518, 19.58442372801899722 ) ) ;
#150017=CARTESIAN_POINT ( 'NONE',  ( 13.97604488694527802, 13.89961937509977652, 84.37390960531433848 ) ) ;
#150018=CARTESIAN_POINT ( 'NONE',  ( 15.80617190586746368, 15.72974639402197994, 44.37390960531435979 ) ) ;
#150020=CARTESIAN_POINT ( 'NONE',  ( 18.62759615963255655, 10.81492255796105972, 101.6677570613523613 ) ) ;
#150021=CARTESIAN_POINT ( 'NONE',  ( -16.53943276465976808, -0.05219959533934237506, 58.75109039468568994 ) ) ;
#150022=CARTESIAN_POINT ( 'NONE',  ( -5.719274019375978568, 21.55341960407610458, 110.2072429386477239 ) ) ;
#150023=CARTESIAN_POINT ( 'NONE',  ( -8.314922557961024197, 14.29746914071037800, 32.91775706135234714 ) ) ;
#150024=CARTESIAN_POINT ( 'NONE',  ( -5.153800228976328057, -19.02544592524343514, 92.29057627198099567 ) ) ;
#150025=CARTESIAN_POINT ( 'NONE',  ( 13.97604488694527802, 13.89961937509977652, 44.37390960531435269 ) ) ;
#150026=CARTESIAN_POINT ( 'NONE',  ( -9.564922557960796823, -16.46253265017161027, 57.08224293864769550 ) ) ;
#150027=CARTESIAN_POINT ( 'NONE',  ( -16.52544592524335698, -4.483927247898792601, 28.95942372801902209 ) ) ;
#150028=CARTESIAN_POINT ( 'NONE',  ( 12.06949235617757843, -12.14591786802309237, 83.12390960531436690 ) ) ;
#150029=CARTESIAN_POINT ( 'NONE',  ( 16.55341960407618274, -4.379528057220086978, 81.04275706135236135 ) ) ;
#150030=CARTESIAN_POINT ( 'NONE',  ( -15.80617190586768217, 15.72974639402176855, 43.12609039468568284 ) ) ;
#150031=CARTESIAN_POINT ( 'NONE',  ( -13.89961937509977652, 13.97604488694528158, 70.62390960531432427 ) ) ;
#150032=CARTESIAN_POINT ( 'NONE',  ( 16.51473224551069308, 9.474510206698969483, 49.16557627198102409 ) ) ;
#150033=CARTESIAN_POINT ( 'NONE',  ( 19.05341960407611168, 5.049401038298154454, 83.95724293864766707 ) ) ;
#150035=CARTESIAN_POINT ( 'NONE',  ( -12.14591786802309592, -12.06949235617757132, 31.87390960531435979 ) ) ;
#150036=CARTESIAN_POINT ( 'NONE',  ( -14.34966873604972548, 8.224510206698743886, 83.33442372801903275 ) ) ;
#150039=CARTESIAN_POINT ( 'NONE',  ( 16.51473224551083163, -9.474510206698727899, 25.83442372801900078 ) ) ;
#150040=CARTESIAN_POINT ( 'NONE',  ( 0.05219959533909260263, 19.03943276465977164, 94.99890960531436690 ) ) ;
#150041=CARTESIAN_POINT ( 'NONE',  ( 13.97604488694527802, 13.89961937509977652, 49.37390960531434558 ) ) ;
#150042=CARTESIAN_POINT ( 'NONE',  ( 16.51473224551083163, -9.474510206698727899, 20.83442372801899722 ) ) ;
#150044=CARTESIAN_POINT ( 'NONE',  ( 14.29746914071037800, 8.314922557961029526, 41.66775706135235424 ) ) ;
#150045=CARTESIAN_POINT ( 'NONE',  ( 19.03943276465977164, 0.05219959533936151252, 66.25109039468567573 ) ) ;
#150046=CARTESIAN_POINT ( 'NONE',  ( 16.53943276465976808, 0.05219959533934440121, 51.25109039468568994 ) ) ;
#150048=CARTESIAN_POINT ( 'NONE',  ( -9.564922557960796823, -16.46253265017161027, 82.08224293864768129 ) ) ;
#150049=CARTESIAN_POINT ( 'NONE',  ( 0.05219959533907565091, 21.53943276465977519, 109.9989096053143527 ) ) ;
#150050=CARTESIAN_POINT ( 'NONE',  ( -19.05341960407617563, 5.049401038297882671, 68.54275706135230450 ) ) ;
#150051=CARTESIAN_POINT ( 'NONE',  ( -13.97604488694527625, -13.89961937509977652, 101.8739096053143811 ) ) ;
#150052=CARTESIAN_POINT ( 'NONE',  ( -9.564922557960796823, -16.46253265017161027, 32.08224293864769550 ) ) ;
#150053=CARTESIAN_POINT ( 'NONE',  ( 13.89961937509977652, -13.97604488694527269, 83.12390960531436690 ) ) ;
#150054=CARTESIAN_POINT ( 'NONE',  ( 12.14591786802309770, 12.06949235617756955, 39.37390960531436690 ) ) ;
#150055=CARTESIAN_POINT ( 'NONE',  ( -13.97604488694527625, -13.89961937509977652, 21.87390960531435979 ) ) ;
#150056=CARTESIAN_POINT ( 'NONE',  ( -9.564922557961040184, 16.46253265017147172, 32.91775706135233293 ) ) ;
#150057=CARTESIAN_POINT ( 'NONE',  ( 8.224510206698953496, -14.34966873604960469, 77.91557627198102409 ) ) ;
#150058=CARTESIAN_POINT ( 'NONE',  ( 19.05341960407617918, -5.049401038297876454, 21.04275706135232582 ) ) ;
#150059=CARTESIAN_POINT ( 'NONE',  ( -19.03943276465977164, 0.05219959533909376836, 51.24890960531436690 ) ) ;
#150061=CARTESIAN_POINT ( 'NONE',  ( 4.483927247898545687, 16.52544592524342804, 59.79057627198103120 ) ) ;
#150062=CARTESIAN_POINT ( 'NONE',  ( -18.67979575497193778, 10.72451020669871902, 108.3344237280190185 ) ) ;
#150063=CARTESIAN_POINT ( 'NONE',  ( 13.89961937509977652, -13.97604488694527269, 98.12390960531433848 ) ) ;
#150064=CARTESIAN_POINT ( 'NONE',  ( -0.05219959533909027116, -19.03943276465977164, 102.4989096053143669 ) ) ;
#150065=CARTESIAN_POINT ( 'NONE',  ( 9.474510206698971260, -16.51473224551069308, 42.91557627198103120 ) ) ;
#150066=CARTESIAN_POINT ( 'NONE',  ( -4.379528057220328563, 16.55341960407611168, 115.2072429386476955 ) ) ;
#150067=CARTESIAN_POINT ( 'NONE',  ( 16.55341960407611168, 4.379528057220329451, 83.95724293864770971 ) ) ;
#150068=CARTESIAN_POINT ( 'NONE',  ( 21.53943276465977519, -0.05219959533907433946, 93.74890960531436690 ) ) ;
#150069=CARTESIAN_POINT ( 'NONE',  ( -13.89961937509977652, 13.97604488694528158, 90.62390960531432427 ) ) ;
#150070=CARTESIAN_POINT ( 'NONE',  ( 18.62759615963271287, -10.81492255796078972, 98.33224293864769550 ) ) ;
#150071=CARTESIAN_POINT ( 'NONE',  ( -5.049401038298153566, 19.05341960407611168, 90.20724293864766707 ) ) ;
#150073=CARTESIAN_POINT ( 'NONE',  ( 8.224510206698953496, -14.34966873604960469, 107.9155762719810241 ) ) ;
#150074=CARTESIAN_POINT ( 'NONE',  ( -0.05219959533909027116, -19.03943276465977164, 67.49890960531436690 ) ) ;
#150075=CARTESIAN_POINT ( 'NONE',  ( -18.62759615963270932, 10.81492255796079327, 80.83224293864769550 ) ) ;
#150077=CARTESIAN_POINT ( 'NONE',  ( 5.823673210054125526, 21.52544592524343514, 24.79057627198103120 ) ) ;
#150078=CARTESIAN_POINT ( 'NONE',  ( 19.36337904590691750, -5.499999999999941380, 67.91494137495620009 ) ) ;
#150079=CARTESIAN_POINT ( 'NONE',  ( 16.55341960407618274, -4.379528057220086978, 31.04275706135234714 ) ) ;
#150080=CARTESIAN_POINT ( 'NONE',  ( -8.224510206698948167, 14.34966873604960824, 95.41557627198102409 ) ) ;
#150082=DIRECTION ( 'NONE',  ( 0.000000000000000000, 0.000000000000000000, -1.000000000000000000 ) ) ;
#150083=CARTESIAN_POINT ( 'NONE',  ( 5.049401038298161559, -19.05341960407611168, 87.70724293864769550 ) ) ;
#150084=CARTESIAN_POINT ( 'NONE',  ( -0.05219959533909027116, -19.03943276465977164, 47.49890960531435979 ) ) ;
#150085=CARTESIAN_POINT ( 'NONE',  ( -4.379528057220328563, 16.55341960407611168, 85.20724293864770971 ) ) ;
#150086=CARTESIAN_POINT ( 'NONE',  ( -5.719274019375978568, 21.55341960407610458, 30.20724293864769550 ) ) ;
#150087=CARTESIAN_POINT ( 'NONE',  ( -12.14591786802309592, -12.06949235617757132, 56.87390960531436690 ) ) ;
#150088=CARTESIAN_POINT ( 'NONE',  ( 13.89961937509957401, 13.97604488694547697, 96.87609039468566152 ) ) ;
#150089=CARTESIAN_POINT ( 'NONE',  ( -0.05219959533937732626, 21.53943276465977519, 62.50109039468568284 ) ) ;
#150092=CARTESIAN_POINT ( 'NONE',  ( -0.05219959533909027116, -19.03943276465977164, 102.4989096053143669 ) ) ;
#150093=CARTESIAN_POINT ( 'NONE',  ( -14.34966873604972548, 8.224510206698743886, 83.33442372801903275 ) ) ;
#150094=CARTESIAN_POINT ( 'NONE',  ( 16.46253265017160672, -9.564922557960803928, 23.33224293864769194 ) ) ;
#150095=CARTESIAN_POINT ( 'NONE',  ( -19.03943276465977164, 0.05219959533909376836, 81.24890960531436690 ) ) ;
#150096=CARTESIAN_POINT ( 'NONE',  ( 10.72451020669898902, -18.67979575497178502, 82.91557627198103830 ) ) ;
#150099=CARTESIAN_POINT ( 'NONE',  ( 19.03943276465977164, 0.05219959533936151252, 106.2510903946856615 ) ) ;
#150100=CARTESIAN_POINT ( 'NONE',  ( 0.05219959533910956823, 16.53943276465976808, 49.99890960531437401 ) ) ;
#150101=CARTESIAN_POINT ( 'NONE',  ( 18.67979575497194134, -10.72451020669871369, 60.83442372801901854 ) ) ;
#150102=CARTESIAN_POINT ( 'NONE',  ( 16.55341960407618274, -4.379528057220086978, 81.04275706135236135 ) ) ;
#150103=CARTESIAN_POINT ( 'NONE',  ( -16.46253265017160317, 9.564922557960807481, 115.8322429386477097 ) ) ;
#150104=CARTESIAN_POINT ( 'NONE',  ( 16.51473224551069308, 9.474510206698969483, 114.1655762719810241 ) ) ;
#150105=CARTESIAN_POINT ( 'NONE',  ( 17.50000000000000000, -5.500000000000000888, 43.29690382534172244 ) ) ;
#150106=CARTESIAN_POINT ( 'NONE',  ( 4.483927247898790824, -16.52544592524335698, 105.2094237280190328 ) ) ;
#150107=CARTESIAN_POINT ( 'NONE',  ( 14.29746914071037800, 8.314922557961029526, 66.66775706135234714 ) ) ;
#150108=CARTESIAN_POINT ( 'NONE',  ( -13.89961937509977652, 13.97604488694528158, 70.62390960531432427 ) ) ;
#150109=CARTESIAN_POINT ( 'NONE',  ( 16.46253265017160672, -9.564922557960803928, 93.33224293864769550 ) ) ;
#150110=CARTESIAN_POINT ( 'NONE',  ( -0.05219959533937732626, 21.53943276465977519, 72.50109039468568994 ) ) ;
#150111=CARTESIAN_POINT ( 'NONE',  ( 16.55341960407618274, -4.379528057220086978, 76.04275706135237556 ) ) ;
#150112=CARTESIAN_POINT ( 'NONE',  ( -16.52544592524342804, 4.483927247898546575, 46.04057627198103830 ) ) ;
#150113=CARTESIAN_POINT ( 'NONE',  ( 13.89961937509977652, -13.97604488694527269, 53.12390960531434558 ) ) ;
#150114=CARTESIAN_POINT ( 'NONE',  ( -16.46253265017160317, 9.564922557960807481, 50.83224293864770260 ) ) ;
#150115=CARTESIAN_POINT ( 'NONE',  ( -8.314922557961024197, 14.29746914071037800, 37.91775706135235424 ) ) ;
#150117=CARTESIAN_POINT ( 'NONE',  ( -0.05219959533936034679, 19.03943276465977164, 92.50109039468566152 ) ) ;
#150118=CARTESIAN_POINT ( 'NONE',  ( -14.29746914071049879, 8.314922557960819915, 100.8322429386477097 ) ) ;
#150119=CARTESIAN_POINT ( 'NONE',  ( -16.51473224551069308, -9.474510206698971260, 61.66557627198103120 ) ) ;
#150120=CARTESIAN_POINT ( 'NONE',  ( 19.02544592524334988, 5.153800228976608722, 96.45942372801897591 ) ) ;
#150122=CARTESIAN_POINT ( 'NONE',  ( -18.62759615963255300, -10.81492255796106328, 104.1677570613523471 ) ) ;
#150123=CARTESIAN_POINT ( 'NONE',  ( -8.314922557961024197, 14.29746914071037800, 67.91775706135234714 ) ) ;
#150125=CARTESIAN_POINT ( 'NONE',  ( -18.62759615963270932, 10.81492255796079327, 65.83224293864769550 ) ) ;
#150126=CARTESIAN_POINT ( 'NONE',  ( -16.53943276465976808, -0.05219959533934237506, 58.75109039468568994 ) ) ;
#150128=CARTESIAN_POINT ( 'NONE',  ( -19.03943276465977164, -0.05219959533935918106, 48.75109039468566863 ) ) ;
#150129=CARTESIAN_POINT ( 'NONE',  ( -19.03943276465977164, 0.05219959533909376836, 91.24890960531436690 ) ) ;
#150130=CARTESIAN_POINT ( 'NONE',  ( -19.03943276465977164, 0.05219959533909376836, 21.24890960531436335 ) ) ;
#150131=CARTESIAN_POINT ( 'NONE',  ( -19.02544592524342804, 5.153800228976336051, 61.04057627198103120 ) ) ;
#150132=CARTESIAN_POINT ( 'NONE',  ( 0.05219959533910956823, 16.53943276465976808, 64.99890960531435269 ) ) ;
#150134=CARTESIAN_POINT ( 'NONE',  ( -21.52544592524334988, -5.823673210054445271, 73.95942372801901854 ) ) ;
#150135=CARTESIAN_POINT ( 'NONE',  ( 19.03943276465977164, 0.05219959533936151252, 51.25109039468567573 ) ) ;
#150136=CARTESIAN_POINT ( 'NONE',  ( -13.89961937509957401, -13.97604488694547875, 34.37609039468566863 ) ) ;
#150137=CARTESIAN_POINT ( 'NONE',  ( -16.51473224551069308, -9.474510206698971260, 51.66557627198102409 ) ) ;
#150138=CARTESIAN_POINT ( 'NONE',  ( 15.72974639402199770, -15.80617190586745480, 28.12390960531435979 ) ) ;
#150139=CARTESIAN_POINT ( 'NONE',  ( 0.05219959533937995610, -21.53943276465977519, 90.00109039468567573 ) ) ;
#150140=CARTESIAN_POINT ( 'NONE',  ( 9.474510206698971260, -16.51473224551069308, 62.91557627198102409 ) ) ;
#150141=CARTESIAN_POINT ( 'NONE',  ( -21.52544592524334988, -5.823673210054445271, 98.95942372801903275 ) ) ;
#150142=CARTESIAN_POINT ( 'NONE',  ( 15.80617190586746368, 15.72974639402197994, 39.37390960531436690 ) ) ;
#150143=CARTESIAN_POINT ( 'NONE',  ( 19.03943276465977164, -0.05219959533909143690, 88.74890960531436690 ) ) ;
#150144=CARTESIAN_POINT ( 'NONE',  ( 19.05341960407617918, -5.049401038297876454, 56.04275706135234714 ) ) ;
#150145=CARTESIAN_POINT ( 'NONE',  ( 9.564922557960805705, 16.46253265017160317, 44.58224293864769550 ) ) ;
#150146=CARTESIAN_POINT ( 'NONE',  ( 5.049401038298161559, -19.05341960407611168, 87.70724293864769550 ) ) ;
#150148=CARTESIAN_POINT ( 'NONE',  ( 8.224510206698742110, 14.34966873604972548, 32.08442372801901854 ) ) ;
#150149=CARTESIAN_POINT ( 'NONE',  ( -16.52544592524342804, 4.483927247898546575, 101.0405762719810383 ) ) ;
#150150=CARTESIAN_POINT ( 'NONE',  ( 16.46253265017160672, -9.564922557960803928, 73.33224293864769550 ) ) ;
#150151=CARTESIAN_POINT ( 'NONE',  ( 21.52544592524344225, -5.823673210054117533, 43.54057627198103830 ) ) ;
#150152=CARTESIAN_POINT ( 'NONE',  ( -12.06949235617739369, -12.14591786802326823, 24.37609039468567573 ) ) ;
#150153=CARTESIAN_POINT ( 'NONE',  ( -21.53943276465977519, -0.05219959533937600094, 18.75109039468568639 ) ) ;
#150154=CARTESIAN_POINT ( 'NONE',  ( -21.53943276465977519, -0.05219959533937600094, 68.75109039468568994 ) ) ;
#150155=CARTESIAN_POINT ( 'NONE',  ( -14.34966873604972548, 8.224510206698743886, 73.33442372801901854 ) ) ;
#150156=CARTESIAN_POINT ( 'NONE',  ( 16.52544592524335698, 4.483927247898782831, 66.45942372801903275 ) ) ;
#150157=CARTESIAN_POINT ( 'NONE',  ( -19.02544592524342804, 5.153800228976336051, 81.04057627198103830 ) ) ;
#150158=CARTESIAN_POINT ( 'NONE',  ( -8.224510206698735004, -14.34966873604973081, 104.5844237280190185 ) ) ;
#150159=CARTESIAN_POINT ( 'NONE',  ( -5.153800228976607833, 19.02544592524334988, 37.70942372801899722 ) ) ;
#150160=CARTESIAN_POINT ( 'NONE',  ( -5.719274019375665041, -21.55341960407619695, 34.79275706135235424 ) ) ;
#150162=CARTESIAN_POINT ( 'NONE',  ( -0.05219959533910754901, -16.53943276465976808, 62.49890960531436690 ) ) ;
#150163=CARTESIAN_POINT ( 'NONE',  ( 19.03943276465977164, -0.05219959533909143690, 98.74890960531436690 ) ) ;
#150164=CARTESIAN_POINT ( 'NONE',  ( -14.34966873604972548, 8.224510206698743886, 83.33442372801903275 ) ) ;
#150165=CARTESIAN_POINT ( 'NONE',  ( 21.53943276465977519, 0.05219959533937863772, 66.25109039468567573 ) ) ;
#150166=CARTESIAN_POINT ( 'NONE',  ( 14.29746914071037800, 8.314922557961029526, 26.66775706135235424 ) ) ;
#150167=CARTESIAN_POINT ( 'NONE',  ( -18.62759615963255300, -10.81492255796106328, 24.16775706135235424 ) ) ;
#150168=CARTESIAN_POINT ( 'NONE',  ( -16.55341960407611168, -4.379528057220339221, 56.45724293864768839 ) ) ;
#150169=ORIENTED_EDGE ( 'NONE', *, *, #198323, .T. ) ;
#150170=CARTESIAN_POINT ( 'NONE',  ( -18.62759615963270932, 10.81492255796079327, 105.8322429386476955 ) ) ;
#150171=CARTESIAN_POINT ( 'NONE',  ( 12.14591786802309770, 12.06949235617756955, 44.37390960531435979 ) ) ;
#150173=CARTESIAN_POINT ( 'NONE',  ( -19.03943276465977164, 0.05219959533909376836, 31.24890960531435979 ) ) ;
#150174=CARTESIAN_POINT ( 'NONE',  ( -15.72974639402197994, 15.80617190586746368, 25.62390960531435624 ) ) ;
#150175=CARTESIAN_POINT ( 'NONE',  ( -18.67979575497193778, 10.72451020669871902, 33.33442372801900433 ) ) ;
#150176=CARTESIAN_POINT ( 'NONE',  ( -8.224510206698948167, 14.34966873604960824, 65.41557627198102409 ) ) ;
#150177=CARTESIAN_POINT ( 'NONE',  ( -21.52544592524343514, 5.823673210054127303, 61.04057627198103120 ) ) ;
#150178=CARTESIAN_POINT ( 'NONE',  ( 19.05341960407611168, 5.049401038298154454, 73.95724293864768129 ) ) ;
#150179=CARTESIAN_POINT ( 'NONE',  ( -9.474510206698964154, 16.51473224551069663, 25.41557627198103120 ) ) ;
#150180=CARTESIAN_POINT ( 'NONE',  ( -19.02544592524334988, -5.153800228976617603, 83.95942372801901854 ) ) ;
#150181=CARTESIAN_POINT ( 'NONE',  ( -0.05219959533907301413, -21.53943276465977519, 47.49890960531435979 ) ) ;
#150182=CARTESIAN_POINT ( 'NONE',  ( -9.474510206698964154, 16.51473224551069663, 40.41557627198103120 ) ) ;
#150183=CARTESIAN_POINT ( 'NONE',  ( 19.02544592524343514, -5.153800228976328945, 78.54057627198099567 ) ) ;
#150185=CARTESIAN_POINT ( 'NONE',  ( -12.14591786802326823, 12.06949235617739902, 38.12609039468567573 ) ) ;
#150186=CARTESIAN_POINT ( 'NONE',  ( 15.72974639402199770, -15.80617190586745480, 113.1239096053143953 ) ) ;
#150188=CARTESIAN_POINT ( 'NONE',  ( 16.53943276465976808, -0.05219959533910856209, 53.74890960531437401 ) ) ;
#150190=CARTESIAN_POINT ( 'NONE',  ( 21.55341960407619695, -5.719274019375665929, 56.04275706135235424 ) ) ;
#150191=CARTESIAN_POINT ( 'NONE',  ( 9.474510206698971260, -16.51473224551069308, 107.9155762719810383 ) ) ;
#150192=CARTESIAN_POINT ( 'NONE',  ( -0.05219959533907301413, -21.53943276465977519, 67.49890960531436690 ) ) ;
#150193=CARTESIAN_POINT ( 'NONE',  ( -10.72451020669898014, 18.67979575497178502, 105.4155762719810383 ) ) ;
#150194=CARTESIAN_POINT ( 'NONE',  ( 4.379528057220092307, 16.55341960407617563, 47.29275706135234003 ) ) ;
#150195=CARTESIAN_POINT ( 'NONE',  ( 5.719274019375991003, -21.55341960407610458, 47.70724293864770260 ) ) ;
#150196=CARTESIAN_POINT ( 'NONE',  ( -18.62759615963255300, -10.81492255796106328, 99.16775706135234714 ) ) ;
#150197=CARTESIAN_POINT ( 'NONE',  ( -5.049401038298153566, 19.05341960407611168, 60.20724293864768129 ) ) ;
#150198=CARTESIAN_POINT ( 'NONE',  ( -16.46253265017160317, 9.564922557960807481, 90.83224293864769550 ) ) ;
#150199=CARTESIAN_POINT ( 'NONE',  ( -9.474510206698964154, 16.51473224551069663, 70.41557627198102409 ) ) ;
#150201=CARTESIAN_POINT ( 'NONE',  ( 13.97604488694548053, -13.89961937509957401, 55.62609039468566863 ) ) ;
#150202=CARTESIAN_POINT ( 'NONE',  ( 13.97604488694548053, -13.89961937509957401, 20.62609039468567573 ) ) ;
#150203=CARTESIAN_POINT ( 'NONE',  ( -18.67979575497178146, -10.72451020669898902, 31.66557627198102054 ) ) ;
#150204=CARTESIAN_POINT ( 'NONE',  ( -12.06949235617739369, -12.14591786802326823, 104.3760903946856899 ) ) ;
#150205=CARTESIAN_POINT ( 'NONE',  ( -13.97604488694547697, 13.89961937509957934, 88.12609039468563310 ) ) ;
#150206=CARTESIAN_POINT ( 'NONE',  ( 9.564922557960805705, 16.46253265017160317, 39.58224293864768839 ) ) ;
#150208=CARTESIAN_POINT ( 'NONE',  ( -5.049401038297874678, -19.05341960407617918, 19.79275706135233293 ) ) ;
#150209=CARTESIAN_POINT ( 'NONE',  ( 5.153800228976615827, -19.02544592524334988, 85.20942372801900433 ) ) ;
#150210=CARTESIAN_POINT ( 'NONE',  ( 13.97604488694548053, -13.89961937509957401, 40.62609039468564731 ) ) ;
#150212=CARTESIAN_POINT ( 'NONE',  ( 16.51473224551069308, 9.474510206698969483, 39.16557627198103120 ) ) ;
#150213=CARTESIAN_POINT ( 'NONE',  ( -8.224510206698948167, 14.34966873604960824, 45.41557627198103830 ) ) ;
#150214=CARTESIAN_POINT ( 'NONE',  ( 5.049401038298161559, -19.05341960407611168, 32.70724293864768129 ) ) ;
#150215=CARTESIAN_POINT ( 'NONE',  ( -14.34966873604960291, -8.224510206698953496, 36.66557627198103120 ) ) ;
#150217=CARTESIAN_POINT ( 'NONE',  ( 16.55341960407618274, -4.379528057220086978, 106.0427570613523471 ) ) ;
#150218=CARTESIAN_POINT ( 'NONE',  ( 9.564922557960805705, 16.46253265017160317, 49.58224293864770260 ) ) ;
#150219=CARTESIAN_POINT ( 'NONE',  ( -18.67979575497193778, 10.72451020669871902, 108.3344237280190185 ) ) ;
#150220=CARTESIAN_POINT ( 'NONE',  ( -12.06949235617739369, -12.14591786802326823, 29.37609039468568284 ) ) ;
#150221=CARTESIAN_POINT ( 'NONE',  ( -21.53943276465977519, 0.05219959533907696930, 36.24890960531435979 ) ) ;
#150222=CARTESIAN_POINT ( 'NONE',  ( 18.67979575497194134, -10.72451020669871369, 95.83442372801903275 ) ) ;
#150224=CARTESIAN_POINT ( 'NONE',  ( 19.05341960407611168, 5.049401038298154454, 103.9572429386476671 ) ) ;
#150225=CARTESIAN_POINT ( 'NONE',  ( -13.97604488694527625, -13.89961937509977652, 81.87390960531436690 ) ) ;
#150227=CARTESIAN_POINT ( 'NONE',  ( 21.55341960407610458, 5.719274019375980345, 108.9572429386476955 ) ) ;
#150229=CARTESIAN_POINT ( 'NONE',  ( 14.34966873604960469, 8.224510206698951720, 84.16557627198103830 ) ) ;
#150230=CARTESIAN_POINT ( 'NONE',  ( 15.72974639402199770, -15.80617190586745480, 78.12390960531436690 ) ) ;
#150231=CARTESIAN_POINT ( 'NONE',  ( -16.51473224551069308, -9.474510206698971260, 66.66557627198102409 ) ) ;
#150232=CARTESIAN_POINT ( 'NONE',  ( 0.05219959533909260263, 19.03943276465977164, 69.99890960531435269 ) ) ;
#150233=CARTESIAN_POINT ( 'NONE',  ( -5.719274019375978568, 21.55341960407610458, 95.20724293864769550 ) ) ;
#150235=CARTESIAN_POINT ( 'NONE',  ( 19.05341960407611168, 5.049401038298154454, 53.95724293864770260 ) ) ;
#150236=CARTESIAN_POINT ( 'NONE',  ( 14.29746914071049879, -8.314922557960816363, 98.33224293864769550 ) ) ;
#150237=CARTESIAN_POINT ( 'NONE',  ( -19.03943276465977164, 0.05219959533909376836, 21.24890960531436335 ) ) ;
#150238=CARTESIAN_POINT ( 'NONE',  ( -5.049401038298153566, 19.05341960407611168, 70.20724293864769550 ) ) ;
#150239=CARTESIAN_POINT ( 'NONE',  ( 0.05219959533936267826, -19.03943276465977164, 80.00109039468567573 ) ) ;
#150241=CARTESIAN_POINT ( 'NONE',  ( 16.52544592524342804, -4.483927247898539470, 98.54057627198105251 ) ) ;
#150242=CARTESIAN_POINT ( 'NONE',  ( -0.05219959533937732626, 21.53943276465977519, 52.50109039468567573 ) ) ;
#150243=CARTESIAN_POINT ( 'NONE',  ( -5.153800228976328057, -19.02544592524343514, 47.29057627198102409 ) ) ;
#150244=CARTESIAN_POINT ( 'NONE',  ( -15.72974639402197994, 15.80617190586746368, 115.6239096053143669 ) ) ;
#150245=CARTESIAN_POINT ( 'NONE',  ( -16.55341960407611168, -4.379528057220339221, 106.4572429386477097 ) ) ;
#150247=CARTESIAN_POINT ( 'NONE',  ( -9.474510206698964154, 16.51473224551069663, 55.41557627198103120 ) ) ;
#150250=CARTESIAN_POINT ( 'NONE',  ( 9.564922557961047289, -16.46253265017146816, 105.4177570613523471 ) ) ;
#150251=CARTESIAN_POINT ( 'NONE',  ( 5.049401038298161559, -19.05341960407611168, 112.7072429386476813 ) ) ;
#150252=CARTESIAN_POINT ( 'NONE',  ( -15.72974639402176322, -15.80617190586768395, 44.37609039468567573 ) ) ;
#150253=CARTESIAN_POINT ( 'NONE',  ( -19.05341960407611168, -5.049401038298163336, 101.4572429386476955 ) ) ;
#150254=CARTESIAN_POINT ( 'NONE',  ( 19.05341960407617918, -5.049401038297876454, 86.04275706135233293 ) ) ;
#150255=CARTESIAN_POINT ( 'NONE',  ( 16.46253265017160672, -9.564922557960803928, 53.33224293864768839 ) ) ;
#150256=CARTESIAN_POINT ( 'NONE',  ( 12.06949235617757843, -12.14591786802309237, 83.12390960531436690 ) ) ;
#150257=CARTESIAN_POINT ( 'NONE',  ( 13.89961937509977652, -13.97604488694527269, 83.12390960531436690 ) ) ;
#150258=CARTESIAN_POINT ( 'NONE',  ( 16.55341960407611168, 4.379528057220329451, 73.95724293864769550 ) ) ;
#150259=CARTESIAN_POINT ( 'NONE',  ( -0.05219959533909027116, -19.03943276465977164, 82.49890960531436690 ) ) ;
#150260=CARTESIAN_POINT ( 'NONE',  ( -5.153800228976607833, 19.02544592524334988, 37.70942372801899722 ) ) ;
#150261=CARTESIAN_POINT ( 'NONE',  ( 16.51473224551069308, 9.474510206698969483, 44.16557627198103120 ) ) ;
#150262=CARTESIAN_POINT ( 'NONE',  ( -4.379528057220328563, 16.55341960407611168, 50.20724293864769550 ) ) ;
#150263=CARTESIAN_POINT ( 'NONE',  ( 16.51473224551069308, 9.474510206698969483, 24.16557627198102765 ) ) ;
#150264=ORIENTED_EDGE ( 'NONE', *, *, #118593, .T. ) ;
#150265=CARTESIAN_POINT ( 'NONE',  ( 10.81492255796106328, -18.62759615963255655, 50.41775706135235424 ) ) ;
#150266=CARTESIAN_POINT ( 'NONE',  ( 19.02544592524334988, 5.153800228976608722, 81.45942372801897591 ) ) ;
#150267=CARTESIAN_POINT ( 'NONE',  ( -4.483927247898539470, -16.52544592524342804, 37.29057627198102409 ) ) ;
#150268=CARTESIAN_POINT ( 'NONE',  ( 0.05219959533907565091, 21.53943276465977519, 99.99890960531436690 ) ) ;
#150269=CARTESIAN_POINT ( 'NONE',  ( -0.05219959533907301413, -21.53943276465977519, 37.49890960531436690 ) ) ;
#150270=CARTESIAN_POINT ( 'NONE',  ( -14.29746914071049879, 8.314922557960819915, 75.83224293864769550 ) ) ;
#150271=CARTESIAN_POINT ( 'NONE',  ( 19.02544592524343514, -5.153800228976328945, 38.54057627198103120 ) ) ;
#150272=CARTESIAN_POINT ( 'NONE',  ( -14.34966873604972548, 8.224510206698743886, 108.3344237280190185 ) ) ;
#150273=CARTESIAN_POINT ( 'NONE',  ( 8.314922557961029526, -14.29746914071037800, 75.41775706135233293 ) ) ;
#150274=CARTESIAN_POINT ( 'NONE',  ( -16.51473224551082808, 9.474510206698731452, 23.33442372801900078 ) ) ;
#150275=CARTESIAN_POINT ( 'NONE',  ( -0.05219959533909027116, -19.03943276465977164, 92.49890960531436690 ) ) ;
#150276=CARTESIAN_POINT ( 'NONE',  ( 13.89961937509977652, -13.97604488694527269, 78.12390960531433848 ) ) ;
#150277=CARTESIAN_POINT ( 'NONE',  ( -14.34966873604972548, 8.224510206698743886, 73.33442372801901854 ) ) ;
#150278=CARTESIAN_POINT ( 'NONE',  ( -19.02544592524342804, 5.153800228976336051, 31.04057627198102409 ) ) ;
#150279=CARTESIAN_POINT ( 'NONE',  ( -14.34966873604960291, -8.224510206698953496, 51.66557627198102409 ) ) ;
#150280=CARTESIAN_POINT ( 'NONE',  ( -19.05341960407611168, -5.049401038298163336, 101.4572429386476955 ) ) ;
#150281=CARTESIAN_POINT ( 'NONE',  ( 19.05341960407611168, 5.049401038298154454, 88.95724293864769550 ) ) ;
#150282=CARTESIAN_POINT ( 'NONE',  ( 15.72974639402199770, -15.80617190586745480, 23.12390960531436335 ) ) ;
#150284=CARTESIAN_POINT ( 'NONE',  ( 14.34966873604960469, 8.224510206698951720, 69.16557627198102409 ) ) ;
#150286=CARTESIAN_POINT ( 'NONE',  ( 12.06949235617757843, -12.14591786802309237, 63.12390960531435979 ) ) ;
#150287=CARTESIAN_POINT ( 'NONE',  ( -4.379528057220086978, -16.55341960407618274, 49.79275706135234714 ) ) ;
#150288=CARTESIAN_POINT ( 'NONE',  ( 17.49999999999999289, -3.305555262949580797, 32.12517152156607381 ) ) ;
#150289=CARTESIAN_POINT ( 'NONE',  ( -16.51473224551082808, 9.474510206698731452, 63.33442372801900433 ) ) ;
#150290=CARTESIAN_POINT ( 'NONE',  ( 16.51473224551069308, 9.474510206698969483, 84.16557627198102409 ) ) ;
#150291=CARTESIAN_POINT ( 'NONE',  ( 19.05341960407617918, -5.049401038297876454, 61.04275706135232582 ) ) ;
#150292=CARTESIAN_POINT ( 'NONE',  ( -5.153800228976607833, 19.02544592524334988, 112.7094237280190043 ) ) ;
#150293=CARTESIAN_POINT ( 'NONE',  ( -4.379528057220086978, -16.55341960407618274, 99.79275706135234714 ) ) ;
#150294=CARTESIAN_POINT ( 'NONE',  ( 13.89961937509977652, -13.97604488694527269, 38.12390960531436690 ) ) ;
#150295=CARTESIAN_POINT ( 'NONE',  ( 0.05219959533907565091, 21.53943276465977519, 24.99890960531435624 ) ) ;
#150296=CARTESIAN_POINT ( 'NONE',  ( 21.52544592524334988, 5.823673210054432836, 56.45942372801902565 ) ) ;
#150297=CARTESIAN_POINT ( 'NONE',  ( -0.05219959533936034679, 19.03943276465977164, 107.5010903946856615 ) ) ;
#150299=CARTESIAN_POINT ( 'NONE',  ( -19.02544592524342804, 5.153800228976336051, 76.04057627198102409 ) ) ;
#150300=CARTESIAN_POINT ( 'NONE',  ( -16.46253265017160317, 9.564922557960807481, 115.8322429386477097 ) ) ;
#150301=CARTESIAN_POINT ( 'NONE',  ( -16.53943276465976808, 0.05219959533911058130, 81.24890960531436690 ) ) ;
#150302=CARTESIAN_POINT ( 'NONE',  ( -19.03943276465977164, 0.05219959533909376836, 76.24890960531435269 ) ) ;
#150303=CARTESIAN_POINT ( 'NONE',  ( 13.97604488694527802, 13.89961937509977652, 79.37390960531435269 ) ) ;
#150304=CARTESIAN_POINT ( 'NONE',  ( -13.97604488694547697, 13.89961937509957934, 83.12609039468564731 ) ) ;
#150305=CARTESIAN_POINT ( 'NONE',  ( -21.53943276465977519, 0.05219959533907696930, 66.24890960531436690 ) ) ;
#150306=CARTESIAN_POINT ( 'NONE',  ( -0.05219959533909027116, -19.03943276465977164, 27.49890960531435624 ) ) ;
#150307=CARTESIAN_POINT ( 'NONE',  ( 0.05219959533936267826, -19.03943276465977164, 55.00109039468566863 ) ) ;
#150308=CARTESIAN_POINT ( 'NONE',  ( -16.51473224551069308, -9.474510206698971260, 56.66557627198103120 ) ) ;
#150309=CARTESIAN_POINT ( 'NONE',  ( 9.564922557960805705, 16.46253265017160317, 94.58224293864769550 ) ) ;
#150310=EDGE_CURVE ( 'NONE', #21338, #190522, #138656, .T. ) ;
#150312=CARTESIAN_POINT ( 'NONE',  ( 5.719274019375991003, -21.55341960407610458, 87.70724293864769550 ) ) ;
#150313=CARTESIAN_POINT ( 'NONE',  ( -12.06949235617756955, 12.14591786802309770, 90.62390960531436690 ) ) ;
#150314=CARTESIAN_POINT ( 'NONE',  ( -16.51473224551082808, 9.474510206698731452, 43.33442372801900433 ) ) ;
#150315=CARTESIAN_POINT ( 'NONE',  ( -21.53943276465977519, 0.05219959533907696930, 81.24890960531436690 ) ) ;
#150316=CARTESIAN_POINT ( 'NONE',  ( 15.80617190586746368, 15.72974639402197994, 54.37390960531435979 ) ) ;
#150318=CARTESIAN_POINT ( 'NONE',  ( 0.05219959533910956823, 16.53943276465976808, 29.99890960531435979 ) ) ;
#150319=CARTESIAN_POINT ( 'NONE',  ( -0.05219959533937732626, 21.53943276465977519, 107.5010903946856899 ) ) ;
#150320=CARTESIAN_POINT ( 'NONE',  ( 19.05341960407611168, 5.049401038298154454, 78.95724293864769550 ) ) ;
#150321=CARTESIAN_POINT ( 'NONE',  ( 13.89961937509977652, -13.97604488694527269, 33.12390960531434558 ) ) ;
#150322=CARTESIAN_POINT ( 'NONE',  ( -21.52544592524334988, -5.823673210054445271, 33.95942372801901143 ) ) ;
#150323=CARTESIAN_POINT ( 'NONE',  ( 18.67979575497194134, -10.72451020669871369, 60.83442372801901854 ) ) ;
#150324=CARTESIAN_POINT ( 'NONE',  ( 19.03943276465977164, -0.05219959533909143690, 48.74890960531435979 ) ) ;
#150325=CARTESIAN_POINT ( 'NONE',  ( 18.62759615963255655, 10.81492255796105972, 26.66775706135235424 ) ) ;
#150326=CARTESIAN_POINT ( 'NONE',  ( 19.05341960407617918, -5.049401038297876454, 56.04275706135234714 ) ) ;
#150327=CARTESIAN_POINT ( 'NONE',  ( -19.05341960407611168, -5.049401038298163336, 31.45724293864769550 ) ) ;
#150328=CARTESIAN_POINT ( 'NONE',  ( -0.05219959533934338120, 16.53943276465976808, 22.50109039468567573 ) ) ;
#150329=CARTESIAN_POINT ( 'NONE',  ( 5.153800228976335163, 19.02544592524342804, 29.79057627198102409 ) ) ;
#150330=CARTESIAN_POINT ( 'NONE',  ( -12.14591786802326823, 12.06949235617739902, 78.12609039468570415 ) ) ;
#150331=CARTESIAN_POINT ( 'NONE',  ( 16.51473224551069308, 9.474510206698969483, 44.16557627198103120 ) ) ;
#150333=CARTESIAN_POINT ( 'NONE',  ( -9.564922557960796823, -16.46253265017161027, 82.08224293864768129 ) ) ;
#150334=CARTESIAN_POINT ( 'NONE',  ( 5.049401038298161559, -19.05341960407611168, 22.70724293864769194 ) ) ;
#150335=CARTESIAN_POINT ( 'NONE',  ( -15.72974639402197994, 15.80617190586746368, 70.62390960531436690 ) ) ;
#150336=CARTESIAN_POINT ( 'NONE',  ( 16.53943276465976808, 0.05219959533934440121, 51.25109039468568994 ) ) ;
#150337=CARTESIAN_POINT ( 'NONE',  ( -21.52544592524334988, -5.823673210054445271, 98.95942372801903275 ) ) ;
#150338=CARTESIAN_POINT ( 'NONE',  ( -19.05341960407611168, -5.049401038298163336, 41.45724293864769550 ) ) ;
#150339=CARTESIAN_POINT ( 'NONE',  ( 4.379528057220339221, -16.55341960407611168, 27.70724293864769905 ) ) ;
#150340=CARTESIAN_POINT ( 'NONE',  ( -14.29746914071049879, 8.314922557960819915, 65.83224293864769550 ) ) ;
#150341=CARTESIAN_POINT ( 'NONE',  ( -13.89961937509977652, 13.97604488694528158, 60.62390960531436690 ) ) ;
#150342=CARTESIAN_POINT ( 'NONE',  ( 16.51473224551083163, -9.474510206698727899, 20.83442372801899722 ) ) ;
#150343=CARTESIAN_POINT ( 'NONE',  ( -5.719274019375665041, -21.55341960407619695, 29.79275706135234358 ) ) ;
#150344=CARTESIAN_POINT ( 'NONE',  ( 0.05219959533909260263, 19.03943276465977164, 79.99890960531436690 ) ) ;
#150345=CARTESIAN_POINT ( 'NONE',  ( 15.72974639402176855, 15.80617190586768217, 81.87609039468568994 ) ) ;
#150346=CARTESIAN_POINT ( 'NONE',  ( 16.55341960407618274, -4.379528057220086978, 71.04275706135234714 ) ) ;
#150347=CARTESIAN_POINT ( 'NONE',  ( -12.06949235617739369, -12.14591786802326823, 24.37609039468567573 ) ) ;
#150348=CARTESIAN_POINT ( 'NONE',  ( 12.06949235617757843, -12.14591786802309237, 93.12390960531436690 ) ) ;
#150349=CARTESIAN_POINT ( 'NONE',  ( -18.67979575497193778, 10.72451020669871902, 103.3344237280190043 ) ) ;
#150350=CARTESIAN_POINT ( 'NONE',  ( 16.52544592524342804, -4.483927247898539470, 38.54057627198103120 ) ) ;
#150351=CARTESIAN_POINT ( 'NONE',  ( -19.02544592524342804, 5.153800228976336051, 26.04057627198103120 ) ) ;
#150352=CARTESIAN_POINT ( 'NONE',  ( 14.29746914071037800, 8.314922557961029526, 46.66775706135234714 ) ) ;
#150353=CARTESIAN_POINT ( 'NONE',  ( 16.55341960407611168, 4.379528057220329451, 53.95724293864770260 ) ) ;
#150354=CARTESIAN_POINT ( 'NONE',  ( 4.483927247898790824, -16.52544592524335698, 100.2094237280190043 ) ) ;
#150355=CARTESIAN_POINT ( 'NONE',  ( 19.03943276465977164, -0.05219959533909143690, 113.7489096053143669 ) ) ;
#150356=CARTESIAN_POINT ( 'NONE',  ( -21.53943276465977519, 0.05219959533907696930, 36.24890960531435979 ) ) ;
#150357=CARTESIAN_POINT ( 'NONE',  ( -9.474510206698720793, -16.51473224551083518, 19.58442372801899722 ) ) ;
#150358=CARTESIAN_POINT ( 'NONE',  ( -0.05219959533910754901, -16.53943276465976808, 82.49890960531436690 ) ) ;
#150359=CARTESIAN_POINT ( 'NONE',  ( -19.05341960407611168, -5.049401038298163336, 101.4572429386476955 ) ) ;
#150362=CARTESIAN_POINT ( 'NONE',  ( -16.55341960407617563, 4.379528057220093196, 43.54275706135235424 ) ) ;
#150363=CARTESIAN_POINT ( 'NONE',  ( 9.564922557960805705, 16.46253265017160317, 44.58224293864769550 ) ) ;
#150364=CARTESIAN_POINT ( 'NONE',  ( 16.53943276465976808, 0.05219959533934440121, 46.25109039468567573 ) ) ;
#150366=CARTESIAN_POINT ( 'NONE',  ( 16.46253265017146816, 9.564922557961045513, 51.66775706135233293 ) ) ;
#150367=CARTESIAN_POINT ( 'NONE',  ( -19.03943276465977164, 0.05219959533909376836, 46.24890960531435979 ) ) ;
#150368=CARTESIAN_POINT ( 'NONE',  ( 8.314922557961029526, -14.29746914071037800, 80.41775706135234714 ) ) ;
#150369=CARTESIAN_POINT ( 'NONE',  ( 19.05341960407617918, -5.049401038297876454, 101.0427570613523045 ) ) ;
#150370=CARTESIAN_POINT ( 'NONE',  ( 13.97604488694548053, -13.89961937509957401, 30.62609039468566863 ) ) ;
#150371=CARTESIAN_POINT ( 'NONE',  ( -13.89961937509977652, 13.97604488694528158, 60.62390960531436690 ) ) ;
#150373=CARTESIAN_POINT ( 'NONE',  ( 4.379528057220339221, -16.55341960407611168, 97.70724293864772392 ) ) ;
#150374=CARTESIAN_POINT ( 'NONE',  ( 19.02544592524334988, 5.153800228976608722, 71.45942372801900433 ) ) ;
#150375=CARTESIAN_POINT ( 'NONE',  ( -10.81492255796078084, -18.62759615963271287, 67.08224293864770971 ) ) ;
#150376=CARTESIAN_POINT ( 'NONE',  ( 19.05341960407617918, -5.049401038297876454, 41.04275706135233293 ) ) ;
#150377=CARTESIAN_POINT ( 'NONE',  ( 19.02544592524343514, -5.153800228976328945, 108.5405762719810383 ) ) ;
#150378=CARTESIAN_POINT ( 'NONE',  ( 5.823673210054125526, 21.52544592524343514, 84.79057627198102409 ) ) ;
#150380=CARTESIAN_POINT ( 'NONE',  ( 13.89961937509957401, 13.97604488694547697, 106.8760903946856757 ) ) ;
#150381=CARTESIAN_POINT ( 'NONE',  ( 5.049401038297881783, 19.05341960407617918, 97.29275706135233293 ) ) ;
#150382=ADVANCED_FACE ( 'NONE', ( #123476 ), #169998, .F. ) ;
#150383=CARTESIAN_POINT ( 'NONE',  ( 12.06949235617739724, 12.14591786802326823, 26.87609039468567218 ) ) ;
#150384=CARTESIAN_POINT ( 'NONE',  ( 0.05219959533909260263, 19.03943276465977164, 44.99890960531435979 ) ) ;
#150385=CARTESIAN_POINT ( 'NONE',  ( -9.474510206698964154, 16.51473224551069663, 115.4155762719810241 ) ) ;
#150386=CARTESIAN_POINT ( 'NONE',  ( 15.80617190586746368, 15.72974639402197994, 89.37390960531435269 ) ) ;
#150387=CARTESIAN_POINT ( 'NONE',  ( 18.62759615963255655, 10.81492255796105972, 56.66775706135235424 ) ) ;
#150388=CARTESIAN_POINT ( 'NONE',  ( 19.02544592524334988, 5.153800228976608722, 106.4594237280190185 ) ) ;
#150389=CARTESIAN_POINT ( 'NONE',  ( 5.823673210054444382, -21.52544592524334988, 105.2094237280190328 ) ) ;
#150390=CARTESIAN_POINT ( 'NONE',  ( -8.314922557961024197, 14.29746914071037800, 112.9177570613523329 ) ) ;
#150391=CARTESIAN_POINT ( 'NONE',  ( -10.81492255796078084, -18.62759615963271287, 97.08224293864770971 ) ) ;
#150392=CARTESIAN_POINT ( 'NONE',  ( 12.14591786802309770, 12.06949235617756955, 54.37390960531435979 ) ) ;
#150393=CARTESIAN_POINT ( 'NONE',  ( 9.564922557961047289, -16.46253265017146816, 85.41775706135233293 ) ) ;
#150394=CARTESIAN_POINT ( 'NONE',  ( 19.02544592524334988, 5.153800228976608722, 51.45942372801900433 ) ) ;
#150395=CARTESIAN_POINT ( 'NONE',  ( 21.52544592524334988, 5.823673210054432836, 66.45942372801903275 ) ) ;
#150396=CARTESIAN_POINT ( 'NONE',  ( 0.05219959533936267826, -19.03943276465977164, 35.00109039468566863 ) ) ;
#150397=CARTESIAN_POINT ( 'NONE',  ( -5.049401038298153566, 19.05341960407611168, 30.20724293864768839 ) ) ;
#150398=CARTESIAN_POINT ( 'NONE',  ( 15.80617190586746368, 15.72974639402197994, 44.37390960531435979 ) ) ;
#150399=CARTESIAN_POINT ( 'NONE',  ( -8.314922557960811034, -14.29746914071050412, 32.08224293864769550 ) ) ;
#150400=CARTESIAN_POINT ( 'NONE',  ( 15.72974639402176855, 15.80617190586768217, 106.8760903946856899 ) ) ;
#150401=CARTESIAN_POINT ( 'NONE',  ( 14.29746914071037800, 8.314922557961029526, 66.66775706135234714 ) ) ;
#150402=CARTESIAN_POINT ( 'NONE',  ( -4.379528057220328563, 16.55341960407611168, 45.20724293864769550 ) ) ;
#150403=CARTESIAN_POINT ( 'NONE',  ( 21.53943276465977519, 0.05219959533937863772, 66.25109039468567573 ) ) ;
#150404=CARTESIAN_POINT ( 'NONE',  ( -5.719274019375665041, -21.55341960407619695, 64.79275706135234714 ) ) ;
#150405=CARTESIAN_POINT ( 'NONE',  ( -21.52544592524343514, 5.823673210054127303, 71.04057627198103830 ) ) ;
#150406=ORIENTED_EDGE ( 'NONE', *, *, #142150, .T. ) ;
#150407=CARTESIAN_POINT ( 'NONE',  ( 19.05341960407611168, 5.049401038298154454, 28.95724293864769550 ) ) ;
#150408=CARTESIAN_POINT ( 'NONE',  ( 10.72451020669871369, 18.67979575497193778, 37.08442372801901143 ) ) ;
#150409=CARTESIAN_POINT ( 'NONE',  ( 13.97604488694527802, 13.89961937509977652, 24.37390960531435624 ) ) ;
#150410=CARTESIAN_POINT ( 'NONE',  ( 9.474510206698971260, -16.51473224551069308, 32.91557627198102409 ) ) ;
#150411=CARTESIAN_POINT ( 'NONE',  ( 8.224510206698953496, -14.34966873604960469, 92.91557627198103830 ) ) ;
#150412=CARTESIAN_POINT ( 'NONE',  ( 9.564922557960805705, 16.46253265017160317, 89.58224293864769550 ) ) ;
#150413=CARTESIAN_POINT ( 'NONE',  ( -12.06949235617756955, 12.14591786802309770, 30.62390960531436335 ) ) ;
#150414=CARTESIAN_POINT ( 'NONE',  ( 12.14591786802309770, 12.06949235617756955, 104.3739096053143669 ) ) ;
#150415=CARTESIAN_POINT ( 'NONE',  ( -5.719274019375978568, 21.55341960407610458, 75.20724293864769550 ) ) ;
#150417=CARTESIAN_POINT ( 'NONE',  ( 15.72974639402199770, -15.80617190586745480, 113.1239096053143953 ) ) ;
#150418=CARTESIAN_POINT ( 'NONE',  ( 9.564922557960805705, 16.46253265017160317, 114.5822429386476955 ) ) ;
#150419=CARTESIAN_POINT ( 'NONE',  ( 19.05341960407611168, 5.049401038298154454, 58.95724293864768129 ) ) ;
#150420=CARTESIAN_POINT ( 'NONE',  ( -8.314922557961024197, 14.29746914071037800, 22.91775706135235069 ) ) ;
#150421=CARTESIAN_POINT ( 'NONE',  ( -21.55341960407610458, -5.719274019375992779, 61.45724293864770260 ) ) ;
#150422=CARTESIAN_POINT ( 'NONE',  ( 0.05219959533937995610, -21.53943276465977519, 85.00109039468568994 ) ) ;
#150423=CARTESIAN_POINT ( 'NONE',  ( 5.049401038298161559, -19.05341960407611168, 82.70724293864770971 ) ) ;
#150424=CARTESIAN_POINT ( 'NONE',  ( -19.02544592524342804, 5.153800228976336051, 106.0405762719810241 ) ) ;
#150425=CARTESIAN_POINT ( 'NONE',  ( -16.53943276465976808, -0.05219959533934237506, 73.75109039468567573 ) ) ;
#150426=CARTESIAN_POINT ( 'NONE',  ( 10.72451020669871369, 18.67979575497193778, 72.08442372801899012 ) ) ;
#150427=CARTESIAN_POINT ( 'NONE',  ( 10.72451020669871369, 18.67979575497193778, 102.0844237280190185 ) ) ;
#150428=CARTESIAN_POINT ( 'NONE',  ( 14.34966873604972726, -8.224510206698740333, 60.83442372801901854 ) ) ;
#150429=CARTESIAN_POINT ( 'NONE',  ( -21.53943276465977519, 0.05219959533907696930, 111.2489096053143669 ) ) ;
#150430=CARTESIAN_POINT ( 'NONE',  ( -5.049401038298153566, 19.05341960407611168, 115.2072429386477097 ) ) ;
#150431=CARTESIAN_POINT ( 'NONE',  ( 10.81492255796078972, 18.62759615963270932, 94.58224293864769550 ) ) ;
#150432=CARTESIAN_POINT ( 'NONE',  ( -9.474510206698720793, -16.51473224551083518, 44.58442372801900433 ) ) ;
#150433=CARTESIAN_POINT ( 'NONE',  ( 10.72451020669898902, -18.67979575497178502, 47.91557627198102409 ) ) ;
#150434=CARTESIAN_POINT ( 'NONE',  ( 13.97604488694527802, 13.89961937509977652, 99.37390960531436690 ) ) ;
#150435=CARTESIAN_POINT ( 'NONE',  ( 14.34966873604960469, 8.224510206698951720, 34.16557627198102409 ) ) ;
#150438=CARTESIAN_POINT ( 'NONE',  ( -16.52544592524335698, -4.483927247898792601, 18.95942372801901143 ) ) ;
#150439=CARTESIAN_POINT ( 'NONE',  ( 0.05219959533907565091, 21.53943276465977519, 84.99890960531436690 ) ) ;
#150440=CARTESIAN_POINT ( 'NONE',  ( 8.224510206698953496, -14.34966873604960469, 57.91557627198103120 ) ) ;
#150441=CARTESIAN_POINT ( 'NONE',  ( 16.52544592524335698, 4.483927247898782831, 31.45942372801901854 ) ) ;
#150442=CARTESIAN_POINT ( 'NONE',  ( 16.46253265017160672, -9.564922557960803928, 38.33224293864768839 ) ) ;
#150443=CARTESIAN_POINT ( 'NONE',  ( 18.62759615963271287, -10.81492255796078972, 113.3322429386476955 ) ) ;
#150444=CARTESIAN_POINT ( 'NONE',  ( -5.049401038297874678, -19.05341960407617918, 84.79275706135233293 ) ) ;
#150445=CARTESIAN_POINT ( 'NONE',  ( 19.02544592524343514, -5.153800228976328945, 83.54057627198100988 ) ) ;
#150446=CARTESIAN_POINT ( 'NONE',  ( 16.51473224551069308, 9.474510206698969483, 74.16557627198103830 ) ) ;
#150447=CARTESIAN_POINT ( 'NONE',  ( 21.55341960407610458, 5.719274019375980345, 78.95724293864769550 ) ) ;
#150448=CARTESIAN_POINT ( 'NONE',  ( -5.049401038298153566, 19.05341960407611168, 35.20724293864768839 ) ) ;
#150450=CARTESIAN_POINT ( 'NONE',  ( -12.06949235617756955, 12.14591786802309770, 55.62390960531436690 ) ) ;
#150451=CARTESIAN_POINT ( 'NONE',  ( 19.05341960407611168, 5.049401038298154454, 83.95724293864766707 ) ) ;
#150453=CARTESIAN_POINT ( 'NONE',  ( 16.51473224551083163, -9.474510206698727899, 65.83442372801900433 ) ) ;
#150455=CARTESIAN_POINT ( 'NONE',  ( 0.05219959533907565091, 21.53943276465977519, 79.99890960531435269 ) ) ;
#150456=CARTESIAN_POINT ( 'NONE',  ( 5.049401038297881783, 19.05341960407617563, 42.29275706135234003 ) ) ;
#150457=CARTESIAN_POINT ( 'NONE',  ( -5.049401038298153566, 19.05341960407611168, 105.2072429386476671 ) ) ;
#150458=CARTESIAN_POINT ( 'NONE',  ( -17.49999999999999645, 4.013004640162621151, 115.4460572099441293 ) ) ;
#150459=CARTESIAN_POINT ( 'NONE',  ( -5.719274019375978568, 21.55341960407610458, 25.20724293864769550 ) ) ;
#150460=CARTESIAN_POINT ( 'NONE',  ( -9.474510206698964154, 16.51473224551069663, 75.41557627198103830 ) ) ;
#150461=CARTESIAN_POINT ( 'NONE',  ( 10.72451020669871369, 18.67979575497193778, 57.08442372801901854 ) ) ;
#150462=CARTESIAN_POINT ( 'NONE',  ( 9.564922557960805705, 16.46253265017160317, 29.58224293864769550 ) ) ;
#150463=CARTESIAN_POINT ( 'NONE',  ( 15.80617190586746368, 15.72974639402197994, 114.3739096053143527 ) ) ;
#150465=CARTESIAN_POINT ( 'NONE',  ( -5.823673210054431948, 21.52544592524334988, 37.70942372801900433 ) ) ;
#150466=ORIENTED_EDGE ( 'NONE', *, *, #12228, .F. ) ;
#150467=CARTESIAN_POINT ( 'NONE',  ( -13.89961937509977652, 13.97604488694528158, 95.62390960531436690 ) ) ;
#150469=CARTESIAN_POINT ( 'NONE',  ( -18.67979575497178146, -10.72451020669898902, 101.6655762719810383 ) ) ;
#150470=CARTESIAN_POINT ( 'NONE',  ( 16.51473224551069308, 9.474510206698969483, 64.16557627198102409 ) ) ;
#150471=CARTESIAN_POINT ( 'NONE',  ( 14.29746914071037800, 8.314922557961029526, 26.66775706135235424 ) ) ;
#150473=CARTESIAN_POINT ( 'NONE',  ( 21.52544592524334988, 5.823673210054432836, 101.4594237280190185 ) ) ;
#150474=CARTESIAN_POINT ( 'NONE',  ( 13.89961937509977652, -13.97604488694527269, 48.12390960531435979 ) ) ;
#150475=CARTESIAN_POINT ( 'NONE',  ( 5.823673210054444382, -21.52544592524334988, 100.2094237280190043 ) ) ;
#150476=CARTESIAN_POINT ( 'NONE',  ( -19.02544592524342804, 5.153800228976336051, 86.04057627198103830 ) ) ;
#150477=CARTESIAN_POINT ( 'NONE',  ( -18.67979575497193778, 10.72451020669871902, 53.33442372801901854 ) ) ;
#150479=CARTESIAN_POINT ( 'NONE',  ( -9.564922557960796823, -16.46253265017161027, 112.0822429386476955 ) ) ;
#150480=DIRECTION ( 'NONE',  ( -1.000000000000000000, 0.000000000000000000, -0.000000000000000000 ) ) ;
#150481=CARTESIAN_POINT ( 'NONE',  ( -4.483927247898782831, 16.52544592524335698, 57.70942372801901143 ) ) ;
#150482=CARTESIAN_POINT ( 'NONE',  ( -8.224510206698735004, -14.34966873604973081, 69.58442372801900433 ) ) ;
#150483=CARTESIAN_POINT ( 'NONE',  ( -21.55341960407619339, 5.719274019375674811, 63.54275706135234003 ) ) ;
#150484=CARTESIAN_POINT ( 'NONE',  ( -15.72974639402176322, -15.80617190586768395, 84.37609039468570415 ) ) ;
#150486=CARTESIAN_POINT ( 'NONE',  ( -12.14591786802326823, 12.06949235617739902, 28.12609039468568284 ) ) ;
#150487=CARTESIAN_POINT ( 'NONE',  ( -9.474510206698964154, 16.51473224551069663, 75.41557627198103830 ) ) ;
#150488=CARTESIAN_POINT ( 'NONE',  ( -19.02544592524342804, 5.153800228976336051, 106.0405762719810241 ) ) ;
#150489=CARTESIAN_POINT ( 'NONE',  ( 17.05116617787827238, 6.768360034955703597, 43.84324446740802017 ) ) ;
#150490=CARTESIAN_POINT ( 'NONE',  ( -13.97604488694527625, -13.89961937509977652, 21.87390960531435979 ) ) ;
#150491=CARTESIAN_POINT ( 'NONE',  ( 18.62759615963271287, -10.81492255796078972, 38.33224293864768839 ) ) ;
#150492=CARTESIAN_POINT ( 'NONE',  ( -4.379528057220086978, -16.55341960407618274, 89.79275706135236135 ) ) ;
#150493=CARTESIAN_POINT ( 'NONE',  ( 16.53943276465976808, -0.05219959533910856209, 88.74890960531436690 ) ) ;
#150494=CARTESIAN_POINT ( 'NONE',  ( -13.97604488694527625, -13.89961937509977652, 61.87390960531435979 ) ) ;
#150495=CARTESIAN_POINT ( 'NONE',  ( -18.62759615963255300, -10.81492255796106328, 84.16775706135234714 ) ) ;
#150497=CARTESIAN_POINT ( 'NONE',  ( -4.483927247898782831, 16.52544592524335698, 27.70942372801901854 ) ) ;
#150498=CARTESIAN_POINT ( 'NONE',  ( -4.379528057220328563, 16.55341960407611168, 70.20724293864769550 ) ) ;
#150499=CARTESIAN_POINT ( 'NONE',  ( -5.719274019375665041, -21.55341960407619695, 44.79275706135234714 ) ) ;
#150500=CARTESIAN_POINT ( 'NONE',  ( 18.67979575497178502, 10.72451020669898547, 69.16557627198102409 ) ) ;
#150501=CARTESIAN_POINT ( 'NONE',  ( 19.03943276465977164, 0.05219959533936151252, 41.25109039468566152 ) ) ;
#150502=CARTESIAN_POINT ( 'NONE',  ( -9.474510206698964154, 16.51473224551069663, 45.41557627198103120 ) ) ;
#150503=CARTESIAN_POINT ( 'NONE',  ( -16.51473224551069308, -9.474510206698971260, 86.66557627198102409 ) ) ;
#150504=CARTESIAN_POINT ( 'NONE',  ( 16.52544592524342804, -4.483927247898539470, 48.54057627198103120 ) ) ;
#150506=CARTESIAN_POINT ( 'NONE',  ( 0.05219959533910956823, 16.53943276465976808, 29.99890960531435979 ) ) ;
#150507=CARTESIAN_POINT ( 'NONE',  ( -14.34966873604972548, 8.224510206698743886, 113.3344237280190328 ) ) ;
#150508=CARTESIAN_POINT ( 'NONE',  ( 0.05219959533936267826, -19.03943276465977164, 65.00109039468567573 ) ) ;
#150509=CARTESIAN_POINT ( 'NONE',  ( 16.62475595723695321, 7.163666690055254804, 46.97286648189537317 ) ) ;
#150510=CARTESIAN_POINT ( 'NONE',  ( -15.72974639402197994, 15.80617190586746368, 25.62390960531435624 ) ) ;
#150511=CARTESIAN_POINT ( 'NONE',  ( -8.314922557960811034, -14.29746914071050412, 87.08224293864769550 ) ) ;
#150513=CARTESIAN_POINT ( 'NONE',  ( 19.02544592524343514, -5.153800228976328945, 43.54057627198103120 ) ) ;
#150514=CARTESIAN_POINT ( 'NONE',  ( -5.823673210054116645, -21.52544592524344225, 32.29057627198102409 ) ) ;
#150515=CARTESIAN_POINT ( 'NONE',  ( 18.62759615963271287, -10.81492255796078972, 63.33224293864770260 ) ) ;
#150516=CARTESIAN_POINT ( 'NONE',  ( -16.52544592524342804, 4.483927247898546575, 106.0405762719810525 ) ) ;
#150517=CARTESIAN_POINT ( 'NONE',  ( 14.34966873604972726, -8.224510206698740333, 70.83442372801901854 ) ) ;
#150518=CARTESIAN_POINT ( 'NONE',  ( 16.46253265017160672, -9.564922557960803928, 53.33224293864768839 ) ) ;
#150519=CARTESIAN_POINT ( 'NONE',  ( -5.719274019375665041, -21.55341960407619695, 59.79275706135234714 ) ) ;
#150520=CARTESIAN_POINT ( 'NONE',  ( 8.224510206698953496, -14.34966873604960469, 102.9155762719810383 ) ) ;
#150521=CARTESIAN_POINT ( 'NONE',  ( 13.97604488694548053, -13.89961937509957401, 90.62609039468567573 ) ) ;
#150524=CARTESIAN_POINT ( 'NONE',  ( 5.719274019375991003, -21.55341960407610458, 37.70724293864769550 ) ) ;
#150525=CARTESIAN_POINT ( 'NONE',  ( -19.03943276465977164, 0.05219959533909376836, 116.2489096053143669 ) ) ;
#150526=CARTESIAN_POINT ( 'NONE',  ( -10.81492255796105439, 18.62759615963255655, 72.91775706135234714 ) ) ;
#150527=CARTESIAN_POINT ( 'NONE',  ( 8.224510206698742110, 14.34966873604972548, 52.08442372801901854 ) ) ;
#150528=CARTESIAN_POINT ( 'NONE',  ( 12.06949235617757843, -12.14591786802309237, 48.12390960531436690 ) ) ;
#150529=CARTESIAN_POINT ( 'NONE',  ( -0.05219959533907301413, -21.53943276465977519, 62.49890960531436690 ) ) ;
#150530=CARTESIAN_POINT ( 'NONE',  ( 21.53943276465977519, -0.05219959533907433946, 63.74890960531435979 ) ) ;
#150531=CARTESIAN_POINT ( 'NONE',  ( -16.46253265017146816, -9.564922557961047289, 89.16775706135234714 ) ) ;
#150532=CARTESIAN_POINT ( 'NONE',  ( 19.02544592524343514, -5.153800228976328945, 108.5405762719810383 ) ) ;
#150533=CARTESIAN_POINT ( 'NONE',  ( -9.474510206698964154, 16.51473224551069663, 55.41557627198103120 ) ) ;
#150534=CARTESIAN_POINT ( 'NONE',  ( -5.153800228976328057, -19.02544592524343514, 22.29057627198102765 ) ) ;
#150535=CARTESIAN_POINT ( 'NONE',  ( -16.51473224551069308, -9.474510206698971260, 111.6655762719810383 ) ) ;
#150537=CARTESIAN_POINT ( 'NONE',  ( 16.55341960407618274, -4.379528057220086978, 71.04275706135234714 ) ) ;
#150538=CARTESIAN_POINT ( 'NONE',  ( -10.81492255796078084, -18.62759615963271287, 107.0822429386476955 ) ) ;
#150539=CARTESIAN_POINT ( 'NONE',  ( -5.049401038298153566, 19.05341960407611168, 70.20724293864769550 ) ) ;
#150540=CARTESIAN_POINT ( 'NONE',  ( 21.53943276465977519, 0.05219959533937863772, 46.25109039468567573 ) ) ;
#150541=CARTESIAN_POINT ( 'NONE',  ( -13.89961937509977652, 13.97604488694528158, 95.62390960531436690 ) ) ;
#150545=CARTESIAN_POINT ( 'NONE',  ( -18.67979575497193778, 10.72451020669871902, 38.33442372801900433 ) ) ;
#150546=CARTESIAN_POINT ( 'NONE',  ( 9.564922557960805705, 16.46253265017160317, 29.58224293864769550 ) ) ;
#150547=CARTESIAN_POINT ( 'NONE',  ( -16.51473224551082808, 9.474510206698731452, 83.33442372801899012 ) ) ;
#150548=CARTESIAN_POINT ( 'NONE',  ( -0.05219959533936034679, 19.03943276465977164, 42.50109039468566152 ) ) ;
#150549=CARTESIAN_POINT ( 'NONE',  ( 5.719274019375673035, 21.55341960407619339, 22.29275706135235069 ) ) ;
#150550=CARTESIAN_POINT ( 'NONE',  ( -9.564922557961040184, 16.46253265017147172, 37.91775706135233293 ) ) ;
#150551=CARTESIAN_POINT ( 'NONE',  ( -5.153800228976607833, 19.02544592524334988, 47.70942372801900433 ) ) ;
#150552=CARTESIAN_POINT ( 'NONE',  ( 16.52544592524335698, 4.483927247898782831, 91.45942372801901854 ) ) ;
#150555=CARTESIAN_POINT ( 'NONE',  ( -13.97604488694527625, -13.89961937509977652, 66.87390960531436690 ) ) ;
#150557=CARTESIAN_POINT ( 'NONE',  ( 15.80617190586769283, -15.72974639402175789, 85.62609039468568994 ) ) ;
#150558=CARTESIAN_POINT ( 'NONE',  ( -10.81492255796105439, 18.62759615963255655, 97.91775706135236135 ) ) ;
#150560=CARTESIAN_POINT ( 'NONE',  ( 19.02544592524343514, -5.153800228976328945, 88.54057627198102409 ) ) ;
#150561=CARTESIAN_POINT ( 'NONE',  ( 21.52544592524334988, 5.823673210054432836, 61.45942372801901854 ) ) ;
#150562=CARTESIAN_POINT ( 'NONE',  ( -5.153800228976607833, 19.02544592524334988, 102.7094237280189759 ) ) ;
#150563=CARTESIAN_POINT ( 'NONE',  ( 9.474510206698971260, -16.51473224551069308, 67.91557627198102409 ) ) ;
#150564=CARTESIAN_POINT ( 'NONE',  ( 18.62759615963271287, -10.81492255796078972, 23.33224293864769194 ) ) ;
#150565=CARTESIAN_POINT ( 'NONE',  ( 16.46253265017160672, -9.564922557960803928, 78.33224293864769550 ) ) ;
#150566=CARTESIAN_POINT ( 'NONE',  ( 13.89961937509978007, -13.97604488694527269, 78.12390960531435269 ) ) ;
#150567=CARTESIAN_POINT ( 'NONE',  ( 16.46253265017160672, -9.564922557960803928, 68.33224293864770971 ) ) ;
#150568=CARTESIAN_POINT ( 'NONE',  ( -16.46253265017160317, 9.564922557960807481, 50.83224293864770260 ) ) ;
#150569=CARTESIAN_POINT ( 'NONE',  ( -18.62759615963270932, 10.81492255796079327, 110.8322429386476955 ) ) ;
#150570=CARTESIAN_POINT ( 'NONE',  ( 8.314922557961029526, -14.29746914071037800, 85.41775706135236135 ) ) ;
#150572=CARTESIAN_POINT ( 'NONE',  ( -5.049401038297874678, -19.05341960407617918, 59.79275706135231871 ) ) ;
#150573=CARTESIAN_POINT ( 'NONE',  ( 0.05219959533909260263, 19.03943276465977164, 79.99890960531436690 ) ) ;
#150574=CARTESIAN_POINT ( 'NONE',  ( 14.29746914071049879, -8.314922557960816363, 78.33224293864770971 ) ) ;
#150575=CARTESIAN_POINT ( 'NONE',  ( 4.379528057220339221, -16.55341960407611168, 112.7072429386476955 ) ) ;
#150576=CARTESIAN_POINT ( 'NONE',  ( 16.46253265017160672, -9.564922557960803928, 113.3322429386476955 ) ) ;
#150577=CARTESIAN_POINT ( 'NONE',  ( -16.46253265017160317, 9.564922557960807481, 110.8322429386476955 ) ) ;
#150578=CARTESIAN_POINT ( 'NONE',  ( -8.224510206698948167, 14.34966873604960824, 75.41557627198102409 ) ) ;
#150579=CARTESIAN_POINT ( 'NONE',  ( 13.97604488694527802, 13.89961937509977652, 114.3739096053143669 ) ) ;
#150580=CARTESIAN_POINT ( 'NONE',  ( -5.049401038297874678, -19.05341960407617918, 29.79275706135232227 ) ) ;
#150581=CARTESIAN_POINT ( 'NONE',  ( 14.34966873604972726, -8.224510206698740333, 105.8344237280190328 ) ) ;
#150582=CARTESIAN_POINT ( 'NONE',  ( 9.474510206698971260, -16.51473224551069308, 87.91557627198102409 ) ) ;
#150583=CARTESIAN_POINT ( 'NONE',  ( -21.55341960407619339, 5.719274019375674811, 53.54275706135234714 ) ) ;
#150584=CARTESIAN_POINT ( 'NONE',  ( 5.719274019375991003, -21.55341960407610458, 42.70724293864770260 ) ) ;
#150585=CARTESIAN_POINT ( 'NONE',  ( 18.62759615963255655, 10.81492255796105972, 21.66775706135235069 ) ) ;
#150586=CARTESIAN_POINT ( 'NONE',  ( 21.55341960407610458, 5.719274019375980345, 63.95724293864770260 ) ) ;
#150587=CARTESIAN_POINT ( 'NONE',  ( 16.52544592524342804, -4.483927247898539470, 88.54057627198103830 ) ) ;
#150588=CARTESIAN_POINT ( 'NONE',  ( -0.05219959533936034679, 19.03943276465977164, 52.50109039468566863 ) ) ;
#150589=CARTESIAN_POINT ( 'NONE',  ( -19.02544592524342804, 5.153800228976336051, 26.04057627198103120 ) ) ;
#150590=CARTESIAN_POINT ( 'NONE',  ( 19.02544592524343514, -5.153800228976328945, 83.54057627198100988 ) ) ;
#150591=CARTESIAN_POINT ( 'NONE',  ( 9.564922557960805705, 16.46253265017160317, 79.58224293864769550 ) ) ;
#150592=CARTESIAN_POINT ( 'NONE',  ( -16.52544592524342804, 4.483927247898546575, 106.0405762719810525 ) ) ;
#150594=VECTOR ( 'NONE', #168124, 1000.000000000000000 ) ;
#150595=CARTESIAN_POINT ( 'NONE',  ( -4.379528057220328563, 16.55341960407611168, 30.20724293864769550 ) ) ;
#150596=CARTESIAN_POINT ( 'NONE',  ( 8.224510206698742110, 14.34966873604972548, 42.08442372801901854 ) ) ;
#150597=CARTESIAN_POINT ( 'NONE',  ( 10.72451020669871369, 18.67979575497193778, 112.0844237280190185 ) ) ;
#150598=CARTESIAN_POINT ( 'NONE',  ( -19.05341960407611168, -5.049401038298163336, 96.45724293864769550 ) ) ;
#150599=CARTESIAN_POINT ( 'NONE',  ( -18.62759615963255300, -10.81492255796106328, 39.16775706135235424 ) ) ;
#150600=CARTESIAN_POINT ( 'NONE',  ( 13.89961937509977652, -13.97604488694527269, 43.12390960531434558 ) ) ;
#150602=CARTESIAN_POINT ( 'NONE',  ( -16.55341960407617563, 4.379528057220093196, 48.54275706135234714 ) ) ;
#150603=CARTESIAN_POINT ( 'NONE',  ( -16.52544592524335698, -4.483927247898792601, 78.95942372801901854 ) ) ;
#150604=CARTESIAN_POINT ( 'NONE',  ( -0.05219959533936034679, 19.03943276465977164, 112.5010903946856757 ) ) ;
#150605=CARTESIAN_POINT ( 'NONE',  ( -9.564922557960796823, -16.46253265017161027, 37.08224293864768839 ) ) ;
#150606=CARTESIAN_POINT ( 'NONE',  ( -8.314922557960811034, -14.29746914071050412, 92.08224293864769550 ) ) ;
#150607=CARTESIAN_POINT ( 'NONE',  ( 5.823673210054125526, 21.52544592524343514, 109.7905762719810383 ) ) ;
#150608=CARTESIAN_POINT ( 'NONE',  ( 19.02544592524334988, 5.153800228976608722, 86.45942372801900433 ) ) ;
#150609=CARTESIAN_POINT ( 'NONE',  ( 16.51473224551069308, 9.474510206698969483, 34.16557627198102409 ) ) ;
#150610=CARTESIAN_POINT ( 'NONE',  ( 19.03943276465977164, -0.05219959533909143690, 93.74890960531435269 ) ) ;
#150611=CARTESIAN_POINT ( 'NONE',  ( 15.72974639402176855, 15.80617190586768217, 26.87609039468567218 ) ) ;
#150613=CARTESIAN_POINT ( 'NONE',  ( 13.89961937509977652, -13.97604488694527269, 98.12390960531433848 ) ) ;
#150614=CARTESIAN_POINT ( 'NONE',  ( 16.29526858892874941, -7.335722546920136367, 111.7032940219980048 ) ) ;
#150615=CARTESIAN_POINT ( 'NONE',  ( 16.46253265017160672, -9.564922557960803928, 88.33224293864769550 ) ) ;
#150616=CARTESIAN_POINT ( 'NONE',  ( -21.52544592524334988, -5.823673210054445271, 38.95942372801901854 ) ) ;
#150617=CARTESIAN_POINT ( 'NONE',  ( -12.06949235617756955, 12.14591786802309770, 85.62390960531436690 ) ) ;
#150618=CARTESIAN_POINT ( 'NONE',  ( -19.02544592524342804, 5.153800228976336051, 96.04057627198103830 ) ) ;
#150619=CARTESIAN_POINT ( 'NONE',  ( -19.03943276465977164, -0.05219959533935918106, 18.75109039468567218 ) ) ;
#150620=CARTESIAN_POINT ( 'NONE',  ( 0.05219959533934541429, -16.53943276465976808, 55.00109039468568284 ) ) ;
#150621=CARTESIAN_POINT ( 'NONE',  ( 10.81492255796106328, -18.62759615963255655, 80.41775706135234714 ) ) ;
#150622=CARTESIAN_POINT ( 'NONE',  ( 14.29746914071037800, 8.314922557961029526, 41.66775706135235424 ) ) ;
#150623=CARTESIAN_POINT ( 'NONE',  ( 9.474510206698971260, -16.51473224551069308, 67.91557627198102409 ) ) ;
#150624=CARTESIAN_POINT ( 'NONE',  ( 19.05341960407617918, -5.049401038297876454, 91.04275706135234714 ) ) ;
#150625=CARTESIAN_POINT ( 'NONE',  ( -12.14591786802326823, 12.06949235617739902, 68.12609039468567573 ) ) ;
#150626=CARTESIAN_POINT ( 'NONE',  ( -15.80617190586768217, 15.72974639402176855, 108.1260903946856757 ) ) ;
#150627=CARTESIAN_POINT ( 'NONE',  ( 16.46253265017146816, 9.564922557961045513, 81.66775706135233293 ) ) ;
#150628=CARTESIAN_POINT ( 'NONE',  ( -9.474510206698964154, 16.51473224551069663, 60.41557627198102409 ) ) ;
#150629=CARTESIAN_POINT ( 'NONE',  ( 10.81492255796078972, 18.62759615963270932, 79.58224293864769550 ) ) ;
#150630=CARTESIAN_POINT ( 'NONE',  ( -16.55341960407611168, -4.379528057220339221, 81.45724293864769550 ) ) ;
#150631=CARTESIAN_POINT ( 'NONE',  ( -19.05341960407617563, 5.049401038297882671, 83.54275706135233293 ) ) ;
#150632=CARTESIAN_POINT ( 'NONE',  ( -18.87580814761074777, 5.500000000000053291, 80.87172394265761000 ) ) ;
#150633=CARTESIAN_POINT ( 'NONE',  ( -0.05219959533936034679, 19.03943276465977164, 62.50109039468566863 ) ) ;
#150634=CARTESIAN_POINT ( 'NONE',  ( 16.53943276465976808, 0.05219959533934440121, 111.2510903946856899 ) ) ;
#150635=CARTESIAN_POINT ( 'NONE',  ( 8.224510206698953496, -14.34966873604960469, 82.91557627198103830 ) ) ;
#150636=CARTESIAN_POINT ( 'NONE',  ( 9.474510206698729675, 16.51473224551082808, 27.08442372801900433 ) ) ;
#150638=CARTESIAN_POINT ( 'NONE',  ( 21.52544592524344225, -5.823673210054117533, 113.5405762719810383 ) ) ;
#150639=CARTESIAN_POINT ( 'NONE',  ( 19.02544592524343514, -5.153800228976328945, 98.54057627198100988 ) ) ;
#150640=CARTESIAN_POINT ( 'NONE',  ( 19.05341960407611168, 5.049401038298154454, 73.95724293864768129 ) ) ;
#150641=CARTESIAN_POINT ( 'NONE',  ( 21.55341960407619695, -5.719274019375665929, 81.04275706135236135 ) ) ;
#150642=CARTESIAN_POINT ( 'NONE',  ( 5.049401038298161559, -19.05341960407611168, 57.70724293864769550 ) ) ;
#150643=CARTESIAN_POINT ( 'NONE',  ( 16.46253265017160672, -9.564922557960803928, 38.33224293864768839 ) ) ;
#150644=CARTESIAN_POINT ( 'NONE',  ( 21.53943276465977519, -0.05219959533907433946, 33.74890960531436690 ) ) ;
#150645=CARTESIAN_POINT ( 'NONE',  ( -8.224510206698948167, 14.34966873604960824, 75.41557627198102409 ) ) ;
#150646=CARTESIAN_POINT ( 'NONE',  ( -13.97604488694527625, -13.89961937509977652, 41.87390960531435979 ) ) ;
#150647=CARTESIAN_POINT ( 'NONE',  ( -12.06949235617756955, 12.14591786802309770, 95.62390960531436690 ) ) ;
#150648=CARTESIAN_POINT ( 'NONE',  ( 5.823673210054125526, 21.52544592524343514, 109.7905762719810383 ) ) ;
#150649=CARTESIAN_POINT ( 'NONE',  ( -21.55341960407619339, 5.719274019375674811, 53.54275706135234714 ) ) ;
#150650=CARTESIAN_POINT ( 'NONE',  ( 13.97604488694527802, 13.89961937509977652, 24.37390960531435624 ) ) ;
#150651=CARTESIAN_POINT ( 'NONE',  ( 14.34966873604972726, -8.224510206698740333, 65.83442372801900433 ) ) ;
#150652=CARTESIAN_POINT ( 'NONE',  ( 18.62759615963271287, -10.81492255796078972, 98.33224293864769550 ) ) ;
#150653=CARTESIAN_POINT ( 'NONE',  ( -21.53943276465977519, 0.05219959533907696930, 101.2489096053143669 ) ) ;
#150654=CARTESIAN_POINT ( 'NONE',  ( 19.05341960407617918, -5.049401038297876454, 41.04275706135233293 ) ) ;
#150655=CARTESIAN_POINT ( 'NONE',  ( -5.153800228976328057, -19.02544592524343514, 47.29057627198102409 ) ) ;
#150656=CARTESIAN_POINT ( 'NONE',  ( 19.03943276465977164, -0.05219959533909143690, 113.7489096053143669 ) ) ;
#150657=CARTESIAN_POINT ( 'NONE',  ( 0.05219959533937995610, -21.53943276465977519, 60.00109039468568284 ) ) ;
#150658=CARTESIAN_POINT ( 'NONE',  ( 5.719274019375991003, -21.55341960407610458, 52.70724293864769550 ) ) ;
#150659=CARTESIAN_POINT ( 'NONE',  ( 14.29746914071049879, -8.314922557960816363, 43.33224293864769550 ) ) ;
#150660=CARTESIAN_POINT ( 'NONE',  ( 21.53943276465977519, 0.05219959533937863772, 81.25109039468568994 ) ) ;
#150661=CARTESIAN_POINT ( 'NONE',  ( -5.719274019375665041, -21.55341960407619695, 109.7927570613523613 ) ) ;
#150662=CARTESIAN_POINT ( 'NONE',  ( -16.51473224551082808, 9.474510206698731452, 43.33442372801900433 ) ) ;
#150663=CARTESIAN_POINT ( 'NONE',  ( -4.483927247898782831, 16.52544592524335698, 102.7094237280190185 ) ) ;
#150664=CARTESIAN_POINT ( 'NONE',  ( 0.05219959533937995610, -21.53943276465977519, 60.00109039468568284 ) ) ;
#150665=CARTESIAN_POINT ( 'NONE',  ( -0.05219959533909027116, -19.03943276465977164, 57.49890960531435979 ) ) ;
#150666=CARTESIAN_POINT ( 'NONE',  ( -19.03943276465977164, -0.05219959533935918106, 28.75109039468566507 ) ) ;
#150667=CARTESIAN_POINT ( 'NONE',  ( -10.81492255796078084, -18.62759615963271287, 37.08224293864768129 ) ) ;
#150668=CARTESIAN_POINT ( 'NONE',  ( -15.72974639402176322, -15.80617190586768395, 29.37609039468568284 ) ) ;
#150669=CARTESIAN_POINT ( 'NONE',  ( 10.81492255796078972, 18.62759615963270932, 89.58224293864768129 ) ) ;
#150670=CARTESIAN_POINT ( 'NONE',  ( 13.97604488694548053, -13.89961937509957401, 90.62609039468567573 ) ) ;
#150671=CARTESIAN_POINT ( 'NONE',  ( -12.06949235617739369, -12.14591786802326823, 59.37609039468568284 ) ) ;
#150672=CARTESIAN_POINT ( 'NONE',  ( -19.03943276465977164, -0.05219959533935946555, 18.75109039468567218 ) ) ;
#150673=CARTESIAN_POINT ( 'NONE',  ( 0.05219959533907565091, 21.53943276465977519, 99.99890960531436690 ) ) ;
#150674=CARTESIAN_POINT ( 'NONE',  ( 16.55341960407618274, -4.379528057220086978, 81.04275706135236135 ) ) ;
#150675=CARTESIAN_POINT ( 'NONE',  ( 16.52544592524342804, -4.483927247898539470, 73.54057627198102409 ) ) ;
#150676=CARTESIAN_POINT ( 'NONE',  ( -16.20579543436678449, -7.371946100355109444, 100.5652083417188152 ) ) ;
#150677=CARTESIAN_POINT ( 'NONE',  ( 5.153800228976615827, -19.02544592524334988, 110.2094237280189901 ) ) ;
#150679=CARTESIAN_POINT ( 'NONE',  ( 0.05219959533907565091, 21.53943276465977519, 29.99890960531435979 ) ) ;
#150681=CARTESIAN_POINT ( 'NONE',  ( 8.224510206698742110, 14.34966873604972548, 52.08442372801901854 ) ) ;
#150682=CARTESIAN_POINT ( 'NONE',  ( 5.719274019375673035, 21.55341960407619339, 32.29275706135235424 ) ) ;
#150683=CARTESIAN_POINT ( 'NONE',  ( -15.80617190586745835, -15.72974639402198527, 51.87390960531437401 ) ) ;
#150684=CARTESIAN_POINT ( 'NONE',  ( 8.224510206698742110, 14.34966873604972548, 67.08442372801901854 ) ) ;
#150685=CARTESIAN_POINT ( 'NONE',  ( 13.89961937509977652, -13.97604488694527269, 83.12390960531436690 ) ) ;
#150686=CARTESIAN_POINT ( 'NONE',  ( -5.823673210054431948, 21.52544592524334988, 52.70942372801902565 ) ) ;
#150687=CARTESIAN_POINT ( 'NONE',  ( -5.049401038298153566, 19.05341960407611168, 30.20724293864768839 ) ) ;
#150688=CARTESIAN_POINT ( 'NONE',  ( 0.05219959533907565091, 21.53943276465977519, 29.99890960531435979 ) ) ;
#150690=CARTESIAN_POINT ( 'NONE',  ( -9.474510206698720793, -16.51473224551083518, 39.58442372801899722 ) ) ;
#150691=CARTESIAN_POINT ( 'NONE',  ( -0.05219959533934338120, 16.53943276465976808, 47.50109039468568994 ) ) ;
#150692=CARTESIAN_POINT ( 'NONE',  ( 21.52544592524344225, -5.823673210054117533, 23.54057627198102765 ) ) ;
#150694=CARTESIAN_POINT ( 'NONE',  ( -9.564922557960796823, -16.46253265017161027, 87.08224293864769550 ) ) ;
#150695=CARTESIAN_POINT ( 'NONE',  ( 16.52544592524335698, 4.483927247898782831, 96.45942372801901854 ) ) ;
#150697=CARTESIAN_POINT ( 'NONE',  ( 0.05219959533910956823, 16.53943276465976808, 99.99890960531436690 ) ) ;
#150698=CARTESIAN_POINT ( 'NONE',  ( -21.55341960407610458, -5.719274019375992779, 31.45724293864769550 ) ) ;
#150699=CARTESIAN_POINT ( 'NONE',  ( -0.05219959533909027116, -19.03943276465977164, 37.49890960531436690 ) ) ;
#150700=CARTESIAN_POINT ( 'NONE',  ( 16.53943276465976808, 0.05219959533934440121, 76.25109039468568994 ) ) ;
#150701=CARTESIAN_POINT ( 'NONE',  ( 10.72451020669871369, 18.67979575497193778, 22.08442372801901143 ) ) ;
#150702=CARTESIAN_POINT ( 'NONE',  ( -13.97604488694547697, 13.89961937509957934, 83.12609039468564731 ) ) ;
#150703=CARTESIAN_POINT ( 'NONE',  ( -13.97604488694527625, -13.89961937509977652, 46.87390960531435979 ) ) ;
#150705=CARTESIAN_POINT ( 'NONE',  ( 16.46253265017160672, -9.564922557960803928, 113.3322429386476955 ) ) ;
#150706=CARTESIAN_POINT ( 'NONE',  ( 15.72974639402176855, 15.80617190586768217, 111.8760903946856615 ) ) ;
#150707=CARTESIAN_POINT ( 'NONE',  ( 16.51473224551069308, 9.474510206698969483, 59.16557627198102409 ) ) ;
#150708=CARTESIAN_POINT ( 'NONE',  ( 4.483927247898790824, -16.52544592524335698, 45.20942372801901854 ) ) ;
#150709=CARTESIAN_POINT ( 'NONE',  ( -21.53943276465977519, -0.05219959533937600094, 93.75109039468567573 ) ) ;
#150710=CARTESIAN_POINT ( 'NONE',  ( 19.02544592524334988, 5.153800228976608722, 41.45942372801900433 ) ) ;
#150711=CARTESIAN_POINT ( 'NONE',  ( -5.153800228976607833, 19.02544592524334988, 57.70942372801899012 ) ) ;
#150713=CARTESIAN_POINT ( 'NONE',  ( -15.72974639402176322, -15.80617190586768395, 44.37609039468567573 ) ) ;
#150714=CARTESIAN_POINT ( 'NONE',  ( -17.58332526062525858, 7.635886036038558977, 55.92334959558466068 ) ) ;
#150715=CARTESIAN_POINT ( 'NONE',  ( -19.02544592524334988, -5.153800228976617603, 43.95942372801899012 ) ) ;
#150716=CARTESIAN_POINT ( 'NONE',  ( 9.564922557960805705, 16.46253265017160317, 99.58224293864770971 ) ) ;
#150717=CARTESIAN_POINT ( 'NONE',  ( 16.46253265017160672, -9.564922557960803928, 78.33224293864769550 ) ) ;
#150718=CARTESIAN_POINT ( 'NONE',  ( -16.55341960407611168, -4.379528057220339221, 31.45724293864769550 ) ) ;
#150719=CARTESIAN_POINT ( 'NONE',  ( -10.72451020669898014, 18.67979575497178502, 35.41557627198102409 ) ) ;
#150722=CARTESIAN_POINT ( 'NONE',  ( -15.80617190586768217, 15.72974639402176855, 93.12609039468568994 ) ) ;
#150724=CARTESIAN_POINT ( 'NONE',  ( 16.51473224551069308, 9.474510206698969483, 34.16557627198102409 ) ) ;
#150725=CARTESIAN_POINT ( 'NONE',  ( 13.97604488694527802, 13.89961937509977652, 109.3739096053143669 ) ) ;
#150727=CARTESIAN_POINT ( 'NONE',  ( 16.55341960407618274, -4.379528057220086978, 61.04275706135234714 ) ) ;
#150728=CARTESIAN_POINT ( 'NONE',  ( -5.719274019375978568, 21.55341960407610458, 85.20724293864770971 ) ) ;
#150729=CARTESIAN_POINT ( 'NONE',  ( 14.34966873604960469, 8.224510206698951720, 44.16557627198103120 ) ) ;
#150730=CARTESIAN_POINT ( 'NONE',  ( 5.049401038298161559, -19.05341960407611168, 32.70724293864768129 ) ) ;
#150731=CARTESIAN_POINT ( 'NONE',  ( 19.03943276465977164, -0.05219959533909143690, 108.7489096053143527 ) ) ;
#150732=CARTESIAN_POINT ( 'NONE',  ( -18.67979575497193778, 10.72451020669871902, 23.33442372801901499 ) ) ;
#150733=CARTESIAN_POINT ( 'NONE',  ( -5.049401038297874678, -19.05341960407617918, 39.79275706135232582 ) ) ;
#150734=CARTESIAN_POINT ( 'NONE',  ( 9.564922557960805705, 16.46253265017160317, 39.58224293864768839 ) ) ;
#150735=CARTESIAN_POINT ( 'NONE',  ( 21.52544592524334988, 5.823673210054432836, 86.45942372801901854 ) ) ;
#150737=CARTESIAN_POINT ( 'NONE',  ( -8.314922557960811034, -14.29746914071050412, 22.08224293864769194 ) ) ;
#150739=CARTESIAN_POINT ( 'NONE',  ( 15.72974639402199770, -15.80617190586745480, 33.12390960531435979 ) ) ;
#150740=CARTESIAN_POINT ( 'NONE',  ( 12.06949235617757843, -12.14591786802309237, 108.1239096053143811 ) ) ;
#150743=CARTESIAN_POINT ( 'NONE',  ( -5.153800228976328057, -19.02544592524343514, 87.29057627198103830 ) ) ;
#150744=CARTESIAN_POINT ( 'NONE',  ( -16.53943276465976808, 0.05219959533911058130, 76.24890960531435269 ) ) ;
#150745=CARTESIAN_POINT ( 'NONE',  ( -5.153800228976607833, 19.02544592524334988, 107.7094237280189759 ) ) ;
#150746=ADVANCED_FACE ( 'NONE', ( #115295 ), #194153, .T. ) ;
#150747=CARTESIAN_POINT ( 'NONE',  ( 18.67979575497178502, 10.72451020669898547, 64.16557627198102409 ) ) ;
#150749=CARTESIAN_POINT ( 'NONE',  ( 16.51473224551069308, 9.474510206698969483, 29.16557627198103475 ) ) ;
#150750=CARTESIAN_POINT ( 'NONE',  ( 13.97604488694527802, 13.89961937509977652, 84.37390960531433848 ) ) ;
#150751=CARTESIAN_POINT ( 'NONE',  ( -21.52544592524343514, 5.823673210054127303, 91.04057627198103830 ) ) ;
#150752=CARTESIAN_POINT ( 'NONE',  ( -12.06949235617739369, -12.14591786802326823, 99.37609039468568994 ) ) ;
#150753=CARTESIAN_POINT ( 'NONE',  ( -0.05219959533909027116, -19.03943276465977164, 92.49890960531436690 ) ) ;
#150754=CARTESIAN_POINT ( 'NONE',  ( 5.049401038297881783, 19.05341960407617563, 82.29275706135229029 ) ) ;
#150755=CARTESIAN_POINT ( 'NONE',  ( 21.55341960407619695, -5.719274019375665929, 101.0427570613523756 ) ) ;
#150756=CARTESIAN_POINT ( 'NONE',  ( 5.823673210054125526, 21.52544592524343514, 79.79057627198102409 ) ) ;
#150757=CARTESIAN_POINT ( 'NONE',  ( -15.80617190586745835, -15.72974639402198527, 36.87390960531435979 ) ) ;
#150758=CARTESIAN_POINT ( 'NONE',  ( -5.153800228976328057, -19.02544592524343514, 47.29057627198102409 ) ) ;
#150759=CARTESIAN_POINT ( 'NONE',  ( 8.224510206698742110, 14.34966873604972548, 112.0844237280190185 ) ) ;
#150760=CARTESIAN_POINT ( 'NONE',  ( 16.51473224551069308, 9.474510206698969483, 69.16557627198102409 ) ) ;
#150761=CARTESIAN_POINT ( 'NONE',  ( 17.58332526062524437, 7.635886036038643354, 81.57665040441534643 ) ) ;
#150762=CARTESIAN_POINT ( 'NONE',  ( 15.72974639402176855, 15.80617190586768217, 106.8760903946856899 ) ) ;
#150763=CARTESIAN_POINT ( 'NONE',  ( -14.34966873604960291, -8.224510206698953496, 76.66557627198103830 ) ) ;
#150764=CARTESIAN_POINT ( 'NONE',  ( 18.62759615963271287, -10.81492255796078972, 108.3322429386477097 ) ) ;
#150765=CARTESIAN_POINT ( 'NONE',  ( -21.52544592524343514, 5.823673210054127303, 111.0405762719810525 ) ) ;
#150766=CARTESIAN_POINT ( 'NONE',  ( -17.49999999999999645, 5.499999999999997335, 120.0000000000000142 ) ) ;
#150767=CARTESIAN_POINT ( 'NONE',  ( -5.823673210054116645, -21.52544592524344225, 57.29057627198103120 ) ) ;
#150768=CARTESIAN_POINT ( 'NONE',  ( 14.29746914071037800, 8.314922557961029526, 96.66775706135234714 ) ) ;
#150769=CARTESIAN_POINT ( 'NONE',  ( -16.52544592524342804, 4.483927247898546575, 111.0405762719810525 ) ) ;
#150770=CARTESIAN_POINT ( 'NONE',  ( -9.474510206698964154, 16.51473224551069663, 55.41557627198103120 ) ) ;
#150772=CARTESIAN_POINT ( 'NONE',  ( 16.53943276465976808, 0.05219959533934440121, 106.2510903946856757 ) ) ;
#150774=CARTESIAN_POINT ( 'NONE',  ( 5.823673210054444382, -21.52544592524334988, 50.20942372801901854 ) ) ;
#150775=CARTESIAN_POINT ( 'NONE',  ( 19.02544592524343514, -5.153800228976328945, 108.5405762719810383 ) ) ;
#150776=CARTESIAN_POINT ( 'NONE',  ( -0.05219959533937732626, 21.53943276465977519, 82.50109039468568994 ) ) ;
#150777=CARTESIAN_POINT ( 'NONE',  ( 13.97604488694527802, 13.89961937509977652, 29.37390960531435979 ) ) ;
#150778=CARTESIAN_POINT ( 'NONE',  ( 19.03943276465977164, -0.05219959533909143690, 43.74890960531435979 ) ) ;
#150780=CARTESIAN_POINT ( 'NONE',  ( 5.719274019375673035, 21.55341960407619339, 77.29275706135234714 ) ) ;
#150781=CARTESIAN_POINT ( 'NONE',  ( -5.823673210054431948, 21.52544592524334988, 67.70942372801901854 ) ) ;
#150782=CARTESIAN_POINT ( 'NONE',  ( -9.474510206698964154, 16.51473224551069663, 105.4155762719810383 ) ) ;
#150783=CARTESIAN_POINT ( 'NONE',  ( -5.049401038297874678, -19.05341960407617918, 74.79275706135231871 ) ) ;
#150784=CARTESIAN_POINT ( 'NONE',  ( -15.72974639402176322, -15.80617190586768395, 54.37609039468568994 ) ) ;
#150785=CARTESIAN_POINT ( 'NONE',  ( -0.05219959533934338120, 16.53943276465976808, 27.50109039468567929 ) ) ;
#150786=CARTESIAN_POINT ( 'NONE',  ( -9.564922557961040184, 16.46253265017147172, 72.91775706135233293 ) ) ;
#150787=CARTESIAN_POINT ( 'NONE',  ( -16.51473224551069308, -9.474510206698971260, 51.66557627198102409 ) ) ;
#150788=CARTESIAN_POINT ( 'NONE',  ( -13.97604488694547697, 13.89961937509957934, 78.12609039468567573 ) ) ;
#150789=CARTESIAN_POINT ( 'NONE',  ( 8.224510206698742110, 14.34966873604972548, 112.0844237280190185 ) ) ;
#150790=CARTESIAN_POINT ( 'NONE',  ( -16.46253265017146816, -9.564922557961047289, 94.16775706135233293 ) ) ;
#150791=CARTESIAN_POINT ( 'NONE',  ( 14.29746914071049879, -8.314922557960816363, 33.33224293864769550 ) ) ;
#150792=CARTESIAN_POINT ( 'NONE',  ( -5.049401038297874678, -19.05341960407617918, 59.79275706135231871 ) ) ;
#150793=CARTESIAN_POINT ( 'NONE',  ( 16.55341960407618274, -4.379528057220086978, 46.04275706135234714 ) ) ;
#150794=CARTESIAN_POINT ( 'NONE',  ( 0.05219959533936267826, -19.03943276465977164, 25.00109039468566152 ) ) ;
#150795=CARTESIAN_POINT ( 'NONE',  ( -13.89961937509977652, 13.97604488694528158, 40.62390960531435979 ) ) ;
#150796=CARTESIAN_POINT ( 'NONE',  ( 18.39635199886970440, -5.499999999999976019, 73.51967076360001840 ) ) ;
#150797=CARTESIAN_POINT ( 'NONE',  ( -12.14591786802326823, 12.06949235617739902, 48.12609039468568284 ) ) ;
#150800=CARTESIAN_POINT ( 'NONE',  ( -16.51473224551069308, -9.474510206698971260, 96.66557627198102409 ) ) ;
#150801=LINE ( 'NONE', #70958, #174947 ) ;
#150802=CARTESIAN_POINT ( 'NONE',  ( -13.89961937509957401, -13.97604488694547875, 99.37609039468567573 ) ) ;
#150803=CARTESIAN_POINT ( 'NONE',  ( -5.823673210054116645, -21.52544592524344225, 27.29057627198103120 ) ) ;
#150804=CARTESIAN_POINT ( 'NONE',  ( -19.03943276465977164, -0.05219959533935918106, 18.75109039468567218 ) ) ;
#150805=CARTESIAN_POINT ( 'NONE',  ( 4.483927247898790824, -16.52544592524335698, 20.20942372801900788 ) ) ;
#150806=CARTESIAN_POINT ( 'NONE',  ( -12.06949235617756955, 12.14591786802309770, 110.6239096053143669 ) ) ;
#150807=CARTESIAN_POINT ( 'NONE',  ( -5.153800228976328057, -19.02544592524343514, 32.29057627198102409 ) ) ;
#150808=CARTESIAN_POINT ( 'NONE',  ( 21.55341960407610458, 5.719274019375980345, 63.95724293864770260 ) ) ;
#150809=CARTESIAN_POINT ( 'NONE',  ( -9.564922557960796823, -16.46253265017161027, 42.08224293864769550 ) ) ;
#150810=DIRECTION ( 'NONE',  ( 0.000000000000000000, 0.000000000000000000, -1.000000000000000000 ) ) ;
#150811=CARTESIAN_POINT ( 'NONE',  ( -13.89961937509957401, -13.97604488694547875, 64.37609039468567573 ) ) ;
#150812=CARTESIAN_POINT ( 'NONE',  ( -4.483927247898539470, -16.52544592524342804, 47.29057627198103120 ) ) ;
#150813=CARTESIAN_POINT ( 'NONE',  ( -18.62759615963270932, 10.81492255796079327, 35.83224293864768839 ) ) ;
#150814=CARTESIAN_POINT ( 'NONE',  ( -5.823673210054431948, 21.52544592524334988, 97.70942372801904696 ) ) ;
#150815=CARTESIAN_POINT ( 'NONE',  ( 15.80617190586746368, 15.72974639402197994, 89.37390960531435269 ) ) ;
#150816=CARTESIAN_POINT ( 'NONE',  ( -5.719274019375665041, -21.55341960407619695, 64.79275706135234714 ) ) ;
#150817=CARTESIAN_POINT ( 'NONE',  ( -10.72451020669870658, -18.67979575497194134, 64.58442372801900433 ) ) ;
#150818=CARTESIAN_POINT ( 'NONE',  ( -9.564922557960796823, -16.46253265017161027, 92.08224293864769550 ) ) ;
#150819=CARTESIAN_POINT ( 'NONE',  ( 8.224510206698742110, 14.34966873604972548, 87.08442372801901854 ) ) ;
#150820=CARTESIAN_POINT ( 'NONE',  ( 10.72451020669871369, 18.67979575497193778, 67.08442372801901854 ) ) ;
#150821=CARTESIAN_POINT ( 'NONE',  ( 13.97604488694527802, 13.89961937509977652, 54.37390960531435979 ) ) ;
#150822=CARTESIAN_POINT ( 'NONE',  ( 13.97604488694527802, 13.89961937509977652, 29.37390960531435979 ) ) ;
#150823=CARTESIAN_POINT ( 'NONE',  ( -19.05341960407611168, -5.049401038298163336, 51.45724293864770260 ) ) ;
#150824=CARTESIAN_POINT ( 'NONE',  ( 8.224510206698953496, -14.34966873604960469, 62.91557627198102409 ) ) ;
#150825=CARTESIAN_POINT ( 'NONE',  ( 16.55341960407611168, 4.379528057220329451, 33.95724293864769550 ) ) ;
#150826=CARTESIAN_POINT ( 'NONE',  ( -15.80617190586745835, -15.72974639402198527, 41.87390960531435979 ) ) ;
#150827=CARTESIAN_POINT ( 'NONE',  ( -9.474510206698964154, 16.51473224551069663, 50.41557627198102409 ) ) ;
#150828=CARTESIAN_POINT ( 'NONE',  ( 15.72974639402199770, -15.80617190586745480, 53.12390960531436690 ) ) ;
#150829=CARTESIAN_POINT ( 'NONE',  ( -19.03943276465977164, -0.05219959533935918106, 53.75109039468566863 ) ) ;
#150831=CARTESIAN_POINT ( 'NONE',  ( -17.40805194822030799, -6.112264579159367273, 39.16628727489390371 ) ) ;
#150832=CARTESIAN_POINT ( 'NONE',  ( 8.224510206698953496, -14.34966873604960469, 52.91557627198103830 ) ) ;
#150833=CARTESIAN_POINT ( 'NONE',  ( -15.80617190586745835, -15.72974639402198527, 26.87390960531435979 ) ) ;
#150834=ORIENTED_EDGE ( 'NONE', *, *, #7150, .F. ) ;
#150835=ORIENTED_EDGE ( 'NONE', *, *, #57463, .T. ) ;
#150837=CARTESIAN_POINT ( 'NONE',  ( -16.52544592524335698, -4.483927247898792601, 88.95942372801901854 ) ) ;
#150838=CARTESIAN_POINT ( 'NONE',  ( -16.46253265017146816, -9.564922557961047289, 69.16775706135233293 ) ) ;
#150839=CARTESIAN_POINT ( 'NONE',  ( 4.483927247898545687, 16.52544592524342804, 59.79057627198103120 ) ) ;
#150840=CARTESIAN_POINT ( 'NONE',  ( -19.25918095147781983, -5.499999999999586109, 59.45284276293935477 ) ) ;
#150841=CARTESIAN_POINT ( 'NONE',  ( 16.55341960407611168, 4.379528057220329451, 33.95724293864769550 ) ) ;
#150842=CARTESIAN_POINT ( 'NONE',  ( 9.474510206698971260, -16.51473224551069308, 47.91557627198102409 ) ) ;
#150843=CARTESIAN_POINT ( 'NONE',  ( 19.02544592524343514, -5.153800228976328945, 68.54057627198103830 ) ) ;
#150844=CARTESIAN_POINT ( 'NONE',  ( 19.05341960407611168, 5.049401038298154454, 38.95724293864767418 ) ) ;
#150845=CARTESIAN_POINT ( 'NONE',  ( 5.823673210054444382, -21.52544592524334988, 45.20942372801901854 ) ) ;
#150846=CARTESIAN_POINT ( 'NONE',  ( 5.153800228976335163, 19.02544592524342804, 74.79057627198103830 ) ) ;
#150847=CARTESIAN_POINT ( 'NONE',  ( -5.153800228976328057, -19.02544592524343514, 22.29057627198102765 ) ) ;
#150849=CARTESIAN_POINT ( 'NONE',  ( -13.89961937509977652, 13.97604488694528158, 60.62390960531436690 ) ) ;
#150850=CARTESIAN_POINT ( 'NONE',  ( -21.52544592524343514, 5.823673210054127303, 56.04057627198102409 ) ) ;
#150852=CARTESIAN_POINT ( 'NONE',  ( -13.97604488694527625, -13.89961937509977652, 41.87390960531435979 ) ) ;
#150853=CARTESIAN_POINT ( 'NONE',  ( -18.67979575497178146, -10.72451020669898902, 46.66557627198102409 ) ) ;
#150854=CARTESIAN_POINT ( 'NONE',  ( 8.224510206698742110, 14.34966873604972548, 102.0844237280190185 ) ) ;
#150855=CARTESIAN_POINT ( 'NONE',  ( -19.02544592524334988, -5.153800228976617603, 18.95942372801899722 ) ) ;
#150857=CARTESIAN_POINT ( 'NONE',  ( 4.483927247898790824, -16.52544592524335698, 45.20942372801901854 ) ) ;
#150858=CARTESIAN_POINT ( 'NONE',  ( -12.14591786802326823, 12.06949235617739902, 83.12609039468568994 ) ) ;
#150860=CARTESIAN_POINT ( 'NONE',  ( -0.05219959533934338120, 16.53943276465976808, 62.50109039468568284 ) ) ;
#150861=CARTESIAN_POINT ( 'NONE',  ( 0.05219959533934541429, -16.53943276465976808, 45.00109039468568284 ) ) ;
#150862=CARTESIAN_POINT ( 'NONE',  ( 16.46253265017160672, -9.564922557960803928, 113.3322429386476955 ) ) ;
#150863=CARTESIAN_POINT ( 'NONE',  ( 16.52544592524335698, 4.483927247898782831, 26.45942372801901854 ) ) ;
#150864=CARTESIAN_POINT ( 'NONE',  ( 16.46253265017160672, -9.564922557960803928, 38.33224293864768839 ) ) ;
#150865=CARTESIAN_POINT ( 'NONE',  ( 18.62759615963255655, 10.81492255796105972, 21.66775706135235069 ) ) ;
#150866=CARTESIAN_POINT ( 'NONE',  ( 0.05219959533934541429, -16.53943276465976808, 40.00109039468567573 ) ) ;
#150867=CARTESIAN_POINT ( 'NONE',  ( -12.06949235617739369, -12.14591786802326823, 94.37609039468568994 ) ) ;
#150869=CARTESIAN_POINT ( 'NONE',  ( 15.80617190586769283, -15.72974639402175789, 100.6260903946857184 ) ) ;
#150870=CARTESIAN_POINT ( 'NONE',  ( -13.89961937509957401, -13.97604488694547875, 99.37609039468567573 ) ) ;
#150871=CARTESIAN_POINT ( 'NONE',  ( -12.14591786802309592, -12.06949235617757132, 56.87390960531436690 ) ) ;
#150872=CARTESIAN_POINT ( 'NONE',  ( 16.46253265017160672, -9.564922557960803928, 23.33224293864769194 ) ) ;
#150873=CARTESIAN_POINT ( 'NONE',  ( -16.51473224551082808, 9.474510206698731452, 58.33442372801900433 ) ) ;
#150875=CARTESIAN_POINT ( 'NONE',  ( 15.80617190586769283, -15.72974639402175789, 55.62609039468568284 ) ) ;
#150876=CARTESIAN_POINT ( 'NONE',  ( 0.05219959533934541429, -16.53943276465976808, 25.00109039468567218 ) ) ;
#150878=CARTESIAN_POINT ( 'NONE',  ( -18.67979575497178146, -10.72451020669898902, 21.66557627198102409 ) ) ;
#150879=CARTESIAN_POINT ( 'NONE',  ( -21.52544592524343514, 5.823673210054127303, 76.04057627198102409 ) ) ;
#150880=CARTESIAN_POINT ( 'NONE',  ( 19.03943276465977164, 0.05219959533936151252, 111.2510903946856757 ) ) ;
#150881=CARTESIAN_POINT ( 'NONE',  ( 5.049401038298161559, -19.05341960407611168, 97.70724293864766707 ) ) ;
#150883=CARTESIAN_POINT ( 'NONE',  ( -9.564922557960796823, -16.46253265017161027, 22.08224293864768839 ) ) ;
#150884=CARTESIAN_POINT ( 'NONE',  ( 10.72451020669871369, 18.67979575497193778, 112.0844237280190185 ) ) ;
#150885=CARTESIAN_POINT ( 'NONE',  ( 5.049401038298161559, -19.05341960407611168, 37.70724293864768839 ) ) ;
#150887=CARTESIAN_POINT ( 'NONE',  ( -15.72974639402176322, -15.80617190586768395, 54.37609039468568994 ) ) ;
#150888=CARTESIAN_POINT ( 'NONE',  ( -15.72974639402176322, -15.80617190586768395, 94.37609039468568994 ) ) ;
#150889=CARTESIAN_POINT ( 'NONE',  ( -4.483927247898782831, 16.52544592524335698, 102.7094237280190185 ) ) ;
#150890=CARTESIAN_POINT ( 'NONE',  ( 5.153800228976335163, 19.02544592524342804, 84.79057627198099567 ) ) ;
#150891=CARTESIAN_POINT ( 'NONE',  ( 21.55341960407619695, -5.719274019375665929, 46.04275706135234714 ) ) ;
#150892=CARTESIAN_POINT ( 'NONE',  ( 21.55341960407619695, -5.719274019375665929, 36.04275706135234714 ) ) ;
#150893=CARTESIAN_POINT ( 'NONE',  ( 19.03943276465977164, 0.05219959533936151252, 81.25109039468567573 ) ) ;
#150894=CARTESIAN_POINT ( 'NONE',  ( -9.564922557960796823, -16.46253265017161027, 97.08224293864769550 ) ) ;
#150895=CARTESIAN_POINT ( 'NONE',  ( 8.314922557960818139, 14.29746914071049879, 104.5822429386477097 ) ) ;
#150896=CARTESIAN_POINT ( 'NONE',  ( -21.52544592524343514, 5.823673210054127303, 101.0405762719810383 ) ) ;
#150897=CARTESIAN_POINT ( 'NONE',  ( 16.55341960407611168, 4.379528057220329451, 83.95724293864770971 ) ) ;
#150898=CARTESIAN_POINT ( 'NONE',  ( 13.97604488694548053, -13.89961937509957401, 25.62609039468566507 ) ) ;
#150899=CARTESIAN_POINT ( 'NONE',  ( 14.29746914071049879, -8.314922557960816363, 98.33224293864769550 ) ) ;
#150900=CARTESIAN_POINT ( 'NONE',  ( -19.05341960407611168, -5.049401038298163336, 46.45724293864768129 ) ) ;
#150901=CARTESIAN_POINT ( 'NONE',  ( -19.03943276465977164, -0.05219959533935918106, 88.75109039468567573 ) ) ;
#150902=CARTESIAN_POINT ( 'NONE',  ( 8.224510206698953496, -14.34966873604960469, 52.91557627198103830 ) ) ;
#150903=CARTESIAN_POINT ( 'NONE',  ( -15.80617190586768217, 15.72974639402176855, 103.1260903946856757 ) ) ;
#150904=CARTESIAN_POINT ( 'NONE',  ( -9.474510206698964154, 16.51473224551069663, 110.4155762719810383 ) ) ;
#150905=CARTESIAN_POINT ( 'NONE',  ( -13.89961937509957401, -13.97604488694547875, 79.37609039468567573 ) ) ;
#150906=CARTESIAN_POINT ( 'NONE',  ( 0.05219959533907565091, 21.53943276465977519, 79.99890960531435269 ) ) ;
#150907=CARTESIAN_POINT ( 'NONE',  ( -15.72974639402176322, -15.80617190586768395, 34.37609039468568284 ) ) ;
#150908=CARTESIAN_POINT ( 'NONE',  ( -14.29746914071037622, -8.314922557961029526, 24.16775706135235424 ) ) ;
#150909=CARTESIAN_POINT ( 'NONE',  ( 8.314922557961029526, -14.29746914071037800, 95.41775706135234714 ) ) ;
#150910=CARTESIAN_POINT ( 'NONE',  ( 9.474510206698971260, -16.51473224551069308, 27.91557627198103120 ) ) ;
#150911=CARTESIAN_POINT ( 'NONE',  ( -10.72451020669870658, -18.67979575497194134, 29.58442372801901854 ) ) ;
#150912=CARTESIAN_POINT ( 'NONE',  ( 9.564922557960805705, 16.46253265017160317, 24.58224293864769194 ) ) ;
#150914=CARTESIAN_POINT ( 'NONE',  ( -16.52544592524335698, -4.483927247898792601, 53.95942372801900433 ) ) ;
#150916=CARTESIAN_POINT ( 'NONE',  ( 16.52544592524342804, -4.483927247898539470, 83.54057627198102409 ) ) ;
#150917=CARTESIAN_POINT ( 'NONE',  ( -10.81492255796078084, -18.62759615963271287, 77.08224293864769550 ) ) ;
#150918=CARTESIAN_POINT ( 'NONE',  ( -12.14591786802309592, -12.06949235617757132, 21.87390960531436690 ) ) ;
#150919=CARTESIAN_POINT ( 'NONE',  ( 16.55341960407618274, -4.379528057220086978, 46.04275706135234714 ) ) ;
#150920=CARTESIAN_POINT ( 'NONE',  ( 9.564922557960805705, 16.46253265017160317, 49.58224293864770260 ) ) ;
#150921=CARTESIAN_POINT ( 'NONE',  ( 16.52544592524335698, 4.483927247898782831, 96.45942372801901854 ) ) ;
#150922=CARTESIAN_POINT ( 'NONE',  ( -5.153800228976607833, 19.02544592524334988, 87.70942372801897591 ) ) ;
#150923=CARTESIAN_POINT ( 'NONE',  ( 21.53943276465977519, -0.05219959533907433946, 83.74890960531435269 ) ) ;
#150924=CARTESIAN_POINT ( 'NONE',  ( -4.379528057220086978, -16.55341960407618274, 104.7927570613523898 ) ) ;
#150927=CARTESIAN_POINT ( 'NONE',  ( -10.81492255796078084, -18.62759615963271287, 62.08224293864769550 ) ) ;
#150929=CARTESIAN_POINT ( 'NONE',  ( -8.314922557961024197, 14.29746914071037800, 87.91775706135234714 ) ) ;
#150931=CARTESIAN_POINT ( 'NONE',  ( 21.52544592524344225, -5.823673210054117533, 33.54057627198102409 ) ) ;
#150932=CARTESIAN_POINT ( 'NONE',  ( -19.52837319214027545, 5.499999999999899636, 74.60471352585540217 ) ) ;
#150933=CARTESIAN_POINT ( 'NONE',  ( -5.823673210054116645, -21.52544592524344225, 77.29057627198102409 ) ) ;
#150934=CARTESIAN_POINT ( 'NONE',  ( 16.52544592524342804, -4.483927247898539470, 23.54057627198102765 ) ) ;
#150935=CARTESIAN_POINT ( 'NONE',  ( -16.52544592524335698, -4.483927247898792601, 18.95942372801901143 ) ) ;
#150936=CARTESIAN_POINT ( 'NONE',  ( -13.89961937509977652, 13.97604488694528158, 35.62390960531435269 ) ) ;
#150937=CARTESIAN_POINT ( 'NONE',  ( -12.14591786802326823, 12.06949235617739902, 33.12609039468569705 ) ) ;
#150938=CARTESIAN_POINT ( 'NONE',  ( -5.153800228976328057, -19.02544592524343514, 47.29057627198102409 ) ) ;
#150940=CARTESIAN_POINT ( 'NONE',  ( 19.02544592524343514, -5.153800228976328945, 108.5405762719810383 ) ) ;
#150941=CARTESIAN_POINT ( 'NONE',  ( -16.51473224551069308, -9.474510206698971260, 106.6655762719810383 ) ) ;
#150942=CARTESIAN_POINT ( 'NONE',  ( 8.314922557961029526, -14.29746914071037800, 95.41775706135234714 ) ) ;
#150943=CARTESIAN_POINT ( 'NONE',  ( -19.05341960407617563, 5.049401038297882671, 88.54275706135230450 ) ) ;
#150944=CARTESIAN_POINT ( 'NONE',  ( 16.51473224551083163, -9.474510206698727899, 35.83442372801899722 ) ) ;
#150945=CARTESIAN_POINT ( 'NONE',  ( 18.67979575497178502, 10.72451020669898547, 79.16557627198103830 ) ) ;
#150946=CARTESIAN_POINT ( 'NONE',  ( 16.52544592524335698, 4.483927247898782831, 96.45942372801901854 ) ) ;
#150947=CARTESIAN_POINT ( 'NONE',  ( -15.80617190586745835, -15.72974639402198527, 36.87390960531435979 ) ) ;
#150948=CARTESIAN_POINT ( 'NONE',  ( -16.46253265017146816, -9.564922557961047289, 89.16775706135234714 ) ) ;
#150949=CARTESIAN_POINT ( 'NONE',  ( -16.46253265017160317, 9.564922557960807481, 45.83224293864769550 ) ) ;
#150950=CARTESIAN_POINT ( 'NONE',  ( -13.89961937509977652, 13.97604488694528158, 95.62390960531436690 ) ) ;
#150951=CARTESIAN_POINT ( 'NONE',  ( 5.719274019375673035, 21.55341960407619339, 67.29275706135234714 ) ) ;
#150952=CARTESIAN_POINT ( 'NONE',  ( -19.02544592524342804, 5.153800228976336051, 56.04057627198100988 ) ) ;
#150953=CARTESIAN_POINT ( 'NONE',  ( 4.379528057220339221, -16.55341960407611168, 97.70724293864772392 ) ) ;
#150955=CARTESIAN_POINT ( 'NONE',  ( -12.14591786802309592, -12.06949235617757132, 76.87390960531439532 ) ) ;
#150956=CARTESIAN_POINT ( 'NONE',  ( 15.72974639402199770, -15.80617190586745480, 73.12390960531436690 ) ) ;
#150957=CARTESIAN_POINT ( 'NONE',  ( -9.564922557961040184, 16.46253265017147172, 92.91775706135233293 ) ) ;
#150958=CARTESIAN_POINT ( 'NONE',  ( 19.52851543214744368, 5.499999999999982236, 92.89357721762581832 ) ) ;
#150959=CARTESIAN_POINT ( 'NONE',  ( 5.153800228976335163, 19.02544592524342804, 59.79057627198100988 ) ) ;
#150960=CARTESIAN_POINT ( 'NONE',  ( 16.81555441253470562, -7.025013491696157075, 73.13685445334213853 ) ) ;
#150961=CARTESIAN_POINT ( 'NONE',  ( 5.153800228976335163, 19.02544592524342804, 79.79057627198102409 ) ) ;
#150962=CARTESIAN_POINT ( 'NONE',  ( -9.564922557960796823, -16.46253265017161027, 82.08224293864768129 ) ) ;
#150963=CARTESIAN_POINT ( 'NONE',  ( 16.55341960407618274, -4.379528057220086978, 66.04275706135236135 ) ) ;
#150964=CARTESIAN_POINT ( 'NONE',  ( -17.31728774477271671, -6.344390552232404445, 49.18093348310683410 ) ) ;
#150965=CARTESIAN_POINT ( 'NONE',  ( -9.474510206698720793, -16.51473224551083518, 39.58442372801899722 ) ) ;
#150967=CARTESIAN_POINT ( 'NONE',  ( -16.46253265017160317, 9.564922557960807481, 110.8322429386476955 ) ) ;
#150968=CARTESIAN_POINT ( 'NONE',  ( -12.06949235617739369, -12.14591786802326823, 104.3760903946856899 ) ) ;
#150970=CARTESIAN_POINT ( 'NONE',  ( -16.53943276465976808, -0.05219959533934237506, 83.75109039468568994 ) ) ;
#150972=CARTESIAN_POINT ( 'NONE',  ( -8.224510206698735004, -14.34966873604973081, 49.58442372801901143 ) ) ;
#150974=CARTESIAN_POINT ( 'NONE',  ( 5.719274019375673035, 21.55341960407619339, 62.29275706135236845 ) ) ;
#150975=CARTESIAN_POINT ( 'NONE',  ( 13.97604488694548053, -13.89961937509957401, 75.62609039468564731 ) ) ;
#150976=CARTESIAN_POINT ( 'NONE',  ( -19.02544592524334988, -5.153800228976617603, 23.95942372801900078 ) ) ;
#150977=CARTESIAN_POINT ( 'NONE',  ( 16.46253265017160672, -9.564922557960803928, 68.33224293864770971 ) ) ;
#150978=CARTESIAN_POINT ( 'NONE',  ( -19.03943276465977164, 0.05219959533909376836, 41.24890960531435269 ) ) ;
#150980=CARTESIAN_POINT ( 'NONE',  ( 5.823673210054125526, 21.52544592524343514, 64.79057627198103830 ) ) ;
#150982=CARTESIAN_POINT ( 'NONE',  ( -21.53943276465977519, 0.05219959533907696930, 36.24890960531435979 ) ) ;
#150983=CARTESIAN_POINT ( 'NONE',  ( -13.89961937509977652, 13.97604488694528158, 25.62390960531434558 ) ) ;
#150984=CARTESIAN_POINT ( 'NONE',  ( 16.55341960407618274, -4.379528057220086978, 46.04275706135234714 ) ) ;
#150985=ADVANCED_FACE ( 'NONE', ( #158792 ), #171923, .T. ) ;
#150987=CARTESIAN_POINT ( 'NONE',  ( 5.719274019375673035, 21.55341960407619339, 32.29275706135235424 ) ) ;
#150988=CARTESIAN_POINT ( 'NONE',  ( 16.52544592524342804, -4.483927247898539470, 48.54057627198103120 ) ) ;
#150990=CARTESIAN_POINT ( 'NONE',  ( -0.05219959533934338120, 16.53943276465976808, 27.50109039468567929 ) ) ;
#150991=CARTESIAN_POINT ( 'NONE',  ( 13.97604488694548053, -13.89961937509957401, 40.62609039468564731 ) ) ;
#150992=CARTESIAN_POINT ( 'NONE',  ( 16.53943276465976808, -0.05219959533910856209, 48.74890960531435979 ) ) ;
#150993=CARTESIAN_POINT ( 'NONE',  ( 10.72451020669871369, 18.67979575497193778, 22.08442372801901143 ) ) ;
#150995=CARTESIAN_POINT ( 'NONE',  ( -18.62759615963270932, 10.81492255796079327, 75.83224293864769550 ) ) ;
#150996=CARTESIAN_POINT ( 'NONE',  ( -13.89961937509977652, 13.97604488694528158, 90.62390960531432427 ) ) ;
#150997=CARTESIAN_POINT ( 'NONE',  ( 8.314922557960818139, 14.29746914071049879, 59.58224293864770260 ) ) ;
#150998=CARTESIAN_POINT ( 'NONE',  ( 5.153800228976335163, 19.02544592524342804, 109.7905762719810099 ) ) ;
#150999=EDGE_CURVE ( 'NONE', #45569, #101009, #40751, .T. ) ;
#151001=CARTESIAN_POINT ( 'NONE',  ( 5.049401038297881783, 19.05341960407617563, 67.29275706135234714 ) ) ;
#151002=CARTESIAN_POINT ( 'NONE',  ( 21.53943276465977519, -0.05219959533907433946, 108.7489096053143669 ) ) ;
#151003=CARTESIAN_POINT ( 'NONE',  ( 19.05341960407611168, 5.049401038298154454, 53.95724293864770260 ) ) ;
#151004=CARTESIAN_POINT ( 'NONE',  ( -16.53943276465976808, 0.05219959533911058130, 116.2489096053143669 ) ) ;
#151005=CARTESIAN_POINT ( 'NONE',  ( 5.823673210054444382, -21.52544592524334988, 50.20942372801901854 ) ) ;
#151007=CARTESIAN_POINT ( 'NONE',  ( 14.34966873604960469, 8.224510206698951720, 39.16557627198102409 ) ) ;
#151008=CARTESIAN_POINT ( 'NONE',  ( 19.05341960407611168, 5.049401038298154454, 43.95724293864769550 ) ) ;
#151009=CARTESIAN_POINT ( 'NONE',  ( -13.97604488694527625, -13.89961937509977652, 96.87390960531433848 ) ) ;
#151010=CARTESIAN_POINT ( 'NONE',  ( 21.53943276465977519, -0.05219959533907433946, 73.74890960531433848 ) ) ;
#151012=CARTESIAN_POINT ( 'NONE',  ( -5.153800228976328057, -19.02544592524343514, 47.29057627198102409 ) ) ;
#151013=CARTESIAN_POINT ( 'NONE',  ( 21.55341960407610458, 5.719274019375980345, 68.95724293864769550 ) ) ;
#151014=CARTESIAN_POINT ( 'NONE',  ( 5.823673210054444382, -21.52544592524334988, 80.20942372801901854 ) ) ;
#151016=CARTESIAN_POINT ( 'NONE',  ( -8.314922557961024197, 14.29746914071037800, 82.91775706135234714 ) ) ;
#151017=CARTESIAN_POINT ( 'NONE',  ( 16.53943276465976808, -0.05219959533910856209, 83.74890960531435269 ) ) ;
#151018=CARTESIAN_POINT ( 'NONE',  ( 9.564922557960805705, 16.46253265017160317, 64.58224293864769550 ) ) ;
#151020=CARTESIAN_POINT ( 'NONE',  ( -13.89961937509957401, -13.97604488694547875, 24.37609039468565442 ) ) ;
#151021=CARTESIAN_POINT ( 'NONE',  ( -12.06949235617739369, -12.14591786802326823, 89.37609039468568994 ) ) ;
#151022=CARTESIAN_POINT ( 'NONE',  ( 13.97604488694548053, -13.89961937509957401, 20.62609039468567573 ) ) ;
#151023=CARTESIAN_POINT ( 'NONE',  ( 16.51473224551069308, 9.474510206698969483, 89.16557627198103830 ) ) ;
#151024=CARTESIAN_POINT ( 'NONE',  ( -0.05219959533907301413, -21.53943276465977519, 47.49890960531435979 ) ) ;
#151025=CARTESIAN_POINT ( 'NONE',  ( -0.05219959533937732626, 21.53943276465977519, 97.50109039468567573 ) ) ;
#151026=CARTESIAN_POINT ( 'NONE',  ( 0.05219959533934541429, -16.53943276465976808, 60.00109039468568284 ) ) ;
#151027=CARTESIAN_POINT ( 'NONE',  ( -21.53943276465977519, 0.05219959533907696930, 111.2489096053143669 ) ) ;
#151028=CARTESIAN_POINT ( 'NONE',  ( 12.06949235617739724, 12.14591786802326823, 21.87609039468567573 ) ) ;
#151029=CARTESIAN_POINT ( 'NONE',  ( -19.03943276465977164, 0.05219959533909376836, 86.24890960531436690 ) ) ;
#151030=CARTESIAN_POINT ( 'NONE',  ( 12.06949235617739724, 12.14591786802326823, 31.87609039468567929 ) ) ;
#151031=CARTESIAN_POINT ( 'NONE',  ( -5.153800228976328057, -19.02544592524343514, 57.29057627198103120 ) ) ;
#151033=CARTESIAN_POINT ( 'NONE',  ( -16.55341960407617563, 4.379528057220093196, 38.54275706135234714 ) ) ;
#151034=CARTESIAN_POINT ( 'NONE',  ( -12.14591786802309592, -12.06949235617757132, 76.87390960531439532 ) ) ;
#151035=CARTESIAN_POINT ( 'NONE',  ( 0.05219959533934541429, -16.53943276465976808, 85.00109039468568994 ) ) ;
#151036=CARTESIAN_POINT ( 'NONE',  ( -21.55341960407619339, 5.719274019375674811, 48.54275706135234714 ) ) ;
#151037=CARTESIAN_POINT ( 'NONE',  ( -13.89961937509977652, 13.97604488694528158, 65.62390960531436690 ) ) ;
#151038=CARTESIAN_POINT ( 'NONE',  ( 16.51473224551069308, 9.474510206698969483, 84.16557627198102409 ) ) ;
#151039=CARTESIAN_POINT ( 'NONE',  ( 16.52544592524335698, 4.483927247898782831, 86.45942372801901854 ) ) ;
#151042=CARTESIAN_POINT ( 'NONE',  ( -13.89961937509957401, -13.97604488694547875, 24.37609039468565442 ) ) ;
#151043=CARTESIAN_POINT ( 'NONE',  ( 16.51473224551069308, 9.474510206698969483, 94.16557627198103830 ) ) ;
#151044=CARTESIAN_POINT ( 'NONE',  ( -9.474510206698964154, 16.51473224551069663, 50.41557627198102409 ) ) ;
#151045=CARTESIAN_POINT ( 'NONE',  ( 19.05341960407611168, 5.049401038298154454, 113.9572429386477097 ) ) ;
#151046=CARTESIAN_POINT ( 'NONE',  ( -4.379528057220086978, -16.55341960407618274, 39.79275706135235424 ) ) ;
#151047=CARTESIAN_POINT ( 'NONE',  ( -0.05219959533936034679, 19.03943276465977164, 62.50109039468566863 ) ) ;
#151048=CARTESIAN_POINT ( 'NONE',  ( 4.379528057220092307, 16.55341960407617563, 62.29275706135236845 ) ) ;
#151049=CARTESIAN_POINT ( 'NONE',  ( -0.05219959533909027116, -19.03943276465977164, 82.49890960531436690 ) ) ;
#151050=CARTESIAN_POINT ( 'NONE',  ( 21.53943276465977519, -0.05219959533907433946, 108.7489096053143669 ) ) ;
#151051=CARTESIAN_POINT ( 'NONE',  ( -19.05341960407617563, 5.049401038297882671, 63.54275706135234003 ) ) ;
#151052=CARTESIAN_POINT ( 'NONE',  ( -5.049401038298153566, 19.05341960407611168, 100.2072429386476955 ) ) ;
#151054=CARTESIAN_POINT ( 'NONE',  ( -19.03943276465977164, 0.05219959533909376836, 71.24890960531435269 ) ) ;
#151055=CARTESIAN_POINT ( 'NONE',  ( -16.53943276465976808, 0.05219959533911058130, 31.24890960531435979 ) ) ;
#151056=DIRECTION ( 'NONE',  ( 1.000000000000000000, -0.000000000000000000, -0.000000000000000000 ) ) ;
#151057=CARTESIAN_POINT ( 'NONE',  ( 19.05341960407617918, -5.049401038297876454, 41.04275706135233293 ) ) ;
#151058=CARTESIAN_POINT ( 'NONE',  ( 0.05219959533910956823, 16.53943276465976808, 69.99890960531435269 ) ) ;
#151059=CARTESIAN_POINT ( 'NONE',  ( -5.719274019375665041, -21.55341960407619695, 99.79275706135234714 ) ) ;
#151060=CARTESIAN_POINT ( 'NONE',  ( 5.049401038298161559, -19.05341960407611168, 37.70724293864768839 ) ) ;
#151061=CARTESIAN_POINT ( 'NONE',  ( 16.53943276465976808, -0.05219959533910856209, 43.74890960531435979 ) ) ;
#151062=CARTESIAN_POINT ( 'NONE',  ( -5.719274019375665041, -21.55341960407619695, 109.7927570613523613 ) ) ;
#151063=CARTESIAN_POINT ( 'NONE',  ( -0.05219959533909027116, -19.03943276465977164, 87.49890960531436690 ) ) ;
#151064=CARTESIAN_POINT ( 'NONE',  ( 5.153800228976335163, 19.02544592524342804, 109.7905762719810099 ) ) ;
#151065=CARTESIAN_POINT ( 'NONE',  ( 9.564922557960805705, 16.46253265017160317, 44.58224293864769550 ) ) ;
#151066=CARTESIAN_POINT ( 'NONE',  ( 12.14591786802309770, 12.06949235617756955, 109.3739096053143811 ) ) ;
#151067=CARTESIAN_POINT ( 'NONE',  ( -14.29746914071049879, 8.314922557960819915, 80.83224293864769550 ) ) ;
#151068=CARTESIAN_POINT ( 'NONE',  ( 21.53943276465977519, -0.05219959533907433946, 88.74890960531436690 ) ) ;
#151069=CARTESIAN_POINT ( 'NONE',  ( 13.97604488694527802, 13.89961937509977652, 89.37390960531436690 ) ) ;
#151070=CARTESIAN_POINT ( 'NONE',  ( -0.05219959533907301413, -21.53943276465977519, 92.49890960531436690 ) ) ;
#151071=CARTESIAN_POINT ( 'NONE',  ( 19.03943276465977164, -0.05219959533909143690, 93.74890960531435269 ) ) ;
#151072=CARTESIAN_POINT ( 'NONE',  ( 19.36337904590692105, -5.499999999999937828, 47.91494137495620720 ) ) ;
#151073=CARTESIAN_POINT ( 'NONE',  ( -16.55341960407611168, -4.379528057220339221, 106.4572429386477097 ) ) ;
#151074=CARTESIAN_POINT ( 'NONE',  ( -19.03943276465977164, 0.05219959533909376836, 66.24890960531436690 ) ) ;
#151075=CARTESIAN_POINT ( 'NONE',  ( -5.719274019375978568, 21.55341960407610458, 80.20724293864769550 ) ) ;
#151077=CARTESIAN_POINT ( 'NONE',  ( -21.55341960407610458, -5.719274019375992779, 26.45724293864768839 ) ) ;
#151079=CARTESIAN_POINT ( 'NONE',  ( -8.224510206698735004, -14.34966873604973081, 19.58442372801901143 ) ) ;
#151080=CARTESIAN_POINT ( 'NONE',  ( -8.224510206698948167, 14.34966873604960824, 100.4155762719810241 ) ) ;
#151081=CARTESIAN_POINT ( 'NONE',  ( -18.22780087662122028, 5.500000000000031086, 43.51540105326107977 ) ) ;
#151082=CARTESIAN_POINT ( 'NONE',  ( 19.05341960407611168, 5.049401038298154454, 93.95724293864769550 ) ) ;
#151083=CARTESIAN_POINT ( 'NONE',  ( -13.97604488694527625, -13.89961937509977652, 46.87390960531435979 ) ) ;
#151084=CARTESIAN_POINT ( 'NONE',  ( -0.05219959533910754901, -16.53943276465976808, 82.49890960531436690 ) ) ;
#151086=CARTESIAN_POINT ( 'NONE',  ( 9.564922557960805705, 16.46253265017160317, 114.5822429386476955 ) ) ;
#151087=CARTESIAN_POINT ( 'NONE',  ( 8.224510206698953496, -14.34966873604960469, 47.91557627198102409 ) ) ;
#151088=CARTESIAN_POINT ( 'NONE',  ( -16.46253265017146816, -9.564922557961047289, 109.1677570613523471 ) ) ;
#151089=CARTESIAN_POINT ( 'NONE',  ( -21.52544592524334988, -5.823673210054445271, 63.95942372801901854 ) ) ;
#151091=CARTESIAN_POINT ( 'NONE',  ( -16.46253265017160317, 9.564922557960807481, 105.8322429386476955 ) ) ;
#151092=CARTESIAN_POINT ( 'NONE',  ( 10.81492255796078972, 18.62759615963270932, 94.58224293864769550 ) ) ;
#151093=CARTESIAN_POINT ( 'NONE',  ( -8.314922557961024197, 14.29746914071037800, 82.91775706135234714 ) ) ;
#151094=CARTESIAN_POINT ( 'NONE',  ( 19.02544592524343514, -5.153800228976328945, 23.54057627198102054 ) ) ;
#151095=CARTESIAN_POINT ( 'NONE',  ( -9.564922557960796823, -16.46253265017161027, 82.08224293864768129 ) ) ;
#151096=CARTESIAN_POINT ( 'NONE',  ( -18.67979575497178146, -10.72451020669898902, 86.66557627198102409 ) ) ;
#151097=CARTESIAN_POINT ( 'NONE',  ( -13.89961937509957401, -13.97604488694547875, 104.3760903946856757 ) ) ;
#151098=CARTESIAN_POINT ( 'NONE',  ( -14.29746914071049879, 8.314922557960819915, 55.83224293864770260 ) ) ;
#151099=CARTESIAN_POINT ( 'NONE',  ( -5.719274019375665041, -21.55341960407619695, 54.79275706135235424 ) ) ;
#151100=CARTESIAN_POINT ( 'NONE',  ( 8.314922557961029526, -14.29746914071037800, 85.41775706135236135 ) ) ;
#151101=CARTESIAN_POINT ( 'NONE',  ( 10.72451020669898902, -18.67979575497178502, 27.91557627198103830 ) ) ;
#151102=CARTESIAN_POINT ( 'NONE',  ( 0.05219959533909260263, 19.03943276465977164, 109.9989096053143669 ) ) ;
#151104=CARTESIAN_POINT ( 'NONE',  ( 12.14591786802327356, -12.06949235617739191, 105.6260903946856899 ) ) ;
#151105=CARTESIAN_POINT ( 'NONE',  ( 12.14591786802327356, -12.06949235617739191, 65.62609039468568994 ) ) ;
#151106=CARTESIAN_POINT ( 'NONE',  ( -13.97604488694527625, -13.89961937509977652, 76.87390960531433848 ) ) ;
#151107=CARTESIAN_POINT ( 'NONE',  ( -16.46253265017160317, 9.564922557960807481, 70.83224293864770971 ) ) ;
#151108=CARTESIAN_POINT ( 'NONE',  ( -14.29746914071037622, -8.314922557961029526, 74.16775706135231871 ) ) ;
#151109=CARTESIAN_POINT ( 'NONE',  ( -4.379528057220328563, 16.55341960407611168, 45.20724293864769550 ) ) ;
#151110=CARTESIAN_POINT ( 'NONE',  ( 16.46253265017160672, -9.564922557960803928, 53.33224293864768839 ) ) ;
#151111=CARTESIAN_POINT ( 'NONE',  ( 19.05341960407611168, 5.049401038298154454, 43.95724293864769550 ) ) ;
#151112=CARTESIAN_POINT ( 'NONE',  ( -16.55341960407617563, 4.379528057220093196, 43.54275706135235424 ) ) ;
#151114=CARTESIAN_POINT ( 'NONE',  ( 9.474510206698729675, 16.51473224551082808, 97.08442372801900433 ) ) ;
#151115=CARTESIAN_POINT ( 'NONE',  ( -12.14591786802309592, -12.06949235617757132, 101.8739096053143811 ) ) ;
#151116=CARTESIAN_POINT ( 'NONE',  ( 13.89961937509977652, -13.97604488694527269, 63.12390960531435979 ) ) ;
#151117=CARTESIAN_POINT ( 'NONE',  ( 9.564922557961047289, -16.46253265017146816, 105.4177570613523471 ) ) ;
#151119=CARTESIAN_POINT ( 'NONE',  ( -21.53943276465977519, -0.05219959533937600094, 108.7510903946857042 ) ) ;
#151120=CARTESIAN_POINT ( 'NONE',  ( -14.34966873604972548, 8.224510206698743886, 63.33442372801900433 ) ) ;
#151121=CARTESIAN_POINT ( 'NONE',  ( 18.67979575497178502, 10.72451020669898547, 69.16557627198102409 ) ) ;
#151122=CARTESIAN_POINT ( 'NONE',  ( -4.483927247898782831, 16.52544592524335698, 57.70942372801901143 ) ) ;
#151123=CARTESIAN_POINT ( 'NONE',  ( -19.03943276465977164, 0.05219959533909376836, 36.24890960531436690 ) ) ;
#151124=CARTESIAN_POINT ( 'NONE',  ( -16.46253265017146816, -9.564922557961047289, 39.16775706135234003 ) ) ;
#151125=CARTESIAN_POINT ( 'NONE',  ( -19.05341960407611168, -5.049401038298163336, 91.45724293864766707 ) ) ;
#151126=CARTESIAN_POINT ( 'NONE',  ( -5.153800228976328057, -19.02544592524343514, 27.29057627198103120 ) ) ;
#151127=CARTESIAN_POINT ( 'NONE',  ( -0.05219959533909027116, -19.03943276465977164, 62.49890960531435979 ) ) ;
#151129=CARTESIAN_POINT ( 'NONE',  ( -5.823673210054431948, 21.52544592524334988, 77.70942372801900433 ) ) ;
#151130=CARTESIAN_POINT ( 'NONE',  ( -16.51473224551082808, 9.474510206698731452, 53.33442372801900433 ) ) ;
#151132=CARTESIAN_POINT ( 'NONE',  ( -16.46253265017146816, -9.564922557961047289, 29.16775706135232937 ) ) ;
#151133=CARTESIAN_POINT ( 'NONE',  ( -16.46253265017160317, 9.564922557960807481, 60.83224293864769550 ) ) ;
#151134=CARTESIAN_POINT ( 'NONE',  ( 19.02544592524343514, -5.153800228976328945, 113.5405762719810241 ) ) ;
#151135=CARTESIAN_POINT ( 'NONE',  ( -5.719274019375665041, -21.55341960407619695, 89.79275706135236135 ) ) ;
#151136=CARTESIAN_POINT ( 'NONE',  ( -0.05219959533909027116, -19.03943276465977164, 62.49890960531435979 ) ) ;
#151137=CARTESIAN_POINT ( 'NONE',  ( 5.719274019375673035, 21.55341960407619339, 92.29275706135236135 ) ) ;
#151138=CARTESIAN_POINT ( 'NONE',  ( -0.05219959533907301413, -21.53943276465977519, 32.49890960531435979 ) ) ;
#151139=CARTESIAN_POINT ( 'NONE',  ( -0.05219959533909027116, -19.03943276465977164, 77.49890960531435269 ) ) ;
#151140=CARTESIAN_POINT ( 'NONE',  ( -21.55341960407619339, 5.719274019375674811, 43.54275706135235424 ) ) ;
#151141=CARTESIAN_POINT ( 'NONE',  ( -16.46253265017146816, -9.564922557961047289, 59.16775706135233293 ) ) ;
#151142=CARTESIAN_POINT ( 'NONE',  ( 9.564922557960805705, 16.46253265017160317, 39.58224293864768839 ) ) ;
#151143=CARTESIAN_POINT ( 'NONE',  ( 13.89961937509977652, -13.97604488694527269, 93.12390960531436690 ) ) ;
#151144=CARTESIAN_POINT ( 'NONE',  ( -8.224510206698735004, -14.34966873604973081, 34.58442372801900433 ) ) ;
#151145=CARTESIAN_POINT ( 'NONE',  ( 16.52544592524342804, -4.483927247898539470, 83.54057627198102409 ) ) ;
#151146=CARTESIAN_POINT ( 'NONE',  ( -19.03943276465977164, 0.05219959533909376836, 66.24890960531436690 ) ) ;
#151147=CARTESIAN_POINT ( 'NONE',  ( 18.62759615963271287, -10.81492255796078972, 53.33224293864769550 ) ) ;
#151148=CARTESIAN_POINT ( 'NONE',  ( 9.564922557961047289, -16.46253265017146816, 110.4177570613523471 ) ) ;
#151149=CARTESIAN_POINT ( 'NONE',  ( -15.80617190586745835, -15.72974639402198527, 111.8739096053143669 ) ) ;
#151150=CARTESIAN_POINT ( 'NONE',  ( -21.52544592524334988, -5.823673210054445271, 68.95942372801901854 ) ) ;
#151151=B_SPLINE_CURVE_WITH_KNOTS ( 'NONE', 3,
 ( #5972, #36308, #162662, #100978 ),
 .UNSPECIFIED., .F., .F.,
 ( 4, 4 ),
 ( 0.001482540648255906276, 0.002244533994399153676 ),
 .UNSPECIFIED. ) ;
#151152=CARTESIAN_POINT ( 'NONE',  ( -16.52544592524335698, -4.483927247898792601, 63.95942372801901854 ) ) ;
#151153=CARTESIAN_POINT ( 'NONE',  ( -4.483927247898782831, 16.52544592524335698, 62.70942372801902565 ) ) ;
#151154=CARTESIAN_POINT ( 'NONE',  ( 19.02544592524343514, -5.153800228976328945, 63.54057627198103830 ) ) ;
#151155=CARTESIAN_POINT ( 'NONE',  ( 8.224510206698742110, 14.34966873604972548, 102.0844237280190185 ) ) ;
#151156=CARTESIAN_POINT ( 'NONE',  ( 5.153800228976615827, -19.02544592524334988, 45.20942372801901143 ) ) ;
#151159=CARTESIAN_POINT ( 'NONE',  ( -5.719274019375978568, 21.55341960407610458, 110.2072429386477239 ) ) ;
#151160=CARTESIAN_POINT ( 'NONE',  ( -0.05219959533910754901, -16.53943276465976808, 67.49890960531436690 ) ) ;
#151161=CARTESIAN_POINT ( 'NONE',  ( -13.97604488694527625, -13.89961937509977652, 91.87390960531432427 ) ) ;
#151162=CARTESIAN_POINT ( 'NONE',  ( -4.483927247898782831, 16.52544592524335698, 82.70942372801900433 ) ) ;
#151163=CARTESIAN_POINT ( 'NONE',  ( -15.72974639402176322, -15.80617190586768395, 59.37609039468568284 ) ) ;
#151164=CARTESIAN_POINT ( 'NONE',  ( 14.29746914071037800, 8.314922557961029526, 36.66775706135234714 ) ) ;
#151165=CARTESIAN_POINT ( 'NONE',  ( -18.67979575497193778, 10.72451020669871902, 33.33442372801900433 ) ) ;
#151166=CARTESIAN_POINT ( 'NONE',  ( -4.379528057220328563, 16.55341960407611168, 55.20724293864770260 ) ) ;
#151168=CARTESIAN_POINT ( 'NONE',  ( -21.55341960407610458, -5.719274019375992779, 106.4572429386477097 ) ) ;
#151169=CARTESIAN_POINT ( 'NONE',  ( 14.29746914071049879, -8.314922557960816363, 33.33224293864769550 ) ) ;
#151170=ORIENTED_EDGE ( 'NONE', *, *, #103145, .T. ) ;
#151172=CARTESIAN_POINT ( 'NONE',  ( -21.52544592524343514, 5.823673210054127303, 26.04057627198103475 ) ) ;
#151173=CARTESIAN_POINT ( 'NONE',  ( -21.55341960407619339, 5.719274019375674811, 43.54275706135235424 ) ) ;
#151174=CARTESIAN_POINT ( 'NONE',  ( -14.34966873604960291, -8.224510206698953496, 66.66557627198102409 ) ) ;
#151175=CARTESIAN_POINT ( 'NONE',  ( 15.72974639402199770, -15.80617190586745480, 68.12390960531436690 ) ) ;
#151176=CARTESIAN_POINT ( 'NONE',  ( 0.05219959533909260263, 19.03943276465977164, 74.99890960531435269 ) ) ;
#151177=CARTESIAN_POINT ( 'NONE',  ( -5.049401038298153566, 19.05341960407611168, 25.20724293864768484 ) ) ;
#151178=CARTESIAN_POINT ( 'NONE',  ( 13.89961937509957401, 13.97604488694547697, 61.87609039468566863 ) ) ;
#151180=CARTESIAN_POINT ( 'NONE',  ( 15.72974639402199770, -15.80617190586745480, 48.12390960531436690 ) ) ;
#151181=CARTESIAN_POINT ( 'NONE',  ( 16.46253265017160672, -9.564922557960803928, 63.33224293864769550 ) ) ;
#151182=CARTESIAN_POINT ( 'NONE',  ( -0.05219959533934338120, 16.53943276465976808, 42.50109039468567573 ) ) ;
#151183=CARTESIAN_POINT ( 'NONE',  ( 0.05219959533907565091, 21.53943276465977519, 109.9989096053143527 ) ) ;
#151184=CARTESIAN_POINT ( 'NONE',  ( 8.224510206698953496, -14.34966873604960469, 52.91557627198103830 ) ) ;
#151185=CARTESIAN_POINT ( 'NONE',  ( -0.05219959533909027116, -19.03943276465977164, 97.49890960531436690 ) ) ;
#151186=CARTESIAN_POINT ( 'NONE',  ( 10.72451020669898902, -18.67979575497178502, 77.91557627198102409 ) ) ;
#151187=CARTESIAN_POINT ( 'NONE',  ( -10.72451020669898014, 18.67979575497178502, 110.4155762719810383 ) ) ;
#151188=CARTESIAN_POINT ( 'NONE',  ( -12.06949235617739369, -12.14591786802326823, 34.37609039468568284 ) ) ;
#151189=CARTESIAN_POINT ( 'NONE',  ( 0.05219959533907565091, 21.53943276465977519, 34.99890960531435979 ) ) ;
#151190=CARTESIAN_POINT ( 'NONE',  ( 21.52544592524334988, 5.823673210054432836, 96.45942372801901854 ) ) ;
#151191=CARTESIAN_POINT ( 'NONE',  ( -19.05341960407611168, -5.049401038298163336, 36.45724293864766707 ) ) ;
#151192=CARTESIAN_POINT ( 'NONE',  ( -13.89961937509977652, 13.97604488694528158, 95.62390960531436690 ) ) ;
#151193=CARTESIAN_POINT ( 'NONE',  ( -0.05219959533909027116, -19.03943276465977164, 82.49890960531436690 ) ) ;
#151196=CARTESIAN_POINT ( 'NONE',  ( 16.51473224551083163, -9.474510206698727899, 55.83442372801899722 ) ) ;
#151197=CARTESIAN_POINT ( 'NONE',  ( 5.153800228976615827, -19.02544592524334988, 20.20942372801899722 ) ) ;
#151198=CARTESIAN_POINT ( 'NONE',  ( -15.80617190586745835, -15.72974639402198527, 36.87390960531435979 ) ) ;
#151199=CARTESIAN_POINT ( 'NONE',  ( 8.224510206698742110, 14.34966873604972548, 107.0844237280190043 ) ) ;
#151200=CARTESIAN_POINT ( 'NONE',  ( 16.46253265017146816, 9.564922557961045513, 91.66775706135234714 ) ) ;
#151201=DIRECTION ( 'NONE',  ( 0.000000000000000000, -0.000000000000000000, 1.000000000000000000 ) ) ;
#151202=CARTESIAN_POINT ( 'NONE',  ( -9.474510206698720793, -16.51473224551083518, 89.58442372801900433 ) ) ;
#151203=CARTESIAN_POINT ( 'NONE',  ( 0.05219959533936267826, -19.03943276465977164, 40.00109039468566152 ) ) ;
#151205=CARTESIAN_POINT ( 'NONE',  ( 0.05219959533909260263, 19.03943276465977164, 44.99890960531435979 ) ) ;
#151206=CARTESIAN_POINT ( 'NONE',  ( -16.52544592524342804, 4.483927247898546575, 56.04057627198102409 ) ) ;
#151207=CARTESIAN_POINT ( 'NONE',  ( 9.474510206698971260, -16.51473224551069308, 37.91557627198102409 ) ) ;
#151208=CARTESIAN_POINT ( 'NONE',  ( -12.14591786802309592, -12.06949235617757132, 26.87390960531435979 ) ) ;
#151209=CARTESIAN_POINT ( 'NONE',  ( 17.60769864724391454, -5.499999999999980460, 46.15024842019165163 ) ) ;
#151210=CARTESIAN_POINT ( 'NONE',  ( -16.53943276465976808, -0.05219959533934237506, 113.7510903946856757 ) ) ;
#151211=CARTESIAN_POINT ( 'NONE',  ( 9.474510206698971260, -16.51473224551069308, 47.91557627198102409 ) ) ;
#151212=CARTESIAN_POINT ( 'NONE',  ( -18.62759615963255300, -10.81492255796106328, 104.1677570613523471 ) ) ;
#151213=CARTESIAN_POINT ( 'NONE',  ( -4.379528057220086978, -16.55341960407618274, 24.79275706135235779 ) ) ;
#151214=CARTESIAN_POINT ( 'NONE',  ( 10.81492255796078972, 18.62759615963270932, 34.58224293864770260 ) ) ;
#151215=CARTESIAN_POINT ( 'NONE',  ( 15.72974639402176855, 15.80617190586768217, 91.87609039468568994 ) ) ;
#151216=CARTESIAN_POINT ( 'NONE',  ( 13.97604488694527802, 13.89961937509977652, 99.37390960531436690 ) ) ;
#151217=CARTESIAN_POINT ( 'NONE',  ( 13.89961937509977652, -13.97604488694527269, 88.12390960531438111 ) ) ;
#151219=CARTESIAN_POINT ( 'NONE',  ( 15.80617190586746368, 15.72974639402197994, 104.3739096053143669 ) ) ;
#151220=CARTESIAN_POINT ( 'NONE',  ( 4.379528057220339221, -16.55341960407611168, 82.70724293864770971 ) ) ;
#151221=CARTESIAN_POINT ( 'NONE',  ( -18.67979575497178146, -10.72451020669898902, 71.66557627198100988 ) ) ;
#151222=CARTESIAN_POINT ( 'NONE',  ( 0.05219959533909260263, 19.03943276465977164, 54.99890960531435979 ) ) ;
#151223=CARTESIAN_POINT ( 'NONE',  ( 21.53943276465977519, -0.05219959533907433946, 98.74890960531438111 ) ) ;
#151225=CARTESIAN_POINT ( 'NONE',  ( -13.89961937509977652, 13.97604488694528158, 60.62390960531436690 ) ) ;
#151226=CARTESIAN_POINT ( 'NONE',  ( -4.483927247898539470, -16.52544592524342804, 92.29057627198103830 ) ) ;
#151228=CARTESIAN_POINT ( 'NONE',  ( -19.02544592524342804, 5.153800228976336051, 66.04057627198103830 ) ) ;
#151229=CARTESIAN_POINT ( 'NONE',  ( -19.02544592524334988, -5.153800228976617603, 73.95942372801900433 ) ) ;
#151230=CARTESIAN_POINT ( 'NONE',  ( -16.52544592524342804, 4.483927247898546575, 86.04057627198102409 ) ) ;
#151231=CARTESIAN_POINT ( 'NONE',  ( 5.719274019375673035, 21.55341960407619339, 52.29275706135236135 ) ) ;
#151232=CARTESIAN_POINT ( 'NONE',  ( -5.049401038298153566, 19.05341960407611168, 45.20724293864769550 ) ) ;
#151233=CARTESIAN_POINT ( 'NONE',  ( -10.81492255796105439, 18.62759615963255655, 22.91775706135235069 ) ) ;
#151234=CARTESIAN_POINT ( 'NONE',  ( 16.55341960407611168, 4.379528057220329451, 103.9572429386476813 ) ) ;
#151236=CARTESIAN_POINT ( 'NONE',  ( -13.89961937509977652, 13.97604488694528158, 65.62390960531436690 ) ) ;
#151237=CARTESIAN_POINT ( 'NONE',  ( 16.62475595723701005, 7.163666690055288555, 111.9728664818952950 ) ) ;
#151238=CARTESIAN_POINT ( 'NONE',  ( -13.97604488694547697, 13.89961937509957934, 113.1260903946856757 ) ) ;
#151239=CARTESIAN_POINT ( 'NONE',  ( 16.51473224551069308, 9.474510206698969483, 109.1655762719810383 ) ) ;
#151240=CARTESIAN_POINT ( 'NONE',  ( 0.05219959533937995610, -21.53943276465977519, 50.00109039468568994 ) ) ;
#151241=CARTESIAN_POINT ( 'NONE',  ( 19.05341960407611168, 5.049401038298154454, 93.95724293864769550 ) ) ;
#151242=CARTESIAN_POINT ( 'NONE',  ( 16.46253265017146816, 9.564922557961045513, 86.66775706135233293 ) ) ;
#151243=CARTESIAN_POINT ( 'NONE',  ( -13.89961937509977652, 13.97604488694528158, 55.62390960531434558 ) ) ;
#151244=CARTESIAN_POINT ( 'NONE',  ( 16.55341960407611168, 4.379528057220329451, 78.95724293864769550 ) ) ;
#151245=CARTESIAN_POINT ( 'NONE',  ( -8.314922557960811034, -14.29746914071050412, 82.08224293864768129 ) ) ;
#151246=CARTESIAN_POINT ( 'NONE',  ( -9.564922557960796823, -16.46253265017161027, 92.08224293864769550 ) ) ;
#151247=CARTESIAN_POINT ( 'NONE',  ( 0.05219959533910956823, 16.53943276465976808, 84.99890960531436690 ) ) ;
#151248=CARTESIAN_POINT ( 'NONE',  ( -0.05219959533909027116, -19.03943276465977164, 87.49890960531436690 ) ) ;
#151249=CARTESIAN_POINT ( 'NONE',  ( -5.049401038297874678, -19.05341960407617918, 34.79275706135233293 ) ) ;
#151250=CARTESIAN_POINT ( 'NONE',  ( 9.474510206698971260, -16.51473224551069308, 47.91557627198102409 ) ) ;
#151251=CARTESIAN_POINT ( 'NONE',  ( -4.379528057220328563, 16.55341960407611168, 25.20724293864769550 ) ) ;
#151252=CARTESIAN_POINT ( 'NONE',  ( -19.02544592524342804, 5.153800228976336051, 26.04057627198103120 ) ) ;
#151254=CARTESIAN_POINT ( 'NONE',  ( 15.72974639402176855, 15.80617190586768217, 46.87609039468568994 ) ) ;
#151255=CARTESIAN_POINT ( 'NONE',  ( -0.05219959533936034679, 19.03943276465977164, 77.50109039468566152 ) ) ;
#151256=CARTESIAN_POINT ( 'NONE',  ( -8.224510206698948167, 14.34966873604960824, 35.41557627198102409 ) ) ;
#151257=CARTESIAN_POINT ( 'NONE',  ( 18.67979575497178502, 10.72451020669898547, 89.16557627198102409 ) ) ;
#151258=CARTESIAN_POINT ( 'NONE',  ( 5.823673210054125526, 21.52544592524343514, 29.79057627198102409 ) ) ;
#151259=CARTESIAN_POINT ( 'NONE',  ( -16.55341960407611168, -4.379528057220339221, 66.45724293864768129 ) ) ;
#151260=CARTESIAN_POINT ( 'NONE',  ( -16.46253265017160317, 9.564922557960807481, 40.83224293864769550 ) ) ;
#151261=CARTESIAN_POINT ( 'NONE',  ( -16.53943276465976808, -0.05219959533934237506, 98.75109039468568994 ) ) ;
#151262=CARTESIAN_POINT ( 'NONE',  ( 12.14591786802327356, -12.06949235617739191, 75.62609039468567573 ) ) ;
#151263=CARTESIAN_POINT ( 'NONE',  ( -18.62759615963270932, 10.81492255796079327, 40.83224293864769550 ) ) ;
#151264=CARTESIAN_POINT ( 'NONE',  ( 5.153800228976615827, -19.02544592524334988, 25.20942372801900433 ) ) ;
#151265=CARTESIAN_POINT ( 'NONE',  ( -13.89961937509977652, 13.97604488694528158, 90.62390960531432427 ) ) ;
#151266=CARTESIAN_POINT ( 'NONE',  ( 12.14591786802327356, -12.06949235617739191, 70.62609039468567573 ) ) ;
#151267=CARTESIAN_POINT ( 'NONE',  ( 16.51473224551069308, 9.474510206698969483, 29.16557627198103475 ) ) ;
#151268=CARTESIAN_POINT ( 'NONE',  ( 0.05219959533910956823, 16.53943276465976808, 39.99890960531436690 ) ) ;
#151269=CARTESIAN_POINT ( 'NONE',  ( -16.46253265017160317, 9.564922557960807481, 100.8322429386477097 ) ) ;
#151270=CARTESIAN_POINT ( 'NONE',  ( -5.049401038298153566, 19.05341960407611168, 90.20724293864766707 ) ) ;
#151271=CARTESIAN_POINT ( 'NONE',  ( -21.55341960407610458, -5.719274019375992779, 21.45724293864769550 ) ) ;
#151272=CARTESIAN_POINT ( 'NONE',  ( -14.29746914071049879, 8.314922557960819915, 75.83224293864769550 ) ) ;
#151274=CARTESIAN_POINT ( 'NONE',  ( -12.06949235617756955, 12.14591786802309770, 50.62390960531435979 ) ) ;
#151276=CARTESIAN_POINT ( 'NONE',  ( 0.05219959533934541429, -16.53943276465976808, 60.00109039468568284 ) ) ;
#151277=CARTESIAN_POINT ( 'NONE',  ( 18.22780087662122384, -5.500000000000022204, 81.01540105326105845 ) ) ;
#151278=CARTESIAN_POINT ( 'NONE',  ( -9.564922557961040184, 16.46253265017147172, 52.91775706135233293 ) ) ;
#151279=CARTESIAN_POINT ( 'NONE',  ( 16.51473224551069308, 9.474510206698969483, 94.16557627198103830 ) ) ;
#151280=CARTESIAN_POINT ( 'NONE',  ( 5.153800228976615827, -19.02544592524334988, 70.20942372801899012 ) ) ;
#151282=CARTESIAN_POINT ( 'NONE',  ( 5.153800228976615827, -19.02544592524334988, 110.2094237280189901 ) ) ;
#151283=CARTESIAN_POINT ( 'NONE',  ( 12.14591786802327356, -12.06949235617739191, 90.62609039468567573 ) ) ;
#151284=CARTESIAN_POINT ( 'NONE',  ( 16.46253265017160672, -9.564922557960803928, 33.33224293864770260 ) ) ;
#151285=( BOUNDED_CURVE ( )  B_SPLINE_CURVE ( 2, ( #109634, #110620, #31810, #79295, #92467, #154155, #140964, #2451, #187500, #93461, #78287, #139961, #45980 ),
 .UNSPECIFIED., .F., .T. ) 
 B_SPLINE_CURVE_WITH_KNOTS ( ( 3, 2, 2, 2, 2, 2, 3 ),
 ( 0.7393182215122932055, 0.7412280701754385692, 0.7456140350877192846, 0.7500000000000000000, 0.7543859649122807154, 0.7587719298245614308, 0.7607274583097971554 ),
 .UNSPECIFIED. ) 
 CURVE ( )  GEOMETRIC_REPRESENTATION_ITEM ( )  RATIONAL_B_SPLINE_CURVE ( ( 0.9832469066685285419, 0.9851625545550100060, 1.000000000000000000, 0.9659258262890683122, 1.000000000000000000, 0.9659258262890683122, 1.000000000000000000, 0.9659258262890683122, 1.000000000000000000, 0.9659258262890683122, 1.000000000000000000, 0.9848076720550078544, 0.9831626618144001517 ) ) 
 REPRESENTATION_ITEM ( '' )  );
#151286=CARTESIAN_POINT ( 'NONE',  ( 16.46253265017160672, -9.564922557960803928, 113.3322429386476955 ) ) ;
#151287=CARTESIAN_POINT ( 'NONE',  ( -21.53943276465977519, -0.05219959533937600094, 48.75109039468568284 ) ) ;
#151288=CARTESIAN_POINT ( 'NONE',  ( -16.51473224551082808, 9.474510206698731452, 98.33442372801900433 ) ) ;
#151289=CARTESIAN_POINT ( 'NONE',  ( 17.50000000000000000, 3.880681150310165251, 22.10217894668021188 ) ) ;
#151290=CARTESIAN_POINT ( 'NONE',  ( -5.049401038298153566, 19.05341960407611168, 55.20724293864769550 ) ) ;
#151293=CARTESIAN_POINT ( 'NONE',  ( -4.483927247898539470, -16.52544592524342804, 72.29057627198102409 ) ) ;
#151294=CARTESIAN_POINT ( 'NONE',  ( 16.51473224551069308, 9.474510206698969483, 64.16557627198102409 ) ) ;
#151295=CARTESIAN_POINT ( 'NONE',  ( 0.05219959533909260263, 19.03943276465977164, 74.99890960531435269 ) ) ;
#151296=CARTESIAN_POINT ( 'NONE',  ( -0.05219959533936034679, 19.03943276465977164, 72.50109039468566152 ) ) ;
#151297=CARTESIAN_POINT ( 'NONE',  ( 5.823673210054125526, 21.52544592524343514, 64.79057627198103830 ) ) ;
#151298=CARTESIAN_POINT ( 'NONE',  ( 12.06949235617757843, -12.14591786802309237, 113.1239096053143953 ) ) ;
#151299=CARTESIAN_POINT ( 'NONE',  ( -5.153800228976607833, 19.02544592524334988, 52.70942372801900433 ) ) ;
#151300=CARTESIAN_POINT ( 'NONE',  ( -0.05219959533909027116, -19.03943276465977164, 57.49890960531435979 ) ) ;
#151301=CARTESIAN_POINT ( 'NONE',  ( 19.05341960407611168, 5.049401038298154454, 98.95724293864766707 ) ) ;
#151302=CARTESIAN_POINT ( 'NONE',  ( 21.53943276465977519, -0.05219959533907433946, 93.74890960531436690 ) ) ;
#151303=CARTESIAN_POINT ( 'NONE',  ( 12.14591786802309770, 12.06949235617756955, 84.37390960531438111 ) ) ;
#151304=CARTESIAN_POINT ( 'NONE',  ( 0.05219959533936267826, -19.03943276465977164, 55.00109039468566863 ) ) ;
#151305=CARTESIAN_POINT ( 'NONE',  ( -18.62759615963270932, 10.81492255796079327, 75.83224293864769550 ) ) ;
#151306=CARTESIAN_POINT ( 'NONE',  ( -5.719274019375978568, 21.55341960407610458, 60.20724293864768839 ) ) ;
#151307=CARTESIAN_POINT ( 'NONE',  ( -0.05219959533910754901, -16.53943276465976808, 27.49890960531435269 ) ) ;
#151308=CARTESIAN_POINT ( 'NONE',  ( 0.05219959533937995610, -21.53943276465977519, 95.00109039468568994 ) ) ;
#151309=CARTESIAN_POINT ( 'NONE',  ( 19.02544592524343514, -5.153800228976328945, 78.54057627198099567 ) ) ;
#151310=CARTESIAN_POINT ( 'NONE',  ( -13.97604488694527625, -13.89961937509977652, 31.87390960531435979 ) ) ;
#151311=CARTESIAN_POINT ( 'NONE',  ( -18.62759615963255300, -10.81492255796106328, 24.16775706135235424 ) ) ;
#151312=CARTESIAN_POINT ( 'NONE',  ( -21.53943276465977519, -0.05219959533937600094, 43.75109039468568284 ) ) ;
#151313=CARTESIAN_POINT ( 'NONE',  ( -16.46253265017160317, 9.564922557960807481, 50.83224293864770260 ) ) ;
#151314=CARTESIAN_POINT ( 'NONE',  ( -21.52544592524334988, -5.823673210054445271, 18.95942372801901143 ) ) ;
#151315=CARTESIAN_POINT ( 'NONE',  ( 9.564922557961047289, -16.46253265017146816, 65.41775706135233293 ) ) ;
#151316=CARTESIAN_POINT ( 'NONE',  ( -5.049401038298153566, 19.05341960407611168, 40.20724293864768839 ) ) ;
#151317=CARTESIAN_POINT ( 'NONE',  ( -12.06949235617739369, -12.14591786802326823, 34.37609039468568284 ) ) ;
#151319=CARTESIAN_POINT ( 'NONE',  ( -12.14591786802326823, 12.06949235617739902, 73.12609039468567573 ) ) ;
#151320=CARTESIAN_POINT ( 'NONE',  ( -0.05219959533909027116, -19.03943276465977164, 37.49890960531436690 ) ) ;
#151322=CARTESIAN_POINT ( 'NONE',  ( -19.02544592524342804, 5.153800228976336051, 86.04057627198103830 ) ) ;
#151323=CARTESIAN_POINT ( 'NONE',  ( -19.02544592524342804, 5.153800228976336051, 26.04057627198103120 ) ) ;
#151324=EDGE_CURVE ( 'NONE', #38283, #135811, #175095, .T. ) ;
#151325=CARTESIAN_POINT ( 'NONE',  ( 10.72451020669898902, -18.67979575497178502, 62.91557627198102409 ) ) ;
#151326=CARTESIAN_POINT ( 'NONE',  ( 0.05219959533934541429, -16.53943276465976808, 45.00109039468568284 ) ) ;
#151327=CARTESIAN_POINT ( 'NONE',  ( -18.62759615963255300, -10.81492255796106328, 94.16775706135237556 ) ) ;
#151328=CARTESIAN_POINT ( 'NONE',  ( -19.05341960407611168, -5.049401038298163336, 36.45724293864766707 ) ) ;
#151329=CARTESIAN_POINT ( 'NONE',  ( -14.29746914071049879, 8.314922557960819915, 35.83224293864768839 ) ) ;
#151330=CARTESIAN_POINT ( 'NONE',  ( 16.52544592524342804, -4.483927247898539470, 68.54057627198103830 ) ) ;
#151331=CARTESIAN_POINT ( 'NONE',  ( -16.46253265017160317, 9.564922557960807481, 65.83224293864769550 ) ) ;
#151332=CARTESIAN_POINT ( 'NONE',  ( -21.52544592524334988, -5.823673210054445271, 108.9594237280190185 ) ) ;
#151333=CARTESIAN_POINT ( 'NONE',  ( 15.72974639402176855, 15.80617190586768217, 26.87609039468567218 ) ) ;
#151334=CARTESIAN_POINT ( 'NONE',  ( -0.05219959533909027116, -19.03943276465977164, 82.49890960531436690 ) ) ;
#151335=CARTESIAN_POINT ( 'NONE',  ( -21.52544592524334988, -5.823673210054445271, 83.95942372801900433 ) ) ;
#151336=CARTESIAN_POINT ( 'NONE',  ( 16.53943276465976808, 0.05219959533934440121, 51.25109039468568994 ) ) ;
#151337=CARTESIAN_POINT ( 'NONE',  ( 14.29746914071037800, 8.314922557961029526, 31.66775706135234358 ) ) ;
#151338=CARTESIAN_POINT ( 'NONE',  ( 0.05219959533910956823, 16.53943276465976808, 94.99890960531436690 ) ) ;
#151339=CARTESIAN_POINT ( 'NONE',  ( 21.52544592524334988, 5.823673210054432836, 96.45942372801901854 ) ) ;
#151340=CARTESIAN_POINT ( 'NONE',  ( 8.224510206698953496, -14.34966873604960469, 32.91557627198102409 ) ) ;
#151341=CARTESIAN_POINT ( 'NONE',  ( 5.049401038298161559, -19.05341960407611168, 22.70724293864769194 ) ) ;
#151342=CARTESIAN_POINT ( 'NONE',  ( -8.224510206698735004, -14.34966873604973081, 59.58442372801901854 ) ) ;
#151343=CARTESIAN_POINT ( 'NONE',  ( -16.53943276465976808, 0.05219959533911058130, 56.24890960531436690 ) ) ;
#151344=CARTESIAN_POINT ( 'NONE',  ( -14.34966873604972548, 8.224510206698743886, 103.3344237280190043 ) ) ;
#151345=CARTESIAN_POINT ( 'NONE',  ( -19.02544592524342804, 5.153800228976336051, 116.0405762719810383 ) ) ;
#151346=CARTESIAN_POINT ( 'NONE',  ( -18.67979575497178146, -10.72451020669898902, 21.66557627198102409 ) ) ;
#151347=CARTESIAN_POINT ( 'NONE',  ( -10.81492255796105439, 18.62759615963255655, 112.9177570613523329 ) ) ;
#151348=CARTESIAN_POINT ( 'NONE',  ( -0.05219959533910754901, -16.53943276465976808, 87.49890960531436690 ) ) ;
#151349=CARTESIAN_POINT ( 'NONE',  ( -5.153800228976328057, -19.02544592524343514, 97.29057627198099567 ) ) ;
#151350=ORIENTED_EDGE ( 'NONE', *, *, #78467, .F. ) ;
#151351=CARTESIAN_POINT ( 'NONE',  ( 0.05219959533934541429, -16.53943276465976808, 40.00109039468567573 ) ) ;
#151352=CARTESIAN_POINT ( 'NONE',  ( -19.03943276465977164, 0.05219959533909376836, 36.24890960531436690 ) ) ;
#151353=CARTESIAN_POINT ( 'NONE',  ( 4.483927247898790824, -16.52544592524335698, 45.20942372801901854 ) ) ;
#151355=CARTESIAN_POINT ( 'NONE',  ( -19.02544592524334988, -5.153800228976617603, 43.95942372801899012 ) ) ;
#151356=CARTESIAN_POINT ( 'NONE',  ( 5.153800228976335163, 19.02544592524342804, 44.79057627198103830 ) ) ;
#151357=CARTESIAN_POINT ( 'NONE',  ( 16.53943276465976808, 0.05219959533934440121, 81.25109039468568994 ) ) ;
#151358=CARTESIAN_POINT ( 'NONE',  ( -19.02544592524334988, -5.153800228976617603, 88.95942372801897591 ) ) ;
#151359=CARTESIAN_POINT ( 'NONE',  ( -19.03943276465977164, -0.05219959533935918106, 23.75109039468566152 ) ) ;
#151360=CARTESIAN_POINT ( 'NONE',  ( -9.564922557960796823, -16.46253265017161027, 57.08224293864769550 ) ) ;
#151361=CARTESIAN_POINT ( 'NONE',  ( -8.224510206698948167, 14.34966873604960824, 95.41557627198102409 ) ) ;
#151362=CARTESIAN_POINT ( 'NONE',  ( -16.46253265017146816, -9.564922557961047289, 69.16775706135233293 ) ) ;
#151363=CARTESIAN_POINT ( 'NONE',  ( 0.05219959533907565091, 21.53943276465977519, 64.99890960531435269 ) ) ;
#151364=CARTESIAN_POINT ( 'NONE',  ( 5.049401038297881783, 19.05341960407617563, 32.29275706135233293 ) ) ;
#151365=CARTESIAN_POINT ( 'NONE',  ( -13.89961937509977652, 13.97604488694528158, 105.6239096053143527 ) ) ;
#151366=CARTESIAN_POINT ( 'NONE',  ( 18.62759615963271287, -10.81492255796078972, 78.33224293864770971 ) ) ;
#151368=CARTESIAN_POINT ( 'NONE',  ( 5.153800228976615827, -19.02544592524334988, 100.2094237280190043 ) ) ;
#151369=CARTESIAN_POINT ( 'NONE',  ( -18.87075004821572222, 5.499999999999904077, 58.67408112101050222 ) ) ;
#151370=CARTESIAN_POINT ( 'NONE',  ( -12.06949235617739369, -12.14591786802326823, 24.37609039468567573 ) ) ;
#151371=CARTESIAN_POINT ( 'NONE',  ( 9.474510206698971260, -16.51473224551069308, 37.91557627198102409 ) ) ;
#151372=CARTESIAN_POINT ( 'NONE',  ( 9.474510206698971260, -16.51473224551069308, 112.9155762719810383 ) ) ;
#151373=CARTESIAN_POINT ( 'NONE',  ( 21.53943276465977519, -0.05219959533907433946, 88.74890960531436690 ) ) ;
#151374=CARTESIAN_POINT ( 'NONE',  ( -10.72451020669870658, -18.67979575497194134, 54.58442372801901143 ) ) ;
#151375=CARTESIAN_POINT ( 'NONE',  ( 0.05219959533936267826, -19.03943276465977164, 110.0010903946856757 ) ) ;
#151376=CARTESIAN_POINT ( 'NONE',  ( 10.72451020669871369, 18.67979575497193778, 107.0844237280190043 ) ) ;
#151377=CARTESIAN_POINT ( 'NONE',  ( -4.379528057220086978, -16.55341960407618274, 109.7927570613523613 ) ) ;
#151379=CARTESIAN_POINT ( 'NONE',  ( -10.72451020669898014, 18.67979575497178502, 105.4155762719810383 ) ) ;
#151380=CARTESIAN_POINT ( 'NONE',  ( 16.53943276465976808, -0.05219959533910856209, 43.74890960531435979 ) ) ;
#151381=CARTESIAN_POINT ( 'NONE',  ( 16.51473224551083163, -9.474510206698727899, 75.83442372801900433 ) ) ;
#151382=CARTESIAN_POINT ( 'NONE',  ( -9.564922557961040184, 16.46253265017147172, 57.91775706135233293 ) ) ;
#151383=CARTESIAN_POINT ( 'NONE',  ( -5.823673210054431948, 21.52544592524334988, 67.70942372801901854 ) ) ;
#151384=CARTESIAN_POINT ( 'NONE',  ( -13.97604488694547697, 13.89961937509957934, 43.12609039468566152 ) ) ;
#151385=CARTESIAN_POINT ( 'NONE',  ( -12.14591786802309592, -12.06949235617757132, 111.8739096053143669 ) ) ;
#151386=CARTESIAN_POINT ( 'NONE',  ( 5.823673210054125526, 21.52544592524343514, 39.79057627198103830 ) ) ;
#151387=CARTESIAN_POINT ( 'NONE',  ( -14.29746914071049879, 8.314922557960819915, 35.83224293864768839 ) ) ;
#151388=CARTESIAN_POINT ( 'NONE',  ( -21.52544592524334988, -5.823673210054445271, 103.9594237280190185 ) ) ;
#151389=CARTESIAN_POINT ( 'NONE',  ( 4.379528057220092307, 16.55341960407617563, 67.29275706135234714 ) ) ;
#151390=CARTESIAN_POINT ( 'NONE',  ( 8.224510206698953496, -14.34966873604960469, 32.91557627198102409 ) ) ;
#151391=CARTESIAN_POINT ( 'NONE',  ( 5.719274019375673035, 21.55341960407619339, 57.29275706135234714 ) ) ;
#151392=CARTESIAN_POINT ( 'NONE',  ( 18.62759615963255655, 10.81492255796105972, 66.66775706135234714 ) ) ;
#151393=CARTESIAN_POINT ( 'NONE',  ( -21.55341960407610458, -5.719274019375992779, 66.45724293864768129 ) ) ;
#151394=ORIENTED_EDGE ( 'NONE', *, *, #51079, .F. ) ;
#151395=CARTESIAN_POINT ( 'NONE',  ( -5.153800228976328057, -19.02544592524343514, 27.29057627198103120 ) ) ;
#151396=CARTESIAN_POINT ( 'NONE',  ( 5.719274019375673035, 21.55341960407619339, 42.29275706135235424 ) ) ;
#151397=CARTESIAN_POINT ( 'NONE',  ( 16.51473224551069308, 9.474510206698969483, 29.16557627198103475 ) ) ;
#151398=CARTESIAN_POINT ( 'NONE',  ( 5.153800228976335163, 19.02544592524342804, 44.79057627198103830 ) ) ;
#151399=CARTESIAN_POINT ( 'NONE',  ( 14.29746914071049879, -8.314922557960816363, 73.33224293864769550 ) ) ;
#151400=CARTESIAN_POINT ( 'NONE',  ( 13.97604488694527802, 13.89961937509977652, 84.37390960531433848 ) ) ;
#151401=CARTESIAN_POINT ( 'NONE',  ( -16.53943276465976808, 0.05219959533911058130, 21.24890960531436690 ) ) ;
#151402=CARTESIAN_POINT ( 'NONE',  ( 14.29746914071049879, -8.314922557960816363, 98.33224293864769550 ) ) ;
#151403=CARTESIAN_POINT ( 'NONE',  ( 15.72974639402199770, -15.80617190586745480, 73.12390960531436690 ) ) ;
#151404=CARTESIAN_POINT ( 'NONE',  ( -10.72451020669898014, 18.67979575497178502, 100.4155762719810241 ) ) ;
#151405=CARTESIAN_POINT ( 'NONE',  ( 16.51473224551069308, 9.474510206698969483, 114.1655762719810241 ) ) ;
#151406=CARTESIAN_POINT ( 'NONE',  ( 9.474510206698971260, -16.51473224551069308, 67.91557627198102409 ) ) ;
#151407=CARTESIAN_POINT ( 'NONE',  ( 8.224510206698742110, 14.34966873604972548, 22.08442372801901143 ) ) ;
#151409=CARTESIAN_POINT ( 'NONE',  ( -21.55341960407610458, -5.719274019375992779, 51.45724293864770260 ) ) ;
#151410=CARTESIAN_POINT ( 'NONE',  ( 10.72451020669871369, 18.67979575497193778, 77.08442372801901854 ) ) ;
#151411=CARTESIAN_POINT ( 'NONE',  ( 19.03943276465977164, -0.05219959533909143690, 68.74890960531436690 ) ) ;
#151412=CARTESIAN_POINT ( 'NONE',  ( -16.46253265017160317, 9.564922557960807481, 100.8322429386477097 ) ) ;
#151413=CARTESIAN_POINT ( 'NONE',  ( 14.34966873604972726, -8.224510206698740333, 75.83442372801900433 ) ) ;
#151414=CARTESIAN_POINT ( 'NONE',  ( -21.53943276465977519, -0.05219959533937600094, 58.75109039468568994 ) ) ;
#151415=CARTESIAN_POINT ( 'NONE',  ( 21.55341960407619695, -5.719274019375665929, 96.04275706135236135 ) ) ;
#151416=CARTESIAN_POINT ( 'NONE',  ( 21.53943276465977519, -0.05219959533907433946, 113.7489096053143527 ) ) ;
#151417=CARTESIAN_POINT ( 'NONE',  ( -19.05341960407611168, -5.049401038298163336, 21.45724293864768839 ) ) ;
#151418=CARTESIAN_POINT ( 'NONE',  ( 21.53943276465977519, -0.05219959533907433946, 88.74890960531436690 ) ) ;
#151419=CARTESIAN_POINT ( 'NONE',  ( 0.05219959533936267826, -19.03943276465977164, 45.00109039468566863 ) ) ;
#151420=CARTESIAN_POINT ( 'NONE',  ( 15.72974639402199770, -15.80617190586745480, 38.12390960531436690 ) ) ;
#151421=CARTESIAN_POINT ( 'NONE',  ( -9.564922557960796823, -16.46253265017161027, 77.08224293864769550 ) ) ;
#151422=CARTESIAN_POINT ( 'NONE',  ( -16.55341960407611168, -4.379528057220339221, 31.45724293864769550 ) ) ;
#151423=CARTESIAN_POINT ( 'NONE',  ( -17.40805194822031154, 6.112264579159341515, 65.83371272510615313 ) ) ;
#151424=CARTESIAN_POINT ( 'NONE',  ( -19.01529144963334872, -5.500000000000081712, 81.23431955728439391 ) ) ;
#151425=CARTESIAN_POINT ( 'NONE',  ( 9.564922557961047289, -16.46253265017146816, 100.4177570613523329 ) ) ;
#151426=CARTESIAN_POINT ( 'NONE',  ( -15.80617190586745835, -15.72974639402198527, 66.87390960531436690 ) ) ;
#151427=CARTESIAN_POINT ( 'NONE',  ( 4.379528057220339221, -16.55341960407611168, 57.70724293864770260 ) ) ;
#151428=CARTESIAN_POINT ( 'NONE',  ( -12.14591786802326823, 12.06949235617739902, 28.12609039468568284 ) ) ;
#151429=CARTESIAN_POINT ( 'NONE',  ( -19.02544592524342804, 5.153800228976336051, 41.04057627198103120 ) ) ;
#151430=CARTESIAN_POINT ( 'NONE',  ( 18.62759615963271287, -10.81492255796078972, 108.3322429386477097 ) ) ;
#151431=CARTESIAN_POINT ( 'NONE',  ( -13.89961937509957401, -13.97604488694547875, 89.37609039468563310 ) ) ;
#151432=CARTESIAN_POINT ( 'NONE',  ( -19.02544592524342804, 5.153800228976336051, 76.04057627198102409 ) ) ;
#151433=CARTESIAN_POINT ( 'NONE',  ( 8.314922557960818139, 14.29746914071049879, 94.58224293864769550 ) ) ;
#151434=CARTESIAN_POINT ( 'NONE',  ( 16.46253265017160672, -9.564922557960803928, 68.33224293864770971 ) ) ;
#151435=CARTESIAN_POINT ( 'NONE',  ( 10.81492255796078972, 18.62759615963270932, 74.58224293864768129 ) ) ;
#151436=CARTESIAN_POINT ( 'NONE',  ( -16.51473224551069308, -9.474510206698971260, 31.66557627198102054 ) ) ;
#151438=CARTESIAN_POINT ( 'NONE',  ( 14.29746914071049879, -8.314922557960816363, 58.33224293864768839 ) ) ;
#151439=CARTESIAN_POINT ( 'NONE',  ( 0.05219959533909260263, 19.03943276465977164, 89.99890960531436690 ) ) ;
#151441=CARTESIAN_POINT ( 'NONE',  ( 0.05219959533936267826, -19.03943276465977164, 55.00109039468566863 ) ) ;
#151442=CARTESIAN_POINT ( 'NONE',  ( 0.05219959533934541429, -16.53943276465976808, 55.00109039468568284 ) ) ;
#151443=CARTESIAN_POINT ( 'NONE',  ( -18.67979575497178146, -10.72451020669898902, 71.66557627198100988 ) ) ;
#151444=CARTESIAN_POINT ( 'NONE',  ( 13.89961937509957401, 13.97604488694547697, 41.87609039468566152 ) ) ;
#151445=CARTESIAN_POINT ( 'NONE',  ( 9.564922557960805705, 16.46253265017160317, 94.58224293864769550 ) ) ;
#151446=CARTESIAN_POINT ( 'NONE',  ( -17.49999999999999645, 5.499999999999997335, 115.7969038253417438 ) ) ;
#151447=CARTESIAN_POINT ( 'NONE',  ( 21.52544592524344225, -5.823673210054117533, 28.54057627198103120 ) ) ;
#151448=CARTESIAN_POINT ( 'NONE',  ( -5.049401038298153566, 19.05341960407611168, 75.20724293864769550 ) ) ;
#151449=CARTESIAN_POINT ( 'NONE',  ( -5.823673210054431948, 21.52544592524334988, 57.70942372801901143 ) ) ;
#151450=CARTESIAN_POINT ( 'NONE',  ( -13.89961937509977652, 13.97604488694528158, 25.62390960531434558 ) ) ;
#151451=CARTESIAN_POINT ( 'NONE',  ( 18.67979575497194134, -10.72451020669871369, 20.83442372801901143 ) ) ;
#151452=CARTESIAN_POINT ( 'NONE',  ( -5.153800228976328057, -19.02544592524343514, 92.29057627198099567 ) ) ;
#151454=CARTESIAN_POINT ( 'NONE',  ( -21.53943276465977519, -0.05219959533937600094, 33.75109039468568284 ) ) ;
#151455=ORIENTED_EDGE ( 'NONE', *, *, #64457, .F. ) ;
#151456=CARTESIAN_POINT ( 'NONE',  ( 16.51473224551069308, 9.474510206698969483, 104.1655762719810241 ) ) ;
#151458=CARTESIAN_POINT ( 'NONE',  ( 21.53943276465977519, -0.05219959533907433946, 113.7489096053143527 ) ) ;
#151459=CARTESIAN_POINT ( 'NONE',  ( -19.03943276465977164, 0.05219959533909376836, 46.24890960531435979 ) ) ;
#151460=CARTESIAN_POINT ( 'NONE',  ( -14.29746914071037622, -8.314922557961029526, 29.16775706135234003 ) ) ;
#151462=CARTESIAN_POINT ( 'NONE',  ( -5.719274019375665041, -21.55341960407619695, 99.79275706135234714 ) ) ;
#151463=CARTESIAN_POINT ( 'NONE',  ( -0.05219959533909027116, -19.03943276465977164, 37.49890960531436690 ) ) ;
#151464=CARTESIAN_POINT ( 'NONE',  ( -18.67979575497193778, 10.72451020669871902, 93.33442372801901854 ) ) ;
#151465=CARTESIAN_POINT ( 'NONE',  ( 16.51473224551069308, 9.474510206698969483, 94.16557627198103830 ) ) ;
#151466=CARTESIAN_POINT ( 'NONE',  ( 10.81492255796106328, -18.62759615963255655, 65.41775706135234714 ) ) ;
#151468=CARTESIAN_POINT ( 'NONE',  ( 5.049401038298161559, -19.05341960407611168, 102.7072429386476955 ) ) ;
#151469=CARTESIAN_POINT ( 'NONE',  ( 18.09867054820434262, 5.499999999999818812, 46.48393025253587041 ) ) ;
#151470=CARTESIAN_POINT ( 'NONE',  ( 0.05219959533934541429, -16.53943276465976808, 55.00109039468568284 ) ) ;
#151471=CARTESIAN_POINT ( 'NONE',  ( -12.14591786802326823, 12.06949235617739902, 63.12609039468568994 ) ) ;
#151472=CARTESIAN_POINT ( 'NONE',  ( -10.81492255796105439, 18.62759615963255655, 57.91775706135234714 ) ) ;
#151473=CARTESIAN_POINT ( 'NONE',  ( -18.62759615963255300, -10.81492255796106328, 84.16775706135234714 ) ) ;
#151474=CARTESIAN_POINT ( 'NONE',  ( 8.314922557961029526, -14.29746914071037800, 30.41775706135234358 ) ) ;
#151475=CARTESIAN_POINT ( 'NONE',  ( -5.153800228976328057, -19.02544592524343514, 77.29057627198099567 ) ) ;
#151476=CARTESIAN_POINT ( 'NONE',  ( 19.03943276465977164, -0.05219959533909143690, 103.7489096053143669 ) ) ;
#151477=CARTESIAN_POINT ( 'NONE',  ( -19.05341960407611168, -5.049401038298163336, 111.4572429386476671 ) ) ;
#151478=CARTESIAN_POINT ( 'NONE',  ( -5.049401038298153566, 19.05341960407611168, 30.20724293864768839 ) ) ;
#151479=CARTESIAN_POINT ( 'NONE',  ( 10.81492255796078972, 18.62759615963270932, 24.58224293864768839 ) ) ;
#151480=CARTESIAN_POINT ( 'NONE',  ( 4.483927247898790824, -16.52544592524335698, 90.20942372801903275 ) ) ;
#151481=CARTESIAN_POINT ( 'NONE',  ( -4.379528057220328563, 16.55341960407611168, 90.20724293864770971 ) ) ;
#151482=CARTESIAN_POINT ( 'NONE',  ( 19.03943276465977164, -0.05219959533909143690, 68.74890960531436690 ) ) ;
#151483=CARTESIAN_POINT ( 'NONE',  ( -10.81492255796105439, 18.62759615963255655, 87.91775706135234714 ) ) ;
#151485=CARTESIAN_POINT ( 'NONE',  ( -8.314922557961024197, 14.29746914071037800, 27.91775706135234358 ) ) ;
#151486=CARTESIAN_POINT ( 'NONE',  ( 8.314922557960818139, 14.29746914071049879, 69.58224293864769550 ) ) ;
#151487=CARTESIAN_POINT ( 'NONE',  ( -21.52544592524334988, -5.823673210054445271, 28.95942372801902209 ) ) ;
#151488=CARTESIAN_POINT ( 'NONE',  ( -5.823673210054116645, -21.52544592524344225, 67.29057627198103830 ) ) ;
#151489=CARTESIAN_POINT ( 'NONE',  ( 19.05341960407617918, -5.049401038297876454, 36.04275706135234003 ) ) ;
#151491=CARTESIAN_POINT ( 'NONE',  ( -13.89961937509977652, 13.97604488694528158, 85.62390960531433848 ) ) ;
#151492=CARTESIAN_POINT ( 'NONE',  ( 14.34966873604960469, 8.224510206698951720, 44.16557627198103120 ) ) ;
#151493=CARTESIAN_POINT ( 'NONE',  ( 16.53943276465976808, -0.05219959533910856209, 38.74890960531435979 ) ) ;
#151494=CARTESIAN_POINT ( 'NONE',  ( -14.29746914071037622, -8.314922557961029526, 109.1677570613523613 ) ) ;
#151495=CARTESIAN_POINT ( 'NONE',  ( -13.89961937509957401, -13.97604488694547875, 69.37609039468564731 ) ) ;
#151496=CARTESIAN_POINT ( 'NONE',  ( 17.40805194822030799, 6.112264579159357503, 46.66628727489389661 ) ) ;
#151497=CARTESIAN_POINT ( 'NONE',  ( 18.62759615963271287, -10.81492255796078972, 23.33224293864769194 ) ) ;
#151498=CARTESIAN_POINT ( 'NONE',  ( 8.314922557960818139, 14.29746914071049879, 69.58224293864769550 ) ) ;
#151500=CARTESIAN_POINT ( 'NONE',  ( -13.97604488694527625, -13.89961937509977652, 31.87390960531435979 ) ) ;
#151501=CARTESIAN_POINT ( 'NONE',  ( 21.55341960407610458, 5.719274019375980345, 33.95724293864769550 ) ) ;
#151502=CARTESIAN_POINT ( 'NONE',  ( 5.719274019375991003, -21.55341960407610458, 72.70724293864769550 ) ) ;
#151503=CARTESIAN_POINT ( 'NONE',  ( -8.224510206698948167, 14.34966873604960824, 110.4155762719810383 ) ) ;
#151504=CARTESIAN_POINT ( 'NONE',  ( -8.314922557961024197, 14.29746914071037800, 67.91775706135234714 ) ) ;
#151505=CARTESIAN_POINT ( 'NONE',  ( 9.564922557960805705, 16.46253265017160317, 44.58224293864769550 ) ) ;
#151506=CARTESIAN_POINT ( 'NONE',  ( -18.62759615963255300, -10.81492255796106328, 54.16775706135235424 ) ) ;
#151507=CARTESIAN_POINT ( 'NONE',  ( -12.14591786802309592, -12.06949235617757132, 106.8739096053143811 ) ) ;
#151509=CARTESIAN_POINT ( 'NONE',  ( 16.19135201231362942, -7.376712067592066546, 37.31319145947968252 ) ) ;
#151511=CARTESIAN_POINT ( 'NONE',  ( -21.53943276465977519, 0.05219959533907696930, 36.24890960531435979 ) ) ;
#151513=CARTESIAN_POINT ( 'NONE',  ( -0.05219959533937732626, 21.53943276465977519, 67.50109039468568994 ) ) ;
#151515=CARTESIAN_POINT ( 'NONE',  ( -4.483927247898782831, 16.52544592524335698, 62.70942372801902565 ) ) ;
#151516=CARTESIAN_POINT ( 'NONE',  ( 12.14591786802309770, 12.06949235617756955, 39.37390960531436690 ) ) ;
#151517=CARTESIAN_POINT ( 'NONE',  ( -15.80617190586745835, -15.72974639402198527, 61.87390960531436690 ) ) ;
#151518=CARTESIAN_POINT ( 'NONE',  ( 5.823673210054125526, 21.52544592524343514, 59.79057627198103120 ) ) ;
#151520=CARTESIAN_POINT ( 'NONE',  ( 9.564922557961047289, -16.46253265017146816, 80.41775706135234714 ) ) ;
#151521=CARTESIAN_POINT ( 'NONE',  ( 13.89961937509977652, -13.97604488694527269, 113.1239096053143527 ) ) ;
#151522=CARTESIAN_POINT ( 'NONE',  ( -9.564922557960796823, -16.46253265017161027, 47.08224293864769550 ) ) ;
#151523=CARTESIAN_POINT ( 'NONE',  ( 14.34966873604960469, 8.224510206698951720, 109.1655762719810383 ) ) ;
#151526=CARTESIAN_POINT ( 'NONE',  ( 13.89961937509977652, -13.97604488694527269, 108.1239096053143669 ) ) ;
#151527=ORIENTED_EDGE ( 'NONE', *, *, #141950, .T. ) ;
#151528=CARTESIAN_POINT ( 'NONE',  ( -8.314922557961024197, 14.29746914071037800, 72.91775706135234714 ) ) ;
#151529=CARTESIAN_POINT ( 'NONE',  ( 18.67979575497178502, 10.72451020669898547, 109.1655762719810383 ) ) ;
#151530=CARTESIAN_POINT ( 'NONE',  ( -0.05219959533909027116, -19.03943276465977164, 52.49890960531436690 ) ) ;
#151531=CARTESIAN_POINT ( 'NONE',  ( 18.67979575497194134, -10.72451020669871369, 40.83442372801901854 ) ) ;
#151532=CARTESIAN_POINT ( 'NONE',  ( 19.03943276465977164, -0.05219959533909143690, 93.74890960531435269 ) ) ;
#151534=ORIENTED_EDGE ( 'NONE', *, *, #67877, .T. ) ;
#151535=CARTESIAN_POINT ( 'NONE',  ( -15.80617190586768217, 15.72974639402176855, 33.12609039468569705 ) ) ;
#151536=CARTESIAN_POINT ( 'NONE',  ( 0.05219959533909260263, 19.03943276465977164, 109.9989096053143669 ) ) ;
#151537=CARTESIAN_POINT ( 'NONE',  ( -13.89961937509957401, -13.97604488694547875, 89.37609039468563310 ) ) ;
#151538=CARTESIAN_POINT ( 'NONE',  ( 16.46253265017146816, 9.564922557961045513, 46.66775706135233293 ) ) ;
#151539=CARTESIAN_POINT ( 'NONE',  ( -10.81492255796078084, -18.62759615963271287, 102.0822429386476955 ) ) ;
#151540=CARTESIAN_POINT ( 'NONE',  ( -0.05219959533936034679, 19.03943276465977164, 37.50109039468567573 ) ) ;
#151541=CARTESIAN_POINT ( 'NONE',  ( -13.97604488694547697, 13.89961937509957934, 43.12609039468566152 ) ) ;
#151542=CARTESIAN_POINT ( 'NONE',  ( 8.314922557961029526, -14.29746914071037800, 95.41775706135234714 ) ) ;
#151544=CARTESIAN_POINT ( 'NONE',  ( 19.02544592524343514, -5.153800228976328945, 68.54057627198103830 ) ) ;
#151545=CARTESIAN_POINT ( 'NONE',  ( 10.81492255796106328, -18.62759615963255655, 75.41775706135233293 ) ) ;
#151546=CARTESIAN_POINT ( 'NONE',  ( -5.719274019375665041, -21.55341960407619695, 79.79275706135236135 ) ) ;
#151548=CARTESIAN_POINT ( 'NONE',  ( 16.51473224551069308, 9.474510206698969483, 94.16557627198103830 ) ) ;
#151549=CARTESIAN_POINT ( 'NONE',  ( 21.55341960407619695, -5.719274019375665929, 56.04275706135235424 ) ) ;
#151550=CARTESIAN_POINT ( 'NONE',  ( 5.049401038297881783, 19.05341960407617563, 107.2927570613523187 ) ) ;
#151551=CARTESIAN_POINT ( 'NONE',  ( -19.02544592524342804, 5.153800228976336051, 71.04057627198099567 ) ) ;
#151552=CARTESIAN_POINT ( 'NONE',  ( 5.049401038298161559, -19.05341960407611168, 107.7072429386476955 ) ) ;
#151553=CARTESIAN_POINT ( 'NONE',  ( 9.474510206698971260, -16.51473224551069308, 77.91557627198103830 ) ) ;
#151555=CARTESIAN_POINT ( 'NONE',  ( -19.03943276465977164, 0.05219959533909376836, 61.24890960531436690 ) ) ;
#151556=ADVANCED_FACE ( 'NONE', ( #109488 ), #39062, .T. ) ;
#151557=CARTESIAN_POINT ( 'NONE',  ( -13.89961937509977652, 13.97604488694528158, 50.62390960531435979 ) ) ;
#151558=CARTESIAN_POINT ( 'NONE',  ( 18.67979575497178502, 10.72451020669898547, 109.1655762719810383 ) ) ;
#151559=CARTESIAN_POINT ( 'NONE',  ( 8.224510206698742110, 14.34966873604972548, 87.08442372801901854 ) ) ;
#151561=CARTESIAN_POINT ( 'NONE',  ( 5.153800228976615827, -19.02544592524334988, 45.20942372801901143 ) ) ;
#151562=CARTESIAN_POINT ( 'NONE',  ( 13.97604488694527802, 13.89961937509977652, 84.37390960531433848 ) ) ;
#151563=CARTESIAN_POINT ( 'NONE',  ( 4.483927247898545687, 16.52544592524342804, 69.79057627198102409 ) ) ;
#151564=CARTESIAN_POINT ( 'NONE',  ( -16.55341960407611168, -4.379528057220339221, 101.4572429386476955 ) ) ;
#151565=CARTESIAN_POINT ( 'NONE',  ( 21.53943276465977519, -0.05219959533907433946, 23.74890960531435269 ) ) ;
#151566=CARTESIAN_POINT ( 'NONE',  ( -13.89961937509977652, 13.97604488694528158, 105.6239096053143527 ) ) ;
#151567=CARTESIAN_POINT ( 'NONE',  ( 0.05219959533910956823, 16.53943276465976808, 79.99890960531435269 ) ) ;
#151569=CARTESIAN_POINT ( 'NONE',  ( 19.03943276465977164, 0.05219959533936151252, 26.25109039468566507 ) ) ;
#151570=CARTESIAN_POINT ( 'NONE',  ( -8.224510206698735004, -14.34966873604973081, 94.58442372801901854 ) ) ;
#151571=CARTESIAN_POINT ( 'NONE',  ( 19.02544592524343514, -5.153800228976328945, 73.54057627198103830 ) ) ;
#151572=CARTESIAN_POINT ( 'NONE',  ( 21.52544592524334988, 5.823673210054432836, 51.45942372801901854 ) ) ;
#151573=CARTESIAN_POINT ( 'NONE',  ( 10.81492255796078972, 18.62759615963270932, 39.58224293864769550 ) ) ;
#151574=CARTESIAN_POINT ( 'NONE',  ( -5.719274019375978568, 21.55341960407610458, 110.2072429386477239 ) ) ;
#151575=CARTESIAN_POINT ( 'NONE',  ( -21.55341960407610458, -5.719274019375992779, 71.45724293864769550 ) ) ;
#151576=CARTESIAN_POINT ( 'NONE',  ( -12.06949235617756955, 12.14591786802309770, 95.62390960531436690 ) ) ;
#151577=CARTESIAN_POINT ( 'NONE',  ( -19.05341960407617563, 5.049401038297882671, 53.54275706135231871 ) ) ;
#151578=CARTESIAN_POINT ( 'NONE',  ( 9.474510206698971260, -16.51473224551069308, 37.91557627198102409 ) ) ;
#151579=CARTESIAN_POINT ( 'NONE',  ( 0.05219959533909260263, 19.03943276465977164, 79.99890960531436690 ) ) ;
#151580=CARTESIAN_POINT ( 'NONE',  ( -0.05219959533909027116, -19.03943276465977164, 87.49890960531436690 ) ) ;
#151581=CARTESIAN_POINT ( 'NONE',  ( -8.314922557960811034, -14.29746914071050412, 97.08224293864770971 ) ) ;
#151582=CARTESIAN_POINT ( 'NONE',  ( -16.55341960407611168, -4.379528057220339221, 31.45724293864769550 ) ) ;
#151583=CARTESIAN_POINT ( 'NONE',  ( 4.483927247898790824, -16.52544592524335698, 30.20942372801902565 ) ) ;
#151584=CARTESIAN_POINT ( 'NONE',  ( -21.55341960407619339, 5.719274019375674811, 108.5427570613523756 ) ) ;
#151585=CARTESIAN_POINT ( 'NONE',  ( -5.049401038298153566, 19.05341960407611168, 105.2072429386476671 ) ) ;
#151586=CARTESIAN_POINT ( 'NONE',  ( 21.52544592524334988, 5.823673210054432836, 26.45942372801901854 ) ) ;
#151587=CARTESIAN_POINT ( 'NONE',  ( -5.049401038298153566, 19.05341960407611168, 50.20724293864770260 ) ) ;
#151588=CARTESIAN_POINT ( 'NONE',  ( 4.379528057220092307, 16.55341960407617563, 47.29275706135234003 ) ) ;
#151589=CARTESIAN_POINT ( 'NONE',  ( 13.89961937509957401, 13.97604488694547697, 111.8760903946856757 ) ) ;
#151590=CARTESIAN_POINT ( 'NONE',  ( 13.89961937509977652, -13.97604488694527269, 38.12390960531436690 ) ) ;
#151591=CARTESIAN_POINT ( 'NONE',  ( 4.483927247898545687, 16.52544592524342804, 94.79057627198105251 ) ) ;
#151592=CARTESIAN_POINT ( 'NONE',  ( 10.81492255796078972, 18.62759615963270932, 104.5822429386477097 ) ) ;
#151593=CARTESIAN_POINT ( 'NONE',  ( 13.97604488694548053, -13.89961937509957401, 80.62609039468567573 ) ) ;
#151595=CARTESIAN_POINT ( 'NONE',  ( -13.89961937509977652, 13.97604488694528158, 85.62390960531433848 ) ) ;
#151596=CARTESIAN_POINT ( 'NONE',  ( 21.52544592524344225, -5.823673210054117533, 113.5405762719810383 ) ) ;
#151598=CARTESIAN_POINT ( 'NONE',  ( -9.564922557960796823, -16.46253265017161027, 87.08224293864769550 ) ) ;
#151599=CARTESIAN_POINT ( 'NONE',  ( 16.81555441253555827, -7.025013491695464296, 113.1368544533426359 ) ) ;
#151600=CARTESIAN_POINT ( 'NONE',  ( 9.564922557960805705, 16.46253265017160317, 84.58224293864769550 ) ) ;
#151601=CARTESIAN_POINT ( 'NONE',  ( -18.67979575497193778, 10.72451020669871902, 28.33442372801902209 ) ) ;
#151602=CARTESIAN_POINT ( 'NONE',  ( -14.34966873604960291, -8.224510206698953496, 76.66557627198103830 ) ) ;
#151603=CARTESIAN_POINT ( 'NONE',  ( -19.03943276465977164, 0.05219959533909376836, 96.24890960531436690 ) ) ;
#151604=CARTESIAN_POINT ( 'NONE',  ( -19.05341960407617563, 5.049401038297882671, 28.54275706135232937 ) ) ;
#151605=CARTESIAN_POINT ( 'NONE',  ( 16.52544592524335698, 4.483927247898782831, 46.45942372801901854 ) ) ;
#151606=CARTESIAN_POINT ( 'NONE',  ( 0.05219959533937995610, -21.53943276465977519, 65.00109039468568994 ) ) ;
#151607=CARTESIAN_POINT ( 'NONE',  ( -4.379528057220086978, -16.55341960407618274, 29.79275706135234358 ) ) ;
#151608=CARTESIAN_POINT ( 'NONE',  ( 0.05219959533909260263, 19.03943276465977164, 64.99890960531436690 ) ) ;
#151609=CARTESIAN_POINT ( 'NONE',  ( 16.51473224551083163, -9.474510206698727899, 90.83442372801900433 ) ) ;
#151610=CARTESIAN_POINT ( 'NONE',  ( 4.379528057220092307, 16.55341960407617563, 72.29275706135236135 ) ) ;
#151611=CARTESIAN_POINT ( 'NONE',  ( -0.05219959533937732626, 21.53943276465977519, 107.5010903946856899 ) ) ;
#151612=CARTESIAN_POINT ( 'NONE',  ( -5.153800228976607833, 19.02544592524334988, 82.70942372801897591 ) ) ;
#151613=CARTESIAN_POINT ( 'NONE',  ( 19.03943276465977164, -0.05219959533909143690, 53.74890960531436690 ) ) ;
#151614=CARTESIAN_POINT ( 'NONE',  ( -15.80617190586745835, -15.72974639402198527, 86.87390960531438111 ) ) ;
#151615=CARTESIAN_POINT ( 'NONE',  ( -12.14591786802309592, -12.06949235617757132, 76.87390960531439532 ) ) ;
#151616=CARTESIAN_POINT ( 'NONE',  ( -5.153800228976607833, 19.02544592524334988, 77.70942372801900433 ) ) ;
#151618=CARTESIAN_POINT ( 'NONE',  ( -19.05341960407617563, 5.049401038297882671, 58.54275706135234003 ) ) ;
#151619=CARTESIAN_POINT ( 'NONE',  ( -4.379528057220086978, -16.55341960407618274, 109.7927570613523613 ) ) ;
#151620=CARTESIAN_POINT ( 'NONE',  ( 4.379528057220339221, -16.55341960407611168, 72.70724293864769550 ) ) ;
#151621=CARTESIAN_POINT ( 'NONE',  ( -10.72451020669870658, -18.67979575497194134, 99.58442372801900433 ) ) ;
#151623=CARTESIAN_POINT ( 'NONE',  ( -5.823673210054116645, -21.52544592524344225, 112.2905762719810241 ) ) ;
#151624=CARTESIAN_POINT ( 'NONE',  ( -0.05219959533909027116, -19.03943276465977164, 62.49890960531435979 ) ) ;
#151625=CARTESIAN_POINT ( 'NONE',  ( -18.67979575497193778, 10.72451020669871902, 78.33442372801901854 ) ) ;
#151626=CARTESIAN_POINT ( 'NONE',  ( -13.89961937509977652, 13.97604488694528158, 65.62390960531436690 ) ) ;
#151627=CARTESIAN_POINT ( 'NONE',  ( -9.564922557960796823, -16.46253265017161027, 22.08224293864768839 ) ) ;
#151628=CARTESIAN_POINT ( 'NONE',  ( 21.55341960407610458, 5.719274019375980345, 28.95724293864769905 ) ) ;
#151629=CARTESIAN_POINT ( 'NONE',  ( 12.06949235617757843, -12.14591786802309237, 73.12390960531436690 ) ) ;
#151630=CARTESIAN_POINT ( 'NONE',  ( 16.46253265017160672, -9.564922557960803928, 48.33224293864769550 ) ) ;
#151631=CARTESIAN_POINT ( 'NONE',  ( 8.314922557960818139, 14.29746914071049879, 104.5822429386477097 ) ) ;
#151632=CARTESIAN_POINT ( 'NONE',  ( -5.719274019375978568, 21.55341960407610458, 110.2072429386477239 ) ) ;
#151633=CARTESIAN_POINT ( 'NONE',  ( -10.72451020669870658, -18.67979575497194134, 49.58442372801901143 ) ) ;
#151634=CARTESIAN_POINT ( 'NONE',  ( -13.97604488694527625, -13.89961937509977652, 31.87390960531435979 ) ) ;
#151635=CARTESIAN_POINT ( 'NONE',  ( 16.55341960407618274, -4.379528057220086978, 61.04275706135234714 ) ) ;
#151636=CARTESIAN_POINT ( 'NONE',  ( -15.72974639402197994, 15.80617190586746368, 100.6239096053143811 ) ) ;
#151637=CARTESIAN_POINT ( 'NONE',  ( -10.81492255796078084, -18.62759615963271287, 92.08224293864769550 ) ) ;
#151638=CARTESIAN_POINT ( 'NONE',  ( -19.05341960407617563, 5.049401038297882671, 23.54275706135233648 ) ) ;
#151639=CARTESIAN_POINT ( 'NONE',  ( 9.474510206698971260, -16.51473224551069308, 52.91557627198102409 ) ) ;
#151640=CARTESIAN_POINT ( 'NONE',  ( -17.50000000001356781, 5.500000000000039968, 40.79690382535057580 ) ) ;
#151641=CARTESIAN_POINT ( 'NONE',  ( 15.72974639402176855, 15.80617190586768217, 56.87609039468568994 ) ) ;
#151642=CARTESIAN_POINT ( 'NONE',  ( 0.05219959533907565091, 21.53943276465977519, 54.99890960531435269 ) ) ;
#151643=CARTESIAN_POINT ( 'NONE',  ( -14.34966873604960291, -8.224510206698953496, 26.66557627198103475 ) ) ;
#151644=CARTESIAN_POINT ( 'NONE',  ( -10.72451020669870658, -18.67979575497194134, 74.58442372801901854 ) ) ;
#151645=CARTESIAN_POINT ( 'NONE',  ( -10.72451020669870658, -18.67979575497194134, 99.58442372801900433 ) ) ;
#151646=CARTESIAN_POINT ( 'NONE',  ( -13.89961937509957401, -13.97604488694547875, 39.37609039468566152 ) ) ;
#151647=CARTESIAN_POINT ( 'NONE',  ( -4.483927247898782831, 16.52544592524335698, 107.7094237280190328 ) ) ;
#151648=CARTESIAN_POINT ( 'NONE',  ( 15.80617190586769283, -15.72974639402175789, 50.62609039468568994 ) ) ;
#151649=CARTESIAN_POINT ( 'NONE',  ( -13.97604488694527625, -13.89961937509977652, 56.87390960531434558 ) ) ;
#151650=CARTESIAN_POINT ( 'NONE',  ( 9.474510206698729675, 16.51473224551082808, 32.08442372801900433 ) ) ;
#151651=CARTESIAN_POINT ( 'NONE',  ( 15.80617190586746368, 15.72974639402197994, 39.37390960531436690 ) ) ;
#151652=CARTESIAN_POINT ( 'NONE',  ( 10.72451020669871369, 18.67979575497193778, 27.08442372801901854 ) ) ;
#151654=CARTESIAN_POINT ( 'NONE',  ( -5.719274019375978568, 21.55341960407610458, 85.20724293864770971 ) ) ;
#151655=CARTESIAN_POINT ( 'NONE',  ( 19.03943276465977164, 0.05219959533936151252, 86.25109039468567573 ) ) ;
#151656=CARTESIAN_POINT ( 'NONE',  ( 8.224510206698742110, 14.34966873604972548, 57.08442372801901854 ) ) ;
#151658=CARTESIAN_POINT ( 'NONE',  ( -21.53943276465977519, 0.05219959533907696930, 86.24890960531436690 ) ) ;
#151659=CARTESIAN_POINT ( 'NONE',  ( 8.314922557961029526, -14.29746914071037800, 75.41775706135233293 ) ) ;
#151660=CARTESIAN_POINT ( 'NONE',  ( -4.483927247898539470, -16.52544592524342804, 77.29057627198102409 ) ) ;
#151662=CARTESIAN_POINT ( 'NONE',  ( -19.05341960407617563, 5.049401038297882671, 108.5427570613523187 ) ) ;
#151663=CARTESIAN_POINT ( 'NONE',  ( 21.53943276465977519, -0.05219959533907433946, 33.74890960531436690 ) ) ;
#151665=CARTESIAN_POINT ( 'NONE',  ( -4.483927247898782831, 16.52544592524335698, 37.70942372801900433 ) ) ;
#151666=CARTESIAN_POINT ( 'NONE',  ( 21.53943276465977519, -0.05219959533907433946, 108.7489096053143669 ) ) ;
#151667=CARTESIAN_POINT ( 'NONE',  ( 5.823673210054125526, 21.52544592524343514, 29.79057627198102409 ) ) ;
#151668=CARTESIAN_POINT ( 'NONE',  ( 16.52544592524335698, 4.483927247898782831, 71.45942372801901854 ) ) ;
#151669=CARTESIAN_POINT ( 'NONE',  ( 0.05219959533909260263, 19.03943276465977164, 89.99890960531436690 ) ) ;
#151670=CARTESIAN_POINT ( 'NONE',  ( 10.81492255796106328, -18.62759615963255655, 60.41775706135235424 ) ) ;
#151671=CARTESIAN_POINT ( 'NONE',  ( -5.153800228976328057, -19.02544592524343514, 27.29057627198103120 ) ) ;
#151673=CARTESIAN_POINT ( 'NONE',  ( -5.823673210054116645, -21.52544592524344225, 22.29057627198102765 ) ) ;
#151674=ORIENTED_EDGE ( 'NONE', *, *, #84216, .T. ) ;
#151675=CARTESIAN_POINT ( 'NONE',  ( -9.474510206698720793, -16.51473224551083518, 34.58442372801899722 ) ) ;
#151676=CARTESIAN_POINT ( 'NONE',  ( -4.379528057220086978, -16.55341960407618274, 49.79275706135234714 ) ) ;
#151677=CARTESIAN_POINT ( 'NONE',  ( -16.46253265017160317, 9.564922557960807481, 115.8322429386477097 ) ) ;
#151678=CARTESIAN_POINT ( 'NONE',  ( -19.05341960407611168, -5.049401038298163336, 71.45724293864766707 ) ) ;
#151679=CARTESIAN_POINT ( 'NONE',  ( -16.53943276465976808, -0.05219959533934237506, 98.75109039468568994 ) ) ;
#151681=CARTESIAN_POINT ( 'NONE',  ( -4.379528057220328563, 16.55341960407611168, 95.20724293864769550 ) ) ;
#151682=CARTESIAN_POINT ( 'NONE',  ( -5.719274019375978568, 21.55341960407610458, 35.20724293864768839 ) ) ;
#151683=CARTESIAN_POINT ( 'NONE',  ( -13.97604488694527625, -13.89961937509977652, 26.87390960531434558 ) ) ;
#151684=CARTESIAN_POINT ( 'NONE',  ( 16.52544592524335698, 4.483927247898782831, 66.45942372801903275 ) ) ;
#151685=CARTESIAN_POINT ( 'NONE',  ( -0.05219959533937732626, 21.53943276465977519, 22.50109039468567573 ) ) ;
#151686=CARTESIAN_POINT ( 'NONE',  ( -19.02544592524334988, -5.153800228976617603, 78.95942372801900433 ) ) ;
#151688=CARTESIAN_POINT ( 'NONE',  ( 19.05341960407611168, 5.049401038298154454, 43.95724293864769550 ) ) ;
#151689=CARTESIAN_POINT ( 'NONE',  ( -0.05219959533907301413, -21.53943276465977519, 72.49890960531435269 ) ) ;
#151691=CARTESIAN_POINT ( 'NONE',  ( -9.474510206698964154, 16.51473224551069663, 110.4155762719810383 ) ) ;
#151692=CARTESIAN_POINT ( 'NONE',  ( -5.823673210054431948, 21.52544592524334988, 97.70942372801904696 ) ) ;
#151693=CARTESIAN_POINT ( 'NONE',  ( -13.97604488694527625, -13.89961937509977652, 66.87390960531436690 ) ) ;
#151694=CARTESIAN_POINT ( 'NONE',  ( -4.483927247898782831, 16.52544592524335698, 47.70942372801902565 ) ) ;
#151695=CARTESIAN_POINT ( 'NONE',  ( -15.72974639402176322, -15.80617190586768395, 84.37609039468570415 ) ) ;
#151696=CARTESIAN_POINT ( 'NONE',  ( 9.474510206698729675, 16.51473224551082808, 37.08442372801899722 ) ) ;
#151697=CARTESIAN_POINT ( 'NONE',  ( -0.05219959533936034679, 19.03943276465977164, 57.50109039468566863 ) ) ;
#151699=CARTESIAN_POINT ( 'NONE',  ( -21.55341960407619339, 5.719274019375674811, 43.54275706135235424 ) ) ;
#151700=CARTESIAN_POINT ( 'NONE',  ( 5.049401038297881783, 19.05341960407617563, 52.29275706135234003 ) ) ;
#151701=CARTESIAN_POINT ( 'NONE',  ( 19.02544592524343514, -5.153800228976328945, 93.54057627198102409 ) ) ;
#151702=CARTESIAN_POINT ( 'NONE',  ( -19.05341960407611168, -5.049401038298163336, 76.45724293864769550 ) ) ;
#151703=CARTESIAN_POINT ( 'NONE',  ( 4.379528057220339221, -16.55341960407611168, 37.70724293864769550 ) ) ;
#151704=CARTESIAN_POINT ( 'NONE',  ( -18.67979575497178146, -10.72451020669898902, 36.66557627198103120 ) ) ;
#151706=CARTESIAN_POINT ( 'NONE',  ( 17.05587630539786304, 6.762274262135712810, 56.75819690962690345 ) ) ;
#151707=CARTESIAN_POINT ( 'NONE',  ( 5.719274019375673035, 21.55341960407619339, 102.2927570613523613 ) ) ;
#151709=CARTESIAN_POINT ( 'NONE',  ( 0.05219959533909260263, 19.03943276465977164, 34.99890960531435979 ) ) ;
#151710=CARTESIAN_POINT ( 'NONE',  ( 19.03943276465977164, -0.05219959533909143690, 113.7489096053143669 ) ) ;
#151712=CARTESIAN_POINT ( 'NONE',  ( -16.55341960407617563, 4.379528057220093196, 53.54275706135234714 ) ) ;
#151713=CARTESIAN_POINT ( 'NONE',  ( 21.52544592524344225, -5.823673210054117533, 68.54057627198103830 ) ) ;
#151714=CARTESIAN_POINT ( 'NONE',  ( 16.55341960407611168, 4.379528057220329451, 33.95724293864769550 ) ) ;
#151715=CARTESIAN_POINT ( 'NONE',  ( -19.05341960407611168, -5.049401038298163336, 26.45724293864769550 ) ) ;
#151716=CARTESIAN_POINT ( 'NONE',  ( 19.05341960407611168, 5.049401038298154454, 103.9572429386476671 ) ) ;
#151717=CARTESIAN_POINT ( 'NONE',  ( -10.81492255796105439, 18.62759615963255655, 32.91775706135234714 ) ) ;
#151718=CARTESIAN_POINT ( 'NONE',  ( -13.97604488694547697, 13.89961937509957934, 38.12609039468566152 ) ) ;
#151719=CARTESIAN_POINT ( 'NONE',  ( -19.05341960407611168, -5.049401038298163336, 26.45724293864769550 ) ) ;
#151720=CARTESIAN_POINT ( 'NONE',  ( 21.55341960407619695, -5.719274019375665929, 81.04275706135236135 ) ) ;
#151721=CARTESIAN_POINT ( 'NONE',  ( 17.05587630539787369, -6.762274262135690606, 33.24180309037313918 ) ) ;
#151722=CARTESIAN_POINT ( 'NONE',  ( -4.379528057220328563, 16.55341960407611168, 30.20724293864769550 ) ) ;
#151723=CARTESIAN_POINT ( 'NONE',  ( 17.50000000000000000, 5.068104630630361207, 111.7718159465997445 ) ) ;
#151724=CARTESIAN_POINT ( 'NONE',  ( -21.55341960407610458, -5.719274019375992779, 31.45724293864769550 ) ) ;
#151725=CARTESIAN_POINT ( 'NONE',  ( -4.379528057220328563, 16.55341960407611168, 90.20724293864770971 ) ) ;
#151726=CARTESIAN_POINT ( 'NONE',  ( -17.49999999999999645, 5.499999999999997335, 120.0000000000000142 ) ) ;
#151727=CARTESIAN_POINT ( 'NONE',  ( 13.89961937509977652, -13.97604488694527269, 78.12390960531433848 ) ) ;
#151728=CARTESIAN_POINT ( 'NONE',  ( 12.06949235617757843, -12.14591786802309237, 73.12390960531436690 ) ) ;
#151729=CARTESIAN_POINT ( 'NONE',  ( -0.05219959533936034679, 19.03943276465977164, 112.5010903946856757 ) ) ;
#151730=CARTESIAN_POINT ( 'NONE',  ( -18.62759615963270932, 10.81492255796079327, 60.83224293864769550 ) ) ;
#151732=CARTESIAN_POINT ( 'NONE',  ( -16.46253265017160317, 9.564922557960807481, 35.83224293864768839 ) ) ;
#151733=CARTESIAN_POINT ( 'NONE',  ( 19.05341960407611168, 5.049401038298154454, 78.95724293864769550 ) ) ;
#151734=CARTESIAN_POINT ( 'NONE',  ( 10.72451020669898902, -18.67979575497178502, 77.91557627198102409 ) ) ;
#151735=CARTESIAN_POINT ( 'NONE',  ( 8.224510206698742110, 14.34966873604972548, 107.0844237280190043 ) ) ;
#151736=CARTESIAN_POINT ( 'NONE',  ( 13.89961937509977652, -13.97604488694527269, 93.12390960531436690 ) ) ;
#151737=CARTESIAN_POINT ( 'NONE',  ( 16.51473224551083163, -9.474510206698727899, 65.83442372801900433 ) ) ;
#151738=CARTESIAN_POINT ( 'NONE',  ( -5.719274019375665041, -21.55341960407619695, 99.79275706135234714 ) ) ;
#151739=CARTESIAN_POINT ( 'NONE',  ( -0.05219959533907301413, -21.53943276465977519, 77.49890960531433848 ) ) ;
#151740=CARTESIAN_POINT ( 'NONE',  ( 18.62759615963271287, -10.81492255796078972, 23.33224293864769194 ) ) ;
#151741=CARTESIAN_POINT ( 'NONE',  ( -19.02544592524342804, 5.153800228976336051, 56.04057627198100988 ) ) ;
#151742=CARTESIAN_POINT ( 'NONE',  ( -0.05219959533910754901, -16.53943276465976808, 27.49890960531435269 ) ) ;
#151743=CARTESIAN_POINT ( 'NONE',  ( 5.049401038298161559, -19.05341960407611168, 67.70724293864769550 ) ) ;
#151744=CYLINDRICAL_SURFACE ( 'NONE', #121559, 2.500000000000002220 ) ;
#151745=CARTESIAN_POINT ( 'NONE',  ( -21.52544592524334988, -5.823673210054445271, 103.9594237280190185 ) ) ;
#151746=CARTESIAN_POINT ( 'NONE',  ( -8.314922557960811034, -14.29746914071050412, 67.08224293864770971 ) ) ;
#151747=CARTESIAN_POINT ( 'NONE',  ( 21.53943276465977519, -0.05219959533907433946, 108.7489096053143669 ) ) ;
#151748=CARTESIAN_POINT ( 'NONE',  ( 18.67979575497178502, 10.72451020669898547, 99.16557627198100988 ) ) ;
#151750=CARTESIAN_POINT ( 'NONE',  ( -15.72974639402197994, 15.80617190586746368, 55.62390960531436690 ) ) ;
#151751=CARTESIAN_POINT ( 'NONE',  ( 12.06949235617739724, 12.14591786802326823, 81.87609039468568994 ) ) ;
#151752=CARTESIAN_POINT ( 'NONE',  ( 4.379528057220339221, -16.55341960407611168, 102.7072429386476955 ) ) ;
#151753=CARTESIAN_POINT ( 'NONE',  ( -9.564922557960796823, -16.46253265017161027, 62.08224293864769550 ) ) ;
#151755=CARTESIAN_POINT ( 'NONE',  ( 16.53943276465976808, 0.05219959533934440121, 111.2510903946856899 ) ) ;
#151756=CARTESIAN_POINT ( 'NONE',  ( 18.62759615963255655, 10.81492255796105972, 51.66775706135234714 ) ) ;
#151757=CARTESIAN_POINT ( 'NONE',  ( 13.89961937509977652, -13.97604488694527269, 108.1239096053143669 ) ) ;
#151758=CARTESIAN_POINT ( 'NONE',  ( 15.80617190586769283, -15.72974639402175789, 85.62609039468568994 ) ) ;
#151759=CARTESIAN_POINT ( 'NONE',  ( -16.51473224551069308, -9.474510206698971260, 31.66557627198102054 ) ) ;
#151760=CARTESIAN_POINT ( 'NONE',  ( 0.05219959533909260263, 19.03943276465977164, 34.99890960531435979 ) ) ;
#151761=ORIENTED_EDGE ( 'NONE', *, *, #142268, .T. ) ;
#151762=CARTESIAN_POINT ( 'NONE',  ( 18.67979575497194134, -10.72451020669871369, 65.83442372801900433 ) ) ;
#151763=CARTESIAN_POINT ( 'NONE',  ( -19.05341960407611168, -5.049401038298163336, 101.4572429386476955 ) ) ;
#151764=CARTESIAN_POINT ( 'NONE',  ( -0.05219959533936034679, 19.03943276465977164, 77.50109039468566152 ) ) ;
#151765=CARTESIAN_POINT ( 'NONE',  ( -15.80617190586768217, 15.72974639402176855, 48.12609039468568284 ) ) ;
#151766=CARTESIAN_POINT ( 'NONE',  ( -12.06949235617739369, -12.14591786802326823, 19.37609039468568639 ) ) ;
#151767=CARTESIAN_POINT ( 'NONE',  ( 5.153800228976615827, -19.02544592524334988, 70.20942372801899012 ) ) ;
#151768=CARTESIAN_POINT ( 'NONE',  ( 13.97604488694527802, 13.89961937509977652, 54.37390960531435979 ) ) ;
#151769=CARTESIAN_POINT ( 'NONE',  ( -19.02544592524334988, -5.153800228976617603, 88.95942372801897591 ) ) ;
#151770=CARTESIAN_POINT ( 'NONE',  ( 16.55341960407611168, 4.379528057220329451, 28.95724293864769905 ) ) ;
#151771=CARTESIAN_POINT ( 'NONE',  ( -0.05219959533936034679, 19.03943276465977164, 92.50109039468566152 ) ) ;
#151772=CARTESIAN_POINT ( 'NONE',  ( 14.34966873604960469, 8.224510206698951720, 44.16557627198103120 ) ) ;
#151773=CARTESIAN_POINT ( 'NONE',  ( -19.02544592524334988, -5.153800228976617603, 58.95942372801900433 ) ) ;
#151774=CARTESIAN_POINT ( 'NONE',  ( 8.224510206698742110, 14.34966873604972548, 52.08442372801901854 ) ) ;
#151775=CARTESIAN_POINT ( 'NONE',  ( -9.474510206698720793, -16.51473224551083518, 24.58442372801900078 ) ) ;
#151776=CARTESIAN_POINT ( 'NONE',  ( 19.05341960407611168, 5.049401038298154454, 38.95724293864767418 ) ) ;
#151777=CARTESIAN_POINT ( 'NONE',  ( -17.05116617787826172, -6.768360034955708038, 66.34324446740804149 ) ) ;
#151778=CARTESIAN_POINT ( 'NONE',  ( 14.29746914071037800, 8.314922557961029526, 46.66775706135234714 ) ) ;
#151781=CARTESIAN_POINT ( 'NONE',  ( -9.564922557960796823, -16.46253265017161027, 92.08224293864769550 ) ) ;
#151782=DIRECTION ( 'NONE',  ( -1.000000000000000000, 0.000000000000000000, 0.000000000000000000 ) ) ;
#151784=CARTESIAN_POINT ( 'NONE',  ( 13.97604488694548053, -13.89961937509957401, 85.62609039468568994 ) ) ;
#151785=AXIS2_PLACEMENT_3D ( 'NONE', #86525, #177559, #148209 ) ;
#151786=CARTESIAN_POINT ( 'NONE',  ( 15.80617190586746368, 15.72974639402197994, 29.37390960531435269 ) ) ;
#151787=CARTESIAN_POINT ( 'NONE',  ( -5.049401038297874678, -19.05341960407617918, 24.79275706135233648 ) ) ;
#151788=CARTESIAN_POINT ( 'NONE',  ( -13.97604488694547697, 13.89961937509957934, 98.12609039468566152 ) ) ;
#151789=CARTESIAN_POINT ( 'NONE',  ( -14.29746914071049879, 8.314922557960819915, 115.8322429386477097 ) ) ;
#151790=CARTESIAN_POINT ( 'NONE',  ( 13.89961937509977652, -13.97604488694527269, 33.12390960531434558 ) ) ;
#151791=CARTESIAN_POINT ( 'NONE',  ( -0.05219959533907301413, -21.53943276465977519, 57.49890960531435979 ) ) ;
#151792=CARTESIAN_POINT ( 'NONE',  ( 9.564922557960805705, 16.46253265017160317, 29.58224293864769550 ) ) ;
#151794=CARTESIAN_POINT ( 'NONE',  ( 19.05341960407617918, -5.049401038297876454, 71.04275706135234714 ) ) ;
#151795=CARTESIAN_POINT ( 'NONE',  ( -16.52544592524342804, 4.483927247898546575, 56.04057627198102409 ) ) ;
#151796=CARTESIAN_POINT ( 'NONE',  ( -21.53943276465977519, 0.05219959533907696930, 31.24890960531435979 ) ) ;
#151797=CARTESIAN_POINT ( 'NONE',  ( 15.80617190586769283, -15.72974639402175789, 95.62609039468568994 ) ) ;
#151798=CARTESIAN_POINT ( 'NONE',  ( 18.67979575497178502, 10.72451020669898547, 89.16557627198102409 ) ) ;
#151799=CARTESIAN_POINT ( 'NONE',  ( 15.80617190586769283, -15.72974639402175789, 60.62609039468567573 ) ) ;
#151800=CARTESIAN_POINT ( 'NONE',  ( 21.53943276465977519, 0.05219959533937863772, 66.25109039468567573 ) ) ;
#151801=CARTESIAN_POINT ( 'NONE',  ( -16.51473224551069308, -9.474510206698971260, 96.66557627198102409 ) ) ;
#151802=CARTESIAN_POINT ( 'NONE',  ( 16.55341960407618274, -4.379528057220086978, 91.04275706135236135 ) ) ;
#151803=CARTESIAN_POINT ( 'NONE',  ( 15.80617190586769283, -15.72974639402175789, 60.62609039468567573 ) ) ;
#151804=CARTESIAN_POINT ( 'NONE',  ( 0.05219959533910956823, 16.53943276465976808, 114.9989096053143669 ) ) ;
#151805=CARTESIAN_POINT ( 'NONE',  ( -14.34966873604960291, -8.224510206698953496, 61.66557627198103120 ) ) ;
#151806=CARTESIAN_POINT ( 'NONE',  ( -14.29746914071049879, 8.314922557960819915, 35.83224293864768839 ) ) ;
#151807=CARTESIAN_POINT ( 'NONE',  ( 18.67979575497178502, 10.72451020669898547, 39.16557627198102409 ) ) ;
#151808=CARTESIAN_POINT ( 'NONE',  ( 9.474510206698971260, -16.51473224551069308, 52.91557627198102409 ) ) ;
#151809=CARTESIAN_POINT ( 'NONE',  ( 21.53943276465977519, -0.05219959533907433946, 58.74890960531436690 ) ) ;
#151810=CARTESIAN_POINT ( 'NONE',  ( -5.049401038297874678, -19.05341960407617918, 49.79275706135231871 ) ) ;
#151811=CARTESIAN_POINT ( 'NONE',  ( -16.20579543436681291, -7.371946100354977105, 40.56520834171877254 ) ) ;
#151812=CARTESIAN_POINT ( 'NONE',  ( 14.29746914071049879, -8.314922557960816363, 43.33224293864769550 ) ) ;
#151813=CARTESIAN_POINT ( 'NONE',  ( 18.67979575497178502, 10.72451020669898547, 24.16557627198103120 ) ) ;
#151817=CARTESIAN_POINT ( 'NONE',  ( -17.49999999999999645, 5.499999999999992895, 83.71769037696435589 ) ) ;
#151818=CARTESIAN_POINT ( 'NONE',  ( -12.14591786802326823, 12.06949235617739902, 73.12609039468567573 ) ) ;
#151819=CARTESIAN_POINT ( 'NONE',  ( 13.89961937509957401, 13.97604488694547697, 76.87609039468566152 ) ) ;
#151820=CARTESIAN_POINT ( 'NONE',  ( -0.05219959533910754901, -16.53943276465976808, 37.49890960531436690 ) ) ;
#151822=CARTESIAN_POINT ( 'NONE',  ( -0.05219959533910754901, -16.53943276465976808, 27.49890960531435269 ) ) ;
#151823=CARTESIAN_POINT ( 'NONE',  ( -19.03943276465977164, 0.05219959533909376836, 51.24890960531436690 ) ) ;
#151824=CARTESIAN_POINT ( 'NONE',  ( -16.51473224551069308, -9.474510206698971260, 76.66557627198103830 ) ) ;
#151825=CARTESIAN_POINT ( 'NONE',  ( 5.153800228976335163, 19.02544592524342804, 34.79057627198102409 ) ) ;
#151826=CARTESIAN_POINT ( 'NONE',  ( 21.53943276465977519, 0.05219959533937863772, 51.25109039468568994 ) ) ;
#151827=CARTESIAN_POINT ( 'NONE',  ( 19.02544592524343514, -5.153800228976328945, 58.54057627198102409 ) ) ;
#151829=CARTESIAN_POINT ( 'NONE',  ( -16.46253265017160317, 9.564922557960807481, 65.83224293864769550 ) ) ;
#151830=CARTESIAN_POINT ( 'NONE',  ( 5.823673210054125526, 21.52544592524343514, 39.79057627198103830 ) ) ;
#151831=CARTESIAN_POINT ( 'NONE',  ( -16.46253265017160317, 9.564922557960807481, 35.83224293864768839 ) ) ;
#151832=CARTESIAN_POINT ( 'NONE',  ( -15.80617190586745835, -15.72974639402198527, 36.87390960531435979 ) ) ;
#151833=CARTESIAN_POINT ( 'NONE',  ( -4.483927247898782831, 16.52544592524335698, 87.70942372801901854 ) ) ;
#151834=CARTESIAN_POINT ( 'NONE',  ( 13.97604488694548053, -13.89961937509957401, 20.62609039468567573 ) ) ;
#151835=CARTESIAN_POINT ( 'NONE',  ( -12.14591786802326823, 12.06949235617739902, 68.12609039468567573 ) ) ;
#151836=CARTESIAN_POINT ( 'NONE',  ( -0.05219959533909027116, -19.03943276465977164, 107.4989096053143527 ) ) ;
#151837=CARTESIAN_POINT ( 'NONE',  ( -16.53943276465976808, -0.05219959533934237506, 58.75109039468568994 ) ) ;
#151838=CARTESIAN_POINT ( 'NONE',  ( 14.34966873604972726, -8.224510206698740333, 40.83442372801901854 ) ) ;
#151839=CARTESIAN_POINT ( 'NONE',  ( -13.89961937509977652, 13.97604488694528158, 110.6239096053143243 ) ) ;
#151840=CARTESIAN_POINT ( 'NONE',  ( 8.314922557961029526, -14.29746914071037800, 20.41775706135234714 ) ) ;
#151841=CARTESIAN_POINT ( 'NONE',  ( -0.05219959533909027116, -19.03943276465977164, 32.49890960531435979 ) ) ;
#151842=CARTESIAN_POINT ( 'NONE',  ( -18.62759615963255300, -10.81492255796106328, 29.16775706135234003 ) ) ;
#151843=CARTESIAN_POINT ( 'NONE',  ( -14.34966873604972548, 8.224510206698743886, 23.33442372801901499 ) ) ;
#151844=CARTESIAN_POINT ( 'NONE',  ( -4.483927247898782831, 16.52544592524335698, 92.70942372801901854 ) ) ;
#151846=CARTESIAN_POINT ( 'NONE',  ( 18.62759615963255655, 10.81492255796105972, 101.6677570613523613 ) ) ;
#151847=CARTESIAN_POINT ( 'NONE',  ( 19.03943276465977164, 0.05219959533936151252, 91.25109039468566152 ) ) ;
#151848=CARTESIAN_POINT ( 'NONE',  ( 16.55341960407611168, 4.379528057220329451, 58.95724293864770971 ) ) ;
#151849=CARTESIAN_POINT ( 'NONE',  ( 9.474510206698971260, -16.51473224551069308, 27.91557627198103120 ) ) ;
#151850=CARTESIAN_POINT ( 'NONE',  ( 19.03943276465977164, 0.05219959533936151252, 51.25109039468567573 ) ) ;
#151852=CARTESIAN_POINT ( 'NONE',  ( 10.72451020669871369, 18.67979575497193778, 52.08442372801901854 ) ) ;
#151853=CARTESIAN_POINT ( 'NONE',  ( 16.53943276465976808, 0.05219959533934440121, 26.25109039468567573 ) ) ;
#151854=CARTESIAN_POINT ( 'NONE',  ( 17.31747979337948706, 6.344076630961015262, 83.87944868065183357 ) ) ;
#151855=CARTESIAN_POINT ( 'NONE',  ( 0.05219959533909260263, 19.03943276465977164, 104.9989096053143669 ) ) ;
#151856=CARTESIAN_POINT ( 'NONE',  ( 21.55341960407610458, 5.719274019375980345, 78.95724293864769550 ) ) ;
#151857=CARTESIAN_POINT ( 'NONE',  ( -5.153800228976607833, 19.02544592524334988, 97.70942372801900433 ) ) ;
#151858=CARTESIAN_POINT ( 'NONE',  ( 19.05341960407611168, 5.049401038298154454, 98.95724293864766707 ) ) ;
#151860=CARTESIAN_POINT ( 'NONE',  ( -8.314922557960811034, -14.29746914071050412, 107.0822429386476955 ) ) ;
#151861=CARTESIAN_POINT ( 'NONE',  ( 0.05219959533937995610, -21.53943276465977519, 100.0010903946857042 ) ) ;
#151862=CARTESIAN_POINT ( 'NONE',  ( 16.46253265017160672, -9.564922557960803928, 48.33224293864769550 ) ) ;
#151863=CARTESIAN_POINT ( 'NONE',  ( -15.80617190586768217, 15.72974639402176855, 58.12609039468568994 ) ) ;
#151865=CARTESIAN_POINT ( 'NONE',  ( 5.823673210054444382, -21.52544592524334988, 90.20942372801903275 ) ) ;
#151866=CARTESIAN_POINT ( 'NONE',  ( -8.224510206698735004, -14.34966873604973081, 104.5844237280190185 ) ) ;
#151867=CARTESIAN_POINT ( 'NONE',  ( 19.03943276465977164, -0.05219959533909143690, 83.74890960531436690 ) ) ;
#151868=CARTESIAN_POINT ( 'NONE',  ( -18.67979575497193778, 10.72451020669871902, 38.33442372801900433 ) ) ;
#151869=CARTESIAN_POINT ( 'NONE',  ( -21.53943276465977519, -0.05219959533937600094, 43.75109039468568284 ) ) ;
#151870=CARTESIAN_POINT ( 'NONE',  ( -9.474510206698720793, -16.51473224551083518, 69.58442372801901854 ) ) ;
#151871=CARTESIAN_POINT ( 'NONE',  ( 0.05219959533909260263, 19.03943276465977164, 89.99890960531436690 ) ) ;
#151872=CARTESIAN_POINT ( 'NONE',  ( 12.14591786802309770, 12.06949235617756955, 99.37390960531436690 ) ) ;
#151873=CARTESIAN_POINT ( 'NONE',  ( -10.72451020669898014, 18.67979575497178502, 100.4155762719810241 ) ) ;
#151874=CARTESIAN_POINT ( 'NONE',  ( 16.55341960407611168, 4.379528057220329451, 68.95724293864769550 ) ) ;
#151875=CARTESIAN_POINT ( 'NONE',  ( -5.153800228976607833, 19.02544592524334988, 22.70942372801899012 ) ) ;
#151876=CARTESIAN_POINT ( 'NONE',  ( -14.34966873604960291, -8.224510206698953496, 81.66557627198103830 ) ) ;
#151877=CARTESIAN_POINT ( 'NONE',  ( -5.049401038298153566, 19.05341960407611168, 35.20724293864768839 ) ) ;
#151878=CARTESIAN_POINT ( 'NONE',  ( -0.05219959533936034679, 19.03943276465977164, 87.50109039468567573 ) ) ;
#151879=CARTESIAN_POINT ( 'NONE',  ( -14.34966873604960291, -8.224510206698953496, 51.66557627198102409 ) ) ;
#151880=CARTESIAN_POINT ( 'NONE',  ( 18.62759615963255655, 10.81492255796105972, 96.66775706135234714 ) ) ;
#151881=CARTESIAN_POINT ( 'NONE',  ( 13.89961937509977652, -13.97604488694527269, 98.12390960531433848 ) ) ;
#151882=CARTESIAN_POINT ( 'NONE',  ( 19.03943276465977164, 0.05219959533936151252, 71.25109039468566152 ) ) ;
#151883=CARTESIAN_POINT ( 'NONE',  ( 5.823673210054125526, 21.52544592524343514, 79.79057627198102409 ) ) ;
#151884=CARTESIAN_POINT ( 'NONE',  ( 5.719274019375673035, 21.55341960407619339, 32.29275706135235424 ) ) ;
#151885=CARTESIAN_POINT ( 'NONE',  ( 16.52544592524335698, 4.483927247898782831, 26.45942372801901854 ) ) ;
#151886=CARTESIAN_POINT ( 'NONE',  ( 4.483927247898790824, -16.52544592524335698, 95.20942372801903275 ) ) ;
#151887=CARTESIAN_POINT ( 'NONE',  ( -5.049401038298153566, 19.05341960407611168, 30.20724293864768839 ) ) ;
#151888=CARTESIAN_POINT ( 'NONE',  ( 10.81492255796106328, -18.62759615963255655, 35.41775706135234003 ) ) ;
#151889=CARTESIAN_POINT ( 'NONE',  ( -13.97604488694527625, -13.89961937509977652, 26.87390960531434558 ) ) ;
#151891=CARTESIAN_POINT ( 'NONE',  ( 16.52544592524335698, 4.483927247898782831, 46.45942372801901854 ) ) ;
#151892=CARTESIAN_POINT ( 'NONE',  ( -16.52544592524342804, 4.483927247898546575, 76.04057627198102409 ) ) ;
#151893=CARTESIAN_POINT ( 'NONE',  ( 10.81492255796078972, 18.62759615963270932, 69.58224293864769550 ) ) ;
#151894=CARTESIAN_POINT ( 'NONE',  ( 14.34966873604960469, 8.224510206698951720, 24.16557627198103120 ) ) ;
#151895=CARTESIAN_POINT ( 'NONE',  ( -12.06949235617739369, -12.14591786802326823, 49.37609039468569705 ) ) ;
#151896=CARTESIAN_POINT ( 'NONE',  ( -16.46253265017160317, 9.564922557960807481, 40.83224293864769550 ) ) ;
#151897=CARTESIAN_POINT ( 'NONE',  ( -8.224510206698735004, -14.34966873604973081, 94.58442372801901854 ) ) ;
#151898=CARTESIAN_POINT ( 'NONE',  ( 13.89961937509957401, 13.97604488694547697, 81.87609039468564731 ) ) ;
#151899=CARTESIAN_POINT ( 'NONE',  ( 15.72974639402199770, -15.80617190586745480, 78.12390960531436690 ) ) ;
#151900=CARTESIAN_POINT ( 'NONE',  ( -4.483927247898539470, -16.52544592524342804, 22.29057627198102765 ) ) ;
#151902=CARTESIAN_POINT ( 'NONE',  ( 5.049401038298161559, -19.05341960407611168, 112.7072429386476813 ) ) ;
#151904=CARTESIAN_POINT ( 'NONE',  ( -10.72451020669898014, 18.67979575497178502, 65.41557627198102409 ) ) ;
#151905=VERTEX_POINT ( 'NONE', #112645 ) ;
#151906=CARTESIAN_POINT ( 'NONE',  ( 4.483927247898790824, -16.52544592524335698, 90.20942372801903275 ) ) ;
#151907=ORIENTED_EDGE ( 'NONE', *, *, #95241, .T. ) ;
#151908=CARTESIAN_POINT ( 'NONE',  ( 13.89961937509977652, -13.97604488694527269, 108.1239096053143669 ) ) ;
#151909=CARTESIAN_POINT ( 'NONE',  ( -18.22780087662123805, 5.499999999999981348, 76.01763182126894947 ) ) ;
#151910=CARTESIAN_POINT ( 'NONE',  ( -18.62759615963270932, 10.81492255796079327, 75.83224293864769550 ) ) ;
#151911=CARTESIAN_POINT ( 'NONE',  ( 14.29746914071037800, 8.314922557961029526, 106.6677570613523756 ) ) ;
#151912=CARTESIAN_POINT ( 'NONE',  ( -12.06949235617739369, -12.14591786802326823, 19.37609039468568639 ) ) ;
#151913=CARTESIAN_POINT ( 'NONE',  ( -19.03943276465977164, 0.05219959533909376836, 26.24890960531435624 ) ) ;
#151914=CARTESIAN_POINT ( 'NONE',  ( -16.55341960407617563, 4.379528057220093196, 33.54275706135234714 ) ) ;
#151915=CARTESIAN_POINT ( 'NONE',  ( 5.049401038298161559, -19.05341960407611168, 52.70724293864767418 ) ) ;
#151917=CARTESIAN_POINT ( 'NONE',  ( 0.05219959533909260263, 19.03943276465977164, 99.99890960531436690 ) ) ;
#151918=CARTESIAN_POINT ( 'NONE',  ( -0.05219959533934338120, 16.53943276465976808, 87.50109039468568994 ) ) ;
#151919=CARTESIAN_POINT ( 'NONE',  ( -16.51473224551082808, 9.474510206698731452, 93.33442372801900433 ) ) ;
#151920=CARTESIAN_POINT ( 'NONE',  ( 16.51473224551083163, -9.474510206698727899, 20.83442372801899722 ) ) ;
#151921=CARTESIAN_POINT ( 'NONE',  ( -5.719274019375978568, 21.55341960407610458, 70.20724293864769550 ) ) ;
#151922=CARTESIAN_POINT ( 'NONE',  ( 16.52544592524335698, 4.483927247898782831, 101.4594237280190185 ) ) ;
#151923=CARTESIAN_POINT ( 'NONE',  ( 13.89961937509957401, 13.97604488694547697, 91.87609039468567573 ) ) ;
#151924=CARTESIAN_POINT ( 'NONE',  ( -13.89961937509977652, 13.97604488694528158, 50.62390960531435979 ) ) ;
#151925=CARTESIAN_POINT ( 'NONE',  ( -5.153800228976328057, -19.02544592524343514, 87.29057627198103830 ) ) ;
#151926=CARTESIAN_POINT ( 'NONE',  ( 5.719274019375673035, 21.55341960407619339, 62.29275706135236845 ) ) ;
#151927=CARTESIAN_POINT ( 'NONE',  ( -19.02544592524342804, 5.153800228976336051, 61.04057627198103120 ) ) ;
#151928=CARTESIAN_POINT ( 'NONE',  ( -12.06949235617756955, 12.14591786802309770, 90.62390960531436690 ) ) ;
#151930=CARTESIAN_POINT ( 'NONE',  ( -16.52544592524342804, 4.483927247898546575, 76.04057627198102409 ) ) ;
#151931=CARTESIAN_POINT ( 'NONE',  ( 10.81492255796078972, 18.62759615963270932, 69.58224293864769550 ) ) ;
#151932=CARTESIAN_POINT ( 'NONE',  ( 9.474510206698729675, 16.51473224551082808, 92.08442372801900433 ) ) ;
#151933=CARTESIAN_POINT ( 'NONE',  ( 19.49671883438227482, 5.500000000000019540, 92.39279849105682274 ) ) ;
#151934=CARTESIAN_POINT ( 'NONE',  ( -19.03943276465977164, -0.05219959533935918106, 43.75109039468566863 ) ) ;
#151936=CARTESIAN_POINT ( 'NONE',  ( 5.049401038298161559, -19.05341960407611168, 77.70724293864765286 ) ) ;
#151937=CARTESIAN_POINT ( 'NONE',  ( 5.049401038298161559, -19.05341960407611168, 92.70724293864769550 ) ) ;
#151938=CARTESIAN_POINT ( 'NONE',  ( 16.55341960407618274, -4.379528057220086978, 71.04275706135234714 ) ) ;
#151939=CARTESIAN_POINT ( 'NONE',  ( -16.79531203550649465, -7.028104445595491079, 51.25244988220442366 ) ) ;
#151940=CARTESIAN_POINT ( 'NONE',  ( 16.51473224551083163, -9.474510206698727899, 45.83442372801900433 ) ) ;
#151942=CARTESIAN_POINT ( 'NONE',  ( -5.049401038298153566, 19.05341960407611168, 105.2072429386476671 ) ) ;
#151943=CARTESIAN_POINT ( 'NONE',  ( 16.55341960407618274, -4.379528057220086978, 106.0427570613523471 ) ) ;
#151944=CARTESIAN_POINT ( 'NONE',  ( 17.49999999999998579, -5.500000000000023981, 68.29690382534171533 ) ) ;
#151945=CARTESIAN_POINT ( 'NONE',  ( -0.05219959533934338120, 16.53943276465976808, 77.50109039468567573 ) ) ;
#151947=CARTESIAN_POINT ( 'NONE',  ( -14.34966873604972548, 8.224510206698743886, 48.33442372801902565 ) ) ;
#151949=CARTESIAN_POINT ( 'NONE',  ( 0.05219959533937995610, -21.53943276465977519, 65.00109039468568994 ) ) ;
#151950=CARTESIAN_POINT ( 'NONE',  ( -19.02544592524334988, -5.153800228976617603, 68.95942372801896170 ) ) ;
#151951=CARTESIAN_POINT ( 'NONE',  ( 16.51473224551083163, -9.474510206698727899, 20.83442372801899722 ) ) ;
#151952=CARTESIAN_POINT ( 'NONE',  ( 13.89961937509977652, -13.97604488694527269, 53.12390960531434558 ) ) ;
#151953=CARTESIAN_POINT ( 'NONE',  ( -19.05341960407611168, -5.049401038298163336, 41.45724293864769550 ) ) ;
#151954=CARTESIAN_POINT ( 'NONE',  ( 17.39620827691126692, -6.149463919001277645, 23.33264299213259108 ) ) ;
#151955=CARTESIAN_POINT ( 'NONE',  ( 18.67979575497178502, 10.72451020669898547, 64.16557627198102409 ) ) ;
#151957=CARTESIAN_POINT ( 'NONE',  ( 5.719274019375991003, -21.55341960407610458, 27.70724293864769905 ) ) ;
#151958=CARTESIAN_POINT ( 'NONE',  ( 16.55341960407611168, 4.379528057220329451, 113.9572429386477239 ) ) ;
#151959=CARTESIAN_POINT ( 'NONE',  ( 14.34966873604972726, -8.224510206698740333, 45.83442372801901854 ) ) ;
#151960=ORIENTED_EDGE ( 'NONE', *, *, #155303, .F. ) ;
#151961=CARTESIAN_POINT ( 'NONE',  ( 0.05219959533907565091, 21.53943276465977519, 109.9989096053143527 ) ) ;
#151962=CARTESIAN_POINT ( 'NONE',  ( -4.483927247898539470, -16.52544592524342804, 52.29057627198102409 ) ) ;
#151964=CARTESIAN_POINT ( 'NONE',  ( 5.049401038297881783, 19.05341960407617563, 112.2927570613523471 ) ) ;
#151965=CARTESIAN_POINT ( 'NONE',  ( 16.51473224551083163, -9.474510206698727899, 40.83442372801900433 ) ) ;
#151966=CARTESIAN_POINT ( 'NONE',  ( -14.29746914071049879, 8.314922557960819915, 40.83224293864769550 ) ) ;
#151967=CARTESIAN_POINT ( 'NONE',  ( 15.72974639402199770, -15.80617190586745480, 113.1239096053143953 ) ) ;
#151969=CARTESIAN_POINT ( 'NONE',  ( -18.62759615963270932, 10.81492255796079327, 60.83224293864769550 ) ) ;
#151970=CARTESIAN_POINT ( 'NONE',  ( 13.89961937509977652, -13.97604488694527269, 88.12390960531438111 ) ) ;
#151971=CARTESIAN_POINT ( 'NONE',  ( -8.314922557960811034, -14.29746914071050412, 62.08224293864769550 ) ) ;
#151972=CARTESIAN_POINT ( 'NONE',  ( 16.46253265017160672, -9.564922557960803928, 108.3322429386476955 ) ) ;
#151973=CARTESIAN_POINT ( 'NONE',  ( -13.89961937509977830, 13.97604488694528158, 80.62390960531436690 ) ) ;
#151974=CARTESIAN_POINT ( 'NONE',  ( -13.89961937509957401, -13.97604488694547875, 59.37609039468566863 ) ) ;
#151975=CARTESIAN_POINT ( 'NONE',  ( 21.53943276465977519, -0.05219959533907433946, 103.7489096053143669 ) ) ;
#151976=CARTESIAN_POINT ( 'NONE',  ( -19.03943276465977164, 0.05219959533909376836, 46.24890960531435979 ) ) ;
#151977=CARTESIAN_POINT ( 'NONE',  ( 8.314922557960818139, 14.29746914071049879, 114.5822429386477097 ) ) ;
#151978=CARTESIAN_POINT ( 'NONE',  ( 10.72451020669871369, 18.67979575497193778, 47.08442372801901854 ) ) ;
#151980=CARTESIAN_POINT ( 'NONE',  ( -8.224510206698948167, 14.34966873604960824, 30.41557627198101699 ) ) ;
#151981=CARTESIAN_POINT ( 'NONE',  ( -16.51473224551069308, -9.474510206698971260, 51.66557627198102409 ) ) ;
#151982=B_SPLINE_CURVE_WITH_KNOTS ( 'NONE', 3,
 ( #178542, #69346, #160362, #22852, #192704, #53175 ),
 .UNSPECIFIED., .F., .F.,
 ( 4, 2, 4 ),
 ( 0.003239945802372246487, 0.003620412082092121231, 0.004000878361811995541 ),
 .UNSPECIFIED. ) ;
#151983=CARTESIAN_POINT ( 'NONE',  ( 16.51473224551069308, 9.474510206698969483, 94.16557627198103830 ) ) ;
#151984=CARTESIAN_POINT ( 'NONE',  ( -10.81492255796078084, -18.62759615963271287, 77.08224293864769550 ) ) ;
#151986=CARTESIAN_POINT ( 'NONE',  ( -13.97604488694527625, -13.89961937509977652, 41.87390960531435979 ) ) ;
#151988=CARTESIAN_POINT ( 'NONE',  ( -0.05219959533907301413, -21.53943276465977519, 47.49890960531435979 ) ) ;
#151989=CARTESIAN_POINT ( 'NONE',  ( 10.72451020669871369, 18.67979575497193778, 92.08442372801901854 ) ) ;
#151991=CARTESIAN_POINT ( 'NONE',  ( 16.52544592524335698, 4.483927247898782831, 81.45942372801900433 ) ) ;
#151992=CARTESIAN_POINT ( 'NONE',  ( 16.55341960407611168, 4.379528057220329451, 63.95724293864770260 ) ) ;
#151993=CARTESIAN_POINT ( 'NONE',  ( -19.02544592524342804, 5.153800228976336051, 71.04057627198099567 ) ) ;
#151995=CARTESIAN_POINT ( 'NONE',  ( 9.474510206698729675, 16.51473224551082808, 27.08442372801900433 ) ) ;
#151996=CARTESIAN_POINT ( 'NONE',  ( 0.05219959533934541429, -16.53943276465976808, 95.00109039468568994 ) ) ;
#151997=CARTESIAN_POINT ( 'NONE',  ( 0.05219959533936267826, -19.03943276465977164, 20.00109039468567218 ) ) ;
#151998=CARTESIAN_POINT ( 'NONE',  ( 0.05219959533909260263, 19.03943276465977164, 69.99890960531435269 ) ) ;
#151999=CARTESIAN_POINT ( 'NONE',  ( -10.72451020669898014, 18.67979575497178502, 45.41557627198103830 ) ) ;
#152000=CARTESIAN_POINT ( 'NONE',  ( 4.483927247898790824, -16.52544592524335698, 30.20942372801902565 ) ) ;
#152001=CARTESIAN_POINT ( 'NONE',  ( 5.719274019375673035, 21.55341960407619339, 92.29275706135236135 ) ) ;
#152002=CARTESIAN_POINT ( 'NONE',  ( -0.05219959533934338120, 16.53943276465976808, 67.50109039468568994 ) ) ;
#152003=CARTESIAN_POINT ( 'NONE',  ( 21.55341960407610458, 5.719274019375980345, 108.9572429386476955 ) ) ;
#152004=CARTESIAN_POINT ( 'NONE',  ( -12.06949235617739369, -12.14591786802326823, 19.37609039468568639 ) ) ;
#152005=CARTESIAN_POINT ( 'NONE',  ( -19.02544592524342804, 5.153800228976336051, 96.04057627198103830 ) ) ;
#152006=CARTESIAN_POINT ( 'NONE',  ( -16.55341960407617563, 4.379528057220093196, 33.54275706135234714 ) ) ;
#152007=CARTESIAN_POINT ( 'NONE',  ( -16.51473224551069308, -9.474510206698971260, 51.66557627198102409 ) ) ;
#152008=CARTESIAN_POINT ( 'NONE',  ( 12.14591786802327356, -12.06949235617739191, 40.62609039468567573 ) ) ;
#152009=CARTESIAN_POINT ( 'NONE',  ( -14.29746914071049879, 8.314922557960819915, 80.83224293864769550 ) ) ;
#152010=CARTESIAN_POINT ( 'NONE',  ( -16.52544592524335698, -4.483927247898792601, 93.95942372801903275 ) ) ;
#152011=CARTESIAN_POINT ( 'NONE',  ( 15.80617190586769283, -15.72974639402175789, 30.62609039468567929 ) ) ;
#152012=CARTESIAN_POINT ( 'NONE',  ( 19.03943276465977164, -0.05219959533909143690, 68.74890960531436690 ) ) ;
#152013=CARTESIAN_POINT ( 'NONE',  ( 5.049401038298161559, -19.05341960407611168, 77.70724293864765286 ) ) ;
#152014=CARTESIAN_POINT ( 'NONE',  ( 16.53943276465976808, 0.05219959533934440121, 81.25109039468568994 ) ) ;
#152017=VERTEX_POINT ( 'NONE', #53980 ) ;
#152018=CARTESIAN_POINT ( 'NONE',  ( -13.97604488694547697, 13.89961937509957934, 33.12609039468566863 ) ) ;
#152019=CARTESIAN_POINT ( 'NONE',  ( 9.474510206698971260, -16.51473224551069308, 92.91557627198103830 ) ) ;
#152020=CARTESIAN_POINT ( 'NONE',  ( -0.05219959533909027116, -19.03943276465977164, 47.49890960531435979 ) ) ;
#152021=CARTESIAN_POINT ( 'NONE',  ( -19.03943276465977164, 0.05219959533909376836, 111.2489096053143669 ) ) ;
#152022=CARTESIAN_POINT ( 'NONE',  ( -8.224510206698735004, -14.34966873604973081, 44.58442372801901854 ) ) ;
#152023=CARTESIAN_POINT ( 'NONE',  ( 19.02544592524334988, 5.153800228976608722, 56.45942372801898301 ) ) ;
#152024=CARTESIAN_POINT ( 'NONE',  ( 14.29746914071037800, 8.314922557961029526, 46.66775706135234714 ) ) ;
#152025=CARTESIAN_POINT ( 'NONE',  ( 13.97604488694527802, 13.89961937509977652, 104.3739096053143385 ) ) ;
#152026=CARTESIAN_POINT ( 'NONE',  ( 19.03943276465977164, -0.05219959533909143690, 73.74890960531435269 ) ) ;
#152027=CARTESIAN_POINT ( 'NONE',  ( -10.72451020669898014, 18.67979575497178502, 105.4155762719810383 ) ) ;
#152028=CARTESIAN_POINT ( 'NONE',  ( -9.474510206698720793, -16.51473224551083518, 64.58442372801900433 ) ) ;
#152029=CARTESIAN_POINT ( 'NONE',  ( -13.97604488694527625, -13.89961937509977652, 86.87390960531436690 ) ) ;
#152030=CARTESIAN_POINT ( 'NONE',  ( 17.46738742707146841, -4.282736719227863809, 21.63625758046896763 ) ) ;
#152031=ADVANCED_FACE ( 'NONE', ( #115653 ), #4455, .T. ) ;
#152032=CARTESIAN_POINT ( 'NONE',  ( 9.474510206698971260, -16.51473224551069308, 62.91557627198102409 ) ) ;
#152033=CARTESIAN_POINT ( 'NONE',  ( 16.55341960407611168, 4.379528057220329451, 38.95724293864768839 ) ) ;
#152034=CARTESIAN_POINT ( 'NONE',  ( 13.89961937509977652, -13.97604488694527269, 28.12390960531435624 ) ) ;
#152035=CARTESIAN_POINT ( 'NONE',  ( -16.51473224551082808, 9.474510206698731452, 38.33442372801899722 ) ) ;
#152036=CARTESIAN_POINT ( 'NONE',  ( -8.224510206698948167, 14.34966873604960824, 80.41557627198103830 ) ) ;
#152037=CARTESIAN_POINT ( 'NONE',  ( 10.72451020669871369, 18.67979575497193778, 97.08442372801904696 ) ) ;
#152038=CARTESIAN_POINT ( 'NONE',  ( 5.153800228976335163, 19.02544592524342804, 44.79057627198103830 ) ) ;
#152039=CARTESIAN_POINT ( 'NONE',  ( 14.34966873604972726, -8.224510206698740333, 50.83442372801901143 ) ) ;
#152040=CARTESIAN_POINT ( 'NONE',  ( 12.14591786802309770, 12.06949235617756955, 44.37390960531435979 ) ) ;
#152041=CARTESIAN_POINT ( 'NONE',  ( 0.05219959533937995610, -21.53943276465977519, 100.0010903946857042 ) ) ;
#152042=CARTESIAN_POINT ( 'NONE',  ( 16.46253265017160672, -9.564922557960803928, 93.33224293864769550 ) ) ;
#152043=CARTESIAN_POINT ( 'NONE',  ( 9.474510206698971260, -16.51473224551069308, 92.91557627198103830 ) ) ;
#152044=CARTESIAN_POINT ( 'NONE',  ( -8.224510206698948167, 14.34966873604960824, 115.4155762719810241 ) ) ;
#152045=CARTESIAN_POINT ( 'NONE',  ( -16.53943276465976808, 0.05219959533911058130, 106.2489096053143811 ) ) ;
#152046=CARTESIAN_POINT ( 'NONE',  ( 14.34966873604960469, 8.224510206698951720, 69.16557627198102409 ) ) ;
#152047=CARTESIAN_POINT ( 'NONE',  ( -21.52544592524343514, 5.823673210054127303, 86.04057627198102409 ) ) ;
#152048=CARTESIAN_POINT ( 'NONE',  ( 0.05219959533909260263, 19.03943276465977164, 89.99890960531436690 ) ) ;
#152049=CARTESIAN_POINT ( 'NONE',  ( 15.80617190586746368, 15.72974639402197994, 94.37390960531436690 ) ) ;
#152050=CARTESIAN_POINT ( 'NONE',  ( 16.51473224551069308, 9.474510206698969483, 84.16557627198102409 ) ) ;
#152051=CARTESIAN_POINT ( 'NONE',  ( 18.87580814761071935, -5.500000000000033751, 48.37172394265761000 ) ) ;
#152052=CARTESIAN_POINT ( 'NONE',  ( 14.29746914071049879, -8.314922557960816363, 88.33224293864769550 ) ) ;
#152053=CARTESIAN_POINT ( 'NONE',  ( 9.564922557960805705, 16.46253265017160317, 59.58224293864769550 ) ) ;
#152054=CARTESIAN_POINT ( 'NONE',  ( -21.52544592524343514, 5.823673210054127303, 66.04057627198103830 ) ) ;
#152055=CARTESIAN_POINT ( 'NONE',  ( 16.88567814943165857, -6.947325034625571050, 26.20998877347415856 ) ) ;
#152056=CARTESIAN_POINT ( 'NONE',  ( 12.06949235617739724, 12.14591786802326823, 106.8760903946856899 ) ) ;
#152058=CARTESIAN_POINT ( 'NONE',  ( 0.05219959533934541429, -16.53943276465976808, 20.00109039468568639 ) ) ;
#152059=CARTESIAN_POINT ( 'NONE',  ( 0.05219959533910956823, 16.53943276465976808, 89.99890960531438111 ) ) ;
#152061=CARTESIAN_POINT ( 'NONE',  ( 5.049401038298161559, -19.05341960407611168, 77.70724293864765286 ) ) ;
#152062=CARTESIAN_POINT ( 'NONE',  ( -5.153800228976328057, -19.02544592524343514, 47.29057627198102409 ) ) ;
#152063=CARTESIAN_POINT ( 'NONE',  ( 4.483927247898545687, 16.52544592524342804, 69.79057627198102409 ) ) ;
#152064=CARTESIAN_POINT ( 'NONE',  ( 15.72974639402199770, -15.80617190586745480, 23.12390960531436335 ) ) ;
#152065=CARTESIAN_POINT ( 'NONE',  ( 13.97604488694548053, -13.89961937509957401, 100.6260903946856615 ) ) ;
#152066=CARTESIAN_POINT ( 'NONE',  ( -18.67979575497193778, 10.72451020669871902, 58.33442372801901143 ) ) ;
#152067=CARTESIAN_POINT ( 'NONE',  ( -13.97604488694527625, -13.89961937509977652, 101.8739096053143811 ) ) ;
#152068=CARTESIAN_POINT ( 'NONE',  ( -21.52544592524343514, 5.823673210054127303, 76.04057627198102409 ) ) ;
#152069=CARTESIAN_POINT ( 'NONE',  ( -4.379528057220086978, -16.55341960407618274, 69.79275706135234714 ) ) ;
#152070=CARTESIAN_POINT ( 'NONE',  ( -19.05341960407611168, -5.049401038298163336, 31.45724293864769550 ) ) ;
#152071=CARTESIAN_POINT ( 'NONE',  ( -13.97604488694527625, -13.89961937509977652, 76.87390960531433848 ) ) ;
#152072=CARTESIAN_POINT ( 'NONE',  ( -18.62759615963270932, 10.81492255796079327, 75.83224293864769550 ) ) ;
#152073=CARTESIAN_POINT ( 'NONE',  ( -13.97604488694547697, 13.89961937509957934, 103.1260903946856473 ) ) ;
#152074=CARTESIAN_POINT ( 'NONE',  ( -16.55341960407611168, -4.379528057220339221, 36.45724293864768839 ) ) ;
#152075=CARTESIAN_POINT ( 'NONE',  ( -15.80617190586768217, 15.72974639402176855, 63.12609039468568994 ) ) ;
#152076=CARTESIAN_POINT ( 'NONE',  ( 4.483927247898790824, -16.52544592524335698, 85.20942372801901854 ) ) ;
#152077=CARTESIAN_POINT ( 'NONE',  ( 13.89961937509977652, -13.97604488694527269, 103.1239096053143527 ) ) ;
#152078=CARTESIAN_POINT ( 'NONE',  ( -9.564922557960796823, -16.46253265017161027, 102.0822429386477097 ) ) ;
#152080=CARTESIAN_POINT ( 'NONE',  ( 8.314922557961029526, -14.29746914071037800, 110.4177570613523756 ) ) ;
#152081=CARTESIAN_POINT ( 'NONE',  ( 0.05219959533934541429, -16.53943276465976808, 45.00109039468568284 ) ) ;
#152082=CARTESIAN_POINT ( 'NONE',  ( 19.03943276465977164, -0.05219959533909143690, 58.74890960531435979 ) ) ;
#152083=CARTESIAN_POINT ( 'NONE',  ( -16.51473224551069308, -9.474510206698971260, 76.66557627198103830 ) ) ;
#152084=CARTESIAN_POINT ( 'NONE',  ( -21.52544592524334988, -5.823673210054445271, 63.95942372801901854 ) ) ;
#152085=CARTESIAN_POINT ( 'NONE',  ( 16.53943276465976808, 0.05219959533934440121, 61.25109039468567573 ) ) ;
#152086=CARTESIAN_POINT ( 'NONE',  ( -4.483927247898539470, -16.52544592524342804, 42.29057627198103120 ) ) ;
#152087=CARTESIAN_POINT ( 'NONE',  ( -13.97604488694527625, -13.89961937509977652, 51.87390960531436690 ) ) ;
#152088=CARTESIAN_POINT ( 'NONE',  ( -5.049401038298153566, 19.05341960407611168, 45.20724293864769550 ) ) ;
#152089=CARTESIAN_POINT ( 'NONE',  ( 4.483927247898790824, -16.52544592524335698, 40.20942372801901854 ) ) ;
#152090=( BOUNDED_CURVE ( )  B_SPLINE_CURVE ( 2, ( #169245, #168263, #9862, #25040, #43939, #15580, #31744, #71521, #105600, #148367, #386, #117020, #178715 ),
 .UNSPECIFIED., .F., .F. ) 
 B_SPLINE_CURVE_WITH_KNOTS ( ( 3, 2, 2, 2, 2, 2, 3 ),
 ( 0.2392725416902030389, 0.2412280701754385970, 0.2456140350877192846, 0.2500000000000000000, 0.2543859649122807154, 0.2587719298245614308, 0.2606817784877069055 ),
 .UNSPECIFIED. ) 
 CURVE ( )  GEOMETRIC_REPRESENTATION_ITEM ( )  RATIONAL_B_SPLINE_CURVE ( ( 0.9831626618144004848, 0.9848076720550091867, 1.000000000000000000, 0.9659258262890683122, 1.000000000000000000, 0.9659258262890683122, 1.000000000000000000, 0.9659258262890683122, 1.000000000000000000, 0.9659258262890683122, 1.000000000000000000, 0.9851625545550088958, 0.9832469066685279868 ) ) 
 REPRESENTATION_ITEM ( '' )  );
#152091=CARTESIAN_POINT ( 'NONE',  ( -19.02544592524334988, -5.153800228976617603, 93.95942372801900433 ) ) ;
#152092=CARTESIAN_POINT ( 'NONE',  ( -16.55341960407611168, -4.379528057220339221, 91.45724293864769550 ) ) ;
#152093=CARTESIAN_POINT ( 'NONE',  ( 19.05341960407611168, 5.049401038298154454, 68.95724293864769550 ) ) ;
#152094=CARTESIAN_POINT ( 'NONE',  ( 19.05341960407617918, -5.049401038297876454, 106.0427570613523471 ) ) ;
#152096=CARTESIAN_POINT ( 'NONE',  ( 15.80617190586769283, -15.72974639402175789, 95.62609039468568994 ) ) ;
#152097=CARTESIAN_POINT ( 'NONE',  ( 16.52544592524335698, 4.483927247898782831, 61.45942372801901854 ) ) ;
#152098=CARTESIAN_POINT ( 'NONE',  ( 17.50000000000000711, -5.499999999999992895, 31.21769037696435589 ) ) ;
#152099=CARTESIAN_POINT ( 'NONE',  ( 18.62759615963271287, -10.81492255796078972, 58.33224293864768839 ) ) ;
#152100=CARTESIAN_POINT ( 'NONE',  ( -4.379528057220086978, -16.55341960407618274, 54.79275706135235424 ) ) ;
#152101=CARTESIAN_POINT ( 'NONE',  ( -19.26498983726237668, 5.499999999999803713, 70.55319577422000066 ) ) ;
#152102=CARTESIAN_POINT ( 'NONE',  ( 9.474510206698729675, 16.51473224551082808, 37.08442372801899722 ) ) ;
#152103=CARTESIAN_POINT ( 'NONE',  ( -16.51473224551069308, -9.474510206698971260, 86.66557627198102409 ) ) ;
#152104=CARTESIAN_POINT ( 'NONE',  ( -0.05219959533909027116, -19.03943276465977164, 27.49890960531435624 ) ) ;
#152105=CARTESIAN_POINT ( 'NONE',  ( -19.03943276465977164, 0.05219959533909376836, 71.24890960531435269 ) ) ;
#152107=CARTESIAN_POINT ( 'NONE',  ( -15.80617190586768217, 15.72974639402176855, 73.12609039468567573 ) ) ;
#152108=CARTESIAN_POINT ( 'NONE',  ( -18.22780087662126647, -5.499999999999827693, 53.98236817873107185 ) ) ;
#152110=CARTESIAN_POINT ( 'NONE',  ( -0.05219959533936034679, 19.03943276465977164, 32.50109039468566863 ) ) ;
#152111=CARTESIAN_POINT ( 'NONE',  ( 16.51473224551083163, -9.474510206698727899, 30.83442372801900433 ) ) ;
#152112=CARTESIAN_POINT ( 'NONE',  ( -12.06949235617756955, 12.14591786802309770, 50.62390960531435979 ) ) ;
#152113=CARTESIAN_POINT ( 'NONE',  ( -5.049401038298153566, 19.05341960407611168, 55.20724293864769550 ) ) ;
#152114=CARTESIAN_POINT ( 'NONE',  ( -5.719274019375978568, 21.55341960407610458, 25.20724293864769550 ) ) ;
#152115=CARTESIAN_POINT ( 'NONE',  ( -10.72451020669870658, -18.67979575497194134, 79.58442372801903275 ) ) ;
#152116=CARTESIAN_POINT ( 'NONE',  ( -5.049401038298153566, 19.05341960407611168, 70.20724293864769550 ) ) ;
#152117=CARTESIAN_POINT ( 'NONE',  ( -15.72974639402176322, -15.80617190586768395, 79.37609039468567573 ) ) ;
#152118=CARTESIAN_POINT ( 'NONE',  ( -21.53943276465977519, 0.05219959533907696930, 31.24890960531435979 ) ) ;
#152119=CARTESIAN_POINT ( 'NONE',  ( 9.474510206698971260, -16.51473224551069308, 67.91557627198102409 ) ) ;
#152120=CARTESIAN_POINT ( 'NONE',  ( 10.81492255796106328, -18.62759615963255655, 45.41775706135234003 ) ) ;
#152121=CARTESIAN_POINT ( 'NONE',  ( 13.97604488694548053, -13.89961937509957401, 55.62609039468566863 ) ) ;
#152122=CARTESIAN_POINT ( 'NONE',  ( 9.474510206698971260, -16.51473224551069308, 47.91557627198102409 ) ) ;
#152123=CARTESIAN_POINT ( 'NONE',  ( -5.049401038298153566, 19.05341960407611168, 80.20724293864769550 ) ) ;
#152124=CARTESIAN_POINT ( 'NONE',  ( 8.314922557961029526, -14.29746914071037800, 25.41775706135235779 ) ) ;
#152125=CARTESIAN_POINT ( 'NONE',  ( -0.05219959533910754901, -16.53943276465976808, 82.49890960531436690 ) ) ;
#152126=CARTESIAN_POINT ( 'NONE',  ( 19.03943276465977164, -0.05219959533909143690, 63.74890960531435979 ) ) ;
#152127=CARTESIAN_POINT ( 'NONE',  ( -18.62759615963270932, 10.81492255796079327, 45.83224293864769550 ) ) ;
#152128=CARTESIAN_POINT ( 'NONE',  ( 5.049401038297881783, 19.05341960407617563, 112.2927570613523471 ) ) ;
#152129=CARTESIAN_POINT ( 'NONE',  ( 21.55341960407619695, -5.719274019375665929, 26.04275706135235779 ) ) ;
#152130=CARTESIAN_POINT ( 'NONE',  ( 10.81492255796106328, -18.62759615963255655, 75.41775706135233293 ) ) ;
#152131=CARTESIAN_POINT ( 'NONE',  ( -12.14591786802326823, 12.06949235617739902, 68.12609039468567573 ) ) ;
#152132=CARTESIAN_POINT ( 'NONE',  ( -4.379528057220086978, -16.55341960407618274, 64.79275706135234714 ) ) ;
#152133=CARTESIAN_POINT ( 'NONE',  ( -5.049401038298153566, 19.05341960407611168, 55.20724293864769550 ) ) ;
#152134=CARTESIAN_POINT ( 'NONE',  ( -12.14591786802326823, 12.06949235617739902, 93.12609039468568994 ) ) ;
#152135=CARTESIAN_POINT ( 'NONE',  ( -19.03943276465977164, -0.05219959533935918106, 38.75109039468566152 ) ) ;
#152136=CARTESIAN_POINT ( 'NONE',  ( 18.67979575497178502, 10.72451020669898547, 109.1655762719810383 ) ) ;
#152137=CARTESIAN_POINT ( 'NONE',  ( -14.29746914071049879, 8.314922557960819915, 65.83224293864769550 ) ) ;
#152138=CARTESIAN_POINT ( 'NONE',  ( 13.89961937509977652, -13.97604488694527269, 83.12390960531436690 ) ) ;
#152139=CARTESIAN_POINT ( 'NONE',  ( -0.05219959533934338120, 16.53943276465976808, 92.50109039468567573 ) ) ;
#152140=CARTESIAN_POINT ( 'NONE',  ( 21.52544592524334988, 5.823673210054432836, 61.45942372801901854 ) ) ;
#152141=CARTESIAN_POINT ( 'NONE',  ( -4.483927247898782831, 16.52544592524335698, 32.70942372801900433 ) ) ;
#152142=CARTESIAN_POINT ( 'NONE',  ( -10.72451020669870658, -18.67979575497194134, 29.58442372801901854 ) ) ;
#152143=CARTESIAN_POINT ( 'NONE',  ( 16.53943276465976808, -0.05219959533910856209, 58.74890960531436690 ) ) ;
#152145=CARTESIAN_POINT ( 'NONE',  ( 10.72451020669898902, -18.67979575497178502, 102.9155762719810383 ) ) ;
#152146=CARTESIAN_POINT ( 'NONE',  ( 8.224510206698953496, -14.34966873604960469, 32.91557627198102409 ) ) ;
#152147=ORIENTED_EDGE ( 'NONE', *, *, #94811, .T. ) ;
#152149=CARTESIAN_POINT ( 'NONE',  ( -5.719274019375978568, 21.55341960407610458, 25.20724293864769550 ) ) ;
#152150=CARTESIAN_POINT ( 'NONE',  ( -15.80617190586768217, 15.72974639402176855, 43.12609039468568284 ) ) ;
#152151=CARTESIAN_POINT ( 'NONE',  ( 12.06949235617757843, -12.14591786802309237, 63.12390960531435979 ) ) ;
#152152=CARTESIAN_POINT ( 'NONE',  ( -13.89961937509977652, 13.97604488694528158, 65.62390960531436690 ) ) ;
#152153=CARTESIAN_POINT ( 'NONE',  ( -0.05219959533909027116, -19.03943276465977164, 22.49890960531436690 ) ) ;
#152154=CARTESIAN_POINT ( 'NONE',  ( -13.97604488694547697, 13.89961937509957934, 63.12609039468566152 ) ) ;
#152155=CARTESIAN_POINT ( 'NONE',  ( 15.72974639402199770, -15.80617190586745480, 43.12390960531435269 ) ) ;
#152157=CARTESIAN_POINT ( 'NONE',  ( -13.97604488694527625, -13.89961937509977652, 61.87390960531435979 ) ) ;
#152158=CARTESIAN_POINT ( 'NONE',  ( 0.05219959533934541429, -16.53943276465976808, 40.00109039468567573 ) ) ;
#152159=CARTESIAN_POINT ( 'NONE',  ( -21.52544592524334988, -5.823673210054445271, 23.95942372801901143 ) ) ;
#152160=CARTESIAN_POINT ( 'NONE',  ( -12.06949235617756955, 12.14591786802309770, 45.62390960531436690 ) ) ;
#152162=CARTESIAN_POINT ( 'NONE',  ( 5.049401038298161559, -19.05341960407611168, 92.70724293864769550 ) ) ;
#152163=CARTESIAN_POINT ( 'NONE',  ( -0.05219959533907301413, -21.53943276465977519, 72.49890960531435269 ) ) ;
#152164=CARTESIAN_POINT ( 'NONE',  ( 0.05219959533907565091, 21.53943276465977519, 114.9989096053143669 ) ) ;
#152165=CARTESIAN_POINT ( 'NONE',  ( -12.06949235617739369, -12.14591786802326823, 44.37609039468567573 ) ) ;
#152166=CARTESIAN_POINT ( 'NONE',  ( -18.62759615963270932, 10.81492255796079327, 40.83224293864769550 ) ) ;
#152167=CARTESIAN_POINT ( 'NONE',  ( 5.823673210054444382, -21.52544592524334988, 105.2094237280190328 ) ) ;
#152168=CARTESIAN_POINT ( 'NONE',  ( 19.05341960407611168, 5.049401038298154454, 93.95724293864769550 ) ) ;
#152169=CARTESIAN_POINT ( 'NONE',  ( 16.51473224551069308, 9.474510206698969483, 44.16557627198103120 ) ) ;
#152170=CARTESIAN_POINT ( 'NONE',  ( -5.049401038298153566, 19.05341960407611168, 95.20724293864770971 ) ) ;
#152171=CARTESIAN_POINT ( 'NONE',  ( -9.474510206698964154, 16.51473224551069663, 80.41557627198103830 ) ) ;
#152172=CARTESIAN_POINT ( 'NONE',  ( 16.62475595723613608, -7.163666690055876529, 88.02713351810406550 ) ) ;
#152173=CARTESIAN_POINT ( 'NONE',  ( 19.05341960407617918, -5.049401038297876454, 56.04275706135234714 ) ) ;
#152174=CARTESIAN_POINT ( 'NONE',  ( 15.80617190586769283, -15.72974639402175789, 105.6260903946856899 ) ) ;
#152175=CARTESIAN_POINT ( 'NONE',  ( 5.719274019375991003, -21.55341960407610458, 27.70724293864769905 ) ) ;
#152176=CARTESIAN_POINT ( 'NONE',  ( 12.14591786802327356, -12.06949235617739191, 105.6260903946856899 ) ) ;
#152177=CARTESIAN_POINT ( 'NONE',  ( 9.474510206698729675, 16.51473224551082808, 77.08442372801900433 ) ) ;
#152178=CARTESIAN_POINT ( 'NONE',  ( -16.61371651742604172, 7.165104196376024248, 58.85415069992998838 ) ) ;
#152179=CARTESIAN_POINT ( 'NONE',  ( -16.46253265017146816, -9.564922557961047289, 89.16775706135234714 ) ) ;
#152180=CARTESIAN_POINT ( 'NONE',  ( 9.564922557961047289, -16.46253265017146816, 30.41775706135232937 ) ) ;
#152181=CARTESIAN_POINT ( 'NONE',  ( -16.19135201231368981, -7.376712067591810751, 45.18680854052031037 ) ) ;
#152182=CARTESIAN_POINT ( 'NONE',  ( 16.51473224551069308, 9.474510206698969483, 44.16557627198103120 ) ) ;
#152183=CARTESIAN_POINT ( 'NONE',  ( -4.379528057220328563, 16.55341960407611168, 45.20724293864769550 ) ) ;
#152184=CARTESIAN_POINT ( 'NONE',  ( 19.05341960407611168, 5.049401038298154454, 23.95724293864769194 ) ) ;
#152185=CARTESIAN_POINT ( 'NONE',  ( 12.14591786802309770, 12.06949235617756955, 24.37390960531435979 ) ) ;
#152187=CARTESIAN_POINT ( 'NONE',  ( -16.53943276465976808, -0.05219959533934237506, 88.75109039468567573 ) ) ;
#152188=CARTESIAN_POINT ( 'NONE',  ( 16.51473224551069308, 9.474510206698969483, 44.16557627198103120 ) ) ;
#152189=CARTESIAN_POINT ( 'NONE',  ( 10.72451020669871369, 18.67979575497193778, 112.0844237280190185 ) ) ;
#152190=CARTESIAN_POINT ( 'NONE',  ( 9.564922557961047289, -16.46253265017146816, 110.4177570613523471 ) ) ;
#152191=CARTESIAN_POINT ( 'NONE',  ( 15.72974639402176855, 15.80617190586768217, 96.87609039468568994 ) ) ;
#152193=CARTESIAN_POINT ( 'NONE',  ( -13.97604488694527625, -13.89961937509977652, 91.87390960531432427 ) ) ;
#152194=CARTESIAN_POINT ( 'NONE',  ( -19.03943276465977164, 0.05219959533909376836, 86.24890960531436690 ) ) ;
#152196=CARTESIAN_POINT ( 'NONE',  ( -15.72974639402197994, 15.80617190586746368, 115.6239096053143669 ) ) ;
#152197=CARTESIAN_POINT ( 'NONE',  ( -0.05219959533910754901, -16.53943276465976808, 82.49890960531436690 ) ) ;
#152198=CARTESIAN_POINT ( 'NONE',  ( 21.55341960407610458, 5.719274019375980345, 78.95724293864769550 ) ) ;
#152199=CARTESIAN_POINT ( 'NONE',  ( 19.02544592524343514, -5.153800228976328945, 53.54057627198102409 ) ) ;
#152200=CARTESIAN_POINT ( 'NONE',  ( 0.05219959533907565091, 21.53943276465977519, 94.99890960531436690 ) ) ;
#152201=CARTESIAN_POINT ( 'NONE',  ( 12.14591786802327356, -12.06949235617739191, 90.62609039468567573 ) ) ;
#152203=CARTESIAN_POINT ( 'NONE',  ( 9.474510206698971260, -16.51473224551069308, 62.91557627198102409 ) ) ;
#152204=CARTESIAN_POINT ( 'NONE',  ( -0.05219959533910754901, -16.53943276465976808, 97.49890960531436690 ) ) ;
#152206=CARTESIAN_POINT ( 'NONE',  ( 0.05219959533909260263, 19.03943276465977164, 49.99890960531435979 ) ) ;
#152207=CARTESIAN_POINT ( 'NONE',  ( -19.03943276465977164, -0.05219959533935918106, 83.75109039468567573 ) ) ;
#152208=CARTESIAN_POINT ( 'NONE',  ( 4.483927247898545687, 16.52544592524342804, 79.79057627198102409 ) ) ;
#152209=CARTESIAN_POINT ( 'NONE',  ( -18.62759615963255300, -10.81492255796106328, 64.16775706135234714 ) ) ;
#152210=CARTESIAN_POINT ( 'NONE',  ( -16.46253265017160317, 9.564922557960807481, 35.83224293864768839 ) ) ;
#152211=CARTESIAN_POINT ( 'NONE',  ( 10.81492255796078972, 18.62759615963270932, 114.5822429386477097 ) ) ;
#152212=CARTESIAN_POINT ( 'NONE',  ( 8.314922557960818139, 14.29746914071049879, 104.5822429386477097 ) ) ;
#152214=CARTESIAN_POINT ( 'NONE',  ( 13.89961937509977652, -13.97604488694527269, 53.12390960531434558 ) ) ;
#152216=CARTESIAN_POINT ( 'NONE',  ( 13.89961937509957401, 13.97604488694547697, 91.87609039468567573 ) ) ;
#152217=CARTESIAN_POINT ( 'NONE',  ( 9.474510206698971260, -16.51473224551069308, 107.9155762719810383 ) ) ;
#152218=CARTESIAN_POINT ( 'NONE',  ( -10.72451020669870658, -18.67979575497194134, 44.58442372801901854 ) ) ;
#152219=CARTESIAN_POINT ( 'NONE',  ( 5.049401038298161559, -19.05341960407611168, 82.70724293864770971 ) ) ;
#152220=CARTESIAN_POINT ( 'NONE',  ( 9.564922557961047289, -16.46253265017146816, 70.41775706135233293 ) ) ;
#152221=CARTESIAN_POINT ( 'NONE',  ( 16.46253265017160672, -9.564922557960803928, 58.33224293864769550 ) ) ;
#152222=CARTESIAN_POINT ( 'NONE',  ( 14.34966873604960469, 8.224510206698951720, 74.16557627198102409 ) ) ;
#152223=CARTESIAN_POINT ( 'NONE',  ( 12.14591786802309770, 12.06949235617756955, 74.37390960531436690 ) ) ;
#152224=CARTESIAN_POINT ( 'NONE',  ( 16.46253265017160672, -9.564922557960803928, 88.33224293864769550 ) ) ;
#152225=CARTESIAN_POINT ( 'NONE',  ( 16.53943276465976808, -0.05219959533910856209, 78.74890960531436690 ) ) ;
#152226=CARTESIAN_POINT ( 'NONE',  ( -9.474510206698964154, 16.51473224551069663, 85.41557627198102409 ) ) ;
#152227=CARTESIAN_POINT ( 'NONE',  ( -0.05219959533936034679, 19.03943276465977164, 32.50109039468566863 ) ) ;
#152228=CARTESIAN_POINT ( 'NONE',  ( -19.02544592524342804, 5.153800228976336051, 56.04057627198100988 ) ) ;
#152229=CARTESIAN_POINT ( 'NONE',  ( 16.55341960407611168, 4.379528057220329451, 23.95724293864769550 ) ) ;
#152230=CARTESIAN_POINT ( 'NONE',  ( 4.379528057220339221, -16.55341960407611168, 107.7072429386476955 ) ) ;
#152232=CARTESIAN_POINT ( 'NONE',  ( 5.719274019375673035, 21.55341960407619339, 42.29275706135235424 ) ) ;
#152233=CARTESIAN_POINT ( 'NONE',  ( -9.564922557961040184, 16.46253265017147172, 72.91775706135233293 ) ) ;
#152234=CARTESIAN_POINT ( 'NONE',  ( 12.06949235617757843, -12.14591786802309237, 33.12390960531435979 ) ) ;
#152235=CARTESIAN_POINT ( 'NONE',  ( -15.72974639402197994, 15.80617190586746368, 80.62390960531438111 ) ) ;
#152236=CARTESIAN_POINT ( 'NONE',  ( 16.51473224551069308, 9.474510206698969483, 109.1655762719810383 ) ) ;
#152237=CARTESIAN_POINT ( 'NONE',  ( -8.314922557960811034, -14.29746914071050412, 72.08224293864769550 ) ) ;
#152238=CARTESIAN_POINT ( 'NONE',  ( -16.46253265017160317, 9.564922557960807481, 45.83224293864769550 ) ) ;
#152239=CARTESIAN_POINT ( 'NONE',  ( -5.153800228976607833, 19.02544592524334988, 37.70942372801899722 ) ) ;
#152240=CARTESIAN_POINT ( 'NONE',  ( 14.34966873604972726, -8.224510206698740333, 105.8344237280190328 ) ) ;
#152241=CARTESIAN_POINT ( 'NONE',  ( -8.314922557961024197, 14.29746914071037800, 52.91775706135235424 ) ) ;
#152242=CARTESIAN_POINT ( 'NONE',  ( -0.05219959533907301413, -21.53943276465977519, 32.49890960531435979 ) ) ;
#152243=CARTESIAN_POINT ( 'NONE',  ( -5.823673210054431948, 21.52544592524334988, 102.7094237280190185 ) ) ;
#152244=CARTESIAN_POINT ( 'NONE',  ( -5.153800228976328057, -19.02544592524343514, 97.29057627198099567 ) ) ;
#152245=CARTESIAN_POINT ( 'NONE',  ( 8.314922557961029526, -14.29746914071037800, 80.41775706135234714 ) ) ;
#152246=CARTESIAN_POINT ( 'NONE',  ( -9.474510206698964154, 16.51473224551069663, 30.41557627198102054 ) ) ;
#152247=CARTESIAN_POINT ( 'NONE',  ( 8.314922557960818139, 14.29746914071049879, 29.58224293864769905 ) ) ;
#152248=CARTESIAN_POINT ( 'NONE',  ( -9.474510206698964154, 16.51473224551069663, 105.4155762719810383 ) ) ;
#152249=CARTESIAN_POINT ( 'NONE',  ( 5.049401038298161559, -19.05341960407611168, 87.70724293864769550 ) ) ;
#152250=CARTESIAN_POINT ( 'NONE',  ( 10.72451020669898902, -18.67979575497178502, 27.91557627198103830 ) ) ;
#152251=CARTESIAN_POINT ( 'NONE',  ( -0.05219959533910754901, -16.53943276465976808, 67.49890960531436690 ) ) ;
#152252=CARTESIAN_POINT ( 'NONE',  ( 4.483927247898545687, 16.52544592524342804, 49.79057627198102409 ) ) ;
#152254=CARTESIAN_POINT ( 'NONE',  ( -14.34966873604972548, 8.224510206698743886, 53.33442372801901854 ) ) ;
#152255=CARTESIAN_POINT ( 'NONE',  ( 17.50000000000001776, -4.658240926743138388, 31.44470417816803831 ) ) ;
#152256=CARTESIAN_POINT ( 'NONE',  ( 13.89961937509957401, 13.97604488694547697, 51.87609039468566863 ) ) ;
#152257=CARTESIAN_POINT ( 'NONE',  ( -5.049401038298153566, 19.05341960407611168, 90.20724293864766707 ) ) ;
#152258=CARTESIAN_POINT ( 'NONE',  ( -9.564922557961040184, 16.46253265017147172, 62.91775706135233293 ) ) ;
#152260=CARTESIAN_POINT ( 'NONE',  ( 19.03943276465977164, 0.05219959533936151252, 51.25109039468567573 ) ) ;
#152261=CARTESIAN_POINT ( 'NONE',  ( -13.97604488694547697, 13.89961937509957934, 98.12609039468566152 ) ) ;
#152262=CARTESIAN_POINT ( 'NONE',  ( 4.483927247898790824, -16.52544592524335698, 100.2094237280190043 ) ) ;
#152264=CARTESIAN_POINT ( 'NONE',  ( -16.46253265017160317, 9.564922557960807481, 25.83224293864769194 ) ) ;
#152265=CARTESIAN_POINT ( 'NONE',  ( 19.03943276465977164, -0.05219959533909143690, 113.7489096053143669 ) ) ;
#152266=CARTESIAN_POINT ( 'NONE',  ( 15.72974639402176855, 15.80617190586768217, 41.87609039468568284 ) ) ;
#152267=CARTESIAN_POINT ( 'NONE',  ( 9.474510206698729675, 16.51473224551082808, 107.0844237280190043 ) ) ;
#152269=CARTESIAN_POINT ( 'NONE',  ( -5.153800228976328057, -19.02544592524343514, 67.29057627198102409 ) ) ;
#152272=CARTESIAN_POINT ( 'NONE',  ( 4.379528057220339221, -16.55341960407611168, 77.70724293864770971 ) ) ;
#152273=CARTESIAN_POINT ( 'NONE',  ( -0.05219959533909027116, -19.03943276465977164, 62.49890960531435979 ) ) ;
#152274=CARTESIAN_POINT ( 'NONE',  ( 13.97604488694527802, 13.89961937509977652, 74.37390960531436690 ) ) ;
#152275=CARTESIAN_POINT ( 'NONE',  ( 13.97604488694548053, -13.89961937509957401, 80.62609039468567573 ) ) ;
#152276=CARTESIAN_POINT ( 'NONE',  ( -21.53943276465977519, 0.05219959533907696930, 61.24890960531435979 ) ) ;
#152277=CARTESIAN_POINT ( 'NONE',  ( 4.483927247898545687, 16.52544592524342804, 109.7905762719810383 ) ) ;
#152278=CARTESIAN_POINT ( 'NONE',  ( 13.97604488694548053, -13.89961937509957401, 40.62609039468564731 ) ) ;
#152279=CARTESIAN_POINT ( 'NONE',  ( -5.049401038298153566, 19.05341960407611168, 75.20724293864769550 ) ) ;
#152280=CARTESIAN_POINT ( 'NONE',  ( -18.62759615963270932, 10.81492255796079327, 95.83224293864770971 ) ) ;
#152281=CARTESIAN_POINT ( 'NONE',  ( 4.483927247898545687, 16.52544592524342804, 79.79057627198102409 ) ) ;
#152282=CARTESIAN_POINT ( 'NONE',  ( 19.05341960407617918, -5.049401038297876454, 51.04275706135231871 ) ) ;
#152283=CARTESIAN_POINT ( 'NONE',  ( 21.53943276465977519, -0.05219959533907433946, 73.74890960531433848 ) ) ;
#152284=CARTESIAN_POINT ( 'NONE',  ( -5.719274019375978568, 21.55341960407610458, 65.20724293864768129 ) ) ;
#152285=CARTESIAN_POINT ( 'NONE',  ( 5.823673210054125526, 21.52544592524343514, 44.79057627198103120 ) ) ;
#152286=CARTESIAN_POINT ( 'NONE',  ( 10.72451020669871369, 18.67979575497193778, 92.08442372801901854 ) ) ;
#152287=CARTESIAN_POINT ( 'NONE',  ( 9.474510206698971260, -16.51473224551069308, 67.91557627198102409 ) ) ;
#152288=CARTESIAN_POINT ( 'NONE',  ( -14.29746914071049879, 8.314922557960819915, 110.8322429386476955 ) ) ;
#152289=CARTESIAN_POINT ( 'NONE',  ( -5.823673210054431948, 21.52544592524334988, 22.70942372801901499 ) ) ;
#152290=CARTESIAN_POINT ( 'NONE',  ( -10.72451020669870658, -18.67979575497194134, 34.58442372801900433 ) ) ;
#152291=CARTESIAN_POINT ( 'NONE',  ( 13.97604488694527802, 13.89961937509977652, 34.37390960531436690 ) ) ;
#152292=CARTESIAN_POINT ( 'NONE',  ( 10.72451020669898902, -18.67979575497178502, 107.9155762719810241 ) ) ;
#152293=CARTESIAN_POINT ( 'NONE',  ( 16.46253265017146816, 9.564922557961045513, 56.66775706135233293 ) ) ;
#152295=CARTESIAN_POINT ( 'NONE',  ( 5.049401038298161559, -19.05341960407611168, 42.70724293864767418 ) ) ;
#152296=CARTESIAN_POINT ( 'NONE',  ( 14.29746914071037800, 8.314922557961029526, 31.66775706135234358 ) ) ;
#152297=CARTESIAN_POINT ( 'NONE',  ( 16.37381404539904750, -7.261601738933634032, 21.61892339308662159 ) ) ;
#152298=CARTESIAN_POINT ( 'NONE',  ( 16.55341960407618274, -4.379528057220086978, 66.04275706135236135 ) ) ;
#152299=CARTESIAN_POINT ( 'NONE',  ( 5.049401038298161559, -19.05341960407611168, 37.70724293864768839 ) ) ;
#152301=CARTESIAN_POINT ( 'NONE',  ( 13.97604488694527802, 13.89961937509977652, 84.37390960531433848 ) ) ;
#152302=CARTESIAN_POINT ( 'NONE',  ( -0.05219959533909027116, -19.03943276465977164, 27.49890960531435624 ) ) ;
#152303=CARTESIAN_POINT ( 'NONE',  ( 18.67979575497178502, 10.72451020669898547, 64.16557627198102409 ) ) ;
#152304=CARTESIAN_POINT ( 'NONE',  ( -14.29746914071037622, -8.314922557961029526, 49.16775706135234003 ) ) ;
#152305=CARTESIAN_POINT ( 'NONE',  ( 15.72974639402176855, 15.80617190586768217, 101.8760903946857042 ) ) ;
#152306=CARTESIAN_POINT ( 'NONE',  ( -13.97604488694527625, -13.89961937509977652, 36.87390960531436690 ) ) ;
#152307=CARTESIAN_POINT ( 'NONE',  ( -8.224510206698948167, 14.34966873604960824, 30.41557627198101699 ) ) ;
#152308=CARTESIAN_POINT ( 'NONE',  ( 4.483927247898545687, 16.52544592524342804, 59.79057627198103120 ) ) ;
#152309=CARTESIAN_POINT ( 'NONE',  ( 16.46253265017160672, -9.564922557960803928, 68.33224293864770971 ) ) ;
#152310=CARTESIAN_POINT ( 'NONE',  ( -5.823673210054431948, 21.52544592524334988, 107.7094237280190328 ) ) ;
#152311=CARTESIAN_POINT ( 'NONE',  ( -5.719274019375665041, -21.55341960407619695, 24.79275706135235779 ) ) ;
#152312=CARTESIAN_POINT ( 'NONE',  ( 0.05219959533937995610, -21.53943276465977519, 90.00109039468567573 ) ) ;
#152313=CARTESIAN_POINT ( 'NONE',  ( -12.14591786802326823, 12.06949235617739902, 53.12609039468568284 ) ) ;
#152314=CARTESIAN_POINT ( 'NONE',  ( 16.55341960407618274, -4.379528057220086978, 31.04275706135234714 ) ) ;
#152315=CARTESIAN_POINT ( 'NONE',  ( 4.483927247898545687, 16.52544592524342804, 74.79057627198105251 ) ) ;
#152316=CARTESIAN_POINT ( 'NONE',  ( -18.67979575497193778, 10.72451020669871902, 98.33442372801901854 ) ) ;
#152317=CARTESIAN_POINT ( 'NONE',  ( 8.224510206698953496, -14.34966873604960469, 37.91557627198102409 ) ) ;
#152318=CARTESIAN_POINT ( 'NONE',  ( 13.89961937509977652, -13.97604488694527269, 33.12390960531434558 ) ) ;
#152319=CARTESIAN_POINT ( 'NONE',  ( -16.52544592524335698, -4.483927247898792601, 43.95942372801902565 ) ) ;
#152320=CARTESIAN_POINT ( 'NONE',  ( 16.53943276465976808, -0.05219959533910856209, 53.74890960531437401 ) ) ;
#152321=CARTESIAN_POINT ( 'NONE',  ( 16.55341960407618274, -4.379528057220086978, 86.04275706135236135 ) ) ;
#152322=CARTESIAN_POINT ( 'NONE',  ( 13.97604488694527802, 13.89961937509977652, 94.37390960531436690 ) ) ;
#152323=CARTESIAN_POINT ( 'NONE',  ( 0.05219959533909260263, 19.03943276465977164, 109.9989096053143669 ) ) ;
#152324=CARTESIAN_POINT ( 'NONE',  ( 19.05341960407617918, -5.049401038297876454, 21.04275706135232582 ) ) ;
#152325=CARTESIAN_POINT ( 'NONE',  ( 16.52544592524342804, -4.483927247898539470, 88.54057627198103830 ) ) ;
#152326=CARTESIAN_POINT ( 'NONE',  ( 9.564922557960805705, 16.46253265017160317, 99.58224293864770971 ) ) ;
#152328=CARTESIAN_POINT ( 'NONE',  ( -12.06949235617739369, -12.14591786802326823, 39.37609039468567573 ) ) ;
#152329=CARTESIAN_POINT ( 'NONE',  ( -13.97604488694527625, -13.89961937509977652, 46.87390960531435979 ) ) ;
#152330=CARTESIAN_POINT ( 'NONE',  ( -16.51473224551069308, -9.474510206698971260, 111.6655762719810383 ) ) ;
#152331=CARTESIAN_POINT ( 'NONE',  ( 16.52544592524335698, 4.483927247898782831, 41.45942372801901143 ) ) ;
#152333=CARTESIAN_POINT ( 'NONE',  ( -9.474510206698720793, -16.51473224551083518, 39.58442372801899722 ) ) ;
#152334=CARTESIAN_POINT ( 'NONE',  ( -19.05341960407611168, -5.049401038298163336, 41.45724293864769550 ) ) ;
#152335=CARTESIAN_POINT ( 'NONE',  ( -12.06949235617739369, -12.14591786802326823, 84.37609039468570415 ) ) ;
#152336=CARTESIAN_POINT ( 'NONE',  ( 5.153800228976615827, -19.02544592524334988, 85.20942372801900433 ) ) ;
#152337=CARTESIAN_POINT ( 'NONE',  ( -19.02544592524334988, -5.153800228976617603, 23.95942372801900078 ) ) ;
#152338=CARTESIAN_POINT ( 'NONE',  ( 9.564922557960805705, 16.46253265017160317, 64.58224293864769550 ) ) ;
#152339=CARTESIAN_POINT ( 'NONE',  ( 12.06949235617757843, -12.14591786802309237, 103.1239096053143811 ) ) ;
#152341=CARTESIAN_POINT ( 'NONE',  ( 19.05341960407617918, -5.049401038297876454, 66.04275706135233293 ) ) ;
#152342=CARTESIAN_POINT ( 'NONE',  ( 21.55341960407610458, 5.719274019375980345, 58.95724293864770971 ) ) ;
#152343=CARTESIAN_POINT ( 'NONE',  ( -9.564922557961040184, 16.46253265017147172, 22.91775706135233648 ) ) ;
#152344=CARTESIAN_POINT ( 'NONE',  ( 19.03943276465977164, -0.05219959533909143690, 108.7489096053143527 ) ) ;
#152345=CARTESIAN_POINT ( 'NONE',  ( -0.05219959533907301413, -21.53943276465977519, 72.49890960531435269 ) ) ;
#152346=CARTESIAN_POINT ( 'NONE',  ( -16.46253265017160317, 9.564922557960807481, 110.8322429386476955 ) ) ;
#152347=CARTESIAN_POINT ( 'NONE',  ( -13.97604488694547697, 13.89961937509957934, 103.1260903946856473 ) ) ;
#152348=CARTESIAN_POINT ( 'NONE',  ( -19.52217212775657629, 5.500000000000115463, 59.93993709005261650 ) ) ;
#152349=CARTESIAN_POINT ( 'NONE',  ( -0.05219959533934338120, 16.53943276465976808, 22.50109039468567573 ) ) ;
#152350=CARTESIAN_POINT ( 'NONE',  ( -5.049401038298153566, 19.05341960407611168, 30.20724293864768839 ) ) ;
#152351=CARTESIAN_POINT ( 'NONE',  ( 5.049401038298161559, -19.05341960407611168, 97.70724293864766707 ) ) ;
#152352=CARTESIAN_POINT ( 'NONE',  ( 21.52544592524344225, -5.823673210054117533, 88.54057627198103830 ) ) ;
#152353=CARTESIAN_POINT ( 'NONE',  ( -21.55341960407619339, 5.719274019375674811, 63.54275706135234003 ) ) ;
#152354=CARTESIAN_POINT ( 'NONE',  ( 16.51473224551083163, -9.474510206698727899, 110.8344237280190043 ) ) ;
#152355=CARTESIAN_POINT ( 'NONE',  ( -18.62759615963255300, -10.81492255796106328, 104.1677570613523471 ) ) ;
#152356=CARTESIAN_POINT ( 'NONE',  ( -8.314922557961024197, 14.29746914071037800, 107.9177570613523471 ) ) ;
#152357=CARTESIAN_POINT ( 'NONE',  ( -21.55341960407610458, -5.719274019375992779, 96.45724293864770971 ) ) ;
#152358=CARTESIAN_POINT ( 'NONE',  ( -16.53943276465976808, 0.05219959533911058130, 41.24890960531435269 ) ) ;
#152359=CARTESIAN_POINT ( 'NONE',  ( 13.89961937509957401, 13.97604488694547697, 81.87609039468564731 ) ) ;
#152360=CARTESIAN_POINT ( 'NONE',  ( -19.05341960407617563, 5.049401038297882671, 58.54275706135234003 ) ) ;
#152361=CARTESIAN_POINT ( 'NONE',  ( 5.719274019375673035, 21.55341960407619339, 57.29275706135234714 ) ) ;
#152362=CARTESIAN_POINT ( 'NONE',  ( -5.049401038297874678, -19.05341960407617918, 39.79275706135232582 ) ) ;
#152363=CARTESIAN_POINT ( 'NONE',  ( 14.29746914071049879, -8.314922557960816363, 108.3322429386477097 ) ) ;
#152364=CARTESIAN_POINT ( 'NONE',  ( 10.72451020669898902, -18.67979575497178502, 32.91557627198102409 ) ) ;
#152365=CARTESIAN_POINT ( 'NONE',  ( 4.483927247898545687, 16.52544592524342804, 39.79057627198103830 ) ) ;
#152366=CARTESIAN_POINT ( 'NONE',  ( 18.67979575497194134, -10.72451020669871369, 100.8344237280190185 ) ) ;
#152367=CARTESIAN_POINT ( 'NONE',  ( 16.53943276465976808, 0.05219959533934440121, 71.25109039468568994 ) ) ;
#152368=CARTESIAN_POINT ( 'NONE',  ( -16.53943276465976808, -0.05219959533934237506, 113.7510903946856757 ) ) ;
#152369=CARTESIAN_POINT ( 'NONE',  ( 21.55341960407619695, -5.719274019375665929, 56.04275706135235424 ) ) ;
#152370=CARTESIAN_POINT ( 'NONE',  ( -21.52544592524334988, -5.823673210054445271, 73.95942372801901854 ) ) ;
#152371=CARTESIAN_POINT ( 'NONE',  ( 21.53943276465977519, -0.05219959533907433946, 68.74890960531435269 ) ) ;
#152373=CARTESIAN_POINT ( 'NONE',  ( -19.02544592524342804, 5.153800228976336051, 31.04057627198102409 ) ) ;
#152374=CARTESIAN_POINT ( 'NONE',  ( 18.62759615963255655, 10.81492255796105972, 46.66775706135234714 ) ) ;
#152375=CARTESIAN_POINT ( 'NONE',  ( 19.02544592524343514, -5.153800228976328945, 28.54057627198102409 ) ) ;
#152376=CARTESIAN_POINT ( 'NONE',  ( 13.97604488694527802, 13.89961937509977652, 34.37390960531436690 ) ) ;
#152377=CARTESIAN_POINT ( 'NONE',  ( 8.314922557960818139, 14.29746914071049879, 84.58224293864769550 ) ) ;
#152378=CARTESIAN_POINT ( 'NONE',  ( -0.05219959533909027116, -19.03943276465977164, 82.49890960531436690 ) ) ;
#152379=CARTESIAN_POINT ( 'NONE',  ( -14.29746914071049879, 8.314922557960819915, 30.83224293864770260 ) ) ;
#152380=CARTESIAN_POINT ( 'NONE',  ( 18.67979575497178502, 10.72451020669898547, 74.16557627198102409 ) ) ;
#152381=CARTESIAN_POINT ( 'NONE',  ( 21.53943276465977519, -0.05219959533907433946, 108.7489096053143669 ) ) ;
#152382=CARTESIAN_POINT ( 'NONE',  ( 0.05219959533909260263, 19.03943276465977164, 114.9989096053143669 ) ) ;
#152383=CARTESIAN_POINT ( 'NONE',  ( 5.049401038298161559, -19.05341960407611168, 67.70724293864769550 ) ) ;
#152384=CARTESIAN_POINT ( 'NONE',  ( 9.564922557961047289, -16.46253265017146816, 105.4177570613523471 ) ) ;
#152385=CARTESIAN_POINT ( 'NONE',  ( 15.72974639402199770, -15.80617190586745480, 53.12390960531436690 ) ) ;
#152386=CARTESIAN_POINT ( 'NONE',  ( 5.719274019375673035, 21.55341960407619339, 82.29275706135234714 ) ) ;
#152387=CARTESIAN_POINT ( 'NONE',  ( -19.03943276465977164, 0.05219959533909376836, 71.24890960531435269 ) ) ;
#152388=CARTESIAN_POINT ( 'NONE',  ( 16.46253265017160672, -9.564922557960803928, 93.33224293864769550 ) ) ;
#152389=CARTESIAN_POINT ( 'NONE',  ( -8.314922557961024197, 14.29746914071037800, 77.91775706135231871 ) ) ;
#152390=CARTESIAN_POINT ( 'NONE',  ( 5.823673210054444382, -21.52544592524334988, 55.20942372801902565 ) ) ;
#152391=CARTESIAN_POINT ( 'NONE',  ( -15.80617190586768217, 15.72974639402176855, 103.1260903946856757 ) ) ;
#152392=CARTESIAN_POINT ( 'NONE',  ( 18.67979575497178502, 10.72451020669898547, 114.1655762719810383 ) ) ;
#152393=CARTESIAN_POINT ( 'NONE',  ( -0.05219959533907301413, -21.53943276465977519, 82.49890960531436690 ) ) ;
#152394=CARTESIAN_POINT ( 'NONE',  ( -0.05219959533936034679, 19.03943276465977164, 47.50109039468566863 ) ) ;
#152395=CARTESIAN_POINT ( 'NONE',  ( -21.53943276465977519, 0.05219959533907696930, 36.24890960531435979 ) ) ;
#152396=CARTESIAN_POINT ( 'NONE',  ( 13.97604488694527802, 13.89961937509977652, 84.37390960531433848 ) ) ;
#152397=CARTESIAN_POINT ( 'NONE',  ( -14.29746914071049879, 8.314922557960819915, 30.83224293864770260 ) ) ;
#152400=CARTESIAN_POINT ( 'NONE',  ( -5.153800228976607833, 19.02544592524334988, 97.70942372801900433 ) ) ;
#152401=CARTESIAN_POINT ( 'NONE',  ( -21.53943276465977519, 0.05219959533907696930, 66.24890960531436690 ) ) ;
#152402=CARTESIAN_POINT ( 'NONE',  ( 14.29746914071049879, -8.314922557960816363, 58.33224293864768839 ) ) ;
#152403=CARTESIAN_POINT ( 'NONE',  ( 0.05219959533934541429, -16.53943276465976808, 30.00109039468568284 ) ) ;
#152404=CARTESIAN_POINT ( 'NONE',  ( 19.02544592524343514, -5.153800228976328945, 43.54057627198103120 ) ) ;
#152405=CARTESIAN_POINT ( 'NONE',  ( -21.52544592524343514, 5.823673210054127303, 106.0405762719810525 ) ) ;
#152406=CARTESIAN_POINT ( 'NONE',  ( 19.03943276465977164, 0.05219959533936151252, 91.25109039468566152 ) ) ;
#152407=CARTESIAN_POINT ( 'NONE',  ( -13.97604488694527625, -13.89961937509977652, 86.87390960531436690 ) ) ;
#152408=CARTESIAN_POINT ( 'NONE',  ( 16.53943276465976808, -0.05219959533910856209, 83.74890960531435269 ) ) ;
#152409=CARTESIAN_POINT ( 'NONE',  ( 0.05219959533909260263, 19.03943276465977164, 64.99890960531436690 ) ) ;
#152410=CARTESIAN_POINT ( 'NONE',  ( -14.34966873604960291, -8.224510206698953496, 71.66557627198100988 ) ) ;
#152411=CARTESIAN_POINT ( 'NONE',  ( 9.564922557960805705, 16.46253265017160317, 29.58224293864769550 ) ) ;
#152413=CARTESIAN_POINT ( 'NONE',  ( 16.52544592524342804, -4.483927247898539470, 48.54057627198103120 ) ) ;
#152414=CARTESIAN_POINT ( 'NONE',  ( 19.03943276465977164, -0.05219959533909143690, 88.74890960531436690 ) ) ;
#152416=CARTESIAN_POINT ( 'NONE',  ( -16.46253265017146816, -9.564922557961047289, 54.16775706135234003 ) ) ;
#152417=CARTESIAN_POINT ( 'NONE',  ( -4.379528057220086978, -16.55341960407618274, 64.79275706135234714 ) ) ;
#152418=CARTESIAN_POINT ( 'NONE',  ( 15.72974639402199770, -15.80617190586745480, 83.12390960531436690 ) ) ;
#152419=CARTESIAN_POINT ( 'NONE',  ( 0.05219959533936267826, -19.03943276465977164, 35.00109039468566863 ) ) ;
#152420=CARTESIAN_POINT ( 'NONE',  ( 19.02544592524343514, -5.153800228976328945, 93.54057627198102409 ) ) ;
#152422=CARTESIAN_POINT ( 'NONE',  ( -21.55341960407610458, -5.719274019375992779, 31.45724293864769550 ) ) ;
#152423=CARTESIAN_POINT ( 'NONE',  ( 0.05219959533909260263, 19.03943276465977164, 54.99890960531435979 ) ) ;
#152424=CARTESIAN_POINT ( 'NONE',  ( 18.67979575497194134, -10.72451020669871369, 55.83442372801901854 ) ) ;
#152425=CARTESIAN_POINT ( 'NONE',  ( -19.03943276465977164, 0.05219959533909376836, 26.24890960531435624 ) ) ;
#152426=CARTESIAN_POINT ( 'NONE',  ( 5.719274019375991003, -21.55341960407610458, 112.7072429386476955 ) ) ;
#152427=CARTESIAN_POINT ( 'NONE',  ( 5.153800228976335163, 19.02544592524342804, 89.79057627198102409 ) ) ;
#152429=CARTESIAN_POINT ( 'NONE',  ( 5.823673210054444382, -21.52544592524334988, 45.20942372801901854 ) ) ;
#152431=CARTESIAN_POINT ( 'NONE',  ( 13.89961937509977652, -13.97604488694527269, 103.1239096053143527 ) ) ;
#152433=CARTESIAN_POINT ( 'NONE',  ( -17.58332526062529411, 7.635886036038502134, 90.92334959558465357 ) ) ;
#152434=CARTESIAN_POINT ( 'NONE',  ( 5.719274019375991003, -21.55341960407610458, 112.7072429386476955 ) ) ;
#152435=CARTESIAN_POINT ( 'NONE',  ( -19.05341960407611168, -5.049401038298163336, 46.45724293864768129 ) ) ;
#152436=CARTESIAN_POINT ( 'NONE',  ( 12.06949235617739724, 12.14591786802326823, 26.87609039468567218 ) ) ;
#152438=CARTESIAN_POINT ( 'NONE',  ( -10.81492255796105439, 18.62759615963255655, 97.91775706135236135 ) ) ;
#152439=CARTESIAN_POINT ( 'NONE',  ( -9.564922557960796823, -16.46253265017161027, 27.08224293864769550 ) ) ;
#152440=CARTESIAN_POINT ( 'NONE',  ( 0.05219959533937995610, -21.53943276465977519, 105.0010903946856757 ) ) ;
#152441=CARTESIAN_POINT ( 'NONE',  ( -9.474510206698964154, 16.51473224551069663, 95.41557627198102409 ) ) ;
#152442=CARTESIAN_POINT ( 'NONE',  ( 21.53943276465977519, 0.05219959533937863772, 56.25109039468568284 ) ) ;
#152444=CARTESIAN_POINT ( 'NONE',  ( -19.03943276465977164, 0.05219959533909376836, 96.24890960531436690 ) ) ;
#152445=CARTESIAN_POINT ( 'NONE',  ( 17.97058386085788229, 5.500000000000048850, 46.50390968646216550 ) ) ;
#152446=CARTESIAN_POINT ( 'NONE',  ( -4.483927247898782831, 16.52544592524335698, 52.70942372801902565 ) ) ;
#152447=CARTESIAN_POINT ( 'NONE',  ( -0.05219959533934338120, 16.53943276465976808, 62.50109039468568284 ) ) ;
#152448=CARTESIAN_POINT ( 'NONE',  ( 10.81492255796106328, -18.62759615963255655, 55.41775706135234714 ) ) ;
#152449=CARTESIAN_POINT ( 'NONE',  ( 21.55341960407619695, -5.719274019375665929, 91.04275706135236135 ) ) ;
#152451=( BOUNDED_CURVE ( )  B_SPLINE_CURVE ( 2, ( #114744, #34916, #113731, #158260, #50099, #159241, #96572, #147093, #176438, #98561, #68234, #54081, #175428 ),
 .UNSPECIFIED., .F., .F. ) 
 B_SPLINE_CURVE_WITH_KNOTS ( ( 3, 2, 2, 2, 2, 2, 3 ),
 ( 0.5287919057228195330, 0.5307017543859648967, 0.5350877192982456121, 0.5394736842105263275, 0.5438596491228070429, 0.5482456140350877583, 0.5502011425203234829 ),
 .UNSPECIFIED. ) 
 CURVE ( )  GEOMETRIC_REPRESENTATION_ITEM ( )  RATIONAL_B_SPLINE_CURVE ( ( 0.9832469066685285419, 0.9851625545550100060, 1.000000000000000000, 0.9659258262890683122, 1.000000000000000000, 0.9659258262890683122, 1.000000000000000000, 0.9659258262890683122, 1.000000000000000000, 0.9659258262890683122, 1.000000000000000000, 0.9848076720550078544, 0.9831626618144001517 ) ) 
 REPRESENTATION_ITEM ( '' )  );
#152452=CARTESIAN_POINT ( 'NONE',  ( -4.483927247898782831, 16.52544592524335698, 22.70942372801901499 ) ) ;
#152453=CARTESIAN_POINT ( 'NONE',  ( 5.153800228976335163, 19.02544592524342804, 74.79057627198103830 ) ) ;
#152454=CARTESIAN_POINT ( 'NONE',  ( 19.02544592524343514, -5.153800228976328945, 93.54057627198102409 ) ) ;
#152455=CARTESIAN_POINT ( 'NONE',  ( -16.53943276465976808, 0.05219959533911058130, 116.2489096053143669 ) ) ;
#152456=CARTESIAN_POINT ( 'NONE',  ( 21.53943276465977519, -0.05219959533907433946, 23.74890960531435269 ) ) ;
#152457=CARTESIAN_POINT ( 'NONE',  ( 16.53943276465976808, 0.05219959533934440121, 96.25109039468568994 ) ) ;
#152458=CARTESIAN_POINT ( 'NONE',  ( -16.53943276465976808, 0.05219959533911058130, 66.24890960531436690 ) ) ;
#152459=CARTESIAN_POINT ( 'NONE',  ( -19.03943276465977164, 0.05219959533909376836, 66.24890960531436690 ) ) ;
#152460=CARTESIAN_POINT ( 'NONE',  ( 0.05219959533937995610, -21.53943276465977519, 90.00109039468567573 ) ) ;
#152462=CARTESIAN_POINT ( 'NONE',  ( 13.97604488694548053, -13.89961937509957401, 105.6260903946856757 ) ) ;
#152463=CARTESIAN_POINT ( 'NONE',  ( -16.55341960407611168, -4.379528057220339221, 81.45724293864769550 ) ) ;
#152464=CARTESIAN_POINT ( 'NONE',  ( -10.81492255796105439, 18.62759615963255655, 22.91775706135235069 ) ) ;
#152465=CARTESIAN_POINT ( 'NONE',  ( 21.53943276465977519, -0.05219959533907433946, 73.74890960531433848 ) ) ;
#152466=CARTESIAN_POINT ( 'NONE',  ( 13.89961937509957401, 13.97604488694547697, 41.87609039468566152 ) ) ;
#152468=CARTESIAN_POINT ( 'NONE',  ( -5.049401038298153566, 19.05341960407611168, 80.20724293864769550 ) ) ;
#152469=CARTESIAN_POINT ( 'NONE',  ( 16.53943276465976808, -0.05219959533910856209, 53.74890960531437401 ) ) ;
#152470=CARTESIAN_POINT ( 'NONE',  ( 8.314922557960818139, 14.29746914071049879, 29.58224293864769905 ) ) ;
#152471=CARTESIAN_POINT ( 'NONE',  ( 4.379528057220092307, 16.55341960407617563, 102.2927570613523613 ) ) ;
#152472=CARTESIAN_POINT ( 'NONE',  ( -9.564922557961040184, 16.46253265017147172, 52.91775706135233293 ) ) ;
#152473=CARTESIAN_POINT ( 'NONE',  ( 19.25176906914649422, 5.499999999999731770, 53.49927264242280245 ) ) ;
#152474=CARTESIAN_POINT ( 'NONE',  ( -9.474510206698964154, 16.51473224551069663, 110.4155762719810383 ) ) ;
#152475=CARTESIAN_POINT ( 'NONE',  ( 8.224510206698953496, -14.34966873604960469, 77.91557627198102409 ) ) ;
#152476=CARTESIAN_POINT ( 'NONE',  ( -19.05341960407617563, 5.049401038297882671, 38.54275706135233293 ) ) ;
#152477=CARTESIAN_POINT ( 'NONE',  ( 9.474510206698971260, -16.51473224551069308, 32.91557627198102409 ) ) ;
#152478=CARTESIAN_POINT ( 'NONE',  ( 15.80617190586746368, 15.72974639402197994, 29.37390960531435269 ) ) ;
#152479=CARTESIAN_POINT ( 'NONE',  ( 10.72451020669898902, -18.67979575497178502, 72.91557627198103830 ) ) ;
#152480=CARTESIAN_POINT ( 'NONE',  ( -12.14591786802309592, -12.06949235617757132, 106.8739096053143811 ) ) ;
#152481=CARTESIAN_POINT ( 'NONE',  ( 8.314922557961029526, -14.29746914071037800, 70.41775706135236135 ) ) ;
#152482=CARTESIAN_POINT ( 'NONE',  ( -19.03943276465977164, 0.05219959533909376836, 46.24890960531435979 ) ) ;
#152483=CARTESIAN_POINT ( 'NONE',  ( -15.72974639402176322, -15.80617190586768395, 39.37609039468567573 ) ) ;
#152484=CARTESIAN_POINT ( 'NONE',  ( -14.34966873604960291, -8.224510206698953496, 86.66557627198102409 ) ) ;
#152485=CARTESIAN_POINT ( 'NONE',  ( -18.22780087662123805, -5.499999999999968026, 93.98236817873105053 ) ) ;
#152486=CARTESIAN_POINT ( 'NONE',  ( -17.44270441346514389, 5.991230190323086013, 48.63664920735773478 ) ) ;
#152487=CARTESIAN_POINT ( 'NONE',  ( 15.80617190586746368, 15.72974639402197994, 29.37390960531435269 ) ) ;
#152490=CARTESIAN_POINT ( 'NONE',  ( -16.53943276465976808, -0.05219959533934237506, 38.75109039468567573 ) ) ;
#152491=CARTESIAN_POINT ( 'NONE',  ( 8.224510206698953496, -14.34966873604960469, 47.91557627198102409 ) ) ;
#152492=CARTESIAN_POINT ( 'NONE',  ( -18.67979575497178146, -10.72451020669898902, 71.66557627198100988 ) ) ;
#152493=CARTESIAN_POINT ( 'NONE',  ( -21.53943276465977519, 0.05219959533907696930, 56.24890960531436690 ) ) ;
#152495=CARTESIAN_POINT ( 'NONE',  ( 19.05341960407617918, -5.049401038297876454, 86.04275706135233293 ) ) ;
#152496=CARTESIAN_POINT ( 'NONE',  ( 5.153800228976335163, 19.02544592524342804, 104.7905762719809957 ) ) ;
#152497=CARTESIAN_POINT ( 'NONE',  ( 19.05341960407611168, 5.049401038298154454, 53.95724293864770260 ) ) ;
#152498=CARTESIAN_POINT ( 'NONE',  ( 0.05219959533909260263, 19.03943276465977164, 24.99890960531435269 ) ) ;
#152499=FACE_BOUND ( 'NONE', #58157, .T. ) ;
#152501=CARTESIAN_POINT ( 'NONE',  ( -16.52544592524335698, -4.483927247898792601, 73.95942372801901854 ) ) ;
#152502=CARTESIAN_POINT ( 'NONE',  ( 10.81492255796078972, 18.62759615963270932, 99.58224293864770971 ) ) ;
#152503=CARTESIAN_POINT ( 'NONE',  ( -19.02544592524342804, 5.153800228976336051, 56.04057627198100988 ) ) ;
#152504=CARTESIAN_POINT ( 'NONE',  ( -21.52544592524334988, -5.823673210054445271, 43.95942372801902565 ) ) ;
#152505=CARTESIAN_POINT ( 'NONE',  ( 16.51473224551069308, 9.474510206698969483, 84.16557627198102409 ) ) ;
#152506=CARTESIAN_POINT ( 'NONE',  ( 16.51473224551069308, 9.474510206698969483, 114.1655762719810241 ) ) ;
#152507=ORIENTED_EDGE ( 'NONE', *, *, #108640, .F. ) ;
#152508=CARTESIAN_POINT ( 'NONE',  ( -21.52544592524334988, -5.823673210054445271, 28.95942372801902209 ) ) ;
#152509=CARTESIAN_POINT ( 'NONE',  ( -0.05219959533909027116, -19.03943276465977164, 112.4989096053143669 ) ) ;
#152510=CARTESIAN_POINT ( 'NONE',  ( -16.51473224551082808, 9.474510206698731452, 88.33442372801900433 ) ) ;
#152512=CARTESIAN_POINT ( 'NONE',  ( -9.474510206698720793, -16.51473224551083518, 44.58442372801900433 ) ) ;
#152513=CARTESIAN_POINT ( 'NONE',  ( -5.719274019375978568, 21.55341960407610458, 100.2072429386476955 ) ) ;
#152514=CARTESIAN_POINT ( 'NONE',  ( 5.049401038297881783, 19.05341960407617563, 32.29275706135233293 ) ) ;
#152515=CARTESIAN_POINT ( 'NONE',  ( -19.05341960407617563, 5.049401038297882671, 33.54275706135231871 ) ) ;
#152516=CARTESIAN_POINT ( 'NONE',  ( -8.224510206698735004, -14.34966873604973081, 94.58442372801901854 ) ) ;
#152518=CARTESIAN_POINT ( 'NONE',  ( -16.46253265017160317, 9.564922557960807481, 60.83224293864769550 ) ) ;
#152519=CARTESIAN_POINT ( 'NONE',  ( 5.719274019375673035, 21.55341960407619339, 67.29275706135234714 ) ) ;
#152520=CARTESIAN_POINT ( 'NONE',  ( -5.823673210054431948, 21.52544592524334988, 82.70942372801900433 ) ) ;
#152522=CARTESIAN_POINT ( 'NONE',  ( 5.049401038298161559, -19.05341960407611168, 82.70724293864770971 ) ) ;
#152523=CARTESIAN_POINT ( 'NONE',  ( -21.55341960407619339, 5.719274019375674811, 68.54275706135234714 ) ) ;
#152524=CARTESIAN_POINT ( 'NONE',  ( -19.03943276465977164, -0.05219959533935918106, 103.7510903946856757 ) ) ;
#152526=CARTESIAN_POINT ( 'NONE',  ( -19.03943276465977164, 0.05219959533909376836, 61.24890960531436690 ) ) ;
#152527=CARTESIAN_POINT ( 'NONE',  ( -16.51473224551069308, -9.474510206698971260, 96.66557627198102409 ) ) ;
#152528=CARTESIAN_POINT ( 'NONE',  ( 19.03943276465977164, -0.05219959533909143690, 73.74890960531435269 ) ) ;
#152529=CARTESIAN_POINT ( 'NONE',  ( -0.05219959533909027116, -19.03943276465977164, 77.49890960531435269 ) ) ;
#152530=CARTESIAN_POINT ( 'NONE',  ( -13.89961937509977652, 13.97604488694528158, 60.62390960531436690 ) ) ;
#152531=CARTESIAN_POINT ( 'NONE',  ( -18.62759615963270932, 10.81492255796079327, 100.8322429386477097 ) ) ;
#152532=CARTESIAN_POINT ( 'NONE',  ( -16.53943276465976808, -0.05219959533934237506, 93.75109039468567573 ) ) ;
#152534=CARTESIAN_POINT ( 'NONE',  ( -19.02544592524334988, -5.153800228976617603, 38.95942372801900433 ) ) ;
#152535=CARTESIAN_POINT ( 'NONE',  ( 13.89961937509977652, -13.97604488694527269, 78.12390960531433848 ) ) ;
#152536=CARTESIAN_POINT ( 'NONE',  ( 14.34966873604960469, 8.224510206698951720, 74.16557627198102409 ) ) ;
#152537=CARTESIAN_POINT ( 'NONE',  ( -0.05219959533910754901, -16.53943276465976808, 107.4989096053143669 ) ) ;
#152538=CARTESIAN_POINT ( 'NONE',  ( 13.89961937509977652, -13.97604488694527269, 108.1239096053143669 ) ) ;
#152539=CARTESIAN_POINT ( 'NONE',  ( 16.51473224551069308, 9.474510206698969483, 109.1655762719810383 ) ) ;
#152541=CARTESIAN_POINT ( 'NONE',  ( -9.564922557961040184, 16.46253265017147172, 32.91775706135233293 ) ) ;
#152542=CARTESIAN_POINT ( 'NONE',  ( -4.483927247898782831, 16.52544592524335698, 92.70942372801901854 ) ) ;
#152543=CARTESIAN_POINT ( 'NONE',  ( -16.46253265017160317, 9.564922557960807481, 70.83224293864770971 ) ) ;
#152544=CARTESIAN_POINT ( 'NONE',  ( -0.05219959533937732626, 21.53943276465977519, 57.50109039468568994 ) ) ;
#152545=CARTESIAN_POINT ( 'NONE',  ( 10.72451020669898902, -18.67979575497178502, 27.91557627198103830 ) ) ;
#152546=CARTESIAN_POINT ( 'NONE',  ( -15.72974639402176322, -15.80617190586768395, 24.37609039468567573 ) ) ;
#152547=CARTESIAN_POINT ( 'NONE',  ( -21.55341960407610458, -5.719274019375992779, 66.45724293864768129 ) ) ;
#152548=CARTESIAN_POINT ( 'NONE',  ( -16.55341960407611168, -4.379528057220339221, 96.45724293864770971 ) ) ;
#152549=CARTESIAN_POINT ( 'NONE',  ( -5.049401038297874678, -19.05341960407617918, 59.79275706135231871 ) ) ;
#152550=CARTESIAN_POINT ( 'NONE',  ( 19.02544592524343514, -5.153800228976328945, 28.54057627198102409 ) ) ;
#152551=CARTESIAN_POINT ( 'NONE',  ( 19.03943276465977164, -0.05219959533909143690, 78.74890960531436690 ) ) ;
#152552=CARTESIAN_POINT ( 'NONE',  ( -16.46253265017160317, 9.564922557960807481, 80.83224293864769550 ) ) ;
#152554=CARTESIAN_POINT ( 'NONE',  ( -4.483927247898539470, -16.52544592524342804, 107.2905762719810525 ) ) ;
#152555=CARTESIAN_POINT ( 'NONE',  ( 14.29746914071049879, -8.314922557960816363, 28.33224293864769550 ) ) ;
#152556=CARTESIAN_POINT ( 'NONE',  ( -14.29746914071037622, -8.314922557961029526, 29.16775706135234003 ) ) ;
#152557=CARTESIAN_POINT ( 'NONE',  ( -10.72451020669870658, -18.67979575497194134, 89.58442372801901854 ) ) ;
#152558=CARTESIAN_POINT ( 'NONE',  ( 9.474510206698971260, -16.51473224551069308, 107.9155762719810383 ) ) ;
#152559=CARTESIAN_POINT ( 'NONE',  ( 5.823673210054444382, -21.52544592524334988, 20.20942372801900788 ) ) ;
#152560=CARTESIAN_POINT ( 'NONE',  ( 13.89961937509977652, -13.97604488694527269, 38.12390960531436690 ) ) ;
#152561=CARTESIAN_POINT ( 'NONE',  ( -16.55341960407617563, 4.379528057220093196, 43.54275706135235424 ) ) ;
#152562=CARTESIAN_POINT ( 'NONE',  ( 13.89961937509957401, 13.97604488694547697, 106.8760903946856757 ) ) ;
#152563=CARTESIAN_POINT ( 'NONE',  ( 19.03943276465977164, -0.05219959533909143690, 33.74890960531435979 ) ) ;
#152564=B_SPLINE_CURVE_WITH_KNOTS ( 'NONE', 3,
 ( #93648, #123974, #185671, #168508, #15826, #187682, #110810, #47162, #49152, #2640, #16821, #153333, #125984, #108821, #48160, #77487, #634, #171501, #1638, #92646, #30006, #198861 ),
 .UNSPECIFIED., .F., .F.,
 ( 4, 2, 2, 2, 2, 2, 2, 2, 2, 2, 4 ),
 ( 2.602085213965210642E-18, 0.001309639967555231059, 0.001964459951332838024, 0.002291869943221640747, 0.002455574939166055553, 0.002619279935110470359, 0.002782984931054886032, 0.002946689926999300404, 0.003274099918888157337, 0.003928919902665849520, 0.005238559870221237355 ),
 .UNSPECIFIED. ) ;
#152565=CARTESIAN_POINT ( 'NONE',  ( -14.29746914071049879, 8.314922557960819915, 90.83224293864769550 ) ) ;
#152566=CARTESIAN_POINT ( 'NONE',  ( 15.72974639402199770, -15.80617190586745480, 108.1239096053143811 ) ) ;
#152567=CARTESIAN_POINT ( 'NONE',  ( -9.474510206698720793, -16.51473224551083518, 69.58442372801901854 ) ) ;
#152568=CARTESIAN_POINT ( 'NONE',  ( 19.03943276465977164, -0.05219959533909143690, 23.74890960531435269 ) ) ;
#152569=CARTESIAN_POINT ( 'NONE',  ( -5.823673210054116645, -21.52544592524344225, 112.2905762719810241 ) ) ;
#152571=CARTESIAN_POINT ( 'NONE',  ( 9.474510206698971260, -16.51473224551069308, 87.91557627198102409 ) ) ;
#152572=CARTESIAN_POINT ( 'NONE',  ( 17.44279575226825330, -5.990770900252416986, 113.3355756751431755 ) ) ;
#152573=CARTESIAN_POINT ( 'NONE',  ( -19.03943276465977164, 0.05219959533909376836, 81.24890960531436690 ) ) ;
#152574=CARTESIAN_POINT ( 'NONE',  ( -18.62759615963255300, -10.81492255796106328, 29.16775706135234003 ) ) ;
#152575=CARTESIAN_POINT ( 'NONE',  ( -0.05219959533910754901, -16.53943276465976808, 82.49890960531436690 ) ) ;
#152576=CARTESIAN_POINT ( 'NONE',  ( -13.97604488694527625, -13.89961937509977652, 76.87390960531433848 ) ) ;
#152577=CARTESIAN_POINT ( 'NONE',  ( -14.34966873604972548, 8.224510206698743886, 48.33442372801902565 ) ) ;
#152578=CARTESIAN_POINT ( 'NONE',  ( -16.46253265017146816, -9.564922557961047289, 49.16775706135233293 ) ) ;
#152579=CARTESIAN_POINT ( 'NONE',  ( 0.05219959533937995610, -21.53943276465977519, 60.00109039468568284 ) ) ;
#152580=CARTESIAN_POINT ( 'NONE',  ( -8.314922557961024197, 14.29746914071037800, 32.91775706135234714 ) ) ;
#152581=CARTESIAN_POINT ( 'NONE',  ( 13.97604488694527802, 13.89961937509977652, 69.37390960531436690 ) ) ;
#152582=CARTESIAN_POINT ( 'NONE',  ( -5.049401038297874678, -19.05341960407617918, 99.79275706135234714 ) ) ;
#152583=CARTESIAN_POINT ( 'NONE',  ( -4.483927247898782831, 16.52544592524335698, 62.70942372801902565 ) ) ;
#152584=CARTESIAN_POINT ( 'NONE',  ( 15.80617190586769283, -15.72974639402175789, 100.6260903946857184 ) ) ;
#152585=CARTESIAN_POINT ( 'NONE',  ( -9.474510206698720793, -16.51473224551083518, 84.58442372801900433 ) ) ;
#152586=CARTESIAN_POINT ( 'NONE',  ( -13.97604488694527625, -13.89961937509977652, 51.87390960531436690 ) ) ;
#152587=CARTESIAN_POINT ( 'NONE',  ( 10.81492255796078972, 18.62759615963270932, 64.58224293864769550 ) ) ;
#152588=CARTESIAN_POINT ( 'NONE',  ( -16.52544592524342804, 4.483927247898546575, 76.04057627198102409 ) ) ;
#152589=CARTESIAN_POINT ( 'NONE',  ( 13.97604488694548053, -13.89961937509957401, 80.62609039468567573 ) ) ;
#152590=CARTESIAN_POINT ( 'NONE',  ( 17.12812012977027720, -6.668231424565975729, 61.14051240676858612 ) ) ;
#152591=CARTESIAN_POINT ( 'NONE',  ( -19.03943276465977164, -0.05219959533935918106, 43.75109039468566863 ) ) ;
#152592=CARTESIAN_POINT ( 'NONE',  ( 4.379528057220092307, 16.55341960407617563, 112.2927570613523471 ) ) ;
#152593=CARTESIAN_POINT ( 'NONE',  ( -4.483927247898539470, -16.52544592524342804, 62.29057627198102409 ) ) ;
#152594=CARTESIAN_POINT ( 'NONE',  ( 5.719274019375673035, 21.55341960407619339, 107.2927570613523471 ) ) ;
#152596=CARTESIAN_POINT ( 'NONE',  ( 15.72974639402199770, -15.80617190586745480, 113.1239096053143953 ) ) ;
#152597=CARTESIAN_POINT ( 'NONE',  ( 16.46253265017160672, -9.564922557960803928, 68.33224293864770971 ) ) ;
#152598=CARTESIAN_POINT ( 'NONE',  ( -18.62759615963255300, -10.81492255796106328, 89.16775706135236135 ) ) ;
#152599=CARTESIAN_POINT ( 'NONE',  ( -5.049401038298153566, 19.05341960407611168, 65.20724293864765286 ) ) ;
#152601=CARTESIAN_POINT ( 'NONE',  ( 14.29746914071049879, -8.314922557960816363, 113.3322429386476955 ) ) ;
#152602=CARTESIAN_POINT ( 'NONE',  ( 18.67979575497178502, 10.72451020669898547, 29.16557627198103120 ) ) ;
#152603=CARTESIAN_POINT ( 'NONE',  ( -16.55341960407611168, -4.379528057220339221, 61.45724293864770260 ) ) ;
#152604=CARTESIAN_POINT ( 'NONE',  ( 13.97604488694527802, 13.89961937509977652, 44.37390960531435269 ) ) ;
#152605=CARTESIAN_POINT ( 'NONE',  ( 4.483927247898545687, 16.52544592524342804, 94.79057627198105251 ) ) ;
#152606=CARTESIAN_POINT ( 'NONE',  ( -21.55341960407610458, -5.719274019375992779, 106.4572429386477097 ) ) ;
#152607=CARTESIAN_POINT ( 'NONE',  ( 15.80617190586769283, -15.72974639402175789, 45.62609039468567573 ) ) ;
#152608=CARTESIAN_POINT ( 'NONE',  ( 9.564922557960805705, 16.46253265017160317, 24.58224293864769194 ) ) ;
#152609=CARTESIAN_POINT ( 'NONE',  ( 16.55341960407618274, -4.379528057220086978, 46.04275706135234714 ) ) ;
#152610=CARTESIAN_POINT ( 'NONE',  ( 5.823673210054125526, 21.52544592524343514, 104.7905762719810241 ) ) ;
#152611=CARTESIAN_POINT ( 'NONE',  ( 10.81492255796078972, 18.62759615963270932, 99.58224293864770971 ) ) ;
#152612=CARTESIAN_POINT ( 'NONE',  ( -0.05219959533936034679, 19.03943276465977164, 27.50109039468566507 ) ) ;
#152613=CARTESIAN_POINT ( 'NONE',  ( -13.89961937509977652, 13.97604488694528158, 50.62390960531435979 ) ) ;
#152614=CARTESIAN_POINT ( 'NONE',  ( -13.97604488694527625, -13.89961937509977652, 111.8739096053143243 ) ) ;
#152615=CARTESIAN_POINT ( 'NONE',  ( 21.52544592524334988, 5.823673210054432836, 56.45942372801902565 ) ) ;
#152616=CARTESIAN_POINT ( 'NONE',  ( -15.80617190586745835, -15.72974639402198527, 41.87390960531435979 ) ) ;
#152617=CARTESIAN_POINT ( 'NONE',  ( 12.06949235617739724, 12.14591786802326823, 111.8760903946856615 ) ) ;
#152618=CARTESIAN_POINT ( 'NONE',  ( 5.719274019375673035, 21.55341960407619339, 67.29275706135234714 ) ) ;
#152619=CARTESIAN_POINT ( 'NONE',  ( -21.53943276465977519, -0.05219959533937600094, 93.75109039468567573 ) ) ;
#152620=CARTESIAN_POINT ( 'NONE',  ( 9.474510206698729675, 16.51473224551082808, 42.08442372801900433 ) ) ;
#152621=CARTESIAN_POINT ( 'NONE',  ( 8.314922557961029526, -14.29746914071037800, 100.4177570613523471 ) ) ;
#152622=CARTESIAN_POINT ( 'NONE',  ( -21.55341960407619339, 5.719274019375674811, 48.54275706135234714 ) ) ;
#152624=CARTESIAN_POINT ( 'NONE',  ( 19.02544592524343514, -5.153800228976328945, 63.54057627198103830 ) ) ;
#152625=CARTESIAN_POINT ( 'NONE',  ( 10.81492255796106328, -18.62759615963255655, 110.4177570613523756 ) ) ;
#152626=CARTESIAN_POINT ( 'NONE',  ( -16.46253265017160317, 9.564922557960807481, 115.8322429386477097 ) ) ;
#152627=CARTESIAN_POINT ( 'NONE',  ( -21.55341960407610458, -5.719274019375992779, 111.4572429386476813 ) ) ;
#152628=CARTESIAN_POINT ( 'NONE',  ( -15.72974639402197994, 15.80617190586746368, 75.62390960531439532 ) ) ;
#152629=CARTESIAN_POINT ( 'NONE',  ( 4.483927247898790824, -16.52544592524335698, 45.20942372801901854 ) ) ;
#152631=CARTESIAN_POINT ( 'NONE',  ( 0.05219959533907565091, 21.53943276465977519, 74.99890960531435269 ) ) ;
#152632=CARTESIAN_POINT ( 'NONE',  ( 16.55341960407618274, -4.379528057220086978, 61.04275706135234714 ) ) ;
#152633=CARTESIAN_POINT ( 'NONE',  ( 16.52544592524342804, -4.483927247898539470, 78.54057627198103830 ) ) ;
#152635=CARTESIAN_POINT ( 'NONE',  ( 9.564922557961047289, -16.46253265017146816, 105.4177570613523471 ) ) ;
#152636=CARTESIAN_POINT ( 'NONE',  ( -21.55341960407610458, -5.719274019375992779, 31.45724293864769550 ) ) ;
#152637=EDGE_CURVE ( 'NONE', #36339, #35831, #67394, .T. ) ;
#152638=CARTESIAN_POINT ( 'NONE',  ( 16.55341960407618274, -4.379528057220086978, 36.04275706135234714 ) ) ;
#152639=CARTESIAN_POINT ( 'NONE',  ( -10.81492255796078084, -18.62759615963271287, 112.0822429386477097 ) ) ;
#152640=CARTESIAN_POINT ( 'NONE',  ( -5.823673210054116645, -21.52544592524344225, 27.29057627198103120 ) ) ;
#152641=CARTESIAN_POINT ( 'NONE',  ( -16.53943276465976808, -0.05219959533934237506, 68.75109039468568994 ) ) ;
#152642=CARTESIAN_POINT ( 'NONE',  ( 19.03943276465977164, -0.05219959533909143690, 88.74890960531436690 ) ) ;
#152643=CARTESIAN_POINT ( 'NONE',  ( -10.72451020669870658, -18.67979575497194134, 59.58442372801901854 ) ) ;
#152644=CARTESIAN_POINT ( 'NONE',  ( 13.89961937509977652, -13.97604488694527269, 23.12390960531436335 ) ) ;
#152645=CARTESIAN_POINT ( 'NONE',  ( -19.03943276465977164, 0.05219959533909376836, 116.2489096053143669 ) ) ;
#152646=ORIENTED_EDGE ( 'NONE', *, *, #131087, .F. ) ;
#152647=CARTESIAN_POINT ( 'NONE',  ( -16.46253265017146816, -9.564922557961047289, 34.16775706135233293 ) ) ;
#152648=CARTESIAN_POINT ( 'NONE',  ( -12.06949235617739369, -12.14591786802326823, 54.37609039468568994 ) ) ;
#152649=CARTESIAN_POINT ( 'NONE',  ( -9.564922557960796823, -16.46253265017161027, 102.0822429386477097 ) ) ;
#152650=CARTESIAN_POINT ( 'NONE',  ( 5.719274019375991003, -21.55341960407610458, 97.70724293864772392 ) ) ;
#152651=CARTESIAN_POINT ( 'NONE',  ( 5.153800228976335163, 19.02544592524342804, 69.79057627198103830 ) ) ;
#152652=CARTESIAN_POINT ( 'NONE',  ( -16.29526858892879204, 7.335722546919972942, 24.20329402199794444 ) ) ;
#152654=CARTESIAN_POINT ( 'NONE',  ( 0.05219959533910956823, 16.53943276465976808, 79.99890960531435269 ) ) ;
#152655=CARTESIAN_POINT ( 'NONE',  ( -18.67979575497178146, -10.72451020669898902, 41.66557627198103120 ) ) ;
#152656=CARTESIAN_POINT ( 'NONE',  ( -16.88567814943165502, 6.947325034625571938, 33.70998877347415146 ) ) ;
#152657=CARTESIAN_POINT ( 'NONE',  ( 16.52544592524335698, 4.483927247898782831, 61.45942372801901854 ) ) ;
#152658=CARTESIAN_POINT ( 'NONE',  ( -10.72451020669870658, -18.67979575497194134, 24.58442372801901499 ) ) ;
#152659=CARTESIAN_POINT ( 'NONE',  ( -5.049401038297874678, -19.05341960407617918, 74.79275706135231871 ) ) ;
#152660=CARTESIAN_POINT ( 'NONE',  ( -5.153800228976328057, -19.02544592524343514, 37.29057627198102409 ) ) ;
#152661=CARTESIAN_POINT ( 'NONE',  ( 15.80617190586746368, 15.72974639402197994, 64.37390960531435269 ) ) ;
#152663=CARTESIAN_POINT ( 'NONE',  ( -21.52544592524334988, -5.823673210054445271, 93.95942372801903275 ) ) ;
#152664=CARTESIAN_POINT ( 'NONE',  ( -13.89961937509977652, 13.97604488694528158, 60.62390960531436690 ) ) ;
#152665=CARTESIAN_POINT ( 'NONE',  ( -8.314922557961024197, 14.29746914071037800, 47.91775706135234714 ) ) ;
#152666=CARTESIAN_POINT ( 'NONE',  ( -9.564922557960796823, -16.46253265017161027, 57.08224293864769550 ) ) ;
#152667=CARTESIAN_POINT ( 'NONE',  ( 15.80617190586769283, -15.72974639402175789, 80.62609039468567573 ) ) ;
#152668=CARTESIAN_POINT ( 'NONE',  ( -5.049401038297874678, -19.05341960407617918, 39.79275706135232582 ) ) ;
#152670=CARTESIAN_POINT ( 'NONE',  ( -5.153800228976607833, 19.02544592524334988, 47.70942372801900433 ) ) ;
#152671=CARTESIAN_POINT ( 'NONE',  ( -0.05219959533937732626, 21.53943276465977519, 52.50109039468567573 ) ) ;
#152672=DIRECTION ( 'NONE',  ( -0.000000000000000000, -0.000000000000000000, 1.000000000000000000 ) ) ;
#152673=CARTESIAN_POINT ( 'NONE',  ( 19.02544592524334988, 5.153800228976608722, 41.45942372801900433 ) ) ;
#152674=CARTESIAN_POINT ( 'NONE',  ( -16.46253265017160317, 9.564922557960807481, 100.8322429386477097 ) ) ;
#152675=CARTESIAN_POINT ( 'NONE',  ( 13.97604488694527802, 13.89961937509977652, 74.37390960531436690 ) ) ;
#152676=CARTESIAN_POINT ( 'NONE',  ( 16.53943276465976808, -0.05219959533910856209, 28.74890960531435624 ) ) ;
#152677=CARTESIAN_POINT ( 'NONE',  ( 18.67979575497178502, 10.72451020669898547, 29.16557627198103120 ) ) ;
#152678=CARTESIAN_POINT ( 'NONE',  ( 5.719274019375673035, 21.55341960407619339, 102.2927570613523613 ) ) ;
#152681=CARTESIAN_POINT ( 'NONE',  ( -5.823673210054431948, 21.52544592524334988, 102.7094237280190185 ) ) ;
#152683=CARTESIAN_POINT ( 'NONE',  ( 4.483927247898545687, 16.52544592524342804, 114.7905762719810383 ) ) ;
#152684=CARTESIAN_POINT ( 'NONE',  ( -16.51473224551069308, -9.474510206698971260, 111.6655762719810383 ) ) ;
#152685=CARTESIAN_POINT ( 'NONE',  ( -22.00000000000000000, -1.132798289211302014E-14, 92.50000000000000000 ) ) ;
#152686=CARTESIAN_POINT ( 'NONE',  ( -0.05219959533934338120, 16.53943276465976808, 52.50109039468567573 ) ) ;
#152687=CARTESIAN_POINT ( 'NONE',  ( 10.81492255796078972, 18.62759615963270932, 74.58224293864768129 ) ) ;
#152688=CARTESIAN_POINT ( 'NONE',  ( -8.224510206698948167, 14.34966873604960824, 45.41557627198103830 ) ) ;
#152689=CARTESIAN_POINT ( 'NONE',  ( -14.34966873604960291, -8.224510206698953496, 106.6655762719810383 ) ) ;
#152690=CARTESIAN_POINT ( 'NONE',  ( -16.51473224551069308, -9.474510206698971260, 111.6655762719810383 ) ) ;
#152691=CARTESIAN_POINT ( 'NONE',  ( 5.823673210054444382, -21.52544592524334988, 30.20942372801902565 ) ) ;
#152692=CARTESIAN_POINT ( 'NONE',  ( -9.564922557961040184, 16.46253265017147172, 37.91775706135233293 ) ) ;
#152693=CARTESIAN_POINT ( 'NONE',  ( -16.51473224551069308, -9.474510206698971260, 21.66557627198102765 ) ) ;
#152694=CARTESIAN_POINT ( 'NONE',  ( -18.67979575497193778, 10.72451020669871902, 68.33442372801900433 ) ) ;
#152695=CARTESIAN_POINT ( 'NONE',  ( 16.38665767535053774, -7.295008042176018392, 32.76400864214546260 ) ) ;
#152696=CARTESIAN_POINT ( 'NONE',  ( -8.314922557960811034, -14.29746914071050412, 32.08224293864769550 ) ) ;
#152698=CARTESIAN_POINT ( 'NONE',  ( 18.62759615963271287, -10.81492255796078972, 33.33224293864769550 ) ) ;
#152699=CARTESIAN_POINT ( 'NONE',  ( 12.14591786802309770, 12.06949235617756955, 84.37390960531438111 ) ) ;
#152701=CARTESIAN_POINT ( 'NONE',  ( -13.89961937509977652, 13.97604488694528158, 80.62390960531436690 ) ) ;
#152702=CARTESIAN_POINT ( 'NONE',  ( 8.314922557960818139, 14.29746914071049879, 69.58224293864769550 ) ) ;
#152703=CARTESIAN_POINT ( 'NONE',  ( 9.474510206698729675, 16.51473224551082808, 107.0844237280190043 ) ) ;
#152704=CARTESIAN_POINT ( 'NONE',  ( -15.72974639402197994, 15.80617190586746368, 45.62390960531436690 ) ) ;
#152705=ORIENTED_EDGE ( 'NONE', *, *, #169362, .F. ) ;
#152706=CARTESIAN_POINT ( 'NONE',  ( -12.06949235617756955, 12.14591786802309770, 110.6239096053143669 ) ) ;
#152707=CARTESIAN_POINT ( 'NONE',  ( 13.89961937509977652, -13.97604488694527269, 68.12390960531436690 ) ) ;
#152708=CARTESIAN_POINT ( 'NONE',  ( -5.823673210054116645, -21.52544592524344225, 77.29057627198102409 ) ) ;
#152709=CARTESIAN_POINT ( 'NONE',  ( 12.14591786802327356, -12.06949235617739191, 100.6260903946857184 ) ) ;
#152710=CARTESIAN_POINT ( 'NONE',  ( 13.97604488694527802, 13.89961937509977652, 84.37390960531433848 ) ) ;
#152711=CARTESIAN_POINT ( 'NONE',  ( 5.049401038297881783, 19.05341960407617563, 67.29275706135234714 ) ) ;
#152712=CARTESIAN_POINT ( 'NONE',  ( 21.53943276465977519, 0.05219959533937863772, 91.25109039468568994 ) ) ;
#152713=CARTESIAN_POINT ( 'NONE',  ( -10.72451020669898014, 18.67979575497178502, 65.41557627198102409 ) ) ;
#152714=CARTESIAN_POINT ( 'NONE',  ( -21.53943276465977519, 0.05219959533907696930, 26.24890960531435624 ) ) ;
#152715=CARTESIAN_POINT ( 'NONE',  ( -13.89961937509977652, 13.97604488694528158, 30.62390960531435269 ) ) ;
#152716=CARTESIAN_POINT ( 'NONE',  ( -16.55341960407617563, 4.379528057220093196, 103.5427570613523613 ) ) ;
#152717=CARTESIAN_POINT ( 'NONE',  ( -16.46253265017160317, 9.564922557960807481, 60.83224293864769550 ) ) ;
#152718=CARTESIAN_POINT ( 'NONE',  ( 16.55341960407618274, -4.379528057220086978, 26.04275706135235779 ) ) ;
#152720=CARTESIAN_POINT ( 'NONE',  ( -5.719274019375665041, -21.55341960407619695, 109.7927570613523613 ) ) ;
#152721=CARTESIAN_POINT ( 'NONE',  ( 16.55341960407611168, 4.379528057220329451, 78.95724293864769550 ) ) ;
#152723=CARTESIAN_POINT ( 'NONE',  ( -15.80617190586745835, -15.72974639402198527, 111.8739096053143669 ) ) ;
#152724=CARTESIAN_POINT ( 'NONE',  ( 18.62759615963271287, -10.81492255796078972, 103.3322429386476955 ) ) ;
#152726=CARTESIAN_POINT ( 'NONE',  ( 10.81492255796078972, 18.62759615963270932, 44.58224293864769550 ) ) ;
#152727=CARTESIAN_POINT ( 'NONE',  ( -16.53943276465976808, -0.05219959533934237506, 83.75109039468568994 ) ) ;
#152728=CARTESIAN_POINT ( 'NONE',  ( -14.29746914071049879, 8.314922557960819915, 100.8322429386477097 ) ) ;
#152729=CARTESIAN_POINT ( 'NONE',  ( 0.05219959533909260263, 19.03943276465977164, 59.99890960531436690 ) ) ;
#152731=CARTESIAN_POINT ( 'NONE',  ( 14.34966873604972726, -8.224510206698740333, 105.8344237280190328 ) ) ;
#152732=CARTESIAN_POINT ( 'NONE',  ( -15.80617190586768217, 15.72974639402176855, 43.12609039468568284 ) ) ;
#152733=CARTESIAN_POINT ( 'NONE',  ( -9.564922557960796823, -16.46253265017161027, 102.0822429386477097 ) ) ;
#152734=CARTESIAN_POINT ( 'NONE',  ( -15.80617190586768217, 15.72974639402176855, 78.12609039468570415 ) ) ;
#152735=CARTESIAN_POINT ( 'NONE',  ( -19.02544592524342804, 5.153800228976336051, 31.04057627198102409 ) ) ;
#152736=CARTESIAN_POINT ( 'NONE',  ( -16.46253265017160317, 9.564922557960807481, 35.83224293864768839 ) ) ;
#152738=CARTESIAN_POINT ( 'NONE',  ( 21.55341960407619695, -5.719274019375665929, 71.04275706135234714 ) ) ;
#152739=CARTESIAN_POINT ( 'NONE',  ( 13.89961937509977652, -13.97604488694527269, 103.1239096053143527 ) ) ;
#152740=CARTESIAN_POINT ( 'NONE',  ( -13.89961937509957401, -13.97604488694547875, 84.37609039468567573 ) ) ;
#152741=CARTESIAN_POINT ( 'NONE',  ( 5.719274019375673035, 21.55341960407619339, 37.29275706135235424 ) ) ;
#152742=CARTESIAN_POINT ( 'NONE',  ( 4.379528057220092307, 16.55341960407617563, 22.29275706135235069 ) ) ;
#152743=CARTESIAN_POINT ( 'NONE',  ( 0.05219959533936267826, -19.03943276465977164, 75.00109039468566152 ) ) ;
#152744=CARTESIAN_POINT ( 'NONE',  ( 5.153800228976335163, 19.02544592524342804, 54.79057627198103120 ) ) ;
#152745=CARTESIAN_POINT ( 'NONE',  ( -16.51473224551082808, 9.474510206698731452, 78.33442372801900433 ) ) ;
#152746=CARTESIAN_POINT ( 'NONE',  ( -12.06949235617756955, 12.14591786802309770, 30.62390960531436335 ) ) ;
#152747=CARTESIAN_POINT ( 'NONE',  ( -5.153800228976607833, 19.02544592524334988, 72.70942372801900433 ) ) ;
#152748=CARTESIAN_POINT ( 'NONE',  ( 16.53943276465976808, -0.05219959533910856209, 43.74890960531435979 ) ) ;
#152749=CARTESIAN_POINT ( 'NONE',  ( 5.049401038297881783, 19.05341960407617563, 67.29275706135234714 ) ) ;
#152750=CARTESIAN_POINT ( 'NONE',  ( -12.14591786802326823, 12.06949235617739902, 43.12609039468568284 ) ) ;
#152751=CARTESIAN_POINT ( 'NONE',  ( -5.823673210054431948, 21.52544592524334988, 112.7094237280190328 ) ) ;
#152752=CARTESIAN_POINT ( 'NONE',  ( 16.51473224551069308, 9.474510206698969483, 34.16557627198102409 ) ) ;
#152753=CARTESIAN_POINT ( 'NONE',  ( -16.20579543436680936, -7.371946100354975329, 65.56520834171874412 ) ) ;
#152754=CARTESIAN_POINT ( 'NONE',  ( 4.483927247898790824, -16.52544592524335698, 50.20942372801901854 ) ) ;
#152758=CARTESIAN_POINT ( 'NONE',  ( 19.02544592524343514, -5.153800228976328945, 88.54057627198102409 ) ) ;
#152761=CARTESIAN_POINT ( 'NONE',  ( -5.049401038297874678, -19.05341960407617918, 79.79275706135233293 ) ) ;
#152762=CARTESIAN_POINT ( 'NONE',  ( 0.05219959533907565091, 21.53943276465977519, 24.99890960531435624 ) ) ;
#152763=CARTESIAN_POINT ( 'NONE',  ( 10.72451020669871369, 18.67979575497193778, 112.0844237280190185 ) ) ;
#152764=CARTESIAN_POINT ( 'NONE',  ( 19.05341960407617918, -5.049401038297876454, 96.04275706135231871 ) ) ;
#152765=CARTESIAN_POINT ( 'NONE',  ( 0.05219959533910956823, 16.53943276465976808, 114.9989096053143669 ) ) ;
#152766=CARTESIAN_POINT ( 'NONE',  ( 19.03943276465977164, -0.05219959533909143690, 43.74890960531435979 ) ) ;
#152767=CARTESIAN_POINT ( 'NONE',  ( 5.823673210054125526, 21.52544592524343514, 54.79057627198104541 ) ) ;
#152768=CARTESIAN_POINT ( 'NONE',  ( 5.823673210054125526, 21.52544592524343514, 49.79057627198102409 ) ) ;
#152769=CARTESIAN_POINT ( 'NONE',  ( -19.02544592524342804, 5.153800228976336051, 26.04057627198103120 ) ) ;
#152771=CARTESIAN_POINT ( 'NONE',  ( 13.97604488694548053, -13.89961937509957401, 70.62609039468567573 ) ) ;
#152772=CARTESIAN_POINT ( 'NONE',  ( 16.55341960407611168, 4.379528057220329451, 38.95724293864768839 ) ) ;
#152773=CARTESIAN_POINT ( 'NONE',  ( -5.719274019375978568, 21.55341960407610458, 25.20724293864769550 ) ) ;
#152774=CARTESIAN_POINT ( 'NONE',  ( 21.53943276465977519, 0.05219959533937863772, 96.25109039468568994 ) ) ;
#152775=CARTESIAN_POINT ( 'NONE',  ( -5.719274019375978568, 21.55341960407610458, 80.20724293864769550 ) ) ;
#152776=CARTESIAN_POINT ( 'NONE',  ( -15.72974639402176322, -15.80617190586768395, 64.37609039468568994 ) ) ;
#152777=CARTESIAN_POINT ( 'NONE',  ( 5.719274019375673035, 21.55341960407619339, 62.29275706135236845 ) ) ;
#152779=CARTESIAN_POINT ( 'NONE',  ( -19.02544592524342804, 5.153800228976336051, 101.0405762719810241 ) ) ;
#152780=CARTESIAN_POINT ( 'NONE',  ( 12.14591786802327356, -12.06949235617739191, 95.62609039468568994 ) ) ;
#152781=CARTESIAN_POINT ( 'NONE',  ( 21.53943276465977519, 0.05219959533937863772, 46.25109039468567573 ) ) ;
#152782=CARTESIAN_POINT ( 'NONE',  ( 9.564922557960805705, 16.46253265017160317, 24.58224293864769194 ) ) ;
#152784=CARTESIAN_POINT ( 'NONE',  ( 12.14591786802309770, 12.06949235617756955, 64.37390960531435269 ) ) ;
#152785=CARTESIAN_POINT ( 'NONE',  ( 0.05219959533910956823, 16.53943276465976808, 39.99890960531436690 ) ) ;
#152786=CARTESIAN_POINT ( 'NONE',  ( -21.52544592524343514, 5.823673210054127303, 41.04057627198103120 ) ) ;
#152787=CARTESIAN_POINT ( 'NONE',  ( -9.564922557960796823, -16.46253265017161027, 72.08224293864770971 ) ) ;
#152788=CARTESIAN_POINT ( 'NONE',  ( 13.97604488694527802, 13.89961937509977652, 49.37390960531434558 ) ) ;
#152789=CARTESIAN_POINT ( 'NONE',  ( -10.72451020669898014, 18.67979575497178502, 55.41557627198102409 ) ) ;
#152790=CARTESIAN_POINT ( 'NONE',  ( -9.564922557961040184, 16.46253265017147172, 37.91775706135233293 ) ) ;
#152792=CARTESIAN_POINT ( 'NONE',  ( -0.05219959533910754901, -16.53943276465976808, 52.49890960531435979 ) ) ;
#152793=CARTESIAN_POINT ( 'NONE',  ( -21.53943276465977519, 0.05219959533907696930, 21.24890960531436690 ) ) ;
#152796=CARTESIAN_POINT ( 'NONE',  ( -0.05219959533934338120, 16.53943276465976808, 67.50109039468568994 ) ) ;
#152797=CARTESIAN_POINT ( 'NONE',  ( -16.46253265017146816, -9.564922557961047289, 79.16775706135234714 ) ) ;
#152798=CARTESIAN_POINT ( 'NONE',  ( -8.314922557960811034, -14.29746914071050412, 37.08224293864768129 ) ) ;
#152799=ORIENTED_EDGE ( 'NONE', *, *, #143157, .T. ) ;
#152801=CARTESIAN_POINT ( 'NONE',  ( -16.53943276465976808, 0.05219959533911058130, 21.24890960531436690 ) ) ;
#152802=CARTESIAN_POINT ( 'NONE',  ( -19.05341960407611168, -5.049401038298163336, 56.45724293864768129 ) ) ;
#152803=CARTESIAN_POINT ( 'NONE',  ( -5.049401038298153566, 19.05341960407611168, 80.20724293864769550 ) ) ;
#152804=CARTESIAN_POINT ( 'NONE',  ( 19.02544592524343514, -5.153800228976328945, 38.54057627198103120 ) ) ;
#152805=CARTESIAN_POINT ( 'NONE',  ( 10.72451020669871369, 18.67979575497193778, 52.08442372801901854 ) ) ;
#152806=CARTESIAN_POINT ( 'NONE',  ( -16.51473224551069308, -9.474510206698971260, 56.66557627198103120 ) ) ;
#152808=CARTESIAN_POINT ( 'NONE',  ( 19.03943276465977164, -0.05219959533909143690, 53.74890960531436690 ) ) ;
#152809=CARTESIAN_POINT ( 'NONE',  ( -18.67979575497178146, -10.72451020669898902, 41.66557627198103120 ) ) ;
#152810=CARTESIAN_POINT ( 'NONE',  ( 9.564922557960805705, 16.46253265017160317, 24.58224293864769194 ) ) ;
#152811=CARTESIAN_POINT ( 'NONE',  ( 10.81492255796078972, 18.62759615963270932, 29.58224293864769905 ) ) ;
#152813=CARTESIAN_POINT ( 'NONE',  ( 8.314922557961029526, -14.29746914071037800, 85.41775706135236135 ) ) ;
#152814=CARTESIAN_POINT ( 'NONE',  ( 0.05219959533937995610, -21.53943276465977519, 105.0010903946856757 ) ) ;
#152815=CARTESIAN_POINT ( 'NONE',  ( -14.34966873604972548, 8.224510206698743886, 63.33442372801900433 ) ) ;
#152816=CARTESIAN_POINT ( 'NONE',  ( 19.02544592524343514, -5.153800228976328945, 108.5405762719810383 ) ) ;
#152817=CARTESIAN_POINT ( 'NONE',  ( 4.379528057220092307, 16.55341960407617563, 57.29275706135234714 ) ) ;
#152818=CARTESIAN_POINT ( 'NONE',  ( -16.53943276465976808, -0.05219959533934237506, 33.75109039468568284 ) ) ;
#152819=CARTESIAN_POINT ( 'NONE',  ( 9.474510206698971260, -16.51473224551069308, 112.9155762719810383 ) ) ;
#152820=CARTESIAN_POINT ( 'NONE',  ( 12.14591786802327356, -12.06949235617739191, 25.62609039468567929 ) ) ;
#152821=CARTESIAN_POINT ( 'NONE',  ( -19.03943276465977164, 0.05219959533909376836, 31.24890960531435979 ) ) ;
#152822=CARTESIAN_POINT ( 'NONE',  ( 15.80617190586769283, -15.72974639402175789, 20.62609039468568639 ) ) ;
#152823=CARTESIAN_POINT ( 'NONE',  ( 14.29746914071037800, 8.314922557961029526, 21.66775706135235069 ) ) ;
#152824=CARTESIAN_POINT ( 'NONE',  ( -4.379528057220086978, -16.55341960407618274, 79.79275706135236135 ) ) ;
#152826=CARTESIAN_POINT ( 'NONE',  ( -10.81492255796105439, 18.62759615963255655, 92.91775706135236135 ) ) ;
#152827=CARTESIAN_POINT ( 'NONE',  ( 16.51473224551083163, -9.474510206698727899, 85.83442372801900433 ) ) ;
#152828=CARTESIAN_POINT ( 'NONE',  ( -4.483927247898539470, -16.52544592524342804, 62.29057627198102409 ) ) ;
#152829=CARTESIAN_POINT ( 'NONE',  ( -4.483927247898539470, -16.52544592524342804, 107.2905762719810525 ) ) ;
#152830=CARTESIAN_POINT ( 'NONE',  ( -9.564922557961040184, 16.46253265017147172, 52.91775706135233293 ) ) ;
#152832=CARTESIAN_POINT ( 'NONE',  ( 21.52544592524334988, 5.823673210054432836, 56.45942372801902565 ) ) ;
#152833=CARTESIAN_POINT ( 'NONE',  ( -5.049401038297874678, -19.05341960407617918, 109.7927570613523187 ) ) ;
#152834=CARTESIAN_POINT ( 'NONE',  ( -18.22780087662122028, 5.500000000000031086, 63.51540105326107266 ) ) ;
#152835=CARTESIAN_POINT ( 'NONE',  ( 13.89961937509977652, -13.97604488694527269, 103.1239096053143527 ) ) ;
#152836=CARTESIAN_POINT ( 'NONE',  ( 10.72451020669898902, -18.67979575497178502, 72.91557627198103830 ) ) ;
#152837=CARTESIAN_POINT ( 'NONE',  ( 16.46253265017146816, 9.564922557961045513, 96.66775706135233293 ) ) ;
#152838=CARTESIAN_POINT ( 'NONE',  ( -5.153800228976328057, -19.02544592524343514, 102.2905762719810383 ) ) ;
#152839=CARTESIAN_POINT ( 'NONE',  ( 18.22780087662125226, -5.499999999999864997, 51.01540105326108687 ) ) ;
#152840=CARTESIAN_POINT ( 'NONE',  ( 12.14591786802309770, 12.06949235617756955, 109.3739096053143811 ) ) ;
#152841=CARTESIAN_POINT ( 'NONE',  ( 10.72451020669871369, 18.67979575497193778, 97.08442372801904696 ) ) ;
#152842=CARTESIAN_POINT ( 'NONE',  ( 13.97604488694527802, 13.89961937509977652, 49.37390960531434558 ) ) ;
#152843=CARTESIAN_POINT ( 'NONE',  ( -21.52544592524334988, -5.823673210054445271, 53.95942372801900433 ) ) ;
#152844=CARTESIAN_POINT ( 'NONE',  ( -10.81492255796105439, 18.62759615963255655, 92.91775706135236135 ) ) ;
#152845=CARTESIAN_POINT ( 'NONE',  ( -16.52544592524335698, -4.483927247898792601, 98.95942372801903275 ) ) ;
#152846=CARTESIAN_POINT ( 'NONE',  ( -10.72451020669870658, -18.67979575497194134, 49.58442372801901143 ) ) ;
#152847=CARTESIAN_POINT ( 'NONE',  ( -21.53943276465977519, -0.05219959533937600094, 33.75109039468568284 ) ) ;
#152848=CARTESIAN_POINT ( 'NONE',  ( -9.564922557961040184, 16.46253265017147172, 62.91775706135233293 ) ) ;
#152849=CARTESIAN_POINT ( 'NONE',  ( 5.049401038298161559, -19.05341960407611168, 97.70724293864766707 ) ) ;
#152850=CARTESIAN_POINT ( 'NONE',  ( 12.14591786802309770, 12.06949235617756955, 109.3739096053143811 ) ) ;
#152851=CARTESIAN_POINT ( 'NONE',  ( 0.05219959533907565091, 21.53943276465977519, 84.99890960531436690 ) ) ;
#152852=CARTESIAN_POINT ( 'NONE',  ( 16.53943276465976808, -0.05219959533910856209, 58.74890960531436690 ) ) ;
#152853=CARTESIAN_POINT ( 'NONE',  ( -15.72974639402176322, -15.80617190586768395, 99.37609039468568994 ) ) ;
#152854=CARTESIAN_POINT ( 'NONE',  ( 16.55341960407611168, 4.379528057220329451, 78.95724293864769550 ) ) ;
#152855=CARTESIAN_POINT ( 'NONE',  ( -13.89961937509977652, 13.97604488694528158, 35.62390960531435269 ) ) ;
#152856=CARTESIAN_POINT ( 'NONE',  ( 16.51473224551083163, -9.474510206698727899, 80.83442372801899012 ) ) ;
#152857=CARTESIAN_POINT ( 'NONE',  ( -14.29746914071049879, 8.314922557960819915, 50.83224293864770971 ) ) ;
#152858=CARTESIAN_POINT ( 'NONE',  ( -21.53943276465977519, -0.05219959533937600094, 98.75109039468568994 ) ) ;
#152859=CARTESIAN_POINT ( 'NONE',  ( 19.03943276465977164, -0.05219959533909143690, 88.74890960531436690 ) ) ;
#152860=CARTESIAN_POINT ( 'NONE',  ( 16.51473224551083163, -9.474510206698727899, 60.83442372801900433 ) ) ;
#152861=CARTESIAN_POINT ( 'NONE',  ( 21.55341960407610458, 5.719274019375980345, 63.95724293864770260 ) ) ;
#152862=CARTESIAN_POINT ( 'NONE',  ( -10.72451020669870658, -18.67979575497194134, 24.58442372801901499 ) ) ;
#152863=CARTESIAN_POINT ( 'NONE',  ( -12.06949235617739369, -12.14591786802326823, 29.37609039468568284 ) ) ;
#152864=CARTESIAN_POINT ( 'NONE',  ( 12.06949235617739724, 12.14591786802326823, 76.87609039468567573 ) ) ;
#152865=CARTESIAN_POINT ( 'NONE',  ( 16.46253265017160672, -9.564922557960803928, 28.33224293864769550 ) ) ;
#152866=CARTESIAN_POINT ( 'NONE',  ( 10.81492255796078972, 18.62759615963270932, 114.5822429386477097 ) ) ;
#152867=CARTESIAN_POINT ( 'NONE',  ( 4.379528057220339221, -16.55341960407611168, 112.7072429386476955 ) ) ;
#152869=CARTESIAN_POINT ( 'NONE',  ( 8.224510206698742110, 14.34966873604972548, 47.08442372801901854 ) ) ;
#152870=CARTESIAN_POINT ( 'NONE',  ( 16.55341960407611168, 4.379528057220329451, 73.95724293864769550 ) ) ;
#152871=CARTESIAN_POINT ( 'NONE',  ( -21.53943276465977519, 0.05219959533907696930, 81.24890960531436690 ) ) ;
#152872=CARTESIAN_POINT ( 'NONE',  ( 12.14591786802309770, 12.06949235617756955, 29.37390960531435269 ) ) ;
#152873=CARTESIAN_POINT ( 'NONE',  ( 8.224510206698742110, 14.34966873604972548, 37.08442372801901143 ) ) ;
#152874=CARTESIAN_POINT ( 'NONE',  ( 9.474510206698971260, -16.51473224551069308, 47.91557627198102409 ) ) ;
#152875=CARTESIAN_POINT ( 'NONE',  ( 8.224510206698742110, 14.34966873604972548, 82.08442372801901854 ) ) ;
#152876=CARTESIAN_POINT ( 'NONE',  ( 19.03943276465977164, 0.05219959533936151252, 76.25109039468566152 ) ) ;
#152877=CARTESIAN_POINT ( 'NONE',  ( -0.05219959533907301413, -21.53943276465977519, 72.49890960531435269 ) ) ;
#152878=CARTESIAN_POINT ( 'NONE',  ( -16.55341960407617563, 4.379528057220093196, 108.5427570613523756 ) ) ;
#152881=CARTESIAN_POINT ( 'NONE',  ( -18.62759615963270932, 10.81492255796079327, 45.83224293864769550 ) ) ;
#152882=EDGE_LOOP ( 'NONE', ( #24973, #106993, #58888, #152799 ) ) ;
#152883=CARTESIAN_POINT ( 'NONE',  ( -16.52544592524335698, -4.483927247898792601, 93.95942372801903275 ) ) ;
#152885=CARTESIAN_POINT ( 'NONE',  ( -18.67979575497178146, -10.72451020669898902, 21.66557627198102409 ) ) ;
#152887=CARTESIAN_POINT ( 'NONE',  ( -21.55341960407610458, -5.719274019375992779, 81.45724293864769550 ) ) ;
#152888=CARTESIAN_POINT ( 'NONE',  ( 12.14591786802327356, -12.06949235617739191, 110.6260903946857042 ) ) ;
#152889=CARTESIAN_POINT ( 'NONE',  ( 19.05341960407617918, -5.049401038297876454, 111.0427570613523329 ) ) ;
#152890=CARTESIAN_POINT ( 'NONE',  ( -14.29746914071049879, 8.314922557960819915, 110.8322429386476955 ) ) ;
#152891=CARTESIAN_POINT ( 'NONE',  ( -14.34966873604972548, 8.224510206698743886, 28.33442372801902209 ) ) ;
#152892=CARTESIAN_POINT ( 'NONE',  ( 19.05341960407611168, 5.049401038298154454, 58.95724293864768129 ) ) ;
#152894=CARTESIAN_POINT ( 'NONE',  ( -16.46253265017160317, 9.564922557960807481, 110.8322429386476955 ) ) ;
#152895=CARTESIAN_POINT ( 'NONE',  ( -12.14591786802326823, 12.06949235617739902, 93.12609039468568994 ) ) ;
#152896=CARTESIAN_POINT ( 'NONE',  ( -19.02544592524334988, -5.153800228976617603, 93.95942372801900433 ) ) ;
#152897=CARTESIAN_POINT ( 'NONE',  ( 9.564922557961047289, -16.46253265017146816, 25.41775706135234003 ) ) ;
#152898=CARTESIAN_POINT ( 'NONE',  ( -10.81492255796078084, -18.62759615963271287, 72.08224293864769550 ) ) ;
#152899=CARTESIAN_POINT ( 'NONE',  ( -16.53943276465976808, -0.05219959533934237506, 98.75109039468568994 ) ) ;
#152900=VECTOR ( 'NONE', #90370, 1000.000000000000000 ) ;
#152901=CARTESIAN_POINT ( 'NONE',  ( -5.153800228976607833, 19.02544592524334988, 92.70942372801901854 ) ) ;
#152902=CARTESIAN_POINT ( 'NONE',  ( 9.474510206698971260, -16.51473224551069308, 47.91557627198102409 ) ) ;
#152903=CARTESIAN_POINT ( 'NONE',  ( -19.03943276465977164, 0.05219959533909376836, 96.24890960531436690 ) ) ;
#152904=CARTESIAN_POINT ( 'NONE',  ( -15.72974639402176322, -15.80617190586768395, 64.37609039468568994 ) ) ;
#152905=CARTESIAN_POINT ( 'NONE',  ( 19.02544592524343514, -5.153800228976328945, 43.54057627198103120 ) ) ;
#152906=CARTESIAN_POINT ( 'NONE',  ( -16.88567814943165502, -6.947325034625698059, 86.29001122652586275 ) ) ;
#152907=CARTESIAN_POINT ( 'NONE',  ( 14.29746914071049879, -8.314922557960816363, 78.33224293864770971 ) ) ;
#152908=CARTESIAN_POINT ( 'NONE',  ( -15.80617190586745835, -15.72974639402198527, 71.87390960531438111 ) ) ;
#152911=CARTESIAN_POINT ( 'NONE',  ( -0.05219959533936034679, 19.03943276465977164, 37.50109039468567573 ) ) ;
#152913=CARTESIAN_POINT ( 'NONE',  ( 19.03943276465977164, -0.05219959533909143690, 73.74890960531435269 ) ) ;
#152914=CARTESIAN_POINT ( 'NONE',  ( -0.05219959533909027116, -19.03943276465977164, 82.49890960531436690 ) ) ;
#152915=CARTESIAN_POINT ( 'NONE',  ( 16.55341960407618274, -4.379528057220086978, 61.04275706135234714 ) ) ;
#152916=CARTESIAN_POINT ( 'NONE',  ( -16.46253265017146816, -9.564922557961047289, 79.16775706135234714 ) ) ;
#152917=CARTESIAN_POINT ( 'NONE',  ( -16.46253265017146816, -9.564922557961047289, 29.16775706135232937 ) ) ;
#152918=CARTESIAN_POINT ( 'NONE',  ( 18.09805431107249873, -5.499999999999973355, 93.51606229291884631 ) ) ;
#152919=CARTESIAN_POINT ( 'NONE',  ( -12.14591786802326823, 12.06949235617739902, 88.12609039468570415 ) ) ;
#152921=CARTESIAN_POINT ( 'NONE',  ( -12.14591786802326823, 12.06949235617739902, 73.12609039468567573 ) ) ;
#152922=CARTESIAN_POINT ( 'NONE',  ( -14.29746914071037622, -8.314922557961029526, 59.16775706135234714 ) ) ;
#152924=CARTESIAN_POINT ( 'NONE',  ( -5.719274019375665041, -21.55341960407619695, 69.79275706135234714 ) ) ;
#152925=CARTESIAN_POINT ( 'NONE',  ( 19.02544592524334988, 5.153800228976608722, 76.45942372801897591 ) ) ;
#152926=CARTESIAN_POINT ( 'NONE',  ( 21.55341960407619695, -5.719274019375665929, 106.0427570613523471 ) ) ;
#152927=CARTESIAN_POINT ( 'NONE',  ( -19.03943276465977164, 0.05219959533909376836, 51.24890960531436690 ) ) ;
#152928=CARTESIAN_POINT ( 'NONE',  ( 9.474510206698971260, -16.51473224551069308, 37.91557627198102409 ) ) ;
#152930=CARTESIAN_POINT ( 'NONE',  ( 21.55341960407610458, 5.719274019375980345, 73.95724293864769550 ) ) ;
#152931=CARTESIAN_POINT ( 'NONE',  ( -19.03943276465977164, 0.05219959533909376836, 116.2489096053143669 ) ) ;
#152932=CARTESIAN_POINT ( 'NONE',  ( -16.51473224551069308, -9.474510206698971260, 21.66557627198102765 ) ) ;
#152933=CARTESIAN_POINT ( 'NONE',  ( -0.05219959533934338120, 16.53943276465976808, 47.50109039468568994 ) ) ;
#152934=CARTESIAN_POINT ( 'NONE',  ( -4.379528057220328563, 16.55341960407611168, 25.20724293864769550 ) ) ;
#152936=CARTESIAN_POINT ( 'NONE',  ( -21.52544592524343514, 5.823673210054127303, 116.0405762719810383 ) ) ;
#152937=CARTESIAN_POINT ( 'NONE',  ( -4.483927247898539470, -16.52544592524342804, 47.29057627198103120 ) ) ;
#152939=CARTESIAN_POINT ( 'NONE',  ( -13.97604488694547697, 13.89961937509957934, 108.1260903946856331 ) ) ;
#152940=CARTESIAN_POINT ( 'NONE',  ( 19.05341960407617918, -5.049401038297876454, 36.04275706135234003 ) ) ;
#152941=CARTESIAN_POINT ( 'NONE',  ( 14.29746914071049879, -8.314922557960816363, 38.33224293864768839 ) ) ;
#152942=CARTESIAN_POINT ( 'NONE',  ( 21.53943276465977519, -0.05219959533907433946, 98.74890960531438111 ) ) ;
#152943=DIRECTION ( 'NONE',  ( 1.000000000000000000, -0.000000000000000000, -0.000000000000000000 ) ) ;
#152944=CARTESIAN_POINT ( 'NONE',  ( -21.53943276465977519, 0.05219959533907696930, 61.24890960531435979 ) ) ;
#152945=CARTESIAN_POINT ( 'NONE',  ( -13.97604488694527625, -13.89961937509977652, 96.87390960531433848 ) ) ;
#152946=CARTESIAN_POINT ( 'NONE',  ( -0.05219959533910754901, -16.53943276465976808, 52.49890960531435979 ) ) ;
#152947=CARTESIAN_POINT ( 'NONE',  ( -19.02544592524342804, 5.153800228976336051, 106.0405762719810241 ) ) ;
#152949=CARTESIAN_POINT ( 'NONE',  ( 13.97604488694548053, -13.89961937509957401, 60.62609039468564731 ) ) ;
#152950=CARTESIAN_POINT ( 'NONE',  ( -5.823673210054116645, -21.52544592524344225, 97.29057627198105251 ) ) ;
#152951=CARTESIAN_POINT ( 'NONE',  ( -0.05219959533909027116, -19.03943276465977164, 42.49890960531435269 ) ) ;
#152952=CARTESIAN_POINT ( 'NONE',  ( -16.51473224551069308, -9.474510206698971260, 21.66557627198102765 ) ) ;
#152954=CARTESIAN_POINT ( 'NONE',  ( 21.55341960407619695, -5.719274019375665929, 56.04275706135235424 ) ) ;
#152956=CARTESIAN_POINT ( 'NONE',  ( -12.14591786802309592, -12.06949235617757132, 21.87390960531436690 ) ) ;
#152957=CARTESIAN_POINT ( 'NONE',  ( 19.05341960407611168, 5.049401038298154454, 53.95724293864770260 ) ) ;
#152958=CARTESIAN_POINT ( 'NONE',  ( 9.474510206698971260, -16.51473224551069308, 92.91557627198103830 ) ) ;
#152959=CARTESIAN_POINT ( 'NONE',  ( -10.81492255796078084, -18.62759615963271287, 62.08224293864769550 ) ) ;
#152961=CARTESIAN_POINT ( 'NONE',  ( 13.89961937509977652, -13.97604488694527269, 48.12390960531435979 ) ) ;
#152962=CARTESIAN_POINT ( 'NONE',  ( -10.72451020669898014, 18.67979575497178502, 55.41557627198102409 ) ) ;
#152963=CARTESIAN_POINT ( 'NONE',  ( -21.53943276465977519, -0.05219959533937600094, 83.75109039468568994 ) ) ;
#152965=CARTESIAN_POINT ( 'NONE',  ( 4.483927247898790824, -16.52544592524335698, 85.20942372801901854 ) ) ;
#152966=CARTESIAN_POINT ( 'NONE',  ( 4.483927247898545687, 16.52544592524342804, 69.79057627198102409 ) ) ;
#152967=CARTESIAN_POINT ( 'NONE',  ( -16.55341960407617563, 4.379528057220093196, 88.54275706135236135 ) ) ;
#152968=CARTESIAN_POINT ( 'NONE',  ( 19.03943276465977164, -0.05219959533909143690, 68.74890960531436690 ) ) ;
#152970=CARTESIAN_POINT ( 'NONE',  ( 0.05219959533936267826, -19.03943276465977164, 20.00109039468567218 ) ) ;
#152971=CARTESIAN_POINT ( 'NONE',  ( -4.483927247898782831, 16.52544592524335698, 92.70942372801901854 ) ) ;
#152972=CARTESIAN_POINT ( 'NONE',  ( -5.719274019375665041, -21.55341960407619695, 109.7927570613523613 ) ) ;
#152973=CARTESIAN_POINT ( 'NONE',  ( -19.05341960407611168, -5.049401038298163336, 81.45724293864769550 ) ) ;
#152974=CARTESIAN_POINT ( 'NONE',  ( 15.80617190586746368, 15.72974639402197994, 49.37390960531436690 ) ) ;
#152975=CARTESIAN_POINT ( 'NONE',  ( 12.06949235617739724, 12.14591786802326823, 31.87609039468567929 ) ) ;
#152976=CARTESIAN_POINT ( 'NONE',  ( -21.53943276465977519, -0.05219959533937600094, 83.75109039468568994 ) ) ;
#152977=CARTESIAN_POINT ( 'NONE',  ( -12.14591786802326823, 12.06949235617739902, 63.12609039468568994 ) ) ;
#152978=CARTESIAN_POINT ( 'NONE',  ( -10.72451020669870658, -18.67979575497194134, 19.58442372801901143 ) ) ;
#152979=CARTESIAN_POINT ( 'NONE',  ( 8.314922557961029526, -14.29746914071037800, 20.41775706135234714 ) ) ;
#152980=CARTESIAN_POINT ( 'NONE',  ( -19.02544592524342804, 5.153800228976336051, 86.04057627198103830 ) ) ;
#152981=CARTESIAN_POINT ( 'NONE',  ( -8.224510206698735004, -14.34966873604973081, 29.58442372801901854 ) ) ;
#152982=CARTESIAN_POINT ( 'NONE',  ( 5.153800228976335163, 19.02544592524342804, 39.79057627198100988 ) ) ;
#152983=CARTESIAN_POINT ( 'NONE',  ( -8.314922557961024197, 14.29746914071037800, 37.91775706135235424 ) ) ;
#152984=CARTESIAN_POINT ( 'NONE',  ( -16.53943276465976808, 0.05219959533911058130, 81.24890960531436690 ) ) ;
#152985=CARTESIAN_POINT ( 'NONE',  ( -12.14591786802326823, 12.06949235617739902, 93.12609039468568994 ) ) ;
#152986=CARTESIAN_POINT ( 'NONE',  ( 21.53943276465977519, 0.05219959533937863772, 26.25109039468567573 ) ) ;
#152987=CARTESIAN_POINT ( 'NONE',  ( -13.97604488694527625, -13.89961937509977652, 61.87390960531435979 ) ) ;
#152988=CARTESIAN_POINT ( 'NONE',  ( 19.05341960407611168, 5.049401038298154454, 63.95724293864769550 ) ) ;
#152989=CARTESIAN_POINT ( 'NONE',  ( -16.53943276465976808, -0.05219959533934237506, 83.75109039468568994 ) ) ;
#152990=CARTESIAN_POINT ( 'NONE',  ( 17.50000000000002132, -5.499999999999878320, 63.29690382534172954 ) ) ;
#152993=CARTESIAN_POINT ( 'NONE',  ( -19.05341960407617563, 5.049401038297882671, 28.54275706135232937 ) ) ;
#152994=CARTESIAN_POINT ( 'NONE',  ( 16.51473224551069308, 9.474510206698969483, 54.16557627198103120 ) ) ;
#152995=EDGE_CURVE ( 'NONE', #95725, #24895, #49760, .T. ) ;
#152998=CARTESIAN_POINT ( 'NONE',  ( -16.55341960407617563, 4.379528057220093196, 23.54275706135235424 ) ) ;
#152999=CARTESIAN_POINT ( 'NONE',  ( -5.153800228976607833, 19.02544592524334988, 52.70942372801900433 ) ) ;
#153000=CARTESIAN_POINT ( 'NONE',  ( -12.06949235617739369, -12.14591786802326823, 39.37609039468567573 ) ) ;
#153001=CARTESIAN_POINT ( 'NONE',  ( -16.51473224551069308, -9.474510206698971260, 101.6655762719810241 ) ) ;
#153002=CARTESIAN_POINT ( 'NONE',  ( -16.51473224551069308, -9.474510206698971260, 81.66557627198103830 ) ) ;
#153003=CARTESIAN_POINT ( 'NONE',  ( 15.72974639402199770, -15.80617190586745480, 93.12390960531436690 ) ) ;
#153004=CARTESIAN_POINT ( 'NONE',  ( -13.97604488694547697, 13.89961937509957934, 63.12609039468566152 ) ) ;
#153005=CARTESIAN_POINT ( 'NONE',  ( -13.89961937509977652, 13.97604488694528158, 85.62390960531433848 ) ) ;
#153006=CARTESIAN_POINT ( 'NONE',  ( 19.05341960407611168, 5.049401038298154454, 23.95724293864769194 ) ) ;
#153007=CARTESIAN_POINT ( 'NONE',  ( -5.153800228976328057, -19.02544592524343514, 57.29057627198103120 ) ) ;
#153008=CARTESIAN_POINT ( 'NONE',  ( 8.224510206698953496, -14.34966873604960469, 27.91557627198103830 ) ) ;
#153009=CARTESIAN_POINT ( 'NONE',  ( 19.02544592524343514, -5.153800228976328945, 28.54057627198102409 ) ) ;
#153010=CARTESIAN_POINT ( 'NONE',  ( 19.05341960407617918, -5.049401038297876454, 36.04275706135234003 ) ) ;
#153011=CARTESIAN_POINT ( 'NONE',  ( -16.52544592524342804, 4.483927247898546575, 76.04057627198102409 ) ) ;
#153012=CARTESIAN_POINT ( 'NONE',  ( -15.80617190586768217, 15.72974639402176855, 93.12609039468568994 ) ) ;
#153013=CARTESIAN_POINT ( 'NONE',  ( 19.03943276465977164, -0.05219959533909143690, 43.74890960531435979 ) ) ;
#153014=CARTESIAN_POINT ( 'NONE',  ( -8.224510206698735004, -14.34966873604973081, 49.58442372801901143 ) ) ;
#153016=CARTESIAN_POINT ( 'NONE',  ( 12.06949235617757843, -12.14591786802309237, 38.12390960531436690 ) ) ;
#153017=CARTESIAN_POINT ( 'NONE',  ( -10.72451020669870658, -18.67979575497194134, 89.58442372801901854 ) ) ;
#153018=CARTESIAN_POINT ( 'NONE',  ( 16.51473224551069308, 9.474510206698969483, 99.16557627198102409 ) ) ;
#153019=CARTESIAN_POINT ( 'NONE',  ( 13.89961937509977652, -13.97604488694527269, 93.12390960531436690 ) ) ;
#153020=CARTESIAN_POINT ( 'NONE',  ( -8.314922557960811034, -14.29746914071050412, 112.0822429386477097 ) ) ;
#153021=CARTESIAN_POINT ( 'NONE',  ( 16.52544592524342804, -4.483927247898539470, 68.54057627198103830 ) ) ;
#153022=CARTESIAN_POINT ( 'NONE',  ( 21.52544592524344225, -5.823673210054117533, 83.54057627198102409 ) ) ;
#153023=CARTESIAN_POINT ( 'NONE',  ( -9.564922557960796823, -16.46253265017161027, 92.08224293864769550 ) ) ;
#153024=CARTESIAN_POINT ( 'NONE',  ( 21.52544592524344225, -5.823673210054117533, 98.54057627198105251 ) ) ;
#153025=CARTESIAN_POINT ( 'NONE',  ( -19.05341960407617563, 5.049401038297882671, 73.54275706135233293 ) ) ;
#153027=CARTESIAN_POINT ( 'NONE',  ( 4.379528057220339221, -16.55341960407611168, 87.70724293864769550 ) ) ;
#153028=CARTESIAN_POINT ( 'NONE',  ( 19.03943276465977164, -0.05219959533909143690, 53.74890960531436690 ) ) ;
#153029=CARTESIAN_POINT ( 'NONE',  ( -21.53943276465977519, 0.05219959533907696930, 71.24890960531435269 ) ) ;
#153030=CARTESIAN_POINT ( 'NONE',  ( 17.40861289039004234, -6.110651285853252901, 26.12767529172568715 ) ) ;
#153031=CARTESIAN_POINT ( 'NONE',  ( -12.14591786802326823, 12.06949235617739902, 113.1260903946856899 ) ) ;
#153033=CARTESIAN_POINT ( 'NONE',  ( 14.29746914071037800, 8.314922557961029526, 26.66775706135235424 ) ) ;
#153034=CARTESIAN_POINT ( 'NONE',  ( -12.14591786802309592, -12.06949235617757132, 86.87390960531438111 ) ) ;
#153036=CARTESIAN_POINT ( 'NONE',  ( -13.89961937509977652, 13.97604488694528158, 75.62390960531438111 ) ) ;
#153037=CARTESIAN_POINT ( 'NONE',  ( -9.564922557960796823, -16.46253265017161027, 52.08224293864768839 ) ) ;
#153038=CARTESIAN_POINT ( 'NONE',  ( -8.224510206698948167, 14.34966873604960824, 70.41557627198102409 ) ) ;
#153040=CARTESIAN_POINT ( 'NONE',  ( -19.05341960407611168, -5.049401038298163336, 111.4572429386476671 ) ) ;
#153041=CARTESIAN_POINT ( 'NONE',  ( 5.049401038297881783, 19.05341960407617563, 97.29275706135233293 ) ) ;
#153042=CARTESIAN_POINT ( 'NONE',  ( 13.97604488694527802, 13.89961937509977652, 104.3739096053143385 ) ) ;
#153043=CARTESIAN_POINT ( 'NONE',  ( 15.72974639402199770, -15.80617190586745480, 73.12390960531436690 ) ) ;
#153044=CARTESIAN_POINT ( 'NONE',  ( -8.224510206698735004, -14.34966873604973081, 74.58442372801901854 ) ) ;
#153045=CARTESIAN_POINT ( 'NONE',  ( -17.12812012977046550, 6.668231424565701282, 93.64051240676855059 ) ) ;
#153046=CARTESIAN_POINT ( 'NONE',  ( 19.02544592524343514, -5.153800228976328945, 68.54057627198103830 ) ) ;
#153047=CARTESIAN_POINT ( 'NONE',  ( -18.62759615963270932, 10.81492255796079327, 85.83224293864768129 ) ) ;
#153048=CARTESIAN_POINT ( 'NONE',  ( -16.53943276465976808, -0.05219959533934237506, 18.75109039468568639 ) ) ;
#153049=CARTESIAN_POINT ( 'NONE',  ( 16.55341960407611168, 4.379528057220329451, 33.95724293864769550 ) ) ;
#153050=CARTESIAN_POINT ( 'NONE',  ( -10.81492255796105439, 18.62759615963255655, 57.91775706135234714 ) ) ;
#153052=CARTESIAN_POINT ( 'NONE',  ( -12.14591786802326823, 12.06949235617739902, 73.12609039468567573 ) ) ;
#153053=CARTESIAN_POINT ( 'NONE',  ( 0.05219959533909260263, 19.03943276465977164, 109.9989096053143669 ) ) ;
#153056=CARTESIAN_POINT ( 'NONE',  ( -14.34966873604972548, 8.224510206698743886, 93.33442372801901854 ) ) ;
#153057=CARTESIAN_POINT ( 'NONE',  ( 16.52544592524335698, 4.483927247898782831, 46.45942372801901854 ) ) ;
#153058=CARTESIAN_POINT ( 'NONE',  ( -9.474510206698964154, 16.51473224551069663, 55.41557627198103120 ) ) ;
#153059=CARTESIAN_POINT ( 'NONE',  ( 16.51473224551069308, 9.474510206698969483, 74.16557627198103830 ) ) ;
#153060=CARTESIAN_POINT ( 'NONE',  ( 15.72974639402176855, 15.80617190586768217, 71.87609039468568994 ) ) ;
#153061=CARTESIAN_POINT ( 'NONE',  ( -16.52544592524335698, -4.483927247898792601, 63.95942372801901854 ) ) ;
#153062=CARTESIAN_POINT ( 'NONE',  ( 16.52544592524342804, -4.483927247898539470, 38.54057627198103120 ) ) ;
#153063=CARTESIAN_POINT ( 'NONE',  ( -13.89961937509977652, 13.97604488694528158, 40.62390960531435979 ) ) ;
#153064=CARTESIAN_POINT ( 'NONE',  ( 5.049401038298161559, -19.05341960407611168, 37.70724293864768839 ) ) ;
#153065=CARTESIAN_POINT ( 'NONE',  ( -16.52544592524335698, -4.483927247898792601, 43.95942372801902565 ) ) ;
#153066=CARTESIAN_POINT ( 'NONE',  ( 9.474510206698729675, 16.51473224551082808, 102.0844237280190043 ) ) ;
#153067=CARTESIAN_POINT ( 'NONE',  ( 16.52544592524342804, -4.483927247898539470, 98.54057627198105251 ) ) ;
#153068=CARTESIAN_POINT ( 'NONE',  ( -19.03943276465977164, 0.05219959533909376836, 51.24890960531436690 ) ) ;
#153069=CARTESIAN_POINT ( 'NONE',  ( -16.46253265017146816, -9.564922557961047289, 84.16775706135233293 ) ) ;
#153071=CARTESIAN_POINT ( 'NONE',  ( -10.72451020669870658, -18.67979575497194134, 94.58442372801901854 ) ) ;
#153072=CARTESIAN_POINT ( 'NONE',  ( -16.53943276465976808, -0.05219959533934237506, 53.75109039468568994 ) ) ;
#153074=CARTESIAN_POINT ( 'NONE',  ( -15.80617190586745835, -15.72974639402198527, 46.87390960531435979 ) ) ;
#153075=CARTESIAN_POINT ( 'NONE',  ( -12.14591786802326823, 12.06949235617739902, 38.12609039468567573 ) ) ;
#153076=CARTESIAN_POINT ( 'NONE',  ( -19.01533133064923931, 5.499999999999444000, 68.76586590595741200 ) ) ;
#153077=CARTESIAN_POINT ( 'NONE',  ( 19.03943276465977164, 0.05219959533936151252, 41.25109039468566152 ) ) ;
#153078=CARTESIAN_POINT ( 'NONE',  ( 9.474510206698971260, -16.51473224551069308, 87.91557627198102409 ) ) ;
#153079=CARTESIAN_POINT ( 'NONE',  ( 16.55341960407611168, 4.379528057220329451, 98.95724293864770971 ) ) ;
#153080=CARTESIAN_POINT ( 'NONE',  ( -9.564922557960796823, -16.46253265017161027, 52.08224293864768839 ) ) ;
#153082=CARTESIAN_POINT ( 'NONE',  ( 18.67979575497194134, -10.72451020669871369, 75.83442372801900433 ) ) ;
#153084=CARTESIAN_POINT ( 'NONE',  ( -5.153800228976607833, 19.02544592524334988, 27.70942372801899722 ) ) ;
#153085=CARTESIAN_POINT ( 'NONE',  ( 18.62759615963255655, 10.81492255796105972, 111.6677570613523613 ) ) ;
#153086=CARTESIAN_POINT ( 'NONE',  ( 14.29746914071049879, -8.314922557960816363, 53.33224293864769550 ) ) ;
#153087=CARTESIAN_POINT ( 'NONE',  ( -5.153800228976328057, -19.02544592524343514, 57.29057627198103120 ) ) ;
#153088=CARTESIAN_POINT ( 'NONE',  ( -19.03943276465977164, 0.05219959533909376836, 111.2489096053143669 ) ) ;
#153089=CARTESIAN_POINT ( 'NONE',  ( 18.67979575497194134, -10.72451020669871369, 85.83442372801901854 ) ) ;
#153090=CARTESIAN_POINT ( 'NONE',  ( 9.564922557960805705, 16.46253265017160317, 59.58224293864769550 ) ) ;
#153091=CARTESIAN_POINT ( 'NONE',  ( 18.62759615963255655, 10.81492255796105972, 81.66775706135236135 ) ) ;
#153092=CARTESIAN_POINT ( 'NONE',  ( 5.823673210054125526, 21.52544592524343514, 34.79057627198103120 ) ) ;
#153093=CARTESIAN_POINT ( 'NONE',  ( 10.81492255796106328, -18.62759615963255655, 35.41775706135234003 ) ) ;
#153094=CARTESIAN_POINT ( 'NONE',  ( 19.03943276465977164, 0.05219959533936151252, 66.25109039468567573 ) ) ;
#153095=CARTESIAN_POINT ( 'NONE',  ( 5.153800228976335163, 19.02544592524342804, 24.79057627198102765 ) ) ;
#153096=CARTESIAN_POINT ( 'NONE',  ( -19.03943276465977164, 0.05219959533909376836, 71.24890960531435269 ) ) ;
#153097=CARTESIAN_POINT ( 'NONE',  ( 4.483927247898790824, -16.52544592524335698, 25.20942372801901854 ) ) ;
#153098=CARTESIAN_POINT ( 'NONE',  ( 4.379528057220339221, -16.55341960407611168, 87.70724293864769550 ) ) ;
#153099=CARTESIAN_POINT ( 'NONE',  ( -9.564922557960796823, -16.46253265017161027, 62.08224293864769550 ) ) ;
#153100=CARTESIAN_POINT ( 'NONE',  ( -18.62759615963270932, 10.81492255796079327, 40.83224293864769550 ) ) ;
#153101=CARTESIAN_POINT ( 'NONE',  ( 14.29746914071037800, 8.314922557961029526, 21.66775706135235069 ) ) ;
#153102=CARTESIAN_POINT ( 'NONE',  ( 18.62759615963255655, 10.81492255796105972, 21.66775706135235069 ) ) ;
#153103=CARTESIAN_POINT ( 'NONE',  ( -10.72451020669870658, -18.67979575497194134, 69.58442372801900433 ) ) ;
#153104=CARTESIAN_POINT ( 'NONE',  ( -4.483927247898782831, 16.52544592524335698, 72.70942372801901854 ) ) ;
#153105=CARTESIAN_POINT ( 'NONE',  ( -8.224510206698735004, -14.34966873604973081, 69.58442372801900433 ) ) ;
#153106=CARTESIAN_POINT ( 'NONE',  ( -9.474510206698964154, 16.51473224551069663, 60.41557627198102409 ) ) ;
#153107=CARTESIAN_POINT ( 'NONE',  ( 4.379528057220092307, 16.55341960407617563, 87.29275706135236135 ) ) ;
#153108=CARTESIAN_POINT ( 'NONE',  ( -16.46253265017146816, -9.564922557961047289, 39.16775706135234003 ) ) ;
#153109=CARTESIAN_POINT ( 'NONE',  ( -18.67979575497178146, -10.72451020669898902, 111.6655762719810525 ) ) ;
#153110=CARTESIAN_POINT ( 'NONE',  ( -16.55341960407611168, -4.379528057220339221, 61.45724293864770260 ) ) ;
#153111=CARTESIAN_POINT ( 'NONE',  ( -9.564922557960796823, -16.46253265017161027, 82.08224293864768129 ) ) ;
#153112=CARTESIAN_POINT ( 'NONE',  ( 14.29746914071037800, 8.314922557961029526, 91.66775706135234714 ) ) ;
#153113=CARTESIAN_POINT ( 'NONE',  ( -5.719274019375665041, -21.55341960407619695, 64.79275706135234714 ) ) ;
#153114=CARTESIAN_POINT ( 'NONE',  ( 16.52544592524335698, 4.483927247898782831, 21.45942372801901499 ) ) ;
#153115=CARTESIAN_POINT ( 'NONE',  ( 5.719274019375991003, -21.55341960407610458, 107.7072429386476955 ) ) ;
#153116=CARTESIAN_POINT ( 'NONE',  ( 8.314922557960818139, 14.29746914071049879, 59.58224293864770260 ) ) ;
#153118=CARTESIAN_POINT ( 'NONE',  ( -18.67979575497178146, -10.72451020669898902, 106.6655762719810383 ) ) ;
#153119=CARTESIAN_POINT ( 'NONE',  ( 14.29746914071049879, -8.314922557960816363, 43.33224293864769550 ) ) ;
#153120=ORIENTED_EDGE ( 'NONE', *, *, #142268, .F. ) ;
#153121=DIRECTION ( 'NONE',  ( 0.000000000000000000, 0.000000000000000000, -1.000000000000000000 ) ) ;
#153122=CARTESIAN_POINT ( 'NONE',  ( -5.719274019375978568, 21.55341960407610458, 110.2072429386477239 ) ) ;
#153123=CARTESIAN_POINT ( 'NONE',  ( -16.46253265017160317, 9.564922557960807481, 115.8322429386477097 ) ) ;
#153124=CARTESIAN_POINT ( 'NONE',  ( -21.55341960407619339, 5.719274019375674811, 38.54275706135234714 ) ) ;
#153125=CARTESIAN_POINT ( 'NONE',  ( -16.55341960407611168, -4.379528057220339221, 46.45724293864769550 ) ) ;
#153127=CARTESIAN_POINT ( 'NONE',  ( 5.049401038298161559, -19.05341960407611168, 57.70724293864769550 ) ) ;
#153128=CARTESIAN_POINT ( 'NONE',  ( -19.03943276465977164, -0.05219959533935918106, 68.75109039468566152 ) ) ;
#153129=CARTESIAN_POINT ( 'NONE',  ( -19.03943276465977164, 0.05219959533909376836, 91.24890960531436690 ) ) ;
#153130=CARTESIAN_POINT ( 'NONE',  ( -15.72974639402197994, 15.80617190586746368, 45.62390960531436690 ) ) ;
#153132=CARTESIAN_POINT ( 'NONE',  ( 5.049401038298161559, -19.05341960407611168, 52.70724293864767418 ) ) ;
#153133=CARTESIAN_POINT ( 'NONE',  ( -8.224510206698735004, -14.34966873604973081, 34.58442372801900433 ) ) ;
#153134=CARTESIAN_POINT ( 'NONE',  ( -13.89961937509957401, -13.97604488694547875, 69.37609039468564731 ) ) ;
#153135=CARTESIAN_POINT ( 'NONE',  ( 5.719274019375991003, -21.55341960407610458, 112.7072429386476955 ) ) ;
#153136=CARTESIAN_POINT ( 'NONE',  ( 14.34966873604960469, 8.224510206698951720, 44.16557627198103120 ) ) ;
#153138=CARTESIAN_POINT ( 'NONE',  ( -9.474510206698964154, 16.51473224551069663, 85.41557627198102409 ) ) ;
#153139=CARTESIAN_POINT ( 'NONE',  ( 5.719274019375991003, -21.55341960407610458, 77.70724293864770971 ) ) ;
#153140=CARTESIAN_POINT ( 'NONE',  ( 0.05219959533907565091, 21.53943276465977519, 109.9989096053143527 ) ) ;
#153141=CARTESIAN_POINT ( 'NONE',  ( 16.53943276465976808, 0.05219959533934440121, 36.25109039468567573 ) ) ;
#153142=CARTESIAN_POINT ( 'NONE',  ( -18.62759615963270932, 10.81492255796079327, 35.83224293864768839 ) ) ;
#153143=CARTESIAN_POINT ( 'NONE',  ( -18.67979575497193778, 10.72451020669871902, 103.3344237280190043 ) ) ;
#153144=CARTESIAN_POINT ( 'NONE',  ( -5.049401038298153566, 19.05341960407611168, 85.20724293864766707 ) ) ;
#153145=CARTESIAN_POINT ( 'NONE',  ( 13.97604488694527802, 13.89961937509977652, 44.37390960531435269 ) ) ;
#153146=CARTESIAN_POINT ( 'NONE',  ( -16.51473224551069308, -9.474510206698971260, 91.66557627198103830 ) ) ;
#153147=CARTESIAN_POINT ( 'NONE',  ( -5.153800228976328057, -19.02544592524343514, 72.29057627198102409 ) ) ;
#153148=CARTESIAN_POINT ( 'NONE',  ( 12.06949235617739724, 12.14591786802326823, 21.87609039468567573 ) ) ;
#153149=EDGE_CURVE ( 'NONE', #163522, #134824, #8415, .T. ) ;
#153150=CARTESIAN_POINT ( 'NONE',  ( -16.46253265017146816, -9.564922557961047289, 54.16775706135234003 ) ) ;
#153151=CARTESIAN_POINT ( 'NONE',  ( 0.05219959533937995610, -21.53943276465977519, 105.0010903946856757 ) ) ;
#153152=CARTESIAN_POINT ( 'NONE',  ( -15.80617190586745835, -15.72974639402198527, 31.87390960531435979 ) ) ;
#153153=CARTESIAN_POINT ( 'NONE',  ( 0.05219959533934541429, -16.53943276465976808, 100.0010903946857042 ) ) ;
#153156=CARTESIAN_POINT ( 'NONE',  ( -9.474510206698720793, -16.51473224551083518, 64.58442372801900433 ) ) ;
#153157=CARTESIAN_POINT ( 'NONE',  ( -9.564922557961040184, 16.46253265017147172, 37.91775706135233293 ) ) ;
#153159=CARTESIAN_POINT ( 'NONE',  ( -13.89961937509977652, 13.97604488694528158, 35.62390960531435269 ) ) ;
#153160=CARTESIAN_POINT ( 'NONE',  ( -8.314922557960811034, -14.29746914071050412, 42.08224293864769550 ) ) ;
#153161=CARTESIAN_POINT ( 'NONE',  ( 9.564922557960805705, 16.46253265017160317, 24.58224293864769194 ) ) ;
#153162=CARTESIAN_POINT ( 'NONE',  ( 8.224510206698953496, -14.34966873604960469, 22.91557627198102765 ) ) ;
#153163=CARTESIAN_POINT ( 'NONE',  ( -30.00000000000000000, -1.163414459189985801E-14, 97.50000000000000000 ) ) ;
#153164=CARTESIAN_POINT ( 'NONE',  ( -14.29746914071037622, -8.314922557961029526, 94.16775706135237556 ) ) ;
#153165=CARTESIAN_POINT ( 'NONE',  ( -16.46253265017160317, 9.564922557960807481, 45.83224293864769550 ) ) ;
#153166=CARTESIAN_POINT ( 'NONE',  ( 18.67979575497194134, -10.72451020669871369, 110.8344237280190043 ) ) ;
#153167=CARTESIAN_POINT ( 'NONE',  ( 4.483927247898790824, -16.52544592524335698, 20.20942372801900788 ) ) ;
#153168=CARTESIAN_POINT ( 'NONE',  ( -21.55341960407619339, 5.719274019375674811, 73.54275706135234714 ) ) ;
#153169=CARTESIAN_POINT ( 'NONE',  ( 13.97604488694548053, -13.89961937509957401, 60.62609039468564731 ) ) ;
#153170=CARTESIAN_POINT ( 'NONE',  ( -5.153800228976328057, -19.02544592524343514, 87.29057627198103830 ) ) ;
#153171=CARTESIAN_POINT ( 'NONE',  ( 0.05219959533909260263, 19.03943276465977164, 89.99890960531436690 ) ) ;
#153173=CARTESIAN_POINT ( 'NONE',  ( -10.72451020669898014, 18.67979575497178502, 110.4155762719810383 ) ) ;
#153174=CARTESIAN_POINT ( 'NONE',  ( -16.55341960407611168, -4.379528057220339221, 66.45724293864768129 ) ) ;
#153175=CARTESIAN_POINT ( 'NONE',  ( -15.80617190586745835, -15.72974639402198527, 61.87390960531436690 ) ) ;
#153176=CARTESIAN_POINT ( 'NONE',  ( 9.474510206698971260, -16.51473224551069308, 62.91557627198102409 ) ) ;
#153177=CARTESIAN_POINT ( 'NONE',  ( 0.05219959533907565091, 21.53943276465977519, 99.99890960531436690 ) ) ;
#153178=CARTESIAN_POINT ( 'NONE',  ( -12.06949235617739369, -12.14591786802326823, 89.37609039468568994 ) ) ;
#153180=CARTESIAN_POINT ( 'NONE',  ( 13.97604488694527802, 13.89961937509977652, 59.37390960531434558 ) ) ;
#153181=CARTESIAN_POINT ( 'NONE',  ( -16.53943276465976808, 0.05219959533911058130, 96.24890960531435269 ) ) ;
#153183=CARTESIAN_POINT ( 'NONE',  ( -16.46253265017160317, 9.564922557960807481, 45.83224293864769550 ) ) ;
#153184=CARTESIAN_POINT ( 'NONE',  ( 9.474510206698729675, 16.51473224551082808, 77.08442372801900433 ) ) ;
#153185=CARTESIAN_POINT ( 'NONE',  ( 16.55341960407611168, 4.379528057220329451, 78.95724293864769550 ) ) ;
#153186=CARTESIAN_POINT ( 'NONE',  ( -18.67979575497193778, 10.72451020669871902, 63.33442372801900433 ) ) ;
#153187=CARTESIAN_POINT ( 'NONE',  ( -19.03943276465977164, 0.05219959533909376836, 31.24890960531435979 ) ) ;
#153188=CARTESIAN_POINT ( 'NONE',  ( -21.53943276465977519, 0.05219959533907696930, 101.2489096053143669 ) ) ;
#153189=CARTESIAN_POINT ( 'NONE',  ( -14.29746914071049879, 8.314922557960819915, 90.83224293864769550 ) ) ;
#153191=CARTESIAN_POINT ( 'NONE',  ( -9.564922557960796823, -16.46253265017161027, 57.08224293864769550 ) ) ;
#153192=CARTESIAN_POINT ( 'NONE',  ( 18.22780087662121673, 5.500000000000056843, 48.98459894673892734 ) ) ;
#153193=CARTESIAN_POINT ( 'NONE',  ( 16.51473224551083163, -9.474510206698727899, 100.8344237280190043 ) ) ;
#153194=CARTESIAN_POINT ( 'NONE',  ( -5.153800228976328057, -19.02544592524343514, 107.2905762719810383 ) ) ;
#153195=CARTESIAN_POINT ( 'NONE',  ( 21.52544592524334988, 5.823673210054432836, 31.45942372801901854 ) ) ;
#153196=CARTESIAN_POINT ( 'NONE',  ( -19.03943276465977164, 0.05219959533909376836, 86.24890960531436690 ) ) ;
#153197=CARTESIAN_POINT ( 'NONE',  ( 16.51473224551083163, -9.474510206698727899, 65.83442372801900433 ) ) ;
#153198=CARTESIAN_POINT ( 'NONE',  ( -19.02544592524342804, 5.153800228976336051, 56.04057627198100988 ) ) ;
#153199=CARTESIAN_POINT ( 'NONE',  ( -0.05219959533910754901, -16.53943276465976808, 77.49890960531433848 ) ) ;
#153200=CARTESIAN_POINT ( 'NONE',  ( -4.483927247898539470, -16.52544592524342804, 72.29057627198102409 ) ) ;
#153201=CARTESIAN_POINT ( 'NONE',  ( 19.02544592524343514, -5.153800228976328945, 93.54057627198102409 ) ) ;
#153202=CARTESIAN_POINT ( 'NONE',  ( 4.483927247898545687, 16.52544592524342804, 74.79057627198105251 ) ) ;
#153203=CARTESIAN_POINT ( 'NONE',  ( 16.51473224551069308, 9.474510206698969483, 89.16557627198103830 ) ) ;
#153205=CARTESIAN_POINT ( 'NONE',  ( 5.049401038297881783, 19.05341960407617563, 37.29275706135232582 ) ) ;
#153206=CARTESIAN_POINT ( 'NONE',  ( 5.153800228976335163, 19.02544592524342804, 34.79057627198102409 ) ) ;
#153207=CARTESIAN_POINT ( 'NONE',  ( -4.379528057220328563, 16.55341960407611168, 35.20724293864768839 ) ) ;
#153208=CARTESIAN_POINT ( 'NONE',  ( -8.224510206698948167, 14.34966873604960824, 105.4155762719810383 ) ) ;
#153209=ORIENTED_EDGE ( 'NONE', *, *, #134802, .F. ) ;
#153210=CARTESIAN_POINT ( 'NONE',  ( -21.53943276465977519, -0.05219959533937600094, 43.75109039468568284 ) ) ;
#153211=CARTESIAN_POINT ( 'NONE',  ( 19.03943276465977164, 0.05219959533936151252, 61.25109039468566863 ) ) ;
#153212=CARTESIAN_POINT ( 'NONE',  ( 0.05219959533910956823, 16.53943276465976808, 34.99890960531435979 ) ) ;
#153213=CARTESIAN_POINT ( 'NONE',  ( -18.62759615963270932, 10.81492255796079327, 80.83224293864769550 ) ) ;
#153214=CARTESIAN_POINT ( 'NONE',  ( -19.03943276465977164, 0.05219959533909376836, 116.2489096053143669 ) ) ;
#153215=CARTESIAN_POINT ( 'NONE',  ( -16.53943276465976808, 0.05219959533911058130, 76.24890960531435269 ) ) ;
#153216=CARTESIAN_POINT ( 'NONE',  ( -19.03943276465977164, 0.05219959533909376836, 46.24890960531435979 ) ) ;
#153217=CARTESIAN_POINT ( 'NONE',  ( 13.89961937509957401, 13.97604488694547697, 26.87609039468566507 ) ) ;
#153218=CARTESIAN_POINT ( 'NONE',  ( -0.05219959533934338120, 16.53943276465976808, 97.50109039468567573 ) ) ;
#153219=CARTESIAN_POINT ( 'NONE',  ( -14.29746914071037622, -8.314922557961029526, 54.16775706135235424 ) ) ;
#153220=CARTESIAN_POINT ( 'NONE',  ( -5.823673210054116645, -21.52544592524344225, 37.29057627198102409 ) ) ;
#153221=CARTESIAN_POINT ( 'NONE',  ( -21.55341960407619339, 5.719274019375674811, 103.5427570613523613 ) ) ;
#153222=CARTESIAN_POINT ( 'NONE',  ( 19.05341960407611168, 5.049401038298154454, 83.95724293864766707 ) ) ;
#153223=CARTESIAN_POINT ( 'NONE',  ( -8.314922557961024197, 14.29746914071037800, 67.91775706135234714 ) ) ;
#153224=CARTESIAN_POINT ( 'NONE',  ( 13.97604488694527802, 13.89961937509977652, 29.37390960531435979 ) ) ;
#153226=CARTESIAN_POINT ( 'NONE',  ( -14.29746914071049879, 8.314922557960819915, 40.83224293864769550 ) ) ;
#153227=CARTESIAN_POINT ( 'NONE',  ( -16.51473224551069308, -9.474510206698971260, 111.6655762719810383 ) ) ;
#153228=CARTESIAN_POINT ( 'NONE',  ( 16.51473224551069308, 9.474510206698969483, 94.16557627198103830 ) ) ;
#153229=CARTESIAN_POINT ( 'NONE',  ( -18.62759615963270932, 10.81492255796079327, 25.83224293864769194 ) ) ;
#153231=CARTESIAN_POINT ( 'NONE',  ( -16.53943276465976808, 0.05219959533911058130, 61.24890960531435979 ) ) ;
#153232=CARTESIAN_POINT ( 'NONE',  ( -0.05219959533910754901, -16.53943276465976808, 32.49890960531435979 ) ) ;
#153234=CARTESIAN_POINT ( 'NONE',  ( -16.52544592524342804, 4.483927247898546575, 56.04057627198102409 ) ) ;
#153235=CARTESIAN_POINT ( 'NONE',  ( -16.55341960407617563, 4.379528057220093196, 43.54275706135235424 ) ) ;
#153237=CARTESIAN_POINT ( 'NONE',  ( 5.049401038297881783, 19.05341960407617563, 47.29275706135231161 ) ) ;
#153238=CARTESIAN_POINT ( 'NONE',  ( -13.97604488694527625, -13.89961937509977652, 91.87390960531432427 ) ) ;
#153239=CARTESIAN_POINT ( 'NONE',  ( 19.02544592524334988, 5.153800228976608722, 66.45942372801899012 ) ) ;
#153241=CARTESIAN_POINT ( 'NONE',  ( -19.03943276465977164, -0.05219959533935918106, 58.75109039468566863 ) ) ;
#153242=CARTESIAN_POINT ( 'NONE',  ( 0.05219959533936267826, -19.03943276465977164, 95.00109039468567573 ) ) ;
#153243=CARTESIAN_POINT ( 'NONE',  ( 14.29746914071037800, 8.314922557961029526, 76.66775706135234714 ) ) ;
#153246=CARTESIAN_POINT ( 'NONE',  ( -0.05219959533909027116, -19.03943276465977164, 27.49890960531435624 ) ) ;
#153247=CARTESIAN_POINT ( 'NONE',  ( 15.80617190586746368, 15.72974639402197994, 24.37390960531435979 ) ) ;
#153248=CARTESIAN_POINT ( 'NONE',  ( -21.55341960407619339, 5.719274019375674811, 38.54275706135234714 ) ) ;
#153249=CARTESIAN_POINT ( 'NONE',  ( -19.05341960407617563, 5.049401038297882671, 108.5427570613523187 ) ) ;
#153250=CARTESIAN_POINT ( 'NONE',  ( 17.49999999999999645, -4.640572885337595821, 108.1378816454884060 ) ) ;
#153251=CARTESIAN_POINT ( 'NONE',  ( 9.474510206698971260, -16.51473224551069308, 67.91557627198102409 ) ) ;
#153252=CARTESIAN_POINT ( 'NONE',  ( 19.03943276465977164, -0.05219959533909143690, 103.7489096053143669 ) ) ;
#153253=CARTESIAN_POINT ( 'NONE',  ( 16.55341960407611168, 4.379528057220329451, 68.95724293864769550 ) ) ;
#153254=CARTESIAN_POINT ( 'NONE',  ( -5.153800228976328057, -19.02544592524343514, 62.29057627198100988 ) ) ;
#153255=CARTESIAN_POINT ( 'NONE',  ( 16.46253265017160672, -9.564922557960803928, 68.33224293864770971 ) ) ;
#153256=CARTESIAN_POINT ( 'NONE',  ( 16.46253265017146816, 9.564922557961045513, 76.66775706135234714 ) ) ;
#153257=CARTESIAN_POINT ( 'NONE',  ( 15.80617190586746368, 15.72974639402197994, 49.37390960531436690 ) ) ;
#153258=CARTESIAN_POINT ( 'NONE',  ( -12.06949235617756955, 12.14591786802309770, 110.6239096053143669 ) ) ;
#153259=CARTESIAN_POINT ( 'NONE',  ( 19.03943276465977164, 0.05219959533936151252, 46.25109039468566863 ) ) ;
#153260=CARTESIAN_POINT ( 'NONE',  ( 9.474510206698971260, -16.51473224551069308, 82.91557627198103830 ) ) ;
#153262=CARTESIAN_POINT ( 'NONE',  ( -5.823673210054116645, -21.52544592524344225, 82.29057627198103830 ) ) ;
#153263=CARTESIAN_POINT ( 'NONE',  ( -4.379528057220328563, 16.55341960407611168, 75.20724293864769550 ) ) ;
#153264=CARTESIAN_POINT ( 'NONE',  ( 9.474510206698729675, 16.51473224551082808, 32.08442372801900433 ) ) ;
#153265=CARTESIAN_POINT ( 'NONE',  ( -10.81492255796078084, -18.62759615963271287, 72.08224293864769550 ) ) ;
#153266=CARTESIAN_POINT ( 'NONE',  ( -5.823673210054116645, -21.52544592524344225, 62.29057627198102409 ) ) ;
#153267=CARTESIAN_POINT ( 'NONE',  ( -21.53943276465977519, 0.05219959533907696930, 46.24890960531435979 ) ) ;
#153268=CARTESIAN_POINT ( 'NONE',  ( -21.52544592524334988, -5.823673210054445271, 88.95942372801901854 ) ) ;
#153269=CARTESIAN_POINT ( 'NONE',  ( 9.474510206698971260, -16.51473224551069308, 72.91557627198102409 ) ) ;
#153270=CARTESIAN_POINT ( 'NONE',  ( -9.564922557960796823, -16.46253265017161027, 22.08224293864768839 ) ) ;
#153272=CARTESIAN_POINT ( 'NONE',  ( 18.62759615963255655, 10.81492255796105972, 21.66775706135235069 ) ) ;
#153274=CARTESIAN_POINT ( 'NONE',  ( -10.81492255796105439, 18.62759615963255655, 42.91775706135235424 ) ) ;
#153275=CARTESIAN_POINT ( 'NONE',  ( 9.474510206698971260, -16.51473224551069308, 32.91557627198102409 ) ) ;
#153276=CARTESIAN_POINT ( 'NONE',  ( -10.72451020669898014, 18.67979575497178502, 110.4155762719810383 ) ) ;
#153277=CARTESIAN_POINT ( 'NONE',  ( 5.153800228976615827, -19.02544592524334988, 50.20942372801897591 ) ) ;
#153278=CARTESIAN_POINT ( 'NONE',  ( -13.97604488694527625, -13.89961937509977652, 31.87390960531435979 ) ) ;
#153281=CARTESIAN_POINT ( 'NONE',  ( -8.224510206698735004, -14.34966873604973081, 59.58442372801901854 ) ) ;
#153282=CARTESIAN_POINT ( 'NONE',  ( -5.153800228976328057, -19.02544592524343514, 32.29057627198102409 ) ) ;
#153284=CARTESIAN_POINT ( 'NONE',  ( 9.564922557960805705, 16.46253265017160317, 79.58224293864769550 ) ) ;
#153285=CARTESIAN_POINT ( 'NONE',  ( 0.05219959533910956823, 16.53943276465976808, 109.9989096053143527 ) ) ;
#153286=CARTESIAN_POINT ( 'NONE',  ( 18.62759615963271287, -10.81492255796078972, 53.33224293864769550 ) ) ;
#153287=CARTESIAN_POINT ( 'NONE',  ( -12.06949235617739369, -12.14591786802326823, 49.37609039468569705 ) ) ;
#153288=CARTESIAN_POINT ( 'NONE',  ( 5.823673210054444382, -21.52544592524334988, 95.20942372801903275 ) ) ;
#153289=CARTESIAN_POINT ( 'NONE',  ( -9.474510206698964154, 16.51473224551069663, 30.41557627198102054 ) ) ;
#153290=CARTESIAN_POINT ( 'NONE',  ( 8.224510206698953496, -14.34966873604960469, 22.91557627198102765 ) ) ;
#153291=CARTESIAN_POINT ( 'NONE',  ( -16.55341960407611168, -4.379528057220339221, 51.45724293864770260 ) ) ;
#153292=CARTESIAN_POINT ( 'NONE',  ( -9.564922557960796823, -16.46253265017161027, 57.08224293864769550 ) ) ;
#153293=CARTESIAN_POINT ( 'NONE',  ( 15.80617190586769283, -15.72974639402175789, 110.6260903946857042 ) ) ;
#153294=CARTESIAN_POINT ( 'NONE',  ( 5.823673210054444382, -21.52544592524334988, 25.20942372801901854 ) ) ;
#153295=CARTESIAN_POINT ( 'NONE',  ( -15.80617190586768217, 15.72974639402176855, 78.12609039468570415 ) ) ;
#153296=CARTESIAN_POINT ( 'NONE',  ( 12.14591786802327356, -12.06949235617739191, 55.62609039468568284 ) ) ;
#153297=CARTESIAN_POINT ( 'NONE',  ( -14.34966873604972548, 8.224510206698743886, 33.33442372801900433 ) ) ;
#153298=CARTESIAN_POINT ( 'NONE',  ( 16.52544592524342804, -4.483927247898539470, 73.54057627198102409 ) ) ;
#153299=CARTESIAN_POINT ( 'NONE',  ( -15.72974639402176322, -15.80617190586768395, 104.3760903946856899 ) ) ;
#153300=CARTESIAN_POINT ( 'NONE',  ( 14.29746914071049879, -8.314922557960816363, 38.33224293864768839 ) ) ;
#153302=CARTESIAN_POINT ( 'NONE',  ( -4.379528057220086978, -16.55341960407618274, 34.79275706135235424 ) ) ;
#153303=CARTESIAN_POINT ( 'NONE',  ( -16.53943276465976808, 0.05219959533911058130, 41.24890960531435269 ) ) ;
#153304=CARTESIAN_POINT ( 'NONE',  ( -14.34966873604972548, 8.224510206698743886, 88.33442372801901854 ) ) ;
#153305=CARTESIAN_POINT ( 'NONE',  ( 19.03943276465977164, -0.05219959533909143690, 98.74890960531436690 ) ) ;
#153306=CARTESIAN_POINT ( 'NONE',  ( -13.89961937509977652, 13.97604488694528158, 115.6239096053143669 ) ) ;
#153307=CARTESIAN_POINT ( 'NONE',  ( 21.55341960407619695, -5.719274019375665929, 96.04275706135236135 ) ) ;
#153308=CARTESIAN_POINT ( 'NONE',  ( 0.05219959533934541429, -16.53943276465976808, 100.0010903946857042 ) ) ;
#153309=CARTESIAN_POINT ( 'NONE',  ( 4.379528057220339221, -16.55341960407611168, 72.70724293864769550 ) ) ;
#153310=CARTESIAN_POINT ( 'NONE',  ( -19.05341960407611168, -5.049401038298163336, 86.45724293864769550 ) ) ;
#153312=CARTESIAN_POINT ( 'NONE',  ( 12.06949235617739724, 12.14591786802326823, 41.87609039468568284 ) ) ;
#153313=CARTESIAN_POINT ( 'NONE',  ( 9.474510206698971260, -16.51473224551069308, 37.91557627198102409 ) ) ;
#153314=CARTESIAN_POINT ( 'NONE',  ( -9.474510206698964154, 16.51473224551069663, 100.4155762719810241 ) ) ;
#153315=CARTESIAN_POINT ( 'NONE',  ( 12.06949235617739724, 12.14591786802326823, 36.87609039468568994 ) ) ;
#153317=CARTESIAN_POINT ( 'NONE',  ( -19.02544592524334988, -5.153800228976617603, 28.95942372801900433 ) ) ;
#153318=CARTESIAN_POINT ( 'NONE',  ( -4.483927247898782831, 16.52544592524335698, 102.7094237280190185 ) ) ;
#153319=CARTESIAN_POINT ( 'NONE',  ( -13.89961937509977652, 13.97604488694528158, 35.62390960531435269 ) ) ;
#153320=CARTESIAN_POINT ( 'NONE',  ( -0.05219959533934338120, 16.53943276465976808, 72.50109039468568994 ) ) ;
#153321=CARTESIAN_POINT ( 'NONE',  ( -0.05219959533936034679, 19.03943276465977164, 87.50109039468567573 ) ) ;
#153322=CARTESIAN_POINT ( 'NONE',  ( -13.97604488694547697, 13.89961937509957934, 33.12609039468566863 ) ) ;
#153323=CARTESIAN_POINT ( 'NONE',  ( 0.05219959533909260263, 19.03943276465977164, 59.99890960531436690 ) ) ;
#153324=CARTESIAN_POINT ( 'NONE',  ( -4.483927247898539470, -16.52544592524342804, 92.29057627198103830 ) ) ;
#153325=CARTESIAN_POINT ( 'NONE',  ( 13.89961937509957401, 13.97604488694547697, 56.87609039468564731 ) ) ;
#153326=CARTESIAN_POINT ( 'NONE',  ( -5.719274019375978568, 21.55341960407610458, 55.20724293864770260 ) ) ;
#153327=CARTESIAN_POINT ( 'NONE',  ( -5.153800228976607833, 19.02544592524334988, 22.70942372801899012 ) ) ;
#153328=CARTESIAN_POINT ( 'NONE',  ( -13.89961937509977652, 13.97604488694528158, 110.6239096053143243 ) ) ;
#153330=CARTESIAN_POINT ( 'NONE',  ( -15.72974639402197994, 15.80617190586746368, 70.62390960531436690 ) ) ;
#153331=CARTESIAN_POINT ( 'NONE',  ( 16.46253265017160672, -9.564922557960803928, 113.3322429386476955 ) ) ;
#153332=CARTESIAN_POINT ( 'NONE',  ( 16.46253265017146816, 9.564922557961045513, 96.66775706135233293 ) ) ;
#153333=CARTESIAN_POINT ( 'NONE',  ( -17.49999999999998934, 3.209263204892635724, 109.7619682560626870 ) ) ;
#153334=CARTESIAN_POINT ( 'NONE',  ( 16.55341960407618274, -4.379528057220086978, 26.04275706135235779 ) ) ;
#153335=CARTESIAN_POINT ( 'NONE',  ( 19.05341960407611168, 5.049401038298154454, 38.95724293864767418 ) ) ;
#153336=CARTESIAN_POINT ( 'NONE',  ( -13.97604488694527625, -13.89961937509977652, 101.8739096053143811 ) ) ;
#153337=CARTESIAN_POINT ( 'NONE',  ( -15.72974639402197994, 15.80617190586746368, 75.62390960531439532 ) ) ;
#153338=CARTESIAN_POINT ( 'NONE',  ( 12.14591786802327356, -12.06949235617739191, 55.62609039468568284 ) ) ;
#153339=CARTESIAN_POINT ( 'NONE',  ( 18.62759615963255655, 10.81492255796105972, 61.66775706135235424 ) ) ;
#153340=CARTESIAN_POINT ( 'NONE',  ( 5.153800228976615827, -19.02544592524334988, 100.2094237280190043 ) ) ;
#153341=CARTESIAN_POINT ( 'NONE',  ( 5.823673210054444382, -21.52544592524334988, 110.2094237280190185 ) ) ;
#153342=CARTESIAN_POINT ( 'NONE',  ( 14.29746914071049879, -8.314922557960816363, 23.33224293864769194 ) ) ;
#153343=CARTESIAN_POINT ( 'NONE',  ( 15.80617190586746368, 15.72974639402197994, 94.37390960531436690 ) ) ;
#153344=CARTESIAN_POINT ( 'NONE',  ( 16.53943276465976808, -0.05219959533910856209, 38.74890960531435979 ) ) ;
#153345=CARTESIAN_POINT ( 'NONE',  ( 19.05341960407617918, -5.049401038297876454, 86.04275706135233293 ) ) ;
#153346=CARTESIAN_POINT ( 'NONE',  ( -0.05219959533937732626, 21.53943276465977519, 52.50109039468567573 ) ) ;
#153347=CARTESIAN_POINT ( 'NONE',  ( -19.03943276465977164, -0.05219959533935918106, 38.75109039468566152 ) ) ;
#153348=CARTESIAN_POINT ( 'NONE',  ( -8.314922557960811034, -14.29746914071050412, 107.0822429386476955 ) ) ;
#153349=CARTESIAN_POINT ( 'NONE',  ( -5.719274019375978568, 21.55341960407610458, 30.20724293864769550 ) ) ;
#153350=CARTESIAN_POINT ( 'NONE',  ( 4.483927247898545687, 16.52544592524342804, 34.79057627198103120 ) ) ;
#153352=CARTESIAN_POINT ( 'NONE',  ( 10.72451020669871369, 18.67979575497193778, 102.0844237280190185 ) ) ;
#153353=CARTESIAN_POINT ( 'NONE',  ( 16.52544592524335698, 4.483927247898782831, 66.45942372801903275 ) ) ;
#153354=CARTESIAN_POINT ( 'NONE',  ( 16.53943276465976808, -0.05219959533910856209, 23.74890960531435269 ) ) ;
#153355=CARTESIAN_POINT ( 'NONE',  ( 21.55341960407619695, -5.719274019375665929, 61.04275706135234714 ) ) ;
#153356=CARTESIAN_POINT ( 'NONE',  ( -18.67979575497193778, 10.72451020669871902, 58.33442372801901143 ) ) ;
#153357=ORIENTED_EDGE ( 'NONE', *, *, #147777, .F. ) ;
#153358=CARTESIAN_POINT ( 'NONE',  ( -5.049401038298153566, 19.05341960407611168, 25.20724293864768484 ) ) ;
#153359=CARTESIAN_POINT ( 'NONE',  ( -18.62759615963255300, -10.81492255796106328, 39.16775706135235424 ) ) ;
#153360=CARTESIAN_POINT ( 'NONE',  ( 9.474510206698971260, -16.51473224551069308, 27.91557627198103120 ) ) ;
#153361=CARTESIAN_POINT ( 'NONE',  ( 16.51473224551069308, 9.474510206698969483, 44.16557627198103120 ) ) ;
#153362=CARTESIAN_POINT ( 'NONE',  ( -16.52544592524342804, 4.483927247898546575, 76.04057627198102409 ) ) ;
#153363=CARTESIAN_POINT ( 'NONE',  ( -16.51473224551069308, -9.474510206698971260, 76.66557627198103830 ) ) ;
#153364=CARTESIAN_POINT ( 'NONE',  ( 4.379528057220339221, -16.55341960407611168, 32.70724293864770260 ) ) ;
#153365=CARTESIAN_POINT ( 'NONE',  ( -5.719274019375978568, 21.55341960407610458, 55.20724293864770260 ) ) ;
#153366=CARTESIAN_POINT ( 'NONE',  ( -4.483927247898539470, -16.52544592524342804, 92.29057627198103830 ) ) ;
#153368=CARTESIAN_POINT ( 'NONE',  ( 21.55341960407610458, 5.719274019375980345, 103.9572429386476813 ) ) ;
#153369=CARTESIAN_POINT ( 'NONE',  ( -0.05219959533909027116, -19.03943276465977164, 97.49890960531436690 ) ) ;
#153370=CARTESIAN_POINT ( 'NONE',  ( -16.51473224551069308, -9.474510206698971260, 61.66557627198103120 ) ) ;
#153371=CARTESIAN_POINT ( 'NONE',  ( -19.05341960407617563, 5.049401038297882671, 103.5427570613523329 ) ) ;
#153372=CARTESIAN_POINT ( 'NONE',  ( -21.52544592524343514, 5.823673210054127303, 56.04057627198102409 ) ) ;
#153373=CARTESIAN_POINT ( 'NONE',  ( -5.719274019375665041, -21.55341960407619695, 79.79275706135236135 ) ) ;
#153374=CARTESIAN_POINT ( 'NONE',  ( -13.97604488694527625, -13.89961937509977652, 66.87390960531436690 ) ) ;
#153375=CARTESIAN_POINT ( 'NONE',  ( -5.153800228976328057, -19.02544592524343514, 97.29057627198099567 ) ) ;
#153376=CARTESIAN_POINT ( 'NONE',  ( 16.53943276465976808, 0.05219959533934440121, 81.25109039468568994 ) ) ;
#153377=CARTESIAN_POINT ( 'NONE',  ( 18.67979575497194134, -10.72451020669871369, 60.83442372801901854 ) ) ;
#153378=CARTESIAN_POINT ( 'NONE',  ( -0.05219959533937732626, 21.53943276465977519, 92.50109039468567573 ) ) ;
#153379=CARTESIAN_POINT ( 'NONE',  ( -18.62759615963270932, 10.81492255796079327, 110.8322429386476955 ) ) ;
#153381=CARTESIAN_POINT ( 'NONE',  ( 12.14591786802327356, -12.06949235617739191, 80.62609039468567573 ) ) ;
#153382=CARTESIAN_POINT ( 'NONE',  ( -10.81492255796078084, -18.62759615963271287, 72.08224293864769550 ) ) ;
#153383=CARTESIAN_POINT ( 'NONE',  ( 19.05341960407617918, -5.049401038297876454, 46.04275706135233293 ) ) ;
#153384=CARTESIAN_POINT ( 'NONE',  ( 15.72974639402199770, -15.80617190586745480, 43.12390960531435269 ) ) ;
#153386=CARTESIAN_POINT ( 'NONE',  ( -13.89961937509977652, 13.97604488694528158, 75.62390960531438111 ) ) ;
#153387=CARTESIAN_POINT ( 'NONE',  ( 8.224510206698953496, -14.34966873604960469, 22.91557627198102765 ) ) ;
#153389=CARTESIAN_POINT ( 'NONE',  ( 14.29746914071049879, -8.314922557960816363, 38.33224293864768839 ) ) ;
#153390=CARTESIAN_POINT ( 'NONE',  ( 10.72451020669898902, -18.67979575497178502, 22.91557627198102765 ) ) ;
#153393=CARTESIAN_POINT ( 'NONE',  ( -5.049401038297874678, -19.05341960407617918, 94.79275706135230450 ) ) ;
#153394=CARTESIAN_POINT ( 'NONE',  ( 18.67979575497178502, 10.72451020669898547, 69.16557627198102409 ) ) ;
#153395=CARTESIAN_POINT ( 'NONE',  ( -8.224510206698948167, 14.34966873604960824, 55.41557627198102409 ) ) ;
#153396=CARTESIAN_POINT ( 'NONE',  ( 16.53943276465976808, 0.05219959533934440121, 21.25109039468567218 ) ) ;
#153397=CARTESIAN_POINT ( 'NONE',  ( 13.97604488694527802, 13.89961937509977652, 49.37390960531434558 ) ) ;
#153398=CARTESIAN_POINT ( 'NONE',  ( 21.53943276465977519, -0.05219959533907433946, 98.74890960531438111 ) ) ;
#153399=CARTESIAN_POINT ( 'NONE',  ( -5.049401038297874678, -19.05341960407617918, 74.79275706135231871 ) ) ;
#153400=CARTESIAN_POINT ( 'NONE',  ( 13.89961937509977652, -13.97604488694527269, 88.12390960531438111 ) ) ;
#153401=CARTESIAN_POINT ( 'NONE',  ( -12.06949235617756955, 12.14591786802309770, 80.62390960531438111 ) ) ;
#153402=CARTESIAN_POINT ( 'NONE',  ( 16.46253265017160672, -9.564922557960803928, 63.33224293864769550 ) ) ;
#153403=CARTESIAN_POINT ( 'NONE',  ( -0.05219959533910754901, -16.53943276465976808, 72.49890960531435269 ) ) ;
#153404=CARTESIAN_POINT ( 'NONE',  ( -13.89961937509977652, 13.97604488694528158, 30.62390960531435269 ) ) ;
#153406=CARTESIAN_POINT ( 'NONE',  ( -8.314922557960811034, -14.29746914071050412, 47.08224293864770260 ) ) ;
#153407=CARTESIAN_POINT ( 'NONE',  ( 16.51473224551069308, 9.474510206698969483, 94.16557627198103830 ) ) ;
#153409=CARTESIAN_POINT ( 'NONE',  ( -13.97604488694547697, 13.89961937509957934, 53.12609039468565442 ) ) ;
#153410=CARTESIAN_POINT ( 'NONE',  ( 16.52544592524335698, 4.483927247898782831, 61.45942372801901854 ) ) ;
#153411=CARTESIAN_POINT ( 'NONE',  ( -21.53943276465977519, 0.05219959533907696930, 61.24890960531435979 ) ) ;
#153412=CARTESIAN_POINT ( 'NONE',  ( -13.97604488694547697, 13.89961937509957934, 43.12609039468566152 ) ) ;
#153413=CARTESIAN_POINT ( 'NONE',  ( 13.89961937509977652, -13.97604488694527269, 93.12390960531436690 ) ) ;
#153415=CARTESIAN_POINT ( 'NONE',  ( 21.55341960407610458, 5.719274019375980345, 28.95724293864769905 ) ) ;
#153417=CARTESIAN_POINT ( 'NONE',  ( -19.03943276465977164, 0.05219959533909376836, 56.24890960531435979 ) ) ;
#153418=CARTESIAN_POINT ( 'NONE',  ( -21.55341960407619339, 5.719274019375674811, 58.54275706135235424 ) ) ;
#153420=CARTESIAN_POINT ( 'NONE',  ( -4.379528057220328563, 16.55341960407611168, 115.2072429386476955 ) ) ;
#153421=CARTESIAN_POINT ( 'NONE',  ( 21.55341960407610458, 5.719274019375980345, 98.95724293864770971 ) ) ;
#153422=CARTESIAN_POINT ( 'NONE',  ( 19.03943276465977164, -0.05219959533909143690, 88.74890960531436690 ) ) ;
#153424=CARTESIAN_POINT ( 'NONE',  ( 21.55341960407619695, -5.719274019375665929, 36.04275706135234714 ) ) ;
#153425=ORIENTED_EDGE ( 'NONE', *, *, #169539, .T. ) ;
#153426=CARTESIAN_POINT ( 'NONE',  ( -9.564922557960796823, -16.46253265017161027, 102.0822429386477097 ) ) ;
#153428=CARTESIAN_POINT ( 'NONE',  ( -0.05219959533907301413, -21.53943276465977519, 107.4989096053143669 ) ) ;
#153429=CARTESIAN_POINT ( 'NONE',  ( -16.51473224551069308, -9.474510206698971260, 51.66557627198102409 ) ) ;
#153430=CARTESIAN_POINT ( 'NONE',  ( -16.55341960407617563, 4.379528057220093196, 23.54275706135235424 ) ) ;
#153432=CARTESIAN_POINT ( 'NONE',  ( 19.03943276465977164, -0.05219959533909143690, 23.74890960531435269 ) ) ;
#153433=CARTESIAN_POINT ( 'NONE',  ( -10.72451020669870658, -18.67979575497194134, 94.58442372801901854 ) ) ;
#153434=CARTESIAN_POINT ( 'NONE',  ( 5.049401038298161559, -19.05341960407611168, 77.70724293864765286 ) ) ;
#153435=CARTESIAN_POINT ( 'NONE',  ( -21.55341960407619339, 5.719274019375674811, 48.54275706135234714 ) ) ;
#153437=CARTESIAN_POINT ( 'NONE',  ( -9.564922557960796823, -16.46253265017161027, 102.0822429386477097 ) ) ;
#153439=CARTESIAN_POINT ( 'NONE',  ( -4.483927247898782831, 16.52544592524335698, 37.70942372801900433 ) ) ;
#153440=CARTESIAN_POINT ( 'NONE',  ( -4.379528057220086978, -16.55341960407618274, 74.79275706135234714 ) ) ;
#153441=CARTESIAN_POINT ( 'NONE',  ( -18.62759615963255300, -10.81492255796106328, 54.16775706135235424 ) ) ;
#153442=CARTESIAN_POINT ( 'NONE',  ( -5.719274019375665041, -21.55341960407619695, 84.79275706135234714 ) ) ;
#153444=CARTESIAN_POINT ( 'NONE',  ( 4.483927247898790824, -16.52544592524335698, 20.20942372801900788 ) ) ;
#153445=CARTESIAN_POINT ( 'NONE',  ( -13.89961937509977652, 13.97604488694528158, 70.62390960531432427 ) ) ;
#153446=CARTESIAN_POINT ( 'NONE',  ( -19.03943276465977164, 0.05219959533909376836, 96.24890960531436690 ) ) ;
#153447=CARTESIAN_POINT ( 'NONE',  ( -16.52544592524342804, 4.483927247898546575, 106.0405762719810525 ) ) ;
#153448=CARTESIAN_POINT ( 'NONE',  ( -15.80617190586745835, -15.72974639402198527, 26.87390960531435979 ) ) ;
#153449=CARTESIAN_POINT ( 'NONE',  ( 16.55341960407618274, -4.379528057220086978, 91.04275706135236135 ) ) ;
#153450=CARTESIAN_POINT ( 'NONE',  ( -16.53943276465976808, 0.05219959533911058130, 76.24890960531435269 ) ) ;
#153451=CARTESIAN_POINT ( 'NONE',  ( 19.02544592524343514, -5.153800228976328945, 53.54057627198102409 ) ) ;
#153452=CARTESIAN_POINT ( 'NONE',  ( -5.719274019375665041, -21.55341960407619695, 74.79275706135234714 ) ) ;
#153454=CARTESIAN_POINT ( 'NONE',  ( 19.03943276465977164, 0.05219959533936151252, 101.2510903946856757 ) ) ;
#153455=CARTESIAN_POINT ( 'NONE',  ( -4.379528057220328563, 16.55341960407611168, 75.20724293864769550 ) ) ;
#153456=CARTESIAN_POINT ( 'NONE',  ( 0.05219959533937995610, -21.53943276465977519, 35.00109039468568284 ) ) ;
#153457=CARTESIAN_POINT ( 'NONE',  ( -21.53943276465977519, 0.05219959533907696930, 56.24890960531436690 ) ) ;
#153459=CARTESIAN_POINT ( 'NONE',  ( -16.61371651742599553, -7.165104196376157475, 106.1458493000700685 ) ) ;
#153461=CARTESIAN_POINT ( 'NONE',  ( -13.97604488694527625, -13.89961937509977652, 86.87390960531436690 ) ) ;
#153462=CARTESIAN_POINT ( 'NONE',  ( 0.05219959533910956823, 16.53943276465976808, 54.99890960531435269 ) ) ;
#153463=CARTESIAN_POINT ( 'NONE',  ( 4.379528057220339221, -16.55341960407611168, 32.70724293864770260 ) ) ;
#153464=CARTESIAN_POINT ( 'NONE',  ( -16.53943276465976808, -0.05219959533934237506, 93.75109039468567573 ) ) ;
#153465=CARTESIAN_POINT ( 'NONE',  ( -5.049401038297874678, -19.05341960407617918, 54.79275706135234003 ) ) ;
#153466=LINE ( 'NONE', #2766, #166758 ) ;
#153467=CARTESIAN_POINT ( 'NONE',  ( -13.89961937509977652, 13.97604488694528158, 100.6239096053143669 ) ) ;
#153469=CARTESIAN_POINT ( 'NONE',  ( 16.52544592524342804, -4.483927247898539470, 78.54057627198103830 ) ) ;
#153470=CARTESIAN_POINT ( 'NONE',  ( -13.97604488694547697, 13.89961937509957934, 38.12609039468566152 ) ) ;
#153471=CARTESIAN_POINT ( 'NONE',  ( 5.049401038298161559, -19.05341960407611168, 37.70724293864768839 ) ) ;
#153472=CARTESIAN_POINT ( 'NONE',  ( -15.80617190586745835, -15.72974639402198527, 36.87390960531435979 ) ) ;
#153473=CARTESIAN_POINT ( 'NONE',  ( -21.55341960407610458, -5.719274019375992779, 61.45724293864770260 ) ) ;
#153474=CARTESIAN_POINT ( 'NONE',  ( -14.34966873604960291, -8.224510206698953496, 96.66557627198102409 ) ) ;
#153475=CARTESIAN_POINT ( 'NONE',  ( 4.379528057220092307, 16.55341960407617563, 57.29275706135234714 ) ) ;
#153476=CARTESIAN_POINT ( 'NONE',  ( -10.72451020669870658, -18.67979575497194134, 39.58442372801901143 ) ) ;
#153477=CARTESIAN_POINT ( 'NONE',  ( 8.224510206698953496, -14.34966873604960469, 97.91557627198103830 ) ) ;
#153478=CARTESIAN_POINT ( 'NONE',  ( 16.61371651742597777, -7.165104196376268497, 36.35415069992995996 ) ) ;
#153479=CARTESIAN_POINT ( 'NONE',  ( -16.52216118717209170, 7.221426719304505859, 48.92400978953009627 ) ) ;
#153480=CARTESIAN_POINT ( 'NONE',  ( 0.05219959533907565091, 21.53943276465977519, 39.99890960531436690 ) ) ;
#153483=CARTESIAN_POINT ( 'NONE',  ( -12.14591786802326823, 12.06949235617739902, 38.12609039468567573 ) ) ;
#153484=CARTESIAN_POINT ( 'NONE',  ( 4.483927247898545687, 16.52544592524342804, 34.79057627198103120 ) ) ;
#153485=CARTESIAN_POINT ( 'NONE',  ( -5.719274019375978568, 21.55341960407610458, 65.20724293864768129 ) ) ;
#153486=CARTESIAN_POINT ( 'NONE',  ( -13.97604488694547697, 13.89961937509957934, 88.12609039468563310 ) ) ;
#153487=CARTESIAN_POINT ( 'NONE',  ( -10.81492255796078084, -18.62759615963271287, 67.08224293864770971 ) ) ;
#153489=CARTESIAN_POINT ( 'NONE',  ( -4.483927247898782831, 16.52544592524335698, 52.70942372801902565 ) ) ;
#153490=CARTESIAN_POINT ( 'NONE',  ( 13.97604488694527802, 13.89961937509977652, 34.37390960531436690 ) ) ;
#153491=CARTESIAN_POINT ( 'NONE',  ( 5.153800228976335163, 19.02544592524342804, 99.79057627198102409 ) ) ;
#153492=CARTESIAN_POINT ( 'NONE',  ( 5.153800228976335163, 19.02544592524342804, 39.79057627198100988 ) ) ;
#153493=CARTESIAN_POINT ( 'NONE',  ( -13.89961937509977652, 13.97604488694528158, 25.62390960531434558 ) ) ;
#153496=CARTESIAN_POINT ( 'NONE',  ( -0.05219959533934338120, 16.53943276465976808, 72.50109039468568994 ) ) ;
#153497=CARTESIAN_POINT ( 'NONE',  ( 0.05219959533907565091, 21.53943276465977519, 94.99890960531436690 ) ) ;
#153498=CARTESIAN_POINT ( 'NONE',  ( 9.564922557960805705, 16.46253265017160317, 59.58224293864769550 ) ) ;
#153499=CARTESIAN_POINT ( 'NONE',  ( -15.80617190586768217, 15.72974639402176855, 23.12609039468567573 ) ) ;
#153500=CARTESIAN_POINT ( 'NONE',  ( 9.564922557960805705, 16.46253265017160317, 79.58224293864769550 ) ) ;
#153501=CARTESIAN_POINT ( 'NONE',  ( 19.03943276465977164, -0.05219959533909143690, 113.7489096053143669 ) ) ;
#153503=CARTESIAN_POINT ( 'NONE',  ( -18.67979575497193778, 10.72451020669871902, 23.33442372801901499 ) ) ;
#153504=CARTESIAN_POINT ( 'NONE',  ( 19.05341960407611168, 5.049401038298154454, 28.95724293864769550 ) ) ;
#153505=CARTESIAN_POINT ( 'NONE',  ( -19.02544592524342804, 5.153800228976336051, 111.0405762719810099 ) ) ;
#153506=CARTESIAN_POINT ( 'NONE',  ( -16.46253265017146816, -9.564922557961047289, 89.16775706135234714 ) ) ;
#153507=CARTESIAN_POINT ( 'NONE',  ( -9.564922557961040184, 16.46253265017147172, 27.91775706135232582 ) ) ;
#153508=CARTESIAN_POINT ( 'NONE',  ( 0.05219959533907565091, 21.53943276465977519, 104.9989096053143669 ) ) ;
#153509=CARTESIAN_POINT ( 'NONE',  ( -9.474510206698720793, -16.51473224551083518, 29.58442372801900433 ) ) ;
#153510=CARTESIAN_POINT ( 'NONE',  ( 0.05219959533934541429, -16.53943276465976808, 75.00109039468568994 ) ) ;
#153511=CARTESIAN_POINT ( 'NONE',  ( 19.03943276465977164, -0.05219959533909143690, 108.7489096053143527 ) ) ;
#153512=CARTESIAN_POINT ( 'NONE',  ( -16.51473224551069308, -9.474510206698971260, 61.66557627198103120 ) ) ;
#153514=CARTESIAN_POINT ( 'NONE',  ( 18.67979575497194134, -10.72451020669871369, 65.83442372801900433 ) ) ;
#153515=CARTESIAN_POINT ( 'NONE',  ( 5.823673210054444382, -21.52544592524334988, 85.20942372801901854 ) ) ;
#153516=CARTESIAN_POINT ( 'NONE',  ( 16.51473224551069308, 9.474510206698969483, 114.1655762719810241 ) ) ;
#153517=CARTESIAN_POINT ( 'NONE',  ( -13.89961937509977652, 13.97604488694528158, 80.62390960531436690 ) ) ;
#153518=CARTESIAN_POINT ( 'NONE',  ( 18.62759615963255655, 10.81492255796105972, 51.66775706135234714 ) ) ;
#153519=CARTESIAN_POINT ( 'NONE',  ( -19.02544592524334988, -5.153800228976617603, 88.95942372801897591 ) ) ;
#153520=CARTESIAN_POINT ( 'NONE',  ( -16.51473224551069308, -9.474510206698971260, 46.66557627198102409 ) ) ;
#153521=CARTESIAN_POINT ( 'NONE',  ( -19.05341960407611168, -5.049401038298163336, 96.45724293864769550 ) ) ;
#153522=CARTESIAN_POINT ( 'NONE',  ( -19.03943276465977164, 0.05219959533909376836, 66.24890960531436690 ) ) ;
#153523=CARTESIAN_POINT ( 'NONE',  ( 17.50000000000000355, -3.786494350217929572, 22.85920472064934117 ) ) ;
#153524=CARTESIAN_POINT ( 'NONE',  ( 13.89961937509977652, -13.97604488694527269, 48.12390960531435979 ) ) ;
#153525=CARTESIAN_POINT ( 'NONE',  ( 15.72974639402199770, -15.80617190586745480, 93.12390960531436690 ) ) ;
#153526=CARTESIAN_POINT ( 'NONE',  ( -0.05219959533934338120, 16.53943276465976808, 87.50109039468568994 ) ) ;
#153528=CARTESIAN_POINT ( 'NONE',  ( 19.05341960407617918, -5.049401038297876454, 41.04275706135233293 ) ) ;
#153529=CARTESIAN_POINT ( 'NONE',  ( 19.05341960407611168, 5.049401038298154454, 78.95724293864769550 ) ) ;
#153530=CARTESIAN_POINT ( 'NONE',  ( -0.05219959533910754901, -16.53943276465976808, 62.49890960531436690 ) ) ;
#153531=CARTESIAN_POINT ( 'NONE',  ( 8.224510206698953496, -14.34966873604960469, 97.91557627198103830 ) ) ;
#153532=VECTOR ( 'NONE', #95038, 1000.000000000000000 ) ;
#153533=CARTESIAN_POINT ( 'NONE',  ( 9.474510206698971260, -16.51473224551069308, 112.9155762719810383 ) ) ;
#153534=CARTESIAN_POINT ( 'NONE',  ( 5.153800228976335163, 19.02544592524342804, 99.79057627198102409 ) ) ;
#153535=CARTESIAN_POINT ( 'NONE',  ( -13.97604488694527625, -13.89961937509977652, 111.8739096053143243 ) ) ;
#153536=CARTESIAN_POINT ( 'NONE',  ( 18.62759615963255655, 10.81492255796105972, 111.6677570613523613 ) ) ;
#153537=CARTESIAN_POINT ( 'NONE',  ( -16.52544592524335698, -4.483927247898792601, 88.95942372801901854 ) ) ;
#153538=CARTESIAN_POINT ( 'NONE',  ( 13.89961937509977652, -13.97604488694527269, 78.12390960531433848 ) ) ;
#153539=CARTESIAN_POINT ( 'NONE',  ( 21.55341960407619695, -5.719274019375665929, 41.04275706135236135 ) ) ;
#153540=CARTESIAN_POINT ( 'NONE',  ( -21.52544592524343514, 5.823673210054127303, 36.04057627198102409 ) ) ;
#153541=CARTESIAN_POINT ( 'NONE',  ( -18.67979575497178146, -10.72451020669898902, 111.6655762719810525 ) ) ;
#153542=CARTESIAN_POINT ( 'NONE',  ( -5.719274019375978568, 21.55341960407610458, 65.20724293864768129 ) ) ;
#153543=CARTESIAN_POINT ( 'NONE',  ( -12.06949235617756955, 12.14591786802309770, 75.62390960531439532 ) ) ;
#153544=CARTESIAN_POINT ( 'NONE',  ( -16.46253265017146816, -9.564922557961047289, 44.16775706135232582 ) ) ;
#153545=CARTESIAN_POINT ( 'NONE',  ( -16.51473224551069308, -9.474510206698971260, 36.66557627198102409 ) ) ;
#153546=CARTESIAN_POINT ( 'NONE',  ( 9.564922557960805705, 16.46253265017160317, 79.58224293864769550 ) ) ;
#153547=CARTESIAN_POINT ( 'NONE',  ( 5.049401038298161559, -19.05341960407611168, 77.70724293864765286 ) ) ;
#153549=CARTESIAN_POINT ( 'NONE',  ( -0.05219959533910754901, -16.53943276465976808, 97.49890960531436690 ) ) ;
#153551=CARTESIAN_POINT ( 'NONE',  ( -8.314922557960811034, -14.29746914071050412, 22.08224293864769194 ) ) ;
#153552=CARTESIAN_POINT ( 'NONE',  ( 12.14591786802327356, -12.06949235617739191, 30.62609039468567929 ) ) ;
#153553=CARTESIAN_POINT ( 'NONE',  ( 15.80617190586769283, -15.72974639402175789, 95.62609039468568994 ) ) ;
#153554=CARTESIAN_POINT ( 'NONE',  ( 16.46253265017160672, -9.564922557960803928, 103.3322429386476955 ) ) ;
#153555=CARTESIAN_POINT ( 'NONE',  ( 0.05219959533937995610, -21.53943276465977519, 25.00109039468567218 ) ) ;
#153556=CARTESIAN_POINT ( 'NONE',  ( -0.05219959533909027116, -19.03943276465977164, 37.49890960531436690 ) ) ;
#153557=CARTESIAN_POINT ( 'NONE',  ( -8.314922557961024197, 14.29746914071037800, 47.91775706135234714 ) ) ;
#153558=CARTESIAN_POINT ( 'NONE',  ( 5.153800228976615827, -19.02544592524334988, 105.2094237280190185 ) ) ;
#153559=EDGE_CURVE ( 'NONE', #99775, #76130, #198474, .T. ) ;
#153560=CARTESIAN_POINT ( 'NONE',  ( 21.53943276465977519, -0.05219959533907433946, 98.74890960531438111 ) ) ;
#153561=CARTESIAN_POINT ( 'NONE',  ( -16.51473224551082808, 9.474510206698731452, 63.33442372801900433 ) ) ;
#153563=CARTESIAN_POINT ( 'NONE',  ( -10.72451020669898014, 18.67979575497178502, 115.4155762719810241 ) ) ;
#153565=CARTESIAN_POINT ( 'NONE',  ( -16.51473224551069308, -9.474510206698971260, 96.66557627198102409 ) ) ;
#153567=CARTESIAN_POINT ( 'NONE',  ( 19.03943276465977164, -0.05219959533909143690, 78.74890960531436690 ) ) ;
#153568=CARTESIAN_POINT ( 'NONE',  ( 0.05219959533937995610, -21.53943276465977519, 30.00109039468568284 ) ) ;
#153569=CARTESIAN_POINT ( 'NONE',  ( 12.06949235617757843, -12.14591786802309237, 83.12390960531436690 ) ) ;
#153570=CARTESIAN_POINT ( 'NONE',  ( -5.153800228976328057, -19.02544592524343514, 87.29057627198103830 ) ) ;
#153571=CARTESIAN_POINT ( 'NONE',  ( -12.06949235617739369, -12.14591786802326823, 54.37609039468568994 ) ) ;
#153572=CARTESIAN_POINT ( 'NONE',  ( -9.474510206698720793, -16.51473224551083518, 54.58442372801899722 ) ) ;
#153573=CARTESIAN_POINT ( 'NONE',  ( 21.53943276465977519, 0.05219959533937863772, 66.25109039468567573 ) ) ;
#153574=CARTESIAN_POINT ( 'NONE',  ( -12.14591786802326823, 12.06949235617739902, 23.12609039468567573 ) ) ;
#153575=CARTESIAN_POINT ( 'NONE',  ( -9.564922557960796823, -16.46253265017161027, 67.08224293864769550 ) ) ;
#153576=CARTESIAN_POINT ( 'NONE',  ( 19.02544592524334988, 5.153800228976608722, 101.4594237280189759 ) ) ;
#153577=CARTESIAN_POINT ( 'NONE',  ( 16.52544592524335698, 4.483927247898782831, 51.45942372801901854 ) ) ;
#153578=CARTESIAN_POINT ( 'NONE',  ( -15.80617190586768217, 15.72974639402176855, 98.12609039468570415 ) ) ;
#153579=CARTESIAN_POINT ( 'NONE',  ( 13.97604488694548053, -13.89961937509957401, 85.62609039468568994 ) ) ;
#153580=CARTESIAN_POINT ( 'NONE',  ( -19.02544592524342804, 5.153800228976336051, 46.04057627198101699 ) ) ;
#153581=CARTESIAN_POINT ( 'NONE',  ( -21.53943276465977519, 0.05219959533907696930, 76.24890960531435269 ) ) ;
#153582=CARTESIAN_POINT ( 'NONE',  ( 4.379528057220339221, -16.55341960407611168, 77.70724293864770971 ) ) ;
#153583=CARTESIAN_POINT ( 'NONE',  ( -0.05219959533936034679, 19.03943276465977164, 82.50109039468567573 ) ) ;
#153584=CARTESIAN_POINT ( 'NONE',  ( -19.39056639909675539, -5.499999999999970690, 70.78948781074340957 ) ) ;
#153585=CARTESIAN_POINT ( 'NONE',  ( 19.03943276465977164, 0.05219959533936151252, 41.25109039468566152 ) ) ;
#153586=CARTESIAN_POINT ( 'NONE',  ( -16.53943276465976808, -0.05219959533934237506, 113.7510903946856757 ) ) ;
#153587=CARTESIAN_POINT ( 'NONE',  ( 0.05219959533910956823, 16.53943276465976808, 64.99890960531435269 ) ) ;
#153588=CARTESIAN_POINT ( 'NONE',  ( 21.53943276465977519, 0.05219959533937863772, 101.2510903946856757 ) ) ;
#153590=CARTESIAN_POINT ( 'NONE',  ( 18.67979575497178502, 10.72451020669898547, 114.1655762719810383 ) ) ;
#153591=CARTESIAN_POINT ( 'NONE',  ( -19.02544592524342804, 5.153800228976336051, 71.04057627198099567 ) ) ;
#153592=B_SPLINE_CURVE_WITH_KNOTS ( 'NONE', 3,
 ( #82341, #67193, #160206, #97505, #19702, #49056 ),
 .UNSPECIFIED., .F., .F.,
 ( 4, 2, 4 ),
 ( 0.003989672132298028098, 0.004372778065220449609, 0.004755883998142871986 ),
 .UNSPECIFIED. ) ;
#153593=CARTESIAN_POINT ( 'NONE',  ( 5.823673210054444382, -21.52544592524334988, 85.20942372801901854 ) ) ;
#153594=CARTESIAN_POINT ( 'NONE',  ( -19.02544592524342804, 5.153800228976336051, 61.04057627198103120 ) ) ;
#153596=CARTESIAN_POINT ( 'NONE',  ( 9.474510206698971260, -16.51473224551069308, 22.91557627198102765 ) ) ;
#153597=CARTESIAN_POINT ( 'NONE',  ( 15.80617190586746368, 15.72974639402197994, 34.37390960531435979 ) ) ;
#153599=CARTESIAN_POINT ( 'NONE',  ( -14.29746914071049879, 8.314922557960819915, 60.83224293864769550 ) ) ;
#153600=CARTESIAN_POINT ( 'NONE',  ( 9.564922557960805705, 16.46253265017160317, 39.58224293864768839 ) ) ;
#153601=CARTESIAN_POINT ( 'NONE',  ( 16.53943276465976808, -0.05219959533910856209, 88.74890960531436690 ) ) ;
#153603=CARTESIAN_POINT ( 'NONE',  ( 5.823673210054125526, 21.52544592524343514, 99.79057627198103830 ) ) ;
#153604=CARTESIAN_POINT ( 'NONE',  ( 0.05219959533937995610, -21.53943276465977519, 55.00109039468568284 ) ) ;
#153606=CARTESIAN_POINT ( 'NONE',  ( -14.29746914071037622, -8.314922557961029526, 54.16775706135235424 ) ) ;
#153607=CARTESIAN_POINT ( 'NONE',  ( 10.72451020669898902, -18.67979575497178502, 102.9155762719810383 ) ) ;
#153608=CARTESIAN_POINT ( 'NONE',  ( 9.564922557961047289, -16.46253265017146816, 25.41775706135234003 ) ) ;
#153609=CARTESIAN_POINT ( 'NONE',  ( -13.97604488694527625, -13.89961937509977652, 41.87390960531435979 ) ) ;
#153610=CARTESIAN_POINT ( 'NONE',  ( -5.153800228976328057, -19.02544592524343514, 102.2905762719810383 ) ) ;
#153611=CARTESIAN_POINT ( 'NONE',  ( -15.80617190586768217, 15.72974639402176855, 53.12609039468568284 ) ) ;
#153612=CARTESIAN_POINT ( 'NONE',  ( 21.52544592524344225, -5.823673210054117533, 48.54057627198103120 ) ) ;
#153613=CARTESIAN_POINT ( 'NONE',  ( 16.55341960407611168, 4.379528057220329451, 23.95724293864769550 ) ) ;
#153614=CARTESIAN_POINT ( 'NONE',  ( 18.62759615963255655, 10.81492255796105972, 66.66775706135234714 ) ) ;
#153615=CARTESIAN_POINT ( 'NONE',  ( 5.719274019375673035, 21.55341960407619339, 92.29275706135236135 ) ) ;
#153616=CARTESIAN_POINT ( 'NONE',  ( 19.03943276465977164, 0.05219959533936151252, 36.25109039468567573 ) ) ;
#153617=CARTESIAN_POINT ( 'NONE',  ( 8.314922557961029526, -14.29746914071037800, 95.41775706135234714 ) ) ;
#153618=CARTESIAN_POINT ( 'NONE',  ( 10.81492255796106328, -18.62759615963255655, 55.41775706135234714 ) ) ;
#153619=CARTESIAN_POINT ( 'NONE',  ( 16.46253265017160672, -9.564922557960803928, 43.33224293864769550 ) ) ;
#153620=CARTESIAN_POINT ( 'NONE',  ( 0.05219959533936267826, -19.03943276465977164, 20.00109039468567218 ) ) ;
#153621=CARTESIAN_POINT ( 'NONE',  ( 10.81492255796078972, 18.62759615963270932, 29.58224293864769905 ) ) ;
#153622=CARTESIAN_POINT ( 'NONE',  ( 5.823673210054444382, -21.52544592524334988, 20.20942372801900788 ) ) ;
#153623=CARTESIAN_POINT ( 'NONE',  ( 0.05219959533907565091, 21.53943276465977519, 69.99890960531435269 ) ) ;
#153624=CARTESIAN_POINT ( 'NONE',  ( 12.06949235617739724, 12.14591786802326823, 41.87609039468568284 ) ) ;
#153626=CARTESIAN_POINT ( 'NONE',  ( -21.52544592524343514, 5.823673210054127303, 81.04057627198102409 ) ) ;
#153627=CARTESIAN_POINT ( 'NONE',  ( 0.05219959533934541429, -16.53943276465976808, 70.00109039468568994 ) ) ;
#153628=B_SPLINE_CURVE_WITH_KNOTS ( 'NONE', 3,
 ( #90789, #43317, #164675, #149497, #151496, #72666, #119170, #42330, #88816, #12007, #150509, #126113, #185810, #33116, #1770, #109947, #138301, #107947, #46290, #188796, #171628, #18946, #35093, #32122, #63448, #199982, #169633, #47296, #108953, #17954, #31129, #94773 ),
 .UNSPECIFIED., .F., .F.,
 ( 4, 2, 2, 2, 2, 2, 2, 2, 2, 2, 2, 2, 2, 2, 2, 4 ),
 ( 2.625112965618923374E-17, 0.0003712461730036948552, 0.0007424923460073634728, 0.001113738519011032253, 0.001484984692014700708, 0.002227477038022038485, 0.002598723211025717565, 0.002969969384029396645, 0.003341215557033075725, 0.003712461730036755239, 0.004083707903040433886, 0.004454954076044113399, 0.004826200249047792046, 0.005197446422051471560, 0.005568692595055150206, 0.005939938768058829720 ),
 .UNSPECIFIED. ) ;
#153629=CARTESIAN_POINT ( 'NONE',  ( -0.05219959533910754901, -16.53943276465976808, 77.49890960531433848 ) ) ;
#153631=CARTESIAN_POINT ( 'NONE',  ( 9.564922557961047289, -16.46253265017146816, 110.4177570613523471 ) ) ;
#153632=CARTESIAN_POINT ( 'NONE',  ( 21.53943276465977519, -0.05219959533907433946, 38.74890960531435979 ) ) ;
#153634=CARTESIAN_POINT ( 'NONE',  ( 16.53943276465976808, 0.05219959533934440121, 41.25109039468568284 ) ) ;
#153635=CARTESIAN_POINT ( 'NONE',  ( -15.72974639402197994, 15.80617190586746368, 115.6239096053143669 ) ) ;
#153636=CARTESIAN_POINT ( 'NONE',  ( 15.72974639402199770, -15.80617190586745480, 28.12390960531435979 ) ) ;
#153637=CARTESIAN_POINT ( 'NONE',  ( -16.55341960407617563, 4.379528057220093196, 58.54275706135235424 ) ) ;
#153638=CARTESIAN_POINT ( 'NONE',  ( 0.05219959533909260263, 19.03943276465977164, 84.99890960531436690 ) ) ;
#153639=CARTESIAN_POINT ( 'NONE',  ( -10.72451020669870658, -18.67979575497194134, 44.58442372801901854 ) ) ;
#153640=CARTESIAN_POINT ( 'NONE',  ( 13.97604488694548053, -13.89961937509957401, 105.6260903946856757 ) ) ;
#153641=CARTESIAN_POINT ( 'NONE',  ( 21.55341960407610458, 5.719274019375980345, 28.95724293864769905 ) ) ;
#153642=ORIENTED_EDGE ( 'NONE', *, *, #158809, .F. ) ;
#153643=CARTESIAN_POINT ( 'NONE',  ( -5.049401038297874678, -19.05341960407617918, 29.79275706135232227 ) ) ;
#153644=CARTESIAN_POINT ( 'NONE',  ( 8.224510206698742110, 14.34966873604972548, 37.08442372801901143 ) ) ;
#153645=CARTESIAN_POINT ( 'NONE',  ( 0.05219959533909260263, 19.03943276465977164, 99.99890960531436690 ) ) ;
#153646=CARTESIAN_POINT ( 'NONE',  ( 10.81492255796078972, 18.62759615963270932, 99.58224293864770971 ) ) ;
#153647=CARTESIAN_POINT ( 'NONE',  ( -16.51473224551069308, -9.474510206698971260, 66.66557627198102409 ) ) ;
#153648=CARTESIAN_POINT ( 'NONE',  ( -17.31747979337950838, 6.344076630961000163, 23.62055131934818064 ) ) ;
#153649=CARTESIAN_POINT ( 'NONE',  ( -16.55341960407611168, -4.379528057220339221, 81.45724293864769550 ) ) ;
#153650=CARTESIAN_POINT ( 'NONE',  ( 18.62759615963271287, -10.81492255796078972, 38.33224293864768839 ) ) ;
#153651=CARTESIAN_POINT ( 'NONE',  ( -16.62475595723696742, 7.163666690055234376, 35.52713351810466946 ) ) ;
#153652=CARTESIAN_POINT ( 'NONE',  ( -0.05219959533934338120, 16.53943276465976808, 62.50109039468568284 ) ) ;
#153653=CARTESIAN_POINT ( 'NONE',  ( -15.80617190586745835, -15.72974639402198527, 111.8739096053143669 ) ) ;
#153654=CARTESIAN_POINT ( 'NONE',  ( -16.46253265017146816, -9.564922557961047289, 79.16775706135234714 ) ) ;
#153655=CARTESIAN_POINT ( 'NONE',  ( -5.049401038298153566, 19.05341960407611168, 30.20724293864768839 ) ) ;
#153656=CARTESIAN_POINT ( 'NONE',  ( 10.81492255796078972, 18.62759615963270932, 69.58224293864769550 ) ) ;
#153657=CARTESIAN_POINT ( 'NONE',  ( 19.02544592524343514, -5.153800228976328945, 98.54057627198100988 ) ) ;
#153658=CARTESIAN_POINT ( 'NONE',  ( -10.81492255796105439, 18.62759615963255655, 92.91775706135236135 ) ) ;
#153659=CARTESIAN_POINT ( 'NONE',  ( -5.049401038298153566, 19.05341960407611168, 70.20724293864769550 ) ) ;
#153661=CARTESIAN_POINT ( 'NONE',  ( -16.55341960407617563, 4.379528057220093196, 43.54275706135235424 ) ) ;
#153662=CARTESIAN_POINT ( 'NONE',  ( 9.474510206698971260, -16.51473224551069308, 62.91557627198102409 ) ) ;
#153663=CARTESIAN_POINT ( 'NONE',  ( -18.67979575497193778, 10.72451020669871902, 83.33442372801903275 ) ) ;
#153665=CARTESIAN_POINT ( 'NONE',  ( -19.05341960407617563, 5.049401038297882671, 33.54275706135231871 ) ) ;
#153666=CARTESIAN_POINT ( 'NONE',  ( -9.564922557961040184, 16.46253265017147172, 57.91775706135233293 ) ) ;
#153667=CARTESIAN_POINT ( 'NONE',  ( 18.62759615963255655, 10.81492255796105972, 56.66775706135235424 ) ) ;
#153669=CARTESIAN_POINT ( 'NONE',  ( 19.03943276465977164, 0.05219959533936151252, 46.25109039468566863 ) ) ;
#153670=CARTESIAN_POINT ( 'NONE',  ( -9.564922557960796823, -16.46253265017161027, 102.0822429386477097 ) ) ;
#153671=CARTESIAN_POINT ( 'NONE',  ( 13.89961937509977652, -13.97604488694527269, 73.12390960531436690 ) ) ;
#153672=CARTESIAN_POINT ( 'NONE',  ( -16.53943276465976808, 0.05219959533911058130, 26.24890960531435624 ) ) ;
#153673=CARTESIAN_POINT ( 'NONE',  ( -9.474510206698964154, 16.51473224551069663, 115.4155762719810241 ) ) ;
#153674=CARTESIAN_POINT ( 'NONE',  ( 21.52544592524334988, 5.823673210054432836, 101.4594237280190185 ) ) ;
#153677=CARTESIAN_POINT ( 'NONE',  ( 21.53943276465977519, 0.05219959533937863772, 96.25109039468568994 ) ) ;
#153680=CARTESIAN_POINT ( 'NONE',  ( 8.314922557960818139, 14.29746914071049879, 114.5822429386477097 ) ) ;
#153683=CARTESIAN_POINT ( 'NONE',  ( -14.29746914071037622, -8.314922557961029526, 54.16775706135235424 ) ) ;
#153684=CARTESIAN_POINT ( 'NONE',  ( -18.67979575497178146, -10.72451020669898902, 66.66557627198102409 ) ) ;
#153685=CARTESIAN_POINT ( 'NONE',  ( 12.14591786802309770, 12.06949235617756955, 39.37390960531436690 ) ) ;
#153686=CARTESIAN_POINT ( 'NONE',  ( 8.224510206698953496, -14.34966873604960469, 112.9155762719810383 ) ) ;
#153687=CARTESIAN_POINT ( 'NONE',  ( 5.049401038298161559, -19.05341960407611168, 92.70724293864769550 ) ) ;
#153688=CARTESIAN_POINT ( 'NONE',  ( 19.02544592524334988, 5.153800228976608722, 41.45942372801900433 ) ) ;
#153689=CARTESIAN_POINT ( 'NONE',  ( -14.34966873604960291, -8.224510206698953496, 111.6655762719810525 ) ) ;
#153690=CARTESIAN_POINT ( 'NONE',  ( 18.62759615963255655, 10.81492255796105972, 71.66775706135234714 ) ) ;
#153692=CARTESIAN_POINT ( 'NONE',  ( -16.53943276465976808, -0.05219959533934237506, 103.7510903946857042 ) ) ;
#153694=CARTESIAN_POINT ( 'NONE',  ( 21.55341960407610458, 5.719274019375980345, 33.95724293864769550 ) ) ;
#153695=CARTESIAN_POINT ( 'NONE',  ( -0.05219959533910754901, -16.53943276465976808, 92.49890960531436690 ) ) ;
#153697=CARTESIAN_POINT ( 'NONE',  ( -13.89961937509957401, -13.97604488694547875, 54.37609039468565442 ) ) ;
#153698=CARTESIAN_POINT ( 'NONE',  ( -9.474510206698964154, 16.51473224551069663, 80.41557627198103830 ) ) ;
#153699=CARTESIAN_POINT ( 'NONE',  ( 12.14591786802309770, 12.06949235617756955, 79.37390960531436690 ) ) ;
#153700=CARTESIAN_POINT ( 'NONE',  ( -19.02544592524334988, -5.153800228976617603, 98.95942372801900433 ) ) ;
#153701=CARTESIAN_POINT ( 'NONE',  ( -21.52544592524343514, 5.823673210054127303, 46.04057627198103830 ) ) ;
#153703=CARTESIAN_POINT ( 'NONE',  ( -8.224510206698948167, 14.34966873604960824, 110.4155762719810383 ) ) ;
#153704=CARTESIAN_POINT ( 'NONE',  ( -16.79531203550650176, -7.028104445595493743, 31.25244988220443076 ) ) ;
#153705=CARTESIAN_POINT ( 'NONE',  ( 9.564922557960805705, 16.46253265017160317, 69.58224293864770971 ) ) ;
#153706=CARTESIAN_POINT ( 'NONE',  ( 5.823673210054125526, 21.52544592524343514, 79.79057627198102409 ) ) ;
#153707=CARTESIAN_POINT ( 'NONE',  ( -4.379528057220086978, -16.55341960407618274, 94.79275706135234714 ) ) ;
#153708=CARTESIAN_POINT ( 'NONE',  ( -16.46253265017160317, 9.564922557960807481, 85.83224293864769550 ) ) ;
#153709=CARTESIAN_POINT ( 'NONE',  ( -13.97604488694547697, 13.89961937509957934, 68.12609039468563310 ) ) ;
#153710=CARTESIAN_POINT ( 'NONE',  ( 21.52544592524334988, 5.823673210054432836, 76.45942372801901854 ) ) ;
#153711=CARTESIAN_POINT ( 'NONE',  ( -0.05219959533907301413, -21.53943276465977519, 57.49890960531435979 ) ) ;
#153712=CARTESIAN_POINT ( 'NONE',  ( -0.05219959533907301413, -21.53943276465977519, 27.49890960531435269 ) ) ;
#153713=CARTESIAN_POINT ( 'NONE',  ( -16.46253265017160317, 9.564922557960807481, 40.83224293864769550 ) ) ;
#153714=CARTESIAN_POINT ( 'NONE',  ( -12.06949235617739369, -12.14591786802326823, 99.37609039468568994 ) ) ;
#153715=CARTESIAN_POINT ( 'NONE',  ( 13.89961937509977652, -13.97604488694527269, 48.12390960531435979 ) ) ;
#153716=CARTESIAN_POINT ( 'NONE',  ( -12.06949235617739369, -12.14591786802326823, 19.37609039468568639 ) ) ;
#153718=CARTESIAN_POINT ( 'NONE',  ( 5.719274019375673035, 21.55341960407619339, 107.2927570613523471 ) ) ;
#153719=CARTESIAN_POINT ( 'NONE',  ( 0.05219959533910956823, 16.53943276465976808, 59.99890960531436690 ) ) ;
#153720=CARTESIAN_POINT ( 'NONE',  ( 18.67979575497178502, 10.72451020669898547, 114.1655762719810383 ) ) ;
#153721=CARTESIAN_POINT ( 'NONE',  ( 15.80617190586746368, 15.72974639402197994, 99.37390960531436690 ) ) ;
#153723=CARTESIAN_POINT ( 'NONE',  ( -10.72451020669898014, 18.67979575497178502, 45.41557627198103830 ) ) ;
#153724=CARTESIAN_POINT ( 'NONE',  ( 4.483927247898790824, -16.52544592524335698, 80.20942372801901854 ) ) ;
#153725=CARTESIAN_POINT ( 'NONE',  ( -12.14591786802309592, -12.06949235617757132, 86.87390960531438111 ) ) ;
#153726=CARTESIAN_POINT ( 'NONE',  ( -19.02544592524342804, 5.153800228976336051, 56.04057627198100988 ) ) ;
#153728=CARTESIAN_POINT ( 'NONE',  ( -12.14591786802326823, 12.06949235617739902, 113.1260903946856899 ) ) ;
#153729=CARTESIAN_POINT ( 'NONE',  ( 5.823673210054444382, -21.52544592524334988, 35.20942372801901854 ) ) ;
#153730=CARTESIAN_POINT ( 'NONE',  ( 5.049401038298161559, -19.05341960407611168, 102.7072429386476955 ) ) ;
#153731=CARTESIAN_POINT ( 'NONE',  ( 5.719274019375673035, 21.55341960407619339, 67.29275706135234714 ) ) ;
#153733=CARTESIAN_POINT ( 'NONE',  ( -16.51473224551069308, -9.474510206698971260, 21.66557627198102765 ) ) ;
#153735=CARTESIAN_POINT ( 'NONE',  ( -0.05219959533937732626, 21.53943276465977519, 77.50109039468567573 ) ) ;
#153736=CARTESIAN_POINT ( 'NONE',  ( -19.05341960407611168, -5.049401038298163336, 46.45724293864768129 ) ) ;
#153737=CARTESIAN_POINT ( 'NONE',  ( 5.153800228976335163, 19.02544592524342804, 84.79057627198099567 ) ) ;
#153738=CARTESIAN_POINT ( 'NONE',  ( 16.46253265017146816, 9.564922557961045513, 76.66775706135234714 ) ) ;
#153739=CARTESIAN_POINT ( 'NONE',  ( 21.52544592524334988, 5.823673210054432836, 36.45942372801901143 ) ) ;
#153740=CARTESIAN_POINT ( 'NONE',  ( -13.97604488694547697, 13.89961937509957934, 108.1260903946856331 ) ) ;
#153742=CARTESIAN_POINT ( 'NONE',  ( 5.049401038297881783, 19.05341960407617563, 77.29275706135231871 ) ) ;
#153743=CARTESIAN_POINT ( 'NONE',  ( -9.564922557960796823, -16.46253265017161027, 37.08224293864768839 ) ) ;
#153744=CARTESIAN_POINT ( 'NONE',  ( 19.02544592524334988, 5.153800228976608722, 81.45942372801897591 ) ) ;
#153745=CARTESIAN_POINT ( 'NONE',  ( 14.34966873604972726, -8.224510206698740333, 105.8344237280190328 ) ) ;
#153746=CARTESIAN_POINT ( 'NONE',  ( 13.89961937509957401, 13.97604488694547697, 76.87609039468566152 ) ) ;
#153747=CARTESIAN_POINT ( 'NONE',  ( 16.55341960407611168, 4.379528057220329451, 38.95724293864768839 ) ) ;
#153748=CARTESIAN_POINT ( 'NONE',  ( 9.474510206698729675, 16.51473224551082808, 47.08442372801900433 ) ) ;
#153749=CARTESIAN_POINT ( 'NONE',  ( -18.67979575497193778, 10.72451020669871902, 103.3344237280190043 ) ) ;
#153750=CARTESIAN_POINT ( 'NONE',  ( 13.89961937509957401, 13.97604488694547697, 21.87609039468566152 ) ) ;
#153751=CARTESIAN_POINT ( 'NONE',  ( -9.474510206698964154, 16.51473224551069663, 35.41557627198102409 ) ) ;
#153752=CARTESIAN_POINT ( 'NONE',  ( 5.823673210054444382, -21.52544592524334988, 85.20942372801901854 ) ) ;
#153753=CARTESIAN_POINT ( 'NONE',  ( 16.52544592524335698, 4.483927247898782831, 41.45942372801901143 ) ) ;
#153754=CARTESIAN_POINT ( 'NONE',  ( 0.05219959533909260263, 19.03943276465977164, 89.99890960531436690 ) ) ;
#153756=CARTESIAN_POINT ( 'NONE',  ( 19.05341960407611168, 5.049401038298154454, 93.95724293864769550 ) ) ;
#153757=EDGE_CURVE ( 'NONE', #198282, #62281, #151151, .T. ) ;
#153760=CARTESIAN_POINT ( 'NONE',  ( -13.89961937509957401, -13.97604488694547875, 79.37609039468567573 ) ) ;
#153761=CARTESIAN_POINT ( 'NONE',  ( -21.52544592524343514, 5.823673210054127303, 31.04057627198102409 ) ) ;
#153762=CARTESIAN_POINT ( 'NONE',  ( -13.89961937509957401, -13.97604488694547875, 19.37609039468566507 ) ) ;
#153763=CARTESIAN_POINT ( 'NONE',  ( 5.049401038297881783, 19.05341960407617563, 102.2927570613523045 ) ) ;
#153764=CARTESIAN_POINT ( 'NONE',  ( 16.55341960407611168, 4.379528057220329451, 98.95724293864770971 ) ) ;
#153765=CARTESIAN_POINT ( 'NONE',  ( 13.89961937509977652, -13.97604488694527269, 23.12390960531436335 ) ) ;
#153766=CARTESIAN_POINT ( 'NONE',  ( -5.719274019375978568, 21.55341960407610458, 65.20724293864768129 ) ) ;
#153767=CARTESIAN_POINT ( 'NONE',  ( 10.81492255796078972, 18.62759615963270932, 54.58224293864769550 ) ) ;
#153768=CARTESIAN_POINT ( 'NONE',  ( 5.153800228976335163, 19.02544592524342804, 24.79057627198102765 ) ) ;
#153770=CARTESIAN_POINT ( 'NONE',  ( 5.153800228976615827, -19.02544592524334988, 65.20942372801900433 ) ) ;
#153771=CARTESIAN_POINT ( 'NONE',  ( -14.29746914071049879, 8.314922557960819915, 45.83224293864769550 ) ) ;
#153772=CARTESIAN_POINT ( 'NONE',  ( -19.02544592524342804, 5.153800228976336051, 116.0405762719810383 ) ) ;
#153773=CARTESIAN_POINT ( 'NONE',  ( -21.52544592524334988, -5.823673210054445271, 78.95942372801901854 ) ) ;
#153774=CARTESIAN_POINT ( 'NONE',  ( -5.719274019375978568, 21.55341960407610458, 70.20724293864769550 ) ) ;
#153775=CARTESIAN_POINT ( 'NONE',  ( 0.05219959533937995610, -21.53943276465977519, 65.00109039468568994 ) ) ;
#153776=CARTESIAN_POINT ( 'NONE',  ( -21.53943276465977519, -0.05219959533937600094, 48.75109039468568284 ) ) ;
#153777=CARTESIAN_POINT ( 'NONE',  ( -9.474510206698964154, 16.51473224551069663, 95.41557627198102409 ) ) ;
#153778=CARTESIAN_POINT ( 'NONE',  ( 12.14591786802327356, -12.06949235617739191, 90.62609039468567573 ) ) ;
#153779=CARTESIAN_POINT ( 'NONE',  ( -8.314922557960811034, -14.29746914071050412, 112.0822429386477097 ) ) ;
#153781=CARTESIAN_POINT ( 'NONE',  ( 14.29746914071049879, -8.314922557960816363, 73.33224293864769550 ) ) ;
#153782=CARTESIAN_POINT ( 'NONE',  ( -8.224510206698948167, 14.34966873604960824, 40.41557627198103120 ) ) ;
#153783=CARTESIAN_POINT ( 'NONE',  ( -19.03943276465977164, 0.05219959533909376836, 61.24890960531436690 ) ) ;
#153784=CARTESIAN_POINT ( 'NONE',  ( 16.46253265017160672, -9.564922557960803928, 38.33224293864768839 ) ) ;
#153785=CARTESIAN_POINT ( 'NONE',  ( 10.81492255796078972, 18.62759615963270932, 54.58224293864769550 ) ) ;
#153786=CARTESIAN_POINT ( 'NONE',  ( -13.89961937509957401, -13.97604488694547875, 39.37609039468566152 ) ) ;
#153788=CARTESIAN_POINT ( 'NONE',  ( -16.52544592524342804, 4.483927247898546575, 51.04057627198103120 ) ) ;
#153789=CARTESIAN_POINT ( 'NONE',  ( 0.05219959533907565091, 21.53943276465977519, 29.99890960531435979 ) ) ;
#153791=CARTESIAN_POINT ( 'NONE',  ( 17.50000000000000000, -5.500000000000000888, 120.0000000000000142 ) ) ;
#153792=CARTESIAN_POINT ( 'NONE',  ( 4.483927247898790824, -16.52544592524335698, 75.20942372801901854 ) ) ;
#153793=CARTESIAN_POINT ( 'NONE',  ( 16.46253265017146816, 9.564922557961045513, 81.66775706135233293 ) ) ;
#153794=CARTESIAN_POINT ( 'NONE',  ( -12.06949235617756955, 12.14591786802309770, 35.62390960531437401 ) ) ;
#153795=CARTESIAN_POINT ( 'NONE',  ( 16.88567814943160172, -6.947325034625743356, 51.20998877347416567 ) ) ;
#153796=CARTESIAN_POINT ( 'NONE',  ( 8.314922557960818139, 14.29746914071049879, 29.58224293864769905 ) ) ;
#153797=CARTESIAN_POINT ( 'NONE',  ( 16.46253265017160672, -9.564922557960803928, 53.33224293864768839 ) ) ;
#153799=CARTESIAN_POINT ( 'NONE',  ( 19.05341960407611168, 5.049401038298154454, 78.95724293864769550 ) ) ;
#153800=CARTESIAN_POINT ( 'NONE',  ( 16.46253265017160672, -9.564922557960803928, 33.33224293864770260 ) ) ;
#153801=CARTESIAN_POINT ( 'NONE',  ( 15.72974639402176855, 15.80617190586768217, 46.87609039468568994 ) ) ;
#153802=CARTESIAN_POINT ( 'NONE',  ( -19.02544592524342804, 5.153800228976336051, 56.04057627198100988 ) ) ;
#153804=CARTESIAN_POINT ( 'NONE',  ( -19.03943276465977164, 0.05219959533909376836, 51.24890960531436690 ) ) ;
#153805=CARTESIAN_POINT ( 'NONE',  ( 0.05219959533907565091, 21.53943276465977519, 34.99890960531435979 ) ) ;
#153806=CARTESIAN_POINT ( 'NONE',  ( -18.67979575497193778, 10.72451020669871902, 68.33442372801900433 ) ) ;
#153807=CARTESIAN_POINT ( 'NONE',  ( 9.474510206698971260, -16.51473224551069308, 22.91557627198102765 ) ) ;
#153808=CARTESIAN_POINT ( 'NONE',  ( 10.72451020669898902, -18.67979575497178502, 27.91557627198103830 ) ) ;
#153809=CARTESIAN_POINT ( 'NONE',  ( 8.314922557961029526, -14.29746914071037800, 90.41775706135236135 ) ) ;
#153810=CARTESIAN_POINT ( 'NONE',  ( 21.53943276465977519, 0.05219959533937863772, 101.2510903946856757 ) ) ;
#153811=CARTESIAN_POINT ( 'NONE',  ( -12.06949235617739369, -12.14591786802326823, 69.37609039468567573 ) ) ;
#153812=CARTESIAN_POINT ( 'NONE',  ( -19.05341960407611168, -5.049401038298163336, 111.4572429386476671 ) ) ;
#153813=CARTESIAN_POINT ( 'NONE',  ( -0.05219959533934338120, 16.53943276465976808, 57.50109039468568994 ) ) ;
#153814=CARTESIAN_POINT ( 'NONE',  ( 16.52544592524335698, 4.483927247898782831, 41.45942372801901143 ) ) ;
#153815=CARTESIAN_POINT ( 'NONE',  ( 16.53943276465976808, 0.05219959533934440121, 101.2510903946856757 ) ) ;
#153816=CARTESIAN_POINT ( 'NONE',  ( 21.53943276465977519, 0.05219959533937863772, 51.25109039468568994 ) ) ;
#153817=CARTESIAN_POINT ( 'NONE',  ( 0.05219959533934541429, -16.53943276465976808, 25.00109039468567218 ) ) ;
#153818=CARTESIAN_POINT ( 'NONE',  ( -18.67979575497178146, -10.72451020669898902, 111.6655762719810525 ) ) ;
#153819=CARTESIAN_POINT ( 'NONE',  ( 19.02544592524334988, 5.153800228976608722, 111.4594237280190043 ) ) ;
#153820=CARTESIAN_POINT ( 'NONE',  ( -8.314922557961024197, 14.29746914071037800, 87.91775706135234714 ) ) ;
#153822=CARTESIAN_POINT ( 'NONE',  ( 15.72974639402176855, 15.80617190586768217, 81.87609039468568994 ) ) ;
#153823=CARTESIAN_POINT ( 'NONE',  ( -19.03943276465977164, -0.05219959533935918106, 78.75109039468567573 ) ) ;
#153824=CARTESIAN_POINT ( 'NONE',  ( -12.06949235617756955, 12.14591786802309770, 60.62390960531437401 ) ) ;
#153825=CARTESIAN_POINT ( 'NONE',  ( 8.314922557960818139, 14.29746914071049879, 39.58224293864769550 ) ) ;
#153826=CARTESIAN_POINT ( 'NONE',  ( -12.06949235617756955, 12.14591786802309770, 100.6239096053143811 ) ) ;
#153827=CARTESIAN_POINT ( 'NONE',  ( 16.46253265017146816, 9.564922557961045513, 46.66775706135233293 ) ) ;
#153829=CARTESIAN_POINT ( 'NONE',  ( -10.81492255796105439, 18.62759615963255655, 47.91775706135234714 ) ) ;
#153830=CARTESIAN_POINT ( 'NONE',  ( -9.474510206698720793, -16.51473224551083518, 109.5844237280190043 ) ) ;
#153831=CARTESIAN_POINT ( 'NONE',  ( -16.51473224551069308, -9.474510206698971260, 101.6655762719810241 ) ) ;
#153832=CARTESIAN_POINT ( 'NONE',  ( 0.05219959533907565091, 21.53943276465977519, 74.99890960531435269 ) ) ;
#153833=CARTESIAN_POINT ( 'NONE',  ( -16.46253265017146816, -9.564922557961047289, 99.16775706135233293 ) ) ;
#153834=CARTESIAN_POINT ( 'NONE',  ( -5.049401038298153566, 19.05341960407611168, 105.2072429386476671 ) ) ;
#153836=CARTESIAN_POINT ( 'NONE',  ( -12.06949235617756955, 12.14591786802309770, 105.6239096053143669 ) ) ;
#153837=CARTESIAN_POINT ( 'NONE',  ( -10.72451020669870658, -18.67979575497194134, 94.58442372801901854 ) ) ;
#153838=CARTESIAN_POINT ( 'NONE',  ( -9.474510206698964154, 16.51473224551069663, 25.41557627198103120 ) ) ;
#153840=CARTESIAN_POINT ( 'NONE',  ( -0.05219959533937732626, 21.53943276465977519, 47.50109039468568994 ) ) ;
#153841=CARTESIAN_POINT ( 'NONE',  ( -15.72974639402176322, -15.80617190586768395, 84.37609039468570415 ) ) ;
#153842=CARTESIAN_POINT ( 'NONE',  ( -8.224510206698735004, -14.34966873604973081, 89.58442372801901854 ) ) ;
#153843=CARTESIAN_POINT ( 'NONE',  ( -21.53943276465977519, -0.05219959533937600094, 48.75109039468568284 ) ) ;
#153844=CARTESIAN_POINT ( 'NONE',  ( -21.53943276465977519, -0.05219959533937600094, 38.75109039468567573 ) ) ;
#153845=CARTESIAN_POINT ( 'NONE',  ( 16.51473224551083163, -9.474510206698727899, 65.83442372801900433 ) ) ;
#153846=CARTESIAN_POINT ( 'NONE',  ( -5.049401038298153566, 19.05341960407611168, 95.20724293864770971 ) ) ;
#153847=CARTESIAN_POINT ( 'NONE',  ( 0.05219959533910956823, 16.53943276465976808, 99.99890960531436690 ) ) ;
#153848=CARTESIAN_POINT ( 'NONE',  ( -15.80617190586745835, -15.72974639402198527, 86.87390960531438111 ) ) ;
#153849=CARTESIAN_POINT ( 'NONE',  ( -16.55341960407611168, -4.379528057220339221, 61.45724293864770260 ) ) ;
#153850=CARTESIAN_POINT ( 'NONE',  ( -18.67979575497193778, 10.72451020669871902, 98.33442372801901854 ) ) ;
#153851=CARTESIAN_POINT ( 'NONE',  ( 14.34966873604960469, 8.224510206698951720, 89.16557627198102409 ) ) ;
#153852=CARTESIAN_POINT ( 'NONE',  ( 16.46253265017160672, -9.564922557960803928, 33.33224293864770260 ) ) ;
#153853=CARTESIAN_POINT ( 'NONE',  ( 9.564922557961047289, -16.46253265017146816, 75.41775706135234714 ) ) ;
#153854=CARTESIAN_POINT ( 'NONE',  ( 4.483927247898545687, 16.52544592524342804, 44.79057627198103120 ) ) ;
#153855=CARTESIAN_POINT ( 'NONE',  ( -15.72974639402176322, -15.80617190586768395, 99.37609039468568994 ) ) ;
#153856=CARTESIAN_POINT ( 'NONE',  ( -9.564922557960796823, -16.46253265017161027, 92.08224293864769550 ) ) ;
#153857=CARTESIAN_POINT ( 'NONE',  ( 19.05341960407617918, -5.049401038297876454, 56.04275706135234714 ) ) ;
#153858=CARTESIAN_POINT ( 'NONE',  ( 21.53943276465977519, -0.05219959533907433946, 58.74890960531436690 ) ) ;
#153859=CARTESIAN_POINT ( 'NONE',  ( -15.80617190586745835, -15.72974639402198527, 111.8739096053143669 ) ) ;
#153860=CARTESIAN_POINT ( 'NONE',  ( -4.379528057220086978, -16.55341960407618274, 19.79275706135235069 ) ) ;
#153861=CARTESIAN_POINT ( 'NONE',  ( -4.483927247898782831, 16.52544592524335698, 77.70942372801900433 ) ) ;
#153862=CARTESIAN_POINT ( 'NONE',  ( 5.049401038298161559, -19.05341960407611168, 27.70724293864769550 ) ) ;
#153863=CARTESIAN_POINT ( 'NONE',  ( 18.67979575497194134, -10.72451020669871369, 20.83442372801901143 ) ) ;
#153864=CARTESIAN_POINT ( 'NONE',  ( -12.14591786802309592, -12.06949235617757132, 111.8739096053143669 ) ) ;
#153866=CARTESIAN_POINT ( 'NONE',  ( -4.379528057220086978, -16.55341960407618274, 49.79275706135234714 ) ) ;
#153867=CARTESIAN_POINT ( 'NONE',  ( -0.05219959533910754901, -16.53943276465976808, 82.49890960531436690 ) ) ;
#153868=CARTESIAN_POINT ( 'NONE',  ( -21.53943276465977519, 0.05219959533907696930, 76.24890960531435269 ) ) ;
#153869=CARTESIAN_POINT ( 'NONE',  ( -8.314922557960811034, -14.29746914071050412, 22.08224293864769194 ) ) ;
#153870=CARTESIAN_POINT ( 'NONE',  ( -16.53943276465976808, -0.05219959533934237506, 33.75109039468568284 ) ) ;
#153871=CARTESIAN_POINT ( 'NONE',  ( 13.97604488694527802, 13.89961937509977652, 39.37390960531435269 ) ) ;
#153872=CARTESIAN_POINT ( 'NONE',  ( -12.06949235617739369, -12.14591786802326823, 74.37609039468568994 ) ) ;
#153873=CARTESIAN_POINT ( 'NONE',  ( 9.474510206698729675, 16.51473224551082808, 72.08442372801900433 ) ) ;
#153874=CARTESIAN_POINT ( 'NONE',  ( -15.80617190586745835, -15.72974639402198527, 66.87390960531436690 ) ) ;
#153875=CARTESIAN_POINT ( 'NONE',  ( 14.29746914071037800, 8.314922557961029526, 106.6677570613523756 ) ) ;
#153877=CARTESIAN_POINT ( 'NONE',  ( 21.52544592524334988, 5.823673210054432836, 76.45942372801901854 ) ) ;
#153878=CARTESIAN_POINT ( 'NONE',  ( -10.81492255796078084, -18.62759615963271287, 42.08224293864769550 ) ) ;
#153879=ORIENTED_EDGE ( 'NONE', *, *, #116955, .F. ) ;
#153881=CARTESIAN_POINT ( 'NONE',  ( -8.314922557961024197, 14.29746914071037800, 92.91775706135236135 ) ) ;
#153882=CARTESIAN_POINT ( 'NONE',  ( 10.81492255796078972, 18.62759615963270932, 39.58224293864769550 ) ) ;
#153884=CARTESIAN_POINT ( 'NONE',  ( 19.02544592524343514, -5.153800228976328945, 108.5405762719810383 ) ) ;
#153885=CARTESIAN_POINT ( 'NONE',  ( 17.50000000000000355, 3.345213924137354411, 107.9123137690565670 ) ) ;
#153886=CARTESIAN_POINT ( 'NONE',  ( -13.97604488694527625, -13.89961937509977652, 26.87390960531434558 ) ) ;
#153887=CARTESIAN_POINT ( 'NONE',  ( -21.53943276465977519, 0.05219959533907696930, 81.24890960531436690 ) ) ;
#153888=CARTESIAN_POINT ( 'NONE',  ( -8.314922557961024197, 14.29746914071037800, 102.9177570613523756 ) ) ;
#153889=CARTESIAN_POINT ( 'NONE',  ( -10.72451020669870658, -18.67979575497194134, 54.58442372801901143 ) ) ;
#153890=CARTESIAN_POINT ( 'NONE',  ( -14.34966873604972548, 8.224510206698743886, 23.33442372801901499 ) ) ;
#153891=CARTESIAN_POINT ( 'NONE',  ( -12.14591786802309592, -12.06949235617757132, 111.8739096053143669 ) ) ;
#153892=CARTESIAN_POINT ( 'NONE',  ( 13.97604488694548053, -13.89961937509957401, 110.6260903946856615 ) ) ;
#153894=CARTESIAN_POINT ( 'NONE',  ( -19.03943276465977164, 0.05219959533909376836, 36.24890960531436690 ) ) ;
#153896=CARTESIAN_POINT ( 'NONE',  ( 0.05219959533909260263, 19.03943276465977164, 104.9989096053143669 ) ) ;
#153898=CARTESIAN_POINT ( 'NONE',  ( -16.52544592524335698, -4.483927247898792601, 83.95942372801900433 ) ) ;
#153899=CARTESIAN_POINT ( 'NONE',  ( 13.97604488694548053, -13.89961937509957401, 80.62609039468567573 ) ) ;
#153900=CARTESIAN_POINT ( 'NONE',  ( -19.02544592524334988, -5.153800228976617603, 28.95942372801900433 ) ) ;
#153901=CARTESIAN_POINT ( 'NONE',  ( 15.80617190586746368, 15.72974639402197994, 74.37390960531436690 ) ) ;
#153902=CARTESIAN_POINT ( 'NONE',  ( -16.53943276465976808, -0.05219959533934237506, 93.75109039468567573 ) ) ;
#153903=CARTESIAN_POINT ( 'NONE',  ( -9.474510206698720793, -16.51473224551083518, 89.58442372801900433 ) ) ;
#153904=CARTESIAN_POINT ( 'NONE',  ( -19.02544592524342804, 5.153800228976336051, 56.04057627198100988 ) ) ;
#153905=CARTESIAN_POINT ( 'NONE',  ( -0.05219959533909027116, -19.03943276465977164, 87.49890960531436690 ) ) ;
#153906=CARTESIAN_POINT ( 'NONE',  ( 0.05219959533937995610, -21.53943276465977519, 50.00109039468568994 ) ) ;
#153907=CARTESIAN_POINT ( 'NONE',  ( 19.02544592524343514, -5.153800228976328945, 48.54057627198103120 ) ) ;
#153908=CARTESIAN_POINT ( 'NONE',  ( -16.18388926212238133, -7.379444403734527924, 85.43953151366152099 ) ) ;
#153909=CARTESIAN_POINT ( 'NONE',  ( -16.51473224551069308, -9.474510206698971260, 106.6655762719810383 ) ) ;
#153910=CARTESIAN_POINT ( 'NONE',  ( 14.29746914071049879, -8.314922557960816363, 63.33224293864770260 ) ) ;
#153911=CARTESIAN_POINT ( 'NONE',  ( 5.719274019375991003, -21.55341960407610458, 77.70724293864770971 ) ) ;
#153913=CARTESIAN_POINT ( 'NONE',  ( -13.97604488694547697, 13.89961937509957934, 48.12609039468566863 ) ) ;
#153915=CARTESIAN_POINT ( 'NONE',  ( -0.05219959533909027116, -19.03943276465977164, 67.49890960531436690 ) ) ;
#153916=CARTESIAN_POINT ( 'NONE',  ( -16.46253265017160317, 9.564922557960807481, 85.83224293864769550 ) ) ;
#153917=CARTESIAN_POINT ( 'NONE',  ( 4.379528057220092307, 16.55341960407617563, 52.29275706135236135 ) ) ;
#153919=CARTESIAN_POINT ( 'NONE',  ( -5.153800228976607833, 19.02544592524334988, 32.70942372801899722 ) ) ;
#153920=CARTESIAN_POINT ( 'NONE',  ( 17.72517630440434289, -5.499999999999968026, 93.42175719257213018 ) ) ;
#153921=CARTESIAN_POINT ( 'NONE',  ( 12.06949235617739724, 12.14591786802326823, 86.87609039468568994 ) ) ;
#153922=EDGE_CURVE ( 'NONE', #199703, #25133, #122099, .T. ) ;
#153924=CARTESIAN_POINT ( 'NONE',  ( -4.379528057220086978, -16.55341960407618274, 84.79275706135234714 ) ) ;
#153925=CARTESIAN_POINT ( 'NONE',  ( -8.224510206698735004, -14.34966873604973081, 59.58442372801901854 ) ) ;
#153926=CARTESIAN_POINT ( 'NONE',  ( -15.80617190586768217, 15.72974639402176855, 113.1260903946856899 ) ) ;
#153927=CARTESIAN_POINT ( 'NONE',  ( 16.46253265017160672, -9.564922557960803928, 53.33224293864768839 ) ) ;
#153928=CARTESIAN_POINT ( 'NONE',  ( 9.564922557960805705, 16.46253265017160317, 74.58224293864769550 ) ) ;
#153929=CARTESIAN_POINT ( 'NONE',  ( 5.823673210054444382, -21.52544592524334988, 65.20942372801901854 ) ) ;
#153930=CARTESIAN_POINT ( 'NONE',  ( 16.46253265017146816, 9.564922557961045513, 76.66775706135234714 ) ) ;
#153931=CARTESIAN_POINT ( 'NONE',  ( -21.52544592524334988, -5.823673210054445271, 103.9594237280190185 ) ) ;
#153932=CARTESIAN_POINT ( 'NONE',  ( 19.03943276465977164, -0.05219959533909143690, 28.74890960531435624 ) ) ;
#153934=CARTESIAN_POINT ( 'NONE',  ( 10.81492255796078972, 18.62759615963270932, 64.58224293864769550 ) ) ;
#153935=CARTESIAN_POINT ( 'NONE',  ( -5.719274019375978568, 21.55341960407610458, 25.20724293864769550 ) ) ;
#153936=CARTESIAN_POINT ( 'NONE',  ( -8.224510206698948167, 14.34966873604960824, 110.4155762719810383 ) ) ;
#153937=CARTESIAN_POINT ( 'NONE',  ( -16.55341960407617563, 4.379528057220093196, 38.54275706135234714 ) ) ;
#153938=CARTESIAN_POINT ( 'NONE',  ( 14.34966873604960469, 8.224510206698951720, 29.16557627198103120 ) ) ;
#153940=CARTESIAN_POINT ( 'NONE',  ( -10.72451020669898014, 18.67979575497178502, 110.4155762719810383 ) ) ;
#153941=CARTESIAN_POINT ( 'NONE',  ( 16.53943276465976808, -0.05219959533910856209, 38.74890960531435979 ) ) ;
#153943=CARTESIAN_POINT ( 'NONE',  ( -19.05341960407617563, 5.049401038297882671, 108.5427570613523187 ) ) ;
#153944=CARTESIAN_POINT ( 'NONE',  ( -0.05219959533936034679, 19.03943276465977164, 27.50109039468566507 ) ) ;
#153945=CARTESIAN_POINT ( 'NONE',  ( -4.379528057220328563, 16.55341960407611168, 50.20724293864769550 ) ) ;
#153946=CARTESIAN_POINT ( 'NONE',  ( 18.62759615963271287, -10.81492255796078972, 108.3322429386477097 ) ) ;
#153947=CARTESIAN_POINT ( 'NONE',  ( 16.19135201231369336, 7.376712067591808974, 32.68680854052032458 ) ) ;
#153948=CARTESIAN_POINT ( 'NONE',  ( -21.55341960407610458, -5.719274019375992779, 61.45724293864770260 ) ) ;
#153949=CARTESIAN_POINT ( 'NONE',  ( 9.474510206698971260, -16.51473224551069308, 82.91557627198103830 ) ) ;
#153950=CARTESIAN_POINT ( 'NONE',  ( 14.34966873604960469, 8.224510206698951720, 44.16557627198103120 ) ) ;
#153951=CARTESIAN_POINT ( 'NONE',  ( -16.51473224551069308, -9.474510206698971260, 106.6655762719810383 ) ) ;
#153953=CARTESIAN_POINT ( 'NONE',  ( 5.153800228976615827, -19.02544592524334988, 60.20942372801899012 ) ) ;
#153954=CARTESIAN_POINT ( 'NONE',  ( 15.80617190586746368, 15.72974639402197994, 94.37390960531436690 ) ) ;
#153955=CARTESIAN_POINT ( 'NONE',  ( -19.05341960407611168, -5.049401038298163336, 41.45724293864769550 ) ) ;
#153956=CARTESIAN_POINT ( 'NONE',  ( 4.483927247898545687, 16.52544592524342804, 109.7905762719810383 ) ) ;
#153957=CARTESIAN_POINT ( 'NONE',  ( 15.72974639402176855, 15.80617190586768217, 46.87609039468568994 ) ) ;
#153959=CARTESIAN_POINT ( 'NONE',  ( 8.224510206698953496, -14.34966873604960469, 32.91557627198102409 ) ) ;
#153960=CARTESIAN_POINT ( 'NONE',  ( -13.89961937509977652, 13.97604488694528158, 50.62390960531435979 ) ) ;
#153961=CARTESIAN_POINT ( 'NONE',  ( 19.03943276465977164, -0.05219959533909143690, 98.74890960531436690 ) ) ;
#153962=CARTESIAN_POINT ( 'NONE',  ( -5.823673210054116645, -21.52544592524344225, 62.29057627198102409 ) ) ;
#153963=CARTESIAN_POINT ( 'NONE',  ( -19.36337904590690329, 5.499999999999949374, 45.41494137495620720 ) ) ;
#153964=CARTESIAN_POINT ( 'NONE',  ( -0.05219959533909027116, -19.03943276465977164, 47.49890960531435979 ) ) ;
#153965=CARTESIAN_POINT ( 'NONE',  ( -5.719274019375978568, 21.55341960407610458, 55.20724293864770260 ) ) ;
#153967=CARTESIAN_POINT ( 'NONE',  ( -10.81492255796105439, 18.62759615963255655, 92.91775706135236135 ) ) ;
#153969=CARTESIAN_POINT ( 'NONE',  ( -12.06949235617739369, -12.14591786802326823, 89.37609039468568994 ) ) ;
#153970=CARTESIAN_POINT ( 'NONE',  ( 4.379528057220092307, 16.55341960407617563, 92.29275706135236135 ) ) ;
#153971=CARTESIAN_POINT ( 'NONE',  ( 9.474510206698971260, -16.51473224551069308, 57.91557627198103120 ) ) ;
#153972=CARTESIAN_POINT ( 'NONE',  ( -13.89961937509977652, 13.97604488694528158, 60.62390960531436690 ) ) ;
#153974=CARTESIAN_POINT ( 'NONE',  ( 19.05341960407617918, -5.049401038297876454, 26.04275706135233293 ) ) ;
#153975=CARTESIAN_POINT ( 'NONE',  ( 8.224510206698742110, 14.34966873604972548, 72.08442372801899012 ) ) ;
#153976=CARTESIAN_POINT ( 'NONE',  ( -18.67979575497193778, 10.72451020669871902, 108.3344237280190185 ) ) ;
#153977=CARTESIAN_POINT ( 'NONE',  ( 5.049401038298161559, -19.05341960407611168, 72.70724293864768129 ) ) ;
#153978=CARTESIAN_POINT ( 'NONE',  ( -0.05219959533907301413, -21.53943276465977519, 52.49890960531435979 ) ) ;
#153979=CARTESIAN_POINT ( 'NONE',  ( -12.06949235617739369, -12.14591786802326823, 29.37609039468568284 ) ) ;
#153980=CARTESIAN_POINT ( 'NONE',  ( 18.67979575497194134, -10.72451020669871369, 75.83442372801900433 ) ) ;
#153981=CARTESIAN_POINT ( 'NONE',  ( 8.224510206698742110, 14.34966873604972548, 47.08442372801901854 ) ) ;
#153982=CARTESIAN_POINT ( 'NONE',  ( -5.823673210054116645, -21.52544592524344225, 107.2905762719810525 ) ) ;
#153983=CARTESIAN_POINT ( 'NONE',  ( -16.53943276465976808, -0.05219959533934237506, 23.75109039468567929 ) ) ;
#153984=CARTESIAN_POINT ( 'NONE',  ( -19.02544592524342804, 5.153800228976336051, 76.04057627198102409 ) ) ;
#153985=CARTESIAN_POINT ( 'NONE',  ( -4.379528057220086978, -16.55341960407618274, 29.79275706135234358 ) ) ;
#153986=CARTESIAN_POINT ( 'NONE',  ( -13.89961937509977652, 13.97604488694528158, 45.62390960531433848 ) ) ;
#153987=CARTESIAN_POINT ( 'NONE',  ( 12.14591786802327356, -12.06949235617739191, 25.62609039468567929 ) ) ;
#153988=CARTESIAN_POINT ( 'NONE',  ( 0.05219959533910956823, 16.53943276465976808, 74.99890960531435269 ) ) ;
#153989=CARTESIAN_POINT ( 'NONE',  ( 14.29746914071037800, 8.314922557961029526, 91.66775706135234714 ) ) ;
#153990=CARTESIAN_POINT ( 'NONE',  ( -21.55341960407619339, 5.719274019375674811, 28.54275706135234358 ) ) ;
#153991=CARTESIAN_POINT ( 'NONE',  ( 16.51473224551069308, 9.474510206698969483, 64.16557627198102409 ) ) ;
#153992=CARTESIAN_POINT ( 'NONE',  ( -5.049401038298153566, 19.05341960407611168, 70.20724293864769550 ) ) ;
#153993=CARTESIAN_POINT ( 'NONE',  ( 4.483927247898790824, -16.52544592524335698, 85.20942372801901854 ) ) ;
#153994=CARTESIAN_POINT ( 'NONE',  ( 17.50000000000000000, 5.499999999999992895, 51.70309617465830598 ) ) ;
#153995=ORIENTED_EDGE ( 'NONE', *, *, #16822, .T. ) ;
#153997=CARTESIAN_POINT ( 'NONE',  ( -0.05219959533936034679, 19.03943276465977164, 32.50109039468566863 ) ) ;
#154000=CARTESIAN_POINT ( 'NONE',  ( -9.564922557960796823, -16.46253265017161027, 32.08224293864769550 ) ) ;
#154001=CARTESIAN_POINT ( 'NONE',  ( 9.474510206698971260, -16.51473224551069308, 112.9155762719810383 ) ) ;
#154003=CARTESIAN_POINT ( 'NONE',  ( -8.314922557961024197, 14.29746914071037800, 22.91775706135235069 ) ) ;
#154004=CARTESIAN_POINT ( 'NONE',  ( -9.564922557961040184, 16.46253265017147172, 52.91775706135233293 ) ) ;
#154005=CARTESIAN_POINT ( 'NONE',  ( -16.53943276465976808, -0.05219959533934237506, 38.75109039468567573 ) ) ;
#154006=CARTESIAN_POINT ( 'NONE',  ( 13.89961937509977652, -13.97604488694527269, 108.1239096053143669 ) ) ;
#154007=CARTESIAN_POINT ( 'NONE',  ( -5.049401038298153566, 19.05341960407611168, 65.20724293864765286 ) ) ;
#154008=CARTESIAN_POINT ( 'NONE',  ( 15.72974639402199770, -15.80617190586745480, 98.12390960531436690 ) ) ;
#154009=CARTESIAN_POINT ( 'NONE',  ( 13.89961937509977652, -13.97604488694527269, 98.12390960531433848 ) ) ;
#154010=CARTESIAN_POINT ( 'NONE',  ( 17.37577197770832527, -5.499999999999936939, 21.30611277022550354 ) ) ;
#154012=CARTESIAN_POINT ( 'NONE',  ( -5.049401038298153566, 19.05341960407611168, 65.20724293864765286 ) ) ;
#154013=CARTESIAN_POINT ( 'NONE',  ( -12.06949235617756955, 12.14591786802309770, 25.62390960531435624 ) ) ;
#154014=CARTESIAN_POINT ( 'NONE',  ( -13.89961937509977652, 13.97604488694528158, 25.62390960531434558 ) ) ;
#154015=CARTESIAN_POINT ( 'NONE',  ( -9.474510206698720793, -16.51473224551083518, 39.58442372801899722 ) ) ;
#154016=CARTESIAN_POINT ( 'NONE',  ( -12.14591786802309592, -12.06949235617757132, 61.87390960531436690 ) ) ;
#154017=CARTESIAN_POINT ( 'NONE',  ( -21.55341960407619339, 5.719274019375674811, 103.5427570613523613 ) ) ;
#154018=CARTESIAN_POINT ( 'NONE',  ( -5.049401038298153566, 19.05341960407611168, 35.20724293864768839 ) ) ;
#154019=CARTESIAN_POINT ( 'NONE',  ( -8.314922557961024197, 14.29746914071037800, 57.91775706135234714 ) ) ;
#154020=CARTESIAN_POINT ( 'NONE',  ( -16.55341960407611168, -4.379528057220339221, 36.45724293864768839 ) ) ;
#154021=CARTESIAN_POINT ( 'NONE',  ( 21.55341960407619695, -5.719274019375665929, 86.04275706135236135 ) ) ;
#154022=CARTESIAN_POINT ( 'NONE',  ( 19.03943276465977164, -0.05219959533909143690, 78.74890960531436690 ) ) ;
#154023=CARTESIAN_POINT ( 'NONE',  ( 9.564922557960805705, 16.46253265017160317, 99.58224293864770971 ) ) ;
#154024=CARTESIAN_POINT ( 'NONE',  ( 14.34966873604960469, 8.224510206698951720, 114.1655762719810383 ) ) ;
#154025=CARTESIAN_POINT ( 'NONE',  ( 4.379528057220339221, -16.55341960407611168, 72.70724293864769550 ) ) ;
#154026=CARTESIAN_POINT ( 'NONE',  ( -5.823673210054116645, -21.52544592524344225, 87.29057627198103830 ) ) ;
#154027=CARTESIAN_POINT ( 'NONE',  ( -9.564922557960796823, -16.46253265017161027, 72.08224293864770971 ) ) ;
#154028=CARTESIAN_POINT ( 'NONE',  ( -0.05219959533907301413, -21.53943276465977519, 102.4989096053143811 ) ) ;
#154029=CARTESIAN_POINT ( 'NONE',  ( 19.02544592524334988, 5.153800228976608722, 76.45942372801897591 ) ) ;
#154030=CARTESIAN_POINT ( 'NONE',  ( 19.48894818550242292, -5.500000000000105693, 47.60307310435243267 ) ) ;
#154031=CARTESIAN_POINT ( 'NONE',  ( 12.06949235617757843, -12.14591786802309237, 93.12390960531436690 ) ) ;
#154033=CARTESIAN_POINT ( 'NONE',  ( -9.474510206698964154, 16.51473224551069663, 60.41557627198102409 ) ) ;
#154034=CARTESIAN_POINT ( 'NONE',  ( 5.719274019375991003, -21.55341960407610458, 72.70724293864769550 ) ) ;
#154035=CARTESIAN_POINT ( 'NONE',  ( 17.50000000000000355, -5.499999999999992006, 26.21769037696436300 ) ) ;
#154036=CARTESIAN_POINT ( 'NONE',  ( 0.05219959533934541429, -16.53943276465976808, 110.0010903946856757 ) ) ;
#154037=CARTESIAN_POINT ( 'NONE',  ( 14.29746914071037800, 8.314922557961029526, 21.66775706135235069 ) ) ;
#154038=CARTESIAN_POINT ( 'NONE',  ( -16.52544592524342804, 4.483927247898546575, 81.04057627198102409 ) ) ;
#154039=CARTESIAN_POINT ( 'NONE',  ( -17.50000000000001066, -5.500000000000021316, 46.28230962303566542 ) ) ;
#154040=CARTESIAN_POINT ( 'NONE',  ( 13.89961937509977652, -13.97604488694527269, 68.12390960531436690 ) ) ;
#154041=CARTESIAN_POINT ( 'NONE',  ( -5.153800228976328057, -19.02544592524343514, 37.29057627198102409 ) ) ;
#154042=CARTESIAN_POINT ( 'NONE',  ( 16.53943276465976808, -0.05219959533910856209, 63.74890960531435979 ) ) ;
#154043=CARTESIAN_POINT ( 'NONE',  ( 0.05219959533909260263, 19.03943276465977164, 109.9989096053143669 ) ) ;
#154044=CARTESIAN_POINT ( 'NONE',  ( -5.153800228976607833, 19.02544592524334988, 92.70942372801901854 ) ) ;
#154045=CARTESIAN_POINT ( 'NONE',  ( -19.02544592524342804, 5.153800228976336051, 106.0405762719810241 ) ) ;
#154046=CARTESIAN_POINT ( 'NONE',  ( -18.62759615963270932, 10.81492255796079327, 70.83224293864770971 ) ) ;
#154047=CARTESIAN_POINT ( 'NONE',  ( 12.06949235617739724, 12.14591786802326823, 66.87609039468568994 ) ) ;
#154048=CARTESIAN_POINT ( 'NONE',  ( -16.88567814943195344, 6.947325034625343676, 93.70998877347403777 ) ) ;
#154049=CARTESIAN_POINT ( 'NONE',  ( 9.474510206698971260, -16.51473224551069308, 57.91557627198103120 ) ) ;
#154050=CARTESIAN_POINT ( 'NONE',  ( -0.05219959533907301413, -21.53943276465977519, 72.49890960531435269 ) ) ;
#154051=CARTESIAN_POINT ( 'NONE',  ( 16.46253265017146816, 9.564922557961045513, 101.6677570613523329 ) ) ;
#154052=CARTESIAN_POINT ( 'NONE',  ( -16.55341960407611168, -4.379528057220339221, 41.45724293864769550 ) ) ;
#154053=CARTESIAN_POINT ( 'NONE',  ( 15.80617190586769283, -15.72974639402175789, 60.62609039468567573 ) ) ;
#154055=CARTESIAN_POINT ( 'NONE',  ( -16.53943276465976808, -0.05219959533934237506, 68.75109039468568994 ) ) ;
#154056=CARTESIAN_POINT ( 'NONE',  ( -13.89961937509977652, 13.97604488694528158, 105.6239096053143527 ) ) ;
#154059=CARTESIAN_POINT ( 'NONE',  ( 12.06949235617739724, 12.14591786802326823, 91.87609039468568994 ) ) ;
#154060=CARTESIAN_POINT ( 'NONE',  ( 4.379528057220092307, 16.55341960407617563, 47.29275706135234003 ) ) ;
#154061=CARTESIAN_POINT ( 'NONE',  ( -5.049401038298153566, 19.05341960407611168, 65.20724293864765286 ) ) ;
#154062=CARTESIAN_POINT ( 'NONE',  ( -9.564922557960796823, -16.46253265017161027, 72.08224293864770971 ) ) ;
#154063=CARTESIAN_POINT ( 'NONE',  ( 10.72451020669871369, 18.67979575497193778, 52.08442372801901854 ) ) ;
#154064=CARTESIAN_POINT ( 'NONE',  ( -0.05219959533934338120, 16.53943276465976808, 57.50109039468568994 ) ) ;
#154065=CARTESIAN_POINT ( 'NONE',  ( 8.224510206698953496, -14.34966873604960469, 27.91557627198103830 ) ) ;
#154066=CARTESIAN_POINT ( 'NONE',  ( -19.05341960407611168, -5.049401038298163336, 36.45724293864766707 ) ) ;
#154067=CARTESIAN_POINT ( 'NONE',  ( -16.51473224551069308, -9.474510206698971260, 31.66557627198102054 ) ) ;
#154068=CARTESIAN_POINT ( 'NONE',  ( -8.224510206698735004, -14.34966873604973081, 29.58442372801901854 ) ) ;
#154070=CARTESIAN_POINT ( 'NONE',  ( 13.89961937509957401, 13.97604488694547697, 81.87609039468564731 ) ) ;
#154071=CARTESIAN_POINT ( 'NONE',  ( 12.06949235617757843, -12.14591786802309237, 78.12390960531436690 ) ) ;
#154072=CARTESIAN_POINT ( 'NONE',  ( -9.564922557960796823, -16.46253265017161027, 47.08224293864769550 ) ) ;
#154073=CARTESIAN_POINT ( 'NONE',  ( 16.46253265017146816, 9.564922557961045513, 86.66775706135233293 ) ) ;
#154075=CARTESIAN_POINT ( 'NONE',  ( -21.52544592524334988, -5.823673210054445271, 83.95942372801900433 ) ) ;
#154076=CARTESIAN_POINT ( 'NONE',  ( 16.55341960407618274, -4.379528057220086978, 56.04275706135235424 ) ) ;
#154077=CARTESIAN_POINT ( 'NONE',  ( -15.49999999999999822, 7.499999999999998224, 120.0000000000000142 ) ) ;
#154078=CARTESIAN_POINT ( 'NONE',  ( -21.52544592524343514, 5.823673210054127303, 46.04057627198103830 ) ) ;
#154079=CARTESIAN_POINT ( 'NONE',  ( 0.05219959533934541429, -16.53943276465976808, 35.00109039468568284 ) ) ;
#154080=CARTESIAN_POINT ( 'NONE',  ( -0.05219959533909027116, -19.03943276465977164, 37.49890960531436690 ) ) ;
#154081=CARTESIAN_POINT ( 'NONE',  ( 19.03943276465977164, 0.05219959533936151252, 36.25109039468567573 ) ) ;
#154082=CARTESIAN_POINT ( 'NONE',  ( -19.02544592524342804, 5.153800228976336051, 91.04057627198100988 ) ) ;
#154083=CARTESIAN_POINT ( 'NONE',  ( 0.05219959533909260263, 19.03943276465977164, 49.99890960531435979 ) ) ;
#154085=CARTESIAN_POINT ( 'NONE',  ( 10.72451020669871369, 18.67979575497193778, 77.08442372801901854 ) ) ;
#154087=CARTESIAN_POINT ( 'NONE',  ( -5.049401038297874678, -19.05341960407617918, 34.79275706135233293 ) ) ;
#154088=CARTESIAN_POINT ( 'NONE',  ( -21.52544592524334988, -5.823673210054445271, 108.9594237280190185 ) ) ;
#154089=CARTESIAN_POINT ( 'NONE',  ( 14.29746914071049879, -8.314922557960816363, 43.33224293864769550 ) ) ;
#154090=CARTESIAN_POINT ( 'NONE',  ( 16.51473224551069308, 9.474510206698969483, 49.16557627198102409 ) ) ;
#154091=CARTESIAN_POINT ( 'NONE',  ( 19.03943276465977164, -0.05219959533909143690, 108.7489096053143527 ) ) ;
#154092=CARTESIAN_POINT ( 'NONE',  ( 21.55341960407619695, -5.719274019375665929, 81.04275706135236135 ) ) ;
#154093=CARTESIAN_POINT ( 'NONE',  ( 0.05219959533909260263, 19.03943276465977164, 59.99890960531436690 ) ) ;
#154094=CARTESIAN_POINT ( 'NONE',  ( 5.823673210054444382, -21.52544592524334988, 80.20942372801901854 ) ) ;
#154095=CARTESIAN_POINT ( 'NONE',  ( -15.72974639402197994, 15.80617190586746368, 40.62390960531435269 ) ) ;
#154096=CARTESIAN_POINT ( 'NONE',  ( 15.72974639402176855, 15.80617190586768217, 31.87609039468567929 ) ) ;
#154097=CARTESIAN_POINT ( 'NONE',  ( -13.89961937509957401, -13.97604488694547875, 49.37609039468567573 ) ) ;
#154098=CARTESIAN_POINT ( 'NONE',  ( 16.46253265017160672, -9.564922557960803928, 23.33224293864769194 ) ) ;
#154099=CARTESIAN_POINT ( 'NONE',  ( -19.03943276465977164, 0.05219959533909376836, 81.24890960531436690 ) ) ;
#154100=CARTESIAN_POINT ( 'NONE',  ( 0.05219959533934541429, -16.53943276465976808, 30.00109039468568284 ) ) ;
#154101=CARTESIAN_POINT ( 'NONE',  ( -4.379528057220328563, 16.55341960407611168, 90.20724293864770971 ) ) ;
#154102=CARTESIAN_POINT ( 'NONE',  ( -5.153800228976328057, -19.02544592524343514, 52.29057627198100988 ) ) ;
#154103=CARTESIAN_POINT ( 'NONE',  ( 10.72451020669898902, -18.67979575497178502, 37.91557627198102409 ) ) ;
#154104=CARTESIAN_POINT ( 'NONE',  ( -5.049401038297874678, -19.05341960407617918, 104.7927570613523471 ) ) ;
#154105=CARTESIAN_POINT ( 'NONE',  ( -18.62759615963270932, 10.81492255796079327, 110.8322429386476955 ) ) ;
#154106=CARTESIAN_POINT ( 'NONE',  ( 10.81492255796106328, -18.62759615963255655, 55.41775706135234714 ) ) ;
#154107=CARTESIAN_POINT ( 'NONE',  ( -16.55341960407617563, 4.379528057220093196, 68.54275706135234714 ) ) ;
#154108=CARTESIAN_POINT ( 'NONE',  ( -12.14591786802326823, 12.06949235617739902, 63.12609039468568994 ) ) ;
#154109=ORIENTED_EDGE ( 'NONE', *, *, #196054, .F. ) ;
#154110=CARTESIAN_POINT ( 'NONE',  ( -19.02544592524342804, 5.153800228976336051, 66.04057627198103830 ) ) ;
#154111=CARTESIAN_POINT ( 'NONE',  ( 8.314922557961029526, -14.29746914071037800, 85.41775706135236135 ) ) ;
#154112=CARTESIAN_POINT ( 'NONE',  ( -18.62759615963270932, 10.81492255796079327, 115.8322429386477097 ) ) ;
#154113=CARTESIAN_POINT ( 'NONE',  ( 12.06949235617757843, -12.14591786802309237, 68.12390960531436690 ) ) ;
#154114=CARTESIAN_POINT ( 'NONE',  ( -19.05341960407611168, -5.049401038298163336, 81.45724293864769550 ) ) ;
#154115=CARTESIAN_POINT ( 'NONE',  ( 14.34966873604972726, -8.224510206698740333, 75.83442372801900433 ) ) ;
#154116=B_SPLINE_CURVE_WITH_KNOTS ( 'NONE', 3,
 ( #29133, #59443, #156176, #155188, #16678, #3477 ),
 .UNSPECIFIED., .F., .F.,
 ( 4, 2, 4 ),
 ( 0.003989672132298151264, 0.004372778065220565835, 0.004755883998142980407 ),
 .UNSPECIFIED. ) ;
#154117=CARTESIAN_POINT ( 'NONE',  ( -10.72451020669870658, -18.67979575497194134, 59.58442372801901854 ) ) ;
#154118=CARTESIAN_POINT ( 'NONE',  ( 16.51473224551083163, -9.474510206698727899, 110.8344237280190043 ) ) ;
#154119=CARTESIAN_POINT ( 'NONE',  ( 18.62759615963271287, -10.81492255796078972, 113.3322429386476955 ) ) ;
#154120=CARTESIAN_POINT ( 'NONE',  ( 4.483927247898545687, 16.52544592524342804, 54.79057627198104541 ) ) ;
#154122=CARTESIAN_POINT ( 'NONE',  ( -21.53943276465977519, 0.05219959533907696930, 86.24890960531436690 ) ) ;
#154123=CARTESIAN_POINT ( 'NONE',  ( -4.379528057220328563, 16.55341960407611168, 35.20724293864768839 ) ) ;
#154126=CARTESIAN_POINT ( 'NONE',  ( -5.719274019375978568, 21.55341960407610458, 115.2072429386476955 ) ) ;
#154127=CARTESIAN_POINT ( 'NONE',  ( -21.53943276465977519, 0.05219959533907696930, 21.24890960531436690 ) ) ;
#154128=CARTESIAN_POINT ( 'NONE',  ( 18.67979575497194134, -10.72451020669871369, 25.83442372801901499 ) ) ;
#154129=CARTESIAN_POINT ( 'NONE',  ( 16.53943276465976808, -0.05219959533910856209, 48.74890960531435979 ) ) ;
#154130=CARTESIAN_POINT ( 'NONE',  ( -16.55341960407617563, 4.379528057220093196, 63.54275706135234003 ) ) ;
#154132=CARTESIAN_POINT ( 'NONE',  ( 13.89961937509977652, -13.97604488694527269, 58.12390960531436690 ) ) ;
#154134=CARTESIAN_POINT ( 'NONE',  ( 5.153800228976615827, -19.02544592524334988, 60.20942372801899012 ) ) ;
#154135=CARTESIAN_POINT ( 'NONE',  ( 9.564922557960805705, 16.46253265017160317, 99.58224293864770971 ) ) ;
#154136=CARTESIAN_POINT ( 'NONE',  ( 10.81492255796078972, 18.62759615963270932, 49.58224293864769550 ) ) ;
#154138=CARTESIAN_POINT ( 'NONE',  ( -9.564922557960796823, -16.46253265017161027, 52.08224293864768839 ) ) ;
#154139=CARTESIAN_POINT ( 'NONE',  ( 16.53943276465976808, 0.05219959533934440121, 36.25109039468567573 ) ) ;
#154140=CARTESIAN_POINT ( 'NONE',  ( 5.153800228976615827, -19.02544592524334988, 60.20942372801899012 ) ) ;
#154141=CARTESIAN_POINT ( 'NONE',  ( 0.05219959533907565091, 21.53943276465977519, 114.9989096053143669 ) ) ;
#154142=CARTESIAN_POINT ( 'NONE',  ( 0.05219959533910956823, 16.53943276465976808, 44.99890960531435979 ) ) ;
#154143=CARTESIAN_POINT ( 'NONE',  ( 16.51473224551069308, 9.474510206698969483, 84.16557627198102409 ) ) ;
#154144=CARTESIAN_POINT ( 'NONE',  ( 21.53943276465977519, -0.05219959533907433946, 63.74890960531435979 ) ) ;
#154145=CARTESIAN_POINT ( 'NONE',  ( -15.80617190586745835, -15.72974639402198527, 101.8739096053143811 ) ) ;
#154146=CARTESIAN_POINT ( 'NONE',  ( 4.483927247898790824, -16.52544592524335698, 35.20942372801901854 ) ) ;
#154147=CARTESIAN_POINT ( 'NONE',  ( -10.81492255796078084, -18.62759615963271287, 42.08224293864769550 ) ) ;
#154148=CARTESIAN_POINT ( 'NONE',  ( 10.81492255796106328, -18.62759615963255655, 95.41775706135234714 ) ) ;
#154149=CARTESIAN_POINT ( 'NONE',  ( 16.51473224551069308, 9.474510206698969483, 84.16557627198102409 ) ) ;
#154150=CARTESIAN_POINT ( 'NONE',  ( 16.46253265017160672, -9.564922557960803928, 38.33224293864768839 ) ) ;
#154151=CARTESIAN_POINT ( 'NONE',  ( 5.049401038298161559, -19.05341960407611168, 102.7072429386476955 ) ) ;
#154152=CARTESIAN_POINT ( 'NONE',  ( 4.483927247898545687, 16.52544592524342804, 104.7905762719810241 ) ) ;
#154153=CARTESIAN_POINT ( 'NONE',  ( -9.564922557960796823, -16.46253265017161027, 67.08224293864769550 ) ) ;
#154154=CARTESIAN_POINT ( 'NONE',  ( 12.06949235617739724, 12.14591786802326823, 26.87609039468567218 ) ) ;
#154155=CARTESIAN_POINT ( 'NONE',  ( -5.153800228976607833, 19.02544592524335343, 42.70942372801900433 ) ) ;
#154156=CARTESIAN_POINT ( 'NONE',  ( 5.049401038297881783, 19.05341960407617563, 57.29275706135231871 ) ) ;
#154158=CARTESIAN_POINT ( 'NONE',  ( -21.55341960407619339, 5.719274019375674811, 93.54275706135234714 ) ) ;
#154159=CARTESIAN_POINT ( 'NONE',  ( 10.72451020669898902, -18.67979575497178502, 27.91557627198103830 ) ) ;
#154160=CARTESIAN_POINT ( 'NONE',  ( -12.06949235617739369, -12.14591786802326823, 89.37609039468568994 ) ) ;
#154161=CARTESIAN_POINT ( 'NONE',  ( -13.97604488694547697, 13.89961937509957934, 68.12609039468563310 ) ) ;
#154162=CARTESIAN_POINT ( 'NONE',  ( -0.05219959533936034679, 19.03943276465977164, 32.50109039468566863 ) ) ;
#154163=CARTESIAN_POINT ( 'NONE',  ( -15.49999999999999822, 5.499999999999998224, 118.0000000000000142 ) ) ;
#154164=CARTESIAN_POINT ( 'NONE',  ( -9.564922557960796823, -16.46253265017161027, 27.08224293864769550 ) ) ;
#154165=CARTESIAN_POINT ( 'NONE',  ( -14.29746914071049879, 8.314922557960819915, 40.83224293864769550 ) ) ;
#154166=EDGE_CURVE ( 'NONE', #182496, #132514, #5380, .T. ) ;
#154167=CARTESIAN_POINT ( 'NONE',  ( 9.474510206698971260, -16.51473224551069308, 22.91557627198102765 ) ) ;
#154168=CARTESIAN_POINT ( 'NONE',  ( -0.05219959533910754901, -16.53943276465976808, 22.49890960531436335 ) ) ;
#154169=CARTESIAN_POINT ( 'NONE',  ( 18.22780087662123805, -5.499999999999976019, 88.51763182126893525 ) ) ;
#154170=CARTESIAN_POINT ( 'NONE',  ( 12.14591786802327356, -12.06949235617739191, 100.6260903946857184 ) ) ;
#154171=CARTESIAN_POINT ( 'NONE',  ( 13.89961937509977652, -13.97604488694527269, 38.12390960531436690 ) ) ;
#154172=CARTESIAN_POINT ( 'NONE',  ( 18.67979575497194134, -10.72451020669871369, 100.8344237280190185 ) ) ;
#154173=CARTESIAN_POINT ( 'NONE',  ( -8.224510206698735004, -14.34966873604973081, 19.58442372801901143 ) ) ;
#154174=CARTESIAN_POINT ( 'NONE',  ( 15.80617190586769283, -15.72974639402175789, 80.62609039468567573 ) ) ;
#154175=CARTESIAN_POINT ( 'NONE',  ( -16.51473224551082808, 9.474510206698731452, 58.33442372801900433 ) ) ;
#154176=CARTESIAN_POINT ( 'NONE',  ( 9.474510206698971260, -16.51473224551069308, 92.91557627198103830 ) ) ;
#154177=CARTESIAN_POINT ( 'NONE',  ( 16.46253265017160672, -9.564922557960803928, 83.33224293864768129 ) ) ;
#154179=CARTESIAN_POINT ( 'NONE',  ( -5.823673210054116645, -21.52544592524344225, 112.2905762719810241 ) ) ;
#154181=CARTESIAN_POINT ( 'NONE',  ( -16.55341960407611168, -4.379528057220339221, 61.45724293864770260 ) ) ;
#154182=CARTESIAN_POINT ( 'NONE',  ( 21.55341960407610458, 5.719274019375980345, 58.95724293864770971 ) ) ;
#154183=CARTESIAN_POINT ( 'NONE',  ( -9.564922557960796823, -16.46253265017161027, 57.08224293864769550 ) ) ;
#154184=CARTESIAN_POINT ( 'NONE',  ( 5.823673210054125526, 21.52544592524343514, 99.79057627198103830 ) ) ;
#154185=CARTESIAN_POINT ( 'NONE',  ( 14.29746914071037800, 8.314922557961029526, 96.66775706135234714 ) ) ;
#154187=CARTESIAN_POINT ( 'NONE',  ( 13.97604488694527802, 13.89961937509977652, 44.37390960531435269 ) ) ;
#154188=CARTESIAN_POINT ( 'NONE',  ( 12.06949235617757843, -12.14591786802309237, 88.12390960531436690 ) ) ;
#154190=CARTESIAN_POINT ( 'NONE',  ( 13.97604488694527802, 13.89961937509977652, 49.37390960531434558 ) ) ;
#154191=CARTESIAN_POINT ( 'NONE',  ( -13.97604488694527625, -13.89961937509977652, 26.87390960531434558 ) ) ;
#154192=CARTESIAN_POINT ( 'NONE',  ( -13.89961937509957401, -13.97604488694547875, 79.37609039468567573 ) ) ;
#154193=CARTESIAN_POINT ( 'NONE',  ( 12.14591786802309770, 12.06949235617756955, 89.37390960531435269 ) ) ;
#154194=CARTESIAN_POINT ( 'NONE',  ( -10.81492255796105439, 18.62759615963255655, 47.91775706135234714 ) ) ;
#154195=CARTESIAN_POINT ( 'NONE',  ( 13.97604488694527802, 13.89961937509977652, 34.37390960531436690 ) ) ;
#154196=CARTESIAN_POINT ( 'NONE',  ( -21.52544592524343514, 5.823673210054127303, 106.0405762719810525 ) ) ;
#154197=CARTESIAN_POINT ( 'NONE',  ( 16.52544592524342804, -4.483927247898539470, 88.54057627198103830 ) ) ;
#154199=CARTESIAN_POINT ( 'NONE',  ( 5.153800228976335163, 19.02544592524342804, 59.79057627198100988 ) ) ;
#154200=CARTESIAN_POINT ( 'NONE',  ( 17.31747979337948706, 6.344076630961062335, 113.8794486806519046 ) ) ;
#154201=CARTESIAN_POINT ( 'NONE',  ( 19.02544592524334988, 5.153800228976608722, 96.45942372801897591 ) ) ;
#154202=CARTESIAN_POINT ( 'NONE',  ( -0.05219959533907301413, -21.53943276465977519, 22.49890960531436335 ) ) ;
#154203=CARTESIAN_POINT ( 'NONE',  ( -10.72451020669870658, -18.67979575497194134, 39.58442372801901143 ) ) ;
#154204=CARTESIAN_POINT ( 'NONE',  ( -16.51473224551069308, -9.474510206698971260, 86.66557627198102409 ) ) ;
#154206=CARTESIAN_POINT ( 'NONE',  ( -19.05341960407617563, 5.049401038297882671, 63.54275706135234003 ) ) ;
#154207=CARTESIAN_POINT ( 'NONE',  ( -9.564922557960796823, -16.46253265017161027, 52.08224293864768839 ) ) ;
#154208=CARTESIAN_POINT ( 'NONE',  ( 8.224510206698953496, -14.34966873604960469, 72.91557627198103830 ) ) ;
#154209=CARTESIAN_POINT ( 'NONE',  ( -12.06949235617756955, 12.14591786802309770, 70.62390960531436690 ) ) ;
#154210=CARTESIAN_POINT ( 'NONE',  ( -9.474510206698964154, 16.51473224551069663, 85.41557627198102409 ) ) ;
#154211=CARTESIAN_POINT ( 'NONE',  ( -10.72451020669898014, 18.67979575497178502, 95.41557627198102409 ) ) ;
#154212=CARTESIAN_POINT ( 'NONE',  ( -5.153800228976328057, -19.02544592524343514, 82.29057627198103830 ) ) ;
#154213=CARTESIAN_POINT ( 'NONE',  ( -9.474510206698720793, -16.51473224551083518, 34.58442372801899722 ) ) ;
#154214=CARTESIAN_POINT ( 'NONE',  ( -9.474510206698964154, 16.51473224551069663, 35.41557627198102409 ) ) ;
#154215=CARTESIAN_POINT ( 'NONE',  ( -14.34966873604960291, -8.224510206698953496, 36.66557627198103120 ) ) ;
#154216=CARTESIAN_POINT ( 'NONE',  ( 14.34966873604960469, 8.224510206698951720, 104.1655762719810241 ) ) ;
#154217=VERTEX_POINT ( 'NONE', #161663 ) ;
#154218=CARTESIAN_POINT ( 'NONE',  ( 10.81492255796106328, -18.62759615963255655, 30.41775706135234358 ) ) ;
#154219=CARTESIAN_POINT ( 'NONE',  ( -5.153800228976607833, 19.02544592524334988, 62.70942372801899722 ) ) ;
#154220=CARTESIAN_POINT ( 'NONE',  ( 12.14591786802309770, 12.06949235617756955, 39.37390960531436690 ) ) ;
#154221=CARTESIAN_POINT ( 'NONE',  ( 5.823673210054125526, 21.52544592524343514, 89.79057627198103830 ) ) ;
#154222=CARTESIAN_POINT ( 'NONE',  ( -5.153800228976328057, -19.02544592524343514, 112.2905762719810099 ) ) ;
#154223=CARTESIAN_POINT ( 'NONE',  ( -16.55341960407611168, -4.379528057220339221, 71.45724293864769550 ) ) ;
#154224=CARTESIAN_POINT ( 'NONE',  ( 19.05341960407611168, 5.049401038298154454, 33.95724293864769550 ) ) ;
#154225=CARTESIAN_POINT ( 'NONE',  ( 16.46253265017146816, 9.564922557961045513, 21.66775706135233648 ) ) ;
#154226=CARTESIAN_POINT ( 'NONE',  ( 8.314922557961029526, -14.29746914071037800, 105.4177570613523613 ) ) ;
#154227=CARTESIAN_POINT ( 'NONE',  ( -0.05219959533934338120, 16.53943276465976808, 62.50109039468568284 ) ) ;
#154228=CARTESIAN_POINT ( 'NONE',  ( -21.52544592524343514, 5.823673210054127303, 36.04057627198102409 ) ) ;
#154229=CARTESIAN_POINT ( 'NONE',  ( -10.72451020669870658, -18.67979575497194134, 104.5844237280190185 ) ) ;
#154230=CARTESIAN_POINT ( 'NONE',  ( 16.46253265017160672, -9.564922557960803928, 73.33224293864769550 ) ) ;
#154231=CARTESIAN_POINT ( 'NONE',  ( -4.379528057220086978, -16.55341960407618274, 54.79275706135235424 ) ) ;
#154232=CARTESIAN_POINT ( 'NONE',  ( 14.34966873604960469, 8.224510206698951720, 114.1655762719810383 ) ) ;
#154233=CARTESIAN_POINT ( 'NONE',  ( -4.379528057220328563, 16.55341960407611168, 40.20724293864769550 ) ) ;
#154235=CARTESIAN_POINT ( 'NONE',  ( -13.97604488694527625, -13.89961937509977652, 106.8739096053143669 ) ) ;
#154236=CARTESIAN_POINT ( 'NONE',  ( -19.02544592524342804, 5.153800228976336051, 96.04057627198103830 ) ) ;
#154237=CARTESIAN_POINT ( 'NONE',  ( 19.02544592524343514, -5.153800228976328945, 103.5405762719809957 ) ) ;
#154238=CARTESIAN_POINT ( 'NONE',  ( 16.55341960407611168, 4.379528057220329451, 58.95724293864770971 ) ) ;
#154239=CARTESIAN_POINT ( 'NONE',  ( 4.483927247898545687, 16.52544592524342804, 34.79057627198103120 ) ) ;
#154240=CARTESIAN_POINT ( 'NONE',  ( 4.379528057220339221, -16.55341960407611168, 47.70724293864770260 ) ) ;
#154241=CARTESIAN_POINT ( 'NONE',  ( -4.483927247898782831, 16.52544592524335698, 37.70942372801900433 ) ) ;
#154242=CARTESIAN_POINT ( 'NONE',  ( 17.50000000000000711, -5.076555817581199115, 31.32048507950228355 ) ) ;
#154243=CARTESIAN_POINT ( 'NONE',  ( -9.564922557961040184, 16.46253265017147172, 47.91775706135233293 ) ) ;
#154244=CARTESIAN_POINT ( 'NONE',  ( -16.46253265017160317, 9.564922557960807481, 75.83224293864769550 ) ) ;
#154245=CARTESIAN_POINT ( 'NONE',  ( -5.153800228976607833, 19.02544592524334988, 67.70942372801900433 ) ) ;
#154247=CARTESIAN_POINT ( 'NONE',  ( 9.564922557961047289, -16.46253265017146816, 60.41775706135233293 ) ) ;
#154248=CARTESIAN_POINT ( 'NONE',  ( -19.05341960407617563, 5.049401038297882671, 103.5427570613523329 ) ) ;
#154249=CARTESIAN_POINT ( 'NONE',  ( 14.34966873604972726, -8.224510206698740333, 85.83442372801901854 ) ) ;
#154251=CARTESIAN_POINT ( 'NONE',  ( 13.97604488694527802, 13.89961937509977652, 29.37390960531435979 ) ) ;
#154252=CARTESIAN_POINT ( 'NONE',  ( -10.81492255796078084, -18.62759615963271287, 27.08224293864769550 ) ) ;
#154253=CARTESIAN_POINT ( 'NONE',  ( 18.62759615963255655, 10.81492255796105972, 41.66775706135235424 ) ) ;
#154254=CARTESIAN_POINT ( 'NONE',  ( 19.03943276465977164, 0.05219959533936151252, 106.2510903946856615 ) ) ;
#154256=CARTESIAN_POINT ( 'NONE',  ( 9.564922557960805705, 16.46253265017160317, 59.58224293864769550 ) ) ;
#154257=CARTESIAN_POINT ( 'NONE',  ( -5.153800228976328057, -19.02544592524343514, 107.2905762719810383 ) ) ;
#154258=CARTESIAN_POINT ( 'NONE',  ( 4.483927247898545687, 16.52544592524342804, 59.79057627198103120 ) ) ;
#154259=CARTESIAN_POINT ( 'NONE',  ( -5.153800228976328057, -19.02544592524343514, 57.29057627198103120 ) ) ;
#154260=CARTESIAN_POINT ( 'NONE',  ( -5.153800228976328057, -19.02544592524343514, 57.29057627198103120 ) ) ;
#154261=CARTESIAN_POINT ( 'NONE',  ( -16.46253265017146816, -9.564922557961047289, 74.16775706135234714 ) ) ;
#154262=CARTESIAN_POINT ( 'NONE',  ( -21.53943276465977519, 0.05219959533907696930, 46.24890960531435979 ) ) ;
#154263=CARTESIAN_POINT ( 'NONE',  ( -16.52544592524342804, 4.483927247898546575, 111.0405762719810525 ) ) ;
#154264=CARTESIAN_POINT ( 'NONE',  ( -13.97604488694547697, 13.89961937509957934, 48.12609039468566863 ) ) ;
#154265=CARTESIAN_POINT ( 'NONE',  ( 13.89961937509977652, -13.97604488694527269, 83.12390960531436690 ) ) ;
#154266=CARTESIAN_POINT ( 'NONE',  ( 18.67979575497178502, 10.72451020669898547, 74.16557627198102409 ) ) ;
#154267=CARTESIAN_POINT ( 'NONE',  ( -14.29746914071049879, 8.314922557960819915, 85.83224293864768129 ) ) ;
#154268=CARTESIAN_POINT ( 'NONE',  ( -16.46253265017146816, -9.564922557961047289, 34.16775706135233293 ) ) ;
#154269=CARTESIAN_POINT ( 'NONE',  ( 15.80617190586746368, 15.72974639402197994, 64.37390960531435269 ) ) ;
#154270=CARTESIAN_POINT ( 'NONE',  ( -21.52544592524343514, 5.823673210054127303, 41.04057627198103120 ) ) ;
#154271=CARTESIAN_POINT ( 'NONE',  ( -21.55341960407619339, 5.719274019375674811, 88.54275706135236135 ) ) ;
#154272=CARTESIAN_POINT ( 'NONE',  ( -9.474510206698964154, 16.51473224551069663, 65.41557627198102409 ) ) ;
#154273=CARTESIAN_POINT ( 'NONE',  ( 4.483927247898545687, 16.52544592524342804, 114.7905762719810383 ) ) ;
#154274=CIRCLE ( 'NONE', #160755, 2.000000000000000000 ) ;
#154275=CARTESIAN_POINT ( 'NONE',  ( -15.72974639402176322, -15.80617190586768395, 24.37609039468567573 ) ) ;
#154277=CARTESIAN_POINT ( 'NONE',  ( -15.80617190586768217, 15.72974639402176855, 43.12609039468568284 ) ) ;
#154278=CARTESIAN_POINT ( 'NONE',  ( -9.474510206698964154, 16.51473224551069663, 30.41557627198102054 ) ) ;
#154279=CARTESIAN_POINT ( 'NONE',  ( -15.72974639402197994, 15.80617190586746368, 105.6239096053143669 ) ) ;
#154280=CARTESIAN_POINT ( 'NONE',  ( 0.05219959533936267826, -19.03943276465977164, 50.00109039468566863 ) ) ;
#154281=CARTESIAN_POINT ( 'NONE',  ( 17.37577197770832527, -5.499999999999936939, 21.30611277022550354 ) ) ;
#154282=CARTESIAN_POINT ( 'NONE',  ( -9.564922557960796823, -16.46253265017161027, 22.08224293864768839 ) ) ;
#154284=CARTESIAN_POINT ( 'NONE',  ( -14.29746914071037622, -8.314922557961029526, 59.16775706135234714 ) ) ;
#154285=CARTESIAN_POINT ( 'NONE',  ( -16.46253265017160317, 9.564922557960807481, 30.83224293864769550 ) ) ;
#154287=CARTESIAN_POINT ( 'NONE',  ( -19.02544592524342804, 5.153800228976336051, 71.04057627198099567 ) ) ;
#154288=CARTESIAN_POINT ( 'NONE',  ( -0.05219959533910754901, -16.53943276465976808, 107.4989096053143669 ) ) ;
#154289=CARTESIAN_POINT ( 'NONE',  ( -18.62759615963270932, 10.81492255796079327, 65.83224293864769550 ) ) ;
#154290=CARTESIAN_POINT ( 'NONE',  ( 14.29746914071037800, 8.314922557961029526, 36.66775706135234714 ) ) ;
#154291=CARTESIAN_POINT ( 'NONE',  ( 18.67979575497194134, -10.72451020669871369, 105.8344237280190328 ) ) ;
#154293=CARTESIAN_POINT ( 'NONE',  ( 12.06949235617739724, 12.14591786802326823, 106.8760903946856899 ) ) ;
#154294=CARTESIAN_POINT ( 'NONE',  ( 12.14591786802309770, 12.06949235617756955, 49.37390960531436690 ) ) ;
#154295=CARTESIAN_POINT ( 'NONE',  ( -16.46253265017160317, 9.564922557960807481, 45.83224293864769550 ) ) ;
#154296=CARTESIAN_POINT ( 'NONE',  ( -18.62759615963255300, -10.81492255796106328, 99.16775706135234714 ) ) ;
#154297=CARTESIAN_POINT ( 'NONE',  ( -10.72451020669898014, 18.67979575497178502, 105.4155762719810383 ) ) ;
#154298=CARTESIAN_POINT ( 'NONE',  ( -15.72974639402176322, -15.80617190586768395, 69.37609039468567573 ) ) ;
#154299=CARTESIAN_POINT ( 'NONE',  ( -8.224510206698735004, -14.34966873604973081, 54.58442372801901143 ) ) ;
#154301=CARTESIAN_POINT ( 'NONE',  ( 12.14591786802309770, 12.06949235617756955, 74.37390960531436690 ) ) ;
#154302=CARTESIAN_POINT ( 'NONE',  ( 15.72974639402176855, 15.80617190586768217, 101.8760903946857042 ) ) ;
#154303=CARTESIAN_POINT ( 'NONE',  ( -14.34966873604960291, -8.224510206698953496, 21.66557627198102409 ) ) ;
#154304=CARTESIAN_POINT ( 'NONE',  ( 17.50000000000000000, -5.499999999999992895, 61.21769037696436300 ) ) ;
#154305=CARTESIAN_POINT ( 'NONE',  ( -8.224510206698735004, -14.34966873604973081, 34.58442372801900433 ) ) ;
#154306=CARTESIAN_POINT ( 'NONE',  ( 16.55341960407611168, 4.379528057220329451, 43.95724293864769550 ) ) ;
#154307=CARTESIAN_POINT ( 'NONE',  ( -14.34966873604972548, 8.224510206698743886, 93.33442372801901854 ) ) ;
#154308=CARTESIAN_POINT ( 'NONE',  ( -16.46253265017160317, 9.564922557960807481, 100.8322429386477097 ) ) ;
#154309=CARTESIAN_POINT ( 'NONE',  ( 18.67979575497178502, 10.72451020669898547, 24.16557627198103120 ) ) ;
#154310=CARTESIAN_POINT ( 'NONE',  ( -5.823673210054431948, 21.52544592524334988, 97.70942372801904696 ) ) ;
#154311=CARTESIAN_POINT ( 'NONE',  ( -14.29746914071037622, -8.314922557961029526, 109.1677570613523613 ) ) ;
#154312=CARTESIAN_POINT ( 'NONE',  ( -16.55341960407611168, -4.379528057220339221, 71.45724293864769550 ) ) ;
#154313=CARTESIAN_POINT ( 'NONE',  ( 9.474510206698971260, -16.51473224551069308, 77.91557627198103830 ) ) ;
#154315=CARTESIAN_POINT ( 'NONE',  ( 4.483927247898790824, -16.52544592524335698, 30.20942372801902565 ) ) ;
#154316=CARTESIAN_POINT ( 'NONE',  ( 19.05341960407611168, 5.049401038298154454, 43.95724293864769550 ) ) ;
#154317=CARTESIAN_POINT ( 'NONE',  ( 16.51473224551069308, 9.474510206698969483, 89.16557627198103830 ) ) ;
#154318=CARTESIAN_POINT ( 'NONE',  ( 12.14591786802327356, -12.06949235617739191, 30.62609039468567929 ) ) ;
#154319=CARTESIAN_POINT ( 'NONE',  ( 17.50000000000000000, 5.500000000000011546, 68.78230962303564411 ) ) ;
#154320=CARTESIAN_POINT ( 'NONE',  ( 19.05341960407617918, -5.049401038297876454, 41.04275706135233293 ) ) ;
#154321=CARTESIAN_POINT ( 'NONE',  ( 14.34966873604972726, -8.224510206698740333, 90.83442372801901854 ) ) ;
#154322=CARTESIAN_POINT ( 'NONE',  ( 19.02544592524343514, -5.153800228976328945, 28.54057627198102409 ) ) ;
#154323=CARTESIAN_POINT ( 'NONE',  ( 8.314922557961029526, -14.29746914071037800, 75.41775706135233293 ) ) ;
#154324=CARTESIAN_POINT ( 'NONE',  ( 16.55341960407618274, -4.379528057220086978, 61.04275706135234714 ) ) ;
#154325=CARTESIAN_POINT ( 'NONE',  ( -5.049401038297874678, -19.05341960407617918, 84.79275706135233293 ) ) ;
#154326=CARTESIAN_POINT ( 'NONE',  ( -0.05219959533936034679, 19.03943276465977164, 32.50109039468566863 ) ) ;
#154327=CARTESIAN_POINT ( 'NONE',  ( 13.89961937509977652, -13.97604488694527269, 48.12390960531435979 ) ) ;
#154328=CARTESIAN_POINT ( 'NONE',  ( 12.14591786802309770, 12.06949235617756955, 89.37390960531435269 ) ) ;
#154329=CARTESIAN_POINT ( 'NONE',  ( 16.51473224551083163, -9.474510206698727899, 50.83442372801899722 ) ) ;
#154330=CARTESIAN_POINT ( 'NONE',  ( 5.719274019375991003, -21.55341960407610458, 52.70724293864769550 ) ) ;
#154331=CARTESIAN_POINT ( 'NONE',  ( -16.46253265017146816, -9.564922557961047289, 29.16775706135232937 ) ) ;
#154332=CARTESIAN_POINT ( 'NONE',  ( -5.049401038298153566, 19.05341960407611168, 100.2072429386476955 ) ) ;
#154333=CARTESIAN_POINT ( 'NONE',  ( 0.05219959533907565091, 21.53943276465977519, 79.99890960531435269 ) ) ;
#154334=CARTESIAN_POINT ( 'NONE',  ( 16.51473224551083163, -9.474510206698727899, 85.83442372801900433 ) ) ;
#154336=CARTESIAN_POINT ( 'NONE',  ( 12.14591786802327356, -12.06949235617739191, 20.62609039468568639 ) ) ;
#154337=CARTESIAN_POINT ( 'NONE',  ( -13.97604488694527625, -13.89961937509977652, 31.87390960531435979 ) ) ;
#154338=CARTESIAN_POINT ( 'NONE',  ( 16.46253265017160672, -9.564922557960803928, 103.3322429386476955 ) ) ;
#154339=CARTESIAN_POINT ( 'NONE',  ( 5.719274019375991003, -21.55341960407610458, 72.70724293864769550 ) ) ;
#154340=CARTESIAN_POINT ( 'NONE',  ( -8.224510206698735004, -14.34966873604973081, 44.58442372801901854 ) ) ;
#154341=CARTESIAN_POINT ( 'NONE',  ( -18.62759615963255300, -10.81492255796106328, 44.16775706135234714 ) ) ;
#154342=CARTESIAN_POINT ( 'NONE',  ( -9.474510206698720793, -16.51473224551083518, 109.5844237280190043 ) ) ;
#154343=CARTESIAN_POINT ( 'NONE',  ( -10.81492255796105439, 18.62759615963255655, 107.9177570613523471 ) ) ;
#154344=CARTESIAN_POINT ( 'NONE',  ( 14.29746914071037800, 8.314922557961029526, 111.6677570613523613 ) ) ;
#154345=CARTESIAN_POINT ( 'NONE',  ( -13.97604488694527625, -13.89961937509977652, 96.87390960531433848 ) ) ;
#154346=CARTESIAN_POINT ( 'NONE',  ( 10.81492255796078972, 18.62759615963270932, 104.5822429386477097 ) ) ;
#154347=CARTESIAN_POINT ( 'NONE',  ( 4.483927247898545687, 16.52544592524342804, 29.79057627198102409 ) ) ;
#154348=CARTESIAN_POINT ( 'NONE',  ( -5.049401038297874678, -19.05341960407617918, 79.79275706135233293 ) ) ;
#154349=CARTESIAN_POINT ( 'NONE',  ( -15.72974639402176322, -15.80617190586768395, 59.37609039468568284 ) ) ;
#154350=CARTESIAN_POINT ( 'NONE',  ( -13.97604488694547697, 13.89961937509957934, 28.12609039468565797 ) ) ;
#154351=CARTESIAN_POINT ( 'NONE',  ( -14.34966873604960291, -8.224510206698953496, 101.6655762719810383 ) ) ;
#154352=CARTESIAN_POINT ( 'NONE',  ( -21.52544592524343514, 5.823673210054127303, 36.04057627198102409 ) ) ;
#154353=CARTESIAN_POINT ( 'NONE',  ( 4.379528057220339221, -16.55341960407611168, 22.70724293864769194 ) ) ;
#154354=CARTESIAN_POINT ( 'NONE',  ( 5.823673210054444382, -21.52544592524334988, 100.2094237280190043 ) ) ;
#154355=CARTESIAN_POINT ( 'NONE',  ( 14.34966873604972726, -8.224510206698740333, 55.83442372801901854 ) ) ;
#154356=CARTESIAN_POINT ( 'NONE',  ( 16.53943276465976808, -0.05219959533910856209, 28.74890960531435624 ) ) ;
#154357=CARTESIAN_POINT ( 'NONE',  ( -10.81492255796105439, 18.62759615963255655, 62.91775706135236135 ) ) ;
#154358=CARTESIAN_POINT ( 'NONE',  ( -21.52544592524334988, -5.823673210054445271, 53.95942372801900433 ) ) ;
#154360=CARTESIAN_POINT ( 'NONE',  ( 9.474510206698971260, -16.51473224551069308, 27.91557627198103120 ) ) ;
#154361=CARTESIAN_POINT ( 'NONE',  ( 10.81492255796106328, -18.62759615963255655, 35.41775706135234003 ) ) ;
#154362=CARTESIAN_POINT ( 'NONE',  ( 16.55341960407611168, 4.379528057220329451, 108.9572429386476955 ) ) ;
#154363=CARTESIAN_POINT ( 'NONE',  ( 19.50973618000807619, -5.499999999999992895, 37.50000000000000000 ) ) ;
#154364=CARTESIAN_POINT ( 'NONE',  ( 12.06949235617757843, -12.14591786802309237, 78.12390960531436690 ) ) ;
#154365=CARTESIAN_POINT ( 'NONE',  ( 19.05341960407611168, 5.049401038298154454, 68.95724293864769550 ) ) ;
#154366=CARTESIAN_POINT ( 'NONE',  ( 4.483927247898545687, 16.52544592524342804, 24.79057627198103120 ) ) ;
#154367=CARTESIAN_POINT ( 'NONE',  ( -18.67979575497178146, -10.72451020669898902, 56.66557627198103830 ) ) ;
#154368=CARTESIAN_POINT ( 'NONE',  ( 12.06949235617757843, -12.14591786802309237, 93.12390960531436690 ) ) ;
#154369=CARTESIAN_POINT ( 'NONE',  ( 18.62759615963271287, -10.81492255796078972, 93.33224293864769550 ) ) ;
#154370=CARTESIAN_POINT ( 'NONE',  ( -13.89961937509977652, 13.97604488694528158, 95.62390960531436690 ) ) ;
#154371=CARTESIAN_POINT ( 'NONE',  ( 5.153800228976335163, 19.02544592524342804, 49.79057627198100988 ) ) ;
#154372=CARTESIAN_POINT ( 'NONE',  ( -16.46253265017146816, -9.564922557961047289, 104.1677570613523329 ) ) ;
#154373=CARTESIAN_POINT ( 'NONE',  ( 5.823673210054125526, 21.52544592524343514, 44.79057627198103120 ) ) ;
#154374=CARTESIAN_POINT ( 'NONE',  ( 5.823673210054444382, -21.52544592524334988, 85.20942372801901854 ) ) ;
#154375=CARTESIAN_POINT ( 'NONE',  ( -13.89961937509977652, 13.97604488694528158, 65.62390960531436690 ) ) ;
#154376=CARTESIAN_POINT ( 'NONE',  ( -9.564922557960796823, -16.46253265017161027, 97.08224293864769550 ) ) ;
#154377=CARTESIAN_POINT ( 'NONE',  ( 0.05219959533934541429, -16.53943276465976808, 80.00109039468568994 ) ) ;
#154378=CARTESIAN_POINT ( 'NONE',  ( -10.81492255796105439, 18.62759615963255655, 62.91775706135236135 ) ) ;
#154379=CARTESIAN_POINT ( 'NONE',  ( -18.62759615963255300, -10.81492255796106328, 84.16775706135234714 ) ) ;
#154380=CARTESIAN_POINT ( 'NONE',  ( -21.55341960407610458, -5.719274019375992779, 106.4572429386477097 ) ) ;
#154381=CARTESIAN_POINT ( 'NONE',  ( -16.52544592524335698, -4.483927247898792601, 78.95942372801901854 ) ) ;
#154382=CARTESIAN_POINT ( 'NONE',  ( 10.81492255796078972, 18.62759615963270932, 74.58224293864768129 ) ) ;
#154383=CARTESIAN_POINT ( 'NONE',  ( -19.03943276465977164, -0.05219959533935918106, 48.75109039468566863 ) ) ;
#154384=CARTESIAN_POINT ( 'NONE',  ( -21.53943276465977519, 0.05219959533907696930, 41.24890960531435269 ) ) ;
#154385=CARTESIAN_POINT ( 'NONE',  ( -0.05219959533909027116, -19.03943276465977164, 77.49890960531435269 ) ) ;
#154386=CARTESIAN_POINT ( 'NONE',  ( 12.14591786802309770, 12.06949235617756955, 24.37390960531435979 ) ) ;
#154387=CARTESIAN_POINT ( 'NONE',  ( -16.31925111598458500, 7.325300261831455551, 65.16424538967254421 ) ) ;
#154388=CARTESIAN_POINT ( 'NONE',  ( 5.153800228976335163, 19.02544592524342804, 114.7905762719810241 ) ) ;
#154390=CARTESIAN_POINT ( 'NONE',  ( 19.02544592524334988, 5.153800228976608722, 101.4594237280189759 ) ) ;
#154391=CARTESIAN_POINT ( 'NONE',  ( 10.72451020669898902, -18.67979575497178502, 77.91557627198102409 ) ) ;
#154392=CARTESIAN_POINT ( 'NONE',  ( 8.314922557960818139, 14.29746914071049879, 44.58224293864769550 ) ) ;
#154393=CARTESIAN_POINT ( 'NONE',  ( -12.06949235617739369, -12.14591786802326823, 19.37609039468568639 ) ) ;
#154394=CARTESIAN_POINT ( 'NONE',  ( -9.564922557960796823, -16.46253265017161027, 37.08224293864768839 ) ) ;
#154395=CARTESIAN_POINT ( 'NONE',  ( 19.02544592524334988, 5.153800228976608722, 106.4594237280190185 ) ) ;
#154396=CARTESIAN_POINT ( 'NONE',  ( 18.67979575497178502, 10.72451020669898547, 104.1655762719810241 ) ) ;
#154397=CARTESIAN_POINT ( 'NONE',  ( -5.049401038297874678, -19.05341960407617918, 69.79275706135233293 ) ) ;
#154398=CARTESIAN_POINT ( 'NONE',  ( -12.06949235617739369, -12.14591786802326823, 84.37609039468570415 ) ) ;
#154399=CARTESIAN_POINT ( 'NONE',  ( 9.474510206698971260, -16.51473224551069308, 87.91557627198102409 ) ) ;
#154400=CARTESIAN_POINT ( 'NONE',  ( -12.06949235617756955, 12.14591786802309770, 70.62390960531436690 ) ) ;
#154402=CARTESIAN_POINT ( 'NONE',  ( 19.02544592524343514, -5.153800228976328945, 63.54057627198103830 ) ) ;
#154403=CARTESIAN_POINT ( 'NONE',  ( 4.379528057220339221, -16.55341960407611168, 72.70724293864769550 ) ) ;
#154404=CARTESIAN_POINT ( 'NONE',  ( -19.03943276465977164, 0.05219959533909376836, 31.24890960531435979 ) ) ;
#154406=CARTESIAN_POINT ( 'NONE',  ( -12.14591786802309592, -12.06949235617757132, 36.87390960531435979 ) ) ;
#154407=CARTESIAN_POINT ( 'NONE',  ( 19.02544592524343514, -5.153800228976328945, 73.54057627198103830 ) ) ;
#154409=CARTESIAN_POINT ( 'NONE',  ( -19.05341960407617563, 5.049401038297882671, 48.54275706135233293 ) ) ;
#154410=CARTESIAN_POINT ( 'NONE',  ( 4.379528057220092307, 16.55341960407617563, 57.29275706135234714 ) ) ;
#154411=CARTESIAN_POINT ( 'NONE',  ( 15.72974639402199770, -15.80617190586745480, 58.12390960531435979 ) ) ;
#154412=CARTESIAN_POINT ( 'NONE',  ( 13.89961937509957401, 13.97604488694547697, 26.87609039468566507 ) ) ;
#154413=CARTESIAN_POINT ( 'NONE',  ( 19.02544592524343514, -5.153800228976328945, 83.54057627198100988 ) ) ;
#154415=CARTESIAN_POINT ( 'NONE',  ( -5.823673210054116645, -21.52544592524344225, 27.29057627198103120 ) ) ;
#154416=CARTESIAN_POINT ( 'NONE',  ( 16.46253265017160672, -9.564922557960803928, 63.33224293864769550 ) ) ;
#154417=CARTESIAN_POINT ( 'NONE',  ( 5.719274019375673035, 21.55341960407619339, 47.29275706135234003 ) ) ;
#154418=CARTESIAN_POINT ( 'NONE',  ( -14.34966873604960291, -8.224510206698953496, 106.6655762719810383 ) ) ;
#154419=CARTESIAN_POINT ( 'NONE',  ( 5.719274019375991003, -21.55341960407610458, 97.70724293864772392 ) ) ;
#154420=CARTESIAN_POINT ( 'NONE',  ( 13.97604488694527802, 13.89961937509977652, 94.37390960531436690 ) ) ;
#154422=CARTESIAN_POINT ( 'NONE',  ( 5.823673210054444382, -21.52544592524334988, 40.20942372801901854 ) ) ;
#154424=CARTESIAN_POINT ( 'NONE',  ( -13.97604488694527625, -13.89961937509977652, 96.87390960531433848 ) ) ;
#154425=CARTESIAN_POINT ( 'NONE',  ( -9.474510206698964154, 16.51473224551069663, 90.41557627198103830 ) ) ;
#154426=CARTESIAN_POINT ( 'NONE',  ( -18.67979575497178146, -10.72451020669898902, 91.66557627198103830 ) ) ;
#154427=CARTESIAN_POINT ( 'NONE',  ( -19.02544592524342804, 5.153800228976336051, 41.04057627198103120 ) ) ;
#154428=CARTESIAN_POINT ( 'NONE',  ( 4.379528057220092307, 16.55341960407617563, 22.29275706135235069 ) ) ;
#154430=CARTESIAN_POINT ( 'NONE',  ( 9.564922557960805705, 16.46253265017160317, 24.58224293864769194 ) ) ;
#154431=CARTESIAN_POINT ( 'NONE',  ( 0.05219959533937995610, -21.53943276465977519, 80.00109039468568994 ) ) ;
#154432=CARTESIAN_POINT ( 'NONE',  ( -19.05341960407611168, -5.049401038298163336, 81.45724293864769550 ) ) ;
#154433=CARTESIAN_POINT ( 'NONE',  ( -5.823673210054431948, 21.52544592524334988, 52.70942372801902565 ) ) ;
#154434=CARTESIAN_POINT ( 'NONE',  ( -5.719274019375665041, -21.55341960407619695, 24.79275706135235779 ) ) ;
#154436=CARTESIAN_POINT ( 'NONE',  ( 19.02544592524343514, -5.153800228976328945, 98.54057627198100988 ) ) ;
#154438=CARTESIAN_POINT ( 'NONE',  ( 4.483927247898790824, -16.52544592524335698, 35.20942372801901854 ) ) ;
#154439=CARTESIAN_POINT ( 'NONE',  ( -12.14591786802326823, 12.06949235617739902, 73.12609039468567573 ) ) ;
#154440=CARTESIAN_POINT ( 'NONE',  ( 21.52544592524334988, 5.823673210054432836, 61.45942372801901854 ) ) ;
#154441=CARTESIAN_POINT ( 'NONE',  ( -18.62759615963255300, -10.81492255796106328, 79.16775706135234714 ) ) ;
#154443=CARTESIAN_POINT ( 'NONE',  ( 9.474510206698729675, 16.51473224551082808, 112.0844237280190043 ) ) ;
#154444=CARTESIAN_POINT ( 'NONE',  ( -5.049401038298153566, 19.05341960407611168, 75.20724293864769550 ) ) ;
#154445=CARTESIAN_POINT ( 'NONE',  ( 0.05219959533909260263, 19.03943276465977164, 99.99890960531436690 ) ) ;
#154446=CONICAL_SURFACE ( 'NONE', #122236, 2.500000000000002220, 1.029744258676656754 ) ;
#154447=CARTESIAN_POINT ( 'NONE',  ( 16.52544592524342804, -4.483927247898539470, 103.5405762719810383 ) ) ;
#154448=CARTESIAN_POINT ( 'NONE',  ( -14.29746914071049879, 8.314922557960819915, 110.8322429386476955 ) ) ;
#154449=CARTESIAN_POINT ( 'NONE',  ( 0.05219959533907565091, 21.53943276465977519, 29.99890960531435979 ) ) ;
#154450=CARTESIAN_POINT ( 'NONE',  ( 16.55341960407618274, -4.379528057220086978, 86.04275706135236135 ) ) ;
#154451=CARTESIAN_POINT ( 'NONE',  ( -14.29746914071049879, 8.314922557960819915, 70.83224293864770971 ) ) ;
#154453=CARTESIAN_POINT ( 'NONE',  ( 19.02544592524343514, -5.153800228976328945, 58.54057627198102409 ) ) ;
#154454=CARTESIAN_POINT ( 'NONE',  ( -0.05219959533937732626, 21.53943276465977519, 72.50109039468568994 ) ) ;
#154455=CARTESIAN_POINT ( 'NONE',  ( 21.52544592524334988, 5.823673210054432836, 71.45942372801901854 ) ) ;
#154456=CARTESIAN_POINT ( 'NONE',  ( -5.153800228976607833, 19.02544592524334988, 112.7094237280190043 ) ) ;
#154457=CARTESIAN_POINT ( 'NONE',  ( -14.29746914071049879, 8.314922557960819915, 75.83224293864769550 ) ) ;
#154458=CARTESIAN_POINT ( 'NONE',  ( -15.72974639402176322, -15.80617190586768395, 24.37609039468567573 ) ) ;
#154459=CARTESIAN_POINT ( 'NONE',  ( 18.67979575497178502, 10.72451020669898547, 59.16557627198103120 ) ) ;
#154460=CARTESIAN_POINT ( 'NONE',  ( -17.12812012977025589, -6.668231424565998822, 106.3594875932314636 ) ) ;
#154462=CARTESIAN_POINT ( 'NONE',  ( 13.97604488694527802, 13.89961937509977652, 74.37390960531436690 ) ) ;
#154463=CARTESIAN_POINT ( 'NONE',  ( -14.29746914071049879, 8.314922557960819915, 55.83224293864770260 ) ) ;
#154464=CARTESIAN_POINT ( 'NONE',  ( -16.53943276465976808, -0.05219959533934237506, 113.7510903946856757 ) ) ;
#154465=CARTESIAN_POINT ( 'NONE',  ( 16.53943276465976808, 0.05219959533934440121, 91.25109039468568994 ) ) ;
#154466=CARTESIAN_POINT ( 'NONE',  ( -5.153800228976607833, 19.02544592524334988, 57.70942372801899012 ) ) ;
#154468=CARTESIAN_POINT ( 'NONE',  ( 0.05219959533909260263, 19.03943276465977164, 109.9989096053143669 ) ) ;
#154469=CARTESIAN_POINT ( 'NONE',  ( -14.34966873604960291, -8.224510206698953496, 76.66557627198103830 ) ) ;
#154470=CARTESIAN_POINT ( 'NONE',  ( 19.03943276465977164, 0.05219959533936151252, 41.25109039468566152 ) ) ;
#154471=CARTESIAN_POINT ( 'NONE',  ( -16.51473224551069308, -9.474510206698971260, 36.66557627198102409 ) ) ;
#154472=CARTESIAN_POINT ( 'NONE',  ( -15.72974639402197994, 15.80617190586746368, 35.62390960531437401 ) ) ;
#154473=CARTESIAN_POINT ( 'NONE',  ( 18.67979575497178502, 10.72451020669898547, 59.16557627198103120 ) ) ;
#154474=CARTESIAN_POINT ( 'NONE',  ( -8.314922557960811034, -14.29746914071050412, 102.0822429386476955 ) ) ;
#154475=CARTESIAN_POINT ( 'NONE',  ( 16.53943276465976808, 0.05219959533934440121, 56.25109039468568284 ) ) ;
#154476=CARTESIAN_POINT ( 'NONE',  ( 12.14591786802309770, 12.06949235617756955, 89.37390960531435269 ) ) ;
#154477=CARTESIAN_POINT ( 'NONE',  ( 17.05587630539787369, -6.762274262135693270, 38.24180309037314629 ) ) ;
#154478=CARTESIAN_POINT ( 'NONE',  ( -17.49999999999999645, 5.500000000000037303, 50.79690382534172244 ) ) ;
#154479=CARTESIAN_POINT ( 'NONE',  ( -10.72451020669898014, 18.67979575497178502, 35.41557627198102409 ) ) ;
#154481=CARTESIAN_POINT ( 'NONE',  ( -17.72696623605163779, 5.499999999999873879, 43.59811031808418136 ) ) ;
#154482=CARTESIAN_POINT ( 'NONE',  ( -16.52544592524335698, -4.483927247898792601, 48.95942372801902565 ) ) ;
#154483=CARTESIAN_POINT ( 'NONE',  ( 0.05219959533910956823, 16.53943276465976808, 24.99890960531435624 ) ) ;
#154484=CARTESIAN_POINT ( 'NONE',  ( 5.719274019375991003, -21.55341960407610458, 57.70724293864770260 ) ) ;
#154485=CARTESIAN_POINT ( 'NONE',  ( 19.05341960407617918, -5.049401038297876454, 86.04275706135233293 ) ) ;
#154486=CARTESIAN_POINT ( 'NONE',  ( 21.52544592524344225, -5.823673210054117533, 58.54057627198103120 ) ) ;
#154487=CARTESIAN_POINT ( 'NONE',  ( 15.72974639402176855, 15.80617190586768217, 86.87609039468568994 ) ) ;
#154489=CARTESIAN_POINT ( 'NONE',  ( -0.05219959533934338120, 16.53943276465976808, 42.50109039468567573 ) ) ;
#154490=CARTESIAN_POINT ( 'NONE',  ( -19.03943276465977164, 0.05219959533909376836, 36.24890960531436690 ) ) ;
#154491=CARTESIAN_POINT ( 'NONE',  ( 0.05219959533909260263, 19.03943276465977164, 94.99890960531436690 ) ) ;
#154492=CARTESIAN_POINT ( 'NONE',  ( 13.97604488694527802, 13.89961937509977652, 34.37390960531436690 ) ) ;
#154493=CARTESIAN_POINT ( 'NONE',  ( -16.52544592524342804, 4.483927247898546575, 96.04057627198102409 ) ) ;
#154495=CARTESIAN_POINT ( 'NONE',  ( -9.474510206698964154, 16.51473224551069663, 115.4155762719810241 ) ) ;
#154497=CARTESIAN_POINT ( 'NONE',  ( 8.314922557961029526, -14.29746914071037800, 65.41775706135234714 ) ) ;
#154498=CARTESIAN_POINT ( 'NONE',  ( -10.72451020669898014, 18.67979575497178502, 85.41557627198102409 ) ) ;
#154499=CARTESIAN_POINT ( 'NONE',  ( 0.05219959533909260263, 19.03943276465977164, 54.99890960531435979 ) ) ;
#154500=CARTESIAN_POINT ( 'NONE',  ( -15.72974639402176322, -15.80617190586768395, 29.37609039468568284 ) ) ;
#154501=CARTESIAN_POINT ( 'NONE',  ( -0.05219959533909027116, -19.03943276465977164, 77.49890960531435269 ) ) ;
#154503=CARTESIAN_POINT ( 'NONE',  ( -21.52544592524343514, 5.823673210054127303, 116.0405762719810383 ) ) ;
#154504=CARTESIAN_POINT ( 'NONE',  ( 13.89961937509977652, -13.97604488694527269, 23.12390960531436335 ) ) ;
#154505=CARTESIAN_POINT ( 'NONE',  ( 9.474510206698971260, -16.51473224551069308, 112.9155762719810383 ) ) ;
#154506=CARTESIAN_POINT ( 'NONE',  ( 16.51473224551083163, -9.474510206698727899, 75.83442372801900433 ) ) ;
#154507=CARTESIAN_POINT ( 'NONE',  ( -13.89961937509957401, -13.97604488694547875, 24.37609039468565442 ) ) ;
#154508=CARTESIAN_POINT ( 'NONE',  ( -15.72974639402197994, 15.80617190586746368, 105.6239096053143669 ) ) ;
#154509=CARTESIAN_POINT ( 'NONE',  ( 9.564922557961047289, -16.46253265017146816, 40.41775706135234003 ) ) ;
#154510=CARTESIAN_POINT ( 'NONE',  ( 14.29746914071037800, 8.314922557961029526, 76.66775706135234714 ) ) ;
#154511=CARTESIAN_POINT ( 'NONE',  ( 5.049401038298161559, -19.05341960407611168, 112.7072429386476813 ) ) ;
#154512=CARTESIAN_POINT ( 'NONE',  ( 19.05341960407611168, 5.049401038298154454, 63.95724293864769550 ) ) ;
#154513=CARTESIAN_POINT ( 'NONE',  ( 18.62759615963255655, 10.81492255796105972, 61.66775706135235424 ) ) ;
#154514=CARTESIAN_POINT ( 'NONE',  ( -15.80617190586768217, 15.72974639402176855, 83.12609039468568994 ) ) ;
#154515=CARTESIAN_POINT ( 'NONE',  ( 13.97604488694527802, 13.89961937509977652, 79.37390960531435269 ) ) ;
#154516=CARTESIAN_POINT ( 'NONE',  ( -5.719274019375665041, -21.55341960407619695, 49.79275706135234714 ) ) ;
#154517=CARTESIAN_POINT ( 'NONE',  ( -5.049401038297874678, -19.05341960407617918, 89.79275706135230450 ) ) ;
#154518=CARTESIAN_POINT ( 'NONE',  ( 19.02544592524343514, -5.153800228976328945, 53.54057627198102409 ) ) ;
#154519=CARTESIAN_POINT ( 'NONE',  ( 5.049401038298161559, -19.05341960407611168, 97.70724293864766707 ) ) ;
#154520=CARTESIAN_POINT ( 'NONE',  ( -16.51473224551069308, -9.474510206698971260, 71.66557627198102409 ) ) ;
#154521=CARTESIAN_POINT ( 'NONE',  ( -13.97604488694527625, -13.89961937509977652, 111.8739096053143243 ) ) ;
#154522=CARTESIAN_POINT ( 'NONE',  ( -19.03943276465977164, 0.05219959533909376836, 46.24890960531435979 ) ) ;
#154523=CARTESIAN_POINT ( 'NONE',  ( -18.62759615963270932, 10.81492255796079327, 105.8322429386476955 ) ) ;
#154524=CARTESIAN_POINT ( 'NONE',  ( 16.55341960407618274, -4.379528057220086978, 86.04275706135236135 ) ) ;
#154526=CARTESIAN_POINT ( 'NONE',  ( 0.05219959533936267826, -19.03943276465977164, 40.00109039468566152 ) ) ;
#154527=CARTESIAN_POINT ( 'NONE',  ( -19.03943276465977164, 0.05219959533909376836, 71.24890960531435269 ) ) ;
#154528=CARTESIAN_POINT ( 'NONE',  ( -8.314922557960811034, -14.29746914071050412, 62.08224293864769550 ) ) ;
#154529=CARTESIAN_POINT ( 'NONE',  ( -4.379528057220328563, 16.55341960407611168, 90.20724293864770971 ) ) ;
#154530=CARTESIAN_POINT ( 'NONE',  ( 21.55341960407610458, 5.719274019375980345, 23.95724293864769550 ) ) ;
#154531=CARTESIAN_POINT ( 'NONE',  ( 9.474510206698971260, -16.51473224551069308, 92.91557627198103830 ) ) ;
#154532=CARTESIAN_POINT ( 'NONE',  ( 0.05219959533909260263, 19.03943276465977164, 99.99890960531436690 ) ) ;
#154533=CARTESIAN_POINT ( 'NONE',  ( -10.81492255796105439, 18.62759615963255655, 107.9177570613523471 ) ) ;
#154534=CARTESIAN_POINT ( 'NONE',  ( 12.14591786802327356, -12.06949235617739191, 90.62609039468567573 ) ) ;
#154535=CARTESIAN_POINT ( 'NONE',  ( -16.46253265017160317, 9.564922557960807481, 80.83224293864769550 ) ) ;
#154537=CARTESIAN_POINT ( 'NONE',  ( 21.53943276465977519, 0.05219959533937863772, 36.25109039468567573 ) ) ;
#154538=CARTESIAN_POINT ( 'NONE',  ( 0.05219959533907565091, 21.53943276465977519, 24.99890960531435624 ) ) ;
#154539=CARTESIAN_POINT ( 'NONE',  ( 10.72451020669898902, -18.67979575497178502, 97.91557627198103830 ) ) ;
#154541=CARTESIAN_POINT ( 'NONE',  ( 14.34966873604960469, 8.224510206698951720, 64.16557627198102409 ) ) ;
#154542=CARTESIAN_POINT ( 'NONE',  ( 19.03943276465977164, -0.05219959533909143690, 58.74890960531435979 ) ) ;
#154543=CARTESIAN_POINT ( 'NONE',  ( -16.55341960407611168, -4.379528057220339221, 76.45724293864769550 ) ) ;
#154544=CARTESIAN_POINT ( 'NONE',  ( -19.02544592524334988, -5.153800228976617603, 43.95942372801899012 ) ) ;
#154545=CARTESIAN_POINT ( 'NONE',  ( -14.29746914071049879, 8.314922557960819915, 110.8322429386476955 ) ) ;
#154546=CARTESIAN_POINT ( 'NONE',  ( 13.89961937509977652, -13.97604488694527269, 88.12390960531438111 ) ) ;
#154547=CARTESIAN_POINT ( 'NONE',  ( 16.51473224551069308, 9.474510206698969483, 84.16557627198102409 ) ) ;
#154549=CARTESIAN_POINT ( 'NONE',  ( -14.29746914071049879, 8.314922557960819915, 95.83224293864770971 ) ) ;
#154551=CARTESIAN_POINT ( 'NONE',  ( 16.53943276465976808, 0.05219959533934440121, 111.2510903946856899 ) ) ;
#154552=CARTESIAN_POINT ( 'NONE',  ( -14.34966873604972548, 8.224510206698743886, 28.33442372801902209 ) ) ;
#154553=CARTESIAN_POINT ( 'NONE',  ( 5.823673210054444382, -21.52544592524334988, 90.20942372801903275 ) ) ;
#154554=CARTESIAN_POINT ( 'NONE',  ( 9.564922557960805705, 16.46253265017160317, 94.58224293864769550 ) ) ;
#154555=CARTESIAN_POINT ( 'NONE',  ( -15.72974639402176322, -15.80617190586768395, 19.37609039468568639 ) ) ;
#154556=CARTESIAN_POINT ( 'NONE',  ( 9.474510206698971260, -16.51473224551069308, 32.91557627198102409 ) ) ;
#154557=CARTESIAN_POINT ( 'NONE',  ( -4.483927247898782831, 16.52544592524335698, 27.70942372801901854 ) ) ;
#154558=CARTESIAN_POINT ( 'NONE',  ( -19.03943276465977164, -0.05219959533935918106, 93.75109039468566152 ) ) ;
#154559=CARTESIAN_POINT ( 'NONE',  ( -5.719274019375978568, 21.55341960407610458, 95.20724293864769550 ) ) ;
#154560=CARTESIAN_POINT ( 'NONE',  ( 0.05219959533936267826, -19.03943276465977164, 70.00109039468566152 ) ) ;
#154562=CARTESIAN_POINT ( 'NONE',  ( -15.72974639402176322, -15.80617190586768395, 24.37609039468567573 ) ) ;
#154564=CARTESIAN_POINT ( 'NONE',  ( -0.05219959533909027116, -19.03943276465977164, 97.49890960531436690 ) ) ;
#154565=CARTESIAN_POINT ( 'NONE',  ( 8.314922557961029526, -14.29746914071037800, 50.41775706135235424 ) ) ;
#154567=CARTESIAN_POINT ( 'NONE',  ( -16.46253265017146816, -9.564922557961047289, 54.16775706135234003 ) ) ;
#154568=CARTESIAN_POINT ( 'NONE',  ( -5.719274019375665041, -21.55341960407619695, 24.79275706135235779 ) ) ;
#154569=CARTESIAN_POINT ( 'NONE',  ( 14.34966873604960469, 8.224510206698951720, 74.16557627198102409 ) ) ;
#154570=CARTESIAN_POINT ( 'NONE',  ( 9.474510206698971260, -16.51473224551069308, 82.91557627198103830 ) ) ;
#154571=CARTESIAN_POINT ( 'NONE',  ( -16.55341960407617563, 4.379528057220093196, 53.54275706135234714 ) ) ;
#154572=CARTESIAN_POINT ( 'NONE',  ( 0.05219959533936267826, -19.03943276465977164, 55.00109039468566863 ) ) ;
#154573=CARTESIAN_POINT ( 'NONE',  ( 10.81492255796106328, -18.62759615963255655, 65.41775706135234714 ) ) ;
#154574=CARTESIAN_POINT ( 'NONE',  ( -4.483927247898782831, 16.52544592524335698, 27.70942372801901854 ) ) ;
#154575=CARTESIAN_POINT ( 'NONE',  ( 19.02544592524343514, -5.153800228976328945, 73.54057627198103830 ) ) ;
#154576=CARTESIAN_POINT ( 'NONE',  ( 9.474510206698729675, 16.51473224551082808, 82.08442372801899012 ) ) ;
#154577=CARTESIAN_POINT ( 'NONE',  ( 16.53943276465976808, 0.05219959533934440121, 56.25109039468568284 ) ) ;
#154578=CARTESIAN_POINT ( 'NONE',  ( 15.80617190586769283, -15.72974639402175789, 95.62609039468568994 ) ) ;
#154579=CARTESIAN_POINT ( 'NONE',  ( 0.05219959533936267826, -19.03943276465977164, 80.00109039468567573 ) ) ;
#154580=CARTESIAN_POINT ( 'NONE',  ( -13.97604488694527625, -13.89961937509977652, 56.87390960531434558 ) ) ;
#154581=CARTESIAN_POINT ( 'NONE',  ( 0.05219959533907565091, 21.53943276465977519, 64.99890960531435269 ) ) ;
#154582=CARTESIAN_POINT ( 'NONE',  ( -16.52544592524342804, 4.483927247898546575, 71.04057627198103830 ) ) ;
#154583=CARTESIAN_POINT ( 'NONE',  ( -9.474510206698720793, -16.51473224551083518, 74.58442372801900433 ) ) ;
#154584=CARTESIAN_POINT ( 'NONE',  ( 16.31925111598454947, -7.325300261831691806, 62.66424538967256552 ) ) ;
#154585=CARTESIAN_POINT ( 'NONE',  ( 13.89961937509957401, 13.97604488694547697, 46.87609039468565442 ) ) ;
#154586=CARTESIAN_POINT ( 'NONE',  ( 8.314922557961029526, -14.29746914071037800, 100.4177570613523471 ) ) ;
#154587=CARTESIAN_POINT ( 'NONE',  ( -4.483927247898539470, -16.52544592524342804, 72.29057627198102409 ) ) ;
#154588=CARTESIAN_POINT ( 'NONE',  ( 5.823673210054444382, -21.52544592524334988, 100.2094237280190043 ) ) ;
#154590=CARTESIAN_POINT ( 'NONE',  ( 18.62759615963271287, -10.81492255796078972, 103.3322429386476955 ) ) ;
#154591=CARTESIAN_POINT ( 'NONE',  ( -13.97604488694527625, -13.89961937509977652, 66.87390960531436690 ) ) ;
#154592=CARTESIAN_POINT ( 'NONE',  ( -18.62759615963255300, -10.81492255796106328, 69.16775706135234714 ) ) ;
#154593=CARTESIAN_POINT ( 'NONE',  ( -9.474510206698964154, 16.51473224551069663, 50.41557627198102409 ) ) ;
#154594=ORIENTED_EDGE ( 'NONE', *, *, #93672, .F. ) ;
#154595=CARTESIAN_POINT ( 'NONE',  ( 5.049401038298161559, -19.05341960407611168, 22.70724293864769194 ) ) ;
#154596=CARTESIAN_POINT ( 'NONE',  ( 0.05219959533909260263, 19.03943276465977164, 109.9989096053143669 ) ) ;
#154597=CARTESIAN_POINT ( 'NONE',  ( 0.05219959533910956823, 16.53943276465976808, 69.99890960531435269 ) ) ;
#154598=CARTESIAN_POINT ( 'NONE',  ( -19.02544592524342804, 5.153800228976336051, 36.04057627198100988 ) ) ;
#154599=CARTESIAN_POINT ( 'NONE',  ( 4.379528057220339221, -16.55341960407611168, 82.70724293864770971 ) ) ;
#154600=CARTESIAN_POINT ( 'NONE',  ( -21.52544592524343514, 5.823673210054127303, 91.04057627198103830 ) ) ;
#154601=CARTESIAN_POINT ( 'NONE',  ( -0.05219959533937732626, 21.53943276465977519, 42.50109039468567573 ) ) ;
#154603=EDGE_CURVE ( 'NONE', #107085, #14621, #93075, .T. ) ;
#154604=CARTESIAN_POINT ( 'NONE',  ( 16.52544592524335698, 4.483927247898782831, 56.45942372801902565 ) ) ;
#154605=CARTESIAN_POINT ( 'NONE',  ( 15.72974639402199770, -15.80617190586745480, 103.1239096053143811 ) ) ;
#154606=CARTESIAN_POINT ( 'NONE',  ( 13.89961937509957401, 13.97604488694547697, 31.87609039468566863 ) ) ;
#154607=CARTESIAN_POINT ( 'NONE',  ( 13.97604488694527802, 13.89961937509977652, 109.3739096053143669 ) ) ;
#154608=CARTESIAN_POINT ( 'NONE',  ( 15.80617190586769283, -15.72974639402175789, 50.62609039468568994 ) ) ;
#154609=CARTESIAN_POINT ( 'NONE',  ( 10.81492255796078972, 18.62759615963270932, 49.58224293864769550 ) ) ;
#154610=CARTESIAN_POINT ( 'NONE',  ( 4.379528057220339221, -16.55341960407611168, 27.70724293864769905 ) ) ;
#154611=CARTESIAN_POINT ( 'NONE',  ( -21.53943276465977519, -0.05219959533937600094, 63.75109039468568284 ) ) ;
#154612=CARTESIAN_POINT ( 'NONE',  ( -21.52544592524334988, -5.823673210054445271, 103.9594237280190185 ) ) ;
#154613=CARTESIAN_POINT ( 'NONE',  ( -16.51473224551082808, 9.474510206698731452, 33.33442372801899722 ) ) ;
#154614=CARTESIAN_POINT ( 'NONE',  ( -4.483927247898782831, 16.52544592524335698, 92.70942372801901854 ) ) ;
#154615=CARTESIAN_POINT ( 'NONE',  ( -0.05219959533937732626, 21.53943276465977519, 52.50109039468567573 ) ) ;
#154616=EDGE_CURVE ( 'NONE', #135352, #61770, #40244, .T. ) ;
#154617=CARTESIAN_POINT ( 'NONE',  ( -13.89961937509977652, 13.97604488694528158, 40.62390960531435979 ) ) ;
#154618=CARTESIAN_POINT ( 'NONE',  ( -5.823673210054431948, 21.52544592524334988, 112.7094237280190328 ) ) ;
#154619=CARTESIAN_POINT ( 'NONE',  ( -21.55341960407610458, -5.719274019375992779, 26.45724293864768839 ) ) ;
#154621=CARTESIAN_POINT ( 'NONE',  ( -5.823673210054116645, -21.52544592524344225, 112.2905762719810241 ) ) ;
#154622=CARTESIAN_POINT ( 'NONE',  ( 21.52544592524344225, -5.823673210054117533, 78.54057627198103830 ) ) ;
#154623=CARTESIAN_POINT ( 'NONE',  ( -4.483927247898782831, 16.52544592524335698, 42.70942372801901854 ) ) ;
#154625=CARTESIAN_POINT ( 'NONE',  ( 10.72451020669898902, -18.67979575497178502, 82.91557627198103830 ) ) ;
#154626=CARTESIAN_POINT ( 'NONE',  ( 14.34966873604972726, -8.224510206698740333, 70.83442372801901854 ) ) ;
#154627=CARTESIAN_POINT ( 'NONE',  ( 4.483927247898545687, 16.52544592524342804, 64.79057627198103830 ) ) ;
#154629=CARTESIAN_POINT ( 'NONE',  ( -19.02544592524334988, -5.153800228976617603, 98.95942372801900433 ) ) ;
#154631=CARTESIAN_POINT ( 'NONE',  ( 4.483927247898790824, -16.52544592524335698, 40.20942372801901854 ) ) ;
#154632=CARTESIAN_POINT ( 'NONE',  ( -10.81492255796078084, -18.62759615963271287, 107.0822429386476955 ) ) ;
#154633=CARTESIAN_POINT ( 'NONE',  ( -0.05219959533907301413, -21.53943276465977519, 32.49890960531435979 ) ) ;
#154634=CARTESIAN_POINT ( 'NONE',  ( -8.224510206698735004, -14.34966873604973081, 59.58442372801901854 ) ) ;
#154635=CARTESIAN_POINT ( 'NONE',  ( -13.97604488694527625, -13.89961937509977652, 71.87390960531433848 ) ) ;
#154636=CARTESIAN_POINT ( 'NONE',  ( 15.72974639402176855, 15.80617190586768217, 41.87609039468568284 ) ) ;
#154637=CARTESIAN_POINT ( 'NONE',  ( -16.51473224551082808, 9.474510206698731452, 108.3344237280190043 ) ) ;
#154638=CARTESIAN_POINT ( 'NONE',  ( -18.67979575497178146, -10.72451020669898902, 26.66557627198103475 ) ) ;
#154640=CARTESIAN_POINT ( 'NONE',  ( 19.03943276465977164, 0.05219959533936151252, 31.25109039468566863 ) ) ;
#154641=CARTESIAN_POINT ( 'NONE',  ( 8.224510206698742110, 14.34966873604972548, 42.08442372801901854 ) ) ;
#154642=CARTESIAN_POINT ( 'NONE',  ( -5.049401038298153566, 19.05341960407611168, 95.20724293864770971 ) ) ;
#154643=CARTESIAN_POINT ( 'NONE',  ( 0.05219959533907565091, 21.53943276465977519, 99.99890960531436690 ) ) ;
#154644=CARTESIAN_POINT ( 'NONE',  ( -19.05341960407611168, -5.049401038298163336, 66.45724293864769550 ) ) ;
#154646=CARTESIAN_POINT ( 'NONE',  ( -14.29746914071049879, 8.314922557960819915, 85.83224293864768129 ) ) ;
#154647=CARTESIAN_POINT ( 'NONE',  ( 18.67979575497178502, 10.72451020669898547, 24.16557627198103120 ) ) ;
#154648=CARTESIAN_POINT ( 'NONE',  ( -16.36317988757058828, 7.306389748694926745, 34.09789608363226421 ) ) ;
#154649=CARTESIAN_POINT ( 'NONE',  ( -4.483927247898782831, 16.52544592524335698, 62.70942372801902565 ) ) ;
#154650=CARTESIAN_POINT ( 'NONE',  ( -21.53943276465977519, 0.05219959533907696930, 101.2489096053143669 ) ) ;
#154651=CARTESIAN_POINT ( 'NONE',  ( 16.46253265017146816, 9.564922557961045513, 66.66775706135233293 ) ) ;
#154652=CARTESIAN_POINT ( 'NONE',  ( -10.72451020669898014, 18.67979575497178502, 35.41557627198102409 ) ) ;
#154653=CARTESIAN_POINT ( 'NONE',  ( -16.51473224551069308, -9.474510206698971260, 31.66557627198102054 ) ) ;
#154654=CARTESIAN_POINT ( 'NONE',  ( 5.719274019375991003, -21.55341960407610458, 67.70724293864769550 ) ) ;
#154655=CARTESIAN_POINT ( 'NONE',  ( 19.02544592524343514, -5.153800228976328945, 93.54057627198102409 ) ) ;
#154656=CARTESIAN_POINT ( 'NONE',  ( 5.719274019375673035, 21.55341960407619339, 92.29275706135236135 ) ) ;
#154657=CARTESIAN_POINT ( 'NONE',  ( -16.51473224551069308, -9.474510206698971260, 51.66557627198102409 ) ) ;
#154658=CARTESIAN_POINT ( 'NONE',  ( 12.06949235617739724, 12.14591786802326823, 36.87609039468568994 ) ) ;
#154659=CARTESIAN_POINT ( 'NONE',  ( 16.46253265017160672, -9.564922557960803928, 53.33224293864768839 ) ) ;
#154660=CARTESIAN_POINT ( 'NONE',  ( 5.719274019375673035, 21.55341960407619339, 82.29275706135234714 ) ) ;
#154662=CARTESIAN_POINT ( 'NONE',  ( -9.474510206698720793, -16.51473224551083518, 39.58442372801899722 ) ) ;
#154663=CARTESIAN_POINT ( 'NONE',  ( 16.46253265017146816, 9.564922557961045513, 46.66775706135233293 ) ) ;
#154664=CARTESIAN_POINT ( 'NONE',  ( -10.81492255796105439, 18.62759615963255655, 42.91775706135235424 ) ) ;
#154666=CARTESIAN_POINT ( 'NONE',  ( 19.03943276465977164, 0.05219959533936151252, 36.25109039468567573 ) ) ;
#154667=CARTESIAN_POINT ( 'NONE',  ( -0.05219959533909027116, -19.03943276465977164, 82.49890960531436690 ) ) ;
#154668=CARTESIAN_POINT ( 'NONE',  ( -5.153800228976328057, -19.02544592524343514, 67.29057627198102409 ) ) ;
#154669=CARTESIAN_POINT ( 'NONE',  ( -14.29746914071049879, 8.314922557960819915, 30.83224293864770260 ) ) ;
#154670=CARTESIAN_POINT ( 'NONE',  ( 19.03943276465977164, -0.05219959533909143690, 113.7489096053143669 ) ) ;
#154671=CARTESIAN_POINT ( 'NONE',  ( -15.72974639402176322, -15.80617190586768395, 89.37609039468568994 ) ) ;
#154674=CARTESIAN_POINT ( 'NONE',  ( 16.62475595723696031, 7.163666690055254804, 56.97286648189535896 ) ) ;
#154675=CARTESIAN_POINT ( 'NONE',  ( -5.823673210054431948, 21.52544592524334988, 97.70942372801904696 ) ) ;
#154676=CARTESIAN_POINT ( 'NONE',  ( 17.49999999999999645, -5.624438216177595429, 43.31670344914645199 ) ) ;
#154677=CARTESIAN_POINT ( 'NONE',  ( 19.03943276465977164, -0.05219959533909143690, 28.74890960531435624 ) ) ;
#154680=CARTESIAN_POINT ( 'NONE',  ( 16.55341960407618274, -4.379528057220086978, 46.04275706135234714 ) ) ;
#154681=CARTESIAN_POINT ( 'NONE',  ( 10.72451020669898902, -18.67979575497178502, 67.91557627198102409 ) ) ;
#154682=CARTESIAN_POINT ( 'NONE',  ( -4.379528057220328563, 16.55341960407611168, 45.20724293864769550 ) ) ;
#154683=CARTESIAN_POINT ( 'NONE',  ( 16.55341960407611168, 4.379528057220329451, 113.9572429386477239 ) ) ;
#154684=CARTESIAN_POINT ( 'NONE',  ( -13.97604488694527625, -13.89961937509977652, 91.87390960531432427 ) ) ;
#154685=CARTESIAN_POINT ( 'NONE',  ( 16.51473224551083163, -9.474510206698727899, 25.83442372801900078 ) ) ;
#154686=CARTESIAN_POINT ( 'NONE',  ( -16.51473224551069308, -9.474510206698971260, 26.66557627198103120 ) ) ;
#154687=CARTESIAN_POINT ( 'NONE',  ( 21.55341960407619695, -5.719274019375665929, 66.04275706135236135 ) ) ;
#154689=CARTESIAN_POINT ( 'NONE',  ( -0.05219959533934338120, 16.53943276465976808, 112.5010903946857042 ) ) ;
#154690=CARTESIAN_POINT ( 'NONE',  ( -19.05341960407617563, 5.049401038297882671, 68.54275706135230450 ) ) ;
#154692=CARTESIAN_POINT ( 'NONE',  ( -0.05219959533907301413, -21.53943276465977519, 27.49890960531435269 ) ) ;
#154693=CARTESIAN_POINT ( 'NONE',  ( -16.52544592524342804, 4.483927247898546575, 86.04057627198102409 ) ) ;
#154694=CARTESIAN_POINT ( 'NONE',  ( 0.05219959533936267826, -19.03943276465977164, 60.00109039468566863 ) ) ;
#154695=CARTESIAN_POINT ( 'NONE',  ( -9.474510206698964154, 16.51473224551069663, 70.41557627198102409 ) ) ;
#154696=CARTESIAN_POINT ( 'NONE',  ( -12.06949235617756955, 12.14591786802309770, 60.62390960531437401 ) ) ;
#154697=CARTESIAN_POINT ( 'NONE',  ( 16.46253265017146816, 9.564922557961045513, 96.66775706135233293 ) ) ;
#154698=CARTESIAN_POINT ( 'NONE',  ( -21.53943276465977519, 0.05219959533907696930, 46.24890960531435979 ) ) ;
#154700=CARTESIAN_POINT ( 'NONE',  ( 13.97604488694527802, 13.89961937509977652, 24.37390960531435624 ) ) ;
#154701=CARTESIAN_POINT ( 'NONE',  ( 16.51473224551083163, -9.474510206698727899, 100.8344237280190043 ) ) ;
#154702=EDGE_CURVE ( 'NONE', #188324, #30166, #153628, .T. ) ;
#154703=CARTESIAN_POINT ( 'NONE',  ( 9.474510206698971260, -16.51473224551069308, 77.91557627198103830 ) ) ;
#154705=CARTESIAN_POINT ( 'NONE',  ( 5.823673210054125526, 21.52544592524343514, 74.79057627198105251 ) ) ;
#154706=CARTESIAN_POINT ( 'NONE',  ( 8.224510206698742110, 14.34966873604972548, 87.08442372801901854 ) ) ;
#154707=CARTESIAN_POINT ( 'NONE',  ( 19.03943276465977164, -0.05219959533909143690, 68.74890960531436690 ) ) ;
#154708=CARTESIAN_POINT ( 'NONE',  ( 5.049401038297881783, 19.05341960407617563, 72.29275706135234714 ) ) ;
#154709=CARTESIAN_POINT ( 'NONE',  ( 15.80617190586769283, -15.72974639402175789, 75.62609039468567573 ) ) ;
#154710=CARTESIAN_POINT ( 'NONE',  ( -21.55341960407610458, -5.719274019375992779, 61.45724293864770260 ) ) ;
#154711=CARTESIAN_POINT ( 'NONE',  ( -18.62759615963270932, 10.81492255796079327, 30.83224293864770260 ) ) ;
#154712=CARTESIAN_POINT ( 'NONE',  ( -19.03943276465977164, 0.05219959533909376836, 31.24890960531435979 ) ) ;
#154713=CARTESIAN_POINT ( 'NONE',  ( -14.29746914071037622, -8.314922557961029526, 99.16775706135234714 ) ) ;
#154714=CARTESIAN_POINT ( 'NONE',  ( -0.05219959533909027116, -19.03943276465977164, 47.49890960531435979 ) ) ;
#154715=CARTESIAN_POINT ( 'NONE',  ( -8.224510206698735004, -14.34966873604973081, 24.58442372801901499 ) ) ;
#154717=CARTESIAN_POINT ( 'NONE',  ( 9.564922557961047289, -16.46253265017146816, 20.41775706135233293 ) ) ;
#154718=CARTESIAN_POINT ( 'NONE',  ( -16.53943276465976808, 0.05219959533911058130, 61.24890960531435979 ) ) ;
#154719=CARTESIAN_POINT ( 'NONE',  ( -21.55341960407610458, -5.719274019375992779, 91.45724293864769550 ) ) ;
#154720=CARTESIAN_POINT ( 'NONE',  ( -18.62759615963270932, 10.81492255796079327, 95.83224293864770971 ) ) ;
#154721=CARTESIAN_POINT ( 'NONE',  ( 17.26172910966780094, -6.454744622555848466, 98.30646908649228521 ) ) ;
#154722=CARTESIAN_POINT ( 'NONE',  ( -5.823673210054116645, -21.52544592524344225, 42.29057627198103120 ) ) ;
#154723=CARTESIAN_POINT ( 'NONE',  ( -14.29746914071037622, -8.314922557961029526, 79.16775706135234714 ) ) ;
#154724=CARTESIAN_POINT ( 'NONE',  ( 0.05219959533910956823, 16.53943276465976808, 94.99890960531436690 ) ) ;
#154725=CARTESIAN_POINT ( 'NONE',  ( 5.049401038298161559, -19.05341960407611168, 47.70724293864770260 ) ) ;
#154727=CARTESIAN_POINT ( 'NONE',  ( -16.53943276465976808, 0.05219959533911058130, 21.24890960531436690 ) ) ;
#154728=CARTESIAN_POINT ( 'NONE',  ( -21.52544592524334988, -5.823673210054445271, 38.95942372801901854 ) ) ;
#154729=CARTESIAN_POINT ( 'NONE',  ( -9.474510206698964154, 16.51473224551069663, 90.41557627198103830 ) ) ;
#154730=CARTESIAN_POINT ( 'NONE',  ( -18.62759615963255300, -10.81492255796106328, 69.16775706135234714 ) ) ;
#154733=EDGE_LOOP ( 'NONE', ( #195705, #181456, #167373, #98148 ) ) ;
#154734=CARTESIAN_POINT ( 'NONE',  ( 15.72974639402176855, 15.80617190586768217, 61.87609039468568284 ) ) ;
#154735=CARTESIAN_POINT ( 'NONE',  ( -9.564922557960796823, -16.46253265017161027, 57.08224293864769550 ) ) ;
#154736=CARTESIAN_POINT ( 'NONE',  ( -13.89961937509977652, 13.97604488694528158, 110.6239096053143243 ) ) ;
#154737=CARTESIAN_POINT ( 'NONE',  ( -16.51473224551069308, -9.474510206698971260, 91.66557627198103830 ) ) ;
#154738=CARTESIAN_POINT ( 'NONE',  ( 19.03943276465977164, 0.05219959533936151252, 66.25109039468567573 ) ) ;
#154739=CARTESIAN_POINT ( 'NONE',  ( -5.823673210054431948, 21.52544592524334988, 42.70942372801901854 ) ) ;
#154740=CARTESIAN_POINT ( 'NONE',  ( -9.564922557961040184, 16.46253265017147172, 102.9177570613523329 ) ) ;
#154741=CARTESIAN_POINT ( 'NONE',  ( -19.02544592524334988, -5.153800228976617603, 73.95942372801900433 ) ) ;
#154742=CARTESIAN_POINT ( 'NONE',  ( 19.02544592524343514, -5.153800228976328945, 33.54057627198102409 ) ) ;
#154743=CARTESIAN_POINT ( 'NONE',  ( -8.224510206698735004, -14.34966873604973081, 104.5844237280190185 ) ) ;
#154744=CARTESIAN_POINT ( 'NONE',  ( 16.46253265017146816, 9.564922557961045513, 71.66775706135233293 ) ) ;
#154745=CARTESIAN_POINT ( 'NONE',  ( 16.52544592524342804, -4.483927247898539470, 28.54057627198103120 ) ) ;
#154746=CARTESIAN_POINT ( 'NONE',  ( -5.049401038297874678, -19.05341960407617918, 54.79275706135234003 ) ) ;
#154747=CARTESIAN_POINT ( 'NONE',  ( 21.55341960407619695, -5.719274019375665929, 101.0427570613523756 ) ) ;
#154748=CARTESIAN_POINT ( 'NONE',  ( 5.049401038297881783, 19.05341960407617563, 27.29275706135232937 ) ) ;
#154749=CARTESIAN_POINT ( 'NONE',  ( 9.474510206698971260, -16.51473224551069308, 22.91557627198102765 ) ) ;
#154750=CARTESIAN_POINT ( 'NONE',  ( -10.81492255796105439, 18.62759615963255655, 82.91775706135234714 ) ) ;
#154751=CARTESIAN_POINT ( 'NONE',  ( -0.05219959533934338120, 16.53943276465976808, 27.50109039468567929 ) ) ;
#154752=CARTESIAN_POINT ( 'NONE',  ( -13.97604488694527625, -13.89961937509977652, 96.87390960531433848 ) ) ;
#154754=CARTESIAN_POINT ( 'NONE',  ( -19.05341960407611168, -5.049401038298163336, 81.45724293864769550 ) ) ;
#154755=CARTESIAN_POINT ( 'NONE',  ( -17.50000000001358202, 5.499999999999951150, 100.7969038253505687 ) ) ;
#154756=CARTESIAN_POINT ( 'NONE',  ( -5.153800228976607833, 19.02544592524334988, 82.70942372801897591 ) ) ;
#154757=CARTESIAN_POINT ( 'NONE',  ( 0.05219959533909260263, 19.03943276465977164, 104.9989096053143669 ) ) ;
#154758=CARTESIAN_POINT ( 'NONE',  ( -21.53943276465977519, -0.05219959533937600094, 108.7510903946857042 ) ) ;
#154759=CARTESIAN_POINT ( 'NONE',  ( 12.14591786802309770, 12.06949235617756955, 94.37390960531436690 ) ) ;
#154760=CARTESIAN_POINT ( 'NONE',  ( -0.05219959533909027116, -19.03943276465977164, 27.49890960531435624 ) ) ;
#154761=CARTESIAN_POINT ( 'NONE',  ( 18.62759615963271287, -10.81492255796078972, 53.33224293864769550 ) ) ;
#154762=CARTESIAN_POINT ( 'NONE',  ( 21.52544592524344225, -5.823673210054117533, 33.54057627198102409 ) ) ;
#154763=CARTESIAN_POINT ( 'NONE',  ( 16.52544592524342804, -4.483927247898539470, 113.5405762719810383 ) ) ;
#154765=CARTESIAN_POINT ( 'NONE',  ( -5.153800228976607833, 19.02544592524334988, 57.70942372801899012 ) ) ;
#154766=CARTESIAN_POINT ( 'NONE',  ( -14.34966873604960291, -8.224510206698953496, 41.66557627198103120 ) ) ;
#154767=CARTESIAN_POINT ( 'NONE',  ( -21.55341960407610458, -5.719274019375992779, 21.45724293864769550 ) ) ;
#154769=CARTESIAN_POINT ( 'NONE',  ( 21.53943276465977519, 0.05219959533937863772, 81.25109039468568994 ) ) ;
#154770=CARTESIAN_POINT ( 'NONE',  ( -21.53943276465977519, 0.05219959533907696930, 76.24890960531435269 ) ) ;
#154771=CARTESIAN_POINT ( 'NONE',  ( -21.55341960407619339, 5.719274019375674811, 63.54275706135234003 ) ) ;
#154772=CARTESIAN_POINT ( 'NONE',  ( 5.823673210054444382, -21.52544592524334988, 50.20942372801901854 ) ) ;
#154773=CARTESIAN_POINT ( 'NONE',  ( 13.97604488694527802, 13.89961937509977652, 89.37390960531436690 ) ) ;
#154774=CARTESIAN_POINT ( 'NONE',  ( 16.53943276465976808, 0.05219959533934440121, 81.25109039468568994 ) ) ;
#154775=CARTESIAN_POINT ( 'NONE',  ( 16.46253265017160672, -9.564922557960803928, 23.33224293864769194 ) ) ;
#154777=CARTESIAN_POINT ( 'NONE',  ( 16.53943276465976808, -0.05219959533910856209, 53.74890960531437401 ) ) ;
#154778=CARTESIAN_POINT ( 'NONE',  ( 12.06949235617757843, -12.14591786802309237, 28.12390960531435979 ) ) ;
#154779=CARTESIAN_POINT ( 'NONE',  ( 13.97604488694527802, 13.89961937509977652, 64.37390960531436690 ) ) ;
#154780=CARTESIAN_POINT ( 'NONE',  ( -13.89961937509977652, 13.97604488694528158, 40.62390960531435979 ) ) ;
#154781=CARTESIAN_POINT ( 'NONE',  ( 21.53943276465977519, -0.05219959533907433946, 38.74890960531435979 ) ) ;
#154782=CARTESIAN_POINT ( 'NONE',  ( -9.474510206698720793, -16.51473224551083518, 44.58442372801900433 ) ) ;
#154783=CARTESIAN_POINT ( 'NONE',  ( -17.49999999999999645, -5.500000000000000888, 39.20309617465829177 ) ) ;
#154784=CARTESIAN_POINT ( 'NONE',  ( -12.06949235617756955, 12.14591786802309770, 50.62390960531435979 ) ) ;
#154785=CARTESIAN_POINT ( 'NONE',  ( 15.72974639402199770, -15.80617190586745480, 23.12390960531436335 ) ) ;
#154786=CARTESIAN_POINT ( 'NONE',  ( 17.69326672847925508, -2.167987141922157690, 37.50000000000000000 ) ) ;
#154787=CARTESIAN_POINT ( 'NONE',  ( -14.34966873604972548, 8.224510206698743886, 68.33442372801900433 ) ) ;
#154788=CARTESIAN_POINT ( 'NONE',  ( 13.97604488694548053, -13.89961937509957401, 75.62609039468564731 ) ) ;
#154790=CARTESIAN_POINT ( 'NONE',  ( 8.314922557960818139, 14.29746914071049879, 39.58224293864769550 ) ) ;
#154792=CARTESIAN_POINT ( 'NONE',  ( 0.05219959533910956823, 16.53943276465976808, 29.99890960531435979 ) ) ;
#154793=CARTESIAN_POINT ( 'NONE',  ( 13.97604488694527802, 13.89961937509977652, 44.37390960531435269 ) ) ;
#154794=CARTESIAN_POINT ( 'NONE',  ( -13.97604488694527625, -13.89961937509977652, 56.87390960531434558 ) ) ;
#154795=CARTESIAN_POINT ( 'NONE',  ( -5.153800228976328057, -19.02544592524343514, 42.29057627198101699 ) ) ;
#154796=CARTESIAN_POINT ( 'NONE',  ( -18.62759615963255300, -10.81492255796106328, 29.16775706135234003 ) ) ;
#154797=CARTESIAN_POINT ( 'NONE',  ( -9.564922557960796823, -16.46253265017161027, 57.08224293864769550 ) ) ;
#154799=CARTESIAN_POINT ( 'NONE',  ( 9.564922557960805705, 16.46253265017160317, 44.58224293864769550 ) ) ;
#154800=CARTESIAN_POINT ( 'NONE',  ( 21.52544592524344225, -5.823673210054117533, 33.54057627198102409 ) ) ;
#154801=CARTESIAN_POINT ( 'NONE',  ( -18.67979575497193778, 10.72451020669871902, 58.33442372801901143 ) ) ;
#154802=CARTESIAN_POINT ( 'NONE',  ( -13.97604488694527625, -13.89961937509977652, 26.87390960531434558 ) ) ;
#154803=CARTESIAN_POINT ( 'NONE',  ( -15.80617190586745835, -15.72974639402198527, 21.87390960531436690 ) ) ;
#154804=CARTESIAN_POINT ( 'NONE',  ( 16.55341960407618274, -4.379528057220086978, 91.04275706135236135 ) ) ;
#154805=CARTESIAN_POINT ( 'NONE',  ( -21.52544592524334988, -5.823673210054445271, 103.9594237280190185 ) ) ;
#154806=CARTESIAN_POINT ( 'NONE',  ( 12.06949235617739724, 12.14591786802326823, 66.87609039468568994 ) ) ;
#154807=CARTESIAN_POINT ( 'NONE',  ( 0.05219959533909260263, 19.03943276465977164, 104.9989096053143669 ) ) ;
#154808=CARTESIAN_POINT ( 'NONE',  ( -12.06949235617739369, -12.14591786802326823, 49.37609039468569705 ) ) ;
#154809=CARTESIAN_POINT ( 'NONE',  ( 0.05219959533934541429, -16.53943276465976808, 40.00109039468567573 ) ) ;
#154810=CARTESIAN_POINT ( 'NONE',  ( -16.55341960407617563, 4.379528057220093196, 93.54275706135234714 ) ) ;
#154811=CARTESIAN_POINT ( 'NONE',  ( 0.05219959533937995610, -21.53943276465977519, 60.00109039468568284 ) ) ;
#154812=CARTESIAN_POINT ( 'NONE',  ( 8.314922557961029526, -14.29746914071037800, 25.41775706135235779 ) ) ;
#154813=CARTESIAN_POINT ( 'NONE',  ( -15.80617190586745835, -15.72974639402198527, 106.8739096053143811 ) ) ;
#154814=CARTESIAN_POINT ( 'NONE',  ( 16.52544592524335698, 4.483927247898782831, 26.45942372801901854 ) ) ;
#154815=CARTESIAN_POINT ( 'NONE',  ( 16.52544592524335698, 4.483927247898782831, 91.45942372801901854 ) ) ;
#154817=CARTESIAN_POINT ( 'NONE',  ( 10.81492255796106328, -18.62759615963255655, 90.41775706135236135 ) ) ;
#154818=CARTESIAN_POINT ( 'NONE',  ( -5.049401038297874678, -19.05341960407617918, 89.79275706135230450 ) ) ;
#154819=CARTESIAN_POINT ( 'NONE',  ( -4.379528057220328563, 16.55341960407611168, 65.20724293864768129 ) ) ;
#154820=CARTESIAN_POINT ( 'NONE',  ( -12.06949235617756955, 12.14591786802309770, 40.62390960531435269 ) ) ;
#154821=CARTESIAN_POINT ( 'NONE',  ( -8.314922557960811034, -14.29746914071050412, 107.0822429386476955 ) ) ;
#154822=CARTESIAN_POINT ( 'NONE',  ( 19.02544592524334988, 5.153800228976608722, 46.45942372801899012 ) ) ;
#154824=CARTESIAN_POINT ( 'NONE',  ( 21.53943276465977519, 0.05219959533937863772, 51.25109039468568994 ) ) ;
#154825=CARTESIAN_POINT ( 'NONE',  ( -9.564922557961040184, 16.46253265017147172, 112.9177570613523329 ) ) ;
#154826=DIRECTION ( 'NONE',  ( 0.000000000000000000, -1.000000000000000000, 0.000000000000000000 ) ) ;
#154827=CARTESIAN_POINT ( 'NONE',  ( -13.89961937509977652, 13.97604488694528158, 100.6239096053143669 ) ) ;
#154828=CARTESIAN_POINT ( 'NONE',  ( -18.67979575497178146, -10.72451020669898902, 66.66557627198102409 ) ) ;
#154829=CARTESIAN_POINT ( 'NONE',  ( -19.03943276465977164, -0.05219959533935918106, 93.75109039468566152 ) ) ;
#154830=CARTESIAN_POINT ( 'NONE',  ( 13.89961937509977652, -13.97604488694527269, 98.12390960531433848 ) ) ;
#154831=CARTESIAN_POINT ( 'NONE',  ( 15.72974639402199770, -15.80617190586745480, 53.12390960531436690 ) ) ;
#154832=CARTESIAN_POINT ( 'NONE',  ( 16.52544592524342804, -4.483927247898539470, 108.5405762719810241 ) ) ;
#154833=CARTESIAN_POINT ( 'NONE',  ( -5.719274019375665041, -21.55341960407619695, 89.79275706135236135 ) ) ;
#154834=CARTESIAN_POINT ( 'NONE',  ( 9.564922557960805705, 16.46253265017160317, 34.58224293864770260 ) ) ;
#154835=CARTESIAN_POINT ( 'NONE',  ( -5.823673210054431948, 21.52544592524334988, 37.70942372801900433 ) ) ;
#154837=CARTESIAN_POINT ( 'NONE',  ( -5.719274019375665041, -21.55341960407619695, 94.79275706135234714 ) ) ;
#154839=CARTESIAN_POINT ( 'NONE',  ( 4.483927247898790824, -16.52544592524335698, 90.20942372801903275 ) ) ;
#154840=CARTESIAN_POINT ( 'NONE',  ( 21.55341960407619695, -5.719274019375665929, 31.04275706135234714 ) ) ;
#154841=CARTESIAN_POINT ( 'NONE',  ( -15.72974639402176322, -15.80617190586768395, 39.37609039468567573 ) ) ;
#154842=CARTESIAN_POINT ( 'NONE',  ( -19.02544592524334988, -5.153800228976617603, 68.95942372801896170 ) ) ;
#154843=CARTESIAN_POINT ( 'NONE',  ( 13.89961937509977652, -13.97604488694527269, 83.12390960531436690 ) ) ;
#154844=CARTESIAN_POINT ( 'NONE',  ( 10.72451020669871369, 18.67979575497193778, 82.08442372801901854 ) ) ;
#154845=CARTESIAN_POINT ( 'NONE',  ( -5.719274019375978568, 21.55341960407610458, 85.20724293864770971 ) ) ;
#154846=CARTESIAN_POINT ( 'NONE',  ( 12.06949235617757843, -12.14591786802309237, 58.12390960531435979 ) ) ;
#154847=CARTESIAN_POINT ( 'NONE',  ( 18.62759615963255655, 10.81492255796105972, 106.6677570613523756 ) ) ;
#154848=CARTESIAN_POINT ( 'NONE',  ( 14.29746914071049879, -8.314922557960816363, 88.33224293864769550 ) ) ;
#154849=CARTESIAN_POINT ( 'NONE',  ( 13.89961937509977652, -13.97604488694527269, 38.12390960531436690 ) ) ;
#154850=CARTESIAN_POINT ( 'NONE',  ( 19.03943276465977164, 0.05219959533936151252, 71.25109039468566152 ) ) ;
#154851=CARTESIAN_POINT ( 'NONE',  ( -8.224510206698948167, 14.34966873604960824, 40.41557627198103120 ) ) ;
#154852=CARTESIAN_POINT ( 'NONE',  ( -0.05219959533937732626, 21.53943276465977519, 97.50109039468567573 ) ) ;
#154853=CARTESIAN_POINT ( 'NONE',  ( -9.474510206698964154, 16.51473224551069663, 95.41557627198102409 ) ) ;
#154854=CARTESIAN_POINT ( 'NONE',  ( -19.02544592524334988, -5.153800228976617603, 63.95942372801899012 ) ) ;
#154855=CARTESIAN_POINT ( 'NONE',  ( 18.62759615963271287, -10.81492255796078972, 68.33224293864769550 ) ) ;
#154856=CARTESIAN_POINT ( 'NONE',  ( 21.55341960407619695, -5.719274019375665929, 21.04275706135234714 ) ) ;
#154857=CARTESIAN_POINT ( 'NONE',  ( -0.05219959533936034679, 19.03943276465977164, 107.5010903946856615 ) ) ;
#154858=CARTESIAN_POINT ( 'NONE',  ( -8.314922557961024197, 14.29746914071037800, 77.91775706135231871 ) ) ;
#154859=CARTESIAN_POINT ( 'NONE',  ( 16.52216118717207749, 7.221426719304521846, 63.57599021046996057 ) ) ;
#154860=CARTESIAN_POINT ( 'NONE',  ( 15.80617190586769283, -15.72974639402175789, 25.62609039468567929 ) ) ;
#154861=CARTESIAN_POINT ( 'NONE',  ( -16.52544592524342804, 4.483927247898546575, 106.0405762719810525 ) ) ;
#154863=CARTESIAN_POINT ( 'NONE',  ( -16.55341960407617563, 4.379528057220093196, 48.54275706135234714 ) ) ;
#154864=CARTESIAN_POINT ( 'NONE',  ( -8.224510206698948167, 14.34966873604960824, 80.41557627198103830 ) ) ;
#154865=CARTESIAN_POINT ( 'NONE',  ( 15.72974639402199770, -15.80617190586745480, 73.12390960531436690 ) ) ;
#154866=CARTESIAN_POINT ( 'NONE',  ( 16.52544592524335698, 4.483927247898782831, 106.4594237280190328 ) ) ;
#154867=CARTESIAN_POINT ( 'NONE',  ( 12.06949235617739724, 12.14591786802326823, 36.87609039468568994 ) ) ;
#154868=CARTESIAN_POINT ( 'NONE',  ( -19.05341960407611168, -5.049401038298163336, 51.45724293864770260 ) ) ;
#154869=CARTESIAN_POINT ( 'NONE',  ( -16.53943276465976808, -0.05219959533934237506, 73.75109039468567573 ) ) ;
#154870=CARTESIAN_POINT ( 'NONE',  ( 16.46253265017146816, 9.564922557961045513, 76.66775706135234714 ) ) ;
#154871=CARTESIAN_POINT ( 'NONE',  ( -18.62759615963270932, 10.81492255796079327, 70.83224293864770971 ) ) ;
#154872=CARTESIAN_POINT ( 'NONE',  ( 12.06949235617739724, 12.14591786802326823, 91.87609039468568994 ) ) ;
#154873=CARTESIAN_POINT ( 'NONE',  ( 18.67979575497194134, -10.72451020669871369, 80.83442372801901854 ) ) ;
#154874=CARTESIAN_POINT ( 'NONE',  ( -21.55341960407610458, -5.719274019375992779, 66.45724293864768129 ) ) ;
#154875=CARTESIAN_POINT ( 'NONE',  ( -15.80617190586745835, -15.72974639402198527, 51.87390960531437401 ) ) ;
#154876=EDGE_LOOP ( 'NONE', ( #151960, #164655, #152147, #83657 ) ) ;
#154877=CARTESIAN_POINT ( 'NONE',  ( 16.55341960407618274, -4.379528057220086978, 81.04275706135236135 ) ) ;
#154878=CARTESIAN_POINT ( 'NONE',  ( 10.81492255796078972, 18.62759615963270932, 44.58224293864769550 ) ) ;
#154879=ORIENTED_EDGE ( 'NONE', *, *, #32834, .F. ) ;
#154880=CARTESIAN_POINT ( 'NONE',  ( 18.67979575497178502, 10.72451020669898547, 24.16557627198103120 ) ) ;
#154882=CARTESIAN_POINT ( 'NONE',  ( -13.89961937509977652, 13.97604488694528158, 25.62390960531434558 ) ) ;
#154883=CARTESIAN_POINT ( 'NONE',  ( -18.67979575497178146, -10.72451020669898902, 76.66557627198103830 ) ) ;
#154884=CARTESIAN_POINT ( 'NONE',  ( 14.34966873604972726, -8.224510206698740333, 110.8344237280190043 ) ) ;
#154885=CARTESIAN_POINT ( 'NONE',  ( -21.53943276465977519, -0.05219959533937600094, 43.75109039468568284 ) ) ;
#154886=CARTESIAN_POINT ( 'NONE',  ( -5.153800228976607833, 19.02544592524334988, 112.7094237280190043 ) ) ;
#154887=CARTESIAN_POINT ( 'NONE',  ( -8.224510206698948167, 14.34966873604960824, 115.4155762719810241 ) ) ;
#154888=CARTESIAN_POINT ( 'NONE',  ( 19.02544592524334988, 5.153800228976608722, 106.4594237280190185 ) ) ;
#154889=CARTESIAN_POINT ( 'NONE',  ( 19.03943276465977164, -0.05219959533909143690, 33.74890960531435979 ) ) ;
#154891=CARTESIAN_POINT ( 'NONE',  ( 9.474510206698971260, -16.51473224551069308, 107.9155762719810383 ) ) ;
#154892=CARTESIAN_POINT ( 'NONE',  ( -0.05219959533934338120, 16.53943276465976808, 92.50109039468567573 ) ) ;
#154893=CARTESIAN_POINT ( 'NONE',  ( -13.97604488694547697, 13.89961937509957934, 83.12609039468564731 ) ) ;
#154894=CARTESIAN_POINT ( 'NONE',  ( 19.05341960407617918, -5.049401038297876454, 21.04275706135232582 ) ) ;
#154895=CARTESIAN_POINT ( 'NONE',  ( -15.72974639402197994, 15.80617190586746368, 55.62390960531436690 ) ) ;
#154896=CARTESIAN_POINT ( 'NONE',  ( -4.483927247898782831, 16.52544592524335698, 82.70942372801900433 ) ) ;
#154897=CARTESIAN_POINT ( 'NONE',  ( 5.049401038297881783, 19.05341960407617563, 82.29275706135229029 ) ) ;
#154898=CARTESIAN_POINT ( 'NONE',  ( 16.51473224551069308, 9.474510206698969483, 39.16557627198103120 ) ) ;
#154899=CARTESIAN_POINT ( 'NONE',  ( -5.153800228976328057, -19.02544592524343514, 92.29057627198099567 ) ) ;
#154900=CARTESIAN_POINT ( 'NONE',  ( -10.72451020669870658, -18.67979575497194134, 49.58442372801901143 ) ) ;
#154901=CARTESIAN_POINT ( 'NONE',  ( 5.049401038298161559, -19.05341960407611168, 47.70724293864770260 ) ) ;
#154903=CARTESIAN_POINT ( 'NONE',  ( -16.46253265017160317, 9.564922557960807481, 115.8322429386477097 ) ) ;
#154904=CARTESIAN_POINT ( 'NONE',  ( -8.224510206698948167, 14.34966873604960824, 65.41557627198102409 ) ) ;
#154905=CARTESIAN_POINT ( 'NONE',  ( -15.72974639402197994, 15.80617190586746368, 60.62390960531437401 ) ) ;
#154907=CARTESIAN_POINT ( 'NONE',  ( 19.02544592524334988, 5.153800228976608722, 41.45942372801900433 ) ) ;
#154909=CARTESIAN_POINT ( 'NONE',  ( -5.049401038298153566, 19.05341960407611168, 60.20724293864768129 ) ) ;
#154910=CARTESIAN_POINT ( 'NONE',  ( -0.05219959533909027116, -19.03943276465977164, 72.49890960531435269 ) ) ;
#154911=CARTESIAN_POINT ( 'NONE',  ( -16.53943276465976808, -0.05219959533934237506, 48.75109039468568284 ) ) ;
#154914=CARTESIAN_POINT ( 'NONE',  ( 4.483927247898790824, -16.52544592524335698, 95.20942372801903275 ) ) ;
#154916=CARTESIAN_POINT ( 'NONE',  ( 8.314922557961029526, -14.29746914071037800, 80.41775706135234714 ) ) ;
#154917=CARTESIAN_POINT ( 'NONE',  ( 16.52544592524335698, 4.483927247898782831, 56.45942372801902565 ) ) ;
#154918=CARTESIAN_POINT ( 'NONE',  ( 5.719274019375673035, 21.55341960407619339, 112.2927570613523471 ) ) ;
#154919=CARTESIAN_POINT ( 'NONE',  ( -16.46253265017160317, 9.564922557960807481, 60.83224293864769550 ) ) ;
#154921=CARTESIAN_POINT ( 'NONE',  ( -15.80617190586768217, 15.72974639402176855, 48.12609039468568284 ) ) ;
#154922=CARTESIAN_POINT ( 'NONE',  ( 9.474510206698729675, 16.51473224551082808, 67.08442372801900433 ) ) ;
#154923=CARTESIAN_POINT ( 'NONE',  ( -0.05219959533937732626, 21.53943276465977519, 107.5010903946856899 ) ) ;
#154924=CARTESIAN_POINT ( 'NONE',  ( -16.51473224551069308, -9.474510206698971260, 26.66557627198103120 ) ) ;
#154926=CARTESIAN_POINT ( 'NONE',  ( -15.80617190586745835, -15.72974639402198527, 71.87390960531438111 ) ) ;
#154927=CARTESIAN_POINT ( 'NONE',  ( 13.89961937509977652, -13.97604488694527269, 113.1239096053143527 ) ) ;
#154928=CARTESIAN_POINT ( 'NONE',  ( -9.474510206698964154, 16.51473224551069663, 25.41557627198103120 ) ) ;
#154929=CARTESIAN_POINT ( 'NONE',  ( -12.14591786802326823, 12.06949235617739902, 38.12609039468567573 ) ) ;
#154930=CARTESIAN_POINT ( 'NONE',  ( -4.379528057220328563, 16.55341960407611168, 35.20724293864768839 ) ) ;
#154933=CARTESIAN_POINT ( 'NONE',  ( 18.67979575497194134, -10.72451020669871369, 20.83442372801901143 ) ) ;
#154934=CARTESIAN_POINT ( 'NONE',  ( 16.52544592524342804, -4.483927247898539470, 43.54057627198103830 ) ) ;
#154935=CARTESIAN_POINT ( 'NONE',  ( -5.049401038298153566, 19.05341960407611168, 110.2072429386476671 ) ) ;
#154936=CARTESIAN_POINT ( 'NONE',  ( -16.51473224551082808, 9.474510206698731452, 113.3344237280190043 ) ) ;
#154937=CARTESIAN_POINT ( 'NONE',  ( 9.474510206698729675, 16.51473224551082808, 27.08442372801900433 ) ) ;
#154938=CARTESIAN_POINT ( 'NONE',  ( 0.05219959533910956823, 16.53943276465976808, 39.99890960531436690 ) ) ;
#154939=CARTESIAN_POINT ( 'NONE',  ( -21.52544592524343514, 5.823673210054127303, 106.0405762719810525 ) ) ;
#154941=CARTESIAN_POINT ( 'NONE',  ( 21.52544592524344225, -5.823673210054117533, 63.54057627198103830 ) ) ;
#154942=CARTESIAN_POINT ( 'NONE',  ( -19.02544592524342804, 5.153800228976336051, 71.04057627198099567 ) ) ;
#154943=CARTESIAN_POINT ( 'NONE',  ( 8.224510206698953496, -14.34966873604960469, 52.91557627198103830 ) ) ;
#154944=CARTESIAN_POINT ( 'NONE',  ( -16.46253265017160317, 9.564922557960807481, 85.83224293864769550 ) ) ;
#154946=LINE ( 'NONE', #167154, #31219 ) ;
#154947=CARTESIAN_POINT ( 'NONE',  ( 19.02544592524334988, 5.153800228976608722, 51.45942372801900433 ) ) ;
#154948=CARTESIAN_POINT ( 'NONE',  ( 5.719274019375991003, -21.55341960407610458, 97.70724293864772392 ) ) ;
#154949=CARTESIAN_POINT ( 'NONE',  ( 8.314922557960818139, 14.29746914071049879, 104.5822429386477097 ) ) ;
#154950=CARTESIAN_POINT ( 'NONE',  ( 10.81492255796106328, -18.62759615963255655, 45.41775706135234003 ) ) ;
#154952=CARTESIAN_POINT ( 'NONE',  ( -16.55341960407611168, -4.379528057220339221, 31.45724293864769550 ) ) ;
#154953=CARTESIAN_POINT ( 'NONE',  ( -13.89961937509977652, 13.97604488694528158, 40.62390960531435979 ) ) ;
#154954=CARTESIAN_POINT ( 'NONE',  ( 13.89961937509977652, -13.97604488694527269, 103.1239096053143527 ) ) ;
#154955=CARTESIAN_POINT ( 'NONE',  ( -5.823673210054116645, -21.52544592524344225, 67.29057627198103830 ) ) ;
#154957=CARTESIAN_POINT ( 'NONE',  ( -13.97604488694527625, -13.89961937509977652, 36.87390960531436690 ) ) ;
#154958=CARTESIAN_POINT ( 'NONE',  ( 21.53943276465977519, -0.05219959533907433946, 48.74890960531435979 ) ) ;
#154959=CARTESIAN_POINT ( 'NONE',  ( -15.80617190586768217, 15.72974639402176855, 73.12609039468567573 ) ) ;
#154961=CARTESIAN_POINT ( 'NONE',  ( 14.29746914071037800, 8.314922557961029526, 81.66775706135236135 ) ) ;
#154962=CARTESIAN_POINT ( 'NONE',  ( 19.05341960407611168, 5.049401038298154454, 58.95724293864768129 ) ) ;
#154963=CARTESIAN_POINT ( 'NONE',  ( -9.564922557960796823, -16.46253265017161027, 67.08224293864769550 ) ) ;
#154965=CARTESIAN_POINT ( 'NONE',  ( 19.03943276465977164, 0.05219959533936151252, 26.25109039468566507 ) ) ;
#154966=CARTESIAN_POINT ( 'NONE',  ( 14.34966873604972726, -8.224510206698740333, 80.83442372801901854 ) ) ;
#154967=CARTESIAN_POINT ( 'NONE',  ( -10.81492255796105439, 18.62759615963255655, 97.91775706135236135 ) ) ;
#154968=CARTESIAN_POINT ( 'NONE',  ( 5.153800228976335163, 19.02544592524342804, 69.79057627198103830 ) ) ;
#154969=CARTESIAN_POINT ( 'NONE',  ( -21.55341960407610458, -5.719274019375992779, 31.45724293864769550 ) ) ;
#154970=CARTESIAN_POINT ( 'NONE',  ( -9.564922557961040184, 16.46253265017147172, 112.9177570613523329 ) ) ;
#154971=CARTESIAN_POINT ( 'NONE',  ( -15.80617190586768217, 15.72974639402176855, 88.12609039468570415 ) ) ;
#154972=CARTESIAN_POINT ( 'NONE',  ( -16.53943276465976808, -0.05219959533934237506, 43.75109039468568284 ) ) ;
#154973=CARTESIAN_POINT ( 'NONE',  ( 18.62759615963271287, -10.81492255796078972, 103.3322429386476955 ) ) ;
#154974=CARTESIAN_POINT ( 'NONE',  ( 16.52544592524335698, 4.483927247898782831, 21.45942372801901499 ) ) ;
#154975=CARTESIAN_POINT ( 'NONE',  ( -19.03943276465977164, 0.05219959533909376836, 81.24890960531436690 ) ) ;
#154976=CARTESIAN_POINT ( 'NONE',  ( 16.55341960407618274, -4.379528057220086978, 26.04275706135235779 ) ) ;
#154977=CARTESIAN_POINT ( 'NONE',  ( -16.51473224551069308, -9.474510206698971260, 41.66557627198103120 ) ) ;
#154979=CARTESIAN_POINT ( 'NONE',  ( 13.89961937509957401, 13.97604488694547697, 111.8760903946856757 ) ) ;
#154980=CARTESIAN_POINT ( 'NONE',  ( -12.06949235617756955, 12.14591786802309770, 70.62390960531436690 ) ) ;
#154981=CARTESIAN_POINT ( 'NONE',  ( 8.224510206698742110, 14.34966873604972548, 72.08442372801899012 ) ) ;
#154982=CARTESIAN_POINT ( 'NONE',  ( -15.80617190586768217, 15.72974639402176855, 28.12609039468568284 ) ) ;
#154983=CARTESIAN_POINT ( 'NONE',  ( 5.049401038298161559, -19.05341960407611168, 47.70724293864770260 ) ) ;
#154984=CARTESIAN_POINT ( 'NONE',  ( 16.46253265017160672, -9.564922557960803928, 73.33224293864769550 ) ) ;
#154985=CARTESIAN_POINT ( 'NONE',  ( 14.34966873604972726, -8.224510206698740333, 75.83442372801900433 ) ) ;
#154988=ORIENTED_EDGE ( 'NONE', *, *, #102901, .F. ) ;
#154989=CARTESIAN_POINT ( 'NONE',  ( 16.46253265017146816, 9.564922557961045513, 21.66775706135233648 ) ) ;
#154990=CARTESIAN_POINT ( 'NONE',  ( 16.46253265017160672, -9.564922557960803928, 38.33224293864768839 ) ) ;
#154991=CARTESIAN_POINT ( 'NONE',  ( -16.46253265017160317, 9.564922557960807481, 110.8322429386476955 ) ) ;
#154992=ORIENTED_EDGE ( 'NONE', *, *, #64542, .F. ) ;
#154993=CARTESIAN_POINT ( 'NONE',  ( -4.483927247898782831, 16.52544592524335698, 32.70942372801900433 ) ) ;
#154994=CARTESIAN_POINT ( 'NONE',  ( -0.05219959533936034679, 19.03943276465977164, 57.50109039468566863 ) ) ;
#154995=CARTESIAN_POINT ( 'NONE',  ( -14.29746914071037622, -8.314922557961029526, 44.16775706135234714 ) ) ;
#154996=CARTESIAN_POINT ( 'NONE',  ( 19.05341960407611168, 5.049401038298154454, 38.95724293864767418 ) ) ;
#154997=CARTESIAN_POINT ( 'NONE',  ( 16.51473224551069308, 9.474510206698969483, 104.1655762719810241 ) ) ;
#154998=CARTESIAN_POINT ( 'NONE',  ( -19.03943276465977164, 0.05219959533909376836, 61.24890960531436690 ) ) ;
#154999=CARTESIAN_POINT ( 'NONE',  ( -15.80617190586745835, -15.72974639402198527, 101.8739096053143811 ) ) ;
#155000=CARTESIAN_POINT ( 'NONE',  ( -9.474510206698964154, 16.51473224551069663, 90.41557627198103830 ) ) ;
#155001=CARTESIAN_POINT ( 'NONE',  ( -16.51473224551069308, -9.474510206698971260, 21.66557627198102765 ) ) ;
#155002=CARTESIAN_POINT ( 'NONE',  ( 13.97604488694527802, 13.89961937509977652, 59.37390960531434558 ) ) ;
#155003=CARTESIAN_POINT ( 'NONE',  ( -0.05219959533910754901, -16.53943276465976808, 22.49890960531436335 ) ) ;
#155005=CARTESIAN_POINT ( 'NONE',  ( 16.51473224551083163, -9.474510206698727899, 100.8344237280190043 ) ) ;
#155006=CARTESIAN_POINT ( 'NONE',  ( 13.97604488694548053, -13.89961937509957401, 25.62609039468566507 ) ) ;
#155007=CARTESIAN_POINT ( 'NONE',  ( 16.53943276465976808, -0.05219959533910856209, 58.74890960531436690 ) ) ;
#155008=CARTESIAN_POINT ( 'NONE',  ( -10.81492255796105439, 18.62759615963255655, 97.91775706135236135 ) ) ;
#155009=CARTESIAN_POINT ( 'NONE',  ( 0.05219959533909260263, 19.03943276465977164, 44.99890960531435979 ) ) ;
#155010=B_SPLINE_CURVE_WITH_KNOTS ( 'NONE', 3,
 ( #180226, #8350, #100348, #134707, #42690, #9361 ),
 .UNSPECIFIED., .F., .F.,
 ( 4, 2, 4 ),
 ( 0.007228050697041582193, 0.007608510107495067287, 0.007988969517948552382 ),
 .UNSPECIFIED. ) ;
#155011=CARTESIAN_POINT ( 'NONE',  ( -12.06949235617756955, 12.14591786802309770, 25.62390960531435624 ) ) ;
#155012=CARTESIAN_POINT ( 'NONE',  ( 18.62759615963255655, 10.81492255796105972, 91.66775706135234714 ) ) ;
#155013=CARTESIAN_POINT ( 'NONE',  ( -9.564922557960796823, -16.46253265017161027, 77.08224293864769550 ) ) ;
#155014=CARTESIAN_POINT ( 'NONE',  ( -0.05219959533909027116, -19.03943276465977164, 97.49890960531436690 ) ) ;
#155015=CARTESIAN_POINT ( 'NONE',  ( 4.483927247898545687, 16.52544592524342804, 104.7905762719810241 ) ) ;
#155016=CARTESIAN_POINT ( 'NONE',  ( -12.06949235617756955, 12.14591786802309770, 75.62390960531439532 ) ) ;
#155017=CARTESIAN_POINT ( 'NONE',  ( -18.67979575497178146, -10.72451020669898902, 81.66557627198103830 ) ) ;
#155018=CARTESIAN_POINT ( 'NONE',  ( -13.97604488694527625, -13.89961937509977652, 76.87390960531433848 ) ) ;
#155019=CARTESIAN_POINT ( 'NONE',  ( 15.72974639402199770, -15.80617190586745480, 83.12390960531436690 ) ) ;
#155020=CARTESIAN_POINT ( 'NONE',  ( 9.564922557961047289, -16.46253265017146816, 80.41775706135234714 ) ) ;
#155021=CARTESIAN_POINT ( 'NONE',  ( 19.02130022317637525, -5.499999999999588773, 48.28188669246576836 ) ) ;
#155022=CARTESIAN_POINT ( 'NONE',  ( 4.379528057220339221, -16.55341960407611168, 92.70724293864770971 ) ) ;
#155023=CARTESIAN_POINT ( 'NONE',  ( 13.97604488694527802, 13.89961937509977652, 59.37390960531434558 ) ) ;
#155024=CARTESIAN_POINT ( 'NONE',  ( 10.72451020669898902, -18.67979575497178502, 62.91557627198102409 ) ) ;
#155026=CARTESIAN_POINT ( 'NONE',  ( 16.55341960407618274, -4.379528057220086978, 111.0427570613523613 ) ) ;
#155028=CARTESIAN_POINT ( 'NONE',  ( 16.55341960407618274, -4.379528057220086978, 26.04275706135235779 ) ) ;
#155030=CARTESIAN_POINT ( 'NONE',  ( 16.55341960407611168, 4.379528057220329451, 78.95724293864769550 ) ) ;
#155032=CARTESIAN_POINT ( 'NONE',  ( 16.46253265017160672, -9.564922557960803928, 73.33224293864769550 ) ) ;
#155033=CARTESIAN_POINT ( 'NONE',  ( -0.05219959533909027116, -19.03943276465977164, 27.49890960531435624 ) ) ;
#155034=CARTESIAN_POINT ( 'NONE',  ( -0.05219959533910754901, -16.53943276465976808, 72.49890960531435269 ) ) ;
#155035=CARTESIAN_POINT ( 'NONE',  ( 16.46253265017160672, -9.564922557960803928, 113.3322429386476955 ) ) ;
#155036=CARTESIAN_POINT ( 'NONE',  ( 0.05219959533936267826, -19.03943276465977164, 95.00109039468567573 ) ) ;
#155037=CARTESIAN_POINT ( 'NONE',  ( 9.474510206698971260, -16.51473224551069308, 72.91557627198102409 ) ) ;
#155038=CARTESIAN_POINT ( 'NONE',  ( -5.049401038298153566, 19.05341960407611168, 85.20724293864766707 ) ) ;
#155039=CARTESIAN_POINT ( 'NONE',  ( 15.72974639402199770, -15.80617190586745480, 78.12390960531436690 ) ) ;
#155040=CARTESIAN_POINT ( 'NONE',  ( -12.06949235617739369, -12.14591786802326823, 74.37609039468568994 ) ) ;
#155041=CARTESIAN_POINT ( 'NONE',  ( 9.474510206698729675, 16.51473224551082808, 112.0844237280190043 ) ) ;
#155042=CARTESIAN_POINT ( 'NONE',  ( -19.02544592524342804, 5.153800228976336051, 56.04057627198100988 ) ) ;
#155043=CARTESIAN_POINT ( 'NONE',  ( -10.72451020669898014, 18.67979575497178502, 70.41557627198102409 ) ) ;
#155044=CARTESIAN_POINT ( 'NONE',  ( -5.049401038297874678, -19.05341960407617918, 99.79275706135234714 ) ) ;
#155045=CARTESIAN_POINT ( 'NONE',  ( 14.29746914071049879, -8.314922557960816363, 33.33224293864769550 ) ) ;
#155046=CARTESIAN_POINT ( 'NONE',  ( 5.719274019375673035, 21.55341960407619339, 52.29275706135236135 ) ) ;
#155048=CARTESIAN_POINT ( 'NONE',  ( -12.06949235617739369, -12.14591786802326823, 74.37609039468568994 ) ) ;
#155049=CARTESIAN_POINT ( 'NONE',  ( 9.564922557960805705, 16.46253265017160317, 109.5822429386476955 ) ) ;
#155051=CARTESIAN_POINT ( 'NONE',  ( 30.00000000000000000, 5.499999999999992895, 102.5000000000000142 ) ) ;
#155052=CARTESIAN_POINT ( 'NONE',  ( 16.52544592524335698, 4.483927247898782831, 96.45942372801901854 ) ) ;
#155053=CARTESIAN_POINT ( 'NONE',  ( -12.06949235617739369, -12.14591786802326823, 44.37609039468567573 ) ) ;
#155054=CARTESIAN_POINT ( 'NONE',  ( -13.89961937509977652, 13.97604488694528158, 65.62390960531436690 ) ) ;
#155055=CARTESIAN_POINT ( 'NONE',  ( -16.51473224551069308, -9.474510206698971260, 71.66557627198102409 ) ) ;
#155056=CARTESIAN_POINT ( 'NONE',  ( 21.53943276465977519, 0.05219959533937863772, 56.25109039468568284 ) ) ;
#155057=CARTESIAN_POINT ( 'NONE',  ( 14.34966873604972726, -8.224510206698740333, 60.83442372801901854 ) ) ;
#155058=CARTESIAN_POINT ( 'NONE',  ( -4.483927247898539470, -16.52544592524342804, 32.29057627198102409 ) ) ;
#155059=CARTESIAN_POINT ( 'NONE',  ( 13.97604488694527802, 13.89961937509977652, 39.37390960531435269 ) ) ;
#155060=CARTESIAN_POINT ( 'NONE',  ( 19.05341960407611168, 5.049401038298154454, 33.95724293864769550 ) ) ;
#155061=CARTESIAN_POINT ( 'NONE',  ( 4.379528057220092307, 16.55341960407617563, 22.29275706135235069 ) ) ;
#155062=CARTESIAN_POINT ( 'NONE',  ( 5.153800228976615827, -19.02544592524334988, 80.20942372801901854 ) ) ;
#155063=CARTESIAN_POINT ( 'NONE',  ( -12.06949235617756955, 12.14591786802309770, 85.62390960531436690 ) ) ;
#155064=CARTESIAN_POINT ( 'NONE',  ( -19.02544592524342804, 5.153800228976336051, 46.04057627198101699 ) ) ;
#155065=CARTESIAN_POINT ( 'NONE',  ( 19.02544592524334988, 5.153800228976608722, 91.45942372801900433 ) ) ;
#155066=LINE ( 'NONE', #16561, #159872 ) ;
#155067=CARTESIAN_POINT ( 'NONE',  ( 10.81492255796106328, -18.62759615963255655, 85.41775706135236135 ) ) ;
#155068=CARTESIAN_POINT ( 'NONE',  ( -14.29746914071037622, -8.314922557961029526, 54.16775706135235424 ) ) ;
#155069=CARTESIAN_POINT ( 'NONE',  ( -17.49999999999999645, 3.209263204892513599, 24.76196825606288598 ) ) ;
#155070=CARTESIAN_POINT ( 'NONE',  ( 18.67979575497178502, 10.72451020669898547, 54.16557627198103120 ) ) ;
#155071=CARTESIAN_POINT ( 'NONE',  ( -14.29746914071037622, -8.314922557961029526, 39.16775706135235424 ) ) ;
#155073=CARTESIAN_POINT ( 'NONE',  ( 19.05341960407617918, -5.049401038297876454, 26.04275706135233293 ) ) ;
#155074=CARTESIAN_POINT ( 'NONE',  ( 13.97604488694527802, 13.89961937509977652, 79.37390960531435269 ) ) ;
#155075=CARTESIAN_POINT ( 'NONE',  ( 5.049401038298161559, -19.05341960407611168, 47.70724293864770260 ) ) ;
#155076=CARTESIAN_POINT ( 'NONE',  ( 30.00000000000000000, -5.204748896376250896E-15, 47.50000000000000000 ) ) ;
#155077=CARTESIAN_POINT ( 'NONE',  ( 13.89961937509977652, -13.97604488694527269, 63.12390960531435979 ) ) ;
#155080=CARTESIAN_POINT ( 'NONE',  ( -9.474510206698720793, -16.51473224551083518, 29.58442372801900433 ) ) ;
#155081=CARTESIAN_POINT ( 'NONE',  ( 21.55341960407619695, -5.719274019375665929, 106.0427570613523471 ) ) ;
#155082=CARTESIAN_POINT ( 'NONE',  ( 14.34966873604960469, 8.224510206698951720, 34.16557627198102409 ) ) ;
#155083=CARTESIAN_POINT ( 'NONE',  ( 19.03943276465977164, -0.05219959533909143690, 43.74890960531435979 ) ) ;
#155084=CARTESIAN_POINT ( 'NONE',  ( -19.03943276465977164, 0.05219959533909376836, 106.2489096053143669 ) ) ;
#155085=CARTESIAN_POINT ( 'NONE',  ( -15.80617190586768217, 15.72974639402176855, 78.12609039468570415 ) ) ;
#155086=CARTESIAN_POINT ( 'NONE',  ( 9.474510206698971260, -16.51473224551069308, 52.91557627198102409 ) ) ;
#155087=CARTESIAN_POINT ( 'NONE',  ( -10.72451020669870658, -18.67979575497194134, 79.58442372801903275 ) ) ;
#155088=CARTESIAN_POINT ( 'NONE',  ( 9.564922557960805705, 16.46253265017160317, 114.5822429386476955 ) ) ;
#155089=CARTESIAN_POINT ( 'NONE',  ( -21.53943276465977519, -0.05219959533937600094, 23.75109039468567929 ) ) ;
#155090=CARTESIAN_POINT ( 'NONE',  ( -13.97604488694547697, 13.89961937509957934, 53.12609039468565442 ) ) ;
#155091=CARTESIAN_POINT ( 'NONE',  ( -19.05341960407611168, -5.049401038298163336, 31.45724293864769550 ) ) ;
#155092=CARTESIAN_POINT ( 'NONE',  ( -13.97604488694527625, -13.89961937509977652, 81.87390960531436690 ) ) ;
#155093=CARTESIAN_POINT ( 'NONE',  ( -12.06949235617739369, -12.14591786802326823, 19.37609039468568639 ) ) ;
#155094=CARTESIAN_POINT ( 'NONE',  ( -12.06949235617756955, 12.14591786802309770, 70.62390960531436690 ) ) ;
#155095=CARTESIAN_POINT ( 'NONE',  ( -15.80617190586745835, -15.72974639402198527, 36.87390960531435979 ) ) ;
#155096=CARTESIAN_POINT ( 'NONE',  ( 9.564922557961047289, -16.46253265017146816, 95.41775706135233293 ) ) ;
#155097=CARTESIAN_POINT ( 'NONE',  ( 10.81492255796078972, 18.62759615963270932, 99.58224293864770971 ) ) ;
#155098=CARTESIAN_POINT ( 'NONE',  ( 21.55341960407619695, -5.719274019375665929, 51.04275706135234714 ) ) ;
#155099=CARTESIAN_POINT ( 'NONE',  ( -12.06949235617739369, -12.14591786802326823, 54.37609039468568994 ) ) ;
#155100=CARTESIAN_POINT ( 'NONE',  ( 16.55341960407618274, -4.379528057220086978, 61.04275706135234714 ) ) ;
#155101=ORIENTED_EDGE ( 'NONE', *, *, #153757, .F. ) ;
#155102=CARTESIAN_POINT ( 'NONE',  ( -5.153800228976328057, -19.02544592524343514, 52.29057627198100988 ) ) ;
#155103=CARTESIAN_POINT ( 'NONE',  ( 16.52544592524335698, 4.483927247898782831, 86.45942372801901854 ) ) ;
#155104=CARTESIAN_POINT ( 'NONE',  ( 18.62759615963271287, -10.81492255796078972, 113.3322429386476955 ) ) ;
#155105=CARTESIAN_POINT ( 'NONE',  ( 12.06949235617757843, -12.14591786802309237, 58.12390960531435979 ) ) ;
#155106=CARTESIAN_POINT ( 'NONE',  ( 19.03943276465977164, -0.05219959533909143690, 88.74890960531436690 ) ) ;
#155107=CARTESIAN_POINT ( 'NONE',  ( 14.29746914071037800, 8.314922557961029526, 71.66775706135234714 ) ) ;
#155108=CARTESIAN_POINT ( 'NONE',  ( -5.823673210054431948, 21.52544592524334988, 57.70942372801901143 ) ) ;
#155109=CARTESIAN_POINT ( 'NONE',  ( -9.564922557961040184, 16.46253265017147172, 107.9177570613523471 ) ) ;
#155110=CARTESIAN_POINT ( 'NONE',  ( -5.823673210054116645, -21.52544592524344225, 112.2905762719810241 ) ) ;
#155111=CARTESIAN_POINT ( 'NONE',  ( 16.52544592524342804, -4.483927247898539470, 43.54057627198103830 ) ) ;
#155113=CARTESIAN_POINT ( 'NONE',  ( -17.40805194822031154, 6.112264579159341515, 75.83371272510613892 ) ) ;
#155114=CARTESIAN_POINT ( 'NONE',  ( -21.55341960407610458, -5.719274019375992779, 81.45724293864769550 ) ) ;
#155115=CARTESIAN_POINT ( 'NONE',  ( -14.29746914071049879, 8.314922557960819915, 25.83224293864769194 ) ) ;
#155117=CARTESIAN_POINT ( 'NONE',  ( 17.50000000000000000, -5.500000000000000888, 120.0000000000000142 ) ) ;
#155118=CARTESIAN_POINT ( 'NONE',  ( -0.05219959533937732626, 21.53943276465977519, 22.50109039468567573 ) ) ;
#155119=CARTESIAN_POINT ( 'NONE',  ( 0.05219959533909260263, 19.03943276465977164, 109.9989096053143669 ) ) ;
#155120=CARTESIAN_POINT ( 'NONE',  ( 15.72974639402176855, 15.80617190586768217, 26.87609039468567218 ) ) ;
#155121=CARTESIAN_POINT ( 'NONE',  ( 16.55341960407611168, 4.379528057220329451, 53.95724293864770260 ) ) ;
#155122=CARTESIAN_POINT ( 'NONE',  ( -4.379528057220086978, -16.55341960407618274, 64.79275706135234714 ) ) ;
#155124=CARTESIAN_POINT ( 'NONE',  ( 13.97604488694527802, 13.89961937509977652, 59.37390960531434558 ) ) ;
#155125=CARTESIAN_POINT ( 'NONE',  ( -19.03943276465977164, -0.05219959533935918106, 63.75109039468566863 ) ) ;
#155126=CARTESIAN_POINT ( 'NONE',  ( -16.51473224551069308, -9.474510206698971260, 86.66557627198102409 ) ) ;
#155127=CARTESIAN_POINT ( 'NONE',  ( 5.719274019375991003, -21.55341960407610458, 32.70724293864770260 ) ) ;
#155129=CARTESIAN_POINT ( 'NONE',  ( 5.049401038298161559, -19.05341960407611168, 57.70724293864769550 ) ) ;
#155130=CARTESIAN_POINT ( 'NONE',  ( 16.55341960407618274, -4.379528057220086978, 26.04275706135235779 ) ) ;
#155131=CARTESIAN_POINT ( 'NONE',  ( 0.05219959533936267826, -19.03943276465977164, 70.00109039468566152 ) ) ;
#155132=CARTESIAN_POINT ( 'NONE',  ( 15.80617190586746368, 15.72974639402197994, 99.37390960531436690 ) ) ;
#155133=CARTESIAN_POINT ( 'NONE',  ( 14.29746914071049879, -8.314922557960816363, 28.33224293864769550 ) ) ;
#155134=CARTESIAN_POINT ( 'NONE',  ( 13.89961937509977652, -13.97604488694527269, 88.12390960531438111 ) ) ;
#155135=CARTESIAN_POINT ( 'NONE',  ( 15.80617190586746368, 15.72974639402197994, 54.37390960531435979 ) ) ;
#155136=CARTESIAN_POINT ( 'NONE',  ( 15.72974639402199770, -15.80617190586745480, 98.12390960531436690 ) ) ;
#155137=CARTESIAN_POINT ( 'NONE',  ( -14.29746914071037622, -8.314922557961029526, 44.16775706135234714 ) ) ;
#155139=CARTESIAN_POINT ( 'NONE',  ( 5.719274019375991003, -21.55341960407610458, 37.70724293864769550 ) ) ;
#155140=CARTESIAN_POINT ( 'NONE',  ( 21.55341960407619695, -5.719274019375665929, 86.04275706135236135 ) ) ;
#155141=CARTESIAN_POINT ( 'NONE',  ( -9.564922557960796823, -16.46253265017161027, 92.08224293864769550 ) ) ;
#155142=CARTESIAN_POINT ( 'NONE',  ( 9.474510206698971260, -16.51473224551069308, 42.91557627198103120 ) ) ;
#155143=CARTESIAN_POINT ( 'NONE',  ( -0.05219959533909027116, -19.03943276465977164, 82.49890960531436690 ) ) ;
#155144=CARTESIAN_POINT ( 'NONE',  ( 12.14591786802309770, 12.06949235617756955, 109.3739096053143811 ) ) ;
#155145=CARTESIAN_POINT ( 'NONE',  ( 19.03943276465977164, -0.05219959533909143690, 63.74890960531435979 ) ) ;
#155146=CARTESIAN_POINT ( 'NONE',  ( 16.46253265017146816, 9.564922557961045513, 111.6677570613523329 ) ) ;
#155147=CARTESIAN_POINT ( 'NONE',  ( 17.48853670773245028, -5.747243402303063853, 86.16671299749992841 ) ) ;
#155148=CARTESIAN_POINT ( 'NONE',  ( 15.80617190586769283, -15.72974639402175789, 95.62609039468568994 ) ) ;
#155149=CARTESIAN_POINT ( 'NONE',  ( 19.02544592524343514, -5.153800228976328945, 108.5405762719810383 ) ) ;
#155150=CARTESIAN_POINT ( 'NONE',  ( 14.29746914071037800, 8.314922557961029526, 96.66775706135234714 ) ) ;
#155151=EDGE_CURVE ( 'NONE', #18983, #167324, #153466, .T. ) ;
#155153=CARTESIAN_POINT ( 'NONE',  ( -5.049401038297874678, -19.05341960407617918, 74.79275706135231871 ) ) ;
#155154=CARTESIAN_POINT ( 'NONE',  ( -9.564922557961040184, 16.46253265017147172, 27.91775706135232582 ) ) ;
#155155=CARTESIAN_POINT ( 'NONE',  ( -17.48853670773242897, -5.747243402303181981, 46.33328700250010712 ) ) ;
#155156=CARTESIAN_POINT ( 'NONE',  ( -0.05219959533909027116, -19.03943276465977164, 32.49890960531435979 ) ) ;
#155157=CARTESIAN_POINT ( 'NONE',  ( -4.483927247898539470, -16.52544592524342804, 42.29057627198103120 ) ) ;
#155158=CARTESIAN_POINT ( 'NONE',  ( -17.26058549869091507, -6.457015423128543929, 111.3774583747606925 ) ) ;
#155159=CARTESIAN_POINT ( 'NONE',  ( 14.29746914071049879, -8.314922557960816363, 33.33224293864769550 ) ) ;
#155160=CARTESIAN_POINT ( 'NONE',  ( -19.52851543214744368, -5.499999999999943157, 85.39357721762581832 ) ) ;
#155161=CARTESIAN_POINT ( 'NONE',  ( 12.14591786802327356, -12.06949235617739191, 90.62609039468567573 ) ) ;
#155162=CARTESIAN_POINT ( 'NONE',  ( 16.46253265017160672, -9.564922557960803928, 43.33224293864769550 ) ) ;
#155163=CARTESIAN_POINT ( 'NONE',  ( -10.72451020669870658, -18.67979575497194134, 94.58442372801901854 ) ) ;
#155164=CARTESIAN_POINT ( 'NONE',  ( 16.46253265017146816, 9.564922557961045513, 111.6677570613523329 ) ) ;
#155165=CARTESIAN_POINT ( 'NONE',  ( 21.55341960407619695, -5.719274019375665929, 81.04275706135236135 ) ) ;
#155166=CARTESIAN_POINT ( 'NONE',  ( -16.46253265017146816, -9.564922557961047289, 59.16775706135233293 ) ) ;
#155167=CARTESIAN_POINT ( 'NONE',  ( 9.474510206698971260, -16.51473224551069308, 87.91557627198102409 ) ) ;
#155168=CARTESIAN_POINT ( 'NONE',  ( 16.51473224551069308, 9.474510206698969483, 69.16557627198102409 ) ) ;
#155169=CARTESIAN_POINT ( 'NONE',  ( 16.52216118717204196, 7.221426719304506747, 73.57599021046989662 ) ) ;
#155170=CARTESIAN_POINT ( 'NONE',  ( -18.62759615963270932, 10.81492255796079327, 90.83224293864769550 ) ) ;
#155171=CARTESIAN_POINT ( 'NONE',  ( -12.14591786802309592, -12.06949235617757132, 71.87390960531438111 ) ) ;
#155172=CARTESIAN_POINT ( 'NONE',  ( -10.81492255796078084, -18.62759615963271287, 67.08224293864770971 ) ) ;
#155173=CARTESIAN_POINT ( 'NONE',  ( 13.89961937509977652, -13.97604488694527269, 58.12390960531436690 ) ) ;
#155174=CARTESIAN_POINT ( 'NONE',  ( 5.823673210054125526, 21.52544592524343514, 79.79057627198102409 ) ) ;
#155175=CARTESIAN_POINT ( 'NONE',  ( -16.53943276465976808, -0.05219959533934237506, 78.75109039468568994 ) ) ;
#155177=CARTESIAN_POINT ( 'NONE',  ( -13.89961937509977652, 13.97604488694528158, 40.62390960531435979 ) ) ;
#155179=CARTESIAN_POINT ( 'NONE',  ( -0.05219959533910754901, -16.53943276465976808, 77.49890960531433848 ) ) ;
#155181=CARTESIAN_POINT ( 'NONE',  ( -0.05219959533909027116, -19.03943276465977164, 52.49890960531436690 ) ) ;
#155182=CARTESIAN_POINT ( 'NONE',  ( 19.05341960407611168, 5.049401038298154454, 23.95724293864769194 ) ) ;
#155183=CARTESIAN_POINT ( 'NONE',  ( 0.05219959533936267826, -19.03943276465977164, 60.00109039468566863 ) ) ;
#155184=CARTESIAN_POINT ( 'NONE',  ( 14.34966873604960469, 8.224510206698951720, 89.16557627198102409 ) ) ;
#155185=CARTESIAN_POINT ( 'NONE',  ( 21.52544592524334988, 5.823673210054432836, 51.45942372801901854 ) ) ;
#155186=CARTESIAN_POINT ( 'NONE',  ( -13.89961937509977652, 13.97604488694528158, 35.62390960531435269 ) ) ;
#155187=CARTESIAN_POINT ( 'NONE',  ( -18.62759615963270932, 10.81492255796079327, 110.8322429386476955 ) ) ;
#155188=CARTESIAN_POINT ( 'NONE',  ( 17.72560187377285601, 5.500000000000007105, 91.57814504131319211 ) ) ;
#155189=CARTESIAN_POINT ( 'NONE',  ( -16.55341960407611168, -4.379528057220339221, 91.45724293864769550 ) ) ;
#155191=CARTESIAN_POINT ( 'NONE',  ( -16.51473224551069308, -9.474510206698971260, 46.66557627198102409 ) ) ;
#155193=CARTESIAN_POINT ( 'NONE',  ( 13.89961937509957401, 13.97604488694547697, 96.87609039468566152 ) ) ;
#155194=CARTESIAN_POINT ( 'NONE',  ( -13.89961937509977652, 13.97604488694528158, 105.6239096053143527 ) ) ;
#155195=CARTESIAN_POINT ( 'NONE',  ( 0.05219959533937995610, -21.53943276465977519, 40.00109039468567573 ) ) ;
#155196=CARTESIAN_POINT ( 'NONE',  ( 5.153800228976335163, 19.02544592524342804, 89.79057627198102409 ) ) ;
#155197=CARTESIAN_POINT ( 'NONE',  ( -19.02544592524334988, -5.153800228976617603, 63.95942372801899012 ) ) ;
#155198=CARTESIAN_POINT ( 'NONE',  ( -0.05219959533909027116, -19.03943276465977164, 42.49890960531435269 ) ) ;
#155199=CARTESIAN_POINT ( 'NONE',  ( -16.53943276465976808, 0.05219959533911058130, 71.24890960531435269 ) ) ;
#155200=CARTESIAN_POINT ( 'NONE',  ( -8.224510206698948167, 14.34966873604960824, 70.41557627198102409 ) ) ;
#155201=CARTESIAN_POINT ( 'NONE',  ( -19.03943276465977164, 0.05219959533909376836, 81.24890960531436690 ) ) ;
#155202=CARTESIAN_POINT ( 'NONE',  ( 10.81492255796078972, 18.62759615963270932, 94.58224293864769550 ) ) ;
#155203=CARTESIAN_POINT ( 'NONE',  ( -16.51473224551069308, -9.474510206698971260, 66.66557627198102409 ) ) ;
#155204=CARTESIAN_POINT ( 'NONE',  ( -21.55341960407619339, 5.719274019375674811, 108.5427570613523756 ) ) ;
#155205=CARTESIAN_POINT ( 'NONE',  ( -5.153800228976328057, -19.02544592524343514, 37.29057627198102409 ) ) ;
#155206=CARTESIAN_POINT ( 'NONE',  ( 4.483927247898545687, 16.52544592524342804, 29.79057627198102409 ) ) ;
#155207=CARTESIAN_POINT ( 'NONE',  ( 4.483927247898545687, 16.52544592524342804, 109.7905762719810383 ) ) ;
#155208=CARTESIAN_POINT ( 'NONE',  ( -5.049401038297874678, -19.05341960407617918, 109.7927570613523187 ) ) ;
#155209=ORIENTED_EDGE ( 'NONE', *, *, #199317, .F. ) ;
#155210=CARTESIAN_POINT ( 'NONE',  ( 10.72451020669871369, 18.67979575497193778, 27.08442372801901854 ) ) ;
#155211=CARTESIAN_POINT ( 'NONE',  ( -0.05219959533936034679, 19.03943276465977164, 67.50109039468566152 ) ) ;
#155212=CARTESIAN_POINT ( 'NONE',  ( 12.06949235617757843, -12.14591786802309237, 23.12390960531436335 ) ) ;
#155213=CARTESIAN_POINT ( 'NONE',  ( -10.81492255796078084, -18.62759615963271287, 82.08224293864768129 ) ) ;
#155214=CARTESIAN_POINT ( 'NONE',  ( 5.153800228976335163, 19.02544592524342804, 109.7905762719810099 ) ) ;
#155215=CARTESIAN_POINT ( 'NONE',  ( 14.29746914071049879, -8.314922557960816363, 58.33224293864768839 ) ) ;
#155216=CARTESIAN_POINT ( 'NONE',  ( -5.153800228976328057, -19.02544592524343514, 32.29057627198102409 ) ) ;
#155217=CARTESIAN_POINT ( 'NONE',  ( 19.02544592524334988, 5.153800228976608722, 21.45942372801899012 ) ) ;
#155218=CARTESIAN_POINT ( 'NONE',  ( -4.379528057220086978, -16.55341960407618274, 84.79275706135234714 ) ) ;
#155219=CARTESIAN_POINT ( 'NONE',  ( -4.483927247898782831, 16.52544592524335698, 52.70942372801902565 ) ) ;
#155220=CARTESIAN_POINT ( 'NONE',  ( -21.53943276465977519, 0.05219959533907696930, 26.24890960531435624 ) ) ;
#155221=CARTESIAN_POINT ( 'NONE',  ( 18.67979575497194134, -10.72451020669871369, 105.8344237280190328 ) ) ;
#155222=CARTESIAN_POINT ( 'NONE',  ( -16.46253265017160317, 9.564922557960807481, 75.83224293864769550 ) ) ;
#155223=CARTESIAN_POINT ( 'NONE',  ( -14.29746914071037622, -8.314922557961029526, 54.16775706135235424 ) ) ;
#155224=CARTESIAN_POINT ( 'NONE',  ( -5.153800228976328057, -19.02544592524343514, 22.29057627198102765 ) ) ;
#155225=CARTESIAN_POINT ( 'NONE',  ( -8.314922557960811034, -14.29746914071050412, 37.08224293864768129 ) ) ;
#155226=CARTESIAN_POINT ( 'NONE',  ( -17.49999999999999645, 5.499999999999985789, 38.71769037696434879 ) ) ;
#155227=CARTESIAN_POINT ( 'NONE',  ( 10.72451020669871369, 18.67979575497193778, 72.08442372801899012 ) ) ;
#155228=CARTESIAN_POINT ( 'NONE',  ( 5.049401038298161559, -19.05341960407611168, 87.70724293864769550 ) ) ;
#155229=CARTESIAN_POINT ( 'NONE',  ( 16.46253265017160672, -9.564922557960803928, 73.33224293864769550 ) ) ;
#155230=CARTESIAN_POINT ( 'NONE',  ( 5.049401038298161559, -19.05341960407611168, 107.7072429386476955 ) ) ;
#155231=CARTESIAN_POINT ( 'NONE',  ( 16.52544592524342804, -4.483927247898539470, 58.54057627198103120 ) ) ;
#155232=CARTESIAN_POINT ( 'NONE',  ( 4.483927247898545687, 16.52544592524342804, 29.79057627198102409 ) ) ;
#155234=CARTESIAN_POINT ( 'NONE',  ( 8.314922557960818139, 14.29746914071049879, 54.58224293864769550 ) ) ;
#155235=CARTESIAN_POINT ( 'NONE',  ( 16.52544592524335698, 4.483927247898782831, 36.45942372801901143 ) ) ;
#155237=CARTESIAN_POINT ( 'NONE',  ( 0.05219959533936267826, -19.03943276465977164, 45.00109039468566863 ) ) ;
#155238=CARTESIAN_POINT ( 'NONE',  ( 5.153800228976335163, 19.02544592524342804, 69.79057627198103830 ) ) ;
#155239=CARTESIAN_POINT ( 'NONE',  ( -16.51473224551082808, 9.474510206698731452, 58.33442372801900433 ) ) ;
#155240=CARTESIAN_POINT ( 'NONE',  ( -9.564922557961040184, 16.46253265017147172, 62.91775706135233293 ) ) ;
#155241=CARTESIAN_POINT ( 'NONE',  ( -16.46253265017146816, -9.564922557961047289, 94.16775706135233293 ) ) ;
#155242=CARTESIAN_POINT ( 'NONE',  ( 0.05219959533934541429, -16.53943276465976808, 85.00109039468568994 ) ) ;
#155244=CARTESIAN_POINT ( 'NONE',  ( 0.05219959533909260263, 19.03943276465977164, 29.99890960531435979 ) ) ;
#155245=CARTESIAN_POINT ( 'NONE',  ( 16.46253265017160672, -9.564922557960803928, 103.3322429386476955 ) ) ;
#155246=CARTESIAN_POINT ( 'NONE',  ( 10.72451020669871369, 18.67979575497193778, 37.08442372801901143 ) ) ;
#155247=CARTESIAN_POINT ( 'NONE',  ( -19.02544592524334988, -5.153800228976617603, 93.95942372801900433 ) ) ;
#155248=CARTESIAN_POINT ( 'NONE',  ( 15.50000000000000178, 0.000000000000000000, 118.0000000000000142 ) ) ;
#155249=CARTESIAN_POINT ( 'NONE',  ( 16.51473224551069308, 9.474510206698969483, 64.16557627198102409 ) ) ;
#155250=CARTESIAN_POINT ( 'NONE',  ( 5.153800228976335163, 19.02544592524342804, 104.7905762719809957 ) ) ;
#155251=CARTESIAN_POINT ( 'NONE',  ( -14.34966873604960291, -8.224510206698953496, 56.66557627198103830 ) ) ;
#155252=CARTESIAN_POINT ( 'NONE',  ( 16.46253265017160672, -9.564922557960803928, 68.33224293864770971 ) ) ;
#155253=CARTESIAN_POINT ( 'NONE',  ( 19.02544592524343514, -5.153800228976328945, 63.54057627198103830 ) ) ;
#155254=CARTESIAN_POINT ( 'NONE',  ( -16.51473224551082808, 9.474510206698731452, 63.33442372801900433 ) ) ;
#155255=CARTESIAN_POINT ( 'NONE',  ( 5.719274019375991003, -21.55341960407610458, 57.70724293864770260 ) ) ;
#155256=CARTESIAN_POINT ( 'NONE',  ( 5.153800228976615827, -19.02544592524334988, 40.20942372801898301 ) ) ;
#155257=CARTESIAN_POINT ( 'NONE',  ( -19.05341960407611168, -5.049401038298163336, 76.45724293864769550 ) ) ;
#155258=CARTESIAN_POINT ( 'NONE',  ( -18.62759615963270932, 10.81492255796079327, 75.83224293864769550 ) ) ;
#155259=CARTESIAN_POINT ( 'NONE',  ( -12.06949235617756955, 12.14591786802309770, 85.62390960531436690 ) ) ;
#155260=CARTESIAN_POINT ( 'NONE',  ( 19.02544592524334988, 5.153800228976608722, 31.45942372801900433 ) ) ;
#155261=CARTESIAN_POINT ( 'NONE',  ( -21.52544592524343514, 5.823673210054127303, 41.04057627198103120 ) ) ;
#155262=CARTESIAN_POINT ( 'NONE',  ( -21.53943276465977519, 0.05219959533907696930, 41.24890960531435269 ) ) ;
#155263=CARTESIAN_POINT ( 'NONE',  ( -16.51473224551069308, -9.474510206698971260, 66.66557627198102409 ) ) ;
#155264=CARTESIAN_POINT ( 'NONE',  ( -5.153800228976328057, -19.02544592524343514, 52.29057627198100988 ) ) ;
#155265=CARTESIAN_POINT ( 'NONE',  ( -4.379528057220328563, 16.55341960407611168, 115.2072429386476955 ) ) ;
#155266=CARTESIAN_POINT ( 'NONE',  ( 0.05219959533937995610, -21.53943276465977519, 25.00109039468567218 ) ) ;
#155269=CARTESIAN_POINT ( 'NONE',  ( -18.62759615963255300, -10.81492255796106328, 24.16775706135235424 ) ) ;
#155270=CARTESIAN_POINT ( 'NONE',  ( -19.05341960407611168, -5.049401038298163336, 31.45724293864769550 ) ) ;
#155271=CARTESIAN_POINT ( 'NONE',  ( -5.719274019375978568, 21.55341960407610458, 110.2072429386477239 ) ) ;
#155272=CARTESIAN_POINT ( 'NONE',  ( -19.02544592524334988, -5.153800228976617603, 43.95942372801899012 ) ) ;
#155273=CARTESIAN_POINT ( 'NONE',  ( 19.02544592524343514, -5.153800228976328945, 28.54057627198102409 ) ) ;
#155274=CARTESIAN_POINT ( 'NONE',  ( 13.97604488694527802, 13.89961937509977652, 24.37390960531435624 ) ) ;
#155275=CARTESIAN_POINT ( 'NONE',  ( 17.37577197770832527, -5.499999999999936939, 21.30611277022550354 ) ) ;
#155276=CARTESIAN_POINT ( 'NONE',  ( -16.53943276465976808, -0.05219959533934237506, 53.75109039468568994 ) ) ;
#155277=CARTESIAN_POINT ( 'NONE',  ( 16.46253265017160672, -9.564922557960803928, 28.33224293864769550 ) ) ;
#155279=CARTESIAN_POINT ( 'NONE',  ( -13.97604488694527625, -13.89961937509977652, 66.87390960531436690 ) ) ;
#155280=CARTESIAN_POINT ( 'NONE',  ( 14.34966873604960469, 8.224510206698951720, 109.1655762719810383 ) ) ;
#155281=CARTESIAN_POINT ( 'NONE',  ( 5.719274019375991003, -21.55341960407610458, 62.70724293864769550 ) ) ;
#155282=CARTESIAN_POINT ( 'NONE',  ( 14.34966873604960469, 8.224510206698951720, 74.16557627198102409 ) ) ;
#155283=CARTESIAN_POINT ( 'NONE',  ( 16.55341960407618274, -4.379528057220086978, 31.04275706135234714 ) ) ;
#155284=CARTESIAN_POINT ( 'NONE',  ( 10.72451020669871369, 18.67979575497193778, 92.08442372801901854 ) ) ;
#155285=CARTESIAN_POINT ( 'NONE',  ( -5.153800228976328057, -19.02544592524343514, 32.29057627198102409 ) ) ;
#155286=CARTESIAN_POINT ( 'NONE',  ( -4.483927247898539470, -16.52544592524342804, 22.29057627198102765 ) ) ;
#155287=CARTESIAN_POINT ( 'NONE',  ( -8.314922557960811034, -14.29746914071050412, 52.08224293864768839 ) ) ;
#155288=CARTESIAN_POINT ( 'NONE',  ( 19.02544592524343514, -5.153800228976328945, 53.54057627198102409 ) ) ;
#155289=CARTESIAN_POINT ( 'NONE',  ( 5.719274019375673035, 21.55341960407619339, 92.29275706135236135 ) ) ;
#155290=CARTESIAN_POINT ( 'NONE',  ( -0.05219959533907301413, -21.53943276465977519, 102.4989096053143811 ) ) ;
#155291=CARTESIAN_POINT ( 'NONE',  ( 15.72974639402176855, 15.80617190586768217, 66.87609039468568994 ) ) ;
#155292=CARTESIAN_POINT ( 'NONE',  ( 12.14591786802327356, -12.06949235617739191, 50.62609039468568994 ) ) ;
#155293=CARTESIAN_POINT ( 'NONE',  ( 12.14591786802309770, 12.06949235617756955, 84.37390960531438111 ) ) ;
#155294=CARTESIAN_POINT ( 'NONE',  ( 21.53943276465977519, 0.05219959533937863772, 91.25109039468568994 ) ) ;
#155295=CARTESIAN_POINT ( 'NONE',  ( -16.55341960407617563, 4.379528057220093196, 113.5427570613523756 ) ) ;
#155297=CARTESIAN_POINT ( 'NONE',  ( -4.379528057220086978, -16.55341960407618274, 44.79275706135234714 ) ) ;
#155298=CARTESIAN_POINT ( 'NONE',  ( -16.55341960407611168, -4.379528057220339221, 36.45724293864768839 ) ) ;
#155299=CARTESIAN_POINT ( 'NONE',  ( -16.53943276465976808, -0.05219959533934237506, 88.75109039468567573 ) ) ;
#155300=CARTESIAN_POINT ( 'NONE',  ( -19.05341960407611168, -5.049401038298163336, 101.4572429386476955 ) ) ;
#155301=CARTESIAN_POINT ( 'NONE',  ( 16.46253265017160672, -9.564922557960803928, 113.3322429386476955 ) ) ;
#155302=CARTESIAN_POINT ( 'NONE',  ( 15.80617190586769283, -15.72974639402175789, 95.62609039468568994 ) ) ;
#155303=EDGE_CURVE ( 'NONE', #27205, #63497, #7731, .T. ) ;
#155304=CARTESIAN_POINT ( 'NONE',  ( 14.34966873604972726, -8.224510206698740333, 105.8344237280190328 ) ) ;
#155305=CARTESIAN_POINT ( 'NONE',  ( 4.379528057220339221, -16.55341960407611168, 77.70724293864770971 ) ) ;
#155306=CARTESIAN_POINT ( 'NONE',  ( -5.049401038298153566, 19.05341960407611168, 75.20724293864769550 ) ) ;
#155307=EDGE_LOOP ( 'NONE', ( #83600, #130587, #58800, #193769 ) ) ;
#155308=CARTESIAN_POINT ( 'NONE',  ( -12.06949235617739369, -12.14591786802326823, 29.37609039468568284 ) ) ;
#155309=CARTESIAN_POINT ( 'NONE',  ( -9.564922557960796823, -16.46253265017161027, 27.08224293864769550 ) ) ;
#155310=CARTESIAN_POINT ( 'NONE',  ( 9.564922557960805705, 16.46253265017160317, 89.58224293864769550 ) ) ;
#155311=CARTESIAN_POINT ( 'NONE',  ( 8.314922557961029526, -14.29746914071037800, 35.41775706135234003 ) ) ;
#155312=CARTESIAN_POINT ( 'NONE',  ( 18.22780087662121673, 5.500000000000056843, 68.98459894673892734 ) ) ;
#155313=CARTESIAN_POINT ( 'NONE',  ( 0.05219959533936267826, -19.03943276465977164, 40.00109039468566152 ) ) ;
#155314=CARTESIAN_POINT ( 'NONE',  ( -4.483927247898782831, 16.52544592524335698, 87.70942372801901854 ) ) ;
#155315=CARTESIAN_POINT ( 'NONE',  ( 5.049401038297881783, 19.05341960407617563, 102.2927570613523045 ) ) ;
#155316=CARTESIAN_POINT ( 'NONE',  ( 9.474510206698971260, -16.51473224551069308, 37.91557627198102409 ) ) ;
#155317=CARTESIAN_POINT ( 'NONE',  ( -16.53943276465976808, -0.05219959533934237506, 73.75109039468567573 ) ) ;
#155318=CARTESIAN_POINT ( 'NONE',  ( -16.55341960407617563, 4.379528057220093196, 63.54275706135234003 ) ) ;
#155319=CARTESIAN_POINT ( 'NONE',  ( 5.049401038297881783, 19.05341960407617563, 82.29275706135229029 ) ) ;
#155320=CARTESIAN_POINT ( 'NONE',  ( 0.05219959533937995610, -21.53943276465977519, 110.0010903946856757 ) ) ;
#155321=CARTESIAN_POINT ( 'NONE',  ( -9.564922557960796823, -16.46253265017161027, 42.08224293864769550 ) ) ;
#155323=CARTESIAN_POINT ( 'NONE',  ( -9.474510206698964154, 16.51473224551069663, 95.41557627198102409 ) ) ;
#155324=CARTESIAN_POINT ( 'NONE',  ( -8.224510206698948167, 14.34966873604960824, 90.41557627198103830 ) ) ;
#155325=CARTESIAN_POINT ( 'NONE',  ( 13.97604488694548053, -13.89961937509957401, 55.62609039468566863 ) ) ;
#155326=CARTESIAN_POINT ( 'NONE',  ( -5.823673210054116645, -21.52544592524344225, 52.29057627198102409 ) ) ;
#155327=CARTESIAN_POINT ( 'NONE',  ( 5.153800228976615827, -19.02544592524334988, 25.20942372801900433 ) ) ;
#155328=CARTESIAN_POINT ( 'NONE',  ( 19.02544592524343514, -5.153800228976328945, 88.54057627198102409 ) ) ;
#155329=CARTESIAN_POINT ( 'NONE',  ( 5.049401038297881783, 19.05341960407617563, 27.29275706135232937 ) ) ;
#155330=CARTESIAN_POINT ( 'NONE',  ( -18.62759615963270932, 10.81492255796079327, 80.83224293864769550 ) ) ;
#155331=CARTESIAN_POINT ( 'NONE',  ( 19.03943276465977164, -0.05219959533909143690, 108.7489096053143527 ) ) ;
#155332=CARTESIAN_POINT ( 'NONE',  ( 5.049401038297881783, 19.05341960407617563, 82.29275706135229029 ) ) ;
#155333=CARTESIAN_POINT ( 'NONE',  ( -19.05341960407611168, -5.049401038298163336, 111.4572429386476671 ) ) ;
#155334=CARTESIAN_POINT ( 'NONE',  ( 0.05219959533934541429, -16.53943276465976808, 20.00109039468568639 ) ) ;
#155335=CARTESIAN_POINT ( 'NONE',  ( -9.474510206698964154, 16.51473224551069663, 30.41557627198102054 ) ) ;
#155336=CARTESIAN_POINT ( 'NONE',  ( 19.02544592524343514, -5.153800228976328945, 93.54057627198102409 ) ) ;
#155337=CARTESIAN_POINT ( 'NONE',  ( -18.67979575497178146, -10.72451020669898902, 71.66557627198100988 ) ) ;
#155338=CARTESIAN_POINT ( 'NONE',  ( -4.483927247898782831, 16.52544592524335698, 52.70942372801902565 ) ) ;
#155339=CARTESIAN_POINT ( 'NONE',  ( -0.05219959533937732626, 21.53943276465977519, 47.50109039468568994 ) ) ;
#155340=CARTESIAN_POINT ( 'NONE',  ( 16.46253265017146816, 9.564922557961045513, 91.66775706135234714 ) ) ;
#155341=CARTESIAN_POINT ( 'NONE',  ( 10.72451020669871369, 18.67979575497193778, 102.0844237280190185 ) ) ;
#155342=CARTESIAN_POINT ( 'NONE',  ( 16.52544592524335698, 4.483927247898782831, 96.45942372801901854 ) ) ;
#155343=CARTESIAN_POINT ( 'NONE',  ( -19.05341960407611168, -5.049401038298163336, 106.4572429386476955 ) ) ;
#155344=CARTESIAN_POINT ( 'NONE',  ( 14.34966873604960469, 8.224510206698951720, 94.16557627198103830 ) ) ;
#155345=CARTESIAN_POINT ( 'NONE',  ( 12.06949235617757843, -12.14591786802309237, 33.12390960531435979 ) ) ;
#155346=CARTESIAN_POINT ( 'NONE',  ( -9.474510206698720793, -16.51473224551083518, 74.58442372801900433 ) ) ;
#155347=CARTESIAN_POINT ( 'NONE',  ( -21.55341960407619339, 5.719274019375674811, 63.54275706135234003 ) ) ;
#155348=CARTESIAN_POINT ( 'NONE',  ( 13.97604488694548053, -13.89961937509957401, 30.62609039468566863 ) ) ;
#155349=CARTESIAN_POINT ( 'NONE',  ( -12.14591786802309592, -12.06949235617757132, 101.8739096053143811 ) ) ;
#155350=CARTESIAN_POINT ( 'NONE',  ( -0.05219959533907301413, -21.53943276465977519, 32.49890960531435979 ) ) ;
#155351=CARTESIAN_POINT ( 'NONE',  ( -12.14591786802326823, 12.06949235617739902, 113.1260903946856899 ) ) ;
#155352=CARTESIAN_POINT ( 'NONE',  ( -21.55341960407619339, 5.719274019375674811, 98.54275706135234714 ) ) ;
#155353=CARTESIAN_POINT ( 'NONE',  ( -16.55341960407617563, 4.379528057220093196, 58.54275706135235424 ) ) ;
#155354=CARTESIAN_POINT ( 'NONE',  ( 14.34966873604960469, 8.224510206698951720, 24.16557627198103120 ) ) ;
#155355=CARTESIAN_POINT ( 'NONE',  ( 21.53943276465977519, 0.05219959533937863772, 46.25109039468567573 ) ) ;
#155356=CARTESIAN_POINT ( 'NONE',  ( 18.62759615963255655, 10.81492255796105972, 56.66775706135235424 ) ) ;
#155358=CARTESIAN_POINT ( 'NONE',  ( -5.719274019375665041, -21.55341960407619695, 34.79275706135235424 ) ) ;
#155359=CARTESIAN_POINT ( 'NONE',  ( 4.483927247898545687, 16.52544592524342804, 99.79057627198103830 ) ) ;
#155360=CARTESIAN_POINT ( 'NONE',  ( -5.049401038298153566, 19.05341960407611168, 25.20724293864768484 ) ) ;
#155361=CARTESIAN_POINT ( 'NONE',  ( 8.314922557960818139, 14.29746914071049879, 74.58224293864768129 ) ) ;
#155362=CARTESIAN_POINT ( 'NONE',  ( 9.564922557960805705, 16.46253265017160317, 74.58224293864769550 ) ) ;
#155363=CARTESIAN_POINT ( 'NONE',  ( 16.53943276465976808, 0.05219959533934440121, 111.2510903946856899 ) ) ;
#155364=CARTESIAN_POINT ( 'NONE',  ( -10.72451020669898014, 18.67979575497178502, 60.41557627198102409 ) ) ;
#155365=CARTESIAN_POINT ( 'NONE',  ( 14.34966873604960469, 8.224510206698951720, 94.16557627198103830 ) ) ;
#155366=CARTESIAN_POINT ( 'NONE',  ( 10.72451020669898902, -18.67979575497178502, 87.91557627198103830 ) ) ;
#155367=CARTESIAN_POINT ( 'NONE',  ( -9.564922557960796823, -16.46253265017161027, 97.08224293864769550 ) ) ;
#155368=CARTESIAN_POINT ( 'NONE',  ( -19.02544592524342804, 5.153800228976336051, 51.04057627198103120 ) ) ;
#155369=CARTESIAN_POINT ( 'NONE',  ( 19.05341960407617918, -5.049401038297876454, 106.0427570613523471 ) ) ;
#155370=CARTESIAN_POINT ( 'NONE',  ( 21.55341960407610458, 5.719274019375980345, 48.95724293864770971 ) ) ;
#155371=CARTESIAN_POINT ( 'NONE',  ( -18.62759615963255300, -10.81492255796106328, 69.16775706135234714 ) ) ;
#155372=CARTESIAN_POINT ( 'NONE',  ( -9.564922557960796823, -16.46253265017161027, 62.08224293864769550 ) ) ;
#155373=CARTESIAN_POINT ( 'NONE',  ( 9.474510206698971260, -16.51473224551069308, 102.9155762719810241 ) ) ;
#155374=CARTESIAN_POINT ( 'NONE',  ( 12.14591786802327356, -12.06949235617739191, 60.62609039468567573 ) ) ;
#155375=CARTESIAN_POINT ( 'NONE',  ( -15.72974639402176322, -15.80617190586768395, 59.37609039468568284 ) ) ;
#155376=CARTESIAN_POINT ( 'NONE',  ( 10.72451020669871369, 18.67979575497193778, 92.08442372801901854 ) ) ;
#155377=CARTESIAN_POINT ( 'NONE',  ( 21.52544592524344225, -5.823673210054117533, 93.54057627198103830 ) ) ;
#155378=CARTESIAN_POINT ( 'NONE',  ( 15.80617190586769283, -15.72974639402175789, 35.62609039468568994 ) ) ;
#155379=CARTESIAN_POINT ( 'NONE',  ( -8.314922557961024197, 14.29746914071037800, 72.91775706135234714 ) ) ;
#155380=CARTESIAN_POINT ( 'NONE',  ( 15.72974639402199770, -15.80617190586745480, 83.12390960531436690 ) ) ;
#155381=CARTESIAN_POINT ( 'NONE',  ( -19.02544592524334988, -5.153800228976617603, 38.95942372801900433 ) ) ;
#155382=CARTESIAN_POINT ( 'NONE',  ( -9.474510206698964154, 16.51473224551069663, 85.41557627198102409 ) ) ;
#155383=CARTESIAN_POINT ( 'NONE',  ( -14.34966873604960291, -8.224510206698953496, 26.66557627198103475 ) ) ;
#155385=CARTESIAN_POINT ( 'NONE',  ( 13.97604488694527802, 13.89961937509977652, 104.3739096053143385 ) ) ;
#155386=CARTESIAN_POINT ( 'NONE',  ( -9.474510206698720793, -16.51473224551083518, 99.58442372801900433 ) ) ;
#155387=CARTESIAN_POINT ( 'NONE',  ( -10.81492255796078084, -18.62759615963271287, 77.08224293864769550 ) ) ;
#155388=CARTESIAN_POINT ( 'NONE',  ( -16.55341960407611168, -4.379528057220339221, 36.45724293864768839 ) ) ;
#155389=CARTESIAN_POINT ( 'NONE',  ( -8.224510206698735004, -14.34966873604973081, 19.58442372801901143 ) ) ;
#155390=CARTESIAN_POINT ( 'NONE',  ( 13.97604488694527802, 13.89961937509977652, 29.37390960531435979 ) ) ;
#155391=CARTESIAN_POINT ( 'NONE',  ( 16.51473224551083163, -9.474510206698727899, 110.8344237280190043 ) ) ;
#155392=CARTESIAN_POINT ( 'NONE',  ( 15.80617190586746368, 15.72974639402197994, 99.37390960531436690 ) ) ;
#155393=CARTESIAN_POINT ( 'NONE',  ( 13.97604488694548053, -13.89961937509957401, 70.62609039468567573 ) ) ;
#155394=CARTESIAN_POINT ( 'NONE',  ( 12.06949235617739724, 12.14591786802326823, 86.87609039468568994 ) ) ;
#155395=CARTESIAN_POINT ( 'NONE',  ( 13.89961937509977652, -13.97604488694527269, 68.12390960531436690 ) ) ;
#155396=CARTESIAN_POINT ( 'NONE',  ( -14.29746914071049879, 8.314922557960819915, 75.83224293864769550 ) ) ;
#155397=CARTESIAN_POINT ( 'NONE',  ( -5.049401038298153566, 19.05341960407611168, 65.20724293864765286 ) ) ;
#155398=CARTESIAN_POINT ( 'NONE',  ( -16.55341960407611168, -4.379528057220339221, 66.45724293864768129 ) ) ;
#155399=CARTESIAN_POINT ( 'NONE',  ( -13.89961937509977652, 13.97604488694528158, 25.62390960531434558 ) ) ;
#155401=CARTESIAN_POINT ( 'NONE',  ( 14.29746914071049879, -8.314922557960816363, 48.33224293864770260 ) ) ;
#155402=CARTESIAN_POINT ( 'NONE',  ( -5.049401038298153566, 19.05341960407611168, 80.20724293864769550 ) ) ;
#155404=CARTESIAN_POINT ( 'NONE',  ( -19.05341960407617563, 5.049401038297882671, 53.54275706135231871 ) ) ;
#155405=CARTESIAN_POINT ( 'NONE',  ( 4.483927247898790824, -16.52544592524335698, 55.20942372801902565 ) ) ;
#155406=CARTESIAN_POINT ( 'NONE',  ( 18.67979575497178502, 10.72451020669898547, 69.16557627198102409 ) ) ;
#155407=CARTESIAN_POINT ( 'NONE',  ( -19.05341960407617563, 5.049401038297882671, 28.54275706135232937 ) ) ;
#155408=CARTESIAN_POINT ( 'NONE',  ( -13.89961937509977652, 13.97604488694528158, 75.62390960531438111 ) ) ;
#155410=CARTESIAN_POINT ( 'NONE',  ( 9.564922557960805705, 16.46253265017160317, 109.5822429386476955 ) ) ;
#155411=CARTESIAN_POINT ( 'NONE',  ( -16.51473224551069308, -9.474510206698971260, 56.66557627198103120 ) ) ;
#155412=CARTESIAN_POINT ( 'NONE',  ( -15.80617190586768217, 15.72974639402176855, 33.12609039468569705 ) ) ;
#155413=CARTESIAN_POINT ( 'NONE',  ( -14.29746914071049879, 8.314922557960819915, 110.8322429386476955 ) ) ;
#155414=CARTESIAN_POINT ( 'NONE',  ( -15.72974639402197994, 15.80617190586746368, 105.6239096053143669 ) ) ;
#155415=CARTESIAN_POINT ( 'NONE',  ( -19.05341960407611168, -5.049401038298163336, 96.45724293864769550 ) ) ;
#155417=CARTESIAN_POINT ( 'NONE',  ( 5.823673210054444382, -21.52544592524334988, 20.20942372801900788 ) ) ;
#155419=CARTESIAN_POINT ( 'NONE',  ( 19.02544592524343514, -5.153800228976328945, 93.54057627198102409 ) ) ;
#155420=CARTESIAN_POINT ( 'NONE',  ( 0.000000000000000000, 5.499999999999998224, 118.0000000000000142 ) ) ;
#155421=CARTESIAN_POINT ( 'NONE',  ( 18.67979575497178502, 10.72451020669898547, 99.16557627198100988 ) ) ;
#155422=CARTESIAN_POINT ( 'NONE',  ( -5.049401038298153566, 19.05341960407611168, 50.20724293864770260 ) ) ;
#155423=CARTESIAN_POINT ( 'NONE',  ( -0.05219959533936034679, 19.03943276465977164, 102.5010903946856757 ) ) ;
#155425=CARTESIAN_POINT ( 'NONE',  ( 16.51473224551069308, 9.474510206698969483, 29.16557627198103475 ) ) ;
#155426=CARTESIAN_POINT ( 'NONE',  ( -21.53943276465977519, -0.05219959533937600094, 88.75109039468567573 ) ) ;
#155427=CARTESIAN_POINT ( 'NONE',  ( 16.51473224551069308, 9.474510206698969483, 79.16557627198103830 ) ) ;
#155428=CARTESIAN_POINT ( 'NONE',  ( -18.67979575497193778, 10.72451020669871902, 43.33442372801901143 ) ) ;
#155429=CARTESIAN_POINT ( 'NONE',  ( -0.05219959533937732626, 21.53943276465977519, 22.50109039468567573 ) ) ;
#155431=CARTESIAN_POINT ( 'NONE',  ( 19.05341960407611168, 5.049401038298154454, 103.9572429386476671 ) ) ;
#155433=CARTESIAN_POINT ( 'NONE',  ( -4.379528057220086978, -16.55341960407618274, 44.79275706135234714 ) ) ;
#155434=CARTESIAN_POINT ( 'NONE',  ( -15.80617190586745835, -15.72974639402198527, 46.87390960531435979 ) ) ;
#155435=CARTESIAN_POINT ( 'NONE',  ( 10.81492255796106328, -18.62759615963255655, 40.41775706135234714 ) ) ;
#155436=CARTESIAN_POINT ( 'NONE',  ( -21.53943276465977519, -0.05219959533937600094, 73.75109039468567573 ) ) ;
#155438=CARTESIAN_POINT ( 'NONE',  ( -9.564922557961040184, 16.46253265017147172, 112.9177570613523329 ) ) ;
#155439=CARTESIAN_POINT ( 'NONE',  ( -19.03943276465977164, 0.05219959533909376836, 66.24890960531436690 ) ) ;
#155440=CARTESIAN_POINT ( 'NONE',  ( 9.474510206698971260, -16.51473224551069308, 92.91557627198103830 ) ) ;
#155441=CARTESIAN_POINT ( 'NONE',  ( -8.314922557960811034, -14.29746914071050412, 107.0822429386476955 ) ) ;
#155442=CARTESIAN_POINT ( 'NONE',  ( 14.29746914071049879, -8.314922557960816363, 108.3322429386477097 ) ) ;
#155443=CARTESIAN_POINT ( 'NONE',  ( -5.719274019375978568, 21.55341960407610458, 30.20724293864769550 ) ) ;
#155444=CARTESIAN_POINT ( 'NONE',  ( 14.29746914071037800, 8.314922557961029526, 81.66775706135236135 ) ) ;
#155445=CARTESIAN_POINT ( 'NONE',  ( -4.379528057220328563, 16.55341960407611168, 65.20724293864768129 ) ) ;
#155446=CARTESIAN_POINT ( 'NONE',  ( 16.51473224551069308, 9.474510206698969483, 49.16557627198102409 ) ) ;
#155447=CARTESIAN_POINT ( 'NONE',  ( 18.67979575497194134, -10.72451020669871369, 70.83442372801901854 ) ) ;
#155448=CARTESIAN_POINT ( 'NONE',  ( 10.72451020669871369, 18.67979575497193778, 77.08442372801901854 ) ) ;
#155449=CARTESIAN_POINT ( 'NONE',  ( 13.89961937509957401, 13.97604488694547697, 101.8760903946856331 ) ) ;
#155450=CARTESIAN_POINT ( 'NONE',  ( 0.05219959533910956823, 16.53943276465976808, 59.99890960531436690 ) ) ;
#155451=CARTESIAN_POINT ( 'NONE',  ( 21.53943276465977519, 0.05219959533937863772, 26.25109039468567573 ) ) ;
#155452=CARTESIAN_POINT ( 'NONE',  ( 18.67979575497178502, 10.72451020669898547, 54.16557627198103120 ) ) ;
#155453=CARTESIAN_POINT ( 'NONE',  ( 18.39639308325437383, 5.500000000000037303, 73.98252246182197212 ) ) ;
#155455=CARTESIAN_POINT ( 'NONE',  ( 19.05341960407611168, 5.049401038298154454, 63.95724293864769550 ) ) ;
#155456=CARTESIAN_POINT ( 'NONE',  ( -16.53943276465976808, 0.05219959533911058130, 31.24890960531435979 ) ) ;
#155457=CARTESIAN_POINT ( 'NONE',  ( -12.14591786802309592, -12.06949235617757132, 21.87390960531436690 ) ) ;
#155458=CARTESIAN_POINT ( 'NONE',  ( -8.224510206698735004, -14.34966873604973081, 94.58442372801901854 ) ) ;
#155459=CARTESIAN_POINT ( 'NONE',  ( 19.05341960407617918, -5.049401038297876454, 51.04275706135231871 ) ) ;
#155461=CARTESIAN_POINT ( 'NONE',  ( -9.564922557960796823, -16.46253265017161027, 102.0822429386477097 ) ) ;
#155462=CARTESIAN_POINT ( 'NONE',  ( 8.224510206698953496, -14.34966873604960469, 72.91557627198103830 ) ) ;
#155463=CARTESIAN_POINT ( 'NONE',  ( -5.049401038297874678, -19.05341960407617918, 39.79275706135232582 ) ) ;
#155464=CARTESIAN_POINT ( 'NONE',  ( -9.564922557960796823, -16.46253265017161027, 32.08224293864769550 ) ) ;
#155465=CARTESIAN_POINT ( 'NONE',  ( -5.823673210054116645, -21.52544592524344225, 27.29057627198103120 ) ) ;
#155466=CARTESIAN_POINT ( 'NONE',  ( -10.81492255796078084, -18.62759615963271287, 52.08224293864768839 ) ) ;
#155467=CARTESIAN_POINT ( 'NONE',  ( -14.29746914071049879, 8.314922557960819915, 100.8322429386477097 ) ) ;
#155468=CARTESIAN_POINT ( 'NONE',  ( -12.14591786802326823, 12.06949235617739902, 48.12609039468568284 ) ) ;
#155469=CARTESIAN_POINT ( 'NONE',  ( -4.483927247898539470, -16.52544592524342804, 87.29057627198103830 ) ) ;
#155471=CARTESIAN_POINT ( 'NONE',  ( -16.81555441253551919, 7.025013491695482948, 50.63685445334259327 ) ) ;
#155472=CARTESIAN_POINT ( 'NONE',  ( -16.51473224551069308, -9.474510206698971260, 111.6655762719810383 ) ) ;
#155475=CARTESIAN_POINT ( 'NONE',  ( 16.52544592524335698, 4.483927247898782831, 46.45942372801901854 ) ) ;
#155476=CARTESIAN_POINT ( 'NONE',  ( -8.224510206698948167, 14.34966873604960824, 25.41557627198103120 ) ) ;
#155477=CARTESIAN_POINT ( 'NONE',  ( -21.52544592524343514, 5.823673210054127303, 51.04057627198103120 ) ) ;
#155478=CARTESIAN_POINT ( 'NONE',  ( 19.02544592524334988, 5.153800228976608722, 86.45942372801900433 ) ) ;
#155479=CARTESIAN_POINT ( 'NONE',  ( -18.67979575497178146, -10.72451020669898902, 46.66557627198102409 ) ) ;
#155480=CARTESIAN_POINT ( 'NONE',  ( -18.67979575497193778, 10.72451020669871902, 88.33442372801901854 ) ) ;
#155482=CARTESIAN_POINT ( 'NONE',  ( 12.06949235617739724, 12.14591786802326823, 51.87609039468568284 ) ) ;
#155483=CARTESIAN_POINT ( 'NONE',  ( -19.05341960407611168, -5.049401038298163336, 41.45724293864769550 ) ) ;
#155484=CARTESIAN_POINT ( 'NONE',  ( -0.05219959533909027116, -19.03943276465977164, 107.4989096053143527 ) ) ;
#155485=CARTESIAN_POINT ( 'NONE',  ( 13.89961937509977652, -13.97604488694527269, 33.12390960531434558 ) ) ;
#155486=CARTESIAN_POINT ( 'NONE',  ( -16.52544592524342804, 4.483927247898546575, 106.0405762719810525 ) ) ;
#155488=CARTESIAN_POINT ( 'NONE',  ( -9.474510206698964154, 16.51473224551069663, 95.41557627198102409 ) ) ;
#155490=CARTESIAN_POINT ( 'NONE',  ( 16.53943276465976808, 0.05219959533934440121, 56.25109039468568284 ) ) ;
#155491=CARTESIAN_POINT ( 'NONE',  ( -10.72451020669898014, 18.67979575497178502, 95.41557627198102409 ) ) ;
#155492=CARTESIAN_POINT ( 'NONE',  ( 9.474510206698971260, -16.51473224551069308, 52.91557627198102409 ) ) ;
#155493=CARTESIAN_POINT ( 'NONE',  ( 15.80617190586769283, -15.72974639402175789, 30.62609039468567929 ) ) ;
#155494=CARTESIAN_POINT ( 'NONE',  ( 9.564922557960805705, 16.46253265017160317, 89.58224293864769550 ) ) ;
#155496=ORIENTED_EDGE ( 'NONE', *, *, #146462, .F. ) ;
#155497=CARTESIAN_POINT ( 'NONE',  ( 10.72451020669898902, -18.67979575497178502, 112.9155762719810383 ) ) ;
#155498=CARTESIAN_POINT ( 'NONE',  ( -16.52544592524342804, 4.483927247898546575, 116.0405762719810383 ) ) ;
#155499=CARTESIAN_POINT ( 'NONE',  ( 19.02544592524343514, -5.153800228976328945, 103.5405762719809957 ) ) ;
#155500=CARTESIAN_POINT ( 'NONE',  ( 9.474510206698729675, 16.51473224551082808, 77.08442372801900433 ) ) ;
#155501=CARTESIAN_POINT ( 'NONE',  ( -9.474510206698720793, -16.51473224551083518, 29.58442372801900433 ) ) ;
#155502=CARTESIAN_POINT ( 'NONE',  ( 18.67979575497178502, 10.72451020669898547, 99.16557627198100988 ) ) ;
#155503=CARTESIAN_POINT ( 'NONE',  ( -16.51473224551082808, 9.474510206698731452, 33.33442372801899722 ) ) ;
#155504=CARTESIAN_POINT ( 'NONE',  ( 12.06949235617739724, 12.14591786802326823, 76.87609039468567573 ) ) ;
#155505=CARTESIAN_POINT ( 'NONE',  ( -16.46253265017160317, 9.564922557960807481, 100.8322429386477097 ) ) ;
#155506=CARTESIAN_POINT ( 'NONE',  ( 19.03943276465977164, -0.05219959533909143690, 63.74890960531435979 ) ) ;
#155507=CARTESIAN_POINT ( 'NONE',  ( 18.62759615963255655, 10.81492255796105972, 71.66775706135234714 ) ) ;
#155508=CARTESIAN_POINT ( 'NONE',  ( -21.52544592524334988, -5.823673210054445271, 83.95942372801900433 ) ) ;
#155509=CARTESIAN_POINT ( 'NONE',  ( 16.51473224551069308, 9.474510206698969483, 74.16557627198103830 ) ) ;
#155510=CARTESIAN_POINT ( 'NONE',  ( 0.05219959533937995610, -21.53943276465977519, 55.00109039468568284 ) ) ;
#155511=CARTESIAN_POINT ( 'NONE',  ( 16.51473224551083163, -9.474510206698727899, 90.83442372801900433 ) ) ;
#155512=CARTESIAN_POINT ( 'NONE',  ( -0.05219959533909027116, -19.03943276465977164, 57.49890960531435979 ) ) ;
#155513=CARTESIAN_POINT ( 'NONE',  ( 19.03943276465977164, -0.05219959533909143690, 98.74890960531436690 ) ) ;
#155514=CARTESIAN_POINT ( 'NONE',  ( 9.564922557960805705, 16.46253265017160317, 59.58224293864769550 ) ) ;
#155515=CARTESIAN_POINT ( 'NONE',  ( -19.03943276465977164, 0.05219959533909376836, 116.2489096053143669 ) ) ;
#155516=CARTESIAN_POINT ( 'NONE',  ( 19.02544592524343514, -5.153800228976328945, 53.54057627198102409 ) ) ;
#155517=CARTESIAN_POINT ( 'NONE',  ( 5.719274019375991003, -21.55341960407610458, 97.70724293864772392 ) ) ;
#155518=CARTESIAN_POINT ( 'NONE',  ( -16.55341960407617563, 4.379528057220093196, 73.54275706135234714 ) ) ;
#155520=CARTESIAN_POINT ( 'NONE',  ( 0.05219959533936267826, -19.03943276465977164, 50.00109039468566863 ) ) ;
#155521=CARTESIAN_POINT ( 'NONE',  ( -16.51473224551069308, -9.474510206698971260, 66.66557627198102409 ) ) ;
#155522=CARTESIAN_POINT ( 'NONE',  ( 8.224510206698953496, -14.34966873604960469, 52.91557627198103830 ) ) ;
#155523=CARTESIAN_POINT ( 'NONE',  ( -8.314922557960811034, -14.29746914071050412, 97.08224293864770971 ) ) ;
#155524=CARTESIAN_POINT ( 'NONE',  ( -19.02544592524342804, 5.153800228976336051, 106.0405762719810241 ) ) ;
#155525=CARTESIAN_POINT ( 'NONE',  ( 13.97604488694527802, 13.89961937509977652, 94.37390960531436690 ) ) ;
#155526=CARTESIAN_POINT ( 'NONE',  ( 19.05341960407611168, 5.049401038298154454, 108.9572429386477097 ) ) ;
#155527=CARTESIAN_POINT ( 'NONE',  ( -21.55341960407619339, 5.719274019375674811, 113.5427570613523756 ) ) ;
#155528=CARTESIAN_POINT ( 'NONE',  ( 12.14591786802327356, -12.06949235617739191, 95.62609039468568994 ) ) ;
#155529=CARTESIAN_POINT ( 'NONE',  ( 18.62759615963255655, 10.81492255796105972, 41.66775706135235424 ) ) ;
#155530=CARTESIAN_POINT ( 'NONE',  ( 5.719274019375991003, -21.55341960407610458, 32.70724293864770260 ) ) ;
#155531=CARTESIAN_POINT ( 'NONE',  ( -21.55341960407610458, -5.719274019375992779, 101.4572429386476955 ) ) ;
#155532=CARTESIAN_POINT ( 'NONE',  ( -16.52544592524342804, 4.483927247898546575, 56.04057627198102409 ) ) ;
#155533=CARTESIAN_POINT ( 'NONE',  ( 19.03943276465977164, -0.05219959533909143690, 53.74890960531436690 ) ) ;
#155534=CARTESIAN_POINT ( 'NONE',  ( -4.483927247898539470, -16.52544592524342804, 77.29057627198102409 ) ) ;
#155535=CARTESIAN_POINT ( 'NONE',  ( -9.564922557961040184, 16.46253265017147172, 42.91775706135234003 ) ) ;
#155537=CARTESIAN_POINT ( 'NONE',  ( 19.03943276465977164, -0.05219959533909143690, 23.74890960531435269 ) ) ;
#155539=CARTESIAN_POINT ( 'NONE',  ( 8.314922557961029526, -14.29746914071037800, 65.41775706135234714 ) ) ;
#155540=CARTESIAN_POINT ( 'NONE',  ( -16.46253265017160317, 9.564922557960807481, 70.83224293864770971 ) ) ;
#155542=CARTESIAN_POINT ( 'NONE',  ( 14.34966873604960469, 8.224510206698951720, 89.16557627198102409 ) ) ;
#155543=CARTESIAN_POINT ( 'NONE',  ( 15.72974639402199770, -15.80617190586745480, 43.12390960531435269 ) ) ;
#155544=ORIENTED_EDGE ( 'NONE', *, *, #109403, .F. ) ;
#155545=CARTESIAN_POINT ( 'NONE',  ( -0.05219959533934338120, 16.53943276465976808, 112.5010903946857042 ) ) ;
#155546=CARTESIAN_POINT ( 'NONE',  ( 16.53943276465976808, 0.05219959533934440121, 26.25109039468567573 ) ) ;
#155547=CARTESIAN_POINT ( 'NONE',  ( 21.55341960407619695, -5.719274019375665929, 91.04275706135236135 ) ) ;
#155548=CARTESIAN_POINT ( 'NONE',  ( 0.05219959533909260263, 19.03943276465977164, 89.99890960531436690 ) ) ;
#155549=CARTESIAN_POINT ( 'NONE',  ( 0.05219959533907565091, 21.53943276465977519, 114.9989096053143669 ) ) ;
#155550=CARTESIAN_POINT ( 'NONE',  ( -16.46253265017160317, 9.564922557960807481, 30.83224293864769550 ) ) ;
#155551=CARTESIAN_POINT ( 'NONE',  ( 12.14591786802327356, -12.06949235617739191, 35.62609039468568994 ) ) ;
#155552=CARTESIAN_POINT ( 'NONE',  ( -5.049401038297874678, -19.05341960407617918, 89.79275706135230450 ) ) ;
#155553=CARTESIAN_POINT ( 'NONE',  ( 18.62759615963271287, -10.81492255796078972, 88.33224293864769550 ) ) ;
#155554=CARTESIAN_POINT ( 'NONE',  ( -13.97604488694547697, 13.89961937509957934, 68.12609039468563310 ) ) ;
#155555=CARTESIAN_POINT ( 'NONE',  ( 16.51473224551069308, 9.474510206698969483, 24.16557627198102765 ) ) ;
#155556=CARTESIAN_POINT ( 'NONE',  ( -21.52544592524343514, 5.823673210054127303, 116.0405762719810383 ) ) ;
#155558=CARTESIAN_POINT ( 'NONE',  ( 9.564922557960805705, 16.46253265017160317, 79.58224293864769550 ) ) ;
#155559=CARTESIAN_POINT ( 'NONE',  ( 14.34966873604972726, -8.224510206698740333, 30.83442372801902209 ) ) ;
#155561=CARTESIAN_POINT ( 'NONE',  ( 9.564922557961047289, -16.46253265017146816, 60.41775706135233293 ) ) ;
#155562=CARTESIAN_POINT ( 'NONE',  ( 21.52544592524344225, -5.823673210054117533, 113.5405762719810383 ) ) ;
#155563=CARTESIAN_POINT ( 'NONE',  ( 12.14591786802309770, 12.06949235617756955, 79.37390960531436690 ) ) ;
#155564=CARTESIAN_POINT ( 'NONE',  ( -19.03943276465977164, 0.05219959533909376836, 81.24890960531436690 ) ) ;
#155565=CARTESIAN_POINT ( 'NONE',  ( 16.55341960407618274, -4.379528057220086978, 36.04275706135234714 ) ) ;
#155566=CARTESIAN_POINT ( 'NONE',  ( 9.474510206698729675, 16.51473224551082808, 42.08442372801900433 ) ) ;
#155567=CARTESIAN_POINT ( 'NONE',  ( -0.05219959533937732626, 21.53943276465977519, 67.50109039468568994 ) ) ;
#155568=CARTESIAN_POINT ( 'NONE',  ( -8.224510206698735004, -14.34966873604973081, 19.58442372801901143 ) ) ;
#155569=CARTESIAN_POINT ( 'NONE',  ( -13.97604488694527625, -13.89961937509977652, 61.87390960531435979 ) ) ;
#155570=CARTESIAN_POINT ( 'NONE',  ( 9.474510206698729675, 16.51473224551082808, 77.08442372801900433 ) ) ;
#155571=CARTESIAN_POINT ( 'NONE',  ( 14.34966873604972726, -8.224510206698740333, 50.83442372801901143 ) ) ;
#155572=CARTESIAN_POINT ( 'NONE',  ( -15.72974639402176322, -15.80617190586768395, 99.37609039468568994 ) ) ;
#155573=CARTESIAN_POINT ( 'NONE',  ( 9.474510206698729675, 16.51473224551082808, 72.08442372801900433 ) ) ;
#155574=CARTESIAN_POINT ( 'NONE',  ( -0.05219959533909027116, -19.03943276465977164, 52.49890960531436690 ) ) ;
#155575=CARTESIAN_POINT ( 'NONE',  ( 5.719274019375991003, -21.55341960407610458, 67.70724293864769550 ) ) ;
#155576=CARTESIAN_POINT ( 'NONE',  ( -8.314922557960811034, -14.29746914071050412, 62.08224293864769550 ) ) ;
#155577=CARTESIAN_POINT ( 'NONE',  ( -19.02544592524334988, -5.153800228976617603, 63.95942372801899012 ) ) ;
#155578=CARTESIAN_POINT ( 'NONE',  ( -19.39720447994790575, -5.500000000000073719, 69.66317477297171479 ) ) ;
#155579=CARTESIAN_POINT ( 'NONE',  ( -19.05341960407617563, 5.049401038297882671, 43.54275706135232582 ) ) ;
#155580=CARTESIAN_POINT ( 'NONE',  ( -4.483927247898782831, 16.52544592524335698, 97.70942372801904696 ) ) ;
#155581=CARTESIAN_POINT ( 'NONE',  ( 8.314922557960818139, 14.29746914071049879, 64.58224293864769550 ) ) ;
#155582=CARTESIAN_POINT ( 'NONE',  ( -5.719274019375665041, -21.55341960407619695, 99.79275706135234714 ) ) ;
#155584=CARTESIAN_POINT ( 'NONE',  ( 18.67979575497178502, 10.72451020669898547, 94.16557627198103830 ) ) ;
#155585=CARTESIAN_POINT ( 'NONE',  ( -9.474510206698964154, 16.51473224551069663, 70.41557627198102409 ) ) ;
#155586=CARTESIAN_POINT ( 'NONE',  ( 18.67979575497194134, -10.72451020669871369, 75.83442372801900433 ) ) ;
#155587=CARTESIAN_POINT ( 'NONE',  ( 9.564922557960805705, 16.46253265017160317, 44.58224293864769550 ) ) ;
#155589=CARTESIAN_POINT ( 'NONE',  ( 13.97604488694527802, 13.89961937509977652, 69.37390960531436690 ) ) ;
#155590=CARTESIAN_POINT ( 'NONE',  ( 19.02544592524343514, -5.153800228976328945, 28.54057627198102409 ) ) ;
#155591=CARTESIAN_POINT ( 'NONE',  ( -5.153800228976328057, -19.02544592524343514, 107.2905762719810383 ) ) ;
#155592=CARTESIAN_POINT ( 'NONE',  ( 8.314922557960818139, 14.29746914071049879, 69.58224293864769550 ) ) ;
#155593=CARTESIAN_POINT ( 'NONE',  ( -16.46253265017160317, 9.564922557960807481, 35.83224293864768839 ) ) ;
#155594=CARTESIAN_POINT ( 'NONE',  ( 12.14591786802309770, 12.06949235617756955, 84.37390960531438111 ) ) ;
#155595=CARTESIAN_POINT ( 'NONE',  ( 0.05219959533907565091, 21.53943276465977519, 94.99890960531436690 ) ) ;
#155596=CARTESIAN_POINT ( 'NONE',  ( 21.55341960407619695, -5.719274019375665929, 41.04275706135236135 ) ) ;
#155598=CARTESIAN_POINT ( 'NONE',  ( 12.06949235617739724, 12.14591786802326823, 46.87609039468568994 ) ) ;
#155599=CARTESIAN_POINT ( 'NONE',  ( -21.55341960407610458, -5.719274019375992779, 86.45724293864770971 ) ) ;
#155600=CARTESIAN_POINT ( 'NONE',  ( -5.153800228976607833, 19.02544592524334988, 27.70942372801899722 ) ) ;
#155601=CARTESIAN_POINT ( 'NONE',  ( -5.049401038298153566, 19.05341960407611168, 100.2072429386476955 ) ) ;
#155602=CARTESIAN_POINT ( 'NONE',  ( -18.67979575497193778, 10.72451020669871902, 38.33442372801900433 ) ) ;
#155603=CARTESIAN_POINT ( 'NONE',  ( -10.81492255796078084, -18.62759615963271287, 42.08224293864769550 ) ) ;
#155604=CARTESIAN_POINT ( 'NONE',  ( 14.34966873604960469, 8.224510206698951720, 24.16557627198103120 ) ) ;
#155606=CARTESIAN_POINT ( 'NONE',  ( 15.72974639402176855, 15.80617190586768217, 66.87609039468568994 ) ) ;
#155607=CARTESIAN_POINT ( 'NONE',  ( 5.823673210054444382, -21.52544592524334988, 100.2094237280190043 ) ) ;
#155608=CARTESIAN_POINT ( 'NONE',  ( 5.153800228976615827, -19.02544592524334988, 30.20942372801900433 ) ) ;
#155609=CARTESIAN_POINT ( 'NONE',  ( 12.14591786802327356, -12.06949235617739191, 85.62609039468568994 ) ) ;
#155610=CARTESIAN_POINT ( 'NONE',  ( -5.823673210054431948, 21.52544592524334988, 47.70942372801902565 ) ) ;
#155611=CARTESIAN_POINT ( 'NONE',  ( 13.97604488694527802, 13.89961937509977652, 49.37390960531434558 ) ) ;
#155612=CARTESIAN_POINT ( 'NONE',  ( -5.049401038297874678, -19.05341960407617918, 24.79275706135233648 ) ) ;
#155613=CARTESIAN_POINT ( 'NONE',  ( 15.80617190586746368, 15.72974639402197994, 24.37390960531435979 ) ) ;
#155614=CARTESIAN_POINT ( 'NONE',  ( -21.52544592524343514, 5.823673210054127303, 116.0405762719810383 ) ) ;
#155615=CARTESIAN_POINT ( 'NONE',  ( 21.53943276465977519, -0.05219959533907433946, 73.74890960531433848 ) ) ;
#155616=CARTESIAN_POINT ( 'NONE',  ( -16.52544592524335698, -4.483927247898792601, 38.95942372801901854 ) ) ;
#155618=CARTESIAN_POINT ( 'NONE',  ( -18.62759615963270932, 10.81492255796079327, 80.83224293864769550 ) ) ;
#155619=CARTESIAN_POINT ( 'NONE',  ( 16.52544592524335698, 4.483927247898782831, 61.45942372801901854 ) ) ;
#155620=CARTESIAN_POINT ( 'NONE',  ( 14.34966873604960469, 8.224510206698951720, 69.16557627198102409 ) ) ;
#155622=CARTESIAN_POINT ( 'NONE',  ( 19.05341960407617918, -5.049401038297876454, 86.04275706135233293 ) ) ;
#155624=CARTESIAN_POINT ( 'NONE',  ( 16.53943276465976808, 0.05219959533934440121, 46.25109039468567573 ) ) ;
#155625=CARTESIAN_POINT ( 'NONE',  ( -21.55341960407610458, -5.719274019375992779, 111.4572429386476813 ) ) ;
#155626=CARTESIAN_POINT ( 'NONE',  ( -5.823673210054116645, -21.52544592524344225, 72.29057627198102409 ) ) ;
#155627=CARTESIAN_POINT ( 'NONE',  ( -18.67979575497178146, -10.72451020669898902, 31.66557627198102054 ) ) ;
#155628=CARTESIAN_POINT ( 'NONE',  ( -4.483927247898782831, 16.52544592524335698, 57.70942372801901143 ) ) ;
#155629=CARTESIAN_POINT ( 'NONE',  ( -0.05219959533909027116, -19.03943276465977164, 67.49890960531436690 ) ) ;
#155630=CARTESIAN_POINT ( 'NONE',  ( 15.72974639402176855, 15.80617190586768217, 46.87609039468568994 ) ) ;
#155631=CARTESIAN_POINT ( 'NONE',  ( 8.314922557961029526, -14.29746914071037800, 20.41775706135234714 ) ) ;
#155632=CARTESIAN_POINT ( 'NONE',  ( -19.03943276465977164, 0.05219959533909376836, 106.2489096053143669 ) ) ;
#155633=CARTESIAN_POINT ( 'NONE',  ( 5.153800228976615827, -19.02544592524334988, 25.20942372801900433 ) ) ;
#155635=CARTESIAN_POINT ( 'NONE',  ( -8.224510206698735004, -14.34966873604973081, 39.58442372801901143 ) ) ;
#155636=CARTESIAN_POINT ( 'NONE',  ( 13.97604488694527802, 13.89961937509977652, 99.37390960531436690 ) ) ;
#155637=CARTESIAN_POINT ( 'NONE',  ( 21.55341960407610458, 5.719274019375980345, 108.9572429386476955 ) ) ;
#155638=CARTESIAN_POINT ( 'NONE',  ( -5.049401038298153566, 19.05341960407611168, 60.20724293864768129 ) ) ;
#155640=CARTESIAN_POINT ( 'NONE',  ( 16.55341960407611168, 4.379528057220329451, 78.95724293864769550 ) ) ;
#155641=CARTESIAN_POINT ( 'NONE',  ( -15.80617190586745835, -15.72974639402198527, 21.87390960531436690 ) ) ;
#155642=CARTESIAN_POINT ( 'NONE',  ( -16.51473224551069308, -9.474510206698971260, 21.66557627198102765 ) ) ;
#155643=CARTESIAN_POINT ( 'NONE',  ( -15.72974639402197994, 15.80617190586746368, 100.6239096053143811 ) ) ;
#155644=CARTESIAN_POINT ( 'NONE',  ( -13.89961937509957401, -13.97604488694547875, 59.37609039468566863 ) ) ;
#155645=CARTESIAN_POINT ( 'NONE',  ( 21.52544592524344225, -5.823673210054117533, 28.54057627198103120 ) ) ;
#155646=CARTESIAN_POINT ( 'NONE',  ( 5.049401038298161559, -19.05341960407611168, 27.70724293864769550 ) ) ;
#155647=CARTESIAN_POINT ( 'NONE',  ( -21.52544592524343514, 5.823673210054127303, 66.04057627198103830 ) ) ;
#155648=CARTESIAN_POINT ( 'NONE',  ( -9.474510206698964154, 16.51473224551069663, 100.4155762719810241 ) ) ;
#155649=CARTESIAN_POINT ( 'NONE',  ( 21.52544592524334988, 5.823673210054432836, 86.45942372801901854 ) ) ;
#155650=CARTESIAN_POINT ( 'NONE',  ( 19.03943276465977164, -0.05219959533909143690, 48.74890960531435979 ) ) ;
#155651=CARTESIAN_POINT ( 'NONE',  ( 14.29746914071049879, -8.314922557960816363, 88.33224293864769550 ) ) ;
#155652=CARTESIAN_POINT ( 'NONE',  ( 12.14591786802327356, -12.06949235617739191, 30.62609039468567929 ) ) ;
#155653=CARTESIAN_POINT ( 'NONE',  ( -13.89961937509977652, 13.97604488694528158, 55.62390960531434558 ) ) ;
#155654=CARTESIAN_POINT ( 'NONE',  ( -10.81492255796105439, 18.62759615963255655, 72.91775706135234714 ) ) ;
#155656=CARTESIAN_POINT ( 'NONE',  ( 13.97604488694548053, -13.89961937509957401, 25.62609039468566507 ) ) ;
#155657=CARTESIAN_POINT ( 'NONE',  ( 5.153800228976615827, -19.02544592524334988, 45.20942372801901143 ) ) ;
#155658=CARTESIAN_POINT ( 'NONE',  ( 18.67979575497194134, -10.72451020669871369, 30.83442372801902209 ) ) ;
#155660=CARTESIAN_POINT ( 'NONE',  ( 19.02544592524334988, 5.153800228976608722, 36.45942372801900433 ) ) ;
#155661=CARTESIAN_POINT ( 'NONE',  ( 13.89961937509977652, -13.97604488694527269, 88.12390960531438111 ) ) ;
#155662=CARTESIAN_POINT ( 'NONE',  ( 19.05341960407611168, 5.049401038298154454, 73.95724293864768129 ) ) ;
#155663=CARTESIAN_POINT ( 'NONE',  ( 12.14591786802309770, 12.06949235617756955, 29.37390960531435269 ) ) ;
#155664=CARTESIAN_POINT ( 'NONE',  ( 15.80617190586746368, 15.72974639402197994, 24.37390960531435979 ) ) ;
#155665=CARTESIAN_POINT ( 'NONE',  ( 18.62759615963255655, 10.81492255796105972, 81.66775706135236135 ) ) ;
#155667=CARTESIAN_POINT ( 'NONE',  ( 17.50000000000000000, 5.622605283950888655, 58.81207310596111881 ) ) ;
#155668=CARTESIAN_POINT ( 'NONE',  ( -21.55341960407619339, 5.719274019375674811, 78.54275706135236135 ) ) ;
#155669=CARTESIAN_POINT ( 'NONE',  ( 16.19135201231362586, -7.376712067592065658, 42.31319145947967542 ) ) ;
#155670=CARTESIAN_POINT ( 'NONE',  ( -19.02544592524342804, 5.153800228976336051, 96.04057627198103830 ) ) ;
#155673=CARTESIAN_POINT ( 'NONE',  ( -21.52544592524343514, 5.823673210054127303, 66.04057627198103830 ) ) ;
#155674=CARTESIAN_POINT ( 'NONE',  ( -14.34966873604960291, -8.224510206698953496, 31.66557627198102054 ) ) ;
#155675=CARTESIAN_POINT ( 'NONE',  ( -12.06949235617756955, 12.14591786802309770, 115.6239096053143669 ) ) ;
#155676=CARTESIAN_POINT ( 'NONE',  ( 9.474510206698971260, -16.51473224551069308, 92.91557627198103830 ) ) ;
#155677=CARTESIAN_POINT ( 'NONE',  ( -0.05219959533937732626, 21.53943276465977519, 112.5010903946857042 ) ) ;
#155678=CARTESIAN_POINT ( 'NONE',  ( 9.474510206698971260, -16.51473224551069308, 22.91557627198102765 ) ) ;
#155679=CARTESIAN_POINT ( 'NONE',  ( -10.81492255796105439, 18.62759615963255655, 62.91775706135236135 ) ) ;
#155680=CARTESIAN_POINT ( 'NONE',  ( -9.564922557960796823, -16.46253265017161027, 97.08224293864769550 ) ) ;
#155681=CARTESIAN_POINT ( 'NONE',  ( -12.06949235617739369, -12.14591786802326823, 109.3760903946857042 ) ) ;
#155682=CARTESIAN_POINT ( 'NONE',  ( -19.02544592524334988, -5.153800228976617603, 68.95942372801896170 ) ) ;
#155684=CARTESIAN_POINT ( 'NONE',  ( 0.05219959533909260263, 19.03943276465977164, 114.9989096053143669 ) ) ;
#155685=CARTESIAN_POINT ( 'NONE',  ( -8.314922557960811034, -14.29746914071050412, 87.08224293864769550 ) ) ;
#155686=CARTESIAN_POINT ( 'NONE',  ( -5.049401038297874678, -19.05341960407617918, 64.79275706135233293 ) ) ;
#155687=CARTESIAN_POINT ( 'NONE',  ( -19.05341960407611168, -5.049401038298163336, 81.45724293864769550 ) ) ;
#155688=CARTESIAN_POINT ( 'NONE',  ( 14.29746914071049879, -8.314922557960816363, 63.33224293864770260 ) ) ;
#155689=CARTESIAN_POINT ( 'NONE',  ( -16.46253265017146816, -9.564922557961047289, 94.16775706135233293 ) ) ;
#155690=CARTESIAN_POINT ( 'NONE',  ( -10.72451020669898014, 18.67979575497178502, 55.41557627198102409 ) ) ;
#155692=CARTESIAN_POINT ( 'NONE',  ( -16.51473224551069308, -9.474510206698971260, 21.66557627198102765 ) ) ;
#155693=CARTESIAN_POINT ( 'NONE',  ( -17.49999999999999645, -5.624438216177606975, 29.18329655085356578 ) ) ;
#155694=CARTESIAN_POINT ( 'NONE',  ( 13.89961937509977652, -13.97604488694527269, 73.12390960531436690 ) ) ;
#155695=CARTESIAN_POINT ( 'NONE',  ( 18.67979575497178502, 10.72451020669898547, 79.16557627198103830 ) ) ;
#155696=CARTESIAN_POINT ( 'NONE',  ( -4.483927247898782831, 16.52544592524335698, 87.70942372801901854 ) ) ;
#155697=CARTESIAN_POINT ( 'NONE',  ( -5.049401038298153566, 19.05341960407611168, 80.20724293864769550 ) ) ;
#155698=CARTESIAN_POINT ( 'NONE',  ( 5.049401038297881783, 19.05341960407617563, 52.29275706135234003 ) ) ;
#155699=CARTESIAN_POINT ( 'NONE',  ( -18.67979575497193778, 10.72451020669871902, 88.33442372801901854 ) ) ;
#155700=CARTESIAN_POINT ( 'NONE',  ( -0.05219959533907301413, -21.53943276465977519, 62.49890960531436690 ) ) ;
#155701=CARTESIAN_POINT ( 'NONE',  ( 18.67979575497178502, 10.72451020669898547, 24.16557627198103120 ) ) ;
#155702=CARTESIAN_POINT ( 'NONE',  ( -9.564922557960796823, -16.46253265017161027, 37.08224293864768839 ) ) ;
#155703=CARTESIAN_POINT ( 'NONE',  ( 8.314922557961029526, -14.29746914071037800, 100.4177570613523471 ) ) ;
#155704=CARTESIAN_POINT ( 'NONE',  ( -14.34966873604972548, 8.224510206698743886, 28.33442372801902209 ) ) ;
#155706=CARTESIAN_POINT ( 'NONE',  ( 18.67979575497194134, -10.72451020669871369, 90.83442372801901854 ) ) ;
#155707=CARTESIAN_POINT ( 'NONE',  ( -0.05219959533910754901, -16.53943276465976808, 62.49890960531436690 ) ) ;
#155708=CARTESIAN_POINT ( 'NONE',  ( -10.72451020669898014, 18.67979575497178502, 90.41557627198103830 ) ) ;
#155709=CARTESIAN_POINT ( 'NONE',  ( 0.05219959533907565091, 21.53943276465977519, 89.99890960531438111 ) ) ;
#155711=CARTESIAN_POINT ( 'NONE',  ( -5.823673210054116645, -21.52544592524344225, 52.29057627198102409 ) ) ;
#155712=CARTESIAN_POINT ( 'NONE',  ( -16.53943276465976808, -0.05219959533934237506, 73.75109039468567573 ) ) ;
#155713=CARTESIAN_POINT ( 'NONE',  ( 16.53943276465976808, -0.05219959533910856209, 93.74890960531436690 ) ) ;
#155714=CARTESIAN_POINT ( 'NONE',  ( -5.153800228976328057, -19.02544592524343514, 52.29057627198100988 ) ) ;
#155716=CARTESIAN_POINT ( 'NONE',  ( 16.53943276465976808, 0.05219959533934440121, 96.25109039468568994 ) ) ;
#155717=CARTESIAN_POINT ( 'NONE',  ( 18.62759615963255655, 10.81492255796105972, 36.66775706135234714 ) ) ;
#155718=CARTESIAN_POINT ( 'NONE',  ( -19.03943276465977164, 0.05219959533909376836, 101.2489096053143669 ) ) ;
#155719=CARTESIAN_POINT ( 'NONE',  ( -5.719274019375665041, -21.55341960407619695, 64.79275706135234714 ) ) ;
#155721=CARTESIAN_POINT ( 'NONE',  ( 0.05219959533909260263, 19.03943276465977164, 24.99890960531435269 ) ) ;
#155722=VERTEX_POINT ( 'NONE', #176615 ) ;
#155723=CARTESIAN_POINT ( 'NONE',  ( -15.80617190586768217, 15.72974639402176855, 58.12609039468568994 ) ) ;
#155724=CARTESIAN_POINT ( 'NONE',  ( 0.05219959533909260263, 19.03943276465977164, 49.99890960531435979 ) ) ;
#155725=CARTESIAN_POINT ( 'NONE',  ( 17.72517630441460312, -5.499999999999974243, 58.42175719257605238 ) ) ;
#155726=CARTESIAN_POINT ( 'NONE',  ( -13.97604488694527625, -13.89961937509977652, 86.87390960531436690 ) ) ;
#155727=CARTESIAN_POINT ( 'NONE',  ( -5.153800228976607833, 19.02544592524334988, 67.70942372801900433 ) ) ;
#155728=CARTESIAN_POINT ( 'NONE',  ( 18.62759615963255655, 10.81492255796105972, 41.66775706135235424 ) ) ;
#155729=CARTESIAN_POINT ( 'NONE',  ( -19.02544592524334988, -5.153800228976617603, 63.95942372801899012 ) ) ;
#155730=CARTESIAN_POINT ( 'NONE',  ( 16.51473224551069308, 9.474510206698969483, 34.16557627198102409 ) ) ;
#155731=CARTESIAN_POINT ( 'NONE',  ( 16.53943276465976808, 0.05219959533934440121, 101.2510903946856757 ) ) ;
#155732=CARTESIAN_POINT ( 'NONE',  ( -16.46253265017146816, -9.564922557961047289, 74.16775706135234714 ) ) ;
#155733=CARTESIAN_POINT ( 'NONE',  ( -14.34966873604960291, -8.224510206698953496, 21.66557627198102409 ) ) ;
#155734=CARTESIAN_POINT ( 'NONE',  ( -5.153800228976607833, 19.02544592524334988, 52.70942372801900433 ) ) ;
#155735=CARTESIAN_POINT ( 'NONE',  ( 0.05219959533909260263, 19.03943276465977164, 99.99890960531436690 ) ) ;
#155736=CARTESIAN_POINT ( 'NONE',  ( 15.80617190586769283, -15.72974639402175789, 110.6260903946857042 ) ) ;
#155737=CARTESIAN_POINT ( 'NONE',  ( 9.564922557961047289, -16.46253265017146816, 25.41775706135234003 ) ) ;
#155739=CARTESIAN_POINT ( 'NONE',  ( 13.97604488694527802, 13.89961937509977652, 29.37390960531435979 ) ) ;
#155740=CARTESIAN_POINT ( 'NONE',  ( -5.823673210054431948, 21.52544592524334988, 82.70942372801900433 ) ) ;
#155741=CARTESIAN_POINT ( 'NONE',  ( 16.52544592524335698, 4.483927247898782831, 31.45942372801901854 ) ) ;
#155742=CARTESIAN_POINT ( 'NONE',  ( -9.474510206698964154, 16.51473224551069663, 95.41557627198102409 ) ) ;
#155744=CARTESIAN_POINT ( 'NONE',  ( -9.564922557960796823, -16.46253265017161027, 82.08224293864768129 ) ) ;
#155746=CARTESIAN_POINT ( 'NONE',  ( -19.03943276465977164, -0.05219959533935918106, 83.75109039468567573 ) ) ;
#155747=CARTESIAN_POINT ( 'NONE',  ( 16.51473224551069308, 9.474510206698969483, 109.1655762719810383 ) ) ;
#155748=CARTESIAN_POINT ( 'NONE',  ( 21.55341960407619695, -5.719274019375665929, 101.0427570613523756 ) ) ;
#155749=CARTESIAN_POINT ( 'NONE',  ( -8.314922557960811034, -14.29746914071050412, 97.08224293864770971 ) ) ;
#155750=CARTESIAN_POINT ( 'NONE',  ( 13.97604488694527802, 13.89961937509977652, 24.37390960531435624 ) ) ;
#155751=CARTESIAN_POINT ( 'NONE',  ( 5.823673210054125526, 21.52544592524343514, 39.79057627198103830 ) ) ;
#155752=CARTESIAN_POINT ( 'NONE',  ( 15.72974639402199770, -15.80617190586745480, 38.12390960531436690 ) ) ;
#155753=CARTESIAN_POINT ( 'NONE',  ( 14.34966873604960469, 8.224510206698951720, 114.1655762719810383 ) ) ;
#155755=CARTESIAN_POINT ( 'NONE',  ( 5.049401038297881783, 19.05341960407617563, 57.29275706135231871 ) ) ;
#155756=CARTESIAN_POINT ( 'NONE',  ( 0.05219959533910956823, 16.53943276465976808, 39.99890960531436690 ) ) ;
#155757=CARTESIAN_POINT ( 'NONE',  ( 9.564922557960805705, 16.46253265017160317, 114.5822429386476955 ) ) ;
#155758=CARTESIAN_POINT ( 'NONE',  ( 15.80617190586769283, -15.72974639402175789, 85.62609039468568994 ) ) ;
#155759=CARTESIAN_POINT ( 'NONE',  ( 15.80617190586746368, 15.72974639402197994, 74.37390960531436690 ) ) ;
#155760=CARTESIAN_POINT ( 'NONE',  ( -15.80617190586768217, 15.72974639402176855, 48.12609039468568284 ) ) ;
#155761=CARTESIAN_POINT ( 'NONE',  ( -5.719274019375978568, 21.55341960407610458, 100.2072429386476955 ) ) ;
#155762=CARTESIAN_POINT ( 'NONE',  ( 5.823673210054444382, -21.52544592524334988, 55.20942372801902565 ) ) ;
#155763=CARTESIAN_POINT ( 'NONE',  ( -19.02544592524342804, 5.153800228976336051, 26.04057627198103120 ) ) ;
#155764=CARTESIAN_POINT ( 'NONE',  ( 19.02544592524343514, -5.153800228976328945, 78.54057627198099567 ) ) ;
#155765=CARTESIAN_POINT ( 'NONE',  ( 8.314922557961029526, -14.29746914071037800, 75.41775706135233293 ) ) ;
#155766=CARTESIAN_POINT ( 'NONE',  ( -16.55341960407611168, -4.379528057220339221, 111.4572429386476813 ) ) ;
#155768=CARTESIAN_POINT ( 'NONE',  ( 4.379528057220339221, -16.55341960407611168, 47.70724293864770260 ) ) ;
#155769=CARTESIAN_POINT ( 'NONE',  ( -12.06949235617756955, 12.14591786802309770, 25.62390960531435624 ) ) ;
#155770=CARTESIAN_POINT ( 'NONE',  ( 0.05219959533909260263, 19.03943276465977164, 64.99890960531436690 ) ) ;
#155771=CARTESIAN_POINT ( 'NONE',  ( -0.05219959533909027116, -19.03943276465977164, 32.49890960531435979 ) ) ;
#155772=CARTESIAN_POINT ( 'NONE',  ( -15.80617190586745835, -15.72974639402198527, 46.87390960531435979 ) ) ;
#155773=CARTESIAN_POINT ( 'NONE',  ( -16.51473224551082808, 9.474510206698731452, 43.33442372801900433 ) ) ;
#155774=CARTESIAN_POINT ( 'NONE',  ( 17.50000000000000000, 5.499999999999992895, 51.70309617465830598 ) ) ;
#155775=CARTESIAN_POINT ( 'NONE',  ( -12.06949235617756955, 12.14591786802309770, 35.62390960531437401 ) ) ;
#155776=CARTESIAN_POINT ( 'NONE',  ( 16.46253265017160672, -9.564922557960803928, 108.3322429386476955 ) ) ;
#155777=CARTESIAN_POINT ( 'NONE',  ( 21.55341960407619695, -5.719274019375665929, 56.04275706135235424 ) ) ;
#155778=B_SPLINE_CURVE_WITH_KNOTS ( 'NONE', 3,
 ( #25437, #193267, #149754, #87078 ),
 .UNSPECIFIED., .F., .F.,
 ( 4, 4 ),
 ( 0.001482540648255936417, 0.002244533994399181866 ),
 .UNSPECIFIED. ) ;
#155780=CARTESIAN_POINT ( 'NONE',  ( -0.05219959533934338120, 16.53943276465976808, 77.50109039468567573 ) ) ;
#155781=CARTESIAN_POINT ( 'NONE',  ( 19.02544592524334988, 5.153800228976608722, 61.45942372801900433 ) ) ;
#155782=CARTESIAN_POINT ( 'NONE',  ( 16.55341960407611168, 4.379528057220329451, 38.95724293864768839 ) ) ;
#155783=LINE ( 'NONE', #15290, #12819 ) ;
#155784=CARTESIAN_POINT ( 'NONE',  ( 12.14591786802309770, 12.06949235617756955, 24.37390960531435979 ) ) ;
#155785=CARTESIAN_POINT ( 'NONE',  ( 16.46253265017160672, -9.564922557960803928, 43.33224293864769550 ) ) ;
#155786=CARTESIAN_POINT ( 'NONE',  ( -16.51473224551069308, -9.474510206698971260, 61.66557627198103120 ) ) ;
#155787=CARTESIAN_POINT ( 'NONE',  ( -19.03943276465977164, 0.05219959533909376836, 26.24890960531435624 ) ) ;
#155788=CARTESIAN_POINT ( 'NONE',  ( 18.62759615963255655, 10.81492255796105972, 26.66775706135235424 ) ) ;
#155789=CARTESIAN_POINT ( 'NONE',  ( 16.51473224551069308, 9.474510206698969483, 54.16557627198103120 ) ) ;
#155791=CARTESIAN_POINT ( 'NONE',  ( 5.049401038298161559, -19.05341960407611168, 52.70724293864767418 ) ) ;
#155792=CARTESIAN_POINT ( 'NONE',  ( -10.81492255796078084, -18.62759615963271287, 32.08224293864769550 ) ) ;
#155793=CARTESIAN_POINT ( 'NONE',  ( -15.72974639402176322, -15.80617190586768395, 54.37609039468568994 ) ) ;
#155794=CARTESIAN_POINT ( 'NONE',  ( 0.05219959533909260263, 19.03943276465977164, 24.99890960531435269 ) ) ;
#155795=CARTESIAN_POINT ( 'NONE',  ( 5.719274019375991003, -21.55341960407610458, 32.70724293864770260 ) ) ;
#155796=CARTESIAN_POINT ( 'NONE',  ( 8.224510206698742110, 14.34966873604972548, 77.08442372801901854 ) ) ;
#155797=CARTESIAN_POINT ( 'NONE',  ( 21.53943276465977519, 0.05219959533937863772, 111.2510903946856899 ) ) ;
#155798=CARTESIAN_POINT ( 'NONE',  ( 12.14591786802327356, -12.06949235617739191, 70.62609039468567573 ) ) ;
#155799=CARTESIAN_POINT ( 'NONE',  ( -9.564922557960796823, -16.46253265017161027, 107.0822429386476955 ) ) ;
#155800=CARTESIAN_POINT ( 'NONE',  ( 14.29746914071037800, 8.314922557961029526, 51.66775706135234714 ) ) ;
#155801=CARTESIAN_POINT ( 'NONE',  ( 16.53943276465976808, 0.05219959533934440121, 26.25109039468567573 ) ) ;
#155802=CARTESIAN_POINT ( 'NONE',  ( -16.53943276465976808, -0.05219959533934237506, 98.75109039468568994 ) ) ;
#155803=CARTESIAN_POINT ( 'NONE',  ( 10.81492255796106328, -18.62759615963255655, 50.41775706135235424 ) ) ;
#155804=CARTESIAN_POINT ( 'NONE',  ( 19.05341960407617918, -5.049401038297876454, 106.0427570613523471 ) ) ;
#155805=CARTESIAN_POINT ( 'NONE',  ( 21.55341960407610458, 5.719274019375980345, 108.9572429386476955 ) ) ;
#155806=CARTESIAN_POINT ( 'NONE',  ( 0.05219959533934541429, -16.53943276465976808, 20.00109039468568639 ) ) ;
#155807=CARTESIAN_POINT ( 'NONE',  ( -4.483927247898782831, 16.52544592524335698, 87.70942372801901854 ) ) ;
#155809=CARTESIAN_POINT ( 'NONE',  ( -10.81492255796105439, 18.62759615963255655, 82.91775706135234714 ) ) ;
#155810=CARTESIAN_POINT ( 'NONE',  ( 9.564922557961047289, -16.46253265017146816, 80.41775706135234714 ) ) ;
#155811=CARTESIAN_POINT ( 'NONE',  ( -14.29746914071049879, 8.314922557960819915, 45.83224293864769550 ) ) ;
#155812=CARTESIAN_POINT ( 'NONE',  ( 4.483927247898545687, 16.52544592524342804, 44.79057627198103120 ) ) ;
#155813=CARTESIAN_POINT ( 'NONE',  ( 14.34966873604960469, 8.224510206698951720, 104.1655762719810241 ) ) ;
#155814=CARTESIAN_POINT ( 'NONE',  ( -19.03943276465977164, -0.05219959533935918106, 43.75109039468566863 ) ) ;
#155816=CARTESIAN_POINT ( 'NONE',  ( -0.05219959533937732626, 21.53943276465977519, 37.50109039468568284 ) ) ;
#155817=CARTESIAN_POINT ( 'NONE',  ( -12.06949235617739369, -12.14591786802326823, 19.37609039468568639 ) ) ;
#155818=DIRECTION ( 'NONE',  ( 0.000000000000000000, -0.000000000000000000, -1.000000000000000000 ) ) ;
#155819=CARTESIAN_POINT ( 'NONE',  ( 19.02544592524343514, -5.153800228976328945, 98.54057627198100988 ) ) ;
#155820=CARTESIAN_POINT ( 'NONE',  ( 15.72974639402199770, -15.80617190586745480, 53.12390960531436690 ) ) ;
#155821=CARTESIAN_POINT ( 'NONE',  ( 13.89961937509957401, 13.97604488694547697, 91.87609039468567573 ) ) ;
#155822=CARTESIAN_POINT ( 'NONE',  ( -16.51473224551069308, -9.474510206698971260, 86.66557627198102409 ) ) ;
#155823=CARTESIAN_POINT ( 'NONE',  ( 21.53943276465977519, -0.05219959533907433946, 53.74890960531437401 ) ) ;
#155824=CARTESIAN_POINT ( 'NONE',  ( 8.224510206698953496, -14.34966873604960469, 102.9155762719810383 ) ) ;
#155825=CARTESIAN_POINT ( 'NONE',  ( -16.46253265017160317, 9.564922557960807481, 75.83224293864769550 ) ) ;
#155826=CARTESIAN_POINT ( 'NONE',  ( -9.564922557960796823, -16.46253265017161027, 32.08224293864769550 ) ) ;
#155827=CARTESIAN_POINT ( 'NONE',  ( -10.81492255796105439, 18.62759615963255655, 32.91775706135234714 ) ) ;
#155828=CARTESIAN_POINT ( 'NONE',  ( -21.53943276465977519, -0.05219959533937600094, 78.75109039468568994 ) ) ;
#155829=CARTESIAN_POINT ( 'NONE',  ( -0.05219959533934338120, 16.53943276465976808, 92.50109039468567573 ) ) ;
#155830=CARTESIAN_POINT ( 'NONE',  ( -21.53943276465977519, -0.05219959533937600094, 33.75109039468568284 ) ) ;
#155831=CARTESIAN_POINT ( 'NONE',  ( -18.67979575497193778, 10.72451020669871902, 23.33442372801901499 ) ) ;
#155832=CARTESIAN_POINT ( 'NONE',  ( 9.564922557961047289, -16.46253265017146816, 60.41775706135233293 ) ) ;
#155833=CARTESIAN_POINT ( 'NONE',  ( 0.05219959533909260263, 19.03943276465977164, 79.99890960531436690 ) ) ;
#155834=CARTESIAN_POINT ( 'NONE',  ( -21.53943276465977519, -0.05219959533937600094, 78.75109039468568994 ) ) ;
#155835=CARTESIAN_POINT ( 'NONE',  ( 0.05219959533907565091, 21.53943276465977519, 89.99890960531438111 ) ) ;
#155836=CARTESIAN_POINT ( 'NONE',  ( -4.379528057220328563, 16.55341960407611168, 70.20724293864769550 ) ) ;
#155837=CARTESIAN_POINT ( 'NONE',  ( 18.67979575497194134, -10.72451020669871369, 100.8344237280190185 ) ) ;
#155838=CARTESIAN_POINT ( 'NONE',  ( 8.224510206698953496, -14.34966873604960469, 87.91557627198103830 ) ) ;
#155839=CARTESIAN_POINT ( 'NONE',  ( -0.05219959533909027116, -19.03943276465977164, 42.49890960531435269 ) ) ;
#155840=CARTESIAN_POINT ( 'NONE',  ( 5.153800228976615827, -19.02544592524334988, 70.20942372801899012 ) ) ;
#155841=CARTESIAN_POINT ( 'NONE',  ( -16.53943276465976808, 0.05219959533911058130, 36.24890960531435979 ) ) ;
#155842=CARTESIAN_POINT ( 'NONE',  ( -10.72451020669870658, -18.67979575497194134, 94.58442372801901854 ) ) ;
#155843=CARTESIAN_POINT ( 'NONE',  ( -19.02544592524342804, 5.153800228976336051, 91.04057627198100988 ) ) ;
#155844=CARTESIAN_POINT ( 'NONE',  ( 19.02544592524334988, 5.153800228976608722, 66.45942372801899012 ) ) ;
#155845=CARTESIAN_POINT ( 'NONE',  ( -15.72974639402197994, 15.80617190586746368, 65.62390960531436690 ) ) ;
#155846=CARTESIAN_POINT ( 'NONE',  ( -0.05219959533937732626, 21.53943276465977519, 22.50109039468567573 ) ) ;
#155847=CARTESIAN_POINT ( 'NONE',  ( 16.53943276465976808, 0.05219959533934440121, 21.25109039468567218 ) ) ;
#155848=CARTESIAN_POINT ( 'NONE',  ( 8.224510206698742110, 14.34966873604972548, 82.08442372801901854 ) ) ;
#155850=CARTESIAN_POINT ( 'NONE',  ( 5.823673210054444382, -21.52544592524334988, 25.20942372801901854 ) ) ;
#155851=CARTESIAN_POINT ( 'NONE',  ( 4.379528057220339221, -16.55341960407611168, 102.7072429386476955 ) ) ;
#155853=CARTESIAN_POINT ( 'NONE',  ( -14.29746914071037622, -8.314922557961029526, 34.16775706135234714 ) ) ;
#155854=CARTESIAN_POINT ( 'NONE',  ( 21.55341960407610458, 5.719274019375980345, 63.95724293864770260 ) ) ;
#155855=CARTESIAN_POINT ( 'NONE',  ( 0.05219959533934541429, -16.53943276465976808, 110.0010903946856757 ) ) ;
#155856=CARTESIAN_POINT ( 'NONE',  ( 14.29746914071037800, 8.314922557961029526, 31.66775706135234358 ) ) ;
#155857=CARTESIAN_POINT ( 'NONE',  ( 13.89961937509977652, -13.97604488694527269, 38.12390960531436690 ) ) ;
#155858=CARTESIAN_POINT ( 'NONE',  ( 8.314922557961029526, -14.29746914071037800, 80.41775706135234714 ) ) ;
#155859=CARTESIAN_POINT ( 'NONE',  ( 19.05341960407617918, -5.049401038297876454, 71.04275706135234714 ) ) ;
#155860=CARTESIAN_POINT ( 'NONE',  ( -15.72974639402197994, 15.80617190586746368, 75.62390960531439532 ) ) ;
#155861=CARTESIAN_POINT ( 'NONE',  ( 14.34966873604972726, -8.224510206698740333, 100.8344237280190185 ) ) ;
#155862=CARTESIAN_POINT ( 'NONE',  ( -15.80617190586768217, 15.72974639402176855, 88.12609039468570415 ) ) ;
#155863=CARTESIAN_POINT ( 'NONE',  ( 21.55341960407610458, 5.719274019375980345, 63.95724293864770260 ) ) ;
#155864=CARTESIAN_POINT ( 'NONE',  ( 10.72451020669898902, -18.67979575497178502, 52.91557627198103830 ) ) ;
#155866=VERTEX_POINT ( 'NONE', #66423 ) ;
#155867=CARTESIAN_POINT ( 'NONE',  ( 0.05219959533934541429, -16.53943276465976808, 80.00109039468568994 ) ) ;
#155868=CARTESIAN_POINT ( 'NONE',  ( -18.67979575497178146, -10.72451020669898902, 51.66557627198102409 ) ) ;
#155869=VERTEX_POINT ( 'NONE', #189788 ) ;
#155870=CARTESIAN_POINT ( 'NONE',  ( 13.97604488694527802, 13.89961937509977652, 109.3739096053143669 ) ) ;
#155872=CARTESIAN_POINT ( 'NONE',  ( -5.049401038298153566, 19.05341960407611168, 25.20724293864768484 ) ) ;
#155873=CARTESIAN_POINT ( 'NONE',  ( 10.72451020669898902, -18.67979575497178502, 62.91557627198102409 ) ) ;
#155874=CARTESIAN_POINT ( 'NONE',  ( -16.53943276465976808, -0.05219959533934237506, 98.75109039468568994 ) ) ;
#155875=CARTESIAN_POINT ( 'NONE',  ( -15.80617190586768217, 15.72974639402176855, 43.12609039468568284 ) ) ;
#155876=CARTESIAN_POINT ( 'NONE',  ( -16.51473224551082808, 9.474510206698731452, 98.33442372801900433 ) ) ;
#155877=CARTESIAN_POINT ( 'NONE',  ( 19.03943276465977164, -0.05219959533909143690, 23.74890960531435269 ) ) ;
#155878=CARTESIAN_POINT ( 'NONE',  ( -4.379528057220086978, -16.55341960407618274, 19.79275706135235069 ) ) ;
#155879=CARTESIAN_POINT ( 'NONE',  ( -13.97604488694527625, -13.89961937509977652, 41.87390960531435979 ) ) ;
#155881=CARTESIAN_POINT ( 'NONE',  ( 19.02544592524343514, -5.153800228976328945, 88.54057627198102409 ) ) ;
#155882=CARTESIAN_POINT ( 'NONE',  ( 8.314922557961029526, -14.29746914071037800, 75.41775706135233293 ) ) ;
#155883=CARTESIAN_POINT ( 'NONE',  ( -19.03943276465977164, -0.05219959533935918106, 73.75109039468566152 ) ) ;
#155884=CARTESIAN_POINT ( 'NONE',  ( 16.46253265017146816, 9.564922557961045513, 26.66775706135234003 ) ) ;
#155885=CARTESIAN_POINT ( 'NONE',  ( -21.53943276465977519, 0.05219959533907696930, 61.24890960531435979 ) ) ;
#155886=CARTESIAN_POINT ( 'NONE',  ( 14.34966873604972726, -8.224510206698740333, 80.83442372801901854 ) ) ;
#155887=CARTESIAN_POINT ( 'NONE',  ( 9.564922557961047289, -16.46253265017146816, 80.41775706135234714 ) ) ;
#155888=CARTESIAN_POINT ( 'NONE',  ( 19.02544592524343514, -5.153800228976328945, 38.54057627198103120 ) ) ;
#155889=CARTESIAN_POINT ( 'NONE',  ( 5.153800228976335163, 19.02544592524342804, 84.79057627198099567 ) ) ;
#155890=CARTESIAN_POINT ( 'NONE',  ( -5.823673210054431948, 21.52544592524334988, 47.70942372801902565 ) ) ;
#155891=CARTESIAN_POINT ( 'NONE',  ( -9.564922557960796823, -16.46253265017161027, 52.08224293864768839 ) ) ;
#155892=CARTESIAN_POINT ( 'NONE',  ( -5.049401038297874678, -19.05341960407617918, 69.79275706135233293 ) ) ;
#155894=CARTESIAN_POINT ( 'NONE',  ( 13.97604488694527802, 13.89961937509977652, 104.3739096053143385 ) ) ;
#155895=CARTESIAN_POINT ( 'NONE',  ( -8.224510206698948167, 14.34966873604960824, 70.41557627198102409 ) ) ;
#155896=CARTESIAN_POINT ( 'NONE',  ( 0.05219959533907565091, 21.53943276465977519, 64.99890960531435269 ) ) ;
#155899=CARTESIAN_POINT ( 'NONE',  ( 9.564922557961047289, -16.46253265017146816, 40.41775706135234003 ) ) ;
#155901=CARTESIAN_POINT ( 'NONE',  ( 9.564922557960805705, 16.46253265017160317, 59.58224293864769550 ) ) ;
#155902=CARTESIAN_POINT ( 'NONE',  ( -9.564922557960796823, -16.46253265017161027, 67.08224293864769550 ) ) ;
#155903=EDGE_CURVE ( 'NONE', #115616, #129907, #81256, .T. ) ;
#155904=CARTESIAN_POINT ( 'NONE',  ( 12.14591786802327356, -12.06949235617739191, 45.62609039468567573 ) ) ;
#155907=CARTESIAN_POINT ( 'NONE',  ( -4.483927247898782831, 16.52544592524335698, 92.70942372801901854 ) ) ;
#155909=CARTESIAN_POINT ( 'NONE',  ( 12.14591786802327356, -12.06949235617739191, 70.62609039468567573 ) ) ;
#155910=CARTESIAN_POINT ( 'NONE',  ( -4.379528057220086978, -16.55341960407618274, 44.79275706135234714 ) ) ;
#155911=CARTESIAN_POINT ( 'NONE',  ( 13.89961937509957401, 13.97604488694547697, 21.87609039468566152 ) ) ;
#155912=CARTESIAN_POINT ( 'NONE',  ( 0.05219959533909260263, 19.03943276465977164, 59.99890960531436690 ) ) ;
#155914=CARTESIAN_POINT ( 'NONE',  ( -0.05219959533937732626, 21.53943276465977519, 47.50109039468568994 ) ) ;
#155915=CARTESIAN_POINT ( 'NONE',  ( 19.05341960407617918, -5.049401038297876454, 66.04275706135233293 ) ) ;
#155916=CARTESIAN_POINT ( 'NONE',  ( -21.55341960407619339, 5.719274019375674811, 113.5427570613523756 ) ) ;
#155917=CARTESIAN_POINT ( 'NONE',  ( 19.02544592524343514, -5.153800228976328945, 28.54057627198102409 ) ) ;
#155918=CARTESIAN_POINT ( 'NONE',  ( 17.47993547923482893, 5.827241545460860372, 23.84623249736978323 ) ) ;
#155919=CARTESIAN_POINT ( 'NONE',  ( -21.53943276465977519, 0.05219959533907696930, 56.24890960531436690 ) ) ;
#155920=CARTESIAN_POINT ( 'NONE',  ( -21.55341960407610458, -5.719274019375992779, 26.45724293864768839 ) ) ;
#155921=CARTESIAN_POINT ( 'NONE',  ( -16.55341960407611168, -4.379528057220339221, 96.45724293864770971 ) ) ;
#155922=CARTESIAN_POINT ( 'NONE',  ( -16.55341960407617563, 4.379528057220093196, 43.54275706135235424 ) ) ;
#155923=CARTESIAN_POINT ( 'NONE',  ( -4.483927247898539470, -16.52544592524342804, 27.29057627198103120 ) ) ;
#155925=CARTESIAN_POINT ( 'NONE',  ( 5.823673210054125526, 21.52544592524343514, 109.7905762719810383 ) ) ;
#155927=CARTESIAN_POINT ( 'NONE',  ( 14.29746914071049879, -8.314922557960816363, 33.33224293864769550 ) ) ;
#155928=CARTESIAN_POINT ( 'NONE',  ( 16.46253265017160672, -9.564922557960803928, 108.3322429386476955 ) ) ;
#155929=CARTESIAN_POINT ( 'NONE',  ( 13.89961937509957401, 13.97604488694547697, 101.8760903946856331 ) ) ;
#155930=CARTESIAN_POINT ( 'NONE',  ( -13.89961937509957401, -13.97604488694547875, 24.37609039468565442 ) ) ;
#155931=CARTESIAN_POINT ( 'NONE',  ( -14.34966873604960291, -8.224510206698953496, 36.66557627198103120 ) ) ;
#155932=CARTESIAN_POINT ( 'NONE',  ( -10.81492255796078084, -18.62759615963271287, 107.0822429386476955 ) ) ;
#155933=CARTESIAN_POINT ( 'NONE',  ( -18.67979575497178146, -10.72451020669898902, 66.66557627198102409 ) ) ;
#155934=CARTESIAN_POINT ( 'NONE',  ( 5.153800228976335163, 19.02544592524342804, 74.79057627198103830 ) ) ;
#155935=CARTESIAN_POINT ( 'NONE',  ( 12.14591786802309770, 12.06949235617756955, 44.37390960531435979 ) ) ;
#155936=CARTESIAN_POINT ( 'NONE',  ( -9.474510206698964154, 16.51473224551069663, 90.41557627198103830 ) ) ;
#155937=CARTESIAN_POINT ( 'NONE',  ( -18.22780087662126647, -5.499999999999827693, 38.98236817873107185 ) ) ;
#155938=CARTESIAN_POINT ( 'NONE',  ( 19.02544592524334988, 5.153800228976608722, 56.45942372801898301 ) ) ;
#155939=CARTESIAN_POINT ( 'NONE',  ( 0.05219959533907565091, 21.53943276465977519, 89.99890960531438111 ) ) ;
#155940=CARTESIAN_POINT ( 'NONE',  ( -16.55341960407611168, -4.379528057220339221, 96.45724293864770971 ) ) ;
#155941=CARTESIAN_POINT ( 'NONE',  ( -21.52544592524334988, -5.823673210054445271, 43.95942372801902565 ) ) ;
#155943=CARTESIAN_POINT ( 'NONE',  ( -16.53943276465976808, 0.05219959533911058130, 26.24890960531435624 ) ) ;
#155944=CARTESIAN_POINT ( 'NONE',  ( -9.474510206698964154, 16.51473224551069663, 30.41557627198102054 ) ) ;
#155945=CARTESIAN_POINT ( 'NONE',  ( -19.02544592524342804, 5.153800228976336051, 91.04057627198100988 ) ) ;
#155946=CARTESIAN_POINT ( 'NONE',  ( 15.80617190586746368, 15.72974639402197994, 59.37390960531436690 ) ) ;
#155947=CARTESIAN_POINT ( 'NONE',  ( 0.05219959533909260263, 19.03943276465977164, 29.99890960531435979 ) ) ;
#155948=CARTESIAN_POINT ( 'NONE',  ( -18.67979575497178146, -10.72451020669898902, 46.66557627198102409 ) ) ;
#155949=CARTESIAN_POINT ( 'NONE',  ( 10.81492255796106328, -18.62759615963255655, 70.41775706135236135 ) ) ;
#155951=CARTESIAN_POINT ( 'NONE',  ( -14.29746914071037622, -8.314922557961029526, 64.16775706135234714 ) ) ;
#155952=CARTESIAN_POINT ( 'NONE',  ( -19.02544592524342804, 5.153800228976336051, 61.04057627198103120 ) ) ;
#155953=CARTESIAN_POINT ( 'NONE',  ( 19.02544592524343514, -5.153800228976328945, 63.54057627198103830 ) ) ;
#155954=ORIENTED_EDGE ( 'NONE', *, *, #152995, .T. ) ;
#155955=CARTESIAN_POINT ( 'NONE',  ( -5.719274019375665041, -21.55341960407619695, 109.7927570613523613 ) ) ;
#155956=CARTESIAN_POINT ( 'NONE',  ( -8.224510206698735004, -14.34966873604973081, 74.58442372801901854 ) ) ;
#155957=CARTESIAN_POINT ( 'NONE',  ( 15.80617190586769283, -15.72974639402175789, 105.6260903946856899 ) ) ;
#155958=CARTESIAN_POINT ( 'NONE',  ( -19.02544592524342804, 5.153800228976336051, 76.04057627198102409 ) ) ;
#155959=CARTESIAN_POINT ( 'NONE',  ( 18.62759615963271287, -10.81492255796078972, 38.33224293864768839 ) ) ;
#155960=CARTESIAN_POINT ( 'NONE',  ( -19.02544592524334988, -5.153800228976617603, 103.9594237280190043 ) ) ;
#155961=CARTESIAN_POINT ( 'NONE',  ( -18.67979575497193778, 10.72451020669871902, 83.33442372801903275 ) ) ;
#155962=CARTESIAN_POINT ( 'NONE',  ( -12.14591786802326823, 12.06949235617739902, 53.12609039468568284 ) ) ;
#155963=CARTESIAN_POINT ( 'NONE',  ( 21.52544592524344225, -5.823673210054117533, 93.54057627198103830 ) ) ;
#155964=CARTESIAN_POINT ( 'NONE',  ( -5.153800228976607833, 19.02544592524334988, 97.70942372801900433 ) ) ;
#155965=CARTESIAN_POINT ( 'NONE',  ( -9.564922557960796823, -16.46253265017161027, 72.08224293864770971 ) ) ;
#155966=CARTESIAN_POINT ( 'NONE',  ( 9.564922557961047289, -16.46253265017146816, 110.4177570613523471 ) ) ;
#155967=CARTESIAN_POINT ( 'NONE',  ( -16.46253265017160317, 9.564922557960807481, 35.83224293864768839 ) ) ;
#155968=CARTESIAN_POINT ( 'NONE',  ( 4.483927247898790824, -16.52544592524335698, 25.20942372801901854 ) ) ;
#155969=CARTESIAN_POINT ( 'NONE',  ( -4.379528057220328563, 16.55341960407611168, 65.20724293864768129 ) ) ;
#155970=CARTESIAN_POINT ( 'NONE',  ( -8.224510206698735004, -14.34966873604973081, 69.58442372801900433 ) ) ;
#155971=EDGE_CURVE ( 'NONE', #27411, #6927, #180166, .T. ) ;
#155972=CARTESIAN_POINT ( 'NONE',  ( 10.81492255796106328, -18.62759615963255655, 30.41775706135234358 ) ) ;
#155973=CARTESIAN_POINT ( 'NONE',  ( -9.474510206698964154, 16.51473224551069663, 45.41557627198103120 ) ) ;
#155974=CARTESIAN_POINT ( 'NONE',  ( 9.564922557960805705, 16.46253265017160317, 69.58224293864770971 ) ) ;
#155975=CARTESIAN_POINT ( 'NONE',  ( -16.52544592524335698, -4.483927247898792601, 73.95942372801901854 ) ) ;
#155978=CARTESIAN_POINT ( 'NONE',  ( 5.153800228976615827, -19.02544592524334988, 20.20942372801899722 ) ) ;
#155979=CARTESIAN_POINT ( 'NONE',  ( -13.89961937509977652, 13.97604488694528158, 30.62390960531435269 ) ) ;
#155980=CARTESIAN_POINT ( 'NONE',  ( 0.05219959533909260263, 19.03943276465977164, 104.9989096053143669 ) ) ;
#155982=CARTESIAN_POINT ( 'NONE',  ( 8.314922557961029526, -14.29746914071037800, 30.41775706135234358 ) ) ;
#155983=CARTESIAN_POINT ( 'NONE',  ( 13.89961937509957401, 13.97604488694547697, 41.87609039468566152 ) ) ;
#155984=CARTESIAN_POINT ( 'NONE',  ( -16.53943276465976808, -0.05219959533934237506, 48.75109039468568284 ) ) ;
#155985=CARTESIAN_POINT ( 'NONE',  ( -5.049401038298153566, 19.05341960407611168, 45.20724293864769550 ) ) ;
#155986=CARTESIAN_POINT ( 'NONE',  ( 5.153800228976335163, 19.02544592524342804, 104.7905762719809957 ) ) ;
#155987=CARTESIAN_POINT ( 'NONE',  ( 9.474510206698971260, -16.51473224551069308, 57.91557627198103120 ) ) ;
#155988=CARTESIAN_POINT ( 'NONE',  ( 10.72451020669898902, -18.67979575497178502, 102.9155762719810383 ) ) ;
#155989=CARTESIAN_POINT ( 'NONE',  ( 0.05219959533909260263, 19.03943276465977164, 89.99890960531436690 ) ) ;
#155990=CARTESIAN_POINT ( 'NONE',  ( -5.153800228976328057, -19.02544592524343514, 112.2905762719810099 ) ) ;
#155991=CARTESIAN_POINT ( 'NONE',  ( 19.05341960407611168, 5.049401038298154454, 63.95724293864769550 ) ) ;
#155992=CARTESIAN_POINT ( 'NONE',  ( 8.314922557960818139, 14.29746914071049879, 24.58224293864768839 ) ) ;
#155994=CARTESIAN_POINT ( 'NONE',  ( 9.564922557961047289, -16.46253265017146816, 95.41775706135233293 ) ) ;
#155995=CARTESIAN_POINT ( 'NONE',  ( 5.153800228976615827, -19.02544592524334988, 30.20942372801900433 ) ) ;
#155996=CARTESIAN_POINT ( 'NONE',  ( 0.05219959533910956823, 16.53943276465976808, 59.99890960531436690 ) ) ;
#155997=CARTESIAN_POINT ( 'NONE',  ( 0.05219959533937995610, -21.53943276465977519, 85.00109039468568994 ) ) ;
#155998=CARTESIAN_POINT ( 'NONE',  ( -0.05219959533909027116, -19.03943276465977164, 22.49890960531436690 ) ) ;
#155999=CARTESIAN_POINT ( 'NONE',  ( -16.53943276465976808, -0.05219959533934237506, 113.7510903946856757 ) ) ;
#156000=CARTESIAN_POINT ( 'NONE',  ( 18.67979575497194134, -10.72451020669871369, 95.83442372801903275 ) ) ;
#156001=CARTESIAN_POINT ( 'NONE',  ( -5.049401038298153566, 19.05341960407611168, 85.20724293864766707 ) ) ;
#156002=CARTESIAN_POINT ( 'NONE',  ( -18.62759615963255300, -10.81492255796106328, 44.16775706135234714 ) ) ;
#156003=CARTESIAN_POINT ( 'NONE',  ( -16.51473224551069308, -9.474510206698971260, 86.66557627198102409 ) ) ;
#156004=CARTESIAN_POINT ( 'NONE',  ( -14.29746914071049879, 8.314922557960819915, 90.83224293864769550 ) ) ;
#156005=CARTESIAN_POINT ( 'NONE',  ( -4.379528057220328563, 16.55341960407611168, 65.20724293864768129 ) ) ;
#156006=CARTESIAN_POINT ( 'NONE',  ( -21.53943276465977519, 0.05219959533907696930, 76.24890960531435269 ) ) ;
#156007=CARTESIAN_POINT ( 'NONE',  ( 16.46253265017160672, -9.564922557960803928, 78.33224293864769550 ) ) ;
#156008=CARTESIAN_POINT ( 'NONE',  ( -18.67979575497178146, -10.72451020669898902, 91.66557627198103830 ) ) ;
#156009=CARTESIAN_POINT ( 'NONE',  ( -5.153800228976607833, 19.02544592524334988, 77.70942372801900433 ) ) ;
#156010=CARTESIAN_POINT ( 'NONE',  ( -19.25918095147782338, -5.499999999999492850, 89.45284276293935477 ) ) ;
#156011=CARTESIAN_POINT ( 'NONE',  ( 8.314922557960818139, 14.29746914071049879, 84.58224293864769550 ) ) ;
#156012=CARTESIAN_POINT ( 'NONE',  ( -9.474510206698964154, 16.51473224551069663, 55.41557627198103120 ) ) ;
#156013=CARTESIAN_POINT ( 'NONE',  ( 15.80617190586746368, 15.72974639402197994, 69.37390960531436690 ) ) ;
#156015=CARTESIAN_POINT ( 'NONE',  ( -4.483927247898539470, -16.52544592524342804, 22.29057627198102765 ) ) ;
#156017=CARTESIAN_POINT ( 'NONE',  ( 0.05219959533936267826, -19.03943276465977164, 100.0010903946856757 ) ) ;
#156018=CARTESIAN_POINT ( 'NONE',  ( -8.224510206698948167, 14.34966873604960824, 85.41557627198102409 ) ) ;
#156019=CARTESIAN_POINT ( 'NONE',  ( -17.50000000000000355, -5.499999999999980460, 96.28230962303564411 ) ) ;
#156020=CARTESIAN_POINT ( 'NONE',  ( -0.05219959533909027116, -19.03943276465977164, 72.49890960531435269 ) ) ;
#156021=CARTESIAN_POINT ( 'NONE',  ( 19.05341960407611168, 5.049401038298154454, 38.95724293864767418 ) ) ;
#156022=CARTESIAN_POINT ( 'NONE',  ( -14.29746914071049879, 8.314922557960819915, 65.83224293864769550 ) ) ;
#156023=CARTESIAN_POINT ( 'NONE',  ( -9.564922557960796823, -16.46253265017161027, 97.08224293864769550 ) ) ;
#156024=CARTESIAN_POINT ( 'NONE',  ( -13.89961937509957401, -13.97604488694547875, 89.37609039468563310 ) ) ;
#156025=CARTESIAN_POINT ( 'NONE',  ( 9.564922557960805705, 16.46253265017160317, 64.58224293864769550 ) ) ;
#156026=CARTESIAN_POINT ( 'NONE',  ( -19.03943276465977164, 0.05219959533909376836, 91.24890960531436690 ) ) ;
#156027=CARTESIAN_POINT ( 'NONE',  ( 5.719274019375991003, -21.55341960407610458, 72.70724293864769550 ) ) ;
#156028=CARTESIAN_POINT ( 'NONE',  ( -12.14591786802326823, 12.06949235617739902, 68.12609039468567573 ) ) ;
#156029=CARTESIAN_POINT ( 'NONE',  ( 16.51473224551083163, -9.474510206698727899, 110.8344237280190043 ) ) ;
#156030=CARTESIAN_POINT ( 'NONE',  ( -19.02544592524342804, 5.153800228976336051, 66.04057627198103830 ) ) ;
#156031=CARTESIAN_POINT ( 'NONE',  ( 5.823673210054125526, 21.52544592524343514, 64.79057627198103830 ) ) ;
#156032=CARTESIAN_POINT ( 'NONE',  ( -16.46253265017146816, -9.564922557961047289, 89.16775706135234714 ) ) ;
#156033=CARTESIAN_POINT ( 'NONE',  ( 8.224510206698953496, -14.34966873604960469, 37.91557627198102409 ) ) ;
#156034=CARTESIAN_POINT ( 'NONE',  ( 15.80617190586769283, -15.72974639402175789, 50.62609039468568994 ) ) ;
#156036=CARTESIAN_POINT ( 'NONE',  ( 16.53943276465976808, 0.05219959533934440121, 71.25109039468568994 ) ) ;
#156037=CARTESIAN_POINT ( 'NONE',  ( -16.46253265017160317, 9.564922557960807481, 110.8322429386476955 ) ) ;
#156038=CARTESIAN_POINT ( 'NONE',  ( 5.049401038298163336, -19.05341960407611168, 102.7072429386476955 ) ) ;
#156039=CARTESIAN_POINT ( 'NONE',  ( -17.49999999999999645, 5.499999999999992895, 78.71769037696437010 ) ) ;
#156040=CARTESIAN_POINT ( 'NONE',  ( -4.483927247898782831, 16.52544592524335698, 92.70942372801901854 ) ) ;
#156041=CARTESIAN_POINT ( 'NONE',  ( 12.14591786802327356, -12.06949235617739191, 50.62609039468568994 ) ) ;
#156042=CARTESIAN_POINT ( 'NONE',  ( 16.51473224551069308, 9.474510206698969483, 54.16557627198103120 ) ) ;
#156043=CARTESIAN_POINT ( 'NONE',  ( -5.049401038298153566, 19.05341960407611168, 55.20724293864769550 ) ) ;
#156044=CARTESIAN_POINT ( 'NONE',  ( 10.72451020669871369, 18.67979575497193778, 47.08442372801901854 ) ) ;
#156045=CARTESIAN_POINT ( 'NONE',  ( -12.06949235617739369, -12.14591786802326823, 59.37609039468568284 ) ) ;
#156046=CARTESIAN_POINT ( 'NONE',  ( -12.06949235617756955, 12.14591786802309770, 35.62390960531437401 ) ) ;
#156047=CARTESIAN_POINT ( 'NONE',  ( 16.46253265017160672, -9.564922557960803928, 43.33224293864769550 ) ) ;
#156048=CARTESIAN_POINT ( 'NONE',  ( -5.153800228976328057, -19.02544592524343514, 37.29057627198102409 ) ) ;
#156049=CARTESIAN_POINT ( 'NONE',  ( 8.314922557961029526, -14.29746914071037800, 30.41775706135234358 ) ) ;
#156051=CARTESIAN_POINT ( 'NONE',  ( 13.97604488694548053, -13.89961937509957401, 80.62609039468567573 ) ) ;
#156052=CARTESIAN_POINT ( 'NONE',  ( -4.483927247898539470, -16.52544592524342804, 82.29057627198103830 ) ) ;
#156053=CARTESIAN_POINT ( 'NONE',  ( 16.46253265017160672, -9.564922557960803928, 48.33224293864769550 ) ) ;
#156054=CARTESIAN_POINT ( 'NONE',  ( -19.05341960407617563, 5.049401038297882671, 93.54275706135234714 ) ) ;
#156056=CARTESIAN_POINT ( 'NONE',  ( 10.81492255796106328, -18.62759615963255655, 95.41775706135234714 ) ) ;
#156057=CARTESIAN_POINT ( 'NONE',  ( 4.483927247898790824, -16.52544592524335698, 50.20942372801901854 ) ) ;
#156058=CARTESIAN_POINT ( 'NONE',  ( 16.21995358207305671, 7.366697692864114799, 37.56448998487844193 ) ) ;
#156059=CARTESIAN_POINT ( 'NONE',  ( 10.81492255796078972, 18.62759615963270932, 44.58224293864769550 ) ) ;
#156060=CARTESIAN_POINT ( 'NONE',  ( -8.314922557961024197, 14.29746914071037800, 37.91775706135235424 ) ) ;
#156061=CARTESIAN_POINT ( 'NONE',  ( -9.474510206698720793, -16.51473224551083518, 24.58442372801900078 ) ) ;
#156062=CARTESIAN_POINT ( 'NONE',  ( 5.153800228976335163, 19.02544592524342804, 74.79057627198103830 ) ) ;
#156064=CARTESIAN_POINT ( 'NONE',  ( 5.153800228976335163, 19.02544592524342804, 49.79057627198100988 ) ) ;
#156066=CARTESIAN_POINT ( 'NONE',  ( -19.03943276465977164, 0.05219959533909376836, 71.24890960531435269 ) ) ;
#156067=CARTESIAN_POINT ( 'NONE',  ( -19.25918095147781628, -5.499999999999586109, 54.45284276293936188 ) ) ;
#156068=CARTESIAN_POINT ( 'NONE',  ( -19.05341960407617563, 5.049401038297882671, 38.54275706135233293 ) ) ;
#156069=CARTESIAN_POINT ( 'NONE',  ( 19.02544592524334988, 5.153800228976608722, 21.45942372801899012 ) ) ;
#156070=CARTESIAN_POINT ( 'NONE',  ( 12.14591786802309770, 12.06949235617756955, 39.37390960531436690 ) ) ;
#156071=CARTESIAN_POINT ( 'NONE',  ( -5.049401038298153566, 19.05341960407611168, 45.20724293864769550 ) ) ;
#156072=CARTESIAN_POINT ( 'NONE',  ( -13.89961937509977652, 13.97604488694528158, 100.6239096053143669 ) ) ;
#156073=CARTESIAN_POINT ( 'NONE',  ( 21.53943276465977519, 0.05219959533937863772, 71.25109039468568994 ) ) ;
#156074=CARTESIAN_POINT ( 'NONE',  ( -16.46253265017160317, 9.564922557960807481, 50.83224293864770260 ) ) ;
#156075=EDGE_CURVE ( 'NONE', #182496, #15494, #16121, .T. ) ;
#156077=CARTESIAN_POINT ( 'NONE',  ( 15.80617190586769283, -15.72974639402175789, 85.62609039468568994 ) ) ;
#156078=CARTESIAN_POINT ( 'NONE',  ( 0.05219959533909260263, 19.03943276465977164, 114.9989096053143669 ) ) ;
#156079=CARTESIAN_POINT ( 'NONE',  ( -16.51473224551069308, -9.474510206698971260, 41.66557627198103120 ) ) ;
#156080=CARTESIAN_POINT ( 'NONE',  ( -5.719274019375665041, -21.55341960407619695, 24.79275706135235779 ) ) ;
#156081=CARTESIAN_POINT ( 'NONE',  ( 13.89961937509957401, 13.97604488694547697, 51.87609039468566863 ) ) ;
#156082=CARTESIAN_POINT ( 'NONE',  ( 16.51473224551069308, 9.474510206698969483, 29.16557627198103475 ) ) ;
#156083=CARTESIAN_POINT ( 'NONE',  ( 9.474510206698971260, -16.51473224551069308, 72.91557627198102409 ) ) ;
#156084=CARTESIAN_POINT ( 'NONE',  ( 16.46253265017146816, 9.564922557961045513, 106.6677570613523471 ) ) ;
#156085=CARTESIAN_POINT ( 'NONE',  ( -8.224510206698948167, 14.34966873604960824, 70.41557627198102409 ) ) ;
#156086=CARTESIAN_POINT ( 'NONE',  ( 10.72451020669898902, -18.67979575497178502, 32.91557627198102409 ) ) ;
#156087=CARTESIAN_POINT ( 'NONE',  ( 19.02544592524334988, 5.153800228976608722, 106.4594237280190185 ) ) ;
#156088=CARTESIAN_POINT ( 'NONE',  ( -10.72451020669898014, 18.67979575497178502, 105.4155762719810383 ) ) ;
#156089=CARTESIAN_POINT ( 'NONE',  ( -10.72451020669870658, -18.67979575497194134, 59.58442372801901854 ) ) ;
#156090=CARTESIAN_POINT ( 'NONE',  ( 8.314922557961029526, -14.29746914071037800, 50.41775706135235424 ) ) ;
#156091=CARTESIAN_POINT ( 'NONE',  ( 12.14591786802327356, -12.06949235617739191, 50.62609039468568994 ) ) ;
#156092=CARTESIAN_POINT ( 'NONE',  ( 15.72974639402199770, -15.80617190586745480, 68.12390960531436690 ) ) ;
#156093=CARTESIAN_POINT ( 'NONE',  ( 9.474510206698971260, -16.51473224551069308, 52.91557627198102409 ) ) ;
#156094=CARTESIAN_POINT ( 'NONE',  ( -0.05219959533934338120, 16.53943276465976808, 82.50109039468568994 ) ) ;
#156095=CARTESIAN_POINT ( 'NONE',  ( 5.719274019375991003, -21.55341960407610458, 107.7072429386476955 ) ) ;
#156096=CARTESIAN_POINT ( 'NONE',  ( 4.379528057220339221, -16.55341960407611168, 52.70724293864769550 ) ) ;
#156097=CARTESIAN_POINT ( 'NONE',  ( 19.03943276465977164, -0.05219959533909143690, 73.74890960531435269 ) ) ;
#156098=CARTESIAN_POINT ( 'NONE',  ( -16.52544592524335698, -4.483927247898792601, 73.95942372801901854 ) ) ;
#156099=CARTESIAN_POINT ( 'NONE',  ( -19.05341960407617563, 5.049401038297882671, 113.5427570613523471 ) ) ;
#156100=CARTESIAN_POINT ( 'NONE',  ( -21.53943276465977519, 0.05219959533907696930, 111.2489096053143669 ) ) ;
#156101=CARTESIAN_POINT ( 'NONE',  ( -16.53943276465976808, 0.05219959533911058130, 41.24890960531435269 ) ) ;
#156103=CARTESIAN_POINT ( 'NONE',  ( -17.49999999999999645, 5.624438216177592764, 75.81670344914645909 ) ) ;
#156104=CARTESIAN_POINT ( 'NONE',  ( 5.719274019375991003, -21.55341960407610458, 92.70724293864770971 ) ) ;
#156106=CARTESIAN_POINT ( 'NONE',  ( 14.29746914071049879, -8.314922557960816363, 28.33224293864769550 ) ) ;
#156109=CARTESIAN_POINT ( 'NONE',  ( -18.67979575497178146, -10.72451020669898902, 101.6655762719810383 ) ) ;
#156110=CARTESIAN_POINT ( 'NONE',  ( -13.97604488694527625, -13.89961937509977652, 106.8739096053143669 ) ) ;
#156111=CARTESIAN_POINT ( 'NONE',  ( -21.53943276465977519, -0.05219959533937600094, 18.75109039468568639 ) ) ;
#156112=CARTESIAN_POINT ( 'NONE',  ( 4.379528057220339221, -16.55341960407611168, 57.70724293864770260 ) ) ;
#156113=CARTESIAN_POINT ( 'NONE',  ( 14.29746914071037800, 8.314922557961029526, 51.66775706135234714 ) ) ;
#156114=CARTESIAN_POINT ( 'NONE',  ( 13.97604488694527802, 13.89961937509977652, 64.37390960531436690 ) ) ;
#156115=CARTESIAN_POINT ( 'NONE',  ( 13.89961937509957401, 13.97604488694547697, 46.87609039468565442 ) ) ;
#156116=CARTESIAN_POINT ( 'NONE',  ( -16.51473224551069308, -9.474510206698971260, 81.66557627198103830 ) ) ;
#156117=CARTESIAN_POINT ( 'NONE',  ( -10.72451020669898014, 18.67979575497178502, 40.41557627198103120 ) ) ;
#156119=CARTESIAN_POINT ( 'NONE',  ( 19.02544592524343514, -5.153800228976328945, 43.54057627198103120 ) ) ;
#156120=CARTESIAN_POINT ( 'NONE',  ( 4.483927247898790824, -16.52544592524335698, 20.20942372801900788 ) ) ;
#156121=CARTESIAN_POINT ( 'NONE',  ( -5.153800228976607833, 19.02544592524334988, 57.70942372801899012 ) ) ;
#156122=CARTESIAN_POINT ( 'NONE',  ( -5.823673210054116645, -21.52544592524344225, 97.29057627198105251 ) ) ;
#156123=CARTESIAN_POINT ( 'NONE',  ( -8.224510206698948167, 14.34966873604960824, 30.41557627198101699 ) ) ;
#156124=CARTESIAN_POINT ( 'NONE',  ( -0.05219959533909027116, -19.03943276465977164, 87.49890960531436690 ) ) ;
#156125=CARTESIAN_POINT ( 'NONE',  ( 10.72451020669898902, -18.67979575497178502, 52.91557627198103830 ) ) ;
#156126=CARTESIAN_POINT ( 'NONE',  ( -15.72974639402197994, 15.80617190586746368, 90.62390960531436690 ) ) ;
#156127=CARTESIAN_POINT ( 'NONE',  ( -12.06949235617739369, -12.14591786802326823, 29.37609039468568284 ) ) ;
#156128=CARTESIAN_POINT ( 'NONE',  ( -21.52544592524343514, 5.823673210054127303, 26.04057627198103475 ) ) ;
#156129=CARTESIAN_POINT ( 'NONE',  ( 0.05219959533937995610, -21.53943276465977519, 90.00109039468567573 ) ) ;
#156130=CARTESIAN_POINT ( 'NONE',  ( -13.97604488694527625, -13.89961937509977652, 86.87390960531436690 ) ) ;
#156131=CARTESIAN_POINT ( 'NONE',  ( -0.05219959533909027116, -19.03943276465977164, 27.49890960531435624 ) ) ;
#156132=CARTESIAN_POINT ( 'NONE',  ( 9.474510206698971260, -16.51473224551069308, 82.91557627198103830 ) ) ;
#156133=CARTESIAN_POINT ( 'NONE',  ( -4.379528057220328563, 16.55341960407611168, 100.2072429386476955 ) ) ;
#156134=CARTESIAN_POINT ( 'NONE',  ( 9.474510206698971260, -16.51473224551069308, 62.91557627198102409 ) ) ;
#156135=CARTESIAN_POINT ( 'NONE',  ( -8.314922557961024197, 14.29746914071037800, 27.91775706135234358 ) ) ;
#156138=CARTESIAN_POINT ( 'NONE',  ( 10.72451020669871369, 18.67979575497193778, 92.08442372801901854 ) ) ;
#156139=CARTESIAN_POINT ( 'NONE',  ( 5.049401038298161559, -19.05341960407611168, 112.7072429386476813 ) ) ;
#156140=CARTESIAN_POINT ( 'NONE',  ( -16.55341960407617563, 4.379528057220093196, 88.54275706135236135 ) ) ;
#156142=CARTESIAN_POINT ( 'NONE',  ( 19.03943276465977164, 0.05219959533936151252, 71.25109039468566152 ) ) ;
#156143=CARTESIAN_POINT ( 'NONE',  ( -9.474510206698720793, -16.51473224551083518, 34.58442372801899722 ) ) ;
#156144=CARTESIAN_POINT ( 'NONE',  ( -17.50000000000001066, -5.500000000000021316, 46.28230962303566542 ) ) ;
#156145=CARTESIAN_POINT ( 'NONE',  ( -13.97604488694527625, -13.89961937509977652, 21.87390960531435979 ) ) ;
#156146=CARTESIAN_POINT ( 'NONE',  ( -4.483927247898539470, -16.52544592524342804, 37.29057627198102409 ) ) ;
#156148=CARTESIAN_POINT ( 'NONE',  ( 16.55341960407618274, -4.379528057220086978, 111.0427570613523613 ) ) ;
#156149=CARTESIAN_POINT ( 'NONE',  ( 17.44279575226823553, 5.990770900252482711, 66.66442432485683867 ) ) ;
#156150=CARTESIAN_POINT ( 'NONE',  ( -8.314922557961024197, 14.29746914071037800, 77.91775706135231871 ) ) ;
#156151=CARTESIAN_POINT ( 'NONE',  ( -13.97604488694527625, -13.89961937509977652, 41.87390960531435979 ) ) ;
#156152=CARTESIAN_POINT ( 'NONE',  ( -10.81492255796105439, 18.62759615963255655, 87.91775706135234714 ) ) ;
#156153=CARTESIAN_POINT ( 'NONE',  ( -9.564922557961040184, 16.46253265017147172, 97.91775706135233293 ) ) ;
#156154=CARTESIAN_POINT ( 'NONE',  ( -10.81492255796105439, 18.62759615963255655, 77.91775706135231871 ) ) ;
#156155=CARTESIAN_POINT ( 'NONE',  ( 16.46253265017146816, 9.564922557961045513, 56.66775706135233293 ) ) ;
#156156=CARTESIAN_POINT ( 'NONE',  ( 5.049401038298161559, -19.05341960407611168, 92.70724293864769550 ) ) ;
#156157=CARTESIAN_POINT ( 'NONE',  ( -16.46253265017160317, 9.564922557960807481, 65.83224293864769550 ) ) ;
#156158=CARTESIAN_POINT ( 'NONE',  ( 16.18388926212237067, 7.379444403734554569, 72.93953151366149257 ) ) ;
#156159=CARTESIAN_POINT ( 'NONE',  ( -14.34966873604960291, -8.224510206698953496, 66.66557627198102409 ) ) ;
#156160=CARTESIAN_POINT ( 'NONE',  ( -5.823673210054116645, -21.52544592524344225, 67.29057627198103830 ) ) ;
#156161=CARTESIAN_POINT ( 'NONE',  ( -5.153800228976328057, -19.02544592524343514, 42.29057627198101699 ) ) ;
#156162=CARTESIAN_POINT ( 'NONE',  ( -21.55341960407610458, -5.719274019375992779, 86.45724293864770971 ) ) ;
#156163=CARTESIAN_POINT ( 'NONE',  ( 12.06949235617739724, 12.14591786802326823, 71.87609039468568994 ) ) ;
#156165=ORIENTED_EDGE ( 'NONE', *, *, #11642, .F. ) ;
#156166=CARTESIAN_POINT ( 'NONE',  ( -13.89961937509977652, 13.97604488694528158, 45.62390960531433848 ) ) ;
#156167=CARTESIAN_POINT ( 'NONE',  ( 16.55341960407611168, 4.379528057220329451, 83.95724293864770971 ) ) ;
#156169=CARTESIAN_POINT ( 'NONE',  ( 5.153800228976335163, 19.02544592524342804, 54.79057627198103120 ) ) ;
#156170=CARTESIAN_POINT ( 'NONE',  ( -9.564922557960796823, -16.46253265017161027, 27.08224293864769550 ) ) ;
#156171=CARTESIAN_POINT ( 'NONE',  ( 13.97604488694548053, -13.89961937509957401, 65.62609039468567573 ) ) ;
#156172=CARTESIAN_POINT ( 'NONE',  ( 4.379528057220339221, -16.55341960407611168, 72.70724293864769550 ) ) ;
#156173=CARTESIAN_POINT ( 'NONE',  ( -21.52544592524334988, -5.823673210054445271, 48.95942372801902565 ) ) ;
#156174=CARTESIAN_POINT ( 'NONE',  ( -13.97604488694527625, -13.89961937509977652, 41.87390960531435979 ) ) ;
#156175=CARTESIAN_POINT ( 'NONE',  ( -5.823673210054116645, -21.52544592524344225, 107.2905762719810525 ) ) ;
#156176=CARTESIAN_POINT ( 'NONE',  ( 17.97058386085786807, 5.500000000000006217, 91.50390968646219392 ) ) ;
#156177=CARTESIAN_POINT ( 'NONE',  ( -12.14591786802309592, -12.06949235617757132, 91.87390960531436690 ) ) ;
#156179=CARTESIAN_POINT ( 'NONE',  ( -13.97604488694527625, -13.89961937509977652, 41.87390960531435979 ) ) ;
#156180=CARTESIAN_POINT ( 'NONE',  ( 19.01529144963331674, 5.500000000000154543, 48.73431955728439391 ) ) ;
#156181=CARTESIAN_POINT ( 'NONE',  ( -16.46253265017146816, -9.564922557961047289, 99.16775706135233293 ) ) ;
#156182=CARTESIAN_POINT ( 'NONE',  ( 19.05341960407611168, 5.049401038298154454, 93.95724293864769550 ) ) ;
#156183=CARTESIAN_POINT ( 'NONE',  ( 18.62759615963255655, 10.81492255796105972, 41.66775706135235424 ) ) ;
#156184=CARTESIAN_POINT ( 'NONE',  ( 9.474510206698971260, -16.51473224551069308, 82.91557627198103830 ) ) ;
#156185=CARTESIAN_POINT ( 'NONE',  ( -13.89961937509957401, -13.97604488694547875, 69.37609039468564731 ) ) ;
#156186=CARTESIAN_POINT ( 'NONE',  ( 13.97604488694527802, 13.89961937509977652, 49.37390960531434558 ) ) ;
#156187=CARTESIAN_POINT ( 'NONE',  ( 14.29746914071049879, -8.314922557960816363, 63.33224293864770260 ) ) ;
#156188=CARTESIAN_POINT ( 'NONE',  ( 14.34966873604960469, 8.224510206698951720, 74.16557627198102409 ) ) ;
#156189=CARTESIAN_POINT ( 'NONE',  ( 16.51473224551069308, 9.474510206698969483, 74.16557627198103830 ) ) ;
#156190=CARTESIAN_POINT ( 'NONE',  ( 15.80617190586746368, 15.72974639402197994, 99.37390960531436690 ) ) ;
#156191=CARTESIAN_POINT ( 'NONE',  ( -19.05341960407611168, -5.049401038298163336, 76.45724293864769550 ) ) ;
#156192=CARTESIAN_POINT ( 'NONE',  ( 10.81492255796106328, -18.62759615963255655, 110.4177570613523756 ) ) ;
#156193=CARTESIAN_POINT ( 'NONE',  ( 19.03943276465977164, -0.05219959533909143690, 33.74890960531435979 ) ) ;
#156194=CARTESIAN_POINT ( 'NONE',  ( 4.483927247898790824, -16.52544592524335698, 105.2094237280190328 ) ) ;
#156195=CARTESIAN_POINT ( 'NONE',  ( 8.314922557960818139, 14.29746914071049879, 109.5822429386476955 ) ) ;
#156196=CARTESIAN_POINT ( 'NONE',  ( 0.05219959533936267826, -19.03943276465977164, 110.0010903946856757 ) ) ;
#156198=CARTESIAN_POINT ( 'NONE',  ( -18.67979575497193778, 10.72451020669871902, 33.33442372801900433 ) ) ;
#156199=CARTESIAN_POINT ( 'NONE',  ( -9.474510206698720793, -16.51473224551083518, 69.58442372801901854 ) ) ;
#156200=CARTESIAN_POINT ( 'NONE',  ( 4.483927247898790824, -16.52544592524335698, 110.2094237280190185 ) ) ;
#156201=CARTESIAN_POINT ( 'NONE',  ( -18.67979575497178146, -10.72451020669898902, 76.66557627198103830 ) ) ;
#156202=CARTESIAN_POINT ( 'NONE',  ( 21.52544592524344225, -5.823673210054117533, 23.54057627198102765 ) ) ;
#156203=CARTESIAN_POINT ( 'NONE',  ( 8.224510206698953496, -14.34966873604960469, 57.91557627198103120 ) ) ;
#156204=CARTESIAN_POINT ( 'NONE',  ( 16.51473224551069308, 9.474510206698969483, 34.16557627198102409 ) ) ;
#156205=CARTESIAN_POINT ( 'NONE',  ( -9.564922557960796823, -16.46253265017161027, 32.08224293864769550 ) ) ;
#156206=CARTESIAN_POINT ( 'NONE',  ( -5.049401038297874678, -19.05341960407617918, 29.79275706135232227 ) ) ;
#156207=CARTESIAN_POINT ( 'NONE',  ( -16.55341960407617563, 4.379528057220093196, 88.54275706135236135 ) ) ;
#156208=CARTESIAN_POINT ( 'NONE',  ( 14.29746914071037800, 8.314922557961029526, 51.66775706135234714 ) ) ;
#156209=CARTESIAN_POINT ( 'NONE',  ( -21.53943276465977519, 0.05219959533907696930, 21.24890960531436690 ) ) ;
#156210=CARTESIAN_POINT ( 'NONE',  ( 19.02544592524343514, -5.153800228976328945, 53.54057627198102409 ) ) ;
#156211=CARTESIAN_POINT ( 'NONE',  ( -18.67979575497193778, 10.72451020669871902, 103.3344237280190043 ) ) ;
#156212=CARTESIAN_POINT ( 'NONE',  ( -13.97604488694527625, -13.89961937509977652, 76.87390960531433848 ) ) ;
#156213=CARTESIAN_POINT ( 'NONE',  ( 16.55341960407618274, -4.379528057220086978, 61.04275706135234714 ) ) ;
#156214=CARTESIAN_POINT ( 'NONE',  ( 12.14591786802309770, 12.06949235617756955, 104.3739096053143669 ) ) ;
#156215=CARTESIAN_POINT ( 'NONE',  ( -4.379528057220328563, 16.55341960407611168, 25.20724293864769550 ) ) ;
#156216=CARTESIAN_POINT ( 'NONE',  ( -17.72696623605164135, 5.499999999999875655, 38.59811031808416004 ) ) ;
#156217=CARTESIAN_POINT ( 'NONE',  ( -5.823673210054431948, 21.52544592524334988, 67.70942372801901854 ) ) ;
#156218=CARTESIAN_POINT ( 'NONE',  ( -9.564922557960796823, -16.46253265017161027, 87.08224293864769550 ) ) ;
#156219=CARTESIAN_POINT ( 'NONE',  ( -9.564922557960796823, -16.46253265017161027, 72.08224293864770971 ) ) ;
#156220=CARTESIAN_POINT ( 'NONE',  ( 19.05341960407611168, 5.049401038298154454, 108.9572429386477097 ) ) ;
#156221=CARTESIAN_POINT ( 'NONE',  ( 4.483927247898545687, 16.52544592524342804, 54.79057627198104541 ) ) ;
#156222=CARTESIAN_POINT ( 'NONE',  ( 8.314922557961029526, -14.29746914071037800, 110.4177570613523756 ) ) ;
#156224=CARTESIAN_POINT ( 'NONE',  ( 16.52544592524342804, -4.483927247898539470, 33.54057627198102409 ) ) ;
#156225=CARTESIAN_POINT ( 'NONE',  ( -16.52544592524335698, -4.483927247898792601, 38.95942372801901854 ) ) ;
#156227=CARTESIAN_POINT ( 'NONE',  ( -5.049401038297874678, -19.05341960407617918, 34.79275706135233293 ) ) ;
#156228=CARTESIAN_POINT ( 'NONE',  ( 19.05341960407611168, 5.049401038298154454, 78.95724293864769550 ) ) ;
#156229=CARTESIAN_POINT ( 'NONE',  ( -16.51473224551082808, 9.474510206698731452, 53.33442372801900433 ) ) ;
#156231=CARTESIAN_POINT ( 'NONE',  ( -9.474510206698720793, -16.51473224551083518, 94.58442372801900433 ) ) ;
#156232=CARTESIAN_POINT ( 'NONE',  ( -16.52544592524335698, -4.483927247898792601, 78.95942372801901854 ) ) ;
#156233=CARTESIAN_POINT ( 'NONE',  ( -19.05341960407611168, -5.049401038298163336, 31.45724293864769550 ) ) ;
#156234=CARTESIAN_POINT ( 'NONE',  ( 19.02544592524343514, -5.153800228976328945, 103.5405762719809957 ) ) ;
#156235=CARTESIAN_POINT ( 'NONE',  ( -0.05219959533937732626, 21.53943276465977519, 42.50109039468567573 ) ) ;
#156236=CARTESIAN_POINT ( 'NONE',  ( -0.05219959533936034679, 19.03943276465977164, 87.50109039468567573 ) ) ;
#156237=DIRECTION ( 'NONE',  ( 0.000000000000000000, 1.000000000000000000, 0.000000000000000000 ) ) ;
#156238=CARTESIAN_POINT ( 'NONE',  ( 13.89961937509977652, -13.97604488694527269, 48.12390960531435979 ) ) ;
#156239=CARTESIAN_POINT ( 'NONE',  ( 19.03943276465977164, -0.05219959533909143690, 108.7489096053143527 ) ) ;
#156240=CARTESIAN_POINT ( 'NONE',  ( -16.55341960407611168, -4.379528057220339221, 56.45724293864768839 ) ) ;
#156241=CARTESIAN_POINT ( 'NONE',  ( -13.89961937509977652, 13.97604488694528158, 45.62390960531433848 ) ) ;
#156242=CARTESIAN_POINT ( 'NONE',  ( -16.51473224551069308, -9.474510206698971260, 66.66557627198102409 ) ) ;
#156243=CARTESIAN_POINT ( 'NONE',  ( 16.51473224551083163, -9.474510206698727899, 65.83442372801900433 ) ) ;
#156244=CARTESIAN_POINT ( 'NONE',  ( 16.51473224551083163, -9.474510206698727899, 30.83442372801900433 ) ) ;
#156245=CARTESIAN_POINT ( 'NONE',  ( 9.564922557961047289, -16.46253265017146816, 45.41775706135232582 ) ) ;
#156246=CARTESIAN_POINT ( 'NONE',  ( -16.51473224551069308, -9.474510206698971260, 81.66557627198103830 ) ) ;
#156247=CARTESIAN_POINT ( 'NONE',  ( 21.53943276465977519, -0.05219959533907433946, 73.74890960531433848 ) ) ;
#156248=CARTESIAN_POINT ( 'NONE',  ( -8.314922557960811034, -14.29746914071050412, 67.08224293864770971 ) ) ;
#156249=CARTESIAN_POINT ( 'NONE',  ( -9.474510206698720793, -16.51473224551083518, 34.58442372801899722 ) ) ;
#156250=CARTESIAN_POINT ( 'NONE',  ( 0.05219959533907565091, 21.53943276465977519, 49.99890960531437401 ) ) ;
#156251=CARTESIAN_POINT ( 'NONE',  ( 21.52544592524344225, -5.823673210054117533, 38.54057627198103120 ) ) ;
#156252=CARTESIAN_POINT ( 'NONE',  ( 0.05219959533909260263, 19.03943276465977164, 69.99890960531435269 ) ) ;
#156253=CARTESIAN_POINT ( 'NONE',  ( -13.89961937509977652, 13.97604488694528158, 35.62390960531435269 ) ) ;
#156254=CARTESIAN_POINT ( 'NONE',  ( 4.483927247898545687, 16.52544592524342804, 94.79057627198105251 ) ) ;
#156255=CARTESIAN_POINT ( 'NONE',  ( 21.53943276465977519, -0.05219959533907433946, 113.7489096053143527 ) ) ;
#156256=CARTESIAN_POINT ( 'NONE',  ( 19.03943276465977164, -0.05219959533909143690, 108.7489096053143527 ) ) ;
#156257=CARTESIAN_POINT ( 'NONE',  ( -5.719274019375665041, -21.55341960407619695, 29.79275706135234358 ) ) ;
#156258=CARTESIAN_POINT ( 'NONE',  ( -16.46253265017160317, 9.564922557960807481, 40.83224293864769550 ) ) ;
#156259=CARTESIAN_POINT ( 'NONE',  ( 21.55341960407610458, 5.719274019375980345, 108.9572429386476955 ) ) ;
#156260=CARTESIAN_POINT ( 'NONE',  ( -0.05219959533936034679, 19.03943276465977164, 52.50109039468566863 ) ) ;
#156261=CARTESIAN_POINT ( 'NONE',  ( 19.05341960407611168, 5.049401038298154454, 28.95724293864769550 ) ) ;
#156262=B_SPLINE_CURVE_WITH_KNOTS ( 'NONE', 3,
 ( #117266, #131430, #177954, #98067, #39422, #79196, #67758, #140865, #9101, #64035, #115269, #161772, #159766, #48872, #85925, #2354, #52588, #147614, #132436, #194128, #125705, #21261, #110527, #55591, #178959, #82916, #144594, #130412, #6080, #129416, #114248, #175954 ),
 .UNSPECIFIED., .F., .F.,
 ( 4, 2, 2, 2, 2, 2, 2, 2, 2, 2, 2, 2, 2, 2, 2, 4 ),
 ( 2.883244014823444873E-17, 0.0003712461730037102509, 0.0007424923460073916620, 0.001113738519011073019, 0.001484984692014754484, 0.002227477038022119150, 0.002598723211025801699, 0.002969969384029484249, 0.003341215557033166798, 0.003712461730036849782, 0.004083707903040531897, 0.004454954076044214881, 0.004826200249047897864, 0.005197446422051580847, 0.005568692595055262963, 0.005939938768058946814 ),
 .UNSPECIFIED. ) ;
#156263=CARTESIAN_POINT ( 'NONE',  ( -16.51473224551069308, -9.474510206698971260, 21.66557627198102765 ) ) ;
#156265=CARTESIAN_POINT ( 'NONE',  ( 12.06949235617739724, 12.14591786802326823, 56.87609039468568994 ) ) ;
#156266=CARTESIAN_POINT ( 'NONE',  ( -9.564922557960796823, -16.46253265017161027, 32.08224293864769550 ) ) ;
#156268=CARTESIAN_POINT ( 'NONE',  ( -16.51473224551069308, -9.474510206698971260, 76.66557627198103830 ) ) ;
#156269=CARTESIAN_POINT ( 'NONE',  ( -4.379528057220328563, 16.55341960407611168, 105.2072429386477097 ) ) ;
#156270=CARTESIAN_POINT ( 'NONE',  ( -21.53943276465977519, 0.05219959533907696930, 41.24890960531435269 ) ) ;
#156271=CARTESIAN_POINT ( 'NONE',  ( -8.224510206698948167, 14.34966873604960824, 80.41557627198103830 ) ) ;
#156272=CARTESIAN_POINT ( 'NONE',  ( 8.224510206698742110, 14.34966873604972548, 37.08442372801901143 ) ) ;
#156273=CARTESIAN_POINT ( 'NONE',  ( 21.55341960407619695, -5.719274019375665929, 81.04275706135236135 ) ) ;
#156275=CARTESIAN_POINT ( 'NONE',  ( -13.97604488694527625, -13.89961937509977652, 21.87390960531435979 ) ) ;
#156276=CARTESIAN_POINT ( 'NONE',  ( 16.55341960407611168, 4.379528057220329451, 23.95724293864769550 ) ) ;
#156277=CARTESIAN_POINT ( 'NONE',  ( -16.53943276465976808, 0.05219959533911058130, 51.24890960531436690 ) ) ;
#156278=CARTESIAN_POINT ( 'NONE',  ( 19.05341960407611168, 5.049401038298154454, 48.95724293864768129 ) ) ;
#156279=CARTESIAN_POINT ( 'NONE',  ( 5.719274019375673035, 21.55341960407619339, 97.29275706135234714 ) ) ;
#156280=CARTESIAN_POINT ( 'NONE',  ( 21.52544592524344225, -5.823673210054117533, 108.5405762719810241 ) ) ;
#156281=CARTESIAN_POINT ( 'NONE',  ( -21.53943276465977519, -0.05219959533937600094, 78.75109039468568994 ) ) ;
#156282=CARTESIAN_POINT ( 'NONE',  ( 14.34966873604972726, -8.224510206698740333, 40.83442372801901854 ) ) ;
#156283=CARTESIAN_POINT ( 'NONE',  ( 14.34966873604960469, 8.224510206698951720, 84.16557627198103830 ) ) ;
#156284=CARTESIAN_POINT ( 'NONE',  ( -10.81492255796105439, 18.62759615963255655, 82.91775706135234714 ) ) ;
#156286=CARTESIAN_POINT ( 'NONE',  ( -14.29746914071037622, -8.314922557961029526, 109.1677570613523613 ) ) ;
#156287=CARTESIAN_POINT ( 'NONE',  ( 4.379528057220092307, 16.55341960407617563, 37.29275706135235424 ) ) ;
#156288=CARTESIAN_POINT ( 'NONE',  ( -8.314922557960811034, -14.29746914071050412, 42.08224293864769550 ) ) ;
#156289=CARTESIAN_POINT ( 'NONE',  ( -14.34966873604972548, 8.224510206698743886, 83.33442372801903275 ) ) ;
#156290=CARTESIAN_POINT ( 'NONE',  ( -19.05341960407611168, -5.049401038298163336, 96.45724293864769550 ) ) ;
#156291=CARTESIAN_POINT ( 'NONE',  ( -16.51473224551069308, -9.474510206698971260, 96.66557627198102409 ) ) ;
#156292=CARTESIAN_POINT ( 'NONE',  ( 15.80617190586769283, -15.72974639402175789, 105.6260903946856899 ) ) ;
#156293=CARTESIAN_POINT ( 'NONE',  ( 8.314922557961029526, -14.29746914071037800, 100.4177570613523471 ) ) ;
#156294=CARTESIAN_POINT ( 'NONE',  ( -4.483927247898539470, -16.52544592524342804, 72.29057627198102409 ) ) ;
#156295=CARTESIAN_POINT ( 'NONE',  ( -13.97604488694527625, -13.89961937509977652, 81.87390960531436690 ) ) ;
#156297=CARTESIAN_POINT ( 'NONE',  ( 8.224510206698742110, 14.34966873604972548, 32.08442372801901854 ) ) ;
#156298=CARTESIAN_POINT ( 'NONE',  ( 19.03943276465977164, -0.05219959533909143690, 28.74890960531435624 ) ) ;
#156299=CARTESIAN_POINT ( 'NONE',  ( -0.05219959533909027116, -19.03943276465977164, 92.49890960531436690 ) ) ;
#156300=CARTESIAN_POINT ( 'NONE',  ( -4.379528057220086978, -16.55341960407618274, 29.79275706135234358 ) ) ;
#156302=CARTESIAN_POINT ( 'NONE',  ( 5.049401038297881783, 19.05341960407617563, 32.29275706135233293 ) ) ;
#156303=CARTESIAN_POINT ( 'NONE',  ( -16.55341960407617563, 4.379528057220093196, 98.54275706135234714 ) ) ;
#156304=CARTESIAN_POINT ( 'NONE',  ( -19.03943276465977164, -0.05219959533935918106, 108.7510903946856615 ) ) ;
#156305=CARTESIAN_POINT ( 'NONE',  ( -9.474510206698964154, 16.51473224551069663, 35.41557627198102409 ) ) ;
#156306=CARTESIAN_POINT ( 'NONE',  ( -14.34966873604972548, 8.224510206698743886, 78.33442372801901854 ) ) ;
#156307=CARTESIAN_POINT ( 'NONE',  ( -4.483927247898782831, 16.52544592524335698, 62.70942372801902565 ) ) ;
#156308=CARTESIAN_POINT ( 'NONE',  ( -5.049401038298153566, 19.05341960407611168, 30.20724293864768839 ) ) ;
#156309=CARTESIAN_POINT ( 'NONE',  ( -9.474510206698720793, -16.51473224551083518, 69.58442372801901854 ) ) ;
#156310=CARTESIAN_POINT ( 'NONE',  ( -21.55341960407619339, 5.719274019375674811, 108.5427570613523756 ) ) ;
#156311=CARTESIAN_POINT ( 'NONE',  ( 19.03943276465977164, -0.05219959533909143690, 53.74890960531436690 ) ) ;
#156312=CARTESIAN_POINT ( 'NONE',  ( -9.474510206698964154, 16.51473224551069663, 90.41557627198103830 ) ) ;
#156313=CARTESIAN_POINT ( 'NONE',  ( 8.224510206698953496, -14.34966873604960469, 82.91557627198103830 ) ) ;
#156315=CARTESIAN_POINT ( 'NONE',  ( 9.564922557961047289, -16.46253265017146816, 60.41775706135233293 ) ) ;
#156316=CARTESIAN_POINT ( 'NONE',  ( -0.05219959533907301413, -21.53943276465977519, 47.49890960531435979 ) ) ;
#156317=CARTESIAN_POINT ( 'NONE',  ( 10.81492255796106328, -18.62759615963255655, 110.4177570613523756 ) ) ;
#156318=CARTESIAN_POINT ( 'NONE',  ( 19.03943276465977164, -0.05219959533909143690, 93.74890960531435269 ) ) ;
#156320=CARTESIAN_POINT ( 'NONE',  ( 16.46253265017146816, 9.564922557961045513, 26.66775706135234003 ) ) ;
#156321=CARTESIAN_POINT ( 'NONE',  ( 10.72451020669898902, -18.67979575497178502, 62.91557627198102409 ) ) ;
#156322=CARTESIAN_POINT ( 'NONE',  ( -5.049401038298153566, 19.05341960407611168, 105.2072429386476671 ) ) ;
#156323=CARTESIAN_POINT ( 'NONE',  ( -0.05219959533936034679, 19.03943276465977164, 87.50109039468567573 ) ) ;
#156325=CARTESIAN_POINT ( 'NONE',  ( -0.05219959533936034679, 19.03943276465977164, 112.5010903946856757 ) ) ;
#156326=CARTESIAN_POINT ( 'NONE',  ( -8.314922557960811034, -14.29746914071050412, 112.0822429386477097 ) ) ;
#156327=CARTESIAN_POINT ( 'NONE',  ( -5.049401038298153566, 19.05341960407611168, 95.20724293864770971 ) ) ;
#156328=CARTESIAN_POINT ( 'NONE',  ( 5.719274019375991003, -21.55341960407610458, 77.70724293864770971 ) ) ;
#156329=CARTESIAN_POINT ( 'NONE',  ( -4.379528057220086978, -16.55341960407618274, 49.79275706135234714 ) ) ;
#156330=CARTESIAN_POINT ( 'NONE',  ( -21.55341960407619339, 5.719274019375674811, 48.54275706135234714 ) ) ;
#156331=CARTESIAN_POINT ( 'NONE',  ( 10.72451020669871369, 18.67979575497193778, 97.08442372801904696 ) ) ;
#156332=CARTESIAN_POINT ( 'NONE',  ( 14.34966873604972726, -8.224510206698740333, 95.83442372801903275 ) ) ;
#156333=CARTESIAN_POINT ( 'NONE',  ( 16.51473224551069308, 9.474510206698969483, 84.16557627198102409 ) ) ;
#156334=CARTESIAN_POINT ( 'NONE',  ( -4.483927247898539470, -16.52544592524342804, 97.29057627198105251 ) ) ;
#156335=CARTESIAN_POINT ( 'NONE',  ( -16.52544592524342804, 4.483927247898546575, 31.04057627198102409 ) ) ;
#156336=CARTESIAN_POINT ( 'NONE',  ( 13.89961937509957401, 13.97604488694547697, 71.87609039468567573 ) ) ;
#156337=CARTESIAN_POINT ( 'NONE',  ( 21.53943276465977519, 0.05219959533937863772, 46.25109039468567573 ) ) ;
#156338=CARTESIAN_POINT ( 'NONE',  ( 9.564922557961047289, -16.46253265017146816, 25.41775706135234003 ) ) ;
#156339=CARTESIAN_POINT ( 'NONE',  ( -8.314922557960811034, -14.29746914071050412, 92.08224293864769550 ) ) ;
#156340=CARTESIAN_POINT ( 'NONE',  ( 5.823673210054125526, 21.52544592524343514, 34.79057627198103120 ) ) ;
#156341=CARTESIAN_POINT ( 'NONE',  ( 12.14591786802309770, 12.06949235617756955, 29.37390960531435269 ) ) ;
#156342=CARTESIAN_POINT ( 'NONE',  ( 21.55341960407619695, -5.719274019375665929, 81.04275706135236135 ) ) ;
#156343=CARTESIAN_POINT ( 'NONE',  ( -8.224510206698735004, -14.34966873604973081, 64.58442372801900433 ) ) ;
#156344=CARTESIAN_POINT ( 'NONE',  ( 0.05219959533934541429, -16.53943276465976808, 105.0010903946856757 ) ) ;
#156345=CARTESIAN_POINT ( 'NONE',  ( -21.53943276465977519, -0.05219959533937600094, 48.75109039468568284 ) ) ;
#156347=CARTESIAN_POINT ( 'NONE',  ( 21.55341960407619695, -5.719274019375665929, 36.04275706135234714 ) ) ;
#156348=CARTESIAN_POINT ( 'NONE',  ( 12.06949235617757843, -12.14591786802309237, 108.1239096053143811 ) ) ;
#156349=CARTESIAN_POINT ( 'NONE',  ( -19.03943276465977164, 0.05219959533909376836, 26.24890960531435624 ) ) ;
#156350=CARTESIAN_POINT ( 'NONE',  ( -4.379528057220328563, 16.55341960407611168, 60.20724293864768839 ) ) ;
#156351=CARTESIAN_POINT ( 'NONE',  ( -19.02544592524342804, 5.153800228976336051, 76.04057627198102409 ) ) ;
#156352=CARTESIAN_POINT ( 'NONE',  ( 16.55341960407618274, -4.379528057220086978, 106.0427570613523471 ) ) ;
#156353=CARTESIAN_POINT ( 'NONE',  ( -21.53943276465977519, 0.05219959533907696930, 56.24890960531436690 ) ) ;
#156354=CARTESIAN_POINT ( 'NONE',  ( 12.06949235617757843, -12.14591786802309237, 98.12390960531436690 ) ) ;
#156355=CARTESIAN_POINT ( 'NONE',  ( -18.67979575497178146, -10.72451020669898902, 91.66557627198103830 ) ) ;
#156356=CARTESIAN_POINT ( 'NONE',  ( -5.049401038298153566, 19.05341960407611168, 95.20724293864770971 ) ) ;
#156357=CARTESIAN_POINT ( 'NONE',  ( -16.46253265017160317, 9.564922557960807481, 55.83224293864769550 ) ) ;
#156358=CARTESIAN_POINT ( 'NONE',  ( 16.51473224551083163, -9.474510206698727899, 100.8344237280190043 ) ) ;
#156359=CARTESIAN_POINT ( 'NONE',  ( 15.72974639402199770, -15.80617190586745480, 43.12390960531435269 ) ) ;
#156360=CARTESIAN_POINT ( 'NONE',  ( 5.719274019375673035, 21.55341960407619339, 62.29275706135236845 ) ) ;
#156361=CARTESIAN_POINT ( 'NONE',  ( 19.05341960407611168, 5.049401038298154454, 53.95724293864770260 ) ) ;
#156362=CARTESIAN_POINT ( 'NONE',  ( 13.97604488694527802, 13.89961937509977652, 84.37390960531433848 ) ) ;
#156363=CARTESIAN_POINT ( 'NONE',  ( 4.379528057220092307, 16.55341960407617563, 57.29275706135234714 ) ) ;
#156364=CARTESIAN_POINT ( 'NONE',  ( -10.72451020669870658, -18.67979575497194134, 39.58442372801901143 ) ) ;
#156365=CARTESIAN_POINT ( 'NONE',  ( 15.80617190586769283, -15.72974639402175789, 85.62609039468568994 ) ) ;
#156366=CARTESIAN_POINT ( 'NONE',  ( -10.81492255796078084, -18.62759615963271287, 102.0822429386476955 ) ) ;
#156367=CARTESIAN_POINT ( 'NONE',  ( -18.67979575497193778, 10.72451020669871902, 33.33442372801900433 ) ) ;
#156368=CARTESIAN_POINT ( 'NONE',  ( -4.379528057220086978, -16.55341960407618274, 69.79275706135234714 ) ) ;
#156369=CARTESIAN_POINT ( 'NONE',  ( 21.52544592524344225, -5.823673210054117533, 73.54057627198102409 ) ) ;
#156370=CARTESIAN_POINT ( 'NONE',  ( -5.049401038297874678, -19.05341960407617918, 39.79275706135232582 ) ) ;
#156371=CARTESIAN_POINT ( 'NONE',  ( 16.51473224551069308, 9.474510206698969483, 64.16557627198102409 ) ) ;
#156372=CARTESIAN_POINT ( 'NONE',  ( -0.05219959533910754901, -16.53943276465976808, 27.49890960531435269 ) ) ;
#156374=CARTESIAN_POINT ( 'NONE',  ( -13.97604488694527625, -13.89961937509977652, 96.87390960531433848 ) ) ;
#156375=CARTESIAN_POINT ( 'NONE',  ( -9.474510206698720793, -16.51473224551083518, 84.58442372801900433 ) ) ;
#156376=CARTESIAN_POINT ( 'NONE',  ( -10.72451020669898014, 18.67979575497178502, 60.41557627198102409 ) ) ;
#156377=CARTESIAN_POINT ( 'NONE',  ( 8.314922557960818139, 14.29746914071049879, 34.58224293864770260 ) ) ;
#156378=CARTESIAN_POINT ( 'NONE',  ( -16.52544592524335698, -4.483927247898792601, 18.95942372801901143 ) ) ;
#156379=CARTESIAN_POINT ( 'NONE',  ( 5.153800228976335163, 19.02544592524342804, 29.79057627198102409 ) ) ;
#156380=CARTESIAN_POINT ( 'NONE',  ( 19.02544592524334988, 5.153800228976608722, 111.4594237280190043 ) ) ;
#156381=CARTESIAN_POINT ( 'NONE',  ( 15.72974639402199770, -15.80617190586745480, 98.12390960531436690 ) ) ;
#156382=CARTESIAN_POINT ( 'NONE',  ( -0.05219959533936034679, 19.03943276465977164, 72.50109039468566152 ) ) ;
#156383=CARTESIAN_POINT ( 'NONE',  ( 16.52544592524335698, 4.483927247898782831, 76.45942372801901854 ) ) ;
#156384=CARTESIAN_POINT ( 'NONE',  ( -13.89961937509977652, 13.97604488694528158, 70.62390960531432427 ) ) ;
#156385=CARTESIAN_POINT ( 'NONE',  ( 4.379528057220339221, -16.55341960407611168, 77.70724293864770971 ) ) ;
#156387=CARTESIAN_POINT ( 'NONE',  ( 5.153800228976335163, 19.02544592524342804, 54.79057627198103120 ) ) ;
#156388=CARTESIAN_POINT ( 'NONE',  ( 16.52544592524342804, -4.483927247898539470, 63.54057627198103830 ) ) ;
#156389=CARTESIAN_POINT ( 'NONE',  ( 9.474510206698971260, -16.51473224551069308, 22.91557627198102765 ) ) ;
#156390=CARTESIAN_POINT ( 'NONE',  ( -17.29957754486504129, -5.500000000000000888, 21.12734848878977445 ) ) ;
#156391=CARTESIAN_POINT ( 'NONE',  ( 16.53943276465976808, -0.05219959533910856209, 38.74890960531435979 ) ) ;
#156392=CARTESIAN_POINT ( 'NONE',  ( 19.02544592524343514, -5.153800228976328945, 83.54057627198100988 ) ) ;
#156394=CARTESIAN_POINT ( 'NONE',  ( 9.564922557961047289, -16.46253265017146816, 40.41775706135234003 ) ) ;
#156395=CARTESIAN_POINT ( 'NONE',  ( -8.224510206698735004, -14.34966873604973081, 44.58442372801901854 ) ) ;
#156396=CARTESIAN_POINT ( 'NONE',  ( -10.72451020669898014, 18.67979575497178502, 65.41557627198102409 ) ) ;
#156397=CARTESIAN_POINT ( 'NONE',  ( -9.564922557961040184, 16.46253265017147172, 22.91775706135233648 ) ) ;
#156398=CARTESIAN_POINT ( 'NONE',  ( 5.049401038298161559, -19.05341960407611168, 77.70724293864765286 ) ) ;
#156400=CARTESIAN_POINT ( 'NONE',  ( -19.02544592524342804, 5.153800228976336051, 106.0405762719810241 ) ) ;
#156401=CARTESIAN_POINT ( 'NONE',  ( 10.72451020669871369, 18.67979575497193778, 32.08442372801901854 ) ) ;
#156402=CARTESIAN_POINT ( 'NONE',  ( -4.379528057220328563, 16.55341960407611168, 110.2072429386477239 ) ) ;
#156403=CARTESIAN_POINT ( 'NONE',  ( -15.72974639402197994, 15.80617190586746368, 100.6239096053143811 ) ) ;
#156404=CARTESIAN_POINT ( 'NONE',  ( 5.153800228976335163, 19.02544592524342804, 84.79057627198099567 ) ) ;
#156406=CARTESIAN_POINT ( 'NONE',  ( -5.823673210054431948, 21.52544592524334988, 22.70942372801901499 ) ) ;
#156410=CARTESIAN_POINT ( 'NONE',  ( -13.89961937509977652, 13.97604488694528158, 85.62390960531433848 ) ) ;
#156412=CARTESIAN_POINT ( 'NONE',  ( 10.81492255796078972, 18.62759615963270932, 94.58224293864769550 ) ) ;
#156413=CARTESIAN_POINT ( 'NONE',  ( 5.049401038298161559, -19.05341960407611168, 32.70724293864768129 ) ) ;
#156414=CARTESIAN_POINT ( 'NONE',  ( -19.05341960407617563, 5.049401038297882671, 103.5427570613523329 ) ) ;
#156417=CARTESIAN_POINT ( 'NONE',  ( 0.05219959533909260263, 19.03943276465977164, 29.99890960531435979 ) ) ;
#156418=CARTESIAN_POINT ( 'NONE',  ( 5.719274019375673035, 21.55341960407619339, 87.29275706135236135 ) ) ;
#156419=CARTESIAN_POINT ( 'NONE',  ( -9.564922557960796823, -16.46253265017161027, 77.08224293864769550 ) ) ;
#156420=CARTESIAN_POINT ( 'NONE',  ( -21.53943276465977519, -0.05219959533937600094, 43.75109039468568284 ) ) ;
#156421=CARTESIAN_POINT ( 'NONE',  ( -5.823673210054431948, 21.52544592524334988, 32.70942372801900433 ) ) ;
#156423=CARTESIAN_POINT ( 'NONE',  ( -19.02544592524342804, 5.153800228976336051, 86.04057627198103830 ) ) ;
#156424=CARTESIAN_POINT ( 'NONE',  ( 19.34837522270365895, 5.499999999999733546, 63.36337684832578532 ) ) ;
#156425=CARTESIAN_POINT ( 'NONE',  ( 16.53943276465976808, 0.05219959533934440121, 36.25109039468567573 ) ) ;
#156426=CARTESIAN_POINT ( 'NONE',  ( -10.81492255796078084, -18.62759615963271287, 42.08224293864769550 ) ) ;
#156427=CARTESIAN_POINT ( 'NONE',  ( 21.55341960407619695, -5.719274019375665929, 46.04275706135234714 ) ) ;
#156428=CARTESIAN_POINT ( 'NONE',  ( 15.80617190586769283, -15.72974639402175789, 75.62609039468567573 ) ) ;
#156431=CARTESIAN_POINT ( 'NONE',  ( 19.02544592524334988, 5.153800228976608722, 106.4594237280190185 ) ) ;
#156432=CARTESIAN_POINT ( 'NONE',  ( -16.51473224551069308, -9.474510206698971260, 61.66557627198103120 ) ) ;
#156433=CARTESIAN_POINT ( 'NONE',  ( 13.97604488694527802, 13.89961937509977652, 89.37390960531436690 ) ) ;
#156434=CARTESIAN_POINT ( 'NONE',  ( 16.52544592524342804, -4.483927247898539470, 113.5405762719810383 ) ) ;
#156435=CARTESIAN_POINT ( 'NONE',  ( -16.52544592524342804, 4.483927247898546575, 111.0405762719810525 ) ) ;
#156436=CARTESIAN_POINT ( 'NONE',  ( 19.03943276465977164, -0.05219959533909143690, 108.7489096053143527 ) ) ;
#156438=CARTESIAN_POINT ( 'NONE',  ( -16.52544592524335698, -4.483927247898792601, 83.95942372801900433 ) ) ;
#156439=CARTESIAN_POINT ( 'NONE',  ( -16.52544592524342804, 4.483927247898546575, 71.04057627198103830 ) ) ;
#156440=CARTESIAN_POINT ( 'NONE',  ( 16.46253265017160672, -9.564922557960803928, 48.33224293864769550 ) ) ;
#156441=CARTESIAN_POINT ( 'NONE',  ( -21.53943276465977519, -0.05219959533937600094, 83.75109039468568994 ) ) ;
#156442=CARTESIAN_POINT ( 'NONE',  ( 10.81492255796106328, -18.62759615963255655, 65.41775706135234714 ) ) ;
#156443=CARTESIAN_POINT ( 'NONE',  ( 9.564922557961047289, -16.46253265017146816, 110.4177570613523471 ) ) ;
#156444=CARTESIAN_POINT ( 'NONE',  ( 16.53943276465976808, -0.05219959533910856209, 58.74890960531436690 ) ) ;
#156445=CARTESIAN_POINT ( 'NONE',  ( -10.81492255796078084, -18.62759615963271287, 112.0822429386477097 ) ) ;
#156446=CARTESIAN_POINT ( 'NONE',  ( 10.72451020669898902, -18.67979575497178502, 57.91557627198103120 ) ) ;
#156447=CARTESIAN_POINT ( 'NONE',  ( -16.52216118717204552, -7.221426719304545827, 106.0759902104699250 ) ) ;
#156449=CARTESIAN_POINT ( 'NONE',  ( 19.05341960407611168, 5.049401038298154454, 68.95724293864769550 ) ) ;
#156450=CARTESIAN_POINT ( 'NONE',  ( 8.224510206698953496, -14.34966873604960469, 42.91557627198103120 ) ) ;
#156451=AXIS2_PLACEMENT_3D ( 'NONE', #195038, #10021, #160686 ) ;
#156452=CARTESIAN_POINT ( 'NONE',  ( -4.483927247898782831, 16.52544592524335698, 112.7094237280190328 ) ) ;
#156453=CARTESIAN_POINT ( 'NONE',  ( 16.55341960407618274, -4.379528057220086978, 101.0427570613523756 ) ) ;
#156454=CARTESIAN_POINT ( 'NONE',  ( 13.89961937509957401, 13.97604488694547697, 51.87609039468566863 ) ) ;
#156456=CARTESIAN_POINT ( 'NONE',  ( 19.03943276465977164, -0.05219959533909143690, 93.74890960531435269 ) ) ;
#156457=CARTESIAN_POINT ( 'NONE',  ( 4.379528057220339221, -16.55341960407611168, 62.70724293864769550 ) ) ;
#156458=CARTESIAN_POINT ( 'NONE',  ( 16.36317988757058473, -7.306389748694911646, 101.5978960836322642 ) ) ;
#156459=CARTESIAN_POINT ( 'NONE',  ( -0.05219959533909027116, -19.03943276465977164, 112.4989096053143669 ) ) ;
#156460=CARTESIAN_POINT ( 'NONE',  ( 21.55341960407610458, 5.719274019375980345, 53.95724293864770260 ) ) ;
#156461=CARTESIAN_POINT ( 'NONE',  ( 4.379528057220339221, -16.55341960407611168, 97.70724293864772392 ) ) ;
#156462=CARTESIAN_POINT ( 'NONE',  ( 12.14591786802327356, -12.06949235617739191, 45.62609039468567573 ) ) ;
#156463=CARTESIAN_POINT ( 'NONE',  ( 4.379528057220339221, -16.55341960407611168, 97.70724293864772392 ) ) ;
#156465=CARTESIAN_POINT ( 'NONE',  ( -13.89961937509957401, -13.97604488694547875, 79.37609039468567573 ) ) ;
#156466=CARTESIAN_POINT ( 'NONE',  ( 10.72451020669898902, -18.67979575497178502, 22.91557627198102765 ) ) ;
#156468=DIRECTION ( 'NONE',  ( -1.000000000000000000, -0.000000000000000000, -0.000000000000000000 ) ) ;
#156469=CARTESIAN_POINT ( 'NONE',  ( 8.224510206698742110, 14.34966873604972548, 47.08442372801901854 ) ) ;
#156470=CARTESIAN_POINT ( 'NONE',  ( 16.53943276465976808, -0.05219959533910856209, 33.74890960531436690 ) ) ;
#156471=CARTESIAN_POINT ( 'NONE',  ( 21.55341960407610458, 5.719274019375980345, 53.95724293864770260 ) ) ;
#156472=CARTESIAN_POINT ( 'NONE',  ( -9.474510206698720793, -16.51473224551083518, 84.58442372801900433 ) ) ;
#156473=CARTESIAN_POINT ( 'NONE',  ( 15.80617190586746368, 15.72974639402197994, 44.37390960531435979 ) ) ;
#156474=CARTESIAN_POINT ( 'NONE',  ( 15.80617190586769283, -15.72974639402175789, 80.62609039468567573 ) ) ;
#156476=CARTESIAN_POINT ( 'NONE',  ( -4.483927247898782831, 16.52544592524335698, 32.70942372801900433 ) ) ;
#156477=CARTESIAN_POINT ( 'NONE',  ( 5.153800228976335163, 19.02544592524342804, 39.79057627198100988 ) ) ;
#156478=CARTESIAN_POINT ( 'NONE',  ( 16.46253265017160672, -9.564922557960803928, 98.33224293864769550 ) ) ;
#156479=CARTESIAN_POINT ( 'NONE',  ( -19.05341960407611168, -5.049401038298163336, 36.45724293864766707 ) ) ;
#156480=CARTESIAN_POINT ( 'NONE',  ( 4.483927247898545687, 16.52544592524342804, 94.79057627198105251 ) ) ;
#156482=CARTESIAN_POINT ( 'NONE',  ( 16.46253265017160672, -9.564922557960803928, 103.3322429386476955 ) ) ;
#156483=ORIENTED_EDGE ( 'NONE', *, *, #177098, .T. ) ;
#156484=CARTESIAN_POINT ( 'NONE',  ( -8.224510206698735004, -14.34966873604973081, 54.58442372801901143 ) ) ;
#156485=CARTESIAN_POINT ( 'NONE',  ( -15.72974639402197994, 15.80617190586746368, 95.62390960531436690 ) ) ;
#156486=CARTESIAN_POINT ( 'NONE',  ( 9.474510206698971260, -16.51473224551069308, 42.91557627198103120 ) ) ;
#156487=CARTESIAN_POINT ( 'NONE',  ( -0.05219959533937732626, 21.53943276465977519, 27.50109039468567929 ) ) ;
#156488=CARTESIAN_POINT ( 'NONE',  ( -5.049401038298153566, 19.05341960407611168, 80.20724293864769550 ) ) ;
#156489=CARTESIAN_POINT ( 'NONE',  ( 5.153800228976335163, 19.02544592524342804, 114.7905762719810241 ) ) ;
#156491=CARTESIAN_POINT ( 'NONE',  ( -12.14591786802326823, 12.06949235617739902, 53.12609039468568284 ) ) ;
#156492=CARTESIAN_POINT ( 'NONE',  ( 21.52544592524334988, 5.823673210054432836, 21.45942372801901499 ) ) ;
#156493=CARTESIAN_POINT ( 'NONE',  ( 8.314922557960818139, 14.29746914071049879, 104.5822429386477097 ) ) ;
#156494=CARTESIAN_POINT ( 'NONE',  ( 9.564922557960805705, 16.46253265017160317, 99.58224293864770971 ) ) ;
#156495=CARTESIAN_POINT ( 'NONE',  ( -0.05219959533936034679, 19.03943276465977164, 77.50109039468566152 ) ) ;
#156496=CARTESIAN_POINT ( 'NONE',  ( 13.89961937509957401, 13.97604488694547697, 26.87609039468566507 ) ) ;
#156497=CARTESIAN_POINT ( 'NONE',  ( 5.719274019375991003, -21.55341960407610458, 82.70724293864770971 ) ) ;
#156498=CARTESIAN_POINT ( 'NONE',  ( 16.46253265017146816, 9.564922557961045513, 41.66775706135234003 ) ) ;
#156499=CARTESIAN_POINT ( 'NONE',  ( 12.06949235617739724, 12.14591786802326823, 81.87609039468568994 ) ) ;
#156500=CARTESIAN_POINT ( 'NONE',  ( -13.89961937509977652, 13.97604488694528158, 100.6239096053143669 ) ) ;
#156501=CARTESIAN_POINT ( 'NONE',  ( 9.474510206698971260, -16.51473224551069308, 62.91557627198102409 ) ) ;
#156502=CARTESIAN_POINT ( 'NONE',  ( 21.52544592524334988, 5.823673210054432836, 66.45942372801903275 ) ) ;
#156503=CARTESIAN_POINT ( 'NONE',  ( -18.62759615963255300, -10.81492255796106328, 69.16775706135234714 ) ) ;
#156504=CARTESIAN_POINT ( 'NONE',  ( 19.05341960407611168, 5.049401038298154454, 73.95724293864768129 ) ) ;
#156505=CARTESIAN_POINT ( 'NONE',  ( 15.72974639402176855, 15.80617190586768217, 51.87609039468568284 ) ) ;
#156507=CARTESIAN_POINT ( 'NONE',  ( -19.05341960407617563, 5.049401038297882671, 88.54275706135230450 ) ) ;
#156508=CARTESIAN_POINT ( 'NONE',  ( 5.153800228976335163, 19.02544592524342804, 49.79057627198100988 ) ) ;
#156509=CARTESIAN_POINT ( 'NONE',  ( 19.02544592524343514, -5.153800228976328945, 98.54057627198100988 ) ) ;
#156510=CARTESIAN_POINT ( 'NONE',  ( 19.02544592524343514, -5.153800228976328945, 63.54057627198103830 ) ) ;
#156511=CARTESIAN_POINT ( 'NONE',  ( 19.02544592524343514, -5.153800228976328945, 108.5405762719810383 ) ) ;
#156512=CARTESIAN_POINT ( 'NONE',  ( -19.02544592524342804, 5.153800228976336051, 46.04057627198101699 ) ) ;
#156514=CARTESIAN_POINT ( 'NONE',  ( 5.719274019375991003, -21.55341960407610458, 92.70724293864770971 ) ) ;
#156515=CARTESIAN_POINT ( 'NONE',  ( 8.314922557961029526, -14.29746914071037800, 70.41775706135236135 ) ) ;
#156517=CARTESIAN_POINT ( 'NONE',  ( 9.564922557961047289, -16.46253265017146816, 35.41775706135233293 ) ) ;
#156519=CARTESIAN_POINT ( 'NONE',  ( 9.564922557960805705, 16.46253265017160317, 69.58224293864770971 ) ) ;
#156520=CARTESIAN_POINT ( 'NONE',  ( 8.224510206698953496, -14.34966873604960469, 62.91557627198102409 ) ) ;
#156521=CARTESIAN_POINT ( 'NONE',  ( 4.483927247898545687, 16.52544592524342804, 99.79057627198103830 ) ) ;
#156522=CARTESIAN_POINT ( 'NONE',  ( -5.153800228976328057, -19.02544592524343514, 102.2905762719810383 ) ) ;
#156523=B_SPLINE_CURVE_WITH_KNOTS ( 'NONE', 3,
 ( #63452, #143254, #109951, #171631, #160435, #65429, #82576, #4738, #186826, #188799, #64446, #110938, #126116, #18949, #95769, #36083, #3752, #127090, #156458, #5744, #48295, #128088, #113908, #174618, #175607, #144257, #189792, #51263, #141280, #21925, #187811, #112923 ),
 .UNSPECIFIED., .F., .F.,
 ( 4, 2, 2, 2, 2, 2, 2, 2, 2, 2, 2, 2, 2, 2, 2, 4 ),
 ( 7.806255641895631925E-18, 0.0003712461730036603234, 0.0007424923460073128405, 0.001113738519010965249, 0.001484984692014617875, 0.002227477038021939172, 0.002598723211025618252, 0.002969969384029296899, 0.003341215557032975545, 0.003712461730036654625, 0.004083707903040333272, 0.004454954076044012785, 0.004826200249047691432, 0.005197446422051370078, 0.005568692595055048725, 0.005939938768058727371 ),
 .UNSPECIFIED. ) ;
#156524=CARTESIAN_POINT ( 'NONE',  ( -16.51473224551069308, -9.474510206698971260, 91.66557627198103830 ) ) ;
#156525=CARTESIAN_POINT ( 'NONE',  ( -5.719274019375665041, -21.55341960407619695, 49.79275706135234714 ) ) ;
#156526=CARTESIAN_POINT ( 'NONE',  ( 13.97604488694527802, 13.89961937509977652, 109.3739096053143669 ) ) ;
#156527=CARTESIAN_POINT ( 'NONE',  ( -16.51473224551082808, 9.474510206698731452, 23.33442372801900078 ) ) ;
#156528=CARTESIAN_POINT ( 'NONE',  ( 16.52544592524335698, 4.483927247898782831, 81.45942372801900433 ) ) ;
#156529=CARTESIAN_POINT ( 'NONE',  ( 18.67979575497194134, -10.72451020669871369, 40.83442372801901854 ) ) ;
#156530=CARTESIAN_POINT ( 'NONE',  ( -21.52544592524343514, 5.823673210054127303, 31.04057627198102409 ) ) ;
#156531=CARTESIAN_POINT ( 'NONE',  ( 18.67979575497178502, 10.72451020669898547, 99.16557627198100988 ) ) ;
#156532=CARTESIAN_POINT ( 'NONE',  ( -16.52544592524342804, 4.483927247898546575, 66.04057627198103830 ) ) ;
#156533=CARTESIAN_POINT ( 'NONE',  ( 9.564922557960805705, 16.46253265017160317, 49.58224293864770260 ) ) ;
#156534=CARTESIAN_POINT ( 'NONE',  ( 8.224510206698953496, -14.34966873604960469, 77.91557627198102409 ) ) ;
#156535=CARTESIAN_POINT ( 'NONE',  ( 10.72451020669898902, -18.67979575497178502, 47.91557627198102409 ) ) ;
#156536=CARTESIAN_POINT ( 'NONE',  ( -16.51473224551082808, 9.474510206698731452, 48.33442372801900433 ) ) ;
#156537=CARTESIAN_POINT ( 'NONE',  ( -19.03943276465977164, 0.05219959533909376836, 21.24890960531436335 ) ) ;
#156539=CARTESIAN_POINT ( 'NONE',  ( -8.224510206698735004, -14.34966873604973081, 69.58442372801900433 ) ) ;
#156540=CARTESIAN_POINT ( 'NONE',  ( 9.474510206698971260, -16.51473224551069308, 62.91557627198102409 ) ) ;
#156542=CARTESIAN_POINT ( 'NONE',  ( 16.53943276465976808, -0.05219959533910856209, 83.74890960531435269 ) ) ;
#156543=CARTESIAN_POINT ( 'NONE',  ( -0.05219959533907301413, -21.53943276465977519, 32.49890960531435979 ) ) ;
#156545=CARTESIAN_POINT ( 'NONE',  ( 8.314922557961029526, -14.29746914071037800, 110.4177570613523756 ) ) ;
#156546=CARTESIAN_POINT ( 'NONE',  ( 13.97604488694548053, -13.89961937509957401, 105.6260903946856757 ) ) ;
#156547=CARTESIAN_POINT ( 'NONE',  ( -21.52544592524334988, -5.823673210054445271, 73.95942372801901854 ) ) ;
#156548=CARTESIAN_POINT ( 'NONE',  ( 19.03943276465977164, -0.05219959533909143690, 93.74890960531435269 ) ) ;
#156549=CARTESIAN_POINT ( 'NONE',  ( -21.53943276465977519, 0.05219959533907696930, 101.2489096053143669 ) ) ;
#156550=CARTESIAN_POINT ( 'NONE',  ( 4.379528057220092307, 16.55341960407617563, 57.29275706135234714 ) ) ;
#156551=CARTESIAN_POINT ( 'NONE',  ( -9.564922557960796823, -16.46253265017161027, 27.08224293864769550 ) ) ;
#156552=CARTESIAN_POINT ( 'NONE',  ( -14.29746914071037622, -8.314922557961029526, 29.16775706135234003 ) ) ;
#156553=CARTESIAN_POINT ( 'NONE',  ( -19.05341960407617563, 5.049401038297882671, 88.54275706135230450 ) ) ;
#156554=CARTESIAN_POINT ( 'NONE',  ( 18.67979575497178502, 10.72451020669898547, 94.16557627198103830 ) ) ;
#156555=CARTESIAN_POINT ( 'NONE',  ( 19.05341960407617918, -5.049401038297876454, 71.04275706135234714 ) ) ;
#156557=CARTESIAN_POINT ( 'NONE',  ( -21.52544592524343514, 5.823673210054127303, 101.0405762719810383 ) ) ;
#156559=CARTESIAN_POINT ( 'NONE',  ( 9.474510206698971260, -16.51473224551069308, 77.91557627198103830 ) ) ;
#156561=CARTESIAN_POINT ( 'NONE',  ( 8.314922557961029526, -14.29746914071037800, 30.41775706135234358 ) ) ;
#156563=CARTESIAN_POINT ( 'NONE',  ( 19.02544592524334988, 5.153800228976608722, 56.45942372801898301 ) ) ;
#156564=CARTESIAN_POINT ( 'NONE',  ( 21.55341960407619695, -5.719274019375665929, 21.04275706135234714 ) ) ;
#156565=CARTESIAN_POINT ( 'NONE',  ( -4.483927247898539470, -16.52544592524342804, 62.29057627198102409 ) ) ;
#156566=CARTESIAN_POINT ( 'NONE',  ( 9.474510206698971260, -16.51473224551069308, 87.91557627198102409 ) ) ;
#156569=CARTESIAN_POINT ( 'NONE',  ( 8.224510206698742110, 14.34966873604972548, 42.08442372801901854 ) ) ;
#156571=CARTESIAN_POINT ( 'NONE',  ( -5.049401038297874678, -19.05341960407617918, 44.79275706135232582 ) ) ;
#156572=CARTESIAN_POINT ( 'NONE',  ( -10.81492255796105439, 18.62759615963255655, 52.91775706135235424 ) ) ;
#156573=CARTESIAN_POINT ( 'NONE',  ( 19.03943276465977164, 0.05219959533936151252, 111.2510903946856757 ) ) ;
#156574=CARTESIAN_POINT ( 'NONE',  ( 5.153800228976335163, 19.02544592524342804, 54.79057627198103120 ) ) ;
#156575=CARTESIAN_POINT ( 'NONE',  ( 19.02544592524334988, 5.153800228976608722, 76.45942372801897591 ) ) ;
#156576=CARTESIAN_POINT ( 'NONE',  ( -5.719274019375665041, -21.55341960407619695, 94.79275706135234714 ) ) ;
#156577=CARTESIAN_POINT ( 'NONE',  ( 19.02544592524334988, 5.153800228976608722, 61.45942372801900433 ) ) ;
#156578=CARTESIAN_POINT ( 'NONE',  ( 19.03943276465977164, -0.05219959533909143690, 38.74890960531436690 ) ) ;
#156579=CARTESIAN_POINT ( 'NONE',  ( -0.05219959533907301413, -21.53943276465977519, 67.49890960531436690 ) ) ;
#156580=CARTESIAN_POINT ( 'NONE',  ( -14.29746914071049879, 8.314922557960819915, 65.83224293864769550 ) ) ;
#156581=CARTESIAN_POINT ( 'NONE',  ( 9.564922557961047289, -16.46253265017146816, 70.41775706135233293 ) ) ;
#156582=CARTESIAN_POINT ( 'NONE',  ( -17.40805194822032220, -6.112264579159275790, 24.16628727489389306 ) ) ;
#156583=CARTESIAN_POINT ( 'NONE',  ( -5.153800228976607833, 19.02544592524334988, 37.70942372801899722 ) ) ;
#156584=CARTESIAN_POINT ( 'NONE',  ( 4.379528057220092307, 16.55341960407617563, 97.29275706135234714 ) ) ;
#156585=CARTESIAN_POINT ( 'NONE',  ( 16.53943276465976808, -0.05219959533910856209, 58.74890960531436690 ) ) ;
#156586=CARTESIAN_POINT ( 'NONE',  ( -18.62759615963255300, -10.81492255796106328, 94.16775706135237556 ) ) ;
#156588=CARTESIAN_POINT ( 'NONE',  ( -21.53943276465977519, 0.05219959533907696930, 101.2489096053143669 ) ) ;
#156589=CARTESIAN_POINT ( 'NONE',  ( 13.97604488694527802, 13.89961937509977652, 49.37390960531434558 ) ) ;
#156590=CARTESIAN_POINT ( 'NONE',  ( 10.72451020669871369, 18.67979575497193778, 72.08442372801899012 ) ) ;
#156591=CARTESIAN_POINT ( 'NONE',  ( 19.02544592524343514, -5.153800228976328945, 43.54057627198103120 ) ) ;
#156592=ORIENTED_EDGE ( 'NONE', *, *, #117399, .F. ) ;
#156593=CARTESIAN_POINT ( 'NONE',  ( 16.51473224551069308, 9.474510206698969483, 59.16557627198102409 ) ) ;
#156594=CARTESIAN_POINT ( 'NONE',  ( -0.05219959533910754901, -16.53943276465976808, 107.4989096053143669 ) ) ;
#156595=CARTESIAN_POINT ( 'NONE',  ( -0.05219959533909027116, -19.03943276465977164, 112.4989096053143669 ) ) ;
#156596=CARTESIAN_POINT ( 'NONE',  ( 16.53943276465976808, -0.05219959533910856209, 53.74890960531437401 ) ) ;
#156597=CARTESIAN_POINT ( 'NONE',  ( 19.03943276465977164, -0.05219959533909143690, 33.74890960531435979 ) ) ;
#156598=CARTESIAN_POINT ( 'NONE',  ( 16.52544592524342804, -4.483927247898539470, 78.54057627198103830 ) ) ;
#156600=CARTESIAN_POINT ( 'NONE',  ( 21.52544592524344225, -5.823673210054117533, 98.54057627198105251 ) ) ;
#156601=CARTESIAN_POINT ( 'NONE',  ( -15.72974639402176322, -15.80617190586768395, 29.37609039468568284 ) ) ;
#156603=CARTESIAN_POINT ( 'NONE',  ( -14.29746914071037622, -8.314922557961029526, 44.16775706135234714 ) ) ;
#156604=CARTESIAN_POINT ( 'NONE',  ( 5.719274019375991003, -21.55341960407610458, 87.70724293864769550 ) ) ;
#156605=CARTESIAN_POINT ( 'NONE',  ( 0.05219959533937995610, -21.53943276465977519, 105.0010903946856757 ) ) ;
#156606=CARTESIAN_POINT ( 'NONE',  ( -16.51473224551069308, -9.474510206698971260, 111.6655762719810383 ) ) ;
#156607=CARTESIAN_POINT ( 'NONE',  ( 21.53943276465977519, 0.05219959533937863772, 41.25109039468568284 ) ) ;
#156608=CARTESIAN_POINT ( 'NONE',  ( -0.05219959533907301413, -21.53943276465977519, 37.49890960531436690 ) ) ;
#156609=CARTESIAN_POINT ( 'NONE',  ( 14.29746914071037800, 8.314922557961029526, 106.6677570613523756 ) ) ;
#156610=CARTESIAN_POINT ( 'NONE',  ( -5.719274019375665041, -21.55341960407619695, 59.79275706135234714 ) ) ;
#156611=CARTESIAN_POINT ( 'NONE',  ( 21.55341960407619695, -5.719274019375665929, 81.04275706135236135 ) ) ;
#156612=CARTESIAN_POINT ( 'NONE',  ( 19.05341960407617918, -5.049401038297876454, 31.04275706135232227 ) ) ;
#156613=CARTESIAN_POINT ( 'NONE',  ( 8.224510206698742110, 14.34966873604972548, 92.08442372801901854 ) ) ;
#156614=CARTESIAN_POINT ( 'NONE',  ( 21.52544592524334988, 5.823673210054432836, 41.45942372801901143 ) ) ;
#156615=CARTESIAN_POINT ( 'NONE',  ( -5.153800228976328057, -19.02544592524343514, 52.29057627198100988 ) ) ;
#156616=CARTESIAN_POINT ( 'NONE',  ( 19.02544592524334988, 5.153800228976608722, 21.45942372801899012 ) ) ;
#156617=CARTESIAN_POINT ( 'NONE',  ( -5.719274019375978568, 21.55341960407610458, 25.20724293864769550 ) ) ;
#156618=CARTESIAN_POINT ( 'NONE',  ( -21.53943276465977519, 0.05219959533907696930, 116.2489096053143669 ) ) ;
#156619=CARTESIAN_POINT ( 'NONE',  ( 21.55341960407610458, 5.719274019375980345, 73.95724293864769550 ) ) ;
#156621=CARTESIAN_POINT ( 'NONE',  ( -5.823673210054116645, -21.52544592524344225, 67.29057627198103830 ) ) ;
#156622=CARTESIAN_POINT ( 'NONE',  ( -8.224510206698735004, -14.34966873604973081, 69.58442372801900433 ) ) ;
#156623=CARTESIAN_POINT ( 'NONE',  ( 16.53943276465976808, -0.05219959533910856209, 63.74890960531435979 ) ) ;
#156625=CARTESIAN_POINT ( 'NONE',  ( 13.97604488694548053, -13.89961937509957401, 90.62609039468567573 ) ) ;
#156627=CARTESIAN_POINT ( 'NONE',  ( 16.52544592524335698, 4.483927247898782831, 31.45942372801901854 ) ) ;
#156628=CARTESIAN_POINT ( 'NONE',  ( -5.823673210054116645, -21.52544592524344225, 102.2905762719810383 ) ) ;
#156629=CARTESIAN_POINT ( 'NONE',  ( 18.67979575497178502, 10.72451020669898547, 74.16557627198102409 ) ) ;
#156630=CARTESIAN_POINT ( 'NONE',  ( 0.05219959533909260263, 19.03943276465977164, 114.9989096053143669 ) ) ;
#156631=CARTESIAN_POINT ( 'NONE',  ( 14.34966873604972726, -8.224510206698740333, 55.83442372801901854 ) ) ;
#156632=CARTESIAN_POINT ( 'NONE',  ( -19.03943276465977164, 0.05219959533909376836, 66.24890960531436690 ) ) ;
#156633=CARTESIAN_POINT ( 'NONE',  ( 21.52544592524334988, 5.823673210054432836, 41.45942372801901143 ) ) ;
#156634=CARTESIAN_POINT ( 'NONE',  ( 12.14591786802327356, -12.06949235617739191, 20.62609039468568639 ) ) ;
#156635=CARTESIAN_POINT ( 'NONE',  ( 9.474510206698971260, -16.51473224551069308, 112.9155762719810383 ) ) ;
#156636=CARTESIAN_POINT ( 'NONE',  ( 16.46253265017146816, 9.564922557961045513, 31.66775706135232937 ) ) ;
#156637=CARTESIAN_POINT ( 'NONE',  ( -16.51473224551069308, -9.474510206698971260, 96.66557627198102409 ) ) ;
#156638=CARTESIAN_POINT ( 'NONE',  ( -18.62759615963270932, 10.81492255796079327, 105.8322429386476955 ) ) ;
#156639=CARTESIAN_POINT ( 'NONE',  ( 0.05219959533909260263, 19.03943276465977164, 54.99890960531435979 ) ) ;
#156640=CARTESIAN_POINT ( 'NONE',  ( -17.48853670773244673, 5.747243402303159776, 23.66671299749991775 ) ) ;
#156641=CARTESIAN_POINT ( 'NONE',  ( -8.224510206698948167, 14.34966873604960824, 80.41557627198103830 ) ) ;
#156642=CARTESIAN_POINT ( 'NONE',  ( -19.05341960407611168, -5.049401038298163336, 111.4572429386476671 ) ) ;
#156643=CARTESIAN_POINT ( 'NONE',  ( -16.81555441253551209, 7.025013491695475842, 35.63685445334257196 ) ) ;
#156645=CARTESIAN_POINT ( 'NONE',  ( -18.62759615963270932, 10.81492255796079327, 100.8322429386477097 ) ) ;
#156646=CARTESIAN_POINT ( 'NONE',  ( -5.049401038297874678, -19.05341960407617918, 59.79275706135231871 ) ) ;
#156647=CARTESIAN_POINT ( 'NONE',  ( 19.05341960407611168, 5.049401038298154454, 113.9572429386477097 ) ) ;
#156648=CARTESIAN_POINT ( 'NONE',  ( -16.46253265017160317, 9.564922557960807481, 25.83224293864769194 ) ) ;
#156649=CARTESIAN_POINT ( 'NONE',  ( 21.53943276465977519, -0.05219959533907433946, 53.74890960531437401 ) ) ;
#156650=CARTESIAN_POINT ( 'NONE',  ( 13.89961937509977652, -13.97604488694527269, 98.12390960531433848 ) ) ;
#156651=CARTESIAN_POINT ( 'NONE',  ( -5.823673210054431948, 21.52544592524334988, 82.70942372801900433 ) ) ;
#156652=CARTESIAN_POINT ( 'NONE',  ( -5.153800228976328057, -19.02544592524343514, 52.29057627198100988 ) ) ;
#156653=CARTESIAN_POINT ( 'NONE',  ( -0.05219959533910754901, -16.53943276465976808, 82.49890960531436690 ) ) ;
#156654=CARTESIAN_POINT ( 'NONE',  ( 4.379528057220092307, 16.55341960407617563, 42.29275706135235424 ) ) ;
#156655=CARTESIAN_POINT ( 'NONE',  ( 10.72451020669871369, 18.67979575497193778, 67.08442372801901854 ) ) ;
#156657=CARTESIAN_POINT ( 'NONE',  ( 9.564922557961047289, -16.46253265017146816, 20.41775706135233293 ) ) ;
#156658=CARTESIAN_POINT ( 'NONE',  ( -5.049401038297874678, -19.05341960407617918, 74.79275706135231871 ) ) ;
#156660=CARTESIAN_POINT ( 'NONE',  ( -13.89961937509957401, -13.97604488694547875, 44.37609039468566863 ) ) ;
#156662=CARTESIAN_POINT ( 'NONE',  ( 18.62759615963255655, 10.81492255796105972, 36.66775706135234714 ) ) ;
#156663=CARTESIAN_POINT ( 'NONE',  ( -18.56399227203345603, -5.499999999999827693, 43.97830131249903474 ) ) ;
#156664=CARTESIAN_POINT ( 'NONE',  ( 5.153800228976615827, -19.02544592524334988, 35.20942372801899722 ) ) ;
#156665=CARTESIAN_POINT ( 'NONE',  ( -19.02544592524342804, 5.153800228976336051, 71.04057627198099567 ) ) ;
#156666=CARTESIAN_POINT ( 'NONE',  ( -14.34966873604960291, -8.224510206698953496, 21.66557627198102409 ) ) ;
#156667=CARTESIAN_POINT ( 'NONE',  ( -5.049401038298153566, 19.05341960407611168, 115.2072429386477097 ) ) ;
#156668=CARTESIAN_POINT ( 'NONE',  ( -21.52544592524334988, -5.823673210054445271, 83.95942372801900433 ) ) ;
#156670=CARTESIAN_POINT ( 'NONE',  ( -17.50000000000002487, -4.658240926743203225, 36.05529582183199722 ) ) ;
#156671=CARTESIAN_POINT ( 'NONE',  ( 10.81492255796106328, -18.62759615963255655, 90.41775706135236135 ) ) ;
#156672=CARTESIAN_POINT ( 'NONE',  ( 16.36317988757059538, -7.306389748694922304, 41.59789608363227842 ) ) ;
#156673=CARTESIAN_POINT ( 'NONE',  ( -13.89961937509977652, 13.97604488694528158, 95.62390960531436690 ) ) ;
#156675=CARTESIAN_POINT ( 'NONE',  ( 13.97604488694527802, 13.89961937509977652, 49.37390960531434558 ) ) ;
#156676=CARTESIAN_POINT ( 'NONE',  ( 15.80617190586746368, 15.72974639402197994, 54.37390960531435979 ) ) ;
#156677=ADVANCED_FACE ( 'NONE', ( #118592 ), #33748, .T. ) ;
#156678=CARTESIAN_POINT ( 'NONE',  ( -8.314922557960811034, -14.29746914071050412, 27.08224293864769550 ) ) ;
#156679=CARTESIAN_POINT ( 'NONE',  ( -19.03943276465977164, 0.05219959533909376836, 21.24890960531436335 ) ) ;
#156680=CARTESIAN_POINT ( 'NONE',  ( -19.05341960407611168, -5.049401038298163336, 91.45724293864766707 ) ) ;
#156681=CARTESIAN_POINT ( 'NONE',  ( -0.05219959533936034679, 19.03943276465977164, 27.50109039468566507 ) ) ;
#156682=CARTESIAN_POINT ( 'NONE',  ( 14.34966873604960469, 8.224510206698951720, 99.16557627198100988 ) ) ;
#156683=CARTESIAN_POINT ( 'NONE',  ( 15.80617190586769283, -15.72974639402175789, 65.62609039468568994 ) ) ;
#156684=CARTESIAN_POINT ( 'NONE',  ( 9.564922557960805705, 16.46253265017160317, 114.5822429386476955 ) ) ;
#156685=CARTESIAN_POINT ( 'NONE',  ( -0.05219959533934338120, 16.53943276465976808, 102.5010903946856899 ) ) ;
#156686=CARTESIAN_POINT ( 'NONE',  ( -9.474510206698720793, -16.51473224551083518, 69.58442372801901854 ) ) ;
#156688=CARTESIAN_POINT ( 'NONE',  ( -9.564922557960796823, -16.46253265017161027, 107.0822429386476955 ) ) ;
#156689=CARTESIAN_POINT ( 'NONE',  ( 12.06949235617757843, -12.14591786802309237, 78.12390960531436690 ) ) ;
#156691=CARTESIAN_POINT ( 'NONE',  ( 9.474510206698729675, 16.51473224551082808, 52.08442372801900433 ) ) ;
#156692=CARTESIAN_POINT ( 'NONE',  ( 9.564922557960805705, 16.46253265017160317, 69.58224293864770971 ) ) ;
#156693=CARTESIAN_POINT ( 'NONE',  ( 16.52544592524342804, -4.483927247898539470, 63.54057627198103830 ) ) ;
#156694=CARTESIAN_POINT ( 'NONE',  ( -9.564922557961040184, 16.46253265017147172, 92.91775706135233293 ) ) ;
#156695=CARTESIAN_POINT ( 'NONE',  ( -0.05219959533907301413, -21.53943276465977519, 47.49890960531435979 ) ) ;
#156697=CARTESIAN_POINT ( 'NONE',  ( 16.46253265017160672, -9.564922557960803928, 23.33224293864769194 ) ) ;
#156698=CARTESIAN_POINT ( 'NONE',  ( -16.19135201231369336, -7.376712067591812527, 30.18680854052031748 ) ) ;
#156699=CARTESIAN_POINT ( 'NONE',  ( 9.564922557960805705, 16.46253265017160317, 64.58224293864769550 ) ) ;
#156700=CARTESIAN_POINT ( 'NONE',  ( 10.81492255796078972, 18.62759615963270932, 59.58224293864770260 ) ) ;
#156701=CARTESIAN_POINT ( 'NONE',  ( 16.53943276465976808, 0.05219959533934440121, 91.25109039468568994 ) ) ;
#156702=CARTESIAN_POINT ( 'NONE',  ( 5.049401038298161559, -19.05341960407611168, 77.70724293864765286 ) ) ;
#156703=CARTESIAN_POINT ( 'NONE',  ( -19.02544592524334988, -5.153800228976617603, 48.95942372801900433 ) ) ;
#156704=CARTESIAN_POINT ( 'NONE',  ( -5.823673210054431948, 21.52544592524334988, 77.70942372801900433 ) ) ;
#156705=CARTESIAN_POINT ( 'NONE',  ( 21.55341960407610458, 5.719274019375980345, 58.95724293864770971 ) ) ;
#156706=CARTESIAN_POINT ( 'NONE',  ( -9.564922557960796823, -16.46253265017161027, 107.0822429386476955 ) ) ;
#156707=AXIS2_PLACEMENT_3D ( 'NONE', #164053, #131701, #85176 ) ;
#156708=CARTESIAN_POINT ( 'NONE',  ( 5.049401038298161559, -19.05341960407611168, 37.70724293864768839 ) ) ;
#156709=CARTESIAN_POINT ( 'NONE',  ( -8.314922557961024197, 14.29746914071037800, 87.91775706135234714 ) ) ;
#156710=CARTESIAN_POINT ( 'NONE',  ( 5.049401038297881783, 19.05341960407617563, 112.2927570613523471 ) ) ;
#156711=CARTESIAN_POINT ( 'NONE',  ( 18.22780087662121673, 5.500000000000056843, 78.98459894673892734 ) ) ;
#156712=CARTESIAN_POINT ( 'NONE',  ( 5.719274019375673035, 21.55341960407619339, 102.2927570613523613 ) ) ;
#156714=CARTESIAN_POINT ( 'NONE',  ( 8.314922557960818139, 14.29746914071049879, 59.58224293864770260 ) ) ;
#156715=CARTESIAN_POINT ( 'NONE',  ( 0.05219959533910956823, 16.53943276465976808, 74.99890960531435269 ) ) ;
#156716=CARTESIAN_POINT ( 'NONE',  ( 21.52544592524344225, -5.823673210054117533, 88.54057627198103830 ) ) ;
#156717=CARTESIAN_POINT ( 'NONE',  ( 18.67979575497178502, 10.72451020669898547, 84.16557627198103830 ) ) ;
#156718=CARTESIAN_POINT ( 'NONE',  ( 17.44279575226823553, -5.990770900252461395, 98.33557567514324660 ) ) ;
#156719=CARTESIAN_POINT ( 'NONE',  ( -0.05219959533907301413, -21.53943276465977519, 52.49890960531435979 ) ) ;
#156720=CARTESIAN_POINT ( 'NONE',  ( -16.52544592524335698, -4.483927247898792601, 63.95942372801901854 ) ) ;
#156721=CARTESIAN_POINT ( 'NONE',  ( 8.224510206698953496, -14.34966873604960469, 92.91557627198103830 ) ) ;
#156722=CARTESIAN_POINT ( 'NONE',  ( -19.03943276465977164, 0.05219959533909376836, 46.24890960531435979 ) ) ;
#156725=CARTESIAN_POINT ( 'NONE',  ( -16.52544592524335698, -4.483927247898792601, 93.95942372801903275 ) ) ;
#156726=CARTESIAN_POINT ( 'NONE',  ( -5.823673210054431948, 21.52544592524334988, 37.70942372801900433 ) ) ;
#156727=CARTESIAN_POINT ( 'NONE',  ( -19.05341960407611168, -5.049401038298163336, 81.45724293864769550 ) ) ;
#156728=CARTESIAN_POINT ( 'NONE',  ( -21.53943276465977519, -0.05219959533937600094, 73.75109039468567573 ) ) ;
#156730=CARTESIAN_POINT ( 'NONE',  ( 16.46253265017160672, -9.564922557960803928, 23.33224293864769194 ) ) ;
#156732=CARTESIAN_POINT ( 'NONE',  ( -21.52544592524334988, -5.823673210054445271, 63.95942372801901854 ) ) ;
#156733=CARTESIAN_POINT ( 'NONE',  ( 5.049401038298161559, -19.05341960407611168, 42.70724293864767418 ) ) ;
#156734=CARTESIAN_POINT ( 'NONE',  ( 17.97161686094259991, -5.499999999999976019, 58.49637206859247840 ) ) ;
#156735=CARTESIAN_POINT ( 'NONE',  ( 9.564922557960805705, 16.46253265017160317, 89.58224293864769550 ) ) ;
#156736=CARTESIAN_POINT ( 'NONE',  ( -5.049401038297874678, -19.05341960407617918, 69.79275706135233293 ) ) ;
#156737=CARTESIAN_POINT ( 'NONE',  ( -10.81492255796105439, 18.62759615963255655, 32.91775706135234714 ) ) ;
#156738=CARTESIAN_POINT ( 'NONE',  ( 9.564922557961047289, -16.46253265017146816, 55.41775706135234003 ) ) ;
#156739=CARTESIAN_POINT ( 'NONE',  ( 16.46253265017160672, -9.564922557960803928, 38.33224293864768839 ) ) ;
#156740=CARTESIAN_POINT ( 'NONE',  ( -12.06949235617739369, -12.14591786802326823, 99.37609039468568994 ) ) ;
#156741=CARTESIAN_POINT ( 'NONE',  ( 16.51473224551083163, -9.474510206698727899, 70.83442372801900433 ) ) ;
#156742=CARTESIAN_POINT ( 'NONE',  ( -0.05219959533910754901, -16.53943276465976808, 22.49890960531436335 ) ) ;
#156743=CARTESIAN_POINT ( 'NONE',  ( 13.97604488694548053, -13.89961937509957401, 55.62609039468566863 ) ) ;
#156744=CARTESIAN_POINT ( 'NONE',  ( -13.89961937509977652, 13.97604488694528158, 105.6239096053143527 ) ) ;
#156745=CARTESIAN_POINT ( 'NONE',  ( -18.62759615963255300, -10.81492255796106328, 104.1677570613523471 ) ) ;
#156747=CARTESIAN_POINT ( 'NONE',  ( -21.52544592524334988, -5.823673210054445271, 103.9594237280190185 ) ) ;
#156748=CARTESIAN_POINT ( 'NONE',  ( -13.89961937509977652, 13.97604488694528158, 25.62390960531434558 ) ) ;
#156749=CARTESIAN_POINT ( 'NONE',  ( -18.62759615963255300, -10.81492255796106328, 94.16775706135237556 ) ) ;
#156750=CARTESIAN_POINT ( 'NONE',  ( 16.55341960407618274, -4.379528057220086978, 31.04275706135234714 ) ) ;
#156751=CARTESIAN_POINT ( 'NONE',  ( 19.05341960407611168, 5.049401038298154454, 98.95724293864766707 ) ) ;
#156752=DIRECTION ( 'NONE',  ( 1.000000000000000000, -0.000000000000000000, -0.000000000000000000 ) ) ;
#156753=CARTESIAN_POINT ( 'NONE',  ( -13.89961937509977652, 13.97604488694528158, 85.62390960531433848 ) ) ;
#156755=CARTESIAN_POINT ( 'NONE',  ( 13.97604488694548053, -13.89961937509957401, 65.62609039468567573 ) ) ;
#156756=CARTESIAN_POINT ( 'NONE',  ( -19.05341960407611168, -5.049401038298163336, 111.4572429386476671 ) ) ;
#156757=CARTESIAN_POINT ( 'NONE',  ( -5.823673210054431948, 21.52544592524334988, 97.70942372801904696 ) ) ;
#156758=CARTESIAN_POINT ( 'NONE',  ( -16.52544592524342804, 4.483927247898546575, 101.0405762719810383 ) ) ;
#156759=CARTESIAN_POINT ( 'NONE',  ( -21.52544592524343514, 5.823673210054127303, 46.04057627198103830 ) ) ;
#156760=CARTESIAN_POINT ( 'NONE',  ( -21.55341960407610458, -5.719274019375992779, 36.45724293864768839 ) ) ;
#156761=CARTESIAN_POINT ( 'NONE',  ( 14.34966873604960469, 8.224510206698951720, 104.1655762719810241 ) ) ;
#156763=CARTESIAN_POINT ( 'NONE',  ( 0.05219959533936267826, -19.03943276465977164, 55.00109039468566863 ) ) ;
#156764=CARTESIAN_POINT ( 'NONE',  ( -16.53943276465976808, -0.05219959533934237506, 113.7510903946856757 ) ) ;
#156765=CARTESIAN_POINT ( 'NONE',  ( 10.72451020669898902, -18.67979575497178502, 22.91557627198102765 ) ) ;
#156766=CARTESIAN_POINT ( 'NONE',  ( 5.719274019375673035, 21.55341960407619339, 77.29275706135234714 ) ) ;
#156767=CARTESIAN_POINT ( 'NONE',  ( 10.81492255796078972, 18.62759615963270932, 69.58224293864769550 ) ) ;
#156768=CARTESIAN_POINT ( 'NONE',  ( 10.81492255796106328, -18.62759615963255655, 45.41775706135234003 ) ) ;
#156769=CARTESIAN_POINT ( 'NONE',  ( 10.72451020669898902, -18.67979575497178502, 92.91557627198103830 ) ) ;
#156770=CARTESIAN_POINT ( 'NONE',  ( 15.72974639402176855, 15.80617190586768217, 51.87609039468568284 ) ) ;
#156771=CARTESIAN_POINT ( 'NONE',  ( -16.53943276465976808, 0.05219959533911058130, 116.2489096053143669 ) ) ;
#156772=CARTESIAN_POINT ( 'NONE',  ( 19.05341960407611168, 5.049401038298154454, 88.95724293864769550 ) ) ;
#156773=CARTESIAN_POINT ( 'NONE',  ( -12.14591786802326823, 12.06949235617739902, 83.12609039468568994 ) ) ;
#156774=CARTESIAN_POINT ( 'NONE',  ( 14.29746914071049879, -8.314922557960816363, 108.3322429386477097 ) ) ;
#156775=CARTESIAN_POINT ( 'NONE',  ( -13.89961937509977652, 13.97604488694528158, 105.6239096053143527 ) ) ;
#156777=CARTESIAN_POINT ( 'NONE',  ( 4.483927247898545687, 16.52544592524342804, 49.79057627198102409 ) ) ;
#156778=CARTESIAN_POINT ( 'NONE',  ( 4.379528057220092307, 16.55341960407617563, 112.2927570613523471 ) ) ;
#156779=CARTESIAN_POINT ( 'NONE',  ( -19.03943276465977164, 0.05219959533909376836, 66.24890960531436690 ) ) ;
#156780=CARTESIAN_POINT ( 'NONE',  ( 13.97604488694527802, 13.89961937509977652, 39.37390960531435269 ) ) ;
#156781=CARTESIAN_POINT ( 'NONE',  ( -21.55341960407610458, -5.719274019375992779, 41.45724293864769550 ) ) ;
#156782=CARTESIAN_POINT ( 'NONE',  ( 9.564922557961047289, -16.46253265017146816, 40.41775706135234003 ) ) ;
#156784=CARTESIAN_POINT ( 'NONE',  ( -16.55341960407611168, -4.379528057220339221, 36.45724293864768839 ) ) ;
#156785=CARTESIAN_POINT ( 'NONE',  ( -16.46253265017160317, 9.564922557960807481, 110.8322429386476955 ) ) ;
#156786=CARTESIAN_POINT ( 'NONE',  ( 5.719274019375673035, 21.55341960407619339, 62.29275706135236845 ) ) ;
#156787=CARTESIAN_POINT ( 'NONE',  ( 9.474510206698971260, -16.51473224551069308, 112.9155762719810383 ) ) ;
#156788=CARTESIAN_POINT ( 'NONE',  ( 4.483927247898790824, -16.52544592524335698, 60.20942372801902565 ) ) ;
#156789=CARTESIAN_POINT ( 'NONE',  ( 9.474510206698729675, 16.51473224551082808, 67.08442372801900433 ) ) ;
#156790=CARTESIAN_POINT ( 'NONE',  ( 8.314922557960818139, 14.29746914071049879, 34.58224293864770260 ) ) ;
#156791=DIRECTION ( 'NONE',  ( 1.000000000000000000, -0.000000000000000000, -0.000000000000000000 ) ) ;
#156792=CARTESIAN_POINT ( 'NONE',  ( 16.53943276465976808, 0.05219959533934440121, 106.2510903946856757 ) ) ;
#156793=CARTESIAN_POINT ( 'NONE',  ( -16.46253265017160317, 9.564922557960807481, 35.83224293864768839 ) ) ;
#156794=CARTESIAN_POINT ( 'NONE',  ( -19.05341960407611168, -5.049401038298163336, 66.45724293864769550 ) ) ;
#156795=CARTESIAN_POINT ( 'NONE',  ( -13.97604488694527625, -13.89961937509977652, 21.87390960531435979 ) ) ;
#156796=CARTESIAN_POINT ( 'NONE',  ( -10.72451020669870658, -18.67979575497194134, 34.58442372801900433 ) ) ;
#156797=CARTESIAN_POINT ( 'NONE',  ( -5.153800228976328057, -19.02544592524343514, 42.29057627198101699 ) ) ;
#156798=CARTESIAN_POINT ( 'NONE',  ( 5.153800228976335163, 19.02544592524342804, 114.7905762719810241 ) ) ;
#156799=CARTESIAN_POINT ( 'NONE',  ( 13.97604488694527802, 13.89961937509977652, 49.37390960531434558 ) ) ;
#156800=CARTESIAN_POINT ( 'NONE',  ( -13.89961937509977652, 13.97604488694528158, 115.6239096053143669 ) ) ;
#156801=CARTESIAN_POINT ( 'NONE',  ( -5.823673210054431948, 21.52544592524334988, 52.70942372801902565 ) ) ;
#156802=CARTESIAN_POINT ( 'NONE',  ( -9.564922557960796823, -16.46253265017161027, 22.08224293864768839 ) ) ;
#156803=CARTESIAN_POINT ( 'NONE',  ( 15.72974639402199770, -15.80617190586745480, 33.12390960531435979 ) ) ;
#156804=CARTESIAN_POINT ( 'NONE',  ( -4.379528057220086978, -16.55341960407618274, 74.79275706135234714 ) ) ;
#156805=ADVANCED_FACE ( 'NONE', ( #178512 ), #102662, .F. ) ;
#156806=CARTESIAN_POINT ( 'NONE',  ( 10.81492255796106328, -18.62759615963255655, 100.4177570613523471 ) ) ;
#156807=CARTESIAN_POINT ( 'NONE',  ( 14.34966873604972726, -8.224510206698740333, 55.83442372801901854 ) ) ;
#156808=CARTESIAN_POINT ( 'NONE',  ( -13.89961937509977652, 13.97604488694528158, 100.6239096053143669 ) ) ;
#156809=CARTESIAN_POINT ( 'NONE',  ( 16.53943276465976808, 0.05219959533934440121, 36.25109039468567573 ) ) ;
#156810=CARTESIAN_POINT ( 'NONE',  ( 12.06949235617739724, 12.14591786802326823, 31.87609039468567929 ) ) ;
#156811=CARTESIAN_POINT ( 'NONE',  ( -8.224510206698735004, -14.34966873604973081, 89.58442372801901854 ) ) ;
#156812=CARTESIAN_POINT ( 'NONE',  ( 10.81492255796106328, -18.62759615963255655, 60.41775706135235424 ) ) ;
#156813=CARTESIAN_POINT ( 'NONE',  ( -9.564922557961040184, 16.46253265017147172, 112.9177570613523329 ) ) ;
#156814=CARTESIAN_POINT ( 'NONE',  ( 10.72451020669898902, -18.67979575497178502, 112.9155762719810383 ) ) ;
#156815=CARTESIAN_POINT ( 'NONE',  ( 12.06949235617757843, -12.14591786802309237, 98.12390960531436690 ) ) ;
#156816=CARTESIAN_POINT ( 'NONE',  ( -16.46253265017146816, -9.564922557961047289, 109.1677570613523471 ) ) ;
#156817=CARTESIAN_POINT ( 'NONE',  ( -12.14591786802326823, 12.06949235617739902, 78.12609039468570415 ) ) ;
#156819=CARTESIAN_POINT ( 'NONE',  ( -5.153800228976607833, 19.02544592524334988, 87.70942372801897591 ) ) ;
#156820=CARTESIAN_POINT ( 'NONE',  ( -8.314922557960811034, -14.29746914071050412, 47.08224293864770260 ) ) ;
#156821=CARTESIAN_POINT ( 'NONE',  ( -8.224510206698948167, 14.34966873604960824, 45.41557627198103830 ) ) ;
#156822=CARTESIAN_POINT ( 'NONE',  ( 8.224510206698953496, -14.34966873604960469, 107.9155762719810241 ) ) ;
#156823=CARTESIAN_POINT ( 'NONE',  ( -16.46253265017146816, -9.564922557961047289, 34.16775706135233293 ) ) ;
#156824=CARTESIAN_POINT ( 'NONE',  ( 15.80617190586769283, -15.72974639402175789, 30.62609039468567929 ) ) ;
#156825=CARTESIAN_POINT ( 'NONE',  ( -16.51473224551082808, 9.474510206698731452, 113.3344237280190043 ) ) ;
#156827=CARTESIAN_POINT ( 'NONE',  ( -9.474510206698964154, 16.51473224551069663, 95.41557627198102409 ) ) ;
#156828=CARTESIAN_POINT ( 'NONE',  ( 5.049401038298161559, -19.05341960407611168, 92.70724293864769550 ) ) ;
#156829=CARTESIAN_POINT ( 'NONE',  ( 5.823673210054125526, 21.52544592524343514, 54.79057627198104541 ) ) ;
#156830=CARTESIAN_POINT ( 'NONE',  ( 0.05219959533910956823, 16.53943276465976808, 94.99890960531436690 ) ) ;
#156831=CARTESIAN_POINT ( 'NONE',  ( 0.05219959533909260263, 19.03943276465977164, 64.99890960531436690 ) ) ;
#156832=CARTESIAN_POINT ( 'NONE',  ( 19.02544592524343514, -5.153800228976328945, 28.54057627198102409 ) ) ;
#156833=CARTESIAN_POINT ( 'NONE',  ( -0.05219959533937732626, 21.53943276465977519, 37.50109039468568284 ) ) ;
#156834=CARTESIAN_POINT ( 'NONE',  ( 15.80617190586769283, -15.72974639402175789, 70.62609039468567573 ) ) ;
#156835=CARTESIAN_POINT ( 'NONE',  ( 8.314922557961029526, -14.29746914071037800, 95.41775706135234714 ) ) ;
#156836=CARTESIAN_POINT ( 'NONE',  ( -21.53943276465977519, -0.05219959533937600094, 23.75109039468567929 ) ) ;
#156837=CARTESIAN_POINT ( 'NONE',  ( 21.52544592524334988, 5.823673210054432836, 21.45942372801901499 ) ) ;
#156838=CARTESIAN_POINT ( 'NONE',  ( -5.153800228976607833, 19.02544592524334988, 57.70942372801899012 ) ) ;
#156839=CARTESIAN_POINT ( 'NONE',  ( 9.474510206698971260, -16.51473224551069308, 72.91557627198102409 ) ) ;
#156840=CARTESIAN_POINT ( 'NONE',  ( 18.62759615963255655, 10.81492255796105972, 81.66775706135236135 ) ) ;
#156841=CARTESIAN_POINT ( 'NONE',  ( -10.72451020669898014, 18.67979575497178502, 80.41557627198103830 ) ) ;
#156842=CARTESIAN_POINT ( 'NONE',  ( -16.52544592524342804, 4.483927247898546575, 46.04057627198103830 ) ) ;
#156843=CARTESIAN_POINT ( 'NONE',  ( -21.55341960407619339, 5.719274019375674811, 108.5427570613523756 ) ) ;
#156844=CARTESIAN_POINT ( 'NONE',  ( 0.05219959533936267826, -19.03943276465977164, 45.00109039468566863 ) ) ;
#156845=CARTESIAN_POINT ( 'NONE',  ( -14.29746914071049879, 8.314922557960819915, 75.83224293864769550 ) ) ;
#156846=CARTESIAN_POINT ( 'NONE',  ( -9.564922557960796823, -16.46253265017161027, 22.08224293864768839 ) ) ;
#156847=CARTESIAN_POINT ( 'NONE',  ( -19.02544592524334988, -5.153800228976617603, 68.95942372801896170 ) ) ;
#156848=CARTESIAN_POINT ( 'NONE',  ( -4.483927247898539470, -16.52544592524342804, 37.29057627198102409 ) ) ;
#156849=CARTESIAN_POINT ( 'NONE',  ( -15.80617190586768217, 15.72974639402176855, 88.12609039468570415 ) ) ;
#156850=CARTESIAN_POINT ( 'NONE',  ( 13.89961937509977652, -13.97604488694527269, 83.12390960531436690 ) ) ;
#156851=CARTESIAN_POINT ( 'NONE',  ( -0.05219959533936034679, 19.03943276465977164, 67.50109039468566152 ) ) ;
#156852=CARTESIAN_POINT ( 'NONE',  ( -21.52544592524343514, 5.823673210054127303, 71.04057627198103830 ) ) ;
#156853=CARTESIAN_POINT ( 'NONE',  ( -5.719274019375978568, 21.55341960407610458, 110.2072429386477239 ) ) ;
#156854=CARTESIAN_POINT ( 'NONE',  ( 4.483927247898790824, -16.52544592524335698, 20.20942372801900788 ) ) ;
#156855=CARTESIAN_POINT ( 'NONE',  ( 4.379528057220092307, 16.55341960407617563, 82.29275706135234714 ) ) ;
#156856=CARTESIAN_POINT ( 'NONE',  ( 17.44270441346512257, 5.991230190323099336, 63.86335079264228654 ) ) ;
#156857=CARTESIAN_POINT ( 'NONE',  ( 21.52544592524334988, 5.823673210054432836, 21.45942372801901499 ) ) ;
#156858=CARTESIAN_POINT ( 'NONE',  ( 4.379528057220339221, -16.55341960407611168, 97.70724293864772392 ) ) ;
#156860=CARTESIAN_POINT ( 'NONE',  ( 14.29746914071037800, 8.314922557961029526, 36.66775706135234714 ) ) ;
#156861=CARTESIAN_POINT ( 'NONE',  ( 21.55341960407610458, 5.719274019375980345, 58.95724293864770971 ) ) ;
#156862=CARTESIAN_POINT ( 'NONE',  ( 14.29746914071037800, 8.314922557961029526, 101.6677570613523613 ) ) ;
#156863=CARTESIAN_POINT ( 'NONE',  ( -0.05219959533934338120, 16.53943276465976808, 37.50109039468568284 ) ) ;
#156864=CARTESIAN_POINT ( 'NONE',  ( -9.474510206698964154, 16.51473224551069663, 35.41557627198102409 ) ) ;
#156865=CARTESIAN_POINT ( 'NONE',  ( 12.14591786802327356, -12.06949235617739191, 85.62609039468568994 ) ) ;
#156866=CARTESIAN_POINT ( 'NONE',  ( 16.51473224551083163, -9.474510206698727899, 70.83442372801900433 ) ) ;
#156867=CARTESIAN_POINT ( 'NONE',  ( -18.62759615963255300, -10.81492255796106328, 34.16775706135234714 ) ) ;
#156868=CARTESIAN_POINT ( 'NONE',  ( -21.55341960407610458, -5.719274019375992779, 56.45724293864768839 ) ) ;
#156869=CARTESIAN_POINT ( 'NONE',  ( -4.379528057220086978, -16.55341960407618274, 94.79275706135234714 ) ) ;
#156870=CARTESIAN_POINT ( 'NONE',  ( 10.72451020669871369, 18.67979575497193778, 77.08442372801901854 ) ) ;
#156871=CARTESIAN_POINT ( 'NONE',  ( -10.72451020669898014, 18.67979575497178502, 55.41557627198102409 ) ) ;
#156872=CARTESIAN_POINT ( 'NONE',  ( 18.67979575497178502, 10.72451020669898547, 44.16557627198103120 ) ) ;
#156873=CARTESIAN_POINT ( 'NONE',  ( -14.29746914071037622, -8.314922557961029526, 74.16775706135231871 ) ) ;
#156874=CARTESIAN_POINT ( 'NONE',  ( -5.719274019375978568, 21.55341960407610458, 50.20724293864769550 ) ) ;
#156875=EDGE_LOOP ( 'NONE', ( #174145, #95610, #116399, #130822, #123438, #7772, #70339, #112352 ) ) ;
#156876=CARTESIAN_POINT ( 'NONE',  ( 9.564922557960805705, 16.46253265017160317, 94.58224293864769550 ) ) ;
#156878=CARTESIAN_POINT ( 'NONE',  ( 0.05219959533909260263, 19.03943276465977164, 29.99890960531435979 ) ) ;
#156879=CARTESIAN_POINT ( 'NONE',  ( -10.72451020669898014, 18.67979575497178502, 55.41557627198102409 ) ) ;
#156880=CARTESIAN_POINT ( 'NONE',  ( -16.52544592524335698, -4.483927247898792601, 93.95942372801903275 ) ) ;
#156881=CARTESIAN_POINT ( 'NONE',  ( -15.80617190586768217, 15.72974639402176855, 48.12609039468568284 ) ) ;
#156882=CARTESIAN_POINT ( 'NONE',  ( 9.474510206698729675, 16.51473224551082808, 97.08442372801900433 ) ) ;
#156883=CARTESIAN_POINT ( 'NONE',  ( 12.14591786802309770, 12.06949235617756955, 104.3739096053143669 ) ) ;
#156884=CARTESIAN_POINT ( 'NONE',  ( 12.06949235617739724, 12.14591786802326823, 21.87609039468567573 ) ) ;
#156886=CARTESIAN_POINT ( 'NONE',  ( 19.02544592524343514, -5.153800228976328945, 38.54057627198103120 ) ) ;
#156889=CARTESIAN_POINT ( 'NONE',  ( -5.049401038298153566, 19.05341960407611168, 85.20724293864766707 ) ) ;
#156890=CARTESIAN_POINT ( 'NONE',  ( 14.34966873604972726, -8.224510206698740333, 80.83442372801901854 ) ) ;
#156891=CARTESIAN_POINT ( 'NONE',  ( 10.72451020669871369, 18.67979575497193778, 102.0844237280190185 ) ) ;
#156892=CARTESIAN_POINT ( 'NONE',  ( -5.719274019375978568, 21.55341960407610458, 65.20724293864768129 ) ) ;
#156893=CARTESIAN_POINT ( 'NONE',  ( 12.14591786802327356, -12.06949235617739191, 90.62609039468567573 ) ) ;
#156894=CARTESIAN_POINT ( 'NONE',  ( -13.89961937509957401, -13.97604488694547875, 74.37609039468566152 ) ) ;
#156895=CARTESIAN_POINT ( 'NONE',  ( -0.05219959533909027116, -19.03943276465977164, 42.49890960531435269 ) ) ;
#156896=CARTESIAN_POINT ( 'NONE',  ( 13.89961937509977652, -13.97604488694527269, 78.12390960531433848 ) ) ;
#156897=CARTESIAN_POINT ( 'NONE',  ( -10.72451020669870658, -18.67979575497194134, 44.58442372801901854 ) ) ;
#156898=CARTESIAN_POINT ( 'NONE',  ( 16.46253265017160672, -9.564922557960803928, 53.33224293864768839 ) ) ;
#156899=CARTESIAN_POINT ( 'NONE',  ( -16.51473224551082808, 9.474510206698731452, 73.33442372801900433 ) ) ;
#156901=CARTESIAN_POINT ( 'NONE',  ( 19.02544592524343514, -5.153800228976328945, 103.5405762719809957 ) ) ;
#156902=CARTESIAN_POINT ( 'NONE',  ( 12.06949235617757843, -12.14591786802309237, 63.12390960531435979 ) ) ;
#156903=CARTESIAN_POINT ( 'NONE',  ( -21.52544592524343514, 5.823673210054127303, 66.04057627198103830 ) ) ;
#156905=CARTESIAN_POINT ( 'NONE',  ( -13.97604488694547697, 13.89961937509957934, 23.12609039468565442 ) ) ;
#156907=CARTESIAN_POINT ( 'NONE',  ( 0.05219959533909260263, 19.03943276465977164, 64.99890960531436690 ) ) ;
#156908=CARTESIAN_POINT ( 'NONE',  ( 9.474510206698971260, -16.51473224551069308, 72.91557627198102409 ) ) ;
#156909=CARTESIAN_POINT ( 'NONE',  ( -8.314922557961024197, 14.29746914071037800, 57.91775706135234714 ) ) ;
#156911=CARTESIAN_POINT ( 'NONE',  ( -16.38665767535055906, 7.295008042176100105, 110.2640086421455123 ) ) ;
#156912=CARTESIAN_POINT ( 'NONE',  ( -0.05219959533934338120, 16.53943276465976808, 77.50109039468567573 ) ) ;
#156913=CARTESIAN_POINT ( 'NONE',  ( 17.60691670004652565, 5.500000000000026645, 96.63333313366440791 ) ) ;
#156914=CARTESIAN_POINT ( 'NONE',  ( 16.53943276465976808, 0.05219959533934440121, 71.25109039468568994 ) ) ;
#156915=CARTESIAN_POINT ( 'NONE',  ( -16.55341960407617563, 4.379528057220093196, 38.54275706135234714 ) ) ;
#156916=CARTESIAN_POINT ( 'NONE',  ( 19.03943276465977164, -0.05219959533909143690, 53.74890960531436690 ) ) ;
#156918=CARTESIAN_POINT ( 'NONE',  ( -5.719274019375665041, -21.55341960407619695, 59.79275706135234714 ) ) ;
#156919=CARTESIAN_POINT ( 'NONE',  ( 13.89961937509957401, 13.97604488694547697, 56.87609039468564731 ) ) ;
#156920=CARTESIAN_POINT ( 'NONE',  ( -21.53943276465977519, -0.05219959533937600094, 108.7510903946857042 ) ) ;
#156921=CARTESIAN_POINT ( 'NONE',  ( 16.51473224551069308, 9.474510206698969483, 34.16557627198102409 ) ) ;
#156923=CARTESIAN_POINT ( 'NONE',  ( 5.823673210054125526, 21.52544592524343514, 59.79057627198103120 ) ) ;
#156924=CARTESIAN_POINT ( 'NONE',  ( 19.05341960407611168, 5.049401038298154454, 103.9572429386476671 ) ) ;
#156925=CARTESIAN_POINT ( 'NONE',  ( 16.52544592524342804, -4.483927247898539470, 103.5405762719810383 ) ) ;
#156926=CARTESIAN_POINT ( 'NONE',  ( -12.06949235617739369, -12.14591786802326823, 34.37609039468568284 ) ) ;
#156927=CARTESIAN_POINT ( 'NONE',  ( -16.52544592524342804, 4.483927247898546575, 31.04057627198102409 ) ) ;
#156929=CARTESIAN_POINT ( 'NONE',  ( -15.80617190586745835, -15.72974639402198527, 96.87390960531436690 ) ) ;
#156930=CARTESIAN_POINT ( 'NONE',  ( 16.52544592524342804, -4.483927247898539470, 38.54057627198103120 ) ) ;
#156931=CARTESIAN_POINT ( 'NONE',  ( -0.05219959533909027116, -19.03943276465977164, 112.4989096053143669 ) ) ;
#156932=CARTESIAN_POINT ( 'NONE',  ( 0.05219959533936267826, -19.03943276465977164, 95.00109039468567573 ) ) ;
#156933=CARTESIAN_POINT ( 'NONE',  ( -13.89961937509957401, -13.97604488694547875, 29.37609039468565797 ) ) ;
#156934=CARTESIAN_POINT ( 'NONE',  ( -4.483927247898539470, -16.52544592524342804, 32.29057627198102409 ) ) ;
#156935=CARTESIAN_POINT ( 'NONE',  ( 15.72974639402199770, -15.80617190586745480, 108.1239096053143811 ) ) ;
#156936=CARTESIAN_POINT ( 'NONE',  ( 21.52544592524344225, -5.823673210054117533, 53.54057627198103120 ) ) ;
#156937=CARTESIAN_POINT ( 'NONE',  ( 5.153800228976335163, 19.02544592524342804, 79.79057627198102409 ) ) ;
#156938=CARTESIAN_POINT ( 'NONE',  ( -14.34966873604960291, -8.224510206698953496, 46.66557627198102409 ) ) ;
#156939=CARTESIAN_POINT ( 'NONE',  ( -19.02544592524342804, 5.153800228976336051, 96.04057627198103830 ) ) ;
#156940=CARTESIAN_POINT ( 'NONE',  ( 19.26498983726237313, -5.499999999999806377, 63.05319577422002908 ) ) ;
#156941=CARTESIAN_POINT ( 'NONE',  ( 19.05341960407617918, -5.049401038297876454, 46.04275706135233293 ) ) ;
#156942=CARTESIAN_POINT ( 'NONE',  ( 10.81492255796078972, 18.62759615963270932, 89.58224293864768129 ) ) ;
#156943=CARTESIAN_POINT ( 'NONE',  ( -0.05219959533910754901, -16.53943276465976808, 97.49890960531436690 ) ) ;
#156944=CARTESIAN_POINT ( 'NONE',  ( 21.52544592524334988, 5.823673210054432836, 36.45942372801901143 ) ) ;
#156946=CARTESIAN_POINT ( 'NONE',  ( -12.14591786802326823, 12.06949235617739902, 113.1260903946856899 ) ) ;
#156947=CARTESIAN_POINT ( 'NONE',  ( -5.153800228976328057, -19.02544592524343514, 32.29057627198102409 ) ) ;
#156948=CARTESIAN_POINT ( 'NONE',  ( 16.46253265017160672, -9.564922557960803928, 83.33224293864768129 ) ) ;
#156949=CARTESIAN_POINT ( 'NONE',  ( -18.22780087662122028, 5.500000000000031086, 93.51540105326107266 ) ) ;
#156950=CARTESIAN_POINT ( 'NONE',  ( 13.89961937509977652, -13.97604488694527269, 38.12390960531436690 ) ) ;
#156951=CARTESIAN_POINT ( 'NONE',  ( 4.379528057220339221, -16.55341960407611168, 42.70724293864770260 ) ) ;
#156952=CARTESIAN_POINT ( 'NONE',  ( -0.05219959533937732626, 21.53943276465977519, 77.50109039468567573 ) ) ;
#156954=CARTESIAN_POINT ( 'NONE',  ( -16.53943276465976808, -0.05219959533934237506, 73.75109039468567573 ) ) ;
#156955=CARTESIAN_POINT ( 'NONE',  ( -16.46253265017160317, 9.564922557960807481, 60.83224293864769550 ) ) ;
#156956=CARTESIAN_POINT ( 'NONE',  ( 0.05219959533909260263, 19.03943276465977164, 69.99890960531435269 ) ) ;
#156958=CARTESIAN_POINT ( 'NONE',  ( -10.81492255796105439, 18.62759615963255655, 102.9177570613523756 ) ) ;
#156959=CARTESIAN_POINT ( 'NONE',  ( 8.314922557961029526, -14.29746914071037800, 70.41775706135236135 ) ) ;
#156960=CARTESIAN_POINT ( 'NONE',  ( 18.62759615963255655, 10.81492255796105972, 101.6677570613523613 ) ) ;
#156961=CARTESIAN_POINT ( 'NONE',  ( -16.46253265017160317, 9.564922557960807481, 60.83224293864769550 ) ) ;
#156962=CARTESIAN_POINT ( 'NONE',  ( 21.52544592524344225, -5.823673210054117533, 38.54057627198103120 ) ) ;
#156963=CARTESIAN_POINT ( 'NONE',  ( 19.03943276465977164, 0.05219959533936151252, 101.2510903946856757 ) ) ;
#156964=CARTESIAN_POINT ( 'NONE',  ( -18.62759615963255300, -10.81492255796106328, 84.16775706135234714 ) ) ;
#156965=CARTESIAN_POINT ( 'NONE',  ( 16.55341960407618274, -4.379528057220086978, 51.04275706135234714 ) ) ;
#156966=CARTESIAN_POINT ( 'NONE',  ( 21.52544592524344225, -5.823673210054117533, 98.54057627198105251 ) ) ;
#156967=CARTESIAN_POINT ( 'NONE',  ( 13.97604488694548053, -13.89961937509957401, 95.62609039468563310 ) ) ;
#156969=CARTESIAN_POINT ( 'NONE',  ( -13.97604488694527625, -13.89961937509977652, 81.87390960531436690 ) ) ;
#156970=CARTESIAN_POINT ( 'NONE',  ( 5.153800228976615827, -19.02544592524334988, 105.2094237280190185 ) ) ;
#156971=CARTESIAN_POINT ( 'NONE',  ( 8.224510206698742110, 14.34966873604972548, 27.08442372801901854 ) ) ;
#156972=CARTESIAN_POINT ( 'NONE',  ( 14.34966873604960469, 8.224510206698951720, 64.16557627198102409 ) ) ;
#156973=CARTESIAN_POINT ( 'NONE',  ( -12.14591786802326823, 12.06949235617739902, 68.12609039468567573 ) ) ;
#156974=CARTESIAN_POINT ( 'NONE',  ( 21.52544592524344225, -5.823673210054117533, 113.5405762719810383 ) ) ;
#156975=CARTESIAN_POINT ( 'NONE',  ( 16.46253265017160672, -9.564922557960803928, 58.33224293864769550 ) ) ;
#156976=CARTESIAN_POINT ( 'NONE',  ( 9.474510206698971260, -16.51473224551069308, 67.91557627198102409 ) ) ;
#156977=CARTESIAN_POINT ( 'NONE',  ( -16.52544592524335698, -4.483927247898792601, 78.95942372801901854 ) ) ;
#156980=CARTESIAN_POINT ( 'NONE',  ( 21.53943276465977519, 0.05219959533937863772, 106.2510903946856757 ) ) ;
#156981=CARTESIAN_POINT ( 'NONE',  ( -5.049401038298153566, 19.05341960407611168, 40.20724293864768839 ) ) ;
#156983=CARTESIAN_POINT ( 'NONE',  ( 0.05219959533934541429, -16.53943276465976808, 20.00109039468568639 ) ) ;
#156984=CARTESIAN_POINT ( 'NONE',  ( 9.564922557961047289, -16.46253265017146816, 40.41775706135234003 ) ) ;
#156985=CARTESIAN_POINT ( 'NONE',  ( -8.224510206698735004, -14.34966873604973081, 24.58442372801901499 ) ) ;
#156986=CARTESIAN_POINT ( 'NONE',  ( -19.03943276465977164, 0.05219959533909376836, 41.24890960531435269 ) ) ;
#156987=CARTESIAN_POINT ( 'NONE',  ( 19.02544592524343514, -5.153800228976328945, 68.54057627198103830 ) ) ;
#156988=CARTESIAN_POINT ( 'NONE',  ( 0.05219959533907565091, 21.53943276465977519, 79.99890960531435269 ) ) ;
#156989=CARTESIAN_POINT ( 'NONE',  ( -19.03943276465977164, 0.05219959533909376836, 116.2489096053143669 ) ) ;
#156990=CARTESIAN_POINT ( 'NONE',  ( 16.51473224551069308, 9.474510206698969483, 44.16557627198103120 ) ) ;
#156992=CARTESIAN_POINT ( 'NONE',  ( -19.03943276465977164, -0.05219959533935918106, 103.7510903946856757 ) ) ;
#156993=CARTESIAN_POINT ( 'NONE',  ( -21.55341960407610458, -5.719274019375992779, 71.45724293864769550 ) ) ;
#156995=CARTESIAN_POINT ( 'NONE',  ( 0.05219959533936267826, -19.03943276465977164, 30.00109039468566863 ) ) ;
#156996=CARTESIAN_POINT ( 'NONE',  ( -12.14591786802309592, -12.06949235617757132, 66.87390960531436690 ) ) ;
#156997=CARTESIAN_POINT ( 'NONE',  ( 10.81492255796106328, -18.62759615963255655, 85.41775706135236135 ) ) ;
#156998=CARTESIAN_POINT ( 'NONE',  ( 4.483927247898545687, 16.52544592524342804, 114.7905762719810383 ) ) ;
#156999=CARTESIAN_POINT ( 'NONE',  ( -8.314922557960811034, -14.29746914071050412, 32.08224293864769550 ) ) ;
#157000=CARTESIAN_POINT ( 'NONE',  ( -15.72974639402176322, -15.80617190586768395, 89.37609039468568994 ) ) ;
#157001=CARTESIAN_POINT ( 'NONE',  ( -19.03943276465977164, 0.05219959533909376836, 81.24890960531436690 ) ) ;
#157002=CARTESIAN_POINT ( 'NONE',  ( 18.62759615963255655, 10.81492255796105972, 41.66775706135235424 ) ) ;
#157003=CARTESIAN_POINT ( 'NONE',  ( 19.05341960407611168, 5.049401038298154454, 78.95724293864769550 ) ) ;
#157004=CARTESIAN_POINT ( 'NONE',  ( 16.55341960407611168, 4.379528057220329451, 88.95724293864769550 ) ) ;
#157005=CARTESIAN_POINT ( 'NONE',  ( -4.483927247898539470, -16.52544592524342804, 62.29057627198102409 ) ) ;
#157006=CARTESIAN_POINT ( 'NONE',  ( 5.823673210054125526, 21.52544592524343514, 69.79057627198102409 ) ) ;
#157007=CARTESIAN_POINT ( 'NONE',  ( 5.049401038298161559, -19.05341960407611168, 77.70724293864765286 ) ) ;
#157008=CARTESIAN_POINT ( 'NONE',  ( 21.52544592524344225, -5.823673210054117533, 88.54057627198103830 ) ) ;
#157009=CARTESIAN_POINT ( 'NONE',  ( 19.03943276465977164, 0.05219959533936151252, 76.25109039468566152 ) ) ;
#157011=CARTESIAN_POINT ( 'NONE',  ( -16.51473224551082808, 9.474510206698731452, 28.33442372801900433 ) ) ;
#157012=CARTESIAN_POINT ( 'NONE',  ( 0.05219959533910956823, 16.53943276465976808, 69.99890960531435269 ) ) ;
#157013=CARTESIAN_POINT ( 'NONE',  ( 5.719274019375991003, -21.55341960407610458, 52.70724293864769550 ) ) ;
#157015=CARTESIAN_POINT ( 'NONE',  ( -16.53943276465976808, -0.05219959533934237506, 98.75109039468568994 ) ) ;
#157017=CARTESIAN_POINT ( 'NONE',  ( -19.05341960407617563, 5.049401038297882671, 98.54275706135233293 ) ) ;
#157018=CARTESIAN_POINT ( 'NONE',  ( 16.53943276465976808, -0.05219959533910856209, 68.74890960531435269 ) ) ;
#157019=CARTESIAN_POINT ( 'NONE',  ( -17.49999999999999645, 5.499999999999997335, 35.79690382534171533 ) ) ;
#157020=CARTESIAN_POINT ( 'NONE',  ( -16.46253265017160317, 9.564922557960807481, 55.83224293864769550 ) ) ;
#157021=CARTESIAN_POINT ( 'NONE',  ( 16.46253265017160672, -9.564922557960803928, 28.33224293864769550 ) ) ;
#157022=CARTESIAN_POINT ( 'NONE',  ( 16.52544592524342804, -4.483927247898539470, 48.54057627198103120 ) ) ;
#157023=CARTESIAN_POINT ( 'NONE',  ( 13.97604488694527802, 13.89961937509977652, 104.3739096053143385 ) ) ;
#157024=CARTESIAN_POINT ( 'NONE',  ( 13.97604488694548053, -13.89961937509957401, 85.62609039468568994 ) ) ;
#157025=CARTESIAN_POINT ( 'NONE',  ( -0.05219959533909027116, -19.03943276465977164, 67.49890960531436690 ) ) ;
#157026=CARTESIAN_POINT ( 'NONE',  ( -12.14591786802326823, 12.06949235617739902, 23.12609039468567573 ) ) ;
#157027=CARTESIAN_POINT ( 'NONE',  ( -19.03943276465977164, 0.05219959533909376836, 81.24890960531436690 ) ) ;
#157028=CARTESIAN_POINT ( 'NONE',  ( -21.55341960407610458, -5.719274019375992779, 66.45724293864768129 ) ) ;
#157029=CARTESIAN_POINT ( 'NONE',  ( 14.34966873604972726, -8.224510206698740333, 55.83442372801901854 ) ) ;
#157030=CARTESIAN_POINT ( 'NONE',  ( -9.564922557961040184, 16.46253265017147172, 107.9177570613523471 ) ) ;
#157031=CARTESIAN_POINT ( 'NONE',  ( 9.474510206698971260, -16.51473224551069308, 62.91557627198102409 ) ) ;
#157032=CARTESIAN_POINT ( 'NONE',  ( -15.80617190586745835, -15.72974639402198527, 61.87390960531436690 ) ) ;
#157033=CARTESIAN_POINT ( 'NONE',  ( -16.51473224551082808, 9.474510206698731452, 88.33442372801900433 ) ) ;
#157034=CARTESIAN_POINT ( 'NONE',  ( 16.52544592524335698, 4.483927247898782831, 111.4594237280190328 ) ) ;
#157035=CARTESIAN_POINT ( 'NONE',  ( 5.823673210054444382, -21.52544592524334988, 50.20942372801901854 ) ) ;
#157038=CARTESIAN_POINT ( 'NONE',  ( -8.314922557961024197, 14.29746914071037800, 67.91775706135234714 ) ) ;
#157039=CARTESIAN_POINT ( 'NONE',  ( -16.52544592524335698, -4.483927247898792601, 98.95942372801903275 ) ) ;
#157040=CARTESIAN_POINT ( 'NONE',  ( 19.53037848336981241, -5.499999999999889866, 42.35532783611441943 ) ) ;
#157041=CARTESIAN_POINT ( 'NONE',  ( -8.314922557961024197, 14.29746914071037800, 77.91775706135231871 ) ) ;
#157042=CARTESIAN_POINT ( 'NONE',  ( 16.53943276465976808, 0.05219959533934440121, 31.25109039468568639 ) ) ;
#157043=CARTESIAN_POINT ( 'NONE',  ( -16.51473224551069308, -9.474510206698971260, 46.66557627198102409 ) ) ;
#157044=CARTESIAN_POINT ( 'NONE',  ( -19.03943276465977164, 0.05219959533909376836, 56.24890960531435979 ) ) ;
#157045=CARTESIAN_POINT ( 'NONE',  ( -19.02544592524342804, 5.153800228976336051, 66.04057627198103830 ) ) ;
#157046=CARTESIAN_POINT ( 'NONE',  ( -0.05219959533937732626, 21.53943276465977519, 57.50109039468568994 ) ) ;
#157047=CARTESIAN_POINT ( 'NONE',  ( -16.55341960407617563, 4.379528057220093196, 48.54275706135234714 ) ) ;
#157048=CARTESIAN_POINT ( 'NONE',  ( 4.483927247898545687, 16.52544592524342804, 39.79057627198103830 ) ) ;
#157049=CARTESIAN_POINT ( 'NONE',  ( 13.97604488694527802, 13.89961937509977652, 24.37390960531435624 ) ) ;
#157050=CARTESIAN_POINT ( 'NONE',  ( 13.89961937509977652, -13.97604488694527269, 33.12390960531434558 ) ) ;
#157051=CARTESIAN_POINT ( 'NONE',  ( -8.314922557961024197, 14.29746914071037800, 27.91775706135234358 ) ) ;
#157052=CARTESIAN_POINT ( 'NONE',  ( -9.564922557961040184, 16.46253265017147172, 82.91775706135233293 ) ) ;
#157053=CARTESIAN_POINT ( 'NONE',  ( 16.53943276465976808, -0.05219959533910856209, 78.74890960531436690 ) ) ;
#157054=CARTESIAN_POINT ( 'NONE',  ( -5.049401038298153566, 19.05341960407611168, 55.20724293864769550 ) ) ;
#157055=CARTESIAN_POINT ( 'NONE',  ( -19.02544592524334988, -5.153800228976617603, 93.95942372801900433 ) ) ;
#157057=CARTESIAN_POINT ( 'NONE',  ( 5.823673210054444382, -21.52544592524334988, 80.20942372801901854 ) ) ;
#157058=CARTESIAN_POINT ( 'NONE',  ( -16.53943276465976808, -0.05219959533934237506, 58.75109039468568994 ) ) ;
#157059=CARTESIAN_POINT ( 'NONE',  ( 17.40805194822031510, 6.112264579159359279, 36.66628727489388950 ) ) ;
#157060=CARTESIAN_POINT ( 'NONE',  ( -21.52544592524343514, 5.823673210054127303, 56.04057627198102409 ) ) ;
#157061=CARTESIAN_POINT ( 'NONE',  ( 4.483927247898790824, -16.52544592524335698, 40.20942372801901854 ) ) ;
#157063=CARTESIAN_POINT ( 'NONE',  ( 9.564922557961047289, -16.46253265017146816, 35.41775706135233293 ) ) ;
#157066=CARTESIAN_POINT ( 'NONE',  ( 16.51473224551069308, 9.474510206698969483, 49.16557627198102409 ) ) ;
#157068=CARTESIAN_POINT ( 'NONE',  ( -16.46253265017160317, 9.564922557960807481, 75.83224293864769550 ) ) ;
#157070=CARTESIAN_POINT ( 'NONE',  ( -19.52837319214026479, 5.499999999999998224, 99.60471352585541638 ) ) ;
#157071=CARTESIAN_POINT ( 'NONE',  ( 13.89961937509957401, 13.97604488694547697, 26.87609039468566507 ) ) ;
#157072=CARTESIAN_POINT ( 'NONE',  ( 8.224510206698953496, -14.34966873604960469, 42.91557627198103120 ) ) ;
#157073=CARTESIAN_POINT ( 'NONE',  ( 19.03943276465977164, -0.05219959533909143690, 48.74890960531435979 ) ) ;
#157074=CARTESIAN_POINT ( 'NONE',  ( -9.564922557960796823, -16.46253265017161027, 112.0822429386476955 ) ) ;
#157075=CARTESIAN_POINT ( 'NONE',  ( -18.67979575497193778, 10.72451020669871902, 73.33442372801901854 ) ) ;
#157076=CARTESIAN_POINT ( 'NONE',  ( 9.474510206698971260, -16.51473224551069308, 47.91557627198102409 ) ) ;
#157077=CARTESIAN_POINT ( 'NONE',  ( -18.67979575497193778, 10.72451020669871902, 63.33442372801900433 ) ) ;
#157078=CARTESIAN_POINT ( 'NONE',  ( -16.46253265017160317, 9.564922557960807481, 115.8322429386477097 ) ) ;
#157079=CARTESIAN_POINT ( 'NONE',  ( -16.51473224551069308, -9.474510206698971260, 31.66557627198102054 ) ) ;
#157080=CARTESIAN_POINT ( 'NONE',  ( 0.05219959533937995610, -21.53943276465977519, 25.00109039468567218 ) ) ;
#157081=CARTESIAN_POINT ( 'NONE',  ( -9.474510206698720793, -16.51473224551083518, 44.58442372801900433 ) ) ;
#157082=CARTESIAN_POINT ( 'NONE',  ( -19.03943276465977164, 0.05219959533909376836, 31.24890960531435979 ) ) ;
#157083=CARTESIAN_POINT ( 'NONE',  ( 16.51473224551069308, 9.474510206698969483, 64.16557627198102409 ) ) ;
#157084=CARTESIAN_POINT ( 'NONE',  ( 4.483927247898790824, -16.52544592524335698, 20.20942372801900788 ) ) ;
#157085=CARTESIAN_POINT ( 'NONE',  ( 12.14591786802309770, 12.06949235617756955, 79.37390960531436690 ) ) ;
#157086=CARTESIAN_POINT ( 'NONE',  ( -21.53943276465977519, 0.05219959533907696930, 31.24890960531435979 ) ) ;
#157087=CARTESIAN_POINT ( 'NONE',  ( 5.049401038297881783, 19.05341960407617563, 97.29275706135233293 ) ) ;
#157088=CARTESIAN_POINT ( 'NONE',  ( 10.72451020669898902, -18.67979575497178502, 107.9155762719810241 ) ) ;
#157089=CARTESIAN_POINT ( 'NONE',  ( -21.55341960407619339, 5.719274019375674811, 53.54275706135234714 ) ) ;
#157090=CARTESIAN_POINT ( 'NONE',  ( 16.55341960407618274, -4.379528057220086978, 61.04275706135234714 ) ) ;
#157091=CARTESIAN_POINT ( 'NONE',  ( 14.34966873604972726, -8.224510206698740333, 50.83442372801901143 ) ) ;
#157092=CARTESIAN_POINT ( 'NONE',  ( -18.67979575497178146, -10.72451020669898902, 56.66557627198103830 ) ) ;
#157093=CARTESIAN_POINT ( 'NONE',  ( -9.474510206698964154, 16.51473224551069663, 45.41557627198103120 ) ) ;
#157094=CARTESIAN_POINT ( 'NONE',  ( 16.52544592524335698, 4.483927247898782831, 71.45942372801901854 ) ) ;
#157095=CARTESIAN_POINT ( 'NONE',  ( 18.67979575497178502, 10.72451020669898547, 99.16557627198100988 ) ) ;
#157096=CARTESIAN_POINT ( 'NONE',  ( 14.34966873604960469, 8.224510206698951720, 54.16557627198103120 ) ) ;
#157097=CARTESIAN_POINT ( 'NONE',  ( 5.049401038298161559, -19.05341960407611168, 77.70724293864765286 ) ) ;
#157098=CARTESIAN_POINT ( 'NONE',  ( -8.224510206698735004, -14.34966873604973081, 79.58442372801903275 ) ) ;
#157099=CARTESIAN_POINT ( 'NONE',  ( 19.03943276465977164, 0.05219959533936151252, 111.2510903946856757 ) ) ;
#157100=CARTESIAN_POINT ( 'NONE',  ( -0.05219959533907301413, -21.53943276465977519, 107.4989096053143669 ) ) ;
#157101=CARTESIAN_POINT ( 'NONE',  ( 14.29746914071049879, -8.314922557960816363, 38.33224293864768839 ) ) ;
#157103=CARTESIAN_POINT ( 'NONE',  ( -16.81555441253553695, 7.025013491695482060, 75.63685445334260748 ) ) ;
#157104=CARTESIAN_POINT ( 'NONE',  ( -0.05219959533907301413, -21.53943276465977519, 92.49890960531436690 ) ) ;
#157105=CARTESIAN_POINT ( 'NONE',  ( -8.224510206698948167, 14.34966873604960824, 30.41557627198101699 ) ) ;
#157108=CARTESIAN_POINT ( 'NONE',  ( -21.52544592524343514, 5.823673210054127303, 101.0405762719810383 ) ) ;
#157109=CARTESIAN_POINT ( 'NONE',  ( 5.153800228976335163, 19.02544592524342804, 104.7905762719809957 ) ) ;
#157110=CARTESIAN_POINT ( 'NONE',  ( 18.67979575497194134, -10.72451020669871369, 20.83442372801901143 ) ) ;
#157111=CARTESIAN_POINT ( 'NONE',  ( 8.224510206698953496, -14.34966873604960469, 47.91557627198102409 ) ) ;
#157112=CARTESIAN_POINT ( 'NONE',  ( 12.14591786802327356, -12.06949235617739191, 45.62609039468567573 ) ) ;
#157113=CARTESIAN_POINT ( 'NONE',  ( -5.049401038298153566, 19.05341960407611168, 50.20724293864770260 ) ) ;
#157114=CARTESIAN_POINT ( 'NONE',  ( 19.02544592524334988, 5.153800228976608722, 56.45942372801898301 ) ) ;
#157115=CARTESIAN_POINT ( 'NONE',  ( 13.97604488694527802, 13.89961937509977652, 84.37390960531433848 ) ) ;
#157116=EDGE_CURVE ( 'NONE', #188457, #89992, #15619, .T. ) ;
#157117=CARTESIAN_POINT ( 'NONE',  ( -18.67979575497178146, -10.72451020669898902, 41.66557627198103120 ) ) ;
#157118=CARTESIAN_POINT ( 'NONE',  ( -18.22780087662119897, 5.500000000000102141, 66.01763182126894947 ) ) ;
#157119=CARTESIAN_POINT ( 'NONE',  ( -14.34966873604972548, 8.224510206698743886, 23.33442372801901499 ) ) ;
#157120=CARTESIAN_POINT ( 'NONE',  ( -13.97604488694547697, 13.89961937509957934, 48.12609039468566863 ) ) ;
#157121=CARTESIAN_POINT ( 'NONE',  ( 18.67979575497178502, 10.72451020669898547, 99.16557627198100988 ) ) ;
#157122=CARTESIAN_POINT ( 'NONE',  ( 4.483927247898545687, 16.52544592524342804, 39.79057627198103830 ) ) ;
#157123=CARTESIAN_POINT ( 'NONE',  ( -16.46253265017160317, 9.564922557960807481, 75.83224293864769550 ) ) ;
#157124=CARTESIAN_POINT ( 'NONE',  ( -5.719274019375978568, 21.55341960407610458, 60.20724293864768839 ) ) ;
#157125=CARTESIAN_POINT ( 'NONE',  ( 5.823673210054125526, 21.52544592524343514, 94.79057627198105251 ) ) ;
#157126=CARTESIAN_POINT ( 'NONE',  ( 16.53943276465976808, 0.05219959533934440121, 26.25109039468567573 ) ) ;
#157127=CARTESIAN_POINT ( 'NONE',  ( 19.05341960407611168, 5.049401038298154454, 113.9572429386477097 ) ) ;
#157128=CARTESIAN_POINT ( 'NONE',  ( -21.53943276465977519, -0.05219959533937600094, 93.75109039468567573 ) ) ;
#157129=CARTESIAN_POINT ( 'NONE',  ( 19.03943276465977164, -0.05219959533909143690, 83.74890960531436690 ) ) ;
#157131=CARTESIAN_POINT ( 'NONE',  ( 19.03943276465977164, -0.05219959533909143690, 28.74890960531435624 ) ) ;
#157132=CARTESIAN_POINT ( 'NONE',  ( 5.049401038298161559, -19.05341960407611168, 82.70724293864770971 ) ) ;
#157133=CARTESIAN_POINT ( 'NONE',  ( 16.52544592524342804, -4.483927247898539470, 108.5405762719810241 ) ) ;
#157134=CARTESIAN_POINT ( 'NONE',  ( 5.153800228976335163, 19.02544592524342804, 59.79057627198100988 ) ) ;
#157135=CARTESIAN_POINT ( 'NONE',  ( -8.314922557961024197, 14.29746914071037800, 22.91775706135235069 ) ) ;
#157137=CARTESIAN_POINT ( 'NONE',  ( 19.02544592524343514, -5.153800228976328945, 73.54057627198103830 ) ) ;
#157138=CARTESIAN_POINT ( 'NONE',  ( -18.62759615963255300, -10.81492255796106328, 104.1677570613523471 ) ) ;
#157139=CARTESIAN_POINT ( 'NONE',  ( -13.89961937509977652, 13.97604488694528158, 115.6239096053143669 ) ) ;
#157140=CARTESIAN_POINT ( 'NONE',  ( -4.379528057220086978, -16.55341960407618274, 89.79275706135236135 ) ) ;
#157141=LINE ( 'NONE', #185494, #77679 ) ;
#157142=CARTESIAN_POINT ( 'NONE',  ( 19.05341960407617918, -5.049401038297876454, 71.04275706135234714 ) ) ;
#157143=CARTESIAN_POINT ( 'NONE',  ( 10.72451020669871369, 18.67979575497193778, 112.0844237280190185 ) ) ;
#157144=B_SPLINE_CURVE_WITH_KNOTS ( 'NONE', 3,
 ( #132480, #166820, #135489, #198140, #120291, #151640 ),
 .UNSPECIFIED., .F., .F.,
 ( 4, 2, 4 ),
 ( 0.000000000000000000, 0.0003837532665554082493, 0.0007675065331108164987 ),
 .UNSPECIFIED. ) ;
#157146=CARTESIAN_POINT ( 'NONE',  ( 9.474510206698971260, -16.51473224551069308, 32.91557627198102409 ) ) ;
#157147=CARTESIAN_POINT ( 'NONE',  ( 12.06949235617757843, -12.14591786802309237, 38.12390960531436690 ) ) ;
#157149=CARTESIAN_POINT ( 'NONE',  ( -14.34966873604972548, 8.224510206698743886, 103.3344237280190043 ) ) ;
#157150=DIRECTION ( 'NONE',  ( 0.000000000000000000, 0.000000000000000000, -1.000000000000000000 ) ) ;
#157151=CARTESIAN_POINT ( 'NONE',  ( 4.379528057220092307, 16.55341960407617563, 77.29275706135234714 ) ) ;
#157152=CARTESIAN_POINT ( 'NONE',  ( -9.474510206698964154, 16.51473224551069663, 40.41557627198103120 ) ) ;
#157153=CARTESIAN_POINT ( 'NONE',  ( -21.53943276465977519, -0.05219959533937600094, 93.75109039468567573 ) ) ;
#157154=CARTESIAN_POINT ( 'NONE',  ( 19.03943276465977164, 0.05219959533936151252, 96.25109039468567573 ) ) ;
#157155=CARTESIAN_POINT ( 'NONE',  ( 21.55341960407619695, -5.719274019375665929, 76.04275706135237556 ) ) ;
#157156=CARTESIAN_POINT ( 'NONE',  ( 13.97604488694548053, -13.89961937509957401, 55.62609039468566863 ) ) ;
#157157=CARTESIAN_POINT ( 'NONE',  ( 5.153800228976335163, 19.02544592524342804, 79.79057627198102409 ) ) ;
#157158=CARTESIAN_POINT ( 'NONE',  ( -13.89961937509977652, 13.97604488694528158, 75.62390960531438111 ) ) ;
#157161=CARTESIAN_POINT ( 'NONE',  ( 16.52544592524342804, -4.483927247898539470, 63.54057627198103830 ) ) ;
#157162=CARTESIAN_POINT ( 'NONE',  ( -15.80617190586745835, -15.72974639402198527, 66.87390960531436690 ) ) ;
#157163=CARTESIAN_POINT ( 'NONE',  ( 16.46253265017160672, -9.564922557960803928, 53.33224293864768839 ) ) ;
#157164=CARTESIAN_POINT ( 'NONE',  ( 21.53943276465977519, -0.05219959533907433946, 83.74890960531435269 ) ) ;
#157165=CARTESIAN_POINT ( 'NONE',  ( 0.05219959533934541429, -16.53943276465976808, 75.00109039468568994 ) ) ;
#157167=CARTESIAN_POINT ( 'NONE',  ( -16.55341960407611168, -4.379528057220339221, 81.45724293864769550 ) ) ;
#157169=CARTESIAN_POINT ( 'NONE',  ( 8.314922557961029526, -14.29746914071037800, 35.41775706135234003 ) ) ;
#157170=CARTESIAN_POINT ( 'NONE',  ( -16.52544592524342804, 4.483927247898546575, 111.0405762719810525 ) ) ;
#157171=CARTESIAN_POINT ( 'NONE',  ( -16.46253265017146816, -9.564922557961047289, 69.16775706135233293 ) ) ;
#157172=CARTESIAN_POINT ( 'NONE',  ( -12.14591786802309592, -12.06949235617757132, 71.87390960531438111 ) ) ;
#157173=CARTESIAN_POINT ( 'NONE',  ( 18.62759615963255655, 10.81492255796105972, 46.66775706135234714 ) ) ;
#157175=CARTESIAN_POINT ( 'NONE',  ( -21.55341960407610458, -5.719274019375992779, 106.4572429386477097 ) ) ;
#157177=CARTESIAN_POINT ( 'NONE',  ( -12.14591786802309592, -12.06949235617757132, 81.87390960531435269 ) ) ;
#157179=CARTESIAN_POINT ( 'NONE',  ( -5.049401038298153566, 19.05341960407611168, 40.20724293864768839 ) ) ;
#157181=CARTESIAN_POINT ( 'NONE',  ( 5.049401038297881783, 19.05341960407617563, 77.29275706135231871 ) ) ;
#157182=CARTESIAN_POINT ( 'NONE',  ( 5.823673210054444382, -21.52544592524334988, 40.20942372801901854 ) ) ;
#157183=CARTESIAN_POINT ( 'NONE',  ( 9.564922557960805705, 16.46253265017160317, 69.58224293864770971 ) ) ;
#157184=CARTESIAN_POINT ( 'NONE',  ( 19.03943276465977164, 0.05219959533936151252, 51.25109039468567573 ) ) ;
#157185=CARTESIAN_POINT ( 'NONE',  ( -19.02544592524342804, 5.153800228976336051, 51.04057627198103120 ) ) ;
#157186=CARTESIAN_POINT ( 'NONE',  ( 4.379528057220339221, -16.55341960407611168, 67.70724293864769550 ) ) ;
#157187=CARTESIAN_POINT ( 'NONE',  ( 16.55341960407611168, 4.379528057220329451, 68.95724293864769550 ) ) ;
#157188=CARTESIAN_POINT ( 'NONE',  ( -16.46253265017160317, 9.564922557960807481, 75.83224293864769550 ) ) ;
#157189=CARTESIAN_POINT ( 'NONE',  ( 21.52544592524344225, -5.823673210054117533, 98.54057627198105251 ) ) ;
#157190=CARTESIAN_POINT ( 'NONE',  ( -13.97604488694527625, -13.89961937509977652, 71.87390960531433848 ) ) ;
#157191=CARTESIAN_POINT ( 'NONE',  ( 18.67979575497178502, 10.72451020669898547, 84.16557627198103830 ) ) ;
#157192=CARTESIAN_POINT ( 'NONE',  ( -16.46253265017146816, -9.564922557961047289, 24.16775706135233648 ) ) ;
#157193=CARTESIAN_POINT ( 'NONE',  ( -5.049401038298153566, 19.05341960407611168, 40.20724293864768839 ) ) ;
#157194=CARTESIAN_POINT ( 'NONE',  ( -8.314922557961024197, 14.29746914071037800, 112.9177570613523329 ) ) ;
#157195=CARTESIAN_POINT ( 'NONE',  ( 12.06949235617757843, -12.14591786802309237, 103.1239096053143811 ) ) ;
#157196=CARTESIAN_POINT ( 'NONE',  ( 9.564922557961047289, -16.46253265017146816, 110.4177570613523471 ) ) ;
#157197=ORIENTED_EDGE ( 'NONE', *, *, #111391, .T. ) ;
#157198=CARTESIAN_POINT ( 'NONE',  ( -10.72451020669870658, -18.67979575497194134, 34.58442372801900433 ) ) ;
#157199=CARTESIAN_POINT ( 'NONE',  ( 9.474510206698729675, 16.51473224551082808, 52.08442372801900433 ) ) ;
#157200=CARTESIAN_POINT ( 'NONE',  ( -14.34966873604960291, -8.224510206698953496, 21.66557627198102409 ) ) ;
#157201=CARTESIAN_POINT ( 'NONE',  ( -18.67979575497178146, -10.72451020669898902, 66.66557627198102409 ) ) ;
#157202=CARTESIAN_POINT ( 'NONE',  ( -19.05341960407611168, -5.049401038298163336, 96.45724293864769550 ) ) ;
#157203=CARTESIAN_POINT ( 'NONE',  ( 14.29746914071049879, -8.314922557960816363, 63.33224293864770260 ) ) ;
#157204=CARTESIAN_POINT ( 'NONE',  ( 5.153800228976335163, 19.02544592524342804, 34.79057627198102409 ) ) ;
#157205=CARTESIAN_POINT ( 'NONE',  ( 5.153800228976335163, 19.02544592524342804, 34.79057627198102409 ) ) ;
#157206=CARTESIAN_POINT ( 'NONE',  ( -19.03943276465977164, -0.05219959533935918106, 23.75109039468566152 ) ) ;
#157207=CARTESIAN_POINT ( 'NONE',  ( 12.14591786802327356, -12.06949235617739191, 95.62609039468568994 ) ) ;
#157208=CARTESIAN_POINT ( 'NONE',  ( -5.719274019375665041, -21.55341960407619695, 44.79275706135234714 ) ) ;
#157209=CARTESIAN_POINT ( 'NONE',  ( -4.483927247898782831, 16.52544592524335698, 47.70942372801902565 ) ) ;
#157210=CARTESIAN_POINT ( 'NONE',  ( 18.62759615963271287, -10.81492255796078972, 28.33224293864769550 ) ) ;
#157211=CARTESIAN_POINT ( 'NONE',  ( -16.46253265017160317, 9.564922557960807481, 55.83224293864769550 ) ) ;
#157212=CARTESIAN_POINT ( 'NONE',  ( -21.55341960407619339, 5.719274019375674811, 98.54275706135234714 ) ) ;
#157213=CARTESIAN_POINT ( 'NONE',  ( -19.05341960407611168, -5.049401038298163336, 81.45724293864769550 ) ) ;
#157215=CARTESIAN_POINT ( 'NONE',  ( -14.34966873604972548, 8.224510206698743886, 63.33442372801900433 ) ) ;
#157216=CARTESIAN_POINT ( 'NONE',  ( -14.34966873604960291, -8.224510206698953496, 101.6655762719810383 ) ) ;
#157217=CARTESIAN_POINT ( 'NONE',  ( 12.06949235617739724, 12.14591786802326823, 111.8760903946856615 ) ) ;
#157219=CARTESIAN_POINT ( 'NONE',  ( 18.62759615963255655, 10.81492255796105972, 66.66775706135234714 ) ) ;
#157220=CARTESIAN_POINT ( 'NONE',  ( -5.153800228976328057, -19.02544592524343514, 92.29057627198099567 ) ) ;
#157221=CARTESIAN_POINT ( 'NONE',  ( 16.51473224551069308, 9.474510206698969483, 79.16557627198103830 ) ) ;
#157222=CARTESIAN_POINT ( 'NONE',  ( 13.97604488694527802, 13.89961937509977652, 104.3739096053143385 ) ) ;
#157223=CARTESIAN_POINT ( 'NONE',  ( -16.55341960407611168, -4.379528057220339221, 56.45724293864768839 ) ) ;
#157225=CARTESIAN_POINT ( 'NONE',  ( -0.05219959533910754901, -16.53943276465976808, 22.49890960531436335 ) ) ;
#157226=CARTESIAN_POINT ( 'NONE',  ( 16.53943276465976808, -0.05219959533910856209, 43.74890960531435979 ) ) ;
#157228=CARTESIAN_POINT ( 'NONE',  ( 16.51473224551083163, -9.474510206698727899, 40.83442372801900433 ) ) ;
#157229=CARTESIAN_POINT ( 'NONE',  ( 9.474510206698971260, -16.51473224551069308, 72.91557627198102409 ) ) ;
#157230=CARTESIAN_POINT ( 'NONE',  ( 5.153800228976615827, -19.02544592524334988, 50.20942372801897591 ) ) ;
#157232=CARTESIAN_POINT ( 'NONE',  ( 17.50000000000000000, 5.499999999999997335, 120.0000000000000142 ) ) ;
#157233=CARTESIAN_POINT ( 'NONE',  ( -13.89961937509957401, -13.97604488694547875, 89.37609039468563310 ) ) ;
#157234=CARTESIAN_POINT ( 'NONE',  ( 16.55341960407618274, -4.379528057220086978, 81.04275706135236135 ) ) ;
#157235=CARTESIAN_POINT ( 'NONE',  ( 19.02544592524343514, -5.153800228976328945, 98.54057627198100988 ) ) ;
#157236=CARTESIAN_POINT ( 'NONE',  ( -18.62759615963255300, -10.81492255796106328, 34.16775706135234714 ) ) ;
#157237=CARTESIAN_POINT ( 'NONE',  ( 19.02544592524334988, 5.153800228976608722, 91.45942372801900433 ) ) ;
#157238=CARTESIAN_POINT ( 'NONE',  ( 16.88567814943163725, 6.947325034625719375, 88.79001122652589117 ) ) ;
#157239=CARTESIAN_POINT ( 'NONE',  ( 5.153800228976335163, 19.02544592524342804, 49.79057627198100988 ) ) ;
#157240=CARTESIAN_POINT ( 'NONE',  ( 19.05341960407611168, 5.049401038298154454, 103.9572429386476671 ) ) ;
#157241=CARTESIAN_POINT ( 'NONE',  ( -16.52544592524342804, 4.483927247898546575, 56.04057627198102409 ) ) ;
#157242=CARTESIAN_POINT ( 'NONE',  ( 19.05341960407611168, 5.049401038298154454, 43.95724293864769550 ) ) ;
#157243=CARTESIAN_POINT ( 'NONE',  ( -19.02544592524342804, 5.153800228976336051, 61.04057627198103120 ) ) ;
#157244=CARTESIAN_POINT ( 'NONE',  ( -16.51473224551082808, 9.474510206698731452, 68.33442372801900433 ) ) ;
#157245=CARTESIAN_POINT ( 'NONE',  ( 19.02544592524334988, 5.153800228976608722, 26.45942372801899722 ) ) ;
#157246=CARTESIAN_POINT ( 'NONE',  ( 13.97604488694527802, 13.89961937509977652, 64.37390960531436690 ) ) ;
#157247=CARTESIAN_POINT ( 'NONE',  ( -0.05219959533907301413, -21.53943276465977519, 72.49890960531435269 ) ) ;
#157248=CARTESIAN_POINT ( 'NONE',  ( -16.52544592524342804, 4.483927247898546575, 71.04057627198103830 ) ) ;
#157249=CARTESIAN_POINT ( 'NONE',  ( -13.89961937509957401, -13.97604488694547875, 34.37609039468566863 ) ) ;
#157250=CARTESIAN_POINT ( 'NONE',  ( -19.02544592524342804, 5.153800228976336051, 116.0405762719810383 ) ) ;
#157251=CARTESIAN_POINT ( 'NONE',  ( -10.72451020669898014, 18.67979575497178502, 40.41557627198103120 ) ) ;
#157252=CARTESIAN_POINT ( 'NONE',  ( 18.67979575497178502, 10.72451020669898547, 24.16557627198103120 ) ) ;
#157253=CARTESIAN_POINT ( 'NONE',  ( 16.46253265017160672, -9.564922557960803928, 53.33224293864768839 ) ) ;
#157254=CARTESIAN_POINT ( 'NONE',  ( 5.153800228976335163, 19.02544592524342804, 34.79057627198102409 ) ) ;
#157255=CARTESIAN_POINT ( 'NONE',  ( 8.314922557960818139, 14.29746914071049879, 104.5822429386477097 ) ) ;
#157256=CARTESIAN_POINT ( 'NONE',  ( -21.53943276465977519, 0.05219959533907696930, 111.2489096053143669 ) ) ;
#157257=CARTESIAN_POINT ( 'NONE',  ( 13.89961937509977652, -13.97604488694527269, 113.1239096053143527 ) ) ;
#157258=CARTESIAN_POINT ( 'NONE',  ( 15.72974639402176855, 15.80617190586768217, 21.87609039468567573 ) ) ;
#157259=CARTESIAN_POINT ( 'NONE',  ( -16.52544592524342804, 4.483927247898546575, 116.0405762719810383 ) ) ;
#157260=CARTESIAN_POINT ( 'NONE',  ( -18.62759615963270932, 10.81492255796079327, 90.83224293864769550 ) ) ;
#157261=CARTESIAN_POINT ( 'NONE',  ( 16.46253265017146816, 9.564922557961045513, 41.66775706135234003 ) ) ;
#157262=CARTESIAN_POINT ( 'NONE',  ( -19.05341960407611168, -5.049401038298163336, 26.45724293864769550 ) ) ;
#157263=CARTESIAN_POINT ( 'NONE',  ( -13.97604488694527625, -13.89961937509977652, 26.87390960531434558 ) ) ;
#157264=CARTESIAN_POINT ( 'NONE',  ( -8.224510206698735004, -14.34966873604973081, 44.58442372801901854 ) ) ;
#157265=CARTESIAN_POINT ( 'NONE',  ( -0.05219959533909027116, -19.03943276465977164, 27.49890960531435624 ) ) ;
#157266=DIRECTION ( 'NONE',  ( 1.000000000000000000, -0.000000000000000000, -0.000000000000000000 ) ) ;
#157267=CARTESIAN_POINT ( 'NONE',  ( -13.97604488694527625, -13.89961937509977652, 76.87390960531433848 ) ) ;
#157268=CARTESIAN_POINT ( 'NONE',  ( -8.314922557960811034, -14.29746914071050412, 107.0822429386476955 ) ) ;
#157269=CARTESIAN_POINT ( 'NONE',  ( 0.05219959533907565091, 21.53943276465977519, 44.99890960531435979 ) ) ;
#157270=CARTESIAN_POINT ( 'NONE',  ( -8.314922557960811034, -14.29746914071050412, 82.08224293864768129 ) ) ;
#157271=CARTESIAN_POINT ( 'NONE',  ( 14.34966873604972726, -8.224510206698740333, 35.83442372801901143 ) ) ;
#157272=CARTESIAN_POINT ( 'NONE',  ( -18.62759615963255300, -10.81492255796106328, 84.16775706135234714 ) ) ;
#157273=CARTESIAN_POINT ( 'NONE',  ( 0.05219959533909260263, 19.03943276465977164, 29.99890960531435979 ) ) ;
#157274=CARTESIAN_POINT ( 'NONE',  ( -16.52544592524335698, -4.483927247898792601, 93.95942372801903275 ) ) ;
#157275=CARTESIAN_POINT ( 'NONE',  ( 16.55341960407611168, 4.379528057220329451, 43.95724293864769550 ) ) ;
#157276=CARTESIAN_POINT ( 'NONE',  ( 9.564922557960805705, 16.46253265017160317, 49.58224293864770260 ) ) ;
#157277=CARTESIAN_POINT ( 'NONE',  ( 5.823673210054444382, -21.52544592524334988, 95.20942372801903275 ) ) ;
#157278=CARTESIAN_POINT ( 'NONE',  ( 18.62759615963271287, -10.81492255796078972, 108.3322429386477097 ) ) ;
#157279=CARTESIAN_POINT ( 'NONE',  ( -0.05219959533937732626, 21.53943276465977519, 67.50109039468568994 ) ) ;
#157280=CARTESIAN_POINT ( 'NONE',  ( 12.06949235617739724, 12.14591786802326823, 41.87609039468568284 ) ) ;
#157281=CARTESIAN_POINT ( 'NONE',  ( 14.29746914071049879, -8.314922557960816363, 68.33224293864769550 ) ) ;
#157282=CARTESIAN_POINT ( 'NONE',  ( -21.55341960407619339, 5.719274019375674811, 88.54275706135236135 ) ) ;
#157284=CARTESIAN_POINT ( 'NONE',  ( 4.379528057220092307, 16.55341960407617563, 107.2927570613523471 ) ) ;
#157285=CARTESIAN_POINT ( 'NONE',  ( -17.12812012977025589, 6.668231424565989052, 113.6405124067685790 ) ) ;
#157287=CARTESIAN_POINT ( 'NONE',  ( -4.379528057220328563, 16.55341960407611168, 35.20724293864768839 ) ) ;
#157288=CARTESIAN_POINT ( 'NONE',  ( -16.55341960407617563, 4.379528057220093196, 68.54275706135234714 ) ) ;
#157289=CARTESIAN_POINT ( 'NONE',  ( -16.51473224551069308, -9.474510206698971260, 81.66557627198103830 ) ) ;
#157290=CARTESIAN_POINT ( 'NONE',  ( 5.049401038298161559, -19.05341960407611168, 102.7072429386476955 ) ) ;
#157291=CARTESIAN_POINT ( 'NONE',  ( 5.823673210054444382, -21.52544592524334988, 100.2094237280190043 ) ) ;
#157292=CARTESIAN_POINT ( 'NONE',  ( -8.224510206698735004, -14.34966873604973081, 99.58442372801900433 ) ) ;
#157293=CARTESIAN_POINT ( 'NONE',  ( 12.14591786802309770, 12.06949235617756955, 79.37390960531436690 ) ) ;
#157294=CARTESIAN_POINT ( 'NONE',  ( 16.51473224551069308, 9.474510206698969483, 84.16557627198102409 ) ) ;
#157296=CARTESIAN_POINT ( 'NONE',  ( 8.314922557961029526, -14.29746914071037800, 25.41775706135235779 ) ) ;
#157297=CARTESIAN_POINT ( 'NONE',  ( 19.03943276465977164, -0.05219959533909143690, 33.74890960531435979 ) ) ;
#157298=CARTESIAN_POINT ( 'NONE',  ( -19.02544592524342804, 5.153800228976336051, 86.04057627198103830 ) ) ;
#157299=CARTESIAN_POINT ( 'NONE',  ( 4.379528057220092307, 16.55341960407617563, 37.29275706135235424 ) ) ;
#157300=CARTESIAN_POINT ( 'NONE',  ( 17.97214573761831247, 5.500000000000079048, 68.96970049038654338 ) ) ;
#157301=CARTESIAN_POINT ( 'NONE',  ( -10.81492255796105439, 18.62759615963255655, 112.9177570613523329 ) ) ;
#157302=CARTESIAN_POINT ( 'NONE',  ( 8.314922557961029526, -14.29746914071037800, 90.41775706135236135 ) ) ;
#157303=CARTESIAN_POINT ( 'NONE',  ( 5.153800228976615827, -19.02544592524334988, 100.2094237280190043 ) ) ;
#157304=CARTESIAN_POINT ( 'NONE',  ( -13.97604488694527625, -13.89961937509977652, 26.87390960531434558 ) ) ;
#157305=CARTESIAN_POINT ( 'NONE',  ( -16.55341960407617563, 4.379528057220093196, 78.54275706135236135 ) ) ;
#157306=CARTESIAN_POINT ( 'NONE',  ( 4.483927247898790824, -16.52544592524335698, 65.20942372801901854 ) ) ;
#157308=CARTESIAN_POINT ( 'NONE',  ( 5.153800228976615827, -19.02544592524334988, 75.20942372801896170 ) ) ;
#157309=CARTESIAN_POINT ( 'NONE',  ( 0.05219959533937995610, -21.53943276465977519, 105.0010903946856757 ) ) ;
#157310=CARTESIAN_POINT ( 'NONE',  ( -19.03943276465977164, 0.05219959533909376836, 51.24890960531436690 ) ) ;
#157311=CARTESIAN_POINT ( 'NONE',  ( 19.02544592524343514, -5.153800228976328945, 98.54057627198100988 ) ) ;
#157312=CARTESIAN_POINT ( 'NONE',  ( 12.14591786802309770, 12.06949235617756955, 84.37390960531438111 ) ) ;
#157315=CARTESIAN_POINT ( 'NONE',  ( -5.153800228976607833, 19.02544592524334988, 57.70942372801899012 ) ) ;
#157316=CARTESIAN_POINT ( 'NONE',  ( -10.81492255796078084, -18.62759615963271287, 47.08224293864770260 ) ) ;
#157317=CARTESIAN_POINT ( 'NONE',  ( 0.05219959533936267826, -19.03943276465977164, 20.00109039468567218 ) ) ;
#157318=CARTESIAN_POINT ( 'NONE',  ( 9.474510206698971260, -16.51473224551069308, 87.91557627198102409 ) ) ;
#157319=CARTESIAN_POINT ( 'NONE',  ( 10.72451020669871369, 18.67979575497193778, 112.0844237280190185 ) ) ;
#157320=CARTESIAN_POINT ( 'NONE',  ( -18.67979575497178146, -10.72451020669898902, 61.66557627198103120 ) ) ;
#157321=CARTESIAN_POINT ( 'NONE',  ( 19.05341960407611168, 5.049401038298154454, 98.95724293864766707 ) ) ;
#157323=CARTESIAN_POINT ( 'NONE',  ( 13.89961937509957401, 13.97604488694547697, 91.87609039468567573 ) ) ;
#157324=CARTESIAN_POINT ( 'NONE',  ( -16.51473224551069308, -9.474510206698971260, 111.6655762719810383 ) ) ;
#157325=CARTESIAN_POINT ( 'NONE',  ( 16.46253265017146816, 9.564922557961045513, 106.6677570613523471 ) ) ;
#157326=CARTESIAN_POINT ( 'NONE',  ( -4.379528057220328563, 16.55341960407611168, 110.2072429386477239 ) ) ;
#157327=CARTESIAN_POINT ( 'NONE',  ( -0.05219959533909027116, -19.03943276465977164, 87.49890960531436690 ) ) ;
#157328=CARTESIAN_POINT ( 'NONE',  ( 0.05219959533907565091, 21.53943276465977519, 74.99890960531435269 ) ) ;
#157329=CARTESIAN_POINT ( 'NONE',  ( 0.05219959533934541429, -16.53943276465976808, 50.00109039468568994 ) ) ;
#157330=CARTESIAN_POINT ( 'NONE',  ( 15.72974639402176855, 15.80617190586768217, 51.87609039468568284 ) ) ;
#157331=CARTESIAN_POINT ( 'NONE',  ( -21.52544592524334988, -5.823673210054445271, 93.95942372801903275 ) ) ;
#157332=CARTESIAN_POINT ( 'NONE',  ( 12.06949235617739724, 12.14591786802326823, 96.87609039468568994 ) ) ;
#157333=CARTESIAN_POINT ( 'NONE',  ( -9.564922557960796823, -16.46253265017161027, 82.08224293864768129 ) ) ;
#157334=CARTESIAN_POINT ( 'NONE',  ( -0.05219959533910754901, -16.53943276465976808, 87.49890960531436690 ) ) ;
#157335=CARTESIAN_POINT ( 'NONE',  ( 14.29746914071049879, -8.314922557960816363, 28.33224293864769550 ) ) ;
#157336=CARTESIAN_POINT ( 'NONE',  ( -5.153800228976607833, 19.02544592524334988, 72.70942372801900433 ) ) ;
#157337=CARTESIAN_POINT ( 'NONE',  ( -21.53943276465977519, -0.05219959533937600094, 43.75109039468568284 ) ) ;
#157338=CARTESIAN_POINT ( 'NONE',  ( -16.51473224551082808, 9.474510206698731452, 23.33442372801900078 ) ) ;
#157339=CARTESIAN_POINT ( 'NONE',  ( 4.483927247898545687, 16.52544592524342804, 94.79057627198105251 ) ) ;
#157340=CARTESIAN_POINT ( 'NONE',  ( -19.03943276465977164, 0.05219959533909376836, 111.2489096053143669 ) ) ;
#157341=CARTESIAN_POINT ( 'NONE',  ( 12.14591786802309770, 12.06949235617756955, 24.37390960531435979 ) ) ;
#157342=CARTESIAN_POINT ( 'NONE',  ( -15.72974639402176322, -15.80617190586768395, 79.37609039468567573 ) ) ;
#157343=CARTESIAN_POINT ( 'NONE',  ( -14.29746914071037622, -8.314922557961029526, 59.16775706135234714 ) ) ;
#157344=CARTESIAN_POINT ( 'NONE',  ( 4.483927247898790824, -16.52544592524335698, 100.2094237280190043 ) ) ;
#157345=CARTESIAN_POINT ( 'NONE',  ( 15.80617190586769283, -15.72974639402175789, 55.62609039468568284 ) ) ;
#157347=CARTESIAN_POINT ( 'NONE',  ( 18.67979575497194134, -10.72451020669871369, 30.83442372801902209 ) ) ;
#157348=CARTESIAN_POINT ( 'NONE',  ( -14.29746914071049879, 8.314922557960819915, 110.8322429386476955 ) ) ;
#157349=CARTESIAN_POINT ( 'NONE',  ( -0.05219959533909027116, -19.03943276465977164, 22.49890960531436690 ) ) ;
#157350=CARTESIAN_POINT ( 'NONE',  ( 4.379528057220339221, -16.55341960407611168, 62.70724293864769550 ) ) ;
#157351=CARTESIAN_POINT ( 'NONE',  ( 16.51473224551069308, 9.474510206698969483, 69.16557627198102409 ) ) ;
#157352=CARTESIAN_POINT ( 'NONE',  ( -0.05219959533934338120, 16.53943276465976808, 102.5010903946856899 ) ) ;
#157353=CARTESIAN_POINT ( 'NONE',  ( 13.89961937509977652, -13.97604488694527269, 33.12390960531434558 ) ) ;
#157354=CARTESIAN_POINT ( 'NONE',  ( -10.81492255796078084, -18.62759615963271287, 52.08224293864768839 ) ) ;
#157355=CARTESIAN_POINT ( 'NONE',  ( -0.05219959533910754901, -16.53943276465976808, 92.49890960531436690 ) ) ;
#157357=CARTESIAN_POINT ( 'NONE',  ( -5.719274019375978568, 21.55341960407610458, 90.20724293864770971 ) ) ;
#157358=CARTESIAN_POINT ( 'NONE',  ( -0.05219959533909027116, -19.03943276465977164, 107.4989096053143527 ) ) ;
#157359=CARTESIAN_POINT ( 'NONE',  ( -13.97604488694527625, -13.89961937509977652, 46.87390960531435979 ) ) ;
#157360=CARTESIAN_POINT ( 'NONE',  ( -13.89961937509957401, -13.97604488694547875, 94.37609039468566152 ) ) ;
#157361=CARTESIAN_POINT ( 'NONE',  ( 21.55341960407610458, 5.719274019375980345, 43.95724293864769550 ) ) ;
#157362=CARTESIAN_POINT ( 'NONE',  ( 15.80617190586769283, -15.72974639402175789, 65.62609039468568994 ) ) ;
#157363=CARTESIAN_POINT ( 'NONE',  ( -9.564922557960796823, -16.46253265017161027, 52.08224293864768839 ) ) ;
#157364=CARTESIAN_POINT ( 'NONE',  ( -9.474510206698964154, 16.51473224551069663, 85.41557627198102409 ) ) ;
#157365=CARTESIAN_POINT ( 'NONE',  ( 8.224510206698742110, 14.34966873604972548, 62.08442372801901143 ) ) ;
#157366=CARTESIAN_POINT ( 'NONE',  ( -21.55341960407619339, 5.719274019375674811, 43.54275706135235424 ) ) ;
#157367=CARTESIAN_POINT ( 'NONE',  ( 5.719274019375673035, 21.55341960407619339, 77.29275706135234714 ) ) ;
#157368=CARTESIAN_POINT ( 'NONE',  ( -13.97604488694527625, -13.89961937509977652, 111.8739096053143243 ) ) ;
#157369=CARTESIAN_POINT ( 'NONE',  ( 0.05219959533907565091, 21.53943276465977519, 94.99890960531436690 ) ) ;
#157370=CARTESIAN_POINT ( 'NONE',  ( 21.53943276465977519, 0.05219959533937863772, 36.25109039468567573 ) ) ;
#157371=CARTESIAN_POINT ( 'NONE',  ( 8.314922557961029526, -14.29746914071037800, 60.41775706135235424 ) ) ;
#157372=CARTESIAN_POINT ( 'NONE',  ( -21.52544592524343514, 5.823673210054127303, 61.04057627198103120 ) ) ;
#157373=CARTESIAN_POINT ( 'NONE',  ( -9.564922557961040184, 16.46253265017147172, 27.91775706135232582 ) ) ;
#157374=B_SPLINE_CURVE_WITH_KNOTS ( 'NONE', 3,
 ( #148128, #164305, #106579, #183438, #153076, #92393, #381, #168256, #44923, #136923, #121746, #29752, #14578, #107561, #152101, #93386, #198610, #169239, #76236, #182451 ),
 .UNSPECIFIED., .F., .F.,
 ( 4, 2, 2, 2, 2, 2, 2, 2, 2, 4 ),
 ( 0.004000878361812006817, 0.004499404418916007169, 0.004997930476020007520, 0.005496456533124007005, 0.005994982590228007356, 0.006244245618780007098, 0.006493508647332007708, 0.006992034704436007192, 0.007490560761540007544, 0.007989086818644007895 ),
 .UNSPECIFIED. ) ;
#157375=CARTESIAN_POINT ( 'NONE',  ( -16.51473224551069308, -9.474510206698971260, 61.66557627198103120 ) ) ;
#157376=CARTESIAN_POINT ( 'NONE',  ( 0.05219959533934541429, -16.53943276465976808, 110.0010903946856757 ) ) ;
#157377=CARTESIAN_POINT ( 'NONE',  ( -17.49999999999999645, -3.305555262949684270, 105.3748284784340967 ) ) ;
#157378=CARTESIAN_POINT ( 'NONE',  ( 13.97604488694527802, 13.89961937509977652, 109.3739096053143669 ) ) ;
#157380=CARTESIAN_POINT ( 'NONE',  ( 19.03943276465977164, 0.05219959533936151252, 86.25109039468567573 ) ) ;
#157381=CARTESIAN_POINT ( 'NONE',  ( -21.55341960407610458, -5.719274019375992779, 56.45724293864768839 ) ) ;
#157382=CARTESIAN_POINT ( 'NONE',  ( 8.224510206698953496, -14.34966873604960469, 37.91557627198102409 ) ) ;
#157383=CARTESIAN_POINT ( 'NONE',  ( 0.05219959533936267826, -19.03943276465977164, 110.0010903946856757 ) ) ;
#157384=CARTESIAN_POINT ( 'NONE',  ( -19.03943276465977164, 0.05219959533909376836, 31.24890960531435979 ) ) ;
#157385=CARTESIAN_POINT ( 'NONE',  ( 13.89961937509957401, 13.97604488694547697, 111.8760903946856757 ) ) ;
#157386=CARTESIAN_POINT ( 'NONE',  ( -21.53943276465977519, 0.05219959533907696930, 91.24890960531436690 ) ) ;
#157387=CARTESIAN_POINT ( 'NONE',  ( 16.46253265017146816, 9.564922557961045513, 56.66775706135233293 ) ) ;
#157388=CARTESIAN_POINT ( 'NONE',  ( 14.29746914071037800, 8.314922557961029526, 81.66775706135236135 ) ) ;
#157389=CARTESIAN_POINT ( 'NONE',  ( -19.03943276465977164, 0.05219959533909376836, 71.24890960531435269 ) ) ;
#157390=CARTESIAN_POINT ( 'NONE',  ( -12.14591786802309592, -12.06949235617757132, 81.87390960531435269 ) ) ;
#157391=CARTESIAN_POINT ( 'NONE',  ( 5.153800228976335163, 19.02544592524342804, 44.79057627198103830 ) ) ;
#157392=CARTESIAN_POINT ( 'NONE',  ( 12.06949235617757843, -12.14591786802309237, 53.12390960531436690 ) ) ;
#157395=CARTESIAN_POINT ( 'NONE',  ( 14.29746914071049879, -8.314922557960816363, 28.33224293864769550 ) ) ;
#157396=CARTESIAN_POINT ( 'NONE',  ( 19.02544592524343514, -5.153800228976328945, 78.54057627198099567 ) ) ;
#157397=CARTESIAN_POINT ( 'NONE',  ( -30.00000000000000000, -5.510910596163089556E-15, 47.50000000000000000 ) ) ;
#157398=CARTESIAN_POINT ( 'NONE',  ( -16.51473224551082808, 9.474510206698731452, 43.33442372801900433 ) ) ;
#157399=CARTESIAN_POINT ( 'NONE',  ( 12.14591786802327356, -12.06949235617739191, 40.62609039468567573 ) ) ;
#157400=CARTESIAN_POINT ( 'NONE',  ( 5.823673210054125526, 21.52544592524343514, 69.79057627198102409 ) ) ;
#157401=CARTESIAN_POINT ( 'NONE',  ( -9.474510206698720793, -16.51473224551083518, 24.58442372801900078 ) ) ;
#157402=CARTESIAN_POINT ( 'NONE',  ( 19.02544592524343514, -5.153800228976328945, 68.54057627198103830 ) ) ;
#157404=CARTESIAN_POINT ( 'NONE',  ( 9.564922557960805705, 16.46253265017160317, 104.5822429386476955 ) ) ;
#157405=CARTESIAN_POINT ( 'NONE',  ( 15.80617190586769283, -15.72974639402175789, 40.62609039468567573 ) ) ;
#157406=CARTESIAN_POINT ( 'NONE',  ( -12.06949235617756955, 12.14591786802309770, 110.6239096053143669 ) ) ;
#157407=CARTESIAN_POINT ( 'NONE',  ( 5.823673210054125526, 21.52544592524343514, 99.79057627198103830 ) ) ;
#157408=CARTESIAN_POINT ( 'NONE',  ( -9.564922557960796823, -16.46253265017161027, 82.08224293864768129 ) ) ;
#157410=CARTESIAN_POINT ( 'NONE',  ( -15.80617190586768217, 15.72974639402176855, 23.12609039468567573 ) ) ;
#157412=CARTESIAN_POINT ( 'NONE',  ( -5.049401038298153566, 19.05341960407611168, 85.20724293864766707 ) ) ;
#157414=CARTESIAN_POINT ( 'NONE',  ( 13.97604488694527802, 13.89961937509977652, 39.37390960531435269 ) ) ;
#157415=CARTESIAN_POINT ( 'NONE',  ( -5.049401038297874678, -19.05341960407617918, 109.7927570613523187 ) ) ;
#157417=CARTESIAN_POINT ( 'NONE',  ( -12.06949235617756955, 12.14591786802309770, 110.6239096053143669 ) ) ;
#157418=CARTESIAN_POINT ( 'NONE',  ( 15.72974639402176855, 15.80617190586768217, 86.87609039468568994 ) ) ;
#157419=CARTESIAN_POINT ( 'NONE',  ( -19.05341960407611168, -5.049401038298163336, 71.45724293864766707 ) ) ;
#157420=CARTESIAN_POINT ( 'NONE',  ( 21.52544592524334988, 5.823673210054432836, 41.45942372801901143 ) ) ;
#157421=CARTESIAN_POINT ( 'NONE',  ( 5.719274019375673035, 21.55341960407619339, 27.29275706135234358 ) ) ;
#157423=CARTESIAN_POINT ( 'NONE',  ( -13.97604488694527625, -13.89961937509977652, 81.87390960531436690 ) ) ;
#157425=CARTESIAN_POINT ( 'NONE',  ( -4.483927247898782831, 16.52544592524335698, 22.70942372801901499 ) ) ;
#157426=CARTESIAN_POINT ( 'NONE',  ( 21.53943276465977519, -0.05219959533907433946, 38.74890960531435979 ) ) ;
#157427=CARTESIAN_POINT ( 'NONE',  ( 5.719274019375673035, 21.55341960407619339, 72.29275706135236135 ) ) ;
#157428=CARTESIAN_POINT ( 'NONE',  ( 19.05341960407611168, 5.049401038298154454, 103.9572429386476671 ) ) ;
#157429=CARTESIAN_POINT ( 'NONE',  ( 16.46253265017146816, 9.564922557961045513, 111.6677570613523329 ) ) ;
#157430=CARTESIAN_POINT ( 'NONE',  ( 0.05219959533909260263, 19.03943276465977164, 64.99890960531436690 ) ) ;
#157431=CARTESIAN_POINT ( 'NONE',  ( 16.51473224551069308, 9.474510206698969483, 84.16557627198102409 ) ) ;
#157432=CARTESIAN_POINT ( 'NONE',  ( -14.34966873604960291, -8.224510206698953496, 101.6655762719810383 ) ) ;
#157433=CARTESIAN_POINT ( 'NONE',  ( -16.55341960407611168, -4.379528057220339221, 111.4572429386476813 ) ) ;
#157434=CARTESIAN_POINT ( 'NONE',  ( -16.51473224551069308, -9.474510206698971260, 106.6655762719810383 ) ) ;
#157435=CARTESIAN_POINT ( 'NONE',  ( -16.52544592524335698, -4.483927247898792601, 78.95942372801901854 ) ) ;
#157436=CARTESIAN_POINT ( 'NONE',  ( 8.314922557960818139, 14.29746914071049879, 59.58224293864770260 ) ) ;
#157437=CARTESIAN_POINT ( 'NONE',  ( -19.02544592524342804, 5.153800228976336051, 56.04057627198100988 ) ) ;
#157438=CARTESIAN_POINT ( 'NONE',  ( -15.80617190586768217, 15.72974639402176855, 78.12609039468570415 ) ) ;
#157439=CARTESIAN_POINT ( 'NONE',  ( 21.55341960407619695, -5.719274019375665929, 71.04275706135234714 ) ) ;
#157440=CARTESIAN_POINT ( 'NONE',  ( 0.05219959533936267826, -19.03943276465977164, 90.00109039468567573 ) ) ;
#157441=CARTESIAN_POINT ( 'NONE',  ( -12.14591786802309592, -12.06949235617757132, 61.87390960531436690 ) ) ;
#157442=CARTESIAN_POINT ( 'NONE',  ( 21.55341960407610458, 5.719274019375980345, 108.9572429386476955 ) ) ;
#157443=CARTESIAN_POINT ( 'NONE',  ( 0.05219959533907565091, 21.53943276465977519, 44.99890960531435979 ) ) ;
#157444=CARTESIAN_POINT ( 'NONE',  ( -16.19135201231367560, -7.376712067591916444, 105.1868085405203175 ) ) ;
#157446=CARTESIAN_POINT ( 'NONE',  ( 5.153800228976335163, 19.02544592524342804, 64.79057627198100988 ) ) ;
#157447=CARTESIAN_POINT ( 'NONE',  ( -14.29746914071049879, 8.314922557960819915, 30.83224293864770260 ) ) ;
#157449=CARTESIAN_POINT ( 'NONE',  ( -12.06949235617739369, -12.14591786802326823, 109.3760903946857042 ) ) ;
#157450=CARTESIAN_POINT ( 'NONE',  ( -4.483927247898782831, 16.52544592524335698, 87.70942372801901854 ) ) ;
#157451=CARTESIAN_POINT ( 'NONE',  ( -19.03943276465977164, -0.05219959533935918106, 33.75109039468566863 ) ) ;
#157453=CARTESIAN_POINT ( 'NONE',  ( -19.02544592524342804, 5.153800228976336051, 96.04057627198103830 ) ) ;
#157454=CARTESIAN_POINT ( 'NONE',  ( 8.224510206698953496, -14.34966873604960469, 57.91557627198103120 ) ) ;
#157455=CARTESIAN_POINT ( 'NONE',  ( 13.97604488694527802, 13.89961937509977652, 24.37390960531435624 ) ) ;
#157456=CARTESIAN_POINT ( 'NONE',  ( 21.52544592524344225, -5.823673210054117533, 28.54057627198103120 ) ) ;
#157457=CARTESIAN_POINT ( 'NONE',  ( 10.81492255796078972, 18.62759615963270932, 59.58224293864770260 ) ) ;
#157459=CARTESIAN_POINT ( 'NONE',  ( -16.55341960407611168, -4.379528057220339221, 101.4572429386476955 ) ) ;
#157460=CARTESIAN_POINT ( 'NONE',  ( 0.05219959533934541429, -16.53943276465976808, 35.00109039468568284 ) ) ;
#157462=CARTESIAN_POINT ( 'NONE',  ( -14.34966873604960291, -8.224510206698953496, 76.66557627198103830 ) ) ;
#157464=CARTESIAN_POINT ( 'NONE',  ( 19.05341960407617918, -5.049401038297876454, 81.04275706135231871 ) ) ;
#157465=CARTESIAN_POINT ( 'NONE',  ( -16.46253265017160317, 9.564922557960807481, 115.8322429386477097 ) ) ;
#157467=CARTESIAN_POINT ( 'NONE',  ( 17.50000000000000000, 5.499999999999997335, 120.0000000000000142 ) ) ;
#157468=CARTESIAN_POINT ( 'NONE',  ( -0.05219959533934338120, 16.53943276465976808, 27.50109039468567929 ) ) ;
#157469=CARTESIAN_POINT ( 'NONE',  ( 8.224510206698953496, -14.34966873604960469, 32.91557627198102409 ) ) ;
#157470=CARTESIAN_POINT ( 'NONE',  ( -5.719274019375978568, 21.55341960407610458, 60.20724293864768839 ) ) ;
#157471=CARTESIAN_POINT ( 'NONE',  ( -19.03943276465977164, -0.05219959533935918106, 88.75109039468567573 ) ) ;
#157472=CARTESIAN_POINT ( 'NONE',  ( 21.52544592524344225, -5.823673210054117533, 43.54057627198103830 ) ) ;
#157473=CARTESIAN_POINT ( 'NONE',  ( 21.53943276465977519, 0.05219959533937863772, 86.25109039468568994 ) ) ;
#157475=CARTESIAN_POINT ( 'NONE',  ( -16.55341960407617563, 4.379528057220093196, 33.54275706135234714 ) ) ;
#157476=CARTESIAN_POINT ( 'NONE',  ( -13.97604488694527625, -13.89961937509977652, 21.87390960531435979 ) ) ;
#157477=CARTESIAN_POINT ( 'NONE',  ( -19.02544592524342804, 5.153800228976336051, 91.04057627198100988 ) ) ;
#157479=CARTESIAN_POINT ( 'NONE',  ( 9.474510206698971260, -16.51473224551069308, 32.91557627198102409 ) ) ;
#157480=CARTESIAN_POINT ( 'NONE',  ( -0.05219959533910754901, -16.53943276465976808, 107.4989096053143669 ) ) ;
#157481=CARTESIAN_POINT ( 'NONE',  ( -19.05341960407611168, -5.049401038298163336, 101.4572429386476955 ) ) ;
#157483=CARTESIAN_POINT ( 'NONE',  ( -8.224510206698735004, -14.34966873604973081, 59.58442372801901854 ) ) ;
#157484=CARTESIAN_POINT ( 'NONE',  ( 18.67979575497178502, 10.72451020669898547, 94.16557627198103830 ) ) ;
#157485=CARTESIAN_POINT ( 'NONE',  ( 5.049401038298161559, -19.05341960407611168, 37.70724293864768839 ) ) ;
#157486=CARTESIAN_POINT ( 'NONE',  ( -5.153800228976607833, 19.02544592524334988, 72.70942372801900433 ) ) ;
#157487=CARTESIAN_POINT ( 'NONE',  ( -18.62759615963255300, -10.81492255796106328, 34.16775706135234714 ) ) ;
#157488=CARTESIAN_POINT ( 'NONE',  ( -5.049401038298153566, 19.05341960407611168, 65.20724293864765286 ) ) ;
#157489=CARTESIAN_POINT ( 'NONE',  ( -19.03943276465977164, 0.05219959533909376836, 101.2489096053143669 ) ) ;
#157491=CARTESIAN_POINT ( 'NONE',  ( 4.483927247898790824, -16.52544592524335698, 40.20942372801901854 ) ) ;
#157492=CARTESIAN_POINT ( 'NONE',  ( -15.72974639402197994, 15.80617190586746368, 115.6239096053143669 ) ) ;
#157493=CARTESIAN_POINT ( 'NONE',  ( -16.52544592524342804, 4.483927247898546575, 101.0405762719810383 ) ) ;
#157494=CARTESIAN_POINT ( 'NONE',  ( -9.564922557960796823, -16.46253265017161027, 92.08224293864769550 ) ) ;
#157495=CARTESIAN_POINT ( 'NONE',  ( 19.02544592524334988, 5.153800228976608722, 76.45942372801897591 ) ) ;
#157496=CARTESIAN_POINT ( 'NONE',  ( 15.80617190586746368, 15.72974639402197994, 89.37390960531435269 ) ) ;
#157497=CARTESIAN_POINT ( 'NONE',  ( -4.483927247898539470, -16.52544592524342804, 47.29057627198103120 ) ) ;
#157498=CARTESIAN_POINT ( 'NONE',  ( -9.564922557961040184, 16.46253265017147172, 22.91775706135233648 ) ) ;
#157499=CARTESIAN_POINT ( 'NONE',  ( -16.53943276465976808, -0.05219959533934237506, 83.75109039468568994 ) ) ;
#157500=CARTESIAN_POINT ( 'NONE',  ( -13.97604488694527625, -13.89961937509977652, 111.8739096053143243 ) ) ;
#157501=CARTESIAN_POINT ( 'NONE',  ( 16.46253265017160672, -9.564922557960803928, 48.33224293864769550 ) ) ;
#157502=CARTESIAN_POINT ( 'NONE',  ( 10.81492255796106328, -18.62759615963255655, 55.41775706135234714 ) ) ;
#157503=CARTESIAN_POINT ( 'NONE',  ( 18.62759615963255655, 10.81492255796105972, 71.66775706135234714 ) ) ;
#157504=CARTESIAN_POINT ( 'NONE',  ( 13.89961937509977652, -13.97604488694527269, 68.12390960531436690 ) ) ;
#157505=CARTESIAN_POINT ( 'NONE',  ( -10.72451020669870658, -18.67979575497194134, 54.58442372801901143 ) ) ;
#157506=CARTESIAN_POINT ( 'NONE',  ( -16.46253265017146816, -9.564922557961047289, 89.16775706135234714 ) ) ;
#157507=CARTESIAN_POINT ( 'NONE',  ( 5.049401038298161559, -19.05341960407611168, 57.70724293864769550 ) ) ;
#157508=CARTESIAN_POINT ( 'NONE',  ( -8.314922557961024197, 14.29746914071037800, 87.91775706135234714 ) ) ;
#157509=CARTESIAN_POINT ( 'NONE',  ( 16.51473224551069308, 9.474510206698969483, 64.16557627198102409 ) ) ;
#157511=CARTESIAN_POINT ( 'NONE',  ( -9.564922557960796823, -16.46253265017161027, 47.08224293864769550 ) ) ;
#157512=CARTESIAN_POINT ( 'NONE',  ( 10.72451020669898902, -18.67979575497178502, 87.91557627198103830 ) ) ;
#157513=CARTESIAN_POINT ( 'NONE',  ( -14.29746914071037622, -8.314922557961029526, 69.16775706135234714 ) ) ;
#157515=CARTESIAN_POINT ( 'NONE',  ( 16.51473224551083163, -9.474510206698727899, 25.83442372801900078 ) ) ;
#157516=CARTESIAN_POINT ( 'NONE',  ( 13.97604488694527802, 13.89961937509977652, 69.37390960531436690 ) ) ;
#157517=CARTESIAN_POINT ( 'NONE',  ( 16.55341960407611168, 4.379528057220329451, 53.95724293864770260 ) ) ;
#157518=CARTESIAN_POINT ( 'NONE',  ( -16.52544592524342804, 4.483927247898546575, 101.0405762719810383 ) ) ;
#157519=CARTESIAN_POINT ( 'NONE',  ( 9.564922557960805705, 16.46253265017160317, 104.5822429386476955 ) ) ;
#157520=CARTESIAN_POINT ( 'NONE',  ( 16.51473224551069308, 9.474510206698969483, 89.16557627198103830 ) ) ;
#157521=CARTESIAN_POINT ( 'NONE',  ( 18.62759615963255655, 10.81492255796105972, 56.66775706135235424 ) ) ;
#157522=CARTESIAN_POINT ( 'NONE',  ( -19.05341960407611168, -5.049401038298163336, 106.4572429386476955 ) ) ;
#157523=CARTESIAN_POINT ( 'NONE',  ( -19.02544592524334988, -5.153800228976617603, 18.95942372801899722 ) ) ;
#157524=CARTESIAN_POINT ( 'NONE',  ( 12.14591786802327356, -12.06949235617739191, 85.62609039468568994 ) ) ;
#157525=CARTESIAN_POINT ( 'NONE',  ( 5.823673210054444382, -21.52544592524334988, 35.20942372801901854 ) ) ;
#157526=CARTESIAN_POINT ( 'NONE',  ( 9.564922557960805705, 16.46253265017160317, 109.5822429386476955 ) ) ;
#157527=CARTESIAN_POINT ( 'NONE',  ( -15.80617190586745835, -15.72974639402198527, 96.87390960531436690 ) ) ;
#157528=CARTESIAN_POINT ( 'NONE',  ( 4.379528057220339221, -16.55341960407611168, 62.70724293864769550 ) ) ;
#157529=CARTESIAN_POINT ( 'NONE',  ( -5.049401038298153566, 19.05341960407611168, 60.20724293864768129 ) ) ;
#157530=CARTESIAN_POINT ( 'NONE',  ( -12.14591786802309592, -12.06949235617757132, 81.87390960531435269 ) ) ;
#157531=CARTESIAN_POINT ( 'NONE',  ( -10.72451020669898014, 18.67979575497178502, 30.41557627198101699 ) ) ;
#157532=CARTESIAN_POINT ( 'NONE',  ( 13.89961937509957401, 13.97604488694547697, 41.87609039468566152 ) ) ;
#157533=CARTESIAN_POINT ( 'NONE',  ( -8.224510206698948167, 14.34966873604960824, 110.4155762719810383 ) ) ;
#157535=CARTESIAN_POINT ( 'NONE',  ( 14.34966873604972726, -8.224510206698740333, 65.83442372801900433 ) ) ;
#157536=CARTESIAN_POINT ( 'NONE',  ( -13.89961937509977652, 13.97604488694528158, 65.62390960531436690 ) ) ;
#157538=CARTESIAN_POINT ( 'NONE',  ( -4.379528057220328563, 16.55341960407611168, 90.20724293864770971 ) ) ;
#157539=CARTESIAN_POINT ( 'NONE',  ( 18.67979575497178502, 10.72451020669898547, 34.16557627198102409 ) ) ;
#157540=CARTESIAN_POINT ( 'NONE',  ( -12.14591786802326823, 12.06949235617739902, 103.1260903946856757 ) ) ;
#157541=CARTESIAN_POINT ( 'NONE',  ( -16.53943276465976808, -0.05219959533934237506, 18.75109039468568639 ) ) ;
#157542=CARTESIAN_POINT ( 'NONE',  ( -18.62759615963255300, -10.81492255796106328, 79.16775706135234714 ) ) ;
#157543=CARTESIAN_POINT ( 'NONE',  ( 19.05341960407611168, 5.049401038298154454, 88.95724293864769550 ) ) ;
#157544=CARTESIAN_POINT ( 'NONE',  ( 18.67979575497178502, 10.72451020669898547, 99.16557627198100988 ) ) ;
#157545=CARTESIAN_POINT ( 'NONE',  ( -12.06949235617739369, -12.14591786802326823, 49.37609039468569705 ) ) ;
#157546=CARTESIAN_POINT ( 'NONE',  ( -9.564922557960796823, -16.46253265017161027, 37.08224293864768839 ) ) ;
#157547=CARTESIAN_POINT ( 'NONE',  ( -16.52544592524335698, -4.483927247898792601, 28.95942372801902209 ) ) ;
#157549=CARTESIAN_POINT ( 'NONE',  ( -19.02544592524334988, -5.153800228976617603, 98.95942372801900433 ) ) ;
#157550=CARTESIAN_POINT ( 'NONE',  ( -18.67979575497178146, -10.72451020669898902, 86.66557627198102409 ) ) ;
#157551=CARTESIAN_POINT ( 'NONE',  ( -19.03943276465977164, -0.05219959533935918106, 58.75109039468566863 ) ) ;
#157552=CARTESIAN_POINT ( 'NONE',  ( 18.87580814761075132, -5.500000000000047073, 88.37172394265761000 ) ) ;
#157553=CARTESIAN_POINT ( 'NONE',  ( 10.72451020669898902, -18.67979575497178502, 97.91557627198103830 ) ) ;
#157554=CARTESIAN_POINT ( 'NONE',  ( -0.05219959533909027116, -19.03943276465977164, 72.49890960531435269 ) ) ;
#157555=CARTESIAN_POINT ( 'NONE',  ( -5.049401038298153566, 19.05341960407611168, 80.20724293864769550 ) ) ;
#157556=CARTESIAN_POINT ( 'NONE',  ( -14.29746914071037622, -8.314922557961029526, 34.16775706135234714 ) ) ;
#157558=CARTESIAN_POINT ( 'NONE',  ( -0.05219959533936034679, 19.03943276465977164, 57.50109039468566863 ) ) ;
#157559=CARTESIAN_POINT ( 'NONE',  ( 15.80617190586746368, 15.72974639402197994, 114.3739096053143527 ) ) ;
#157560=CARTESIAN_POINT ( 'NONE',  ( 12.14591786802309770, 12.06949235617756955, 59.37390960531436690 ) ) ;
#157561=CARTESIAN_POINT ( 'NONE',  ( -5.153800228976328057, -19.02544592524343514, 67.29057627198102409 ) ) ;
#157562=CARTESIAN_POINT ( 'NONE',  ( 8.224510206698742110, 14.34966873604972548, 32.08442372801901854 ) ) ;
#157563=CARTESIAN_POINT ( 'NONE',  ( 19.05341960407617918, -5.049401038297876454, 36.04275706135234003 ) ) ;
#157564=CARTESIAN_POINT ( 'NONE',  ( 15.72974639402176855, 15.80617190586768217, 51.87609039468568284 ) ) ;
#157565=CARTESIAN_POINT ( 'NONE',  ( -19.03943276465977164, -0.05219959533935918106, 108.7510903946856615 ) ) ;
#157566=CARTESIAN_POINT ( 'NONE',  ( -19.03943276465977164, 0.05219959533909376836, 61.24890960531436690 ) ) ;
#157567=CARTESIAN_POINT ( 'NONE',  ( -13.89961937509957401, -13.97604488694547875, 84.37609039468567573 ) ) ;
#157568=CARTESIAN_POINT ( 'NONE',  ( 21.55341960407619695, -5.719274019375665929, 91.04275706135236135 ) ) ;
#157569=CARTESIAN_POINT ( 'NONE',  ( 19.03943276465977164, 0.05219959533936151252, 61.25109039468566863 ) ) ;
#157570=CARTESIAN_POINT ( 'NONE',  ( -13.89961937509977652, 13.97604488694528158, 30.62390960531435269 ) ) ;
#157571=CARTESIAN_POINT ( 'NONE',  ( 5.719274019375991003, -21.55341960407610458, 62.70724293864769550 ) ) ;
#157572=CARTESIAN_POINT ( 'NONE',  ( 16.53943276465976808, -0.05219959533910856209, 63.74890960531435979 ) ) ;
#157573=CARTESIAN_POINT ( 'NONE',  ( -9.474510206698720793, -16.51473224551083518, 69.58442372801901854 ) ) ;
#157574=CARTESIAN_POINT ( 'NONE',  ( -17.13100169013301155, -6.664070546373100257, 24.23210164300151703 ) ) ;
#157575=CARTESIAN_POINT ( 'NONE',  ( -9.474510206698720793, -16.51473224551083518, 34.58442372801899722 ) ) ;
#157576=CARTESIAN_POINT ( 'NONE',  ( -14.29746914071037622, -8.314922557961029526, 94.16775706135237556 ) ) ;
#157577=CARTESIAN_POINT ( 'NONE',  ( 12.06949235617757843, -12.14591786802309237, 48.12390960531436690 ) ) ;
#157578=CARTESIAN_POINT ( 'NONE',  ( 18.67979575497194134, -10.72451020669871369, 90.83442372801901854 ) ) ;
#157580=CARTESIAN_POINT ( 'NONE',  ( -5.719274019375978568, 21.55341960407610458, 90.20724293864770971 ) ) ;
#157581=CARTESIAN_POINT ( 'NONE',  ( -13.89961937509977652, 13.97604488694528158, 50.62390960531435979 ) ) ;
#157582=CARTESIAN_POINT ( 'NONE',  ( 10.81492255796106328, -18.62759615963255655, 70.41775706135236135 ) ) ;
#157583=CARTESIAN_POINT ( 'NONE',  ( -16.46253265017160317, 9.564922557960807481, 55.83224293864769550 ) ) ;
#157584=ORIENTED_EDGE ( 'NONE', *, *, #136149, .F. ) ;
#157585=CARTESIAN_POINT ( 'NONE',  ( 13.97604488694527802, 13.89961937509977652, 64.37390960531436690 ) ) ;
#157586=CARTESIAN_POINT ( 'NONE',  ( -4.379528057220328563, 16.55341960407611168, 105.2072429386477097 ) ) ;
#157587=CARTESIAN_POINT ( 'NONE',  ( 15.72974639402199770, -15.80617190586745480, 23.12390960531436335 ) ) ;
#157588=CARTESIAN_POINT ( 'NONE',  ( -16.55341960407611168, -4.379528057220339221, 56.45724293864768839 ) ) ;
#157589=CARTESIAN_POINT ( 'NONE',  ( 19.02544592524343514, -5.153800228976328945, 28.54057627198102409 ) ) ;
#157590=CARTESIAN_POINT ( 'NONE',  ( -16.55341960407611168, -4.379528057220339221, 91.45724293864769550 ) ) ;
#157592=CARTESIAN_POINT ( 'NONE',  ( -21.52544592524343514, 5.823673210054127303, 101.0405762719810383 ) ) ;
#157593=CARTESIAN_POINT ( 'NONE',  ( 18.62759615963255655, 10.81492255796105972, 41.66775706135235424 ) ) ;
#157594=CARTESIAN_POINT ( 'NONE',  ( -8.224510206698735004, -14.34966873604973081, 34.58442372801900433 ) ) ;
#157595=CARTESIAN_POINT ( 'NONE',  ( -15.80617190586745835, -15.72974639402198527, 81.87390960531435269 ) ) ;
#157596=CARTESIAN_POINT ( 'NONE',  ( -21.53943276465977519, -0.05219959533937600094, 113.7510903946856757 ) ) ;
#157597=CARTESIAN_POINT ( 'NONE',  ( -0.05219959533909027116, -19.03943276465977164, 97.49890960531436690 ) ) ;
#157598=CARTESIAN_POINT ( 'NONE',  ( 5.823673210054444382, -21.52544592524334988, 40.20942372801901854 ) ) ;
#157600=CARTESIAN_POINT ( 'NONE',  ( 21.52544592524344225, -5.823673210054117533, 28.54057627198103120 ) ) ;
#157601=CARTESIAN_POINT ( 'NONE',  ( 16.52544592524335698, 4.483927247898782831, 101.4594237280190185 ) ) ;
#157602=CARTESIAN_POINT ( 'NONE',  ( 15.72974639402176855, 15.80617190586768217, 51.87609039468568284 ) ) ;
#157603=CARTESIAN_POINT ( 'NONE',  ( -5.823673210054431948, 21.52544592524334988, 77.70942372801900433 ) ) ;
#157604=CARTESIAN_POINT ( 'NONE',  ( -16.46253265017146816, -9.564922557961047289, 29.16775706135232937 ) ) ;
#157605=CARTESIAN_POINT ( 'NONE',  ( -16.53943276465976808, -0.05219959533934237506, 93.75109039468567573 ) ) ;
#157606=CARTESIAN_POINT ( 'NONE',  ( -18.67979575497193778, 10.72451020669871902, 48.33442372801902565 ) ) ;
#157607=CARTESIAN_POINT ( 'NONE',  ( 16.46253265017160672, -9.564922557960803928, 48.33224293864769550 ) ) ;
#157608=CARTESIAN_POINT ( 'NONE',  ( -21.53943276465977519, -0.05219959533937600094, 98.75109039468568994 ) ) ;
#157609=CARTESIAN_POINT ( 'NONE',  ( 16.46253265017160672, -9.564922557960803928, 108.3322429386476955 ) ) ;
#157610=CARTESIAN_POINT ( 'NONE',  ( -15.80617190586745835, -15.72974639402198527, 101.8739096053143811 ) ) ;
#157611=CARTESIAN_POINT ( 'NONE',  ( -5.719274019375978568, 21.55341960407610458, 55.20724293864770260 ) ) ;
#157613=CARTESIAN_POINT ( 'NONE',  ( 18.62759615963271287, -10.81492255796078972, 63.33224293864770260 ) ) ;
#157614=CARTESIAN_POINT ( 'NONE',  ( -16.55341960407617563, 4.379528057220093196, 48.54275706135234714 ) ) ;
#157615=CARTESIAN_POINT ( 'NONE',  ( 4.483927247898545687, 16.52544592524342804, 69.79057627198102409 ) ) ;
#157617=CARTESIAN_POINT ( 'NONE',  ( 5.153800228976615827, -19.02544592524334988, 90.20942372801900433 ) ) ;
#157620=CARTESIAN_POINT ( 'NONE',  ( 14.34966873604972726, -8.224510206698740333, 20.83442372801901143 ) ) ;
#157621=CARTESIAN_POINT ( 'NONE',  ( 18.62759615963271287, -10.81492255796078972, 103.3322429386476955 ) ) ;
#157622=CARTESIAN_POINT ( 'NONE',  ( 15.80617190586746368, 15.72974639402197994, 79.37390960531436690 ) ) ;
#157623=CARTESIAN_POINT ( 'NONE',  ( -9.474510206698964154, 16.51473224551069663, 115.4155762719810241 ) ) ;
#157624=CARTESIAN_POINT ( 'NONE',  ( -12.06949235617739369, -12.14591786802326823, 54.37609039468568994 ) ) ;
#157625=CARTESIAN_POINT ( 'NONE',  ( 0.05219959533909260263, 19.03943276465977164, 64.99890960531436690 ) ) ;
#157626=CARTESIAN_POINT ( 'NONE',  ( -5.823673210054431948, 21.52544592524334988, 37.70942372801900433 ) ) ;
#157627=CARTESIAN_POINT ( 'NONE',  ( -13.97604488694547697, 13.89961937509957934, 113.1260903946856757 ) ) ;
#157628=CARTESIAN_POINT ( 'NONE',  ( 9.564922557960805705, 16.46253265017160317, 114.5822429386476955 ) ) ;
#157630=CARTESIAN_POINT ( 'NONE',  ( 13.97604488694527802, 13.89961937509977652, 94.37390960531436690 ) ) ;
#157631=CARTESIAN_POINT ( 'NONE',  ( 10.72451020669898902, -18.67979575497178502, 87.91557627198103830 ) ) ;
#157632=CARTESIAN_POINT ( 'NONE',  ( -19.02544592524342804, 5.153800228976336051, 61.04057627198103120 ) ) ;
#157634=CARTESIAN_POINT ( 'NONE',  ( 4.379528057220339221, -16.55341960407611168, 72.70724293864769550 ) ) ;
#157635=CARTESIAN_POINT ( 'NONE',  ( 16.51473224551069308, 9.474510206698969483, 114.1655762719810241 ) ) ;
#157637=CARTESIAN_POINT ( 'NONE',  ( 10.72451020669898902, -18.67979575497178502, 102.9155762719810383 ) ) ;
#157638=CARTESIAN_POINT ( 'NONE',  ( 9.474510206698729675, 16.51473224551082808, 67.08442372801900433 ) ) ;
#157639=CARTESIAN_POINT ( 'NONE',  ( 19.03943276465977164, -0.05219959533909143690, 108.7489096053143527 ) ) ;
#157640=CARTESIAN_POINT ( 'NONE',  ( -16.46253265017160317, 9.564922557960807481, 30.83224293864769550 ) ) ;
#157641=CARTESIAN_POINT ( 'NONE',  ( 18.67979575497178502, 10.72451020669898547, 59.16557627198103120 ) ) ;
#157642=CARTESIAN_POINT ( 'NONE',  ( 9.474510206698971260, -16.51473224551069308, 97.91557627198102409 ) ) ;
#157643=CARTESIAN_POINT ( 'NONE',  ( -0.05219959533937732626, 21.53943276465977519, 77.50109039468567573 ) ) ;
#157644=CARTESIAN_POINT ( 'NONE',  ( 13.97604488694527802, 13.89961937509977652, 54.37390960531435979 ) ) ;
#157645=CARTESIAN_POINT ( 'NONE',  ( 12.06949235617757843, -12.14591786802309237, 93.12390960531436690 ) ) ;
#157646=CARTESIAN_POINT ( 'NONE',  ( 12.06949235617739724, 12.14591786802326823, 41.87609039468568284 ) ) ;
#157647=CARTESIAN_POINT ( 'NONE',  ( -5.719274019375665041, -21.55341960407619695, 59.79275706135234714 ) ) ;
#157649=CARTESIAN_POINT ( 'NONE',  ( -9.474510206698720793, -16.51473224551083518, 24.58442372801900078 ) ) ;
#157650=CARTESIAN_POINT ( 'NONE',  ( -13.89961937509957401, -13.97604488694547875, 79.37609039468567573 ) ) ;
#157651=CARTESIAN_POINT ( 'NONE',  ( -5.049401038297874678, -19.05341960407617918, 39.79275706135232582 ) ) ;
#157653=CARTESIAN_POINT ( 'NONE',  ( 21.55341960407619695, -5.719274019375665929, 36.04275706135234714 ) ) ;
#157656=CARTESIAN_POINT ( 'NONE',  ( -19.02544592524334988, -5.153800228976617603, 38.95942372801900433 ) ) ;
#157657=CARTESIAN_POINT ( 'NONE',  ( -16.46253265017160317, 9.564922557960807481, 60.83224293864769550 ) ) ;
#157658=CARTESIAN_POINT ( 'NONE',  ( 13.97604488694548053, -13.89961937509957401, 30.62609039468566863 ) ) ;
#157659=CARTESIAN_POINT ( 'NONE',  ( -8.224510206698735004, -14.34966873604973081, 99.58442372801900433 ) ) ;
#157660=CARTESIAN_POINT ( 'NONE',  ( -5.049401038298153566, 19.05341960407611168, 110.2072429386476671 ) ) ;
#157661=CARTESIAN_POINT ( 'NONE',  ( 21.52544592524334988, 5.823673210054432836, 86.45942372801901854 ) ) ;
#157664=CARTESIAN_POINT ( 'NONE',  ( -18.62759615963255300, -10.81492255796106328, 89.16775706135236135 ) ) ;
#157666=CARTESIAN_POINT ( 'NONE',  ( 19.03943276465977164, -0.05219959533909143690, 93.74890960531435269 ) ) ;
#157669=CARTESIAN_POINT ( 'NONE',  ( -16.46253265017160317, 9.564922557960807481, 55.83224293864769550 ) ) ;
#157670=CARTESIAN_POINT ( 'NONE',  ( -15.80617190586745835, -15.72974639402198527, 61.87390960531436690 ) ) ;
#157671=CARTESIAN_POINT ( 'NONE',  ( 8.224510206698953496, -14.34966873604960469, 32.91557627198102409 ) ) ;
#157672=CARTESIAN_POINT ( 'NONE',  ( -16.55341960407611168, -4.379528057220339221, 101.4572429386476955 ) ) ;
#157673=CARTESIAN_POINT ( 'NONE',  ( -9.474510206698964154, 16.51473224551069663, 95.41557627198102409 ) ) ;
#157674=CARTESIAN_POINT ( 'NONE',  ( 13.97604488694548053, -13.89961937509957401, 20.62609039468567573 ) ) ;
#157675=CARTESIAN_POINT ( 'NONE',  ( -16.53943276465976808, 0.05219959533911058130, 101.2489096053143669 ) ) ;
#157676=CARTESIAN_POINT ( 'NONE',  ( 21.53943276465977519, 0.05219959533937863772, 61.25109039468567573 ) ) ;
#157677=CARTESIAN_POINT ( 'NONE',  ( -16.53943276465976808, -0.05219959533934237506, 113.7510903946856757 ) ) ;
#157678=CARTESIAN_POINT ( 'NONE',  ( -13.89961937509957401, -13.97604488694547875, 69.37609039468564731 ) ) ;
#157680=CARTESIAN_POINT ( 'NONE',  ( -9.474510206698964154, 16.51473224551069663, 110.4155762719810383 ) ) ;
#157681=CARTESIAN_POINT ( 'NONE',  ( -14.29746914071049879, 8.314922557960819915, 75.83224293864769550 ) ) ;
#157682=CARTESIAN_POINT ( 'NONE',  ( -16.46253265017146816, -9.564922557961047289, 59.16775706135233293 ) ) ;
#157683=CARTESIAN_POINT ( 'NONE',  ( 5.153800228976335163, 19.02544592524342804, 64.79057627198100988 ) ) ;
#157684=CARTESIAN_POINT ( 'NONE',  ( 12.14591786802309770, 12.06949235617756955, 59.37390960531436690 ) ) ;
#157685=CARTESIAN_POINT ( 'NONE',  ( 13.97604488694548053, -13.89961937509957401, 95.62609039468563310 ) ) ;
#157686=CARTESIAN_POINT ( 'NONE',  ( -5.823673210054116645, -21.52544592524344225, 42.29057627198103120 ) ) ;
#157688=CARTESIAN_POINT ( 'NONE',  ( -0.05219959533910754901, -16.53943276465976808, 102.4989096053143811 ) ) ;
#157689=CARTESIAN_POINT ( 'NONE',  ( 18.22780087662122384, -5.500000000000022204, 76.01540105326107266 ) ) ;
#157690=CARTESIAN_POINT ( 'NONE',  ( -9.474510206698964154, 16.51473224551069663, 65.41557627198102409 ) ) ;
#157691=CARTESIAN_POINT ( 'NONE',  ( -18.67979575497178146, -10.72451020669898902, 66.66557627198102409 ) ) ;
#157692=CARTESIAN_POINT ( 'NONE',  ( -16.46253265017160317, 9.564922557960807481, 40.83224293864769550 ) ) ;
#157693=CARTESIAN_POINT ( 'NONE',  ( 12.06949235617739724, 12.14591786802326823, 86.87609039468568994 ) ) ;
#157694=CARTESIAN_POINT ( 'NONE',  ( -9.474510206698964154, 16.51473224551069663, 80.41557627198103830 ) ) ;
#157695=CARTESIAN_POINT ( 'NONE',  ( 5.049401038297881783, 19.05341960407617563, 47.29275706135231161 ) ) ;
#157696=EDGE_CURVE ( 'NONE', #106494, #160325, #17605, .T. ) ;
#157697=CARTESIAN_POINT ( 'NONE',  ( 10.72451020669871369, 18.67979575497193778, 82.08442372801901854 ) ) ;
#157698=CARTESIAN_POINT ( 'NONE',  ( 10.72451020669898902, -18.67979575497178502, 52.91557627198103830 ) ) ;
#157699=CARTESIAN_POINT ( 'NONE',  ( -5.153800228976328057, -19.02544592524343514, 102.2905762719810383 ) ) ;
#157700=CARTESIAN_POINT ( 'NONE',  ( -9.474510206698964154, 16.51473224551069663, 25.41557627198103120 ) ) ;
#157701=CARTESIAN_POINT ( 'NONE',  ( -16.52544592524335698, -4.483927247898792601, 83.95942372801900433 ) ) ;
#157702=CARTESIAN_POINT ( 'NONE',  ( -9.474510206698720793, -16.51473224551083518, 104.5844237280190043 ) ) ;
#157703=CARTESIAN_POINT ( 'NONE',  ( -9.564922557960796823, -16.46253265017161027, 22.08224293864768839 ) ) ;
#157704=CARTESIAN_POINT ( 'NONE',  ( 19.01529144963336648, 5.499999999999969802, 78.73431955728439391 ) ) ;
#157705=CARTESIAN_POINT ( 'NONE',  ( 21.55341960407619695, -5.719274019375665929, 101.0427570613523756 ) ) ;
#157707=CARTESIAN_POINT ( 'NONE',  ( -16.53943276465976808, 0.05219959533911058130, 56.24890960531436690 ) ) ;
#157708=CARTESIAN_POINT ( 'NONE',  ( -16.53943276465976808, 0.05219959533911058130, 66.24890960531436690 ) ) ;
#157709=CARTESIAN_POINT ( 'NONE',  ( -5.719274019375978568, 21.55341960407610458, 100.2072429386476955 ) ) ;
#157710=CARTESIAN_POINT ( 'NONE',  ( -18.67979575497178146, -10.72451020669898902, 86.66557627198102409 ) ) ;
#157711=CARTESIAN_POINT ( 'NONE',  ( 17.26058549869091507, -6.457015423128540377, 96.12254162523933587 ) ) ;
#157712=CARTESIAN_POINT ( 'NONE',  ( 10.81492255796078972, 18.62759615963270932, 34.58224293864770260 ) ) ;
#157713=CARTESIAN_POINT ( 'NONE',  ( 4.379528057220092307, 16.55341960407617563, 62.29275706135236845 ) ) ;
#157714=CARTESIAN_POINT ( 'NONE',  ( -4.379528057220328563, 16.55341960407611168, 95.20724293864769550 ) ) ;
#157715=CARTESIAN_POINT ( 'NONE',  ( -5.153800228976328057, -19.02544592524343514, 42.29057627198101699 ) ) ;
#157718=CARTESIAN_POINT ( 'NONE',  ( 14.34966873604972726, -8.224510206698740333, 90.83442372801901854 ) ) ;
#157719=CARTESIAN_POINT ( 'NONE',  ( -21.53943276465977519, -0.05219959533937600094, 38.75109039468567573 ) ) ;
#157720=CARTESIAN_POINT ( 'NONE',  ( -9.564922557960796823, -16.46253265017161027, 82.08224293864768129 ) ) ;
#157721=CARTESIAN_POINT ( 'NONE',  ( 18.67979575497194134, -10.72451020669871369, 65.83442372801900433 ) ) ;
#157723=CARTESIAN_POINT ( 'NONE',  ( 5.153800228976335163, 19.02544592524342804, 24.79057627198102765 ) ) ;
#157724=ORIENTED_EDGE ( 'NONE', *, *, #52038, .T. ) ;
#157725=CARTESIAN_POINT ( 'NONE',  ( -15.72974639402176322, -15.80617190586768395, 54.37609039468568994 ) ) ;
#157726=CARTESIAN_POINT ( 'NONE',  ( -19.05341960407611168, -5.049401038298163336, 41.45724293864769550 ) ) ;
#157728=CARTESIAN_POINT ( 'NONE',  ( -5.153800228976328057, -19.02544592524343514, 87.29057627198103830 ) ) ;
#157729=CARTESIAN_POINT ( 'NONE',  ( -13.97604488694547697, 13.89961937509957934, 63.12609039468566152 ) ) ;
#157730=CARTESIAN_POINT ( 'NONE',  ( -10.72451020669870658, -18.67979575497194134, 24.58442372801901499 ) ) ;
#157731=CARTESIAN_POINT ( 'NONE',  ( -5.049401038297874678, -19.05341960407617918, 64.79275706135233293 ) ) ;
#157732=CARTESIAN_POINT ( 'NONE',  ( -5.049401038298153566, 19.05341960407611168, 40.20724293864768839 ) ) ;
#157733=CARTESIAN_POINT ( 'NONE',  ( 8.314922557961029526, -14.29746914071037800, 110.4177570613523756 ) ) ;
#157734=CARTESIAN_POINT ( 'NONE',  ( -16.51473224551082808, 9.474510206698731452, 68.33442372801900433 ) ) ;
#157735=CARTESIAN_POINT ( 'NONE',  ( -12.06949235617756955, 12.14591786802309770, 30.62390960531436335 ) ) ;
#157736=CARTESIAN_POINT ( 'NONE',  ( 19.02544592524334988, 5.153800228976608722, 56.45942372801898301 ) ) ;
#157738=CARTESIAN_POINT ( 'NONE',  ( 19.03943276465977164, -0.05219959533909143690, 83.74890960531436690 ) ) ;
#157739=CARTESIAN_POINT ( 'NONE',  ( -21.55341960407619339, 5.719274019375674811, 98.54275706135234714 ) ) ;
#157740=CARTESIAN_POINT ( 'NONE',  ( -0.05219959533937732626, 21.53943276465977519, 112.5010903946857042 ) ) ;
#157742=CARTESIAN_POINT ( 'NONE',  ( 5.823673210054444382, -21.52544592524334988, 95.20942372801903275 ) ) ;
#157743=CARTESIAN_POINT ( 'NONE',  ( -12.06949235617739369, -12.14591786802326823, 34.37609039468568284 ) ) ;
#157744=CARTESIAN_POINT ( 'NONE',  ( 13.89961937509977652, -13.97604488694527269, 98.12390960531433848 ) ) ;
#157746=CARTESIAN_POINT ( 'NONE',  ( 16.51473224551069308, 9.474510206698969483, 84.16557627198102409 ) ) ;
#157748=CARTESIAN_POINT ( 'NONE',  ( -13.89961937509957401, -13.97604488694547875, 69.37609039468564731 ) ) ;
#157749=CARTESIAN_POINT ( 'NONE',  ( -19.02544592524342804, 5.153800228976336051, 101.0405762719810241 ) ) ;
#157750=CARTESIAN_POINT ( 'NONE',  ( 21.53943276465977519, 0.05219959533937863772, 106.2510903946856757 ) ) ;
#157751=CARTESIAN_POINT ( 'NONE',  ( -16.53943276465976808, 0.05219959533911058130, 101.2489096053143669 ) ) ;
#157752=CARTESIAN_POINT ( 'NONE',  ( 21.53943276465977519, -0.05219959533907433946, 48.74890960531435979 ) ) ;
#157753=( BOUNDED_SURFACE ( )  B_SPLINE_SURFACE ( 3, 2, ( 
 ( #199012, #135371, #14991, #13988, #154495, #75654, #169663, #60481, #200011, #138330, #137332, #122156, #45333, #27197, #76652, #119198, #88843, #197041, #15990, #106985, #168658, #123148, #150535, #57529, #73699, #198022, #31158, #42358, #105015, #104021, #30158, #61477, #184836, #44340, #58509, #121165, #91801, #120175, #181865, #151526, #13015, #2795, #81592, #64473, #126140, #18974, #141306, #94803, #110964, #173654, #20941, #96773, #47327, #109976, #170663, #49305, #35121, #187836, #50306, #127117, #4762, #172648, #156482, #51287, #159446, #19950, #80620, #158462, #142297, #16980, #108983, #157481, #97758, #34136, #171656, #95795, #63477, #17984, #3777, #185840, #124141, #62469, #78634, #143277, #33145, #79637, #32151, #93808, #65454, #66450, #188823, #111962, #128111, #189815, #112948, #174641, #82598, #36106, #796, #140309, #155488, #1799, #125153, #186852, #48321, #85607, #147294, #148294, #69446, #53272, #7763, #101780, #116947, #100769, #130094, #54284, #133115, #99774, #8783, #179651, #194804, #98765, #70453, #176644, #177645, #191791, #131113, #25965, #114951, #52274, #67443, #9788, #163468, #56278, #39113, #102785, #132118, #162451, #144279, #84597, #117960, #37105, #83599, #193811, #38120, #175631, #86611, #115956, #160458, #71450, #5768, #161459, #41121, #23952, #22949, #129101, #146276, #55276, #145278, #164471, #178639, #190800, #21950, #113932, #6761, #192801, #68440, #40102, #24965, #44110, #13758, #57291, #46083, #103788, #134130, #89606, #197791, #150303, #91567, #120926, #87608, #167455, #181632, #149294, #76418, #166468, #14757, #169419, #182625, #45100, #104780, #75426, #26964, #88607, #137100, #198786, #121923, #27966, #151295, #11800, #183617, #152274, #118968, #28951, #73464, #138094, #199775, #72456, #43112, #135137, #12784, #105768, #74449, #90592, #59257, #196811, #136115, #42126, #107738, #195819, #29928, #60252, #58278, #180651, #106757, #168432, #61242, #122914, #119947, #10788, #153255, #184602, #165468, #109739, #34885, #63234, #32909, #111728, #156242, #185596, #124913, #186611, #18737, #48083, #171423, #79401, #94563, #140067, #17744, #172410, #96540, #95556, #15751, #155253, #139080, #141072, #33899, #2557, #49073, #187604, #142056, #64239, #1558, #126880, #173414, #157243, #125905, #80384, #110729, #123897, #77410, #3542, #30924, #65220, #78391, #188586, #31914, #50067, #92572, #558, #62229, #47085, #108746, #154260, #170422, #93567, #16742, #57938, #14398, #153904, #91211, #28603, #136744, #105419, #76064, #92218, #170071, #46732, #122564, #208, #11445, #30567, #169061, #134786, #199423, #108394, #137739, #29580, #167102, #45736, #75077, #166115, #119609, #59902, #77056, #151924, #184254, #42770, #73117, #123547, #93213, #12443, #183265, #61877, #181292, #15399, #31562, #196468, #152902, #89257, #107388, #106401, #104432, #168083, #185241, #60888, #138728, #27618, #150949, #74105, #44745, #135775, #197446, #58912, #120580, #182273, #43755, #90241, #13413, #198428, #121570, #51695, #47732, #95208, #156895, #143695, #109385, #94209, #19378, #63887, #186254, #97179, #126537, #171065, #158865, #16397, #2206, #66859, #188236, #187255, #154898, #48724, #65861, #155888, #113358, #157889, #20354, #32555, #1200, #82002, #18391, #5178, #33547, #173064, #111375, #81027, #124557, #175050, #17386, #62876, #80042, #64876, #79041, #128522, #49711, #78043, #34541, #110377, #139712, #190216, #141711, #36514, #140716, #96200, #112371, #172060, #142703, #125558, #3202, #4182, #127532, #189235, #50713, #174063, #35531, #30444, #104308, #150822, #119487, #31437, #1077, #120456, #91094, #169946, #27491, #138603, #77924, #181169, #60768, #197324, #15274, #14273, #16272, #75942, #93091, #122440, #61755, #85, #199301, #184132, #152782, #89134, #123423, #42646, #12319, #58788, #154775, #45614, #107266, #185116, #73984, #139591, #135653, #59780, #165991, #108267, #105295 ),
 ( #182148, #28486, #43632, #166983, #46606, #90120, #151804, #137617, #13295, #168937, #74960, #136622, #198303, #121449, #183141, #44626, #92090, #106278, #167963, #29462, #153779, #76934, #51572, #155766, #2084, #127408, #171938, #94087, #5053, #34421, #17264, #66739, #124432, #110257, #174927, #96080, #95086, #62752, #156774, #173941, #63764, #21238, #65740, #128400, #78917, #109262, #190097, #3081, #113236, #141594, #80906, #19260, #189117, #32433, #82893, #140594, #170941, #64757, #172942, #125437, #36390, #157769, #186129, #142583, #18268, #47608, #98044, #126419, #159742, #144571, #4062, #20231, #79921, #50590, #187133, #48605, #112249, #35408, #97060, #188117, #49588, #111251, #33427, #158742, #81879, #143571, #192084, #136159, #120969, #191089, #100063, #145570, #23243, #27008, #161748, #88652, #119012, #7047, #57336, #160746, #28993, #114223, #151338, #180695, #53566, #175928, #42171, #104823, #197834, #68729, #103831, #150348, #44151, #182667, #135181, #11844, #73509, #12827, #134176, #115244, #72502, #166512, #181675, #165512, #176936, #196855, #59300, #84887, #58321, #105810, #167497, #22238, #119989, #38406, #43156, #146566, #195864, #90633, #10832, #37399, #28010, #89650, #99058, #74493, #6057, #67735, #130387, #129393, #52563, #83887, #64277, #78432, #93608, #155293, #156283, #77450, #61285, #15790, #109778, #124954, #108784, #138136, #62268, #141110, #107777, #16783, #187642, #2598, #106799, #140107, #184642, #185634, #199817, #139121, #33939, #122954, #60292, #75467, #17784, #171461, #125944, #47126, #121965, #49113, #110770, #46123, #92610, #172452, #45142, #91610, #1598, #169462, #183658, #94604, #123936, #168473, #79439, #13801, #30963, #152315, #170462, #154301, #137140, #597, #63274, #153298, #198828, #186650, #29971, #14799, #76460, #31953, #48121, #32949, #174445, #113738, #52082, #21752, #65260, #54088, #111767, #142097, #97560, #5568, #158269, #99577, #128906, #95597, #175435, #189618, #157281, #84402, #35914, #22753, #177450, #190606, #53073, #112751, #83403, #34925, #96580, #145081, #6564, #129894, #159248, #20744, #82399, #188627, #50107, #173456, #36905, #81399, #146078, #7563, #80424, #51091, #19758, #144087, #98568, #67247, #160262, #68241, #143085, #191594, #4564, #115762, #3582, #37918, #69249, #114751, #130915, #18777, #176445, #161259, #192606, #126920, #66256, #127916, #165270, #26764, #73269, #179454, #117762, #25772, #131927, #193611, #116753, #180457, #24769, #166268, #151098, #23758, #132922, #178444, #56081, #57094, #194609, #118768, #149103, #39911, #87418, #55083, #59060, #147100, #181439, #10593, #86416, #8585, #72254, #134938, #27766, #101578, #133932, #41929, #74254, #12589, #88404, #103595, #150100, #42918, #164278, #148101, #102593, #196616, #11601, #195622, #9593, #58086, #89409, #40920, #119756, #135924, #197594, #163267, #104583, #71258, #120727, #38920, #100577, #162259, #85408, #70259, #105568, #186401, #1345, #32703, #77205, #90389, #17530, #140859, #76209, #122710, #171213, #75226, #121720, #46878, #91358, #13559, #124704, #154052, #136897, #47878, #43905, #29725, #94354, #15547, #14551, #182427, #137888, #93359, #183412, #2348, #185387, #109531, #198584, #28753, #156033, #184400, #79189, #61038, #354, #138874, #108538, #152074, #64029, #60052, #44895, #45880, #92366, #106552, #167254, #62024, #168228, #123688, #199569, #153049, #170217, #31710, #155045, #107534, #169210, #30719, #16540, #78187, #139857, #63026, #129652, #159004, #125699, #5320, #19516, #187398, #114495, #4322, #52826, #7316, #20497, #83162, #142843, #51835, #65017, #126673, #113494, #175189, #160013, #66006, #127674, #112508, #18532, #80179, #3342, #67004, #111519, #176197, #37666, #110521, #81161, #188377, #189374, #143841, #50851, #128663, #35670, #49854, #174202, #141851, #145834, #33687, #67999, #97318, #173205, #95350, #82145, #21501, #99331, #34680, #190358 ),
 ( #84155, #36655, #144836, #191348, #98313, #48866, #6320, #161014, #22508, #172202, #96338, #157034, #158025, #149847, #71013, #194369, #87175, #9348, #163014, #179206, #146843, #117509, #165025, #166022, #178200, #38679, #40674, #41682, #55836, #118523, #195368, #73022, #132681, #24521, #119518, #27522, #88163, #148856, #26518, #10347, #85157, #177206, #25531, #89163, #102344, #39664, #164033, #131681, #86172, #72004, #53844, #192361, #130667, #8337, #100335, #133677, #150854, #56847, #101325, #180212, #193362, #147862, #103346, #115518, #162013, #23509, #70012, #11351, #134693, #196377, #54838, #116513, #57846, #181200, #42677, #104338, #69001, #106308, #76963, #93119, #170971, #47639, #123453, #1106, #12348, #31467, #169975, #135682, #115, #109292, #138634, #30471, #167993, #46636, #75972, #167013, #120486, #137645, #197354, #185146, #58818, #43663, #74012, #124462, #94117, #13323, #184161, #62781, #182177, #154804, #32464, #105325, #153809, #90149, #108296, #107294, #28514, #168966, #186159, #15303, #16302, #77952, #92121, #61784, #45642, #151833, #139619, #74988, #136652, #198333, #59809, #121479, #183172, #44655, #29490, #91123, #152813, #14305, #199332, #60797, #122470, #114255, #5083, #113262, #159771, #142611, #175960, #172971, #65769, #52594, #50617, #33457, #157797, #19288, #36417, #80935, #4090, #173968, #96108, #49619, #127438, #95115, #189144, #51598, #37429, #64787, #125467, #112276, #128426, #35436, #66765, #81906, #21266, #97088, #111281, #6086, #155796, #174954, #158771, #98072, #20260, #143599, #190122, #63794, #82923, #17294, #187164, #156804, #191120, #144600, #67765, #129422, #48635, #78947, #110287, #171969, #140623, #2113, #34449, #18297, #79952, #141622, #3111, #126448, #188146, #116270, #9107, #196139, #194134, #176968, #101088, #162774, #179974, #24282, #85931, #117272, #39428, #193122, #70774, #38438, #147620, #195128, #57610, #8090, #68761, #132443, #71768, #55597, #148617, #25291, #103107, #178966, #54596, #149611, #119279, #118283, #40433, #56609, #102105, #115275, #7080, #163790, #180962, #86934, #69767, #10108, #161778, #177960, #133438, #83919, #22269, #160780, #100094, #41440, #131436, #164788, #130419, #145601, #26282, #87924, #11109, #72784, #134454, #99089, #192117, #53599, #23273, #84917, #146597, #31235, #42439, #61553, #200085, #165785, #30237, #139391, #168733, #60558, #136424, #76729, #106075, #197121, #150620, #167762, #27281, #153571, #88928, #73779, #104102, #154571, #124224, #43428, #14067, #92884, #12116, #123222, #873, #135452, #183924, #120254, #138404, #137410, #62548, #199090, #16067, #45409, #184912, #46397, #122233, #181945, #44422, #29260, #108056, #90891, #152577, #107062, #182939, #198104, #75734, #105097, #91880, #169740, #58588, #151605, #166783, #15068, #77725, #28284, #89923, #13096, #74762, #59570, #121245, #36186, #144364, #4850, #65537, #143358, #3858, #1878, #93887, #142379, #82680, #172736, #156569, #187916, #48401, #2877, #19055, #170739, #109061, #47405, #63559, #20033, #18065, #64556, #17059, #32229, #188911, #128197, #127197, #126220, #111048, #79720, #50389, #66534, #5851, #21027, #96859, #174723, #185920, #189895, #51370, #155565, #173737, #67527, #112049, #35206, #141389, #81675, #49385, #140390, #78714, #34216, #125233, #158543, #186931, #110058, #171738, #97840, #33226, #94886, #157562, #159528, #95879, #113031, #80702, #10869, #70533, #6844, #25048, #24036, #26043, #85691, #41204, #132202, #71530, #9870, #8866, #193893, #162532, #37191, #148375, #190882, #98848, #68523, #164550, #55358, #117028, #194887, #22032, #87688, #83684, #160543, #133196, #175712, #84679, #149373, #178723, #86691, #56361, #116036, #129184, #146358, #39194, #52358, #147377, #130177, #177725, #118044, #114015, #38201, #145362, #100850, #101865, #54364, #40185, #163548, #179734, #69532, #23034, #102865, #191874, #53358, #115035, #176728, #99857 ),
 ( #7845, #161541, #131196, #192886, #42208, #31004, #88692, #119050, #74531, #182706, #135220, #76504, #105850, #72539, #152354, #166550, #134216, #61327, #151375, #199862, #154342, #167537, #30013, #89690, #198867, #11884, #73547, #60334, #122008, #106840, #12866, #136196, #59338, #165549, #27046, #150388, #13839, #58359, #122998, #184684, #57377, #28049, #196892, #197871, #90672, #121008, #75506, #44191, #120026, #29032, #181711, #92653, #180732, #14841, #137179, #43193, #103868, #183699, #168515, #46167, #104861, #45186, #91651, #107821, #169505, #153340, #138180, #195902, #22548, #143882, #127715, #82189, #99370, #190402, #145874, #185679, #128705, #7357, #174245, #160056, #53883, #69042, #170507, #21543, #50892, #51878, #1645, #5363, #100375, #189417, #123981, #139164, #84194, #37708, #130707, #113537, #93655, #20540, #67047, #161053, #175231, #36696, #98357, #159046, #112550, #83203, #155340, #144878, #114537, #115558, #35713, #47169, #6360, #191389, #68040, #129692, #52866, #192401, #176237, #97360, #177245, #38717, #15835, #77494, #641, #62311, #31998, #108828, #16829, #78480, #140153, #63323, #164070, #24560, #179247, #195408, #146885, #85197, #23549, #178240, #196413, #132717, #40713, #193402, #8377, #165062, #104376, #41720, #102382, #87213, #55875, #26556, #42714, #120523, #197391, #73059, #150893, #162053, #181238, #119555, #70052, #149883, #58856, #88199, #180250, #117548, #57883, #25569, #116551, #131720, #148895, #54877, #134731, #39701, #101364, #163053, #74049, #43700, #86209, #133716, #12387, #147899, #166059, #182216, #9385, #103384, #71051, #27560, #56886, #194405, #118560, #135720, #11389, #89200, #10385, #72042, #170013, #138671, #13360, #124501, #167049, #75024, #183210, #140659, #185183, #31504, #171010, #198371, #2151, #59848, #136689, #109328, #151870, #60832, #63829, #154842, #62817, #32501, #92158, #125501, #122507, #15343, #187199, #151, #186196, #123490, #121515, #44691, #61820, #105362, #153845, #76008, #107330, #168029, #184197, #46673, #90187, #28550, #106345, #29526, #139655, #137683, #45679, #91159, #152848, #108333, #47677, #93157, #169003, #30507, #199368, #16339, #94153, #14342, #76999, #77988, #155832, #1143, #17329, #78984, #172003, #36453, #145636, #174989, #66799, #142646, #82960, #112312, #3147, #156838, #174002, #33491, #159808, #95149, #79988, #48670, #160817, #130457, #49653, #20294, #99127, #18333, #67803, #7116, #110322, #190158, #126483, #144637, #143633, #68798, #5117, #22305, #51634, #191157, #129458, #128462, #113298, #81942, #141656, #52630, #64821, #188181, #111317, #83956, #98111, #21303, #114294, #173006, #34485, #96143, #157832, #175996, #19323, #4125, #80970, #6120, #37466, #65804, #35473, #127472, #189178, #158805, #50651, #97122, #69802, #194167, #55631, #72819, #117304, #179000, #10143, #132478, #85965, #102140, #131470, #40468, #87959, #88964, #101121, #161811, #163825, #164823, #25326, #41477, #118317, #196175, #86968, #147654, #42475, #150654, #11145, #71803, #134488, #149647, #115312, #180010, #12152, #103141, #133472, #9142, #26319, #148655, #146632, #100130, #195163, #177004, #57647, #38473, #23306, #192154, #104138, #73817, #193157, #56644, #165820, #84950, #119313, #53635, #8124, #180999, #54629, #27317, #116304, #177993, #39460, #162807, #24316, #70809, #16101, #15104, #200119, #168767, #43464, #154606, #197157, #105132, #13133, #170775, #76765, #61588, #907, #28319, #32265, #89958, #166818, #139425, #181982, #90926, #93922, #184947, #92920, #62582, #122269, #155600, #152612, #45444, #17095, #30270, #74795, #137448, #199127, #77759, #60594, #183957, #153608, #75770, #29296, #107097, #136457, #91915, #31269, #135487, #44458, #151638, #138438, #108091, #123256, #46432, #169775, #124260, #185955, #14102, #47439, #58622, #109096, #120289, #198138, #59608, #121281, #182974, #106112, #167796, #65573, #49420, #80736, #141425, #95912 ),
 ( #157596, #3894, #172772, #143395, #159564, #37226, #114050, #189928, #67561, #78748, #171772, #18099, #4884, #187951, #110094, #21062, #50424, #33261, #82717, #140425, #126254, #190916, #112083, #111082, #1915, #34253, #51403, #79754, #98883, #81709, #144399, #94920, #125269, #5885, #19088, #129219, #142415, #96893, #35239, #66566, #48437, #160577, #156605, #186967, #127233, #188947, #2911, #52393, #173773, #63594, #158576, #20066, #64590, #175749, #128231, #113063, #174755, #36220, #97872, #39227, #148409, #161574, #23067, #9904, #71564, #56396, #162566, #100883, #8900, #115070, #176762, #99889, #163581, #7880, #149406, #134249, #6878, #116070, #84713, #24070, #40222, #177758, #101899, #132236, #146391, #70568, #38234, #42240, #130212, #164583, #193928, #69565, #191907, #55391, #118078, #10901, #131231, #117061, #25081, #57410, #195936, #133229, #86724, #194920, #26077, #147412, #192920, #85725, #102898, #178756, #72575, #53392, #179768, #119082, #41237, #87721, #180764, #103901, #54398, #22066, #83717, #145395, #68556, #90703, #47201, #74562, #73581, #88727, #169537, #184715, #15868, #60368, #135253, #673, #124013, #59373, #105883, #154374, #150422, #11917, #27080, #181746, #199894, #136229, #182741, #196925, #58392, #168544, #107852, #45216, #44225, #152386, #121045, #30042, #46199, #185711, #62344, #76536, #77526, #165582, #31037, #123029, #120059, #153373, #43228, #91681, #183730, #167570, #61358, #29064, #104895, #166584, #13871, #28084, #138212, #89724, #151410, #12898, #139198, #197904, #75538, #137213, #198900, #122040, #92686, #106871, #14875, #50186, #186728, #4641, #3659, #5646, #65337, #20820, #111843, #51169, #189696, #188704, #173533, #142175, #16860, #127993, #170540, #78511, #48199, #144161, #35002, #96657, #174521, #1677, #67323, #63355, #140185, #112829, #155371, #64354, #128985, #158344, #66332, #35988, #95676, #190683, #126023, #18856, #108861, #126997, #109853, #110848, #172532, #97635, #34018, #157362, #19833, #49190, #2677, #80502, #171538, #81474, #159324, #32030, #17863, #125032, #143161, #82476, #93688, #33026, #94681, #156360, #79518, #187719, #141188, #194689, #178519, #162334, #39986, #100652, #145159, #98646, #38996, #132998, #192682, #37999, #7640, #191671, #22830, #115838, #69324, #53150, #84477, #177527, #175510, #113815, #36984, #6643, #55158, #99654, #146154, #21829, #160340, #23835, #101657, #85484, #130990, #54165, #161338, #147173, #163348, #56159, #71336, #132002, #86493, #52158, #9671, #148178, #68321, #24844, #83481, #117841, #129971, #8662, #114829, #193690, #70335, #116828, #176523, #17499, #143808, #79156, #63998, #32671, #144806, #114462, #33656, #4292, #83130, #140827, #51804, #191317, #94324, #174171, #110489, #128633, #127643, #129622, #189343, #6289, #35641, #175157, #113463, #112478, #97287, #65974, #2316, #36624, #156002, #125668, #172171, #67968, #158974, #20466, #98281, #187366, #52794, #48835, #95317, #159982, #157002, #188346, #18500, #82116, #190327, #21469, #19486, #80148, #49824, #142812, #141819, #50821, #3312, #34649, #96308, #64985, #157994, #81131, #5290, #173173, #126643, #66973, #111488, #24490, #71973, #72992, #85127, #145804, #86141, #148827, #101296, #25500, #102314, #180183, #116481, #69982, #26490, #134661, #195338, #55807, #133647, #194339, #192330, #84125, #132651, #196347, #162985, #146811, #57815, #8305, #7287, #99298, #41652, #56818, #88132, #70983, #68971, #11322, #176164, #131650, #178170, #164996, #130635, #115486, #40645, #193332, #53811, #118492, #147832, #177174, #103316, #37634, #23478, #149816, #9318, #54806, #160983, #39635, #87144, #38647, #22477, #179177, #100304, #161982, #117479, #164004, #10317, #41282, #44266, #42286, #10946, #103945, #118124, #133275, #89766, #29105, #166624, #165624, #11958, #180807, #151451, #167609, #45259, #122082, #197945, #75580, #86772, #105924, #90743, #9950, #74603 ),
 ( #28126, #72620, #13914, #198942, #71609, #27123, #26123, #88770, #104938, #150463, #12938, #196965, #87765, #135293, #102944, #106913, #194966, #152426, #58433, #134295, #56445, #120100, #182783, #137259, #149450, #181789, #136270, #183773, #60409, #59415, #121089, #168586, #148456, #73623, #195981, #43269, #179812, #164628, #57454, #119126, #140230, #18900, #185761, #171582, #65382, #80546, #184759, #33070, #62390, #63399, #15913, #155414, #188749, #124060, #170586, #142220, #123073, #169585, #94725, #139243, #61402, #172576, #1723, #46244, #34062, #91725, #77571, #3704, #125076, #47249, #30084, #108906, #141230, #31083, #50234, #156403, #95721, #107898, #76579, #157407, #32076, #127042, #111889, #153421, #14919, #79563, #199938, #138255, #92731, #154419, #93733, #186773, #718, #16904, #48244, #78555, #109898, #17907, #2721, #64398, #126067, #187763, #49233, #110891, #131040, #190730, #99701, #112875, #174568, #161385, #22876, #7686, #113861, #52203, #160388, #66379, #128040, #51214, #114877, #159373, #100697, #85532, #158390, #67370, #36034, #175557, #191716, #129029, #53200, #83527, #97683, #21877, #189741, #193737, #81520, #115883, #145205, #20869, #143206, #6688, #69370, #162378, #82527, #68366, #176571, #8711, #147220, #84523, #38045, #146200, #177573, #98694, #144209, #37033, #54212, #130017, #23880, #4687, #192730, #70380, #39040, #132048, #55205, #173578, #5694, #35047, #96701, #19879, #102713, #42053, #198709, #25894, #24891, #40030, #120850, #136041, #167379, #11726, #86539, #152198, #118894, #179578, #134055, #150230, #101704, #163394, #71381, #74376, #72380, #41049, #195747, #148223, #9717, #119877, #59181, #196741, #57221, #103717, #10717, #181562, #197716, #75349, #13682, #27892, #105693, #116874, #182550, #44032, #133045, #104706, #137019, #43040, #135065, #180579, #151221, #165397, #194735, #56205, #26890, #117888, #89534, #164402, #87539, #178565, #28876, #149226, #88533, #73394, #90516, #58208, #166396, #12710, #141975, #1473, #138016, #156160, #155172, #157162, #16663, #30846, #187525, #91488, #29851, #108665, #17658, #48990, #199699, #93486, #63152, #95475, #172326, #186531, #124831, #48004, #64157, #185514, #169337, #123816, #140988, #31835, #110645, #153175, #170343, #33815, #15672, #109660, #18656, #80302, #14678, #171340, #92493, #78311, #46005, #47006, #60176, #154182, #168355, #183538, #125822, #79318, #121845, #139984, #76340, #45023, #106682, #77332, #478, #61165, #122836, #184525, #32828, #138999, #107660, #2476, #94479, #62152, #7441, #65140, #50973, #115641, #36781, #35795, #3463, #97442, #114624, #4443, #162138, #34805, #69126, #49982, #159127, #23634, #52949, #161136, #130792, #190489, #85283, #20625, #113620, #100458, #98446, #81281, #5447, #67130, #84279, #128788, #51960, #21629, #143967, #82274, #175314, #142964, #160140, #99456, #126797, #112633, #173332, #83285, #176324, #144959, #37793, #129774, #192485, #6441, #68122, #53967, #188503, #22633, #191470, #145960, #177330, #19639, #111646, #38802, #96460, #158148, #174326, #66131, #127796, #189497, #180337, #131807, #70136, #101452, #104465, #102469, #71137, #164156, #178324, #193486, #149974, #89290, #26642, #25654, #72132, #40799, #11479, #27651, #105452, #182309, #57970, #135808, #146974, #166149, #150982, #54964, #134821, #43788, #73150, #165151, #87299, #181324, #10471, #163143, #116635, #133807, #39787, #119642, #24646, #86295, #8462, #58945, #28636, #147984, #118646, #197478, #9473, #12475, #167137, #132802, #88285, #194489, #42803, #41805, #55961, #74136, #120613, #117638, #179336, #148982, #196500, #195498, #103473, #56972, #109416, #151957, #59934, #168113, #125586, #170099, #16425, #155920, #183297, #187283, #44778, #92251, #171095, #153935, #15430, #108423, #30598, #184284, #239, #29609, #138757, #186283, #48754, #199453, #121601, #61906, #62908, #77088, #139740, #78072, #94240, #123577, #45766 ),
 ( #152931, #107418, #185272, #75109, #13445, #106431, #47763, #169091, #14430, #46764, #91241, #136777, #93242, #32587, #31593, #154927, #1229, #124588, #17415, #79073, #110407, #172089, #140746, #2234, #90273, #63917, #198463, #76093, #137768, #60921, #122595, #51723, #127564, #67889, #97208, #188264, #141740, #158894, #18421, #144723, #80071, #64904, #33576, #145726, #115405, #34571, #5207, #84047, #3230, #52716, #192248, #95238, #175076, #111408, #129542, #128549, #130551, #37554, #176084, #156924, #173093, #114380, #113386, #98198, #66888, #126565, #99216, #49739, #96228, #157916, #68891, #36542, #159902, #160904, #19406, #53730, #81055, #142732, #22397, #4211, #189265, #65889, #83049, #191242, #7207, #20384, #50740, #112399, #143728, #174091, #190246, #35560, #82031, #21390, #6209, #179095, #87060, #39553, #181090, #10233, #177093, #56739, #70901, #38565, #165909, #55724, #104228, #58707, #71893, #134582, #194257, #103234, #116395, #178084, #164916, #26410, #11238, #117396, #40564, #163922, #69898, #131565, #54722, #118410, #162900, #27407, #89053, #161902, #132568, #101211, #102234, #195254, #25418, #180103, #148745, #24409, #133564, #193249, #197246, #150743, #147747, #12242, #8221, #146724, #41571, #72912, #73904, #86058, #88049, #149737, #135574, #100221, #196268, #57737, #119407, #42565, #23396, #9234, #85043, #995, #92004, #47528, #90045, #30361, #109183, #75860, #61675, #155687, #170862, #74883, #123344, #152701, #153698, #106201, #45531, #2004, #29384, #28406, #43553, #124350, #139512, #32353, #15193, #151727, #17182, #78836, #14190, #60684, #94006, #13220, #59698, #185037, #91015, #136545, #62669, #76852, #198226, #186045, #182070, #167885, #140514, #138523, #137536, #120377, #199218, #31359, #121370, #105219, #46524, #166907, #183063, #44546, #122359, #184048, #107185, #168856, #1, #108184, #169865, #93009, #154695, #16190, #77845, #160661, #156692, #95004, #67648, #110178, #19173, #22152, #113150, #21149, #129306, #50506, #83802, #80822, #173858, #145483, #158659, #141512, #65658, #127320, #144486, #189032, #112170, #81795, #3978, #157683, #35324, #2997, #96978, #159652, #63683, #172857, #33345, #20150, #36305, #143482, #174840, #190015, #191002, #4967, #142500, #114137, #125357, #82804, #66653, #5969, #128315, #79843, #171857, #51488, #187054, #97960, #34338, #52478, #126337, #175838, #37312, #48524, #18186, #64675, #98970, #188034, #49504, #111167, #95999, #56236, #12739, #152228, #89564, #26920, #135093, #103747, #74405, #90546, #168386, #45054, #120881, #198741, #6963, #28906, #167410, #130299, #197745, #106712, #136071, #27921, #165426, #44063, #73422, #164430, #117917, #196769, #191993, #182580, #179606, #41078, #68643, #121876, #91519, #10746, #181591, #60206, #102742, #13713, #29881, #25924, #151250, #87567, #105723, #104735, #149254, #75379, #137051, #72410, #134087, #183569, #59212, #195777, #43068, #57250, #118924, #180609, #42082, #88563, #150261, #11755, #58237, #119905, #166426, #186563, #61195, #172357, #14711, #122867, #30878, #188536, #32861, #79350, #18687, #46036, #50014, #107691, #184555, #157193, #199729, #108696, #111679, #2508, #110677, #80334, #140018, #173366, #170375, #63184, #34836, #48036, #92525, #155205, #16694, #33847, #78344, #1507, #171374, #93520, #47039, #124864, #154214, #109692, #49022, #153206, #62183, #169370, #94511, #125855, #156193, #64188, #141021, #142006, #17693, #31866, #3495, #76371, #95507, #187555, #65171, #126830, #15704, #77364, #138048, #139032, #511, #123847, #185545, #159159, #113651, #129806, #81313, #19671, #51004, #54000, #51992, #20654, #175345, #127826, #142996, #99489, #38833, #176356, #36813, #21662, #190518, #161169, #177362, #54996, #131838, #7475, #85316, #96491, #115674, #100491, #4474, #84313, #193521, #22666, #114660, #98479, #130826, #160172, #112665, #66164, #83316, #189532, #69159, #174357, #35827 ) ),
 .UNSPECIFIED., .T., .F., .T. ) 
 B_SPLINE_SURFACE_WITH_KNOTS ( ( 4, 3, 4 ),
 ( 3, 2, 2, 2, 2, 2, 2, 2, 2, 2, 2, 2, 2, 2, 2, 2, 2, 2, 2, 2, 2, 2, 2, 2, 2, 2, 2, 2, 2, 2, 2, 2, 2, 2, 2, 2, 2, 2, 2, 2, 2, 2, 2, 2, 2, 2, 2, 2, 2, 2, 2, 2, 2, 2, 2, 2, 2, 2, 2, 2, 2, 2, 2, 2, 2, 2, 2, 2, 2, 2, 2, 2, 2, 2, 2, 2, 2, 2, 2, 2, 2, 2, 2, 2, 2, 2, 2, 2, 2, 2, 2, 2, 2, 2, 2, 2, 2, 2, 2, 2, 2, 2, 2, 2, 2, 2, 2, 2, 2, 2, 2, 2, 2, 2, 2, 2, 2, 2, 2, 2, 2, 2, 2, 2, 2, 2, 2, 2, 2, 2, 2, 2, 2, 2, 2, 2, 2, 2, 2, 2, 2, 2, 2, 2, 2, 2, 2, 2, 2, 2, 2, 2, 2, 2, 2, 2, 2, 2, 2, 2, 2, 2, 2, 2, 2, 2, 2, 2, 2, 2, 2, 2, 2, 2, 2, 2, 2, 2, 2, 2, 2, 2, 2, 2, 2, 2, 2, 2, 2, 2, 2, 2, 2, 2, 2, 2, 2, 2, 2, 2, 2, 2, 2, 2, 2, 2, 2, 2, 2, 2, 2, 2, 2, 2, 2, 2, 2, 2, 2, 2, 2, 2, 2, 2, 2, 2, 2, 2, 3 ),
 ( 0.000000000000000000, 0.5000000000000000000, 1.000000000000000000 ),
 ( 0.000000000000000000, 0.004385964912280701511, 0.008771929824561403022, 0.01315789473684210453, 0.01754385964912280604, 0.02192982456140350755, 0.02631578947368420907, 0.03070175438596491058, 0.03508771929824561209, 0.03947368421052631360, 0.04385964912280701511, 0.04824561403508771662, 0.05263157894736841813, 0.05701754385964911964, 0.06140350877192982115, 0.06578947368421052266, 0.07017543859649122417, 0.07456140350877192569, 0.07894736842105262720, 0.08333333333333332871, 0.08771929824561403022, 0.09210526315789473173, 0.09649122807017543324, 0.1008771929824561348, 0.1052631578947368363, 0.1096491228070175378, 0.1140350877192982393, 0.1184210526315789408, 0.1228070175438596423, 0.1271929824561403577, 0.1315789473684210453, 0.1359649122807017607, 0.1403508771929824483, 0.1447368421052631637, 0.1491228070175438514, 0.1535087719298245668, 0.1578947368421052544, 0.1622807017543859698, 0.1666666666666666574, 0.1710526315789473728, 0.1754385964912280604, 0.1798245614035087758, 0.1842105263157894635, 0.1885964912280701788, 0.1929824561403508665, 0.1973684210526315819, 0.2017543859649122695, 0.2061403508771929849, 0.2105263157894736725, 0.2149122807017543879, 0.2192982456140350755, 0.2236842105263157909, 0.2280701754385964786, 0.2324561403508771940, 0.2368421052631578816, 0.2412280701754385970, 0.2456140350877192846, 0.2500000000000000000, 0.2543859649122807154, 0.2587719298245614308, 0.2631578947368420907, 0.2675438596491228060, 0.2719298245614035214, 0.2763157894736842368, 0.2807017543859648967, 0.2850877192982456121, 0.2894736842105263275, 0.2938596491228070429, 0.2982456140350877027, 0.3026315789473684181, 0.3070175438596491335, 0.3114035087719298489, 0.3157894736842105088, 0.3201754385964912242, 0.3245614035087719396, 0.3289473684210526550, 0.3333333333333333148, 0.3377192982456140302, 0.3421052631578947456, 0.3464912280701754610, 0.3508771929824561209, 0.3552631578947368363, 0.3596491228070175517, 0.3640350877192982670, 0.3684210526315789269, 0.3728070175438596423, 0.3771929824561403577, 0.3815789473684210731, 0.3859649122807017330, 0.3903508771929824483, 0.3947368421052631637, 0.3991228070175438791, 0.4035087719298245390, 0.4078947368421052544, 0.4122807017543859698, 0.4166666666666666852, 0.4210526315789473450, 0.4254385964912280604, 0.4298245614035087758, 0.4342105263157894912, 0.4385964912280701511, 0.4429824561403508665, 0.4473684210526315819, 0.4517543859649122973, 0.4561403508771929571, 0.4605263157894736725, 0.4649122807017543879, 0.4692982456140351033, 0.4736842105263157632, 0.4780701754385964786, 0.4824561403508771940, 0.4868421052631579093, 0.4912280701754385692, 0.4956140350877192846, 0.5000000000000000000, 0.5043859649122807154, 0.5087719298245614308, 0.5131578947368421462, 0.5175438596491228616, 0.5219298245614034659, 0.5263157894736841813, 0.5307017543859648967, 0.5350877192982456121, 0.5394736842105263275, 0.5438596491228070429, 0.5482456140350877583, 0.5526315789473684736, 0.5570175438596490780, 0.5614035087719297934, 0.5657894736842105088, 0.5701754385964912242, 0.5745614035087719396, 0.5789473684210526550, 0.5833333333333333703, 0.5877192982456140857, 0.5921052631578946901, 0.5964912280701754055, 0.6008771929824561209, 0.6052631578947368363, 0.6096491228070175517, 0.6140350877192982670, 0.6184210526315789824, 0.6228070175438596978, 0.6271929824561403022, 0.6315789473684210176, 0.6359649122807017330, 0.6403508771929824483, 0.6447368421052631637, 0.6491228070175438791, 0.6535087719298245945, 0.6578947368421053099, 0.6622807017543859143, 0.6666666666666666297, 0.6710526315789473450, 0.6754385964912280604, 0.6798245614035087758, 0.6842105263157894912, 0.6885964912280702066, 0.6929824561403509220, 0.6973684210526315264, 0.7017543859649122417, 0.7061403508771929571, 0.7105263157894736725, 0.7149122807017543879, 0.7192982456140351033, 0.7236842105263158187, 0.7280701754385965341, 0.7324561403508771384, 0.7368421052631578538, 0.7412280701754385692, 0.7456140350877192846, 0.7500000000000000000, 0.7543859649122807154, 0.7587719298245614308, 0.7631578947368421462, 0.7675438596491228616, 0.7719298245614034659, 0.7763157894736841813, 0.7807017543859648967, 0.7850877192982456121, 0.7894736842105263275, 0.7938596491228070429, 0.7982456140350877583, 0.8026315789473684736, 0.8070175438596490780, 0.8114035087719297934, 0.8157894736842105088, 0.8201754385964912242, 0.8245614035087719396, 0.8289473684210526550, 0.8333333333333333703, 0.8377192982456140857, 0.8421052631578946901, 0.8464912280701754055, 0.8508771929824561209, 0.8552631578947368363, 0.8596491228070175517, 0.8640350877192982670, 0.8684210526315789824, 0.8728070175438596978, 0.8771929824561403022, 0.8815789473684210176, 0.8859649122807017330, 0.8903508771929824483, 0.8947368421052631637, 0.8991228070175438791, 0.9035087719298245945, 0.9078947368421053099, 0.9122807017543859143, 0.9166666666666666297, 0.9210526315789473450, 0.9254385964912280604, 0.9298245614035087758, 0.9342105263157894912, 0.9385964912280702066, 0.9429824561403509220, 0.9473684210526315264, 0.9517543859649122417, 0.9561403508771929571, 0.9605263157894736725, 0.9649122807017543879, 0.9692982456140351033, 0.9736842105263158187, 0.9780701754385965341, 0.9824561403508771384, 0.9868421052631578538, 0.9912280701754385692, 0.9956140350877192846, 1.000000000000000000 ),
 .UNSPECIFIED. ) 
 GEOMETRIC_REPRESENTATION_ITEM ( )  RATIONAL_B_SPLINE_SURFACE ( (
 ( 1.000000000000000000, 0.9659258262890683122, 1.000000000000000000, 0.9659258262890683122, 1.000000000000000000, 0.9659258262890683122, 1.000000000000000000, 0.9659258262890683122, 1.000000000000000000, 0.9659258262890683122, 1.000000000000000000, 0.9659258262890683122, 1.000000000000000000, 0.9659258262890683122, 1.000000000000000000, 0.9659258262890683122, 1.000000000000000000, 0.9659258262890683122, 1.000000000000000000, 0.9659258262890683122, 1.000000000000000000, 0.9659258262890683122, 1.000000000000000000, 0.9659258262890683122, 1.000000000000000000, 0.9659258262890683122, 1.000000000000000000, 0.9659258262890683122, 1.000000000000000000, 0.9659258262890683122, 1.000000000000000000, 0.9659258262890683122, 1.000000000000000000, 0.9659258262890683122, 1.000000000000000000, 0.9659258262890683122, 1.000000000000000000, 0.9659258262890683122, 1.000000000000000000, 0.9659258262890683122, 1.000000000000000000, 0.9659258262890683122, 1.000000000000000000, 0.9659258262890683122, 1.000000000000000000, 0.9659258262890683122, 1.000000000000000000, 0.9659258262890683122, 1.000000000000000000, 0.9659258262890683122, 1.000000000000000000, 0.9659258262890683122, 1.000000000000000000, 0.9659258262890683122, 1.000000000000000000, 0.9659258262890683122, 1.000000000000000000, 0.9659258262890683122, 1.000000000000000000, 0.9659258262890683122, 1.000000000000000000, 0.9659258262890683122, 1.000000000000000000, 0.9659258262890683122, 1.000000000000000000, 0.9659258262890683122, 1.000000000000000000, 0.9659258262890683122, 1.000000000000000000, 0.9659258262890683122, 1.000000000000000000, 0.9659258262890683122, 1.000000000000000000, 0.9659258262890683122, 1.000000000000000000, 0.9659258262890683122, 1.000000000000000000, 0.9659258262890683122, 1.000000000000000000, 0.9659258262890683122, 1.000000000000000000, 0.9659258262890683122, 1.000000000000000000, 0.9659258262890683122, 1.000000000000000000, 0.9659258262890683122, 1.000000000000000000, 0.9659258262890683122, 1.000000000000000000, 0.9659258262890683122, 1.000000000000000000, 0.9659258262890683122, 1.000000000000000000, 0.9659258262890683122, 1.000000000000000000, 0.9659258262890683122, 1.000000000000000000, 0.9659258262890683122, 1.000000000000000000, 0.9659258262890683122, 1.000000000000000000, 0.9659258262890683122, 1.000000000000000000, 0.9659258262890683122, 1.000000000000000000, 0.9659258262890683122, 1.000000000000000000, 0.9659258262890683122, 1.000000000000000000, 0.9659258262890683122, 1.000000000000000000, 0.9659258262890683122, 1.000000000000000000, 0.9659258262890683122, 1.000000000000000000, 0.9659258262890683122, 1.000000000000000000, 0.9659258262890683122, 1.000000000000000000, 0.9659258262890683122, 1.000000000000000000, 0.9659258262890683122, 1.000000000000000000, 0.9659258262890683122, 1.000000000000000000, 0.9659258262890683122, 1.000000000000000000, 0.9659258262890683122, 1.000000000000000000, 0.9659258262890683122, 1.000000000000000000, 0.9659258262890683122, 1.000000000000000000, 0.9659258262890683122, 1.000000000000000000, 0.9659258262890683122, 1.000000000000000000, 0.9659258262890683122, 1.000000000000000000, 0.9659258262890683122, 1.000000000000000000, 0.9659258262890683122, 1.000000000000000000, 0.9659258262890683122, 1.000000000000000000, 0.9659258262890683122, 1.000000000000000000, 0.9659258262890683122, 1.000000000000000000, 0.9659258262890683122, 1.000000000000000000, 0.9659258262890683122, 1.000000000000000000, 0.9659258262890683122, 1.000000000000000000, 0.9659258262890683122, 1.000000000000000000, 0.9659258262890683122, 1.000000000000000000, 0.9659258262890683122, 1.000000000000000000, 0.9659258262890683122, 1.000000000000000000, 0.9659258262890683122, 1.000000000000000000, 0.9659258262890683122, 1.000000000000000000, 0.9659258262890683122, 1.000000000000000000, 0.9659258262890683122, 1.000000000000000000, 0.9659258262890683122, 1.000000000000000000, 0.9659258262890683122, 1.000000000000000000, 0.9659258262890683122, 1.000000000000000000, 0.9659258262890683122, 1.000000000000000000, 0.9659258262890683122, 1.000000000000000000, 0.9659258262890683122, 1.000000000000000000, 0.9659258262890683122, 1.000000000000000000, 0.9659258262890683122, 1.000000000000000000, 0.9659258262890683122, 1.000000000000000000, 0.9659258262890683122, 1.000000000000000000, 0.9659258262890683122, 1.000000000000000000, 0.9659258262890683122, 1.000000000000000000, 0.9659258262890683122, 1.000000000000000000, 0.9659258262890683122, 1.000000000000000000, 0.9659258262890683122, 1.000000000000000000, 0.9659258262890683122, 1.000000000000000000, 0.9659258262890683122, 1.000000000000000000, 0.9659258262890683122, 1.000000000000000000, 0.9659258262890683122, 1.000000000000000000, 0.9659258262890683122, 1.000000000000000000, 0.9659258262890683122, 1.000000000000000000, 0.9659258262890683122, 1.000000000000000000, 0.9659258262890683122, 1.000000000000000000, 0.9659258262890683122, 1.000000000000000000, 0.9659258262890683122, 1.000000000000000000, 0.9659258262890683122, 1.000000000000000000, 0.9659258262890683122, 1.000000000000000000, 0.9659258262890683122, 1.000000000000000000, 0.9659258262890683122, 1.000000000000000000, 0.9659258262890683122, 1.000000000000000000, 0.9659258262890683122, 1.000000000000000000, 0.9659258262890683122, 1.000000000000000000, 0.9659258262890683122, 1.000000000000000000, 0.9659258262890683122, 1.000000000000000000, 0.9659258262890683122, 1.000000000000000000, 0.9659258262890683122, 1.000000000000000000, 0.9659258262890683122, 1.000000000000000000, 0.9659258262890683122, 1.000000000000000000, 0.9659258262890683122, 1.000000000000000000, 0.9659258262890683122, 1.000000000000000000, 0.9659258262890683122, 1.000000000000000000, 0.9659258262890683122, 1.000000000000000000, 0.9659258262890683122, 1.000000000000000000, 0.9659258262890683122, 1.000000000000000000, 0.9659258262890683122, 1.000000000000000000, 0.9659258262890683122, 1.000000000000000000, 0.9659258262890683122, 1.000000000000000000, 0.9659258262890683122, 1.000000000000000000, 0.9659258262890683122, 1.000000000000000000, 0.9659258262890683122, 1.000000000000000000, 0.9659258262890683122, 1.000000000000000000, 0.9659258262890683122, 1.000000000000000000, 0.9659258262890683122, 1.000000000000000000, 0.9659258262890683122, 1.000000000000000000, 0.9659258262890683122, 1.000000000000000000, 0.9659258262890683122, 1.000000000000000000, 0.9659258262890683122, 1.000000000000000000, 0.9659258262890683122, 1.000000000000000000, 0.9659258262890683122, 1.000000000000000000, 0.9659258262890683122, 1.000000000000000000, 0.9659258262890683122, 1.000000000000000000, 0.9659258262890683122, 1.000000000000000000, 0.9659258262890683122, 1.000000000000000000, 0.9659258262890683122, 1.000000000000000000, 0.9659258262890683122, 1.000000000000000000, 0.9659258262890683122, 1.000000000000000000, 0.9659258262890683122, 1.000000000000000000, 0.9659258262890683122, 1.000000000000000000, 0.9659258262890683122, 1.000000000000000000, 0.9659258262890683122, 1.000000000000000000, 0.9659258262890683122, 1.000000000000000000, 0.9659258262890683122, 1.000000000000000000, 0.9659258262890683122, 1.000000000000000000, 0.9659258262890683122, 1.000000000000000000, 0.9659258262890683122, 1.000000000000000000, 0.9659258262890683122, 1.000000000000000000, 0.9659258262890683122, 1.000000000000000000, 0.9659258262890683122, 1.000000000000000000, 0.9659258262890683122, 1.000000000000000000, 0.9659258262890683122, 1.000000000000000000, 0.9659258262890683122, 1.000000000000000000, 0.9659258262890683122, 1.000000000000000000, 0.9659258262890683122, 1.000000000000000000, 0.9659258262890683122, 1.000000000000000000, 0.9659258262890683122, 1.000000000000000000, 0.9659258262890683122, 1.000000000000000000, 0.9659258262890683122, 1.000000000000000000, 0.9659258262890683122, 1.000000000000000000, 0.9659258262890683122, 1.000000000000000000, 0.9659258262890683122, 1.000000000000000000, 0.9659258262890683122, 1.000000000000000000, 0.9659258262890683122, 1.000000000000000000, 0.9659258262890683122, 1.000000000000000000, 0.9659258262890683122, 1.000000000000000000, 0.9659258262890683122, 1.000000000000000000, 0.9659258262890683122, 1.000000000000000000, 0.9659258262890683122, 1.000000000000000000, 0.9659258262890683122, 1.000000000000000000, 0.9659258262890683122, 1.000000000000000000, 0.9659258262890683122, 1.000000000000000000, 0.9659258262890683122, 1.000000000000000000, 0.9659258262890683122, 1.000000000000000000, 0.9659258262890683122, 1.000000000000000000, 0.9659258262890683122, 1.000000000000000000, 0.9659258262890683122, 1.000000000000000000, 0.9659258262890683122, 1.000000000000000000, 0.9659258262890683122, 1.000000000000000000, 0.9659258262890683122, 1.000000000000000000, 0.9659258262890683122, 1.000000000000000000, 0.9659258262890683122, 1.000000000000000000, 0.9659258262890683122, 1.000000000000000000, 0.9659258262890683122, 1.000000000000000000, 0.9659258262890683122, 1.000000000000000000, 0.9659258262890683122, 1.000000000000000000, 0.9659258262890683122, 1.000000000000000000, 0.9659258262890683122, 1.000000000000000000, 0.9659258262890683122, 1.000000000000000000, 0.9659258262890683122, 1.000000000000000000, 0.9659258262890683122, 1.000000000000000000, 0.9659258262890683122, 1.000000000000000000, 0.9659258262890683122, 1.000000000000000000, 0.9659258262890683122, 1.000000000000000000, 0.9659258262890683122, 1.000000000000000000, 0.9659258262890683122, 1.000000000000000000, 0.9659258262890683122, 1.000000000000000000, 0.9659258262890683122, 1.000000000000000000, 0.9659258262890683122, 1.000000000000000000, 0.9659258262890683122, 1.000000000000000000, 0.9659258262890683122, 1.000000000000000000, 0.9659258262890683122, 1.000000000000000000, 0.9659258262890683122, 1.000000000000000000, 0.9659258262890683122, 1.000000000000000000, 0.9659258262890683122, 1.000000000000000000, 0.9659258262890683122, 1.000000000000000000, 0.9659258262890683122, 1.000000000000000000, 0.9659258262890683122, 1.000000000000000000, 0.9659258262890683122, 1.000000000000000000, 0.9659258262890683122, 1.000000000000000000, 0.9659258262890683122, 1.000000000000000000, 0.9659258262890683122, 1.000000000000000000, 0.9659258262890683122, 1.000000000000000000, 0.9659258262890683122, 1.000000000000000000, 0.9659258262890683122, 1.000000000000000000),
 ( 0.3333333333333333703, 0.3219752754296894559, 0.3333333333333333703, 0.3219752754296894559, 0.3333333333333333703, 0.3219752754296894559, 0.3333333333333333703, 0.3219752754296894559, 0.3333333333333333703, 0.3219752754296894559, 0.3333333333333333703, 0.3219752754296894559, 0.3333333333333333703, 0.3219752754296894559, 0.3333333333333333703, 0.3219752754296894559, 0.3333333333333333703, 0.3219752754296894559, 0.3333333333333333703, 0.3219752754296894559, 0.3333333333333333703, 0.3219752754296894559, 0.3333333333333333703, 0.3219752754296894559, 0.3333333333333333703, 0.3219752754296894559, 0.3333333333333333703, 0.3219752754296894559, 0.3333333333333333703, 0.3219752754296894559, 0.3333333333333333703, 0.3219752754296894559, 0.3333333333333333703, 0.3219752754296894559, 0.3333333333333333703, 0.3219752754296894559, 0.3333333333333333703, 0.3219752754296894559, 0.3333333333333333703, 0.3219752754296894559, 0.3333333333333333703, 0.3219752754296894559, 0.3333333333333333703, 0.3219752754296894559, 0.3333333333333333703, 0.3219752754296894559, 0.3333333333333333703, 0.3219752754296894559, 0.3333333333333333703, 0.3219752754296894559, 0.3333333333333333703, 0.3219752754296894559, 0.3333333333333333703, 0.3219752754296894559, 0.3333333333333333703, 0.3219752754296894559, 0.3333333333333333703, 0.3219752754296894559, 0.3333333333333333703, 0.3219752754296894559, 0.3333333333333333703, 0.3219752754296894559, 0.3333333333333333703, 0.3219752754296894559, 0.3333333333333333703, 0.3219752754296894559, 0.3333333333333333703, 0.3219752754296894559, 0.3333333333333333703, 0.3219752754296894559, 0.3333333333333333703, 0.3219752754296894559, 0.3333333333333333703, 0.3219752754296894559, 0.3333333333333333703, 0.3219752754296894559, 0.3333333333333333703, 0.3219752754296894559, 0.3333333333333333703, 0.3219752754296894559, 0.3333333333333333703, 0.3219752754296894559, 0.3333333333333333703, 0.3219752754296894559, 0.3333333333333333703, 0.3219752754296894559, 0.3333333333333333703, 0.3219752754296894559, 0.3333333333333333703, 0.3219752754296894559, 0.3333333333333333703, 0.3219752754296894559, 0.3333333333333333703, 0.3219752754296894559, 0.3333333333333333703, 0.3219752754296894559, 0.3333333333333333703, 0.3219752754296894559, 0.3333333333333333703, 0.3219752754296894559, 0.3333333333333333703, 0.3219752754296894559, 0.3333333333333333703, 0.3219752754296894559, 0.3333333333333333703, 0.3219752754296894559, 0.3333333333333333703, 0.3219752754296894559, 0.3333333333333333703, 0.3219752754296894559, 0.3333333333333333703, 0.3219752754296894559, 0.3333333333333333703, 0.3219752754296894559, 0.3333333333333333703, 0.3219752754296894559, 0.3333333333333333703, 0.3219752754296894559, 0.3333333333333333703, 0.3219752754296894559, 0.3333333333333333703, 0.3219752754296894559, 0.3333333333333333703, 0.3219752754296894559, 0.3333333333333333703, 0.3219752754296894559, 0.3333333333333333703, 0.3219752754296894559, 0.3333333333333333703, 0.3219752754296894559, 0.3333333333333333703, 0.3219752754296894559, 0.3333333333333333703, 0.3219752754296894559, 0.3333333333333333703, 0.3219752754296894559, 0.3333333333333333703, 0.3219752754296894559, 0.3333333333333333703, 0.3219752754296894559, 0.3333333333333333703, 0.3219752754296894559, 0.3333333333333333703, 0.3219752754296894559, 0.3333333333333333703, 0.3219752754296894559, 0.3333333333333333703, 0.3219752754296894559, 0.3333333333333333703, 0.3219752754296894559, 0.3333333333333333703, 0.3219752754296894559, 0.3333333333333333703, 0.3219752754296894559, 0.3333333333333333703, 0.3219752754296894559, 0.3333333333333333703, 0.3219752754296894559, 0.3333333333333333703, 0.3219752754296894559, 0.3333333333333333703, 0.3219752754296894559, 0.3333333333333333703, 0.3219752754296894559, 0.3333333333333333703, 0.3219752754296894559, 0.3333333333333333703, 0.3219752754296894559, 0.3333333333333333703, 0.3219752754296894559, 0.3333333333333333703, 0.3219752754296894559, 0.3333333333333333703, 0.3219752754296894559, 0.3333333333333333703, 0.3219752754296894559, 0.3333333333333333703, 0.3219752754296894559, 0.3333333333333333703, 0.3219752754296894559, 0.3333333333333333703, 0.3219752754296894559, 0.3333333333333333703, 0.3219752754296894559, 0.3333333333333333703, 0.3219752754296894559, 0.3333333333333333703, 0.3219752754296894559, 0.3333333333333333703, 0.3219752754296894559, 0.3333333333333333703, 0.3219752754296894559, 0.3333333333333333703, 0.3219752754296894559, 0.3333333333333333703, 0.3219752754296894559, 0.3333333333333333703, 0.3219752754296894559, 0.3333333333333333703, 0.3219752754296894559, 0.3333333333333333703, 0.3219752754296894559, 0.3333333333333333703, 0.3219752754296894559, 0.3333333333333333703, 0.3219752754296894559, 0.3333333333333333703, 0.3219752754296894559, 0.3333333333333333703, 0.3219752754296894559, 0.3333333333333333703, 0.3219752754296894559, 0.3333333333333333703, 0.3219752754296894559, 0.3333333333333333703, 0.3219752754296894559, 0.3333333333333333703, 0.3219752754296894559, 0.3333333333333333703, 0.3219752754296894559, 0.3333333333333333703, 0.3219752754296894559, 0.3333333333333333703, 0.3219752754296894559, 0.3333333333333333703, 0.3219752754296894559, 0.3333333333333333703, 0.3219752754296894559, 0.3333333333333333703, 0.3219752754296894559, 0.3333333333333333703, 0.3219752754296894559, 0.3333333333333333703, 0.3219752754296894559, 0.3333333333333333703, 0.3219752754296894559, 0.3333333333333333703, 0.3219752754296894559, 0.3333333333333333703, 0.3219752754296894559, 0.3333333333333333703, 0.3219752754296894559, 0.3333333333333333703, 0.3219752754296894559, 0.3333333333333333703, 0.3219752754296894559, 0.3333333333333333703, 0.3219752754296894559, 0.3333333333333333703, 0.3219752754296894559, 0.3333333333333333703, 0.3219752754296894559, 0.3333333333333333703, 0.3219752754296894559, 0.3333333333333333703, 0.3219752754296894559, 0.3333333333333333703, 0.3219752754296894559, 0.3333333333333333703, 0.3219752754296894559, 0.3333333333333333703, 0.3219752754296894559, 0.3333333333333333703, 0.3219752754296894559, 0.3333333333333333703, 0.3219752754296894559, 0.3333333333333333703, 0.3219752754296894559, 0.3333333333333333703, 0.3219752754296894559, 0.3333333333333333703, 0.3219752754296894559, 0.3333333333333333703, 0.3219752754296894559, 0.3333333333333333703, 0.3219752754296894559, 0.3333333333333333703, 0.3219752754296894559, 0.3333333333333333703, 0.3219752754296894559, 0.3333333333333333703, 0.3219752754296894559, 0.3333333333333333703, 0.3219752754296894559, 0.3333333333333333703, 0.3219752754296894559, 0.3333333333333333703, 0.3219752754296894559, 0.3333333333333333703, 0.3219752754296894559, 0.3333333333333333703, 0.3219752754296894559, 0.3333333333333333703, 0.3219752754296894559, 0.3333333333333333703, 0.3219752754296894559, 0.3333333333333333703, 0.3219752754296894559, 0.3333333333333333703, 0.3219752754296894559, 0.3333333333333333703, 0.3219752754296894559, 0.3333333333333333703, 0.3219752754296894559, 0.3333333333333333703, 0.3219752754296894559, 0.3333333333333333703, 0.3219752754296894559, 0.3333333333333333703, 0.3219752754296894559, 0.3333333333333333703, 0.3219752754296894559, 0.3333333333333333703, 0.3219752754296894559, 0.3333333333333333703, 0.3219752754296894559, 0.3333333333333333703, 0.3219752754296894559, 0.3333333333333333703, 0.3219752754296894559, 0.3333333333333333703, 0.3219752754296894559, 0.3333333333333333703, 0.3219752754296894559, 0.3333333333333333703, 0.3219752754296894559, 0.3333333333333333703, 0.3219752754296894559, 0.3333333333333333703, 0.3219752754296894559, 0.3333333333333333703, 0.3219752754296894559, 0.3333333333333333703, 0.3219752754296894559, 0.3333333333333333703, 0.3219752754296894559, 0.3333333333333333703, 0.3219752754296894559, 0.3333333333333333703, 0.3219752754296894559, 0.3333333333333333703, 0.3219752754296894559, 0.3333333333333333703, 0.3219752754296894559, 0.3333333333333333703, 0.3219752754296894559, 0.3333333333333333703, 0.3219752754296894559, 0.3333333333333333703, 0.3219752754296894559, 0.3333333333333333703, 0.3219752754296894559, 0.3333333333333333703, 0.3219752754296894559, 0.3333333333333333703, 0.3219752754296894559, 0.3333333333333333703, 0.3219752754296894559, 0.3333333333333333703, 0.3219752754296894559, 0.3333333333333333703, 0.3219752754296894559, 0.3333333333333333703, 0.3219752754296894559, 0.3333333333333333703, 0.3219752754296894559, 0.3333333333333333703, 0.3219752754296894559, 0.3333333333333333703, 0.3219752754296894559, 0.3333333333333333703, 0.3219752754296894559, 0.3333333333333333703, 0.3219752754296894559, 0.3333333333333333703, 0.3219752754296894559, 0.3333333333333333703, 0.3219752754296894559, 0.3333333333333333703, 0.3219752754296894559, 0.3333333333333333703, 0.3219752754296894559, 0.3333333333333333703, 0.3219752754296894559, 0.3333333333333333703, 0.3219752754296894559, 0.3333333333333333703, 0.3219752754296894559, 0.3333333333333333703, 0.3219752754296894559, 0.3333333333333333703, 0.3219752754296894559, 0.3333333333333333703, 0.3219752754296894559, 0.3333333333333333703, 0.3219752754296894559, 0.3333333333333333703, 0.3219752754296894559, 0.3333333333333333703, 0.3219752754296894559, 0.3333333333333333703, 0.3219752754296894559, 0.3333333333333333703, 0.3219752754296894559, 0.3333333333333333703, 0.3219752754296894559, 0.3333333333333333703, 0.3219752754296894559, 0.3333333333333333703, 0.3219752754296894559, 0.3333333333333333703, 0.3219752754296894559, 0.3333333333333333703, 0.3219752754296894559, 0.3333333333333333703, 0.3219752754296894559, 0.3333333333333333703, 0.3219752754296894559, 0.3333333333333333703, 0.3219752754296894559, 0.3333333333333333703, 0.3219752754296894559, 0.3333333333333333703, 0.3219752754296894559, 0.3333333333333333703, 0.3219752754296894559, 0.3333333333333333703, 0.3219752754296894559, 0.3333333333333333703, 0.3219752754296894559, 0.3333333333333333703, 0.3219752754296894559, 0.3333333333333333703, 0.3219752754296894559, 0.3333333333333333703, 0.3219752754296894559, 0.3333333333333333703, 0.3219752754296894559, 0.3333333333333333703, 0.3219752754296894559, 0.3333333333333333703, 0.3219752754296894559, 0.3333333333333333703, 0.3219752754296894559, 0.3333333333333333703, 0.3219752754296894559, 0.3333333333333333703, 0.3219752754296894559, 0.3333333333333333703, 0.3219752754296894559, 0.3333333333333333703, 0.3219752754296894559, 0.3333333333333333703, 0.3219752754296894559, 0.3333333333333333703, 0.3219752754296894559, 0.3333333333333333703),
 ( 0.3333333333333333703, 0.3219752754296894559, 0.3333333333333333703, 0.3219752754296894559, 0.3333333333333333703, 0.3219752754296894559, 0.3333333333333333703, 0.3219752754296894559, 0.3333333333333333703, 0.3219752754296894559, 0.3333333333333333703, 0.3219752754296894559, 0.3333333333333333703, 0.3219752754296894559, 0.3333333333333333703, 0.3219752754296894559, 0.3333333333333333703, 0.3219752754296894559, 0.3333333333333333703, 0.3219752754296894559, 0.3333333333333333703, 0.3219752754296894559, 0.3333333333333333703, 0.3219752754296894559, 0.3333333333333333703, 0.3219752754296894559, 0.3333333333333333703, 0.3219752754296894559, 0.3333333333333333703, 0.3219752754296894559, 0.3333333333333333703, 0.3219752754296894559, 0.3333333333333333703, 0.3219752754296894559, 0.3333333333333333703, 0.3219752754296894559, 0.3333333333333333703, 0.3219752754296894559, 0.3333333333333333703, 0.3219752754296894559, 0.3333333333333333703, 0.3219752754296894559, 0.3333333333333333703, 0.3219752754296894559, 0.3333333333333333703, 0.3219752754296894559, 0.3333333333333333703, 0.3219752754296894559, 0.3333333333333333703, 0.3219752754296894559, 0.3333333333333333703, 0.3219752754296894559, 0.3333333333333333703, 0.3219752754296894559, 0.3333333333333333703, 0.3219752754296894559, 0.3333333333333333703, 0.3219752754296894559, 0.3333333333333333703, 0.3219752754296894559, 0.3333333333333333703, 0.3219752754296894559, 0.3333333333333333703, 0.3219752754296894559, 0.3333333333333333703, 0.3219752754296894559, 0.3333333333333333703, 0.3219752754296894559, 0.3333333333333333703, 0.3219752754296894559, 0.3333333333333333703, 0.3219752754296894559, 0.3333333333333333703, 0.3219752754296894559, 0.3333333333333333703, 0.3219752754296894559, 0.3333333333333333703, 0.3219752754296894559, 0.3333333333333333703, 0.3219752754296894559, 0.3333333333333333703, 0.3219752754296894559, 0.3333333333333333703, 0.3219752754296894559, 0.3333333333333333703, 0.3219752754296894559, 0.3333333333333333703, 0.3219752754296894559, 0.3333333333333333703, 0.3219752754296894559, 0.3333333333333333703, 0.3219752754296894559, 0.3333333333333333703, 0.3219752754296894559, 0.3333333333333333703, 0.3219752754296894559, 0.3333333333333333703, 0.3219752754296894559, 0.3333333333333333703, 0.3219752754296894559, 0.3333333333333333703, 0.3219752754296894559, 0.3333333333333333703, 0.3219752754296894559, 0.3333333333333333703, 0.3219752754296894559, 0.3333333333333333703, 0.3219752754296894559, 0.3333333333333333703, 0.3219752754296894559, 0.3333333333333333703, 0.3219752754296894559, 0.3333333333333333703, 0.3219752754296894559, 0.3333333333333333703, 0.3219752754296894559, 0.3333333333333333703, 0.3219752754296894559, 0.3333333333333333703, 0.3219752754296894559, 0.3333333333333333703, 0.3219752754296894559, 0.3333333333333333703, 0.3219752754296894559, 0.3333333333333333703, 0.3219752754296894559, 0.3333333333333333703, 0.3219752754296894559, 0.3333333333333333703, 0.3219752754296894559, 0.3333333333333333703, 0.3219752754296894559, 0.3333333333333333703, 0.3219752754296894559, 0.3333333333333333703, 0.3219752754296894559, 0.3333333333333333703, 0.3219752754296894559, 0.3333333333333333703, 0.3219752754296894559, 0.3333333333333333703, 0.3219752754296894559, 0.3333333333333333703, 0.3219752754296894559, 0.3333333333333333703, 0.3219752754296894559, 0.3333333333333333703, 0.3219752754296894559, 0.3333333333333333703, 0.3219752754296894559, 0.3333333333333333703, 0.3219752754296894559, 0.3333333333333333703, 0.3219752754296894559, 0.3333333333333333703, 0.3219752754296894559, 0.3333333333333333703, 0.3219752754296894559, 0.3333333333333333703, 0.3219752754296894559, 0.3333333333333333703, 0.3219752754296894559, 0.3333333333333333703, 0.3219752754296894559, 0.3333333333333333703, 0.3219752754296894559, 0.3333333333333333703, 0.3219752754296894559, 0.3333333333333333703, 0.3219752754296894559, 0.3333333333333333703, 0.3219752754296894559, 0.3333333333333333703, 0.3219752754296894559, 0.3333333333333333703, 0.3219752754296894559, 0.3333333333333333703, 0.3219752754296894559, 0.3333333333333333703, 0.3219752754296894559, 0.3333333333333333703, 0.3219752754296894559, 0.3333333333333333703, 0.3219752754296894559, 0.3333333333333333703, 0.3219752754296894559, 0.3333333333333333703, 0.3219752754296894559, 0.3333333333333333703, 0.3219752754296894559, 0.3333333333333333703, 0.3219752754296894559, 0.3333333333333333703, 0.3219752754296894559, 0.3333333333333333703, 0.3219752754296894559, 0.3333333333333333703, 0.3219752754296894559, 0.3333333333333333703, 0.3219752754296894559, 0.3333333333333333703, 0.3219752754296894559, 0.3333333333333333703, 0.3219752754296894559, 0.3333333333333333703, 0.3219752754296894559, 0.3333333333333333703, 0.3219752754296894559, 0.3333333333333333703, 0.3219752754296894559, 0.3333333333333333703, 0.3219752754296894559, 0.3333333333333333703, 0.3219752754296894559, 0.3333333333333333703, 0.3219752754296894559, 0.3333333333333333703, 0.3219752754296894559, 0.3333333333333333703, 0.3219752754296894559, 0.3333333333333333703, 0.3219752754296894559, 0.3333333333333333703, 0.3219752754296894559, 0.3333333333333333703, 0.3219752754296894559, 0.3333333333333333703, 0.3219752754296894559, 0.3333333333333333703, 0.3219752754296894559, 0.3333333333333333703, 0.3219752754296894559, 0.3333333333333333703, 0.3219752754296894559, 0.3333333333333333703, 0.3219752754296894559, 0.3333333333333333703, 0.3219752754296894559, 0.3333333333333333703, 0.3219752754296894559, 0.3333333333333333703, 0.3219752754296894559, 0.3333333333333333703, 0.3219752754296894559, 0.3333333333333333703, 0.3219752754296894559, 0.3333333333333333703, 0.3219752754296894559, 0.3333333333333333703, 0.3219752754296894559, 0.3333333333333333703, 0.3219752754296894559, 0.3333333333333333703, 0.3219752754296894559, 0.3333333333333333703, 0.3219752754296894559, 0.3333333333333333703, 0.3219752754296894559, 0.3333333333333333703, 0.3219752754296894559, 0.3333333333333333703, 0.3219752754296894559, 0.3333333333333333703, 0.3219752754296894559, 0.3333333333333333703, 0.3219752754296894559, 0.3333333333333333703, 0.3219752754296894559, 0.3333333333333333703, 0.3219752754296894559, 0.3333333333333333703, 0.3219752754296894559, 0.3333333333333333703, 0.3219752754296894559, 0.3333333333333333703, 0.3219752754296894559, 0.3333333333333333703, 0.3219752754296894559, 0.3333333333333333703, 0.3219752754296894559, 0.3333333333333333703, 0.3219752754296894559, 0.3333333333333333703, 0.3219752754296894559, 0.3333333333333333703, 0.3219752754296894559, 0.3333333333333333703, 0.3219752754296894559, 0.3333333333333333703, 0.3219752754296894559, 0.3333333333333333703, 0.3219752754296894559, 0.3333333333333333703, 0.3219752754296894559, 0.3333333333333333703, 0.3219752754296894559, 0.3333333333333333703, 0.3219752754296894559, 0.3333333333333333703, 0.3219752754296894559, 0.3333333333333333703, 0.3219752754296894559, 0.3333333333333333703, 0.3219752754296894559, 0.3333333333333333703, 0.3219752754296894559, 0.3333333333333333703, 0.3219752754296894559, 0.3333333333333333703, 0.3219752754296894559, 0.3333333333333333703, 0.3219752754296894559, 0.3333333333333333703, 0.3219752754296894559, 0.3333333333333333703, 0.3219752754296894559, 0.3333333333333333703, 0.3219752754296894559, 0.3333333333333333703, 0.3219752754296894559, 0.3333333333333333703, 0.3219752754296894559, 0.3333333333333333703, 0.3219752754296894559, 0.3333333333333333703, 0.3219752754296894559, 0.3333333333333333703, 0.3219752754296894559, 0.3333333333333333703, 0.3219752754296894559, 0.3333333333333333703, 0.3219752754296894559, 0.3333333333333333703, 0.3219752754296894559, 0.3333333333333333703, 0.3219752754296894559, 0.3333333333333333703, 0.3219752754296894559, 0.3333333333333333703, 0.3219752754296894559, 0.3333333333333333703, 0.3219752754296894559, 0.3333333333333333703, 0.3219752754296894559, 0.3333333333333333703, 0.3219752754296894559, 0.3333333333333333703, 0.3219752754296894559, 0.3333333333333333703, 0.3219752754296894559, 0.3333333333333333703, 0.3219752754296894559, 0.3333333333333333703, 0.3219752754296894559, 0.3333333333333333703, 0.3219752754296894559, 0.3333333333333333703, 0.3219752754296894559, 0.3333333333333333703, 0.3219752754296894559, 0.3333333333333333703, 0.3219752754296894559, 0.3333333333333333703, 0.3219752754296894559, 0.3333333333333333703, 0.3219752754296894559, 0.3333333333333333703, 0.3219752754296894559, 0.3333333333333333703, 0.3219752754296894559, 0.3333333333333333703, 0.3219752754296894559, 0.3333333333333333703, 0.3219752754296894559, 0.3333333333333333703, 0.3219752754296894559, 0.3333333333333333703, 0.3219752754296894559, 0.3333333333333333703, 0.3219752754296894559, 0.3333333333333333703, 0.3219752754296894559, 0.3333333333333333703, 0.3219752754296894559, 0.3333333333333333703, 0.3219752754296894559, 0.3333333333333333703, 0.3219752754296894559, 0.3333333333333333703, 0.3219752754296894559, 0.3333333333333333703, 0.3219752754296894559, 0.3333333333333333703, 0.3219752754296894559, 0.3333333333333333703, 0.3219752754296894559, 0.3333333333333333703, 0.3219752754296894559, 0.3333333333333333703, 0.3219752754296894559, 0.3333333333333333703, 0.3219752754296894559, 0.3333333333333333703, 0.3219752754296894559, 0.3333333333333333703, 0.3219752754296894559, 0.3333333333333333703, 0.3219752754296894559, 0.3333333333333333703, 0.3219752754296894559, 0.3333333333333333703, 0.3219752754296894559, 0.3333333333333333703, 0.3219752754296894559, 0.3333333333333333703, 0.3219752754296894559, 0.3333333333333333703, 0.3219752754296894559, 0.3333333333333333703, 0.3219752754296894559, 0.3333333333333333703, 0.3219752754296894559, 0.3333333333333333703, 0.3219752754296894559, 0.3333333333333333703, 0.3219752754296894559, 0.3333333333333333703, 0.3219752754296894559, 0.3333333333333333703, 0.3219752754296894559, 0.3333333333333333703, 0.3219752754296894559, 0.3333333333333333703, 0.3219752754296894559, 0.3333333333333333703, 0.3219752754296894559, 0.3333333333333333703, 0.3219752754296894559, 0.3333333333333333703, 0.3219752754296894559, 0.3333333333333333703, 0.3219752754296894559, 0.3333333333333333703, 0.3219752754296894559, 0.3333333333333333703, 0.3219752754296894559, 0.3333333333333333703, 0.3219752754296894559, 0.3333333333333333703, 0.3219752754296894559, 0.3333333333333333703, 0.3219752754296894559, 0.3333333333333333703, 0.3219752754296894559, 0.3333333333333333703, 0.3219752754296894559, 0.3333333333333333703),
 ( 1.000000000000000000, 0.9659258262890683122, 1.000000000000000000, 0.9659258262890683122, 1.000000000000000000, 0.9659258262890683122, 1.000000000000000000, 0.9659258262890683122, 1.000000000000000000, 0.9659258262890683122, 1.000000000000000000, 0.9659258262890683122, 1.000000000000000000, 0.9659258262890683122, 1.000000000000000000, 0.9659258262890683122, 1.000000000000000000, 0.9659258262890683122, 1.000000000000000000, 0.9659258262890683122, 1.000000000000000000, 0.9659258262890683122, 1.000000000000000000, 0.9659258262890683122, 1.000000000000000000, 0.9659258262890683122, 1.000000000000000000, 0.9659258262890683122, 1.000000000000000000, 0.9659258262890683122, 1.000000000000000000, 0.9659258262890683122, 1.000000000000000000, 0.9659258262890683122, 1.000000000000000000, 0.9659258262890683122, 1.000000000000000000, 0.9659258262890683122, 1.000000000000000000, 0.9659258262890683122, 1.000000000000000000, 0.9659258262890683122, 1.000000000000000000, 0.9659258262890683122, 1.000000000000000000, 0.9659258262890683122, 1.000000000000000000, 0.9659258262890683122, 1.000000000000000000, 0.9659258262890683122, 1.000000000000000000, 0.9659258262890683122, 1.000000000000000000, 0.9659258262890683122, 1.000000000000000000, 0.9659258262890683122, 1.000000000000000000, 0.9659258262890683122, 1.000000000000000000, 0.9659258262890683122, 1.000000000000000000, 0.9659258262890683122, 1.000000000000000000, 0.9659258262890683122, 1.000000000000000000, 0.9659258262890683122, 1.000000000000000000, 0.9659258262890683122, 1.000000000000000000, 0.9659258262890683122, 1.000000000000000000, 0.9659258262890683122, 1.000000000000000000, 0.9659258262890683122, 1.000000000000000000, 0.9659258262890683122, 1.000000000000000000, 0.9659258262890683122, 1.000000000000000000, 0.9659258262890683122, 1.000000000000000000, 0.9659258262890683122, 1.000000000000000000, 0.9659258262890683122, 1.000000000000000000, 0.9659258262890683122, 1.000000000000000000, 0.9659258262890683122, 1.000000000000000000, 0.9659258262890683122, 1.000000000000000000, 0.9659258262890683122, 1.000000000000000000, 0.9659258262890683122, 1.000000000000000000, 0.9659258262890683122, 1.000000000000000000, 0.9659258262890683122, 1.000000000000000000, 0.9659258262890683122, 1.000000000000000000, 0.9659258262890683122, 1.000000000000000000, 0.9659258262890683122, 1.000000000000000000, 0.9659258262890683122, 1.000000000000000000, 0.9659258262890683122, 1.000000000000000000, 0.9659258262890683122, 1.000000000000000000, 0.9659258262890683122, 1.000000000000000000, 0.9659258262890683122, 1.000000000000000000, 0.9659258262890683122, 1.000000000000000000, 0.9659258262890683122, 1.000000000000000000, 0.9659258262890683122, 1.000000000000000000, 0.9659258262890683122, 1.000000000000000000, 0.9659258262890683122, 1.000000000000000000, 0.9659258262890683122, 1.000000000000000000, 0.9659258262890683122, 1.000000000000000000, 0.9659258262890683122, 1.000000000000000000, 0.9659258262890683122, 1.000000000000000000, 0.9659258262890683122, 1.000000000000000000, 0.9659258262890683122, 1.000000000000000000, 0.9659258262890683122, 1.000000000000000000, 0.9659258262890683122, 1.000000000000000000, 0.9659258262890683122, 1.000000000000000000, 0.9659258262890683122, 1.000000000000000000, 0.9659258262890683122, 1.000000000000000000, 0.9659258262890683122, 1.000000000000000000, 0.9659258262890683122, 1.000000000000000000, 0.9659258262890683122, 1.000000000000000000, 0.9659258262890683122, 1.000000000000000000, 0.9659258262890683122, 1.000000000000000000, 0.9659258262890683122, 1.000000000000000000, 0.9659258262890683122, 1.000000000000000000, 0.9659258262890683122, 1.000000000000000000, 0.9659258262890683122, 1.000000000000000000, 0.9659258262890683122, 1.000000000000000000, 0.9659258262890683122, 1.000000000000000000, 0.9659258262890683122, 1.000000000000000000, 0.9659258262890683122, 1.000000000000000000, 0.9659258262890683122, 1.000000000000000000, 0.9659258262890683122, 1.000000000000000000, 0.9659258262890683122, 1.000000000000000000, 0.9659258262890683122, 1.000000000000000000, 0.9659258262890683122, 1.000000000000000000, 0.9659258262890683122, 1.000000000000000000, 0.9659258262890683122, 1.000000000000000000, 0.9659258262890683122, 1.000000000000000000, 0.9659258262890683122, 1.000000000000000000, 0.9659258262890683122, 1.000000000000000000, 0.9659258262890683122, 1.000000000000000000, 0.9659258262890683122, 1.000000000000000000, 0.9659258262890683122, 1.000000000000000000, 0.9659258262890683122, 1.000000000000000000, 0.9659258262890683122, 1.000000000000000000, 0.9659258262890683122, 1.000000000000000000, 0.9659258262890683122, 1.000000000000000000, 0.9659258262890683122, 1.000000000000000000, 0.9659258262890683122, 1.000000000000000000, 0.9659258262890683122, 1.000000000000000000, 0.9659258262890683122, 1.000000000000000000, 0.9659258262890683122, 1.000000000000000000, 0.9659258262890683122, 1.000000000000000000, 0.9659258262890683122, 1.000000000000000000, 0.9659258262890683122, 1.000000000000000000, 0.9659258262890683122, 1.000000000000000000, 0.9659258262890683122, 1.000000000000000000, 0.9659258262890683122, 1.000000000000000000, 0.9659258262890683122, 1.000000000000000000, 0.9659258262890683122, 1.000000000000000000, 0.9659258262890683122, 1.000000000000000000, 0.9659258262890683122, 1.000000000000000000, 0.9659258262890683122, 1.000000000000000000, 0.9659258262890683122, 1.000000000000000000, 0.9659258262890683122, 1.000000000000000000, 0.9659258262890683122, 1.000000000000000000, 0.9659258262890683122, 1.000000000000000000, 0.9659258262890683122, 1.000000000000000000, 0.9659258262890683122, 1.000000000000000000, 0.9659258262890683122, 1.000000000000000000, 0.9659258262890683122, 1.000000000000000000, 0.9659258262890683122, 1.000000000000000000, 0.9659258262890683122, 1.000000000000000000, 0.9659258262890683122, 1.000000000000000000, 0.9659258262890683122, 1.000000000000000000, 0.9659258262890683122, 1.000000000000000000, 0.9659258262890683122, 1.000000000000000000, 0.9659258262890683122, 1.000000000000000000, 0.9659258262890683122, 1.000000000000000000, 0.9659258262890683122, 1.000000000000000000, 0.9659258262890683122, 1.000000000000000000, 0.9659258262890683122, 1.000000000000000000, 0.9659258262890683122, 1.000000000000000000, 0.9659258262890683122, 1.000000000000000000, 0.9659258262890683122, 1.000000000000000000, 0.9659258262890683122, 1.000000000000000000, 0.9659258262890683122, 1.000000000000000000, 0.9659258262890683122, 1.000000000000000000, 0.9659258262890683122, 1.000000000000000000, 0.9659258262890683122, 1.000000000000000000, 0.9659258262890683122, 1.000000000000000000, 0.9659258262890683122, 1.000000000000000000, 0.9659258262890683122, 1.000000000000000000, 0.9659258262890683122, 1.000000000000000000, 0.9659258262890683122, 1.000000000000000000, 0.9659258262890683122, 1.000000000000000000, 0.9659258262890683122, 1.000000000000000000, 0.9659258262890683122, 1.000000000000000000, 0.9659258262890683122, 1.000000000000000000, 0.9659258262890683122, 1.000000000000000000, 0.9659258262890683122, 1.000000000000000000, 0.9659258262890683122, 1.000000000000000000, 0.9659258262890683122, 1.000000000000000000, 0.9659258262890683122, 1.000000000000000000, 0.9659258262890683122, 1.000000000000000000, 0.9659258262890683122, 1.000000000000000000, 0.9659258262890683122, 1.000000000000000000, 0.9659258262890683122, 1.000000000000000000, 0.9659258262890683122, 1.000000000000000000, 0.9659258262890683122, 1.000000000000000000, 0.9659258262890683122, 1.000000000000000000, 0.9659258262890683122, 1.000000000000000000, 0.9659258262890683122, 1.000000000000000000, 0.9659258262890683122, 1.000000000000000000, 0.9659258262890683122, 1.000000000000000000, 0.9659258262890683122, 1.000000000000000000, 0.9659258262890683122, 1.000000000000000000, 0.9659258262890683122, 1.000000000000000000, 0.9659258262890683122, 1.000000000000000000, 0.9659258262890683122, 1.000000000000000000, 0.9659258262890683122, 1.000000000000000000, 0.9659258262890683122, 1.000000000000000000, 0.9659258262890683122, 1.000000000000000000, 0.9659258262890683122, 1.000000000000000000, 0.9659258262890683122, 1.000000000000000000, 0.9659258262890683122, 1.000000000000000000, 0.9659258262890683122, 1.000000000000000000, 0.9659258262890683122, 1.000000000000000000, 0.9659258262890683122, 1.000000000000000000, 0.9659258262890683122, 1.000000000000000000, 0.9659258262890683122, 1.000000000000000000, 0.9659258262890683122, 1.000000000000000000, 0.9659258262890683122, 1.000000000000000000, 0.9659258262890683122, 1.000000000000000000, 0.9659258262890683122, 1.000000000000000000, 0.9659258262890683122, 1.000000000000000000, 0.9659258262890683122, 1.000000000000000000, 0.9659258262890683122, 1.000000000000000000, 0.9659258262890683122, 1.000000000000000000, 0.9659258262890683122, 1.000000000000000000, 0.9659258262890683122, 1.000000000000000000, 0.9659258262890683122, 1.000000000000000000, 0.9659258262890683122, 1.000000000000000000, 0.9659258262890683122, 1.000000000000000000, 0.9659258262890683122, 1.000000000000000000, 0.9659258262890683122, 1.000000000000000000, 0.9659258262890683122, 1.000000000000000000, 0.9659258262890683122, 1.000000000000000000, 0.9659258262890683122, 1.000000000000000000, 0.9659258262890683122, 1.000000000000000000, 0.9659258262890683122, 1.000000000000000000, 0.9659258262890683122, 1.000000000000000000, 0.9659258262890683122, 1.000000000000000000, 0.9659258262890683122, 1.000000000000000000, 0.9659258262890683122, 1.000000000000000000, 0.9659258262890683122, 1.000000000000000000, 0.9659258262890683122, 1.000000000000000000, 0.9659258262890683122, 1.000000000000000000, 0.9659258262890683122, 1.000000000000000000, 0.9659258262890683122, 1.000000000000000000, 0.9659258262890683122, 1.000000000000000000, 0.9659258262890683122, 1.000000000000000000, 0.9659258262890683122, 1.000000000000000000, 0.9659258262890683122, 1.000000000000000000, 0.9659258262890683122, 1.000000000000000000, 0.9659258262890683122, 1.000000000000000000, 0.9659258262890683122, 1.000000000000000000, 0.9659258262890683122, 1.000000000000000000, 0.9659258262890683122, 1.000000000000000000, 0.9659258262890683122, 1.000000000000000000, 0.9659258262890683122, 1.000000000000000000, 0.9659258262890683122, 1.000000000000000000),
 ( 0.3333333333333333703, 0.3219752754296894559, 0.3333333333333333703, 0.3219752754296894559, 0.3333333333333333703, 0.3219752754296894559, 0.3333333333333333703, 0.3219752754296894559, 0.3333333333333333703, 0.3219752754296894559, 0.3333333333333333703, 0.3219752754296894559, 0.3333333333333333703, 0.3219752754296894559, 0.3333333333333333703, 0.3219752754296894559, 0.3333333333333333703, 0.3219752754296894559, 0.3333333333333333703, 0.3219752754296894559, 0.3333333333333333703, 0.3219752754296894559, 0.3333333333333333703, 0.3219752754296894559, 0.3333333333333333703, 0.3219752754296894559, 0.3333333333333333703, 0.3219752754296894559, 0.3333333333333333703, 0.3219752754296894559, 0.3333333333333333703, 0.3219752754296894559, 0.3333333333333333703, 0.3219752754296894559, 0.3333333333333333703, 0.3219752754296894559, 0.3333333333333333703, 0.3219752754296894559, 0.3333333333333333703, 0.3219752754296894559, 0.3333333333333333703, 0.3219752754296894559, 0.3333333333333333703, 0.3219752754296894559, 0.3333333333333333703, 0.3219752754296894559, 0.3333333333333333703, 0.3219752754296894559, 0.3333333333333333703, 0.3219752754296894559, 0.3333333333333333703, 0.3219752754296894559, 0.3333333333333333703, 0.3219752754296894559, 0.3333333333333333703, 0.3219752754296894559, 0.3333333333333333703, 0.3219752754296894559, 0.3333333333333333703, 0.3219752754296894559, 0.3333333333333333703, 0.3219752754296894559, 0.3333333333333333703, 0.3219752754296894559, 0.3333333333333333703, 0.3219752754296894559, 0.3333333333333333703, 0.3219752754296894559, 0.3333333333333333703, 0.3219752754296894559, 0.3333333333333333703, 0.3219752754296894559, 0.3333333333333333703, 0.3219752754296894559, 0.3333333333333333703, 0.3219752754296894559, 0.3333333333333333703, 0.3219752754296894559, 0.3333333333333333703, 0.3219752754296894559, 0.3333333333333333703, 0.3219752754296894559, 0.3333333333333333703, 0.3219752754296894559, 0.3333333333333333703, 0.3219752754296894559, 0.3333333333333333703, 0.3219752754296894559, 0.3333333333333333703, 0.3219752754296894559, 0.3333333333333333703, 0.3219752754296894559, 0.3333333333333333703, 0.3219752754296894559, 0.3333333333333333703, 0.3219752754296894559, 0.3333333333333333703, 0.3219752754296894559, 0.3333333333333333703, 0.3219752754296894559, 0.3333333333333333703, 0.3219752754296894559, 0.3333333333333333703, 0.3219752754296894559, 0.3333333333333333703, 0.3219752754296894559, 0.3333333333333333703, 0.3219752754296894559, 0.3333333333333333703, 0.3219752754296894559, 0.3333333333333333703, 0.3219752754296894559, 0.3333333333333333703, 0.3219752754296894559, 0.3333333333333333703, 0.3219752754296894559, 0.3333333333333333703, 0.3219752754296894559, 0.3333333333333333703, 0.3219752754296894559, 0.3333333333333333703, 0.3219752754296894559, 0.3333333333333333703, 0.3219752754296894559, 0.3333333333333333703, 0.3219752754296894559, 0.3333333333333333703, 0.3219752754296894559, 0.3333333333333333703, 0.3219752754296894559, 0.3333333333333333703, 0.3219752754296894559, 0.3333333333333333703, 0.3219752754296894559, 0.3333333333333333703, 0.3219752754296894559, 0.3333333333333333703, 0.3219752754296894559, 0.3333333333333333703, 0.3219752754296894559, 0.3333333333333333703, 0.3219752754296894559, 0.3333333333333333703, 0.3219752754296894559, 0.3333333333333333703, 0.3219752754296894559, 0.3333333333333333703, 0.3219752754296894559, 0.3333333333333333703, 0.3219752754296894559, 0.3333333333333333703, 0.3219752754296894559, 0.3333333333333333703, 0.3219752754296894559, 0.3333333333333333703, 0.3219752754296894559, 0.3333333333333333703, 0.3219752754296894559, 0.3333333333333333703, 0.3219752754296894559, 0.3333333333333333703, 0.3219752754296894559, 0.3333333333333333703, 0.3219752754296894559, 0.3333333333333333703, 0.3219752754296894559, 0.3333333333333333703, 0.3219752754296894559, 0.3333333333333333703, 0.3219752754296894559, 0.3333333333333333703, 0.3219752754296894559, 0.3333333333333333703, 0.3219752754296894559, 0.3333333333333333703, 0.3219752754296894559, 0.3333333333333333703, 0.3219752754296894559, 0.3333333333333333703, 0.3219752754296894559, 0.3333333333333333703, 0.3219752754296894559, 0.3333333333333333703, 0.3219752754296894559, 0.3333333333333333703, 0.3219752754296894559, 0.3333333333333333703, 0.3219752754296894559, 0.3333333333333333703, 0.3219752754296894559, 0.3333333333333333703, 0.3219752754296894559, 0.3333333333333333703, 0.3219752754296894559, 0.3333333333333333703, 0.3219752754296894559, 0.3333333333333333703, 0.3219752754296894559, 0.3333333333333333703, 0.3219752754296894559, 0.3333333333333333703, 0.3219752754296894559, 0.3333333333333333703, 0.3219752754296894559, 0.3333333333333333703, 0.3219752754296894559, 0.3333333333333333703, 0.3219752754296894559, 0.3333333333333333703, 0.3219752754296894559, 0.3333333333333333703, 0.3219752754296894559, 0.3333333333333333703, 0.3219752754296894559, 0.3333333333333333703, 0.3219752754296894559, 0.3333333333333333703, 0.3219752754296894559, 0.3333333333333333703, 0.3219752754296894559, 0.3333333333333333703, 0.3219752754296894559, 0.3333333333333333703, 0.3219752754296894559, 0.3333333333333333703, 0.3219752754296894559, 0.3333333333333333703, 0.3219752754296894559, 0.3333333333333333703, 0.3219752754296894559, 0.3333333333333333703, 0.3219752754296894559, 0.3333333333333333703, 0.3219752754296894559, 0.3333333333333333703, 0.3219752754296894559, 0.3333333333333333703, 0.3219752754296894559, 0.3333333333333333703, 0.3219752754296894559, 0.3333333333333333703, 0.3219752754296894559, 0.3333333333333333703, 0.3219752754296894559, 0.3333333333333333703, 0.3219752754296894559, 0.3333333333333333703, 0.3219752754296894559, 0.3333333333333333703, 0.3219752754296894559, 0.3333333333333333703, 0.3219752754296894559, 0.3333333333333333703, 0.3219752754296894559, 0.3333333333333333703, 0.3219752754296894559, 0.3333333333333333703, 0.3219752754296894559, 0.3333333333333333703, 0.3219752754296894559, 0.3333333333333333703, 0.3219752754296894559, 0.3333333333333333703, 0.3219752754296894559, 0.3333333333333333703, 0.3219752754296894559, 0.3333333333333333703, 0.3219752754296894559, 0.3333333333333333703, 0.3219752754296894559, 0.3333333333333333703, 0.3219752754296894559, 0.3333333333333333703, 0.3219752754296894559, 0.3333333333333333703, 0.3219752754296894559, 0.3333333333333333703, 0.3219752754296894559, 0.3333333333333333703, 0.3219752754296894559, 0.3333333333333333703, 0.3219752754296894559, 0.3333333333333333703, 0.3219752754296894559, 0.3333333333333333703, 0.3219752754296894559, 0.3333333333333333703, 0.3219752754296894559, 0.3333333333333333703, 0.3219752754296894559, 0.3333333333333333703, 0.3219752754296894559, 0.3333333333333333703, 0.3219752754296894559, 0.3333333333333333703, 0.3219752754296894559, 0.3333333333333333703, 0.3219752754296894559, 0.3333333333333333703, 0.3219752754296894559, 0.3333333333333333703, 0.3219752754296894559, 0.3333333333333333703, 0.3219752754296894559, 0.3333333333333333703, 0.3219752754296894559, 0.3333333333333333703, 0.3219752754296894559, 0.3333333333333333703, 0.3219752754296894559, 0.3333333333333333703, 0.3219752754296894559, 0.3333333333333333703, 0.3219752754296894559, 0.3333333333333333703, 0.3219752754296894559, 0.3333333333333333703, 0.3219752754296894559, 0.3333333333333333703, 0.3219752754296894559, 0.3333333333333333703, 0.3219752754296894559, 0.3333333333333333703, 0.3219752754296894559, 0.3333333333333333703, 0.3219752754296894559, 0.3333333333333333703, 0.3219752754296894559, 0.3333333333333333703, 0.3219752754296894559, 0.3333333333333333703, 0.3219752754296894559, 0.3333333333333333703, 0.3219752754296894559, 0.3333333333333333703, 0.3219752754296894559, 0.3333333333333333703, 0.3219752754296894559, 0.3333333333333333703, 0.3219752754296894559, 0.3333333333333333703, 0.3219752754296894559, 0.3333333333333333703, 0.3219752754296894559, 0.3333333333333333703, 0.3219752754296894559, 0.3333333333333333703, 0.3219752754296894559, 0.3333333333333333703, 0.3219752754296894559, 0.3333333333333333703, 0.3219752754296894559, 0.3333333333333333703, 0.3219752754296894559, 0.3333333333333333703, 0.3219752754296894559, 0.3333333333333333703, 0.3219752754296894559, 0.3333333333333333703, 0.3219752754296894559, 0.3333333333333333703, 0.3219752754296894559, 0.3333333333333333703, 0.3219752754296894559, 0.3333333333333333703, 0.3219752754296894559, 0.3333333333333333703, 0.3219752754296894559, 0.3333333333333333703, 0.3219752754296894559, 0.3333333333333333703, 0.3219752754296894559, 0.3333333333333333703, 0.3219752754296894559, 0.3333333333333333703, 0.3219752754296894559, 0.3333333333333333703, 0.3219752754296894559, 0.3333333333333333703, 0.3219752754296894559, 0.3333333333333333703, 0.3219752754296894559, 0.3333333333333333703, 0.3219752754296894559, 0.3333333333333333703, 0.3219752754296894559, 0.3333333333333333703, 0.3219752754296894559, 0.3333333333333333703, 0.3219752754296894559, 0.3333333333333333703, 0.3219752754296894559, 0.3333333333333333703, 0.3219752754296894559, 0.3333333333333333703, 0.3219752754296894559, 0.3333333333333333703, 0.3219752754296894559, 0.3333333333333333703, 0.3219752754296894559, 0.3333333333333333703, 0.3219752754296894559, 0.3333333333333333703, 0.3219752754296894559, 0.3333333333333333703, 0.3219752754296894559, 0.3333333333333333703, 0.3219752754296894559, 0.3333333333333333703, 0.3219752754296894559, 0.3333333333333333703, 0.3219752754296894559, 0.3333333333333333703, 0.3219752754296894559, 0.3333333333333333703, 0.3219752754296894559, 0.3333333333333333703, 0.3219752754296894559, 0.3333333333333333703, 0.3219752754296894559, 0.3333333333333333703, 0.3219752754296894559, 0.3333333333333333703, 0.3219752754296894559, 0.3333333333333333703, 0.3219752754296894559, 0.3333333333333333703, 0.3219752754296894559, 0.3333333333333333703, 0.3219752754296894559, 0.3333333333333333703, 0.3219752754296894559, 0.3333333333333333703, 0.3219752754296894559, 0.3333333333333333703, 0.3219752754296894559, 0.3333333333333333703, 0.3219752754296894559, 0.3333333333333333703, 0.3219752754296894559, 0.3333333333333333703, 0.3219752754296894559, 0.3333333333333333703, 0.3219752754296894559, 0.3333333333333333703, 0.3219752754296894559, 0.3333333333333333703, 0.3219752754296894559, 0.3333333333333333703, 0.3219752754296894559, 0.3333333333333333703, 0.3219752754296894559, 0.3333333333333333703, 0.3219752754296894559, 0.3333333333333333703, 0.3219752754296894559, 0.3333333333333333703),
 ( 0.3333333333333333703, 0.3219752754296894559, 0.3333333333333333703, 0.3219752754296894559, 0.3333333333333333703, 0.3219752754296894559, 0.3333333333333333703, 0.3219752754296894559, 0.3333333333333333703, 0.3219752754296894559, 0.3333333333333333703, 0.3219752754296894559, 0.3333333333333333703, 0.3219752754296894559, 0.3333333333333333703, 0.3219752754296894559, 0.3333333333333333703, 0.3219752754296894559, 0.3333333333333333703, 0.3219752754296894559, 0.3333333333333333703, 0.3219752754296894559, 0.3333333333333333703, 0.3219752754296894559, 0.3333333333333333703, 0.3219752754296894559, 0.3333333333333333703, 0.3219752754296894559, 0.3333333333333333703, 0.3219752754296894559, 0.3333333333333333703, 0.3219752754296894559, 0.3333333333333333703, 0.3219752754296894559, 0.3333333333333333703, 0.3219752754296894559, 0.3333333333333333703, 0.3219752754296894559, 0.3333333333333333703, 0.3219752754296894559, 0.3333333333333333703, 0.3219752754296894559, 0.3333333333333333703, 0.3219752754296894559, 0.3333333333333333703, 0.3219752754296894559, 0.3333333333333333703, 0.3219752754296894559, 0.3333333333333333703, 0.3219752754296894559, 0.3333333333333333703, 0.3219752754296894559, 0.3333333333333333703, 0.3219752754296894559, 0.3333333333333333703, 0.3219752754296894559, 0.3333333333333333703, 0.3219752754296894559, 0.3333333333333333703, 0.3219752754296894559, 0.3333333333333333703, 0.3219752754296894559, 0.3333333333333333703, 0.3219752754296894559, 0.3333333333333333703, 0.3219752754296894559, 0.3333333333333333703, 0.3219752754296894559, 0.3333333333333333703, 0.3219752754296894559, 0.3333333333333333703, 0.3219752754296894559, 0.3333333333333333703, 0.3219752754296894559, 0.3333333333333333703, 0.3219752754296894559, 0.3333333333333333703, 0.3219752754296894559, 0.3333333333333333703, 0.3219752754296894559, 0.3333333333333333703, 0.3219752754296894559, 0.3333333333333333703, 0.3219752754296894559, 0.3333333333333333703, 0.3219752754296894559, 0.3333333333333333703, 0.3219752754296894559, 0.3333333333333333703, 0.3219752754296894559, 0.3333333333333333703, 0.3219752754296894559, 0.3333333333333333703, 0.3219752754296894559, 0.3333333333333333703, 0.3219752754296894559, 0.3333333333333333703, 0.3219752754296894559, 0.3333333333333333703, 0.3219752754296894559, 0.3333333333333333703, 0.3219752754296894559, 0.3333333333333333703, 0.3219752754296894559, 0.3333333333333333703, 0.3219752754296894559, 0.3333333333333333703, 0.3219752754296894559, 0.3333333333333333703, 0.3219752754296894559, 0.3333333333333333703, 0.3219752754296894559, 0.3333333333333333703, 0.3219752754296894559, 0.3333333333333333703, 0.3219752754296894559, 0.3333333333333333703, 0.3219752754296894559, 0.3333333333333333703, 0.3219752754296894559, 0.3333333333333333703, 0.3219752754296894559, 0.3333333333333333703, 0.3219752754296894559, 0.3333333333333333703, 0.3219752754296894559, 0.3333333333333333703, 0.3219752754296894559, 0.3333333333333333703, 0.3219752754296894559, 0.3333333333333333703, 0.3219752754296894559, 0.3333333333333333703, 0.3219752754296894559, 0.3333333333333333703, 0.3219752754296894559, 0.3333333333333333703, 0.3219752754296894559, 0.3333333333333333703, 0.3219752754296894559, 0.3333333333333333703, 0.3219752754296894559, 0.3333333333333333703, 0.3219752754296894559, 0.3333333333333333703, 0.3219752754296894559, 0.3333333333333333703, 0.3219752754296894559, 0.3333333333333333703, 0.3219752754296894559, 0.3333333333333333703, 0.3219752754296894559, 0.3333333333333333703, 0.3219752754296894559, 0.3333333333333333703, 0.3219752754296894559, 0.3333333333333333703, 0.3219752754296894559, 0.3333333333333333703, 0.3219752754296894559, 0.3333333333333333703, 0.3219752754296894559, 0.3333333333333333703, 0.3219752754296894559, 0.3333333333333333703, 0.3219752754296894559, 0.3333333333333333703, 0.3219752754296894559, 0.3333333333333333703, 0.3219752754296894559, 0.3333333333333333703, 0.3219752754296894559, 0.3333333333333333703, 0.3219752754296894559, 0.3333333333333333703, 0.3219752754296894559, 0.3333333333333333703, 0.3219752754296894559, 0.3333333333333333703, 0.3219752754296894559, 0.3333333333333333703, 0.3219752754296894559, 0.3333333333333333703, 0.3219752754296894559, 0.3333333333333333703, 0.3219752754296894559, 0.3333333333333333703, 0.3219752754296894559, 0.3333333333333333703, 0.3219752754296894559, 0.3333333333333333703, 0.3219752754296894559, 0.3333333333333333703, 0.3219752754296894559, 0.3333333333333333703, 0.3219752754296894559, 0.3333333333333333703, 0.3219752754296894559, 0.3333333333333333703, 0.3219752754296894559, 0.3333333333333333703, 0.3219752754296894559, 0.3333333333333333703, 0.3219752754296894559, 0.3333333333333333703, 0.3219752754296894559, 0.3333333333333333703, 0.3219752754296894559, 0.3333333333333333703, 0.3219752754296894559, 0.3333333333333333703, 0.3219752754296894559, 0.3333333333333333703, 0.3219752754296894559, 0.3333333333333333703, 0.3219752754296894559, 0.3333333333333333703, 0.3219752754296894559, 0.3333333333333333703, 0.3219752754296894559, 0.3333333333333333703, 0.3219752754296894559, 0.3333333333333333703, 0.3219752754296894559, 0.3333333333333333703, 0.3219752754296894559, 0.3333333333333333703, 0.3219752754296894559, 0.3333333333333333703, 0.3219752754296894559, 0.3333333333333333703, 0.3219752754296894559, 0.3333333333333333703, 0.3219752754296894559, 0.3333333333333333703, 0.3219752754296894559, 0.3333333333333333703, 0.3219752754296894559, 0.3333333333333333703, 0.3219752754296894559, 0.3333333333333333703, 0.3219752754296894559, 0.3333333333333333703, 0.3219752754296894559, 0.3333333333333333703, 0.3219752754296894559, 0.3333333333333333703, 0.3219752754296894559, 0.3333333333333333703, 0.3219752754296894559, 0.3333333333333333703, 0.3219752754296894559, 0.3333333333333333703, 0.3219752754296894559, 0.3333333333333333703, 0.3219752754296894559, 0.3333333333333333703, 0.3219752754296894559, 0.3333333333333333703, 0.3219752754296894559, 0.3333333333333333703, 0.3219752754296894559, 0.3333333333333333703, 0.3219752754296894559, 0.3333333333333333703, 0.3219752754296894559, 0.3333333333333333703, 0.3219752754296894559, 0.3333333333333333703, 0.3219752754296894559, 0.3333333333333333703, 0.3219752754296894559, 0.3333333333333333703, 0.3219752754296894559, 0.3333333333333333703, 0.3219752754296894559, 0.3333333333333333703, 0.3219752754296894559, 0.3333333333333333703, 0.3219752754296894559, 0.3333333333333333703, 0.3219752754296894559, 0.3333333333333333703, 0.3219752754296894559, 0.3333333333333333703, 0.3219752754296894559, 0.3333333333333333703, 0.3219752754296894559, 0.3333333333333333703, 0.3219752754296894559, 0.3333333333333333703, 0.3219752754296894559, 0.3333333333333333703, 0.3219752754296894559, 0.3333333333333333703, 0.3219752754296894559, 0.3333333333333333703, 0.3219752754296894559, 0.3333333333333333703, 0.3219752754296894559, 0.3333333333333333703, 0.3219752754296894559, 0.3333333333333333703, 0.3219752754296894559, 0.3333333333333333703, 0.3219752754296894559, 0.3333333333333333703, 0.3219752754296894559, 0.3333333333333333703, 0.3219752754296894559, 0.3333333333333333703, 0.3219752754296894559, 0.3333333333333333703, 0.3219752754296894559, 0.3333333333333333703, 0.3219752754296894559, 0.3333333333333333703, 0.3219752754296894559, 0.3333333333333333703, 0.3219752754296894559, 0.3333333333333333703, 0.3219752754296894559, 0.3333333333333333703, 0.3219752754296894559, 0.3333333333333333703, 0.3219752754296894559, 0.3333333333333333703, 0.3219752754296894559, 0.3333333333333333703, 0.3219752754296894559, 0.3333333333333333703, 0.3219752754296894559, 0.3333333333333333703, 0.3219752754296894559, 0.3333333333333333703, 0.3219752754296894559, 0.3333333333333333703, 0.3219752754296894559, 0.3333333333333333703, 0.3219752754296894559, 0.3333333333333333703, 0.3219752754296894559, 0.3333333333333333703, 0.3219752754296894559, 0.3333333333333333703, 0.3219752754296894559, 0.3333333333333333703, 0.3219752754296894559, 0.3333333333333333703, 0.3219752754296894559, 0.3333333333333333703, 0.3219752754296894559, 0.3333333333333333703, 0.3219752754296894559, 0.3333333333333333703, 0.3219752754296894559, 0.3333333333333333703, 0.3219752754296894559, 0.3333333333333333703, 0.3219752754296894559, 0.3333333333333333703, 0.3219752754296894559, 0.3333333333333333703, 0.3219752754296894559, 0.3333333333333333703, 0.3219752754296894559, 0.3333333333333333703, 0.3219752754296894559, 0.3333333333333333703, 0.3219752754296894559, 0.3333333333333333703, 0.3219752754296894559, 0.3333333333333333703, 0.3219752754296894559, 0.3333333333333333703, 0.3219752754296894559, 0.3333333333333333703, 0.3219752754296894559, 0.3333333333333333703, 0.3219752754296894559, 0.3333333333333333703, 0.3219752754296894559, 0.3333333333333333703, 0.3219752754296894559, 0.3333333333333333703, 0.3219752754296894559, 0.3333333333333333703, 0.3219752754296894559, 0.3333333333333333703, 0.3219752754296894559, 0.3333333333333333703, 0.3219752754296894559, 0.3333333333333333703, 0.3219752754296894559, 0.3333333333333333703, 0.3219752754296894559, 0.3333333333333333703, 0.3219752754296894559, 0.3333333333333333703, 0.3219752754296894559, 0.3333333333333333703, 0.3219752754296894559, 0.3333333333333333703, 0.3219752754296894559, 0.3333333333333333703, 0.3219752754296894559, 0.3333333333333333703, 0.3219752754296894559, 0.3333333333333333703, 0.3219752754296894559, 0.3333333333333333703, 0.3219752754296894559, 0.3333333333333333703, 0.3219752754296894559, 0.3333333333333333703, 0.3219752754296894559, 0.3333333333333333703, 0.3219752754296894559, 0.3333333333333333703, 0.3219752754296894559, 0.3333333333333333703, 0.3219752754296894559, 0.3333333333333333703, 0.3219752754296894559, 0.3333333333333333703, 0.3219752754296894559, 0.3333333333333333703, 0.3219752754296894559, 0.3333333333333333703, 0.3219752754296894559, 0.3333333333333333703, 0.3219752754296894559, 0.3333333333333333703, 0.3219752754296894559, 0.3333333333333333703, 0.3219752754296894559, 0.3333333333333333703, 0.3219752754296894559, 0.3333333333333333703, 0.3219752754296894559, 0.3333333333333333703, 0.3219752754296894559, 0.3333333333333333703, 0.3219752754296894559, 0.3333333333333333703, 0.3219752754296894559, 0.3333333333333333703, 0.3219752754296894559, 0.3333333333333333703, 0.3219752754296894559, 0.3333333333333333703, 0.3219752754296894559, 0.3333333333333333703, 0.3219752754296894559, 0.3333333333333333703, 0.3219752754296894559, 0.3333333333333333703),
 ( 1.000000000000000000, 0.9659258262890683122, 1.000000000000000000, 0.9659258262890683122, 1.000000000000000000, 0.9659258262890683122, 1.000000000000000000, 0.9659258262890683122, 1.000000000000000000, 0.9659258262890683122, 1.000000000000000000, 0.9659258262890683122, 1.000000000000000000, 0.9659258262890683122, 1.000000000000000000, 0.9659258262890683122, 1.000000000000000000, 0.9659258262890683122, 1.000000000000000000, 0.9659258262890683122, 1.000000000000000000, 0.9659258262890683122, 1.000000000000000000, 0.9659258262890683122, 1.000000000000000000, 0.9659258262890683122, 1.000000000000000000, 0.9659258262890683122, 1.000000000000000000, 0.9659258262890683122, 1.000000000000000000, 0.9659258262890683122, 1.000000000000000000, 0.9659258262890683122, 1.000000000000000000, 0.9659258262890683122, 1.000000000000000000, 0.9659258262890683122, 1.000000000000000000, 0.9659258262890683122, 1.000000000000000000, 0.9659258262890683122, 1.000000000000000000, 0.9659258262890683122, 1.000000000000000000, 0.9659258262890683122, 1.000000000000000000, 0.9659258262890683122, 1.000000000000000000, 0.9659258262890683122, 1.000000000000000000, 0.9659258262890683122, 1.000000000000000000, 0.9659258262890683122, 1.000000000000000000, 0.9659258262890683122, 1.000000000000000000, 0.9659258262890683122, 1.000000000000000000, 0.9659258262890683122, 1.000000000000000000, 0.9659258262890683122, 1.000000000000000000, 0.9659258262890683122, 1.000000000000000000, 0.9659258262890683122, 1.000000000000000000, 0.9659258262890683122, 1.000000000000000000, 0.9659258262890683122, 1.000000000000000000, 0.9659258262890683122, 1.000000000000000000, 0.9659258262890683122, 1.000000000000000000, 0.9659258262890683122, 1.000000000000000000, 0.9659258262890683122, 1.000000000000000000, 0.9659258262890683122, 1.000000000000000000, 0.9659258262890683122, 1.000000000000000000, 0.9659258262890683122, 1.000000000000000000, 0.9659258262890683122, 1.000000000000000000, 0.9659258262890683122, 1.000000000000000000, 0.9659258262890683122, 1.000000000000000000, 0.9659258262890683122, 1.000000000000000000, 0.9659258262890683122, 1.000000000000000000, 0.9659258262890683122, 1.000000000000000000, 0.9659258262890683122, 1.000000000000000000, 0.9659258262890683122, 1.000000000000000000, 0.9659258262890683122, 1.000000000000000000, 0.9659258262890683122, 1.000000000000000000, 0.9659258262890683122, 1.000000000000000000, 0.9659258262890683122, 1.000000000000000000, 0.9659258262890683122, 1.000000000000000000, 0.9659258262890683122, 1.000000000000000000, 0.9659258262890683122, 1.000000000000000000, 0.9659258262890683122, 1.000000000000000000, 0.9659258262890683122, 1.000000000000000000, 0.9659258262890683122, 1.000000000000000000, 0.9659258262890683122, 1.000000000000000000, 0.9659258262890683122, 1.000000000000000000, 0.9659258262890683122, 1.000000000000000000, 0.9659258262890683122, 1.000000000000000000, 0.9659258262890683122, 1.000000000000000000, 0.9659258262890683122, 1.000000000000000000, 0.9659258262890683122, 1.000000000000000000, 0.9659258262890683122, 1.000000000000000000, 0.9659258262890683122, 1.000000000000000000, 0.9659258262890683122, 1.000000000000000000, 0.9659258262890683122, 1.000000000000000000, 0.9659258262890683122, 1.000000000000000000, 0.9659258262890683122, 1.000000000000000000, 0.9659258262890683122, 1.000000000000000000, 0.9659258262890683122, 1.000000000000000000, 0.9659258262890683122, 1.000000000000000000, 0.9659258262890683122, 1.000000000000000000, 0.9659258262890683122, 1.000000000000000000, 0.9659258262890683122, 1.000000000000000000, 0.9659258262890683122, 1.000000000000000000, 0.9659258262890683122, 1.000000000000000000, 0.9659258262890683122, 1.000000000000000000, 0.9659258262890683122, 1.000000000000000000, 0.9659258262890683122, 1.000000000000000000, 0.9659258262890683122, 1.000000000000000000, 0.9659258262890683122, 1.000000000000000000, 0.9659258262890683122, 1.000000000000000000, 0.9659258262890683122, 1.000000000000000000, 0.9659258262890683122, 1.000000000000000000, 0.9659258262890683122, 1.000000000000000000, 0.9659258262890683122, 1.000000000000000000, 0.9659258262890683122, 1.000000000000000000, 0.9659258262890683122, 1.000000000000000000, 0.9659258262890683122, 1.000000000000000000, 0.9659258262890683122, 1.000000000000000000, 0.9659258262890683122, 1.000000000000000000, 0.9659258262890683122, 1.000000000000000000, 0.9659258262890683122, 1.000000000000000000, 0.9659258262890683122, 1.000000000000000000, 0.9659258262890683122, 1.000000000000000000, 0.9659258262890683122, 1.000000000000000000, 0.9659258262890683122, 1.000000000000000000, 0.9659258262890683122, 1.000000000000000000, 0.9659258262890683122, 1.000000000000000000, 0.9659258262890683122, 1.000000000000000000, 0.9659258262890683122, 1.000000000000000000, 0.9659258262890683122, 1.000000000000000000, 0.9659258262890683122, 1.000000000000000000, 0.9659258262890683122, 1.000000000000000000, 0.9659258262890683122, 1.000000000000000000, 0.9659258262890683122, 1.000000000000000000, 0.9659258262890683122, 1.000000000000000000, 0.9659258262890683122, 1.000000000000000000, 0.9659258262890683122, 1.000000000000000000, 0.9659258262890683122, 1.000000000000000000, 0.9659258262890683122, 1.000000000000000000, 0.9659258262890683122, 1.000000000000000000, 0.9659258262890683122, 1.000000000000000000, 0.9659258262890683122, 1.000000000000000000, 0.9659258262890683122, 1.000000000000000000, 0.9659258262890683122, 1.000000000000000000, 0.9659258262890683122, 1.000000000000000000, 0.9659258262890683122, 1.000000000000000000, 0.9659258262890683122, 1.000000000000000000, 0.9659258262890683122, 1.000000000000000000, 0.9659258262890683122, 1.000000000000000000, 0.9659258262890683122, 1.000000000000000000, 0.9659258262890683122, 1.000000000000000000, 0.9659258262890683122, 1.000000000000000000, 0.9659258262890683122, 1.000000000000000000, 0.9659258262890683122, 1.000000000000000000, 0.9659258262890683122, 1.000000000000000000, 0.9659258262890683122, 1.000000000000000000, 0.9659258262890683122, 1.000000000000000000, 0.9659258262890683122, 1.000000000000000000, 0.9659258262890683122, 1.000000000000000000, 0.9659258262890683122, 1.000000000000000000, 0.9659258262890683122, 1.000000000000000000, 0.9659258262890683122, 1.000000000000000000, 0.9659258262890683122, 1.000000000000000000, 0.9659258262890683122, 1.000000000000000000, 0.9659258262890683122, 1.000000000000000000, 0.9659258262890683122, 1.000000000000000000, 0.9659258262890683122, 1.000000000000000000, 0.9659258262890683122, 1.000000000000000000, 0.9659258262890683122, 1.000000000000000000, 0.9659258262890683122, 1.000000000000000000, 0.9659258262890683122, 1.000000000000000000, 0.9659258262890683122, 1.000000000000000000, 0.9659258262890683122, 1.000000000000000000, 0.9659258262890683122, 1.000000000000000000, 0.9659258262890683122, 1.000000000000000000, 0.9659258262890683122, 1.000000000000000000, 0.9659258262890683122, 1.000000000000000000, 0.9659258262890683122, 1.000000000000000000, 0.9659258262890683122, 1.000000000000000000, 0.9659258262890683122, 1.000000000000000000, 0.9659258262890683122, 1.000000000000000000, 0.9659258262890683122, 1.000000000000000000, 0.9659258262890683122, 1.000000000000000000, 0.9659258262890683122, 1.000000000000000000, 0.9659258262890683122, 1.000000000000000000, 0.9659258262890683122, 1.000000000000000000, 0.9659258262890683122, 1.000000000000000000, 0.9659258262890683122, 1.000000000000000000, 0.9659258262890683122, 1.000000000000000000, 0.9659258262890683122, 1.000000000000000000, 0.9659258262890683122, 1.000000000000000000, 0.9659258262890683122, 1.000000000000000000, 0.9659258262890683122, 1.000000000000000000, 0.9659258262890683122, 1.000000000000000000, 0.9659258262890683122, 1.000000000000000000, 0.9659258262890683122, 1.000000000000000000, 0.9659258262890683122, 1.000000000000000000, 0.9659258262890683122, 1.000000000000000000, 0.9659258262890683122, 1.000000000000000000, 0.9659258262890683122, 1.000000000000000000, 0.9659258262890683122, 1.000000000000000000, 0.9659258262890683122, 1.000000000000000000, 0.9659258262890683122, 1.000000000000000000, 0.9659258262890683122, 1.000000000000000000, 0.9659258262890683122, 1.000000000000000000, 0.9659258262890683122, 1.000000000000000000, 0.9659258262890683122, 1.000000000000000000, 0.9659258262890683122, 1.000000000000000000, 0.9659258262890683122, 1.000000000000000000, 0.9659258262890683122, 1.000000000000000000, 0.9659258262890683122, 1.000000000000000000, 0.9659258262890683122, 1.000000000000000000, 0.9659258262890683122, 1.000000000000000000, 0.9659258262890683122, 1.000000000000000000, 0.9659258262890683122, 1.000000000000000000, 0.9659258262890683122, 1.000000000000000000, 0.9659258262890683122, 1.000000000000000000, 0.9659258262890683122, 1.000000000000000000, 0.9659258262890683122, 1.000000000000000000, 0.9659258262890683122, 1.000000000000000000, 0.9659258262890683122, 1.000000000000000000, 0.9659258262890683122, 1.000000000000000000, 0.9659258262890683122, 1.000000000000000000, 0.9659258262890683122, 1.000000000000000000, 0.9659258262890683122, 1.000000000000000000, 0.9659258262890683122, 1.000000000000000000, 0.9659258262890683122, 1.000000000000000000, 0.9659258262890683122, 1.000000000000000000, 0.9659258262890683122, 1.000000000000000000, 0.9659258262890683122, 1.000000000000000000, 0.9659258262890683122, 1.000000000000000000, 0.9659258262890683122, 1.000000000000000000, 0.9659258262890683122, 1.000000000000000000, 0.9659258262890683122, 1.000000000000000000, 0.9659258262890683122, 1.000000000000000000, 0.9659258262890683122, 1.000000000000000000, 0.9659258262890683122, 1.000000000000000000, 0.9659258262890683122, 1.000000000000000000, 0.9659258262890683122, 1.000000000000000000, 0.9659258262890683122, 1.000000000000000000, 0.9659258262890683122, 1.000000000000000000, 0.9659258262890683122, 1.000000000000000000, 0.9659258262890683122, 1.000000000000000000, 0.9659258262890683122, 1.000000000000000000, 0.9659258262890683122, 1.000000000000000000, 0.9659258262890683122, 1.000000000000000000, 0.9659258262890683122, 1.000000000000000000, 0.9659258262890683122, 1.000000000000000000, 0.9659258262890683122, 1.000000000000000000, 0.9659258262890683122, 1.000000000000000000, 0.9659258262890683122, 1.000000000000000000) ) ) 
 REPRESENTATION_ITEM ( '' )  SURFACE ( )  );
#157754=CARTESIAN_POINT ( 'NONE',  ( 10.81492255796078972, 18.62759615963270932, 39.58224293864769550 ) ) ;
#157755=CARTESIAN_POINT ( 'NONE',  ( -14.29746914071049879, 8.314922557960819915, 100.8322429386477097 ) ) ;
#157757=CARTESIAN_POINT ( 'NONE',  ( -0.05219959533936034679, 19.03943276465977164, 57.50109039468566863 ) ) ;
#157758=CARTESIAN_POINT ( 'NONE',  ( 14.34966873604960469, 8.224510206698951720, 24.16557627198103120 ) ) ;
#157760=CARTESIAN_POINT ( 'NONE',  ( -9.564922557960796823, -16.46253265017161027, 97.08224293864769550 ) ) ;
#157761=CARTESIAN_POINT ( 'NONE',  ( 21.52544592524334988, 5.823673210054432836, 81.45942372801900433 ) ) ;
#157762=CARTESIAN_POINT ( 'NONE',  ( -5.823673210054116645, -21.52544592524344225, 67.29057627198103830 ) ) ;
#157763=CARTESIAN_POINT ( 'NONE',  ( -0.05219959533937732626, 21.53943276465977519, 42.50109039468567573 ) ) ;
#157764=CARTESIAN_POINT ( 'NONE',  ( 5.823673210054125526, 21.52544592524343514, 94.79057627198105251 ) ) ;
#157765=CARTESIAN_POINT ( 'NONE',  ( 10.72451020669871369, 18.67979575497193778, 57.08442372801901854 ) ) ;
#157766=CARTESIAN_POINT ( 'NONE',  ( 16.46253265017160672, -9.564922557960803928, 23.33224293864769194 ) ) ;
#157767=CARTESIAN_POINT ( 'NONE',  ( 16.51473224551069308, 9.474510206698969483, 84.16557627198102409 ) ) ;
#157768=CARTESIAN_POINT ( 'NONE',  ( -4.483927247898782831, 16.52544592524335698, 77.70942372801900433 ) ) ;
#157769=CARTESIAN_POINT ( 'NONE',  ( 16.52544592524342804, -4.483927247898539470, 103.5405762719810383 ) ) ;
#157770=CARTESIAN_POINT ( 'NONE',  ( -5.153800228976328057, -19.02544592524343514, 102.2905762719810383 ) ) ;
#157771=CARTESIAN_POINT ( 'NONE',  ( 8.314922557960818139, 14.29746914071049879, 49.58224293864769550 ) ) ;
#157772=CARTESIAN_POINT ( 'NONE',  ( -4.483927247898782831, 16.52544592524335698, 107.7094237280190328 ) ) ;
#157773=CARTESIAN_POINT ( 'NONE',  ( -16.51473224551069308, -9.474510206698971260, 56.66557627198103120 ) ) ;
#157774=CARTESIAN_POINT ( 'NONE',  ( 5.153800228976335163, 19.02544592524342804, 29.79057627198102409 ) ) ;
#157775=CARTESIAN_POINT ( 'NONE',  ( -15.80617190586745835, -15.72974639402198527, 51.87390960531437401 ) ) ;
#157776=CARTESIAN_POINT ( 'NONE',  ( -13.97604488694547697, 13.89961937509957934, 23.12609039468565442 ) ) ;
#157777=CARTESIAN_POINT ( 'NONE',  ( 17.97058386085788229, 5.500000000000048850, 51.50390968646216550 ) ) ;
#157778=CARTESIAN_POINT ( 'NONE',  ( 14.34966873604960469, 8.224510206698951720, 39.16557627198102409 ) ) ;
#157779=CARTESIAN_POINT ( 'NONE',  ( 21.52544592524334988, 5.823673210054432836, 41.45942372801901143 ) ) ;
#157780=EDGE_CURVE ( 'NONE', #10418, #166568, #174353, .T. ) ;
#157782=CARTESIAN_POINT ( 'NONE',  ( -8.224510206698735004, -14.34966873604973081, 59.58442372801901854 ) ) ;
#157783=CARTESIAN_POINT ( 'NONE',  ( 16.51473224551083163, -9.474510206698727899, 60.83442372801900433 ) ) ;
#157784=CARTESIAN_POINT ( 'NONE',  ( -16.55341960407611168, -4.379528057220339221, 26.45724293864768839 ) ) ;
#157785=CARTESIAN_POINT ( 'NONE',  ( 16.52544592524335698, 4.483927247898782831, 101.4594237280190185 ) ) ;
#157786=CARTESIAN_POINT ( 'NONE',  ( 16.46253265017160672, -9.564922557960803928, 33.33224293864770260 ) ) ;
#157787=CARTESIAN_POINT ( 'NONE',  ( 5.049401038298161559, -19.05341960407611168, 67.70724293864769550 ) ) ;
#157788=CARTESIAN_POINT ( 'NONE',  ( 13.89961937509977652, -13.97604488694527269, 28.12390960531435624 ) ) ;
#157789=CARTESIAN_POINT ( 'NONE',  ( 5.823673210054444382, -21.52544592524334988, 35.20942372801901854 ) ) ;
#157790=CARTESIAN_POINT ( 'NONE',  ( -13.89961937509977652, 13.97604488694528158, 40.62390960531435979 ) ) ;
#157792=CARTESIAN_POINT ( 'NONE',  ( 19.02544592524343514, -5.153800228976328945, 43.54057627198103120 ) ) ;
#157793=CARTESIAN_POINT ( 'NONE',  ( 9.564922557960805705, 16.46253265017160317, 114.5822429386476955 ) ) ;
#157794=CARTESIAN_POINT ( 'NONE',  ( -15.80617190586768217, 15.72974639402176855, 63.12609039468568994 ) ) ;
#157795=CARTESIAN_POINT ( 'NONE',  ( 16.52544592524342804, -4.483927247898539470, 108.5405762719810241 ) ) ;
#157796=CARTESIAN_POINT ( 'NONE',  ( 16.51473224551069308, 9.474510206698969483, 109.1655762719810383 ) ) ;
#157797=CARTESIAN_POINT ( 'NONE',  ( 8.224510206698742110, 14.34966873604972548, 82.08442372801901854 ) ) ;
#157798=CARTESIAN_POINT ( 'NONE',  ( 10.81492255796106328, -18.62759615963255655, 95.41775706135234714 ) ) ;
#157799=CARTESIAN_POINT ( 'NONE',  ( 8.224510206698742110, 14.34966873604972548, 57.08442372801901854 ) ) ;
#157800=CARTESIAN_POINT ( 'NONE',  ( 5.153800228976335163, 19.02544592524342804, 89.79057627198102409 ) ) ;
#157801=CARTESIAN_POINT ( 'NONE',  ( 8.314922557961029526, -14.29746914071037800, 35.41775706135234003 ) ) ;
#157802=CARTESIAN_POINT ( 'NONE',  ( -8.314922557961024197, 14.29746914071037800, 27.91775706135234358 ) ) ;
#157803=CARTESIAN_POINT ( 'NONE',  ( 16.55341960407618274, -4.379528057220086978, 101.0427570613523756 ) ) ;
#157804=CARTESIAN_POINT ( 'NONE',  ( -5.049401038297874678, -19.05341960407617918, 109.7927570613523187 ) ) ;
#157805=CARTESIAN_POINT ( 'NONE',  ( 10.81492255796078972, 18.62759615963270932, 114.5822429386477097 ) ) ;
#157806=CARTESIAN_POINT ( 'NONE',  ( -12.06949235617756955, 12.14591786802309770, 105.6239096053143669 ) ) ;
#157807=CARTESIAN_POINT ( 'NONE',  ( 13.97604488694548053, -13.89961937509957401, 100.6260903946856615 ) ) ;
#157808=CARTESIAN_POINT ( 'NONE',  ( 4.379528057220092307, 16.55341960407617563, 72.29275706135236135 ) ) ;
#157810=CARTESIAN_POINT ( 'NONE',  ( 13.89961937509957401, 13.97604488694547697, 71.87609039468567573 ) ) ;
#157812=CARTESIAN_POINT ( 'NONE',  ( 14.34966873604960469, 8.224510206698951720, 39.16557627198102409 ) ) ;
#157813=CARTESIAN_POINT ( 'NONE',  ( -14.34966873604960291, -8.224510206698953496, 41.66557627198103120 ) ) ;
#157814=CARTESIAN_POINT ( 'NONE',  ( -12.14591786802309592, -12.06949235617757132, 91.87390960531436690 ) ) ;
#157815=CARTESIAN_POINT ( 'NONE',  ( -19.05341960407617563, 5.049401038297882671, 28.54275706135232937 ) ) ;
#157817=CARTESIAN_POINT ( 'NONE',  ( -15.80617190586768217, 15.72974639402176855, 38.12609039468567573 ) ) ;
#157818=CARTESIAN_POINT ( 'NONE',  ( 0.05219959533936267826, -19.03943276465977164, 95.00109039468567573 ) ) ;
#157820=CARTESIAN_POINT ( 'NONE',  ( -13.89961937509977652, 13.97604488694528158, 85.62390960531433848 ) ) ;
#157821=CARTESIAN_POINT ( 'NONE',  ( 9.474510206698971260, -16.51473224551069308, 92.91557627198103830 ) ) ;
#157822=CARTESIAN_POINT ( 'NONE',  ( -18.62759615963270932, 10.81492255796079327, 55.83224293864770260 ) ) ;
#157823=CARTESIAN_POINT ( 'NONE',  ( 16.55341960407611168, 4.379528057220329451, 88.95724293864769550 ) ) ;
#157824=CARTESIAN_POINT ( 'NONE',  ( 5.153800228976335163, 19.02544592524342804, 69.79057627198103830 ) ) ;
#157825=CARTESIAN_POINT ( 'NONE',  ( 16.51473224551069308, 9.474510206698969483, 34.16557627198102409 ) ) ;
#157826=CARTESIAN_POINT ( 'NONE',  ( 5.719274019375673035, 21.55341960407619339, 42.29275706135235424 ) ) ;
#157827=CARTESIAN_POINT ( 'NONE',  ( 21.55341960407619695, -5.719274019375665929, 76.04275706135237556 ) ) ;
#157828=CARTESIAN_POINT ( 'NONE',  ( -16.51473224551069308, -9.474510206698971260, 56.66557627198103120 ) ) ;
#157829=CARTESIAN_POINT ( 'NONE',  ( 14.34966873604972726, -8.224510206698740333, 80.83442372801901854 ) ) ;
#157830=CARTESIAN_POINT ( 'NONE',  ( -15.80617190586768217, 15.72974639402176855, 33.12609039468569705 ) ) ;
#157831=CARTESIAN_POINT ( 'NONE',  ( 15.80617190586769283, -15.72974639402175789, 20.62609039468568639 ) ) ;
#157832=CARTESIAN_POINT ( 'NONE',  ( -16.46253265017146816, -9.564922557961047289, 49.16775706135233293 ) ) ;
#157833=CARTESIAN_POINT ( 'NONE',  ( -16.46253265017160317, 9.564922557960807481, 80.83224293864769550 ) ) ;
#157834=CARTESIAN_POINT ( 'NONE',  ( 13.89961937509957401, 13.97604488694547697, 31.87609039468566863 ) ) ;
#157835=CARTESIAN_POINT ( 'NONE',  ( -21.55341960407619339, 5.719274019375674811, 88.54275706135236135 ) ) ;
#157836=CARTESIAN_POINT ( 'NONE',  ( -5.823673210054116645, -21.52544592524344225, 72.29057627198102409 ) ) ;
#157837=CARTESIAN_POINT ( 'NONE',  ( 8.314922557960818139, 14.29746914071049879, 44.58224293864769550 ) ) ;
#157838=CARTESIAN_POINT ( 'NONE',  ( 10.81492255796106328, -18.62759615963255655, 95.41775706135234714 ) ) ;
#157839=CARTESIAN_POINT ( 'NONE',  ( 16.46253265017146816, 9.564922557961045513, 31.66775706135232937 ) ) ;
#157840=CARTESIAN_POINT ( 'NONE',  ( 8.314922557960818139, 14.29746914071049879, 69.58224293864769550 ) ) ;
#157841=CARTESIAN_POINT ( 'NONE',  ( 16.55341960407611168, 4.379528057220329451, 113.9572429386477239 ) ) ;
#157842=CARTESIAN_POINT ( 'NONE',  ( 13.89961937509957401, 13.97604488694547697, 66.87609039468567573 ) ) ;
#157843=CARTESIAN_POINT ( 'NONE',  ( -8.314922557960811034, -14.29746914071050412, 37.08224293864768129 ) ) ;
#157844=CARTESIAN_POINT ( 'NONE',  ( -18.62759615963255300, -10.81492255796106328, 84.16775706135234714 ) ) ;
#157845=CARTESIAN_POINT ( 'NONE',  ( 13.97604488694527802, 13.89961937509977652, 74.37390960531436690 ) ) ;
#157846=CARTESIAN_POINT ( 'NONE',  ( -19.02544592524334988, -5.153800228976617603, 43.95942372801899012 ) ) ;
#157847=CARTESIAN_POINT ( 'NONE',  ( 10.72451020669898902, -18.67979575497178502, 47.91557627198102409 ) ) ;
#157848=CARTESIAN_POINT ( 'NONE',  ( -15.72974639402197994, 15.80617190586746368, 110.6239096053143669 ) ) ;
#157849=CARTESIAN_POINT ( 'NONE',  ( -19.03943276465977164, -0.05219959533935918106, 108.7510903946856615 ) ) ;
#157850=CARTESIAN_POINT ( 'NONE',  ( -8.224510206698735004, -14.34966873604973081, 69.58442372801900433 ) ) ;
#157851=CARTESIAN_POINT ( 'NONE',  ( 16.19135201231370047, 7.376712067591811639, 62.68680854052030327 ) ) ;
#157852=CARTESIAN_POINT ( 'NONE',  ( 18.62759615963271287, -10.81492255796078972, 103.3322429386476955 ) ) ;
#157853=CARTESIAN_POINT ( 'NONE',  ( -4.379528057220328563, 16.55341960407611168, 105.2072429386477097 ) ) ;
#157855=CARTESIAN_POINT ( 'NONE',  ( -8.314922557961024197, 14.29746914071037800, 32.91775706135234714 ) ) ;
#157857=CARTESIAN_POINT ( 'NONE',  ( -21.52544592524343514, 5.823673210054127303, 66.04057627198103830 ) ) ;
#157858=CARTESIAN_POINT ( 'NONE',  ( -4.483927247898782831, 16.52544592524335698, 102.7094237280190185 ) ) ;
#157859=CARTESIAN_POINT ( 'NONE',  ( 16.46253265017160672, -9.564922557960803928, 33.33224293864770260 ) ) ;
#157860=CARTESIAN_POINT ( 'NONE',  ( -4.379528057220086978, -16.55341960407618274, 69.79275706135234714 ) ) ;
#157861=CARTESIAN_POINT ( 'NONE',  ( -5.153800228976607833, 19.02544592524334988, 62.70942372801899722 ) ) ;
#157862=CARTESIAN_POINT ( 'NONE',  ( 21.53943276465977519, 0.05219959533937863772, 41.25109039468568284 ) ) ;
#157863=CARTESIAN_POINT ( 'NONE',  ( 18.67979575497178502, 10.72451020669898547, 54.16557627198103120 ) ) ;
#157864=CARTESIAN_POINT ( 'NONE',  ( 4.379528057220092307, 16.55341960407617563, 92.29275706135236135 ) ) ;
#157865=CARTESIAN_POINT ( 'NONE',  ( -21.55341960407619339, 5.719274019375674811, 88.54275706135236135 ) ) ;
#157866=CARTESIAN_POINT ( 'NONE',  ( -21.55341960407610458, -5.719274019375992779, 51.45724293864770260 ) ) ;
#157867=CARTESIAN_POINT ( 'NONE',  ( 0.05219959533907565091, 21.53943276465977519, 29.99890960531435979 ) ) ;
#157869=CARTESIAN_POINT ( 'NONE',  ( 16.55341960407618274, -4.379528057220086978, 76.04275706135237556 ) ) ;
#157870=CARTESIAN_POINT ( 'NONE',  ( 18.67979575497178502, 10.72451020669898547, 44.16557627198103120 ) ) ;
#157872=CARTESIAN_POINT ( 'NONE',  ( 19.05341960407611168, 5.049401038298154454, 103.9572429386476671 ) ) ;
#157874=CARTESIAN_POINT ( 'NONE',  ( -5.153800228976328057, -19.02544592524343514, 32.29057627198102409 ) ) ;
#157875=CARTESIAN_POINT ( 'NONE',  ( -21.52544592524343514, 5.823673210054127303, 66.04057627198103830 ) ) ;
#157876=CARTESIAN_POINT ( 'NONE',  ( -8.314922557961024197, 14.29746914071037800, 87.91775706135234714 ) ) ;
#157877=CARTESIAN_POINT ( 'NONE',  ( -0.05219959533937732626, 21.53943276465977519, 47.50109039468568994 ) ) ;
#157878=CARTESIAN_POINT ( 'NONE',  ( -13.89961937509957401, -13.97604488694547875, 109.3760903946856331 ) ) ;
#157879=CARTESIAN_POINT ( 'NONE',  ( 16.55341960407611168, 4.379528057220329451, 103.9572429386476813 ) ) ;
#157880=CARTESIAN_POINT ( 'NONE',  ( 19.03943276465977164, 0.05219959533936151252, 111.2510903946856757 ) ) ;
#157881=CARTESIAN_POINT ( 'NONE',  ( -13.97604488694527625, -13.89961937509977652, 46.87390960531435979 ) ) ;
#157882=CARTESIAN_POINT ( 'NONE',  ( -30.00000000000000000, 0.000000000000000000, 0.000000000000000000 ) ) ;
#157883=CARTESIAN_POINT ( 'NONE',  ( 13.89961937509977652, -13.97604488694527269, 93.12390960531436690 ) ) ;
#157884=CARTESIAN_POINT ( 'NONE',  ( -8.224510206698735004, -14.34966873604973081, 79.58442372801903275 ) ) ;
#157885=CARTESIAN_POINT ( 'NONE',  ( 18.62759615963255655, 10.81492255796105972, 101.6677570613523613 ) ) ;
#157886=CARTESIAN_POINT ( 'NONE',  ( 10.72451020669898902, -18.67979575497178502, 57.91557627198103120 ) ) ;
#157887=CARTESIAN_POINT ( 'NONE',  ( 16.55341960407618274, -4.379528057220086978, 86.04275706135236135 ) ) ;
#157888=CARTESIAN_POINT ( 'NONE',  ( 5.153800228976615827, -19.02544592524334988, 80.20942372801901854 ) ) ;
#157889=CARTESIAN_POINT ( 'NONE',  ( 13.89961937509977652, -13.97604488694527269, 38.12390960531436690 ) ) ;
#157890=CARTESIAN_POINT ( 'NONE',  ( 19.03943276465977164, -0.05219959533909143690, 73.74890960531435269 ) ) ;
#157891=CARTESIAN_POINT ( 'NONE',  ( 16.46253265017160672, -9.564922557960803928, 28.33224293864769550 ) ) ;
#157892=CARTESIAN_POINT ( 'NONE',  ( -0.05219959533936034679, 19.03943276465977164, 72.50109039468566152 ) ) ;
#157894=CARTESIAN_POINT ( 'NONE',  ( -5.153800228976328057, -19.02544592524343514, 107.2905762719810383 ) ) ;
#157895=CARTESIAN_POINT ( 'NONE',  ( 14.29746914071049879, -8.314922557960816363, 58.33224293864768839 ) ) ;
#157896=CARTESIAN_POINT ( 'NONE',  ( 15.72974639402199770, -15.80617190586745480, 63.12390960531435979 ) ) ;
#157897=CARTESIAN_POINT ( 'NONE',  ( -17.49999999999999289, 4.013004640162588288, 105.4460572099440725 ) ) ;
#157898=CARTESIAN_POINT ( 'NONE',  ( -5.049401038297874678, -19.05341960407617918, 24.79275706135233648 ) ) ;
#157900=CARTESIAN_POINT ( 'NONE',  ( 9.474510206698971260, -16.51473224551069308, 62.91557627198102409 ) ) ;
#157901=CARTESIAN_POINT ( 'NONE',  ( -19.02544592524342804, 5.153800228976336051, 76.04057627198102409 ) ) ;
#157902=CARTESIAN_POINT ( 'NONE',  ( -16.53943276465976808, -0.05219959533934237506, 33.75109039468568284 ) ) ;
#157905=CARTESIAN_POINT ( 'NONE',  ( 14.34966873604972726, -8.224510206698740333, 80.83442372801901854 ) ) ;
#157906=CARTESIAN_POINT ( 'NONE',  ( 0.05219959533934541429, -16.53943276465976808, 60.00109039468568284 ) ) ;
#157907=CARTESIAN_POINT ( 'NONE',  ( -4.379528057220086978, -16.55341960407618274, 34.79275706135235424 ) ) ;
#157908=CARTESIAN_POINT ( 'NONE',  ( -16.46253265017160317, 9.564922557960807481, 45.83224293864769550 ) ) ;
#157910=CARTESIAN_POINT ( 'NONE',  ( -5.719274019375665041, -21.55341960407619695, 49.79275706135234714 ) ) ;
#157911=CARTESIAN_POINT ( 'NONE',  ( -9.474510206698720793, -16.51473224551083518, 64.58442372801900433 ) ) ;
#157912=CARTESIAN_POINT ( 'NONE',  ( 18.62759615963255655, 10.81492255796105972, 96.66775706135234714 ) ) ;
#157913=CARTESIAN_POINT ( 'NONE',  ( -0.05219959533909027116, -19.03943276465977164, 27.49890960531435624 ) ) ;
#157915=CARTESIAN_POINT ( 'NONE',  ( -18.62759615963270932, 10.81492255796079327, 60.83224293864769550 ) ) ;
#157916=CARTESIAN_POINT ( 'NONE',  ( -13.97604488694527625, -13.89961937509977652, 101.8739096053143811 ) ) ;
#157917=CARTESIAN_POINT ( 'NONE',  ( 12.14591786802309770, 12.06949235617756955, 99.37390960531436690 ) ) ;
#157918=CARTESIAN_POINT ( 'NONE',  ( 8.224510206698742110, 14.34966873604972548, 42.08442372801901854 ) ) ;
#157919=CARTESIAN_POINT ( 'NONE',  ( 16.55341960407618274, -4.379528057220086978, 111.0427570613523613 ) ) ;
#157921=CARTESIAN_POINT ( 'NONE',  ( 10.72451020669898902, -18.67979575497178502, 97.91557627198103830 ) ) ;
#157922=CARTESIAN_POINT ( 'NONE',  ( 4.379528057220339221, -16.55341960407611168, 37.70724293864769550 ) ) ;
#157923=CARTESIAN_POINT ( 'NONE',  ( 13.89961937509977652, -13.97604488694527269, 113.1239096053143527 ) ) ;
#157924=CARTESIAN_POINT ( 'NONE',  ( -19.02544592524334988, -5.153800228976617603, 93.95942372801900433 ) ) ;
#157925=CARTESIAN_POINT ( 'NONE',  ( 19.03943276465977164, 0.05219959533936151252, 31.25109039468566863 ) ) ;
#157926=CARTESIAN_POINT ( 'NONE',  ( 8.224510206698953496, -14.34966873604960469, 32.91557627198102409 ) ) ;
#157927=CARTESIAN_POINT ( 'NONE',  ( 15.72974639402199770, -15.80617190586745480, 88.12390960531436690 ) ) ;
#157928=CARTESIAN_POINT ( 'NONE',  ( 5.823673210054125526, 21.52544592524343514, 54.79057627198104541 ) ) ;
#157929=CARTESIAN_POINT ( 'NONE',  ( 16.51473224551069308, 9.474510206698969483, 74.16557627198103830 ) ) ;
#157930=CARTESIAN_POINT ( 'NONE',  ( 16.55341960407611168, 4.379528057220329451, 38.95724293864768839 ) ) ;
#157931=CARTESIAN_POINT ( 'NONE',  ( -19.02544592524342804, 5.153800228976336051, 86.04057627198103830 ) ) ;
#157932=CARTESIAN_POINT ( 'NONE',  ( 18.22780087662121673, 5.500000000000056843, 58.98459894673892023 ) ) ;
#157933=CARTESIAN_POINT ( 'NONE',  ( 13.89961937509957401, 13.97604488694547697, 46.87609039468565442 ) ) ;
#157934=CARTESIAN_POINT ( 'NONE',  ( -21.52544592524343514, 5.823673210054127303, 76.04057627198102409 ) ) ;
#157935=CARTESIAN_POINT ( 'NONE',  ( -14.34966873604960291, -8.224510206698953496, 101.6655762719810383 ) ) ;
#157936=CARTESIAN_POINT ( 'NONE',  ( -10.81492255796105439, 18.62759615963255655, 37.91775706135235424 ) ) ;
#157938=CARTESIAN_POINT ( 'NONE',  ( 4.379528057220092307, 16.55341960407617563, 102.2927570613523613 ) ) ;
#157939=CARTESIAN_POINT ( 'NONE',  ( -19.05341960407611168, -5.049401038298163336, 36.45724293864766707 ) ) ;
#157940=CARTESIAN_POINT ( 'NONE',  ( 5.153800228976335163, 19.02544592524342804, 89.79057627198102409 ) ) ;
#157941=CARTESIAN_POINT ( 'NONE',  ( -19.48894818550241936, 5.500000000000114575, 45.10307310435242556 ) ) ;
#157942=CARTESIAN_POINT ( 'NONE',  ( -13.89961937509977652, 13.97604488694528158, 35.62390960531435269 ) ) ;
#157943=CARTESIAN_POINT ( 'NONE',  ( -4.379528057220328563, 16.55341960407611168, 45.20724293864769550 ) ) ;
#157944=CARTESIAN_POINT ( 'NONE',  ( -5.823673210054431948, 21.52544592524334988, 72.70942372801901854 ) ) ;
#157946=CARTESIAN_POINT ( 'NONE',  ( 16.55341960407618274, -4.379528057220086978, 76.04275706135237556 ) ) ;
#157947=CARTESIAN_POINT ( 'NONE',  ( 13.89961937509977652, -13.97604488694527269, 58.12390960531436690 ) ) ;
#157948=CARTESIAN_POINT ( 'NONE',  ( -0.05219959533909027116, -19.03943276465977164, 62.49890960531435979 ) ) ;
#157950=CARTESIAN_POINT ( 'NONE',  ( -10.72451020669870658, -18.67979575497194134, 104.5844237280190185 ) ) ;
#157951=CARTESIAN_POINT ( 'NONE',  ( -4.483927247898782831, 16.52544592524335698, 77.70942372801900433 ) ) ;
#157952=CARTESIAN_POINT ( 'NONE',  ( 21.52544592524334988, 5.823673210054432836, 101.4594237280190185 ) ) ;
#157953=CARTESIAN_POINT ( 'NONE',  ( 13.89961937509977652, -13.97604488694527269, 63.12390960531435979 ) ) ;
#157954=CARTESIAN_POINT ( 'NONE',  ( -21.53943276465977519, 0.05219959533907696930, 36.24890960531435979 ) ) ;
#157955=CARTESIAN_POINT ( 'NONE',  ( -5.049401038297874678, -19.05341960407617918, 109.7927570613523187 ) ) ;
#157956=CARTESIAN_POINT ( 'NONE',  ( 18.67979575497194134, -10.72451020669871369, 65.83442372801900433 ) ) ;
#157957=CARTESIAN_POINT ( 'NONE',  ( 8.224510206698742110, 14.34966873604972548, 52.08442372801901854 ) ) ;
#157958=CARTESIAN_POINT ( 'NONE',  ( 15.72974639402199770, -15.80617190586745480, 98.12390960531436690 ) ) ;
#157959=CARTESIAN_POINT ( 'NONE',  ( -16.51473224551082808, 9.474510206698731452, 93.33442372801900433 ) ) ;
#157960=CARTESIAN_POINT ( 'NONE',  ( -19.02544592524342804, 5.153800228976336051, 81.04057627198103830 ) ) ;
#157961=CARTESIAN_POINT ( 'NONE',  ( -19.02544592524334988, -5.153800228976617603, 103.9594237280190043 ) ) ;
#157962=CARTESIAN_POINT ( 'NONE',  ( -14.29746914071037622, -8.314922557961029526, 24.16775706135235424 ) ) ;
#157963=CARTESIAN_POINT ( 'NONE',  ( -14.29746914071049879, 8.314922557960819915, 70.83224293864770971 ) ) ;
#157964=CARTESIAN_POINT ( 'NONE',  ( 4.379528057220092307, 16.55341960407617563, 77.29275706135234714 ) ) ;
#157965=CARTESIAN_POINT ( 'NONE',  ( -18.62759615963270932, 10.81492255796079327, 110.8322429386476955 ) ) ;
#157966=CARTESIAN_POINT ( 'NONE',  ( -5.153800228976328057, -19.02544592524343514, 57.29057627198103120 ) ) ;
#157967=CARTESIAN_POINT ( 'NONE',  ( -9.474510206698964154, 16.51473224551069663, 55.41557627198103120 ) ) ;
#157968=CARTESIAN_POINT ( 'NONE',  ( -4.379528057220086978, -16.55341960407618274, 69.79275706135234714 ) ) ;
#157971=CARTESIAN_POINT ( 'NONE',  ( -21.52544592524334988, -5.823673210054445271, 108.9594237280190185 ) ) ;
#157972=CARTESIAN_POINT ( 'NONE',  ( 19.02544592524343514, -5.153800228976328945, 33.54057627198102409 ) ) ;
#157974=CARTESIAN_POINT ( 'NONE',  ( 8.314922557961029526, -14.29746914071037800, 20.41775706135234714 ) ) ;
#157976=CARTESIAN_POINT ( 'NONE',  ( 16.51473224551083163, -9.474510206698727899, 40.83442372801900433 ) ) ;
#157977=CARTESIAN_POINT ( 'NONE',  ( 0.05219959533934541429, -16.53943276465976808, 30.00109039468568284 ) ) ;
#157978=CARTESIAN_POINT ( 'NONE',  ( 16.46253265017160672, -9.564922557960803928, 48.33224293864769550 ) ) ;
#157979=CARTESIAN_POINT ( 'NONE',  ( -13.89961937509977652, 13.97604488694528158, 60.62390960531436690 ) ) ;
#157980=CARTESIAN_POINT ( 'NONE',  ( -10.72451020669898014, 18.67979575497178502, 90.41557627198103830 ) ) ;
#157981=CARTESIAN_POINT ( 'NONE',  ( 9.564922557960805705, 16.46253265017160317, 114.5822429386476955 ) ) ;
#157982=CARTESIAN_POINT ( 'NONE',  ( 19.03943276465977164, -0.05219959533909143690, 53.74890960531436690 ) ) ;
#157984=CARTESIAN_POINT ( 'NONE',  ( -13.89961937509957401, -13.97604488694547875, 99.37609039468567573 ) ) ;
#157985=CARTESIAN_POINT ( 'NONE',  ( -12.14591786802309592, -12.06949235617757132, 66.87390960531436690 ) ) ;
#157986=CARTESIAN_POINT ( 'NONE',  ( 19.03943276465977164, 0.05219959533936151252, 21.25109039468565797 ) ) ;
#157987=CARTESIAN_POINT ( 'NONE',  ( -14.34966873604960291, -8.224510206698953496, 66.66557627198102409 ) ) ;
#157988=CARTESIAN_POINT ( 'NONE',  ( -10.81492255796105439, 18.62759615963255655, 87.91775706135234714 ) ) ;
#157989=CARTESIAN_POINT ( 'NONE',  ( -9.474510206698964154, 16.51473224551069663, 30.41557627198102054 ) ) ;
#157990=CARTESIAN_POINT ( 'NONE',  ( 0.05219959533937995610, -21.53943276465977519, 85.00109039468568994 ) ) ;
#157991=CARTESIAN_POINT ( 'NONE',  ( -0.05219959533910754901, -16.53943276465976808, 32.49890960531435979 ) ) ;
#157992=CARTESIAN_POINT ( 'NONE',  ( 21.55341960407619695, -5.719274019375665929, 71.04275706135234714 ) ) ;
#157993=CARTESIAN_POINT ( 'NONE',  ( 19.05341960407611168, 5.049401038298154454, 73.95724293864768129 ) ) ;
#157994=CARTESIAN_POINT ( 'NONE',  ( -18.67979575497193778, 10.72451020669871902, 38.33442372801900433 ) ) ;
#157995=CARTESIAN_POINT ( 'NONE',  ( 0.05219959533909260263, 19.03943276465977164, 74.99890960531435269 ) ) ;
#157996=CARTESIAN_POINT ( 'NONE',  ( 14.29746914071049879, -8.314922557960816363, 88.33224293864769550 ) ) ;
#157997=CARTESIAN_POINT ( 'NONE',  ( -14.34966873604960291, -8.224510206698953496, 61.66557627198103120 ) ) ;
#157998=CARTESIAN_POINT ( 'NONE',  ( -0.05219959533907301413, -21.53943276465977519, 67.49890960531436690 ) ) ;
#157999=CARTESIAN_POINT ( 'NONE',  ( 13.97604488694527802, 13.89961937509977652, 74.37390960531436690 ) ) ;
#158000=CARTESIAN_POINT ( 'NONE',  ( -21.55341960407610458, -5.719274019375992779, 86.45724293864770971 ) ) ;
#158001=CARTESIAN_POINT ( 'NONE',  ( 16.51473224551083163, -9.474510206698727899, 65.83442372801900433 ) ) ;
#158002=CARTESIAN_POINT ( 'NONE',  ( 19.02544592524335343, 5.153800228976608722, 36.45942372801900433 ) ) ;
#158003=CARTESIAN_POINT ( 'NONE',  ( 8.224510206698953496, -14.34966873604960469, 72.91557627198103830 ) ) ;
#158004=CARTESIAN_POINT ( 'NONE',  ( 10.72451020669898902, -18.67979575497178502, 57.91557627198103120 ) ) ;
#158007=CARTESIAN_POINT ( 'NONE',  ( 0.05219959533934541429, -16.53943276465976808, 100.0010903946857042 ) ) ;
#158009=CARTESIAN_POINT ( 'NONE',  ( 5.049401038297881783, 19.05341960407617563, 107.2927570613523187 ) ) ;
#158010=CARTESIAN_POINT ( 'NONE',  ( 12.14591786802309770, 12.06949235617756955, 64.37390960531435269 ) ) ;
#158011=CARTESIAN_POINT ( 'NONE',  ( -17.49999999999995381, 3.512728167237034516, 35.22809995181123810 ) ) ;
#158012=CARTESIAN_POINT ( 'NONE',  ( -19.05341960407611168, -5.049401038298163336, 66.45724293864769550 ) ) ;
#158013=CARTESIAN_POINT ( 'NONE',  ( 4.483927247898545687, 16.52544592524342804, 59.79057627198103120 ) ) ;
#158014=CARTESIAN_POINT ( 'NONE',  ( 13.89961937509977652, -13.97604488694527269, 108.1239096053143669 ) ) ;
#158015=CARTESIAN_POINT ( 'NONE',  ( -16.46253265017146816, -9.564922557961047289, 84.16775706135233293 ) ) ;
#158016=CARTESIAN_POINT ( 'NONE',  ( -13.97604488694527625, -13.89961937509977652, 66.87390960531436690 ) ) ;
#158017=CARTESIAN_POINT ( 'NONE',  ( 19.03943276465977164, -0.05219959533909143690, 88.74890960531436690 ) ) ;
#158018=CARTESIAN_POINT ( 'NONE',  ( -16.46253265017160317, 9.564922557960807481, 85.83224293864769550 ) ) ;
#158019=CARTESIAN_POINT ( 'NONE',  ( 5.719274019375991003, -21.55341960407610458, 57.70724293864770260 ) ) ;
#158020=CARTESIAN_POINT ( 'NONE',  ( 16.55341960407618274, -4.379528057220086978, 61.04275706135234714 ) ) ;
#158021=CARTESIAN_POINT ( 'NONE',  ( 17.50000000000002132, 5.499999999999984013, 98.78230962303568674 ) ) ;
#158022=CARTESIAN_POINT ( 'NONE',  ( 16.51473224551069308, 9.474510206698969483, 49.16557627198102409 ) ) ;
#158023=CARTESIAN_POINT ( 'NONE',  ( 10.72451020669898902, -18.67979575497178502, 67.91557627198102409 ) ) ;
#158024=CARTESIAN_POINT ( 'NONE',  ( 0.05219959533936267826, -19.03943276465977164, 95.00109039468567573 ) ) ;
#158025=CARTESIAN_POINT ( 'NONE',  ( 16.53943276465976808, 0.05219959533934440121, 111.2510903946856899 ) ) ;
#158026=CARTESIAN_POINT ( 'NONE',  ( 5.719274019375673035, 21.55341960407619339, 42.29275706135235424 ) ) ;
#158027=CARTESIAN_POINT ( 'NONE',  ( -9.564922557961040184, 16.46253265017147172, 37.91775706135233293 ) ) ;
#158028=CARTESIAN_POINT ( 'NONE',  ( -14.29746914071037622, -8.314922557961029526, 54.16775706135235424 ) ) ;
#158029=CARTESIAN_POINT ( 'NONE',  ( -8.314922557961024197, 14.29746914071037800, 92.91775706135236135 ) ) ;
#158031=CARTESIAN_POINT ( 'NONE',  ( 16.55341960407618274, -4.379528057220086978, 76.04275706135237556 ) ) ;
#158032=CARTESIAN_POINT ( 'NONE',  ( -12.06949235617739369, -12.14591786802326823, 39.37609039468567573 ) ) ;
#158033=CARTESIAN_POINT ( 'NONE',  ( -5.153800228976328057, -19.02544592524343514, 42.29057627198101699 ) ) ;
#158034=CARTESIAN_POINT ( 'NONE',  ( -19.02544592524342804, 5.153800228976336051, 46.04057627198101699 ) ) ;
#158035=CARTESIAN_POINT ( 'NONE',  ( -9.474510206698964154, 16.51473224551069663, 60.41557627198102409 ) ) ;
#158036=CARTESIAN_POINT ( 'NONE',  ( -15.80617190586768217, 15.72974639402176855, 58.12609039468568994 ) ) ;
#158037=CARTESIAN_POINT ( 'NONE',  ( -8.224510206698735004, -14.34966873604973081, 44.58442372801901854 ) ) ;
#158038=CARTESIAN_POINT ( 'NONE',  ( 12.06949235617739724, 12.14591786802326823, 111.8760903946856615 ) ) ;
#158039=CARTESIAN_POINT ( 'NONE',  ( -19.03943276465977164, 0.05219959533909376836, 31.24890960531435979 ) ) ;
#158040=CARTESIAN_POINT ( 'NONE',  ( 5.719274019375673035, 21.55341960407619339, 112.2927570613523471 ) ) ;
#158041=CARTESIAN_POINT ( 'NONE',  ( 0.05219959533934541429, -16.53943276465976808, 35.00109039468568284 ) ) ;
#158043=CARTESIAN_POINT ( 'NONE',  ( -16.51473224551082808, 9.474510206698731452, 88.33442372801900433 ) ) ;
#158044=CARTESIAN_POINT ( 'NONE',  ( -8.314922557960811034, -14.29746914071050412, 82.08224293864768129 ) ) ;
#158045=CARTESIAN_POINT ( 'NONE',  ( -19.03943276465977164, 0.05219959533909376836, 36.24890960531436690 ) ) ;
#158046=CARTESIAN_POINT ( 'NONE',  ( 19.02544592524334988, 5.153800228976608722, 76.45942372801897591 ) ) ;
#158047=CARTESIAN_POINT ( 'NONE',  ( 17.13100169013299734, 6.664070546373172199, 76.73210164300155611 ) ) ;
#158048=CARTESIAN_POINT ( 'NONE',  ( 15.80617190586769283, -15.72974639402175789, 70.62609039468567573 ) ) ;
#158049=CARTESIAN_POINT ( 'NONE',  ( -16.52544592524335698, -4.483927247898792601, 43.95942372801902565 ) ) ;
#158051=CARTESIAN_POINT ( 'NONE',  ( -21.53943276465977519, 0.05219959533907696930, 31.24890960531435979 ) ) ;
#158052=CARTESIAN_POINT ( 'NONE',  ( 16.53943276465976808, 0.05219959533934440121, 31.25109039468568639 ) ) ;
#158053=CARTESIAN_POINT ( 'NONE',  ( -13.97604488694527625, -13.89961937509977830, 26.87390960531435269 ) ) ;
#158054=CARTESIAN_POINT ( 'NONE',  ( 9.474510206698729675, 16.51473224551082808, 27.08442372801900433 ) ) ;
#158056=CARTESIAN_POINT ( 'NONE',  ( 13.89961937509977652, -13.97604488694527269, 43.12390960531434558 ) ) ;
#158058=CARTESIAN_POINT ( 'NONE',  ( -13.89961937509977652, 13.97604488694528158, 65.62390960531436690 ) ) ;
#158059=CARTESIAN_POINT ( 'NONE',  ( -18.22780087662119541, 5.500000000000102141, 66.01763182126894947 ) ) ;
#158060=CARTESIAN_POINT ( 'NONE',  ( 5.153800228976615827, -19.02544592524334988, 25.20942372801900433 ) ) ;
#158061=CARTESIAN_POINT ( 'NONE',  ( 14.34966873604960469, 8.224510206698951720, 39.16557627198102409 ) ) ;
#158062=CARTESIAN_POINT ( 'NONE',  ( 19.03943276465977164, -0.05219959533909143690, 38.74890960531436690 ) ) ;
#158063=CARTESIAN_POINT ( 'NONE',  ( -19.02544592524342804, 5.153800228976336051, 96.04057627198103830 ) ) ;
#158064=CARTESIAN_POINT ( 'NONE',  ( -5.719274019375665041, -21.55341960407619695, 69.79275706135234714 ) ) ;
#158065=CARTESIAN_POINT ( 'NONE',  ( 9.564922557960805705, 16.46253265017160317, 44.58224293864769550 ) ) ;
#158066=CARTESIAN_POINT ( 'NONE',  ( 10.81492255796106328, -18.62759615963255655, 60.41775706135235424 ) ) ;
#158067=CARTESIAN_POINT ( 'NONE',  ( 21.53943276465977519, -0.05219959533907433946, 28.74890960531435624 ) ) ;
#158068=CARTESIAN_POINT ( 'NONE',  ( 19.05341960407611168, 5.049401038298154454, 33.95724293864769550 ) ) ;
#158069=CARTESIAN_POINT ( 'NONE',  ( 18.62759615963255655, 10.81492255796105972, 26.66775706135235424 ) ) ;
#158070=CARTESIAN_POINT ( 'NONE',  ( -13.97604488694547697, 13.89961937509957934, 43.12609039468566152 ) ) ;
#158071=CARTESIAN_POINT ( 'NONE',  ( -4.379528057220328563, 16.55341960407611168, 110.2072429386477239 ) ) ;
#158072=CARTESIAN_POINT ( 'NONE',  ( -16.51473224551069308, -9.474510206698971260, 56.66557627198103120 ) ) ;
#158073=CARTESIAN_POINT ( 'NONE',  ( 19.03943276465977164, 0.05219959533936151252, 106.2510903946856615 ) ) ;
#158074=CARTESIAN_POINT ( 'NONE',  ( -16.52544592524342804, 4.483927247898546575, 81.04057627198102409 ) ) ;
#158075=CARTESIAN_POINT ( 'NONE',  ( -18.67979575497178146, -10.72451020669898902, 21.66557627198102409 ) ) ;
#158076=CARTESIAN_POINT ( 'NONE',  ( -0.05219959533936034679, 19.03943276465977164, 87.50109039468567573 ) ) ;
#158077=CARTESIAN_POINT ( 'NONE',  ( -10.81492255796078084, -18.62759615963271287, 102.0822429386476955 ) ) ;
#158078=CARTESIAN_POINT ( 'NONE',  ( 5.719274019375673035, 21.55341960407619339, 57.29275706135234714 ) ) ;
#158079=CARTESIAN_POINT ( 'NONE',  ( 8.314922557961029526, -14.29746914071037800, 60.41775706135235424 ) ) ;
#158080=CARTESIAN_POINT ( 'NONE',  ( -16.53943276465976808, -0.05219959533934237506, 53.75109039468568994 ) ) ;
#158081=CARTESIAN_POINT ( 'NONE',  ( 18.67979575497178502, 10.72451020669898547, 49.16557627198102409 ) ) ;
#158082=CARTESIAN_POINT ( 'NONE',  ( 9.474510206698971260, -16.51473224551069308, 42.91557627198103120 ) ) ;
#158084=CARTESIAN_POINT ( 'NONE',  ( 8.314922557961029526, -14.29746914071037800, 80.41775706135234714 ) ) ;
#158085=CARTESIAN_POINT ( 'NONE',  ( 5.823673210054125526, 21.52544592524343514, 99.79057627198103830 ) ) ;
#158086=CARTESIAN_POINT ( 'NONE',  ( 4.379528057220339221, -16.55341960407611168, 57.70724293864770260 ) ) ;
#158087=CARTESIAN_POINT ( 'NONE',  ( -16.51473224551069308, -9.474510206698971260, 66.66557627198102409 ) ) ;
#158088=CARTESIAN_POINT ( 'NONE',  ( 8.314922557961029526, -14.29746914071037800, 75.41775706135233293 ) ) ;
#158089=CARTESIAN_POINT ( 'NONE',  ( -19.02544592524334988, -5.153800228976617603, 93.95942372801900433 ) ) ;
#158090=CARTESIAN_POINT ( 'NONE',  ( 5.719274019375991003, -21.55341960407610458, 102.7072429386476955 ) ) ;
#158091=CARTESIAN_POINT ( 'NONE',  ( -16.53943276465976808, 0.05219959533911058130, 51.24890960531436690 ) ) ;
#158093=CARTESIAN_POINT ( 'NONE',  ( 19.01533133064925352, -5.499999999999442224, 91.26586590595742621 ) ) ;
#158094=CARTESIAN_POINT ( 'NONE',  ( 10.72451020669898902, -18.67979575497178502, 67.91557627198102409 ) ) ;
#158095=CARTESIAN_POINT ( 'NONE',  ( -12.06949235617756955, 12.14591786802309770, 25.62390960531435624 ) ) ;
#158097=CARTESIAN_POINT ( 'NONE',  ( -17.40805194822029733, -6.112264579159361944, 54.16628727489391792 ) ) ;
#158098=CARTESIAN_POINT ( 'NONE',  ( -5.719274019375978568, 21.55341960407610458, 105.2072429386477097 ) ) ;
#158099=CARTESIAN_POINT ( 'NONE',  ( -15.72974639402176322, -15.80617190586768395, 29.37609039468568284 ) ) ;
#158100=CARTESIAN_POINT ( 'NONE',  ( -12.06949235617756955, 12.14591786802309770, 40.62390960531435269 ) ) ;
#158101=CARTESIAN_POINT ( 'NONE',  ( -8.224510206698735004, -14.34966873604973081, 49.58442372801901143 ) ) ;
#158102=CARTESIAN_POINT ( 'NONE',  ( 16.51473224551069308, 9.474510206698969483, 44.16557627198103120 ) ) ;
#158103=CARTESIAN_POINT ( 'NONE',  ( -0.05219959533936034679, 19.03943276465977164, 57.50109039468566863 ) ) ;
#158104=CARTESIAN_POINT ( 'NONE',  ( -16.51473224551069308, -9.474510206698971260, 76.66557627198103830 ) ) ;
#158106=CARTESIAN_POINT ( 'NONE',  ( 21.52544592524344225, -5.823673210054117533, 33.54057627198102409 ) ) ;
#158108=CARTESIAN_POINT ( 'NONE',  ( 8.224510206698742110, 14.34966873604972548, 27.08442372801901854 ) ) ;
#158109=CARTESIAN_POINT ( 'NONE',  ( -5.049401038297874678, -19.05341960407617918, 54.79275706135234003 ) ) ;
#158110=CARTESIAN_POINT ( 'NONE',  ( -21.53943276465977519, 0.05219959533907696930, 106.2489096053143811 ) ) ;
#158111=CARTESIAN_POINT ( 'NONE',  ( 4.379528057220339221, -16.55341960407611168, 37.70724293864769550 ) ) ;
#158112=CARTESIAN_POINT ( 'NONE',  ( 13.97604488694527802, 13.89961937509977652, 74.37390960531436690 ) ) ;
#158113=CARTESIAN_POINT ( 'NONE',  ( 21.55341960407610458, 5.719274019375980345, 53.95724293864770260 ) ) ;
#158114=CARTESIAN_POINT ( 'NONE',  ( 21.53943276465977519, -0.05219959533907433946, 88.74890960531436690 ) ) ;
#158115=CARTESIAN_POINT ( 'NONE',  ( 12.14591786802327356, -12.06949235617739191, 25.62609039468567929 ) ) ;
#158116=CARTESIAN_POINT ( 'NONE',  ( -16.46253265017160317, 9.564922557960807481, 115.8322429386477097 ) ) ;
#158117=CARTESIAN_POINT ( 'NONE',  ( 0.05219959533937995610, -21.53943276465977519, 85.00109039468568994 ) ) ;
#158118=CARTESIAN_POINT ( 'NONE',  ( -9.564922557960796823, -16.46253265017161027, 77.08224293864769550 ) ) ;
#158120=CARTESIAN_POINT ( 'NONE',  ( 16.46253265017160672, -9.564922557960803928, 28.33224293864769550 ) ) ;
#158121=CARTESIAN_POINT ( 'NONE',  ( 13.89961937509977652, -13.97604488694527269, 83.12390960531436690 ) ) ;
#158122=CARTESIAN_POINT ( 'NONE',  ( -4.483927247898539470, -16.52544592524342804, 102.2905762719810383 ) ) ;
#158123=CARTESIAN_POINT ( 'NONE',  ( 13.89961937509957401, 13.97604488694547697, 101.8760903946856331 ) ) ;
#158125=CARTESIAN_POINT ( 'NONE',  ( 13.89961937509977652, -13.97604488694527269, 78.12390960531433848 ) ) ;
#158126=CARTESIAN_POINT ( 'NONE',  ( 5.823673210054444382, -21.52544592524334988, 95.20942372801903275 ) ) ;
#158127=CARTESIAN_POINT ( 'NONE',  ( -16.51473224551069308, -9.474510206698971260, 111.6655762719810383 ) ) ;
#158128=CARTESIAN_POINT ( 'NONE',  ( 16.52544592524335698, 4.483927247898782831, 91.45942372801901854 ) ) ;
#158130=CARTESIAN_POINT ( 'NONE',  ( 13.97604488694548053, -13.89961937509957401, 60.62609039468564731 ) ) ;
#158131=CARTESIAN_POINT ( 'NONE',  ( -5.823673210054431948, 21.52544592524334988, 112.7094237280190328 ) ) ;
#158133=CARTESIAN_POINT ( 'NONE',  ( 19.05341960407611168, 5.049401038298154454, 28.95724293864769550 ) ) ;
#158134=CARTESIAN_POINT ( 'NONE',  ( 16.53943276465976808, -0.05219959533910856209, 28.74890960531435624 ) ) ;
#158135=CARTESIAN_POINT ( 'NONE',  ( 15.50000000000000178, -5.500000000000000888, 120.0000000000000142 ) ) ;
#158136=CARTESIAN_POINT ( 'NONE',  ( 4.483927247898790824, -16.52544592524335698, 100.2094237280190043 ) ) ;
#158138=CARTESIAN_POINT ( 'NONE',  ( -4.379528057220086978, -16.55341960407618274, 74.79275706135234714 ) ) ;
#158139=CARTESIAN_POINT ( 'NONE',  ( 9.564922557960805705, 16.46253265017160317, 84.58224293864769550 ) ) ;
#158140=CARTESIAN_POINT ( 'NONE',  ( 18.67979575497194134, -10.72451020669871369, 95.83442372801903275 ) ) ;
#158141=CARTESIAN_POINT ( 'NONE',  ( 13.97604488694548053, -13.89961937509957401, 105.6260903946856757 ) ) ;
#158142=CARTESIAN_POINT ( 'NONE',  ( 15.80617190586769283, -15.72974639402175789, 65.62609039468568994 ) ) ;
#158143=CARTESIAN_POINT ( 'NONE',  ( -0.05219959533936034679, 19.03943276465977164, 47.50109039468566863 ) ) ;
#158144=CARTESIAN_POINT ( 'NONE',  ( -9.474510206698964154, 16.51473224551069663, 75.41557627198103830 ) ) ;
#158145=CARTESIAN_POINT ( 'NONE',  ( -13.89961937509977652, 13.97604488694528158, 70.62390960531432427 ) ) ;
#158146=CARTESIAN_POINT ( 'NONE',  ( 16.29526858892873165, 7.335722546920136367, 73.29670597800203780 ) ) ;
#158148=CARTESIAN_POINT ( 'NONE',  ( -5.823673210054116645, -21.52544592524344225, 42.29057627198103120 ) ) ;
#158149=CARTESIAN_POINT ( 'NONE',  ( -9.474510206698964154, 16.51473224551069663, 40.41557627198103120 ) ) ;
#158150=CARTESIAN_POINT ( 'NONE',  ( -10.72451020669898014, 18.67979575497178502, 80.41557627198103830 ) ) ;
#158151=CARTESIAN_POINT ( 'NONE',  ( -4.379528057220086978, -16.55341960407618274, 74.79275706135234714 ) ) ;
#158153=CARTESIAN_POINT ( 'NONE',  ( 14.34966873604960469, 8.224510206698951720, 79.16557627198103830 ) ) ;
#158155=CARTESIAN_POINT ( 'NONE',  ( 4.379528057220092307, 16.55341960407617563, 32.29275706135235424 ) ) ;
#158156=CARTESIAN_POINT ( 'NONE',  ( -9.474510206698964154, 16.51473224551069663, 25.41557627198103120 ) ) ;
#158157=CARTESIAN_POINT ( 'NONE',  ( -9.564922557961040184, 16.46253265017147172, 62.91775706135233293 ) ) ;
#158158=CARTESIAN_POINT ( 'NONE',  ( -4.483927247898539470, -16.52544592524342804, 72.29057627198102409 ) ) ;
#158159=CARTESIAN_POINT ( 'NONE',  ( 5.823673210054444382, -21.52544592524334988, 50.20942372801901854 ) ) ;
#158161=CARTESIAN_POINT ( 'NONE',  ( -5.719274019375978568, 21.55341960407610458, 95.20724293864769550 ) ) ;
#158163=CARTESIAN_POINT ( 'NONE',  ( 16.55341960407611168, 4.379528057220329451, 78.95724293864769550 ) ) ;
#158165=CARTESIAN_POINT ( 'NONE',  ( 19.03943276465977164, -0.05219959533909143690, 43.74890960531435979 ) ) ;
#158167=CARTESIAN_POINT ( 'NONE',  ( 16.51473224551083163, -9.474510206698727899, 75.83442372801900433 ) ) ;
#158168=CARTESIAN_POINT ( 'NONE',  ( -5.719274019375665041, -21.55341960407619695, 24.79275706135235779 ) ) ;
#158169=CARTESIAN_POINT ( 'NONE',  ( -5.153800228976328057, -19.02544592524343514, 72.29057627198102409 ) ) ;
#158170=CARTESIAN_POINT ( 'NONE',  ( -5.049401038297874678, -19.05341960407617918, 59.79275706135231871 ) ) ;
#158171=CARTESIAN_POINT ( 'NONE',  ( -9.474510206698964154, 16.51473224551069663, 50.41557627198102409 ) ) ;
#158173=CARTESIAN_POINT ( 'NONE',  ( -12.14591786802309592, -12.06949235617757132, 66.87390960531436690 ) ) ;
#158174=CARTESIAN_POINT ( 'NONE',  ( 14.34966873604960469, 8.224510206698951720, 59.16557627198103120 ) ) ;
#158175=CARTESIAN_POINT ( 'NONE',  ( 0.05219959533909260263, 19.03943276465977164, 74.99890960531435269 ) ) ;
#158177=CARTESIAN_POINT ( 'NONE',  ( -18.67979575497178146, -10.72451020669898902, 101.6655762719810383 ) ) ;
#158178=CARTESIAN_POINT ( 'NONE',  ( 19.03943276465977164, -0.05219959533909143690, 68.74890960531436690 ) ) ;
#158179=CARTESIAN_POINT ( 'NONE',  ( 15.80617190586746368, 15.72974639402197994, 74.37390960531436690 ) ) ;
#158180=CARTESIAN_POINT ( 'NONE',  ( -16.46253265017146816, -9.564922557961047289, 19.16775706135233293 ) ) ;
#158182=CARTESIAN_POINT ( 'NONE',  ( 8.224510206698742110, 14.34966873604972548, 112.0844237280190185 ) ) ;
#158183=CARTESIAN_POINT ( 'NONE',  ( -4.379528057220328563, 16.55341960407611168, 95.20724293864769550 ) ) ;
#158184=CARTESIAN_POINT ( 'NONE',  ( -16.46253265017146816, -9.564922557961047289, 109.1677570613523471 ) ) ;
#158186=CARTESIAN_POINT ( 'NONE',  ( 5.719274019375673035, 21.55341960407619339, 32.29275706135235424 ) ) ;
#158187=CARTESIAN_POINT ( 'NONE',  ( -19.05341960407617563, 5.049401038297882671, 53.54275706135231871 ) ) ;
#158188=CARTESIAN_POINT ( 'NONE',  ( -16.53943276465976808, 0.05219959533911058130, 26.24890960531435624 ) ) ;
#158189=CARTESIAN_POINT ( 'NONE',  ( 5.719274019375991003, -21.55341960407610458, 72.70724293864769550 ) ) ;
#158190=CARTESIAN_POINT ( 'NONE',  ( 13.89961937509977652, -13.97604488694527269, 103.1239096053143527 ) ) ;
#158191=CARTESIAN_POINT ( 'NONE',  ( 14.34966873604960469, 8.224510206698951720, 54.16557627198103120 ) ) ;
#158192=CARTESIAN_POINT ( 'NONE',  ( 16.46253265017160672, -9.564922557960803928, 28.33224293864769550 ) ) ;
#158193=CARTESIAN_POINT ( 'NONE',  ( -0.05219959533909027116, -19.03943276465977164, 27.49890960531435624 ) ) ;
#158194=CARTESIAN_POINT ( 'NONE',  ( -0.05219959533937732626, 21.53943276465977519, 107.5010903946856899 ) ) ;
#158195=CARTESIAN_POINT ( 'NONE',  ( 14.34966873604972726, -8.224510206698740333, 90.83442372801901854 ) ) ;
#158196=CARTESIAN_POINT ( 'NONE',  ( 21.52544592524334988, 5.823673210054432836, 36.45942372801901143 ) ) ;
#158197=CARTESIAN_POINT ( 'NONE',  ( 0.05219959533934541429, -16.53943276465976808, 40.00109039468567573 ) ) ;
#158198=CARTESIAN_POINT ( 'NONE',  ( -5.153800228976328057, -19.02544592524343514, 112.2905762719810099 ) ) ;
#158199=CARTESIAN_POINT ( 'NONE',  ( -5.153800228976328057, -19.02544592524343514, 52.29057627198100988 ) ) ;
#158200=CARTESIAN_POINT ( 'NONE',  ( 9.564922557960805705, 16.46253265017160317, 64.58224293864769550 ) ) ;
#158201=CARTESIAN_POINT ( 'NONE',  ( -0.05219959533934338120, 16.53943276465976808, 62.50109039468568284 ) ) ;
#158202=CARTESIAN_POINT ( 'NONE',  ( 4.483927247898545687, 16.52544592524342804, 99.79057627198103830 ) ) ;
#158203=CARTESIAN_POINT ( 'NONE',  ( 14.34966873604960469, 8.224510206698951720, 24.16557627198103120 ) ) ;
#158205=CARTESIAN_POINT ( 'NONE',  ( -18.67979575497193778, 10.72451020669871902, 58.33442372801901143 ) ) ;
#158206=CARTESIAN_POINT ( 'NONE',  ( -19.03943276465977164, 0.05219959533909376836, 91.24890960531436690 ) ) ;
#158207=CARTESIAN_POINT ( 'NONE',  ( -0.05219959533909027116, -19.03943276465977164, 82.49890960531436690 ) ) ;
#158208=CARTESIAN_POINT ( 'NONE',  ( -13.97604488694527625, -13.89961937509977652, 106.8739096053143669 ) ) ;
#158209=CARTESIAN_POINT ( 'NONE',  ( -16.55341960407611168, -4.379528057220339221, 51.45724293864770260 ) ) ;
#158210=CARTESIAN_POINT ( 'NONE',  ( -16.52544592524342804, 4.483927247898546575, 26.04057627198103475 ) ) ;
#158211=CARTESIAN_POINT ( 'NONE',  ( 12.06949235617757843, -12.14591786802309237, 33.12390960531435979 ) ) ;
#158213=CARTESIAN_POINT ( 'NONE',  ( 19.02544592524334988, 5.153800228976608722, 31.45942372801900433 ) ) ;
#158214=CARTESIAN_POINT ( 'NONE',  ( 13.89961937509977652, -13.97604488694527269, 73.12390960531436690 ) ) ;
#158215=CARTESIAN_POINT ( 'NONE',  ( -13.97604488694547697, 13.89961937509957934, 48.12609039468566863 ) ) ;
#158218=CARTESIAN_POINT ( 'NONE',  ( 9.474510206698729675, 16.51473224551082808, 82.08442372801899012 ) ) ;
#158219=CARTESIAN_POINT ( 'NONE',  ( -4.379528057220086978, -16.55341960407618274, 74.79275706135234714 ) ) ;
#158221=CARTESIAN_POINT ( 'NONE',  ( 13.97604488694527802, 13.89961937509977652, 99.37390960531436690 ) ) ;
#158222=CARTESIAN_POINT ( 'NONE',  ( -18.67979575497193778, 10.72451020669871902, 28.33442372801902209 ) ) ;
#158223=CARTESIAN_POINT ( 'NONE',  ( 5.049401038297881783, 19.05341960407617563, 92.29275706135234714 ) ) ;
#158224=CARTESIAN_POINT ( 'NONE',  ( 13.89961937509977652, -13.97604488694527269, 113.1239096053143527 ) ) ;
#158225=CARTESIAN_POINT ( 'NONE',  ( -5.153800228976328057, -19.02544592524343514, 47.29057627198102409 ) ) ;
#158226=CARTESIAN_POINT ( 'NONE',  ( -9.564922557960796823, -16.46253265017161027, 87.08224293864769550 ) ) ;
#158227=CARTESIAN_POINT ( 'NONE',  ( -8.224510206698948167, 14.34966873604960824, 45.41557627198103830 ) ) ;
#158228=CARTESIAN_POINT ( 'NONE',  ( -9.474510206698964154, 16.51473224551069663, 45.41557627198103120 ) ) ;
#158229=CARTESIAN_POINT ( 'NONE',  ( 13.97604488694548053, -13.89961937509957401, 65.62609039468567573 ) ) ;
#158230=CARTESIAN_POINT ( 'NONE',  ( 19.03943276465977164, 0.05219959533936151252, 36.25109039468567573 ) ) ;
#158231=CARTESIAN_POINT ( 'NONE',  ( -13.89961937509977652, 13.97604488694528158, 65.62390960531436690 ) ) ;
#158232=CARTESIAN_POINT ( 'NONE',  ( -18.67979575497178146, -10.72451020669898902, 61.66557627198103120 ) ) ;
#158233=CARTESIAN_POINT ( 'NONE',  ( 12.14591786802309770, 12.06949235617756955, 69.37390960531436690 ) ) ;
#158234=CARTESIAN_POINT ( 'NONE',  ( 19.05341960407617918, -5.049401038297876454, 26.04275706135233293 ) ) ;
#158235=CARTESIAN_POINT ( 'NONE',  ( -17.97058386085787163, -5.500000000000058620, 54.00390968646216550 ) ) ;
#158236=CARTESIAN_POINT ( 'NONE',  ( -21.55341960407610458, -5.719274019375992779, 21.45724293864769550 ) ) ;
#158237=CARTESIAN_POINT ( 'NONE',  ( -16.51473224551069308, -9.474510206698971260, 56.66557627198103120 ) ) ;
#158238=CARTESIAN_POINT ( 'NONE',  ( -0.05219959533909027116, -19.03943276465977164, 37.49890960531436690 ) ) ;
#158239=CARTESIAN_POINT ( 'NONE',  ( -0.05219959533910754901, -16.53943276465976808, 102.4989096053143811 ) ) ;
#158240=CARTESIAN_POINT ( 'NONE',  ( -21.53943276465977519, -0.05219959533937600094, 18.75109039468568639 ) ) ;
#158241=CARTESIAN_POINT ( 'NONE',  ( -13.89961937509977652, 13.97604488694528158, 115.6239096053143669 ) ) ;
#158242=CARTESIAN_POINT ( 'NONE',  ( 15.72974639402176855, 15.80617190586768217, 26.87609039468567218 ) ) ;
#158243=CARTESIAN_POINT ( 'NONE',  ( -12.06949235617756955, 12.14591786802309770, 110.6239096053143669 ) ) ;
#158244=CARTESIAN_POINT ( 'NONE',  ( 10.81492255796106328, -18.62759615963255655, 75.41775706135233293 ) ) ;
#158245=CARTESIAN_POINT ( 'NONE',  ( -15.80617190586745835, -15.72974639402198527, 86.87390960531438111 ) ) ;
#158247=CARTESIAN_POINT ( 'NONE',  ( 13.97604488694548053, -13.89961937509957401, 35.62609039468567573 ) ) ;
#158248=CARTESIAN_POINT ( 'NONE',  ( -5.153800228976328057, -19.02544592524343514, 22.29057627198102765 ) ) ;
#158249=FACE_OUTER_BOUND ( 'NONE', #35620, .T. ) ;
#158250=CARTESIAN_POINT ( 'NONE',  ( -16.46253265017160317, 9.564922557960807481, 60.83224293864769550 ) ) ;
#158251=CARTESIAN_POINT ( 'NONE',  ( -14.34966873604972548, 8.224510206698743886, 48.33442372801902565 ) ) ;
#158252=CARTESIAN_POINT ( 'NONE',  ( 8.224510206698953496, -14.34966873604960469, 102.9155762719810383 ) ) ;
#158254=CARTESIAN_POINT ( 'NONE',  ( -16.46253265017160317, 9.564922557960807481, 65.83224293864769550 ) ) ;
#158255=CARTESIAN_POINT ( 'NONE',  ( -4.483927247898539470, -16.52544592524342804, 87.29057627198103830 ) ) ;
#158256=CARTESIAN_POINT ( 'NONE',  ( -10.72451020669898014, 18.67979575497178502, 45.41557627198103830 ) ) ;
#158257=CARTESIAN_POINT ( 'NONE',  ( -12.06949235617756955, 12.14591786802309770, 60.62390960531437401 ) ) ;
#158258=CARTESIAN_POINT ( 'NONE',  ( 12.14591786802327356, -12.06949235617739191, 40.62609039468567573 ) ) ;
#158259=CARTESIAN_POINT ( 'NONE',  ( 21.53943276465977519, 0.05219959533937863772, 91.25109039468568994 ) ) ;
#158260=CARTESIAN_POINT ( 'NONE',  ( -13.97604488694547520, 13.89961937509957934, 63.12609039468566863 ) ) ;
#158261=CARTESIAN_POINT ( 'NONE',  ( -14.29746914071037622, -8.314922557961029526, 104.1677570613523471 ) ) ;
#158262=CARTESIAN_POINT ( 'NONE',  ( -12.14591786802309592, -12.06949235617757132, 41.87390960531435979 ) ) ;
#158263=CONICAL_SURFACE ( 'NONE', #80751, 2.500000000000002220, 1.029744258676656754 ) ;
#158264=CARTESIAN_POINT ( 'NONE',  ( 16.46253265017160672, -9.564922557960803928, 38.33224293864768839 ) ) ;
#158265=CARTESIAN_POINT ( 'NONE',  ( 15.72974639402176855, 15.80617190586768217, 96.87609039468568994 ) ) ;
#158266=CARTESIAN_POINT ( 'NONE',  ( 21.53943276465977519, -0.05219959533907433946, 113.7489096053143527 ) ) ;
#158267=CARTESIAN_POINT ( 'NONE',  ( 0.05219959533937995610, -21.53943276465977519, 60.00109039468568284 ) ) ;
#158268=CARTESIAN_POINT ( 'NONE',  ( 0.05219959533934541429, -16.53943276465976808, 40.00109039468567573 ) ) ;
#158269=CARTESIAN_POINT ( 'NONE',  ( 8.314922557960818139, 14.29746914071049879, 69.58224293864769550 ) ) ;
#158270=CARTESIAN_POINT ( 'NONE',  ( 15.80617190586769283, -15.72974639402175789, 80.62609039468567573 ) ) ;
#158271=CARTESIAN_POINT ( 'NONE',  ( -16.55341960407611168, -4.379528057220339221, 26.45724293864768839 ) ) ;
#158272=CARTESIAN_POINT ( 'NONE',  ( 16.29526858892879204, 7.335722546919999587, 28.29670597800209464 ) ) ;
#158274=CARTESIAN_POINT ( 'NONE',  ( 16.52544592524342804, -4.483927247898539470, 23.54057627198102765 ) ) ;
#158275=CARTESIAN_POINT ( 'NONE',  ( 12.14591786802327356, -12.06949235617739191, 75.62609039468567573 ) ) ;
#158276=CARTESIAN_POINT ( 'NONE',  ( 9.564922557960805705, 16.46253265017160317, 79.58224293864769550 ) ) ;
#158277=CARTESIAN_POINT ( 'NONE',  ( 19.03943276465977164, -0.05219959533909143690, 103.7489096053143669 ) ) ;
#158278=CARTESIAN_POINT ( 'NONE',  ( 15.72974639402176855, 15.80617190586768217, 81.87609039468568994 ) ) ;
#158279=CARTESIAN_POINT ( 'NONE',  ( -8.314922557961024197, 14.29746914071037800, 82.91775706135234714 ) ) ;
#158280=CARTESIAN_POINT ( 'NONE',  ( -16.55341960407611168, -4.379528057220339221, 61.45724293864770260 ) ) ;
#158281=CARTESIAN_POINT ( 'NONE',  ( -19.02544592524342804, 5.153800228976336051, 71.04057627198099567 ) ) ;
#158283=CARTESIAN_POINT ( 'NONE',  ( 16.55341960407618274, -4.379528057220086978, 21.04275706135234714 ) ) ;
#158284=CARTESIAN_POINT ( 'NONE',  ( 9.564922557960805705, 16.46253265017160317, 34.58224293864770260 ) ) ;
#158285=CARTESIAN_POINT ( 'NONE',  ( 19.03943276465977164, -0.05219959533909143690, 73.74890960531435269 ) ) ;
#158286=CARTESIAN_POINT ( 'NONE',  ( 16.53943276465976808, 0.05219959533934440121, 21.25109039468567218 ) ) ;
#158288=CARTESIAN_POINT ( 'NONE',  ( -13.97604488694547697, 13.89961937509957934, 23.12609039468565442 ) ) ;
#158289=CARTESIAN_POINT ( 'NONE',  ( -16.53943276465976808, -0.05219959533934237506, 98.75109039468568994 ) ) ;
#158290=CARTESIAN_POINT ( 'NONE',  ( 0.05219959533936267826, -19.03943276465977164, 105.0010903946856615 ) ) ;
#158291=CARTESIAN_POINT ( 'NONE',  ( -5.049401038298153566, 19.05341960407611168, 25.20724293864768484 ) ) ;
#158292=CARTESIAN_POINT ( 'NONE',  ( 16.55341960407618274, -4.379528057220086978, 66.04275706135236135 ) ) ;
#158293=CARTESIAN_POINT ( 'NONE',  ( -12.06949235617739369, -12.14591786802326823, 54.37609039468568994 ) ) ;
#158295=CARTESIAN_POINT ( 'NONE',  ( 19.02544592524334988, 5.153800228976608722, 66.45942372801899012 ) ) ;
#158296=CARTESIAN_POINT ( 'NONE',  ( 5.823673210054444382, -21.52544592524334988, 110.2094237280190185 ) ) ;
#158297=CARTESIAN_POINT ( 'NONE',  ( 16.46253265017160672, -9.564922557960803928, 48.33224293864769550 ) ) ;
#158298=CARTESIAN_POINT ( 'NONE',  ( -0.05219959533909027116, -19.03943276465977164, 82.49890960531436690 ) ) ;
#158299=CARTESIAN_POINT ( 'NONE',  ( -8.314922557960811034, -14.29746914071050412, 77.08224293864769550 ) ) ;
#158301=CARTESIAN_POINT ( 'NONE',  ( -19.02544592524334988, -5.153800228976617603, 43.95942372801899012 ) ) ;
#158302=CARTESIAN_POINT ( 'NONE',  ( -21.52544592524343514, 5.823673210054127303, 31.04057627198102409 ) ) ;
#158303=CARTESIAN_POINT ( 'NONE',  ( 9.564922557961047289, -16.46253265017146816, 20.41775706135233293 ) ) ;
#158304=CARTESIAN_POINT ( 'NONE',  ( -5.153800228976328057, -19.02544592524343514, 97.29057627198099567 ) ) ;
#158305=CARTESIAN_POINT ( 'NONE',  ( -21.52544592524334988, -5.823673210054445271, 108.9594237280190185 ) ) ;
#158306=CARTESIAN_POINT ( 'NONE',  ( -21.53943276465977519, 0.05219959533907696930, 66.24890960531436690 ) ) ;
#158307=CARTESIAN_POINT ( 'NONE',  ( -19.03943276465977164, 0.05219959533909376836, 91.24890960531436690 ) ) ;
#158308=CARTESIAN_POINT ( 'NONE',  ( 13.97604488694548053, -13.89961937509957401, 90.62609039468567573 ) ) ;
#158309=CARTESIAN_POINT ( 'NONE',  ( -13.97604488694527625, -13.89961937509977652, 106.8739096053143669 ) ) ;
#158310=CARTESIAN_POINT ( 'NONE',  ( -13.97604488694547697, 13.89961937509957934, 103.1260903946856473 ) ) ;
#158311=CARTESIAN_POINT ( 'NONE',  ( 9.474510206698971260, -16.51473224551069308, 22.91557627198102765 ) ) ;
#158312=CARTESIAN_POINT ( 'NONE',  ( 9.564922557960805705, 16.46253265017160317, 89.58224293864769550 ) ) ;
#158313=CARTESIAN_POINT ( 'NONE',  ( 18.62759615963271287, -10.81492255796078972, 58.33224293864768839 ) ) ;
#158314=CARTESIAN_POINT ( 'NONE',  ( 14.34966873604972726, -8.224510206698740333, 40.83442372801901854 ) ) ;
#158315=CARTESIAN_POINT ( 'NONE',  ( 21.55341960407619695, -5.719274019375665929, 41.04275706135236135 ) ) ;
#158316=CARTESIAN_POINT ( 'NONE',  ( 15.72974639402176855, 15.80617190586768217, 91.87609039468568994 ) ) ;
#158317=CARTESIAN_POINT ( 'NONE',  ( 12.14591786802327356, -12.06949235617739191, 100.6260903946857184 ) ) ;
#158318=CARTESIAN_POINT ( 'NONE',  ( -13.89961937509977652, 13.97604488694528158, 90.62390960531432427 ) ) ;
#158319=CARTESIAN_POINT ( 'NONE',  ( -8.314922557960811034, -14.29746914071050412, 92.08224293864769550 ) ) ;
#158320=CARTESIAN_POINT ( 'NONE',  ( -14.34966873604972548, 8.224510206698743886, 113.3344237280190328 ) ) ;
#158321=CARTESIAN_POINT ( 'NONE',  ( 13.97604488694548053, -13.89961937509957401, 65.62609039468567573 ) ) ;
#158322=CARTESIAN_POINT ( 'NONE',  ( 15.80617190586769283, -15.72974639402175789, 45.62609039468567573 ) ) ;
#158323=CARTESIAN_POINT ( 'NONE',  ( -12.06949235617756955, 12.14591786802309770, 85.62390960531436690 ) ) ;
#158324=CARTESIAN_POINT ( 'NONE',  ( -9.564922557960796823, -16.46253265017161027, 107.0822429386476955 ) ) ;
#158325=CARTESIAN_POINT ( 'NONE',  ( -8.224510206698735004, -14.34966873604973081, 109.5844237280190328 ) ) ;
#158326=CARTESIAN_POINT ( 'NONE',  ( 0.05219959533937995610, -21.53943276465977519, 85.00109039468568994 ) ) ;
#158327=CARTESIAN_POINT ( 'NONE',  ( -0.05219959533934338120, 16.53943276465976808, 62.50109039468568284 ) ) ;
#158328=CARTESIAN_POINT ( 'NONE',  ( -5.719274019375665041, -21.55341960407619695, 44.79275706135234714 ) ) ;
#158330=CARTESIAN_POINT ( 'NONE',  ( -0.05219959533937732626, 21.53943276465977519, 32.50109039468568284 ) ) ;
#158331=CARTESIAN_POINT ( 'NONE',  ( -14.29746914071049879, 8.314922557960819915, 105.8322429386476955 ) ) ;
#158332=CARTESIAN_POINT ( 'NONE',  ( -13.97604488694527625, -13.89961937509977652, 21.87390960531435979 ) ) ;
#158333=CARTESIAN_POINT ( 'NONE',  ( 0.05219959533910956823, 16.53943276465976808, 69.99890960531435269 ) ) ;
#158334=CARTESIAN_POINT ( 'NONE',  ( 16.46253265017160672, -9.564922557960803928, 63.33224293864769550 ) ) ;
#158335=CARTESIAN_POINT ( 'NONE',  ( 12.14591786802327356, -12.06949235617739191, 100.6260903946857184 ) ) ;
#158336=CARTESIAN_POINT ( 'NONE',  ( 19.03943276465977164, -0.05219959533909143690, 33.74890960531435979 ) ) ;
#158337=CARTESIAN_POINT ( 'NONE',  ( 5.719274019375991003, -21.55341960407610458, 37.70724293864769550 ) ) ;
#158338=CARTESIAN_POINT ( 'NONE',  ( -16.52544592524342804, 4.483927247898546575, 81.04057627198102409 ) ) ;
#158339=CARTESIAN_POINT ( 'NONE',  ( -15.80617190586745835, -15.72974639402198527, 86.87390960531438111 ) ) ;
#158340=CARTESIAN_POINT ( 'NONE',  ( -19.05341960407611168, -5.049401038298163336, 91.45724293864766707 ) ) ;
#158341=CARTESIAN_POINT ( 'NONE',  ( -9.474510206698964154, 16.51473224551069663, 55.41557627198103120 ) ) ;
#158342=CARTESIAN_POINT ( 'NONE',  ( -19.02544592524334988, -5.153800228976617603, 88.95942372801897591 ) ) ;
#158343=CARTESIAN_POINT ( 'NONE',  ( 21.55341960407610458, 5.719274019375980345, 38.95724293864768839 ) ) ;
#158344=CARTESIAN_POINT ( 'NONE',  ( -21.55341960407619339, 5.719274019375674811, 68.54275706135234714 ) ) ;
#158345=CARTESIAN_POINT ( 'NONE',  ( 5.049401038298161559, -19.05341960407611168, 57.70724293864769550 ) ) ;
#158346=CARTESIAN_POINT ( 'NONE',  ( -5.153800228976328057, -19.02544592524343514, 82.29057627198103830 ) ) ;
#158347=ORIENTED_EDGE ( 'NONE', *, *, #158649, .T. ) ;
#158348=CARTESIAN_POINT ( 'NONE',  ( -12.06949235617739369, -12.14591786802326823, 69.37609039468567573 ) ) ;
#158349=CARTESIAN_POINT ( 'NONE',  ( 21.52544592524334988, 5.823673210054432836, 41.45942372801901143 ) ) ;
#158350=CARTESIAN_POINT ( 'NONE',  ( 0.05219959533937995610, -21.53943276465977519, 75.00109039468568994 ) ) ;
#158351=CARTESIAN_POINT ( 'NONE',  ( -19.02544592524342804, 5.153800228976336051, 111.0405762719810099 ) ) ;
#158352=CARTESIAN_POINT ( 'NONE',  ( -18.67979575497178146, -10.72451020669898902, 101.6655762719810383 ) ) ;
#158353=CARTESIAN_POINT ( 'NONE',  ( -21.55341960407619339, 5.719274019375674811, 43.54275706135235424 ) ) ;
#158354=CARTESIAN_POINT ( 'NONE',  ( -14.34966873604972548, 8.224510206698743886, 63.33442372801900433 ) ) ;
#158356=CARTESIAN_POINT ( 'NONE',  ( -10.81492255796078084, -18.62759615963271287, 62.08224293864769550 ) ) ;
#158357=CARTESIAN_POINT ( 'NONE',  ( -13.97604488694547697, 13.89961937509957934, 28.12609039468565797 ) ) ;
#158358=CARTESIAN_POINT ( 'NONE',  ( 19.03943276465977164, -0.05219959533909143690, 73.74890960531435269 ) ) ;
#158359=CARTESIAN_POINT ( 'NONE',  ( -14.34966873604972548, 8.224510206698743886, 108.3344237280190185 ) ) ;
#158360=CARTESIAN_POINT ( 'NONE',  ( -17.49999999999999645, -5.068104630630367424, 104.2718159465997161 ) ) ;
#158361=CARTESIAN_POINT ( 'NONE',  ( -13.89961937509977652, 13.97604488694528158, 105.6239096053143527 ) ) ;
#158363=CARTESIAN_POINT ( 'NONE',  ( 13.89961937509957401, 13.97604488694547697, 76.87609039468566152 ) ) ;
#158364=CARTESIAN_POINT ( 'NONE',  ( 15.72974639402199770, -15.80617190586745480, 53.12390960531436690 ) ) ;
#158365=CARTESIAN_POINT ( 'NONE',  ( -14.34966873604960291, -8.224510206698953496, 41.66557627198103120 ) ) ;
#158366=CARTESIAN_POINT ( 'NONE',  ( 16.51473224551083163, -9.474510206698727899, 95.83442372801900433 ) ) ;
#158367=CARTESIAN_POINT ( 'NONE',  ( -0.05219959533909027116, -19.03943276465977164, 37.49890960531436690 ) ) ;
#158368=CARTESIAN_POINT ( 'NONE',  ( -16.52544592524335698, -4.483927247898792601, 18.95942372801901143 ) ) ;
#158369=CARTESIAN_POINT ( 'NONE',  ( 18.62759615963271287, -10.81492255796078972, 83.33224293864769550 ) ) ;
#158370=CARTESIAN_POINT ( 'NONE',  ( -9.564922557961040184, 16.46253265017147172, 52.91775706135233293 ) ) ;
#158371=CARTESIAN_POINT ( 'NONE',  ( -16.52544592524335698, -4.483927247898792601, 73.95942372801901854 ) ) ;
#158372=CARTESIAN_POINT ( 'NONE',  ( 13.97604488694527802, 13.89961937509977652, 69.37390960531436690 ) ) ;
#158373=CARTESIAN_POINT ( 'NONE',  ( 16.53943276465976808, -0.05219959533910856209, 63.74890960531435979 ) ) ;
#158374=CARTESIAN_POINT ( 'NONE',  ( 19.02544592524343514, -5.153800228976328945, 43.54057627198103120 ) ) ;
#158375=CARTESIAN_POINT ( 'NONE',  ( 16.53943276465976808, -0.05219959533910856209, 58.74890960531436690 ) ) ;
#158376=CARTESIAN_POINT ( 'NONE',  ( 5.153800228976335163, 19.02544592524342804, 24.79057627198102765 ) ) ;
#158378=CARTESIAN_POINT ( 'NONE',  ( -8.314922557960811034, -14.29746914071050412, 22.08224293864769194 ) ) ;
#158379=CARTESIAN_POINT ( 'NONE',  ( -19.05341960407611168, -5.049401038298163336, 81.45724293864769550 ) ) ;
#158381=CARTESIAN_POINT ( 'NONE',  ( -19.05341960407617563, 5.049401038297882671, 33.54275706135231871 ) ) ;
#158382=CARTESIAN_POINT ( 'NONE',  ( -16.55341960407617563, 4.379528057220093196, 48.54275706135234714 ) ) ;
#158383=CARTESIAN_POINT ( 'NONE',  ( -21.52544592524343514, 5.823673210054127303, 46.04057627198103830 ) ) ;
#158384=CARTESIAN_POINT ( 'NONE',  ( -21.53943276465977519, -0.05219959533937600094, 113.7510903946856757 ) ) ;
#158385=CARTESIAN_POINT ( 'NONE',  ( 16.46253265017160672, -9.564922557960803928, 78.33224293864769550 ) ) ;
#158387=CARTESIAN_POINT ( 'NONE',  ( 9.474510206698971260, -16.51473224551069308, 107.9155762719810383 ) ) ;
#158388=CARTESIAN_POINT ( 'NONE',  ( 5.719274019375673035, 21.55341960407619339, 42.29275706135235424 ) ) ;
#158389=CARTESIAN_POINT ( 'NONE',  ( -12.14591786802309592, -12.06949235617757132, 111.8739096053143669 ) ) ;
#158390=CARTESIAN_POINT ( 'NONE',  ( -18.62759615963270932, 10.81492255796079327, 90.83224293864769550 ) ) ;
#158391=CARTESIAN_POINT ( 'NONE',  ( -16.46253265017160317, 9.564922557960807481, 85.83224293864769550 ) ) ;
#158393=CARTESIAN_POINT ( 'NONE',  ( 10.72451020669871369, 18.67979575497193778, 32.08442372801901854 ) ) ;
#158395=CARTESIAN_POINT ( 'NONE',  ( -19.05341960407611168, -5.049401038298163336, 86.45724293864769550 ) ) ;
#158397=CARTESIAN_POINT ( 'NONE',  ( 9.474510206698971260, -16.51473224551069308, 27.91557627198103120 ) ) ;
#158398=CARTESIAN_POINT ( 'NONE',  ( -13.97604488694527625, -13.89961937509977652, 36.87390960531436690 ) ) ;
#158399=CARTESIAN_POINT ( 'NONE',  ( 5.049401038297881783, 19.05341960407617563, 112.2927570613523471 ) ) ;
#158401=CARTESIAN_POINT ( 'NONE',  ( -8.314922557960811034, -14.29746914071050412, 107.0822429386476955 ) ) ;
#158402=CARTESIAN_POINT ( 'NONE',  ( -5.823673210054431948, 21.52544592524334988, 87.70942372801901854 ) ) ;
#158403=CARTESIAN_POINT ( 'NONE',  ( 19.02544592524343514, -5.153800228976328945, 63.54057627198103830 ) ) ;
#158404=CARTESIAN_POINT ( 'NONE',  ( -15.80617190586768217, 15.72974639402176855, 38.12609039468567573 ) ) ;
#158405=CARTESIAN_POINT ( 'NONE',  ( 15.80617190586769283, -15.72974639402175789, 30.62609039468567929 ) ) ;
#158407=CARTESIAN_POINT ( 'NONE',  ( -16.46253265017160317, 9.564922557960807481, 80.83224293864769550 ) ) ;
#158409=CARTESIAN_POINT ( 'NONE',  ( 12.06949235617739724, 12.14591786802326823, 21.87609039468567573 ) ) ;
#158410=CARTESIAN_POINT ( 'NONE',  ( -18.67979575497178146, -10.72451020669898902, 46.66557627198102409 ) ) ;
#158411=CARTESIAN_POINT ( 'NONE',  ( -0.05219959533937732626, 21.53943276465977519, 77.50109039468567573 ) ) ;
#158412=CARTESIAN_POINT ( 'NONE',  ( -13.89961937509977652, 13.97604488694528158, 105.6239096053143527 ) ) ;
#158413=CARTESIAN_POINT ( 'NONE',  ( -9.474510206698720793, -16.51473224551083518, 94.58442372801900433 ) ) ;
#158414=CARTESIAN_POINT ( 'NONE',  ( -13.97604488694527625, -13.89961937509977652, 56.87390960531434558 ) ) ;
#158415=CARTESIAN_POINT ( 'NONE',  ( 19.02544592524343514, -5.153800228976328945, 83.54057627198100988 ) ) ;
#158417=CARTESIAN_POINT ( 'NONE',  ( -12.14591786802309592, -12.06949235617757132, 96.87390960531436690 ) ) ;
#158418=CARTESIAN_POINT ( 'NONE',  ( 14.29746914071049879, -8.314922557960816363, 103.3322429386476955 ) ) ;
#158419=CARTESIAN_POINT ( 'NONE',  ( 19.05341960407611168, 5.049401038298154454, 113.9572429386477097 ) ) ;
#158420=CARTESIAN_POINT ( 'NONE',  ( -12.14591786802309592, -12.06949235617757132, 51.87390960531437401 ) ) ;
#158421=CARTESIAN_POINT ( 'NONE',  ( 16.51473224551069308, 9.474510206698969483, 44.16557627198103120 ) ) ;
#158422=CARTESIAN_POINT ( 'NONE',  ( -21.55341960407619339, 5.719274019375674811, 68.54275706135234714 ) ) ;
#158423=CARTESIAN_POINT ( 'NONE',  ( -9.564922557961040184, 16.46253265017147172, 87.91775706135233293 ) ) ;
#158424=CARTESIAN_POINT ( 'NONE',  ( -16.53943276465976808, 0.05219959533911058130, 66.24890960531436690 ) ) ;
#158425=CARTESIAN_POINT ( 'NONE',  ( -5.719274019375978568, 21.55341960407610458, 110.2072429386477239 ) ) ;
#158426=CARTESIAN_POINT ( 'NONE',  ( 5.719274019375991003, -21.55341960407610458, 42.70724293864770260 ) ) ;
#158427=CARTESIAN_POINT ( 'NONE',  ( 19.05341960407611168, 5.049401038298154454, 108.9572429386477097 ) ) ;
#158429=CARTESIAN_POINT ( 'NONE',  ( -13.97604488694527625, -13.89961937509977652, 66.87390960531436690 ) ) ;
#158430=CARTESIAN_POINT ( 'NONE',  ( 12.14591786802309770, 12.06949235617756955, 34.37390960531435979 ) ) ;
#158432=CARTESIAN_POINT ( 'NONE',  ( -16.53943276465976808, -0.05219959533934237506, 108.7510903946857042 ) ) ;
#158433=CARTESIAN_POINT ( 'NONE',  ( 12.14591786802327356, -12.06949235617739191, 80.62609039468567573 ) ) ;
#158434=CARTESIAN_POINT ( 'NONE',  ( 13.97604488694548053, -13.89961937509957401, 45.62609039468566863 ) ) ;
#158436=CARTESIAN_POINT ( 'NONE',  ( -19.05341960407611168, -5.049401038298163336, 96.45724293864769550 ) ) ;
#158437=CARTESIAN_POINT ( 'NONE',  ( -5.153800228976328057, -19.02544592524343514, 52.29057627198100988 ) ) ;
#158438=CARTESIAN_POINT ( 'NONE',  ( 4.379528057220339221, -16.55341960407611168, 67.70724293864769550 ) ) ;
#158439=CARTESIAN_POINT ( 'NONE',  ( -9.564922557960796823, -16.46253265017161027, 22.08224293864768839 ) ) ;
#158440=CARTESIAN_POINT ( 'NONE',  ( 10.72451020669898902, -18.67979575497178502, 27.91557627198103830 ) ) ;
#158441=CARTESIAN_POINT ( 'NONE',  ( 10.72451020669898902, -18.67979575497178502, 52.91557627198103830 ) ) ;
#158442=CARTESIAN_POINT ( 'NONE',  ( 8.314922557960818139, 14.29746914071049879, 84.58224293864769550 ) ) ;
#158443=CARTESIAN_POINT ( 'NONE',  ( -16.53943276465976808, -0.05219959533934237506, 38.75109039468567573 ) ) ;
#158444=CARTESIAN_POINT ( 'NONE',  ( 14.34966873604960469, 8.224510206698951720, 79.16557627198103830 ) ) ;
#158446=CARTESIAN_POINT ( 'NONE',  ( 0.05219959533936267826, -19.03943276465977164, 75.00109039468566152 ) ) ;
#158447=CARTESIAN_POINT ( 'NONE',  ( -21.53943276465977519, 0.05219959533907696930, 21.24890960531436690 ) ) ;
#158449=LINE ( 'NONE', #157467, #9256 ) ;
#158450=CARTESIAN_POINT ( 'NONE',  ( 12.14591786802327356, -12.06949235617739191, 25.62609039468567929 ) ) ;
#158451=CARTESIAN_POINT ( 'NONE',  ( -4.483927247898782831, 16.52544592524335698, 107.7094237280190328 ) ) ;
#158452=CARTESIAN_POINT ( 'NONE',  ( 13.97604488694548053, -13.89961937509957401, 65.62609039468567573 ) ) ;
#158453=CARTESIAN_POINT ( 'NONE',  ( -10.81492255796078084, -18.62759615963271287, 47.08224293864770260 ) ) ;
#158454=CARTESIAN_POINT ( 'NONE',  ( 15.80617190586769283, -15.72974639402175789, 65.62609039468568994 ) ) ;
#158456=CARTESIAN_POINT ( 'NONE',  ( 8.314922557961029526, -14.29746914071037800, 30.41775706135234358 ) ) ;
#158457=CARTESIAN_POINT ( 'NONE',  ( -9.474510206698964154, 16.51473224551069663, 25.41557627198103120 ) ) ;
#158458=CARTESIAN_POINT ( 'NONE',  ( -9.564922557960796823, -16.46253265017161027, 87.08224293864769550 ) ) ;
#158460=CARTESIAN_POINT ( 'NONE',  ( 14.29746914071049879, -8.314922557960816363, 98.33224293864769550 ) ) ;
#158462=CARTESIAN_POINT ( 'NONE',  ( -5.153800228976328057, -19.02544592524343514, 102.2905762719810383 ) ) ;
#158464=CARTESIAN_POINT ( 'NONE',  ( 14.34966873604972726, -8.224510206698740333, 60.83442372801901854 ) ) ;
#158465=CARTESIAN_POINT ( 'NONE',  ( -16.46253265017146816, -9.564922557961047289, 109.1677570613523471 ) ) ;
#158466=CARTESIAN_POINT ( 'NONE',  ( -10.81492255796078084, -18.62759615963271287, 82.08224293864768129 ) ) ;
#158467=CARTESIAN_POINT ( 'NONE',  ( -16.51473224551069308, -9.474510206698971260, 41.66557627198103120 ) ) ;
#158468=CARTESIAN_POINT ( 'NONE',  ( -19.05341960407617563, 5.049401038297882671, 68.54275706135230450 ) ) ;
#158469=CARTESIAN_POINT ( 'NONE',  ( -15.80617190586745835, -15.72974639402198527, 111.8739096053143669 ) ) ;
#158470=CARTESIAN_POINT ( 'NONE',  ( -9.564922557960796823, -16.46253265017161027, 72.08224293864770971 ) ) ;
#158471=CARTESIAN_POINT ( 'NONE',  ( 9.564922557960805705, 16.46253265017160317, 99.58224293864770971 ) ) ;
#158472=ORIENTED_EDGE ( 'NONE', *, *, #146153, .F. ) ;
#158473=CARTESIAN_POINT ( 'NONE',  ( 8.224510206698742110, 14.34966873604972548, 32.08442372801901854 ) ) ;
#158474=CARTESIAN_POINT ( 'NONE',  ( 10.72451020669898902, -18.67979575497178502, 107.9155762719810241 ) ) ;
#158475=CARTESIAN_POINT ( 'NONE',  ( -8.224510206698948167, 14.34966873604960824, 105.4155762719810383 ) ) ;
#158476=CARTESIAN_POINT ( 'NONE',  ( 13.89961937509977652, -13.97604488694527269, 98.12390960531433848 ) ) ;
#158477=CARTESIAN_POINT ( 'NONE',  ( 19.03943276465977164, 0.05219959533936151252, 76.25109039468566152 ) ) ;
#158478=CARTESIAN_POINT ( 'NONE',  ( 18.62759615963271287, -10.81492255796078972, 88.33224293864769550 ) ) ;
#158479=CARTESIAN_POINT ( 'NONE',  ( 12.14591786802309770, 12.06949235617756955, 44.37390960531435979 ) ) ;
#158480=CARTESIAN_POINT ( 'NONE',  ( 9.564922557961047289, -16.46253265017146816, 25.41775706135234003 ) ) ;
#158481=CARTESIAN_POINT ( 'NONE',  ( 8.314922557961029526, -14.29746914071037800, 70.41775706135236135 ) ) ;
#158482=CARTESIAN_POINT ( 'NONE',  ( 5.049401038298161559, -19.05341960407611168, 92.70724293864769550 ) ) ;
#158483=CARTESIAN_POINT ( 'NONE',  ( 13.97604488694527802, 13.89961937509977652, 44.37390960531435269 ) ) ;
#158484=CARTESIAN_POINT ( 'NONE',  ( -15.72974639402176322, -15.80617190586768395, 54.37609039468568994 ) ) ;
#158485=CARTESIAN_POINT ( 'NONE',  ( -15.80617190586768217, 15.72974639402176855, 63.12609039468568994 ) ) ;
#158486=CARTESIAN_POINT ( 'NONE',  ( 13.89961937509977652, -13.97604488694527269, 63.12390960531435979 ) ) ;
#158487=CARTESIAN_POINT ( 'NONE',  ( -10.81492255796105439, 18.62759615963255655, 32.91775706135234714 ) ) ;
#158489=CARTESIAN_POINT ( 'NONE',  ( -5.153800228976607833, 19.02544592524334988, 77.70942372801900433 ) ) ;
#158490=CARTESIAN_POINT ( 'NONE',  ( 5.153800228976335163, 19.02544592524342804, 44.79057627198103830 ) ) ;
#158491=CARTESIAN_POINT ( 'NONE',  ( -4.483927247898782831, 16.52544592524335698, 87.70942372801901854 ) ) ;
#158492=CARTESIAN_POINT ( 'NONE',  ( -19.02544592524342804, 5.153800228976336051, 56.04057627198100988 ) ) ;
#158493=CARTESIAN_POINT ( 'NONE',  ( -9.564922557960796823, -16.46253265017161027, 107.0822429386476955 ) ) ;
#158494=CARTESIAN_POINT ( 'NONE',  ( 16.46253265017160672, -9.564922557960803928, 43.33224293864769550 ) ) ;
#158495=CARTESIAN_POINT ( 'NONE',  ( -15.72974639402197994, 15.80617190586746368, 90.62390960531436690 ) ) ;
#158496=CARTESIAN_POINT ( 'NONE',  ( -14.34966873604972548, 8.224510206698743886, 73.33442372801901854 ) ) ;
#158498=CARTESIAN_POINT ( 'NONE',  ( -5.049401038297874678, -19.05341960407617918, 34.79275706135233293 ) ) ;
#158499=CARTESIAN_POINT ( 'NONE',  ( -9.564922557960796823, -16.46253265017161027, 72.08224293864770971 ) ) ;
#158500=CARTESIAN_POINT ( 'NONE',  ( 8.314922557960818139, 14.29746914071049879, 44.58224293864769550 ) ) ;
#158501=CARTESIAN_POINT ( 'NONE',  ( 8.224510206698953496, -14.34966873604960469, 77.91557627198102409 ) ) ;
#158502=CARTESIAN_POINT ( 'NONE',  ( -9.564922557960796823, -16.46253265017161027, 102.0822429386477097 ) ) ;
#158503=CARTESIAN_POINT ( 'NONE',  ( 13.89961937509977652, -13.97604488694527269, 88.12390960531438111 ) ) ;
#158504=CARTESIAN_POINT ( 'NONE',  ( -5.823673210054431948, 21.52544592524334988, 52.70942372801902565 ) ) ;
#158505=CARTESIAN_POINT ( 'NONE',  ( 9.474510206698971260, -16.51473224551069308, 97.91557627198102409 ) ) ;
#158506=CARTESIAN_POINT ( 'NONE',  ( 10.81492255796106328, -18.62759615963255655, 100.4177570613523471 ) ) ;
#158507=CARTESIAN_POINT ( 'NONE',  ( 4.483927247898790824, -16.52544592524335698, 85.20942372801901854 ) ) ;
#158508=CARTESIAN_POINT ( 'NONE',  ( 21.55341960407619695, -5.719274019375665929, 26.04275706135235779 ) ) ;
#158509=CARTESIAN_POINT ( 'NONE',  ( 21.53943276465977519, -0.05219959533907433946, 103.7489096053143669 ) ) ;
#158510=CARTESIAN_POINT ( 'NONE',  ( 4.483927247898545687, 16.52544592524342804, 59.79057627198103120 ) ) ;
#158511=CARTESIAN_POINT ( 'NONE',  ( 19.02544592524343514, -5.153800228976328945, 43.54057627198103120 ) ) ;
#158512=CARTESIAN_POINT ( 'NONE',  ( 16.53943276465976808, -0.05219959533910856209, 68.74890960531435269 ) ) ;
#158513=CARTESIAN_POINT ( 'NONE',  ( -18.62759615963270932, 10.81492255796079327, 25.83224293864769194 ) ) ;
#158514=CARTESIAN_POINT ( 'NONE',  ( 5.153800228976615827, -19.02544592524334988, 35.20942372801899722 ) ) ;
#158515=CARTESIAN_POINT ( 'NONE',  ( 16.52544592524342804, -4.483927247898539470, 108.5405762719810241 ) ) ;
#158517=CARTESIAN_POINT ( 'NONE',  ( 8.314922557961029526, -14.29746914071037800, 60.41775706135235424 ) ) ;
#158518=CARTESIAN_POINT ( 'NONE',  ( -13.97604488694527625, -13.89961937509977652, 71.87390960531433848 ) ) ;
#158519=LINE ( 'NONE', #113991, #24234 ) ;
#158520=CARTESIAN_POINT ( 'NONE',  ( 16.52544592524342804, -4.483927247898539470, 93.54057627198103830 ) ) ;
#158521=CARTESIAN_POINT ( 'NONE',  ( 5.823673210054125526, 21.52544592524343514, 34.79057627198103120 ) ) ;
#158523=CARTESIAN_POINT ( 'NONE',  ( -8.314922557961024197, 14.29746914071037800, 112.9177570613523329 ) ) ;
#158524=CARTESIAN_POINT ( 'NONE',  ( 16.51473224551083163, -9.474510206698727899, 105.8344237280190043 ) ) ;
#158525=CARTESIAN_POINT ( 'NONE',  ( 18.67979575497194134, -10.72451020669871369, 75.83442372801900433 ) ) ;
#158526=CARTESIAN_POINT ( 'NONE',  ( 16.51473224551069308, 9.474510206698969483, 89.16557627198103830 ) ) ;
#158527=CARTESIAN_POINT ( 'NONE',  ( 10.81492255796078972, 18.62759615963270932, 99.58224293864770971 ) ) ;
#158528=CARTESIAN_POINT ( 'NONE',  ( -16.55341960407617563, 4.379528057220093196, 48.54275706135234714 ) ) ;
#158529=CARTESIAN_POINT ( 'NONE',  ( -19.03943276465977164, 0.05219959533909376836, 31.24890960531435979 ) ) ;
#158530=CARTESIAN_POINT ( 'NONE',  ( 12.06949235617739724, 12.14591786802326823, 31.87609039468567929 ) ) ;
#158531=CARTESIAN_POINT ( 'NONE',  ( 19.05341960407617918, -5.049401038297876454, 91.04275706135234714 ) ) ;
#158532=CARTESIAN_POINT ( 'NONE',  ( 10.72451020669898902, -18.67979575497178502, 87.91557627198103830 ) ) ;
#158533=CARTESIAN_POINT ( 'NONE',  ( 16.46253265017146816, 9.564922557961045513, 56.66775706135233293 ) ) ;
#158535=CARTESIAN_POINT ( 'NONE',  ( 21.53943276465977519, -0.05219959533907433946, 98.74890960531438111 ) ) ;
#158536=CARTESIAN_POINT ( 'NONE',  ( -5.153800228976328057, -19.02544592524343514, 82.29057627198103830 ) ) ;
#158538=CARTESIAN_POINT ( 'NONE',  ( 16.52544592524335698, 4.483927247898782831, 31.45942372801901854 ) ) ;
#158540=CARTESIAN_POINT ( 'NONE',  ( -0.05219959533937732626, 21.53943276465977519, 22.50109039468567573 ) ) ;
#158541=CARTESIAN_POINT ( 'NONE',  ( 4.379528057220339221, -16.55341960407611168, 62.70724293864769550 ) ) ;
#158542=CARTESIAN_POINT ( 'NONE',  ( -9.474510206698964154, 16.51473224551069663, 65.41557627198102409 ) ) ;
#158543=CARTESIAN_POINT ( 'NONE',  ( -16.55341960407617563, 4.379528057220093196, 33.54275706135234714 ) ) ;
#158544=CARTESIAN_POINT ( 'NONE',  ( -19.02544592524334988, -5.153800228976617603, 43.95942372801899012 ) ) ;
#158545=CARTESIAN_POINT ( 'NONE',  ( 18.62759615963255655, 10.81492255796105972, 51.66775706135234714 ) ) ;
#158546=CARTESIAN_POINT ( 'NONE',  ( 8.314922557961029526, -14.29746914071037800, 20.41775706135234714 ) ) ;
#158547=CARTESIAN_POINT ( 'NONE',  ( 9.474510206698971260, -16.51473224551069308, 57.91557627198103120 ) ) ;
#158548=CARTESIAN_POINT ( 'NONE',  ( -9.564922557961040184, 16.46253265017147172, 82.91775706135233293 ) ) ;
#158549=CARTESIAN_POINT ( 'NONE',  ( -21.55341960407619339, 5.719274019375674811, 88.54275706135236135 ) ) ;
#158550=CARTESIAN_POINT ( 'NONE',  ( -19.02544592524334988, -5.153800228976617603, 63.95942372801899012 ) ) ;
#158551=CARTESIAN_POINT ( 'NONE',  ( -16.46253265017160317, 9.564922557960807481, 40.83224293864769550 ) ) ;
#158552=CARTESIAN_POINT ( 'NONE',  ( 15.72974639402199770, -15.80617190586745480, 63.12390960531435979 ) ) ;
#158553=CARTESIAN_POINT ( 'NONE',  ( 12.06949235617757843, -12.14591786802309237, 58.12390960531435979 ) ) ;
#158555=CARTESIAN_POINT ( 'NONE',  ( 19.03943276465977164, 0.05219959533936151252, 36.25109039468567573 ) ) ;
#158556=CARTESIAN_POINT ( 'NONE',  ( -4.483927247898782831, 16.52544592524335698, 102.7094237280190185 ) ) ;
#158557=CARTESIAN_POINT ( 'NONE',  ( -14.34966873604960291, -8.224510206698953496, 51.66557627198102409 ) ) ;
#158558=CARTESIAN_POINT ( 'NONE',  ( 15.80617190586769283, -15.72974639402175789, 85.62609039468568994 ) ) ;
#158559=CARTESIAN_POINT ( 'NONE',  ( 18.67979575497194134, -10.72451020669871369, 80.83442372801901854 ) ) ;
#158560=CARTESIAN_POINT ( 'NONE',  ( 18.62759615963271287, -10.81492255796078972, 88.33224293864769550 ) ) ;
#158561=( BOUNDED_SURFACE ( )  B_SPLINE_SURFACE ( 3, 2, ( 
 ( #42400, #104063, #165744, #122196, #30200, #27238, #183888, #45373, #107026, #150579, #73741, #168698, #91841, #118243, #164748, #179934, #41401, #138368, #125195, #35165, #112008, #153535, #94845, #15032, #76692, #140350, #108016, #61518, #95838, #127158, #124180, #186891, #139355, #156526, #50349, #155526, #3818, #79678, #48362, #18025, #17021, #141349, #173697, #47367, #171697, #49344, #78674, #157522, #16029, #34177, #1838, #65496, #200049, #33186, #185882, #836, #77687, #62509, #109022, #123187, #111006, #19016, #2836, #169702, #80662, #184876, #142338, #110016, #170701, #64514, #63520, #126181, #46358, #188866, #187876, #32190, #31196, #92847, #154532, #172692, #93848, #96820, #51331, #37148, #4805, #38162, #7806, #68482, #158505, #99817, #146317, #192844, #132160, #67487, #85650, #19992, #175674, #22992, #143318, #162492, #130137, #128157, #189857, #113976, #66494, #129145, #174684, #69490, #191834, #190842, #112991, #116988, #23993, #81635, #36149, #145321, #131155, #100809, #161502, #178681, #83644, #53315, #54324, #97801, #52318, #147337, #115996, #6804, #114993, #159490, #176687, #177685, #20983, #84640, #82640, #39153, #8824, #70493, #193852, #144323, #5812, #55317, #98807, #160501, #21991, #101821, #87648, #181671, #196851, #195860, #139848, #102827, #149334, #89646, #163509, #148335, #78179, #135177, #27003, #197830, #40144, #88648, #151334, #74489, #1337, #133156, #58317, #119985, #43150, #73505, #123680, #46869, #16532, #165507, #150344, #63017, #104819, #25007, #166508, #124696, #86651, #136155, #9830, #10828, #26006, #71490, #11840, #185379, #194847, #72498, #62016, #108530, #12823, #170209, #42167, #179692, #56320, #134172, #28006, #31702, #57332, #118003, #164513, #119008, #93351, #41164, #180691, #103827, #155037, #173195, #143831, #186393, #34671, #97309, #20488, #21492, #79180, #81152, #142834, #4313, #19507, #66995, #190349, #160004, #111509, #96329, #83153, #127665, #47870, #112499, #144827, #109523, #82137, #171205, #157025, #172193, #17522, #158016, #128654, #32695, #18523, #5311, #51825, #35661, #113485, #188368, #65996, #6311, #156025, #189365, #80170, #50842, #175179, #174193, #158995, #95340, #36645, #141842, #3333, #98304, #94346, #140851, #126664, #2340, #67989, #64021, #125690, #187389, #48857, #110512, #33678, #65007, #49845, #118514, #129643, #8327, #55828, #176188, #195360, #101317, #161006, #22500, #146834, #37657, #100325, #7309, #40666, #163006, #162004, #84147, #149839, #56839, #114485, #99322, #178191, #164025, #133669, #71005, #11343, #116503, #24513, #87167, #145826, #23500, #180204, #179198, #39656, #86163, #191339, #147853, #102335, #53835, #9340, #68994, #132673, #194361, #117501, #25521, #130659, #192352, #148848, #10339, #115509, #88154, #71995, #52817, #177197, #38670, #41673, #85148, #103337, #54829, #70002, #131672, #193353, #165017, #26510, #31458, #75964, #137637, #57837, #28506, #61775, #123443, #60789, #29483, #76954, #15294, #199324, #43655, #13314, #91114, #45634, #44647, #136642, #154795, #93110, #185136, #198325, #122460, #167985, #135674, #89155, #167004, #138624, #73014, #197346, #46627, #108287, #168957, #105317, #150844, #134683, #152804, #184153, #166014, #107286, #90140, #119510, #106299, #196369, #181191, #42669, #14296, #104330, #27514, #59801, #12340, #74004, #105, #169965, #151825, #30463, #58809, #92111, #120478, #74980, #182169, #153800, #121471, #183163, #18288, #80925, #113253, #110278, #34440, #112267, #79943, #20251, #78938, #97079, #3100, #128417, #98061, #96099, #187154, #2104, #140614, #63785, #125457, #174944, #173959, #81897, #157788, #32455, #143590, #36406, #5073, #64778, #62772, #141613, #48626, #155787, #19278, #126439, #142602, #4081, #17284, #95106, #16293, #188137, #171959, #65759, #49608, #127428, #139610, #66756, #111271, #33447, #158760, #190113, #189136, #172962, #156795, #77943, #1096, #35426 ),
 ( #50608, #51588, #124453, #186149, #47628, #109283, #170961, #94108, #10095, #84905, #24269, #54584, #22257, #175948, #53587, #163777, #179960, #83906, #71755, #195113, #55584, #192104, #37417, #118270, #116257, #85918, #52582, #9094, #130406, #144588, #131424, #41427, #159760, #21255, #101075, #82910, #6074, #146584, #114241, #67752, #102092, #133425, #115263, #193110, #145589, #162760, #56596, #161766, #129410, #147606, #177948, #70761, #23261, #132429, #191107, #176956, #39416, #117259, #8078, #25278, #7067, #40421, #69754, #99077, #160767, #194121, #38425, #68749, #100081, #178951, #86921, #148603, #167749, #14054, #13082, #196126, #75721, #45397, #137397, #43413, #149598, #58575, #165771, #119266, #136410, #105083, #74747, #198090, #180949, #135438, #103093, #28270, #73765, #121233, #166769, #59555, #87911, #199078, #89909, #88914, #60546, #122221, #107050, #151591, #26269, #164775, #11095, #106063, #27265, #72771, #182926, #29247, #42426, #168723, #44409, #104088, #150606, #90881, #12102, #120241, #197108, #183912, #152565, #181932, #134441, #57597, #10755, #68403, #130055, #132086, #117926, #87576, #24931, #103756, #70419, #116912, #41088, #176608, #54249, #149263, #133081, #193775, #55244, #145244, #101745, #194771, #7725, #178605, #191755, #86576, #163434, #40068, #148260, #22914, #99738, #9753, #164439, #69411, #84560, #6725, #131077, #71417, #56245, #39079, #180618, #146238, #192766, #179616, #53238, #114915, #118933, #102751, #25933, #72419, #83565, #134096, #195787, #57259, #42091, #38082, #165435, #161422, #115921, #177611, #100735, #162416, #23918, #8749, #85572, #147259, #168395, #88572, #153215, #62193, #150270, #61204, #11765, #197754, #12749, #58246, #137060, #169379, #73431, #59221, #122876, #107700, #76380, #92534, #28915, #121885, #185555, #196778, #152237, #120890, #106721, #154223, #29890, #183578, #136080, #15713, #182589, #44073, #138057, #26930, #181600, #167419, #135102, #91528, #199738, #198750, #119914, #14720, #184564, #46045, #123857, #105732, #77373, #13722, #30887, #151259, #166435, #43077, #74414, #139041, #45063, #90555, #47049, #89573, #75388, #521, #104744, #27930, #108706, #60215, #157203, #127836, #170385, #18697, #81323, #4484, #5489, #63194, #65181, #126840, #188546, #3505, #51014, #174367, #144008, #95517, #80344, #67172, #111689, #31876, #96501, #128829, #93530, #66174, #155215, #141031, #156203, #1517, #142016, #112675, #16704, #2518, #189542, #35837, #19681, #97483, #172367, #50024, #190528, #140028, #173376, #64198, #34846, #159169, #158191, #143006, #79360, #20664, #125865, #187565, #82318, #78354, #124874, #110687, #186573, #52002, #48046, #109702, #171384, #32871, #94521, #17703, #49032, #33857, #188294, #112428, #52742, #114409, #51751, #20412, #67917, #6238, #66917, #34598, #4240, #82062, #36571, #35589, #127593, #145752, #84073, #176111, #189292, #128581, #158922, #126592, #80099, #157943, #129570, #63946, #49771, #37581, #99244, #159930, #96256, #141767, #22423, #143755, #190275, #156951, #113412, #19434, #48784, #97235, #125614, #187313, #110438, #5236, #172119, #33605, #175103, #65920, #98227, #160932, #81081, #21417, #83077, #50769, #191267, #111436, #144753, #174118, #95268, #18448, #3259, #142760, #173123, #64933, #69928, #131593, #165938, #164944, #72940, #87088, #23425, #134609, #104256, #196294, #55752, #53757, #9263, #54752, #146755, #10263, #117426, #148774, #71921, #8249, #86086, #7234, #179124, #162930, #133592, #40592, #195284, #130581, #57764, #194286, #116426, #149765, #119434, #27438, #102263, #68919, #192275, #89081, #56765, #85072, #118437, #132596, #193278, #115431, #177122, #26437, #180130, #38593, #11267, #181118, #178114, #163951, #42592, #100249, #41599, #25448, #161930, #39582, #103263, #101241, #147776, #88079, #24437, #70929, #14221, #32383, #170891, #1027, #75890, #15224, #45562, #13248, #166934, #44574, #154727 ),
 ( #74911, #199249, #197273, #153728, #168886, #60716, #122390, #90072, #28436, #137565, #31390, #136574, #151755, #12268, #198254, #92039, #107216, #106230, #47559, #59730, #121399, #32, #73933, #109212, #120405, #184078, #183093, #30392, #77875, #76883, #138554, #167913, #16223, #29413, #91044, #61705, #150772, #105248, #152731, #58735, #123375, #185067, #46555, #135602, #108217, #169897, #93040, #186077, #182098, #139542, #62699, #124382, #43582, #140545, #159686, #65690, #125388, #187085, #111200, #2033, #64708, #171889, #5004, #127355, #126370, #48555, #114171, #21184, #78865, #63713, #142533, #128349, #97993, #35360, #175874, #80857, #189068, #51522, #110208, #188067, #82840, #143515, #4012, #50540, #155716, #112201, #66687, #18217, #173891, #33376, #97012, #158693, #20182, #81828, #95034, #156725, #190047, #174874, #79874, #141543, #17213, #3032, #113185, #36340, #49538, #191037, #172892, #34371, #144519, #96031, #157718, #129342, #6004, #67684, #52510, #94038, #19207, #148537, #71688, #72699, #130333, #132363, #194056, #55517, #70695, #118202, #41359, #11024, #162694, #24200, #134372, #178883, #99004, #163708, #196058, #160695, #133355, #22186, #8004, #23192, #68678, #147538, #179893, #83834, #69687, #195045, #103024, #86853, #164707, #39350, #117190, #40351, #9026, #102025, #25211, #176883, #116193, #37346, #10028, #193043, #56524, #26202, #87841, #145516, #149529, #85849, #146514, #57531, #119200, #6996, #192031, #53513, #115191, #38354, #100009, #161695, #84835, #131354, #54520, #177882, #101010, #138332, #91804, #139318, #106000, #46323, #199014, #169665, #106987, #27199, #107977, #152501, #12037, #73701, #198024, #88845, #151528, #58511, #153496, #13990, #13017, #135373, #798, #31160, #165702, #150537, #29184, #14993, #184838, #122158, #62471, #167687, #75657, #200012, #197043, #74682, #92810, #30160, #90818, #137334, #42360, #60483, #76653, #105017, #183847, #120177, #45335, #168660, #61479, #123150, #181867, #43346, #154497, #15992, #166701, #28204, #104023, #89845, #77650, #180885, #136348, #59492, #121167, #182861, #44342, #47329, #32153, #162206, #18976, #110966, #81594, #124143, #172650, #35123, #158464, #23704, #16982, #80622, #142299, #3779, #157483, #4764, #130863, #100527, #49307, #34138, #85352, #65456, #185842, #50308, #147045, #108984, #19952, #170665, #94805, #109978, #155490, #95797, #192554, #126142, #127119, #8529, #93810, #188825, #156484, #111964, #54037, #173656, #96775, #33147, #115711, #17986, #79639, #143278, #78636, #140311, #64475, #1801, #69196, #177399, #38871, #63479, #125155, #186854, #48323, #171658, #141308, #2797, #187838, #59009, #196563, #116701, #135870, #41875, #101521, #163211, #87365, #178391, #40865, #148048, #181387, #103542, #102539, #24714, #90337, #197541, #55031, #39855, #118713, #104531, #74201, #11549, #152022, #57040, #165217, #27713, #86363, #164222, #120676, #119704, #180403, #26712, #131874, #88351, #42866, #194557, #150044, #9538, #73216, #134887, #58034, #166212, #71205, #132868, #89356, #151046, #56027, #117705, #193559, #179401, #12536, #182375, #25719, #167203, #149050, #10538, #43852, #72202, #133876, #105518, #28701, #70207, #195566, #13508, #61974, #124652, #47828, #48816, #106501, #108487, #170166, #31659, #46827, #94304, #17479, #187346, #138826, #306, #110469, #154993, #75173, #139806, #172151, #136845, #109479, #198530, #184350, #199520, #44845, #123640, #155982, #60001, #45832, #171163, #79136, #62972, #33637, #15499, #63979, #1294, #93308, #16489, #77155, #78138, #95299, #107483, #186348, #32650, #185337, #140807, #76159, #2297, #125648, #121668, #183363, #168178, #169161, #60987, #137839, #122662, #30665, #29674, #91306, #152998, #14497, #92318, #154003, #53788, #22455, #5269, #3293, #158954, #4272, #96288, #159961, #66951, #98259, #21448, #157974, #35621, #156983, #128613, #112458, #83109, #190305, #144785, #80130 ),
 ( #82095, #19467, #115463, #18481, #114442, #67947, #177152, #38624, #51782, #84104, #143787, #145783, #7264, #6268, #113442, #160962, #99275, #129601, #127623, #97266, #175135, #191297, #36602, #20444, #141799, #64965, #68949, #52773, #176143, #37613, #81112, #173154, #50800, #130612, #126624, #142792, #192308, #188325, #49804, #189323, #34629, #111469, #65952, #174149, #193310, #149796, #70960, #85103, #71953, #182128, #58767, #100281, #41631, #161960, #23456, #87120, #54783, #8282, #42624, #73964, #132629, #133625, #86118, #103295, #146789, #27471, #148806, #9295, #104288, #150802, #120435, #195317, #69960, #131626, #116459, #164975, #178147, #180161, #25479, #39613, #101272, #162962, #57795, #11301, #24468, #197303, #10296, #89113, #56798, #12298, #135632, #88112, #118470, #165969, #147809, #26470, #194317, #40623, #72972, #134641, #196327, #163982, #55784, #117456, #179155, #119465, #181149, #102293, #106260, #59761, #137597, #47588, #63743, #167943, #94066, #78896, #139572, #75922, #121429, #2064, #138584, #108247, #136603, #93071, #14251, #28466, #15255, #125417, #43612, #105276, #185097, #166963, #90101, #30424, #198283, #151784, #186107, #17244, #199280, #76913, #29442, #46586, #140574, #45593, #155746, #169927, #64, #31419, #107247, #154756, #13276, #60747, #61736, #1057, #168918, #109241, #91074, #124413, #92071, #74940, #183122, #123404, #122420, #152761, #184111, #153760, #16253, #44605, #62731, #170920, #77905, #32412, #52544, #83869, #114205, #35390, #33408, #189098, #34402, #126400, #190078, #97041, #128382, #51554, #188096, #65720, #187113, #158722, #142564, #113218, #20213, #174908, #36372, #145551, #50571, #37381, #98026, #81861, #159722, #112231, #21218, #7029, #80887, #5035, #82875, #173921, #191071, #49569, #67717, #143550, #99038, #68711, #66721, #157748, #172923, #111232, #96060, #19239, #48585, #144553, #175910, #6038, #3061, #160728, #110237, #22220, #129374, #95067, #171918, #4043, #127388, #156755, #18249, #79902, #141573, #64738, #9058, #130368, #102059, #85885, #56560, #40386, #71720, #53547, #57564, #117224, #39384, #72735, #180918, #88880, #163744, #192065, #115225, #12071, #195080, #8040, #10060, #55551, #69721, #150572, #176917, #87875, #41394, #38388, #27231, #25244, #119234, #178918, #42393, #104056, #118236, #86885, #134407, #196094, #133389, #101043, #70729, #148570, #103059, #179927, #194089, #100044, #161730, #165736, #164741, #26236, #149563, #193077, #146546, #24235, #23225, #84868, #54552, #131388, #116225, #11059, #162729, #177916, #147573, #132396, #138362, #166734, #123181, #44376, #58544, #45367, #155520, #32184, #73733, #15025, #135406, #197077, #60515, #28238, #181900, #16023, #47361, #106032, #107020, #59523, #184870, #167718, #120210, #168692, #43378, #93841, #105050, #76686, #89878, #151561, #122190, #13050, #74717, #77681, #109016, #29216, #30193, #121200, #200043, #170695, #75687, #124174, #61512, #91835, #46352, #137366, #108010, #136380, #90849, #153528, #169695, #199045, #139349, #198057, #154526, #183882, #185875, #182892, #31189, #152534, #14021, #92841, #828, #62503, #175667, #174677, #82633, #96812, #33179, #144316, #113968, #5805, #65489, #63514, #19009, #64507, #156517, #19985, #127151, #158498, #81628, #18018, #95831, #17015, #188859, #172685, #143311, #50342, #4798, #140344, #67478, #3811, #126174, #159482, #129138, #37142, #112000, #78667, #1832, #98801, #66487, #94838, #128150, #142331, #79671, #125189, #186885, #36142, #189849, #48355, #110009, #173690, #190835, #35156, #52311, #171690, #51323, #112984, #20976, #141342, #97794, #187869, #157515, #2829, #49337, #110999, #80655, #34169, #180684, #10821, #85644, #25001, #55310, #22984, #176681, #54318, #164505, #42160, #84634, #72491, #195853, #56313, #192838, #38156, #119001, #116982, #86645, #53309, #21985, #7800, #101815, #178674, #115990, #57325, #146311, #69484, #9823 ),
 ( #134164, #160495, #40138, #131149, #177679, #39147, #100802, #162486, #83637, #117996, #25999, #163503, #99810, #87641, #145314, #149327, #8818, #6798, #23987, #147330, #161496, #148328, #70487, #71484, #133149, #132153, #193846, #68476, #194840, #179685, #41157, #102820, #130131, #191828, #114987, #90623, #12815, #46114, #154291, #62259, #75456, #165500, #26996, #185625, #168463, #181664, #183648, #28982, #43143, #123927, #103820, #61274, #14789, #88641, #587, #13790, #30954, #152305, #92601, #15781, #91598, #60282, #107767, #169452, #106789, #74482, #44141, #121955, #76449, #137130, #167486, #150337, #11832, #77440, #198817, #29961, #45130, #166501, #119978, #197823, #139112, #73498, #27999, #135170, #196843, #199807, #136147, #104812, #58310, #153288, #138126, #89638, #122944, #59289, #151327, #184633, #120958, #182657, #105800, #188617, #47116, #108775, #33930, #1589, #155284, #189609, #20734, #50098, #158259, #18768, #170453, #111758, #96571, #143076, #82391, #172442, #112743, #65251, #35906, #173447, #93598, #174436, #80415, #78422, #140098, #64268, #16774, #17775, #124944, #19749, #142087, #79430, #63264, #67239, #97552, #31944, #186641, #95588, #81390, #51083, #34915, #128898, #157272, #3573, #4554, #48112, #141101, #159240, #66247, #126911, #127907, #109768, #144079, #5560, #171452, #32940, #94595, #156273, #2588, #125934, #187633, #49103, #110761, #177442, #71250, #114743, #129886, #52074, #37911, #131919, #147092, #146070, #87410, #53064, #99570, #39903, #113730, #98560, #25764, #85399, #38912, #148093, #190597, #100569, #101568, #24761, #149095, #83396, #8576, #70251, #193603, #23750, #132914, #194601, #164269, #115754, #162251, #10585, #55075, #175427, #116745, #72246, #36895, #86408, #160254, #161251, #176437, #21744, #178435, #56073, #145073, #22745, #9584, #117753, #163259, #179446, #192597, #40912, #6555, #68233, #102585, #84394, #191586, #7555, #69241, #130907, #54080, #2095, #42909, #27757, #47619, #133923, #88396, #74245, #41921, #63776, #105560, #165262, #26756, #151089, #180449, #104575, #11593, #109273, #167246, #166257, #150089, #156786, #125448, #118760, #103587, #182417, #170952, #140605, #75217, #18279, #120719, #28745, #94098, #73261, #89400, #187144, #186140, #43897, #90381, #195614, #152066, #32445, #58078, #13551, #134930, #136889, #198574, #60044, #124444, #196607, #119748, #155777, #17275, #181431, #12580, #57086, #135914, #78929, #48617, #197585, #33438, #59052, #110268, #171949, #95097, #81889, #144581, #176948, #173951, #98053, #175940, #143582, #83898, #142593, #160758, #66749, #192096, #161759, #159753, #50600, #65750, #4073, #127419, #189128, #38417, #37411, #145581, #21248, #96091, #7059, #100074, #68740, #128410, #126430, #5064, #112259, #19270, #82902, #190106, #6067, #67745, #80917, #158752, #79933, #51581, #35418, #129403, #113245, #191099, #3091, #130398, #174936, #97071, #22249, #53578, #141604, #36399, #64768, #188127, #49598, #52574, #157779, #114234, #99069, #20241, #111262, #172953, #115255, #34431, #181926, #120235, #133417, #150599, #10088, #12097, #73760, #9087, #54578, #195106, #165764, #84897, #194114, #57589, #104082, #72764, #88908, #25271, #118263, #43407, #193104, #148596, #55578, #103086, #135432, #26262, #179953, #132423, #197103, #117252, #178944, #134434, #23254, #177942, #163770, #131416, #164767, #196119, #56589, #146576, #87903, #119259, #180943, #58570, #71746, #105077, #41420, #8071, #149589, #69747, #116250, #11087, #39409, #101069, #40415, #162754, #102086, #24263, #42419, #27258, #86913, #85912, #147600, #70755, #151586, #13075, #15052, #857, #170722, #108038, #186913, #153555, #200070, #124204, #59550, #137392, #32214, #16050, #76713, #138388, #28265, #184897, #77709, #90875, #61538, #74742, #169724, #46379, #123207, #31217, #106058, #182919, #92868, #47389, #152559, #167744, #89903, #14048, #154555, #139375, #125217, #29242 ),
 ( #1861, #121228, #62531, #185904, #109044, #93870, #155549, #17043, #140374, #91862, #78697, #63543, #48384, #136405, #166763, #198083, #44404, #75714, #199072, #60541, #122217, #183908, #45393, #107046, #168718, #30220, #49366, #68503, #110041, #67509, #21006, #130158, #6825, #20015, #37169, #96842, #98828, #160522, #97821, #66516, #113996, #52340, #113012, #80685, #50371, #128178, #82661, #81658, #173720, #191855, #171720, #22013, #35188, #174705, #4828, #172716, #126203, #3841, #175694, #33209, #34199, #83665, #145343, #5833, #142361, #187899, #94868, #189877, #36169, #2859, #159510, #65520, #156549, #143341, #18048, #79701, #141372, #51352, #64537, #111030, #158527, #95861, #157544, #19038, #127180, #188890, #144345, #112031, #129166, #190863, #41187, #85673, #9853, #178706, #25030, #8848, #148357, #195886, #100833, #101844, #56343, #70516, #164535, #192868, #102850, #193875, #10854, #119034, #163530, #39175, #54347, #116018, #177708, #162516, #57360, #118025, #26028, #86674, #146339, #87673, #53336, #149357, #55341, #161523, #132184, #24018, #131178, #71512, #117011, #133180, #194870, #147360, #40168, #115015, #179715, #72523, #134198, #176709, #38183, #23015, #99839, #84661, #7827, #69512, #84311, #192514, #5477, #95505, #33845, #67160, #189530, #160170, #143996, #175343, #157191, #161167, #20652, #142994, #176354, #145990, #53998, #128817, #18685, #80332, #115672, #98477, #111677, #113649, #159156, #173364, #142004, #3492, #191503, #144991, #65169, #130823, #190516, #22664, #82306, #7473, #69157, #21660, #51990, #37827, #99487, #36810, #4472, #174355, #83314, #6472, #68152, #97471, #126828, #188534, #50012, #129804, #52979, #114657, #96489, #34834, #127824, #158179, #19669, #81310, #66162, #51002, #112663, #35825, #54994, #135838, #72163, #41836, #70167, #26676, #148012, #162168, #149013, #58974, #197507, #177360, #118676, #38831, #100489, #164185, #131836, #85314, #119671, #151013, #9502, #10501, #163172, #150005, #132832, #58001, #55991, #103504, #133838, #180368, #179365, #165181, #74167, #71167, #195528, #73181, #40828, #181353, #39817, #42833, #25682, #89321, #23665, #57002, #194518, #24676, #101483, #86326, #117669, #147005, #134852, #104498, #88316, #193518, #166179, #8491, #27680, #87328, #116663, #102500, #11511, #178354, #196531, #12504, #61938, #185302, #59965, #199485, #13475, #170128, #91271, #105482, #92281, #2263, #79101, #120642, #123607, #182340, #43818, #107449, #75139, #28667, #62937, #94270, #152962, #153965, #106463, #93273, #76123, #1260, #60951, #46793, #15463, #108452, #122626, #31623, #17445, #14460, #138789, #16454, #184316, #124617, #183327, #186312, #169123, #32616, #167168, #270, #137801, #168142, #44808, #29638, #45797, #140774, #78103, #47793, #154958, #136808, #109444, #90302, #171127, #30628, #151988, #77119, #139772, #121631, #155948, #198493, #153267, #137111, #17753, #48091, #184612, #77420, #141080, #152285, #107748, #14769, #62238, #109747, #185605, #139092, #91578, #171431, #76429, #138105, #93577, #182638, #198798, #122924, #90603, #123906, #155262, #154270, #44121, #47095, #31923, #78400, #79410, #169430, #32918, #567, #94573, #108755, #28962, #156251, #15761, #13769, #75437, #199786, #60263, #61254, #121934, #16752, #170431, #46093, #183629, #2565, #64247, #167467, #45111, #30935, #140076, #186619, #1567, #105780, #92582, #63243, #124922, #106768, #168443, #29939, #175404, #112721, #174414, #187612, #110739, #172420, #35883, #160231, #129864, #67217, #146048, #97530, #159217, #83374, #18746, #96549, #191562, #36872, #20712, #82368, #49082, #144057, #98537, #50076, #5538, #33908, #128875, #190575, #52051, #113707, #65229, #142065, #21721, #6532, #111737, #126889, #95566, #173424, #145051, #68212, #84371, #188595, #157252, #53041, #114721, #80393, #3551, #161229, #176414, #37889, #99547, #125914, #22723, #7532, #34893, #158236, #19727 ),
 ( #81368, #143052, #4531, #66223, #127884, #189587, #51059, #116722, #8551, #72222, #58053, #100547, #88370, #119724, #148068, #69217, #40886, #24734, #195588, #179421, #10558, #192575, #196583, #56047, #178411, #11569, #181407, #27732, #102559, #130885, #54058, #151064, #133897, #147067, #149070, #194577, #70227, #89375, #115732, #26731, #180423, #177419, #166232, #164244, #42885, #117726, #104550, #38890, #57060, #25739, #73235, #134906, #118735, #39875, #9559, #87385, #41896, #103562, #132888, #162226, #23725, #85374, #131895, #165237, #193579, #55051, #150064, #101542, #163234, #86384, #71225, #183384, #184370, #198551, #185356, #168199, #93329, #91327, #138845, #45851, #154023, #14518, #77175, #109501, #106522, #30686, #108507, #76179, #16510, #75194, #155014, #199539, #124672, #94325, #92337, #44866, #60021, #136865, #121688, #29696, #171183, #170186, #78158, #15518, #28721, #139826, #32672, #1315, #61009, #59028, #137859, #153019, #152043, #325, #62994, #43872, #31680, #186369, #122681, #12555, #107504, #169180, #61993, #123659, #46847, #135889, #47848, #74221, #197561, #120695, #182394, #105537, #167223, #90358, #13528, #37635, #20467, #33657, #35642, #81132, #95318, #114463, #156003, #113464, #66974, #176165, #52795, #65975, #83131, #142813, #144807, #6290, #143809, #112479, #159983, #98282, #158975, #126644, #96309, #174172, #128634, #127644, #19487, #17500, #79157, #67969, #4293, #82117, #50822, #18501, #172172, #49825, #21470, #140828, #80149, #129623, #191318, #51805, #188347, #157003, #2317, #97288, #5291, #48836, #190328, #111489, #63999, #189344, #125669, #187367, #110490, #141820, #175158, #36625, #3313, #64986, #173174, #34650, #157995, #88133, #149817, #87145, #55808, #103317, #41653, #102315, #69983, #39636, #117480, #71974, #70984, #162986, #181170, #119488, #11323, #24491, #164005, #194340, #161983, #115487, #193333, #164997, #99299, #23479, #72993, #134662, #195339, #131651, #177175, #57816, #179178, #25501, #192331, #148828, #54807, #84126, #132652, #160984, #22478, #145805, #40646, #7288, #68972, #86142, #53812, #130636, #26491, #196348, #116482, #10318, #85128, #133648, #178171, #180184, #101297, #56819, #118493, #38648, #147833, #100305, #146812, #9319, #8306, #141356, #47375, #49351, #108024, #126188, #32199, #157529, #127165, #125202, #16037, #31204, #169711, #92855, #154542, #3825, #2843, #111013, #186898, #58789, #172700, #142345, #34184, #93856, #89135, #109030, #77695, #184884, #48369, #95845, #73985, #64521, #19023, #124189, #42647, #17028, #844, #171704, #155533, #110026, #165992, #80669, #78681, #139363, #187884, #65504, #104309, #140357, #27492, #150823, #12320, #33193, #120457, #94852, #170709, #46366, #1845, #63527, #156533, #18032, #135654, #197325, #62517, #79686, #185890, #24000, #130144, #50356, #115001, #85656, #112015, #23001, #173704, #159496, #174691, #19998, #98814, #131162, #35172, #147343, #20992, #143326, #8831, #54331, #190848, #83651, #70499, #158511, #113982, #82646, #68489, #116002, #191841, #145329, #97807, #177691, #144329, #5818, #99824, #188874, #4813, #129151, #96827, #53322, #161509, #160508, #81642, #176695, #38169, #84647, #66500, #175680, #39159, #6811, #100816, #146324, #128163, #162499, #21998, #189863, #51337, #67494, #112997, #52325, #36155, #7813, #69497, #37155, #192852, #104826, #57340, #196858, #27011, #194853, #148340, #26011, #136162, #152318, #56326, #182670, #167501, #28013, #164518, #9836, #90636, #88655, #58324, #25013, #181678, #102832, #116994, #103834, #13804, #132167, #193858, #73513, #55323, #178689, #119015, #86656, #40151, #74496, #105814, #87654, #165515, #118008, #166515, #149339, #12830, #10835, #119992, #150351, #135184, #134180, #43159, #28996, #72505, #11848, #89655, #195867, #197837, #179697, #59303, #180698, #42174, #44154, #101827, #151341, #120972, #41169, #163514, #71495, #133161, #33942, #32952 ) ),
 .UNSPECIFIED., .T., .F., .F. ) 
 B_SPLINE_SURFACE_WITH_KNOTS ( ( 4, 3, 4 ),
 ( 3, 2, 2, 2, 2, 2, 2, 2, 2, 2, 2, 2, 2, 2, 2, 2, 2, 2, 2, 2, 2, 2, 2, 2, 2, 2, 2, 2, 2, 2, 2, 2, 2, 2, 2, 2, 2, 2, 2, 2, 2, 2, 2, 2, 2, 2, 2, 2, 2, 2, 2, 2, 2, 2, 2, 2, 2, 2, 2, 2, 2, 2, 2, 2, 2, 2, 2, 2, 2, 2, 2, 2, 2, 2, 2, 2, 2, 2, 2, 2, 2, 2, 2, 2, 2, 2, 2, 2, 2, 2, 2, 2, 2, 2, 2, 2, 2, 2, 2, 2, 2, 2, 2, 2, 2, 2, 2, 2, 2, 2, 2, 2, 2, 2, 2, 2, 2, 2, 2, 2, 2, 2, 2, 2, 2, 2, 2, 2, 2, 2, 2, 2, 2, 2, 2, 2, 2, 2, 2, 2, 2, 2, 2, 2, 2, 2, 2, 2, 2, 2, 2, 2, 2, 2, 2, 2, 2, 2, 2, 2, 2, 2, 2, 2, 2, 2, 2, 2, 2, 2, 2, 2, 2, 2, 2, 2, 2, 2, 2, 2, 2, 2, 2, 2, 2, 2, 2, 2, 2, 2, 2, 2, 2, 2, 2, 2, 2, 2, 2, 2, 2, 2, 2, 2, 2, 2, 2, 2, 2, 2, 2, 2, 2, 2, 2, 2, 2, 2, 2, 2, 2, 2, 2, 2, 2, 2, 2, 2, 3 ),
 ( 0.000000000000000000, 0.5000000000000000000, 1.000000000000000000 ),
 ( 0.000000000000000000, 0.004385964912280701511, 0.008771929824561403022, 0.01315789473684210453, 0.01754385964912280604, 0.02192982456140350755, 0.02631578947368420907, 0.03070175438596491058, 0.03508771929824561209, 0.03947368421052631360, 0.04385964912280701511, 0.04824561403508771662, 0.05263157894736841813, 0.05701754385964911964, 0.06140350877192982115, 0.06578947368421052266, 0.07017543859649122417, 0.07456140350877192569, 0.07894736842105262720, 0.08333333333333332871, 0.08771929824561403022, 0.09210526315789473173, 0.09649122807017543324, 0.1008771929824561348, 0.1052631578947368363, 0.1096491228070175378, 0.1140350877192982393, 0.1184210526315789408, 0.1228070175438596423, 0.1271929824561403577, 0.1315789473684210453, 0.1359649122807017607, 0.1403508771929824483, 0.1447368421052631637, 0.1491228070175438514, 0.1535087719298245668, 0.1578947368421052544, 0.1622807017543859698, 0.1666666666666666574, 0.1710526315789473728, 0.1754385964912280604, 0.1798245614035087758, 0.1842105263157894635, 0.1885964912280701788, 0.1929824561403508665, 0.1973684210526315819, 0.2017543859649122695, 0.2061403508771929849, 0.2105263157894736725, 0.2149122807017543879, 0.2192982456140350755, 0.2236842105263157909, 0.2280701754385964786, 0.2324561403508771940, 0.2368421052631578816, 0.2412280701754385970, 0.2456140350877192846, 0.2500000000000000000, 0.2543859649122807154, 0.2587719298245614308, 0.2631578947368420907, 0.2675438596491228060, 0.2719298245614035214, 0.2763157894736842368, 0.2807017543859648967, 0.2850877192982456121, 0.2894736842105263275, 0.2938596491228070429, 0.2982456140350877027, 0.3026315789473684181, 0.3070175438596491335, 0.3114035087719298489, 0.3157894736842105088, 0.3201754385964912242, 0.3245614035087719396, 0.3289473684210526550, 0.3333333333333333148, 0.3377192982456140302, 0.3421052631578947456, 0.3464912280701754610, 0.3508771929824561209, 0.3552631578947368363, 0.3596491228070175517, 0.3640350877192982670, 0.3684210526315789269, 0.3728070175438596423, 0.3771929824561403577, 0.3815789473684210731, 0.3859649122807017330, 0.3903508771929824483, 0.3947368421052631637, 0.3991228070175438791, 0.4035087719298245390, 0.4078947368421052544, 0.4122807017543859698, 0.4166666666666666852, 0.4210526315789473450, 0.4254385964912280604, 0.4298245614035087758, 0.4342105263157894912, 0.4385964912280701511, 0.4429824561403508665, 0.4473684210526315819, 0.4517543859649122973, 0.4561403508771929571, 0.4605263157894736725, 0.4649122807017543879, 0.4692982456140351033, 0.4736842105263157632, 0.4780701754385964786, 0.4824561403508771940, 0.4868421052631579093, 0.4912280701754385692, 0.4956140350877192846, 0.5000000000000000000, 0.5043859649122807154, 0.5087719298245614308, 0.5131578947368421462, 0.5175438596491228616, 0.5219298245614034659, 0.5263157894736841813, 0.5307017543859648967, 0.5350877192982456121, 0.5394736842105263275, 0.5438596491228070429, 0.5482456140350877583, 0.5526315789473684736, 0.5570175438596490780, 0.5614035087719297934, 0.5657894736842105088, 0.5701754385964912242, 0.5745614035087719396, 0.5789473684210526550, 0.5833333333333333703, 0.5877192982456140857, 0.5921052631578946901, 0.5964912280701754055, 0.6008771929824561209, 0.6052631578947368363, 0.6096491228070175517, 0.6140350877192982670, 0.6184210526315789824, 0.6228070175438596978, 0.6271929824561403022, 0.6315789473684210176, 0.6359649122807017330, 0.6403508771929824483, 0.6447368421052631637, 0.6491228070175438791, 0.6535087719298245945, 0.6578947368421053099, 0.6622807017543859143, 0.6666666666666666297, 0.6710526315789473450, 0.6754385964912280604, 0.6798245614035087758, 0.6842105263157894912, 0.6885964912280702066, 0.6929824561403509220, 0.6973684210526315264, 0.7017543859649122417, 0.7061403508771929571, 0.7105263157894736725, 0.7149122807017543879, 0.7192982456140351033, 0.7236842105263158187, 0.7280701754385965341, 0.7324561403508771384, 0.7368421052631578538, 0.7412280701754385692, 0.7456140350877192846, 0.7500000000000000000, 0.7543859649122807154, 0.7587719298245614308, 0.7631578947368421462, 0.7675438596491228616, 0.7719298245614034659, 0.7763157894736841813, 0.7807017543859648967, 0.7850877192982456121, 0.7894736842105263275, 0.7938596491228070429, 0.7982456140350877583, 0.8026315789473684736, 0.8070175438596490780, 0.8114035087719297934, 0.8157894736842105088, 0.8201754385964912242, 0.8245614035087719396, 0.8289473684210526550, 0.8333333333333333703, 0.8377192982456140857, 0.8421052631578946901, 0.8464912280701754055, 0.8508771929824561209, 0.8552631578947368363, 0.8596491228070175517, 0.8640350877192982670, 0.8684210526315789824, 0.8728070175438596978, 0.8771929824561403022, 0.8815789473684210176, 0.8859649122807017330, 0.8903508771929824483, 0.8947368421052631637, 0.8991228070175438791, 0.9035087719298245945, 0.9078947368421053099, 0.9122807017543859143, 0.9166666666666666297, 0.9210526315789473450, 0.9254385964912280604, 0.9298245614035087758, 0.9342105263157894912, 0.9385964912280702066, 0.9429824561403509220, 0.9473684210526315264, 0.9517543859649122417, 0.9561403508771929571, 0.9605263157894736725, 0.9649122807017543879, 0.9692982456140351033, 0.9736842105263158187, 0.9780701754385965341, 0.9824561403508771384, 0.9868421052631578538, 0.9912280701754385692, 0.9956140350877192846, 1.000000000000000000 ),
 .UNSPECIFIED. ) 
 GEOMETRIC_REPRESENTATION_ITEM ( )  RATIONAL_B_SPLINE_SURFACE ( (
 ( 1.000000000000000000, 0.9659258262890683122, 1.000000000000000000, 0.9659258262890683122, 1.000000000000000000, 0.9659258262890683122, 1.000000000000000000, 0.9659258262890683122, 1.000000000000000000, 0.9659258262890683122, 1.000000000000000000, 0.9659258262890683122, 1.000000000000000000, 0.9659258262890683122, 1.000000000000000000, 0.9659258262890683122, 1.000000000000000000, 0.9659258262890683122, 1.000000000000000000, 0.9659258262890683122, 1.000000000000000000, 0.9659258262890683122, 1.000000000000000000, 0.9659258262890683122, 1.000000000000000000, 0.9659258262890683122, 1.000000000000000000, 0.9659258262890683122, 1.000000000000000000, 0.9659258262890683122, 1.000000000000000000, 0.9659258262890683122, 1.000000000000000000, 0.9659258262890683122, 1.000000000000000000, 0.9659258262890683122, 1.000000000000000000, 0.9659258262890683122, 1.000000000000000000, 0.9659258262890683122, 1.000000000000000000, 0.9659258262890683122, 1.000000000000000000, 0.9659258262890683122, 1.000000000000000000, 0.9659258262890683122, 1.000000000000000000, 0.9659258262890683122, 1.000000000000000000, 0.9659258262890683122, 1.000000000000000000, 0.9659258262890683122, 1.000000000000000000, 0.9659258262890683122, 1.000000000000000000, 0.9659258262890683122, 1.000000000000000000, 0.9659258262890683122, 1.000000000000000000, 0.9659258262890683122, 1.000000000000000000, 0.9659258262890683122, 1.000000000000000000, 0.9659258262890683122, 1.000000000000000000, 0.9659258262890683122, 1.000000000000000000, 0.9659258262890683122, 1.000000000000000000, 0.9659258262890683122, 1.000000000000000000, 0.9659258262890683122, 1.000000000000000000, 0.9659258262890683122, 1.000000000000000000, 0.9659258262890683122, 1.000000000000000000, 0.9659258262890683122, 1.000000000000000000, 0.9659258262890683122, 1.000000000000000000, 0.9659258262890683122, 1.000000000000000000, 0.9659258262890683122, 1.000000000000000000, 0.9659258262890683122, 1.000000000000000000, 0.9659258262890683122, 1.000000000000000000, 0.9659258262890683122, 1.000000000000000000, 0.9659258262890683122, 1.000000000000000000, 0.9659258262890683122, 1.000000000000000000, 0.9659258262890683122, 1.000000000000000000, 0.9659258262890683122, 1.000000000000000000, 0.9659258262890683122, 1.000000000000000000, 0.9659258262890683122, 1.000000000000000000, 0.9659258262890683122, 1.000000000000000000, 0.9659258262890683122, 1.000000000000000000, 0.9659258262890683122, 1.000000000000000000, 0.9659258262890683122, 1.000000000000000000, 0.9659258262890683122, 1.000000000000000000, 0.9659258262890683122, 1.000000000000000000, 0.9659258262890683122, 1.000000000000000000, 0.9659258262890683122, 1.000000000000000000, 0.9659258262890683122, 1.000000000000000000, 0.9659258262890683122, 1.000000000000000000, 0.9659258262890683122, 1.000000000000000000, 0.9659258262890683122, 1.000000000000000000, 0.9659258262890683122, 1.000000000000000000, 0.9659258262890683122, 1.000000000000000000, 0.9659258262890683122, 1.000000000000000000, 0.9659258262890683122, 1.000000000000000000, 0.9659258262890683122, 1.000000000000000000, 0.9659258262890683122, 1.000000000000000000, 0.9659258262890683122, 1.000000000000000000, 0.9659258262890683122, 1.000000000000000000, 0.9659258262890683122, 1.000000000000000000, 0.9659258262890683122, 1.000000000000000000, 0.9659258262890683122, 1.000000000000000000, 0.9659258262890683122, 1.000000000000000000, 0.9659258262890683122, 1.000000000000000000, 0.9659258262890683122, 1.000000000000000000, 0.9659258262890683122, 1.000000000000000000, 0.9659258262890683122, 1.000000000000000000, 0.9659258262890683122, 1.000000000000000000, 0.9659258262890683122, 1.000000000000000000, 0.9659258262890683122, 1.000000000000000000, 0.9659258262890683122, 1.000000000000000000, 0.9659258262890683122, 1.000000000000000000, 0.9659258262890683122, 1.000000000000000000, 0.9659258262890683122, 1.000000000000000000, 0.9659258262890683122, 1.000000000000000000, 0.9659258262890683122, 1.000000000000000000, 0.9659258262890683122, 1.000000000000000000, 0.9659258262890683122, 1.000000000000000000, 0.9659258262890683122, 1.000000000000000000, 0.9659258262890683122, 1.000000000000000000, 0.9659258262890683122, 1.000000000000000000, 0.9659258262890683122, 1.000000000000000000, 0.9659258262890683122, 1.000000000000000000, 0.9659258262890683122, 1.000000000000000000, 0.9659258262890683122, 1.000000000000000000, 0.9659258262890683122, 1.000000000000000000, 0.9659258262890683122, 1.000000000000000000, 0.9659258262890683122, 1.000000000000000000, 0.9659258262890683122, 1.000000000000000000, 0.9659258262890683122, 1.000000000000000000, 0.9659258262890683122, 1.000000000000000000, 0.9659258262890683122, 1.000000000000000000, 0.9659258262890683122, 1.000000000000000000, 0.9659258262890683122, 1.000000000000000000, 0.9659258262890683122, 1.000000000000000000, 0.9659258262890683122, 1.000000000000000000, 0.9659258262890683122, 1.000000000000000000, 0.9659258262890683122, 1.000000000000000000, 0.9659258262890683122, 1.000000000000000000, 0.9659258262890683122, 1.000000000000000000, 0.9659258262890683122, 1.000000000000000000, 0.9659258262890683122, 1.000000000000000000, 0.9659258262890683122, 1.000000000000000000, 0.9659258262890683122, 1.000000000000000000, 0.9659258262890683122, 1.000000000000000000, 0.9659258262890683122, 1.000000000000000000, 0.9659258262890683122, 1.000000000000000000, 0.9659258262890683122, 1.000000000000000000, 0.9659258262890683122, 1.000000000000000000, 0.9659258262890683122, 1.000000000000000000, 0.9659258262890683122, 1.000000000000000000, 0.9659258262890683122, 1.000000000000000000, 0.9659258262890683122, 1.000000000000000000, 0.9659258262890683122, 1.000000000000000000, 0.9659258262890683122, 1.000000000000000000, 0.9659258262890683122, 1.000000000000000000, 0.9659258262890683122, 1.000000000000000000, 0.9659258262890683122, 1.000000000000000000, 0.9659258262890683122, 1.000000000000000000, 0.9659258262890683122, 1.000000000000000000, 0.9659258262890683122, 1.000000000000000000, 0.9659258262890683122, 1.000000000000000000, 0.9659258262890683122, 1.000000000000000000, 0.9659258262890683122, 1.000000000000000000, 0.9659258262890683122, 1.000000000000000000, 0.9659258262890683122, 1.000000000000000000, 0.9659258262890683122, 1.000000000000000000, 0.9659258262890683122, 1.000000000000000000, 0.9659258262890683122, 1.000000000000000000, 0.9659258262890683122, 1.000000000000000000, 0.9659258262890683122, 1.000000000000000000, 0.9659258262890683122, 1.000000000000000000, 0.9659258262890683122, 1.000000000000000000, 0.9659258262890683122, 1.000000000000000000, 0.9659258262890683122, 1.000000000000000000, 0.9659258262890683122, 1.000000000000000000, 0.9659258262890683122, 1.000000000000000000, 0.9659258262890683122, 1.000000000000000000, 0.9659258262890683122, 1.000000000000000000, 0.9659258262890683122, 1.000000000000000000, 0.9659258262890683122, 1.000000000000000000, 0.9659258262890683122, 1.000000000000000000, 0.9659258262890683122, 1.000000000000000000, 0.9659258262890683122, 1.000000000000000000, 0.9659258262890683122, 1.000000000000000000, 0.9659258262890683122, 1.000000000000000000, 0.9659258262890683122, 1.000000000000000000, 0.9659258262890683122, 1.000000000000000000, 0.9659258262890683122, 1.000000000000000000, 0.9659258262890683122, 1.000000000000000000, 0.9659258262890683122, 1.000000000000000000, 0.9659258262890683122, 1.000000000000000000, 0.9659258262890683122, 1.000000000000000000, 0.9659258262890683122, 1.000000000000000000, 0.9659258262890683122, 1.000000000000000000, 0.9659258262890683122, 1.000000000000000000, 0.9659258262890683122, 1.000000000000000000, 0.9659258262890683122, 1.000000000000000000, 0.9659258262890683122, 1.000000000000000000, 0.9659258262890683122, 1.000000000000000000, 0.9659258262890683122, 1.000000000000000000, 0.9659258262890683122, 1.000000000000000000, 0.9659258262890683122, 1.000000000000000000, 0.9659258262890683122, 1.000000000000000000, 0.9659258262890683122, 1.000000000000000000, 0.9659258262890683122, 1.000000000000000000, 0.9659258262890683122, 1.000000000000000000, 0.9659258262890683122, 1.000000000000000000, 0.9659258262890683122, 1.000000000000000000, 0.9659258262890683122, 1.000000000000000000, 0.9659258262890683122, 1.000000000000000000, 0.9659258262890683122, 1.000000000000000000, 0.9659258262890683122, 1.000000000000000000, 0.9659258262890683122, 1.000000000000000000, 0.9659258262890683122, 1.000000000000000000, 0.9659258262890683122, 1.000000000000000000, 0.9659258262890683122, 1.000000000000000000, 0.9659258262890683122, 1.000000000000000000, 0.9659258262890683122, 1.000000000000000000, 0.9659258262890683122, 1.000000000000000000, 0.9659258262890683122, 1.000000000000000000, 0.9659258262890683122, 1.000000000000000000, 0.9659258262890683122, 1.000000000000000000, 0.9659258262890683122, 1.000000000000000000, 0.9659258262890683122, 1.000000000000000000, 0.9659258262890683122, 1.000000000000000000, 0.9659258262890683122, 1.000000000000000000, 0.9659258262890683122, 1.000000000000000000, 0.9659258262890683122, 1.000000000000000000, 0.9659258262890683122, 1.000000000000000000, 0.9659258262890683122, 1.000000000000000000, 0.9659258262890683122, 1.000000000000000000, 0.9659258262890683122, 1.000000000000000000, 0.9659258262890683122, 1.000000000000000000, 0.9659258262890683122, 1.000000000000000000, 0.9659258262890683122, 1.000000000000000000, 0.9659258262890683122, 1.000000000000000000, 0.9659258262890683122, 1.000000000000000000, 0.9659258262890683122, 1.000000000000000000, 0.9659258262890683122, 1.000000000000000000, 0.9659258262890683122, 1.000000000000000000, 0.9659258262890683122, 1.000000000000000000, 0.9659258262890683122, 1.000000000000000000, 0.9659258262890683122, 1.000000000000000000, 0.9659258262890683122, 1.000000000000000000, 0.9659258262890683122, 1.000000000000000000, 0.9659258262890683122, 1.000000000000000000, 0.9659258262890683122, 1.000000000000000000, 0.9659258262890683122, 1.000000000000000000, 0.9659258262890683122, 1.000000000000000000, 0.9659258262890683122, 1.000000000000000000, 0.9659258262890683122, 1.000000000000000000, 0.9659258262890683122, 1.000000000000000000, 0.9659258262890683122, 1.000000000000000000, 0.9659258262890683122, 1.000000000000000000, 0.9659258262890683122, 1.000000000000000000),
 ( 0.3333333333333333703, 0.3219752754296894559, 0.3333333333333333703, 0.3219752754296894559, 0.3333333333333333703, 0.3219752754296894559, 0.3333333333333333703, 0.3219752754296894559, 0.3333333333333333703, 0.3219752754296894559, 0.3333333333333333703, 0.3219752754296894559, 0.3333333333333333703, 0.3219752754296894559, 0.3333333333333333703, 0.3219752754296894559, 0.3333333333333333703, 0.3219752754296894559, 0.3333333333333333703, 0.3219752754296894559, 0.3333333333333333703, 0.3219752754296894559, 0.3333333333333333703, 0.3219752754296894559, 0.3333333333333333703, 0.3219752754296894559, 0.3333333333333333703, 0.3219752754296894559, 0.3333333333333333703, 0.3219752754296894559, 0.3333333333333333703, 0.3219752754296894559, 0.3333333333333333703, 0.3219752754296894559, 0.3333333333333333703, 0.3219752754296894559, 0.3333333333333333703, 0.3219752754296894559, 0.3333333333333333703, 0.3219752754296894559, 0.3333333333333333703, 0.3219752754296894559, 0.3333333333333333703, 0.3219752754296894559, 0.3333333333333333703, 0.3219752754296894559, 0.3333333333333333703, 0.3219752754296894559, 0.3333333333333333703, 0.3219752754296894559, 0.3333333333333333703, 0.3219752754296894559, 0.3333333333333333703, 0.3219752754296894559, 0.3333333333333333703, 0.3219752754296894559, 0.3333333333333333703, 0.3219752754296894559, 0.3333333333333333703, 0.3219752754296894559, 0.3333333333333333703, 0.3219752754296894559, 0.3333333333333333703, 0.3219752754296894559, 0.3333333333333333703, 0.3219752754296894559, 0.3333333333333333703, 0.3219752754296894559, 0.3333333333333333703, 0.3219752754296894559, 0.3333333333333333703, 0.3219752754296894559, 0.3333333333333333703, 0.3219752754296894559, 0.3333333333333333703, 0.3219752754296894559, 0.3333333333333333703, 0.3219752754296894559, 0.3333333333333333703, 0.3219752754296894559, 0.3333333333333333703, 0.3219752754296894559, 0.3333333333333333703, 0.3219752754296894559, 0.3333333333333333703, 0.3219752754296894559, 0.3333333333333333703, 0.3219752754296894559, 0.3333333333333333703, 0.3219752754296894559, 0.3333333333333333703, 0.3219752754296894559, 0.3333333333333333703, 0.3219752754296894559, 0.3333333333333333703, 0.3219752754296894559, 0.3333333333333333703, 0.3219752754296894559, 0.3333333333333333703, 0.3219752754296894559, 0.3333333333333333703, 0.3219752754296894559, 0.3333333333333333703, 0.3219752754296894559, 0.3333333333333333703, 0.3219752754296894559, 0.3333333333333333703, 0.3219752754296894559, 0.3333333333333333703, 0.3219752754296894559, 0.3333333333333333703, 0.3219752754296894559, 0.3333333333333333703, 0.3219752754296894559, 0.3333333333333333703, 0.3219752754296894559, 0.3333333333333333703, 0.3219752754296894559, 0.3333333333333333703, 0.3219752754296894559, 0.3333333333333333703, 0.3219752754296894559, 0.3333333333333333703, 0.3219752754296894559, 0.3333333333333333703, 0.3219752754296894559, 0.3333333333333333703, 0.3219752754296894559, 0.3333333333333333703, 0.3219752754296894559, 0.3333333333333333703, 0.3219752754296894559, 0.3333333333333333703, 0.3219752754296894559, 0.3333333333333333703, 0.3219752754296894559, 0.3333333333333333703, 0.3219752754296894559, 0.3333333333333333703, 0.3219752754296894559, 0.3333333333333333703, 0.3219752754296894559, 0.3333333333333333703, 0.3219752754296894559, 0.3333333333333333703, 0.3219752754296894559, 0.3333333333333333703, 0.3219752754296894559, 0.3333333333333333703, 0.3219752754296894559, 0.3333333333333333703, 0.3219752754296894559, 0.3333333333333333703, 0.3219752754296894559, 0.3333333333333333703, 0.3219752754296894559, 0.3333333333333333703, 0.3219752754296894559, 0.3333333333333333703, 0.3219752754296894559, 0.3333333333333333703, 0.3219752754296894559, 0.3333333333333333703, 0.3219752754296894559, 0.3333333333333333703, 0.3219752754296894559, 0.3333333333333333703, 0.3219752754296894559, 0.3333333333333333703, 0.3219752754296894559, 0.3333333333333333703, 0.3219752754296894559, 0.3333333333333333703, 0.3219752754296894559, 0.3333333333333333703, 0.3219752754296894559, 0.3333333333333333703, 0.3219752754296894559, 0.3333333333333333703, 0.3219752754296894559, 0.3333333333333333703, 0.3219752754296894559, 0.3333333333333333703, 0.3219752754296894559, 0.3333333333333333703, 0.3219752754296894559, 0.3333333333333333703, 0.3219752754296894559, 0.3333333333333333703, 0.3219752754296894559, 0.3333333333333333703, 0.3219752754296894559, 0.3333333333333333703, 0.3219752754296894559, 0.3333333333333333703, 0.3219752754296894559, 0.3333333333333333703, 0.3219752754296894559, 0.3333333333333333703, 0.3219752754296894559, 0.3333333333333333703, 0.3219752754296894559, 0.3333333333333333703, 0.3219752754296894559, 0.3333333333333333703, 0.3219752754296894559, 0.3333333333333333703, 0.3219752754296894559, 0.3333333333333333703, 0.3219752754296894559, 0.3333333333333333703, 0.3219752754296894559, 0.3333333333333333703, 0.3219752754296894559, 0.3333333333333333703, 0.3219752754296894559, 0.3333333333333333703, 0.3219752754296894559, 0.3333333333333333703, 0.3219752754296894559, 0.3333333333333333703, 0.3219752754296894559, 0.3333333333333333703, 0.3219752754296894559, 0.3333333333333333703, 0.3219752754296894559, 0.3333333333333333703, 0.3219752754296894559, 0.3333333333333333703, 0.3219752754296894559, 0.3333333333333333703, 0.3219752754296894559, 0.3333333333333333703, 0.3219752754296894559, 0.3333333333333333703, 0.3219752754296894559, 0.3333333333333333703, 0.3219752754296894559, 0.3333333333333333703, 0.3219752754296894559, 0.3333333333333333703, 0.3219752754296894559, 0.3333333333333333703, 0.3219752754296894559, 0.3333333333333333703, 0.3219752754296894559, 0.3333333333333333703, 0.3219752754296894559, 0.3333333333333333703, 0.3219752754296894559, 0.3333333333333333703, 0.3219752754296894559, 0.3333333333333333703, 0.3219752754296894559, 0.3333333333333333703, 0.3219752754296894559, 0.3333333333333333703, 0.3219752754296894559, 0.3333333333333333703, 0.3219752754296894559, 0.3333333333333333703, 0.3219752754296894559, 0.3333333333333333703, 0.3219752754296894559, 0.3333333333333333703, 0.3219752754296894559, 0.3333333333333333703, 0.3219752754296894559, 0.3333333333333333703, 0.3219752754296894559, 0.3333333333333333703, 0.3219752754296894559, 0.3333333333333333703, 0.3219752754296894559, 0.3333333333333333703, 0.3219752754296894559, 0.3333333333333333703, 0.3219752754296894559, 0.3333333333333333703, 0.3219752754296894559, 0.3333333333333333703, 0.3219752754296894559, 0.3333333333333333703, 0.3219752754296894559, 0.3333333333333333703, 0.3219752754296894559, 0.3333333333333333703, 0.3219752754296894559, 0.3333333333333333703, 0.3219752754296894559, 0.3333333333333333703, 0.3219752754296894559, 0.3333333333333333703, 0.3219752754296894559, 0.3333333333333333703, 0.3219752754296894559, 0.3333333333333333703, 0.3219752754296894559, 0.3333333333333333703, 0.3219752754296894559, 0.3333333333333333703, 0.3219752754296894559, 0.3333333333333333703, 0.3219752754296894559, 0.3333333333333333703, 0.3219752754296894559, 0.3333333333333333703, 0.3219752754296894559, 0.3333333333333333703, 0.3219752754296894559, 0.3333333333333333703, 0.3219752754296894559, 0.3333333333333333703, 0.3219752754296894559, 0.3333333333333333703, 0.3219752754296894559, 0.3333333333333333703, 0.3219752754296894559, 0.3333333333333333703, 0.3219752754296894559, 0.3333333333333333703, 0.3219752754296894559, 0.3333333333333333703, 0.3219752754296894559, 0.3333333333333333703, 0.3219752754296894559, 0.3333333333333333703, 0.3219752754296894559, 0.3333333333333333703, 0.3219752754296894559, 0.3333333333333333703, 0.3219752754296894559, 0.3333333333333333703, 0.3219752754296894559, 0.3333333333333333703, 0.3219752754296894559, 0.3333333333333333703, 0.3219752754296894559, 0.3333333333333333703, 0.3219752754296894559, 0.3333333333333333703, 0.3219752754296894559, 0.3333333333333333703, 0.3219752754296894559, 0.3333333333333333703, 0.3219752754296894559, 0.3333333333333333703, 0.3219752754296894559, 0.3333333333333333703, 0.3219752754296894559, 0.3333333333333333703, 0.3219752754296894559, 0.3333333333333333703, 0.3219752754296894559, 0.3333333333333333703, 0.3219752754296894559, 0.3333333333333333703, 0.3219752754296894559, 0.3333333333333333703, 0.3219752754296894559, 0.3333333333333333703, 0.3219752754296894559, 0.3333333333333333703, 0.3219752754296894559, 0.3333333333333333703, 0.3219752754296894559, 0.3333333333333333703, 0.3219752754296894559, 0.3333333333333333703, 0.3219752754296894559, 0.3333333333333333703, 0.3219752754296894559, 0.3333333333333333703, 0.3219752754296894559, 0.3333333333333333703, 0.3219752754296894559, 0.3333333333333333703, 0.3219752754296894559, 0.3333333333333333703, 0.3219752754296894559, 0.3333333333333333703, 0.3219752754296894559, 0.3333333333333333703, 0.3219752754296894559, 0.3333333333333333703, 0.3219752754296894559, 0.3333333333333333703, 0.3219752754296894559, 0.3333333333333333703, 0.3219752754296894559, 0.3333333333333333703, 0.3219752754296894559, 0.3333333333333333703, 0.3219752754296894559, 0.3333333333333333703, 0.3219752754296894559, 0.3333333333333333703, 0.3219752754296894559, 0.3333333333333333703, 0.3219752754296894559, 0.3333333333333333703, 0.3219752754296894559, 0.3333333333333333703, 0.3219752754296894559, 0.3333333333333333703, 0.3219752754296894559, 0.3333333333333333703, 0.3219752754296894559, 0.3333333333333333703, 0.3219752754296894559, 0.3333333333333333703, 0.3219752754296894559, 0.3333333333333333703, 0.3219752754296894559, 0.3333333333333333703, 0.3219752754296894559, 0.3333333333333333703, 0.3219752754296894559, 0.3333333333333333703, 0.3219752754296894559, 0.3333333333333333703, 0.3219752754296894559, 0.3333333333333333703, 0.3219752754296894559, 0.3333333333333333703, 0.3219752754296894559, 0.3333333333333333703, 0.3219752754296894559, 0.3333333333333333703, 0.3219752754296894559, 0.3333333333333333703, 0.3219752754296894559, 0.3333333333333333703, 0.3219752754296894559, 0.3333333333333333703, 0.3219752754296894559, 0.3333333333333333703, 0.3219752754296894559, 0.3333333333333333703, 0.3219752754296894559, 0.3333333333333333703, 0.3219752754296894559, 0.3333333333333333703, 0.3219752754296894559, 0.3333333333333333703, 0.3219752754296894559, 0.3333333333333333703, 0.3219752754296894559, 0.3333333333333333703, 0.3219752754296894559, 0.3333333333333333703, 0.3219752754296894559, 0.3333333333333333703, 0.3219752754296894559, 0.3333333333333333703, 0.3219752754296894559, 0.3333333333333333703),
 ( 0.3333333333333333703, 0.3219752754296894559, 0.3333333333333333703, 0.3219752754296894559, 0.3333333333333333703, 0.3219752754296894559, 0.3333333333333333703, 0.3219752754296894559, 0.3333333333333333703, 0.3219752754296894559, 0.3333333333333333703, 0.3219752754296894559, 0.3333333333333333703, 0.3219752754296894559, 0.3333333333333333703, 0.3219752754296894559, 0.3333333333333333703, 0.3219752754296894559, 0.3333333333333333703, 0.3219752754296894559, 0.3333333333333333703, 0.3219752754296894559, 0.3333333333333333703, 0.3219752754296894559, 0.3333333333333333703, 0.3219752754296894559, 0.3333333333333333703, 0.3219752754296894559, 0.3333333333333333703, 0.3219752754296894559, 0.3333333333333333703, 0.3219752754296894559, 0.3333333333333333703, 0.3219752754296894559, 0.3333333333333333703, 0.3219752754296894559, 0.3333333333333333703, 0.3219752754296894559, 0.3333333333333333703, 0.3219752754296894559, 0.3333333333333333703, 0.3219752754296894559, 0.3333333333333333703, 0.3219752754296894559, 0.3333333333333333703, 0.3219752754296894559, 0.3333333333333333703, 0.3219752754296894559, 0.3333333333333333703, 0.3219752754296894559, 0.3333333333333333703, 0.3219752754296894559, 0.3333333333333333703, 0.3219752754296894559, 0.3333333333333333703, 0.3219752754296894559, 0.3333333333333333703, 0.3219752754296894559, 0.3333333333333333703, 0.3219752754296894559, 0.3333333333333333703, 0.3219752754296894559, 0.3333333333333333703, 0.3219752754296894559, 0.3333333333333333703, 0.3219752754296894559, 0.3333333333333333703, 0.3219752754296894559, 0.3333333333333333703, 0.3219752754296894559, 0.3333333333333333703, 0.3219752754296894559, 0.3333333333333333703, 0.3219752754296894559, 0.3333333333333333703, 0.3219752754296894559, 0.3333333333333333703, 0.3219752754296894559, 0.3333333333333333703, 0.3219752754296894559, 0.3333333333333333703, 0.3219752754296894559, 0.3333333333333333703, 0.3219752754296894559, 0.3333333333333333703, 0.3219752754296894559, 0.3333333333333333703, 0.3219752754296894559, 0.3333333333333333703, 0.3219752754296894559, 0.3333333333333333703, 0.3219752754296894559, 0.3333333333333333703, 0.3219752754296894559, 0.3333333333333333703, 0.3219752754296894559, 0.3333333333333333703, 0.3219752754296894559, 0.3333333333333333703, 0.3219752754296894559, 0.3333333333333333703, 0.3219752754296894559, 0.3333333333333333703, 0.3219752754296894559, 0.3333333333333333703, 0.3219752754296894559, 0.3333333333333333703, 0.3219752754296894559, 0.3333333333333333703, 0.3219752754296894559, 0.3333333333333333703, 0.3219752754296894559, 0.3333333333333333703, 0.3219752754296894559, 0.3333333333333333703, 0.3219752754296894559, 0.3333333333333333703, 0.3219752754296894559, 0.3333333333333333703, 0.3219752754296894559, 0.3333333333333333703, 0.3219752754296894559, 0.3333333333333333703, 0.3219752754296894559, 0.3333333333333333703, 0.3219752754296894559, 0.3333333333333333703, 0.3219752754296894559, 0.3333333333333333703, 0.3219752754296894559, 0.3333333333333333703, 0.3219752754296894559, 0.3333333333333333703, 0.3219752754296894559, 0.3333333333333333703, 0.3219752754296894559, 0.3333333333333333703, 0.3219752754296894559, 0.3333333333333333703, 0.3219752754296894559, 0.3333333333333333703, 0.3219752754296894559, 0.3333333333333333703, 0.3219752754296894559, 0.3333333333333333703, 0.3219752754296894559, 0.3333333333333333703, 0.3219752754296894559, 0.3333333333333333703, 0.3219752754296894559, 0.3333333333333333703, 0.3219752754296894559, 0.3333333333333333703, 0.3219752754296894559, 0.3333333333333333703, 0.3219752754296894559, 0.3333333333333333703, 0.3219752754296894559, 0.3333333333333333703, 0.3219752754296894559, 0.3333333333333333703, 0.3219752754296894559, 0.3333333333333333703, 0.3219752754296894559, 0.3333333333333333703, 0.3219752754296894559, 0.3333333333333333703, 0.3219752754296894559, 0.3333333333333333703, 0.3219752754296894559, 0.3333333333333333703, 0.3219752754296894559, 0.3333333333333333703, 0.3219752754296894559, 0.3333333333333333703, 0.3219752754296894559, 0.3333333333333333703, 0.3219752754296894559, 0.3333333333333333703, 0.3219752754296894559, 0.3333333333333333703, 0.3219752754296894559, 0.3333333333333333703, 0.3219752754296894559, 0.3333333333333333703, 0.3219752754296894559, 0.3333333333333333703, 0.3219752754296894559, 0.3333333333333333703, 0.3219752754296894559, 0.3333333333333333703, 0.3219752754296894559, 0.3333333333333333703, 0.3219752754296894559, 0.3333333333333333703, 0.3219752754296894559, 0.3333333333333333703, 0.3219752754296894559, 0.3333333333333333703, 0.3219752754296894559, 0.3333333333333333703, 0.3219752754296894559, 0.3333333333333333703, 0.3219752754296894559, 0.3333333333333333703, 0.3219752754296894559, 0.3333333333333333703, 0.3219752754296894559, 0.3333333333333333703, 0.3219752754296894559, 0.3333333333333333703, 0.3219752754296894559, 0.3333333333333333703, 0.3219752754296894559, 0.3333333333333333703, 0.3219752754296894559, 0.3333333333333333703, 0.3219752754296894559, 0.3333333333333333703, 0.3219752754296894559, 0.3333333333333333703, 0.3219752754296894559, 0.3333333333333333703, 0.3219752754296894559, 0.3333333333333333703, 0.3219752754296894559, 0.3333333333333333703, 0.3219752754296894559, 0.3333333333333333703, 0.3219752754296894559, 0.3333333333333333703, 0.3219752754296894559, 0.3333333333333333703, 0.3219752754296894559, 0.3333333333333333703, 0.3219752754296894559, 0.3333333333333333703, 0.3219752754296894559, 0.3333333333333333703, 0.3219752754296894559, 0.3333333333333333703, 0.3219752754296894559, 0.3333333333333333703, 0.3219752754296894559, 0.3333333333333333703, 0.3219752754296894559, 0.3333333333333333703, 0.3219752754296894559, 0.3333333333333333703, 0.3219752754296894559, 0.3333333333333333703, 0.3219752754296894559, 0.3333333333333333703, 0.3219752754296894559, 0.3333333333333333703, 0.3219752754296894559, 0.3333333333333333703, 0.3219752754296894559, 0.3333333333333333703, 0.3219752754296894559, 0.3333333333333333703, 0.3219752754296894559, 0.3333333333333333703, 0.3219752754296894559, 0.3333333333333333703, 0.3219752754296894559, 0.3333333333333333703, 0.3219752754296894559, 0.3333333333333333703, 0.3219752754296894559, 0.3333333333333333703, 0.3219752754296894559, 0.3333333333333333703, 0.3219752754296894559, 0.3333333333333333703, 0.3219752754296894559, 0.3333333333333333703, 0.3219752754296894559, 0.3333333333333333703, 0.3219752754296894559, 0.3333333333333333703, 0.3219752754296894559, 0.3333333333333333703, 0.3219752754296894559, 0.3333333333333333703, 0.3219752754296894559, 0.3333333333333333703, 0.3219752754296894559, 0.3333333333333333703, 0.3219752754296894559, 0.3333333333333333703, 0.3219752754296894559, 0.3333333333333333703, 0.3219752754296894559, 0.3333333333333333703, 0.3219752754296894559, 0.3333333333333333703, 0.3219752754296894559, 0.3333333333333333703, 0.3219752754296894559, 0.3333333333333333703, 0.3219752754296894559, 0.3333333333333333703, 0.3219752754296894559, 0.3333333333333333703, 0.3219752754296894559, 0.3333333333333333703, 0.3219752754296894559, 0.3333333333333333703, 0.3219752754296894559, 0.3333333333333333703, 0.3219752754296894559, 0.3333333333333333703, 0.3219752754296894559, 0.3333333333333333703, 0.3219752754296894559, 0.3333333333333333703, 0.3219752754296894559, 0.3333333333333333703, 0.3219752754296894559, 0.3333333333333333703, 0.3219752754296894559, 0.3333333333333333703, 0.3219752754296894559, 0.3333333333333333703, 0.3219752754296894559, 0.3333333333333333703, 0.3219752754296894559, 0.3333333333333333703, 0.3219752754296894559, 0.3333333333333333703, 0.3219752754296894559, 0.3333333333333333703, 0.3219752754296894559, 0.3333333333333333703, 0.3219752754296894559, 0.3333333333333333703, 0.3219752754296894559, 0.3333333333333333703, 0.3219752754296894559, 0.3333333333333333703, 0.3219752754296894559, 0.3333333333333333703, 0.3219752754296894559, 0.3333333333333333703, 0.3219752754296894559, 0.3333333333333333703, 0.3219752754296894559, 0.3333333333333333703, 0.3219752754296894559, 0.3333333333333333703, 0.3219752754296894559, 0.3333333333333333703, 0.3219752754296894559, 0.3333333333333333703, 0.3219752754296894559, 0.3333333333333333703, 0.3219752754296894559, 0.3333333333333333703, 0.3219752754296894559, 0.3333333333333333703, 0.3219752754296894559, 0.3333333333333333703, 0.3219752754296894559, 0.3333333333333333703, 0.3219752754296894559, 0.3333333333333333703, 0.3219752754296894559, 0.3333333333333333703, 0.3219752754296894559, 0.3333333333333333703, 0.3219752754296894559, 0.3333333333333333703, 0.3219752754296894559, 0.3333333333333333703, 0.3219752754296894559, 0.3333333333333333703, 0.3219752754296894559, 0.3333333333333333703, 0.3219752754296894559, 0.3333333333333333703, 0.3219752754296894559, 0.3333333333333333703, 0.3219752754296894559, 0.3333333333333333703, 0.3219752754296894559, 0.3333333333333333703, 0.3219752754296894559, 0.3333333333333333703, 0.3219752754296894559, 0.3333333333333333703, 0.3219752754296894559, 0.3333333333333333703, 0.3219752754296894559, 0.3333333333333333703, 0.3219752754296894559, 0.3333333333333333703, 0.3219752754296894559, 0.3333333333333333703, 0.3219752754296894559, 0.3333333333333333703, 0.3219752754296894559, 0.3333333333333333703, 0.3219752754296894559, 0.3333333333333333703, 0.3219752754296894559, 0.3333333333333333703, 0.3219752754296894559, 0.3333333333333333703, 0.3219752754296894559, 0.3333333333333333703, 0.3219752754296894559, 0.3333333333333333703, 0.3219752754296894559, 0.3333333333333333703, 0.3219752754296894559, 0.3333333333333333703, 0.3219752754296894559, 0.3333333333333333703, 0.3219752754296894559, 0.3333333333333333703, 0.3219752754296894559, 0.3333333333333333703, 0.3219752754296894559, 0.3333333333333333703, 0.3219752754296894559, 0.3333333333333333703, 0.3219752754296894559, 0.3333333333333333703, 0.3219752754296894559, 0.3333333333333333703, 0.3219752754296894559, 0.3333333333333333703, 0.3219752754296894559, 0.3333333333333333703, 0.3219752754296894559, 0.3333333333333333703, 0.3219752754296894559, 0.3333333333333333703, 0.3219752754296894559, 0.3333333333333333703, 0.3219752754296894559, 0.3333333333333333703, 0.3219752754296894559, 0.3333333333333333703, 0.3219752754296894559, 0.3333333333333333703, 0.3219752754296894559, 0.3333333333333333703, 0.3219752754296894559, 0.3333333333333333703, 0.3219752754296894559, 0.3333333333333333703, 0.3219752754296894559, 0.3333333333333333703, 0.3219752754296894559, 0.3333333333333333703),
 ( 1.000000000000000000, 0.9659258262890683122, 1.000000000000000000, 0.9659258262890683122, 1.000000000000000000, 0.9659258262890683122, 1.000000000000000000, 0.9659258262890683122, 1.000000000000000000, 0.9659258262890683122, 1.000000000000000000, 0.9659258262890683122, 1.000000000000000000, 0.9659258262890683122, 1.000000000000000000, 0.9659258262890683122, 1.000000000000000000, 0.9659258262890683122, 1.000000000000000000, 0.9659258262890683122, 1.000000000000000000, 0.9659258262890683122, 1.000000000000000000, 0.9659258262890683122, 1.000000000000000000, 0.9659258262890683122, 1.000000000000000000, 0.9659258262890683122, 1.000000000000000000, 0.9659258262890683122, 1.000000000000000000, 0.9659258262890683122, 1.000000000000000000, 0.9659258262890683122, 1.000000000000000000, 0.9659258262890683122, 1.000000000000000000, 0.9659258262890683122, 1.000000000000000000, 0.9659258262890683122, 1.000000000000000000, 0.9659258262890683122, 1.000000000000000000, 0.9659258262890683122, 1.000000000000000000, 0.9659258262890683122, 1.000000000000000000, 0.9659258262890683122, 1.000000000000000000, 0.9659258262890683122, 1.000000000000000000, 0.9659258262890683122, 1.000000000000000000, 0.9659258262890683122, 1.000000000000000000, 0.9659258262890683122, 1.000000000000000000, 0.9659258262890683122, 1.000000000000000000, 0.9659258262890683122, 1.000000000000000000, 0.9659258262890683122, 1.000000000000000000, 0.9659258262890683122, 1.000000000000000000, 0.9659258262890683122, 1.000000000000000000, 0.9659258262890683122, 1.000000000000000000, 0.9659258262890683122, 1.000000000000000000, 0.9659258262890683122, 1.000000000000000000, 0.9659258262890683122, 1.000000000000000000, 0.9659258262890683122, 1.000000000000000000, 0.9659258262890683122, 1.000000000000000000, 0.9659258262890683122, 1.000000000000000000, 0.9659258262890683122, 1.000000000000000000, 0.9659258262890683122, 1.000000000000000000, 0.9659258262890683122, 1.000000000000000000, 0.9659258262890683122, 1.000000000000000000, 0.9659258262890683122, 1.000000000000000000, 0.9659258262890683122, 1.000000000000000000, 0.9659258262890683122, 1.000000000000000000, 0.9659258262890683122, 1.000000000000000000, 0.9659258262890683122, 1.000000000000000000, 0.9659258262890683122, 1.000000000000000000, 0.9659258262890683122, 1.000000000000000000, 0.9659258262890683122, 1.000000000000000000, 0.9659258262890683122, 1.000000000000000000, 0.9659258262890683122, 1.000000000000000000, 0.9659258262890683122, 1.000000000000000000, 0.9659258262890683122, 1.000000000000000000, 0.9659258262890683122, 1.000000000000000000, 0.9659258262890683122, 1.000000000000000000, 0.9659258262890683122, 1.000000000000000000, 0.9659258262890683122, 1.000000000000000000, 0.9659258262890683122, 1.000000000000000000, 0.9659258262890683122, 1.000000000000000000, 0.9659258262890683122, 1.000000000000000000, 0.9659258262890683122, 1.000000000000000000, 0.9659258262890683122, 1.000000000000000000, 0.9659258262890683122, 1.000000000000000000, 0.9659258262890683122, 1.000000000000000000, 0.9659258262890683122, 1.000000000000000000, 0.9659258262890683122, 1.000000000000000000, 0.9659258262890683122, 1.000000000000000000, 0.9659258262890683122, 1.000000000000000000, 0.9659258262890683122, 1.000000000000000000, 0.9659258262890683122, 1.000000000000000000, 0.9659258262890683122, 1.000000000000000000, 0.9659258262890683122, 1.000000000000000000, 0.9659258262890683122, 1.000000000000000000, 0.9659258262890683122, 1.000000000000000000, 0.9659258262890683122, 1.000000000000000000, 0.9659258262890683122, 1.000000000000000000, 0.9659258262890683122, 1.000000000000000000, 0.9659258262890683122, 1.000000000000000000, 0.9659258262890683122, 1.000000000000000000, 0.9659258262890683122, 1.000000000000000000, 0.9659258262890683122, 1.000000000000000000, 0.9659258262890683122, 1.000000000000000000, 0.9659258262890683122, 1.000000000000000000, 0.9659258262890683122, 1.000000000000000000, 0.9659258262890683122, 1.000000000000000000, 0.9659258262890683122, 1.000000000000000000, 0.9659258262890683122, 1.000000000000000000, 0.9659258262890683122, 1.000000000000000000, 0.9659258262890683122, 1.000000000000000000, 0.9659258262890683122, 1.000000000000000000, 0.9659258262890683122, 1.000000000000000000, 0.9659258262890683122, 1.000000000000000000, 0.9659258262890683122, 1.000000000000000000, 0.9659258262890683122, 1.000000000000000000, 0.9659258262890683122, 1.000000000000000000, 0.9659258262890683122, 1.000000000000000000, 0.9659258262890683122, 1.000000000000000000, 0.9659258262890683122, 1.000000000000000000, 0.9659258262890683122, 1.000000000000000000, 0.9659258262890683122, 1.000000000000000000, 0.9659258262890683122, 1.000000000000000000, 0.9659258262890683122, 1.000000000000000000, 0.9659258262890683122, 1.000000000000000000, 0.9659258262890683122, 1.000000000000000000, 0.9659258262890683122, 1.000000000000000000, 0.9659258262890683122, 1.000000000000000000, 0.9659258262890683122, 1.000000000000000000, 0.9659258262890683122, 1.000000000000000000, 0.9659258262890683122, 1.000000000000000000, 0.9659258262890683122, 1.000000000000000000, 0.9659258262890683122, 1.000000000000000000, 0.9659258262890683122, 1.000000000000000000, 0.9659258262890683122, 1.000000000000000000, 0.9659258262890683122, 1.000000000000000000, 0.9659258262890683122, 1.000000000000000000, 0.9659258262890683122, 1.000000000000000000, 0.9659258262890683122, 1.000000000000000000, 0.9659258262890683122, 1.000000000000000000, 0.9659258262890683122, 1.000000000000000000, 0.9659258262890683122, 1.000000000000000000, 0.9659258262890683122, 1.000000000000000000, 0.9659258262890683122, 1.000000000000000000, 0.9659258262890683122, 1.000000000000000000, 0.9659258262890683122, 1.000000000000000000, 0.9659258262890683122, 1.000000000000000000, 0.9659258262890683122, 1.000000000000000000, 0.9659258262890683122, 1.000000000000000000, 0.9659258262890683122, 1.000000000000000000, 0.9659258262890683122, 1.000000000000000000, 0.9659258262890683122, 1.000000000000000000, 0.9659258262890683122, 1.000000000000000000, 0.9659258262890683122, 1.000000000000000000, 0.9659258262890683122, 1.000000000000000000, 0.9659258262890683122, 1.000000000000000000, 0.9659258262890683122, 1.000000000000000000, 0.9659258262890683122, 1.000000000000000000, 0.9659258262890683122, 1.000000000000000000, 0.9659258262890683122, 1.000000000000000000, 0.9659258262890683122, 1.000000000000000000, 0.9659258262890683122, 1.000000000000000000, 0.9659258262890683122, 1.000000000000000000, 0.9659258262890683122, 1.000000000000000000, 0.9659258262890683122, 1.000000000000000000, 0.9659258262890683122, 1.000000000000000000, 0.9659258262890683122, 1.000000000000000000, 0.9659258262890683122, 1.000000000000000000, 0.9659258262890683122, 1.000000000000000000, 0.9659258262890683122, 1.000000000000000000, 0.9659258262890683122, 1.000000000000000000, 0.9659258262890683122, 1.000000000000000000, 0.9659258262890683122, 1.000000000000000000, 0.9659258262890683122, 1.000000000000000000, 0.9659258262890683122, 1.000000000000000000, 0.9659258262890683122, 1.000000000000000000, 0.9659258262890683122, 1.000000000000000000, 0.9659258262890683122, 1.000000000000000000, 0.9659258262890683122, 1.000000000000000000, 0.9659258262890683122, 1.000000000000000000, 0.9659258262890683122, 1.000000000000000000, 0.9659258262890683122, 1.000000000000000000, 0.9659258262890683122, 1.000000000000000000, 0.9659258262890683122, 1.000000000000000000, 0.9659258262890683122, 1.000000000000000000, 0.9659258262890683122, 1.000000000000000000, 0.9659258262890683122, 1.000000000000000000, 0.9659258262890683122, 1.000000000000000000, 0.9659258262890683122, 1.000000000000000000, 0.9659258262890683122, 1.000000000000000000, 0.9659258262890683122, 1.000000000000000000, 0.9659258262890683122, 1.000000000000000000, 0.9659258262890683122, 1.000000000000000000, 0.9659258262890683122, 1.000000000000000000, 0.9659258262890683122, 1.000000000000000000, 0.9659258262890683122, 1.000000000000000000, 0.9659258262890683122, 1.000000000000000000, 0.9659258262890683122, 1.000000000000000000, 0.9659258262890683122, 1.000000000000000000, 0.9659258262890683122, 1.000000000000000000, 0.9659258262890683122, 1.000000000000000000, 0.9659258262890683122, 1.000000000000000000, 0.9659258262890683122, 1.000000000000000000, 0.9659258262890683122, 1.000000000000000000, 0.9659258262890683122, 1.000000000000000000, 0.9659258262890683122, 1.000000000000000000, 0.9659258262890683122, 1.000000000000000000, 0.9659258262890683122, 1.000000000000000000, 0.9659258262890683122, 1.000000000000000000, 0.9659258262890683122, 1.000000000000000000, 0.9659258262890683122, 1.000000000000000000, 0.9659258262890683122, 1.000000000000000000, 0.9659258262890683122, 1.000000000000000000, 0.9659258262890683122, 1.000000000000000000, 0.9659258262890683122, 1.000000000000000000, 0.9659258262890683122, 1.000000000000000000, 0.9659258262890683122, 1.000000000000000000, 0.9659258262890683122, 1.000000000000000000, 0.9659258262890683122, 1.000000000000000000, 0.9659258262890683122, 1.000000000000000000, 0.9659258262890683122, 1.000000000000000000, 0.9659258262890683122, 1.000000000000000000, 0.9659258262890683122, 1.000000000000000000, 0.9659258262890683122, 1.000000000000000000, 0.9659258262890683122, 1.000000000000000000, 0.9659258262890683122, 1.000000000000000000, 0.9659258262890683122, 1.000000000000000000, 0.9659258262890683122, 1.000000000000000000, 0.9659258262890683122, 1.000000000000000000, 0.9659258262890683122, 1.000000000000000000, 0.9659258262890683122, 1.000000000000000000, 0.9659258262890683122, 1.000000000000000000, 0.9659258262890683122, 1.000000000000000000, 0.9659258262890683122, 1.000000000000000000, 0.9659258262890683122, 1.000000000000000000, 0.9659258262890683122, 1.000000000000000000, 0.9659258262890683122, 1.000000000000000000, 0.9659258262890683122, 1.000000000000000000, 0.9659258262890683122, 1.000000000000000000, 0.9659258262890683122, 1.000000000000000000, 0.9659258262890683122, 1.000000000000000000, 0.9659258262890683122, 1.000000000000000000, 0.9659258262890683122, 1.000000000000000000, 0.9659258262890683122, 1.000000000000000000, 0.9659258262890683122, 1.000000000000000000, 0.9659258262890683122, 1.000000000000000000, 0.9659258262890683122, 1.000000000000000000),
 ( 0.3333333333333333703, 0.3219752754296894559, 0.3333333333333333703, 0.3219752754296894559, 0.3333333333333333703, 0.3219752754296894559, 0.3333333333333333703, 0.3219752754296894559, 0.3333333333333333703, 0.3219752754296894559, 0.3333333333333333703, 0.3219752754296894559, 0.3333333333333333703, 0.3219752754296894559, 0.3333333333333333703, 0.3219752754296894559, 0.3333333333333333703, 0.3219752754296894559, 0.3333333333333333703, 0.3219752754296894559, 0.3333333333333333703, 0.3219752754296894559, 0.3333333333333333703, 0.3219752754296894559, 0.3333333333333333703, 0.3219752754296894559, 0.3333333333333333703, 0.3219752754296894559, 0.3333333333333333703, 0.3219752754296894559, 0.3333333333333333703, 0.3219752754296894559, 0.3333333333333333703, 0.3219752754296894559, 0.3333333333333333703, 0.3219752754296894559, 0.3333333333333333703, 0.3219752754296894559, 0.3333333333333333703, 0.3219752754296894559, 0.3333333333333333703, 0.3219752754296894559, 0.3333333333333333703, 0.3219752754296894559, 0.3333333333333333703, 0.3219752754296894559, 0.3333333333333333703, 0.3219752754296894559, 0.3333333333333333703, 0.3219752754296894559, 0.3333333333333333703, 0.3219752754296894559, 0.3333333333333333703, 0.3219752754296894559, 0.3333333333333333703, 0.3219752754296894559, 0.3333333333333333703, 0.3219752754296894559, 0.3333333333333333703, 0.3219752754296894559, 0.3333333333333333703, 0.3219752754296894559, 0.3333333333333333703, 0.3219752754296894559, 0.3333333333333333703, 0.3219752754296894559, 0.3333333333333333703, 0.3219752754296894559, 0.3333333333333333703, 0.3219752754296894559, 0.3333333333333333703, 0.3219752754296894559, 0.3333333333333333703, 0.3219752754296894559, 0.3333333333333333703, 0.3219752754296894559, 0.3333333333333333703, 0.3219752754296894559, 0.3333333333333333703, 0.3219752754296894559, 0.3333333333333333703, 0.3219752754296894559, 0.3333333333333333703, 0.3219752754296894559, 0.3333333333333333703, 0.3219752754296894559, 0.3333333333333333703, 0.3219752754296894559, 0.3333333333333333703, 0.3219752754296894559, 0.3333333333333333703, 0.3219752754296894559, 0.3333333333333333703, 0.3219752754296894559, 0.3333333333333333703, 0.3219752754296894559, 0.3333333333333333703, 0.3219752754296894559, 0.3333333333333333703, 0.3219752754296894559, 0.3333333333333333703, 0.3219752754296894559, 0.3333333333333333703, 0.3219752754296894559, 0.3333333333333333703, 0.3219752754296894559, 0.3333333333333333703, 0.3219752754296894559, 0.3333333333333333703, 0.3219752754296894559, 0.3333333333333333703, 0.3219752754296894559, 0.3333333333333333703, 0.3219752754296894559, 0.3333333333333333703, 0.3219752754296894559, 0.3333333333333333703, 0.3219752754296894559, 0.3333333333333333703, 0.3219752754296894559, 0.3333333333333333703, 0.3219752754296894559, 0.3333333333333333703, 0.3219752754296894559, 0.3333333333333333703, 0.3219752754296894559, 0.3333333333333333703, 0.3219752754296894559, 0.3333333333333333703, 0.3219752754296894559, 0.3333333333333333703, 0.3219752754296894559, 0.3333333333333333703, 0.3219752754296894559, 0.3333333333333333703, 0.3219752754296894559, 0.3333333333333333703, 0.3219752754296894559, 0.3333333333333333703, 0.3219752754296894559, 0.3333333333333333703, 0.3219752754296894559, 0.3333333333333333703, 0.3219752754296894559, 0.3333333333333333703, 0.3219752754296894559, 0.3333333333333333703, 0.3219752754296894559, 0.3333333333333333703, 0.3219752754296894559, 0.3333333333333333703, 0.3219752754296894559, 0.3333333333333333703, 0.3219752754296894559, 0.3333333333333333703, 0.3219752754296894559, 0.3333333333333333703, 0.3219752754296894559, 0.3333333333333333703, 0.3219752754296894559, 0.3333333333333333703, 0.3219752754296894559, 0.3333333333333333703, 0.3219752754296894559, 0.3333333333333333703, 0.3219752754296894559, 0.3333333333333333703, 0.3219752754296894559, 0.3333333333333333703, 0.3219752754296894559, 0.3333333333333333703, 0.3219752754296894559, 0.3333333333333333703, 0.3219752754296894559, 0.3333333333333333703, 0.3219752754296894559, 0.3333333333333333703, 0.3219752754296894559, 0.3333333333333333703, 0.3219752754296894559, 0.3333333333333333703, 0.3219752754296894559, 0.3333333333333333703, 0.3219752754296894559, 0.3333333333333333703, 0.3219752754296894559, 0.3333333333333333703, 0.3219752754296894559, 0.3333333333333333703, 0.3219752754296894559, 0.3333333333333333703, 0.3219752754296894559, 0.3333333333333333703, 0.3219752754296894559, 0.3333333333333333703, 0.3219752754296894559, 0.3333333333333333703, 0.3219752754296894559, 0.3333333333333333703, 0.3219752754296894559, 0.3333333333333333703, 0.3219752754296894559, 0.3333333333333333703, 0.3219752754296894559, 0.3333333333333333703, 0.3219752754296894559, 0.3333333333333333703, 0.3219752754296894559, 0.3333333333333333703, 0.3219752754296894559, 0.3333333333333333703, 0.3219752754296894559, 0.3333333333333333703, 0.3219752754296894559, 0.3333333333333333703, 0.3219752754296894559, 0.3333333333333333703, 0.3219752754296894559, 0.3333333333333333703, 0.3219752754296894559, 0.3333333333333333703, 0.3219752754296894559, 0.3333333333333333703, 0.3219752754296894559, 0.3333333333333333703, 0.3219752754296894559, 0.3333333333333333703, 0.3219752754296894559, 0.3333333333333333703, 0.3219752754296894559, 0.3333333333333333703, 0.3219752754296894559, 0.3333333333333333703, 0.3219752754296894559, 0.3333333333333333703, 0.3219752754296894559, 0.3333333333333333703, 0.3219752754296894559, 0.3333333333333333703, 0.3219752754296894559, 0.3333333333333333703, 0.3219752754296894559, 0.3333333333333333703, 0.3219752754296894559, 0.3333333333333333703, 0.3219752754296894559, 0.3333333333333333703, 0.3219752754296894559, 0.3333333333333333703, 0.3219752754296894559, 0.3333333333333333703, 0.3219752754296894559, 0.3333333333333333703, 0.3219752754296894559, 0.3333333333333333703, 0.3219752754296894559, 0.3333333333333333703, 0.3219752754296894559, 0.3333333333333333703, 0.3219752754296894559, 0.3333333333333333703, 0.3219752754296894559, 0.3333333333333333703, 0.3219752754296894559, 0.3333333333333333703, 0.3219752754296894559, 0.3333333333333333703, 0.3219752754296894559, 0.3333333333333333703, 0.3219752754296894559, 0.3333333333333333703, 0.3219752754296894559, 0.3333333333333333703, 0.3219752754296894559, 0.3333333333333333703, 0.3219752754296894559, 0.3333333333333333703, 0.3219752754296894559, 0.3333333333333333703, 0.3219752754296894559, 0.3333333333333333703, 0.3219752754296894559, 0.3333333333333333703, 0.3219752754296894559, 0.3333333333333333703, 0.3219752754296894559, 0.3333333333333333703, 0.3219752754296894559, 0.3333333333333333703, 0.3219752754296894559, 0.3333333333333333703, 0.3219752754296894559, 0.3333333333333333703, 0.3219752754296894559, 0.3333333333333333703, 0.3219752754296894559, 0.3333333333333333703, 0.3219752754296894559, 0.3333333333333333703, 0.3219752754296894559, 0.3333333333333333703, 0.3219752754296894559, 0.3333333333333333703, 0.3219752754296894559, 0.3333333333333333703, 0.3219752754296894559, 0.3333333333333333703, 0.3219752754296894559, 0.3333333333333333703, 0.3219752754296894559, 0.3333333333333333703, 0.3219752754296894559, 0.3333333333333333703, 0.3219752754296894559, 0.3333333333333333703, 0.3219752754296894559, 0.3333333333333333703, 0.3219752754296894559, 0.3333333333333333703, 0.3219752754296894559, 0.3333333333333333703, 0.3219752754296894559, 0.3333333333333333703, 0.3219752754296894559, 0.3333333333333333703, 0.3219752754296894559, 0.3333333333333333703, 0.3219752754296894559, 0.3333333333333333703, 0.3219752754296894559, 0.3333333333333333703, 0.3219752754296894559, 0.3333333333333333703, 0.3219752754296894559, 0.3333333333333333703, 0.3219752754296894559, 0.3333333333333333703, 0.3219752754296894559, 0.3333333333333333703, 0.3219752754296894559, 0.3333333333333333703, 0.3219752754296894559, 0.3333333333333333703, 0.3219752754296894559, 0.3333333333333333703, 0.3219752754296894559, 0.3333333333333333703, 0.3219752754296894559, 0.3333333333333333703, 0.3219752754296894559, 0.3333333333333333703, 0.3219752754296894559, 0.3333333333333333703, 0.3219752754296894559, 0.3333333333333333703, 0.3219752754296894559, 0.3333333333333333703, 0.3219752754296894559, 0.3333333333333333703, 0.3219752754296894559, 0.3333333333333333703, 0.3219752754296894559, 0.3333333333333333703, 0.3219752754296894559, 0.3333333333333333703, 0.3219752754296894559, 0.3333333333333333703, 0.3219752754296894559, 0.3333333333333333703, 0.3219752754296894559, 0.3333333333333333703, 0.3219752754296894559, 0.3333333333333333703, 0.3219752754296894559, 0.3333333333333333703, 0.3219752754296894559, 0.3333333333333333703, 0.3219752754296894559, 0.3333333333333333703, 0.3219752754296894559, 0.3333333333333333703, 0.3219752754296894559, 0.3333333333333333703, 0.3219752754296894559, 0.3333333333333333703, 0.3219752754296894559, 0.3333333333333333703, 0.3219752754296894559, 0.3333333333333333703, 0.3219752754296894559, 0.3333333333333333703, 0.3219752754296894559, 0.3333333333333333703, 0.3219752754296894559, 0.3333333333333333703, 0.3219752754296894559, 0.3333333333333333703, 0.3219752754296894559, 0.3333333333333333703, 0.3219752754296894559, 0.3333333333333333703, 0.3219752754296894559, 0.3333333333333333703, 0.3219752754296894559, 0.3333333333333333703, 0.3219752754296894559, 0.3333333333333333703, 0.3219752754296894559, 0.3333333333333333703, 0.3219752754296894559, 0.3333333333333333703, 0.3219752754296894559, 0.3333333333333333703, 0.3219752754296894559, 0.3333333333333333703, 0.3219752754296894559, 0.3333333333333333703, 0.3219752754296894559, 0.3333333333333333703, 0.3219752754296894559, 0.3333333333333333703, 0.3219752754296894559, 0.3333333333333333703, 0.3219752754296894559, 0.3333333333333333703, 0.3219752754296894559, 0.3333333333333333703, 0.3219752754296894559, 0.3333333333333333703, 0.3219752754296894559, 0.3333333333333333703, 0.3219752754296894559, 0.3333333333333333703, 0.3219752754296894559, 0.3333333333333333703, 0.3219752754296894559, 0.3333333333333333703, 0.3219752754296894559, 0.3333333333333333703, 0.3219752754296894559, 0.3333333333333333703, 0.3219752754296894559, 0.3333333333333333703, 0.3219752754296894559, 0.3333333333333333703, 0.3219752754296894559, 0.3333333333333333703, 0.3219752754296894559, 0.3333333333333333703, 0.3219752754296894559, 0.3333333333333333703, 0.3219752754296894559, 0.3333333333333333703, 0.3219752754296894559, 0.3333333333333333703, 0.3219752754296894559, 0.3333333333333333703),
 ( 0.3333333333333333703, 0.3219752754296894559, 0.3333333333333333703, 0.3219752754296894559, 0.3333333333333333703, 0.3219752754296894559, 0.3333333333333333703, 0.3219752754296894559, 0.3333333333333333703, 0.3219752754296894559, 0.3333333333333333703, 0.3219752754296894559, 0.3333333333333333703, 0.3219752754296894559, 0.3333333333333333703, 0.3219752754296894559, 0.3333333333333333703, 0.3219752754296894559, 0.3333333333333333703, 0.3219752754296894559, 0.3333333333333333703, 0.3219752754296894559, 0.3333333333333333703, 0.3219752754296894559, 0.3333333333333333703, 0.3219752754296894559, 0.3333333333333333703, 0.3219752754296894559, 0.3333333333333333703, 0.3219752754296894559, 0.3333333333333333703, 0.3219752754296894559, 0.3333333333333333703, 0.3219752754296894559, 0.3333333333333333703, 0.3219752754296894559, 0.3333333333333333703, 0.3219752754296894559, 0.3333333333333333703, 0.3219752754296894559, 0.3333333333333333703, 0.3219752754296894559, 0.3333333333333333703, 0.3219752754296894559, 0.3333333333333333703, 0.3219752754296894559, 0.3333333333333333703, 0.3219752754296894559, 0.3333333333333333703, 0.3219752754296894559, 0.3333333333333333703, 0.3219752754296894559, 0.3333333333333333703, 0.3219752754296894559, 0.3333333333333333703, 0.3219752754296894559, 0.3333333333333333703, 0.3219752754296894559, 0.3333333333333333703, 0.3219752754296894559, 0.3333333333333333703, 0.3219752754296894559, 0.3333333333333333703, 0.3219752754296894559, 0.3333333333333333703, 0.3219752754296894559, 0.3333333333333333703, 0.3219752754296894559, 0.3333333333333333703, 0.3219752754296894559, 0.3333333333333333703, 0.3219752754296894559, 0.3333333333333333703, 0.3219752754296894559, 0.3333333333333333703, 0.3219752754296894559, 0.3333333333333333703, 0.3219752754296894559, 0.3333333333333333703, 0.3219752754296894559, 0.3333333333333333703, 0.3219752754296894559, 0.3333333333333333703, 0.3219752754296894559, 0.3333333333333333703, 0.3219752754296894559, 0.3333333333333333703, 0.3219752754296894559, 0.3333333333333333703, 0.3219752754296894559, 0.3333333333333333703, 0.3219752754296894559, 0.3333333333333333703, 0.3219752754296894559, 0.3333333333333333703, 0.3219752754296894559, 0.3333333333333333703, 0.3219752754296894559, 0.3333333333333333703, 0.3219752754296894559, 0.3333333333333333703, 0.3219752754296894559, 0.3333333333333333703, 0.3219752754296894559, 0.3333333333333333703, 0.3219752754296894559, 0.3333333333333333703, 0.3219752754296894559, 0.3333333333333333703, 0.3219752754296894559, 0.3333333333333333703, 0.3219752754296894559, 0.3333333333333333703, 0.3219752754296894559, 0.3333333333333333703, 0.3219752754296894559, 0.3333333333333333703, 0.3219752754296894559, 0.3333333333333333703, 0.3219752754296894559, 0.3333333333333333703, 0.3219752754296894559, 0.3333333333333333703, 0.3219752754296894559, 0.3333333333333333703, 0.3219752754296894559, 0.3333333333333333703, 0.3219752754296894559, 0.3333333333333333703, 0.3219752754296894559, 0.3333333333333333703, 0.3219752754296894559, 0.3333333333333333703, 0.3219752754296894559, 0.3333333333333333703, 0.3219752754296894559, 0.3333333333333333703, 0.3219752754296894559, 0.3333333333333333703, 0.3219752754296894559, 0.3333333333333333703, 0.3219752754296894559, 0.3333333333333333703, 0.3219752754296894559, 0.3333333333333333703, 0.3219752754296894559, 0.3333333333333333703, 0.3219752754296894559, 0.3333333333333333703, 0.3219752754296894559, 0.3333333333333333703, 0.3219752754296894559, 0.3333333333333333703, 0.3219752754296894559, 0.3333333333333333703, 0.3219752754296894559, 0.3333333333333333703, 0.3219752754296894559, 0.3333333333333333703, 0.3219752754296894559, 0.3333333333333333703, 0.3219752754296894559, 0.3333333333333333703, 0.3219752754296894559, 0.3333333333333333703, 0.3219752754296894559, 0.3333333333333333703, 0.3219752754296894559, 0.3333333333333333703, 0.3219752754296894559, 0.3333333333333333703, 0.3219752754296894559, 0.3333333333333333703, 0.3219752754296894559, 0.3333333333333333703, 0.3219752754296894559, 0.3333333333333333703, 0.3219752754296894559, 0.3333333333333333703, 0.3219752754296894559, 0.3333333333333333703, 0.3219752754296894559, 0.3333333333333333703, 0.3219752754296894559, 0.3333333333333333703, 0.3219752754296894559, 0.3333333333333333703, 0.3219752754296894559, 0.3333333333333333703, 0.3219752754296894559, 0.3333333333333333703, 0.3219752754296894559, 0.3333333333333333703, 0.3219752754296894559, 0.3333333333333333703, 0.3219752754296894559, 0.3333333333333333703, 0.3219752754296894559, 0.3333333333333333703, 0.3219752754296894559, 0.3333333333333333703, 0.3219752754296894559, 0.3333333333333333703, 0.3219752754296894559, 0.3333333333333333703, 0.3219752754296894559, 0.3333333333333333703, 0.3219752754296894559, 0.3333333333333333703, 0.3219752754296894559, 0.3333333333333333703, 0.3219752754296894559, 0.3333333333333333703, 0.3219752754296894559, 0.3333333333333333703, 0.3219752754296894559, 0.3333333333333333703, 0.3219752754296894559, 0.3333333333333333703, 0.3219752754296894559, 0.3333333333333333703, 0.3219752754296894559, 0.3333333333333333703, 0.3219752754296894559, 0.3333333333333333703, 0.3219752754296894559, 0.3333333333333333703, 0.3219752754296894559, 0.3333333333333333703, 0.3219752754296894559, 0.3333333333333333703, 0.3219752754296894559, 0.3333333333333333703, 0.3219752754296894559, 0.3333333333333333703, 0.3219752754296894559, 0.3333333333333333703, 0.3219752754296894559, 0.3333333333333333703, 0.3219752754296894559, 0.3333333333333333703, 0.3219752754296894559, 0.3333333333333333703, 0.3219752754296894559, 0.3333333333333333703, 0.3219752754296894559, 0.3333333333333333703, 0.3219752754296894559, 0.3333333333333333703, 0.3219752754296894559, 0.3333333333333333703, 0.3219752754296894559, 0.3333333333333333703, 0.3219752754296894559, 0.3333333333333333703, 0.3219752754296894559, 0.3333333333333333703, 0.3219752754296894559, 0.3333333333333333703, 0.3219752754296894559, 0.3333333333333333703, 0.3219752754296894559, 0.3333333333333333703, 0.3219752754296894559, 0.3333333333333333703, 0.3219752754296894559, 0.3333333333333333703, 0.3219752754296894559, 0.3333333333333333703, 0.3219752754296894559, 0.3333333333333333703, 0.3219752754296894559, 0.3333333333333333703, 0.3219752754296894559, 0.3333333333333333703, 0.3219752754296894559, 0.3333333333333333703, 0.3219752754296894559, 0.3333333333333333703, 0.3219752754296894559, 0.3333333333333333703, 0.3219752754296894559, 0.3333333333333333703, 0.3219752754296894559, 0.3333333333333333703, 0.3219752754296894559, 0.3333333333333333703, 0.3219752754296894559, 0.3333333333333333703, 0.3219752754296894559, 0.3333333333333333703, 0.3219752754296894559, 0.3333333333333333703, 0.3219752754296894559, 0.3333333333333333703, 0.3219752754296894559, 0.3333333333333333703, 0.3219752754296894559, 0.3333333333333333703, 0.3219752754296894559, 0.3333333333333333703, 0.3219752754296894559, 0.3333333333333333703, 0.3219752754296894559, 0.3333333333333333703, 0.3219752754296894559, 0.3333333333333333703, 0.3219752754296894559, 0.3333333333333333703, 0.3219752754296894559, 0.3333333333333333703, 0.3219752754296894559, 0.3333333333333333703, 0.3219752754296894559, 0.3333333333333333703, 0.3219752754296894559, 0.3333333333333333703, 0.3219752754296894559, 0.3333333333333333703, 0.3219752754296894559, 0.3333333333333333703, 0.3219752754296894559, 0.3333333333333333703, 0.3219752754296894559, 0.3333333333333333703, 0.3219752754296894559, 0.3333333333333333703, 0.3219752754296894559, 0.3333333333333333703, 0.3219752754296894559, 0.3333333333333333703, 0.3219752754296894559, 0.3333333333333333703, 0.3219752754296894559, 0.3333333333333333703, 0.3219752754296894559, 0.3333333333333333703, 0.3219752754296894559, 0.3333333333333333703, 0.3219752754296894559, 0.3333333333333333703, 0.3219752754296894559, 0.3333333333333333703, 0.3219752754296894559, 0.3333333333333333703, 0.3219752754296894559, 0.3333333333333333703, 0.3219752754296894559, 0.3333333333333333703, 0.3219752754296894559, 0.3333333333333333703, 0.3219752754296894559, 0.3333333333333333703, 0.3219752754296894559, 0.3333333333333333703, 0.3219752754296894559, 0.3333333333333333703, 0.3219752754296894559, 0.3333333333333333703, 0.3219752754296894559, 0.3333333333333333703, 0.3219752754296894559, 0.3333333333333333703, 0.3219752754296894559, 0.3333333333333333703, 0.3219752754296894559, 0.3333333333333333703, 0.3219752754296894559, 0.3333333333333333703, 0.3219752754296894559, 0.3333333333333333703, 0.3219752754296894559, 0.3333333333333333703, 0.3219752754296894559, 0.3333333333333333703, 0.3219752754296894559, 0.3333333333333333703, 0.3219752754296894559, 0.3333333333333333703, 0.3219752754296894559, 0.3333333333333333703, 0.3219752754296894559, 0.3333333333333333703, 0.3219752754296894559, 0.3333333333333333703, 0.3219752754296894559, 0.3333333333333333703, 0.3219752754296894559, 0.3333333333333333703, 0.3219752754296894559, 0.3333333333333333703, 0.3219752754296894559, 0.3333333333333333703, 0.3219752754296894559, 0.3333333333333333703, 0.3219752754296894559, 0.3333333333333333703, 0.3219752754296894559, 0.3333333333333333703, 0.3219752754296894559, 0.3333333333333333703, 0.3219752754296894559, 0.3333333333333333703, 0.3219752754296894559, 0.3333333333333333703, 0.3219752754296894559, 0.3333333333333333703, 0.3219752754296894559, 0.3333333333333333703, 0.3219752754296894559, 0.3333333333333333703, 0.3219752754296894559, 0.3333333333333333703, 0.3219752754296894559, 0.3333333333333333703, 0.3219752754296894559, 0.3333333333333333703, 0.3219752754296894559, 0.3333333333333333703, 0.3219752754296894559, 0.3333333333333333703, 0.3219752754296894559, 0.3333333333333333703, 0.3219752754296894559, 0.3333333333333333703, 0.3219752754296894559, 0.3333333333333333703, 0.3219752754296894559, 0.3333333333333333703, 0.3219752754296894559, 0.3333333333333333703, 0.3219752754296894559, 0.3333333333333333703, 0.3219752754296894559, 0.3333333333333333703, 0.3219752754296894559, 0.3333333333333333703, 0.3219752754296894559, 0.3333333333333333703, 0.3219752754296894559, 0.3333333333333333703, 0.3219752754296894559, 0.3333333333333333703, 0.3219752754296894559, 0.3333333333333333703, 0.3219752754296894559, 0.3333333333333333703, 0.3219752754296894559, 0.3333333333333333703, 0.3219752754296894559, 0.3333333333333333703, 0.3219752754296894559, 0.3333333333333333703, 0.3219752754296894559, 0.3333333333333333703, 0.3219752754296894559, 0.3333333333333333703),
 ( 1.000000000000000000, 0.9659258262890683122, 1.000000000000000000, 0.9659258262890683122, 1.000000000000000000, 0.9659258262890683122, 1.000000000000000000, 0.9659258262890683122, 1.000000000000000000, 0.9659258262890683122, 1.000000000000000000, 0.9659258262890683122, 1.000000000000000000, 0.9659258262890683122, 1.000000000000000000, 0.9659258262890683122, 1.000000000000000000, 0.9659258262890683122, 1.000000000000000000, 0.9659258262890683122, 1.000000000000000000, 0.9659258262890683122, 1.000000000000000000, 0.9659258262890683122, 1.000000000000000000, 0.9659258262890683122, 1.000000000000000000, 0.9659258262890683122, 1.000000000000000000, 0.9659258262890683122, 1.000000000000000000, 0.9659258262890683122, 1.000000000000000000, 0.9659258262890683122, 1.000000000000000000, 0.9659258262890683122, 1.000000000000000000, 0.9659258262890683122, 1.000000000000000000, 0.9659258262890683122, 1.000000000000000000, 0.9659258262890683122, 1.000000000000000000, 0.9659258262890683122, 1.000000000000000000, 0.9659258262890683122, 1.000000000000000000, 0.9659258262890683122, 1.000000000000000000, 0.9659258262890683122, 1.000000000000000000, 0.9659258262890683122, 1.000000000000000000, 0.9659258262890683122, 1.000000000000000000, 0.9659258262890683122, 1.000000000000000000, 0.9659258262890683122, 1.000000000000000000, 0.9659258262890683122, 1.000000000000000000, 0.9659258262890683122, 1.000000000000000000, 0.9659258262890683122, 1.000000000000000000, 0.9659258262890683122, 1.000000000000000000, 0.9659258262890683122, 1.000000000000000000, 0.9659258262890683122, 1.000000000000000000, 0.9659258262890683122, 1.000000000000000000, 0.9659258262890683122, 1.000000000000000000, 0.9659258262890683122, 1.000000000000000000, 0.9659258262890683122, 1.000000000000000000, 0.9659258262890683122, 1.000000000000000000, 0.9659258262890683122, 1.000000000000000000, 0.9659258262890683122, 1.000000000000000000, 0.9659258262890683122, 1.000000000000000000, 0.9659258262890683122, 1.000000000000000000, 0.9659258262890683122, 1.000000000000000000, 0.9659258262890683122, 1.000000000000000000, 0.9659258262890683122, 1.000000000000000000, 0.9659258262890683122, 1.000000000000000000, 0.9659258262890683122, 1.000000000000000000, 0.9659258262890683122, 1.000000000000000000, 0.9659258262890683122, 1.000000000000000000, 0.9659258262890683122, 1.000000000000000000, 0.9659258262890683122, 1.000000000000000000, 0.9659258262890683122, 1.000000000000000000, 0.9659258262890683122, 1.000000000000000000, 0.9659258262890683122, 1.000000000000000000, 0.9659258262890683122, 1.000000000000000000, 0.9659258262890683122, 1.000000000000000000, 0.9659258262890683122, 1.000000000000000000, 0.9659258262890683122, 1.000000000000000000, 0.9659258262890683122, 1.000000000000000000, 0.9659258262890683122, 1.000000000000000000, 0.9659258262890683122, 1.000000000000000000, 0.9659258262890683122, 1.000000000000000000, 0.9659258262890683122, 1.000000000000000000, 0.9659258262890683122, 1.000000000000000000, 0.9659258262890683122, 1.000000000000000000, 0.9659258262890683122, 1.000000000000000000, 0.9659258262890683122, 1.000000000000000000, 0.9659258262890683122, 1.000000000000000000, 0.9659258262890683122, 1.000000000000000000, 0.9659258262890683122, 1.000000000000000000, 0.9659258262890683122, 1.000000000000000000, 0.9659258262890683122, 1.000000000000000000, 0.9659258262890683122, 1.000000000000000000, 0.9659258262890683122, 1.000000000000000000, 0.9659258262890683122, 1.000000000000000000, 0.9659258262890683122, 1.000000000000000000, 0.9659258262890683122, 1.000000000000000000, 0.9659258262890683122, 1.000000000000000000, 0.9659258262890683122, 1.000000000000000000, 0.9659258262890683122, 1.000000000000000000, 0.9659258262890683122, 1.000000000000000000, 0.9659258262890683122, 1.000000000000000000, 0.9659258262890683122, 1.000000000000000000, 0.9659258262890683122, 1.000000000000000000, 0.9659258262890683122, 1.000000000000000000, 0.9659258262890683122, 1.000000000000000000, 0.9659258262890683122, 1.000000000000000000, 0.9659258262890683122, 1.000000000000000000, 0.9659258262890683122, 1.000000000000000000, 0.9659258262890683122, 1.000000000000000000, 0.9659258262890683122, 1.000000000000000000, 0.9659258262890683122, 1.000000000000000000, 0.9659258262890683122, 1.000000000000000000, 0.9659258262890683122, 1.000000000000000000, 0.9659258262890683122, 1.000000000000000000, 0.9659258262890683122, 1.000000000000000000, 0.9659258262890683122, 1.000000000000000000, 0.9659258262890683122, 1.000000000000000000, 0.9659258262890683122, 1.000000000000000000, 0.9659258262890683122, 1.000000000000000000, 0.9659258262890683122, 1.000000000000000000, 0.9659258262890683122, 1.000000000000000000, 0.9659258262890683122, 1.000000000000000000, 0.9659258262890683122, 1.000000000000000000, 0.9659258262890683122, 1.000000000000000000, 0.9659258262890683122, 1.000000000000000000, 0.9659258262890683122, 1.000000000000000000, 0.9659258262890683122, 1.000000000000000000, 0.9659258262890683122, 1.000000000000000000, 0.9659258262890683122, 1.000000000000000000, 0.9659258262890683122, 1.000000000000000000, 0.9659258262890683122, 1.000000000000000000, 0.9659258262890683122, 1.000000000000000000, 0.9659258262890683122, 1.000000000000000000, 0.9659258262890683122, 1.000000000000000000, 0.9659258262890683122, 1.000000000000000000, 0.9659258262890683122, 1.000000000000000000, 0.9659258262890683122, 1.000000000000000000, 0.9659258262890683122, 1.000000000000000000, 0.9659258262890683122, 1.000000000000000000, 0.9659258262890683122, 1.000000000000000000, 0.9659258262890683122, 1.000000000000000000, 0.9659258262890683122, 1.000000000000000000, 0.9659258262890683122, 1.000000000000000000, 0.9659258262890683122, 1.000000000000000000, 0.9659258262890683122, 1.000000000000000000, 0.9659258262890683122, 1.000000000000000000, 0.9659258262890683122, 1.000000000000000000, 0.9659258262890683122, 1.000000000000000000, 0.9659258262890683122, 1.000000000000000000, 0.9659258262890683122, 1.000000000000000000, 0.9659258262890683122, 1.000000000000000000, 0.9659258262890683122, 1.000000000000000000, 0.9659258262890683122, 1.000000000000000000, 0.9659258262890683122, 1.000000000000000000, 0.9659258262890683122, 1.000000000000000000, 0.9659258262890683122, 1.000000000000000000, 0.9659258262890683122, 1.000000000000000000, 0.9659258262890683122, 1.000000000000000000, 0.9659258262890683122, 1.000000000000000000, 0.9659258262890683122, 1.000000000000000000, 0.9659258262890683122, 1.000000000000000000, 0.9659258262890683122, 1.000000000000000000, 0.9659258262890683122, 1.000000000000000000, 0.9659258262890683122, 1.000000000000000000, 0.9659258262890683122, 1.000000000000000000, 0.9659258262890683122, 1.000000000000000000, 0.9659258262890683122, 1.000000000000000000, 0.9659258262890683122, 1.000000000000000000, 0.9659258262890683122, 1.000000000000000000, 0.9659258262890683122, 1.000000000000000000, 0.9659258262890683122, 1.000000000000000000, 0.9659258262890683122, 1.000000000000000000, 0.9659258262890683122, 1.000000000000000000, 0.9659258262890683122, 1.000000000000000000, 0.9659258262890683122, 1.000000000000000000, 0.9659258262890683122, 1.000000000000000000, 0.9659258262890683122, 1.000000000000000000, 0.9659258262890683122, 1.000000000000000000, 0.9659258262890683122, 1.000000000000000000, 0.9659258262890683122, 1.000000000000000000, 0.9659258262890683122, 1.000000000000000000, 0.9659258262890683122, 1.000000000000000000, 0.9659258262890683122, 1.000000000000000000, 0.9659258262890683122, 1.000000000000000000, 0.9659258262890683122, 1.000000000000000000, 0.9659258262890683122, 1.000000000000000000, 0.9659258262890683122, 1.000000000000000000, 0.9659258262890683122, 1.000000000000000000, 0.9659258262890683122, 1.000000000000000000, 0.9659258262890683122, 1.000000000000000000, 0.9659258262890683122, 1.000000000000000000, 0.9659258262890683122, 1.000000000000000000, 0.9659258262890683122, 1.000000000000000000, 0.9659258262890683122, 1.000000000000000000, 0.9659258262890683122, 1.000000000000000000, 0.9659258262890683122, 1.000000000000000000, 0.9659258262890683122, 1.000000000000000000, 0.9659258262890683122, 1.000000000000000000, 0.9659258262890683122, 1.000000000000000000, 0.9659258262890683122, 1.000000000000000000, 0.9659258262890683122, 1.000000000000000000, 0.9659258262890683122, 1.000000000000000000, 0.9659258262890683122, 1.000000000000000000, 0.9659258262890683122, 1.000000000000000000, 0.9659258262890683122, 1.000000000000000000, 0.9659258262890683122, 1.000000000000000000, 0.9659258262890683122, 1.000000000000000000, 0.9659258262890683122, 1.000000000000000000, 0.9659258262890683122, 1.000000000000000000, 0.9659258262890683122, 1.000000000000000000, 0.9659258262890683122, 1.000000000000000000, 0.9659258262890683122, 1.000000000000000000, 0.9659258262890683122, 1.000000000000000000, 0.9659258262890683122, 1.000000000000000000, 0.9659258262890683122, 1.000000000000000000, 0.9659258262890683122, 1.000000000000000000, 0.9659258262890683122, 1.000000000000000000, 0.9659258262890683122, 1.000000000000000000, 0.9659258262890683122, 1.000000000000000000, 0.9659258262890683122, 1.000000000000000000, 0.9659258262890683122, 1.000000000000000000, 0.9659258262890683122, 1.000000000000000000, 0.9659258262890683122, 1.000000000000000000, 0.9659258262890683122, 1.000000000000000000, 0.9659258262890683122, 1.000000000000000000, 0.9659258262890683122, 1.000000000000000000, 0.9659258262890683122, 1.000000000000000000, 0.9659258262890683122, 1.000000000000000000, 0.9659258262890683122, 1.000000000000000000, 0.9659258262890683122, 1.000000000000000000, 0.9659258262890683122, 1.000000000000000000, 0.9659258262890683122, 1.000000000000000000, 0.9659258262890683122, 1.000000000000000000, 0.9659258262890683122, 1.000000000000000000, 0.9659258262890683122, 1.000000000000000000, 0.9659258262890683122, 1.000000000000000000, 0.9659258262890683122, 1.000000000000000000, 0.9659258262890683122, 1.000000000000000000, 0.9659258262890683122, 1.000000000000000000, 0.9659258262890683122, 1.000000000000000000, 0.9659258262890683122, 1.000000000000000000, 0.9659258262890683122, 1.000000000000000000, 0.9659258262890683122, 1.000000000000000000, 0.9659258262890683122, 1.000000000000000000, 0.9659258262890683122, 1.000000000000000000) ) ) 
 REPRESENTATION_ITEM ( '' )  SURFACE ( )  );
#158562=CARTESIAN_POINT ( 'NONE',  ( -9.564922557960796823, -16.46253265017161027, 57.08224293864769550 ) ) ;
#158563=CARTESIAN_POINT ( 'NONE',  ( -5.823673210054431948, 21.52544592524334988, 67.70942372801901854 ) ) ;
#158564=CARTESIAN_POINT ( 'NONE',  ( -19.02544592524342804, 5.153800228976336051, 46.04057627198101699 ) ) ;
#158565=CARTESIAN_POINT ( 'NONE',  ( -13.97604488694527625, -13.89961937509977652, 71.87390960531433848 ) ) ;
#158566=CARTESIAN_POINT ( 'NONE',  ( -12.06949235617756955, 12.14591786802309770, 105.6239096053143669 ) ) ;
#158567=CARTESIAN_POINT ( 'NONE',  ( 19.02544592524343514, -5.153800228976328945, 113.5405762719810241 ) ) ;
#158568=CARTESIAN_POINT ( 'NONE',  ( 14.29746914071049879, -8.314922557960816363, 48.33224293864770260 ) ) ;
#158569=CARTESIAN_POINT ( 'NONE',  ( -4.483927247898539470, -16.52544592524342804, 112.2905762719810241 ) ) ;
#158570=CARTESIAN_POINT ( 'NONE',  ( 8.314922557960818139, 14.29746914071049879, 74.58224293864768129 ) ) ;
#158571=CARTESIAN_POINT ( 'NONE',  ( -5.719274019375978568, 21.55341960407610458, 85.20724293864770971 ) ) ;
#158572=CARTESIAN_POINT ( 'NONE',  ( -0.05219959533937732626, 21.53943276465977519, 32.50109039468568284 ) ) ;
#158574=CARTESIAN_POINT ( 'NONE',  ( 16.55341960407618274, -4.379528057220086978, 31.04275706135234714 ) ) ;
#158575=CARTESIAN_POINT ( 'NONE',  ( 18.62759615963271287, -10.81492255796078972, 83.33224293864769550 ) ) ;
#158576=CARTESIAN_POINT ( 'NONE',  ( -18.67979575497193778, 10.72451020669871902, 103.3344237280190043 ) ) ;
#158577=CARTESIAN_POINT ( 'NONE',  ( -9.564922557960796823, -16.46253265017161027, 92.08224293864769550 ) ) ;
#158578=CARTESIAN_POINT ( 'NONE',  ( 15.72974639402176855, 15.80617190586768217, 46.87609039468568994 ) ) ;
#158579=EDGE_CURVE ( 'NONE', #187465, #81647, #17495, .T. ) ;
#158580=CARTESIAN_POINT ( 'NONE',  ( 21.52544592524344225, -5.823673210054117533, 23.54057627198102765 ) ) ;
#158581=CARTESIAN_POINT ( 'NONE',  ( 16.55341960407618274, -4.379528057220086978, 101.0427570613523756 ) ) ;
#158582=CARTESIAN_POINT ( 'NONE',  ( 5.719274019375673035, 21.55341960407619339, 47.29275706135234003 ) ) ;
#158583=CARTESIAN_POINT ( 'NONE',  ( -15.80617190586768217, 15.72974639402176855, 83.12609039468568994 ) ) ;
#158584=CARTESIAN_POINT ( 'NONE',  ( 10.72451020669871369, 18.67979575497193778, 112.0844237280190185 ) ) ;
#158585=CARTESIAN_POINT ( 'NONE',  ( -4.483927247898782831, 16.52544592524335698, 72.70942372801901854 ) ) ;
#158586=CARTESIAN_POINT ( 'NONE',  ( -18.67979575497193778, 10.72451020669871902, 43.33442372801901143 ) ) ;
#158587=CARTESIAN_POINT ( 'NONE',  ( 13.97604488694527802, 13.89961937509977652, 39.37390960531435269 ) ) ;
#158588=CARTESIAN_POINT ( 'NONE',  ( 5.719274019375673035, 21.55341960407619339, 97.29275706135234714 ) ) ;
#158589=CARTESIAN_POINT ( 'NONE',  ( -19.05341960407611168, -5.049401038298163336, 106.4572429386476955 ) ) ;
#158590=CARTESIAN_POINT ( 'NONE',  ( 21.55341960407610458, 5.719274019375980345, 98.95724293864770971 ) ) ;
#158591=CARTESIAN_POINT ( 'NONE',  ( 18.56101223717332616, 5.499999999999948486, 83.94978406935679516 ) ) ;
#158592=CARTESIAN_POINT ( 'NONE',  ( -10.81492255796078084, -18.62759615963271287, 62.08224293864769550 ) ) ;
#158593=CARTESIAN_POINT ( 'NONE',  ( 16.52544592524335698, 4.483927247898782831, 51.45942372801901854 ) ) ;
#158594=CARTESIAN_POINT ( 'NONE',  ( -12.14591786802309592, -12.06949235617757132, 46.87390960531435979 ) ) ;
#158595=CARTESIAN_POINT ( 'NONE',  ( 19.54388014595539858, -5.500000000000015099, 102.3151885665635774 ) ) ;
#158596=CARTESIAN_POINT ( 'NONE',  ( 13.89961937509957401, 13.97604488694547697, 96.87609039468566152 ) ) ;
#158598=CARTESIAN_POINT ( 'NONE',  ( 8.314922557961029526, -14.29746914071037800, 25.41775706135235779 ) ) ;
#158599=CARTESIAN_POINT ( 'NONE',  ( -0.05219959533907301413, -21.53943276465977519, 102.4989096053143811 ) ) ;
#158600=CARTESIAN_POINT ( 'NONE',  ( -10.72451020669898014, 18.67979575497178502, 80.41557627198103830 ) ) ;
#158601=CARTESIAN_POINT ( 'NONE',  ( -5.823673210054116645, -21.52544592524344225, 22.29057627198102765 ) ) ;
#158602=CARTESIAN_POINT ( 'NONE',  ( 4.483927247898790824, -16.52544592524335698, 45.20942372801901854 ) ) ;
#158603=CARTESIAN_POINT ( 'NONE',  ( 9.474510206698971260, -16.51473224551069308, 77.91557627198103830 ) ) ;
#158604=CARTESIAN_POINT ( 'NONE',  ( -18.67979575497193778, 10.72451020669871902, 33.33442372801900433 ) ) ;
#158605=CARTESIAN_POINT ( 'NONE',  ( 13.89961937509957401, 13.97604488694547697, 96.87609039468566152 ) ) ;
#158606=CARTESIAN_POINT ( 'NONE',  ( -19.03943276465977164, 0.05219959533909376836, 111.2489096053143669 ) ) ;
#158607=CARTESIAN_POINT ( 'NONE',  ( 13.89961937509977652, -13.97604488694527269, 88.12390960531438111 ) ) ;
#158608=CARTESIAN_POINT ( 'NONE',  ( 15.72974639402199770, -15.80617190586745480, 88.12390960531436690 ) ) ;
#158609=CARTESIAN_POINT ( 'NONE',  ( -5.049401038298153566, 19.05341960407611168, 65.20724293864765286 ) ) ;
#158611=CARTESIAN_POINT ( 'NONE',  ( -4.379528057220328563, 16.55341960407611168, 75.20724293864769550 ) ) ;
#158612=CARTESIAN_POINT ( 'NONE',  ( -21.55341960407610458, -5.719274019375992779, 26.45724293864768839 ) ) ;
#158614=CARTESIAN_POINT ( 'NONE',  ( 5.823673210054125526, 21.52544592524343514, 104.7905762719810241 ) ) ;
#158615=CARTESIAN_POINT ( 'NONE',  ( -5.153800228976607833, 19.02544592524334988, 62.70942372801899722 ) ) ;
#158616=CARTESIAN_POINT ( 'NONE',  ( 16.51473224551069308, 9.474510206698969483, 109.1655762719810383 ) ) ;
#158618=CARTESIAN_POINT ( 'NONE',  ( -10.72451020669898014, 18.67979575497178502, 55.41557627198102409 ) ) ;
#158619=CARTESIAN_POINT ( 'NONE',  ( 13.97604488694527802, 13.89961937509977652, 84.37390960531433848 ) ) ;
#158620=CARTESIAN_POINT ( 'NONE',  ( 18.62759615963255655, 10.81492255796105972, 76.66775706135234714 ) ) ;
#158621=CARTESIAN_POINT ( 'NONE',  ( -19.03943276465977164, 0.05219959533909376836, 46.24890960531435979 ) ) ;
#158622=CARTESIAN_POINT ( 'NONE',  ( 12.14591786802309770, 12.06949235617756955, 84.37390960531438111 ) ) ;
#158623=CARTESIAN_POINT ( 'NONE',  ( -14.34966873604972548, 8.224510206698743886, 33.33442372801900433 ) ) ;
#158624=CARTESIAN_POINT ( 'NONE',  ( -5.823673210054431948, 21.52544592524334988, 67.70942372801901854 ) ) ;
#158626=CARTESIAN_POINT ( 'NONE',  ( 13.97604488694548053, -13.89961937509957401, 20.62609039468567573 ) ) ;
#158627=CARTESIAN_POINT ( 'NONE',  ( 9.564922557961047289, -16.46253265017146816, 80.41775706135234714 ) ) ;
#158628=CARTESIAN_POINT ( 'NONE',  ( -17.72662750342728444, -5.500000000000021316, 91.40179492283749596 ) ) ;
#158629=CARTESIAN_POINT ( 'NONE',  ( 18.67979575497194134, -10.72451020669871369, 40.83442372801901854 ) ) ;
#158631=CARTESIAN_POINT ( 'NONE',  ( -16.46253265017146816, -9.564922557961047289, 29.16775706135232937 ) ) ;
#158632=CARTESIAN_POINT ( 'NONE',  ( 19.05341960407611168, 5.049401038298154454, 53.95724293864770260 ) ) ;
#158633=CARTESIAN_POINT ( 'NONE',  ( -16.46253265017146816, -9.564922557961047289, 24.16775706135233648 ) ) ;
#158634=CARTESIAN_POINT ( 'NONE',  ( -12.06949235617739369, -12.14591786802326823, 109.3760903946857042 ) ) ;
#158635=CARTESIAN_POINT ( 'NONE',  ( 9.564922557960805705, 16.46253265017160317, 104.5822429386476955 ) ) ;
#158636=CARTESIAN_POINT ( 'NONE',  ( 18.67979575497194134, -10.72451020669871369, 90.83442372801901854 ) ) ;
#158638=CARTESIAN_POINT ( 'NONE',  ( -17.50000000000149925, -3.254303733634381857, 34.97604106928617540 ) ) ;
#158639=CARTESIAN_POINT ( 'NONE',  ( 18.62759615963255655, 10.81492255796105972, 86.66775706135234714 ) ) ;
#158641=CARTESIAN_POINT ( 'NONE',  ( -13.89961937509977652, 13.97604488694528158, 105.6239096053143527 ) ) ;
#158643=CARTESIAN_POINT ( 'NONE',  ( -5.153800228976328057, -19.02544592524343514, 37.29057627198102409 ) ) ;
#158644=CARTESIAN_POINT ( 'NONE',  ( -15.72974639402197994, 15.80617190586746368, 60.62390960531437401 ) ) ;
#158645=CARTESIAN_POINT ( 'NONE',  ( -4.483927247898539470, -16.52544592524342804, 27.29057627198103120 ) ) ;
#158646=CARTESIAN_POINT ( 'NONE',  ( -0.05219959533910754901, -16.53943276465976808, 92.49890960531436690 ) ) ;
#158647=CARTESIAN_POINT ( 'NONE',  ( 9.564922557960805705, 16.46253265017160317, 79.58224293864769550 ) ) ;
#158648=CARTESIAN_POINT ( 'NONE',  ( -16.46253265017146816, -9.564922557961047289, 19.16775706135233293 ) ) ;
#158649=EDGE_CURVE ( 'NONE', #199255, #15160, #53918, .T. ) ;
#158650=CARTESIAN_POINT ( 'NONE',  ( 9.564922557960805705, 16.46253265017160317, 39.58224293864768839 ) ) ;
#158651=CARTESIAN_POINT ( 'NONE',  ( 12.06949235617757843, -12.14591786802309237, 108.1239096053143811 ) ) ;
#158652=CARTESIAN_POINT ( 'NONE',  ( -18.67979575497193778, 10.72451020669871902, 53.33442372801901854 ) ) ;
#158653=CARTESIAN_POINT ( 'NONE',  ( -21.52544592524343514, 5.823673210054127303, 81.04057627198102409 ) ) ;
#158654=CARTESIAN_POINT ( 'NONE',  ( -19.05341960407617563, 5.049401038297882671, 63.54275706135234003 ) ) ;
#158656=CARTESIAN_POINT ( 'NONE',  ( 13.97604488694527802, 13.89961937509977652, 114.3739096053143669 ) ) ;
#158657=CARTESIAN_POINT ( 'NONE',  ( -12.14591786802309592, -12.06949235617757132, 76.87390960531439532 ) ) ;
#158658=CARTESIAN_POINT ( 'NONE',  ( -13.89961937509957401, -13.97604488694547875, 39.37609039468566152 ) ) ;
#158659=CARTESIAN_POINT ( 'NONE',  ( -16.51473224551069308, -9.474510206698971260, 66.66557627198102409 ) ) ;
#158660=CARTESIAN_POINT ( 'NONE',  ( -4.379528057220328563, 16.55341960407611168, 60.20724293864768839 ) ) ;
#158661=CARTESIAN_POINT ( 'NONE',  ( -9.474510206698720793, -16.51473224551083518, 74.58442372801900433 ) ) ;
#158662=CARTESIAN_POINT ( 'NONE',  ( 17.05116617787826172, 6.768360034955700044, 33.84324446740802728 ) ) ;
#158663=CARTESIAN_POINT ( 'NONE',  ( -10.72451020669898014, 18.67979575497178502, 40.41557627198103120 ) ) ;
#158664=ORIENTED_EDGE ( 'NONE', *, *, #153149, .F. ) ;
#158665=EDGE_CURVE ( 'NONE', #12092, #112608, #32201, .T. ) ;
#158666=CARTESIAN_POINT ( 'NONE',  ( -8.224510206698948167, 14.34966873604960824, 95.41557627198102409 ) ) ;
#158668=CARTESIAN_POINT ( 'NONE',  ( 19.05341960407611168, 5.049401038298154454, 53.95724293864770260 ) ) ;
#158669=CARTESIAN_POINT ( 'NONE',  ( -21.55341960407610458, -5.719274019375992779, 56.45724293864768839 ) ) ;
#158670=CARTESIAN_POINT ( 'NONE',  ( -5.153800228976328057, -19.02544592524343514, 37.29057627198102409 ) ) ;
#158671=CARTESIAN_POINT ( 'NONE',  ( 16.55341960407618274, -4.379528057220086978, 81.04275706135236135 ) ) ;
#158672=CARTESIAN_POINT ( 'NONE',  ( -13.89961937509977652, 13.97604488694528158, 80.62390960531436690 ) ) ;
#158673=CARTESIAN_POINT ( 'NONE',  ( -9.474510206698720793, -16.51473224551083518, 54.58442372801899722 ) ) ;
#158674=CARTESIAN_POINT ( 'NONE',  ( -21.55341960407619339, 5.719274019375674811, 63.54275706135234003 ) ) ;
#158675=ORIENTED_EDGE ( 'NONE', *, *, #11833, .T. ) ;
#158676=CARTESIAN_POINT ( 'NONE',  ( 21.53943276465977519, -0.05219959533907433946, 48.74890960531435979 ) ) ;
#158677=CARTESIAN_POINT ( 'NONE',  ( -5.153800228976328057, -19.02544592524343514, 27.29057627198103120 ) ) ;
#158678=CARTESIAN_POINT ( 'NONE',  ( -12.14591786802326823, 12.06949235617739902, 93.12609039468568994 ) ) ;
#158679=CARTESIAN_POINT ( 'NONE',  ( -0.05219959533936034679, 19.03943276465977164, 102.5010903946856757 ) ) ;
#158681=CARTESIAN_POINT ( 'NONE',  ( 18.89770734986044687, 5.500000000000083489, 76.60214472496639360 ) ) ;
#158682=CARTESIAN_POINT ( 'NONE',  ( -15.80617190586768217, 15.72974639402176855, 93.12609039468568994 ) ) ;
#158683=CARTESIAN_POINT ( 'NONE',  ( -12.06949235617756955, 12.14591786802309770, 40.62390960531435269 ) ) ;
#158684=CARTESIAN_POINT ( 'NONE',  ( -8.314922557960811034, -14.29746914071050412, 72.08224293864769550 ) ) ;
#158685=CARTESIAN_POINT ( 'NONE',  ( -18.67979575497178146, -10.72451020669898902, 96.66557627198102409 ) ) ;
#158686=CARTESIAN_POINT ( 'NONE',  ( -18.62759615963270932, 10.81492255796079327, 90.83224293864769550 ) ) ;
#158687=CARTESIAN_POINT ( 'NONE',  ( 17.12812012977027720, -6.668231424565983723, 96.14051240676860743 ) ) ;
#158688=CARTESIAN_POINT ( 'NONE',  ( 15.72974639402199770, -15.80617190586745480, 28.12390960531435979 ) ) ;
#158689=CARTESIAN_POINT ( 'NONE',  ( -14.34966873604972548, 8.224510206698743886, 68.33442372801900433 ) ) ;
#158690=CARTESIAN_POINT ( 'NONE',  ( -12.06949235617756955, 12.14591786802309770, 80.62390960531438111 ) ) ;
#158691=CARTESIAN_POINT ( 'NONE',  ( 9.564922557960805705, 16.46253265017160317, 39.58224293864768839 ) ) ;
#158693=CARTESIAN_POINT ( 'NONE',  ( -4.379528057220086978, -16.55341960407618274, 94.79275706135234714 ) ) ;
#158694=CARTESIAN_POINT ( 'NONE',  ( -5.823673210054116645, -21.52544592524344225, 112.2905762719810241 ) ) ;
#158695=CARTESIAN_POINT ( 'NONE',  ( 19.02544592524343514, -5.153800228976328945, 78.54057627198099567 ) ) ;
#158696=CARTESIAN_POINT ( 'NONE',  ( -18.62759615963255300, -10.81492255796106328, 59.16775706135234714 ) ) ;
#158697=CARTESIAN_POINT ( 'NONE',  ( -16.46253265017160317, 9.564922557960807481, 105.8322429386476955 ) ) ;
#158699=ORIENTED_EDGE ( 'NONE', *, *, #184816, .T. ) ;
#158700=CARTESIAN_POINT ( 'NONE',  ( -10.81492255796105439, 18.62759615963255655, 47.91775706135234714 ) ) ;
#158701=CARTESIAN_POINT ( 'NONE',  ( -9.564922557960796823, -16.46253265017161027, 37.08224293864768839 ) ) ;
#158702=CARTESIAN_POINT ( 'NONE',  ( 13.89961937509977652, -13.97604488694527269, 23.12390960531436335 ) ) ;
#158703=CARTESIAN_POINT ( 'NONE',  ( -13.89961937509957401, -13.97604488694547875, 69.37609039468564731 ) ) ;
#158704=CARTESIAN_POINT ( 'NONE',  ( -15.80617190586768217, 15.72974639402176855, 28.12609039468568284 ) ) ;
#158705=CARTESIAN_POINT ( 'NONE',  ( -13.97604488694547697, 13.89961937509957934, 58.12609039468566863 ) ) ;
#158706=CARTESIAN_POINT ( 'NONE',  ( 19.02544592524343514, -5.153800228976328945, 23.54057627198102054 ) ) ;
#158707=CARTESIAN_POINT ( 'NONE',  ( -4.483927247898782831, 16.52544592524335698, 97.70942372801904696 ) ) ;
#158708=CARTESIAN_POINT ( 'NONE',  ( 19.02544592524334988, 5.153800228976608722, 66.45942372801899012 ) ) ;
#158709=CARTESIAN_POINT ( 'NONE',  ( 8.224510206698953496, -14.34966873604960469, 27.91557627198103830 ) ) ;
#158711=CARTESIAN_POINT ( 'NONE',  ( 0.05219959533909260263, 19.03943276465977164, 79.99890960531436690 ) ) ;
#158712=CARTESIAN_POINT ( 'NONE',  ( -21.53943276465977519, -0.05219959533937600094, 88.75109039468567573 ) ) ;
#158713=CARTESIAN_POINT ( 'NONE',  ( 21.53943276465977519, 0.05219959533937863772, 106.2510903946856757 ) ) ;
#158715=CARTESIAN_POINT ( 'NONE',  ( -10.81492255796105439, 18.62759615963255655, 72.91775706135234714 ) ) ;
#158716=CARTESIAN_POINT ( 'NONE',  ( -8.224510206698735004, -14.34966873604973081, 34.58442372801900433 ) ) ;
#158717=CARTESIAN_POINT ( 'NONE',  ( 16.51473224551069308, 9.474510206698969483, 74.16557627198103830 ) ) ;
#158718=CARTESIAN_POINT ( 'NONE',  ( -21.52544592524343514, 5.823673210054127303, 31.04057627198102409 ) ) ;
#158720=CARTESIAN_POINT ( 'NONE',  ( 13.89961937509977652, -13.97604488694527269, 63.12390960531435979 ) ) ;
#158721=CARTESIAN_POINT ( 'NONE',  ( -17.26058549869106429, 6.457015423128241949, 98.62254162523932166 ) ) ;
#158722=CARTESIAN_POINT ( 'NONE',  ( -5.049401038297874678, -19.05341960407617918, 74.79275706135231871 ) ) ;
#158724=CARTESIAN_POINT ( 'NONE',  ( -0.05219959533909027116, -19.03943276465977164, 102.4989096053143669 ) ) ;
#158725=CARTESIAN_POINT ( 'NONE',  ( 5.719274019375673035, 21.55341960407619339, 102.2927570613523613 ) ) ;
#158726=CARTESIAN_POINT ( 'NONE',  ( -4.379528057220328563, 16.55341960407611168, 80.20724293864769550 ) ) ;
#158727=CARTESIAN_POINT ( 'NONE',  ( -21.53943276465977519, 0.05219959533907696930, 46.24890960531435979 ) ) ;
#158728=CARTESIAN_POINT ( 'NONE',  ( 18.62759615963271287, -10.81492255796078972, 43.33224293864769550 ) ) ;
#158729=CARTESIAN_POINT ( 'NONE',  ( 14.34966873604960469, 8.224510206698951720, 99.16557627198100988 ) ) ;
#158731=CARTESIAN_POINT ( 'NONE',  ( 13.97604488694548053, -13.89961937509957401, 60.62609039468564731 ) ) ;
#158732=CARTESIAN_POINT ( 'NONE',  ( 4.379528057220339221, -16.55341960407611168, 22.70724293864769194 ) ) ;
#158733=CARTESIAN_POINT ( 'NONE',  ( -13.97604488694527625, -13.89961937509977652, 101.8739096053143811 ) ) ;
#158734=CARTESIAN_POINT ( 'NONE',  ( -5.719274019375665041, -21.55341960407619695, 69.79275706135234714 ) ) ;
#158735=CARTESIAN_POINT ( 'NONE',  ( -5.823673210054116645, -21.52544592524344225, 57.29057627198103120 ) ) ;
#158736=B_SPLINE_CURVE_WITH_KNOTS ( 'NONE', 3,
 ( #26151, #196007, #69638, #55467, #147487, #56471, #118150, #27149, #120127, #73649, #148487, #88796, #165651, #132312, #9978, #71638, #100958, #119152, #180834, #131304, #8978, #135321, #70646, #150489, #85801, #41311, #117137, #194004, #179840, #196993, #133305, #194994 ),
 .UNSPECIFIED., .F., .F.,
 ( 4, 2, 2, 2, 2, 2, 2, 2, 2, 2, 2, 2, 2, 2, 2, 4 ),
 ( 4.563344992840995729E-17, 0.0003712461730037242913, 0.0007424923460074029377, 0.001113738519011081476, 0.001484984692014760122, 0.002227477038022111343, 0.002598723211025783918, 0.002969969384029456493, 0.003341215557033128634, 0.003712461730036799908, 0.004083707903040472917, 0.004454954076044144624, 0.004826200249047817199, 0.005197446422051488907, 0.005568692595055160614, 0.005939938768058833189 ),
 .UNSPECIFIED. ) ;
#158737=CARTESIAN_POINT ( 'NONE',  ( -18.62759615963255300, -10.81492255796106328, 49.16775706135234003 ) ) ;
#158738=CARTESIAN_POINT ( 'NONE',  ( 10.81492255796078972, 18.62759615963270932, 99.58224293864770971 ) ) ;
#158739=CARTESIAN_POINT ( 'NONE',  ( -15.80617190586768217, 15.72974639402176855, 38.12609039468567573 ) ) ;
#158740=CARTESIAN_POINT ( 'NONE',  ( 0.05219959533910956823, 16.53943276465976808, 114.9989096053143669 ) ) ;
#158741=CARTESIAN_POINT ( 'NONE',  ( -5.049401038298153566, 19.05341960407611168, 85.20724293864766707 ) ) ;
#158742=CARTESIAN_POINT ( 'NONE',  ( 16.55341960407611168, 4.379528057220329451, 98.95724293864770971 ) ) ;
#158743=CARTESIAN_POINT ( 'NONE',  ( 5.153800228976335163, 19.02544592524342804, 109.7905762719810099 ) ) ;
#158744=CARTESIAN_POINT ( 'NONE',  ( 4.379528057220339221, -16.55341960407611168, 57.70724293864770260 ) ) ;
#158745=CARTESIAN_POINT ( 'NONE',  ( 16.55341960407618274, -4.379528057220086978, 111.0427570613523613 ) ) ;
#158746=CARTESIAN_POINT ( 'NONE',  ( -16.51473224551069308, -9.474510206698971260, 46.66557627198102409 ) ) ;
#158747=CARTESIAN_POINT ( 'NONE',  ( -19.03943276465977164, 0.05219959533909376836, 21.24890960531436335 ) ) ;
#158748=CARTESIAN_POINT ( 'NONE',  ( -18.62759615963270932, 10.81492255796079327, 35.83224293864768839 ) ) ;
#158749=CARTESIAN_POINT ( 'NONE',  ( -5.049401038297874678, -19.05341960407617918, 19.79275706135233293 ) ) ;
#158750=CARTESIAN_POINT ( 'NONE',  ( -16.61371651742603461, -7.165104196376044676, 41.14584930007004004 ) ) ;
#158751=CARTESIAN_POINT ( 'NONE',  ( 16.53943276465976808, -0.05219959533910856209, 38.74890960531435979 ) ) ;
#158752=CARTESIAN_POINT ( 'NONE',  ( 10.81492255796106328, -18.62759615963255655, 45.41775706135234003 ) ) ;
#158753=CARTESIAN_POINT ( 'NONE',  ( 19.02544592524343514, -5.153800228976328945, 113.5405762719810241 ) ) ;
#158754=CARTESIAN_POINT ( 'NONE',  ( 14.34966873604972726, -8.224510206698740333, 55.83442372801901854 ) ) ;
#158755=CARTESIAN_POINT ( 'NONE',  ( -13.89961937509957401, -13.97604488694547875, 64.37609039468567573 ) ) ;
#158756=CARTESIAN_POINT ( 'NONE',  ( -4.483927247898539470, -16.52544592524342804, 32.29057627198102409 ) ) ;
#158757=CARTESIAN_POINT ( 'NONE',  ( 4.483927247898790824, -16.52544592524335698, 105.2094237280190328 ) ) ;
#158758=CARTESIAN_POINT ( 'NONE',  ( 9.564922557960805705, 16.46253265017160317, 44.58224293864769550 ) ) ;
#158759=CARTESIAN_POINT ( 'NONE',  ( 13.89961937509977652, -13.97604488694527269, 68.12390960531436690 ) ) ;
#158760=CARTESIAN_POINT ( 'NONE',  ( 5.049401038298161559, -19.05341960407611168, 22.70724293864769194 ) ) ;
#158761=CARTESIAN_POINT ( 'NONE',  ( 10.81492255796106328, -18.62759615963255655, 35.41775706135234003 ) ) ;
#158762=CARTESIAN_POINT ( 'NONE',  ( -13.97604488694527625, -13.89961937509977652, 41.87390960531435979 ) ) ;
#158765=CARTESIAN_POINT ( 'NONE',  ( 9.474510206698971260, -16.51473224551069308, 32.91557627198102409 ) ) ;
#158767=CARTESIAN_POINT ( 'NONE',  ( 9.474510206698971260, -16.51473224551069308, 112.9155762719810383 ) ) ;
#158768=CARTESIAN_POINT ( 'NONE',  ( -18.62759615963255300, -10.81492255796106328, 64.16775706135234714 ) ) ;
#158769=CARTESIAN_POINT ( 'NONE',  ( 14.34966873604960469, 8.224510206698951720, 109.1655762719810383 ) ) ;
#158770=CARTESIAN_POINT ( 'NONE',  ( -19.02544592524342804, 5.153800228976336051, 111.0405762719810099 ) ) ;
#158771=CARTESIAN_POINT ( 'NONE',  ( 14.29746914071037800, 8.314922557961029526, 76.66775706135234714 ) ) ;
#158772=CARTESIAN_POINT ( 'NONE',  ( 5.719274019375673035, 21.55341960407619339, 87.29275706135236135 ) ) ;
#158773=CARTESIAN_POINT ( 'NONE',  ( -0.05219959533934338120, 16.53943276465976808, 57.50109039468568994 ) ) ;
#158774=CARTESIAN_POINT ( 'NONE',  ( -9.474510206698964154, 16.51473224551069663, 100.4155762719810241 ) ) ;
#158776=CARTESIAN_POINT ( 'NONE',  ( 4.483927247898790824, -16.52544592524335698, 40.20942372801901854 ) ) ;
#158777=CARTESIAN_POINT ( 'NONE',  ( -14.29746914071037622, -8.314922557961029526, 29.16775706135234003 ) ) ;
#158778=CARTESIAN_POINT ( 'NONE',  ( -14.34966873604972548, 8.224510206698743886, 88.33442372801901854 ) ) ;
#158779=CARTESIAN_POINT ( 'NONE',  ( -13.97604488694547697, 13.89961937509957934, 103.1260903946856473 ) ) ;
#158780=CARTESIAN_POINT ( 'NONE',  ( 10.72451020669898902, -18.67979575497178502, 97.91557627198103830 ) ) ;
#158781=CARTESIAN_POINT ( 'NONE',  ( -4.379528057220328563, 16.55341960407611168, 100.2072429386476955 ) ) ;
#158782=CARTESIAN_POINT ( 'NONE',  ( 16.51473224551083163, -9.474510206698727899, 100.8344237280190043 ) ) ;
#158783=CARTESIAN_POINT ( 'NONE',  ( 16.52544592524335698, 4.483927247898782831, 66.45942372801903275 ) ) ;
#158785=CARTESIAN_POINT ( 'NONE',  ( -16.46253265017146816, -9.564922557961047289, 64.16775706135233293 ) ) ;
#158786=CARTESIAN_POINT ( 'NONE',  ( -12.14591786802309592, -12.06949235617757132, 46.87390960531435979 ) ) ;
#158787=CARTESIAN_POINT ( 'NONE',  ( -14.34966873604960291, -8.224510206698953496, 26.66557627198103475 ) ) ;
#158788=CARTESIAN_POINT ( 'NONE',  ( 4.379528057220339221, -16.55341960407611168, 87.70724293864769550 ) ) ;
#158789=CARTESIAN_POINT ( 'NONE',  ( -5.049401038297874678, -19.05341960407617918, 34.79275706135233293 ) ) ;
#158790=CARTESIAN_POINT ( 'NONE',  ( -15.72974639402176322, -15.80617190586768395, 39.37609039468567573 ) ) ;
#158791=CARTESIAN_POINT ( 'NONE',  ( -19.05341960407617563, 5.049401038297882671, 98.54275706135233293 ) ) ;
#158792=FACE_OUTER_BOUND ( 'NONE', #165625, .T. ) ;
#158793=CARTESIAN_POINT ( 'NONE',  ( -5.049401038298153566, 19.05341960407611168, 85.20724293864766707 ) ) ;
#158794=CARTESIAN_POINT ( 'NONE',  ( 9.564922557960805705, 16.46253265017160317, 89.58224293864769550 ) ) ;
#158795=CARTESIAN_POINT ( 'NONE',  ( 18.67979575497178502, 10.72451020669898547, 59.16557627198103120 ) ) ;
#158796=CARTESIAN_POINT ( 'NONE',  ( 14.34966873604960469, 8.224510206698951720, 99.16557627198100988 ) ) ;
#158797=CARTESIAN_POINT ( 'NONE',  ( 9.564922557960805705, 16.46253265017160317, 69.58224293864770971 ) ) ;
#158798=CARTESIAN_POINT ( 'NONE',  ( -16.55341960407611168, -4.379528057220339221, 111.4572429386476813 ) ) ;
#158799=CARTESIAN_POINT ( 'NONE',  ( -15.72974639402176322, -15.80617190586768395, 44.37609039468567573 ) ) ;
#158800=CARTESIAN_POINT ( 'NONE',  ( -5.719274019375665041, -21.55341960407619695, 74.79275706135234714 ) ) ;
#158801=CARTESIAN_POINT ( 'NONE',  ( -13.97604488694527625, -13.89961937509977652, 56.87390960531434558 ) ) ;
#158802=CARTESIAN_POINT ( 'NONE',  ( 4.483927247898790824, -16.52544592524335698, 75.20942372801901854 ) ) ;
#158803=CARTESIAN_POINT ( 'NONE',  ( -5.719274019375665041, -21.55341960407619695, 29.79275706135234358 ) ) ;
#158804=CARTESIAN_POINT ( 'NONE',  ( -15.80617190586768217, 15.72974639402176855, 23.12609039468567573 ) ) ;
#158805=CARTESIAN_POINT ( 'NONE',  ( 13.89961937509957401, 13.97604488694547697, 46.87609039468565442 ) ) ;
#158806=CARTESIAN_POINT ( 'NONE',  ( -16.51473224551069308, -9.474510206698971260, 76.66557627198103830 ) ) ;
#158807=CARTESIAN_POINT ( 'NONE',  ( 5.049401038297881783, 19.05341960407617563, 27.29275706135232937 ) ) ;
#158808=CARTESIAN_POINT ( 'NONE',  ( -10.81492255796105439, 18.62759615963255655, 77.91775706135231871 ) ) ;
#158809=EDGE_CURVE ( 'NONE', #183245, #47139, #102026, .T. ) ;
#158810=CARTESIAN_POINT ( 'NONE',  ( -21.52544592524343514, 5.823673210054127303, 66.04057627198103830 ) ) ;
#158811=CARTESIAN_POINT ( 'NONE',  ( -12.06949235617756955, 12.14591786802309770, 50.62390960531435979 ) ) ;
#158812=CARTESIAN_POINT ( 'NONE',  ( -21.55341960407619339, 5.719274019375674811, 88.54275706135236135 ) ) ;
#158813=CARTESIAN_POINT ( 'NONE',  ( -5.049401038297874678, -19.05341960407617918, 29.79275706135232227 ) ) ;
#158814=CARTESIAN_POINT ( 'NONE',  ( 12.14591786802309770, 12.06949235617756955, 74.37390960531436690 ) ) ;
#158815=CARTESIAN_POINT ( 'NONE',  ( -19.02544592524342804, 5.153800228976336051, 26.04057627198103120 ) ) ;
#158816=CARTESIAN_POINT ( 'NONE',  ( 19.03943276465977164, 0.05219959533936151252, 56.25109039468566863 ) ) ;
#158817=CARTESIAN_POINT ( 'NONE',  ( 12.14591786802309770, 12.06949235617756955, 39.37390960531436690 ) ) ;
#158818=CARTESIAN_POINT ( 'NONE',  ( 0.05219959533937995610, -21.53943276465977519, 80.00109039468568994 ) ) ;
#158819=CARTESIAN_POINT ( 'NONE',  ( 5.049401038298161559, -19.05341960407611168, 72.70724293864768129 ) ) ;
#158820=CARTESIAN_POINT ( 'NONE',  ( 5.049401038297881783, 19.05341960407617563, 52.29275706135234003 ) ) ;
#158821=CARTESIAN_POINT ( 'NONE',  ( -10.81492255796078084, -18.62759615963271287, 47.08224293864770260 ) ) ;
#158822=CARTESIAN_POINT ( 'NONE',  ( 18.62759615963255655, 10.81492255796105972, 46.66775706135234714 ) ) ;
#158823=CARTESIAN_POINT ( 'NONE',  ( 0.05219959533907565091, 21.53943276465977519, 99.99890960531436690 ) ) ;
#158824=CARTESIAN_POINT ( 'NONE',  ( -0.05219959533936034679, 19.03943276465977164, 97.50109039468567573 ) ) ;
#158825=CARTESIAN_POINT ( 'NONE',  ( -16.52544592524335698, -4.483927247898792601, 63.95942372801901854 ) ) ;
#158827=CARTESIAN_POINT ( 'NONE',  ( -10.72451020669898014, 18.67979575497178502, 105.4155762719810383 ) ) ;
#158828=CARTESIAN_POINT ( 'NONE',  ( -0.05219959533910754901, -16.53943276465976808, 97.49890960531436690 ) ) ;
#158829=CARTESIAN_POINT ( 'NONE',  ( -17.49999999999999645, -4.640572885337608255, 29.36211835451158692 ) ) ;
#158830=CARTESIAN_POINT ( 'NONE',  ( -14.34966873604972548, 8.224510206698743886, 38.33442372801900433 ) ) ;
#158831=CARTESIAN_POINT ( 'NONE',  ( -5.719274019375978568, 21.55341960407610458, 65.20724293864768129 ) ) ;
#158832=CARTESIAN_POINT ( 'NONE',  ( -14.29746914071037622, -8.314922557961029526, 109.1677570613523613 ) ) ;
#158833=CARTESIAN_POINT ( 'NONE',  ( 9.564922557960805705, 16.46253265017160317, 34.58224293864770260 ) ) ;
#158834=CARTESIAN_POINT ( 'NONE',  ( 14.29746914071037800, 8.314922557961029526, 61.66775706135235424 ) ) ;
#158835=CARTESIAN_POINT ( 'NONE',  ( 13.89961937509957401, 13.97604488694547697, 56.87609039468564731 ) ) ;
#158836=CARTESIAN_POINT ( 'NONE',  ( 15.72974639402176855, 15.80617190586768217, 36.87609039468568994 ) ) ;
#158837=CARTESIAN_POINT ( 'NONE',  ( 18.67979575497178502, 10.72451020669898547, 64.16557627198102409 ) ) ;
#158838=CARTESIAN_POINT ( 'NONE',  ( 14.34966873604972726, -8.224510206698740333, 95.83442372801903275 ) ) ;
#158839=CARTESIAN_POINT ( 'NONE',  ( 5.823673210054444382, -21.52544592524334988, 75.20942372801901854 ) ) ;
#158840=CARTESIAN_POINT ( 'NONE',  ( -0.05219959533907301413, -21.53943276465977519, 57.49890960531435979 ) ) ;
#158841=CARTESIAN_POINT ( 'NONE',  ( 10.72451020669898902, -18.67979575497178502, 27.91557627198103830 ) ) ;
#158843=CARTESIAN_POINT ( 'NONE',  ( 14.34966873604972726, -8.224510206698740333, 80.83442372801901854 ) ) ;
#158844=CARTESIAN_POINT ( 'NONE',  ( 18.67979575497178502, 10.72451020669898547, 29.16557627198103120 ) ) ;
#158845=ORIENTED_EDGE ( 'NONE', *, *, #20984, .T. ) ;
#158846=CARTESIAN_POINT ( 'NONE',  ( -16.46253265017160317, 9.564922557960807481, 105.8322429386476955 ) ) ;
#158847=CARTESIAN_POINT ( 'NONE',  ( -14.34966873604972548, 8.224510206698743886, 108.3344237280190185 ) ) ;
#158849=CARTESIAN_POINT ( 'NONE',  ( 12.14591786802309770, 12.06949235617756955, 109.3739096053143811 ) ) ;
#158850=CARTESIAN_POINT ( 'NONE',  ( 0.05219959533907565091, 21.53943276465977519, 59.99890960531436690 ) ) ;
#158851=CARTESIAN_POINT ( 'NONE',  ( 0.05219959533934541429, -16.53943276465976808, 85.00109039468568994 ) ) ;
#158852=CARTESIAN_POINT ( 'NONE',  ( -21.55341960407619339, 5.719274019375674811, 48.54275706135234714 ) ) ;
#158853=CARTESIAN_POINT ( 'NONE',  ( 9.564922557961047289, -16.46253265017146816, 100.4177570613523329 ) ) ;
#158854=CARTESIAN_POINT ( 'NONE',  ( -16.55341960407611168, -4.379528057220339221, 106.4572429386477097 ) ) ;
#158855=CARTESIAN_POINT ( 'NONE',  ( -19.05341960407611168, -5.049401038298163336, 56.45724293864768129 ) ) ;
#158856=CARTESIAN_POINT ( 'NONE',  ( 9.564922557960805705, 16.46253265017160317, 24.58224293864769194 ) ) ;
#158858=CARTESIAN_POINT ( 'NONE',  ( 9.474510206698971260, -16.51473224551069308, 92.91557627198103830 ) ) ;
#158859=CARTESIAN_POINT ( 'NONE',  ( 12.14591786802327356, -12.06949235617739191, 75.62609039468567573 ) ) ;
#158860=CARTESIAN_POINT ( 'NONE',  ( -0.05219959533937732626, 21.53943276465977519, 102.5010903946856899 ) ) ;
#158861=CARTESIAN_POINT ( 'NONE',  ( -10.72451020669898014, 18.67979575497178502, 65.41557627198102409 ) ) ;
#158862=CARTESIAN_POINT ( 'NONE',  ( 8.224510206698742110, 14.34966873604972548, 92.08442372801901854 ) ) ;
#158863=CARTESIAN_POINT ( 'NONE',  ( 16.46253265017146816, 9.564922557961045513, 86.66775706135233293 ) ) ;
#158865=CARTESIAN_POINT ( 'NONE',  ( -9.474510206698964154, 16.51473224551069663, 40.41557627198103120 ) ) ;
#158866=CARTESIAN_POINT ( 'NONE',  ( 13.89961937509977652, -13.97604488694527269, 83.12390960531436690 ) ) ;
#158867=CARTESIAN_POINT ( 'NONE',  ( 13.97604488694527802, 13.89961937509977652, 39.37390960531435269 ) ) ;
#158868=CARTESIAN_POINT ( 'NONE',  ( -19.05341960407617563, 5.049401038297882671, 78.54275706135233293 ) ) ;
#158870=CARTESIAN_POINT ( 'NONE',  ( 19.05341960407611168, 5.049401038298154454, 93.95724293864769550 ) ) ;
#158871=CARTESIAN_POINT ( 'NONE',  ( -8.224510206698948167, 14.34966873604960824, 55.41557627198102409 ) ) ;
#158872=CARTESIAN_POINT ( 'NONE',  ( -15.72974639402197994, 15.80617190586746368, 55.62390960531436690 ) ) ;
#158874=CARTESIAN_POINT ( 'NONE',  ( 9.474510206698729675, 16.51473224551082808, 32.08442372801900433 ) ) ;
#158876=CARTESIAN_POINT ( 'NONE',  ( -9.564922557960796823, -16.46253265017161027, 57.08224293864769550 ) ) ;
#158877=CARTESIAN_POINT ( 'NONE',  ( -5.153800228976328057, -19.02544592524343514, 77.29057627198099567 ) ) ;
#158878=CARTESIAN_POINT ( 'NONE',  ( 14.29746914071037800, 8.314922557961029526, 31.66775706135234358 ) ) ;
#158881=CARTESIAN_POINT ( 'NONE',  ( 8.314922557961029526, -14.29746914071037800, 70.41775706135236135 ) ) ;
#158882=CARTESIAN_POINT ( 'NONE',  ( -5.719274019375978568, 21.55341960407610458, 100.2072429386476955 ) ) ;
#158883=CARTESIAN_POINT ( 'NONE',  ( -12.06949235617739369, -12.14591786802326823, 44.37609039468567573 ) ) ;
#158884=CARTESIAN_POINT ( 'NONE',  ( -9.474510206698964154, 16.51473224551069663, 40.41557627198103120 ) ) ;
#158886=CARTESIAN_POINT ( 'NONE',  ( 5.823673210054444382, -21.52544592524334988, 60.20942372801902565 ) ) ;
#158887=CARTESIAN_POINT ( 'NONE',  ( -13.89961937509957401, -13.97604488694547875, 64.37609039468567573 ) ) ;
#158888=CARTESIAN_POINT ( 'NONE',  ( -21.55341960407619339, 5.719274019375674811, 88.54275706135236135 ) ) ;
#158889=CARTESIAN_POINT ( 'NONE',  ( -17.49999999999999645, 5.499999999999992895, 48.71769037696437010 ) ) ;
#158890=CARTESIAN_POINT ( 'NONE',  ( 14.34966873604960469, 8.224510206698951720, 39.16557627198102409 ) ) ;
#158891=CARTESIAN_POINT ( 'NONE',  ( 19.39056639909672342, 5.500000000000043521, 43.28948781074344510 ) ) ;
#158892=CARTESIAN_POINT ( 'NONE',  ( -10.72451020669898014, 18.67979575497178502, 50.41557627198103120 ) ) ;
#158894=CARTESIAN_POINT ( 'NONE',  ( 19.02544592524343514, -5.153800228976328945, 108.5405762719810383 ) ) ;
#158895=CARTESIAN_POINT ( 'NONE',  ( -16.52544592524342804, 4.483927247898546575, 106.0405762719810525 ) ) ;
#158896=CARTESIAN_POINT ( 'NONE',  ( -16.53943276465976808, -0.05219959533934237506, 28.75109039468567929 ) ) ;
#158897=CARTESIAN_POINT ( 'NONE',  ( 14.34966873604972726, -8.224510206698740333, 105.8344237280190328 ) ) ;
#158898=VERTEX_POINT ( 'NONE', #106386 ) ;
#158899=CARTESIAN_POINT ( 'NONE',  ( -0.05219959533907301413, -21.53943276465977519, 107.4989096053143669 ) ) ;
#158900=CARTESIAN_POINT ( 'NONE',  ( -16.52544592524342804, 4.483927247898546575, 26.04057627198103475 ) ) ;
#158901=CARTESIAN_POINT ( 'NONE',  ( -19.02544592524342804, 5.153800228976336051, 116.0405762719810383 ) ) ;
#158902=CARTESIAN_POINT ( 'NONE',  ( 5.153800228976615827, -19.02544592524334988, 90.20942372801900433 ) ) ;
#158903=CARTESIAN_POINT ( 'NONE',  ( -10.81492255796105439, 18.62759615963255655, 102.9177570613523756 ) ) ;
#158904=CARTESIAN_POINT ( 'NONE',  ( 14.34966873604960469, 8.224510206698951720, 29.16557627198103120 ) ) ;
#158905=CARTESIAN_POINT ( 'NONE',  ( 21.52544592524344225, -5.823673210054117533, 88.54057627198103830 ) ) ;
#158906=CARTESIAN_POINT ( 'NONE',  ( -21.52544592524343514, 5.823673210054127303, 56.04057627198102409 ) ) ;
#158907=CARTESIAN_POINT ( 'NONE',  ( 13.97604488694527802, 13.89961937509977652, 59.37390960531434558 ) ) ;
#158908=CARTESIAN_POINT ( 'NONE',  ( -14.34966873604960291, -8.224510206698953496, 36.66557627198103120 ) ) ;
#158909=CARTESIAN_POINT ( 'NONE',  ( 19.03943276465977164, -0.05219959533909143690, 73.74890960531435269 ) ) ;
#158910=ORIENTED_EDGE ( 'NONE', *, *, #124931, .F. ) ;
#158911=CARTESIAN_POINT ( 'NONE',  ( 19.19724070472091171, 5.500000000000159872, 58.56193348274382515 ) ) ;
#158912=CARTESIAN_POINT ( 'NONE',  ( -13.89961937509957401, -13.97604488694547875, 44.37609039468566863 ) ) ;
#158913=CARTESIAN_POINT ( 'NONE',  ( 18.62759615963271287, -10.81492255796078972, 78.33224293864770971 ) ) ;
#158914=CARTESIAN_POINT ( 'NONE',  ( -16.52544592524342804, 4.483927247898546575, 106.0405762719810525 ) ) ;
#158916=CARTESIAN_POINT ( 'NONE',  ( -15.72974639402176322, -15.80617190586768395, 39.37609039468567573 ) ) ;
#158918=CARTESIAN_POINT ( 'NONE',  ( -0.05219959533934338120, 16.53943276465976808, 102.5010903946856899 ) ) ;
#158919=CARTESIAN_POINT ( 'NONE',  ( 9.474510206698971260, -16.51473224551069308, 32.91557627198102409 ) ) ;
#158920=CARTESIAN_POINT ( 'NONE',  ( 0.05219959533909260263, 19.03943276465977164, 84.99890960531436690 ) ) ;
#158921=CARTESIAN_POINT ( 'NONE',  ( 9.474510206698971260, -16.51473224551069308, 37.91557627198102409 ) ) ;
#158922=CARTESIAN_POINT ( 'NONE',  ( -14.29746914071049879, 8.314922557960819915, 45.83224293864769550 ) ) ;
#158923=EDGE_CURVE ( 'NONE', #9532, #107482, #20000, .T. ) ;
#158924=CARTESIAN_POINT ( 'NONE',  ( -21.53943276465977519, -0.05219959533937600094, 78.75109039468568994 ) ) ;
#158926=CARTESIAN_POINT ( 'NONE',  ( 16.53943276465976808, 0.05219959533934440121, 66.25109039468567573 ) ) ;
#158927=CARTESIAN_POINT ( 'NONE',  ( -19.05341960407611168, -5.049401038298163336, 46.45724293864768129 ) ) ;
#158928=CARTESIAN_POINT ( 'NONE',  ( -13.97604488694527625, -13.89961937509977652, 51.87390960531436690 ) ) ;
#158930=CARTESIAN_POINT ( 'NONE',  ( -18.67979575497193778, 10.72451020669871902, 103.3344237280190043 ) ) ;
#158931=CARTESIAN_POINT ( 'NONE',  ( -16.52544592524335698, -4.483927247898792601, 58.95942372801902565 ) ) ;
#158932=CARTESIAN_POINT ( 'NONE',  ( 10.81492255796106328, -18.62759615963255655, 105.4177570613523613 ) ) ;
#158933=CARTESIAN_POINT ( 'NONE',  ( -21.52544592524343514, 5.823673210054127303, 41.04057627198103120 ) ) ;
#158934=CARTESIAN_POINT ( 'NONE',  ( 19.03943276465977164, 0.05219959533936151252, 111.2510903946856757 ) ) ;
#158935=CARTESIAN_POINT ( 'NONE',  ( -5.719274019375665041, -21.55341960407619695, 69.79275706135234714 ) ) ;
#158936=CARTESIAN_POINT ( 'NONE',  ( -12.14591786802326823, 12.06949235617739902, 33.12609039468569705 ) ) ;
#158937=CARTESIAN_POINT ( 'NONE',  ( 10.81492255796078972, 18.62759615963270932, 104.5822429386477097 ) ) ;
#158938=CARTESIAN_POINT ( 'NONE',  ( -9.564922557961040184, 16.46253265017147172, 97.91775706135233293 ) ) ;
#158939=CARTESIAN_POINT ( 'NONE',  ( -9.474510206698964154, 16.51473224551069663, 70.41557627198102409 ) ) ;
#158940=CARTESIAN_POINT ( 'NONE',  ( 4.483927247898790824, -16.52544592524335698, 20.20942372801900788 ) ) ;
#158941=CARTESIAN_POINT ( 'NONE',  ( 9.564922557961047289, -16.46253265017146816, 105.4177570613523471 ) ) ;
#158942=CARTESIAN_POINT ( 'NONE',  ( -12.14591786802309592, -12.06949235617757132, 66.87390960531436690 ) ) ;
#158943=CARTESIAN_POINT ( 'NONE',  ( -16.55341960407617563, 4.379528057220093196, 73.54275706135234714 ) ) ;
#158944=CARTESIAN_POINT ( 'NONE',  ( -15.80617190586768217, 15.72974639402176855, 23.12609039468567573 ) ) ;
#158945=CARTESIAN_POINT ( 'NONE',  ( -16.51473224551069308, -9.474510206698971260, 46.66557627198102409 ) ) ;
#158946=CARTESIAN_POINT ( 'NONE',  ( 19.02544592524343514, -5.153800228976328945, 53.54057627198102409 ) ) ;
#158947=CARTESIAN_POINT ( 'NONE',  ( -16.55341960407617563, 4.379528057220093196, 68.54275706135234714 ) ) ;
#158951=CARTESIAN_POINT ( 'NONE',  ( -13.97604488694547697, 13.89961937509957934, 23.12609039468565442 ) ) ;
#158952=CARTESIAN_POINT ( 'NONE',  ( 9.564922557960805705, 16.46253265017160317, 24.58224293864769194 ) ) ;
#158954=CARTESIAN_POINT ( 'NONE',  ( 12.06949235617739724, 12.14591786802326823, 21.87609039468567573 ) ) ;
#158955=CARTESIAN_POINT ( 'NONE',  ( 21.55341960407610458, 5.719274019375980345, 53.95724293864770260 ) ) ;
#158956=CARTESIAN_POINT ( 'NONE',  ( 19.02544592524334988, 5.153800228976608722, 51.45942372801900433 ) ) ;
#158957=CARTESIAN_POINT ( 'NONE',  ( 8.224510206698742110, 14.34966873604972548, 32.08442372801901854 ) ) ;
#158958=CARTESIAN_POINT ( 'NONE',  ( 9.474510206698971260, -16.51473224551069308, 42.91557627198103120 ) ) ;
#158959=CARTESIAN_POINT ( 'NONE',  ( -0.05219959533909027116, -19.03943276465977164, 47.49890960531435979 ) ) ;
#158960=CARTESIAN_POINT ( 'NONE',  ( 10.72451020669898902, -18.67979575497178502, 87.91557627198103830 ) ) ;
#158961=CARTESIAN_POINT ( 'NONE',  ( -9.474510206698964154, 16.51473224551069663, 110.4155762719810383 ) ) ;
#158962=CARTESIAN_POINT ( 'NONE',  ( -5.153800228976328057, -19.02544592524343514, 52.29057627198100988 ) ) ;
#158963=CARTESIAN_POINT ( 'NONE',  ( 17.49999999999999289, 5.500000000000006217, 48.78230962303565121 ) ) ;
#158964=CARTESIAN_POINT ( 'NONE',  ( -13.97604488694547697, 13.89961937509957934, 98.12609039468566152 ) ) ;
#158965=CARTESIAN_POINT ( 'NONE',  ( -12.14591786802309592, -12.06949235617757132, 61.87390960531436690 ) ) ;
#158966=CARTESIAN_POINT ( 'NONE',  ( 19.05341960407617918, -5.049401038297876454, 31.04275706135232227 ) ) ;
#158967=CARTESIAN_POINT ( 'NONE',  ( -10.81492255796078084, -18.62759615963271287, 102.0822429386476955 ) ) ;
#158968=CARTESIAN_POINT ( 'NONE',  ( 5.823673210054444382, -21.52544592524334988, 90.20942372801903275 ) ) ;
#158969=CARTESIAN_POINT ( 'NONE',  ( 19.03943276465977164, -0.05219959533909143690, 23.74890960531435269 ) ) ;
#158970=CARTESIAN_POINT ( 'NONE',  ( -15.72974639402176322, -15.80617190586768395, 74.37609039468568994 ) ) ;
#158971=CARTESIAN_POINT ( 'NONE',  ( -8.314922557960811034, -14.29746914071050412, 22.08224293864769194 ) ) ;
#158972=CARTESIAN_POINT ( 'NONE',  ( 5.719274019375673035, 21.55341960407619339, 77.29275706135234714 ) ) ;
#158973=CARTESIAN_POINT ( 'NONE',  ( -16.46253265017160317, 9.564922557960807481, 70.83224293864770971 ) ) ;
#158974=CARTESIAN_POINT ( 'NONE',  ( -18.67979575497193778, 10.72451020669871902, 43.33442372801901143 ) ) ;
#158975=CARTESIAN_POINT ( 'NONE',  ( 19.03943276465977164, -0.05219959533909143690, 83.74890960531436690 ) ) ;
#158976=CARTESIAN_POINT ( 'NONE',  ( 4.379528057220339221, -16.55341960407611168, 87.70724293864769550 ) ) ;
#158977=CARTESIAN_POINT ( 'NONE',  ( 8.224510206698953496, -14.34966873604960469, 57.91557627198103120 ) ) ;
#158978=CARTESIAN_POINT ( 'NONE',  ( -15.80617190586745835, -15.72974639402198527, 76.87390960531439532 ) ) ;
#158979=CARTESIAN_POINT ( 'NONE',  ( 5.153800228976335163, 19.02544592524342804, 59.79057627198100988 ) ) ;
#158980=CARTESIAN_POINT ( 'NONE',  ( -5.823673210054116645, -21.52544592524344225, 87.29057627198103830 ) ) ;
#158981=CARTESIAN_POINT ( 'NONE',  ( 16.46253265017146816, 9.564922557961045513, 61.66775706135234003 ) ) ;
#158982=CARTESIAN_POINT ( 'NONE',  ( -9.564922557961040184, 16.46253265017147172, 27.91775706135232582 ) ) ;
#158983=CARTESIAN_POINT ( 'NONE',  ( -16.53943276465976808, 0.05219959533911058130, 81.24890960531436690 ) ) ;
#158984=CARTESIAN_POINT ( 'NONE',  ( 5.719274019375991003, -21.55341960407610458, 47.70724293864770260 ) ) ;
#158986=CARTESIAN_POINT ( 'NONE',  ( -14.29746914071037622, -8.314922557961029526, 104.1677570613523471 ) ) ;
#158988=CARTESIAN_POINT ( 'NONE',  ( -16.46253265017146816, -9.564922557961047289, 104.1677570613523329 ) ) ;
#158989=CARTESIAN_POINT ( 'NONE',  ( -16.55341960407611168, -4.379528057220339221, 61.45724293864770260 ) ) ;
#158990=CARTESIAN_POINT ( 'NONE',  ( -17.50000000000001776, 3.565345528327884317, 34.42494486806472054 ) ) ;
#158991=CARTESIAN_POINT ( 'NONE',  ( -13.97604488694527625, -13.89961937509977652, 61.87390960531435979 ) ) ;
#158992=CARTESIAN_POINT ( 'NONE',  ( -0.05219959533910754901, -16.53943276465976808, 47.49890960531435979 ) ) ;
#158993=CARTESIAN_POINT ( 'NONE',  ( -5.049401038298153566, 19.05341960407611168, 100.2072429386476955 ) ) ;
#158994=CARTESIAN_POINT ( 'NONE',  ( -13.89961937509957401, -13.97604488694547875, 74.37609039468566152 ) ) ;
#158995=CARTESIAN_POINT ( 'NONE',  ( 16.46253265017160672, -9.564922557960803928, 63.33224293864769550 ) ) ;
#158996=CARTESIAN_POINT ( 'NONE',  ( -16.51473224551069308, -9.474510206698971260, 81.66557627198103830 ) ) ;
#158997=CARTESIAN_POINT ( 'NONE',  ( 5.153800228976335163, 19.02544592524342804, 79.79057627198102409 ) ) ;
#158998=CARTESIAN_POINT ( 'NONE',  ( 21.53943276465977519, -0.05219959533907433946, 58.74890960531436690 ) ) ;
#158999=CARTESIAN_POINT ( 'NONE',  ( -16.52544592524335698, -4.483927247898792601, 53.95942372801900433 ) ) ;
#159000=CARTESIAN_POINT ( 'NONE',  ( 0.05219959533936267826, -19.03943276465977164, 105.0010903946856615 ) ) ;
#159001=CARTESIAN_POINT ( 'NONE',  ( 0.05219959533909260263, 19.03943276465977164, 49.99890960531435979 ) ) ;
#159002=CARTESIAN_POINT ( 'NONE',  ( -15.80617190586745835, -15.72974639402198527, 51.87390960531437401 ) ) ;
#159003=CARTESIAN_POINT ( 'NONE',  ( -16.46253265017146816, -9.564922557961047289, 94.16775706135233293 ) ) ;
#159004=CARTESIAN_POINT ( 'NONE',  ( -16.55341960407611168, -4.379528057220339221, 31.45724293864769550 ) ) ;
#159005=CARTESIAN_POINT ( 'NONE',  ( 21.55341960407619695, -5.719274019375665929, 41.04275706135236135 ) ) ;
#159006=CARTESIAN_POINT ( 'NONE',  ( -19.05341960407617563, 5.049401038297882671, 33.54275706135231871 ) ) ;
#159007=CARTESIAN_POINT ( 'NONE',  ( -14.34966873604972548, 8.224510206698743886, 53.33442372801901854 ) ) ;
#159008=CARTESIAN_POINT ( 'NONE',  ( -16.53943276465976808, -0.05219959533934237506, 88.75109039468567573 ) ) ;
#159010=CARTESIAN_POINT ( 'NONE',  ( -12.06949235617739369, -12.14591786802326823, 74.37609039468568994 ) ) ;
#159011=CARTESIAN_POINT ( 'NONE',  ( -5.823673210054116645, -21.52544592524344225, 32.29057627198102409 ) ) ;
#159012=CARTESIAN_POINT ( 'NONE',  ( -8.314922557961024197, 14.29746914071037800, 37.91775706135235424 ) ) ;
#159013=CARTESIAN_POINT ( 'NONE',  ( -16.51473224551069308, -9.474510206698971260, 41.66557627198103120 ) ) ;
#159014=CARTESIAN_POINT ( 'NONE',  ( 19.02544592524343514, -5.153800228976328945, 43.54057627198103120 ) ) ;
#159015=CARTESIAN_POINT ( 'NONE',  ( 19.03943276465977164, -0.05219959533909143690, 58.74890960531435979 ) ) ;
#159016=CARTESIAN_POINT ( 'NONE',  ( 0.05219959533937995610, -21.53943276465977519, 35.00109039468568284 ) ) ;
#159017=CARTESIAN_POINT ( 'NONE',  ( -16.52544592524335698, -4.483927247898792601, 53.95942372801900433 ) ) ;
#159018=CARTESIAN_POINT ( 'NONE',  ( 12.06949235617739724, 12.14591786802326823, 106.8760903946856899 ) ) ;
#159019=CARTESIAN_POINT ( 'NONE',  ( -9.564922557960796823, -16.46253265017161027, 22.08224293864768839 ) ) ;
#159020=CARTESIAN_POINT ( 'NONE',  ( -21.53943276465977519, -0.05219959533937600094, 108.7510903946857042 ) ) ;
#159021=CARTESIAN_POINT ( 'NONE',  ( -8.224510206698735004, -14.34966873604973081, 19.58442372801901143 ) ) ;
#159022=CARTESIAN_POINT ( 'NONE',  ( 19.03943276465977164, 0.05219959533936151252, 66.25109039468567573 ) ) ;
#159023=CARTESIAN_POINT ( 'NONE',  ( 8.314922557960818139, 14.29746914071049879, 64.58224293864769550 ) ) ;
#159024=CARTESIAN_POINT ( 'NONE',  ( -16.51473224551069308, -9.474510206698971260, 41.66557627198103120 ) ) ;
#159025=CARTESIAN_POINT ( 'NONE',  ( 9.564922557961047289, -16.46253265017146816, 70.41775706135233293 ) ) ;
#159026=CARTESIAN_POINT ( 'NONE',  ( 17.05587630539786304, 6.762274262135719027, 76.75819690962691766 ) ) ;
#159027=CARTESIAN_POINT ( 'NONE',  ( 10.81492255796106328, -18.62759615963255655, 80.41775706135234714 ) ) ;
#159028=CARTESIAN_POINT ( 'NONE',  ( 16.55341960407618274, -4.379528057220086978, 41.04275706135236135 ) ) ;
#159030=CARTESIAN_POINT ( 'NONE',  ( -5.823673210054116645, -21.52544592524344225, 37.29057627198102409 ) ) ;
#159031=CARTESIAN_POINT ( 'NONE',  ( 8.224510206698742110, 14.34966873604972548, 27.08442372801901854 ) ) ;
#159032=CARTESIAN_POINT ( 'NONE',  ( 17.72662750342729510, 5.499999999999909406, 88.90179492283745333 ) ) ;
#159033=CARTESIAN_POINT ( 'NONE',  ( 0.05219959533936267826, -19.03943276465977164, 30.00109039468566863 ) ) ;
#159035=CARTESIAN_POINT ( 'NONE',  ( 0.05219959533909260263, 19.03943276465977164, 44.99890960531435979 ) ) ;
#159036=CARTESIAN_POINT ( 'NONE',  ( -16.51473224551082808, 9.474510206698731452, 58.33442372801900433 ) ) ;
#159037=CARTESIAN_POINT ( 'NONE',  ( 16.51473224551069308, 9.474510206698969483, 64.16557627198102409 ) ) ;
#159038=CARTESIAN_POINT ( 'NONE',  ( -19.02130022317636815, 5.499999999999802824, 100.7818866924657897 ) ) ;
#159039=CARTESIAN_POINT ( 'NONE',  ( 13.89961937509957401, 13.97604488694547697, 21.87609039468566152 ) ) ;
#159040=CARTESIAN_POINT ( 'NONE',  ( 0.05219959533910956823, 16.53943276465976808, 24.99890960531435624 ) ) ;
#159041=CARTESIAN_POINT ( 'NONE',  ( -9.474510206698964154, 16.51473224551069663, 30.41557627198102054 ) ) ;
#159042=CARTESIAN_POINT ( 'NONE',  ( -5.049401038298153566, 19.05341960407611168, 95.20724293864770971 ) ) ;
#159043=CARTESIAN_POINT ( 'NONE',  ( 15.80617190586769283, -15.72974639402175789, 75.62609039468567573 ) ) ;
#159044=CARTESIAN_POINT ( 'NONE',  ( 19.05341960407611168, 5.049401038298154454, 53.95724293864770260 ) ) ;
#159045=CARTESIAN_POINT ( 'NONE',  ( -21.52544592524334988, -5.823673210054445271, 68.95942372801901854 ) ) ;
#159046=CARTESIAN_POINT ( 'NONE',  ( 5.049401038297881783, 19.05341960407617563, 92.29275706135234714 ) ) ;
#159047=CARTESIAN_POINT ( 'NONE',  ( 21.55341960407610458, 5.719274019375980345, 23.95724293864769550 ) ) ;
#159048=CARTESIAN_POINT ( 'NONE',  ( -16.51473224551069308, -9.474510206698971260, 36.66557627198102409 ) ) ;
#159049=CARTESIAN_POINT ( 'NONE',  ( -21.53943276465977519, 0.05219959533907696930, 116.2489096053143669 ) ) ;
#159050=CARTESIAN_POINT ( 'NONE',  ( -16.46253265017146816, -9.564922557961047289, 39.16775706135234003 ) ) ;
#159051=CARTESIAN_POINT ( 'NONE',  ( -8.314922557960811034, -14.29746914071050412, 112.0822429386477097 ) ) ;
#159052=CARTESIAN_POINT ( 'NONE',  ( -16.51473224551069308, -9.474510206698971260, 66.66557627198102409 ) ) ;
#159053=CARTESIAN_POINT ( 'NONE',  ( -13.97604488694547697, 13.89961937509957934, 113.1260903946856757 ) ) ;
#159054=CARTESIAN_POINT ( 'NONE',  ( -16.55341960407611168, -4.379528057220339221, 81.45724293864769550 ) ) ;
#159055=CARTESIAN_POINT ( 'NONE',  ( 15.80617190586746368, 15.72974639402197994, 29.37390960531435269 ) ) ;
#159056=CARTESIAN_POINT ( 'NONE',  ( -19.03943276465977164, -0.05219959533935918106, 83.75109039468567573 ) ) ;
#159057=CARTESIAN_POINT ( 'NONE',  ( 21.53943276465977519, -0.05219959533907433946, 93.74890960531436690 ) ) ;
#159058=CARTESIAN_POINT ( 'NONE',  ( -10.81492255796105439, 18.62759615963255655, 42.91775706135235424 ) ) ;
#159059=CARTESIAN_POINT ( 'NONE',  ( 12.06949235617739724, 12.14591786802326823, 61.87609039468568284 ) ) ;
#159060=CARTESIAN_POINT ( 'NONE',  ( 16.53943276465976808, 0.05219959533934440121, 51.25109039468568994 ) ) ;
#159061=CARTESIAN_POINT ( 'NONE',  ( 5.823673210054444382, -21.52544592524334988, 50.20942372801901854 ) ) ;
#159062=CARTESIAN_POINT ( 'NONE',  ( -15.80617190586745835, -15.72974639402198527, 51.87390960531437401 ) ) ;
#159063=CARTESIAN_POINT ( 'NONE',  ( 0.05219959533909260263, 19.03943276465977164, 49.99890960531435979 ) ) ;
#159065=CARTESIAN_POINT ( 'NONE',  ( 16.52544592524335698, 4.483927247898782831, 76.45942372801901854 ) ) ;
#159066=CARTESIAN_POINT ( 'NONE',  ( -21.55341960407610458, -5.719274019375992779, 101.4572429386476955 ) ) ;
#159067=CARTESIAN_POINT ( 'NONE',  ( -16.55341960407611168, -4.379528057220339221, 46.45724293864769550 ) ) ;
#159068=CARTESIAN_POINT ( 'NONE',  ( 0.05219959533934541429, -16.53943276465976808, 60.00109039468568284 ) ) ;
#159069=CARTESIAN_POINT ( 'NONE',  ( 16.46253265017146816, 9.564922557961045513, 96.66775706135233293 ) ) ;
#159070=CARTESIAN_POINT ( 'NONE',  ( 5.823673210054125526, 21.52544592524343514, 94.79057627198105251 ) ) ;
#159071=CARTESIAN_POINT ( 'NONE',  ( -4.483927247898539470, -16.52544592524342804, 42.29057627198103120 ) ) ;
#159072=EDGE_LOOP ( 'NONE', ( #23697, #188753, #170671, #158347 ) ) ;
#159073=CARTESIAN_POINT ( 'NONE',  ( -17.49999999999999289, 5.500000000000036415, 75.79690382534175797 ) ) ;
#159074=CARTESIAN_POINT ( 'NONE',  ( -0.05219959533907301413, -21.53943276465977519, 77.49890960531433848 ) ) ;
#159075=CARTESIAN_POINT ( 'NONE',  ( -16.52544592524342804, 4.483927247898546575, 31.04057627198102409 ) ) ;
#159078=CARTESIAN_POINT ( 'NONE',  ( -10.81492255796078084, -18.62759615963271287, 107.0822429386476955 ) ) ;
#159079=CARTESIAN_POINT ( 'NONE',  ( -10.72451020669898014, 18.67979575497178502, 110.4155762719810383 ) ) ;
#159080=CARTESIAN_POINT ( 'NONE',  ( -4.483927247898539470, -16.52544592524342804, 32.29057627198102409 ) ) ;
#159081=CARTESIAN_POINT ( 'NONE',  ( -12.14591786802326823, 12.06949235617739902, 53.12609039468568284 ) ) ;
#159082=CARTESIAN_POINT ( 'NONE',  ( 9.474510206698971260, -16.51473224551069308, 47.91557627198102409 ) ) ;
#159083=CARTESIAN_POINT ( 'NONE',  ( 9.474510206698971260, -16.51473224551069308, 62.91557627198102409 ) ) ;
#159085=CARTESIAN_POINT ( 'NONE',  ( -15.72974639402197994, 15.80617190586746368, 40.62390960531435269 ) ) ;
#159087=CARTESIAN_POINT ( 'NONE',  ( -16.55341960407617563, 4.379528057220093196, 23.54275706135235424 ) ) ;
#159088=CARTESIAN_POINT ( 'NONE',  ( -9.474510206698720793, -16.51473224551083518, 44.58442372801900433 ) ) ;
#159089=CARTESIAN_POINT ( 'NONE',  ( 10.72451020669898902, -18.67979575497178502, 107.9155762719810241 ) ) ;
#159090=CARTESIAN_POINT ( 'NONE',  ( 12.14591786802309770, 12.06949235617756955, 34.37390960531435979 ) ) ;
#159092=CARTESIAN_POINT ( 'NONE',  ( 19.03943276465977164, -0.05219959533909143690, 83.74890960531436690 ) ) ;
#159093=CARTESIAN_POINT ( 'NONE',  ( -10.72451020669898014, 18.67979575497178502, 45.41557627198103830 ) ) ;
#159094=CARTESIAN_POINT ( 'NONE',  ( -10.72451020669898014, 18.67979575497178502, 80.41557627198103830 ) ) ;
#159095=CARTESIAN_POINT ( 'NONE',  ( -16.53943276465976808, -0.05219959533934237506, 23.75109039468567929 ) ) ;
#159096=CARTESIAN_POINT ( 'NONE',  ( -0.05219959533907301413, -21.53943276465977519, 22.49890960531436335 ) ) ;
#159097=CARTESIAN_POINT ( 'NONE',  ( -15.72974639402176322, -15.80617190586768395, 74.37609039468568994 ) ) ;
#159098=CARTESIAN_POINT ( 'NONE',  ( 13.89961937509977652, -13.97604488694527269, 78.12390960531433848 ) ) ;
#159099=CARTESIAN_POINT ( 'NONE',  ( -19.02544592524342804, 5.153800228976336051, 31.04057627198102409 ) ) ;
#159100=CARTESIAN_POINT ( 'NONE',  ( -5.153800228976328057, -19.02544592524343514, 82.29057627198103830 ) ) ;
#159101=CARTESIAN_POINT ( 'NONE',  ( -16.55341960407611168, -4.379528057220339221, 86.45724293864770971 ) ) ;
#159103=CARTESIAN_POINT ( 'NONE',  ( -5.049401038297874678, -19.05341960407617918, 109.7927570613523187 ) ) ;
#159105=CARTESIAN_POINT ( 'NONE',  ( 13.89961937509977652, -13.97604488694527269, 68.12390960531436690 ) ) ;
#159106=CARTESIAN_POINT ( 'NONE',  ( -15.72974639402176322, -15.80617190586768395, 89.37609039468568994 ) ) ;
#159107=CARTESIAN_POINT ( 'NONE',  ( 5.153800228976335163, 19.02544592524342804, 114.7905762719810241 ) ) ;
#159108=CARTESIAN_POINT ( 'NONE',  ( -8.224510206698735004, -14.34966873604973081, 79.58442372801903275 ) ) ;
#159109=CARTESIAN_POINT ( 'NONE',  ( -17.05587630539786659, -6.762274262135682612, 74.25819690962691766 ) ) ;
#159110=CARTESIAN_POINT ( 'NONE',  ( 0.05219959533936267826, -19.03943276465977164, 55.00109039468566863 ) ) ;
#159111=CARTESIAN_POINT ( 'NONE',  ( 13.97604488694548053, -13.89961937509957401, 20.62609039468567573 ) ) ;
#159115=CARTESIAN_POINT ( 'NONE',  ( 0.05219959533910956823, 16.53943276465976808, 24.99890960531435624 ) ) ;
#159117=CARTESIAN_POINT ( 'NONE',  ( -4.483927247898782831, 16.52544592524335698, 107.7094237280190328 ) ) ;
#159119=CARTESIAN_POINT ( 'NONE',  ( -16.53943276465976808, -0.05219959533934237506, 83.75109039468568994 ) ) ;
#159120=CARTESIAN_POINT ( 'NONE',  ( -5.719274019375665041, -21.55341960407619695, 89.79275706135236135 ) ) ;
#159121=CARTESIAN_POINT ( 'NONE',  ( 19.02544592524334988, 5.153800228976608722, 101.4594237280189759 ) ) ;
#159122=CARTESIAN_POINT ( 'NONE',  ( 15.72974639402176855, 15.80617190586768217, 61.87609039468568284 ) ) ;
#159123=CARTESIAN_POINT ( 'NONE',  ( 13.97604488694548053, -13.89961937509957401, 40.62609039468564731 ) ) ;
#159124=CARTESIAN_POINT ( 'NONE',  ( -13.89961937509977652, 13.97604488694528158, 85.62390960531433848 ) ) ;
#159125=CARTESIAN_POINT ( 'NONE',  ( 5.049401038298161559, -19.05341960407611168, 72.70724293864768129 ) ) ;
#159126=CARTESIAN_POINT ( 'NONE',  ( -17.49999999999999645, 5.499999999999997335, 120.0000000000000142 ) ) ;
#159127=CARTESIAN_POINT ( 'NONE',  ( -18.67979575497178146, -10.72451020669898902, 51.66557627198102409 ) ) ;
#159128=CARTESIAN_POINT ( 'NONE',  ( -0.05219959533909027116, -19.03943276465977164, 47.49890960531435979 ) ) ;
#159129=CARTESIAN_POINT ( 'NONE',  ( -14.34966873604972548, 8.224510206698743886, 83.33442372801903275 ) ) ;
#159132=CARTESIAN_POINT ( 'NONE',  ( 12.14591786802309770, 12.06949235617756955, 79.37390960531436690 ) ) ;
#159134=CARTESIAN_POINT ( 'NONE',  ( -16.53943276465976808, -0.05219959533934237506, 43.75109039468568284 ) ) ;
#159135=CARTESIAN_POINT ( 'NONE',  ( -8.314922557960811034, -14.29746914071050412, 102.0822429386476955 ) ) ;
#159136=CARTESIAN_POINT ( 'NONE',  ( -9.474510206698720793, -16.51473224551083518, 69.58442372801901854 ) ) ;
#159137=CARTESIAN_POINT ( 'NONE',  ( 16.55341960407611168, 4.379528057220329451, 73.95724293864769550 ) ) ;
#159138=CARTESIAN_POINT ( 'NONE',  ( -5.719274019375665041, -21.55341960407619695, 29.79275706135234358 ) ) ;
#159139=CARTESIAN_POINT ( 'NONE',  ( 16.46253265017160672, -9.564922557960803928, 23.33224293864769194 ) ) ;
#159140=CARTESIAN_POINT ( 'NONE',  ( -10.81492255796078084, -18.62759615963271287, 87.08224293864769550 ) ) ;
#159141=CARTESIAN_POINT ( 'NONE',  ( -16.51473224551069308, -9.474510206698971260, 101.6655762719810241 ) ) ;
#159142=CARTESIAN_POINT ( 'NONE',  ( -12.14591786802309592, -12.06949235617757132, 71.87390960531438111 ) ) ;
#159144=CARTESIAN_POINT ( 'NONE',  ( -16.51473224551069308, -9.474510206698971260, 51.66557627198102409 ) ) ;
#159146=CARTESIAN_POINT ( 'NONE',  ( 16.51473224551083163, -9.474510206698727899, 80.83442372801899012 ) ) ;
#159147=CARTESIAN_POINT ( 'NONE',  ( -10.72451020669898014, 18.67979575497178502, 115.4155762719810241 ) ) ;
#159148=CARTESIAN_POINT ( 'NONE',  ( 19.02544592524343514, -5.153800228976328945, 73.54057627198103830 ) ) ;
#159149=CARTESIAN_POINT ( 'NONE',  ( 16.51473224551083163, -9.474510206698727899, 60.83442372801900433 ) ) ;
#159150=CARTESIAN_POINT ( 'NONE',  ( 13.97604488694527802, 13.89961937509977652, 39.37390960531435269 ) ) ;
#159151=CARTESIAN_POINT ( 'NONE',  ( 16.53943276465976808, -0.05219959533910856209, 68.74890960531435269 ) ) ;
#159152=CARTESIAN_POINT ( 'NONE',  ( 12.14591786802309770, 12.06949235617756955, 49.37390960531436690 ) ) ;
#159153=CARTESIAN_POINT ( 'NONE',  ( -9.474510206698964154, 16.51473224551069663, 75.41557627198103830 ) ) ;
#159154=CARTESIAN_POINT ( 'NONE',  ( -21.55341960407610458, -5.719274019375992779, 81.45724293864769550 ) ) ;
#159155=CARTESIAN_POINT ( 'NONE',  ( -16.46253265017160317, 9.564922557960807481, 70.83224293864770971 ) ) ;
#159156=CARTESIAN_POINT ( 'NONE',  ( -21.53943276465977519, 0.05219959533907696930, 81.24890960531436690 ) ) ;
#159158=CARTESIAN_POINT ( 'NONE',  ( -9.474510206698720793, -16.51473224551083518, 24.58442372801900078 ) ) ;
#159159=CARTESIAN_POINT ( 'NONE',  ( 5.153800228976335163, 19.02544592524342804, 29.79057627198102409 ) ) ;
#159160=CARTESIAN_POINT ( 'NONE',  ( 12.14591786802327356, -12.06949235617739191, 110.6260903946857042 ) ) ;
#159161=CARTESIAN_POINT ( 'NONE',  ( -14.29746914071049879, 8.314922557960819915, 95.83224293864770971 ) ) ;
#159162=CARTESIAN_POINT ( 'NONE',  ( 5.153800228976615827, -19.02544592524334988, 100.2094237280190043 ) ) ;
#159164=CARTESIAN_POINT ( 'NONE',  ( 15.72974639402199770, -15.80617190586745480, 113.1239096053143953 ) ) ;
#159165=CARTESIAN_POINT ( 'NONE',  ( 19.05341960407617918, -5.049401038297876454, 56.04275706135234714 ) ) ;
#159166=CARTESIAN_POINT ( 'NONE',  ( -16.52544592524342804, 4.483927247898546575, 26.04057627198103475 ) ) ;
#159167=CARTESIAN_POINT ( 'NONE',  ( 13.89961937509957401, 13.97604488694547697, 41.87609039468566152 ) ) ;
#159168=CARTESIAN_POINT ( 'NONE',  ( -19.03943276465977164, 0.05219959533909376836, 106.2489096053143669 ) ) ;
#159169=CARTESIAN_POINT ( 'NONE',  ( 12.14591786802309770, 12.06949235617756955, 54.37390960531435979 ) ) ;
#159170=CARTESIAN_POINT ( 'NONE',  ( -19.05341960407611168, -5.049401038298163336, 21.45724293864768839 ) ) ;
#159171=CARTESIAN_POINT ( 'NONE',  ( 19.02544592524343514, -5.153800228976328945, 33.54057627198102409 ) ) ;
#159172=CARTESIAN_POINT ( 'NONE',  ( 0.05219959533936267826, -19.03943276465977164, 20.00109039468567218 ) ) ;
#159173=CARTESIAN_POINT ( 'NONE',  ( 4.379528057220092307, 16.55341960407617563, 87.29275706135236135 ) ) ;
#159174=CARTESIAN_POINT ( 'NONE',  ( -18.67979575497193778, 10.72451020669871902, 43.33442372801901143 ) ) ;
#159175=CARTESIAN_POINT ( 'NONE',  ( -12.14591786802326823, 12.06949235617739902, 38.12609039468567573 ) ) ;
#159176=CARTESIAN_POINT ( 'NONE',  ( 5.049401038298161559, -19.05341960407611168, 102.7072429386476955 ) ) ;
#159177=CARTESIAN_POINT ( 'NONE',  ( -9.474510206698964154, 16.51473224551069663, 50.41557627198102409 ) ) ;
#159178=CARTESIAN_POINT ( 'NONE',  ( -13.89961937509977652, 13.97604488694528158, 70.62390960531432427 ) ) ;
#159179=CARTESIAN_POINT ( 'NONE',  ( -16.53943276465976808, -0.05219959533934237506, 53.75109039468568994 ) ) ;
#159180=CARTESIAN_POINT ( 'NONE',  ( -14.29746914071049879, 8.314922557960819915, 105.8322429386476955 ) ) ;
#159181=CARTESIAN_POINT ( 'NONE',  ( 0.05219959533934541429, -16.53943276465976808, 110.0010903946856757 ) ) ;
#159183=CARTESIAN_POINT ( 'NONE',  ( -10.72451020669870658, -18.67979575497194134, 59.58442372801901854 ) ) ;
#159184=CARTESIAN_POINT ( 'NONE',  ( -13.89961937509977652, 13.97604488694528158, 95.62390960531436690 ) ) ;
#159185=CARTESIAN_POINT ( 'NONE',  ( -13.89961937509977652, 13.97604488694528158, 80.62390960531436690 ) ) ;
#159186=CARTESIAN_POINT ( 'NONE',  ( -16.46253265017160317, 9.564922557960807481, 95.83224293864769550 ) ) ;
#159187=CARTESIAN_POINT ( 'NONE',  ( -12.14591786802309592, -12.06949235617757132, 46.87390960531435979 ) ) ;
#159188=CARTESIAN_POINT ( 'NONE',  ( 8.224510206698742110, 14.34966873604972548, 107.0844237280190043 ) ) ;
#159189=CARTESIAN_POINT ( 'NONE',  ( 16.53943276465976808, -0.05219959533910856209, 38.74890960531435979 ) ) ;
#159192=CARTESIAN_POINT ( 'NONE',  ( -13.97604488694547697, 13.89961937509957934, 43.12609039468566152 ) ) ;
#159193=CARTESIAN_POINT ( 'NONE',  ( 5.153800228976335163, 19.02544592524342804, 64.79057627198100988 ) ) ;
#159194=CARTESIAN_POINT ( 'NONE',  ( -16.46253265017146816, -9.564922557961047289, 54.16775706135234003 ) ) ;
#159196=LINE ( 'NONE', #157232, #105502 ) ;
#159197=CARTESIAN_POINT ( 'NONE',  ( 0.05219959533936267826, -19.03943276465977164, 85.00109039468567573 ) ) ;
#159198=CARTESIAN_POINT ( 'NONE',  ( 16.55341960407618274, -4.379528057220086978, 66.04275706135236135 ) ) ;
#159200=CARTESIAN_POINT ( 'NONE',  ( -19.02544592524342804, 5.153800228976336051, 86.04057627198103830 ) ) ;
#159201=CARTESIAN_POINT ( 'NONE',  ( -21.55341960407619339, 5.719274019375674811, 28.54275706135234358 ) ) ;
#159203=CARTESIAN_POINT ( 'NONE',  ( -9.474510206698720793, -16.51473224551083518, 84.58442372801900433 ) ) ;
#159204=CARTESIAN_POINT ( 'NONE',  ( -5.153800228976328057, -19.02544592524343514, 112.2905762719810099 ) ) ;
#159205=CARTESIAN_POINT ( 'NONE',  ( -19.05341960407611168, -5.049401038298163336, 46.45724293864768129 ) ) ;
#159206=CARTESIAN_POINT ( 'NONE',  ( -13.89961937509977652, 13.97604488694528158, 95.62390960531436690 ) ) ;
#159207=CARTESIAN_POINT ( 'NONE',  ( 14.29746914071049879, -8.314922557960816363, 43.33224293864769550 ) ) ;
#159208=CARTESIAN_POINT ( 'NONE',  ( -13.97604488694527625, -13.89961937509977652, 46.87390960531435979 ) ) ;
#159209=CARTESIAN_POINT ( 'NONE',  ( 9.564922557961047289, -16.46253265017146816, 60.41775706135233293 ) ) ;
#159211=CARTESIAN_POINT ( 'NONE',  ( -5.049401038297874678, -19.05341960407617918, 24.79275706135233648 ) ) ;
#159212=CARTESIAN_POINT ( 'NONE',  ( -9.474510206698964154, 16.51473224551069663, 65.41557627198102409 ) ) ;
#159213=CARTESIAN_POINT ( 'NONE',  ( 10.72451020669898902, -18.67979575497178502, 67.91557627198102409 ) ) ;
#159214=CARTESIAN_POINT ( 'NONE',  ( 16.55341960407611168, 4.379528057220329451, 63.95724293864770260 ) ) ;
#159215=CARTESIAN_POINT ( 'NONE',  ( -5.049401038297874678, -19.05341960407617918, 24.79275706135233648 ) ) ;
#159216=CARTESIAN_POINT ( 'NONE',  ( 5.153800228976335163, 19.02544592524342804, 104.7905762719809957 ) ) ;
#159217=CARTESIAN_POINT ( 'NONE',  ( -10.72451020669898014, 18.67979575497178502, 30.41557627198101699 ) ) ;
#159218=CARTESIAN_POINT ( 'NONE',  ( 9.564922557960805705, 16.46253265017160317, 49.58224293864770260 ) ) ;
#159219=CARTESIAN_POINT ( 'NONE',  ( 9.474510206698971260, -16.51473224551069308, 37.91557627198102409 ) ) ;
#159220=CARTESIAN_POINT ( 'NONE',  ( -12.14591786802309592, -12.06949235617757132, 106.8739096053143811 ) ) ;
#159221=CARTESIAN_POINT ( 'NONE',  ( -15.80617190586745835, -15.72974639402198527, 106.8739096053143811 ) ) ;
#159222=CARTESIAN_POINT ( 'NONE',  ( -5.153800228976328057, -19.02544592524343514, 112.2905762719810099 ) ) ;
#159223=CARTESIAN_POINT ( 'NONE',  ( -15.72974639402176322, -15.80617190586768395, 24.37609039468567573 ) ) ;
#159224=CARTESIAN_POINT ( 'NONE',  ( 16.46253265017160672, -9.564922557960803928, 108.3322429386476955 ) ) ;
#159225=CARTESIAN_POINT ( 'NONE',  ( 14.29746914071049879, -8.314922557960816363, 113.3322429386476955 ) ) ;
#159226=CARTESIAN_POINT ( 'NONE',  ( -0.05219959533937732626, 21.53943276465977519, 72.50109039468568994 ) ) ;
#159227=CARTESIAN_POINT ( 'NONE',  ( 21.52544592524344225, -5.823673210054117533, 93.54057627198103830 ) ) ;
#159228=CARTESIAN_POINT ( 'NONE',  ( 17.31747979337947285, -6.344076630961067664, 106.1205513193481664 ) ) ;
#159229=CARTESIAN_POINT ( 'NONE',  ( 19.53037848336980886, -5.499999999999890754, 77.35532783611445495 ) ) ;
#159230=CARTESIAN_POINT ( 'NONE',  ( -9.474510206698964154, 16.51473224551069663, 60.41557627198102409 ) ) ;
#159231=CARTESIAN_POINT ( 'NONE',  ( -4.483927247898782831, 16.52544592524335698, 47.70942372801902565 ) ) ;
#159232=CARTESIAN_POINT ( 'NONE',  ( 12.06949235617757843, -12.14591786802309237, 108.1239096053143811 ) ) ;
#159234=CARTESIAN_POINT ( 'NONE',  ( 19.03943276465977164, -0.05219959533909143690, 53.74890960531436690 ) ) ;
#159235=CARTESIAN_POINT ( 'NONE',  ( 16.55341960407611168, 4.379528057220329451, 98.95724293864770971 ) ) ;
#159236=CIRCLE ( 'NONE', #1053, 2.000000000000001776 ) ;
#159237=CARTESIAN_POINT ( 'NONE',  ( 15.80617190586746368, 15.72974639402197994, 44.37390960531435979 ) ) ;
#159238=CARTESIAN_POINT ( 'NONE',  ( 12.14591786802309770, 12.06949235617756955, 59.37390960531436690 ) ) ;
#159239=CARTESIAN_POINT ( 'NONE',  ( -9.474510206698720793, -16.51473224551083518, 109.5844237280190043 ) ) ;
#159240=CARTESIAN_POINT ( 'NONE',  ( -15.80617190586768217, 15.72974639402176855, 83.12609039468568994 ) ) ;
#159241=CARTESIAN_POINT ( 'NONE',  ( -5.153800228976607833, 19.02544592524335343, 62.70942372801899012 ) ) ;
#159242=CARTESIAN_POINT ( 'NONE',  ( 8.314922557961029526, -14.29746914071037800, 95.41775706135234714 ) ) ;
#159243=CARTESIAN_POINT ( 'NONE',  ( 8.224510206698953496, -14.34966873604960469, 37.91557627198102409 ) ) ;
#159244=CARTESIAN_POINT ( 'NONE',  ( 19.02544592524343514, -5.153800228976328945, 43.54057627198103120 ) ) ;
#159245=CARTESIAN_POINT ( 'NONE',  ( 0.05219959533909260263, 19.03943276465977164, 89.99890960531436690 ) ) ;
#159246=CARTESIAN_POINT ( 'NONE',  ( -10.72451020669898014, 18.67979575497178502, 90.41557627198103830 ) ) ;
#159247=CARTESIAN_POINT ( 'NONE',  ( -14.29746914071037622, -8.314922557961029526, 39.16775706135235424 ) ) ;
#159248=CARTESIAN_POINT ( 'NONE',  ( -8.224510206698948167, 14.34966873604960824, 65.41557627198102409 ) ) ;
#159249=CARTESIAN_POINT ( 'NONE',  ( 5.823673210054444382, -21.52544592524334988, 90.20942372801903275 ) ) ;
#159250=CARTESIAN_POINT ( 'NONE',  ( 8.314922557961029526, -14.29746914071037800, 95.41775706135234714 ) ) ;
#159251=CARTESIAN_POINT ( 'NONE',  ( 17.40805194822030089, 6.112264579159360167, 26.66628727489388950 ) ) ;
#159253=CARTESIAN_POINT ( 'NONE',  ( -8.224510206698948167, 14.34966873604960824, 25.41557627198103120 ) ) ;
#159254=CARTESIAN_POINT ( 'NONE',  ( -14.29746914071037622, -8.314922557961029526, 74.16775706135231871 ) ) ;
#159255=CARTESIAN_POINT ( 'NONE',  ( -19.02544592524342804, 5.153800228976336051, 81.04057627198103830 ) ) ;
#159256=CARTESIAN_POINT ( 'NONE',  ( 19.03943276465977164, -0.05219959533909143690, 98.74890960531436690 ) ) ;
#159257=CARTESIAN_POINT ( 'NONE',  ( 5.719274019375673035, 21.55341960407619339, 87.29275706135236135 ) ) ;
#159258=CARTESIAN_POINT ( 'NONE',  ( 4.379528057220092307, 16.55341960407617563, 92.29275706135236135 ) ) ;
#159259=CARTESIAN_POINT ( 'NONE',  ( 12.14591786802309770, 12.06949235617756955, 64.37390960531435269 ) ) ;
#159260=CARTESIAN_POINT ( 'NONE',  ( 5.153800228976335163, 19.02544592524342804, 69.79057627198103830 ) ) ;
#159262=CARTESIAN_POINT ( 'NONE',  ( 0.05219959533936267826, -19.03943276465977164, 110.0010903946856757 ) ) ;
#159263=CARTESIAN_POINT ( 'NONE',  ( 19.05341960407611168, 5.049401038298154454, 33.95724293864769550 ) ) ;
#159264=CARTESIAN_POINT ( 'NONE',  ( 19.03943276465977164, -0.05219959533909143690, 78.74890960531436690 ) ) ;
#159265=CARTESIAN_POINT ( 'NONE',  ( 0.05219959533936267826, -19.03943276465977164, 110.0010903946856757 ) ) ;
#159267=CARTESIAN_POINT ( 'NONE',  ( -9.564922557961040184, 16.46253265017147172, 27.91775706135232582 ) ) ;
#159268=CARTESIAN_POINT ( 'NONE',  ( -0.05219959533934338120, 16.53943276465976808, 82.50109039468568994 ) ) ;
#159269=CARTESIAN_POINT ( 'NONE',  ( 9.474510206698729675, 16.51473224551082808, 107.0844237280190043 ) ) ;
#159270=CARTESIAN_POINT ( 'NONE',  ( 4.483927247898545687, 16.52544592524342804, 114.7905762719810383 ) ) ;
#159271=CARTESIAN_POINT ( 'NONE',  ( -14.29746914071037622, -8.314922557961029526, 69.16775706135234714 ) ) ;
#159272=CARTESIAN_POINT ( 'NONE',  ( -14.34966873604972548, 8.224510206698743886, 48.33442372801902565 ) ) ;
#159273=CARTESIAN_POINT ( 'NONE',  ( -19.05341960407611168, -5.049401038298163336, 26.45724293864769550 ) ) ;
#159274=CARTESIAN_POINT ( 'NONE',  ( 5.153800228976615827, -19.02544592524334988, 65.20942372801900433 ) ) ;
#159275=CARTESIAN_POINT ( 'NONE',  ( 10.72451020669871369, 18.67979575497193778, 112.0844237280190185 ) ) ;
#159276=CARTESIAN_POINT ( 'NONE',  ( 5.049401038298161559, -19.05341960407611168, 37.70724293864768839 ) ) ;
#159277=CARTESIAN_POINT ( 'NONE',  ( 16.46253265017160672, -9.564922557960803928, 73.33224293864769550 ) ) ;
#159278=CARTESIAN_POINT ( 'NONE',  ( -16.52544592524342804, 4.483927247898546575, 66.04057627198103830 ) ) ;
#159279=CARTESIAN_POINT ( 'NONE',  ( 13.97604488694548053, -13.89961937509957401, 45.62609039468566863 ) ) ;
#159280=CARTESIAN_POINT ( 'NONE',  ( 10.81492255796078972, 18.62759615963270932, 34.58224293864770260 ) ) ;
#159281=CARTESIAN_POINT ( 'NONE',  ( -5.823673210054431948, 21.52544592524334988, 112.7094237280190328 ) ) ;
#159282=CARTESIAN_POINT ( 'NONE',  ( -19.03943276465977164, 0.05219959533909376836, 91.24890960531436690 ) ) ;
#159283=CARTESIAN_POINT ( 'NONE',  ( 5.823673210054444382, -21.52544592524334988, 105.2094237280190328 ) ) ;
#159284=CARTESIAN_POINT ( 'NONE',  ( 18.62759615963271287, -10.81492255796078972, 68.33224293864769550 ) ) ;
#159285=CARTESIAN_POINT ( 'NONE',  ( -19.03943276465977164, 0.05219959533909376836, 101.2489096053143669 ) ) ;
#159286=CARTESIAN_POINT ( 'NONE',  ( 5.153800228976615827, -19.02544592524334988, 80.20942372801901854 ) ) ;
#159287=CARTESIAN_POINT ( 'NONE',  ( 16.51473224551069308, 9.474510206698969483, 99.16557627198102409 ) ) ;
#159288=CARTESIAN_POINT ( 'NONE',  ( -19.02544592524334988, -5.153800228976617603, 98.95942372801900433 ) ) ;
#159289=CARTESIAN_POINT ( 'NONE',  ( 16.52544592524335698, 4.483927247898782831, 61.45942372801901854 ) ) ;
#159290=CARTESIAN_POINT ( 'NONE',  ( 0.05219959533909260263, 19.03943276465977164, 24.99890960531435269 ) ) ;
#159291=CARTESIAN_POINT ( 'NONE',  ( 5.049401038298161559, -19.05341960407611168, 87.70724293864769550 ) ) ;
#159292=CARTESIAN_POINT ( 'NONE',  ( 15.72974639402199770, -15.80617190586745480, 68.12390960531436690 ) ) ;
#159293=CARTESIAN_POINT ( 'NONE',  ( -12.06949235617739369, -12.14591786802326823, 29.37609039468568284 ) ) ;
#159294=CARTESIAN_POINT ( 'NONE',  ( -10.72451020669870658, -18.67979575497194134, 34.58442372801900433 ) ) ;
#159295=CARTESIAN_POINT ( 'NONE',  ( -10.81492255796105439, 18.62759615963255655, 97.91775706135236135 ) ) ;
#159296=CARTESIAN_POINT ( 'NONE',  ( -8.224510206698735004, -14.34966873604973081, 94.58442372801901854 ) ) ;
#159297=VECTOR ( 'NONE', #54218, 1000.000000000000000 ) ;
#159298=CARTESIAN_POINT ( 'NONE',  ( -5.049401038298153566, 19.05341960407611168, 85.20724293864766707 ) ) ;
#159299=CARTESIAN_POINT ( 'NONE',  ( -8.224510206698948167, 14.34966873604960824, 75.41557627198102409 ) ) ;
#159300=CARTESIAN_POINT ( 'NONE',  ( -14.29746914071049879, 8.314922557960819915, 25.83224293864769194 ) ) ;
#159301=CARTESIAN_POINT ( 'NONE',  ( 5.049401038297881783, 19.05341960407617563, 72.29275706135234714 ) ) ;
#159303=CARTESIAN_POINT ( 'NONE',  ( 5.719274019375673035, 21.55341960407619339, 42.29275706135235424 ) ) ;
#159304=CARTESIAN_POINT ( 'NONE',  ( 4.379528057220339221, -16.55341960407611168, 87.70724293864769550 ) ) ;
#159305=CARTESIAN_POINT ( 'NONE',  ( 5.049401038298161559, -19.05341960407611168, 112.7072429386476813 ) ) ;
#159306=CARTESIAN_POINT ( 'NONE',  ( -4.379528057220086978, -16.55341960407618274, 99.79275706135234714 ) ) ;
#159307=CARTESIAN_POINT ( 'NONE',  ( 18.62759615963255655, 10.81492255796105972, 86.66775706135234714 ) ) ;
#159308=CARTESIAN_POINT ( 'NONE',  ( -4.483927247898782831, 16.52544592524335698, 47.70942372801902565 ) ) ;
#159309=CARTESIAN_POINT ( 'NONE',  ( 18.62759615963255655, 10.81492255796105972, 41.66775706135235424 ) ) ;
#159311=CARTESIAN_POINT ( 'NONE',  ( 10.81492255796106328, -18.62759615963255655, 20.41775706135234714 ) ) ;
#159312=CARTESIAN_POINT ( 'NONE',  ( 16.52544592524342804, -4.483927247898539470, 88.54057627198103830 ) ) ;
#159314=CARTESIAN_POINT ( 'NONE',  ( -4.379528057220328563, 16.55341960407611168, 65.20724293864768129 ) ) ;
#159315=CARTESIAN_POINT ( 'NONE',  ( 8.224510206698742110, 14.34966873604972548, 112.0844237280190185 ) ) ;
#159316=CARTESIAN_POINT ( 'NONE',  ( -16.46253265017160317, 9.564922557960807481, 35.83224293864768839 ) ) ;
#159317=CARTESIAN_POINT ( 'NONE',  ( -5.823673210054116645, -21.52544592524344225, 37.29057627198102409 ) ) ;
#159318=CARTESIAN_POINT ( 'NONE',  ( 4.483927247898545687, 16.52544592524342804, 84.79057627198102409 ) ) ;
#159319=CARTESIAN_POINT ( 'NONE',  ( 21.52544592524344225, -5.823673210054117533, 83.54057627198102409 ) ) ;
#159320=CARTESIAN_POINT ( 'NONE',  ( -9.564922557960796823, -16.46253265017161027, 92.08224293864769550 ) ) ;
#159321=CARTESIAN_POINT ( 'NONE',  ( 19.05341960407611168, 5.049401038298154454, 43.95724293864769550 ) ) ;
#159322=CARTESIAN_POINT ( 'NONE',  ( 5.049401038297881783, 19.05341960407617563, 92.29275706135234714 ) ) ;
#159323=CARTESIAN_POINT ( 'NONE',  ( 10.72451020669898902, -18.67979575497178502, 27.91557627198103830 ) ) ;
#159324=CARTESIAN_POINT ( 'NONE',  ( -18.62759615963255300, -10.81492255796106328, 64.16775706135234714 ) ) ;
#159325=CARTESIAN_POINT ( 'NONE',  ( -16.46253265017160317, 9.564922557960807481, 50.83224293864770260 ) ) ;
#159326=CARTESIAN_POINT ( 'NONE',  ( -19.05341960407611168, -5.049401038298163336, 91.45724293864766707 ) ) ;
#159328=CARTESIAN_POINT ( 'NONE',  ( -16.53943276465976808, -0.05219959533934237506, 63.75109039468568284 ) ) ;
#159329=CARTESIAN_POINT ( 'NONE',  ( 5.823673210054444382, -21.52544592524334988, 45.20942372801901854 ) ) ;
#159330=CARTESIAN_POINT ( 'NONE',  ( -5.719274019375665041, -21.55341960407619695, 74.79275706135234714 ) ) ;
#159331=CARTESIAN_POINT ( 'NONE',  ( 19.05341960407611168, 5.049401038298154454, 113.9572429386477097 ) ) ;
#159332=CARTESIAN_POINT ( 'NONE',  ( -5.823673210054116645, -21.52544592524344225, 102.2905762719810383 ) ) ;
#159333=CARTESIAN_POINT ( 'NONE',  ( -5.719274019375665041, -21.55341960407619695, 29.79275706135234358 ) ) ;
#159334=CARTESIAN_POINT ( 'NONE',  ( -16.53943276465976808, -0.05219959533934237506, 63.75109039468568284 ) ) ;
#159335=CARTESIAN_POINT ( 'NONE',  ( -21.52544592524343514, 5.823673210054127303, 66.04057627198103830 ) ) ;
#159336=CARTESIAN_POINT ( 'NONE',  ( 21.53943276465977519, 0.05219959533937863772, 111.2510903946856899 ) ) ;
#159337=CARTESIAN_POINT ( 'NONE',  ( -9.564922557960796823, -16.46253265017161027, 67.08224293864769550 ) ) ;
#159338=CARTESIAN_POINT ( 'NONE',  ( 0.05219959533934541429, -16.53943276465976808, 105.0010903946856757 ) ) ;
#159339=CARTESIAN_POINT ( 'NONE',  ( -17.50000000000015277, -3.417042746626872685, 104.8261960376753450 ) ) ;
#159340=CARTESIAN_POINT ( 'NONE',  ( -13.89961937509977652, 13.97604488694528158, 100.6239096053143669 ) ) ;
#159342=CARTESIAN_POINT ( 'NONE',  ( -14.34966873604972548, 8.224510206698743886, 43.33442372801901143 ) ) ;
#159344=CARTESIAN_POINT ( 'NONE',  ( 19.02544592524334988, 5.153800228976608722, 81.45942372801897591 ) ) ;
#159345=CARTESIAN_POINT ( 'NONE',  ( -21.52544592524343514, 5.823673210054127303, 61.04057627198103120 ) ) ;
#159346=CARTESIAN_POINT ( 'NONE',  ( -12.14591786802309592, -12.06949235617757132, 26.87390960531435979 ) ) ;
#159347=CARTESIAN_POINT ( 'NONE',  ( -19.05341960407617563, 5.049401038297882671, 98.54275706135233293 ) ) ;
#159348=LINE ( 'NONE', #20844, #162836 ) ;
#159349=CARTESIAN_POINT ( 'NONE',  ( 13.97604488694548053, -13.89961937509957401, 95.62609039468563310 ) ) ;
#159350=CARTESIAN_POINT ( 'NONE',  ( 21.53943276465977519, -0.05219959533907433946, 93.74890960531436690 ) ) ;
#159351=CARTESIAN_POINT ( 'NONE',  ( -5.153800228976607833, 19.02544592524334988, 57.70942372801899012 ) ) ;
#159353=CARTESIAN_POINT ( 'NONE',  ( 9.564922557960805705, 16.46253265017160317, 74.58224293864769550 ) ) ;
#159354=CARTESIAN_POINT ( 'NONE',  ( 12.14591786802309770, 12.06949235617756955, 59.37390960531436690 ) ) ;
#159355=CARTESIAN_POINT ( 'NONE',  ( -19.05341960407611168, -5.049401038298163336, 51.45724293864770260 ) ) ;
#159356=CARTESIAN_POINT ( 'NONE',  ( -8.224510206698948167, 14.34966873604960824, 50.41557627198103120 ) ) ;
#159359=CARTESIAN_POINT ( 'NONE',  ( 8.314922557960818139, 14.29746914071049879, 29.58224293864769905 ) ) ;
#159360=CARTESIAN_POINT ( 'NONE',  ( 19.03943276465977164, -0.05219959533909143690, 68.74890960531436690 ) ) ;
#159361=CARTESIAN_POINT ( 'NONE',  ( -17.49999999999999645, 5.500000000000037303, 50.79690382534172244 ) ) ;
#159362=CARTESIAN_POINT ( 'NONE',  ( 16.46253265017146816, 9.564922557961045513, 36.66775706135233293 ) ) ;
#159363=CARTESIAN_POINT ( 'NONE',  ( 4.483927247898790824, -16.52544592524335698, 50.20942372801901854 ) ) ;
#159364=CARTESIAN_POINT ( 'NONE',  ( -18.67979575497178146, -10.72451020669898902, 56.66557627198103830 ) ) ;
#159365=CARTESIAN_POINT ( 'NONE',  ( -5.719274019375665041, -21.55341960407619695, 99.79275706135234714 ) ) ;
#159366=CARTESIAN_POINT ( 'NONE',  ( 16.46253265017160672, -9.564922557960803928, 73.33224293864769550 ) ) ;
#159368=CARTESIAN_POINT ( 'NONE',  ( -5.049401038298153566, 19.05341960407611168, 115.2072429386477097 ) ) ;
#159370=CARTESIAN_POINT ( 'NONE',  ( 5.823673210054444382, -21.52544592524334988, 35.20942372801901854 ) ) ;
#159371=CARTESIAN_POINT ( 'NONE',  ( 16.55341960407611168, 4.379528057220329451, 93.95724293864770971 ) ) ;
#159373=CARTESIAN_POINT ( 'NONE',  ( -21.55341960407610458, -5.719274019375992779, 91.45724293864769550 ) ) ;
#159374=CARTESIAN_POINT ( 'NONE',  ( -16.51473224551069308, -9.474510206698971260, 76.66557627198103830 ) ) ;
#159376=CARTESIAN_POINT ( 'NONE',  ( -19.02544592524342804, 5.153800228976336051, 86.04057627198103830 ) ) ;
#159377=CARTESIAN_POINT ( 'NONE',  ( 18.67979575497194134, -10.72451020669871369, 30.83442372801902209 ) ) ;
#159379=CARTESIAN_POINT ( 'NONE',  ( 19.02544592524343514, -5.153800228976328945, 78.54057627198099567 ) ) ;
#159381=LINE ( 'NONE', #23887, #159297 ) ;
#159382=CARTESIAN_POINT ( 'NONE',  ( -9.474510206698964154, 16.51473224551069663, 30.41557627198102054 ) ) ;
#159383=CARTESIAN_POINT ( 'NONE',  ( 13.97604488694527802, 13.89961937509977652, 34.37390960531436690 ) ) ;
#159384=CARTESIAN_POINT ( 'NONE',  ( -19.03943276465977164, -0.05219959533935918106, 108.7510903946856615 ) ) ;
#159386=CARTESIAN_POINT ( 'NONE',  ( -0.05219959533910754901, -16.53943276465976808, 112.4989096053143669 ) ) ;
#159387=CARTESIAN_POINT ( 'NONE',  ( -21.53943276465977519, -0.05219959533937600094, 68.75109039468568994 ) ) ;
#159388=CARTESIAN_POINT ( 'NONE',  ( 9.474510206698971260, -16.51473224551069308, 67.91557627198102409 ) ) ;
#159389=CARTESIAN_POINT ( 'NONE',  ( -21.52544592524334988, -5.823673210054445271, 38.95942372801901854 ) ) ;
#159390=CARTESIAN_POINT ( 'NONE',  ( -21.53943276465977519, 0.05219959533907696930, 116.2489096053143669 ) ) ;
#159392=CARTESIAN_POINT ( 'NONE',  ( 5.049401038298161559, -19.05341960407611168, 82.70724293864770971 ) ) ;
#159394=CARTESIAN_POINT ( 'NONE',  ( -4.379528057220086978, -16.55341960407618274, 19.79275706135235069 ) ) ;
#159395=CARTESIAN_POINT ( 'NONE',  ( -15.72974639402197994, 15.80617190586746368, 45.62390960531436690 ) ) ;
#159396=CARTESIAN_POINT ( 'NONE',  ( -5.823673210054431948, 21.52544592524334988, 67.70942372801901854 ) ) ;
#159397=FACE_OUTER_BOUND ( 'NONE', #62526, .T. ) ;
#159398=CARTESIAN_POINT ( 'NONE',  ( 0.05219959533936267826, -19.03943276465977164, 95.00109039468567573 ) ) ;
#159399=CARTESIAN_POINT ( 'NONE',  ( 13.89961937509977652, -13.97604488694527269, 63.12390960531435979 ) ) ;
#159400=CARTESIAN_POINT ( 'NONE',  ( 5.153800228976335163, 19.02544592524342804, 84.79057627198099567 ) ) ;
#159401=CARTESIAN_POINT ( 'NONE',  ( 12.06949235617757843, -12.14591786802309237, 98.12390960531436690 ) ) ;
#159402=CARTESIAN_POINT ( 'NONE',  ( 8.314922557960818139, 14.29746914071049879, 89.58224293864768129 ) ) ;
#159403=CARTESIAN_POINT ( 'NONE',  ( 10.72451020669898902, -18.67979575497178502, 22.91557627198102765 ) ) ;
#159404=CARTESIAN_POINT ( 'NONE',  ( 4.379528057220339221, -16.55341960407611168, 62.70724293864769550 ) ) ;
#159405=CARTESIAN_POINT ( 'NONE',  ( 5.049401038298161559, -19.05341960407611168, 37.70724293864768839 ) ) ;
#159406=CARTESIAN_POINT ( 'NONE',  ( 5.823673210054444382, -21.52544592524334988, 60.20942372801902565 ) ) ;
#159407=CARTESIAN_POINT ( 'NONE',  ( 13.89961937509957401, 13.97604488694547697, 86.87609039468567573 ) ) ;
#159408=CARTESIAN_POINT ( 'NONE',  ( 16.52544592524342804, -4.483927247898539470, 68.54057627198103830 ) ) ;
#159409=CARTESIAN_POINT ( 'NONE',  ( -15.72974639402176322, -15.80617190586768395, 19.37609039468568639 ) ) ;
#159410=CARTESIAN_POINT ( 'NONE',  ( -21.52544592524343514, 5.823673210054127303, 41.04057627198103120 ) ) ;
#159411=CARTESIAN_POINT ( 'NONE',  ( -16.46253265017160317, 9.564922557960807481, 110.8322429386476955 ) ) ;
#159413=CARTESIAN_POINT ( 'NONE',  ( -0.05219959533909027116, -19.03943276465977164, 57.49890960531435979 ) ) ;
#159414=CARTESIAN_POINT ( 'NONE',  ( -8.314922557960811034, -14.29746914071050412, 32.08224293864769550 ) ) ;
#159415=CARTESIAN_POINT ( 'NONE',  ( 16.52544592524335698, 4.483927247898782831, 101.4594237280190185 ) ) ;
#159416=CARTESIAN_POINT ( 'NONE',  ( -0.05219959533934338120, 16.53943276465976808, 82.50109039468568994 ) ) ;
#159417=CARTESIAN_POINT ( 'NONE',  ( -16.46253265017146816, -9.564922557961047289, 39.16775706135234003 ) ) ;
#159418=DIRECTION ( 'NONE',  ( -1.000000000000000000, -0.000000000000000000, -0.000000000000000000 ) ) ;
#159419=CARTESIAN_POINT ( 'NONE',  ( -9.474510206698964154, 16.51473224551069663, 90.41557627198103830 ) ) ;
#159420=CARTESIAN_POINT ( 'NONE',  ( 9.474510206698971260, -16.51473224551069308, 52.91557627198102409 ) ) ;
#159421=CARTESIAN_POINT ( 'NONE',  ( 16.53943276465976808, -0.05219959533910856209, 63.74890960531435979 ) ) ;
#159422=CARTESIAN_POINT ( 'NONE',  ( -0.05219959533909027116, -19.03943276465977164, 22.49890960531436690 ) ) ;
#159423=CARTESIAN_POINT ( 'NONE',  ( -10.81492255796078084, -18.62759615963271287, 27.08224293864769550 ) ) ;
#159424=CARTESIAN_POINT ( 'NONE',  ( -5.719274019375978568, 21.55341960407610458, 45.20724293864769550 ) ) ;
#159425=CARTESIAN_POINT ( 'NONE',  ( 16.52544592524342804, -4.483927247898539470, 83.54057627198102409 ) ) ;
#159426=CARTESIAN_POINT ( 'NONE',  ( -8.314922557961024197, 14.29746914071037800, 32.91775706135234714 ) ) ;
#159427=CARTESIAN_POINT ( 'NONE',  ( 8.224510206698953496, -14.34966873604960469, 82.91557627198103830 ) ) ;
#159428=CARTESIAN_POINT ( 'NONE',  ( -18.56453257813359770, 5.500000000000041744, 65.99000423690688422 ) ) ;
#159429=CARTESIAN_POINT ( 'NONE',  ( -13.97604488694547697, 13.89961937509957934, 73.12609039468568994 ) ) ;
#159430=CARTESIAN_POINT ( 'NONE',  ( 21.53943276465977519, -0.05219959533907433946, 23.74890960531435269 ) ) ;
#159433=CARTESIAN_POINT ( 'NONE',  ( -14.34966873604972548, 8.224510206698743886, 23.33442372801901499 ) ) ;
#159434=CARTESIAN_POINT ( 'NONE',  ( -14.29746914071037622, -8.314922557961029526, 104.1677570613523471 ) ) ;
#159436=CARTESIAN_POINT ( 'NONE',  ( -13.97604488694547697, 13.89961937509957934, 73.12609039468568994 ) ) ;
#159437=CARTESIAN_POINT ( 'NONE',  ( 10.81492255796078972, 18.62759615963270932, 44.58224293864769550 ) ) ;
#159438=CARTESIAN_POINT ( 'NONE',  ( -21.55341960407619339, 5.719274019375674811, 73.54275706135234714 ) ) ;
#159440=CARTESIAN_POINT ( 'NONE',  ( -4.379528057220086978, -16.55341960407618274, 34.79275706135235424 ) ) ;
#159441=CARTESIAN_POINT ( 'NONE',  ( 9.564922557960805705, 16.46253265017160317, 24.58224293864769194 ) ) ;
#159442=CARTESIAN_POINT ( 'NONE',  ( -0.05219959533909027116, -19.03943276465977164, 92.49890960531436690 ) ) ;
#159443=CARTESIAN_POINT ( 'NONE',  ( 16.46253265017160672, -9.564922557960803928, 23.33224293864769194 ) ) ;
#159444=CARTESIAN_POINT ( 'NONE',  ( -12.06949235617756955, 12.14591786802309770, 90.62390960531436690 ) ) ;
#159446=CARTESIAN_POINT ( 'NONE',  ( 9.474510206698971260, -16.51473224551069308, 102.9155762719810241 ) ) ;
#159447=CARTESIAN_POINT ( 'NONE',  ( -19.05341960407617563, 5.049401038297882671, 108.5427570613523187 ) ) ;
#159448=CARTESIAN_POINT ( 'NONE',  ( 21.55341960407610458, 5.719274019375980345, 83.95724293864770971 ) ) ;
#159449=CARTESIAN_POINT ( 'NONE',  ( 13.89961937509977652, -13.97604488694527269, 43.12390960531434558 ) ) ;
#159450=CARTESIAN_POINT ( 'NONE',  ( 9.474510206698729675, 16.51473224551082808, 67.08442372801900433 ) ) ;
#159451=CARTESIAN_POINT ( 'NONE',  ( -10.72451020669870658, -18.67979575497194134, 19.58442372801901143 ) ) ;
#159452=CARTESIAN_POINT ( 'NONE',  ( -9.474510206698964154, 16.51473224551069663, 70.41557627198102409 ) ) ;
#159453=CARTESIAN_POINT ( 'NONE',  ( 0.05219959533909260263, 19.03943276465977164, 109.9989096053143669 ) ) ;
#159455=CARTESIAN_POINT ( 'NONE',  ( -8.314922557961024197, 14.29746914071037800, 37.91775706135235424 ) ) ;
#159456=CARTESIAN_POINT ( 'NONE',  ( -0.05219959533907301413, -21.53943276465977519, 107.4989096053143669 ) ) ;
#159457=CARTESIAN_POINT ( 'NONE',  ( -12.14591786802309592, -12.06949235617757132, 111.8739096053143669 ) ) ;
#159458=CARTESIAN_POINT ( 'NONE',  ( -19.05341960407611168, -5.049401038298163336, 96.45724293864769550 ) ) ;
#159459=CARTESIAN_POINT ( 'NONE',  ( 16.51473224551083163, -9.474510206698727899, 55.83442372801899722 ) ) ;
#159460=CARTESIAN_POINT ( 'NONE',  ( -15.72974639402197994, 15.80617190586746368, 90.62390960531436690 ) ) ;
#159461=CARTESIAN_POINT ( 'NONE',  ( -12.14591786802309592, -12.06949235617757132, 41.87390960531435979 ) ) ;
#159462=CARTESIAN_POINT ( 'NONE',  ( -0.05219959533936034679, 19.03943276465977164, 22.50109039468566152 ) ) ;
#159463=CARTESIAN_POINT ( 'NONE',  ( -14.29746914071037622, -8.314922557961029526, 59.16775706135234714 ) ) ;
#159464=CARTESIAN_POINT ( 'NONE',  ( 16.46253265017160672, -9.564922557960803928, 88.33224293864769550 ) ) ;
#159465=CARTESIAN_POINT ( 'NONE',  ( -0.05219959533909027116, -19.03943276465977164, 42.49890960531435269 ) ) ;
#159467=CARTESIAN_POINT ( 'NONE',  ( -10.81492255796105439, 18.62759615963255655, 47.91775706135234714 ) ) ;
#159468=CARTESIAN_POINT ( 'NONE',  ( 21.52544592524334988, 5.823673210054432836, 66.45942372801903275 ) ) ;
#159469=CARTESIAN_POINT ( 'NONE',  ( 0.05219959533909260263, 19.03943276465977164, 54.99890960531435979 ) ) ;
#159470=CARTESIAN_POINT ( 'NONE',  ( 18.67979575497194134, -10.72451020669871369, 30.83442372801902209 ) ) ;
#159471=CARTESIAN_POINT ( 'NONE',  ( -5.049401038297874678, -19.05341960407617918, 74.79275706135231871 ) ) ;
#159473=CARTESIAN_POINT ( 'NONE',  ( 5.153800228976615827, -19.02544592524334988, 80.20942372801901854 ) ) ;
#159474=CARTESIAN_POINT ( 'NONE',  ( -19.03943276465977164, 0.05219959533909376836, 36.24890960531436690 ) ) ;
#159475=CARTESIAN_POINT ( 'NONE',  ( -4.483927247898782831, 16.52544592524335698, 92.70942372801901854 ) ) ;
#159476=CARTESIAN_POINT ( 'NONE',  ( 0.05219959533909260263, 19.03943276465977164, 54.99890960531435979 ) ) ;
#159477=CARTESIAN_POINT ( 'NONE',  ( -19.03943276465977164, 0.05219959533909376836, 21.24890960531436335 ) ) ;
#159478=CARTESIAN_POINT ( 'NONE',  ( -19.03943276465977164, 0.05219959533909376836, 101.2489096053143669 ) ) ;
#159479=CARTESIAN_POINT ( 'NONE',  ( 5.049401038298161559, -19.05341960407611168, 32.70724293864768129 ) ) ;
#159480=CARTESIAN_POINT ( 'NONE',  ( -21.53943276465977519, 0.05219959533907696930, 86.24890960531436690 ) ) ;
#159481=CARTESIAN_POINT ( 'NONE',  ( 0.05219959533934541429, -16.53943276465976808, 75.00109039468568994 ) ) ;
#159482=CARTESIAN_POINT ( 'NONE',  ( 13.89961937509957401, 13.97604488694547697, 31.87609039468566863 ) ) ;
#159483=CARTESIAN_POINT ( 'NONE',  ( 16.51473224551069308, 9.474510206698969483, 49.16557627198102409 ) ) ;
#159484=CARTESIAN_POINT ( 'NONE',  ( 14.29746914071049879, -8.314922557960816363, 48.33224293864770260 ) ) ;
#159485=CARTESIAN_POINT ( 'NONE',  ( -8.314922557960811034, -14.29746914071050412, 87.08224293864769550 ) ) ;
#159486=B_SPLINE_CURVE_WITH_KNOTS ( 'NONE', 3,
 ( #83189, #32729, #159032, #6346, #129677, #94381 ),
 .UNSPECIFIED., .F., .F.,
 ( 4, 2, 4 ),
 ( 0.007228050697041539692, 0.007608510107495016980, 0.007988969517948495136 ),
 .UNSPECIFIED. ) ;
#159487=CARTESIAN_POINT ( 'NONE',  ( -19.05341960407611168, -5.049401038298163336, 96.45724293864769550 ) ) ;
#159488=CARTESIAN_POINT ( 'NONE',  ( -9.564922557960796823, -16.46253265017161027, 82.08224293864768129 ) ) ;
#159489=CARTESIAN_POINT ( 'NONE',  ( 10.81492255796106328, -18.62759615963255655, 40.41775706135234714 ) ) ;
#159490=CARTESIAN_POINT ( 'NONE',  ( 13.97604488694527802, 13.89961937509977652, 89.37390960531436690 ) ) ;
#159491=CARTESIAN_POINT ( 'NONE',  ( -21.55341960407619339, 5.719274019375674811, 93.54275706135234714 ) ) ;
#159492=CARTESIAN_POINT ( 'NONE',  ( 4.483927247898790824, -16.52544592524335698, 75.20942372801901854 ) ) ;
#159493=CARTESIAN_POINT ( 'NONE',  ( -18.62759615963255300, -10.81492255796106328, 24.16775706135235424 ) ) ;
#159494=CARTESIAN_POINT ( 'NONE',  ( 21.52544592524344225, -5.823673210054117533, 93.54057627198103830 ) ) ;
#159495=CARTESIAN_POINT ( 'NONE',  ( 4.379528057220339221, -16.55341960407611168, 47.70724293864770260 ) ) ;
#159496=CARTESIAN_POINT ( 'NONE',  ( -19.05341960407611168, -5.049401038298163336, 46.45724293864768129 ) ) ;
#159497=CARTESIAN_POINT ( 'NONE',  ( 16.52544592524342804, -4.483927247898539470, 68.54057627198103830 ) ) ;
#159498=CARTESIAN_POINT ( 'NONE',  ( -0.05219959533907301413, -21.53943276465977519, 27.49890960531435269 ) ) ;
#159499=CARTESIAN_POINT ( 'NONE',  ( -9.474510206698720793, -16.51473224551083518, 34.58442372801899722 ) ) ;
#159500=CARTESIAN_POINT ( 'NONE',  ( 4.483927247898545687, 16.52544592524342804, 94.79057627198105251 ) ) ;
#159502=CARTESIAN_POINT ( 'NONE',  ( -14.29746914071037622, -8.314922557961029526, 69.16775706135234714 ) ) ;
#159503=CARTESIAN_POINT ( 'NONE',  ( 19.03943276465977164, -0.05219959533909143690, 63.74890960531435979 ) ) ;
#159505=CARTESIAN_POINT ( 'NONE',  ( -21.53943276465977519, 0.05219959533907696930, 36.24890960531435979 ) ) ;
#159506=CARTESIAN_POINT ( 'NONE',  ( -14.29746914071037622, -8.314922557961029526, 94.16775706135237556 ) ) ;
#159507=CARTESIAN_POINT ( 'NONE',  ( 5.153800228976615827, -19.02544592524334988, 110.2094237280189901 ) ) ;
#159508=CARTESIAN_POINT ( 'NONE',  ( -5.823673210054431948, 21.52544592524334988, 77.70942372801900433 ) ) ;
#159509=CARTESIAN_POINT ( 'NONE',  ( 19.05341960407611168, 5.049401038298154454, 73.95724293864768129 ) ) ;
#159510=CARTESIAN_POINT ( 'NONE',  ( -18.67979575497178146, -10.72451020669898902, 101.6655762719810383 ) ) ;
#159511=CARTESIAN_POINT ( 'NONE',  ( -16.53943276465976808, -0.05219959533934237506, 58.75109039468568994 ) ) ;
#159512=CARTESIAN_POINT ( 'NONE',  ( -4.483927247898539470, -16.52544592524342804, 112.2905762719810241 ) ) ;
#159513=CARTESIAN_POINT ( 'NONE',  ( -0.05219959533934338120, 16.53943276465976808, 22.50109039468567573 ) ) ;
#159514=CARTESIAN_POINT ( 'NONE',  ( 9.474510206698729675, 16.51473224551082808, 82.08442372801899012 ) ) ;
#159515=CARTESIAN_POINT ( 'NONE',  ( 21.52544592524344225, -5.823673210054117533, 78.54057627198103830 ) ) ;
#159516=CARTESIAN_POINT ( 'NONE',  ( -5.049401038297874678, -19.05341960407617918, 49.79275706135231871 ) ) ;
#159518=CARTESIAN_POINT ( 'NONE',  ( -0.05219959533907301413, -21.53943276465977519, 97.49890960531436690 ) ) ;
#159520=CARTESIAN_POINT ( 'NONE',  ( -9.474510206698964154, 16.51473224551069663, 75.41557627198103830 ) ) ;
#159522=CARTESIAN_POINT ( 'NONE',  ( -4.379528057220086978, -16.55341960407618274, 34.79275706135235424 ) ) ;
#159524=CARTESIAN_POINT ( 'NONE',  ( -0.05219959533907301413, -21.53943276465977519, 97.49890960531436690 ) ) ;
#159525=CARTESIAN_POINT ( 'NONE',  ( 14.34966873604960469, 8.224510206698951720, 64.16557627198102409 ) ) ;
#159526=CARTESIAN_POINT ( 'NONE',  ( 19.02544592524343514, -5.153800228976328945, 63.54057627198103830 ) ) ;
#159527=CARTESIAN_POINT ( 'NONE',  ( -5.823673210054431948, 21.52544592524334988, 92.70942372801901854 ) ) ;
#159528=CARTESIAN_POINT ( 'NONE',  ( 12.06949235617739724, 12.14591786802326823, 31.87609039468567929 ) ) ;
#159529=CARTESIAN_POINT ( 'NONE',  ( -19.05341960407617563, 5.049401038297882671, 38.54275706135233293 ) ) ;
#159530=CARTESIAN_POINT ( 'NONE',  ( 21.52544592524334988, 5.823673210054432836, 46.45942372801901854 ) ) ;
#159531=CARTESIAN_POINT ( 'NONE',  ( 5.719274019375991003, -21.55341960407610458, 62.70724293864769550 ) ) ;
#159532=CARTESIAN_POINT ( 'NONE',  ( -9.564922557961040184, 16.46253265017147172, 102.9177570613523329 ) ) ;
#159533=CARTESIAN_POINT ( 'NONE',  ( -19.03943276465977164, 0.05219959533909376836, 51.24890960531436690 ) ) ;
#159535=CARTESIAN_POINT ( 'NONE',  ( 5.153800228976615827, -19.02544592524334988, 65.20942372801900433 ) ) ;
#159536=CARTESIAN_POINT ( 'NONE',  ( 21.55341960407619695, -5.719274019375665929, 81.04275706135236135 ) ) ;
#159537=CARTESIAN_POINT ( 'NONE',  ( -9.474510206698720793, -16.51473224551083518, 69.58442372801901854 ) ) ;
#159538=CARTESIAN_POINT ( 'NONE',  ( -13.97604488694527625, -13.89961937509977652, 31.87390960531435979 ) ) ;
#159539=CARTESIAN_POINT ( 'NONE',  ( -15.80617190586745835, -15.72974639402198527, 51.87390960531437401 ) ) ;
#159540=CARTESIAN_POINT ( 'NONE',  ( -8.314922557960811034, -14.29746914071050412, 57.08224293864769550 ) ) ;
#159542=CARTESIAN_POINT ( 'NONE',  ( 0.05219959533936267826, -19.03943276465977164, 35.00109039468566863 ) ) ;
#159543=CARTESIAN_POINT ( 'NONE',  ( -8.224510206698735004, -14.34966873604973081, 84.58442372801903275 ) ) ;
#159544=CARTESIAN_POINT ( 'NONE',  ( -4.379528057220328563, 16.55341960407611168, 55.20724293864770260 ) ) ;
#159545=CARTESIAN_POINT ( 'NONE',  ( 18.62759615963255655, 10.81492255796105972, 91.66775706135234714 ) ) ;
#159546=CARTESIAN_POINT ( 'NONE',  ( -5.719274019375665041, -21.55341960407619695, 79.79275706135236135 ) ) ;
#159547=CARTESIAN_POINT ( 'NONE',  ( -18.62759615963270932, 10.81492255796079327, 95.83224293864770971 ) ) ;
#159548=CIRCLE ( 'NONE', #63150, 2.500000000000002220 ) ;
#159549=CARTESIAN_POINT ( 'NONE',  ( -9.564922557960796823, -16.46253265017161027, 52.08224293864768839 ) ) ;
#159550=CARTESIAN_POINT ( 'NONE',  ( 18.62759615963255655, 10.81492255796105972, 61.66775706135235424 ) ) ;
#159551=CARTESIAN_POINT ( 'NONE',  ( -5.049401038298153566, 19.05341960407611168, 35.20724293864768839 ) ) ;
#159552=CARTESIAN_POINT ( 'NONE',  ( 5.153800228976335163, 19.02544592524342804, 54.79057627198103120 ) ) ;
#159553=CARTESIAN_POINT ( 'NONE',  ( -16.52544592524342804, 4.483927247898546575, 111.0405762719810525 ) ) ;
#159554=CARTESIAN_POINT ( 'NONE',  ( -19.03943276465977164, 0.05219959533909376836, 96.24890960531436690 ) ) ;
#159555=CARTESIAN_POINT ( 'NONE',  ( 12.06949235617757843, -12.14591786802309237, 53.12390960531436690 ) ) ;
#159556=CARTESIAN_POINT ( 'NONE',  ( -12.14591786802309592, -12.06949235617757132, 111.8739096053143669 ) ) ;
#159557=CARTESIAN_POINT ( 'NONE',  ( 18.67979575497178502, 10.72451020669898547, 79.16557627198103830 ) ) ;
#159558=CARTESIAN_POINT ( 'NONE',  ( -18.67979575497193778, 10.72451020669871902, 33.33442372801900433 ) ) ;
#159560=CARTESIAN_POINT ( 'NONE',  ( -14.34966873604972548, 8.224510206698743886, 43.33442372801901143 ) ) ;
#159561=VERTEX_POINT ( 'NONE', #34524 ) ;
#159562=CARTESIAN_POINT ( 'NONE',  ( 21.55341960407610458, 5.719274019375980345, 78.95724293864769550 ) ) ;
#159564=CARTESIAN_POINT ( 'NONE',  ( -10.81492255796105439, 18.62759615963255655, 112.9177570613523329 ) ) ;
#159565=CARTESIAN_POINT ( 'NONE',  ( 16.51473224551069308, 9.474510206698969483, 99.16557627198102409 ) ) ;
#159566=CARTESIAN_POINT ( 'NONE',  ( 0.05219959533937995610, -21.53943276465977519, 30.00109039468568284 ) ) ;
#159567=CARTESIAN_POINT ( 'NONE',  ( 21.53943276465977519, -0.05219959533907433946, 33.74890960531436690 ) ) ;
#159568=CARTESIAN_POINT ( 'NONE',  ( -16.52544592524335698, -4.483927247898792601, 98.95942372801903275 ) ) ;
#159569=CARTESIAN_POINT ( 'NONE',  ( -5.823673210054431948, 21.52544592524334988, 52.70942372801902565 ) ) ;
#159570=CARTESIAN_POINT ( 'NONE',  ( -21.53943276465977519, -0.05219959533937600094, 78.75109039468568994 ) ) ;
#159571=CARTESIAN_POINT ( 'NONE',  ( -0.05219959533936034679, 19.03943276465977164, 22.50109039468566152 ) ) ;
#159572=CARTESIAN_POINT ( 'NONE',  ( -14.29746914071037622, -8.314922557961029526, 69.16775706135234714 ) ) ;
#159573=CARTESIAN_POINT ( 'NONE',  ( -10.81492255796105439, 18.62759615963255655, 42.91775706135235424 ) ) ;
#159575=CARTESIAN_POINT ( 'NONE',  ( -16.51473224551069308, -9.474510206698971260, 36.66557627198102409 ) ) ;
#159576=CARTESIAN_POINT ( 'NONE',  ( 18.67979575497194134, -10.72451020669871369, 105.8344237280190328 ) ) ;
#159577=CARTESIAN_POINT ( 'NONE',  ( -16.51473224551069308, -9.474510206698971260, 106.6655762719810383 ) ) ;
#159578=CARTESIAN_POINT ( 'NONE',  ( -21.55341960407610458, -5.719274019375992779, 101.4572429386476955 ) ) ;
#159580=CARTESIAN_POINT ( 'NONE',  ( -5.719274019375978568, 21.55341960407610458, 65.20724293864768129 ) ) ;
#159581=CARTESIAN_POINT ( 'NONE',  ( 16.53943276465976808, 0.05219959533934440121, 51.25109039468568994 ) ) ;
#159582=CARTESIAN_POINT ( 'NONE',  ( 16.53943276465976808, -0.05219959533910856209, 48.74890960531435979 ) ) ;
#159584=CARTESIAN_POINT ( 'NONE',  ( -16.51473224551082808, 9.474510206698731452, 88.33442372801900433 ) ) ;
#159585=CARTESIAN_POINT ( 'NONE',  ( -16.29526858892876007, 7.335722546920112386, 104.2032940219980048 ) ) ;
#159586=CARTESIAN_POINT ( 'NONE',  ( 12.14591786802327356, -12.06949235617739191, 25.62609039468567929 ) ) ;
#159587=CARTESIAN_POINT ( 'NONE',  ( 5.719274019375991003, -21.55341960407610458, 102.7072429386476955 ) ) ;
#159588=CARTESIAN_POINT ( 'NONE',  ( 10.81492255796078972, 18.62759615963270932, 69.58224293864769550 ) ) ;
#159589=CARTESIAN_POINT ( 'NONE',  ( -13.89961937509977652, 13.97604488694528158, 110.6239096053143243 ) ) ;
#159590=CARTESIAN_POINT ( 'NONE',  ( 0.05219959533934541429, -16.53943276465976808, 40.00109039468567573 ) ) ;
#159591=CARTESIAN_POINT ( 'NONE',  ( 13.97604488694527802, 13.89961937509977652, 59.37390960531434558 ) ) ;
#159592=CARTESIAN_POINT ( 'NONE',  ( 0.05219959533937995610, -21.53943276465977519, 30.00109039468568284 ) ) ;
#159593=CARTESIAN_POINT ( 'NONE',  ( -5.153800228976607833, 19.02544592524334988, 97.70942372801900433 ) ) ;
#159594=CARTESIAN_POINT ( 'NONE',  ( 13.97604488694527802, 13.89961937509977652, 104.3739096053143385 ) ) ;
#159595=CARTESIAN_POINT ( 'NONE',  ( 19.03943276465977164, -0.05219959533909143690, 83.74890960531436690 ) ) ;
#159596=CARTESIAN_POINT ( 'NONE',  ( -15.80617190586745835, -15.72974639402198527, 91.87390960531436690 ) ) ;
#159597=CARTESIAN_POINT ( 'NONE',  ( -19.05341960407611168, -5.049401038298163336, 61.45724293864769550 ) ) ;
#159599=CARTESIAN_POINT ( 'NONE',  ( -12.06949235617756955, 12.14591786802309770, 70.62390960531436690 ) ) ;
#159600=CARTESIAN_POINT ( 'NONE',  ( 9.564922557960805705, 16.46253265017160317, 99.58224293864770971 ) ) ;
#159602=CARTESIAN_POINT ( 'NONE',  ( -19.03943276465977164, -0.05219959533935918106, 83.75109039468567573 ) ) ;
#159603=CARTESIAN_POINT ( 'NONE',  ( -0.05219959533907301413, -21.53943276465977519, 87.49890960531436690 ) ) ;
#159604=CARTESIAN_POINT ( 'NONE',  ( 13.97604488694548053, -13.89961937509957401, 50.62609039468566152 ) ) ;
#159605=CARTESIAN_POINT ( 'NONE',  ( -19.03943276465977164, 0.05219959533909376836, 111.2489096053143669 ) ) ;
#159606=CARTESIAN_POINT ( 'NONE',  ( 18.39639308325437383, 5.500000000000037303, 68.98252246182197212 ) ) ;
#159607=CARTESIAN_POINT ( 'NONE',  ( -15.72974639402197994, 15.80617190586746368, 60.62390960531437401 ) ) ;
#159609=CARTESIAN_POINT ( 'NONE',  ( -9.474510206698964154, 16.51473224551069663, 80.41557627198103830 ) ) ;
#159610=CARTESIAN_POINT ( 'NONE',  ( -10.72451020669870658, -18.67979575497194134, 79.58442372801903275 ) ) ;
#159612=CARTESIAN_POINT ( 'NONE',  ( -5.049401038298153566, 19.05341960407611168, 40.20724293864768839 ) ) ;
#159614=CARTESIAN_POINT ( 'NONE',  ( 12.06949235617757843, -12.14591786802309237, 68.12390960531436690 ) ) ;
#159615=CARTESIAN_POINT ( 'NONE',  ( -0.05219959533934338120, 16.53943276465976808, 27.50109039468567929 ) ) ;
#159616=CARTESIAN_POINT ( 'NONE',  ( -21.55341960407619339, 5.719274019375674811, 68.54275706135234714 ) ) ;
#159617=ORIENTED_EDGE ( 'NONE', *, *, #19140, .F. ) ;
#159618=CARTESIAN_POINT ( 'NONE',  ( -9.564922557961040184, 16.46253265017147172, 22.91775706135233648 ) ) ;
#159619=CARTESIAN_POINT ( 'NONE',  ( -13.89961937509957401, -13.97604488694547875, 74.37609039468566152 ) ) ;
#159621=CARTESIAN_POINT ( 'NONE',  ( -18.67979575497193778, 10.72451020669871902, 28.33442372801902209 ) ) ;
#159622=CARTESIAN_POINT ( 'NONE',  ( -19.19724070472091526, -5.500000000000168754, 46.06193348274383936 ) ) ;
#159623=CARTESIAN_POINT ( 'NONE',  ( -10.81492255796105439, 18.62759615963255655, 112.9177570613523329 ) ) ;
#159624=CARTESIAN_POINT ( 'NONE',  ( -19.03943276465977164, 0.05219959533909376836, 51.24890960531436690 ) ) ;
#159625=CARTESIAN_POINT ( 'NONE',  ( 13.89961937509957401, 13.97604488694547697, 36.87609039468565442 ) ) ;
#159626=CARTESIAN_POINT ( 'NONE',  ( 8.314922557961029526, -14.29746914071037800, 110.4177570613523756 ) ) ;
#159627=CARTESIAN_POINT ( 'NONE',  ( -9.564922557960796823, -16.46253265017161027, 97.08224293864769550 ) ) ;
#159628=CARTESIAN_POINT ( 'NONE',  ( 5.719274019375673035, 21.55341960407619339, 67.29275706135234714 ) ) ;
#159631=CARTESIAN_POINT ( 'NONE',  ( 10.72451020669871369, 18.67979575497193778, 87.08442372801901854 ) ) ;
#159632=CARTESIAN_POINT ( 'NONE',  ( -15.80617190586768217, 15.72974639402176855, 108.1260903946856757 ) ) ;
#159634=CARTESIAN_POINT ( 'NONE',  ( -16.46253265017160317, 9.564922557960807481, 100.8322429386477097 ) ) ;
#159635=CARTESIAN_POINT ( 'NONE',  ( -19.02544592524334988, -5.153800228976617603, 18.95942372801899722 ) ) ;
#159637=CARTESIAN_POINT ( 'NONE',  ( 9.474510206698971260, -16.51473224551069308, 42.91557627198103120 ) ) ;
#159638=CARTESIAN_POINT ( 'NONE',  ( -0.05219959533907301413, -21.53943276465977519, 52.49890960531435979 ) ) ;
#159639=CARTESIAN_POINT ( 'NONE',  ( -0.05219959533910754901, -16.53943276465976808, 22.49890960531436335 ) ) ;
#159640=CARTESIAN_POINT ( 'NONE',  ( -8.224510206698948167, 14.34966873604960824, 90.41557627198103830 ) ) ;
#159641=CARTESIAN_POINT ( 'NONE',  ( -16.46253265017160317, 9.564922557960807481, 80.83224293864769550 ) ) ;
#159642=CARTESIAN_POINT ( 'NONE',  ( 10.81492255796106328, -18.62759615963255655, 110.4177570613523756 ) ) ;
#159643=CARTESIAN_POINT ( 'NONE',  ( 19.02544592524343514, -5.153800228976328945, 38.54057627198103120 ) ) ;
#159644=CARTESIAN_POINT ( 'NONE',  ( -8.314922557960811034, -14.29746914071050412, 107.0822429386476955 ) ) ;
#159645=CARTESIAN_POINT ( 'NONE',  ( -21.52544592524334988, -5.823673210054445271, 58.95942372801902565 ) ) ;
#159646=CARTESIAN_POINT ( 'NONE',  ( 5.719274019375991003, -21.55341960407610458, 87.70724293864769550 ) ) ;
#159647=CARTESIAN_POINT ( 'NONE',  ( 19.03943276465977164, 0.05219959533936151252, 56.25109039468566863 ) ) ;
#159649=CARTESIAN_POINT ( 'NONE',  ( 5.049401038298161559, -19.05341960407611168, 112.7072429386476813 ) ) ;
#159650=CARTESIAN_POINT ( 'NONE',  ( -0.05219959533910754901, -16.53943276465976808, 72.49890960531435269 ) ) ;
#159651=CARTESIAN_POINT ( 'NONE',  ( -16.46253265017146816, -9.564922557961047289, 49.16775706135233293 ) ) ;
#159652=CARTESIAN_POINT ( 'NONE',  ( 19.05341960407611168, 5.049401038298154454, 63.95724293864769550 ) ) ;
#159653=CARTESIAN_POINT ( 'NONE',  ( 4.379528057220339221, -16.55341960407611168, 47.70724293864770260 ) ) ;
#159654=CARTESIAN_POINT ( 'NONE',  ( 13.89961937509957401, 13.97604488694547697, 81.87609039468564731 ) ) ;
#159655=CARTESIAN_POINT ( 'NONE',  ( -19.46398650005391318, 5.499999999999953815, 85.18269651486372140 ) ) ;
#159656=CARTESIAN_POINT ( 'NONE',  ( -15.72974639402197994, 15.80617190586746368, 40.62390960531435269 ) ) ;
#159657=CARTESIAN_POINT ( 'NONE',  ( 16.55341960407611168, 4.379528057220329451, 103.9572429386476813 ) ) ;
#159658=CARTESIAN_POINT ( 'NONE',  ( -17.50000000000015632, -3.292511757969812436, 24.93479729789453003 ) ) ;
#159659=CARTESIAN_POINT ( 'NONE',  ( 19.05341960407611168, 5.049401038298154454, 63.95724293864769550 ) ) ;
#159660=CARTESIAN_POINT ( 'NONE',  ( 0.05219959533907565091, 21.53943276465977519, 64.99890960531435269 ) ) ;
#159661=CARTESIAN_POINT ( 'NONE',  ( -16.51473224551069308, -9.474510206698971260, 36.66557627198102409 ) ) ;
#159662=CARTESIAN_POINT ( 'NONE',  ( -16.53943276465976808, -0.05219959533934237506, 73.75109039468567573 ) ) ;
#159663=CARTESIAN_POINT ( 'NONE',  ( -19.02544592524342804, 5.153800228976336051, 61.04057627198103120 ) ) ;
#159664=CARTESIAN_POINT ( 'NONE',  ( 13.89961937509957401, 13.97604488694547697, 56.87609039468564731 ) ) ;
#159666=CARTESIAN_POINT ( 'NONE',  ( 10.72451020669871369, 18.67979575497193778, 62.08442372801901143 ) ) ;
#159667=CARTESIAN_POINT ( 'NONE',  ( -0.05219959533907301413, -21.53943276465977519, 52.49890960531435979 ) ) ;
#159668=CARTESIAN_POINT ( 'NONE',  ( 0.05219959533909260263, 19.03943276465977164, 29.99890960531435979 ) ) ;
#159669=CARTESIAN_POINT ( 'NONE',  ( -16.52544592524335698, -4.483927247898792601, 93.95942372801903275 ) ) ;
#159670=CARTESIAN_POINT ( 'NONE',  ( 0.05219959533936267826, -19.03943276465977164, 100.0010903946856757 ) ) ;
#159672=CARTESIAN_POINT ( 'NONE',  ( 19.35543954521080678, 5.499999999999573674, 77.08901960356448058 ) ) ;
#159673=CARTESIAN_POINT ( 'NONE',  ( -5.823673210054116645, -21.52544592524344225, 57.29057627198103120 ) ) ;
#159674=CARTESIAN_POINT ( 'NONE',  ( 5.719274019375673035, 21.55341960407619339, 97.29275706135234714 ) ) ;
#159676=CARTESIAN_POINT ( 'NONE',  ( -16.52544592524342804, 4.483927247898546575, 41.04057627198103120 ) ) ;
#159677=CARTESIAN_POINT ( 'NONE',  ( 4.379528057220339221, -16.55341960407611168, 57.70724293864770260 ) ) ;
#159678=CARTESIAN_POINT ( 'NONE',  ( 10.81492255796078972, 18.62759615963270932, 84.58224293864769550 ) ) ;
#159679=CARTESIAN_POINT ( 'NONE',  ( -10.81492255796078084, -18.62759615963271287, 87.08224293864769550 ) ) ;
#159681=CARTESIAN_POINT ( 'NONE',  ( 21.55341960407610458, 5.719274019375980345, 28.95724293864769905 ) ) ;
#159682=CARTESIAN_POINT ( 'NONE',  ( 16.53943276465976808, 0.05219959533934440121, 71.25109039468568994 ) ) ;
#159683=CARTESIAN_POINT ( 'NONE',  ( 16.53943276465976808, -0.05219959533910856209, 73.74890960531433848 ) ) ;
#159684=CARTESIAN_POINT ( 'NONE',  ( 5.153800228976335163, 19.02544592524342804, 34.79057627198102409 ) ) ;
#159686=CARTESIAN_POINT ( 'NONE',  ( -0.05219959533934338120, 16.53943276465976808, 102.5010903946856899 ) ) ;
#159687=CARTESIAN_POINT ( 'NONE',  ( -5.719274019375665041, -21.55341960407619695, 24.79275706135235779 ) ) ;
#159688=CARTESIAN_POINT ( 'NONE',  ( -0.05219959533909027116, -19.03943276465977164, 87.49890960531436690 ) ) ;
#159689=CARTESIAN_POINT ( 'NONE',  ( 0.05219959533937995610, -21.53943276465977519, 60.00109039468568284 ) ) ;
#159690=CARTESIAN_POINT ( 'NONE',  ( -13.89961937509977652, 13.97604488694528158, 115.6239096053143669 ) ) ;
#159694=CARTESIAN_POINT ( 'NONE',  ( -18.67979575497193778, 10.72451020669871902, 43.33442372801901143 ) ) ;
#159695=CARTESIAN_POINT ( 'NONE',  ( -19.03943276465977164, 0.05219959533909376836, 36.24890960531436690 ) ) ;
#159696=CARTESIAN_POINT ( 'NONE',  ( -16.46253265017160317, 9.564922557960807481, 105.8322429386476955 ) ) ;
#159697=CARTESIAN_POINT ( 'NONE',  ( 16.46253265017146816, 9.564922557961045513, 51.66775706135233293 ) ) ;
#159698=CARTESIAN_POINT ( 'NONE',  ( 21.52544592524334988, 5.823673210054432836, 31.45942372801901854 ) ) ;
#159699=CARTESIAN_POINT ( 'NONE',  ( -13.89961937509957401, -13.97604488694547875, 59.37609039468566863 ) ) ;
#159701=CARTESIAN_POINT ( 'NONE',  ( 4.483927247898790824, -16.52544592524335698, 95.20942372801903275 ) ) ;
#159702=CARTESIAN_POINT ( 'NONE',  ( 5.153800228976615827, -19.02544592524334988, 60.20942372801899012 ) ) ;
#159703=CARTESIAN_POINT ( 'NONE',  ( 8.314922557961029526, -14.29746914071037800, 105.4177570613523613 ) ) ;
#159705=CARTESIAN_POINT ( 'NONE',  ( -0.05219959533909027116, -19.03943276465977164, 82.49890960531436690 ) ) ;
#159706=CARTESIAN_POINT ( 'NONE',  ( 21.53943276465977519, 0.05219959533937863772, 86.25109039468568994 ) ) ;
#159707=CARTESIAN_POINT ( 'NONE',  ( 21.53943276465977519, 0.05219959533937863772, 111.2510903946856899 ) ) ;
#159708=CARTESIAN_POINT ( 'NONE',  ( -13.89961937509977652, 13.97604488694528158, 95.62390960531436690 ) ) ;
#159709=CARTESIAN_POINT ( 'NONE',  ( -0.05219959533937732626, 21.53943276465977519, 77.50109039468567573 ) ) ;
#159710=CARTESIAN_POINT ( 'NONE',  ( 8.314922557961029526, -14.29746914071037800, 25.41775706135235779 ) ) ;
#159712=CARTESIAN_POINT ( 'NONE',  ( -13.89961937509977652, 13.97604488694528158, 80.62390960531436690 ) ) ;
#159713=CARTESIAN_POINT ( 'NONE',  ( 21.53943276465977519, -0.05219959533907433946, 33.74890960531436690 ) ) ;
#159715=CARTESIAN_POINT ( 'NONE',  ( -9.564922557960796823, -16.46253265017161027, 97.08224293864769550 ) ) ;
#159717=CARTESIAN_POINT ( 'NONE',  ( 0.05219959533909260263, 19.03943276465977164, 74.99890960531435269 ) ) ;
#159718=CARTESIAN_POINT ( 'NONE',  ( -0.05219959533909027116, -19.03943276465977164, 62.49890960531435979 ) ) ;
#159719=CARTESIAN_POINT ( 'NONE',  ( -4.379528057220328563, 16.55341960407611168, 25.20724293864769550 ) ) ;
#159722=CARTESIAN_POINT ( 'NONE',  ( -0.05219959533936034679, 19.03943276465977164, 72.50109039468566152 ) ) ;
#159723=CARTESIAN_POINT ( 'NONE',  ( 16.46253265017160672, -9.564922557960803928, 93.33224293864769550 ) ) ;
#159724=CARTESIAN_POINT ( 'NONE',  ( -16.55341960407611168, -4.379528057220339221, 91.45724293864769550 ) ) ;
#159725=CARTESIAN_POINT ( 'NONE',  ( 10.72451020669898902, -18.67979575497178502, 42.91557627198103120 ) ) ;
#159727=CARTESIAN_POINT ( 'NONE',  ( 21.53943276465977519, -0.05219959533907433946, 28.74890960531435624 ) ) ;
#159728=CARTESIAN_POINT ( 'NONE',  ( 8.224510206698953496, -14.34966873604960469, 102.9155762719810383 ) ) ;
#159729=CARTESIAN_POINT ( 'NONE',  ( -16.62475595723696387, 7.163666690055236153, 55.52713351810467657 ) ) ;
#159730=CARTESIAN_POINT ( 'NONE',  ( 19.03943276465977164, 0.05219959533936151252, 46.25109039468566863 ) ) ;
#159731=CARTESIAN_POINT ( 'NONE',  ( -16.53943276465976808, 0.05219959533911058130, 31.24890960531435979 ) ) ;
#159732=CARTESIAN_POINT ( 'NONE',  ( 5.153800228976335163, 19.02544592524342804, 99.79057627198102409 ) ) ;
#159733=CARTESIAN_POINT ( 'NONE',  ( 18.62759615963255655, 10.81492255796105972, 61.66775706135235424 ) ) ;
#159734=CARTESIAN_POINT ( 'NONE',  ( 5.719274019375991003, -21.55341960407610458, 52.70724293864769550 ) ) ;
#159735=CARTESIAN_POINT ( 'NONE',  ( 5.719274019375673035, 21.55341960407619339, 47.29275706135234003 ) ) ;
#159736=CARTESIAN_POINT ( 'NONE',  ( 18.67979575497178502, 10.72451020669898547, 99.16557627198100988 ) ) ;
#159737=CARTESIAN_POINT ( 'NONE',  ( 15.80617190586769283, -15.72974639402175789, 35.62609039468568994 ) ) ;
#159738=CARTESIAN_POINT ( 'NONE',  ( -8.224510206698948167, 14.34966873604960824, 110.4155762719810383 ) ) ;
#159739=CARTESIAN_POINT ( 'NONE',  ( -0.05219959533936034679, 19.03943276465977164, 72.50109039468566152 ) ) ;
#159740=CARTESIAN_POINT ( 'NONE',  ( -19.03943276465977164, 0.05219959533909376836, 46.24890960531435979 ) ) ;
#159742=CARTESIAN_POINT ( 'NONE',  ( -8.314922557960811034, -14.29746914071050412, 102.0822429386476955 ) ) ;
#159743=CARTESIAN_POINT ( 'NONE',  ( -0.05219959533909027116, -19.03943276465977164, 107.4989096053143527 ) ) ;
#159744=CARTESIAN_POINT ( 'NONE',  ( 8.224510206698953496, -14.34966873604960469, 37.91557627198102409 ) ) ;
#159745=CARTESIAN_POINT ( 'NONE',  ( 16.52544592524335698, 4.483927247898782831, 101.4594237280190185 ) ) ;
#159746=CARTESIAN_POINT ( 'NONE',  ( -16.46253265017160317, 9.564922557960807481, 50.83224293864770260 ) ) ;
#159747=CARTESIAN_POINT ( 'NONE',  ( 8.224510206698953496, -14.34966873604960469, 112.9155762719810383 ) ) ;
#159749=CARTESIAN_POINT ( 'NONE',  ( 13.89961937509957401, 13.97604488694547697, 21.87609039468566152 ) ) ;
#159750=CONICAL_SURFACE ( 'NONE', #37075, 2.500000000000002220, 1.029744260000000189 ) ;
#159752=CARTESIAN_POINT ( 'NONE',  ( 16.55341960407611168, 4.379528057220329451, 38.95724293864768839 ) ) ;
#159753=CARTESIAN_POINT ( 'NONE',  ( 10.81492255796106328, -18.62759615963255655, 50.41775706135235424 ) ) ;
#159754=PLANE ( 'NONE',  #32280 ) ;
#159755=CARTESIAN_POINT ( 'NONE',  ( -14.29746914071037622, -8.314922557961029526, 54.16775706135235424 ) ) ;
#159756=CARTESIAN_POINT ( 'NONE',  ( 16.53943276465976808, -0.05219959533910856209, 28.74890960531435624 ) ) ;
#159757=CARTESIAN_POINT ( 'NONE',  ( -8.224510206698735004, -14.34966873604973081, 109.5844237280190328 ) ) ;
#159758=CARTESIAN_POINT ( 'NONE',  ( 0.05219959533934541429, -16.53943276465976808, 30.00109039468568284 ) ) ;
#159759=CARTESIAN_POINT ( 'NONE',  ( -19.03943276465977164, 0.05219959533909376836, 46.24890960531435979 ) ) ;
#159760=CARTESIAN_POINT ( 'NONE',  ( 8.314922557960818139, 14.29746914071049879, 109.5822429386476955 ) ) ;
#159761=CARTESIAN_POINT ( 'NONE',  ( 18.62759615963271287, -10.81492255796078972, 113.3322429386476955 ) ) ;
#159762=CARTESIAN_POINT ( 'NONE',  ( -19.02544592524342804, 5.153800228976336051, 41.04057627198103120 ) ) ;
#159763=CARTESIAN_POINT ( 'NONE',  ( 16.46253265017160672, -9.564922557960803928, 113.3322429386476955 ) ) ;
#159764=CARTESIAN_POINT ( 'NONE',  ( -19.05341960407611168, -5.049401038298163336, 31.45724293864769550 ) ) ;
#159765=CARTESIAN_POINT ( 'NONE',  ( -21.53943276465977519, 0.05219959533907696930, 21.24890960531436690 ) ) ;
#159766=CARTESIAN_POINT ( 'NONE',  ( -16.31925111598458855, -7.325300261831428905, 34.83575461032747711 ) ) ;
#159767=CARTESIAN_POINT ( 'NONE',  ( 13.97604488694527802, 13.89961937509977652, 104.3739096053143385 ) ) ;
#159768=CARTESIAN_POINT ( 'NONE',  ( 18.62759615963255655, 10.81492255796105972, 51.66775706135234714 ) ) ;
#159769=CARTESIAN_POINT ( 'NONE',  ( -4.483927247898539470, -16.52544592524342804, 102.2905762719810383 ) ) ;
#159770=CARTESIAN_POINT ( 'NONE',  ( 16.51473224551069308, 9.474510206698969483, 104.1655762719810241 ) ) ;
#159771=CARTESIAN_POINT ( 'NONE',  ( -16.53943276465976808, -0.05219959533934237506, 83.75109039468568994 ) ) ;
#159772=CARTESIAN_POINT ( 'NONE',  ( -15.72974639402176322, -15.80617190586768395, 94.37609039468568994 ) ) ;
#159773=CARTESIAN_POINT ( 'NONE',  ( 16.52544592524335698, 4.483927247898782831, 56.45942372801902565 ) ) ;
#159774=CARTESIAN_POINT ( 'NONE',  ( -9.474510206698964154, 16.51473224551069663, 95.41557627198102409 ) ) ;
#159775=CARTESIAN_POINT ( 'NONE',  ( 16.52544592524335698, 4.483927247898782831, 46.45942372801901854 ) ) ;
#159776=CARTESIAN_POINT ( 'NONE',  ( 14.34966873604972726, -8.224510206698740333, 20.83442372801901143 ) ) ;
#159777=CARTESIAN_POINT ( 'NONE',  ( 16.55341960407618274, -4.379528057220086978, 86.04275706135236135 ) ) ;
#159778=CARTESIAN_POINT ( 'NONE',  ( -5.153800228976607833, 19.02544592524334988, 102.7094237280189759 ) ) ;
#159779=CARTESIAN_POINT ( 'NONE',  ( 13.89961937509977652, -13.97604488694527269, 78.12390960531433848 ) ) ;
#159780=CARTESIAN_POINT ( 'NONE',  ( -21.55341960407610458, -5.719274019375992779, 101.4572429386476955 ) ) ;
#159781=CARTESIAN_POINT ( 'NONE',  ( 16.53943276465976808, -0.05219959533910856209, 108.7489096053143669 ) ) ;
#159782=CARTESIAN_POINT ( 'NONE',  ( -13.97604488694547697, 13.89961937509957934, 98.12609039468566152 ) ) ;
#159783=CARTESIAN_POINT ( 'NONE',  ( -8.314922557961024197, 14.29746914071037800, 67.91775706135234714 ) ) ;
#159785=CARTESIAN_POINT ( 'NONE',  ( -5.153800228976607833, 19.02544592524334988, 67.70942372801900433 ) ) ;
#159786=CARTESIAN_POINT ( 'NONE',  ( -16.53943276465976808, 0.05219959533911058130, 41.24890960531435269 ) ) ;
#159787=CARTESIAN_POINT ( 'NONE',  ( 16.55341960407611168, 4.379528057220329451, 98.95724293864770971 ) ) ;
#159788=CARTESIAN_POINT ( 'NONE',  ( 9.474510206698729675, 16.51473224551082808, 32.08442372801900433 ) ) ;
#159789=CARTESIAN_POINT ( 'NONE',  ( -16.18388926212237777, 7.379444403734526148, 89.56046848633847901 ) ) ;
#159790=CARTESIAN_POINT ( 'NONE',  ( 18.62759615963255655, 10.81492255796105972, 41.66775706135235424 ) ) ;
#159791=CARTESIAN_POINT ( 'NONE',  ( -13.89961937509957401, -13.97604488694547875, 99.37609039468567573 ) ) ;
#159792=CARTESIAN_POINT ( 'NONE',  ( 19.02544592524343514, -5.153800228976328945, 113.5405762719810241 ) ) ;
#159793=CARTESIAN_POINT ( 'NONE',  ( 5.153800228976335163, 19.02544592524342804, 94.79057627198103830 ) ) ;
#159794=CARTESIAN_POINT ( 'NONE',  ( 18.67979575497194134, -10.72451020669871369, 110.8344237280190043 ) ) ;
#159795=CARTESIAN_POINT ( 'NONE',  ( 5.049401038298161559, -19.05341960407611168, 87.70724293864769550 ) ) ;
#159796=CARTESIAN_POINT ( 'NONE',  ( 15.80617190586746368, 15.72974639402197994, 49.37390960531436690 ) ) ;
#159797=CARTESIAN_POINT ( 'NONE',  ( 4.379528057220339221, -16.55341960407611168, 92.70724293864770971 ) ) ;
#159798=CARTESIAN_POINT ( 'NONE',  ( 16.46253265017160672, -9.564922557960803928, 63.33224293864769550 ) ) ;
#159799=CARTESIAN_POINT ( 'NONE',  ( -16.53943276465976808, 0.05219959533911058130, 106.2489096053143811 ) ) ;
#159800=CARTESIAN_POINT ( 'NONE',  ( 15.72974639402176855, 15.80617190586768217, 21.87609039468567573 ) ) ;
#159801=CARTESIAN_POINT ( 'NONE',  ( 18.62759615963255655, 10.81492255796105972, 71.66775706135234714 ) ) ;
#159802=CARTESIAN_POINT ( 'NONE',  ( -5.153800228976328057, -19.02544592524343514, 42.29057627198101699 ) ) ;
#159803=CARTESIAN_POINT ( 'NONE',  ( -0.05219959533934338120, 16.53943276465976808, 77.50109039468567573 ) ) ;
#159805=CARTESIAN_POINT ( 'NONE',  ( 18.62759615963255655, 10.81492255796105972, 21.66775706135235069 ) ) ;
#159807=CARTESIAN_POINT ( 'NONE',  ( -10.81492255796105439, 18.62759615963255655, 22.91775706135235069 ) ) ;
#159808=CARTESIAN_POINT ( 'NONE',  ( 9.474510206698729675, 16.51473224551082808, 57.08442372801900433 ) ) ;
#159809=CARTESIAN_POINT ( 'NONE',  ( -13.89961937509977652, 13.97604488694528158, 65.62390960531436690 ) ) ;
#159810=CARTESIAN_POINT ( 'NONE',  ( -5.153800228976607833, 19.02544592524334988, 37.70942372801899722 ) ) ;
#159811=CARTESIAN_POINT ( 'NONE',  ( 5.719274019375673035, 21.55341960407619339, 67.29275706135234714 ) ) ;
#159812=CARTESIAN_POINT ( 'NONE',  ( 0.05219959533907565091, 21.53943276465977519, 64.99890960531435269 ) ) ;
#159813=CARTESIAN_POINT ( 'NONE',  ( 12.14591786802309770, 12.06949235617756955, 49.37390960531436690 ) ) ;
#159814=CARTESIAN_POINT ( 'NONE',  ( -15.72974639402176322, -15.80617190586768395, 89.37609039468568994 ) ) ;
#159815=CARTESIAN_POINT ( 'NONE',  ( 13.97604488694548053, -13.89961937509957401, 35.62609039468567573 ) ) ;
#159816=CARTESIAN_POINT ( 'NONE',  ( 16.53943276465976808, -0.05219959533910856209, 68.74890960531435269 ) ) ;
#159817=CARTESIAN_POINT ( 'NONE',  ( -19.03943276465977164, 0.05219959533909376836, 21.24890960531436335 ) ) ;
#159818=CARTESIAN_POINT ( 'NONE',  ( -9.564922557961040184, 16.46253265017147172, 52.91775706135233293 ) ) ;
#159819=CARTESIAN_POINT ( 'NONE',  ( 12.06949235617757843, -12.14591786802309237, 23.12390960531436335 ) ) ;
#159820=CARTESIAN_POINT ( 'NONE',  ( -5.719274019375665041, -21.55341960407619695, 79.79275706135236135 ) ) ;
#159821=CARTESIAN_POINT ( 'NONE',  ( -0.05219959533909027116, -19.03943276465977164, 82.49890960531436690 ) ) ;
#159822=CARTESIAN_POINT ( 'NONE',  ( -9.564922557961040184, 16.46253265017147172, 52.91775706135233293 ) ) ;
#159823=CARTESIAN_POINT ( 'NONE',  ( 10.81492255796078972, 18.62759615963270932, 54.58224293864769550 ) ) ;
#159824=CARTESIAN_POINT ( 'NONE',  ( -18.67979575497193778, 10.72451020669871902, 48.33442372801902565 ) ) ;
#159825=CARTESIAN_POINT ( 'NONE',  ( 15.80617190586746368, 15.72974639402197994, 104.3739096053143669 ) ) ;
#159826=CARTESIAN_POINT ( 'NONE',  ( -19.05341960407617563, 5.049401038297882671, 98.54275706135233293 ) ) ;
#159827=CARTESIAN_POINT ( 'NONE',  ( 0.05219959533934541429, -16.53943276465976808, 70.00109039468568994 ) ) ;
#159829=CARTESIAN_POINT ( 'NONE',  ( -21.55341960407610458, -5.719274019375992779, 106.4572429386477097 ) ) ;
#159830=CARTESIAN_POINT ( 'NONE',  ( 0.05219959533910956823, 16.53943276465976808, 89.99890960531438111 ) ) ;
#159831=CARTESIAN_POINT ( 'NONE',  ( -17.50000000000002132, -4.658240926743158816, 31.05529582183199011 ) ) ;
#159832=CARTESIAN_POINT ( 'NONE',  ( 16.55341960407618274, -4.379528057220086978, 36.04275706135234714 ) ) ;
#159834=CARTESIAN_POINT ( 'NONE',  ( 0.05219959533907565091, 21.53943276465977519, 49.99890960531437401 ) ) ;
#159835=CARTESIAN_POINT ( 'NONE',  ( 16.53943276465976808, 0.05219959533934440121, 91.25109039468568994 ) ) ;
#159836=CARTESIAN_POINT ( 'NONE',  ( 13.97604488694527802, 13.89961937509977652, 34.37390960531436690 ) ) ;
#159837=CARTESIAN_POINT ( 'NONE',  ( 4.483927247898790824, -16.52544592524335698, 70.20942372801904696 ) ) ;
#159838=CARTESIAN_POINT ( 'NONE',  ( -18.62759615963255300, -10.81492255796106328, 39.16775706135235424 ) ) ;
#159840=CARTESIAN_POINT ( 'NONE',  ( -18.62759615963270932, 10.81492255796079327, 55.83224293864770260 ) ) ;
#159841=CARTESIAN_POINT ( 'NONE',  ( -4.379528057220086978, -16.55341960407618274, 89.79275706135236135 ) ) ;
#159842=CARTESIAN_POINT ( 'NONE',  ( 10.81492255796106328, -18.62759615963255655, 65.41775706135234714 ) ) ;
#159843=CARTESIAN_POINT ( 'NONE',  ( -15.80617190586745835, -15.72974639402198527, 56.87390960531436690 ) ) ;
#159844=CARTESIAN_POINT ( 'NONE',  ( -15.72974639402197994, 15.80617190586746368, 40.62390960531435269 ) ) ;
#159846=CARTESIAN_POINT ( 'NONE',  ( 14.29746914071037800, 8.314922557961029526, 61.66775706135235424 ) ) ;
#159847=CARTESIAN_POINT ( 'NONE',  ( -21.52544592524343514, 5.823673210054127303, 26.04057627198103475 ) ) ;
#159849=CARTESIAN_POINT ( 'NONE',  ( -19.03943276465977164, 0.05219959533909376836, 96.24890960531436690 ) ) ;
#159850=CARTESIAN_POINT ( 'NONE',  ( -4.483927247898782831, 16.52544592524335698, 112.7094237280190328 ) ) ;
#159852=CARTESIAN_POINT ( 'NONE',  ( 4.379528057220339221, -16.55341960407611168, 107.7072429386476955 ) ) ;
#159853=CARTESIAN_POINT ( 'NONE',  ( 18.62759615963271287, -10.81492255796078972, 58.33224293864768839 ) ) ;
#159854=CARTESIAN_POINT ( 'NONE',  ( 5.153800228976335163, 19.02544592524342804, 39.79057627198100988 ) ) ;
#159855=CARTESIAN_POINT ( 'NONE',  ( 14.34966873604972726, -8.224510206698740333, 90.83442372801901854 ) ) ;
#159856=CARTESIAN_POINT ( 'NONE',  ( -15.80617190586768217, 15.72974639402176855, 38.12609039468567573 ) ) ;
#159857=CARTESIAN_POINT ( 'NONE',  ( -19.05341960407617563, 5.049401038297882671, 103.5427570613523329 ) ) ;
#159858=CARTESIAN_POINT ( 'NONE',  ( -16.55341960407611168, -4.379528057220339221, 101.4572429386476955 ) ) ;
#159859=CARTESIAN_POINT ( 'NONE',  ( 16.46253265017160672, -9.564922557960803928, 48.33224293864769550 ) ) ;
#159861=CARTESIAN_POINT ( 'NONE',  ( -16.51473224551069308, -9.474510206698971260, 21.66557627198102765 ) ) ;
#159863=CARTESIAN_POINT ( 'NONE',  ( -5.153800228976328057, -19.02544592524343514, 77.29057627198099567 ) ) ;
#159864=CARTESIAN_POINT ( 'NONE',  ( -14.34966873604972548, 8.224510206698743886, 73.33442372801901854 ) ) ;
#159865=CARTESIAN_POINT ( 'NONE',  ( 21.52544592524334988, 5.823673210054432836, 106.4594237280190328 ) ) ;
#159866=CARTESIAN_POINT ( 'NONE',  ( 10.81492255796078972, 18.62759615963270932, 54.58224293864769550 ) ) ;
#159867=CARTESIAN_POINT ( 'NONE',  ( -4.483927247898782831, 16.52544592524335698, 77.70942372801900433 ) ) ;
#159868=CARTESIAN_POINT ( 'NONE',  ( 9.474510206698729675, 16.51473224551082808, 67.08442372801900433 ) ) ;
#159870=CARTESIAN_POINT ( 'NONE',  ( -10.72451020669870658, -18.67979575497194134, 59.58442372801901854 ) ) ;
#159871=CARTESIAN_POINT ( 'NONE',  ( 5.049401038298161559, -19.05341960407611168, 77.70724293864765286 ) ) ;
#159872=VECTOR ( 'NONE', #139878, 1000.000000000000000 ) ;
#159873=CARTESIAN_POINT ( 'NONE',  ( -5.153800228976328057, -19.02544592524343514, 37.29057627198102409 ) ) ;
#159874=CARTESIAN_POINT ( 'NONE',  ( -5.153800228976607833, 19.02544592524334988, 57.70942372801899012 ) ) ;
#159875=CARTESIAN_POINT ( 'NONE',  ( -19.02544592524342804, 5.153800228976336051, 111.0405762719810099 ) ) ;
#159876=CARTESIAN_POINT ( 'NONE',  ( 13.89961937509977652, -13.97604488694527269, 93.12390960531436690 ) ) ;
#159877=CARTESIAN_POINT ( 'NONE',  ( 0.05219959533910956823, 16.53943276465976808, 44.99890960531435979 ) ) ;
#159878=CARTESIAN_POINT ( 'NONE',  ( -18.62759615963270932, 10.81492255796079327, 50.83224293864770971 ) ) ;
#159881=CARTESIAN_POINT ( 'NONE',  ( 15.80617190586746368, 15.72974639402197994, 69.37390960531436690 ) ) ;
#159882=CARTESIAN_POINT ( 'NONE',  ( -19.03943276465977164, -0.05219959533935918106, 28.75109039468566507 ) ) ;
#159883=CARTESIAN_POINT ( 'NONE',  ( -17.40861289039004944, -6.110651285853239578, 81.37232470827431996 ) ) ;
#159884=CARTESIAN_POINT ( 'NONE',  ( -5.049401038298153566, 19.05341960407611168, 45.20724293864769550 ) ) ;
#159885=CARTESIAN_POINT ( 'NONE',  ( -16.55341960407617563, 4.379528057220093196, 33.54275706135234714 ) ) ;
#159888=CARTESIAN_POINT ( 'NONE',  ( 16.55341960407618274, -4.379528057220086978, 76.04275706135237556 ) ) ;
#159889=CARTESIAN_POINT ( 'NONE',  ( 18.67979575497178502, 10.72451020669898547, 99.16557627198100988 ) ) ;
#159890=CARTESIAN_POINT ( 'NONE',  ( -19.03943276465977164, 0.05219959533909376836, 36.24890960531436690 ) ) ;
#159892=CARTESIAN_POINT ( 'NONE',  ( 10.72451020669871369, 18.67979575497193778, 42.08442372801901854 ) ) ;
#159893=CARTESIAN_POINT ( 'NONE',  ( 16.51473224551083163, -9.474510206698727899, 50.83442372801899722 ) ) ;
#159894=CARTESIAN_POINT ( 'NONE',  ( 19.03943276465977164, -0.05219959533909143690, 48.74890960531435979 ) ) ;
#159895=CARTESIAN_POINT ( 'NONE',  ( 21.53943276465977519, 0.05219959533937863772, 91.25109039468568994 ) ) ;
#159896=CARTESIAN_POINT ( 'NONE',  ( 16.36317988757059894, 7.306389748694943620, 98.40210391636779264 ) ) ;
#159897=CARTESIAN_POINT ( 'NONE',  ( 0.05219959533910956823, 16.53943276465976808, 44.99890960531435979 ) ) ;
#159899=CARTESIAN_POINT ( 'NONE',  ( 10.81492255796078972, 18.62759615963270932, 49.58224293864769550 ) ) ;
#159902=CARTESIAN_POINT ( 'NONE',  ( -19.03943276465977164, 0.05219959533909376836, 101.2489096053143669 ) ) ;
#159903=CARTESIAN_POINT ( 'NONE',  ( -4.483927247898539470, -16.52544592524342804, 102.2905762719810383 ) ) ;
#159904=CARTESIAN_POINT ( 'NONE',  ( 14.29746914071037800, 8.314922557961029526, 26.66775706135235424 ) ) ;
#159905=CARTESIAN_POINT ( 'NONE',  ( -16.52544592524335698, -4.483927247898792601, 108.9594237280190185 ) ) ;
#159906=ORIENTED_EDGE ( 'NONE', *, *, #147658, .T. ) ;
#159907=CARTESIAN_POINT ( 'NONE',  ( 16.46253265017160672, -9.564922557960803928, 103.3322429386476955 ) ) ;
#159908=CARTESIAN_POINT ( 'NONE',  ( -5.719274019375978568, 21.55341960407610458, 100.2072429386476955 ) ) ;
#159909=CARTESIAN_POINT ( 'NONE',  ( -12.06949235617756955, 12.14591786802309770, 25.62390960531435624 ) ) ;
#159910=CARTESIAN_POINT ( 'NONE',  ( -9.474510206698964154, 16.51473224551069663, 105.4155762719810383 ) ) ;
#159911=CARTESIAN_POINT ( 'NONE',  ( 16.46253265017146816, 9.564922557961045513, 96.66775706135233293 ) ) ;
#159912=CARTESIAN_POINT ( 'NONE',  ( -18.62759615963255300, -10.81492255796106328, 109.1677570613523613 ) ) ;
#159913=CARTESIAN_POINT ( 'NONE',  ( -10.72451020669898014, 18.67979575497178502, 95.41557627198102409 ) ) ;
#159914=CARTESIAN_POINT ( 'NONE',  ( -18.62759615963270932, 10.81492255796079327, 45.83224293864769550 ) ) ;
#159915=CARTESIAN_POINT ( 'NONE',  ( 16.46253265017160672, -9.564922557960803928, 58.33224293864769550 ) ) ;
#159916=CARTESIAN_POINT ( 'NONE',  ( -12.06949235617756955, 12.14591786802309770, 30.62390960531436335 ) ) ;
#159917=CARTESIAN_POINT ( 'NONE',  ( 19.02544592524343514, -5.153800228976328945, 83.54057627198100988 ) ) ;
#159918=ORIENTED_EDGE ( 'NONE', *, *, #62342, .F. ) ;
#159919=CARTESIAN_POINT ( 'NONE',  ( 19.46398650005386699, -5.500000000000144773, 62.68269651486372851 ) ) ;
#159920=CARTESIAN_POINT ( 'NONE',  ( -0.05219959533936034679, 19.03943276465977164, 37.50109039468567573 ) ) ;
#159921=CARTESIAN_POINT ( 'NONE',  ( 5.823673210054125526, 21.52544592524343514, 79.79057627198102409 ) ) ;
#159922=CARTESIAN_POINT ( 'NONE',  ( -8.314922557960811034, -14.29746914071050412, 82.08224293864768129 ) ) ;
#159923=CARTESIAN_POINT ( 'NONE',  ( -10.72451020669870658, -18.67979575497194134, 34.58442372801900433 ) ) ;
#159925=CARTESIAN_POINT ( 'NONE',  ( -4.483927247898782831, 16.52544592524335698, 107.7094237280190328 ) ) ;
#159926=CARTESIAN_POINT ( 'NONE',  ( 16.52544592524342804, -4.483927247898539470, 113.5405762719810383 ) ) ;
#159927=CARTESIAN_POINT ( 'NONE',  ( 5.049401038298161559, -19.05341960407611168, 87.70724293864769550 ) ) ;
#159928=CARTESIAN_POINT ( 'NONE',  ( 18.10062525802553779, -5.500000000000023093, 71.01383468041922242 ) ) ;
#159930=CARTESIAN_POINT ( 'NONE',  ( 16.55341960407611168, 4.379528057220329451, 43.95724293864769550 ) ) ;
#159931=CARTESIAN_POINT ( 'NONE',  ( 21.52544592524334988, 5.823673210054432836, 56.45942372801902565 ) ) ;
#159933=CARTESIAN_POINT ( 'NONE',  ( -0.05219959533909027116, -19.03943276465977164, 47.49890960531435979 ) ) ;
#159934=CARTESIAN_POINT ( 'NONE',  ( -5.153800228976328057, -19.02544592524343514, 47.29057627198102409 ) ) ;
#159936=CARTESIAN_POINT ( 'NONE',  ( 15.72974639402176855, 15.80617190586768217, 111.8760903946856615 ) ) ;
#159937=CARTESIAN_POINT ( 'NONE',  ( 8.314922557961029526, -14.29746914071037800, 65.41775706135234714 ) ) ;
#159938=CARTESIAN_POINT ( 'NONE',  ( 5.823673210054444382, -21.52544592524334988, 90.20942372801903275 ) ) ;
#159939=CARTESIAN_POINT ( 'NONE',  ( -19.02544592524342804, 5.153800228976336051, 111.0405762719810099 ) ) ;
#159940=CARTESIAN_POINT ( 'NONE',  ( 9.474510206698729675, 16.51473224551082808, 92.08442372801900433 ) ) ;
#159941=CARTESIAN_POINT ( 'NONE',  ( 21.53943276465977519, 0.05219959533937863772, 71.25109039468568994 ) ) ;
#159942=CARTESIAN_POINT ( 'NONE',  ( 12.06949235617739724, 12.14591786802326823, 36.87609039468568994 ) ) ;
#159943=CARTESIAN_POINT ( 'NONE',  ( -18.67979575497178146, -10.72451020669898902, 86.66557627198102409 ) ) ;
#159944=CARTESIAN_POINT ( 'NONE',  ( -19.03943276465977164, -0.05219959533935918106, 93.75109039468566152 ) ) ;
#159945=CARTESIAN_POINT ( 'NONE',  ( -9.474510206698964154, 16.51473224551069663, 65.41557627198102409 ) ) ;
#159946=CARTESIAN_POINT ( 'NONE',  ( -4.379528057220086978, -16.55341960407618274, 19.79275706135235069 ) ) ;
#159947=CARTESIAN_POINT ( 'NONE',  ( 16.46253265017146816, 9.564922557961045513, 106.6677570613523471 ) ) ;
#159948=CARTESIAN_POINT ( 'NONE',  ( -14.29746914071049879, 8.314922557960819915, 55.83224293864770260 ) ) ;
#159949=CARTESIAN_POINT ( 'NONE',  ( -9.474510206698720793, -16.51473224551083518, 79.58442372801899012 ) ) ;
#159950=CARTESIAN_POINT ( 'NONE',  ( -4.483927247898782831, 16.52544592524335698, 62.70942372801902565 ) ) ;
#159951=CARTESIAN_POINT ( 'NONE',  ( -5.719274019375665041, -21.55341960407619695, 19.79275706135235069 ) ) ;
#159952=CARTESIAN_POINT ( 'NONE',  ( -19.02544592524342804, 5.153800228976336051, 41.04057627198103120 ) ) ;
#159953=CARTESIAN_POINT ( 'NONE',  ( -9.474510206698964154, 16.51473224551069663, 50.41557627198102409 ) ) ;
#159954=CARTESIAN_POINT ( 'NONE',  ( 4.483927247898790824, -16.52544592524335698, 65.20942372801901854 ) ) ;
#159958=CARTESIAN_POINT ( 'NONE',  ( 5.153800228976335163, 19.02544592524342804, 104.7905762719809957 ) ) ;
#159961=CARTESIAN_POINT ( 'NONE',  ( 16.53943276465976808, 0.05219959533934440121, 21.25109039468567218 ) ) ;
#159962=CARTESIAN_POINT ( 'NONE',  ( 10.72451020669898902, -18.67979575497178502, 42.91557627198103120 ) ) ;
#159963=CARTESIAN_POINT ( 'NONE',  ( -5.153800228976607833, 19.02544592524334988, 42.70942372801901143 ) ) ;
#159964=CARTESIAN_POINT ( 'NONE',  ( -4.483927247898782831, 16.52544592524335698, 32.70942372801900433 ) ) ;
#159965=CARTESIAN_POINT ( 'NONE',  ( -13.89961937509977652, 13.97604488694528158, 25.62390960531434558 ) ) ;
#159966=CARTESIAN_POINT ( 'NONE',  ( -9.564922557960796823, -16.46253265017161027, 57.08224293864769550 ) ) ;
#159967=CARTESIAN_POINT ( 'NONE',  ( -21.55341960407610458, -5.719274019375992779, 91.45724293864769550 ) ) ;
#159968=CARTESIAN_POINT ( 'NONE',  ( -9.474510206698964154, 16.51473224551069663, 115.4155762719810241 ) ) ;
#159969=CARTESIAN_POINT ( 'NONE',  ( -16.46253265017160317, 9.564922557960807481, 50.83224293864770260 ) ) ;
#159971=CARTESIAN_POINT ( 'NONE',  ( -13.97604488694547697, 13.89961937509957934, 78.12609039468567573 ) ) ;
#159972=CARTESIAN_POINT ( 'NONE',  ( 16.52544592524342804, -4.483927247898539470, 68.54057627198103830 ) ) ;
#159973=CARTESIAN_POINT ( 'NONE',  ( -10.81492255796105439, 18.62759615963255655, 107.9177570613523471 ) ) ;
#159974=CARTESIAN_POINT ( 'NONE',  ( -21.53943276465977519, 0.05219959533907696930, 101.2489096053143669 ) ) ;
#159975=CARTESIAN_POINT ( 'NONE',  ( 0.05219959533937995610, -21.53943276465977519, 80.00109039468568994 ) ) ;
#159976=CARTESIAN_POINT ( 'NONE',  ( -19.02544592524342804, 5.153800228976336051, 31.04057627198102409 ) ) ;
#159977=CARTESIAN_POINT ( 'NONE',  ( 18.62759615963255655, 10.81492255796105972, 71.66775706135234714 ) ) ;
#159978=CARTESIAN_POINT ( 'NONE',  ( 19.03943276465977164, -0.05219959533909143690, 108.7489096053143527 ) ) ;
#159979=CARTESIAN_POINT ( 'NONE',  ( 0.05219959533934541429, -16.53943276465976808, 100.0010903946857042 ) ) ;
#159980=CARTESIAN_POINT ( 'NONE',  ( -18.67979575497193778, 10.72451020669871902, 78.33442372801901854 ) ) ;
#159981=CARTESIAN_POINT ( 'NONE',  ( 16.46253265017160672, -9.564922557960803928, 63.33224293864769550 ) ) ;
#159982=CARTESIAN_POINT ( 'NONE',  ( 15.72974639402176855, 15.80617190586768217, 41.87609039468568284 ) ) ;
#159983=CARTESIAN_POINT ( 'NONE',  ( 16.51473224551069308, 9.474510206698969483, 84.16557627198102409 ) ) ;
#159984=CARTESIAN_POINT ( 'NONE',  ( -16.55341960407611168, -4.379528057220339221, 91.45724293864769550 ) ) ;
#159985=CARTESIAN_POINT ( 'NONE',  ( -4.379528057220328563, 16.55341960407611168, 55.20724293864770260 ) ) ;
#159986=CARTESIAN_POINT ( 'NONE',  ( 0.05219959533907565091, 21.53943276465977519, 64.99890960531435269 ) ) ;
#159987=CARTESIAN_POINT ( 'NONE',  ( -19.02544592524342804, 5.153800228976336051, 66.04057627198103830 ) ) ;
#159988=CARTESIAN_POINT ( 'NONE',  ( 21.52544592524344225, -5.823673210054117533, 73.54057627198102409 ) ) ;
#159990=CARTESIAN_POINT ( 'NONE',  ( 0.05219959533936267826, -19.03943276465977164, 65.00109039468567573 ) ) ;
#159991=CARTESIAN_POINT ( 'NONE',  ( -18.56399227203342761, -5.499999999999929834, 88.97830131249907026 ) ) ;
#159992=CARTESIAN_POINT ( 'NONE',  ( 0.05219959533910956823, 16.53943276465976808, 79.99890960531435269 ) ) ;
#159993=CARTESIAN_POINT ( 'NONE',  ( 21.52544592524344225, -5.823673210054117533, 58.54057627198103120 ) ) ;
#159995=CARTESIAN_POINT ( 'NONE',  ( -8.224510206698735004, -14.34966873604973081, 99.58442372801900433 ) ) ;
#159997=CARTESIAN_POINT ( 'NONE',  ( -16.51473224551082808, 9.474510206698731452, 103.3344237280190043 ) ) ;
#159998=CARTESIAN_POINT ( 'NONE',  ( 16.52544592524342804, -4.483927247898539470, 68.54057627198103830 ) ) ;
#159999=CARTESIAN_POINT ( 'NONE',  ( -17.50000000000004263, 4.049696124445827827, 34.18039670665945806 ) ) ;
#160000=CARTESIAN_POINT ( 'NONE',  ( -19.03943276465977164, 0.05219959533909376836, 66.24890960531436690 ) ) ;
#160001=CARTESIAN_POINT ( 'NONE',  ( -16.53943276465976808, 0.05219959533911058130, 51.24890960531436690 ) ) ;
#160002=CARTESIAN_POINT ( 'NONE',  ( 19.02544592524343514, -5.153800228976328945, 88.54057627198102409 ) ) ;
#160003=CARTESIAN_POINT ( 'NONE',  ( 19.02544592524334988, 5.153800228976608722, 71.45942372801900433 ) ) ;
#160004=CARTESIAN_POINT ( 'NONE',  ( 5.153800228976335163, 19.02544592524342804, 69.79057627198103830 ) ) ;
#160005=CARTESIAN_POINT ( 'NONE',  ( 5.049401038298161559, -19.05341960407611168, 87.70724293864769550 ) ) ;
#160006=CARTESIAN_POINT ( 'NONE',  ( 16.46253265017160672, -9.564922557960803928, 73.33224293864769550 ) ) ;
#160007=CARTESIAN_POINT ( 'NONE',  ( 21.53943276465977519, -0.05219959533907433946, 63.74890960531435979 ) ) ;
#160008=CARTESIAN_POINT ( 'NONE',  ( 12.14591786802327356, -12.06949235617739191, 60.62609039468567573 ) ) ;
#160010=CARTESIAN_POINT ( 'NONE',  ( 5.049401038298161559, -19.05341960407611168, 42.70724293864767418 ) ) ;
#160011=CARTESIAN_POINT ( 'NONE',  ( -18.62759615963270932, 10.81492255796079327, 55.83224293864770260 ) ) ;
#160012=CARTESIAN_POINT ( 'NONE',  ( -9.564922557961040184, 16.46253265017147172, 87.91775706135233293 ) ) ;
#160013=CARTESIAN_POINT ( 'NONE',  ( 8.224510206698953496, -14.34966873604960469, 27.91557627198103830 ) ) ;
#160014=CARTESIAN_POINT ( 'NONE',  ( -15.72974639402176322, -15.80617190586768395, 29.37609039468568284 ) ) ;
#160015=CARTESIAN_POINT ( 'NONE',  ( 9.474510206698729675, 16.51473224551082808, 37.08442372801899722 ) ) ;
#160016=CARTESIAN_POINT ( 'NONE',  ( -12.14591786802326823, 12.06949235617739902, 63.12609039468568994 ) ) ;
#160017=CARTESIAN_POINT ( 'NONE',  ( 8.314922557961029526, -14.29746914071037800, 95.41775706135234714 ) ) ;
#160019=CARTESIAN_POINT ( 'NONE',  ( -0.05219959533934338120, 16.53943276465976808, 87.50109039468568994 ) ) ;
#160020=CARTESIAN_POINT ( 'NONE',  ( 0.05219959533907565091, 21.53943276465977519, 29.99890960531435979 ) ) ;
#160021=CARTESIAN_POINT ( 'NONE',  ( -12.14591786802326823, 12.06949235617739902, 33.12609039468569705 ) ) ;
#160022=CARTESIAN_POINT ( 'NONE',  ( -19.03943276465977164, 0.05219959533909376836, 51.24890960531436690 ) ) ;
#160023=CARTESIAN_POINT ( 'NONE',  ( 16.51473224551069308, 9.474510206698969483, 54.16557627198103120 ) ) ;
#160024=CARTESIAN_POINT ( 'NONE',  ( -13.89961937509977652, 13.97604488694528158, 65.62390960531436690 ) ) ;
#160025=CARTESIAN_POINT ( 'NONE',  ( 10.72451020669871369, 18.67979575497193778, 42.08442372801901854 ) ) ;
#160026=CARTESIAN_POINT ( 'NONE',  ( -12.06949235617739369, -12.14591786802326823, 44.37609039468567573 ) ) ;
#160027=CARTESIAN_POINT ( 'NONE',  ( -14.34966873604960291, -8.224510206698953496, 21.66557627198102409 ) ) ;
#160028=CARTESIAN_POINT ( 'NONE',  ( -5.049401038298153566, 19.05341960407611168, 25.20724293864768484 ) ) ;
#160029=CARTESIAN_POINT ( 'NONE',  ( 18.67979575497194134, -10.72451020669871369, 110.8344237280190043 ) ) ;
#160030=CARTESIAN_POINT ( 'NONE',  ( 12.14591786802327356, -12.06949235617739191, 20.62609039468568639 ) ) ;
#160031=CARTESIAN_POINT ( 'NONE',  ( 19.02544592524334988, 5.153800228976608722, 71.45942372801900433 ) ) ;
#160032=CARTESIAN_POINT ( 'NONE',  ( 14.29746914071049879, -8.314922557960816363, 68.33224293864769550 ) ) ;
#160033=CARTESIAN_POINT ( 'NONE',  ( 19.03943276465977164, -0.05219959533909143690, 43.74890960531435979 ) ) ;
#160034=CARTESIAN_POINT ( 'NONE',  ( -19.03943276465977164, -0.05219959533935918106, 78.75109039468567573 ) ) ;
#160035=CARTESIAN_POINT ( 'NONE',  ( 17.12812012977027010, -6.668231424565981058, 91.14051240676852217 ) ) ;
#160036=CARTESIAN_POINT ( 'NONE',  ( 15.80617190586769283, -15.72974639402175789, 80.62609039468567573 ) ) ;
#160037=CARTESIAN_POINT ( 'NONE',  ( -14.34966873604972548, 8.224510206698743886, 38.33442372801900433 ) ) ;
#160038=CARTESIAN_POINT ( 'NONE',  ( 17.40861289039003879, 6.110651285853278658, 38.87232470827432707 ) ) ;
#160039=CARTESIAN_POINT ( 'NONE',  ( -21.53943276465977519, 0.05219959533907696930, 36.24890960531435979 ) ) ;
#160040=CARTESIAN_POINT ( 'NONE',  ( 8.314922557961029526, -14.29746914071037800, 30.41775706135234358 ) ) ;
#160041=CARTESIAN_POINT ( 'NONE',  ( -16.51473224551069308, -9.474510206698971260, 21.66557627198102765 ) ) ;
#160042=CARTESIAN_POINT ( 'NONE',  ( 15.72974639402176855, 15.80617190586768217, 106.8760903946856899 ) ) ;
#160044=CARTESIAN_POINT ( 'NONE',  ( 16.46253265017160672, -9.564922557960803928, 38.33224293864768839 ) ) ;
#160046=CARTESIAN_POINT ( 'NONE',  ( -9.474510206698964154, 16.51473224551069663, 55.41557627198103120 ) ) ;
#160047=CARTESIAN_POINT ( 'NONE',  ( -15.80617190586768217, 15.72974639402176855, 68.12609039468567573 ) ) ;
#160048=CARTESIAN_POINT ( 'NONE',  ( 9.564922557961047289, -16.46253265017146816, 25.41775706135234003 ) ) ;
#160049=CARTESIAN_POINT ( 'NONE',  ( -0.05219959533910754901, -16.53943276465976808, 27.49890960531435269 ) ) ;
#160050=CARTESIAN_POINT ( 'NONE',  ( 19.03943276465977164, -0.05219959533909143690, 33.74890960531435979 ) ) ;
#160052=CARTESIAN_POINT ( 'NONE',  ( 16.46253265017160672, -9.564922557960803928, 98.33224293864769550 ) ) ;
#160053=CARTESIAN_POINT ( 'NONE',  ( 21.53943276465977519, 0.05219959533937863772, 66.25109039468567573 ) ) ;
#160054=CARTESIAN_POINT ( 'NONE',  ( 9.474510206698971260, -16.51473224551069308, 42.91557627198103120 ) ) ;
#160055=CARTESIAN_POINT ( 'NONE',  ( 21.52544592524334988, 5.823673210054432836, 66.45942372801903275 ) ) ;
#160056=CARTESIAN_POINT ( 'NONE',  ( 5.049401038297881783, 19.05341960407617563, 97.29275706135233293 ) ) ;
#160057=CARTESIAN_POINT ( 'NONE',  ( -13.89961937509977652, 13.97604488694528158, 100.6239096053143669 ) ) ;
#160058=CARTESIAN_POINT ( 'NONE',  ( 5.153800228976335163, 19.02544592524342804, 39.79057627198100988 ) ) ;
#160059=CARTESIAN_POINT ( 'NONE',  ( -0.05219959533907301413, -21.53943276465977519, 112.4989096053143669 ) ) ;
#160060=CARTESIAN_POINT ( 'NONE',  ( 0.05219959533936267826, -19.03943276465977164, 40.00109039468566152 ) ) ;
#160061=CARTESIAN_POINT ( 'NONE',  ( 16.53943276465976808, -0.05219959533910856209, 113.7489096053143527 ) ) ;
#160062=CARTESIAN_POINT ( 'NONE',  ( 19.02544592524343514, -5.153800228976328945, 63.54057627198103830 ) ) ;
#160063=CARTESIAN_POINT ( 'NONE',  ( 9.564922557961047289, -16.46253265017146816, 100.4177570613523329 ) ) ;
#160064=CARTESIAN_POINT ( 'NONE',  ( 4.379528057220339221, -16.55341960407611168, 57.70724293864770260 ) ) ;
#160065=CARTESIAN_POINT ( 'NONE',  ( 18.62759615963271287, -10.81492255796078972, 23.33224293864769194 ) ) ;
#160066=CARTESIAN_POINT ( 'NONE',  ( -13.89961937509957401, -13.97604488694547875, 84.37609039468567573 ) ) ;
#160067=CARTESIAN_POINT ( 'NONE',  ( -15.80617190586745835, -15.72974639402198527, 96.87390960531436690 ) ) ;
#160068=CARTESIAN_POINT ( 'NONE',  ( -21.52544592524334988, -5.823673210054445271, 43.95942372801902565 ) ) ;
#160069=CARTESIAN_POINT ( 'NONE',  ( 14.29746914071037800, 8.314922557961029526, 41.66775706135235424 ) ) ;
#160070=CARTESIAN_POINT ( 'NONE',  ( 4.483927247898790824, -16.52544592524335698, 40.20942372801901854 ) ) ;
#160071=CARTESIAN_POINT ( 'NONE',  ( 15.72974639402176855, 15.80617190586768217, 51.87609039468568284 ) ) ;
#160072=CARTESIAN_POINT ( 'NONE',  ( -21.52544592524343514, 5.823673210054127303, 56.04057627198102409 ) ) ;
#160073=CARTESIAN_POINT ( 'NONE',  ( 0.05219959533909260263, 19.03943276465977164, 39.99890960531436690 ) ) ;
#160075=CARTESIAN_POINT ( 'NONE',  ( -16.53943276465976808, -0.05219959533934237506, 78.75109039468568994 ) ) ;
#160076=CARTESIAN_POINT ( 'NONE',  ( -21.53943276465977519, 0.05219959533907696930, 106.2489096053143811 ) ) ;
#160077=CARTESIAN_POINT ( 'NONE',  ( 14.29746914071049879, -8.314922557960816363, 38.33224293864768839 ) ) ;
#160078=CARTESIAN_POINT ( 'NONE',  ( -12.14591786802326823, 12.06949235617739902, 68.12609039468567573 ) ) ;
#160079=CARTESIAN_POINT ( 'NONE',  ( -16.46253265017146816, -9.564922557961047289, 94.16775706135233293 ) ) ;
#160080=CARTESIAN_POINT ( 'NONE',  ( 15.80617190586746368, 15.72974639402197994, 104.3739096053143669 ) ) ;
#160081=CARTESIAN_POINT ( 'NONE',  ( -16.55341960407611168, -4.379528057220339221, 26.45724293864768839 ) ) ;
#160084=CARTESIAN_POINT ( 'NONE',  ( -14.34966873604972548, 8.224510206698743886, 78.33442372801901854 ) ) ;
#160085=CARTESIAN_POINT ( 'NONE',  ( 19.26498983726236602, -5.499999999999790390, 93.05319577422004329 ) ) ;
#160086=CARTESIAN_POINT ( 'NONE',  ( 21.53943276465977519, -0.05219959533907433946, 73.74890960531433848 ) ) ;
#160087=CARTESIAN_POINT ( 'NONE',  ( 8.224510206698742110, 14.34966873604972548, 107.0844237280190043 ) ) ;
#160089=CARTESIAN_POINT ( 'NONE',  ( -17.26172910966778318, -6.454744622555873335, 54.19353091350776452 ) ) ;
#160090=CARTESIAN_POINT ( 'NONE',  ( 18.62759615963271287, -10.81492255796078972, 98.33224293864769550 ) ) ;
#160092=CARTESIAN_POINT ( 'NONE',  ( -5.823673210054116645, -21.52544592524344225, 107.2905762719810525 ) ) ;
#160093=CARTESIAN_POINT ( 'NONE',  ( -12.06949235617756955, 12.14591786802309770, 35.62390960531437401 ) ) ;
#160094=CARTESIAN_POINT ( 'NONE',  ( -0.05219959533934338120, 16.53943276465976808, 42.50109039468567573 ) ) ;
#160095=CARTESIAN_POINT ( 'NONE',  ( 16.46253265017160672, -9.564922557960803928, 43.33224293864769550 ) ) ;
#160096=CARTESIAN_POINT ( 'NONE',  ( 16.46253265017160672, -9.564922557960803928, 63.33224293864769550 ) ) ;
#160097=CARTESIAN_POINT ( 'NONE',  ( -16.51473224551069308, -9.474510206698971260, 111.6655762719810383 ) ) ;
#160099=CARTESIAN_POINT ( 'NONE',  ( 0.05219959533936267826, -19.03943276465977164, 100.0010903946856757 ) ) ;
#160100=CARTESIAN_POINT ( 'NONE',  ( 16.51473224551083163, -9.474510206698727899, 50.83442372801899722 ) ) ;
#160101=CARTESIAN_POINT ( 'NONE',  ( 15.72974639402199770, -15.80617190586745480, 93.12390960531436690 ) ) ;
#160102=CARTESIAN_POINT ( 'NONE',  ( 12.14591786802309770, 12.06949235617756955, 24.37390960531435979 ) ) ;
#160103=CARTESIAN_POINT ( 'NONE',  ( 16.51473224551069308, 9.474510206698969483, 79.16557627198103830 ) ) ;
#160104=CARTESIAN_POINT ( 'NONE',  ( -5.823673210054116645, -21.52544592524344225, 52.29057627198102409 ) ) ;
#160105=CARTESIAN_POINT ( 'NONE',  ( 18.62759615963271287, -10.81492255796078972, 88.33224293864769550 ) ) ;
#160106=CARTESIAN_POINT ( 'NONE',  ( -4.379528057220086978, -16.55341960407618274, 24.79275706135235779 ) ) ;
#160107=CARTESIAN_POINT ( 'NONE',  ( 18.62759615963271287, -10.81492255796078972, 23.33224293864769194 ) ) ;
#160108=CARTESIAN_POINT ( 'NONE',  ( -5.719274019375665041, -21.55341960407619695, 69.79275706135234714 ) ) ;
#160109=CARTESIAN_POINT ( 'NONE',  ( 19.05341960407611168, 5.049401038298154454, 78.95724293864769550 ) ) ;
#160110=CARTESIAN_POINT ( 'NONE',  ( 9.474510206698971260, -16.51473224551069308, 32.91557627198102409 ) ) ;
#160111=CARTESIAN_POINT ( 'NONE',  ( -13.89961937509977652, 13.97604488694528158, 75.62390960531438111 ) ) ;
#160112=CARTESIAN_POINT ( 'NONE',  ( -14.34966873604960291, -8.224510206698953496, 96.66557627198102409 ) ) ;
#160113=ORIENTED_EDGE ( 'NONE', *, *, #178569, .F. ) ;
#160114=CARTESIAN_POINT ( 'NONE',  ( -19.03943276465977164, -0.05219959533935918106, 98.75109039468567573 ) ) ;
#160117=CARTESIAN_POINT ( 'NONE',  ( -5.153800228976328057, -19.02544592524343514, 77.29057627198099567 ) ) ;
#160118=CARTESIAN_POINT ( 'NONE',  ( 10.81492255796106328, -18.62759615963255655, 80.41775706135234714 ) ) ;
#160119=CARTESIAN_POINT ( 'NONE',  ( 13.89961937509977652, -13.97604488694527269, 103.1239096053143527 ) ) ;
#160120=CARTESIAN_POINT ( 'NONE',  ( -16.53943276465976808, -0.05219959533934237506, 78.75109039468568994 ) ) ;
#160122=CARTESIAN_POINT ( 'NONE',  ( 9.474510206698729675, 16.51473224551082808, 57.08442372801900433 ) ) ;
#160123=CARTESIAN_POINT ( 'NONE',  ( 0.05219959533937995610, -21.53943276465977519, 110.0010903946856757 ) ) ;
#160125=CARTESIAN_POINT ( 'NONE',  ( 16.62544781628812274, 7.153289815129877383, 22.00000000000000000 ) ) ;
#160127=CARTESIAN_POINT ( 'NONE',  ( -8.314922557960811034, -14.29746914071050412, 27.08224293864769550 ) ) ;
#160129=CARTESIAN_POINT ( 'NONE',  ( -4.379528057220086978, -16.55341960407618274, 109.7927570613523613 ) ) ;
#160130=CARTESIAN_POINT ( 'NONE',  ( 17.31747979337950127, 6.344076630961018815, 68.87944868065181936 ) ) ;
#160131=CARTESIAN_POINT ( 'NONE',  ( 12.06949235617739724, 12.14591786802326823, 81.87609039468568994 ) ) ;
#160132=CARTESIAN_POINT ( 'NONE',  ( 5.719274019375673035, 21.55341960407619339, 77.29275706135234714 ) ) ;
#160133=CARTESIAN_POINT ( 'NONE',  ( -9.474510206698720793, -16.51473224551083518, 99.58442372801900433 ) ) ;
#160134=CARTESIAN_POINT ( 'NONE',  ( -21.52544592524334988, -5.823673210054445271, 63.95942372801901854 ) ) ;
#160135=CARTESIAN_POINT ( 'NONE',  ( -19.03943276465977164, -0.05219959533935918106, 38.75109039468566152 ) ) ;
#160136=CARTESIAN_POINT ( 'NONE',  ( -5.049401038298153566, 19.05341960407611168, 75.20724293864769550 ) ) ;
#160137=CARTESIAN_POINT ( 'NONE',  ( -9.474510206698964154, 16.51473224551069663, 60.41557627198102409 ) ) ;
#160138=CARTESIAN_POINT ( 'NONE',  ( 18.10062525802546674, -5.499999999999985789, 41.01383468041921532 ) ) ;
#160139=CARTESIAN_POINT ( 'NONE',  ( -21.55341960407610458, -5.719274019375992779, 91.45724293864769550 ) ) ;
#160140=CARTESIAN_POINT ( 'NONE',  ( -10.81492255796078084, -18.62759615963271287, 47.08224293864770260 ) ) ;
#160141=CARTESIAN_POINT ( 'NONE',  ( -13.89961937509977652, 13.97604488694528158, 50.62390960531435979 ) ) ;
#160142=CARTESIAN_POINT ( 'NONE',  ( -16.53943276465976808, -0.05219959533934237506, 58.75109039468568994 ) ) ;
#160143=ORIENTED_EDGE ( 'NONE', *, *, #142697, .F. ) ;
#160144=CARTESIAN_POINT ( 'NONE',  ( -21.55341960407619339, 5.719274019375674811, 38.54275706135234714 ) ) ;
#160145=CARTESIAN_POINT ( 'NONE',  ( -12.14591786802309592, -12.06949235617757132, 71.87390960531438111 ) ) ;
#160147=CARTESIAN_POINT ( 'NONE',  ( 12.06949235617739724, 12.14591786802326823, 36.87609039468568994 ) ) ;
#160148=CARTESIAN_POINT ( 'NONE',  ( -16.55341960407611168, -4.379528057220339221, 106.4572429386477097 ) ) ;
#160149=CARTESIAN_POINT ( 'NONE',  ( -5.153800228976607833, 19.02544592524334988, 57.70942372801899012 ) ) ;
#160150=CARTESIAN_POINT ( 'NONE',  ( -0.05219959533910754901, -16.53943276465976808, 72.49890960531435269 ) ) ;
#160151=CARTESIAN_POINT ( 'NONE',  ( -18.67979575497193778, 10.72451020669871902, 33.33442372801900433 ) ) ;
#160153=CARTESIAN_POINT ( 'NONE',  ( -16.51473224551069308, -9.474510206698971260, 21.66557627198102765 ) ) ;
#160154=CARTESIAN_POINT ( 'NONE',  ( 15.72974639402199770, -15.80617190586745480, 88.12390960531436690 ) ) ;
#160155=CARTESIAN_POINT ( 'NONE',  ( -5.153800228976328057, -19.02544592524343514, 102.2905762719810383 ) ) ;
#160156=CARTESIAN_POINT ( 'NONE',  ( -16.53943276465976808, 0.05219959533911058130, 81.24890960531436690 ) ) ;
#160159=CARTESIAN_POINT ( 'NONE',  ( 9.474510206698729675, 16.51473224551082808, 87.08442372801900433 ) ) ;
#160160=CARTESIAN_POINT ( 'NONE',  ( 5.719274019375673035, 21.55341960407619339, 22.29275706135235069 ) ) ;
#160161=CARTESIAN_POINT ( 'NONE',  ( -9.474510206698964154, 16.51473224551069663, 65.41557627198102409 ) ) ;
#160162=CARTESIAN_POINT ( 'NONE',  ( -9.564922557961040184, 16.46253265017147172, 52.91775706135233293 ) ) ;
#160163=CARTESIAN_POINT ( 'NONE',  ( -5.153800228976328057, -19.02544592524343514, 27.29057627198103120 ) ) ;
#160164=CARTESIAN_POINT ( 'NONE',  ( -8.314922557960811034, -14.29746914071050412, 57.08224293864769550 ) ) ;
#160166=CARTESIAN_POINT ( 'NONE',  ( 16.55341960407611168, 4.379528057220329451, 53.95724293864770260 ) ) ;
#160167=CARTESIAN_POINT ( 'NONE',  ( 19.05341960407611168, 5.049401038298154454, 68.95724293864769550 ) ) ;
#160168=CARTESIAN_POINT ( 'NONE',  ( -21.52544592524343514, 5.823673210054127303, 81.04057627198102409 ) ) ;
#160169=CARTESIAN_POINT ( 'NONE',  ( 16.51473224551069308, 9.474510206698969483, 59.16557627198102409 ) ) ;
#160170=CARTESIAN_POINT ( 'NONE',  ( 5.823673210054125526, 21.52544592524343514, 84.79057627198102409 ) ) ;
#160171=CARTESIAN_POINT ( 'NONE',  ( -18.67979575497193778, 10.72451020669871902, 98.33442372801901854 ) ) ;
#160172=CARTESIAN_POINT ( 'NONE',  ( 5.049401038298161559, -19.05341960407611168, 22.70724293864769194 ) ) ;
#160173=CARTESIAN_POINT ( 'NONE',  ( -14.29746914071037622, -8.314922557961029526, 109.1677570613523613 ) ) ;
#160174=CARTESIAN_POINT ( 'NONE',  ( -12.06949235617756955, 12.14591786802309770, 100.6239096053143811 ) ) ;
#160175=CARTESIAN_POINT ( 'NONE',  ( 19.05341960407617918, -5.049401038297876454, 86.04275706135233293 ) ) ;
#160177=CARTESIAN_POINT ( 'NONE',  ( 5.823673210054125526, 21.52544592524343514, 114.7905762719810383 ) ) ;
#160178=CARTESIAN_POINT ( 'NONE',  ( -19.02544592524334988, -5.153800228976617603, 48.95942372801900433 ) ) ;
#160179=CARTESIAN_POINT ( 'NONE',  ( -12.06949235617739369, -12.14591786802326823, 99.37609039468568994 ) ) ;
#160180=CARTESIAN_POINT ( 'NONE',  ( 19.05341960407617918, -5.049401038297876454, 26.04275706135233293 ) ) ;
#160181=CARTESIAN_POINT ( 'NONE',  ( 9.474510206698971260, -16.51473224551069308, 102.9155762719810241 ) ) ;
#160182=CARTESIAN_POINT ( 'NONE',  ( -5.823673210054116645, -21.52544592524344225, 67.29057627198103830 ) ) ;
#160183=CARTESIAN_POINT ( 'NONE',  ( -19.46398650005391318, 5.499999999999952927, 50.18269651486372851 ) ) ;
#160184=CARTESIAN_POINT ( 'NONE',  ( 16.46253265017160672, -9.564922557960803928, 33.33224293864770260 ) ) ;
#160185=CARTESIAN_POINT ( 'NONE',  ( -21.53943276465977519, -0.05219959533937600094, 108.7510903946857042 ) ) ;
#160186=CARTESIAN_POINT ( 'NONE',  ( 8.224510206698742110, 14.34966873604972548, 77.08442372801901854 ) ) ;
#160187=CARTESIAN_POINT ( 'NONE',  ( 0.05219959533937995610, -21.53943276465977519, 35.00109039468568284 ) ) ;
#160188=CARTESIAN_POINT ( 'NONE',  ( -14.29746914071037622, -8.314922557961029526, 49.16775706135234003 ) ) ;
#160189=CARTESIAN_POINT ( 'NONE',  ( -13.89961937509977652, 13.97604488694528158, 100.6239096053143669 ) ) ;
#160190=CARTESIAN_POINT ( 'NONE',  ( 16.46253265017160672, -9.564922557960803928, 58.33224293864769550 ) ) ;
#160191=CARTESIAN_POINT ( 'NONE',  ( 9.474510206698971260, -16.51473224551069308, 67.91557627198102409 ) ) ;
#160193=CARTESIAN_POINT ( 'NONE',  ( -14.29746914071037622, -8.314922557961029526, 44.16775706135234714 ) ) ;
#160194=CARTESIAN_POINT ( 'NONE',  ( -0.05219959533910754901, -16.53943276465976808, 102.4989096053143811 ) ) ;
#160195=CARTESIAN_POINT ( 'NONE',  ( 14.29746914071037800, 8.314922557961029526, 111.6677570613523613 ) ) ;
#160196=CARTESIAN_POINT ( 'NONE',  ( -18.22780087662119897, 5.500000000000102141, 51.01763182126894947 ) ) ;
#160197=CARTESIAN_POINT ( 'NONE',  ( 15.72974639402176855, 15.80617190586768217, 61.87609039468568284 ) ) ;
#160198=CARTESIAN_POINT ( 'NONE',  ( 0.05219959533909260263, 19.03943276465977164, 84.99890960531436690 ) ) ;
#160199=CARTESIAN_POINT ( 'NONE',  ( 19.05341960407611168, 5.049401038298154454, 68.95724293864769550 ) ) ;
#160200=CARTESIAN_POINT ( 'NONE',  ( -13.89961937509977652, 13.97604488694528158, 90.62390960531432427 ) ) ;
#160201=CARTESIAN_POINT ( 'NONE',  ( -14.34966873604960291, -8.224510206698953496, 46.66557627198102409 ) ) ;
#160202=CARTESIAN_POINT ( 'NONE',  ( -4.483927247898539470, -16.52544592524342804, 22.29057627198102765 ) ) ;
#160203=CARTESIAN_POINT ( 'NONE',  ( 14.34966873604960469, 8.224510206698951720, 39.16557627198102409 ) ) ;
#160204=ORIENTED_EDGE ( 'NONE', *, *, #115041, .T. ) ;
#160205=CARTESIAN_POINT ( 'NONE',  ( 0.05219959533936267826, -19.03943276465977164, 45.00109039468566863 ) ) ;
#160206=CARTESIAN_POINT ( 'NONE',  ( 17.97058386085787873, 5.500000000000048850, 56.50390968646217260 ) ) ;
#160207=CARTESIAN_POINT ( 'NONE',  ( 0.05219959533909260263, 19.03943276465977164, 64.99890960531436690 ) ) ;
#160208=CARTESIAN_POINT ( 'NONE',  ( -5.153800228976607833, 19.02544592524334988, 32.70942372801899722 ) ) ;
#160211=CARTESIAN_POINT ( 'NONE',  ( 13.97604488694548053, -13.89961937509957401, 90.62609039468567573 ) ) ;
#160212=CARTESIAN_POINT ( 'NONE',  ( 4.483927247898790824, -16.52544592524335698, 65.20942372801901854 ) ) ;
#160213=CARTESIAN_POINT ( 'NONE',  ( 16.36317988757057762, 7.306389748694928521, 93.40210391636776421 ) ) ;
#160214=CARTESIAN_POINT ( 'NONE',  ( 0.05219959533909260263, 19.03943276465977164, 89.99890960531436690 ) ) ;
#160215=CARTESIAN_POINT ( 'NONE',  ( -5.823673210054431948, 21.52544592524334988, 32.70942372801900433 ) ) ;
#160216=CARTESIAN_POINT ( 'NONE',  ( 9.564922557961047289, -16.46253265017146816, 75.41775706135234714 ) ) ;
#160218=CARTESIAN_POINT ( 'NONE',  ( 19.03943276465977164, -0.05219959533909143690, 48.74890960531435979 ) ) ;
#160219=CARTESIAN_POINT ( 'NONE',  ( 19.05341960407611168, 5.049401038298154454, 83.95724293864766707 ) ) ;
#160220=CARTESIAN_POINT ( 'NONE',  ( 12.14591786802309770, 12.06949235617756955, 49.37390960531436690 ) ) ;
#160221=CARTESIAN_POINT ( 'NONE',  ( -5.049401038298153566, 19.05341960407611168, 55.20724293864769550 ) ) ;
#160222=CARTESIAN_POINT ( 'NONE',  ( -13.89961937509957401, -13.97604488694547875, 54.37609039468565442 ) ) ;
#160223=CARTESIAN_POINT ( 'NONE',  ( 16.52544592524342804, -4.483927247898539470, 88.54057627198103830 ) ) ;
#160224=CARTESIAN_POINT ( 'NONE',  ( -16.51473224551082808, 9.474510206698731452, 28.33442372801900433 ) ) ;
#160225=CARTESIAN_POINT ( 'NONE',  ( 9.474510206698971260, -16.51473224551069308, 67.91557627198102409 ) ) ;
#160226=CARTESIAN_POINT ( 'NONE',  ( 15.80617190586746368, 15.72974639402197994, 69.37390960531436690 ) ) ;
#160227=CARTESIAN_POINT ( 'NONE',  ( 8.224510206698953496, -14.34966873604960469, 67.91557627198102409 ) ) ;
#160228=CARTESIAN_POINT ( 'NONE',  ( -19.05341960407617563, 5.049401038297882671, 23.54275706135233648 ) ) ;
#160229=CARTESIAN_POINT ( 'NONE',  ( -9.564922557960796823, -16.46253265017161027, 107.0822429386476955 ) ) ;
#160231=CARTESIAN_POINT ( 'NONE',  ( -21.55341960407610458, -5.719274019375992779, 31.45724293864769550 ) ) ;
#160232=CARTESIAN_POINT ( 'NONE',  ( 16.51473224551069308, 9.474510206698969483, 59.16557627198102409 ) ) ;
#160233=CARTESIAN_POINT ( 'NONE',  ( -5.049401038298153566, 19.05341960407611168, 40.20724293864768839 ) ) ;
#160234=CARTESIAN_POINT ( 'NONE',  ( -16.52544592524342804, 4.483927247898546575, 101.0405762719810383 ) ) ;
#160235=CARTESIAN_POINT ( 'NONE',  ( 21.53943276465977519, -0.05219959533907433946, 108.7489096053143669 ) ) ;
#160236=CARTESIAN_POINT ( 'NONE',  ( -0.05219959533909027116, -19.03943276465977164, 102.4989096053143669 ) ) ;
#160237=CARTESIAN_POINT ( 'NONE',  ( 5.719274019375991003, -21.55341960407610458, 112.7072429386476955 ) ) ;
#160238=CARTESIAN_POINT ( 'NONE',  ( -9.474510206698964154, 16.51473224551069663, 100.4155762719810241 ) ) ;
#160239=CARTESIAN_POINT ( 'NONE',  ( -9.474510206698964154, 16.51473224551069663, 25.41557627198103120 ) ) ;
#160241=CARTESIAN_POINT ( 'NONE',  ( -5.823673210054431948, 21.52544592524334988, 77.70942372801900433 ) ) ;
#160242=CARTESIAN_POINT ( 'NONE',  ( 18.67979575497178502, 10.72451020669898547, 99.16557627198100988 ) ) ;
#160244=CARTESIAN_POINT ( 'NONE',  ( 19.02130022317637881, -5.499999999999793054, 78.28188669246573284 ) ) ;
#160246=CARTESIAN_POINT ( 'NONE',  ( 0.05219959533934541429, -16.53943276465976808, 50.00109039468568994 ) ) ;
#160247=CARTESIAN_POINT ( 'NONE',  ( -16.52544592524342804, 4.483927247898546575, 111.0405762719810525 ) ) ;
#160249=CARTESIAN_POINT ( 'NONE',  ( 5.049401038298161559, -19.05341960407611168, 57.70724293864769550 ) ) ;
#160250=CARTESIAN_POINT ( 'NONE',  ( -14.29746914071049879, 8.314922557960819915, 95.83224293864770971 ) ) ;
#160251=CARTESIAN_POINT ( 'NONE',  ( 5.823673210054125526, 21.52544592524343514, 49.79057627198102409 ) ) ;
#160252=CARTESIAN_POINT ( 'NONE',  ( -16.52544592524342804, 4.483927247898546575, 71.04057627198103830 ) ) ;
#160253=CARTESIAN_POINT ( 'NONE',  ( 8.314922557961029526, -14.29746914071037800, 20.41775706135234714 ) ) ;
#160254=CARTESIAN_POINT ( 'NONE',  ( 21.53943276465977519, 0.05219959533937863772, 71.25109039468568994 ) ) ;
#160255=CARTESIAN_POINT ( 'NONE',  ( 17.13100169013300800, -6.664070546373153547, 78.26789835699852915 ) ) ;
#160256=CARTESIAN_POINT ( 'NONE',  ( -16.55341960407617563, 4.379528057220093196, 98.54275706135234714 ) ) ;
#160257=CARTESIAN_POINT ( 'NONE',  ( -0.05219959533910754901, -16.53943276465976808, 42.49890960531435979 ) ) ;
#160258=CARTESIAN_POINT ( 'NONE',  ( -9.474510206698964154, 16.51473224551069663, 35.41557627198102409 ) ) ;
#160259=CARTESIAN_POINT ( 'NONE',  ( -13.97604488694527625, -13.89961937509977652, 86.87390960531436690 ) ) ;
#160260=CARTESIAN_POINT ( 'NONE',  ( -21.53943276465977519, 0.05219959533907696930, 96.24890960531435269 ) ) ;
#160261=CARTESIAN_POINT ( 'NONE',  ( 14.34966873604972726, -8.224510206698740333, 20.83442372801901143 ) ) ;
#160262=CARTESIAN_POINT ( 'NONE',  ( -8.314922557960811034, -14.29746914071050412, 62.08224293864769550 ) ) ;
#160263=CARTESIAN_POINT ( 'NONE',  ( -10.81492255796105439, 18.62759615963255655, 77.91775706135231871 ) ) ;
#160264=CARTESIAN_POINT ( 'NONE',  ( -4.483927247898782831, 16.52544592524335698, 97.70942372801904696 ) ) ;
#160265=CARTESIAN_POINT ( 'NONE',  ( 17.13100169013228324, -6.664070546374126103, 48.26789835699824494 ) ) ;
#160267=CARTESIAN_POINT ( 'NONE',  ( 8.224510206698953496, -14.34966873604960469, 27.91557627198103830 ) ) ;
#160268=CARTESIAN_POINT ( 'NONE',  ( -12.14591786802326823, 12.06949235617739902, 68.12609039468567573 ) ) ;
#160269=CARTESIAN_POINT ( 'NONE',  ( -19.03943276465977164, 0.05219959533909376836, 86.24890960531436690 ) ) ;
#160270=CARTESIAN_POINT ( 'NONE',  ( 5.153800228976335163, 19.02544592524342804, 104.7905762719809957 ) ) ;
#160271=CARTESIAN_POINT ( 'NONE',  ( 21.53943276465977519, 0.05219959533937863772, 91.25109039468568994 ) ) ;
#160272=CARTESIAN_POINT ( 'NONE',  ( -8.314922557961024197, 14.29746914071037800, 92.91775706135236135 ) ) ;
#160273=CARTESIAN_POINT ( 'NONE',  ( -16.52544592524342804, 4.483927247898546575, 66.04057627198103830 ) ) ;
#160274=CARTESIAN_POINT ( 'NONE',  ( 9.564922557960805705, 16.46253265017160317, 64.58224293864769550 ) ) ;
#160276=CARTESIAN_POINT ( 'NONE',  ( -13.97604488694547697, 13.89961937509957934, 113.1260903946856757 ) ) ;
#160277=CARTESIAN_POINT ( 'NONE',  ( 8.314922557960818139, 14.29746914071049879, 104.5822429386477097 ) ) ;
#160278=CARTESIAN_POINT ( 'NONE',  ( -19.05341960407611168, -5.049401038298163336, 76.45724293864769550 ) ) ;
#160279=CARTESIAN_POINT ( 'NONE',  ( -14.29746914071037622, -8.314922557961029526, 19.16775706135234714 ) ) ;
#160281=CARTESIAN_POINT ( 'NONE',  ( -0.05219959533937732626, 21.53943276465977519, 112.5010903946857042 ) ) ;
#160282=CARTESIAN_POINT ( 'NONE',  ( -8.314922557961024197, 14.29746914071037800, 82.91775706135234714 ) ) ;
#160283=CARTESIAN_POINT ( 'NONE',  ( -5.049401038297874678, -19.05341960407617918, 99.79275706135234714 ) ) ;
#160284=CARTESIAN_POINT ( 'NONE',  ( 13.89961937509977652, -13.97604488694527269, 23.12390960531436335 ) ) ;
#160285=CARTESIAN_POINT ( 'NONE',  ( -12.14591786802326823, 12.06949235617739902, 68.12609039468567573 ) ) ;
#160286=CARTESIAN_POINT ( 'NONE',  ( 12.06949235617739724, 12.14591786802326823, 56.87609039468568994 ) ) ;
#160288=CARTESIAN_POINT ( 'NONE',  ( -13.89961937509957401, -13.97604488694547875, 74.37609039468566152 ) ) ;
#160289=CARTESIAN_POINT ( 'NONE',  ( 10.72451020669871369, 18.67979575497193778, 97.08442372801904696 ) ) ;
#160290=CARTESIAN_POINT ( 'NONE',  ( 9.564922557960805705, 16.46253265017160317, 34.58224293864770260 ) ) ;
#160291=CARTESIAN_POINT ( 'NONE',  ( 9.474510206698971260, -16.51473224551069308, 72.91557627198102409 ) ) ;
#160292=CARTESIAN_POINT ( 'NONE',  ( -16.52544592524342804, 4.483927247898546575, 76.04057627198102409 ) ) ;
#160294=CARTESIAN_POINT ( 'NONE',  ( 18.67979575497194134, -10.72451020669871369, 95.83442372801903275 ) ) ;
#160295=CARTESIAN_POINT ( 'NONE',  ( 0.05219959533936267826, -19.03943276465977164, 35.00109039468566863 ) ) ;
#160296=CARTESIAN_POINT ( 'NONE',  ( -10.72451020669898014, 18.67979575497178502, 40.41557627198103120 ) ) ;
#160297=CARTESIAN_POINT ( 'NONE',  ( -9.474510206698720793, -16.51473224551083518, 19.58442372801899722 ) ) ;
#160298=CARTESIAN_POINT ( 'NONE',  ( 5.049401038298161559, -19.05341960407611168, 82.70724293864770971 ) ) ;
#160299=CARTESIAN_POINT ( 'NONE',  ( -5.823673210054431948, 21.52544592524334988, 112.7094237280190328 ) ) ;
#160300=CARTESIAN_POINT ( 'NONE',  ( -5.719274019375978568, 21.55341960407610458, 60.20724293864768839 ) ) ;
#160301=CARTESIAN_POINT ( 'NONE',  ( -19.05341960407611168, -5.049401038298163336, 101.4572429386476955 ) ) ;
#160302=CARTESIAN_POINT ( 'NONE',  ( 16.51473224551083163, -9.474510206698727899, 70.83442372801900433 ) ) ;
#160303=CARTESIAN_POINT ( 'NONE',  ( 19.02544592524343514, -5.153800228976328945, 98.54057627198100988 ) ) ;
#160304=CARTESIAN_POINT ( 'NONE',  ( 16.51473224551083163, -9.474510206698727899, 90.83442372801900433 ) ) ;
#160305=CARTESIAN_POINT ( 'NONE',  ( 0.05219959533934541429, -16.53943276465976808, 45.00109039468568284 ) ) ;
#160306=CARTESIAN_POINT ( 'NONE',  ( -14.29746914071049879, 8.314922557960819915, 115.8322429386477097 ) ) ;
#160307=CARTESIAN_POINT ( 'NONE',  ( -19.05341960407611168, -5.049401038298163336, 81.45724293864769550 ) ) ;
#160308=CARTESIAN_POINT ( 'NONE',  ( -5.823673210054116645, -21.52544592524344225, 57.29057627198103120 ) ) ;
#160309=CARTESIAN_POINT ( 'NONE',  ( 8.224510206698742110, 14.34966873604972548, 27.08442372801901854 ) ) ;
#160310=CARTESIAN_POINT ( 'NONE',  ( -10.81492255796105439, 18.62759615963255655, 27.91775706135234358 ) ) ;
#160311=CARTESIAN_POINT ( 'NONE',  ( 21.52544592524334988, 5.823673210054432836, 81.45942372801900433 ) ) ;
#160312=CARTESIAN_POINT ( 'NONE',  ( -16.53943276465976808, -0.05219959533934237506, 88.75109039468567573 ) ) ;
#160313=CARTESIAN_POINT ( 'NONE',  ( -13.97604488694527625, -13.89961937509977652, 91.87390960531432427 ) ) ;
#160314=CARTESIAN_POINT ( 'NONE',  ( 8.224510206698953496, -14.34966873604960469, 82.91557627198103830 ) ) ;
#160315=CARTESIAN_POINT ( 'NONE',  ( 16.55341960407611168, 4.379528057220329451, 23.95724293864769550 ) ) ;
#160316=CARTESIAN_POINT ( 'NONE',  ( -19.02544592524334988, -5.153800228976617603, 58.95942372801900433 ) ) ;
#160317=CARTESIAN_POINT ( 'NONE',  ( 15.72974639402176855, 15.80617190586768217, 41.87609039468568284 ) ) ;
#160318=CARTESIAN_POINT ( 'NONE',  ( -14.34966873604960291, -8.224510206698953496, 96.66557627198102409 ) ) ;
#160319=CARTESIAN_POINT ( 'NONE',  ( -9.474510206698964154, 16.51473224551069663, 110.4155762719810383 ) ) ;
#160320=CARTESIAN_POINT ( 'NONE',  ( -14.34966873604972548, 8.224510206698743886, 98.33442372801901854 ) ) ;
#160321=CARTESIAN_POINT ( 'NONE',  ( -5.719274019375665041, -21.55341960407619695, 84.79275706135234714 ) ) ;
#160322=CARTESIAN_POINT ( 'NONE',  ( -16.53943276465976808, -0.05219959533934237506, 48.75109039468568284 ) ) ;
#160323=CARTESIAN_POINT ( 'NONE',  ( 15.72974639402176855, 15.80617190586768217, 36.87609039468568994 ) ) ;
#160325=VERTEX_POINT ( 'NONE', #21344 ) ;
#160326=CARTESIAN_POINT ( 'NONE',  ( 10.72451020669871369, 18.67979575497193778, 22.08442372801901143 ) ) ;
#160327=CARTESIAN_POINT ( 'NONE',  ( 12.06949235617757843, -12.14591786802309237, 98.12390960531436690 ) ) ;
#160328=CARTESIAN_POINT ( 'NONE',  ( -18.56399227203345959, -5.499999999999828582, 48.97830131249904895 ) ) ;
#160329=CARTESIAN_POINT ( 'NONE',  ( 12.14591786802309770, 12.06949235617756955, 69.37390960531436690 ) ) ;
#160330=CARTESIAN_POINT ( 'NONE',  ( -12.06949235617739369, -12.14591786802326823, 94.37609039468568994 ) ) ;
#160331=CARTESIAN_POINT ( 'NONE',  ( 16.46253265017160672, -9.564922557960803928, 33.33224293864770260 ) ) ;
#160332=CARTESIAN_POINT ( 'NONE',  ( -15.80617190586745835, -15.72974639402198527, 41.87390960531435979 ) ) ;
#160333=CARTESIAN_POINT ( 'NONE',  ( -16.53943276465976808, 0.05219959533911058130, 81.24890960531436690 ) ) ;
#160335=CARTESIAN_POINT ( 'NONE',  ( 10.81492255796078972, 18.62759615963270932, 74.58224293864768129 ) ) ;
#160336=CARTESIAN_POINT ( 'NONE',  ( 9.474510206698971260, -16.51473224551069308, 87.91557627198102409 ) ) ;
#160337=CARTESIAN_POINT ( 'NONE',  ( -19.02544592524342804, 5.153800228976336051, 41.04057627198103120 ) ) ;
#160338=CARTESIAN_POINT ( 'NONE',  ( 13.89961937509957401, 13.97604488694547697, 96.87609039468566152 ) ) ;
#160339=CARTESIAN_POINT ( 'NONE',  ( -15.80617190586745835, -15.72974639402198527, 26.87390960531435979 ) ) ;
#160340=CARTESIAN_POINT ( 'NONE',  ( 18.67979575497194134, -10.72451020669871369, 55.83442372801901854 ) ) ;
#160341=CARTESIAN_POINT ( 'NONE',  ( 5.153800228976335163, 19.02544592524342804, 49.79057627198100988 ) ) ;
#160342=CARTESIAN_POINT ( 'NONE',  ( 13.89961937509977652, -13.97604488694527269, 83.12390960531436690 ) ) ;
#160344=CARTESIAN_POINT ( 'NONE',  ( -4.379528057220086978, -16.55341960407618274, 44.79275706135234714 ) ) ;
#160345=CARTESIAN_POINT ( 'NONE',  ( -18.62759615963255300, -10.81492255796106328, 39.16775706135235424 ) ) ;
#160346=CARTESIAN_POINT ( 'NONE',  ( 18.62759615963255655, 10.81492255796105972, 71.66775706135234714 ) ) ;
#160347=CARTESIAN_POINT ( 'NONE',  ( -19.02544592524342804, 5.153800228976336051, 116.0405762719810383 ) ) ;
#160348=CARTESIAN_POINT ( 'NONE',  ( -0.05219959533907301413, -21.53943276465977519, 92.49890960531436690 ) ) ;
#160349=CARTESIAN_POINT ( 'NONE',  ( -21.52544592524334988, -5.823673210054445271, 23.95942372801901143 ) ) ;
#160350=CARTESIAN_POINT ( 'NONE',  ( 0.05219959533934541429, -16.53943276465976808, 65.00109039468568994 ) ) ;
#160351=CARTESIAN_POINT ( 'NONE',  ( 10.72451020669898902, -18.67979575497178502, 67.91557627198102409 ) ) ;
#160352=CARTESIAN_POINT ( 'NONE',  ( -5.823673210054431948, 21.52544592524334988, 112.7094237280190328 ) ) ;
#160353=CARTESIAN_POINT ( 'NONE',  ( 5.049401038298161559, -19.05341960407611168, 67.70724293864769550 ) ) ;
#160354=CARTESIAN_POINT ( 'NONE',  ( 4.379528057220092307, 16.55341960407617563, 107.2927570613523471 ) ) ;
#160356=CARTESIAN_POINT ( 'NONE',  ( -5.153800228976328057, -19.02544592524343514, 87.29057627198103830 ) ) ;
#160357=CARTESIAN_POINT ( 'NONE',  ( -5.153800228976607833, 19.02544592524335343, 52.70942372801900433 ) ) ;
#160358=CARTESIAN_POINT ( 'NONE',  ( 5.049401038297881783, 19.05341960407617563, 82.29275706135229029 ) ) ;
#160359=CARTESIAN_POINT ( 'NONE',  ( 0.05219959533907565091, 21.53943276465977519, 44.99890960531435979 ) ) ;
#160360=CARTESIAN_POINT ( 'NONE',  ( 4.379528057220092307, 16.55341960407617563, 112.2927570613523471 ) ) ;
#160361=CARTESIAN_POINT ( 'NONE',  ( -13.89961937509957401, -13.97604488694547875, 99.37609039468567573 ) ) ;
#160362=CARTESIAN_POINT ( 'NONE',  ( 17.72696623605160227, -5.500000000000076383, 51.09811031808416004 ) ) ;
#160363=CARTESIAN_POINT ( 'NONE',  ( 19.02544592524334988, 5.153800228976608722, 91.45942372801900433 ) ) ;
#160364=CARTESIAN_POINT ( 'NONE',  ( -5.823673210054116645, -21.52544592524344225, 92.29057627198103830 ) ) ;
#160365=CARTESIAN_POINT ( 'NONE',  ( 5.153800228976615827, -19.02544592524334988, 55.20942372801899722 ) ) ;
#160366=CARTESIAN_POINT ( 'NONE',  ( 17.13100169013301155, 6.664070546373133119, 106.7321016430015561 ) ) ;
#160367=CARTESIAN_POINT ( 'NONE',  ( 19.02544592524343514, -5.153800228976328945, 48.54057627198103120 ) ) ;
#160368=CARTESIAN_POINT ( 'NONE',  ( -14.34966873604960291, -8.224510206698953496, 56.66557627198103830 ) ) ;
#160369=CARTESIAN_POINT ( 'NONE',  ( -9.474510206698964154, 16.51473224551069663, 45.41557627198103120 ) ) ;
#160370=CARTESIAN_POINT ( 'NONE',  ( -4.483927247898539470, -16.52544592524342804, 52.29057627198102409 ) ) ;
#160373=CARTESIAN_POINT ( 'NONE',  ( 8.314922557960818139, 14.29746914071049879, 34.58224293864770260 ) ) ;
#160374=CARTESIAN_POINT ( 'NONE',  ( -13.97604488694527625, -13.89961937509977652, 66.87390960531436690 ) ) ;
#160376=CARTESIAN_POINT ( 'NONE',  ( -0.05219959533936034679, 19.03943276465977164, 42.50109039468566152 ) ) ;
#160377=CARTESIAN_POINT ( 'NONE',  ( -14.34966873604972548, 8.224510206698743886, 48.33442372801902565 ) ) ;
#160378=CARTESIAN_POINT ( 'NONE',  ( 0.05219959533907565091, 21.53943276465977519, 44.99890960531435979 ) ) ;
#160379=CARTESIAN_POINT ( 'NONE',  ( -5.719274019375665041, -21.55341960407619695, 104.7927570613523898 ) ) ;
#160381=CARTESIAN_POINT ( 'NONE',  ( -9.474510206698964154, 16.51473224551069663, 65.41557627198102409 ) ) ;
#160383=CARTESIAN_POINT ( 'NONE',  ( -16.51473224551069308, -9.474510206698971260, 101.6655762719810241 ) ) ;
#160385=CARTESIAN_POINT ( 'NONE',  ( 15.80617190586769283, -15.72974639402175789, 20.62609039468568639 ) ) ;
#160386=VECTOR ( 'NONE', #197494, 1000.000000000000000 ) ;
#160387=CARTESIAN_POINT ( 'NONE',  ( 16.53943276465976808, -0.05219959533910856209, 88.74890960531436690 ) ) ;
#160388=CARTESIAN_POINT ( 'NONE',  ( -0.05219959533907301413, -21.53943276465977519, 92.49890960531436690 ) ) ;
#160389=CARTESIAN_POINT ( 'NONE',  ( -5.049401038298153566, 19.05341960407611168, 80.20724293864769550 ) ) ;
#160390=CARTESIAN_POINT ( 'NONE',  ( -0.05219959533909027116, -19.03943276465977164, 92.49890960531436690 ) ) ;
#160391=CARTESIAN_POINT ( 'NONE',  ( -18.62759615963270932, 10.81492255796079327, 105.8322429386476955 ) ) ;
#160393=CARTESIAN_POINT ( 'NONE',  ( -5.153800228976328057, -19.02544592524343514, 72.29057627198102409 ) ) ;
#160395=CARTESIAN_POINT ( 'NONE',  ( -16.53943276465976808, 0.05219959533911058130, 101.2489096053143669 ) ) ;
#160396=CARTESIAN_POINT ( 'NONE',  ( 5.153800228976335163, 19.02544592524342804, 34.79057627198102409 ) ) ;
#160397=CARTESIAN_POINT ( 'NONE',  ( -5.153800228976607833, 19.02544592524334988, 97.70942372801900433 ) ) ;
#160398=CARTESIAN_POINT ( 'NONE',  ( -4.379528057220328563, 16.55341960407611168, 105.2072429386477097 ) ) ;
#160399=CARTESIAN_POINT ( 'NONE',  ( -5.823673210054431948, 21.52544592524334988, 67.70942372801901854 ) ) ;
#160400=CARTESIAN_POINT ( 'NONE',  ( 9.564922557960805705, 16.46253265017160317, 59.58224293864769550 ) ) ;
#160401=CARTESIAN_POINT ( 'NONE',  ( -21.53943276465977519, -0.05219959533937600094, 38.75109039468567573 ) ) ;
#160402=CARTESIAN_POINT ( 'NONE',  ( 5.823673210054125526, 21.52544592524343514, 114.7905762719810383 ) ) ;
#160404=CARTESIAN_POINT ( 'NONE',  ( 9.474510206698971260, -16.51473224551069308, 87.91557627198102409 ) ) ;
#160406=CARTESIAN_POINT ( 'NONE',  ( 16.55341960407618274, -4.379528057220086978, 26.04275706135235779 ) ) ;
#160407=CARTESIAN_POINT ( 'NONE',  ( -10.81492255796078084, -18.62759615963271287, 37.08224293864768129 ) ) ;
#160408=CARTESIAN_POINT ( 'NONE',  ( -21.55341960407619339, 5.719274019375674811, 68.54275706135234714 ) ) ;
#160409=CARTESIAN_POINT ( 'NONE',  ( 5.153800228976335163, 19.02544592524342804, 104.7905762719809957 ) ) ;
#160410=CARTESIAN_POINT ( 'NONE',  ( -9.564922557961040184, 16.46253265017147172, 102.9177570613523329 ) ) ;
#160411=CARTESIAN_POINT ( 'NONE',  ( -19.03943276465977164, 0.05219959533909376836, 46.24890960531435979 ) ) ;
#160412=CARTESIAN_POINT ( 'NONE',  ( 0.05219959533909260263, 19.03943276465977164, 64.99890960531436690 ) ) ;
#160413=CARTESIAN_POINT ( 'NONE',  ( 8.224510206698953496, -14.34966873604960469, 92.91557627198103830 ) ) ;
#160414=CARTESIAN_POINT ( 'NONE',  ( -9.564922557960796823, -16.46253265017161027, 112.0822429386476955 ) ) ;
#160415=CARTESIAN_POINT ( 'NONE',  ( -12.06949235617756955, 12.14591786802309770, 85.62390960531436690 ) ) ;
#160416=CARTESIAN_POINT ( 'NONE',  ( -9.474510206698964154, 16.51473224551069663, 110.4155762719810383 ) ) ;
#160417=CARTESIAN_POINT ( 'NONE',  ( 8.224510206698953496, -14.34966873604960469, 57.91557627198103120 ) ) ;
#160418=CARTESIAN_POINT ( 'NONE',  ( -0.05219959533909027116, -19.03943276465977164, 37.49890960531436690 ) ) ;
#160419=CARTESIAN_POINT ( 'NONE',  ( 5.719274019375673035, 21.55341960407619339, 57.29275706135234714 ) ) ;
#160420=CARTESIAN_POINT ( 'NONE',  ( -19.05341960407617563, 5.049401038297882671, 98.54275706135233293 ) ) ;
#160421=CARTESIAN_POINT ( 'NONE',  ( 14.29746914071049879, -8.314922557960816363, 53.33224293864769550 ) ) ;
#160422=CARTESIAN_POINT ( 'NONE',  ( 15.80617190586746368, 15.72974639402197994, 114.3739096053143527 ) ) ;
#160423=CARTESIAN_POINT ( 'NONE',  ( 21.55341960407610458, 5.719274019375980345, 43.95724293864769550 ) ) ;
#160424=CARTESIAN_POINT ( 'NONE',  ( -5.153800228976328057, -19.02544592524343514, 112.2905762719810099 ) ) ;
#160426=CARTESIAN_POINT ( 'NONE',  ( -9.474510206698964154, 16.51473224551069663, 50.41557627198102409 ) ) ;
#160427=CARTESIAN_POINT ( 'NONE',  ( 16.52544592524335698, 4.483927247898782831, 111.4594237280190328 ) ) ;
#160428=CARTESIAN_POINT ( 'NONE',  ( 8.224510206698742110, 14.34966873604972548, 102.0844237280190185 ) ) ;
#160429=CARTESIAN_POINT ( 'NONE',  ( -12.14591786802326823, 12.06949235617739902, 88.12609039468570415 ) ) ;
#160430=CARTESIAN_POINT ( 'NONE',  ( -5.153800228976607833, 19.02544592524334988, 32.70942372801899722 ) ) ;
#160432=CARTESIAN_POINT ( 'NONE',  ( 5.049401038298161559, -19.05341960407611168, 87.70724293864769550 ) ) ;
#160433=CARTESIAN_POINT ( 'NONE',  ( 19.02544592524343514, -5.153800228976328945, 53.54057627198102409 ) ) ;
#160434=CARTESIAN_POINT ( 'NONE',  ( 16.52544592524342804, -4.483927247898539470, 63.54057627198103830 ) ) ;
#160435=CARTESIAN_POINT ( 'NONE',  ( 17.40805194822030799, -6.112264579159331745, 103.3337127251061105 ) ) ;
#160436=CARTESIAN_POINT ( 'NONE',  ( 9.564922557960805705, 16.46253265017160317, 104.5822429386476955 ) ) ;
#160437=CARTESIAN_POINT ( 'NONE',  ( -5.823673210054116645, -21.52544592524344225, 47.29057627198103120 ) ) ;
#160438=CARTESIAN_POINT ( 'NONE',  ( 14.29746914071049879, -8.314922557960816363, 83.33224293864769550 ) ) ;
#160439=CARTESIAN_POINT ( 'NONE',  ( 8.314922557961029526, -14.29746914071037800, 35.41775706135234003 ) ) ;
#160440=CARTESIAN_POINT ( 'NONE',  ( -14.29746914071049879, 8.314922557960819915, 80.83224293864769550 ) ) ;
#160442=CARTESIAN_POINT ( 'NONE',  ( -9.564922557961040184, 16.46253265017147172, 77.91775706135234714 ) ) ;
#160443=CARTESIAN_POINT ( 'NONE',  ( 5.049401038298161559, -19.05341960407611168, 102.7072429386476955 ) ) ;
#160444=CARTESIAN_POINT ( 'NONE',  ( 16.51473224551083163, -9.474510206698727899, 80.83442372801899012 ) ) ;
#160446=CARTESIAN_POINT ( 'NONE',  ( 8.224510206698742110, 14.34966873604972548, 27.08442372801901854 ) ) ;
#160447=CARTESIAN_POINT ( 'NONE',  ( -8.314922557961024197, 14.29746914071037800, 112.9177570613523329 ) ) ;
#160448=CARTESIAN_POINT ( 'NONE',  ( 9.474510206698729675, 16.51473224551082808, 72.08442372801900433 ) ) ;
#160449=CARTESIAN_POINT ( 'NONE',  ( -15.80617190586745835, -15.72974639402198527, 36.87390960531435979 ) ) ;
#160450=CARTESIAN_POINT ( 'NONE',  ( 21.52544592524334988, 5.823673210054432836, 71.45942372801901854 ) ) ;
#160452=CARTESIAN_POINT ( 'NONE',  ( -12.06949235617739369, -12.14591786802326823, 39.37609039468567573 ) ) ;
#160453=CARTESIAN_POINT ( 'NONE',  ( -19.05341960407611168, -5.049401038298163336, 21.45724293864768839 ) ) ;
#160454=CARTESIAN_POINT ( 'NONE',  ( 19.05341960407611168, 5.049401038298154454, 93.95724293864769550 ) ) ;
#160456=CARTESIAN_POINT ( 'NONE',  ( 8.224510206698953496, -14.34966873604960469, 82.91557627198103830 ) ) ;
#160458=CARTESIAN_POINT ( 'NONE',  ( -9.474510206698964154, 16.51473224551069663, 85.41557627198102409 ) ) ;
#160459=ORIENTED_EDGE ( 'NONE', *, *, #196667, .T. ) ;
#160460=CARTESIAN_POINT ( 'NONE',  ( 19.03943276465977164, 0.05219959533936151252, 111.2510903946856757 ) ) ;
#160461=CARTESIAN_POINT ( 'NONE',  ( 15.80617190586746368, 15.72974639402197994, 79.37390960531436690 ) ) ;
#160462=CARTESIAN_POINT ( 'NONE',  ( 19.02544592524343514, -5.153800228976328945, 38.54057627198103120 ) ) ;
#160463=CARTESIAN_POINT ( 'NONE',  ( -13.97604488694547697, 13.89961937509957934, 73.12609039468568994 ) ) ;
#160464=CARTESIAN_POINT ( 'NONE',  ( 0.05219959533937995610, -21.53943276465977519, 20.00109039468568639 ) ) ;
#160465=CARTESIAN_POINT ( 'NONE',  ( -5.049401038298153566, 19.05341960407611168, 70.20724293864769550 ) ) ;
#160466=CARTESIAN_POINT ( 'NONE',  ( -9.474510206698964154, 16.51473224551069663, 110.4155762719810383 ) ) ;
#160468=CARTESIAN_POINT ( 'NONE',  ( -14.29746914071037622, -8.314922557961029526, 34.16775706135234714 ) ) ;
#160469=CARTESIAN_POINT ( 'NONE',  ( 21.52544592524344225, -5.823673210054117533, 108.5405762719810241 ) ) ;
#160470=CARTESIAN_POINT ( 'NONE',  ( 12.06949235617757843, -12.14591786802309237, 108.1239096053143811 ) ) ;
#160471=CARTESIAN_POINT ( 'NONE',  ( -13.89961937509977652, 13.97604488694528158, 95.62390960531436690 ) ) ;
#160472=CARTESIAN_POINT ( 'NONE',  ( -5.153800228976607833, 19.02544592524334988, 57.70942372801899012 ) ) ;
#160473=CARTESIAN_POINT ( 'NONE',  ( 21.53943276465977519, -0.05219959533907433946, 83.74890960531435269 ) ) ;
#160474=CARTESIAN_POINT ( 'NONE',  ( 5.719274019375991003, -21.55341960407610458, 92.70724293864770971 ) ) ;
#160475=CARTESIAN_POINT ( 'NONE',  ( 4.483927247898545687, 16.52544592524342804, 44.79057627198103120 ) ) ;
#160476=CARTESIAN_POINT ( 'NONE',  ( -13.97604488694547697, 13.89961937509957934, 23.12609039468565442 ) ) ;
#160477=CARTESIAN_POINT ( 'NONE',  ( -16.53943276465976808, -0.05219959533934237506, 68.75109039468568994 ) ) ;
#160478=CARTESIAN_POINT ( 'NONE',  ( 19.02544592524343514, -5.153800228976328945, 98.54057627198100988 ) ) ;
#160479=CARTESIAN_POINT ( 'NONE',  ( 19.05341960407611168, 5.049401038298154454, 48.95724293864768129 ) ) ;
#160481=CARTESIAN_POINT ( 'NONE',  ( -21.53943276465977519, -0.05219959533937600094, 48.75109039468568284 ) ) ;
#160482=CARTESIAN_POINT ( 'NONE',  ( -5.719274019375665041, -21.55341960407619695, 64.79275706135234714 ) ) ;
#160483=CARTESIAN_POINT ( 'NONE',  ( -5.153800228976328057, -19.02544592524343514, 62.29057627198100988 ) ) ;
#160484=CARTESIAN_POINT ( 'NONE',  ( -21.52544592524334988, -5.823673210054445271, 28.95942372801902209 ) ) ;
#160485=CARTESIAN_POINT ( 'NONE',  ( -9.564922557961040184, 16.46253265017147172, 77.91775706135234714 ) ) ;
#160486=CARTESIAN_POINT ( 'NONE',  ( -19.05341960407617563, 5.049401038297882671, 73.54275706135233293 ) ) ;
#160487=CARTESIAN_POINT ( 'NONE',  ( 16.46253265017160672, -9.564922557960803928, 33.33224293864770260 ) ) ;
#160488=CARTESIAN_POINT ( 'NONE',  ( -8.314922557961024197, 14.29746914071037800, 82.91775706135234714 ) ) ;
#160489=CARTESIAN_POINT ( 'NONE',  ( -19.05341960407611168, -5.049401038298163336, 56.45724293864768129 ) ) ;
#160490=CARTESIAN_POINT ( 'NONE',  ( 0.05219959533909260263, 19.03943276465977164, 29.99890960531435979 ) ) ;
#160491=CARTESIAN_POINT ( 'NONE',  ( 9.564922557960805705, 16.46253265017160317, 94.58224293864769550 ) ) ;
#160492=CARTESIAN_POINT ( 'NONE',  ( 19.02544592524343514, -5.153800228976328945, 38.54057627198103120 ) ) ;
#160493=CARTESIAN_POINT ( 'NONE',  ( 5.719274019375991003, -21.55341960407610458, 82.70724293864770971 ) ) ;
#160494=CARTESIAN_POINT ( 'NONE',  ( 4.483927247898790824, -16.52544592524335698, 65.20942372801901854 ) ) ;
#160495=CARTESIAN_POINT ( 'NONE',  ( -21.55341960407619339, 5.719274019375674811, 113.5427570613523756 ) ) ;
#160496=CARTESIAN_POINT ( 'NONE',  ( -13.89961937509977652, 13.97604488694528158, 50.62390960531435979 ) ) ;
#160497=CARTESIAN_POINT ( 'NONE',  ( 4.379528057220339221, -16.55341960407611168, 42.70724293864770260 ) ) ;
#160498=CARTESIAN_POINT ( 'NONE',  ( 0.05219959533910956823, 16.53943276465976808, 84.99890960531436690 ) ) ;
#160499=CARTESIAN_POINT ( 'NONE',  ( 19.02544592524343514, -5.153800228976328945, 73.54057627198103830 ) ) ;
#160500=CARTESIAN_POINT ( 'NONE',  ( -15.80617190586768217, 15.72974639402176855, 38.12609039468567573 ) ) ;
#160501=CARTESIAN_POINT ( 'NONE',  ( -19.05341960407611168, -5.049401038298163336, 86.45724293864769550 ) ) ;
#160502=CARTESIAN_POINT ( 'NONE',  ( -21.52544592524334988, -5.823673210054445271, 98.95942372801903275 ) ) ;
#160503=CARTESIAN_POINT ( 'NONE',  ( -0.05219959533934338120, 16.53943276465976808, 77.50109039468567573 ) ) ;
#160504=CARTESIAN_POINT ( 'NONE',  ( 15.72974639402176855, 15.80617190586768217, 31.87609039468567929 ) ) ;
#160505=CARTESIAN_POINT ( 'NONE',  ( 13.97604488694527802, 13.89961937509977652, 114.3739096053143669 ) ) ;
#160506=CARTESIAN_POINT ( 'NONE',  ( -21.52544592524343514, 5.823673210054127303, 86.04057627198102409 ) ) ;
#160507=CARTESIAN_POINT ( 'NONE',  ( -8.314922557960811034, -14.29746914071050412, 42.08224293864769550 ) ) ;
#160508=CARTESIAN_POINT ( 'NONE',  ( 5.153800228976335163, 19.02544592524342804, 39.79057627198100988 ) ) ;
#160509=CARTESIAN_POINT ( 'NONE',  ( 8.224510206698953496, -14.34966873604960469, 72.91557627198103830 ) ) ;
#160510=CARTESIAN_POINT ( 'NONE',  ( 21.53943276465977519, -0.05219959533907433946, 28.74890960531435624 ) ) ;
#160511=CARTESIAN_POINT ( 'NONE',  ( -16.46253265017146816, -9.564922557961047289, 34.16775706135233293 ) ) ;
#160512=CARTESIAN_POINT ( 'NONE',  ( -14.29746914071049879, 8.314922557960819915, 100.8322429386477097 ) ) ;
#160513=CARTESIAN_POINT ( 'NONE',  ( -19.05341960407611168, -5.049401038298163336, 106.4572429386476955 ) ) ;
#160515=CARTESIAN_POINT ( 'NONE',  ( -4.483927247898782831, 16.52544592524335698, 47.70942372801902565 ) ) ;
#160516=CARTESIAN_POINT ( 'NONE',  ( 9.474510206698971260, -16.51473224551069308, 52.91557627198102409 ) ) ;
#160518=CARTESIAN_POINT ( 'NONE',  ( -12.14591786802326823, 12.06949235617739902, 88.12609039468570415 ) ) ;
#160519=CARTESIAN_POINT ( 'NONE',  ( 19.02544592524334988, 5.153800228976608722, 106.4594237280190185 ) ) ;
#160520=CARTESIAN_POINT ( 'NONE',  ( 15.80617190586769283, -15.72974639402175789, 80.62609039468567573 ) ) ;
#160521=CARTESIAN_POINT ( 'NONE',  ( 19.02544592524343514, -5.153800228976328945, 78.54057627198099567 ) ) ;
#160522=CARTESIAN_POINT ( 'NONE',  ( 21.52544592524344225, -5.823673210054117533, 108.5405762719810241 ) ) ;
#160523=CARTESIAN_POINT ( 'NONE',  ( -16.55341960407617563, 4.379528057220093196, 58.54275706135235424 ) ) ;
#160524=CARTESIAN_POINT ( 'NONE',  ( 16.53943276465976808, -0.05219959533910856209, 113.7489096053143527 ) ) ;
#160526=EDGE_CURVE ( 'NONE', #1176, #8743, #181543, .T. ) ;
#160527=CARTESIAN_POINT ( 'NONE',  ( -16.52544592524335698, -4.483927247898792601, 18.95942372801901143 ) ) ;
#160528=CARTESIAN_POINT ( 'NONE',  ( -19.02544592524334988, -5.153800228976617603, 78.95942372801900433 ) ) ;
#160529=CARTESIAN_POINT ( 'NONE',  ( 18.67979575497178502, 10.72451020669898547, 79.16557627198103830 ) ) ;
#160530=CARTESIAN_POINT ( 'NONE',  ( -19.02544592524334988, -5.153800228976617603, 48.95942372801900433 ) ) ;
#160532=CARTESIAN_POINT ( 'NONE',  ( 15.80617190586746368, 15.72974639402197994, 104.3739096053143669 ) ) ;
#160533=CARTESIAN_POINT ( 'NONE',  ( 17.50000000000002132, 3.305555262949611439, 27.87482847843411804 ) ) ;
#160534=CARTESIAN_POINT ( 'NONE',  ( -13.97604488694527625, -13.89961937509977652, 66.87390960531436690 ) ) ;
#160536=CARTESIAN_POINT ( 'NONE',  ( 13.89961937509957401, 13.97604488694547697, 111.8760903946856757 ) ) ;
#160538=CARTESIAN_POINT ( 'NONE',  ( -18.62759615963255300, -10.81492255796106328, 54.16775706135235424 ) ) ;
#160539=CARTESIAN_POINT ( 'NONE',  ( 21.52544592524344225, -5.823673210054117533, 98.54057627198105251 ) ) ;
#160540=CARTESIAN_POINT ( 'NONE',  ( -14.29746914071049879, 8.314922557960819915, 65.83224293864769550 ) ) ;
#160541=CARTESIAN_POINT ( 'NONE',  ( 16.46253265017160672, -9.564922557960803928, 68.33224293864770971 ) ) ;
#160542=CARTESIAN_POINT ( 'NONE',  ( 21.53943276465977519, 0.05219959533937863772, 76.25109039468568994 ) ) ;
#160543=CARTESIAN_POINT ( 'NONE',  ( 12.14591786802327356, -12.06949235617739191, 25.62609039468567929 ) ) ;
#160544=CARTESIAN_POINT ( 'NONE',  ( -5.049401038297874678, -19.05341960407617918, 34.79275706135233293 ) ) ;
#160545=CARTESIAN_POINT ( 'NONE',  ( -15.80617190586768217, 15.72974639402176855, 58.12609039468568994 ) ) ;
#160546=CARTESIAN_POINT ( 'NONE',  ( 21.52544592524344225, -5.823673210054117533, 108.5405762719810241 ) ) ;
#160547=CARTESIAN_POINT ( 'NONE',  ( -10.72451020669898014, 18.67979575497178502, 65.41557627198102409 ) ) ;
#160548=CARTESIAN_POINT ( 'NONE',  ( 5.153800228976615827, -19.02544592524334988, 100.2094237280190043 ) ) ;
#160549=CARTESIAN_POINT ( 'NONE',  ( -9.474510206698720793, -16.51473224551083518, 64.58442372801900433 ) ) ;
#160550=CARTESIAN_POINT ( 'NONE',  ( -21.52544592524334988, -5.823673210054445271, 88.95942372801901854 ) ) ;
#160551=CARTESIAN_POINT ( 'NONE',  ( 13.97604488694548053, -13.89961937509957401, 50.62609039468566152 ) ) ;
#160552=CARTESIAN_POINT ( 'NONE',  ( 0.05219959533909260263, 19.03943276465977164, 39.99890960531436690 ) ) ;
#160553=CARTESIAN_POINT ( 'NONE',  ( 18.67979575497178502, 10.72451020669898547, 64.16557627198102409 ) ) ;
#160554=CARTESIAN_POINT ( 'NONE',  ( 4.379528057220339221, -16.55341960407611168, 47.70724293864770260 ) ) ;
#160555=CARTESIAN_POINT ( 'NONE',  ( -16.61371651742599553, -7.165104196376250734, 26.14584930007006491 ) ) ;
#160556=CARTESIAN_POINT ( 'NONE',  ( 19.05341960407617918, -5.049401038297876454, 31.04275706135232227 ) ) ;
#160557=CARTESIAN_POINT ( 'NONE',  ( 8.314922557961029526, -14.29746914071037800, 80.41775706135234714 ) ) ;
#160558=CARTESIAN_POINT ( 'NONE',  ( -4.379528057220328563, 16.55341960407611168, 60.20724293864768839 ) ) ;
#160559=CARTESIAN_POINT ( 'NONE',  ( -15.80617190586768217, 15.72974639402176855, 93.12609039468568994 ) ) ;
#160560=CARTESIAN_POINT ( 'NONE',  ( -10.81492255796105439, 18.62759615963255655, 77.91775706135231871 ) ) ;
#160561=CARTESIAN_POINT ( 'NONE',  ( -0.05219959533907301413, -21.53943276465977519, 77.49890960531433848 ) ) ;
#160563=CARTESIAN_POINT ( 'NONE',  ( 13.97604488694527802, 13.89961937509977652, 54.37390960531435979 ) ) ;
#160564=CARTESIAN_POINT ( 'NONE',  ( 10.72451020669871369, 18.67979575497193778, 52.08442372801901854 ) ) ;
#160565=CARTESIAN_POINT ( 'NONE',  ( -9.564922557960796823, -16.46253265017161027, 32.08224293864769550 ) ) ;
#160566=CARTESIAN_POINT ( 'NONE',  ( -5.049401038298153566, 19.05341960407611168, 50.20724293864770260 ) ) ;
#160567=CARTESIAN_POINT ( 'NONE',  ( 0.05219959533910956823, 16.53943276465976808, 104.9989096053143669 ) ) ;
#160568=CARTESIAN_POINT ( 'NONE',  ( -9.564922557960796823, -16.46253265017161027, 97.08224293864769550 ) ) ;
#160569=CARTESIAN_POINT ( 'NONE',  ( -12.06949235617756955, 12.14591786802309770, 55.62390960531436690 ) ) ;
#160570=CARTESIAN_POINT ( 'NONE',  ( -4.483927247898539470, -16.52544592524342804, 107.2905762719810525 ) ) ;
#160571=CARTESIAN_POINT ( 'NONE',  ( -0.05219959533907301413, -21.53943276465977519, 77.49890960531433848 ) ) ;
#160572=CARTESIAN_POINT ( 'NONE',  ( 10.81492255796106328, -18.62759615963255655, 25.41775706135235779 ) ) ;
#160574=CARTESIAN_POINT ( 'NONE',  ( -16.55341960407617563, 4.379528057220093196, 38.54275706135234714 ) ) ;
#160576=CARTESIAN_POINT ( 'NONE',  ( 21.52544592524344225, -5.823673210054117533, 68.54057627198103830 ) ) ;
#160577=CARTESIAN_POINT ( 'NONE',  ( 5.823673210054444382, -21.52544592524334988, 105.2094237280190328 ) ) ;
#160578=CARTESIAN_POINT ( 'NONE',  ( 13.97604488694527802, 13.89961937509977652, 94.37390960531436690 ) ) ;
#160579=CARTESIAN_POINT ( 'NONE',  ( -15.72974639402176322, -15.80617190586768395, 29.37609039468568284 ) ) ;
#160580=CARTESIAN_POINT ( 'NONE',  ( -5.823673210054116645, -21.52544592524344225, 27.29057627198103120 ) ) ;
#160581=CARTESIAN_POINT ( 'NONE',  ( -14.29746914071037622, -8.314922557961029526, 104.1677570613523471 ) ) ;
#160582=CARTESIAN_POINT ( 'NONE',  ( 21.52544592524334988, 5.823673210054432836, 86.45942372801901854 ) ) ;
#160583=CARTESIAN_POINT ( 'NONE',  ( -19.03943276465977164, -0.05219959533935918106, 23.75109039468566152 ) ) ;
#160584=CARTESIAN_POINT ( 'NONE',  ( 16.55341960407618274, -4.379528057220086978, 76.04275706135237556 ) ) ;
#160585=CARTESIAN_POINT ( 'NONE',  ( 0.05219959533937995610, -21.53943276465977519, 35.00109039468568284 ) ) ;
#160586=CARTESIAN_POINT ( 'NONE',  ( -16.51473224551069308, -9.474510206698971260, 31.66557627198102054 ) ) ;
#160587=CARTESIAN_POINT ( 'NONE',  ( 5.823673210054444382, -21.52544592524334988, 100.2094237280190043 ) ) ;
#160588=CARTESIAN_POINT ( 'NONE',  ( 16.46253265017160672, -9.564922557960803928, 103.3322429386476955 ) ) ;
#160589=CARTESIAN_POINT ( 'NONE',  ( -5.719274019375978568, 21.55341960407610458, 100.2072429386476955 ) ) ;
#160590=CARTESIAN_POINT ( 'NONE',  ( 19.19724070472096855, 5.499999999999978684, 83.56193348274379673 ) ) ;
#160591=CARTESIAN_POINT ( 'NONE',  ( 5.719274019375991003, -21.55341960407610458, 72.70724293864769550 ) ) ;
#160592=CARTESIAN_POINT ( 'NONE',  ( 12.06949235617739724, 12.14591786802326823, 56.87609039468568994 ) ) ;
#160593=CARTESIAN_POINT ( 'NONE',  ( 12.14591786802309770, 12.06949235617756955, 54.37390960531435979 ) ) ;
#160595=CARTESIAN_POINT ( 'NONE',  ( 9.564922557961047289, -16.46253265017146816, 80.41775706135234714 ) ) ;
#160597=CARTESIAN_POINT ( 'NONE',  ( -8.314922557961024197, 14.29746914071037800, 22.91775706135235069 ) ) ;
#160598=CARTESIAN_POINT ( 'NONE',  ( 5.823673210054125526, 21.52544592524343514, 94.79057627198105251 ) ) ;
#160599=CARTESIAN_POINT ( 'NONE',  ( -14.29746914071049879, 8.314922557960819915, 70.83224293864770971 ) ) ;
#160600=CARTESIAN_POINT ( 'NONE',  ( -5.719274019375978568, 21.55341960407610458, 25.20724293864769550 ) ) ;
#160601=CARTESIAN_POINT ( 'NONE',  ( -8.224510206698735004, -14.34966873604973081, 39.58442372801901143 ) ) ;
#160602=CARTESIAN_POINT ( 'NONE',  ( -16.51473224551069308, -9.474510206698971260, 51.66557627198102409 ) ) ;
#160603=CARTESIAN_POINT ( 'NONE',  ( 21.55341960407619695, -5.719274019375665929, 36.04275706135234714 ) ) ;
#160604=CARTESIAN_POINT ( 'NONE',  ( 16.46253265017146816, 9.564922557961045513, 96.66775706135233293 ) ) ;
#160605=CARTESIAN_POINT ( 'NONE',  ( 19.02544592524343514, -5.153800228976328945, 98.54057627198100988 ) ) ;
#160606=CARTESIAN_POINT ( 'NONE',  ( 19.02544592524343514, -5.153800228976328945, 93.54057627198102409 ) ) ;
#160607=CARTESIAN_POINT ( 'NONE',  ( -0.05219959533907301413, -21.53943276465977519, 92.49890960531436690 ) ) ;
#160608=CARTESIAN_POINT ( 'NONE',  ( 5.049401038298161559, -19.05341960407611168, 42.70724293864767418 ) ) ;
#160609=CARTESIAN_POINT ( 'NONE',  ( -16.31925111598457079, -7.325300261831483972, 59.83575461032751264 ) ) ;
#160610=CARTESIAN_POINT ( 'NONE',  ( -12.14591786802309592, -12.06949235617757132, 66.87390960531436690 ) ) ;
#160611=CARTESIAN_POINT ( 'NONE',  ( -13.97604488694527625, -13.89961937509977652, 106.8739096053143669 ) ) ;
#160613=CARTESIAN_POINT ( 'NONE',  ( 13.89961937509957401, 13.97604488694547697, 81.87609039468564731 ) ) ;
#160614=CARTESIAN_POINT ( 'NONE',  ( -18.62759615963270932, 10.81492255796079327, 95.83224293864770971 ) ) ;
#160615=CARTESIAN_POINT ( 'NONE',  ( -13.89961937509957401, -13.97604488694547875, 49.37609039468567573 ) ) ;
#160616=CARTESIAN_POINT ( 'NONE',  ( -16.46253265017160317, 9.564922557960807481, 110.8322429386476955 ) ) ;
#160617=CARTESIAN_POINT ( 'NONE',  ( -18.67979575497178146, -10.72451020669898902, 56.66557627198103830 ) ) ;
#160618=CARTESIAN_POINT ( 'NONE',  ( 0.05219959533909260263, 19.03943276465977164, 89.99890960531436690 ) ) ;
#160619=CARTESIAN_POINT ( 'NONE',  ( 15.80617190586769283, -15.72974639402175789, 60.62609039468567573 ) ) ;
#160620=CARTESIAN_POINT ( 'NONE',  ( -0.05219959533909027116, -19.03943276465977164, 37.49890960531436690 ) ) ;
#160621=CARTESIAN_POINT ( 'NONE',  ( 8.224510206698953496, -14.34966873604960469, 72.91557627198103830 ) ) ;
#160622=CARTESIAN_POINT ( 'NONE',  ( -16.53943276465976808, -0.05219959533934237506, 18.75109039468568639 ) ) ;
#160623=CARTESIAN_POINT ( 'NONE',  ( -5.823673210054431948, 21.52544592524334988, 57.70942372801901143 ) ) ;
#160624=VERTEX_POINT ( 'NONE', #100173 ) ;
#160625=CARTESIAN_POINT ( 'NONE',  ( 16.51473224551069308, 9.474510206698969483, 114.1655762719810241 ) ) ;
#160626=CARTESIAN_POINT ( 'NONE',  ( -19.05341960407617563, 5.049401038297882671, 73.54275706135233293 ) ) ;
#160628=CARTESIAN_POINT ( 'NONE',  ( 0.05219959533907565091, 21.53943276465977519, 114.9989096053143669 ) ) ;
#160630=CARTESIAN_POINT ( 'NONE',  ( -9.474510206698720793, -16.51473224551083518, 19.58442372801899722 ) ) ;
#160631=CARTESIAN_POINT ( 'NONE',  ( -13.89961937509977652, 13.97604488694528158, 60.62390960531436690 ) ) ;
#160632=CARTESIAN_POINT ( 'NONE',  ( 21.53943276465977519, 0.05219959533937863772, 106.2510903946856757 ) ) ;
#160633=CARTESIAN_POINT ( 'NONE',  ( 16.55341960407618274, -4.379528057220086978, 106.0427570613523471 ) ) ;
#160634=CARTESIAN_POINT ( 'NONE',  ( 5.049401038298161559, -19.05341960407611168, 102.7072429386476955 ) ) ;
#160635=CARTESIAN_POINT ( 'NONE',  ( 0.05219959533937995610, -21.53943276465977519, 70.00109039468568994 ) ) ;
#160639=CARTESIAN_POINT ( 'NONE',  ( 0.05219959533937995610, -21.53943276465977519, 75.00109039468568994 ) ) ;
#160640=CARTESIAN_POINT ( 'NONE',  ( 21.55341960407619695, -5.719274019375665929, 106.0427570613523471 ) ) ;
#160642=CARTESIAN_POINT ( 'NONE',  ( -9.474510206698964154, 16.51473224551069663, 90.41557627198103830 ) ) ;
#160643=CARTESIAN_POINT ( 'NONE',  ( -5.153800228976607833, 19.02544592524334988, 22.70942372801899012 ) ) ;
#160645=CARTESIAN_POINT ( 'NONE',  ( 19.02544592524343514, -5.153800228976328945, 43.54057627198103120 ) ) ;
#160646=CARTESIAN_POINT ( 'NONE',  ( 21.52544592524344225, -5.823673210054117533, 58.54057627198103120 ) ) ;
#160647=CARTESIAN_POINT ( 'NONE',  ( -14.34966873604972548, 8.224510206698743886, 108.3344237280190185 ) ) ;
#160648=CARTESIAN_POINT ( 'NONE',  ( -14.34966873604960291, -8.224510206698953496, 101.6655762719810383 ) ) ;
#160649=CARTESIAN_POINT ( 'NONE',  ( -13.97604488694527625, -13.89961937509977652, 86.87390960531436690 ) ) ;
#160650=CARTESIAN_POINT ( 'NONE',  ( -5.823673210054431948, 21.52544592524334988, 97.70942372801904696 ) ) ;
#160651=CARTESIAN_POINT ( 'NONE',  ( 9.474510206698971260, -16.51473224551069308, 37.91557627198102409 ) ) ;
#160652=CARTESIAN_POINT ( 'NONE',  ( -4.483927247898539470, -16.52544592524342804, 97.29057627198105251 ) ) ;
#160653=CARTESIAN_POINT ( 'NONE',  ( 15.80617190586769283, -15.72974639402175789, 50.62609039468568994 ) ) ;
#160654=CARTESIAN_POINT ( 'NONE',  ( -15.80617190586745835, -15.72974639402198527, 91.87390960531436690 ) ) ;
#160655=CARTESIAN_POINT ( 'NONE',  ( 5.153800228976615827, -19.02544592524334988, 55.20942372801899722 ) ) ;
#160656=CARTESIAN_POINT ( 'NONE',  ( -0.05219959533909027116, -19.03943276465977164, 47.49890960531435979 ) ) ;
#160657=CARTESIAN_POINT ( 'NONE',  ( 9.474510206698971260, -16.51473224551069308, 92.91557627198103830 ) ) ;
#160658=CARTESIAN_POINT ( 'NONE',  ( -8.314922557960811034, -14.29746914071050412, 72.08224293864769550 ) ) ;
#160659=CARTESIAN_POINT ( 'NONE',  ( -5.049401038297874678, -19.05341960407617918, 49.79275706135231871 ) ) ;
#160661=CARTESIAN_POINT ( 'NONE',  ( 5.153800228976335163, 19.02544592524342804, 69.79057627198103830 ) ) ;
#160662=CARTESIAN_POINT ( 'NONE',  ( 16.55341960407611168, 4.379528057220329451, 48.95724293864770971 ) ) ;
#160663=CARTESIAN_POINT ( 'NONE',  ( 19.03943276465977164, 0.05219959533936151252, 81.25109039468567573 ) ) ;
#160664=CARTESIAN_POINT ( 'NONE',  ( -15.80617190586745835, -15.72974639402198527, 31.87390960531435979 ) ) ;
#160665=CARTESIAN_POINT ( 'NONE',  ( 8.314922557960818139, 14.29746914071049879, 99.58224293864770971 ) ) ;
#160666=CARTESIAN_POINT ( 'NONE',  ( -17.50000000000000000, -3.471454075611492218, 25.51667418855629421 ) ) ;
#160667=CARTESIAN_POINT ( 'NONE',  ( 19.03943276465977164, -0.05219959533909143690, 63.74890960531435979 ) ) ;
#160668=CARTESIAN_POINT ( 'NONE',  ( 10.81492255796078972, 18.62759615963270932, 64.58224293864769550 ) ) ;
#160669=CARTESIAN_POINT ( 'NONE',  ( 19.02544592524343514, -5.153800228976328945, 28.54057627198102409 ) ) ;
#160670=CARTESIAN_POINT ( 'NONE',  ( 0.05219959533934541429, -16.53943276465976808, 85.00109039468568994 ) ) ;
#160671=CARTESIAN_POINT ( 'NONE',  ( 0.05219959533909260263, 19.03943276465977164, 54.99890960531435979 ) ) ;
#160672=CARTESIAN_POINT ( 'NONE',  ( 9.474510206698729675, 16.51473224551082808, 47.08442372801900433 ) ) ;
#160673=CARTESIAN_POINT ( 'NONE',  ( -10.72451020669870658, -18.67979575497194134, 69.58442372801900433 ) ) ;
#160674=CARTESIAN_POINT ( 'NONE',  ( -18.62759615963270932, 10.81492255796079327, 55.83224293864770260 ) ) ;
#160675=CARTESIAN_POINT ( 'NONE',  ( 19.02544592524343514, -5.153800228976328945, 23.54057627198102054 ) ) ;
#160676=CARTESIAN_POINT ( 'NONE',  ( -8.224510206698735004, -14.34966873604973081, 84.58442372801903275 ) ) ;
#160677=CARTESIAN_POINT ( 'NONE',  ( -19.03943276465977164, -0.05219959533935918106, 98.75109039468567573 ) ) ;
#160678=CARTESIAN_POINT ( 'NONE',  ( -19.03943276465977164, 0.05219959533909376836, 21.24890960531436335 ) ) ;
#160680=CARTESIAN_POINT ( 'NONE',  ( 21.52544592524344225, -5.823673210054117533, 48.54057627198103120 ) ) ;
#160681=CARTESIAN_POINT ( 'NONE',  ( 5.823673210054444382, -21.52544592524334988, 80.20942372801901854 ) ) ;
#160682=CARTESIAN_POINT ( 'NONE',  ( 14.34966873604960469, 8.224510206698951720, 44.16557627198103120 ) ) ;
#160683=CARTESIAN_POINT ( 'NONE',  ( -12.06949235617756955, 12.14591786802309770, 55.62390960531436690 ) ) ;
#160684=CARTESIAN_POINT ( 'NONE',  ( 21.53943276465977519, -0.05219959533907433946, 83.74890960531435269 ) ) ;
#160685=CARTESIAN_POINT ( 'NONE',  ( -21.52544592524343514, 5.823673210054127303, 81.04057627198102409 ) ) ;
#160686=DIRECTION ( 'NONE',  ( 0.000000000000000000, 0.000000000000000000, 1.000000000000000000 ) ) ;
#160687=CARTESIAN_POINT ( 'NONE',  ( -21.55341960407610458, -5.719274019375992779, 31.45724293864769550 ) ) ;
#160688=EDGE_CURVE ( 'NONE', #165125, #178804, #46509, .T. ) ;
#160689=CARTESIAN_POINT ( 'NONE',  ( -16.55341960407617563, 4.379528057220093196, 63.54275706135234003 ) ) ;
#160690=CARTESIAN_POINT ( 'NONE',  ( 12.14591786802309770, 12.06949235617756955, 79.37390960531436690 ) ) ;
#160691=CARTESIAN_POINT ( 'NONE',  ( 16.51473224551069308, 9.474510206698969483, 29.16557627198103475 ) ) ;
#160694=ORIENTED_EDGE ( 'NONE', *, *, #120448, .T. ) ;
#160695=CARTESIAN_POINT ( 'NONE',  ( 12.14591786802327356, -12.06949235617739191, 85.62609039468568994 ) ) ;
#160696=CARTESIAN_POINT ( 'NONE',  ( -21.52544592524334988, -5.823673210054445271, 18.95942372801901143 ) ) ;
#160697=CARTESIAN_POINT ( 'NONE',  ( -13.89961937509977652, 13.97604488694528158, 85.62390960531433848 ) ) ;
#160698=CARTESIAN_POINT ( 'NONE',  ( 18.62759615963255655, 10.81492255796105972, 56.66775706135235424 ) ) ;
#160699=CARTESIAN_POINT ( 'NONE',  ( -5.153800228976328057, -19.02544592524343514, 107.2905762719810383 ) ) ;
#160702=CARTESIAN_POINT ( 'NONE',  ( 5.823673210054444382, -21.52544592524334988, 40.20942372801901854 ) ) ;
#160703=CARTESIAN_POINT ( 'NONE',  ( 13.89961937509977652, -13.97604488694527269, 38.12390960531436690 ) ) ;
#160704=CARTESIAN_POINT ( 'NONE',  ( -9.474510206698964154, 16.51473224551069663, 105.4155762719810383 ) ) ;
#160705=CARTESIAN_POINT ( 'NONE',  ( -16.51473224551082808, 9.474510206698731452, 48.33442372801900433 ) ) ;
#160706=CARTESIAN_POINT ( 'NONE',  ( -15.72974639402176322, -15.80617190586768395, 34.37609039468568284 ) ) ;
#160707=CARTESIAN_POINT ( 'NONE',  ( -5.153800228976607833, 19.02544592524334988, 42.70942372801901143 ) ) ;
#160708=CARTESIAN_POINT ( 'NONE',  ( 16.51473224551069308, 9.474510206698969483, 29.16557627198103475 ) ) ;
#160709=CARTESIAN_POINT ( 'NONE',  ( 8.224510206698742110, 14.34966873604972548, 92.08442372801901854 ) ) ;
#160710=CARTESIAN_POINT ( 'NONE',  ( 9.474510206698729675, 16.51473224551082808, 57.08442372801900433 ) ) ;
#160711=CARTESIAN_POINT ( 'NONE',  ( 16.55341960407618274, -4.379528057220086978, 106.0427570613523471 ) ) ;
#160713=CARTESIAN_POINT ( 'NONE',  ( 19.02544592524343514, -5.153800228976328945, 88.54057627198102409 ) ) ;
#160714=CARTESIAN_POINT ( 'NONE',  ( -5.823673210054431948, 21.52544592524334988, 92.70942372801901854 ) ) ;
#160715=CARTESIAN_POINT ( 'NONE',  ( -15.80617190586768217, 15.72974639402176855, 108.1260903946856757 ) ) ;
#160717=CARTESIAN_POINT ( 'NONE',  ( -19.02544592524342804, 5.153800228976336051, 106.0405762719810241 ) ) ;
#160718=CARTESIAN_POINT ( 'NONE',  ( 0.05219959533937995610, -21.53943276465977519, 70.00109039468568994 ) ) ;
#160719=CARTESIAN_POINT ( 'NONE',  ( -14.29746914071037622, -8.314922557961029526, 19.16775706135234714 ) ) ;
#160720=CARTESIAN_POINT ( 'NONE',  ( 13.89961937509977652, -13.97604488694527269, 73.12390960531436690 ) ) ;
#160721=CARTESIAN_POINT ( 'NONE',  ( 21.53943276465977519, -0.05219959533907433946, 28.74890960531435624 ) ) ;
#160722=CARTESIAN_POINT ( 'NONE',  ( 16.46253265017160672, -9.564922557960803928, 93.33224293864769550 ) ) ;
#160723=CARTESIAN_POINT ( 'NONE',  ( -16.38665767535051643, -7.295008042176172935, 89.73599135785457293 ) ) ;
#160724=CARTESIAN_POINT ( 'NONE',  ( 16.46253265017160672, -9.564922557960803928, 78.33224293864769550 ) ) ;
#160725=CARTESIAN_POINT ( 'NONE',  ( 5.049401038298161559, -19.05341960407611168, 62.70724293864769550 ) ) ;
#160726=CARTESIAN_POINT ( 'NONE',  ( 12.14591786802327356, -12.06949235617739191, 95.62609039468568994 ) ) ;
#160728=CARTESIAN_POINT ( 'NONE',  ( 5.049401038297881783, 19.05341960407617563, 67.29275706135234714 ) ) ;
#160729=CARTESIAN_POINT ( 'NONE',  ( -13.97604488694527625, -13.89961937509977652, 86.87390960531436690 ) ) ;
#160730=CARTESIAN_POINT ( 'NONE',  ( -0.05219959533910754901, -16.53943276465976808, 82.49890960531436690 ) ) ;
#160731=CARTESIAN_POINT ( 'NONE',  ( 10.81492255796078972, 18.62759615963270932, 34.58224293864770260 ) ) ;
#160732=CARTESIAN_POINT ( 'NONE',  ( -16.46253265017160317, 9.564922557960807481, 115.8322429386477097 ) ) ;
#160733=CARTESIAN_POINT ( 'NONE',  ( 12.14591786802309770, 12.06949235617756955, 109.3739096053143811 ) ) ;
#160735=CARTESIAN_POINT ( 'NONE',  ( -13.97604488694547697, 13.89961937509957934, 43.12609039468566152 ) ) ;
#160736=CARTESIAN_POINT ( 'NONE',  ( 16.55341960407611168, 4.379528057220329451, 23.95724293864769550 ) ) ;
#160737=CARTESIAN_POINT ( 'NONE',  ( -19.03943276465977164, 0.05219959533909376836, 106.2489096053143669 ) ) ;
#160738=CARTESIAN_POINT ( 'NONE',  ( 21.55341960407619695, -5.719274019375665929, 71.04275706135234714 ) ) ;
#160739=CARTESIAN_POINT ( 'NONE',  ( 21.53943276465977519, -0.05219959533907433946, 63.74890960531435979 ) ) ;
#160740=CARTESIAN_POINT ( 'NONE',  ( 21.53943276465977519, 0.05219959533937863772, 36.25109039468567573 ) ) ;
#160741=CARTESIAN_POINT ( 'NONE',  ( -0.05219959533907301413, -21.53943276465977519, 77.49890960531433848 ) ) ;
#160742=CARTESIAN_POINT ( 'NONE',  ( -21.55341960407619339, 5.719274019375674811, 43.54275706135235424 ) ) ;
#160743=CARTESIAN_POINT ( 'NONE',  ( 8.224510206698953496, -14.34966873604960469, 107.9155762719810241 ) ) ;
#160744=CARTESIAN_POINT ( 'NONE',  ( 9.564922557961047289, -16.46253265017146816, 75.41775706135234714 ) ) ;
#160745=CARTESIAN_POINT ( 'NONE',  ( -9.474510206698964154, 16.51473224551069663, 50.41557627198102409 ) ) ;
#160746=CARTESIAN_POINT ( 'NONE',  ( -12.06949235617756955, 12.14591786802309770, 95.62390960531436690 ) ) ;
#160747=CARTESIAN_POINT ( 'NONE',  ( 5.153800228976335163, 19.02544592524342804, 94.79057627198103830 ) ) ;
#160748=CARTESIAN_POINT ( 'NONE',  ( 5.153800228976335163, 19.02544592524342804, 94.79057627198103830 ) ) ;
#160749=CARTESIAN_POINT ( 'NONE',  ( -5.153800228976328057, -19.02544592524343514, 22.29057627198102765 ) ) ;
#160750=CARTESIAN_POINT ( 'NONE',  ( -4.483927247898539470, -16.52544592524342804, 47.29057627198103120 ) ) ;
#160751=CARTESIAN_POINT ( 'NONE',  ( -16.52544592524335698, -4.483927247898792601, 98.95942372801903275 ) ) ;
#160752=CARTESIAN_POINT ( 'NONE',  ( 5.049401038298161559, -19.05341960407611168, 52.70724293864767418 ) ) ;
#160753=CARTESIAN_POINT ( 'NONE',  ( 9.474510206698971260, -16.51473224551069308, 27.91557627198103120 ) ) ;
#160754=CARTESIAN_POINT ( 'NONE',  ( -19.05341960407617563, 5.049401038297882671, 23.54275706135233648 ) ) ;
#160755=AXIS2_PLACEMENT_3D ( 'NONE', #89323, #166181, #43820 ) ;
#160756=FACE_OUTER_BOUND ( 'NONE', #5483, .T. ) ;
#160757=CARTESIAN_POINT ( 'NONE',  ( -12.14591786802309592, -12.06949235617757132, 26.87390960531435979 ) ) ;
#160758=CARTESIAN_POINT ( 'NONE',  ( 21.53943276465977519, 0.05219959533937863772, 51.25109039468568994 ) ) ;
#160760=CARTESIAN_POINT ( 'NONE',  ( 4.379528057220092307, 16.55341960407617563, 52.29275706135236135 ) ) ;
#160761=EDGE_CURVE ( 'NONE', #25133, #50018, #82648, .T. ) ;
#160762=CARTESIAN_POINT ( 'NONE',  ( 16.53943276465976808, -0.05219959533910856209, 33.74890960531436690 ) ) ;
#160763=CARTESIAN_POINT ( 'NONE',  ( -9.474510206698964154, 16.51473224551069663, 40.41557627198103120 ) ) ;
#160764=CARTESIAN_POINT ( 'NONE',  ( -16.52544592524335698, -4.483927247898792601, 103.9594237280190185 ) ) ;
#160765=CARTESIAN_POINT ( 'NONE',  ( 14.34966873604972726, -8.224510206698740333, 20.83442372801901143 ) ) ;
#160766=CARTESIAN_POINT ( 'NONE',  ( -16.51473224551069308, -9.474510206698971260, 46.66557627198102409 ) ) ;
#160767=CARTESIAN_POINT ( 'NONE',  ( 8.224510206698953496, -14.34966873604960469, 102.9155762719810383 ) ) ;
#160768=CARTESIAN_POINT ( 'NONE',  ( 15.80617190586746368, 15.72974639402197994, 114.3739096053143527 ) ) ;
#160769=CARTESIAN_POINT ( 'NONE',  ( -9.564922557960796823, -16.46253265017161027, 52.08224293864768839 ) ) ;
#160770=CARTESIAN_POINT ( 'NONE',  ( -13.89961937509977652, 13.97604488694528158, 100.6239096053143669 ) ) ;
#160771=CARTESIAN_POINT ( 'NONE',  ( 13.89961937509977652, -13.97604488694527269, 33.12390960531434558 ) ) ;
#160772=CARTESIAN_POINT ( 'NONE',  ( 0.05219959533909260263, 19.03943276465977164, 99.99890960531436690 ) ) ;
#160775=CARTESIAN_POINT ( 'NONE',  ( 13.89961937509977652, -13.97604488694527269, 93.12390960531436690 ) ) ;
#160776=CARTESIAN_POINT ( 'NONE',  ( 15.80617190586769283, -15.72974639402175789, 40.62609039468567573 ) ) ;
#160777=CARTESIAN_POINT ( 'NONE',  ( -4.379528057220328563, 16.55341960407611168, 100.2072429386476955 ) ) ;
#160778=CARTESIAN_POINT ( 'NONE',  ( -13.89961937509977652, 13.97604488694528158, 110.6239096053143243 ) ) ;
#160779=CARTESIAN_POINT ( 'NONE',  ( 16.51473224551083163, -9.474510206698727899, 70.83442372801900433 ) ) ;
#160780=CARTESIAN_POINT ( 'NONE',  ( 16.52544592524335698, 4.483927247898782831, 61.45942372801901854 ) ) ;
#160781=CARTESIAN_POINT ( 'NONE',  ( 15.72974639402176855, 15.80617190586768217, 96.87609039468568994 ) ) ;
#160783=CARTESIAN_POINT ( 'NONE',  ( 16.53943276465976808, 0.05219959533934440121, 56.25109039468568284 ) ) ;
#160784=CARTESIAN_POINT ( 'NONE',  ( -19.02544592524342804, 5.153800228976336051, 101.0405762719810241 ) ) ;
#160785=CARTESIAN_POINT ( 'NONE',  ( -16.53943276465976808, -0.05219959533934237506, 43.75109039468568284 ) ) ;
#160786=CARTESIAN_POINT ( 'NONE',  ( 0.05219959533936267826, -19.03943276465977164, 110.0010903946856757 ) ) ;
#160787=CARTESIAN_POINT ( 'NONE',  ( -0.05219959533934338120, 16.53943276465976808, 87.50109039468568994 ) ) ;
#160788=CARTESIAN_POINT ( 'NONE',  ( -5.153800228976607833, 19.02544592524334988, 97.70942372801900433 ) ) ;
#160789=CARTESIAN_POINT ( 'NONE',  ( -19.03943276465977164, 0.05219959533909376836, 81.24890960531436690 ) ) ;
#160790=CARTESIAN_POINT ( 'NONE',  ( 0.05219959533907565091, 21.53943276465977519, 99.99890960531436690 ) ) ;
#160791=CARTESIAN_POINT ( 'NONE',  ( 4.379528057220339221, -16.55341960407611168, 87.70724293864769550 ) ) ;
#160792=CARTESIAN_POINT ( 'NONE',  ( 9.474510206698729675, 16.51473224551082808, 107.0844237280190043 ) ) ;
#160793=CARTESIAN_POINT ( 'NONE',  ( -0.05219959533934338120, 16.53943276465976808, 67.50109039468568994 ) ) ;
#160795=CARTESIAN_POINT ( 'NONE',  ( -5.049401038297874678, -19.05341960407617918, 74.79275706135231871 ) ) ;
#160796=CARTESIAN_POINT ( 'NONE',  ( 12.06949235617757843, -12.14591786802309237, 38.12390960531436690 ) ) ;
#160797=CARTESIAN_POINT ( 'NONE',  ( -12.06949235617756955, 12.14591786802309770, 95.62390960531436690 ) ) ;
#160798=CARTESIAN_POINT ( 'NONE',  ( 19.05341960407617918, -5.049401038297876454, 36.04275706135234003 ) ) ;
#160799=CARTESIAN_POINT ( 'NONE',  ( -16.31925111598456368, 7.325300261831606541, 90.16424538967254421 ) ) ;
#160800=CARTESIAN_POINT ( 'NONE',  ( -21.53943276465977519, -0.05219959533937600094, 23.75109039468567929 ) ) ;
#160801=CARTESIAN_POINT ( 'NONE',  ( 5.049401038297881783, 19.05341960407617563, 102.2927570613523045 ) ) ;
#160802=CARTESIAN_POINT ( 'NONE',  ( 9.564922557960805705, 16.46253265017160317, 114.5822429386476955 ) ) ;
#160803=CARTESIAN_POINT ( 'NONE',  ( -13.97604488694527625, -13.89961937509977652, 86.87390960531436690 ) ) ;
#160804=CARTESIAN_POINT ( 'NONE',  ( -5.719274019375665041, -21.55341960407619695, 99.79275706135234714 ) ) ;
#160805=CARTESIAN_POINT ( 'NONE',  ( -0.05219959533909027116, -19.03943276465977164, 72.49890960531435269 ) ) ;
#160806=CARTESIAN_POINT ( 'NONE',  ( -15.80617190586745835, -15.72974639402198527, 36.87390960531435979 ) ) ;
#160807=CARTESIAN_POINT ( 'NONE',  ( -12.14591786802309592, -12.06949235617757132, 96.87390960531436690 ) ) ;
#160808=CARTESIAN_POINT ( 'NONE',  ( -19.02544592524342804, 5.153800228976336051, 51.04057627198103120 ) ) ;
#160809=CARTESIAN_POINT ( 'NONE',  ( 4.483927247898545687, 16.52544592524342804, 114.7905762719810383 ) ) ;
#160810=CARTESIAN_POINT ( 'NONE',  ( 10.81492255796106328, -18.62759615963255655, 20.41775706135234714 ) ) ;
#160811=CARTESIAN_POINT ( 'NONE',  ( -18.62759615963255300, -10.81492255796106328, 59.16775706135234714 ) ) ;
#160812=CARTESIAN_POINT ( 'NONE',  ( 16.51473224551069308, 9.474510206698969483, 39.16557627198103120 ) ) ;
#160813=CARTESIAN_POINT ( 'NONE',  ( 16.55341960407618274, -4.379528057220086978, 71.04275706135234714 ) ) ;
#160814=CARTESIAN_POINT ( 'NONE',  ( -5.719274019375665041, -21.55341960407619695, 19.79275706135235069 ) ) ;
#160816=CARTESIAN_POINT ( 'NONE',  ( -5.719274019375978568, 21.55341960407610458, 115.2072429386476955 ) ) ;
#160817=CARTESIAN_POINT ( 'NONE',  ( 19.03943276465977164, 0.05219959533936151252, 56.25109039468566863 ) ) ;
#160818=CARTESIAN_POINT ( 'NONE',  ( 19.03943276465977164, -0.05219959533909143690, 63.74890960531435979 ) ) ;
#160819=CARTESIAN_POINT ( 'NONE',  ( -16.51473224551082808, 9.474510206698731452, 33.33442372801899722 ) ) ;
#160820=CARTESIAN_POINT ( 'NONE',  ( 5.823673210054444382, -21.52544592524334988, 65.20942372801901854 ) ) ;
#160821=CARTESIAN_POINT ( 'NONE',  ( 5.719274019375991003, -21.55341960407610458, 72.70724293864769550 ) ) ;
#160822=CARTESIAN_POINT ( 'NONE',  ( 4.483927247898545687, 16.52544592524342804, 54.79057627198104541 ) ) ;
#160823=CARTESIAN_POINT ( 'NONE',  ( 18.67979575497194134, -10.72451020669871369, 90.83442372801901854 ) ) ;
#160824=CARTESIAN_POINT ( 'NONE',  ( 0.05219959533936267826, -19.03943276465977164, 25.00109039468566152 ) ) ;
#160825=CARTESIAN_POINT ( 'NONE',  ( -16.53943276465976808, 0.05219959533911058130, 76.24890960531435269 ) ) ;
#160826=CARTESIAN_POINT ( 'NONE',  ( 14.34966873604960469, 8.224510206698951720, 114.1655762719810383 ) ) ;
#160827=CARTESIAN_POINT ( 'NONE',  ( 16.46253265017146816, 9.564922557961045513, 61.66775706135234003 ) ) ;
#160828=CARTESIAN_POINT ( 'NONE',  ( -0.05219959533910754901, -16.53943276465976808, 22.49890960531436335 ) ) ;
#160829=CARTESIAN_POINT ( 'NONE',  ( 10.81492255796106328, -18.62759615963255655, 75.41775706135233293 ) ) ;
#160830=CARTESIAN_POINT ( 'NONE',  ( -16.51473224551082808, 9.474510206698731452, 43.33442372801900433 ) ) ;
#160831=CARTESIAN_POINT ( 'NONE',  ( 5.823673210054125526, 21.52544592524343514, 54.79057627198104541 ) ) ;
#160832=CARTESIAN_POINT ( 'NONE',  ( 15.80617190586769283, -15.72974639402175789, 40.62609039468567573 ) ) ;
#160833=CARTESIAN_POINT ( 'NONE',  ( -5.719274019375978568, 21.55341960407610458, 95.20724293864769550 ) ) ;
#160834=CARTESIAN_POINT ( 'NONE',  ( -19.03943276465977164, -0.05219959533935918106, 103.7510903946856757 ) ) ;
#160835=CARTESIAN_POINT ( 'NONE',  ( 8.224510206698742110, 14.34966873604972548, 67.08442372801901854 ) ) ;
#160837=CARTESIAN_POINT ( 'NONE',  ( 18.67979575497178502, 10.72451020669898547, 104.1655762719810241 ) ) ;
#160838=CARTESIAN_POINT ( 'NONE',  ( -8.314922557960811034, -14.29746914071050412, 87.08224293864769550 ) ) ;
#160839=CARTESIAN_POINT ( 'NONE',  ( -17.05587630539786304, -6.762274262135706593, 99.25819690962688924 ) ) ;
#160840=CARTESIAN_POINT ( 'NONE',  ( 12.06949235617739724, 12.14591786802326823, 21.87609039468567573 ) ) ;
#160841=CARTESIAN_POINT ( 'NONE',  ( 5.719274019375991003, -21.55341960407610458, 47.70724293864770260 ) ) ;
#160842=CARTESIAN_POINT ( 'NONE',  ( -4.483927247898782831, 16.52544592524335698, 87.70942372801901854 ) ) ;
#160843=CARTESIAN_POINT ( 'NONE',  ( -9.564922557960796823, -16.46253265017161027, 22.08224293864768839 ) ) ;
#160844=CARTESIAN_POINT ( 'NONE',  ( -8.314922557961024197, 14.29746914071037800, 62.91775706135236135 ) ) ;
#160845=CARTESIAN_POINT ( 'NONE',  ( -10.72451020669870658, -18.67979575497194134, 44.58442372801901854 ) ) ;
#160846=CARTESIAN_POINT ( 'NONE',  ( 21.53943276465977519, -0.05219959533907433946, 63.74890960531435979 ) ) ;
#160847=CARTESIAN_POINT ( 'NONE',  ( -4.483927247898782831, 16.52544592524335698, 82.70942372801900433 ) ) ;
#160848=CARTESIAN_POINT ( 'NONE',  ( 16.51473224551069308, 9.474510206698969483, 94.16557627198103830 ) ) ;
#160849=CARTESIAN_POINT ( 'NONE',  ( 18.67979575497194134, -10.72451020669871369, 75.83442372801900433 ) ) ;
#160850=CARTESIAN_POINT ( 'NONE',  ( 18.62759615963271287, -10.81492255796078972, 58.33224293864768839 ) ) ;
#160851=CARTESIAN_POINT ( 'NONE',  ( -5.823673210054116645, -21.52544592524344225, 37.29057627198102409 ) ) ;
#160852=ORIENTED_EDGE ( 'NONE', *, *, #128318, .F. ) ;
#160853=CARTESIAN_POINT ( 'NONE',  ( -4.379528057220086978, -16.55341960407618274, 59.79275706135234714 ) ) ;
#160854=CARTESIAN_POINT ( 'NONE',  ( -10.72451020669898014, 18.67979575497178502, 35.41557627198102409 ) ) ;
#160856=CARTESIAN_POINT ( 'NONE',  ( 9.474510206698971260, -16.51473224551069308, 102.9155762719810241 ) ) ;
#160857=CARTESIAN_POINT ( 'NONE',  ( -0.05219959533910754901, -16.53943276465976808, 22.49890960531436335 ) ) ;
#160859=CARTESIAN_POINT ( 'NONE',  ( 16.53943276465976808, -0.05219959533910856209, 108.7489096053143669 ) ) ;
#160860=CARTESIAN_POINT ( 'NONE',  ( 10.81492255796078972, 18.62759615963270932, 49.58224293864769550 ) ) ;
#160861=CARTESIAN_POINT ( 'NONE',  ( -19.02544592524342804, 5.153800228976336051, 41.04057627198103120 ) ) ;
#160862=CARTESIAN_POINT ( 'NONE',  ( 16.55341960407618274, -4.379528057220086978, 96.04275706135236135 ) ) ;
#160863=CARTESIAN_POINT ( 'NONE',  ( 18.62759615963255655, 10.81492255796105972, 36.66775706135234714 ) ) ;
#160864=CARTESIAN_POINT ( 'NONE',  ( -16.46253265017146816, -9.564922557961047289, 94.16775706135233293 ) ) ;
#160865=CARTESIAN_POINT ( 'NONE',  ( 4.379528057220339221, -16.55341960407611168, 107.7072429386476955 ) ) ;
#160866=CARTESIAN_POINT ( 'NONE',  ( 16.46253265017160672, -9.564922557960803928, 53.33224293864768839 ) ) ;
#160867=CARTESIAN_POINT ( 'NONE',  ( 13.89961937509977652, -13.97604488694527269, 33.12390960531434558 ) ) ;
#160869=CARTESIAN_POINT ( 'NONE',  ( 19.05341960407611168, 5.049401038298154454, 73.95724293864768129 ) ) ;
#160870=CARTESIAN_POINT ( 'NONE',  ( -14.34966873604972548, 8.224510206698743886, 63.33442372801900433 ) ) ;
#160871=CARTESIAN_POINT ( 'NONE',  ( 18.62759615963255655, 10.81492255796105972, 111.6677570613523613 ) ) ;
#160872=CARTESIAN_POINT ( 'NONE',  ( -21.53943276465977519, 0.05219959533907696930, 46.24890960531435979 ) ) ;
#160873=CARTESIAN_POINT ( 'NONE',  ( -16.52544592524335698, -4.483927247898792601, 78.95942372801901854 ) ) ;
#160874=CARTESIAN_POINT ( 'NONE',  ( -16.46253265017146816, -9.564922557961047289, 49.16775706135233293 ) ) ;
#160875=CARTESIAN_POINT ( 'NONE',  ( 13.89961937509957401, 13.97604488694547697, 61.87609039468566863 ) ) ;
#160876=CARTESIAN_POINT ( 'NONE',  ( -0.05219959533937732626, 21.53943276465977519, 57.50109039468568994 ) ) ;
#160877=CARTESIAN_POINT ( 'NONE',  ( 16.51473224551069308, 9.474510206698969483, 64.16557627198102409 ) ) ;
#160878=CARTESIAN_POINT ( 'NONE',  ( -9.564922557960796823, -16.46253265017161027, 32.08224293864769550 ) ) ;
#160879=CARTESIAN_POINT ( 'NONE',  ( -13.89961937509957401, -13.97604488694547875, 64.37609039468567573 ) ) ;
#160880=CARTESIAN_POINT ( 'NONE',  ( 13.89961937509977652, -13.97604488694527269, 108.1239096053143669 ) ) ;
#160881=CARTESIAN_POINT ( 'NONE',  ( -19.02544592524342804, 5.153800228976336051, 96.04057627198103830 ) ) ;
#160882=CARTESIAN_POINT ( 'NONE',  ( 4.483927247898545687, 16.52544592524342804, 54.79057627198104541 ) ) ;
#160883=CARTESIAN_POINT ( 'NONE',  ( 21.52544592524344225, -5.823673210054117533, 53.54057627198103120 ) ) ;
#160884=CARTESIAN_POINT ( 'NONE',  ( 17.60769864724391809, -5.499999999999981348, 91.15024842019167295 ) ) ;
#160885=CARTESIAN_POINT ( 'NONE',  ( -19.02544592524334988, -5.153800228976617603, 33.95942372801897591 ) ) ;
#160886=CARTESIAN_POINT ( 'NONE',  ( -17.44279575226823198, -5.990770900252435638, 79.16442432485685288 ) ) ;
#160887=CARTESIAN_POINT ( 'NONE',  ( 16.51473224551069308, 9.474510206698969483, 54.16557627198103120 ) ) ;
#160888=CARTESIAN_POINT ( 'NONE',  ( -19.35543954521080678, -5.499999999999533706, 99.58901960356450900 ) ) ;
#160890=CARTESIAN_POINT ( 'NONE',  ( 4.483927247898790824, -16.52544592524335698, 75.20942372801901854 ) ) ;
#160891=CARTESIAN_POINT ( 'NONE',  ( 10.72451020669898902, -18.67979575497178502, 97.91557627198103830 ) ) ;
#160892=CARTESIAN_POINT ( 'NONE',  ( -16.53943276465976808, 0.05219959533911058130, 56.24890960531436690 ) ) ;
#160893=CARTESIAN_POINT ( 'NONE',  ( -5.049401038298153566, 19.05341960407611168, 40.20724293864768839 ) ) ;
#160894=CARTESIAN_POINT ( 'NONE',  ( -13.89961937509977652, 13.97604488694528158, 115.6239096053143669 ) ) ;
#160895=CARTESIAN_POINT ( 'NONE',  ( 5.719274019375673035, 21.55341960407619339, 42.29275706135235424 ) ) ;
#160896=CARTESIAN_POINT ( 'NONE',  ( 0.05219959533936267826, -19.03943276465977164, 50.00109039468566863 ) ) ;
#160897=CARTESIAN_POINT ( 'NONE',  ( 0.05219959533909260263, 19.03943276465977164, 44.99890960531435979 ) ) ;
#160898=CARTESIAN_POINT ( 'NONE',  ( -10.81492255796105439, 18.62759615963255655, 92.91775706135236135 ) ) ;
#160899=CARTESIAN_POINT ( 'NONE',  ( 17.26058549869091863, 6.457015423128549259, 98.87745837476064992 ) ) ;
#160900=CARTESIAN_POINT ( 'NONE',  ( -16.53943276465976808, 0.05219959533911058130, 41.24890960531435269 ) ) ;
#160902=CARTESIAN_POINT ( 'NONE',  ( 18.67979575497178502, 10.72451020669898547, 44.16557627198103120 ) ) ;
#160904=CARTESIAN_POINT ( 'NONE',  ( -19.02544592524342804, 5.153800228976336051, 101.0405762719810241 ) ) ;
#160905=CARTESIAN_POINT ( 'NONE',  ( 12.06949235617757843, -12.14591786802309237, 93.12390960531436690 ) ) ;
#160906=CARTESIAN_POINT ( 'NONE',  ( -16.52544592524335698, -4.483927247898792601, 28.95942372801902209 ) ) ;
#160907=CARTESIAN_POINT ( 'NONE',  ( -8.314922557960811034, -14.29746914071050412, 22.08224293864769194 ) ) ;
#160909=CARTESIAN_POINT ( 'NONE',  ( 5.153800228976335163, 19.02544592524342804, 94.79057627198103830 ) ) ;
#160910=CARTESIAN_POINT ( 'NONE',  ( -0.05219959533907301413, -21.53943276465977519, 102.4989096053143811 ) ) ;
#160911=CARTESIAN_POINT ( 'NONE',  ( -14.29746914071049879, 8.314922557960819915, 30.83224293864770260 ) ) ;
#160912=CARTESIAN_POINT ( 'NONE',  ( -13.97604488694527625, -13.89961937509977652, 96.87390960531433848 ) ) ;
#160913=CARTESIAN_POINT ( 'NONE',  ( -16.46253265017146816, -9.564922557961047289, 99.16775706135233293 ) ) ;
#160914=CARTESIAN_POINT ( 'NONE',  ( 18.62759615963255655, 10.81492255796105972, 106.6677570613523756 ) ) ;
#160915=CARTESIAN_POINT ( 'NONE',  ( 5.719274019375991003, -21.55341960407610458, 92.70724293864770971 ) ) ;
#160916=CARTESIAN_POINT ( 'NONE',  ( 5.823673210054125526, 21.52544592524343514, 44.79057627198103120 ) ) ;
#160917=CARTESIAN_POINT ( 'NONE',  ( -5.049401038298153566, 19.05341960407611168, 65.20724293864765286 ) ) ;
#160918=CARTESIAN_POINT ( 'NONE',  ( 12.14591786802309770, 12.06949235617756955, 34.37390960531435979 ) ) ;
#160919=CARTESIAN_POINT ( 'NONE',  ( 19.02544592524343514, -5.153800228976328945, 73.54057627198103830 ) ) ;
#160921=CARTESIAN_POINT ( 'NONE',  ( 18.39635199886970796, -5.499999999999989342, 63.51967076360001840 ) ) ;
#160922=CARTESIAN_POINT ( 'NONE',  ( -13.89961937509957401, -13.97604488694547875, 34.37609039468566863 ) ) ;
#160923=CARTESIAN_POINT ( 'NONE',  ( 0.05219959533910956823, 16.53943276465976808, 79.99890960531435269 ) ) ;
#160924=CARTESIAN_POINT ( 'NONE',  ( -10.72451020669870658, -18.67979575497194134, 24.58442372801901499 ) ) ;
#160928=CARTESIAN_POINT ( 'NONE',  ( -0.05219959533934338120, 16.53943276465976808, 107.5010903946856899 ) ) ;
#160929=CARTESIAN_POINT ( 'NONE',  ( -0.05219959533910754901, -16.53943276465976808, 112.4989096053143669 ) ) ;
#160930=CARTESIAN_POINT ( 'NONE',  ( 5.153800228976335163, 19.02544592524342804, 74.79057627198103830 ) ) ;
#160931=CARTESIAN_POINT ( 'NONE',  ( -13.97604488694527625, -13.89961937509977652, 21.87390960531435979 ) ) ;
#160932=CARTESIAN_POINT ( 'NONE',  ( 4.483927247898545687, 16.52544592524342804, 39.79057627198103830 ) ) ;
#160933=CARTESIAN_POINT ( 'NONE',  ( -15.72974639402176322, -15.80617190586768395, 54.37609039468568994 ) ) ;
#160934=CARTESIAN_POINT ( 'NONE',  ( 21.53943276465977519, 0.05219959533937863772, 96.25109039468568994 ) ) ;
#160935=CARTESIAN_POINT ( 'NONE',  ( 0.05219959533909260263, 19.03943276465977164, 49.99890960531435979 ) ) ;
#160936=CARTESIAN_POINT ( 'NONE',  ( -5.049401038298153566, 19.05341960407611168, 45.20724293864769550 ) ) ;
#160938=CARTESIAN_POINT ( 'NONE',  ( 21.52544592524334988, 5.823673210054432836, 91.45942372801901854 ) ) ;
#160939=CARTESIAN_POINT ( 'NONE',  ( 12.06949235617739724, 12.14591786802326823, 56.87609039468568994 ) ) ;
#160940=CARTESIAN_POINT ( 'NONE',  ( 18.62759615963255655, 10.81492255796105972, 81.66775706135236135 ) ) ;
#160941=CARTESIAN_POINT ( 'NONE',  ( -21.53943276465977519, 0.05219959533907696930, 21.24890960531436690 ) ) ;
#160942=CARTESIAN_POINT ( 'NONE',  ( -16.51473224551082808, 9.474510206698731452, 98.33442372801900433 ) ) ;
#160943=CARTESIAN_POINT ( 'NONE',  ( -18.67979575497193778, 10.72451020669871902, 73.33442372801901854 ) ) ;
#160944=CARTESIAN_POINT ( 'NONE',  ( -16.52544592524335698, -4.483927247898792601, 38.95942372801901854 ) ) ;
#160945=CARTESIAN_POINT ( 'NONE',  ( -18.62759615963270932, 10.81492255796079327, 90.83224293864769550 ) ) ;
#160946=CARTESIAN_POINT ( 'NONE',  ( 0.05219959533936267826, -19.03943276465977164, 80.00109039468567573 ) ) ;
#160947=CARTESIAN_POINT ( 'NONE',  ( 19.03943276465977164, -0.05219959533909143690, 58.74890960531435979 ) ) ;
#160948=CARTESIAN_POINT ( 'NONE',  ( -13.89961937509957401, -13.97604488694547875, 99.37609039468567573 ) ) ;
#160949=CARTESIAN_POINT ( 'NONE',  ( 19.03943276465977164, 0.05219959533936151252, 96.25109039468567573 ) ) ;
#160950=CARTESIAN_POINT ( 'NONE',  ( -16.55341960407611168, -4.379528057220339221, 46.45724293864769550 ) ) ;
#160951=CARTESIAN_POINT ( 'NONE',  ( 19.05341960407617918, -5.049401038297876454, 71.04275706135234714 ) ) ;
#160952=CARTESIAN_POINT ( 'NONE',  ( 14.29746914071037800, 8.314922557961029526, 56.66775706135235424 ) ) ;
#160953=CARTESIAN_POINT ( 'NONE',  ( 16.46253265017160672, -9.564922557960803928, 33.33224293864770260 ) ) ;
#160954=CARTESIAN_POINT ( 'NONE',  ( -19.02544592524342804, 5.153800228976336051, 61.04057627198103120 ) ) ;
#160956=CARTESIAN_POINT ( 'NONE',  ( -16.55341960407617563, 4.379528057220093196, 63.54275706135234003 ) ) ;
#160959=CARTESIAN_POINT ( 'NONE',  ( -13.89961937509977652, 13.97604488694528158, 105.6239096053143527 ) ) ;
#160961=ORIENTED_EDGE ( 'NONE', *, *, #35450, .F. ) ;
#160962=CARTESIAN_POINT ( 'NONE',  ( 13.97604488694548053, -13.89961937509957401, 110.6260903946856615 ) ) ;
#160963=CARTESIAN_POINT ( 'NONE',  ( 5.719274019375991003, -21.55341960407610458, 37.70724293864769550 ) ) ;
#160964=CARTESIAN_POINT ( 'NONE',  ( 5.049401038297881783, 19.05341960407617563, 27.29275706135232937 ) ) ;
#160965=CARTESIAN_POINT ( 'NONE',  ( 8.224510206698742110, 14.34966873604972548, 27.08442372801901854 ) ) ;
#160966=CARTESIAN_POINT ( 'NONE',  ( 0.05219959533909260263, 19.03943276465977164, 24.99890960531435269 ) ) ;
#160967=CARTESIAN_POINT ( 'NONE',  ( -13.89961937509977652, 13.97604488694528158, 45.62390960531433848 ) ) ;
#160968=CARTESIAN_POINT ( 'NONE',  ( -10.81492255796078084, -18.62759615963271287, 92.08224293864769550 ) ) ;
#160969=CARTESIAN_POINT ( 'NONE',  ( -13.89961937509977652, 13.97604488694528158, 100.6239096053143669 ) ) ;
#160970=CARTESIAN_POINT ( 'NONE',  ( 0.05219959533909260263, 19.03943276465977164, 54.99890960531435979 ) ) ;
#160972=CARTESIAN_POINT ( 'NONE',  ( -16.51473224551082808, 9.474510206698731452, 78.33442372801900433 ) ) ;
#160973=CARTESIAN_POINT ( 'NONE',  ( -14.29746914071049879, 8.314922557960819915, 70.83224293864770971 ) ) ;
#160974=CARTESIAN_POINT ( 'NONE',  ( 15.72974639402199770, -15.80617190586745480, 43.12390960531435269 ) ) ;
#160975=CARTESIAN_POINT ( 'NONE',  ( 5.823673210054444382, -21.52544592524334988, 100.2094237280190043 ) ) ;
#160976=CARTESIAN_POINT ( 'NONE',  ( 5.823673210054125526, 21.52544592524343514, 94.79057627198105251 ) ) ;
#160977=CARTESIAN_POINT ( 'NONE',  ( -0.05219959533937732626, 21.53943276465977519, 77.50109039468567573 ) ) ;
#160978=CARTESIAN_POINT ( 'NONE',  ( 5.719274019375673035, 21.55341960407619339, 82.29275706135234714 ) ) ;
#160979=CARTESIAN_POINT ( 'NONE',  ( 9.474510206698971260, -16.51473224551069308, 107.9155762719810383 ) ) ;
#160980=CARTESIAN_POINT ( 'NONE',  ( -8.224510206698735004, -14.34966873604973081, 104.5844237280190185 ) ) ;
#160981=CARTESIAN_POINT ( 'NONE',  ( 0.05219959533937995610, -21.53943276465977519, 80.00109039468568994 ) ) ;
#160982=CARTESIAN_POINT ( 'NONE',  ( -5.049401038298153566, 19.05341960407611168, 60.20724293864768129 ) ) ;
#160983=CARTESIAN_POINT ( 'NONE',  ( 18.67979575497194134, -10.72451020669871369, 25.83442372801901499 ) ) ;
#160984=CARTESIAN_POINT ( 'NONE',  ( -13.97604488694527625, -13.89961937509977652, 66.87390960531436690 ) ) ;
#160985=CARTESIAN_POINT ( 'NONE',  ( -4.379528057220328563, 16.55341960407611168, 75.20724293864769550 ) ) ;
#160986=CARTESIAN_POINT ( 'NONE',  ( 16.55341960407611168, 4.379528057220329451, 48.95724293864770971 ) ) ;
#160987=CARTESIAN_POINT ( 'NONE',  ( -10.81492255796078084, -18.62759615963271287, 57.08224293864769550 ) ) ;
#160988=CARTESIAN_POINT ( 'NONE',  ( 5.049401038298161559, -19.05341960407611168, 57.70724293864769550 ) ) ;
#160989=CARTESIAN_POINT ( 'NONE',  ( -15.80617190586745835, -15.72974639402198527, 66.87390960531436690 ) ) ;
#160990=CARTESIAN_POINT ( 'NONE',  ( -5.049401038297874678, -19.05341960407617918, 69.79275706135233293 ) ) ;
#160991=CARTESIAN_POINT ( 'NONE',  ( 16.46253265017146816, 9.564922557961045513, 21.66775706135233648 ) ) ;
#160992=CARTESIAN_POINT ( 'NONE',  ( 0.05219959533910956823, 16.53943276465976808, 74.99890960531435269 ) ) ;
#160993=CARTESIAN_POINT ( 'NONE',  ( -18.62759615963270932, 10.81492255796079327, 50.83224293864770971 ) ) ;
#160995=CARTESIAN_POINT ( 'NONE',  ( -17.50000000000000711, -5.499999999999956479, 36.28230962303565121 ) ) ;
#160996=CARTESIAN_POINT ( 'NONE',  ( -14.34966873604972548, 8.224510206698743886, 93.33442372801901854 ) ) ;
#160999=CARTESIAN_POINT ( 'NONE',  ( 16.51473224551083163, -9.474510206698727899, 85.83442372801900433 ) ) ;
#161000=CARTESIAN_POINT ( 'NONE',  ( -0.05219959533910754901, -16.53943276465976808, 62.49890960531436690 ) ) ;
#161002=CARTESIAN_POINT ( 'NONE',  ( -16.46253265017160317, 9.564922557960807481, 65.83224293864769550 ) ) ;
#161003=CARTESIAN_POINT ( 'NONE',  ( 16.52544592524342804, -4.483927247898539470, 58.54057627198103120 ) ) ;
#161004=CARTESIAN_POINT ( 'NONE',  ( 16.51473224551069308, 9.474510206698969483, 84.16557627198102409 ) ) ;
#161005=CARTESIAN_POINT ( 'NONE',  ( 9.564922557961047289, -16.46253265017146816, 75.41775706135234714 ) ) ;
#161006=CARTESIAN_POINT ( 'NONE',  ( 9.474510206698971260, -16.51473224551069308, 57.91557627198103120 ) ) ;
#161007=CARTESIAN_POINT ( 'NONE',  ( 5.049401038298161559, -19.05341960407611168, 82.70724293864770971 ) ) ;
#161008=CARTESIAN_POINT ( 'NONE',  ( -13.97604488694527625, -13.89961937509977652, 71.87390960531433848 ) ) ;
#161009=CARTESIAN_POINT ( 'NONE',  ( 10.81492255796078972, 18.62759615963270932, 59.58224293864770260 ) ) ;
#161010=SPHERICAL_SURFACE ( 'NONE', #42003, 2.000000000000000000 ) ;
#161011=CARTESIAN_POINT ( 'NONE',  ( 19.02544592524343514, -5.153800228976328945, 53.54057627198102409 ) ) ;
#161012=CARTESIAN_POINT ( 'NONE',  ( -15.72974639402197994, 15.80617190586746368, 55.62390960531436690 ) ) ;
#161013=CARTESIAN_POINT ( 'NONE',  ( 5.153800228976615827, -19.02544592524334988, 85.20942372801900433 ) ) ;
#161014=CARTESIAN_POINT ( 'NONE',  ( 4.379528057220092307, 16.55341960407617563, 112.2927570613523471 ) ) ;
#161015=CARTESIAN_POINT ( 'NONE',  ( 9.564922557961047289, -16.46253265017146816, 40.41775706135234003 ) ) ;
#161016=CARTESIAN_POINT ( 'NONE',  ( 16.55341960407618274, -4.379528057220086978, 66.04275706135236135 ) ) ;
#161017=CARTESIAN_POINT ( 'NONE',  ( -16.55341960407617563, 4.379528057220093196, 88.54275706135236135 ) ) ;
#161019=CARTESIAN_POINT ( 'NONE',  ( 16.55341960407618274, -4.379528057220086978, 81.04275706135236135 ) ) ;
#161020=CARTESIAN_POINT ( 'NONE',  ( -0.05219959533907301413, -21.53943276465977519, 27.49890960531435269 ) ) ;
#161021=CARTESIAN_POINT ( 'NONE',  ( 19.05341960407611168, 5.049401038298154454, 28.95724293864769550 ) ) ;
#161022=CARTESIAN_POINT ( 'NONE',  ( 9.474510206698971260, -16.51473224551069308, 47.91557627198102409 ) ) ;
#161023=CARTESIAN_POINT ( 'NONE',  ( -13.89961937509977652, 13.97604488694528158, 40.62390960531435979 ) ) ;
#161024=CARTESIAN_POINT ( 'NONE',  ( -18.67979575497193778, 10.72451020669871902, 33.33442372801900433 ) ) ;
#161025=CARTESIAN_POINT ( 'NONE',  ( -0.05219959533934338120, 16.53943276465976808, 52.50109039468567573 ) ) ;
#161026=CARTESIAN_POINT ( 'NONE',  ( 4.379528057220339221, -16.55341960407611168, 22.70724293864769194 ) ) ;
#161027=CARTESIAN_POINT ( 'NONE',  ( -16.51473224551069308, -9.474510206698971260, 31.66557627198102054 ) ) ;
#161028=CARTESIAN_POINT ( 'NONE',  ( 5.049401038297881783, 19.05341960407617563, 22.29275706135233648 ) ) ;
#161029=CARTESIAN_POINT ( 'NONE',  ( -13.97604488694547697, 13.89961937509957934, 108.1260903946856331 ) ) ;
#161030=CARTESIAN_POINT ( 'NONE',  ( -16.46253265017146816, -9.564922557961047289, 69.16775706135233293 ) ) ;
#161031=CARTESIAN_POINT ( 'NONE',  ( -8.224510206698948167, 14.34966873604960824, 75.41557627198102409 ) ) ;
#161032=CARTESIAN_POINT ( 'NONE',  ( 13.89961937509977652, -13.97604488694527269, 43.12390960531434558 ) ) ;
#161033=CARTESIAN_POINT ( 'NONE',  ( -16.51473224551082808, 9.474510206698731452, 68.33442372801900433 ) ) ;
#161034=DIRECTION ( 'NONE',  ( -0.000000000000000000, -0.000000000000000000, 1.000000000000000000 ) ) ;
#161035=CARTESIAN_POINT ( 'NONE',  ( 5.719274019375673035, 21.55341960407619339, 82.29275706135234714 ) ) ;
#161036=CARTESIAN_POINT ( 'NONE',  ( -4.483927247898782831, 16.52544592524335698, 42.70942372801901854 ) ) ;
#161037=CARTESIAN_POINT ( 'NONE',  ( 17.97161686094261768, -5.499999999999982236, 73.49637206859250682 ) ) ;
#161038=CARTESIAN_POINT ( 'NONE',  ( 21.55341960407610458, 5.719274019375980345, 33.95724293864769550 ) ) ;
#161039=CARTESIAN_POINT ( 'NONE',  ( 12.14591786802327356, -12.06949235617739191, 25.62609039468567929 ) ) ;
#161040=CARTESIAN_POINT ( 'NONE',  ( -19.02544592524342804, 5.153800228976336051, 116.0405762719810383 ) ) ;
#161042=CARTESIAN_POINT ( 'NONE',  ( -13.97604488694527625, -13.89961937509977652, 36.87390960531436690 ) ) ;
#161043=CARTESIAN_POINT ( 'NONE',  ( -0.05219959533936034679, 19.03943276465977164, 57.50109039468566863 ) ) ;
#161044=CARTESIAN_POINT ( 'NONE',  ( 16.46253265017160672, -9.564922557960803928, 53.33224293864768839 ) ) ;
#161045=CARTESIAN_POINT ( 'NONE',  ( -18.67979575497193778, 10.72451020669871902, 63.33442372801900433 ) ) ;
#161046=CARTESIAN_POINT ( 'NONE',  ( 9.564922557961047289, -16.46253265017146816, 20.41775706135233293 ) ) ;
#161047=CARTESIAN_POINT ( 'NONE',  ( 16.55341960407611168, 4.379528057220329451, 23.95724293864769550 ) ) ;
#161048=CARTESIAN_POINT ( 'NONE',  ( 13.97604488694527802, 13.89961937509977652, 34.37390960531436690 ) ) ;
#161049=CARTESIAN_POINT ( 'NONE',  ( 13.97604488694527802, 13.89961937509977652, 94.37390960531436690 ) ) ;
#161050=CARTESIAN_POINT ( 'NONE',  ( 5.719274019375673035, 21.55341960407619339, 52.29275706135236135 ) ) ;
#161051=CARTESIAN_POINT ( 'NONE',  ( 9.474510206698971260, -16.51473224551069308, 32.91557627198102409 ) ) ;
#161052=CARTESIAN_POINT ( 'NONE',  ( 10.81492255796106328, -18.62759615963255655, 70.41775706135236135 ) ) ;
#161053=CARTESIAN_POINT ( 'NONE',  ( -13.97604488694547697, 13.89961937509957934, 93.12609039468566152 ) ) ;
#161054=CARTESIAN_POINT ( 'NONE',  ( 19.03943276465977164, -0.05219959533909143690, 103.7489096053143669 ) ) ;
#161055=CARTESIAN_POINT ( 'NONE',  ( -16.52544592524342804, 4.483927247898546575, 116.0405762719810383 ) ) ;
#161056=CARTESIAN_POINT ( 'NONE',  ( -5.719274019375978568, 21.55341960407610458, 115.2072429386476955 ) ) ;
#161057=CARTESIAN_POINT ( 'NONE',  ( -19.02544592524334988, -5.153800228976617603, 33.95942372801897591 ) ) ;
#161058=CARTESIAN_POINT ( 'NONE',  ( 8.224510206698953496, -14.34966873604960469, 107.9155762719810241 ) ) ;
#161059=CARTESIAN_POINT ( 'NONE',  ( 13.97604488694527802, 13.89961937509977652, 64.37390960531436690 ) ) ;
#161060=CARTESIAN_POINT ( 'NONE',  ( -5.153800228976607833, 19.02544592524334988, 97.70942372801900433 ) ) ;
#161061=CARTESIAN_POINT ( 'NONE',  ( 16.52544592524342804, -4.483927247898539470, 58.54057627198103120 ) ) ;
#161062=CARTESIAN_POINT ( 'NONE',  ( 9.474510206698729675, 16.51473224551082808, 22.08442372801899722 ) ) ;
#161063=CARTESIAN_POINT ( 'NONE',  ( 21.53943276465977519, -0.05219959533907433946, 23.74890960531435269 ) ) ;
#161064=CARTESIAN_POINT ( 'NONE',  ( -13.97604488694547697, 13.89961937509957934, 88.12609039468563310 ) ) ;
#161065=CARTESIAN_POINT ( 'NONE',  ( -10.72451020669898014, 18.67979575497178502, 90.41557627198103830 ) ) ;
#161066=CARTESIAN_POINT ( 'NONE',  ( 21.55341960407619695, -5.719274019375665929, 46.04275706135234714 ) ) ;
#161067=CARTESIAN_POINT ( 'NONE',  ( 8.314922557961029526, -14.29746914071037800, 40.41775706135234714 ) ) ;
#161068=CARTESIAN_POINT ( 'NONE',  ( -0.05219959533934338120, 16.53943276465976808, 107.5010903946856899 ) ) ;
#161069=CARTESIAN_POINT ( 'NONE',  ( -16.53943276465976808, -0.05219959533934237506, 38.75109039468567573 ) ) ;
#161070=CARTESIAN_POINT ( 'NONE',  ( -21.55341960407619339, 5.719274019375674811, 48.54275706135234714 ) ) ;
#161071=CARTESIAN_POINT ( 'NONE',  ( 5.719274019375991003, -21.55341960407610458, 52.70724293864769550 ) ) ;
#161072=CARTESIAN_POINT ( 'NONE',  ( 5.153800228976335163, 19.02544592524342804, 29.79057627198102409 ) ) ;
#161074=CARTESIAN_POINT ( 'NONE',  ( 12.14591786802327356, -12.06949235617739191, 80.62609039468567573 ) ) ;
#161075=CARTESIAN_POINT ( 'NONE',  ( 18.67979575497178502, 10.72451020669898547, 94.16557627198103830 ) ) ;
#161076=CARTESIAN_POINT ( 'NONE',  ( 12.14591786802309770, 12.06949235617756955, 34.37390960531435979 ) ) ;
#161077=CARTESIAN_POINT ( 'NONE',  ( 16.52544592524335698, 4.483927247898782831, 61.45942372801901854 ) ) ;
#161078=CARTESIAN_POINT ( 'NONE',  ( 13.89961937509957401, 13.97604488694547697, 106.8760903946856757 ) ) ;
#161079=CARTESIAN_POINT ( 'NONE',  ( 15.72974639402199770, -15.80617190586745480, 103.1239096053143811 ) ) ;
#161080=CARTESIAN_POINT ( 'NONE',  ( -8.224510206698948167, 14.34966873604960824, 25.41557627198103120 ) ) ;
#161082=CARTESIAN_POINT ( 'NONE',  ( -8.314922557961024197, 14.29746914071037800, 82.91775706135234714 ) ) ;
#161084=CARTESIAN_POINT ( 'NONE',  ( -21.55341960407610458, -5.719274019375992779, 71.45724293864769550 ) ) ;
#161085=CARTESIAN_POINT ( 'NONE',  ( 0.05219959533934541429, -16.53943276465976808, 100.0010903946857042 ) ) ;
#161087=CARTESIAN_POINT ( 'NONE',  ( 19.35543954521079968, 5.499999999999572786, 87.08901960356450900 ) ) ;
#161088=CARTESIAN_POINT ( 'NONE',  ( 15.80617190586746368, 15.72974639402197994, 94.37390960531436690 ) ) ;
#161089=CARTESIAN_POINT ( 'NONE',  ( -5.719274019375978568, 21.55341960407610458, 105.2072429386477097 ) ) ;
#161090=CARTESIAN_POINT ( 'NONE',  ( -16.52544592524342804, 4.483927247898546575, 41.04057627198103120 ) ) ;
#161091=CARTESIAN_POINT ( 'NONE',  ( -12.14591786802326823, 12.06949235617739902, 38.12609039468567573 ) ) ;
#161092=CARTESIAN_POINT ( 'NONE',  ( -19.02544592524342804, 5.153800228976336051, 46.04057627198101699 ) ) ;
#161093=CARTESIAN_POINT ( 'NONE',  ( -9.474510206698964154, 16.51473224551069663, 60.41557627198102409 ) ) ;
#161095=CARTESIAN_POINT ( 'NONE',  ( -9.474510206698964154, 16.51473224551069663, 115.4155762719810241 ) ) ;
#161096=CARTESIAN_POINT ( 'NONE',  ( 19.02544592524343514, -5.153800228976328945, 113.5405762719810241 ) ) ;
#161097=CARTESIAN_POINT ( 'NONE',  ( -19.03943276465977164, -0.05219959533935918106, 108.7510903946856615 ) ) ;
#161098=CARTESIAN_POINT ( 'NONE',  ( 5.049401038297881783, 19.05341960407617563, 57.29275706135231871 ) ) ;
#161099=CARTESIAN_POINT ( 'NONE',  ( -10.81492255796078084, -18.62759615963271287, 82.08224293864768129 ) ) ;
#161101=CARTESIAN_POINT ( 'NONE',  ( -8.224510206698948167, 14.34966873604960824, 25.41557627198103120 ) ) ;
#161102=CARTESIAN_POINT ( 'NONE',  ( -21.53943276465977519, 0.05219959533907696930, 41.24890960531435269 ) ) ;
#161103=CARTESIAN_POINT ( 'NONE',  ( -5.823673210054116645, -21.52544592524344225, 77.29057627198102409 ) ) ;
#161104=CARTESIAN_POINT ( 'NONE',  ( -9.474510206698720793, -16.51473224551083518, 104.5844237280190043 ) ) ;
#161105=CARTESIAN_POINT ( 'NONE',  ( -9.474510206698964154, 16.51473224551069663, 105.4155762719810383 ) ) ;
#161106=CARTESIAN_POINT ( 'NONE',  ( -0.05219959533937732626, 21.53943276465977519, 72.50109039468568994 ) ) ;
#161107=CARTESIAN_POINT ( 'NONE',  ( -9.474510206698964154, 16.51473224551069663, 70.41557627198102409 ) ) ;
#161109=CARTESIAN_POINT ( 'NONE',  ( 19.05341960407611168, 5.049401038298154454, 73.95724293864768129 ) ) ;
#161110=CARTESIAN_POINT ( 'NONE',  ( -16.53943276465976808, 0.05219959533911058130, 96.24890960531435269 ) ) ;
#161112=CARTESIAN_POINT ( 'NONE',  ( 19.03943276465977164, 0.05219959533936151252, 111.2510903946856757 ) ) ;
#161114=CARTESIAN_POINT ( 'NONE',  ( -19.02544592524342804, 5.153800228976336051, 71.04057627198099567 ) ) ;
#161115=CARTESIAN_POINT ( 'NONE',  ( -10.72451020669870658, -18.67979575497194134, 79.58442372801903275 ) ) ;
#161116=CARTESIAN_POINT ( 'NONE',  ( -9.474510206698964154, 16.51473224551069663, 95.41557627198102409 ) ) ;
#161117=CARTESIAN_POINT ( 'NONE',  ( -12.14591786802326823, 12.06949235617739902, 78.12609039468570415 ) ) ;
#161118=CARTESIAN_POINT ( 'NONE',  ( -16.18388926212238488, -7.379444403734526148, 75.43953151366153520 ) ) ;
#161119=CARTESIAN_POINT ( 'NONE',  ( 19.05341960407617918, -5.049401038297876454, 51.04275706135231871 ) ) ;
#161120=CARTESIAN_POINT ( 'NONE',  ( -21.52544592524334988, -5.823673210054445271, 108.9594237280190185 ) ) ;
#161124=CARTESIAN_POINT ( 'NONE',  ( 16.53943276465976808, 0.05219959533934440121, 111.2510903946856899 ) ) ;
#161126=CARTESIAN_POINT ( 'NONE',  ( -14.34966873604972548, 8.224510206698743886, 93.33442372801901854 ) ) ;
#161128=CARTESIAN_POINT ( 'NONE',  ( 12.06949235617739724, 12.14591786802326823, 61.87609039468568284 ) ) ;
#161129=CARTESIAN_POINT ( 'NONE',  ( -10.72451020669870658, -18.67979575497194134, 84.58442372801903275 ) ) ;
#161130=CARTESIAN_POINT ( 'NONE',  ( 5.153800228976615827, -19.02544592524334988, 95.20942372801897591 ) ) ;
#161131=CARTESIAN_POINT ( 'NONE',  ( -13.89961937509957401, -13.97604488694547875, 39.37609039468566152 ) ) ;
#161132=CARTESIAN_POINT ( 'NONE',  ( 19.02544592524343514, -5.153800228976328945, 83.54057627198100988 ) ) ;
#161133=CARTESIAN_POINT ( 'NONE',  ( 13.97604488694527802, 13.89961937509977652, 59.37390960531434558 ) ) ;
#161134=CARTESIAN_POINT ( 'NONE',  ( 9.474510206698971260, -16.51473224551069308, 87.91557627198102409 ) ) ;
#161135=CARTESIAN_POINT ( 'NONE',  ( 18.67979575497178502, 10.72451020669898547, 84.16557627198103830 ) ) ;
#161136=CARTESIAN_POINT ( 'NONE',  ( -21.52544592524343514, 5.823673210054127303, 51.04057627198103120 ) ) ;
#161137=CARTESIAN_POINT ( 'NONE',  ( 0.05219959533909260263, 19.03943276465977164, 34.99890960531435979 ) ) ;
#161138=CARTESIAN_POINT ( 'NONE',  ( 14.29746914071037800, 8.314922557961029526, 61.66775706135235424 ) ) ;
#161141=CARTESIAN_POINT ( 'NONE',  ( -10.81492255796105439, 18.62759615963255655, 42.91775706135235424 ) ) ;
#161142=CARTESIAN_POINT ( 'NONE',  ( -12.06949235617756955, 12.14591786802309770, 65.62390960531436690 ) ) ;
#161144=CARTESIAN_POINT ( 'NONE',  ( 0.05219959533934541429, -16.53943276465976808, 40.00109039468567573 ) ) ;
#161145=CARTESIAN_POINT ( 'NONE',  ( -0.05219959533910754901, -16.53943276465976808, 107.4989096053143669 ) ) ;
#161146=CARTESIAN_POINT ( 'NONE',  ( 19.02544592524334988, 5.153800228976608722, 56.45942372801898301 ) ) ;
#161147=CARTESIAN_POINT ( 'NONE',  ( 12.14591786802309770, 12.06949235617756955, 59.37390960531436690 ) ) ;
#161148=CARTESIAN_POINT ( 'NONE',  ( 21.53943276465977519, 0.05219959533937863772, 31.25109039468568639 ) ) ;
#161149=CARTESIAN_POINT ( 'NONE',  ( -5.153800228976328057, -19.02544592524343514, 27.29057627198103120 ) ) ;
#161150=CARTESIAN_POINT ( 'NONE',  ( -5.823673210054116645, -21.52544592524344225, 92.29057627198103830 ) ) ;
#161151=CARTESIAN_POINT ( 'NONE',  ( 16.51473224551069308, 9.474510206698969483, 99.16557627198102409 ) ) ;
#161152=CARTESIAN_POINT ( 'NONE',  ( -8.314922557960811034, -14.29746914071050412, 77.08224293864769550 ) ) ;
#161153=CARTESIAN_POINT ( 'NONE',  ( -13.97604488694527625, -13.89961937509977652, 111.8739096053143243 ) ) ;
#161156=CARTESIAN_POINT ( 'NONE',  ( -16.46253265017146816, -9.564922557961047289, 79.16775706135234714 ) ) ;
#161157=CARTESIAN_POINT ( 'NONE',  ( -18.62759615963255300, -10.81492255796106328, 24.16775706135235424 ) ) ;
#161158=CARTESIAN_POINT ( 'NONE',  ( 0.05219959533909260263, 19.03943276465977164, 64.99890960531436690 ) ) ;
#161159=CARTESIAN_POINT ( 'NONE',  ( -0.05219959533936034679, 19.03943276465977164, 57.50109039468566863 ) ) ;
#161160=CARTESIAN_POINT ( 'NONE',  ( -19.05341960407611168, -5.049401038298163336, 31.45724293864769550 ) ) ;
#161161=CARTESIAN_POINT ( 'NONE',  ( -21.52544592524334988, -5.823673210054445271, 68.95942372801901854 ) ) ;
#161163=CARTESIAN_POINT ( 'NONE',  ( 0.05219959533910956823, 16.53943276465976808, 54.99890960531435269 ) ) ;
#161164=CARTESIAN_POINT ( 'NONE',  ( -16.46253265017160317, 9.564922557960807481, 60.83224293864769550 ) ) ;
#161165=CARTESIAN_POINT ( 'NONE',  ( 5.719274019375991003, -21.55341960407610458, 82.70724293864770971 ) ) ;
#161166=CARTESIAN_POINT ( 'NONE',  ( 19.05341960407611168, 5.049401038298154454, 58.95724293864768129 ) ) ;
#161167=CARTESIAN_POINT ( 'NONE',  ( 21.55341960407610458, 5.719274019375980345, 83.95724293864770971 ) ) ;
#161168=CARTESIAN_POINT ( 'NONE',  ( -15.72974639402176322, -15.80617190586768395, 94.37609039468568994 ) ) ;
#161169=CARTESIAN_POINT ( 'NONE',  ( -19.02544592524342804, 5.153800228976336051, 26.04057627198103120 ) ) ;
#161170=CARTESIAN_POINT ( 'NONE',  ( -12.06949235617739369, -12.14591786802326823, 99.37609039468568994 ) ) ;
#161171=CARTESIAN_POINT ( 'NONE',  ( 16.53943276465976808, -0.05219959533910856209, 98.74890960531438111 ) ) ;
#161172=CARTESIAN_POINT ( 'NONE',  ( -19.02544592524334988, -5.153800228976617603, 93.95942372801900433 ) ) ;
#161174=CARTESIAN_POINT ( 'NONE',  ( -18.67979575497193778, 10.72451020669871902, 23.33442372801901499 ) ) ;
#161175=CARTESIAN_POINT ( 'NONE',  ( 13.97604488694548053, -13.89961937509957401, 50.62609039468566152 ) ) ;
#161176=CARTESIAN_POINT ( 'NONE',  ( -8.224510206698735004, -14.34966873604973081, 104.5844237280190185 ) ) ;
#161178=CARTESIAN_POINT ( 'NONE',  ( 13.97604488694548053, -13.89961937509957401, 25.62609039468566507 ) ) ;
#161179=CARTESIAN_POINT ( 'NONE',  ( -13.97604488694527625, -13.89961937509977652, 106.8739096053143669 ) ) ;
#161180=CARTESIAN_POINT ( 'NONE',  ( 5.719274019375991003, -21.55341960407610458, 62.70724293864769550 ) ) ;
#161182=CARTESIAN_POINT ( 'NONE',  ( 14.34966873604960469, 8.224510206698951720, 114.1655762719810383 ) ) ;
#161183=CARTESIAN_POINT ( 'NONE',  ( -21.55341960407619339, 5.719274019375674811, 108.5427570613523756 ) ) ;
#161184=CARTESIAN_POINT ( 'NONE',  ( 12.14591786802327356, -12.06949235617739191, 75.62609039468567573 ) ) ;
#161185=CARTESIAN_POINT ( 'NONE',  ( -0.05219959533937732626, 21.53943276465977519, 32.50109039468568284 ) ) ;
#161186=CARTESIAN_POINT ( 'NONE',  ( -16.52544592524335698, -4.483927247898792601, 38.95942372801901854 ) ) ;
#161187=CARTESIAN_POINT ( 'NONE',  ( 13.97604488694527802, 13.89961937509977652, 104.3739096053143385 ) ) ;
#161188=CARTESIAN_POINT ( 'NONE',  ( -19.03943276465977164, 0.05219959533909376836, 41.24890960531435269 ) ) ;
#161189=CARTESIAN_POINT ( 'NONE',  ( -13.97604488694527625, -13.89961937509977652, 61.87390960531435979 ) ) ;
#161190=CARTESIAN_POINT ( 'NONE',  ( 14.34966873604972726, -8.224510206698740333, 40.83442372801901854 ) ) ;
#161191=CARTESIAN_POINT ( 'NONE',  ( -4.483927247898539470, -16.52544592524342804, 92.29057627198103830 ) ) ;
#161192=CARTESIAN_POINT ( 'NONE',  ( 4.379528057220092307, 16.55341960407617563, 102.2927570613523613 ) ) ;
#161193=CARTESIAN_POINT ( 'NONE',  ( 5.153800228976335163, 19.02544592524342804, 49.79057627198101699 ) ) ;
#161194=CARTESIAN_POINT ( 'NONE',  ( -0.05219959533937732626, 21.53943276465977519, 52.50109039468567573 ) ) ;
#161195=CARTESIAN_POINT ( 'NONE',  ( -19.05341960407611168, -5.049401038298163336, 76.45724293864769550 ) ) ;
#161196=CARTESIAN_POINT ( 'NONE',  ( 16.51473224551069308, 9.474510206698969483, 69.16557627198102409 ) ) ;
#161197=CARTESIAN_POINT ( 'NONE',  ( -13.89961937509977652, 13.97604488694528158, 100.6239096053143669 ) ) ;
#161199=CARTESIAN_POINT ( 'NONE',  ( 14.34966873604960469, 8.224510206698951720, 49.16557627198102409 ) ) ;
#161200=CARTESIAN_POINT ( 'NONE',  ( -16.53943276465976808, -0.05219959533934237506, 103.7510903946857042 ) ) ;
#161201=CARTESIAN_POINT ( 'NONE',  ( -16.53943276465976808, -0.05219959533934237506, 113.7510903946856757 ) ) ;
#161202=VERTEX_POINT ( 'NONE', #164868 ) ;
#161203=CARTESIAN_POINT ( 'NONE',  ( -19.02544592524334988, -5.153800228976617603, 43.95942372801899012 ) ) ;
#161204=CARTESIAN_POINT ( 'NONE',  ( -5.153800228976328057, -19.02544592524343514, 112.2905762719810099 ) ) ;
#161205=CARTESIAN_POINT ( 'NONE',  ( 16.46253265017160672, -9.564922557960803928, 63.33224293864769550 ) ) ;
#161206=CARTESIAN_POINT ( 'NONE',  ( -16.51473224551082808, 9.474510206698731452, 38.33442372801899722 ) ) ;
#161209=CARTESIAN_POINT ( 'NONE',  ( 0.05219959533936267826, -19.03943276465977164, 90.00109039468567573 ) ) ;
#161210=CARTESIAN_POINT ( 'NONE',  ( 8.314922557961029526, -14.29746914071037800, 70.41775706135236135 ) ) ;
#161211=CARTESIAN_POINT ( 'NONE',  ( 17.05116617787825462, 6.768360034955822613, 93.84324446740806991 ) ) ;
#161212=CARTESIAN_POINT ( 'NONE',  ( 0.05219959533909260263, 19.03943276465977164, 84.99890960531436690 ) ) ;
#161213=CARTESIAN_POINT ( 'NONE',  ( -10.81492255796105439, 18.62759615963255655, 32.91775706135234714 ) ) ;
#161214=CARTESIAN_POINT ( 'NONE',  ( 13.97604488694548053, -13.89961937509957401, 70.62609039468567573 ) ) ;
#161216=CARTESIAN_POINT ( 'NONE',  ( 5.153800228976335163, 19.02544592524342804, 29.79057627198102409 ) ) ;
#161217=CARTESIAN_POINT ( 'NONE',  ( 19.03943276465977164, -0.05219959533909143690, 88.74890960531436690 ) ) ;
#161218=CARTESIAN_POINT ( 'NONE',  ( 16.52544592524342804, -4.483927247898539470, 53.54057627198103120 ) ) ;
#161219=CARTESIAN_POINT ( 'NONE',  ( -13.97604488694527625, -13.89961937509977652, 36.87390960531436690 ) ) ;
#161220=CARTESIAN_POINT ( 'NONE',  ( 16.51473224551083163, -9.474510206698727899, 45.83442372801900433 ) ) ;
#161222=CARTESIAN_POINT ( 'NONE',  ( -16.55341960407611168, -4.379528057220339221, 86.45724293864770971 ) ) ;
#161223=CARTESIAN_POINT ( 'NONE',  ( 19.02544592524334988, 5.153800228976608722, 36.45942372801900433 ) ) ;
#161224=CARTESIAN_POINT ( 'NONE',  ( 5.153800228976335163, 19.02544592524342804, 69.79057627198103830 ) ) ;
#161225=CARTESIAN_POINT ( 'NONE',  ( -5.719274019375978568, 21.55341960407610458, 65.20724293864768129 ) ) ;
#161226=CARTESIAN_POINT ( 'NONE',  ( 12.06949235617757843, -12.14591786802309237, 58.12390960531435979 ) ) ;
#161227=CARTESIAN_POINT ( 'NONE',  ( 10.72451020669871369, 18.67979575497193778, 112.0844237280190185 ) ) ;
#161228=CARTESIAN_POINT ( 'NONE',  ( -5.049401038298153566, 19.05341960407611168, 110.2072429386476671 ) ) ;
#161229=CARTESIAN_POINT ( 'NONE',  ( 15.72974639402199770, -15.80617190586745480, 23.12390960531436335 ) ) ;
#161230=CARTESIAN_POINT ( 'NONE',  ( 9.564922557960805705, 16.46253265017160317, 54.58224293864769550 ) ) ;
#161231=CARTESIAN_POINT ( 'NONE',  ( -16.53943276465976808, 0.05219959533911058130, 116.2489096053143669 ) ) ;
#161232=CARTESIAN_POINT ( 'NONE',  ( -0.05219959533910754901, -16.53943276465976808, 92.49890960531436690 ) ) ;
#161233=CARTESIAN_POINT ( 'NONE',  ( 5.719274019375991003, -21.55341960407610458, 102.7072429386476955 ) ) ;
#161234=CARTESIAN_POINT ( 'NONE',  ( 0.05219959533909260263, 19.03943276465977164, 104.9989096053143669 ) ) ;
#161235=CARTESIAN_POINT ( 'NONE',  ( -18.62759615963270932, 10.81492255796079327, 105.8322429386476955 ) ) ;
#161236=CARTESIAN_POINT ( 'NONE',  ( -13.97604488694527625, -13.89961937509977652, 106.8739096053143669 ) ) ;
#161237=CARTESIAN_POINT ( 'NONE',  ( -0.05219959533909027116, -19.03943276465977164, 27.49890960531435624 ) ) ;
#161238=CARTESIAN_POINT ( 'NONE',  ( 5.823673210054444382, -21.52544592524334988, 75.20942372801901854 ) ) ;
#161239=CARTESIAN_POINT ( 'NONE',  ( -18.62759615963270932, 10.81492255796079327, 95.83224293864770971 ) ) ;
#161240=CARTESIAN_POINT ( 'NONE',  ( 17.44279575226824974, -5.990770900252421427, 108.3355756751431898 ) ) ;
#161241=CARTESIAN_POINT ( 'NONE',  ( -17.49999999999999645, 5.500000000000001776, 103.7176903769643701 ) ) ;
#161243=CARTESIAN_POINT ( 'NONE',  ( -8.314922557961024197, 14.29746914071037800, 52.91775706135235424 ) ) ;
#161244=CARTESIAN_POINT ( 'NONE',  ( 16.53943276465976808, -0.05219959533910856209, 108.7489096053143669 ) ) ;
#161246=CARTESIAN_POINT ( 'NONE',  ( 5.049401038298161559, -19.05341960407611168, 52.70724293864767418 ) ) ;
#161247=CARTESIAN_POINT ( 'NONE',  ( 8.314922557960818139, 14.29746914071049879, 89.58224293864768129 ) ) ;
#161248=CARTESIAN_POINT ( 'NONE',  ( -15.72974639402197994, 15.80617190586746368, 30.62390960531436335 ) ) ;
#161249=CARTESIAN_POINT ( 'NONE',  ( -8.314922557960811034, -14.29746914071050412, 72.08224293864769550 ) ) ;
#161250=CARTESIAN_POINT ( 'NONE',  ( -12.14591786802326823, 12.06949235617739902, 23.12609039468567573 ) ) ;
#161251=CARTESIAN_POINT ( 'NONE',  ( 21.55341960407619695, -5.719274019375665929, 71.04275706135234714 ) ) ;
#161252=CARTESIAN_POINT ( 'NONE',  ( 17.48847506799967988, -5.747544572773781724, 78.32697437843279431 ) ) ;
#161253=CARTESIAN_POINT ( 'NONE',  ( 21.53943276465977519, -0.05219959533907433946, 23.74890960531435269 ) ) ;
#161254=CARTESIAN_POINT ( 'NONE',  ( -12.14591786802326823, 12.06949235617739902, 98.12609039468570415 ) ) ;
#161255=CARTESIAN_POINT ( 'NONE',  ( 0.05219959533909260263, 19.03943276465977164, 34.99890960531435979 ) ) ;
#161256=CARTESIAN_POINT ( 'NONE',  ( 9.474510206698971260, -16.51473224551069308, 87.91557627198102409 ) ) ;
#161257=CARTESIAN_POINT ( 'NONE',  ( -10.72451020669898014, 18.67979575497178502, 100.4155762719810241 ) ) ;
#161258=CARTESIAN_POINT ( 'NONE',  ( -16.52544592524335698, -4.483927247898792601, 23.95942372801901143 ) ) ;
#161259=CARTESIAN_POINT ( 'NONE',  ( 12.14591786802309770, 12.06949235617756955, 59.37390960531436690 ) ) ;
#161260=CARTESIAN_POINT ( 'NONE',  ( 21.52544592524334988, 5.823673210054432836, 76.45942372801901854 ) ) ;
#161261=CARTESIAN_POINT ( 'NONE',  ( -14.34966873604972548, 8.224510206698743886, 93.33442372801901854 ) ) ;
#161262=CARTESIAN_POINT ( 'NONE',  ( 16.36317988757094710, -7.306389748694845920, 46.59789608363175262 ) ) ;
#161263=CARTESIAN_POINT ( 'NONE',  ( -19.25918095147780207, -5.499999999999585221, 64.45284276293934056 ) ) ;
#161264=CARTESIAN_POINT ( 'NONE',  ( 16.55341960407611168, 4.379528057220329451, 28.95724293864769905 ) ) ;
#161265=CARTESIAN_POINT ( 'NONE',  ( 4.379528057220092307, 16.55341960407617563, 72.29275706135236135 ) ) ;
#161266=CARTESIAN_POINT ( 'NONE',  ( -9.474510206698964154, 16.51473224551069663, 80.41557627198103830 ) ) ;
#161267=CARTESIAN_POINT ( 'NONE',  ( -13.89961937509977652, 13.97604488694528158, 90.62390960531432427 ) ) ;
#161268=CARTESIAN_POINT ( 'NONE',  ( -21.55341960407619339, 5.719274019375674811, 88.54275706135236135 ) ) ;
#161269=CARTESIAN_POINT ( 'NONE',  ( 0.05219959533934541429, -16.53943276465976808, 85.00109039468568994 ) ) ;
#161270=CARTESIAN_POINT ( 'NONE',  ( -12.06949235617756955, 12.14591786802309770, 60.62390960531437401 ) ) ;
#161271=CARTESIAN_POINT ( 'NONE',  ( -9.564922557960796823, -16.46253265017161027, 62.08224293864769550 ) ) ;
#161273=CARTESIAN_POINT ( 'NONE',  ( 19.05341960407617918, -5.049401038297876454, 111.0427570613523329 ) ) ;
#161274=CARTESIAN_POINT ( 'NONE',  ( -19.03943276465977164, 0.05219959533909376836, 21.24890960531436335 ) ) ;
#161275=CARTESIAN_POINT ( 'NONE',  ( -13.97604488694527625, -13.89961937509977652, 81.87390960531436690 ) ) ;
#161276=CARTESIAN_POINT ( 'NONE',  ( 16.46253265017146816, 9.564922557961045513, 111.6677570613523329 ) ) ;
#161278=CARTESIAN_POINT ( 'NONE',  ( 5.049401038297881783, 19.05341960407617563, 27.29275706135232937 ) ) ;
#161279=CARTESIAN_POINT ( 'NONE',  ( 14.34966873604972726, -8.224510206698740333, 80.83442372801901854 ) ) ;
#161280=CARTESIAN_POINT ( 'NONE',  ( 13.89961937509957401, 13.97604488694547697, 91.87609039468567573 ) ) ;
#161281=CARTESIAN_POINT ( 'NONE',  ( -19.05341960407611168, -5.049401038298163336, 21.45724293864768839 ) ) ;
#161282=CARTESIAN_POINT ( 'NONE',  ( 12.14591786802327356, -12.06949235617739191, 60.62609039468567573 ) ) ;
#161283=CARTESIAN_POINT ( 'NONE',  ( 8.314922557961029526, -14.29746914071037800, 55.41775706135234714 ) ) ;
#161285=CARTESIAN_POINT ( 'NONE',  ( 9.564922557961047289, -16.46253265017146816, 50.41775706135233293 ) ) ;
#161286=CARTESIAN_POINT ( 'NONE',  ( -10.81492255796105439, 18.62759615963255655, 102.9177570613523756 ) ) ;
#161287=CARTESIAN_POINT ( 'NONE',  ( 16.46253265017160672, -9.564922557960803928, 38.33224293864768839 ) ) ;
#161288=CARTESIAN_POINT ( 'NONE',  ( 13.89961937509977652, -13.97604488694527269, 83.12390960531436690 ) ) ;
#161289=CARTESIAN_POINT ( 'NONE',  ( 14.29746914071049879, -8.314922557960816363, 78.33224293864770971 ) ) ;
#161290=CARTESIAN_POINT ( 'NONE',  ( 10.81492255796106328, -18.62759615963255655, 85.41775706135236135 ) ) ;
#161291=CARTESIAN_POINT ( 'NONE',  ( -16.46253265017146816, -9.564922557961047289, 64.16775706135233293 ) ) ;
#161292=CARTESIAN_POINT ( 'NONE',  ( 19.02544592524334988, 5.153800228976608722, 46.45942372801899012 ) ) ;
#161293=CARTESIAN_POINT ( 'NONE',  ( -21.52544592524343514, 5.823673210054127303, 41.04057627198103120 ) ) ;
#161294=CARTESIAN_POINT ( 'NONE',  ( 21.53943276465977519, 0.05219959533937863772, 101.2510903946856757 ) ) ;
#161295=CARTESIAN_POINT ( 'NONE',  ( 19.02544592524343514, -5.153800228976328945, 83.54057627198100988 ) ) ;
#161296=CARTESIAN_POINT ( 'NONE',  ( 21.55341960407619695, -5.719274019375665929, 101.0427570613523756 ) ) ;
#161297=CARTESIAN_POINT ( 'NONE',  ( 10.72451020669898902, -18.67979575497178502, 47.91557627198102409 ) ) ;
#161298=CARTESIAN_POINT ( 'NONE',  ( 5.153800228976335163, 19.02544592524342804, 94.79057627198103830 ) ) ;
#161299=CARTESIAN_POINT ( 'NONE',  ( 19.02544592524334988, 5.153800228976608722, 81.45942372801897591 ) ) ;
#161300=CARTESIAN_POINT ( 'NONE',  ( -19.03943276465977164, 0.05219959533909376836, 101.2489096053143669 ) ) ;
#161302=CARTESIAN_POINT ( 'NONE',  ( -9.564922557961040184, 16.46253265017147172, 97.91775706135233293 ) ) ;
#161303=CARTESIAN_POINT ( 'NONE',  ( -16.55341960407617563, 4.379528057220093196, 38.54275706135234714 ) ) ;
#161304=CARTESIAN_POINT ( 'NONE',  ( -8.314922557960811034, -14.29746914071050412, 102.0822429386476955 ) ) ;
#161305=CARTESIAN_POINT ( 'NONE',  ( -19.05341960407611168, -5.049401038298163336, 86.45724293864769550 ) ) ;
#161306=CARTESIAN_POINT ( 'NONE',  ( -18.62759615963270932, 10.81492255796079327, 60.83224293864769550 ) ) ;
#161308=CARTESIAN_POINT ( 'NONE',  ( -8.224510206698735004, -14.34966873604973081, 34.58442372801900433 ) ) ;
#161309=CARTESIAN_POINT ( 'NONE',  ( 15.72974639402176855, 15.80617190586768217, 31.87609039468567929 ) ) ;
#161310=CARTESIAN_POINT ( 'NONE',  ( 10.81492255796106328, -18.62759615963255655, 90.41775706135236135 ) ) ;
#161311=CARTESIAN_POINT ( 'NONE',  ( 14.29746914071037800, 8.314922557961029526, 76.66775706135234714 ) ) ;
#161312=CARTESIAN_POINT ( 'NONE',  ( 13.97604488694527802, 13.89961937509977652, 79.37390960531435269 ) ) ;
#161313=CARTESIAN_POINT ( 'NONE',  ( 14.34966873604960469, 8.224510206698951720, 74.16557627198102409 ) ) ;
#161314=CARTESIAN_POINT ( 'NONE',  ( 12.14591786802327356, -12.06949235617739191, 110.6260903946857042 ) ) ;
#161315=CARTESIAN_POINT ( 'NONE',  ( 9.474510206698729675, 16.51473224551082808, 62.08442372801899722 ) ) ;
#161316=CARTESIAN_POINT ( 'NONE',  ( -18.67979575497193778, 10.72451020669871902, 33.33442372801900433 ) ) ;
#161317=ADVANCED_FACE ( 'NONE', ( #89998 ), #102255, .T. ) ;
#161318=CARTESIAN_POINT ( 'NONE',  ( -4.483927247898539470, -16.52544592524342804, 72.29057627198102409 ) ) ;
#161319=CARTESIAN_POINT ( 'NONE',  ( 18.62759615963271287, -10.81492255796078972, 23.33224293864769194 ) ) ;
#161320=CARTESIAN_POINT ( 'NONE',  ( -14.29746914071037622, -8.314922557961029526, 99.16775706135234714 ) ) ;
#161321=CARTESIAN_POINT ( 'NONE',  ( -5.719274019375665041, -21.55341960407619695, 69.79275706135234714 ) ) ;
#161322=CARTESIAN_POINT ( 'NONE',  ( -14.29746914071037622, -8.314922557961029526, 39.16775706135235424 ) ) ;
#161323=CARTESIAN_POINT ( 'NONE',  ( 10.81492255796106328, -18.62759615963255655, 35.41775706135234003 ) ) ;
#161324=ORIENTED_EDGE ( 'NONE', *, *, #193913, .T. ) ;
#161325=CARTESIAN_POINT ( 'NONE',  ( -18.62759615963270932, 10.81492255796079327, 110.8322429386476955 ) ) ;
#161326=CARTESIAN_POINT ( 'NONE',  ( -12.06949235617756955, 12.14591786802309770, 85.62390960531436690 ) ) ;
#161327=CARTESIAN_POINT ( 'NONE',  ( -18.87255363501903105, -5.499999999999950262, 51.32513748171828638 ) ) ;
#161328=CARTESIAN_POINT ( 'NONE',  ( -8.314922557960811034, -14.29746914071050412, 52.08224293864768839 ) ) ;
#161329=CARTESIAN_POINT ( 'NONE',  ( -16.46253265017160317, 9.564922557960807481, 25.83224293864769194 ) ) ;
#161330=CARTESIAN_POINT ( 'NONE',  ( 21.52544592524344225, -5.823673210054117533, 48.54057627198103120 ) ) ;
#161331=CARTESIAN_POINT ( 'NONE',  ( 12.06949235617757843, -12.14591786802309237, 83.12390960531436690 ) ) ;
#161332=AXIS2_PLACEMENT_3D ( 'NONE', #13833, #105843, #101858 ) ;
#161333=CARTESIAN_POINT ( 'NONE',  ( -21.55341960407610458, -5.719274019375992779, 81.45724293864769550 ) ) ;
#161334=CARTESIAN_POINT ( 'NONE',  ( 0.05219959533909260263, 19.03943276465977164, 84.99890960531436690 ) ) ;
#161335=CARTESIAN_POINT ( 'NONE',  ( 13.97604488694527802, 13.89961937509977652, 39.37390960531435269 ) ) ;
#161336=CARTESIAN_POINT ( 'NONE',  ( -5.153800228976607833, 19.02544592524334988, 72.70942372801900433 ) ) ;
#161337=CARTESIAN_POINT ( 'NONE',  ( -15.80617190586745835, -15.72974639402198527, 36.87390960531435979 ) ) ;
#161338=CARTESIAN_POINT ( 'NONE',  ( -10.72451020669870658, -18.67979575497194134, 54.58442372801901143 ) ) ;
#161339=CARTESIAN_POINT ( 'NONE',  ( -15.72974639402197994, 15.80617190586746368, 65.62390960531436690 ) ) ;
#161340=CARTESIAN_POINT ( 'NONE',  ( -16.51473224551069308, -9.474510206698971260, 36.66557627198102409 ) ) ;
#161341=CARTESIAN_POINT ( 'NONE',  ( -13.97604488694527625, -13.89961937509977652, 71.87390960531433848 ) ) ;
#161342=ORIENTED_EDGE ( 'NONE', *, *, #38220, .F. ) ;
#161343=CARTESIAN_POINT ( 'NONE',  ( 14.34966873604972726, -8.224510206698740333, 45.83442372801901854 ) ) ;
#161344=CARTESIAN_POINT ( 'NONE',  ( 5.719274019375673035, 21.55341960407619339, 32.29275706135235424 ) ) ;
#161346=CARTESIAN_POINT ( 'NONE',  ( 15.80617190586769283, -15.72974639402175789, 70.62609039468567573 ) ) ;
#161347=CARTESIAN_POINT ( 'NONE',  ( 13.89961937509977652, -13.97604488694527269, 113.1239096053143527 ) ) ;
#161348=CARTESIAN_POINT ( 'NONE',  ( 18.67979575497178502, 10.72451020669898547, 84.16557627198103830 ) ) ;
#161349=CARTESIAN_POINT ( 'NONE',  ( -18.62759615963270932, 10.81492255796079327, 115.8322429386477097 ) ) ;
#161350=CARTESIAN_POINT ( 'NONE',  ( 12.14591786802327356, -12.06949235617739191, 55.62609039468568284 ) ) ;
#161351=CARTESIAN_POINT ( 'NONE',  ( 21.55341960407610458, 5.719274019375980345, 63.95724293864770260 ) ) ;
#161352=CARTESIAN_POINT ( 'NONE',  ( 9.564922557961047289, -16.46253265017146816, 20.41775706135233293 ) ) ;
#161353=CARTESIAN_POINT ( 'NONE',  ( 19.05341960407611168, 5.049401038298154454, 48.95724293864768129 ) ) ;
#161354=CARTESIAN_POINT ( 'NONE',  ( -16.51473224551069308, -9.474510206698971260, 111.6655762719810383 ) ) ;
#161355=CARTESIAN_POINT ( 'NONE',  ( 9.474510206698971260, -16.51473224551069308, 92.91557627198103830 ) ) ;
#161357=CARTESIAN_POINT ( 'NONE',  ( 13.97604488694548053, -13.89961937509957401, 65.62609039468567573 ) ) ;
#161358=CARTESIAN_POINT ( 'NONE',  ( -10.81492255796078084, -18.62759615963271287, 42.08224293864769550 ) ) ;
#161359=CARTESIAN_POINT ( 'NONE',  ( -12.06949235617756955, 12.14591786802309770, 25.62390960531435624 ) ) ;
#161360=CARTESIAN_POINT ( 'NONE',  ( 0.05219959533936267826, -19.03943276465977164, 105.0010903946856615 ) ) ;
#161361=CARTESIAN_POINT ( 'NONE',  ( -0.05219959533909027116, -19.03943276465977164, 22.49890960531436690 ) ) ;
#161362=CARTESIAN_POINT ( 'NONE',  ( -5.049401038297874678, -19.05341960407617918, 24.79275706135233648 ) ) ;
#161363=CARTESIAN_POINT ( 'NONE',  ( 16.46253265017146816, 9.564922557961045513, 96.66775706135233293 ) ) ;
#161364=CARTESIAN_POINT ( 'NONE',  ( -10.81492255796078084, -18.62759615963271287, 87.08224293864769550 ) ) ;
#161365=CARTESIAN_POINT ( 'NONE',  ( -19.05341960407617563, 5.049401038297882671, 53.54275706135231871 ) ) ;
#161367=CARTESIAN_POINT ( 'NONE',  ( 13.97604488694527802, 13.89961937509977652, 54.37390960531435979 ) ) ;
#161368=CARTESIAN_POINT ( 'NONE',  ( 16.55341960407611168, 4.379528057220329451, 63.95724293864770260 ) ) ;
#161369=CARTESIAN_POINT ( 'NONE',  ( 5.049401038298161559, -19.05341960407611168, 47.70724293864770260 ) ) ;
#161370=CARTESIAN_POINT ( 'NONE',  ( 14.29746914071049879, -8.314922557960816363, 53.33224293864769550 ) ) ;
#161372=CARTESIAN_POINT ( 'NONE',  ( -8.224510206698948167, 14.34966873604960824, 25.41557627198103120 ) ) ;
#161373=CARTESIAN_POINT ( 'NONE',  ( 5.049401038298161559, -19.05341960407611168, 62.70724293864769550 ) ) ;
#161374=CARTESIAN_POINT ( 'NONE',  ( -16.46253265017146816, -9.564922557961047289, 29.16775706135232937 ) ) ;
#161375=CARTESIAN_POINT ( 'NONE',  ( -4.483927247898782831, 16.52544592524335698, 32.70942372801900433 ) ) ;
#161376=CARTESIAN_POINT ( 'NONE',  ( -10.72451020669898014, 18.67979575497178502, 45.41557627198103830 ) ) ;
#161377=CARTESIAN_POINT ( 'NONE',  ( 21.53943276465977519, 0.05219959533937863772, 111.2510903946856899 ) ) ;
#161378=ORIENTED_EDGE ( 'NONE', *, *, #128983, .T. ) ;
#161379=CARTESIAN_POINT ( 'NONE',  ( 19.03943276465977164, -0.05219959533909143690, 58.74890960531435979 ) ) ;
#161381=CARTESIAN_POINT ( 'NONE',  ( -5.153800228976328057, -19.02544592524343514, 92.29057627198099567 ) ) ;
#161383=CARTESIAN_POINT ( 'NONE',  ( 21.52544592524334988, 5.823673210054432836, 26.45942372801901854 ) ) ;
#161384=CARTESIAN_POINT ( 'NONE',  ( 14.34966873604960469, 8.224510206698951720, 99.16557627198100988 ) ) ;
#161385=CARTESIAN_POINT ( 'NONE',  ( 21.52544592524344225, -5.823673210054117533, 93.54057627198103830 ) ) ;
#161386=CARTESIAN_POINT ( 'NONE',  ( 5.049401038298161559, -19.05341960407611168, 72.70724293864768129 ) ) ;
#161387=CARTESIAN_POINT ( 'NONE',  ( 16.46253265017160672, -9.564922557960803928, 88.33224293864769550 ) ) ;
#161388=CARTESIAN_POINT ( 'NONE',  ( -21.55341960407610458, -5.719274019375992779, 111.4572429386476813 ) ) ;
#161390=CARTESIAN_POINT ( 'NONE',  ( -16.51473224551069308, -9.474510206698971260, 71.66557627198102409 ) ) ;
#161391=CARTESIAN_POINT ( 'NONE',  ( 19.01533133064924286, -5.499999999999438671, 96.26586590595742621 ) ) ;
#161392=CARTESIAN_POINT ( 'NONE',  ( 8.314922557960818139, 14.29746914071049879, 109.5822429386476955 ) ) ;
#161393=CARTESIAN_POINT ( 'NONE',  ( 5.049401038298161559, -19.05341960407611168, 22.70724293864769194 ) ) ;
#161394=CARTESIAN_POINT ( 'NONE',  ( -0.05219959533936034679, 19.03943276465977164, 97.50109039468567573 ) ) ;
#161395=CARTESIAN_POINT ( 'NONE',  ( 14.29746914071049879, -8.314922557960816363, 113.3322429386476955 ) ) ;
#161396=CARTESIAN_POINT ( 'NONE',  ( -5.823673210054431948, 21.52544592524334988, 72.70942372801901854 ) ) ;
#161397=CARTESIAN_POINT ( 'NONE',  ( -19.05341960407611168, -5.049401038298163336, 61.45724293864769550 ) ) ;
#161398=CARTESIAN_POINT ( 'NONE',  ( -21.55341960407619339, 5.719274019375674811, 28.54275706135234358 ) ) ;
#161399=CARTESIAN_POINT ( 'NONE',  ( 0.05219959533907565091, 21.53943276465977519, 104.9989096053143669 ) ) ;
#161401=CARTESIAN_POINT ( 'NONE',  ( 9.564922557960805705, 16.46253265017160317, 74.58224293864769550 ) ) ;
#161403=CARTESIAN_POINT ( 'NONE',  ( 4.379528057220092307, 16.55341960407617563, 32.29275706135235424 ) ) ;
#161404=CARTESIAN_POINT ( 'NONE',  ( -5.719274019375978568, 21.55341960407610458, 25.20724293864769550 ) ) ;
#161405=CARTESIAN_POINT ( 'NONE',  ( -0.05219959533937732626, 21.53943276465977519, 57.50109039468568994 ) ) ;
#161406=CARTESIAN_POINT ( 'NONE',  ( -0.05219959533909027116, -19.03943276465977164, 107.4989096053143527 ) ) ;
#161407=CARTESIAN_POINT ( 'NONE',  ( 5.153800228976615827, -19.02544592524334988, 100.2094237280190043 ) ) ;
#161408=CARTESIAN_POINT ( 'NONE',  ( 9.564922557960805705, 16.46253265017160317, 49.58224293864770260 ) ) ;
#161409=CARTESIAN_POINT ( 'NONE',  ( -13.89961937509977652, 13.97604488694528158, 70.62390960531432427 ) ) ;
#161410=CARTESIAN_POINT ( 'NONE',  ( -16.55341960407611168, -4.379528057220339221, 96.45724293864770971 ) ) ;
#161411=CARTESIAN_POINT ( 'NONE',  ( -5.049401038298153566, 19.05341960407611168, 100.2072429386476955 ) ) ;
#161412=CARTESIAN_POINT ( 'NONE',  ( -12.14591786802309592, -12.06949235617757132, 86.87390960531438111 ) ) ;
#161413=CARTESIAN_POINT ( 'NONE',  ( 9.564922557960805705, 16.46253265017160317, 94.58224293864769550 ) ) ;
#161414=CARTESIAN_POINT ( 'NONE',  ( 16.52544592524342804, -4.483927247898539470, 48.54057627198103120 ) ) ;
#161415=CARTESIAN_POINT ( 'NONE',  ( -9.564922557960796823, -16.46253265017161027, 42.08224293864769550 ) ) ;
#161416=CARTESIAN_POINT ( 'NONE',  ( 10.81492255796106328, -18.62759615963255655, 60.41775706135235424 ) ) ;
#161417=CARTESIAN_POINT ( 'NONE',  ( -13.97604488694547697, 13.89961937509957934, 93.12609039468566152 ) ) ;
#161418=CARTESIAN_POINT ( 'NONE',  ( 16.52544592524342804, -4.483927247898539470, 53.54057627198103120 ) ) ;
#161419=CARTESIAN_POINT ( 'NONE',  ( 21.55341960407610458, 5.719274019375980345, 93.95724293864770971 ) ) ;
#161420=CARTESIAN_POINT ( 'NONE',  ( -5.823673210054116645, -21.52544592524344225, 47.29057627198103120 ) ) ;
#161421=CARTESIAN_POINT ( 'NONE',  ( 19.53091890409951503, 5.500000000000032863, 72.56097431831418021 ) ) ;
#161422=CARTESIAN_POINT ( 'NONE',  ( 16.52544592524342804, -4.483927247898539470, 78.54057627198103830 ) ) ;
#161424=CARTESIAN_POINT ( 'NONE',  ( 5.153800228976335163, 19.02544592524342804, 49.79057627198100988 ) ) ;
#161425=CARTESIAN_POINT ( 'NONE',  ( 8.224510206698742110, 14.34966873604972548, 112.0844237280190185 ) ) ;
#161426=CARTESIAN_POINT ( 'NONE',  ( -4.379528057220086978, -16.55341960407618274, 94.79275706135234714 ) ) ;
#161427=CARTESIAN_POINT ( 'NONE',  ( 16.52544592524335698, 4.483927247898782831, 81.45942372801900433 ) ) ;
#161428=CARTESIAN_POINT ( 'NONE',  ( -19.05341960407617563, 5.049401038297882671, 38.54275706135233293 ) ) ;
#161430=CARTESIAN_POINT ( 'NONE',  ( 5.049401038298161559, -19.05341960407611168, 107.7072429386476955 ) ) ;
#161431=CARTESIAN_POINT ( 'NONE',  ( 19.05341960407611168, 5.049401038298154454, 78.95724293864769550 ) ) ;
#161432=CARTESIAN_POINT ( 'NONE',  ( 9.474510206698971260, -16.51473224551069308, 42.91557627198103120 ) ) ;
#161433=CARTESIAN_POINT ( 'NONE',  ( -14.29746914071049879, 8.314922557960819915, 50.83224293864770971 ) ) ;
#161435=CARTESIAN_POINT ( 'NONE',  ( -5.153800228976328057, -19.02544592524343514, 107.2905762719810383 ) ) ;
#161436=CARTESIAN_POINT ( 'NONE',  ( 10.81492255796078972, 18.62759615963270932, 34.58224293864770260 ) ) ;
#161437=CARTESIAN_POINT ( 'NONE',  ( 16.53943276465976808, -0.05219959533910856209, 83.74890960531435269 ) ) ;
#161438=CARTESIAN_POINT ( 'NONE',  ( -16.52544592524335698, -4.483927247898792601, 38.95942372801901854 ) ) ;
#161439=CARTESIAN_POINT ( 'NONE',  ( -8.224510206698948167, 14.34966873604960824, 75.41557627198102409 ) ) ;
#161440=CARTESIAN_POINT ( 'NONE',  ( 17.50000000000002487, -4.013004640162650460, 32.94605720994412934 ) ) ;
#161441=CARTESIAN_POINT ( 'NONE',  ( 16.51473224551083163, -9.474510206698727899, 60.83442372801900433 ) ) ;
#161442=CARTESIAN_POINT ( 'NONE',  ( -19.05341960407611168, -5.049401038298163336, 96.45724293864769550 ) ) ;
#161443=CARTESIAN_POINT ( 'NONE',  ( 13.89961937509957401, 13.97604488694547697, 81.87609039468564731 ) ) ;
#161444=CARTESIAN_POINT ( 'NONE',  ( 17.50000000000000000, 5.499999999999992895, 76.70309617465829888 ) ) ;
#161445=VECTOR ( 'NONE', #120838, 1000.000000000000000 ) ;
#161446=CARTESIAN_POINT ( 'NONE',  ( -16.52544592524335698, -4.483927247898792601, 28.95942372801902209 ) ) ;
#161447=CARTESIAN_POINT ( 'NONE',  ( -8.314922557961024197, 14.29746914071037800, 107.9177570613523471 ) ) ;
#161448=CARTESIAN_POINT ( 'NONE',  ( 5.049401038297881783, 19.05341960407617563, 77.29275706135231871 ) ) ;
#161449=CARTESIAN_POINT ( 'NONE',  ( -18.67979575497178146, -10.72451020669898902, 31.66557627198102054 ) ) ;
#161450=CARTESIAN_POINT ( 'NONE',  ( 21.53943276465977519, 0.05219959533937863772, 66.25109039468567573 ) ) ;
#161452=CARTESIAN_POINT ( 'NONE',  ( 12.06949235617739724, 12.14591786802326823, 26.87609039468567218 ) ) ;
#161453=CARTESIAN_POINT ( 'NONE',  ( 5.049401038298161559, -19.05341960407611168, 27.70724293864769550 ) ) ;
#161454=CARTESIAN_POINT ( 'NONE',  ( 13.97604488694527802, 13.89961937509977652, 89.37390960531436690 ) ) ;
#161455=CARTESIAN_POINT ( 'NONE',  ( -16.51473224551069308, -9.474510206698971260, 26.66557627198103120 ) ) ;
#161456=CARTESIAN_POINT ( 'NONE',  ( -4.379528057220328563, 16.55341960407611168, 90.20724293864770971 ) ) ;
#161457=CARTESIAN_POINT ( 'NONE',  ( -9.474510206698964154, 16.51473224551069663, 75.41557627198103830 ) ) ;
#161459=CARTESIAN_POINT ( 'NONE',  ( 5.153800228976335163, 19.02544592524342804, 84.79057627198099567 ) ) ;
#161461=CARTESIAN_POINT ( 'NONE',  ( 9.564922557961047289, -16.46253265017146816, 95.41775706135233293 ) ) ;
#161462=CARTESIAN_POINT ( 'NONE',  ( 21.52544592524344225, -5.823673210054117533, 83.54057627198102409 ) ) ;
#161463=CARTESIAN_POINT ( 'NONE',  ( -16.46253265017160317, 9.564922557960807481, 35.83224293864768839 ) ) ;
#161464=CARTESIAN_POINT ( 'NONE',  ( -9.564922557961040184, 16.46253265017147172, 67.91775706135233293 ) ) ;
#161465=CARTESIAN_POINT ( 'NONE',  ( -18.62759615963270932, 10.81492255796079327, 110.8322429386476955 ) ) ;
#161466=CARTESIAN_POINT ( 'NONE',  ( -0.05219959533909027116, -19.03943276465977164, 67.49890960531436690 ) ) ;
#161467=CARTESIAN_POINT ( 'NONE',  ( 5.049401038298161559, -19.05341960407611168, 112.7072429386476813 ) ) ;
#161470=CARTESIAN_POINT ( 'NONE',  ( 18.62759615963271287, -10.81492255796078972, 103.3322429386476955 ) ) ;
#161471=CARTESIAN_POINT ( 'NONE',  ( -16.55341960407611168, -4.379528057220339221, 91.45724293864769550 ) ) ;
#161472=CARTESIAN_POINT ( 'NONE',  ( -19.03943276465977164, 0.05219959533909376836, 81.24890960531436690 ) ) ;
#161473=CARTESIAN_POINT ( 'NONE',  ( 19.03943276465977164, 0.05219959533936151252, 61.25109039468566863 ) ) ;
#161474=CARTESIAN_POINT ( 'NONE',  ( -0.05219959533907301413, -21.53943276465977519, 92.49890960531436690 ) ) ;
#161475=CARTESIAN_POINT ( 'NONE',  ( -21.53943276465977519, 0.05219959533907696930, 71.24890960531435269 ) ) ;
#161476=CARTESIAN_POINT ( 'NONE',  ( 4.379528057220339221, -16.55341960407611168, 52.70724293864769550 ) ) ;
#161477=CARTESIAN_POINT ( 'NONE',  ( -19.03943276465977164, -0.05219959533935918106, 28.75109039468566507 ) ) ;
#161478=CARTESIAN_POINT ( 'NONE',  ( 12.14591786802327356, -12.06949235617739191, 70.62609039468567573 ) ) ;
#161480=CARTESIAN_POINT ( 'NONE',  ( 19.03943276465977164, -0.05219959533909143690, 98.74890960531436690 ) ) ;
#161481=CARTESIAN_POINT ( 'NONE',  ( 0.05219959533909260263, 19.03943276465977164, 39.99890960531436690 ) ) ;
#161482=CARTESIAN_POINT ( 'NONE',  ( -18.62759615963255300, -10.81492255796106328, 49.16775706135234003 ) ) ;
#161483=CARTESIAN_POINT ( 'NONE',  ( -18.67979575497193778, 10.72451020669871902, 48.33442372801902565 ) ) ;
#161484=CARTESIAN_POINT ( 'NONE',  ( -0.05219959533909027116, -19.03943276465977164, 62.49890960531435979 ) ) ;
#161485=CARTESIAN_POINT ( 'NONE',  ( 10.72451020669871369, 18.67979575497193778, 42.08442372801901854 ) ) ;
#161486=CARTESIAN_POINT ( 'NONE',  ( -5.049401038297874678, -19.05341960407617918, 79.79275706135233293 ) ) ;
#161487=CARTESIAN_POINT ( 'NONE',  ( -0.05219959533936034679, 19.03943276465977164, 67.50109039468566152 ) ) ;
#161488=CARTESIAN_POINT ( 'NONE',  ( 5.049401038298161559, -19.05341960407611168, 37.70724293864768839 ) ) ;
#161489=CARTESIAN_POINT ( 'NONE',  ( 4.483927247898790824, -16.52544592524335698, 80.20942372801901854 ) ) ;
#161490=CARTESIAN_POINT ( 'NONE',  ( 16.51473224551069308, 9.474510206698969483, 54.16557627198103120 ) ) ;
#161492=CARTESIAN_POINT ( 'NONE',  ( 19.03943276465977164, -0.05219959533909143690, 98.74890960531436690 ) ) ;
#161493=CARTESIAN_POINT ( 'NONE',  ( -13.97604488694527625, -13.89961937509977652, 41.87390960531435979 ) ) ;
#161494=CARTESIAN_POINT ( 'NONE',  ( -21.53943276465977519, 0.05219959533907696930, 71.24890960531435269 ) ) ;
#161495=CARTESIAN_POINT ( 'NONE',  ( 4.379528057220092307, 16.55341960407617563, 62.29275706135236845 ) ) ;
#161496=CARTESIAN_POINT ( 'NONE',  ( -10.72451020669870658, -18.67979575497194134, 109.5844237280190328 ) ) ;
#161497=CARTESIAN_POINT ( 'NONE',  ( -19.05341960407611168, -5.049401038298163336, 51.45724293864770260 ) ) ;
#161498=CARTESIAN_POINT ( 'NONE',  ( -16.55341960407611168, -4.379528057220339221, 51.45724293864770260 ) ) ;
#161499=CARTESIAN_POINT ( 'NONE',  ( -14.29746914071049879, 8.314922557960819915, 85.83224293864768129 ) ) ;
#161500=CARTESIAN_POINT ( 'NONE',  ( -9.564922557960796823, -16.46253265017161027, 72.08224293864770971 ) ) ;
#161501=CARTESIAN_POINT ( 'NONE',  ( 21.53943276465977519, 0.05219959533937863772, 31.25109039468568639 ) ) ;
#161502=CARTESIAN_POINT ( 'NONE',  ( -16.51473224551069308, -9.474510206698971260, 91.66557627198103830 ) ) ;
#161503=CARTESIAN_POINT ( 'NONE',  ( -18.62759615963255300, -10.81492255796106328, 99.16775706135234714 ) ) ;
#161504=CARTESIAN_POINT ( 'NONE',  ( 12.06949235617739724, 12.14591786802326823, 66.87609039468568994 ) ) ;
#161505=CARTESIAN_POINT ( 'NONE',  ( 10.81492255796106328, -18.62759615963255655, 25.41775706135235779 ) ) ;
#161506=CARTESIAN_POINT ( 'NONE',  ( 19.03943276465977164, -0.05219959533909143690, 108.7489096053143527 ) ) ;
#161507=CARTESIAN_POINT ( 'NONE',  ( -10.81492255796078084, -18.62759615963271287, 87.08224293864769550 ) ) ;
#161508=CARTESIAN_POINT ( 'NONE',  ( -14.29746914071049879, 8.314922557960819915, 40.83224293864769550 ) ) ;
#161509=CARTESIAN_POINT ( 'NONE',  ( 0.05219959533909260263, 19.03943276465977164, 39.99890960531436690 ) ) ;
#161510=CARTESIAN_POINT ( 'NONE',  ( -0.05219959533910754901, -16.53943276465976808, 67.49890960531436690 ) ) ;
#161511=CARTESIAN_POINT ( 'NONE',  ( 18.67979575497178502, 10.72451020669898547, 24.16557627198103120 ) ) ;
#161512=CARTESIAN_POINT ( 'NONE',  ( -19.03943276465977164, -0.05219959533935918106, 28.75109039468566507 ) ) ;
#161513=CARTESIAN_POINT ( 'NONE',  ( 4.483927247898545687, 16.52544592524342804, 99.79057627198103830 ) ) ;
#161514=CARTESIAN_POINT ( 'NONE',  ( -19.03943276465977164, 0.05219959533909376836, 111.2489096053143669 ) ) ;
#161516=CARTESIAN_POINT ( 'NONE',  ( 14.29746914071037800, 8.314922557961029526, 56.66775706135235424 ) ) ;
#161517=CARTESIAN_POINT ( 'NONE',  ( 5.153800228976335163, 19.02544592524342804, 49.79057627198100988 ) ) ;
#161518=CARTESIAN_POINT ( 'NONE',  ( -16.78782133324386905, -5.971338504361712651, 20.53800302010647982 ) ) ;
#161519=CARTESIAN_POINT ( 'NONE',  ( -8.314922557961024197, 14.29746914071037800, 97.91775706135236135 ) ) ;
#161520=CARTESIAN_POINT ( 'NONE',  ( 16.46253265017146816, 9.564922557961045513, 101.6677570613523329 ) ) ;
#161521=CARTESIAN_POINT ( 'NONE',  ( -15.72974639402176322, -15.80617190586768395, 69.37609039468567573 ) ) ;
#161522=CARTESIAN_POINT ( 'NONE',  ( -16.51473224551069308, -9.474510206698971260, 76.66557627198103830 ) ) ;
#161523=CARTESIAN_POINT ( 'NONE',  ( -15.72974639402197994, 15.80617190586746368, 90.62390960531436690 ) ) ;
#161524=CARTESIAN_POINT ( 'NONE',  ( 14.34966873604972726, -8.224510206698740333, 40.83442372801901854 ) ) ;
#161525=CARTESIAN_POINT ( 'NONE',  ( 12.14591786802309770, 12.06949235617756955, 109.3739096053143811 ) ) ;
#161526=CARTESIAN_POINT ( 'NONE',  ( 19.03943276465977164, 0.05219959533936151252, 81.25109039468567573 ) ) ;
#161527=CARTESIAN_POINT ( 'NONE',  ( -15.72974639402197994, 15.80617190586746368, 75.62390960531439532 ) ) ;
#161528=CARTESIAN_POINT ( 'NONE',  ( 0.05219959533936267826, -19.03943276465977164, 55.00109039468566863 ) ) ;
#161529=CARTESIAN_POINT ( 'NONE',  ( 16.46253265017160672, -9.564922557960803928, 113.3322429386476955 ) ) ;
#161530=CARTESIAN_POINT ( 'NONE',  ( 21.55341960407610458, 5.719274019375980345, 83.95724293864770971 ) ) ;
#161531=CARTESIAN_POINT ( 'NONE',  ( 17.50000000000002487, 3.237210098469580632, 27.78763012620467521 ) ) ;
#161532=CARTESIAN_POINT ( 'NONE',  ( -16.51473224551069308, -9.474510206698971260, 61.66557627198103120 ) ) ;
#161534=CARTESIAN_POINT ( 'NONE',  ( -9.564922557961040184, 16.46253265017147172, 112.9177570613523329 ) ) ;
#161536=CARTESIAN_POINT ( 'NONE',  ( -19.03943276465977164, 0.05219959533909376836, 41.24890960531435269 ) ) ;
#161537=CARTESIAN_POINT ( 'NONE',  ( -21.55341960407610458, -5.719274019375992779, 101.4572429386476955 ) ) ;
#161538=CARTESIAN_POINT ( 'NONE',  ( 12.06949235617757843, -12.14591786802309237, 48.12390960531436690 ) ) ;
#161539=CARTESIAN_POINT ( 'NONE',  ( -13.97604488694527625, -13.89961937509977652, 66.87390960531436690 ) ) ;
#161540=CARTESIAN_POINT ( 'NONE',  ( 18.67979575497194134, -10.72451020669871369, 70.83442372801901854 ) ) ;
#161541=CARTESIAN_POINT ( 'NONE',  ( -19.05341960407617563, 5.049401038297882671, 113.5427570613523471 ) ) ;
#161542=CARTESIAN_POINT ( 'NONE',  ( 9.564922557961047289, -16.46253265017146816, 30.41775706135232937 ) ) ;
#161543=CARTESIAN_POINT ( 'NONE',  ( -15.80617190586768217, 15.72974639402176855, 38.12609039468567573 ) ) ;
#161544=CARTESIAN_POINT ( 'NONE',  ( -21.53943276465977519, 0.05219959533907696930, 111.2489096053143669 ) ) ;
#161545=CARTESIAN_POINT ( 'NONE',  ( 5.823673210054125526, 21.52544592524343514, 54.79057627198104541 ) ) ;
#161546=CARTESIAN_POINT ( 'NONE',  ( 9.564922557961047289, -16.46253265017146816, 90.41775706135234714 ) ) ;
#161547=CARTESIAN_POINT ( 'NONE',  ( -9.564922557961040184, 16.46253265017147172, 62.91775706135233293 ) ) ;
#161548=CARTESIAN_POINT ( 'NONE',  ( 15.72974639402176855, 15.80617190586768217, 81.87609039468568994 ) ) ;
#161549=CARTESIAN_POINT ( 'NONE',  ( 19.02544592524334988, 5.153800228976608722, 51.45942372801900433 ) ) ;
#161550=CARTESIAN_POINT ( 'NONE',  ( 16.46253265017160672, -9.564922557960803928, 23.33224293864769194 ) ) ;
#161551=CARTESIAN_POINT ( 'NONE',  ( -0.05219959533907301413, -21.53943276465977519, 62.49890960531436690 ) ) ;
#161552=CARTESIAN_POINT ( 'NONE',  ( 14.34966873604960469, 8.224510206698951720, 44.16557627198103120 ) ) ;
#161553=CARTESIAN_POINT ( 'NONE',  ( -17.72662750342725602, -5.500000000000090594, 51.40179492283743201 ) ) ;
#161554=CARTESIAN_POINT ( 'NONE',  ( -19.03943276465977164, -0.05219959533935918106, 28.75109039468566507 ) ) ;
#161555=CARTESIAN_POINT ( 'NONE',  ( -8.224510206698735004, -14.34966873604973081, 89.58442372801901854 ) ) ;
#161556=CARTESIAN_POINT ( 'NONE',  ( -16.53943276465976808, 0.05219959533911058130, 46.24890960531435979 ) ) ;
#161557=CARTESIAN_POINT ( 'NONE',  ( 5.823673210054444382, -21.52544592524334988, 75.20942372801901854 ) ) ;
#161558=CARTESIAN_POINT ( 'NONE',  ( 15.80617190586769283, -15.72974639402175789, 80.62609039468567573 ) ) ;
#161559=CARTESIAN_POINT ( 'NONE',  ( 21.52544592524344225, -5.823673210054117533, 78.54057627198103830 ) ) ;
#161560=CARTESIAN_POINT ( 'NONE',  ( -0.05219959533909027116, -19.03943276465977164, 37.49890960531436690 ) ) ;
#161561=CARTESIAN_POINT ( 'NONE',  ( 21.53943276465977519, 0.05219959533937863772, 56.25109039468568284 ) ) ;
#161562=CARTESIAN_POINT ( 'NONE',  ( -13.89961937509977652, 13.97604488694528158, 30.62390960531435269 ) ) ;
#161563=ORIENTED_EDGE ( 'NONE', *, *, #73579, .T. ) ;
#161564=CARTESIAN_POINT ( 'NONE',  ( -9.564922557960796823, -16.46253265017161027, 57.08224293864769550 ) ) ;
#161565=CARTESIAN_POINT ( 'NONE',  ( -12.06949235617756955, 12.14591786802309770, 90.62390960531436690 ) ) ;
#161566=CARTESIAN_POINT ( 'NONE',  ( 19.03943276465977164, -0.05219959533909143690, 103.7489096053143669 ) ) ;
#161567=CARTESIAN_POINT ( 'NONE',  ( -12.14591786802309592, -12.06949235617757132, 41.87390960531435979 ) ) ;
#161568=CARTESIAN_POINT ( 'NONE',  ( -8.314922557960811034, -14.29746914071050412, 112.0822429386477097 ) ) ;
#161569=CARTESIAN_POINT ( 'NONE',  ( 5.823673210054125526, 21.52544592524343514, 84.79057627198102409 ) ) ;
#161570=CARTESIAN_POINT ( 'NONE',  ( -5.719274019375665041, -21.55341960407619695, 24.79275706135235779 ) ) ;
#161572=CARTESIAN_POINT ( 'NONE',  ( -12.14591786802326823, 12.06949235617739902, 43.12609039468568284 ) ) ;
#161573=CARTESIAN_POINT ( 'NONE',  ( -15.80617190586745835, -15.72974639402198527, 76.87390960531439532 ) ) ;
#161574=CARTESIAN_POINT ( 'NONE',  ( 21.55341960407619695, -5.719274019375665929, 101.0427570613523756 ) ) ;
#161575=CARTESIAN_POINT ( 'NONE',  ( -13.89961937509977652, 13.97604488694528158, 90.62390960531432427 ) ) ;
#161576=CARTESIAN_POINT ( 'NONE',  ( -21.52544592524334988, -5.823673210054445271, 28.95942372801902209 ) ) ;
#161577=CARTESIAN_POINT ( 'NONE',  ( -5.719274019375978568, 21.55341960407610458, 30.20724293864769550 ) ) ;
#161578=CARTESIAN_POINT ( 'NONE',  ( 16.53943276465976808, 0.05219959533934440121, 96.25109039468568994 ) ) ;
#161579=CARTESIAN_POINT ( 'NONE',  ( 5.823673210054444382, -21.52544592524334988, 65.20942372801901854 ) ) ;
#161580=CARTESIAN_POINT ( 'NONE',  ( 18.67979575497194134, -10.72451020669871369, 110.8344237280190043 ) ) ;
#161581=CARTESIAN_POINT ( 'NONE',  ( 16.52544592524335698, 4.483927247898782831, 76.45942372801901854 ) ) ;
#161582=CARTESIAN_POINT ( 'NONE',  ( 5.719274019375673035, 21.55341960407619339, 32.29275706135235424 ) ) ;
#161583=CARTESIAN_POINT ( 'NONE',  ( 19.05341960407611168, 5.049401038298154454, 38.95724293864767418 ) ) ;
#161584=CARTESIAN_POINT ( 'NONE',  ( -18.62759615963255300, -10.81492255796106328, 94.16775706135237556 ) ) ;
#161585=CARTESIAN_POINT ( 'NONE',  ( -13.97604488694527625, -13.89961937509977652, 106.8739096053143669 ) ) ;
#161586=CARTESIAN_POINT ( 'NONE',  ( 18.67979575497178502, 10.72451020669898547, 109.1655762719810383 ) ) ;
#161587=CARTESIAN_POINT ( 'NONE',  ( 18.89770734986046463, 5.500000000000088818, 81.60214472496643623 ) ) ;
#161588=CARTESIAN_POINT ( 'NONE',  ( -18.62759615963270932, 10.81492255796079327, 55.83224293864770260 ) ) ;
#161589=CARTESIAN_POINT ( 'NONE',  ( 16.51473224551069308, 9.474510206698969483, 99.16557627198102409 ) ) ;
#161590=CARTESIAN_POINT ( 'NONE',  ( -14.34966873604960291, -8.224510206698953496, 46.66557627198102409 ) ) ;
#161592=CARTESIAN_POINT ( 'NONE',  ( -19.02544592524334988, -5.153800228976617603, 78.95942372801900433 ) ) ;
#161594=CARTESIAN_POINT ( 'NONE',  ( -16.51473224551082808, 9.474510206698731452, 108.3344237280190043 ) ) ;
#161595=CARTESIAN_POINT ( 'NONE',  ( 0.05219959533907565091, 21.53943276465977519, 79.99890960531435269 ) ) ;
#161596=CARTESIAN_POINT ( 'NONE',  ( 4.483927247898545687, 16.52544592524342804, 64.79057627198103830 ) ) ;
#161597=CARTESIAN_POINT ( 'NONE',  ( -16.51473224551069308, -9.474510206698971260, 106.6655762719810383 ) ) ;
#161598=CARTESIAN_POINT ( 'NONE',  ( -4.379528057220086978, -16.55341960407618274, 44.79275706135234714 ) ) ;
#161599=CARTESIAN_POINT ( 'NONE',  ( 16.51473224551069308, 9.474510206698969483, 54.16557627198103120 ) ) ;
#161600=CARTESIAN_POINT ( 'NONE',  ( -15.72974639402176322, -15.80617190586768395, 29.37609039468568284 ) ) ;
#161601=CARTESIAN_POINT ( 'NONE',  ( 13.89961937509957401, 13.97604488694547697, 91.87609039468567573 ) ) ;
#161602=CARTESIAN_POINT ( 'NONE',  ( 9.564922557960805705, 16.46253265017160317, 94.58224293864769550 ) ) ;
#161603=CARTESIAN_POINT ( 'NONE',  ( 9.474510206698971260, -16.51473224551069308, 87.91557627198102409 ) ) ;
#161604=CARTESIAN_POINT ( 'NONE',  ( 15.80617190586746368, 15.72974639402197994, 94.37390960531436690 ) ) ;
#161605=CARTESIAN_POINT ( 'NONE',  ( -16.51473224551069308, -9.474510206698971260, 46.66557627198102409 ) ) ;
#161607=CARTESIAN_POINT ( 'NONE',  ( 12.14591786802309770, 12.06949235617756955, 64.37390960531435269 ) ) ;
#161608=CARTESIAN_POINT ( 'NONE',  ( 13.89961937509977652, -13.97604488694527269, 103.1239096053143527 ) ) ;
#161610=CARTESIAN_POINT ( 'NONE',  ( 16.46253265017146816, 9.564922557961045513, 61.66775706135234003 ) ) ;
#161611=CARTESIAN_POINT ( 'NONE',  ( -15.80617190586745835, -15.72974639402198527, 86.87390960531438111 ) ) ;
#161612=CARTESIAN_POINT ( 'NONE',  ( -9.564922557961040184, 16.46253265017147172, 52.91775706135233293 ) ) ;
#161613=CARTESIAN_POINT ( 'NONE',  ( 13.89961937509977652, -13.97604488694527269, 103.1239096053143527 ) ) ;
#161614=CARTESIAN_POINT ( 'NONE',  ( 19.20446147854521968, 5.500000000000079936, 66.88999695167673565 ) ) ;
#161615=CARTESIAN_POINT ( 'NONE',  ( -15.80617190586745835, -15.72974639402198527, 36.87390960531435979 ) ) ;
#161617=CARTESIAN_POINT ( 'NONE',  ( 5.153800228976335163, 19.02544592524342804, 89.79057627198102409 ) ) ;
#161618=CARTESIAN_POINT ( 'NONE',  ( -5.823673210054431948, 21.52544592524334988, 62.70942372801902565 ) ) ;
#161619=CARTESIAN_POINT ( 'NONE',  ( 0.05219959533909260263, 19.03943276465977164, 34.99890960531435979 ) ) ;
#161620=CARTESIAN_POINT ( 'NONE',  ( -14.29746914071049879, 8.314922557960819915, 70.83224293864770971 ) ) ;
#161621=CARTESIAN_POINT ( 'NONE',  ( 16.53943276465976808, 0.05219959533934440121, 26.25109039468567573 ) ) ;
#161622=CARTESIAN_POINT ( 'NONE',  ( -21.53943276465977519, -0.05219959533937600094, 53.75109039468568994 ) ) ;
#161625=CARTESIAN_POINT ( 'NONE',  ( -13.97604488694547697, 13.89961937509957934, 73.12609039468568994 ) ) ;
#161627=CARTESIAN_POINT ( 'NONE',  ( 0.05219959533937995610, -21.53943276465977519, 30.00109039468568284 ) ) ;
#161629=CARTESIAN_POINT ( 'NONE',  ( -13.89961937509957401, -13.97604488694547875, 24.37609039468565442 ) ) ;
#161630=CARTESIAN_POINT ( 'NONE',  ( -16.51473224551069308, -9.474510206698971260, 56.66557627198103120 ) ) ;
#161631=CARTESIAN_POINT ( 'NONE',  ( -0.05219959533937732626, 21.53943276465977519, 112.5010903946857042 ) ) ;
#161632=CARTESIAN_POINT ( 'NONE',  ( 4.379528057220092307, 16.55341960407617563, 107.2927570613523471 ) ) ;
#161633=CARTESIAN_POINT ( 'NONE',  ( -19.03943276465977164, 0.05219959533909376836, 101.2489096053143669 ) ) ;
#161634=CARTESIAN_POINT ( 'NONE',  ( 21.55341960407619695, -5.719274019375665929, 76.04275706135237556 ) ) ;
#161636=FACE_OUTER_BOUND ( 'NONE', #126141, .T. ) ;
#161637=CARTESIAN_POINT ( 'NONE',  ( -18.22780087662122028, 5.500000000000031086, 78.51540105326107266 ) ) ;
#161638=CARTESIAN_POINT ( 'NONE',  ( 4.379528057220092307, 16.55341960407617563, 72.29275706135236135 ) ) ;
#161639=CARTESIAN_POINT ( 'NONE',  ( 15.80617190586769283, -15.72974639402175789, 65.62609039468568994 ) ) ;
#161640=CARTESIAN_POINT ( 'NONE',  ( -15.80617190586768217, 15.72974639402176855, 98.12609039468570415 ) ) ;
#161641=CARTESIAN_POINT ( 'NONE',  ( 17.31747979337951548, -6.344076630960995722, 41.12055131934816643 ) ) ;
#161642=CARTESIAN_POINT ( 'NONE',  ( 19.05341960407611168, 5.049401038298154454, 88.95724293864769550 ) ) ;
#161643=CARTESIAN_POINT ( 'NONE',  ( -13.89961937509977652, 13.97604488694528158, 105.6239096053143527 ) ) ;
#161644=CARTESIAN_POINT ( 'NONE',  ( 15.50000000000000355, -7.500000000000000888, 120.0000000000000142 ) ) ;
#161645=CARTESIAN_POINT ( 'NONE',  ( 13.89961937509977652, -13.97604488694527269, 33.12390960531434558 ) ) ;
#161646=CARTESIAN_POINT ( 'NONE',  ( 10.72451020669898902, -18.67979575497178502, 37.91557627198102409 ) ) ;
#161647=CARTESIAN_POINT ( 'NONE',  ( 8.314922557961029526, -14.29746914071037800, 100.4177570613523471 ) ) ;
#161648=CARTESIAN_POINT ( 'NONE',  ( 14.34966873604960469, 8.224510206698951720, 99.16557627198100988 ) ) ;
#161649=CARTESIAN_POINT ( 'NONE',  ( 19.05341960407611168, 5.049401038298154454, 78.95724293864769550 ) ) ;
#161650=CARTESIAN_POINT ( 'NONE',  ( 10.81492255796106328, -18.62759615963255655, 105.4177570613523613 ) ) ;
#161651=CARTESIAN_POINT ( 'NONE',  ( -13.89961937509977652, 13.97604488694528158, 30.62390960531435269 ) ) ;
#161652=CARTESIAN_POINT ( 'NONE',  ( 16.55341960407611168, 4.379528057220329451, 88.95724293864769550 ) ) ;
#161653=CARTESIAN_POINT ( 'NONE',  ( -18.67979575497193778, 10.72451020669871902, 58.33442372801901143 ) ) ;
#161654=CARTESIAN_POINT ( 'NONE',  ( -18.67979575497178146, -10.72451020669898902, 86.66557627198102409 ) ) ;
#161655=CARTESIAN_POINT ( 'NONE',  ( 19.02544592524334988, 5.153800228976608722, 51.45942372801900433 ) ) ;
#161657=CARTESIAN_POINT ( 'NONE',  ( 16.51473224551069308, 9.474510206698969483, 99.16557627198102409 ) ) ;
#161658=CARTESIAN_POINT ( 'NONE',  ( -16.55341960407611168, -4.379528057220339221, 61.45724293864770260 ) ) ;
#161659=CARTESIAN_POINT ( 'NONE',  ( -16.46253265017146816, -9.564922557961047289, 44.16775706135232582 ) ) ;
#161660=CARTESIAN_POINT ( 'NONE',  ( 8.224510206698953496, -14.34966873604960469, 47.91557627198102409 ) ) ;
#161661=CARTESIAN_POINT ( 'NONE',  ( 13.89961937509957401, 13.97604488694547697, 76.87609039468566152 ) ) ;
#161663=CARTESIAN_POINT ( 'NONE',  ( 18.22780087662119897, -5.500000000000096811, 48.51763182126894236 ) ) ;
#161664=CARTESIAN_POINT ( 'NONE',  ( -10.72451020669898014, 18.67979575497178502, 35.41557627198102409 ) ) ;
#161665=CARTESIAN_POINT ( 'NONE',  ( 0.05219959533910956823, 16.53943276465976808, 99.99890960531436690 ) ) ;
#161666=CARTESIAN_POINT ( 'NONE',  ( -17.50000000000147438, -3.202012800152302052, 25.07177583972721280 ) ) ;
#161667=CARTESIAN_POINT ( 'NONE',  ( 5.153800228976335163, 19.02544592524342804, 49.79057627198100988 ) ) ;
#161668=CARTESIAN_POINT ( 'NONE',  ( 21.52544592524344225, -5.823673210054117533, 43.54057627198103830 ) ) ;
#161669=CARTESIAN_POINT ( 'NONE',  ( -13.89961937509977652, 13.97604488694528158, 35.62390960531435269 ) ) ;
#161670=CARTESIAN_POINT ( 'NONE',  ( -4.483927247898782831, 16.52544592524335698, 82.70942372801900433 ) ) ;
#161671=CARTESIAN_POINT ( 'NONE',  ( 5.153800228976335163, 19.02544592524342804, 64.79057627198100988 ) ) ;
#161672=CARTESIAN_POINT ( 'NONE',  ( 16.51473224551083163, -9.474510206698727899, 35.83442372801899722 ) ) ;
#161673=CARTESIAN_POINT ( 'NONE',  ( -15.80617190586768217, 15.72974639402176855, 63.12609039468568994 ) ) ;
#161674=CARTESIAN_POINT ( 'NONE',  ( -10.72451020669898014, 18.67979575497178502, 55.41557627198102409 ) ) ;
#161675=CARTESIAN_POINT ( 'NONE',  ( 16.51473224551069308, 9.474510206698969483, 29.16557627198103475 ) ) ;
#161676=CARTESIAN_POINT ( 'NONE',  ( -16.46253265017146816, -9.564922557961047289, 109.1677570613523471 ) ) ;
#161677=CARTESIAN_POINT ( 'NONE',  ( 5.049401038298161559, -19.05341960407611168, 22.70724293864769194 ) ) ;
#161679=CARTESIAN_POINT ( 'NONE',  ( 21.55341960407610458, 5.719274019375980345, 53.95724293864770260 ) ) ;
#161680=CARTESIAN_POINT ( 'NONE',  ( -9.474510206698964154, 16.51473224551069663, 25.41557627198103120 ) ) ;
#161681=CARTESIAN_POINT ( 'NONE',  ( -5.823673210054431948, 21.52544592524334988, 77.70942372801900433 ) ) ;
#161682=CARTESIAN_POINT ( 'NONE',  ( -16.53943276465976808, 0.05219959533911058130, 51.24890960531436690 ) ) ;
#161683=CARTESIAN_POINT ( 'NONE',  ( -0.05219959533910754901, -16.53943276465976808, 52.49890960531435979 ) ) ;
#161684=CARTESIAN_POINT ( 'NONE',  ( -18.67979575497178146, -10.72451020669898902, 76.66557627198103830 ) ) ;
#161686=CARTESIAN_POINT ( 'NONE',  ( 21.53943276465977519, -0.05219959533907433946, 78.74890960531436690 ) ) ;
#161688=B_SPLINE_CURVE_WITH_KNOTS ( 'NONE', 3,
 ( #148363, #149363, #180722, #177713, #70521, #178711, #40173, #54352, #103858, #101852, #115023, #39181, #24024, #85678, #99845, #192874, #42197, #102855, #100838, #164541 ),
 .UNSPECIFIED., .F., .F.,
 ( 4, 2, 2, 2, 2, 2, 2, 2, 2, 4 ),
 ( 0.000000000000000000, 0.0004987090165372657638, 0.0009974180330745315275, 0.001246772541343167933, 0.001496127049611804555, 0.001994836066149077800, 0.002493545082686351045, 0.002742899590954987667, 0.002992254099223623856, 0.003989672132298142590 ),
 .UNSPECIFIED. ) ;
#161689=CARTESIAN_POINT ( 'NONE',  ( 10.72451020669898902, -18.67979575497178502, 27.91557627198103830 ) ) ;
#161690=CARTESIAN_POINT ( 'NONE',  ( 0.05219959533934541429, -16.53943276465976808, 50.00109039468568994 ) ) ;
#161691=CARTESIAN_POINT ( 'NONE',  ( -4.379528057220328563, 16.55341960407611168, 80.20724293864769550 ) ) ;
#161692=CARTESIAN_POINT ( 'NONE',  ( -5.049401038298153566, 19.05341960407611168, 60.20724293864768129 ) ) ;
#161693=CARTESIAN_POINT ( 'NONE',  ( -5.049401038298153566, 19.05341960407611168, 35.20724293864768839 ) ) ;
#161695=CARTESIAN_POINT ( 'NONE',  ( 4.379528057220092307, 16.55341960407617563, 77.29275706135234714 ) ) ;
#161696=CARTESIAN_POINT ( 'NONE',  ( -21.53943276465977519, -0.05219959533937600094, 18.75109039468568639 ) ) ;
#161697=CARTESIAN_POINT ( 'NONE',  ( 5.153800228976335163, 19.02544592524342804, 74.79057627198103830 ) ) ;
#161698=CARTESIAN_POINT ( 'NONE',  ( -5.719274019375665041, -21.55341960407619695, 59.79275706135234714 ) ) ;
#161699=CARTESIAN_POINT ( 'NONE',  ( 5.153800228976335163, 19.02544592524342804, 104.7905762719809957 ) ) ;
#161703=CARTESIAN_POINT ( 'NONE',  ( 10.72451020669871369, 18.67979575497193778, 52.08442372801901854 ) ) ;
#161704=CARTESIAN_POINT ( 'NONE',  ( -13.97604488694527625, -13.89961937509977652, 21.87390960531435979 ) ) ;
#161705=CARTESIAN_POINT ( 'NONE',  ( 13.97604488694527802, 13.89961937509977652, 99.37390960531436690 ) ) ;
#161706=CARTESIAN_POINT ( 'NONE',  ( -5.153800228976607833, 19.02544592524334988, 47.70942372801900433 ) ) ;
#161707=CARTESIAN_POINT ( 'NONE',  ( -10.72451020669870658, -18.67979575497194134, 19.58442372801901143 ) ) ;
#161708=CARTESIAN_POINT ( 'NONE',  ( -13.97604488694547697, 13.89961937509957934, 48.12609039468566863 ) ) ;
#161709=CARTESIAN_POINT ( 'NONE',  ( -19.03943276465977164, 0.05219959533909376836, 31.24890960531435979 ) ) ;
#161710=CARTESIAN_POINT ( 'NONE',  ( -4.483927247898782831, 16.52544592524335698, 92.70942372801901854 ) ) ;
#161711=CARTESIAN_POINT ( 'NONE',  ( -16.46253265017146816, -9.564922557961047289, 69.16775706135233293 ) ) ;
#161712=CARTESIAN_POINT ( 'NONE',  ( -16.53943276465976808, -0.05219959533934237506, 103.7510903946857042 ) ) ;
#161715=CARTESIAN_POINT ( 'NONE',  ( -19.05341960407611168, -5.049401038298163336, 81.45724293864769550 ) ) ;
#161716=CARTESIAN_POINT ( 'NONE',  ( -21.55341960407619339, 5.719274019375674811, 88.54275706135236135 ) ) ;
#161717=CARTESIAN_POINT ( 'NONE',  ( 15.80617190586769283, -15.72974639402175789, 100.6260903946857184 ) ) ;
#161718=CARTESIAN_POINT ( 'NONE',  ( 18.22780087662123805, -5.499999999999976019, 98.51763182126896368 ) ) ;
#161719=CARTESIAN_POINT ( 'NONE',  ( 5.153800228976335163, 19.02544592524342804, 99.79057627198102409 ) ) ;
#161720=CARTESIAN_POINT ( 'NONE',  ( -15.72974639402176322, -15.80617190586768395, 79.37609039468567573 ) ) ;
#161721=CARTESIAN_POINT ( 'NONE',  ( -13.89961937509957401, -13.97604488694547875, 109.3760903946856331 ) ) ;
#161722=CARTESIAN_POINT ( 'NONE',  ( 9.474510206698971260, -16.51473224551069308, 82.91557627198103830 ) ) ;
#161723=CARTESIAN_POINT ( 'NONE',  ( -15.72974639402197994, 15.80617190586746368, 30.62390960531436335 ) ) ;
#161724=CARTESIAN_POINT ( 'NONE',  ( 5.049401038298161559, -19.05341960407611168, 92.70724293864769550 ) ) ;
#161726=CARTESIAN_POINT ( 'NONE',  ( 19.02544592524343514, -5.153800228976328945, 83.54057627198100988 ) ) ;
#161727=CARTESIAN_POINT ( 'NONE',  ( 13.97604488694527802, 13.89961937509977652, 69.37390960531436690 ) ) ;
#161728=CARTESIAN_POINT ( 'NONE',  ( -12.06949235617739369, -12.14591786802326823, 104.3760903946856899 ) ) ;
#161729=CARTESIAN_POINT ( 'NONE',  ( -16.61371651742644318, 7.165104196375866152, 98.85415069992970416 ) ) ;
#161730=CARTESIAN_POINT ( 'NONE',  ( 0.05219959533936267826, -19.03943276465977164, 55.00109039468566863 ) ) ;
#161731=CARTESIAN_POINT ( 'NONE',  ( 9.564922557960805705, 16.46253265017160317, 94.58224293864769550 ) ) ;
#161732=CARTESIAN_POINT ( 'NONE',  ( -4.379528057220328563, 16.55341960407611168, 90.20724293864770971 ) ) ;
#161733=CARTESIAN_POINT ( 'NONE',  ( -18.67979575497178146, -10.72451020669898902, 26.66557627198103475 ) ) ;
#161734=CARTESIAN_POINT ( 'NONE',  ( 9.474510206698971260, -16.51473224551069308, 112.9155762719810383 ) ) ;
#161735=CARTESIAN_POINT ( 'NONE',  ( -12.06949235617756955, 12.14591786802309770, 85.62390960531436690 ) ) ;
#161736=CARTESIAN_POINT ( 'NONE',  ( -16.19135201231369692, 7.376712067591781441, 54.81319145947971094 ) ) ;
#161737=CARTESIAN_POINT ( 'NONE',  ( -13.97604488694547697, 13.89961937509957934, 48.12609039468566863 ) ) ;
#161738=CARTESIAN_POINT ( 'NONE',  ( 14.29746914071037800, 8.314922557961029526, 101.6677570613523613 ) ) ;
#161739=CARTESIAN_POINT ( 'NONE',  ( 13.89961937509977652, -13.97604488694527269, 103.1239096053143527 ) ) ;
#161740=CARTESIAN_POINT ( 'NONE',  ( 10.72451020669871369, 18.67979575497193778, 72.08442372801899012 ) ) ;
#161741=CARTESIAN_POINT ( 'NONE',  ( 21.55341960407610458, 5.719274019375980345, 53.95724293864770260 ) ) ;
#161742=CARTESIAN_POINT ( 'NONE',  ( -21.52544592524334988, -5.823673210054445271, 33.95942372801901143 ) ) ;
#161743=CARTESIAN_POINT ( 'NONE',  ( 18.67979575497178502, 10.72451020669898547, 89.16557627198102409 ) ) ;
#161744=CARTESIAN_POINT ( 'NONE',  ( 15.72974639402176855, 15.80617190586768217, 36.87609039468568994 ) ) ;
#161745=CARTESIAN_POINT ( 'NONE',  ( -16.53943276465976808, 0.05219959533911058130, 111.2489096053143669 ) ) ;
#161746=CARTESIAN_POINT ( 'NONE',  ( 13.89961937509957401, 13.97604488694547697, 66.87609039468567573 ) ) ;
#161747=CARTESIAN_POINT ( 'NONE',  ( 5.153800228976335163, 19.02544592524342804, 44.79057627198103830 ) ) ;
#161748=CARTESIAN_POINT ( 'NONE',  ( -14.34966873604960291, -8.224510206698953496, 96.66557627198102409 ) ) ;
#161749=CARTESIAN_POINT ( 'NONE',  ( 19.02544592524343514, -5.153800228976328945, 103.5405762719809957 ) ) ;
#161750=CARTESIAN_POINT ( 'NONE',  ( 13.97604488694527802, 13.89961937509977652, 89.37390960531436690 ) ) ;
#161751=CARTESIAN_POINT ( 'NONE',  ( -14.29746914071049879, 8.314922557960819915, 115.8322429386477097 ) ) ;
#161752=CARTESIAN_POINT ( 'NONE',  ( 4.483927247898545687, 16.52544592524342804, 34.79057627198103120 ) ) ;
#161753=CARTESIAN_POINT ( 'NONE',  ( -8.224510206698735004, -14.34966873604973081, 104.5844237280190185 ) ) ;
#161754=CARTESIAN_POINT ( 'NONE',  ( 9.474510206698971260, -16.51473224551069308, 52.91557627198102409 ) ) ;
#161755=CARTESIAN_POINT ( 'NONE',  ( 19.03943276465977164, -0.05219959533909143690, 23.74890960531435269 ) ) ;
#161756=CARTESIAN_POINT ( 'NONE',  ( -13.89961937509957401, -13.97604488694547875, 24.37609039468565442 ) ) ;
#161757=CARTESIAN_POINT ( 'NONE',  ( -0.05219959533909027116, -19.03943276465977164, 112.4989096053143669 ) ) ;
#161758=CARTESIAN_POINT ( 'NONE',  ( 12.14591786802327356, -12.06949235617739191, 110.6260903946857042 ) ) ;
#161759=CARTESIAN_POINT ( 'NONE',  ( 15.80617190586769283, -15.72974639402175789, 50.62609039468568994 ) ) ;
#161760=CARTESIAN_POINT ( 'NONE',  ( 16.46253265017160672, -9.564922557960803928, 108.3322429386476955 ) ) ;
#161761=CARTESIAN_POINT ( 'NONE',  ( -8.314922557961024197, 14.29746914071037800, 42.91775706135235424 ) ) ;
#161762=CARTESIAN_POINT ( 'NONE',  ( -16.52544592524335698, -4.483927247898792601, 103.9594237280190185 ) ) ;
#161763=CARTESIAN_POINT ( 'NONE',  ( -4.483927247898782831, 16.52544592524335698, 87.70942372801901854 ) ) ;
#161764=CARTESIAN_POINT ( 'NONE',  ( 16.55341960407618274, -4.379528057220086978, 31.04275706135234714 ) ) ;
#161765=CARTESIAN_POINT ( 'NONE',  ( -5.153800228976328057, -19.02544592524343514, 42.29057627198101699 ) ) ;
#161766=CARTESIAN_POINT ( 'NONE',  ( -16.55341960407611168, -4.379528057220339221, 106.4572429386477097 ) ) ;
#161767=CARTESIAN_POINT ( 'NONE',  ( -5.719274019375978568, 21.55341960407610458, 115.2072429386476955 ) ) ;
#161768=CARTESIAN_POINT ( 'NONE',  ( 19.05341960407611168, 5.049401038298154454, 28.95724293864769550 ) ) ;
#161769=CARTESIAN_POINT ( 'NONE',  ( 0.05219959533909260263, 19.03943276465977164, 99.99890960531436690 ) ) ;
#161770=CARTESIAN_POINT ( 'NONE',  ( -5.153800228976328057, -19.02544592524343514, 32.29057627198102409 ) ) ;
#161771=CARTESIAN_POINT ( 'NONE',  ( 9.564922557960805705, 16.46253265017160317, 99.58224293864770971 ) ) ;
#161772=CARTESIAN_POINT ( 'NONE',  ( -16.38665767535055906, -7.295008042175999741, 34.73599135785454450 ) ) ;
#161773=CARTESIAN_POINT ( 'NONE',  ( 9.564922557960805705, 16.46253265017160317, 99.58224293864770971 ) ) ;
#161774=CARTESIAN_POINT ( 'NONE',  ( 10.81492255796106328, -18.62759615963255655, 40.41775706135234714 ) ) ;
#161775=CARTESIAN_POINT ( 'NONE',  ( 16.53943276465976808, -0.05219959533910856209, 108.7489096053143669 ) ) ;
#161776=CARTESIAN_POINT ( 'NONE',  ( 9.564922557960805705, 16.46253265017160317, 114.5822429386476955 ) ) ;
#161778=CARTESIAN_POINT ( 'NONE',  ( -0.05219959533934338120, 16.53943276465976808, 62.50109039468568284 ) ) ;
#161779=CARTESIAN_POINT ( 'NONE',  ( 0.05219959533937995610, -21.53943276465977519, 75.00109039468568994 ) ) ;
#161780=CARTESIAN_POINT ( 'NONE',  ( 12.14591786802327356, -12.06949235617739191, 45.62609039468567573 ) ) ;
#161781=CARTESIAN_POINT ( 'NONE',  ( -19.02544592524342804, 5.153800228976336051, 76.04057627198102409 ) ) ;
#161782=CARTESIAN_POINT ( 'NONE',  ( -19.05341960407617563, 5.049401038297882671, 108.5427570613523187 ) ) ;
#161783=CARTESIAN_POINT ( 'NONE',  ( 16.52544592524335698, 4.483927247898782831, 76.45942372801901854 ) ) ;
#161784=CARTESIAN_POINT ( 'NONE',  ( -0.05219959533936034679, 19.03943276465977164, 87.50109039468567573 ) ) ;
#161785=CARTESIAN_POINT ( 'NONE',  ( -16.46253265017160317, 9.564922557960807481, 80.83224293864769550 ) ) ;
#161786=CARTESIAN_POINT ( 'NONE',  ( -5.823673210054116645, -21.52544592524344225, 97.29057627198105251 ) ) ;
#161787=CARTESIAN_POINT ( 'NONE',  ( 16.55341960407611168, 4.379528057220329451, 83.95724293864770971 ) ) ;
#161788=CARTESIAN_POINT ( 'NONE',  ( 0.05219959533936267826, -19.03943276465977164, 85.00109039468567573 ) ) ;
#161789=CARTESIAN_POINT ( 'NONE',  ( -16.53943276465976808, -0.05219959533934237506, 63.75109039468568284 ) ) ;
#161790=CARTESIAN_POINT ( 'NONE',  ( -19.01533133064924996, 5.499999999999451106, 78.76586590595742621 ) ) ;
#161791=CARTESIAN_POINT ( 'NONE',  ( -13.89961937509957401, -13.97604488694547875, 69.37609039468564731 ) ) ;
#161792=CARTESIAN_POINT ( 'NONE',  ( -0.05219959533910754901, -16.53943276465976808, 27.49890960531435269 ) ) ;
#161793=CARTESIAN_POINT ( 'NONE',  ( 16.55341960407611168, 4.379528057220329451, 78.95724293864769550 ) ) ;
#161794=CARTESIAN_POINT ( 'NONE',  ( 13.97604488694548053, -13.89961937509957401, 20.62609039468567573 ) ) ;
#161795=CARTESIAN_POINT ( 'NONE',  ( -19.26498983726238379, 5.499999999999807265, 90.55319577422004329 ) ) ;
#161796=CARTESIAN_POINT ( 'NONE',  ( -18.62759615963255300, -10.81492255796106328, 24.16775706135235424 ) ) ;
#161797=CARTESIAN_POINT ( 'NONE',  ( 19.05341960407611168, 5.049401038298154454, 108.9572429386477097 ) ) ;
#161798=CARTESIAN_POINT ( 'NONE',  ( -9.474510206698964154, 16.51473224551069663, 80.41557627198103830 ) ) ;
#161799=CARTESIAN_POINT ( 'NONE',  ( -0.05219959533937732626, 21.53943276465977519, 97.50109039468567573 ) ) ;
#161800=CARTESIAN_POINT ( 'NONE',  ( -5.153800228976328057, -19.02544592524343514, 72.29057627198102409 ) ) ;
#161801=CARTESIAN_POINT ( 'NONE',  ( -18.62759615963270932, 10.81492255796079327, 45.83224293864769550 ) ) ;
#161802=CARTESIAN_POINT ( 'NONE',  ( 8.224510206698953496, -14.34966873604960469, 82.91557627198103830 ) ) ;
#161803=CARTESIAN_POINT ( 'NONE',  ( -9.564922557960796823, -16.46253265017161027, 62.08224293864769550 ) ) ;
#161804=CARTESIAN_POINT ( 'NONE',  ( -16.53943276465976808, 0.05219959533911058130, 111.2489096053143669 ) ) ;
#161805=CARTESIAN_POINT ( 'NONE',  ( -10.72451020669870658, -18.67979575497194134, 24.58442372801901499 ) ) ;
#161806=CARTESIAN_POINT ( 'NONE',  ( 5.719274019375673035, 21.55341960407619339, 57.29275706135234714 ) ) ;
#161807=CARTESIAN_POINT ( 'NONE',  ( 9.564922557960805705, 16.46253265017160317, 44.58224293864769550 ) ) ;
#161808=CARTESIAN_POINT ( 'NONE',  ( -16.55341960407617563, 4.379528057220093196, 83.54275706135234714 ) ) ;
#161809=CARTESIAN_POINT ( 'NONE',  ( 10.72451020669898902, -18.67979575497178502, 107.9155762719810241 ) ) ;
#161810=CARTESIAN_POINT ( 'NONE',  ( 5.823673210054125526, 21.52544592524343514, 104.7905762719810241 ) ) ;
#161811=CARTESIAN_POINT ( 'NONE',  ( -13.97604488694547697, 13.89961937509957934, 43.12609039468566152 ) ) ;
#161812=CARTESIAN_POINT ( 'NONE',  ( 19.03943276465977164, -0.05219959533909143690, 68.74890960531436690 ) ) ;
#161813=CARTESIAN_POINT ( 'NONE',  ( -19.03943276465977164, -0.05219959533935918106, 38.75109039468566152 ) ) ;
#161814=CARTESIAN_POINT ( 'NONE',  ( 15.80617190586769283, -15.72974639402175789, 70.62609039468567573 ) ) ;
#161815=CARTESIAN_POINT ( 'NONE',  ( 21.55341960407610458, 5.719274019375980345, 63.95724293864770260 ) ) ;
#161816=CARTESIAN_POINT ( 'NONE',  ( 16.52544592524342804, -4.483927247898539470, 33.54057627198102409 ) ) ;
#161817=CARTESIAN_POINT ( 'NONE',  ( -21.55341960407619339, 5.719274019375674811, 93.54275706135234714 ) ) ;
#161818=CARTESIAN_POINT ( 'NONE',  ( 21.53943276465977519, 0.05219959533937863772, 106.2510903946856757 ) ) ;
#161819=CARTESIAN_POINT ( 'NONE',  ( -4.379528057220328563, 16.55341960407611168, 60.20724293864768839 ) ) ;
#161820=CARTESIAN_POINT ( 'NONE',  ( -4.483927247898539470, -16.52544592524342804, 102.2905762719810383 ) ) ;
#161821=CARTESIAN_POINT ( 'NONE',  ( -9.564922557961040184, 16.46253265017147172, 57.91775706135233293 ) ) ;
#161822=CARTESIAN_POINT ( 'NONE',  ( 16.52544592524342804, -4.483927247898539470, 28.54057627198103120 ) ) ;
#161823=CARTESIAN_POINT ( 'NONE',  ( -21.52544592524334988, -5.823673210054445271, 63.95942372801901854 ) ) ;
#161824=CARTESIAN_POINT ( 'NONE',  ( -13.89961937509977652, 13.97604488694528158, 75.62390960531438111 ) ) ;
#161825=CARTESIAN_POINT ( 'NONE',  ( -13.97604488694547697, 13.89961937509957934, 43.12609039468566152 ) ) ;
#161826=CARTESIAN_POINT ( 'NONE',  ( 15.80617190586746368, 15.72974639402197994, 49.37390960531436690 ) ) ;
#161827=CARTESIAN_POINT ( 'NONE',  ( 21.52544592524334988, 5.823673210054432836, 46.45942372801901854 ) ) ;
#161828=CARTESIAN_POINT ( 'NONE',  ( 15.72974639402199770, -15.80617190586745480, 103.1239096053143811 ) ) ;
#161829=CARTESIAN_POINT ( 'NONE',  ( -13.97604488694547697, 13.89961937509957934, 103.1260903946856473 ) ) ;
#161830=CARTESIAN_POINT ( 'NONE',  ( 16.53943276465976808, 0.05219959533934440121, 71.25109039468568994 ) ) ;
#161832=CARTESIAN_POINT ( 'NONE',  ( -15.72974639402197994, 15.80617190586746368, 110.6239096053143669 ) ) ;
#161833=CARTESIAN_POINT ( 'NONE',  ( -4.483927247898539470, -16.52544592524342804, 92.29057627198103830 ) ) ;
#161835=CARTESIAN_POINT ( 'NONE',  ( -8.314922557961024197, 14.29746914071037800, 27.91775706135234358 ) ) ;
#161837=CARTESIAN_POINT ( 'NONE',  ( -15.72974639402197994, 15.80617190586746368, 45.62390960531436690 ) ) ;
#161838=CARTESIAN_POINT ( 'NONE',  ( 12.06949235617739724, 12.14591786802326823, 86.87609039468568994 ) ) ;
#161839=DIRECTION ( 'NONE',  ( 0.5150380749100522682, 0.000000000000000000, -0.8571673007021134438 ) ) ;
#161840=CARTESIAN_POINT ( 'NONE',  ( -8.314922557961024197, 14.29746914071037800, 67.91775706135234714 ) ) ;
#161841=CARTESIAN_POINT ( 'NONE',  ( -5.719274019375665041, -21.55341960407619695, 29.79275706135234358 ) ) ;
#161842=CARTESIAN_POINT ( 'NONE',  ( -18.67979575497178146, -10.72451020669898902, 46.66557627198102409 ) ) ;
#161843=CARTESIAN_POINT ( 'NONE',  ( 8.314922557961029526, -14.29746914071037800, 85.41775706135236135 ) ) ;
#161844=CARTESIAN_POINT ( 'NONE',  ( -5.049401038298153566, 19.05341960407611168, 100.2072429386476955 ) ) ;
#161845=CARTESIAN_POINT ( 'NONE',  ( -5.823673210054431948, 21.52544592524334988, 72.70942372801901854 ) ) ;
#161846=CARTESIAN_POINT ( 'NONE',  ( 18.62759615963271287, -10.81492255796078972, 43.33224293864769550 ) ) ;
#161847=CARTESIAN_POINT ( 'NONE',  ( -0.05219959533907301413, -21.53943276465977519, 32.49890960531435979 ) ) ;
#161849=CARTESIAN_POINT ( 'NONE',  ( 19.03943276465977164, 0.05219959533936151252, 46.25109039468566863 ) ) ;
#161850=CARTESIAN_POINT ( 'NONE',  ( 16.53943276465976808, 0.05219959533934440121, 66.25109039468567573 ) ) ;
#161851=CARTESIAN_POINT ( 'NONE',  ( 5.719274019375991003, -21.55341960407610458, 37.70724293864769550 ) ) ;
#161853=CARTESIAN_POINT ( 'NONE',  ( 13.89961937509977652, -13.97604488694527269, 88.12390960531438111 ) ) ;
#161854=CARTESIAN_POINT ( 'NONE',  ( 0.05219959533910956823, 16.53943276465976808, 24.99890960531435624 ) ) ;
#161856=CARTESIAN_POINT ( 'NONE',  ( -4.379528057220328563, 16.55341960407611168, 110.2072429386477239 ) ) ;
#161857=CARTESIAN_POINT ( 'NONE',  ( -0.05219959533907301413, -21.53943276465977519, 42.49890960531435979 ) ) ;
#161858=CARTESIAN_POINT ( 'NONE',  ( 13.97604488694527802, 13.89961937509977652, 49.37390960531434558 ) ) ;
#161859=CARTESIAN_POINT ( 'NONE',  ( -4.483927247898782831, 16.52544592524335698, 77.70942372801900433 ) ) ;
#161860=CARTESIAN_POINT ( 'NONE',  ( 15.72974639402176855, 15.80617190586768217, 26.87609039468567218 ) ) ;
#161861=CARTESIAN_POINT ( 'NONE',  ( -19.03943276465977164, -0.05219959533935918106, 83.75109039468567573 ) ) ;
#161862=CARTESIAN_POINT ( 'NONE',  ( 16.52544592524342804, -4.483927247898539470, 93.54057627198103830 ) ) ;
#161863=CARTESIAN_POINT ( 'NONE',  ( 13.97604488694527802, 13.89961937509977652, 49.37390960531434558 ) ) ;
#161864=CARTESIAN_POINT ( 'NONE',  ( 19.05341960407611168, 5.049401038298154454, 28.95724293864769550 ) ) ;
#161865=CARTESIAN_POINT ( 'NONE',  ( 21.53943276465977519, 0.05219959533937863772, 111.2510903946856899 ) ) ;
#161866=CARTESIAN_POINT ( 'NONE',  ( 9.564922557960805705, 16.46253265017160317, 74.58224293864769550 ) ) ;
#161867=CARTESIAN_POINT ( 'NONE',  ( -16.55341960407617563, 4.379528057220093196, 68.54275706135234714 ) ) ;
#161868=CARTESIAN_POINT ( 'NONE',  ( -15.72974639402176322, -15.80617190586768395, 89.37609039468568994 ) ) ;
#161869=CARTESIAN_POINT ( 'NONE',  ( -18.62759615963270932, 10.81492255796079327, 50.83224293864770971 ) ) ;
#161870=CARTESIAN_POINT ( 'NONE',  ( -4.483927247898782831, 16.52544592524335698, 67.70942372801901854 ) ) ;
#161871=CARTESIAN_POINT ( 'NONE',  ( -19.05341960407617563, 5.049401038297882671, 53.54275706135231871 ) ) ;
#161872=CARTESIAN_POINT ( 'NONE',  ( 13.97604488694548053, -13.89961937509957401, 70.62609039468567573 ) ) ;
#161874=CARTESIAN_POINT ( 'NONE',  ( 10.81492255796106328, -18.62759615963255655, 65.41775706135234714 ) ) ;
#161875=CARTESIAN_POINT ( 'NONE',  ( -9.474510206698964154, 16.51473224551069663, 65.41557627198102409 ) ) ;
#161876=CARTESIAN_POINT ( 'NONE',  ( 9.564922557960805705, 16.46253265017160317, 39.58224293864768839 ) ) ;
#161877=CARTESIAN_POINT ( 'NONE',  ( 19.02544592524334988, 5.153800228976608722, 56.45942372801898301 ) ) ;
#161878=CARTESIAN_POINT ( 'NONE',  ( -5.153800228976328057, -19.02544592524343514, 107.2905762719810383 ) ) ;
#161879=CARTESIAN_POINT ( 'NONE',  ( -19.02544592524342804, 5.153800228976336051, 91.04057627198100988 ) ) ;
#161880=CARTESIAN_POINT ( 'NONE',  ( -16.55341960407611168, -4.379528057220339221, 56.45724293864768839 ) ) ;
#161881=CARTESIAN_POINT ( 'NONE',  ( 15.80617190586746368, 15.72974639402197994, 49.37390960531436690 ) ) ;
#161883=CARTESIAN_POINT ( 'NONE',  ( 0.05219959533937995610, -21.53943276465977519, 110.0010903946856757 ) ) ;
#161884=CARTESIAN_POINT ( 'NONE',  ( 19.03943276465977164, -0.05219959533909143690, 48.74890960531435979 ) ) ;
#161887=CARTESIAN_POINT ( 'NONE',  ( 14.34966873604972726, -8.224510206698740333, 65.83442372801900433 ) ) ;
#161888=CARTESIAN_POINT ( 'NONE',  ( -18.67979575497178146, -10.72451020669898902, 91.66557627198103830 ) ) ;
#161889=CARTESIAN_POINT ( 'NONE',  ( 12.14591786802309770, 12.06949235617756955, 49.37390960531436690 ) ) ;
#161890=CARTESIAN_POINT ( 'NONE',  ( 13.89961937509977652, -13.97604488694527269, 43.12390960531434558 ) ) ;
#161892=CARTESIAN_POINT ( 'NONE',  ( 15.72974639402176855, 15.80617190586768217, 41.87609039468568284 ) ) ;
#161893=CARTESIAN_POINT ( 'NONE',  ( -13.97604488694547697, 13.89961937509957934, 48.12609039468566863 ) ) ;
#161894=CARTESIAN_POINT ( 'NONE',  ( -16.46253265017160317, 9.564922557960807481, 35.83224293864768839 ) ) ;
#161895=CARTESIAN_POINT ( 'NONE',  ( 15.80617190586769283, -15.72974639402175789, 100.6260903946857184 ) ) ;
#161898=CARTESIAN_POINT ( 'NONE',  ( -0.05219959533910754901, -16.53943276465976808, 37.49890960531436690 ) ) ;
#161899=CARTESIAN_POINT ( 'NONE',  ( 19.34837522270364829, 5.499999999999730882, 43.36337684832574979 ) ) ;
#161900=CARTESIAN_POINT ( 'NONE',  ( -5.719274019375978568, 21.55341960407610458, 35.20724293864768839 ) ) ;
#161902=CARTESIAN_POINT ( 'NONE',  ( 5.153800228976335163, 19.02544592524342804, 89.79057627198102409 ) ) ;
#161903=CARTESIAN_POINT ( 'NONE',  ( 4.483927247898545687, 16.52544592524342804, 84.79057627198102409 ) ) ;
#161904=CARTESIAN_POINT ( 'NONE',  ( -16.55341960407617563, 4.379528057220093196, 23.54275706135235424 ) ) ;
#161905=EDGE_CURVE ( 'NONE', #194969, #152017, #155010, .T. ) ;
#161906=CARTESIAN_POINT ( 'NONE',  ( 8.224510206698742110, 14.34966873604972548, 112.0844237280190185 ) ) ;
#161908=CARTESIAN_POINT ( 'NONE',  ( 5.049401038298161559, -19.05341960407611168, 102.7072429386476955 ) ) ;
#161909=CARTESIAN_POINT ( 'NONE',  ( -5.719274019375978568, 21.55341960407610458, 85.20724293864770971 ) ) ;
#161910=CARTESIAN_POINT ( 'NONE',  ( 16.52544592524342804, -4.483927247898539470, 23.54057627198102765 ) ) ;
#161911=CARTESIAN_POINT ( 'NONE',  ( -13.89961937509977652, 13.97604488694528158, 105.6239096053143527 ) ) ;
#161912=CARTESIAN_POINT ( 'NONE',  ( 19.02544592524334988, 5.153800228976608722, 76.45942372801897591 ) ) ;
#161913=CARTESIAN_POINT ( 'NONE',  ( 15.80617190586769283, -15.72974639402175789, 105.6260903946856899 ) ) ;
#161914=CARTESIAN_POINT ( 'NONE',  ( 5.719274019375991003, -21.55341960407610458, 87.70724293864769550 ) ) ;
#161915=CARTESIAN_POINT ( 'NONE',  ( -21.53943276465977519, 0.05219959533907696930, 36.24890960531435979 ) ) ;
#161916=CARTESIAN_POINT ( 'NONE',  ( -9.474510206698964154, 16.51473224551069663, 65.41557627198102409 ) ) ;
#161917=CARTESIAN_POINT ( 'NONE',  ( -14.29746914071049879, 8.314922557960819915, 40.83224293864769550 ) ) ;
#161918=CARTESIAN_POINT ( 'NONE',  ( -19.05341960407611168, -5.049401038298163336, 76.45724293864769550 ) ) ;
#161921=CARTESIAN_POINT ( 'NONE',  ( -16.51473224551082808, 9.474510206698731452, 23.33442372801900078 ) ) ;
#161922=CARTESIAN_POINT ( 'NONE',  ( 4.483927247898545687, 16.52544592524342804, 84.79057627198102409 ) ) ;
#161923=CARTESIAN_POINT ( 'NONE',  ( 18.62759615963255655, 10.81492255796105972, 26.66775706135235424 ) ) ;
#161925=CARTESIAN_POINT ( 'NONE',  ( 10.81492255796078972, 18.62759615963270932, 74.58224293864768129 ) ) ;
#161926=CARTESIAN_POINT ( 'NONE',  ( -8.314922557961024197, 14.29746914071037800, 92.91775706135236135 ) ) ;
#161927=CARTESIAN_POINT ( 'NONE',  ( 19.03943276465977164, -0.05219959533909143690, 23.74890960531435269 ) ) ;
#161928=CARTESIAN_POINT ( 'NONE',  ( 5.049401038298161559, -19.05341960407611168, 67.70724293864769550 ) ) ;
#161929=CARTESIAN_POINT ( 'NONE',  ( 19.03943276465977164, -0.05219959533909143690, 23.74890960531435269 ) ) ;
#161930=CARTESIAN_POINT ( 'NONE',  ( 0.05219959533910956823, 16.53943276465976808, 24.99890960531435624 ) ) ;
#161931=CARTESIAN_POINT ( 'NONE',  ( -21.52544592524334988, -5.823673210054445271, 58.95942372801902565 ) ) ;
#161933=CARTESIAN_POINT ( 'NONE',  ( 15.80617190586769283, -15.72974639402175789, 95.62609039468568994 ) ) ;
#161934=CARTESIAN_POINT ( 'NONE',  ( -13.89961937509977652, 13.97604488694528158, 40.62390960531435979 ) ) ;
#161935=CARTESIAN_POINT ( 'NONE',  ( -16.51473224551069308, -9.474510206698971260, 51.66557627198102409 ) ) ;
#161937=CARTESIAN_POINT ( 'NONE',  ( -21.53943276465977519, -0.05219959533937600094, 88.75109039468567573 ) ) ;
#161938=CARTESIAN_POINT ( 'NONE',  ( 16.53943276465976808, 0.05219959533934440121, 66.25109039468567573 ) ) ;
#161939=CARTESIAN_POINT ( 'NONE',  ( 21.53943276465977519, 0.05219959533937863772, 81.25109039468568994 ) ) ;
#161940=CARTESIAN_POINT ( 'NONE',  ( 0.05219959533909260263, 19.03943276465977164, 114.9989096053143669 ) ) ;
#161941=CARTESIAN_POINT ( 'NONE',  ( 9.564922557961047289, -16.46253265017146816, 100.4177570613523329 ) ) ;
#161942=CARTESIAN_POINT ( 'NONE',  ( 18.62759615963255655, 10.81492255796105972, 56.66775706135235424 ) ) ;
#161943=CARTESIAN_POINT ( 'NONE',  ( 16.53943276465976808, 0.05219959533934440121, 36.25109039468567573 ) ) ;
#161944=CARTESIAN_POINT ( 'NONE',  ( -21.53943276465977519, 0.05219959533907696930, 91.24890960531436690 ) ) ;
#161945=CARTESIAN_POINT ( 'NONE',  ( -19.02544592524334988, -5.153800228976617603, 88.95942372801897591 ) ) ;
#161946=CARTESIAN_POINT ( 'NONE',  ( -13.89961937509977652, 13.97604488694528158, 60.62390960531436690 ) ) ;
#161947=CARTESIAN_POINT ( 'NONE',  ( -5.049401038297874678, -19.05341960407617918, 94.79275706135230450 ) ) ;
#161948=CARTESIAN_POINT ( 'NONE',  ( -9.474510206698720793, -16.51473224551083518, 99.58442372801900433 ) ) ;
#161949=CARTESIAN_POINT ( 'NONE',  ( 12.06949235617757843, -12.14591786802309237, 53.12390960531436690 ) ) ;
#161950=CARTESIAN_POINT ( 'NONE',  ( -13.97604488694547697, 13.89961937509957934, 73.12609039468568994 ) ) ;
#161951=CARTESIAN_POINT ( 'NONE',  ( 16.55341960407618274, -4.379528057220086978, 56.04275706135235424 ) ) ;
#161952=CARTESIAN_POINT ( 'NONE',  ( 16.46253265017160672, -9.564922557960803928, 38.33224293864768839 ) ) ;
#161953=CARTESIAN_POINT ( 'NONE',  ( 19.02544592524343514, -5.153800228976328945, 58.54057627198102409 ) ) ;
#161954=CARTESIAN_POINT ( 'NONE',  ( 0.05219959533934541429, -16.53943276465976808, 60.00109039468568284 ) ) ;
#161957=CARTESIAN_POINT ( 'NONE',  ( -16.46253265017160317, 9.564922557960807481, 105.8322429386476955 ) ) ;
#161960=CARTESIAN_POINT ( 'NONE',  ( -5.153800228976607833, 19.02544592524334988, 102.7094237280189759 ) ) ;
#161961=CARTESIAN_POINT ( 'NONE',  ( -5.823673210054116645, -21.52544592524344225, 42.29057627198103120 ) ) ;
#161962=CARTESIAN_POINT ( 'NONE',  ( -5.153800228976607833, 19.02544592524334988, 32.70942372801899722 ) ) ;
#161963=CARTESIAN_POINT ( 'NONE',  ( -4.379528057220086978, -16.55341960407618274, 19.79275706135235069 ) ) ;
#161964=CARTESIAN_POINT ( 'NONE',  ( 16.46253265017160672, -9.564922557960803928, 23.33224293864769194 ) ) ;
#161965=CARTESIAN_POINT ( 'NONE',  ( 0.05219959533909260263, 19.03943276465977164, 49.99890960531435979 ) ) ;
#161966=CARTESIAN_POINT ( 'NONE',  ( -21.52544592524343514, 5.823673210054127303, 71.04057627198103830 ) ) ;
#161967=CARTESIAN_POINT ( 'NONE',  ( 19.05341960407611168, 5.049401038298154454, 103.9572429386476671 ) ) ;
#161968=CARTESIAN_POINT ( 'NONE',  ( -16.46253265017160317, 9.564922557960807481, 35.83224293864768839 ) ) ;
#161970=CARTESIAN_POINT ( 'NONE',  ( -5.153800228976607833, 19.02544592524334988, 87.70942372801897591 ) ) ;
#161971=CARTESIAN_POINT ( 'NONE',  ( -0.05219959533910754901, -16.53943276465976808, 67.49890960531436690 ) ) ;
#161972=CARTESIAN_POINT ( 'NONE',  ( -21.52544592524343514, 5.823673210054127303, 51.04057627198103120 ) ) ;
#161973=CARTESIAN_POINT ( 'NONE',  ( -18.62759615963255300, -10.81492255796106328, 104.1677570613523471 ) ) ;
#161974=CARTESIAN_POINT ( 'NONE',  ( 15.80617190586746368, 15.72974639402197994, 94.37390960531436690 ) ) ;
#161975=CARTESIAN_POINT ( 'NONE',  ( -5.823673210054431948, 21.52544592524334988, 67.70942372801901854 ) ) ;
#161976=CARTESIAN_POINT ( 'NONE',  ( -21.55341960407619339, 5.719274019375674811, 83.54275706135234714 ) ) ;
#161977=CARTESIAN_POINT ( 'NONE',  ( 19.02544592524343514, -5.153800228976328945, 108.5405762719810383 ) ) ;
#161978=CARTESIAN_POINT ( 'NONE',  ( -4.379528057220086978, -16.55341960407618274, 109.7927570613523613 ) ) ;
#161979=CARTESIAN_POINT ( 'NONE',  ( -0.05219959533937732626, 21.53943276465977519, 82.50109039468568994 ) ) ;
#161980=CARTESIAN_POINT ( 'NONE',  ( -16.51473224551069308, -9.474510206698971260, 66.66557627198102409 ) ) ;
#161981=CARTESIAN_POINT ( 'NONE',  ( -19.02544592524334988, -5.153800228976617603, 33.95942372801897591 ) ) ;
#161982=CARTESIAN_POINT ( 'NONE',  ( -15.72974639402176322, -15.80617190586768395, 24.37609039468567573 ) ) ;
#161983=CARTESIAN_POINT ( 'NONE',  ( -16.46253265017160317, 9.564922557960807481, 70.83224293864770971 ) ) ;
#161984=CARTESIAN_POINT ( 'NONE',  ( -12.14591786802309592, -12.06949235617757132, 86.87390960531438111 ) ) ;
#161985=CARTESIAN_POINT ( 'NONE',  ( -4.379528057220328563, 16.55341960407611168, 45.20724293864769550 ) ) ;
#161986=CARTESIAN_POINT ( 'NONE',  ( 21.52544592524344225, -5.823673210054117533, 53.54057627198103120 ) ) ;
#161987=CARTESIAN_POINT ( 'NONE',  ( -19.05341960407611168, -5.049401038298163336, 66.45724293864769550 ) ) ;
#161988=CARTESIAN_POINT ( 'NONE',  ( 18.62759615963271287, -10.81492255796078972, 73.33224293864769550 ) ) ;
#161989=CARTESIAN_POINT ( 'NONE',  ( -13.97604488694547697, 13.89961937509957934, 68.12609039468563310 ) ) ;
#161990=CARTESIAN_POINT ( 'NONE',  ( 5.153800228976617603, -19.02544592524335343, 25.20942372801900433 ) ) ;
#161991=CARTESIAN_POINT ( 'NONE',  ( -16.52544592524342804, 4.483927247898546575, 66.04057627198103830 ) ) ;
#161992=CARTESIAN_POINT ( 'NONE',  ( 15.80617190586746368, 15.72974639402197994, 44.37390960531435979 ) ) ;
#161994=CARTESIAN_POINT ( 'NONE',  ( 16.62475595723698873, 7.163666690055318753, 101.9728664818952666 ) ) ;
#161995=CARTESIAN_POINT ( 'NONE',  ( -8.314922557961024197, 14.29746914071037800, 87.91775706135234714 ) ) ;
#161997=CARTESIAN_POINT ( 'NONE',  ( 9.564922557961047289, -16.46253265017146816, 90.41775706135234714 ) ) ;
#161998=CARTESIAN_POINT ( 'NONE',  ( -16.53943276465976808, 0.05219959533911058130, 51.24890960531436690 ) ) ;
#161999=CARTESIAN_POINT ( 'NONE',  ( -19.39056639909674118, -5.500000000000059508, 60.78948781074343088 ) ) ;
#162000=CARTESIAN_POINT ( 'NONE',  ( -0.05219959533909027116, -19.03943276465977164, 47.49890960531435979 ) ) ;
#162001=CARTESIAN_POINT ( 'NONE',  ( 0.05219959533910956823, 16.53943276465976808, 34.99890960531435979 ) ) ;
#162002=CARTESIAN_POINT ( 'NONE',  ( -19.03943276465977164, 0.05219959533909376836, 86.24890960531436690 ) ) ;
#162003=CARTESIAN_POINT ( 'NONE',  ( -9.564922557961040184, 16.46253265017147172, 77.91775706135234714 ) ) ;
#162004=CARTESIAN_POINT ( 'NONE',  ( -19.03943276465977164, 0.05219959533909376836, 56.24890960531435979 ) ) ;
#162005=CARTESIAN_POINT ( 'NONE',  ( -10.81492255796105439, 18.62759615963255655, 62.91775706135236135 ) ) ;
#162006=CARTESIAN_POINT ( 'NONE',  ( -19.02544592524342804, 5.153800228976336051, 66.04057627198103830 ) ) ;
#162007=CARTESIAN_POINT ( 'NONE',  ( -13.97604488694527625, -13.89961937509977652, 31.87390960531435979 ) ) ;
#162008=CARTESIAN_POINT ( 'NONE',  ( 16.46253265017160672, -9.564922557960803928, 78.33224293864769550 ) ) ;
#162009=CARTESIAN_POINT ( 'NONE',  ( 21.52544592524344225, -5.823673210054117533, 53.54057627198103120 ) ) ;
#162010=CARTESIAN_POINT ( 'NONE',  ( 16.46253265017160672, -9.564922557960803928, 43.33224293864769550 ) ) ;
#162011=CARTESIAN_POINT ( 'NONE',  ( -5.719274019375978568, 21.55341960407610458, 60.20724293864768839 ) ) ;
#162012=CARTESIAN_POINT ( 'NONE',  ( -5.049401038297874678, -19.05341960407617918, 84.79275706135233293 ) ) ;
#162013=CARTESIAN_POINT ( 'NONE',  ( 8.314922557961029526, -14.29746914071037800, 100.4177570613523471 ) ) ;
#162014=CARTESIAN_POINT ( 'NONE',  ( 13.97604488694548053, -13.89961937509957401, 30.62609039468566863 ) ) ;
#162015=EDGE_CURVE ( 'NONE', #65144, #61486, #39677, .T. ) ;
#162016=CARTESIAN_POINT ( 'NONE',  ( 4.483927247898790824, -16.52544592524335698, 55.20942372801902565 ) ) ;
#162017=CARTESIAN_POINT ( 'NONE',  ( 16.53943276465976808, 0.05219959533934440121, 86.25109039468568994 ) ) ;
#162018=CARTESIAN_POINT ( 'NONE',  ( 0.000000000000000000, 0.000000000000000000, 20.00000000000000000 ) ) ;
#162019=CARTESIAN_POINT ( 'NONE',  ( 14.29746914071037800, 8.314922557961029526, 71.66775706135234714 ) ) ;
#162020=CARTESIAN_POINT ( 'NONE',  ( 21.55341960407610458, 5.719274019375980345, 23.95724293864769550 ) ) ;
#162021=CARTESIAN_POINT ( 'NONE',  ( 19.05341960407611168, 5.049401038298154454, 38.95724293864767418 ) ) ;
#162022=CARTESIAN_POINT ( 'NONE',  ( 4.483927247898790824, -16.52544592524335698, 35.20942372801901854 ) ) ;
#162023=CARTESIAN_POINT ( 'NONE',  ( -19.02544592524342804, 5.153800228976336051, 51.04057627198103120 ) ) ;
#162024=CARTESIAN_POINT ( 'NONE',  ( -18.62759615963255300, -10.81492255796106328, 44.16775706135234714 ) ) ;
#162025=CARTESIAN_POINT ( 'NONE',  ( 0.05219959533934541429, -16.53943276465976808, 30.00109039468568284 ) ) ;
#162026=CARTESIAN_POINT ( 'NONE',  ( 0.05219959533910956823, 16.53943276465976808, 24.99890960531435624 ) ) ;
#162028=CARTESIAN_POINT ( 'NONE',  ( -10.81492255796105439, 18.62759615963255655, 112.9177570613523329 ) ) ;
#162029=CARTESIAN_POINT ( 'NONE',  ( 16.46253265017146816, 9.564922557961045513, 106.6677570613523471 ) ) ;
#162030=CARTESIAN_POINT ( 'NONE',  ( 13.97604488694548053, -13.89961937509957401, 65.62609039468567573 ) ) ;
#162031=CARTESIAN_POINT ( 'NONE',  ( -16.52544592524342804, 4.483927247898546575, 76.04057627198102409 ) ) ;
#162032=CARTESIAN_POINT ( 'NONE',  ( 13.97604488694527802, 13.89961937509977652, 44.37390960531435269 ) ) ;
#162033=CARTESIAN_POINT ( 'NONE',  ( 16.51473224551083163, -9.474510206698727899, 75.83442372801900433 ) ) ;
#162034=CARTESIAN_POINT ( 'NONE',  ( 17.44279575226787671, -5.990770900253882481, 58.33557567514320397 ) ) ;
#162035=CARTESIAN_POINT ( 'NONE',  ( 21.55341960407619695, -5.719274019375665929, 61.04275706135234714 ) ) ;
#162036=CARTESIAN_POINT ( 'NONE',  ( 4.379528057220092307, 16.55341960407617563, 37.29275706135235424 ) ) ;
#162037=CARTESIAN_POINT ( 'NONE',  ( 19.46398650005389896, -5.499999999999940492, 57.68269651486372851 ) ) ;
#162038=CARTESIAN_POINT ( 'NONE',  ( -13.97604488694527625, -13.89961937509977652, 111.8739096053143243 ) ) ;
#162039=CARTESIAN_POINT ( 'NONE',  ( 12.06949235617739724, 12.14591786802326823, 31.87609039468567929 ) ) ;
#162042=CARTESIAN_POINT ( 'NONE',  ( -9.474510206698964154, 16.51473224551069663, 35.41557627198102409 ) ) ;
#162043=CARTESIAN_POINT ( 'NONE',  ( -5.719274019375665041, -21.55341960407619695, 104.7927570613523898 ) ) ;
#162044=CARTESIAN_POINT ( 'NONE',  ( 13.89961937509977652, -13.97604488694527269, 53.12390960531434558 ) ) ;
#162045=CARTESIAN_POINT ( 'NONE',  ( 21.55341960407619695, -5.719274019375665929, 61.04275706135234714 ) ) ;
#162046=CARTESIAN_POINT ( 'NONE',  ( -10.81492255796105439, 18.62759615963255655, 97.91775706135236135 ) ) ;
#162047=CARTESIAN_POINT ( 'NONE',  ( 14.29746914071049879, -8.314922557960816363, 23.33224293864769194 ) ) ;
#162048=CARTESIAN_POINT ( 'NONE',  ( -9.564922557960796823, -16.46253265017161027, 27.08224293864769550 ) ) ;
#162049=CARTESIAN_POINT ( 'NONE',  ( -0.05219959533909027116, -19.03943276465977164, 87.49890960531436690 ) ) ;
#162050=CARTESIAN_POINT ( 'NONE',  ( -10.72451020669870658, -18.67979575497194134, 59.58442372801901854 ) ) ;
#162051=CARTESIAN_POINT ( 'NONE',  ( -13.97604488694527625, -13.89961937509977652, 31.87390960531435979 ) ) ;
#162052=CARTESIAN_POINT ( 'NONE',  ( 21.53943276465977519, 0.05219959533937863772, 56.25109039468568284 ) ) ;
#162053=CARTESIAN_POINT ( 'NONE',  ( 19.05341960407617918, -5.049401038297876454, 81.04275706135231871 ) ) ;
#162054=CARTESIAN_POINT ( 'NONE',  ( -19.03943276465977164, 0.05219959533909376836, 111.2489096053143669 ) ) ;
#162055=CARTESIAN_POINT ( 'NONE',  ( 9.474510206698971260, -16.51473224551069308, 22.91557627198102765 ) ) ;
#162056=CARTESIAN_POINT ( 'NONE',  ( 18.67979575497178502, 10.72451020669898547, 114.1655762719810383 ) ) ;
#162057=CARTESIAN_POINT ( 'NONE',  ( 16.51473224551083163, -9.474510206698727899, 30.83442372801900433 ) ) ;
#162058=CARTESIAN_POINT ( 'NONE',  ( 16.53943276465976808, -0.05219959533910856209, 108.7489096053143669 ) ) ;
#162059=CARTESIAN_POINT ( 'NONE',  ( 16.46253265017160672, -9.564922557960803928, 53.33224293864768839 ) ) ;
#162060=CARTESIAN_POINT ( 'NONE',  ( 13.89961937509957401, 13.97604488694547697, 101.8760903946856331 ) ) ;
#162061=CARTESIAN_POINT ( 'NONE',  ( -8.314922557960811034, -14.29746914071050412, 57.08224293864769550 ) ) ;
#162062=CARTESIAN_POINT ( 'NONE',  ( 18.62759615963255655, 10.81492255796105972, 111.6677570613523613 ) ) ;
#162063=CARTESIAN_POINT ( 'NONE',  ( 15.72974639402199770, -15.80617190586745480, 28.12390960531435979 ) ) ;
#162064=CARTESIAN_POINT ( 'NONE',  ( 0.05219959533936267826, -19.03943276465977164, 85.00109039468567573 ) ) ;
#162065=CARTESIAN_POINT ( 'NONE',  ( -21.52544592524343514, 5.823673210054127303, 96.04057627198102409 ) ) ;
#162066=CARTESIAN_POINT ( 'NONE',  ( 21.52544592524334988, 5.823673210054432836, 46.45942372801901854 ) ) ;
#162067=CARTESIAN_POINT ( 'NONE',  ( 4.379528057220092307, 16.55341960407617563, 42.29275706135235424 ) ) ;
#162068=CARTESIAN_POINT ( 'NONE',  ( -8.224510206698735004, -14.34966873604973081, 104.5844237280190185 ) ) ;
#162069=CARTESIAN_POINT ( 'NONE',  ( -16.52544592524335698, -4.483927247898792601, 38.95942372801901854 ) ) ;
#162070=CARTESIAN_POINT ( 'NONE',  ( -21.52544592524334988, -5.823673210054445271, 43.95942372801902565 ) ) ;
#162071=CARTESIAN_POINT ( 'NONE',  ( 10.72451020669898902, -18.67979575497178502, 42.91557627198103120 ) ) ;
#162072=CARTESIAN_POINT ( 'NONE',  ( 19.02544592524343514, -5.153800228976328945, 38.54057627198103120 ) ) ;
#162074=CARTESIAN_POINT ( 'NONE',  ( 14.34966873604972726, -8.224510206698740333, 65.83442372801900433 ) ) ;
#162077=CARTESIAN_POINT ( 'NONE',  ( -10.81492255796078084, -18.62759615963271287, 92.08224293864769550 ) ) ;
#162078=CARTESIAN_POINT ( 'NONE',  ( 12.14591786802309770, 12.06949235617756955, 39.37390960531436690 ) ) ;
#162079=CARTESIAN_POINT ( 'NONE',  ( 16.55341960407618274, -4.379528057220086978, 56.04275706135235424 ) ) ;
#162080=CARTESIAN_POINT ( 'NONE',  ( 19.03943276465977164, -0.05219959533909143690, 53.74890960531436690 ) ) ;
#162081=CARTESIAN_POINT ( 'NONE',  ( 5.049401038297881783, 19.05341960407617563, 102.2927570613523045 ) ) ;
#162082=CARTESIAN_POINT ( 'NONE',  ( -10.72451020669898014, 18.67979575497178502, 85.41557627198102409 ) ) ;
#162083=CARTESIAN_POINT ( 'NONE',  ( 4.483927247898545687, 16.52544592524342804, 34.79057627198103120 ) ) ;
#162085=CARTESIAN_POINT ( 'NONE',  ( -4.483927247898782831, 16.52544592524335698, 82.70942372801900433 ) ) ;
#162087=CARTESIAN_POINT ( 'NONE',  ( -18.62759615963270932, 10.81492255796079327, 75.83224293864769550 ) ) ;
#162088=CARTESIAN_POINT ( 'NONE',  ( -16.52544592524335698, -4.483927247898792601, 98.95942372801903275 ) ) ;
#162091=CARTESIAN_POINT ( 'NONE',  ( 0.05219959533907565091, 21.53943276465977519, 84.99890960531436690 ) ) ;
#162092=CARTESIAN_POINT ( 'NONE',  ( -5.823673210054116645, -21.52544592524344225, 112.2905762719810241 ) ) ;
#162093=CARTESIAN_POINT ( 'NONE',  ( -8.314922557960811034, -14.29746914071050412, 37.08224293864768129 ) ) ;
#162094=CARTESIAN_POINT ( 'NONE',  ( 4.483927247898790824, -16.52544592524335698, 35.20942372801901854 ) ) ;
#162095=CARTESIAN_POINT ( 'NONE',  ( 5.049401038298161559, -19.05341960407611168, 37.70724293864768839 ) ) ;
#162096=CARTESIAN_POINT ( 'NONE',  ( 13.89961937509977652, -13.97604488694527269, 68.12390960531436690 ) ) ;
#162098=CARTESIAN_POINT ( 'NONE',  ( -21.53943276465977519, 0.05219959533907696930, 21.24890960531436690 ) ) ;
#162100=CARTESIAN_POINT ( 'NONE',  ( -19.05341960407617563, 5.049401038297882671, 103.5427570613523329 ) ) ;
#162101=CARTESIAN_POINT ( 'NONE',  ( -16.46253265017146816, -9.564922557961047289, 44.16775706135232582 ) ) ;
#162102=CARTESIAN_POINT ( 'NONE',  ( 18.62759615963271287, -10.81492255796078972, 88.33224293864769550 ) ) ;
#162103=CARTESIAN_POINT ( 'NONE',  ( -12.14591786802326823, 12.06949235617739902, 113.1260903946856899 ) ) ;
#162104=CARTESIAN_POINT ( 'NONE',  ( 5.823673210054125526, 21.52544592524343514, 44.79057627198103120 ) ) ;
#162105=CARTESIAN_POINT ( 'NONE',  ( -18.62759615963270932, 10.81492255796079327, 80.83224293864769550 ) ) ;
#162106=CARTESIAN_POINT ( 'NONE',  ( -19.02544592524334988, -5.153800228976617603, 108.9594237280189759 ) ) ;
#162107=CARTESIAN_POINT ( 'NONE',  ( -19.03943276465977164, 0.05219959533909376836, 111.2489096053143669 ) ) ;
#162108=CARTESIAN_POINT ( 'NONE',  ( 15.72974639402176855, 15.80617190586768217, 71.87609039468568994 ) ) ;
#162109=CARTESIAN_POINT ( 'NONE',  ( 5.049401038298161559, -19.05341960407611168, 72.70724293864768129 ) ) ;
#162110=CARTESIAN_POINT ( 'NONE',  ( -12.06949235617756955, 12.14591786802309770, 105.6239096053143669 ) ) ;
#162112=CARTESIAN_POINT ( 'NONE',  ( 9.564922557960805705, 16.46253265017160317, 64.58224293864769550 ) ) ;
#162113=CARTESIAN_POINT ( 'NONE',  ( 0.05219959533910956823, 16.53943276465976808, 84.99890960531436690 ) ) ;
#162115=CARTESIAN_POINT ( 'NONE',  ( 19.03943276465977164, 0.05219959533936151252, 101.2510903946856757 ) ) ;
#162117=CARTESIAN_POINT ( 'NONE',  ( 0.05219959533909260263, 19.03943276465977164, 54.99890960531435979 ) ) ;
#162118=CARTESIAN_POINT ( 'NONE',  ( -0.05219959533937732626, 21.53943276465977519, 82.50109039468568994 ) ) ;
#162119=CARTESIAN_POINT ( 'NONE',  ( 9.564922557960805705, 16.46253265017160317, 104.5822429386476955 ) ) ;
#162120=CARTESIAN_POINT ( 'NONE',  ( 0.05219959533934541429, -16.53943276465976808, 80.00109039468568994 ) ) ;
#162121=CARTESIAN_POINT ( 'NONE',  ( -17.48847506799967988, -5.747544572773758631, 74.17302562156723411 ) ) ;
#162122=CARTESIAN_POINT ( 'NONE',  ( 13.89961937509957401, 13.97604488694547697, 61.87609039468566863 ) ) ;
#162123=CARTESIAN_POINT ( 'NONE',  ( -5.823673210054431948, 21.52544592524334988, 97.70942372801904696 ) ) ;
#162126=CARTESIAN_POINT ( 'NONE',  ( -12.06949235617739369, -12.14591786802326823, 109.3760903946857042 ) ) ;
#162128=CARTESIAN_POINT ( 'NONE',  ( -14.29746914071037622, -8.314922557961029526, 89.16775706135236135 ) ) ;
#162130=CARTESIAN_POINT ( 'NONE',  ( -14.29746914071037622, -8.314922557961029526, 64.16775706135234714 ) ) ;
#162131=CARTESIAN_POINT ( 'NONE',  ( 10.72451020669871369, 18.67979575497193778, 82.08442372801901854 ) ) ;
#162132=CARTESIAN_POINT ( 'NONE',  ( -13.97604488694547697, 13.89961937509957934, 93.12609039468566152 ) ) ;
#162133=CARTESIAN_POINT ( 'NONE',  ( 19.03943276465977164, 0.05219959533936151252, 41.25109039468566152 ) ) ;
#162134=CARTESIAN_POINT ( 'NONE',  ( 19.05341960407611168, 5.049401038298154454, 68.95724293864769550 ) ) ;
#162135=CARTESIAN_POINT ( 'NONE',  ( 13.89961937509977652, -13.97604488694527269, 63.12390960531435979 ) ) ;
#162137=CARTESIAN_POINT ( 'NONE',  ( 21.52544592524344225, -5.823673210054117533, 83.54057627198102409 ) ) ;
#162138=CARTESIAN_POINT ( 'NONE',  ( -0.05219959533907301413, -21.53943276465977519, 52.49890960531435979 ) ) ;
#162139=CARTESIAN_POINT ( 'NONE',  ( 19.02544592524343514, -5.153800228976328945, 33.54057627198102409 ) ) ;
#162140=CARTESIAN_POINT ( 'NONE',  ( -14.34966873604972548, 8.224510206698743886, 58.33442372801901143 ) ) ;
#162142=ORIENTED_EDGE ( 'NONE', *, *, #61248, .T. ) ;
#162143=CARTESIAN_POINT ( 'NONE',  ( 0.05219959533937995610, -21.53943276465977519, 50.00109039468568994 ) ) ;
#162144=CARTESIAN_POINT ( 'NONE',  ( -4.483927247898539470, -16.52544592524342804, 67.29057627198103830 ) ) ;
#162146=CARTESIAN_POINT ( 'NONE',  ( 14.34966873604972726, -8.224510206698740333, 30.83442372801902209 ) ) ;
#162147=CARTESIAN_POINT ( 'NONE',  ( -5.049401038297874678, -19.05341960407617918, 59.79275706135231871 ) ) ;
#162148=CARTESIAN_POINT ( 'NONE',  ( -14.29746914071049879, 8.314922557960819915, 55.83224293864770260 ) ) ;
#162149=CARTESIAN_POINT ( 'NONE',  ( 10.72451020669871369, 18.67979575497193778, 27.08442372801901854 ) ) ;
#162151=CARTESIAN_POINT ( 'NONE',  ( -18.67979575497178146, -10.72451020669898902, 96.66557627198102409 ) ) ;
#162152=CARTESIAN_POINT ( 'NONE',  ( 9.474510206698971260, -16.51473224551069308, 102.9155762719810241 ) ) ;
#162153=CARTESIAN_POINT ( 'NONE',  ( 12.06949235617757843, -12.14591786802309237, 73.12390960531436690 ) ) ;
#162156=CARTESIAN_POINT ( 'NONE',  ( 5.153800228976615827, -19.02544592524334988, 65.20942372801900433 ) ) ;
#162157=CARTESIAN_POINT ( 'NONE',  ( 18.67979575497178502, 10.72451020669898547, 114.1655762719810383 ) ) ;
#162158=CARTESIAN_POINT ( 'NONE',  ( 13.97604488694527802, 13.89961937509977652, 59.37390960531434558 ) ) ;
#162159=CARTESIAN_POINT ( 'NONE',  ( -9.564922557961040184, 16.46253265017147172, 42.91775706135234003 ) ) ;
#162160=CARTESIAN_POINT ( 'NONE',  ( 19.03943276465977164, -0.05219959533909143690, 33.74890960531435979 ) ) ;
#162161=CARTESIAN_POINT ( 'NONE',  ( -5.719274019375665041, -21.55341960407619695, 69.79275706135234714 ) ) ;
#162162=CARTESIAN_POINT ( 'NONE',  ( -17.50000000000001066, -5.622605283950844246, 71.31207310596111881 ) ) ;
#162163=CARTESIAN_POINT ( 'NONE',  ( -0.05219959533910754901, -16.53943276465976808, 42.49890960531435979 ) ) ;
#162164=CARTESIAN_POINT ( 'NONE',  ( -19.02544592524342804, 5.153800228976336051, 61.04057627198103120 ) ) ;
#162165=CARTESIAN_POINT ( 'NONE',  ( 15.80617190586746368, 15.72974639402197994, 89.37390960531435269 ) ) ;
#162166=CARTESIAN_POINT ( 'NONE',  ( -5.049401038298153566, 19.05341960407611168, 60.20724293864768129 ) ) ;
#162168=CARTESIAN_POINT ( 'NONE',  ( -21.55341960407610458, -5.719274019375992779, 71.45724293864769550 ) ) ;
#162169=CARTESIAN_POINT ( 'NONE',  ( 10.81492255796106328, -18.62759615963255655, 100.4177570613523471 ) ) ;
#162171=CARTESIAN_POINT ( 'NONE',  ( -8.314922557961024197, 14.29746914071037800, 97.91775706135236135 ) ) ;
#162172=CARTESIAN_POINT ( 'NONE',  ( -8.224510206698948167, 14.34966873604960824, 85.41557627198102409 ) ) ;
#162173=CARTESIAN_POINT ( 'NONE',  ( -19.02544592524334988, -5.153800228976617603, 98.95942372801900433 ) ) ;
#162175=CARTESIAN_POINT ( 'NONE',  ( -18.67979575497178146, -10.72451020669898902, 111.6655762719810525 ) ) ;
#162176=CARTESIAN_POINT ( 'NONE',  ( -0.05219959533936034679, 19.03943276465977164, 42.50109039468566152 ) ) ;
#162177=CARTESIAN_POINT ( 'NONE',  ( -12.14591786802326823, 12.06949235617739902, 98.12609039468570415 ) ) ;
#162178=CARTESIAN_POINT ( 'NONE',  ( -16.46253265017146816, -9.564922557961047289, 24.16775706135233648 ) ) ;
#162179=CARTESIAN_POINT ( 'NONE',  ( 0.05219959533909260263, 19.03943276465977164, 89.99890960531436690 ) ) ;
#162180=CARTESIAN_POINT ( 'NONE',  ( 0.05219959533907565091, 21.53943276465977519, 64.99890960531435269 ) ) ;
#162182=CARTESIAN_POINT ( 'NONE',  ( -19.05341960407611168, -5.049401038298163336, 26.45724293864769550 ) ) ;
#162183=CARTESIAN_POINT ( 'NONE',  ( -18.67979575497193778, 10.72451020669871902, 113.3344237280190328 ) ) ;
#162184=CARTESIAN_POINT ( 'NONE',  ( -12.06949235617739369, -12.14591786802326823, 79.37609039468567573 ) ) ;
#162185=CARTESIAN_POINT ( 'NONE',  ( 0.05219959533937995610, -21.53943276465977519, 30.00109039468568284 ) ) ;
#162186=CARTESIAN_POINT ( 'NONE',  ( -14.34966873604972548, 8.224510206698743886, 28.33442372801902209 ) ) ;
#162187=CARTESIAN_POINT ( 'NONE',  ( 19.02544592524343514, -5.153800228976328945, 108.5405762719810383 ) ) ;
#162188=CARTESIAN_POINT ( 'NONE',  ( -19.05341960407611168, -5.049401038298163336, 36.45724293864766707 ) ) ;
#162189=CARTESIAN_POINT ( 'NONE',  ( -5.049401038298153566, 19.05341960407611168, 65.20724293864765286 ) ) ;
#162190=CARTESIAN_POINT ( 'NONE',  ( -16.53943276465976808, -0.05219959533934237506, 48.75109039468568284 ) ) ;
#162191=CARTESIAN_POINT ( 'NONE',  ( -16.53943276465976808, 0.05219959533911058130, 96.24890960531435269 ) ) ;
#162192=CARTESIAN_POINT ( 'NONE',  ( 12.14591786802327356, -12.06949235617739191, 95.62609039468568994 ) ) ;
#162193=CARTESIAN_POINT ( 'NONE',  ( 10.81492255796106328, -18.62759615963255655, 55.41775706135234714 ) ) ;
#162194=CARTESIAN_POINT ( 'NONE',  ( 19.02544592524343514, -5.153800228976328945, 73.54057627198103830 ) ) ;
#162195=CARTESIAN_POINT ( 'NONE',  ( 9.564922557960805705, 16.46253265017160317, 69.58224293864770971 ) ) ;
#162196=CARTESIAN_POINT ( 'NONE',  ( 0.05219959533909260263, 19.03943276465977164, 94.99890960531436690 ) ) ;
#162197=CARTESIAN_POINT ( 'NONE',  ( 14.34966873604960469, 8.224510206698951720, 39.16557627198102409 ) ) ;
#162198=CARTESIAN_POINT ( 'NONE',  ( -12.06949235617739369, -12.14591786802326823, 104.3760903946856899 ) ) ;
#162200=CARTESIAN_POINT ( 'NONE',  ( 9.564922557961047289, -16.46253265017146816, 40.41775706135234003 ) ) ;
#162201=CARTESIAN_POINT ( 'NONE',  ( 0.05219959533909260263, 19.03943276465977164, 109.9989096053143669 ) ) ;
#162202=CARTESIAN_POINT ( 'NONE',  ( -0.05219959533909027116, -19.03943276465977164, 57.49890960531435979 ) ) ;
#162203=CARTESIAN_POINT ( 'NONE',  ( 19.05341960407617918, -5.049401038297876454, 41.04275706135233293 ) ) ;
#162205=CARTESIAN_POINT ( 'NONE',  ( 18.87075004821567248, -5.500000000000077272, 71.17408112101045958 ) ) ;
#162206=CARTESIAN_POINT ( 'NONE',  ( 4.379528057220092307, 16.55341960407617563, 62.29275706135236845 ) ) ;
#162207=CARTESIAN_POINT ( 'NONE',  ( -9.474510206698720793, -16.51473224551083518, 69.58442372801901854 ) ) ;
#162208=CARTESIAN_POINT ( 'NONE',  ( 16.52544592524335698, 4.483927247898782831, 66.45942372801903275 ) ) ;
#162210=CARTESIAN_POINT ( 'NONE',  ( -5.049401038298153566, 19.05341960407611168, 90.20724293864766707 ) ) ;
#162211=CARTESIAN_POINT ( 'NONE',  ( 5.823673210054444382, -21.52544592524334988, 20.20942372801900788 ) ) ;
#162212=CARTESIAN_POINT ( 'NONE',  ( 16.46253265017146816, 9.564922557961045513, 76.66775706135234714 ) ) ;
#162213=CARTESIAN_POINT ( 'NONE',  ( -9.474510206698964154, 16.51473224551069663, 100.4155762719810241 ) ) ;
#162214=CARTESIAN_POINT ( 'NONE',  ( -19.05341960407611168, -5.049401038298163336, 36.45724293864766707 ) ) ;
#162215=CARTESIAN_POINT ( 'NONE',  ( -19.05341960407611168, -5.049401038298163336, 91.45724293864766707 ) ) ;
#162216=CARTESIAN_POINT ( 'NONE',  ( 4.483927247898545687, 16.52544592524342804, 49.79057627198102409 ) ) ;
#162217=CARTESIAN_POINT ( 'NONE',  ( 5.049401038298161559, -19.05341960407611168, 37.70724293864768839 ) ) ;
#162218=CARTESIAN_POINT ( 'NONE',  ( 5.049401038297881783, 19.05341960407617563, 52.29275706135234003 ) ) ;
#162219=CARTESIAN_POINT ( 'NONE',  ( 8.314922557960818139, 14.29746914071049879, 84.58224293864769550 ) ) ;
#162220=CARTESIAN_POINT ( 'NONE',  ( -10.81492255796105439, 18.62759615963255655, 112.9177570613523329 ) ) ;
#162221=CARTESIAN_POINT ( 'NONE',  ( -9.474510206698964154, 16.51473224551069663, 50.41557627198102409 ) ) ;
#162222=CARTESIAN_POINT ( 'NONE',  ( -5.719274019375978568, 21.55341960407610458, 55.20724293864770260 ) ) ;
#162223=CARTESIAN_POINT ( 'NONE',  ( 12.06949235617757843, -12.14591786802309237, 48.12390960531436690 ) ) ;
#162224=CARTESIAN_POINT ( 'NONE',  ( -16.46253265017146816, -9.564922557961047289, 24.16775706135233648 ) ) ;
#162225=CARTESIAN_POINT ( 'NONE',  ( -19.05341960407611168, -5.049401038298163336, 106.4572429386476955 ) ) ;
#162226=CARTESIAN_POINT ( 'NONE',  ( 19.05341960407611168, 5.049401038298154454, 103.9572429386476671 ) ) ;
#162227=CARTESIAN_POINT ( 'NONE',  ( 16.51473224551069308, 9.474510206698969483, 39.16557627198103120 ) ) ;
#162228=CARTESIAN_POINT ( 'NONE',  ( -9.474510206698964154, 16.51473224551069663, 30.41557627198102054 ) ) ;
#162229=CARTESIAN_POINT ( 'NONE',  ( -8.314922557960811034, -14.29746914071050412, 82.08224293864768129 ) ) ;
#162230=CARTESIAN_POINT ( 'NONE',  ( -15.80617190586745835, -15.72974639402198527, 91.87390960531436690 ) ) ;
#162231=CARTESIAN_POINT ( 'NONE',  ( -13.89961937509977652, 13.97604488694528158, 105.6239096053143527 ) ) ;
#162232=CARTESIAN_POINT ( 'NONE',  ( 5.823673210054125526, 21.52544592524343514, 109.7905762719810383 ) ) ;
#162233=CARTESIAN_POINT ( 'NONE',  ( -9.564922557960796823, -16.46253265017161027, 102.0822429386477097 ) ) ;
#162234=CARTESIAN_POINT ( 'NONE',  ( 16.53943276465976808, -0.05219959533910856209, 103.7489096053143669 ) ) ;
#162235=CARTESIAN_POINT ( 'NONE',  ( -15.72974639402176322, -15.80617190586768395, 74.37609039468568994 ) ) ;
#162236=CARTESIAN_POINT ( 'NONE',  ( -21.55341960407610458, -5.719274019375992779, 86.45724293864770971 ) ) ;
#162237=CARTESIAN_POINT ( 'NONE',  ( 17.40861289039002457, -6.110651285853328396, 106.1276752917256516 ) ) ;
#162239=CARTESIAN_POINT ( 'NONE',  ( 0.05219959533907565091, 21.53943276465977519, 34.99890960531435979 ) ) ;
#162241=CARTESIAN_POINT ( 'NONE',  ( -12.06949235617739369, -12.14591786802326823, 29.37609039468568284 ) ) ;
#162242=CARTESIAN_POINT ( 'NONE',  ( -0.05219959533910754901, -16.53943276465976808, 112.4989096053143669 ) ) ;
#162244=CARTESIAN_POINT ( 'NONE',  ( 19.03943276465977164, -0.05219959533909143690, 58.74890960531435979 ) ) ;
#162245=CARTESIAN_POINT ( 'NONE',  ( 12.06949235617757843, -12.14591786802309237, 88.12390960531436690 ) ) ;
#162248=CARTESIAN_POINT ( 'NONE',  ( 18.67979575497178502, 10.72451020669898547, 34.16557627198102409 ) ) ;
#162249=CARTESIAN_POINT ( 'NONE',  ( -14.34966873604960291, -8.224510206698953496, 61.66557627198103120 ) ) ;
#162250=CARTESIAN_POINT ( 'NONE',  ( 4.483927247898790824, -16.52544592524335698, 25.20942372801901854 ) ) ;
#162251=CARTESIAN_POINT ( 'NONE',  ( -10.81492255796105439, 18.62759615963255655, 72.91775706135234714 ) ) ;
#162252=CARTESIAN_POINT ( 'NONE',  ( 17.31728774477272736, -6.344390552232384017, 78.31906651689315879 ) ) ;
#162253=CARTESIAN_POINT ( 'NONE',  ( 16.51473224551069308, 9.474510206698969483, 109.1655762719810383 ) ) ;
#162254=CARTESIAN_POINT ( 'NONE',  ( 14.29746914071037800, 8.314922557961029526, 81.66775706135236135 ) ) ;
#162255=CARTESIAN_POINT ( 'NONE',  ( 16.51473224551069308, 9.474510206698969483, 39.16557627198103120 ) ) ;
#162256=CARTESIAN_POINT ( 'NONE',  ( 0.05219959533909260263, 19.03943276465977164, 84.99890960531436690 ) ) ;
#162257=CARTESIAN_POINT ( 'NONE',  ( 15.80617190586746368, 15.72974639402197994, 89.37390960531435269 ) ) ;
#162258=CARTESIAN_POINT ( 'NONE',  ( 8.224510206698742110, 14.34966873604972548, 22.08442372801901143 ) ) ;
#162259=CARTESIAN_POINT ( 'NONE',  ( -12.06949235617756955, 12.14591786802309770, 45.62390960531436690 ) ) ;
#162260=CARTESIAN_POINT ( 'NONE',  ( 21.52544592524334988, 5.823673210054432836, 66.45942372801903275 ) ) ;
#162261=CARTESIAN_POINT ( 'NONE',  ( -14.34966873604972548, 8.224510206698743886, 103.3344237280190043 ) ) ;
#162262=CARTESIAN_POINT ( 'NONE',  ( 19.05341960407611168, 5.049401038298154454, 113.9572429386476955 ) ) ;
#162264=CARTESIAN_POINT ( 'NONE',  ( 4.379528057220339221, -16.55341960407611168, 22.70724293864769194 ) ) ;
#162265=CARTESIAN_POINT ( 'NONE',  ( 0.05219959533934541429, -16.53943276465976808, 55.00109039468568284 ) ) ;
#162266=CARTESIAN_POINT ( 'NONE',  ( 9.474510206698971260, -16.51473224551069308, 72.91557627198102409 ) ) ;
#162267=CARTESIAN_POINT ( 'NONE',  ( -19.05341960407611168, -5.049401038298163336, 86.45724293864769550 ) ) ;
#162268=CARTESIAN_POINT ( 'NONE',  ( 5.823673210054444382, -21.52544592524334988, 80.20942372801901854 ) ) ;
#162269=CARTESIAN_POINT ( 'NONE',  ( 8.224510206698742110, 14.34966873604972548, 92.08442372801901854 ) ) ;
#162270=CARTESIAN_POINT ( 'NONE',  ( -4.483927247898539470, -16.52544592524342804, 57.29057627198103120 ) ) ;
#162271=CARTESIAN_POINT ( 'NONE',  ( 13.97604488694527802, 13.89961937509977652, 74.37390960531436690 ) ) ;
#162273=CARTESIAN_POINT ( 'NONE',  ( 9.564922557961047289, -16.46253265017146816, 110.4177570613523471 ) ) ;
#162274=CARTESIAN_POINT ( 'NONE',  ( 4.379528057220339221, -16.55341960407611168, 107.7072429386476955 ) ) ;
#162275=CARTESIAN_POINT ( 'NONE',  ( 19.02544592524343514, -5.153800228976328945, 78.54057627198099567 ) ) ;
#162276=CARTESIAN_POINT ( 'NONE',  ( -19.05341960407617563, 5.049401038297882671, 113.5427570613523471 ) ) ;
#162278=CARTESIAN_POINT ( 'NONE',  ( 15.80617190586769283, -15.72974639402175789, 105.6260903946856899 ) ) ;
#162279=CARTESIAN_POINT ( 'NONE',  ( -14.34966873604972548, 8.224510206698743886, 83.33442372801903275 ) ) ;
#162280=CARTESIAN_POINT ( 'NONE',  ( 9.564922557961047289, -16.46253265017146816, 90.41775706135234714 ) ) ;
#162281=CARTESIAN_POINT ( 'NONE',  ( 12.14591786802309770, 12.06949235617756955, 109.3739096053143811 ) ) ;
#162282=CARTESIAN_POINT ( 'NONE',  ( -12.06949235617739369, -12.14591786802326823, 69.37609039468567573 ) ) ;
#162284=CARTESIAN_POINT ( 'NONE',  ( 16.46253265017146816, 9.564922557961045513, 51.66775706135233293 ) ) ;
#162285=CARTESIAN_POINT ( 'NONE',  ( -5.823673210054431948, 21.52544592524334988, 102.7094237280190185 ) ) ;
#162286=CARTESIAN_POINT ( 'NONE',  ( 16.51473224551069308, 9.474510206698969483, 34.16557627198102409 ) ) ;
#162287=CARTESIAN_POINT ( 'NONE',  ( 9.564922557960805705, 16.46253265017160317, 74.58224293864769550 ) ) ;
#162288=CARTESIAN_POINT ( 'NONE',  ( -14.29746914071049879, 8.314922557960819915, 75.83224293864769550 ) ) ;
#162290=CARTESIAN_POINT ( 'NONE',  ( 0.05219959533937995610, -21.53943276465977519, 85.00109039468568994 ) ) ;
#162291=CARTESIAN_POINT ( 'NONE',  ( 5.153800228976615827, -19.02544592524334988, 50.20942372801897591 ) ) ;
#162292=CARTESIAN_POINT ( 'NONE',  ( -0.05219959533936034679, 19.03943276465977164, 37.50109039468567573 ) ) ;
#162293=CARTESIAN_POINT ( 'NONE',  ( 21.55341960407610458, 5.719274019375980345, 38.95724293864768839 ) ) ;
#162294=CARTESIAN_POINT ( 'NONE',  ( -15.72974639402176322, -15.80617190586768395, 99.37609039468568994 ) ) ;
#162295=CARTESIAN_POINT ( 'NONE',  ( 16.46253265017160672, -9.564922557960803928, 83.33224293864768129 ) ) ;
#162296=CARTESIAN_POINT ( 'NONE',  ( 5.823673210054444382, -21.52544592524334988, 90.20942372801903275 ) ) ;
#162297=CARTESIAN_POINT ( 'NONE',  ( 21.52544592524344225, -5.823673210054117533, 48.54057627198103120 ) ) ;
#162298=CARTESIAN_POINT ( 'NONE',  ( 13.89961937509977652, -13.97604488694527269, 83.12390960531436690 ) ) ;
#162299=CARTESIAN_POINT ( 'NONE',  ( 0.05219959533936267826, -19.03943276465977164, 75.00109039468566152 ) ) ;
#162300=CARTESIAN_POINT ( 'NONE',  ( 9.474510206698971260, -16.51473224551069308, 97.91557627198102409 ) ) ;
#162301=CARTESIAN_POINT ( 'NONE',  ( 9.564922557961047289, -16.46253265017146816, 100.4177570613523329 ) ) ;
#162302=CARTESIAN_POINT ( 'NONE',  ( -8.314922557961024197, 14.29746914071037800, 47.91775706135234714 ) ) ;
#162303=CARTESIAN_POINT ( 'NONE',  ( 16.53943276465976808, -0.05219959533910856209, 98.74890960531438111 ) ) ;
#162304=CARTESIAN_POINT ( 'NONE',  ( 13.97604488694527802, 13.89961937509977652, 69.37390960531436690 ) ) ;
#162305=CARTESIAN_POINT ( 'NONE',  ( 0.05219959533907565091, 21.53943276465977519, 69.99890960531435269 ) ) ;
#162306=CARTESIAN_POINT ( 'NONE',  ( -14.29746914071037622, -8.314922557961029526, 34.16775706135234714 ) ) ;
#162307=CARTESIAN_POINT ( 'NONE',  ( 0.05219959533937995610, -21.53943276465977519, 35.00109039468568284 ) ) ;
#162308=CARTESIAN_POINT ( 'NONE',  ( -21.53943276465977519, -0.05219959533937600094, 83.75109039468568994 ) ) ;
#162309=CARTESIAN_POINT ( 'NONE',  ( -12.14591786802326823, 12.06949235617739902, 88.12609039468570415 ) ) ;
#162310=CARTESIAN_POINT ( 'NONE',  ( 16.51473224551069308, 9.474510206698969483, 69.16557627198102409 ) ) ;
#162311=CARTESIAN_POINT ( 'NONE',  ( 16.52544592524342804, -4.483927247898539470, 83.54057627198102409 ) ) ;
#162312=CARTESIAN_POINT ( 'NONE',  ( 4.483927247898790824, -16.52544592524335698, 105.2094237280190328 ) ) ;
#162313=CARTESIAN_POINT ( 'NONE',  ( 0.05219959533936267826, -19.03943276465977164, 50.00109039468566863 ) ) ;
#162314=CARTESIAN_POINT ( 'NONE',  ( 5.719274019375673035, 21.55341960407619339, 32.29275706135235424 ) ) ;
#162315=CARTESIAN_POINT ( 'NONE',  ( 4.483927247898545687, 16.52544592524342804, 84.79057627198102409 ) ) ;
#162316=CARTESIAN_POINT ( 'NONE',  ( -5.049401038298153566, 19.05341960407611168, 105.2072429386476671 ) ) ;
#162317=CARTESIAN_POINT ( 'NONE',  ( 12.06949235617739724, 12.14591786802326823, 96.87609039468568994 ) ) ;
#162318=CARTESIAN_POINT ( 'NONE',  ( -10.81492255796105439, 18.62759615963255655, 72.91775706135234714 ) ) ;
#162319=CARTESIAN_POINT ( 'NONE',  ( 16.55341960407618274, -4.379528057220086978, 41.04275706135236135 ) ) ;
#162320=CARTESIAN_POINT ( 'NONE',  ( -10.81492255796105439, 18.62759615963255655, 37.91775706135235424 ) ) ;
#162321=CARTESIAN_POINT ( 'NONE',  ( 16.53943276465976808, -0.05219959533910856209, 68.74890960531435269 ) ) ;
#162323=CARTESIAN_POINT ( 'NONE',  ( 15.72974639402176855, 15.80617190586768217, 21.87609039468567573 ) ) ;
#162325=CARTESIAN_POINT ( 'NONE',  ( 14.29746914071049879, -8.314922557960816363, 48.33224293864770260 ) ) ;
#162326=CARTESIAN_POINT ( 'NONE',  ( -19.03943276465977164, 0.05219959533909376836, 21.24890960531436335 ) ) ;
#162327=CARTESIAN_POINT ( 'NONE',  ( 18.62759615963271287, -10.81492255796078972, 43.33224293864769550 ) ) ;
#162328=CARTESIAN_POINT ( 'NONE',  ( -0.05219959533910754901, -16.53943276465976808, 77.49890960531433848 ) ) ;
#162329=CARTESIAN_POINT ( 'NONE',  ( 15.80617190586746368, 15.72974639402197994, 79.37390960531436690 ) ) ;
#162330=CARTESIAN_POINT ( 'NONE',  ( -5.049401038298153566, 19.05341960407611168, 90.20724293864766707 ) ) ;
#162331=CARTESIAN_POINT ( 'NONE',  ( -13.89961937509977652, 13.97604488694528158, 35.62390960531435269 ) ) ;
#162332=CARTESIAN_POINT ( 'NONE',  ( 5.049401038297881783, 19.05341960407617563, 82.29275706135229029 ) ) ;
#162334=CARTESIAN_POINT ( 'NONE',  ( 21.55341960407619695, -5.719274019375665929, 61.04275706135234714 ) ) ;
#162335=CARTESIAN_POINT ( 'NONE',  ( 18.62759615963271287, -10.81492255796078972, 68.33224293864769550 ) ) ;
#162336=CARTESIAN_POINT ( 'NONE',  ( 19.03943276465977164, -0.05219959533909143690, 43.74890960531435979 ) ) ;
#162337=CARTESIAN_POINT ( 'NONE',  ( -9.564922557960796823, -16.46253265017161027, 72.08224293864770971 ) ) ;
#162339=CARTESIAN_POINT ( 'NONE',  ( 16.55341960407618274, -4.379528057220086978, 51.04275706135234714 ) ) ;
#162340=CARTESIAN_POINT ( 'NONE',  ( -18.67979575497193778, 10.72451020669871902, 33.33442372801900433 ) ) ;
#162341=CARTESIAN_POINT ( 'NONE',  ( 21.53943276465977519, 0.05219959533937863772, 66.25109039468567573 ) ) ;
#162342=CARTESIAN_POINT ( 'NONE',  ( 16.46253265017160672, -9.564922557960803928, 108.3322429386476955 ) ) ;
#162343=CARTESIAN_POINT ( 'NONE',  ( -21.52544592524343514, 5.823673210054127303, 81.04057627198102409 ) ) ;
#162344=CARTESIAN_POINT ( 'NONE',  ( -15.80617190586768217, 15.72974639402176855, 28.12609039468568284 ) ) ;
#162345=CARTESIAN_POINT ( 'NONE',  ( 12.06949235617739724, 12.14591786802326823, 46.87609039468568994 ) ) ;
#162346=CARTESIAN_POINT ( 'NONE',  ( -21.52544592524343514, 5.823673210054127303, 56.04057627198102409 ) ) ;
#162347=CARTESIAN_POINT ( 'NONE',  ( -0.05219959533936034679, 19.03943276465977164, 22.50109039468566152 ) ) ;
#162348=CARTESIAN_POINT ( 'NONE',  ( 16.46253265017160672, -9.564922557960803928, 48.33224293864769550 ) ) ;
#162349=CARTESIAN_POINT ( 'NONE',  ( 16.46253265017160672, -9.564922557960803928, 108.3322429386476955 ) ) ;
#162350=CARTESIAN_POINT ( 'NONE',  ( -13.89961937509977652, 13.97604488694528158, 95.62390960531436690 ) ) ;
#162352=CARTESIAN_POINT ( 'NONE',  ( 5.049401038297881783, 19.05341960407617563, 62.29275706135234003 ) ) ;
#162353=CARTESIAN_POINT ( 'NONE',  ( 5.719274019375991003, -21.55341960407610458, 42.70724293864770260 ) ) ;
#162354=CARTESIAN_POINT ( 'NONE',  ( 16.53943276465976808, -0.05219959533910856209, 23.74890960531435269 ) ) ;
#162355=CARTESIAN_POINT ( 'NONE',  ( 9.564922557961047289, -16.46253265017146816, 100.4177570613523329 ) ) ;
#162357=CARTESIAN_POINT ( 'NONE',  ( -5.153800228976607833, 19.02544592524334988, 27.70942372801899722 ) ) ;
#162358=CARTESIAN_POINT ( 'NONE',  ( -13.97604488694547697, 13.89961937509957934, 103.1260903946856473 ) ) ;
#162359=CARTESIAN_POINT ( 'NONE',  ( -0.05219959533936034679, 19.03943276465977164, 47.50109039468566863 ) ) ;
#162360=CARTESIAN_POINT ( 'NONE',  ( 17.44279575226825330, 5.990770900252411657, 106.6644243248568102 ) ) ;
#162361=CARTESIAN_POINT ( 'NONE',  ( -9.564922557960796823, -16.46253265017161027, 57.08224293864769550 ) ) ;
#162362=CARTESIAN_POINT ( 'NONE',  ( -8.224510206698948167, 14.34966873604960824, 60.41557627198102409 ) ) ;
#162363=CARTESIAN_POINT ( 'NONE',  ( 16.46253265017160672, -9.564922557960803928, 33.33224293864770260 ) ) ;
#162364=CARTESIAN_POINT ( 'NONE',  ( -16.55341960407611168, -4.379528057220339221, 46.45724293864769550 ) ) ;
#162366=CARTESIAN_POINT ( 'NONE',  ( 4.379528057220092307, 16.55341960407617563, 107.2927570613523471 ) ) ;
#162367=CARTESIAN_POINT ( 'NONE',  ( 16.51473224551069308, 9.474510206698969483, 64.16557627198102409 ) ) ;
#162368=CARTESIAN_POINT ( 'NONE',  ( -9.474510206698720793, -16.51473224551083518, 29.58442372801900433 ) ) ;
#162369=CARTESIAN_POINT ( 'NONE',  ( -8.224510206698735004, -14.34966873604973081, 39.58442372801901143 ) ) ;
#162370=CARTESIAN_POINT ( 'NONE',  ( -18.67979575497178146, -10.72451020669898902, 51.66557627198102409 ) ) ;
#162371=CARTESIAN_POINT ( 'NONE',  ( -15.72974639402176322, -15.80617190586768395, 104.3760903946856899 ) ) ;
#162372=CARTESIAN_POINT ( 'NONE',  ( 9.474510206698971260, -16.51473224551069308, 62.91557627198102409 ) ) ;
#162373=CARTESIAN_POINT ( 'NONE',  ( -9.474510206698964154, 16.51473224551069663, 110.4155762719810383 ) ) ;
#162374=CARTESIAN_POINT ( 'NONE',  ( -19.02544592524342804, 5.153800228976336051, 96.04057627198103830 ) ) ;
#162376=CARTESIAN_POINT ( 'NONE',  ( 10.81492255796106328, -18.62759615963255655, 30.41775706135234358 ) ) ;
#162377=CARTESIAN_POINT ( 'NONE',  ( 16.55341960407611168, 4.379528057220329451, 98.95724293864770971 ) ) ;
#162378=CARTESIAN_POINT ( 'NONE',  ( -15.80617190586745835, -15.72974639402198527, 86.87390960531438111 ) ) ;
#162379=CARTESIAN_POINT ( 'NONE',  ( 16.51473224551069308, 9.474510206698969483, 64.16557627198102409 ) ) ;
#162380=CARTESIAN_POINT ( 'NONE',  ( -19.02544592524342804, 5.153800228976336051, 76.04057627198102409 ) ) ;
#162381=CARTESIAN_POINT ( 'NONE',  ( 21.55341960407610458, 5.719274019375980345, 113.9572429386477239 ) ) ;
#162383=CARTESIAN_POINT ( 'NONE',  ( -13.89961937509977652, 13.97604488694528158, 70.62390960531432427 ) ) ;
#162385=CARTESIAN_POINT ( 'NONE',  ( -4.379528057220328563, 16.55341960407611168, 110.2072429386477239 ) ) ;
#162387=CARTESIAN_POINT ( 'NONE',  ( 0.05219959533936267826, -19.03943276465977164, 90.00109039468567573 ) ) ;
#162388=CARTESIAN_POINT ( 'NONE',  ( 8.314922557960818139, 14.29746914071049879, 99.58224293864770971 ) ) ;
#162389=CARTESIAN_POINT ( 'NONE',  ( -18.67979575497193778, 10.72451020669871902, 68.33442372801900433 ) ) ;
#162390=CARTESIAN_POINT ( 'NONE',  ( -19.03943276465977164, 0.05219959533909376836, 56.24890960531435979 ) ) ;
#162391=CARTESIAN_POINT ( 'NONE',  ( -15.80617190586768217, 15.72974639402176855, 28.12609039468568284 ) ) ;
#162392=CARTESIAN_POINT ( 'NONE',  ( -18.62759615963270932, 10.81492255796079327, 110.8322429386476955 ) ) ;
#162394=CARTESIAN_POINT ( 'NONE',  ( -16.51473224551069308, -9.474510206698971260, 71.66557627198102409 ) ) ;
#162396=CARTESIAN_POINT ( 'NONE',  ( 13.89961937509957401, 13.97604488694547697, 111.8760903946856757 ) ) ;
#162397=CARTESIAN_POINT ( 'NONE',  ( -18.67979575497178146, -10.72451020669898902, 31.66557627198102054 ) ) ;
#162398=CARTESIAN_POINT ( 'NONE',  ( 0.05219959533937995610, -21.53943276465977519, 60.00109039468568284 ) ) ;
#162399=CARTESIAN_POINT ( 'NONE',  ( -16.46253265017160317, 9.564922557960807481, 95.83224293864769550 ) ) ;
#162400=CARTESIAN_POINT ( 'NONE',  ( -16.46253265017146816, -9.564922557961047289, 79.16775706135234714 ) ) ;
#162402=CARTESIAN_POINT ( 'NONE',  ( 13.89961937509977652, -13.97604488694527269, 43.12390960531434558 ) ) ;
#162403=CARTESIAN_POINT ( 'NONE',  ( 0.05219959533909260263, 19.03943276465977164, 69.99890960531435269 ) ) ;
#162404=CARTESIAN_POINT ( 'NONE',  ( -16.52544592524342804, 4.483927247898546575, 91.04057627198103830 ) ) ;
#162405=CARTESIAN_POINT ( 'NONE',  ( 16.46253265017160672, -9.564922557960803928, 98.33224293864769550 ) ) ;
#162406=CARTESIAN_POINT ( 'NONE',  ( 14.29746914071049879, -8.314922557960816363, 88.33224293864769550 ) ) ;
#162407=CARTESIAN_POINT ( 'NONE',  ( 5.153800228976335163, 19.02544592524342804, 99.79057627198102409 ) ) ;
#162408=CARTESIAN_POINT ( 'NONE',  ( 8.224510206698953496, -14.34966873604960469, 42.91557627198103120 ) ) ;
#162409=CARTESIAN_POINT ( 'NONE',  ( 9.474510206698971260, -16.51473224551069308, 22.91557627198102765 ) ) ;
#162410=EDGE_LOOP ( 'NONE', ( #50949, #47335, #166094, #121166, #58565, #154109, #91278, #149230 ) ) ;
#162411=CARTESIAN_POINT ( 'NONE',  ( 10.72451020669871369, 18.67979575497193778, 57.08442372801901854 ) ) ;
#162412=CARTESIAN_POINT ( 'NONE',  ( 13.97604488694548053, -13.89961937509957401, 80.62609039468567573 ) ) ;
#162413=CARTESIAN_POINT ( 'NONE',  ( -4.483927247898539470, -16.52544592524342804, 47.29057627198103120 ) ) ;
#162414=CARTESIAN_POINT ( 'NONE',  ( -18.67979575497178146, -10.72451020669898902, 96.66557627198102409 ) ) ;
#162415=CARTESIAN_POINT ( 'NONE',  ( 10.72451020669898902, -18.67979575497178502, 37.91557627198102409 ) ) ;
#162416=CARTESIAN_POINT ( 'NONE',  ( 4.379528057220339221, -16.55341960407611168, 77.70724293864770971 ) ) ;
#162417=CARTESIAN_POINT ( 'NONE',  ( 19.02544592524343514, -5.153800228976328945, 58.54057627198102409 ) ) ;
#162418=CARTESIAN_POINT ( 'NONE',  ( -4.483927247898539470, -16.52544592524342804, 27.29057627198103120 ) ) ;
#162419=CARTESIAN_POINT ( 'NONE',  ( -14.34966873604972548, 8.224510206698743886, 103.3344237280190043 ) ) ;
#162420=CARTESIAN_POINT ( 'NONE',  ( -16.55341960407617563, 4.379528057220093196, 73.54275706135234714 ) ) ;
#162421=CARTESIAN_POINT ( 'NONE',  ( -13.89961937509957401, -13.97604488694547875, 29.37609039468565797 ) ) ;
#162423=CARTESIAN_POINT ( 'NONE',  ( -19.02544592524342804, 5.153800228976336051, 106.0405762719810241 ) ) ;
#162424=CARTESIAN_POINT ( 'NONE',  ( -9.564922557960796823, -16.46253265017161027, 72.08224293864770971 ) ) ;
#162425=CARTESIAN_POINT ( 'NONE',  ( 5.049401038298161559, -19.05341960407611168, 42.70724293864767418 ) ) ;
#162426=CARTESIAN_POINT ( 'NONE',  ( -14.34966873604960291, -8.224510206698953496, 41.66557627198103120 ) ) ;
#162428=CARTESIAN_POINT ( 'NONE',  ( -13.89961937509977652, 13.97604488694528158, 110.6239096053143243 ) ) ;
#162429=CARTESIAN_POINT ( 'NONE',  ( -10.72451020669898014, 18.67979575497178502, 40.41557627198103120 ) ) ;
#162430=CARTESIAN_POINT ( 'NONE',  ( 0.05219959533910956823, 16.53943276465976808, 79.99890960531435269 ) ) ;
#162431=CARTESIAN_POINT ( 'NONE',  ( 12.06949235617739724, 12.14591786802326823, 21.87609039468567573 ) ) ;
#162433=CARTESIAN_POINT ( 'NONE',  ( 8.224510206698953496, -14.34966873604960469, 67.91557627198102409 ) ) ;
#162434=CARTESIAN_POINT ( 'NONE',  ( 17.50000000000000000, -5.499999999999992895, 86.21769037696435589 ) ) ;
#162435=CARTESIAN_POINT ( 'NONE',  ( 19.02544592524334988, 5.153800228976608722, 61.45942372801900433 ) ) ;
#162436=CARTESIAN_POINT ( 'NONE',  ( 13.97604488694527802, 13.89961937509977652, 109.3739096053143669 ) ) ;
#162437=CARTESIAN_POINT ( 'NONE',  ( -13.89961937509957401, -13.97604488694547875, 84.37609039468567573 ) ) ;
#162438=CARTESIAN_POINT ( 'NONE',  ( 13.97604488694548053, -13.89961937509957401, 95.62609039468566152 ) ) ;
#162439=CARTESIAN_POINT ( 'NONE',  ( -16.51473224551082808, 9.474510206698731452, 108.3344237280190043 ) ) ;
#162440=CARTESIAN_POINT ( 'NONE',  ( 4.483927247898790824, -16.52544592524335698, 110.2094237280190185 ) ) ;
#162441=CARTESIAN_POINT ( 'NONE',  ( -0.05219959533936034679, 19.03943276465977164, 67.50109039468566152 ) ) ;
#162442=CARTESIAN_POINT ( 'NONE',  ( -18.62759615963270932, 10.81492255796079327, 40.83224293864769550 ) ) ;
#162443=CARTESIAN_POINT ( 'NONE',  ( -18.62759615963255300, -10.81492255796106328, 64.16775706135234714 ) ) ;
#162445=CARTESIAN_POINT ( 'NONE',  ( 8.224510206698742110, 14.34966873604972548, 22.08442372801901143 ) ) ;
#162446=CARTESIAN_POINT ( 'NONE',  ( 17.50000000000000711, 3.442889716078282092, 22.31504430846741727 ) ) ;
#162447=CARTESIAN_POINT ( 'NONE',  ( 13.89961937509977652, -13.97604488694527269, 78.12390960531433848 ) ) ;
#162449=CARTESIAN_POINT ( 'NONE',  ( 16.52544592524342804, -4.483927247898539470, 93.54057627198103830 ) ) ;
#162450=CARTESIAN_POINT ( 'NONE',  ( -13.89961937509977652, 13.97604488694528158, 70.62390960531432427 ) ) ;
#162451=CARTESIAN_POINT ( 'NONE',  ( 5.049401038298161559, -19.05341960407611168, 87.70724293864769550 ) ) ;
#162452=VERTEX_POINT ( 'NONE', #72018 ) ;
#162453=CARTESIAN_POINT ( 'NONE',  ( -19.05341960407617563, 5.049401038297882671, 88.54275706135230450 ) ) ;
#162454=CARTESIAN_POINT ( 'NONE',  ( 21.53943276465977519, -0.05219959533907433946, 73.74890960531433848 ) ) ;
#162455=CARTESIAN_POINT ( 'NONE',  ( 13.97604488694527802, 13.89961937509977652, 24.37390960531435624 ) ) ;
#162456=CARTESIAN_POINT ( 'NONE',  ( 9.564922557961047289, -16.46253265017146816, 60.41775706135233293 ) ) ;
#162457=CARTESIAN_POINT ( 'NONE',  ( -19.05341960407611168, -5.049401038298163336, 56.45724293864768129 ) ) ;
#162458=CARTESIAN_POINT ( 'NONE',  ( -16.46253265017160317, 9.564922557960807481, 90.83224293864769550 ) ) ;
#162459=ORIENTED_EDGE ( 'NONE', *, *, #199317, .T. ) ;
#162460=CARTESIAN_POINT ( 'NONE',  ( -5.823673210054116645, -21.52544592524344225, 107.2905762719810525 ) ) ;
#162461=CARTESIAN_POINT ( 'NONE',  ( -0.05219959533910754901, -16.53943276465976808, 87.49890960531436690 ) ) ;
#162462=CARTESIAN_POINT ( 'NONE',  ( -5.049401038298153566, 19.05341960407611168, 85.20724293864766707 ) ) ;
#162463=CARTESIAN_POINT ( 'NONE',  ( -13.89961937509957401, -13.97604488694547875, 64.37609039468567573 ) ) ;
#162464=CARTESIAN_POINT ( 'NONE',  ( 21.52544592524344225, -5.823673210054117533, 93.54057627198103830 ) ) ;
#162465=CARTESIAN_POINT ( 'NONE',  ( -5.719274019375978568, 21.55341960407610458, 75.20724293864769550 ) ) ;
#162466=CARTESIAN_POINT ( 'NONE',  ( -14.29746914071049879, 8.314922557960819915, 35.83224293864768839 ) ) ;
#162467=CARTESIAN_POINT ( 'NONE',  ( 18.67979575497194134, -10.72451020669871369, 100.8344237280190185 ) ) ;
#162468=CARTESIAN_POINT ( 'NONE',  ( 4.379528057220092307, 16.55341960407617563, 67.29275706135234714 ) ) ;
#162469=CARTESIAN_POINT ( 'NONE',  ( 16.51473224551069308, 9.474510206698969483, 99.16557627198102409 ) ) ;
#162470=CARTESIAN_POINT ( 'NONE',  ( 19.03943276465977164, -0.05219959533909143690, 28.74890960531435624 ) ) ;
#162471=CARTESIAN_POINT ( 'NONE',  ( 5.823673210054444382, -21.52544592524334988, 35.20942372801901854 ) ) ;
#162472=CARTESIAN_POINT ( 'NONE',  ( 21.52544592524334988, 5.823673210054432836, 51.45942372801901854 ) ) ;
#162473=CARTESIAN_POINT ( 'NONE',  ( 5.049401038298161559, -19.05341960407611168, 47.70724293864770260 ) ) ;
#162474=CARTESIAN_POINT ( 'NONE',  ( 21.55341960407619695, -5.719274019375665929, 36.04275706135234714 ) ) ;
#162475=CARTESIAN_POINT ( 'NONE',  ( 13.89961937509957401, 13.97604488694547697, 71.87609039468567573 ) ) ;
#162476=CARTESIAN_POINT ( 'NONE',  ( -5.049401038297874678, -19.05341960407617918, 79.79275706135233293 ) ) ;
#162477=CARTESIAN_POINT ( 'NONE',  ( 9.564922557960805705, 16.46253265017160317, 39.58224293864768839 ) ) ;
#162478=CARTESIAN_POINT ( 'NONE',  ( -16.55341960407617563, 4.379528057220093196, 68.54275706135234714 ) ) ;
#162479=CARTESIAN_POINT ( 'NONE',  ( -9.564922557960796823, -16.46253265017161027, 52.08224293864768839 ) ) ;
#162481=CARTESIAN_POINT ( 'NONE',  ( 0.05219959533909260263, 19.03943276465977164, 99.99890960531436690 ) ) ;
#162482=CARTESIAN_POINT ( 'NONE',  ( 5.153800228976335163, 19.02544592524342804, 44.79057627198103830 ) ) ;
#162484=CARTESIAN_POINT ( 'NONE',  ( 15.72974639402199770, -15.80617190586745480, 68.12390960531436690 ) ) ;
#162485=CARTESIAN_POINT ( 'NONE',  ( -14.29746914071037622, -8.314922557961029526, 59.16775706135234714 ) ) ;
#162486=CARTESIAN_POINT ( 'NONE',  ( 5.719274019375673035, 21.55341960407619339, 112.2927570613523471 ) ) ;
#162487=CARTESIAN_POINT ( 'NONE',  ( -13.89961937509977652, 13.97604488694528158, 55.62390960531434558 ) ) ;
#162488=CARTESIAN_POINT ( 'NONE',  ( 4.483927247898545687, 16.52544592524342804, 39.79057627198103830 ) ) ;
#162489=CARTESIAN_POINT ( 'NONE',  ( -4.483927247898539470, -16.52544592524342804, 87.29057627198103830 ) ) ;
#162490=CARTESIAN_POINT ( 'NONE',  ( -0.05219959533909027116, -19.03943276465977164, 77.49890960531435269 ) ) ;
#162491=CARTESIAN_POINT ( 'NONE',  ( -5.823673210054431948, 21.52544592524334988, 32.70942372801900433 ) ) ;
#162492=CARTESIAN_POINT ( 'NONE',  ( -13.89961937509977652, 13.97604488694528158, 95.62390960531436690 ) ) ;
#162494=CARTESIAN_POINT ( 'NONE',  ( -0.05219959533937732626, 21.53943276465977519, 97.50109039468567573 ) ) ;
#162495=CARTESIAN_POINT ( 'NONE',  ( 12.14591786802327356, -12.06949235617739191, 60.62609039468567573 ) ) ;
#162496=CARTESIAN_POINT ( 'NONE',  ( -9.564922557960796823, -16.46253265017161027, 102.0822429386477097 ) ) ;
#162497=CARTESIAN_POINT ( 'NONE',  ( -18.67979575497178146, -10.72451020669898902, 86.66557627198102409 ) ) ;
#162498=CARTESIAN_POINT ( 'NONE',  ( -12.06949235617756955, 12.14591786802309770, 50.62390960531435979 ) ) ;
#162499=CARTESIAN_POINT ( 'NONE',  ( -5.153800228976328057, -19.02544592524343514, 37.29057627198102409 ) ) ;
#162500=CARTESIAN_POINT ( 'NONE',  ( -16.55341960407617563, 4.379528057220093196, 58.54275706135235424 ) ) ;
#162501=CARTESIAN_POINT ( 'NONE',  ( 4.379528057220339221, -16.55341960407611168, 67.70724293864769550 ) ) ;
#162502=CARTESIAN_POINT ( 'NONE',  ( 19.02544592524343514, -5.153800228976328945, 108.5405762719810383 ) ) ;
#162503=CARTESIAN_POINT ( 'NONE',  ( -21.53943276465977519, 0.05219959533907696930, 31.24890960531435979 ) ) ;
#162504=CARTESIAN_POINT ( 'NONE',  ( -5.153800228976607833, 19.02544592524334988, 32.70942372801899722 ) ) ;
#162505=CARTESIAN_POINT ( 'NONE',  ( 16.53943276465976808, -0.05219959533910856209, 103.7489096053143669 ) ) ;
#162506=CARTESIAN_POINT ( 'NONE',  ( 13.97604488694527802, 13.89961937509977652, 109.3739096053143669 ) ) ;
#162508=CARTESIAN_POINT ( 'NONE',  ( -12.06949235617739369, -12.14591786802326823, 49.37609039468569705 ) ) ;
#162509=CARTESIAN_POINT ( 'NONE',  ( -9.474510206698964154, 16.51473224551069663, 55.41557627198103120 ) ) ;
#162511=CARTESIAN_POINT ( 'NONE',  ( -0.05219959533936034679, 19.03943276465977164, 67.50109039468566152 ) ) ;
#162512=CARTESIAN_POINT ( 'NONE',  ( 8.224510206698742110, 14.34966873604972548, 87.08442372801901854 ) ) ;
#162513=CARTESIAN_POINT ( 'NONE',  ( 19.05341960407617918, -5.049401038297876454, 91.04275706135234714 ) ) ;
#162514=CARTESIAN_POINT ( 'NONE',  ( -10.81492255796105439, 18.62759615963255655, 72.91775706135234714 ) ) ;
#162515=CARTESIAN_POINT ( 'NONE',  ( -9.474510206698964154, 16.51473224551069663, 70.41557627198102409 ) ) ;
#162516=CARTESIAN_POINT ( 'NONE',  ( 5.719274019375991003, -21.55341960407610458, 92.70724293864770971 ) ) ;
#162517=CARTESIAN_POINT ( 'NONE',  ( -4.379528057220328563, 16.55341960407611168, 115.2072429386476955 ) ) ;
#162518=CARTESIAN_POINT ( 'NONE',  ( 13.97604488694548053, -13.89961937509957401, 80.62609039468567573 ) ) ;
#162519=CARTESIAN_POINT ( 'NONE',  ( 21.53943276465977519, -0.05219959533907433946, 83.74890960531435269 ) ) ;
#162520=CARTESIAN_POINT ( 'NONE',  ( -9.564922557961040184, 16.46253265017147172, 42.91775706135234003 ) ) ;
#162521=FACE_BOUND ( 'NONE', #90079, .T. ) ;
#162522=CARTESIAN_POINT ( 'NONE',  ( 0.05219959533907565091, 21.53943276465977519, 94.99890960531436690 ) ) ;
#162523=CARTESIAN_POINT ( 'NONE',  ( -15.49999999999999822, 7.499999999999999112, 20.00000000000000000 ) ) ;
#162524=CARTESIAN_POINT ( 'NONE',  ( -19.02544592524342804, 5.153800228976336051, 61.04057627198103120 ) ) ;
#162526=CARTESIAN_POINT ( 'NONE',  ( 8.314922557961029526, -14.29746914071037800, 25.41775706135235779 ) ) ;
#162528=CARTESIAN_POINT ( 'NONE',  ( -5.153800228976328057, -19.02544592524343514, 52.29057627198100988 ) ) ;
#162529=CARTESIAN_POINT ( 'NONE',  ( -15.80617190586745835, -15.72974639402198527, 101.8739096053143811 ) ) ;
#162530=CARTESIAN_POINT ( 'NONE',  ( 16.52544592524342804, -4.483927247898539470, 48.54057627198103120 ) ) ;
#162531=CARTESIAN_POINT ( 'NONE',  ( -10.81492255796105439, 18.62759615963255655, 77.91775706135231871 ) ) ;
#162532=CARTESIAN_POINT ( 'NONE',  ( -14.34966873604972548, 8.224510206698743886, 28.33442372801902209 ) ) ;
#162533=CARTESIAN_POINT ( 'NONE',  ( -19.03943276465977164, -0.05219959533935918106, 28.75109039468566507 ) ) ;
#162534=CARTESIAN_POINT ( 'NONE',  ( -14.34966873604960291, -8.224510206698953496, 36.66557627198103120 ) ) ;
#162535=CARTESIAN_POINT ( 'NONE',  ( 0.05219959533937995610, -21.53943276465977519, 45.00109039468568284 ) ) ;
#162536=CARTESIAN_POINT ( 'NONE',  ( -10.72451020669898014, 18.67979575497178502, 115.4155762719810241 ) ) ;
#162537=CARTESIAN_POINT ( 'NONE',  ( -21.55341960407610458, -5.719274019375992779, 61.45724293864770260 ) ) ;
#162538=CARTESIAN_POINT ( 'NONE',  ( -9.474510206698720793, -16.51473224551083518, 89.58442372801900433 ) ) ;
#162539=CARTESIAN_POINT ( 'NONE',  ( 0.05219959533936267826, -19.03943276465977164, 75.00109039468566152 ) ) ;
#162540=CARTESIAN_POINT ( 'NONE',  ( 10.72451020669871369, 18.67979575497193778, 77.08442372801901854 ) ) ;
#162541=CARTESIAN_POINT ( 'NONE',  ( 0.05219959533936267826, -19.03943276465977164, 50.00109039468566863 ) ) ;
#162542=CARTESIAN_POINT ( 'NONE',  ( 19.05341960407611168, 5.049401038298154454, 23.95724293864769194 ) ) ;
#162543=CARTESIAN_POINT ( 'NONE',  ( 5.823673210054125526, 21.52544592524343514, 44.79057627198103120 ) ) ;
#162544=CARTESIAN_POINT ( 'NONE',  ( -14.29746914071049879, 8.314922557960819915, 45.83224293864769550 ) ) ;
#162545=CARTESIAN_POINT ( 'NONE',  ( -17.97214573761829470, -5.500000000000090594, 51.46970049038655048 ) ) ;
#162546=CARTESIAN_POINT ( 'NONE',  ( -5.153800228976607833, 19.02544592524334988, 22.70942372801899012 ) ) ;
#162547=CARTESIAN_POINT ( 'NONE',  ( -8.314922557961024197, 14.29746914071037800, 82.91775706135234714 ) ) ;
#162548=CARTESIAN_POINT ( 'NONE',  ( 4.483927247898545687, 16.52544592524342804, 39.79057627198103830 ) ) ;
#162549=CARTESIAN_POINT ( 'NONE',  ( 15.72974639402176855, 15.80617190586768217, 71.87609039468568994 ) ) ;
#162550=CARTESIAN_POINT ( 'NONE',  ( 0.05219959533937995610, -21.53943276465977519, 85.00109039468568994 ) ) ;
#162551=CARTESIAN_POINT ( 'NONE',  ( -5.719274019375978568, 21.55341960407610458, 85.20724293864770971 ) ) ;
#162552=CARTESIAN_POINT ( 'NONE',  ( -0.05219959533909027116, -19.03943276465977164, 32.49890960531435979 ) ) ;
#162553=CARTESIAN_POINT ( 'NONE',  ( -15.80617190586768217, 15.72974639402176855, 58.12609039468568994 ) ) ;
#162554=CARTESIAN_POINT ( 'NONE',  ( -5.153800228976328057, -19.02544592524343514, 32.29057627198102409 ) ) ;
#162555=CARTESIAN_POINT ( 'NONE',  ( -13.89961937509977652, 13.97604488694528158, 50.62390960531435979 ) ) ;
#162556=CARTESIAN_POINT ( 'NONE',  ( -12.14591786802309592, -12.06949235617757132, 86.87390960531438111 ) ) ;
#162557=CARTESIAN_POINT ( 'NONE',  ( -19.02544592524342804, 5.153800228976336051, 96.04057627198103830 ) ) ;
#162558=CARTESIAN_POINT ( 'NONE',  ( -4.483927247898539470, -16.52544592524342804, 37.29057627198102409 ) ) ;
#162559=CARTESIAN_POINT ( 'NONE',  ( 4.483927247898545687, 16.52544592524342804, 114.7905762719810383 ) ) ;
#162560=CARTESIAN_POINT ( 'NONE',  ( -5.823673210054116645, -21.52544592524344225, 77.29057627198102409 ) ) ;
#162561=CARTESIAN_POINT ( 'NONE',  ( 10.81492255796106328, -18.62759615963255655, 20.41775706135234714 ) ) ;
#162563=CARTESIAN_POINT ( 'NONE',  ( 0.05219959533934541429, -16.53943276465976808, 20.00109039468568639 ) ) ;
#162565=CARTESIAN_POINT ( 'NONE',  ( 0.05219959533907565091, 21.53943276465977519, 64.99890960531435269 ) ) ;
#162566=CARTESIAN_POINT ( 'NONE',  ( 0.05219959533937995610, -21.53943276465977519, 100.0010903946857042 ) ) ;
#162567=CARTESIAN_POINT ( 'NONE',  ( -16.51473224551069308, -9.474510206698971260, 81.66557627198103830 ) ) ;
#162568=CARTESIAN_POINT ( 'NONE',  ( -15.72974639402176322, -15.80617190586768395, 34.37609039468568284 ) ) ;
#162570=CARTESIAN_POINT ( 'NONE',  ( 19.02544592524343514, -5.153800228976328945, 113.5405762719810241 ) ) ;
#162571=CARTESIAN_POINT ( 'NONE',  ( -14.29746914071037622, -8.314922557961029526, 89.16775706135236135 ) ) ;
#162572=CARTESIAN_POINT ( 'NONE',  ( -5.823673210054431948, 21.52544592524334988, 67.70942372801901854 ) ) ;
#162573=CARTESIAN_POINT ( 'NONE',  ( -16.51473224551082808, 9.474510206698731452, 23.33442372801900078 ) ) ;
#162574=CARTESIAN_POINT ( 'NONE',  ( -16.53943276465976808, -0.05219959533934237506, 78.75109039468568994 ) ) ;
#162575=CARTESIAN_POINT ( 'NONE',  ( -5.719274019375665041, -21.55341960407619695, 34.79275706135235424 ) ) ;
#162576=CARTESIAN_POINT ( 'NONE',  ( 19.03943276465977164, -0.05219959533909143690, 28.74890960531435624 ) ) ;
#162577=CARTESIAN_POINT ( 'NONE',  ( 10.81492255796106328, -18.62759615963255655, 90.41775706135236135 ) ) ;
#162578=CARTESIAN_POINT ( 'NONE',  ( 13.89961937509977652, -13.97604488694527269, 93.12390960531436690 ) ) ;
#162579=CARTESIAN_POINT ( 'NONE',  ( 21.53943276465977519, -0.05219959533907433946, 83.74890960531435269 ) ) ;
#162580=CARTESIAN_POINT ( 'NONE',  ( 13.97604488694548053, -13.89961937509957401, 65.62609039468567573 ) ) ;
#162582=CARTESIAN_POINT ( 'NONE',  ( 21.52544592524344225, -5.823673210054117533, 48.54057627198103120 ) ) ;
#162583=CARTESIAN_POINT ( 'NONE',  ( -16.51473224551069308, -9.474510206698971260, 91.66557627198103830 ) ) ;
#162584=CARTESIAN_POINT ( 'NONE',  ( 0.05219959533910956823, 16.53943276465976808, 44.99890960531435979 ) ) ;
#162586=CARTESIAN_POINT ( 'NONE',  ( -13.97604488694547697, 13.89961937509957934, 73.12609039468568994 ) ) ;
#162587=CARTESIAN_POINT ( 'NONE',  ( -17.12812012977026299, 6.668231424565975729, 103.6405124067685506 ) ) ;
#162588=CARTESIAN_POINT ( 'NONE',  ( -16.51473224551082808, 9.474510206698731452, 103.3344237280190043 ) ) ;
#162589=CARTESIAN_POINT ( 'NONE',  ( -0.05219959533907301413, -21.53943276465977519, 87.49890960531436690 ) ) ;
#162590=CARTESIAN_POINT ( 'NONE',  ( -14.29746914071049879, 8.314922557960819915, 65.83224293864769550 ) ) ;
#162591=CARTESIAN_POINT ( 'NONE',  ( 16.46253265017160672, -9.564922557960803928, 98.33224293864769550 ) ) ;
#162592=CARTESIAN_POINT ( 'NONE',  ( -16.52544592524335698, -4.483927247898792601, 43.95942372801902565 ) ) ;
#162593=CARTESIAN_POINT ( 'NONE',  ( 9.564922557960805705, 16.46253265017160317, 54.58224293864769550 ) ) ;
#162594=CARTESIAN_POINT ( 'NONE',  ( 15.80617190586769283, -15.72974639402175789, 35.62609039468568994 ) ) ;
#162595=CARTESIAN_POINT ( 'NONE',  ( -5.153800228976607833, 19.02544592524334988, 92.70942372801901854 ) ) ;
#162597=CARTESIAN_POINT ( 'NONE',  ( -9.564922557960796823, -16.46253265017161027, 97.08224293864769550 ) ) ;
#162598=CARTESIAN_POINT ( 'NONE',  ( 19.03943276465977164, -0.05219959533909143690, 73.74890960531435269 ) ) ;
#162599=CARTESIAN_POINT ( 'NONE',  ( -18.62759615963270932, 10.81492255796079327, 80.83224293864769550 ) ) ;
#162600=CARTESIAN_POINT ( 'NONE',  ( -16.46253265017160317, 9.564922557960807481, 40.83224293864769550 ) ) ;
#162602=CARTESIAN_POINT ( 'NONE',  ( 0.05219959533910956823, 16.53943276465976808, 54.99890960531435269 ) ) ;
#162603=CARTESIAN_POINT ( 'NONE',  ( 16.46253265017160672, -9.564922557960803928, 108.3322429386476955 ) ) ;
#162605=CARTESIAN_POINT ( 'NONE',  ( 19.05341960407617918, -5.049401038297876454, 71.04275706135234714 ) ) ;
#162606=CARTESIAN_POINT ( 'NONE',  ( -0.05219959533907301413, -21.53943276465977519, 92.49890960531436690 ) ) ;
#162607=CARTESIAN_POINT ( 'NONE',  ( 9.564922557961047289, -16.46253265017146816, 45.41775706135232582 ) ) ;
#162608=CARTESIAN_POINT ( 'NONE',  ( -5.153800228976328057, -19.02544592524343514, 107.2905762719810383 ) ) ;
#162609=CARTESIAN_POINT ( 'NONE',  ( 17.50000000000000000, 5.499999999999992895, 76.70309617465829888 ) ) ;
#162610=CARTESIAN_POINT ( 'NONE',  ( -5.823673210054116645, -21.52544592524344225, 37.29057627198102409 ) ) ;
#162611=CARTESIAN_POINT ( 'NONE',  ( 5.153800228976335163, 19.02544592524342804, 69.79057627198103830 ) ) ;
#162612=CARTESIAN_POINT ( 'NONE',  ( -5.719274019375665041, -21.55341960407619695, 59.79275706135234714 ) ) ;
#162613=CARTESIAN_POINT ( 'NONE',  ( 13.97604488694527802, 13.89961937509977652, 44.37390960531435269 ) ) ;
#162614=CARTESIAN_POINT ( 'NONE',  ( -4.483927247898539470, -16.52544592524342804, 77.29057627198102409 ) ) ;
#162616=CARTESIAN_POINT ( 'NONE',  ( -4.379528057220086978, -16.55341960407618274, 24.79275706135235779 ) ) ;
#162617=CARTESIAN_POINT ( 'NONE',  ( 21.52544592524334988, 5.823673210054432836, 46.45942372801901854 ) ) ;
#162619=CARTESIAN_POINT ( 'NONE',  ( -0.05219959533909027116, -19.03943276465977164, 112.4989096053143669 ) ) ;
#162620=CARTESIAN_POINT ( 'NONE',  ( -5.049401038297874678, -19.05341960407617918, 69.79275706135233293 ) ) ;
#162622=CARTESIAN_POINT ( 'NONE',  ( -21.52544592524334988, -5.823673210054445271, 28.95942372801902209 ) ) ;
#162623=CARTESIAN_POINT ( 'NONE',  ( -9.564922557960796823, -16.46253265017161027, 62.08224293864769550 ) ) ;
#162625=CARTESIAN_POINT ( 'NONE',  ( 18.67979575497194134, -10.72451020669871369, 110.8344237280190043 ) ) ;
#162626=CARTESIAN_POINT ( 'NONE',  ( 13.89961937509977652, -13.97604488694527269, 43.12390960531434558 ) ) ;
#162627=CARTESIAN_POINT ( 'NONE',  ( 19.05341960407617918, -5.049401038297876454, 21.04275706135232582 ) ) ;
#162628=CARTESIAN_POINT ( 'NONE',  ( 16.52544592524335698, 4.483927247898782831, 86.45942372801901854 ) ) ;
#162629=CARTESIAN_POINT ( 'NONE',  ( -19.05341960407611168, -5.049401038298163336, 106.4572429386476955 ) ) ;
#162630=CARTESIAN_POINT ( 'NONE',  ( 5.823673210054444382, -21.52544592524334988, 75.20942372801901854 ) ) ;
#162632=CARTESIAN_POINT ( 'NONE',  ( 5.153800228976335163, 19.02544592524342804, 114.7905762719810241 ) ) ;
#162634=CARTESIAN_POINT ( 'NONE',  ( 8.224510206698742110, 14.34966873604972548, 62.08442372801901143 ) ) ;
#162635=CARTESIAN_POINT ( 'NONE',  ( 0.05219959533937995610, -21.53943276465977519, 65.00109039468568994 ) ) ;
#162636=CARTESIAN_POINT ( 'NONE',  ( 21.53943276465977519, 0.05219959533937863772, 101.2510903946856757 ) ) ;
#162639=CARTESIAN_POINT ( 'NONE',  ( 16.52544592524335698, 4.483927247898782831, 41.45942372801901143 ) ) ;
#162640=CARTESIAN_POINT ( 'NONE',  ( 16.51473224551069308, 9.474510206698969483, 89.16557627198103830 ) ) ;
#162644=CARTESIAN_POINT ( 'NONE',  ( 13.97604488694527802, 13.89961937509977652, 44.37390960531435269 ) ) ;
#162645=CARTESIAN_POINT ( 'NONE',  ( -18.67979575497178146, -10.72451020669898902, 36.66557627198103120 ) ) ;
#162647=CARTESIAN_POINT ( 'NONE',  ( 12.14591786802327356, -12.06949235617739191, 110.6260903946857042 ) ) ;
#162648=CARTESIAN_POINT ( 'NONE',  ( 8.314922557960818139, 14.29746914071049879, 84.58224293864769550 ) ) ;
#162649=CARTESIAN_POINT ( 'NONE',  ( -5.049401038298153566, 19.05341960407611168, 85.20724293864766707 ) ) ;
#162650=CARTESIAN_POINT ( 'NONE',  ( -5.719274019375665041, -21.55341960407619695, 109.7927570613523613 ) ) ;
#162651=CARTESIAN_POINT ( 'NONE',  ( -12.14591786802326823, 12.06949235617739902, 23.12609039468567573 ) ) ;
#162652=CARTESIAN_POINT ( 'NONE',  ( 14.29746914071049879, -8.314922557960816363, 83.33224293864769550 ) ) ;
#162653=CARTESIAN_POINT ( 'NONE',  ( -18.62759615963255300, -10.81492255796106328, 39.16775706135235424 ) ) ;
#162654=CARTESIAN_POINT ( 'NONE',  ( 18.67979575497178502, 10.72451020669898547, 84.16557627198103830 ) ) ;
#162655=CARTESIAN_POINT ( 'NONE',  ( -19.03943276465977164, -0.05219959533935918106, 53.75109039468566863 ) ) ;
#162657=CARTESIAN_POINT ( 'NONE',  ( -19.05341960407611168, -5.049401038298163336, 96.45724293864769550 ) ) ;
#162658=CARTESIAN_POINT ( 'NONE',  ( -14.29746914071049879, 8.314922557960819915, 60.83224293864769550 ) ) ;
#162659=CARTESIAN_POINT ( 'NONE',  ( 12.14591786802309770, 12.06949235617756955, 54.37390960531435979 ) ) ;
#162660=CARTESIAN_POINT ( 'NONE',  ( -12.14591786802309592, -12.06949235617757132, 31.87390960531435979 ) ) ;
#162661=CARTESIAN_POINT ( 'NONE',  ( -5.153800228976607833, 19.02544592524334988, 82.70942372801897591 ) ) ;
#162662=CARTESIAN_POINT ( 'NONE',  ( 17.97394159160245408, -5.500000000000022204, 101.0122743667617442 ) ) ;
#162663=CARTESIAN_POINT ( 'NONE',  ( 9.564922557960805705, 16.46253265017160317, 114.5822429386476955 ) ) ;
#162664=CARTESIAN_POINT ( 'NONE',  ( -0.05219959533910754901, -16.53943276465976808, 87.49890960531436690 ) ) ;
#162666=CARTESIAN_POINT ( 'NONE',  ( -9.474510206698964154, 16.51473224551069663, 50.41557627198102409 ) ) ;
#162667=CARTESIAN_POINT ( 'NONE',  ( 15.72974639402199770, -15.80617190586745480, 43.12390960531435269 ) ) ;
#162668=CARTESIAN_POINT ( 'NONE',  ( 0.05219959533909260263, 19.03943276465977164, 29.99890960531435979 ) ) ;
#162669=CARTESIAN_POINT ( 'NONE',  ( -8.314922557961024197, 14.29746914071037800, 82.91775706135234714 ) ) ;
#162670=CARTESIAN_POINT ( 'NONE',  ( 13.89961937509977652, -13.97604488694527269, 58.12390960531436690 ) ) ;
#162671=CARTESIAN_POINT ( 'NONE',  ( 13.97604488694548053, -13.89961937509957401, 40.62609039468564731 ) ) ;
#162672=CARTESIAN_POINT ( 'NONE',  ( 0.05219959533937995610, -21.53943276465977519, 65.00109039468568994 ) ) ;
#162673=CARTESIAN_POINT ( 'NONE',  ( 21.55341960407610458, 5.719274019375980345, 33.95724293864769550 ) ) ;
#162674=CARTESIAN_POINT ( 'NONE',  ( 16.53943276465976808, -0.05219959533910856209, 103.7489096053143669 ) ) ;
#162676=CARTESIAN_POINT ( 'NONE',  ( 5.049401038297881783, 19.05341960407617563, 97.29275706135233293 ) ) ;
#162678=CARTESIAN_POINT ( 'NONE',  ( 17.50000000000001066, 3.307050604927454618, 37.42089634664176856 ) ) ;
#162679=CARTESIAN_POINT ( 'NONE',  ( 5.719274019375991003, -21.55341960407610458, 52.70724293864769550 ) ) ;
#162680=CARTESIAN_POINT ( 'NONE',  ( -0.05219959533909027116, -19.03943276465977164, 22.49890960531436690 ) ) ;
#162681=CARTESIAN_POINT ( 'NONE',  ( -21.53943276465977519, -0.05219959533937600094, 83.75109039468568994 ) ) ;
#162682=CARTESIAN_POINT ( 'NONE',  ( -12.06949235617756955, 12.14591786802309770, 45.62390960531436690 ) ) ;
#162683=CARTESIAN_POINT ( 'NONE',  ( -4.379528057220086978, -16.55341960407618274, 64.79275706135234714 ) ) ;
#162684=CARTESIAN_POINT ( 'NONE',  ( 8.314922557960818139, 14.29746914071049879, 59.58224293864770260 ) ) ;
#162685=CARTESIAN_POINT ( 'NONE',  ( -5.823673210054116645, -21.52544592524344225, 87.29057627198103830 ) ) ;
#162686=CARTESIAN_POINT ( 'NONE',  ( -10.81492255796078084, -18.62759615963271287, 72.08224293864769550 ) ) ;
#162688=CARTESIAN_POINT ( 'NONE',  ( -16.46253265017160317, 9.564922557960807481, 110.8322429386476955 ) ) ;
#162689=CARTESIAN_POINT ( 'NONE',  ( 9.474510206698971260, -16.51473224551069308, 57.91557627198103120 ) ) ;
#162690=CARTESIAN_POINT ( 'NONE',  ( 0.05219959533909260263, 19.03943276465977164, 29.99890960531435979 ) ) ;
#162694=CARTESIAN_POINT ( 'NONE',  ( 8.224510206698742110, 14.34966873604972548, 87.08442372801901854 ) ) ;
#162695=CARTESIAN_POINT ( 'NONE',  ( -21.52544592524334988, -5.823673210054445271, 23.95942372801901143 ) ) ;
#162696=CARTESIAN_POINT ( 'NONE',  ( -19.02544592524342804, 5.153800228976336051, 76.04057627198102409 ) ) ;
#162697=CARTESIAN_POINT ( 'NONE',  ( -21.52544592524334988, -5.823673210054445271, 58.95942372801902565 ) ) ;
#162699=CARTESIAN_POINT ( 'NONE',  ( -19.05341960407611168, -5.049401038298163336, 106.4572429386476955 ) ) ;
#162702=CARTESIAN_POINT ( 'NONE',  ( 10.81492255796106328, -18.62759615963255655, 45.41775706135234003 ) ) ;
#162703=CARTESIAN_POINT ( 'NONE',  ( -5.049401038298153566, 19.05341960407611168, 115.2072429386477097 ) ) ;
#162704=CARTESIAN_POINT ( 'NONE',  ( 19.05341960407611168, 5.049401038298154454, 108.9572429386477097 ) ) ;
#162705=CARTESIAN_POINT ( 'NONE',  ( -9.474510206698720793, -16.51473224551083518, 59.58442372801900433 ) ) ;
#162706=CARTESIAN_POINT ( 'NONE',  ( 5.823673210054444382, -21.52544592524334988, 20.20942372801900788 ) ) ;
#162707=CARTESIAN_POINT ( 'NONE',  ( 19.03943276465977164, 0.05219959533936151252, 46.25109039468566863 ) ) ;
#162708=CARTESIAN_POINT ( 'NONE',  ( 9.564922557961047289, -16.46253265017146816, 55.41775706135234003 ) ) ;
#162709=CARTESIAN_POINT ( 'NONE',  ( 0.05219959533934541429, -16.53943276465976808, 100.0010903946857042 ) ) ;
#162712=CARTESIAN_POINT ( 'NONE',  ( -13.89961937509977652, 13.97604488694528158, 75.62390960531438111 ) ) ;
#162713=CARTESIAN_POINT ( 'NONE',  ( -10.81492255796105439, 18.62759615963255655, 82.91775706135234714 ) ) ;
#162714=CARTESIAN_POINT ( 'NONE',  ( -10.81492255796105439, 18.62759615963255655, 87.91775706135234714 ) ) ;
#162716=CARTESIAN_POINT ( 'NONE',  ( 5.049401038298161559, -19.05341960407611168, 97.70724293864766707 ) ) ;
#162717=CARTESIAN_POINT ( 'NONE',  ( 21.52544592524334988, 5.823673210054432836, 81.45942372801900433 ) ) ;
#162718=CARTESIAN_POINT ( 'NONE',  ( 9.564922557961047289, -16.46253265017146816, 110.4177570613523471 ) ) ;
#162719=CARTESIAN_POINT ( 'NONE',  ( 9.564922557960805705, 16.46253265017160317, 74.58224293864769550 ) ) ;
#162720=CARTESIAN_POINT ( 'NONE',  ( -19.05341960407611168, -5.049401038298163336, 106.4572429386476955 ) ) ;
#162722=CARTESIAN_POINT ( 'NONE',  ( -16.51473224551069308, -9.474510206698971260, 91.66557627198103830 ) ) ;
#162723=CARTESIAN_POINT ( 'NONE',  ( -18.22780087662122028, 5.500000000000031086, 88.51540105326107266 ) ) ;
#162724=CARTESIAN_POINT ( 'NONE',  ( -13.97604488694527625, -13.89961937509977652, 81.87390960531436690 ) ) ;
#162725=CARTESIAN_POINT ( 'NONE',  ( -5.153800228976328057, -19.02544592524343514, 62.29057627198100988 ) ) ;
#162726=CARTESIAN_POINT ( 'NONE',  ( -5.719274019375665041, -21.55341960407619695, 19.79275706135235069 ) ) ;
#162727=CARTESIAN_POINT ( 'NONE',  ( -14.29746914071037622, -8.314922557961029526, 94.16775706135237556 ) ) ;
#162729=CARTESIAN_POINT ( 'NONE',  ( 9.474510206698729675, 16.51473224551082808, 52.08442372801900433 ) ) ;
#162730=CARTESIAN_POINT ( 'NONE',  ( 19.02544592524343514, -5.153800228976328945, 98.54057627198100988 ) ) ;
#162731=CARTESIAN_POINT ( 'NONE',  ( 8.224510206698953496, -14.34966873604960469, 87.91557627198103830 ) ) ;
#162732=CARTESIAN_POINT ( 'NONE',  ( -15.72974639402197994, 15.80617190586746368, 35.62390960531437401 ) ) ;
#162733=CARTESIAN_POINT ( 'NONE',  ( -0.05219959533907301413, -21.53943276465977519, 22.49890960531436335 ) ) ;
#162734=CARTESIAN_POINT ( 'NONE',  ( 12.06949235617757843, -12.14591786802309237, 98.12390960531436690 ) ) ;
#162736=CARTESIAN_POINT ( 'NONE',  ( 13.97604488694548053, -13.89961937509957401, 50.62609039468566152 ) ) ;
#162737=CARTESIAN_POINT ( 'NONE',  ( -16.55341960407617563, 4.379528057220093196, 103.5427570613523613 ) ) ;
#162738=CARTESIAN_POINT ( 'NONE',  ( 5.153800228976335163, 19.02544592524342804, 94.79057627198103830 ) ) ;
#162739=CARTESIAN_POINT ( 'NONE',  ( 18.62759615963255655, 10.81492255796105972, 66.66775706135234714 ) ) ;
#162740=CARTESIAN_POINT ( 'NONE',  ( -18.62759615963270932, 10.81492255796079327, 60.83224293864769550 ) ) ;
#162741=CARTESIAN_POINT ( 'NONE',  ( 5.823673210054444382, -21.52544592524334988, 30.20942372801902565 ) ) ;
#162742=CARTESIAN_POINT ( 'NONE',  ( 5.823673210054125526, 21.52544592524343514, 84.79057627198102409 ) ) ;
#162743=CARTESIAN_POINT ( 'NONE',  ( 4.379528057220339221, -16.55341960407611168, 112.7072429386476955 ) ) ;
#162744=CARTESIAN_POINT ( 'NONE',  ( 16.46253265017146816, 9.564922557961045513, 66.66775706135233293 ) ) ;
#162745=CARTESIAN_POINT ( 'NONE',  ( -16.51473224551069308, -9.474510206698971260, 41.66557627198103120 ) ) ;
#162746=CARTESIAN_POINT ( 'NONE',  ( 13.97604488694527802, 13.89961937509977652, 94.37390960531436690 ) ) ;
#162747=CARTESIAN_POINT ( 'NONE',  ( 0.05219959533909260263, 19.03943276465977164, 89.99890960531436690 ) ) ;
#162748=CARTESIAN_POINT ( 'NONE',  ( 13.97604488694527802, 13.89961937509977652, 24.37390960531435624 ) ) ;
#162749=CARTESIAN_POINT ( 'NONE',  ( 16.53943276465976808, -0.05219959533910856209, 38.74890960531435979 ) ) ;
#162750=CARTESIAN_POINT ( 'NONE',  ( -12.06949235617739369, -12.14591786802326823, 44.37609039468567573 ) ) ;
#162751=CARTESIAN_POINT ( 'NONE',  ( 18.62759615963255655, 10.81492255796105972, 111.6677570613523613 ) ) ;
#162752=CARTESIAN_POINT ( 'NONE',  ( -9.474510206698964154, 16.51473224551069663, 115.4155762719810241 ) ) ;
#162753=CARTESIAN_POINT ( 'NONE',  ( 14.29746914071037800, 8.314922557961029526, 111.6677570613523613 ) ) ;
#162754=CARTESIAN_POINT ( 'NONE',  ( -18.67979575497193778, 10.72451020669871902, 28.33442372801902209 ) ) ;
#162755=CARTESIAN_POINT ( 'NONE',  ( -13.89961937509977652, 13.97604488694528158, 110.6239096053143243 ) ) ;
#162756=CARTESIAN_POINT ( 'NONE',  ( -14.34966873604972548, 8.224510206698743886, 113.3344237280190328 ) ) ;
#162757=CARTESIAN_POINT ( 'NONE',  ( -16.55341960407617563, 4.379528057220093196, 98.54275706135234714 ) ) ;
#162758=CARTESIAN_POINT ( 'NONE',  ( 14.34966873604972726, -8.224510206698740333, 25.83442372801901499 ) ) ;
#162759=CARTESIAN_POINT ( 'NONE',  ( -19.02544592524342804, 5.153800228976336051, 46.04057627198101699 ) ) ;
#162760=CARTESIAN_POINT ( 'NONE',  ( -12.14591786802309592, -12.06949235617757132, 106.8739096053143811 ) ) ;
#162761=CARTESIAN_POINT ( 'NONE',  ( 15.80617190586769283, -15.72974639402175789, 25.62609039468567929 ) ) ;
#162762=CARTESIAN_POINT ( 'NONE',  ( -16.51473224551069308, -9.474510206698971260, 36.66557627198102409 ) ) ;
#162763=CARTESIAN_POINT ( 'NONE',  ( -19.02544592524342804, 5.153800228976336051, 106.0405762719810241 ) ) ;
#162764=CARTESIAN_POINT ( 'NONE',  ( 5.049401038298161559, -19.05341960407611168, 32.70724293864768129 ) ) ;
#162765=CARTESIAN_POINT ( 'NONE',  ( -9.474510206698964154, 16.51473224551069663, 110.4155762719810383 ) ) ;
#162768=CARTESIAN_POINT ( 'NONE',  ( 13.89961937509977652, -13.97604488694527269, 103.1239096053143527 ) ) ;
#162769=CARTESIAN_POINT ( 'NONE',  ( -5.823673210054431948, 21.52544592524334988, 47.70942372801902565 ) ) ;
#162770=CARTESIAN_POINT ( 'NONE',  ( -14.34966873604960291, -8.224510206698953496, 96.66557627198102409 ) ) ;
#162771=CARTESIAN_POINT ( 'NONE',  ( 9.564922557960805705, 16.46253265017160317, 99.58224293864770971 ) ) ;
#162774=CARTESIAN_POINT ( 'NONE',  ( -4.379528057220086978, -16.55341960407618274, 69.79275706135234714 ) ) ;
#162775=CARTESIAN_POINT ( 'NONE',  ( 10.72451020669871369, 18.67979575497193778, 82.08442372801901854 ) ) ;
#162776=CARTESIAN_POINT ( 'NONE',  ( -14.29746914071037622, -8.314922557961029526, 39.16775706135235424 ) ) ;
#162777=CARTESIAN_POINT ( 'NONE',  ( 5.153800228976335163, 19.02544592524342804, 79.79057627198102409 ) ) ;
#162778=CARTESIAN_POINT ( 'NONE',  ( -16.52544592524335698, -4.483927247898792601, 18.95942372801901143 ) ) ;
#162779=CARTESIAN_POINT ( 'NONE',  ( 4.483927247898790824, -16.52544592524335698, 85.20942372801901854 ) ) ;
#162780=CARTESIAN_POINT ( 'NONE',  ( -19.02544592524334988, -5.153800228976617603, 98.95942372801900433 ) ) ;
#162781=CARTESIAN_POINT ( 'NONE',  ( -5.049401038298153566, 19.05341960407611168, 65.20724293864765286 ) ) ;
#162782=CARTESIAN_POINT ( 'NONE',  ( 18.62759615963271287, -10.81492255796078972, 78.33224293864770971 ) ) ;
#162783=CARTESIAN_POINT ( 'NONE',  ( 14.29746914071049879, -8.314922557960816363, 83.33224293864769550 ) ) ;
#162784=CARTESIAN_POINT ( 'NONE',  ( -5.049401038297874678, -19.05341960407617918, 94.79275706135230450 ) ) ;
#162785=CARTESIAN_POINT ( 'NONE',  ( -8.224510206698735004, -14.34966873604973081, 54.58442372801901143 ) ) ;
#162786=CARTESIAN_POINT ( 'NONE',  ( -19.52837319214028611, 5.499999999999900524, 79.60471352585538796 ) ) ;
#162787=CARTESIAN_POINT ( 'NONE',  ( -19.03943276465977164, -0.05219959533935918106, 58.75109039468566863 ) ) ;
#162788=CARTESIAN_POINT ( 'NONE',  ( 14.34966873604960469, 8.224510206698951720, 29.16557627198103120 ) ) ;
#162789=CARTESIAN_POINT ( 'NONE',  ( -16.52544592524342804, 4.483927247898546575, 86.04057627198102409 ) ) ;
#162790=CARTESIAN_POINT ( 'NONE',  ( 10.72451020669871369, 18.67979575497193778, 112.0844237280190185 ) ) ;
#162791=CARTESIAN_POINT ( 'NONE',  ( -17.49999999999999289, 5.624438216177559902, 40.81670344914644488 ) ) ;
#162792=CARTESIAN_POINT ( 'NONE',  ( -21.52544592524334988, -5.823673210054445271, 23.95942372801901143 ) ) ;
#162793=CARTESIAN_POINT ( 'NONE',  ( -5.153800228976328057, -19.02544592524343514, 112.2905762719810099 ) ) ;
#162794=CARTESIAN_POINT ( 'NONE',  ( -19.05341960407611168, -5.049401038298163336, 81.45724293864769550 ) ) ;
#162795=CARTESIAN_POINT ( 'NONE',  ( -15.80617190586768217, 15.72974639402176855, 93.12609039468568994 ) ) ;
#162796=CARTESIAN_POINT ( 'NONE',  ( 19.03943276465977164, -0.05219959533909143690, 78.74890960531436690 ) ) ;
#162797=CARTESIAN_POINT ( 'NONE',  ( 18.67979575497178502, 10.72451020669898547, 44.16557627198103120 ) ) ;
#162798=CARTESIAN_POINT ( 'NONE',  ( 0.05219959533910956823, 16.53943276465976808, 79.99890960531435269 ) ) ;
#162799=CARTESIAN_POINT ( 'NONE',  ( 16.51473224551069308, 9.474510206698969483, 54.16557627198103120 ) ) ;
#162800=CARTESIAN_POINT ( 'NONE',  ( -9.564922557960796823, -16.46253265017161027, 22.08224293864768839 ) ) ;
#162801=CARTESIAN_POINT ( 'NONE',  ( 18.62759615963255655, 10.81492255796105972, 21.66775706135235069 ) ) ;
#162802=CARTESIAN_POINT ( 'NONE',  ( -21.55341960407619339, 5.719274019375674811, 68.54275706135234714 ) ) ;
#162803=CARTESIAN_POINT ( 'NONE',  ( 13.97604488694527802, 13.89961937509977652, 39.37390960531435269 ) ) ;
#162804=CARTESIAN_POINT ( 'NONE',  ( -8.314922557961024197, 14.29746914071037800, 67.91775706135234714 ) ) ;
#162805=CARTESIAN_POINT ( 'NONE',  ( 18.62759615963271287, -10.81492255796078972, 113.3322429386476955 ) ) ;
#162806=CARTESIAN_POINT ( 'NONE',  ( -21.52544592524343514, 5.823673210054127303, 111.0405762719810525 ) ) ;
#162807=CARTESIAN_POINT ( 'NONE',  ( -19.05341960407617563, 5.049401038297882671, 33.54275706135231871 ) ) ;
#162808=CARTESIAN_POINT ( 'NONE',  ( -19.02544592524342804, 5.153800228976336051, 71.04057627198099567 ) ) ;
#162810=CARTESIAN_POINT ( 'NONE',  ( -0.05219959533937732626, 21.53943276465977519, 67.50109039468568994 ) ) ;
#162811=CARTESIAN_POINT ( 'NONE',  ( -15.80617190586745835, -15.72974639402198527, 61.87390960531436690 ) ) ;
#162812=CARTESIAN_POINT ( 'NONE',  ( -14.29746914071049879, 8.314922557960819915, 40.83224293864769550 ) ) ;
#162813=CARTESIAN_POINT ( 'NONE',  ( -18.67979575497193778, 10.72451020669871902, 73.33442372801901854 ) ) ;
#162814=CARTESIAN_POINT ( 'NONE',  ( 10.81492255796106328, -18.62759615963255655, 105.4177570613523613 ) ) ;
#162815=CARTESIAN_POINT ( 'NONE',  ( 4.483927247898545687, 16.52544592524342804, 59.79057627198103120 ) ) ;
#162816=CARTESIAN_POINT ( 'NONE',  ( 14.34966873604960469, 8.224510206698951720, 104.1655762719810241 ) ) ;
#162817=CARTESIAN_POINT ( 'NONE',  ( 0.05219959533936267826, -19.03943276465977164, 60.00109039468566863 ) ) ;
#162818=CARTESIAN_POINT ( 'NONE',  ( -12.14591786802309592, -12.06949235617757132, 26.87390960531435979 ) ) ;
#162819=CARTESIAN_POINT ( 'NONE',  ( -21.55341960407619339, 5.719274019375674811, 68.54275706135234714 ) ) ;
#162820=CARTESIAN_POINT ( 'NONE',  ( 13.89961937509977652, -13.97604488694527269, 68.12390960531436690 ) ) ;
#162821=CARTESIAN_POINT ( 'NONE',  ( 19.02544592524334988, 5.153800228976608722, 36.45942372801900433 ) ) ;
#162822=CARTESIAN_POINT ( 'NONE',  ( 21.53943276465977519, -0.05219959533907433946, 38.74890960531435979 ) ) ;
#162823=CARTESIAN_POINT ( 'NONE',  ( 0.05219959533937995610, -21.53943276465977519, 40.00109039468567573 ) ) ;
#162824=CARTESIAN_POINT ( 'NONE',  ( 21.55341960407610458, 5.719274019375980345, 98.95724293864770971 ) ) ;
#162825=CARTESIAN_POINT ( 'NONE',  ( -19.05341960407617563, 5.049401038297882671, 103.5427570613523329 ) ) ;
#162826=CARTESIAN_POINT ( 'NONE',  ( -0.05219959533934338120, 16.53943276465976808, 57.50109039468568994 ) ) ;
#162828=CARTESIAN_POINT ( 'NONE',  ( 21.52544592524344225, -5.823673210054117533, 93.54057627198103830 ) ) ;
#162829=CARTESIAN_POINT ( 'NONE',  ( 14.29746914071049879, -8.314922557960816363, 88.33224293864769550 ) ) ;
#162831=CARTESIAN_POINT ( 'NONE',  ( -0.05219959533936034679, 19.03943276465977164, 112.5010903946856757 ) ) ;
#162832=CARTESIAN_POINT ( 'NONE',  ( 18.67979575497178502, 10.72451020669898547, 54.16557627198103120 ) ) ;
#162833=CARTESIAN_POINT ( 'NONE',  ( 8.314922557961029526, -14.29746914071037800, 95.41775706135234714 ) ) ;
#162835=CARTESIAN_POINT ( 'NONE',  ( -14.34966873604972548, 8.224510206698743886, 48.33442372801902565 ) ) ;
#162836=VECTOR ( 'NONE', #82502, 1000.000000000000000 ) ;
#162837=CARTESIAN_POINT ( 'NONE',  ( 21.52544592524334988, 5.823673210054432836, 21.45942372801901499 ) ) ;
#162838=CARTESIAN_POINT ( 'NONE',  ( -0.05219959533907301413, -21.53943276465977519, 42.49890960531435979 ) ) ;
#162839=CARTESIAN_POINT ( 'NONE',  ( 16.53943276465976808, 0.05219959533934440121, 81.25109039468568994 ) ) ;
#162840=CARTESIAN_POINT ( 'NONE',  ( 19.03943276465977164, -0.05219959533909143690, 103.7489096053143669 ) ) ;
#162841=CARTESIAN_POINT ( 'NONE',  ( 21.53943276465977519, 0.05219959533937863772, 71.25109039468568994 ) ) ;
#162843=CARTESIAN_POINT ( 'NONE',  ( 21.55341960407610458, 5.719274019375980345, 33.95724293864769550 ) ) ;
#162844=CARTESIAN_POINT ( 'NONE',  ( -15.80617190586745835, -15.72974639402198527, 26.87390960531435979 ) ) ;
#162846=CARTESIAN_POINT ( 'NONE',  ( 16.51473224551083163, -9.474510206698727899, 45.83442372801900433 ) ) ;
#162847=CARTESIAN_POINT ( 'NONE',  ( -0.05219959533934338120, 16.53943276465976808, 67.50109039468568994 ) ) ;
#162848=CARTESIAN_POINT ( 'NONE',  ( -18.67979575497178146, -10.72451020669898902, 31.66557627198102054 ) ) ;
#162850=CARTESIAN_POINT ( 'NONE',  ( -9.474510206698964154, 16.51473224551069663, 80.41557627198103830 ) ) ;
#162851=CARTESIAN_POINT ( 'NONE',  ( 16.52544592524335698, 4.483927247898782831, 111.4594237280190328 ) ) ;
#162853=CARTESIAN_POINT ( 'NONE',  ( 16.52544592524342804, -4.483927247898539470, 108.5405762719810241 ) ) ;
#162854=CARTESIAN_POINT ( 'NONE',  ( -18.67979575497178146, -10.72451020669898902, 46.66557627198102409 ) ) ;
#162855=CARTESIAN_POINT ( 'NONE',  ( 13.97604488694527802, 13.89961937509977652, 44.37390960531435269 ) ) ;
#162856=CARTESIAN_POINT ( 'NONE',  ( 16.52544592524335698, 4.483927247898782831, 81.45942372801900433 ) ) ;
#162857=CARTESIAN_POINT ( 'NONE',  ( 10.72451020669871369, 18.67979575497193778, 32.08442372801901854 ) ) ;
#162858=CARTESIAN_POINT ( 'NONE',  ( 19.05341960407617918, -5.049401038297876454, 86.04275706135233293 ) ) ;
#162859=CARTESIAN_POINT ( 'NONE',  ( -8.224510206698948167, 14.34966873604960824, 95.41557627198102409 ) ) ;
#162860=CARTESIAN_POINT ( 'NONE',  ( 19.03943276465977164, -0.05219959533909143690, 53.74890960531436690 ) ) ;
#162861=CARTESIAN_POINT ( 'NONE',  ( 16.51473224551069308, 9.474510206698969483, 24.16557627198102765 ) ) ;
#162862=CARTESIAN_POINT ( 'NONE',  ( 0.05219959533937995610, -21.53943276465977519, 110.0010903946856757 ) ) ;
#162863=CARTESIAN_POINT ( 'NONE',  ( -5.049401038298153566, 19.05341960407611168, 80.20724293864769550 ) ) ;
#162864=CARTESIAN_POINT ( 'NONE',  ( 8.224510206698742110, 14.34966873604972548, 62.08442372801901143 ) ) ;
#162865=CARTESIAN_POINT ( 'NONE',  ( -15.80617190586768217, 15.72974639402176855, 88.12609039468570415 ) ) ;
#162866=CARTESIAN_POINT ( 'NONE',  ( 5.823673210054125526, 21.52544592524343514, 54.79057627198104541 ) ) ;
#162867=CARTESIAN_POINT ( 'NONE',  ( -14.34966873604972548, 8.224510206698743886, 68.33442372801900433 ) ) ;
#162868=CARTESIAN_POINT ( 'NONE',  ( 16.46253265017146816, 9.564922557961045513, 56.66775706135233293 ) ) ;
#162869=CARTESIAN_POINT ( 'NONE',  ( -13.97604488694547697, 13.89961937509957934, 73.12609039468568994 ) ) ;
#162870=EDGE_LOOP ( 'NONE', ( #142766, #160694, #8190, #105394 ) ) ;
#162871=CARTESIAN_POINT ( 'NONE',  ( 21.53943276465977519, 0.05219959533937863772, 66.25109039468567573 ) ) ;
#162872=CARTESIAN_POINT ( 'NONE',  ( 19.02544592524343514, -5.153800228976328945, 68.54057627198103830 ) ) ;
#162873=CARTESIAN_POINT ( 'NONE',  ( -0.05219959533909027116, -19.03943276465977164, 57.49890960531435979 ) ) ;
#162874=CARTESIAN_POINT ( 'NONE',  ( -19.02544592524334988, -5.153800228976617603, 63.95942372801899012 ) ) ;
#162875=CARTESIAN_POINT ( 'NONE',  ( 16.51473224551069308, 9.474510206698969483, 114.1655762719810241 ) ) ;
#162876=CARTESIAN_POINT ( 'NONE',  ( -9.564922557960796823, -16.46253265017161027, 82.08224293864768129 ) ) ;
#162877=CARTESIAN_POINT ( 'NONE',  ( -12.14591786802309592, -12.06949235617757132, 36.87390960531435979 ) ) ;
#162878=CARTESIAN_POINT ( 'NONE',  ( -18.67979575497178146, -10.72451020669898902, 46.66557627198102409 ) ) ;
#162879=DIRECTION ( 'NONE',  ( 0.000000000000000000, 0.000000000000000000, -1.000000000000000000 ) ) ;
#162880=CARTESIAN_POINT ( 'NONE',  ( -5.823673210054431948, 21.52544592524334988, 107.7094237280190328 ) ) ;
#162881=CARTESIAN_POINT ( 'NONE',  ( -17.49999999999999645, -5.499999999999992895, 79.20309617465829888 ) ) ;
#162882=CARTESIAN_POINT ( 'NONE',  ( 9.564922557960805705, 16.46253265017160317, 44.58224293864769550 ) ) ;
#162883=CARTESIAN_POINT ( 'NONE',  ( -5.153800228976328057, -19.02544592524343514, 27.29057627198103120 ) ) ;
#162886=CARTESIAN_POINT ( 'NONE',  ( -12.14591786802326823, 12.06949235617739902, 58.12609039468568994 ) ) ;
#162887=CARTESIAN_POINT ( 'NONE',  ( 15.72974639402199770, -15.80617190586745480, 78.12390960531436690 ) ) ;
#162888=CARTESIAN_POINT ( 'NONE',  ( 0.05219959533910956823, 16.53943276465976808, 49.99890960531437401 ) ) ;
#162889=CARTESIAN_POINT ( 'NONE',  ( 9.474510206698971260, -16.51473224551069308, 27.91557627198103120 ) ) ;
#162891=CARTESIAN_POINT ( 'NONE',  ( 21.52544592524334988, 5.823673210054432836, 41.45942372801901143 ) ) ;
#162892=CARTESIAN_POINT ( 'NONE',  ( 0.05219959533936267826, -19.03943276465977164, 45.00109039468566863 ) ) ;
#162893=CARTESIAN_POINT ( 'NONE',  ( 13.97604488694527802, 13.89961937509977652, 29.37390960531435979 ) ) ;
#162894=CARTESIAN_POINT ( 'NONE',  ( 5.823673210054444382, -21.52544592524334988, 75.20942372801901854 ) ) ;
#162895=CARTESIAN_POINT ( 'NONE',  ( 16.38665767535053419, 7.295008042176124086, 97.23599135785455871 ) ) ;
#162896=CARTESIAN_POINT ( 'NONE',  ( 14.34966873604960469, 8.224510206698951720, 44.16557627198103120 ) ) ;
#162898=CARTESIAN_POINT ( 'NONE',  ( 10.72451020669898902, -18.67979575497178502, 37.91557627198102409 ) ) ;
#162900=CARTESIAN_POINT ( 'NONE',  ( -9.474510206698964154, 16.51473224551069663, 90.41557627198103830 ) ) ;
#162901=CARTESIAN_POINT ( 'NONE',  ( 14.34966873604960469, 8.224510206698951720, 84.16557627198103830 ) ) ;
#162902=CARTESIAN_POINT ( 'NONE',  ( -12.06949235617739369, -12.14591786802326823, 24.37609039468567573 ) ) ;
#162903=CARTESIAN_POINT ( 'NONE',  ( 21.53943276465977519, -0.05219959533907433946, 63.74890960531435979 ) ) ;
#162905=CARTESIAN_POINT ( 'NONE',  ( 16.46253265017160672, -9.564922557960803928, 38.33224293864768839 ) ) ;
#162907=CARTESIAN_POINT ( 'NONE',  ( 13.97604488694527802, 13.89961937509977652, 89.37390960531436690 ) ) ;
#162908=CARTESIAN_POINT ( 'NONE',  ( 21.53943276465977519, -0.05219959533907433946, 83.74890960531435269 ) ) ;
#162909=CARTESIAN_POINT ( 'NONE',  ( -4.483927247898782831, 16.52544592524335698, 112.7094237280190328 ) ) ;
#162910=CARTESIAN_POINT ( 'NONE',  ( 16.51473224551069308, 9.474510206698969483, 99.16557627198102409 ) ) ;
#162911=CARTESIAN_POINT ( 'NONE',  ( -9.564922557961040184, 16.46253265017147172, 82.91775706135233293 ) ) ;
#162912=CARTESIAN_POINT ( 'NONE',  ( -21.55341960407619339, 5.719274019375674811, 103.5427570613523613 ) ) ;
#162913=CARTESIAN_POINT ( 'NONE',  ( 5.823673210054125526, 21.52544592524343514, 74.79057627198105251 ) ) ;
#162914=CARTESIAN_POINT ( 'NONE',  ( -21.52544592524343514, 5.823673210054127303, 36.04057627198102409 ) ) ;
#162915=CARTESIAN_POINT ( 'NONE',  ( -16.46253265017160317, 9.564922557960807481, 55.83224293864769550 ) ) ;
#162916=CARTESIAN_POINT ( 'NONE',  ( 16.53943276465976808, -0.05219959533910856209, 23.74890960531435269 ) ) ;
#162917=CARTESIAN_POINT ( 'NONE',  ( 16.51473224551069308, 9.474510206698969483, 74.16557627198103830 ) ) ;
#162919=CARTESIAN_POINT ( 'NONE',  ( 16.46253265017146816, 9.564922557961045513, 21.66775706135233648 ) ) ;
#162920=CARTESIAN_POINT ( 'NONE',  ( 16.52544592524342804, -4.483927247898539470, 88.54057627198103830 ) ) ;
#162922=CARTESIAN_POINT ( 'NONE',  ( 15.80617190586769283, -15.72974639402175789, 30.62609039468567929 ) ) ;
#162924=CARTESIAN_POINT ( 'NONE',  ( -21.53943276465977519, 0.05219959533907696930, 71.24890960531435269 ) ) ;
#162925=CARTESIAN_POINT ( 'NONE',  ( -14.34966873604972548, 8.224510206698743886, 88.33442372801901854 ) ) ;
#162926=CARTESIAN_POINT ( 'NONE',  ( 12.06949235617757843, -12.14591786802309237, 113.1239096053143953 ) ) ;
#162927=CARTESIAN_POINT ( 'NONE',  ( 9.564922557960805705, 16.46253265017160317, 74.58224293864769550 ) ) ;
#162928=CARTESIAN_POINT ( 'NONE',  ( 18.22780087662123805, 5.499999999999960032, 91.48236817873106475 ) ) ;
#162930=CARTESIAN_POINT ( 'NONE',  ( -12.14591786802309592, -12.06949235617757132, 31.87390960531435979 ) ) ;
#162931=CARTESIAN_POINT ( 'NONE',  ( 18.62759615963255655, 10.81492255796105972, 56.66775706135235424 ) ) ;
#162932=CARTESIAN_POINT ( 'NONE',  ( 9.474510206698971260, -16.51473224551069308, 107.9155762719810383 ) ) ;
#162933=CARTESIAN_POINT ( 'NONE',  ( -5.823673210054431948, 21.52544592524334988, 92.70942372801901854 ) ) ;
#162934=CARTESIAN_POINT ( 'NONE',  ( 5.049401038298161559, -19.05341960407611168, 42.70724293864767418 ) ) ;
#162935=CARTESIAN_POINT ( 'NONE',  ( 13.89961937509977652, -13.97604488694527269, 53.12390960531434558 ) ) ;
#162937=CARTESIAN_POINT ( 'NONE',  ( 5.823673210054444382, -21.52544592524334988, 90.20942372801903275 ) ) ;
#162938=CARTESIAN_POINT ( 'NONE',  ( -14.34966873604972548, 8.224510206698743886, 68.33442372801900433 ) ) ;
#162939=CARTESIAN_POINT ( 'NONE',  ( 18.67979575497194134, -10.72451020669871369, 90.83442372801901854 ) ) ;
#162940=CARTESIAN_POINT ( 'NONE',  ( -15.72974639402197994, 15.80617190586746368, 25.62390960531435624 ) ) ;
#162941=CARTESIAN_POINT ( 'NONE',  ( -9.474510206698720793, -16.51473224551083518, 94.58442372801900433 ) ) ;
#162942=CARTESIAN_POINT ( 'NONE',  ( 5.823673210054444382, -21.52544592524334988, 60.20942372801902565 ) ) ;
#162943=CARTESIAN_POINT ( 'NONE',  ( 16.55341960407618274, -4.379528057220086978, 41.04275706135236135 ) ) ;
#162944=CARTESIAN_POINT ( 'NONE',  ( -15.72974639402197994, 15.80617190586746368, 85.62390960531436690 ) ) ;
#162945=CARTESIAN_POINT ( 'NONE',  ( -13.89961937509957401, -13.97604488694547875, 84.37609039468567573 ) ) ;
#162946=CARTESIAN_POINT ( 'NONE',  ( -19.05341960407611168, -5.049401038298163336, 66.45724293864769550 ) ) ;
#162947=CARTESIAN_POINT ( 'NONE',  ( 16.46253265017146816, 9.564922557961045513, 96.66775706135233293 ) ) ;
#162949=CARTESIAN_POINT ( 'NONE',  ( -13.89961937509957401, -13.97604488694547875, 94.37609039468566152 ) ) ;
#162950=CARTESIAN_POINT ( 'NONE',  ( -8.224510206698948167, 14.34966873604960824, 55.41557627198102409 ) ) ;
#162951=CARTESIAN_POINT ( 'NONE',  ( -16.51473224551082808, 9.474510206698731452, 78.33442372801900433 ) ) ;
#162952=CARTESIAN_POINT ( 'NONE',  ( -16.52544592524335698, -4.483927247898792601, 63.95942372801901854 ) ) ;
#162953=CARTESIAN_POINT ( 'NONE',  ( 13.89961937509957401, 13.97604488694547697, 41.87609039468566152 ) ) ;
#162954=CARTESIAN_POINT ( 'NONE',  ( 0.05219959533909260263, 19.03943276465977164, 34.99890960531435979 ) ) ;
#162955=CARTESIAN_POINT ( 'NONE',  ( 5.153800228976335163, 19.02544592524342804, 44.79057627198103830 ) ) ;
#162956=CARTESIAN_POINT ( 'NONE',  ( 8.314922557961029526, -14.29746914071037800, 55.41775706135234714 ) ) ;
#162959=CARTESIAN_POINT ( 'NONE',  ( 13.89961937509977652, -13.97604488694527269, 103.1239096053143527 ) ) ;
#162960=CARTESIAN_POINT ( 'NONE',  ( -0.05219959533909027116, -19.03943276465977164, 22.49890960531436690 ) ) ;
#162962=CARTESIAN_POINT ( 'NONE',  ( 13.89961937509957401, 13.97604488694547697, 96.87609039468566152 ) ) ;
#162963=CARTESIAN_POINT ( 'NONE',  ( 21.55341960407610458, 5.719274019375980345, 38.95724293864768839 ) ) ;
#162964=CARTESIAN_POINT ( 'NONE',  ( 13.97604488694548053, -13.89961937509957401, 25.62609039468566507 ) ) ;
#162965=CARTESIAN_POINT ( 'NONE',  ( -9.474510206698720793, -16.51473224551083518, 109.5844237280190043 ) ) ;
#162966=CARTESIAN_POINT ( 'NONE',  ( -0.05219959533909027116, -19.03943276465977164, 32.49890960531435979 ) ) ;
#162967=CARTESIAN_POINT ( 'NONE',  ( -9.474510206698964154, 16.51473224551069663, 50.41557627198102409 ) ) ;
#162968=CARTESIAN_POINT ( 'NONE',  ( -18.67979575497178146, -10.72451020669898902, 66.66557627198102409 ) ) ;
#162969=CARTESIAN_POINT ( 'NONE',  ( 13.97604488694527802, 13.89961937509977652, 104.3739096053143385 ) ) ;
#162971=CARTESIAN_POINT ( 'NONE',  ( 13.97604488694527802, 13.89961937509977652, 34.37390960531436690 ) ) ;
#162973=CARTESIAN_POINT ( 'NONE',  ( -13.89961937509957401, -13.97604488694547875, 89.37609039468563310 ) ) ;
#162974=CARTESIAN_POINT ( 'NONE',  ( -14.34966873604960291, -8.224510206698953496, 56.66557627198103830 ) ) ;
#162975=CARTESIAN_POINT ( 'NONE',  ( -10.81492255796078084, -18.62759615963271287, 37.08224293864768129 ) ) ;
#162976=CARTESIAN_POINT ( 'NONE',  ( -21.55341960407619339, 5.719274019375674811, 108.5427570613523756 ) ) ;
#162977=CARTESIAN_POINT ( 'NONE',  ( 18.67979575497178502, 10.72451020669898547, 94.16557627198103830 ) ) ;
#162978=CARTESIAN_POINT ( 'NONE',  ( 18.67979575497194134, -10.72451020669871369, 65.83442372801900433 ) ) ;
#162979=CARTESIAN_POINT ( 'NONE',  ( -5.719274019375665041, -21.55341960407619695, 79.79275706135236135 ) ) ;
#162980=CARTESIAN_POINT ( 'NONE',  ( -16.51473224551069308, -9.474510206698971260, 106.6655762719810383 ) ) ;
#162981=CARTESIAN_POINT ( 'NONE',  ( 14.29746914071037800, 8.314922557961029526, 106.6677570613523756 ) ) ;
#162982=CARTESIAN_POINT ( 'NONE',  ( -15.80617190586768217, 15.72974639402176855, 58.12609039468568994 ) ) ;
#162983=CARTESIAN_POINT ( 'NONE',  ( -5.153800228976328057, -19.02544592524343514, 62.29057627198100988 ) ) ;
#162984=CARTESIAN_POINT ( 'NONE',  ( -9.564922557961040184, 16.46253265017147172, 37.91775706135233293 ) ) ;
#162985=CARTESIAN_POINT ( 'NONE',  ( 10.72451020669871369, 18.67979575497193778, 32.08442372801901854 ) ) ;
#162986=CARTESIAN_POINT ( 'NONE',  ( -5.153800228976328057, -19.02544592524343514, 72.29057627198102409 ) ) ;
#162987=CARTESIAN_POINT ( 'NONE',  ( 12.14591786802309770, 12.06949235617756955, 84.37390960531438111 ) ) ;
#162988=CARTESIAN_POINT ( 'NONE',  ( 16.52544592524342804, -4.483927247898539470, 43.54057627198103830 ) ) ;
#162989=CARTESIAN_POINT ( 'NONE',  ( -21.52544592524343514, 5.823673210054127303, 51.04057627198103120 ) ) ;
#162990=CARTESIAN_POINT ( 'NONE',  ( -5.153800228976328057, -19.02544592524343514, 62.29057627198100988 ) ) ;
#162991=CARTESIAN_POINT ( 'NONE',  ( 5.823673210054125526, 21.52544592524343514, 74.79057627198105251 ) ) ;
#162992=CARTESIAN_POINT ( 'NONE',  ( -0.05219959533936034679, 19.03943276465977164, 47.50109039468566863 ) ) ;
#162993=CARTESIAN_POINT ( 'NONE',  ( -0.05219959533936034679, 19.03943276465977164, 22.50109039468566152 ) ) ;
#162994=CARTESIAN_POINT ( 'NONE',  ( -14.29746914071049879, 8.314922557960819915, 60.83224293864769550 ) ) ;
#162995=CARTESIAN_POINT ( 'NONE',  ( 0.05219959533907565091, 21.53943276465977519, 44.99890960531435979 ) ) ;
#162998=CARTESIAN_POINT ( 'NONE',  ( 14.34966873604972726, -8.224510206698740333, 90.83442372801901854 ) ) ;
#163000=CARTESIAN_POINT ( 'NONE',  ( -9.474510206698720793, -16.51473224551083518, 94.58442372801900433 ) ) ;
#163001=CARTESIAN_POINT ( 'NONE',  ( -14.29746914071049879, 8.314922557960819915, 55.83224293864770260 ) ) ;
#163003=CARTESIAN_POINT ( 'NONE',  ( -9.474510206698964154, 16.51473224551069663, 45.41557627198103120 ) ) ;
#163004=CARTESIAN_POINT ( 'NONE',  ( 4.483927247898545687, 16.52544592524342804, 34.79057627198103120 ) ) ;
#163005=CARTESIAN_POINT ( 'NONE',  ( -5.153800228976328057, -19.02544592524343514, 92.29057627198099567 ) ) ;
#163006=CARTESIAN_POINT ( 'NONE',  ( -19.05341960407611168, -5.049401038298163336, 56.45724293864768129 ) ) ;
#163007=CARTESIAN_POINT ( 'NONE',  ( -21.52544592524334988, -5.823673210054445271, 63.95942372801901854 ) ) ;
#163008=CARTESIAN_POINT ( 'NONE',  ( -13.89961937509977652, 13.97604488694528158, 75.62390960531438111 ) ) ;
#163010=CARTESIAN_POINT ( 'NONE',  ( -16.46253265017160317, 9.564922557960807481, 70.83224293864770971 ) ) ;
#163011=CARTESIAN_POINT ( 'NONE',  ( -18.62759615963270932, 10.81492255796079327, 55.83224293864770260 ) ) ;
#163012=CARTESIAN_POINT ( 'NONE',  ( -16.46253265017160317, 9.564922557960807481, 40.83224293864769550 ) ) ;
#163013=CARTESIAN_POINT ( 'NONE',  ( 0.05219959533907565091, 21.53943276465977519, 39.99890960531436690 ) ) ;
#163014=CARTESIAN_POINT ( 'NONE',  ( 0.05219959533934541429, -16.53943276465976808, 110.0010903946856757 ) ) ;
#163015=CARTESIAN_POINT ( 'NONE',  ( -13.89961937509957401, -13.97604488694547875, 19.37609039468566507 ) ) ;
#163016=CARTESIAN_POINT ( 'NONE',  ( -16.52544592524335698, -4.483927247898792601, 48.95942372801902565 ) ) ;
#163017=CARTESIAN_POINT ( 'NONE',  ( 12.06949235617739724, 12.14591786802326823, 76.87609039468567573 ) ) ;
#163019=CARTESIAN_POINT ( 'NONE',  ( -8.224510206698735004, -14.34966873604973081, 64.58442372801900433 ) ) ;
#163020=CARTESIAN_POINT ( 'NONE',  ( -21.55341960407610458, -5.719274019375992779, 26.45724293864768839 ) ) ;
#163022=CARTESIAN_POINT ( 'NONE',  ( -5.153800228976328057, -19.02544592524343514, 32.29057627198102409 ) ) ;
#163023=CARTESIAN_POINT ( 'NONE',  ( -8.314922557961024197, 14.29746914071037800, 37.91775706135235424 ) ) ;
#163024=CARTESIAN_POINT ( 'NONE',  ( 0.05219959533909260263, 19.03943276465977164, 44.99890960531435979 ) ) ;
#163025=CARTESIAN_POINT ( 'NONE',  ( 5.823673210054444382, -21.52544592524334988, 35.20942372801901854 ) ) ;
#163026=CARTESIAN_POINT ( 'NONE',  ( 14.29746914071037800, 8.314922557961029526, 41.66775706135235424 ) ) ;
#163027=CARTESIAN_POINT ( 'NONE',  ( 12.14591786802327356, -12.06949235617739191, 95.62609039468568994 ) ) ;
#163029=CARTESIAN_POINT ( 'NONE',  ( 21.52544592524334988, 5.823673210054432836, 96.45942372801901854 ) ) ;
#163030=CARTESIAN_POINT ( 'NONE',  ( 13.97604488694548053, -13.89961937509957401, 90.62609039468567573 ) ) ;
#163031=CARTESIAN_POINT ( 'NONE',  ( 16.51473224551083163, -9.474510206698727899, 65.83442372801900433 ) ) ;
#163032=CARTESIAN_POINT ( 'NONE',  ( 8.314922557960818139, 14.29746914071049879, 69.58224293864769550 ) ) ;
#163033=CARTESIAN_POINT ( 'NONE',  ( -19.05341960407611168, -5.049401038298163336, 21.45724293864768839 ) ) ;
#163034=CARTESIAN_POINT ( 'NONE',  ( 13.97604488694548053, -13.89961937509957401, 60.62609039468564731 ) ) ;
#163035=CARTESIAN_POINT ( 'NONE',  ( 17.26058549869092928, 6.457015423128504850, 78.87745837476070676 ) ) ;
#163036=CARTESIAN_POINT ( 'NONE',  ( -10.81492255796105439, 18.62759615963255655, 57.91775706135234714 ) ) ;
#163037=CARTESIAN_POINT ( 'NONE',  ( 14.34966873604972726, -8.224510206698740333, 25.83442372801901499 ) ) ;
#163039=CARTESIAN_POINT ( 'NONE',  ( -21.55341960407610458, -5.719274019375992779, 21.45724293864769550 ) ) ;
#163040=CARTESIAN_POINT ( 'NONE',  ( -16.46253265017146816, -9.564922557961047289, 104.1677570613523329 ) ) ;
#163041=CARTESIAN_POINT ( 'NONE',  ( 18.22780087662123805, -5.499999999999976019, 98.51763182126896368 ) ) ;
#163043=CARTESIAN_POINT ( 'NONE',  ( -19.05341960407611168, -5.049401038298163336, 26.45724293864769550 ) ) ;
#163044=CARTESIAN_POINT ( 'NONE',  ( -21.53943276465977519, -0.05219959533937600094, 103.7510903946857042 ) ) ;
#163045=CARTESIAN_POINT ( 'NONE',  ( 5.153800228976335163, 19.02544592524342804, 49.79057627198100988 ) ) ;
#163047=CARTESIAN_POINT ( 'NONE',  ( -5.719274019375665041, -21.55341960407619695, 69.79275706135234714 ) ) ;
#163048=CARTESIAN_POINT ( 'NONE',  ( 18.62759615963255655, 10.81492255796105972, 106.6677570613523756 ) ) ;
#163049=CARTESIAN_POINT ( 'NONE',  ( -16.53943276465976808, 0.05219959533911058130, 26.24890960531435624 ) ) ;
#163050=CARTESIAN_POINT ( 'NONE',  ( -9.474510206698964154, 16.51473224551069663, 80.41557627198103830 ) ) ;
#163051=CARTESIAN_POINT ( 'NONE',  ( 10.72451020669871369, 18.67979575497193778, 62.08442372801901143 ) ) ;
#163052=CARTESIAN_POINT ( 'NONE',  ( -21.55341960407619339, 5.719274019375674811, 53.54275706135234714 ) ) ;
#163053=CARTESIAN_POINT ( 'NONE',  ( 5.049401038297881783, 19.05341960407617563, 77.29275706135231871 ) ) ;
#163054=CARTESIAN_POINT ( 'NONE',  ( 13.97604488694527802, 13.89961937509977652, 109.3739096053143669 ) ) ;
#163055=CARTESIAN_POINT ( 'NONE',  ( -16.53943276465976808, 0.05219959533911058130, 116.2489096053143669 ) ) ;
#163056=CARTESIAN_POINT ( 'NONE',  ( 0.05219959533907565091, 21.53943276465977519, 104.9989096053143669 ) ) ;
#163057=CARTESIAN_POINT ( 'NONE',  ( 16.51473224551083163, -9.474510206698727899, 35.83442372801899722 ) ) ;
#163058=CARTESIAN_POINT ( 'NONE',  ( -16.52544592524342804, 4.483927247898546575, 91.04057627198103830 ) ) ;
#163059=CARTESIAN_POINT ( 'NONE',  ( 13.89961937509977652, -13.97604488694527269, 43.12390960531434558 ) ) ;
#163060=CARTESIAN_POINT ( 'NONE',  ( -13.89961937509957401, -13.97604488694547875, 94.37609039468566152 ) ) ;
#163061=CIRCLE ( 'NONE', #72733, 2.000000000000000000 ) ;
#163062=CARTESIAN_POINT ( 'NONE',  ( -12.14591786802309592, -12.06949235617757132, 66.87390960531436690 ) ) ;
#163063=CARTESIAN_POINT ( 'NONE',  ( 21.53943276465977519, 0.05219959533937863772, 111.2510903946856899 ) ) ;
#163064=CARTESIAN_POINT ( 'NONE',  ( -9.474510206698964154, 16.51473224551069663, 100.4155762719810241 ) ) ;
#163065=CARTESIAN_POINT ( 'NONE',  ( -5.049401038297874678, -19.05341960407617918, 79.79275706135233293 ) ) ;
#163066=CARTESIAN_POINT ( 'NONE',  ( 18.62759615963271287, -10.81492255796078972, 88.33224293864769550 ) ) ;
#163068=CARTESIAN_POINT ( 'NONE',  ( -21.53943276465977519, -0.05219959533937600094, 48.75109039468568284 ) ) ;
#163069=CARTESIAN_POINT ( 'NONE',  ( -12.14591786802326823, 12.06949235617739902, 43.12609039468568284 ) ) ;
#163070=CARTESIAN_POINT ( 'NONE',  ( -14.34966873604972548, 8.224510206698743886, 108.3344237280190185 ) ) ;
#163071=CARTESIAN_POINT ( 'NONE',  ( 12.06949235617739724, 12.14591786802326823, 36.87609039468568994 ) ) ;
#163072=CARTESIAN_POINT ( 'NONE',  ( -15.80617190586768217, 15.72974639402176855, 33.12609039468569705 ) ) ;
#163073=CARTESIAN_POINT ( 'NONE',  ( -18.67979575497178146, -10.72451020669898902, 41.66557627198103120 ) ) ;
#163076=CARTESIAN_POINT ( 'NONE',  ( 5.153800228976335163, 19.02544592524342804, 39.79057627198100988 ) ) ;
#163078=CARTESIAN_POINT ( 'NONE',  ( -4.379528057220086978, -16.55341960407618274, 64.79275706135234714 ) ) ;
#163079=CARTESIAN_POINT ( 'NONE',  ( 15.80617190586746368, 15.72974639402197994, 94.37390960531436690 ) ) ;
#163080=CARTESIAN_POINT ( 'NONE',  ( -0.05219959533910754901, -16.53943276465976808, 32.49890960531435979 ) ) ;
#163081=CARTESIAN_POINT ( 'NONE',  ( -4.483927247898782831, 16.52544592524335698, 67.70942372801901854 ) ) ;
#163082=CARTESIAN_POINT ( 'NONE',  ( 9.564922557960805705, 16.46253265017160317, 64.58224293864769550 ) ) ;
#163083=CARTESIAN_POINT ( 'NONE',  ( 16.46253265017146816, 9.564922557961045513, 91.66775706135234714 ) ) ;
#163084=CARTESIAN_POINT ( 'NONE',  ( 15.80617190586746368, 15.72974639402197994, 79.37390960531436690 ) ) ;
#163085=CARTESIAN_POINT ( 'NONE',  ( 4.483927247898545687, 16.52544592524342804, 29.79057627198102409 ) ) ;
#163086=ORIENTED_EDGE ( 'NONE', *, *, #199224, .T. ) ;
#163089=CARTESIAN_POINT ( 'NONE',  ( -10.72451020669898014, 18.67979575497178502, 60.41557627198102409 ) ) ;
#163090=CARTESIAN_POINT ( 'NONE',  ( -16.52544592524335698, -4.483927247898792601, 103.9594237280190185 ) ) ;
#163091=VERTEX_POINT ( 'NONE', #184173 ) ;
#163093=CARTESIAN_POINT ( 'NONE',  ( -5.823673210054116645, -21.52544592524344225, 87.29057627198103830 ) ) ;
#163094=CARTESIAN_POINT ( 'NONE',  ( 10.72451020669898902, -18.67979575497178502, 107.9155762719810241 ) ) ;
#163095=CARTESIAN_POINT ( 'NONE',  ( -14.29746914071049879, 8.314922557960819915, 30.83224293864770260 ) ) ;
#163097=CARTESIAN_POINT ( 'NONE',  ( -14.34966873604972548, 8.224510206698743886, 33.33442372801900433 ) ) ;
#163098=CARTESIAN_POINT ( 'NONE',  ( 0.05219959533909260263, 19.03943276465977164, 34.99890960531435979 ) ) ;
#163099=CARTESIAN_POINT ( 'NONE',  ( 13.97604488694527802, 13.89961937509977652, 69.37390960531436690 ) ) ;
#163101=CARTESIAN_POINT ( 'NONE',  ( -5.719274019375978568, 21.55341960407610458, 25.20724293864769550 ) ) ;
#163102=CARTESIAN_POINT ( 'NONE',  ( -5.049401038297874678, -19.05341960407617918, 109.7927570613523187 ) ) ;
#163103=CARTESIAN_POINT ( 'NONE',  ( -16.46253265017146816, -9.564922557961047289, 34.16775706135233293 ) ) ;
#163104=CARTESIAN_POINT ( 'NONE',  ( 21.53943276465977519, -0.05219959533907433946, 93.74890960531436690 ) ) ;
#163105=CARTESIAN_POINT ( 'NONE',  ( -14.29746914071049879, 8.314922557960819915, 25.83224293864769194 ) ) ;
#163106=B_SPLINE_CURVE_WITH_KNOTS ( 'NONE', 3,
 ( #170328, #105678, #183524, #137005, #198695, #74361, #46991, #60161, #77317, #30830, #197701, #121830, #31821, #93471, #14662, #122821, #138985, #45007, #28862, #199684, #59167, #76323, #123802, #185500, #120836, #155158, #63138, #182535, #124817, #44017, #167364, #114611 ),
 .UNSPECIFIED., .F., .F.,
 ( 4, 2, 2, 2, 2, 2, 2, 2, 2, 2, 2, 2, 2, 2, 2, 4 ),
 ( 8.673617379884035472E-19, 0.0003712461730036809775, 0.0007424923460073610875, 0.001113738519011041143, 0.001484984692014721308, 0.002227477038022088358, 0.002598723211025757464, 0.002969969384029427437, 0.003341215557033096542, 0.003712461730036766515, 0.004083707903040435620, 0.004454954076044105593, 0.004826200249047775566, 0.005197446422051444671, 0.005568692595055114644, 0.005939938768058783750 ),
 .UNSPECIFIED. ) ;
#163107=CARTESIAN_POINT ( 'NONE',  ( 15.72974639402199770, -15.80617190586745480, 48.12390960531436690 ) ) ;
#163108=CARTESIAN_POINT ( 'NONE',  ( 10.72451020669898902, -18.67979575497178502, 77.91557627198102409 ) ) ;
#163109=CARTESIAN_POINT ( 'NONE',  ( 19.02544592524334988, 5.153800228976608722, 106.4594237280190185 ) ) ;
#163110=CARTESIAN_POINT ( 'NONE',  ( -9.474510206698964154, 16.51473224551069663, 100.4155762719810241 ) ) ;
#163111=CARTESIAN_POINT ( 'NONE',  ( -15.72974639402176322, -15.80617190586768395, 69.37609039468567573 ) ) ;
#163112=CARTESIAN_POINT ( 'NONE',  ( -9.564922557960796823, -16.46253265017161027, 62.08224293864769550 ) ) ;
#163113=CARTESIAN_POINT ( 'NONE',  ( -14.29746914071049879, 8.314922557960819915, 105.8322429386476955 ) ) ;
#163115=CARTESIAN_POINT ( 'NONE',  ( 0.05219959533909260263, 19.03943276465977164, 69.99890960531435269 ) ) ;
#163116=CARTESIAN_POINT ( 'NONE',  ( 16.55341960407611168, 4.379528057220329451, 93.95724293864770971 ) ) ;
#163118=CARTESIAN_POINT ( 'NONE',  ( 13.89961937509957401, 13.97604488694547697, 91.87609039468567573 ) ) ;
#163120=CARTESIAN_POINT ( 'NONE',  ( 9.474510206698971260, -16.51473224551069308, 57.91557627198103120 ) ) ;
#163121=CARTESIAN_POINT ( 'NONE',  ( 21.55341960407619695, -5.719274019375665929, 91.04275706135236135 ) ) ;
#163122=CARTESIAN_POINT ( 'NONE',  ( 5.049401038298161559, -19.05341960407611168, 97.70724293864766707 ) ) ;
#163123=CARTESIAN_POINT ( 'NONE',  ( 16.52544592524335698, 4.483927247898782831, 81.45942372801900433 ) ) ;
#163124=CARTESIAN_POINT ( 'NONE',  ( -17.48853670773242541, -5.747243402303182869, 51.33328700250012133 ) ) ;
#163125=CARTESIAN_POINT ( 'NONE',  ( -0.05219959533936034679, 19.03943276465977164, 37.50109039468567573 ) ) ;
#163126=CARTESIAN_POINT ( 'NONE',  ( 21.55341960407619695, -5.719274019375665929, 106.0427570613523471 ) ) ;
#163129=CARTESIAN_POINT ( 'NONE',  ( 8.314922557961029526, -14.29746914071037800, 100.4177570613523471 ) ) ;
#163131=CARTESIAN_POINT ( 'NONE',  ( 16.53943276465976808, 0.05219959533934440121, 96.25109039468568994 ) ) ;
#163132=CARTESIAN_POINT ( 'NONE',  ( 17.40861289039003523, 6.110651285853279546, 68.87232470827430575 ) ) ;
#163133=CARTESIAN_POINT ( 'NONE',  ( -8.224510206698735004, -14.34966873604973081, 64.58442372801900433 ) ) ;
#163135=CARTESIAN_POINT ( 'NONE',  ( 15.72974639402176855, 15.80617190586768217, 81.87609039468568994 ) ) ;
#163136=CARTESIAN_POINT ( 'NONE',  ( 9.564922557961047289, -16.46253265017146816, 85.41775706135233293 ) ) ;
#163137=CARTESIAN_POINT ( 'NONE',  ( 9.564922557961047289, -16.46253265017146816, 35.41775706135233293 ) ) ;
#163139=CARTESIAN_POINT ( 'NONE',  ( -16.51473224551069308, -9.474510206698971260, 66.66557627198102409 ) ) ;
#163140=CARTESIAN_POINT ( 'NONE',  ( -13.97604488694527625, -13.89961937509977652, 56.87390960531434558 ) ) ;
#163141=CARTESIAN_POINT ( 'NONE',  ( -18.56453257813359770, 5.500000000000040856, 40.99000423690688422 ) ) ;
#163142=CARTESIAN_POINT ( 'NONE',  ( -15.80617190586745835, -15.72974639402198527, 76.87390960531439532 ) ) ;
#163143=CARTESIAN_POINT ( 'NONE',  ( 15.80617190586746368, 15.72974639402197994, 34.37390960531435979 ) ) ;
#163144=CARTESIAN_POINT ( 'NONE',  ( 19.03943276465977164, -0.05219959533909143690, 33.74890960531435979 ) ) ;
#163145=CARTESIAN_POINT ( 'NONE',  ( -8.224510206698735004, -14.34966873604973081, 59.58442372801901854 ) ) ;
#163147=CARTESIAN_POINT ( 'NONE',  ( 21.52544592524334988, 5.823673210054432836, 26.45942372801901854 ) ) ;
#163148=CARTESIAN_POINT ( 'NONE',  ( -8.224510206698948167, 14.34966873604960824, 70.41557627198102409 ) ) ;
#163150=CARTESIAN_POINT ( 'NONE',  ( 16.52544592524335698, 4.483927247898782831, 21.45942372801901499 ) ) ;
#163151=CARTESIAN_POINT ( 'NONE',  ( -16.46253265017146816, -9.564922557961047289, 54.16775706135234003 ) ) ;
#163152=CARTESIAN_POINT ( 'NONE',  ( -8.314922557960811034, -14.29746914071050412, 57.08224293864769550 ) ) ;
#163153=CARTESIAN_POINT ( 'NONE',  ( -0.05219959533937732626, 21.53943276465977519, 37.50109039468568284 ) ) ;
#163155=CARTESIAN_POINT ( 'NONE',  ( 10.81492255796078972, 18.62759615963270932, 79.58224293864769550 ) ) ;
#163156=CARTESIAN_POINT ( 'NONE',  ( 16.46253265017160672, -9.564922557960803928, 103.3322429386476955 ) ) ;
#163157=CARTESIAN_POINT ( 'NONE',  ( -4.379528057220328563, 16.55341960407611168, 65.20724293864768129 ) ) ;
#163159=CARTESIAN_POINT ( 'NONE',  ( 17.72662750342724181, 5.500000000000073719, 43.90179492283744622 ) ) ;
#163160=CARTESIAN_POINT ( 'NONE',  ( -5.049401038297874678, -19.05341960407617918, 69.79275706135233293 ) ) ;
#163161=CARTESIAN_POINT ( 'NONE',  ( -5.719274019375978568, 21.55341960407610458, 110.2072429386477239 ) ) ;
#163162=CARTESIAN_POINT ( 'NONE',  ( 9.474510206698971260, -16.51473224551069308, 52.91557627198102409 ) ) ;
#163163=CARTESIAN_POINT ( 'NONE',  ( 16.51473224551083163, -9.474510206698727899, 40.83442372801900433 ) ) ;
#163164=CARTESIAN_POINT ( 'NONE',  ( 0.05219959533909260263, 19.03943276465977164, 29.99890960531435979 ) ) ;
#163165=CARTESIAN_POINT ( 'NONE',  ( 21.52544592524334988, 5.823673210054432836, 61.45942372801901854 ) ) ;
#163167=CARTESIAN_POINT ( 'NONE',  ( 14.29746914071049879, -8.314922557960816363, 38.33224293864768839 ) ) ;
#163168=CARTESIAN_POINT ( 'NONE',  ( -5.049401038298153566, 19.05341960407611168, 65.20724293864765286 ) ) ;
#163169=CARTESIAN_POINT ( 'NONE',  ( 15.80617190586746368, 15.72974639402197994, 84.37390960531438111 ) ) ;
#163170=CARTESIAN_POINT ( 'NONE',  ( -19.02544592524342804, 5.153800228976336051, 56.04057627198100988 ) ) ;
#163172=CARTESIAN_POINT ( 'NONE',  ( 18.62759615963271287, -10.81492255796078972, 68.33224293864769550 ) ) ;
#163173=VERTEX_POINT ( 'NONE', #16314 ) ;
#163174=CARTESIAN_POINT ( 'NONE',  ( -5.823673210054431948, 21.52544592524334988, 97.70942372801904696 ) ) ;
#163176=CARTESIAN_POINT ( 'NONE',  ( 0.05219959533934541429, -16.53943276465976808, 90.00109039468567573 ) ) ;
#163177=CARTESIAN_POINT ( 'NONE',  ( -0.05219959533910754901, -16.53943276465976808, 77.49890960531433848 ) ) ;
#163178=CARTESIAN_POINT ( 'NONE',  ( 9.564922557961047289, -16.46253265017146816, 90.41775706135234714 ) ) ;
#163180=CARTESIAN_POINT ( 'NONE',  ( -0.05219959533936034679, 19.03943276465977164, 37.50109039468567573 ) ) ;
#163181=CARTESIAN_POINT ( 'NONE',  ( 4.483927247898790824, -16.52544592524335698, 95.20942372801903275 ) ) ;
#163182=CARTESIAN_POINT ( 'NONE',  ( -5.049401038297874678, -19.05341960407617918, 29.79275706135232227 ) ) ;
#163183=CARTESIAN_POINT ( 'NONE',  ( 19.05341960407611168, 5.049401038298154454, 83.95724293864766707 ) ) ;
#163184=CARTESIAN_POINT ( 'NONE',  ( -18.67979575497178146, -10.72451020669898902, 61.66557627198103120 ) ) ;
#163185=CARTESIAN_POINT ( 'NONE',  ( -13.97604488694527625, -13.89961937509977652, 21.87390960531435979 ) ) ;
#163186=CARTESIAN_POINT ( 'NONE',  ( 16.46253265017160672, -9.564922557960803928, 23.33224293864769194 ) ) ;
#163187=CARTESIAN_POINT ( 'NONE',  ( -18.62759615963255300, -10.81492255796106328, 94.16775706135237556 ) ) ;
#163188=CARTESIAN_POINT ( 'NONE',  ( 0.05219959533934541429, -16.53943276465976808, 80.00109039468568994 ) ) ;
#163189=CARTESIAN_POINT ( 'NONE',  ( -21.53943276465977519, -0.05219959533937600094, 33.75109039468568284 ) ) ;
#163190=CARTESIAN_POINT ( 'NONE',  ( 16.52544592524335698, 4.483927247898782831, 26.45942372801901854 ) ) ;
#163191=CARTESIAN_POINT ( 'NONE',  ( 5.153800228976335163, 19.02544592524342804, 104.7905762719809957 ) ) ;
#163192=CARTESIAN_POINT ( 'NONE',  ( -9.474510206698964154, 16.51473224551069663, 45.41557627198103120 ) ) ;
#163193=CARTESIAN_POINT ( 'NONE',  ( -16.51473224551069308, -9.474510206698971260, 46.66557627198102409 ) ) ;
#163195=CARTESIAN_POINT ( 'NONE',  ( 8.224510206698742110, 14.34966873604972548, 52.08442372801901854 ) ) ;
#163196=CARTESIAN_POINT ( 'NONE',  ( 14.34966873604960469, 8.224510206698951720, 94.16557627198103830 ) ) ;
#163197=CARTESIAN_POINT ( 'NONE',  ( 8.224510206698742110, 14.34966873604972548, 107.0844237280190043 ) ) ;
#163198=CARTESIAN_POINT ( 'NONE',  ( 10.72451020669871369, 18.67979575497193778, 47.08442372801901854 ) ) ;
#163199=CARTESIAN_POINT ( 'NONE',  ( -19.03943276465977164, 0.05219959533909376836, 81.24890960531436690 ) ) ;
#163200=CARTESIAN_POINT ( 'NONE',  ( 16.46253265017160672, -9.564922557960803928, 68.33224293864770971 ) ) ;
#163201=CARTESIAN_POINT ( 'NONE',  ( -9.564922557960796823, -16.46253265017161027, 97.08224293864769550 ) ) ;
#163202=CARTESIAN_POINT ( 'NONE',  ( -4.483927247898539470, -16.52544592524342804, 32.29057627198102409 ) ) ;
#163203=CARTESIAN_POINT ( 'NONE',  ( -16.52544592524335698, -4.483927247898792601, 98.95942372801903275 ) ) ;
#163205=CARTESIAN_POINT ( 'NONE',  ( -16.46253265017146816, -9.564922557961047289, 49.16775706135233293 ) ) ;
#163206=CARTESIAN_POINT ( 'NONE',  ( -16.46253265017160317, 9.564922557960807481, 115.8322429386477097 ) ) ;
#163207=CARTESIAN_POINT ( 'NONE',  ( 19.03943276465977164, -0.05219959533909143690, 68.74890960531436690 ) ) ;
#163208=CARTESIAN_POINT ( 'NONE',  ( 19.03943276465977164, 0.05219959533936151252, 36.25109039468567573 ) ) ;
#163210=CARTESIAN_POINT ( 'NONE',  ( 19.02130022317636104, -5.499999999999790390, 73.28188669246573284 ) ) ;
#163211=CARTESIAN_POINT ( 'NONE',  ( -12.14591786802326823, 12.06949235617739902, 48.12609039468568284 ) ) ;
#163212=AXIS2_PLACEMENT_3D ( 'NONE', #99960, #116141, #177832 ) ;
#163213=CARTESIAN_POINT ( 'NONE',  ( 9.474510206698729675, 16.51473224551082808, 77.08442372801900433 ) ) ;
#163214=CARTESIAN_POINT ( 'NONE',  ( -0.05219959533934338120, 16.53943276465976808, 52.50109039468567573 ) ) ;
#163215=CARTESIAN_POINT ( 'NONE',  ( 13.97604488694527802, 13.89961937509977652, 114.3739096053143669 ) ) ;
#163216=CARTESIAN_POINT ( 'NONE',  ( 19.03943276465977164, -0.05219959533909143690, 88.74890960531436690 ) ) ;
#163217=CARTESIAN_POINT ( 'NONE',  ( -15.72974639402197994, 15.80617190586746368, 115.6239096053143669 ) ) ;
#163218=CARTESIAN_POINT ( 'NONE',  ( -19.05341960407617563, 5.049401038297882671, 73.54275706135233293 ) ) ;
#163219=CARTESIAN_POINT ( 'NONE',  ( -9.474510206698964154, 16.51473224551069663, 110.4155762719810383 ) ) ;
#163220=CARTESIAN_POINT ( 'NONE',  ( -19.03943276465977164, 0.05219959533909376836, 41.24890960531435269 ) ) ;
#163222=CARTESIAN_POINT ( 'NONE',  ( -16.51473224551069308, -9.474510206698971260, 71.66557627198102409 ) ) ;
#163223=CARTESIAN_POINT ( 'NONE',  ( 12.14591786802309770, 12.06949235617756955, 34.37390960531435979 ) ) ;
#163224=CARTESIAN_POINT ( 'NONE',  ( -13.89961937509977652, 13.97604488694528158, 35.62390960531435269 ) ) ;
#163226=CARTESIAN_POINT ( 'NONE',  ( -19.03943276465977164, -0.05219959533935918106, 53.75109039468566863 ) ) ;
#163227=CARTESIAN_POINT ( 'NONE',  ( 16.52544592524342804, -4.483927247898539470, 83.54057627198102409 ) ) ;
#163228=CARTESIAN_POINT ( 'NONE',  ( 15.80617190586769283, -15.72974639402175789, 105.6260903946856899 ) ) ;
#163229=CARTESIAN_POINT ( 'NONE',  ( 5.049401038298161559, -19.05341960407611168, 47.70724293864770260 ) ) ;
#163230=CARTESIAN_POINT ( 'NONE',  ( 0.05219959533907565091, 21.53943276465977519, 49.99890960531437401 ) ) ;
#163231=CARTESIAN_POINT ( 'NONE',  ( -4.379528057220328563, 16.55341960407611168, 50.20724293864769550 ) ) ;
#163232=CARTESIAN_POINT ( 'NONE',  ( 21.52544592524334988, 5.823673210054432836, 106.4594237280190328 ) ) ;
#163233=CARTESIAN_POINT ( 'NONE',  ( 19.05341960407611168, 5.049401038298154454, 103.9572429386476671 ) ) ;
#163234=CARTESIAN_POINT ( 'NONE',  ( -9.564922557960796823, -16.46253265017161027, 102.0822429386477097 ) ) ;
#163235=CARTESIAN_POINT ( 'NONE',  ( -5.049401038298153566, 19.05341960407611168, 40.20724293864768839 ) ) ;
#163236=CARTESIAN_POINT ( 'NONE',  ( 9.564922557960805705, 16.46253265017160317, 24.58224293864769194 ) ) ;
#163237=CARTESIAN_POINT ( 'NONE',  ( -16.53943276465976808, 0.05219959533911058130, 91.24890960531436690 ) ) ;
#163238=CARTESIAN_POINT ( 'NONE',  ( -21.52544592524343514, 5.823673210054127303, 91.04057627198103830 ) ) ;
#163239=CARTESIAN_POINT ( 'NONE',  ( 19.03943276465977164, -0.05219959533909143690, 103.7489096053143669 ) ) ;
#163240=CARTESIAN_POINT ( 'NONE',  ( 15.80617190586746368, 15.72974639402197994, 114.3739096053143527 ) ) ;
#163241=CARTESIAN_POINT ( 'NONE',  ( 5.049401038298161559, -19.05341960407611168, 97.70724293864766707 ) ) ;
#163242=CARTESIAN_POINT ( 'NONE',  ( 16.51473224551083163, -9.474510206698727899, 65.83442372801900433 ) ) ;
#163243=CARTESIAN_POINT ( 'NONE',  ( -16.53943276465976808, 0.05219959533911058130, 101.2489096053143669 ) ) ;
#163244=CARTESIAN_POINT ( 'NONE',  ( 9.474510206698971260, -16.51473224551069308, 77.91557627198103830 ) ) ;
#163245=CARTESIAN_POINT ( 'NONE',  ( -21.55341960407610458, -5.719274019375992779, 81.45724293864769550 ) ) ;
#163246=CARTESIAN_POINT ( 'NONE',  ( 17.05587630539787369, -6.762274262135683500, 108.2418030903731818 ) ) ;
#163248=CARTESIAN_POINT ( 'NONE',  ( 21.55341960407610458, 5.719274019375980345, 23.95724293864769550 ) ) ;
#163249=CARTESIAN_POINT ( 'NONE',  ( 18.39635199886966177, -5.500000000000095923, 68.51967076359998998 ) ) ;
#163250=CARTESIAN_POINT ( 'NONE',  ( -14.29746914071037622, -8.314922557961029526, 39.16775706135235424 ) ) ;
#163251=CARTESIAN_POINT ( 'NONE',  ( 16.55341960407611168, 4.379528057220329451, 98.95724293864770971 ) ) ;
#163253=CARTESIAN_POINT ( 'NONE',  ( -9.564922557960796823, -16.46253265017161027, 92.08224293864769550 ) ) ;
#163254=CARTESIAN_POINT ( 'NONE',  ( 16.51473224551069308, 9.474510206698969483, 59.16557627198102409 ) ) ;
#163255=CARTESIAN_POINT ( 'NONE',  ( 16.55341960407611168, 4.379528057220329451, 83.95724293864770971 ) ) ;
#163256=CARTESIAN_POINT ( 'NONE',  ( 21.55341960407610458, 5.719274019375980345, 38.95724293864768839 ) ) ;
#163257=CARTESIAN_POINT ( 'NONE',  ( -12.06949235617756955, 12.14591786802309770, 55.62390960531436690 ) ) ;
#163258=CARTESIAN_POINT ( 'NONE',  ( 14.34966873604972726, -8.224510206698740333, 25.83442372801901499 ) ) ;
#163259=CARTESIAN_POINT ( 'NONE',  ( -18.62759615963255300, -10.81492255796106328, 69.16775706135234714 ) ) ;
#163261=CARTESIAN_POINT ( 'NONE',  ( 15.72974639402199770, -15.80617190586745480, 23.12390960531436335 ) ) ;
#163262=CARTESIAN_POINT ( 'NONE',  ( -8.314922557961024197, 14.29746914071037800, 77.91775706135231871 ) ) ;
#163263=CARTESIAN_POINT ( 'NONE',  ( 16.51473224551069308, 9.474510206698969483, 24.16557627198102765 ) ) ;
#163264=CARTESIAN_POINT ( 'NONE',  ( -9.474510206698964154, 16.51473224551069663, 85.41557627198102409 ) ) ;
#163265=CARTESIAN_POINT ( 'NONE',  ( -21.52544592524343514, 5.823673210054127303, 101.0405762719810383 ) ) ;
#163266=CARTESIAN_POINT ( 'NONE',  ( -16.55341960407617563, 4.379528057220093196, 28.54275706135234358 ) ) ;
#163267=CARTESIAN_POINT ( 'NONE',  ( -12.14591786802309592, -12.06949235617757132, 46.87390960531435979 ) ) ;
#163268=CARTESIAN_POINT ( 'NONE',  ( 18.62759615963255655, 10.81492255796105972, 71.66775706135234714 ) ) ;
#163269=CARTESIAN_POINT ( 'NONE',  ( 0.05219959533934541429, -16.53943276465976808, 100.0010903946857042 ) ) ;
#163270=CARTESIAN_POINT ( 'NONE',  ( 18.62759615963271287, -10.81492255796078972, 28.33224293864769550 ) ) ;
#163271=CARTESIAN_POINT ( 'NONE',  ( 0.05219959533909260263, 19.03943276465977164, 114.9989096053143669 ) ) ;
#163272=CARTESIAN_POINT ( 'NONE',  ( -16.21995358207303539, 7.366697692864245361, 79.93551001512159360 ) ) ;
#163273=CARTESIAN_POINT ( 'NONE',  ( 16.55341960407618274, -4.379528057220086978, 106.0427570613523471 ) ) ;
#163274=CARTESIAN_POINT ( 'NONE',  ( -16.53943276465976808, -0.05219959533934237506, 53.75109039468568994 ) ) ;
#163275=CARTESIAN_POINT ( 'NONE',  ( -9.564922557960796823, -16.46253265017161027, 67.08224293864769550 ) ) ;
#163277=CARTESIAN_POINT ( 'NONE',  ( 19.03943276465977164, -0.05219959533909143690, 93.74890960531435269 ) ) ;
#163278=CARTESIAN_POINT ( 'NONE',  ( 15.80617190586769283, -15.72974639402175789, 75.62609039468567573 ) ) ;
#163279=CARTESIAN_POINT ( 'NONE',  ( 16.55341960407618274, -4.379528057220086978, 71.04275706135234714 ) ) ;
#163280=CARTESIAN_POINT ( 'NONE',  ( -14.29746914071049879, 8.314922557960819915, 50.83224293864770971 ) ) ;
#163281=CARTESIAN_POINT ( 'NONE',  ( 19.05341960407611168, 5.049401038298154454, 53.95724293864770260 ) ) ;
#163283=CARTESIAN_POINT ( 'NONE',  ( 16.46253265017146816, 9.564922557961045513, 111.6677570613523329 ) ) ;
#163284=CARTESIAN_POINT ( 'NONE',  ( 0.05219959533910956823, 16.53943276465976808, 104.9989096053143669 ) ) ;
#163285=CARTESIAN_POINT ( 'NONE',  ( 19.03943276465977164, -0.05219959533909143690, 63.74890960531435979 ) ) ;
#163286=CARTESIAN_POINT ( 'NONE',  ( 19.05341960407617918, -5.049401038297876454, 96.04275706135231871 ) ) ;
#163288=CARTESIAN_POINT ( 'NONE',  ( -10.72451020669870658, -18.67979575497194134, 99.58442372801900433 ) ) ;
#163289=CARTESIAN_POINT ( 'NONE',  ( -16.52544592524335698, -4.483927247898792601, 68.95942372801901854 ) ) ;
#163290=CARTESIAN_POINT ( 'NONE',  ( -16.51473224551082808, 9.474510206698731452, 98.33442372801900433 ) ) ;
#163291=CARTESIAN_POINT ( 'NONE',  ( -15.80617190586745835, -15.72974639402198527, 61.87390960531436690 ) ) ;
#163293=CARTESIAN_POINT ( 'NONE',  ( 8.314922557961029526, -14.29746914071037800, 50.41775706135235424 ) ) ;
#163295=CARTESIAN_POINT ( 'NONE',  ( 5.153800228976615827, -19.02544592524334988, 55.20942372801899722 ) ) ;
#163297=CARTESIAN_POINT ( 'NONE',  ( 21.55341960407619695, -5.719274019375665929, 91.04275706135236135 ) ) ;
#163298=CARTESIAN_POINT ( 'NONE',  ( -19.03943276465977164, 0.05219959533909376836, 41.24890960531435269 ) ) ;
#163299=CARTESIAN_POINT ( 'NONE',  ( -5.153800228976328057, -19.02544592524343514, 67.29057627198102409 ) ) ;
#163300=CARTESIAN_POINT ( 'NONE',  ( 4.483927247898545687, 16.52544592524342804, 64.79057627198103830 ) ) ;
#163301=CARTESIAN_POINT ( 'NONE',  ( 0.05219959533937995610, -21.53943276465977519, 95.00109039468568994 ) ) ;
#163303=CARTESIAN_POINT ( 'NONE',  ( -13.97604488694547697, 13.89961937509957934, 48.12609039468566863 ) ) ;
#163304=CARTESIAN_POINT ( 'NONE',  ( 13.89961937509957401, 13.97604488694547697, 21.87609039468566152 ) ) ;
#163305=CARTESIAN_POINT ( 'NONE',  ( 19.05341960407611168, 5.049401038298154454, 113.9572429386477097 ) ) ;
#163306=CARTESIAN_POINT ( 'NONE',  ( 21.55341960407619695, -5.719274019375665929, 91.04275706135236135 ) ) ;
#163307=CARTESIAN_POINT ( 'NONE',  ( 13.89961937509977652, -13.97604488694527269, 73.12390960531436690 ) ) ;
#163308=CARTESIAN_POINT ( 'NONE',  ( 21.52544592524334988, 5.823673210054432836, 96.45942372801901854 ) ) ;
#163309=CARTESIAN_POINT ( 'NONE',  ( -5.719274019375978568, 21.55341960407610458, 50.20724293864769550 ) ) ;
#163310=CARTESIAN_POINT ( 'NONE',  ( 19.02544592524343514, -5.153800228976328945, 78.54057627198099567 ) ) ;
#163311=CARTESIAN_POINT ( 'NONE',  ( 19.05341960407617918, -5.049401038297876454, 76.04275706135230450 ) ) ;
#163312=CARTESIAN_POINT ( 'NONE',  ( -19.02544592524342804, 5.153800228976336051, 41.04057627198103120 ) ) ;
#163313=CARTESIAN_POINT ( 'NONE',  ( -13.97604488694527625, -13.89961937509977652, 86.87390960531436690 ) ) ;
#163314=CARTESIAN_POINT ( 'NONE',  ( -19.05341960407617563, 5.049401038297882671, 88.54275706135230450 ) ) ;
#163315=CARTESIAN_POINT ( 'NONE',  ( -16.53943276465976808, -0.05219959533934237506, 43.75109039468568284 ) ) ;
#163316=CARTESIAN_POINT ( 'NONE',  ( -12.06949235617756955, 12.14591786802309770, 105.6239096053143669 ) ) ;
#163317=CARTESIAN_POINT ( 'NONE',  ( 0.05219959533909260263, 19.03943276465977164, 64.99890960531436690 ) ) ;
#163318=EDGE_CURVE ( 'NONE', #155722, #53380, #75137, .T. ) ;
#163319=CARTESIAN_POINT ( 'NONE',  ( 15.80617190586746368, 15.72974639402197994, 49.37390960531436690 ) ) ;
#163320=CARTESIAN_POINT ( 'NONE',  ( 16.55341960407618274, -4.379528057220086978, 36.04275706135234714 ) ) ;
#163321=CARTESIAN_POINT ( 'NONE',  ( -21.52544592524334988, -5.823673210054445271, 38.95942372801901854 ) ) ;
#163322=CARTESIAN_POINT ( 'NONE',  ( -21.53943276465977519, -0.05219959533937600094, 78.75109039468568994 ) ) ;
#163324=CARTESIAN_POINT ( 'NONE',  ( -14.29746914071037622, -8.314922557961029526, 84.16775706135234714 ) ) ;
#163325=CARTESIAN_POINT ( 'NONE',  ( -19.05341960407611168, -5.049401038298163336, 71.45724293864766707 ) ) ;
#163326=CARTESIAN_POINT ( 'NONE',  ( 8.224510206698742110, 14.34966873604972548, 107.0844237280190043 ) ) ;
#163327=CARTESIAN_POINT ( 'NONE',  ( 5.153800228976615827, -19.02544592524334988, 60.20942372801899012 ) ) ;
#163328=CARTESIAN_POINT ( 'NONE',  ( -21.53943276465977519, -0.05219959533937600094, 33.75109039468568284 ) ) ;
#163329=CARTESIAN_POINT ( 'NONE',  ( 8.314922557960818139, 14.29746914071049879, 79.58224293864769550 ) ) ;
#163330=CARTESIAN_POINT ( 'NONE',  ( 19.05341960407611168, 5.049401038298154454, 98.95724293864766707 ) ) ;
#163331=CARTESIAN_POINT ( 'NONE',  ( 8.224510206698742110, 14.34966873604972548, 107.0844237280190043 ) ) ;
#163332=CARTESIAN_POINT ( 'NONE',  ( 18.62759615963255655, 10.81492255796105972, 76.66775706135234714 ) ) ;
#163333=CARTESIAN_POINT ( 'NONE',  ( -8.314922557961024197, 14.29746914071037800, 47.91775706135234714 ) ) ;
#163334=CARTESIAN_POINT ( 'NONE',  ( 15.80617190586769283, -15.72974639402175789, 30.62609039468567929 ) ) ;
#163335=CARTESIAN_POINT ( 'NONE',  ( 14.29746914071049879, -8.314922557960816363, 73.33224293864769550 ) ) ;
#163336=ORIENTED_EDGE ( 'NONE', *, *, #185965, .T. ) ;
#163338=CARTESIAN_POINT ( 'NONE',  ( -21.52544592524343514, 5.823673210054127303, 111.0405762719810525 ) ) ;
#163339=CARTESIAN_POINT ( 'NONE',  ( 14.34966873604960469, 8.224510206698951720, 54.16557627198103120 ) ) ;
#163341=CARTESIAN_POINT ( 'NONE',  ( -5.719274019375978568, 21.55341960407610458, 30.20724293864769550 ) ) ;
#163342=CARTESIAN_POINT ( 'NONE',  ( -10.81492255796105439, 18.62759615963255655, 52.91775706135235424 ) ) ;
#163343=CARTESIAN_POINT ( 'NONE',  ( -8.224510206698948167, 14.34966873604960824, 70.41557627198102409 ) ) ;
#163344=CARTESIAN_POINT ( 'NONE',  ( 15.72974639402199770, -15.80617190586745480, 78.12390960531436690 ) ) ;
#163345=CARTESIAN_POINT ( 'NONE',  ( -19.03943276465977164, 0.05219959533909376836, 81.24890960531436690 ) ) ;
#163346=CARTESIAN_POINT ( 'NONE',  ( 9.474510206698971260, -16.51473224551069308, 32.91557627198102409 ) ) ;
#163347=CARTESIAN_POINT ( 'NONE',  ( 5.049401038297881783, 19.05341960407617563, 77.29275706135231871 ) ) ;
#163348=CARTESIAN_POINT ( 'NONE',  ( -18.62759615963255300, -10.81492255796106328, 54.16775706135235424 ) ) ;
#163349=CARTESIAN_POINT ( 'NONE',  ( -18.67979575497178146, -10.72451020669898902, 66.66557627198102409 ) ) ;
#163350=CARTESIAN_POINT ( 'NONE',  ( -16.46253265017160317, 9.564922557960807481, 45.83224293864769550 ) ) ;
#163351=CARTESIAN_POINT ( 'NONE',  ( -16.46253265017160317, 9.564922557960807481, 70.83224293864770971 ) ) ;
#163353=CARTESIAN_POINT ( 'NONE',  ( -4.379528057220086978, -16.55341960407618274, 49.79275706135234714 ) ) ;
#163354=CARTESIAN_POINT ( 'NONE',  ( 18.62759615963255655, 10.81492255796105972, 31.66775706135234358 ) ) ;
#163355=CARTESIAN_POINT ( 'NONE',  ( 18.62759615963255655, 10.81492255796105972, 56.66775706135235424 ) ) ;
#163356=CARTESIAN_POINT ( 'NONE',  ( -16.46253265017160317, 9.564922557960807481, 105.8322429386476955 ) ) ;
#163357=CARTESIAN_POINT ( 'NONE',  ( 5.823673210054125526, 21.52544592524343514, 89.79057627198103830 ) ) ;
#163358=CARTESIAN_POINT ( 'NONE',  ( -18.62759615963255300, -10.81492255796106328, 29.16775706135234003 ) ) ;
#163359=CARTESIAN_POINT ( 'NONE',  ( 14.29746914071037800, 8.314922557961029526, 56.66775706135235424 ) ) ;
#163360=CARTESIAN_POINT ( 'NONE',  ( 21.52544592524344225, -5.823673210054117533, 43.54057627198103830 ) ) ;
#163361=CARTESIAN_POINT ( 'NONE',  ( 0.05219959533936267826, -19.03943276465977164, 20.00109039468567218 ) ) ;
#163362=CARTESIAN_POINT ( 'NONE',  ( -16.51473224551069308, -9.474510206698971260, 51.66557627198102409 ) ) ;
#163363=CARTESIAN_POINT ( 'NONE',  ( 9.564922557960805705, 16.46253265017160317, 109.5822429386476955 ) ) ;
#163364=CARTESIAN_POINT ( 'NONE',  ( 0.05219959533909260263, 19.03943276465977164, 84.99890960531436690 ) ) ;
#163365=CARTESIAN_POINT ( 'NONE',  ( 17.50000000000002132, 5.272787497354016750, 103.7271518416984435 ) ) ;
#163366=CARTESIAN_POINT ( 'NONE',  ( 13.89961937509957401, 13.97604488694547697, 71.87609039468567573 ) ) ;
#163367=CARTESIAN_POINT ( 'NONE',  ( -5.719274019375978568, 21.55341960407610458, 50.20724293864769550 ) ) ;
#163368=CARTESIAN_POINT ( 'NONE',  ( 8.314922557960818139, 14.29746914071049879, 29.58224293864769905 ) ) ;
#163369=CARTESIAN_POINT ( 'NONE',  ( 19.02544592524334988, 5.153800228976608722, 91.45942372801900433 ) ) ;
#163371=CARTESIAN_POINT ( 'NONE',  ( -16.46253265017146816, -9.564922557961047289, 19.16775706135233293 ) ) ;
#163372=CARTESIAN_POINT ( 'NONE',  ( -13.97604488694547697, 13.89961937509957934, 98.12609039468566152 ) ) ;
#163373=CARTESIAN_POINT ( 'NONE',  ( -13.89961937509957401, -13.97604488694547875, 39.37609039468566152 ) ) ;
#163375=CARTESIAN_POINT ( 'NONE',  ( 19.02544592524343514, -5.153800228976328945, 58.54057627198102409 ) ) ;
#163376=CARTESIAN_POINT ( 'NONE',  ( -8.314922557960811034, -14.29746914071050412, 47.08224293864770260 ) ) ;
#163377=CARTESIAN_POINT ( 'NONE',  ( -16.51473224551069308, -9.474510206698971260, 36.66557627198102409 ) ) ;
#163378=CARTESIAN_POINT ( 'NONE',  ( -12.06949235617756955, 12.14591786802309770, 40.62390960531435269 ) ) ;
#163380=CARTESIAN_POINT ( 'NONE',  ( 16.52544592524335698, 4.483927247898782831, 101.4594237280190185 ) ) ;
#163381=CARTESIAN_POINT ( 'NONE',  ( -16.51473224551069308, -9.474510206698971260, 66.66557627198102409 ) ) ;
#163382=CARTESIAN_POINT ( 'NONE',  ( -16.51473224551082808, 9.474510206698731452, 28.33442372801900433 ) ) ;
#163383=CARTESIAN_POINT ( 'NONE',  ( 8.224510206698742110, 14.34966873604972548, 37.08442372801901143 ) ) ;
#163384=CARTESIAN_POINT ( 'NONE',  ( 0.05219959533907565091, 21.53943276465977519, 34.99890960531435979 ) ) ;
#163385=CARTESIAN_POINT ( 'NONE',  ( 15.80617190586769283, -15.72974639402175789, 100.6260903946857184 ) ) ;
#163387=CARTESIAN_POINT ( 'NONE',  ( 13.97604488694527802, 13.89961937509977652, 64.37390960531436690 ) ) ;
#163388=CARTESIAN_POINT ( 'NONE',  ( -19.03943276465977164, 0.05219959533909376836, 101.2489096053143669 ) ) ;
#163389=CARTESIAN_POINT ( 'NONE',  ( 16.51473224551069308, 9.474510206698969483, 99.16557627198102409 ) ) ;
#163390=CARTESIAN_POINT ( 'NONE',  ( -18.09867054820434262, -5.499999999999827693, 43.98393025253587041 ) ) ;
#163391=CARTESIAN_POINT ( 'NONE',  ( 0.05219959533937995610, -21.53943276465977519, 25.00109039468567218 ) ) ;
#163393=CARTESIAN_POINT ( 'NONE',  ( -12.06949235617756955, 12.14591786802309770, 80.62390960531438111 ) ) ;
#163394=CARTESIAN_POINT ( 'NONE',  ( 5.719274019375991003, -21.55341960407610458, 77.70724293864770971 ) ) ;
#163395=CARTESIAN_POINT ( 'NONE',  ( 13.97604488694527802, 13.89961937509977652, 69.37390960531436690 ) ) ;
#163396=CARTESIAN_POINT ( 'NONE',  ( -5.153800228976328057, -19.02544592524343514, 77.29057627198099567 ) ) ;
#163397=CARTESIAN_POINT ( 'NONE',  ( 21.53943276465977519, -0.05219959533907433946, 113.7489096053143527 ) ) ;
#163399=CARTESIAN_POINT ( 'NONE',  ( 19.05341960407611168, 5.049401038298154454, 78.95724293864769550 ) ) ;
#163402=CARTESIAN_POINT ( 'NONE',  ( 14.29746914071049879, -8.314922557960816363, 103.3322429386476955 ) ) ;
#163404=CARTESIAN_POINT ( 'NONE',  ( 5.049401038298161559, -19.05341960407611168, 62.70724293864769550 ) ) ;
#163405=CARTESIAN_POINT ( 'NONE',  ( -19.03943276465977164, -0.05219959533935918106, 98.75109039468567573 ) ) ;
#163406=CARTESIAN_POINT ( 'NONE',  ( 0.05219959533910956823, 16.53943276465976808, 99.99890960531436690 ) ) ;
#163407=CARTESIAN_POINT ( 'NONE',  ( 21.55341960407619695, -5.719274019375665929, 66.04275706135236135 ) ) ;
#163408=CARTESIAN_POINT ( 'NONE',  ( 9.474510206698971260, -16.51473224551069308, 52.91557627198102409 ) ) ;
#163409=CARTESIAN_POINT ( 'NONE',  ( -10.72451020669898014, 18.67979575497178502, 115.4155762719810241 ) ) ;
#163410=CARTESIAN_POINT ( 'NONE',  ( -21.55341960407610458, -5.719274019375992779, 106.4572429386477097 ) ) ;
#163412=CARTESIAN_POINT ( 'NONE',  ( 19.02544592524343514, -5.153800228976328945, 73.54057627198103830 ) ) ;
#163413=CARTESIAN_POINT ( 'NONE',  ( 17.26172910966780094, 6.454744622555824485, 111.6935309135077290 ) ) ;
#163414=CARTESIAN_POINT ( 'NONE',  ( 9.474510206698729675, 16.51473224551082808, 102.0844237280190043 ) ) ;
#163415=CARTESIAN_POINT ( 'NONE',  ( 21.52544592524344225, -5.823673210054117533, 33.54057627198102409 ) ) ;
#163416=CARTESIAN_POINT ( 'NONE',  ( 15.72974639402176855, 15.80617190586768217, 46.87609039468568994 ) ) ;
#163417=CARTESIAN_POINT ( 'NONE',  ( -5.153800228976328057, -19.02544592524343514, 97.29057627198099567 ) ) ;
#163418=CARTESIAN_POINT ( 'NONE',  ( -19.03943276465977164, -0.05219959533935918106, 88.75109039468567573 ) ) ;
#163419=CARTESIAN_POINT ( 'NONE',  ( 13.97604488694527802, 13.89961937509977652, 44.37390960531435269 ) ) ;
#163420=CARTESIAN_POINT ( 'NONE',  ( -5.153800228976328057, -19.02544592524343514, 72.29057627198102409 ) ) ;
#163421=CARTESIAN_POINT ( 'NONE',  ( 12.14591786802309770, 12.06949235617756955, 84.37390960531438111 ) ) ;
#163422=CARTESIAN_POINT ( 'NONE',  ( -16.51473224551069308, -9.474510206698971260, 106.6655762719810383 ) ) ;
#163423=CARTESIAN_POINT ( 'NONE',  ( 4.379528057220339221, -16.55341960407611168, 92.70724293864770971 ) ) ;
#163424=CARTESIAN_POINT ( 'NONE',  ( 19.02544592524343514, -5.153800228976328945, 98.54057627198100988 ) ) ;
#163425=CARTESIAN_POINT ( 'NONE',  ( -4.483927247898539470, -16.52544592524342804, 37.29057627198102409 ) ) ;
#163426=CARTESIAN_POINT ( 'NONE',  ( 19.05341960407611168, 5.049401038298154454, 23.95724293864769194 ) ) ;
#163428=CARTESIAN_POINT ( 'NONE',  ( 21.53943276465977519, 0.05219959533937863772, 56.25109039468568284 ) ) ;
#163429=CARTESIAN_POINT ( 'NONE',  ( -19.05341960407617563, 5.049401038297882671, 73.54275706135233293 ) ) ;
#163430=CARTESIAN_POINT ( 'NONE',  ( 8.224510206698953496, -14.34966873604960469, 42.91557627198103120 ) ) ;
#163431=CARTESIAN_POINT ( 'NONE',  ( -10.72451020669898014, 18.67979575497178502, 105.4155762719810383 ) ) ;
#163432=CARTESIAN_POINT ( 'NONE',  ( 21.52544592524344225, -5.823673210054117533, 38.54057627198103120 ) ) ;
#163434=CARTESIAN_POINT ( 'NONE',  ( 0.05219959533910956823, 16.53943276465976808, 84.99890960531436690 ) ) ;
#163435=CARTESIAN_POINT ( 'NONE',  ( 16.51473224551069308, 9.474510206698969483, 54.16557627198103120 ) ) ;
#163436=CARTESIAN_POINT ( 'NONE',  ( 14.34966873604960469, 8.224510206698951720, 24.16557627198103120 ) ) ;
#163437=CARTESIAN_POINT ( 'NONE',  ( -8.224510206698735004, -14.34966873604973081, 104.5844237280190185 ) ) ;
#163438=CARTESIAN_POINT ( 'NONE',  ( -12.14591786802326823, 12.06949235617739902, 68.12609039468567573 ) ) ;
#163439=CARTESIAN_POINT ( 'NONE',  ( 13.89961937509957401, 13.97604488694547697, 26.87609039468566507 ) ) ;
#163440=CARTESIAN_POINT ( 'NONE',  ( -9.564922557960796823, -16.46253265017161027, 102.0822429386477097 ) ) ;
#163441=CARTESIAN_POINT ( 'NONE',  ( 5.049401038298161559, -19.05341960407611168, 82.70724293864770971 ) ) ;
#163442=CARTESIAN_POINT ( 'NONE',  ( -5.049401038298153566, 19.05341960407611168, 40.20724293864768839 ) ) ;
#163443=CARTESIAN_POINT ( 'NONE',  ( -4.483927247898539470, -16.52544592524342804, 42.29057627198103120 ) ) ;
#163445=CARTESIAN_POINT ( 'NONE',  ( 9.564922557960805705, 16.46253265017160317, 99.58224293864770971 ) ) ;
#163446=CARTESIAN_POINT ( 'NONE',  ( -21.53943276465977519, 0.05219959533907696930, 41.24890960531435269 ) ) ;
#163447=CARTESIAN_POINT ( 'NONE',  ( -4.483927247898539470, -16.52544592524342804, 67.29057627198103830 ) ) ;
#163448=CARTESIAN_POINT ( 'NONE',  ( 8.314922557961029526, -14.29746914071037800, 20.41775706135234714 ) ) ;
#163449=CARTESIAN_POINT ( 'NONE',  ( 0.05219959533910956823, 16.53943276465976808, 59.99890960531436690 ) ) ;
#163450=CARTESIAN_POINT ( 'NONE',  ( 17.50000000000000355, -5.068104630630418050, 33.22818405340032655 ) ) ;
#163451=CARTESIAN_POINT ( 'NONE',  ( -19.03943276465977164, -0.05219959533935918106, 63.75109039468566863 ) ) ;
#163452=CARTESIAN_POINT ( 'NONE',  ( -13.89961937509977652, 13.97604488694528158, 100.6239096053143669 ) ) ;
#163453=CARTESIAN_POINT ( 'NONE',  ( 9.564922557961047289, -16.46253265017146816, 85.41775706135233293 ) ) ;
#163455=CARTESIAN_POINT ( 'NONE',  ( -0.05219959533934338120, 16.53943276465976808, 22.50109039468567573 ) ) ;
#163456=CARTESIAN_POINT ( 'NONE',  ( -16.52544592524335698, -4.483927247898792601, 98.95942372801903275 ) ) ;
#163457=CARTESIAN_POINT ( 'NONE',  ( -16.46253265017160317, 9.564922557960807481, 45.83224293864769550 ) ) ;
#163458=CARTESIAN_POINT ( 'NONE',  ( 21.52544592524344225, -5.823673210054117533, 38.54057627198103120 ) ) ;
#163459=CARTESIAN_POINT ( 'NONE',  ( 15.72974639402176855, 15.80617190586768217, 51.87609039468568284 ) ) ;
#163461=CARTESIAN_POINT ( 'NONE',  ( 4.483927247898790824, -16.52544592524335698, 20.20942372801900788 ) ) ;
#163463=CARTESIAN_POINT ( 'NONE',  ( 19.03943276465977164, -0.05219959533909143690, 68.74890960531436690 ) ) ;
#163465=CARTESIAN_POINT ( 'NONE',  ( 0.05219959533909260263, 19.03943276465977164, 114.9989096053143669 ) ) ;
#163466=CARTESIAN_POINT ( 'NONE',  ( 16.53943276465976808, -0.05219959533910856209, 93.74890960531436690 ) ) ;
#163467=CARTESIAN_POINT ( 'NONE',  ( 19.02544592524343514, -5.153800228976328945, 78.54057627198099567 ) ) ;
#163468=CARTESIAN_POINT ( 'NONE',  ( 19.03943276465977164, -0.05219959533909143690, 88.74890960531436690 ) ) ;
#163469=ORIENTED_EDGE ( 'NONE', *, *, #23111, .F. ) ;
#163470=CARTESIAN_POINT ( 'NONE',  ( -5.153800228976607833, 19.02544592524334988, 92.70942372801901854 ) ) ;
#163471=CARTESIAN_POINT ( 'NONE',  ( -15.72974639402197994, 15.80617190586746368, 65.62390960531436690 ) ) ;
#163472=CARTESIAN_POINT ( 'NONE',  ( 9.564922557960805705, 16.46253265017160317, 24.58224293864769194 ) ) ;
#163473=CARTESIAN_POINT ( 'NONE',  ( 19.05341960407617918, -5.049401038297876454, 51.04275706135231871 ) ) ;
#163474=CARTESIAN_POINT ( 'NONE',  ( 13.89961937509977652, -13.97604488694527269, 63.12390960531435979 ) ) ;
#163475=CARTESIAN_POINT ( 'NONE',  ( -19.03943276465977164, 0.05219959533909376836, 91.24890960531436690 ) ) ;
#163477=CARTESIAN_POINT ( 'NONE',  ( 10.72451020669898902, -18.67979575497178502, 92.91557627198103830 ) ) ;
#163478=CARTESIAN_POINT ( 'NONE',  ( -14.34966873604960291, -8.224510206698953496, 91.66557627198103830 ) ) ;
#163479=CARTESIAN_POINT ( 'NONE',  ( 9.564922557961047289, -16.46253265017146816, 60.41775706135233293 ) ) ;
#163480=CARTESIAN_POINT ( 'NONE',  ( -21.52544592524343514, 5.823673210054127303, 96.04057627198102409 ) ) ;
#163481=CARTESIAN_POINT ( 'NONE',  ( -18.67979575497178146, -10.72451020669898902, 76.66557627198103830 ) ) ;
#163482=CARTESIAN_POINT ( 'NONE',  ( -8.314922557960811034, -14.29746914071050412, 27.08224293864769550 ) ) ;
#163483=CARTESIAN_POINT ( 'NONE',  ( -5.823673210054431948, 21.52544592524334988, 102.7094237280190185 ) ) ;
#163484=CARTESIAN_POINT ( 'NONE',  ( -16.55341960407617563, 4.379528057220093196, 58.54275706135235424 ) ) ;
#163485=CARTESIAN_POINT ( 'NONE',  ( 5.049401038298161559, -19.05341960407611168, 82.70724293864770971 ) ) ;
#163486=CARTESIAN_POINT ( 'NONE',  ( -13.89961937509977652, 13.97604488694528158, 30.62390960531435269 ) ) ;
#163487=CARTESIAN_POINT ( 'NONE',  ( -21.55341960407619339, 5.719274019375674811, 38.54275706135234714 ) ) ;
#163488=CARTESIAN_POINT ( 'NONE',  ( 21.55341960407619695, -5.719274019375665929, 56.04275706135235424 ) ) ;
#163489=CARTESIAN_POINT ( 'NONE',  ( 5.153800228976335163, 19.02544592524342804, 49.79057627198100988 ) ) ;
#163490=CARTESIAN_POINT ( 'NONE',  ( -21.53943276465977519, -0.05219959533937600094, 23.75109039468567929 ) ) ;
#163491=CARTESIAN_POINT ( 'NONE',  ( 5.153800228976615827, -19.02544592524334988, 55.20942372801899722 ) ) ;
#163492=EDGE_CURVE ( 'NONE', #135352, #194071, #111290, .T. ) ;
#163493=CARTESIAN_POINT ( 'NONE',  ( 13.89961937509957401, 13.97604488694547697, 76.87609039468566152 ) ) ;
#163494=CARTESIAN_POINT ( 'NONE',  ( 0.05219959533934541429, -16.53943276465976808, 35.00109039468568284 ) ) ;
#163496=CARTESIAN_POINT ( 'NONE',  ( -4.483927247898782831, 16.52544592524335698, 67.70942372801901854 ) ) ;
#163497=CARTESIAN_POINT ( 'NONE',  ( -9.564922557960796823, -16.46253265017161027, 42.08224293864769550 ) ) ;
#163499=CARTESIAN_POINT ( 'NONE',  ( 16.46253265017160672, -9.564922557960803928, 103.3322429386476955 ) ) ;
#163500=CARTESIAN_POINT ( 'NONE',  ( -19.05341960407611168, -5.049401038298163336, 26.45724293864769550 ) ) ;
#163501=CARTESIAN_POINT ( 'NONE',  ( -21.55341960407610458, -5.719274019375992779, 66.45724293864768129 ) ) ;
#163502=CARTESIAN_POINT ( 'NONE',  ( -4.483927247898782831, 16.52544592524335698, 57.70942372801901143 ) ) ;
#163503=CARTESIAN_POINT ( 'NONE',  ( 21.52544592524334988, 5.823673210054432836, 111.4594237280190328 ) ) ;
#163504=CARTESIAN_POINT ( 'NONE',  ( -5.049401038298153566, 19.05341960407611168, 45.20724293864769550 ) ) ;
#163505=CARTESIAN_POINT ( 'NONE',  ( -16.52544592524342804, 4.483927247898546575, 31.04057627198102409 ) ) ;
#163506=CARTESIAN_POINT ( 'NONE',  ( 12.06949235617757843, -12.14591786802309237, 73.12390960531436690 ) ) ;
#163507=CARTESIAN_POINT ( 'NONE',  ( 19.02544592524343514, -5.153800228976328945, 83.54057627198100988 ) ) ;
#163508=CARTESIAN_POINT ( 'NONE',  ( -5.823673210054431948, 21.52544592524334988, 42.70942372801901854 ) ) ;
#163509=CARTESIAN_POINT ( 'NONE',  ( 16.51473224551069308, 9.474510206698969483, 84.16557627198102409 ) ) ;
#163510=CARTESIAN_POINT ( 'NONE',  ( -10.81492255796105439, 18.62759615963255655, 82.91775706135234714 ) ) ;
#163511=CARTESIAN_POINT ( 'NONE',  ( -8.314922557961024197, 14.29746914071037800, 62.91775706135236135 ) ) ;
#163512=CARTESIAN_POINT ( 'NONE',  ( -19.05341960407611168, -5.049401038298163336, 106.4572429386476955 ) ) ;
#163513=CARTESIAN_POINT ( 'NONE',  ( -16.53943276465976808, 0.05219959533911058130, 46.24890960531435979 ) ) ;
#163514=CARTESIAN_POINT ( 'NONE',  ( -9.564922557960796823, -16.46253265017161027, 22.08224293864768839 ) ) ;
#163515=CARTESIAN_POINT ( 'NONE',  ( 8.224510206698742110, 14.34966873604972548, 52.08442372801901854 ) ) ;
#163516=CARTESIAN_POINT ( 'NONE',  ( -16.55341960407611168, -4.379528057220339221, 51.45724293864770260 ) ) ;
#163517=CARTESIAN_POINT ( 'NONE',  ( -0.05219959533909027116, -19.03943276465977164, 107.4989096053143527 ) ) ;
#163518=CARTESIAN_POINT ( 'NONE',  ( -21.55341960407610458, -5.719274019375992779, 31.45724293864769550 ) ) ;
#163519=CARTESIAN_POINT ( 'NONE',  ( -18.67979575497193778, 10.72451020669871902, 108.3344237280190185 ) ) ;
#163520=CARTESIAN_POINT ( 'NONE',  ( -12.14591786802309592, -12.06949235617757132, 101.8739096053143811 ) ) ;
#163521=CARTESIAN_POINT ( 'NONE',  ( -9.564922557960796823, -16.46253265017161027, 92.08224293864769550 ) ) ;
#163522=VERTEX_POINT ( 'NONE', #192131 ) ;
#163523=CARTESIAN_POINT ( 'NONE',  ( -16.55341960407617563, 4.379528057220093196, 48.54275706135234714 ) ) ;
#163524=CARTESIAN_POINT ( 'NONE',  ( 5.049401038298161559, -19.05341960407611168, 52.70724293864767418 ) ) ;
#163525=CARTESIAN_POINT ( 'NONE',  ( -9.564922557961040184, 16.46253265017147172, 47.91775706135233293 ) ) ;
#163526=CARTESIAN_POINT ( 'NONE',  ( 16.55341960407618274, -4.379528057220086978, 91.04275706135236135 ) ) ;
#163527=CARTESIAN_POINT ( 'NONE',  ( 16.51473224551083163, -9.474510206698727899, 100.8344237280190043 ) ) ;
#163528=CARTESIAN_POINT ( 'NONE',  ( -18.62759615963255300, -10.81492255796106328, 64.16775706135234714 ) ) ;
#163529=CARTESIAN_POINT ( 'NONE',  ( -19.03943276465977164, 0.05219959533909376836, 81.24890960531436690 ) ) ;
#163530=CARTESIAN_POINT ( 'NONE',  ( 21.53943276465977519, -0.05219959533907433946, 93.74890960531436690 ) ) ;
#163531=CARTESIAN_POINT ( 'NONE',  ( 4.379528057220339221, -16.55341960407611168, 107.7072429386476955 ) ) ;
#163533=CARTESIAN_POINT ( 'NONE',  ( 16.46253265017146816, 9.564922557961045513, 86.66775706135233293 ) ) ;
#163534=CARTESIAN_POINT ( 'NONE',  ( 21.53943276465977519, -0.05219959533907433946, 78.74890960531436690 ) ) ;
#163535=CARTESIAN_POINT ( 'NONE',  ( 16.46253265017146816, 9.564922557961045513, 36.66775706135233293 ) ) ;
#163536=FACE_BOUND ( 'NONE', #105166, .T. ) ;
#163537=CARTESIAN_POINT ( 'NONE',  ( -21.52544592524343514, 5.823673210054127303, 96.04057627198102409 ) ) ;
#163539=CARTESIAN_POINT ( 'NONE',  ( 19.02544592524343514, -5.153800228976328945, 63.54057627198103830 ) ) ;
#163541=CARTESIAN_POINT ( 'NONE',  ( 14.29746914071037800, 8.314922557961029526, 21.66775706135235069 ) ) ;
#163542=CARTESIAN_POINT ( 'NONE',  ( -18.22780087662122028, 5.500000000000031086, 58.51540105326107977 ) ) ;
#163543=CARTESIAN_POINT ( 'NONE',  ( 0.05219959533909260263, 19.03943276465977164, 49.99890960531435979 ) ) ;
#163544=CARTESIAN_POINT ( 'NONE',  ( 9.564922557960805705, 16.46253265017160317, 114.5822429386476955 ) ) ;
#163545=CARTESIAN_POINT ( 'NONE',  ( -21.53943276465977519, 0.05219959533907696930, 101.2489096053143669 ) ) ;
#163546=CARTESIAN_POINT ( 'NONE',  ( 0.05219959533910956823, 16.53943276465976808, 49.99890960531437401 ) ) ;
#163547=CARTESIAN_POINT ( 'NONE',  ( -18.62759615963255300, -10.81492255796106328, 79.16775706135234714 ) ) ;
#163548=CARTESIAN_POINT ( 'NONE',  ( 12.14591786802327356, -12.06949235617739191, 20.62609039468568639 ) ) ;
#163549=CARTESIAN_POINT ( 'NONE',  ( -9.564922557961040184, 16.46253265017147172, 32.91775706135233293 ) ) ;
#163550=CARTESIAN_POINT ( 'NONE',  ( -12.14591786802309592, -12.06949235617757132, 36.87390960531435979 ) ) ;
#163551=CARTESIAN_POINT ( 'NONE',  ( 5.823673210054125526, 21.52544592524343514, 114.7905762719810383 ) ) ;
#163552=CARTESIAN_POINT ( 'NONE',  ( -16.52544592524342804, 4.483927247898546575, 46.04057627198103830 ) ) ;
#163553=CARTESIAN_POINT ( 'NONE',  ( 13.89961937509957401, 13.97604488694547697, 96.87609039468566152 ) ) ;
#163554=CARTESIAN_POINT ( 'NONE',  ( 19.05341960407617918, -5.049401038297876454, 66.04275706135233293 ) ) ;
#163555=CARTESIAN_POINT ( 'NONE',  ( 0.05219959533937995610, -21.53943276465977519, 65.00109039468568994 ) ) ;
#163556=CARTESIAN_POINT ( 'NONE',  ( 19.03943276465977164, 0.05219959533936151252, 51.25109039468567573 ) ) ;
#163557=CARTESIAN_POINT ( 'NONE',  ( 14.29746914071049879, -8.314922557960816363, 113.3322429386476955 ) ) ;
#163558=CARTESIAN_POINT ( 'NONE',  ( 15.80617190586746368, 15.72974639402197994, 39.37390960531436690 ) ) ;
#163559=CARTESIAN_POINT ( 'NONE',  ( -12.06949235617756955, 12.14591786802309770, 50.62390960531435979 ) ) ;
#163560=CARTESIAN_POINT ( 'NONE',  ( -18.56197773271729901, 5.499999999999997335, 93.55066217314454491 ) ) ;
#163561=CARTESIAN_POINT ( 'NONE',  ( -0.05219959533936034679, 19.03943276465977164, 22.50109039468566152 ) ) ;
#163562=CARTESIAN_POINT ( 'NONE',  ( -14.29746914071037622, -8.314922557961029526, 79.16775706135234714 ) ) ;
#163563=CARTESIAN_POINT ( 'NONE',  ( -12.14591786802309592, -12.06949235617757132, 41.87390960531435979 ) ) ;
#163564=CARTESIAN_POINT ( 'NONE',  ( 5.823673210054444382, -21.52544592524334988, 80.20942372801901854 ) ) ;
#163565=CARTESIAN_POINT ( 'NONE',  ( -5.719274019375665041, -21.55341960407619695, 69.79275706135234714 ) ) ;
#163566=CARTESIAN_POINT ( 'NONE',  ( -5.719274019375978568, 21.55341960407610458, 80.20724293864769550 ) ) ;
#163567=CARTESIAN_POINT ( 'NONE',  ( 16.46253265017160672, -9.564922557960803928, 43.33224293864769550 ) ) ;
#163568=CARTESIAN_POINT ( 'NONE',  ( -15.72974639402176322, -15.80617190586768395, 54.37609039468568994 ) ) ;
#163569=CARTESIAN_POINT ( 'NONE',  ( 19.02544592524343514, -5.153800228976328945, 33.54057627198102409 ) ) ;
#163570=CARTESIAN_POINT ( 'NONE',  ( 13.89961937509977652, -13.97604488694527269, 48.12390960531435979 ) ) ;
#163571=CARTESIAN_POINT ( 'NONE',  ( -12.14591786802309592, -12.06949235617757132, 91.87390960531436690 ) ) ;
#163572=CARTESIAN_POINT ( 'NONE',  ( 19.02544592524343514, -5.153800228976328945, 93.54057627198102409 ) ) ;
#163573=CARTESIAN_POINT ( 'NONE',  ( -16.55341960407611168, -4.379528057220339221, 36.45724293864768839 ) ) ;
#163574=CARTESIAN_POINT ( 'NONE',  ( -16.52544592524342804, 4.483927247898546575, 101.0405762719810383 ) ) ;
#163575=CARTESIAN_POINT ( 'NONE',  ( 18.62759615963271287, -10.81492255796078972, 68.33224293864769550 ) ) ;
#163576=CARTESIAN_POINT ( 'NONE',  ( -10.72451020669870658, -18.67979575497194134, 19.58442372801901143 ) ) ;
#163577=CARTESIAN_POINT ( 'NONE',  ( -19.02544592524342804, 5.153800228976336051, 116.0405762719810383 ) ) ;
#163578=CARTESIAN_POINT ( 'NONE',  ( -19.02544592524342804, 5.153800228976336051, 76.04057627198102409 ) ) ;
#163579=CARTESIAN_POINT ( 'NONE',  ( -4.379528057220086978, -16.55341960407618274, 29.79275706135234358 ) ) ;
#163580=CARTESIAN_POINT ( 'NONE',  ( -21.52544592524343514, 5.823673210054127303, 66.04057627198103830 ) ) ;
#163581=CARTESIAN_POINT ( 'NONE',  ( -21.53943276465977519, -0.05219959533937600094, 98.75109039468568994 ) ) ;
#163582=CARTESIAN_POINT ( 'NONE',  ( -5.049401038298153566, 19.05341960407611168, 75.20724293864769550 ) ) ;
#163583=CARTESIAN_POINT ( 'NONE',  ( 18.67979575497194134, -10.72451020669871369, 30.83442372801902209 ) ) ;
#163584=CARTESIAN_POINT ( 'NONE',  ( 5.153800228976335163, 19.02544592524342804, 114.7905762719810241 ) ) ;
#163585=CARTESIAN_POINT ( 'NONE',  ( 12.14591786802327356, -12.06949235617739191, 95.62609039468568994 ) ) ;
#163586=CARTESIAN_POINT ( 'NONE',  ( -0.05219959533937732626, 21.53943276465977519, 77.50109039468567573 ) ) ;
#163587=CARTESIAN_POINT ( 'NONE',  ( -10.72451020669870658, -18.67979575497194134, 94.58442372801901854 ) ) ;
#163588=CARTESIAN_POINT ( 'NONE',  ( -8.314922557961024197, 14.29746914071037800, 57.91775706135234714 ) ) ;
#163589=CARTESIAN_POINT ( 'NONE',  ( -21.52544592524334988, -5.823673210054445271, 23.95942372801901143 ) ) ;
#163590=CARTESIAN_POINT ( 'NONE',  ( 19.03943276465977164, -0.05219959533909143690, 113.7489096053143669 ) ) ;
#163591=CARTESIAN_POINT ( 'NONE',  ( 18.62759615963255655, 10.81492255796105972, 91.66775706135234714 ) ) ;
#163592=CARTESIAN_POINT ( 'NONE',  ( -9.564922557960796823, -16.46253265017161027, 87.08224293864769550 ) ) ;
#163593=CARTESIAN_POINT ( 'NONE',  ( 21.52544592524344225, -5.823673210054117533, 83.54057627198102409 ) ) ;
#163594=CARTESIAN_POINT ( 'NONE',  ( -13.89961937509957401, -13.97604488694547875, 59.37609039468566863 ) ) ;
#163596=CARTESIAN_POINT ( 'NONE',  ( -5.823673210054116645, -21.52544592524344225, 57.29057627198103120 ) ) ;
#163597=CARTESIAN_POINT ( 'NONE',  ( 16.51473224551069308, 9.474510206698969483, 89.16557627198103830 ) ) ;
#163598=CARTESIAN_POINT ( 'NONE',  ( 4.483927247898545687, 16.52544592524342804, 39.79057627198103830 ) ) ;
#163600=CARTESIAN_POINT ( 'NONE',  ( -9.564922557961040184, 16.46253265017147172, 72.91775706135233293 ) ) ;
#163601=CARTESIAN_POINT ( 'NONE',  ( -17.26058549869090797, 6.457015423128532383, 103.6225416252393643 ) ) ;
#163602=CARTESIAN_POINT ( 'NONE',  ( -4.379528057220086978, -16.55341960407618274, 19.79275706135235069 ) ) ;
#163603=CARTESIAN_POINT ( 'NONE',  ( 21.53943276465977519, -0.05219959533907433946, 88.74890960531436690 ) ) ;
#163604=CARTESIAN_POINT ( 'NONE',  ( 12.14591786802309770, 12.06949235617756955, 64.37390960531435269 ) ) ;
#163605=CARTESIAN_POINT ( 'NONE',  ( -19.03943276465977164, 0.05219959533909376836, 106.2489096053143669 ) ) ;
#163606=CARTESIAN_POINT ( 'NONE',  ( 0.05219959533934541429, -16.53943276465976808, 35.00109039468568284 ) ) ;
#163607=CARTESIAN_POINT ( 'NONE',  ( 9.474510206698971260, -16.51473224551069308, 57.91557627198103120 ) ) ;
#163608=CARTESIAN_POINT ( 'NONE',  ( -18.62759615963255300, -10.81492255796106328, 19.16775706135234714 ) ) ;
#163609=CARTESIAN_POINT ( 'NONE',  ( 16.51473224551083163, -9.474510206698727899, 90.83442372801900433 ) ) ;
#163610=CARTESIAN_POINT ( 'NONE',  ( 16.51473224551069308, 9.474510206698969483, 89.16557627198103830 ) ) ;
#163611=CARTESIAN_POINT ( 'NONE',  ( 5.153800228976335163, 19.02544592524342804, 79.79057627198102409 ) ) ;
#163612=CARTESIAN_POINT ( 'NONE',  ( 21.52544592524344225, -5.823673210054117533, 78.54057627198103830 ) ) ;
#163613=CARTESIAN_POINT ( 'NONE',  ( -5.153800228976328057, -19.02544592524343514, 52.29057627198100988 ) ) ;
#163615=CARTESIAN_POINT ( 'NONE',  ( -12.06949235617756955, 12.14591786802309770, 50.62390960531435979 ) ) ;
#163616=CARTESIAN_POINT ( 'NONE',  ( -19.02544592524342804, 5.153800228976336051, 106.0405762719810241 ) ) ;
#163617=CARTESIAN_POINT ( 'NONE',  ( -18.22780087662119541, 5.500000000000102141, 41.01763182126894236 ) ) ;
#163618=CARTESIAN_POINT ( 'NONE',  ( -9.474510206698720793, -16.51473224551083518, 69.58442372801901854 ) ) ;
#163619=CARTESIAN_POINT ( 'NONE',  ( 10.72451020669898902, -18.67979575497178502, 72.91557627198103830 ) ) ;
#163620=CARTESIAN_POINT ( 'NONE',  ( 19.05341960407617918, -5.049401038297876454, 51.04275706135231871 ) ) ;
#163621=CARTESIAN_POINT ( 'NONE',  ( 5.153800228976335163, 19.02544592524342804, 104.7905762719809957 ) ) ;
#163622=CARTESIAN_POINT ( 'NONE',  ( -17.49999999999999645, 4.640572885337594933, 115.6378816454884486 ) ) ;
#163623=CARTESIAN_POINT ( 'NONE',  ( 21.53943276465977519, -0.05219959533907433946, 38.74890960531435979 ) ) ;
#163624=CARTESIAN_POINT ( 'NONE',  ( -19.03943276465977164, 0.05219959533909376836, 71.24890960531435269 ) ) ;
#163625=CARTESIAN_POINT ( 'NONE',  ( 10.81492255796106328, -18.62759615963255655, 65.41775706135234714 ) ) ;
#163626=CARTESIAN_POINT ( 'NONE',  ( 16.51473224551069308, 9.474510206698969483, 34.16557627198102409 ) ) ;
#163627=CARTESIAN_POINT ( 'NONE',  ( 12.06949235617757843, -12.14591786802309237, 73.12390960531436690 ) ) ;
#163629=CARTESIAN_POINT ( 'NONE',  ( 18.67979575497194134, -10.72451020669871369, 55.83442372801901854 ) ) ;
#163630=ORIENTED_EDGE ( 'NONE', *, *, #158665, .T. ) ;
#163631=CARTESIAN_POINT ( 'NONE',  ( 19.03943276465977164, -0.05219959533909143690, 108.7489096053143527 ) ) ;
#163632=CARTESIAN_POINT ( 'NONE',  ( -5.153800228976607833, 19.02544592524334988, 62.70942372801899722 ) ) ;
#163633=EDGE_CURVE ( 'NONE', #50923, #192458, #179033, .T. ) ;
#163635=CARTESIAN_POINT ( 'NONE',  ( 5.823673210054125526, 21.52544592524343514, 114.7905762719810383 ) ) ;
#163636=CARTESIAN_POINT ( 'NONE',  ( 19.05341960407611168, 5.049401038298154454, 53.95724293864770260 ) ) ;
#163637=CARTESIAN_POINT ( 'NONE',  ( -16.53943276465976808, -0.05219959533934237506, 43.75109039468568284 ) ) ;
#163639=CARTESIAN_POINT ( 'NONE',  ( -19.02544592524334988, -5.153800228976617603, 23.95942372801900078 ) ) ;
#163640=CARTESIAN_POINT ( 'NONE',  ( -19.03943276465977164, 0.05219959533909376836, 46.24890960531435979 ) ) ;
#163641=CARTESIAN_POINT ( 'NONE',  ( 19.02544592524334988, 5.153800228976608722, 21.45942372801899012 ) ) ;
#163642=CARTESIAN_POINT ( 'NONE',  ( -8.224510206698735004, -14.34966873604973081, 94.58442372801901854 ) ) ;
#163643=CARTESIAN_POINT ( 'NONE',  ( -19.03943276465977164, 0.05219959533909376836, 91.24890960531436690 ) ) ;
#163644=CARTESIAN_POINT ( 'NONE',  ( 15.80617190586769283, -15.72974639402175789, 55.62609039468568284 ) ) ;
#163646=CARTESIAN_POINT ( 'NONE',  ( 0.05219959533909260263, 19.03943276465977164, 109.9989096053143669 ) ) ;
#163647=CARTESIAN_POINT ( 'NONE',  ( -17.50000000000017764, 3.417042746626915317, 30.17380396232480066 ) ) ;
#163648=CARTESIAN_POINT ( 'NONE',  ( 0.05219959533934541429, -16.53943276465976808, 50.00109039468568994 ) ) ;
#163649=CARTESIAN_POINT ( 'NONE',  ( 18.62759615963255655, 10.81492255796105972, 76.66775706135234714 ) ) ;
#163650=CARTESIAN_POINT ( 'NONE',  ( 10.72451020669871369, 18.67979575497193778, 107.0844237280190043 ) ) ;
#163652=CARTESIAN_POINT ( 'NONE',  ( 14.29746914071037800, 8.314922557961029526, 31.66775706135234358 ) ) ;
#163653=CARTESIAN_POINT ( 'NONE',  ( -19.03943276465977164, 0.05219959533909376836, 81.24890960531436690 ) ) ;
#163654=CARTESIAN_POINT ( 'NONE',  ( 16.51473224551069308, 9.474510206698969483, 114.1655762719810241 ) ) ;
#163655=EDGE_LOOP ( 'NONE', ( #194739, #87840, #129341, #18476, #138150, #69076, #38830, #72270, #39547, #52898, #169475, #119699, #186860, #17420, #155496, #176360, #158675, #149919, #86238, #136602, #182040, #117699, #44604, #108910, #192216, #82532, #86285, #134610, #52095, #51727, #184322, #150004, #69070, #104319, #152646, #42658, #79018, #179042, #126519, #151394, #131169, #148117, #174107, #123126, #75353, #95796, #132119, #166389, #71110, #38129, #6243, #27504, #93975, #133116, #118016, #164629 ) ) ;
#163656=DIRECTION ( 'NONE',  ( 0.000000000000000000, 0.000000000000000000, 1.000000000000000000 ) ) ;
#163657=CARTESIAN_POINT ( 'NONE',  ( 13.89961937509977652, -13.97604488694527269, 28.12390960531435624 ) ) ;
#163658=CARTESIAN_POINT ( 'NONE',  ( 15.80617190586746368, 15.72974639402197994, 44.37390960531435979 ) ) ;
#163659=CARTESIAN_POINT ( 'NONE',  ( 8.224510206698742110, 14.34966873604972548, 107.0844237280190043 ) ) ;
#163660=CARTESIAN_POINT ( 'NONE',  ( 4.379528057220339221, -16.55341960407611168, 82.70724293864770971 ) ) ;
#163661=CARTESIAN_POINT ( 'NONE',  ( 16.46253265017160672, -9.564922557960803928, 73.33224293864769550 ) ) ;
#163662=CARTESIAN_POINT ( 'NONE',  ( 5.719274019375673035, 21.55341960407619339, 102.2927570613523613 ) ) ;
#163664=CARTESIAN_POINT ( 'NONE',  ( -4.379528057220086978, -16.55341960407618274, 19.79275706135235069 ) ) ;
#163665=CARTESIAN_POINT ( 'NONE',  ( 12.06949235617757843, -12.14591786802309237, 93.12390960531436690 ) ) ;
#163666=CARTESIAN_POINT ( 'NONE',  ( -15.72974639402176322, -15.80617190586768395, 44.37609039468567573 ) ) ;
#163667=CARTESIAN_POINT ( 'NONE',  ( 15.72974639402199770, -15.80617190586745480, 78.12390960531436690 ) ) ;
#163668=CARTESIAN_POINT ( 'NONE',  ( 13.97604488694548053, -13.89961937509957401, 55.62609039468566863 ) ) ;
#163669=CARTESIAN_POINT ( 'NONE',  ( 16.51473224551069308, 9.474510206698969483, 44.16557627198103120 ) ) ;
#163670=CARTESIAN_POINT ( 'NONE',  ( 5.153800228976335163, 19.02544592524342804, 94.79057627198103830 ) ) ;
#163671=CARTESIAN_POINT ( 'NONE',  ( 8.224510206698953496, -14.34966873604960469, 67.91557627198102409 ) ) ;
#163672=CARTESIAN_POINT ( 'NONE',  ( -16.52544592524342804, 4.483927247898546575, 51.04057627198103120 ) ) ;
#163673=CARTESIAN_POINT ( 'NONE',  ( 4.379528057220339221, -16.55341960407611168, 22.70724293864769194 ) ) ;
#163674=CARTESIAN_POINT ( 'NONE',  ( 16.46253265017146816, 9.564922557961045513, 71.66775706135233293 ) ) ;
#163675=CARTESIAN_POINT ( 'NONE',  ( -19.48894818550246200, 5.499999999999919176, 85.10307310435239003 ) ) ;
#163676=CARTESIAN_POINT ( 'NONE',  ( 5.719274019375991003, -21.55341960407610458, 22.70724293864769194 ) ) ;
#163677=CARTESIAN_POINT ( 'NONE',  ( 16.53943276465976808, -0.05219959533910856209, 83.74890960531435269 ) ) ;
#163679=CARTESIAN_POINT ( 'NONE',  ( 9.564922557960805705, 16.46253265017160317, 44.58224293864769550 ) ) ;
#163680=CARTESIAN_POINT ( 'NONE',  ( 18.67979575497178502, 10.72451020669898547, 54.16557627198103120 ) ) ;
#163681=CARTESIAN_POINT ( 'NONE',  ( -18.62759615963270932, 10.81492255796079327, 75.83224293864769550 ) ) ;
#163682=CARTESIAN_POINT ( 'NONE',  ( -14.34966873604960291, -8.224510206698953496, 111.6655762719810525 ) ) ;
#163683=CARTESIAN_POINT ( 'NONE',  ( 4.483927247898790824, -16.52544592524335698, 70.20942372801904696 ) ) ;
#163684=CARTESIAN_POINT ( 'NONE',  ( -9.474510206698964154, 16.51473224551069663, 60.41557627198102409 ) ) ;
#163685=CARTESIAN_POINT ( 'NONE',  ( 19.05341960407617918, -5.049401038297876454, 36.04275706135234003 ) ) ;
#163686=CARTESIAN_POINT ( 'NONE',  ( -5.823673210054431948, 21.52544592524334988, 52.70942372801902565 ) ) ;
#163688=CARTESIAN_POINT ( 'NONE',  ( 12.14591786802309770, 12.06949235617756955, 104.3739096053143669 ) ) ;
#163689=CARTESIAN_POINT ( 'NONE',  ( -19.05341960407617563, 5.049401038297882671, 93.54275706135234714 ) ) ;
#163692=CARTESIAN_POINT ( 'NONE',  ( -5.719274019375978568, 21.55341960407610458, 50.20724293864769550 ) ) ;
#163693=CARTESIAN_POINT ( 'NONE',  ( -16.51473224551069308, -9.474510206698971260, 21.66557627198102765 ) ) ;
#163694=CARTESIAN_POINT ( 'NONE',  ( 0.05219959533937995610, -21.53943276465977519, 90.00109039468567573 ) ) ;
#163695=CARTESIAN_POINT ( 'NONE',  ( -8.314922557960811034, -14.29746914071050412, 27.08224293864769550 ) ) ;
#163696=CARTESIAN_POINT ( 'NONE',  ( 16.53943276465976808, 0.05219959533934440121, 61.25109039468567573 ) ) ;
#163697=CARTESIAN_POINT ( 'NONE',  ( 14.34966873604960469, 8.224510206698951720, 59.16557627198103120 ) ) ;
#163698=B_SPLINE_CURVE_WITH_KNOTS ( 'NONE', 3,
 ( #17957, #79611, #20918, #37083, #173627, #129075 ),
 .UNSPECIFIED., .F., .F.,
 ( 4, 2, 4 ),
 ( 0.000000000000000000, 0.0003837532665553974615, 0.0007675065331107949231 ),
 .UNSPECIFIED. ) ;
#163699=CARTESIAN_POINT ( 'NONE',  ( -21.53943276465977519, 0.05219959533907696930, 76.24890960531435269 ) ) ;
#163700=CARTESIAN_POINT ( 'NONE',  ( -5.719274019375978568, 21.55341960407610458, 75.20724293864769550 ) ) ;
#163702=CARTESIAN_POINT ( 'NONE',  ( -13.89961937509957401, -13.97604488694547875, 79.37609039468567573 ) ) ;
#163703=CARTESIAN_POINT ( 'NONE',  ( -9.474510206698964154, 16.51473224551069663, 115.4155762719810241 ) ) ;
#163704=CARTESIAN_POINT ( 'NONE',  ( 19.03943276465977164, -0.05219959533909143690, 53.74890960531436690 ) ) ;
#163705=CARTESIAN_POINT ( 'NONE',  ( -9.564922557960796823, -16.46253265017161027, 27.08224293864769550 ) ) ;
#163708=CARTESIAN_POINT ( 'NONE',  ( 16.55341960407618274, -4.379528057220086978, 86.04275706135236135 ) ) ;
#163709=CARTESIAN_POINT ( 'NONE',  ( 0.05219959533907565091, 21.53943276465977519, 104.9989096053143669 ) ) ;
#163710=CARTESIAN_POINT ( 'NONE',  ( -16.51473224551069308, -9.474510206698971260, 71.66557627198102409 ) ) ;
#163711=CARTESIAN_POINT ( 'NONE',  ( 21.52544592524334988, 5.823673210054432836, 46.45942372801901854 ) ) ;
#163712=CARTESIAN_POINT ( 'NONE',  ( -13.89961937509977652, 13.97604488694528158, 90.62390960531432427 ) ) ;
#163715=VERTEX_POINT ( 'NONE', #135464 ) ;
#163716=CARTESIAN_POINT ( 'NONE',  ( 5.719274019375673035, 21.55341960407619339, 27.29275706135234358 ) ) ;
#163717=CARTESIAN_POINT ( 'NONE',  ( -13.89961937509977652, 13.97604488694528158, 25.62390960531434558 ) ) ;
#163718=CARTESIAN_POINT ( 'NONE',  ( 19.02544592524343514, -5.153800228976328945, 98.54057627198100988 ) ) ;
#163719=CARTESIAN_POINT ( 'NONE',  ( -16.51473224551082808, 9.474510206698731452, 43.33442372801900433 ) ) ;
#163720=CARTESIAN_POINT ( 'NONE',  ( -18.67979575497178146, -10.72451020669898902, 111.6655762719810525 ) ) ;
#163721=CARTESIAN_POINT ( 'NONE',  ( 0.05219959533936267826, -19.03943276465977164, 50.00109039468566863 ) ) ;
#163722=CARTESIAN_POINT ( 'NONE',  ( 0.05219959533936267826, -19.03943276465977164, 50.00109039468566863 ) ) ;
#163723=CARTESIAN_POINT ( 'NONE',  ( -4.379528057220086978, -16.55341960407618274, 99.79275706135234714 ) ) ;
#163726=CARTESIAN_POINT ( 'NONE',  ( -19.05341960407611168, -5.049401038298163336, 76.45724293864769550 ) ) ;
#163728=CARTESIAN_POINT ( 'NONE',  ( -21.53943276465977519, -0.05219959533937600094, 83.75109039468568994 ) ) ;
#163729=CARTESIAN_POINT ( 'NONE',  ( -5.823673210054431948, 21.52544592524334988, 97.70942372801904696 ) ) ;
#163731=CARTESIAN_POINT ( 'NONE',  ( -0.05219959533909027116, -19.03943276465977164, 92.49890960531436690 ) ) ;
#163732=CARTESIAN_POINT ( 'NONE',  ( -15.80617190586768217, 15.72974639402176855, 58.12609039468568994 ) ) ;
#163733=CARTESIAN_POINT ( 'NONE',  ( 8.224510206698742110, 14.34966873604972548, 22.08442372801901143 ) ) ;
#163734=EDGE_CURVE ( 'NONE', #199255, #14026, #69855, .T. ) ;
#163735=CARTESIAN_POINT ( 'NONE',  ( 19.02544592524343514, -5.153800228976328945, 63.54057627198103830 ) ) ;
#163736=CARTESIAN_POINT ( 'NONE',  ( 13.89961937509977652, -13.97604488694527269, 113.1239096053143527 ) ) ;
#163737=CARTESIAN_POINT ( 'NONE',  ( -9.564922557960796823, -16.46253265017161027, 87.08224293864769550 ) ) ;
#163739=CARTESIAN_POINT ( 'NONE',  ( -5.049401038298153566, 19.05341960407611168, 65.20724293864765286 ) ) ;
#163740=CARTESIAN_POINT ( 'NONE',  ( 19.05341960407611168, 5.049401038298154454, 53.95724293864770260 ) ) ;
#163741=CARTESIAN_POINT ( 'NONE',  ( -5.719274019375978568, 21.55341960407610458, 110.2072429386477239 ) ) ;
#163742=CARTESIAN_POINT ( 'NONE',  ( 14.34966873604972726, -8.224510206698740333, 105.8344237280190328 ) ) ;
#163744=CARTESIAN_POINT ( 'NONE',  ( 16.46253265017146816, 9.564922557961045513, 61.66775706135234003 ) ) ;
#163745=CARTESIAN_POINT ( 'NONE',  ( -16.51473224551069308, -9.474510206698971260, 91.66557627198103830 ) ) ;
#163746=CARTESIAN_POINT ( 'NONE',  ( -12.14591786802309592, -12.06949235617757132, 76.87390960531439532 ) ) ;
#163747=CARTESIAN_POINT ( 'NONE',  ( 4.379528057220339221, -16.55341960407611168, 102.7072429386476955 ) ) ;
#163748=CARTESIAN_POINT ( 'NONE',  ( -15.72974639402197994, 15.80617190586746368, 30.62390960531436335 ) ) ;
#163749=CARTESIAN_POINT ( 'NONE',  ( 5.153800228976335163, 19.02544592524342804, 114.7905762719810241 ) ) ;
#163750=CARTESIAN_POINT ( 'NONE',  ( -14.34966873604960291, -8.224510206698953496, 91.66557627198103830 ) ) ;
#163751=CARTESIAN_POINT ( 'NONE',  ( -17.50000000000001421, 5.622605283950871780, 53.68792689403890250 ) ) ;
#163752=CARTESIAN_POINT ( 'NONE',  ( 16.51473224551083163, -9.474510206698727899, 40.83442372801900433 ) ) ;
#163753=CARTESIAN_POINT ( 'NONE',  ( 4.483927247898790824, -16.52544592524335698, 100.2094237280190043 ) ) ;
#163754=CARTESIAN_POINT ( 'NONE',  ( -19.05341960407611168, -5.049401038298163336, 91.45724293864766707 ) ) ;
#163755=CARTESIAN_POINT ( 'NONE',  ( 18.67979575497194134, -10.72451020669871369, 50.83442372801901143 ) ) ;
#163756=CARTESIAN_POINT ( 'NONE',  ( 15.80617190586746368, 15.72974639402197994, 49.37390960531436690 ) ) ;
#163757=CARTESIAN_POINT ( 'NONE',  ( 21.53943276465977519, 0.05219959533937863772, 31.25109039468568639 ) ) ;
#163758=CARTESIAN_POINT ( 'NONE',  ( -5.719274019375978568, 21.55341960407610458, 80.20724293864769550 ) ) ;
#163759=CARTESIAN_POINT ( 'NONE',  ( 16.53943276465976808, -0.05219959533910856209, 108.7489096053143669 ) ) ;
#163760=CARTESIAN_POINT ( 'NONE',  ( 5.049401038297881783, 19.05341960407617563, 62.29275706135234003 ) ) ;
#163761=CARTESIAN_POINT ( 'NONE',  ( -16.51473224551069308, -9.474510206698971260, 46.66557627198102409 ) ) ;
#163762=CARTESIAN_POINT ( 'NONE',  ( -19.03943276465977164, 0.05219959533909376836, 96.24890960531436690 ) ) ;
#163763=CARTESIAN_POINT ( 'NONE',  ( 19.02544592524343514, -5.153800228976328945, 93.54057627198102409 ) ) ;
#163764=CARTESIAN_POINT ( 'NONE',  ( 19.02544592524343514, -5.153800228976328945, 23.54057627198102054 ) ) ;
#163765=CARTESIAN_POINT ( 'NONE',  ( 8.314922557960818139, 14.29746914071049879, 44.58224293864769550 ) ) ;
#163766=CARTESIAN_POINT ( 'NONE',  ( 16.52544592524335698, 4.483927247898782831, 41.45942372801901143 ) ) ;
#163767=CARTESIAN_POINT ( 'NONE',  ( -15.80617190586768217, 15.72974639402176855, 108.1260903946856757 ) ) ;
#163768=CARTESIAN_POINT ( 'NONE',  ( -5.049401038298153566, 19.05341960407611168, 115.2072429386477097 ) ) ;
#163769=CARTESIAN_POINT ( 'NONE',  ( 12.06949235617757843, -12.14591786802309237, 23.12390960531436335 ) ) ;
#163770=CARTESIAN_POINT ( 'NONE',  ( -5.823673210054431948, 21.52544592524334988, 32.70942372801900433 ) ) ;
#163771=CARTESIAN_POINT ( 'NONE',  ( 13.97604488694527802, 13.89961937509977652, 109.3739096053143669 ) ) ;
#163772=CARTESIAN_POINT ( 'NONE',  ( 16.53943276465976808, 0.05219959533934440121, 56.25109039468568284 ) ) ;
#163773=CARTESIAN_POINT ( 'NONE',  ( 4.379528057220092307, 16.55341960407617563, 102.2927570613523613 ) ) ;
#163774=CARTESIAN_POINT ( 'NONE',  ( -12.06949235617739369, -12.14591786802326823, 99.37609039468568994 ) ) ;
#163775=CARTESIAN_POINT ( 'NONE',  ( -4.483927247898782831, 16.52544592524335698, 22.70942372801901499 ) ) ;
#163776=CARTESIAN_POINT ( 'NONE',  ( -9.474510206698964154, 16.51473224551069663, 45.41557627198103120 ) ) ;
#163777=CARTESIAN_POINT ( 'NONE',  ( 12.06949235617757843, -12.14591786802309237, 113.1239096053143953 ) ) ;
#163778=CARTESIAN_POINT ( 'NONE',  ( 0.05219959533937995610, -21.53943276465977519, 20.00109039468568639 ) ) ;
#163779=CARTESIAN_POINT ( 'NONE',  ( -19.02544592524342804, 5.153800228976336051, 36.04057627198100988 ) ) ;
#163780=CARTESIAN_POINT ( 'NONE',  ( -5.153800228976328057, -19.02544592524343514, 107.2905762719810383 ) ) ;
#163781=CARTESIAN_POINT ( 'NONE',  ( 15.80617190586769283, -15.72974639402175789, 35.62609039468568994 ) ) ;
#163782=CARTESIAN_POINT ( 'NONE',  ( -19.02544592524342804, 5.153800228976336051, 26.04057627198103120 ) ) ;
#163783=CARTESIAN_POINT ( 'NONE',  ( 13.97604488694527802, 13.89961937509977652, 109.3739096053143669 ) ) ;
#163784=CARTESIAN_POINT ( 'NONE',  ( 16.62475595723700650, -7.163666690055283226, 113.0271335181047050 ) ) ;
#163785=CARTESIAN_POINT ( 'NONE',  ( 13.97604488694527802, 13.89961937509977652, 99.37390960531436690 ) ) ;
#163786=CARTESIAN_POINT ( 'NONE',  ( -5.719274019375665041, -21.55341960407619695, 39.79275706135235424 ) ) ;
#163787=CARTESIAN_POINT ( 'NONE',  ( 16.52544592524342804, -4.483927247898539470, 93.54057627198103830 ) ) ;
#163788=CARTESIAN_POINT ( 'NONE',  ( -16.51473224551069308, -9.474510206698971260, 101.6655762719810241 ) ) ;
#163789=CARTESIAN_POINT ( 'NONE',  ( 17.59860650958994555, -7.585241751806880650, 70.92337014262493256 ) ) ;
#163790=CARTESIAN_POINT ( 'NONE',  ( -16.55341960407617563, 4.379528057220093196, 63.54275706135234003 ) ) ;
#163791=CARTESIAN_POINT ( 'NONE',  ( 21.53943276465977519, 0.05219959533937863772, 81.25109039468568994 ) ) ;
#163792=CARTESIAN_POINT ( 'NONE',  ( -4.483927247898782831, 16.52544592524335698, 37.70942372801900433 ) ) ;
#163793=CARTESIAN_POINT ( 'NONE',  ( 5.049401038298161559, -19.05341960407611168, 82.70724293864770971 ) ) ;
#163794=CARTESIAN_POINT ( 'NONE',  ( 13.89961937509957401, 13.97604488694547697, 106.8760903946856757 ) ) ;
#163795=CARTESIAN_POINT ( 'NONE',  ( -4.483927247898782831, 16.52544592524335698, 67.70942372801901854 ) ) ;
#163796=CARTESIAN_POINT ( 'NONE',  ( -16.46253265017146816, -9.564922557961047289, 19.16775706135233293 ) ) ;
#163797=CARTESIAN_POINT ( 'NONE',  ( -13.97604488694547697, 13.89961937509957934, 93.12609039468566152 ) ) ;
#163798=CARTESIAN_POINT ( 'NONE',  ( -19.03943276465977164, 0.05219959533909376836, 66.24890960531436690 ) ) ;
#163799=CARTESIAN_POINT ( 'NONE',  ( -0.05219959533907301413, -21.53943276465977519, 82.49890960531436690 ) ) ;
#163800=CARTESIAN_POINT ( 'NONE',  ( 14.34966873604960469, 8.224510206698951720, 94.16557627198103830 ) ) ;
#163801=CARTESIAN_POINT ( 'NONE',  ( 9.564922557961047289, -16.46253265017146816, 95.41775706135233293 ) ) ;
#163802=CARTESIAN_POINT ( 'NONE',  ( 4.483927247898790824, -16.52544592524335698, 65.20942372801901854 ) ) ;
#163804=CARTESIAN_POINT ( 'NONE',  ( 9.474510206698729675, 16.51473224551082808, 52.08442372801900433 ) ) ;
#163805=CARTESIAN_POINT ( 'NONE',  ( 16.52544592524342804, -4.483927247898539470, 33.54057627198102409 ) ) ;
#163806=CARTESIAN_POINT ( 'NONE',  ( 16.53943276465976808, -0.05219959533910856209, 83.74890960531435269 ) ) ;
#163807=CARTESIAN_POINT ( 'NONE',  ( 0.05219959533937995610, -21.53943276465977519, 110.0010903946856757 ) ) ;
#163808=CARTESIAN_POINT ( 'NONE',  ( 16.51473224551083163, -9.474510206698727899, 45.83442372801900433 ) ) ;
#163809=CARTESIAN_POINT ( 'NONE',  ( 18.67979575497194134, -10.72451020669871369, 25.83442372801901499 ) ) ;
#163810=CARTESIAN_POINT ( 'NONE',  ( -5.049401038298153566, 19.05341960407611168, 95.20724293864770971 ) ) ;
#163811=CARTESIAN_POINT ( 'NONE',  ( -5.153800228976328057, -19.02544592524343514, 77.29057627198099567 ) ) ;
#163812=CARTESIAN_POINT ( 'NONE',  ( -15.72974639402176322, -15.80617190586768395, 94.37609039468568994 ) ) ;
#163813=CARTESIAN_POINT ( 'NONE',  ( 19.05341960407611168, 5.049401038298154454, 78.95724293864769550 ) ) ;
#163814=CARTESIAN_POINT ( 'NONE',  ( 18.67979575497178502, 10.72451020669898547, 39.16557627198102409 ) ) ;
#163815=CARTESIAN_POINT ( 'NONE',  ( 16.52544592524342804, -4.483927247898539470, 83.54057627198102409 ) ) ;
#163816=CARTESIAN_POINT ( 'NONE',  ( 19.02544592524343514, -5.153800228976328945, 58.54057627198102409 ) ) ;
#163817=CARTESIAN_POINT ( 'NONE',  ( -12.06949235617756955, 12.14591786802309770, 100.6239096053143811 ) ) ;
#163819=CARTESIAN_POINT ( 'NONE',  ( -15.72974639402176322, -15.80617190586768395, 24.37609039468567573 ) ) ;
#163820=CARTESIAN_POINT ( 'NONE',  ( 5.823673210054444382, -21.52544592524334988, 65.20942372801901854 ) ) ;
#163821=CARTESIAN_POINT ( 'NONE',  ( -0.05219959533909027116, -19.03943276465977164, 47.49890960531435979 ) ) ;
#163822=CARTESIAN_POINT ( 'NONE',  ( -12.06949235617739369, -12.14591786802326823, 59.37609039468568284 ) ) ;
#163823=CARTESIAN_POINT ( 'NONE',  ( 18.67979575497178502, 10.72451020669898547, 114.1655762719810383 ) ) ;
#163824=CARTESIAN_POINT ( 'NONE',  ( -21.55341960407610458, -5.719274019375992779, 111.4572429386476813 ) ) ;
#163825=CARTESIAN_POINT ( 'NONE',  ( -9.564922557961040184, 16.46253265017147172, 42.91775706135234003 ) ) ;
#163826=CARTESIAN_POINT ( 'NONE',  ( 9.474510206698971260, -16.51473224551069308, 62.91557627198102409 ) ) ;
#163828=CARTESIAN_POINT ( 'NONE',  ( -21.53943276465977519, -0.05219959533937600094, 68.75109039468568994 ) ) ;
#163829=CARTESIAN_POINT ( 'NONE',  ( -0.05219959533907301413, -21.53943276465977519, 57.49890960531435979 ) ) ;
#163830=CARTESIAN_POINT ( 'NONE',  ( 14.34966873604960469, 8.224510206698951720, 44.16557627198103120 ) ) ;
#163831=CARTESIAN_POINT ( 'NONE',  ( 21.53943276465977519, 0.05219959533937863772, 71.25109039468568994 ) ) ;
#163832=CARTESIAN_POINT ( 'NONE',  ( 16.51473224551083163, -9.474510206698727899, 20.83442372801899722 ) ) ;
#163833=CARTESIAN_POINT ( 'NONE',  ( 12.06949235617757843, -12.14591786802309237, 58.12390960531435979 ) ) ;
#163834=CARTESIAN_POINT ( 'NONE',  ( 16.52544592524342804, -4.483927247898539470, 103.5405762719810383 ) ) ;
#163835=CARTESIAN_POINT ( 'NONE',  ( -5.153800228976607833, 19.02544592524334988, 47.70942372801900433 ) ) ;
#163836=CARTESIAN_POINT ( 'NONE',  ( -16.52544592524342804, 4.483927247898546575, 26.04057627198103475 ) ) ;
#163837=CARTESIAN_POINT ( 'NONE',  ( -5.823673210054431948, 21.52544592524334988, 72.70942372801901854 ) ) ;
#163839=CARTESIAN_POINT ( 'NONE',  ( -19.02544592524342804, 5.153800228976336051, 61.04057627198103120 ) ) ;
#163840=CARTESIAN_POINT ( 'NONE',  ( -16.51473224551082808, 9.474510206698731452, 28.33442372801900433 ) ) ;
#163841=CARTESIAN_POINT ( 'NONE',  ( 5.823673210054125526, 21.52544592524343514, 34.79057627198103120 ) ) ;
#163842=CARTESIAN_POINT ( 'NONE',  ( 21.53943276465977519, 0.05219959533937863772, 36.25109039468567573 ) ) ;
#163843=CARTESIAN_POINT ( 'NONE',  ( 10.72451020669898902, -18.67979575497178502, 92.91557627198103830 ) ) ;
#163844=CARTESIAN_POINT ( 'NONE',  ( 16.51473224551083163, -9.474510206698727899, 80.83442372801899012 ) ) ;
#163845=CARTESIAN_POINT ( 'NONE',  ( 14.29746914071037800, 8.314922557961029526, 46.66775706135234714 ) ) ;
#163847=CARTESIAN_POINT ( 'NONE',  ( 18.62759615963271287, -10.81492255796078972, 88.33224293864769550 ) ) ;
#163848=CARTESIAN_POINT ( 'NONE',  ( 16.52544592524342804, -4.483927247898539470, 93.54057627198103830 ) ) ;
#163850=CARTESIAN_POINT ( 'NONE',  ( 12.14591786802327356, -12.06949235617739191, 25.62609039468567929 ) ) ;
#163851=CARTESIAN_POINT ( 'NONE',  ( 10.72451020669898902, -18.67979575497178502, 47.91557627198102409 ) ) ;
#163853=CARTESIAN_POINT ( 'NONE',  ( 12.06949235617739724, 12.14591786802326823, 91.87609039468568994 ) ) ;
#163854=CARTESIAN_POINT ( 'NONE',  ( 19.05341960407611168, 5.049401038298154454, 23.95724293864769194 ) ) ;
#163855=EDGE_CURVE ( 'NONE', #24501, #55198, #185933, .T. ) ;
#163856=CARTESIAN_POINT ( 'NONE',  ( 14.34966873604972726, -8.224510206698740333, 55.83442372801901854 ) ) ;
#163857=CARTESIAN_POINT ( 'NONE',  ( 21.52544592524334988, 5.823673210054432836, 31.45942372801901854 ) ) ;
#163858=CARTESIAN_POINT ( 'NONE',  ( 10.72451020669898902, -18.67979575497178502, 47.91557627198102409 ) ) ;
#163859=CARTESIAN_POINT ( 'NONE',  ( -0.05219959533934338120, 16.53943276465976808, 87.50109039468568994 ) ) ;
#163860=CARTESIAN_POINT ( 'NONE',  ( 0.05219959533909260263, 19.03943276465977164, 99.99890960531436690 ) ) ;
#163861=CARTESIAN_POINT ( 'NONE',  ( 15.72974639402176855, 15.80617190586768217, 61.87609039468568284 ) ) ;
#163862=CARTESIAN_POINT ( 'NONE',  ( -13.89961937509977652, 13.97604488694528158, 25.62390960531434558 ) ) ;
#163863=CARTESIAN_POINT ( 'NONE',  ( -10.72451020669898014, 18.67979575497178502, 45.41557627198103830 ) ) ;
#163864=CARTESIAN_POINT ( 'NONE',  ( 0.05219959533909260263, 19.03943276465977164, 109.9989096053143669 ) ) ;
#163866=CARTESIAN_POINT ( 'NONE',  ( -0.05219959533936034679, 19.03943276465977164, 42.50109039468566152 ) ) ;
#163867=CARTESIAN_POINT ( 'NONE',  ( 12.14591786802327356, -12.06949235617739191, 60.62609039468567573 ) ) ;
#163868=CARTESIAN_POINT ( 'NONE',  ( 9.564922557960805705, 16.46253265017160317, 114.5822429386476955 ) ) ;
#163870=CARTESIAN_POINT ( 'NONE',  ( 9.564922557960805705, 16.46253265017160317, 89.58224293864769550 ) ) ;
#163871=CARTESIAN_POINT ( 'NONE',  ( 14.29746914071037800, 8.314922557961029526, 106.6677570613523756 ) ) ;
#163873=CARTESIAN_POINT ( 'NONE',  ( -4.483927247898539470, -16.52544592524342804, 97.29057627198105251 ) ) ;
#163874=CARTESIAN_POINT ( 'NONE',  ( 18.62759615963271287, -10.81492255796078972, 48.33224293864770260 ) ) ;
#163875=CARTESIAN_POINT ( 'NONE',  ( 9.564922557960805705, 16.46253265017160317, 34.58224293864770260 ) ) ;
#163876=CARTESIAN_POINT ( 'NONE',  ( -8.314922557961024197, 14.29746914071037800, 77.91775706135231871 ) ) ;
#163877=CARTESIAN_POINT ( 'NONE',  ( 0.05219959533937995610, -21.53943276465977519, 35.00109039468568284 ) ) ;
#163878=CARTESIAN_POINT ( 'NONE',  ( 19.03943276465977164, 0.05219959533936151252, 96.25109039468567573 ) ) ;
#163879=CARTESIAN_POINT ( 'NONE',  ( 16.53943276465976808, -0.05219959533910856209, 88.74890960531436690 ) ) ;
#163880=CARTESIAN_POINT ( 'NONE',  ( 9.474510206698971260, -16.51473224551069308, 42.91557627198103120 ) ) ;
#163882=CARTESIAN_POINT ( 'NONE',  ( 9.474510206698971260, -16.51473224551069308, 107.9155762719810383 ) ) ;
#163883=CARTESIAN_POINT ( 'NONE',  ( 21.53943276465977519, 0.05219959533937863772, 101.2510903946856757 ) ) ;
#163884=CARTESIAN_POINT ( 'NONE',  ( -9.564922557960796823, -16.46253265017161027, 72.08224293864770971 ) ) ;
#163885=CARTESIAN_POINT ( 'NONE',  ( 14.29746914071037800, 8.314922557961029526, 61.66775706135235424 ) ) ;
#163886=CARTESIAN_POINT ( 'NONE',  ( 10.81492255796106328, -18.62759615963255655, 95.41775706135234714 ) ) ;
#163887=CARTESIAN_POINT ( 'NONE',  ( -16.52544592524335698, -4.483927247898792601, 58.95942372801902565 ) ) ;
#163888=CARTESIAN_POINT ( 'NONE',  ( 19.03943276465977164, 0.05219959533936151252, 51.25109039468567573 ) ) ;
#163889=EDGE_CURVE ( 'NONE', #152017, #78021, #39191, .T. ) ;
#163890=CARTESIAN_POINT ( 'NONE',  ( 16.51473224551083163, -9.474510206698727899, 70.83442372801900433 ) ) ;
#163892=CARTESIAN_POINT ( 'NONE',  ( 21.55341960407619695, -5.719274019375665929, 61.04275706135234714 ) ) ;
#163893=CARTESIAN_POINT ( 'NONE',  ( 9.474510206698971260, -16.51473224551069308, 67.91557627198102409 ) ) ;
#163894=CARTESIAN_POINT ( 'NONE',  ( -9.564922557960796823, -16.46253265017161027, 22.08224293864768839 ) ) ;
#163895=CARTESIAN_POINT ( 'NONE',  ( -9.564922557961040184, 16.46253265017147172, 57.91775706135233293 ) ) ;
#163896=CARTESIAN_POINT ( 'NONE',  ( -16.46253265017160317, 9.564922557960807481, 110.8322429386476955 ) ) ;
#163897=CARTESIAN_POINT ( 'NONE',  ( -0.05219959533909027116, -19.03943276465977164, 87.49890960531436690 ) ) ;
#163898=CARTESIAN_POINT ( 'NONE',  ( 16.52544592524342804, -4.483927247898539470, 33.54057627198102409 ) ) ;
#163899=CARTESIAN_POINT ( 'NONE',  ( -18.62759615963270932, 10.81492255796079327, 45.83224293864769550 ) ) ;
#163900=CARTESIAN_POINT ( 'NONE',  ( -17.60779699588839264, -5.499999999999979572, 96.34981316670102558 ) ) ;
#163901=CARTESIAN_POINT ( 'NONE',  ( 15.72974639402176855, 15.80617190586768217, 106.8760903946856899 ) ) ;
#163903=CARTESIAN_POINT ( 'NONE',  ( 5.153800228976335163, 19.02544592524342804, 39.79057627198100988 ) ) ;
#163904=CARTESIAN_POINT ( 'NONE',  ( 5.049401038298161559, -19.05341960407611168, 27.70724293864769550 ) ) ;
#163906=CARTESIAN_POINT ( 'NONE',  ( 15.72974639402176855, 15.80617190586768217, 71.87609039468568994 ) ) ;
#163908=CARTESIAN_POINT ( 'NONE',  ( -0.05219959533934338120, 16.53943276465976808, 57.50109039468568994 ) ) ;
#163909=CARTESIAN_POINT ( 'NONE',  ( -18.67979575497178146, -10.72451020669898902, 81.66557627198103830 ) ) ;
#163910=CARTESIAN_POINT ( 'NONE',  ( 12.14591786802309770, 12.06949235617756955, 54.37390960531435979 ) ) ;
#163911=CARTESIAN_POINT ( 'NONE',  ( 19.05341960407611168, 5.049401038298154454, 23.95724293864769194 ) ) ;
#163912=CARTESIAN_POINT ( 'NONE',  ( -0.05219959533909027116, -19.03943276465977164, 102.4989096053143669 ) ) ;
#163913=CARTESIAN_POINT ( 'NONE',  ( 21.55341960407619695, -5.719274019375665929, 36.04275706135234714 ) ) ;
#163914=CARTESIAN_POINT ( 'NONE',  ( -19.05341960407617563, 5.049401038297882671, 43.54275706135232582 ) ) ;
#163915=CARTESIAN_POINT ( 'NONE',  ( -16.51473224551069308, -9.474510206698971260, 31.66557627198102054 ) ) ;
#163916=CARTESIAN_POINT ( 'NONE',  ( 5.719274019375673035, 21.55341960407619339, 82.29275706135234714 ) ) ;
#163917=CARTESIAN_POINT ( 'NONE',  ( 17.26172910966779384, -6.454744622555846689, 33.30646908649223548 ) ) ;
#163918=CARTESIAN_POINT ( 'NONE',  ( -16.52544592524342804, 4.483927247898546575, 31.04057627198102409 ) ) ;
#163919=CARTESIAN_POINT ( 'NONE',  ( 17.50000000000000355, 3.565345528327992231, 113.0750551319353292 ) ) ;
#163920=CARTESIAN_POINT ( 'NONE',  ( -0.05219959533907301413, -21.53943276465977519, 37.49890960531436690 ) ) ;
#163922=CARTESIAN_POINT ( 'NONE',  ( -19.05341960407611168, -5.049401038298163336, 91.45724293864766707 ) ) ;
#163923=CARTESIAN_POINT ( 'NONE',  ( 4.379528057220339221, -16.55341960407611168, 92.70724293864770971 ) ) ;
#163924=CARTESIAN_POINT ( 'NONE',  ( -19.05341960407617563, 5.049401038297882671, 108.5427570613523187 ) ) ;
#163925=CARTESIAN_POINT ( 'NONE',  ( 18.62759615963271287, -10.81492255796078972, 58.33224293864768839 ) ) ;
#163927=CARTESIAN_POINT ( 'NONE',  ( -19.02544592524342804, 5.153800228976336051, 36.04057627198100988 ) ) ;
#163928=CARTESIAN_POINT ( 'NONE',  ( 19.05341960407611168, 5.049401038298154454, 83.95724293864766707 ) ) ;
#163929=CARTESIAN_POINT ( 'NONE',  ( -15.80617190586745835, -15.72974639402198527, 86.87390960531438111 ) ) ;
#163930=CARTESIAN_POINT ( 'NONE',  ( -12.14591786802326823, 12.06949235617739902, 108.1260903946856757 ) ) ;
#163931=CARTESIAN_POINT ( 'NONE',  ( -13.97604488694527625, -13.89961937509977652, 101.8739096053143811 ) ) ;
#163932=CARTESIAN_POINT ( 'NONE',  ( -5.049401038297874678, -19.05341960407617918, 84.79275706135233293 ) ) ;
#163933=CARTESIAN_POINT ( 'NONE',  ( 0.05219959533937995610, -21.53943276465977519, 95.00109039468568994 ) ) ;
#163934=CARTESIAN_POINT ( 'NONE',  ( 15.80617190586746368, 15.72974639402197994, 79.37390960531436690 ) ) ;
#163935=CARTESIAN_POINT ( 'NONE',  ( 18.62759615963271287, -10.81492255796078972, 43.33224293864769550 ) ) ;
#163936=CARTESIAN_POINT ( 'NONE',  ( 13.97604488694527802, 13.89961937509977652, 49.37390960531434558 ) ) ;
#163937=CARTESIAN_POINT ( 'NONE',  ( 12.06949235617739724, 12.14591786802326823, 111.8760903946856615 ) ) ;
#163938=CARTESIAN_POINT ( 'NONE',  ( -13.97604488694527625, -13.89961937509977652, 61.87390960531435979 ) ) ;
#163941=CARTESIAN_POINT ( 'NONE',  ( -0.05219959533936034679, 19.03943276465977164, 27.50109039468566507 ) ) ;
#163942=CARTESIAN_POINT ( 'NONE',  ( -16.53943276465976808, 0.05219959533911058130, 76.24890960531435269 ) ) ;
#163943=CARTESIAN_POINT ( 'NONE',  ( -21.53943276465977519, 0.05219959533907696930, 116.2489096053143669 ) ) ;
#163945=CARTESIAN_POINT ( 'NONE',  ( 18.62759615963271287, -10.81492255796078972, 63.33224293864770260 ) ) ;
#163946=CARTESIAN_POINT ( 'NONE',  ( -12.06949235617739369, -12.14591786802326823, 99.37609039468568994 ) ) ;
#163947=CARTESIAN_POINT ( 'NONE',  ( -16.51473224551069308, -9.474510206698971260, 21.66557627198102765 ) ) ;
#163948=CARTESIAN_POINT ( 'NONE',  ( 13.97604488694527802, 13.89961937509977652, 69.37390960531436690 ) ) ;
#163951=CARTESIAN_POINT ( 'NONE',  ( -16.52544592524342804, 4.483927247898546575, 26.04057627198103475 ) ) ;
#163952=CARTESIAN_POINT ( 'NONE',  ( 10.81492255796106328, -18.62759615963255655, 60.41775706135235424 ) ) ;
#163953=CARTESIAN_POINT ( 'NONE',  ( 0.05219959533909260263, 19.03943276465977164, 114.9989096053143669 ) ) ;
#163954=CARTESIAN_POINT ( 'NONE',  ( -5.719274019375665041, -21.55341960407619695, 99.79275706135234714 ) ) ;
#163955=CARTESIAN_POINT ( 'NONE',  ( 9.564922557960805705, 16.46253265017160317, 34.58224293864770260 ) ) ;
#163956=CARTESIAN_POINT ( 'NONE',  ( 13.89961937509977652, -13.97604488694527269, 33.12390960531434558 ) ) ;
#163958=CARTESIAN_POINT ( 'NONE',  ( -15.72974639402176322, -15.80617190586768395, 94.37609039468568994 ) ) ;
#163959=CARTESIAN_POINT ( 'NONE',  ( -8.314922557961024197, 14.29746914071037800, 52.91775706135235424 ) ) ;
#163960=CARTESIAN_POINT ( 'NONE',  ( -21.53943276465977519, -0.05219959533937600094, 83.75109039468568994 ) ) ;
#163961=CARTESIAN_POINT ( 'NONE',  ( -16.51473224551069308, -9.474510206698971260, 111.6655762719810383 ) ) ;
#163962=CARTESIAN_POINT ( 'NONE',  ( -16.46253265017146816, -9.564922557961047289, 89.16775706135234714 ) ) ;
#163963=CARTESIAN_POINT ( 'NONE',  ( -15.72974639402176322, -15.80617190586768395, 59.37609039468568284 ) ) ;
#163964=CARTESIAN_POINT ( 'NONE',  ( -14.29746914071037622, -8.314922557961029526, 29.16775706135234003 ) ) ;
#163965=CARTESIAN_POINT ( 'NONE',  ( -16.46253265017146816, -9.564922557961047289, 89.16775706135234714 ) ) ;
#163966=CARTESIAN_POINT ( 'NONE',  ( -5.153800228976328057, -19.02544592524343514, 47.29057627198102409 ) ) ;
#163967=CARTESIAN_POINT ( 'NONE',  ( 19.03943276465977164, 0.05219959533936151252, 101.2510903946856757 ) ) ;
#163968=CARTESIAN_POINT ( 'NONE',  ( -16.46253265017146816, -9.564922557961047289, 89.16775706135234714 ) ) ;
#163969=CARTESIAN_POINT ( 'NONE',  ( -14.34966873604960291, -8.224510206698953496, 51.66557627198102409 ) ) ;
#163971=CARTESIAN_POINT ( 'NONE',  ( -19.05341960407617563, 5.049401038297882671, 73.54275706135233293 ) ) ;
#163972=CARTESIAN_POINT ( 'NONE',  ( -8.224510206698735004, -14.34966873604973081, 59.58442372801901854 ) ) ;
#163973=CARTESIAN_POINT ( 'NONE',  ( 0.05219959533936267826, -19.03943276465977164, 20.00109039468567218 ) ) ;
#163974=CARTESIAN_POINT ( 'NONE',  ( -5.049401038298153566, 19.05341960407611168, 40.20724293864768839 ) ) ;
#163975=CARTESIAN_POINT ( 'NONE',  ( -13.97604488694527625, -13.89961937509977652, 41.87390960531435979 ) ) ;
#163976=CARTESIAN_POINT ( 'NONE',  ( -12.14591786802326823, 12.06949235617739902, 63.12609039468568994 ) ) ;
#163977=CARTESIAN_POINT ( 'NONE',  ( 18.22780087662126647, 5.499999999999818812, 41.48236817873107185 ) ) ;
#163979=CARTESIAN_POINT ( 'NONE',  ( 16.51473224551069308, 9.474510206698969483, 104.1655762719810241 ) ) ;
#163980=CARTESIAN_POINT ( 'NONE',  ( 17.59860650958994555, -7.585241751806880650, 85.92337014262491834 ) ) ;
#163982=CARTESIAN_POINT ( 'NONE',  ( -5.153800228976607833, 19.02544592524334988, 92.70942372801901854 ) ) ;
#163983=CARTESIAN_POINT ( 'NONE',  ( 15.72974639402199770, -15.80617190586745480, 38.12390960531436690 ) ) ;
#163984=CARTESIAN_POINT ( 'NONE',  ( -16.51473224551082808, 9.474510206698731452, 28.33442372801900433 ) ) ;
#163985=CARTESIAN_POINT ( 'NONE',  ( 16.46253265017146816, 9.564922557961045513, 106.6677570613523471 ) ) ;
#163986=CARTESIAN_POINT ( 'NONE',  ( 9.474510206698971260, -16.51473224551069308, 27.91557627198103120 ) ) ;
#163987=CARTESIAN_POINT ( 'NONE',  ( 19.03943276465977164, -0.05219959533909143690, 38.74890960531436690 ) ) ;
#163988=CARTESIAN_POINT ( 'NONE',  ( -21.52544592524343514, 5.823673210054127303, 76.04057627198102409 ) ) ;
#163989=CARTESIAN_POINT ( 'NONE',  ( -19.02544592524342804, 5.153800228976336051, 31.04057627198102409 ) ) ;
#163991=CARTESIAN_POINT ( 'NONE',  ( 9.474510206698729675, 16.51473224551082808, 87.08442372801900433 ) ) ;
#163992=CARTESIAN_POINT ( 'NONE',  ( 16.55341960407611168, 4.379528057220329451, 58.95724293864770971 ) ) ;
#163993=CARTESIAN_POINT ( 'NONE',  ( 18.62759615963271287, -10.81492255796078972, 33.33224293864769550 ) ) ;
#163994=CARTESIAN_POINT ( 'NONE',  ( -10.72451020669870658, -18.67979575497194134, 104.5844237280190185 ) ) ;
#163995=CARTESIAN_POINT ( 'NONE',  ( 21.52544592524344225, -5.823673210054117533, 78.54057627198103830 ) ) ;
#163996=CARTESIAN_POINT ( 'NONE',  ( 5.823673210054444382, -21.52544592524334988, 70.20942372801904696 ) ) ;
#163997=CARTESIAN_POINT ( 'NONE',  ( 21.55341960407619695, -5.719274019375665929, 61.04275706135234714 ) ) ;
#163999=CARTESIAN_POINT ( 'NONE',  ( -9.564922557960796823, -16.46253265017161027, 107.0822429386476955 ) ) ;
#164000=CARTESIAN_POINT ( 'NONE',  ( 14.34966873604972726, -8.224510206698740333, 100.8344237280190185 ) ) ;
#164001=CARTESIAN_POINT ( 'NONE',  ( 10.72451020669871369, 18.67979575497193778, 57.08442372801901854 ) ) ;
#164002=CARTESIAN_POINT ( 'NONE',  ( 13.89961937509977652, -13.97604488694527269, 53.12390960531434558 ) ) ;
#164003=CARTESIAN_POINT ( 'NONE',  ( 5.153800228976615827, -19.02544592524334988, 30.20942372801900433 ) ) ;
#164004=CARTESIAN_POINT ( 'NONE',  ( -21.52544592524334988, -5.823673210054445271, 23.95942372801901143 ) ) ;
#164005=CARTESIAN_POINT ( 'NONE',  ( -19.03943276465977164, 0.05219959533909376836, 71.24890960531435269 ) ) ;
#164006=CARTESIAN_POINT ( 'NONE',  ( -16.52544592524342804, 4.483927247898546575, 76.04057627198102409 ) ) ;
#164007=CARTESIAN_POINT ( 'NONE',  ( -16.53943276465976808, 0.05219959533911058130, 51.24890960531436690 ) ) ;
#164008=CARTESIAN_POINT ( 'NONE',  ( 15.72974639402199770, -15.80617190586745480, 63.12390960531435979 ) ) ;
#164009=CARTESIAN_POINT ( 'NONE',  ( 9.564922557960805705, 16.46253265017160317, 54.58224293864769550 ) ) ;
#164010=CARTESIAN_POINT ( 'NONE',  ( -10.72451020669898014, 18.67979575497178502, 70.41557627198102409 ) ) ;
#164011=CARTESIAN_POINT ( 'NONE',  ( 16.46253265017146816, 9.564922557961045513, 56.66775706135233293 ) ) ;
#164013=CARTESIAN_POINT ( 'NONE',  ( 8.224510206698953496, -14.34966873604960469, 57.91557627198103120 ) ) ;
#164014=CARTESIAN_POINT ( 'NONE',  ( -21.52544592524343514, 5.823673210054127303, 41.04057627198103120 ) ) ;
#164016=CARTESIAN_POINT ( 'NONE',  ( 17.48853670773245028, 5.747243402303093163, 103.8332870025000858 ) ) ;
#164017=CARTESIAN_POINT ( 'NONE',  ( -14.29746914071037622, -8.314922557961029526, 84.16775706135234714 ) ) ;
#164019=CARTESIAN_POINT ( 'NONE',  ( 19.05341960407617918, -5.049401038297876454, 91.04275706135234714 ) ) ;
#164020=CARTESIAN_POINT ( 'NONE',  ( 4.483927247898545687, 16.52544592524342804, 54.79057627198104541 ) ) ;
#164022=CARTESIAN_POINT ( 'NONE',  ( 19.03943276465977164, -0.05219959533909143690, 43.74890960531435979 ) ) ;
#164023=CARTESIAN_POINT ( 'NONE',  ( -8.224510206698948167, 14.34966873604960824, 45.41557627198103830 ) ) ;
#164024=CARTESIAN_POINT ( 'NONE',  ( -19.02544592524342804, 5.153800228976336051, 86.04057627198103830 ) ) ;
#164025=CARTESIAN_POINT ( 'NONE',  ( 5.153800228976335163, 19.02544592524342804, 54.79057627198103120 ) ) ;
#164026=CARTESIAN_POINT ( 'NONE',  ( 0.05219959533937995610, -21.53943276465977519, 55.00109039468568284 ) ) ;
#164027=CARTESIAN_POINT ( 'NONE',  ( -19.02544592524342804, 5.153800228976336051, 71.04057627198099567 ) ) ;
#164028=CARTESIAN_POINT ( 'NONE',  ( 16.51473224551069308, 9.474510206698969483, 29.16557627198103475 ) ) ;
#164029=CARTESIAN_POINT ( 'NONE',  ( 0.05219959533909260263, 19.03943276465977164, 69.99890960531435269 ) ) ;
#164030=CARTESIAN_POINT ( 'NONE',  ( 10.72451020669898902, -18.67979575497178502, 52.91557627198103830 ) ) ;
#164031=CARTESIAN_POINT ( 'NONE',  ( -19.03943276465977164, 0.05219959533909376836, 31.24890960531435979 ) ) ;
#164032=CARTESIAN_POINT ( 'NONE',  ( -10.81492255796078084, -18.62759615963271287, 37.08224293864768129 ) ) ;
#164033=CARTESIAN_POINT ( 'NONE',  ( -14.29746914071037622, -8.314922557961029526, 104.1677570613523471 ) ) ;
#164034=CARTESIAN_POINT ( 'NONE',  ( 16.51473224551083163, -9.474510206698727899, 20.83442372801899722 ) ) ;
#164035=CARTESIAN_POINT ( 'NONE',  ( 8.224510206698742110, 14.34966873604972548, 42.08442372801901854 ) ) ;
#164036=CARTESIAN_POINT ( 'NONE',  ( 16.55341960407618274, -4.379528057220086978, 81.04275706135236135 ) ) ;
#164038=CARTESIAN_POINT ( 'NONE',  ( 16.55341960407618274, -4.379528057220086978, 61.04275706135234714 ) ) ;
#164039=CARTESIAN_POINT ( 'NONE',  ( -5.049401038298153566, 19.05341960407611168, 105.2072429386476671 ) ) ;
#164040=CARTESIAN_POINT ( 'NONE',  ( -19.02544592524342804, 5.153800228976336051, 36.04057627198100988 ) ) ;
#164041=CARTESIAN_POINT ( 'NONE',  ( 4.379528057220092307, 16.55341960407617563, 42.29275706135235424 ) ) ;
#164042=CARTESIAN_POINT ( 'NONE',  ( 5.049401038298161559, -19.05341960407611168, 42.70724293864767418 ) ) ;
#164043=CARTESIAN_POINT ( 'NONE',  ( -15.72974639402176322, -15.80617190586768395, 24.37609039468567573 ) ) ;
#164044=CARTESIAN_POINT ( 'NONE',  ( -14.29746914071037622, -8.314922557961029526, 39.16775706135235424 ) ) ;
#164045=CARTESIAN_POINT ( 'NONE',  ( 16.52544592524335698, 4.483927247898782831, 101.4594237280190185 ) ) ;
#164047=CARTESIAN_POINT ( 'NONE',  ( -10.72451020669870658, -18.67979575497194134, 94.58442372801901854 ) ) ;
#164048=CARTESIAN_POINT ( 'NONE',  ( 19.05341960407617918, -5.049401038297876454, 101.0427570613523045 ) ) ;
#164049=CARTESIAN_POINT ( 'NONE',  ( 19.05341960407617918, -5.049401038297876454, 51.04275706135231871 ) ) ;
#164050=CARTESIAN_POINT ( 'NONE',  ( -16.55341960407611168, -4.379528057220339221, 56.45724293864768839 ) ) ;
#164051=CARTESIAN_POINT ( 'NONE',  ( 5.049401038298161559, -19.05341960407611168, 27.70724293864769550 ) ) ;
#164052=CARTESIAN_POINT ( 'NONE',  ( 0.05219959533936267826, -19.03943276465977164, 60.00109039468566863 ) ) ;
#164053=CARTESIAN_POINT ( 'NONE',  ( -15.49999999999999822, 5.499999999999997335, 118.0000000000000142 ) ) ;
#164054=CARTESIAN_POINT ( 'NONE',  ( -21.55341960407619339, 5.719274019375674811, 63.54275706135234003 ) ) ;
#164055=CARTESIAN_POINT ( 'NONE',  ( 16.55341960407618274, -4.379528057220086978, 21.04275706135234714 ) ) ;
#164056=CARTESIAN_POINT ( 'NONE',  ( 19.48894818550242647, -5.500000000000105693, 57.60307310435242556 ) ) ;
#164057=CARTESIAN_POINT ( 'NONE',  ( -9.474510206698964154, 16.51473224551069663, 115.4155762719810241 ) ) ;
#164058=CARTESIAN_POINT ( 'NONE',  ( -19.05341960407617563, 5.049401038297882671, 103.5427570613523329 ) ) ;
#164059=CARTESIAN_POINT ( 'NONE',  ( -0.05219959533909027116, -19.03943276465977164, 112.4989096053143669 ) ) ;
#164061=CARTESIAN_POINT ( 'NONE',  ( -19.03943276465977164, 0.05219959533909376836, 21.24890960531436335 ) ) ;
#164062=CARTESIAN_POINT ( 'NONE',  ( 0.05219959533937995610, -21.53943276465977519, 110.0010903946856757 ) ) ;
#164063=CARTESIAN_POINT ( 'NONE',  ( -16.51473224551069308, -9.474510206698971260, 61.66557627198103120 ) ) ;
#164064=CARTESIAN_POINT ( 'NONE',  ( -21.52544592524334988, -5.823673210054445271, 63.95942372801901854 ) ) ;
#164065=CARTESIAN_POINT ( 'NONE',  ( 21.53943276465977519, 0.05219959533937863772, 106.2510903946856757 ) ) ;
#164066=CARTESIAN_POINT ( 'NONE',  ( -0.05219959533934338120, 16.53943276465976808, 107.5010903946856899 ) ) ;
#164067=CARTESIAN_POINT ( 'NONE',  ( 19.05341960407611168, 5.049401038298154454, 73.95724293864768129 ) ) ;
#164068=CARTESIAN_POINT ( 'NONE',  ( 21.53943276465977519, 0.05219959533937863772, 56.25109039468568284 ) ) ;
#164069=CARTESIAN_POINT ( 'NONE',  ( -15.72974639402176322, -15.80617190586768395, 59.37609039468568284 ) ) ;
#164070=CARTESIAN_POINT ( 'NONE',  ( 19.03943276465977164, 0.05219959533936151252, 86.25109039468567573 ) ) ;
#164071=CARTESIAN_POINT ( 'NONE',  ( 5.049401038298161559, -19.05341960407611168, 102.7072429386476955 ) ) ;
#164072=CARTESIAN_POINT ( 'NONE',  ( -12.14591786802309592, -12.06949235617757132, 111.8739096053143669 ) ) ;
#164073=CARTESIAN_POINT ( 'NONE',  ( 10.72451020669898902, -18.67979575497178502, 92.91557627198103830 ) ) ;
#164074=CARTESIAN_POINT ( 'NONE',  ( 16.51473224551083163, -9.474510206698727899, 20.83442372801899722 ) ) ;
#164075=CARTESIAN_POINT ( 'NONE',  ( 16.52544592524342804, -4.483927247898539470, 103.5405762719810383 ) ) ;
#164076=CARTESIAN_POINT ( 'NONE',  ( 13.97604488694527802, 13.89961937509977652, 49.37390960531434558 ) ) ;
#164077=CARTESIAN_POINT ( 'NONE',  ( -13.97604488694547697, 13.89961937509957934, 93.12609039468566152 ) ) ;
#164078=CARTESIAN_POINT ( 'NONE',  ( 16.52544592524342804, -4.483927247898539470, 68.54057627198103830 ) ) ;
#164079=CARTESIAN_POINT ( 'NONE',  ( 15.72974639402176855, 15.80617190586768217, 111.8760903946856615 ) ) ;
#164080=CARTESIAN_POINT ( 'NONE',  ( 19.05341960407611168, 5.049401038298154454, 103.9572429386476671 ) ) ;
#164081=CARTESIAN_POINT ( 'NONE',  ( 5.049401038297881783, 19.05341960407617563, 77.29275706135231871 ) ) ;
#164082=CARTESIAN_POINT ( 'NONE',  ( 21.52544592524344225, -5.823673210054117533, 83.54057627198102409 ) ) ;
#164083=CARTESIAN_POINT ( 'NONE',  ( -15.80617190586768217, 15.72974639402176855, 33.12609039468569705 ) ) ;
#164084=CARTESIAN_POINT ( 'NONE',  ( -0.05219959533934338120, 16.53943276465976808, 37.50109039468568284 ) ) ;
#164085=CARTESIAN_POINT ( 'NONE',  ( 16.53943276465976808, 0.05219959533934440121, 91.25109039468568994 ) ) ;
#164086=CARTESIAN_POINT ( 'NONE',  ( 14.29746914071037800, 8.314922557961029526, 46.66775706135234714 ) ) ;
#164087=CARTESIAN_POINT ( 'NONE',  ( -5.719274019375665041, -21.55341960407619695, 39.79275706135235424 ) ) ;
#164088=CARTESIAN_POINT ( 'NONE',  ( 0.05219959533907565091, 21.53943276465977519, 39.99890960531436690 ) ) ;
#164089=CARTESIAN_POINT ( 'NONE',  ( -16.51473224551069308, -9.474510206698971260, 31.66557627198102054 ) ) ;
#164091=CARTESIAN_POINT ( 'NONE',  ( 4.483927247898790824, -16.52544592524335698, 60.20942372801902565 ) ) ;
#164092=CARTESIAN_POINT ( 'NONE',  ( -18.67979575497178146, -10.72451020669898902, 91.66557627198103830 ) ) ;
#164093=CARTESIAN_POINT ( 'NONE',  ( -14.34966873604960291, -8.224510206698953496, 41.66557627198103120 ) ) ;
#164094=CARTESIAN_POINT ( 'NONE',  ( -16.52544592524335698, -4.483927247898792601, 43.95942372801902565 ) ) ;
#164095=CARTESIAN_POINT ( 'NONE',  ( -16.46253265017160317, 9.564922557960807481, 55.83224293864769550 ) ) ;
#164096=CARTESIAN_POINT ( 'NONE',  ( 4.483927247898790824, -16.52544592524335698, 90.20942372801903275 ) ) ;
#164097=CARTESIAN_POINT ( 'NONE',  ( 16.51473224551083163, -9.474510206698727899, 90.83442372801900433 ) ) ;
#164098=CARTESIAN_POINT ( 'NONE',  ( 10.72451020669898902, -18.67979575497178502, 87.91557627198103830 ) ) ;
#164099=CARTESIAN_POINT ( 'NONE',  ( 16.52544592524342804, -4.483927247898539470, 28.54057627198103120 ) ) ;
#164102=CARTESIAN_POINT ( 'NONE',  ( -5.719274019375978568, 21.55341960407610458, 55.20724293864770260 ) ) ;
#164103=CARTESIAN_POINT ( 'NONE',  ( 16.55341960407618274, -4.379528057220086978, 101.0427570613523756 ) ) ;
#164105=CARTESIAN_POINT ( 'NONE',  ( 17.50000000000000711, -3.427582784585717413, 102.6734475746479092 ) ) ;
#164106=CARTESIAN_POINT ( 'NONE',  ( 18.67979575497178502, 10.72451020669898547, 84.16557627198103830 ) ) ;
#164107=CARTESIAN_POINT ( 'NONE',  ( 16.55341960407611168, 4.379528057220329451, 23.95724293864769550 ) ) ;
#164108=CARTESIAN_POINT ( 'NONE',  ( -4.483927247898782831, 16.52544592524335698, 37.70942372801900433 ) ) ;
#164109=VECTOR ( 'NONE', #161839, 1000.000000000000000 ) ;
#164110=CARTESIAN_POINT ( 'NONE',  ( -0.05219959533909027116, -19.03943276465977164, 37.49890960531436690 ) ) ;
#164111=CARTESIAN_POINT ( 'NONE',  ( 19.05341960407611168, 5.049401038298154454, 48.95724293864768129 ) ) ;
#164113=CARTESIAN_POINT ( 'NONE',  ( 10.81492255796078972, 18.62759615963270932, 24.58224293864768839 ) ) ;
#164115=CARTESIAN_POINT ( 'NONE',  ( -8.314922557961024197, 14.29746914071037800, 97.91775706135236135 ) ) ;
#164116=CARTESIAN_POINT ( 'NONE',  ( -9.474510206698720793, -16.51473224551083518, 104.5844237280190043 ) ) ;
#164117=CARTESIAN_POINT ( 'NONE',  ( 19.03943276465977164, 0.05219959533936151252, 31.25109039468566863 ) ) ;
#164118=CARTESIAN_POINT ( 'NONE',  ( -0.05219959533907301413, -21.53943276465977519, 87.49890960531436690 ) ) ;
#164119=CARTESIAN_POINT ( 'NONE',  ( 12.14591786802327356, -12.06949235617739191, 110.6260903946857042 ) ) ;
#164120=CARTESIAN_POINT ( 'NONE',  ( -0.05219959533907301413, -21.53943276465977519, 32.49890960531435979 ) ) ;
#164121=CARTESIAN_POINT ( 'NONE',  ( -19.03943276465977164, -0.05219959533935918106, 103.7510903946856757 ) ) ;
#164122=CARTESIAN_POINT ( 'NONE',  ( -13.89961937509977652, 13.97604488694528158, 110.6239096053143243 ) ) ;
#164123=CARTESIAN_POINT ( 'NONE',  ( 10.81492255796106328, -18.62759615963255655, 60.41775706135235424 ) ) ;
#164124=CARTESIAN_POINT ( 'NONE',  ( 19.05341960407611168, 5.049401038298154454, 53.95724293864770260 ) ) ;
#164125=CARTESIAN_POINT ( 'NONE',  ( -14.29746914071049879, 8.314922557960819915, 95.83224293864770971 ) ) ;
#164127=CARTESIAN_POINT ( 'NONE',  ( 9.564922557960805705, 16.46253265017160317, 74.58224293864769550 ) ) ;
#164128=CARTESIAN_POINT ( 'NONE',  ( 14.34966873604960469, 8.224510206698951720, 74.16557627198102409 ) ) ;
#164129=ORIENTED_EDGE ( 'NONE', *, *, #190442, .F. ) ;
#164130=CARTESIAN_POINT ( 'NONE',  ( 19.03943276465977164, 0.05219959533936151252, 86.25109039468567573 ) ) ;
#164131=CARTESIAN_POINT ( 'NONE',  ( 19.20446147854526231, 5.499999999999948486, 91.88999695167677828 ) ) ;
#164132=CARTESIAN_POINT ( 'NONE',  ( -19.02544592524342804, 5.153800228976336051, 61.04057627198103120 ) ) ;
#164134=VECTOR ( 'NONE', #116425, 1000.000000000000000 ) ;
#164135=CARTESIAN_POINT ( 'NONE',  ( -19.05341960407611168, -5.049401038298163336, 71.45724293864766707 ) ) ;
#164136=CARTESIAN_POINT ( 'NONE',  ( 5.153800228976335163, 19.02544592524342804, 99.79057627198102409 ) ) ;
#164137=CARTESIAN_POINT ( 'NONE',  ( -8.224510206698735004, -14.34966873604973081, 59.58442372801901854 ) ) ;
#164139=CARTESIAN_POINT ( 'NONE',  ( 19.02544592524334988, 5.153800228976608722, 46.45942372801899012 ) ) ;
#164140=CARTESIAN_POINT ( 'NONE',  ( 5.719274019375673035, 21.55341960407619339, 97.29275706135234714 ) ) ;
#164142=CARTESIAN_POINT ( 'NONE',  ( -9.564922557960796823, -16.46253265017161027, 112.0822429386476955 ) ) ;
#164143=CARTESIAN_POINT ( 'NONE',  ( -0.05219959533934338120, 16.53943276465976808, 102.5010903946856899 ) ) ;
#164145=CARTESIAN_POINT ( 'NONE',  ( -14.34966873604972548, 8.224510206698743886, 98.33442372801901854 ) ) ;
#164146=CARTESIAN_POINT ( 'NONE',  ( -16.38665767535054485, 7.295008042176025498, 30.26400864214545905 ) ) ;
#164147=CARTESIAN_POINT ( 'NONE',  ( 12.14591786802327356, -12.06949235617739191, 70.62609039468567573 ) ) ;
#164149=CARTESIAN_POINT ( 'NONE',  ( -18.62759615963255300, -10.81492255796106328, 74.16775706135231871 ) ) ;
#164150=CARTESIAN_POINT ( 'NONE',  ( -19.05341960407617563, 5.049401038297882671, 83.54275706135233293 ) ) ;
#164151=CARTESIAN_POINT ( 'NONE',  ( 19.05341960407617918, -5.049401038297876454, 31.04275706135232227 ) ) ;
#164152=CARTESIAN_POINT ( 'NONE',  ( 16.51473224551069308, 9.474510206698969483, 64.16557627198102409 ) ) ;
#164153=CARTESIAN_POINT ( 'NONE',  ( -16.51473224551069308, -9.474510206698971260, 51.66557627198102409 ) ) ;
#164155=CARTESIAN_POINT ( 'NONE',  ( -15.72974639402197994, 15.80617190586746368, 80.62390960531438111 ) ) ;
#164156=CARTESIAN_POINT ( 'NONE',  ( 5.823673210054125526, 21.52544592524343514, 39.79057627198103830 ) ) ;
#164157=CARTESIAN_POINT ( 'NONE',  ( 16.51473224551069308, 9.474510206698969483, 39.16557627198103120 ) ) ;
#164158=CARTESIAN_POINT ( 'NONE',  ( 14.34966873604972726, -8.224510206698740333, 60.83442372801901854 ) ) ;
#164160=CARTESIAN_POINT ( 'NONE',  ( 10.81492255796106328, -18.62759615963255655, 25.41775706135235779 ) ) ;
#164161=CARTESIAN_POINT ( 'NONE',  ( 16.53943276465976808, -0.05219959533910856209, 63.74890960531435979 ) ) ;
#164163=CARTESIAN_POINT ( 'NONE',  ( -4.379528057220086978, -16.55341960407618274, 19.79275706135235069 ) ) ;
#164164=CARTESIAN_POINT ( 'NONE',  ( -19.03943276465977164, -0.05219959533935918106, 38.75109039468566152 ) ) ;
#164165=CARTESIAN_POINT ( 'NONE',  ( 14.34966873604960469, 8.224510206698951720, 64.16557627198102409 ) ) ;
#164166=CARTESIAN_POINT ( 'NONE',  ( 0.05219959533937995610, -21.53943276465977519, 25.00109039468567218 ) ) ;
#164168=CARTESIAN_POINT ( 'NONE',  ( 21.52544592524344225, -5.823673210054117533, 73.54057627198102409 ) ) ;
#164169=CARTESIAN_POINT ( 'NONE',  ( 9.564922557960805705, 16.46253265017160317, 94.58224293864769550 ) ) ;
#164170=CARTESIAN_POINT ( 'NONE',  ( -12.06949235617756955, 12.14591786802309770, 60.62390960531437401 ) ) ;
#164173=CARTESIAN_POINT ( 'NONE',  ( -9.474510206698720793, -16.51473224551083518, 74.58442372801900433 ) ) ;
#164174=CARTESIAN_POINT ( 'NONE',  ( -10.81492255796078084, -18.62759615963271287, 102.0822429386476955 ) ) ;
#164175=CARTESIAN_POINT ( 'NONE',  ( -13.89961937509977652, 13.97604488694528158, 50.62390960531435979 ) ) ;
#164176=CARTESIAN_POINT ( 'NONE',  ( -19.05341960407617563, 5.049401038297882671, 48.54275706135233293 ) ) ;
#164177=CARTESIAN_POINT ( 'NONE',  ( -13.89961937509977652, 13.97604488694528158, 25.62390960531434558 ) ) ;
#164178=CARTESIAN_POINT ( 'NONE',  ( -18.67979575497193778, 10.72451020669871902, 68.33442372801900433 ) ) ;
#164179=CARTESIAN_POINT ( 'NONE',  ( -17.50000000000000000, -5.624438216177585659, 69.18329655085355512 ) ) ;
#164180=CARTESIAN_POINT ( 'NONE',  ( -12.14591786802309592, -12.06949235617757132, 46.87390960531435979 ) ) ;
#164181=CARTESIAN_POINT ( 'NONE',  ( 9.474510206698971260, -16.51473224551069308, 67.91557627198102409 ) ) ;
#164182=CARTESIAN_POINT ( 'NONE',  ( 15.80617190586746368, 15.72974639402197994, 74.37390960531436690 ) ) ;
#164183=CARTESIAN_POINT ( 'NONE',  ( 5.049401038298161559, -19.05341960407611168, 62.70724293864769550 ) ) ;
#164185=CARTESIAN_POINT ( 'NONE',  ( 5.823673210054125526, 21.52544592524343514, 69.79057627198102409 ) ) ;
#164186=CARTESIAN_POINT ( 'NONE',  ( -15.80617190586768217, 15.72974639402176855, 103.1260903946856757 ) ) ;
#164188=CARTESIAN_POINT ( 'NONE',  ( 0.05219959533934541429, -16.53943276465976808, 95.00109039468568994 ) ) ;
#164189=CARTESIAN_POINT ( 'NONE',  ( 4.483927247898545687, 16.52544592524342804, 89.79057627198103830 ) ) ;
#164190=CARTESIAN_POINT ( 'NONE',  ( -0.05219959533936034679, 19.03943276465977164, 87.50109039468567573 ) ) ;
#164192=CARTESIAN_POINT ( 'NONE',  ( -16.46253265017146816, -9.564922557961047289, 44.16775706135232582 ) ) ;
#164193=CARTESIAN_POINT ( 'NONE',  ( -16.52544592524335698, -4.483927247898792601, 103.9594237280190185 ) ) ;
#164194=CARTESIAN_POINT ( 'NONE',  ( -5.153800228976607833, 19.02544592524334988, 32.70942372801899722 ) ) ;
#164195=CARTESIAN_POINT ( 'NONE',  ( -13.89961937509977652, 13.97604488694528158, 95.62390960531436690 ) ) ;
#164196=CARTESIAN_POINT ( 'NONE',  ( -18.62759615963270932, 10.81492255796079327, 55.83224293864770260 ) ) ;
#164198=CARTESIAN_POINT ( 'NONE',  ( -12.14591786802309592, -12.06949235617757132, 111.8739096053143669 ) ) ;
#164199=CARTESIAN_POINT ( 'NONE',  ( 21.55341960407619695, -5.719274019375665929, 101.0427570613523756 ) ) ;
#164200=CARTESIAN_POINT ( 'NONE',  ( 14.34966873604972726, -8.224510206698740333, 75.83442372801900433 ) ) ;
#164201=CARTESIAN_POINT ( 'NONE',  ( -10.81492255796105439, 18.62759615963255655, 27.91775706135234358 ) ) ;
#164202=CARTESIAN_POINT ( 'NONE',  ( -4.379528057220086978, -16.55341960407618274, 29.79275706135234358 ) ) ;
#164203=CARTESIAN_POINT ( 'NONE',  ( 19.03943276465977164, -0.05219959533909143690, 93.74890960531435269 ) ) ;
#164204=CARTESIAN_POINT ( 'NONE',  ( 13.97604488694527802, 13.89961937509977652, 39.37390960531435269 ) ) ;
#164205=CARTESIAN_POINT ( 'NONE',  ( -9.564922557960796823, -16.46253265017161027, 47.08224293864769550 ) ) ;
#164206=CARTESIAN_POINT ( 'NONE',  ( -4.379528057220086978, -16.55341960407618274, 29.79275706135234358 ) ) ;
#164207=CARTESIAN_POINT ( 'NONE',  ( -14.29746914071049879, 8.314922557960819915, 90.83224293864769550 ) ) ;
#164209=CARTESIAN_POINT ( 'NONE',  ( 14.34966873604972726, -8.224510206698740333, 100.8344237280190185 ) ) ;
#164210=CARTESIAN_POINT ( 'NONE',  ( -5.719274019375665041, -21.55341960407619695, 39.79275706135235424 ) ) ;
#164211=CARTESIAN_POINT ( 'NONE',  ( 19.05341960407611168, 5.049401038298154454, 83.95724293864766707 ) ) ;
#164212=CARTESIAN_POINT ( 'NONE',  ( -5.049401038298153566, 19.05341960407611168, 60.20724293864768129 ) ) ;
#164213=CARTESIAN_POINT ( 'NONE',  ( -16.46253265017160317, 9.564922557960807481, 80.83224293864769550 ) ) ;
#164214=CARTESIAN_POINT ( 'NONE',  ( 12.06949235617757843, -12.14591786802309237, 38.12390960531436690 ) ) ;
#164215=CARTESIAN_POINT ( 'NONE',  ( 0.05219959533934541429, -16.53943276465976808, 105.0010903946856757 ) ) ;
#164217=CARTESIAN_POINT ( 'NONE',  ( -19.02544592524334988, -5.153800228976617603, 48.95942372801900433 ) ) ;
#164219=CARTESIAN_POINT ( 'NONE',  ( 9.564922557960805705, 16.46253265017160317, 44.58224293864769550 ) ) ;
#164220=CARTESIAN_POINT ( 'NONE',  ( -5.049401038297874678, -19.05341960407617918, 34.79275706135233293 ) ) ;
#164222=CARTESIAN_POINT ( 'NONE',  ( -16.55341960407617563, 4.379528057220093196, 43.54275706135235424 ) ) ;
#164223=CARTESIAN_POINT ( 'NONE',  ( -16.46253265017146816, -9.564922557961047289, 74.16775706135234714 ) ) ;
#164224=CARTESIAN_POINT ( 'NONE',  ( 12.14591786802327356, -12.06949235617739191, 50.62609039468568994 ) ) ;
#164226=CARTESIAN_POINT ( 'NONE',  ( 19.05341960407611168, 5.049401038298154454, 73.95724293864768129 ) ) ;
#164227=CARTESIAN_POINT ( 'NONE',  ( 15.80617190586769283, -15.72974639402175789, 20.62609039468568639 ) ) ;
#164228=CARTESIAN_POINT ( 'NONE',  ( 9.474510206698729675, 16.51473224551082808, 77.08442372801900433 ) ) ;
#164229=CARTESIAN_POINT ( 'NONE',  ( -13.89961937509977652, 13.97604488694528158, 110.6239096053143243 ) ) ;
#164230=CARTESIAN_POINT ( 'NONE',  ( 5.049401038298161559, -19.05341960407611168, 32.70724293864768129 ) ) ;
#164232=CARTESIAN_POINT ( 'NONE',  ( -16.46253265017160317, 9.564922557960807481, 75.83224293864769550 ) ) ;
#164233=CARTESIAN_POINT ( 'NONE',  ( -12.06949235617756955, 12.14591786802309770, 40.62390960531435269 ) ) ;
#164234=CARTESIAN_POINT ( 'NONE',  ( 19.03943276465977164, -0.05219959533909143690, 33.74890960531435979 ) ) ;
#164235=CARTESIAN_POINT ( 'NONE',  ( 13.97604488694548053, -13.89961937509957401, 55.62609039468566863 ) ) ;
#164236=CARTESIAN_POINT ( 'NONE',  ( -16.55341960407611168, -4.379528057220339221, 91.45724293864769550 ) ) ;
#164237=CARTESIAN_POINT ( 'NONE',  ( -16.51473224551082808, 9.474510206698731452, 23.33442372801900078 ) ) ;
#164238=CARTESIAN_POINT ( 'NONE',  ( -13.89961937509977652, 13.97604488694528158, 50.62390960531435979 ) ) ;
#164240=CARTESIAN_POINT ( 'NONE',  ( -10.81492255796078084, -18.62759615963271287, 52.08224293864768839 ) ) ;
#164241=CARTESIAN_POINT ( 'NONE',  ( 16.53943276465976808, -0.05219959533910856209, 58.74890960531436690 ) ) ;
#164242=CARTESIAN_POINT ( 'NONE',  ( 5.719274019375673035, 21.55341960407619339, 102.2927570613523613 ) ) ;
#164243=CARTESIAN_POINT ( 'NONE',  ( 19.05341960407611168, 5.049401038298154454, 93.95724293864769550 ) ) ;
#164244=CARTESIAN_POINT ( 'NONE',  ( -5.153800228976328057, -19.02544592524343514, 107.2905762719810383 ) ) ;
#164245=CARTESIAN_POINT ( 'NONE',  ( 19.05341960407611168, 5.049401038298154454, 33.95724293864769550 ) ) ;
#164246=CARTESIAN_POINT ( 'NONE',  ( -12.06949235617756955, 12.14591786802309770, 115.6239096053143669 ) ) ;
#164247=CARTESIAN_POINT ( 'NONE',  ( 16.53943276465976808, -0.05219959533910856209, 93.74890960531436690 ) ) ;
#164248=CARTESIAN_POINT ( 'NONE',  ( 15.72974639402199770, -15.80617190586745480, 103.1239096053143811 ) ) ;
#164249=CARTESIAN_POINT ( 'NONE',  ( 16.46253265017160672, -9.564922557960803928, 98.33224293864769550 ) ) ;
#164250=CARTESIAN_POINT ( 'NONE',  ( 15.80617190586746368, 15.72974639402197994, 109.3739096053143811 ) ) ;
#164251=CARTESIAN_POINT ( 'NONE',  ( -13.89961937509977652, 13.97604488694528158, 90.62390960531432427 ) ) ;
#164253=CARTESIAN_POINT ( 'NONE',  ( -12.14591786802309592, -12.06949235617757132, 106.8739096053143811 ) ) ;
#164254=CARTESIAN_POINT ( 'NONE',  ( 0.05219959533909260263, 19.03943276465977164, 74.99890960531435269 ) ) ;
#164255=CARTESIAN_POINT ( 'NONE',  ( 10.81492255796078972, 18.62759615963270932, 84.58224293864769550 ) ) ;
#164258=CARTESIAN_POINT ( 'NONE',  ( -5.719274019375978568, 21.55341960407610458, 30.20724293864769550 ) ) ;
#164260=CARTESIAN_POINT ( 'NONE',  ( -12.06949235617739369, -12.14591786802326823, 39.37609039468567573 ) ) ;
#164261=CARTESIAN_POINT ( 'NONE',  ( 16.53943276465976808, -0.05219959533910856209, 88.74890960531436690 ) ) ;
#164262=CARTESIAN_POINT ( 'NONE',  ( 19.46398650005387410, -5.500000000000147438, 52.68269651486371430 ) ) ;
#164263=CARTESIAN_POINT ( 'NONE',  ( -19.03943276465977164, 0.05219959533909376836, 86.24890960531436690 ) ) ;
#164264=CARTESIAN_POINT ( 'NONE',  ( -19.02544592524342804, 5.153800228976336051, 46.04057627198101699 ) ) ;
#164265=CARTESIAN_POINT ( 'NONE',  ( 8.314922557960818139, 14.29746914071049879, 84.58224293864769550 ) ) ;
#164266=CARTESIAN_POINT ( 'NONE',  ( 10.72451020669898902, -18.67979575497178502, 27.91557627198103830 ) ) ;
#164267=CARTESIAN_POINT ( 'NONE',  ( 16.55341960407611168, 4.379528057220329451, 48.95724293864770971 ) ) ;
#164268=CARTESIAN_POINT ( 'NONE',  ( 9.474510206698729675, 16.51473224551082808, 102.0844237280190043 ) ) ;
#164269=CARTESIAN_POINT ( 'NONE',  ( -18.67979575497193778, 10.72451020669871902, 73.33442372801901854 ) ) ;
#164271=CARTESIAN_POINT ( 'NONE',  ( -21.55341960407610458, -5.719274019375992779, 21.45724293864769550 ) ) ;
#164272=CARTESIAN_POINT ( 'NONE',  ( -16.53943276465976808, -0.05219959533934237506, 78.75109039468568994 ) ) ;
#164273=CARTESIAN_POINT ( 'NONE',  ( 19.05341960407611168, 5.049401038298154454, 23.95724293864769194 ) ) ;
#164274=CARTESIAN_POINT ( 'NONE',  ( -19.02544592524342804, 5.153800228976336051, 76.04057627198102409 ) ) ;
#164275=CARTESIAN_POINT ( 'NONE',  ( 5.823673210054125526, 21.52544592524343514, 79.79057627198102409 ) ) ;
#164276=( BOUNDED_SURFACE ( )  B_SPLINE_SURFACE ( 3, 2, ( 
 ( #195165, #119315, #26321, #12154, #87961, #27319, #118319, #181001, #180012, #88966, #41479, #103143, #150656, #73819, #110095, #199129, #92921, #908, #94921, #44460, #14104, #152614, #156606, #77760, #109097, #167798, #124261, #184948, #46433, #106114, #1916, #139426, #63595, #154607, #32266, #18101, #171773, #75772, #62583, #107099, #33262, #108092, #140426, #45446, #125270, #29298, #93923, #186968, #78749, #79755, #16102, #141426, #30272, #169776, #137450, #200120, #48438, #60596, #122271, #185956, #168769, #90928, #59610, #15106, #121283, #183959, #91917, #153610, #182976, #47440, #76767, #138439, #170776, #61589, #123257, #31270, #17096, #155601, #95913, #114051, #19089, #113064, #159565, #81710, #21063, #82718, #129220, #65574, #144400, #20067, #157597, #130213, #176763, #51404, #115071, #36221, #2912, #5886, #96894, #64591, #191908, #143396, #53393, #84714, #97873, #160578, #4885, #38235, #66567, #128232, #189929, #190917, #37227, #174756, #67562, #173774, #158577, #52394, #175750, #98884, #22067, #188948, #99890, #161575, #83718, #23068, #145396, #126255, #6879, #68557, #187952, #49421, #111083, #172773, #34254, #80737, #142416, #3895, #127234, #50425, #35240, #112084, #58393, #196926, #85726, #179769, #87722, #181748, #131233, #100884, #39228, #43229, #164584, #195937, #54399, #10902, #71565, #133230, #192921, #88728, #26078, #150423, #41238, #119084, #104896, #120060, #162567, #149407, #193929, #166585, #194921, #27081, #132237, #11918, #116071, #180765, #73582, #165583, #28085, #102899, #146392, #117062, #56397, #24071, #86725, #135254, #147413, #8901, #72576, #55392, #177759, #7881, #101900, #69566, #70569, #178757, #40223, #163582, #134250, #25082, #148410, #57411, #9905, #118079, #42241, #103902, #29065, #182742, #674, #105884, #199895, #46200, #168545, #107853, #169538, #15869, #152387, #31038, #106872, #44227, #16861, #63356, #138213, #1678, #123030, #89725, #92687, #183731, #151411, #78512, #30043, #140186, #171539, #184716, #47202, #91682, #125033, #153374, #14876, #76537, #77527, #124014, #61359, #154375, #60369, #45217, #186729, #74563, #167571, #90704, #48200, #139199, #62345, #197905, #185712, #108862, #170541, #136230, #32032, #93689, #155372, #109854, #12899, #59374, #121046, #13872, #75539, #137214, #198901, #122041, #113816, #18857, #36985, #2678, #5647, #98647, #52159, #83482, #127994, #53152, #3660, #158345, #49191, #173534, #21830, #126024, #172533, #97636, #142176, #64355, #175511, #188705, #114831, #17864, #187720, #80503, #145160, #66333, #65338, #156361, #112830, #35003, #110849, #96658, #190684, #34019, #95677, #144162, #157363, #143162, #189697, #111844, #51170, #174522, #159325, #126998, #35989, #50187, #19834, #160341, #6644, #81475, #68322, #20821, #33027, #82478, #4642, #94682, #129972, #67324, #191672, #79519, #128986, #141189, #193692, #103674, #116830, #55160, #163350, #102671, #10672, #178521, #39988, #147175, #132004, #101659, #24846, #117843, #162336, #165352, #88487, #164356, #26846, #194691, #60871, #56161, #86495, #179535, #148180, #72336, #9673, #25852, #69326, #41004, #150182, #133001, #11683, #8664, #73349, #135022, #196697, #115840, #71338, #87495, #176525, #149184, #134011, #38001, #99656, #146156, #195703, #57175, #161340, #177529, #118852, #180535, #22832, #84479, #130992, #192684, #7642, #42009, #54167, #38998, #100654, #23837, #85486, #70337, #64860, #140699, #126522, #17369, #95192, #157874, #173048, #77040, #63871, #170054, #34525, #47716, #3187, #108378, #188221, #92202, #156878, #49694, #141696, #96185, #79024, #142687, #93197, #109367, #138711, #62859, #111359, #15383, #61861, #187238, #31545, #153886, #19363, #78027, #4167, #107372, #192, #154882, #81012, #155872, #16380, #45719, #2189, #124541, #123530, #186238, #80027, #185224, #46715, #33530, #139696, #32539, #125542, #1182, #48708, #110361, #172043, #171049, #18375 ),
 ( #122548, #184238, #169044, #30550, #94192, #193201, #6163, #83003, #52673, #192199, #100174, #67843, #144678, #36498, #21345, #129498, #114336, #7161, #51679, #54674, #178037, #53681, #116348, #84000, #147700, #145679, #191198, #68844, #176039, #161856, #37507, #130503, #99169, #158849, #39505, #101165, #160859, #162853, #22349, #65845, #115358, #159852, #127515, #24360, #177048, #86011, #189219, #38518, #23350, #84995, #50697, #146676, #8171, #69847, #131515, #112356, #174047, #35516, #98152, #97164, #20337, #81986, #143679, #113341, #5160, #66843, #128506, #190201, #175033, #90967, #27360, #164869, #89006, #119360, #105173, #181044, #58663, #102185, #150697, #136499, #165864, #198179, #120329, #12195, #72865, #132522, #148700, #42519, #73860, #44499, #194211, #163873, #25372, #106155, #135529, #182024, #117350, #197200, #134534, #196222, #55676, #151681, #43507, #13173, #104182, #166859, #167837, #59649, #87014, #28361, #56689, #121323, #57692, #89999, #195209, #74836, #179046, #183015, #29338, #9188, #70853, #40514, #10188, #180056, #71848, #133517, #149692, #118363, #41525, #103188, #26364, #88004, #11190, #94957, #108132, #34288, #137489, #184001, #200158, #64627, #185995, #184988, #75811, #32306, #92960, #45484, #154646, #110131, #91956, #107139, #63633, #168809, #62620, #109135, #31307, #170813, #93960, #78787, #15144, #2948, #47478, #172807, #123296, #77796, #30313, #16141, #141464, #153649, #76806, #17135, #61628, #138477, #156641, #169816, #152654, #199169, #46472, #139465, #126289, #155640, #945, #60636, #140464, #124298, #1954, #125309, #171810, #187005, #48475, #33298, #18137, #79791, #187986, #49456, #111118, #14144, #122310, #158611, #37260, #113098, #188982, #23101, #69599, #144433, #7915, #129255, #95948, #175786, #189963, #157634, #84747, #174789, #146424, #177791, #190950, #53426, #36255, #131266, #97908, #159599, #82753, #22100, #130246, #21096, #5919, #66601, #51438, #67596, #52427, #98918, #81745, #192954, #54433, #83750, #116103, #114085, #19123, #160610, #145429, #6912, #68590, #191941, #115103, #176795, #50458, #38268, #80773, #99922, #142451, #161607, #3929, #65609, #127269, #35274, #112117, #173809, #96929, #20101, #143432, #4918, #128265, #57441, #88757, #147447, #103932, #164616, #26110, #85760, #181776, #119114, #43257, #134281, #11946, #74589, #89752, #193962, #180795, #86760, #151438, #87753, #120088, #25116, #104925, #8935, #73610, #166612, #58421, #42274, #28114, #195969, #12925, #150450, #165612, #102931, #162602, #178791, #72607, #27111, #136257, #24106, #55425, #132271, #197933, #135281, #196953, #70604, #59401, #149438, #10934, #117096, #121075, #39261, #100917, #40260, #101933, #163615, #148443, #9938, #71597, #133263, #194954, #56431, #118111, #179800, #41269, #152413, #155401, #186760, #1710, #33058, #77558, #2709, #153406, #107885, #198928, #123060, #171569, #75567, #122068, #47234, #91712, #13901, #125063, #138241, #64386, #167596, #137243, #30071, #94713, #15900, #14904, #105910, #62377, #184746, #60396, #46231, #140217, #183760, #45246, #93719, #106900, #92717, #139230, #61388, #705, #124047, #108893, #168573, #185746, #199925, #76566, #109885, #156391, #31069, #17895, #170572, #182769, #32063, #169572, #44253, #79549, #154406, #141218, #29091, #16891, #63386, #78542, #90730, #48230, #143195, #112863, #52190, #160373, #66367, #4675, #96690, #81507, #128027, #174554, #67357, #111876, #53187, #38032, #113848, #114862, #144195, #7673, #5681, #189729, #129017, #36021, #21864, #97670, #175544, #18888, #19867, #159359, #176557, #190717, #95707, #37019, #35035, #157395, #20856, #98680, #51202, #83514, #145191, #130003, #50222, #80534, #84510, #6674, #68352, #191703, #99688, #161372, #22863, #146188, #126054, #187751, #82513, #49221, #110879, #172564, #142208, #34050, #3691, #65370, #127030, #188737, #173566, #158378, #72368, #117875, #85518, #119865 ),
 ( #151210, #164389, #26878, #86526, #196729, #9704, #148210, #56192, #195735, #103705, #71368, #133032, #40018, #24877, #194722, #179565, #10705, #55192, #58197, #181550, #57208, #43029, #87527, #69357, #149214, #41035, #134042, #102701, #165385, #25882, #118883, #162366, #180567, #104695, #42041, #166383, #88521, #150217, #11714, #192715, #8697, #73381, #135053, #27879, #54199, #23867, #147206, #89520, #131026, #115871, #177560, #39029, #100684, #70367, #132035, #193724, #116861, #178552, #101691, #163380, #47994, #63141, #167367, #154170, #60164, #124820, #138003, #93474, #198698, #16653, #182538, #185503, #78300, #31824, #122824, #169326, #91476, #30833, #92481, #138988, #75338, #15661, #29839, #105681, #139974, #186520, #61152, #109648, #45994, #12698, #77320, #106670, #74364, #1463, #153164, #171330, #94469, #107649, #170331, #14665, #32818, #76326, #199687, #184514, #466, #46994, #62141, #123805, #183527, #168343, #108653, #155161, #136030, #121833, #197704, #59170, #120839, #44020, #28865, #90505, #152187, #13671, #137008, #45010, #51951, #66122, #5437, #48980, #174316, #83276, #112624, #144951, #67121, #35786, #19630, #79308, #95465, #189487, #97433, #191462, #140977, #110635, #172316, #52940, #159119, #128779, #64147, #20614, #81272, #142954, #2465, #98435, #82265, #160131, #50965, #190479, #114614, #6432, #33805, #143957, #3453, #68114, #4434, #36771, #141964, #21619, #125811, #113611, #129766, #175305, #176314, #37784, #156150, #126787, #127787, #157151, #96451, #17648, #18646, #80292, #187514, #65130, #188493, #49972, #111636, #173321, #34796, #158138, #146965, #11470, #132793, #131798, #22624, #179326, #39778, #130783, #101442, #56963, #38793, #192475, #10462, #115633, #53958, #134811, #117628, #148973, #7433, #164147, #24636, #86284, #145952, #41796, #40790, #103463, #194480, #72123, #196491, #149964, #177322, #102459, #8453, #73141, #147975, #180328, #85274, #165142, #69117, #133797, #26633, #118636, #57961, #55952, #119632, #70126, #9464, #100450, #163133, #88276, #162130, #23626, #25644, #193477, #54954, #181315, #116626, #99448, #84271, #178315, #71127, #161128, #87289, #195488, #166139, #122586, #183287, #74127, #44769, #229, #182298, #135798, #153925, #58935, #152922, #199442, #121592, #60910, #184273, #169081, #105443, #45756, #59924, #197469, #170088, #16415, #91232, #154917, #76082, #42794, #107408, #136767, #104456, #31582, #106422, #93232, #124577, #137758, #61897, #168103, #78062, #29600, #14418, #30587, #92239, #77078, #15419, #138747, #13436, #198453, #123567, #185262, #46754, #28627, #139730, #1219, #108413, #62897, #27641, #89282, #150972, #12466, #120604, #43778, #167127, #90264, #151947, #75100, #4202, #113375, #142722, #177827, #97197, #65880, #49730, #109406, #125577, #19397, #127554, #24145, #171085, #140736, #95229, #155910, #34562, #158883, #111398, #35550, #112390, #190235, #110398, #79063, #147483, #174081, #5195, #189255, #143716, #50731, #20373, #162639, #100954, #8973, #81046, #82021, #39297, #66877, #17406, #128539, #51712, #85797, #47752, #2225, #70642, #156915, #186273, #96218, #63907, #32576, #94229, #187275, #48745, #172080, #80061, #33567, #18412, #141731, #3221, #64895, #126556, #188256, #173083, #157907, #55462, #120124, #196990, #41306, #43294, #101971, #166649, #196004, #86796, #40297, #44290, #164652, #88793, #194000, #163652, #132308, #105948, #13937, #57477, #25154, #151474, #148483, #12964, #90768, #117133, #73646, #74628, #104962, #136294, #121113, #27146, #150486, #29130, #182807, #119149, #28150, #135317, #58456, #9974, #197970, #178827, #71634, #11981, #167633, #133300, #89790, #194991, #165648, #59440, #56468, #10970, #42308, #118146, #179836, #102967, #181815, #26147, #152452, #180831, #87789, #149474, #103969, #72643, #134318, #76602, #62415, #94750, #187785, #198965, #153444, #93757, #15937, #169609, #185786, #64420, #16928, #45283 ),
 ( #124087, #49255, #108930, #75604, #155438, #31107, #137283, #126089, #154443, #2743, #157429, #170610, #33094, #92755, #110913, #77596, #139267, #47273, #1747, #109924, #743, #32100, #46269, #78581, #140255, #63425, #125100, #61426, #172599, #34085, #186798, #95744, #48269, #60432, #171606, #156431, #17931, #79585, #141254, #122106, #183796, #168609, #106936, #30109, #91749, #14942, #138279, #199961, #123097, #184783, #107924, #52226, #160410, #54234, #3728, #173601, #111913, #115905, #37057, #68388, #127066, #83549, #144233, #5717, #65405, #161407, #98716, #22899, #113882, #191739, #177595, #69394, #35070, #21899, #66402, #131062, #67395, #99723, #4713, #84545, #188774, #53223, #146222, #38067, #192751, #175580, #39063, #189766, #129051, #96725, #159398, #7710, #158413, #19902, #145228, #128064, #50257, #100720, #174593, #18923, #81544, #143230, #51238, #80568, #6710, #112899, #142243, #130040, #20893, #36058, #82551, #176593, #97707, #190752, #114899, #178589, #179600, #72403, #166419, #197737, #163418, #149248, #181583, #74397, #85557, #40053, #180601, #102735, #56229, #134080, #151242, #103739, #132071, #150254, #71403, #193760, #10739, #135086, #87561, #11748, #88555, #27913, #86561, #55228, #120872, #73415, #43061, #42075, #119898, #165419, #196762, #136062, #59203, #182572, #195769, #26912, #12731, #58229, #116897, #57243, #104727, #89556, #23903, #101730, #44055, #133067, #162400, #118917, #24915, #147242, #8734, #70403, #148245, #9739, #117911, #194757, #41072, #164424, #25917, #16686, #94503, #105715, #124855, #63176, #28898, #93511, #170366, #14701, #78336, #75371, #140010, #169360, #60198, #13704, #17684, #138040, #62175, #167402, #137041, #90538, #79342, #187547, #30870, #198732, #186555, #121868, #48027, #64180, #152220, #47030, #109684, #1498, #171365, #156185, #503, #123839, #2499, #141012, #92516, #32853, #108688, #31858, #183560, #125846, #45046, #106704, #185537, #168378, #29873, #91510, #153197, #139023, #76363, #199721, #184547, #15695, #61187, #122859, #46027, #155197, #107683, #154206, #77356, #69147, #18678, #143989, #37817, #172349, #144983, #141997, #82298, #114647, #130814, #127817, #159149, #95498, #65162, #34827, #5470, #158170, #67152, #35817, #49014, #66154, #20645, #52970, #84302, #50004, #97463, #68144, #161159, #33838, #126821, #128810, #189522, #142987, #190509, #99478, #51983, #80324, #36803, #19662, #3485, #113641, #21653, #174347, #98468, #175336, #176345, #173357, #188527, #7463, #160162, #129795, #83306, #6463, #191492, #22655, #145981, #110669, #157184, #111669, #96482, #81303, #4465, #50995, #112656, #56992, #40819, #53989, #85303, #133828, #178345, #164176, #71157, #146995, #26664, #118666, #196520, #41826, #149994, #39807, #25674, #180357, #73171, #11500, #10492, #165171, #192505, #103493, #88306, #177352, #72152, #149003, #101473, #195519, #23655, #134841, #132823, #8482, #162159, #115662, #24666, #87319, #100480, #70157, #38822, #131827, #193508, #54985, #163163, #116654, #55982, #86316, #148004, #9494, #194509, #117659, #179356, #102489, #161813, #67805, #129460, #69804, #23308, #159810, #7118, #175998, #37468, #80972, #192156, #34487, #54631, #191159, #128464, #52632, #82962, #68800, #144639, #22307, #65806, #114296, #100132, #99129, #84952, #83958, #160819, #36455, #96145, #112314, #6122, #145638, #8126, #157834, #127474, #189180, #131472, #130459, #53637, #142648, #115314, #98113, #21305, #19325, #177006, #38475, #146634, #193159, #173008, #4127, #50653, #174004, #35475, #20296, #97124, #158807, #81944, #143635, #5119, #66801, #190160, #51636, #113300, #174991, #145849, #193376, #69015, #19531, #82161, #142858, #21516, #7331, #98329, #22522, #99345, #177220, #97334, #66021, #131695, #161028, #192375, #52840, #130681, #191362, #84169, #146858, #85170, #54852, #6334, #37680, #23524, #53858, #4337, #68014, #115532, #114509, #34696 ),
 ( #173220, #176211, #67020, #96353, #162028, #51851, #100349, #158040, #129666, #38693, #190376, #8351, #113510, #175205, #160029, #70026, #81176, #36670, #83177, #143857, #128679, #144851, #127689, #189389, #159020, #50866, #112524, #174218, #35686, #20513, #5336, #132694, #26533, #73036, #195385, #134708, #196391, #42691, #179222, #57859, #133692, #9362, #43676, #90163, #165040, #28527, #149861, #116526, #119532, #10362, #178214, #105338, #56863, #167025, #198348, #11366, #74026, #118538, #151846, #180227, #41697, #103362, #104352, #150869, #88177, #181215, #87190, #72019, #166036, #27536, #89177, #102357, #13336, #75001, #12363, #136666, #135696, #39678, #197368, #58833, #120500, #182191, #101340, #163029, #24535, #71027, #86186, #147876, #194383, #55850, #117524, #40688, #164047, #25546, #148871, #93132, #1120, #97839, #44668, #14320, #152826, #159527, #77965, #109305, #168007, #124475, #185159, #46649, #106321, #4848, #139632, #66533, #154817, #32477, #21025, #113030, #75985, #62794, #107307, #174722, #108309, #140637, #45656, #128196, #29503, #94130, #189894, #78962, #36185, #16315, #82679, #186172, #47654, #59822, #128, #51369, #137658, #199345, #170984, #168979, #91136, #144363, #15317, #121492, #60810, #122483, #30484, #183186, #155809, #92135, #184174, #17307, #61797, #153822, #123467, #76976, #138647, #169989, #31480, #39193, #38200, #129183, #85689, #146357, #37190, #7844, #163547, #145361, #98847, #117027, #22031, #116035, #162531, #84678, #24035, #147376, #132201, #68522, #8865, #23033, #160542, #133195, #179733, #54363, #118043, #100849, #5850, #70532, #99856, #67526, #194886, #69531, #56360, #87687, #193892, #25047, #131195, #41203, #192885, #177724, #55357, #178722, #40184, #101864, #86690, #176727, #161540, #148374, #9869, #71528, #191873, #102864, #164549, #26042, #190881, #52357, #114013, #175711, #83683, #6843, #130176, #53357, #115034, #198866, #42207, #167536, #76503, #105849, #138179, #60333, #29031, #12865, #72538, #88691, #182705, #90671, #184683, #134215, #103867, #165548, #46166, #152353, #122007, #57376, #13838, #74530, #136195, #195901, #91650, #75505, #153339, #44190, #183698, #107820, #199861, #27045, #137178, #196891, #61326, #197870, #30012, #135219, #14840, #119049, #45185, #122997, #168514, #169504, #106839, #31003, #149372, #10868, #180731, #89689, #150387, #11883, #73546, #58358, #120025, #181710, #43191, #104860, #166549, #28048, #151374, #59337, #121007, #143130, #187688, #51138, #18825, #49158, #92652, #32996, #81444, #185678, #31997, #157330, #1644, #123980, #34974, #48167, #174492, #77493, #47168, #140152, #4610, #125990, #125001, #15834, #172499, #94650, #108827, #156330, #50154, #93654, #170506, #3627, #155339, #2646, #110816, #171507, #33986, #95642, #80470, #16828, #142143, #109824, #78479, #19803, #66302, #141157, #127962, #65306, #154341, #126965, #186696, #139163, #189665, #17830, #112799, #640, #188674, #111813, #79488, #62310, #64323, #173501, #96627, #158315, #63322, #176493, #114800, #6613, #191642, #37969, #84449, #177500, #21800, #163321, #148152, #23807, #24818, #54136, #117814, #115810, #53122, #38969, #146127, #131976, #7612, #85458, #128954, #100625, #86467, #192653, #9644, #147147, #162307, #99627, #159294, #175482, #69297, #8635, #71310, #20791, #190654, #52130, #132973, #70307, #193661, #144134, #55132, #161309, #22803, #82446, #178494, #116802, #39960, #130963, #101631, #194663, #56132, #113787, #35959, #83452, #97606, #5616, #67295, #145130, #36954, #98616, #160310, #68292, #129943, #102644, #57146, #197645, #119807, #73320, #89461, #152129, #199624, #75279, #25823, #88457, #149155, #27819, #13611, #104633, #28804, #105620, #183465, #103647, #72306, #137940, #167308, #198638, #59111, #136949, #120776, #90444, #153102, #91415, #61091, #12640, #43958, #29779, #60104, #10645, #74307, #121772, #182477, #40975, #195675, #44951, #150153 ),
 ( #106607, #168282, #179507, #14606, #76262, #164329, #87468, #133984, #11654, #118823, #180508, #41981, #42970, #165325, #26817, #134991, #196670, #135974, #58139, #181492, #166322, #151149, #4375, #186455, #92419, #141902, #154105, #3393, #81212, #122764, #64081, #65068, #33742, #126725, #111573, #17585, #79245, #19568, #173257, #109585, #157088, #125751, #187451, #30772, #188429, #184453, #15599, #140916, #34732, #45933, #18584, #77257, #156088, #49907, #107588, #1400, #32756, #169266, #138926, #108591, #2403, #31762, #48919, #171268, #142893, #139910, #94407, #96390, #158077, #123743, #110573, #406, #172254, #62078, #185442, #170268, #95402, #93411, #80231, #46932, #155097, #63080, #16591, #78239, #124759, #47931, #52878, #85209, #178252, #189428, #143893, #84206, #6371, #160067, #176249, #38729, #86221, #162065, #112561, #175242, #35724, #114550, #100387, #191401, #115570, #192413, #70064, #190413, #159057, #24572, #53895, #146898, #145886, #23561, #7369, #177257, #39713, #101376, #147911, #99382, #130720, #116563, #8389, #97371, #161065, #131732, #69054, #127726, #82201, #193414, #36707, #54889, #37720, #5374, #163066, #66059, #50903, #174256, #20551, #21554, #67058, #128716, #51889, #113548, #98369, #83214, #144889, #68051, #129705, #22560, #197404, #74062, #118572, #120536, #179260, #43714, #73071, #164082, #117560, #121528, #41732, #166072, #71063, #40725, #9397, #183223, #91172, #134743, #102394, #28563, #25581, #90200, #168042, #132729, #150906, #151883, #182229, #13373, #198384, #104389, #27574, #106358, #59861, #196425, #105375, #12400, #135733, #87225, #75037, #194417, #148907, #89213, #44704, #55887, #167062, #10397, #42727, #136703, #72054, #88211, #133728, #195420, #58870, #149895, #103396, #119567, #29539, #56898, #180262, #165074, #26568, #11402, #57895, #181250, #78001, #2164, #78998, #156852, #77012, #45692, #111331, #63843, #165, #64835, #186210, #185196, #76021, #32514, #93170, #184210, #154855, #110335, #92172, #107343, #125515, #169016, #62831, #109341, #31517, #171023, #94166, #140672, #15356, #155845, #170027, #30521, #80002, #126497, #1156, #188195, #47691, #152861, #17342, #46687, #14356, #141671, #16353, #3162, #34500, #187212, #172016, #139668, #49667, #124514, #48683, #33505, #95164, #18347, #173021, #137696, #123503, #108347, #199381, #60845, #122520, #138684, #153858, #61833, #83970, #84965, #114309, #178008, #176011, #51649, #37480, #6134, #192170, #67817, #145650, #189193, #99142, #23321, #52645, #146647, #7131, #160831, #159823, #19339, #35488, #129472, #22319, #131485, #80986, #50667, #112327, #193172, #68814, #130473, #4140, #53650, #21318, #82976, #142661, #38488, #115328, #100145, #191171, #177019, #54644, #8141, #174017, #161826, #143649, #69818, #144652, #116319, #81957, #96158, #157847, #65819, #127488, #97138, #158821, #20309, #5132, #66815, #128477, #190173, #113313, #175005, #36469, #98126, #164838, #120302, #25342, #43477, #9158, #12165, #105145, #58636, #89971, #134504, #198151, #165834, #196190, #39475, #180025, #28332, #132493, #179015, #104152, #148670, #70824, #181995, #136471, #41493, #181015, #88977, #86983, #151651, #72834, #71818, #162822, #119329, #103157, #194182, #26334, #197171, #40483, #55646, #150667, #117319, #149662, #57662, #118332, #42489, #27331, #73830, #102155, #135500, #56659, #163841, #166831, #13146, #87974, #74809, #59621, #101136, #121294, #133486, #24331, #85981, #11160, #147670, #10158, #195178, #140437, #200131, #110106, #123269, #61600, #169788, #109108, #17108, #184960, #46444, #153621, #138450, #108104, #31281, #124272, #168781, #171785, #94932, #170787, #33273, #920, #64602, #62594, #92932, #185968, #154619, #78760, #16113, #32277, #75783, #47452, #156617, #139438, #18112, #93934, #155613, #77771, #106125, #122282, #1927, #63606, #79766, #167809, #137461, #199140, #141437, #125282, #186979, #90939, #2924, #182987 ),
 ( #48449, #44471, #152626, #29309, #14116, #60607, #183970, #45457, #107111, #30284, #91929, #15117, #76778, #176773, #80749, #67573, #173785, #38245, #51415, #6889, #112095, #130224, #95924, #98894, #191920, #145407, #99900, #21074, #84724, #52405, #82730, #126266, #66578, #115081, #19100, #65586, #190928, #35252, #157609, #68567, #23079, #128243, #129231, #175762, #96905, #161585, #159577, #158589, #49433, #5897, #189940, #142427, #113075, #83728, #127246, #3906, #37238, #188959, #36233, #144411, #4896, #114064, #160588, #22077, #50436, #53403, #143408, #20078, #146402, #7892, #174767, #187963, #111094, #172784, #34265, #81722, #97885, #61117, #148420, #199651, #154135, #164594, #29805, #86735, #122791, #9915, #71574, #56408, #195947, #106635, #133240, #194932, #40234, #25093, #118089, #179779, #10913, #55402, #184480, #45959, #60131, #107614, #87732, #69577, #149417, #41248, #72586, #102910, #168308, #26088, #121799, #162578, #134260, #169292, #30798, #183492, #92447, #44976, #91441, #131243, #153129, #192931, #24082, #8911, #14632, #178768, #100894, #76291, #54409, #137969, #116081, #177769, #117072, #39238, #85737, #101910, #147424, #70579, #132247, #193939, #163592, #173286, #155126, #108619, #126754, #31790, #125778, #172282, #94435, #33771, #95431, #141929, #78267, #157115, #32783, #170297, #142919, #189453, #64112, #127752, #48947, #15627, #18612, #109613, #77284, #4401, #156116, #66086, #97397, #110600, #34760, #17614, #50931, #79273, #140944, #2432, #3420, #49937, #187480, #80259, #186485, #171297, #65096, #188456, #111602, #1429, #112588, #174282, #96418, #35751, #158104, #138954, #19596, #81238, #433, #62107, #123770, #185470, #46960, #93439, #16619, #139939, #63108, #124786, #47961, #115599, #22588, #82230, #98399, #192442, #100415, #194444, #143920, #113575, #51916, #55915, #177288, #8420, #67085, #23591, #84236, #145914, #5401, #101405, #38758, #163099, #53924, #131761, #117589, #9425, #175269, #162096, #6399, #71090, #7399, #39743, #144916, #24602, #128744, #193443, #86249, #178280, #54919, #69083, #70092, #36735, #85239, #147939, #146930, #132757, #116591, #179290, #130750, #190440, #160096, #40755, #159083, #20578, #21582, #83241, #68078, #129732, #191429, #52905, #114581, #176279, #37750, #99411, #161093, #44736, #120567, #106392, #197435, #75068, #137730, #152892, #56929, #43746, #149927, #14388, #27606, #183255, #88242, #168073, #72086, #136734, #29571, #121560, #76054, #58901, #60878, #28594, #182261, #102424, #42758, #91202, #195455, #41762, #167093, #11434, #133760, #199414, #122555, #104421, #105409, #151915, #73105, #184245, #135764, #134774, #25609, #90231, #166104, #118604, #89246, #59893, #103427, #180294, #13404, #165106, #12431, #198416, #181281, #164111, #87253, #148938, #26599, #10428, #119598, #196457, #57927, #150938, #74094, #157881, #79031, #45726, #125549, #139703, #107379, #34533, #124548, #173056, #127523, #140707, #3194, #62866, #96192, #186245, #47723, #32546, #172050, #80034, #109374, #171056, #16387, #1189, #94199, #155879, #187245, #31552, #19370, #81019, #33537, #142694, #63878, #169051, #48715, #17376, #110368, #2197, #30557, #95200, #64867, #156886, #4174, #18383, #141703, #126529, #188228, #49701, #111367, #65852, #78034, #92209, #153894, #15390, #77047, #93204, #138718, #199, #61868, #123537, #185231, #46722, #108385, #170062, #154889, #99178, #85003, #160867, #38526, #81993, #7169, #116356, #145687, #178045, #100182, #68852, #52681, #112363, #128513, #22357, #130511, #24369, #174054, #143686, #5168, #86020, #192207, #161864, #97171, #53689, #114344, #176048, #35523, #131524, #115367, #193209, #84009, #23358, #147709, #39513, #66851, #177056, #36506, #101173, #37516, #69856, #175041, #54683, #158856, #146684, #162861, #8180, #9196, #70862, #189227, #50705, #20344, #190208, #129506, #51687, #113349, #98160, #159861, #21354, #83011 ) ),
 .UNSPECIFIED., .T., .F., .F. ) 
 B_SPLINE_SURFACE_WITH_KNOTS ( ( 4, 3, 4 ),
 ( 3, 2, 2, 2, 2, 2, 2, 2, 2, 2, 2, 2, 2, 2, 2, 2, 2, 2, 2, 2, 2, 2, 2, 2, 2, 2, 2, 2, 2, 2, 2, 2, 2, 2, 2, 2, 2, 2, 2, 2, 2, 2, 2, 2, 2, 2, 2, 2, 2, 2, 2, 2, 2, 2, 2, 2, 2, 2, 2, 2, 2, 2, 2, 2, 2, 2, 2, 2, 2, 2, 2, 2, 2, 2, 2, 2, 2, 2, 2, 2, 2, 2, 2, 2, 2, 2, 2, 2, 2, 2, 2, 2, 2, 2, 2, 2, 2, 2, 2, 2, 2, 2, 2, 2, 2, 2, 2, 2, 2, 2, 2, 2, 2, 2, 2, 2, 2, 2, 2, 2, 2, 2, 2, 2, 2, 2, 2, 2, 2, 2, 2, 2, 2, 2, 2, 2, 2, 2, 2, 2, 2, 2, 2, 2, 2, 2, 2, 2, 2, 2, 2, 2, 2, 2, 2, 2, 2, 2, 2, 2, 2, 2, 2, 2, 2, 2, 2, 2, 2, 2, 2, 2, 2, 2, 2, 2, 2, 2, 2, 2, 2, 2, 2, 2, 2, 2, 2, 2, 2, 2, 2, 2, 2, 2, 2, 2, 2, 2, 2, 2, 2, 2, 2, 2, 2, 2, 2, 2, 2, 2, 2, 2, 2, 2, 2, 2, 2, 2, 2, 2, 2, 2, 2, 2, 2, 2, 2, 2, 3 ),
 ( 0.000000000000000000, 0.5000000000000000000, 1.000000000000000000 ),
 ( 0.000000000000000000, 0.004385964912280701511, 0.008771929824561403022, 0.01315789473684210453, 0.01754385964912280604, 0.02192982456140350755, 0.02631578947368420907, 0.03070175438596491058, 0.03508771929824561209, 0.03947368421052631360, 0.04385964912280701511, 0.04824561403508771662, 0.05263157894736841813, 0.05701754385964911964, 0.06140350877192982115, 0.06578947368421052266, 0.07017543859649122417, 0.07456140350877192569, 0.07894736842105262720, 0.08333333333333332871, 0.08771929824561403022, 0.09210526315789473173, 0.09649122807017543324, 0.1008771929824561348, 0.1052631578947368363, 0.1096491228070175378, 0.1140350877192982393, 0.1184210526315789408, 0.1228070175438596423, 0.1271929824561403577, 0.1315789473684210453, 0.1359649122807017607, 0.1403508771929824483, 0.1447368421052631637, 0.1491228070175438514, 0.1535087719298245668, 0.1578947368421052544, 0.1622807017543859698, 0.1666666666666666574, 0.1710526315789473728, 0.1754385964912280604, 0.1798245614035087758, 0.1842105263157894635, 0.1885964912280701788, 0.1929824561403508665, 0.1973684210526315819, 0.2017543859649122695, 0.2061403508771929849, 0.2105263157894736725, 0.2149122807017543879, 0.2192982456140350755, 0.2236842105263157909, 0.2280701754385964786, 0.2324561403508771940, 0.2368421052631578816, 0.2412280701754385970, 0.2456140350877192846, 0.2500000000000000000, 0.2543859649122807154, 0.2587719298245614308, 0.2631578947368420907, 0.2675438596491228060, 0.2719298245614035214, 0.2763157894736842368, 0.2807017543859648967, 0.2850877192982456121, 0.2894736842105263275, 0.2938596491228070429, 0.2982456140350877027, 0.3026315789473684181, 0.3070175438596491335, 0.3114035087719298489, 0.3157894736842105088, 0.3201754385964912242, 0.3245614035087719396, 0.3289473684210526550, 0.3333333333333333148, 0.3377192982456140302, 0.3421052631578947456, 0.3464912280701754610, 0.3508771929824561209, 0.3552631578947368363, 0.3596491228070175517, 0.3640350877192982670, 0.3684210526315789269, 0.3728070175438596423, 0.3771929824561403577, 0.3815789473684210731, 0.3859649122807017330, 0.3903508771929824483, 0.3947368421052631637, 0.3991228070175438791, 0.4035087719298245390, 0.4078947368421052544, 0.4122807017543859698, 0.4166666666666666852, 0.4210526315789473450, 0.4254385964912280604, 0.4298245614035087758, 0.4342105263157894912, 0.4385964912280701511, 0.4429824561403508665, 0.4473684210526315819, 0.4517543859649122973, 0.4561403508771929571, 0.4605263157894736725, 0.4649122807017543879, 0.4692982456140351033, 0.4736842105263157632, 0.4780701754385964786, 0.4824561403508771940, 0.4868421052631579093, 0.4912280701754385692, 0.4956140350877192846, 0.5000000000000000000, 0.5043859649122807154, 0.5087719298245614308, 0.5131578947368421462, 0.5175438596491228616, 0.5219298245614034659, 0.5263157894736841813, 0.5307017543859648967, 0.5350877192982456121, 0.5394736842105263275, 0.5438596491228070429, 0.5482456140350877583, 0.5526315789473684736, 0.5570175438596490780, 0.5614035087719297934, 0.5657894736842105088, 0.5701754385964912242, 0.5745614035087719396, 0.5789473684210526550, 0.5833333333333333703, 0.5877192982456140857, 0.5921052631578946901, 0.5964912280701754055, 0.6008771929824561209, 0.6052631578947368363, 0.6096491228070175517, 0.6140350877192982670, 0.6184210526315789824, 0.6228070175438596978, 0.6271929824561403022, 0.6315789473684210176, 0.6359649122807017330, 0.6403508771929824483, 0.6447368421052631637, 0.6491228070175438791, 0.6535087719298245945, 0.6578947368421053099, 0.6622807017543859143, 0.6666666666666666297, 0.6710526315789473450, 0.6754385964912280604, 0.6798245614035087758, 0.6842105263157894912, 0.6885964912280702066, 0.6929824561403509220, 0.6973684210526315264, 0.7017543859649122417, 0.7061403508771929571, 0.7105263157894736725, 0.7149122807017543879, 0.7192982456140351033, 0.7236842105263158187, 0.7280701754385965341, 0.7324561403508771384, 0.7368421052631578538, 0.7412280701754385692, 0.7456140350877192846, 0.7500000000000000000, 0.7543859649122807154, 0.7587719298245614308, 0.7631578947368421462, 0.7675438596491228616, 0.7719298245614034659, 0.7763157894736841813, 0.7807017543859648967, 0.7850877192982456121, 0.7894736842105263275, 0.7938596491228070429, 0.7982456140350877583, 0.8026315789473684736, 0.8070175438596490780, 0.8114035087719297934, 0.8157894736842105088, 0.8201754385964912242, 0.8245614035087719396, 0.8289473684210526550, 0.8333333333333333703, 0.8377192982456140857, 0.8421052631578946901, 0.8464912280701754055, 0.8508771929824561209, 0.8552631578947368363, 0.8596491228070175517, 0.8640350877192982670, 0.8684210526315789824, 0.8728070175438596978, 0.8771929824561403022, 0.8815789473684210176, 0.8859649122807017330, 0.8903508771929824483, 0.8947368421052631637, 0.8991228070175438791, 0.9035087719298245945, 0.9078947368421053099, 0.9122807017543859143, 0.9166666666666666297, 0.9210526315789473450, 0.9254385964912280604, 0.9298245614035087758, 0.9342105263157894912, 0.9385964912280702066, 0.9429824561403509220, 0.9473684210526315264, 0.9517543859649122417, 0.9561403508771929571, 0.9605263157894736725, 0.9649122807017543879, 0.9692982456140351033, 0.9736842105263158187, 0.9780701754385965341, 0.9824561403508771384, 0.9868421052631578538, 0.9912280701754385692, 0.9956140350877192846, 1.000000000000000000 ),
 .UNSPECIFIED. ) 
 GEOMETRIC_REPRESENTATION_ITEM ( )  RATIONAL_B_SPLINE_SURFACE ( (
 ( 1.000000000000000000, 0.9659258262890683122, 1.000000000000000000, 0.9659258262890683122, 1.000000000000000000, 0.9659258262890683122, 1.000000000000000000, 0.9659258262890683122, 1.000000000000000000, 0.9659258262890683122, 1.000000000000000000, 0.9659258262890683122, 1.000000000000000000, 0.9659258262890683122, 1.000000000000000000, 0.9659258262890683122, 1.000000000000000000, 0.9659258262890683122, 1.000000000000000000, 0.9659258262890683122, 1.000000000000000000, 0.9659258262890683122, 1.000000000000000000, 0.9659258262890683122, 1.000000000000000000, 0.9659258262890683122, 1.000000000000000000, 0.9659258262890683122, 1.000000000000000000, 0.9659258262890683122, 1.000000000000000000, 0.9659258262890683122, 1.000000000000000000, 0.9659258262890683122, 1.000000000000000000, 0.9659258262890683122, 1.000000000000000000, 0.9659258262890683122, 1.000000000000000000, 0.9659258262890683122, 1.000000000000000000, 0.9659258262890683122, 1.000000000000000000, 0.9659258262890683122, 1.000000000000000000, 0.9659258262890683122, 1.000000000000000000, 0.9659258262890683122, 1.000000000000000000, 0.9659258262890683122, 1.000000000000000000, 0.9659258262890683122, 1.000000000000000000, 0.9659258262890683122, 1.000000000000000000, 0.9659258262890683122, 1.000000000000000000, 0.9659258262890683122, 1.000000000000000000, 0.9659258262890683122, 1.000000000000000000, 0.9659258262890683122, 1.000000000000000000, 0.9659258262890683122, 1.000000000000000000, 0.9659258262890683122, 1.000000000000000000, 0.9659258262890683122, 1.000000000000000000, 0.9659258262890683122, 1.000000000000000000, 0.9659258262890683122, 1.000000000000000000, 0.9659258262890683122, 1.000000000000000000, 0.9659258262890683122, 1.000000000000000000, 0.9659258262890683122, 1.000000000000000000, 0.9659258262890683122, 1.000000000000000000, 0.9659258262890683122, 1.000000000000000000, 0.9659258262890683122, 1.000000000000000000, 0.9659258262890683122, 1.000000000000000000, 0.9659258262890683122, 1.000000000000000000, 0.9659258262890683122, 1.000000000000000000, 0.9659258262890683122, 1.000000000000000000, 0.9659258262890683122, 1.000000000000000000, 0.9659258262890683122, 1.000000000000000000, 0.9659258262890683122, 1.000000000000000000, 0.9659258262890683122, 1.000000000000000000, 0.9659258262890683122, 1.000000000000000000, 0.9659258262890683122, 1.000000000000000000, 0.9659258262890683122, 1.000000000000000000, 0.9659258262890683122, 1.000000000000000000, 0.9659258262890683122, 1.000000000000000000, 0.9659258262890683122, 1.000000000000000000, 0.9659258262890683122, 1.000000000000000000, 0.9659258262890683122, 1.000000000000000000, 0.9659258262890683122, 1.000000000000000000, 0.9659258262890683122, 1.000000000000000000, 0.9659258262890683122, 1.000000000000000000, 0.9659258262890683122, 1.000000000000000000, 0.9659258262890683122, 1.000000000000000000, 0.9659258262890683122, 1.000000000000000000, 0.9659258262890683122, 1.000000000000000000, 0.9659258262890683122, 1.000000000000000000, 0.9659258262890683122, 1.000000000000000000, 0.9659258262890683122, 1.000000000000000000, 0.9659258262890683122, 1.000000000000000000, 0.9659258262890683122, 1.000000000000000000, 0.9659258262890683122, 1.000000000000000000, 0.9659258262890683122, 1.000000000000000000, 0.9659258262890683122, 1.000000000000000000, 0.9659258262890683122, 1.000000000000000000, 0.9659258262890683122, 1.000000000000000000, 0.9659258262890683122, 1.000000000000000000, 0.9659258262890683122, 1.000000000000000000, 0.9659258262890683122, 1.000000000000000000, 0.9659258262890683122, 1.000000000000000000, 0.9659258262890683122, 1.000000000000000000, 0.9659258262890683122, 1.000000000000000000, 0.9659258262890683122, 1.000000000000000000, 0.9659258262890683122, 1.000000000000000000, 0.9659258262890683122, 1.000000000000000000, 0.9659258262890683122, 1.000000000000000000, 0.9659258262890683122, 1.000000000000000000, 0.9659258262890683122, 1.000000000000000000, 0.9659258262890683122, 1.000000000000000000, 0.9659258262890683122, 1.000000000000000000, 0.9659258262890683122, 1.000000000000000000, 0.9659258262890683122, 1.000000000000000000, 0.9659258262890683122, 1.000000000000000000, 0.9659258262890683122, 1.000000000000000000, 0.9659258262890683122, 1.000000000000000000, 0.9659258262890683122, 1.000000000000000000, 0.9659258262890683122, 1.000000000000000000, 0.9659258262890683122, 1.000000000000000000, 0.9659258262890683122, 1.000000000000000000, 0.9659258262890683122, 1.000000000000000000, 0.9659258262890683122, 1.000000000000000000, 0.9659258262890683122, 1.000000000000000000, 0.9659258262890683122, 1.000000000000000000, 0.9659258262890683122, 1.000000000000000000, 0.9659258262890683122, 1.000000000000000000, 0.9659258262890683122, 1.000000000000000000, 0.9659258262890683122, 1.000000000000000000, 0.9659258262890683122, 1.000000000000000000, 0.9659258262890683122, 1.000000000000000000, 0.9659258262890683122, 1.000000000000000000, 0.9659258262890683122, 1.000000000000000000, 0.9659258262890683122, 1.000000000000000000, 0.9659258262890683122, 1.000000000000000000, 0.9659258262890683122, 1.000000000000000000, 0.9659258262890683122, 1.000000000000000000, 0.9659258262890683122, 1.000000000000000000, 0.9659258262890683122, 1.000000000000000000, 0.9659258262890683122, 1.000000000000000000, 0.9659258262890683122, 1.000000000000000000, 0.9659258262890683122, 1.000000000000000000, 0.9659258262890683122, 1.000000000000000000, 0.9659258262890683122, 1.000000000000000000, 0.9659258262890683122, 1.000000000000000000, 0.9659258262890683122, 1.000000000000000000, 0.9659258262890683122, 1.000000000000000000, 0.9659258262890683122, 1.000000000000000000, 0.9659258262890683122, 1.000000000000000000, 0.9659258262890683122, 1.000000000000000000, 0.9659258262890683122, 1.000000000000000000, 0.9659258262890683122, 1.000000000000000000, 0.9659258262890683122, 1.000000000000000000, 0.9659258262890683122, 1.000000000000000000, 0.9659258262890683122, 1.000000000000000000, 0.9659258262890683122, 1.000000000000000000, 0.9659258262890683122, 1.000000000000000000, 0.9659258262890683122, 1.000000000000000000, 0.9659258262890683122, 1.000000000000000000, 0.9659258262890683122, 1.000000000000000000, 0.9659258262890683122, 1.000000000000000000, 0.9659258262890683122, 1.000000000000000000, 0.9659258262890683122, 1.000000000000000000, 0.9659258262890683122, 1.000000000000000000, 0.9659258262890683122, 1.000000000000000000, 0.9659258262890683122, 1.000000000000000000, 0.9659258262890683122, 1.000000000000000000, 0.9659258262890683122, 1.000000000000000000, 0.9659258262890683122, 1.000000000000000000, 0.9659258262890683122, 1.000000000000000000, 0.9659258262890683122, 1.000000000000000000, 0.9659258262890683122, 1.000000000000000000, 0.9659258262890683122, 1.000000000000000000, 0.9659258262890683122, 1.000000000000000000, 0.9659258262890683122, 1.000000000000000000, 0.9659258262890683122, 1.000000000000000000, 0.9659258262890683122, 1.000000000000000000, 0.9659258262890683122, 1.000000000000000000, 0.9659258262890683122, 1.000000000000000000, 0.9659258262890683122, 1.000000000000000000, 0.9659258262890683122, 1.000000000000000000, 0.9659258262890683122, 1.000000000000000000, 0.9659258262890683122, 1.000000000000000000, 0.9659258262890683122, 1.000000000000000000, 0.9659258262890683122, 1.000000000000000000, 0.9659258262890683122, 1.000000000000000000, 0.9659258262890683122, 1.000000000000000000, 0.9659258262890683122, 1.000000000000000000, 0.9659258262890683122, 1.000000000000000000, 0.9659258262890683122, 1.000000000000000000, 0.9659258262890683122, 1.000000000000000000, 0.9659258262890683122, 1.000000000000000000, 0.9659258262890683122, 1.000000000000000000, 0.9659258262890683122, 1.000000000000000000, 0.9659258262890683122, 1.000000000000000000, 0.9659258262890683122, 1.000000000000000000, 0.9659258262890683122, 1.000000000000000000, 0.9659258262890683122, 1.000000000000000000, 0.9659258262890683122, 1.000000000000000000, 0.9659258262890683122, 1.000000000000000000, 0.9659258262890683122, 1.000000000000000000, 0.9659258262890683122, 1.000000000000000000, 0.9659258262890683122, 1.000000000000000000, 0.9659258262890683122, 1.000000000000000000, 0.9659258262890683122, 1.000000000000000000, 0.9659258262890683122, 1.000000000000000000, 0.9659258262890683122, 1.000000000000000000, 0.9659258262890683122, 1.000000000000000000, 0.9659258262890683122, 1.000000000000000000, 0.9659258262890683122, 1.000000000000000000, 0.9659258262890683122, 1.000000000000000000, 0.9659258262890683122, 1.000000000000000000, 0.9659258262890683122, 1.000000000000000000, 0.9659258262890683122, 1.000000000000000000, 0.9659258262890683122, 1.000000000000000000, 0.9659258262890683122, 1.000000000000000000, 0.9659258262890683122, 1.000000000000000000, 0.9659258262890683122, 1.000000000000000000, 0.9659258262890683122, 1.000000000000000000, 0.9659258262890683122, 1.000000000000000000, 0.9659258262890683122, 1.000000000000000000, 0.9659258262890683122, 1.000000000000000000, 0.9659258262890683122, 1.000000000000000000, 0.9659258262890683122, 1.000000000000000000, 0.9659258262890683122, 1.000000000000000000, 0.9659258262890683122, 1.000000000000000000, 0.9659258262890683122, 1.000000000000000000, 0.9659258262890683122, 1.000000000000000000, 0.9659258262890683122, 1.000000000000000000, 0.9659258262890683122, 1.000000000000000000, 0.9659258262890683122, 1.000000000000000000, 0.9659258262890683122, 1.000000000000000000, 0.9659258262890683122, 1.000000000000000000, 0.9659258262890683122, 1.000000000000000000, 0.9659258262890683122, 1.000000000000000000, 0.9659258262890683122, 1.000000000000000000, 0.9659258262890683122, 1.000000000000000000, 0.9659258262890683122, 1.000000000000000000, 0.9659258262890683122, 1.000000000000000000, 0.9659258262890683122, 1.000000000000000000, 0.9659258262890683122, 1.000000000000000000, 0.9659258262890683122, 1.000000000000000000, 0.9659258262890683122, 1.000000000000000000, 0.9659258262890683122, 1.000000000000000000, 0.9659258262890683122, 1.000000000000000000, 0.9659258262890683122, 1.000000000000000000, 0.9659258262890683122, 1.000000000000000000, 0.9659258262890683122, 1.000000000000000000, 0.9659258262890683122, 1.000000000000000000, 0.9659258262890683122, 1.000000000000000000, 0.9659258262890683122, 1.000000000000000000),
 ( 0.3333333333333333703, 0.3219752754296894559, 0.3333333333333333703, 0.3219752754296894559, 0.3333333333333333703, 0.3219752754296894559, 0.3333333333333333703, 0.3219752754296894559, 0.3333333333333333703, 0.3219752754296894559, 0.3333333333333333703, 0.3219752754296894559, 0.3333333333333333703, 0.3219752754296894559, 0.3333333333333333703, 0.3219752754296894559, 0.3333333333333333703, 0.3219752754296894559, 0.3333333333333333703, 0.3219752754296894559, 0.3333333333333333703, 0.3219752754296894559, 0.3333333333333333703, 0.3219752754296894559, 0.3333333333333333703, 0.3219752754296894559, 0.3333333333333333703, 0.3219752754296894559, 0.3333333333333333703, 0.3219752754296894559, 0.3333333333333333703, 0.3219752754296894559, 0.3333333333333333703, 0.3219752754296894559, 0.3333333333333333703, 0.3219752754296894559, 0.3333333333333333703, 0.3219752754296894559, 0.3333333333333333703, 0.3219752754296894559, 0.3333333333333333703, 0.3219752754296894559, 0.3333333333333333703, 0.3219752754296894559, 0.3333333333333333703, 0.3219752754296894559, 0.3333333333333333703, 0.3219752754296894559, 0.3333333333333333703, 0.3219752754296894559, 0.3333333333333333703, 0.3219752754296894559, 0.3333333333333333703, 0.3219752754296894559, 0.3333333333333333703, 0.3219752754296894559, 0.3333333333333333703, 0.3219752754296894559, 0.3333333333333333703, 0.3219752754296894559, 0.3333333333333333703, 0.3219752754296894559, 0.3333333333333333703, 0.3219752754296894559, 0.3333333333333333703, 0.3219752754296894559, 0.3333333333333333703, 0.3219752754296894559, 0.3333333333333333703, 0.3219752754296894559, 0.3333333333333333703, 0.3219752754296894559, 0.3333333333333333703, 0.3219752754296894559, 0.3333333333333333703, 0.3219752754296894559, 0.3333333333333333703, 0.3219752754296894559, 0.3333333333333333703, 0.3219752754296894559, 0.3333333333333333703, 0.3219752754296894559, 0.3333333333333333703, 0.3219752754296894559, 0.3333333333333333703, 0.3219752754296894559, 0.3333333333333333703, 0.3219752754296894559, 0.3333333333333333703, 0.3219752754296894559, 0.3333333333333333703, 0.3219752754296894559, 0.3333333333333333703, 0.3219752754296894559, 0.3333333333333333703, 0.3219752754296894559, 0.3333333333333333703, 0.3219752754296894559, 0.3333333333333333703, 0.3219752754296894559, 0.3333333333333333703, 0.3219752754296894559, 0.3333333333333333703, 0.3219752754296894559, 0.3333333333333333703, 0.3219752754296894559, 0.3333333333333333703, 0.3219752754296894559, 0.3333333333333333703, 0.3219752754296894559, 0.3333333333333333703, 0.3219752754296894559, 0.3333333333333333703, 0.3219752754296894559, 0.3333333333333333703, 0.3219752754296894559, 0.3333333333333333703, 0.3219752754296894559, 0.3333333333333333703, 0.3219752754296894559, 0.3333333333333333703, 0.3219752754296894559, 0.3333333333333333703, 0.3219752754296894559, 0.3333333333333333703, 0.3219752754296894559, 0.3333333333333333703, 0.3219752754296894559, 0.3333333333333333703, 0.3219752754296894559, 0.3333333333333333703, 0.3219752754296894559, 0.3333333333333333703, 0.3219752754296894559, 0.3333333333333333703, 0.3219752754296894559, 0.3333333333333333703, 0.3219752754296894559, 0.3333333333333333703, 0.3219752754296894559, 0.3333333333333333703, 0.3219752754296894559, 0.3333333333333333703, 0.3219752754296894559, 0.3333333333333333703, 0.3219752754296894559, 0.3333333333333333703, 0.3219752754296894559, 0.3333333333333333703, 0.3219752754296894559, 0.3333333333333333703, 0.3219752754296894559, 0.3333333333333333703, 0.3219752754296894559, 0.3333333333333333703, 0.3219752754296894559, 0.3333333333333333703, 0.3219752754296894559, 0.3333333333333333703, 0.3219752754296894559, 0.3333333333333333703, 0.3219752754296894559, 0.3333333333333333703, 0.3219752754296894559, 0.3333333333333333703, 0.3219752754296894559, 0.3333333333333333703, 0.3219752754296894559, 0.3333333333333333703, 0.3219752754296894559, 0.3333333333333333703, 0.3219752754296894559, 0.3333333333333333703, 0.3219752754296894559, 0.3333333333333333703, 0.3219752754296894559, 0.3333333333333333703, 0.3219752754296894559, 0.3333333333333333703, 0.3219752754296894559, 0.3333333333333333703, 0.3219752754296894559, 0.3333333333333333703, 0.3219752754296894559, 0.3333333333333333703, 0.3219752754296894559, 0.3333333333333333703, 0.3219752754296894559, 0.3333333333333333703, 0.3219752754296894559, 0.3333333333333333703, 0.3219752754296894559, 0.3333333333333333703, 0.3219752754296894559, 0.3333333333333333703, 0.3219752754296894559, 0.3333333333333333703, 0.3219752754296894559, 0.3333333333333333703, 0.3219752754296894559, 0.3333333333333333703, 0.3219752754296894559, 0.3333333333333333703, 0.3219752754296894559, 0.3333333333333333703, 0.3219752754296894559, 0.3333333333333333703, 0.3219752754296894559, 0.3333333333333333703, 0.3219752754296894559, 0.3333333333333333703, 0.3219752754296894559, 0.3333333333333333703, 0.3219752754296894559, 0.3333333333333333703, 0.3219752754296894559, 0.3333333333333333703, 0.3219752754296894559, 0.3333333333333333703, 0.3219752754296894559, 0.3333333333333333703, 0.3219752754296894559, 0.3333333333333333703, 0.3219752754296894559, 0.3333333333333333703, 0.3219752754296894559, 0.3333333333333333703, 0.3219752754296894559, 0.3333333333333333703, 0.3219752754296894559, 0.3333333333333333703, 0.3219752754296894559, 0.3333333333333333703, 0.3219752754296894559, 0.3333333333333333703, 0.3219752754296894559, 0.3333333333333333703, 0.3219752754296894559, 0.3333333333333333703, 0.3219752754296894559, 0.3333333333333333703, 0.3219752754296894559, 0.3333333333333333703, 0.3219752754296894559, 0.3333333333333333703, 0.3219752754296894559, 0.3333333333333333703, 0.3219752754296894559, 0.3333333333333333703, 0.3219752754296894559, 0.3333333333333333703, 0.3219752754296894559, 0.3333333333333333703, 0.3219752754296894559, 0.3333333333333333703, 0.3219752754296894559, 0.3333333333333333703, 0.3219752754296894559, 0.3333333333333333703, 0.3219752754296894559, 0.3333333333333333703, 0.3219752754296894559, 0.3333333333333333703, 0.3219752754296894559, 0.3333333333333333703, 0.3219752754296894559, 0.3333333333333333703, 0.3219752754296894559, 0.3333333333333333703, 0.3219752754296894559, 0.3333333333333333703, 0.3219752754296894559, 0.3333333333333333703, 0.3219752754296894559, 0.3333333333333333703, 0.3219752754296894559, 0.3333333333333333703, 0.3219752754296894559, 0.3333333333333333703, 0.3219752754296894559, 0.3333333333333333703, 0.3219752754296894559, 0.3333333333333333703, 0.3219752754296894559, 0.3333333333333333703, 0.3219752754296894559, 0.3333333333333333703, 0.3219752754296894559, 0.3333333333333333703, 0.3219752754296894559, 0.3333333333333333703, 0.3219752754296894559, 0.3333333333333333703, 0.3219752754296894559, 0.3333333333333333703, 0.3219752754296894559, 0.3333333333333333703, 0.3219752754296894559, 0.3333333333333333703, 0.3219752754296894559, 0.3333333333333333703, 0.3219752754296894559, 0.3333333333333333703, 0.3219752754296894559, 0.3333333333333333703, 0.3219752754296894559, 0.3333333333333333703, 0.3219752754296894559, 0.3333333333333333703, 0.3219752754296894559, 0.3333333333333333703, 0.3219752754296894559, 0.3333333333333333703, 0.3219752754296894559, 0.3333333333333333703, 0.3219752754296894559, 0.3333333333333333703, 0.3219752754296894559, 0.3333333333333333703, 0.3219752754296894559, 0.3333333333333333703, 0.3219752754296894559, 0.3333333333333333703, 0.3219752754296894559, 0.3333333333333333703, 0.3219752754296894559, 0.3333333333333333703, 0.3219752754296894559, 0.3333333333333333703, 0.3219752754296894559, 0.3333333333333333703, 0.3219752754296894559, 0.3333333333333333703, 0.3219752754296894559, 0.3333333333333333703, 0.3219752754296894559, 0.3333333333333333703, 0.3219752754296894559, 0.3333333333333333703, 0.3219752754296894559, 0.3333333333333333703, 0.3219752754296894559, 0.3333333333333333703, 0.3219752754296894559, 0.3333333333333333703, 0.3219752754296894559, 0.3333333333333333703, 0.3219752754296894559, 0.3333333333333333703, 0.3219752754296894559, 0.3333333333333333703, 0.3219752754296894559, 0.3333333333333333703, 0.3219752754296894559, 0.3333333333333333703, 0.3219752754296894559, 0.3333333333333333703, 0.3219752754296894559, 0.3333333333333333703, 0.3219752754296894559, 0.3333333333333333703, 0.3219752754296894559, 0.3333333333333333703, 0.3219752754296894559, 0.3333333333333333703, 0.3219752754296894559, 0.3333333333333333703, 0.3219752754296894559, 0.3333333333333333703, 0.3219752754296894559, 0.3333333333333333703, 0.3219752754296894559, 0.3333333333333333703, 0.3219752754296894559, 0.3333333333333333703, 0.3219752754296894559, 0.3333333333333333703, 0.3219752754296894559, 0.3333333333333333703, 0.3219752754296894559, 0.3333333333333333703, 0.3219752754296894559, 0.3333333333333333703, 0.3219752754296894559, 0.3333333333333333703, 0.3219752754296894559, 0.3333333333333333703, 0.3219752754296894559, 0.3333333333333333703, 0.3219752754296894559, 0.3333333333333333703, 0.3219752754296894559, 0.3333333333333333703, 0.3219752754296894559, 0.3333333333333333703, 0.3219752754296894559, 0.3333333333333333703, 0.3219752754296894559, 0.3333333333333333703, 0.3219752754296894559, 0.3333333333333333703, 0.3219752754296894559, 0.3333333333333333703, 0.3219752754296894559, 0.3333333333333333703, 0.3219752754296894559, 0.3333333333333333703, 0.3219752754296894559, 0.3333333333333333703, 0.3219752754296894559, 0.3333333333333333703, 0.3219752754296894559, 0.3333333333333333703, 0.3219752754296894559, 0.3333333333333333703, 0.3219752754296894559, 0.3333333333333333703, 0.3219752754296894559, 0.3333333333333333703, 0.3219752754296894559, 0.3333333333333333703, 0.3219752754296894559, 0.3333333333333333703, 0.3219752754296894559, 0.3333333333333333703, 0.3219752754296894559, 0.3333333333333333703, 0.3219752754296894559, 0.3333333333333333703, 0.3219752754296894559, 0.3333333333333333703, 0.3219752754296894559, 0.3333333333333333703, 0.3219752754296894559, 0.3333333333333333703, 0.3219752754296894559, 0.3333333333333333703, 0.3219752754296894559, 0.3333333333333333703, 0.3219752754296894559, 0.3333333333333333703, 0.3219752754296894559, 0.3333333333333333703, 0.3219752754296894559, 0.3333333333333333703, 0.3219752754296894559, 0.3333333333333333703, 0.3219752754296894559, 0.3333333333333333703, 0.3219752754296894559, 0.3333333333333333703, 0.3219752754296894559, 0.3333333333333333703, 0.3219752754296894559, 0.3333333333333333703, 0.3219752754296894559, 0.3333333333333333703),
 ( 0.3333333333333333703, 0.3219752754296894559, 0.3333333333333333703, 0.3219752754296894559, 0.3333333333333333703, 0.3219752754296894559, 0.3333333333333333703, 0.3219752754296894559, 0.3333333333333333703, 0.3219752754296894559, 0.3333333333333333703, 0.3219752754296894559, 0.3333333333333333703, 0.3219752754296894559, 0.3333333333333333703, 0.3219752754296894559, 0.3333333333333333703, 0.3219752754296894559, 0.3333333333333333703, 0.3219752754296894559, 0.3333333333333333703, 0.3219752754296894559, 0.3333333333333333703, 0.3219752754296894559, 0.3333333333333333703, 0.3219752754296894559, 0.3333333333333333703, 0.3219752754296894559, 0.3333333333333333703, 0.3219752754296894559, 0.3333333333333333703, 0.3219752754296894559, 0.3333333333333333703, 0.3219752754296894559, 0.3333333333333333703, 0.3219752754296894559, 0.3333333333333333703, 0.3219752754296894559, 0.3333333333333333703, 0.3219752754296894559, 0.3333333333333333703, 0.3219752754296894559, 0.3333333333333333703, 0.3219752754296894559, 0.3333333333333333703, 0.3219752754296894559, 0.3333333333333333703, 0.3219752754296894559, 0.3333333333333333703, 0.3219752754296894559, 0.3333333333333333703, 0.3219752754296894559, 0.3333333333333333703, 0.3219752754296894559, 0.3333333333333333703, 0.3219752754296894559, 0.3333333333333333703, 0.3219752754296894559, 0.3333333333333333703, 0.3219752754296894559, 0.3333333333333333703, 0.3219752754296894559, 0.3333333333333333703, 0.3219752754296894559, 0.3333333333333333703, 0.3219752754296894559, 0.3333333333333333703, 0.3219752754296894559, 0.3333333333333333703, 0.3219752754296894559, 0.3333333333333333703, 0.3219752754296894559, 0.3333333333333333703, 0.3219752754296894559, 0.3333333333333333703, 0.3219752754296894559, 0.3333333333333333703, 0.3219752754296894559, 0.3333333333333333703, 0.3219752754296894559, 0.3333333333333333703, 0.3219752754296894559, 0.3333333333333333703, 0.3219752754296894559, 0.3333333333333333703, 0.3219752754296894559, 0.3333333333333333703, 0.3219752754296894559, 0.3333333333333333703, 0.3219752754296894559, 0.3333333333333333703, 0.3219752754296894559, 0.3333333333333333703, 0.3219752754296894559, 0.3333333333333333703, 0.3219752754296894559, 0.3333333333333333703, 0.3219752754296894559, 0.3333333333333333703, 0.3219752754296894559, 0.3333333333333333703, 0.3219752754296894559, 0.3333333333333333703, 0.3219752754296894559, 0.3333333333333333703, 0.3219752754296894559, 0.3333333333333333703, 0.3219752754296894559, 0.3333333333333333703, 0.3219752754296894559, 0.3333333333333333703, 0.3219752754296894559, 0.3333333333333333703, 0.3219752754296894559, 0.3333333333333333703, 0.3219752754296894559, 0.3333333333333333703, 0.3219752754296894559, 0.3333333333333333703, 0.3219752754296894559, 0.3333333333333333703, 0.3219752754296894559, 0.3333333333333333703, 0.3219752754296894559, 0.3333333333333333703, 0.3219752754296894559, 0.3333333333333333703, 0.3219752754296894559, 0.3333333333333333703, 0.3219752754296894559, 0.3333333333333333703, 0.3219752754296894559, 0.3333333333333333703, 0.3219752754296894559, 0.3333333333333333703, 0.3219752754296894559, 0.3333333333333333703, 0.3219752754296894559, 0.3333333333333333703, 0.3219752754296894559, 0.3333333333333333703, 0.3219752754296894559, 0.3333333333333333703, 0.3219752754296894559, 0.3333333333333333703, 0.3219752754296894559, 0.3333333333333333703, 0.3219752754296894559, 0.3333333333333333703, 0.3219752754296894559, 0.3333333333333333703, 0.3219752754296894559, 0.3333333333333333703, 0.3219752754296894559, 0.3333333333333333703, 0.3219752754296894559, 0.3333333333333333703, 0.3219752754296894559, 0.3333333333333333703, 0.3219752754296894559, 0.3333333333333333703, 0.3219752754296894559, 0.3333333333333333703, 0.3219752754296894559, 0.3333333333333333703, 0.3219752754296894559, 0.3333333333333333703, 0.3219752754296894559, 0.3333333333333333703, 0.3219752754296894559, 0.3333333333333333703, 0.3219752754296894559, 0.3333333333333333703, 0.3219752754296894559, 0.3333333333333333703, 0.3219752754296894559, 0.3333333333333333703, 0.3219752754296894559, 0.3333333333333333703, 0.3219752754296894559, 0.3333333333333333703, 0.3219752754296894559, 0.3333333333333333703, 0.3219752754296894559, 0.3333333333333333703, 0.3219752754296894559, 0.3333333333333333703, 0.3219752754296894559, 0.3333333333333333703, 0.3219752754296894559, 0.3333333333333333703, 0.3219752754296894559, 0.3333333333333333703, 0.3219752754296894559, 0.3333333333333333703, 0.3219752754296894559, 0.3333333333333333703, 0.3219752754296894559, 0.3333333333333333703, 0.3219752754296894559, 0.3333333333333333703, 0.3219752754296894559, 0.3333333333333333703, 0.3219752754296894559, 0.3333333333333333703, 0.3219752754296894559, 0.3333333333333333703, 0.3219752754296894559, 0.3333333333333333703, 0.3219752754296894559, 0.3333333333333333703, 0.3219752754296894559, 0.3333333333333333703, 0.3219752754296894559, 0.3333333333333333703, 0.3219752754296894559, 0.3333333333333333703, 0.3219752754296894559, 0.3333333333333333703, 0.3219752754296894559, 0.3333333333333333703, 0.3219752754296894559, 0.3333333333333333703, 0.3219752754296894559, 0.3333333333333333703, 0.3219752754296894559, 0.3333333333333333703, 0.3219752754296894559, 0.3333333333333333703, 0.3219752754296894559, 0.3333333333333333703, 0.3219752754296894559, 0.3333333333333333703, 0.3219752754296894559, 0.3333333333333333703, 0.3219752754296894559, 0.3333333333333333703, 0.3219752754296894559, 0.3333333333333333703, 0.3219752754296894559, 0.3333333333333333703, 0.3219752754296894559, 0.3333333333333333703, 0.3219752754296894559, 0.3333333333333333703, 0.3219752754296894559, 0.3333333333333333703, 0.3219752754296894559, 0.3333333333333333703, 0.3219752754296894559, 0.3333333333333333703, 0.3219752754296894559, 0.3333333333333333703, 0.3219752754296894559, 0.3333333333333333703, 0.3219752754296894559, 0.3333333333333333703, 0.3219752754296894559, 0.3333333333333333703, 0.3219752754296894559, 0.3333333333333333703, 0.3219752754296894559, 0.3333333333333333703, 0.3219752754296894559, 0.3333333333333333703, 0.3219752754296894559, 0.3333333333333333703, 0.3219752754296894559, 0.3333333333333333703, 0.3219752754296894559, 0.3333333333333333703, 0.3219752754296894559, 0.3333333333333333703, 0.3219752754296894559, 0.3333333333333333703, 0.3219752754296894559, 0.3333333333333333703, 0.3219752754296894559, 0.3333333333333333703, 0.3219752754296894559, 0.3333333333333333703, 0.3219752754296894559, 0.3333333333333333703, 0.3219752754296894559, 0.3333333333333333703, 0.3219752754296894559, 0.3333333333333333703, 0.3219752754296894559, 0.3333333333333333703, 0.3219752754296894559, 0.3333333333333333703, 0.3219752754296894559, 0.3333333333333333703, 0.3219752754296894559, 0.3333333333333333703, 0.3219752754296894559, 0.3333333333333333703, 0.3219752754296894559, 0.3333333333333333703, 0.3219752754296894559, 0.3333333333333333703, 0.3219752754296894559, 0.3333333333333333703, 0.3219752754296894559, 0.3333333333333333703, 0.3219752754296894559, 0.3333333333333333703, 0.3219752754296894559, 0.3333333333333333703, 0.3219752754296894559, 0.3333333333333333703, 0.3219752754296894559, 0.3333333333333333703, 0.3219752754296894559, 0.3333333333333333703, 0.3219752754296894559, 0.3333333333333333703, 0.3219752754296894559, 0.3333333333333333703, 0.3219752754296894559, 0.3333333333333333703, 0.3219752754296894559, 0.3333333333333333703, 0.3219752754296894559, 0.3333333333333333703, 0.3219752754296894559, 0.3333333333333333703, 0.3219752754296894559, 0.3333333333333333703, 0.3219752754296894559, 0.3333333333333333703, 0.3219752754296894559, 0.3333333333333333703, 0.3219752754296894559, 0.3333333333333333703, 0.3219752754296894559, 0.3333333333333333703, 0.3219752754296894559, 0.3333333333333333703, 0.3219752754296894559, 0.3333333333333333703, 0.3219752754296894559, 0.3333333333333333703, 0.3219752754296894559, 0.3333333333333333703, 0.3219752754296894559, 0.3333333333333333703, 0.3219752754296894559, 0.3333333333333333703, 0.3219752754296894559, 0.3333333333333333703, 0.3219752754296894559, 0.3333333333333333703, 0.3219752754296894559, 0.3333333333333333703, 0.3219752754296894559, 0.3333333333333333703, 0.3219752754296894559, 0.3333333333333333703, 0.3219752754296894559, 0.3333333333333333703, 0.3219752754296894559, 0.3333333333333333703, 0.3219752754296894559, 0.3333333333333333703, 0.3219752754296894559, 0.3333333333333333703, 0.3219752754296894559, 0.3333333333333333703, 0.3219752754296894559, 0.3333333333333333703, 0.3219752754296894559, 0.3333333333333333703, 0.3219752754296894559, 0.3333333333333333703, 0.3219752754296894559, 0.3333333333333333703, 0.3219752754296894559, 0.3333333333333333703, 0.3219752754296894559, 0.3333333333333333703, 0.3219752754296894559, 0.3333333333333333703, 0.3219752754296894559, 0.3333333333333333703, 0.3219752754296894559, 0.3333333333333333703, 0.3219752754296894559, 0.3333333333333333703, 0.3219752754296894559, 0.3333333333333333703, 0.3219752754296894559, 0.3333333333333333703, 0.3219752754296894559, 0.3333333333333333703, 0.3219752754296894559, 0.3333333333333333703, 0.3219752754296894559, 0.3333333333333333703, 0.3219752754296894559, 0.3333333333333333703, 0.3219752754296894559, 0.3333333333333333703, 0.3219752754296894559, 0.3333333333333333703, 0.3219752754296894559, 0.3333333333333333703, 0.3219752754296894559, 0.3333333333333333703, 0.3219752754296894559, 0.3333333333333333703, 0.3219752754296894559, 0.3333333333333333703, 0.3219752754296894559, 0.3333333333333333703, 0.3219752754296894559, 0.3333333333333333703, 0.3219752754296894559, 0.3333333333333333703, 0.3219752754296894559, 0.3333333333333333703, 0.3219752754296894559, 0.3333333333333333703, 0.3219752754296894559, 0.3333333333333333703, 0.3219752754296894559, 0.3333333333333333703, 0.3219752754296894559, 0.3333333333333333703, 0.3219752754296894559, 0.3333333333333333703, 0.3219752754296894559, 0.3333333333333333703, 0.3219752754296894559, 0.3333333333333333703, 0.3219752754296894559, 0.3333333333333333703, 0.3219752754296894559, 0.3333333333333333703, 0.3219752754296894559, 0.3333333333333333703, 0.3219752754296894559, 0.3333333333333333703, 0.3219752754296894559, 0.3333333333333333703, 0.3219752754296894559, 0.3333333333333333703, 0.3219752754296894559, 0.3333333333333333703, 0.3219752754296894559, 0.3333333333333333703, 0.3219752754296894559, 0.3333333333333333703, 0.3219752754296894559, 0.3333333333333333703, 0.3219752754296894559, 0.3333333333333333703),
 ( 1.000000000000000000, 0.9659258262890683122, 1.000000000000000000, 0.9659258262890683122, 1.000000000000000000, 0.9659258262890683122, 1.000000000000000000, 0.9659258262890683122, 1.000000000000000000, 0.9659258262890683122, 1.000000000000000000, 0.9659258262890683122, 1.000000000000000000, 0.9659258262890683122, 1.000000000000000000, 0.9659258262890683122, 1.000000000000000000, 0.9659258262890683122, 1.000000000000000000, 0.9659258262890683122, 1.000000000000000000, 0.9659258262890683122, 1.000000000000000000, 0.9659258262890683122, 1.000000000000000000, 0.9659258262890683122, 1.000000000000000000, 0.9659258262890683122, 1.000000000000000000, 0.9659258262890683122, 1.000000000000000000, 0.9659258262890683122, 1.000000000000000000, 0.9659258262890683122, 1.000000000000000000, 0.9659258262890683122, 1.000000000000000000, 0.9659258262890683122, 1.000000000000000000, 0.9659258262890683122, 1.000000000000000000, 0.9659258262890683122, 1.000000000000000000, 0.9659258262890683122, 1.000000000000000000, 0.9659258262890683122, 1.000000000000000000, 0.9659258262890683122, 1.000000000000000000, 0.9659258262890683122, 1.000000000000000000, 0.9659258262890683122, 1.000000000000000000, 0.9659258262890683122, 1.000000000000000000, 0.9659258262890683122, 1.000000000000000000, 0.9659258262890683122, 1.000000000000000000, 0.9659258262890683122, 1.000000000000000000, 0.9659258262890683122, 1.000000000000000000, 0.9659258262890683122, 1.000000000000000000, 0.9659258262890683122, 1.000000000000000000, 0.9659258262890683122, 1.000000000000000000, 0.9659258262890683122, 1.000000000000000000, 0.9659258262890683122, 1.000000000000000000, 0.9659258262890683122, 1.000000000000000000, 0.9659258262890683122, 1.000000000000000000, 0.9659258262890683122, 1.000000000000000000, 0.9659258262890683122, 1.000000000000000000, 0.9659258262890683122, 1.000000000000000000, 0.9659258262890683122, 1.000000000000000000, 0.9659258262890683122, 1.000000000000000000, 0.9659258262890683122, 1.000000000000000000, 0.9659258262890683122, 1.000000000000000000, 0.9659258262890683122, 1.000000000000000000, 0.9659258262890683122, 1.000000000000000000, 0.9659258262890683122, 1.000000000000000000, 0.9659258262890683122, 1.000000000000000000, 0.9659258262890683122, 1.000000000000000000, 0.9659258262890683122, 1.000000000000000000, 0.9659258262890683122, 1.000000000000000000, 0.9659258262890683122, 1.000000000000000000, 0.9659258262890683122, 1.000000000000000000, 0.9659258262890683122, 1.000000000000000000, 0.9659258262890683122, 1.000000000000000000, 0.9659258262890683122, 1.000000000000000000, 0.9659258262890683122, 1.000000000000000000, 0.9659258262890683122, 1.000000000000000000, 0.9659258262890683122, 1.000000000000000000, 0.9659258262890683122, 1.000000000000000000, 0.9659258262890683122, 1.000000000000000000, 0.9659258262890683122, 1.000000000000000000, 0.9659258262890683122, 1.000000000000000000, 0.9659258262890683122, 1.000000000000000000, 0.9659258262890683122, 1.000000000000000000, 0.9659258262890683122, 1.000000000000000000, 0.9659258262890683122, 1.000000000000000000, 0.9659258262890683122, 1.000000000000000000, 0.9659258262890683122, 1.000000000000000000, 0.9659258262890683122, 1.000000000000000000, 0.9659258262890683122, 1.000000000000000000, 0.9659258262890683122, 1.000000000000000000, 0.9659258262890683122, 1.000000000000000000, 0.9659258262890683122, 1.000000000000000000, 0.9659258262890683122, 1.000000000000000000, 0.9659258262890683122, 1.000000000000000000, 0.9659258262890683122, 1.000000000000000000, 0.9659258262890683122, 1.000000000000000000, 0.9659258262890683122, 1.000000000000000000, 0.9659258262890683122, 1.000000000000000000, 0.9659258262890683122, 1.000000000000000000, 0.9659258262890683122, 1.000000000000000000, 0.9659258262890683122, 1.000000000000000000, 0.9659258262890683122, 1.000000000000000000, 0.9659258262890683122, 1.000000000000000000, 0.9659258262890683122, 1.000000000000000000, 0.9659258262890683122, 1.000000000000000000, 0.9659258262890683122, 1.000000000000000000, 0.9659258262890683122, 1.000000000000000000, 0.9659258262890683122, 1.000000000000000000, 0.9659258262890683122, 1.000000000000000000, 0.9659258262890683122, 1.000000000000000000, 0.9659258262890683122, 1.000000000000000000, 0.9659258262890683122, 1.000000000000000000, 0.9659258262890683122, 1.000000000000000000, 0.9659258262890683122, 1.000000000000000000, 0.9659258262890683122, 1.000000000000000000, 0.9659258262890683122, 1.000000000000000000, 0.9659258262890683122, 1.000000000000000000, 0.9659258262890683122, 1.000000000000000000, 0.9659258262890683122, 1.000000000000000000, 0.9659258262890683122, 1.000000000000000000, 0.9659258262890683122, 1.000000000000000000, 0.9659258262890683122, 1.000000000000000000, 0.9659258262890683122, 1.000000000000000000, 0.9659258262890683122, 1.000000000000000000, 0.9659258262890683122, 1.000000000000000000, 0.9659258262890683122, 1.000000000000000000, 0.9659258262890683122, 1.000000000000000000, 0.9659258262890683122, 1.000000000000000000, 0.9659258262890683122, 1.000000000000000000, 0.9659258262890683122, 1.000000000000000000, 0.9659258262890683122, 1.000000000000000000, 0.9659258262890683122, 1.000000000000000000, 0.9659258262890683122, 1.000000000000000000, 0.9659258262890683122, 1.000000000000000000, 0.9659258262890683122, 1.000000000000000000, 0.9659258262890683122, 1.000000000000000000, 0.9659258262890683122, 1.000000000000000000, 0.9659258262890683122, 1.000000000000000000, 0.9659258262890683122, 1.000000000000000000, 0.9659258262890683122, 1.000000000000000000, 0.9659258262890683122, 1.000000000000000000, 0.9659258262890683122, 1.000000000000000000, 0.9659258262890683122, 1.000000000000000000, 0.9659258262890683122, 1.000000000000000000, 0.9659258262890683122, 1.000000000000000000, 0.9659258262890683122, 1.000000000000000000, 0.9659258262890683122, 1.000000000000000000, 0.9659258262890683122, 1.000000000000000000, 0.9659258262890683122, 1.000000000000000000, 0.9659258262890683122, 1.000000000000000000, 0.9659258262890683122, 1.000000000000000000, 0.9659258262890683122, 1.000000000000000000, 0.9659258262890683122, 1.000000000000000000, 0.9659258262890683122, 1.000000000000000000, 0.9659258262890683122, 1.000000000000000000, 0.9659258262890683122, 1.000000000000000000, 0.9659258262890683122, 1.000000000000000000, 0.9659258262890683122, 1.000000000000000000, 0.9659258262890683122, 1.000000000000000000, 0.9659258262890683122, 1.000000000000000000, 0.9659258262890683122, 1.000000000000000000, 0.9659258262890683122, 1.000000000000000000, 0.9659258262890683122, 1.000000000000000000, 0.9659258262890683122, 1.000000000000000000, 0.9659258262890683122, 1.000000000000000000, 0.9659258262890683122, 1.000000000000000000, 0.9659258262890683122, 1.000000000000000000, 0.9659258262890683122, 1.000000000000000000, 0.9659258262890683122, 1.000000000000000000, 0.9659258262890683122, 1.000000000000000000, 0.9659258262890683122, 1.000000000000000000, 0.9659258262890683122, 1.000000000000000000, 0.9659258262890683122, 1.000000000000000000, 0.9659258262890683122, 1.000000000000000000, 0.9659258262890683122, 1.000000000000000000, 0.9659258262890683122, 1.000000000000000000, 0.9659258262890683122, 1.000000000000000000, 0.9659258262890683122, 1.000000000000000000, 0.9659258262890683122, 1.000000000000000000, 0.9659258262890683122, 1.000000000000000000, 0.9659258262890683122, 1.000000000000000000, 0.9659258262890683122, 1.000000000000000000, 0.9659258262890683122, 1.000000000000000000, 0.9659258262890683122, 1.000000000000000000, 0.9659258262890683122, 1.000000000000000000, 0.9659258262890683122, 1.000000000000000000, 0.9659258262890683122, 1.000000000000000000, 0.9659258262890683122, 1.000000000000000000, 0.9659258262890683122, 1.000000000000000000, 0.9659258262890683122, 1.000000000000000000, 0.9659258262890683122, 1.000000000000000000, 0.9659258262890683122, 1.000000000000000000, 0.9659258262890683122, 1.000000000000000000, 0.9659258262890683122, 1.000000000000000000, 0.9659258262890683122, 1.000000000000000000, 0.9659258262890683122, 1.000000000000000000, 0.9659258262890683122, 1.000000000000000000, 0.9659258262890683122, 1.000000000000000000, 0.9659258262890683122, 1.000000000000000000, 0.9659258262890683122, 1.000000000000000000, 0.9659258262890683122, 1.000000000000000000, 0.9659258262890683122, 1.000000000000000000, 0.9659258262890683122, 1.000000000000000000, 0.9659258262890683122, 1.000000000000000000, 0.9659258262890683122, 1.000000000000000000, 0.9659258262890683122, 1.000000000000000000, 0.9659258262890683122, 1.000000000000000000, 0.9659258262890683122, 1.000000000000000000, 0.9659258262890683122, 1.000000000000000000, 0.9659258262890683122, 1.000000000000000000, 0.9659258262890683122, 1.000000000000000000, 0.9659258262890683122, 1.000000000000000000, 0.9659258262890683122, 1.000000000000000000, 0.9659258262890683122, 1.000000000000000000, 0.9659258262890683122, 1.000000000000000000, 0.9659258262890683122, 1.000000000000000000, 0.9659258262890683122, 1.000000000000000000, 0.9659258262890683122, 1.000000000000000000, 0.9659258262890683122, 1.000000000000000000, 0.9659258262890683122, 1.000000000000000000, 0.9659258262890683122, 1.000000000000000000, 0.9659258262890683122, 1.000000000000000000, 0.9659258262890683122, 1.000000000000000000, 0.9659258262890683122, 1.000000000000000000, 0.9659258262890683122, 1.000000000000000000, 0.9659258262890683122, 1.000000000000000000, 0.9659258262890683122, 1.000000000000000000, 0.9659258262890683122, 1.000000000000000000, 0.9659258262890683122, 1.000000000000000000, 0.9659258262890683122, 1.000000000000000000, 0.9659258262890683122, 1.000000000000000000, 0.9659258262890683122, 1.000000000000000000, 0.9659258262890683122, 1.000000000000000000, 0.9659258262890683122, 1.000000000000000000, 0.9659258262890683122, 1.000000000000000000, 0.9659258262890683122, 1.000000000000000000, 0.9659258262890683122, 1.000000000000000000, 0.9659258262890683122, 1.000000000000000000, 0.9659258262890683122, 1.000000000000000000, 0.9659258262890683122, 1.000000000000000000, 0.9659258262890683122, 1.000000000000000000, 0.9659258262890683122, 1.000000000000000000, 0.9659258262890683122, 1.000000000000000000, 0.9659258262890683122, 1.000000000000000000, 0.9659258262890683122, 1.000000000000000000),
 ( 0.3333333333333333703, 0.3219752754296894559, 0.3333333333333333703, 0.3219752754296894559, 0.3333333333333333703, 0.3219752754296894559, 0.3333333333333333703, 0.3219752754296894559, 0.3333333333333333703, 0.3219752754296894559, 0.3333333333333333703, 0.3219752754296894559, 0.3333333333333333703, 0.3219752754296894559, 0.3333333333333333703, 0.3219752754296894559, 0.3333333333333333703, 0.3219752754296894559, 0.3333333333333333703, 0.3219752754296894559, 0.3333333333333333703, 0.3219752754296894559, 0.3333333333333333703, 0.3219752754296894559, 0.3333333333333333703, 0.3219752754296894559, 0.3333333333333333703, 0.3219752754296894559, 0.3333333333333333703, 0.3219752754296894559, 0.3333333333333333703, 0.3219752754296894559, 0.3333333333333333703, 0.3219752754296894559, 0.3333333333333333703, 0.3219752754296894559, 0.3333333333333333703, 0.3219752754296894559, 0.3333333333333333703, 0.3219752754296894559, 0.3333333333333333703, 0.3219752754296894559, 0.3333333333333333703, 0.3219752754296894559, 0.3333333333333333703, 0.3219752754296894559, 0.3333333333333333703, 0.3219752754296894559, 0.3333333333333333703, 0.3219752754296894559, 0.3333333333333333703, 0.3219752754296894559, 0.3333333333333333703, 0.3219752754296894559, 0.3333333333333333703, 0.3219752754296894559, 0.3333333333333333703, 0.3219752754296894559, 0.3333333333333333703, 0.3219752754296894559, 0.3333333333333333703, 0.3219752754296894559, 0.3333333333333333703, 0.3219752754296894559, 0.3333333333333333703, 0.3219752754296894559, 0.3333333333333333703, 0.3219752754296894559, 0.3333333333333333703, 0.3219752754296894559, 0.3333333333333333703, 0.3219752754296894559, 0.3333333333333333703, 0.3219752754296894559, 0.3333333333333333703, 0.3219752754296894559, 0.3333333333333333703, 0.3219752754296894559, 0.3333333333333333703, 0.3219752754296894559, 0.3333333333333333703, 0.3219752754296894559, 0.3333333333333333703, 0.3219752754296894559, 0.3333333333333333703, 0.3219752754296894559, 0.3333333333333333703, 0.3219752754296894559, 0.3333333333333333703, 0.3219752754296894559, 0.3333333333333333703, 0.3219752754296894559, 0.3333333333333333703, 0.3219752754296894559, 0.3333333333333333703, 0.3219752754296894559, 0.3333333333333333703, 0.3219752754296894559, 0.3333333333333333703, 0.3219752754296894559, 0.3333333333333333703, 0.3219752754296894559, 0.3333333333333333703, 0.3219752754296894559, 0.3333333333333333703, 0.3219752754296894559, 0.3333333333333333703, 0.3219752754296894559, 0.3333333333333333703, 0.3219752754296894559, 0.3333333333333333703, 0.3219752754296894559, 0.3333333333333333703, 0.3219752754296894559, 0.3333333333333333703, 0.3219752754296894559, 0.3333333333333333703, 0.3219752754296894559, 0.3333333333333333703, 0.3219752754296894559, 0.3333333333333333703, 0.3219752754296894559, 0.3333333333333333703, 0.3219752754296894559, 0.3333333333333333703, 0.3219752754296894559, 0.3333333333333333703, 0.3219752754296894559, 0.3333333333333333703, 0.3219752754296894559, 0.3333333333333333703, 0.3219752754296894559, 0.3333333333333333703, 0.3219752754296894559, 0.3333333333333333703, 0.3219752754296894559, 0.3333333333333333703, 0.3219752754296894559, 0.3333333333333333703, 0.3219752754296894559, 0.3333333333333333703, 0.3219752754296894559, 0.3333333333333333703, 0.3219752754296894559, 0.3333333333333333703, 0.3219752754296894559, 0.3333333333333333703, 0.3219752754296894559, 0.3333333333333333703, 0.3219752754296894559, 0.3333333333333333703, 0.3219752754296894559, 0.3333333333333333703, 0.3219752754296894559, 0.3333333333333333703, 0.3219752754296894559, 0.3333333333333333703, 0.3219752754296894559, 0.3333333333333333703, 0.3219752754296894559, 0.3333333333333333703, 0.3219752754296894559, 0.3333333333333333703, 0.3219752754296894559, 0.3333333333333333703, 0.3219752754296894559, 0.3333333333333333703, 0.3219752754296894559, 0.3333333333333333703, 0.3219752754296894559, 0.3333333333333333703, 0.3219752754296894559, 0.3333333333333333703, 0.3219752754296894559, 0.3333333333333333703, 0.3219752754296894559, 0.3333333333333333703, 0.3219752754296894559, 0.3333333333333333703, 0.3219752754296894559, 0.3333333333333333703, 0.3219752754296894559, 0.3333333333333333703, 0.3219752754296894559, 0.3333333333333333703, 0.3219752754296894559, 0.3333333333333333703, 0.3219752754296894559, 0.3333333333333333703, 0.3219752754296894559, 0.3333333333333333703, 0.3219752754296894559, 0.3333333333333333703, 0.3219752754296894559, 0.3333333333333333703, 0.3219752754296894559, 0.3333333333333333703, 0.3219752754296894559, 0.3333333333333333703, 0.3219752754296894559, 0.3333333333333333703, 0.3219752754296894559, 0.3333333333333333703, 0.3219752754296894559, 0.3333333333333333703, 0.3219752754296894559, 0.3333333333333333703, 0.3219752754296894559, 0.3333333333333333703, 0.3219752754296894559, 0.3333333333333333703, 0.3219752754296894559, 0.3333333333333333703, 0.3219752754296894559, 0.3333333333333333703, 0.3219752754296894559, 0.3333333333333333703, 0.3219752754296894559, 0.3333333333333333703, 0.3219752754296894559, 0.3333333333333333703, 0.3219752754296894559, 0.3333333333333333703, 0.3219752754296894559, 0.3333333333333333703, 0.3219752754296894559, 0.3333333333333333703, 0.3219752754296894559, 0.3333333333333333703, 0.3219752754296894559, 0.3333333333333333703, 0.3219752754296894559, 0.3333333333333333703, 0.3219752754296894559, 0.3333333333333333703, 0.3219752754296894559, 0.3333333333333333703, 0.3219752754296894559, 0.3333333333333333703, 0.3219752754296894559, 0.3333333333333333703, 0.3219752754296894559, 0.3333333333333333703, 0.3219752754296894559, 0.3333333333333333703, 0.3219752754296894559, 0.3333333333333333703, 0.3219752754296894559, 0.3333333333333333703, 0.3219752754296894559, 0.3333333333333333703, 0.3219752754296894559, 0.3333333333333333703, 0.3219752754296894559, 0.3333333333333333703, 0.3219752754296894559, 0.3333333333333333703, 0.3219752754296894559, 0.3333333333333333703, 0.3219752754296894559, 0.3333333333333333703, 0.3219752754296894559, 0.3333333333333333703, 0.3219752754296894559, 0.3333333333333333703, 0.3219752754296894559, 0.3333333333333333703, 0.3219752754296894559, 0.3333333333333333703, 0.3219752754296894559, 0.3333333333333333703, 0.3219752754296894559, 0.3333333333333333703, 0.3219752754296894559, 0.3333333333333333703, 0.3219752754296894559, 0.3333333333333333703, 0.3219752754296894559, 0.3333333333333333703, 0.3219752754296894559, 0.3333333333333333703, 0.3219752754296894559, 0.3333333333333333703, 0.3219752754296894559, 0.3333333333333333703, 0.3219752754296894559, 0.3333333333333333703, 0.3219752754296894559, 0.3333333333333333703, 0.3219752754296894559, 0.3333333333333333703, 0.3219752754296894559, 0.3333333333333333703, 0.3219752754296894559, 0.3333333333333333703, 0.3219752754296894559, 0.3333333333333333703, 0.3219752754296894559, 0.3333333333333333703, 0.3219752754296894559, 0.3333333333333333703, 0.3219752754296894559, 0.3333333333333333703, 0.3219752754296894559, 0.3333333333333333703, 0.3219752754296894559, 0.3333333333333333703, 0.3219752754296894559, 0.3333333333333333703, 0.3219752754296894559, 0.3333333333333333703, 0.3219752754296894559, 0.3333333333333333703, 0.3219752754296894559, 0.3333333333333333703, 0.3219752754296894559, 0.3333333333333333703, 0.3219752754296894559, 0.3333333333333333703, 0.3219752754296894559, 0.3333333333333333703, 0.3219752754296894559, 0.3333333333333333703, 0.3219752754296894559, 0.3333333333333333703, 0.3219752754296894559, 0.3333333333333333703, 0.3219752754296894559, 0.3333333333333333703, 0.3219752754296894559, 0.3333333333333333703, 0.3219752754296894559, 0.3333333333333333703, 0.3219752754296894559, 0.3333333333333333703, 0.3219752754296894559, 0.3333333333333333703, 0.3219752754296894559, 0.3333333333333333703, 0.3219752754296894559, 0.3333333333333333703, 0.3219752754296894559, 0.3333333333333333703, 0.3219752754296894559, 0.3333333333333333703, 0.3219752754296894559, 0.3333333333333333703, 0.3219752754296894559, 0.3333333333333333703, 0.3219752754296894559, 0.3333333333333333703, 0.3219752754296894559, 0.3333333333333333703, 0.3219752754296894559, 0.3333333333333333703, 0.3219752754296894559, 0.3333333333333333703, 0.3219752754296894559, 0.3333333333333333703, 0.3219752754296894559, 0.3333333333333333703, 0.3219752754296894559, 0.3333333333333333703, 0.3219752754296894559, 0.3333333333333333703, 0.3219752754296894559, 0.3333333333333333703, 0.3219752754296894559, 0.3333333333333333703, 0.3219752754296894559, 0.3333333333333333703, 0.3219752754296894559, 0.3333333333333333703, 0.3219752754296894559, 0.3333333333333333703, 0.3219752754296894559, 0.3333333333333333703, 0.3219752754296894559, 0.3333333333333333703, 0.3219752754296894559, 0.3333333333333333703, 0.3219752754296894559, 0.3333333333333333703, 0.3219752754296894559, 0.3333333333333333703, 0.3219752754296894559, 0.3333333333333333703, 0.3219752754296894559, 0.3333333333333333703, 0.3219752754296894559, 0.3333333333333333703, 0.3219752754296894559, 0.3333333333333333703, 0.3219752754296894559, 0.3333333333333333703, 0.3219752754296894559, 0.3333333333333333703, 0.3219752754296894559, 0.3333333333333333703, 0.3219752754296894559, 0.3333333333333333703, 0.3219752754296894559, 0.3333333333333333703, 0.3219752754296894559, 0.3333333333333333703, 0.3219752754296894559, 0.3333333333333333703, 0.3219752754296894559, 0.3333333333333333703, 0.3219752754296894559, 0.3333333333333333703, 0.3219752754296894559, 0.3333333333333333703, 0.3219752754296894559, 0.3333333333333333703, 0.3219752754296894559, 0.3333333333333333703, 0.3219752754296894559, 0.3333333333333333703, 0.3219752754296894559, 0.3333333333333333703, 0.3219752754296894559, 0.3333333333333333703, 0.3219752754296894559, 0.3333333333333333703, 0.3219752754296894559, 0.3333333333333333703, 0.3219752754296894559, 0.3333333333333333703, 0.3219752754296894559, 0.3333333333333333703, 0.3219752754296894559, 0.3333333333333333703, 0.3219752754296894559, 0.3333333333333333703, 0.3219752754296894559, 0.3333333333333333703, 0.3219752754296894559, 0.3333333333333333703, 0.3219752754296894559, 0.3333333333333333703, 0.3219752754296894559, 0.3333333333333333703, 0.3219752754296894559, 0.3333333333333333703, 0.3219752754296894559, 0.3333333333333333703, 0.3219752754296894559, 0.3333333333333333703, 0.3219752754296894559, 0.3333333333333333703, 0.3219752754296894559, 0.3333333333333333703, 0.3219752754296894559, 0.3333333333333333703, 0.3219752754296894559, 0.3333333333333333703),
 ( 0.3333333333333333703, 0.3219752754296894559, 0.3333333333333333703, 0.3219752754296894559, 0.3333333333333333703, 0.3219752754296894559, 0.3333333333333333703, 0.3219752754296894559, 0.3333333333333333703, 0.3219752754296894559, 0.3333333333333333703, 0.3219752754296894559, 0.3333333333333333703, 0.3219752754296894559, 0.3333333333333333703, 0.3219752754296894559, 0.3333333333333333703, 0.3219752754296894559, 0.3333333333333333703, 0.3219752754296894559, 0.3333333333333333703, 0.3219752754296894559, 0.3333333333333333703, 0.3219752754296894559, 0.3333333333333333703, 0.3219752754296894559, 0.3333333333333333703, 0.3219752754296894559, 0.3333333333333333703, 0.3219752754296894559, 0.3333333333333333703, 0.3219752754296894559, 0.3333333333333333703, 0.3219752754296894559, 0.3333333333333333703, 0.3219752754296894559, 0.3333333333333333703, 0.3219752754296894559, 0.3333333333333333703, 0.3219752754296894559, 0.3333333333333333703, 0.3219752754296894559, 0.3333333333333333703, 0.3219752754296894559, 0.3333333333333333703, 0.3219752754296894559, 0.3333333333333333703, 0.3219752754296894559, 0.3333333333333333703, 0.3219752754296894559, 0.3333333333333333703, 0.3219752754296894559, 0.3333333333333333703, 0.3219752754296894559, 0.3333333333333333703, 0.3219752754296894559, 0.3333333333333333703, 0.3219752754296894559, 0.3333333333333333703, 0.3219752754296894559, 0.3333333333333333703, 0.3219752754296894559, 0.3333333333333333703, 0.3219752754296894559, 0.3333333333333333703, 0.3219752754296894559, 0.3333333333333333703, 0.3219752754296894559, 0.3333333333333333703, 0.3219752754296894559, 0.3333333333333333703, 0.3219752754296894559, 0.3333333333333333703, 0.3219752754296894559, 0.3333333333333333703, 0.3219752754296894559, 0.3333333333333333703, 0.3219752754296894559, 0.3333333333333333703, 0.3219752754296894559, 0.3333333333333333703, 0.3219752754296894559, 0.3333333333333333703, 0.3219752754296894559, 0.3333333333333333703, 0.3219752754296894559, 0.3333333333333333703, 0.3219752754296894559, 0.3333333333333333703, 0.3219752754296894559, 0.3333333333333333703, 0.3219752754296894559, 0.3333333333333333703, 0.3219752754296894559, 0.3333333333333333703, 0.3219752754296894559, 0.3333333333333333703, 0.3219752754296894559, 0.3333333333333333703, 0.3219752754296894559, 0.3333333333333333703, 0.3219752754296894559, 0.3333333333333333703, 0.3219752754296894559, 0.3333333333333333703, 0.3219752754296894559, 0.3333333333333333703, 0.3219752754296894559, 0.3333333333333333703, 0.3219752754296894559, 0.3333333333333333703, 0.3219752754296894559, 0.3333333333333333703, 0.3219752754296894559, 0.3333333333333333703, 0.3219752754296894559, 0.3333333333333333703, 0.3219752754296894559, 0.3333333333333333703, 0.3219752754296894559, 0.3333333333333333703, 0.3219752754296894559, 0.3333333333333333703, 0.3219752754296894559, 0.3333333333333333703, 0.3219752754296894559, 0.3333333333333333703, 0.3219752754296894559, 0.3333333333333333703, 0.3219752754296894559, 0.3333333333333333703, 0.3219752754296894559, 0.3333333333333333703, 0.3219752754296894559, 0.3333333333333333703, 0.3219752754296894559, 0.3333333333333333703, 0.3219752754296894559, 0.3333333333333333703, 0.3219752754296894559, 0.3333333333333333703, 0.3219752754296894559, 0.3333333333333333703, 0.3219752754296894559, 0.3333333333333333703, 0.3219752754296894559, 0.3333333333333333703, 0.3219752754296894559, 0.3333333333333333703, 0.3219752754296894559, 0.3333333333333333703, 0.3219752754296894559, 0.3333333333333333703, 0.3219752754296894559, 0.3333333333333333703, 0.3219752754296894559, 0.3333333333333333703, 0.3219752754296894559, 0.3333333333333333703, 0.3219752754296894559, 0.3333333333333333703, 0.3219752754296894559, 0.3333333333333333703, 0.3219752754296894559, 0.3333333333333333703, 0.3219752754296894559, 0.3333333333333333703, 0.3219752754296894559, 0.3333333333333333703, 0.3219752754296894559, 0.3333333333333333703, 0.3219752754296894559, 0.3333333333333333703, 0.3219752754296894559, 0.3333333333333333703, 0.3219752754296894559, 0.3333333333333333703, 0.3219752754296894559, 0.3333333333333333703, 0.3219752754296894559, 0.3333333333333333703, 0.3219752754296894559, 0.3333333333333333703, 0.3219752754296894559, 0.3333333333333333703, 0.3219752754296894559, 0.3333333333333333703, 0.3219752754296894559, 0.3333333333333333703, 0.3219752754296894559, 0.3333333333333333703, 0.3219752754296894559, 0.3333333333333333703, 0.3219752754296894559, 0.3333333333333333703, 0.3219752754296894559, 0.3333333333333333703, 0.3219752754296894559, 0.3333333333333333703, 0.3219752754296894559, 0.3333333333333333703, 0.3219752754296894559, 0.3333333333333333703, 0.3219752754296894559, 0.3333333333333333703, 0.3219752754296894559, 0.3333333333333333703, 0.3219752754296894559, 0.3333333333333333703, 0.3219752754296894559, 0.3333333333333333703, 0.3219752754296894559, 0.3333333333333333703, 0.3219752754296894559, 0.3333333333333333703, 0.3219752754296894559, 0.3333333333333333703, 0.3219752754296894559, 0.3333333333333333703, 0.3219752754296894559, 0.3333333333333333703, 0.3219752754296894559, 0.3333333333333333703, 0.3219752754296894559, 0.3333333333333333703, 0.3219752754296894559, 0.3333333333333333703, 0.3219752754296894559, 0.3333333333333333703, 0.3219752754296894559, 0.3333333333333333703, 0.3219752754296894559, 0.3333333333333333703, 0.3219752754296894559, 0.3333333333333333703, 0.3219752754296894559, 0.3333333333333333703, 0.3219752754296894559, 0.3333333333333333703, 0.3219752754296894559, 0.3333333333333333703, 0.3219752754296894559, 0.3333333333333333703, 0.3219752754296894559, 0.3333333333333333703, 0.3219752754296894559, 0.3333333333333333703, 0.3219752754296894559, 0.3333333333333333703, 0.3219752754296894559, 0.3333333333333333703, 0.3219752754296894559, 0.3333333333333333703, 0.3219752754296894559, 0.3333333333333333703, 0.3219752754296894559, 0.3333333333333333703, 0.3219752754296894559, 0.3333333333333333703, 0.3219752754296894559, 0.3333333333333333703, 0.3219752754296894559, 0.3333333333333333703, 0.3219752754296894559, 0.3333333333333333703, 0.3219752754296894559, 0.3333333333333333703, 0.3219752754296894559, 0.3333333333333333703, 0.3219752754296894559, 0.3333333333333333703, 0.3219752754296894559, 0.3333333333333333703, 0.3219752754296894559, 0.3333333333333333703, 0.3219752754296894559, 0.3333333333333333703, 0.3219752754296894559, 0.3333333333333333703, 0.3219752754296894559, 0.3333333333333333703, 0.3219752754296894559, 0.3333333333333333703, 0.3219752754296894559, 0.3333333333333333703, 0.3219752754296894559, 0.3333333333333333703, 0.3219752754296894559, 0.3333333333333333703, 0.3219752754296894559, 0.3333333333333333703, 0.3219752754296894559, 0.3333333333333333703, 0.3219752754296894559, 0.3333333333333333703, 0.3219752754296894559, 0.3333333333333333703, 0.3219752754296894559, 0.3333333333333333703, 0.3219752754296894559, 0.3333333333333333703, 0.3219752754296894559, 0.3333333333333333703, 0.3219752754296894559, 0.3333333333333333703, 0.3219752754296894559, 0.3333333333333333703, 0.3219752754296894559, 0.3333333333333333703, 0.3219752754296894559, 0.3333333333333333703, 0.3219752754296894559, 0.3333333333333333703, 0.3219752754296894559, 0.3333333333333333703, 0.3219752754296894559, 0.3333333333333333703, 0.3219752754296894559, 0.3333333333333333703, 0.3219752754296894559, 0.3333333333333333703, 0.3219752754296894559, 0.3333333333333333703, 0.3219752754296894559, 0.3333333333333333703, 0.3219752754296894559, 0.3333333333333333703, 0.3219752754296894559, 0.3333333333333333703, 0.3219752754296894559, 0.3333333333333333703, 0.3219752754296894559, 0.3333333333333333703, 0.3219752754296894559, 0.3333333333333333703, 0.3219752754296894559, 0.3333333333333333703, 0.3219752754296894559, 0.3333333333333333703, 0.3219752754296894559, 0.3333333333333333703, 0.3219752754296894559, 0.3333333333333333703, 0.3219752754296894559, 0.3333333333333333703, 0.3219752754296894559, 0.3333333333333333703, 0.3219752754296894559, 0.3333333333333333703, 0.3219752754296894559, 0.3333333333333333703, 0.3219752754296894559, 0.3333333333333333703, 0.3219752754296894559, 0.3333333333333333703, 0.3219752754296894559, 0.3333333333333333703, 0.3219752754296894559, 0.3333333333333333703, 0.3219752754296894559, 0.3333333333333333703, 0.3219752754296894559, 0.3333333333333333703, 0.3219752754296894559, 0.3333333333333333703, 0.3219752754296894559, 0.3333333333333333703, 0.3219752754296894559, 0.3333333333333333703, 0.3219752754296894559, 0.3333333333333333703, 0.3219752754296894559, 0.3333333333333333703, 0.3219752754296894559, 0.3333333333333333703, 0.3219752754296894559, 0.3333333333333333703, 0.3219752754296894559, 0.3333333333333333703, 0.3219752754296894559, 0.3333333333333333703, 0.3219752754296894559, 0.3333333333333333703, 0.3219752754296894559, 0.3333333333333333703, 0.3219752754296894559, 0.3333333333333333703, 0.3219752754296894559, 0.3333333333333333703, 0.3219752754296894559, 0.3333333333333333703, 0.3219752754296894559, 0.3333333333333333703, 0.3219752754296894559, 0.3333333333333333703, 0.3219752754296894559, 0.3333333333333333703, 0.3219752754296894559, 0.3333333333333333703, 0.3219752754296894559, 0.3333333333333333703, 0.3219752754296894559, 0.3333333333333333703, 0.3219752754296894559, 0.3333333333333333703, 0.3219752754296894559, 0.3333333333333333703, 0.3219752754296894559, 0.3333333333333333703, 0.3219752754296894559, 0.3333333333333333703, 0.3219752754296894559, 0.3333333333333333703, 0.3219752754296894559, 0.3333333333333333703, 0.3219752754296894559, 0.3333333333333333703, 0.3219752754296894559, 0.3333333333333333703, 0.3219752754296894559, 0.3333333333333333703, 0.3219752754296894559, 0.3333333333333333703, 0.3219752754296894559, 0.3333333333333333703, 0.3219752754296894559, 0.3333333333333333703, 0.3219752754296894559, 0.3333333333333333703, 0.3219752754296894559, 0.3333333333333333703, 0.3219752754296894559, 0.3333333333333333703, 0.3219752754296894559, 0.3333333333333333703, 0.3219752754296894559, 0.3333333333333333703, 0.3219752754296894559, 0.3333333333333333703, 0.3219752754296894559, 0.3333333333333333703, 0.3219752754296894559, 0.3333333333333333703, 0.3219752754296894559, 0.3333333333333333703, 0.3219752754296894559, 0.3333333333333333703, 0.3219752754296894559, 0.3333333333333333703, 0.3219752754296894559, 0.3333333333333333703, 0.3219752754296894559, 0.3333333333333333703, 0.3219752754296894559, 0.3333333333333333703, 0.3219752754296894559, 0.3333333333333333703),
 ( 1.000000000000000000, 0.9659258262890683122, 1.000000000000000000, 0.9659258262890683122, 1.000000000000000000, 0.9659258262890683122, 1.000000000000000000, 0.9659258262890683122, 1.000000000000000000, 0.9659258262890683122, 1.000000000000000000, 0.9659258262890683122, 1.000000000000000000, 0.9659258262890683122, 1.000000000000000000, 0.9659258262890683122, 1.000000000000000000, 0.9659258262890683122, 1.000000000000000000, 0.9659258262890683122, 1.000000000000000000, 0.9659258262890683122, 1.000000000000000000, 0.9659258262890683122, 1.000000000000000000, 0.9659258262890683122, 1.000000000000000000, 0.9659258262890683122, 1.000000000000000000, 0.9659258262890683122, 1.000000000000000000, 0.9659258262890683122, 1.000000000000000000, 0.9659258262890683122, 1.000000000000000000, 0.9659258262890683122, 1.000000000000000000, 0.9659258262890683122, 1.000000000000000000, 0.9659258262890683122, 1.000000000000000000, 0.9659258262890683122, 1.000000000000000000, 0.9659258262890683122, 1.000000000000000000, 0.9659258262890683122, 1.000000000000000000, 0.9659258262890683122, 1.000000000000000000, 0.9659258262890683122, 1.000000000000000000, 0.9659258262890683122, 1.000000000000000000, 0.9659258262890683122, 1.000000000000000000, 0.9659258262890683122, 1.000000000000000000, 0.9659258262890683122, 1.000000000000000000, 0.9659258262890683122, 1.000000000000000000, 0.9659258262890683122, 1.000000000000000000, 0.9659258262890683122, 1.000000000000000000, 0.9659258262890683122, 1.000000000000000000, 0.9659258262890683122, 1.000000000000000000, 0.9659258262890683122, 1.000000000000000000, 0.9659258262890683122, 1.000000000000000000, 0.9659258262890683122, 1.000000000000000000, 0.9659258262890683122, 1.000000000000000000, 0.9659258262890683122, 1.000000000000000000, 0.9659258262890683122, 1.000000000000000000, 0.9659258262890683122, 1.000000000000000000, 0.9659258262890683122, 1.000000000000000000, 0.9659258262890683122, 1.000000000000000000, 0.9659258262890683122, 1.000000000000000000, 0.9659258262890683122, 1.000000000000000000, 0.9659258262890683122, 1.000000000000000000, 0.9659258262890683122, 1.000000000000000000, 0.9659258262890683122, 1.000000000000000000, 0.9659258262890683122, 1.000000000000000000, 0.9659258262890683122, 1.000000000000000000, 0.9659258262890683122, 1.000000000000000000, 0.9659258262890683122, 1.000000000000000000, 0.9659258262890683122, 1.000000000000000000, 0.9659258262890683122, 1.000000000000000000, 0.9659258262890683122, 1.000000000000000000, 0.9659258262890683122, 1.000000000000000000, 0.9659258262890683122, 1.000000000000000000, 0.9659258262890683122, 1.000000000000000000, 0.9659258262890683122, 1.000000000000000000, 0.9659258262890683122, 1.000000000000000000, 0.9659258262890683122, 1.000000000000000000, 0.9659258262890683122, 1.000000000000000000, 0.9659258262890683122, 1.000000000000000000, 0.9659258262890683122, 1.000000000000000000, 0.9659258262890683122, 1.000000000000000000, 0.9659258262890683122, 1.000000000000000000, 0.9659258262890683122, 1.000000000000000000, 0.9659258262890683122, 1.000000000000000000, 0.9659258262890683122, 1.000000000000000000, 0.9659258262890683122, 1.000000000000000000, 0.9659258262890683122, 1.000000000000000000, 0.9659258262890683122, 1.000000000000000000, 0.9659258262890683122, 1.000000000000000000, 0.9659258262890683122, 1.000000000000000000, 0.9659258262890683122, 1.000000000000000000, 0.9659258262890683122, 1.000000000000000000, 0.9659258262890683122, 1.000000000000000000, 0.9659258262890683122, 1.000000000000000000, 0.9659258262890683122, 1.000000000000000000, 0.9659258262890683122, 1.000000000000000000, 0.9659258262890683122, 1.000000000000000000, 0.9659258262890683122, 1.000000000000000000, 0.9659258262890683122, 1.000000000000000000, 0.9659258262890683122, 1.000000000000000000, 0.9659258262890683122, 1.000000000000000000, 0.9659258262890683122, 1.000000000000000000, 0.9659258262890683122, 1.000000000000000000, 0.9659258262890683122, 1.000000000000000000, 0.9659258262890683122, 1.000000000000000000, 0.9659258262890683122, 1.000000000000000000, 0.9659258262890683122, 1.000000000000000000, 0.9659258262890683122, 1.000000000000000000, 0.9659258262890683122, 1.000000000000000000, 0.9659258262890683122, 1.000000000000000000, 0.9659258262890683122, 1.000000000000000000, 0.9659258262890683122, 1.000000000000000000, 0.9659258262890683122, 1.000000000000000000, 0.9659258262890683122, 1.000000000000000000, 0.9659258262890683122, 1.000000000000000000, 0.9659258262890683122, 1.000000000000000000, 0.9659258262890683122, 1.000000000000000000, 0.9659258262890683122, 1.000000000000000000, 0.9659258262890683122, 1.000000000000000000, 0.9659258262890683122, 1.000000000000000000, 0.9659258262890683122, 1.000000000000000000, 0.9659258262890683122, 1.000000000000000000, 0.9659258262890683122, 1.000000000000000000, 0.9659258262890683122, 1.000000000000000000, 0.9659258262890683122, 1.000000000000000000, 0.9659258262890683122, 1.000000000000000000, 0.9659258262890683122, 1.000000000000000000, 0.9659258262890683122, 1.000000000000000000, 0.9659258262890683122, 1.000000000000000000, 0.9659258262890683122, 1.000000000000000000, 0.9659258262890683122, 1.000000000000000000, 0.9659258262890683122, 1.000000000000000000, 0.9659258262890683122, 1.000000000000000000, 0.9659258262890683122, 1.000000000000000000, 0.9659258262890683122, 1.000000000000000000, 0.9659258262890683122, 1.000000000000000000, 0.9659258262890683122, 1.000000000000000000, 0.9659258262890683122, 1.000000000000000000, 0.9659258262890683122, 1.000000000000000000, 0.9659258262890683122, 1.000000000000000000, 0.9659258262890683122, 1.000000000000000000, 0.9659258262890683122, 1.000000000000000000, 0.9659258262890683122, 1.000000000000000000, 0.9659258262890683122, 1.000000000000000000, 0.9659258262890683122, 1.000000000000000000, 0.9659258262890683122, 1.000000000000000000, 0.9659258262890683122, 1.000000000000000000, 0.9659258262890683122, 1.000000000000000000, 0.9659258262890683122, 1.000000000000000000, 0.9659258262890683122, 1.000000000000000000, 0.9659258262890683122, 1.000000000000000000, 0.9659258262890683122, 1.000000000000000000, 0.9659258262890683122, 1.000000000000000000, 0.9659258262890683122, 1.000000000000000000, 0.9659258262890683122, 1.000000000000000000, 0.9659258262890683122, 1.000000000000000000, 0.9659258262890683122, 1.000000000000000000, 0.9659258262890683122, 1.000000000000000000, 0.9659258262890683122, 1.000000000000000000, 0.9659258262890683122, 1.000000000000000000, 0.9659258262890683122, 1.000000000000000000, 0.9659258262890683122, 1.000000000000000000, 0.9659258262890683122, 1.000000000000000000, 0.9659258262890683122, 1.000000000000000000, 0.9659258262890683122, 1.000000000000000000, 0.9659258262890683122, 1.000000000000000000, 0.9659258262890683122, 1.000000000000000000, 0.9659258262890683122, 1.000000000000000000, 0.9659258262890683122, 1.000000000000000000, 0.9659258262890683122, 1.000000000000000000, 0.9659258262890683122, 1.000000000000000000, 0.9659258262890683122, 1.000000000000000000, 0.9659258262890683122, 1.000000000000000000, 0.9659258262890683122, 1.000000000000000000, 0.9659258262890683122, 1.000000000000000000, 0.9659258262890683122, 1.000000000000000000, 0.9659258262890683122, 1.000000000000000000, 0.9659258262890683122, 1.000000000000000000, 0.9659258262890683122, 1.000000000000000000, 0.9659258262890683122, 1.000000000000000000, 0.9659258262890683122, 1.000000000000000000, 0.9659258262890683122, 1.000000000000000000, 0.9659258262890683122, 1.000000000000000000, 0.9659258262890683122, 1.000000000000000000, 0.9659258262890683122, 1.000000000000000000, 0.9659258262890683122, 1.000000000000000000, 0.9659258262890683122, 1.000000000000000000, 0.9659258262890683122, 1.000000000000000000, 0.9659258262890683122, 1.000000000000000000, 0.9659258262890683122, 1.000000000000000000, 0.9659258262890683122, 1.000000000000000000, 0.9659258262890683122, 1.000000000000000000, 0.9659258262890683122, 1.000000000000000000, 0.9659258262890683122, 1.000000000000000000, 0.9659258262890683122, 1.000000000000000000, 0.9659258262890683122, 1.000000000000000000, 0.9659258262890683122, 1.000000000000000000, 0.9659258262890683122, 1.000000000000000000, 0.9659258262890683122, 1.000000000000000000, 0.9659258262890683122, 1.000000000000000000, 0.9659258262890683122, 1.000000000000000000, 0.9659258262890683122, 1.000000000000000000, 0.9659258262890683122, 1.000000000000000000, 0.9659258262890683122, 1.000000000000000000, 0.9659258262890683122, 1.000000000000000000, 0.9659258262890683122, 1.000000000000000000, 0.9659258262890683122, 1.000000000000000000, 0.9659258262890683122, 1.000000000000000000, 0.9659258262890683122, 1.000000000000000000, 0.9659258262890683122, 1.000000000000000000, 0.9659258262890683122, 1.000000000000000000, 0.9659258262890683122, 1.000000000000000000, 0.9659258262890683122, 1.000000000000000000, 0.9659258262890683122, 1.000000000000000000, 0.9659258262890683122, 1.000000000000000000, 0.9659258262890683122, 1.000000000000000000, 0.9659258262890683122, 1.000000000000000000, 0.9659258262890683122, 1.000000000000000000, 0.9659258262890683122, 1.000000000000000000, 0.9659258262890683122, 1.000000000000000000, 0.9659258262890683122, 1.000000000000000000, 0.9659258262890683122, 1.000000000000000000, 0.9659258262890683122, 1.000000000000000000, 0.9659258262890683122, 1.000000000000000000, 0.9659258262890683122, 1.000000000000000000, 0.9659258262890683122, 1.000000000000000000, 0.9659258262890683122, 1.000000000000000000, 0.9659258262890683122, 1.000000000000000000, 0.9659258262890683122, 1.000000000000000000, 0.9659258262890683122, 1.000000000000000000, 0.9659258262890683122, 1.000000000000000000, 0.9659258262890683122, 1.000000000000000000, 0.9659258262890683122, 1.000000000000000000, 0.9659258262890683122, 1.000000000000000000, 0.9659258262890683122, 1.000000000000000000, 0.9659258262890683122, 1.000000000000000000, 0.9659258262890683122, 1.000000000000000000, 0.9659258262890683122, 1.000000000000000000, 0.9659258262890683122, 1.000000000000000000, 0.9659258262890683122, 1.000000000000000000, 0.9659258262890683122, 1.000000000000000000, 0.9659258262890683122, 1.000000000000000000, 0.9659258262890683122, 1.000000000000000000, 0.9659258262890683122, 1.000000000000000000) ) ) 
 REPRESENTATION_ITEM ( '' )  SURFACE ( )  );
#164277=CARTESIAN_POINT ( 'NONE',  ( 0.05219959533934541429, -16.53943276465976808, 25.00109039468567218 ) ) ;
#164278=CARTESIAN_POINT ( 'NONE',  ( 8.314922557960818139, 14.29746914071049879, 49.58224293864769550 ) ) ;
#164279=CARTESIAN_POINT ( 'NONE',  ( -15.72974639402176322, -15.80617190586768395, 79.37609039468567573 ) ) ;
#164281=CARTESIAN_POINT ( 'NONE',  ( -8.314922557961024197, 14.29746914071037800, 87.91775706135234714 ) ) ;
#164282=CARTESIAN_POINT ( 'NONE',  ( -18.62759615963270932, 10.81492255796079327, 25.83224293864769194 ) ) ;
#164283=CARTESIAN_POINT ( 'NONE',  ( -19.05341960407611168, -5.049401038298164224, 111.4572429386476813 ) ) ;
#164285=CARTESIAN_POINT ( 'NONE',  ( 0.05219959533934541429, -16.53943276465976808, 105.0010903946856757 ) ) ;
#164286=CARTESIAN_POINT ( 'NONE',  ( 14.34966873604972726, -8.224510206698740333, 55.83442372801901854 ) ) ;
#164287=CARTESIAN_POINT ( 'NONE',  ( -16.46253265017160317, 9.564922557960807481, 70.83224293864770971 ) ) ;
#164288=CARTESIAN_POINT ( 'NONE',  ( 13.97604488694527802, 13.89961937509977652, 89.37390960531436690 ) ) ;
#164289=CARTESIAN_POINT ( 'NONE',  ( 5.823673210054444382, -21.52544592524334988, 75.20942372801901854 ) ) ;
#164290=CARTESIAN_POINT ( 'NONE',  ( -4.483927247898782831, 16.52544592524335698, 72.70942372801901854 ) ) ;
#164291=CARTESIAN_POINT ( 'NONE',  ( 8.224510206698953496, -14.34966873604960469, 42.91557627198103120 ) ) ;
#164292=CARTESIAN_POINT ( 'NONE',  ( -13.89961937509977652, 13.97604488694528158, 60.62390960531436690 ) ) ;
#164293=CARTESIAN_POINT ( 'NONE',  ( 5.049401038298161559, -19.05341960407611168, 42.70724293864767418 ) ) ;
#164295=CARTESIAN_POINT ( 'NONE',  ( 5.153800228976615827, -19.02544592524334988, 95.20942372801897591 ) ) ;
#164296=CARTESIAN_POINT ( 'NONE',  ( -12.06949235617756955, 12.14591786802309770, 95.62390960531436690 ) ) ;
#164297=CARTESIAN_POINT ( 'NONE',  ( -9.564922557960796823, -16.46253265017161027, 62.08224293864769550 ) ) ;
#164298=CARTESIAN_POINT ( 'NONE',  ( -5.153800228976607833, 19.02544592524334988, 102.7094237280189759 ) ) ;
#164300=CARTESIAN_POINT ( 'NONE',  ( 10.72451020669871369, 18.67979575497193778, 102.0844237280190185 ) ) ;
#164301=CARTESIAN_POINT ( 'NONE',  ( 12.06949235617739724, 12.14591786802326823, 61.87609039468568284 ) ) ;
#164302=CARTESIAN_POINT ( 'NONE',  ( 9.474510206698729675, 16.51473224551082808, 97.08442372801900433 ) ) ;
#164303=CARTESIAN_POINT ( 'NONE',  ( -5.719274019375978568, 21.55341960407610458, 65.20724293864768129 ) ) ;
#164304=CARTESIAN_POINT ( 'NONE',  ( 12.06949235617739724, 12.14591786802326823, 46.87609039468568994 ) ) ;
#164305=CARTESIAN_POINT ( 'NONE',  ( -18.39443945427638738, 5.500000000000033751, 68.51745347608652992 ) ) ;
#164306=CARTESIAN_POINT ( 'NONE',  ( 16.46253265017146816, 9.564922557961045513, 56.66775706135233293 ) ) ;
#164307=CARTESIAN_POINT ( 'NONE',  ( -15.80617190586768217, 15.72974639402176855, 103.1260903946856757 ) ) ;
#164308=CARTESIAN_POINT ( 'NONE',  ( -4.483927247898539470, -16.52544592524342804, 112.2905762719810241 ) ) ;
#164309=CARTESIAN_POINT ( 'NONE',  ( 9.474510206698971260, -16.51473224551069308, 62.91557627198102409 ) ) ;
#164310=CARTESIAN_POINT ( 'NONE',  ( 8.224510206698953496, -14.34966873604960469, 62.91557627198102409 ) ) ;
#164311=CARTESIAN_POINT ( 'NONE',  ( -15.72974639402176322, -15.80617190586768395, 94.37609039468568994 ) ) ;
#164312=CARTESIAN_POINT ( 'NONE',  ( -9.564922557961040184, 16.46253265017147172, 42.91775706135234003 ) ) ;
#164313=CARTESIAN_POINT ( 'NONE',  ( -13.89961937509957401, -13.97604488694547875, 24.37609039468565442 ) ) ;
#164314=CARTESIAN_POINT ( 'NONE',  ( 10.81492255796078972, 18.62759615963270932, 24.58224293864768839 ) ) ;
#164315=CARTESIAN_POINT ( 'NONE',  ( -18.67979575497193778, 10.72451020669871902, 93.33442372801901854 ) ) ;
#164316=CARTESIAN_POINT ( 'NONE',  ( -9.564922557960796823, -16.46253265017161027, 72.08224293864770971 ) ) ;
#164317=CARTESIAN_POINT ( 'NONE',  ( -15.72974639402176322, -15.80617190586768395, 94.37609039468568994 ) ) ;
#164318=CARTESIAN_POINT ( 'NONE',  ( 0.05219959533907565091, 21.53943276465977519, 49.99890960531437401 ) ) ;
#164319=CARTESIAN_POINT ( 'NONE',  ( 19.03943276465977164, -0.05219959533909143690, 83.74890960531436690 ) ) ;
#164320=CARTESIAN_POINT ( 'NONE',  ( -13.89961937509957401, -13.97604488694547875, 64.37609039468567573 ) ) ;
#164321=CARTESIAN_POINT ( 'NONE',  ( 5.049401038298161559, -19.05341960407611168, 42.70724293864767418 ) ) ;
#164322=CARTESIAN_POINT ( 'NONE',  ( -13.89961937509977652, 13.97604488694528158, 85.62390960531433848 ) ) ;
#164323=CARTESIAN_POINT ( 'NONE',  ( 16.51473224551083163, -9.474510206698727899, 85.83442372801900433 ) ) ;
#164324=CARTESIAN_POINT ( 'NONE',  ( 12.14591786802327356, -12.06949235617739191, 40.62609039468567573 ) ) ;
#164325=CARTESIAN_POINT ( 'NONE',  ( -16.55341960407611168, -4.379528057220339221, 106.4572429386477097 ) ) ;
#164326=CARTESIAN_POINT ( 'NONE',  ( 13.97604488694527802, 13.89961937509977652, 64.37390960531436690 ) ) ;
#164327=CARTESIAN_POINT ( 'NONE',  ( 18.67979575497178502, 10.72451020669898547, 49.16557627198102409 ) ) ;
#164328=CARTESIAN_POINT ( 'NONE',  ( 8.314922557961029526, -14.29746914071037800, 20.41775706135234714 ) ) ;
#164329=CARTESIAN_POINT ( 'NONE',  ( -5.719274019375978568, 21.55341960407610458, 115.2072429386476955 ) ) ;
#164330=CARTESIAN_POINT ( 'NONE',  ( -10.72451020669870658, -18.67979575497194134, 79.58442372801903275 ) ) ;
#164331=CARTESIAN_POINT ( 'NONE',  ( -8.224510206698735004, -14.34966873604973081, 79.58442372801903275 ) ) ;
#164332=CARTESIAN_POINT ( 'NONE',  ( 0.05219959533909260263, 19.03943276465977164, 79.99890960531436690 ) ) ;
#164333=CARTESIAN_POINT ( 'NONE',  ( 8.314922557961029526, -14.29746914071037800, 105.4177570613523613 ) ) ;
#164334=CARTESIAN_POINT ( 'NONE',  ( 13.89961937509957401, 13.97604488694547697, 61.87609039468566863 ) ) ;
#164335=CARTESIAN_POINT ( 'NONE',  ( 21.52544592524334988, 5.823673210054432836, 31.45942372801901854 ) ) ;
#164336=CARTESIAN_POINT ( 'NONE',  ( -4.379528057220328563, 16.55341960407611168, 75.20724293864769550 ) ) ;
#164337=CARTESIAN_POINT ( 'NONE',  ( -16.51473224551069308, -9.474510206698971260, 101.6655762719810241 ) ) ;
#164338=CARTESIAN_POINT ( 'NONE',  ( -14.34966873604972548, 8.224510206698743886, 93.33442372801901854 ) ) ;
#164339=CARTESIAN_POINT ( 'NONE',  ( -21.53943276465977519, -0.05219959533937600094, 73.75109039468567573 ) ) ;
#164340=CARTESIAN_POINT ( 'NONE',  ( -4.379528057220086978, -16.55341960407618274, 34.79275706135235424 ) ) ;
#164341=CARTESIAN_POINT ( 'NONE',  ( -18.67979575497193778, 10.72451020669871902, 23.33442372801901499 ) ) ;
#164342=CARTESIAN_POINT ( 'NONE',  ( -16.52544592524342804, 4.483927247898546575, 66.04057627198103830 ) ) ;
#164343=ORIENTED_EDGE ( 'NONE', *, *, #164865, .T. ) ;
#164344=CARTESIAN_POINT ( 'NONE',  ( 5.719274019375991003, -21.55341960407610458, 97.70724293864772392 ) ) ;
#164345=CARTESIAN_POINT ( 'NONE',  ( 0.05219959533910956823, 16.53943276465976808, 49.99890960531437401 ) ) ;
#164348=CARTESIAN_POINT ( 'NONE',  ( 21.52544592524344225, -5.823673210054117533, 23.54057627198102765 ) ) ;
#164349=CARTESIAN_POINT ( 'NONE',  ( -0.05219959533937732626, 21.53943276465977519, 52.50109039468567573 ) ) ;
#164350=CARTESIAN_POINT ( 'NONE',  ( 16.52544592524342804, -4.483927247898539470, 58.54057627198103120 ) ) ;
#164351=CARTESIAN_POINT ( 'NONE',  ( -5.823673210054116645, -21.52544592524344225, 62.29057627198102409 ) ) ;
#164352=CARTESIAN_POINT ( 'NONE',  ( 19.02544592524343514, -5.153800228976328945, 68.54057627198103830 ) ) ;
#164353=CARTESIAN_POINT ( 'NONE',  ( 19.05341960407611168, 5.049401038298154454, 23.95724293864769194 ) ) ;
#164354=CARTESIAN_POINT ( 'NONE',  ( -9.564922557961040184, 16.46253265017147172, 77.91775706135234714 ) ) ;
#164355=CARTESIAN_POINT ( 'NONE',  ( 5.823673210054125526, 21.52544592524343514, 59.79057627198103120 ) ) ;
#164356=CARTESIAN_POINT ( 'NONE',  ( 13.89961937509977652, -13.97604488694527269, 43.12390960531434558 ) ) ;
#164357=CARTESIAN_POINT ( 'NONE',  ( 5.049401038298161559, -19.05341960407611168, 67.70724293864769550 ) ) ;
#164359=CARTESIAN_POINT ( 'NONE',  ( 4.483927247898790824, -16.52544592524335698, 55.20942372801902565 ) ) ;
#164360=CARTESIAN_POINT ( 'NONE',  ( -10.72451020669870658, -18.67979575497194134, 34.58442372801900433 ) ) ;
#164361=CARTESIAN_POINT ( 'NONE',  ( 5.823673210054444382, -21.52544592524334988, 60.20942372801902565 ) ) ;
#164362=CARTESIAN_POINT ( 'NONE',  ( 16.46253265017160672, -9.564922557960803928, 103.3322429386476955 ) ) ;
#164363=CARTESIAN_POINT ( 'NONE',  ( -5.719274019375978568, 21.55341960407610458, 90.20724293864770971 ) ) ;
#164364=CARTESIAN_POINT ( 'NONE',  ( 15.72974639402199770, -15.80617190586745480, 103.1239096053143811 ) ) ;
#164365=CARTESIAN_POINT ( 'NONE',  ( -8.224510206698735004, -14.34966873604973081, 54.58442372801901143 ) ) ;
#164366=CARTESIAN_POINT ( 'NONE',  ( -21.55341960407610458, -5.719274019375992779, 56.45724293864768839 ) ) ;
#164367=CARTESIAN_POINT ( 'NONE',  ( 15.72974639402176855, 15.80617190586768217, 101.8760903946857042 ) ) ;
#164369=CARTESIAN_POINT ( 'NONE',  ( 9.474510206698971260, -16.51473224551069308, 52.91557627198102409 ) ) ;
#164370=CARTESIAN_POINT ( 'NONE',  ( -13.97604488694527625, -13.89961937509977652, 106.8739096053143669 ) ) ;
#164371=CARTESIAN_POINT ( 'NONE',  ( 5.153800228976335163, 19.02544592524342804, 79.79057627198102409 ) ) ;
#164375=CARTESIAN_POINT ( 'NONE',  ( 16.46253265017146816, 9.564922557961045513, 66.66775706135233293 ) ) ;
#164376=CARTESIAN_POINT ( 'NONE',  ( -21.55341960407610458, -5.719274019375992779, 41.45724293864769550 ) ) ;
#164377=CARTESIAN_POINT ( 'NONE',  ( -8.224510206698735004, -14.34966873604973081, 104.5844237280190185 ) ) ;
#164378=CARTESIAN_POINT ( 'NONE',  ( -16.51473224551082808, 9.474510206698731452, 88.33442372801900433 ) ) ;
#164380=CARTESIAN_POINT ( 'NONE',  ( 19.02544592524334988, 5.153800228976608722, 21.45942372801899012 ) ) ;
#164381=CARTESIAN_POINT ( 'NONE',  ( -19.03943276465977164, -0.05219959533935918106, 88.75109039468567573 ) ) ;
#164382=CARTESIAN_POINT ( 'NONE',  ( -13.97604488694547697, 13.89961937509957934, 48.12609039468566863 ) ) ;
#164383=CARTESIAN_POINT ( 'NONE',  ( 17.26058549869091507, 6.457015423128556364, 108.8774583747606783 ) ) ;
#164384=CARTESIAN_POINT ( 'NONE',  ( 19.03943276465977164, -0.05219959533909143690, 58.74890960531435979 ) ) ;
#164385=CARTESIAN_POINT ( 'NONE',  ( -16.55341960407611168, -4.379528057220339221, 46.45724293864769550 ) ) ;
#164386=CARTESIAN_POINT ( 'NONE',  ( 13.89961937509977652, -13.97604488694527269, 28.12390960531435624 ) ) ;
#164387=CARTESIAN_POINT ( 'NONE',  ( -16.52544592524342804, 4.483927247898546575, 41.04057627198103120 ) ) ;
#164389=CARTESIAN_POINT ( 'NONE',  ( -16.55341960407617563, 4.379528057220093196, 113.5427570613523756 ) ) ;
#164390=CARTESIAN_POINT ( 'NONE',  ( -13.97604488694527625, -13.89961937509977652, 51.87390960531436690 ) ) ;
#164391=CARTESIAN_POINT ( 'NONE',  ( -19.05341960407617563, 5.049401038297882671, 23.54275706135233648 ) ) ;
#164392=CARTESIAN_POINT ( 'NONE',  ( -8.314922557961024197, 14.29746914071037800, 32.91775706135234714 ) ) ;
#164393=CARTESIAN_POINT ( 'NONE',  ( -10.72451020669898014, 18.67979575497178502, 35.41557627198102409 ) ) ;
#164394=CARTESIAN_POINT ( 'NONE',  ( -0.05219959533937732626, 21.53943276465977519, 92.50109039468567573 ) ) ;
#164396=CARTESIAN_POINT ( 'NONE',  ( 13.89961937509977652, -13.97604488694527269, 63.12390960531435979 ) ) ;
#164397=CARTESIAN_POINT ( 'NONE',  ( -16.46253265017160317, 9.564922557960807481, 105.8322429386476955 ) ) ;
#164398=CARTESIAN_POINT ( 'NONE',  ( 19.02544592524343514, -5.153800228976328945, 93.54057627198102409 ) ) ;
#164400=CARTESIAN_POINT ( 'NONE',  ( -5.719274019375665041, -21.55341960407619695, 19.79275706135235069 ) ) ;
#164401=CARTESIAN_POINT ( 'NONE',  ( 8.314922557960818139, 14.29746914071049879, 74.58224293864768129 ) ) ;
#164402=CARTESIAN_POINT ( 'NONE',  ( -5.719274019375978568, 21.55341960407610458, 70.20724293864769550 ) ) ;
#164403=CARTESIAN_POINT ( 'NONE',  ( -13.97604488694527625, -13.89961937509977652, 66.87390960531436690 ) ) ;
#164404=CARTESIAN_POINT ( 'NONE',  ( -13.97604488694527625, -13.89961937509977652, 76.87390960531433848 ) ) ;
#164405=CARTESIAN_POINT ( 'NONE',  ( -21.53943276465977519, 0.05219959533907696930, 111.2489096053143669 ) ) ;
#164406=VERTEX_POINT ( 'NONE', #66546 ) ;
#164407=CARTESIAN_POINT ( 'NONE',  ( -19.02544592524342804, 5.153800228976336051, 56.04057627198100988 ) ) ;
#164408=CARTESIAN_POINT ( 'NONE',  ( 8.314922557960818139, 14.29746914071049879, 104.5822429386477097 ) ) ;
#164410=CARTESIAN_POINT ( 'NONE',  ( 19.03943276465977164, -0.05219959533909143690, 58.74890960531435979 ) ) ;
#164411=CARTESIAN_POINT ( 'NONE',  ( 13.97604488694548053, -13.89961937509957401, 90.62609039468567573 ) ) ;
#164412=CARTESIAN_POINT ( 'NONE',  ( 16.52544592524342804, -4.483927247898539470, 93.54057627198103830 ) ) ;
#164413=CARTESIAN_POINT ( 'NONE',  ( 5.823673210054444382, -21.52544592524334988, 65.20942372801901854 ) ) ;
#164414=CARTESIAN_POINT ( 'NONE',  ( 19.03943276465977164, -0.05219959533909143690, 53.74890960531436690 ) ) ;
#164415=CARTESIAN_POINT ( 'NONE',  ( 21.53943276465977519, -0.05219959533907433946, 113.7489096053143527 ) ) ;
#164416=CARTESIAN_POINT ( 'NONE',  ( 8.314922557960818139, 14.29746914071049879, 99.58224293864770971 ) ) ;
#164418=CARTESIAN_POINT ( 'NONE',  ( 16.46253265017160672, -9.564922557960803928, 68.33224293864770971 ) ) ;
#164419=CARTESIAN_POINT ( 'NONE',  ( 16.61371651742599553, 7.165104196376170798, 113.6458493000700543 ) ) ;
#164420=CARTESIAN_POINT ( 'NONE',  ( -16.46253265017146816, -9.564922557961047289, 109.1677570613523471 ) ) ;
#164421=CARTESIAN_POINT ( 'NONE',  ( 21.53943276465977519, -0.05219959533907433946, 28.74890960531435624 ) ) ;
#164422=CARTESIAN_POINT ( 'NONE',  ( -10.81492255796105439, 18.62759615963255655, 47.91775706135234714 ) ) ;
#164423=CARTESIAN_POINT ( 'NONE',  ( 5.049401038298161559, -19.05341960407611168, 102.7072429386476955 ) ) ;
#164424=CARTESIAN_POINT ( 'NONE',  ( 13.89961937509957401, 13.97604488694547697, 76.87609039468566152 ) ) ;
#164425=CARTESIAN_POINT ( 'NONE',  ( -9.474510206698964154, 16.51473224551069663, 75.41557627198103830 ) ) ;
#164426=CARTESIAN_POINT ( 'NONE',  ( 12.14591786802309770, 12.06949235617756955, 79.37390960531436690 ) ) ;
#164427=CARTESIAN_POINT ( 'NONE',  ( -16.51473224551069308, -9.474510206698971260, 101.6655762719810241 ) ) ;
#164428=CARTESIAN_POINT ( 'NONE',  ( -16.52544592524342804, 4.483927247898546575, 76.04057627198102409 ) ) ;
#164429=CARTESIAN_POINT ( 'NONE',  ( -13.97604488694527625, -13.89961937509977652, 101.8739096053143811 ) ) ;
#164430=CARTESIAN_POINT ( 'NONE',  ( -19.05341960407611168, -5.049401038298163336, 51.45724293864770260 ) ) ;
#164431=CARTESIAN_POINT ( 'NONE',  ( -14.34966873604960291, -8.224510206698953496, 41.66557627198103120 ) ) ;
#164432=CARTESIAN_POINT ( 'NONE',  ( -9.474510206698964154, 16.51473224551069663, 30.41557627198102054 ) ) ;
#164434=CARTESIAN_POINT ( 'NONE',  ( -10.72451020669870658, -18.67979575497194134, 49.58442372801901143 ) ) ;
#164435=CARTESIAN_POINT ( 'NONE',  ( 19.05341960407617918, -5.049401038297876454, 81.04275706135231871 ) ) ;
#164436=CARTESIAN_POINT ( 'NONE',  ( -0.05219959533910754901, -16.53943276465976808, 52.49890960531435979 ) ) ;
#164437=CARTESIAN_POINT ( 'NONE',  ( 10.72451020669898902, -18.67979575497178502, 92.91557627198103830 ) ) ;
#164438=CARTESIAN_POINT ( 'NONE',  ( 18.67979575497178502, 10.72451020669898547, 29.16557627198103120 ) ) ;
#164439=CARTESIAN_POINT ( 'NONE',  ( 16.53943276465976808, -0.05219959533910856209, 83.74890960531435269 ) ) ;
#164440=CARTESIAN_POINT ( 'NONE',  ( 19.05341960407611168, 5.049401038298154454, 48.95724293864768129 ) ) ;
#164441=CARTESIAN_POINT ( 'NONE',  ( -16.52544592524342804, 4.483927247898546575, 26.04057627198103475 ) ) ;
#164442=CARTESIAN_POINT ( 'NONE',  ( -4.379528057220086978, -16.55341960407618274, 89.79275706135236135 ) ) ;
#164443=CARTESIAN_POINT ( 'NONE',  ( 4.483927247898790824, -16.52544592524335698, 70.20942372801904696 ) ) ;
#164444=CARTESIAN_POINT ( 'NONE',  ( -9.474510206698720793, -16.51473224551083518, 29.58442372801900433 ) ) ;
#164445=CARTESIAN_POINT ( 'NONE',  ( -19.02544592524342804, 5.153800228976336051, 91.04057627198100988 ) ) ;
#164446=CARTESIAN_POINT ( 'NONE',  ( 19.03943276465977164, -0.05219959533909143690, 78.74890960531436690 ) ) ;
#164447=CARTESIAN_POINT ( 'NONE',  ( -4.483927247898782831, 16.52544592524335698, 77.70942372801900433 ) ) ;
#164448=CARTESIAN_POINT ( 'NONE',  ( 19.05341960407611168, 5.049401038298154454, 43.95724293864769550 ) ) ;
#164449=EDGE_CURVE ( 'NONE', #91848, #155866, #121204, .T. ) ;
#164450=CARTESIAN_POINT ( 'NONE',  ( -8.224510206698948167, 14.34966873604960824, 50.41557627198103120 ) ) ;
#164451=CARTESIAN_POINT ( 'NONE',  ( 19.05341960407611168, 5.049401038298154454, 98.95724293864766707 ) ) ;
#164452=CARTESIAN_POINT ( 'NONE',  ( 10.81492255796078972, 18.62759615963270932, 29.58224293864769905 ) ) ;
#164453=CARTESIAN_POINT ( 'NONE',  ( -8.314922557960811034, -14.29746914071050412, 67.08224293864770971 ) ) ;
#164454=CARTESIAN_POINT ( 'NONE',  ( 8.314922557960818139, 14.29746914071049879, 69.58224293864769550 ) ) ;
#164455=CARTESIAN_POINT ( 'NONE',  ( 17.50000000000018474, -3.292511757969704522, 32.56520270210548773 ) ) ;
#164456=CARTESIAN_POINT ( 'NONE',  ( -13.89961937509957401, -13.97604488694547875, 64.37609039468567573 ) ) ;
#164457=CARTESIAN_POINT ( 'NONE',  ( 0.05219959533909260263, 19.03943276465977164, 99.99890960531436690 ) ) ;
#164458=CARTESIAN_POINT ( 'NONE',  ( 9.474510206698729675, 16.51473224551082808, 77.08442372801900433 ) ) ;
#164459=CARTESIAN_POINT ( 'NONE',  ( -17.58332526062525147, -7.635886036038636249, 94.07665040441534643 ) ) ;
#164460=CARTESIAN_POINT ( 'NONE',  ( -19.05341960407617563, 5.049401038297882671, 113.5427570613523471 ) ) ;
#164461=CARTESIAN_POINT ( 'NONE',  ( 16.55341960407618274, -4.379528057220086978, 91.04275706135236135 ) ) ;
#164462=CARTESIAN_POINT ( 'NONE',  ( 5.049401038298161559, -19.05341960407611168, 42.70724293864767418 ) ) ;
#164463=CARTESIAN_POINT ( 'NONE',  ( 21.53943276465977519, -0.05219959533907433946, 38.74890960531435979 ) ) ;
#164464=CARTESIAN_POINT ( 'NONE',  ( -18.67979575497193778, 10.72451020669871902, 53.33442372801901854 ) ) ;
#164465=CARTESIAN_POINT ( 'NONE',  ( 8.224510206698742110, 14.34966873604972548, 27.08442372801901854 ) ) ;
#164467=CARTESIAN_POINT ( 'NONE',  ( -9.474510206698964154, 16.51473224551069663, 80.41557627198103830 ) ) ;
#164468=CARTESIAN_POINT ( 'NONE',  ( 13.97604488694527802, 13.89961937509977652, 114.3739096053143669 ) ) ;
#164469=CARTESIAN_POINT ( 'NONE',  ( -12.06949235617756955, 12.14591786802309770, 80.62390960531438111 ) ) ;
#164470=CARTESIAN_POINT ( 'NONE',  ( 0.05219959533909260263, 19.03943276465977164, 79.99890960531436690 ) ) ;
#164471=CARTESIAN_POINT ( 'NONE',  ( 13.89961937509977652, -13.97604488694527269, 83.12390960531436690 ) ) ;
#164473=CARTESIAN_POINT ( 'NONE',  ( 5.049401038297881783, 19.05341960407617563, 87.29275706135234714 ) ) ;
#164474=CARTESIAN_POINT ( 'NONE',  ( 21.52544592524344225, -5.823673210054117533, 58.54057627198103120 ) ) ;
#164475=CARTESIAN_POINT ( 'NONE',  ( -19.02544592524342804, 5.153800228976336051, 31.04057627198102409 ) ) ;
#164476=CARTESIAN_POINT ( 'NONE',  ( 19.02544592524334988, 5.153800228976608722, 61.45942372801900433 ) ) ;
#164477=CARTESIAN_POINT ( 'NONE',  ( -13.89961937509977652, 13.97604488694528158, 60.62390960531436690 ) ) ;
#164478=CARTESIAN_POINT ( 'NONE',  ( -16.51473224551069308, -9.474510206698971260, 86.66557627198102409 ) ) ;
#164480=CARTESIAN_POINT ( 'NONE',  ( -10.72451020669898014, 18.67979575497178502, 85.41557627198102409 ) ) ;
#164481=CARTESIAN_POINT ( 'NONE',  ( 14.34966873604960469, 8.224510206698951720, 94.16557627198103830 ) ) ;
#164482=CARTESIAN_POINT ( 'NONE',  ( 5.153800228976615827, -19.02544592524334988, 50.20942372801897591 ) ) ;
#164483=CARTESIAN_POINT ( 'NONE',  ( 21.55341960407610458, 5.719274019375980345, 93.95724293864770971 ) ) ;
#164484=CARTESIAN_POINT ( 'NONE',  ( 21.53943276465977519, -0.05219959533907433946, 78.74890960531436690 ) ) ;
#164485=CARTESIAN_POINT ( 'NONE',  ( -4.483927247898539470, -16.52544592524342804, 37.29057627198102409 ) ) ;
#164486=CARTESIAN_POINT ( 'NONE',  ( 21.52544592524334988, 5.823673210054432836, 101.4594237280190185 ) ) ;
#164487=CARTESIAN_POINT ( 'NONE',  ( -16.55341960407617563, 4.379528057220093196, 53.54275706135234714 ) ) ;
#164488=CARTESIAN_POINT ( 'NONE',  ( 19.03943276465977164, -0.05219959533909143690, 78.74890960531436690 ) ) ;
#164489=CARTESIAN_POINT ( 'NONE',  ( -16.51473224551069308, -9.474510206698971260, 26.66557627198103120 ) ) ;
#164490=CARTESIAN_POINT ( 'NONE',  ( -5.719274019375665041, -21.55341960407619695, 44.79275706135234714 ) ) ;
#164491=CARTESIAN_POINT ( 'NONE',  ( 10.72451020669871369, 18.67979575497193778, 52.08442372801901854 ) ) ;
#164492=CARTESIAN_POINT ( 'NONE',  ( -13.89961937509977652, 13.97604488694528158, 50.62390960531435979 ) ) ;
#164493=CARTESIAN_POINT ( 'NONE',  ( -10.72451020669898014, 18.67979575497178502, 115.4155762719810241 ) ) ;
#164494=CARTESIAN_POINT ( 'NONE',  ( 9.474510206698729675, 16.51473224551082808, 67.08442372801900433 ) ) ;
#164495=CARTESIAN_POINT ( 'NONE',  ( 19.05341960407611168, 5.049401038298154454, 38.95724293864767418 ) ) ;
#164496=CARTESIAN_POINT ( 'NONE',  ( 0.05219959533934541429, -16.53943276465976808, 25.00109039468567218 ) ) ;
#164497=CARTESIAN_POINT ( 'NONE',  ( -19.03943276465977164, 0.05219959533909376836, 26.24890960531435624 ) ) ;
#164498=CARTESIAN_POINT ( 'NONE',  ( -4.483927247898782831, 16.52544592524335698, 72.70942372801901854 ) ) ;
#164499=CARTESIAN_POINT ( 'NONE',  ( 9.564922557960805705, 16.46253265017160317, 44.58224293864769550 ) ) ;
#164501=CARTESIAN_POINT ( 'NONE',  ( 13.89961937509977652, -13.97604488694527269, 88.12390960531438111 ) ) ;
#164502=CARTESIAN_POINT ( 'NONE',  ( -0.05219959533909027116, -19.03943276465977164, 22.49890960531436690 ) ) ;
#164503=CARTESIAN_POINT ( 'NONE',  ( 10.81492255796078972, 18.62759615963270932, 79.58224293864769550 ) ) ;
#164504=CARTESIAN_POINT ( 'NONE',  ( 12.14591786802327356, -12.06949235617739191, 50.62609039468568994 ) ) ;
#164505=CARTESIAN_POINT ( 'NONE',  ( -9.564922557961040184, 16.46253265017147172, 22.91775706135233648 ) ) ;
#164506=CARTESIAN_POINT ( 'NONE',  ( -9.564922557960796823, -16.46253265017161027, 37.08224293864768839 ) ) ;
#164507=CARTESIAN_POINT ( 'NONE',  ( 16.52544592524342804, -4.483927247898539470, 28.54057627198103120 ) ) ;
#164508=CARTESIAN_POINT ( 'NONE',  ( 16.52544592524342804, -4.483927247898539470, 63.54057627198103830 ) ) ;
#164510=CARTESIAN_POINT ( 'NONE',  ( -13.89961937509977652, 13.97604488694528158, 65.62390960531436690 ) ) ;
#164511=CARTESIAN_POINT ( 'NONE',  ( -18.62759615963255300, -10.81492255796106328, 109.1677570613523613 ) ) ;
#164512=CARTESIAN_POINT ( 'NONE',  ( 0.05219959533937995610, -21.53943276465977519, 30.00109039468568284 ) ) ;
#164513=CARTESIAN_POINT ( 'NONE',  ( 16.51473224551069308, 9.474510206698969483, 74.16557627198103830 ) ) ;
#164514=CARTESIAN_POINT ( 'NONE',  ( 21.55341960407619695, -5.719274019375665929, 81.04275706135236135 ) ) ;
#164515=CARTESIAN_POINT ( 'NONE',  ( -0.05219959533934338120, 16.53943276465976808, 72.50109039468568994 ) ) ;
#164516=CARTESIAN_POINT ( 'NONE',  ( 16.51473224551069308, 9.474510206698969483, 109.1655762719810383 ) ) ;
#164517=CARTESIAN_POINT ( 'NONE',  ( 12.06949235617757843, -12.14591786802309237, 33.12390960531435979 ) ) ;
#164518=CARTESIAN_POINT ( 'NONE',  ( -9.564922557960796823, -16.46253265017161027, 32.08224293864769550 ) ) ;
#164519=CARTESIAN_POINT ( 'NONE',  ( -4.379528057220086978, -16.55341960407618274, 54.79275706135235424 ) ) ;
#164520=CARTESIAN_POINT ( 'NONE',  ( 4.483927247898545687, 16.52544592524342804, 54.79057627198104541 ) ) ;
#164521=CARTESIAN_POINT ( 'NONE',  ( -19.02544592524342804, 5.153800228976336051, 106.0405762719810241 ) ) ;
#164522=CARTESIAN_POINT ( 'NONE',  ( 10.72451020669898902, -18.67979575497178502, 37.91557627198102409 ) ) ;
#164523=CARTESIAN_POINT ( 'NONE',  ( 18.62759615963255655, 10.81492255796105972, 106.6677570613523756 ) ) ;
#164524=CARTESIAN_POINT ( 'NONE',  ( -4.483927247898539470, -16.52544592524342804, 87.29057627198103830 ) ) ;
#164525=CARTESIAN_POINT ( 'NONE',  ( -19.03943276465977164, 0.05219959533909376836, 96.24890960531436690 ) ) ;
#164526=EDGE_LOOP ( 'NONE', ( #43847, #124149, #172147, #73004 ) ) ;
#164527=CARTESIAN_POINT ( 'NONE',  ( 16.53943276465976808, 0.05219959533934440121, 56.25109039468568284 ) ) ;
#164528=CARTESIAN_POINT ( 'NONE',  ( 16.46253265017160672, -9.564922557960803928, 58.33224293864769550 ) ) ;
#164529=CARTESIAN_POINT ( 'NONE',  ( 13.89961937509957401, 13.97604488694547697, 51.87609039468566863 ) ) ;
#164530=CARTESIAN_POINT ( 'NONE',  ( -16.51473224551069308, -9.474510206698971260, 51.66557627198102409 ) ) ;
#164531=CARTESIAN_POINT ( 'NONE',  ( -14.34966873604972548, 8.224510206698743886, 78.33442372801901854 ) ) ;
#164532=CARTESIAN_POINT ( 'NONE',  ( -5.049401038297874678, -19.05341960407617918, 94.79275706135230450 ) ) ;
#164533=CARTESIAN_POINT ( 'NONE',  ( -0.05219959533937732626, 21.53943276465977519, 62.50109039468568284 ) ) ;
#164534=CARTESIAN_POINT ( 'NONE',  ( -0.05219959533909027116, -19.03943276465977164, 57.49890960531435979 ) ) ;
#164535=CARTESIAN_POINT ( 'NONE',  ( 0.05219959533907565091, 21.53943276465977519, 94.99890960531436690 ) ) ;
#164536=CARTESIAN_POINT ( 'NONE',  ( 14.29746914071049879, -8.314922557960816363, 98.33224293864769550 ) ) ;
#164538=CARTESIAN_POINT ( 'NONE',  ( -13.89961937509957401, -13.97604488694547875, 69.37609039468564731 ) ) ;
#164539=CARTESIAN_POINT ( 'NONE',  ( 5.823673210054125526, 21.52544592524343514, 64.79057627198103830 ) ) ;
#164540=CARTESIAN_POINT ( 'NONE',  ( 19.02544592524334988, 5.153800228976608722, 36.45942372801900433 ) ) ;
#164541=CARTESIAN_POINT ( 'NONE',  ( 18.22780087662123805, 5.499999999999960032, 96.48236817873105053 ) ) ;
#164542=CARTESIAN_POINT ( 'NONE',  ( -18.67979575497178146, -10.72451020669898902, 91.66557627198103830 ) ) ;
#164543=CARTESIAN_POINT ( 'NONE',  ( -19.02130022317638236, 5.499999999999601208, 55.78188669246575415 ) ) ;
#164544=CARTESIAN_POINT ( 'NONE',  ( 4.483927247898790824, -16.52544592524335698, 20.20942372801900788 ) ) ;
#164545=CARTESIAN_POINT ( 'NONE',  ( -4.379528057220086978, -16.55341960407618274, 24.79275706135235779 ) ) ;
#164546=CARTESIAN_POINT ( 'NONE',  ( -19.02544592524342804, 5.153800228976336051, 46.04057627198101699 ) ) ;
#164547=CARTESIAN_POINT ( 'NONE',  ( -16.46253265017160317, 9.564922557960807481, 110.8322429386476955 ) ) ;
#164548=CARTESIAN_POINT ( 'NONE',  ( -5.719274019375978568, 21.55341960407610458, 85.20724293864770971 ) ) ;
#164549=CARTESIAN_POINT ( 'NONE',  ( -10.72451020669870658, -18.67979575497194134, 69.58442372801900433 ) ) ;
#164550=CARTESIAN_POINT ( 'NONE',  ( 8.224510206698742110, 14.34966873604972548, 27.08442372801901854 ) ) ;
#164551=CARTESIAN_POINT ( 'NONE',  ( 5.049401038297881783, 19.05341960407617563, 22.29275706135233648 ) ) ;
#164552=CARTESIAN_POINT ( 'NONE',  ( -16.52544592524342804, 4.483927247898546575, 31.04057627198102409 ) ) ;
#164553=CARTESIAN_POINT ( 'NONE',  ( 5.719274019375991003, -21.55341960407610458, 112.7072429386476955 ) ) ;
#164554=CARTESIAN_POINT ( 'NONE',  ( 0.05219959533910956823, 16.53943276465976808, 44.99890960531435979 ) ) ;
#164555=CARTESIAN_POINT ( 'NONE',  ( 16.46253265017146816, 9.564922557961045513, 91.66775706135234714 ) ) ;
#164556=CARTESIAN_POINT ( 'NONE',  ( -16.46253265017146816, -9.564922557961047289, 54.16775706135234003 ) ) ;
#164557=CARTESIAN_POINT ( 'NONE',  ( -21.53943276465977519, -0.05219959533937600094, 68.75109039468568994 ) ) ;
#164558=CARTESIAN_POINT ( 'NONE',  ( -16.46253265017146816, -9.564922557961047289, 54.16775706135234003 ) ) ;
#164559=CARTESIAN_POINT ( 'NONE',  ( 5.153800228976335163, 19.02544592524342804, 29.79057627198102409 ) ) ;
#164560=CARTESIAN_POINT ( 'NONE',  ( 21.55341960407610458, 5.719274019375980345, 43.95724293864769550 ) ) ;
#164561=CARTESIAN_POINT ( 'NONE',  ( 12.06949235617757843, -12.14591786802309237, 48.12390960531436690 ) ) ;
#164562=CARTESIAN_POINT ( 'NONE',  ( -16.79531203550646268, -7.028104445595714900, 26.25244988220445919 ) ) ;
#164563=CARTESIAN_POINT ( 'NONE',  ( 13.97604488694548053, -13.89961937509957401, 20.62609039468567573 ) ) ;
#164564=CARTESIAN_POINT ( 'NONE',  ( 16.55341960407618274, -4.379528057220086978, 71.04275706135234714 ) ) ;
#164565=CARTESIAN_POINT ( 'NONE',  ( -8.224510206698948167, 14.34966873604960824, 45.41557627198103830 ) ) ;
#164566=CARTESIAN_POINT ( 'NONE',  ( -5.823673210054431948, 21.52544592524334988, 77.70942372801900433 ) ) ;
#164567=CARTESIAN_POINT ( 'NONE',  ( 10.81492255796106328, -18.62759615963255655, 70.41775706135236135 ) ) ;
#164568=CARTESIAN_POINT ( 'NONE',  ( 10.81492255796078972, 18.62759615963270932, 84.58224293864769550 ) ) ;
#164569=CARTESIAN_POINT ( 'NONE',  ( -19.05341960407611168, -5.049401038298163336, 36.45724293864766707 ) ) ;
#164570=CARTESIAN_POINT ( 'NONE',  ( 10.81492255796106328, -18.62759615963255655, 40.41775706135234714 ) ) ;
#164571=CARTESIAN_POINT ( 'NONE',  ( 16.46253265017160672, -9.564922557960803928, 23.33224293864769194 ) ) ;
#164572=CARTESIAN_POINT ( 'NONE',  ( 5.153800228976335163, 19.02544592524342804, 34.79057627198102409 ) ) ;
#164573=CARTESIAN_POINT ( 'NONE',  ( -12.14591786802309592, -12.06949235617757132, 96.87390960531436690 ) ) ;
#164574=CARTESIAN_POINT ( 'NONE',  ( 0.05219959533909260263, 19.03943276465977164, 89.99890960531436690 ) ) ;
#164575=CARTESIAN_POINT ( 'NONE',  ( 8.314922557960818139, 14.29746914071049879, 44.58224293864769550 ) ) ;
#164576=CARTESIAN_POINT ( 'NONE',  ( -8.224510206698948167, 14.34966873604960824, 105.4155762719810383 ) ) ;
#164577=CARTESIAN_POINT ( 'NONE',  ( 0.05219959533907565091, 21.53943276465977519, 64.99890960531435269 ) ) ;
#164578=CARTESIAN_POINT ( 'NONE',  ( 21.53943276465977519, -0.05219959533907433946, 113.7489096053143527 ) ) ;
#164579=CARTESIAN_POINT ( 'NONE',  ( -5.049401038298153566, 19.05341960407611168, 110.2072429386476671 ) ) ;
#164580=CARTESIAN_POINT ( 'NONE',  ( -9.474510206698964154, 16.51473224551069663, 60.41557627198102409 ) ) ;
#164581=CARTESIAN_POINT ( 'NONE',  ( 14.29746914071037800, 8.314922557961029526, 21.66775706135235069 ) ) ;
#164582=CARTESIAN_POINT ( 'NONE',  ( 18.67979575497178502, 10.72451020669898547, 69.16557627198102409 ) ) ;
#164583=CARTESIAN_POINT ( 'NONE',  ( 5.823673210054444382, -21.52544592524334988, 95.20942372801903275 ) ) ;
#164584=CARTESIAN_POINT ( 'NONE',  ( 9.564922557960805705, 16.46253265017160317, 84.58224293864769550 ) ) ;
#164585=CARTESIAN_POINT ( 'NONE',  ( 10.72451020669898902, -18.67979575497178502, 112.9155762719810383 ) ) ;
#164586=CARTESIAN_POINT ( 'NONE',  ( -19.03943276465977164, 0.05219959533909376836, 111.2489096053143669 ) ) ;
#164587=CARTESIAN_POINT ( 'NONE',  ( 12.14591786802327356, -12.06949235617739191, 85.62609039468568994 ) ) ;
#164588=CARTESIAN_POINT ( 'NONE',  ( 21.52544592524334988, 5.823673210054432836, 71.45942372801901854 ) ) ;
#164589=CARTESIAN_POINT ( 'NONE',  ( 15.80617190586769283, -15.72974639402175789, 105.6260903946856899 ) ) ;
#164590=CARTESIAN_POINT ( 'NONE',  ( 12.14591786802327356, -12.06949235617739191, 55.62609039468568284 ) ) ;
#164591=CARTESIAN_POINT ( 'NONE',  ( 21.53943276465977519, 0.05219959533937863772, 26.25109039468567573 ) ) ;
#164592=CARTESIAN_POINT ( 'NONE',  ( -5.153800228976328057, -19.02544592524343514, 112.2905762719810099 ) ) ;
#164593=CARTESIAN_POINT ( 'NONE',  ( -21.55341960407619339, 5.719274019375674811, 88.54275706135236135 ) ) ;
#164594=CARTESIAN_POINT ( 'NONE',  ( 13.97604488694527802, 13.89961937509977652, 99.37390960531436690 ) ) ;
#164595=CARTESIAN_POINT ( 'NONE',  ( -18.67979575497178146, -10.72451020669898902, 86.66557627198102409 ) ) ;
#164596=CARTESIAN_POINT ( 'NONE',  ( -9.474510206698720793, -16.51473224551083518, 64.58442372801900433 ) ) ;
#164597=CARTESIAN_POINT ( 'NONE',  ( -21.53943276465977519, 0.05219959533907696930, 56.24890960531436690 ) ) ;
#164598=CARTESIAN_POINT ( 'NONE',  ( -5.153800228976328057, -19.02544592524343514, 92.29057627198099567 ) ) ;
#164599=CARTESIAN_POINT ( 'NONE',  ( -8.224510206698948167, 14.34966873604960824, 35.41557627198102409 ) ) ;
#164601=CARTESIAN_POINT ( 'NONE',  ( -19.05341960407617563, 5.049401038297882671, 83.54275706135233293 ) ) ;
#164604=CARTESIAN_POINT ( 'NONE',  ( 13.97604488694548053, -13.89961937509957401, 110.6260903946856615 ) ) ;
#164605=CARTESIAN_POINT ( 'NONE',  ( -15.72974639402197994, 15.80617190586746368, 85.62390960531436690 ) ) ;
#164606=CARTESIAN_POINT ( 'NONE',  ( -16.53943276465976808, 0.05219959533911058130, 71.24890960531435269 ) ) ;
#164607=CARTESIAN_POINT ( 'NONE',  ( 12.14591786802327356, -12.06949235617739191, 35.62609039468568994 ) ) ;
#164608=CARTESIAN_POINT ( 'NONE',  ( 16.46253265017160672, -9.564922557960803928, 43.33224293864769550 ) ) ;
#164609=CARTESIAN_POINT ( 'NONE',  ( 5.823673210054125526, 21.52544592524343514, 109.7905762719810383 ) ) ;
#164610=CARTESIAN_POINT ( 'NONE',  ( -5.049401038297874678, -19.05341960407617918, 89.79275706135230450 ) ) ;
#164611=CARTESIAN_POINT ( 'NONE',  ( 19.05341960407611168, 5.049401038298154454, 98.95724293864766707 ) ) ;
#164612=CARTESIAN_POINT ( 'NONE',  ( 19.05341960407611168, 5.049401038298154454, 68.95724293864769550 ) ) ;
#164613=CARTESIAN_POINT ( 'NONE',  ( 15.80617190586746368, 15.72974639402197994, 79.37390960531436690 ) ) ;
#164614=CARTESIAN_POINT ( 'NONE',  ( -13.89961937509977652, 13.97604488694528158, 40.62390960531435979 ) ) ;
#164616=CARTESIAN_POINT ( 'NONE',  ( -16.52544592524342804, 4.483927247898546575, 61.04057627198103120 ) ) ;
#164617=CARTESIAN_POINT ( 'NONE',  ( -19.03943276465977164, 0.05219959533909376836, 96.24890960531436690 ) ) ;
#164619=CARTESIAN_POINT ( 'NONE',  ( -13.97604488694547697, 13.89961937509957934, 68.12609039468563310 ) ) ;
#164620=CARTESIAN_POINT ( 'NONE',  ( 21.53943276465977519, -0.05219959533907433946, 73.74890960531433848 ) ) ;
#164621=CARTESIAN_POINT ( 'NONE',  ( -9.474510206698720793, -16.51473224551083518, 39.58442372801899722 ) ) ;
#164622=CARTESIAN_POINT ( 'NONE',  ( 19.03943276465977164, -0.05219959533909143690, 103.7489096053143669 ) ) ;
#164624=CARTESIAN_POINT ( 'NONE',  ( -21.52544592524343514, 5.823673210054127303, 41.04057627198103120 ) ) ;
#164625=CARTESIAN_POINT ( 'NONE',  ( -19.03943276465977164, 0.05219959533909376836, 66.24890960531436690 ) ) ;
#164626=CARTESIAN_POINT ( 'NONE',  ( -21.53943276465977519, -0.05219959533937600094, 68.75109039468568994 ) ) ;
#164627=CARTESIAN_POINT ( 'NONE',  ( 5.049401038298161559, -19.05341960407611168, 27.70724293864769550 ) ) ;
#164628=CARTESIAN_POINT ( 'NONE',  ( 21.52544592524344225, -5.823673210054117533, 108.5405762719810241 ) ) ;
#164629=ORIENTED_EDGE ( 'NONE', *, *, #164449, .F. ) ;
#164630=CARTESIAN_POINT ( 'NONE',  ( 18.62759615963255655, 10.81492255796105972, 51.66775706135234714 ) ) ;
#164633=CARTESIAN_POINT ( 'NONE',  ( -16.46253265017146816, -9.564922557961047289, 64.16775706135233293 ) ) ;
#164635=CARTESIAN_POINT ( 'NONE',  ( 0.05219959533907565091, 21.53943276465977519, 104.9989096053143669 ) ) ;
#164636=CARTESIAN_POINT ( 'NONE',  ( -0.05219959533909027116, -19.03943276465977164, 62.49890960531435979 ) ) ;
#164637=CARTESIAN_POINT ( 'NONE',  ( 4.483927247898790824, -16.52544592524335698, 40.20942372801901854 ) ) ;
#164639=CARTESIAN_POINT ( 'NONE',  ( 10.72451020669871369, 18.67979575497193778, 102.0844237280190185 ) ) ;
#164640=CARTESIAN_POINT ( 'NONE',  ( -19.03943276465977164, 0.05219959533909376836, 36.24890960531436690 ) ) ;
#164641=CARTESIAN_POINT ( 'NONE',  ( -21.53943276465977519, -0.05219959533937600094, 108.7510903946857042 ) ) ;
#164642=CARTESIAN_POINT ( 'NONE',  ( -5.049401038298153566, 19.05341960407611168, 85.20724293864766707 ) ) ;
#164643=CARTESIAN_POINT ( 'NONE',  ( -5.719274019375665041, -21.55341960407619695, 64.79275706135234714 ) ) ;
#164646=CARTESIAN_POINT ( 'NONE',  ( 16.46253265017160672, -9.564922557960803928, 113.3322429386476955 ) ) ;
#164647=CARTESIAN_POINT ( 'NONE',  ( -17.49999999999998224, 3.512728167237041621, 30.22809995181128428 ) ) ;
#164648=CARTESIAN_POINT ( 'NONE',  ( -16.55341960407617563, 4.379528057220093196, 58.54275706135235424 ) ) ;
#164649=CARTESIAN_POINT ( 'NONE',  ( 10.72451020669871369, 18.67979575497193778, 72.08442372801899012 ) ) ;
#164650=CARTESIAN_POINT ( 'NONE',  ( 18.67979575497194134, -10.72451020669871369, 90.83442372801901854 ) ) ;
#164652=CARTESIAN_POINT ( 'NONE',  ( 4.379528057220092307, 16.55341960407617563, 32.29275706135235424 ) ) ;
#164653=CARTESIAN_POINT ( 'NONE',  ( 5.153800228976335163, 19.02544592524342804, 89.79057627198102409 ) ) ;
#164655=ORIENTED_EDGE ( 'NONE', *, *, #96611, .T. ) ;
#164657=CARTESIAN_POINT ( 'NONE',  ( -5.153800228976328057, -19.02544592524343514, 22.29057627198102765 ) ) ;
#164658=CARTESIAN_POINT ( 'NONE',  ( -21.52544592524343514, 5.823673210054127303, 46.04057627198103830 ) ) ;
#164659=CARTESIAN_POINT ( 'NONE',  ( 14.34966873604972726, -8.224510206698740333, 110.8344237280190043 ) ) ;
#164660=CARTESIAN_POINT ( 'NONE',  ( 8.224510206698953496, -14.34966873604960469, 82.91557627198103830 ) ) ;
#164661=CARTESIAN_POINT ( 'NONE',  ( 9.564922557960805705, 16.46253265017160317, 74.58224293864769550 ) ) ;
#164662=CARTESIAN_POINT ( 'NONE',  ( 18.67979575497194134, -10.72451020669871369, 95.83442372801903275 ) ) ;
#164663=CARTESIAN_POINT ( 'NONE',  ( 0.05219959533934541429, -16.53943276465976808, 30.00109039468568284 ) ) ;
#164664=CARTESIAN_POINT ( 'NONE',  ( 12.14591786802309770, 12.06949235617756955, 89.37390960531435269 ) ) ;
#164665=CARTESIAN_POINT ( 'NONE',  ( -5.823673210054431948, 21.52544592524334988, 42.70942372801901854 ) ) ;
#164666=CARTESIAN_POINT ( 'NONE',  ( -21.53943276465977519, 0.05219959533907696930, 71.24890960531435269 ) ) ;
#164667=CARTESIAN_POINT ( 'NONE',  ( 5.049401038297881783, 19.05341960407617563, 42.29275706135234003 ) ) ;
#164669=CARTESIAN_POINT ( 'NONE',  ( -9.564922557960796823, -16.46253265017161027, 82.08224293864768129 ) ) ;
#164670=CARTESIAN_POINT ( 'NONE',  ( -4.379528057220328563, 16.55341960407611168, 60.20724293864768839 ) ) ;
#164671=AXIS2_PLACEMENT_3D ( 'NONE', #59804, #186152, #32458 ) ;
#164672=CARTESIAN_POINT ( 'NONE',  ( -16.52544592524342804, 4.483927247898546575, 41.04057627198103120 ) ) ;
#164673=CARTESIAN_POINT ( 'NONE',  ( -4.379528057220086978, -16.55341960407618274, 109.7927570613523613 ) ) ;
#164674=CARTESIAN_POINT ( 'NONE',  ( 9.474510206698729675, 16.51473224551082808, 62.08442372801899722 ) ) ;
#164675=CARTESIAN_POINT ( 'NONE',  ( 17.48847506799968698, 5.747544572773807481, 46.67302562156721280 ) ) ;
#164676=CARTESIAN_POINT ( 'NONE',  ( -18.62759615963270932, 10.81492255796079327, 25.83224293864769194 ) ) ;
#164678=CARTESIAN_POINT ( 'NONE',  ( 8.314922557960818139, 14.29746914071049879, 84.58224293864769550 ) ) ;
#164679=CARTESIAN_POINT ( 'NONE',  ( 18.52568451169414843, -5.500000000000145661, 38.52123528320487367 ) ) ;
#164680=CARTESIAN_POINT ( 'NONE',  ( -9.564922557960796823, -16.46253265017161027, 47.08224293864769550 ) ) ;
#164681=CARTESIAN_POINT ( 'NONE',  ( -10.81492255796078084, -18.62759615963271287, 47.08224293864770260 ) ) ;
#164682=CARTESIAN_POINT ( 'NONE',  ( 5.719274019375991003, -21.55341960407610458, 82.70724293864770971 ) ) ;
#164683=CARTESIAN_POINT ( 'NONE',  ( 8.224510206698953496, -14.34966873604960469, 107.9155762719810241 ) ) ;
#164684=CARTESIAN_POINT ( 'NONE',  ( -16.52544592524335698, -4.483927247898792601, 63.95942372801901854 ) ) ;
#164685=CARTESIAN_POINT ( 'NONE',  ( -16.51473224551069308, -9.474510206698971260, 41.66557627198103120 ) ) ;
#164686=CARTESIAN_POINT ( 'NONE',  ( 21.52544592524334988, 5.823673210054432836, 51.45942372801901854 ) ) ;
#164687=CARTESIAN_POINT ( 'NONE',  ( -16.53943276465976808, 0.05219959533911058130, 101.2489096053143669 ) ) ;
#164688=CARTESIAN_POINT ( 'NONE',  ( -9.474510206698720793, -16.51473224551083518, 84.58442372801900433 ) ) ;
#164691=CARTESIAN_POINT ( 'NONE',  ( -15.72974639402197994, 15.80617190586746368, 50.62390960531435979 ) ) ;
#164692=CARTESIAN_POINT ( 'NONE',  ( 16.21995358207306737, -7.366697692864089042, 67.43551001512162202 ) ) ;
#164693=CARTESIAN_POINT ( 'NONE',  ( -15.72974639402176322, -15.80617190586768395, 79.37609039468567573 ) ) ;
#164694=CARTESIAN_POINT ( 'NONE',  ( 16.55341960407611168, 4.379528057220329451, 38.95724293864768839 ) ) ;
#164695=CARTESIAN_POINT ( 'NONE',  ( -8.314922557961024197, 14.29746914071037800, 52.91775706135235424 ) ) ;
#164696=CARTESIAN_POINT ( 'NONE',  ( 12.14591786802309770, 12.06949235617756955, 44.37390960531435979 ) ) ;
#164697=CARTESIAN_POINT ( 'NONE',  ( 10.81492255796078972, 18.62759615963270932, 74.58224293864768129 ) ) ;
#164698=CARTESIAN_POINT ( 'NONE',  ( 0.05219959533907565091, 21.53943276465977519, 69.99890960531435269 ) ) ;
#164700=CARTESIAN_POINT ( 'NONE',  ( 5.153800228976615827, -19.02544592524334988, 90.20942372801900433 ) ) ;
#164701=CARTESIAN_POINT ( 'NONE',  ( 21.55341960407610458, 5.719274019375980345, 23.95724293864769550 ) ) ;
#164702=CARTESIAN_POINT ( 'NONE',  ( -19.05341960407611168, -5.049401038298163336, 51.45724293864770260 ) ) ;
#164703=CARTESIAN_POINT ( 'NONE',  ( -16.51473224551069308, -9.474510206698971260, 21.66557627198102765 ) ) ;
#164706=ORIENTED_EDGE ( 'NONE', *, *, #33627, .T. ) ;
#164707=CARTESIAN_POINT ( 'NONE',  ( -8.314922557961024197, 14.29746914071037800, 82.91775706135234714 ) ) ;
#164708=CARTESIAN_POINT ( 'NONE',  ( 21.52544592524344225, -5.823673210054117533, 108.5405762719810241 ) ) ;
#164709=CARTESIAN_POINT ( 'NONE',  ( -19.03943276465977164, 0.05219959533909376836, 66.24890960531436690 ) ) ;
#164710=CARTESIAN_POINT ( 'NONE',  ( -18.67979575497193778, 10.72451020669871902, 43.33442372801901143 ) ) ;
#164711=CARTESIAN_POINT ( 'NONE',  ( -0.05219959533909027116, -19.03943276465977164, 92.49890960531436690 ) ) ;
#164714=CARTESIAN_POINT ( 'NONE',  ( -15.80617190586768217, 15.72974639402176855, 38.12609039468567573 ) ) ;
#164715=CARTESIAN_POINT ( 'NONE',  ( -9.564922557960796823, -16.46253265017161027, 27.08224293864769550 ) ) ;
#164716=CARTESIAN_POINT ( 'NONE',  ( -19.03943276465977164, -0.05219959533935918106, 93.75109039468566152 ) ) ;
#164717=CARTESIAN_POINT ( 'NONE',  ( 5.049401038297881783, 19.05341960407617563, 37.29275706135232582 ) ) ;
#164718=CARTESIAN_POINT ( 'NONE',  ( 21.55341960407610458, 5.719274019375980345, 108.9572429386476955 ) ) ;
#164719=CARTESIAN_POINT ( 'NONE',  ( 9.474510206698729675, 16.51473224551082808, 47.08442372801900433 ) ) ;
#164720=CARTESIAN_POINT ( 'NONE',  ( -16.46253265017146816, -9.564922557961047289, 49.16775706135233293 ) ) ;
#164721=CARTESIAN_POINT ( 'NONE',  ( -0.05219959533934338120, 16.53943276465976808, 92.50109039468567573 ) ) ;
#164724=CARTESIAN_POINT ( 'NONE',  ( -0.05219959533909027116, -19.03943276465977164, 77.49890960531435269 ) ) ;
#164725=CARTESIAN_POINT ( 'NONE',  ( -15.72974639402176322, -15.80617190586768395, 74.37609039468568994 ) ) ;
#164726=CARTESIAN_POINT ( 'NONE',  ( 10.72451020669871369, 18.67979575497193778, 97.08442372801904696 ) ) ;
#164728=CARTESIAN_POINT ( 'NONE',  ( 19.03943276465977164, -0.05219959533909143690, 93.74890960531435269 ) ) ;
#164729=CARTESIAN_POINT ( 'NONE',  ( -5.823673210054431948, 21.52544592524334988, 67.70942372801901854 ) ) ;
#164730=CARTESIAN_POINT ( 'NONE',  ( 19.02544592524334988, 5.153800228976608722, 96.45942372801897591 ) ) ;
#164731=CARTESIAN_POINT ( 'NONE',  ( 0.05219959533909260263, 19.03943276465977164, 64.99890960531436690 ) ) ;
#164732=CARTESIAN_POINT ( 'NONE',  ( -19.02544592524342804, 5.153800228976336051, 116.0405762719810383 ) ) ;
#164733=CARTESIAN_POINT ( 'NONE',  ( 5.153800228976335163, 19.02544592524342804, 79.79057627198102409 ) ) ;
#164735=CARTESIAN_POINT ( 'NONE',  ( 19.03943276465977164, -0.05219959533909143690, 68.74890960531436690 ) ) ;
#164736=CARTESIAN_POINT ( 'NONE',  ( 16.46253265017160672, -9.564922557960803928, 48.33224293864769550 ) ) ;
#164737=CARTESIAN_POINT ( 'NONE',  ( 5.719274019375991003, -21.55341960407610458, 112.7072429386476955 ) ) ;
#164738=CARTESIAN_POINT ( 'NONE',  ( 12.06949235617739724, 12.14591786802326823, 96.87609039468568994 ) ) ;
#164739=CARTESIAN_POINT ( 'NONE',  ( -18.22780087662126647, -5.499999999999827693, 38.98236817873107185 ) ) ;
#164741=CARTESIAN_POINT ( 'NONE',  ( -9.474510206698720793, -16.51473224551083518, 54.58442372801899722 ) ) ;
#164742=CARTESIAN_POINT ( 'NONE',  ( 5.049401038298161559, -19.05341960407611168, 82.70724293864770971 ) ) ;
#164743=CARTESIAN_POINT ( 'NONE',  ( -0.05219959533910754901, -16.53943276465976808, 77.49890960531433848 ) ) ;
#164744=CARTESIAN_POINT ( 'NONE',  ( 16.52544592524342804, -4.483927247898539470, 108.5405762719810241 ) ) ;
#164745=CARTESIAN_POINT ( 'NONE',  ( 21.52544592524344225, -5.823673210054117533, 38.54057627198103120 ) ) ;
#164746=CARTESIAN_POINT ( 'NONE',  ( 19.05341960407611168, 5.049401038298154454, 103.9572429386476671 ) ) ;
#164747=CARTESIAN_POINT ( 'NONE',  ( 12.06949235617757843, -12.14591786802309237, 88.12390960531436690 ) ) ;
#164748=CARTESIAN_POINT ( 'NONE',  ( 16.46253265017160672, -9.564922557960803928, 113.3322429386476955 ) ) ;
#164749=CARTESIAN_POINT ( 'NONE',  ( -13.97604488694547697, 13.89961937509957934, 28.12609039468565797 ) ) ;
#164750=CARTESIAN_POINT ( 'NONE',  ( 16.55341960407618274, -4.379528057220086978, 111.0427570613523613 ) ) ;
#164751=CARTESIAN_POINT ( 'NONE',  ( -0.05219959533909027116, -19.03943276465977164, 92.49890960531436690 ) ) ;
#164752=CARTESIAN_POINT ( 'NONE',  ( 5.719274019375673035, 21.55341960407619339, 47.29275706135234003 ) ) ;
#164753=CARTESIAN_POINT ( 'NONE',  ( 0.05219959533907565091, 21.53943276465977519, 39.99890960531436690 ) ) ;
#164754=CARTESIAN_POINT ( 'NONE',  ( 21.55341960407619695, -5.719274019375665929, 26.04275706135235779 ) ) ;
#164755=CARTESIAN_POINT ( 'NONE',  ( 18.67979575497178502, 10.72451020669898547, 74.16557627198102409 ) ) ;
#164756=CARTESIAN_POINT ( 'NONE',  ( -16.53943276465976808, 0.05219959533911058130, 91.24890960531436690 ) ) ;
#164757=CARTESIAN_POINT ( 'NONE',  ( -0.05219959533936034679, 19.03943276465977164, 62.50109039468566863 ) ) ;
#164758=CARTESIAN_POINT ( 'NONE',  ( 19.05341960407611168, 5.049401038298154454, 33.95724293864769550 ) ) ;
#164759=CARTESIAN_POINT ( 'NONE',  ( -16.46253265017160317, 9.564922557960807481, 100.8322429386477097 ) ) ;
#164760=CARTESIAN_POINT ( 'NONE',  ( 19.05341960407611168, 5.049401038298154454, 98.95724293864766707 ) ) ;
#164761=CARTESIAN_POINT ( 'NONE',  ( 12.14591786802309770, 12.06949235617756955, 109.3739096053143811 ) ) ;
#164762=CARTESIAN_POINT ( 'NONE',  ( 16.53943276465976808, -0.05219959533910856209, 33.74890960531436690 ) ) ;
#164763=CARTESIAN_POINT ( 'NONE',  ( 0.05219959533934541429, -16.53943276465976808, 45.00109039468568284 ) ) ;
#164764=CARTESIAN_POINT ( 'NONE',  ( 0.05219959533937995610, -21.53943276465977519, 110.0010903946856757 ) ) ;
#164765=CARTESIAN_POINT ( 'NONE',  ( -16.46253265017160317, 9.564922557960807481, 110.8322429386476955 ) ) ;
#164766=CARTESIAN_POINT ( 'NONE',  ( -16.53943276465976808, 0.05219959533911058130, 21.24890960531436690 ) ) ;
#164767=CARTESIAN_POINT ( 'NONE',  ( 5.719274019375673035, 21.55341960407619339, 32.29275706135235424 ) ) ;
#164768=CARTESIAN_POINT ( 'NONE',  ( -5.049401038298153566, 19.05341960407611168, 45.20724293864769550 ) ) ;
#164769=CARTESIAN_POINT ( 'NONE',  ( -16.53943276465976808, -0.05219959533934237506, 48.75109039468568284 ) ) ;
#164770=CARTESIAN_POINT ( 'NONE',  ( 14.34966873604972726, -8.224510206698740333, 105.8344237280190328 ) ) ;
#164771=CARTESIAN_POINT ( 'NONE',  ( -4.379528057220086978, -16.55341960407618274, 94.79275706135234714 ) ) ;
#164772=CARTESIAN_POINT ( 'NONE',  ( 9.564922557961047289, -16.46253265017146816, 110.4177570613523471 ) ) ;
#164773=EDGE_CURVE ( 'NONE', #78133, #18983, #46129, .T. ) ;
#164774=CARTESIAN_POINT ( 'NONE',  ( -5.049401038298153566, 19.05341960407611168, 40.20724293864768839 ) ) ;
#164775=CARTESIAN_POINT ( 'NONE',  ( 12.14591786802309770, 12.06949235617756955, 94.37390960531436690 ) ) ;
#164776=CARTESIAN_POINT ( 'NONE',  ( -10.81492255796078084, -18.62759615963271287, 102.0822429386476955 ) ) ;
#164777=CARTESIAN_POINT ( 'NONE',  ( 5.049401038298161559, -19.05341960407611168, 37.70724293864768839 ) ) ;
#164778=CARTESIAN_POINT ( 'NONE',  ( -9.564922557960796823, -16.46253265017161027, 107.0822429386476955 ) ) ;
#164779=CARTESIAN_POINT ( 'NONE',  ( -5.719274019375665041, -21.55341960407619695, 29.79275706135234358 ) ) ;
#164781=CARTESIAN_POINT ( 'NONE',  ( 19.02544592524343514, -5.153800228976328945, 108.5405762719810383 ) ) ;
#164783=CARTESIAN_POINT ( 'NONE',  ( -19.02544592524342804, 5.153800228976336051, 81.04057627198103830 ) ) ;
#164784=CARTESIAN_POINT ( 'NONE',  ( -21.55341960407619339, 5.719274019375674811, 28.54275706135234358 ) ) ;
#164785=CARTESIAN_POINT ( 'NONE',  ( -16.53943276465976808, 0.05219959533911058130, 86.24890960531436690 ) ) ;
#164786=CARTESIAN_POINT ( 'NONE',  ( -13.89961937509977652, 13.97604488694528158, 100.6239096053143669 ) ) ;
#164788=CARTESIAN_POINT ( 'NONE',  ( 12.14591786802327356, -12.06949235617739191, 60.62609039468567573 ) ) ;
#164789=CARTESIAN_POINT ( 'NONE',  ( -5.719274019375665041, -21.55341960407619695, 74.79275706135234714 ) ) ;
#164790=CARTESIAN_POINT ( 'NONE',  ( -12.06949235617739369, -12.14591786802326823, 44.37609039468567573 ) ) ;
#164791=CARTESIAN_POINT ( 'NONE',  ( -19.05341960407611168, -5.049401038298163336, 81.45724293864769550 ) ) ;
#164792=CARTESIAN_POINT ( 'NONE',  ( -19.03943276465977164, -0.05219959533935918106, 108.7510903946856615 ) ) ;
#164793=CARTESIAN_POINT ( 'NONE',  ( -16.53943276465976808, -0.05219959533934237506, 63.75109039468568284 ) ) ;
#164794=CARTESIAN_POINT ( 'NONE',  ( 19.02544592524334988, 5.153800228976608722, 21.45942372801899012 ) ) ;
#164795=CARTESIAN_POINT ( 'NONE',  ( -9.564922557961040184, 16.46253265017147172, 87.91775706135233293 ) ) ;
#164796=CARTESIAN_POINT ( 'NONE',  ( 9.564922557960805705, 16.46253265017160317, 64.58224293864769550 ) ) ;
#164797=CARTESIAN_POINT ( 'NONE',  ( 15.72974639402199770, -15.80617190586745480, 88.12390960531436690 ) ) ;
#164798=CARTESIAN_POINT ( 'NONE',  ( -4.483927247898539470, -16.52544592524342804, 87.29057627198103830 ) ) ;
#164799=CARTESIAN_POINT ( 'NONE',  ( -5.153800228976607833, 19.02544592524334988, 87.70942372801897591 ) ) ;
#164800=CARTESIAN_POINT ( 'NONE',  ( -14.29746914071037622, -8.314922557961029526, 64.16775706135234714 ) ) ;
#164801=CARTESIAN_POINT ( 'NONE',  ( -19.36337904590693171, 5.499999999999953815, 80.41494137495621430 ) ) ;
#164802=CARTESIAN_POINT ( 'NONE',  ( 9.474510206698729675, 16.51473224551082808, 62.08442372801899722 ) ) ;
#164803=CARTESIAN_POINT ( 'NONE',  ( -14.34966873604960291, -8.224510206698953496, 26.66557627198103475 ) ) ;
#164804=CARTESIAN_POINT ( 'NONE',  ( 16.52544592524342804, -4.483927247898539470, 78.54057627198103830 ) ) ;
#164805=CARTESIAN_POINT ( 'NONE',  ( 9.564922557961047289, -16.46253265017146816, 25.41775706135234003 ) ) ;
#164806=CARTESIAN_POINT ( 'NONE',  ( 18.22780087662122384, -5.500000000000022204, 46.01540105326107266 ) ) ;
#164807=CARTESIAN_POINT ( 'NONE',  ( 5.823673210054444382, -21.52544592524334988, 30.20942372801902565 ) ) ;
#164808=CARTESIAN_POINT ( 'NONE',  ( -16.51473224551069308, -9.474510206698971260, 96.66557627198102409 ) ) ;
#164809=CARTESIAN_POINT ( 'NONE',  ( -19.02544592524342804, 5.153800228976336051, 81.04057627198103830 ) ) ;
#164810=CARTESIAN_POINT ( 'NONE',  ( 18.67979575497194134, -10.72451020669871369, 90.83442372801901854 ) ) ;
#164811=CARTESIAN_POINT ( 'NONE',  ( 13.97604488694527802, 13.89961937509977652, 79.37390960531435269 ) ) ;
#164812=CARTESIAN_POINT ( 'NONE',  ( 10.72451020669898902, -18.67979575497178502, 32.91557627198102409 ) ) ;
#164813=CARTESIAN_POINT ( 'NONE',  ( -12.06949235617756955, 12.14591786802309770, 85.62390960531436690 ) ) ;
#164814=CARTESIAN_POINT ( 'NONE',  ( 19.02544592524343514, -5.153800228976328945, 48.54057627198103120 ) ) ;
#164815=CARTESIAN_POINT ( 'NONE',  ( -12.14591786802309592, -12.06949235617757132, 96.87390960531436690 ) ) ;
#164816=CARTESIAN_POINT ( 'NONE',  ( -15.72974639402197994, 15.80617190586746368, 105.6239096053143669 ) ) ;
#164818=CARTESIAN_POINT ( 'NONE',  ( -10.72451020669870658, -18.67979575497194134, 64.58442372801900433 ) ) ;
#164819=CARTESIAN_POINT ( 'NONE',  ( -9.564922557960796823, -16.46253265017161027, 27.08224293864769550 ) ) ;
#164820=CARTESIAN_POINT ( 'NONE',  ( -14.29746914071037622, -8.314922557961029526, 64.16775706135234714 ) ) ;
#164821=CARTESIAN_POINT ( 'NONE',  ( -15.80617190586745835, -15.72974639402198527, 101.8739096053143811 ) ) ;
#164822=CARTESIAN_POINT ( 'NONE',  ( 10.72451020669898902, -18.67979575497178502, 112.9155762719810383 ) ) ;
#164823=CARTESIAN_POINT ( 'NONE',  ( -5.153800228976607833, 19.02544592524334988, 42.70942372801901143 ) ) ;
#164824=CARTESIAN_POINT ( 'NONE',  ( 0.05219959533909260263, 19.03943276465977164, 49.99890960531435979 ) ) ;
#164826=CARTESIAN_POINT ( 'NONE',  ( 10.81492255796106328, -18.62759615963255655, 55.41775706135234714 ) ) ;
#164827=CARTESIAN_POINT ( 'NONE',  ( -0.05219959533907301413, -21.53943276465977519, 62.49890960531436690 ) ) ;
#164828=CARTESIAN_POINT ( 'NONE',  ( 14.34966873604960469, 8.224510206698951720, 39.16557627198102409 ) ) ;
#164829=CARTESIAN_POINT ( 'NONE',  ( -15.80617190586768217, 15.72974639402176855, 73.12609039468567573 ) ) ;
#164830=CARTESIAN_POINT ( 'NONE',  ( 19.03943276465977164, 0.05219959533936151252, 21.25109039468565797 ) ) ;
#164831=CARTESIAN_POINT ( 'NONE',  ( 16.53943276465976808, -0.05219959533910856209, 63.74890960531435979 ) ) ;
#164832=CARTESIAN_POINT ( 'NONE',  ( -14.29746914071049879, 8.314922557960819915, 105.8322429386476955 ) ) ;
#164833=CARTESIAN_POINT ( 'NONE',  ( 9.564922557961047289, -16.46253265017146816, 40.41775706135234003 ) ) ;
#164834=CARTESIAN_POINT ( 'NONE',  ( 16.52544592524335698, 4.483927247898782831, 101.4594237280190185 ) ) ;
#164835=CARTESIAN_POINT ( 'NONE',  ( -10.81492255796105439, 18.62759615963255655, 67.91775706135234714 ) ) ;
#164836=CARTESIAN_POINT ( 'NONE',  ( 19.05341960407611168, 5.049401038298154454, 53.95724293864770260 ) ) ;
#164837=CARTESIAN_POINT ( 'NONE',  ( -9.564922557961040184, 16.46253265017147172, 32.91775706135233293 ) ) ;
#164838=CARTESIAN_POINT ( 'NONE',  ( 0.05219959533907565091, 21.53943276465977519, 44.99890960531435979 ) ) ;
#164839=CARTESIAN_POINT ( 'NONE',  ( 18.67979575497194134, -10.72451020669871369, 25.83442372801901499 ) ) ;
#164840=CARTESIAN_POINT ( 'NONE',  ( 21.53943276465977519, -0.05219959533907433946, 83.74890960531435269 ) ) ;
#164841=CARTESIAN_POINT ( 'NONE',  ( -16.51473224551082808, 9.474510206698731452, 88.33442372801900433 ) ) ;
#164842=CARTESIAN_POINT ( 'NONE',  ( -4.483927247898782831, 16.52544592524335698, 52.70942372801902565 ) ) ;
#164844=CARTESIAN_POINT ( 'NONE',  ( 21.55341960407610458, 5.719274019375980345, 93.95724293864770971 ) ) ;
#164845=CARTESIAN_POINT ( 'NONE',  ( 0.05219959533910956823, 16.53943276465976808, 79.99890960531435269 ) ) ;
#164846=CARTESIAN_POINT ( 'NONE',  ( 17.60691670004651854, 5.500000000000061284, 41.63333313366439370 ) ) ;
#164847=CARTESIAN_POINT ( 'NONE',  ( 8.314922557961029526, -14.29746914071037800, 25.41775706135235779 ) ) ;
#164848=CARTESIAN_POINT ( 'NONE',  ( 18.67979575497178502, 10.72451020669898547, 34.16557627198102409 ) ) ;
#164849=CARTESIAN_POINT ( 'NONE',  ( -0.05219959533934338120, 16.53943276465976808, 72.50109039468568994 ) ) ;
#164850=CARTESIAN_POINT ( 'NONE',  ( -5.049401038298153566, 19.05341960407611168, 25.20724293864768484 ) ) ;
#164851=CARTESIAN_POINT ( 'NONE',  ( -16.53943276465976808, -0.05219959533934237506, 53.75109039468568994 ) ) ;
#164852=CARTESIAN_POINT ( 'NONE',  ( -10.81492255796105439, 18.62759615963255655, 22.91775706135235069 ) ) ;
#164853=CARTESIAN_POINT ( 'NONE',  ( -21.53943276465977519, 0.05219959533907696930, 46.24890960531435979 ) ) ;
#164854=CARTESIAN_POINT ( 'NONE',  ( -4.483927247898782831, 16.52544592524335698, 67.70942372801901854 ) ) ;
#164855=CARTESIAN_POINT ( 'NONE',  ( -13.97604488694527625, -13.89961937509977652, 81.87390960531436690 ) ) ;
#164856=CARTESIAN_POINT ( 'NONE',  ( 18.62759615963255655, 10.81492255796105972, 51.66775706135234714 ) ) ;
#164857=CARTESIAN_POINT ( 'NONE',  ( -19.02544592524342804, 5.153800228976336051, 31.04057627198102409 ) ) ;
#164858=CARTESIAN_POINT ( 'NONE',  ( 10.81492255796078972, 18.62759615963270932, 44.58224293864769550 ) ) ;
#164859=CARTESIAN_POINT ( 'NONE',  ( 18.67979575497178502, 10.72451020669898547, 24.16557627198103120 ) ) ;
#164861=CARTESIAN_POINT ( 'NONE',  ( -9.564922557961040184, 16.46253265017147172, 37.91775706135233293 ) ) ;
#164862=CARTESIAN_POINT ( 'NONE',  ( 0.05219959533934541429, -16.53943276465976808, 50.00109039468568994 ) ) ;
#164863=CARTESIAN_POINT ( 'NONE',  ( 9.474510206698971260, -16.51473224551069308, 112.9155762719810383 ) ) ;
#164865=EDGE_CURVE ( 'NONE', #198671, #85061, #29325, .T. ) ;
#164866=CARTESIAN_POINT ( 'NONE',  ( -13.89961937509977652, 13.97604488694528158, 90.62390960531432427 ) ) ;
#164867=CARTESIAN_POINT ( 'NONE',  ( 8.314922557961029526, -14.29746914071037800, 100.4177570613523471 ) ) ;
#164868=CARTESIAN_POINT ( 'NONE',  ( -18.22780087662122028, 5.500000000000031086, 93.51540105326107266 ) ) ;
#164869=CARTESIAN_POINT ( 'NONE',  ( -16.55341960407611168, -4.379528057220339221, 101.4572429386476955 ) ) ;
#164870=CARTESIAN_POINT ( 'NONE',  ( 10.81492255796078972, 18.62759615963270932, 44.58224293864769550 ) ) ;
#164871=CARTESIAN_POINT ( 'NONE',  ( -9.474510206698964154, 16.51473224551069663, 35.41557627198102409 ) ) ;
#164872=CARTESIAN_POINT ( 'NONE',  ( -4.379528057220086978, -16.55341960407618274, 79.79275706135236135 ) ) ;
#164873=CARTESIAN_POINT ( 'NONE',  ( -18.62759615963270932, 10.81492255796079327, 115.8322429386477097 ) ) ;
#164874=CARTESIAN_POINT ( 'NONE',  ( 19.03943276465977164, 0.05219959533936151252, 76.25109039468566152 ) ) ;
#164875=CARTESIAN_POINT ( 'NONE',  ( 5.153800228976335163, 19.02544592524342804, 39.79057627198100988 ) ) ;
#164876=CARTESIAN_POINT ( 'NONE',  ( -19.03943276465977164, 0.05219959533909376836, 106.2489096053143669 ) ) ;
#164877=CARTESIAN_POINT ( 'NONE',  ( -18.67979575497193778, 10.72451020669871902, 103.3344237280190043 ) ) ;
#164878=CARTESIAN_POINT ( 'NONE',  ( 16.51473224551069308, 9.474510206698969483, 64.16557627198102409 ) ) ;
#164879=EDGE_CURVE ( 'NONE', #161202, #92863, #34321, .T. ) ;
#164880=CARTESIAN_POINT ( 'NONE',  ( -4.483927247898782831, 16.52544592524335698, 52.70942372801902565 ) ) ;
#164881=CARTESIAN_POINT ( 'NONE',  ( -21.52544592524334988, -5.823673210054445271, 88.95942372801901854 ) ) ;
#164882=CARTESIAN_POINT ( 'NONE',  ( -16.51473224551082808, 9.474510206698731452, 53.33442372801900433 ) ) ;
#164883=CARTESIAN_POINT ( 'NONE',  ( 0.05219959533936267826, -19.03943276465977164, 50.00109039468566863 ) ) ;
#164885=CARTESIAN_POINT ( 'NONE',  ( 21.52544592524334988, 5.823673210054432836, 51.45942372801901854 ) ) ;
#164888=CARTESIAN_POINT ( 'NONE',  ( -19.03943276465977164, -0.05219959533935918106, 43.75109039468566863 ) ) ;
#164889=CARTESIAN_POINT ( 'NONE',  ( -19.02544592524342804, 5.153800228976336051, 106.0405762719810241 ) ) ;
#164890=CARTESIAN_POINT ( 'NONE',  ( 19.03943276465977164, -0.05219959533909143690, 78.74890960531436690 ) ) ;
#164891=CARTESIAN_POINT ( 'NONE',  ( 12.06949235617757843, -12.14591786802309237, 43.12390960531435269 ) ) ;
#164892=CARTESIAN_POINT ( 'NONE',  ( 10.81492255796078972, 18.62759615963270932, 39.58224293864769550 ) ) ;
#164894=CARTESIAN_POINT ( 'NONE',  ( -18.22780087662122384, -5.500000000000025757, 96.48459894673894155 ) ) ;
#164895=CARTESIAN_POINT ( 'NONE',  ( -10.81492255796105439, 18.62759615963255655, 107.9177570613523471 ) ) ;
#164897=CARTESIAN_POINT ( 'NONE',  ( 19.02544592524343514, -5.153800228976328945, 43.54057627198103120 ) ) ;
#164898=CARTESIAN_POINT ( 'NONE',  ( 0.05219959533909260263, 19.03943276465977164, 24.99890960531435269 ) ) ;
#164901=CARTESIAN_POINT ( 'NONE',  ( -16.53943276465976808, -0.05219959533934237506, 68.75109039468568994 ) ) ;
#164902=CARTESIAN_POINT ( 'NONE',  ( 18.67979575497178502, 10.72451020669898547, 79.16557627198103830 ) ) ;
#164903=CARTESIAN_POINT ( 'NONE',  ( -12.14591786802309592, -12.06949235617757132, 51.87390960531437401 ) ) ;
#164904=CARTESIAN_POINT ( 'NONE',  ( -5.153800228976328057, -19.02544592524343514, 22.29057627198102765 ) ) ;
#164905=CARTESIAN_POINT ( 'NONE',  ( 16.46253265017160672, -9.564922557960803928, 108.3322429386476955 ) ) ;
#164906=CARTESIAN_POINT ( 'NONE',  ( -18.62759615963255300, -10.81492255796106328, 24.16775706135235424 ) ) ;
#164907=CARTESIAN_POINT ( 'NONE',  ( -0.05219959533936034679, 19.03943276465977164, 32.50109039468566863 ) ) ;
#164908=CARTESIAN_POINT ( 'NONE',  ( -0.05219959533909027116, -19.03943276465977164, 27.49890960531435624 ) ) ;
#164909=CARTESIAN_POINT ( 'NONE',  ( -18.67979575497193778, 10.72451020669871902, 83.33442372801903275 ) ) ;
#164911=CARTESIAN_POINT ( 'NONE',  ( -14.34966873604960291, -8.224510206698953496, 26.66557627198103475 ) ) ;
#164912=CARTESIAN_POINT ( 'NONE',  ( 17.50000000000001066, 3.850315288878835229, 113.2337086939655677 ) ) ;
#164913=CARTESIAN_POINT ( 'NONE',  ( -10.81492255796078084, -18.62759615963271287, 42.08224293864769550 ) ) ;
#164914=CARTESIAN_POINT ( 'NONE',  ( 16.52544592524342804, -4.483927247898539470, 98.54057627198105251 ) ) ;
#164916=CARTESIAN_POINT ( 'NONE',  ( -0.05219959533909027116, -19.03943276465977164, 92.49890960531436690 ) ) ;
#164917=CARTESIAN_POINT ( 'NONE',  ( -0.05219959533910754901, -16.53943276465976808, 92.49890960531436690 ) ) ;
#164918=CARTESIAN_POINT ( 'NONE',  ( 19.02544592524334988, 5.153800228976608722, 101.4594237280189759 ) ) ;
#164919=CARTESIAN_POINT ( 'NONE',  ( -18.67979575497178146, -10.72451020669898902, 66.66557627198102409 ) ) ;
#164921=CARTESIAN_POINT ( 'NONE',  ( 9.474510206698971260, -16.51473224551069308, 32.91557627198102409 ) ) ;
#164922=B_SPLINE_CURVE_WITH_KNOTS ( 'NONE', 3,
 ( #8696, #179564, #116860, #21862, #192714, #70366 ),
 .UNSPECIFIED., .F., .F.,
 ( 4, 2, 4 ),
 ( 0.003239945802372221333, 0.003620412082092075261, 0.004000878361811928755 ),
 .UNSPECIFIED. ) ;
#164923=CARTESIAN_POINT ( 'NONE',  ( -9.564922557960796823, -16.46253265017161027, 92.08224293864769550 ) ) ;
#164924=CARTESIAN_POINT ( 'NONE',  ( -15.80617190586745835, -15.72974639402198527, 91.87390960531436690 ) ) ;
#164925=CARTESIAN_POINT ( 'NONE',  ( -12.14591786802326823, 12.06949235617739902, 103.1260903946856757 ) ) ;
#164926=CARTESIAN_POINT ( 'NONE',  ( -5.153800228976328057, -19.02544592524343514, 87.29057627198103830 ) ) ;
#164927=CARTESIAN_POINT ( 'NONE',  ( 9.474510206698729675, 16.51473224551082808, 82.08442372801899012 ) ) ;
#164928=CARTESIAN_POINT ( 'NONE',  ( 10.81492255796106328, -18.62759615963255655, 100.4177570613523471 ) ) ;
#164929=CARTESIAN_POINT ( 'NONE',  ( 0.05219959533907565091, 21.53943276465977519, 69.99890960531435269 ) ) ;
#164930=CARTESIAN_POINT ( 'NONE',  ( -5.823673210054116645, -21.52544592524344225, 42.29057627198103120 ) ) ;
#164931=CARTESIAN_POINT ( 'NONE',  ( -16.51473224551069308, -9.474510206698971260, 46.66557627198102409 ) ) ;
#164932=CARTESIAN_POINT ( 'NONE',  ( 4.483927247898790824, -16.52544592524335698, 110.2094237280190185 ) ) ;
#164933=CARTESIAN_POINT ( 'NONE',  ( 19.03943276465977164, -0.05219959533909143690, 68.74890960531436690 ) ) ;
#164936=CARTESIAN_POINT ( 'NONE',  ( 13.97604488694548053, -13.89961937509957401, 30.62609039468566863 ) ) ;
#164937=CARTESIAN_POINT ( 'NONE',  ( 4.379528057220339221, -16.55341960407611168, 67.70724293864769550 ) ) ;
#164938=CARTESIAN_POINT ( 'NONE',  ( -21.55341960407619339, 5.719274019375674811, 28.54275706135234358 ) ) ;
#164940=CARTESIAN_POINT ( 'NONE',  ( 18.67979575497178502, 10.72451020669898547, 64.16557627198102409 ) ) ;
#164941=CARTESIAN_POINT ( 'NONE',  ( 16.52544592524335698, 4.483927247898782831, 96.45942372801901854 ) ) ;
#164942=CARTESIAN_POINT ( 'NONE',  ( 14.29746914071049879, -8.314922557960816363, 103.3322429386476955 ) ) ;
#164943=CARTESIAN_POINT ( 'NONE',  ( 16.46253265017160672, -9.564922557960803928, 68.33224293864770971 ) ) ;
#164944=CARTESIAN_POINT ( 'NONE',  ( -16.52544592524342804, 4.483927247898546575, 36.04057627198102409 ) ) ;
#164945=CARTESIAN_POINT ( 'NONE',  ( 5.719274019375673035, 21.55341960407619339, 42.29275706135235424 ) ) ;
#164946=CARTESIAN_POINT ( 'NONE',  ( 16.46253265017160672, -9.564922557960803928, 108.3322429386476955 ) ) ;
#164947=CARTESIAN_POINT ( 'NONE',  ( 18.67979575497194134, -10.72451020669871369, 75.83442372801900433 ) ) ;
#164948=CARTESIAN_POINT ( 'NONE',  ( 16.51473224551069308, 9.474510206698969483, 29.16557627198103475 ) ) ;
#164949=CARTESIAN_POINT ( 'NONE',  ( 13.89961937509977652, -13.97604488694527269, 43.12390960531434558 ) ) ;
#164950=ORIENTED_EDGE ( 'NONE', *, *, #125615, .T. ) ;
#164951=CARTESIAN_POINT ( 'NONE',  ( 21.53943276465977519, 0.05219959533937863772, 91.25109039468568994 ) ) ;
#164952=CARTESIAN_POINT ( 'NONE',  ( -16.55341960407617563, 4.379528057220093196, 48.54275706135234714 ) ) ;
#164953=CARTESIAN_POINT ( 'NONE',  ( -21.55341960407619339, 5.719274019375674811, 73.54275706135234714 ) ) ;
#164954=CARTESIAN_POINT ( 'NONE',  ( 9.474510206698971260, -16.51473224551069308, 97.91557627198102409 ) ) ;
#164955=CARTESIAN_POINT ( 'NONE',  ( -16.46253265017146816, -9.564922557961047289, 84.16775706135233293 ) ) ;
#164956=CARTESIAN_POINT ( 'NONE',  ( 21.53943276465977519, 0.05219959533937863772, 56.25109039468568284 ) ) ;
#164957=CARTESIAN_POINT ( 'NONE',  ( -8.314922557961024197, 14.29746914071037800, 27.91775706135234358 ) ) ;
#164958=CARTESIAN_POINT ( 'NONE',  ( 19.03943276465977164, 0.05219959533936151252, 91.25109039468566152 ) ) ;
#164959=CARTESIAN_POINT ( 'NONE',  ( -9.474510206698964154, 16.51473224551069663, 45.41557627198103120 ) ) ;
#164960=CARTESIAN_POINT ( 'NONE',  ( 5.049401038297881783, 19.05341960407617563, 92.29275706135234714 ) ) ;
#164961=CARTESIAN_POINT ( 'NONE',  ( -16.55341960407611168, -4.379528057220339221, 21.45724293864769550 ) ) ;
#164962=CARTESIAN_POINT ( 'NONE',  ( -9.474510206698720793, -16.51473224551083518, 84.58442372801900433 ) ) ;
#164963=CARTESIAN_POINT ( 'NONE',  ( 8.224510206698953496, -14.34966873604960469, 42.91557627198103120 ) ) ;
#164964=CARTESIAN_POINT ( 'NONE',  ( -0.05219959533936034679, 19.03943276465977164, 62.50109039468566863 ) ) ;
#164965=CARTESIAN_POINT ( 'NONE',  ( -16.52544592524335698, -4.483927247898792601, 53.95942372801900433 ) ) ;
#164966=CARTESIAN_POINT ( 'NONE',  ( 19.05341960407617918, -5.049401038297876454, 26.04275706135233293 ) ) ;
#164967=CARTESIAN_POINT ( 'NONE',  ( -9.564922557960796823, -16.46253265017161027, 27.08224293864769550 ) ) ;
#164968=CARTESIAN_POINT ( 'NONE',  ( 13.89961937509977652, -13.97604488694527269, 38.12390960531436690 ) ) ;
#164969=CARTESIAN_POINT ( 'NONE',  ( 12.06949235617739724, 12.14591786802326823, 41.87609039468568284 ) ) ;
#164972=CARTESIAN_POINT ( 'NONE',  ( -5.153800228976328057, -19.02544592524343514, 92.29057627198099567 ) ) ;
#164974=CARTESIAN_POINT ( 'NONE',  ( -17.97058386085788584, -5.499999999999976019, 69.00390968646215129 ) ) ;
#164975=CARTESIAN_POINT ( 'NONE',  ( -13.97604488694547697, 13.89961937509957934, 98.12609039468566152 ) ) ;
#164976=CARTESIAN_POINT ( 'NONE',  ( 0.05219959533907565091, 21.53943276465977519, 29.99890960531435979 ) ) ;
#164977=CARTESIAN_POINT ( 'NONE',  ( 19.02544592524334988, 5.153800228976608722, 36.45942372801900433 ) ) ;
#164978=CARTESIAN_POINT ( 'NONE',  ( 13.89961937509957401, 13.97604488694547697, 111.8760903946856757 ) ) ;
#164979=CARTESIAN_POINT ( 'NONE',  ( 14.34966873604960469, 8.224510206698951720, 114.1655762719810383 ) ) ;
#164980=CARTESIAN_POINT ( 'NONE',  ( -5.049401038298153566, 19.05341960407611168, 35.20724293864768839 ) ) ;
#164981=CARTESIAN_POINT ( 'NONE',  ( 15.80617190586746368, 15.72974639402197994, 74.37390960531436690 ) ) ;
#164982=CARTESIAN_POINT ( 'NONE',  ( 9.474510206698971260, -16.51473224551069308, 42.91557627198103120 ) ) ;
#164984=CARTESIAN_POINT ( 'NONE',  ( 16.51473224551083163, -9.474510206698727899, 75.83442372801900433 ) ) ;
#164985=CARTESIAN_POINT ( 'NONE',  ( -0.05219959533910754901, -16.53943276465976808, 57.49890960531435979 ) ) ;
#164986=CARTESIAN_POINT ( 'NONE',  ( 15.80617190586746368, 15.72974639402197994, 39.37390960531436690 ) ) ;
#164987=CARTESIAN_POINT ( 'NONE',  ( -21.53943276465977519, -0.05219959533937600094, 93.75109039468567573 ) ) ;
#164989=CARTESIAN_POINT ( 'NONE',  ( 5.719274019375991003, -21.55341960407610458, 77.70724293864770971 ) ) ;
#164990=CARTESIAN_POINT ( 'NONE',  ( -15.72974639402176322, -15.80617190586768395, 74.37609039468568994 ) ) ;
#164991=CARTESIAN_POINT ( 'NONE',  ( -5.719274019375665041, -21.55341960407619695, 69.79275706135234714 ) ) ;
#164992=CARTESIAN_POINT ( 'NONE',  ( 16.46253265017160672, -9.564922557960803928, 98.33224293864769550 ) ) ;
#164993=CARTESIAN_POINT ( 'NONE',  ( -14.29746914071037622, -8.314922557961029526, 89.16775706135236135 ) ) ;
#164994=CARTESIAN_POINT ( 'NONE',  ( -0.05219959533937732626, 21.53943276465977519, 67.50109039468568994 ) ) ;
#164995=CARTESIAN_POINT ( 'NONE',  ( -16.51473224551069308, -9.474510206698971260, 51.66557627198102409 ) ) ;
#164996=CARTESIAN_POINT ( 'NONE',  ( -21.52544592524334988, -5.823673210054445271, 28.95942372801902209 ) ) ;
#164997=CARTESIAN_POINT ( 'NONE',  ( -5.049401038298153566, 19.05341960407611168, 70.20724293864769550 ) ) ;
#164998=CARTESIAN_POINT ( 'NONE',  ( -8.314922557960811034, -14.29746914071050412, 67.08224293864770971 ) ) ;
#164999=CARTESIAN_POINT ( 'NONE',  ( -4.379528057220328563, 16.55341960407611168, 50.20724293864769550 ) ) ;
#165000=CARTESIAN_POINT ( 'NONE',  ( -21.52544592524343514, 5.823673210054127303, 56.04057627198102409 ) ) ;
#165001=CARTESIAN_POINT ( 'NONE',  ( -9.564922557960796823, -16.46253265017161027, 42.08224293864769550 ) ) ;
#165002=CARTESIAN_POINT ( 'NONE',  ( -21.53943276465977519, 0.05219959533907696930, 56.24890960531436690 ) ) ;
#165003=CARTESIAN_POINT ( 'NONE',  ( 5.049401038297881783, 19.05341960407617563, 57.29275706135231871 ) ) ;
#165005=CARTESIAN_POINT ( 'NONE',  ( 12.06949235617757843, -12.14591786802309237, 68.12390960531436690 ) ) ;
#165006=CARTESIAN_POINT ( 'NONE',  ( 15.80617190586746368, 15.72974639402197994, 34.37390960531435979 ) ) ;
#165007=VERTEX_POINT ( 'NONE', #8879 ) ;
#165009=CARTESIAN_POINT ( 'NONE',  ( -12.06949235617739369, -12.14591786802326823, 84.37609039468570415 ) ) ;
#165010=CARTESIAN_POINT ( 'NONE',  ( 5.049401038297881783, 19.05341960407617563, 92.29275706135234714 ) ) ;
#165011=CARTESIAN_POINT ( 'NONE',  ( 16.53943276465976808, -0.05219959533910856209, 53.74890960531437401 ) ) ;
#165012=CARTESIAN_POINT ( 'NONE',  ( -18.56399227203345959, -5.499999999999827693, 58.97830131249904184 ) ) ;
#165013=CARTESIAN_POINT ( 'NONE',  ( 13.89961937509977652, -13.97604488694527269, 53.12390960531434558 ) ) ;
#165014=CARTESIAN_POINT ( 'NONE',  ( -14.29746914071049879, 8.314922557960819915, 45.83224293864769550 ) ) ;
#165016=CARTESIAN_POINT ( 'NONE',  ( 5.049401038298161559, -19.05341960407611168, 77.70724293864765286 ) ) ;
#165017=CARTESIAN_POINT ( 'NONE',  ( -19.05341960407611168, -5.049401038298163336, 46.45724293864768129 ) ) ;
#165018=CARTESIAN_POINT ( 'NONE',  ( -21.53943276465977519, -0.05219959533937600094, 53.75109039468568994 ) ) ;
#165019=CARTESIAN_POINT ( 'NONE',  ( 16.46253265017160672, -9.564922557960803928, 73.33224293864769550 ) ) ;
#165020=CARTESIAN_POINT ( 'NONE',  ( 16.46253265017160672, -9.564922557960803928, 33.33224293864770260 ) ) ;
#165021=CARTESIAN_POINT ( 'NONE',  ( -19.03943276465977164, 0.05219959533909376836, 56.24890960531435979 ) ) ;
#165022=CARTESIAN_POINT ( 'NONE',  ( 5.823673210054125526, 21.52544592524343514, 54.79057627198104541 ) ) ;
#165023=CARTESIAN_POINT ( 'NONE',  ( -5.153800228976328057, -19.02544592524343514, 32.29057627198102409 ) ) ;
#165024=CARTESIAN_POINT ( 'NONE',  ( -15.72974639402197994, 15.80617190586746368, 35.62390960531437401 ) ) ;
#165025=CARTESIAN_POINT ( 'NONE',  ( -14.29746914071037622, -8.314922557961029526, 109.1677570613523613 ) ) ;
#165026=CARTESIAN_POINT ( 'NONE',  ( -5.823673210054431948, 21.52544592524334988, 112.7094237280190328 ) ) ;
#165027=CARTESIAN_POINT ( 'NONE',  ( 12.14591786802327356, -12.06949235617739191, 40.62609039468567573 ) ) ;
#165028=CARTESIAN_POINT ( 'NONE',  ( 14.34966873604972726, -8.224510206698740333, 75.83442372801900433 ) ) ;
#165030=CARTESIAN_POINT ( 'NONE',  ( 12.14591786802327356, -12.06949235617739191, 65.62609039468568994 ) ) ;
#165031=CARTESIAN_POINT ( 'NONE',  ( -14.34966873604972548, 8.224510206698743886, 58.33442372801901143 ) ) ;
#165032=CARTESIAN_POINT ( 'NONE',  ( -16.51473224551069308, -9.474510206698971260, 111.6655762719810383 ) ) ;
#165033=CARTESIAN_POINT ( 'NONE',  ( 13.97604488694527802, 13.89961937509977652, 29.37390960531435979 ) ) ;
#165034=CARTESIAN_POINT ( 'NONE',  ( -4.379528057220086978, -16.55341960407618274, 39.79275706135235424 ) ) ;
#165035=CARTESIAN_POINT ( 'NONE',  ( -13.97604488694527625, -13.89961937509977652, 36.87390960531436690 ) ) ;
#165036=CARTESIAN_POINT ( 'NONE',  ( 18.67979575497194134, -10.72451020669871369, 30.83442372801902209 ) ) ;
#165037=CARTESIAN_POINT ( 'NONE',  ( 14.29746914071037800, 8.314922557961029526, 36.66775706135234714 ) ) ;
#165038=CARTESIAN_POINT ( 'NONE',  ( -8.224510206698735004, -14.34966873604973081, 99.58442372801900433 ) ) ;
#165040=CARTESIAN_POINT ( 'NONE',  ( -10.72451020669870658, -18.67979575497194134, 104.5844237280190185 ) ) ;
#165041=CARTESIAN_POINT ( 'NONE',  ( -19.02544592524334988, -5.153800228976617603, 98.95942372801900433 ) ) ;
#165042=CARTESIAN_POINT ( 'NONE',  ( -14.29746914071049879, 8.314922557960819915, 50.83224293864770971 ) ) ;
#165043=CARTESIAN_POINT ( 'NONE',  ( -9.564922557960796823, -16.46253265017161027, 27.08224293864769550 ) ) ;
#165044=CARTESIAN_POINT ( 'NONE',  ( 5.153800228976615827, -19.02544592524334988, 60.20942372801899012 ) ) ;
#165045=CARTESIAN_POINT ( 'NONE',  ( 16.19135201231366139, 7.376712067591951083, 77.68680854052031748 ) ) ;
#165046=CARTESIAN_POINT ( 'NONE',  ( -10.72451020669870658, -18.67979575497194134, 69.58442372801900433 ) ) ;
#165047=CARTESIAN_POINT ( 'NONE',  ( -8.224510206698735004, -14.34966873604973081, 24.58442372801901499 ) ) ;
#165048=CARTESIAN_POINT ( 'NONE',  ( 17.05587630539785593, 6.762274262135716363, 81.75819690962686082 ) ) ;
#165049=CARTESIAN_POINT ( 'NONE',  ( -15.72974639402197994, 15.80617190586746368, 25.62390960531435624 ) ) ;
#165050=CARTESIAN_POINT ( 'NONE',  ( -5.153800228976607833, 19.02544592524334988, 107.7094237280189759 ) ) ;
#165051=CARTESIAN_POINT ( 'NONE',  ( 5.153800228976335163, 19.02544592524342804, 114.7905762719810241 ) ) ;
#165053=CARTESIAN_POINT ( 'NONE',  ( 16.51473224551069308, 9.474510206698969483, 29.16557627198103475 ) ) ;
#165054=CARTESIAN_POINT ( 'NONE',  ( 21.52544592524334988, 5.823673210054432836, 101.4594237280190185 ) ) ;
#165055=CARTESIAN_POINT ( 'NONE',  ( 13.89961937509977652, -13.97604488694527269, 48.12390960531435979 ) ) ;
#165056=CARTESIAN_POINT ( 'NONE',  ( -5.823673210054431948, 21.52544592524334988, 52.70942372801902565 ) ) ;
#165057=CARTESIAN_POINT ( 'NONE',  ( -5.823673210054431948, 21.52544592524334988, 107.7094237280190328 ) ) ;
#165058=CARTESIAN_POINT ( 'NONE',  ( -16.55341960407617563, 4.379528057220093196, 98.54275706135234714 ) ) ;
#165059=CARTESIAN_POINT ( 'NONE',  ( -0.05219959533909027116, -19.03943276465977164, 72.49890960531435269 ) ) ;
#165060=CARTESIAN_POINT ( 'NONE',  ( -18.62759615963255300, -10.81492255796106328, 59.16775706135234714 ) ) ;
#165061=CARTESIAN_POINT ( 'NONE',  ( 18.67979575497194134, -10.72451020669871369, 55.83442372801901854 ) ) ;
#165062=CARTESIAN_POINT ( 'NONE',  ( -19.05341960407617563, 5.049401038297882671, 83.54275706135233293 ) ) ;
#165063=CARTESIAN_POINT ( 'NONE',  ( 19.05341960407611168, 5.049401038298154454, 88.95724293864769550 ) ) ;
#165064=CARTESIAN_POINT ( 'NONE',  ( -9.564922557960796823, -16.46253265017161027, 27.08224293864769550 ) ) ;
#165065=CARTESIAN_POINT ( 'NONE',  ( -0.05219959533907301413, -21.53943276465977519, 97.49890960531436690 ) ) ;
#165066=CARTESIAN_POINT ( 'NONE',  ( -9.564922557961040184, 16.46253265017147172, 27.91775706135232582 ) ) ;
#165067=CARTESIAN_POINT ( 'NONE',  ( 0.05219959533910956823, 16.53943276465976808, 99.99890960531436690 ) ) ;
#165068=CARTESIAN_POINT ( 'NONE',  ( -19.05341960407611168, -5.049401038298163336, 51.45724293864770260 ) ) ;
#165069=CARTESIAN_POINT ( 'NONE',  ( -19.05341960407617563, 5.049401038297882671, 78.54275706135233293 ) ) ;
#165070=CARTESIAN_POINT ( 'NONE',  ( -0.05219959533910754901, -16.53943276465976808, 47.49890960531435979 ) ) ;
#165071=CARTESIAN_POINT ( 'NONE',  ( 15.80617190586769283, -15.72974639402175789, 105.6260903946856899 ) ) ;
#165072=CARTESIAN_POINT ( 'NONE',  ( -13.89961937509977652, 13.97604488694528158, 105.6239096053143527 ) ) ;
#165073=CARTESIAN_POINT ( 'NONE',  ( 9.564922557961047289, -16.46253265017146816, 70.41775706135233293 ) ) ;
#165074=CARTESIAN_POINT ( 'NONE',  ( 5.719274019375991003, -21.55341960407610458, 72.70724293864769550 ) ) ;
#165075=CARTESIAN_POINT ( 'NONE',  ( -0.05219959533937732626, 21.53943276465977519, 32.50109039468568284 ) ) ;
#165076=CARTESIAN_POINT ( 'NONE',  ( 16.55341960407618274, -4.379528057220086978, 36.04275706135234714 ) ) ;
#165077=CARTESIAN_POINT ( 'NONE',  ( 12.06949235617739724, 12.14591786802326823, 91.87609039468568994 ) ) ;
#165078=CARTESIAN_POINT ( 'NONE',  ( -16.46253265017160317, 9.564922557960807481, 30.83224293864769550 ) ) ;
#165079=CARTESIAN_POINT ( 'NONE',  ( 18.67979575497194134, -10.72451020669871369, 40.83442372801901854 ) ) ;
#165080=CARTESIAN_POINT ( 'NONE',  ( -15.72974639402197994, 15.80617190586746368, 40.62390960531435269 ) ) ;
#165081=CARTESIAN_POINT ( 'NONE',  ( -9.564922557960796823, -16.46253265017161027, 22.08224293864768839 ) ) ;
#165083=CARTESIAN_POINT ( 'NONE',  ( 8.224510206698742110, 14.34966873604972548, 62.08442372801901143 ) ) ;
#165084=CARTESIAN_POINT ( 'NONE',  ( -12.14591786802309592, -12.06949235617757132, 96.87390960531436690 ) ) ;
#165085=CARTESIAN_POINT ( 'NONE',  ( 0.05219959533907565091, 21.53943276465977519, 84.99890960531436690 ) ) ;
#165086=CARTESIAN_POINT ( 'NONE',  ( -4.483927247898782831, 16.52544592524335698, 112.7094237280190328 ) ) ;
#165087=CARTESIAN_POINT ( 'NONE',  ( 4.483927247898790824, -16.52544592524335698, 50.20942372801901854 ) ) ;
#165088=CARTESIAN_POINT ( 'NONE',  ( -16.46253265017160317, 9.564922557960807481, 60.83224293864769550 ) ) ;
#165089=CARTESIAN_POINT ( 'NONE',  ( 12.14591786802327356, -12.06949235617739191, 95.62609039468568994 ) ) ;
#165090=CARTESIAN_POINT ( 'NONE',  ( 9.564922557961047289, -16.46253265017146816, 85.41775706135233293 ) ) ;
#165091=CARTESIAN_POINT ( 'NONE',  ( 15.80617190586746368, 15.72974639402197994, 84.37390960531438111 ) ) ;
#165092=CARTESIAN_POINT ( 'NONE',  ( 8.314922557960818139, 14.29746914071049879, 24.58224293864768839 ) ) ;
#165096=CARTESIAN_POINT ( 'NONE',  ( 15.72974639402199770, -15.80617190586745480, 63.12390960531435979 ) ) ;
#165097=CARTESIAN_POINT ( 'NONE',  ( 12.06949235617739724, 12.14591786802326823, 91.87609039468568994 ) ) ;
#165099=CARTESIAN_POINT ( 'NONE',  ( -21.52544592524343514, 5.823673210054127303, 36.04057627198102409 ) ) ;
#165100=CARTESIAN_POINT ( 'NONE',  ( 18.56101223717332971, 5.499999999999949374, 88.94978406935679516 ) ) ;
#165101=CARTESIAN_POINT ( 'NONE',  ( 10.81492255796078972, 18.62759615963270932, 89.58224293864768129 ) ) ;
#165102=CARTESIAN_POINT ( 'NONE',  ( 16.53943276465976808, 0.05219959533934440121, 111.2510903946856899 ) ) ;
#165103=CARTESIAN_POINT ( 'NONE',  ( 12.06949235617739724, 12.14591786802326823, 31.87609039468567929 ) ) ;
#165104=CARTESIAN_POINT ( 'NONE',  ( 19.03943276465977164, -0.05219959533909143690, 28.74890960531435624 ) ) ;
#165105=CARTESIAN_POINT ( 'NONE',  ( -4.379528057220086978, -16.55341960407618274, 34.79275706135235424 ) ) ;
#165106=CARTESIAN_POINT ( 'NONE',  ( 5.153800228976335163, 19.02544592524342804, 49.79057627198100988 ) ) ;
#165108=CARTESIAN_POINT ( 'NONE',  ( 9.474510206698971260, -16.51473224551069308, 107.9155762719810383 ) ) ;
#165109=CARTESIAN_POINT ( 'NONE',  ( 9.474510206698971260, -16.51473224551069308, 112.9155762719810383 ) ) ;
#165111=CARTESIAN_POINT ( 'NONE',  ( -12.14591786802326823, 12.06949235617739902, 108.1260903946856757 ) ) ;
#165112=CARTESIAN_POINT ( 'NONE',  ( -19.03943276465977164, -0.05219959533935918106, 98.75109039468567573 ) ) ;
#165113=CARTESIAN_POINT ( 'NONE',  ( -19.03943276465977164, -0.05219959533935918106, 43.75109039468566863 ) ) ;
#165114=CARTESIAN_POINT ( 'NONE',  ( 5.719274019375991003, -21.55341960407610458, 72.70724293864769550 ) ) ;
#165115=CARTESIAN_POINT ( 'NONE',  ( -8.224510206698735004, -14.34966873604973081, 99.58442372801900433 ) ) ;
#165116=CARTESIAN_POINT ( 'NONE',  ( 10.72451020669898902, -18.67979575497178502, 27.91557627198103830 ) ) ;
#165117=CARTESIAN_POINT ( 'NONE',  ( -5.153800228976607833, 19.02544592524334988, 102.7094237280189759 ) ) ;
#165118=CARTESIAN_POINT ( 'NONE',  ( 19.05341960407611168, 5.049401038298154454, 108.9572429386477097 ) ) ;
#165119=CARTESIAN_POINT ( 'NONE',  ( -10.81492255796105439, 18.62759615963255655, 57.91775706135234714 ) ) ;
#165120=CARTESIAN_POINT ( 'NONE',  ( -19.05341960407611168, -5.049401038298163336, 66.45724293864769550 ) ) ;
#165121=CARTESIAN_POINT ( 'NONE',  ( 4.483927247898545687, 16.52544592524342804, 99.79057627198103830 ) ) ;
#165123=CARTESIAN_POINT ( 'NONE',  ( -14.29746914071049879, 8.314922557960819915, 75.83224293864769550 ) ) ;
#165124=CARTESIAN_POINT ( 'NONE',  ( 15.72974639402199770, -15.80617190586745480, 78.12390960531436690 ) ) ;
#165125=VERTEX_POINT ( 'NONE', #145030 ) ;
#165126=CARTESIAN_POINT ( 'NONE',  ( 19.05341960407617918, -5.049401038297876454, 96.04275706135231871 ) ) ;
#165128=CARTESIAN_POINT ( 'NONE',  ( -5.049401038298153566, 19.05341960407611168, 60.20724293864768129 ) ) ;
#165129=CARTESIAN_POINT ( 'NONE',  ( 16.52216118717250026, -7.221426719304218089, 71.42400978952970547 ) ) ;
#165130=CARTESIAN_POINT ( 'NONE',  ( 16.46253265017160672, -9.564922557960803928, 83.33224293864768129 ) ) ;
#165131=CARTESIAN_POINT ( 'NONE',  ( 19.02544592524343514, -5.153800228976328945, 83.54057627198100988 ) ) ;
#165132=CARTESIAN_POINT ( 'NONE',  ( -16.53943276465976808, -0.05219959533934237506, 58.75109039468568994 ) ) ;
#165133=CARTESIAN_POINT ( 'NONE',  ( -16.29526858892876717, -7.335722546919996034, 50.79670597800200937 ) ) ;
#165134=CARTESIAN_POINT ( 'NONE',  ( 9.474510206698729675, 16.51473224551082808, 37.08442372801899722 ) ) ;
#165136=CARTESIAN_POINT ( 'NONE',  ( -9.564922557960796823, -16.46253265017161027, 107.0822429386476955 ) ) ;
#165137=CARTESIAN_POINT ( 'NONE',  ( -12.14591786802326823, 12.06949235617739902, 103.1260903946856757 ) ) ;
#165140=CARTESIAN_POINT ( 'NONE',  ( 16.52544592524335698, 4.483927247898782831, 91.45942372801901854 ) ) ;
#165141=CARTESIAN_POINT ( 'NONE',  ( -16.18388926212241685, 7.379444403734382263, 29.56046848633847901 ) ) ;
#165142=CARTESIAN_POINT ( 'NONE',  ( 12.06949235617739724, 12.14591786802326823, 66.87609039468568994 ) ) ;
#165144=CARTESIAN_POINT ( 'NONE',  ( 21.52544592524334988, 5.823673210054432836, 66.45942372801903275 ) ) ;
#165145=CARTESIAN_POINT ( 'NONE',  ( 19.02544592524334988, 5.153800228976608722, 91.45942372801900433 ) ) ;
#165146=CARTESIAN_POINT ( 'NONE',  ( 16.51473224551083163, -9.474510206698727899, 30.83442372801900433 ) ) ;
#165147=CARTESIAN_POINT ( 'NONE',  ( -5.153800228976328057, -19.02544592524343514, 67.29057627198102409 ) ) ;
#165148=CARTESIAN_POINT ( 'NONE',  ( 19.02544592524343514, -5.153800228976328945, 48.54057627198103120 ) ) ;
#165149=CARTESIAN_POINT ( 'NONE',  ( 16.82725176010342949, -7.001296733591735766, 23.13668599133183079 ) ) ;
#165150=CARTESIAN_POINT ( 'NONE',  ( -5.719274019375978568, 21.55341960407610458, 80.20724293864769550 ) ) ;
#165151=CARTESIAN_POINT ( 'NONE',  ( -5.719274019375978568, 21.55341960407610458, 35.20724293864768839 ) ) ;
#165152=CARTESIAN_POINT ( 'NONE',  ( 19.05341960407611168, 5.049401038298154454, 28.95724293864769550 ) ) ;
#165153=CARTESIAN_POINT ( 'NONE',  ( 14.34966873604972726, -8.224510206698740333, 50.83442372801901143 ) ) ;
#165155=CARTESIAN_POINT ( 'NONE',  ( 21.52544592524334988, 5.823673210054432836, 31.45942372801901854 ) ) ;
#165156=CARTESIAN_POINT ( 'NONE',  ( -16.55341960407611168, -4.379528057220339221, 51.45724293864770260 ) ) ;
#165158=CARTESIAN_POINT ( 'NONE',  ( 4.483927247898790824, -16.52544592524335698, 30.20942372801902565 ) ) ;
#165159=CARTESIAN_POINT ( 'NONE',  ( -16.51473224551082808, 9.474510206698731452, 33.33442372801899722 ) ) ;
#165160=CARTESIAN_POINT ( 'NONE',  ( -8.314922557960811034, -14.29746914071050412, 52.08224293864768839 ) ) ;
#165161=CARTESIAN_POINT ( 'NONE',  ( -10.81492255796078084, -18.62759615963271287, 112.0822429386477097 ) ) ;
#165163=CARTESIAN_POINT ( 'NONE',  ( 21.55341960407610458, 5.719274019375980345, 73.95724293864769550 ) ) ;
#165164=CARTESIAN_POINT ( 'NONE',  ( 9.474510206698971260, -16.51473224551069308, 87.91557627198102409 ) ) ;
#165165=CARTESIAN_POINT ( 'NONE',  ( -14.34966873604960291, -8.224510206698953496, 61.66557627198103120 ) ) ;
#165166=CARTESIAN_POINT ( 'NONE',  ( 19.05341960407611168, 5.049401038298154454, 108.9572429386477097 ) ) ;
#165168=CARTESIAN_POINT ( 'NONE',  ( 5.049401038297881783, 19.05341960407617563, 62.29275706135234003 ) ) ;
#165169=CARTESIAN_POINT ( 'NONE',  ( -10.81492255796078084, -18.62759615963271287, 107.0822429386476955 ) ) ;
#165170=CARTESIAN_POINT ( 'NONE',  ( -13.97604488694527625, -13.89961937509977652, 51.87390960531436690 ) ) ;
#165171=CARTESIAN_POINT ( 'NONE',  ( 13.97604488694548053, -13.89961937509957401, 45.62609039468566863 ) ) ;
#165172=CARTESIAN_POINT ( 'NONE',  ( 8.224510206698953496, -14.34966873604960469, 112.9155762719810383 ) ) ;
#165173=CARTESIAN_POINT ( 'NONE',  ( -15.80617190586768217, 15.72974639402176855, 68.12609039468567573 ) ) ;
#165174=CARTESIAN_POINT ( 'NONE',  ( -16.38665767535051998, -7.295008042176176488, 69.73599135785454450 ) ) ;
#165175=CARTESIAN_POINT ( 'NONE',  ( -4.379528057220328563, 16.55341960407611168, 35.20724293864768839 ) ) ;
#165176=CARTESIAN_POINT ( 'NONE',  ( 5.049401038298161559, -19.05341960407611168, 52.70724293864767418 ) ) ;
#165177=CARTESIAN_POINT ( 'NONE',  ( -5.823673210054116645, -21.52544592524344225, 72.29057627198102409 ) ) ;
#165179=CARTESIAN_POINT ( 'NONE',  ( -19.03943276465977164, 0.05219959533909376836, 51.24890960531436690 ) ) ;
#165180=VERTEX_POINT ( 'NONE', #49061 ) ;
#165181=CARTESIAN_POINT ( 'NONE',  ( -21.55341960407610458, -5.719274019375992779, 66.45724293864768129 ) ) ;
#165182=CARTESIAN_POINT ( 'NONE',  ( 21.52544592524334988, 5.823673210054432836, 91.45942372801901854 ) ) ;
#165184=CARTESIAN_POINT ( 'NONE',  ( 14.34966873604972726, -8.224510206698740333, 100.8344237280190185 ) ) ;
#165185=CARTESIAN_POINT ( 'NONE',  ( 12.06949235617757843, -12.14591786802309237, 83.12390960531436690 ) ) ;
#165186=CARTESIAN_POINT ( 'NONE',  ( 5.153800228976335163, 19.02544592524342804, 64.79057627198100988 ) ) ;
#165187=VERTEX_POINT ( 'NONE', #34873 ) ;
#165188=CARTESIAN_POINT ( 'NONE',  ( 19.05341960407617918, -5.049401038297876454, 46.04275706135233293 ) ) ;
#165189=CARTESIAN_POINT ( 'NONE',  ( -16.53943276465976808, -0.05219959533934237506, 88.75109039468567573 ) ) ;
#165190=CARTESIAN_POINT ( 'NONE',  ( -5.823673210054431948, 21.52544592524334988, 107.7094237280190328 ) ) ;
#165191=CARTESIAN_POINT ( 'NONE',  ( -19.03943276465977164, 0.05219959533909376836, 91.24890960531436690 ) ) ;
#165192=CARTESIAN_POINT ( 'NONE',  ( 15.72974639402199770, -15.80617190586745480, 48.12390960531436690 ) ) ;
#165194=CARTESIAN_POINT ( 'NONE',  ( -15.72974639402176322, -15.80617190586768395, 99.37609039468568994 ) ) ;
#165195=CARTESIAN_POINT ( 'NONE',  ( -4.379528057220086978, -16.55341960407618274, 64.79275706135234714 ) ) ;
#165196=CARTESIAN_POINT ( 'NONE',  ( 15.80617190586746368, 15.72974639402197994, 114.3739096053143527 ) ) ;
#165197=CARTESIAN_POINT ( 'NONE',  ( 12.14591786802327356, -12.06949235617739191, 35.62609039468568994 ) ) ;
#165198=CARTESIAN_POINT ( 'NONE',  ( 19.02544592524343514, -5.153800228976328945, 93.54057627198102409 ) ) ;
#165199=CARTESIAN_POINT ( 'NONE',  ( -9.564922557960796823, -16.46253265017161027, 37.08224293864768839 ) ) ;
#165200=CARTESIAN_POINT ( 'NONE',  ( 5.153800228976335163, 19.02544592524342804, 49.79057627198100988 ) ) ;
#165201=CARTESIAN_POINT ( 'NONE',  ( -14.29746914071037622, -8.314922557961029526, 39.16775706135235424 ) ) ;
#165202=CARTESIAN_POINT ( 'NONE',  ( 12.06949235617757843, -12.14591786802309237, 78.12390960531436690 ) ) ;
#165203=CARTESIAN_POINT ( 'NONE',  ( -16.55341960407617563, 4.379528057220093196, 103.5427570613523613 ) ) ;
#165204=CARTESIAN_POINT ( 'NONE',  ( -5.823673210054431948, 21.52544592524334988, 47.70942372801902565 ) ) ;
#165205=CARTESIAN_POINT ( 'NONE',  ( 5.153800228976335163, 19.02544592524342804, 64.79057627198100988 ) ) ;
#165206=CARTESIAN_POINT ( 'NONE',  ( -5.049401038298153566, 19.05341960407611168, 50.20724293864770260 ) ) ;
#165207=CARTESIAN_POINT ( 'NONE',  ( 16.51473224551069308, 9.474510206698969483, 89.16557627198103830 ) ) ;
#165208=CARTESIAN_POINT ( 'NONE',  ( -16.55341960407611168, -4.379528057220339221, 36.45724293864768839 ) ) ;
#165209=CARTESIAN_POINT ( 'NONE',  ( 14.29746914071037800, 8.314922557961029526, 96.66775706135234714 ) ) ;
#165211=CARTESIAN_POINT ( 'NONE',  ( 19.02544592524334988, 5.153800228976608722, 26.45942372801899722 ) ) ;
#165212=CARTESIAN_POINT ( 'NONE',  ( -19.03943276465977164, 0.05219959533909376836, 106.2489096053143669 ) ) ;
#165214=CARTESIAN_POINT ( 'NONE',  ( 19.05341960407611168, 5.049401038298154454, 48.95724293864768129 ) ) ;
#165215=CARTESIAN_POINT ( 'NONE',  ( 19.02544592524334988, 5.153800228976608722, 26.45942372801899722 ) ) ;
#165217=CARTESIAN_POINT ( 'NONE',  ( -14.29746914071037622, -8.314922557961029526, 44.16775706135234714 ) ) ;
#165218=CARTESIAN_POINT ( 'NONE',  ( 9.474510206698729675, 16.51473224551082808, 67.08442372801900433 ) ) ;
#165219=CARTESIAN_POINT ( 'NONE',  ( -8.224510206698735004, -14.34966873604973081, 49.58442372801901143 ) ) ;
#165221=CARTESIAN_POINT ( 'NONE',  ( 9.474510206698971260, -16.51473224551069308, 72.91557627198102409 ) ) ;
#165222=CARTESIAN_POINT ( 'NONE',  ( -10.72451020669898014, 18.67979575497178502, 110.4155762719810383 ) ) ;
#165223=CARTESIAN_POINT ( 'NONE',  ( 9.564922557961047289, -16.46253265017146816, 65.41775706135233293 ) ) ;
#165224=CARTESIAN_POINT ( 'NONE',  ( 5.049401038298161559, -19.05341960407611168, 102.7072429386476955 ) ) ;
#165225=CARTESIAN_POINT ( 'NONE',  ( -0.05219959533909027116, -19.03943276465977164, 32.49890960531435979 ) ) ;
#165226=CARTESIAN_POINT ( 'NONE',  ( -19.02544592524342804, 5.153800228976336051, 71.04057627198099567 ) ) ;
#165227=CARTESIAN_POINT ( 'NONE',  ( 4.483927247898545687, 16.52544592524342804, 34.79057627198103120 ) ) ;
#165228=CARTESIAN_POINT ( 'NONE',  ( 9.474510206698971260, -16.51473224551069308, 37.91557627198102409 ) ) ;
#165229=CARTESIAN_POINT ( 'NONE',  ( -13.89961937509957401, -13.97604488694547875, 34.37609039468566863 ) ) ;
#165230=CARTESIAN_POINT ( 'NONE',  ( -16.53943276465976808, 0.05219959533911058130, 76.24890960531435269 ) ) ;
#165231=CARTESIAN_POINT ( 'NONE',  ( 21.52544592524334988, 5.823673210054432836, 111.4594237280190328 ) ) ;
#165232=CARTESIAN_POINT ( 'NONE',  ( -19.03943276465977164, 0.05219959533909376836, 56.24890960531435979 ) ) ;
#165233=CARTESIAN_POINT ( 'NONE',  ( -21.53943276465977519, 0.05219959533907696930, 51.24890960531436690 ) ) ;
#165234=CARTESIAN_POINT ( 'NONE',  ( 0.05219959533910956823, 16.53943276465976808, 49.99890960531437401 ) ) ;
#165235=CARTESIAN_POINT ( 'NONE',  ( -10.81492255796105439, 18.62759615963255655, 97.91775706135236135 ) ) ;
#165236=CARTESIAN_POINT ( 'NONE',  ( -16.51473224551069308, -9.474510206698971260, 96.66557627198102409 ) ) ;
#165237=CARTESIAN_POINT ( 'NONE',  ( 13.89961937509977652, -13.97604488694527269, 103.1239096053143527 ) ) ;
#165238=CARTESIAN_POINT ( 'NONE',  ( -19.03943276465977164, 0.05219959533909376836, 46.24890960531435979 ) ) ;
#165239=CARTESIAN_POINT ( 'NONE',  ( -19.02544592524342804, 5.153800228976336051, 26.04057627198103120 ) ) ;
#165240=CARTESIAN_POINT ( 'NONE',  ( -12.14591786802309592, -12.06949235617757132, 86.87390960531438111 ) ) ;
#165241=CARTESIAN_POINT ( 'NONE',  ( -21.55341960407610458, -5.719274019375992779, 96.45724293864770971 ) ) ;
#165242=CARTESIAN_POINT ( 'NONE',  ( -5.153800228976328057, -19.02544592524343514, 87.29057627198103830 ) ) ;
#165243=CARTESIAN_POINT ( 'NONE',  ( -15.72974639402197994, 15.80617190586746368, 95.62390960531436690 ) ) ;
#165244=CARTESIAN_POINT ( 'NONE',  ( 9.564922557960805705, 16.46253265017160317, 94.58224293864769550 ) ) ;
#165245=DIRECTION ( 'NONE',  ( -1.000000000000000000, -0.000000000000000000, -0.000000000000000000 ) ) ;
#165246=CARTESIAN_POINT ( 'NONE',  ( -14.29746914071049879, 8.314922557960819915, 105.8322429386476955 ) ) ;
#165247=CARTESIAN_POINT ( 'NONE',  ( 5.049401038298161559, -19.05341960407611168, 67.70724293864769550 ) ) ;
#165248=CARTESIAN_POINT ( 'NONE',  ( 21.53943276465977519, -0.05219959533907433946, 73.74890960531433848 ) ) ;
#165251=CARTESIAN_POINT ( 'NONE',  ( -10.81492255796078084, -18.62759615963271287, 32.08224293864769550 ) ) ;
#165252=CARTESIAN_POINT ( 'NONE',  ( 19.25663599770060941, -5.499999999999441336, 66.49419308057197497 ) ) ;
#165253=CARTESIAN_POINT ( 'NONE',  ( 0.05219959533934541429, -16.53943276465976808, 30.00109039468568284 ) ) ;
#165254=CARTESIAN_POINT ( 'NONE',  ( -14.34966873604960291, -8.224510206698953496, 91.66557627198103830 ) ) ;
#165255=CARTESIAN_POINT ( 'NONE',  ( -17.44279575226823198, -5.990770900252464060, 94.16442432485685288 ) ) ;
#165256=CARTESIAN_POINT ( 'NONE',  ( 19.03943276465977164, -0.05219959533909143690, 93.74890960531435269 ) ) ;
#165257=CARTESIAN_POINT ( 'NONE',  ( -16.46253265017160317, 9.564922557960807481, 40.83224293864769550 ) ) ;
#165258=CARTESIAN_POINT ( 'NONE',  ( 14.29746914071049879, -8.314922557960816363, 78.33224293864770971 ) ) ;
#165259=CARTESIAN_POINT ( 'NONE',  ( 21.52544592524344225, -5.823673210054117533, 38.54057627198103120 ) ) ;
#165260=CARTESIAN_POINT ( 'NONE',  ( 14.34966873604960469, 8.224510206698951720, 49.16557627198102409 ) ) ;
#165261=CARTESIAN_POINT ( 'NONE',  ( -0.05219959533936034679, 19.03943276465977164, 97.50109039468567573 ) ) ;
#165262=CARTESIAN_POINT ( 'NONE',  ( -15.72974639402176322, -15.80617190586768395, 64.37609039468568994 ) ) ;
#165264=CARTESIAN_POINT ( 'NONE',  ( -0.05219959533909027116, -19.03943276465977164, 97.49890960531436690 ) ) ;
#165265=CARTESIAN_POINT ( 'NONE',  ( -16.55341960407617563, 4.379528057220093196, 88.54275706135236135 ) ) ;
#165266=CARTESIAN_POINT ( 'NONE',  ( -0.05219959533909027116, -19.03943276465977164, 27.49890960531435624 ) ) ;
#165267=CARTESIAN_POINT ( 'NONE',  ( -9.474510206698964154, 16.51473224551069663, 75.41557627198103830 ) ) ;
#165268=CARTESIAN_POINT ( 'NONE',  ( 0.05219959533907565091, 21.53943276465977519, 74.99890960531435269 ) ) ;
#165269=CARTESIAN_POINT ( 'NONE',  ( -13.89961937509957401, -13.97604488694547875, 109.3760903946856331 ) ) ;
#165270=CARTESIAN_POINT ( 'NONE',  ( 14.29746914071049879, -8.314922557960816363, 58.33224293864768839 ) ) ;
#165271=CARTESIAN_POINT ( 'NONE',  ( 15.80617190586769283, -15.72974639402175789, 55.62609039468568284 ) ) ;
#165272=CARTESIAN_POINT ( 'NONE',  ( 14.34966873604972726, -8.224510206698740333, 80.83442372801901854 ) ) ;
#165273=CARTESIAN_POINT ( 'NONE',  ( 21.52544592524344225, -5.823673210054117533, 23.54057627198102765 ) ) ;
#165276=CARTESIAN_POINT ( 'NONE',  ( -16.53943276465976808, -0.05219959533934237506, 113.7510903946856757 ) ) ;
#165277=CARTESIAN_POINT ( 'NONE',  ( -16.52544592524335698, -4.483927247898792601, 58.95942372801902565 ) ) ;
#165278=CARTESIAN_POINT ( 'NONE',  ( 16.51473224551069308, 9.474510206698969483, 74.16557627198103830 ) ) ;
#165280=CARTESIAN_POINT ( 'NONE',  ( -19.02544592524342804, 5.153800228976336051, 86.04057627198103830 ) ) ;
#165281=CARTESIAN_POINT ( 'NONE',  ( 15.80617190586769283, -15.72974639402175789, 70.62609039468567573 ) ) ;
#165282=CARTESIAN_POINT ( 'NONE',  ( 16.52544592524335698, 4.483927247898782831, 81.45942372801900433 ) ) ;
#165283=CARTESIAN_POINT ( 'NONE',  ( 16.53943276465976808, -0.05219959533910856209, 48.74890960531435979 ) ) ;
#165284=CARTESIAN_POINT ( 'NONE',  ( -9.474510206698964154, 16.51473224551069663, 55.41557627198103120 ) ) ;
#165285=CARTESIAN_POINT ( 'NONE',  ( 16.46253265017160672, -9.564922557960803928, 53.33224293864768839 ) ) ;
#165286=CARTESIAN_POINT ( 'NONE',  ( 16.55341960407618274, -4.379528057220086978, 36.04275706135234714 ) ) ;
#165288=CARTESIAN_POINT ( 'NONE',  ( -13.97604488694547697, 13.89961937509957934, 93.12609039468566152 ) ) ;
#165289=CARTESIAN_POINT ( 'NONE',  ( -12.14591786802309592, -12.06949235617757132, 91.87390960531436690 ) ) ;
#165290=CARTESIAN_POINT ( 'NONE',  ( 13.89961937509977652, -13.97604488694527269, 68.12390960531436690 ) ) ;
#165291=CARTESIAN_POINT ( 'NONE',  ( -5.153800228976607833, 19.02544592524334988, 97.70942372801900433 ) ) ;
#165293=CARTESIAN_POINT ( 'NONE',  ( -18.67979575497193778, 10.72451020669871902, 103.3344237280190043 ) ) ;
#165294=CARTESIAN_POINT ( 'NONE',  ( 14.29746914071037800, 8.314922557961029526, 61.66775706135235424 ) ) ;
#165295=CARTESIAN_POINT ( 'NONE',  ( -17.50000000000002842, 4.013004640162660230, 25.44605720994415066 ) ) ;
#165296=CARTESIAN_POINT ( 'NONE',  ( 21.53943276465977519, -0.05219959533907433946, 68.74890960531435269 ) ) ;
#165297=CARTESIAN_POINT ( 'NONE',  ( 14.34966873604972726, -8.224510206698740333, 55.83442372801901854 ) ) ;
#165299=CARTESIAN_POINT ( 'NONE',  ( -19.03943276465977164, -0.05219959533935918106, 58.75109039468566863 ) ) ;
#165300=CARTESIAN_POINT ( 'NONE',  ( -0.05219959533909027116, -19.03943276465977164, 87.49890960531436690 ) ) ;
#165301=CARTESIAN_POINT ( 'NONE',  ( 5.049401038298161559, -19.05341960407611168, 22.70724293864769194 ) ) ;
#165302=CARTESIAN_POINT ( 'NONE',  ( -9.474510206698964154, 16.51473224551069663, 60.41557627198102409 ) ) ;
#165303=CARTESIAN_POINT ( 'NONE',  ( 12.06949235617757843, -12.14591786802309237, 53.12390960531436690 ) ) ;
#165304=CARTESIAN_POINT ( 'NONE',  ( 15.80617190586769283, -15.72974639402175789, 75.62609039468567573 ) ) ;
#165305=CARTESIAN_POINT ( 'NONE',  ( 13.89961937509957401, 13.97604488694547697, 41.87609039468566152 ) ) ;
#165306=CARTESIAN_POINT ( 'NONE',  ( 13.89961937509957401, 13.97604488694547697, 31.87609039468566863 ) ) ;
#165307=CARTESIAN_POINT ( 'NONE',  ( 19.05341960407611168, 5.049401038298154454, 53.95724293864770260 ) ) ;
#165308=CARTESIAN_POINT ( 'NONE',  ( -15.80617190586745835, -15.72974639402198527, 21.87390960531436690 ) ) ;
#165309=B_SPLINE_CURVE_WITH_KNOTS ( 'NONE', 3,
 ( #63440, #124102, #94765, #76616, #107939, #61440, #138294, #111929, #171621, #80584, #14956, #187801, #46283, #33109, #157444, #91764, #142258, #169626, #123112, #156447, #153459, #17947, #64435, #77611, #154460, #15952, #65419, #139282, #759, #62430, #185802, #170626 ),
 .UNSPECIFIED., .F., .F.,
 ( 4, 2, 2, 2, 2, 2, 2, 2, 2, 2, 2, 2, 2, 2, 2, 4 ),
 ( 8.673617379884035472E-19, 0.0003712461730036752312, 0.0007424923460073495950, 0.001113738519011024013, 0.001484984692014698323, 0.002227477038022067542, 0.002598723211025740550, 0.002969969384029413993, 0.003341215557033087868, 0.003712461730036761311, 0.004083707903040434753, 0.004454954076044109063, 0.004826200249047782505, 0.005197446422051455947, 0.005568692595055130257, 0.005939938768058803699 ),
 .UNSPECIFIED. ) ;
#165310=CARTESIAN_POINT ( 'NONE',  ( 5.823673210054444382, -21.52544592524334988, 95.20942372801903275 ) ) ;
#165311=CARTESIAN_POINT ( 'NONE',  ( 16.46253265017160672, -9.564922557960803928, 58.33224293864769550 ) ) ;
#165312=CARTESIAN_POINT ( 'NONE',  ( -0.05219959533937732626, 21.53943276465977519, 92.50109039468567573 ) ) ;
#165313=CARTESIAN_POINT ( 'NONE',  ( -18.62759615963270932, 10.81492255796079327, 55.83224293864770260 ) ) ;
#165315=CARTESIAN_POINT ( 'NONE',  ( 5.153800228976335163, 19.02544592524342804, 79.79057627198102409 ) ) ;
#165316=CARTESIAN_POINT ( 'NONE',  ( 9.474510206698729675, 16.51473224551082808, 57.08442372801900433 ) ) ;
#165317=CARTESIAN_POINT ( 'NONE',  ( -19.05341960407611168, -5.049401038298163336, 46.45724293864768129 ) ) ;
#165318=CARTESIAN_POINT ( 'NONE',  ( 9.474510206698971260, -16.51473224551069308, 87.91557627198102409 ) ) ;
#165319=CARTESIAN_POINT ( 'NONE',  ( -0.05219959533936034679, 19.03943276465977164, 87.50109039468567573 ) ) ;
#165320=CARTESIAN_POINT ( 'NONE',  ( -16.53943276465976808, -0.05219959533934237506, 33.75109039468568284 ) ) ;
#165321=CARTESIAN_POINT ( 'NONE',  ( -4.379528057220328563, 16.55341960407611168, 100.2072429386476955 ) ) ;
#165322=CARTESIAN_POINT ( 'NONE',  ( -16.46253265017160317, 9.564922557960807481, 65.83224293864769550 ) ) ;
#165323=CARTESIAN_POINT ( 'NONE',  ( 15.72974639402199770, -15.80617190586745480, 48.12390960531436690 ) ) ;
#165324=CARTESIAN_POINT ( 'NONE',  ( -16.46253265017146816, -9.564922557961047289, 109.1677570613523471 ) ) ;
#165325=CARTESIAN_POINT ( 'NONE',  ( 21.52544592524344225, -5.823673210054117533, 113.5405762719810383 ) ) ;
#165326=CARTESIAN_POINT ( 'NONE',  ( 0.05219959533937995610, -21.53943276465977519, 65.00109039468568994 ) ) ;
#165327=CARTESIAN_POINT ( 'NONE',  ( 8.314922557961029526, -14.29746914071037800, 65.41775706135234714 ) ) ;
#165328=CARTESIAN_POINT ( 'NONE',  ( -16.46253265017160317, 9.564922557960807481, 70.83224293864770971 ) ) ;
#165329=CARTESIAN_POINT ( 'NONE',  ( -14.34966873604972548, 8.224510206698743886, 103.3344237280190043 ) ) ;
#165330=CARTESIAN_POINT ( 'NONE',  ( 19.02544592524334988, 5.153800228976608722, 46.45942372801899012 ) ) ;
#165331=CARTESIAN_POINT ( 'NONE',  ( -15.72974639402176322, -15.80617190586768395, 29.37609039468568284 ) ) ;
#165332=CARTESIAN_POINT ( 'NONE',  ( -12.06949235617756955, 12.14591786802309770, 80.62390960531438111 ) ) ;
#165333=CARTESIAN_POINT ( 'NONE',  ( -9.474510206698964154, 16.51473224551069663, 95.41557627198102409 ) ) ;
#165334=CARTESIAN_POINT ( 'NONE',  ( 8.314922557961029526, -14.29746914071037800, 85.41775706135236135 ) ) ;
#165335=CARTESIAN_POINT ( 'NONE',  ( 15.72974639402176855, 15.80617190586768217, 66.87609039468568994 ) ) ;
#165336=CARTESIAN_POINT ( 'NONE',  ( 4.379528057220092307, 16.55341960407617563, 27.29275706135234358 ) ) ;
#165337=CARTESIAN_POINT ( 'NONE',  ( -21.52544592524334988, -5.823673210054445271, 28.95942372801902209 ) ) ;
#165338=CARTESIAN_POINT ( 'NONE',  ( -12.06949235617756955, 12.14591786802309770, 65.62390960531436690 ) ) ;
#165339=ORIENTED_EDGE ( 'NONE', *, *, #9292, .T. ) ;
#165340=CARTESIAN_POINT ( 'NONE',  ( 5.719274019375991003, -21.55341960407610458, 107.7072429386476955 ) ) ;
#165341=CARTESIAN_POINT ( 'NONE',  ( 12.06949235617757843, -12.14591786802309237, 48.12390960531436690 ) ) ;
#165343=CARTESIAN_POINT ( 'NONE',  ( 19.02544592524343514, -5.153800228976328945, 23.54057627198102054 ) ) ;
#165344=CARTESIAN_POINT ( 'NONE',  ( 10.81492255796078972, 18.62759615963270932, 34.58224293864770260 ) ) ;
#165345=CARTESIAN_POINT ( 'NONE',  ( 5.823673210054444382, -21.52544592524334988, 40.20942372801901854 ) ) ;
#165346=CARTESIAN_POINT ( 'NONE',  ( 4.483927247898545687, 16.52544592524342804, 69.79057627198102409 ) ) ;
#165347=CARTESIAN_POINT ( 'NONE',  ( 0.05219959533907565091, 21.53943276465977519, 64.99890960531435269 ) ) ;
#165348=CARTESIAN_POINT ( 'NONE',  ( 13.89961937509977652, -13.97604488694527269, 78.12390960531433848 ) ) ;
#165349=CARTESIAN_POINT ( 'NONE',  ( 16.46253265017160672, -9.564922557960803928, 28.33224293864769550 ) ) ;
#165350=CARTESIAN_POINT ( 'NONE',  ( -16.46253265017146816, -9.564922557961047289, 74.16775706135234714 ) ) ;
#165351=CARTESIAN_POINT ( 'NONE',  ( -5.823673210054116645, -21.52544592524344225, 52.29057627198102409 ) ) ;
#165352=CARTESIAN_POINT ( 'NONE',  ( 19.02544592524343514, -5.153800228976328945, 43.54057627198103120 ) ) ;
#165353=CARTESIAN_POINT ( 'NONE',  ( -19.05341960407611168, -5.049401038298163336, 71.45724293864766707 ) ) ;
#165355=CARTESIAN_POINT ( 'NONE',  ( 12.14591786802327356, -12.06949235617739191, 30.62609039468567929 ) ) ;
#165356=CARTESIAN_POINT ( 'NONE',  ( 18.67979575497178502, 10.72451020669898547, 114.1655762719810383 ) ) ;
#165357=CARTESIAN_POINT ( 'NONE',  ( 8.224510206698953496, -14.34966873604960469, 47.91557627198102409 ) ) ;
#165358=CARTESIAN_POINT ( 'NONE',  ( -21.55341960407619339, 5.719274019375674811, 63.54275706135234003 ) ) ;
#165359=CARTESIAN_POINT ( 'NONE',  ( -9.564922557960796823, -16.46253265017161027, 107.0822429386476955 ) ) ;
#165360=CARTESIAN_POINT ( 'NONE',  ( 15.80617190586746368, 15.72974639402197994, 74.37390960531436690 ) ) ;
#165361=CARTESIAN_POINT ( 'NONE',  ( 10.81492255796078972, 18.62759615963270932, 104.5822429386477097 ) ) ;
#165362=CARTESIAN_POINT ( 'NONE',  ( -16.55341960407617563, 4.379528057220093196, 53.54275706135234714 ) ) ;
#165363=CARTESIAN_POINT ( 'NONE',  ( -10.72451020669898014, 18.67979575497178502, 55.41557627198102409 ) ) ;
#165364=CARTESIAN_POINT ( 'NONE',  ( -15.72974639402176322, -15.80617190586768395, 99.37609039468568994 ) ) ;
#165365=CARTESIAN_POINT ( 'NONE',  ( -9.564922557960796823, -16.46253265017161027, 52.08224293864768839 ) ) ;
#165366=CARTESIAN_POINT ( 'NONE',  ( 19.02544592524343514, -5.153800228976328945, 108.5405762719810383 ) ) ;
#165367=CARTESIAN_POINT ( 'NONE',  ( -19.05341960407611168, -5.049401038298163336, 71.45724293864766707 ) ) ;
#165369=CARTESIAN_POINT ( 'NONE',  ( -16.46253265017146816, -9.564922557961047289, 64.16775706135233293 ) ) ;
#165370=CARTESIAN_POINT ( 'NONE',  ( -19.02544592524334988, -5.153800228976617603, 18.95942372801899722 ) ) ;
#165371=CARTESIAN_POINT ( 'NONE',  ( -15.80617190586745835, -15.72974639402198527, 26.87390960531435979 ) ) ;
#165372=CARTESIAN_POINT ( 'NONE',  ( 4.379528057220092307, 16.55341960407617563, 107.2927570613523471 ) ) ;
#165373=CARTESIAN_POINT ( 'NONE',  ( 5.049401038297881783, 19.05341960407617563, 82.29275706135229029 ) ) ;
#165374=CARTESIAN_POINT ( 'NONE',  ( -16.31925111598458855, 7.325300261831458215, 60.16424538967254421 ) ) ;
#165375=CARTESIAN_POINT ( 'NONE',  ( -19.02544592524334988, -5.153800228976617603, 18.95942372801899722 ) ) ;
#165376=CARTESIAN_POINT ( 'NONE',  ( 9.474510206698729675, 16.51473224551082808, 77.08442372801900433 ) ) ;
#165377=CARTESIAN_POINT ( 'NONE',  ( 13.89961937509957401, 13.97604488694547697, 41.87609039468566152 ) ) ;
#165379=CARTESIAN_POINT ( 'NONE',  ( -19.02544592524342804, 5.153800228976336051, 46.04057627198101699 ) ) ;
#165380=CARTESIAN_POINT ( 'NONE',  ( 8.314922557960818139, 14.29746914071049879, 54.58224293864769550 ) ) ;
#165382=CARTESIAN_POINT ( 'NONE',  ( -13.89961937509977652, 13.97604488694528158, 40.62390960531435979 ) ) ;
#165383=CARTESIAN_POINT ( 'NONE',  ( 8.224510206698953496, -14.34966873604960469, 37.91557627198102409 ) ) ;
#165384=CARTESIAN_POINT ( 'NONE',  ( 18.10062525802554489, -5.500000000000022204, 46.01383468041920821 ) ) ;
#165385=CARTESIAN_POINT ( 'NONE',  ( -8.314922557961024197, 14.29746914071037800, 107.9177570613523471 ) ) ;
#165386=CARTESIAN_POINT ( 'NONE',  ( 0.05219959533909260263, 19.03943276465977164, 49.99890960531435979 ) ) ;
#165387=CARTESIAN_POINT ( 'NONE',  ( -19.02544592524334988, -5.153800228976617603, 28.95942372801900433 ) ) ;
#165388=CARTESIAN_POINT ( 'NONE',  ( -14.29746914071037622, -8.314922557961029526, 39.16775706135235424 ) ) ;
#165389=CARTESIAN_POINT ( 'NONE',  ( -21.53943276465977519, 0.05219959533907696930, 41.24890960531435269 ) ) ;
#165390=CARTESIAN_POINT ( 'NONE',  ( -21.52544592524334988, -5.823673210054445271, 88.95942372801901854 ) ) ;
#165392=CARTESIAN_POINT ( 'NONE',  ( -13.89961937509977652, 13.97604488694528158, 105.6239096053143527 ) ) ;
#165393=CARTESIAN_POINT ( 'NONE',  ( 5.049401038298161559, -19.05341960407611168, 82.70724293864770971 ) ) ;
#165395=CARTESIAN_POINT ( 'NONE',  ( 10.72451020669898902, -18.67979575497178502, 112.9155762719810383 ) ) ;
#165396=CARTESIAN_POINT ( 'NONE',  ( -4.379528057220328563, 16.55341960407611168, 75.20724293864769550 ) ) ;
#165397=CARTESIAN_POINT ( 'NONE',  ( -21.55341960407610458, -5.719274019375992779, 71.45724293864769550 ) ) ;
#165398=CARTESIAN_POINT ( 'NONE',  ( 19.05341960407611168, 5.049401038298154454, 68.95724293864769550 ) ) ;
#165399=CARTESIAN_POINT ( 'NONE',  ( 9.564922557960805705, 16.46253265017160317, 79.58224293864769550 ) ) ;
#165400=CARTESIAN_POINT ( 'NONE',  ( -21.52544592524343514, 5.823673210054127303, 91.04057627198103830 ) ) ;
#165401=ORIENTED_EDGE ( 'NONE', *, *, #54823, .T. ) ;
#165402=CARTESIAN_POINT ( 'NONE',  ( 16.51473224551069308, 9.474510206698969483, 64.16557627198102409 ) ) ;
#165403=CARTESIAN_POINT ( 'NONE',  ( 4.483927247898545687, 16.52544592524342804, 94.79057627198105251 ) ) ;
#165404=CARTESIAN_POINT ( 'NONE',  ( -16.46253265017160317, 9.564922557960807481, 25.83224293864769194 ) ) ;
#165405=CARTESIAN_POINT ( 'NONE',  ( 5.153800228976335163, 19.02544592524342804, 59.79057627198100988 ) ) ;
#165406=CARTESIAN_POINT ( 'NONE',  ( 19.05341960407617918, -5.049401038297876454, 81.04275706135231871 ) ) ;
#165407=CARTESIAN_POINT ( 'NONE',  ( -14.34966873604960291, -8.224510206698953496, 91.66557627198103830 ) ) ;
#165408=CARTESIAN_POINT ( 'NONE',  ( -15.80617190586768217, 15.72974639402176855, 53.12609039468568284 ) ) ;
#165409=CARTESIAN_POINT ( 'NONE',  ( -19.03943276465977164, 0.05219959533909376836, 51.24890960531436690 ) ) ;
#165410=CARTESIAN_POINT ( 'NONE',  ( 15.72974639402176855, 15.80617190586768217, 21.87609039468567573 ) ) ;
#165411=CARTESIAN_POINT ( 'NONE',  ( -12.06949235617756955, 12.14591786802309770, 105.6239096053143669 ) ) ;
#165413=CARTESIAN_POINT ( 'NONE',  ( 16.46253265017160672, -9.564922557960803928, 58.33224293864769550 ) ) ;
#165414=DIRECTION ( 'NONE',  ( -0.000000000000000000, -0.000000000000000000, 1.000000000000000000 ) ) ;
#165415=CARTESIAN_POINT ( 'NONE',  ( 9.474510206698729675, 16.51473224551082808, 107.0844237280190043 ) ) ;
#165416=CARTESIAN_POINT ( 'NONE',  ( 5.719274019375991003, -21.55341960407610458, 22.70724293864769194 ) ) ;
#165417=CARTESIAN_POINT ( 'NONE',  ( -21.53943276465977519, -0.05219959533937600094, 43.75109039468568284 ) ) ;
#165418=CARTESIAN_POINT ( 'NONE',  ( 16.46253265017160672, -9.564922557960803928, 98.33224293864769550 ) ) ;
#165419=CARTESIAN_POINT ( 'NONE',  ( -5.153800228976607833, 19.02544592524334988, 82.70942372801897591 ) ) ;
#165420=CARTESIAN_POINT ( 'NONE',  ( 0.05219959533909260263, 19.03943276465977164, 59.99890960531436690 ) ) ;
#165421=CARTESIAN_POINT ( 'NONE',  ( -16.52544592524342804, 4.483927247898546575, 81.04057627198102409 ) ) ;
#165422=CARTESIAN_POINT ( 'NONE',  ( 19.03943276465977164, -0.05219959533909143690, 103.7489096053143669 ) ) ;
#165423=CARTESIAN_POINT ( 'NONE',  ( -16.53943276465976808, 0.05219959533911058130, 81.24890960531436690 ) ) ;
#165424=CARTESIAN_POINT ( 'NONE',  ( -9.564922557960796823, -16.46253265017161027, 97.08224293864769550 ) ) ;
#165425=CARTESIAN_POINT ( 'NONE',  ( 9.474510206698729675, 16.51473224551082808, 47.08442372801900433 ) ) ;
#165426=CARTESIAN_POINT ( 'NONE',  ( -9.564922557960796823, -16.46253265017161027, 52.08224293864768839 ) ) ;
#165427=CARTESIAN_POINT ( 'NONE',  ( 14.29746914071049879, -8.314922557960816363, 43.33224293864769550 ) ) ;
#165428=CARTESIAN_POINT ( 'NONE',  ( 16.51473224551069308, 9.474510206698969483, 34.16557627198102409 ) ) ;
#165430=CARTESIAN_POINT ( 'NONE',  ( -10.81492255796105439, 18.62759615963255655, 47.91775706135234714 ) ) ;
#165431=CARTESIAN_POINT ( 'NONE',  ( -16.51473224551082808, 9.474510206698731452, 83.33442372801899012 ) ) ;
#165432=CARTESIAN_POINT ( 'NONE',  ( -16.52544592524342804, 4.483927247898546575, 41.04057627198103120 ) ) ;
#165433=CARTESIAN_POINT ( 'NONE',  ( -18.62759615963270932, 10.81492255796079327, 105.8322429386476955 ) ) ;
#165434=CARTESIAN_POINT ( 'NONE',  ( -21.55341960407610458, -5.719274019375992779, 31.45724293864769550 ) ) ;
#165435=CARTESIAN_POINT ( 'NONE',  ( 16.53943276465976808, -0.05219959533910856209, 78.74890960531436690 ) ) ;
#165436=CARTESIAN_POINT ( 'NONE',  ( -5.153800228976328057, -19.02544592524343514, 37.29057627198102409 ) ) ;
#165437=CARTESIAN_POINT ( 'NONE',  ( -16.55341960407617563, 4.379528057220093196, 98.54275706135234714 ) ) ;
#165438=CARTESIAN_POINT ( 'NONE',  ( 16.55341960407618274, -4.379528057220086978, 71.04275706135234714 ) ) ;
#165439=CARTESIAN_POINT ( 'NONE',  ( 0.05219959533936267826, -19.03943276465977164, 30.00109039468566863 ) ) ;
#165440=CARTESIAN_POINT ( 'NONE',  ( -19.02544592524342804, 5.153800228976336051, 96.04057627198103830 ) ) ;
#165441=CARTESIAN_POINT ( 'NONE',  ( 9.474510206698971260, -16.51473224551069308, 72.91557627198102409 ) ) ;
#165442=CARTESIAN_POINT ( 'NONE',  ( -14.29746914071037622, -8.314922557961029526, 69.16775706135234714 ) ) ;
#165443=CARTESIAN_POINT ( 'NONE',  ( 13.97604488694527802, 13.89961937509977652, 39.37390960531435269 ) ) ;
#165444=CARTESIAN_POINT ( 'NONE',  ( 14.34966873604960469, 8.224510206698951720, 44.16557627198103120 ) ) ;
#165445=CARTESIAN_POINT ( 'NONE',  ( 15.50000000000000355, 7.499999999999998224, 22.00000000000000711 ) ) ;
#165446=CARTESIAN_POINT ( 'NONE',  ( 5.153800228976335163, 19.02544592524342804, 84.79057627198099567 ) ) ;
#165447=CARTESIAN_POINT ( 'NONE',  ( 21.52544592524344225, -5.823673210054117533, 23.54057627198102765 ) ) ;
#165448=CARTESIAN_POINT ( 'NONE',  ( 16.53943276465976808, -0.05219959533910856209, 73.74890960531433848 ) ) ;
#165449=CARTESIAN_POINT ( 'NONE',  ( -16.53943276465976808, 0.05219959533911058130, 61.24890960531435979 ) ) ;
#165450=CARTESIAN_POINT ( 'NONE',  ( -4.379528057220086978, -16.55341960407618274, 54.79275706135235424 ) ) ;
#165451=CARTESIAN_POINT ( 'NONE',  ( 17.50000000000149569, -3.254303733634584361, 32.52395893071417277 ) ) ;
#165452=CARTESIAN_POINT ( 'NONE',  ( -13.89961937509957401, -13.97604488694547875, 69.37609039468564731 ) ) ;
#165453=CARTESIAN_POINT ( 'NONE',  ( -16.46253265017160317, 9.564922557960807481, 85.83224293864769550 ) ) ;
#165454=CARTESIAN_POINT ( 'NONE',  ( -16.46253265017146816, -9.564922557961047289, 64.16775706135233293 ) ) ;
#165455=CARTESIAN_POINT ( 'NONE',  ( 13.97604488694548053, -13.89961937509957401, 40.62609039468565442 ) ) ;
#165456=CARTESIAN_POINT ( 'NONE',  ( 4.483927247898790824, -16.52544592524335698, 20.20942372801900788 ) ) ;
#165457=CARTESIAN_POINT ( 'NONE',  ( 0.05219959533934541429, -16.53943276465976808, 95.00109039468568994 ) ) ;
#165458=CARTESIAN_POINT ( 'NONE',  ( -16.46253265017160317, 9.564922557960807481, 40.83224293864769550 ) ) ;
#165460=CARTESIAN_POINT ( 'NONE',  ( -21.53943276465977519, 0.05219959533907696930, 21.24890960531436690 ) ) ;
#165461=CARTESIAN_POINT ( 'NONE',  ( 18.67979575497194134, -10.72451020669871369, 55.83442372801901854 ) ) ;
#165462=CARTESIAN_POINT ( 'NONE',  ( -14.34966873604972548, 8.224510206698743886, 23.33442372801901499 ) ) ;
#165463=CARTESIAN_POINT ( 'NONE',  ( -17.58332526062528345, -7.635886036038592728, 54.07665040441535353 ) ) ;
#165464=CARTESIAN_POINT ( 'NONE',  ( -16.46253265017160317, 9.564922557960807481, 75.83224293864769550 ) ) ;
#165466=CARTESIAN_POINT ( 'NONE',  ( -16.52544592524342804, 4.483927247898546575, 81.04057627198102409 ) ) ;
#165467=CARTESIAN_POINT ( 'NONE',  ( 19.03943276465977164, -0.05219959533909143690, 78.74890960531436690 ) ) ;
#165468=CARTESIAN_POINT ( 'NONE',  ( 9.474510206698971260, -16.51473224551069308, 67.91557627198102409 ) ) ;
#165469=CARTESIAN_POINT ( 'NONE',  ( -0.05219959533936034679, 19.03943276465977164, 92.50109039468566152 ) ) ;
#165470=CARTESIAN_POINT ( 'NONE',  ( -10.81492255796078084, -18.62759615963271287, 67.08224293864770971 ) ) ;
#165471=CARTESIAN_POINT ( 'NONE',  ( 19.02544592524343514, -5.153800228976328945, 33.54057627198102409 ) ) ;
#165472=CARTESIAN_POINT ( 'NONE',  ( 19.03943276465977164, 0.05219959533936151252, 56.25109039468566863 ) ) ;
#165473=CARTESIAN_POINT ( 'NONE',  ( -9.474510206698964154, 16.51473224551069663, 60.41557627198102409 ) ) ;
#165474=CARTESIAN_POINT ( 'NONE',  ( 13.97604488694527802, 13.89961937509977652, 94.37390960531436690 ) ) ;
#165476=CARTESIAN_POINT ( 'NONE',  ( 10.72451020669898902, -18.67979575497178502, 87.91557627198103830 ) ) ;
#165477=CARTESIAN_POINT ( 'NONE',  ( -16.52544592524342804, 4.483927247898546575, 91.04057627198103830 ) ) ;
#165478=CARTESIAN_POINT ( 'NONE',  ( -9.564922557961040184, 16.46253265017147172, 52.91775706135233293 ) ) ;
#165479=CARTESIAN_POINT ( 'NONE',  ( -18.62759615963270932, 10.81492255796079327, 80.83224293864769550 ) ) ;
#165480=CARTESIAN_POINT ( 'NONE',  ( -0.05219959533907301413, -21.53943276465977519, 57.49890960531435979 ) ) ;
#165481=CARTESIAN_POINT ( 'NONE',  ( -16.53943276465976808, 0.05219959533911058130, 36.24890960531435979 ) ) ;
#165482=CARTESIAN_POINT ( 'NONE',  ( 5.719274019375673035, 21.55341960407619339, 107.2927570613523471 ) ) ;
#165483=CARTESIAN_POINT ( 'NONE',  ( 19.03943276465977164, -0.05219959533909143690, 83.74890960531436690 ) ) ;
#165484=CARTESIAN_POINT ( 'NONE',  ( 5.049401038298161559, -19.05341960407611168, 37.70724293864768839 ) ) ;
#165485=CARTESIAN_POINT ( 'NONE',  ( 5.823673210054444382, -21.52544592524334988, 45.20942372801901854 ) ) ;
#165486=CARTESIAN_POINT ( 'NONE',  ( -15.72974639402176322, -15.80617190586768395, 49.37609039468569705 ) ) ;
#165487=CARTESIAN_POINT ( 'NONE',  ( 13.89961937509977652, -13.97604488694527269, 53.12390960531434558 ) ) ;
#165488=CARTESIAN_POINT ( 'NONE',  ( -21.53943276465977519, -0.05219959533937600094, 28.75109039468567929 ) ) ;
#165489=CARTESIAN_POINT ( 'NONE',  ( -19.05341960407617563, 5.049401038297882671, 63.54275706135234003 ) ) ;
#165490=CARTESIAN_POINT ( 'NONE',  ( 5.049401038298161559, -19.05341960407611168, 32.70724293864768129 ) ) ;
#165491=CARTESIAN_POINT ( 'NONE',  ( 14.29746914071037800, 8.314922557961029526, 26.66775706135235424 ) ) ;
#165493=CARTESIAN_POINT ( 'NONE',  ( 14.29746914071037800, 8.314922557961029526, 76.66775706135234714 ) ) ;
#165494=CARTESIAN_POINT ( 'NONE',  ( 19.05341960407611168, 5.049401038298154454, 33.95724293864769550 ) ) ;
#165496=CARTESIAN_POINT ( 'NONE',  ( 19.05341960407611168, 5.049401038298154454, 83.95724293864766707 ) ) ;
#165497=CARTESIAN_POINT ( 'NONE',  ( -19.03943276465977164, 0.05219959533909376836, 26.24890960531435624 ) ) ;
#165498=CARTESIAN_POINT ( 'NONE',  ( 5.719274019375991003, -21.55341960407610458, 72.70724293864769550 ) ) ;
#165499=CARTESIAN_POINT ( 'NONE',  ( 12.06949235617739724, 12.14591786802326823, 46.87609039468568994 ) ) ;
#165500=CARTESIAN_POINT ( 'NONE',  ( 5.823673210054444382, -21.52544592524334988, 105.2094237280190328 ) ) ;
#165501=CARTESIAN_POINT ( 'NONE',  ( 5.049401038298161559, -19.05341960407611168, 37.70724293864768839 ) ) ;
#165502=CARTESIAN_POINT ( 'NONE',  ( 16.55341960407611168, 4.379528057220329451, 28.95724293864769905 ) ) ;
#165503=CARTESIAN_POINT ( 'NONE',  ( -0.05219959533910754901, -16.53943276465976808, 67.49890960531436690 ) ) ;
#165504=CARTESIAN_POINT ( 'NONE',  ( -13.97604488694527625, -13.89961937509977652, 61.87390960531435979 ) ) ;
#165505=CARTESIAN_POINT ( 'NONE',  ( -18.67979575497193778, 10.72451020669871902, 103.3344237280190043 ) ) ;
#165506=CARTESIAN_POINT ( 'NONE',  ( -21.53943276465977519, -0.05219959533937600094, 28.75109039468567929 ) ) ;
#165507=CARTESIAN_POINT ( 'NONE',  ( -5.049401038298153566, 19.05341960407611168, 80.20724293864769550 ) ) ;
#165508=CARTESIAN_POINT ( 'NONE',  ( -21.55341960407619339, 5.719274019375674811, 83.54275706135234714 ) ) ;
#165509=CARTESIAN_POINT ( 'NONE',  ( 12.06949235617739724, 12.14591786802326823, 61.87609039468568284 ) ) ;
#165510=CARTESIAN_POINT ( 'NONE',  ( 14.29746914071037800, 8.314922557961029526, 26.66775706135235424 ) ) ;
#165511=EDGE_CURVE ( 'NONE', #99775, #162452, #198343, .T. ) ;
#165512=CARTESIAN_POINT ( 'NONE',  ( -12.06949235617756955, 12.14591786802309770, 90.62390960531436690 ) ) ;
#165513=CARTESIAN_POINT ( 'NONE',  ( -5.823673210054431948, 21.52544592524334988, 102.7094237280190185 ) ) ;
#165514=CARTESIAN_POINT ( 'NONE',  ( 12.14591786802309770, 12.06949235617756955, 39.37390960531436690 ) ) ;
#165515=CARTESIAN_POINT ( 'NONE',  ( -0.05219959533909027116, -19.03943276465977164, 27.49890960531435624 ) ) ;
#165516=CARTESIAN_POINT ( 'NONE',  ( 8.224510206698742110, 14.34966873604972548, 57.08442372801901854 ) ) ;
#165517=CARTESIAN_POINT ( 'NONE',  ( 0.05219959533910956823, 16.53943276465976808, 54.99890960531435269 ) ) ;
#165518=CARTESIAN_POINT ( 'NONE',  ( 16.53943276465976808, 0.05219959533934440121, 101.2510903946856757 ) ) ;
#165519=CARTESIAN_POINT ( 'NONE',  ( 5.719274019375991003, -21.55341960407610458, 22.70724293864769194 ) ) ;
#165520=CARTESIAN_POINT ( 'NONE',  ( -10.81492255796078084, -18.62759615963271287, 32.08224293864769550 ) ) ;
#165521=CARTESIAN_POINT ( 'NONE',  ( -19.05341960407617563, 5.049401038297882671, 23.54275706135233648 ) ) ;
#165522=CARTESIAN_POINT ( 'NONE',  ( -12.06949235617756955, 12.14591786802309770, 80.62390960531438111 ) ) ;
#165523=CARTESIAN_POINT ( 'NONE',  ( -9.564922557960796823, -16.46253265017161027, 97.08224293864769550 ) ) ;
#165524=VERTEX_POINT ( 'NONE', #22703 ) ;
#165525=CARTESIAN_POINT ( 'NONE',  ( 14.34966873604972726, -8.224510206698740333, 35.83442372801901143 ) ) ;
#165526=CARTESIAN_POINT ( 'NONE',  ( -16.46253265017160317, 9.564922557960807481, 45.83224293864769550 ) ) ;
#165527=CARTESIAN_POINT ( 'NONE',  ( -12.14591786802326823, 12.06949235617739902, 43.12609039468568284 ) ) ;
#165529=CARTESIAN_POINT ( 'NONE',  ( -19.05341960407617563, 5.049401038297882671, 53.54275706135231871 ) ) ;
#165530=CARTESIAN_POINT ( 'NONE',  ( 5.049401038298161559, -19.05341960407611168, 52.70724293864767418 ) ) ;
#165531=CARTESIAN_POINT ( 'NONE',  ( 16.55341960407618274, -4.379528057220086978, 86.04275706135236135 ) ) ;
#165532=CARTESIAN_POINT ( 'NONE',  ( -5.049401038297874678, -19.05341960407617918, 89.79275706135230450 ) ) ;
#165533=CARTESIAN_POINT ( 'NONE',  ( -9.564922557961040184, 16.46253265017147172, 27.91775706135232582 ) ) ;
#165534=CARTESIAN_POINT ( 'NONE',  ( -0.05219959533909027116, -19.03943276465977164, 67.49890960531436690 ) ) ;
#165535=CARTESIAN_POINT ( 'NONE',  ( -4.379528057220328563, 16.55341960407611168, 105.2072429386477097 ) ) ;
#165536=CARTESIAN_POINT ( 'NONE',  ( -9.474510206698720793, -16.51473224551083518, 74.58442372801900433 ) ) ;
#165537=CARTESIAN_POINT ( 'NONE',  ( -15.80617190586745835, -15.72974639402198527, 66.87390960531436690 ) ) ;
#165538=CARTESIAN_POINT ( 'NONE',  ( -19.05341960407617563, 5.049401038297882671, 43.54275706135232582 ) ) ;
#165539=CARTESIAN_POINT ( 'NONE',  ( 19.02544592524343514, -5.153800228976328945, 98.54057627198100988 ) ) ;
#165540=CARTESIAN_POINT ( 'NONE',  ( -21.53943276465977519, 0.05219959533907696930, 91.24890960531436690 ) ) ;
#165541=CARTESIAN_POINT ( 'NONE',  ( -16.19135201231366139, 7.376712067591929767, 84.81319145947969673 ) ) ;
#165542=CARTESIAN_POINT ( 'NONE',  ( -9.474510206698720793, -16.51473224551083518, 99.58442372801900433 ) ) ;
#165543=CARTESIAN_POINT ( 'NONE',  ( -18.22780087662119541, 5.500000000000102141, 61.01763182126894947 ) ) ;
#165544=CARTESIAN_POINT ( 'NONE',  ( 16.53943276465976808, 0.05219959533934440121, 26.25109039468567573 ) ) ;
#165545=CARTESIAN_POINT ( 'NONE',  ( -19.02544592524342804, 5.153800228976336051, 51.04057627198103120 ) ) ;
#165546=CARTESIAN_POINT ( 'NONE',  ( 19.03943276465977164, -0.05219959533909143690, 108.7489096053143527 ) ) ;
#165547=CARTESIAN_POINT ( 'NONE',  ( -15.72974639402197994, 15.80617190586746368, 90.62390960531436690 ) ) ;
#165548=CARTESIAN_POINT ( 'NONE',  ( -21.52544592524334988, -5.823673210054445271, 63.95942372801901854 ) ) ;
#165549=CARTESIAN_POINT ( 'NONE',  ( 13.89961937509957401, 13.97604488694547697, 106.8760903946856757 ) ) ;
#165550=CARTESIAN_POINT ( 'NONE',  ( 15.80617190586769283, -15.72974639402175789, 110.6260903946857042 ) ) ;
#165551=CARTESIAN_POINT ( 'NONE',  ( 14.34966873604960469, 8.224510206698951720, 34.16557627198102409 ) ) ;
#165552=CARTESIAN_POINT ( 'NONE',  ( 15.72974639402199770, -15.80617190586745480, 98.12390960531436690 ) ) ;
#165553=CARTESIAN_POINT ( 'NONE',  ( -4.379528057220328563, 16.55341960407611168, 45.20724293864769550 ) ) ;
#165554=CARTESIAN_POINT ( 'NONE',  ( -9.564922557961040184, 16.46253265017147172, 87.91775706135233293 ) ) ;
#165555=CARTESIAN_POINT ( 'NONE',  ( 9.474510206698729675, 16.51473224551082808, 62.08442372801899722 ) ) ;
#165556=CARTESIAN_POINT ( 'NONE',  ( 0.05219959533937995610, -21.53943276465977519, 70.00109039468568994 ) ) ;
#165557=CARTESIAN_POINT ( 'NONE',  ( 9.474510206698729675, 16.51473224551082808, 42.08442372801900433 ) ) ;
#165558=CARTESIAN_POINT ( 'NONE',  ( -0.05219959533909027116, -19.03943276465977164, 27.49890960531435624 ) ) ;
#165559=CARTESIAN_POINT ( 'NONE',  ( 5.719274019375991003, -21.55341960407610458, 42.70724293864770260 ) ) ;
#165560=CARTESIAN_POINT ( 'NONE',  ( 16.53943276465976808, -0.05219959533910856209, 33.74890960531436690 ) ) ;
#165561=CARTESIAN_POINT ( 'NONE',  ( 19.05341960407617918, -5.049401038297876454, 21.04275706135232582 ) ) ;
#165562=CARTESIAN_POINT ( 'NONE',  ( -16.53943276465976808, -0.05219959533934237506, 68.75109039468568994 ) ) ;
#165563=CARTESIAN_POINT ( 'NONE',  ( 14.29746914071049879, -8.314922557960816363, 43.33224293864769550 ) ) ;
#165564=CARTESIAN_POINT ( 'NONE',  ( -0.05219959533937732626, 21.53943276465977519, 82.50109039468568994 ) ) ;
#165565=CARTESIAN_POINT ( 'NONE',  ( 15.72974639402176855, 15.80617190586768217, 71.87609039468568994 ) ) ;
#165566=CARTESIAN_POINT ( 'NONE',  ( 21.55341960407610458, 5.719274019375980345, 68.95724293864769550 ) ) ;
#165567=CARTESIAN_POINT ( 'NONE',  ( 9.474510206698971260, -16.51473224551069308, 22.91557627198102765 ) ) ;
#165568=CARTESIAN_POINT ( 'NONE',  ( -15.72974639402176322, -15.80617190586768395, 44.37609039468567573 ) ) ;
#165569=CARTESIAN_POINT ( 'NONE',  ( 13.89961937509977652, -13.97604488694527269, 23.12390960531436335 ) ) ;
#165570=CARTESIAN_POINT ( 'NONE',  ( 19.02544592524343514, -5.153800228976328945, 33.54057627198102409 ) ) ;
#165571=CARTESIAN_POINT ( 'NONE',  ( -0.05219959533910754901, -16.53943276465976808, 97.49890960531436690 ) ) ;
#165572=CARTESIAN_POINT ( 'NONE',  ( -9.564922557960796823, -16.46253265017161027, 82.08224293864768129 ) ) ;
#165573=CARTESIAN_POINT ( 'NONE',  ( 14.29746914071049879, -8.314922557960816363, 43.33224293864769550 ) ) ;
#165574=CARTESIAN_POINT ( 'NONE',  ( 16.53943276465976808, -0.05219959533910856209, 103.7489096053143669 ) ) ;
#165575=CARTESIAN_POINT ( 'NONE',  ( 18.67979575497178502, 10.72451020669898547, 69.16557627198102409 ) ) ;
#165576=CARTESIAN_POINT ( 'NONE',  ( -21.52544592524343514, 5.823673210054127303, 101.0405762719810383 ) ) ;
#165577=CARTESIAN_POINT ( 'NONE',  ( -13.89961937509977652, 13.97604488694528158, 110.6239096053143243 ) ) ;
#165579=CARTESIAN_POINT ( 'NONE',  ( -16.46253265017160317, 9.564922557960807481, 60.83224293864769550 ) ) ;
#165580=CARTESIAN_POINT ( 'NONE',  ( -16.53943276465976808, -0.05219959533934237506, 23.75109039468567929 ) ) ;
#165581=CARTESIAN_POINT ( 'NONE',  ( -21.55341960407610458, -5.719274019375992779, 56.45724293864768839 ) ) ;
#165582=CARTESIAN_POINT ( 'NONE',  ( 15.80617190586769283, -15.72974639402175789, 80.62609039468567573 ) ) ;
#165583=CARTESIAN_POINT ( 'NONE',  ( 13.97604488694527802, 13.89961937509977652, 79.37390960531435269 ) ) ;
#165584=CARTESIAN_POINT ( 'NONE',  ( 15.80617190586769283, -15.72974639402175789, 20.62609039468568639 ) ) ;
#165585=CARTESIAN_POINT ( 'NONE',  ( 13.89961937509977652, -13.97604488694527269, 113.1239096053143527 ) ) ;
#165586=CARTESIAN_POINT ( 'NONE',  ( -4.379528057220086978, -16.55341960407618274, 79.79275706135236135 ) ) ;
#165587=CARTESIAN_POINT ( 'NONE',  ( -5.823673210054431948, 21.52544592524334988, 72.70942372801901854 ) ) ;
#165588=CARTESIAN_POINT ( 'NONE',  ( 15.80617190586769283, -15.72974639402175789, 100.6260903946857184 ) ) ;
#165589=CARTESIAN_POINT ( 'NONE',  ( 0.05219959533934541429, -16.53943276465976808, 55.00109039468568284 ) ) ;
#165590=CARTESIAN_POINT ( 'NONE',  ( -21.53943276465977519, 0.05219959533907696930, 116.2489096053143669 ) ) ;
#165591=CARTESIAN_POINT ( 'NONE',  ( 16.51473224551069308, 9.474510206698969483, 114.1655762719810241 ) ) ;
#165592=CARTESIAN_POINT ( 'NONE',  ( -0.05219959533937732626, 21.53943276465977519, 92.50109039468567573 ) ) ;
#165593=CARTESIAN_POINT ( 'NONE',  ( 10.81492255796078972, 18.62759615963270932, 84.58224293864769550 ) ) ;
#165594=CARTESIAN_POINT ( 'NONE',  ( 9.564922557961047289, -16.46253265017146816, 50.41775706135233293 ) ) ;
#165595=CARTESIAN_POINT ( 'NONE',  ( -15.72974639402197994, 15.80617190586746368, 50.62390960531435979 ) ) ;
#165596=CARTESIAN_POINT ( 'NONE',  ( 19.05341960407611168, 5.049401038298154454, 93.95724293864769550 ) ) ;
#165597=CARTESIAN_POINT ( 'NONE',  ( 16.52544592524342804, -4.483927247898539470, 38.54057627198103120 ) ) ;
#165598=CARTESIAN_POINT ( 'NONE',  ( -18.22780087662121673, -5.500000000000063061, 41.48459894673893444 ) ) ;
#165600=CARTESIAN_POINT ( 'NONE',  ( 9.474510206698729675, 16.51473224551082808, 102.0844237280190043 ) ) ;
#165601=CARTESIAN_POINT ( 'NONE',  ( 21.55341960407610458, 5.719274019375980345, 88.95724293864769550 ) ) ;
#165602=CARTESIAN_POINT ( 'NONE',  ( -16.52544592524342804, 4.483927247898546575, 46.04057627198103830 ) ) ;
#165603=CARTESIAN_POINT ( 'NONE',  ( 8.314922557961029526, -14.29746914071037800, 25.41775706135235779 ) ) ;
#165604=CARTESIAN_POINT ( 'NONE',  ( 19.03943276465977164, -0.05219959533909143690, 38.74890960531436690 ) ) ;
#165605=CARTESIAN_POINT ( 'NONE',  ( -15.72974639402197994, 15.80617190586746368, 110.6239096053143669 ) ) ;
#165606=CARTESIAN_POINT ( 'NONE',  ( 9.564922557961047289, -16.46253265017146816, 80.41775706135234714 ) ) ;
#165607=CARTESIAN_POINT ( 'NONE',  ( 9.474510206698971260, -16.51473224551069308, 82.91557627198103830 ) ) ;
#165608=CARTESIAN_POINT ( 'NONE',  ( 0.05219959533909260263, 19.03943276465977164, 79.99890960531436690 ) ) ;
#165609=CARTESIAN_POINT ( 'NONE',  ( 15.80617190586746368, 15.72974639402197994, 74.37390960531436690 ) ) ;
#165610=CARTESIAN_POINT ( 'NONE',  ( 13.89961937509977652, -13.97604488694527269, 33.12390960531434558 ) ) ;
#165612=CARTESIAN_POINT ( 'NONE',  ( -8.224510206698948167, 14.34966873604960824, 55.41557627198102409 ) ) ;
#165613=CARTESIAN_POINT ( 'NONE',  ( 9.564922557960805705, 16.46253265017160317, 84.58224293864769550 ) ) ;
#165615=CARTESIAN_POINT ( 'NONE',  ( 9.564922557961047289, -16.46253265017146816, 60.41775706135233293 ) ) ;
#165616=CARTESIAN_POINT ( 'NONE',  ( 21.52544592524344225, -5.823673210054117533, 78.54057627198103830 ) ) ;
#165617=CARTESIAN_POINT ( 'NONE',  ( 13.97604488694548053, -13.89961937509957401, 40.62609039468564731 ) ) ;
#165618=CARTESIAN_POINT ( 'NONE',  ( 16.46253265017160672, -9.564922557960803928, 103.3322429386476955 ) ) ;
#165619=CARTESIAN_POINT ( 'NONE',  ( -17.49999999999999645, 3.805241302050293761, 115.3735247278259095 ) ) ;
#165620=CARTESIAN_POINT ( 'NONE',  ( -21.52544592524343514, 5.823673210054127303, 26.04057627198103475 ) ) ;
#165621=CARTESIAN_POINT ( 'NONE',  ( 9.564922557960805705, 16.46253265017160317, 74.58224293864769550 ) ) ;
#165622=CARTESIAN_POINT ( 'NONE',  ( 21.55341960407619695, -5.719274019375665929, 51.04275706135234714 ) ) ;
#165623=CARTESIAN_POINT ( 'NONE',  ( 19.03943276465977164, -0.05219959533909143690, 28.74890960531435624 ) ) ;
#165624=CARTESIAN_POINT ( 'NONE',  ( 21.52544592524334988, 5.823673210054432836, 21.45942372801901499 ) ) ;
#165625=EDGE_LOOP ( 'NONE', ( #170897, #106053, #10015, #179571 ) ) ;
#165626=CARTESIAN_POINT ( 'NONE',  ( -21.53943276465977519, -0.05219959533937600094, 43.75109039468568284 ) ) ;
#165627=ORIENTED_EDGE ( 'NONE', *, *, #119374, .T. ) ;
#165628=CARTESIAN_POINT ( 'NONE',  ( -0.05219959533909027116, -19.03943276465977164, 97.49890960531436690 ) ) ;
#165629=VECTOR ( 'NONE', #165245, 1000.000000000000000 ) ;
#165631=CARTESIAN_POINT ( 'NONE',  ( 15.72974639402199770, -15.80617190586745480, 113.1239096053143953 ) ) ;
#165632=CARTESIAN_POINT ( 'NONE',  ( 13.89961937509977652, -13.97604488694527269, 63.12390960531435979 ) ) ;
#165633=CARTESIAN_POINT ( 'NONE',  ( 14.29746914071037800, 8.314922557961029526, 21.66775706135235069 ) ) ;
#165635=CARTESIAN_POINT ( 'NONE',  ( 21.52544592524334988, 5.823673210054432836, 106.4594237280190328 ) ) ;
#165636=CARTESIAN_POINT ( 'NONE',  ( -19.05341960407611168, -5.049401038298163336, 46.45724293864768129 ) ) ;
#165637=CARTESIAN_POINT ( 'NONE',  ( -10.72451020669870658, -18.67979575497194134, 104.5844237280190185 ) ) ;
#165638=CARTESIAN_POINT ( 'NONE',  ( -9.564922557960796823, -16.46253265017161027, 87.08224293864769550 ) ) ;
#165639=CARTESIAN_POINT ( 'NONE',  ( -5.719274019375665041, -21.55341960407619695, 54.79275706135235424 ) ) ;
#165641=CARTESIAN_POINT ( 'NONE',  ( 5.049401038298161559, -19.05341960407611168, 107.7072429386476955 ) ) ;
#165642=CARTESIAN_POINT ( 'NONE',  ( -17.49999999999999645, 5.068104630630415386, 30.72818405340029813 ) ) ;
#165643=CARTESIAN_POINT ( 'NONE',  ( 4.483927247898790824, -16.52544592524335698, 55.20942372801902565 ) ) ;
#165644=CARTESIAN_POINT ( 'NONE',  ( 0.05219959533934541429, -16.53943276465976808, 75.00109039468568994 ) ) ;
#165645=CARTESIAN_POINT ( 'NONE',  ( -18.67979575497193778, 10.72451020669871902, 53.33442372801901854 ) ) ;
#165646=CARTESIAN_POINT ( 'NONE',  ( -18.62759615963255300, -10.81492255796106328, 94.16775706135237556 ) ) ;
#165648=CARTESIAN_POINT ( 'NONE',  ( -4.379528057220086978, -16.55341960407618274, 24.79275706135235779 ) ) ;
#165649=CARTESIAN_POINT ( 'NONE',  ( -19.02544592524342804, 5.153800228976336051, 76.04057627198102409 ) ) ;
#165650=CARTESIAN_POINT ( 'NONE',  ( -16.46253265017160317, 9.564922557960807481, 105.8322429386476955 ) ) ;
#165651=CARTESIAN_POINT ( 'NONE',  ( 16.31925111598457079, 7.325300261831479531, 42.33575461032752685 ) ) ;
#165652=CARTESIAN_POINT ( 'NONE',  ( 19.02544592524343514, -5.153800228976328945, 28.54057627198102409 ) ) ;
#165653=CARTESIAN_POINT ( 'NONE',  ( 18.67979575497178502, 10.72451020669898547, 39.16557627198102409 ) ) ;
#165654=CARTESIAN_POINT ( 'NONE',  ( 4.379528057220092307, 16.55341960407617563, 92.29275706135236135 ) ) ;
#165655=CARTESIAN_POINT ( 'NONE',  ( 12.06949235617757843, -12.14591786802309237, 78.12390960531436690 ) ) ;
#165656=CARTESIAN_POINT ( 'NONE',  ( -13.89961937509977652, 13.97604488694528158, 65.62390960531436690 ) ) ;
#165657=CARTESIAN_POINT ( 'NONE',  ( -15.72974639402176322, -15.80617190586768395, 84.37609039468570415 ) ) ;
#165659=CARTESIAN_POINT ( 'NONE',  ( 14.29746914071037800, 8.314922557961029526, 26.66775706135235424 ) ) ;
#165660=CARTESIAN_POINT ( 'NONE',  ( -16.55341960407611168, -4.379528057220339221, 71.45724293864769550 ) ) ;
#165661=CARTESIAN_POINT ( 'NONE',  ( -21.52544592524334988, -5.823673210054445271, 38.95942372801901854 ) ) ;
#165662=CARTESIAN_POINT ( 'NONE',  ( 21.53943276465977519, -0.05219959533907433946, 78.74890960531436690 ) ) ;
#165663=CARTESIAN_POINT ( 'NONE',  ( -9.474510206698720793, -16.51473224551083518, 44.58442372801900433 ) ) ;
#165665=CARTESIAN_POINT ( 'NONE',  ( 5.049401038298161559, -19.05341960407611168, 77.70724293864765286 ) ) ;
#165666=CARTESIAN_POINT ( 'NONE',  ( 12.06949235617757843, -12.14591786802309237, 68.12390960531436690 ) ) ;
#165667=CARTESIAN_POINT ( 'NONE',  ( -8.224510206698948167, 14.34966873604960824, 30.41557627198101699 ) ) ;
#165668=CARTESIAN_POINT ( 'NONE',  ( -16.55341960407617563, 4.379528057220093196, 113.5427570613523756 ) ) ;
#165669=CARTESIAN_POINT ( 'NONE',  ( 9.564922557961047289, -16.46253265017146816, 65.41775706135233293 ) ) ;
#165671=CARTESIAN_POINT ( 'NONE',  ( 19.05341960407611168, 5.049401038298154454, 113.9572429386477097 ) ) ;
#165672=CARTESIAN_POINT ( 'NONE',  ( 4.379528057220339221, -16.55341960407611168, 82.70724293864770971 ) ) ;
#165673=CARTESIAN_POINT ( 'NONE',  ( -17.97182807773875268, 5.499999999999872990, 58.53038844047289047 ) ) ;
#165674=CARTESIAN_POINT ( 'NONE',  ( -5.049401038298153566, 19.05341960407611168, 40.20724293864768839 ) ) ;
#165675=CARTESIAN_POINT ( 'NONE',  ( 15.80617190586746368, 15.72974639402197994, 44.37390960531435979 ) ) ;
#165676=CARTESIAN_POINT ( 'NONE',  ( 10.81492255796078972, 18.62759615963270932, 64.58224293864769550 ) ) ;
#165677=CARTESIAN_POINT ( 'NONE',  ( -12.06949235617756955, 12.14591786802309770, 105.6239096053143669 ) ) ;
#165678=CARTESIAN_POINT ( 'NONE',  ( 12.14591786802327356, -12.06949235617739191, 65.62609039468568994 ) ) ;
#165679=CARTESIAN_POINT ( 'NONE',  ( 9.474510206698971260, -16.51473224551069308, 42.91557627198103120 ) ) ;
#165680=CARTESIAN_POINT ( 'NONE',  ( -15.72974639402176322, -15.80617190586768395, 59.37609039468568284 ) ) ;
#165682=CARTESIAN_POINT ( 'NONE',  ( 0.05219959533910956823, 16.53943276465976808, 104.9989096053143669 ) ) ;
#165683=CARTESIAN_POINT ( 'NONE',  ( -13.89961937509957401, -13.97604488694547875, 94.37609039468566152 ) ) ;
#165685=CARTESIAN_POINT ( 'NONE',  ( -17.60769864724391454, 5.499999999999988454, 38.65024842019165874 ) ) ;
#165686=CARTESIAN_POINT ( 'NONE',  ( 21.52544592524344225, -5.823673210054117533, 38.54057627198103120 ) ) ;
#165687=CARTESIAN_POINT ( 'NONE',  ( -13.97604488694527625, -13.89961937509977652, 26.87390960531434558 ) ) ;
#165688=CARTESIAN_POINT ( 'NONE',  ( -18.62759615963255300, -10.81492255796106328, 74.16775706135231871 ) ) ;
#165689=CARTESIAN_POINT ( 'NONE',  ( 14.34966873604972726, -8.224510206698740333, 60.83442372801901854 ) ) ;
#165690=CARTESIAN_POINT ( 'NONE',  ( 14.29746914071049879, -8.314922557960816363, 48.33224293864770260 ) ) ;
#165691=CARTESIAN_POINT ( 'NONE',  ( -21.55341960407610458, -5.719274019375992779, 71.45724293864769550 ) ) ;
#165692=CARTESIAN_POINT ( 'NONE',  ( -5.823673210054116645, -21.52544592524344225, 67.29057627198103830 ) ) ;
#165693=DIRECTION ( 'NONE',  ( -1.000000000000000000, 0.000000000000000000, -0.000000000000000000 ) ) ;
#165694=CARTESIAN_POINT ( 'NONE',  ( 16.51473224551083163, -9.474510206698727899, 85.83442372801900433 ) ) ;
#165695=CARTESIAN_POINT ( 'NONE',  ( 9.564922557960805705, 16.46253265017160317, 109.5822429386476955 ) ) ;
#165697=CARTESIAN_POINT ( 'NONE',  ( 9.564922557960805705, 16.46253265017160317, 44.58224293864769550 ) ) ;
#165698=CARTESIAN_POINT ( 'NONE',  ( -8.224510206698948167, 14.34966873604960824, 110.4155762719810383 ) ) ;
#165700=FACE_BOUND ( 'NONE', #85286, .T. ) ;
#165701=ORIENTED_EDGE ( 'NONE', *, *, #82301, .T. ) ;
#165702=CARTESIAN_POINT ( 'NONE',  ( 16.53943276465976808, 0.05219959533934440121, 71.25109039468568994 ) ) ;
#165703=CARTESIAN_POINT ( 'NONE',  ( 21.55341960407610458, 5.719274019375980345, 98.95724293864770971 ) ) ;
#165704=CARTESIAN_POINT ( 'NONE',  ( 19.05341960407611168, 5.049401038298154454, 63.95724293864769550 ) ) ;
#165705=CARTESIAN_POINT ( 'NONE',  ( -5.719274019375665041, -21.55341960407619695, 44.79275706135234714 ) ) ;
#165706=CARTESIAN_POINT ( 'NONE',  ( -13.89961937509977652, 13.97604488694528158, 100.6239096053143669 ) ) ;
#165709=CARTESIAN_POINT ( 'NONE',  ( -21.53943276465977519, -0.05219959533937600094, 33.75109039468568284 ) ) ;
#165710=CARTESIAN_POINT ( 'NONE',  ( -19.02544592524342804, 5.153800228976336051, 31.04057627198102409 ) ) ;
#165711=CARTESIAN_POINT ( 'NONE',  ( -19.05341960407617563, 5.049401038297882671, 83.54275706135233293 ) ) ;
#165712=CARTESIAN_POINT ( 'NONE',  ( -9.474510206698720793, -16.51473224551083518, 34.58442372801899722 ) ) ;
#165713=CARTESIAN_POINT ( 'NONE',  ( 21.53943276465977519, -0.05219959533907433946, 113.7489096053143527 ) ) ;
#165714=CARTESIAN_POINT ( 'NONE',  ( -19.02544592524334988, -5.153800228976617603, 33.95942372801897591 ) ) ;
#165715=CARTESIAN_POINT ( 'NONE',  ( -16.46253265017146816, -9.564922557961047289, 54.16775706135234003 ) ) ;
#165716=CARTESIAN_POINT ( 'NONE',  ( 8.224510206698742110, 14.34966873604972548, 87.08442372801901854 ) ) ;
#165717=PLANE ( 'NONE',  #8709 ) ;
#165718=ORIENTED_EDGE ( 'NONE', *, *, #131252, .F. ) ;
#165719=CARTESIAN_POINT ( 'NONE',  ( 5.049401038298161559, -19.05341960407611168, 72.70724293864768129 ) ) ;
#165720=CARTESIAN_POINT ( 'NONE',  ( 0.05219959533937995610, -21.53943276465977519, 80.00109039468568994 ) ) ;
#165721=CARTESIAN_POINT ( 'NONE',  ( 21.53943276465977519, 0.05219959533937863772, 96.25109039468568994 ) ) ;
#165722=CARTESIAN_POINT ( 'NONE',  ( 18.22780087662121673, 5.500000000000056843, 38.98459894673893444 ) ) ;
#165723=CARTESIAN_POINT ( 'NONE',  ( -0.05219959533909027116, -19.03943276465977164, 82.49890960531436690 ) ) ;
#165724=CARTESIAN_POINT ( 'NONE',  ( 5.719274019375673035, 21.55341960407619339, 57.29275706135234714 ) ) ;
#165725=CARTESIAN_POINT ( 'NONE',  ( 16.51473224551083163, -9.474510206698727899, 105.8344237280190043 ) ) ;
#165726=CARTESIAN_POINT ( 'NONE',  ( -13.89961937509977652, 13.97604488694528158, 70.62390960531432427 ) ) ;
#165727=CARTESIAN_POINT ( 'NONE',  ( 5.719274019375991003, -21.55341960407610458, 22.70724293864769194 ) ) ;
#165728=CARTESIAN_POINT ( 'NONE',  ( 9.474510206698971260, -16.51473224551069308, 72.91557627198102409 ) ) ;
#165729=CARTESIAN_POINT ( 'NONE',  ( 17.49999999999997513, -3.905042442100252309, 22.90465208775962935 ) ) ;
#165730=CARTESIAN_POINT ( 'NONE',  ( 9.474510206698971260, -16.51473224551069308, 67.91557627198102409 ) ) ;
#165731=CARTESIAN_POINT ( 'NONE',  ( 9.474510206698971260, -16.51473224551069308, 52.91557627198102409 ) ) ;
#165732=CARTESIAN_POINT ( 'NONE',  ( 10.81492255796106328, -18.62759615963255655, 20.41775706135234714 ) ) ;
#165733=CARTESIAN_POINT ( 'NONE',  ( 14.29746914071037800, 8.314922557961029526, 86.66775706135234714 ) ) ;
#165736=CARTESIAN_POINT ( 'NONE',  ( -5.049401038297874678, -19.05341960407617918, 54.79275706135234003 ) ) ;
#165737=CARTESIAN_POINT ( 'NONE',  ( 19.02544592524343514, -5.153800228976328945, 73.54057627198103830 ) ) ;
#165738=CARTESIAN_POINT ( 'NONE',  ( 16.55341960407611168, 4.379528057220329451, 73.95724293864769550 ) ) ;
#165739=CARTESIAN_POINT ( 'NONE',  ( -12.14591786802309592, -12.06949235617757132, 101.8739096053143811 ) ) ;
#165740=CARTESIAN_POINT ( 'NONE',  ( -21.52544592524343514, 5.823673210054127303, 26.04057627198103475 ) ) ;
#165741=CARTESIAN_POINT ( 'NONE',  ( 19.05341960407611168, 5.049401038298154454, 98.95724293864766707 ) ) ;
#165743=CARTESIAN_POINT ( 'NONE',  ( 4.379528057220339221, -16.55341960407611168, 92.70724293864770971 ) ) ;
#165744=CARTESIAN_POINT ( 'NONE',  ( -16.46253265017160317, 9.564922557960807481, 115.8322429386477097 ) ) ;
#165745=CARTESIAN_POINT ( 'NONE',  ( -16.46253265017146816, -9.564922557961047289, 34.16775706135233293 ) ) ;
#165746=CARTESIAN_POINT ( 'NONE',  ( 16.53943276465976808, 0.05219959533934440121, 111.2510903946856899 ) ) ;
#165747=CARTESIAN_POINT ( 'NONE',  ( 13.97604488694527802, 13.89961937509977652, 89.37390960531436690 ) ) ;
#165748=EDGE_CURVE ( 'NONE', #24895, #109664, #159196, .T. ) ;
#165749=CARTESIAN_POINT ( 'NONE',  ( -15.72974639402176322, -15.80617190586768395, 54.37609039468568994 ) ) ;
#165750=CARTESIAN_POINT ( 'NONE',  ( 21.55341960407610458, 5.719274019375980345, 48.95724293864770971 ) ) ;
#165751=CARTESIAN_POINT ( 'NONE',  ( 21.53943276465977519, -0.05219959533907433946, 113.7489096053143527 ) ) ;
#165752=CARTESIAN_POINT ( 'NONE',  ( 21.52544592524344225, -5.823673210054117533, 73.54057627198102409 ) ) ;
#165753=CARTESIAN_POINT ( 'NONE',  ( 16.53943276465976808, -0.05219959533910856209, 98.74890960531438111 ) ) ;
#165754=CARTESIAN_POINT ( 'NONE',  ( 19.02544592524334988, 5.153800228976608722, 56.45942372801898301 ) ) ;
#165755=CARTESIAN_POINT ( 'NONE',  ( -16.51473224551069308, -9.474510206698971260, 26.66557627198103120 ) ) ;
#165756=CARTESIAN_POINT ( 'NONE',  ( 16.46253265017160672, -9.564922557960803928, 83.33224293864768129 ) ) ;
#165757=CARTESIAN_POINT ( 'NONE',  ( -5.049401038298153566, 19.05341960407611168, 80.20724293864769550 ) ) ;
#165758=CARTESIAN_POINT ( 'NONE',  ( 8.224510206698953496, -14.34966873604960469, 102.9155762719810383 ) ) ;
#165760=CARTESIAN_POINT ( 'NONE',  ( 8.314922557960818139, 14.29746914071049879, 29.58224293864769905 ) ) ;
#165761=CARTESIAN_POINT ( 'NONE',  ( -14.29746914071037622, -8.314922557961029526, 34.16775706135234714 ) ) ;
#165762=CARTESIAN_POINT ( 'NONE',  ( -0.05219959533937732626, 21.53943276465977519, 102.5010903946856899 ) ) ;
#165763=CARTESIAN_POINT ( 'NONE',  ( 9.564922557960805705, 16.46253265017160317, 104.5822429386476955 ) ) ;
#165764=CARTESIAN_POINT ( 'NONE',  ( -5.823673210054431948, 21.52544592524334988, 37.70942372801900433 ) ) ;
#165765=CARTESIAN_POINT ( 'NONE',  ( 19.03943276465977164, -0.05219959533909143690, 43.74890960531435979 ) ) ;
#165766=CARTESIAN_POINT ( 'NONE',  ( -12.14591786802326823, 12.06949235617739902, 43.12609039468568284 ) ) ;
#165767=CARTESIAN_POINT ( 'NONE',  ( -12.14591786802326823, 12.06949235617739902, 98.12609039468570415 ) ) ;
#165768=CARTESIAN_POINT ( 'NONE',  ( -9.474510206698720793, -16.51473224551083518, 109.5844237280190043 ) ) ;
#165769=CARTESIAN_POINT ( 'NONE',  ( -19.02544592524342804, 5.153800228976336051, 41.04057627198103120 ) ) ;
#165771=CARTESIAN_POINT ( 'NONE',  ( 14.34966873604960469, 8.224510206698951720, 99.16557627198100988 ) ) ;
#165772=CARTESIAN_POINT ( 'NONE',  ( 15.80617190586746368, 15.72974639402197994, 99.37390960531436690 ) ) ;
#165773=CARTESIAN_POINT ( 'NONE',  ( 19.02544592524334988, 5.153800228976608722, 76.45942372801897591 ) ) ;
#165774=CARTESIAN_POINT ( 'NONE',  ( -19.02544592524342804, 5.153800228976336051, 26.04057627198103120 ) ) ;
#165775=CARTESIAN_POINT ( 'NONE',  ( 9.564922557960805705, 16.46253265017160317, 89.58224293864769550 ) ) ;
#165776=CARTESIAN_POINT ( 'NONE',  ( 10.72451020669871369, 18.67979575497193778, 37.08442372801901143 ) ) ;
#165778=CARTESIAN_POINT ( 'NONE',  ( -9.564922557960796823, -16.46253265017161027, 92.08224293864769550 ) ) ;
#165780=CARTESIAN_POINT ( 'NONE',  ( -5.049401038298153566, 19.05341960407611168, 90.20724293864766707 ) ) ;
#165781=CARTESIAN_POINT ( 'NONE',  ( 18.67979575497194134, -10.72451020669871369, 25.83442372801901499 ) ) ;
#165782=CARTESIAN_POINT ( 'NONE',  ( -12.06949235617756955, 12.14591786802309770, 90.62390960531436690 ) ) ;
#165783=CARTESIAN_POINT ( 'NONE',  ( -9.474510206698964154, 16.51473224551069663, 90.41557627198103830 ) ) ;
#165784=CARTESIAN_POINT ( 'NONE',  ( -9.564922557961040184, 16.46253265017147172, 27.91775706135232582 ) ) ;
#165785=CARTESIAN_POINT ( 'NONE',  ( 12.06949235617739724, 12.14591786802326823, 56.87609039468568994 ) ) ;
#165786=CARTESIAN_POINT ( 'NONE',  ( -10.81492255796105439, 18.62759615963255655, 77.91775706135231871 ) ) ;
#165787=CARTESIAN_POINT ( 'NONE',  ( 0.05219959533934541429, -16.53943276465976808, 40.00109039468567573 ) ) ;
#165788=CARTESIAN_POINT ( 'NONE',  ( -19.02544592524342804, 5.153800228976336051, 71.04057627198099567 ) ) ;
#165789=CARTESIAN_POINT ( 'NONE',  ( 0.05219959533936267826, -19.03943276465977164, 95.00109039468567573 ) ) ;
#165790=CARTESIAN_POINT ( 'NONE',  ( 8.314922557961029526, -14.29746914071037800, 75.41775706135233293 ) ) ;
#165791=CARTESIAN_POINT ( 'NONE',  ( 0.05219959533936267826, -19.03943276465977164, 20.00109039468567218 ) ) ;
#165792=CARTESIAN_POINT ( 'NONE',  ( -5.049401038297874678, -19.05341960407617918, 84.79275706135233293 ) ) ;
#165793=CARTESIAN_POINT ( 'NONE',  ( -0.05219959533909027116, -19.03943276465977164, 67.49890960531436690 ) ) ;
#165794=CARTESIAN_POINT ( 'NONE',  ( -5.823673210054116645, -21.52544592524344225, 87.29057627198103830 ) ) ;
#165795=CARTESIAN_POINT ( 'NONE',  ( 12.06949235617757843, -12.14591786802309237, 73.12390960531436690 ) ) ;
#165796=CARTESIAN_POINT ( 'NONE',  ( -9.474510206698720793, -16.51473224551083518, 94.58442372801900433 ) ) ;
#165798=CARTESIAN_POINT ( 'NONE',  ( 5.049401038297881783, 19.05341960407617563, 57.29275706135231871 ) ) ;
#165799=CARTESIAN_POINT ( 'NONE',  ( -14.34966873604972548, 8.224510206698743886, 113.3344237280190328 ) ) ;
#165800=CARTESIAN_POINT ( 'NONE',  ( -4.379528057220328563, 16.55341960407611168, 75.20724293864769550 ) ) ;
#165801=CARTESIAN_POINT ( 'NONE',  ( 5.049401038297881783, 19.05341960407617563, 27.29275706135232937 ) ) ;
#165802=CARTESIAN_POINT ( 'NONE',  ( -17.40805194821983903, 6.112264579160790134, 40.83371272510607497 ) ) ;
#165803=CARTESIAN_POINT ( 'NONE',  ( -0.05219959533907301413, -21.53943276465977519, 107.4989096053143669 ) ) ;
#165804=CARTESIAN_POINT ( 'NONE',  ( 5.049401038298161559, -19.05341960407611168, 97.70724293864766707 ) ) ;
#165805=CARTESIAN_POINT ( 'NONE',  ( 13.97604488694527802, 13.89961937509977652, 74.37390960531436690 ) ) ;
#165806=CARTESIAN_POINT ( 'NONE',  ( -18.67979575497193778, 10.72451020669871902, 83.33442372801903275 ) ) ;
#165807=CARTESIAN_POINT ( 'NONE',  ( 16.46253265017160672, -9.564922557960803928, 68.33224293864770971 ) ) ;
#165808=CARTESIAN_POINT ( 'NONE',  ( 19.02544592524343514, -5.153800228976328945, 43.54057627198103120 ) ) ;
#165809=CARTESIAN_POINT ( 'NONE',  ( -21.53943276465977519, 0.05219959533907696930, 26.24890960531435624 ) ) ;
#165810=CARTESIAN_POINT ( 'NONE',  ( 16.53943276465976808, -0.05219959533910856209, 78.74890960531436690 ) ) ;
#165811=CARTESIAN_POINT ( 'NONE',  ( 9.564922557960805705, 16.46253265017160317, 49.58224293864770260 ) ) ;
#165812=CARTESIAN_POINT ( 'NONE',  ( -14.34966873604960291, -8.224510206698953496, 101.6655762719810383 ) ) ;
#165813=CARTESIAN_POINT ( 'NONE',  ( 21.52544592524344225, -5.823673210054117533, 103.5405762719810383 ) ) ;
#165814=CARTESIAN_POINT ( 'NONE',  ( 5.719274019375673035, 21.55341960407619339, 47.29275706135234003 ) ) ;
#165815=CARTESIAN_POINT ( 'NONE',  ( -5.049401038298153566, 19.05341960407611168, 25.20724293864768484 ) ) ;
#165817=CARTESIAN_POINT ( 'NONE',  ( 0.05219959533934541429, -16.53943276465976808, 70.00109039468568994 ) ) ;
#165818=CARTESIAN_POINT ( 'NONE',  ( -10.81492255796078084, -18.62759615963271287, 97.08224293864770971 ) ) ;
#165819=CARTESIAN_POINT ( 'NONE',  ( -21.55341960407610458, -5.719274019375992779, 101.4572429386476955 ) ) ;
#165820=CARTESIAN_POINT ( 'NONE',  ( 16.51473224551083163, -9.474510206698727899, 35.83442372801899722 ) ) ;
#165821=CARTESIAN_POINT ( 'NONE',  ( 19.03943276465977164, -0.05219959533909143690, 48.74890960531435979 ) ) ;
#165823=CARTESIAN_POINT ( 'NONE',  ( 21.55341960407619695, -5.719274019375665929, 51.04275706135234714 ) ) ;
#165824=CARTESIAN_POINT ( 'NONE',  ( 10.72451020669898902, -18.67979575497178502, 52.91557627198103830 ) ) ;
#165825=CARTESIAN_POINT ( 'NONE',  ( -8.314922557960811034, -14.29746914071050412, 42.08224293864769550 ) ) ;
#165826=CARTESIAN_POINT ( 'NONE',  ( -15.72974639402176322, -15.80617190586768395, 79.37609039468567573 ) ) ;
#165827=CARTESIAN_POINT ( 'NONE',  ( 21.52544592524334988, 5.823673210054432836, 106.4594237280190328 ) ) ;
#165828=CARTESIAN_POINT ( 'NONE',  ( -16.53943276465976808, 0.05219959533911058130, 101.2489096053143669 ) ) ;
#165829=CARTESIAN_POINT ( 'NONE',  ( -19.02544592524334988, -5.153800228976617603, 38.95942372801900433 ) ) ;
#165830=CARTESIAN_POINT ( 'NONE',  ( 16.53943276465976808, 0.05219959533934440121, 106.2510903946856757 ) ) ;
#165831=CARTESIAN_POINT ( 'NONE',  ( -21.53943276465977519, -0.05219959533937600094, 68.75109039468568994 ) ) ;
#165832=CARTESIAN_POINT ( 'NONE',  ( 19.02544592524343514, -5.153800228976328945, 53.54057627198102409 ) ) ;
#165833=CARTESIAN_POINT ( 'NONE',  ( -19.05341960407617563, 5.049401038297882671, 28.54275706135232937 ) ) ;
#165834=CARTESIAN_POINT ( 'NONE',  ( 5.719274019375991003, -21.55341960407610458, 42.70724293864770260 ) ) ;
#165835=CARTESIAN_POINT ( 'NONE',  ( 21.52544592524334988, 5.823673210054432836, 31.45942372801901854 ) ) ;
#165836=CARTESIAN_POINT ( 'NONE',  ( 0.05219959533907565091, 21.53943276465977519, 94.99890960531436690 ) ) ;
#165837=CARTESIAN_POINT ( 'NONE',  ( -19.03943276465977164, -0.05219959533935918106, 83.75109039468567573 ) ) ;
#165838=CARTESIAN_POINT ( 'NONE',  ( 16.53943276465976808, 0.05219959533934440121, 56.25109039468568284 ) ) ;
#165840=CARTESIAN_POINT ( 'NONE',  ( -21.52544592524343514, 5.823673210054127303, 96.04057627198102409 ) ) ;
#165841=CARTESIAN_POINT ( 'NONE',  ( 16.52544592524335698, 4.483927247898782831, 81.45942372801900433 ) ) ;
#165842=CARTESIAN_POINT ( 'NONE',  ( -14.29746914071049879, 8.314922557960819915, 75.83224293864769550 ) ) ;
#165843=CARTESIAN_POINT ( 'NONE',  ( -17.49999999999998579, -5.499999999999973355, 101.2823096230356583 ) ) ;
#165844=CARTESIAN_POINT ( 'NONE',  ( -5.153800228976607833, 19.02544592524334988, 107.7094237280189759 ) ) ;
#165846=CARTESIAN_POINT ( 'NONE',  ( -18.67979575497178146, -10.72451020669898902, 31.66557627198102054 ) ) ;
#165848=CARTESIAN_POINT ( 'NONE',  ( 8.314922557961029526, -14.29746914071037800, 55.41775706135234714 ) ) ;
#165849=CARTESIAN_POINT ( 'NONE',  ( -0.05219959533937732626, 21.53943276465977519, 32.50109039468568284 ) ) ;
#165850=CARTESIAN_POINT ( 'NONE',  ( -18.62759615963270932, 10.81492255796079327, 40.83224293864769550 ) ) ;
#165851=CARTESIAN_POINT ( 'NONE',  ( 12.06949235617739724, 12.14591786802326823, 76.87609039468567573 ) ) ;
#165852=CARTESIAN_POINT ( 'NONE',  ( -19.03943276465977164, 0.05219959533909376836, 86.24890960531436690 ) ) ;
#165853=CARTESIAN_POINT ( 'NONE',  ( -18.67979575497193778, 10.72451020669871902, 53.33442372801901854 ) ) ;
#165854=CARTESIAN_POINT ( 'NONE',  ( -13.97604488694527625, -13.89961937509977652, 21.87390960531435979 ) ) ;
#165855=CARTESIAN_POINT ( 'NONE',  ( -21.53943276465977519, 0.05219959533907696930, 36.24890960531435979 ) ) ;
#165856=ORIENTED_EDGE ( 'NONE', *, *, #132474, .F. ) ;
#165857=CARTESIAN_POINT ( 'NONE',  ( 16.51473224551083163, -9.474510206698727899, 35.83442372801899722 ) ) ;
#165858=CARTESIAN_POINT ( 'NONE',  ( 14.34966873604972726, -8.224510206698740333, 55.83442372801901854 ) ) ;
#165859=CARTESIAN_POINT ( 'NONE',  ( 10.72451020669898902, -18.67979575497178502, 22.91557627198102765 ) ) ;
#165861=CARTESIAN_POINT ( 'NONE',  ( -19.03943276465977164, 0.05219959533909376836, 91.24890960531436690 ) ) ;
#165862=CARTESIAN_POINT ( 'NONE',  ( -0.05219959533934338120, 16.53943276465976808, 97.50109039468567573 ) ) ;
#165863=CARTESIAN_POINT ( 'NONE',  ( -16.46253265017160317, 9.564922557960807481, 115.8322429386477097 ) ) ;
#165864=CARTESIAN_POINT ( 'NONE',  ( 8.314922557960818139, 14.29746914071049879, 99.58224293864770971 ) ) ;
#165865=CARTESIAN_POINT ( 'NONE',  ( 10.81492255796078972, 18.62759615963270932, 39.58224293864769550 ) ) ;
#165866=CARTESIAN_POINT ( 'NONE',  ( 9.564922557960805705, 16.46253265017160317, 29.58224293864769550 ) ) ;
#165867=CARTESIAN_POINT ( 'NONE',  ( 12.14591786802327356, -12.06949235617739191, 75.62609039468567573 ) ) ;
#165868=CARTESIAN_POINT ( 'NONE',  ( -21.55341960407610458, -5.719274019375992779, 111.4572429386476813 ) ) ;
#165869=CARTESIAN_POINT ( 'NONE',  ( 16.51473224551083163, -9.474510206698727899, 70.83442372801900433 ) ) ;
#165870=CARTESIAN_POINT ( 'NONE',  ( -19.02544592524342804, 5.153800228976336051, 41.04057627198103120 ) ) ;
#165871=CARTESIAN_POINT ( 'NONE',  ( -5.049401038298153566, 19.05341960407611168, 115.2072429386477097 ) ) ;
#165872=CARTESIAN_POINT ( 'NONE',  ( -5.719274019375665041, -21.55341960407619695, 99.79275706135234714 ) ) ;
#165873=CARTESIAN_POINT ( 'NONE',  ( 5.153800228976335163, 19.02544592524342804, 59.79057627198100988 ) ) ;
#165874=CARTESIAN_POINT ( 'NONE',  ( -16.53943276465976808, -0.05219959533934237506, 48.75109039468568284 ) ) ;
#165875=CARTESIAN_POINT ( 'NONE',  ( 15.72974639402176855, 15.80617190586768217, 91.87609039468568994 ) ) ;
#165876=CARTESIAN_POINT ( 'NONE',  ( 5.049401038297881783, 19.05341960407617563, 37.29275706135232582 ) ) ;
#165877=CARTESIAN_POINT ( 'NONE',  ( 5.049401038297881783, 19.05341960407617563, 57.29275706135231871 ) ) ;
#165879=CARTESIAN_POINT ( 'NONE',  ( 0.05219959533937995610, -21.53943276465977519, 45.00109039468568284 ) ) ;
#165880=CARTESIAN_POINT ( 'NONE',  ( -13.97604488694527625, -13.89961937509977830, 56.87390960531435269 ) ) ;
#165881=CARTESIAN_POINT ( 'NONE',  ( -0.05219959533936034679, 19.03943276465977164, 47.50109039468566863 ) ) ;
#165882=CARTESIAN_POINT ( 'NONE',  ( -16.51473224551069308, -9.474510206698971260, 106.6655762719810383 ) ) ;
#165883=CARTESIAN_POINT ( 'NONE',  ( -19.02544592524342804, 5.153800228976336051, 81.04057627198103830 ) ) ;
#165884=CARTESIAN_POINT ( 'NONE',  ( -16.53943276465976808, 0.05219959533911058130, 41.24890960531435269 ) ) ;
#165885=CARTESIAN_POINT ( 'NONE',  ( 15.80617190586746368, 15.72974639402197994, 39.37390960531436690 ) ) ;
#165888=CARTESIAN_POINT ( 'NONE',  ( -21.53943276465977519, -0.05219959533937600094, 98.75109039468568994 ) ) ;
#165890=CARTESIAN_POINT ( 'NONE',  ( -5.153800228976328057, -19.02544592524343514, 37.29057627198102409 ) ) ;
#165891=CARTESIAN_POINT ( 'NONE',  ( -13.89961937509977652, 13.97604488694528158, 110.6239096053143243 ) ) ;
#165894=CARTESIAN_POINT ( 'NONE',  ( -8.224510206698735004, -14.34966873604973081, 64.58442372801900433 ) ) ;
#165895=CARTESIAN_POINT ( 'NONE',  ( -0.05219959533907301413, -21.53943276465977519, 87.49890960531436690 ) ) ;
#165896=CARTESIAN_POINT ( 'NONE',  ( 4.379528057220339221, -16.55341960407611168, 42.70724293864770260 ) ) ;
#165897=CARTESIAN_POINT ( 'NONE',  ( 13.89961937509977652, -13.97604488694527269, 28.12390960531435624 ) ) ;
#165898=CARTESIAN_POINT ( 'NONE',  ( -19.05341960407611168, -5.049401038298163336, 111.4572429386476671 ) ) ;
#165899=CARTESIAN_POINT ( 'NONE',  ( -10.72451020669870658, -18.67979575497194134, 24.58442372801901499 ) ) ;
#165900=CARTESIAN_POINT ( 'NONE',  ( -5.049401038297874678, -19.05341960407617918, 29.79275706135232227 ) ) ;
#165901=CARTESIAN_POINT ( 'NONE',  ( 9.564922557960805705, 16.46253265017160317, 29.58224293864769550 ) ) ;
#165902=CARTESIAN_POINT ( 'NONE',  ( 10.72451020669871369, 18.67979575497193778, 77.08442372801901854 ) ) ;
#165904=CARTESIAN_POINT ( 'NONE',  ( -12.14591786802309592, -12.06949235617757132, 21.87390960531436690 ) ) ;
#165906=CARTESIAN_POINT ( 'NONE',  ( 10.81492255796078972, 18.62759615963270932, 29.58224293864769905 ) ) ;
#165907=CARTESIAN_POINT ( 'NONE',  ( 14.34966873604960469, 8.224510206698951720, 104.1655762719810241 ) ) ;
#165908=CARTESIAN_POINT ( 'NONE',  ( -17.97058386085787163, -5.500000000000058620, 39.00390968646216550 ) ) ;
#165909=CARTESIAN_POINT ( 'NONE',  ( 9.564922557960805705, 16.46253265017160317, 94.58224293864769550 ) ) ;
#165910=CARTESIAN_POINT ( 'NONE',  ( 4.379528057220339221, -16.55341960407611168, 77.70724293864770971 ) ) ;
#165911=CARTESIAN_POINT ( 'NONE',  ( -5.049401038297874678, -19.05341960407617918, 99.79275706135234714 ) ) ;
#165912=CARTESIAN_POINT ( 'NONE',  ( 21.53943276465977519, -0.05219959533907433946, 68.74890960531435269 ) ) ;
#165914=CARTESIAN_POINT ( 'NONE',  ( 0.05219959533909260263, 19.03943276465977164, 34.99890960531435979 ) ) ;
#165916=CARTESIAN_POINT ( 'NONE',  ( 19.05341960407611168, 5.049401038298154454, 88.95724293864769550 ) ) ;
#165917=CARTESIAN_POINT ( 'NONE',  ( 10.81492255796078972, 18.62759615963270932, 89.58224293864768129 ) ) ;
#165919=CARTESIAN_POINT ( 'NONE',  ( -4.379528057220086978, -16.55341960407618274, 99.79275706135234714 ) ) ;
#165920=CARTESIAN_POINT ( 'NONE',  ( -9.564922557960796823, -16.46253265017161027, 82.08224293864768129 ) ) ;
#165921=CARTESIAN_POINT ( 'NONE',  ( 0.05219959533936267826, -19.03943276465977164, 85.00109039468567573 ) ) ;
#165922=CARTESIAN_POINT ( 'NONE',  ( -21.52544592524334988, -5.823673210054445271, 88.95942372801901854 ) ) ;
#165923=CARTESIAN_POINT ( 'NONE',  ( -21.53943276465977519, 0.05219959533907696930, 76.24890960531435269 ) ) ;
#165924=CARTESIAN_POINT ( 'NONE',  ( 5.719274019375991003, -21.55341960407610458, 32.70724293864770260 ) ) ;
#165925=CARTESIAN_POINT ( 'NONE',  ( 16.51473224551069308, 9.474510206698969483, 49.16557627198102409 ) ) ;
#165926=CARTESIAN_POINT ( 'NONE',  ( -16.55341960407611168, -4.379528057220339221, 26.45724293864768839 ) ) ;
#165927=CARTESIAN_POINT ( 'NONE',  ( -9.474510206698964154, 16.51473224551069663, 70.41557627198102409 ) ) ;
#165928=DIRECTION ( 'NONE',  ( 0.000000000000000000, 0.000000000000000000, 1.000000000000000000 ) ) ;
#165929=CARTESIAN_POINT ( 'NONE',  ( -16.46253265017146816, -9.564922557961047289, 19.16775706135233293 ) ) ;
#165930=CARTESIAN_POINT ( 'NONE',  ( 0.05219959533910956823, 16.53943276465976808, 69.99890960531435269 ) ) ;
#165931=CARTESIAN_POINT ( 'NONE',  ( -5.823673210054116645, -21.52544592524344225, 107.2905762719810525 ) ) ;
#165932=CARTESIAN_POINT ( 'NONE',  ( -21.55341960407610458, -5.719274019375992779, 111.4572429386476813 ) ) ;
#165934=CARTESIAN_POINT ( 'NONE',  ( -18.67979575497178146, -10.72451020669898902, 61.66557627198103120 ) ) ;
#165935=CARTESIAN_POINT ( 'NONE',  ( 8.314922557961029526, -14.29746914071037800, 90.41775706135236135 ) ) ;
#165936=CARTESIAN_POINT ( 'NONE',  ( 16.53943276465976808, -0.05219959533910856209, 98.74890960531438111 ) ) ;
#165937=CARTESIAN_POINT ( 'NONE',  ( -16.46253265017160317, 9.564922557960807481, 55.83224293864769550 ) ) ;
#165938=CARTESIAN_POINT ( 'NONE',  ( -16.53943276465976808, 0.05219959533911058130, 36.24890960531435979 ) ) ;
#165939=ORIENTED_EDGE ( 'NONE', *, *, #115128, .T. ) ;
#165940=CARTESIAN_POINT ( 'NONE',  ( -5.823673210054431948, 21.52544592524334988, 42.70942372801901854 ) ) ;
#165941=CARTESIAN_POINT ( 'NONE',  ( -19.05341960407611168, -5.049401038298163336, 111.4572429386476671 ) ) ;
#165942=CARTESIAN_POINT ( 'NONE',  ( 15.80617190586769283, -15.72974639402175789, 75.62609039468567573 ) ) ;
#165943=CARTESIAN_POINT ( 'NONE',  ( -16.51473224551069308, -9.474510206698971260, 26.66557627198103120 ) ) ;
#165944=CARTESIAN_POINT ( 'NONE',  ( -19.05341960407611168, -5.049401038298163336, 41.45724293864769550 ) ) ;
#165946=CARTESIAN_POINT ( 'NONE',  ( -5.823673210054431948, 21.52544592524334988, 82.70942372801900433 ) ) ;
#165947=CARTESIAN_POINT ( 'NONE',  ( 16.53943276465976808, 0.05219959533934440121, 51.25109039468568994 ) ) ;
#165948=CARTESIAN_POINT ( 'NONE',  ( -18.67979575497193778, 10.72451020669871902, 68.33442372801900433 ) ) ;
#165949=CARTESIAN_POINT ( 'NONE',  ( 5.153800228976335163, 19.02544592524342804, 99.79057627198102409 ) ) ;
#165950=CARTESIAN_POINT ( 'NONE',  ( 19.03943276465977164, 0.05219959533936151252, 81.25109039468567573 ) ) ;
#165951=CARTESIAN_POINT ( 'NONE',  ( 5.823673210054444382, -21.52544592524334988, 55.20942372801902565 ) ) ;
#165952=CARTESIAN_POINT ( 'NONE',  ( -0.05219959533934338120, 16.53943276465976808, 22.50109039468567573 ) ) ;
#165953=CARTESIAN_POINT ( 'NONE',  ( 19.05341960407617918, -5.049401038297876454, 76.04275706135230450 ) ) ;
#165954=CARTESIAN_POINT ( 'NONE',  ( -0.05219959533909027116, -19.03943276465977164, 57.49890960531435979 ) ) ;
#165955=CARTESIAN_POINT ( 'NONE',  ( -5.049401038297874678, -19.05341960407617918, 89.79275706135230450 ) ) ;
#165956=CARTESIAN_POINT ( 'NONE',  ( -4.483927247898539470, -16.52544592524342804, 27.29057627198103120 ) ) ;
#165957=CARTESIAN_POINT ( 'NONE',  ( -13.89961937509957401, -13.97604488694547875, 89.37609039468563310 ) ) ;
#165958=CARTESIAN_POINT ( 'NONE',  ( 16.52544592524342804, -4.483927247898539470, 33.54057627198102409 ) ) ;
#165959=CARTESIAN_POINT ( 'NONE',  ( 19.05341960407617918, -5.049401038297876454, 61.04275706135232582 ) ) ;
#165960=CARTESIAN_POINT ( 'NONE',  ( -16.55341960407617563, 4.379528057220093196, 48.54275706135234714 ) ) ;
#165961=CARTESIAN_POINT ( 'NONE',  ( -9.474510206698720793, -16.51473224551083518, 29.58442372801900433 ) ) ;
#165962=CARTESIAN_POINT ( 'NONE',  ( 19.05341960407611168, 5.049401038298154454, 48.95724293864768129 ) ) ;
#165963=CARTESIAN_POINT ( 'NONE',  ( 4.483927247898790824, -16.52544592524335698, 40.20942372801901854 ) ) ;
#165966=CARTESIAN_POINT ( 'NONE',  ( 16.46253265017160672, -9.564922557960803928, 98.33224293864769550 ) ) ;
#165967=CARTESIAN_POINT ( 'NONE',  ( 5.153800228976617603, -19.02544592524335343, 85.20942372801900433 ) ) ;
#165969=CARTESIAN_POINT ( 'NONE',  ( -13.89961937509957401, -13.97604488694547875, 94.37609039468566152 ) ) ;
#165970=CARTESIAN_POINT ( 'NONE',  ( 21.55341960407610458, 5.719274019375980345, 28.95724293864769905 ) ) ;
#165971=CARTESIAN_POINT ( 'NONE',  ( -15.80617190586768217, 15.72974639402176855, 108.1260903946856757 ) ) ;
#165972=CARTESIAN_POINT ( 'NONE',  ( -16.53943276465976808, -0.05219959533934237506, 18.75109039468568639 ) ) ;
#165973=CARTESIAN_POINT ( 'NONE',  ( -14.34966873604960291, -8.224510206698953496, 111.6655762719810525 ) ) ;
#165974=CARTESIAN_POINT ( 'NONE',  ( -16.51473224551069308, -9.474510206698971260, 36.66557627198102409 ) ) ;
#165975=CARTESIAN_POINT ( 'NONE',  ( 0.05219959533907565091, 21.53943276465977519, 74.99890960531435269 ) ) ;
#165977=CARTESIAN_POINT ( 'NONE',  ( 0.05219959533909260263, 19.03943276465977164, 39.99890960531436690 ) ) ;
#165979=CARTESIAN_POINT ( 'NONE',  ( 19.05341960407617918, -5.049401038297876454, 66.04275706135233293 ) ) ;
#165980=CARTESIAN_POINT ( 'NONE',  ( -12.14591786802309592, -12.06949235617757132, 56.87390960531436690 ) ) ;
#165981=CARTESIAN_POINT ( 'NONE',  ( -5.719274019375978568, 21.55341960407610458, 30.20724293864769550 ) ) ;
#165982=EDGE_CURVE ( 'NONE', #2008, #86900, #197917, .T. ) ;
#165983=CARTESIAN_POINT ( 'NONE',  ( 15.72974639402176855, 15.80617190586768217, 86.87609039468568994 ) ) ;
#165984=CARTESIAN_POINT ( 'NONE',  ( 21.55341960407610458, 5.719274019375980345, 88.95724293864769550 ) ) ;
#165985=CARTESIAN_POINT ( 'NONE',  ( 5.719274019375673035, 21.55341960407619339, 57.29275706135234714 ) ) ;
#165986=CARTESIAN_POINT ( 'NONE',  ( -15.80617190586768217, 15.72974639402176855, 58.12609039468568994 ) ) ;
#165987=CARTESIAN_POINT ( 'NONE',  ( 9.474510206698971260, -16.51473224551069308, 102.9155762719810241 ) ) ;
#165988=CARTESIAN_POINT ( 'NONE',  ( -0.05219959533934338120, 16.53943276465976808, 87.50109039468568994 ) ) ;
#165989=CARTESIAN_POINT ( 'NONE',  ( -5.719274019375665041, -21.55341960407619695, 69.79275706135234714 ) ) ;
#165990=CARTESIAN_POINT ( 'NONE',  ( 19.05341960407611168, 5.049401038298154454, 58.95724293864768129 ) ) ;
#165991=CARTESIAN_POINT ( 'NONE',  ( -16.51473224551069308, -9.474510206698971260, 21.66557627198102765 ) ) ;
#165992=CARTESIAN_POINT ( 'NONE',  ( 16.46253265017160672, -9.564922557960803928, 53.33224293864768839 ) ) ;
#165993=CARTESIAN_POINT ( 'NONE',  ( 16.53943276465976808, -0.05219959533910856209, 63.74890960531435979 ) ) ;
#165994=CARTESIAN_POINT ( 'NONE',  ( 14.29746914071049879, -8.314922557960816363, 38.33224293864768839 ) ) ;
#165995=CARTESIAN_POINT ( 'NONE',  ( 15.80617190586746368, 15.72974639402197994, 44.37390960531435979 ) ) ;
#165996=CARTESIAN_POINT ( 'NONE',  ( -13.89961937509977652, 13.97604488694528158, 50.62390960531435979 ) ) ;
#165997=CARTESIAN_POINT ( 'NONE',  ( -15.72974639402197994, 15.80617190586746368, 55.62390960531436690 ) ) ;
#165998=CARTESIAN_POINT ( 'NONE',  ( 9.564922557961047289, -16.46253265017146816, 55.41775706135234003 ) ) ;
#166001=CARTESIAN_POINT ( 'NONE',  ( 4.483927247898545687, 16.52544592524342804, 49.79057627198102409 ) ) ;
#166002=CARTESIAN_POINT ( 'NONE',  ( -18.62759615963270932, 10.81492255796079327, 35.83224293864768839 ) ) ;
#166004=ORIENTED_EDGE ( 'NONE', *, *, #63061, .T. ) ;
#166006=CARTESIAN_POINT ( 'NONE',  ( -8.224510206698735004, -14.34966873604973081, 79.58442372801903275 ) ) ;
#166007=CARTESIAN_POINT ( 'NONE',  ( -13.89961937509957401, -13.97604488694547875, 74.37609039468566152 ) ) ;
#166008=EDGE_CURVE ( 'NONE', #196699, #104654, #130628, .T. ) ;
#166009=CARTESIAN_POINT ( 'NONE',  ( 14.34966873604960469, 8.224510206698951720, 49.16557627198102409 ) ) ;
#166010=CARTESIAN_POINT ( 'NONE',  ( 17.48847506799972251, -5.747544572773699123, 53.32697437843280852 ) ) ;
#166011=CARTESIAN_POINT ( 'NONE',  ( -8.314922557960811034, -14.29746914071050412, 37.08224293864768129 ) ) ;
#166012=CARTESIAN_POINT ( 'NONE',  ( 13.97604488694527802, 13.89961937509977652, 54.37390960531435979 ) ) ;
#166013=CARTESIAN_POINT ( 'NONE',  ( -9.474510206698964154, 16.51473224551069663, 75.41557627198103830 ) ) ;
#166014=CARTESIAN_POINT ( 'NONE',  ( 13.89961937509977652, -13.97604488694527269, 38.12390960531436690 ) ) ;
#166015=CARTESIAN_POINT ( 'NONE',  ( 5.823673210054444382, -21.52544592524334988, 40.20942372801901854 ) ) ;
#166016=CARTESIAN_POINT ( 'NONE',  ( 5.049401038298161559, -19.05341960407611168, 72.70724293864768129 ) ) ;
#166017=CARTESIAN_POINT ( 'NONE',  ( -0.05219959533909027116, -19.03943276465977164, 22.49890960531436690 ) ) ;
#166018=CARTESIAN_POINT ( 'NONE',  ( 13.97604488694527802, 13.89961937509977652, 54.37390960531435979 ) ) ;
#166019=CARTESIAN_POINT ( 'NONE',  ( -21.53943276465977519, 0.05219959533907696930, 51.24890960531436690 ) ) ;
#166020=CARTESIAN_POINT ( 'NONE',  ( 16.51473224551069308, 9.474510206698969483, 39.16557627198103120 ) ) ;
#166021=CARTESIAN_POINT ( 'NONE',  ( 5.719274019375991003, -21.55341960407610458, 37.70724293864769550 ) ) ;
#166022=CARTESIAN_POINT ( 'NONE',  ( -16.52544592524335698, -4.483927247898792601, 108.9594237280190185 ) ) ;
#166023=CARTESIAN_POINT ( 'NONE',  ( -21.53943276465977519, -0.05219959533937600094, 113.7510903946856757 ) ) ;
#166024=CARTESIAN_POINT ( 'NONE',  ( 12.06949235617739724, 12.14591786802326823, 51.87609039468568284 ) ) ;
#166025=CARTESIAN_POINT ( 'NONE',  ( 0.05219959533934541429, -16.53943276465976808, 80.00109039468568994 ) ) ;
#166027=CARTESIAN_POINT ( 'NONE',  ( -16.55341960407617563, 4.379528057220093196, 63.54275706135234003 ) ) ;
#166028=CARTESIAN_POINT ( 'NONE',  ( 16.53943276465976808, 0.05219959533934440121, 36.25109039468567573 ) ) ;
#166029=CARTESIAN_POINT ( 'NONE',  ( -13.97604488694527625, -13.89961937509977652, 101.8739096053143811 ) ) ;
#166030=CARTESIAN_POINT ( 'NONE',  ( 8.224510206698742110, 14.34966873604972548, 27.08442372801901854 ) ) ;
#166031=CARTESIAN_POINT ( 'NONE',  ( 5.153800228976335163, 19.02544592524342804, 29.79057627198102409 ) ) ;
#166032=CARTESIAN_POINT ( 'NONE',  ( 10.72451020669871369, 18.67979575497193778, 22.08442372801901143 ) ) ;
#166033=CARTESIAN_POINT ( 'NONE',  ( 8.224510206698742110, 14.34966873604972548, 37.08442372801901143 ) ) ;
#166034=CARTESIAN_POINT ( 'NONE',  ( -8.314922557961024197, 14.29746914071037800, 102.9177570613523756 ) ) ;
#166035=CARTESIAN_POINT ( 'NONE',  ( 17.50000000000000000, -5.500000000000000888, 120.0000000000000142 ) ) ;
#166036=CARTESIAN_POINT ( 'NONE',  ( -10.72451020669870658, -18.67979575497194134, 99.58442372801900433 ) ) ;
#166037=CARTESIAN_POINT ( 'NONE',  ( -19.05341960407617563, 5.049401038297882671, 98.54275706135233293 ) ) ;
#166038=CARTESIAN_POINT ( 'NONE',  ( -16.53943276465976808, 0.05219959533911058130, 56.24890960531436690 ) ) ;
#166039=CARTESIAN_POINT ( 'NONE',  ( -13.89961937509977652, 13.97604488694528158, 25.62390960531434558 ) ) ;
#166040=CARTESIAN_POINT ( 'NONE',  ( 9.564922557961047289, -16.46253265017146816, 65.41775706135233293 ) ) ;
#166042=CARTESIAN_POINT ( 'NONE',  ( -21.53943276465977519, -0.05219959533937600094, 58.75109039468568994 ) ) ;
#166043=CARTESIAN_POINT ( 'NONE',  ( 16.55341960407618274, -4.379528057220086978, 26.04275706135235779 ) ) ;
#166045=CARTESIAN_POINT ( 'NONE',  ( 15.72974639402199770, -15.80617190586745480, 23.12390960531436335 ) ) ;
#166046=CARTESIAN_POINT ( 'NONE',  ( 10.72451020669898902, -18.67979575497178502, 77.91557627198102409 ) ) ;
#166047=CARTESIAN_POINT ( 'NONE',  ( 19.05341960407617918, -5.049401038297876454, 106.0427570613523471 ) ) ;
#166048=CARTESIAN_POINT ( 'NONE',  ( 9.474510206698971260, -16.51473224551069308, 107.9155762719810383 ) ) ;
#166050=CARTESIAN_POINT ( 'NONE',  ( 14.34966873604960469, 8.224510206698951720, 114.1655762719810383 ) ) ;
#166051=CARTESIAN_POINT ( 'NONE',  ( -18.62759615963255300, -10.81492255796106328, 109.1677570613523613 ) ) ;
#166052=CARTESIAN_POINT ( 'NONE',  ( -9.564922557960796823, -16.46253265017161027, 47.08224293864769550 ) ) ;
#166053=CARTESIAN_POINT ( 'NONE',  ( 15.72974639402176855, 15.80617190586768217, 56.87609039468568994 ) ) ;
#166054=CARTESIAN_POINT ( 'NONE',  ( -18.67979575497193778, 10.72451020669871902, 83.33442372801903275 ) ) ;
#166055=CARTESIAN_POINT ( 'NONE',  ( -16.52544592524335698, -4.483927247898792601, 108.9594237280190185 ) ) ;
#166056=CARTESIAN_POINT ( 'NONE',  ( -0.05219959533909027116, -19.03943276465977164, 82.49890960531436690 ) ) ;
#166057=CARTESIAN_POINT ( 'NONE',  ( 21.55341960407619695, -5.719274019375665929, 41.04275706135236135 ) ) ;
#166058=CARTESIAN_POINT ( 'NONE',  ( -15.80617190586768217, 15.72974639402176855, 58.12609039468568994 ) ) ;
#166059=CARTESIAN_POINT ( 'NONE',  ( 16.51473224551083163, -9.474510206698727899, 75.83442372801900433 ) ) ;
#166060=CARTESIAN_POINT ( 'NONE',  ( 13.97604488694527802, 13.89961937509977652, 94.37390960531436690 ) ) ;
#166061=CARTESIAN_POINT ( 'NONE',  ( 8.224510206698953496, -14.34966873604960469, 97.91557627198103830 ) ) ;
#166062=CARTESIAN_POINT ( 'NONE',  ( -18.67979575497178146, -10.72451020669898902, 101.6655762719810383 ) ) ;
#166063=CARTESIAN_POINT ( 'NONE',  ( -4.483927247898539470, -16.52544592524342804, 77.29057627198102409 ) ) ;
#166064=CARTESIAN_POINT ( 'NONE',  ( 16.46253265017146816, 9.564922557961045513, 21.66775706135233648 ) ) ;
#166065=CARTESIAN_POINT ( 'NONE',  ( 16.53943276465976808, -0.05219959533910856209, 103.7489096053143669 ) ) ;
#166066=CARTESIAN_POINT ( 'NONE',  ( 5.153800228976335163, 19.02544592524342804, 49.79057627198100988 ) ) ;
#166067=CARTESIAN_POINT ( 'NONE',  ( -13.97604488694547697, 13.89961937509957934, 88.12609039468563310 ) ) ;
#166068=CARTESIAN_POINT ( 'NONE',  ( 4.483927247898545687, 16.52544592524342804, 54.79057627198104541 ) ) ;
#166069=CARTESIAN_POINT ( 'NONE',  ( 10.81492255796106328, -18.62759615963255655, 110.4177570613523756 ) ) ;
#166070=CARTESIAN_POINT ( 'NONE',  ( 16.46253265017160672, -9.564922557960803928, 103.3322429386476955 ) ) ;
#166071=CARTESIAN_POINT ( 'NONE',  ( -9.564922557961040184, 16.46253265017147172, 77.91775706135234714 ) ) ;
#166072=CARTESIAN_POINT ( 'NONE',  ( 5.719274019375991003, -21.55341960407610458, 82.70724293864770971 ) ) ;
#166073=CARTESIAN_POINT ( 'NONE',  ( 21.53943276465977519, 0.05219959533937863772, 36.25109039468567573 ) ) ;
#166074=CARTESIAN_POINT ( 'NONE',  ( -0.05219959533934338120, 16.53943276465976808, 27.50109039468567929 ) ) ;
#166075=CARTESIAN_POINT ( 'NONE',  ( 16.52544592524335698, 4.483927247898782831, 91.45942372801901854 ) ) ;
#166076=CARTESIAN_POINT ( 'NONE',  ( 17.26172910966779384, 6.454744622555874223, 61.69353091350775742 ) ) ;
#166077=CARTESIAN_POINT ( 'NONE',  ( 21.52544592524334988, 5.823673210054432836, 31.45942372801901854 ) ) ;
#166078=CARTESIAN_POINT ( 'NONE',  ( -16.53943276465976808, 0.05219959533911058130, 116.2489096053143669 ) ) ;
#166080=CARTESIAN_POINT ( 'NONE',  ( 4.379528057220092307, 16.55341960407617563, 67.29275706135234714 ) ) ;
#166081=CARTESIAN_POINT ( 'NONE',  ( 4.483927247898545687, 16.52544592524342804, 89.79057627198103830 ) ) ;
#166082=CARTESIAN_POINT ( 'NONE',  ( -15.72974639402197994, 15.80617190586746368, 80.62390960531438111 ) ) ;
#166083=CARTESIAN_POINT ( 'NONE',  ( 14.29746914071049879, -8.314922557960816363, 28.33224293864769550 ) ) ;
#166084=CARTESIAN_POINT ( 'NONE',  ( -16.53943276465976808, -0.05219959533934237506, 48.75109039468568284 ) ) ;
#166085=CARTESIAN_POINT ( 'NONE',  ( -16.46253265017160317, 9.564922557960807481, 45.83224293864769550 ) ) ;
#166086=CARTESIAN_POINT ( 'NONE',  ( -4.379528057220086978, -16.55341960407618274, 94.79275706135234714 ) ) ;
#166087=CARTESIAN_POINT ( 'NONE',  ( -9.564922557961040184, 16.46253265017147172, 87.91775706135233293 ) ) ;
#166088=CARTESIAN_POINT ( 'NONE',  ( -18.62759615963270932, 10.81492255796079327, 90.83224293864769550 ) ) ;
#166089=CARTESIAN_POINT ( 'NONE',  ( -12.06949235617739369, -12.14591786802326823, 104.3760903946856899 ) ) ;
#166091=CARTESIAN_POINT ( 'NONE',  ( 16.46253265017160672, -9.564922557960803928, 113.3322429386476955 ) ) ;
#166093=CARTESIAN_POINT ( 'NONE',  ( 21.53943276465977519, -0.05219959533907433946, 58.74890960531436690 ) ) ;
#166094=ORIENTED_EDGE ( 'NONE', *, *, #114637, .T. ) ;
#166095=CARTESIAN_POINT ( 'NONE',  ( 4.483927247898790824, -16.52544592524335698, 95.20942372801903275 ) ) ;
#166096=ORIENTED_EDGE ( 'NONE', *, *, #142697, .T. ) ;
#166097=CARTESIAN_POINT ( 'NONE',  ( -21.55341960407610458, -5.719274019375992779, 36.45724293864768839 ) ) ;
#166098=CARTESIAN_POINT ( 'NONE',  ( -18.22780087662122028, 5.500000000000031086, 73.51540105326107266 ) ) ;
#166099=CARTESIAN_POINT ( 'NONE',  ( -5.719274019375978568, 21.55341960407610458, 80.20724293864769550 ) ) ;
#166100=CARTESIAN_POINT ( 'NONE',  ( 4.379528057220339221, -16.55341960407611168, 22.70724293864769194 ) ) ;
#166101=CARTESIAN_POINT ( 'NONE',  ( -4.483927247898782831, 16.52544592524335698, 27.70942372801901854 ) ) ;
#166102=CARTESIAN_POINT ( 'NONE',  ( -19.05341960407611168, -5.049401038298163336, 31.45724293864769550 ) ) ;
#166103=CARTESIAN_POINT ( 'NONE',  ( 12.06949235617739724, 12.14591786802326823, 26.87609039468567218 ) ) ;
#166104=CARTESIAN_POINT ( 'NONE',  ( -19.03943276465977164, 0.05219959533909376836, 51.24890960531436690 ) ) ;
#166106=CARTESIAN_POINT ( 'NONE',  ( -0.05219959533909027116, -19.03943276465977164, 107.4989096053143527 ) ) ;
#166107=CARTESIAN_POINT ( 'NONE',  ( 19.05341960407611168, 5.049401038298154454, 103.9572429386476671 ) ) ;
#166108=CARTESIAN_POINT ( 'NONE',  ( 12.14591786802327356, -12.06949235617739191, 85.62609039468568994 ) ) ;
#166109=CARTESIAN_POINT ( 'NONE',  ( -13.97604488694547697, 13.89961937509957934, 93.12609039468566152 ) ) ;
#166110=CARTESIAN_POINT ( 'NONE',  ( 19.02544592524334988, 5.153800228976608722, 41.45942372801900433 ) ) ;
#166111=CARTESIAN_POINT ( 'NONE',  ( 10.81492255796078972, 18.62759615963270932, 79.58224293864769550 ) ) ;
#166112=CARTESIAN_POINT ( 'NONE',  ( 14.34966873604972726, -8.224510206698740333, 95.83442372801903275 ) ) ;
#166113=CARTESIAN_POINT ( 'NONE',  ( 15.72974639402199770, -15.80617190586745480, 38.12390960531436690 ) ) ;
#166114=CARTESIAN_POINT ( 'NONE',  ( 9.564922557961047289, -16.46253265017146816, 90.41775706135234714 ) ) ;
#166115=CARTESIAN_POINT ( 'NONE',  ( -19.05341960407611168, -5.049401038298163336, 51.45724293864770260 ) ) ;
#166116=CARTESIAN_POINT ( 'NONE',  ( 16.46253265017160672, -9.564922557960803928, 93.33224293864769550 ) ) ;
#166118=CARTESIAN_POINT ( 'NONE',  ( -21.55341960407619339, 5.719274019375674811, 68.54275706135234714 ) ) ;
#166119=CARTESIAN_POINT ( 'NONE',  ( -9.564922557960796823, -16.46253265017161027, 57.08224293864769550 ) ) ;
#166120=CARTESIAN_POINT ( 'NONE',  ( 14.29746914071049879, -8.314922557960816363, 98.33224293864769550 ) ) ;
#166122=CARTESIAN_POINT ( 'NONE',  ( 0.05219959533910956823, 16.53943276465976808, 74.99890960531435269 ) ) ;
#166123=CARTESIAN_POINT ( 'NONE',  ( 21.55341960407610458, 5.719274019375980345, 73.95724293864769550 ) ) ;
#166124=CARTESIAN_POINT ( 'NONE',  ( -19.03943276465977164, -0.05219959533935918106, 93.75109039468566152 ) ) ;
#166126=CARTESIAN_POINT ( 'NONE',  ( -16.46253265017160317, 9.564922557960807481, 55.83224293864769550 ) ) ;
#166127=CARTESIAN_POINT ( 'NONE',  ( 18.22780087662121673, 5.500000000000056843, 68.98459894673892734 ) ) ;
#166128=CARTESIAN_POINT ( 'NONE',  ( -19.03943276465977164, 0.05219959533909376836, 71.24890960531435269 ) ) ;
#166129=CARTESIAN_POINT ( 'NONE',  ( -16.51473224551069308, -9.474510206698971260, 86.66557627198102409 ) ) ;
#166130=CARTESIAN_POINT ( 'NONE',  ( -14.29746914071037622, -8.314922557961029526, 64.16775706135234714 ) ) ;
#166131=CARTESIAN_POINT ( 'NONE',  ( -16.61371651742603817, -7.165104196376042900, 51.14584930007003294 ) ) ;
#166132=CARTESIAN_POINT ( 'NONE',  ( 5.153800228976615827, -19.02544592524334988, 50.20942372801897591 ) ) ;
#166134=CARTESIAN_POINT ( 'NONE',  ( -13.97604488694527625, -13.89961937509977652, 111.8739096053143243 ) ) ;
#166135=CARTESIAN_POINT ( 'NONE',  ( 16.53943276465976808, 0.05219959533934440121, 101.2510903946856757 ) ) ;
#166137=CARTESIAN_POINT ( 'NONE',  ( 8.224510206698742110, 14.34966873604972548, 82.08442372801901854 ) ) ;
#166138=CARTESIAN_POINT ( 'NONE',  ( 18.22780087662122384, -5.500000000000022204, 66.01540105326107266 ) ) ;
#166139=CARTESIAN_POINT ( 'NONE',  ( 16.53943276465976808, 0.05219959533934440121, 61.25109039468567573 ) ) ;
#166141=CARTESIAN_POINT ( 'NONE',  ( -0.05219959533937732626, 21.53943276465977519, 62.50109039468568284 ) ) ;
#166142=CARTESIAN_POINT ( 'NONE',  ( -19.02544592524334988, -5.153800228976617603, 73.95942372801900433 ) ) ;
#166143=CARTESIAN_POINT ( 'NONE',  ( -19.02544592524334988, -5.153800228976617603, 28.95942372801900433 ) ) ;
#166144=CARTESIAN_POINT ( 'NONE',  ( 9.564922557960805705, 16.46253265017160317, 69.58224293864770971 ) ) ;
#166145=CARTESIAN_POINT ( 'NONE',  ( 9.564922557960805705, 16.46253265017160317, 49.58224293864770260 ) ) ;
#166147=CARTESIAN_POINT ( 'NONE',  ( -21.52544592524343514, 5.823673210054127303, 71.04057627198103830 ) ) ;
#166149=CARTESIAN_POINT ( 'NONE',  ( -21.55341960407610458, -5.719274019375992779, 36.45724293864768839 ) ) ;
#166150=CARTESIAN_POINT ( 'NONE',  ( 16.55341960407611168, 4.379528057220329451, 108.9572429386476955 ) ) ;
#166151=CARTESIAN_POINT ( 'NONE',  ( 0.05219959533934541429, -16.53943276465976808, 50.00109039468568994 ) ) ;
#166154=CARTESIAN_POINT ( 'NONE',  ( -18.62759615963255300, -10.81492255796106328, 29.16775706135234003 ) ) ;
#166155=CARTESIAN_POINT ( 'NONE',  ( 16.55341960407611168, 4.379528057220329451, 48.95724293864770971 ) ) ;
#166157=CARTESIAN_POINT ( 'NONE',  ( -4.483927247898782831, 16.52544592524335698, 22.70942372801901499 ) ) ;
#166158=CARTESIAN_POINT ( 'NONE',  ( -19.05341960407617563, 5.049401038297882671, 38.54275706135233293 ) ) ;
#166159=CARTESIAN_POINT ( 'NONE',  ( -4.379528057220328563, 16.55341960407611168, 45.20724293864769550 ) ) ;
#166160=CARTESIAN_POINT ( 'NONE',  ( 0.05219959533907565091, 21.53943276465977519, 109.9989096053143527 ) ) ;
#166162=CARTESIAN_POINT ( 'NONE',  ( -18.62759615963270932, 10.81492255796079327, 80.83224293864769550 ) ) ;
#166163=CARTESIAN_POINT ( 'NONE',  ( 13.97604488694527802, 13.89961937509977652, 94.37390960531436690 ) ) ;
#166164=CARTESIAN_POINT ( 'NONE',  ( 14.34966873604960469, 8.224510206698951720, 64.16557627198102409 ) ) ;
#166165=CARTESIAN_POINT ( 'NONE',  ( 0.05219959533909260263, 19.03943276465977164, 104.9989096053143669 ) ) ;
#166167=CARTESIAN_POINT ( 'NONE',  ( -16.46253265017146816, -9.564922557961047289, 74.16775706135234714 ) ) ;
#166168=CARTESIAN_POINT ( 'NONE',  ( 18.62759615963271287, -10.81492255796078972, 103.3322429386476955 ) ) ;
#166169=CARTESIAN_POINT ( 'NONE',  ( -19.03943276465977164, 0.05219959533909376836, 61.24890960531436690 ) ) ;
#166170=CARTESIAN_POINT ( 'NONE',  ( -19.03943276465977164, 0.05219959533909376836, 21.24890960531436335 ) ) ;
#166171=CARTESIAN_POINT ( 'NONE',  ( 18.62759615963255655, 10.81492255796105972, 51.66775706135234714 ) ) ;
#166173=CARTESIAN_POINT ( 'NONE',  ( 0.05219959533910956823, 16.53943276465976808, 44.99890960531435979 ) ) ;
#166174=CARTESIAN_POINT ( 'NONE',  ( -5.049401038298153566, 19.05341960407611168, 45.20724293864769550 ) ) ;
#166175=CARTESIAN_POINT ( 'NONE',  ( 5.153800228976335163, 19.02544592524342804, 99.79057627198102409 ) ) ;
#166176=CARTESIAN_POINT ( 'NONE',  ( 10.72451020669898902, -18.67979575497178502, 67.91557627198102409 ) ) ;
#166178=CARTESIAN_POINT ( 'NONE',  ( 19.02544592524343514, -5.153800228976328945, 38.54057627198103120 ) ) ;
#166179=CARTESIAN_POINT ( 'NONE',  ( -18.67979575497178146, -10.72451020669898902, 61.66557627198103120 ) ) ;
#166180=CARTESIAN_POINT ( 'NONE',  ( 10.81492255796106328, -18.62759615963255655, 80.41775706135234714 ) ) ;
#166181=DIRECTION ( 'NONE',  ( -0.000000000000000000, -0.000000000000000000, -1.000000000000000000 ) ) ;
#166182=CARTESIAN_POINT ( 'NONE',  ( -8.224510206698735004, -14.34966873604973081, 89.58442372801901854 ) ) ;
#166183=CARTESIAN_POINT ( 'NONE',  ( -16.55341960407611168, -4.379528057220339221, 81.45724293864769550 ) ) ;
#166184=CARTESIAN_POINT ( 'NONE',  ( -0.05219959533909027116, -19.03943276465977164, 67.49890960531436690 ) ) ;
#166186=CARTESIAN_POINT ( 'NONE',  ( -9.564922557961040184, 16.46253265017147172, 32.91775706135233293 ) ) ;
#166187=CARTESIAN_POINT ( 'NONE',  ( -12.06949235617739369, -12.14591786802326823, 94.37609039468568994 ) ) ;
#166188=CARTESIAN_POINT ( 'NONE',  ( 5.719274019375673035, 21.55341960407619339, 107.2927570613523471 ) ) ;
#166189=CARTESIAN_POINT ( 'NONE',  ( 19.05341960407611168, 5.049401038298154454, 88.95724293864769550 ) ) ;
#166190=CARTESIAN_POINT ( 'NONE',  ( -21.55341960407610458, -5.719274019375992779, 46.45724293864769550 ) ) ;
#166191=CARTESIAN_POINT ( 'NONE',  ( 18.67979575497194134, -10.72451020669871369, 95.83442372801903275 ) ) ;
#166192=CARTESIAN_POINT ( 'NONE',  ( 4.379528057220092307, 16.55341960407617563, 57.29275706135234714 ) ) ;
#166193=CARTESIAN_POINT ( 'NONE',  ( -21.53943276465977519, 0.05219959533907696930, 106.2489096053143811 ) ) ;
#166194=CARTESIAN_POINT ( 'NONE',  ( 16.53943276465976808, 0.05219959533934440121, 26.25109039468567573 ) ) ;
#166195=CARTESIAN_POINT ( 'NONE',  ( -19.05341960407611168, -5.049401038298163336, 86.45724293864769550 ) ) ;
#166196=CARTESIAN_POINT ( 'NONE',  ( 0.05219959533934541429, -16.53943276465976808, 25.00109039468567218 ) ) ;
#166197=CARTESIAN_POINT ( 'NONE',  ( -16.51473224551069308, -9.474510206698971260, 56.66557627198103120 ) ) ;
#166198=CARTESIAN_POINT ( 'NONE',  ( -4.483927247898782831, 16.52544592524335698, 27.70942372801901854 ) ) ;
#166199=CARTESIAN_POINT ( 'NONE',  ( -14.29746914071049879, 8.314922557960819915, 75.83224293864769550 ) ) ;
#166200=CARTESIAN_POINT ( 'NONE',  ( 12.06949235617739724, 12.14591786802326823, 86.87609039468568994 ) ) ;
#166201=CARTESIAN_POINT ( 'NONE',  ( -21.52544592524334988, -5.823673210054445271, 43.95942372801902565 ) ) ;
#166202=CARTESIAN_POINT ( 'NONE',  ( -19.02544592524342804, 5.153800228976336051, 71.04057627198099567 ) ) ;
#166203=CARTESIAN_POINT ( 'NONE',  ( 0.05219959533909260263, 19.03943276465977164, 84.99890960531436690 ) ) ;
#166204=CARTESIAN_POINT ( 'NONE',  ( 16.55341960407611168, 4.379528057220329451, 28.95724293864769905 ) ) ;
#166205=CARTESIAN_POINT ( 'NONE',  ( -4.379528057220086978, -16.55341960407618274, 79.79275706135236135 ) ) ;
#166208=CARTESIAN_POINT ( 'NONE',  ( 19.03943276465977164, 0.05219959533936151252, 36.25109039468567573 ) ) ;
#166209=CARTESIAN_POINT ( 'NONE',  ( 5.153800228976335163, 19.02544592524342804, 104.7905762719809957 ) ) ;
#166210=CARTESIAN_POINT ( 'NONE',  ( -9.474510206698964154, 16.51473224551069663, 55.41557627198103120 ) ) ;
#166211=LINE ( 'NONE', #122660, #26913 ) ;
#166212=CARTESIAN_POINT ( 'NONE',  ( 12.14591786802327356, -12.06949235617739191, 40.62609039468567573 ) ) ;
#166213=CARTESIAN_POINT ( 'NONE',  ( -13.89961937509957401, -13.97604488694547875, 74.37609039468566152 ) ) ;
#166214=CARTESIAN_POINT ( 'NONE',  ( -16.53943276465976808, -0.05219959533934237506, 53.75109039468568994 ) ) ;
#166215=DIRECTION ( 'NONE',  ( 3.469446951953611033E-15, 0.000000000000000000, -1.000000000000000000 ) ) ;
#166216=CARTESIAN_POINT ( 'NONE',  ( -0.05219959533909027116, -19.03943276465977164, 77.49890960531435269 ) ) ;
#166217=CARTESIAN_POINT ( 'NONE',  ( 18.67979575497178502, 10.72451020669898547, 114.1655762719810383 ) ) ;
#166218=CARTESIAN_POINT ( 'NONE',  ( -13.89961937509957401, -13.97604488694547875, 69.37609039468564731 ) ) ;
#166219=CARTESIAN_POINT ( 'NONE',  ( -16.46253265017160317, 9.564922557960807481, 100.8322429386477097 ) ) ;
#166220=CARTESIAN_POINT ( 'NONE',  ( -0.05219959533909027116, -19.03943276465977164, 27.49890960531435624 ) ) ;
#166221=CARTESIAN_POINT ( 'NONE',  ( 16.46253265017160672, -9.564922557960803928, 78.33224293864769550 ) ) ;
#166222=CARTESIAN_POINT ( 'NONE',  ( -0.05219959533910754901, -16.53943276465976808, 32.49890960531435979 ) ) ;
#166223=CARTESIAN_POINT ( 'NONE',  ( -5.153800228976328057, -19.02544592524343514, 22.29057627198102765 ) ) ;
#166224=CARTESIAN_POINT ( 'NONE',  ( 0.05219959533936267826, -19.03943276465977164, 40.00109039468566152 ) ) ;
#166225=CARTESIAN_POINT ( 'NONE',  ( -0.05219959533910754901, -16.53943276465976808, 77.49890960531433848 ) ) ;
#166226=CARTESIAN_POINT ( 'NONE',  ( -13.97604488694547697, 13.89961937509957934, 23.12609039468565442 ) ) ;
#166227=CARTESIAN_POINT ( 'NONE',  ( 16.51473224551069308, 9.474510206698969483, 34.16557627198102409 ) ) ;
#166229=CARTESIAN_POINT ( 'NONE',  ( -16.53943276465976808, 0.05219959533911058130, 46.24890960531435979 ) ) ;
#166230=CARTESIAN_POINT ( 'NONE',  ( -18.67979575497193778, 10.72451020669871902, 103.3344237280190043 ) ) ;
#166231=CARTESIAN_POINT ( 'NONE',  ( -16.46253265017160317, 9.564922557960807481, 95.83224293864769550 ) ) ;
#166232=CARTESIAN_POINT ( 'NONE',  ( -0.05219959533909027116, -19.03943276465977164, 107.4989096053143527 ) ) ;
#166233=CARTESIAN_POINT ( 'NONE',  ( -19.05341960407611168, -5.049401038298163336, 36.45724293864766707 ) ) ;
#166234=CARTESIAN_POINT ( 'NONE',  ( -14.29746914071049879, 8.314922557960819915, 110.8322429386476955 ) ) ;
#166235=CARTESIAN_POINT ( 'NONE',  ( -4.483927247898539470, -16.52544592524342804, 72.29057627198102409 ) ) ;
#166236=CARTESIAN_POINT ( 'NONE',  ( -21.55341960407610458, -5.719274019375992779, 86.45724293864770971 ) ) ;
#166237=CARTESIAN_POINT ( 'NONE',  ( 19.03943276465977164, -0.05219959533909143690, 83.74890960531436690 ) ) ;
#166238=CARTESIAN_POINT ( 'NONE',  ( 15.72974639402199770, -15.80617190586745480, 98.12390960531436690 ) ) ;
#166239=CARTESIAN_POINT ( 'NONE',  ( -19.05341960407611168, -5.049401038298163336, 96.45724293864769550 ) ) ;
#166240=CARTESIAN_POINT ( 'NONE',  ( 19.35633801406907750, -5.499999999999772626, 46.63373818172765795 ) ) ;
#166241=CARTESIAN_POINT ( 'NONE',  ( -8.314922557960811034, -14.29746914071050412, 107.0822429386476955 ) ) ;
#166242=CARTESIAN_POINT ( 'NONE',  ( 19.02544592524343514, -5.153800228976328945, 68.54057627198103830 ) ) ;
#166243=CARTESIAN_POINT ( 'NONE',  ( 10.72451020669898902, -18.67979575497178502, 77.91557627198102409 ) ) ;
#166245=CARTESIAN_POINT ( 'NONE',  ( 0.05219959533907565091, 21.53943276465977519, 29.99890960531435979 ) ) ;
#166246=CARTESIAN_POINT ( 'NONE',  ( 19.52217212775656563, -5.500000000000102141, 67.43993709005262360 ) ) ;
#166247=CARTESIAN_POINT ( 'NONE',  ( 19.03943276465977164, 0.05219959533936151252, 111.2510903946856757 ) ) ;
#166249=CARTESIAN_POINT ( 'NONE',  ( 12.06949235617757843, -12.14591786802309237, 98.12390960531436690 ) ) ;
#166250=CARTESIAN_POINT ( 'NONE',  ( -16.31925111598456368, -7.325300261831544368, 94.83575461032751264 ) ) ;
#166251=CARTESIAN_POINT ( 'NONE',  ( -19.05341960407611168, -5.049401038298163336, 86.45724293864769550 ) ) ;
#166252=CARTESIAN_POINT ( 'NONE',  ( 9.564922557960805705, 16.46253265017160317, 49.58224293864770260 ) ) ;
#166253=CARTESIAN_POINT ( 'NONE',  ( 12.06949235617757843, -12.14591786802309237, 83.12390960531436690 ) ) ;
#166254=CARTESIAN_POINT ( 'NONE',  ( 21.53943276465977519, -0.05219959533907433946, 23.74890960531435269 ) ) ;
#166255=CARTESIAN_POINT ( 'NONE',  ( -16.52544592524342804, 4.483927247898546575, 51.04057627198103120 ) ) ;
#166256=CARTESIAN_POINT ( 'NONE',  ( -16.46253265017146816, -9.564922557961047289, 104.1677570613523329 ) ) ;
#166257=CARTESIAN_POINT ( 'NONE',  ( -5.823673210054431948, 21.52544592524334988, 62.70942372801902565 ) ) ;
#166260=CARTESIAN_POINT ( 'NONE',  ( 9.564922557960805705, 16.46253265017160317, 94.58224293864769550 ) ) ;
#166261=CARTESIAN_POINT ( 'NONE',  ( -15.80617190586745835, -15.72974639402198527, 86.87390960531438111 ) ) ;
#166262=CARTESIAN_POINT ( 'NONE',  ( 16.55341960407618274, -4.379528057220086978, 91.04275706135236135 ) ) ;
#166263=CARTESIAN_POINT ( 'NONE',  ( 9.564922557960805705, 16.46253265017160317, 29.58224293864769550 ) ) ;
#166264=CARTESIAN_POINT ( 'NONE',  ( -19.02544592524342804, 5.153800228976336051, 81.04057627198103830 ) ) ;
#166265=CARTESIAN_POINT ( 'NONE',  ( -10.72451020669898014, 18.67979575497178502, 85.41557627198102409 ) ) ;
#166267=CARTESIAN_POINT ( 'NONE',  ( 0.05219959533936267826, -19.03943276465977164, 105.0010903946856615 ) ) ;
#166268=CARTESIAN_POINT ( 'NONE',  ( -16.52544592524342804, 4.483927247898546575, 56.04057627198102409 ) ) ;
#166269=CARTESIAN_POINT ( 'NONE',  ( 5.823673210054444382, -21.52544592524334988, 55.20942372801902565 ) ) ;
#166270=CARTESIAN_POINT ( 'NONE',  ( -8.224510206698735004, -14.34966873604973081, 89.58442372801901854 ) ) ;
#166271=CARTESIAN_POINT ( 'NONE',  ( 13.97604488694527802, 13.89961937509977652, 114.3739096053143669 ) ) ;
#166272=CARTESIAN_POINT ( 'NONE',  ( -19.03943276465977164, 0.05219959533909376836, 111.2489096053143669 ) ) ;
#166273=CARTESIAN_POINT ( 'NONE',  ( -16.62475595723700650, 7.163666690055234376, 80.52713351810471920 ) ) ;
#166274=CARTESIAN_POINT ( 'NONE',  ( -16.52544592524335698, -4.483927247898792601, 108.9594237280190185 ) ) ;
#166275=CARTESIAN_POINT ( 'NONE',  ( -16.55341960407617563, 4.379528057220093196, 63.54275706135234003 ) ) ;
#166276=CARTESIAN_POINT ( 'NONE',  ( 19.03943276465977164, -0.05219959533909143690, 68.74890960531436690 ) ) ;
#166277=CARTESIAN_POINT ( 'NONE',  ( 13.97604488694527802, 13.89961937509977652, 79.37390960531435269 ) ) ;
#166278=CARTESIAN_POINT ( 'NONE',  ( 18.67979575497194134, -10.72451020669871369, 70.83442372801901854 ) ) ;
#166280=CARTESIAN_POINT ( 'NONE',  ( -8.224510206698735004, -14.34966873604973081, 74.58442372801901854 ) ) ;
#166281=CARTESIAN_POINT ( 'NONE',  ( -4.379528057220328563, 16.55341960407611168, 50.20724293864769550 ) ) ;
#166282=CARTESIAN_POINT ( 'NONE',  ( -16.51473224551069308, -9.474510206698971260, 51.66557627198102409 ) ) ;
#166283=CARTESIAN_POINT ( 'NONE',  ( 16.51473224551069308, 9.474510206698969483, 54.16557627198103120 ) ) ;
#166284=CARTESIAN_POINT ( 'NONE',  ( 16.53943276465976808, 0.05219959533934440121, 41.25109039468568284 ) ) ;
#166287=CARTESIAN_POINT ( 'NONE',  ( 13.89961937509957401, 13.97604488694547697, 91.87609039468567573 ) ) ;
#166288=CARTESIAN_POINT ( 'NONE',  ( 4.379528057220339221, -16.55341960407611168, 102.7072429386476955 ) ) ;
#166289=CARTESIAN_POINT ( 'NONE',  ( 13.97604488694527802, 13.89961937509977652, 64.37390960531436690 ) ) ;
#166290=CARTESIAN_POINT ( 'NONE',  ( -0.05219959533936034679, 19.03943276465977164, 97.50109039468567573 ) ) ;
#166292=CARTESIAN_POINT ( 'NONE',  ( -5.719274019375665041, -21.55341960407619695, 99.79275706135234714 ) ) ;
#166293=CARTESIAN_POINT ( 'NONE',  ( -14.34966873604972548, 8.224510206698743886, 68.33442372801900433 ) ) ;
#166295=CARTESIAN_POINT ( 'NONE',  ( -21.53943276465977519, 0.05219959533907696930, 61.24890960531435979 ) ) ;
#166296=CARTESIAN_POINT ( 'NONE',  ( -8.314922557961024197, 14.29746914071037800, 47.91775706135234714 ) ) ;
#166297=CARTESIAN_POINT ( 'NONE',  ( -9.564922557960796823, -16.46253265017161027, 32.08224293864769550 ) ) ;
#166298=CARTESIAN_POINT ( 'NONE',  ( 19.03943276465977164, 0.05219959533936151252, 46.25109039468566863 ) ) ;
#166299=CARTESIAN_POINT ( 'NONE',  ( 19.02544592524343514, -5.153800228976328945, 93.54057627198102409 ) ) ;
#166300=CARTESIAN_POINT ( 'NONE',  ( -4.379528057220328563, 16.55341960407611168, 115.2072429386476955 ) ) ;
#166301=CARTESIAN_POINT ( 'NONE',  ( 0.05219959533909260263, 19.03943276465977164, 64.99890960531436690 ) ) ;
#166303=CARTESIAN_POINT ( 'NONE',  ( -10.72451020669870658, -18.67979575497194134, 79.58442372801903275 ) ) ;
#166304=CARTESIAN_POINT ( 'NONE',  ( -19.03943276465977164, -0.05219959533935918106, 48.75109039468566863 ) ) ;
#166305=CARTESIAN_POINT ( 'NONE',  ( -19.05341960407617563, 5.049401038297882671, 33.54275706135231871 ) ) ;
#166306=CARTESIAN_POINT ( 'NONE',  ( 9.474510206698971260, -16.51473224551069308, 57.91557627198103120 ) ) ;
#166307=CARTESIAN_POINT ( 'NONE',  ( 0.05219959533907565091, 21.53943276465977519, 24.99890960531435624 ) ) ;
#166308=CARTESIAN_POINT ( 'NONE',  ( -18.67979575497193778, 10.72451020669871902, 88.33442372801901854 ) ) ;
#166309=CARTESIAN_POINT ( 'NONE',  ( -19.02544592524342804, 5.153800228976336051, 66.04057627198103830 ) ) ;
#166310=CARTESIAN_POINT ( 'NONE',  ( -18.62759615963255300, -10.81492255796106328, 99.16775706135234714 ) ) ;
#166311=CARTESIAN_POINT ( 'NONE',  ( 18.62759615963271287, -10.81492255796078972, 33.33224293864769550 ) ) ;
#166312=CARTESIAN_POINT ( 'NONE',  ( 13.89961937509977652, -13.97604488694527269, 78.12390960531433848 ) ) ;
#166313=CARTESIAN_POINT ( 'NONE',  ( 18.67979575497194134, -10.72451020669871369, 40.83442372801901854 ) ) ;
#166314=CARTESIAN_POINT ( 'NONE',  ( 0.05219959533936267826, -19.03943276465977164, 60.00109039468566863 ) ) ;
#166315=CARTESIAN_POINT ( 'NONE',  ( -13.97604488694527625, -13.89961937509977652, 41.87390960531435979 ) ) ;
#166316=CARTESIAN_POINT ( 'NONE',  ( 0.05219959533909260263, 19.03943276465977164, 94.99890960531436690 ) ) ;
#166317=CARTESIAN_POINT ( 'NONE',  ( -8.224510206698735004, -14.34966873604973081, 29.58442372801901854 ) ) ;
#166318=CARTESIAN_POINT ( 'NONE',  ( 12.14591786802309770, 12.06949235617756955, 84.37390960531438111 ) ) ;
#166319=CARTESIAN_POINT ( 'NONE',  ( -16.51473224551069308, -9.474510206698971260, 66.66557627198102409 ) ) ;
#166320=CARTESIAN_POINT ( 'NONE',  ( 21.52544592524344225, -5.823673210054117533, 53.54057627198103120 ) ) ;
#166321=CARTESIAN_POINT ( 'NONE',  ( -14.29746914071037622, -8.314922557961029526, 19.16775706135234714 ) ) ;
#166322=CARTESIAN_POINT ( 'NONE',  ( -10.81492255796078084, -18.62759615963271287, 112.0822429386477097 ) ) ;
#166323=CARTESIAN_POINT ( 'NONE',  ( 21.52544592524334988, 5.823673210054432836, 71.45942372801901854 ) ) ;
#166324=CARTESIAN_POINT ( 'NONE',  ( -8.224510206698735004, -14.34966873604973081, 64.58442372801900433 ) ) ;
#166325=CARTESIAN_POINT ( 'NONE',  ( -0.05219959533934338120, 16.53943276465976808, 72.50109039468568994 ) ) ;
#166326=CARTESIAN_POINT ( 'NONE',  ( -0.05219959533909027116, -19.03943276465977164, 67.49890960531436690 ) ) ;
#166327=CARTESIAN_POINT ( 'NONE',  ( 16.55341960407618274, -4.379528057220086978, 96.04275706135236135 ) ) ;
#166328=CARTESIAN_POINT ( 'NONE',  ( 13.89961937509957401, 13.97604488694547697, 41.87609039468566152 ) ) ;
#166329=CARTESIAN_POINT ( 'NONE',  ( -21.53943276465977519, 0.05219959533907696930, 116.2489096053143669 ) ) ;
#166330=CARTESIAN_POINT ( 'NONE',  ( 8.224510206698953496, -14.34966873604960469, 62.91557627198102409 ) ) ;
#166331=CARTESIAN_POINT ( 'NONE',  ( -5.049401038298153566, 19.05341960407611168, 80.20724293864769550 ) ) ;
#166332=CARTESIAN_POINT ( 'NONE',  ( -8.224510206698735004, -14.34966873604973081, 84.58442372801903275 ) ) ;
#166333=CARTESIAN_POINT ( 'NONE',  ( -21.55341960407619339, 5.719274019375674811, 53.54275706135234714 ) ) ;
#166334=CARTESIAN_POINT ( 'NONE',  ( 4.483927247898790824, -16.52544592524335698, 25.20942372801901854 ) ) ;
#166335=CARTESIAN_POINT ( 'NONE',  ( 18.62759615963255655, 10.81492255796105972, 21.66775706135235069 ) ) ;
#166336=CARTESIAN_POINT ( 'NONE',  ( -12.14591786802309592, -12.06949235617757132, 51.87390960531437401 ) ) ;
#166338=CARTESIAN_POINT ( 'NONE',  ( -10.81492255796078084, -18.62759615963271287, 97.08224293864770971 ) ) ;
#166339=CARTESIAN_POINT ( 'NONE',  ( 16.52544592524342804, -4.483927247898539470, 33.54057627198102409 ) ) ;
#166343=CARTESIAN_POINT ( 'NONE',  ( -15.72974639402197994, 15.80617190586746368, 35.62390960531437401 ) ) ;
#166344=CARTESIAN_POINT ( 'NONE',  ( -5.719274019375665041, -21.55341960407619695, 39.79275706135235424 ) ) ;
#166345=CARTESIAN_POINT ( 'NONE',  ( -4.483927247898539470, -16.52544592524342804, 62.29057627198102409 ) ) ;
#166346=CARTESIAN_POINT ( 'NONE',  ( 15.80617190586746368, 15.72974639402197994, 69.37390960531436690 ) ) ;
#166347=CARTESIAN_POINT ( 'NONE',  ( 9.474510206698971260, -16.51473224551069308, 72.91557627198102409 ) ) ;
#166348=CARTESIAN_POINT ( 'NONE',  ( 5.153800228976335163, 19.02544592524342804, 29.79057627198102409 ) ) ;
#166349=CARTESIAN_POINT ( 'NONE',  ( -9.564922557961040184, 16.46253265017147172, 67.91775706135233293 ) ) ;
#166350=CARTESIAN_POINT ( 'NONE',  ( 10.72451020669898902, -18.67979575497178502, 52.91557627198103830 ) ) ;
#166351=CARTESIAN_POINT ( 'NONE',  ( -16.46253265017160317, 9.564922557960807481, 55.83224293864769550 ) ) ;
#166353=CARTESIAN_POINT ( 'NONE',  ( -16.55341960407617563, 4.379528057220093196, 33.54275706135234714 ) ) ;
#166354=CARTESIAN_POINT ( 'NONE',  ( 15.80617190586769283, -15.72974639402175789, 20.62609039468568639 ) ) ;
#166355=CARTESIAN_POINT ( 'NONE',  ( -16.55341960407611168, -4.379528057220339221, 41.45724293864769550 ) ) ;
#166357=CARTESIAN_POINT ( 'NONE',  ( -0.05219959533909027116, -19.03943276465977164, 102.4989096053143669 ) ) ;
#166358=CARTESIAN_POINT ( 'NONE',  ( -15.72974639402197994, 15.80617190586746368, 70.62390960531436690 ) ) ;
#166359=CARTESIAN_POINT ( 'NONE',  ( -10.81492255796078084, -18.62759615963271287, 102.0822429386476955 ) ) ;
#166360=CARTESIAN_POINT ( 'NONE',  ( -14.29746914071037622, -8.314922557961029526, 34.16775706135234714 ) ) ;
#166361=EDGE_CURVE ( 'NONE', #163173, #112403, #128114, .T. ) ;
#166362=CARTESIAN_POINT ( 'NONE',  ( -21.52544592524343514, 5.823673210054127303, 46.04057627198103830 ) ) ;
#166363=CARTESIAN_POINT ( 'NONE',  ( -21.53943276465977519, -0.05219959533937600094, 98.75109039468568994 ) ) ;
#166364=CARTESIAN_POINT ( 'NONE',  ( -9.474510206698964154, 16.51473224551069663, 35.41557627198102409 ) ) ;
#166365=CARTESIAN_POINT ( 'NONE',  ( -5.153800228976328057, -19.02544592524343514, 102.2905762719810383 ) ) ;
#166366=CARTESIAN_POINT ( 'NONE',  ( 5.049401038298161559, -19.05341960407611168, 77.70724293864765286 ) ) ;
#166367=CARTESIAN_POINT ( 'NONE',  ( 17.50000000001358202, -5.500000000000038192, 88.29690382535061133 ) ) ;
#166368=CARTESIAN_POINT ( 'NONE',  ( -13.97604488694547697, 13.89961937509957934, 53.12609039468565442 ) ) ;
#166369=CARTESIAN_POINT ( 'NONE',  ( 18.62759615963255655, 10.81492255796105972, 106.6677570613523756 ) ) ;
#166370=CARTESIAN_POINT ( 'NONE',  ( 10.72451020669898902, -18.67979575497178502, 32.91557627198102409 ) ) ;
#166371=CARTESIAN_POINT ( 'NONE',  ( -16.53943276465976808, -0.05219959533934237506, 98.75109039468568994 ) ) ;
#166372=EDGE_CURVE ( 'NONE', #68158, #83853, #157144, .T. ) ;
#166373=CARTESIAN_POINT ( 'NONE',  ( -5.153800228976607833, 19.02544592524334988, 82.70942372801897591 ) ) ;
#166375=CARTESIAN_POINT ( 'NONE',  ( -5.153800228976607833, 19.02544592524334988, 82.70942372801897591 ) ) ;
#166376=CARTESIAN_POINT ( 'NONE',  ( 9.474510206698729675, 16.51473224551082808, 42.08442372801900433 ) ) ;
#166378=CARTESIAN_POINT ( 'NONE',  ( 19.02544592524343514, -5.153800228976328945, 38.54057627198103120 ) ) ;
#166379=CARTESIAN_POINT ( 'NONE',  ( 16.53943276465976808, -0.05219959533910856209, 53.74890960531437401 ) ) ;
#166380=CARTESIAN_POINT ( 'NONE',  ( -16.46253265017160317, 9.564922557960807481, 35.83224293864768839 ) ) ;
#166381=CARTESIAN_POINT ( 'NONE',  ( 16.53943276465976808, -0.05219959533910856209, 43.74890960531435979 ) ) ;
#166382=CARTESIAN_POINT ( 'NONE',  ( 17.72696623605164845, -5.499999999999870326, 46.09811031808416715 ) ) ;
#166383=CARTESIAN_POINT ( 'NONE',  ( 16.52544592524335698, 4.483927247898782831, 106.4594237280190328 ) ) ;
#166384=CARTESIAN_POINT ( 'NONE',  ( -16.46253265017160317, 9.564922557960807481, 50.83224293864770260 ) ) ;
#166385=CARTESIAN_POINT ( 'NONE',  ( -21.52544592524334988, -5.823673210054445271, 108.9594237280190185 ) ) ;
#166386=CARTESIAN_POINT ( 'NONE',  ( -14.29746914071037622, -8.314922557961029526, 19.16775706135234714 ) ) ;
#166387=CARTESIAN_POINT ( 'NONE',  ( -21.52544592524343514, 5.823673210054127303, 41.04057627198103120 ) ) ;
#166388=CARTESIAN_POINT ( 'NONE',  ( 18.67979575497194134, -10.72451020669871369, 85.83442372801901854 ) ) ;
#166389=ORIENTED_EDGE ( 'NONE', *, *, #187948, .F. ) ;
#166390=CARTESIAN_POINT ( 'NONE',  ( -5.049401038298153566, 19.05341960407611168, 100.2072429386476955 ) ) ;
#166391=CARTESIAN_POINT ( 'NONE',  ( 13.89961937509977652, -13.97604488694527269, 78.12390960531433848 ) ) ;
#166393=CARTESIAN_POINT ( 'NONE',  ( 18.67979575497178502, 10.72451020669898547, 109.1655762719810383 ) ) ;
#166395=CARTESIAN_POINT ( 'NONE',  ( -8.224510206698948167, 14.34966873604960824, 80.41557627198103830 ) ) ;
#166396=CARTESIAN_POINT ( 'NONE',  ( 18.62759615963271287, -10.81492255796078972, 68.33224293864769550 ) ) ;
#166397=CARTESIAN_POINT ( 'NONE',  ( 13.89961937509977652, -13.97604488694527269, 73.12390960531436690 ) ) ;
#166398=CARTESIAN_POINT ( 'NONE',  ( -21.53943276465977519, 0.05219959533907696930, 96.24890960531435269 ) ) ;
#166400=CARTESIAN_POINT ( 'NONE',  ( -19.02544592524342804, 5.153800228976336051, 61.04057627198103120 ) ) ;
#166401=CARTESIAN_POINT ( 'NONE',  ( 0.05219959533910956823, 16.53943276465976808, 89.99890960531438111 ) ) ;
#166403=CARTESIAN_POINT ( 'NONE',  ( -19.03943276465977164, 0.05219959533909376836, 61.24890960531436690 ) ) ;
#166404=CARTESIAN_POINT ( 'NONE',  ( 13.89961937509957401, 13.97604488694547697, 76.87609039468566152 ) ) ;
#166406=CARTESIAN_POINT ( 'NONE',  ( 16.52544592524342804, -4.483927247898539470, 83.54057627198102409 ) ) ;
#166407=CARTESIAN_POINT ( 'NONE',  ( -10.72451020669870658, -18.67979575497194134, 54.58442372801901143 ) ) ;
#166408=CARTESIAN_POINT ( 'NONE',  ( -5.049401038298153566, 19.05341960407611168, 50.20724293864770260 ) ) ;
#166409=CARTESIAN_POINT ( 'NONE',  ( 10.81492255796106328, -18.62759615963255655, 20.41775706135234714 ) ) ;
#166410=CARTESIAN_POINT ( 'NONE',  ( 16.53943276465976808, -0.05219959533910856209, 103.7489096053143669 ) ) ;
#166411=FACE_OUTER_BOUND ( 'NONE', #78257, .T. ) ;
#166412=CARTESIAN_POINT ( 'NONE',  ( 5.153800228976335163, 19.02544592524342804, 54.79057627198103120 ) ) ;
#166414=CARTESIAN_POINT ( 'NONE',  ( 16.18388926212238133, 7.379444403734521707, 112.9395315136614926 ) ) ;
#166415=CARTESIAN_POINT ( 'NONE',  ( -9.564922557961040184, 16.46253265017147172, 102.9177570613523329 ) ) ;
#166416=CARTESIAN_POINT ( 'NONE',  ( 19.02544592524343514, -5.153800228976328945, 108.5405762719810383 ) ) ;
#166417=CARTESIAN_POINT ( 'NONE',  ( 18.67979575497194134, -10.72451020669871369, 50.83442372801901143 ) ) ;
#166418=CARTESIAN_POINT ( 'NONE',  ( 13.97604488694527802, 13.89961937509977652, 94.37390960531436690 ) ) ;
#166419=CARTESIAN_POINT ( 'NONE',  ( -16.46253265017146816, -9.564922557961047289, 89.16775706135234714 ) ) ;
#166420=CARTESIAN_POINT ( 'NONE',  ( -5.153800228976328057, -19.02544592524343514, 52.29057627198100988 ) ) ;
#166421=CARTESIAN_POINT ( 'NONE',  ( -8.314922557960811034, -14.29746914071050412, 87.08224293864769550 ) ) ;
#166422=CARTESIAN_POINT ( 'NONE',  ( 13.89961937509977652, -13.97604488694527269, 93.12390960531436690 ) ) ;
#166423=CARTESIAN_POINT ( 'NONE',  ( 14.34966873604960469, 8.224510206698951720, 84.16557627198103830 ) ) ;
#166424=CARTESIAN_POINT ( 'NONE',  ( 19.02544592524343514, -5.153800228976328945, 88.54057627198102409 ) ) ;
#166425=CARTESIAN_POINT ( 'NONE',  ( -19.05341960407617563, 5.049401038297882671, 28.54275706135232937 ) ) ;
#166426=CARTESIAN_POINT ( 'NONE',  ( 16.46253265017160672, -9.564922557960803928, 43.33224293864769550 ) ) ;
#166427=CARTESIAN_POINT ( 'NONE',  ( -16.53943276465976808, 0.05219959533911058130, 26.24890960531435624 ) ) ;
#166428=CARTESIAN_POINT ( 'NONE',  ( 19.02544592524343514, -5.153800228976328945, 33.54057627198102409 ) ) ;
#166429=ORIENTED_EDGE ( 'NONE', *, *, #174036, .T. ) ;
#166430=CARTESIAN_POINT ( 'NONE',  ( 18.62759615963255655, 10.81492255796105972, 41.66775706135235424 ) ) ;
#166431=CARTESIAN_POINT ( 'NONE',  ( -5.049401038297874678, -19.05341960407617918, 79.79275706135233293 ) ) ;
#166432=CARTESIAN_POINT ( 'NONE',  ( -12.14591786802309592, -12.06949235617757132, 36.87390960531435979 ) ) ;
#166433=CARTESIAN_POINT ( 'NONE',  ( -5.719274019375978568, 21.55341960407610458, 85.20724293864770971 ) ) ;
#166434=CARTESIAN_POINT ( 'NONE',  ( 5.719274019375991003, -21.55341960407610458, 32.70724293864770260 ) ) ;
#166435=CARTESIAN_POINT ( 'NONE',  ( -16.53943276465976808, 0.05219959533911058130, 66.24890960531436690 ) ) ;
#166436=CARTESIAN_POINT ( 'NONE',  ( 5.049401038298161559, -19.05341960407611168, 42.70724293864767418 ) ) ;
#166437=CARTESIAN_POINT ( 'NONE',  ( -0.05219959533934338120, 16.53943276465976808, 107.5010903946856899 ) ) ;
#166438=CARTESIAN_POINT ( 'NONE',  ( -16.52544592524335698, -4.483927247898792601, 63.95942372801901854 ) ) ;
#166439=CARTESIAN_POINT ( 'NONE',  ( -15.72974639402197994, 15.80617190586746368, 40.62390960531435269 ) ) ;
#166440=CARTESIAN_POINT ( 'NONE',  ( 13.89961937509957401, 13.97604488694547697, 21.87609039468566152 ) ) ;
#166441=CARTESIAN_POINT ( 'NONE',  ( -9.564922557960796823, -16.46253265017161027, 97.08224293864769550 ) ) ;
#166442=CARTESIAN_POINT ( 'NONE',  ( 4.483927247898790824, -16.52544592524335698, 75.20942372801901854 ) ) ;
#166443=CARTESIAN_POINT ( 'NONE',  ( 5.049401038298161559, -19.05341960407611168, 22.70724293864769194 ) ) ;
#166444=CARTESIAN_POINT ( 'NONE',  ( -12.14591786802309592, -12.06949235617757132, 36.87390960531435979 ) ) ;
#166445=CARTESIAN_POINT ( 'NONE',  ( -5.049401038298153566, 19.05341960407611168, 105.2072429386476671 ) ) ;
#166446=CARTESIAN_POINT ( 'NONE',  ( 5.049401038298161559, -19.05341960407611168, 97.70724293864766707 ) ) ;
#166447=CARTESIAN_POINT ( 'NONE',  ( -10.81492255796078084, -18.62759615963271287, 22.08224293864769194 ) ) ;
#166448=CARTESIAN_POINT ( 'NONE',  ( -4.483927247898539470, -16.52544592524342804, 72.29057627198102409 ) ) ;
#166449=ORIENTED_EDGE ( 'NONE', *, *, #114142, .T. ) ;
#166450=CARTESIAN_POINT ( 'NONE',  ( 12.14591786802309770, 12.06949235617756955, 54.37390960531435979 ) ) ;
#166451=CARTESIAN_POINT ( 'NONE',  ( 4.483927247898790824, -16.52544592524335698, 50.20942372801901854 ) ) ;
#166453=CARTESIAN_POINT ( 'NONE',  ( 16.46253265017146816, 9.564922557961045513, 56.66775706135233293 ) ) ;
#166454=CARTESIAN_POINT ( 'NONE',  ( 9.474510206698971260, -16.51473224551069308, 87.91557627198102409 ) ) ;
#166455=CARTESIAN_POINT ( 'NONE',  ( 9.474510206698729675, 16.51473224551082808, 72.08442372801900433 ) ) ;
#166457=CARTESIAN_POINT ( 'NONE',  ( -16.53943276465976808, -0.05219959533934237506, 18.75109039468568639 ) ) ;
#166458=CARTESIAN_POINT ( 'NONE',  ( -8.224510206698735004, -14.34966873604973081, 99.58442372801900433 ) ) ;
#166459=CARTESIAN_POINT ( 'NONE',  ( -5.049401038298153566, 19.05341960407611168, 35.20724293864768839 ) ) ;
#166460=CARTESIAN_POINT ( 'NONE',  ( -18.67979575497178146, -10.72451020669898902, 26.66557627198103475 ) ) ;
#166461=CARTESIAN_POINT ( 'NONE',  ( 18.67979575497194134, -10.72451020669871369, 60.83442372801901854 ) ) ;
#166462=CARTESIAN_POINT ( 'NONE',  ( -0.05219959533936034679, 19.03943276465977164, 102.5010903946856757 ) ) ;
#166463=CYLINDRICAL_SURFACE ( 'NONE', #134820, 2.500000000000002220 ) ;
#166464=CARTESIAN_POINT ( 'NONE',  ( 9.564922557960805705, 16.46253265017160317, 79.58224293864769550 ) ) ;
#166465=CARTESIAN_POINT ( 'NONE',  ( -13.89961937509977652, 13.97604488694528158, 115.6239096053143669 ) ) ;
#166466=CARTESIAN_POINT ( 'NONE',  ( -4.379528057220328563, 16.55341960407611168, 70.20724293864769550 ) ) ;
#166467=CARTESIAN_POINT ( 'NONE',  ( 0.05219959533909260263, 19.03943276465977164, 59.99890960531436690 ) ) ;
#166468=CARTESIAN_POINT ( 'NONE',  ( 5.049401038298161559, -19.05341960407611168, 77.70724293864765286 ) ) ;
#166469=CARTESIAN_POINT ( 'NONE',  ( -13.97604488694547697, 13.89961937509957934, 73.12609039468568994 ) ) ;
#166470=CARTESIAN_POINT ( 'NONE',  ( 0.05219959533907565091, 21.53943276465977519, 59.99890960531436690 ) ) ;
#166471=CARTESIAN_POINT ( 'NONE',  ( 14.29746914071049879, -8.314922557960816363, 113.3322429386476955 ) ) ;
#166472=CARTESIAN_POINT ( 'NONE',  ( 9.564922557961047289, -16.46253265017146816, 55.41775706135234003 ) ) ;
#166473=CARTESIAN_POINT ( 'NONE',  ( -9.564922557960796823, -16.46253265017161027, 52.08224293864768839 ) ) ;
#166474=CARTESIAN_POINT ( 'NONE',  ( 19.03943276465977164, -0.05219959533909143690, 98.74890960531436690 ) ) ;
#166475=CARTESIAN_POINT ( 'NONE',  ( 15.80617190586746368, 15.72974639402197994, 94.37390960531436690 ) ) ;
#166476=CARTESIAN_POINT ( 'NONE',  ( 14.34966873604960469, 8.224510206698951720, 74.16557627198102409 ) ) ;
#166477=CARTESIAN_POINT ( 'NONE',  ( -0.05219959533936034679, 19.03943276465977164, 47.50109039468566863 ) ) ;
#166478=CARTESIAN_POINT ( 'NONE',  ( -21.55341960407610458, -5.719274019375992779, 76.45724293864769550 ) ) ;
#166479=CARTESIAN_POINT ( 'NONE',  ( -15.72974639402197994, 15.80617190586746368, 65.62390960531436690 ) ) ;
#166481=CARTESIAN_POINT ( 'NONE',  ( -12.06949235617756955, 12.14591786802309770, 30.62390960531436335 ) ) ;
#166482=CARTESIAN_POINT ( 'NONE',  ( 18.62759615963255655, 10.81492255796105972, 91.66775706135234714 ) ) ;
#166483=CARTESIAN_POINT ( 'NONE',  ( 19.03943276465977164, -0.05219959533909143690, 73.74890960531435269 ) ) ;
#166484=CARTESIAN_POINT ( 'NONE',  ( 5.153800228976335163, 19.02544592524342804, 29.79057627198102409 ) ) ;
#166485=CARTESIAN_POINT ( 'NONE',  ( 21.52544592524334988, 5.823673210054432836, 36.45942372801901143 ) ) ;
#166487=CARTESIAN_POINT ( 'NONE',  ( -21.52544592524334988, -5.823673210054445271, 38.95942372801901854 ) ) ;
#166488=CARTESIAN_POINT ( 'NONE',  ( -5.049401038298153566, 19.05341960407611168, 45.20724293864769550 ) ) ;
#166489=CARTESIAN_POINT ( 'NONE',  ( 21.52544592524344225, -5.823673210054117533, 113.5405762719810383 ) ) ;
#166490=CARTESIAN_POINT ( 'NONE',  ( -19.02544592524334988, -5.153800228976617603, 58.95942372801900433 ) ) ;
#166491=CARTESIAN_POINT ( 'NONE',  ( -9.474510206698964154, 16.51473224551069663, 40.41557627198103120 ) ) ;
#166492=CARTESIAN_POINT ( 'NONE',  ( -14.34966873604972548, 8.224510206698743886, 33.33442372801900433 ) ) ;
#166493=CARTESIAN_POINT ( 'NONE',  ( 0.05219959533909260263, 19.03943276465977164, 24.99890960531435269 ) ) ;
#166494=CARTESIAN_POINT ( 'NONE',  ( -4.379528057220086978, -16.55341960407618274, 69.79275706135234714 ) ) ;
#166495=CARTESIAN_POINT ( 'NONE',  ( 16.46253265017160672, -9.564922557960803928, 43.33224293864769550 ) ) ;
#166497=CARTESIAN_POINT ( 'NONE',  ( -19.03943276465977164, 0.05219959533909376836, 86.24890960531436690 ) ) ;
#166498=CARTESIAN_POINT ( 'NONE',  ( 9.474510206698971260, -16.51473224551069308, 22.91557627198102765 ) ) ;
#166499=CARTESIAN_POINT ( 'NONE',  ( 5.823673210054125526, 21.52544592524343514, 64.79057627198103830 ) ) ;
#166500=CARTESIAN_POINT ( 'NONE',  ( 12.06949235617739724, 12.14591786802326823, 51.87609039468568284 ) ) ;
#166501=CARTESIAN_POINT ( 'NONE',  ( -5.823673210054431948, 21.52544592524334988, 97.70942372801904696 ) ) ;
#166502=CARTESIAN_POINT ( 'NONE',  ( -16.46253265017160317, 9.564922557960807481, 35.83224293864768839 ) ) ;
#166503=CARTESIAN_POINT ( 'NONE',  ( -12.06949235617756955, 12.14591786802309770, 30.62390960531436335 ) ) ;
#166504=CARTESIAN_POINT ( 'NONE',  ( 4.379528057220339221, -16.55341960407611168, 67.70724293864769550 ) ) ;
#166505=CARTESIAN_POINT ( 'NONE',  ( 5.049401038298161559, -19.05341960407611168, 67.70724293864769550 ) ) ;
#166506=CARTESIAN_POINT ( 'NONE',  ( 18.62759615963255655, 10.81492255796105972, 111.6677570613523613 ) ) ;
#166507=CARTESIAN_POINT ( 'NONE',  ( -0.05219959533937732626, 21.53943276465977519, 27.50109039468567929 ) ) ;
#166508=CARTESIAN_POINT ( 'NONE',  ( 16.51473224551069308, 9.474510206698969483, 79.16557627198103830 ) ) ;
#166509=CARTESIAN_POINT ( 'NONE',  ( -5.823673210054431948, 21.52544592524334988, 82.70942372801900433 ) ) ;
#166510=CARTESIAN_POINT ( 'NONE',  ( -16.55341960407617563, 4.379528057220093196, 58.54275706135235424 ) ) ;
#166511=CARTESIAN_POINT ( 'NONE',  ( 14.34966873604972726, -8.224510206698740333, 30.83442372801902209 ) ) ;
#166512=CARTESIAN_POINT ( 'NONE',  ( -16.52544592524342804, 4.483927247898546575, 91.04057627198103830 ) ) ;
#166513=CARTESIAN_POINT ( 'NONE',  ( -0.05219959533937732626, 21.53943276465977519, 97.50109039468567573 ) ) ;
#166514=CARTESIAN_POINT ( 'NONE',  ( 12.14591786802309770, 12.06949235617756955, 34.37390960531435979 ) ) ;
#166515=CARTESIAN_POINT ( 'NONE',  ( -9.564922557960796823, -16.46253265017161027, 27.08224293864769550 ) ) ;
#166516=CARTESIAN_POINT ( 'NONE',  ( 0.05219959533934541429, -16.53943276465976808, 50.00109039468568994 ) ) ;
#166517=CARTESIAN_POINT ( 'NONE',  ( 8.224510206698953496, -14.34966873604960469, 57.91557627198103120 ) ) ;
#166518=CARTESIAN_POINT ( 'NONE',  ( 14.34966873604972726, -8.224510206698740333, 100.8344237280190185 ) ) ;
#166519=CARTESIAN_POINT ( 'NONE',  ( -9.474510206698964154, 16.51473224551069663, 110.4155762719810383 ) ) ;
#166520=CARTESIAN_POINT ( 'NONE',  ( -5.049401038298153566, 19.05341960407611168, 110.2072429386476671 ) ) ;
#166521=CARTESIAN_POINT ( 'NONE',  ( 13.89961937509957401, 13.97604488694547697, 21.87609039468566152 ) ) ;
#166522=EDGE_CURVE ( 'NONE', #116638, #199703, #85021, .T. ) ;
#166523=CARTESIAN_POINT ( 'NONE',  ( -12.14591786802309592, -12.06949235617757132, 86.87390960531438111 ) ) ;
#166524=CARTESIAN_POINT ( 'NONE',  ( -16.51473224551069308, -9.474510206698971260, 96.66557627198102409 ) ) ;
#166526=CARTESIAN_POINT ( 'NONE',  ( 14.29746914071037800, 8.314922557961029526, 46.66775706135234714 ) ) ;
#166527=CARTESIAN_POINT ( 'NONE',  ( -19.02544592524342804, 5.153800228976336051, 46.04057627198101699 ) ) ;
#166528=CARTESIAN_POINT ( 'NONE',  ( 14.29746914071037800, 8.314922557961029526, 51.66775706135234714 ) ) ;
#166529=DIRECTION ( 'NONE',  ( 0.000000000000000000, 0.000000000000000000, 1.000000000000000000 ) ) ;
#166530=CARTESIAN_POINT ( 'NONE',  ( -0.05219959533936034679, 19.03943276465977164, 52.50109039468566863 ) ) ;
#166531=CARTESIAN_POINT ( 'NONE',  ( 13.97604488694527802, 13.89961937509977652, 44.37390960531435269 ) ) ;
#166532=CARTESIAN_POINT ( 'NONE',  ( -4.483927247898782831, 16.52544592524335698, 82.70942372801900433 ) ) ;
#166533=CARTESIAN_POINT ( 'NONE',  ( 16.51473224551083163, -9.474510206698727899, 80.83442372801899012 ) ) ;
#166534=CARTESIAN_POINT ( 'NONE',  ( 9.564922557961047289, -16.46253265017146816, 30.41775706135232937 ) ) ;
#166535=CARTESIAN_POINT ( 'NONE',  ( 5.049401038298161559, -19.05341960407611168, 57.70724293864769550 ) ) ;
#166536=CARTESIAN_POINT ( 'NONE',  ( -8.314922557960811034, -14.29746914071050412, 102.0822429386476955 ) ) ;
#166537=CARTESIAN_POINT ( 'NONE',  ( 13.97604488694548053, -13.89961937509957401, 70.62609039468567573 ) ) ;
#166538=CARTESIAN_POINT ( 'NONE',  ( 21.53943276465977519, -0.05219959533907433946, 63.74890960531435979 ) ) ;
#166539=CARTESIAN_POINT ( 'NONE',  ( -13.97604488694547697, 13.89961937509957934, 23.12609039468565442 ) ) ;
#166540=CARTESIAN_POINT ( 'NONE',  ( -0.05219959533909027116, -19.03943276465977164, 102.4989096053143669 ) ) ;
#166541=CARTESIAN_POINT ( 'NONE',  ( 18.62759615963271287, -10.81492255796078972, 83.33224293864769550 ) ) ;
#166542=DIRECTION ( 'NONE',  ( -0.000000000000000000, -0.000000000000000000, 1.000000000000000000 ) ) ;
#166543=CARTESIAN_POINT ( 'NONE',  ( 0.05219959533936267826, -19.03943276465977164, 105.0010903946856615 ) ) ;
#166545=CARTESIAN_POINT ( 'NONE',  ( 8.224510206698742110, 14.34966873604972548, 22.08442372801901143 ) ) ;
#166546=CARTESIAN_POINT ( 'NONE',  ( 5.049401038298161559, -19.05341960407611168, 27.70724293864769550 ) ) ;
#166547=CARTESIAN_POINT ( 'NONE',  ( -16.46253265017160317, 9.564922557960807481, 105.8322429386476955 ) ) ;
#166548=CARTESIAN_POINT ( 'NONE',  ( 10.81492255796078972, 18.62759615963270932, 94.58224293864769550 ) ) ;
#166549=CARTESIAN_POINT ( 'NONE',  ( 0.05219959533937995610, -21.53943276465977519, 55.00109039468568284 ) ) ;
#166550=CARTESIAN_POINT ( 'NONE',  ( 13.97604488694548053, -13.89961937509957401, 110.6260903946856615 ) ) ;
#166551=CARTESIAN_POINT ( 'NONE',  ( -21.52544592524334988, -5.823673210054445271, 108.9594237280190185 ) ) ;
#166552=CARTESIAN_POINT ( 'NONE',  ( -14.29746914071037622, -8.314922557961029526, 104.1677570613523471 ) ) ;
#166553=CARTESIAN_POINT ( 'NONE',  ( -10.72451020669898014, 18.67979575497178502, 95.41557627198102409 ) ) ;
#166554=CARTESIAN_POINT ( 'NONE',  ( -8.224510206698948167, 14.34966873604960824, 50.41557627198103120 ) ) ;
#166555=CARTESIAN_POINT ( 'NONE',  ( 5.153800228976615827, -19.02544592524334988, 80.20942372801901854 ) ) ;
#166556=CARTESIAN_POINT ( 'NONE',  ( 13.89961937509957401, 13.97604488694547697, 61.87609039468566863 ) ) ;
#166557=CARTESIAN_POINT ( 'NONE',  ( 18.67979575497194134, -10.72451020669871369, 70.83442372801901854 ) ) ;
#166558=CARTESIAN_POINT ( 'NONE',  ( 19.05341960407617918, -5.049401038297876454, 41.04275706135233293 ) ) ;
#166559=CARTESIAN_POINT ( 'NONE',  ( -4.379528057220328563, 16.55341960407611168, 105.2072429386477097 ) ) ;
#166560=CARTESIAN_POINT ( 'NONE',  ( -5.823673210054116645, -21.52544592524344225, 42.29057627198103120 ) ) ;
#166561=CARTESIAN_POINT ( 'NONE',  ( -12.06949235617756955, 12.14591786802309770, 30.62390960531436335 ) ) ;
#166562=CARTESIAN_POINT ( 'NONE',  ( 10.81492255796106328, -18.62759615963255655, 100.4177570613523471 ) ) ;
#166563=CARTESIAN_POINT ( 'NONE',  ( 14.34966873604972726, -8.224510206698740333, 70.83442372801901854 ) ) ;
#166564=CARTESIAN_POINT ( 'NONE',  ( 8.224510206698953496, -14.34966873604960469, 22.91557627198102765 ) ) ;
#166565=CARTESIAN_POINT ( 'NONE',  ( -15.72974639402176322, -15.80617190586768395, 59.37609039468568284 ) ) ;
#166566=CARTESIAN_POINT ( 'NONE',  ( -18.67979575497193778, 10.72451020669871902, 63.33442372801900433 ) ) ;
#166567=CARTESIAN_POINT ( 'NONE',  ( 5.823673210054125526, 21.52544592524343514, 74.79057627198105251 ) ) ;
#166568=VERTEX_POINT ( 'NONE', #194169 ) ;
#166569=CARTESIAN_POINT ( 'NONE',  ( 16.51473224551069308, 9.474510206698969483, 29.16557627198103475 ) ) ;
#166570=CARTESIAN_POINT ( 'NONE',  ( 10.81492255796106328, -18.62759615963255655, 45.41775706135234003 ) ) ;
#166571=CARTESIAN_POINT ( 'NONE',  ( -5.153800228976328057, -19.02544592524343514, 27.29057627198103120 ) ) ;
#166572=CARTESIAN_POINT ( 'NONE',  ( 0.05219959533909260263, 19.03943276465977164, 39.99890960531436690 ) ) ;
#166573=CARTESIAN_POINT ( 'NONE',  ( 16.52544592524342804, -4.483927247898539470, 83.54057627198102409 ) ) ;
#166574=CARTESIAN_POINT ( 'NONE',  ( 19.03943276465977164, -0.05219959533909143690, 88.74890960531436690 ) ) ;
#166575=CARTESIAN_POINT ( 'NONE',  ( 14.34966873604960469, 8.224510206698951720, 29.16557627198103120 ) ) ;
#166576=CARTESIAN_POINT ( 'NONE',  ( 12.06949235617757843, -12.14591786802309237, 103.1239096053143811 ) ) ;
#166577=CARTESIAN_POINT ( 'NONE',  ( 15.72974639402199770, -15.80617190586745480, 68.12390960531436690 ) ) ;
#166579=CARTESIAN_POINT ( 'NONE',  ( -10.81492255796078084, -18.62759615963271287, 102.0822429386476955 ) ) ;
#166580=CARTESIAN_POINT ( 'NONE',  ( 13.89961937509977652, -13.97604488694527269, 108.1239096053143669 ) ) ;
#166581=CARTESIAN_POINT ( 'NONE',  ( -19.02544592524342804, 5.153800228976336051, 71.04057627198099567 ) ) ;
#166582=CARTESIAN_POINT ( 'NONE',  ( -14.34966873604972548, 8.224510206698743886, 28.33442372801902209 ) ) ;
#166583=CARTESIAN_POINT ( 'NONE',  ( 21.53943276465977519, -0.05219959533907433946, 58.74890960531436690 ) ) ;
#166584=CARTESIAN_POINT ( 'NONE',  ( -15.80617190586768217, 15.72974639402176855, 78.12609039468570415 ) ) ;
#166585=CARTESIAN_POINT ( 'NONE',  ( -19.02544592524342804, 5.153800228976336051, 81.04057627198103830 ) ) ;
#166586=CARTESIAN_POINT ( 'NONE',  ( -13.89961937509977652, 13.97604488694528158, 105.6239096053143527 ) ) ;
#166587=CARTESIAN_POINT ( 'NONE',  ( -0.05219959533934338120, 16.53943276465976808, 77.50109039468567573 ) ) ;
#166588=CARTESIAN_POINT ( 'NONE',  ( 21.52544592524334988, 5.823673210054432836, 51.45942372801901854 ) ) ;
#166589=CARTESIAN_POINT ( 'NONE',  ( -21.52544592524334988, -5.823673210054445271, 98.95942372801903275 ) ) ;
#166590=CARTESIAN_POINT ( 'NONE',  ( -4.379528057220086978, -16.55341960407618274, 59.79275706135234714 ) ) ;
#166591=CARTESIAN_POINT ( 'NONE',  ( -5.719274019375665041, -21.55341960407619695, 19.79275706135235069 ) ) ;
#166592=CARTESIAN_POINT ( 'NONE',  ( -5.153800228976328057, -19.02544592524343514, 22.29057627198102765 ) ) ;
#166593=CARTESIAN_POINT ( 'NONE',  ( -21.53943276465977519, 0.05219959533907696930, 91.24890960531436690 ) ) ;
#166594=CARTESIAN_POINT ( 'NONE',  ( -5.153800228976607833, 19.02544592524334988, 42.70942372801901143 ) ) ;
#166595=CARTESIAN_POINT ( 'NONE',  ( 21.55341960407610458, 5.719274019375980345, 38.95724293864768839 ) ) ;
#166596=CARTESIAN_POINT ( 'NONE',  ( 19.03943276465977164, -0.05219959533909143690, 78.74890960531436690 ) ) ;
#166597=CARTESIAN_POINT ( 'NONE',  ( -14.34966873604960291, -8.224510206698953496, 41.66557627198103120 ) ) ;
#166598=CARTESIAN_POINT ( 'NONE',  ( -16.20579543436675252, 7.371946100355232900, 64.43479165828124167 ) ) ;
#166600=CARTESIAN_POINT ( 'NONE',  ( 5.153800228976615827, -19.02544592524334988, 95.20942372801897591 ) ) ;
#166601=CARTESIAN_POINT ( 'NONE',  ( 10.72451020669898902, -18.67979575497178502, 67.91557627198102409 ) ) ;
#166602=CARTESIAN_POINT ( 'NONE',  ( 14.34966873604960469, 8.224510206698951720, 54.16557627198103120 ) ) ;
#166603=CARTESIAN_POINT ( 'NONE',  ( -4.379528057220086978, -16.55341960407618274, 29.79275706135234358 ) ) ;
#166604=CARTESIAN_POINT ( 'NONE',  ( -19.05341960407611168, -5.049401038298163336, 51.45724293864770260 ) ) ;
#166605=CARTESIAN_POINT ( 'NONE',  ( 18.62759615963255655, 10.81492255796105972, 21.66775706135235069 ) ) ;
#166606=CARTESIAN_POINT ( 'NONE',  ( -16.51473224551082808, 9.474510206698731452, 78.33442372801900433 ) ) ;
#166607=CARTESIAN_POINT ( 'NONE',  ( -13.97604488694527625, -13.89961937509977652, 76.87390960531433848 ) ) ;
#166608=CARTESIAN_POINT ( 'NONE',  ( -13.97604488694527625, -13.89961937509977652, 71.87390960531433848 ) ) ;
#166609=CARTESIAN_POINT ( 'NONE',  ( 5.719274019375991003, -21.55341960407610458, 82.70724293864770971 ) ) ;
#166610=CARTESIAN_POINT ( 'NONE',  ( 0.05219959533909260263, 19.03943276465977164, 29.99890960531435979 ) ) ;
#166611=CARTESIAN_POINT ( 'NONE',  ( -18.22780087662123094, -5.499999999999984901, 81.48459894673892734 ) ) ;
#166612=CARTESIAN_POINT ( 'NONE',  ( -12.14591786802309592, -12.06949235617757132, 56.87390960531436690 ) ) ;
#166613=CARTESIAN_POINT ( 'NONE',  ( 19.05341960407611168, 5.049401038298154454, 93.95724293864769550 ) ) ;
#166614=CARTESIAN_POINT ( 'NONE',  ( 5.049401038297881783, 19.05341960407617563, 52.29275706135234003 ) ) ;
#166616=CARTESIAN_POINT ( 'NONE',  ( 5.719274019375991003, -21.55341960407610458, 72.70724293864769550 ) ) ;
#166617=CARTESIAN_POINT ( 'NONE',  ( -5.049401038297874678, -19.05341960407617918, 39.79275706135232582 ) ) ;
#166618=CARTESIAN_POINT ( 'NONE',  ( 19.03943276465977164, -0.05219959533909143690, 93.74890960531435269 ) ) ;
#166620=CARTESIAN_POINT ( 'NONE',  ( 18.67979575497178502, 10.72451020669898547, 24.16557627198103120 ) ) ;
#166621=CARTESIAN_POINT ( 'NONE',  ( -0.05219959533909027116, -19.03943276465977164, 77.49890960531435269 ) ) ;
#166622=CARTESIAN_POINT ( 'NONE',  ( -21.55341960407619339, 5.719274019375674811, 53.54275706135234714 ) ) ;
#166623=CARTESIAN_POINT ( 'NONE',  ( -12.06949235617756955, 12.14591786802309770, 115.6239096053143669 ) ) ;
#166624=CARTESIAN_POINT ( 'NONE',  ( 18.62759615963255655, 10.81492255796105972, 21.66775706135235069 ) ) ;
#166625=CARTESIAN_POINT ( 'NONE',  ( 9.474510206698971260, -16.51473224551069308, 97.91557627198102409 ) ) ;
#166627=CARTESIAN_POINT ( 'NONE',  ( 21.52544592524334988, 5.823673210054432836, 41.45942372801901143 ) ) ;
#166629=CARTESIAN_POINT ( 'NONE',  ( -0.05219959533909027116, -19.03943276465977164, 102.4989096053143669 ) ) ;
#166631=CARTESIAN_POINT ( 'NONE',  ( -5.719274019375978568, 21.55341960407610458, 105.2072429386477097 ) ) ;
#166632=CARTESIAN_POINT ( 'NONE',  ( 0.05219959533909260263, 19.03943276465977164, 49.99890960531435979 ) ) ;
#166633=CARTESIAN_POINT ( 'NONE',  ( 14.34966873604972726, -8.224510206698740333, 30.83442372801902209 ) ) ;
#166635=CARTESIAN_POINT ( 'NONE',  ( 0.05219959533937995610, -21.53943276465977519, 100.0010903946857042 ) ) ;
#166636=CARTESIAN_POINT ( 'NONE',  ( 13.89961937509977652, -13.97604488694527269, 38.12390960531436690 ) ) ;
#166637=CARTESIAN_POINT ( 'NONE',  ( -21.52544592524334988, -5.823673210054445271, 93.95942372801903275 ) ) ;
#166638=CARTESIAN_POINT ( 'NONE',  ( -13.89961937509977652, 13.97604488694528158, 90.62390960531432427 ) ) ;
#166639=CARTESIAN_POINT ( 'NONE',  ( 21.52544592524334988, 5.823673210054432836, 66.45942372801903275 ) ) ;
#166641=CARTESIAN_POINT ( 'NONE',  ( -9.474510206698964154, 16.51473224551069663, 100.4155762719810241 ) ) ;
#166642=CARTESIAN_POINT ( 'NONE',  ( -17.50000000000017408, 3.292511757969708519, 30.06520270210541668 ) ) ;
#166643=CARTESIAN_POINT ( 'NONE',  ( -8.224510206698735004, -14.34966873604973081, 49.58442372801901143 ) ) ;
#166644=CARTESIAN_POINT ( 'NONE',  ( -4.379528057220086978, -16.55341960407618274, 69.79275706135234714 ) ) ;
#166645=CARTESIAN_POINT ( 'NONE',  ( 5.719274019375673035, 21.55341960407619339, 62.29275706135236845 ) ) ;
#166646=CARTESIAN_POINT ( 'NONE',  ( 10.81492255796106328, -18.62759615963255655, 85.41775706135236135 ) ) ;
#166649=CARTESIAN_POINT ( 'NONE',  ( -14.34966873604972548, 8.224510206698743886, 33.33442372801900433 ) ) ;
#166650=CARTESIAN_POINT ( 'NONE',  ( -9.474510206698964154, 16.51473224551069663, 70.41557627198102409 ) ) ;
#166651=CARTESIAN_POINT ( 'NONE',  ( 9.564922557960805705, 16.46253265017160317, 99.58224293864770971 ) ) ;
#166652=CARTESIAN_POINT ( 'NONE',  ( 17.49999999999999289, 5.500000000000063061, 41.70309617465829177 ) ) ;
#166653=CARTESIAN_POINT ( 'NONE',  ( 9.564922557960805705, 16.46253265017160317, 24.58224293864769194 ) ) ;
#166654=CARTESIAN_POINT ( 'NONE',  ( -21.52544592524343514, 5.823673210054127303, 31.04057627198102409 ) ) ;
#166655=CARTESIAN_POINT ( 'NONE',  ( -0.05219959533934338120, 16.53943276465976808, 87.50109039468568994 ) ) ;
#166656=CARTESIAN_POINT ( 'NONE',  ( 12.14591786802309770, 12.06949235617756955, 89.37390960531435269 ) ) ;
#166657=CARTESIAN_POINT ( 'NONE',  ( -0.05219959533909027116, -19.03943276465977164, 67.49890960531436690 ) ) ;
#166658=CARTESIAN_POINT ( 'NONE',  ( 21.53943276465977519, 0.05219959533937863772, 96.25109039468568994 ) ) ;
#166660=CARTESIAN_POINT ( 'NONE',  ( 16.55341960407618274, -4.379528057220086978, 31.04275706135234714 ) ) ;
#166661=CARTESIAN_POINT ( 'NONE',  ( -14.29746914071049879, 8.314922557960819915, 70.83224293864770971 ) ) ;
#166662=CARTESIAN_POINT ( 'NONE',  ( -10.72451020669870658, -18.67979575497194134, 44.58442372801901854 ) ) ;
#166663=CARTESIAN_POINT ( 'NONE',  ( 21.55341960407610458, 5.719274019375980345, 68.95724293864769550 ) ) ;
#166664=CARTESIAN_POINT ( 'NONE',  ( -19.02544592524334988, -5.153800228976617603, 38.95942372801900433 ) ) ;
#166666=CARTESIAN_POINT ( 'NONE',  ( 16.51473224551069308, 9.474510206698969483, 84.16557627198102409 ) ) ;
#166667=CARTESIAN_POINT ( 'NONE',  ( 14.29746914071049879, -8.314922557960816363, 48.33224293864770260 ) ) ;
#166668=CARTESIAN_POINT ( 'NONE',  ( 4.483927247898545687, 16.52544592524342804, 29.79057627198102409 ) ) ;
#166669=CARTESIAN_POINT ( 'NONE',  ( 16.55341960407618274, -4.379528057220086978, 106.0427570613523471 ) ) ;
#166670=CARTESIAN_POINT ( 'NONE',  ( -16.46253265017146816, -9.564922557961047289, 64.16775706135233293 ) ) ;
#166671=CARTESIAN_POINT ( 'NONE',  ( 13.89961937509957579, 13.97604488694547520, 76.87609039468566152 ) ) ;
#166672=CARTESIAN_POINT ( 'NONE',  ( 0.05219959533909260263, 19.03943276465977164, 114.9989096053143669 ) ) ;
#166673=CARTESIAN_POINT ( 'NONE',  ( 16.53943276465976808, -0.05219959533910856209, 88.74890960531436690 ) ) ;
#166676=CARTESIAN_POINT ( 'NONE',  ( 19.03943276465977164, -0.05219959533909143690, 28.74890960531435624 ) ) ;
#166677=CARTESIAN_POINT ( 'NONE',  ( -5.719274019375978568, 21.55341960407610458, 35.20724293864768839 ) ) ;
#166678=CARTESIAN_POINT ( 'NONE',  ( 5.823673210054125526, 21.52544592524343514, 64.79057627198103830 ) ) ;
#166679=CARTESIAN_POINT ( 'NONE',  ( -16.53943276465976808, 0.05219959533911058130, 111.2489096053143669 ) ) ;
#166680=CARTESIAN_POINT ( 'NONE',  ( -16.53943276465976808, -0.05219959533934237506, 68.75109039468568994 ) ) ;
#166681=CARTESIAN_POINT ( 'NONE',  ( -5.153800228976328057, -19.02544592524343514, 47.29057627198102409 ) ) ;
#166682=CARTESIAN_POINT ( 'NONE',  ( 18.62759615963255655, 10.81492255796105972, 61.66775706135235424 ) ) ;
#166683=CARTESIAN_POINT ( 'NONE',  ( -8.224510206698948167, 14.34966873604960824, 105.4155762719810383 ) ) ;
#166684=CARTESIAN_POINT ( 'NONE',  ( -13.97604488694547697, 13.89961937509957934, 88.12609039468563310 ) ) ;
#166687=CARTESIAN_POINT ( 'NONE',  ( -15.72974639402197994, 15.80617190586746368, 30.62390960531436335 ) ) ;
#166688=CARTESIAN_POINT ( 'NONE',  ( 0.05219959533937995610, -21.53943276465977519, 75.00109039468568994 ) ) ;
#166689=CARTESIAN_POINT ( 'NONE',  ( -12.14591786802326823, 12.06949235617739902, 58.12609039468568994 ) ) ;
#166690=CARTESIAN_POINT ( 'NONE',  ( 0.05219959533910956823, 16.53943276465976808, 39.99890960531436690 ) ) ;
#166691=CARTESIAN_POINT ( 'NONE',  ( 5.719274019375991003, -21.55341960407610458, 72.70724293864769550 ) ) ;
#166692=CARTESIAN_POINT ( 'NONE',  ( -10.72451020669898014, 18.67979575497178502, 60.41557627198102409 ) ) ;
#166694=CARTESIAN_POINT ( 'NONE',  ( -16.51473224551082808, 9.474510206698731452, 83.33442372801899012 ) ) ;
#166695=CARTESIAN_POINT ( 'NONE',  ( -5.719274019375978568, 21.55341960407610458, 25.20724293864769550 ) ) ;
#166696=CARTESIAN_POINT ( 'NONE',  ( -19.05341960407611168, -5.049401038298163336, 46.45724293864768129 ) ) ;
#166697=CARTESIAN_POINT ( 'NONE',  ( 19.05341960407611168, 5.049401038298154454, 23.95724293864769194 ) ) ;
#166699=FACE_BOUND ( 'NONE', #7931, .T. ) ;
#166701=CARTESIAN_POINT ( 'NONE',  ( 0.05219959533934541429, -16.53943276465976808, 65.00109039468568994 ) ) ;
#166702=CARTESIAN_POINT ( 'NONE',  ( -21.53943276465977519, 0.05219959533907696930, 106.2489096053143811 ) ) ;
#166703=CARTESIAN_POINT ( 'NONE',  ( -9.564922557960796823, -16.46253265017161027, 52.08224293864768839 ) ) ;
#166704=CARTESIAN_POINT ( 'NONE',  ( 5.823673210054444382, -21.52544592524334988, 40.20942372801901854 ) ) ;
#166705=CARTESIAN_POINT ( 'NONE',  ( 16.51473224551069308, 9.474510206698969483, 94.16557627198103830 ) ) ;
#166708=CARTESIAN_POINT ( 'NONE',  ( -10.81492255796105439, 18.62759615963255655, 37.91775706135235424 ) ) ;
#166709=CARTESIAN_POINT ( 'NONE',  ( -9.564922557960796823, -16.46253265017161027, 112.0822429386476955 ) ) ;
#166710=CARTESIAN_POINT ( 'NONE',  ( -5.049401038297874678, -19.05341960407617918, 94.79275706135230450 ) ) ;
#166711=CARTESIAN_POINT ( 'NONE',  ( -16.46253265017146816, -9.564922557961047289, 44.16775706135232582 ) ) ;
#166712=CARTESIAN_POINT ( 'NONE',  ( -18.62759615963270932, 10.81492255796079327, 95.83224293864770971 ) ) ;
#166713=CARTESIAN_POINT ( 'NONE',  ( 5.153800228976615827, -19.02544592524334988, 30.20942372801900433 ) ) ;
#166714=CARTESIAN_POINT ( 'NONE',  ( 5.153800228976615827, -19.02544592524334988, 45.20942372801901143 ) ) ;
#166715=CARTESIAN_POINT ( 'NONE',  ( -16.52544592524335698, -4.483927247898792601, 93.95942372801903275 ) ) ;
#166716=CARTESIAN_POINT ( 'NONE',  ( -18.22780087662126647, -5.499999999999827693, 43.98236817873107185 ) ) ;
#166717=CARTESIAN_POINT ( 'NONE',  ( -16.46253265017160317, 9.564922557960807481, 75.83224293864769550 ) ) ;
#166719=CARTESIAN_POINT ( 'NONE',  ( 10.72451020669871369, 18.67979575497193778, 77.08442372801901854 ) ) ;
#166720=CARTESIAN_POINT ( 'NONE',  ( 5.719274019375673035, 21.55341960407619339, 82.29275706135234714 ) ) ;
#166722=CARTESIAN_POINT ( 'NONE',  ( -19.02544592524342804, 5.153800228976336051, 86.04057627198103830 ) ) ;
#166723=CARTESIAN_POINT ( 'NONE',  ( 21.53943276465977519, 0.05219959533937863772, 56.25109039468568284 ) ) ;
#166724=CARTESIAN_POINT ( 'NONE',  ( -5.049401038297874678, -19.05341960407617918, 104.7927570613523471 ) ) ;
#166725=CARTESIAN_POINT ( 'NONE',  ( -9.474510206698964154, 16.51473224551069663, 70.41557627198102409 ) ) ;
#166726=CARTESIAN_POINT ( 'NONE',  ( 16.46253265017160672, -9.564922557960803928, 108.3322429386476955 ) ) ;
#166727=CARTESIAN_POINT ( 'NONE',  ( -0.05219959533909027116, -19.03943276465977164, 82.49890960531436690 ) ) ;
#166728=CARTESIAN_POINT ( 'NONE',  ( -17.48853670773246805, -5.747243402303017668, 91.33328700250007159 ) ) ;
#166729=CARTESIAN_POINT ( 'NONE',  ( 5.153800228976335163, 19.02544592524342804, 64.79057627198100988 ) ) ;
#166730=CARTESIAN_POINT ( 'NONE',  ( 19.02544592524343514, -5.153800228976328945, 58.54057627198102409 ) ) ;
#166731=CARTESIAN_POINT ( 'NONE',  ( -21.52544592524343514, 5.823673210054127303, 111.0405762719810525 ) ) ;
#166732=CARTESIAN_POINT ( 'NONE',  ( -12.14591786802326823, 12.06949235617739902, 93.12609039468568994 ) ) ;
#166734=CARTESIAN_POINT ( 'NONE',  ( 19.05341960407617918, -5.049401038297876454, 51.04275706135231871 ) ) ;
#166735=CARTESIAN_POINT ( 'NONE',  ( -19.03943276465977164, 0.05219959533909376836, 81.24890960531436690 ) ) ;
#166736=CARTESIAN_POINT ( 'NONE',  ( 14.29746914071049879, -8.314922557960816363, 73.33224293864769550 ) ) ;
#166737=CARTESIAN_POINT ( 'NONE',  ( 12.14591786802309770, 12.06949235617756955, 104.3739096053143669 ) ) ;
#166738=CARTESIAN_POINT ( 'NONE',  ( -5.049401038298153566, 19.05341960407611168, 110.2072429386476671 ) ) ;
#166740=CARTESIAN_POINT ( 'NONE',  ( -13.97604488694527625, -13.89961937509977652, 101.8739096053143811 ) ) ;
#166741=CARTESIAN_POINT ( 'NONE',  ( -16.52544592524342804, 4.483927247898546575, 76.04057627198102409 ) ) ;
#166743=CARTESIAN_POINT ( 'NONE',  ( 5.153800228976615827, -19.02544592524334988, 35.20942372801899722 ) ) ;
#166744=CARTESIAN_POINT ( 'NONE',  ( -14.34966873604972548, 8.224510206698743886, 93.33442372801901854 ) ) ;
#166745=CARTESIAN_POINT ( 'NONE',  ( 16.51473224551069308, 9.474510206698969483, 84.16557627198102409 ) ) ;
#166746=CARTESIAN_POINT ( 'NONE',  ( -18.62759615963255300, -10.81492255796106328, 59.16775706135234714 ) ) ;
#166747=CARTESIAN_POINT ( 'NONE',  ( -15.72974639402197994, 15.80617190586746368, 40.62390960531435269 ) ) ;
#166748=CARTESIAN_POINT ( 'NONE',  ( -21.53943276465977519, 0.05219959533907696930, 116.2489096053143669 ) ) ;
#166749=CARTESIAN_POINT ( 'NONE',  ( 0.05219959533907565091, 21.53943276465977519, 69.99890960531435269 ) ) ;
#166750=CARTESIAN_POINT ( 'NONE',  ( -14.29746914071049879, 8.314922557960819915, 95.83224293864770971 ) ) ;
#166751=CARTESIAN_POINT ( 'NONE',  ( 13.97604488694548053, -13.89961937509957401, 55.62609039468566863 ) ) ;
#166753=CARTESIAN_POINT ( 'NONE',  ( -19.03943276465977164, 0.05219959533909376836, 31.24890960531435979 ) ) ;
#166754=CARTESIAN_POINT ( 'NONE',  ( -13.89961937509977652, 13.97604488694528158, 85.62390960531433848 ) ) ;
#166755=CARTESIAN_POINT ( 'NONE',  ( 5.049401038298161559, -19.05341960407611168, 87.70724293864769550 ) ) ;
#166756=CARTESIAN_POINT ( 'NONE',  ( -0.05219959533910754901, -16.53943276465976808, 102.4989096053143811 ) ) ;
#166758=VECTOR ( 'NONE', #127087, 1000.000000000000000 ) ;
#166759=CARTESIAN_POINT ( 'NONE',  ( 0.05219959533910956823, 16.53943276465976808, 24.99890960531435624 ) ) ;
#166760=CARTESIAN_POINT ( 'NONE',  ( -16.53943276465976808, -0.05219959533934237506, 43.75109039468568284 ) ) ;
#166761=CARTESIAN_POINT ( 'NONE',  ( 21.53943276465977519, 0.05219959533937863772, 106.2510903946856757 ) ) ;
#166762=CARTESIAN_POINT ( 'NONE',  ( 13.97604488694527802, 13.89961937509977652, 104.3739096053143385 ) ) ;
#166763=CARTESIAN_POINT ( 'NONE',  ( 18.62759615963271287, -10.81492255796078972, 113.3322429386476955 ) ) ;
#166764=CARTESIAN_POINT ( 'NONE',  ( -0.05219959533909027116, -19.03943276465977164, 47.49890960531435979 ) ) ;
#166766=CARTESIAN_POINT ( 'NONE',  ( 12.14591786802327356, -12.06949235617739191, 40.62609039468567573 ) ) ;
#166767=CARTESIAN_POINT ( 'NONE',  ( 9.474510206698729675, 16.51473224551082808, 102.0844237280190043 ) ) ;
#166768=CARTESIAN_POINT ( 'NONE',  ( -19.03943276465977164, 0.05219959533909376836, 41.24890960531435269 ) ) ;
#166769=CARTESIAN_POINT ( 'NONE',  ( -14.34966873604960291, -8.224510206698953496, 96.66557627198102409 ) ) ;
#166770=CARTESIAN_POINT ( 'NONE',  ( -15.72974639402197994, 15.80617190586746368, 100.6239096053143811 ) ) ;
#166771=CARTESIAN_POINT ( 'NONE',  ( 9.474510206698729675, 16.51473224551082808, 77.08442372801900433 ) ) ;
#166773=CARTESIAN_POINT ( 'NONE',  ( -16.46253265017160317, 9.564922557960807481, 85.83224293864769550 ) ) ;
#166774=CARTESIAN_POINT ( 'NONE',  ( -21.53943276465977519, -0.05219959533937600094, 18.75109039468568639 ) ) ;
#166775=CARTESIAN_POINT ( 'NONE',  ( -5.153800228976328057, -19.02544592524343514, 22.29057627198102765 ) ) ;
#166776=CARTESIAN_POINT ( 'NONE',  ( 19.05341960407611168, 5.049401038298154454, 88.95724293864769550 ) ) ;
#166777=CARTESIAN_POINT ( 'NONE',  ( -17.50000000000000711, -5.499999999999944045, 81.28230962303565832 ) ) ;
#166778=CARTESIAN_POINT ( 'NONE',  ( -19.02544592524342804, 5.153800228976336051, 86.04057627198103830 ) ) ;
#166779=CARTESIAN_POINT ( 'NONE',  ( -5.823673210054431948, 21.52544592524334988, 32.70942372801900433 ) ) ;
#166780=CARTESIAN_POINT ( 'NONE',  ( -8.224510206698948167, 14.34966873604960824, 90.41557627198103830 ) ) ;
#166781=CARTESIAN_POINT ( 'NONE',  ( -13.89961937509977652, 13.97604488694528158, 95.62390960531436690 ) ) ;
#166782=CARTESIAN_POINT ( 'NONE',  ( -5.153800228976607833, 19.02544592524334988, 27.70942372801899722 ) ) ;
#166783=CARTESIAN_POINT ( 'NONE',  ( 16.53943276465976808, 0.05219959533934440121, 46.25109039468567573 ) ) ;
#166784=CARTESIAN_POINT ( 'NONE',  ( 21.55341960407619695, -5.719274019375665929, 71.04275706135234714 ) ) ;
#166785=CARTESIAN_POINT ( 'NONE',  ( 4.483927247898790824, -16.52544592524335698, 25.20942372801901854 ) ) ;
#166786=CARTESIAN_POINT ( 'NONE',  ( -16.51473224551069308, -9.474510206698971260, 66.66557627198102409 ) ) ;
#166787=CARTESIAN_POINT ( 'NONE',  ( 19.05341960407617918, -5.049401038297876454, 101.0427570613523045 ) ) ;
#166788=CARTESIAN_POINT ( 'NONE',  ( 16.53943276465976808, 0.05219959533934440121, 71.25109039468568994 ) ) ;
#166789=CARTESIAN_POINT ( 'NONE',  ( -5.719274019375665041, -21.55341960407619695, 109.7927570613523613 ) ) ;
#166790=CARTESIAN_POINT ( 'NONE',  ( 5.153800228976615827, -19.02544592524334988, 85.20942372801900433 ) ) ;
#166791=CARTESIAN_POINT ( 'NONE',  ( 19.03943276465977164, -0.05219959533909143690, 48.74890960531435979 ) ) ;
#166792=CARTESIAN_POINT ( 'NONE',  ( 21.53943276465977519, -0.05219959533907433946, 78.74890960531436690 ) ) ;
#166793=CARTESIAN_POINT ( 'NONE',  ( -14.29746914071049879, 8.314922557960819915, 80.83224293864769550 ) ) ;
#166794=CARTESIAN_POINT ( 'NONE',  ( -13.97604488694547697, 13.89961937509957934, 73.12609039468568994 ) ) ;
#166795=CARTESIAN_POINT ( 'NONE',  ( -19.34837522270365895, -5.499999999999857003, 70.86337684832579953 ) ) ;
#166796=CARTESIAN_POINT ( 'NONE',  ( 13.97604488694548053, -13.89961937509957401, 50.62609039468566152 ) ) ;
#166797=CARTESIAN_POINT ( 'NONE',  ( -16.52544592524335698, -4.483927247898792601, 108.9594237280190185 ) ) ;
#166798=CARTESIAN_POINT ( 'NONE',  ( -16.52544592524342804, 4.483927247898546575, 61.04057627198103120 ) ) ;
#166799=CARTESIAN_POINT ( 'NONE',  ( 21.53943276465977519, 0.05219959533937863772, 106.2510903946856757 ) ) ;
#166801=CARTESIAN_POINT ( 'NONE',  ( -5.823673210054116645, -21.52544592524344225, 107.2905762719810525 ) ) ;
#166802=CARTESIAN_POINT ( 'NONE',  ( 9.474510206698971260, -16.51473224551069308, 107.9155762719810383 ) ) ;
#166803=CARTESIAN_POINT ( 'NONE',  ( 13.97604488694527802, 13.89961937509977652, 64.37390960531436690 ) ) ;
#166804=CARTESIAN_POINT ( 'NONE',  ( -21.53943276465977519, -0.05219959533937600094, 78.75109039468568994 ) ) ;
#166805=CARTESIAN_POINT ( 'NONE',  ( 9.474510206698971260, -16.51473224551069308, 67.91557627198102409 ) ) ;
#166807=CARTESIAN_POINT ( 'NONE',  ( 19.03943276465977164, -0.05219959533909143690, 33.74890960531435979 ) ) ;
#166808=CARTESIAN_POINT ( 'NONE',  ( 18.67979575497178502, 10.72451020669898547, 24.16557627198103120 ) ) ;
#166809=CARTESIAN_POINT ( 'NONE',  ( -8.314922557960811034, -14.29746914071050412, 67.08224293864770971 ) ) ;
#166810=CARTESIAN_POINT ( 'NONE',  ( -9.474510206698964154, 16.51473224551069663, 45.41557627198103120 ) ) ;
#166811=CARTESIAN_POINT ( 'NONE',  ( 0.05219959533910956823, 16.53943276465976808, 94.99890960531436690 ) ) ;
#166812=CARTESIAN_POINT ( 'NONE',  ( -10.72451020669898014, 18.67979575497178502, 110.4155762719810383 ) ) ;
#166813=CARTESIAN_POINT ( 'NONE',  ( -15.72974639402176322, -15.80617190586768395, 49.37609039468569705 ) ) ;
#166814=CARTESIAN_POINT ( 'NONE',  ( 5.049401038298161559, -19.05341960407611168, 27.70724293864769550 ) ) ;
#166815=CARTESIAN_POINT ( 'NONE',  ( 14.29746914071037800, 8.314922557961029526, 66.66775706135234714 ) ) ;
#166816=CARTESIAN_POINT ( 'NONE',  ( -10.72451020669898014, 18.67979575497178502, 105.4155762719810383 ) ) ;
#166817=CARTESIAN_POINT ( 'NONE',  ( 18.67979575497178502, 10.72451020669898547, 94.16557627198103830 ) ) ;
#166818=CARTESIAN_POINT ( 'NONE',  ( -9.474510206698720793, -16.51473224551083518, 29.58442372801900433 ) ) ;
#166819=CARTESIAN_POINT ( 'NONE',  ( -19.03943276465977164, 0.05219959533909376836, 56.24890960531435979 ) ) ;
#166820=CARTESIAN_POINT ( 'NONE',  ( -18.09805431107519880, 5.500000000000101252, 41.01606229291888894 ) ) ;
#166821=CARTESIAN_POINT ( 'NONE',  ( -21.53943276465977519, -0.05219959533937600094, 58.75109039468568994 ) ) ;
#166822=CARTESIAN_POINT ( 'NONE',  ( -15.80617190586745835, -15.72974639402198527, 56.87390960531436690 ) ) ;
#166823=CARTESIAN_POINT ( 'NONE',  ( 16.53943276465976808, -0.05219959533910856209, 23.74890960531435269 ) ) ;
#166824=CARTESIAN_POINT ( 'NONE',  ( -5.719274019375665041, -21.55341960407619695, 79.79275706135236135 ) ) ;
#166825=CARTESIAN_POINT ( 'NONE',  ( -18.67979575497193778, 10.72451020669871902, 103.3344237280190043 ) ) ;
#166826=CARTESIAN_POINT ( 'NONE',  ( 19.02544592524334988, 5.153800228976608722, 41.45942372801900433 ) ) ;
#166827=CARTESIAN_POINT ( 'NONE',  ( 16.52544592524335698, 4.483927247898782831, 96.45942372801901854 ) ) ;
#166828=CARTESIAN_POINT ( 'NONE',  ( 21.55341960407619695, -5.719274019375665929, 51.04275706135234714 ) ) ;
#166829=CARTESIAN_POINT ( 'NONE',  ( 9.474510206698971260, -16.51473224551069308, 57.91557627198103120 ) ) ;
#166830=CARTESIAN_POINT ( 'NONE',  ( -16.51473224551082808, 9.474510206698731452, 38.33442372801899722 ) ) ;
#166831=CARTESIAN_POINT ( 'NONE',  ( 10.81492255796078972, 18.62759615963270932, 34.58224293864770260 ) ) ;
#166832=CARTESIAN_POINT ( 'NONE',  ( -15.72974639402176322, -15.80617190586768395, 34.37609039468568284 ) ) ;
#166833=CARTESIAN_POINT ( 'NONE',  ( -10.72451020669898014, 18.67979575497178502, 85.41557627198102409 ) ) ;
#166834=CARTESIAN_POINT ( 'NONE',  ( 9.474510206698729675, 16.51473224551082808, 82.08442372801899012 ) ) ;
#166835=CARTESIAN_POINT ( 'NONE',  ( 4.483927247898790824, -16.52544592524335698, 50.20942372801901854 ) ) ;
#166837=CARTESIAN_POINT ( 'NONE',  ( 15.80617190586746368, 15.72974639402197994, 99.37390960531436690 ) ) ;
#166838=CARTESIAN_POINT ( 'NONE',  ( -16.53943276465976808, -0.05219959533934237506, 83.75109039468568994 ) ) ;
#166839=CARTESIAN_POINT ( 'NONE',  ( -16.52544592524342804, 4.483927247898546575, 76.04057627198102409 ) ) ;
#166840=CARTESIAN_POINT ( 'NONE',  ( -16.29526858892875651, -7.335722546920136367, 100.7967059780020520 ) ) ;
#166841=CARTESIAN_POINT ( 'NONE',  ( -16.46253265017146816, -9.564922557961047289, 104.1677570613523329 ) ) ;
#166842=CARTESIAN_POINT ( 'NONE',  ( -5.719274019375978568, 21.55341960407610458, 35.20724293864768839 ) ) ;
#166844=CARTESIAN_POINT ( 'NONE',  ( -16.55341960407617563, 4.379528057220093196, 48.54275706135234714 ) ) ;
#166845=CARTESIAN_POINT ( 'NONE',  ( 0.05219959533907565091, 21.53943276465977519, 109.9989096053143527 ) ) ;
#166846=CARTESIAN_POINT ( 'NONE',  ( -15.80617190586745835, -15.72974639402198527, 31.87390960531435979 ) ) ;
#166847=CARTESIAN_POINT ( 'NONE',  ( 14.29746914071037800, 8.314922557961029526, 76.66775706135234714 ) ) ;
#166848=CARTESIAN_POINT ( 'NONE',  ( 19.03943276465977164, -0.05219959533909143690, 78.74890960531436690 ) ) ;
#166849=CARTESIAN_POINT ( 'NONE',  ( 21.52544592524334988, 5.823673210054432836, 61.45942372801901854 ) ) ;
#166850=CARTESIAN_POINT ( 'NONE',  ( -13.97604488694527625, -13.89961937509977652, 31.87390960531435979 ) ) ;
#166851=CARTESIAN_POINT ( 'NONE',  ( 18.67979575497178502, 10.72451020669898547, 24.16557627198103120 ) ) ;
#166852=ORIENTED_EDGE ( 'NONE', *, *, #197067, .T. ) ;
#166853=CARTESIAN_POINT ( 'NONE',  ( 16.51473224551083163, -9.474510206698727899, 40.83442372801900433 ) ) ;
#166854=CARTESIAN_POINT ( 'NONE',  ( -4.379528057220086978, -16.55341960407618274, 54.79275706135235424 ) ) ;
#166855=CARTESIAN_POINT ( 'NONE',  ( -16.51473224551069308, -9.474510206698971260, 111.6655762719810383 ) ) ;
#166856=CARTESIAN_POINT ( 'NONE',  ( 5.049401038298161559, -19.05341960407611168, 72.70724293864768129 ) ) ;
#166857=CARTESIAN_POINT ( 'NONE',  ( -14.34966873604972548, 8.224510206698743886, 103.3344237280190043 ) ) ;
#166859=CARTESIAN_POINT ( 'NONE',  ( 12.14591786802309770, 12.06949235617756955, 94.37390960531436690 ) ) ;
#166860=CARTESIAN_POINT ( 'NONE',  ( -21.53943276465977519, 0.05219959533907696930, 41.24890960531435269 ) ) ;
#166861=CARTESIAN_POINT ( 'NONE',  ( -9.474510206698964154, 16.51473224551069663, 25.41557627198103120 ) ) ;
#166862=CARTESIAN_POINT ( 'NONE',  ( 4.483927247898790824, -16.52544592524335698, 65.20942372801901854 ) ) ;
#166863=CARTESIAN_POINT ( 'NONE',  ( 0.05219959533937995610, -21.53943276465977519, 25.00109039468567218 ) ) ;
#166864=CARTESIAN_POINT ( 'NONE',  ( 19.03943276465977164, 0.05219959533936151252, 71.25109039468566152 ) ) ;
#166865=CARTESIAN_POINT ( 'NONE',  ( 16.51473224551069308, 9.474510206698969483, 39.16557627198103120 ) ) ;
#166866=CARTESIAN_POINT ( 'NONE',  ( -21.52544592524343514, 5.823673210054127303, 71.04057627198103830 ) ) ;
#166868=CARTESIAN_POINT ( 'NONE',  ( -16.51473224551069308, -9.474510206698971260, 111.6655762719810383 ) ) ;
#166869=CARTESIAN_POINT ( 'NONE',  ( -15.80617190586768217, 15.72974639402176855, 98.12609039468570415 ) ) ;
#166870=CARTESIAN_POINT ( 'NONE',  ( -19.05341960407611168, -5.049401038298163336, 66.45724293864769550 ) ) ;
#166871=CARTESIAN_POINT ( 'NONE',  ( -8.314922557961024197, 14.29746914071037800, 52.91775706135235424 ) ) ;
#166872=CARTESIAN_POINT ( 'NONE',  ( -5.719274019375665041, -21.55341960407619695, 84.79275706135234714 ) ) ;
#166873=CARTESIAN_POINT ( 'NONE',  ( 9.564922557961047289, -16.46253265017146816, 35.41775706135233293 ) ) ;
#166874=CARTESIAN_POINT ( 'NONE',  ( -19.03943276465977164, -0.05219959533935918106, 58.75109039468566863 ) ) ;
#166876=CARTESIAN_POINT ( 'NONE',  ( -21.53943276465977519, -0.05219959533937600094, 53.75109039468568994 ) ) ;
#166877=CARTESIAN_POINT ( 'NONE',  ( -19.05341960407611168, -5.049401038298163336, 26.45724293864769550 ) ) ;
#166878=CARTESIAN_POINT ( 'NONE',  ( 5.153800228976615827, -19.02544592524334988, 45.20942372801901143 ) ) ;
#166879=CARTESIAN_POINT ( 'NONE',  ( 19.03943276465977164, -0.05219959533909143690, 93.74890960531435269 ) ) ;
#166880=CARTESIAN_POINT ( 'NONE',  ( -9.564922557960796823, -16.46253265017161027, 77.08224293864769550 ) ) ;
#166881=CARTESIAN_POINT ( 'NONE',  ( 14.34966873604960469, 8.224510206698951720, 39.16557627198102409 ) ) ;
#166882=CARTESIAN_POINT ( 'NONE',  ( 0.05219959533907565091, 21.53943276465977519, 39.99890960531436690 ) ) ;
#166884=CARTESIAN_POINT ( 'NONE',  ( 17.31747979337948706, 6.344076630961012597, 58.87944868065186199 ) ) ;
#166885=CARTESIAN_POINT ( 'NONE',  ( -0.05219959533937732626, 21.53943276465977519, 92.50109039468567573 ) ) ;
#166887=CARTESIAN_POINT ( 'NONE',  ( -16.46253265017160317, 9.564922557960807481, 35.83224293864768839 ) ) ;
#166888=CARTESIAN_POINT ( 'NONE',  ( -19.03943276465977164, 0.05219959533909376836, 111.2489096053143669 ) ) ;
#166891=CARTESIAN_POINT ( 'NONE',  ( 8.314922557961029526, -14.29746914071037800, 45.41775706135234003 ) ) ;
#166892=CARTESIAN_POINT ( 'NONE',  ( 18.62759615963271287, -10.81492255796078972, 63.33224293864770260 ) ) ;
#166893=CARTESIAN_POINT ( 'NONE',  ( -0.05219959533910754901, -16.53943276465976808, 37.49890960531436690 ) ) ;
#166894=CARTESIAN_POINT ( 'NONE',  ( -9.564922557960796823, -16.46253265017161027, 27.08224293864769550 ) ) ;
#166895=CARTESIAN_POINT ( 'NONE',  ( 5.153800228976335163, 19.02544592524342804, 109.7905762719810099 ) ) ;
#166896=CARTESIAN_POINT ( 'NONE',  ( -21.52544592524334988, -5.823673210054445271, 28.95942372801902209 ) ) ;
#166897=CARTESIAN_POINT ( 'NONE',  ( -5.153800228976607833, 19.02544592524334988, 37.70942372801899722 ) ) ;
#166898=CARTESIAN_POINT ( 'NONE',  ( 13.89961937509977652, -13.97604488694527269, 23.12390960531436335 ) ) ;
#166899=CARTESIAN_POINT ( 'NONE',  ( 21.53943276465977519, 0.05219959533937863772, 76.25109039468568994 ) ) ;
#166901=CARTESIAN_POINT ( 'NONE',  ( -16.53943276465976808, 0.05219959533911058130, 31.24890960531435979 ) ) ;
#166902=CARTESIAN_POINT ( 'NONE',  ( 17.50000000000014566, 3.292511757969652120, 112.4347972978947325 ) ) ;
#166903=CARTESIAN_POINT ( 'NONE',  ( 0.05219959533907565091, 21.53943276465977519, 29.99890960531435979 ) ) ;
#166904=CARTESIAN_POINT ( 'NONE',  ( 0.05219959533910956823, 16.53943276465976808, 84.99890960531436690 ) ) ;
#166906=AXIS2_PLACEMENT_3D ( 'NONE', #143503, #4987, #25193 ) ;
#166907=CARTESIAN_POINT ( 'NONE',  ( 5.049401038298161559, -19.05341960407611168, 72.70724293864768129 ) ) ;
#166908=CARTESIAN_POINT ( 'NONE',  ( 12.14591786802309770, 12.06949235617756955, 74.37390960531436690 ) ) ;
#166909=CARTESIAN_POINT ( 'NONE',  ( -5.049401038297874678, -19.05341960407617918, 104.7927570613523471 ) ) ;
#166910=CARTESIAN_POINT ( 'NONE',  ( -15.80617190586745835, -15.72974639402198527, 61.87390960531436690 ) ) ;
#166912=CARTESIAN_POINT ( 'NONE',  ( -13.89961937509977652, 13.97604488694528158, 35.62390960531435269 ) ) ;
#166913=CARTESIAN_POINT ( 'NONE',  ( 9.474510206698971260, -16.51473224551069308, 87.91557627198102409 ) ) ;
#166914=CARTESIAN_POINT ( 'NONE',  ( -15.72974639402197994, 15.80617190586746368, 80.62390960531438111 ) ) ;
#166915=CARTESIAN_POINT ( 'NONE',  ( 12.06949235617739724, 12.14591786802326823, 101.8760903946857042 ) ) ;
#166916=CARTESIAN_POINT ( 'NONE',  ( -16.46253265017160317, 9.564922557960807481, 80.83224293864769550 ) ) ;
#166917=CARTESIAN_POINT ( 'NONE',  ( 19.03943276465977164, 0.05219959533936151252, 61.25109039468566863 ) ) ;
#166918=CARTESIAN_POINT ( 'NONE',  ( -10.81492255796105439, 18.62759615963255655, 97.91775706135236135 ) ) ;
#166919=CARTESIAN_POINT ( 'NONE',  ( 10.81492255796078972, 18.62759615963270932, 79.58224293864769550 ) ) ;
#166920=CARTESIAN_POINT ( 'NONE',  ( 19.05341960407611168, 5.049401038298154454, 113.9572429386477097 ) ) ;
#166921=CARTESIAN_POINT ( 'NONE',  ( 5.049401038298161559, -19.05341960407611168, 52.70724293864767418 ) ) ;
#166922=CARTESIAN_POINT ( 'NONE',  ( -16.55341960407617563, 4.379528057220093196, 113.5427570613523756 ) ) ;
#166923=CARTESIAN_POINT ( 'NONE',  ( 0.05219959533909260263, 19.03943276465977164, 69.99890960531435269 ) ) ;
#166924=CARTESIAN_POINT ( 'NONE',  ( -13.97604488694547520, 13.89961937509957934, 83.12609039468566152 ) ) ;
#166925=CARTESIAN_POINT ( 'NONE',  ( -18.62759615963255300, -10.81492255796106328, 104.1677570613523471 ) ) ;
#166926=CARTESIAN_POINT ( 'NONE',  ( 14.34966873604960469, 8.224510206698951720, 69.16557627198102409 ) ) ;
#166927=CARTESIAN_POINT ( 'NONE',  ( 5.823673210054125526, 21.52544592524343514, 109.7905762719810383 ) ) ;
#166928=CARTESIAN_POINT ( 'NONE',  ( 18.67979575497178502, 10.72451020669898547, 104.1655762719810241 ) ) ;
#166930=CARTESIAN_POINT ( 'NONE',  ( -15.72974639402197994, 15.80617190586746368, 60.62390960531437401 ) ) ;
#166931=CARTESIAN_POINT ( 'NONE',  ( -16.55341960407617563, 4.379528057220093196, 83.54275706135234714 ) ) ;
#166932=CARTESIAN_POINT ( 'NONE',  ( -14.29746914071049879, 8.314922557960819915, 110.8322429386476955 ) ) ;
#166933=CARTESIAN_POINT ( 'NONE',  ( 13.89961937509977652, -13.97604488694527269, 53.12390960531434558 ) ) ;
#166934=CARTESIAN_POINT ( 'NONE',  ( -14.34966873604960291, -8.224510206698953496, 21.66557627198102409 ) ) ;
#166935=CARTESIAN_POINT ( 'NONE',  ( -10.81492255796105439, 18.62759615963255655, 47.91775706135234714 ) ) ;
#166936=CARTESIAN_POINT ( 'NONE',  ( -9.474510206698964154, 16.51473224551069663, 110.4155762719810383 ) ) ;
#166937=CARTESIAN_POINT ( 'NONE',  ( 21.53943276465977519, 0.05219959533937863772, 81.25109039468568994 ) ) ;
#166938=CARTESIAN_POINT ( 'NONE',  ( 16.51473224551069308, 9.474510206698969483, 34.16557627198102409 ) ) ;
#166939=CARTESIAN_POINT ( 'NONE',  ( 9.474510206698971260, -16.51473224551069308, 37.91557627198102409 ) ) ;
#166941=CARTESIAN_POINT ( 'NONE',  ( 21.53943276465977519, 0.05219959533937863772, 66.25109039468567573 ) ) ;
#166942=CARTESIAN_POINT ( 'NONE',  ( 16.51473224551069308, 9.474510206698969483, 104.1655762719810241 ) ) ;
#166943=CARTESIAN_POINT ( 'NONE',  ( -19.03943276465977164, -0.05219959533935918106, 78.75109039468567573 ) ) ;
#166944=CARTESIAN_POINT ( 'NONE',  ( 5.823673210054444382, -21.52544592524334988, 45.20942372801901854 ) ) ;
#166945=CARTESIAN_POINT ( 'NONE',  ( -12.14591786802326823, 12.06949235617739902, 28.12609039468568284 ) ) ;
#166946=CARTESIAN_POINT ( 'NONE',  ( 19.05341960407617918, -5.049401038297876454, 71.04275706135234714 ) ) ;
#166947=CARTESIAN_POINT ( 'NONE',  ( -9.564922557960796823, -16.46253265017161027, 57.08224293864769550 ) ) ;
#166948=CARTESIAN_POINT ( 'NONE',  ( 5.153800228976615827, -19.02544592524334988, 85.20942372801900433 ) ) ;
#166949=CARTESIAN_POINT ( 'NONE',  ( -16.55341960407611168, -4.379528057220339221, 31.45724293864769550 ) ) ;
#166950=CARTESIAN_POINT ( 'NONE',  ( -16.51473224551082808, 9.474510206698731452, 88.33442372801900433 ) ) ;
#166951=CARTESIAN_POINT ( 'NONE',  ( -12.06949235617756955, 12.14591786802309770, 40.62390960531435269 ) ) ;
#166952=CARTESIAN_POINT ( 'NONE',  ( 9.474510206698729675, 16.51473224551082808, 67.08442372801900433 ) ) ;
#166953=CARTESIAN_POINT ( 'NONE',  ( 4.379528057220092307, 16.55341960407617563, 42.29275706135235424 ) ) ;
#166954=CARTESIAN_POINT ( 'NONE',  ( -5.049401038297874678, -19.05341960407617918, 19.79275706135233293 ) ) ;
#166956=CARTESIAN_POINT ( 'NONE',  ( -9.474510206698964154, 16.51473224551069663, 40.41557627198103120 ) ) ;
#166958=CARTESIAN_POINT ( 'NONE',  ( -16.53943276465976808, -0.05219959533934237506, 48.75109039468568284 ) ) ;
#166961=CARTESIAN_POINT ( 'NONE',  ( 0.05219959533909260263, 19.03943276465977164, 89.99890960531436690 ) ) ;
#166963=CARTESIAN_POINT ( 'NONE',  ( 19.02544592524334988, 5.153800228976608722, 86.45942372801900433 ) ) ;
#166965=CARTESIAN_POINT ( 'NONE',  ( -10.72451020669898014, 18.67979575497178502, 30.41557627198101699 ) ) ;
#166966=CARTESIAN_POINT ( 'NONE',  ( 15.72974639402176855, 15.80617190586768217, 106.8760903946856899 ) ) ;
#166967=CARTESIAN_POINT ( 'NONE',  ( -16.46253265017146816, -9.564922557961047289, 99.16775706135233293 ) ) ;
#166968=CARTESIAN_POINT ( 'NONE',  ( -8.224510206698948167, 14.34966873604960824, 110.4155762719810383 ) ) ;
#166969=CARTESIAN_POINT ( 'NONE',  ( 0.05219959533909260263, 19.03943276465977164, 39.99890960531436690 ) ) ;
#166970=CARTESIAN_POINT ( 'NONE',  ( 21.55341960407610458, 5.719274019375980345, 58.95724293864770971 ) ) ;
#166971=CARTESIAN_POINT ( 'NONE',  ( 9.474510206698971260, -16.51473224551069308, 22.91557627198102765 ) ) ;
#166973=CARTESIAN_POINT ( 'NONE',  ( 19.02544592524334988, 5.153800228976608722, 76.45942372801897591 ) ) ;
#166974=CARTESIAN_POINT ( 'NONE',  ( 4.483927247898545687, 16.52544592524342804, 49.79057627198102409 ) ) ;
#166975=CARTESIAN_POINT ( 'NONE',  ( -15.80617190586745835, -15.72974639402198527, 31.87390960531435979 ) ) ;
#166976=CARTESIAN_POINT ( 'NONE',  ( -15.80617190586768217, 15.72974639402176855, 98.12609039468570415 ) ) ;
#166977=CARTESIAN_POINT ( 'NONE',  ( -15.80617190586745835, -15.72974639402198527, 86.87390960531438111 ) ) ;
#166978=CARTESIAN_POINT ( 'NONE',  ( -15.80617190586768217, 15.72974639402176855, 53.12609039468568284 ) ) ;
#166979=CARTESIAN_POINT ( 'NONE',  ( 15.80617190586769283, -15.72974639402175789, 70.62609039468567573 ) ) ;
#166980=CARTESIAN_POINT ( 'NONE',  ( 5.049401038298161559, -19.05341960407611168, 102.7072429386476955 ) ) ;
#166981=CARTESIAN_POINT ( 'NONE',  ( 0.05219959533934541429, -16.53943276465976808, 95.00109039468568994 ) ) ;
#166982=CARTESIAN_POINT ( 'NONE',  ( 10.81492255796106328, -18.62759615963255655, 65.41775706135234714 ) ) ;
#166983=CARTESIAN_POINT ( 'NONE',  ( -12.06949235617756955, 12.14591786802309770, 115.6239096053143669 ) ) ;
#166984=CARTESIAN_POINT ( 'NONE',  ( 8.224510206698953496, -14.34966873604960469, 72.91557627198103830 ) ) ;
#166985=CARTESIAN_POINT ( 'NONE',  ( -4.483927247898539470, -16.52544592524342804, 37.29057627198102409 ) ) ;
#166986=CARTESIAN_POINT ( 'NONE',  ( 18.67979575497178502, 10.72451020669898547, 44.16557627198103120 ) ) ;
#166987=CARTESIAN_POINT ( 'NONE',  ( 9.564922557960805705, 16.46253265017160317, 49.58224293864770260 ) ) ;
#166988=CARTESIAN_POINT ( 'NONE',  ( 5.719274019375991003, -21.55341960407610458, 62.70724293864769550 ) ) ;
#166989=CARTESIAN_POINT ( 'NONE',  ( 16.46253265017146816, 9.564922557961045513, 51.66775706135233293 ) ) ;
#166991=CARTESIAN_POINT ( 'NONE',  ( -16.18388926212241330, -7.379444403734408908, 40.43953151366154231 ) ) ;
#166992=CARTESIAN_POINT ( 'NONE',  ( -4.379528057220328563, 16.55341960407611168, 45.20724293864769550 ) ) ;
#166993=CARTESIAN_POINT ( 'NONE',  ( -10.81492255796078084, -18.62759615963271287, 27.08224293864769550 ) ) ;
#166997=CARTESIAN_POINT ( 'NONE',  ( 8.224510206698742110, 14.34966873604972548, 72.08442372801899012 ) ) ;
#166998=CARTESIAN_POINT ( 'NONE',  ( 16.51473224551083163, -9.474510206698727899, 75.83442372801900433 ) ) ;
#166999=CARTESIAN_POINT ( 'NONE',  ( 14.29746914071049879, -8.314922557960816363, 38.33224293864768839 ) ) ;
#167000=CARTESIAN_POINT ( 'NONE',  ( 16.81555441253556893, -7.025013491695413670, 53.13685445334258617 ) ) ;
#167001=CARTESIAN_POINT ( 'NONE',  ( 14.29746914071049879, -8.314922557960816363, 33.33224293864769550 ) ) ;
#167002=CARTESIAN_POINT ( 'NONE',  ( -16.51473224551069308, -9.474510206698971260, 46.66557627198102409 ) ) ;
#167003=CARTESIAN_POINT ( 'NONE',  ( -19.02544592524342804, 5.153800228976336051, 71.04057627198099567 ) ) ;
#167004=CARTESIAN_POINT ( 'NONE',  ( -13.89961937509977652, 13.97604488694528158, 40.62390960531435979 ) ) ;
#167005=CARTESIAN_POINT ( 'NONE',  ( 10.81492255796106328, -18.62759615963255655, 45.41775706135234003 ) ) ;
#167006=CARTESIAN_POINT ( 'NONE',  ( -19.02544592524342804, 5.153800228976336051, 61.04057627198103120 ) ) ;
#167009=CARTESIAN_POINT ( 'NONE',  ( -5.153800228976328057, -19.02544592524343514, 62.29057627198100988 ) ) ;
#167010=CARTESIAN_POINT ( 'NONE',  ( -5.719274019375978568, 21.55341960407610458, 40.20724293864769550 ) ) ;
#167011=CARTESIAN_POINT ( 'NONE',  ( 19.05341960407611168, 5.049401038298154454, 38.95724293864767418 ) ) ;
#167012=CARTESIAN_POINT ( 'NONE',  ( -5.823673210054116645, -21.52544592524344225, 37.29057627198102409 ) ) ;
#167013=CARTESIAN_POINT ( 'NONE',  ( -16.52544592524335698, -4.483927247898792601, 93.95942372801903275 ) ) ;
#167014=CARTESIAN_POINT ( 'NONE',  ( -15.80617190586768217, 15.72974639402176855, 113.1260903946856899 ) ) ;
#167015=CARTESIAN_POINT ( 'NONE',  ( 8.224510206698742110, 14.34966873604972548, 72.08442372801899012 ) ) ;
#167016=CARTESIAN_POINT ( 'NONE',  ( -5.049401038298153566, 19.05341960407611168, 105.2072429386476671 ) ) ;
#167017=CARTESIAN_POINT ( 'NONE',  ( 14.34966873604972726, -8.224510206698740333, 60.83442372801901854 ) ) ;
#167018=CARTESIAN_POINT ( 'NONE',  ( -12.14591786802326823, 12.06949235617739902, 38.12609039468567573 ) ) ;
#167019=CARTESIAN_POINT ( 'NONE',  ( 5.153800228976335163, 19.02544592524342804, 104.7905762719809957 ) ) ;
#167020=CARTESIAN_POINT ( 'NONE',  ( -0.05219959533934338120, 16.53943276465976808, 27.50109039468567929 ) ) ;
#167021=CARTESIAN_POINT ( 'NONE',  ( -9.474510206698964154, 16.51473224551069663, 40.41557627198103120 ) ) ;
#167022=CARTESIAN_POINT ( 'NONE',  ( 5.823673210054444382, -21.52544592524334988, 25.20942372801901854 ) ) ;
#167023=CARTESIAN_POINT ( 'NONE',  ( -4.483927247898782831, 16.52544592524335698, 27.70942372801901854 ) ) ;
#167024=CARTESIAN_POINT ( 'NONE',  ( 0.05219959533934541429, -16.53943276465976808, 105.0010903946856757 ) ) ;
#167025=CARTESIAN_POINT ( 'NONE',  ( -5.823673210054431948, 21.52544592524334988, 102.7094237280190185 ) ) ;
#167026=CARTESIAN_POINT ( 'NONE',  ( 9.474510206698729675, 16.51473224551082808, 102.0844237280190043 ) ) ;
#167027=CARTESIAN_POINT ( 'NONE',  ( -8.224510206698948167, 14.34966873604960824, 55.41557627198102409 ) ) ;
#167028=CARTESIAN_POINT ( 'NONE',  ( -16.51473224551069308, -9.474510206698971260, 31.66557627198102054 ) ) ;
#167029=CARTESIAN_POINT ( 'NONE',  ( -9.474510206698720793, -16.51473224551083518, 54.58442372801899722 ) ) ;
#167031=CARTESIAN_POINT ( 'NONE',  ( 18.67979575497194134, -10.72451020669871369, 50.83442372801901143 ) ) ;
#167032=CARTESIAN_POINT ( 'NONE',  ( -14.34966873604972548, 8.224510206698743886, 23.33442372801901499 ) ) ;
#167034=CARTESIAN_POINT ( 'NONE',  ( 19.02544592524343514, -5.153800228976328945, 108.5405762719810383 ) ) ;
#167035=CARTESIAN_POINT ( 'NONE',  ( -0.05219959533907301413, -21.53943276465977519, 67.49890960531436690 ) ) ;
#167036=CARTESIAN_POINT ( 'NONE',  ( 9.564922557961047289, -16.46253265017146816, 105.4177570613523471 ) ) ;
#167037=CARTESIAN_POINT ( 'NONE',  ( -19.05341960407611168, -5.049401038298163336, 96.45724293864769550 ) ) ;
#167039=CARTESIAN_POINT ( 'NONE',  ( 4.483927247898545687, 16.52544592524342804, 104.7905762719810241 ) ) ;
#167040=CARTESIAN_POINT ( 'NONE',  ( -21.53943276465977519, -0.05219959533937600094, 93.75109039468567573 ) ) ;
#167041=CARTESIAN_POINT ( 'NONE',  ( -16.46253265017160317, 9.564922557960807481, 45.83224293864769550 ) ) ;
#167043=CARTESIAN_POINT ( 'NONE',  ( 21.53943276465977519, 0.05219959533937863772, 51.25109039468568994 ) ) ;
#167044=CARTESIAN_POINT ( 'NONE',  ( 0.05219959533937995610, -21.53943276465977519, 95.00109039468568994 ) ) ;
#167045=CARTESIAN_POINT ( 'NONE',  ( 12.06949235617739724, 12.14591786802326823, 106.8760903946856899 ) ) ;
#167046=CARTESIAN_POINT ( 'NONE',  ( -16.51473224551069308, -9.474510206698971260, 76.66557627198103830 ) ) ;
#167047=CARTESIAN_POINT ( 'NONE',  ( 0.05219959533937995610, -21.53943276465977519, 45.00109039468568284 ) ) ;
#167048=CARTESIAN_POINT ( 'NONE',  ( 10.81492255796106328, -18.62759615963255655, 40.41775706135234714 ) ) ;
#167049=CARTESIAN_POINT ( 'NONE',  ( 9.474510206698729675, 16.51473224551082808, 72.08442372801900433 ) ) ;
#167050=CARTESIAN_POINT ( 'NONE',  ( -19.03943276465977164, 0.05219959533909376836, 86.24890960531436690 ) ) ;
#167051=CARTESIAN_POINT ( 'NONE',  ( -14.29746914071049879, 8.314922557960819915, 110.8322429386476955 ) ) ;
#167052=CARTESIAN_POINT ( 'NONE',  ( 15.80617190586746368, 15.72974639402197994, 94.37390960531436690 ) ) ;
#167053=CARTESIAN_POINT ( 'NONE',  ( -8.224510206698948167, 14.34966873604960824, 60.41557627198102409 ) ) ;
#167054=CARTESIAN_POINT ( 'NONE',  ( -9.564922557961040184, 16.46253265017147172, 22.91775706135233648 ) ) ;
#167055=CARTESIAN_POINT ( 'NONE',  ( -4.379528057220328563, 16.55341960407611168, 100.2072429386476955 ) ) ;
#167056=CARTESIAN_POINT ( 'NONE',  ( -5.153800228976328057, -19.02544592524343514, 32.29057627198102409 ) ) ;
#167057=CARTESIAN_POINT ( 'NONE',  ( -16.51473224551082808, 9.474510206698731452, 83.33442372801899012 ) ) ;
#167058=CARTESIAN_POINT ( 'NONE',  ( -4.483927247898539470, -16.52544592524342804, 42.29057627198103120 ) ) ;
#167059=CARTESIAN_POINT ( 'NONE',  ( -5.823673210054431948, 21.52544592524334988, 92.70942372801901854 ) ) ;
#167060=CARTESIAN_POINT ( 'NONE',  ( 9.564922557960805705, 16.46253265017160317, 104.5822429386476955 ) ) ;
#167061=CARTESIAN_POINT ( 'NONE',  ( -19.02544592524334988, -5.153800228976617603, 68.95942372801896170 ) ) ;
#167062=CARTESIAN_POINT ( 'NONE',  ( -18.62759615963270932, 10.81492255796079327, 75.83224293864769550 ) ) ;
#167063=CARTESIAN_POINT ( 'NONE',  ( 21.55341960407619695, -5.719274019375665929, 36.04275706135234714 ) ) ;
#167064=CARTESIAN_POINT ( 'NONE',  ( 4.483927247898790824, -16.52544592524335698, 30.20942372801902565 ) ) ;
#167065=CARTESIAN_POINT ( 'NONE',  ( 12.14591786802327356, -12.06949235617739191, 90.62609039468567573 ) ) ;
#167066=CARTESIAN_POINT ( 'NONE',  ( -19.05341960407611168, -5.049401038298163336, 26.45724293864769550 ) ) ;
#167067=CARTESIAN_POINT ( 'NONE',  ( -0.05219959533937732626, 21.53943276465977519, 37.50109039468568284 ) ) ;
#167068=CARTESIAN_POINT ( 'NONE',  ( -19.05341960407611168, -5.049401038298163336, 21.45724293864768839 ) ) ;
#167070=CARTESIAN_POINT ( 'NONE',  ( -12.06949235617739369, -12.14591786802326823, 54.37609039468568994 ) ) ;
#167071=CARTESIAN_POINT ( 'NONE',  ( 8.224510206698953496, -14.34966873604960469, 77.91557627198102409 ) ) ;
#167072=CARTESIAN_POINT ( 'NONE',  ( -21.53943276465977519, 0.05219959533907696930, 71.24890960531435269 ) ) ;
#167073=CARTESIAN_POINT ( 'NONE',  ( -14.29746914071049879, 8.314922557960819915, 30.83224293864770260 ) ) ;
#167074=CARTESIAN_POINT ( 'NONE',  ( 12.14591786802327356, -12.06949235617739191, 55.62609039468568284 ) ) ;
#167075=CARTESIAN_POINT ( 'NONE',  ( -13.97604488694527625, -13.89961937509977652, 46.87390960531435979 ) ) ;
#167076=CARTESIAN_POINT ( 'NONE',  ( 0.05219959533934541429, -16.53943276465976808, 90.00109039468567573 ) ) ;
#167077=CARTESIAN_POINT ( 'NONE',  ( -19.05341960407617563, 5.049401038297882671, 93.54275706135234714 ) ) ;
#167078=CARTESIAN_POINT ( 'NONE',  ( 5.823673210054125526, 21.52544592524343514, 69.79057627198102409 ) ) ;
#167079=CARTESIAN_POINT ( 'NONE',  ( 16.55341960407618274, -4.379528057220086978, 111.0427570613523613 ) ) ;
#167082=CARTESIAN_POINT ( 'NONE',  ( -21.55341960407610458, -5.719274019375992779, 61.45724293864770260 ) ) ;
#167084=CARTESIAN_POINT ( 'NONE',  ( 12.14591786802327356, -12.06949235617739191, 95.62609039468568994 ) ) ;
#167086=CARTESIAN_POINT ( 'NONE',  ( 21.55341960407610458, 5.719274019375980345, 23.95724293864769550 ) ) ;
#167087=CARTESIAN_POINT ( 'NONE',  ( 17.49999999999999289, 3.805241302050251573, 107.1264752721741615 ) ) ;
#167088=CARTESIAN_POINT ( 'NONE',  ( -21.55341960407610458, -5.719274019375992779, 71.45724293864769550 ) ) ;
#167089=CARTESIAN_POINT ( 'NONE',  ( -16.55341960407611168, -4.379528057220339221, 31.45724293864769550 ) ) ;
#167090=CARTESIAN_POINT ( 'NONE',  ( -16.52544592524335698, -4.483927247898792601, 23.95942372801901143 ) ) ;
#167091=CARTESIAN_POINT ( 'NONE',  ( -0.05219959533909027116, -19.03943276465977164, 27.49890960531435624 ) ) ;
#167092=CARTESIAN_POINT ( 'NONE',  ( -0.05219959533934338120, 16.53943276465976808, 32.50109039468568284 ) ) ;
#167093=CARTESIAN_POINT ( 'NONE',  ( 16.51473224551069308, 9.474510206698969483, 54.16557627198103120 ) ) ;
#167095=CARTESIAN_POINT ( 'NONE',  ( -9.474510206698964154, 16.51473224551069663, 100.4155762719810241 ) ) ;
#167096=CARTESIAN_POINT ( 'NONE',  ( 4.483927247898790824, -16.52544592524335698, 95.20942372801903275 ) ) ;
#167097=CARTESIAN_POINT ( 'NONE',  ( -13.97604488694547697, 13.89961937509957934, 98.12609039468566152 ) ) ;
#167098=CARTESIAN_POINT ( 'NONE',  ( 19.05341960407617918, -5.049401038297876454, 26.04275706135233293 ) ) ;
#167099=CARTESIAN_POINT ( 'NONE',  ( -10.72451020669898014, 18.67979575497178502, 80.41557627198103830 ) ) ;
#167100=CARTESIAN_POINT ( 'NONE',  ( -4.379528057220086978, -16.55341960407618274, 99.79275706135234714 ) ) ;
#167101=CARTESIAN_POINT ( 'NONE',  ( -19.05341960407617563, 5.049401038297882671, 98.54275706135233293 ) ) ;
#167102=CARTESIAN_POINT ( 'NONE',  ( -9.564922557960796823, -16.46253265017161027, 52.08224293864768839 ) ) ;
#167103=CARTESIAN_POINT ( 'NONE',  ( -19.03943276465977164, 0.05219959533909376836, 86.24890960531436690 ) ) ;
#167104=CARTESIAN_POINT ( 'NONE',  ( -15.80617190586768217, 15.72974639402176855, 63.12609039468568994 ) ) ;
#167105=CARTESIAN_POINT ( 'NONE',  ( -5.049401038298153566, 19.05341960407611168, 60.20724293864768129 ) ) ;
#167106=CARTESIAN_POINT ( 'NONE',  ( -16.52544592524342804, 4.483927247898546575, 86.04057627198102409 ) ) ;
#167107=CARTESIAN_POINT ( 'NONE',  ( -17.26172910966779739, -6.454744622555837807, 84.19353091350780005 ) ) ;
#167108=CARTESIAN_POINT ( 'NONE',  ( 12.06949235617757843, -12.14591786802309237, 78.12390960531436690 ) ) ;
#167109=CARTESIAN_POINT ( 'NONE',  ( -10.72451020669898014, 18.67979575497178502, 80.41557627198103830 ) ) ;
#167110=CARTESIAN_POINT ( 'NONE',  ( -19.02544592524334988, -5.153800228976617603, 93.95942372801900433 ) ) ;
#167111=CARTESIAN_POINT ( 'NONE',  ( 17.05116617787825462, -6.768360034955811955, 81.15675553259195851 ) ) ;
#167112=CARTESIAN_POINT ( 'NONE',  ( -19.02544592524334988, -5.153800228976617603, 38.95942372801900433 ) ) ;
#167114=CARTESIAN_POINT ( 'NONE',  ( -9.474510206698964154, 16.51473224551069663, 75.41557627198103830 ) ) ;
#167115=CARTESIAN_POINT ( 'NONE',  ( 9.474510206698971260, -16.51473224551069308, 87.91557627198102409 ) ) ;
#167116=B_SPLINE_CURVE_WITH_KNOTS ( 'NONE', 3,
 ( #142210, #65372, #174556, #6676, #68354, #159361 ),
 .UNSPECIFIED., .F., .F.,
 ( 4, 2, 4 ),
 ( 0.000000000000000000, 0.0003837532665634982949, 0.0007675065331269965898 ),
 .UNSPECIFIED. ) ;
#167117=EDGE_CURVE ( 'NONE', #198282, #95422, #117306, .T. ) ;
#167118=CARTESIAN_POINT ( 'NONE',  ( 12.14591786802327356, -12.06949235617739191, 60.62609039468567573 ) ) ;
#167120=CARTESIAN_POINT ( 'NONE',  ( -19.03943276465977164, -0.05219959533935918106, 38.75109039468566152 ) ) ;
#167122=CARTESIAN_POINT ( 'NONE',  ( -19.02544592524342804, 5.153800228976336051, 111.0405762719810099 ) ) ;
#167123=CARTESIAN_POINT ( 'NONE',  ( -4.483927247898782831, 16.52544592524335698, 107.7094237280190328 ) ) ;
#167125=CARTESIAN_POINT ( 'NONE',  ( -4.379528057220086978, -16.55341960407618274, 74.79275706135234714 ) ) ;
#167126=CARTESIAN_POINT ( 'NONE',  ( -17.44270441346513678, 5.991230190323086013, 28.63664920735772057 ) ) ;
#167127=CARTESIAN_POINT ( 'NONE',  ( -16.53943276465976808, -0.05219959533934237506, 48.75109039468568284 ) ) ;
#167129=CARTESIAN_POINT ( 'NONE',  ( 5.719274019375673035, 21.55341960407619339, 67.29275706135234714 ) ) ;
#167130=CARTESIAN_POINT ( 'NONE',  ( 5.153800228976615827, -19.02544592524334988, 75.20942372801896170 ) ) ;
#167131=CARTESIAN_POINT ( 'NONE',  ( -13.89961937509957401, -13.97604488694547875, 29.37609039468565797 ) ) ;
#167132=CARTESIAN_POINT ( 'NONE',  ( -9.564922557960796823, -16.46253265017161027, 57.08224293864769550 ) ) ;
#167133=CARTESIAN_POINT ( 'NONE',  ( 5.049401038298161559, -19.05341960407611168, 47.70724293864770260 ) ) ;
#167135=CARTESIAN_POINT ( 'NONE',  ( -21.53943276465977519, 0.05219959533907696930, 66.24890960531436690 ) ) ;
#167137=CARTESIAN_POINT ( 'NONE',  ( -21.53943276465977519, 0.05219959533907696930, 31.24890960531435979 ) ) ;
#167138=CARTESIAN_POINT ( 'NONE',  ( 5.153800228976335163, 19.02544592524342804, 24.79057627198102765 ) ) ;
#167139=CARTESIAN_POINT ( 'NONE',  ( 12.06949235617739724, 12.14591786802326823, 51.87609039468568284 ) ) ;
#167142=CARTESIAN_POINT ( 'NONE',  ( -21.53943276465977519, -0.05219959533937600094, 28.75109039468567929 ) ) ;
#167143=CARTESIAN_POINT ( 'NONE',  ( -4.483927247898539470, -16.52544592524342804, 57.29057627198103120 ) ) ;
#167145=CARTESIAN_POINT ( 'NONE',  ( 13.97604488694548053, -13.89961937509957401, 110.6260903946856615 ) ) ;
#167146=CARTESIAN_POINT ( 'NONE',  ( -19.02544592524334988, -5.153800228976617603, 38.95942372801900433 ) ) ;
#167147=CARTESIAN_POINT ( 'NONE',  ( 14.29746914071049879, -8.314922557960816363, 48.33224293864770260 ) ) ;
#167148=CARTESIAN_POINT ( 'NONE',  ( 10.81492255796106328, -18.62759615963255655, 25.41775706135235779 ) ) ;
#167150=CARTESIAN_POINT ( 'NONE',  ( 21.55341960407610458, 5.719274019375980345, 58.95724293864770971 ) ) ;
#167151=CARTESIAN_POINT ( 'NONE',  ( -5.153800228976328057, -19.02544592524343514, 92.29057627198099567 ) ) ;
#167152=CARTESIAN_POINT ( 'NONE',  ( 16.52544592524342804, -4.483927247898539470, 63.54057627198103830 ) ) ;
#167153=CARTESIAN_POINT ( 'NONE',  ( -5.049401038298153566, 19.05341960407611168, 110.2072429386476671 ) ) ;
#167154=CARTESIAN_POINT ( 'NONE',  ( -17.49999999999999645, -5.500000000000000888, 120.0000000000000142 ) ) ;
#167155=CARTESIAN_POINT ( 'NONE',  ( -9.474510206698720793, -16.51473224551083518, 49.58442372801899722 ) ) ;
#167156=CARTESIAN_POINT ( 'NONE',  ( -5.719274019375978568, 21.55341960407610458, 105.2072429386477097 ) ) ;
#167157=CARTESIAN_POINT ( 'NONE',  ( -13.89961937509977652, 13.97604488694528158, 40.62390960531435979 ) ) ;
#167158=CARTESIAN_POINT ( 'NONE',  ( -13.97604488694527625, -13.89961937509977652, 21.87390960531435979 ) ) ;
#167159=CARTESIAN_POINT ( 'NONE',  ( 15.80617190586769283, -15.72974639402175789, 50.62609039468568994 ) ) ;
#167162=CARTESIAN_POINT ( 'NONE',  ( 12.06949235617757843, -12.14591786802309237, 23.12390960531436335 ) ) ;
#167163=CARTESIAN_POINT ( 'NONE',  ( -13.89961937509977652, 13.97604488694528158, 45.62390960531433848 ) ) ;
#167164=CARTESIAN_POINT ( 'NONE',  ( 0.05219959533909260263, 19.03943276465977164, 94.99890960531436690 ) ) ;
#167165=CARTESIAN_POINT ( 'NONE',  ( 0.05219959533907565091, 21.53943276465977519, 79.99890960531435269 ) ) ;
#167167=CARTESIAN_POINT ( 'NONE',  ( -19.05341960407611168, -5.049401038298163336, 46.45724293864768129 ) ) ;
#167168=CARTESIAN_POINT ( 'NONE',  ( -18.62759615963270932, 10.81492255796079327, 50.83224293864770971 ) ) ;
#167169=CARTESIAN_POINT ( 'NONE',  ( -18.67979575497193778, 10.72451020669871902, 83.33442372801903275 ) ) ;
#167170=CARTESIAN_POINT ( 'NONE',  ( 18.22780087662121673, 5.500000000000056843, 53.98459894673893444 ) ) ;
#167171=CARTESIAN_POINT ( 'NONE',  ( -4.483927247898782831, 16.52544592524335698, 82.70942372801900433 ) ) ;
#167172=CARTESIAN_POINT ( 'NONE',  ( -14.29746914071049879, 8.314922557960819915, 65.83224293864769550 ) ) ;
#167173=CARTESIAN_POINT ( 'NONE',  ( -19.05341960407611168, -5.049401038298163336, 76.45724293864769550 ) ) ;
#167175=CARTESIAN_POINT ( 'NONE',  ( 19.02544592524334988, 5.153800228976608722, 21.45942372801899012 ) ) ;
#167176=CARTESIAN_POINT ( 'NONE',  ( -12.14591786802326823, 12.06949235617739902, 93.12609039468568994 ) ) ;
#167177=CARTESIAN_POINT ( 'NONE',  ( -15.80617190586768217, 15.72974639402176855, 108.1260903946856757 ) ) ;
#167178=CARTESIAN_POINT ( 'NONE',  ( -0.05219959533909027116, -19.03943276465977164, 77.49890960531435269 ) ) ;
#167179=CARTESIAN_POINT ( 'NONE',  ( -5.719274019375978568, 21.55341960407610458, 50.20724293864769550 ) ) ;
#167180=CARTESIAN_POINT ( 'NONE',  ( 4.483927247898790824, -16.52544592524335698, 25.20942372801901854 ) ) ;
#167181=CARTESIAN_POINT ( 'NONE',  ( -21.53943276465977519, -0.05219959533937600094, 93.75109039468567573 ) ) ;
#167182=CARTESIAN_POINT ( 'NONE',  ( -14.29746914071037622, -8.314922557961029526, 69.16775706135234714 ) ) ;
#167183=CARTESIAN_POINT ( 'NONE',  ( 10.81492255796106328, -18.62759615963255655, 20.41775706135234714 ) ) ;
#167184=CARTESIAN_POINT ( 'NONE',  ( -16.46253265017146816, -9.564922557961047289, 109.1677570613523471 ) ) ;
#167185=CARTESIAN_POINT ( 'NONE',  ( -13.89961937509977652, 13.97604488694528158, 95.62390960531436690 ) ) ;
#167186=CARTESIAN_POINT ( 'NONE',  ( 4.483927247898790824, -16.52544592524335698, 30.20942372801902565 ) ) ;
#167187=CARTESIAN_POINT ( 'NONE',  ( 0.05219959533909260263, 19.03943276465977164, 49.99890960531435979 ) ) ;
#167189=CARTESIAN_POINT ( 'NONE',  ( 14.29746914071037800, 8.314922557961029526, 31.66775706135234358 ) ) ;
#167190=CARTESIAN_POINT ( 'NONE',  ( 4.379528057220339221, -16.55341960407611168, 72.70724293864769550 ) ) ;
#167191=CARTESIAN_POINT ( 'NONE',  ( 12.06949235617739724, 12.14591786802326823, 81.87609039468568994 ) ) ;
#167193=CARTESIAN_POINT ( 'NONE',  ( -10.81492255796105439, 18.62759615963255655, 32.91775706135234714 ) ) ;
#167194=CARTESIAN_POINT ( 'NONE',  ( -5.049401038298153566, 19.05341960407611168, 65.20724293864765286 ) ) ;
#167195=CARTESIAN_POINT ( 'NONE',  ( -9.564922557960796823, -16.46253265017161027, 82.08224293864768129 ) ) ;
#167196=CARTESIAN_POINT ( 'NONE',  ( -12.06949235617739369, -12.14591786802326823, 84.37609039468570415 ) ) ;
#167199=CARTESIAN_POINT ( 'NONE',  ( -19.05341960407617563, 5.049401038297882671, 33.54275706135231871 ) ) ;
#167200=CARTESIAN_POINT ( 'NONE',  ( -19.02544592524342804, 5.153800228976336051, 101.0405762719810241 ) ) ;
#167201=CARTESIAN_POINT ( 'NONE',  ( -0.05219959533909027116, -19.03943276465977164, 52.49890960531436690 ) ) ;
#167203=CARTESIAN_POINT ( 'NONE',  ( -12.14591786802326823, 12.06949235617739902, 38.12609039468567573 ) ) ;
#167204=CARTESIAN_POINT ( 'NONE',  ( -9.564922557961040184, 16.46253265017147172, 57.91775706135233293 ) ) ;
#167205=CARTESIAN_POINT ( 'NONE',  ( 12.14591786802327356, -12.06949235617739191, 55.62609039468568284 ) ) ;
#167206=CARTESIAN_POINT ( 'NONE',  ( -16.46253265017160317, 9.564922557960807481, 105.8322429386476955 ) ) ;
#167208=CARTESIAN_POINT ( 'NONE',  ( -5.153800228976328057, -19.02544592524343514, 82.29057627198103830 ) ) ;
#167209=CARTESIAN_POINT ( 'NONE',  ( 0.05219959533907565091, 21.53943276465977519, 99.99890960531436690 ) ) ;
#167210=CARTESIAN_POINT ( 'NONE',  ( -9.474510206698720793, -16.51473224551083518, 69.58442372801901854 ) ) ;
#167211=CARTESIAN_POINT ( 'NONE',  ( -0.05219959533909027116, -19.03943276465977164, 87.49890960531436690 ) ) ;
#167213=CARTESIAN_POINT ( 'NONE',  ( 19.02544592524343514, -5.153800228976328945, 63.54057627198103830 ) ) ;
#167214=CARTESIAN_POINT ( 'NONE',  ( 12.14591786802309770, 12.06949235617756955, 29.37390960531435269 ) ) ;
#167215=CARTESIAN_POINT ( 'NONE',  ( 16.46253265017160672, -9.564922557960803928, 23.33224293864769194 ) ) ;
#167216=CARTESIAN_POINT ( 'NONE',  ( 9.474510206698729675, 16.51473224551082808, 42.08442372801900433 ) ) ;
#167217=CARTESIAN_POINT ( 'NONE',  ( 14.29746914071049879, -8.314922557960816363, 68.33224293864769550 ) ) ;
#167218=CARTESIAN_POINT ( 'NONE',  ( -21.53943276465977519, -0.05219959533937600094, 98.75109039468568994 ) ) ;
#167219=CARTESIAN_POINT ( 'NONE',  ( -19.03943276465977164, 0.05219959533909376836, 36.24890960531436690 ) ) ;
#167220=CARTESIAN_POINT ( 'NONE',  ( -4.483927247898539470, -16.52544592524342804, 37.29057627198102409 ) ) ;
#167221=CARTESIAN_POINT ( 'NONE',  ( 15.80617190586769283, -15.72974639402175789, 105.6260903946856899 ) ) ;
#167222=CARTESIAN_POINT ( 'NONE',  ( -5.153800228976328057, -19.02544592524343514, 87.29057627198103830 ) ) ;
#167223=CARTESIAN_POINT ( 'NONE',  ( 19.03943276465977164, -0.05219959533909143690, 88.74890960531436690 ) ) ;
#167224=CARTESIAN_POINT ( 'NONE',  ( 19.02544592524343514, -5.153800228976328945, 23.54057627198102054 ) ) ;
#167225=CARTESIAN_POINT ( 'NONE',  ( -4.483927247898539470, -16.52544592524342804, 112.2905762719810241 ) ) ;
#167226=CARTESIAN_POINT ( 'NONE',  ( -16.53943276465976808, 0.05219959533911058130, 76.24890960531435269 ) ) ;
#167227=CARTESIAN_POINT ( 'NONE',  ( 0.05219959533907565091, 21.53943276465977519, 89.99890960531438111 ) ) ;
#167228=CARTESIAN_POINT ( 'NONE',  ( 5.153800228976335163, 19.02544592524342804, 84.79057627198099567 ) ) ;
#167229=CARTESIAN_POINT ( 'NONE',  ( -5.719274019375978568, 21.55341960407610458, 100.2072429386476955 ) ) ;
#167230=CARTESIAN_POINT ( 'NONE',  ( -19.05341960407611168, -5.049401038298163336, 91.45724293864766707 ) ) ;
#167231=CARTESIAN_POINT ( 'NONE',  ( -5.049401038297874678, -19.05341960407618274, 64.79275706135233293 ) ) ;
#167232=CARTESIAN_POINT ( 'NONE',  ( -14.29746914071049879, 8.314922557960819915, 85.83224293864768129 ) ) ;
#167233=CARTESIAN_POINT ( 'NONE',  ( -9.474510206698964154, 16.51473224551069663, 65.41557627198102409 ) ) ;
#167234=CARTESIAN_POINT ( 'NONE',  ( -18.67979575497178146, -10.72451020669898902, 71.66557627198100988 ) ) ;
#167236=CARTESIAN_POINT ( 'NONE',  ( -4.483927247898782831, 16.52544592524335698, 112.7094237280190328 ) ) ;
#167238=CARTESIAN_POINT ( 'NONE',  ( 16.53943276465976808, 0.05219959533934440121, 26.25109039468567573 ) ) ;
#167239=CARTESIAN_POINT ( 'NONE',  ( 12.06949235617757843, -12.14591786802309237, 93.12390960531436690 ) ) ;
#167240=CARTESIAN_POINT ( 'NONE',  ( -17.50000000000000711, -5.622605283950870003, 96.31207310596111881 ) ) ;
#167241=CARTESIAN_POINT ( 'NONE',  ( 16.46253265017160672, -9.564922557960803928, 83.33224293864768129 ) ) ;
#167242=CARTESIAN_POINT ( 'NONE',  ( -13.89961937509977652, 13.97604488694528158, 50.62390960531435979 ) ) ;
#167243=CARTESIAN_POINT ( 'NONE',  ( 4.379528057220339221, -16.55341960407611168, 67.70724293864769550 ) ) ;
#167244=CARTESIAN_POINT ( 'NONE',  ( 19.03943276465977164, -0.05219959533909143690, 108.7489096053143527 ) ) ;
#167245=CARTESIAN_POINT ( 'NONE',  ( 16.51473224551083163, -9.474510206698727899, 105.8344237280190043 ) ) ;
#167246=CARTESIAN_POINT ( 'NONE',  ( -10.81492255796105439, 18.62759615963255655, 62.91775706135236135 ) ) ;
#167247=CARTESIAN_POINT ( 'NONE',  ( 13.89961937509977652, -13.97604488694527269, 93.12390960531436690 ) ) ;
#167248=CARTESIAN_POINT ( 'NONE',  ( -15.72974639402197994, 15.80617190586746368, 80.62390960531438111 ) ) ;
#167249=CARTESIAN_POINT ( 'NONE',  ( 12.14591786802327356, -12.06949235617739191, 65.62609039468568994 ) ) ;
#167250=CARTESIAN_POINT ( 'NONE',  ( 30.00000000000000000, 5.499999999999992895, 37.50000000000000000 ) ) ;
#167251=CARTESIAN_POINT ( 'NONE',  ( -19.02544592524342804, 5.153800228976336051, 71.04057627198099567 ) ) ;
#167252=CARTESIAN_POINT ( 'NONE',  ( -15.80617190586745835, -15.72974639402198527, 86.87390960531438111 ) ) ;
#167253=CARTESIAN_POINT ( 'NONE',  ( -5.049401038297874678, -19.05341960407617918, 109.7927570613523187 ) ) ;
#167254=CARTESIAN_POINT ( 'NONE',  ( 0.05219959533910956823, 16.53943276465976808, 34.99890960531435979 ) ) ;
#167255=CARTESIAN_POINT ( 'NONE',  ( -10.72451020669870658, -18.67979575497194134, 64.58442372801900433 ) ) ;
#167256=CARTESIAN_POINT ( 'NONE',  ( -14.34966873604972548, 8.224510206698743886, 88.33442372801901854 ) ) ;
#167257=CARTESIAN_POINT ( 'NONE',  ( -18.67979575497178146, -10.72451020669898902, 26.66557627198103475 ) ) ;
#167258=CARTESIAN_POINT ( 'NONE',  ( 5.049401038298163336, -19.05341960407611168, 107.7072429386476955 ) ) ;
#167260=CARTESIAN_POINT ( 'NONE',  ( 8.224510206698742110, 14.34966873604972548, 112.0844237280190185 ) ) ;
#167261=CARTESIAN_POINT ( 'NONE',  ( 14.29746914071037800, 8.314922557961029526, 46.66775706135234714 ) ) ;
#167262=CARTESIAN_POINT ( 'NONE',  ( -9.474510206698964154, 16.51473224551069663, 60.41557627198102409 ) ) ;
#167263=CARTESIAN_POINT ( 'NONE',  ( 5.049401038298161559, -19.05341960407611168, 72.70724293864768129 ) ) ;
#167264=CARTESIAN_POINT ( 'NONE',  ( 0.05219959533934541429, -16.53943276465976808, 70.00109039468568994 ) ) ;
#167265=CARTESIAN_POINT ( 'NONE',  ( 12.06949235617757843, -12.14591786802309237, 43.12390960531435269 ) ) ;
#167266=CARTESIAN_POINT ( 'NONE',  ( -9.564922557960796823, -16.46253265017161027, 52.08224293864768839 ) ) ;
#167267=CARTESIAN_POINT ( 'NONE',  ( -13.89961937509977652, 13.97604488694528158, 45.62390960531433848 ) ) ;
#167268=CARTESIAN_POINT ( 'NONE',  ( -12.06949235617739369, -12.14591786802326823, 39.37609039468567573 ) ) ;
#167269=CARTESIAN_POINT ( 'NONE',  ( 19.05341960407617918, -5.049401038297876454, 91.04275706135234714 ) ) ;
#167270=CARTESIAN_POINT ( 'NONE',  ( 14.29746914071049879, -8.314922557960816363, 103.3322429386476955 ) ) ;
#167271=CARTESIAN_POINT ( 'NONE',  ( -9.474510206698964154, 16.51473224551069663, 70.41557627198102409 ) ) ;
#167272=CARTESIAN_POINT ( 'NONE',  ( -16.46253265017146816, -9.564922557961047289, 104.1677570613523329 ) ) ;
#167274=CARTESIAN_POINT ( 'NONE',  ( 15.80617190586769283, -15.72974639402175789, 85.62609039468568994 ) ) ;
#167275=CARTESIAN_POINT ( 'NONE',  ( -8.314922557961024197, 14.29746914071037800, 62.91775706135236135 ) ) ;
#167276=CARTESIAN_POINT ( 'NONE',  ( -17.50000000000000000, -5.500000000000000000, 106.2823096230357010 ) ) ;
#167277=CARTESIAN_POINT ( 'NONE',  ( -10.72451020669898014, 18.67979575497178502, 65.41557627198102409 ) ) ;
#167278=CARTESIAN_POINT ( 'NONE',  ( -12.06949235617739369, -12.14591786802326823, 49.37609039468569705 ) ) ;
#167279=CARTESIAN_POINT ( 'NONE',  ( 19.03943276465977164, -0.05219959533909143690, 33.74890960531435979 ) ) ;
#167280=CARTESIAN_POINT ( 'NONE',  ( -0.05219959533936034679, 19.03943276465977164, 47.50109039468566863 ) ) ;
#167281=CARTESIAN_POINT ( 'NONE',  ( 19.03943276465977164, -0.05219959533909143690, 88.74890960531436690 ) ) ;
#167282=CARTESIAN_POINT ( 'NONE',  ( 4.379528057220339221, -16.55341960407611168, 112.7072429386476955 ) ) ;
#167283=CARTESIAN_POINT ( 'NONE',  ( 5.153800228976335163, 19.02544592524342804, 64.79057627198100988 ) ) ;
#167285=CARTESIAN_POINT ( 'NONE',  ( -17.49999999999999645, 5.499999999999992895, 53.71769037696436300 ) ) ;
#167286=CARTESIAN_POINT ( 'NONE',  ( -18.62759615963255300, -10.81492255796106328, 74.16775706135231871 ) ) ;
#167288=CARTESIAN_POINT ( 'NONE',  ( -19.03943276465977164, -0.05219959533935918106, 33.75109039468566863 ) ) ;
#167289=CARTESIAN_POINT ( 'NONE',  ( -9.564922557961040184, 16.46253265017147172, 27.91775706135232582 ) ) ;
#167290=CARTESIAN_POINT ( 'NONE',  ( 4.379528057220339221, -16.55341960407611168, 57.70724293864770260 ) ) ;
#167291=CARTESIAN_POINT ( 'NONE',  ( 5.049401038298161559, -19.05341960407611168, 57.70724293864769550 ) ) ;
#167292=CARTESIAN_POINT ( 'NONE',  ( -10.72451020669898014, 18.67979575497178502, 25.41557627198103120 ) ) ;
#167293=CARTESIAN_POINT ( 'NONE',  ( -21.53943276465977519, -0.05219959533937600094, 83.75109039468568994 ) ) ;
#167294=CARTESIAN_POINT ( 'NONE',  ( 16.46253265017160672, -9.564922557960803928, 68.33224293864770971 ) ) ;
#167295=ADVANCED_FACE ( 'NONE', ( #71805 ), #164276, .T. ) ;
#167296=CARTESIAN_POINT ( 'NONE',  ( -21.53943276465977519, -0.05219959533937600094, 83.75109039468568994 ) ) ;
#167297=CARTESIAN_POINT ( 'NONE',  ( -18.67979575497178146, -10.72451020669898902, 31.66557627198102054 ) ) ;
#167298=CARTESIAN_POINT ( 'NONE',  ( -16.46253265017160317, 9.564922557960807481, 65.83224293864769550 ) ) ;
#167299=CARTESIAN_POINT ( 'NONE',  ( 15.80617190586769283, -15.72974639402175789, 40.62609039468567573 ) ) ;
#167300=CARTESIAN_POINT ( 'NONE',  ( -19.03943276465977164, -0.05219959533935918106, 63.75109039468566863 ) ) ;
#167301=CARTESIAN_POINT ( 'NONE',  ( 19.02544592524343514, -5.153800228976328945, 38.54057627198103120 ) ) ;
#167302=CARTESIAN_POINT ( 'NONE',  ( 5.049401038298161559, -19.05341960407611168, 72.70724293864768129 ) ) ;
#167303=CARTESIAN_POINT ( 'NONE',  ( -16.55341960407617563, 4.379528057220093196, 28.54275706135234358 ) ) ;
#167304=CARTESIAN_POINT ( 'NONE',  ( -8.224510206698948167, 14.34966873604960824, 90.41557627198103830 ) ) ;
#167305=CARTESIAN_POINT ( 'NONE',  ( 16.46253265017160672, -9.564922557960803928, 53.33224293864768839 ) ) ;
#167306=CARTESIAN_POINT ( 'NONE',  ( -21.55341960407610458, -5.719274019375992779, 51.45724293864770260 ) ) ;
#167307=CARTESIAN_POINT ( 'NONE',  ( 4.483927247898790824, -16.52544592524335698, 20.20942372801900788 ) ) ;
#167308=CARTESIAN_POINT ( 'NONE',  ( -10.81492255796105439, 18.62759615963255655, 22.91775706135235069 ) ) ;
#167309=CARTESIAN_POINT ( 'NONE',  ( 18.67979575497194134, -10.72451020669871369, 70.83442372801901854 ) ) ;
#167310=CARTESIAN_POINT ( 'NONE',  ( -16.52544592524335698, -4.483927247898792601, 73.95942372801901854 ) ) ;
#167311=CARTESIAN_POINT ( 'NONE',  ( -16.52544592524335698, -4.483927247898792601, 73.95942372801901854 ) ) ;
#167312=CARTESIAN_POINT ( 'NONE',  ( -13.89961937509977652, 13.97604488694528158, 55.62390960531434558 ) ) ;
#167313=CARTESIAN_POINT ( 'NONE',  ( 8.224510206698742110, 14.34966873604972548, 92.08442372801901854 ) ) ;
#167314=CARTESIAN_POINT ( 'NONE',  ( 9.564922557961047289, -16.46253265017146816, 40.41775706135234003 ) ) ;
#167316=CARTESIAN_POINT ( 'NONE',  ( -5.823673210054431948, 21.52544592524334988, 22.70942372801901499 ) ) ;
#167317=CARTESIAN_POINT ( 'NONE',  ( 4.379528057220339221, -16.55341960407611168, 67.70724293864769550 ) ) ;
#167318=CARTESIAN_POINT ( 'NONE',  ( 13.97604488694527802, 13.89961937509977652, 84.37390960531433848 ) ) ;
#167319=CARTESIAN_POINT ( 'NONE',  ( 4.483927247898790824, -16.52544592524335698, 90.20942372801903275 ) ) ;
#167320=CARTESIAN_POINT ( 'NONE',  ( 18.67979575497194134, -10.72451020669871369, 60.83442372801901854 ) ) ;
#167321=CARTESIAN_POINT ( 'NONE',  ( 16.53943276465976808, 0.05219959533934440121, 36.25109039468567573 ) ) ;
#167322=CARTESIAN_POINT ( 'NONE',  ( -0.05219959533937732626, 21.53943276465977519, 32.50109039468568284 ) ) ;
#167323=CARTESIAN_POINT ( 'NONE',  ( -4.483927247898539470, -16.52544592524342804, 57.29057627198103120 ) ) ;
#167324=VERTEX_POINT ( 'NONE', #144686 ) ;
#167325=CARTESIAN_POINT ( 'NONE',  ( 5.823673210054125526, 21.52544592524343514, 99.79057627198103830 ) ) ;
#167326=CARTESIAN_POINT ( 'NONE',  ( 16.52544592524342804, -4.483927247898539470, 38.54057627198103120 ) ) ;
#167329=CARTESIAN_POINT ( 'NONE',  ( -18.62759615963270932, 10.81492255796079327, 25.83224293864769194 ) ) ;
#167330=CARTESIAN_POINT ( 'NONE',  ( 5.719274019375673035, 21.55341960407619339, 42.29275706135235424 ) ) ;
#167331=CARTESIAN_POINT ( 'NONE',  ( 14.34966873604960469, 8.224510206698951720, 69.16557627198102409 ) ) ;
#167332=CARTESIAN_POINT ( 'NONE',  ( 16.51473224551069308, 9.474510206698969483, 74.16557627198103830 ) ) ;
#167333=CARTESIAN_POINT ( 'NONE',  ( -16.51473224551069308, -9.474510206698971260, 26.66557627198103120 ) ) ;
#167334=CARTESIAN_POINT ( 'NONE',  ( -9.474510206698720793, -16.51473224551083518, 69.58442372801901854 ) ) ;
#167335=CARTESIAN_POINT ( 'NONE',  ( -5.823673210054116645, -21.52544592524344225, 47.29057627198103120 ) ) ;
#167337=CARTESIAN_POINT ( 'NONE',  ( -19.05341960407611168, -5.049401038298163336, 56.45724293864768129 ) ) ;
#167338=CARTESIAN_POINT ( 'NONE',  ( 4.379528057220092307, 16.55341960407617563, 42.29275706135235424 ) ) ;
#167339=CARTESIAN_POINT ( 'NONE',  ( 21.52544592524344225, -5.823673210054117533, 113.5405762719810383 ) ) ;
#167340=CARTESIAN_POINT ( 'NONE',  ( -4.379528057220328563, 16.55341960407611168, 50.20724293864769550 ) ) ;
#167342=CARTESIAN_POINT ( 'NONE',  ( -19.02544592524342804, 5.153800228976336051, 96.04057627198103830 ) ) ;
#167343=CARTESIAN_POINT ( 'NONE',  ( 18.62759615963271287, -10.81492255796078972, 78.33224293864770971 ) ) ;
#167344=CARTESIAN_POINT ( 'NONE',  ( 10.81492255796078972, 18.62759615963270932, 114.5822429386477097 ) ) ;
#167345=CARTESIAN_POINT ( 'NONE',  ( 12.06949235617739724, 12.14591786802326823, 31.87609039468567929 ) ) ;
#167346=CARTESIAN_POINT ( 'NONE',  ( -5.719274019375978568, 21.55341960407610458, 40.20724293864769550 ) ) ;
#167347=CARTESIAN_POINT ( 'NONE',  ( -21.53943276465977519, -0.05219959533937600094, 108.7510903946857042 ) ) ;
#167348=CARTESIAN_POINT ( 'NONE',  ( 9.564922557960805705, 16.46253265017160317, 104.5822429386476955 ) ) ;
#167349=CARTESIAN_POINT ( 'NONE',  ( -19.02544592524342804, 5.153800228976336051, 36.04057627198100988 ) ) ;
#167350=CARTESIAN_POINT ( 'NONE',  ( 9.474510206698971260, -16.51473224551069308, 97.91557627198102409 ) ) ;
#167351=CARTESIAN_POINT ( 'NONE',  ( 5.153800228976335163, 19.02544592524342804, 74.79057627198103830 ) ) ;
#167353=CARTESIAN_POINT ( 'NONE',  ( 13.97604488694548053, -13.89961937509957401, 50.62609039468566152 ) ) ;
#167354=CARTESIAN_POINT ( 'NONE',  ( -18.67979575497193778, 10.72451020669871902, 108.3344237280190185 ) ) ;
#167355=CARTESIAN_POINT ( 'NONE',  ( -15.72974639402197994, 15.80617190586746368, 25.62390960531435624 ) ) ;
#167356=CARTESIAN_POINT ( 'NONE',  ( 16.53943276465976808, 0.05219959533934440121, 106.2510903946856757 ) ) ;
#167357=CARTESIAN_POINT ( 'NONE',  ( 9.474510206698729675, 16.51473224551082808, 92.08442372801900433 ) ) ;
#167358=CARTESIAN_POINT ( 'NONE',  ( -16.21995358207306737, 7.366697692864095259, 59.93551001512161491 ) ) ;
#167359=CARTESIAN_POINT ( 'NONE',  ( -13.97604488694547697, 13.89961937509957934, 88.12609039468563310 ) ) ;
#167360=CARTESIAN_POINT ( 'NONE',  ( 19.05341960407617918, -5.049401038297876454, 36.04275706135234003 ) ) ;
#167361=CARTESIAN_POINT ( 'NONE',  ( -16.18388926212241330, -7.379444403734407132, 45.43953151366152809 ) ) ;
#167362=CARTESIAN_POINT ( 'NONE',  ( 16.46253265017160672, -9.564922557960803928, 43.33224293864769550 ) ) ;
#167363=CARTESIAN_POINT ( 'NONE',  ( 14.29746914071049879, -8.314922557960816363, 53.33224293864769550 ) ) ;
#167364=CARTESIAN_POINT ( 'NONE',  ( -17.50000000000000711, -5.622605283950883326, 111.3120731059611330 ) ) ;
#167365=CARTESIAN_POINT ( 'NONE',  ( 4.379528057220339221, -16.55341960407611168, 22.70724293864769194 ) ) ;
#167367=CARTESIAN_POINT ( 'NONE',  ( 14.34966873604972726, -8.224510206698740333, 100.8344237280190185 ) ) ;
#167368=CARTESIAN_POINT ( 'NONE',  ( -13.89961937509977652, 13.97604488694528158, 45.62390960531433848 ) ) ;
#167370=CARTESIAN_POINT ( 'NONE',  ( -15.80617190586768217, 15.72974639402176855, 108.1260903946856757 ) ) ;
#167371=CARTESIAN_POINT ( 'NONE',  ( 12.06949235617739724, 12.14591786802326823, 26.87609039468567218 ) ) ;
#167372=CARTESIAN_POINT ( 'NONE',  ( -15.80617190586768217, 15.72974639402176855, 93.12609039468568994 ) ) ;
#167373=ORIENTED_EDGE ( 'NONE', *, *, #60920, .T. ) ;
#167374=CARTESIAN_POINT ( 'NONE',  ( -16.51473224551069308, -9.474510206698971260, 86.66557627198102409 ) ) ;
#167375=CARTESIAN_POINT ( 'NONE',  ( 9.564922557960805705, 16.46253265017160317, 79.58224293864769550 ) ) ;
#167377=CARTESIAN_POINT ( 'NONE',  ( -18.62759615963270932, 10.81492255796079327, 105.8322429386476955 ) ) ;
#167378=CARTESIAN_POINT ( 'NONE',  ( 16.52544592524342804, -4.483927247898539470, 78.54057627198103830 ) ) ;
#167379=CARTESIAN_POINT ( 'NONE',  ( 10.81492255796078972, 18.62759615963270932, 79.58224293864769550 ) ) ;
#167380=CARTESIAN_POINT ( 'NONE',  ( 5.153800228976335163, 19.02544592524342804, 64.79057627198100988 ) ) ;
#167381=CARTESIAN_POINT ( 'NONE',  ( 15.72974639402199770, -15.80617190586745480, 98.12390960531436690 ) ) ;
#167382=CARTESIAN_POINT ( 'NONE',  ( 8.224510206698742110, 14.34966873604972548, 97.08442372801904696 ) ) ;
#167385=CARTESIAN_POINT ( 'NONE',  ( -19.03943276465977164, 0.05219959533909376836, 66.24890960531436690 ) ) ;
#167386=CARTESIAN_POINT ( 'NONE',  ( -12.14591786802309592, -12.06949235617757132, 86.87390960531438111 ) ) ;
#167388=CARTESIAN_POINT ( 'NONE',  ( 13.89961937509977652, -13.97604488694527269, 68.12390960531436690 ) ) ;
#167389=CARTESIAN_POINT ( 'NONE',  ( 19.02544592524334988, 5.153800228976608722, 76.45942372801897591 ) ) ;
#167390=CARTESIAN_POINT ( 'NONE',  ( -12.14591786802309592, -12.06949235617757132, 86.87390960531438111 ) ) ;
#167391=CARTESIAN_POINT ( 'NONE',  ( -15.72974639402176322, -15.80617190586768395, 59.37609039468568284 ) ) ;
#167392=CARTESIAN_POINT ( 'NONE',  ( 0.05219959533909260263, 19.03943276465977164, 54.99890960531435979 ) ) ;
#167393=CARTESIAN_POINT ( 'NONE',  ( -21.53943276465977519, 0.05219959533907696930, 116.2489096053143669 ) ) ;
#167394=CARTESIAN_POINT ( 'NONE',  ( 16.52544592524342804, -4.483927247898539470, 98.54057627198105251 ) ) ;
#167396=CARTESIAN_POINT ( 'NONE',  ( 19.03943276465977164, -0.05219959533909143690, 53.74890960531436690 ) ) ;
#167397=CYLINDRICAL_SURFACE ( 'NONE', #21534, 2.500000000000002220 ) ;
#167398=CARTESIAN_POINT ( 'NONE',  ( 0.05219959533936267826, -19.03943276465977164, 100.0010903946856757 ) ) ;
#167399=CARTESIAN_POINT ( 'NONE',  ( 15.72974639402199770, -15.80617190586745480, 23.12390960531436335 ) ) ;
#167400=CARTESIAN_POINT ( 'NONE',  ( 21.53943276465977519, 0.05219959533937863772, 46.25109039468567573 ) ) ;
#167401=CARTESIAN_POINT ( 'NONE',  ( -19.05341960407611168, -5.049401038298163336, 86.45724293864769550 ) ) ;
#167402=CARTESIAN_POINT ( 'NONE',  ( -5.153800228976607833, 19.02544592524334988, 72.70942372801900433 ) ) ;
#167403=CARTESIAN_POINT ( 'NONE',  ( 19.03943276465977164, -0.05219959533909143690, 58.74890960531435979 ) ) ;
#167404=CARTESIAN_POINT ( 'NONE',  ( -4.483927247898539470, -16.52544592524342804, 82.29057627198103830 ) ) ;
#167405=CARTESIAN_POINT ( 'NONE',  ( 8.224510206698953496, -14.34966873604960469, 77.91557627198102409 ) ) ;
#167406=CARTESIAN_POINT ( 'NONE',  ( -19.02544592524342804, 5.153800228976336051, 91.04057627198100988 ) ) ;
#167407=CARTESIAN_POINT ( 'NONE',  ( -8.314922557960811034, -14.29746914071050412, 77.08224293864769550 ) ) ;
#167408=CARTESIAN_POINT ( 'NONE',  ( 5.153800228976335163, 19.02544592524342804, 84.79057627198099567 ) ) ;
#167409=CARTESIAN_POINT ( 'NONE',  ( 9.564922557961047289, -16.46253265017146816, 25.41775706135234003 ) ) ;
#167410=CARTESIAN_POINT ( 'NONE',  ( 16.46253265017160672, -9.564922557960803928, 53.33224293864768839 ) ) ;
#167411=CARTESIAN_POINT ( 'NONE',  ( 14.34966873604960469, 8.224510206698951720, 24.16557627198103120 ) ) ;
#167412=CARTESIAN_POINT ( 'NONE',  ( 12.06949235617757843, -12.14591786802309237, 108.1239096053143811 ) ) ;
#167414=CARTESIAN_POINT ( 'NONE',  ( 18.67979575497194134, -10.72451020669871369, 45.83442372801901854 ) ) ;
#167415=CARTESIAN_POINT ( 'NONE',  ( -19.02544592524334988, -5.153800228976617603, 68.95942372801896170 ) ) ;
#167416=CARTESIAN_POINT ( 'NONE',  ( -14.29746914071049879, 8.314922557960819915, 40.83224293864769550 ) ) ;
#167417=CARTESIAN_POINT ( 'NONE',  ( -21.55341960407610458, -5.719274019375992779, 81.45724293864769550 ) ) ;
#167418=CARTESIAN_POINT ( 'NONE',  ( 19.03943276465977164, -0.05219959533909143690, 113.7489096053143669 ) ) ;
#167419=CARTESIAN_POINT ( 'NONE',  ( 12.14591786802309770, 12.06949235617756955, 69.37390960531436690 ) ) ;
#167420=CARTESIAN_POINT ( 'NONE',  ( -9.564922557960796823, -16.46253265017161027, 42.08224293864769550 ) ) ;
#167421=CARTESIAN_POINT ( 'NONE',  ( 16.51473224551083163, -9.474510206698727899, 45.83442372801900433 ) ) ;
#167422=CARTESIAN_POINT ( 'NONE',  ( -16.52544592524335698, -4.483927247898792601, 103.9594237280190185 ) ) ;
#167423=CARTESIAN_POINT ( 'NONE',  ( 12.06949235617739724, 12.14591786802326823, 61.87609039468568284 ) ) ;
#167424=CARTESIAN_POINT ( 'NONE',  ( -15.72974639402197994, 15.80617190586746368, 35.62390960531437401 ) ) ;
#167425=CARTESIAN_POINT ( 'NONE',  ( -18.67979575497193778, 10.72451020669871902, 108.3344237280190185 ) ) ;
#167426=CARTESIAN_POINT ( 'NONE',  ( -16.51473224551069308, -9.474510206698971260, 91.66557627198103830 ) ) ;
#167427=CARTESIAN_POINT ( 'NONE',  ( 14.29746914071037800, 8.314922557961029526, 71.66775706135234714 ) ) ;
#167428=CARTESIAN_POINT ( 'NONE',  ( 19.05341960407611168, 5.049401038298154454, 23.95724293864769194 ) ) ;
#167429=CARTESIAN_POINT ( 'NONE',  ( 0.05219959533910956823, 16.53943276465976808, 29.99890960531435979 ) ) ;
#167430=CARTESIAN_POINT ( 'NONE',  ( 13.89961937509977652, -13.97604488694527269, 103.1239096053143527 ) ) ;
#167431=CARTESIAN_POINT ( 'NONE',  ( -5.049401038298153566, 19.05341960407611168, 95.20724293864770971 ) ) ;
#167432=CARTESIAN_POINT ( 'NONE',  ( -18.67979575497178146, -10.72451020669898902, 26.66557627198103475 ) ) ;
#167433=CARTESIAN_POINT ( 'NONE',  ( 12.06949235617757843, -12.14591786802309237, 68.12390960531436690 ) ) ;
#167434=CARTESIAN_POINT ( 'NONE',  ( 8.224510206698953496, -14.34966873604960469, 47.91557627198102409 ) ) ;
#167435=CARTESIAN_POINT ( 'NONE',  ( -14.29746914071037622, -8.314922557961029526, 54.16775706135235424 ) ) ;
#167436=CARTESIAN_POINT ( 'NONE',  ( -17.72662750342724891, -5.500000000000087041, 56.40179492283746043 ) ) ;
#167437=CARTESIAN_POINT ( 'NONE',  ( 5.153800228976615827, -19.02544592524334988, 55.20942372801899722 ) ) ;
#167438=CARTESIAN_POINT ( 'NONE',  ( 9.474510206698971260, -16.51473224551069308, 92.91557627198103830 ) ) ;
#167439=CARTESIAN_POINT ( 'NONE',  ( 9.564922557961047289, -16.46253265017146816, 65.41775706135233293 ) ) ;
#167441=CARTESIAN_POINT ( 'NONE',  ( 9.474510206698729675, 16.51473224551082808, 52.08442372801900433 ) ) ;
#167442=CARTESIAN_POINT ( 'NONE',  ( -9.564922557961040184, 16.46253265017147172, 102.9177570613523329 ) ) ;
#167443=CARTESIAN_POINT ( 'NONE',  ( 4.379528057220092307, 16.55341960407617563, 92.29275706135236135 ) ) ;
#167445=CARTESIAN_POINT ( 'NONE',  ( 19.05341960407611168, 5.049401038298154454, 38.95724293864767418 ) ) ;
#167446=CARTESIAN_POINT ( 'NONE',  ( -5.823673210054116645, -21.52544592524344225, 27.29057627198103120 ) ) ;
#167447=CARTESIAN_POINT ( 'NONE',  ( 15.80617190586769283, -15.72974639402175789, 50.62609039468568994 ) ) ;
#167448=CARTESIAN_POINT ( 'NONE',  ( -16.51473224551082808, 9.474510206698731452, 103.3344237280190043 ) ) ;
#167450=CARTESIAN_POINT ( 'NONE',  ( 16.51473224551069308, 9.474510206698969483, 59.16557627198102409 ) ) ;
#167453=CARTESIAN_POINT ( 'NONE',  ( 4.379528057220339221, -16.55341960407611168, 72.70724293864769550 ) ) ;
#167454=CARTESIAN_POINT ( 'NONE',  ( -9.564922557960796823, -16.46253265017161027, 62.08224293864769550 ) ) ;
#167455=CARTESIAN_POINT ( 'NONE',  ( 19.02544592524343514, -5.153800228976328945, 78.54057627198099567 ) ) ;
#167456=CARTESIAN_POINT ( 'NONE',  ( -9.474510206698720793, -16.51473224551083518, 84.58442372801900433 ) ) ;
#167457=CARTESIAN_POINT ( 'NONE',  ( 18.67979575497178502, 10.72451020669898547, 69.16557627198102409 ) ) ;
#167458=CARTESIAN_POINT ( 'NONE',  ( 14.34966873604960469, 8.224510206698951720, 109.1655762719810383 ) ) ;
#167459=CARTESIAN_POINT ( 'NONE',  ( 5.153800228976615827, -19.02544592524334988, 45.20942372801901143 ) ) ;
#167460=CARTESIAN_POINT ( 'NONE',  ( 19.02544592524343514, -5.153800228976328945, 73.54057627198103830 ) ) ;
#167462=CARTESIAN_POINT ( 'NONE',  ( -18.67979575497178146, -10.72451020669898902, 86.66557627198102409 ) ) ;
#167463=CARTESIAN_POINT ( 'NONE',  ( 16.55341960407611168, 4.379528057220329451, 73.95724293864769550 ) ) ;
#167464=CARTESIAN_POINT ( 'NONE',  ( 19.02544592524334988, 5.153800228976608722, 51.45942372801900433 ) ) ;
#167465=CARTESIAN_POINT ( 'NONE',  ( -10.81492255796078084, -18.62759615963271287, 77.08224293864769550 ) ) ;
#167466=CARTESIAN_POINT ( 'NONE',  ( -21.55341960407610458, -5.719274019375992779, 61.45724293864770260 ) ) ;
#167467=CARTESIAN_POINT ( 'NONE',  ( -15.72974639402197994, 15.80617190586746368, 35.62390960531437401 ) ) ;
#167468=CARTESIAN_POINT ( 'NONE',  ( -15.80617190586768217, 15.72974639402176855, 88.12609039468570415 ) ) ;
#167469=CARTESIAN_POINT ( 'NONE',  ( -9.474510206698964154, 16.51473224551069663, 80.41557627198103830 ) ) ;
#167470=CARTESIAN_POINT ( 'NONE',  ( 12.14591786802309770, 12.06949235617756955, 114.3739096053143527 ) ) ;
#167471=CARTESIAN_POINT ( 'NONE',  ( 21.55341960407619695, -5.719274019375665929, 26.04275706135235779 ) ) ;
#167472=CARTESIAN_POINT ( 'NONE',  ( 5.719274019375673035, 21.55341960407619339, 37.29275706135235424 ) ) ;
#167473=CARTESIAN_POINT ( 'NONE',  ( -16.51473224551069308, -9.474510206698971260, 31.66557627198102054 ) ) ;
#167474=CARTESIAN_POINT ( 'NONE',  ( 18.67979575497194134, -10.72451020669871369, 20.83442372801901143 ) ) ;
#167475=CARTESIAN_POINT ( 'NONE',  ( 16.46253265017146816, 9.564922557961045513, 66.66775706135233293 ) ) ;
#167476=CARTESIAN_POINT ( 'NONE',  ( 13.97604488694527802, 13.89961937509977652, 39.37390960531435269 ) ) ;
#167477=CARTESIAN_POINT ( 'NONE',  ( 16.52544592524335698, 4.483927247898782831, 31.45942372801901854 ) ) ;
#167478=CARTESIAN_POINT ( 'NONE',  ( 17.50000000000000000, 5.499999999999997335, 120.0000000000000142 ) ) ;
#167479=CARTESIAN_POINT ( 'NONE',  ( 4.483927247898790824, -16.52544592524335698, 65.20942372801901854 ) ) ;
#167480=CARTESIAN_POINT ( 'NONE',  ( 9.564922557960805705, 16.46253265017160317, 39.58224293864768839 ) ) ;
#167482=CARTESIAN_POINT ( 'NONE',  ( -16.51473224551069308, -9.474510206698971260, 86.66557627198102409 ) ) ;
#167483=CARTESIAN_POINT ( 'NONE',  ( -19.03943276465977164, 0.05219959533909376836, 21.24890960531436335 ) ) ;
#167484=CARTESIAN_POINT ( 'NONE',  ( -21.52544592524343514, 5.823673210054127303, 56.04057627198102409 ) ) ;
#167485=CARTESIAN_POINT ( 'NONE',  ( -12.14591786802326823, 12.06949235617739902, 48.12609039468568284 ) ) ;
#167486=CARTESIAN_POINT ( 'NONE',  ( -18.62759615963255300, -10.81492255796106328, 99.16775706135234714 ) ) ;
#167488=CARTESIAN_POINT ( 'NONE',  ( 19.03943276465977164, -0.05219959533909143690, 43.74890960531435979 ) ) ;
#167489=CARTESIAN_POINT ( 'NONE',  ( 16.53943276465976808, -0.05219959533910856209, 28.74890960531435624 ) ) ;
#167490=CARTESIAN_POINT ( 'NONE',  ( -14.29746914071049879, 8.314922557960819915, 70.83224293864770971 ) ) ;
#167491=CARTESIAN_POINT ( 'NONE',  ( -5.049401038298153566, 19.05341960407611168, 60.20724293864768129 ) ) ;
#167492=CARTESIAN_POINT ( 'NONE',  ( 5.823673210054444382, -21.52544592524334988, 110.2094237280190185 ) ) ;
#167493=CARTESIAN_POINT ( 'NONE',  ( -10.81492255796105439, 18.62759615963255655, 22.91775706135235069 ) ) ;
#167494=CARTESIAN_POINT ( 'NONE',  ( 21.52544592524334988, 5.823673210054432836, 86.45942372801901854 ) ) ;
#167495=CARTESIAN_POINT ( 'NONE',  ( -4.483927247898782831, 16.52544592524335698, 47.70942372801902565 ) ) ;
#167496=CARTESIAN_POINT ( 'NONE',  ( 16.53943276465976808, 0.05219959533934440121, 26.25109039468567573 ) ) ;
#167497=CARTESIAN_POINT ( 'NONE',  ( 14.34966873604960469, 8.224510206698951720, 89.16557627198102409 ) ) ;
#167498=CARTESIAN_POINT ( 'NONE',  ( -10.72451020669870658, -18.67979575497194134, 94.58442372801901854 ) ) ;
#167499=ADVANCED_FACE ( 'NONE', ( #27367 ), #80375, .T. ) ;
#167500=CARTESIAN_POINT ( 'NONE',  ( 4.379528057220339221, -16.55341960407611168, 32.70724293864770260 ) ) ;
#167501=CARTESIAN_POINT ( 'NONE',  ( -0.05219959533909027116, -19.03943276465977164, 32.49890960531435979 ) ) ;
#167502=CARTESIAN_POINT ( 'NONE',  ( 14.34966873604972726, -8.224510206698740333, 45.83442372801901854 ) ) ;
#167503=CARTESIAN_POINT ( 'NONE',  ( 12.06949235617757843, -12.14591786802309237, 58.12390960531435979 ) ) ;
#167504=CARTESIAN_POINT ( 'NONE',  ( -4.483927247898782831, 16.52544592524335698, 92.70942372801901854 ) ) ;
#167505=CARTESIAN_POINT ( 'NONE',  ( -13.97604488694527625, -13.89961937509977652, 96.87390960531433848 ) ) ;
#167506=CARTESIAN_POINT ( 'NONE',  ( 10.72451020669898902, -18.67979575497178502, 22.91557627198102765 ) ) ;
#167507=CARTESIAN_POINT ( 'NONE',  ( -15.72974639402176322, -15.80617190586768395, 109.3760903946857042 ) ) ;
#167508=CARTESIAN_POINT ( 'NONE',  ( 16.55341960407611168, 4.379528057220329451, 83.95724293864770971 ) ) ;
#167509=CARTESIAN_POINT ( 'NONE',  ( -13.89961937509977652, 13.97604488694528158, 100.6239096053143669 ) ) ;
#167511=CARTESIAN_POINT ( 'NONE',  ( -16.52544592524335698, -4.483927247898792601, 38.95942372801901854 ) ) ;
#167512=CARTESIAN_POINT ( 'NONE',  ( -5.153800228976328057, -19.02544592524343514, 42.29057627198101699 ) ) ;
#167513=CARTESIAN_POINT ( 'NONE',  ( 13.89961937509977652, -13.97604488694527269, 103.1239096053143527 ) ) ;
#167514=CARTESIAN_POINT ( 'NONE',  ( 12.06949235617739724, 12.14591786802326823, 41.87609039468568284 ) ) ;
#167516=CARTESIAN_POINT ( 'NONE',  ( 9.564922557961047289, -16.46253265017146816, 50.41775706135233293 ) ) ;
#167517=CARTESIAN_POINT ( 'NONE',  ( 16.46253265017160672, -9.564922557960803928, 48.33224293864769550 ) ) ;
#167518=CARTESIAN_POINT ( 'NONE',  ( -4.379528057220086978, -16.55341960407618274, 79.79275706135236135 ) ) ;
#167519=CARTESIAN_POINT ( 'NONE',  ( 19.02544592524334988, 5.153800228976608722, 86.45942372801900433 ) ) ;
#167520=CARTESIAN_POINT ( 'NONE',  ( -9.474510206698720793, -16.51473224551083518, 34.58442372801899722 ) ) ;
#167521=CARTESIAN_POINT ( 'NONE',  ( -19.02544592524342804, 5.153800228976336051, 66.04057627198103830 ) ) ;
#167522=CARTESIAN_POINT ( 'NONE',  ( -0.05219959533910754901, -16.53943276465976808, 97.49890960531436690 ) ) ;
#167523=CARTESIAN_POINT ( 'NONE',  ( 19.03943276465977164, 0.05219959533936151252, 71.25109039468566152 ) ) ;
#167524=CARTESIAN_POINT ( 'NONE',  ( 18.67979575497178502, 10.72451020669898547, 69.16557627198102409 ) ) ;
#167525=CARTESIAN_POINT ( 'NONE',  ( 16.51473224551083163, -9.474510206698727899, 25.83442372801900078 ) ) ;
#167526=CARTESIAN_POINT ( 'NONE',  ( -9.474510206698964154, 16.51473224551069663, 105.4155762719810383 ) ) ;
#167528=CARTESIAN_POINT ( 'NONE',  ( -15.80617190586745835, -15.72974639402198527, 81.87390960531435269 ) ) ;
#167529=CARTESIAN_POINT ( 'NONE',  ( -18.22780087662122028, 5.500000000000031086, 53.51540105326106556 ) ) ;
#167530=CARTESIAN_POINT ( 'NONE',  ( -19.02544592524334988, -5.153800228976617603, 103.9594237280190043 ) ) ;
#167531=CARTESIAN_POINT ( 'NONE',  ( -19.25663599770061296, 5.499999999999452882, 58.99419308057201050 ) ) ;
#167532=CARTESIAN_POINT ( 'NONE',  ( 8.314922557961029526, -14.29746914071037800, 25.41775706135235779 ) ) ;
#167533=CARTESIAN_POINT ( 'NONE',  ( 5.153800228976335163, 19.02544592524342804, 34.79057627198102409 ) ) ;
#167534=CARTESIAN_POINT ( 'NONE',  ( 19.03943276465977164, -0.05219959533909143690, 103.7489096053143669 ) ) ;
#167535=CARTESIAN_POINT ( 'NONE',  ( -15.80617190586745835, -15.72974639402198527, 91.87390960531436690 ) ) ;
#167536=CARTESIAN_POINT ( 'NONE',  ( 15.72974639402176855, 15.80617190586768217, 66.87609039468568994 ) ) ;
#167537=CARTESIAN_POINT ( 'NONE',  ( -13.89961937509957401, -13.97604488694547875, 109.3760903946856331 ) ) ;
#167538=CARTESIAN_POINT ( 'NONE',  ( 15.72974639402176855, 15.80617190586768217, 106.8760903946856899 ) ) ;
#167539=CARTESIAN_POINT ( 'NONE',  ( -0.05219959533910754901, -16.53943276465976808, 22.49890960531436335 ) ) ;
#167540=CARTESIAN_POINT ( 'NONE',  ( -0.05219959533907301413, -21.53943276465977519, 97.49890960531436690 ) ) ;
#167541=CARTESIAN_POINT ( 'NONE',  ( 12.06949235617757843, -12.14591786802309237, 53.12390960531436690 ) ) ;
#167542=CARTESIAN_POINT ( 'NONE',  ( 19.03943276465977164, 0.05219959533936151252, 81.25109039468567573 ) ) ;
#167543=CARTESIAN_POINT ( 'NONE',  ( 19.05341960407617918, -5.049401038297876454, 56.04275706135234714 ) ) ;
#167544=CARTESIAN_POINT ( 'NONE',  ( 21.55341960407619695, -5.719274019375665929, 61.04275706135234714 ) ) ;
#167545=CARTESIAN_POINT ( 'NONE',  ( 13.97604488694548053, -13.89961937509957401, 40.62609039468564731 ) ) ;
#167546=CARTESIAN_POINT ( 'NONE',  ( -16.52544592524342804, 4.483927247898546575, 111.0405762719810525 ) ) ;
#167547=CARTESIAN_POINT ( 'NONE',  ( 15.80617190586746368, 15.72974639402197994, 34.37390960531435979 ) ) ;
#167548=CARTESIAN_POINT ( 'NONE',  ( -4.483927247898539470, -16.52544592524342804, 42.29057627198103120 ) ) ;
#167549=CARTESIAN_POINT ( 'NONE',  ( 5.823673210054444382, -21.52544592524334988, 95.20942372801903275 ) ) ;
#167550=CARTESIAN_POINT ( 'NONE',  ( 16.52544592524335698, 4.483927247898782831, 76.45942372801901854 ) ) ;
#167551=CARTESIAN_POINT ( 'NONE',  ( -16.55341960407611168, -4.379528057220339221, 21.45724293864769550 ) ) ;
#167552=CARTESIAN_POINT ( 'NONE',  ( 21.53943276465977519, 0.05219959533937863772, 56.25109039468568284 ) ) ;
#167553=CARTESIAN_POINT ( 'NONE',  ( 5.823673210054444382, -21.52544592524334988, 70.20942372801904696 ) ) ;
#167554=CARTESIAN_POINT ( 'NONE',  ( -21.53943276465977519, 0.05219959533907696930, 66.24890960531436690 ) ) ;
#167556=CARTESIAN_POINT ( 'NONE',  ( 19.03943276465977164, -0.05219959533909143690, 23.74890960531435269 ) ) ;
#167557=CARTESIAN_POINT ( 'NONE',  ( -10.81492255796105439, 18.62759615963255655, 42.91775706135235424 ) ) ;
#167558=CARTESIAN_POINT ( 'NONE',  ( -16.53943276465976808, 0.05219959533911058130, 116.2489096053143669 ) ) ;
#167559=CARTESIAN_POINT ( 'NONE',  ( -13.89961937509977652, 13.97604488694528158, 45.62390960531433848 ) ) ;
#167560=CARTESIAN_POINT ( 'NONE',  ( 4.483927247898545687, 16.52544592524342804, 79.79057627198102409 ) ) ;
#167561=CARTESIAN_POINT ( 'NONE',  ( 13.97604488694527802, 13.89961937509977652, 89.37390960531436690 ) ) ;
#167562=CARTESIAN_POINT ( 'NONE',  ( 16.55341960407611168, 4.379528057220329451, 23.95724293864769550 ) ) ;
#167563=CARTESIAN_POINT ( 'NONE',  ( 14.34966873604960469, 8.224510206698951720, 104.1655762719810241 ) ) ;
#167564=CARTESIAN_POINT ( 'NONE',  ( 5.823673210054125526, 21.52544592524343514, 74.79057627198105251 ) ) ;
#167565=CARTESIAN_POINT ( 'NONE',  ( 10.81492255796078972, 18.62759615963270932, 109.5822429386476955 ) ) ;
#167566=CARTESIAN_POINT ( 'NONE',  ( 19.02544592524343514, -5.153800228976328945, 108.5405762719810383 ) ) ;
#167567=CARTESIAN_POINT ( 'NONE',  ( 19.02544592524343514, -5.153800228976328945, 63.54057627198103830 ) ) ;
#167568=CARTESIAN_POINT ( 'NONE',  ( -19.02544592524334988, -5.153800228976617603, 108.9594237280189759 ) ) ;
#167569=CARTESIAN_POINT ( 'NONE',  ( -21.53943276465977519, 0.05219959533907696930, 56.24890960531436690 ) ) ;
#167570=CARTESIAN_POINT ( 'NONE',  ( -21.52544592524334988, -5.823673210054445271, 78.95942372801901854 ) ) ;
#167571=CARTESIAN_POINT ( 'NONE',  ( 9.564922557960805705, 16.46253265017160317, 64.58224293864769550 ) ) ;
#167572=CARTESIAN_POINT ( 'NONE',  ( 13.97604488694527802, 13.89961937509977652, 104.3739096053143385 ) ) ;
#167573=CARTESIAN_POINT ( 'NONE',  ( 14.29746914071037800, 8.314922557961029526, 71.66775706135234714 ) ) ;
#167574=CARTESIAN_POINT ( 'NONE',  ( 15.80617190586769283, -15.72974639402175789, 55.62609039468568284 ) ) ;
#167575=CARTESIAN_POINT ( 'NONE',  ( 21.53943276465977519, 0.05219959533937863772, 106.2510903946856757 ) ) ;
#167576=CARTESIAN_POINT ( 'NONE',  ( -21.52544592524343514, 5.823673210054127303, 111.0405762719810525 ) ) ;
#167577=CARTESIAN_POINT ( 'NONE',  ( 21.52544592524344225, -5.823673210054117533, 78.54057627198103830 ) ) ;
#167578=CARTESIAN_POINT ( 'NONE',  ( 13.97604488694548053, -13.89961937509957401, 45.62609039468566863 ) ) ;
#167579=CARTESIAN_POINT ( 'NONE',  ( -5.823673210054116645, -21.52544592524344225, 42.29057627198103120 ) ) ;
#167580=CARTESIAN_POINT ( 'NONE',  ( -13.97604488694527625, -13.89961937509977652, 76.87390960531433848 ) ) ;
#167581=CARTESIAN_POINT ( 'NONE',  ( 16.55341960407611168, 4.379528057220329451, 33.95724293864769550 ) ) ;
#167583=CARTESIAN_POINT ( 'NONE',  ( 16.46253265017146816, 9.564922557961045513, 91.66775706135234714 ) ) ;
#167584=CARTESIAN_POINT ( 'NONE',  ( -15.72974639402197994, 15.80617190586746368, 65.62390960531436690 ) ) ;
#167585=CARTESIAN_POINT ( 'NONE',  ( 16.53943276465976808, -0.05219959533910856209, 48.74890960531435979 ) ) ;
#167586=CARTESIAN_POINT ( 'NONE',  ( 16.55341960407618274, -4.379528057220086978, 31.04275706135234714 ) ) ;
#167587=CARTESIAN_POINT ( 'NONE',  ( -0.05219959533909027116, -19.03943276465977164, 42.49890960531435269 ) ) ;
#167588=CARTESIAN_POINT ( 'NONE',  ( 5.719274019375991003, -21.55341960407610458, 97.70724293864772392 ) ) ;
#167589=CARTESIAN_POINT ( 'NONE',  ( -0.05219959533936034679, 19.03943276465977164, 82.50109039468567573 ) ) ;
#167590=CARTESIAN_POINT ( 'NONE',  ( 19.05341960407611168, 5.049401038298154454, 78.95724293864769550 ) ) ;
#167591=CARTESIAN_POINT ( 'NONE',  ( -14.29746914071049879, 8.314922557960819915, 90.83224293864769550 ) ) ;
#167592=CARTESIAN_POINT ( 'NONE',  ( -16.51473224551069308, -9.474510206698971260, 66.66557627198102409 ) ) ;
#167593=CARTESIAN_POINT ( 'NONE',  ( -4.483927247898539470, -16.52544592524342804, 67.29057627198103830 ) ) ;
#167594=CARTESIAN_POINT ( 'NONE',  ( -5.153800228976328057, -19.02544592524343514, 37.29057627198102409 ) ) ;
#167596=CARTESIAN_POINT ( 'NONE',  ( 12.14591786802309770, 12.06949235617756955, 44.37390960531435979 ) ) ;
#167597=CARTESIAN_POINT ( 'NONE',  ( 16.46253265017160672, -9.564922557960803928, 88.33224293864769550 ) ) ;
#167599=CARTESIAN_POINT ( 'NONE',  ( 5.049401038297881783, 19.05341960407617563, 57.29275706135231871 ) ) ;
#167600=CARTESIAN_POINT ( 'NONE',  ( 14.34966873604972726, -8.224510206698740333, 65.83442372801900433 ) ) ;
#167601=CARTESIAN_POINT ( 'NONE',  ( 15.80617190586746368, 15.72974639402197994, 74.37390960531436690 ) ) ;
#167602=CARTESIAN_POINT ( 'NONE',  ( 0.05219959533936267826, -19.03943276465977164, 40.00109039468566152 ) ) ;
#167603=CARTESIAN_POINT ( 'NONE',  ( 5.153800228976335163, 19.02544592524342804, 89.79057627198102409 ) ) ;
#167605=CARTESIAN_POINT ( 'NONE',  ( 5.823673210054125526, 21.52544592524343514, 29.79057627198102409 ) ) ;
#167606=CARTESIAN_POINT ( 'NONE',  ( -9.474510206698964154, 16.51473224551069663, 55.41557627198103120 ) ) ;
#167607=CARTESIAN_POINT ( 'NONE',  ( 21.53943276465977519, 0.05219959533937863772, 56.25109039468568284 ) ) ;
#167608=CARTESIAN_POINT ( 'NONE',  ( 16.46253265017160672, -9.564922557960803928, 28.33224293864769550 ) ) ;
#167609=CARTESIAN_POINT ( 'NONE',  ( 15.80617190586769283, -15.72974639402175789, 20.62609039468568639 ) ) ;
#167610=CARTESIAN_POINT ( 'NONE',  ( -5.049401038298153566, 19.05341960407611168, 90.20724293864766707 ) ) ;
#167612=CARTESIAN_POINT ( 'NONE',  ( -15.72974639402176322, -15.80617190586768395, 44.37609039468567573 ) ) ;
#167614=CARTESIAN_POINT ( 'NONE',  ( 9.564922557960805705, 16.46253265017160317, 94.58224293864769550 ) ) ;
#167616=CARTESIAN_POINT ( 'NONE',  ( -10.72451020669898014, 18.67979575497178502, 105.4155762719810383 ) ) ;
#167617=CARTESIAN_POINT ( 'NONE',  ( -9.474510206698964154, 16.51473224551069663, 45.41557627198103120 ) ) ;
#167618=CARTESIAN_POINT ( 'NONE',  ( 16.52544592524335698, 4.483927247898782831, 26.45942372801901854 ) ) ;
#167620=CARTESIAN_POINT ( 'NONE',  ( 21.55341960407619695, -5.719274019375665929, 106.0427570613523471 ) ) ;
#167621=CARTESIAN_POINT ( 'NONE',  ( 13.97604488694527802, 13.89961937509977652, 29.37390960531435979 ) ) ;
#167622=CARTESIAN_POINT ( 'NONE',  ( 21.52544592524334988, 5.823673210054432836, 101.4594237280190185 ) ) ;
#167623=CARTESIAN_POINT ( 'NONE',  ( -9.474510206698964154, 16.51473224551069663, 90.41557627198103830 ) ) ;
#167624=CARTESIAN_POINT ( 'NONE',  ( 21.55341960407619695, -5.719274019375665929, 66.04275706135236135 ) ) ;
#167626=CARTESIAN_POINT ( 'NONE',  ( -19.05341960407611168, -5.049401038298163336, 96.45724293864769550 ) ) ;
#167627=CARTESIAN_POINT ( 'NONE',  ( -17.50000000000001421, 4.049696124445815393, 29.18039670665949004 ) ) ;
#167628=CARTESIAN_POINT ( 'NONE',  ( 4.379528057220092307, 16.55341960407617563, 52.29275706135236135 ) ) ;
#167629=CARTESIAN_POINT ( 'NONE',  ( 8.314922557961029526, -14.29746914071037800, 70.41775706135236135 ) ) ;
#167630=CARTESIAN_POINT ( 'NONE',  ( 15.72974639402176855, 15.80617190586768217, 61.87609039468568284 ) ) ;
#167631=CARTESIAN_POINT ( 'NONE',  ( 15.72974639402176855, 15.80617190586768217, 86.87609039468568994 ) ) ;
#167633=CARTESIAN_POINT ( 'NONE',  ( 12.14591786802327356, -12.06949235617739191, 25.62609039468567929 ) ) ;
#167634=CARTESIAN_POINT ( 'NONE',  ( 16.51473224551069308, 9.474510206698969483, 79.16557627198103830 ) ) ;
#167635=CARTESIAN_POINT ( 'NONE',  ( 5.153800228976335163, 19.02544592524342804, 99.79057627198102409 ) ) ;
#167637=CARTESIAN_POINT ( 'NONE',  ( -19.05341960407611168, -5.049401038298163336, 21.45724293864768839 ) ) ;
#167638=CARTESIAN_POINT ( 'NONE',  ( -0.05219959533907301413, -21.53943276465977519, 27.49890960531435269 ) ) ;
#167640=CARTESIAN_POINT ( 'NONE',  ( -14.29746914071037622, -8.314922557961029526, 99.16775706135234714 ) ) ;
#167641=CARTESIAN_POINT ( 'NONE',  ( 12.14591786802309770, 12.06949235617756955, 69.37390960531436690 ) ) ;
#167642=CARTESIAN_POINT ( 'NONE',  ( 19.03943276465977164, -0.05219959533909143690, 73.74890960531435269 ) ) ;
#167643=CARTESIAN_POINT ( 'NONE',  ( 21.53943276465977519, 0.05219959533937863772, 91.25109039468568994 ) ) ;
#167644=CARTESIAN_POINT ( 'NONE',  ( 17.48464627749218536, 5.278740712515454625, 21.75031283919550162 ) ) ;
#167645=CARTESIAN_POINT ( 'NONE',  ( 0.05219959533936267826, -19.03943276465977164, 105.0010903946856615 ) ) ;
#167646=CARTESIAN_POINT ( 'NONE',  ( -4.483927247898539470, -16.52544592524342804, 82.29057627198103830 ) ) ;
#167647=CARTESIAN_POINT ( 'NONE',  ( 0.05219959533937995610, -21.53943276465977519, 30.00109039468568284 ) ) ;
#167648=CARTESIAN_POINT ( 'NONE',  ( 10.81492255796078972, 18.62759615963270932, 69.58224293864769550 ) ) ;
#167649=CARTESIAN_POINT ( 'NONE',  ( -16.51473224551082808, 9.474510206698731452, 33.33442372801899722 ) ) ;
#167651=CARTESIAN_POINT ( 'NONE',  ( 5.153800228976335163, 19.02544592524342804, 79.79057627198102409 ) ) ;
#167652=CARTESIAN_POINT ( 'NONE',  ( -12.06949235617756955, 12.14591786802309770, 55.62390960531436690 ) ) ;
#167653=CARTESIAN_POINT ( 'NONE',  ( 0.05219959533910956823, 16.53943276465976808, 34.99890960531435979 ) ) ;
#167654=CARTESIAN_POINT ( 'NONE',  ( -12.06949235617739369, -12.14591786802326823, 104.3760903946856899 ) ) ;
#167655=CARTESIAN_POINT ( 'NONE',  ( -5.049401038297874678, -19.05341960407617918, 59.79275706135231871 ) ) ;
#167656=CARTESIAN_POINT ( 'NONE',  ( 19.34837522270366605, 5.499999999999732658, 53.36337684832579953 ) ) ;
#167657=CARTESIAN_POINT ( 'NONE',  ( 13.97604488694527802, 13.89961937509977652, 109.3739096053143669 ) ) ;
#167658=CARTESIAN_POINT ( 'NONE',  ( -8.224510206698948167, 14.34966873604960824, 70.41557627198102409 ) ) ;
#167659=CARTESIAN_POINT ( 'NONE',  ( 19.42893418801164529, -5.499999999999810818, 37.78583261411539240 ) ) ;
#167660=CARTESIAN_POINT ( 'NONE',  ( -16.46253265017160317, 9.564922557960807481, 25.83224293864769194 ) ) ;
#167661=CARTESIAN_POINT ( 'NONE',  ( -5.719274019375978568, 21.55341960407610458, 30.20724293864769550 ) ) ;
#167662=CARTESIAN_POINT ( 'NONE',  ( -15.80617190586745835, -15.72974639402198527, 66.87390960531436690 ) ) ;
#167663=CARTESIAN_POINT ( 'NONE',  ( 16.53943276465976808, -0.05219959533910856209, 108.7489096053143669 ) ) ;
#167664=CARTESIAN_POINT ( 'NONE',  ( 0.05219959533934541429, -16.53943276465976808, 65.00109039468568994 ) ) ;
#167665=CARTESIAN_POINT ( 'NONE',  ( 16.51473224551069308, 9.474510206698969483, 49.16557627198102409 ) ) ;
#167666=CARTESIAN_POINT ( 'NONE',  ( -15.80617190586768217, 15.72974639402176855, 43.12609039468568284 ) ) ;
#167667=CARTESIAN_POINT ( 'NONE',  ( -4.379528057220328563, 16.55341960407611168, 90.20724293864770971 ) ) ;
#167668=CARTESIAN_POINT ( 'NONE',  ( 17.31728774477274868, -6.344390552232389346, 38.31906651689320142 ) ) ;
#167670=CARTESIAN_POINT ( 'NONE',  ( 10.81492255796078972, 18.62759615963270932, 29.58224293864769905 ) ) ;
#167671=CARTESIAN_POINT ( 'NONE',  ( 18.09805431107249873, -5.499999999999975131, 78.51606229291886052 ) ) ;
#167674=CARTESIAN_POINT ( 'NONE',  ( -16.52544592524335698, -4.483927247898792601, 38.95942372801901854 ) ) ;
#167675=CARTESIAN_POINT ( 'NONE',  ( -4.483927247898539470, -16.52544592524342804, 42.29057627198103120 ) ) ;
#167676=CARTESIAN_POINT ( 'NONE',  ( 0.05219959533907565091, 21.53943276465977519, 69.99890960531435269 ) ) ;
#167677=CARTESIAN_POINT ( 'NONE',  ( -15.80617190586745835, -15.72974639402198527, 61.87390960531436690 ) ) ;
#167679=CARTESIAN_POINT ( 'NONE',  ( -9.564922557961040184, 16.46253265017147172, 77.91775706135234714 ) ) ;
#167680=CARTESIAN_POINT ( 'NONE',  ( 9.564922557960805705, 16.46253265017160317, 104.5822429386476955 ) ) ;
#167681=B_SPLINE_CURVE_WITH_KNOTS ( 'NONE', 3,
 ( #184621, #169442, #111747, #31933, #34905, #33919 ),
 .UNSPECIFIED., .F., .F.,
 ( 4, 2, 4 ),
 ( 0.003239945802372249956, 0.003620412082092100414, 0.004000878361811950439 ),
 .UNSPECIFIED. ) ;
#167682=CARTESIAN_POINT ( 'NONE',  ( -13.89961937509977652, 13.97604488694528158, 50.62390960531435979 ) ) ;
#167683=CARTESIAN_POINT ( 'NONE',  ( -0.05219959533909027116, -19.03943276465977164, 22.49890960531436690 ) ) ;
#167685=FACE_BOUND ( 'NONE', #131032, .T. ) ;
#167687=CARTESIAN_POINT ( 'NONE',  ( -4.379528057220086978, -16.55341960407618274, 69.79275706135234714 ) ) ;
#167688=CARTESIAN_POINT ( 'NONE',  ( -0.05219959533907301413, -21.53943276465977519, 102.4989096053143811 ) ) ;
#167689=CARTESIAN_POINT ( 'NONE',  ( -9.474510206698964154, 16.51473224551069663, 50.41557627198102409 ) ) ;
#167690=CARTESIAN_POINT ( 'NONE',  ( 10.72451020669871369, 18.67979575497193778, 42.08442372801901854 ) ) ;
#167691=CARTESIAN_POINT ( 'NONE',  ( -19.05341960407611168, -5.049401038298163336, 91.45724293864766707 ) ) ;
#167694=CARTESIAN_POINT ( 'NONE',  ( -0.05219959533937732626, 21.53943276465977519, 37.50109039468568284 ) ) ;
#167695=CARTESIAN_POINT ( 'NONE',  ( 13.89961937509977652, -13.97604488694527269, 113.1239096053143527 ) ) ;
#167696=CARTESIAN_POINT ( 'NONE',  ( -5.153800228976607833, 19.02544592524334988, 92.70942372801901854 ) ) ;
#167697=CARTESIAN_POINT ( 'NONE',  ( 16.46253265017146816, 9.564922557961045513, 36.66775706135233293 ) ) ;
#167698=CARTESIAN_POINT ( 'NONE',  ( -18.67979575497178146, -10.72451020669898902, 101.6655762719810383 ) ) ;
#167699=CARTESIAN_POINT ( 'NONE',  ( -5.153800228976607833, 19.02544592524334988, 32.70942372801899722 ) ) ;
#167700=CARTESIAN_POINT ( 'NONE',  ( 19.03943276465977164, 0.05219959533936151252, 41.25109039468566152 ) ) ;
#167701=CARTESIAN_POINT ( 'NONE',  ( -12.14591786802326823, 12.06949235617739902, 93.12609039468568994 ) ) ;
#167703=CARTESIAN_POINT ( 'NONE',  ( 13.97604488694527802, 13.89961937509977652, 64.37390960531436690 ) ) ;
#167705=CARTESIAN_POINT ( 'NONE',  ( -15.72974639402176322, -15.80617190586768395, 64.37609039468568994 ) ) ;
#167706=CARTESIAN_POINT ( 'NONE',  ( -18.67979575497193778, 10.72451020669871902, 83.33442372801903275 ) ) ;
#167707=CARTESIAN_POINT ( 'NONE',  ( -17.49999999999999645, -5.499999999999992895, 54.20309617465830598 ) ) ;
#167708=CARTESIAN_POINT ( 'NONE',  ( 9.474510206698971260, -16.51473224551069308, 92.91557627198103830 ) ) ;
#167709=CARTESIAN_POINT ( 'NONE',  ( -18.67979575497193778, 10.72451020669871902, 68.33442372801900433 ) ) ;
#167710=CARTESIAN_POINT ( 'NONE',  ( 9.474510206698729675, 16.51473224551082808, 102.0844237280190043 ) ) ;
#167711=CARTESIAN_POINT ( 'NONE',  ( -16.51473224551069308, -9.474510206698971260, 61.66557627198103120 ) ) ;
#167712=CARTESIAN_POINT ( 'NONE',  ( -0.05219959533909027116, -19.03943276465977164, 102.4989096053143669 ) ) ;
#167713=CARTESIAN_POINT ( 'NONE',  ( -9.564922557960796823, -16.46253265017161027, 82.08224293864768129 ) ) ;
#167714=CARTESIAN_POINT ( 'NONE',  ( -19.02544592524342804, 5.153800228976336051, 71.04057627198099567 ) ) ;
#167715=CARTESIAN_POINT ( 'NONE',  ( 5.823673210054125526, 21.52544592524343514, 99.79057627198103830 ) ) ;
#167716=CARTESIAN_POINT ( 'NONE',  ( 12.14591786802327356, -12.06949235617739191, 90.62609039468567573 ) ) ;
#167718=CARTESIAN_POINT ( 'NONE',  ( 13.89961937509957401, 13.97604488694547697, 46.87609039468565442 ) ) ;
#167719=CARTESIAN_POINT ( 'NONE',  ( 9.564922557960805705, 16.46253265017160317, 79.58224293864769550 ) ) ;
#167720=CARTESIAN_POINT ( 'NONE',  ( -0.05219959533910754901, -16.53943276465976808, 72.49890960531435269 ) ) ;
#167721=CARTESIAN_POINT ( 'NONE',  ( -14.29746914071049879, 8.314922557960819915, 110.8322429386476955 ) ) ;
#167722=CARTESIAN_POINT ( 'NONE',  ( -13.89961937509977652, 13.97604488694528158, 115.6239096053143669 ) ) ;
#167723=CARTESIAN_POINT ( 'NONE',  ( -9.474510206698964154, 16.51473224551069663, 100.4155762719810241 ) ) ;
#167725=CARTESIAN_POINT ( 'NONE',  ( 19.03943276465977164, 0.05219959533936151252, 31.25109039468566863 ) ) ;
#167726=CARTESIAN_POINT ( 'NONE',  ( -12.06949235617739369, -12.14591786802326823, 99.37609039468568994 ) ) ;
#167727=CARTESIAN_POINT ( 'NONE',  ( 19.02544592524343514, -5.153800228976328945, 78.54057627198099567 ) ) ;
#167728=CARTESIAN_POINT ( 'NONE',  ( -15.80617190586768217, 15.72974639402176855, 58.12609039468568994 ) ) ;
#167729=CARTESIAN_POINT ( 'NONE',  ( 10.72451020669898902, -18.67979575497178502, 47.91557627198102409 ) ) ;
#167730=CARTESIAN_POINT ( 'NONE',  ( -5.719274019375665041, -21.55341960407619695, 19.79275706135235069 ) ) ;
#167731=CARTESIAN_POINT ( 'NONE',  ( 10.72451020669898902, -18.67979575497178502, 67.91557627198102409 ) ) ;
#167732=CARTESIAN_POINT ( 'NONE',  ( -16.52544592524342804, 4.483927247898546575, 91.04057627198103830 ) ) ;
#167733=CARTESIAN_POINT ( 'NONE',  ( 16.46253265017146816, 9.564922557961045513, 61.66775706135234003 ) ) ;
#167734=CARTESIAN_POINT ( 'NONE',  ( 0.05219959533909260263, 19.03943276465977164, 29.99890960531435979 ) ) ;
#167735=CARTESIAN_POINT ( 'NONE',  ( 19.05341960407611168, 5.049401038298154454, 83.95724293864766707 ) ) ;
#167736=CARTESIAN_POINT ( 'NONE',  ( -5.049401038298153566, 19.05341960407611168, 85.20724293864766707 ) ) ;
#167738=CARTESIAN_POINT ( 'NONE',  ( 0.05219959533910956823, 16.53943276465976808, 99.99890960531436690 ) ) ;
#167740=CARTESIAN_POINT ( 'NONE',  ( -8.314922557960811034, -14.29746914071050412, 32.08224293864769550 ) ) ;
#167741=CARTESIAN_POINT ( 'NONE',  ( 4.379528057220092307, 16.55341960407617563, 27.29275706135234358 ) ) ;
#167742=CARTESIAN_POINT ( 'NONE',  ( 21.52544592524334988, 5.823673210054432836, 96.45942372801901854 ) ) ;
#167743=CARTESIAN_POINT ( 'NONE',  ( -9.564922557960796823, -16.46253265017161027, 107.0822429386476955 ) ) ;
#167744=CARTESIAN_POINT ( 'NONE',  ( 0.05219959533937995610, -21.53943276465977519, 20.00109039468568639 ) ) ;
#167745=CARTESIAN_POINT ( 'NONE',  ( 0.05219959533909260263, 19.03943276465977164, 44.99890960531435979 ) ) ;
#167746=CARTESIAN_POINT ( 'NONE',  ( -0.05219959533934338120, 16.53943276465976808, 42.50109039468567573 ) ) ;
#167747=CARTESIAN_POINT ( 'NONE',  ( -13.97604488694547697, 13.89961937509957934, 113.1260903946856757 ) ) ;
#167748=CARTESIAN_POINT ( 'NONE',  ( -5.153800228976328057, -19.02544592524343514, 32.29057627198102409 ) ) ;
#167749=CARTESIAN_POINT ( 'NONE',  ( -16.53943276465976808, 0.05219959533911058130, 101.2489096053143669 ) ) ;
#167750=CARTESIAN_POINT ( 'NONE',  ( -18.62759615963270932, 10.81492255796079327, 100.8322429386477097 ) ) ;
#167751=CARTESIAN_POINT ( 'NONE',  ( -9.564922557961040184, 16.46253265017147172, 62.91775706135233293 ) ) ;
#167753=CARTESIAN_POINT ( 'NONE',  ( 10.81492255796078972, 18.62759615963270932, 114.5822429386477097 ) ) ;
#167754=CARTESIAN_POINT ( 'NONE',  ( 0.05219959533909260263, 19.03943276465977164, 24.99890960531435269 ) ) ;
#167755=CARTESIAN_POINT ( 'NONE',  ( 5.049401038298161559, -19.05341960407611168, 97.70724293864766707 ) ) ;
#167757=CARTESIAN_POINT ( 'NONE',  ( -5.049401038298153566, 19.05341960407611168, 85.20724293864766707 ) ) ;
#167758=CARTESIAN_POINT ( 'NONE',  ( 21.52544592524334988, 5.823673210054432836, 31.45942372801901854 ) ) ;
#167759=CARTESIAN_POINT ( 'NONE',  ( -8.314922557960811034, -14.29746914071050412, 77.08224293864769550 ) ) ;
#167760=CARTESIAN_POINT ( 'NONE',  ( 5.153800228976335163, 19.02544592524342804, 79.79057627198102409 ) ) ;
#167761=CARTESIAN_POINT ( 'NONE',  ( 9.564922557961047289, -16.46253265017146816, 30.41775706135232937 ) ) ;
#167762=CARTESIAN_POINT ( 'NONE',  ( -4.379528057220086978, -16.55341960407618274, 54.79275706135235424 ) ) ;
#167763=CARTESIAN_POINT ( 'NONE',  ( -19.05341960407617563, 5.049401038297882671, 53.54275706135231871 ) ) ;
#167764=CARTESIAN_POINT ( 'NONE',  ( -21.53943276465977519, -0.05219959533937600094, 68.75109039468568994 ) ) ;
#167765=CARTESIAN_POINT ( 'NONE',  ( -16.55341960407617563, 4.379528057220093196, 33.54275706135234714 ) ) ;
#167766=CARTESIAN_POINT ( 'NONE',  ( 9.474510206698971260, -16.51473224551069308, 72.91557627198102409 ) ) ;
#167767=CARTESIAN_POINT ( 'NONE',  ( -0.05219959533936034679, 19.03943276465977164, 92.50109039468566152 ) ) ;
#167768=CARTESIAN_POINT ( 'NONE',  ( -12.06949235617739369, -12.14591786802326823, 74.37609039468568994 ) ) ;
#167769=CARTESIAN_POINT ( 'NONE',  ( -15.72974639402176322, -15.80617190586768395, 94.37609039468568994 ) ) ;
#167770=CARTESIAN_POINT ( 'NONE',  ( -13.97604488694547697, 13.89961937509957934, 78.12609039468567573 ) ) ;
#167771=CARTESIAN_POINT ( 'NONE',  ( -5.153800228976328057, -19.02544592524343514, 47.29057627198102409 ) ) ;
#167772=CARTESIAN_POINT ( 'NONE',  ( -10.81492255796078084, -18.62759615963271287, 77.08224293864769550 ) ) ;
#167773=CARTESIAN_POINT ( 'NONE',  ( 16.53943276465976808, -0.05219959533910856209, 78.74890960531436690 ) ) ;
#167774=CARTESIAN_POINT ( 'NONE',  ( -16.51473224551082808, 9.474510206698731452, 83.33442372801899012 ) ) ;
#167775=CARTESIAN_POINT ( 'NONE',  ( 16.62475595723702781, -7.163666690055162434, 63.02713351810474052 ) ) ;
#167776=CARTESIAN_POINT ( 'NONE',  ( 19.05341960407617918, -5.049401038297876454, 41.04275706135233293 ) ) ;
#167777=CARTESIAN_POINT ( 'NONE',  ( 12.14591786802309770, 12.06949235617756955, 24.37390960531435979 ) ) ;
#167778=CARTESIAN_POINT ( 'NONE',  ( -12.14591786802309592, -12.06949235617757132, 71.87390960531438111 ) ) ;
#167779=CARTESIAN_POINT ( 'NONE',  ( -0.05219959533937732626, 21.53943276465977519, 107.5010903946856899 ) ) ;
#167781=CARTESIAN_POINT ( 'NONE',  ( 21.52544592524344225, -5.823673210054117533, 108.5405762719810241 ) ) ;
#167782=CARTESIAN_POINT ( 'NONE',  ( -16.46253265017160317, 9.564922557960807481, 65.83224293864769550 ) ) ;
#167783=CARTESIAN_POINT ( 'NONE',  ( 15.72974639402176855, 15.80617190586768217, 86.87609039468568994 ) ) ;
#167784=CARTESIAN_POINT ( 'NONE',  ( 16.46253265017160672, -9.564922557960803928, 63.33224293864769550 ) ) ;
#167785=CARTESIAN_POINT ( 'NONE',  ( 0.05219959533909260263, 19.03943276465977164, 29.99890960531435979 ) ) ;
#167786=CARTESIAN_POINT ( 'NONE',  ( -18.62759615963270932, 10.81492255796079327, 35.83224293864768839 ) ) ;
#167787=CARTESIAN_POINT ( 'NONE',  ( 12.14591786802309770, 12.06949235617756955, 64.37390960531435269 ) ) ;
#167788=CARTESIAN_POINT ( 'NONE',  ( -5.049401038298153566, 19.05341960407611168, 45.20724293864769550 ) ) ;
#167789=CARTESIAN_POINT ( 'NONE',  ( 14.29746914071049879, -8.314922557960816363, 103.3322429386476955 ) ) ;
#167790=CARTESIAN_POINT ( 'NONE',  ( 10.81492255796078972, 18.62759615963270932, 109.5822429386476955 ) ) ;
#167791=CARTESIAN_POINT ( 'NONE',  ( -0.05219959533937732626, 21.53943276465977519, 52.50109039468567573 ) ) ;
#167792=CARTESIAN_POINT ( 'NONE',  ( 9.474510206698971260, -16.51473224551069308, 32.91557627198102409 ) ) ;
#167793=CARTESIAN_POINT ( 'NONE',  ( -8.314922557961024197, 14.29746914071037800, 52.91775706135235424 ) ) ;
#167794=CARTESIAN_POINT ( 'NONE',  ( 10.72451020669898902, -18.67979575497178502, 102.9155762719810383 ) ) ;
#167795=CARTESIAN_POINT ( 'NONE',  ( -21.55341960407610458, -5.719274019375992779, 91.45724293864769550 ) ) ;
#167796=CARTESIAN_POINT ( 'NONE',  ( -5.049401038297874678, -19.05341960407617918, 19.79275706135233293 ) ) ;
#167797=CARTESIAN_POINT ( 'NONE',  ( 19.02544592524343514, -5.153800228976328945, 53.54057627198102409 ) ) ;
#167798=CARTESIAN_POINT ( 'NONE',  ( -19.02544592524342804, 5.153800228976336051, 111.0405762719810099 ) ) ;
#167799=CARTESIAN_POINT ( 'NONE',  ( -5.823673210054431948, 21.52544592524334988, 52.70942372801902565 ) ) ;
#167800=CARTESIAN_POINT ( 'NONE',  ( 21.53943276465977519, -0.05219959533907433946, 43.74890960531435979 ) ) ;
#167801=CARTESIAN_POINT ( 'NONE',  ( 4.379528057220092307, 16.55341960407617563, 112.2927570613523471 ) ) ;
#167802=CARTESIAN_POINT ( 'NONE',  ( 15.72974639402176855, 15.80617190586768217, 61.87609039468568284 ) ) ;
#167803=CARTESIAN_POINT ( 'NONE',  ( 21.53943276465977519, 0.05219959533937863772, 96.25109039468568994 ) ) ;
#167804=CARTESIAN_POINT ( 'NONE',  ( -19.05341960407617563, 5.049401038297882671, 38.54275706135233293 ) ) ;
#167805=CARTESIAN_POINT ( 'NONE',  ( -16.53943276465976808, -0.05219959533934237506, 103.7510903946857042 ) ) ;
#167806=CARTESIAN_POINT ( 'NONE',  ( 10.81492255796106328, -18.62759615963255655, 60.41775706135235424 ) ) ;
#167807=CARTESIAN_POINT ( 'NONE',  ( -19.02544592524342804, 5.153800228976336051, 66.04057627198103830 ) ) ;
#167808=CARTESIAN_POINT ( 'NONE',  ( 21.52544592524334988, 5.823673210054432836, 111.4594237280190328 ) ) ;
#167809=CARTESIAN_POINT ( 'NONE',  ( 10.72451020669898902, -18.67979575497178502, 22.91557627198102765 ) ) ;
#167810=CARTESIAN_POINT ( 'NONE',  ( 21.55341960407619695, -5.719274019375665929, 36.04275706135234714 ) ) ;
#167812=CARTESIAN_POINT ( 'NONE',  ( 10.72451020669898902, -18.67979575497178502, 82.91557627198103830 ) ) ;
#167813=CARTESIAN_POINT ( 'NONE',  ( -4.483927247898782831, 16.52544592524335698, 37.70942372801900433 ) ) ;
#167814=CARTESIAN_POINT ( 'NONE',  ( 18.09918380851993192, 5.500000000000035527, 63.98618307335613054 ) ) ;
#167815=CARTESIAN_POINT ( 'NONE',  ( -0.05219959533907301413, -21.53943276465977519, 77.49890960531433848 ) ) ;
#167816=CARTESIAN_POINT ( 'NONE',  ( -12.06949235617739369, -12.14591786802326823, 59.37609039468568284 ) ) ;
#167817=CARTESIAN_POINT ( 'NONE',  ( -12.06949235617756955, 12.14591786802309770, 75.62390960531439532 ) ) ;
#167819=CARTESIAN_POINT ( 'NONE',  ( 9.474510206698729675, 16.51473224551082808, 107.0844237280190043 ) ) ;
#167820=CARTESIAN_POINT ( 'NONE',  ( 21.55341960407610458, 5.719274019375980345, 33.95724293864769550 ) ) ;
#167822=CARTESIAN_POINT ( 'NONE',  ( 0.05219959533934541429, -16.53943276465976808, 40.00109039468567573 ) ) ;
#167823=CARTESIAN_POINT ( 'NONE',  ( -21.55341960407610458, -5.719274019375992779, 106.4572429386477097 ) ) ;
#167824=CARTESIAN_POINT ( 'NONE',  ( 15.80617190586746368, 15.72974639402197994, 34.37390960531435979 ) ) ;
#167825=CARTESIAN_POINT ( 'NONE',  ( 4.483927247898790824, -16.52544592524335698, 65.20942372801901854 ) ) ;
#167826=CARTESIAN_POINT ( 'NONE',  ( -9.474510206698964154, 16.51473224551069663, 90.41557627198103830 ) ) ;
#167827=CARTESIAN_POINT ( 'NONE',  ( -10.81492255796105439, 18.62759615963255655, 52.91775706135235424 ) ) ;
#167828=CARTESIAN_POINT ( 'NONE',  ( -5.049401038298153566, 19.05341960407611168, 25.20724293864768484 ) ) ;
#167829=CARTESIAN_POINT ( 'NONE',  ( -5.049401038298153566, 19.05341960407611168, 115.2072429386477097 ) ) ;
#167831=CARTESIAN_POINT ( 'NONE',  ( -16.51473224551082808, 9.474510206698731452, 43.33442372801900433 ) ) ;
#167832=CARTESIAN_POINT ( 'NONE',  ( 16.55341960407618274, -4.379528057220086978, 46.04275706135234714 ) ) ;
#167833=CARTESIAN_POINT ( 'NONE',  ( 19.03943276465977164, -0.05219959533909143690, 113.7489096053143669 ) ) ;
#167834=CARTESIAN_POINT ( 'NONE',  ( 13.89961937509977652, -13.97604488694527269, 78.12390960531433848 ) ) ;
#167835=CARTESIAN_POINT ( 'NONE',  ( -16.52544592524335698, -4.483927247898792601, 93.95942372801903275 ) ) ;
#167837=CARTESIAN_POINT ( 'NONE',  ( 14.34966873604960469, 8.224510206698951720, 94.16557627198103830 ) ) ;
#167838=CARTESIAN_POINT ( 'NONE',  ( -21.55341960407610458, -5.719274019375992779, 41.45724293864769550 ) ) ;
#167839=CARTESIAN_POINT ( 'NONE',  ( 16.46253265017160672, -9.564922557960803928, 28.33224293864769550 ) ) ;
#167840=CARTESIAN_POINT ( 'NONE',  ( 8.224510206698742110, 14.34966873604972548, 67.08442372801901854 ) ) ;
#167841=CARTESIAN_POINT ( 'NONE',  ( 18.67979575497194134, -10.72451020669871369, 20.83442372801901143 ) ) ;
#167842=CARTESIAN_POINT ( 'NONE',  ( -0.05219959533936034679, 19.03943276465977164, 77.50109039468566152 ) ) ;
#167843=CARTESIAN_POINT ( 'NONE',  ( 13.89961937509977652, -13.97604488694527269, 38.12390960531436690 ) ) ;
#167844=CARTESIAN_POINT ( 'NONE',  ( 5.823673210054125526, 21.52544592524343514, 64.79057627198103830 ) ) ;
#167846=CARTESIAN_POINT ( 'NONE',  ( 5.049401038298161559, -19.05341960407611168, 112.7072429386476813 ) ) ;
#167847=CARTESIAN_POINT ( 'NONE',  ( -10.81492255796105439, 18.62759615963255655, 87.91775706135234714 ) ) ;
#167848=CARTESIAN_POINT ( 'NONE',  ( 9.474510206698971260, -16.51473224551069308, 62.91557627198102409 ) ) ;
#167849=CARTESIAN_POINT ( 'NONE',  ( 8.314922557961029526, -14.29746914071037800, 45.41775706135234003 ) ) ;
#167850=CARTESIAN_POINT ( 'NONE',  ( -16.46253265017160317, 9.564922557960807481, 55.83224293864769550 ) ) ;
#167851=CARTESIAN_POINT ( 'NONE',  ( -0.05219959533937732626, 21.53943276465977519, 77.50109039468567573 ) ) ;
#167852=CARTESIAN_POINT ( 'NONE',  ( 5.153800228976615827, -19.02544592524334988, 40.20942372801898301 ) ) ;
#167853=CARTESIAN_POINT ( 'NONE',  ( -19.03943276465977164, -0.05219959533935918106, 48.75109039468566863 ) ) ;
#167854=CARTESIAN_POINT ( 'NONE',  ( -18.67979575497193778, 10.72451020669871902, 53.33442372801901854 ) ) ;
#167856=CARTESIAN_POINT ( 'NONE',  ( -16.46253265017146816, -9.564922557961047289, 49.16775706135233293 ) ) ;
#167857=CARTESIAN_POINT ( 'NONE',  ( -19.03943276465977164, 0.05219959533909376836, 96.24890960531436690 ) ) ;
#167858=CARTESIAN_POINT ( 'NONE',  ( -19.02544592524342804, 5.153800228976336051, 66.04057627198103830 ) ) ;
#167859=CARTESIAN_POINT ( 'NONE',  ( 4.483927247898545687, 16.52544592524342804, 29.79057627198102409 ) ) ;
#167860=CARTESIAN_POINT ( 'NONE',  ( 15.80617190586746368, 15.72974639402197994, 29.37390960531435269 ) ) ;
#167861=CARTESIAN_POINT ( 'NONE',  ( 21.52544592524334988, 5.823673210054432836, 106.4594237280190328 ) ) ;
#167864=CARTESIAN_POINT ( 'NONE',  ( 21.52544592524334988, 5.823673210054432836, 96.45942372801901854 ) ) ;
#167866=CARTESIAN_POINT ( 'NONE',  ( 13.97604488694527802, 13.89961937509977652, 39.37390960531435269 ) ) ;
#167869=CARTESIAN_POINT ( 'NONE',  ( 16.52544592524335698, 4.483927247898782831, 46.45942372801901854 ) ) ;
#167870=CARTESIAN_POINT ( 'NONE',  ( -15.80617190586745835, -15.72974639402198527, 66.87390960531436690 ) ) ;
#167872=CARTESIAN_POINT ( 'NONE',  ( 16.53943276465976808, -0.05219959533910856209, 43.74890960531435979 ) ) ;
#167873=CARTESIAN_POINT ( 'NONE',  ( -0.05219959533910754901, -16.53943276465976808, 107.4989096053143669 ) ) ;
#167874=CARTESIAN_POINT ( 'NONE',  ( -0.05219959533909027116, -19.03943276465977164, 107.4989096053143527 ) ) ;
#167875=CARTESIAN_POINT ( 'NONE',  ( -5.719274019375665041, -21.55341960407619695, 29.79275706135234358 ) ) ;
#167876=CARTESIAN_POINT ( 'NONE',  ( 0.05219959533936267826, -19.03943276465977164, 40.00109039468566152 ) ) ;
#167877=CARTESIAN_POINT ( 'NONE',  ( 16.52544592524342804, -4.483927247898539470, 113.5405762719810383 ) ) ;
#167878=CARTESIAN_POINT ( 'NONE',  ( -10.72451020669870658, -18.67979575497194134, 74.58442372801901854 ) ) ;
#167879=CARTESIAN_POINT ( 'NONE',  ( 17.44270441346514389, -5.991230190323083349, 31.13664920735773478 ) ) ;
#167880=CARTESIAN_POINT ( 'NONE',  ( 4.379528057220339221, -16.55341960407611168, 22.70724293864769194 ) ) ;
#167882=CARTESIAN_POINT ( 'NONE',  ( -21.53943276465977519, 0.05219959533907696930, 31.24890960531435979 ) ) ;
#167883=CARTESIAN_POINT ( 'NONE',  ( -8.224510206698948167, 14.34966873604960824, 95.41557627198102409 ) ) ;
#167885=CARTESIAN_POINT ( 'NONE',  ( 5.153800228976335163, 19.02544592524342804, 74.79057627198103830 ) ) ;
#167886=CARTESIAN_POINT ( 'NONE',  ( 14.29746914071049879, -8.314922557960816363, 78.33224293864770971 ) ) ;
#167887=CARTESIAN_POINT ( 'NONE',  ( 16.46253265017146816, 9.564922557961045513, 111.6677570613523329 ) ) ;
#167888=CARTESIAN_POINT ( 'NONE',  ( -21.52544592524343514, 5.823673210054127303, 51.04057627198103120 ) ) ;
#167890=CARTESIAN_POINT ( 'NONE',  ( -9.564922557960796823, -16.46253265017161027, 22.08224293864768839 ) ) ;
#167891=CARTESIAN_POINT ( 'NONE',  ( 19.05341960407611168, 5.049401038298154454, 73.95724293864768129 ) ) ;
#167892=CARTESIAN_POINT ( 'NONE',  ( -18.62759615963270932, 10.81492255796079327, 70.83224293864770971 ) ) ;
#167893=CARTESIAN_POINT ( 'NONE',  ( -12.06949235617739369, -12.14591786802326823, 109.3760903946857042 ) ) ;
#167894=CARTESIAN_POINT ( 'NONE',  ( 5.153800228976335163, 19.02544592524342804, 89.79057627198102409 ) ) ;
#167895=CARTESIAN_POINT ( 'NONE',  ( 5.153800228976615827, -19.02544592524334988, 70.20942372801899012 ) ) ;
#167896=CARTESIAN_POINT ( 'NONE',  ( -0.05219959533937732626, 21.53943276465977519, 92.50109039468567573 ) ) ;
#167897=CARTESIAN_POINT ( 'NONE',  ( -21.55341960407610458, -5.719274019375992779, 66.45724293864768129 ) ) ;
#167898=CARTESIAN_POINT ( 'NONE',  ( 9.474510206698971260, -16.51473224551069308, 112.9155762719810383 ) ) ;
#167899=CARTESIAN_POINT ( 'NONE',  ( 19.03943276465977164, -0.05219959533909143690, 33.74890960531435979 ) ) ;
#167900=CARTESIAN_POINT ( 'NONE',  ( 14.29746914071037800, 8.314922557961029526, 101.6677570613523613 ) ) ;
#167901=CARTESIAN_POINT ( 'NONE',  ( -16.46253265017160317, 9.564922557960807481, 65.83224293864769550 ) ) ;
#167902=CARTESIAN_POINT ( 'NONE',  ( 14.34966873604972726, -8.224510206698740333, 20.83442372801901143 ) ) ;
#167903=CARTESIAN_POINT ( 'NONE',  ( 16.38665767535053774, 7.295008042176050367, 52.23599135785457293 ) ) ;
#167904=CARTESIAN_POINT ( 'NONE',  ( 15.80617190586769283, -15.72974639402175789, 110.6260903946857042 ) ) ;
#167905=CARTESIAN_POINT ( 'NONE',  ( -12.14591786802309592, -12.06949235617757132, 76.87390960531439532 ) ) ;
#167906=CARTESIAN_POINT ( 'NONE',  ( 5.823673210054125526, 21.52544592524343514, 114.7905762719810383 ) ) ;
#167907=CARTESIAN_POINT ( 'NONE',  ( 15.72974639402199770, -15.80617190586745480, 103.1239096053143811 ) ) ;
#167909=CARTESIAN_POINT ( 'NONE',  ( 10.81492255796078972, 18.62759615963270932, 54.58224293864769550 ) ) ;
#167910=CARTESIAN_POINT ( 'NONE',  ( 16.52544592524335698, 4.483927247898782831, 76.45942372801901854 ) ) ;
#167911=CARTESIAN_POINT ( 'NONE',  ( 12.06949235617757843, -12.14591786802309237, 108.1239096053143811 ) ) ;
#167912=CARTESIAN_POINT ( 'NONE',  ( 19.02544592524343514, -5.153800228976328945, 58.54057627198102409 ) ) ;
#167913=CARTESIAN_POINT ( 'NONE',  ( 4.379528057220092307, 16.55341960407617563, 107.2927570613523471 ) ) ;
#167914=CARTESIAN_POINT ( 'NONE',  ( 10.72451020669871369, 18.67979575497193778, 47.08442372801901854 ) ) ;
#167915=CARTESIAN_POINT ( 'NONE',  ( -16.46253265017160317, 9.564922557960807481, 100.8322429386477097 ) ) ;
#167916=CARTESIAN_POINT ( 'NONE',  ( -10.72451020669870658, -18.67979575497194134, 79.58442372801903275 ) ) ;
#167917=CARTESIAN_POINT ( 'NONE',  ( -13.89961937509977652, 13.97604488694528158, 35.62390960531435269 ) ) ;
#167918=CARTESIAN_POINT ( 'NONE',  ( 0.05219959533909260263, 19.03943276465977164, 39.99890960531436690 ) ) ;
#167920=CARTESIAN_POINT ( 'NONE',  ( -10.72451020669870658, -18.67979575497194134, 74.58442372801901854 ) ) ;
#167921=CARTESIAN_POINT ( 'NONE',  ( -19.02544592524342804, 5.153800228976336051, 106.0405762719810241 ) ) ;
#167922=CARTESIAN_POINT ( 'NONE',  ( 19.02544592524334988, 5.153800228976608722, 76.45942372801897591 ) ) ;
#167923=CARTESIAN_POINT ( 'NONE',  ( -10.81492255796105439, 18.62759615963255655, 37.91775706135235424 ) ) ;
#167924=CARTESIAN_POINT ( 'NONE',  ( 12.14591786802327356, -12.06949235617739191, 20.62609039468568639 ) ) ;
#167925=CARTESIAN_POINT ( 'NONE',  ( -5.153800228976607833, 19.02544592524334988, 67.70942372801900433 ) ) ;
#167926=CARTESIAN_POINT ( 'NONE',  ( -13.89961937509977652, 13.97604488694528158, 50.62390960531435979 ) ) ;
#167927=CARTESIAN_POINT ( 'NONE',  ( 5.153800228976615827, -19.02544592524334988, 80.20942372801901854 ) ) ;
#167928=CARTESIAN_POINT ( 'NONE',  ( 16.52544592524342804, -4.483927247898539470, 28.54057627198103120 ) ) ;
#167929=CARTESIAN_POINT ( 'NONE',  ( -9.564922557961040184, 16.46253265017147172, 72.91775706135233293 ) ) ;
#167930=CARTESIAN_POINT ( 'NONE',  ( 16.55341960407611168, 4.379528057220329451, 43.95724293864769550 ) ) ;
#167931=CARTESIAN_POINT ( 'NONE',  ( -5.049401038297874678, -19.05341960407617918, 69.79275706135233293 ) ) ;
#167932=CARTESIAN_POINT ( 'NONE',  ( -4.379528057220086978, -16.55341960407618274, 44.79275706135234714 ) ) ;
#167933=CARTESIAN_POINT ( 'NONE',  ( 16.51473224551083163, -9.474510206698727899, 25.83442372801900078 ) ) ;
#167935=CARTESIAN_POINT ( 'NONE',  ( 13.89961937509977652, -13.97604488694527269, 33.12390960531434558 ) ) ;
#167936=CARTESIAN_POINT ( 'NONE',  ( -16.19135201231369692, -7.376712067591814304, 65.18680854052030327 ) ) ;
#167937=CARTESIAN_POINT ( 'NONE',  ( 12.14591786802327356, -12.06949235617739191, 45.62609039468567573 ) ) ;
#167940=CARTESIAN_POINT ( 'NONE',  ( 9.474510206698971260, -16.51473224551069308, 92.91557627198103830 ) ) ;
#167941=CARTESIAN_POINT ( 'NONE',  ( 13.97604488694548053, -13.89961937509957401, 85.62609039468567573 ) ) ;
#167943=CARTESIAN_POINT ( 'NONE',  ( 5.153800228976615827, -19.02544592524334988, 90.20942372801900433 ) ) ;
#167944=AXIS2_PLACEMENT_3D ( 'NONE', #79547, #188735, #35033 ) ;
#167945=CARTESIAN_POINT ( 'NONE',  ( 10.81492255796078972, 18.62759615963270932, 24.58224293864768839 ) ) ;
#167946=CARTESIAN_POINT ( 'NONE',  ( -9.474510206698720793, -16.51473224551083518, 19.58442372801899722 ) ) ;
#167947=CARTESIAN_POINT ( 'NONE',  ( -13.89961937509957401, -13.97604488694547875, 104.3760903946856757 ) ) ;
#167948=CARTESIAN_POINT ( 'NONE',  ( 12.06949235617757843, -12.14591786802309237, 108.1239096053143811 ) ) ;
#167949=CARTESIAN_POINT ( 'NONE',  ( 9.474510206698971260, -16.51473224551069308, 32.91557627198102409 ) ) ;
#167950=CARTESIAN_POINT ( 'NONE',  ( 21.52544592524344225, -5.823673210054117533, 53.54057627198103120 ) ) ;
#167951=CARTESIAN_POINT ( 'NONE',  ( 19.03943276465977164, -0.05219959533909143690, 28.74890960531435624 ) ) ;
#167953=CARTESIAN_POINT ( 'NONE',  ( -16.51473224551082808, 9.474510206698731452, 73.33442372801900433 ) ) ;
#167954=CARTESIAN_POINT ( 'NONE',  ( 4.483927247898545687, 16.52544592524342804, 34.79057627198103120 ) ) ;
#167955=CARTESIAN_POINT ( 'NONE',  ( 19.05341960407611168, 5.049401038298154454, 108.9572429386477097 ) ) ;
#167956=CARTESIAN_POINT ( 'NONE',  ( -18.67979575497193778, 10.72451020669871902, 93.33442372801901854 ) ) ;
#167957=CARTESIAN_POINT ( 'NONE',  ( -10.72451020669898014, 18.67979575497178502, 80.41557627198103830 ) ) ;
#167958=CARTESIAN_POINT ( 'NONE',  ( 5.823673210054444382, -21.52544592524334988, 55.20942372801902565 ) ) ;
#167959=CARTESIAN_POINT ( 'NONE',  ( 21.53943276465977519, 0.05219959533937863772, 61.25109039468567573 ) ) ;
#167960=CARTESIAN_POINT ( 'NONE',  ( -13.97604488694527625, -13.89961937509977652, 91.87390960531432427 ) ) ;
#167961=CARTESIAN_POINT ( 'NONE',  ( -16.52544592524335698, -4.483927247898792601, 93.95942372801903275 ) ) ;
#167962=CARTESIAN_POINT ( 'NONE',  ( 15.72974639402176855, 15.80617190586768217, 51.87609039468568284 ) ) ;
#167963=CARTESIAN_POINT ( 'NONE',  ( -0.05219959533910754901, -16.53943276465976808, 112.4989096053143669 ) ) ;
#167964=CARTESIAN_POINT ( 'NONE',  ( -12.06949235617756955, 12.14591786802309770, 70.62390960531436690 ) ) ;
#167965=CARTESIAN_POINT ( 'NONE',  ( -8.314922557960811034, -14.29746914071050412, 32.08224293864769550 ) ) ;
#167966=CARTESIAN_POINT ( 'NONE',  ( 15.72974639402199770, -15.80617190586745480, 43.12390960531435269 ) ) ;
#167967=CARTESIAN_POINT ( 'NONE',  ( -19.05341960407611168, -5.049401038298163336, 61.45724293864769550 ) ) ;
#167968=CARTESIAN_POINT ( 'NONE',  ( 5.153800228976335163, 19.02544592524342804, 49.79057627198100988 ) ) ;
#167969=CARTESIAN_POINT ( 'NONE',  ( 5.719274019375991003, -21.55341960407610458, 57.70724293864770260 ) ) ;
#167970=CARTESIAN_POINT ( 'NONE',  ( 19.02544592524334988, 5.153800228976608722, 41.45942372801900433 ) ) ;
#167971=CARTESIAN_POINT ( 'NONE',  ( -17.05587630539784882, -6.762274262135712810, 39.25819690962689634 ) ) ;
#167972=CARTESIAN_POINT ( 'NONE',  ( 8.224510206698953496, -14.34966873604960469, 47.91557627198102409 ) ) ;
#167973=CARTESIAN_POINT ( 'NONE',  ( 10.81492255796078972, 18.62759615963270932, 24.58224293864768839 ) ) ;
#167975=ORIENTED_EDGE ( 'NONE', *, *, #98443, .F. ) ;
#167978=CARTESIAN_POINT ( 'NONE',  ( 12.14591786802327356, -12.06949235617739191, 75.62609039468567573 ) ) ;
#167979=CARTESIAN_POINT ( 'NONE',  ( 9.474510206698729675, 16.51473224551082808, 77.08442372801900433 ) ) ;
#167980=CARTESIAN_POINT ( 'NONE',  ( -4.379528057220328563, 16.55341960407611168, 35.20724293864768839 ) ) ;
#167982=CARTESIAN_POINT ( 'NONE',  ( 12.06949235617757843, -12.14591786802309237, 23.12390960531436335 ) ) ;
#167983=CARTESIAN_POINT ( 'NONE',  ( -19.02544592524342804, 5.153800228976336051, 46.04057627198101699 ) ) ;
#167984=CARTESIAN_POINT ( 'NONE',  ( 16.51473224551069308, 9.474510206698969483, 79.16557627198103830 ) ) ;
#167985=CARTESIAN_POINT ( 'NONE',  ( -19.03943276465977164, 0.05219959533909376836, 41.24890960531435269 ) ) ;
#167986=CARTESIAN_POINT ( 'NONE',  ( 21.55341960407619695, -5.719274019375665929, 51.04275706135234714 ) ) ;
#167987=CARTESIAN_POINT ( 'NONE',  ( -0.05219959533909027116, -19.03943276465977164, 52.49890960531436690 ) ) ;
#167989=CARTESIAN_POINT ( 'NONE',  ( 9.564922557960805705, 16.46253265017160317, 54.58224293864769550 ) ) ;
#167990=CARTESIAN_POINT ( 'NONE',  ( -15.80617190586745835, -15.72974639402198527, 41.87390960531435979 ) ) ;
#167991=CARTESIAN_POINT ( 'NONE',  ( 8.224510206698953496, -14.34966873604960469, 112.9155762719810383 ) ) ;
#167992=CARTESIAN_POINT ( 'NONE',  ( -5.719274019375978568, 21.55341960407610458, 30.20724293864769550 ) ) ;
#167993=CARTESIAN_POINT ( 'NONE',  ( -8.224510206698735004, -14.34966873604973081, 94.58442372801901854 ) ) ;
#167995=CARTESIAN_POINT ( 'NONE',  ( 18.67979575497194134, -10.72451020669871369, 110.8344237280190043 ) ) ;
#167996=CARTESIAN_POINT ( 'NONE',  ( 4.483927247898790824, -16.52544592524335698, 65.20942372801901854 ) ) ;
#167997=CARTESIAN_POINT ( 'NONE',  ( 13.97604488694527802, 13.89961937509977652, 109.3739096053143669 ) ) ;
#167998=CARTESIAN_POINT ( 'NONE',  ( 12.14591786802327356, -12.06949235617739191, 50.62609039468568994 ) ) ;
#167999=CARTESIAN_POINT ( 'NONE',  ( -16.55341960407617563, 4.379528057220093196, 43.54275706135235424 ) ) ;
#168000=CARTESIAN_POINT ( 'NONE',  ( 5.049401038298161559, -19.05341960407611168, 112.7072429386476813 ) ) ;
#168001=CARTESIAN_POINT ( 'NONE',  ( -16.53943276465976808, -0.05219959533934237506, 23.75109039468567929 ) ) ;
#168002=CARTESIAN_POINT ( 'NONE',  ( 13.97604488694527802, 13.89961937509977652, 34.37390960531436690 ) ) ;
#168003=CARTESIAN_POINT ( 'NONE',  ( -10.81492255796105439, 18.62759615963255655, 27.91775706135234358 ) ) ;
#168004=CARTESIAN_POINT ( 'NONE',  ( -12.14591786802326823, 12.06949235617739902, 28.12609039468568284 ) ) ;
#168005=CARTESIAN_POINT ( 'NONE',  ( -12.06949235617739369, -12.14591786802326823, 84.37609039468570415 ) ) ;
#168006=CARTESIAN_POINT ( 'NONE',  ( -17.50000000001357847, 5.500000000000046185, 45.79690382535059001 ) ) ;
#168007=CARTESIAN_POINT ( 'NONE',  ( 10.72451020669871369, 18.67979575497193778, 92.08442372801901854 ) ) ;
#168008=CARTESIAN_POINT ( 'NONE',  ( -13.97604488694547697, 13.89961937509957934, 83.12609039468564731 ) ) ;
#168009=CARTESIAN_POINT ( 'NONE',  ( -4.483927247898539470, -16.52544592524342804, 52.29057627198102409 ) ) ;
#168010=CARTESIAN_POINT ( 'NONE',  ( 16.52544592524342804, -4.483927247898539470, 108.5405762719810241 ) ) ;
#168011=CARTESIAN_POINT ( 'NONE',  ( -19.03943276465977164, -0.05219959533935918106, 53.75109039468566863 ) ) ;
#168013=CARTESIAN_POINT ( 'NONE',  ( -10.72451020669870658, -18.67979575497194134, 54.58442372801901143 ) ) ;
#168014=CARTESIAN_POINT ( 'NONE',  ( 19.03943276465977164, 0.05219959533936151252, 111.2510903946856757 ) ) ;
#168015=CARTESIAN_POINT ( 'NONE',  ( 17.44279575226823553, 5.990770900252481823, 81.66442432485685288 ) ) ;
#168016=CARTESIAN_POINT ( 'NONE',  ( 19.03943276465977164, -0.05219959533909143690, 103.7489096053143669 ) ) ;
#168017=CARTESIAN_POINT ( 'NONE',  ( -18.67979575497178146, -10.72451020669898902, 76.66557627198103830 ) ) ;
#168018=CARTESIAN_POINT ( 'NONE',  ( -0.05219959533936034679, 19.03943276465977164, 97.50109039468567573 ) ) ;
#168019=CARTESIAN_POINT ( 'NONE',  ( -0.05219959533909027116, -19.03943276465977164, 102.4989096053143669 ) ) ;
#168021=CARTESIAN_POINT ( 'NONE',  ( -16.53943276465976808, 0.05219959533911058130, 101.2489096053143669 ) ) ;
#168022=CARTESIAN_POINT ( 'NONE',  ( 5.823673210054444382, -21.52544592524334988, 95.20942372801903275 ) ) ;
#168023=CARTESIAN_POINT ( 'NONE',  ( -5.153800228976328057, -19.02544592524343514, 42.29057627198101699 ) ) ;
#168024=CARTESIAN_POINT ( 'NONE',  ( -21.53943276465977519, -0.05219959533937600094, 48.75109039468568284 ) ) ;
#168025=CARTESIAN_POINT ( 'NONE',  ( -5.823673210054431948, 21.52544592524334988, 82.70942372801900433 ) ) ;
#168026=CARTESIAN_POINT ( 'NONE',  ( -8.224510206698735004, -14.34966873604973081, 99.58442372801900433 ) ) ;
#168027=CARTESIAN_POINT ( 'NONE',  ( -0.05219959533937732626, 21.53943276465977519, 37.50109039468568284 ) ) ;
#168028=CARTESIAN_POINT ( 'NONE',  ( 15.72974639402176855, 15.80617190586768217, 41.87609039468568284 ) ) ;
#168029=CARTESIAN_POINT ( 'NONE',  ( 5.153800228976615827, -19.02544592524334988, 65.20942372801900433 ) ) ;
#168030=CARTESIAN_POINT ( 'NONE',  ( -19.02544592524342804, 5.153800228976336051, 96.04057627198103830 ) ) ;
#168031=CARTESIAN_POINT ( 'NONE',  ( -12.06949235617756955, 12.14591786802309770, 105.6239096053143669 ) ) ;
#168032=CARTESIAN_POINT ( 'NONE',  ( -21.52544592524343514, 5.823673210054127303, 81.04057627198102409 ) ) ;
#168033=CARTESIAN_POINT ( 'NONE',  ( -12.06949235617756955, 12.14591786802309770, 70.62390960531436690 ) ) ;
#168034=CARTESIAN_POINT ( 'NONE',  ( 21.52544592524334988, 5.823673210054432836, 111.4594237280190328 ) ) ;
#168035=CARTESIAN_POINT ( 'NONE',  ( -4.483927247898539470, -16.52544592524342804, 82.29057627198103830 ) ) ;
#168036=CARTESIAN_POINT ( 'NONE',  ( 0.05219959533909260263, 19.03943276465977164, 29.99890960531435979 ) ) ;
#168037=CARTESIAN_POINT ( 'NONE',  ( 9.564922557961047289, -16.46253265017146816, 90.41775706135234714 ) ) ;
#168038=CARTESIAN_POINT ( 'NONE',  ( -8.224510206698948167, 14.34966873604960824, 45.41557627198103830 ) ) ;
#168039=CARTESIAN_POINT ( 'NONE',  ( 15.80617190586769283, -15.72974639402175789, 90.62609039468567573 ) ) ;
#168040=CARTESIAN_POINT ( 'NONE',  ( 0.05219959533909260263, 19.03943276465977164, 89.99890960531436690 ) ) ;
#168041=CARTESIAN_POINT ( 'NONE',  ( -5.153800228976607833, 19.02544592524334988, 62.70942372801899722 ) ) ;
#168042=CARTESIAN_POINT ( 'NONE',  ( -10.72451020669898014, 18.67979575497178502, 80.41557627198103830 ) ) ;
#168043=CARTESIAN_POINT ( 'NONE',  ( 18.62759615963255655, 10.81492255796105972, 26.66775706135235424 ) ) ;
#168044=CARTESIAN_POINT ( 'NONE',  ( -16.52544592524335698, -4.483927247898792601, 33.95942372801901143 ) ) ;
#168045=CARTESIAN_POINT ( 'NONE',  ( -16.55341960407617563, 4.379528057220093196, 83.54275706135234714 ) ) ;
#168046=CARTESIAN_POINT ( 'NONE',  ( 13.97604488694527802, 13.89961937509977652, 29.37390960531435979 ) ) ;
#168047=CARTESIAN_POINT ( 'NONE',  ( -10.72451020669898014, 18.67979575497178502, 115.4155762719810241 ) ) ;
#168048=CARTESIAN_POINT ( 'NONE',  ( 16.53943276465976808, -0.05219959533910856209, 113.7489096053143527 ) ) ;
#168050=CARTESIAN_POINT ( 'NONE',  ( -14.34966873604972548, 8.224510206698743886, 43.33442372801901143 ) ) ;
#168051=CARTESIAN_POINT ( 'NONE',  ( 4.483927247898545687, 16.52544592524342804, 84.79057627198102409 ) ) ;
#168052=CARTESIAN_POINT ( 'NONE',  ( -21.52544592524343514, 5.823673210054127303, 71.04057627198103830 ) ) ;
#168053=CARTESIAN_POINT ( 'NONE',  ( -4.379528057220328563, 16.55341960407611168, 25.20724293864769550 ) ) ;
#168054=CARTESIAN_POINT ( 'NONE',  ( 12.14591786802327356, -12.06949235617739191, 45.62609039468567573 ) ) ;
#168055=CARTESIAN_POINT ( 'NONE',  ( 5.049401038298161559, -19.05341960407611168, 47.70724293864770260 ) ) ;
#168056=CARTESIAN_POINT ( 'NONE',  ( -14.29746914071037622, -8.314922557961029526, 79.16775706135234714 ) ) ;
#168057=CARTESIAN_POINT ( 'NONE',  ( -19.03943276465977164, -0.05219959533935918106, 68.75109039468566152 ) ) ;
#168058=CARTESIAN_POINT ( 'NONE',  ( -10.81492255796078084, -18.62759615963271287, 67.08224293864770971 ) ) ;
#168059=CARTESIAN_POINT ( 'NONE',  ( -14.34966873604972548, 8.224510206698743886, 108.3344237280190185 ) ) ;
#168061=CARTESIAN_POINT ( 'NONE',  ( -19.02544592524342804, 5.153800228976336051, 116.0405762719810383 ) ) ;
#168062=CARTESIAN_POINT ( 'NONE',  ( 0.05219959533907565091, 21.53943276465977519, 49.99890960531437401 ) ) ;
#168063=VERTEX_POINT ( 'NONE', #149129 ) ;
#168064=CARTESIAN_POINT ( 'NONE',  ( -16.53943276465976808, -0.05219959533934237506, 88.75109039468567573 ) ) ;
#168065=ORIENTED_EDGE ( 'NONE', *, *, #85112, .F. ) ;
#168066=CARTESIAN_POINT ( 'NONE',  ( -16.51473224551069308, -9.474510206698971260, 106.6655762719810383 ) ) ;
#168067=CARTESIAN_POINT ( 'NONE',  ( 17.50000000000000000, 3.850315288878781050, 108.2337086939655109 ) ) ;
#168068=CARTESIAN_POINT ( 'NONE',  ( 21.52544592524344225, -5.823673210054117533, 73.54057627198102409 ) ) ;
#168069=CARTESIAN_POINT ( 'NONE',  ( 8.224510206698742110, 14.34966873604972548, 102.0844237280190185 ) ) ;
#168070=CARTESIAN_POINT ( 'NONE',  ( -0.05219959533936034679, 19.03943276465977164, 112.5010903946856757 ) ) ;
#168071=CARTESIAN_POINT ( 'NONE',  ( -9.564922557960796823, -16.46253265017161027, 27.08224293864769550 ) ) ;
#168072=CARTESIAN_POINT ( 'NONE',  ( -14.29746914071037622, -8.314922557961029526, 24.16775706135235424 ) ) ;
#168073=CARTESIAN_POINT ( 'NONE',  ( -5.153800228976328057, -19.02544592524343514, 57.29057627198103120 ) ) ;
#168076=CARTESIAN_POINT ( 'NONE',  ( 19.03943276465977164, -0.05219959533909143690, 98.74890960531436690 ) ) ;
#168077=CARTESIAN_POINT ( 'NONE',  ( -8.314922557961024197, 14.29746914071037800, 87.91775706135234714 ) ) ;
#168078=CARTESIAN_POINT ( 'NONE',  ( 16.51473224551083163, -9.474510206698727899, 85.83442372801900433 ) ) ;
#168079=CARTESIAN_POINT ( 'NONE',  ( -21.53943276465977519, -0.05219959533937600094, 113.7510903946856757 ) ) ;
#168080=CARTESIAN_POINT ( 'NONE',  ( 18.62759615963271287, -10.81492255796078972, 73.33224293864769550 ) ) ;
#168081=CARTESIAN_POINT ( 'NONE',  ( 12.06949235617739724, 12.14591786802326823, 101.8760903946857042 ) ) ;
#168082=CARTESIAN_POINT ( 'NONE',  ( 19.03943276465977164, 0.05219959533936151252, 96.25109039468567573 ) ) ;
#168083=CARTESIAN_POINT ( 'NONE',  ( -13.97604488694527625, -13.89961937509977652, 46.87390960531435979 ) ) ;
#168084=CARTESIAN_POINT ( 'NONE',  ( -5.153800228976328057, -19.02544592524343514, 97.29057627198099567 ) ) ;
#168085=CARTESIAN_POINT ( 'NONE',  ( 21.52544592524334988, 5.823673210054432836, 66.45942372801903275 ) ) ;
#168086=CARTESIAN_POINT ( 'NONE',  ( 19.05341960407611168, 5.049401038298154454, 43.95724293864769550 ) ) ;
#168088=CARTESIAN_POINT ( 'NONE',  ( -14.34966873604960291, -8.224510206698953496, 76.66557627198103830 ) ) ;
#168089=CARTESIAN_POINT ( 'NONE',  ( 21.55341960407610458, 5.719274019375980345, 78.95724293864769550 ) ) ;
#168091=CARTESIAN_POINT ( 'NONE',  ( 19.03943276465977164, 0.05219959533936151252, 41.25109039468566152 ) ) ;
#168092=CARTESIAN_POINT ( 'NONE',  ( 16.61371651742642186, -7.165104196375917667, 71.35415069992967574 ) ) ;
#168093=CARTESIAN_POINT ( 'NONE',  ( -5.049401038298153566, 19.05341960407611168, 75.20724293864769550 ) ) ;
#168094=CARTESIAN_POINT ( 'NONE',  ( 13.89961937509977652, -13.97604488694527269, 83.12390960531436690 ) ) ;
#168095=CARTESIAN_POINT ( 'NONE',  ( 12.14591786802327356, -12.06949235617739191, 65.62609039468568994 ) ) ;
#168097=CARTESIAN_POINT ( 'NONE',  ( -19.03943276465977164, -0.05219959533935918106, 23.75109039468566152 ) ) ;
#168098=CARTESIAN_POINT ( 'NONE',  ( 17.49999999999999645, -5.500000000000031974, 93.29690382534172954 ) ) ;
#168099=CARTESIAN_POINT ( 'NONE',  ( -8.224510206698735004, -14.34966873604973081, 84.58442372801903275 ) ) ;
#168101=CARTESIAN_POINT ( 'NONE',  ( 12.14591786802327356, -12.06949235617739191, 85.62609039468568994 ) ) ;
#168102=CARTESIAN_POINT ( 'NONE',  ( -16.52216118717208460, 7.221426719304501418, 28.92400978953008561 ) ) ;
#168103=CARTESIAN_POINT ( 'NONE',  ( -16.52544592524335698, -4.483927247898792601, 53.95942372801900433 ) ) ;
#168104=CARTESIAN_POINT ( 'NONE',  ( -9.474510206698964154, 16.51473224551069663, 75.41557627198103830 ) ) ;
#168105=CARTESIAN_POINT ( 'NONE',  ( 18.62759615963255655, 10.81492255796105972, 66.66775706135234714 ) ) ;
#168106=CARTESIAN_POINT ( 'NONE',  ( -5.153800228976607833, 19.02544592524334988, 72.70942372801900433 ) ) ;
#168107=CARTESIAN_POINT ( 'NONE',  ( -5.719274019375665041, -21.55341960407619695, 104.7927570613523898 ) ) ;
#168108=CARTESIAN_POINT ( 'NONE',  ( -5.049401038298153566, 19.05341960407611168, 55.20724293864769550 ) ) ;
#168109=CARTESIAN_POINT ( 'NONE',  ( -13.97604488694527625, -13.89961937509977652, 46.87390960531435979 ) ) ;
#168110=CARTESIAN_POINT ( 'NONE',  ( 16.40734927747358540, 7.283318515949404492, 22.21415419577492045 ) ) ;
#168111=CARTESIAN_POINT ( 'NONE',  ( -0.05219959533907301413, -21.53943276465977519, 62.49890960531436690 ) ) ;
#168113=CARTESIAN_POINT ( 'NONE',  ( -5.823673210054116645, -21.52544592524344225, 27.29057627198103120 ) ) ;
#168114=CARTESIAN_POINT ( 'NONE',  ( 19.02544592524343514, -5.153800228976328945, 23.54057627198102054 ) ) ;
#168115=CARTESIAN_POINT ( 'NONE',  ( -16.55341960407617563, 4.379528057220093196, 53.54275706135234714 ) ) ;
#168117=CARTESIAN_POINT ( 'NONE',  ( 18.67979575497178502, 10.72451020669898547, 114.1655762719810383 ) ) ;
#168118=CARTESIAN_POINT ( 'NONE',  ( 8.314922557960818139, 14.29746914071049879, 54.58224293864769550 ) ) ;
#168120=CARTESIAN_POINT ( 'NONE',  ( 0.05219959533936267826, -19.03943276465977164, 105.0010903946856615 ) ) ;
#168121=CARTESIAN_POINT ( 'NONE',  ( 5.153800228976615827, -19.02544592524334988, 45.20942372801901143 ) ) ;
#168122=CARTESIAN_POINT ( 'NONE',  ( 16.53943276465976808, -0.05219959533910856209, 38.74890960531435979 ) ) ;
#168123=CARTESIAN_POINT ( 'NONE',  ( -0.05219959533937732626, 21.53943276465977519, 22.50109039468567573 ) ) ;
#168124=DIRECTION ( 'NONE',  ( -0.000000000000000000, -0.000000000000000000, 1.000000000000000000 ) ) ;
#168125=CARTESIAN_POINT ( 'NONE',  ( 10.72451020669898902, -18.67979575497178502, 62.91557627198102409 ) ) ;
#168126=CARTESIAN_POINT ( 'NONE',  ( 19.02544592524343514, -5.153800228976328945, 88.54057627198102409 ) ) ;
#168127=CARTESIAN_POINT ( 'NONE',  ( 14.29746914071049879, -8.314922557960816363, 53.33224293864769550 ) ) ;
#168128=CARTESIAN_POINT ( 'NONE',  ( -19.03943276465977164, 0.05219959533909376836, 101.2489096053143669 ) ) ;
#168130=CARTESIAN_POINT ( 'NONE',  ( -0.05219959533936034679, 19.03943276465977164, 57.50109039468566863 ) ) ;
#168131=CARTESIAN_POINT ( 'NONE',  ( 18.67979575497178502, 10.72451020669898547, 99.16557627198100988 ) ) ;
#168132=CARTESIAN_POINT ( 'NONE',  ( 9.564922557960805705, 16.46253265017160317, 49.58224293864770260 ) ) ;
#168133=CARTESIAN_POINT ( 'NONE',  ( 13.89961937509977652, -13.97604488694527269, 23.12390960531436335 ) ) ;
#168134=CARTESIAN_POINT ( 'NONE',  ( 18.62759615963255655, 10.81492255796105972, 56.66775706135235424 ) ) ;
#168136=CARTESIAN_POINT ( 'NONE',  ( -8.314922557960811034, -14.29746914071050412, 22.08224293864769194 ) ) ;
#168137=CARTESIAN_POINT ( 'NONE',  ( -5.049401038298153566, 19.05341960407611168, 50.20724293864770260 ) ) ;
#168138=CARTESIAN_POINT ( 'NONE',  ( 19.05341960407611168, 5.049401038298154454, 98.95724293864766707 ) ) ;
#168139=CARTESIAN_POINT ( 'NONE',  ( 0.05219959533907565091, 21.53943276465977519, 54.99890960531435269 ) ) ;
#168141=CARTESIAN_POINT ( 'NONE',  ( 19.05341960407611168, 5.049401038298154454, 48.95724293864768129 ) ) ;
#168142=CARTESIAN_POINT ( 'NONE',  ( -5.719274019375978568, 21.55341960407610458, 50.20724293864769550 ) ) ;
#168143=CARTESIAN_POINT ( 'NONE',  ( 10.81492255796106328, -18.62759615963255655, 85.41775706135236135 ) ) ;
#168145=CARTESIAN_POINT ( 'NONE',  ( 16.52544592524335698, 4.483927247898782831, 86.45942372801901854 ) ) ;
#168146=CARTESIAN_POINT ( 'NONE',  ( -14.29746914071049879, 8.314922557960819915, 75.83224293864769550 ) ) ;
#168147=CARTESIAN_POINT ( 'NONE',  ( 14.29746914071037800, 8.314922557961029526, 86.66775706135234714 ) ) ;
#168148=CARTESIAN_POINT ( 'NONE',  ( 9.564922557960805705, 16.46253265017160317, 69.58224293864770971 ) ) ;
#168150=CARTESIAN_POINT ( 'NONE',  ( 16.51473224551083163, -9.474510206698727899, 20.83442372801899722 ) ) ;
#168151=CARTESIAN_POINT ( 'NONE',  ( 4.483927247898790824, -16.52544592524335698, 90.20942372801903275 ) ) ;
#168152=CARTESIAN_POINT ( 'NONE',  ( 5.153800228976615827, -19.02544592524334988, 20.20942372801899722 ) ) ;
#168153=CARTESIAN_POINT ( 'NONE',  ( -5.153800228976328057, -19.02544592524343514, 82.29057627198103830 ) ) ;
#168154=CARTESIAN_POINT ( 'NONE',  ( -10.81492255796078084, -18.62759615963271287, 42.08224293864769550 ) ) ;
#168155=CARTESIAN_POINT ( 'NONE',  ( 0.05219959533934541429, -16.53943276465976808, 30.00109039468568284 ) ) ;
#168156=CARTESIAN_POINT ( 'NONE',  ( 5.719274019375673035, 21.55341960407619339, 87.29275706135236135 ) ) ;
#168157=CARTESIAN_POINT ( 'NONE',  ( 16.52544592524335698, 4.483927247898782831, 66.45942372801903275 ) ) ;
#168158=CARTESIAN_POINT ( 'NONE',  ( 0.05219959533907565091, 21.53943276465977519, 114.9989096053143669 ) ) ;
#168159=CARTESIAN_POINT ( 'NONE',  ( 4.483927247898790824, -16.52544592524335698, 20.20942372801900788 ) ) ;
#168160=CARTESIAN_POINT ( 'NONE',  ( 16.46253265017160672, -9.564922557960803928, 93.33224293864769550 ) ) ;
#168161=CARTESIAN_POINT ( 'NONE',  ( -0.05219959533934338120, 16.53943276465976808, 27.50109039468567929 ) ) ;
#168162=CARTESIAN_POINT ( 'NONE',  ( -9.474510206698964154, 16.51473224551069663, 40.41557627198103120 ) ) ;
#168163=CARTESIAN_POINT ( 'NONE',  ( -12.06949235617739369, -12.14591786802326823, 39.37609039468567573 ) ) ;
#168164=CARTESIAN_POINT ( 'NONE',  ( 4.483927247898545687, 16.52544592524342804, 74.79057627198105251 ) ) ;
#168165=CARTESIAN_POINT ( 'NONE',  ( 4.379528057220092307, 16.55341960407617563, 82.29275706135234714 ) ) ;
#168166=CARTESIAN_POINT ( 'NONE',  ( -15.72974639402176322, -15.80617190586768395, 24.37609039468567573 ) ) ;
#168167=CARTESIAN_POINT ( 'NONE',  ( 5.049401038298161559, -19.05341960407611168, 67.70724293864769550 ) ) ;
#168168=CARTESIAN_POINT ( 'NONE',  ( 19.03943276465977164, -0.05219959533909143690, 88.74890960531436690 ) ) ;
#168169=CARTESIAN_POINT ( 'NONE',  ( 4.379528057220092307, 16.55341960407617563, 92.29275706135236135 ) ) ;
#168173=CARTESIAN_POINT ( 'NONE',  ( -13.89961937509957401, -13.97604488694547875, 34.37609039468566863 ) ) ;
#168174=CARTESIAN_POINT ( 'NONE',  ( -0.05219959533909027116, -19.03943276465977164, 92.49890960531436690 ) ) ;
#168175=CARTESIAN_POINT ( 'NONE',  ( 13.97604488694527802, 13.89961937509977652, 54.37390960531435979 ) ) ;
#168176=CARTESIAN_POINT ( 'NONE',  ( -5.153800228976328057, -19.02544592524343514, 112.2905762719810099 ) ) ;
#168177=ORIENTED_EDGE ( 'NONE', *, *, #95827, .F. ) ;
#168178=CARTESIAN_POINT ( 'NONE',  ( 4.483927247898790824, -16.52544592524335698, 25.20942372801901854 ) ) ;
#168179=CARTESIAN_POINT ( 'NONE',  ( -16.51473224551082808, 9.474510206698731452, 53.33442372801900433 ) ) ;
#168180=CARTESIAN_POINT ( 'NONE',  ( 16.55341960407618274, -4.379528057220086978, 36.04275706135234714 ) ) ;
#168181=CARTESIAN_POINT ( 'NONE',  ( -19.02544592524342804, 5.153800228976336051, 106.0405762719810241 ) ) ;
#168182=CARTESIAN_POINT ( 'NONE',  ( -13.89961937509977652, 13.97604488694528158, 80.62390960531436690 ) ) ;
#168183=CARTESIAN_POINT ( 'NONE',  ( 21.55341960407610458, 5.719274019375980345, 93.95724293864770971 ) ) ;
#168184=CARTESIAN_POINT ( 'NONE',  ( -13.89961937509957401, -13.97604488694547875, 59.37609039468566863 ) ) ;
#168185=CARTESIAN_POINT ( 'NONE',  ( 5.049401038298161559, -19.05341960407611168, 87.70724293864769550 ) ) ;
#168187=CARTESIAN_POINT ( 'NONE',  ( 13.89961937509977652, -13.97604488694527269, 58.12390960531436690 ) ) ;
#168188=CARTESIAN_POINT ( 'NONE',  ( -0.05219959533934338120, 16.53943276465976808, 112.5010903946857042 ) ) ;
#168189=CARTESIAN_POINT ( 'NONE',  ( -19.03943276465977164, 0.05219959533909376836, 26.24890960531435624 ) ) ;
#168191=CARTESIAN_POINT ( 'NONE',  ( -13.89961937509957401, -13.97604488694547875, 39.37609039468566152 ) ) ;
#168192=CARTESIAN_POINT ( 'NONE',  ( -8.224510206698948167, 14.34966873604960824, 70.41557627198102409 ) ) ;
#168193=CARTESIAN_POINT ( 'NONE',  ( 5.823673210054444382, -21.52544592524334988, 105.2094237280190328 ) ) ;
#168194=CARTESIAN_POINT ( 'NONE',  ( -5.153800228976328057, -19.02544592524343514, 42.29057627198101699 ) ) ;
#168195=CARTESIAN_POINT ( 'NONE',  ( -16.53943276465976808, -0.05219959533934237506, 53.75109039468568994 ) ) ;
#168196=CARTESIAN_POINT ( 'NONE',  ( -14.34966873604960291, -8.224510206698953496, 41.66557627198103120 ) ) ;
#168197=CARTESIAN_POINT ( 'NONE',  ( 15.80617190586769283, -15.72974639402175789, 90.62609039468567573 ) ) ;
#168198=CARTESIAN_POINT ( 'NONE',  ( -13.97604488694527625, -13.89961937509977652, 86.87390960531436690 ) ) ;
#168199=CARTESIAN_POINT ( 'NONE',  ( -13.89961937509977652, 13.97604488694528158, 100.6239096053143669 ) ) ;
#168200=CARTESIAN_POINT ( 'NONE',  ( -14.29746914071049879, 8.314922557960819915, 105.8322429386476955 ) ) ;
#168201=CARTESIAN_POINT ( 'NONE',  ( 16.53943276465976808, -0.05219959533910856209, 73.74890960531433848 ) ) ;
#168202=CARTESIAN_POINT ( 'NONE',  ( 10.72451020669898902, -18.67979575497178502, 77.91557627198102409 ) ) ;
#168203=CARTESIAN_POINT ( 'NONE',  ( 9.474510206698971260, -16.51473224551069308, 92.91557627198103830 ) ) ;
#168204=CARTESIAN_POINT ( 'NONE',  ( -15.72974639402197994, 15.80617190586746368, 100.6239096053143811 ) ) ;
#168205=CARTESIAN_POINT ( 'NONE',  ( 19.02544592524343514, -5.153800228976328945, 93.54057627198102409 ) ) ;
#168206=CARTESIAN_POINT ( 'NONE',  ( -19.52851543214744368, -5.499999999999942268, 90.39357721762578990 ) ) ;
#168207=CARTESIAN_POINT ( 'NONE',  ( -16.52544592524342804, 4.483927247898546575, 91.04057627198103830 ) ) ;
#168208=CARTESIAN_POINT ( 'NONE',  ( -5.049401038298153566, 19.05341960407611168, 55.20724293864769550 ) ) ;
#168209=CARTESIAN_POINT ( 'NONE',  ( -15.72974639402197994, 15.80617190586746368, 60.62390960531437401 ) ) ;
#168211=CARTESIAN_POINT ( 'NONE',  ( 16.52544592524342804, -4.483927247898539470, 23.54057627198102765 ) ) ;
#168212=LINE ( 'NONE', #44879, #179255 ) ;
#168213=CARTESIAN_POINT ( 'NONE',  ( 4.379528057220092307, 16.55341960407617563, 22.29275706135235069 ) ) ;
#168214=CARTESIAN_POINT ( 'NONE',  ( 8.224510206698953496, -14.34966873604960469, 82.91557627198103830 ) ) ;
#168215=CARTESIAN_POINT ( 'NONE',  ( -16.38665767535051998, -7.295008042176110763, 94.73599135785453029 ) ) ;
#168216=CARTESIAN_POINT ( 'NONE',  ( -19.03943276465977164, 0.05219959533909376836, 81.24890960531436690 ) ) ;
#168217=CARTESIAN_POINT ( 'NONE',  ( 13.97604488694527802, 13.89961937509977652, 39.37390960531435269 ) ) ;
#168218=CARTESIAN_POINT ( 'NONE',  ( 4.379528057220339221, -16.55341960407611168, 72.70724293864769550 ) ) ;
#168219=CARTESIAN_POINT ( 'NONE',  ( 5.823673210054125526, 21.52544592524343514, 24.79057627198103120 ) ) ;
#168220=CARTESIAN_POINT ( 'NONE',  ( -9.564922557961040184, 16.46253265017147172, 97.91775706135233293 ) ) ;
#168221=CARTESIAN_POINT ( 'NONE',  ( -16.51473224551069308, -9.474510206698971260, 101.6655762719810241 ) ) ;
#168222=CARTESIAN_POINT ( 'NONE',  ( -21.53943276465977519, 0.05219959533907696930, 76.24890960531435269 ) ) ;
#168223=CARTESIAN_POINT ( 'NONE',  ( 16.52544592524335698, 4.483927247898782831, 76.45942372801901854 ) ) ;
#168224=CARTESIAN_POINT ( 'NONE',  ( -16.61371651742643252, 7.165104196375864376, 93.85415069992970416 ) ) ;
#168225=CARTESIAN_POINT ( 'NONE',  ( -13.89961937509977652, 13.97604488694528158, 75.62390960531438111 ) ) ;
#168226=CARTESIAN_POINT ( 'NONE',  ( -15.80617190586745835, -15.72974639402198527, 76.87390960531439532 ) ) ;
#168227=CARTESIAN_POINT ( 'NONE',  ( 19.05341960407617918, -5.049401038297876454, 106.0427570613523471 ) ) ;
#168228=CARTESIAN_POINT ( 'NONE',  ( 8.314922557960818139, 14.29746914071049879, 34.58224293864770260 ) ) ;
#168229=CARTESIAN_POINT ( 'NONE',  ( -18.67979575497193778, 10.72451020669871902, 53.33442372801901854 ) ) ;
#168232=CARTESIAN_POINT ( 'NONE',  ( 14.29746914071037800, 8.314922557961029526, 66.66775706135234714 ) ) ;
#168233=CARTESIAN_POINT ( 'NONE',  ( -13.97604488694527625, -13.89961937509977652, 106.8739096053143669 ) ) ;
#168235=CARTESIAN_POINT ( 'NONE',  ( -17.31747979337950127, 6.344076630960996610, 78.62055131934819485 ) ) ;
#168236=CARTESIAN_POINT ( 'NONE',  ( -12.14591786802326823, 12.06949235617739902, 93.12609039468568994 ) ) ;
#168237=CARTESIAN_POINT ( 'NONE',  ( 12.06949235617739724, 12.14591786802326823, 41.87609039468568284 ) ) ;
#168238=CARTESIAN_POINT ( 'NONE',  ( -16.51473224551069308, -9.474510206698971260, 56.66557627198103120 ) ) ;
#168239=CARTESIAN_POINT ( 'NONE',  ( 16.51473224551069308, 9.474510206698969483, 79.16557627198103830 ) ) ;
#168240=CARTESIAN_POINT ( 'NONE',  ( 10.81492255796106328, -18.62759615963255655, 60.41775706135235424 ) ) ;
#168241=CARTESIAN_POINT ( 'NONE',  ( 16.52544592524335698, 4.483927247898782831, 61.45942372801901854 ) ) ;
#168242=CARTESIAN_POINT ( 'NONE',  ( 4.379528057220339221, -16.55341960407611168, 37.70724293864769550 ) ) ;
#168243=CARTESIAN_POINT ( 'NONE',  ( 9.474510206698971260, -16.51473224551069308, 42.91557627198103120 ) ) ;
#168244=CARTESIAN_POINT ( 'NONE',  ( 9.474510206698971260, -16.51473224551069308, 52.91557627198102409 ) ) ;
#168245=CARTESIAN_POINT ( 'NONE',  ( -12.06949235617739369, -12.14591786802326823, 44.37609039468567573 ) ) ;
#168246=CARTESIAN_POINT ( 'NONE',  ( -9.564922557961040184, 16.46253265017147172, 97.91775706135233293 ) ) ;
#168247=CARTESIAN_POINT ( 'NONE',  ( -0.05219959533910754901, -16.53943276465976808, 102.4989096053143811 ) ) ;
#168248=CARTESIAN_POINT ( 'NONE',  ( 16.46253265017160672, -9.564922557960803928, 53.33224293864768839 ) ) ;
#168249=CARTESIAN_POINT ( 'NONE',  ( -9.474510206698720793, -16.51473224551083518, 84.58442372801900433 ) ) ;
#168250=CARTESIAN_POINT ( 'NONE',  ( 17.49999999999999645, -5.624438216177591876, 93.31670344914644488 ) ) ;
#168251=CARTESIAN_POINT ( 'NONE',  ( 21.52544592524334988, 5.823673210054432836, 96.45942372801901854 ) ) ;
#168252=CARTESIAN_POINT ( 'NONE',  ( -14.29746914071037622, -8.314922557961029526, 49.16775706135234003 ) ) ;
#168254=CARTESIAN_POINT ( 'NONE',  ( 15.72974639402199770, -15.80617190586745480, 48.12390960531436690 ) ) ;
#168255=CARTESIAN_POINT ( 'NONE',  ( 12.14591786802327356, -12.06949235617739191, 45.62609039468567573 ) ) ;
#168256=CARTESIAN_POINT ( 'NONE',  ( -19.49149378614661643, 5.499999999999580780, 69.43757513605359577 ) ) ;
#168257=CARTESIAN_POINT ( 'NONE',  ( 19.02544592524334988, 5.153800228976608722, 46.45942372801899012 ) ) ;
#168258=CARTESIAN_POINT ( 'NONE',  ( 16.46253265017160672, -9.564922557960803928, 88.33224293864769550 ) ) ;
#168259=CARTESIAN_POINT ( 'NONE',  ( 16.46253265017160672, -9.564922557960803928, 23.33224293864769194 ) ) ;
#168260=CARTESIAN_POINT ( 'NONE',  ( -16.46253265017160317, 9.564922557960807481, 55.83224293864769550 ) ) ;
#168262=CARTESIAN_POINT ( 'NONE',  ( 5.719274019375673035, 21.55341960407619339, 82.29275706135234714 ) ) ;
#168263=CARTESIAN_POINT ( 'NONE',  ( 17.58332526062529411, -7.635886036038496805, 93.42334959558465357 ) ) ;
#168264=CARTESIAN_POINT ( 'NONE',  ( -19.02544592524334988, -5.153800228976617603, 33.95942372801897591 ) ) ;
#168265=CARTESIAN_POINT ( 'NONE',  ( -21.53943276465977519, -0.05219959533937600094, 108.7510903946857042 ) ) ;
#168266=CARTESIAN_POINT ( 'NONE',  ( 16.55341960407611168, 4.379528057220329451, 53.95724293864770260 ) ) ;
#168267=CARTESIAN_POINT ( 'NONE',  ( -5.153800228976328057, -19.02544592524343514, 62.29057627198100988 ) ) ;
#168268=CARTESIAN_POINT ( 'NONE',  ( -0.05219959533909027116, -19.03943276465977164, 102.4989096053143669 ) ) ;
#168269=CARTESIAN_POINT ( 'NONE',  ( 18.62759615963255655, 10.81492255796105972, 76.66775706135234714 ) ) ;
#168270=CARTESIAN_POINT ( 'NONE',  ( 5.049401038298161559, -19.05341960407611168, 62.70724293864769550 ) ) ;
#168271=CARTESIAN_POINT ( 'NONE',  ( -21.53943276465977519, -0.05219959533937600094, 73.75109039468567573 ) ) ;
#168272=CARTESIAN_POINT ( 'NONE',  ( -21.53943276465977519, 0.05219959533907696930, 36.24890960531435979 ) ) ;
#168273=CARTESIAN_POINT ( 'NONE',  ( -10.72451020669870658, -18.67979575497194134, 34.58442372801900433 ) ) ;
#168274=CARTESIAN_POINT ( 'NONE',  ( -0.05219959533936034679, 19.03943276465977164, 57.50109039468566863 ) ) ;
#168275=CARTESIAN_POINT ( 'NONE',  ( 0.05219959533909260263, 19.03943276465977164, 29.99890960531435979 ) ) ;
#168276=CARTESIAN_POINT ( 'NONE',  ( -5.049401038298153566, 19.05341960407611168, 75.20724293864769550 ) ) ;
#168277=CARTESIAN_POINT ( 'NONE',  ( 0.05219959533934541429, -16.53943276465976808, 35.00109039468568284 ) ) ;
#168278=CARTESIAN_POINT ( 'NONE',  ( 4.483927247898545687, 16.52544592524342804, 94.79057627198105251 ) ) ;
#168279=CARTESIAN_POINT ( 'NONE',  ( 9.474510206698971260, -16.51473224551069308, 62.91557627198102409 ) ) ;
#168280=CARTESIAN_POINT ( 'NONE',  ( -15.72974639402197994, 15.80617190586746368, 30.62390960531436335 ) ) ;
#168281=CARTESIAN_POINT ( 'NONE',  ( -0.05219959533934338120, 16.53943276465976808, 22.50109039468567573 ) ) ;
#168282=CARTESIAN_POINT ( 'NONE',  ( -21.52544592524343514, 5.823673210054127303, 116.0405762719810383 ) ) ;
#168283=CARTESIAN_POINT ( 'NONE',  ( 21.53943276465977519, 0.05219959533937863772, 66.25109039468567573 ) ) ;
#168284=CARTESIAN_POINT ( 'NONE',  ( 12.14591786802327356, -12.06949235617739191, 70.62609039468567573 ) ) ;
#168285=CARTESIAN_POINT ( 'NONE',  ( -4.379528057220086978, -16.55341960407618274, 69.79275706135234714 ) ) ;
#168286=EDGE_LOOP ( 'NONE', ( #177151, #118707, #124868, #179062, #99003, #135296, #153425, #9414 ) ) ;
#168287=CARTESIAN_POINT ( 'NONE',  ( 9.474510206698971260, -16.51473224551069308, 62.91557627198102409 ) ) ;
#168288=CARTESIAN_POINT ( 'NONE',  ( -0.05219959533934338120, 16.53943276465976808, 87.50109039468568994 ) ) ;
#168289=CARTESIAN_POINT ( 'NONE',  ( -5.049401038297874678, -19.05341960407617918, 39.79275706135232582 ) ) ;
#168290=CARTESIAN_POINT ( 'NONE',  ( -15.80617190586745835, -15.72974639402198527, 111.8739096053143669 ) ) ;
#168291=CARTESIAN_POINT ( 'NONE',  ( -16.52544592524342804, 4.483927247898546575, 71.04057627198103830 ) ) ;
#168292=CARTESIAN_POINT ( 'NONE',  ( 0.05219959533909260263, 19.03943276465977164, 89.99890960531436690 ) ) ;
#168293=CARTESIAN_POINT ( 'NONE',  ( -8.314922557961024197, 14.29746914071037800, 92.91775706135236135 ) ) ;
#168294=CARTESIAN_POINT ( 'NONE',  ( -21.53943276465977519, -0.05219959533937600094, 53.75109039468568994 ) ) ;
#168295=CARTESIAN_POINT ( 'NONE',  ( -14.34966873604972548, 8.224510206698743886, 28.33442372801902209 ) ) ;
#168296=CARTESIAN_POINT ( 'NONE',  ( 18.62759615963271287, -10.81492255796078972, 108.3322429386477097 ) ) ;
#168297=CARTESIAN_POINT ( 'NONE',  ( 16.55341960407611168, 4.379528057220329451, 63.95724293864770260 ) ) ;
#168299=CARTESIAN_POINT ( 'NONE',  ( 0.05219959533907565091, 21.53943276465977519, 94.99890960531436690 ) ) ;
#168300=CARTESIAN_POINT ( 'NONE',  ( 8.224510206698953496, -14.34966873604960469, 37.91557627198102409 ) ) ;
#168303=CARTESIAN_POINT ( 'NONE',  ( 9.474510206698971260, -16.51473224551069308, 112.9155762719810383 ) ) ;
#168304=CARTESIAN_POINT ( 'NONE',  ( 0.05219959533937995610, -21.53943276465977519, 40.00109039468567573 ) ) ;
#168305=CARTESIAN_POINT ( 'NONE',  ( -4.379528057220328563, 16.55341960407611168, 50.20724293864769550 ) ) ;
#168306=CARTESIAN_POINT ( 'NONE',  ( -13.97604488694527625, -13.89961937509977652, 61.87390960531435979 ) ) ;
#168307=CARTESIAN_POINT ( 'NONE',  ( 0.05219959533936267826, -19.03943276465977164, 65.00109039468567573 ) ) ;
#168308=CARTESIAN_POINT ( 'NONE',  ( 19.03943276465977164, -0.05219959533909143690, 93.74890960531435269 ) ) ;
#168310=CARTESIAN_POINT ( 'NONE',  ( 5.719274019375991003, -21.55341960407610458, 47.70724293864770260 ) ) ;
#168312=CARTESIAN_POINT ( 'NONE',  ( 19.03943276465977164, -0.05219959533909143690, 53.74890960531436690 ) ) ;
#168313=CARTESIAN_POINT ( 'NONE',  ( -16.52544592524335698, -4.483927247898792601, 38.95942372801901854 ) ) ;
#168314=CARTESIAN_POINT ( 'NONE',  ( 13.97604488694548053, -13.89961937509957401, 60.62609039468564731 ) ) ;
#168315=CARTESIAN_POINT ( 'NONE',  ( 5.823673210054444382, -21.52544592524334988, 20.20942372801900788 ) ) ;
#168316=CARTESIAN_POINT ( 'NONE',  ( -8.224510206698948167, 14.34966873604960824, 50.41557627198103120 ) ) ;
#168317=CARTESIAN_POINT ( 'NONE',  ( -9.564922557960796823, -16.46253265017161027, 87.08224293864769550 ) ) ;
#168318=CARTESIAN_POINT ( 'NONE',  ( 15.80617190586746368, 15.72974639402197994, 79.37390960531436690 ) ) ;
#168319=CARTESIAN_POINT ( 'NONE',  ( -21.55341960407610458, -5.719274019375992779, 111.4572429386476813 ) ) ;
#168320=CARTESIAN_POINT ( 'NONE',  ( -0.05219959533934338120, 16.53943276465976808, 37.50109039468568284 ) ) ;
#168321=CARTESIAN_POINT ( 'NONE',  ( 21.52544592524344225, -5.823673210054117533, 38.54057627198103120 ) ) ;
#168322=CARTESIAN_POINT ( 'NONE',  ( -18.62759615963255300, -10.81492255796106328, 104.1677570613523471 ) ) ;
#168323=CARTESIAN_POINT ( 'NONE',  ( 5.153800228976335163, 19.02544592524342804, 89.79057627198102409 ) ) ;
#168324=CARTESIAN_POINT ( 'NONE',  ( -16.51473224551069308, -9.474510206698971260, 41.66557627198103120 ) ) ;
#168325=CARTESIAN_POINT ( 'NONE',  ( -13.97604488694527625, -13.89961937509977652, 101.8739096053143811 ) ) ;
#168326=B_SPLINE_CURVE_WITH_KNOTS ( 'NONE', 3,
 ( #176220, #38701, #115541, #114519, #25555, #100358, #102367, #132703, #130690, #52848, #116535, #164056, #162037, #87199, #22531, #144860, #98339, #85179, #192384, #5345 ),
 .UNSPECIFIED., .F., .F.,
 ( 4, 2, 2, 2, 2, 2, 2, 2, 2, 4 ),
 ( 0.004000878361811928755, 0.004499404418915952525, 0.004997930476019976295, 0.005496456533124000066, 0.005994982590228023836, 0.006244245618780026180, 0.006493508647332026790, 0.006992034704436006325, 0.007490560761539986727, 0.007989086818643966262 ),
 .UNSPECIFIED. ) ;
#168327=CARTESIAN_POINT ( 'NONE',  ( 19.05341960407611168, 5.049401038298154454, 73.95724293864768129 ) ) ;
#168328=CARTESIAN_POINT ( 'NONE',  ( -0.05219959533934338120, 16.53943276465976808, 27.50109039468567929 ) ) ;
#168330=CARTESIAN_POINT ( 'NONE',  ( 16.46253265017146816, 9.564922557961045513, 56.66775706135233293 ) ) ;
#168331=CARTESIAN_POINT ( 'NONE',  ( 5.823673210054444382, -21.52544592524334988, 105.2094237280190328 ) ) ;
#168332=CARTESIAN_POINT ( 'NONE',  ( -0.05219959533907301413, -21.53943276465977519, 37.49890960531436690 ) ) ;
#168333=CARTESIAN_POINT ( 'NONE',  ( 16.55341960407618274, -4.379528057220086978, 101.0427570613523756 ) ) ;
#168335=CARTESIAN_POINT ( 'NONE',  ( -13.97604488694547697, 13.89961937509957934, 78.12609039468567573 ) ) ;
#168336=CARTESIAN_POINT ( 'NONE',  ( -5.049401038297874678, -19.05341960407617918, 24.79275706135233648 ) ) ;
#168337=FACE_OUTER_BOUND ( 'NONE', #176750, .T. ) ;
#168338=CARTESIAN_POINT ( 'NONE',  ( 9.474510206698971260, -16.51473224551069308, 37.91557627198102409 ) ) ;
#168339=CARTESIAN_POINT ( 'NONE',  ( -4.379528057220328563, 16.55341960407611168, 40.20724293864769550 ) ) ;
#168340=CARTESIAN_POINT ( 'NONE',  ( -19.03943276465977164, 0.05219959533909376836, 26.24890960531435624 ) ) ;
#168341=CARTESIAN_POINT ( 'NONE',  ( -16.53943276465976808, -0.05219959533934237506, 113.7510903946856757 ) ) ;
#168343=CARTESIAN_POINT ( 'NONE',  ( 16.55341960407618274, -4.379528057220086978, 91.04275706135236135 ) ) ;
#168344=CARTESIAN_POINT ( 'NONE',  ( -19.05341960407611168, -5.049401038298163336, 46.45724293864768129 ) ) ;
#168345=CARTESIAN_POINT ( 'NONE',  ( 21.52544592524334988, 5.823673210054432836, 101.4594237280190185 ) ) ;
#168346=CARTESIAN_POINT ( 'NONE',  ( 14.34966873604972726, -8.224510206698740333, 25.83442372801901499 ) ) ;
#168347=CARTESIAN_POINT ( 'NONE',  ( 10.72451020669871369, 18.67979575497193778, 77.08442372801901854 ) ) ;
#168349=CARTESIAN_POINT ( 'NONE',  ( 19.03943276465977164, 0.05219959533936151252, 61.25109039468566863 ) ) ;
#168350=CARTESIAN_POINT ( 'NONE',  ( -19.03943276465977164, 0.05219959533909376836, 86.24890960531436690 ) ) ;
#168351=CARTESIAN_POINT ( 'NONE',  ( 13.89961937509977652, -13.97604488694527269, 83.12390960531436690 ) ) ;
#168353=CARTESIAN_POINT ( 'NONE',  ( -5.719274019375978568, 21.55341960407610458, 115.2072429386476955 ) ) ;
#168354=CARTESIAN_POINT ( 'NONE',  ( -14.34966873604960291, -8.224510206698953496, 71.66557627198100988 ) ) ;
#168355=CARTESIAN_POINT ( 'NONE',  ( 21.53943276465977519, -0.05219959533907433946, 58.74890960531436690 ) ) ;
#168356=CARTESIAN_POINT ( 'NONE',  ( -19.05341960407611168, -5.049401038298163336, 56.45724293864768129 ) ) ;
#168357=CARTESIAN_POINT ( 'NONE',  ( 18.62759615963271287, -10.81492255796078972, 93.33224293864769550 ) ) ;
#168358=CARTESIAN_POINT ( 'NONE',  ( -12.06949235617739369, -12.14591786802326823, 84.37609039468570415 ) ) ;
#168360=CARTESIAN_POINT ( 'NONE',  ( -5.153800228976328057, -19.02544592524343514, 57.29057627198103120 ) ) ;
#168361=CARTESIAN_POINT ( 'NONE',  ( -8.224510206698948167, 14.34966873604960824, 95.41557627198102409 ) ) ;
#168363=CARTESIAN_POINT ( 'NONE',  ( -16.51473224551069308, -9.474510206698971260, 51.66557627198102409 ) ) ;
#168364=CARTESIAN_POINT ( 'NONE',  ( -0.05219959533936034679, 19.03943276465977164, 77.50109039468566152 ) ) ;
#168365=CARTESIAN_POINT ( 'NONE',  ( 16.53943276465976808, -0.05219959533910856209, 78.74890960531436690 ) ) ;
#168366=CARTESIAN_POINT ( 'NONE',  ( -10.72451020669870658, -18.67979575497194134, 64.58442372801900433 ) ) ;
#168367=CARTESIAN_POINT ( 'NONE',  ( 0.05219959533909260263, 19.03943276465977164, 39.99890960531436690 ) ) ;
#168368=CARTESIAN_POINT ( 'NONE',  ( 5.719274019375991003, -21.55341960407610458, 102.7072429386476955 ) ) ;
#168369=CARTESIAN_POINT ( 'NONE',  ( 12.06949235617757843, -12.14591786802309237, 98.12390960531436690 ) ) ;
#168371=CARTESIAN_POINT ( 'NONE',  ( 9.564922557960805705, 16.46253265017160317, 54.58224293864769550 ) ) ;
#168373=CARTESIAN_POINT ( 'NONE',  ( -5.049401038297874678, -19.05341960407617918, 94.79275706135230450 ) ) ;
#168374=CARTESIAN_POINT ( 'NONE',  ( 9.564922557960805705, 16.46253265017160317, 114.5822429386476955 ) ) ;
#168375=CARTESIAN_POINT ( 'NONE',  ( -15.80617190586768217, 15.72974639402176855, 33.12609039468569705 ) ) ;
#168376=CARTESIAN_POINT ( 'NONE',  ( -5.153800228976328057, -19.02544592524343514, 82.29057627198103830 ) ) ;
#168378=CARTESIAN_POINT ( 'NONE',  ( 19.02544592524334988, 5.153800228976608722, 66.45942372801899012 ) ) ;
#168379=CARTESIAN_POINT ( 'NONE',  ( -19.03943276465977164, 0.05219959533909376836, 61.24890960531436690 ) ) ;
#168380=CARTESIAN_POINT ( 'NONE',  ( 16.53943276465976808, -0.05219959533910856209, 78.74890960531436690 ) ) ;
#168381=CARTESIAN_POINT ( 'NONE',  ( 14.29746914071049879, -8.314922557960816363, 68.33224293864769550 ) ) ;
#168382=CARTESIAN_POINT ( 'NONE',  ( 19.03943276465977164, -0.05219959533909143690, 83.74890960531436690 ) ) ;
#168383=CARTESIAN_POINT ( 'NONE',  ( 16.52544592524342804, -4.483927247898539470, 83.54057627198102409 ) ) ;
#168384=CARTESIAN_POINT ( 'NONE',  ( 16.51473224551069308, 9.474510206698969483, 79.16557627198103830 ) ) ;
#168385=CARTESIAN_POINT ( 'NONE',  ( -13.89961937509957401, -13.97604488694547875, 34.37609039468566863 ) ) ;
#168386=CARTESIAN_POINT ( 'NONE',  ( 9.564922557960805705, 16.46253265017160317, 54.58224293864769550 ) ) ;
#168387=CARTESIAN_POINT ( 'NONE',  ( -16.53943276465976808, 0.05219959533911058130, 31.24890960531435979 ) ) ;
#168388=CARTESIAN_POINT ( 'NONE',  ( -0.05219959533910754901, -16.53943276465976808, 107.4989096053143669 ) ) ;
#168390=CARTESIAN_POINT ( 'NONE',  ( -21.55341960407619339, 5.719274019375674811, 48.54275706135234714 ) ) ;
#168391=CARTESIAN_POINT ( 'NONE',  ( -13.89961937509957401, -13.97604488694547875, 64.37609039468567573 ) ) ;
#168392=CARTESIAN_POINT ( 'NONE',  ( -12.06949235617756955, 12.14591786802309770, 40.62390960531435269 ) ) ;
#168393=CARTESIAN_POINT ( 'NONE',  ( 10.81492255796078972, 18.62759615963270932, 89.58224293864768129 ) ) ;
#168394=CARTESIAN_POINT ( 'NONE',  ( -18.62759615963270932, 10.81492255796079327, 25.83224293864769194 ) ) ;
#168395=CARTESIAN_POINT ( 'NONE',  ( -14.34966873604960291, -8.224510206698953496, 76.66557627198103830 ) ) ;
#168396=CARTESIAN_POINT ( 'NONE',  ( -13.97604488694527625, -13.89961937509977652, 46.87390960531435979 ) ) ;
#168397=CARTESIAN_POINT ( 'NONE',  ( -13.89961937509957401, -13.97604488694547875, 29.37609039468565797 ) ) ;
#168398=CARTESIAN_POINT ( 'NONE',  ( -4.483927247898782831, 16.52544592524335698, 97.70942372801904696 ) ) ;
#168399=CARTESIAN_POINT ( 'NONE',  ( 0.05219959533934541429, -16.53943276465976808, 55.00109039468568284 ) ) ;
#168400=CARTESIAN_POINT ( 'NONE',  ( -5.719274019375978568, 21.55341960407610458, 30.20724293864769550 ) ) ;
#168401=CARTESIAN_POINT ( 'NONE',  ( -0.05219959533937732626, 21.53943276465977519, 112.5010903946857042 ) ) ;
#168402=CARTESIAN_POINT ( 'NONE',  ( 16.51473224551069308, 9.474510206698969483, 99.16557627198102409 ) ) ;
#168403=CARTESIAN_POINT ( 'NONE',  ( -8.224510206698735004, -14.34966873604973081, 69.58442372801900433 ) ) ;
#168404=CARTESIAN_POINT ( 'NONE',  ( -5.153800228976328057, -19.02544592524343514, 27.29057627198103120 ) ) ;
#168405=CARTESIAN_POINT ( 'NONE',  ( 16.52544592524342804, -4.483927247898539470, 28.54057627198103120 ) ) ;
#168406=CARTESIAN_POINT ( 'NONE',  ( 5.049401038298161559, -19.05341960407611168, 102.7072429386476955 ) ) ;
#168407=CARTESIAN_POINT ( 'NONE',  ( 5.049401038298161559, -19.05341960407611168, 92.70724293864769550 ) ) ;
#168408=CARTESIAN_POINT ( 'NONE',  ( -15.72974639402197994, 15.80617190586746368, 25.62390960531435624 ) ) ;
#168409=CARTESIAN_POINT ( 'NONE',  ( -14.29746914071049879, 8.314922557960819915, 60.83224293864769550 ) ) ;
#168411=CARTESIAN_POINT ( 'NONE',  ( -16.52544592524342804, 4.483927247898546575, 36.04057627198102409 ) ) ;
#168412=CARTESIAN_POINT ( 'NONE',  ( -16.52544592524342804, 4.483927247898546575, 46.04057627198103830 ) ) ;
#168413=CARTESIAN_POINT ( 'NONE',  ( 14.34966873604972726, -8.224510206698740333, 45.83442372801901854 ) ) ;
#168415=CARTESIAN_POINT ( 'NONE',  ( 9.564922557961047289, -16.46253265017146816, 55.41775706135234003 ) ) ;
#168416=CARTESIAN_POINT ( 'NONE',  ( 5.153800228976335163, 19.02544592524342804, 94.79057627198103830 ) ) ;
#168417=CARTESIAN_POINT ( 'NONE',  ( -0.05219959533936034679, 19.03943276465977164, 67.50109039468566152 ) ) ;
#168419=CARTESIAN_POINT ( 'NONE',  ( -13.97604488694547697, 13.89961937509957934, 58.12609039468566863 ) ) ;
#168420=CARTESIAN_POINT ( 'NONE',  ( -0.05219959533936034679, 19.03943276465977164, 92.50109039468566152 ) ) ;
#168421=CARTESIAN_POINT ( 'NONE',  ( 16.53943276465976808, 0.05219959533934440121, 81.25109039468568994 ) ) ;
#168423=CARTESIAN_POINT ( 'NONE',  ( 19.03943276465977164, -0.05219959533909143690, 23.74890960531435269 ) ) ;
#168424=CARTESIAN_POINT ( 'NONE',  ( 19.02544592524343514, -5.153800228976328945, 113.5405762719810241 ) ) ;
#168425=CARTESIAN_POINT ( 'NONE',  ( -10.72451020669870658, -18.67979575497194134, 39.58442372801901143 ) ) ;
#168426=CARTESIAN_POINT ( 'NONE',  ( 19.03943276465977164, 0.05219959533936151252, 101.2510903946856757 ) ) ;
#168428=CARTESIAN_POINT ( 'NONE',  ( 19.03943276465977164, -0.05219959533909143690, 58.74890960531435979 ) ) ;
#168429=CARTESIAN_POINT ( 'NONE',  ( 16.46253265017160672, -9.564922557960803928, 108.3322429386476955 ) ) ;
#168430=CARTESIAN_POINT ( 'NONE',  ( -12.06949235617756955, 12.14591786802309770, 75.62390960531439532 ) ) ;
#168431=CARTESIAN_POINT ( 'NONE',  ( 19.02544592524343514, -5.153800228976328945, 63.54057627198103830 ) ) ;
#168432=CARTESIAN_POINT ( 'NONE',  ( 13.97604488694527802, 13.89961937509977652, 69.37390960531436690 ) ) ;
#168433=CARTESIAN_POINT ( 'NONE',  ( 9.474510206698729675, 16.51473224551082808, 77.08442372801900433 ) ) ;
#168434=CARTESIAN_POINT ( 'NONE',  ( 18.62759615963271287, -10.81492255796078972, 53.33224293864769550 ) ) ;
#168435=CARTESIAN_POINT ( 'NONE',  ( 9.474510206698971260, -16.51473224551069308, 22.91557627198102765 ) ) ;
#168436=CARTESIAN_POINT ( 'NONE',  ( 5.049401038297881783, 19.05341960407617563, 37.29275706135232582 ) ) ;
#168437=CARTESIAN_POINT ( 'NONE',  ( 5.153800228976335163, 19.02544592524342804, 74.79057627198103830 ) ) ;
#168438=CARTESIAN_POINT ( 'NONE',  ( -18.67979575497178146, -10.72451020669898902, 71.66557627198100988 ) ) ;
#168439=CARTESIAN_POINT ( 'NONE',  ( -16.55341960407611168, -4.379528057220339221, 76.45724293864769550 ) ) ;
#168440=CARTESIAN_POINT ( 'NONE',  ( 19.05341960407617918, -5.049401038297876454, 46.04275706135233293 ) ) ;
#168441=CARTESIAN_POINT ( 'NONE',  ( -0.05219959533907301413, -21.53943276465977519, 72.49890960531435269 ) ) ;
#168442=CARTESIAN_POINT ( 'NONE',  ( -21.52544592524343514, 5.823673210054127303, 61.04057627198103120 ) ) ;
#168443=CARTESIAN_POINT ( 'NONE',  ( 18.62759615963271287, -10.81492255796078972, 33.33224293864769550 ) ) ;
#168444=CARTESIAN_POINT ( 'NONE',  ( 21.53943276465977519, 0.05219959533937863772, 96.25109039468568994 ) ) ;
#168445=CARTESIAN_POINT ( 'NONE',  ( -9.564922557960796823, -16.46253265017161027, 67.08224293864769550 ) ) ;
#168446=CARTESIAN_POINT ( 'NONE',  ( 4.483927247898545687, 16.52544592524342804, 109.7905762719810383 ) ) ;
#168448=CARTESIAN_POINT ( 'NONE',  ( -10.81492255796105439, 18.62759615963255655, 22.91775706135235069 ) ) ;
#168449=CARTESIAN_POINT ( 'NONE',  ( -5.823673210054431948, 21.52544592524334988, 37.70942372801900433 ) ) ;
#168450=CARTESIAN_POINT ( 'NONE',  ( -0.05219959533909027116, -19.03943276465977164, 37.49890960531436690 ) ) ;
#168451=CARTESIAN_POINT ( 'NONE',  ( -18.62759615963270932, 10.81492255796079327, 105.8322429386476955 ) ) ;
#168452=CARTESIAN_POINT ( 'NONE',  ( -16.51473224551082808, 9.474510206698731452, 48.33442372801900433 ) ) ;
#168453=CARTESIAN_POINT ( 'NONE',  ( -9.474510206698964154, 16.51473224551069663, 35.41557627198102409 ) ) ;
#168454=CARTESIAN_POINT ( 'NONE',  ( -19.03943276465977164, 0.05219959533909376836, 26.24890960531435624 ) ) ;
#168455=CARTESIAN_POINT ( 'NONE',  ( 30.00000000000000000, -1.163414459189985801E-14, 95.00000000000000000 ) ) ;
#168456=CARTESIAN_POINT ( 'NONE',  ( -16.52544592524335698, -4.483927247898792601, 58.95942372801902565 ) ) ;
#168457=CARTESIAN_POINT ( 'NONE',  ( -16.46253265017160317, 9.564922557960807481, 25.83224293864769194 ) ) ;
#168459=CARTESIAN_POINT ( 'NONE',  ( 5.153800228976335163, 19.02544592524342804, 79.79057627198102409 ) ) ;
#168460=CARTESIAN_POINT ( 'NONE',  ( -12.14591786802309592, -12.06949235617757132, 101.8739096053143811 ) ) ;
#168461=CARTESIAN_POINT ( 'NONE',  ( 18.67979575497178502, 10.72451020669898547, 54.16557627198103120 ) ) ;
#168462=CARTESIAN_POINT ( 'NONE',  ( -0.05219959533934338120, 16.53943276465976808, 52.50109039468567573 ) ) ;
#168463=CARTESIAN_POINT ( 'NONE',  ( -10.72451020669870658, -18.67979575497194134, 104.5844237280190185 ) ) ;
#168464=CARTESIAN_POINT ( 'NONE',  ( 19.05341960407611168, 5.049401038298154454, 23.95724293864769194 ) ) ;
#168465=CARTESIAN_POINT ( 'NONE',  ( 4.379528057220092307, 16.55341960407617563, 107.2927570613523471 ) ) ;
#168466=CARTESIAN_POINT ( 'NONE',  ( 12.06949235617757843, -12.14591786802309237, 53.12390960531436690 ) ) ;
#168467=CARTESIAN_POINT ( 'NONE',  ( -16.51473224551069308, -9.474510206698971260, 46.66557627198102409 ) ) ;
#168468=CARTESIAN_POINT ( 'NONE',  ( -15.80617190586768217, 15.72974639402176855, 113.1260903946856899 ) ) ;
#168469=CARTESIAN_POINT ( 'NONE',  ( -15.80617190586768217, 15.72974639402176855, 28.12609039468568284 ) ) ;
#168470=CARTESIAN_POINT ( 'NONE',  ( -18.62759615963255300, -10.81492255796106328, 74.16775706135231871 ) ) ;
#168471=CARTESIAN_POINT ( 'NONE',  ( -16.53943276465976808, -0.05219959533934237506, 53.75109039468568994 ) ) ;
#168472=CARTESIAN_POINT ( 'NONE',  ( -4.379528057220086978, -16.55341960407618274, 34.79275706135235424 ) ) ;
#168473=CARTESIAN_POINT ( 'NONE',  ( -12.06949235617756955, 12.14591786802309770, 75.62390960531439532 ) ) ;
#168474=CARTESIAN_POINT ( 'NONE',  ( -21.52544592524334988, -5.823673210054445271, 103.9594237280190185 ) ) ;
#168475=CARTESIAN_POINT ( 'NONE',  ( 14.34966873604960469, 8.224510206698951720, 29.16557627198103120 ) ) ;
#168476=CARTESIAN_POINT ( 'NONE',  ( -16.21995358207305671, 7.366697692864169866, 114.9355100151216078 ) ) ;
#168477=CARTESIAN_POINT ( 'NONE',  ( 8.314922557961029526, -14.29746914071037800, 35.41775706135234003 ) ) ;
#168478=CARTESIAN_POINT ( 'NONE',  ( 12.06949235617757843, -12.14591786802309237, 48.12390960531436690 ) ) ;
#168479=CARTESIAN_POINT ( 'NONE',  ( 12.06949235617739724, 12.14591786802326823, 81.87609039468568994 ) ) ;
#168480=CARTESIAN_POINT ( 'NONE',  ( 16.51473224551069308, 9.474510206698969483, 99.16557627198102409 ) ) ;
#168481=CARTESIAN_POINT ( 'NONE',  ( 13.89961937509977652, -13.97604488694527269, 113.1239096053143527 ) ) ;
#168482=CARTESIAN_POINT ( 'NONE',  ( 21.53943276465977519, 0.05219959533937863772, 96.25109039468568994 ) ) ;
#168483=CARTESIAN_POINT ( 'NONE',  ( -16.55341960407617563, 4.379528057220093196, 98.54275706135234714 ) ) ;
#168484=CARTESIAN_POINT ( 'NONE',  ( -16.55341960407611168, -4.379528057220339221, 81.45724293864769550 ) ) ;
#168485=CARTESIAN_POINT ( 'NONE',  ( 13.97604488694527802, 13.89961937509977652, 84.37390960531433848 ) ) ;
#168487=CARTESIAN_POINT ( 'NONE',  ( 16.52544592524335698, 4.483927247898782831, 41.45942372801901143 ) ) ;
#168488=CARTESIAN_POINT ( 'NONE',  ( -13.89961937509977652, 13.97604488694528158, 45.62390960531433848 ) ) ;
#168489=CARTESIAN_POINT ( 'NONE',  ( 16.46253265017160672, -9.564922557960803928, 103.3322429386476955 ) ) ;
#168490=CARTESIAN_POINT ( 'NONE',  ( 8.224510206698742110, 14.34966873604972548, 27.08442372801901854 ) ) ;
#168492=CARTESIAN_POINT ( 'NONE',  ( 19.02544592524334988, 5.153800228976608722, 41.45942372801900433 ) ) ;
#168493=CARTESIAN_POINT ( 'NONE',  ( -16.55341960407617563, 4.379528057220093196, 103.5427570613523613 ) ) ;
#168494=CARTESIAN_POINT ( 'NONE',  ( 16.51473224551069308, 9.474510206698969483, 29.16557627198103475 ) ) ;
#168495=CARTESIAN_POINT ( 'NONE',  ( -14.34966873604972548, 8.224510206698743886, 73.33442372801901854 ) ) ;
#168496=CARTESIAN_POINT ( 'NONE',  ( -5.049401038297874678, -19.05341960407617918, 79.79275706135233293 ) ) ;
#168497=CARTESIAN_POINT ( 'NONE',  ( -9.564922557961040184, 16.46253265017147172, 32.91775706135233293 ) ) ;
#168498=CARTESIAN_POINT ( 'NONE',  ( 19.03943276465977164, -0.05219959533909143690, 63.74890960531435979 ) ) ;
#168499=CARTESIAN_POINT ( 'NONE',  ( -16.53943276465976808, 0.05219959533911058130, 101.2489096053143669 ) ) ;
#168501=CARTESIAN_POINT ( 'NONE',  ( -0.05219959533936034679, 19.03943276465977164, 62.50109039468566863 ) ) ;
#168502=CARTESIAN_POINT ( 'NONE',  ( -5.823673210054116645, -21.52544592524344225, 67.29057627198103830 ) ) ;
#168503=CARTESIAN_POINT ( 'NONE',  ( 13.89961937509957401, 13.97604488694547697, 21.87609039468566152 ) ) ;
#168504=CARTESIAN_POINT ( 'NONE',  ( 0.05219959533909260263, 19.03943276465977164, 109.9989096053143669 ) ) ;
#168505=CARTESIAN_POINT ( 'NONE',  ( -21.52544592524343514, 5.823673210054127303, 71.04057627198103830 ) ) ;
#168506=CARTESIAN_POINT ( 'NONE',  ( 0.05219959533909260263, 19.03943276465977164, 109.9989096053143669 ) ) ;
#168507=CARTESIAN_POINT ( 'NONE',  ( -9.564922557961040184, 16.46253265017147172, 102.9177570613523329 ) ) ;
#168508=CARTESIAN_POINT ( 'NONE',  ( -17.50000000000000355, 4.013004640162589176, 110.4460572099441009 ) ) ;
#168509=CARTESIAN_POINT ( 'NONE',  ( 16.55341960407618274, -4.379528057220086978, 21.04275706135234714 ) ) ;
#168510=CARTESIAN_POINT ( 'NONE',  ( -5.049401038298153566, 19.05341960407611168, 35.20724293864768839 ) ) ;
#168511=CARTESIAN_POINT ( 'NONE',  ( -5.153800228976328057, -19.02544592524343514, 92.29057627198099567 ) ) ;
#168512=CARTESIAN_POINT ( 'NONE',  ( -15.72974639402197994, 15.80617190586746368, 85.62390960531436690 ) ) ;
#168513=CARTESIAN_POINT ( 'NONE',  ( -14.34966873604972548, 8.224510206698743886, 58.33442372801901143 ) ) ;
#168514=CARTESIAN_POINT ( 'NONE',  ( -18.67979575497193778, 10.72451020669871902, 58.33442372801901143 ) ) ;
#168515=CARTESIAN_POINT ( 'NONE',  ( 16.46253265017146816, 9.564922557961045513, 101.6677570613523329 ) ) ;
#168516=CARTESIAN_POINT ( 'NONE',  ( -10.72451020669870658, -18.67979575497194134, 109.5844237280190328 ) ) ;
#168517=CARTESIAN_POINT ( 'NONE',  ( -8.314922557960811034, -14.29746914071050412, 22.08224293864769194 ) ) ;
#168518=CARTESIAN_POINT ( 'NONE',  ( 21.55341960407610458, 5.719274019375980345, 98.95724293864770971 ) ) ;
#168519=CARTESIAN_POINT ( 'NONE',  ( -14.34966873604960291, -8.224510206698953496, 41.66557627198103120 ) ) ;
#168520=CARTESIAN_POINT ( 'NONE',  ( -13.97604488694547697, 13.89961937509957934, 88.12609039468563310 ) ) ;
#168521=CARTESIAN_POINT ( 'NONE',  ( -21.53943276465977519, -0.05219959533937600094, 53.75109039468568994 ) ) ;
#168522=CARTESIAN_POINT ( 'NONE',  ( 19.05341960407617918, -5.049401038297876454, 46.04275706135233293 ) ) ;
#168523=CARTESIAN_POINT ( 'NONE',  ( -14.29746914071049879, 8.314922557960819915, 110.8322429386476955 ) ) ;
#168524=CARTESIAN_POINT ( 'NONE',  ( 18.62759615963271287, -10.81492255796078972, 28.33224293864769550 ) ) ;
#168525=CARTESIAN_POINT ( 'NONE',  ( 16.53943276465976808, -0.05219959533910856209, 38.74890960531435979 ) ) ;
#168526=CARTESIAN_POINT ( 'NONE',  ( 10.81492255796106328, -18.62759615963255655, 105.4177570613523613 ) ) ;
#168527=CARTESIAN_POINT ( 'NONE',  ( -14.34966873604972548, 8.224510206698743886, 68.33442372801900433 ) ) ;
#168528=CARTESIAN_POINT ( 'NONE',  ( 14.29746914071049879, -8.314922557960816363, 28.33224293864769550 ) ) ;
#168529=CARTESIAN_POINT ( 'NONE',  ( -0.05219959533937732626, 21.53943276465977519, 62.50109039468568284 ) ) ;
#168530=CARTESIAN_POINT ( 'NONE',  ( -21.55341960407619339, 5.719274019375674811, 53.54275706135234714 ) ) ;
#168531=CARTESIAN_POINT ( 'NONE',  ( 13.97604488694527802, 13.89961937509977652, 29.37390960531435979 ) ) ;
#168532=CARTESIAN_POINT ( 'NONE',  ( 0.05219959533937995610, -21.53943276465977519, 40.00109039468567573 ) ) ;
#168533=CARTESIAN_POINT ( 'NONE',  ( 12.06949235617757843, -12.14591786802309237, 113.1239096053143953 ) ) ;
#168534=CARTESIAN_POINT ( 'NONE',  ( -16.46253265017160317, 9.564922557960807481, 40.83224293864769550 ) ) ;
#168535=CARTESIAN_POINT ( 'NONE',  ( -4.483927247898539470, -16.52544592524342804, 82.29057627198103830 ) ) ;
#168536=CARTESIAN_POINT ( 'NONE',  ( -5.049401038298153566, 19.05341960407611168, 85.20724293864766707 ) ) ;
#168537=CARTESIAN_POINT ( 'NONE',  ( -12.14591786802309592, -12.06949235617757132, 31.87390960531435979 ) ) ;
#168538=CARTESIAN_POINT ( 'NONE',  ( 0.05219959533907565091, 21.53943276465977519, 54.99890960531435269 ) ) ;
#168539=CARTESIAN_POINT ( 'NONE',  ( 5.823673210054125526, 21.52544592524343514, 104.7905762719810241 ) ) ;
#168540=CARTESIAN_POINT ( 'NONE',  ( 13.97604488694527802, 13.89961937509977652, 99.37390960531436690 ) ) ;
#168541=CARTESIAN_POINT ( 'NONE',  ( 5.049401038298161559, -19.05341960407611168, 62.70724293864769550 ) ) ;
#168542=CARTESIAN_POINT ( 'NONE',  ( -5.049401038297874678, -19.05341960407617918, 99.79275706135234714 ) ) ;
#168543=CARTESIAN_POINT ( 'NONE',  ( 15.72974639402199770, -15.80617190586745480, 63.12390960531435979 ) ) ;
#168544=CARTESIAN_POINT ( 'NONE',  ( -15.80617190586768217, 15.72974639402176855, 83.12609039468568994 ) ) ;
#168545=CARTESIAN_POINT ( 'NONE',  ( -9.564922557960796823, -16.46253265017161027, 72.08224293864770971 ) ) ;
#168546=CARTESIAN_POINT ( 'NONE',  ( -9.564922557960796823, -16.46253265017161027, 92.08224293864769550 ) ) ;
#168547=CARTESIAN_POINT ( 'NONE',  ( -14.34966873604972548, 8.224510206698743886, 73.33442372801901854 ) ) ;
#168548=CARTESIAN_POINT ( 'NONE',  ( -5.719274019375665041, -21.55341960407619695, 59.79275706135234714 ) ) ;
#168549=CARTESIAN_POINT ( 'NONE',  ( 21.52544592524334988, 5.823673210054432836, 91.45942372801901854 ) ) ;
#168550=CARTESIAN_POINT ( 'NONE',  ( 21.52544592524344225, -5.823673210054117533, 108.5405762719810241 ) ) ;
#168551=CARTESIAN_POINT ( 'NONE',  ( -8.224510206698735004, -14.34966873604973081, 79.58442372801903275 ) ) ;
#168552=CARTESIAN_POINT ( 'NONE',  ( -15.72974639402197994, 15.80617190586746368, 70.62390960531436690 ) ) ;
#168553=CARTESIAN_POINT ( 'NONE',  ( -9.564922557961040184, 16.46253265017147172, 47.91775706135233293 ) ) ;
#168554=CARTESIAN_POINT ( 'NONE',  ( -10.72451020669898014, 18.67979575497178502, 40.41557627198103120 ) ) ;
#168555=CARTESIAN_POINT ( 'NONE',  ( -0.05219959533909027116, -19.03943276465977164, 87.49890960531436690 ) ) ;
#168556=CARTESIAN_POINT ( 'NONE',  ( 16.53943276465976808, -0.05219959533910856209, 23.74890960531435269 ) ) ;
#168557=CARTESIAN_POINT ( 'NONE',  ( -17.31728774477274158, 6.344390552232390235, 65.81906651689320142 ) ) ;
#168558=CARTESIAN_POINT ( 'NONE',  ( -0.05219959533907301413, -21.53943276465977519, 27.49890960531435269 ) ) ;
#168559=CARTESIAN_POINT ( 'NONE',  ( -18.56399227203343472, -5.499999999999927169, 78.97830131249902763 ) ) ;
#168560=CARTESIAN_POINT ( 'NONE',  ( 13.97604488694548053, -13.89961937509957401, 100.6260903946856615 ) ) ;
#168561=CARTESIAN_POINT ( 'NONE',  ( 18.62759615963271287, -10.81492255796078972, 68.33224293864769550 ) ) ;
#168562=CARTESIAN_POINT ( 'NONE',  ( -16.52544592524342804, 4.483927247898546575, 51.04057627198103120 ) ) ;
#168563=CARTESIAN_POINT ( 'NONE',  ( 9.474510206698729675, 16.51473224551082808, 107.0844237280190043 ) ) ;
#168564=CARTESIAN_POINT ( 'NONE',  ( 0.05219959533909260263, 19.03943276465977164, 39.99890960531436690 ) ) ;
#168565=CARTESIAN_POINT ( 'NONE',  ( 15.72974639402199770, -15.80617190586745480, 103.1239096053143811 ) ) ;
#168566=CARTESIAN_POINT ( 'NONE',  ( 9.474510206698729675, 16.51473224551082808, 72.08442372801900433 ) ) ;
#168567=CARTESIAN_POINT ( 'NONE',  ( -5.049401038298153566, 19.05341960407611168, 80.20724293864769550 ) ) ;
#168568=CARTESIAN_POINT ( 'NONE',  ( 14.34966873604960469, 8.224510206698951720, 94.16557627198103830 ) ) ;
#168569=CARTESIAN_POINT ( 'NONE',  ( 0.05219959533909260263, 19.03943276465977164, 59.99890960531436690 ) ) ;
#168570=CARTESIAN_POINT ( 'NONE',  ( 12.06949235617757843, -12.14591786802309237, 73.12390960531436690 ) ) ;
#168571=CARTESIAN_POINT ( 'NONE',  ( 19.03943276465977164, -0.05219959533909143690, 33.74890960531435979 ) ) ;
#168573=CARTESIAN_POINT ( 'NONE',  ( 4.483927247898545687, 16.52544592524342804, 39.79057627198103830 ) ) ;
#168574=CARTESIAN_POINT ( 'NONE',  ( -9.474510206698964154, 16.51473224551069663, 90.41557627198103830 ) ) ;
#168576=CARTESIAN_POINT ( 'NONE',  ( -19.03943276465977164, -0.05219959533935918106, 48.75109039468566863 ) ) ;
#168577=CARTESIAN_POINT ( 'NONE',  ( 16.55341960407618274, -4.379528057220086978, 66.04275706135236135 ) ) ;
#168578=CARTESIAN_POINT ( 'NONE',  ( 0.05219959533907565091, 21.53943276465977519, 69.99890960531435269 ) ) ;
#168579=CARTESIAN_POINT ( 'NONE',  ( 9.474510206698729675, 16.51473224551082808, 32.08442372801900433 ) ) ;
#168580=CARTESIAN_POINT ( 'NONE',  ( -13.89961937509977652, 13.97604488694528158, 85.62390960531433848 ) ) ;
#168582=CARTESIAN_POINT ( 'NONE',  ( -15.80617190586745835, -15.72974639402198527, 31.87390960531435979 ) ) ;
#168583=CARTESIAN_POINT ( 'NONE',  ( -16.46253265017160317, 9.564922557960807481, 65.83224293864769550 ) ) ;
#168584=CARTESIAN_POINT ( 'NONE',  ( -0.05219959533937732626, 21.53943276465977519, 47.50109039468568994 ) ) ;
#168585=CARTESIAN_POINT ( 'NONE',  ( -16.52544592524342804, 4.483927247898546575, 116.0405762719810383 ) ) ;
#168586=CARTESIAN_POINT ( 'NONE',  ( 5.823673210054125526, 21.52544592524343514, 109.7905762719810383 ) ) ;
#168587=CARTESIAN_POINT ( 'NONE',  ( 16.51473224551069308, 9.474510206698969483, 89.16557627198103830 ) ) ;
#168589=CARTESIAN_POINT ( 'NONE',  ( 15.80617190586769283, -15.72974639402175789, 45.62609039468567573 ) ) ;
#168591=CARTESIAN_POINT ( 'NONE',  ( -5.049401038298153566, 19.05341960407611168, 95.20724293864770971 ) ) ;
#168592=CARTESIAN_POINT ( 'NONE',  ( 18.22780087662121673, 5.500000000000056843, 88.98459894673892734 ) ) ;
#168593=CARTESIAN_POINT ( 'NONE',  ( -15.72974639402197994, 15.80617190586746368, 110.6239096053143669 ) ) ;
#168594=CARTESIAN_POINT ( 'NONE',  ( 16.46253265017160672, -9.564922557960803928, 43.33224293864769550 ) ) ;
#168595=CARTESIAN_POINT ( 'NONE',  ( 4.483927247898790824, -16.52544592524335698, 25.20942372801901854 ) ) ;
#168597=CARTESIAN_POINT ( 'NONE',  ( -5.153800228976328057, -19.02544592524343514, 32.29057627198102409 ) ) ;
#168598=CARTESIAN_POINT ( 'NONE',  ( -10.72451020669870658, -18.67979575497194134, 99.58442372801900433 ) ) ;
#168599=CARTESIAN_POINT ( 'NONE',  ( -16.51473224551069308, -9.474510206698971260, 76.66557627198103830 ) ) ;
#168600=CARTESIAN_POINT ( 'NONE',  ( 10.81492255796106328, -18.62759615963255655, 45.41775706135234003 ) ) ;
#168602=CARTESIAN_POINT ( 'NONE',  ( 16.46253265017160672, -9.564922557960803928, 103.3322429386476955 ) ) ;
#168603=CARTESIAN_POINT ( 'NONE',  ( 18.56101223717332616, 5.499999999999942268, 63.94978406935678095 ) ) ;
#168604=CARTESIAN_POINT ( 'NONE',  ( -4.379528057220086978, -16.55341960407618274, 39.79275706135235424 ) ) ;
#168605=CARTESIAN_POINT ( 'NONE',  ( 0.05219959533934541429, -16.53943276465976808, 70.00109039468568994 ) ) ;
#168606=CARTESIAN_POINT ( 'NONE',  ( 10.72451020669871369, 18.67979575497193778, 57.08442372801901854 ) ) ;
#168607=CARTESIAN_POINT ( 'NONE',  ( -15.72974639402176322, -15.80617190586768395, 94.37609039468568994 ) ) ;
#168609=CARTESIAN_POINT ( 'NONE',  ( 5.153800228976615827, -19.02544592524334988, 105.2094237280190185 ) ) ;
#168610=CARTESIAN_POINT ( 'NONE',  ( 9.474510206698971260, -16.51473224551069308, 72.91557627198102409 ) ) ;
#168611=CARTESIAN_POINT ( 'NONE',  ( -13.97604488694527625, -13.89961937509977652, 96.87390960531433848 ) ) ;
#168612=CARTESIAN_POINT ( 'NONE',  ( 14.29746914071049879, -8.314922557960816363, 108.3322429386477097 ) ) ;
#168613=CARTESIAN_POINT ( 'NONE',  ( -21.53943276465977519, 0.05219959533907696930, 31.24890960531435979 ) ) ;
#168614=CARTESIAN_POINT ( 'NONE',  ( -0.05219959533934338120, 16.53943276465976808, 97.50109039468567573 ) ) ;
#168615=CARTESIAN_POINT ( 'NONE',  ( -12.14591786802309592, -12.06949235617757132, 76.87390960531439532 ) ) ;
#168616=CARTESIAN_POINT ( 'NONE',  ( -19.05341960407611168, -5.049401038298163336, 56.45724293864768129 ) ) ;
#168617=CARTESIAN_POINT ( 'NONE',  ( -10.81492255796105439, 18.62759615963255655, 92.91775706135236135 ) ) ;
#168619=CARTESIAN_POINT ( 'NONE',  ( -0.05219959533936034679, 19.03943276465977164, 102.5010903946856757 ) ) ;
#168620=CARTESIAN_POINT ( 'NONE',  ( -16.55341960407611168, -4.379528057220339221, 76.45724293864769550 ) ) ;
#168621=CARTESIAN_POINT ( 'NONE',  ( 18.67979575497194134, -10.72451020669871369, 30.83442372801902209 ) ) ;
#168622=CARTESIAN_POINT ( 'NONE',  ( 18.62759615963271287, -10.81492255796078972, 58.33224293864768839 ) ) ;
#168623=CARTESIAN_POINT ( 'NONE',  ( -19.03943276465977164, -0.05219959533935918106, 33.75109039468566863 ) ) ;
#168625=CARTESIAN_POINT ( 'NONE',  ( -16.46253265017160317, 9.564922557960807481, 85.83224293864769550 ) ) ;
#168626=CARTESIAN_POINT ( 'NONE',  ( 14.29746914071049879, -8.314922557960816363, 53.33224293864769550 ) ) ;
#168627=CARTESIAN_POINT ( 'NONE',  ( -12.06949235617756955, 12.14591786802309770, 35.62390960531437401 ) ) ;
#168628=CARTESIAN_POINT ( 'NONE',  ( -4.379528057220086978, -16.55341960407618274, 94.79275706135234714 ) ) ;
#168629=CARTESIAN_POINT ( 'NONE',  ( -5.153800228976607833, 19.02544592524334988, 47.70942372801900433 ) ) ;
#168630=CARTESIAN_POINT ( 'NONE',  ( -0.05219959533936034679, 19.03943276465977164, 77.50109039468566152 ) ) ;
#168631=CARTESIAN_POINT ( 'NONE',  ( 16.51473224551069308, 9.474510206698969483, 99.16557627198102409 ) ) ;
#168632=CARTESIAN_POINT ( 'NONE',  ( 4.483927247898545687, 16.52544592524342804, 69.79057627198102409 ) ) ;
#168633=CARTESIAN_POINT ( 'NONE',  ( 19.02544592524334988, 5.153800228976608722, 46.45942372801899012 ) ) ;
#168634=CARTESIAN_POINT ( 'NONE',  ( -0.05219959533909027116, -19.03943276465977164, 37.49890960531436690 ) ) ;
#168635=CARTESIAN_POINT ( 'NONE',  ( 10.81492255796078972, 18.62759615963270932, 39.58224293864769550 ) ) ;
#168636=CARTESIAN_POINT ( 'NONE',  ( 15.72974639402199770, -15.80617190586745480, 63.12390960531435979 ) ) ;
#168637=CARTESIAN_POINT ( 'NONE',  ( -12.14591786802309592, -12.06949235617757132, 101.8739096053143811 ) ) ;
#168638=CARTESIAN_POINT ( 'NONE',  ( -14.34966873604972548, 8.224510206698743886, 53.33442372801901854 ) ) ;
#168640=CARTESIAN_POINT ( 'NONE',  ( 5.719274019375673035, 21.55341960407619339, 37.29275706135235424 ) ) ;
#168641=CARTESIAN_POINT ( 'NONE',  ( 16.52544592524342804, -4.483927247898539470, 88.54057627198103830 ) ) ;
#168644=CARTESIAN_POINT ( 'NONE',  ( -5.719274019375978568, 21.55341960407610458, 40.20724293864769550 ) ) ;
#168647=CARTESIAN_POINT ( 'NONE',  ( -14.29746914071037622, -8.314922557961029526, 49.16775706135234003 ) ) ;
#168648=CARTESIAN_POINT ( 'NONE',  ( 14.34966873604960469, 8.224510206698951720, 34.16557627198102409 ) ) ;
#168649=CARTESIAN_POINT ( 'NONE',  ( -15.72974639402197994, 15.80617190586746368, 65.62390960531436690 ) ) ;
#168650=CARTESIAN_POINT ( 'NONE',  ( 19.03943276465977164, 0.05219959533936151252, 91.25109039468566152 ) ) ;
#168651=CARTESIAN_POINT ( 'NONE',  ( -21.52544592524343514, 5.823673210054127303, 61.04057627198103120 ) ) ;
#168653=CARTESIAN_POINT ( 'NONE',  ( -19.05341960407611168, -5.049401038298163336, 36.45724293864766707 ) ) ;
#168654=CARTESIAN_POINT ( 'NONE',  ( -13.97604488694527625, -13.89961937509977652, 96.87390960531433848 ) ) ;
#168655=CARTESIAN_POINT ( 'NONE',  ( -9.474510206698964154, 16.51473224551069663, 40.41557627198103120 ) ) ;
#168656=CARTESIAN_POINT ( 'NONE',  ( 12.06949235617757843, -12.14591786802309237, 108.1239096053143811 ) ) ;
#168658=CARTESIAN_POINT ( 'NONE',  ( -9.564922557960796823, -16.46253265017161027, 112.0822429386476955 ) ) ;
#168660=CARTESIAN_POINT ( 'NONE',  ( 16.52544592524335698, 4.483927247898782831, 66.45942372801903275 ) ) ;
#168661=CARTESIAN_POINT ( 'NONE',  ( -5.823673210054116645, -21.52544592524344225, 97.29057627198105251 ) ) ;
#168662=CARTESIAN_POINT ( 'NONE',  ( 13.89961937509977652, -13.97604488694527269, 58.12390960531436690 ) ) ;
#168663=CARTESIAN_POINT ( 'NONE',  ( -15.72974639402176322, -15.80617190586768395, 24.37609039468567573 ) ) ;
#168664=CARTESIAN_POINT ( 'NONE',  ( 16.46253265017160672, -9.564922557960803928, 78.33224293864769550 ) ) ;
#168665=CARTESIAN_POINT ( 'NONE',  ( -19.02544592524342804, 5.153800228976336051, 116.0405762719810383 ) ) ;
#168667=CARTESIAN_POINT ( 'NONE',  ( -15.72974639402197994, 15.80617190586746368, 110.6239096053143669 ) ) ;
#168668=CARTESIAN_POINT ( 'NONE',  ( 16.53943276465976808, -0.05219959533910856209, 113.7489096053143527 ) ) ;
#168669=CARTESIAN_POINT ( 'NONE',  ( -0.05219959533909027116, -19.03943276465977164, 102.4989096053143669 ) ) ;
#168670=CARTESIAN_POINT ( 'NONE',  ( 13.89961937509957401, 13.97604488694547697, 91.87609039468567573 ) ) ;
#168671=CARTESIAN_POINT ( 'NONE',  ( -19.05341960407617563, 5.049401038297882671, 28.54275706135232937 ) ) ;
#168672=CARTESIAN_POINT ( 'NONE',  ( 10.72451020669898902, -18.67979575497178502, 102.9155762719810383 ) ) ;
#168673=CARTESIAN_POINT ( 'NONE',  ( 19.05341960407617918, -5.049401038297876454, 31.04275706135232227 ) ) ;
#168674=CARTESIAN_POINT ( 'NONE',  ( 13.97604488694548053, -13.89961937509957401, 35.62609039468567573 ) ) ;
#168675=CARTESIAN_POINT ( 'NONE',  ( -8.314922557961024197, 14.29746914071037800, 77.91775706135231871 ) ) ;
#168676=CARTESIAN_POINT ( 'NONE',  ( 13.89961937509977652, -13.97604488694527269, 103.1239096053143527 ) ) ;
#168677=CARTESIAN_POINT ( 'NONE',  ( -19.05341960407611168, -5.049401038298163336, 61.45724293864769550 ) ) ;
#168678=CARTESIAN_POINT ( 'NONE',  ( -5.719274019375665041, -21.55341960407619695, 69.79275706135234714 ) ) ;
#168679=CARTESIAN_POINT ( 'NONE',  ( 18.67979575497194134, -10.72451020669871369, 85.83442372801901854 ) ) ;
#168681=CARTESIAN_POINT ( 'NONE',  ( -16.51473224551069308, -9.474510206698971260, 76.66557627198103830 ) ) ;
#168682=CARTESIAN_POINT ( 'NONE',  ( -18.67979575497193778, 10.72451020669871902, 53.33442372801901854 ) ) ;
#168683=CARTESIAN_POINT ( 'NONE',  ( 16.46253265017146816, 9.564922557961045513, 96.66775706135233293 ) ) ;
#168684=CARTESIAN_POINT ( 'NONE',  ( -19.05341960407611168, -5.049401038298163336, 56.45724293864768129 ) ) ;
#168685=CARTESIAN_POINT ( 'NONE',  ( 19.02544592524343514, -5.153800228976328945, 93.54057627198102409 ) ) ;
#168686=CARTESIAN_POINT ( 'NONE',  ( 16.46253265017160672, -9.564922557960803928, 83.33224293864768129 ) ) ;
#168687=CARTESIAN_POINT ( 'NONE',  ( 17.50000000000000000, -5.500000000000000888, 23.29690382534171889 ) ) ;
#168688=CARTESIAN_POINT ( 'NONE',  ( -16.46253265017160317, 9.564922557960807481, 55.83224293864769550 ) ) ;
#168689=CARTESIAN_POINT ( 'NONE',  ( 21.55341960407610458, 5.719274019375980345, 103.9572429386476813 ) ) ;
#168690=CARTESIAN_POINT ( 'NONE',  ( -14.34966873604972548, 8.224510206698743886, 88.33442372801901854 ) ) ;
#168692=CARTESIAN_POINT ( 'NONE',  ( 19.02544592524334988, 5.153800228976608722, 46.45942372801899012 ) ) ;
#168693=CARTESIAN_POINT ( 'NONE',  ( -0.05219959533909027116, -19.03943276465977164, 82.49890960531436690 ) ) ;
#168694=CARTESIAN_POINT ( 'NONE',  ( 12.14591786802309770, 12.06949235617756955, 64.37390960531435269 ) ) ;
#168695=CARTESIAN_POINT ( 'NONE',  ( 16.52544592524342804, -4.483927247898539470, 98.54057627198105251 ) ) ;
#168696=CARTESIAN_POINT ( 'NONE',  ( -15.72974639402197994, 15.80617190586746368, 25.62390960531435624 ) ) ;
#168697=CARTESIAN_POINT ( 'NONE',  ( -16.51473224551069308, -9.474510206698971260, 111.6655762719810383 ) ) ;
#168698=CARTESIAN_POINT ( 'NONE',  ( 19.05341960407611168, 5.049401038298154454, 113.9572429386477097 ) ) ;
#168699=CARTESIAN_POINT ( 'NONE',  ( -5.049401038297874678, -19.05341960407617918, 34.79275706135233293 ) ) ;
#168700=CARTESIAN_POINT ( 'NONE',  ( 16.52544592524335698, 4.483927247898782831, 91.45942372801901854 ) ) ;
#168701=CARTESIAN_POINT ( 'NONE',  ( 16.51473224551069308, 9.474510206698969483, 79.16557627198103830 ) ) ;
#168702=CARTESIAN_POINT ( 'NONE',  ( 21.52544592524334988, 5.823673210054432836, 46.45942372801901854 ) ) ;
#168703=CARTESIAN_POINT ( 'NONE',  ( -21.55341960407610458, -5.719274019375992779, 31.45724293864769550 ) ) ;
#168704=CARTESIAN_POINT ( 'NONE',  ( 5.823673210054444382, -21.52544592524334988, 20.20942372801900788 ) ) ;
#168705=CARTESIAN_POINT ( 'NONE',  ( -18.67979575497178146, -10.72451020669898902, 71.66557627198100988 ) ) ;
#168706=CARTESIAN_POINT ( 'NONE',  ( -4.379528057220328563, 16.55341960407611168, 95.20724293864769550 ) ) ;
#168707=CARTESIAN_POINT ( 'NONE',  ( -16.51473224551082808, 9.474510206698731452, 38.33442372801899722 ) ) ;
#168708=CARTESIAN_POINT ( 'NONE',  ( 9.474510206698971260, -16.51473224551069308, 27.91557627198103120 ) ) ;
#168709=CARTESIAN_POINT ( 'NONE',  ( -19.03943276465977164, 0.05219959533909376836, 86.24890960531436690 ) ) ;
#168710=CARTESIAN_POINT ( 'NONE',  ( 13.97604488694527802, 13.89961937509977652, 79.37390960531435269 ) ) ;
#168712=CARTESIAN_POINT ( 'NONE',  ( -12.14591786802309592, -12.06949235617757132, 101.8739096053143811 ) ) ;
#168714=CARTESIAN_POINT ( 'NONE',  ( 16.53943276465976808, -0.05219959533910856209, 28.74890960531435624 ) ) ;
#168715=CARTESIAN_POINT ( 'NONE',  ( -16.53943276465976808, -0.05219959533934237506, 33.75109039468568284 ) ) ;
#168716=CARTESIAN_POINT ( 'NONE',  ( 10.81492255796106328, -18.62759615963255655, 95.41775706135234714 ) ) ;
#168717=CARTESIAN_POINT ( 'NONE',  ( -0.05219959533909027116, -19.03943276465977164, 97.49890960531436690 ) ) ;
#168718=CARTESIAN_POINT ( 'NONE',  ( -21.53943276465977519, 0.05219959533907696930, 111.2489096053143669 ) ) ;
#168719=CARTESIAN_POINT ( 'NONE',  ( -19.02544592524342804, 5.153800228976336051, 41.04057627198103120 ) ) ;
#168720=CARTESIAN_POINT ( 'NONE',  ( 4.379528057220092307, 16.55341960407617563, 42.29275706135235424 ) ) ;
#168722=CARTESIAN_POINT ( 'NONE',  ( -8.224510206698735004, -14.34966873604973081, 19.58442372801901143 ) ) ;
#168723=CARTESIAN_POINT ( 'NONE',  ( 4.379528057220339221, -16.55341960407611168, 92.70724293864770971 ) ) ;
#168724=CARTESIAN_POINT ( 'NONE',  ( -21.55341960407610458, -5.719274019375992779, 101.4572429386476955 ) ) ;
#168725=CARTESIAN_POINT ( 'NONE',  ( 13.89961937509957401, 13.97604488694547697, 61.87609039468566863 ) ) ;
#168726=CARTESIAN_POINT ( 'NONE',  ( -18.67979575497178146, -10.72451020669898902, 111.6655762719810525 ) ) ;
#168727=CARTESIAN_POINT ( 'NONE',  ( -16.46253265017160317, 9.564922557960807481, 90.83224293864769550 ) ) ;
#168729=CARTESIAN_POINT ( 'NONE',  ( -0.05219959533909027116, -19.03943276465977164, 87.49890960531436690 ) ) ;
#168730=CARTESIAN_POINT ( 'NONE',  ( -15.80617190586768217, 15.72974639402176855, 28.12609039468568284 ) ) ;
#168731=CARTESIAN_POINT ( 'NONE',  ( 12.14591786802309770, 12.06949235617756955, 74.37390960531436690 ) ) ;
#168732=CARTESIAN_POINT ( 'NONE',  ( -16.51473224551069308, -9.474510206698971260, 81.66557627198103830 ) ) ;
#168733=CARTESIAN_POINT ( 'NONE',  ( 16.53943276465976808, 0.05219959533934440121, 56.25109039468568284 ) ) ;
#168734=CARTESIAN_POINT ( 'NONE',  ( 5.049401038297881783, 19.05341960407617563, 57.29275706135231871 ) ) ;
#168735=CARTESIAN_POINT ( 'NONE',  ( 18.62759615963255655, 10.81492255796105972, 71.66775706135234714 ) ) ;
#168736=CARTESIAN_POINT ( 'NONE',  ( 4.379528057220092307, 16.55341960407617563, 32.29275706135235424 ) ) ;
#168737=CARTESIAN_POINT ( 'NONE',  ( -5.153800228976328057, -19.02544592524343514, 72.29057627198102409 ) ) ;
#168738=CARTESIAN_POINT ( 'NONE',  ( -5.153800228976607833, 19.02544592524334988, 92.70942372801901854 ) ) ;
#168739=CARTESIAN_POINT ( 'NONE',  ( -4.483927247898782831, 16.52544592524335698, 57.70942372801901143 ) ) ;
#168740=CARTESIAN_POINT ( 'NONE',  ( 21.55341960407619695, -5.719274019375665929, 96.04275706135236135 ) ) ;
#168741=CARTESIAN_POINT ( 'NONE',  ( -13.89961937509957401, -13.97604488694547875, 79.37609039468567573 ) ) ;
#168742=CARTESIAN_POINT ( 'NONE',  ( 0.05219959533909260263, 19.03943276465977164, 44.99890960531435979 ) ) ;
#168743=CARTESIAN_POINT ( 'NONE',  ( 21.55341960407610458, 5.719274019375980345, 73.95724293864769550 ) ) ;
#168744=CARTESIAN_POINT ( 'NONE',  ( -12.06949235617756955, 12.14591786802309770, 75.62390960531439532 ) ) ;
#168745=CARTESIAN_POINT ( 'NONE',  ( 0.05219959533936267826, -19.03943276465977164, 80.00109039468567573 ) ) ;
#168747=CARTESIAN_POINT ( 'NONE',  ( -19.05341960407617563, 5.049401038297882671, 48.54275706135233293 ) ) ;
#168749=CARTESIAN_POINT ( 'NONE',  ( 8.314922557961029526, -14.29746914071037800, 110.4177570613523756 ) ) ;
#168750=CARTESIAN_POINT ( 'NONE',  ( -4.483927247898539470, -16.52544592524342804, 67.29057627198103830 ) ) ;
#168751=CARTESIAN_POINT ( 'NONE',  ( 5.823673210054444382, -21.52544592524334988, 105.2094237280190328 ) ) ;
#168753=CARTESIAN_POINT ( 'NONE',  ( -18.62759615963270932, 10.81492255796079327, 105.8322429386476955 ) ) ;
#168754=CARTESIAN_POINT ( 'NONE',  ( -9.474510206698964154, 16.51473224551069663, 60.41557627198102409 ) ) ;
#168755=CARTESIAN_POINT ( 'NONE',  ( -10.72451020669870658, -18.67979575497194134, 89.58442372801901854 ) ) ;
#168756=CARTESIAN_POINT ( 'NONE',  ( 9.564922557960805705, 16.46253265017160317, 64.58224293864769550 ) ) ;
#168757=CARTESIAN_POINT ( 'NONE',  ( 5.153800228976335163, 19.02544592524342804, 24.79057627198102765 ) ) ;
#168758=CARTESIAN_POINT ( 'NONE',  ( -21.55341960407610458, -5.719274019375992779, 31.45724293864769550 ) ) ;
#168759=CARTESIAN_POINT ( 'NONE',  ( -12.14591786802309592, -12.06949235617757132, 61.87390960531436690 ) ) ;
#168760=CARTESIAN_POINT ( 'NONE',  ( 19.03943276465977164, -0.05219959533909143690, 48.74890960531435979 ) ) ;
#168761=CARTESIAN_POINT ( 'NONE',  ( -16.53943276465976808, 0.05219959533911058130, 81.24890960531436690 ) ) ;
#168762=CARTESIAN_POINT ( 'NONE',  ( 15.80617190586746368, 15.72974639402197994, 109.3739096053143811 ) ) ;
#168763=CARTESIAN_POINT ( 'NONE',  ( -18.67979575497193778, 10.72451020669871902, 48.33442372801902565 ) ) ;
#168764=CARTESIAN_POINT ( 'NONE',  ( 9.564922557960805705, 16.46253265017160317, 34.58224293864770260 ) ) ;
#168765=CARTESIAN_POINT ( 'NONE',  ( 14.29746914071037800, 8.314922557961029526, 46.66775706135234714 ) ) ;
#168766=CARTESIAN_POINT ( 'NONE',  ( 21.52544592524344225, -5.823673210054117533, 93.54057627198103830 ) ) ;
#168767=CARTESIAN_POINT ( 'NONE',  ( 5.049401038297881783, 19.05341960407617563, 32.29275706135233293 ) ) ;
#168768=CARTESIAN_POINT ( 'NONE',  ( -0.05219959533909027116, -19.03943276465977164, 52.49890960531436690 ) ) ;
#168769=CARTESIAN_POINT ( 'NONE',  ( 19.03943276465977164, -0.05219959533909143690, 103.7489096053143669 ) ) ;
#168770=CARTESIAN_POINT ( 'NONE',  ( 10.81492255796106328, -18.62759615963255655, 60.41775706135235424 ) ) ;
#168771=VECTOR ( 'NONE', #197569, 1000.000000000000000 ) ;
#168772=CARTESIAN_POINT ( 'NONE',  ( 15.72974639402199770, -15.80617190586745480, 43.12390960531435269 ) ) ;
#168773=CARTESIAN_POINT ( 'NONE',  ( 8.314922557960818139, 14.29746914071049879, 24.58224293864768839 ) ) ;
#168774=CARTESIAN_POINT ( 'NONE',  ( 10.72451020669871369, 18.67979575497193778, 57.08442372801901854 ) ) ;
#168775=CARTESIAN_POINT ( 'NONE',  ( 10.81492255796106328, -18.62759615963255655, 100.4177570613523471 ) ) ;
#168776=CARTESIAN_POINT ( 'NONE',  ( -9.564922557961040184, 16.46253265017147172, 37.91775706135233293 ) ) ;
#168777=CARTESIAN_POINT ( 'NONE',  ( -8.314922557961024197, 14.29746914071037800, 97.91775706135236135 ) ) ;
#168778=CARTESIAN_POINT ( 'NONE',  ( 15.80617190586769283, -15.72974639402175789, 60.62609039468567573 ) ) ;
#168779=CARTESIAN_POINT ( 'NONE',  ( -0.05219959533909027116, -19.03943276465977164, 52.49890960531436690 ) ) ;
#168780=CARTESIAN_POINT ( 'NONE',  ( -9.564922557961040184, 16.46253265017147172, 22.91775706135233648 ) ) ;
#168781=CARTESIAN_POINT ( 'NONE',  ( 21.52544592524344225, -5.823673210054117533, 28.54057627198103120 ) ) ;
#168783=CARTESIAN_POINT ( 'NONE',  ( 5.719274019375991003, -21.55341960407610458, 112.7072429386476955 ) ) ;
#168784=CARTESIAN_POINT ( 'NONE',  ( -21.53943276465977519, 0.05219959533907696930, 81.24890960531436690 ) ) ;
#168785=CARTESIAN_POINT ( 'NONE',  ( 14.34966873604972726, -8.224510206698740333, 45.83442372801901854 ) ) ;
#168787=CARTESIAN_POINT ( 'NONE',  ( 21.52544592524344225, -5.823673210054117533, 78.54057627198103830 ) ) ;
#168788=CARTESIAN_POINT ( 'NONE',  ( 12.14591786802327356, -12.06949235617739191, 70.62609039468567573 ) ) ;
#168789=CARTESIAN_POINT ( 'NONE',  ( -12.06949235617756955, 12.14591786802309770, 70.62390960531436690 ) ) ;
#168791=CARTESIAN_POINT ( 'NONE',  ( 19.02544592524334988, 5.153800228976608722, 101.4594237280189759 ) ) ;
#168792=CARTESIAN_POINT ( 'NONE',  ( -0.05219959533907301413, -21.53943276465977519, 37.49890960531436690 ) ) ;
#168793=LINE ( 'NONE', #11172, #5458 ) ;
#168794=CARTESIAN_POINT ( 'NONE',  ( 0.05219959533934541429, -16.53943276465976808, 45.00109039468568284 ) ) ;
#168795=CARTESIAN_POINT ( 'NONE',  ( -21.53943276465977519, 0.05219959533907696930, 111.2489096053143669 ) ) ;
#168796=CARTESIAN_POINT ( 'NONE',  ( -0.05219959533907301413, -21.53943276465977519, 37.49890960531436690 ) ) ;
#168797=CARTESIAN_POINT ( 'NONE',  ( 12.14591786802327356, -12.06949235617739191, 70.62609039468567573 ) ) ;
#168798=CARTESIAN_POINT ( 'NONE',  ( 5.049401038298161559, -19.05341960407611168, 82.70724293864770971 ) ) ;
#168799=CARTESIAN_POINT ( 'NONE',  ( 10.72451020669871369, 18.67979575497193778, 47.08442372801901854 ) ) ;
#168800=CARTESIAN_POINT ( 'NONE',  ( 14.29746914071037800, 8.314922557961029526, 21.66775706135235069 ) ) ;
#168801=CARTESIAN_POINT ( 'NONE',  ( 18.67979575497178502, 10.72451020669898547, 29.16557627198103120 ) ) ;
#168803=CARTESIAN_POINT ( 'NONE',  ( -13.97604488694547697, 13.89961937509957934, 28.12609039468565797 ) ) ;
#168804=CARTESIAN_POINT ( 'NONE',  ( -16.53943276465976808, -0.05219959533934237506, 58.75109039468568994 ) ) ;
#168805=CARTESIAN_POINT ( 'NONE',  ( -19.05341960407611168, -5.049401038298163336, 106.4572429386476955 ) ) ;
#168806=CARTESIAN_POINT ( 'NONE',  ( 15.80617190586746368, 15.72974639402197994, 99.37390960531436690 ) ) ;
#168807=CARTESIAN_POINT ( 'NONE',  ( -16.46253265017160317, 9.564922557960807481, 70.83224293864770971 ) ) ;
#168808=CARTESIAN_POINT ( 'NONE',  ( -17.05116617787826883, 6.768360034955676952, 23.65675553259199759 ) ) ;
#168809=CARTESIAN_POINT ( 'NONE',  ( 4.483927247898545687, 16.52544592524342804, 84.79057627198102409 ) ) ;
#168810=CARTESIAN_POINT ( 'NONE',  ( 10.81492255796078972, 18.62759615963270932, 34.58224293864770260 ) ) ;
#168811=CARTESIAN_POINT ( 'NONE',  ( 9.564922557960805705, 16.46253265017160317, 24.58224293864769194 ) ) ;
#168812=CARTESIAN_POINT ( 'NONE',  ( -0.05219959533934338120, 16.53943276465976808, 67.50109039468568994 ) ) ;
#168813=CARTESIAN_POINT ( 'NONE',  ( 18.67979575497178502, 10.72451020669898547, 114.1655762719810383 ) ) ;
#168814=CARTESIAN_POINT ( 'NONE',  ( -19.05341960407617563, 5.049401038297882671, 78.54275706135233293 ) ) ;
#168815=CARTESIAN_POINT ( 'NONE',  ( 19.03943276465977164, -0.05219959533909143690, 23.74890960531435269 ) ) ;
#168816=CARTESIAN_POINT ( 'NONE',  ( 10.81492255796078972, 18.62759615963270932, 74.58224293864768129 ) ) ;
#168817=CARTESIAN_POINT ( 'NONE',  ( 19.05341960407611168, 5.049401038298154454, 103.9572429386476671 ) ) ;
#168818=CARTESIAN_POINT ( 'NONE',  ( -18.62759615963255300, -10.81492255796106328, 89.16775706135236135 ) ) ;
#168819=CARTESIAN_POINT ( 'NONE',  ( 19.05341960407611168, 5.049401038298154454, 63.95724293864769550 ) ) ;
#168820=CARTESIAN_POINT ( 'NONE',  ( -12.06949235617739369, -12.14591786802326823, 54.37609039468568994 ) ) ;
#168821=CARTESIAN_POINT ( 'NONE',  ( 13.89961937509977652, -13.97604488694527269, 58.12390960531436690 ) ) ;
#168822=CARTESIAN_POINT ( 'NONE',  ( 10.81492255796106328, -18.62759615963255655, 80.41775706135234714 ) ) ;
#168824=CARTESIAN_POINT ( 'NONE',  ( 16.51473224551083163, -9.474510206698727899, 35.83442372801899722 ) ) ;
#168825=CARTESIAN_POINT ( 'NONE',  ( 19.05341960407617918, -5.049401038297876454, 51.04275706135231871 ) ) ;
#168826=CARTESIAN_POINT ( 'NONE',  ( 18.67979575497194134, -10.72451020669871369, 45.83442372801901854 ) ) ;
#168829=CARTESIAN_POINT ( 'NONE',  ( 5.153800228976615827, -19.02544592524334988, 50.20942372801897591 ) ) ;
#168830=CARTESIAN_POINT ( 'NONE',  ( 0.05219959533909260263, 19.03943276465977164, 94.99890960531436690 ) ) ;
#168831=CARTESIAN_POINT ( 'NONE',  ( -13.89961937509977652, 13.97604488694528158, 70.62390960531432427 ) ) ;
#168832=CARTESIAN_POINT ( 'NONE',  ( -4.379528057220328563, 16.55341960407611168, 25.20724293864769550 ) ) ;
#168833=CARTESIAN_POINT ( 'NONE',  ( -21.52544592524343514, 5.823673210054127303, 36.04057627198102409 ) ) ;
#168834=CARTESIAN_POINT ( 'NONE',  ( 0.05219959533937995610, -21.53943276465977519, 100.0010903946857042 ) ) ;
#168837=CARTESIAN_POINT ( 'NONE',  ( -21.52544592524334988, -5.823673210054445271, 103.9594237280190185 ) ) ;
#168839=CARTESIAN_POINT ( 'NONE',  ( -16.51473224551069308, -9.474510206698971260, 21.66557627198102765 ) ) ;
#168840=CARTESIAN_POINT ( 'NONE',  ( -19.02544592524342804, 5.153800228976336051, 116.0405762719810383 ) ) ;
#168842=CARTESIAN_POINT ( 'NONE',  ( -12.14591786802326823, 12.06949235617739902, 53.12609039468568284 ) ) ;
#168843=CARTESIAN_POINT ( 'NONE',  ( 15.80617190586746368, 15.72974639402197994, 64.37390960531435269 ) ) ;
#168844=CARTESIAN_POINT ( 'NONE',  ( 16.55341960407611168, 4.379528057220329451, 43.95724293864769550 ) ) ;
#168845=CARTESIAN_POINT ( 'NONE',  ( -16.53943276465976808, 0.05219959533911058130, 111.2489096053143669 ) ) ;
#168846=CARTESIAN_POINT ( 'NONE',  ( -13.89961937509977652, 13.97604488694528158, 95.62390960531436690 ) ) ;
#168847=CARTESIAN_POINT ( 'NONE',  ( -9.564922557961040184, 16.46253265017147172, 32.91775706135233293 ) ) ;
#168848=CARTESIAN_POINT ( 'NONE',  ( -8.224510206698948167, 14.34966873604960824, 115.4155762719810241 ) ) ;
#168849=CARTESIAN_POINT ( 'NONE',  ( 21.53943276465977519, 0.05219959533937863772, 71.25109039468568994 ) ) ;
#168851=CARTESIAN_POINT ( 'NONE',  ( 4.483927247898790824, -16.52544592524335698, 105.2094237280190328 ) ) ;
#168853=CARTESIAN_POINT ( 'NONE',  ( -5.719274019375978568, 21.55341960407610458, 30.20724293864769550 ) ) ;
#168854=CARTESIAN_POINT ( 'NONE',  ( 16.52544592524342804, -4.483927247898539470, 88.54057627198103830 ) ) ;
#168855=CARTESIAN_POINT ( 'NONE',  ( 5.049401038297881783, 19.05341960407617563, 57.29275706135231871 ) ) ;
#168856=CARTESIAN_POINT ( 'NONE',  ( -19.05341960407611168, -5.049401038298163336, 71.45724293864766707 ) ) ;
#168857=CARTESIAN_POINT ( 'NONE',  ( -12.06949235617756955, 12.14591786802309770, 75.62390960531439532 ) ) ;
#168858=CARTESIAN_POINT ( 'NONE',  ( 16.46253265017146816, 9.564922557961045513, 86.66775706135233293 ) ) ;
#168859=CARTESIAN_POINT ( 'NONE',  ( 21.53943276465977519, -0.05219959533907433946, 48.74890960531435979 ) ) ;
#168861=CARTESIAN_POINT ( 'NONE',  ( -19.02544592524342804, 5.153800228976336051, 26.04057627198103120 ) ) ;
#168863=CARTESIAN_POINT ( 'NONE',  ( -5.153800228976328057, -19.02544592524343514, 72.29057627198102409 ) ) ;
#168864=CARTESIAN_POINT ( 'NONE',  ( 15.80617190586746368, 15.72974639402197994, 74.37390960531436690 ) ) ;
#168865=CARTESIAN_POINT ( 'NONE',  ( -16.55341960407617563, 4.379528057220093196, 98.54275706135234714 ) ) ;
#168866=CARTESIAN_POINT ( 'NONE',  ( -9.474510206698964154, 16.51473224551069663, 90.41557627198103830 ) ) ;
#168867=CARTESIAN_POINT ( 'NONE',  ( 19.03943276465977164, 0.05219959533936151252, 71.25109039468566152 ) ) ;
#168868=CARTESIAN_POINT ( 'NONE',  ( -18.62759615963255300, -10.81492255796106328, 79.16775706135234714 ) ) ;
#168869=CARTESIAN_POINT ( 'NONE',  ( 21.53943276465977519, -0.05219959533907433946, 58.74890960531436690 ) ) ;
#168870=CARTESIAN_POINT ( 'NONE',  ( 5.823673210054125526, 21.52544592524343514, 29.79057627198102409 ) ) ;
#168871=CARTESIAN_POINT ( 'NONE',  ( -19.02544592524342804, 5.153800228976336051, 41.04057627198103120 ) ) ;
#168872=CARTESIAN_POINT ( 'NONE',  ( -4.379528057220086978, -16.55341960407618274, 104.7927570613523898 ) ) ;
#168873=CARTESIAN_POINT ( 'NONE',  ( -13.97604488694527625, -13.89961937509977652, 56.87390960531434558 ) ) ;
#168874=CARTESIAN_POINT ( 'NONE',  ( 4.379528057220092307, 16.55341960407617563, 27.29275706135234358 ) ) ;
#168876=CARTESIAN_POINT ( 'NONE',  ( 13.97604488694548053, -13.89961937509957401, 20.62609039468567573 ) ) ;
#168877=CARTESIAN_POINT ( 'NONE',  ( -4.483927247898539470, -16.52544592524342804, 62.29057627198102409 ) ) ;
#168878=CARTESIAN_POINT ( 'NONE',  ( -10.81492255796078084, -18.62759615963271287, 112.0822429386477097 ) ) ;
#168879=CARTESIAN_POINT ( 'NONE',  ( -15.80617190586745835, -15.72974639402198527, 101.8739096053143811 ) ) ;
#168880=CARTESIAN_POINT ( 'NONE',  ( 17.49999999999999645, -5.624438216177592764, 98.31670344914645909 ) ) ;
#168881=CARTESIAN_POINT ( 'NONE',  ( -15.72974639402197994, 15.80617190586746368, 45.62390960531436690 ) ) ;
#168882=CARTESIAN_POINT ( 'NONE',  ( -12.14591786802326823, 12.06949235617739902, 78.12609039468570415 ) ) ;
#168883=CARTESIAN_POINT ( 'NONE',  ( -4.379528057220328563, 16.55341960407611168, 110.2072429386477239 ) ) ;
#168884=CARTESIAN_POINT ( 'NONE',  ( 16.46253265017160672, -9.564922557960803928, 63.33224293864769550 ) ) ;
#168886=CARTESIAN_POINT ( 'NONE',  ( -8.314922557961024197, 14.29746914071037800, 112.9177570613523329 ) ) ;
#168888=CARTESIAN_POINT ( 'NONE',  ( 15.80617190586769283, -15.72974639402175789, 50.62609039468568994 ) ) ;
#168889=CARTESIAN_POINT ( 'NONE',  ( 16.51473224551069308, 9.474510206698969483, 99.16557627198102409 ) ) ;
#168890=CARTESIAN_POINT ( 'NONE',  ( -21.55341960407619339, 5.719274019375674811, 83.54275706135234714 ) ) ;
#168892=CARTESIAN_POINT ( 'NONE',  ( -5.049401038298153566, 19.05341960407611168, 30.20724293864768839 ) ) ;
#168894=CARTESIAN_POINT ( 'NONE',  ( 21.52544592524334988, 5.823673210054432836, 66.45942372801903275 ) ) ;
#168895=CARTESIAN_POINT ( 'NONE',  ( -19.05341960407611168, -5.049401038298163336, 51.45724293864770260 ) ) ;
#168896=CARTESIAN_POINT ( 'NONE',  ( 19.05341960407611168, 5.049401038298154454, 98.95724293864766707 ) ) ;
#168897=CARTESIAN_POINT ( 'NONE',  ( -13.97604488694547697, 13.89961937509957934, 78.12609039468567573 ) ) ;
#168898=CARTESIAN_POINT ( 'NONE',  ( -15.72974639402176322, -15.80617190586768395, 39.37609039468567573 ) ) ;
#168899=CARTESIAN_POINT ( 'NONE',  ( 0.05219959533936267826, -19.03943276465977164, 110.0010903946856757 ) ) ;
#168900=CARTESIAN_POINT ( 'NONE',  ( -19.05341960407617563, 5.049401038297882671, 73.54275706135233293 ) ) ;
#168901=CARTESIAN_POINT ( 'NONE',  ( 19.02544592524343514, -5.153800228976328945, 38.54057627198103120 ) ) ;
#168902=CARTESIAN_POINT ( 'NONE',  ( -9.474510206698720793, -16.51473224551083518, 84.58442372801900433 ) ) ;
#168903=CARTESIAN_POINT ( 'NONE',  ( -12.14591786802326823, 12.06949235617739902, 103.1260903946856757 ) ) ;
#168904=CARTESIAN_POINT ( 'NONE',  ( 16.51473224551083163, -9.474510206698727899, 80.83442372801899012 ) ) ;
#168905=CARTESIAN_POINT ( 'NONE',  ( -8.314922557960811034, -14.29746914071050412, 42.08224293864769550 ) ) ;
#168906=CARTESIAN_POINT ( 'NONE',  ( 5.153800228976615827, -19.02544592524334988, 70.20942372801899012 ) ) ;
#168907=CARTESIAN_POINT ( 'NONE',  ( 21.55341960407619695, -5.719274019375665929, 111.0427570613523613 ) ) ;
#168908=CARTESIAN_POINT ( 'NONE',  ( -16.51473224551082808, 9.474510206698731452, 23.33442372801900078 ) ) ;
#168909=CARTESIAN_POINT ( 'NONE',  ( -19.03943276465977164, 0.05219959533909376836, 26.24890960531435624 ) ) ;
#168911=CARTESIAN_POINT ( 'NONE',  ( 14.29746914071037800, 8.314922557961029526, 41.66775706135235424 ) ) ;
#168912=CARTESIAN_POINT ( 'NONE',  ( 13.97604488694527802, 13.89961937509977652, 94.37390960531436690 ) ) ;
#168915=CARTESIAN_POINT ( 'NONE',  ( -19.05341960407611168, -5.049401038298163336, 91.45724293864766707 ) ) ;
#168916=CARTESIAN_POINT ( 'NONE',  ( -17.31728774477210564, 6.344390552233735825, 100.8190665168930593 ) ) ;
#168918=CARTESIAN_POINT ( 'NONE',  ( 16.46253265017146816, 9.564922557961045513, 81.66775706135233293 ) ) ;
#168919=CARTESIAN_POINT ( 'NONE',  ( -21.52544592524343514, 5.823673210054127303, 26.04057627198103475 ) ) ;
#168920=CARTESIAN_POINT ( 'NONE',  ( 18.67979575497194134, -10.72451020669871369, 110.8344237280190043 ) ) ;
#168921=CARTESIAN_POINT ( 'NONE',  ( 19.02544592524334988, 5.153800228976608722, 101.4594237280189759 ) ) ;
#168922=CARTESIAN_POINT ( 'NONE',  ( -4.483927247898539470, -16.52544592524342804, 107.2905762719810525 ) ) ;
#168923=CARTESIAN_POINT ( 'NONE',  ( -5.049401038298153566, 19.05341960407611168, 25.20724293864768484 ) ) ;
#168924=CARTESIAN_POINT ( 'NONE',  ( 15.72974639402199770, -15.80617190586745480, 58.12390960531435979 ) ) ;
#168925=CARTESIAN_POINT ( 'NONE',  ( 21.53943276465977519, -0.05219959533907433946, 43.74890960531435979 ) ) ;
#168926=CARTESIAN_POINT ( 'NONE',  ( 19.02544592524343514, -5.153800228976328945, 28.54057627198102409 ) ) ;
#168928=CARTESIAN_POINT ( 'NONE',  ( 0.05219959533936267826, -19.03943276465977164, 70.00109039468566152 ) ) ;
#168929=CARTESIAN_POINT ( 'NONE',  ( -16.52544592524342804, 4.483927247898546575, 41.04057627198103120 ) ) ;
#168930=CARTESIAN_POINT ( 'NONE',  ( 19.03943276465977164, -0.05219959533909143690, 108.7489096053143527 ) ) ;
#168931=CARTESIAN_POINT ( 'NONE',  ( -21.55341960407619339, 5.719274019375674811, 98.54275706135234714 ) ) ;
#168932=CARTESIAN_POINT ( 'NONE',  ( -18.62759615963270932, 10.81492255796079327, 70.83224293864770971 ) ) ;
#168933=CARTESIAN_POINT ( 'NONE',  ( 10.72451020669871369, 18.67979575497193778, 52.08442372801901854 ) ) ;
#168934=CARTESIAN_POINT ( 'NONE',  ( 18.62759615963255655, 10.81492255796105972, 46.66775706135234714 ) ) ;
#168935=CARTESIAN_POINT ( 'NONE',  ( -19.03943276465977164, 0.05219959533909376836, 91.24890960531436690 ) ) ;
#168936=CARTESIAN_POINT ( 'NONE',  ( -14.34966873604972548, 8.224510206698743886, 98.33442372801901854 ) ) ;
#168937=CARTESIAN_POINT ( 'NONE',  ( 12.14591786802309770, 12.06949235617756955, 114.3739096053143527 ) ) ;
#168939=CARTESIAN_POINT ( 'NONE',  ( -0.05219959533910754901, -16.53943276465976808, 67.49890960531436690 ) ) ;
#168940=CARTESIAN_POINT ( 'NONE',  ( 14.29746914071049879, -8.314922557960816363, 33.33224293864769550 ) ) ;
#168941=CARTESIAN_POINT ( 'NONE',  ( -0.05219959533909027116, -19.03943276465977164, 62.49890960531435979 ) ) ;
#168942=CARTESIAN_POINT ( 'NONE',  ( -19.05341960407611168, -5.049401038298163336, 36.45724293864766707 ) ) ;
#168943=CARTESIAN_POINT ( 'NONE',  ( 18.67979575497178502, 10.72451020669898547, 64.16557627198102409 ) ) ;
#168944=CARTESIAN_POINT ( 'NONE',  ( -19.05341960407617563, 5.049401038297882671, 33.54275706135231871 ) ) ;
#168946=CARTESIAN_POINT ( 'NONE',  ( -16.53943276465976808, 0.05219959533911058130, 56.24890960531436690 ) ) ;
#168947=CARTESIAN_POINT ( 'NONE',  ( -10.81492255796078084, -18.62759615963271287, 32.08224293864769550 ) ) ;
#168948=ORIENTED_EDGE ( 'NONE', *, *, #120571, .T. ) ;
#168949=CARTESIAN_POINT ( 'NONE',  ( 17.49999999999999645, 3.242565516156353134, 37.49999999998637179 ) ) ;
#168950=CARTESIAN_POINT ( 'NONE',  ( 8.224510206698742110, 14.34966873604972548, 77.08442372801901854 ) ) ;
#168951=CARTESIAN_POINT ( 'NONE',  ( 16.46253265017146816, 9.564922557961045513, 71.66775706135233293 ) ) ;
#168952=CARTESIAN_POINT ( 'NONE',  ( 16.52544592524342804, -4.483927247898539470, 38.54057627198103120 ) ) ;
#168953=CARTESIAN_POINT ( 'NONE',  ( -18.22780087662124160, -5.499999999999927169, 73.98236817873106475 ) ) ;
#168954=CARTESIAN_POINT ( 'NONE',  ( -14.34966873604960291, -8.224510206698953496, 31.66557627198102054 ) ) ;
#168955=CARTESIAN_POINT ( 'NONE',  ( 16.46253265017160672, -9.564922557960803928, 58.33224293864769550 ) ) ;
#168956=CARTESIAN_POINT ( 'NONE',  ( -13.97604488694527625, -13.89961937509977652, 71.87390960531433848 ) ) ;
#168957=CARTESIAN_POINT ( 'NONE',  ( 13.97604488694527802, 13.89961937509977652, 39.37390960531435269 ) ) ;
#168958=CARTESIAN_POINT ( 'NONE',  ( 10.72451020669871369, 18.67979575497193778, 42.08442372801901854 ) ) ;
#168959=CARTESIAN_POINT ( 'NONE',  ( 13.97604488694527802, 13.89961937509977652, 59.37390960531434558 ) ) ;
#168961=CARTESIAN_POINT ( 'NONE',  ( 13.97604488694527802, 13.89961937509977652, 59.37390960531434558 ) ) ;
#168962=CARTESIAN_POINT ( 'NONE',  ( 10.72451020669898902, -18.67979575497178502, 37.91557627198102409 ) ) ;
#168963=CARTESIAN_POINT ( 'NONE',  ( 8.314922557960818139, 14.29746914071049879, 114.5822429386477097 ) ) ;
#168964=CARTESIAN_POINT ( 'NONE',  ( 18.62759615963271287, -10.81492255796078972, 28.33224293864769550 ) ) ;
#168965=AXIS2_PLACEMENT_3D ( 'NONE', #146872, #68028, #194395 ) ;
#168966=CARTESIAN_POINT ( 'NONE',  ( -12.06949235617739369, -12.14591786802326823, 89.37609039468568994 ) ) ;
#168967=CARTESIAN_POINT ( 'NONE',  ( 15.72974639402176855, 15.80617190586768217, 101.8760903946857042 ) ) ;
#168968=CARTESIAN_POINT ( 'NONE',  ( 12.14591786802327356, -12.06949235617739191, 65.62609039468568994 ) ) ;
#168969=CARTESIAN_POINT ( 'NONE',  ( 5.049401038298161559, -19.05341960407611168, 112.7072429386476813 ) ) ;
#168970=CARTESIAN_POINT ( 'NONE',  ( 4.483927247898790824, -16.52544592524335698, 60.20942372801902565 ) ) ;
#168971=CARTESIAN_POINT ( 'NONE',  ( -16.52544592524335698, -4.483927247898792601, 43.95942372801902565 ) ) ;
#168972=CARTESIAN_POINT ( 'NONE',  ( -0.05219959533934338120, 16.53943276465976808, 92.50109039468567573 ) ) ;
#168973=CARTESIAN_POINT ( 'NONE',  ( -8.314922557961024197, 14.29746914071037800, 27.91775706135234358 ) ) ;
#168974=CARTESIAN_POINT ( 'NONE',  ( 16.46253265017160672, -9.564922557960803928, 33.33224293864770260 ) ) ;
#168975=CARTESIAN_POINT ( 'NONE',  ( -18.62759615963255300, -10.81492255796106328, 19.16775706135234714 ) ) ;
#168976=CARTESIAN_POINT ( 'NONE',  ( -4.379528057220086978, -16.55341960407618274, 24.79275706135235779 ) ) ;
#168977=CARTESIAN_POINT ( 'NONE',  ( 8.224510206698742110, 14.34966873604972548, 82.08442372801901854 ) ) ;
#168979=CARTESIAN_POINT ( 'NONE',  ( -5.719274019375665041, -21.55341960407619695, 84.79275706135234714 ) ) ;
#168980=CARTESIAN_POINT ( 'NONE',  ( -16.51473224551082808, 9.474510206698731452, 78.33442372801900433 ) ) ;
#168982=CARTESIAN_POINT ( 'NONE',  ( -16.52544592524342804, 4.483927247898546575, 56.04057627198102409 ) ) ;
#168983=CARTESIAN_POINT ( 'NONE',  ( 4.379528057220339221, -16.55341960407611168, 42.70724293864770260 ) ) ;
#168984=CARTESIAN_POINT ( 'NONE',  ( -16.53943276465976808, 0.05219959533911058130, 101.2489096053143669 ) ) ;
#168985=CARTESIAN_POINT ( 'NONE',  ( 19.05341960407617918, -5.049401038297876454, 41.04275706135233293 ) ) ;
#168987=CARTESIAN_POINT ( 'NONE',  ( 21.53943276465977519, 0.05219959533937863772, 56.25109039468568284 ) ) ;
#168988=CARTESIAN_POINT ( 'NONE',  ( -13.97604488694547697, 13.89961937509957934, 113.1260903946856757 ) ) ;
#168990=CARTESIAN_POINT ( 'NONE',  ( 19.05341960407611168, 5.049401038298154454, 108.9572429386477097 ) ) ;
#168991=CARTESIAN_POINT ( 'NONE',  ( 0.05219959533907565091, 21.53943276465977519, 69.99890960531435269 ) ) ;
#168992=CARTESIAN_POINT ( 'NONE',  ( 9.474510206698729675, 16.51473224551082808, 97.08442372801900433 ) ) ;
#168993=CARTESIAN_POINT ( 'NONE',  ( 19.05341960407611168, 5.049401038298154454, 108.9572429386477097 ) ) ;
#168995=CARTESIAN_POINT ( 'NONE',  ( 16.52544592524342804, -4.483927247898539470, 103.5405762719810383 ) ) ;
#168996=CARTESIAN_POINT ( 'NONE',  ( -10.81492255796105439, 18.62759615963255655, 97.91775706135236135 ) ) ;
#168997=CARTESIAN_POINT ( 'NONE',  ( 9.564922557960805705, 16.46253265017160317, 29.58224293864769550 ) ) ;
#168998=CARTESIAN_POINT ( 'NONE',  ( 0.05219959533937995610, -21.53943276465977519, 55.00109039468568284 ) ) ;
#168999=CARTESIAN_POINT ( 'NONE',  ( 10.72451020669871369, 18.67979575497193778, 87.08442372801901854 ) ) ;
#169000=CARTESIAN_POINT ( 'NONE',  ( -12.14591786802326823, 12.06949235617739902, 88.12609039468570415 ) ) ;
#169001=CARTESIAN_POINT ( 'NONE',  ( 10.72451020669871369, 18.67979575497193778, 37.08442372801901143 ) ) ;
#169002=CARTESIAN_POINT ( 'NONE',  ( -15.72974639402176322, -15.80617190586768395, 44.37609039468567573 ) ) ;
#169003=CARTESIAN_POINT ( 'NONE',  ( 9.474510206698729675, 16.51473224551082808, 62.08442372801899722 ) ) ;
#169004=CARTESIAN_POINT ( 'NONE',  ( 9.474510206698971260, -16.51473224551069308, 92.91557627198103830 ) ) ;
#169005=CARTESIAN_POINT ( 'NONE',  ( -16.53943276465976808, 0.05219959533911058130, 101.2489096053143669 ) ) ;
#169006=CARTESIAN_POINT ( 'NONE',  ( 5.719274019375991003, -21.55341960407610458, 87.70724293864769550 ) ) ;
#169007=CARTESIAN_POINT ( 'NONE',  ( 14.29746914071049879, -8.314922557960816363, 63.33224293864770260 ) ) ;
#169008=CARTESIAN_POINT ( 'NONE',  ( 10.72451020669871369, 18.67979575497193778, 107.0844237280190043 ) ) ;
#169009=CARTESIAN_POINT ( 'NONE',  ( 8.224510206698953496, -14.34966873604960469, 77.91557627198102409 ) ) ;
#169010=CARTESIAN_POINT ( 'NONE',  ( 19.05341960407611168, 5.049401038298154454, 33.95724293864769550 ) ) ;
#169011=CARTESIAN_POINT ( 'NONE',  ( 16.46253265017146816, 9.564922557961045513, 86.66775706135233293 ) ) ;
#169012=CARTESIAN_POINT ( 'NONE',  ( 0.05219959533910956823, 16.53943276465976808, 44.99890960531435979 ) ) ;
#169013=CARTESIAN_POINT ( 'NONE',  ( -15.80617190586768217, 15.72974639402176855, 93.12609039468568994 ) ) ;
#169014=CARTESIAN_POINT ( 'NONE',  ( -5.153800228976328057, -19.02544592524343514, 97.29057627198099567 ) ) ;
#169015=CARTESIAN_POINT ( 'NONE',  ( 16.46253265017146816, 9.564922557961045513, 56.66775706135233293 ) ) ;
#169016=CARTESIAN_POINT ( 'NONE',  ( -5.823673210054116645, -21.52544592524344225, 67.29057627198103830 ) ) ;
#169017=CARTESIAN_POINT ( 'NONE',  ( -10.72451020669898014, 18.67979575497178502, 115.4155762719810241 ) ) ;
#169018=CARTESIAN_POINT ( 'NONE',  ( 0.05219959533934541429, -16.53943276465976808, 25.00109039468567218 ) ) ;
#169019=CARTESIAN_POINT ( 'NONE',  ( -12.06949235617739369, -12.14591786802326823, 79.37609039468567573 ) ) ;
#169020=CARTESIAN_POINT ( 'NONE',  ( -16.51473224551069308, -9.474510206698971260, 31.66557627198102054 ) ) ;
#169021=CARTESIAN_POINT ( 'NONE',  ( 15.80617190586769283, -15.72974639402175789, 20.62609039468568639 ) ) ;
#169022=CARTESIAN_POINT ( 'NONE',  ( -12.06949235617756955, 12.14591786802309770, 115.6239096053143669 ) ) ;
#169024=CARTESIAN_POINT ( 'NONE',  ( -16.53943276465976808, -0.05219959533934237506, 53.75109039468568994 ) ) ;
#169025=CARTESIAN_POINT ( 'NONE',  ( -8.314922557960811034, -14.29746914071050412, 77.08224293864769550 ) ) ;
#169026=CARTESIAN_POINT ( 'NONE',  ( 0.05219959533907565091, 21.53943276465977519, 74.99890960531435269 ) ) ;
#169027=CARTESIAN_POINT ( 'NONE',  ( 0.05219959533910956823, 16.53943276465976808, 29.99890960531435979 ) ) ;
#169028=CARTESIAN_POINT ( 'NONE',  ( 8.314922557961029526, -14.29746914071037800, 35.41775706135234003 ) ) ;
#169029=CARTESIAN_POINT ( 'NONE',  ( 13.97604488694527802, 13.89961937509977652, 44.37390960531435269 ) ) ;
#169030=CARTESIAN_POINT ( 'NONE',  ( -4.379528057220086978, -16.55341960407618274, 74.79275706135234714 ) ) ;
#169031=CARTESIAN_POINT ( 'NONE',  ( -9.474510206698720793, -16.51473224551083518, 79.58442372801899012 ) ) ;
#169032=CARTESIAN_POINT ( 'NONE',  ( 18.62759615963271287, -10.81492255796078972, 73.33224293864769550 ) ) ;
#169033=CARTESIAN_POINT ( 'NONE',  ( -0.05219959533934338120, 16.53943276465976808, 107.5010903946856899 ) ) ;
#169035=CARTESIAN_POINT ( 'NONE',  ( -18.62759615963255300, -10.81492255796106328, 79.16775706135234714 ) ) ;
#169036=CARTESIAN_POINT ( 'NONE',  ( 10.72451020669898902, -18.67979575497178502, 42.91557627198103120 ) ) ;
#169038=VERTEX_POINT ( 'NONE', #69273 ) ;
#169039=CARTESIAN_POINT ( 'NONE',  ( 12.06949235617739724, 12.14591786802326823, 86.87609039468568994 ) ) ;
#169040=CARTESIAN_POINT ( 'NONE',  ( -5.719274019375978568, 21.55341960407610458, 45.20724293864769550 ) ) ;
#169041=ORIENTED_EDGE ( 'NONE', *, *, #126300, .T. ) ;
#169042=CARTESIAN_POINT ( 'NONE',  ( -19.05341960407611168, -5.049401038298163336, 106.4572429386476955 ) ) ;
#169044=CARTESIAN_POINT ( 'NONE',  ( -14.29746914071049879, 8.314922557960819915, 115.8322429386477097 ) ) ;
#169045=CARTESIAN_POINT ( 'NONE',  ( -15.80617190586745835, -15.72974639402198527, 76.87390960531439532 ) ) ;
#169046=CARTESIAN_POINT ( 'NONE',  ( 8.314922557961029526, -14.29746914071037800, 110.4177570613523756 ) ) ;
#169047=CARTESIAN_POINT ( 'NONE',  ( -10.81492255796105439, 18.62759615963255655, 57.91775706135234714 ) ) ;
#169048=CARTESIAN_POINT ( 'NONE',  ( 16.52544592524335698, 4.483927247898782831, 21.45942372801901499 ) ) ;
#169049=CARTESIAN_POINT ( 'NONE',  ( 5.049401038298161559, -19.05341960407611168, 27.70724293864769550 ) ) ;
#169050=CARTESIAN_POINT ( 'NONE',  ( 12.06949235617739724, 12.14591786802326823, 31.87609039468567929 ) ) ;
#169051=CARTESIAN_POINT ( 'NONE',  ( -5.049401038298153566, 19.05341960407611168, 40.20724293864768839 ) ) ;
#169053=CARTESIAN_POINT ( 'NONE',  ( -19.03943276465977164, 0.05219959533909376836, 106.2489096053143669 ) ) ;
#169054=CARTESIAN_POINT ( 'NONE',  ( 4.483927247898790824, -16.52544592524335698, 85.20942372801901854 ) ) ;
#169055=CARTESIAN_POINT ( 'NONE',  ( 13.97604488694548053, -13.89961937509957401, 75.62609039468564731 ) ) ;
#169056=CARTESIAN_POINT ( 'NONE',  ( 16.46253265017146816, 9.564922557961045513, 21.66775706135233648 ) ) ;
#169057=CARTESIAN_POINT ( 'NONE',  ( 0.05219959533907565091, 21.53943276465977519, 79.99890960531435269 ) ) ;
#169058=CARTESIAN_POINT ( 'NONE',  ( 12.14591786802327356, -12.06949235617739191, 95.62609039468568994 ) ) ;
#169060=CARTESIAN_POINT ( 'NONE',  ( -5.049401038297874678, -19.05341960407617918, 89.79275706135230450 ) ) ;
#169061=CARTESIAN_POINT ( 'NONE',  ( 16.46253265017160672, -9.564922557960803928, 53.33224293864768839 ) ) ;
#169062=CARTESIAN_POINT ( 'NONE',  ( 13.89961937509977652, -13.97604488694527269, 88.12390960531438111 ) ) ;
#169063=CARTESIAN_POINT ( 'NONE',  ( -5.719274019375665041, -21.55341960407619695, 54.79275706135235424 ) ) ;
#169064=CARTESIAN_POINT ( 'NONE',  ( 13.89961937509977652, -13.97604488694527269, 53.12390960531434558 ) ) ;
#169065=CARTESIAN_POINT ( 'NONE',  ( -16.81555441253551919, -7.025013491695472290, 84.36314554665739252 ) ) ;
#169066=CARTESIAN_POINT ( 'NONE',  ( -19.03943276465977164, 0.05219959533909376836, 111.2489096053143669 ) ) ;
#169067=CARTESIAN_POINT ( 'NONE',  ( 14.34966873604960469, 8.224510206698951720, 64.16557627198102409 ) ) ;
#169068=CARTESIAN_POINT ( 'NONE',  ( 21.53943276465977519, -0.05219959533907433946, 78.74890960531436690 ) ) ;
#169070=CARTESIAN_POINT ( 'NONE',  ( 16.51473224551083163, -9.474510206698727899, 40.83442372801900433 ) ) ;
#169072=CARTESIAN_POINT ( 'NONE',  ( -16.51473224551069308, -9.474510206698971260, 66.66557627198102409 ) ) ;
#169073=CARTESIAN_POINT ( 'NONE',  ( 13.89961937509977652, -13.97604488694527269, 88.12390960531438111 ) ) ;
#169074=CARTESIAN_POINT ( 'NONE',  ( -16.55341960407617563, 4.379528057220093196, 48.54275706135234714 ) ) ;
#169076=CARTESIAN_POINT ( 'NONE',  ( -19.02544592524334988, -5.153800228976617603, 33.95942372801897591 ) ) ;
#169078=CARTESIAN_POINT ( 'NONE',  ( 14.34966873604972726, -8.224510206698740333, 95.83442372801903275 ) ) ;
#169080=CARTESIAN_POINT ( 'NONE',  ( -8.224510206698735004, -14.34966873604973081, 79.58442372801903275 ) ) ;
#169081=CARTESIAN_POINT ( 'NONE',  ( -12.14591786802326823, 12.06949235617739902, 58.12609039468568994 ) ) ;
#169082=CARTESIAN_POINT ( 'NONE',  ( -9.474510206698720793, -16.51473224551083518, 19.58442372801899722 ) ) ;
#169083=CARTESIAN_POINT ( 'NONE',  ( 0.05219959533909260263, 19.03943276465977164, 54.99890960531435979 ) ) ;
#169084=CARTESIAN_POINT ( 'NONE',  ( -18.22780087662126647, -5.499999999999827693, 58.98236817873108606 ) ) ;
#169085=CARTESIAN_POINT ( 'NONE',  ( -21.55341960407619339, 5.719274019375674811, 73.54275706135234714 ) ) ;
#169086=CARTESIAN_POINT ( 'NONE',  ( -19.05341960407617563, 5.049401038297882671, 78.54275706135233293 ) ) ;
#169087=CARTESIAN_POINT ( 'NONE',  ( 18.67979575497194134, -10.72451020669871369, 105.8344237280190328 ) ) ;
#169088=CARTESIAN_POINT ( 'NONE',  ( -5.153800228976328057, -19.02544592524343514, 32.29057627198102409 ) ) ;
#169090=CARTESIAN_POINT ( 'NONE',  ( 21.52544592524344225, -5.823673210054117533, 68.54057627198103830 ) ) ;
#169091=CARTESIAN_POINT ( 'NONE',  ( 5.153800228976335163, 19.02544592524342804, 114.7905762719810241 ) ) ;
#169092=CARTESIAN_POINT ( 'NONE',  ( -8.314922557960811034, -14.29746914071050412, 112.0822429386477097 ) ) ;
#169093=CARTESIAN_POINT ( 'NONE',  ( -12.14591786802326823, 12.06949235617739902, 43.12609039468568284 ) ) ;
#169094=CARTESIAN_POINT ( 'NONE',  ( -16.55341960407611168, -4.379528057220339221, 26.45724293864768839 ) ) ;
#169096=CARTESIAN_POINT ( 'NONE',  ( -5.719274019375665041, -21.55341960407619695, 19.79275706135235069 ) ) ;
#169097=CARTESIAN_POINT ( 'NONE',  ( -16.52544592524342804, 4.483927247898546575, 46.04057627198103830 ) ) ;
#169099=CARTESIAN_POINT ( 'NONE',  ( -16.51473224551082808, 9.474510206698731452, 108.3344237280190043 ) ) ;
#169100=CARTESIAN_POINT ( 'NONE',  ( 13.97604488694548053, -13.89961937509957401, 30.62609039468566863 ) ) ;
#169101=CARTESIAN_POINT ( 'NONE',  ( 16.52544592524342804, -4.483927247898539470, 48.54057627198103120 ) ) ;
#169102=CARTESIAN_POINT ( 'NONE',  ( -10.81492255796078084, -18.62759615963271287, 102.0822429386476955 ) ) ;
#169103=CARTESIAN_POINT ( 'NONE',  ( 16.38665767535053064, 7.295008042176040597, 32.23599135785455871 ) ) ;
#169104=CARTESIAN_POINT ( 'NONE',  ( 10.72451020669898902, -18.67979575497178502, 67.91557627198102409 ) ) ;
#169105=CARTESIAN_POINT ( 'NONE',  ( -13.89961937509977652, 13.97604488694528158, 75.62390960531438111 ) ) ;
#169106=CARTESIAN_POINT ( 'NONE',  ( -4.379528057220328563, 16.55341960407611168, 45.20724293864769550 ) ) ;
#169107=CARTESIAN_POINT ( 'NONE',  ( 16.51473224551069308, 9.474510206698969483, 104.1655762719810241 ) ) ;
#169109=CARTESIAN_POINT ( 'NONE',  ( 19.03943276465977164, 0.05219959533936151252, 56.25109039468566863 ) ) ;
#169110=CARTESIAN_POINT ( 'NONE',  ( -15.80617190586745835, -15.72974639402198527, 91.87390960531436690 ) ) ;
#169111=CARTESIAN_POINT ( 'NONE',  ( -5.153800228976328057, -19.02544592524343514, 42.29057627198101699 ) ) ;
#169112=CARTESIAN_POINT ( 'NONE',  ( -14.29746914071049879, 8.314922557960819915, 115.8322429386477097 ) ) ;
#169115=CARTESIAN_POINT ( 'NONE',  ( 21.52544592524334988, 5.823673210054432836, 51.45942372801901854 ) ) ;
#169117=CARTESIAN_POINT ( 'NONE',  ( 12.14591786802309770, 12.06949235617756955, 24.37390960531435979 ) ) ;
#169118=CARTESIAN_POINT ( 'NONE',  ( -13.97604488694527625, -13.89961937509977652, 46.87390960531435979 ) ) ;
#169119=CARTESIAN_POINT ( 'NONE',  ( -16.46253265017160317, 9.564922557960807481, 105.8322429386476955 ) ) ;
#169120=CARTESIAN_POINT ( 'NONE',  ( 5.719274019375991003, -21.55341960407610458, 57.70724293864770260 ) ) ;
#169121=CARTESIAN_POINT ( 'NONE',  ( -13.97604488694547520, 13.89961937509957934, 93.12609039468566152 ) ) ;
#169122=CARTESIAN_POINT ( 'NONE',  ( -13.89961937509977652, 13.97604488694528158, 40.62390960531435979 ) ) ;
#169123=CARTESIAN_POINT ( 'NONE',  ( -21.53943276465977519, 0.05219959533907696930, 51.24890960531436690 ) ) ;
#169125=CARTESIAN_POINT ( 'NONE',  ( -21.52544592524334988, -5.823673210054445271, 88.95942372801901854 ) ) ;
#169127=CARTESIAN_POINT ( 'NONE',  ( 4.379528057220092307, 16.55341960407617563, 77.29275706135234714 ) ) ;
#169128=CARTESIAN_POINT ( 'NONE',  ( 16.53943276465976808, 0.05219959533934440121, 91.25109039468568994 ) ) ;
#169129=CARTESIAN_POINT ( 'NONE',  ( -13.89961937509977652, 13.97604488694528158, 65.62390960531436690 ) ) ;
#169130=CARTESIAN_POINT ( 'NONE',  ( 13.97604488694527802, 13.89961937509977652, 69.37390960531436690 ) ) ;
#169131=ORIENTED_EDGE ( 'NONE', *, *, #184219, .T. ) ;
#169132=CARTESIAN_POINT ( 'NONE',  ( -9.564922557961040184, 16.46253265017147172, 27.91775706135232582 ) ) ;
#169133=CARTESIAN_POINT ( 'NONE',  ( 8.314922557961029526, -14.29746914071037800, 75.41775706135233293 ) ) ;
#169134=CARTESIAN_POINT ( 'NONE',  ( -13.89961937509957401, -13.97604488694547875, 19.37609039468566507 ) ) ;
#169135=CARTESIAN_POINT ( 'NONE',  ( -19.03943276465977164, 0.05219959533909376836, 81.24890960531436690 ) ) ;
#169136=CARTESIAN_POINT ( 'NONE',  ( -10.81492255796078084, -18.62759615963271287, 47.08224293864770260 ) ) ;
#169137=CARTESIAN_POINT ( 'NONE',  ( -14.34966873604972548, 8.224510206698743886, 28.33442372801902209 ) ) ;
#169138=CARTESIAN_POINT ( 'NONE',  ( 10.72451020669871369, 18.67979575497193778, 82.08442372801901854 ) ) ;
#169139=CARTESIAN_POINT ( 'NONE',  ( -14.29746914071037622, -8.314922557961029526, 64.16775706135234714 ) ) ;
#169140=CARTESIAN_POINT ( 'NONE',  ( 10.81492255796078972, 18.62759615963270932, 114.5822429386477097 ) ) ;
#169141=CARTESIAN_POINT ( 'NONE',  ( 16.46253265017146816, 9.564922557961045513, 106.6677570613523471 ) ) ;
#169142=CARTESIAN_POINT ( 'NONE',  ( -13.97604488694527625, -13.89961937509977652, 76.87390960531433848 ) ) ;
#169143=CARTESIAN_POINT ( 'NONE',  ( 14.34966873604972726, -8.224510206698740333, 25.83442372801901499 ) ) ;
#169144=CARTESIAN_POINT ( 'NONE',  ( -5.049401038298153566, 19.05341960407611168, 45.20724293864769550 ) ) ;
#169146=CARTESIAN_POINT ( 'NONE',  ( -0.05219959533934338120, 16.53943276465976808, 22.50109039468567573 ) ) ;
#169147=CARTESIAN_POINT ( 'NONE',  ( -14.34966873604960291, -8.224510206698953496, 76.66557627198103830 ) ) ;
#169148=CARTESIAN_POINT ( 'NONE',  ( -4.379528057220086978, -16.55341960407618274, 84.79275706135234714 ) ) ;
#169149=CARTESIAN_POINT ( 'NONE',  ( 15.80617190586769283, -15.72974639402175789, 35.62609039468568994 ) ) ;
#169150=CARTESIAN_POINT ( 'NONE',  ( -9.474510206698964154, 16.51473224551069663, 60.41557627198102409 ) ) ;
#169151=CARTESIAN_POINT ( 'NONE',  ( 13.97604488694527802, 13.89961937509977652, 74.37390960531436690 ) ) ;
#169152=B_SPLINE_CURVE_WITH_KNOTS ( 'NONE', 3,
 ( #158889, #128544, #69891, #190241, #193244, #85038 ),
 .UNSPECIFIED., .F., .F.,
 ( 4, 2, 4 ),
 ( 0.003239945802372207456, 0.003620412082092024954, 0.004000878361811842886 ),
 .UNSPECIFIED. ) ;
#169153=CARTESIAN_POINT ( 'NONE',  ( -14.29746914071037622, -8.314922557961029526, 89.16775706135236135 ) ) ;
#169157=CARTESIAN_POINT ( 'NONE',  ( 19.02544592524334988, 5.153800228976608722, 36.45942372801900433 ) ) ;
#169158=CARTESIAN_POINT ( 'NONE',  ( 5.049401038298161559, -19.05341960407611168, 32.70724293864768129 ) ) ;
#169161=CARTESIAN_POINT ( 'NONE',  ( 0.05219959533934541429, -16.53943276465976808, 25.00109039468567218 ) ) ;
#169162=CARTESIAN_POINT ( 'NONE',  ( 5.049401038297881783, 19.05341960407617563, 62.29275706135234003 ) ) ;
#169163=CARTESIAN_POINT ( 'NONE',  ( 8.224510206698742110, 14.34966873604972548, 42.08442372801901854 ) ) ;
#169164=CARTESIAN_POINT ( 'NONE',  ( -0.05219959533909027116, -19.03943276465977164, 112.4989096053143669 ) ) ;
#169165=CARTESIAN_POINT ( 'NONE',  ( 19.03943276465977164, -0.05219959533909143690, 68.74890960531436690 ) ) ;
#169166=CARTESIAN_POINT ( 'NONE',  ( -21.53943276465977519, 0.05219959533907696930, 96.24890960531435269 ) ) ;
#169167=CARTESIAN_POINT ( 'NONE',  ( 13.97604488694527802, 13.89961937509977652, 94.37390960531436690 ) ) ;
#169168=CARTESIAN_POINT ( 'NONE',  ( -19.02544592524342804, 5.153800228976336051, 26.04057627198103120 ) ) ;
#169169=CARTESIAN_POINT ( 'NONE',  ( 19.05341960407611168, 5.049401038298154454, 68.95724293864769550 ) ) ;
#169170=CARTESIAN_POINT ( 'NONE',  ( 8.224510206698953496, -14.34966873604960469, 22.91557627198102765 ) ) ;
#169171=CARTESIAN_POINT ( 'NONE',  ( 5.153800228976335163, 19.02544592524342804, 69.79057627198102409 ) ) ;
#169172=CARTESIAN_POINT ( 'NONE',  ( -16.46253265017146816, -9.564922557961047289, 44.16775706135232582 ) ) ;
#169173=CARTESIAN_POINT ( 'NONE',  ( 16.55341960407611168, 4.379528057220329451, 63.95724293864770260 ) ) ;
#169174=CARTESIAN_POINT ( 'NONE',  ( 10.72451020669871369, 18.67979575497193778, 92.08442372801901854 ) ) ;
#169175=CARTESIAN_POINT ( 'NONE',  ( -19.05341960407611168, -5.049401038298163336, 36.45724293864766707 ) ) ;
#169176=CARTESIAN_POINT ( 'NONE',  ( 14.29746914071037800, 8.314922557961029526, 56.66775706135235424 ) ) ;
#169177=CARTESIAN_POINT ( 'NONE',  ( 16.52544592524342804, -4.483927247898539470, 43.54057627198103830 ) ) ;
#169178=CARTESIAN_POINT ( 'NONE',  ( -15.80617190586768217, 15.72974639402176855, 93.12609039468568994 ) ) ;
#169179=CARTESIAN_POINT ( 'NONE',  ( 13.97604488694527802, 13.89961937509977652, 74.37390960531436690 ) ) ;
#169180=CARTESIAN_POINT ( 'NONE',  ( -19.02544592524342804, 5.153800228976336051, 91.04057627198100988 ) ) ;
#169181=CARTESIAN_POINT ( 'NONE',  ( 12.06949235617757843, -12.14591786802309237, 108.1239096053143811 ) ) ;
#169182=CARTESIAN_POINT ( 'NONE',  ( -4.379528057220328563, 16.55341960407611168, 75.20724293864769550 ) ) ;
#169183=CARTESIAN_POINT ( 'NONE',  ( 18.67979575497178502, 10.72451020669898547, 89.16557627198102409 ) ) ;
#169184=CARTESIAN_POINT ( 'NONE',  ( 13.89961937509977652, -13.97604488694527269, 93.12390960531436690 ) ) ;
#169185=CARTESIAN_POINT ( 'NONE',  ( 10.72451020669898902, -18.67979575497178502, 102.9155762719810383 ) ) ;
#169186=CARTESIAN_POINT ( 'NONE',  ( 19.03943276465977164, 0.05219959533936151252, 81.25109039468567573 ) ) ;
#169187=CARTESIAN_POINT ( 'NONE',  ( -19.01529144963339846, -5.499999999999896083, 91.23431955728437970 ) ) ;
#169188=CARTESIAN_POINT ( 'NONE',  ( -8.314922557960811034, -14.29746914071050412, 87.08224293864769550 ) ) ;
#169189=CARTESIAN_POINT ( 'NONE',  ( -0.05219959533909027116, -19.03943276465977164, 52.49890960531436690 ) ) ;
#169190=CARTESIAN_POINT ( 'NONE',  ( 21.55341960407610458, 5.719274019375980345, 68.95724293864769550 ) ) ;
#169192=CARTESIAN_POINT ( 'NONE',  ( 12.14591786802327356, -12.06949235617739191, 105.6260903946856899 ) ) ;
#169194=CARTESIAN_POINT ( 'NONE',  ( -8.224510206698735004, -14.34966873604973081, 24.58442372801901499 ) ) ;
#169195=CARTESIAN_POINT ( 'NONE',  ( -14.29746914071049879, 8.314922557960819915, 75.83224293864769550 ) ) ;
#169196=CARTESIAN_POINT ( 'NONE',  ( -18.22780087662126647, -5.499999999999827693, 63.98236817873107185 ) ) ;
#169197=CARTESIAN_POINT ( 'NONE',  ( 19.02544592524343514, -5.153800228976328945, 68.54057627198103830 ) ) ;
#169198=CARTESIAN_POINT ( 'NONE',  ( 19.05341960407611168, 5.049401038298154454, 28.95724293864769550 ) ) ;
#169199=CARTESIAN_POINT ( 'NONE',  ( 14.34966873604960469, 8.224510206698951720, 69.16557627198102409 ) ) ;
#169201=CARTESIAN_POINT ( 'NONE',  ( 18.67979575497178502, 10.72451020669898547, 24.16557627198103120 ) ) ;
#169202=CARTESIAN_POINT ( 'NONE',  ( -9.474510206698720793, -16.51473224551083518, 94.58442372801900433 ) ) ;
#169203=CARTESIAN_POINT ( 'NONE',  ( 16.51473224551069308, 9.474510206698969483, 99.16557627198102409 ) ) ;
#169204=CARTESIAN_POINT ( 'NONE',  ( -21.55341960407610458, -5.719274019375992779, 76.45724293864769550 ) ) ;
#169205=CARTESIAN_POINT ( 'NONE',  ( 8.314922557961029526, -14.29746914071037800, 65.41775706135234714 ) ) ;
#169206=CARTESIAN_POINT ( 'NONE',  ( 19.02544592524335343, 5.153800228976608722, 106.4594237280190043 ) ) ;
#169207=CARTESIAN_POINT ( 'NONE',  ( 19.02544592524343514, -5.153800228976328945, 58.54057627198102409 ) ) ;
#169208=CARTESIAN_POINT ( 'NONE',  ( -0.05219959533907301413, -21.53943276465977519, 62.49890960531436690 ) ) ;
#169209=CARTESIAN_POINT ( 'NONE',  ( -9.564922557961040184, 16.46253265017147172, 112.9177570613523329 ) ) ;
#169210=CARTESIAN_POINT ( 'NONE',  ( 8.224510206698953496, -14.34966873604960469, 32.91557627198102409 ) ) ;
#169211=CARTESIAN_POINT ( 'NONE',  ( -18.62759615963255300, -10.81492255796106328, 64.16775706135234714 ) ) ;
#169212=CARTESIAN_POINT ( 'NONE',  ( 17.97214573761830536, 5.500000000000079048, 83.96970049038658601 ) ) ;
#169213=CARTESIAN_POINT ( 'NONE',  ( -16.52544592524335698, -4.483927247898792601, 68.95942372801901854 ) ) ;
#169214=CARTESIAN_POINT ( 'NONE',  ( -9.474510206698964154, 16.51473224551069663, 110.4155762719810383 ) ) ;
#169217=CARTESIAN_POINT ( 'NONE',  ( -14.34966873604972548, 8.224510206698743886, 98.33442372801901854 ) ) ;
#169218=CARTESIAN_POINT ( 'NONE',  ( -16.55341960407617563, 4.379528057220093196, 48.54275706135234714 ) ) ;
#169219=CARTESIAN_POINT ( 'NONE',  ( 19.02544592524343514, -5.153800228976328945, 53.54057627198102409 ) ) ;
#169220=CARTESIAN_POINT ( 'NONE',  ( -9.564922557960796823, -16.46253265017161027, 77.08224293864769550 ) ) ;
#169221=CARTESIAN_POINT ( 'NONE',  ( 15.80617190586769283, -15.72974639402175789, 55.62609039468568284 ) ) ;
#169222=CARTESIAN_POINT ( 'NONE',  ( 0.05219959533934541429, -16.53943276465976808, 65.00109039468568994 ) ) ;
#169223=CARTESIAN_POINT ( 'NONE',  ( 12.14591786802309770, 12.06949235617756955, 29.37390960531435269 ) ) ;
#169224=CARTESIAN_POINT ( 'NONE',  ( -0.05219959533909027116, -19.03943276465977164, 37.49890960531436690 ) ) ;
#169225=CARTESIAN_POINT ( 'NONE',  ( 5.049401038298161559, -19.05341960407611168, 32.70724293864768129 ) ) ;
#169226=CARTESIAN_POINT ( 'NONE',  ( -0.05219959533934338120, 16.53943276465976808, 32.50109039468568284 ) ) ;
#169229=CARTESIAN_POINT ( 'NONE',  ( 13.97604488694548053, -13.89961937509957401, 85.62609039468568994 ) ) ;
#169230=CARTESIAN_POINT ( 'NONE',  ( -16.53943276465976808, 0.05219959533911058130, 81.24890960531436690 ) ) ;
#169231=CARTESIAN_POINT ( 'NONE',  ( 13.89961937509977652, -13.97604488694527269, 48.12390960531435979 ) ) ;
#169232=CARTESIAN_POINT ( 'NONE',  ( 19.02544592524334988, 5.153800228976608722, 81.45942372801897591 ) ) ;
#169234=CARTESIAN_POINT ( 'NONE',  ( 18.67979575497194134, -10.72451020669871369, 95.83442372801903275 ) ) ;
#169235=CARTESIAN_POINT ( 'NONE',  ( 4.483927247898790824, -16.52544592524335698, 55.20942372801902565 ) ) ;
#169237=CARTESIAN_POINT ( 'NONE',  ( -10.72451020669898014, 18.67979575497178502, 50.41557627198103120 ) ) ;
#169238=CARTESIAN_POINT ( 'NONE',  ( 4.379528057220092307, 16.55341960407617563, 42.29275706135235424 ) ) ;
#169239=CARTESIAN_POINT ( 'NONE',  ( -18.56453257813364388, 5.500000000000057732, 70.99000423690689843 ) ) ;
#169240=CARTESIAN_POINT ( 'NONE',  ( -9.564922557961040184, 16.46253265017147172, 37.91775706135233293 ) ) ;
#169241=CARTESIAN_POINT ( 'NONE',  ( -9.474510206698964154, 16.51473224551069663, 85.41557627198102409 ) ) ;
#169242=CARTESIAN_POINT ( 'NONE',  ( -16.51473224551069308, -9.474510206698971260, 51.66557627198102409 ) ) ;
#169244=CARTESIAN_POINT ( 'NONE',  ( 21.55341960407619695, -5.719274019375665929, 71.04275706135234714 ) ) ;
#169245=CARTESIAN_POINT ( 'NONE',  ( 18.22780087662123805, -5.499999999999976019, 93.51763182126896368 ) ) ;
#169246=CARTESIAN_POINT ( 'NONE',  ( -16.51473224551082808, 9.474510206698731452, 33.33442372801899722 ) ) ;
#169247=CARTESIAN_POINT ( 'NONE',  ( 5.823673210054444382, -21.52544592524334988, 105.2094237280190328 ) ) ;
#169248=CARTESIAN_POINT ( 'NONE',  ( -12.14591786802309592, -12.06949235617757132, 36.87390960531435979 ) ) ;
#169249=CARTESIAN_POINT ( 'NONE',  ( 16.46253265017160672, -9.564922557960803928, 43.33224293864769550 ) ) ;
#169251=CARTESIAN_POINT ( 'NONE',  ( -19.05341960407611168, -5.049401038298163336, 101.4572429386476955 ) ) ;
#169252=CARTESIAN_POINT ( 'NONE',  ( 10.72451020669871369, 18.67979575497193778, 87.08442372801901854 ) ) ;
#169253=CARTESIAN_POINT ( 'NONE',  ( 16.51473224551069308, 9.474510206698969483, 64.16557627198102409 ) ) ;
#169254=CARTESIAN_POINT ( 'NONE',  ( 18.67979575497194134, -10.72451020669871369, 80.83442372801901854 ) ) ;
#169255=CARTESIAN_POINT ( 'NONE',  ( -10.81492255796078084, -18.62759615963271287, 37.08224293864768129 ) ) ;
#169256=CARTESIAN_POINT ( 'NONE',  ( 21.53943276465977519, 0.05219959533937863772, 21.25109039468567218 ) ) ;
#169257=CARTESIAN_POINT ( 'NONE',  ( -16.46253265017146816, -9.564922557961047289, 44.16775706135232582 ) ) ;
#169258=CARTESIAN_POINT ( 'NONE',  ( 16.51473224551069308, 9.474510206698969483, 24.16557627198102765 ) ) ;
#169259=CARTESIAN_POINT ( 'NONE',  ( -5.153800228976328057, -19.02544592524343514, 77.29057627198099567 ) ) ;
#169260=CARTESIAN_POINT ( 'NONE',  ( 14.29746914071037800, 8.314922557961029526, 31.66775706135234358 ) ) ;
#169262=CARTESIAN_POINT ( 'NONE',  ( 8.314922557960818139, 14.29746914071049879, 84.58224293864769550 ) ) ;
#169263=CARTESIAN_POINT ( 'NONE',  ( 5.049401038298161559, -19.05341960407611168, 62.70724293864769550 ) ) ;
#169264=CARTESIAN_POINT ( 'NONE',  ( -21.55341960407610458, -5.719274019375992779, 31.45724293864769550 ) ) ;
#169265=CARTESIAN_POINT ( 'NONE',  ( 16.46253265017146816, 9.564922557961045513, 96.66775706135233293 ) ) ;
#169266=CARTESIAN_POINT ( 'NONE',  ( 15.80617190586746368, 15.72974639402197994, 104.3739096053143669 ) ) ;
#169267=CARTESIAN_POINT ( 'NONE',  ( 5.719274019375673035, 21.55341960407619339, 77.29275706135234714 ) ) ;
#169268=CARTESIAN_POINT ( 'NONE',  ( 0.05219959533934541429, -16.53943276465976808, 70.00109039468568994 ) ) ;
#169269=CARTESIAN_POINT ( 'NONE',  ( -8.314922557961024197, 14.29746914071037800, 62.91775706135236135 ) ) ;
#169270=CARTESIAN_POINT ( 'NONE',  ( 5.153800228976335163, 19.02544592524342804, 64.79057627198100988 ) ) ;
#169271=CARTESIAN_POINT ( 'NONE',  ( -14.34966873604972548, 8.224510206698743886, 93.33442372801901854 ) ) ;
#169272=CARTESIAN_POINT ( 'NONE',  ( -9.564922557961040184, 16.46253265017147172, 47.91775706135233293 ) ) ;
#169273=CARTESIAN_POINT ( 'NONE',  ( 0.05219959533937995610, -21.53943276465977519, 20.00109039468568639 ) ) ;
#169274=CARTESIAN_POINT ( 'NONE',  ( -14.29746914071049879, 8.314922557960819915, 70.83224293864770971 ) ) ;
#169275=CARTESIAN_POINT ( 'NONE',  ( 16.51473224551069308, 9.474510206698969483, 89.16557627198103830 ) ) ;
#169276=CARTESIAN_POINT ( 'NONE',  ( 4.379528057220092307, 16.55341960407617563, 77.29275706135234714 ) ) ;
#169277=CARTESIAN_POINT ( 'NONE',  ( 15.80617190586769283, -15.72974639402175789, 55.62609039468568284 ) ) ;
#169278=CARTESIAN_POINT ( 'NONE',  ( -14.29746914071037622, -8.314922557961029526, 19.16775706135234714 ) ) ;
#169279=CARTESIAN_POINT ( 'NONE',  ( -18.67979575497178146, -10.72451020669898902, 111.6655762719810525 ) ) ;
#169280=CARTESIAN_POINT ( 'NONE',  ( 16.52544592524342804, -4.483927247898539470, 53.54057627198103120 ) ) ;
#169282=CARTESIAN_POINT ( 'NONE',  ( 21.52544592524344225, -5.823673210054117533, 93.54057627198103830 ) ) ;
#169283=CARTESIAN_POINT ( 'NONE',  ( -4.379528057220328563, 16.55341960407611168, 40.20724293864769550 ) ) ;
#169286=CARTESIAN_POINT ( 'NONE',  ( 18.67979575497178502, 10.72451020669898547, 109.1655762719810383 ) ) ;
#169287=CARTESIAN_POINT ( 'NONE',  ( -15.80617190586745835, -15.72974639402198527, 21.87390960531436690 ) ) ;
#169288=CARTESIAN_POINT ( 'NONE',  ( 10.72451020669871369, 18.67979575497193778, 37.08442372801901143 ) ) ;
#169289=CARTESIAN_POINT ( 'NONE',  ( -14.34966873604960291, -8.224510206698953496, 56.66557627198103830 ) ) ;
#169290=CARTESIAN_POINT ( 'NONE',  ( -9.564922557960796823, -16.46253265017161027, 62.08224293864769550 ) ) ;
#169291=CARTESIAN_POINT ( 'NONE',  ( 19.03943276465977164, 0.05219959533936151252, 66.25109039468567573 ) ) ;
#169292=CARTESIAN_POINT ( 'NONE',  ( 5.049401038298161559, -19.05341960407611168, 92.70724293864769550 ) ) ;
#169293=CARTESIAN_POINT ( 'NONE',  ( 0.05219959533907565091, 21.53943276465977519, 49.99890960531437401 ) ) ;
#169295=CARTESIAN_POINT ( 'NONE',  ( 19.02544592524343514, -5.153800228976328945, 63.54057627198103830 ) ) ;
#169296=CARTESIAN_POINT ( 'NONE',  ( -8.314922557961024197, 14.29746914071037800, 42.91775706135235424 ) ) ;
#169297=CARTESIAN_POINT ( 'NONE',  ( 5.049401038297881783, 19.05341960407617563, 67.29275706135234714 ) ) ;
#169298=CARTESIAN_POINT ( 'NONE',  ( 21.52544592524334988, 5.823673210054432836, 21.45942372801901499 ) ) ;
#169299=CARTESIAN_POINT ( 'NONE',  ( 16.55341960407611168, 4.379528057220329451, 43.95724293864769550 ) ) ;
#169300=CARTESIAN_POINT ( 'NONE',  ( -9.474510206698964154, 16.51473224551069663, 90.41557627198103830 ) ) ;
#169301=CARTESIAN_POINT ( 'NONE',  ( 21.55341960407610458, 5.719274019375980345, 73.95724293864769550 ) ) ;
#169302=CARTESIAN_POINT ( 'NONE',  ( 18.62759615963271287, -10.81492255796078972, 93.33224293864769550 ) ) ;
#169303=CARTESIAN_POINT ( 'NONE',  ( -4.379528057220086978, -16.55341960407618274, 44.79275706135234714 ) ) ;
#169304=CARTESIAN_POINT ( 'NONE',  ( 18.62759615963271287, -10.81492255796078972, 38.33224293864768839 ) ) ;
#169305=CARTESIAN_POINT ( 'NONE',  ( -18.67979575497193778, 10.72451020669871902, 93.33442372801901854 ) ) ;
#169306=CARTESIAN_POINT ( 'NONE',  ( -9.564922557960796823, -16.46253265017161027, 87.08224293864769550 ) ) ;
#169307=CARTESIAN_POINT ( 'NONE',  ( -0.05219959533909027116, -19.03943276465977164, 47.49890960531435979 ) ) ;
#169308=CARTESIAN_POINT ( 'NONE',  ( 0.05219959533909260263, 19.03943276465977164, 94.99890960531436690 ) ) ;
#169309=CARTESIAN_POINT ( 'NONE',  ( -16.52544592524342804, 4.483927247898546575, 111.0405762719810525 ) ) ;
#169310=CARTESIAN_POINT ( 'NONE',  ( 0.05219959533909260263, 19.03943276465977164, 59.99890960531436690 ) ) ;
#169311=CARTESIAN_POINT ( 'NONE',  ( -12.06949235617739369, -12.14591786802326823, 19.37609039468568639 ) ) ;
#169312=CARTESIAN_POINT ( 'NONE',  ( 17.50000000000147082, 3.254303733634585694, 32.47604106928593382 ) ) ;
#169313=CARTESIAN_POINT ( 'NONE',  ( -19.05341960407617563, 5.049401038297882671, 58.54275706135234003 ) ) ;
#169314=CARTESIAN_POINT ( 'NONE',  ( 15.72974639402176855, 15.80617190586768217, 111.8760903946856615 ) ) ;
#169315=CARTESIAN_POINT ( 'NONE',  ( -15.72974639402197994, 15.80617190586746368, 30.62390960531436335 ) ) ;
#169316=CARTESIAN_POINT ( 'NONE',  ( 12.06949235617739724, 12.14591786802326823, 96.87609039468568994 ) ) ;
#169318=CARTESIAN_POINT ( 'NONE',  ( 16.51473224551083163, -9.474510206698727899, 65.83442372801900433 ) ) ;
#169319=CARTESIAN_POINT ( 'NONE',  ( -5.153800228976607833, 19.02544592524334988, 32.70942372801899722 ) ) ;
#169320=CARTESIAN_POINT ( 'NONE',  ( -17.05116617787826172, -6.768360034955700044, 46.34324446740803438 ) ) ;
#169321=CARTESIAN_POINT ( 'NONE',  ( -19.03943276465977164, 0.05219959533909376836, 41.24890960531435269 ) ) ;
#169322=CARTESIAN_POINT ( 'NONE',  ( -0.05219959533910754901, -16.53943276465976808, 37.49890960531436690 ) ) ;
#169323=CARTESIAN_POINT ( 'NONE',  ( -9.564922557960796823, -16.46253265017161027, 27.08224293864769550 ) ) ;
#169324=CARTESIAN_POINT ( 'NONE',  ( 16.53943276465976808, -0.05219959533910856209, 23.74890960531435269 ) ) ;
#169326=CARTESIAN_POINT ( 'NONE',  ( -12.14591786802326823, 12.06949235617739902, 98.12609039468570415 ) ) ;
#169327=CARTESIAN_POINT ( 'NONE',  ( 16.46253265017160672, -9.564922557960803928, 33.33224293864770260 ) ) ;
#169328=CARTESIAN_POINT ( 'NONE',  ( 21.53943276465977519, 0.05219959533937863772, 101.2510903946856757 ) ) ;
#169329=CARTESIAN_POINT ( 'NONE',  ( 0.05219959533934541429, -16.53943276465976808, 20.00109039468568639 ) ) ;
#169330=CARTESIAN_POINT ( 'NONE',  ( -18.62759615963255300, -10.81492255796106328, 74.16775706135231871 ) ) ;
#169331=CARTESIAN_POINT ( 'NONE',  ( -9.564922557961040184, 16.46253265017147172, 57.91775706135233293 ) ) ;
#169332=CARTESIAN_POINT ( 'NONE',  ( -16.51473224551069308, -9.474510206698971260, 91.66557627198103830 ) ) ;
#169333=CARTESIAN_POINT ( 'NONE',  ( 16.51473224551069308, 9.474510206698969483, 79.16557627198103830 ) ) ;
#169334=CARTESIAN_POINT ( 'NONE',  ( 16.62475595723699939, 7.163666690055260133, 71.97286648189529501 ) ) ;
#169335=CARTESIAN_POINT ( 'NONE',  ( 18.67979575497178502, 10.72451020669898547, 114.1655762719810383 ) ) ;
#169336=CARTESIAN_POINT ( 'NONE',  ( -8.314922557960811034, -14.29746914071050412, 62.08224293864769550 ) ) ;
#169337=CARTESIAN_POINT ( 'NONE',  ( 10.72451020669898902, -18.67979575497178502, 62.91557627198102409 ) ) ;
#169338=CARTESIAN_POINT ( 'NONE',  ( 13.97604488694527802, 13.89961937509977652, 64.37390960531436690 ) ) ;
#169339=CARTESIAN_POINT ( 'NONE',  ( 15.72974639402199770, -15.80617190586745480, 93.12390960531436690 ) ) ;
#169340=CARTESIAN_POINT ( 'NONE',  ( -4.379528057220086978, -16.55341960407618274, 94.79275706135234714 ) ) ;
#169341=ORIENTED_EDGE ( 'NONE', *, *, #42638, .F. ) ;
#169342=CARTESIAN_POINT ( 'NONE',  ( 16.51473224551069308, 9.474510206698969483, 49.16557627198102409 ) ) ;
#169343=CARTESIAN_POINT ( 'NONE',  ( -4.379528057220328563, 16.55341960407611168, 95.20724293864769550 ) ) ;
#169345=CARTESIAN_POINT ( 'NONE',  ( 9.474510206698971260, -16.51473224551069308, 47.91557627198102409 ) ) ;
#169346=CARTESIAN_POINT ( 'NONE',  ( -19.05341960407611168, -5.049401038298163336, 21.45724293864768839 ) ) ;
#169347=CARTESIAN_POINT ( 'NONE',  ( -19.03943276465977164, -0.05219959533935918106, 78.75109039468567573 ) ) ;
#169348=CARTESIAN_POINT ( 'NONE',  ( 8.314922557960818139, 14.29746914071049879, 84.58224293864769550 ) ) ;
#169349=CARTESIAN_POINT ( 'NONE',  ( 10.81492255796106328, -18.62759615963255655, 50.41775706135235424 ) ) ;
#169350=CARTESIAN_POINT ( 'NONE',  ( 16.46253265017160672, -9.564922557960803928, 38.33224293864768839 ) ) ;
#169351=CARTESIAN_POINT ( 'NONE',  ( -15.72974639402197994, 15.80617190586746368, 110.6239096053143669 ) ) ;
#169352=CARTESIAN_POINT ( 'NONE',  ( -8.224510206698948167, 14.34966873604960824, 90.41557627198103830 ) ) ;
#169354=CARTESIAN_POINT ( 'NONE',  ( -9.474510206698964154, 16.51473224551069663, 60.41557627198102409 ) ) ;
#169355=CARTESIAN_POINT ( 'NONE',  ( 18.22780087662126647, 5.499999999999818812, 46.48236817873107185 ) ) ;
#169356=CARTESIAN_POINT ( 'NONE',  ( 16.51473224551083163, -9.474510206698727899, 90.83442372801900433 ) ) ;
#169357=CARTESIAN_POINT ( 'NONE',  ( 13.97604488694527802, 13.89961937509977652, 114.3739096053143669 ) ) ;
#169358=CARTESIAN_POINT ( 'NONE',  ( 15.80617190586769283, -15.72974639402175789, 30.62609039468567929 ) ) ;
#169359=CARTESIAN_POINT ( 'NONE',  ( 16.46253265017160672, -9.564922557960803928, 78.33224293864769550 ) ) ;
#169360=CARTESIAN_POINT ( 'NONE',  ( -19.02544592524334988, -5.153800228976617603, 73.95942372801900433 ) ) ;
#169361=CARTESIAN_POINT ( 'NONE',  ( 13.97604488694527802, 13.89961937509977652, 54.37390960531435979 ) ) ;
#169362=EDGE_CURVE ( 'NONE', #49283, #105512, #157374, .T. ) ;
#169363=CARTESIAN_POINT ( 'NONE',  ( -12.06949235617756955, 12.14591786802309770, 75.62390960531439532 ) ) ;
#169364=CARTESIAN_POINT ( 'NONE',  ( -16.52544592524342804, 4.483927247898546575, 66.04057627198103830 ) ) ;
#169365=CARTESIAN_POINT ( 'NONE',  ( -19.02544592524342804, 5.153800228976336051, 96.04057627198103830 ) ) ;
#169366=CARTESIAN_POINT ( 'NONE',  ( 5.719274019375991003, -21.55341960407610458, 97.70724293864772392 ) ) ;
#169367=CARTESIAN_POINT ( 'NONE',  ( -19.03943276465977164, 0.05219959533909376836, 86.24890960531436690 ) ) ;
#169369=CARTESIAN_POINT ( 'NONE',  ( 16.51473224551083163, -9.474510206698727899, 25.83442372801900078 ) ) ;
#169370=CARTESIAN_POINT ( 'NONE',  ( 13.97604488694527802, 13.89961937509977652, 34.37390960531436690 ) ) ;
#169371=CARTESIAN_POINT ( 'NONE',  ( 8.314922557960818139, 14.29746914071049879, 29.58224293864769905 ) ) ;
#169372=CARTESIAN_POINT ( 'NONE',  ( -8.224510206698948167, 14.34966873604960824, 115.4155762719810241 ) ) ;
#169374=CARTESIAN_POINT ( 'NONE',  ( -10.72451020669870658, -18.67979575497194134, 29.58442372801901854 ) ) ;
#169375=CARTESIAN_POINT ( 'NONE',  ( 13.89961937509957401, 13.97604488694547697, 71.87609039468567573 ) ) ;
#169376=CARTESIAN_POINT ( 'NONE',  ( -16.55341960407611168, -4.379528057220339221, 31.45724293864769550 ) ) ;
#169377=CARTESIAN_POINT ( 'NONE',  ( -10.72451020669898014, 18.67979575497178502, 85.41557627198102409 ) ) ;
#169378=CARTESIAN_POINT ( 'NONE',  ( 18.62759615963271287, -10.81492255796078972, 23.33224293864769194 ) ) ;
#169379=CARTESIAN_POINT ( 'NONE',  ( 12.14591786802309770, 12.06949235617756955, 74.37390960531436690 ) ) ;
#169380=CARTESIAN_POINT ( 'NONE',  ( -9.474510206698964154, 16.51473224551069663, 30.41557627198102054 ) ) ;
#169381=CARTESIAN_POINT ( 'NONE',  ( -0.05219959533936034679, 19.03943276465977164, 22.50109039468566152 ) ) ;
#169382=CARTESIAN_POINT ( 'NONE',  ( -8.314922557961024197, 14.29746914071037800, 102.9177570613523756 ) ) ;
#169383=CARTESIAN_POINT ( 'NONE',  ( -16.55341960407617563, 4.379528057220093196, 53.54275706135234714 ) ) ;
#169384=CARTESIAN_POINT ( 'NONE',  ( -18.67979575497178146, -10.72451020669898902, 36.66557627198103120 ) ) ;
#169385=CARTESIAN_POINT ( 'NONE',  ( -21.55341960407619339, 5.719274019375674811, 113.5427570613523756 ) ) ;
#169386=CARTESIAN_POINT ( 'NONE',  ( -13.89961937509977652, 13.97604488694528158, 85.62390960531433848 ) ) ;
#169387=CARTESIAN_POINT ( 'NONE',  ( 8.314922557961029526, -14.29746914071037800, 55.41775706135234714 ) ) ;
#169388=CARTESIAN_POINT ( 'NONE',  ( 9.564922557960805705, 16.46253265017160317, 24.58224293864769194 ) ) ;
#169389=CARTESIAN_POINT ( 'NONE',  ( 14.29746914071049879, -8.314922557960816363, 33.33224293864769550 ) ) ;
#169390=CARTESIAN_POINT ( 'NONE',  ( -9.564922557960796823, -16.46253265017161027, 107.0822429386476955 ) ) ;
#169391=CARTESIAN_POINT ( 'NONE',  ( 13.89961937509977652, -13.97604488694527269, 93.12390960531436690 ) ) ;
#169392=CARTESIAN_POINT ( 'NONE',  ( 19.05341960407611168, 5.049401038298154454, 103.9572429386476671 ) ) ;
#169394=CARTESIAN_POINT ( 'NONE',  ( 12.06949235617757843, -12.14591786802309237, 58.12390960531435979 ) ) ;
#169395=B_SPLINE_CURVE_WITH_KNOTS ( 'NONE', 3,
 ( #134747, #41736, #57899, #181254, #42731, #104393, #166076, #27579, #89217, #31521, #126501, #111335, #1160, #93174, #157851, #188199, #65823, #189197, #172020, #154859, #96162, #3166, #139672, #50672, #95168, #34504, #2168, #140676, #156856, #64839, #17346, #112332 ),
 .UNSPECIFIED., .F., .F.,
 ( 4, 2, 2, 2, 2, 2, 2, 2, 2, 2, 2, 2, 2, 2, 2, 4 ),
 ( 2.711112516444420852E-17, 0.0003712461730037074862, 0.0007424923460073878673, 0.001113738519011068248, 0.001484984692014748630, 0.002227477038022109609, 0.002598723211025793026, 0.002969969384029457361, 0.003341215557033121696, 0.003712461730036786031, 0.004083707903040450365, 0.004454954076044115134, 0.004826200249047779903, 0.005197446422051443804, 0.005568692595055108573, 0.005939938768058773341 ),
 .UNSPECIFIED. ) ;
#169396=CARTESIAN_POINT ( 'NONE',  ( 14.34966873604960469, 8.224510206698951720, 39.16557627198102409 ) ) ;
#169397=CARTESIAN_POINT ( 'NONE',  ( 14.29746914071049879, -8.314922557960816363, 48.33224293864770260 ) ) ;
#169398=CARTESIAN_POINT ( 'NONE',  ( 4.483927247898790824, -16.52544592524335698, 40.20942372801901854 ) ) ;
#169401=CARTESIAN_POINT ( 'NONE',  ( 16.51473224551083163, -9.474510206698727899, 45.83442372801900433 ) ) ;
#169402=CARTESIAN_POINT ( 'NONE',  ( 19.03943276465977164, -0.05219959533909143690, 83.74890960531436690 ) ) ;
#169403=CARTESIAN_POINT ( 'NONE',  ( -13.97604488694547697, 13.89961937509957934, 68.12609039468563310 ) ) ;
#169405=CARTESIAN_POINT ( 'NONE',  ( -5.049401038297874678, -19.05341960407617918, 54.79275706135234003 ) ) ;
#169406=CARTESIAN_POINT ( 'NONE',  ( 5.049401038297881783, 19.05341960407617563, 97.29275706135233293 ) ) ;
#169407=CARTESIAN_POINT ( 'NONE',  ( -0.05219959533934338120, 16.53943276465976808, 82.50109039468568994 ) ) ;
#169411=CARTESIAN_POINT ( 'NONE',  ( -5.823673210054116645, -21.52544592524344225, 22.29057627198102765 ) ) ;
#169412=CARTESIAN_POINT ( 'NONE',  ( 15.72974639402176855, 15.80617190586768217, 36.87609039468568994 ) ) ;
#169413=CARTESIAN_POINT ( 'NONE',  ( -5.153800228976607833, 19.02544592524334988, 107.7094237280189759 ) ) ;
#169414=CARTESIAN_POINT ( 'NONE',  ( 15.50000000000000178, 5.499999999999998224, 22.00000000000000000 ) ) ;
#169415=CARTESIAN_POINT ( 'NONE',  ( 5.153800228976335163, 19.02544592524342804, 64.79057627198100988 ) ) ;
#169416=CARTESIAN_POINT ( 'NONE',  ( -0.05219959533909027116, -19.03943276465977164, 107.4989096053143527 ) ) ;
#169417=CARTESIAN_POINT ( 'NONE',  ( -16.52544592524342804, 4.483927247898546575, 61.04057627198103120 ) ) ;
#169418=CARTESIAN_POINT ( 'NONE',  ( -16.51473224551069308, -9.474510206698971260, 66.66557627198102409 ) ) ;
#169419=CARTESIAN_POINT ( 'NONE',  ( -5.153800228976328057, -19.02544592524343514, 77.29057627198099567 ) ) ;
#169420=CARTESIAN_POINT ( 'NONE',  ( 9.564922557961047289, -16.46253265017146816, 75.41775706135234714 ) ) ;
#169421=CARTESIAN_POINT ( 'NONE',  ( -10.72451020669898014, 18.67979575497178502, 50.41557627198103120 ) ) ;
#169422=CARTESIAN_POINT ( 'NONE',  ( -14.34966873604960291, -8.224510206698953496, 111.6655762719810525 ) ) ;
#169423=CARTESIAN_POINT ( 'NONE',  ( 13.89961937509957401, 13.97604488694547697, 46.87609039468565442 ) ) ;
#169424=CARTESIAN_POINT ( 'NONE',  ( 9.564922557960805705, 16.46253265017160317, 79.58224293864769550 ) ) ;
#169425=CARTESIAN_POINT ( 'NONE',  ( -0.05219959533907301413, -21.53943276465977519, 82.49890960531436690 ) ) ;
#169426=CARTESIAN_POINT ( 'NONE',  ( -14.34966873604960291, -8.224510206698953496, 86.66557627198102409 ) ) ;
#169427=CARTESIAN_POINT ( 'NONE',  ( -19.03943276465977164, -0.05219959533935918106, 28.75109039468566507 ) ) ;
#169428=CARTESIAN_POINT ( 'NONE',  ( -18.62759615963270932, 10.81492255796079327, 55.83224293864770260 ) ) ;
#169430=CARTESIAN_POINT ( 'NONE',  ( 5.823673210054125526, 21.52544592524343514, 39.79057627198103830 ) ) ;
#169431=CARTESIAN_POINT ( 'NONE',  ( 10.72451020669871369, 18.67979575497193778, 97.08442372801904696 ) ) ;
#169432=CARTESIAN_POINT ( 'NONE',  ( -5.049401038298153566, 19.05341960407611168, 60.20724293864768129 ) ) ;
#169433=CARTESIAN_POINT ( 'NONE',  ( -9.474510206698964154, 16.51473224551069663, 25.41557627198103120 ) ) ;
#169435=CARTESIAN_POINT ( 'NONE',  ( 10.81492255796106328, -18.62759615963255655, 25.41775706135235779 ) ) ;
#169436=CARTESIAN_POINT ( 'NONE',  ( -19.35543954521081389, -5.499999999999585221, 39.58901960356453031 ) ) ;
#169437=CARTESIAN_POINT ( 'NONE',  ( 15.72974639402176855, 15.80617190586768217, 46.87609039468568994 ) ) ;
#169438=CARTESIAN_POINT ( 'NONE',  ( -13.89961937509977652, 13.97604488694528158, 40.62390960531435979 ) ) ;
#169439=CARTESIAN_POINT ( 'NONE',  ( -21.53943276465977519, 0.05219959533907696930, 111.2489096053143669 ) ) ;
#169441=CARTESIAN_POINT ( 'NONE',  ( 19.02544592524334988, 5.153800228976608722, 46.45942372801899012 ) ) ;
#169442=CARTESIAN_POINT ( 'NONE',  ( 17.60769864724391098, -5.499999999999979572, 76.15024842019164453 ) ) ;
#169443=CARTESIAN_POINT ( 'NONE',  ( 19.03943276465977164, -0.05219959533909143690, 28.74890960531435624 ) ) ;
#169444=FACE_OUTER_BOUND ( 'NONE', #92735, .T. ) ;
#169445=CARTESIAN_POINT ( 'NONE',  ( -4.483927247898782831, 16.52544592524335698, 57.70942372801901143 ) ) ;
#169446=CARTESIAN_POINT ( 'NONE',  ( -5.049401038298153566, 19.05341960407611168, 25.20724293864768484 ) ) ;
#169448=CARTESIAN_POINT ( 'NONE',  ( 9.474510206698971260, -16.51473224551069308, 72.91557627198102409 ) ) ;
#169449=CARTESIAN_POINT ( 'NONE',  ( -8.314922557960811034, -14.29746914071050412, 112.0822429386477097 ) ) ;
#169450=CARTESIAN_POINT ( 'NONE',  ( 15.72974639402199770, -15.80617190586745480, 58.12390960531435979 ) ) ;
#169451=CARTESIAN_POINT ( 'NONE',  ( -14.29746914071037622, -8.314922557961029526, 39.16775706135235424 ) ) ;
#169452=CARTESIAN_POINT ( 'NONE',  ( 15.80617190586769283, -15.72974639402175789, 100.6260903946857184 ) ) ;
#169453=CARTESIAN_POINT ( 'NONE',  ( -5.153800228976328057, -19.02544592524343514, 22.29057627198102765 ) ) ;
#169454=ADVANCED_FACE ( 'NONE', ( #16567 ), #185415, .T. ) ;
#169455=CARTESIAN_POINT ( 'NONE',  ( -12.14591786802309592, -12.06949235617757132, 21.87390960531436690 ) ) ;
#169456=CARTESIAN_POINT ( 'NONE',  ( 4.483927247898545687, 16.52544592524342804, 49.79057627198102409 ) ) ;
#169457=CARTESIAN_POINT ( 'NONE',  ( -19.05341960407611168, -5.049401038298163336, 46.45724293864768129 ) ) ;
#169458=CARTESIAN_POINT ( 'NONE',  ( 10.81492255796106328, -18.62759615963255655, 100.4177570613523471 ) ) ;
#169459=CARTESIAN_POINT ( 'NONE',  ( -15.80617190586745835, -15.72974639402198527, 106.8739096053143811 ) ) ;
#169460=CARTESIAN_POINT ( 'NONE',  ( 5.719274019375673035, 21.55341960407619339, 67.29275706135234714 ) ) ;
#169461=CARTESIAN_POINT ( 'NONE',  ( -16.52544592524335698, -4.483927247898792601, 53.95942372801900433 ) ) ;
#169462=CARTESIAN_POINT ( 'NONE',  ( -16.55341960407611168, -4.379528057220339221, 76.45724293864769550 ) ) ;
#169463=CARTESIAN_POINT ( 'NONE',  ( 15.80617190586769283, -15.72974639402175789, 100.6260903946857184 ) ) ;
#169464=CARTESIAN_POINT ( 'NONE',  ( -8.314922557960811034, -14.29746914071050412, 22.08224293864769194 ) ) ;
#169465=CARTESIAN_POINT ( 'NONE',  ( -16.79531203550645557, 7.028104445595627858, 113.7475501177956119 ) ) ;
#169466=CARTESIAN_POINT ( 'NONE',  ( 4.483927247898790824, -16.52544592524335698, 35.20942372801901854 ) ) ;
#169467=CARTESIAN_POINT ( 'NONE',  ( 12.06949235617757843, -12.14591786802309237, 43.12390960531435269 ) ) ;
#169468=CARTESIAN_POINT ( 'NONE',  ( 16.52544592524335698, 4.483927247898782831, 91.45942372801901854 ) ) ;
#169469=CARTESIAN_POINT ( 'NONE',  ( 13.97604488694527802, 13.89961937509977652, 99.37390960531436690 ) ) ;
#169470=CARTESIAN_POINT ( 'NONE',  ( 21.55341960407610458, 5.719274019375980345, 23.95724293864769550 ) ) ;
#169471=CARTESIAN_POINT ( 'NONE',  ( -10.81492255796105439, 18.62759615963255655, 92.91775706135236135 ) ) ;
#169472=CARTESIAN_POINT ( 'NONE',  ( -16.53943276465976808, -0.05219959533934237506, 98.75109039468568994 ) ) ;
#169473=CARTESIAN_POINT ( 'NONE',  ( 12.14591786802309770, 12.06949235617756955, 74.37390960531436690 ) ) ;
#169474=CARTESIAN_POINT ( 'NONE',  ( 19.05341960407611168, 5.049401038298154454, 78.95724293864769550 ) ) ;
#169475=ORIENTED_EDGE ( 'NONE', *, *, #193154, .F. ) ;
#169476=CARTESIAN_POINT ( 'NONE',  ( 16.55341960407618274, -4.379528057220086978, 26.04275706135235779 ) ) ;
#169477=CARTESIAN_POINT ( 'NONE',  ( 16.46253265017160672, -9.564922557960803928, 43.33224293864769550 ) ) ;
#169478=CARTESIAN_POINT ( 'NONE',  ( -19.02544592524342804, 5.153800228976336051, 96.04057627198103830 ) ) ;
#169479=CARTESIAN_POINT ( 'NONE',  ( -0.05219959533934338120, 16.53943276465976808, 37.50109039468568284 ) ) ;
#169481=CARTESIAN_POINT ( 'NONE',  ( -16.51473224551082808, 9.474510206698731452, 33.33442372801899722 ) ) ;
#169482=CARTESIAN_POINT ( 'NONE',  ( 12.14591786802327356, -12.06949235617739191, 95.62609039468568994 ) ) ;
#169483=CARTESIAN_POINT ( 'NONE',  ( 16.46253265017160672, -9.564922557960803928, 38.33224293864768839 ) ) ;
#169484=CARTESIAN_POINT ( 'NONE',  ( 8.224510206698742110, 14.34966873604972548, 77.08442372801901854 ) ) ;
#169485=CARTESIAN_POINT ( 'NONE',  ( -12.14591786802326823, 12.06949235617739902, 73.12609039468567573 ) ) ;
#169486=CARTESIAN_POINT ( 'NONE',  ( -9.474510206698720793, -16.51473224551083518, 79.58442372801899012 ) ) ;
#169487=CARTESIAN_POINT ( 'NONE',  ( -0.05219959533936034679, 19.03943276465977164, 22.50109039468566152 ) ) ;
#169488=CARTESIAN_POINT ( 'NONE',  ( -16.51473224551069308, -9.474510206698971260, 51.66557627198102409 ) ) ;
#169489=CARTESIAN_POINT ( 'NONE',  ( -8.224510206698948167, 14.34966873604960824, 85.41557627198102409 ) ) ;
#169490=CARTESIAN_POINT ( 'NONE',  ( -19.03943276465977164, -0.05219959533935918106, 58.75109039468566863 ) ) ;
#169491=CARTESIAN_POINT ( 'NONE',  ( -10.81492255796078084, -18.62759615963271287, 57.08224293864769550 ) ) ;
#169492=CARTESIAN_POINT ( 'NONE',  ( 9.564922557961047289, -16.46253265017146816, 30.41775706135232937 ) ) ;
#169493=CARTESIAN_POINT ( 'NONE',  ( -9.474510206698964154, 16.51473224551069663, 100.4155762719810241 ) ) ;
#169495=CARTESIAN_POINT ( 'NONE',  ( -5.823673210054116645, -21.52544592524344225, 82.29057627198103830 ) ) ;
#169496=CARTESIAN_POINT ( 'NONE',  ( 13.97604488694527802, 13.89961937509977652, 109.3739096053143669 ) ) ;
#169497=CARTESIAN_POINT ( 'NONE',  ( -5.153800228976607833, 19.02544592524334988, 97.70942372801900433 ) ) ;
#169498=CARTESIAN_POINT ( 'NONE',  ( -16.46253265017160317, 9.564922557960807481, 115.8322429386477097 ) ) ;
#169499=CARTESIAN_POINT ( 'NONE',  ( -9.564922557961040184, 16.46253265017147172, 112.9177570613523329 ) ) ;
#169500=CARTESIAN_POINT ( 'NONE',  ( -9.564922557960796823, -16.46253265017161027, 32.08224293864769550 ) ) ;
#169501=CARTESIAN_POINT ( 'NONE',  ( 19.05341960407611168, 5.049401038298154454, 98.95724293864766707 ) ) ;
#169502=CARTESIAN_POINT ( 'NONE',  ( 21.52544592524344225, -5.823673210054117533, 73.54057627198102409 ) ) ;
#169503=CARTESIAN_POINT ( 'NONE',  ( -12.06949235617739369, -12.14591786802326823, 44.37609039468567573 ) ) ;
#169504=CARTESIAN_POINT ( 'NONE',  ( -15.80617190586768217, 15.72974639402176855, 58.12609039468568994 ) ) ;
#169505=CARTESIAN_POINT ( 'NONE',  ( 9.564922557961047289, -16.46253265017146816, 100.4177570613523329 ) ) ;
#169506=CARTESIAN_POINT ( 'NONE',  ( -0.05219959533937732626, 21.53943276465977519, 107.5010903946856899 ) ) ;
#169507=CARTESIAN_POINT ( 'NONE',  ( 16.52544592524342804, -4.483927247898539470, 23.54057627198102765 ) ) ;
#169508=CARTESIAN_POINT ( 'NONE',  ( -21.52544592524343514, 5.823673210054127303, 106.0405762719810525 ) ) ;
#169509=CARTESIAN_POINT ( 'NONE',  ( 8.224510206698953496, -14.34966873604960469, 37.91557627198102409 ) ) ;
#169510=CARTESIAN_POINT ( 'NONE',  ( -13.97604488694547697, 13.89961937509957934, 78.12609039468567573 ) ) ;
#169511=CARTESIAN_POINT ( 'NONE',  ( 10.81492255796106328, -18.62759615963255655, 55.41775706135234714 ) ) ;
#169512=CARTESIAN_POINT ( 'NONE',  ( 0.05219959533936267826, -19.03943276465977164, 25.00109039468566152 ) ) ;
#169513=CARTESIAN_POINT ( 'NONE',  ( 14.34966873604960469, 8.224510206698951720, 99.16557627198100988 ) ) ;
#169514=CARTESIAN_POINT ( 'NONE',  ( -5.823673210054116645, -21.52544592524344225, 37.29057627198102409 ) ) ;
#169515=CARTESIAN_POINT ( 'NONE',  ( -14.29746914071049879, 8.314922557960819915, 40.83224293864769550 ) ) ;
#169516=CARTESIAN_POINT ( 'NONE',  ( -5.719274019375665041, -21.55341960407619695, 99.79275706135234714 ) ) ;
#169517=CARTESIAN_POINT ( 'NONE',  ( 4.379528057220092307, 16.55341960407617563, 57.29275706135234714 ) ) ;
#169518=CARTESIAN_POINT ( 'NONE',  ( -14.34966873604972548, 8.224510206698743886, 113.3344237280190328 ) ) ;
#169519=CARTESIAN_POINT ( 'NONE',  ( -5.823673210054431948, 21.52544592524334988, 67.70942372801901854 ) ) ;
#169520=CARTESIAN_POINT ( 'NONE',  ( 10.81492255796106328, -18.62759615963255655, 50.41775706135235424 ) ) ;
#169522=CARTESIAN_POINT ( 'NONE',  ( 16.46253265017160672, -9.564922557960803928, 28.33224293864769550 ) ) ;
#169523=CARTESIAN_POINT ( 'NONE',  ( 18.62759615963255655, 10.81492255796105972, 36.66775706135234714 ) ) ;
#169524=CARTESIAN_POINT ( 'NONE',  ( 8.314922557960818139, 14.29746914071049879, 109.5822429386476955 ) ) ;
#169525=CARTESIAN_POINT ( 'NONE',  ( 9.564922557960805705, 16.46253265017160317, 24.58224293864769194 ) ) ;
#169526=CARTESIAN_POINT ( 'NONE',  ( -14.34966873604960291, -8.224510206698953496, 81.66557627198103830 ) ) ;
#169527=CARTESIAN_POINT ( 'NONE',  ( 0.05219959533909260263, 19.03943276465977164, 69.99890960531435269 ) ) ;
#169528=CARTESIAN_POINT ( 'NONE',  ( 16.53943276465976808, -0.05219959533910856209, 23.74890960531435269 ) ) ;
#169529=CARTESIAN_POINT ( 'NONE',  ( 18.67979575497178502, 10.72451020669898547, 59.16557627198103120 ) ) ;
#169530=CARTESIAN_POINT ( 'NONE',  ( 4.379528057220339221, -16.55341960407611168, 87.70724293864769550 ) ) ;
#169532=CARTESIAN_POINT ( 'NONE',  ( 10.72451020669898902, -18.67979575497178502, 97.91557627198103830 ) ) ;
#169533=CARTESIAN_POINT ( 'NONE',  ( 16.51473224551069308, 9.474510206698969483, 104.1655762719810241 ) ) ;
#169534=CARTESIAN_POINT ( 'NONE',  ( 19.02544592524343514, -5.153800228976328945, 58.54057627198102409 ) ) ;
#169535=CARTESIAN_POINT ( 'NONE',  ( 9.564922557961047289, -16.46253265017146816, 110.4177570613523471 ) ) ;
#169536=CARTESIAN_POINT ( 'NONE',  ( 10.72451020669898902, -18.67979575497178502, 52.91557627198103830 ) ) ;
#169537=CARTESIAN_POINT ( 'NONE',  ( 10.72451020669871369, 18.67979575497193778, 87.08442372801901854 ) ) ;
#169538=CARTESIAN_POINT ( 'NONE',  ( -16.51473224551069308, -9.474510206698971260, 71.66557627198102409 ) ) ;
#169539=EDGE_CURVE ( 'NONE', #196449, #11730, #115229, .T. ) ;
#169540=CARTESIAN_POINT ( 'NONE',  ( 19.03943276465977164, -0.05219959533909143690, 98.74890960531436690 ) ) ;
#169541=CARTESIAN_POINT ( 'NONE',  ( 8.224510206698742110, 14.34966873604972548, 82.08442372801901854 ) ) ;
#169542=CARTESIAN_POINT ( 'NONE',  ( -10.72451020669870658, -18.67979575497194134, 54.58442372801901143 ) ) ;
#169543=CARTESIAN_POINT ( 'NONE',  ( 18.62759615963255655, 10.81492255796105972, 81.66775706135236135 ) ) ;
#169544=CARTESIAN_POINT ( 'NONE',  ( 15.80617190586746368, 15.72974639402197994, 114.3739096053143527 ) ) ;
#169545=CARTESIAN_POINT ( 'NONE',  ( 14.29746914071037800, 8.314922557961029526, 71.66775706135234714 ) ) ;
#169546=CARTESIAN_POINT ( 'NONE',  ( 10.72451020669898902, -18.67979575497178502, 82.91557627198103830 ) ) ;
#169547=CARTESIAN_POINT ( 'NONE',  ( 13.97604488694548053, -13.89961937509957401, 40.62609039468564731 ) ) ;
#169548=CARTESIAN_POINT ( 'NONE',  ( -18.67979575497178146, -10.72451020669898902, 41.66557627198103120 ) ) ;
#169549=AXIS2_PLACEMENT_3D ( 'NONE', #12692, #106664, #11708 ) ;
#169550=CARTESIAN_POINT ( 'NONE',  ( -13.89961937509977652, 13.97604488694528158, 80.62390960531436690 ) ) ;
#169551=CARTESIAN_POINT ( 'NONE',  ( -8.314922557960811034, -14.29746914071050412, 27.08224293864769550 ) ) ;
#169552=CARTESIAN_POINT ( 'NONE',  ( -16.29526858892873875, 7.335722546920271370, 64.20329402199794799 ) ) ;
#169554=( BOUNDED_SURFACE ( )  B_SPLINE_SURFACE ( 3, 2, ( 
 ( #142216, #127038, #20864, #188745, #7681, #50230, #111884, #35043, #129024, #69365, #131034, #96697, #81515, #143202, #66375, #174562, #82521, #144203, #190725, #179573, #194730, #40025, #72375, #9712, #135060, #70375, #134049, #27886, #162373, #196736, #132043, #195741, #104701, #120845, #117882, #149221, #85526, #100692, #57215, #59176, #181557, #23875, #118889, #41043, #133040, #10712, #147214, #116869, #119872, #102708, #164397, #165392, #180574, #71376, #8705, #24885, #193732, #12705, #86534, #150224, #197711, #42048, #136036, #56200, #178560, #55200, #103712, #25889, #39036, #26885, #101698, #87534, #163388, #58203, #148218, #43035, #88528, #166390, #11720, #73388, #89528, #151216, #74371, #64153, #1469, #16659, #63147, #47000, #15667, #122831, #106677, #124826, #14672, #182544, #92487, #61159, #44026, #76333, #186526, #79314, #75344, #62147, #138994, #60170, #17654, #138010, #170337, #199694, #473, #109654, #184520, #107655, #154176, #156156, #46000, #90511, #2471, #152193, #169332, #13677, #48000, #137013, #198703, #121839, #77326, #31830, #171336, #93480, #32824, #94475, #108659, #105687, #123811, #30840, #140983, #185509, #155167, #183533, #78307, #153170, #139980, #45017, #167374, #28870, #168350, #29846, #91483, #159124, #191466, #7437, #4440, #35792, #172322, #141970, #84275, #66128, #81278, #161132, #5442, #128784, #65136, #127793, #34802, #189493, #143962, #125817, #67126, #174322, #114619, #50971, #142960, #126793, #20620, #96457, #21624, #157157, #82270, #176318, #48986, #83281, #18652, #190484, #52944, #187520, #112630, #97439, #33811, #3459, #145956, #51956, #113616, #22628, #175310, #36776, #188499, #98441, #158144, #160136, #144955, #110641, #6436, #95471, #68118, #80298, #129770, #37788, #19636, #99452, #49978, #111642, #173327, #71132, #147980, #195494, #40795, #101447, #115637, #54959, #23630, #42799, #116631, #180333, #27647, #102464, #166144, #86290, #8458, #162134, #148978, #194485, #150977, #10467, #131803, #9469, #100454, #165147, #85278, #26638, #163139, #134816, #130788, #146970, #103468, #39783, #132798, #69121, #88281, #149969, #11475, #133802, #164152, #55957, #193482, #73146, #24642, #192479, #179332, #117633, #53962, #25649, #196496, #89286, #70131, #72128, #87294, #178320, #104461, #56968, #118641, #41801, #57966, #119637, #181320, #177326, #38797, #189016, #14424, #120609, #35309, #182303, #76089, #43784, #34322, #105448, #167132, #28632, #48509, #64660, #95984, #126322, #157669, #3963, #79827, #168108, #13441, #110163, #183292, #111153, #90269, #171842, #65643, #135803, #172842, #151952, #33330, #80806, #96963, #91237, #125341, #58940, #75105, #173843, #152927, #29605, #50490, #94990, #18170, #136772, #137764, #121597, #199448, #156675, #74132, #141497, #12471, #19158, #197474, #2981, #60916, #106427, #187039, #198458, #59930, #142485, #188019, #49491, #127305, #112153, #44774, #128299, #54472, #131305, #66636, #113135, #116142, #162644, #23140, #189998, #82788, #160645, #100959, #39301, #159637, #190987, #51473, #36289, #177833, #194005, #130284, #176835, #174825, #22137, #175823, #37296, #38306, #115142, #84785, #24151, #69639, #70647, #143467, #40301, #191978, #97945, #21133, #146464, #144470, #85802, #83787, #158643, #20135, #192995, #145466, #5954, #114121, #52463, #147488, #98955, #6948, #67631, #8979, #4951, #7956, #68628, #129291, #132313, #53465, #99961, #55468, #161645, #117138, #178832, #81780, #89795, #90771, #120128, #183799, #118151, #73650, #56472, #121117, #197974, #11986, #151478, #194995, #135322, #59444, #101977, #41312, #29134, #103973, #165652, #181819, #163657, #196994, #122110, #44294, #86802, #43298, #42312, #196008, #58461, #25160, #179841, #182811, #27150, #180835, #28154, #104966, #134322, #166653, #137286, #105953, #88797, #149479, #12969, #60435, #74633, #198968, #119153, #102972, #164657, #136299, #150490, #148488, #167637, #26152 ),
 ( #152455, #13941, #9979, #71639, #75607, #133306, #87794, #10975, #72648, #57483, #170614, #127069, #45286, #156434, #108933, #169613, #746, #139270, #79588, #124090, #62418, #14945, #49258, #30112, #171609, #185789, #199964, #187789, #47277, #61429, #33097, #76605, #91753, #123100, #106939, #94753, #34088, #63428, #168612, #184786, #16931, #46272, #64423, #141257, #155441, #17934, #138283, #78584, #2747, #153447, #107927, #172602, #32103, #3731, #126092, #77599, #125104, #93760, #1750, #31110, #92758, #154447, #80572, #186802, #110916, #15940, #109927, #140258, #48272, #95747, #157432, #18927, #142246, #65408, #174596, #6713, #188777, #176596, #114902, #177598, #37060, #192754, #7713, #39066, #83552, #98719, #8737, #159401, #21902, #84548, #20896, #129054, #190755, #158417, #146226, #161410, #96728, #143233, #69398, #54237, #53226, #19905, #112902, #52229, #131065, #115908, #189769, #82554, #81547, #66405, #100723, #23906, #160413, #68391, #4716, #113886, #5720, #67398, #130043, #145231, #38070, #162404, #99726, #85560, #173604, #70406, #191743, #128067, #51242, #22902, #36062, #147246, #175584, #50260, #111916, #35074, #97710, #144236, #87563, #25919, #166421, #10741, #149250, #101733, #136066, #116900, #58232, #72405, #86564, #74400, #134082, #148247, #119900, #163421, #178593, #9741, #13708, #181585, #120875, #150256, #132074, #71405, #103741, #133069, #151245, #27916, #42077, #43063, #24919, #165421, #89559, #193763, #194759, #59206, #195772, #90541, #104729, #164426, #11750, #180604, #88557, #40056, #56231, #117913, #167405, #73417, #12734, #179602, #196764, #57245, #118919, #41074, #197740, #102738, #182575, #44058, #26915, #135088, #55231, #105718, #28901, #152223, #156188, #141016, #140013, #171368, #108691, #17687, #76366, #107686, #183564, #153200, #32856, #110672, #47034, #93514, #106707, #77359, #92519, #154209, #155200, #31861, #1501, #79345, #186558, #187550, #60201, #157187, #170369, #45049, #168381, #63179, #14705, #2503, #506, #75374, #137044, #48030, #139027, #199724, #30873, #169364, #109687, #15698, #62178, #29876, #64183, #121871, #124859, #123842, #91514, #125849, #185540, #138043, #94506, #61190, #122862, #184550, #198736, #49017, #172352, #16689, #46031, #78339, #33841, #95501, #37822, #114651, #128813, #68148, #111673, #51986, #176349, #100484, #158174, #145985, #20648, #177356, #191498, #50998, #98472, #67156, #175339, #3488, #173360, #34830, #53993, #36806, #129799, #126824, #83309, #143992, #5473, #65165, #161163, #188530, #144986, #52974, #4468, #160166, #18681, #6467, #99482, #21656, #22659, #84306, #7468, #69152, #113645, #130818, #190512, #192509, #115667, #38826, #80328, #142000, #50007, #189526, #96485, #19665, #112659, #159152, #82302, #81306, #142990, #66157, #127820, #174350, #35821, #97467, #26669, #70162, #86321, #164180, #104491, #193513, #25678, #179360, #40823, #180362, #118671, #88310, #166173, #73175, #74160, #147000, #43812, #133832, #131831, #54989, #149998, #39812, #89314, #87323, #162163, #23660, #134846, #149008, #148008, #117663, #55987, #196524, #102495, #10496, #116658, #27674, #8486, #11504, #72157, #178349, #151007, #195523, #101477, #57995, #163167, #24671, #9498, #85308, #119665, #12498, #41830, #71162, #132827, #56996, #194513, #181347, #42826, #103497, #135832, #165175, #197501, #58968, #120636, #182334, #32610, #107443, #63940, #78097, #137795, #185296, #153959, #61932, #90296, #59959, #198486, #140768, #123601, #154952, #13469, #170122, #30622, #92275, #151980, #47787, #75132, #31617, #139766, #91265, #46787, #105475, #93267, #16448, #108446, #186306, #171121, #1254, #62931, #138783, #94264, #15457, #109438, #124611, #155943, #264, #77113, #125608, #76117, #17439, #79095, #199479, #45791, #169117, #136802, #2257, #187307, #121625, #183321, #167162, #28661, #44802, #106457, #29632, #168136, #152956, #14454, #60945, #122620 ),
 ( #184310, #144748, #21414, #156946, #3254, #6233, #52738, #113408, #18443, #173118, #50765, #191263, #129565, #49766, #81076, #80094, #126587, #67912, #84069, #20408, #66912, #141762, #112423, #65915, #127588, #128576, #5231, #175099, #114405, #159925, #160928, #33600, #130576, #82057, #64927, #188289, #36567, #111431, #176106, #174114, #48778, #110432, #83072, #35584, #34593, #4235, #142755, #37576, #189287, #97230, #96251, #99239, #95263, #98222, #158918, #157938, #22419, #143751, #19429, #145748, #190270, #51747, #7229, #172114, #68914, #181115, #10258, #73929, #8245, #163946, #146750, #11264, #88075, #102259, #41595, #85068, #25444, #149761, #192271, #131589, #119431, #194282, #150768, #164941, #24433, #71918, #40588, #148769, #177118, #69923, #193274, #27434, #133589, #103259, #100244, #56762, #117422, #179120, #38589, #134605, #161926, #118434, #26434, #178109, #195280, #53753, #180127, #72936, #196291, #57761, #42589, #104252, #165935, #87084, #89077, #12265, #115427, #23420, #54747, #116421, #39577, #101236, #162925, #86081, #147772, #9259, #70925, #132592, #55748, #43579, #105244, #123370, #13244, #62695, #60711, #17208, #135598, #46551, #199244, #59726, #91040, #29410, #169892, #14217, #152727, #166931, #139538, #120402, #61701, #75886, #90069, #77871, #137561, #151751, #185063, #28432, #182095, #74907, #197270, #108213, #124377, #153724, #58732, #136571, #107212, #198251, #154723, #31386, #45558, #93035, #121396, #168882, #16217, #183089, #44571, #186072, #122385, #94033, #1022, #167910, #15220, #184074, #92034, #106226, #30387, #76879, #170887, #138550, #47555, #27, #109208, #32379, #155712, #125384, #21178, #187081, #4998, #51517, #64704, #97007, #78861, #66682, #128344, #35356, #159682, #144514, #143511, #174869, #112197, #67678, #127350, #82834, #97988, #129336, #173887, #189063, #98999, #49533, #158689, #36335, #111195, #19203, #80852, #48550, #5999, #113179, #110204, #33372, #191031, #52506, #190043, #171884, #3028, #142529, #114166, #175869, #79870, #172886, #95030, #156720, #37341, #160689, #50535, #20178, #18212, #4007, #96027, #157713, #81824, #140541, #2029, #141539, #63709, #65686, #126366, #188062, #34366, #130327, #151276, #197772, #7998, #43094, #22180, #12765, #74429, #181615, #105749, #90573, #89589, #120907, #58261, #13739, #73446, #28932, #44091, #75408, #119930, #135119, #45081, #193037, #104762, #182606, #54514, #165450, #26947, #192024, #167435, #59238, #53508, #176878, #152254, #137078, #136096, #115185, #146508, #88588, #198767, #60233, #23185, #116187, #38348, #100003, #121904, #183597, #196793, #166451, #161690, #150287, #42109, #103771, #27948, #106738, #83830, #145511, #6992, #68673, #84828, #69682, #131349, #180634, #11782, #186594, #122894, #141053, #185575, #33880, #168413, #109722, #47067, #30905, #139061, #77391, #32892, #62211, #539, #138075, #2539, #153235, #48066, #123878, #61223, #79384, #108727, #184583, #171406, #199756, #14738, #46064, #29908, #94544, #187586, #140049, #91548, #169398, #1538, #92553, #64221, #125886, #78373, #156225, #107718, #63215, #49055, #76399, #170404, #154241, #17725, #15732, #31896, #110710, #93549, #155235, #16725, #172392, #124895, #41761, #184244, #58900, #195454, #165105, #107378, #89244, #104420, #45725, #28593, #151914, #88241, #150937, #57926, #12430, #167092, #10427, #43745, #169050, #91201, #133759, #90230, #74093, #42757, #120566, #72085, #26598, #29570, #135763, #27605, #75067, #182260, #181280, #105407, #30556, #152891, #197434, #196456, #59892, #148937, #13403, #56928, #166103, #149926, #103426, #136733, #198415, #118603, #121558, #11433, #183254, #180293, #44735, #73103, #106391, #168072, #14387, #134773, #119597, #76053, #137729, #199413, #60877, #122554, #126528, #111365, #156884, #173054, #142693, #80033, #170060, #19369, #17375, #174053, #92208, #3193, #155878, #16386, #47722, #186244, #188227, #171055 ),
 ( #112362, #198, #79030, #61867, #34531, #123536, #185230, #46721, #125548, #141702, #96191, #64866, #157880, #81018, #18381, #153892, #110367, #140705, #4173, #32545, #109373, #93203, #187244, #62865, #49700, #108384, #48714, #65851, #15389, #127521, #31551, #172049, #189225, #77046, #94198, #154888, #50703, #124547, #2195, #138717, #78033, #139702, #1188, #63877, #33536, #95198, #31671, #34638, #156992, #186360, #51793, #170178, #81121, #33647, #94316, #125659, #63989, #4282, #48826, #187356, #139818, #174161, #155005, #96298, #110479, #124664, #112468, #172162, #47840, #157984, #1306, #16502, #109492, #93321, #19475, #158964, #188335, #78150, #171175, #141809, #32662, #189333, #65962, #80139, #142801, #62985, #3302, #127633, #155994, #17490, #97276, #95308, #128623, #50810, #2308, #49813, #18491, #126633, #79147, #140819, #64974, #5280, #111478, #35631, #173163, #20455, #82105, #143797, #66962, #190316, #21458, #39623, #86128, #99285, #131636, #113452, #101283, #162973, #69970, #194327, #179165, #178158, #9305, #146799, #102302, #161970, #117467, #132639, #163991, #8292, #23466, #133636, #84114, #193320, #70971, #145793, #53798, #115473, #83119, #55795, #147819, #144796, #67957, #40633, #25488, #24478, #6279, #37623, #177162, #87130, #148815, #114452, #7276, #129612, #191307, #10305, #71962, #85115, #54794, #52783, #38635, #130622, #192318, #175145, #68960, #195327, #36613, #176153, #116469, #98269, #160972, #159971, #100292, #22466, #89123, #74949, #184122, #73973, #182138, #166973, #30434, #58776, #164984, #76923, #26479, #120444, #88121, #75932, #149805, #11311, #72981, #90110, #106268, #137607, #167953, #199290, #45604, #121438, #138594, #136612, #105285, #107257, #197312, #12307, #57804, #151794, #27480, #152771, #134650, #13285, #168928, #180171, #14263, #196336, #198293, #122430, #56807, #135642, #28476, #103305, #119475, #15265, #43621, #59770, #92081, #183131, #44614, #181158, #29452, #165979, #91084, #60757, #118481, #153770, #41640, #42634, #104297, #150811, #140583, #94076, #110245, #123414, #77914, #80895, #2073, #78906, #126408, #171927, #32421, #95075, #35398, #4051, #125426, #47597, #111240, #158731, #33416, #97049, #17253, #139581, #93081, #79910, #187122, #81869, #141581, #62741, #63752, #31428, #96068, #154765, #157757, #155755, #65728, #61746, #16263, #34410, #170930, #48594, #76, #19248, #142572, #109250, #156763, #18257, #169937, #173929, #1066, #3069, #64746, #188104, #49577, #172931, #127397, #189106, #50579, #112239, #20221, #185107, #108257, #46597, #124421, #186117, #113225, #162736, #174915, #36379, #98033, #176924, #193084, #24244, #54559, #85893, #132404, #8049, #25252, #161737, #192073, #194097, #83876, #99045, #144560, #38395, #114212, #39391, #159730, #100051, #55559, #66729, #101051, #21226, #23232, #9067, #143560, #22227, #53554, #190085, #82882, #102067, #145558, #160735, #178926, #84876, #146553, #6046, #7036, #52551, #68718, #69728, #5043, #131396, #163752, #147581, #128389, #116232, #130375, #37388, #115233, #51561, #67724, #70737, #177923, #117233, #40396, #129382, #175917, #191078, #122197, #90856, #12079, #134416, #198065, #45374, #120218, #183889, #104064, #26244, #179935, #166743, #73742, #168699, #28246, #149571, #165745, #118244, #182900, #41402, #44384, #119242, #152541, #148578, #103067, #121209, #57572, #88888, #86894, #106039, #167725, #196102, #27239, #197085, #56570, #60522, #87883, #150580, #180926, #58552, #135414, #10068, #42401, #29223, #107027, #164749, #89886, #43387, #11067, #71728, #181908, #74724, #105059, #72745, #151569, #13058, #14029, #136388, #59531, #75694, #137374, #133398, #199052, #195087, #184877, #172693, #32191, #46359, #156527, #61519, #15033, #108017, #112009, #18026, #19017, #48363, #30201, #169703, #1839, #31197, #49345, #126182, #140351, #79679, #123188, #63521, #187877, #91842, #92848, #157523, #93849 ),
 ( #94846, #155527, #17022, #76693, #34178, #138370, #141350, #2837, #16030, #110018, #153536, #64515, #111007, #186892, #95839, #80663, #142339, #3819, #125196, #65497, #78675, #127159, #188867, #50350, #171698, #33187, #200050, #837, #154533, #77688, #62510, #170702, #139356, #124182, #185883, #47368, #109023, #128158, #69491, #177686, #38163, #81637, #97802, #175675, #115997, #54325, #174686, #5813, #143319, #51332, #131156, #8825, #145322, #191835, #4806, #37149, #190843, #52319, #53316, #130138, #99818, #39154, #84641, #85651, #158506, #114994, #70494, #192845, #23994, #35166, #161503, #160502, #189858, #55318, #173698, #146318, #98808, #100810, #162494, #22993, #147338, #6805, #132161, #21992, #193853, #96821, #19993, #68483, #83645, #66495, #144324, #176688, #112992, #67488, #113977, #7807, #36150, #159491, #20985, #82641, #129146, #12824, #120965, #181672, #25008, #41165, #119009, #59297, #197831, #118004, #149335, #86652, #194849, #74490, #152312, #88649, #135178, #148336, #180692, #134173, #195861, #196852, #73506, #43152, #182664, #28007, #28990, #101822, #58318, #13798, #136156, #167494, #178683, #104820, #103828, #133157, #198824, #116989, #89647, #42168, #102828, #72499, #10830, #151335, #57333, #165508, #9831, #44148, #163510, #166509, #27005, #71491, #105807, #150345, #56321, #90630, #179693, #164514, #26007, #40145, #75464, #137137, #119986, #87649, #11841, #31951, #14796, #79437, #156281, #170460, #109776, #153295, #93606, #17782, #142095, #199814, #187640, #62266, #18775, #32947, #92608, #140105, #108782, #16781, #45139, #76456, #138133, #95595, #78430, #171459, #168470, #124952, #185632, #47124, #106796, #2596, #29968, #186648, #94602, #46121, #1596, #60289, #48119, #141108, #63272, #121962, #64275, #122952, #77448, #91607, #125942, #61282, #49111, #154298, #110768, #183655, #184640, #172450, #30961, #123934, #107775, #33937, #157279, #169460, #595, #155291, #15788, #80422, #139119, #8328, #115510, #116504, #85149, #65258, #100326, #25522, #103338, #96578, #86164, #163007, #81397, #41674, #38671, #194362, #162005, #24514, #133670, #23501, #131673, #178192, #180205, #70003, #111765, #26511, #173454, #193354, #34923, #87168, #158267, #19756, #143083, #39657, #55829, #148849, #117502, #10340, #195361, #71006, #88155, #147854, #54830, #56840, #146835, #101318, #4562, #9341, #177198, #102336, #66254, #132674, #118515, #126918, #164026, #127914, #179199, #71996, #3580, #40667, #165018, #50105, #189616, #188625, #53836, #105318, #185137, #29484, #152805, #89156, #90141, #58810, #151826, #167986, #11344, #44648, #169966, #92112, #134684, #91115, #13315, #43656, #59802, #73015, #27515, #30464, #74981, #28507, #75965, #121472, #182170, #106300, #46628, #153801, #136643, #197347, #60790, #108288, #183164, #31459, #167005, #150845, #42670, #14297, #198326, #149840, #137638, #199325, #57838, #122461, #184154, #45635, #196370, #15295, #119511, #107287, #168958, #135675, #76955, #181192, #138625, #106, #61776, #123444, #104331, #166015, #12341, #74005, #120479, #141614, #97080, #112268, #143591, #188138, #3101, #113254, #63786, #126440, #189137, #125458, #33448, #95107, #62773, #50609, #65760, #1097, #47629, #173960, #158761, #157789, #124454, #17285, #156796, #35427, #20252, #94109, #187155, #186150, #170962, #81898, #128418, #64779, #111272, #109284, #18289, #110279, #171960, #172963, #49609, #19279, #5074, #4082, #66757, #77944, #34441, #190114, #51589, #174945, #154796, #80926, #79944, #32456, #93111, #16294, #127429, #96100, #78939, #48627, #142603, #139611, #155788, #140615, #2105, #40422, #21256, #162761, #53588, #191108, #178952, #38426, #52583, #24270, #67753, #82911, #114242, #118271, #85919, #25279, #54585, #36407, #175949, #8079, #37418, #55585, #132430, #146585, #147607, #129411, #69755, #194122, #98062, #99078, #163778, #100082, #195114, #9095, #68750, #116258, #84906 ),
 ( #71756, #177949, #70762, #144589, #101076, #161767, #23262, #6075, #102093, #160768, #117260, #86922, #22258, #39417, #159761, #148604, #10096, #193111, #133426, #56597, #83907, #145590, #131425, #7068, #130407, #192105, #115264, #176957, #74748, #28271, #200074, #150607, #13083, #75722, #12103, #120242, #181933, #149599, #137398, #152566, #87912, #134442, #199079, #183913, #44410, #11096, #104089, #43414, #122222, #60547, #180950, #73766, #72772, #57598, #45398, #15057, #151592, #198091, #196127, #105084, #197109, #58576, #59556, #136411, #106064, #107051, #90882, #91867, #164776, #121234, #76717, #168724, #30225, #41428, #167750, #166770, #119267, #61542, #179961, #14055, #89910, #165772, #135439, #182927, #153560, #29248, #138393, #42427, #103094, #26270, #27266, #88915, #140379, #48389, #33214, #96847, #125221, #31223, #143346, #92872, #186919, #154559, #142367, #16055, #77713, #139379, #156554, #172722, #3846, #34204, #65525, #112037, #187904, #4834, #141377, #171726, #173725, #63547, #184901, #18054, #123211, #127185, #108043, #2865, #110046, #17047, #94874, #46385, #861, #188896, #79708, #1866, #49373, #64543, #155553, #126208, #158532, #50377, #111036, #170726, #95867, #81663, #157550, #20021, #19043, #62536, #124210, #80690, #35194, #169728, #185908, #47394, #109049, #32218, #93875, #78702, #162519, #98834, #132188, #128184, #82667, #100836, #37175, #68509, #148361, #85676, #24022, #114001, #6830, #176714, #36174, #40171, #5838, #130163, #175699, #38187, #145348, #189882, #160529, #147363, #163534, #159515, #146344, #144351, #22018, #117014, #83670, #54350, #191860, #84665, #193879, #53342, #115021, #99843, #101850, #161527, #174710, #86677, #97827, #23019, #21011, #8852, #67514, #129171, #190869, #7831, #116022, #70519, #177711, #55344, #178709, #131182, #66521, #69517, #192872, #25034, #39179, #51357, #52345, #113018, #180720, #105837, #41191, #104848, #198855, #133183, #167524, #102853, #43180, #75493, #91638, #88679, #120014, #56346, #26031, #168502, #150375, #165537, #45172, #89677, #12854, #149361, #11871, #119038, #73535, #28036, #151363, #164539, #135208, #27034, #196880, #74519, #166538, #136184, #13827, #120995, #121996, #194873, #197859, #106827, #29020, #60321, #71515, #59326, #58346, #87676, #9856, #118029, #182694, #181699, #134202, #44179, #103856, #90660, #10857, #152342, #30000, #137166, #179720, #183686, #72526, #195890, #57365, #42195, #169491, #79475, #184671, #138167, #107809, #34961, #141143, #142130, #171494, #153326, #30991, #124987, #92640, #172485, #49145, #63308, #2633, #46154, #186683, #110803, #14828, #154330, #80456, #155326, #111799, #125977, #185665, #32983, #1631, #109811, #199848, #15820, #77481, #188661, #94636, #64309, #61314, #17817, #78464, #140139, #122984, #95629, #139150, #187675, #33972, #627, #156316, #76490, #157316, #18812, #3614, #65293, #126952, #50140, #173488, #48153, #62298, #123968, #47156, #108815, #170494, #31984, #93641, #16814, #67280, #129929, #192639, #128939, #36940, #98602, #66289, #54122, #69283, #4597, #51125, #115795, #100610, #161293, #127948, #20777, #160296, #38954, #177485, #97592, #190640, #189651, #174479, #162293, #131961, #68278, #23793, #85443, #6599, #146113, #112785, #191628, #147133, #178478, #35946, #8621, #21786, #55118, #130949, #52116, #176479, #145114, #53108, #81431, #159280, #82432, #193646, #114786, #7597, #144120, #22788, #83437, #37955, #143117, #70293, #5601, #84435, #116787, #113772, #99613, #96613, #158302, #19790, #175468, #120761, #105605, #104618, #135959, #73306, #28789, #88443, #43943, #59095, #90428, #134977, #150138, #60090, #10629, #196654, #197629, #72290, #180493, #41965, #9628, #182462, #12625, #148137, #194646, #167292, #152114, #166307, #71295, #164314, #103632, #13597, #75264, #40957, #133968, #132958, #117799, #136935, #198624, #11639, #58123, #56116, #165308, #57131, #118807, #119792 ),
 ( #149139, #181476, #26802, #101616, #195660, #121758, #39945, #179492, #42954, #102629, #27803, #163305, #89444, #151134, #74290, #24803, #86452, #25807, #87453, #93398, #157074, #185428, #91399, #3379, #153088, #46918, #14592, #2388, #76248, #137926, #199610, #16578, #32741, #138911, #184439, #78225, #154091, #79231, #61076, #139896, #172240, #106592, #140902, #122748, #1385, #48905, #65054, #62064, #155084, #29765, #45919, #141888, #123729, #391, #18570, #63066, #186441, #107573, #108578, #92405, #170255, #124745, #44935, #47917, #183451, #125737, #168268, #109571, #31749, #77243, #171254, #169251, #30758, #64067, #94393, #156072, #17570, #187437, #15585, #110559, #80217, #33726, #95388, #174241, #37704, #85192, #160052, #23545, #143878, #66044, #19554, #6356, #51874, #8373, #68036, #189412, #5359, #158063, #22543, #81198, #84190, #159042, #192397, #188414, #142879, #161049, #97356, #128701, #126711, #145870, #7353, #35709, #67042, #36692, #96376, #100370, #127711, #190398, #20535, #98353, #113533, #49892, #82185, #69037, #146881, #4360, #129688, #50888, #175227, #177241, #21539, #114533, #83199, #144873, #53879, #191385, #52861, #176233, #162049, #99366, #34718, #111558, #112546, #130702, #115554, #38713, #173243, #101360, #39698, #103381, #119552, #150890, #181235, #12384, #58853, #134728, #151867, #88196, #118557, #120520, #10382, #24557, #166056, #74046, #196410, #178235, #194402, #72039, #135717, #197388, #71048, #102379, #163050, #147896, #27557, #105359, #41716, #149880, #86206, #133712, #87210, #148892, #11386, #26553, #57880, #182213, #42711, #43697, #54873, #73056, #167046, #89197, #28547, #131716, #104373, #56883, #9382, #70048, #193398, #90184, #195405, #55870, #25566, #164067, #116547, #132714, #117544, #179243, #40710, #180247, #165059, #33250, #170764, #158565, #18087, #32253, #142404, #44688, #198368, #93911, #97862, #3882, #4873, #34240, #13357, #155589, #187939, #17084, #35228, #112072, #126243, #65561, #106342, #49408, #173761, #75021, #78737, #143381, #79743, #174745, #188935, #48426, #95901, #64578, #172760, #59845, #140413, #1903, #51393, #157585, #127221, #121512, #80725, #141412, #2900, #183207, #20054, #63583, #50412, #96882, #125257, #19077, #136686, #81698, #66556, #128221, #189918, #113053, #36209, #186955, #111071, #110082, #171761, #94908, #156593, #9892, #54387, #7869, #179756, #130201, #192910, #55380, #191896, #99879, #161564, #129207, #117050, #132224, #67550, #144388, #114039, #41226, #147401, #148398, #177748, #159552, #175737, #131219, #37214, #178745, #40209, #69555, #8889, #52382, #116060, #101888, #21049, #98870, #86713, #23057, #118066, #193917, #53381, #39217, #100873, #162555, #5873, #160566, #22055, #194909, #24060, #70557, #190905, #85715, #84702, #146381, #83706, #163570, #145384, #25070, #71553, #6866, #133218, #82704, #56384, #68545, #115058, #176751, #38224, #167559, #198889, #136218, #91670, #151398, #106860, #122030, #153361, #197893, #12888, #123018, #73569, #59362, #60357, #135242, #43216, #104884, #72563, #183720, #75528, #10890, #57399, #45206, #168534, #29053, #134238, #27069, #166572, #30032, #14863, #103890, #196914, #195923, #180753, #76524, #138201, #74551, #121031, #119071, #28072, #120048, #181735, #182729, #44213, #90693, #199883, #13861, #61347, #87709, #105872, #184703, #102887, #164572, #26066, #152376, #89713, #42229, #149395, #165570, #137203, #88715, #150410, #58381, #11905, #80489, #185700, #172520, #143148, #173519, #31025, #34005, #63344, #662, #188692, #48187, #62332, #95662, #77515, #142163, #124002, #3647, #78500, #111830, #107841, #47189, #65325, #16849, #109842, #127980, #126985, #50173, #93677, #186717, #156349, #15857, #19821, #108849, #171527, #155360, #17850, #125021, #169525, #140173, #34990, #4629, #139187, #126011, #170529, #1666, #96644, #33015, #157349, #94670, #64342, #158332, #79506, #141175, #2665 ) ),
 .UNSPECIFIED., .T., .F., .T. ) 
 B_SPLINE_SURFACE_WITH_KNOTS ( ( 4, 3, 4 ),
 ( 3, 2, 2, 2, 2, 2, 2, 2, 2, 2, 2, 2, 2, 2, 2, 2, 2, 2, 2, 2, 2, 2, 2, 2, 2, 2, 2, 2, 2, 2, 2, 2, 2, 2, 2, 2, 2, 2, 2, 2, 2, 2, 2, 2, 2, 2, 2, 2, 2, 2, 2, 2, 2, 2, 2, 2, 2, 2, 2, 2, 2, 2, 2, 2, 2, 2, 2, 2, 2, 2, 2, 2, 2, 2, 2, 2, 2, 2, 2, 2, 2, 2, 2, 2, 2, 2, 2, 2, 2, 2, 2, 2, 2, 2, 2, 2, 2, 2, 2, 2, 2, 2, 2, 2, 2, 2, 2, 2, 2, 2, 2, 2, 2, 2, 2, 2, 2, 2, 2, 2, 2, 2, 2, 2, 2, 2, 2, 2, 2, 2, 2, 2, 2, 2, 2, 2, 2, 2, 2, 2, 2, 2, 2, 2, 2, 2, 2, 2, 2, 2, 2, 2, 2, 2, 2, 2, 2, 2, 2, 2, 2, 2, 2, 2, 2, 2, 2, 2, 2, 2, 2, 2, 2, 2, 2, 2, 2, 2, 2, 2, 2, 2, 2, 2, 2, 2, 2, 2, 2, 2, 2, 2, 2, 2, 2, 2, 2, 2, 2, 2, 2, 2, 2, 2, 2, 2, 2, 2, 2, 2, 2, 2, 2, 2, 2, 2, 2, 2, 2, 2, 2, 2, 2, 2, 2, 2, 2, 2, 3 ),
 ( 0.000000000000000000, 0.5000000000000000000, 1.000000000000000000 ),
 ( 0.000000000000000000, 0.004385964912280701511, 0.008771929824561403022, 0.01315789473684210453, 0.01754385964912280604, 0.02192982456140350755, 0.02631578947368420907, 0.03070175438596491058, 0.03508771929824561209, 0.03947368421052631360, 0.04385964912280701511, 0.04824561403508771662, 0.05263157894736841813, 0.05701754385964911964, 0.06140350877192982115, 0.06578947368421052266, 0.07017543859649122417, 0.07456140350877192569, 0.07894736842105262720, 0.08333333333333332871, 0.08771929824561403022, 0.09210526315789473173, 0.09649122807017543324, 0.1008771929824561348, 0.1052631578947368363, 0.1096491228070175378, 0.1140350877192982393, 0.1184210526315789408, 0.1228070175438596423, 0.1271929824561403577, 0.1315789473684210453, 0.1359649122807017607, 0.1403508771929824483, 0.1447368421052631637, 0.1491228070175438514, 0.1535087719298245668, 0.1578947368421052544, 0.1622807017543859698, 0.1666666666666666574, 0.1710526315789473728, 0.1754385964912280604, 0.1798245614035087758, 0.1842105263157894635, 0.1885964912280701788, 0.1929824561403508665, 0.1973684210526315819, 0.2017543859649122695, 0.2061403508771929849, 0.2105263157894736725, 0.2149122807017543879, 0.2192982456140350755, 0.2236842105263157909, 0.2280701754385964786, 0.2324561403508771940, 0.2368421052631578816, 0.2412280701754385970, 0.2456140350877192846, 0.2500000000000000000, 0.2543859649122807154, 0.2587719298245614308, 0.2631578947368420907, 0.2675438596491228060, 0.2719298245614035214, 0.2763157894736842368, 0.2807017543859648967, 0.2850877192982456121, 0.2894736842105263275, 0.2938596491228070429, 0.2982456140350877027, 0.3026315789473684181, 0.3070175438596491335, 0.3114035087719298489, 0.3157894736842105088, 0.3201754385964912242, 0.3245614035087719396, 0.3289473684210526550, 0.3333333333333333148, 0.3377192982456140302, 0.3421052631578947456, 0.3464912280701754610, 0.3508771929824561209, 0.3552631578947368363, 0.3596491228070175517, 0.3640350877192982670, 0.3684210526315789269, 0.3728070175438596423, 0.3771929824561403577, 0.3815789473684210731, 0.3859649122807017330, 0.3903508771929824483, 0.3947368421052631637, 0.3991228070175438791, 0.4035087719298245390, 0.4078947368421052544, 0.4122807017543859698, 0.4166666666666666852, 0.4210526315789473450, 0.4254385964912280604, 0.4298245614035087758, 0.4342105263157894912, 0.4385964912280701511, 0.4429824561403508665, 0.4473684210526315819, 0.4517543859649122973, 0.4561403508771929571, 0.4605263157894736725, 0.4649122807017543879, 0.4692982456140351033, 0.4736842105263157632, 0.4780701754385964786, 0.4824561403508771940, 0.4868421052631579093, 0.4912280701754385692, 0.4956140350877192846, 0.5000000000000000000, 0.5043859649122807154, 0.5087719298245614308, 0.5131578947368421462, 0.5175438596491228616, 0.5219298245614034659, 0.5263157894736841813, 0.5307017543859648967, 0.5350877192982456121, 0.5394736842105263275, 0.5438596491228070429, 0.5482456140350877583, 0.5526315789473684736, 0.5570175438596490780, 0.5614035087719297934, 0.5657894736842105088, 0.5701754385964912242, 0.5745614035087719396, 0.5789473684210526550, 0.5833333333333333703, 0.5877192982456140857, 0.5921052631578946901, 0.5964912280701754055, 0.6008771929824561209, 0.6052631578947368363, 0.6096491228070175517, 0.6140350877192982670, 0.6184210526315789824, 0.6228070175438596978, 0.6271929824561403022, 0.6315789473684210176, 0.6359649122807017330, 0.6403508771929824483, 0.6447368421052631637, 0.6491228070175438791, 0.6535087719298245945, 0.6578947368421053099, 0.6622807017543859143, 0.6666666666666666297, 0.6710526315789473450, 0.6754385964912280604, 0.6798245614035087758, 0.6842105263157894912, 0.6885964912280702066, 0.6929824561403509220, 0.6973684210526315264, 0.7017543859649122417, 0.7061403508771929571, 0.7105263157894736725, 0.7149122807017543879, 0.7192982456140351033, 0.7236842105263158187, 0.7280701754385965341, 0.7324561403508771384, 0.7368421052631578538, 0.7412280701754385692, 0.7456140350877192846, 0.7500000000000000000, 0.7543859649122807154, 0.7587719298245614308, 0.7631578947368421462, 0.7675438596491228616, 0.7719298245614034659, 0.7763157894736841813, 0.7807017543859648967, 0.7850877192982456121, 0.7894736842105263275, 0.7938596491228070429, 0.7982456140350877583, 0.8026315789473684736, 0.8070175438596490780, 0.8114035087719297934, 0.8157894736842105088, 0.8201754385964912242, 0.8245614035087719396, 0.8289473684210526550, 0.8333333333333333703, 0.8377192982456140857, 0.8421052631578946901, 0.8464912280701754055, 0.8508771929824561209, 0.8552631578947368363, 0.8596491228070175517, 0.8640350877192982670, 0.8684210526315789824, 0.8728070175438596978, 0.8771929824561403022, 0.8815789473684210176, 0.8859649122807017330, 0.8903508771929824483, 0.8947368421052631637, 0.8991228070175438791, 0.9035087719298245945, 0.9078947368421053099, 0.9122807017543859143, 0.9166666666666666297, 0.9210526315789473450, 0.9254385964912280604, 0.9298245614035087758, 0.9342105263157894912, 0.9385964912280702066, 0.9429824561403509220, 0.9473684210526315264, 0.9517543859649122417, 0.9561403508771929571, 0.9605263157894736725, 0.9649122807017543879, 0.9692982456140351033, 0.9736842105263158187, 0.9780701754385965341, 0.9824561403508771384, 0.9868421052631578538, 0.9912280701754385692, 0.9956140350877192846, 1.000000000000000000 ),
 .UNSPECIFIED. ) 
 GEOMETRIC_REPRESENTATION_ITEM ( )  RATIONAL_B_SPLINE_SURFACE ( (
 ( 1.000000000000000000, 0.9659258262890683122, 1.000000000000000000, 0.9659258262890683122, 1.000000000000000000, 0.9659258262890683122, 1.000000000000000000, 0.9659258262890683122, 1.000000000000000000, 0.9659258262890683122, 1.000000000000000000, 0.9659258262890683122, 1.000000000000000000, 0.9659258262890683122, 1.000000000000000000, 0.9659258262890683122, 1.000000000000000000, 0.9659258262890683122, 1.000000000000000000, 0.9659258262890683122, 1.000000000000000000, 0.9659258262890683122, 1.000000000000000000, 0.9659258262890683122, 1.000000000000000000, 0.9659258262890683122, 1.000000000000000000, 0.9659258262890683122, 1.000000000000000000, 0.9659258262890683122, 1.000000000000000000, 0.9659258262890683122, 1.000000000000000000, 0.9659258262890683122, 1.000000000000000000, 0.9659258262890683122, 1.000000000000000000, 0.9659258262890683122, 1.000000000000000000, 0.9659258262890683122, 1.000000000000000000, 0.9659258262890683122, 1.000000000000000000, 0.9659258262890683122, 1.000000000000000000, 0.9659258262890683122, 1.000000000000000000, 0.9659258262890683122, 1.000000000000000000, 0.9659258262890683122, 1.000000000000000000, 0.9659258262890683122, 1.000000000000000000, 0.9659258262890683122, 1.000000000000000000, 0.9659258262890683122, 1.000000000000000000, 0.9659258262890683122, 1.000000000000000000, 0.9659258262890683122, 1.000000000000000000, 0.9659258262890683122, 1.000000000000000000, 0.9659258262890683122, 1.000000000000000000, 0.9659258262890683122, 1.000000000000000000, 0.9659258262890683122, 1.000000000000000000, 0.9659258262890683122, 1.000000000000000000, 0.9659258262890683122, 1.000000000000000000, 0.9659258262890683122, 1.000000000000000000, 0.9659258262890683122, 1.000000000000000000, 0.9659258262890683122, 1.000000000000000000, 0.9659258262890683122, 1.000000000000000000, 0.9659258262890683122, 1.000000000000000000, 0.9659258262890683122, 1.000000000000000000, 0.9659258262890683122, 1.000000000000000000, 0.9659258262890683122, 1.000000000000000000, 0.9659258262890683122, 1.000000000000000000, 0.9659258262890683122, 1.000000000000000000, 0.9659258262890683122, 1.000000000000000000, 0.9659258262890683122, 1.000000000000000000, 0.9659258262890683122, 1.000000000000000000, 0.9659258262890683122, 1.000000000000000000, 0.9659258262890683122, 1.000000000000000000, 0.9659258262890683122, 1.000000000000000000, 0.9659258262890683122, 1.000000000000000000, 0.9659258262890683122, 1.000000000000000000, 0.9659258262890683122, 1.000000000000000000, 0.9659258262890683122, 1.000000000000000000, 0.9659258262890683122, 1.000000000000000000, 0.9659258262890683122, 1.000000000000000000, 0.9659258262890683122, 1.000000000000000000, 0.9659258262890683122, 1.000000000000000000, 0.9659258262890683122, 1.000000000000000000, 0.9659258262890683122, 1.000000000000000000, 0.9659258262890683122, 1.000000000000000000, 0.9659258262890683122, 1.000000000000000000, 0.9659258262890683122, 1.000000000000000000, 0.9659258262890683122, 1.000000000000000000, 0.9659258262890683122, 1.000000000000000000, 0.9659258262890683122, 1.000000000000000000, 0.9659258262890683122, 1.000000000000000000, 0.9659258262890683122, 1.000000000000000000, 0.9659258262890683122, 1.000000000000000000, 0.9659258262890683122, 1.000000000000000000, 0.9659258262890683122, 1.000000000000000000, 0.9659258262890683122, 1.000000000000000000, 0.9659258262890683122, 1.000000000000000000, 0.9659258262890683122, 1.000000000000000000, 0.9659258262890683122, 1.000000000000000000, 0.9659258262890683122, 1.000000000000000000, 0.9659258262890683122, 1.000000000000000000, 0.9659258262890683122, 1.000000000000000000, 0.9659258262890683122, 1.000000000000000000, 0.9659258262890683122, 1.000000000000000000, 0.9659258262890683122, 1.000000000000000000, 0.9659258262890683122, 1.000000000000000000, 0.9659258262890683122, 1.000000000000000000, 0.9659258262890683122, 1.000000000000000000, 0.9659258262890683122, 1.000000000000000000, 0.9659258262890683122, 1.000000000000000000, 0.9659258262890683122, 1.000000000000000000, 0.9659258262890683122, 1.000000000000000000, 0.9659258262890683122, 1.000000000000000000, 0.9659258262890683122, 1.000000000000000000, 0.9659258262890683122, 1.000000000000000000, 0.9659258262890683122, 1.000000000000000000, 0.9659258262890683122, 1.000000000000000000, 0.9659258262890683122, 1.000000000000000000, 0.9659258262890683122, 1.000000000000000000, 0.9659258262890683122, 1.000000000000000000, 0.9659258262890683122, 1.000000000000000000, 0.9659258262890683122, 1.000000000000000000, 0.9659258262890683122, 1.000000000000000000, 0.9659258262890683122, 1.000000000000000000, 0.9659258262890683122, 1.000000000000000000, 0.9659258262890683122, 1.000000000000000000, 0.9659258262890683122, 1.000000000000000000, 0.9659258262890683122, 1.000000000000000000, 0.9659258262890683122, 1.000000000000000000, 0.9659258262890683122, 1.000000000000000000, 0.9659258262890683122, 1.000000000000000000, 0.9659258262890683122, 1.000000000000000000, 0.9659258262890683122, 1.000000000000000000, 0.9659258262890683122, 1.000000000000000000, 0.9659258262890683122, 1.000000000000000000, 0.9659258262890683122, 1.000000000000000000, 0.9659258262890683122, 1.000000000000000000, 0.9659258262890683122, 1.000000000000000000, 0.9659258262890683122, 1.000000000000000000, 0.9659258262890683122, 1.000000000000000000, 0.9659258262890683122, 1.000000000000000000, 0.9659258262890683122, 1.000000000000000000, 0.9659258262890683122, 1.000000000000000000, 0.9659258262890683122, 1.000000000000000000, 0.9659258262890683122, 1.000000000000000000, 0.9659258262890683122, 1.000000000000000000, 0.9659258262890683122, 1.000000000000000000, 0.9659258262890683122, 1.000000000000000000, 0.9659258262890683122, 1.000000000000000000, 0.9659258262890683122, 1.000000000000000000, 0.9659258262890683122, 1.000000000000000000, 0.9659258262890683122, 1.000000000000000000, 0.9659258262890683122, 1.000000000000000000, 0.9659258262890683122, 1.000000000000000000, 0.9659258262890683122, 1.000000000000000000, 0.9659258262890683122, 1.000000000000000000, 0.9659258262890683122, 1.000000000000000000, 0.9659258262890683122, 1.000000000000000000, 0.9659258262890683122, 1.000000000000000000, 0.9659258262890683122, 1.000000000000000000, 0.9659258262890683122, 1.000000000000000000, 0.9659258262890683122, 1.000000000000000000, 0.9659258262890683122, 1.000000000000000000, 0.9659258262890683122, 1.000000000000000000, 0.9659258262890683122, 1.000000000000000000, 0.9659258262890683122, 1.000000000000000000, 0.9659258262890683122, 1.000000000000000000, 0.9659258262890683122, 1.000000000000000000, 0.9659258262890683122, 1.000000000000000000, 0.9659258262890683122, 1.000000000000000000, 0.9659258262890683122, 1.000000000000000000, 0.9659258262890683122, 1.000000000000000000, 0.9659258262890683122, 1.000000000000000000, 0.9659258262890683122, 1.000000000000000000, 0.9659258262890683122, 1.000000000000000000, 0.9659258262890683122, 1.000000000000000000, 0.9659258262890683122, 1.000000000000000000, 0.9659258262890683122, 1.000000000000000000, 0.9659258262890683122, 1.000000000000000000, 0.9659258262890683122, 1.000000000000000000, 0.9659258262890683122, 1.000000000000000000, 0.9659258262890683122, 1.000000000000000000, 0.9659258262890683122, 1.000000000000000000, 0.9659258262890683122, 1.000000000000000000, 0.9659258262890683122, 1.000000000000000000, 0.9659258262890683122, 1.000000000000000000, 0.9659258262890683122, 1.000000000000000000, 0.9659258262890683122, 1.000000000000000000, 0.9659258262890683122, 1.000000000000000000, 0.9659258262890683122, 1.000000000000000000, 0.9659258262890683122, 1.000000000000000000, 0.9659258262890683122, 1.000000000000000000, 0.9659258262890683122, 1.000000000000000000, 0.9659258262890683122, 1.000000000000000000, 0.9659258262890683122, 1.000000000000000000, 0.9659258262890683122, 1.000000000000000000, 0.9659258262890683122, 1.000000000000000000, 0.9659258262890683122, 1.000000000000000000, 0.9659258262890683122, 1.000000000000000000, 0.9659258262890683122, 1.000000000000000000, 0.9659258262890683122, 1.000000000000000000, 0.9659258262890683122, 1.000000000000000000, 0.9659258262890683122, 1.000000000000000000, 0.9659258262890683122, 1.000000000000000000, 0.9659258262890683122, 1.000000000000000000, 0.9659258262890683122, 1.000000000000000000, 0.9659258262890683122, 1.000000000000000000, 0.9659258262890683122, 1.000000000000000000, 0.9659258262890683122, 1.000000000000000000, 0.9659258262890683122, 1.000000000000000000, 0.9659258262890683122, 1.000000000000000000, 0.9659258262890683122, 1.000000000000000000, 0.9659258262890683122, 1.000000000000000000, 0.9659258262890683122, 1.000000000000000000, 0.9659258262890683122, 1.000000000000000000, 0.9659258262890683122, 1.000000000000000000, 0.9659258262890683122, 1.000000000000000000, 0.9659258262890683122, 1.000000000000000000, 0.9659258262890683122, 1.000000000000000000, 0.9659258262890683122, 1.000000000000000000, 0.9659258262890683122, 1.000000000000000000, 0.9659258262890683122, 1.000000000000000000, 0.9659258262890683122, 1.000000000000000000, 0.9659258262890683122, 1.000000000000000000, 0.9659258262890683122, 1.000000000000000000, 0.9659258262890683122, 1.000000000000000000, 0.9659258262890683122, 1.000000000000000000, 0.9659258262890683122, 1.000000000000000000, 0.9659258262890683122, 1.000000000000000000, 0.9659258262890683122, 1.000000000000000000, 0.9659258262890683122, 1.000000000000000000, 0.9659258262890683122, 1.000000000000000000, 0.9659258262890683122, 1.000000000000000000, 0.9659258262890683122, 1.000000000000000000, 0.9659258262890683122, 1.000000000000000000, 0.9659258262890683122, 1.000000000000000000, 0.9659258262890683122, 1.000000000000000000, 0.9659258262890683122, 1.000000000000000000, 0.9659258262890683122, 1.000000000000000000, 0.9659258262890683122, 1.000000000000000000, 0.9659258262890683122, 1.000000000000000000, 0.9659258262890683122, 1.000000000000000000, 0.9659258262890683122, 1.000000000000000000, 0.9659258262890683122, 1.000000000000000000, 0.9659258262890683122, 1.000000000000000000, 0.9659258262890683122, 1.000000000000000000, 0.9659258262890683122, 1.000000000000000000, 0.9659258262890683122, 1.000000000000000000, 0.9659258262890683122, 1.000000000000000000, 0.9659258262890683122, 1.000000000000000000),
 ( 0.3333333333333333703, 0.3219752754296894559, 0.3333333333333333703, 0.3219752754296894559, 0.3333333333333333703, 0.3219752754296894559, 0.3333333333333333703, 0.3219752754296894559, 0.3333333333333333703, 0.3219752754296894559, 0.3333333333333333703, 0.3219752754296894559, 0.3333333333333333703, 0.3219752754296894559, 0.3333333333333333703, 0.3219752754296894559, 0.3333333333333333703, 0.3219752754296894559, 0.3333333333333333703, 0.3219752754296894559, 0.3333333333333333703, 0.3219752754296894559, 0.3333333333333333703, 0.3219752754296894559, 0.3333333333333333703, 0.3219752754296894559, 0.3333333333333333703, 0.3219752754296894559, 0.3333333333333333703, 0.3219752754296894559, 0.3333333333333333703, 0.3219752754296894559, 0.3333333333333333703, 0.3219752754296894559, 0.3333333333333333703, 0.3219752754296894559, 0.3333333333333333703, 0.3219752754296894559, 0.3333333333333333703, 0.3219752754296894559, 0.3333333333333333703, 0.3219752754296894559, 0.3333333333333333703, 0.3219752754296894559, 0.3333333333333333703, 0.3219752754296894559, 0.3333333333333333703, 0.3219752754296894559, 0.3333333333333333703, 0.3219752754296894559, 0.3333333333333333703, 0.3219752754296894559, 0.3333333333333333703, 0.3219752754296894559, 0.3333333333333333703, 0.3219752754296894559, 0.3333333333333333703, 0.3219752754296894559, 0.3333333333333333703, 0.3219752754296894559, 0.3333333333333333703, 0.3219752754296894559, 0.3333333333333333703, 0.3219752754296894559, 0.3333333333333333703, 0.3219752754296894559, 0.3333333333333333703, 0.3219752754296894559, 0.3333333333333333703, 0.3219752754296894559, 0.3333333333333333703, 0.3219752754296894559, 0.3333333333333333703, 0.3219752754296894559, 0.3333333333333333703, 0.3219752754296894559, 0.3333333333333333703, 0.3219752754296894559, 0.3333333333333333703, 0.3219752754296894559, 0.3333333333333333703, 0.3219752754296894559, 0.3333333333333333703, 0.3219752754296894559, 0.3333333333333333703, 0.3219752754296894559, 0.3333333333333333703, 0.3219752754296894559, 0.3333333333333333703, 0.3219752754296894559, 0.3333333333333333703, 0.3219752754296894559, 0.3333333333333333703, 0.3219752754296894559, 0.3333333333333333703, 0.3219752754296894559, 0.3333333333333333703, 0.3219752754296894559, 0.3333333333333333703, 0.3219752754296894559, 0.3333333333333333703, 0.3219752754296894559, 0.3333333333333333703, 0.3219752754296894559, 0.3333333333333333703, 0.3219752754296894559, 0.3333333333333333703, 0.3219752754296894559, 0.3333333333333333703, 0.3219752754296894559, 0.3333333333333333703, 0.3219752754296894559, 0.3333333333333333703, 0.3219752754296894559, 0.3333333333333333703, 0.3219752754296894559, 0.3333333333333333703, 0.3219752754296894559, 0.3333333333333333703, 0.3219752754296894559, 0.3333333333333333703, 0.3219752754296894559, 0.3333333333333333703, 0.3219752754296894559, 0.3333333333333333703, 0.3219752754296894559, 0.3333333333333333703, 0.3219752754296894559, 0.3333333333333333703, 0.3219752754296894559, 0.3333333333333333703, 0.3219752754296894559, 0.3333333333333333703, 0.3219752754296894559, 0.3333333333333333703, 0.3219752754296894559, 0.3333333333333333703, 0.3219752754296894559, 0.3333333333333333703, 0.3219752754296894559, 0.3333333333333333703, 0.3219752754296894559, 0.3333333333333333703, 0.3219752754296894559, 0.3333333333333333703, 0.3219752754296894559, 0.3333333333333333703, 0.3219752754296894559, 0.3333333333333333703, 0.3219752754296894559, 0.3333333333333333703, 0.3219752754296894559, 0.3333333333333333703, 0.3219752754296894559, 0.3333333333333333703, 0.3219752754296894559, 0.3333333333333333703, 0.3219752754296894559, 0.3333333333333333703, 0.3219752754296894559, 0.3333333333333333703, 0.3219752754296894559, 0.3333333333333333703, 0.3219752754296894559, 0.3333333333333333703, 0.3219752754296894559, 0.3333333333333333703, 0.3219752754296894559, 0.3333333333333333703, 0.3219752754296894559, 0.3333333333333333703, 0.3219752754296894559, 0.3333333333333333703, 0.3219752754296894559, 0.3333333333333333703, 0.3219752754296894559, 0.3333333333333333703, 0.3219752754296894559, 0.3333333333333333703, 0.3219752754296894559, 0.3333333333333333703, 0.3219752754296894559, 0.3333333333333333703, 0.3219752754296894559, 0.3333333333333333703, 0.3219752754296894559, 0.3333333333333333703, 0.3219752754296894559, 0.3333333333333333703, 0.3219752754296894559, 0.3333333333333333703, 0.3219752754296894559, 0.3333333333333333703, 0.3219752754296894559, 0.3333333333333333703, 0.3219752754296894559, 0.3333333333333333703, 0.3219752754296894559, 0.3333333333333333703, 0.3219752754296894559, 0.3333333333333333703, 0.3219752754296894559, 0.3333333333333333703, 0.3219752754296894559, 0.3333333333333333703, 0.3219752754296894559, 0.3333333333333333703, 0.3219752754296894559, 0.3333333333333333703, 0.3219752754296894559, 0.3333333333333333703, 0.3219752754296894559, 0.3333333333333333703, 0.3219752754296894559, 0.3333333333333333703, 0.3219752754296894559, 0.3333333333333333703, 0.3219752754296894559, 0.3333333333333333703, 0.3219752754296894559, 0.3333333333333333703, 0.3219752754296894559, 0.3333333333333333703, 0.3219752754296894559, 0.3333333333333333703, 0.3219752754296894559, 0.3333333333333333703, 0.3219752754296894559, 0.3333333333333333703, 0.3219752754296894559, 0.3333333333333333703, 0.3219752754296894559, 0.3333333333333333703, 0.3219752754296894559, 0.3333333333333333703, 0.3219752754296894559, 0.3333333333333333703, 0.3219752754296894559, 0.3333333333333333703, 0.3219752754296894559, 0.3333333333333333703, 0.3219752754296894559, 0.3333333333333333703, 0.3219752754296894559, 0.3333333333333333703, 0.3219752754296894559, 0.3333333333333333703, 0.3219752754296894559, 0.3333333333333333703, 0.3219752754296894559, 0.3333333333333333703, 0.3219752754296894559, 0.3333333333333333703, 0.3219752754296894559, 0.3333333333333333703, 0.3219752754296894559, 0.3333333333333333703, 0.3219752754296894559, 0.3333333333333333703, 0.3219752754296894559, 0.3333333333333333703, 0.3219752754296894559, 0.3333333333333333703, 0.3219752754296894559, 0.3333333333333333703, 0.3219752754296894559, 0.3333333333333333703, 0.3219752754296894559, 0.3333333333333333703, 0.3219752754296894559, 0.3333333333333333703, 0.3219752754296894559, 0.3333333333333333703, 0.3219752754296894559, 0.3333333333333333703, 0.3219752754296894559, 0.3333333333333333703, 0.3219752754296894559, 0.3333333333333333703, 0.3219752754296894559, 0.3333333333333333703, 0.3219752754296894559, 0.3333333333333333703, 0.3219752754296894559, 0.3333333333333333703, 0.3219752754296894559, 0.3333333333333333703, 0.3219752754296894559, 0.3333333333333333703, 0.3219752754296894559, 0.3333333333333333703, 0.3219752754296894559, 0.3333333333333333703, 0.3219752754296894559, 0.3333333333333333703, 0.3219752754296894559, 0.3333333333333333703, 0.3219752754296894559, 0.3333333333333333703, 0.3219752754296894559, 0.3333333333333333703, 0.3219752754296894559, 0.3333333333333333703, 0.3219752754296894559, 0.3333333333333333703, 0.3219752754296894559, 0.3333333333333333703, 0.3219752754296894559, 0.3333333333333333703, 0.3219752754296894559, 0.3333333333333333703, 0.3219752754296894559, 0.3333333333333333703, 0.3219752754296894559, 0.3333333333333333703, 0.3219752754296894559, 0.3333333333333333703, 0.3219752754296894559, 0.3333333333333333703, 0.3219752754296894559, 0.3333333333333333703, 0.3219752754296894559, 0.3333333333333333703, 0.3219752754296894559, 0.3333333333333333703, 0.3219752754296894559, 0.3333333333333333703, 0.3219752754296894559, 0.3333333333333333703, 0.3219752754296894559, 0.3333333333333333703, 0.3219752754296894559, 0.3333333333333333703, 0.3219752754296894559, 0.3333333333333333703, 0.3219752754296894559, 0.3333333333333333703, 0.3219752754296894559, 0.3333333333333333703, 0.3219752754296894559, 0.3333333333333333703, 0.3219752754296894559, 0.3333333333333333703, 0.3219752754296894559, 0.3333333333333333703, 0.3219752754296894559, 0.3333333333333333703, 0.3219752754296894559, 0.3333333333333333703, 0.3219752754296894559, 0.3333333333333333703, 0.3219752754296894559, 0.3333333333333333703, 0.3219752754296894559, 0.3333333333333333703, 0.3219752754296894559, 0.3333333333333333703, 0.3219752754296894559, 0.3333333333333333703, 0.3219752754296894559, 0.3333333333333333703, 0.3219752754296894559, 0.3333333333333333703, 0.3219752754296894559, 0.3333333333333333703, 0.3219752754296894559, 0.3333333333333333703, 0.3219752754296894559, 0.3333333333333333703, 0.3219752754296894559, 0.3333333333333333703, 0.3219752754296894559, 0.3333333333333333703, 0.3219752754296894559, 0.3333333333333333703, 0.3219752754296894559, 0.3333333333333333703, 0.3219752754296894559, 0.3333333333333333703, 0.3219752754296894559, 0.3333333333333333703, 0.3219752754296894559, 0.3333333333333333703, 0.3219752754296894559, 0.3333333333333333703, 0.3219752754296894559, 0.3333333333333333703, 0.3219752754296894559, 0.3333333333333333703, 0.3219752754296894559, 0.3333333333333333703, 0.3219752754296894559, 0.3333333333333333703, 0.3219752754296894559, 0.3333333333333333703, 0.3219752754296894559, 0.3333333333333333703, 0.3219752754296894559, 0.3333333333333333703, 0.3219752754296894559, 0.3333333333333333703, 0.3219752754296894559, 0.3333333333333333703, 0.3219752754296894559, 0.3333333333333333703, 0.3219752754296894559, 0.3333333333333333703, 0.3219752754296894559, 0.3333333333333333703, 0.3219752754296894559, 0.3333333333333333703, 0.3219752754296894559, 0.3333333333333333703, 0.3219752754296894559, 0.3333333333333333703, 0.3219752754296894559, 0.3333333333333333703, 0.3219752754296894559, 0.3333333333333333703, 0.3219752754296894559, 0.3333333333333333703, 0.3219752754296894559, 0.3333333333333333703, 0.3219752754296894559, 0.3333333333333333703, 0.3219752754296894559, 0.3333333333333333703, 0.3219752754296894559, 0.3333333333333333703, 0.3219752754296894559, 0.3333333333333333703, 0.3219752754296894559, 0.3333333333333333703, 0.3219752754296894559, 0.3333333333333333703, 0.3219752754296894559, 0.3333333333333333703, 0.3219752754296894559, 0.3333333333333333703, 0.3219752754296894559, 0.3333333333333333703, 0.3219752754296894559, 0.3333333333333333703, 0.3219752754296894559, 0.3333333333333333703, 0.3219752754296894559, 0.3333333333333333703, 0.3219752754296894559, 0.3333333333333333703, 0.3219752754296894559, 0.3333333333333333703, 0.3219752754296894559, 0.3333333333333333703, 0.3219752754296894559, 0.3333333333333333703, 0.3219752754296894559, 0.3333333333333333703),
 ( 0.3333333333333333703, 0.3219752754296894559, 0.3333333333333333703, 0.3219752754296894559, 0.3333333333333333703, 0.3219752754296894559, 0.3333333333333333703, 0.3219752754296894559, 0.3333333333333333703, 0.3219752754296894559, 0.3333333333333333703, 0.3219752754296894559, 0.3333333333333333703, 0.3219752754296894559, 0.3333333333333333703, 0.3219752754296894559, 0.3333333333333333703, 0.3219752754296894559, 0.3333333333333333703, 0.3219752754296894559, 0.3333333333333333703, 0.3219752754296894559, 0.3333333333333333703, 0.3219752754296894559, 0.3333333333333333703, 0.3219752754296894559, 0.3333333333333333703, 0.3219752754296894559, 0.3333333333333333703, 0.3219752754296894559, 0.3333333333333333703, 0.3219752754296894559, 0.3333333333333333703, 0.3219752754296894559, 0.3333333333333333703, 0.3219752754296894559, 0.3333333333333333703, 0.3219752754296894559, 0.3333333333333333703, 0.3219752754296894559, 0.3333333333333333703, 0.3219752754296894559, 0.3333333333333333703, 0.3219752754296894559, 0.3333333333333333703, 0.3219752754296894559, 0.3333333333333333703, 0.3219752754296894559, 0.3333333333333333703, 0.3219752754296894559, 0.3333333333333333703, 0.3219752754296894559, 0.3333333333333333703, 0.3219752754296894559, 0.3333333333333333703, 0.3219752754296894559, 0.3333333333333333703, 0.3219752754296894559, 0.3333333333333333703, 0.3219752754296894559, 0.3333333333333333703, 0.3219752754296894559, 0.3333333333333333703, 0.3219752754296894559, 0.3333333333333333703, 0.3219752754296894559, 0.3333333333333333703, 0.3219752754296894559, 0.3333333333333333703, 0.3219752754296894559, 0.3333333333333333703, 0.3219752754296894559, 0.3333333333333333703, 0.3219752754296894559, 0.3333333333333333703, 0.3219752754296894559, 0.3333333333333333703, 0.3219752754296894559, 0.3333333333333333703, 0.3219752754296894559, 0.3333333333333333703, 0.3219752754296894559, 0.3333333333333333703, 0.3219752754296894559, 0.3333333333333333703, 0.3219752754296894559, 0.3333333333333333703, 0.3219752754296894559, 0.3333333333333333703, 0.3219752754296894559, 0.3333333333333333703, 0.3219752754296894559, 0.3333333333333333703, 0.3219752754296894559, 0.3333333333333333703, 0.3219752754296894559, 0.3333333333333333703, 0.3219752754296894559, 0.3333333333333333703, 0.3219752754296894559, 0.3333333333333333703, 0.3219752754296894559, 0.3333333333333333703, 0.3219752754296894559, 0.3333333333333333703, 0.3219752754296894559, 0.3333333333333333703, 0.3219752754296894559, 0.3333333333333333703, 0.3219752754296894559, 0.3333333333333333703, 0.3219752754296894559, 0.3333333333333333703, 0.3219752754296894559, 0.3333333333333333703, 0.3219752754296894559, 0.3333333333333333703, 0.3219752754296894559, 0.3333333333333333703, 0.3219752754296894559, 0.3333333333333333703, 0.3219752754296894559, 0.3333333333333333703, 0.3219752754296894559, 0.3333333333333333703, 0.3219752754296894559, 0.3333333333333333703, 0.3219752754296894559, 0.3333333333333333703, 0.3219752754296894559, 0.3333333333333333703, 0.3219752754296894559, 0.3333333333333333703, 0.3219752754296894559, 0.3333333333333333703, 0.3219752754296894559, 0.3333333333333333703, 0.3219752754296894559, 0.3333333333333333703, 0.3219752754296894559, 0.3333333333333333703, 0.3219752754296894559, 0.3333333333333333703, 0.3219752754296894559, 0.3333333333333333703, 0.3219752754296894559, 0.3333333333333333703, 0.3219752754296894559, 0.3333333333333333703, 0.3219752754296894559, 0.3333333333333333703, 0.3219752754296894559, 0.3333333333333333703, 0.3219752754296894559, 0.3333333333333333703, 0.3219752754296894559, 0.3333333333333333703, 0.3219752754296894559, 0.3333333333333333703, 0.3219752754296894559, 0.3333333333333333703, 0.3219752754296894559, 0.3333333333333333703, 0.3219752754296894559, 0.3333333333333333703, 0.3219752754296894559, 0.3333333333333333703, 0.3219752754296894559, 0.3333333333333333703, 0.3219752754296894559, 0.3333333333333333703, 0.3219752754296894559, 0.3333333333333333703, 0.3219752754296894559, 0.3333333333333333703, 0.3219752754296894559, 0.3333333333333333703, 0.3219752754296894559, 0.3333333333333333703, 0.3219752754296894559, 0.3333333333333333703, 0.3219752754296894559, 0.3333333333333333703, 0.3219752754296894559, 0.3333333333333333703, 0.3219752754296894559, 0.3333333333333333703, 0.3219752754296894559, 0.3333333333333333703, 0.3219752754296894559, 0.3333333333333333703, 0.3219752754296894559, 0.3333333333333333703, 0.3219752754296894559, 0.3333333333333333703, 0.3219752754296894559, 0.3333333333333333703, 0.3219752754296894559, 0.3333333333333333703, 0.3219752754296894559, 0.3333333333333333703, 0.3219752754296894559, 0.3333333333333333703, 0.3219752754296894559, 0.3333333333333333703, 0.3219752754296894559, 0.3333333333333333703, 0.3219752754296894559, 0.3333333333333333703, 0.3219752754296894559, 0.3333333333333333703, 0.3219752754296894559, 0.3333333333333333703, 0.3219752754296894559, 0.3333333333333333703, 0.3219752754296894559, 0.3333333333333333703, 0.3219752754296894559, 0.3333333333333333703, 0.3219752754296894559, 0.3333333333333333703, 0.3219752754296894559, 0.3333333333333333703, 0.3219752754296894559, 0.3333333333333333703, 0.3219752754296894559, 0.3333333333333333703, 0.3219752754296894559, 0.3333333333333333703, 0.3219752754296894559, 0.3333333333333333703, 0.3219752754296894559, 0.3333333333333333703, 0.3219752754296894559, 0.3333333333333333703, 0.3219752754296894559, 0.3333333333333333703, 0.3219752754296894559, 0.3333333333333333703, 0.3219752754296894559, 0.3333333333333333703, 0.3219752754296894559, 0.3333333333333333703, 0.3219752754296894559, 0.3333333333333333703, 0.3219752754296894559, 0.3333333333333333703, 0.3219752754296894559, 0.3333333333333333703, 0.3219752754296894559, 0.3333333333333333703, 0.3219752754296894559, 0.3333333333333333703, 0.3219752754296894559, 0.3333333333333333703, 0.3219752754296894559, 0.3333333333333333703, 0.3219752754296894559, 0.3333333333333333703, 0.3219752754296894559, 0.3333333333333333703, 0.3219752754296894559, 0.3333333333333333703, 0.3219752754296894559, 0.3333333333333333703, 0.3219752754296894559, 0.3333333333333333703, 0.3219752754296894559, 0.3333333333333333703, 0.3219752754296894559, 0.3333333333333333703, 0.3219752754296894559, 0.3333333333333333703, 0.3219752754296894559, 0.3333333333333333703, 0.3219752754296894559, 0.3333333333333333703, 0.3219752754296894559, 0.3333333333333333703, 0.3219752754296894559, 0.3333333333333333703, 0.3219752754296894559, 0.3333333333333333703, 0.3219752754296894559, 0.3333333333333333703, 0.3219752754296894559, 0.3333333333333333703, 0.3219752754296894559, 0.3333333333333333703, 0.3219752754296894559, 0.3333333333333333703, 0.3219752754296894559, 0.3333333333333333703, 0.3219752754296894559, 0.3333333333333333703, 0.3219752754296894559, 0.3333333333333333703, 0.3219752754296894559, 0.3333333333333333703, 0.3219752754296894559, 0.3333333333333333703, 0.3219752754296894559, 0.3333333333333333703, 0.3219752754296894559, 0.3333333333333333703, 0.3219752754296894559, 0.3333333333333333703, 0.3219752754296894559, 0.3333333333333333703, 0.3219752754296894559, 0.3333333333333333703, 0.3219752754296894559, 0.3333333333333333703, 0.3219752754296894559, 0.3333333333333333703, 0.3219752754296894559, 0.3333333333333333703, 0.3219752754296894559, 0.3333333333333333703, 0.3219752754296894559, 0.3333333333333333703, 0.3219752754296894559, 0.3333333333333333703, 0.3219752754296894559, 0.3333333333333333703, 0.3219752754296894559, 0.3333333333333333703, 0.3219752754296894559, 0.3333333333333333703, 0.3219752754296894559, 0.3333333333333333703, 0.3219752754296894559, 0.3333333333333333703, 0.3219752754296894559, 0.3333333333333333703, 0.3219752754296894559, 0.3333333333333333703, 0.3219752754296894559, 0.3333333333333333703, 0.3219752754296894559, 0.3333333333333333703, 0.3219752754296894559, 0.3333333333333333703, 0.3219752754296894559, 0.3333333333333333703, 0.3219752754296894559, 0.3333333333333333703, 0.3219752754296894559, 0.3333333333333333703, 0.3219752754296894559, 0.3333333333333333703, 0.3219752754296894559, 0.3333333333333333703, 0.3219752754296894559, 0.3333333333333333703, 0.3219752754296894559, 0.3333333333333333703, 0.3219752754296894559, 0.3333333333333333703, 0.3219752754296894559, 0.3333333333333333703, 0.3219752754296894559, 0.3333333333333333703, 0.3219752754296894559, 0.3333333333333333703, 0.3219752754296894559, 0.3333333333333333703, 0.3219752754296894559, 0.3333333333333333703, 0.3219752754296894559, 0.3333333333333333703, 0.3219752754296894559, 0.3333333333333333703, 0.3219752754296894559, 0.3333333333333333703, 0.3219752754296894559, 0.3333333333333333703, 0.3219752754296894559, 0.3333333333333333703, 0.3219752754296894559, 0.3333333333333333703, 0.3219752754296894559, 0.3333333333333333703, 0.3219752754296894559, 0.3333333333333333703, 0.3219752754296894559, 0.3333333333333333703, 0.3219752754296894559, 0.3333333333333333703, 0.3219752754296894559, 0.3333333333333333703, 0.3219752754296894559, 0.3333333333333333703, 0.3219752754296894559, 0.3333333333333333703, 0.3219752754296894559, 0.3333333333333333703, 0.3219752754296894559, 0.3333333333333333703, 0.3219752754296894559, 0.3333333333333333703, 0.3219752754296894559, 0.3333333333333333703, 0.3219752754296894559, 0.3333333333333333703, 0.3219752754296894559, 0.3333333333333333703, 0.3219752754296894559, 0.3333333333333333703, 0.3219752754296894559, 0.3333333333333333703, 0.3219752754296894559, 0.3333333333333333703, 0.3219752754296894559, 0.3333333333333333703, 0.3219752754296894559, 0.3333333333333333703, 0.3219752754296894559, 0.3333333333333333703, 0.3219752754296894559, 0.3333333333333333703, 0.3219752754296894559, 0.3333333333333333703, 0.3219752754296894559, 0.3333333333333333703, 0.3219752754296894559, 0.3333333333333333703, 0.3219752754296894559, 0.3333333333333333703, 0.3219752754296894559, 0.3333333333333333703, 0.3219752754296894559, 0.3333333333333333703, 0.3219752754296894559, 0.3333333333333333703, 0.3219752754296894559, 0.3333333333333333703, 0.3219752754296894559, 0.3333333333333333703, 0.3219752754296894559, 0.3333333333333333703, 0.3219752754296894559, 0.3333333333333333703, 0.3219752754296894559, 0.3333333333333333703, 0.3219752754296894559, 0.3333333333333333703, 0.3219752754296894559, 0.3333333333333333703, 0.3219752754296894559, 0.3333333333333333703, 0.3219752754296894559, 0.3333333333333333703, 0.3219752754296894559, 0.3333333333333333703, 0.3219752754296894559, 0.3333333333333333703),
 ( 1.000000000000000000, 0.9659258262890683122, 1.000000000000000000, 0.9659258262890683122, 1.000000000000000000, 0.9659258262890683122, 1.000000000000000000, 0.9659258262890683122, 1.000000000000000000, 0.9659258262890683122, 1.000000000000000000, 0.9659258262890683122, 1.000000000000000000, 0.9659258262890683122, 1.000000000000000000, 0.9659258262890683122, 1.000000000000000000, 0.9659258262890683122, 1.000000000000000000, 0.9659258262890683122, 1.000000000000000000, 0.9659258262890683122, 1.000000000000000000, 0.9659258262890683122, 1.000000000000000000, 0.9659258262890683122, 1.000000000000000000, 0.9659258262890683122, 1.000000000000000000, 0.9659258262890683122, 1.000000000000000000, 0.9659258262890683122, 1.000000000000000000, 0.9659258262890683122, 1.000000000000000000, 0.9659258262890683122, 1.000000000000000000, 0.9659258262890683122, 1.000000000000000000, 0.9659258262890683122, 1.000000000000000000, 0.9659258262890683122, 1.000000000000000000, 0.9659258262890683122, 1.000000000000000000, 0.9659258262890683122, 1.000000000000000000, 0.9659258262890683122, 1.000000000000000000, 0.9659258262890683122, 1.000000000000000000, 0.9659258262890683122, 1.000000000000000000, 0.9659258262890683122, 1.000000000000000000, 0.9659258262890683122, 1.000000000000000000, 0.9659258262890683122, 1.000000000000000000, 0.9659258262890683122, 1.000000000000000000, 0.9659258262890683122, 1.000000000000000000, 0.9659258262890683122, 1.000000000000000000, 0.9659258262890683122, 1.000000000000000000, 0.9659258262890683122, 1.000000000000000000, 0.9659258262890683122, 1.000000000000000000, 0.9659258262890683122, 1.000000000000000000, 0.9659258262890683122, 1.000000000000000000, 0.9659258262890683122, 1.000000000000000000, 0.9659258262890683122, 1.000000000000000000, 0.9659258262890683122, 1.000000000000000000, 0.9659258262890683122, 1.000000000000000000, 0.9659258262890683122, 1.000000000000000000, 0.9659258262890683122, 1.000000000000000000, 0.9659258262890683122, 1.000000000000000000, 0.9659258262890683122, 1.000000000000000000, 0.9659258262890683122, 1.000000000000000000, 0.9659258262890683122, 1.000000000000000000, 0.9659258262890683122, 1.000000000000000000, 0.9659258262890683122, 1.000000000000000000, 0.9659258262890683122, 1.000000000000000000, 0.9659258262890683122, 1.000000000000000000, 0.9659258262890683122, 1.000000000000000000, 0.9659258262890683122, 1.000000000000000000, 0.9659258262890683122, 1.000000000000000000, 0.9659258262890683122, 1.000000000000000000, 0.9659258262890683122, 1.000000000000000000, 0.9659258262890683122, 1.000000000000000000, 0.9659258262890683122, 1.000000000000000000, 0.9659258262890683122, 1.000000000000000000, 0.9659258262890683122, 1.000000000000000000, 0.9659258262890683122, 1.000000000000000000, 0.9659258262890683122, 1.000000000000000000, 0.9659258262890683122, 1.000000000000000000, 0.9659258262890683122, 1.000000000000000000, 0.9659258262890683122, 1.000000000000000000, 0.9659258262890683122, 1.000000000000000000, 0.9659258262890683122, 1.000000000000000000, 0.9659258262890683122, 1.000000000000000000, 0.9659258262890683122, 1.000000000000000000, 0.9659258262890683122, 1.000000000000000000, 0.9659258262890683122, 1.000000000000000000, 0.9659258262890683122, 1.000000000000000000, 0.9659258262890683122, 1.000000000000000000, 0.9659258262890683122, 1.000000000000000000, 0.9659258262890683122, 1.000000000000000000, 0.9659258262890683122, 1.000000000000000000, 0.9659258262890683122, 1.000000000000000000, 0.9659258262890683122, 1.000000000000000000, 0.9659258262890683122, 1.000000000000000000, 0.9659258262890683122, 1.000000000000000000, 0.9659258262890683122, 1.000000000000000000, 0.9659258262890683122, 1.000000000000000000, 0.9659258262890683122, 1.000000000000000000, 0.9659258262890683122, 1.000000000000000000, 0.9659258262890683122, 1.000000000000000000, 0.9659258262890683122, 1.000000000000000000, 0.9659258262890683122, 1.000000000000000000, 0.9659258262890683122, 1.000000000000000000, 0.9659258262890683122, 1.000000000000000000, 0.9659258262890683122, 1.000000000000000000, 0.9659258262890683122, 1.000000000000000000, 0.9659258262890683122, 1.000000000000000000, 0.9659258262890683122, 1.000000000000000000, 0.9659258262890683122, 1.000000000000000000, 0.9659258262890683122, 1.000000000000000000, 0.9659258262890683122, 1.000000000000000000, 0.9659258262890683122, 1.000000000000000000, 0.9659258262890683122, 1.000000000000000000, 0.9659258262890683122, 1.000000000000000000, 0.9659258262890683122, 1.000000000000000000, 0.9659258262890683122, 1.000000000000000000, 0.9659258262890683122, 1.000000000000000000, 0.9659258262890683122, 1.000000000000000000, 0.9659258262890683122, 1.000000000000000000, 0.9659258262890683122, 1.000000000000000000, 0.9659258262890683122, 1.000000000000000000, 0.9659258262890683122, 1.000000000000000000, 0.9659258262890683122, 1.000000000000000000, 0.9659258262890683122, 1.000000000000000000, 0.9659258262890683122, 1.000000000000000000, 0.9659258262890683122, 1.000000000000000000, 0.9659258262890683122, 1.000000000000000000, 0.9659258262890683122, 1.000000000000000000, 0.9659258262890683122, 1.000000000000000000, 0.9659258262890683122, 1.000000000000000000, 0.9659258262890683122, 1.000000000000000000, 0.9659258262890683122, 1.000000000000000000, 0.9659258262890683122, 1.000000000000000000, 0.9659258262890683122, 1.000000000000000000, 0.9659258262890683122, 1.000000000000000000, 0.9659258262890683122, 1.000000000000000000, 0.9659258262890683122, 1.000000000000000000, 0.9659258262890683122, 1.000000000000000000, 0.9659258262890683122, 1.000000000000000000, 0.9659258262890683122, 1.000000000000000000, 0.9659258262890683122, 1.000000000000000000, 0.9659258262890683122, 1.000000000000000000, 0.9659258262890683122, 1.000000000000000000, 0.9659258262890683122, 1.000000000000000000, 0.9659258262890683122, 1.000000000000000000, 0.9659258262890683122, 1.000000000000000000, 0.9659258262890683122, 1.000000000000000000, 0.9659258262890683122, 1.000000000000000000, 0.9659258262890683122, 1.000000000000000000, 0.9659258262890683122, 1.000000000000000000, 0.9659258262890683122, 1.000000000000000000, 0.9659258262890683122, 1.000000000000000000, 0.9659258262890683122, 1.000000000000000000, 0.9659258262890683122, 1.000000000000000000, 0.9659258262890683122, 1.000000000000000000, 0.9659258262890683122, 1.000000000000000000, 0.9659258262890683122, 1.000000000000000000, 0.9659258262890683122, 1.000000000000000000, 0.9659258262890683122, 1.000000000000000000, 0.9659258262890683122, 1.000000000000000000, 0.9659258262890683122, 1.000000000000000000, 0.9659258262890683122, 1.000000000000000000, 0.9659258262890683122, 1.000000000000000000, 0.9659258262890683122, 1.000000000000000000, 0.9659258262890683122, 1.000000000000000000, 0.9659258262890683122, 1.000000000000000000, 0.9659258262890683122, 1.000000000000000000, 0.9659258262890683122, 1.000000000000000000, 0.9659258262890683122, 1.000000000000000000, 0.9659258262890683122, 1.000000000000000000, 0.9659258262890683122, 1.000000000000000000, 0.9659258262890683122, 1.000000000000000000, 0.9659258262890683122, 1.000000000000000000, 0.9659258262890683122, 1.000000000000000000, 0.9659258262890683122, 1.000000000000000000, 0.9659258262890683122, 1.000000000000000000, 0.9659258262890683122, 1.000000000000000000, 0.9659258262890683122, 1.000000000000000000, 0.9659258262890683122, 1.000000000000000000, 0.9659258262890683122, 1.000000000000000000, 0.9659258262890683122, 1.000000000000000000, 0.9659258262890683122, 1.000000000000000000, 0.9659258262890683122, 1.000000000000000000, 0.9659258262890683122, 1.000000000000000000, 0.9659258262890683122, 1.000000000000000000, 0.9659258262890683122, 1.000000000000000000, 0.9659258262890683122, 1.000000000000000000, 0.9659258262890683122, 1.000000000000000000, 0.9659258262890683122, 1.000000000000000000, 0.9659258262890683122, 1.000000000000000000, 0.9659258262890683122, 1.000000000000000000, 0.9659258262890683122, 1.000000000000000000, 0.9659258262890683122, 1.000000000000000000, 0.9659258262890683122, 1.000000000000000000, 0.9659258262890683122, 1.000000000000000000, 0.9659258262890683122, 1.000000000000000000, 0.9659258262890683122, 1.000000000000000000, 0.9659258262890683122, 1.000000000000000000, 0.9659258262890683122, 1.000000000000000000, 0.9659258262890683122, 1.000000000000000000, 0.9659258262890683122, 1.000000000000000000, 0.9659258262890683122, 1.000000000000000000, 0.9659258262890683122, 1.000000000000000000, 0.9659258262890683122, 1.000000000000000000, 0.9659258262890683122, 1.000000000000000000, 0.9659258262890683122, 1.000000000000000000, 0.9659258262890683122, 1.000000000000000000, 0.9659258262890683122, 1.000000000000000000, 0.9659258262890683122, 1.000000000000000000, 0.9659258262890683122, 1.000000000000000000, 0.9659258262890683122, 1.000000000000000000, 0.9659258262890683122, 1.000000000000000000, 0.9659258262890683122, 1.000000000000000000, 0.9659258262890683122, 1.000000000000000000, 0.9659258262890683122, 1.000000000000000000, 0.9659258262890683122, 1.000000000000000000, 0.9659258262890683122, 1.000000000000000000, 0.9659258262890683122, 1.000000000000000000, 0.9659258262890683122, 1.000000000000000000, 0.9659258262890683122, 1.000000000000000000, 0.9659258262890683122, 1.000000000000000000, 0.9659258262890683122, 1.000000000000000000, 0.9659258262890683122, 1.000000000000000000, 0.9659258262890683122, 1.000000000000000000, 0.9659258262890683122, 1.000000000000000000, 0.9659258262890683122, 1.000000000000000000, 0.9659258262890683122, 1.000000000000000000, 0.9659258262890683122, 1.000000000000000000, 0.9659258262890683122, 1.000000000000000000, 0.9659258262890683122, 1.000000000000000000, 0.9659258262890683122, 1.000000000000000000, 0.9659258262890683122, 1.000000000000000000, 0.9659258262890683122, 1.000000000000000000, 0.9659258262890683122, 1.000000000000000000, 0.9659258262890683122, 1.000000000000000000, 0.9659258262890683122, 1.000000000000000000, 0.9659258262890683122, 1.000000000000000000, 0.9659258262890683122, 1.000000000000000000, 0.9659258262890683122, 1.000000000000000000, 0.9659258262890683122, 1.000000000000000000, 0.9659258262890683122, 1.000000000000000000, 0.9659258262890683122, 1.000000000000000000, 0.9659258262890683122, 1.000000000000000000),
 ( 0.3333333333333333703, 0.3219752754296894559, 0.3333333333333333703, 0.3219752754296894559, 0.3333333333333333703, 0.3219752754296894559, 0.3333333333333333703, 0.3219752754296894559, 0.3333333333333333703, 0.3219752754296894559, 0.3333333333333333703, 0.3219752754296894559, 0.3333333333333333703, 0.3219752754296894559, 0.3333333333333333703, 0.3219752754296894559, 0.3333333333333333703, 0.3219752754296894559, 0.3333333333333333703, 0.3219752754296894559, 0.3333333333333333703, 0.3219752754296894559, 0.3333333333333333703, 0.3219752754296894559, 0.3333333333333333703, 0.3219752754296894559, 0.3333333333333333703, 0.3219752754296894559, 0.3333333333333333703, 0.3219752754296894559, 0.3333333333333333703, 0.3219752754296894559, 0.3333333333333333703, 0.3219752754296894559, 0.3333333333333333703, 0.3219752754296894559, 0.3333333333333333703, 0.3219752754296894559, 0.3333333333333333703, 0.3219752754296894559, 0.3333333333333333703, 0.3219752754296894559, 0.3333333333333333703, 0.3219752754296894559, 0.3333333333333333703, 0.3219752754296894559, 0.3333333333333333703, 0.3219752754296894559, 0.3333333333333333703, 0.3219752754296894559, 0.3333333333333333703, 0.3219752754296894559, 0.3333333333333333703, 0.3219752754296894559, 0.3333333333333333703, 0.3219752754296894559, 0.3333333333333333703, 0.3219752754296894559, 0.3333333333333333703, 0.3219752754296894559, 0.3333333333333333703, 0.3219752754296894559, 0.3333333333333333703, 0.3219752754296894559, 0.3333333333333333703, 0.3219752754296894559, 0.3333333333333333703, 0.3219752754296894559, 0.3333333333333333703, 0.3219752754296894559, 0.3333333333333333703, 0.3219752754296894559, 0.3333333333333333703, 0.3219752754296894559, 0.3333333333333333703, 0.3219752754296894559, 0.3333333333333333703, 0.3219752754296894559, 0.3333333333333333703, 0.3219752754296894559, 0.3333333333333333703, 0.3219752754296894559, 0.3333333333333333703, 0.3219752754296894559, 0.3333333333333333703, 0.3219752754296894559, 0.3333333333333333703, 0.3219752754296894559, 0.3333333333333333703, 0.3219752754296894559, 0.3333333333333333703, 0.3219752754296894559, 0.3333333333333333703, 0.3219752754296894559, 0.3333333333333333703, 0.3219752754296894559, 0.3333333333333333703, 0.3219752754296894559, 0.3333333333333333703, 0.3219752754296894559, 0.3333333333333333703, 0.3219752754296894559, 0.3333333333333333703, 0.3219752754296894559, 0.3333333333333333703, 0.3219752754296894559, 0.3333333333333333703, 0.3219752754296894559, 0.3333333333333333703, 0.3219752754296894559, 0.3333333333333333703, 0.3219752754296894559, 0.3333333333333333703, 0.3219752754296894559, 0.3333333333333333703, 0.3219752754296894559, 0.3333333333333333703, 0.3219752754296894559, 0.3333333333333333703, 0.3219752754296894559, 0.3333333333333333703, 0.3219752754296894559, 0.3333333333333333703, 0.3219752754296894559, 0.3333333333333333703, 0.3219752754296894559, 0.3333333333333333703, 0.3219752754296894559, 0.3333333333333333703, 0.3219752754296894559, 0.3333333333333333703, 0.3219752754296894559, 0.3333333333333333703, 0.3219752754296894559, 0.3333333333333333703, 0.3219752754296894559, 0.3333333333333333703, 0.3219752754296894559, 0.3333333333333333703, 0.3219752754296894559, 0.3333333333333333703, 0.3219752754296894559, 0.3333333333333333703, 0.3219752754296894559, 0.3333333333333333703, 0.3219752754296894559, 0.3333333333333333703, 0.3219752754296894559, 0.3333333333333333703, 0.3219752754296894559, 0.3333333333333333703, 0.3219752754296894559, 0.3333333333333333703, 0.3219752754296894559, 0.3333333333333333703, 0.3219752754296894559, 0.3333333333333333703, 0.3219752754296894559, 0.3333333333333333703, 0.3219752754296894559, 0.3333333333333333703, 0.3219752754296894559, 0.3333333333333333703, 0.3219752754296894559, 0.3333333333333333703, 0.3219752754296894559, 0.3333333333333333703, 0.3219752754296894559, 0.3333333333333333703, 0.3219752754296894559, 0.3333333333333333703, 0.3219752754296894559, 0.3333333333333333703, 0.3219752754296894559, 0.3333333333333333703, 0.3219752754296894559, 0.3333333333333333703, 0.3219752754296894559, 0.3333333333333333703, 0.3219752754296894559, 0.3333333333333333703, 0.3219752754296894559, 0.3333333333333333703, 0.3219752754296894559, 0.3333333333333333703, 0.3219752754296894559, 0.3333333333333333703, 0.3219752754296894559, 0.3333333333333333703, 0.3219752754296894559, 0.3333333333333333703, 0.3219752754296894559, 0.3333333333333333703, 0.3219752754296894559, 0.3333333333333333703, 0.3219752754296894559, 0.3333333333333333703, 0.3219752754296894559, 0.3333333333333333703, 0.3219752754296894559, 0.3333333333333333703, 0.3219752754296894559, 0.3333333333333333703, 0.3219752754296894559, 0.3333333333333333703, 0.3219752754296894559, 0.3333333333333333703, 0.3219752754296894559, 0.3333333333333333703, 0.3219752754296894559, 0.3333333333333333703, 0.3219752754296894559, 0.3333333333333333703, 0.3219752754296894559, 0.3333333333333333703, 0.3219752754296894559, 0.3333333333333333703, 0.3219752754296894559, 0.3333333333333333703, 0.3219752754296894559, 0.3333333333333333703, 0.3219752754296894559, 0.3333333333333333703, 0.3219752754296894559, 0.3333333333333333703, 0.3219752754296894559, 0.3333333333333333703, 0.3219752754296894559, 0.3333333333333333703, 0.3219752754296894559, 0.3333333333333333703, 0.3219752754296894559, 0.3333333333333333703, 0.3219752754296894559, 0.3333333333333333703, 0.3219752754296894559, 0.3333333333333333703, 0.3219752754296894559, 0.3333333333333333703, 0.3219752754296894559, 0.3333333333333333703, 0.3219752754296894559, 0.3333333333333333703, 0.3219752754296894559, 0.3333333333333333703, 0.3219752754296894559, 0.3333333333333333703, 0.3219752754296894559, 0.3333333333333333703, 0.3219752754296894559, 0.3333333333333333703, 0.3219752754296894559, 0.3333333333333333703, 0.3219752754296894559, 0.3333333333333333703, 0.3219752754296894559, 0.3333333333333333703, 0.3219752754296894559, 0.3333333333333333703, 0.3219752754296894559, 0.3333333333333333703, 0.3219752754296894559, 0.3333333333333333703, 0.3219752754296894559, 0.3333333333333333703, 0.3219752754296894559, 0.3333333333333333703, 0.3219752754296894559, 0.3333333333333333703, 0.3219752754296894559, 0.3333333333333333703, 0.3219752754296894559, 0.3333333333333333703, 0.3219752754296894559, 0.3333333333333333703, 0.3219752754296894559, 0.3333333333333333703, 0.3219752754296894559, 0.3333333333333333703, 0.3219752754296894559, 0.3333333333333333703, 0.3219752754296894559, 0.3333333333333333703, 0.3219752754296894559, 0.3333333333333333703, 0.3219752754296894559, 0.3333333333333333703, 0.3219752754296894559, 0.3333333333333333703, 0.3219752754296894559, 0.3333333333333333703, 0.3219752754296894559, 0.3333333333333333703, 0.3219752754296894559, 0.3333333333333333703, 0.3219752754296894559, 0.3333333333333333703, 0.3219752754296894559, 0.3333333333333333703, 0.3219752754296894559, 0.3333333333333333703, 0.3219752754296894559, 0.3333333333333333703, 0.3219752754296894559, 0.3333333333333333703, 0.3219752754296894559, 0.3333333333333333703, 0.3219752754296894559, 0.3333333333333333703, 0.3219752754296894559, 0.3333333333333333703, 0.3219752754296894559, 0.3333333333333333703, 0.3219752754296894559, 0.3333333333333333703, 0.3219752754296894559, 0.3333333333333333703, 0.3219752754296894559, 0.3333333333333333703, 0.3219752754296894559, 0.3333333333333333703, 0.3219752754296894559, 0.3333333333333333703, 0.3219752754296894559, 0.3333333333333333703, 0.3219752754296894559, 0.3333333333333333703, 0.3219752754296894559, 0.3333333333333333703, 0.3219752754296894559, 0.3333333333333333703, 0.3219752754296894559, 0.3333333333333333703, 0.3219752754296894559, 0.3333333333333333703, 0.3219752754296894559, 0.3333333333333333703, 0.3219752754296894559, 0.3333333333333333703, 0.3219752754296894559, 0.3333333333333333703, 0.3219752754296894559, 0.3333333333333333703, 0.3219752754296894559, 0.3333333333333333703, 0.3219752754296894559, 0.3333333333333333703, 0.3219752754296894559, 0.3333333333333333703, 0.3219752754296894559, 0.3333333333333333703, 0.3219752754296894559, 0.3333333333333333703, 0.3219752754296894559, 0.3333333333333333703, 0.3219752754296894559, 0.3333333333333333703, 0.3219752754296894559, 0.3333333333333333703, 0.3219752754296894559, 0.3333333333333333703, 0.3219752754296894559, 0.3333333333333333703, 0.3219752754296894559, 0.3333333333333333703, 0.3219752754296894559, 0.3333333333333333703, 0.3219752754296894559, 0.3333333333333333703, 0.3219752754296894559, 0.3333333333333333703, 0.3219752754296894559, 0.3333333333333333703, 0.3219752754296894559, 0.3333333333333333703, 0.3219752754296894559, 0.3333333333333333703, 0.3219752754296894559, 0.3333333333333333703, 0.3219752754296894559, 0.3333333333333333703, 0.3219752754296894559, 0.3333333333333333703, 0.3219752754296894559, 0.3333333333333333703, 0.3219752754296894559, 0.3333333333333333703, 0.3219752754296894559, 0.3333333333333333703, 0.3219752754296894559, 0.3333333333333333703, 0.3219752754296894559, 0.3333333333333333703, 0.3219752754296894559, 0.3333333333333333703, 0.3219752754296894559, 0.3333333333333333703, 0.3219752754296894559, 0.3333333333333333703, 0.3219752754296894559, 0.3333333333333333703, 0.3219752754296894559, 0.3333333333333333703, 0.3219752754296894559, 0.3333333333333333703, 0.3219752754296894559, 0.3333333333333333703, 0.3219752754296894559, 0.3333333333333333703, 0.3219752754296894559, 0.3333333333333333703, 0.3219752754296894559, 0.3333333333333333703, 0.3219752754296894559, 0.3333333333333333703, 0.3219752754296894559, 0.3333333333333333703, 0.3219752754296894559, 0.3333333333333333703, 0.3219752754296894559, 0.3333333333333333703, 0.3219752754296894559, 0.3333333333333333703, 0.3219752754296894559, 0.3333333333333333703, 0.3219752754296894559, 0.3333333333333333703, 0.3219752754296894559, 0.3333333333333333703, 0.3219752754296894559, 0.3333333333333333703, 0.3219752754296894559, 0.3333333333333333703, 0.3219752754296894559, 0.3333333333333333703, 0.3219752754296894559, 0.3333333333333333703, 0.3219752754296894559, 0.3333333333333333703, 0.3219752754296894559, 0.3333333333333333703, 0.3219752754296894559, 0.3333333333333333703, 0.3219752754296894559, 0.3333333333333333703, 0.3219752754296894559, 0.3333333333333333703, 0.3219752754296894559, 0.3333333333333333703, 0.3219752754296894559, 0.3333333333333333703, 0.3219752754296894559, 0.3333333333333333703, 0.3219752754296894559, 0.3333333333333333703, 0.3219752754296894559, 0.3333333333333333703),
 ( 0.3333333333333333703, 0.3219752754296894559, 0.3333333333333333703, 0.3219752754296894559, 0.3333333333333333703, 0.3219752754296894559, 0.3333333333333333703, 0.3219752754296894559, 0.3333333333333333703, 0.3219752754296894559, 0.3333333333333333703, 0.3219752754296894559, 0.3333333333333333703, 0.3219752754296894559, 0.3333333333333333703, 0.3219752754296894559, 0.3333333333333333703, 0.3219752754296894559, 0.3333333333333333703, 0.3219752754296894559, 0.3333333333333333703, 0.3219752754296894559, 0.3333333333333333703, 0.3219752754296894559, 0.3333333333333333703, 0.3219752754296894559, 0.3333333333333333703, 0.3219752754296894559, 0.3333333333333333703, 0.3219752754296894559, 0.3333333333333333703, 0.3219752754296894559, 0.3333333333333333703, 0.3219752754296894559, 0.3333333333333333703, 0.3219752754296894559, 0.3333333333333333703, 0.3219752754296894559, 0.3333333333333333703, 0.3219752754296894559, 0.3333333333333333703, 0.3219752754296894559, 0.3333333333333333703, 0.3219752754296894559, 0.3333333333333333703, 0.3219752754296894559, 0.3333333333333333703, 0.3219752754296894559, 0.3333333333333333703, 0.3219752754296894559, 0.3333333333333333703, 0.3219752754296894559, 0.3333333333333333703, 0.3219752754296894559, 0.3333333333333333703, 0.3219752754296894559, 0.3333333333333333703, 0.3219752754296894559, 0.3333333333333333703, 0.3219752754296894559, 0.3333333333333333703, 0.3219752754296894559, 0.3333333333333333703, 0.3219752754296894559, 0.3333333333333333703, 0.3219752754296894559, 0.3333333333333333703, 0.3219752754296894559, 0.3333333333333333703, 0.3219752754296894559, 0.3333333333333333703, 0.3219752754296894559, 0.3333333333333333703, 0.3219752754296894559, 0.3333333333333333703, 0.3219752754296894559, 0.3333333333333333703, 0.3219752754296894559, 0.3333333333333333703, 0.3219752754296894559, 0.3333333333333333703, 0.3219752754296894559, 0.3333333333333333703, 0.3219752754296894559, 0.3333333333333333703, 0.3219752754296894559, 0.3333333333333333703, 0.3219752754296894559, 0.3333333333333333703, 0.3219752754296894559, 0.3333333333333333703, 0.3219752754296894559, 0.3333333333333333703, 0.3219752754296894559, 0.3333333333333333703, 0.3219752754296894559, 0.3333333333333333703, 0.3219752754296894559, 0.3333333333333333703, 0.3219752754296894559, 0.3333333333333333703, 0.3219752754296894559, 0.3333333333333333703, 0.3219752754296894559, 0.3333333333333333703, 0.3219752754296894559, 0.3333333333333333703, 0.3219752754296894559, 0.3333333333333333703, 0.3219752754296894559, 0.3333333333333333703, 0.3219752754296894559, 0.3333333333333333703, 0.3219752754296894559, 0.3333333333333333703, 0.3219752754296894559, 0.3333333333333333703, 0.3219752754296894559, 0.3333333333333333703, 0.3219752754296894559, 0.3333333333333333703, 0.3219752754296894559, 0.3333333333333333703, 0.3219752754296894559, 0.3333333333333333703, 0.3219752754296894559, 0.3333333333333333703, 0.3219752754296894559, 0.3333333333333333703, 0.3219752754296894559, 0.3333333333333333703, 0.3219752754296894559, 0.3333333333333333703, 0.3219752754296894559, 0.3333333333333333703, 0.3219752754296894559, 0.3333333333333333703, 0.3219752754296894559, 0.3333333333333333703, 0.3219752754296894559, 0.3333333333333333703, 0.3219752754296894559, 0.3333333333333333703, 0.3219752754296894559, 0.3333333333333333703, 0.3219752754296894559, 0.3333333333333333703, 0.3219752754296894559, 0.3333333333333333703, 0.3219752754296894559, 0.3333333333333333703, 0.3219752754296894559, 0.3333333333333333703, 0.3219752754296894559, 0.3333333333333333703, 0.3219752754296894559, 0.3333333333333333703, 0.3219752754296894559, 0.3333333333333333703, 0.3219752754296894559, 0.3333333333333333703, 0.3219752754296894559, 0.3333333333333333703, 0.3219752754296894559, 0.3333333333333333703, 0.3219752754296894559, 0.3333333333333333703, 0.3219752754296894559, 0.3333333333333333703, 0.3219752754296894559, 0.3333333333333333703, 0.3219752754296894559, 0.3333333333333333703, 0.3219752754296894559, 0.3333333333333333703, 0.3219752754296894559, 0.3333333333333333703, 0.3219752754296894559, 0.3333333333333333703, 0.3219752754296894559, 0.3333333333333333703, 0.3219752754296894559, 0.3333333333333333703, 0.3219752754296894559, 0.3333333333333333703, 0.3219752754296894559, 0.3333333333333333703, 0.3219752754296894559, 0.3333333333333333703, 0.3219752754296894559, 0.3333333333333333703, 0.3219752754296894559, 0.3333333333333333703, 0.3219752754296894559, 0.3333333333333333703, 0.3219752754296894559, 0.3333333333333333703, 0.3219752754296894559, 0.3333333333333333703, 0.3219752754296894559, 0.3333333333333333703, 0.3219752754296894559, 0.3333333333333333703, 0.3219752754296894559, 0.3333333333333333703, 0.3219752754296894559, 0.3333333333333333703, 0.3219752754296894559, 0.3333333333333333703, 0.3219752754296894559, 0.3333333333333333703, 0.3219752754296894559, 0.3333333333333333703, 0.3219752754296894559, 0.3333333333333333703, 0.3219752754296894559, 0.3333333333333333703, 0.3219752754296894559, 0.3333333333333333703, 0.3219752754296894559, 0.3333333333333333703, 0.3219752754296894559, 0.3333333333333333703, 0.3219752754296894559, 0.3333333333333333703, 0.3219752754296894559, 0.3333333333333333703, 0.3219752754296894559, 0.3333333333333333703, 0.3219752754296894559, 0.3333333333333333703, 0.3219752754296894559, 0.3333333333333333703, 0.3219752754296894559, 0.3333333333333333703, 0.3219752754296894559, 0.3333333333333333703, 0.3219752754296894559, 0.3333333333333333703, 0.3219752754296894559, 0.3333333333333333703, 0.3219752754296894559, 0.3333333333333333703, 0.3219752754296894559, 0.3333333333333333703, 0.3219752754296894559, 0.3333333333333333703, 0.3219752754296894559, 0.3333333333333333703, 0.3219752754296894559, 0.3333333333333333703, 0.3219752754296894559, 0.3333333333333333703, 0.3219752754296894559, 0.3333333333333333703, 0.3219752754296894559, 0.3333333333333333703, 0.3219752754296894559, 0.3333333333333333703, 0.3219752754296894559, 0.3333333333333333703, 0.3219752754296894559, 0.3333333333333333703, 0.3219752754296894559, 0.3333333333333333703, 0.3219752754296894559, 0.3333333333333333703, 0.3219752754296894559, 0.3333333333333333703, 0.3219752754296894559, 0.3333333333333333703, 0.3219752754296894559, 0.3333333333333333703, 0.3219752754296894559, 0.3333333333333333703, 0.3219752754296894559, 0.3333333333333333703, 0.3219752754296894559, 0.3333333333333333703, 0.3219752754296894559, 0.3333333333333333703, 0.3219752754296894559, 0.3333333333333333703, 0.3219752754296894559, 0.3333333333333333703, 0.3219752754296894559, 0.3333333333333333703, 0.3219752754296894559, 0.3333333333333333703, 0.3219752754296894559, 0.3333333333333333703, 0.3219752754296894559, 0.3333333333333333703, 0.3219752754296894559, 0.3333333333333333703, 0.3219752754296894559, 0.3333333333333333703, 0.3219752754296894559, 0.3333333333333333703, 0.3219752754296894559, 0.3333333333333333703, 0.3219752754296894559, 0.3333333333333333703, 0.3219752754296894559, 0.3333333333333333703, 0.3219752754296894559, 0.3333333333333333703, 0.3219752754296894559, 0.3333333333333333703, 0.3219752754296894559, 0.3333333333333333703, 0.3219752754296894559, 0.3333333333333333703, 0.3219752754296894559, 0.3333333333333333703, 0.3219752754296894559, 0.3333333333333333703, 0.3219752754296894559, 0.3333333333333333703, 0.3219752754296894559, 0.3333333333333333703, 0.3219752754296894559, 0.3333333333333333703, 0.3219752754296894559, 0.3333333333333333703, 0.3219752754296894559, 0.3333333333333333703, 0.3219752754296894559, 0.3333333333333333703, 0.3219752754296894559, 0.3333333333333333703, 0.3219752754296894559, 0.3333333333333333703, 0.3219752754296894559, 0.3333333333333333703, 0.3219752754296894559, 0.3333333333333333703, 0.3219752754296894559, 0.3333333333333333703, 0.3219752754296894559, 0.3333333333333333703, 0.3219752754296894559, 0.3333333333333333703, 0.3219752754296894559, 0.3333333333333333703, 0.3219752754296894559, 0.3333333333333333703, 0.3219752754296894559, 0.3333333333333333703, 0.3219752754296894559, 0.3333333333333333703, 0.3219752754296894559, 0.3333333333333333703, 0.3219752754296894559, 0.3333333333333333703, 0.3219752754296894559, 0.3333333333333333703, 0.3219752754296894559, 0.3333333333333333703, 0.3219752754296894559, 0.3333333333333333703, 0.3219752754296894559, 0.3333333333333333703, 0.3219752754296894559, 0.3333333333333333703, 0.3219752754296894559, 0.3333333333333333703, 0.3219752754296894559, 0.3333333333333333703, 0.3219752754296894559, 0.3333333333333333703, 0.3219752754296894559, 0.3333333333333333703, 0.3219752754296894559, 0.3333333333333333703, 0.3219752754296894559, 0.3333333333333333703, 0.3219752754296894559, 0.3333333333333333703, 0.3219752754296894559, 0.3333333333333333703, 0.3219752754296894559, 0.3333333333333333703, 0.3219752754296894559, 0.3333333333333333703, 0.3219752754296894559, 0.3333333333333333703, 0.3219752754296894559, 0.3333333333333333703, 0.3219752754296894559, 0.3333333333333333703, 0.3219752754296894559, 0.3333333333333333703, 0.3219752754296894559, 0.3333333333333333703, 0.3219752754296894559, 0.3333333333333333703, 0.3219752754296894559, 0.3333333333333333703, 0.3219752754296894559, 0.3333333333333333703, 0.3219752754296894559, 0.3333333333333333703, 0.3219752754296894559, 0.3333333333333333703, 0.3219752754296894559, 0.3333333333333333703, 0.3219752754296894559, 0.3333333333333333703, 0.3219752754296894559, 0.3333333333333333703, 0.3219752754296894559, 0.3333333333333333703, 0.3219752754296894559, 0.3333333333333333703, 0.3219752754296894559, 0.3333333333333333703, 0.3219752754296894559, 0.3333333333333333703, 0.3219752754296894559, 0.3333333333333333703, 0.3219752754296894559, 0.3333333333333333703, 0.3219752754296894559, 0.3333333333333333703, 0.3219752754296894559, 0.3333333333333333703, 0.3219752754296894559, 0.3333333333333333703, 0.3219752754296894559, 0.3333333333333333703, 0.3219752754296894559, 0.3333333333333333703, 0.3219752754296894559, 0.3333333333333333703, 0.3219752754296894559, 0.3333333333333333703, 0.3219752754296894559, 0.3333333333333333703, 0.3219752754296894559, 0.3333333333333333703, 0.3219752754296894559, 0.3333333333333333703, 0.3219752754296894559, 0.3333333333333333703, 0.3219752754296894559, 0.3333333333333333703, 0.3219752754296894559, 0.3333333333333333703, 0.3219752754296894559, 0.3333333333333333703, 0.3219752754296894559, 0.3333333333333333703, 0.3219752754296894559, 0.3333333333333333703, 0.3219752754296894559, 0.3333333333333333703),
 ( 1.000000000000000000, 0.9659258262890683122, 1.000000000000000000, 0.9659258262890683122, 1.000000000000000000, 0.9659258262890683122, 1.000000000000000000, 0.9659258262890683122, 1.000000000000000000, 0.9659258262890683122, 1.000000000000000000, 0.9659258262890683122, 1.000000000000000000, 0.9659258262890683122, 1.000000000000000000, 0.9659258262890683122, 1.000000000000000000, 0.9659258262890683122, 1.000000000000000000, 0.9659258262890683122, 1.000000000000000000, 0.9659258262890683122, 1.000000000000000000, 0.9659258262890683122, 1.000000000000000000, 0.9659258262890683122, 1.000000000000000000, 0.9659258262890683122, 1.000000000000000000, 0.9659258262890683122, 1.000000000000000000, 0.9659258262890683122, 1.000000000000000000, 0.9659258262890683122, 1.000000000000000000, 0.9659258262890683122, 1.000000000000000000, 0.9659258262890683122, 1.000000000000000000, 0.9659258262890683122, 1.000000000000000000, 0.9659258262890683122, 1.000000000000000000, 0.9659258262890683122, 1.000000000000000000, 0.9659258262890683122, 1.000000000000000000, 0.9659258262890683122, 1.000000000000000000, 0.9659258262890683122, 1.000000000000000000, 0.9659258262890683122, 1.000000000000000000, 0.9659258262890683122, 1.000000000000000000, 0.9659258262890683122, 1.000000000000000000, 0.9659258262890683122, 1.000000000000000000, 0.9659258262890683122, 1.000000000000000000, 0.9659258262890683122, 1.000000000000000000, 0.9659258262890683122, 1.000000000000000000, 0.9659258262890683122, 1.000000000000000000, 0.9659258262890683122, 1.000000000000000000, 0.9659258262890683122, 1.000000000000000000, 0.9659258262890683122, 1.000000000000000000, 0.9659258262890683122, 1.000000000000000000, 0.9659258262890683122, 1.000000000000000000, 0.9659258262890683122, 1.000000000000000000, 0.9659258262890683122, 1.000000000000000000, 0.9659258262890683122, 1.000000000000000000, 0.9659258262890683122, 1.000000000000000000, 0.9659258262890683122, 1.000000000000000000, 0.9659258262890683122, 1.000000000000000000, 0.9659258262890683122, 1.000000000000000000, 0.9659258262890683122, 1.000000000000000000, 0.9659258262890683122, 1.000000000000000000, 0.9659258262890683122, 1.000000000000000000, 0.9659258262890683122, 1.000000000000000000, 0.9659258262890683122, 1.000000000000000000, 0.9659258262890683122, 1.000000000000000000, 0.9659258262890683122, 1.000000000000000000, 0.9659258262890683122, 1.000000000000000000, 0.9659258262890683122, 1.000000000000000000, 0.9659258262890683122, 1.000000000000000000, 0.9659258262890683122, 1.000000000000000000, 0.9659258262890683122, 1.000000000000000000, 0.9659258262890683122, 1.000000000000000000, 0.9659258262890683122, 1.000000000000000000, 0.9659258262890683122, 1.000000000000000000, 0.9659258262890683122, 1.000000000000000000, 0.9659258262890683122, 1.000000000000000000, 0.9659258262890683122, 1.000000000000000000, 0.9659258262890683122, 1.000000000000000000, 0.9659258262890683122, 1.000000000000000000, 0.9659258262890683122, 1.000000000000000000, 0.9659258262890683122, 1.000000000000000000, 0.9659258262890683122, 1.000000000000000000, 0.9659258262890683122, 1.000000000000000000, 0.9659258262890683122, 1.000000000000000000, 0.9659258262890683122, 1.000000000000000000, 0.9659258262890683122, 1.000000000000000000, 0.9659258262890683122, 1.000000000000000000, 0.9659258262890683122, 1.000000000000000000, 0.9659258262890683122, 1.000000000000000000, 0.9659258262890683122, 1.000000000000000000, 0.9659258262890683122, 1.000000000000000000, 0.9659258262890683122, 1.000000000000000000, 0.9659258262890683122, 1.000000000000000000, 0.9659258262890683122, 1.000000000000000000, 0.9659258262890683122, 1.000000000000000000, 0.9659258262890683122, 1.000000000000000000, 0.9659258262890683122, 1.000000000000000000, 0.9659258262890683122, 1.000000000000000000, 0.9659258262890683122, 1.000000000000000000, 0.9659258262890683122, 1.000000000000000000, 0.9659258262890683122, 1.000000000000000000, 0.9659258262890683122, 1.000000000000000000, 0.9659258262890683122, 1.000000000000000000, 0.9659258262890683122, 1.000000000000000000, 0.9659258262890683122, 1.000000000000000000, 0.9659258262890683122, 1.000000000000000000, 0.9659258262890683122, 1.000000000000000000, 0.9659258262890683122, 1.000000000000000000, 0.9659258262890683122, 1.000000000000000000, 0.9659258262890683122, 1.000000000000000000, 0.9659258262890683122, 1.000000000000000000, 0.9659258262890683122, 1.000000000000000000, 0.9659258262890683122, 1.000000000000000000, 0.9659258262890683122, 1.000000000000000000, 0.9659258262890683122, 1.000000000000000000, 0.9659258262890683122, 1.000000000000000000, 0.9659258262890683122, 1.000000000000000000, 0.9659258262890683122, 1.000000000000000000, 0.9659258262890683122, 1.000000000000000000, 0.9659258262890683122, 1.000000000000000000, 0.9659258262890683122, 1.000000000000000000, 0.9659258262890683122, 1.000000000000000000, 0.9659258262890683122, 1.000000000000000000, 0.9659258262890683122, 1.000000000000000000, 0.9659258262890683122, 1.000000000000000000, 0.9659258262890683122, 1.000000000000000000, 0.9659258262890683122, 1.000000000000000000, 0.9659258262890683122, 1.000000000000000000, 0.9659258262890683122, 1.000000000000000000, 0.9659258262890683122, 1.000000000000000000, 0.9659258262890683122, 1.000000000000000000, 0.9659258262890683122, 1.000000000000000000, 0.9659258262890683122, 1.000000000000000000, 0.9659258262890683122, 1.000000000000000000, 0.9659258262890683122, 1.000000000000000000, 0.9659258262890683122, 1.000000000000000000, 0.9659258262890683122, 1.000000000000000000, 0.9659258262890683122, 1.000000000000000000, 0.9659258262890683122, 1.000000000000000000, 0.9659258262890683122, 1.000000000000000000, 0.9659258262890683122, 1.000000000000000000, 0.9659258262890683122, 1.000000000000000000, 0.9659258262890683122, 1.000000000000000000, 0.9659258262890683122, 1.000000000000000000, 0.9659258262890683122, 1.000000000000000000, 0.9659258262890683122, 1.000000000000000000, 0.9659258262890683122, 1.000000000000000000, 0.9659258262890683122, 1.000000000000000000, 0.9659258262890683122, 1.000000000000000000, 0.9659258262890683122, 1.000000000000000000, 0.9659258262890683122, 1.000000000000000000, 0.9659258262890683122, 1.000000000000000000, 0.9659258262890683122, 1.000000000000000000, 0.9659258262890683122, 1.000000000000000000, 0.9659258262890683122, 1.000000000000000000, 0.9659258262890683122, 1.000000000000000000, 0.9659258262890683122, 1.000000000000000000, 0.9659258262890683122, 1.000000000000000000, 0.9659258262890683122, 1.000000000000000000, 0.9659258262890683122, 1.000000000000000000, 0.9659258262890683122, 1.000000000000000000, 0.9659258262890683122, 1.000000000000000000, 0.9659258262890683122, 1.000000000000000000, 0.9659258262890683122, 1.000000000000000000, 0.9659258262890683122, 1.000000000000000000, 0.9659258262890683122, 1.000000000000000000, 0.9659258262890683122, 1.000000000000000000, 0.9659258262890683122, 1.000000000000000000, 0.9659258262890683122, 1.000000000000000000, 0.9659258262890683122, 1.000000000000000000, 0.9659258262890683122, 1.000000000000000000, 0.9659258262890683122, 1.000000000000000000, 0.9659258262890683122, 1.000000000000000000, 0.9659258262890683122, 1.000000000000000000, 0.9659258262890683122, 1.000000000000000000, 0.9659258262890683122, 1.000000000000000000, 0.9659258262890683122, 1.000000000000000000, 0.9659258262890683122, 1.000000000000000000, 0.9659258262890683122, 1.000000000000000000, 0.9659258262890683122, 1.000000000000000000, 0.9659258262890683122, 1.000000000000000000, 0.9659258262890683122, 1.000000000000000000, 0.9659258262890683122, 1.000000000000000000, 0.9659258262890683122, 1.000000000000000000, 0.9659258262890683122, 1.000000000000000000, 0.9659258262890683122, 1.000000000000000000, 0.9659258262890683122, 1.000000000000000000, 0.9659258262890683122, 1.000000000000000000, 0.9659258262890683122, 1.000000000000000000, 0.9659258262890683122, 1.000000000000000000, 0.9659258262890683122, 1.000000000000000000, 0.9659258262890683122, 1.000000000000000000, 0.9659258262890683122, 1.000000000000000000, 0.9659258262890683122, 1.000000000000000000, 0.9659258262890683122, 1.000000000000000000, 0.9659258262890683122, 1.000000000000000000, 0.9659258262890683122, 1.000000000000000000, 0.9659258262890683122, 1.000000000000000000, 0.9659258262890683122, 1.000000000000000000, 0.9659258262890683122, 1.000000000000000000, 0.9659258262890683122, 1.000000000000000000, 0.9659258262890683122, 1.000000000000000000, 0.9659258262890683122, 1.000000000000000000, 0.9659258262890683122, 1.000000000000000000, 0.9659258262890683122, 1.000000000000000000, 0.9659258262890683122, 1.000000000000000000, 0.9659258262890683122, 1.000000000000000000, 0.9659258262890683122, 1.000000000000000000, 0.9659258262890683122, 1.000000000000000000, 0.9659258262890683122, 1.000000000000000000, 0.9659258262890683122, 1.000000000000000000, 0.9659258262890683122, 1.000000000000000000, 0.9659258262890683122, 1.000000000000000000, 0.9659258262890683122, 1.000000000000000000, 0.9659258262890683122, 1.000000000000000000, 0.9659258262890683122, 1.000000000000000000, 0.9659258262890683122, 1.000000000000000000, 0.9659258262890683122, 1.000000000000000000, 0.9659258262890683122, 1.000000000000000000, 0.9659258262890683122, 1.000000000000000000, 0.9659258262890683122, 1.000000000000000000, 0.9659258262890683122, 1.000000000000000000, 0.9659258262890683122, 1.000000000000000000, 0.9659258262890683122, 1.000000000000000000, 0.9659258262890683122, 1.000000000000000000, 0.9659258262890683122, 1.000000000000000000, 0.9659258262890683122, 1.000000000000000000, 0.9659258262890683122, 1.000000000000000000, 0.9659258262890683122, 1.000000000000000000, 0.9659258262890683122, 1.000000000000000000, 0.9659258262890683122, 1.000000000000000000, 0.9659258262890683122, 1.000000000000000000, 0.9659258262890683122, 1.000000000000000000, 0.9659258262890683122, 1.000000000000000000, 0.9659258262890683122, 1.000000000000000000, 0.9659258262890683122, 1.000000000000000000, 0.9659258262890683122, 1.000000000000000000, 0.9659258262890683122, 1.000000000000000000, 0.9659258262890683122, 1.000000000000000000, 0.9659258262890683122, 1.000000000000000000, 0.9659258262890683122, 1.000000000000000000, 0.9659258262890683122, 1.000000000000000000) ) ) 
 REPRESENTATION_ITEM ( '' )  SURFACE ( )  );
#169555=CARTESIAN_POINT ( 'NONE',  ( -9.474510206698964154, 16.51473224551069663, 110.4155762719810383 ) ) ;
#169557=CARTESIAN_POINT ( 'NONE',  ( 19.05341960407617918, -5.049401038297876454, 96.04275706135231871 ) ) ;
#169558=CARTESIAN_POINT ( 'NONE',  ( 5.719274019375991003, -21.55341960407610458, 67.70724293864769550 ) ) ;
#169559=CARTESIAN_POINT ( 'NONE',  ( 0.05219959533910956823, 16.53943276465976808, 54.99890960531435269 ) ) ;
#169560=CARTESIAN_POINT ( 'NONE',  ( 0.05219959533934541429, -16.53943276465976808, 20.00109039468568639 ) ) ;
#169561=CARTESIAN_POINT ( 'NONE',  ( 19.02544592524343514, -5.153800228976328945, 33.54057627198102409 ) ) ;
#169562=CARTESIAN_POINT ( 'NONE',  ( 5.153800228976615827, -19.02544592524334988, 105.2094237280190185 ) ) ;
#169563=CARTESIAN_POINT ( 'NONE',  ( 5.823673210054125526, 21.52544592524343514, 99.79057627198103830 ) ) ;
#169564=CARTESIAN_POINT ( 'NONE',  ( -13.89961937509957401, -13.97604488694547875, 69.37609039468564731 ) ) ;
#169565=CARTESIAN_POINT ( 'NONE',  ( -16.55341960407617563, 4.379528057220093196, 83.54275706135234714 ) ) ;
#169566=CARTESIAN_POINT ( 'NONE',  ( -19.05341960407611168, -5.049401038298163336, 76.45724293864769550 ) ) ;
#169567=CARTESIAN_POINT ( 'NONE',  ( 0.05219959533910956823, 16.53943276465976808, 79.99890960531435269 ) ) ;
#169568=CARTESIAN_POINT ( 'NONE',  ( -13.97604488694527625, -13.89961937509977652, 61.87390960531435979 ) ) ;
#169569=CARTESIAN_POINT ( 'NONE',  ( -14.34966873604960291, -8.224510206698953496, 66.66557627198102409 ) ) ;
#169570=CARTESIAN_POINT ( 'NONE',  ( 16.51473224551069308, 9.474510206698969483, 34.16557627198102409 ) ) ;
#169572=CARTESIAN_POINT ( 'NONE',  ( -0.05219959533910754901, -16.53943276465976808, 37.49890960531436690 ) ) ;
#169573=CARTESIAN_POINT ( 'NONE',  ( -5.153800228976328057, -19.02544592524343514, 82.29057627198103830 ) ) ;
#169575=CARTESIAN_POINT ( 'NONE',  ( -5.049401038297874678, -19.05341960407617918, 54.79275706135234003 ) ) ;
#169576=CARTESIAN_POINT ( 'NONE',  ( -0.05219959533934338120, 16.53943276465976808, 57.50109039468568994 ) ) ;
#169577=CARTESIAN_POINT ( 'NONE',  ( 21.53943276465977519, -0.05219959533907433946, 58.74890960531436690 ) ) ;
#169578=CARTESIAN_POINT ( 'NONE',  ( -19.02544592524334988, -5.153800228976617603, 28.95942372801900433 ) ) ;
#169579=CARTESIAN_POINT ( 'NONE',  ( -16.51473224551069308, -9.474510206698971260, 86.66557627198102409 ) ) ;
#169581=CARTESIAN_POINT ( 'NONE',  ( 15.80617190586746368, 15.72974639402197994, 29.37390960531435269 ) ) ;
#169582=CARTESIAN_POINT ( 'NONE',  ( -0.05219959533909027116, -19.03943276465977164, 57.49890960531435979 ) ) ;
#169583=CARTESIAN_POINT ( 'NONE',  ( -5.823673210054431948, 21.52544592524334988, 52.70942372801902565 ) ) ;
#169584=CARTESIAN_POINT ( 'NONE',  ( -0.05219959533910754901, -16.53943276465976808, 112.4989096053143669 ) ) ;
#169585=CARTESIAN_POINT ( 'NONE',  ( 15.80617190586746368, 15.72974639402197994, 104.3739096053143669 ) ) ;
#169586=CARTESIAN_POINT ( 'NONE',  ( -9.564922557960796823, -16.46253265017161027, 97.08224293864769550 ) ) ;
#169587=ORIENTED_EDGE ( 'NONE', *, *, #118593, .F. ) ;
#169588=CARTESIAN_POINT ( 'NONE',  ( -21.55341960407619339, 5.719274019375674811, 38.54275706135234714 ) ) ;
#169589=ORIENTED_EDGE ( 'NONE', *, *, #185663, .T. ) ;
#169590=CARTESIAN_POINT ( 'NONE',  ( 0.05219959533909260263, 19.03943276465977164, 99.99890960531436690 ) ) ;
#169592=CARTESIAN_POINT ( 'NONE',  ( 21.53943276465977519, -0.05219959533907433946, 88.74890960531436690 ) ) ;
#169593=CARTESIAN_POINT ( 'NONE',  ( -19.03943276465977164, 0.05219959533909376836, 51.24890960531436690 ) ) ;
#169594=CARTESIAN_POINT ( 'NONE',  ( 8.224510206698742110, 14.34966873604972548, 27.08442372801901854 ) ) ;
#169596=CARTESIAN_POINT ( 'NONE',  ( -13.89961937509977652, 13.97604488694528158, 35.62390960531435269 ) ) ;
#169597=CARTESIAN_POINT ( 'NONE',  ( 5.719274019375673035, 21.55341960407619339, 97.29275706135234714 ) ) ;
#169598=CARTESIAN_POINT ( 'NONE',  ( -0.05219959533909027116, -19.03943276465977164, 72.49890960531435269 ) ) ;
#169599=CARTESIAN_POINT ( 'NONE',  ( -21.52544592524334988, -5.823673210054445271, 48.95942372801902565 ) ) ;
#169600=CARTESIAN_POINT ( 'NONE',  ( 18.67979575497194134, -10.72451020669871369, 25.83442372801901499 ) ) ;
#169602=CARTESIAN_POINT ( 'NONE',  ( 0.05219959533909260263, 19.03943276465977164, 99.99890960531436690 ) ) ;
#169604=CARTESIAN_POINT ( 'NONE',  ( -16.53943276465976808, -0.05219959533934237506, 33.75109039468568284 ) ) ;
#169605=CARTESIAN_POINT ( 'NONE',  ( -4.483927247898782831, 16.52544592524335698, 72.70942372801901854 ) ) ;
#169606=CARTESIAN_POINT ( 'NONE',  ( -10.72451020669870658, -18.67979575497194134, 59.58442372801901854 ) ) ;
#169607=CARTESIAN_POINT ( 'NONE',  ( -5.823673210054431948, 21.52544592524334988, 82.70942372801900433 ) ) ;
#169608=CARTESIAN_POINT ( 'NONE',  ( 15.50000000000000178, -5.500000000000000888, 118.0000000000000142 ) ) ;
#169609=CARTESIAN_POINT ( 'NONE',  ( -8.224510206698735004, -14.34966873604973081, 19.58442372801901143 ) ) ;
#169610=CARTESIAN_POINT ( 'NONE',  ( -5.049401038298153566, 19.05341960407611168, 70.20724293864769550 ) ) ;
#169611=CARTESIAN_POINT ( 'NONE',  ( -13.97604488694527625, -13.89961937509977652, 101.8739096053143811 ) ) ;
#169613=CARTESIAN_POINT ( 'NONE',  ( 12.06949235617757843, -12.14591786802309237, 113.1239096053143953 ) ) ;
#169614=CARTESIAN_POINT ( 'NONE',  ( -12.14591786802309592, -12.06949235617757132, 111.8739096053143669 ) ) ;
#169615=CARTESIAN_POINT ( 'NONE',  ( 21.52544592524344225, -5.823673210054117533, 28.54057627198103120 ) ) ;
#169616=CARTESIAN_POINT ( 'NONE',  ( 0.05219959533934541429, -16.53943276465976808, 75.00109039468568994 ) ) ;
#169617=CARTESIAN_POINT ( 'NONE',  ( 4.483927247898545687, 16.52544592524342804, 69.79057627198102409 ) ) ;
#169618=CARTESIAN_POINT ( 'NONE',  ( 13.89961937509977652, -13.97604488694527269, 53.12390960531434558 ) ) ;
#169619=CARTESIAN_POINT ( 'NONE',  ( -18.67979575497193778, 10.72451020669871902, 73.33442372801901854 ) ) ;
#169621=CARTESIAN_POINT ( 'NONE',  ( 13.89961937509957401, 13.97604488694547697, 106.8760903946856757 ) ) ;
#169622=CARTESIAN_POINT ( 'NONE',  ( 12.06949235617757843, -12.14591786802309237, 78.12390960531436690 ) ) ;
#169623=CARTESIAN_POINT ( 'NONE',  ( -10.81492255796105439, 18.62759615963255655, 27.91775706135234358 ) ) ;
#169624=CARTESIAN_POINT ( 'NONE',  ( -0.05219959533907301413, -21.53943276465977519, 57.49890960531435979 ) ) ;
#169626=CARTESIAN_POINT ( 'NONE',  ( -16.29526858892874586, -7.335722546920136367, 105.7967059780020520 ) ) ;
#169628=CARTESIAN_POINT ( 'NONE',  ( -13.89961937509977652, 13.97604488694528158, 75.62390960531438111 ) ) ;
#169629=CARTESIAN_POINT ( 'NONE',  ( 8.224510206698953496, -14.34966873604960469, 47.91557627198102409 ) ) ;
#169630=CARTESIAN_POINT ( 'NONE',  ( 8.224510206698953496, -14.34966873604960469, 27.91557627198103830 ) ) ;
#169631=CARTESIAN_POINT ( 'NONE',  ( 12.06949235617739724, 12.14591786802326823, 91.87609039468568994 ) ) ;
#169632=CARTESIAN_POINT ( 'NONE',  ( 19.05341960407617918, -5.049401038297876454, 46.04275706135233293 ) ) ;
#169633=CARTESIAN_POINT ( 'NONE',  ( 17.31747979337950838, 6.344076630961018815, 48.87944868065186910 ) ) ;
#169634=CARTESIAN_POINT ( 'NONE',  ( -16.51473224551069308, -9.474510206698971260, 111.6655762719810383 ) ) ;
#169635=EDGE_CURVE ( 'NONE', #91449, #187465, #159486, .T. ) ;
#169636=CARTESIAN_POINT ( 'NONE',  ( -12.14591786802309592, -12.06949235617757132, 71.87390960531438111 ) ) ;
#169637=CARTESIAN_POINT ( 'NONE',  ( 5.049401038297881783, 19.05341960407617563, 42.29275706135234003 ) ) ;
#169638=CARTESIAN_POINT ( 'NONE',  ( -13.89961937509977652, 13.97604488694528158, 30.62390960531435269 ) ) ;
#169639=CARTESIAN_POINT ( 'NONE',  ( -0.05219959533907301413, -21.53943276465977519, 37.49890960531436690 ) ) ;
#169640=CARTESIAN_POINT ( 'NONE',  ( 5.719274019375991003, -21.55341960407610458, 57.70724293864770260 ) ) ;
#169642=CARTESIAN_POINT ( 'NONE',  ( 8.314922557960818139, 14.29746914071049879, 104.5822429386477097 ) ) ;
#169643=CARTESIAN_POINT ( 'NONE',  ( 16.53943276465976808, 0.05219959533934440121, 51.25109039468568994 ) ) ;
#169644=CARTESIAN_POINT ( 'NONE',  ( 4.379528057220339221, -16.55341960407611168, 92.70724293864770971 ) ) ;
#169645=DIRECTION ( 'NONE',  ( 1.000000000000000000, -0.000000000000000000, -0.000000000000000000 ) ) ;
#169646=CARTESIAN_POINT ( 'NONE',  ( -17.50000000000000000, 5.622605283950872668, 48.68792689403888829 ) ) ;
#169647=CARTESIAN_POINT ( 'NONE',  ( -21.53943276465977519, 0.05219959533907696930, 31.24890960531435979 ) ) ;
#169650=CARTESIAN_POINT ( 'NONE',  ( 12.06949235617739724, 12.14591786802326823, 36.87609039468568994 ) ) ;
#169651=CARTESIAN_POINT ( 'NONE',  ( -16.53943276465976808, 0.05219959533911058130, 26.24890960531435624 ) ) ;
#169652=CARTESIAN_POINT ( 'NONE',  ( 21.53943276465977519, -0.05219959533907433946, 53.74890960531437401 ) ) ;
#169653=CARTESIAN_POINT ( 'NONE',  ( -9.474510206698720793, -16.51473224551083518, 79.58442372801899012 ) ) ;
#169654=CARTESIAN_POINT ( 'NONE',  ( -21.55341960407610458, -5.719274019375992779, 61.45724293864770260 ) ) ;
#169655=CARTESIAN_POINT ( 'NONE',  ( 21.53943276465977519, 0.05219959533937863772, 76.25109039468568994 ) ) ;
#169657=CARTESIAN_POINT ( 'NONE',  ( -12.14591786802326823, 12.06949235617739902, 43.12609039468568284 ) ) ;
#169658=CARTESIAN_POINT ( 'NONE',  ( -16.51473224551069308, -9.474510206698971260, 31.66557627198102054 ) ) ;
#169659=CARTESIAN_POINT ( 'NONE',  ( 13.97604488694527802, 13.89961937509977652, 99.37390960531436690 ) ) ;
#169660=CARTESIAN_POINT ( 'NONE',  ( 5.049401038298161559, -19.05341960407611168, 32.70724293864768129 ) ) ;
#169661=CARTESIAN_POINT ( 'NONE',  ( -4.483927247898539470, -16.52544592524342804, 97.29057627198105251 ) ) ;
#169663=CARTESIAN_POINT ( 'NONE',  ( 0.05219959533909260263, 19.03943276465977164, 114.9989096053143669 ) ) ;
#169664=ORIENTED_EDGE ( 'NONE', *, *, #185663, .F. ) ;
#169665=CARTESIAN_POINT ( 'NONE',  ( -4.379528057220086978, -16.55341960407618274, 74.79275706135234714 ) ) ;
#169666=CARTESIAN_POINT ( 'NONE',  ( -21.55341960407610458, -5.719274019375992779, 86.45724293864770971 ) ) ;
#169667=CARTESIAN_POINT ( 'NONE',  ( 9.474510206698971260, -16.51473224551069308, 62.91557627198102409 ) ) ;
#169668=CARTESIAN_POINT ( 'NONE',  ( -21.53943276465977519, -0.05219959533937600094, 23.75109039468567929 ) ) ;
#169669=CARTESIAN_POINT ( 'NONE',  ( 19.02544592524343514, -5.153800228976328945, 78.54057627198099567 ) ) ;
#169671=CARTESIAN_POINT ( 'NONE',  ( 15.80617190586746368, 15.72974639402197994, 114.3739096053143527 ) ) ;
#169672=CARTESIAN_POINT ( 'NONE',  ( -5.049401038298153566, 19.05341960407611168, 30.20724293864768839 ) ) ;
#169673=CARTESIAN_POINT ( 'NONE',  ( 19.05341960407611168, 5.049401038298154454, 108.9572429386477097 ) ) ;
#169674=CARTESIAN_POINT ( 'NONE',  ( -16.51473224551082808, 9.474510206698731452, 73.33442372801900433 ) ) ;
#169675=CARTESIAN_POINT ( 'NONE',  ( 9.564922557961047289, -16.46253265017146816, 30.41775706135232937 ) ) ;
#169676=CARTESIAN_POINT ( 'NONE',  ( -15.80617190586745835, -15.72974639402198527, 101.8739096053143811 ) ) ;
#169677=CARTESIAN_POINT ( 'NONE',  ( -19.05341960407617563, 5.049401038297882671, 38.54275706135233293 ) ) ;
#169678=CARTESIAN_POINT ( 'NONE',  ( -16.52544592524335698, -4.483927247898792601, 78.95942372801901854 ) ) ;
#169679=CARTESIAN_POINT ( 'NONE',  ( -19.02544592524342804, 5.153800228976336051, 111.0405762719810099 ) ) ;
#169680=CARTESIAN_POINT ( 'NONE',  ( 9.564922557960805705, 16.46253265017160317, 64.58224293864769550 ) ) ;
#169682=CARTESIAN_POINT ( 'NONE',  ( -0.05219959533937732626, 21.53943276465977519, 67.50109039468568994 ) ) ;
#169683=CARTESIAN_POINT ( 'NONE',  ( 15.72974639402176855, 15.80617190586768217, 86.87609039468568994 ) ) ;
#169684=CARTESIAN_POINT ( 'NONE',  ( -16.46253265017160317, 9.564922557960807481, 70.83224293864770971 ) ) ;
#169685=CARTESIAN_POINT ( 'NONE',  ( 0.05219959533937995610, -21.53943276465977519, 45.00109039468568284 ) ) ;
#169686=CARTESIAN_POINT ( 'NONE',  ( -9.564922557961040184, 16.46253265017147172, 82.91775706135233293 ) ) ;
#169687=CARTESIAN_POINT ( 'NONE',  ( 16.46253265017160672, -9.564922557960803928, 53.33224293864768839 ) ) ;
#169688=CARTESIAN_POINT ( 'NONE',  ( 13.89961937509977652, -13.97604488694527269, 103.1239096053143527 ) ) ;
#169689=CARTESIAN_POINT ( 'NONE',  ( -13.97604488694527625, -13.89961937509977652, 66.87390960531436690 ) ) ;
#169690=CARTESIAN_POINT ( 'NONE',  ( 16.46253265017160672, -9.564922557960803928, 78.33224293864769550 ) ) ;
#169691=CARTESIAN_POINT ( 'NONE',  ( -13.97604488694527625, -13.89961937509977652, 56.87390960531434558 ) ) ;
#169692=CARTESIAN_POINT ( 'NONE',  ( -10.81492255796078084, -18.62759615963271287, 102.0822429386476955 ) ) ;
#169693=CARTESIAN_POINT ( 'NONE',  ( -16.55341960407617563, 4.379528057220093196, 88.54275706135236135 ) ) ;
#169695=CARTESIAN_POINT ( 'NONE',  ( 16.51473224551083163, -9.474510206698727899, 40.83442372801900433 ) ) ;
#169696=CARTESIAN_POINT ( 'NONE',  ( -19.02544592524342804, 5.153800228976336051, 66.04057627198103830 ) ) ;
#169697=CARTESIAN_POINT ( 'NONE',  ( 14.34966873604960469, 8.224510206698951720, 54.16557627198103120 ) ) ;
#169698=CARTESIAN_POINT ( 'NONE',  ( 16.52544592524342804, -4.483927247898539470, 93.54057627198103830 ) ) ;
#169700=CARTESIAN_POINT ( 'NONE',  ( -19.03943276465977164, 0.05219959533909376836, 111.2489096053143669 ) ) ;
#169701=CARTESIAN_POINT ( 'NONE',  ( 9.564922557960805705, 16.46253265017160317, 94.58224293864769550 ) ) ;
#169702=CARTESIAN_POINT ( 'NONE',  ( 13.89961937509977652, -13.97604488694527269, 103.1239096053143527 ) ) ;
#169703=CARTESIAN_POINT ( 'NONE',  ( 19.02544592524334988, 5.153800228976608722, 21.45942372801899012 ) ) ;
#169704=CARTESIAN_POINT ( 'NONE',  ( 16.55341960407618274, -4.379528057220086978, 96.04275706135236135 ) ) ;
#169705=CARTESIAN_POINT ( 'NONE',  ( 5.049401038298161559, -19.05341960407611168, 72.70724293864768129 ) ) ;
#169706=CARTESIAN_POINT ( 'NONE',  ( 15.72974639402176855, 15.80617190586768217, 41.87609039468568284 ) ) ;
#169708=CARTESIAN_POINT ( 'NONE',  ( -0.05219959533907301413, -21.53943276465977519, 32.49890960531435979 ) ) ;
#169709=CARTESIAN_POINT ( 'NONE',  ( -21.53943276465977519, -0.05219959533937600094, 23.75109039468567929 ) ) ;
#169710=CARTESIAN_POINT ( 'NONE',  ( -4.483927247898539470, -16.52544592524342804, 62.29057627198102409 ) ) ;
#169711=CARTESIAN_POINT ( 'NONE',  ( 16.51473224551069308, 9.474510206698969483, 59.16557627198102409 ) ) ;
#169712=CARTESIAN_POINT ( 'NONE',  ( 0.05219959533910956823, 16.53943276465976808, 79.99890960531435269 ) ) ;
#169713=CARTESIAN_POINT ( 'NONE',  ( -0.05219959533936034679, 19.03943276465977164, 47.50109039468566863 ) ) ;
#169714=CARTESIAN_POINT ( 'NONE',  ( 5.049401038298161559, -19.05341960407611168, 22.70724293864769194 ) ) ;
#169715=CARTESIAN_POINT ( 'NONE',  ( 9.474510206698971260, -16.51473224551069308, 82.91557627198103830 ) ) ;
#169716=CARTESIAN_POINT ( 'NONE',  ( -13.97604488694527625, -13.89961937509977652, 86.87390960531436690 ) ) ;
#169718=CARTESIAN_POINT ( 'NONE',  ( -12.14591786802309592, -12.06949235617757132, 106.8739096053143811 ) ) ;
#169720=CARTESIAN_POINT ( 'NONE',  ( 14.29746914071037800, 8.314922557961029526, 101.6677570613523613 ) ) ;
#169721=CARTESIAN_POINT ( 'NONE',  ( 16.52544592524335698, 4.483927247898782831, 31.45942372801901854 ) ) ;
#169722=CARTESIAN_POINT ( 'NONE',  ( -10.81492255796105439, 18.62759615963255655, 92.91775706135236135 ) ) ;
#169723=CARTESIAN_POINT ( 'NONE',  ( 13.97604488694527802, 13.89961937509977652, 84.37390960531433848 ) ) ;
#169724=CARTESIAN_POINT ( 'NONE',  ( 15.72974639402176855, 15.80617190586768217, 21.87609039468567573 ) ) ;
#169725=CARTESIAN_POINT ( 'NONE',  ( -16.51473224551069308, -9.474510206698971260, 31.66557627198102054 ) ) ;
#169726=CARTESIAN_POINT ( 'NONE',  ( 14.29746914071037800, 8.314922557961029526, 31.66775706135234358 ) ) ;
#169727=CARTESIAN_POINT ( 'NONE',  ( 19.03943276465977164, 0.05219959533936151252, 96.25109039468567573 ) ) ;
#169728=CARTESIAN_POINT ( 'NONE',  ( -5.719274019375978568, 21.55341960407610458, 85.20724293864770971 ) ) ;
#169729=CARTESIAN_POINT ( 'NONE',  ( -5.153800228976607833, 19.02544592524334988, 67.70942372801900433 ) ) ;
#169730=CARTESIAN_POINT ( 'NONE',  ( -13.97604488694527625, -13.89961937509977652, 21.87390960531435979 ) ) ;
#169731=CARTESIAN_POINT ( 'NONE',  ( 5.823673210054444382, -21.52544592524334988, 25.20942372801901854 ) ) ;
#169733=CARTESIAN_POINT ( 'NONE',  ( 16.46253265017160672, -9.564922557960803928, 88.33224293864769550 ) ) ;
#169734=CARTESIAN_POINT ( 'NONE',  ( -0.05219959533934338120, 16.53943276465976808, 47.50109039468568994 ) ) ;
#169736=CARTESIAN_POINT ( 'NONE',  ( 0.05219959533936267826, -19.03943276465977164, 55.00109039468566863 ) ) ;
#169737=CARTESIAN_POINT ( 'NONE',  ( -10.72451020669898014, 18.67979575497178502, 110.4155762719810383 ) ) ;
#169738=CARTESIAN_POINT ( 'NONE',  ( 0.05219959533910956823, 16.53943276465976808, 79.99890960531435269 ) ) ;
#169739=CARTESIAN_POINT ( 'NONE',  ( 0.05219959533909260263, 19.03943276465977164, 84.99890960531436690 ) ) ;
#169740=CARTESIAN_POINT ( 'NONE',  ( 12.06949235617739724, 12.14591786802326823, 46.87609039468568994 ) ) ;
#169741=CARTESIAN_POINT ( 'NONE',  ( 9.564922557961047289, -16.46253265017146816, 55.41775706135234003 ) ) ;
#169742=CARTESIAN_POINT ( 'NONE',  ( -18.62759615963255300, -10.81492255796106328, 69.16775706135234714 ) ) ;
#169743=CARTESIAN_POINT ( 'NONE',  ( 16.55341960407618274, -4.379528057220086978, 21.04275706135234714 ) ) ;
#169744=CARTESIAN_POINT ( 'NONE',  ( 19.03943276465977164, -0.05219959533909143690, 63.74890960531435979 ) ) ;
#169745=CARTESIAN_POINT ( 'NONE',  ( 19.03943276465977164, 0.05219959533936151252, 101.2510903946856757 ) ) ;
#169746=CARTESIAN_POINT ( 'NONE',  ( -8.224510206698735004, -14.34966873604973081, 49.58442372801901143 ) ) ;
#169747=CARTESIAN_POINT ( 'NONE',  ( 21.53943276465977519, 0.05219959533937863772, 96.25109039468568994 ) ) ;
#169748=CARTESIAN_POINT ( 'NONE',  ( -5.049401038297874678, -19.05341960407617918, 74.79275706135231871 ) ) ;
#169749=CARTESIAN_POINT ( 'NONE',  ( 5.049401038298161559, -19.05341960407611168, 47.70724293864770260 ) ) ;
#169750=CARTESIAN_POINT ( 'NONE',  ( -21.53943276465977519, 0.05219959533907696930, 66.24890960531436690 ) ) ;
#169751=CARTESIAN_POINT ( 'NONE',  ( -12.14591786802309592, -12.06949235617757132, 71.87390960531438111 ) ) ;
#169752=CARTESIAN_POINT ( 'NONE',  ( 16.51473224551083163, -9.474510206698727899, 75.83442372801900433 ) ) ;
#169753=CARTESIAN_POINT ( 'NONE',  ( -19.25176906914649777, -5.499999999999856115, 70.99927264242278113 ) ) ;
#169754=CARTESIAN_POINT ( 'NONE',  ( 5.153800228976615827, -19.02544592524334988, 50.20942372801897591 ) ) ;
#169755=CARTESIAN_POINT ( 'NONE',  ( -12.06949235617756955, 12.14591786802309770, 25.62390960531435624 ) ) ;
#169756=CARTESIAN_POINT ( 'NONE',  ( -14.34966873604960291, -8.224510206698953496, 71.66557627198100988 ) ) ;
#169757=CARTESIAN_POINT ( 'NONE',  ( 10.72451020669871369, 18.67979575497193778, 107.0844237280190043 ) ) ;
#169759=CARTESIAN_POINT ( 'NONE',  ( 15.80617190586746368, 15.72974639402197994, 109.3739096053143811 ) ) ;
#169760=CARTESIAN_POINT ( 'NONE',  ( 0.05219959533909260263, 19.03943276465977164, 69.99890960531435269 ) ) ;
#169761=CARTESIAN_POINT ( 'NONE',  ( -18.67979575497193778, 10.72451020669871902, 88.33442372801901854 ) ) ;
#169762=CARTESIAN_POINT ( 'NONE',  ( 9.474510206698971260, -16.51473224551069308, 52.91557627198102409 ) ) ;
#169764=CARTESIAN_POINT ( 'NONE',  ( 19.05341960407611168, 5.049401038298154454, 23.95724293864769194 ) ) ;
#169765=CARTESIAN_POINT ( 'NONE',  ( -16.51473224551069308, -9.474510206698971260, 111.6655762719810383 ) ) ;
#169767=CARTESIAN_POINT ( 'NONE',  ( -8.314922557960811034, -14.29746914071050412, 72.08224293864769550 ) ) ;
#169768=CARTESIAN_POINT ( 'NONE',  ( -9.564922557960796823, -16.46253265017161027, 27.08224293864769550 ) ) ;
#169769=CARTESIAN_POINT ( 'NONE',  ( -14.34966873604960291, -8.224510206698953496, 81.66557627198103830 ) ) ;
#169770=CARTESIAN_POINT ( 'NONE',  ( -15.80617190586745835, -15.72974639402198527, 101.8739096053143811 ) ) ;
#169771=CARTESIAN_POINT ( 'NONE',  ( -18.67979575497193778, 10.72451020669871902, 43.33442372801901143 ) ) ;
#169773=CARTESIAN_POINT ( 'NONE',  ( 16.55341960407618274, -4.379528057220086978, 51.04275706135234714 ) ) ;
#169774=CARTESIAN_POINT ( 'NONE',  ( -5.719274019375978568, 21.55341960407610458, 100.2072429386476955 ) ) ;
#169775=CARTESIAN_POINT ( 'NONE',  ( -0.05219959533936034679, 19.03943276465977164, 22.50109039468566152 ) ) ;
#169776=CARTESIAN_POINT ( 'NONE',  ( -5.049401038298153566, 19.05341960407611168, 105.2072429386476671 ) ) ;
#169777=CARTESIAN_POINT ( 'NONE',  ( 21.55341960407619695, -5.719274019375665929, 41.04275706135236135 ) ) ;
#169779=CARTESIAN_POINT ( 'NONE',  ( 10.72451020669898902, -18.67979575497178502, 47.91557627198102409 ) ) ;
#169780=CARTESIAN_POINT ( 'NONE',  ( 14.34966873604960469, 8.224510206698951720, 29.16557627198103120 ) ) ;
#169781=CARTESIAN_POINT ( 'NONE',  ( -10.72451020669870658, -18.67979575497194134, 69.58442372801900433 ) ) ;
#169782=CARTESIAN_POINT ( 'NONE',  ( 5.719274019375673035, 21.55341960407619339, 102.2927570613523613 ) ) ;
#169783=CARTESIAN_POINT ( 'NONE',  ( -0.05219959533936034679, 19.03943276465977164, 27.50109039468566507 ) ) ;
#169784=CARTESIAN_POINT ( 'NONE',  ( -4.483927247898782831, 16.52544592524335698, 82.70942372801900433 ) ) ;
#169785=CARTESIAN_POINT ( 'NONE',  ( -5.719274019375665041, -21.55341960407619695, 54.79275706135235424 ) ) ;
#169786=CARTESIAN_POINT ( 'NONE',  ( -9.474510206698964154, 16.51473224551069663, 50.41557627198102409 ) ) ;
#169787=CARTESIAN_POINT ( 'NONE',  ( -19.05341960407617563, 5.049401038297882671, 23.54275706135233648 ) ) ;
#169788=CARTESIAN_POINT ( 'NONE',  ( -15.72974639402197994, 15.80617190586746368, 30.62390960531436335 ) ) ;
#169789=CARTESIAN_POINT ( 'NONE',  ( -10.81492255796105439, 18.62759615963255655, 22.91775706135235069 ) ) ;
#169790=CARTESIAN_POINT ( 'NONE',  ( -18.67979575497178146, -10.72451020669898902, 81.66557627198103830 ) ) ;
#169791=CARTESIAN_POINT ( 'NONE',  ( -8.314922557961024197, 14.29746914071037800, 42.91775706135235424 ) ) ;
#169793=CARTESIAN_POINT ( 'NONE',  ( -21.55341960407610458, -5.719274019375992779, 81.45724293864769550 ) ) ;
#169794=CARTESIAN_POINT ( 'NONE',  ( -12.06949235617739369, -12.14591786802326823, 69.37609039468567573 ) ) ;
#169795=CARTESIAN_POINT ( 'NONE',  ( -8.314922557960811034, -14.29746914071050412, 62.08224293864769550 ) ) ;
#169797=CARTESIAN_POINT ( 'NONE',  ( 9.564922557961047289, -16.46253265017146816, 100.4177570613523329 ) ) ;
#169798=CARTESIAN_POINT ( 'NONE',  ( -9.564922557960796823, -16.46253265017161027, 112.0822429386476955 ) ) ;
#169800=CARTESIAN_POINT ( 'NONE',  ( 16.55341960407618274, -4.379528057220086978, 46.04275706135234714 ) ) ;
#169801=CARTESIAN_POINT ( 'NONE',  ( -15.72974639402197994, 15.80617190586746368, 110.6239096053143669 ) ) ;
#169802=CARTESIAN_POINT ( 'NONE',  ( -21.52544592524343514, 5.823673210054127303, 26.04057627198103475 ) ) ;
#169803=CARTESIAN_POINT ( 'NONE',  ( 4.379528057220092307, 16.55341960407617563, 52.29275706135236135 ) ) ;
#169804=CARTESIAN_POINT ( 'NONE',  ( 5.049401038298161559, -19.05341960407611168, 67.70724293864769550 ) ) ;
#169805=CARTESIAN_POINT ( 'NONE',  ( -15.72974639402176322, -15.80617190586768395, 44.37609039468567573 ) ) ;
#169806=CARTESIAN_POINT ( 'NONE',  ( 9.564922557961047289, -16.46253265017146816, 110.4177570613523471 ) ) ;
#169807=CARTESIAN_POINT ( 'NONE',  ( -21.55341960407610458, -5.719274019375992779, 31.45724293864769550 ) ) ;
#169809=CARTESIAN_POINT ( 'NONE',  ( 0.05219959533936267826, -19.03943276465977164, 30.00109039468566863 ) ) ;
#169811=CARTESIAN_POINT ( 'NONE',  ( 16.52544592524335698, 4.483927247898782831, 36.45942372801901143 ) ) ;
#169812=CARTESIAN_POINT ( 'NONE',  ( 19.03943276465977164, -0.05219959533909143690, 103.7489096053143669 ) ) ;
#169813=CARTESIAN_POINT ( 'NONE',  ( 18.62759615963271287, -10.81492255796078972, 98.33224293864769550 ) ) ;
#169814=CARTESIAN_POINT ( 'NONE',  ( -5.153800228976328057, -19.02544592524343514, 67.29057627198102409 ) ) ;
#169815=CARTESIAN_POINT ( 'NONE',  ( -17.05587630539786304, 6.762274262135694158, 25.74180309037313208 ) ) ;
#169816=CARTESIAN_POINT ( 'NONE',  ( -4.379528057220328563, 16.55341960407611168, 80.20724293864769550 ) ) ;
#169817=CARTESIAN_POINT ( 'NONE',  ( 5.719274019375991003, -21.55341960407610458, 37.70724293864769550 ) ) ;
#169818=CARTESIAN_POINT ( 'NONE',  ( -5.049401038298153566, 19.05341960407611168, 25.20724293864768484 ) ) ;
#169819=CARTESIAN_POINT ( 'NONE',  ( -4.379528057220086978, -16.55341960407618274, 59.79275706135234714 ) ) ;
#169820=CARTESIAN_POINT ( 'NONE',  ( -21.52544592524343514, 5.823673210054127303, 106.0405762719810525 ) ) ;
#169821=CARTESIAN_POINT ( 'NONE',  ( 19.02544592524334988, 5.153800228976608722, 61.45942372801900433 ) ) ;
#169822=CARTESIAN_POINT ( 'NONE',  ( 0.05219959533907565091, 21.53943276465977519, 29.99890960531435979 ) ) ;
#169823=CARTESIAN_POINT ( 'NONE',  ( -0.05219959533909027116, -19.03943276465977164, 22.49890960531436690 ) ) ;
#169824=CARTESIAN_POINT ( 'NONE',  ( 21.52544592524344225, -5.823673210054117533, 73.54057627198102409 ) ) ;
#169825=CARTESIAN_POINT ( 'NONE',  ( -5.153800228976328057, -19.02544592524343514, 97.29057627198099567 ) ) ;
#169826=CARTESIAN_POINT ( 'NONE',  ( -21.55341960407619339, 5.719274019375674811, 93.54275706135234714 ) ) ;
#169827=CARTESIAN_POINT ( 'NONE',  ( 9.564922557960805705, 16.46253265017160317, 54.58224293864769550 ) ) ;
#169828=CARTESIAN_POINT ( 'NONE',  ( 16.53943276465976808, 0.05219959533934440121, 36.25109039468567573 ) ) ;
#169829=CARTESIAN_POINT ( 'NONE',  ( -16.46253265017160317, 9.564922557960807481, 60.83224293864769550 ) ) ;
#169830=CARTESIAN_POINT ( 'NONE',  ( 21.55341960407619695, -5.719274019375665929, 76.04275706135237556 ) ) ;
#169831=VERTEX_POINT ( 'NONE', #102370 ) ;
#169832=CARTESIAN_POINT ( 'NONE',  ( -13.89961937509957401, -13.97604488694547875, 44.37609039468566863 ) ) ;
#169833=CARTESIAN_POINT ( 'NONE',  ( 19.02544592524334988, 5.153800228976608722, 36.45942372801900433 ) ) ;
#169834=CARTESIAN_POINT ( 'NONE',  ( 10.72451020669871369, 18.67979575497193778, 32.08442372801901854 ) ) ;
#169836=CARTESIAN_POINT ( 'NONE',  ( -19.03943276465977164, -0.05219959533935918106, 28.75109039468566507 ) ) ;
#169837=CARTESIAN_POINT ( 'NONE',  ( 16.51473224551069308, 9.474510206698969483, 84.16557627198102409 ) ) ;
#169838=CARTESIAN_POINT ( 'NONE',  ( -16.51473224551069308, -9.474510206698971260, 71.66557627198102409 ) ) ;
#169839=CARTESIAN_POINT ( 'NONE',  ( 16.55341960407618274, -4.379528057220086978, 111.0427570613523613 ) ) ;
#169840=CARTESIAN_POINT ( 'NONE',  ( 5.153800228976335163, 19.02544592524342804, 114.7905762719810241 ) ) ;
#169841=CARTESIAN_POINT ( 'NONE',  ( 21.55341960407619695, -5.719274019375665929, 86.04275706135236135 ) ) ;
#169844=CARTESIAN_POINT ( 'NONE',  ( -5.719274019375665041, -21.55341960407619695, 94.79275706135234714 ) ) ;
#169846=CARTESIAN_POINT ( 'NONE',  ( 12.06949235617757843, -12.14591786802309237, 113.1239096053143953 ) ) ;
#169849=CARTESIAN_POINT ( 'NONE',  ( 0.05219959533934541429, -16.53943276465976808, 55.00109039468568284 ) ) ;
#169850=CARTESIAN_POINT ( 'NONE',  ( 10.81492255796078972, 18.62759615963270932, 69.58224293864769550 ) ) ;
#169851=CARTESIAN_POINT ( 'NONE',  ( -4.483927247898539470, -16.52544592524342804, 37.29057627198102409 ) ) ;
#169852=CARTESIAN_POINT ( 'NONE',  ( -8.314922557960811034, -14.29746914071050412, 112.0822429386477097 ) ) ;
#169853=CARTESIAN_POINT ( 'NONE',  ( -9.474510206698964154, 16.51473224551069663, 90.41557627198103830 ) ) ;
#169854=CARTESIAN_POINT ( 'NONE',  ( 5.153800228976615827, -19.02544592524334988, 20.20942372801899722 ) ) ;
#169855=CARTESIAN_POINT ( 'NONE',  ( 16.53943276465976808, -0.05219959533910856209, 113.7489096053143527 ) ) ;
#169856=CARTESIAN_POINT ( 'NONE',  ( -21.55341960407619339, 5.719274019375674811, 73.54275706135234714 ) ) ;
#169857=CARTESIAN_POINT ( 'NONE',  ( -19.03943276465977164, 0.05219959533909376836, 111.2489096053143669 ) ) ;
#169858=CARTESIAN_POINT ( 'NONE',  ( -14.29746914071037622, -8.314922557961029526, 109.1677570613523613 ) ) ;
#169859=CARTESIAN_POINT ( 'NONE',  ( 16.46253265017146816, 9.564922557961045513, 61.66775706135234003 ) ) ;
#169861=CARTESIAN_POINT ( 'NONE',  ( -5.823673210054116645, -21.52544592524344225, 27.29057627198103120 ) ) ;
#169862=CARTESIAN_POINT ( 'NONE',  ( -4.483927247898539470, -16.52544592524342804, 87.29057627198103830 ) ) ;
#169864=CARTESIAN_POINT ( 'NONE',  ( 13.89961937509957401, 13.97604488694547697, 56.87609039468564731 ) ) ;
#169865=CARTESIAN_POINT ( 'NONE',  ( -16.46253265017160317, 9.564922557960807481, 70.83224293864770971 ) ) ;
#169866=CARTESIAN_POINT ( 'NONE',  ( -16.52544592524342804, 4.483927247898546575, 71.04057627198103830 ) ) ;
#169867=CARTESIAN_POINT ( 'NONE',  ( -13.97604488694547697, 13.89961937509957934, 98.12609039468566152 ) ) ;
#169868=CARTESIAN_POINT ( 'NONE',  ( 10.81492255796078972, 18.62759615963270932, 49.58224293864769550 ) ) ;
#169871=CARTESIAN_POINT ( 'NONE',  ( -19.03943276465977164, 0.05219959533909376836, 21.24890960531436335 ) ) ;
#169872=CARTESIAN_POINT ( 'NONE',  ( -17.26172910966778673, -6.454744622555875111, 29.19353091350778229 ) ) ;
#169873=CARTESIAN_POINT ( 'NONE',  ( -13.97604488694527625, -13.89961937509977652, 71.87390960531433848 ) ) ;
#169874=CARTESIAN_POINT ( 'NONE',  ( -10.81492255796078084, -18.62759615963271287, 72.08224293864769550 ) ) ;
#169875=CARTESIAN_POINT ( 'NONE',  ( -14.29746914071037622, -8.314922557961029526, 89.16775706135236135 ) ) ;
#169876=CARTESIAN_POINT ( 'NONE',  ( -19.05341960407611168, -5.049401038298163336, 71.45724293864766707 ) ) ;
#169877=CARTESIAN_POINT ( 'NONE',  ( 19.02544592524334988, 5.153800228976608722, 66.45942372801899012 ) ) ;
#169878=CARTESIAN_POINT ( 'NONE',  ( 21.55341960407619695, -5.719274019375665929, 76.04275706135237556 ) ) ;
#169879=CARTESIAN_POINT ( 'NONE',  ( 21.53943276465977519, -0.05219959533907433946, 63.74890960531435979 ) ) ;
#169880=CARTESIAN_POINT ( 'NONE',  ( -19.02544592524342804, 5.153800228976336051, 116.0405762719810383 ) ) ;
#169881=CARTESIAN_POINT ( 'NONE',  ( -16.51473224551069308, -9.474510206698971260, 36.66557627198102409 ) ) ;
#169882=CARTESIAN_POINT ( 'NONE',  ( 14.34966873604972726, -8.224510206698740333, 105.8344237280190328 ) ) ;
#169883=CARTESIAN_POINT ( 'NONE',  ( 5.153800228976335163, 19.02544592524342804, 54.79057627198103120 ) ) ;
#169884=CARTESIAN_POINT ( 'NONE',  ( -4.483927247898782831, 16.52544592524335698, 22.70942372801901499 ) ) ;
#169885=CARTESIAN_POINT ( 'NONE',  ( 16.19135201231370047, 7.376712067591809863, 52.68680854052031748 ) ) ;
#169886=CARTESIAN_POINT ( 'NONE',  ( 5.823673210054444382, -21.52544592524334988, 105.2094237280190328 ) ) ;
#169887=CARTESIAN_POINT ( 'NONE',  ( 14.34966873604960469, 8.224510206698951720, 59.16557627198103120 ) ) ;
#169888=CARTESIAN_POINT ( 'NONE',  ( 10.72451020669898902, -18.67979575497178502, 102.9155762719810383 ) ) ;
#169889=CARTESIAN_POINT ( 'NONE',  ( -18.62759615963270932, 10.81492255796079327, 100.8322429386477097 ) ) ;
#169891=CARTESIAN_POINT ( 'NONE',  ( 5.823673210054125526, 21.52544592524343514, 44.79057627198103120 ) ) ;
#169892=CARTESIAN_POINT ( 'NONE',  ( -14.29746914071037622, -8.314922557961029526, 84.16775706135234714 ) ) ;
#169893=CARTESIAN_POINT ( 'NONE',  ( -12.14591786802309592, -12.06949235617757132, 96.87390960531436690 ) ) ;
#169894=CARTESIAN_POINT ( 'NONE',  ( 0.05219959533909260263, 19.03943276465977164, 64.99890960531436690 ) ) ;
#169897=CARTESIAN_POINT ( 'NONE',  ( -12.06949235617739369, -12.14591786802326823, 104.3760903946856899 ) ) ;
#169898=CARTESIAN_POINT ( 'NONE',  ( -5.823673210054431948, 21.52544592524334988, 32.70942372801900433 ) ) ;
#169899=CARTESIAN_POINT ( 'NONE',  ( -0.05219959533909027116, -19.03943276465977164, 92.49890960531436690 ) ) ;
#169900=CARTESIAN_POINT ( 'NONE',  ( -10.81492255796105439, 18.62759615963255655, 62.91775706135236135 ) ) ;
#169901=CARTESIAN_POINT ( 'NONE',  ( -30.00000000000000000, 5.499999999999992895, 102.5000000000000142 ) ) ;
#169904=CARTESIAN_POINT ( 'NONE',  ( -10.81492255796105439, 18.62759615963255655, 62.91775706135236135 ) ) ;
#169905=CARTESIAN_POINT ( 'NONE',  ( -13.97604488694527625, -13.89961937509977652, 56.87390960531434558 ) ) ;
#169906=CARTESIAN_POINT ( 'NONE',  ( 19.03943276465977164, -0.05219959533909143690, 83.74890960531436690 ) ) ;
#169907=CARTESIAN_POINT ( 'NONE',  ( -16.46253265017146816, -9.564922557961047289, 69.16775706135233293 ) ) ;
#169908=CARTESIAN_POINT ( 'NONE',  ( 21.55341960407619695, -5.719274019375665929, 46.04275706135234714 ) ) ;
#169909=CARTESIAN_POINT ( 'NONE',  ( 19.03943276465977164, 0.05219959533936151252, 106.2510903946856615 ) ) ;
#169911=CARTESIAN_POINT ( 'NONE',  ( 16.51473224551083163, -9.474510206698727899, 65.83442372801900433 ) ) ;
#169912=CARTESIAN_POINT ( 'NONE',  ( 0.05219959533909260263, 19.03943276465977164, 34.99890960531435979 ) ) ;
#169913=CARTESIAN_POINT ( 'NONE',  ( -8.314922557961024197, 14.29746914071037800, 107.9177570613523471 ) ) ;
#169914=CARTESIAN_POINT ( 'NONE',  ( 13.89961937509957401, 13.97604488694547697, 81.87609039468564731 ) ) ;
#169915=CARTESIAN_POINT ( 'NONE',  ( 0.05219959533910956823, 16.53943276465976808, 29.99890960531435979 ) ) ;
#169916=CARTESIAN_POINT ( 'NONE',  ( 19.03943276465977164, 0.05219959533936151252, 46.25109039468566863 ) ) ;
#169917=CARTESIAN_POINT ( 'NONE',  ( 0.05219959533937995610, -21.53943276465977519, 100.0010903946857042 ) ) ;
#169918=CARTESIAN_POINT ( 'NONE',  ( 19.03943276465977164, 0.05219959533936151252, 26.25109039468566507 ) ) ;
#169919=CARTESIAN_POINT ( 'NONE',  ( 16.46253265017160672, -9.564922557960803928, 23.33224293864769194 ) ) ;
#169920=CARTESIAN_POINT ( 'NONE',  ( -5.823673210054431948, 21.52544592524334988, 87.70942372801901854 ) ) ;
#169921=CARTESIAN_POINT ( 'NONE',  ( 8.314922557961029526, -14.29746914071037800, 35.41775706135234003 ) ) ;
#169922=CARTESIAN_POINT ( 'NONE',  ( 0.05219959533909260263, 19.03943276465977164, 94.99890960531436690 ) ) ;
#169924=CARTESIAN_POINT ( 'NONE',  ( 5.153800228976335163, 19.02544592524342804, 79.79057627198102409 ) ) ;
#169927=CARTESIAN_POINT ( 'NONE',  ( -19.05341960407617563, 5.049401038297882671, 83.54275706135233293 ) ) ;
#169928=CARTESIAN_POINT ( 'NONE',  ( 13.97604488694527802, 13.89961937509977652, 109.3739096053143669 ) ) ;
#169929=CARTESIAN_POINT ( 'NONE',  ( 19.03943276465977164, 0.05219959533936151252, 21.25109039468565797 ) ) ;
#169930=CARTESIAN_POINT ( 'NONE',  ( -19.03943276465977164, -0.05219959533935918106, 98.75109039468567573 ) ) ;
#169931=CARTESIAN_POINT ( 'NONE',  ( 4.379528057220339221, -16.55341960407611168, 92.70724293864770971 ) ) ;
#169932=CARTESIAN_POINT ( 'NONE',  ( -5.153800228976328057, -19.02544592524343514, 27.29057627198103120 ) ) ;
#169933=CARTESIAN_POINT ( 'NONE',  ( 15.72974639402199770, -15.80617190586745480, 63.12390960531435979 ) ) ;
#169934=CARTESIAN_POINT ( 'NONE',  ( -5.823673210054116645, -21.52544592524344225, 42.29057627198103120 ) ) ;
#169935=CARTESIAN_POINT ( 'NONE',  ( 16.55341960407611168, 4.379528057220329451, 113.9572429386477239 ) ) ;
#169937=CARTESIAN_POINT ( 'NONE',  ( -9.474510206698720793, -16.51473224551083518, 54.58442372801899722 ) ) ;
#169938=CARTESIAN_POINT ( 'NONE',  ( -16.52544592524342804, 4.483927247898546575, 46.04057627198103830 ) ) ;
#169939=CARTESIAN_POINT ( 'NONE',  ( -10.72451020669898014, 18.67979575497178502, 25.41557627198103120 ) ) ;
#169940=CARTESIAN_POINT ( 'NONE',  ( 15.72974639402176855, 15.80617190586768217, 76.87609039468567573 ) ) ;
#169941=CARTESIAN_POINT ( 'NONE',  ( -15.80617190586745835, -15.72974639402198527, 71.87390960531438111 ) ) ;
#169942=CARTESIAN_POINT ( 'NONE',  ( -15.80617190586768217, 15.72974639402176855, 58.12609039468568994 ) ) ;
#169943=CARTESIAN_POINT ( 'NONE',  ( -5.823673210054431948, 21.52544592524334988, 52.70942372801902565 ) ) ;
#169944=CARTESIAN_POINT ( 'NONE',  ( 16.46253265017160672, -9.564922557960803928, 88.33224293864769550 ) ) ;
#169945=CARTESIAN_POINT ( 'NONE',  ( -8.314922557961024197, 14.29746914071037800, 77.91775706135231871 ) ) ;
#169946=CARTESIAN_POINT ( 'NONE',  ( 13.89961937509977652, -13.97604488694527269, 28.12390960531435624 ) ) ;
#169948=CARTESIAN_POINT ( 'NONE',  ( 16.52544592524342804, -4.483927247898539470, 48.54057627198103120 ) ) ;
#169949=CARTESIAN_POINT ( 'NONE',  ( 16.53943276465976808, -0.05219959533910856209, 28.74890960531435624 ) ) ;
#169950=CARTESIAN_POINT ( 'NONE',  ( -5.153800228976328057, -19.02544592524343514, 72.29057627198102409 ) ) ;
#169951=CARTESIAN_POINT ( 'NONE',  ( -16.51473224551069308, -9.474510206698971260, 36.66557627198102409 ) ) ;
#169952=CARTESIAN_POINT ( 'NONE',  ( -21.52544592524343514, 5.823673210054127303, 51.04057627198103120 ) ) ;
#169953=CARTESIAN_POINT ( 'NONE',  ( 16.46253265017146816, 9.564922557961045513, 31.66775706135232937 ) ) ;
#169955=CARTESIAN_POINT ( 'NONE',  ( -8.314922557960811034, -14.29746914071050412, 52.08224293864768839 ) ) ;
#169956=CARTESIAN_POINT ( 'NONE',  ( -5.823673210054116645, -21.52544592524344225, 22.29057627198102765 ) ) ;
#169958=CARTESIAN_POINT ( 'NONE',  ( -12.14591786802326823, 12.06949235617739902, 78.12609039468570415 ) ) ;
#169959=CARTESIAN_POINT ( 'NONE',  ( 9.564922557961047289, -16.46253265017146816, 70.41775706135233293 ) ) ;
#169960=CARTESIAN_POINT ( 'NONE',  ( -12.06949235617756955, 12.14591786802309770, 40.62390960531435269 ) ) ;
#169961=CARTESIAN_POINT ( 'NONE',  ( -19.20446147854525876, -5.500000000000005329, 74.38999695167674986 ) ) ;
#169962=CARTESIAN_POINT ( 'NONE',  ( 4.483927247898545687, 16.52544592524342804, 29.79057627198102409 ) ) ;
#169963=CARTESIAN_POINT ( 'NONE',  ( -9.564922557960796823, -16.46253265017161027, 57.08224293864769550 ) ) ;
#169964=CARTESIAN_POINT ( 'NONE',  ( 19.05341960407611168, 5.049401038298154454, 63.95724293864769550 ) ) ;
#169965=CARTESIAN_POINT ( 'NONE',  ( 0.05219959533909260263, 19.03943276465977164, 34.99890960531435979 ) ) ;
#169966=CARTESIAN_POINT ( 'NONE',  ( 10.81492255796106328, -18.62759615963255655, 50.41775706135235424 ) ) ;
#169967=CARTESIAN_POINT ( 'NONE',  ( 0.05219959533909260263, 19.03943276465977164, 59.99890960531436690 ) ) ;
#169969=CARTESIAN_POINT ( 'NONE',  ( -16.46253265017160317, 9.564922557960807481, 40.83224293864769550 ) ) ;
#169970=EDGE_CURVE ( 'NONE', #132379, #95422, #96816, .T. ) ;
#169971=CARTESIAN_POINT ( 'NONE',  ( 15.72974639402199770, -15.80617190586745480, 38.12390960531436690 ) ) ;
#169972=CARTESIAN_POINT ( 'NONE',  ( -21.52544592524334988, -5.823673210054445271, 63.95942372801901854 ) ) ;
#169973=CARTESIAN_POINT ( 'NONE',  ( -0.05219959533909027116, -19.03943276465977164, 27.49890960531435624 ) ) ;
#169974=CARTESIAN_POINT ( 'NONE',  ( -0.05219959533907301413, -21.53943276465977519, 22.49890960531436335 ) ) ;
#169975=CARTESIAN_POINT ( 'NONE',  ( 14.34966873604972726, -8.224510206698740333, 95.83442372801903275 ) ) ;
#169976=CARTESIAN_POINT ( 'NONE',  ( 0.05219959533937995610, -21.53943276465977519, 110.0010903946856757 ) ) ;
#169977=CARTESIAN_POINT ( 'NONE',  ( 16.55341960407618274, -4.379528057220086978, 71.04275706135234714 ) ) ;
#169978=CARTESIAN_POINT ( 'NONE',  ( 19.02544592524343514, -5.153800228976328945, 103.5405762719809957 ) ) ;
#169980=CARTESIAN_POINT ( 'NONE',  ( 8.314922557961029526, -14.29746914071037800, 55.41775706135234714 ) ) ;
#169981=CARTESIAN_POINT ( 'NONE',  ( 16.53943276465976808, 0.05219959533934440121, 46.25109039468567573 ) ) ;
#169982=CARTESIAN_POINT ( 'NONE',  ( 8.314922557961029526, -14.29746914071037800, 100.4177570613523471 ) ) ;
#169983=CARTESIAN_POINT ( 'NONE',  ( -10.72451020669870658, -18.67979575497194134, 54.58442372801901143 ) ) ;
#169984=CARTESIAN_POINT ( 'NONE',  ( 14.34966873604972726, -8.224510206698740333, 20.83442372801901143 ) ) ;
#169985=CARTESIAN_POINT ( 'NONE',  ( 18.62759615963271287, -10.81492255796078972, 108.3322429386477097 ) ) ;
#169986=CARTESIAN_POINT ( 'NONE',  ( -16.52544592524335698, -4.483927247898792601, 28.95942372801902209 ) ) ;
#169987=CARTESIAN_POINT ( 'NONE',  ( -16.53943276465976808, -0.05219959533934237506, 88.75109039468567573 ) ) ;
#169988=CARTESIAN_POINT ( 'NONE',  ( -16.38665767534995510, 7.295008042176403862, 45.26400864214468811 ) ) ;
#169989=CARTESIAN_POINT ( 'NONE',  ( 21.55341960407619695, -5.719274019375665929, 81.04275706135236135 ) ) ;
#169990=CARTESIAN_POINT ( 'NONE',  ( -19.02544592524334988, -5.153800228976617603, 83.95942372801901854 ) ) ;
#169991=CARTESIAN_POINT ( 'NONE',  ( -12.14591786802309592, -12.06949235617757132, 56.87390960531436690 ) ) ;
#169992=CARTESIAN_POINT ( 'NONE',  ( 0.05219959533910956823, 16.53943276465976808, 44.99890960531435979 ) ) ;
#169993=CARTESIAN_POINT ( 'NONE',  ( 12.14591786802309770, 12.06949235617756955, 109.3739096053143811 ) ) ;
#169994=CARTESIAN_POINT ( 'NONE',  ( 9.474510206698729675, 16.51473224551082808, 52.08442372801900433 ) ) ;
#169995=CARTESIAN_POINT ( 'NONE',  ( 17.48853670773249291, -5.747243402302947501, 56.16671299749993551 ) ) ;
#169996=CARTESIAN_POINT ( 'NONE',  ( 5.823673210054444382, -21.52544592524334988, 55.20942372801902565 ) ) ;
#169997=CARTESIAN_POINT ( 'NONE',  ( -19.05341960407617563, 5.049401038297882671, 108.5427570613523187 ) ) ;
#169998=PLANE ( 'NONE',  #14768 ) ;
#169999=CARTESIAN_POINT ( 'NONE',  ( 16.46253265017160672, -9.564922557960803928, 103.3322429386476955 ) ) ;
#170000=CARTESIAN_POINT ( 'NONE',  ( -15.72974639402197994, 15.80617190586746368, 70.62390960531436690 ) ) ;
#170001=CARTESIAN_POINT ( 'NONE',  ( -13.89961937509957401, -13.97604488694547875, 94.37609039468566152 ) ) ;
#170002=CARTESIAN_POINT ( 'NONE',  ( -5.049401038298153566, 19.05341960407611168, 100.2072429386476955 ) ) ;
#170003=CARTESIAN_POINT ( 'NONE',  ( 21.53943276465977519, -0.05219959533907433946, 58.74890960531436690 ) ) ;
#170004=CARTESIAN_POINT ( 'NONE',  ( 4.379528057220339221, -16.55341960407611168, 112.7072429386476955 ) ) ;
#170005=CARTESIAN_POINT ( 'NONE',  ( -10.72451020669870658, -18.67979575497194134, 99.58442372801900433 ) ) ;
#170006=CARTESIAN_POINT ( 'NONE',  ( 9.564922557960805705, 16.46253265017160317, 24.58224293864769194 ) ) ;
#170008=CARTESIAN_POINT ( 'NONE',  ( -10.81492255796105439, 18.62759615963255655, 37.91775706135235424 ) ) ;
#170009=CARTESIAN_POINT ( 'NONE',  ( -21.55341960407619339, 5.719274019375674811, 93.54275706135234714 ) ) ;
#170010=CARTESIAN_POINT ( 'NONE',  ( -14.29746914071037622, -8.314922557961029526, 84.16775706135234714 ) ) ;
#170011=CARTESIAN_POINT ( 'NONE',  ( -18.67979575497193778, 10.72451020669871902, 33.33442372801900433 ) ) ;
#170012=CARTESIAN_POINT ( 'NONE',  ( 21.55341960407619695, -5.719274019375665929, 41.04275706135236135 ) ) ;
#170013=CARTESIAN_POINT ( 'NONE',  ( -9.564922557961040184, 16.46253265017147172, 72.91775706135233293 ) ) ;
#170014=CARTESIAN_POINT ( 'NONE',  ( 16.51473224551069308, 9.474510206698969483, 74.16557627198103830 ) ) ;
#170015=CARTESIAN_POINT ( 'NONE',  ( -14.34966873604960291, -8.224510206698953496, 106.6655762719810383 ) ) ;
#170017=CARTESIAN_POINT ( 'NONE',  ( -10.81492255796078084, -18.62759615963271287, 77.08224293864769550 ) ) ;
#170018=CARTESIAN_POINT ( 'NONE',  ( 8.224510206698953496, -14.34966873604960469, 62.91557627198102409 ) ) ;
#170019=CARTESIAN_POINT ( 'NONE',  ( 15.80617190586769283, -15.72974639402175789, 100.6260903946857184 ) ) ;
#170020=CARTESIAN_POINT ( 'NONE',  ( 16.55341960407611168, 4.379528057220329451, 83.95724293864770971 ) ) ;
#170021=CARTESIAN_POINT ( 'NONE',  ( 19.03943276465977164, -0.05219959533909143690, 33.74890960531435979 ) ) ;
#170022=CARTESIAN_POINT ( 'NONE',  ( 9.474510206698729675, 16.51473224551082808, 77.08442372801900433 ) ) ;
#170023=CARTESIAN_POINT ( 'NONE',  ( 16.55341960407611168, 4.379528057220329451, 28.95724293864769905 ) ) ;
#170024=CARTESIAN_POINT ( 'NONE',  ( -0.05219959533937732626, 21.53943276465977519, 92.50109039468567573 ) ) ;
#170025=CARTESIAN_POINT ( 'NONE',  ( -19.03943276465977164, 0.05219959533909376836, 96.24890960531436690 ) ) ;
#170026=CARTESIAN_POINT ( 'NONE',  ( -16.46253265017146816, -9.564922557961047289, 64.16775706135233293 ) ) ;
#170027=CARTESIAN_POINT ( 'NONE',  ( -10.72451020669898014, 18.67979575497178502, 65.41557627198102409 ) ) ;
#170028=CARTESIAN_POINT ( 'NONE',  ( 21.55341960407610458, 5.719274019375980345, 113.9572429386477239 ) ) ;
#170029=CARTESIAN_POINT ( 'NONE',  ( 19.05341960407617918, -5.049401038297876454, 111.0427570613523329 ) ) ;
#170030=CARTESIAN_POINT ( 'NONE',  ( -12.06949235617739369, -12.14591786802326823, 84.37609039468570415 ) ) ;
#170032=CARTESIAN_POINT ( 'NONE',  ( 5.719274019375673035, 21.55341960407619339, 27.29275706135234358 ) ) ;
#170033=CARTESIAN_POINT ( 'NONE',  ( -4.483927247898539470, -16.52544592524342804, 107.2905762719810525 ) ) ;
#170035=CARTESIAN_POINT ( 'NONE',  ( -14.29746914071037622, -8.314922557961029526, 44.16775706135234714 ) ) ;
#170036=CARTESIAN_POINT ( 'NONE',  ( -12.14591786802309592, -12.06949235617757132, 81.87390960531435269 ) ) ;
#170037=CARTESIAN_POINT ( 'NONE',  ( -15.72974639402197994, 15.80617190586746368, 70.62390960531436690 ) ) ;
#170038=CARTESIAN_POINT ( 'NONE',  ( -12.14591786802326823, 12.06949235617739902, 108.1260903946856757 ) ) ;
#170039=CARTESIAN_POINT ( 'NONE',  ( 8.224510206698742110, 14.34966873604972548, 32.08442372801901854 ) ) ;
#170040=CARTESIAN_POINT ( 'NONE',  ( 0.05219959533909260263, 19.03943276465977164, 44.99890960531435979 ) ) ;
#170041=CARTESIAN_POINT ( 'NONE',  ( -16.55341960407617563, 4.379528057220093196, 83.54275706135234714 ) ) ;
#170042=CARTESIAN_POINT ( 'NONE',  ( 0.05219959533936267826, -19.03943276465977164, 75.00109039468566152 ) ) ;
#170043=CARTESIAN_POINT ( 'NONE',  ( -18.67979575497178146, -10.72451020669898902, 76.66557627198103830 ) ) ;
#170044=CARTESIAN_POINT ( 'NONE',  ( -16.53943276465976808, -0.05219959533934237506, 93.75109039468567573 ) ) ;
#170045=CARTESIAN_POINT ( 'NONE',  ( -15.80617190586768217, 15.72974639402176855, 83.12609039468568994 ) ) ;
#170046=CARTESIAN_POINT ( 'NONE',  ( -21.52544592524343514, 5.823673210054127303, 66.04057627198103830 ) ) ;
#170047=CARTESIAN_POINT ( 'NONE',  ( -21.53943276465977519, 0.05219959533907696930, 41.24890960531435269 ) ) ;
#170049=CARTESIAN_POINT ( 'NONE',  ( -4.379528057220086978, -16.55341960407618274, 84.79275706135234714 ) ) ;
#170050=CARTESIAN_POINT ( 'NONE',  ( 18.67979575497178502, 10.72451020669898547, 49.16557627198102409 ) ) ;
#170052=CARTESIAN_POINT ( 'NONE',  ( -19.03943276465977164, 0.05219959533909376836, 116.2489096053143669 ) ) ;
#170054=CARTESIAN_POINT ( 'NONE',  ( -19.05341960407611168, -5.049401038298163336, 31.45724293864769550 ) ) ;
#170055=CARTESIAN_POINT ( 'NONE',  ( -15.72974639402197994, 15.80617190586746368, 75.62390960531439532 ) ) ;
#170056=CARTESIAN_POINT ( 'NONE',  ( -4.379528057220086978, -16.55341960407618274, 109.7927570613523613 ) ) ;
#170057=CARTESIAN_POINT ( 'NONE',  ( -0.05219959533937732626, 21.53943276465977519, 52.50109039468567573 ) ) ;
#170058=CARTESIAN_POINT ( 'NONE',  ( -12.14591786802326823, 12.06949235617739902, 28.12609039468568284 ) ) ;
#170059=CARTESIAN_POINT ( 'NONE',  ( -9.564922557960796823, -16.46253265017161027, 22.08224293864768839 ) ) ;
#170060=CARTESIAN_POINT ( 'NONE',  ( 16.55341960407618274, -4.379528057220086978, 21.04275706135234714 ) ) ;
#170062=CARTESIAN_POINT ( 'NONE',  ( 19.05341960407611168, 5.049401038298154454, 33.95724293864769550 ) ) ;
#170064=CARTESIAN_POINT ( 'NONE',  ( -5.049401038298153566, 19.05341960407611168, 110.2072429386476671 ) ) ;
#170065=CARTESIAN_POINT ( 'NONE',  ( -14.29746914071037622, -8.314922557961029526, 89.16775706135236135 ) ) ;
#170066=CARTESIAN_POINT ( 'NONE',  ( 16.46253265017146816, 9.564922557961045513, 76.66775706135234714 ) ) ;
#170067=CARTESIAN_POINT ( 'NONE',  ( 19.02544592524334988, 5.153800228976608722, 21.45942372801899012 ) ) ;
#170068=CARTESIAN_POINT ( 'NONE',  ( -18.62759615963270932, 10.81492255796079327, 55.83224293864770260 ) ) ;
#170069=CARTESIAN_POINT ( 'NONE',  ( -4.483927247898782831, 16.52544592524335698, 92.70942372801901854 ) ) ;
#170070=CARTESIAN_POINT ( 'NONE',  ( 5.153800228976615827, -19.02544592524334988, 90.20942372801900433 ) ) ;
#170071=CARTESIAN_POINT ( 'NONE',  ( 9.564922557960805705, 16.46253265017160317, 54.58224293864769550 ) ) ;
#170072=CARTESIAN_POINT ( 'NONE',  ( -9.564922557960796823, -16.46253265017161027, 97.08224293864769550 ) ) ;
#170073=CARTESIAN_POINT ( 'NONE',  ( -21.52544592524334988, -5.823673210054445271, 53.95942372801900433 ) ) ;
#170074=CARTESIAN_POINT ( 'NONE',  ( -16.51473224551069308, -9.474510206698971260, 41.66557627198103120 ) ) ;
#170076=CARTESIAN_POINT ( 'NONE',  ( 9.474510206698971260, -16.51473224551069308, 102.9155762719810241 ) ) ;
#170077=CARTESIAN_POINT ( 'NONE',  ( 16.55341960407611168, 4.379528057220329451, 68.95724293864769550 ) ) ;
#170078=CARTESIAN_POINT ( 'NONE',  ( -21.52544592524343514, 5.823673210054127303, 56.04057627198102409 ) ) ;
#170079=CARTESIAN_POINT ( 'NONE',  ( 20.22402473803820300, -1.857821124618943331, 102.5000000000000284 ) ) ;
#170080=CARTESIAN_POINT ( 'NONE',  ( -19.05341960407617563, 5.049401038297882671, 43.54275706135232582 ) ) ;
#170081=CARTESIAN_POINT ( 'NONE',  ( -19.05341960407611168, -5.049401038298163336, 61.45724293864769550 ) ) ;
#170082=CARTESIAN_POINT ( 'NONE',  ( 0.05219959533909260263, 19.03943276465977164, 74.99890960531435269 ) ) ;
#170083=CARTESIAN_POINT ( 'NONE',  ( -16.53943276465976808, -0.05219959533934237506, 53.75109039468568994 ) ) ;
#170084=CARTESIAN_POINT ( 'NONE',  ( -17.29957754486504129, -5.500000000000000888, 21.12734848878977445 ) ) ;
#170085=CARTESIAN_POINT ( 'NONE',  ( -12.06949235617739369, -12.14591786802326823, 84.37609039468570415 ) ) ;
#170087=CARTESIAN_POINT ( 'NONE',  ( -4.483927247898782831, 16.52544592524335698, 77.70942372801900433 ) ) ;
#170088=CARTESIAN_POINT ( 'NONE',  ( 8.224510206698742110, 14.34966873604972548, 57.08442372801901854 ) ) ;
#170089=CARTESIAN_POINT ( 'NONE',  ( 0.05219959533936267826, -19.03943276465977164, 20.00109039468567218 ) ) ;
#170090=CARTESIAN_POINT ( 'NONE',  ( -19.02544592524342804, 5.153800228976336051, 51.04057627198103120 ) ) ;
#170092=CARTESIAN_POINT ( 'NONE',  ( -21.52544592524334988, -5.823673210054445271, 58.95942372801902565 ) ) ;
#170093=CARTESIAN_POINT ( 'NONE',  ( 16.46253265017146816, 9.564922557961045513, 61.66775706135234003 ) ) ;
#170094=CARTESIAN_POINT ( 'NONE',  ( 15.72974639402176855, 15.80617190586768217, 111.8760903946856615 ) ) ;
#170095=CARTESIAN_POINT ( 'NONE',  ( 9.474510206698971260, -16.51473224551069308, 27.91557627198103120 ) ) ;
#170097=CARTESIAN_POINT ( 'NONE',  ( 21.53943276465977519, -0.05219959533907433946, 73.74890960531433848 ) ) ;
#170099=CARTESIAN_POINT ( 'NONE',  ( -15.80617190586745835, -15.72974639402198527, 26.87390960531435979 ) ) ;
#170100=CARTESIAN_POINT ( 'NONE',  ( -16.53943276465976808, 0.05219959533911058130, 116.2489096053143669 ) ) ;
#170101=CARTESIAN_POINT ( 'NONE',  ( 14.29746914071037800, 8.314922557961029526, 31.66775706135234358 ) ) ;
#170102=CARTESIAN_POINT ( 'NONE',  ( -16.53943276465976808, 0.05219959533911058130, 36.24890960531435979 ) ) ;
#170104=CARTESIAN_POINT ( 'NONE',  ( -21.53943276465977519, 0.05219959533907696930, 111.2489096053143669 ) ) ;
#170105=CARTESIAN_POINT ( 'NONE',  ( 12.06949235617757843, -12.14591786802309237, 43.12390960531435269 ) ) ;
#170106=CARTESIAN_POINT ( 'NONE',  ( -13.89961937509977652, 13.97604488694528158, 110.6239096053143243 ) ) ;
#170107=CARTESIAN_POINT ( 'NONE',  ( -13.97604488694547697, 13.89961937509957934, 103.1260903946856473 ) ) ;
#170108=CARTESIAN_POINT ( 'NONE',  ( -13.97604488694547697, 13.89961937509957934, 23.12609039468565442 ) ) ;
#170109=CARTESIAN_POINT ( 'NONE',  ( -16.52544592524342804, 4.483927247898546575, 41.04057627198103120 ) ) ;
#170110=CARTESIAN_POINT ( 'NONE',  ( -0.05219959533907301413, -21.53943276465977519, 97.49890960531436690 ) ) ;
#170112=CARTESIAN_POINT ( 'NONE',  ( 10.81492255796078972, 18.62759615963270932, 64.58224293864769550 ) ) ;
#170113=CARTESIAN_POINT ( 'NONE',  ( 0.05219959533909260263, 19.03943276465977164, 79.99890960531436690 ) ) ;
#170114=CARTESIAN_POINT ( 'NONE',  ( -16.53943276465976808, 0.05219959533911058130, 51.24890960531436690 ) ) ;
#170115=CARTESIAN_POINT ( 'NONE',  ( -13.97604488694527625, -13.89961937509977652, 86.87390960531436690 ) ) ;
#170117=CARTESIAN_POINT ( 'NONE',  ( 13.89961937509957401, 13.97604488694547697, 51.87609039468566863 ) ) ;
#170118=CARTESIAN_POINT ( 'NONE',  ( -5.719274019375978568, 21.55341960407610458, 95.20724293864769550 ) ) ;
#170119=CARTESIAN_POINT ( 'NONE',  ( -14.29746914071049879, 8.314922557960819915, 95.83224293864770971 ) ) ;
#170120=CARTESIAN_POINT ( 'NONE',  ( 10.72451020669871369, 18.67979575497193778, 57.08442372801901854 ) ) ;
#170122=CARTESIAN_POINT ( 'NONE',  ( -16.52544592524342804, 4.483927247898546575, 31.04057627198102409 ) ) ;
#170123=CARTESIAN_POINT ( 'NONE',  ( 13.97604488694527802, 13.89961937509977652, 39.37390960531435269 ) ) ;
#170124=CARTESIAN_POINT ( 'NONE',  ( -19.02544592524342804, 5.153800228976336051, 101.0405762719810241 ) ) ;
#170125=CARTESIAN_POINT ( 'NONE',  ( 18.67979575497178502, 10.72451020669898547, 59.16557627198103120 ) ) ;
#170126=CARTESIAN_POINT ( 'NONE',  ( -18.87075004821571866, 5.499999999999904077, 43.67408112101048090 ) ) ;
#170127=CARTESIAN_POINT ( 'NONE',  ( -19.05341960407611168, -5.049401038298163336, 31.45724293864769550 ) ) ;
#170128=CARTESIAN_POINT ( 'NONE',  ( 21.52544592524344225, -5.823673210054117533, 58.54057627198103120 ) ) ;
#170130=CARTESIAN_POINT ( 'NONE',  ( 18.62759615963255655, 10.81492255796105972, 71.66775706135234714 ) ) ;
#170132=CARTESIAN_POINT ( 'NONE',  ( 14.34966873604972726, -8.224510206698740333, 80.83442372801901854 ) ) ;
#170133=CARTESIAN_POINT ( 'NONE',  ( -19.02544592524342804, 5.153800228976336051, 56.04057627198100988 ) ) ;
#170134=CARTESIAN_POINT ( 'NONE',  ( -19.05341960407611168, -5.049401038298163336, 71.45724293864766707 ) ) ;
#170136=CARTESIAN_POINT ( 'NONE',  ( 13.89961937509957401, 13.97604488694547697, 26.87609039468566507 ) ) ;
#170137=CARTESIAN_POINT ( 'NONE',  ( -12.06949235617739369, -12.14591786802326823, 74.37609039468568994 ) ) ;
#170138=CARTESIAN_POINT ( 'NONE',  ( 0.05219959533937995610, -21.53943276465977519, 95.00109039468568994 ) ) ;
#170139=CARTESIAN_POINT ( 'NONE',  ( -9.474510206698964154, 16.51473224551069663, 70.41557627198102409 ) ) ;
#170140=CARTESIAN_POINT ( 'NONE',  ( -0.05219959533907301413, -21.53943276465977519, 32.49890960531435979 ) ) ;
#170141=CARTESIAN_POINT ( 'NONE',  ( 0.05219959533936267826, -19.03943276465977164, 110.0010903946856757 ) ) ;
#170142=CARTESIAN_POINT ( 'NONE',  ( -21.52544592524334988, -5.823673210054445271, 83.95942372801900433 ) ) ;
#170143=CARTESIAN_POINT ( 'NONE',  ( -4.379528057220086978, -16.55341960407618274, 49.79275706135234714 ) ) ;
#170144=CARTESIAN_POINT ( 'NONE',  ( -10.72451020669898014, 18.67979575497178502, 95.41557627198102409 ) ) ;
#170145=CARTESIAN_POINT ( 'NONE',  ( 19.05341960407617918, -5.049401038297876454, 106.0427570613523471 ) ) ;
#170146=CARTESIAN_POINT ( 'NONE',  ( 0.05219959533909260263, 19.03943276465977164, 84.99890960531436690 ) ) ;
#170147=ADVANCED_FACE ( 'NONE', ( #11377 ), #4191, .T. ) ;
#170148=CARTESIAN_POINT ( 'NONE',  ( 12.06949235617739724, 12.14591786802326823, 26.87609039468567218 ) ) ;
#170149=CARTESIAN_POINT ( 'NONE',  ( -16.51473224551069308, -9.474510206698971260, 36.66557627198102409 ) ) ;
#170151=CARTESIAN_POINT ( 'NONE',  ( 13.97604488694548053, -13.89961937509957401, 110.6260903946856615 ) ) ;
#170152=CARTESIAN_POINT ( 'NONE',  ( -16.55341960407611168, -4.379528057220339221, 71.45724293864769550 ) ) ;
#170153=CARTESIAN_POINT ( 'NONE',  ( -0.05219959533934338120, 16.53943276465976808, 87.50109039468568994 ) ) ;
#170154=CARTESIAN_POINT ( 'NONE',  ( 21.55341960407619695, -5.719274019375665929, 31.04275706135234714 ) ) ;
#170155=CARTESIAN_POINT ( 'NONE',  ( 9.564922557960805705, 16.46253265017160317, 54.58224293864769550 ) ) ;
#170156=CARTESIAN_POINT ( 'NONE',  ( -9.474510206698964154, 16.51473224551069663, 70.41557627198102409 ) ) ;
#170157=CARTESIAN_POINT ( 'NONE',  ( 14.29746914071037800, 8.314922557961029526, 66.66775706135234714 ) ) ;
#170161=CARTESIAN_POINT ( 'NONE',  ( 21.55341960407619695, -5.719274019375665929, 111.0427570613523613 ) ) ;
#170163=CARTESIAN_POINT ( 'NONE',  ( -5.153800228976328057, -19.02544592524343514, 37.29057627198102409 ) ) ;
#170164=CARTESIAN_POINT ( 'NONE',  ( -9.474510206698964154, 16.51473224551069663, 110.4155762719810383 ) ) ;
#170166=CARTESIAN_POINT ( 'NONE',  ( -8.224510206698735004, -14.34966873604973081, 34.58442372801900433 ) ) ;
#170167=CARTESIAN_POINT ( 'NONE',  ( 9.474510206698729675, 16.51473224551082808, 62.08442372801899722 ) ) ;
#170168=CARTESIAN_POINT ( 'NONE',  ( -12.14591786802326823, 12.06949235617739902, 43.12609039468568284 ) ) ;
#170169=CARTESIAN_POINT ( 'NONE',  ( -5.049401038298153566, 19.05341960407611168, 40.20724293864768839 ) ) ;
#170170=CARTESIAN_POINT ( 'NONE',  ( -16.51473224551069308, -9.474510206698971260, 106.6655762719810383 ) ) ;
#170171=CARTESIAN_POINT ( 'NONE',  ( -13.97604488694527625, -13.89961937509977652, 61.87390960531435979 ) ) ;
#170172=CARTESIAN_POINT ( 'NONE',  ( 15.80617190586746368, 15.72974639402197994, 104.3739096053143669 ) ) ;
#170173=CARTESIAN_POINT ( 'NONE',  ( -13.89961937509977652, 13.97604488694528158, 95.62390960531436690 ) ) ;
#170174=CARTESIAN_POINT ( 'NONE',  ( 5.153800228976335163, 19.02544592524342804, 24.79057627198102765 ) ) ;
#170175=CARTESIAN_POINT ( 'NONE',  ( 0.05219959533909260263, 19.03943276465977164, 69.99890960531435269 ) ) ;
#170176=CARTESIAN_POINT ( 'NONE',  ( 16.52544592524342804, -4.483927247898539470, 23.54057627198102765 ) ) ;
#170177=CARTESIAN_POINT ( 'NONE',  ( 13.89961937509977652, -13.97604488694527269, 23.12390960531436335 ) ) ;
#170178=CARTESIAN_POINT ( 'NONE',  ( -13.97604488694547697, 13.89961937509957934, 103.1260903946856473 ) ) ;
#170179=CARTESIAN_POINT ( 'NONE',  ( -21.55341960407619339, 5.719274019375674811, 113.5427570613523756 ) ) ;
#170180=CARTESIAN_POINT ( 'NONE',  ( -12.14591786802309592, -12.06949235617757132, 56.87390960531436690 ) ) ;
#170181=CARTESIAN_POINT ( 'NONE',  ( -21.55341960407619339, 5.719274019375674811, 98.54275706135234714 ) ) ;
#170182=CARTESIAN_POINT ( 'NONE',  ( 13.89961937509977652, -13.97604488694527269, 38.12390960531436690 ) ) ;
#170183=CARTESIAN_POINT ( 'NONE',  ( 8.314922557960818139, 14.29746914071049879, 39.58224293864769550 ) ) ;
#170184=CARTESIAN_POINT ( 'NONE',  ( 0.05219959533937995610, -21.53943276465977519, 85.00109039468568994 ) ) ;
#170185=CARTESIAN_POINT ( 'NONE',  ( -9.564922557960796823, -16.46253265017161027, 82.08224293864768129 ) ) ;
#170186=CARTESIAN_POINT ( 'NONE',  ( -5.049401038298153566, 19.05341960407611168, 95.20724293864770971 ) ) ;
#170187=CARTESIAN_POINT ( 'NONE',  ( -14.34966873604960291, -8.224510206698953496, 106.6655762719810383 ) ) ;
#170188=CARTESIAN_POINT ( 'NONE',  ( -12.06949235617756955, 12.14591786802309770, 80.62390960531438111 ) ) ;
#170189=CARTESIAN_POINT ( 'NONE',  ( 10.72451020669898902, -18.67979575497178502, 82.91557627198103830 ) ) ;
#170190=CARTESIAN_POINT ( 'NONE',  ( 19.05341960407611168, 5.049401038298154454, 68.95724293864769550 ) ) ;
#170191=CARTESIAN_POINT ( 'NONE',  ( -21.53943276465977519, 0.05219959533907696930, 86.24890960531436690 ) ) ;
#170192=CARTESIAN_POINT ( 'NONE',  ( 9.474510206698729675, 16.51473224551082808, 77.08442372801900433 ) ) ;
#170193=CARTESIAN_POINT ( 'NONE',  ( -9.474510206698720793, -16.51473224551083518, 64.58442372801900433 ) ) ;
#170194=CARTESIAN_POINT ( 'NONE',  ( -12.06949235617756955, 12.14591786802309770, 90.62390960531436690 ) ) ;
#170195=VECTOR ( 'NONE', #170396, 1000.000000000000000 ) ;
#170196=CARTESIAN_POINT ( 'NONE',  ( 5.153800228976335163, 19.02544592524342804, 59.79057627198100988 ) ) ;
#170197=CARTESIAN_POINT ( 'NONE',  ( -5.719274019375978568, 21.55341960407610458, 65.20724293864768129 ) ) ;
#170198=CARTESIAN_POINT ( 'NONE',  ( -17.49999999999999645, -5.499999999999992895, 84.20309617465829888 ) ) ;
#170199=CARTESIAN_POINT ( 'NONE',  ( 16.55341960407611168, 4.379528057220329451, 23.95724293864769550 ) ) ;
#170201=CARTESIAN_POINT ( 'NONE',  ( -16.53943276465976808, -0.05219959533934237506, 23.75109039468567929 ) ) ;
#170202=CARTESIAN_POINT ( 'NONE',  ( 0.05219959533910956823, 16.53943276465976808, 79.99890960531435269 ) ) ;
#170203=CARTESIAN_POINT ( 'NONE',  ( -18.22780087662122384, -5.500000000000025757, 96.48459894673894155 ) ) ;
#170204=CARTESIAN_POINT ( 'NONE',  ( -19.05341960407611168, -5.049401038298163336, 76.45724293864769550 ) ) ;
#170205=CARTESIAN_POINT ( 'NONE',  ( -5.049401038298153566, 19.05341960407611168, 35.20724293864768839 ) ) ;
#170206=CARTESIAN_POINT ( 'NONE',  ( -4.379528057220328563, 16.55341960407611168, 65.20724293864768129 ) ) ;
#170207=CARTESIAN_POINT ( 'NONE',  ( 21.52544592524344225, -5.823673210054117533, 23.54057627198102765 ) ) ;
#170208=CARTESIAN_POINT ( 'NONE',  ( 13.89961937509957401, 13.97604488694547697, 86.87609039468567573 ) ) ;
#170209=CARTESIAN_POINT ( 'NONE',  ( -19.02544592524342804, 5.153800228976336051, 76.04057627198102409 ) ) ;
#170210=CARTESIAN_POINT ( 'NONE',  ( 13.97604488694527802, 13.89961937509977652, 84.37390960531433848 ) ) ;
#170211=CARTESIAN_POINT ( 'NONE',  ( 10.72451020669898902, -18.67979575497178502, 82.91557627198103830 ) ) ;
#170212=CARTESIAN_POINT ( 'NONE',  ( 0.05219959533934541429, -16.53943276465976808, 65.00109039468568994 ) ) ;
#170213=CARTESIAN_POINT ( 'NONE',  ( -9.564922557961040184, 16.46253265017147172, 112.9177570613523329 ) ) ;
#170214=CARTESIAN_POINT ( 'NONE',  ( 19.03943276465977164, -0.05219959533909143690, 68.74890960531436690 ) ) ;
#170215=CARTESIAN_POINT ( 'NONE',  ( -10.81492255796078084, -18.62759615963271287, 72.08224293864769550 ) ) ;
#170216=CARTESIAN_POINT ( 'NONE',  ( 13.97604488694548053, -13.89961937509957401, 90.62609039468567573 ) ) ;
#170217=CARTESIAN_POINT ( 'NONE',  ( 16.53943276465976808, -0.05219959533910856209, 33.74890960531436690 ) ) ;
#170218=CARTESIAN_POINT ( 'NONE',  ( -18.62759615963255300, -10.81492255796106328, 49.16775706135234003 ) ) ;
#170220=CARTESIAN_POINT ( 'NONE',  ( -16.52544592524335698, -4.483927247898792601, 73.95942372801901854 ) ) ;
#170221=CARTESIAN_POINT ( 'NONE',  ( 0.05219959533909260263, 19.03943276465977164, 99.99890960531436690 ) ) ;
#170222=CARTESIAN_POINT ( 'NONE',  ( -17.59860650958990647, -7.585241751807021870, 101.5766298573750817 ) ) ;
#170224=CARTESIAN_POINT ( 'NONE',  ( 8.314922557961029526, -14.29746914071037800, 95.41775706135234714 ) ) ;
#170225=CARTESIAN_POINT ( 'NONE',  ( -8.224510206698735004, -14.34966873604973081, 44.58442372801901854 ) ) ;
#170226=CARTESIAN_POINT ( 'NONE',  ( 19.02544592524343514, -5.153800228976328945, 58.54057627198102409 ) ) ;
#170227=CARTESIAN_POINT ( 'NONE',  ( -19.03943276465977164, 0.05219959533909376836, 76.24890960531435269 ) ) ;
#170228=CARTESIAN_POINT ( 'NONE',  ( 0.05219959533937995610, -21.53943276465977519, 50.00109039468568994 ) ) ;
#170229=CARTESIAN_POINT ( 'NONE',  ( -12.14591786802326823, 12.06949235617739902, 63.12609039468568994 ) ) ;
#170230=CARTESIAN_POINT ( 'NONE',  ( 16.53943276465976808, -0.05219959533910856209, 33.74890960531436690 ) ) ;
#170231=CARTESIAN_POINT ( 'NONE',  ( -9.564922557960796823, -16.46253265017161027, 42.08224293864769550 ) ) ;
#170232=CARTESIAN_POINT ( 'NONE',  ( 13.97604488694527802, 13.89961937509977652, 29.37390960531435979 ) ) ;
#170233=CARTESIAN_POINT ( 'NONE',  ( -4.483927247898782831, 16.52544592524335698, 22.70942372801901499 ) ) ;
#170234=CARTESIAN_POINT ( 'NONE',  ( 19.02544592524334988, 5.153800228976608722, 81.45942372801897591 ) ) ;
#170235=CARTESIAN_POINT ( 'NONE',  ( -0.05219959533910754901, -16.53943276465976808, 87.49890960531436690 ) ) ;
#170236=CARTESIAN_POINT ( 'NONE',  ( -9.564922557960796823, -16.46253265017161027, 52.08224293864768839 ) ) ;
#170237=CARTESIAN_POINT ( 'NONE',  ( -5.049401038297874678, -19.05341960407617918, 89.79275706135230450 ) ) ;
#170239=CARTESIAN_POINT ( 'NONE',  ( 15.80617190586769283, -15.72974639402175789, 90.62609039468567573 ) ) ;
#170240=CARTESIAN_POINT ( 'NONE',  ( -12.06949235617739369, -12.14591786802326823, 49.37609039468569705 ) ) ;
#170241=CARTESIAN_POINT ( 'NONE',  ( -17.49999999999999645, 3.512728167237046950, 25.22809995181131271 ) ) ;
#170242=CARTESIAN_POINT ( 'NONE',  ( -0.05219959533907301413, -21.53943276465977519, 52.49890960531435979 ) ) ;
#170243=CARTESIAN_POINT ( 'NONE',  ( 16.55341960407618274, -4.379528057220086978, 41.04275706135236135 ) ) ;
#170244=CARTESIAN_POINT ( 'NONE',  ( 13.89961937509978007, -13.97604488694527269, 33.12390960531435269 ) ) ;
#170245=CARTESIAN_POINT ( 'NONE',  ( 5.153800228976615827, -19.02544592524334988, 40.20942372801898301 ) ) ;
#170246=CARTESIAN_POINT ( 'NONE',  ( -0.05219959533909027116, -19.03943276465977164, 82.49890960531436690 ) ) ;
#170247=CARTESIAN_POINT ( 'NONE',  ( -9.474510206698964154, 16.51473224551069663, 55.41557627198103120 ) ) ;
#170249=CARTESIAN_POINT ( 'NONE',  ( 19.03943276465977164, -0.05219959533909143690, 68.74890960531436690 ) ) ;
#170251=CARTESIAN_POINT ( 'NONE',  ( -19.05341960407617563, 5.049401038297882671, 33.54275706135231871 ) ) ;
#170252=CARTESIAN_POINT ( 'NONE',  ( 15.72974639402176855, 15.80617190586768217, 111.8760903946856615 ) ) ;
#170253=CARTESIAN_POINT ( 'NONE',  ( 16.52544592524342804, -4.483927247898539470, 38.54057627198103120 ) ) ;
#170254=CARTESIAN_POINT ( 'NONE',  ( -13.97604488694527625, -13.89961937509977652, 36.87390960531436690 ) ) ;
#170255=CARTESIAN_POINT ( 'NONE',  ( 19.03943276465977164, -0.05219959533909143690, 103.7489096053143669 ) ) ;
#170256=CARTESIAN_POINT ( 'NONE',  ( -21.52544592524334988, -5.823673210054445271, 78.95942372801901854 ) ) ;
#170257=CARTESIAN_POINT ( 'NONE',  ( -5.049401038298153566, 19.05341960407611168, 50.20724293864770260 ) ) ;
#170258=CARTESIAN_POINT ( 'NONE',  ( 15.80617190586769283, -15.72974639402175789, 80.62609039468567573 ) ) ;
#170259=CARTESIAN_POINT ( 'NONE',  ( -15.80617190586745835, -15.72974639402198527, 26.87390960531435979 ) ) ;
#170260=CARTESIAN_POINT ( 'NONE',  ( 5.823673210054444382, -21.52544592524334988, 20.20942372801900788 ) ) ;
#170261=CARTESIAN_POINT ( 'NONE',  ( 16.51473224551083163, -9.474510206698727899, 45.83442372801900433 ) ) ;
#170262=CARTESIAN_POINT ( 'NONE',  ( 19.02544592524343514, -5.153800228976328945, 33.54057627198102409 ) ) ;
#170263=CARTESIAN_POINT ( 'NONE',  ( 19.02544592524343514, -5.153800228976328945, 78.54057627198099567 ) ) ;
#170264=CARTESIAN_POINT ( 'NONE',  ( 4.379528057220092307, 16.55341960407617563, 22.29275706135235069 ) ) ;
#170265=CARTESIAN_POINT ( 'NONE',  ( -16.55341960407611168, -4.379528057220339221, 86.45724293864770971 ) ) ;
#170266=CARTESIAN_POINT ( 'NONE',  ( 18.67979575497178502, 10.72451020669898547, 39.16557627198102409 ) ) ;
#170267=CARTESIAN_POINT ( 'NONE',  ( -5.153800228976607833, 19.02544592524334988, 102.7094237280189759 ) ) ;
#170268=CARTESIAN_POINT ( 'NONE',  ( -15.72974639402197994, 15.80617190586746368, 100.6239096053143811 ) ) ;
#170269=CARTESIAN_POINT ( 'NONE',  ( 21.52544592524334988, 5.823673210054432836, 51.45942372801901854 ) ) ;
#170270=CARTESIAN_POINT ( 'NONE',  ( -4.483927247898782831, 16.52544592524335698, 62.70942372801902565 ) ) ;
#170271=CARTESIAN_POINT ( 'NONE',  ( 8.224510206698742110, 14.34966873604972548, 67.08442372801901854 ) ) ;
#170273=CARTESIAN_POINT ( 'NONE',  ( -9.564922557960796823, -16.46253265017161027, 57.08224293864769550 ) ) ;
#170274=CARTESIAN_POINT ( 'NONE',  ( -14.29746914071037622, -8.314922557961029526, 89.16775706135236135 ) ) ;
#170275=CARTESIAN_POINT ( 'NONE',  ( 5.719274019375991003, -21.55341960407610458, 112.7072429386476955 ) ) ;
#170276=CARTESIAN_POINT ( 'NONE',  ( -12.06949235617756955, 12.14591786802309770, 50.62390960531435979 ) ) ;
#170277=CARTESIAN_POINT ( 'NONE',  ( -13.89961937509977652, 13.97604488694528158, 80.62390960531436690 ) ) ;
#170278=CARTESIAN_POINT ( 'NONE',  ( -8.314922557961024197, 14.29746914071037800, 72.91775706135234714 ) ) ;
#170279=CARTESIAN_POINT ( 'NONE',  ( -10.81492255796105439, 18.62759615963255655, 52.91775706135235424 ) ) ;
#170280=CARTESIAN_POINT ( 'NONE',  ( -13.89961937509957401, -13.97604488694547875, 109.3760903946856331 ) ) ;
#170281=CARTESIAN_POINT ( 'NONE',  ( 15.72974639402199770, -15.80617190586745480, 108.1239096053143811 ) ) ;
#170282=CARTESIAN_POINT ( 'NONE',  ( -4.483927247898539470, -16.52544592524342804, 52.29057627198102409 ) ) ;
#170284=CARTESIAN_POINT ( 'NONE',  ( -17.48853670773247515, 5.747243402303043425, 68.66671299749995683 ) ) ;
#170285=CARTESIAN_POINT ( 'NONE',  ( -15.80617190586745835, -15.72974639402198527, 81.87390960531435269 ) ) ;
#170286=CARTESIAN_POINT ( 'NONE',  ( 12.06949235617757843, -12.14591786802309237, 43.12390960531435269 ) ) ;
#170289=CARTESIAN_POINT ( 'NONE',  ( 21.55341960407610458, 5.719274019375980345, 108.9572429386476955 ) ) ;
#170290=CARTESIAN_POINT ( 'NONE',  ( 5.719274019375991003, -21.55341960407610458, 22.70724293864769194 ) ) ;
#170291=CARTESIAN_POINT ( 'NONE',  ( -10.81492255796105439, 18.62759615963255655, 27.91775706135234358 ) ) ;
#170292=CARTESIAN_POINT ( 'NONE',  ( -8.314922557960811034, -14.29746914071050412, 52.08224293864768839 ) ) ;
#170293=CARTESIAN_POINT ( 'NONE',  ( -12.06949235617739369, -12.14591786802326823, 59.37609039468568284 ) ) ;
#170295=CARTESIAN_POINT ( 'NONE',  ( -0.05219959533909027116, -19.03943276465977164, 57.49890960531435979 ) ) ;
#170296=CARTESIAN_POINT ( 'NONE',  ( -16.51473224551082808, 9.474510206698731452, 63.33442372801900433 ) ) ;
#170297=CARTESIAN_POINT ( 'NONE',  ( 19.05341960407611168, 5.049401038298154454, 83.95724293864766707 ) ) ;
#170298=CARTESIAN_POINT ( 'NONE',  ( 15.80617190586746368, 15.72974639402197994, 34.37390960531435979 ) ) ;
#170300=CARTESIAN_POINT ( 'NONE',  ( -5.153800228976328057, -19.02544592524343514, 62.29057627198100988 ) ) ;
#170301=CARTESIAN_POINT ( 'NONE',  ( -12.14591786802326823, 12.06949235617739902, 23.12609039468567573 ) ) ;
#170302=CARTESIAN_POINT ( 'NONE',  ( -19.05341960407617563, 5.049401038297882671, 63.54275706135234003 ) ) ;
#170303=CARTESIAN_POINT ( 'NONE',  ( 18.67979575497178502, 10.72451020669898547, 104.1655762719810241 ) ) ;
#170304=CARTESIAN_POINT ( 'NONE',  ( 14.34966873604960469, 8.224510206698951720, 34.16557627198102409 ) ) ;
#170305=CARTESIAN_POINT ( 'NONE',  ( -16.51473224551069308, -9.474510206698971260, 96.66557627198102409 ) ) ;
#170306=CARTESIAN_POINT ( 'NONE',  ( -5.823673210054116645, -21.52544592524344225, 62.29057627198102409 ) ) ;
#170307=CARTESIAN_POINT ( 'NONE',  ( -18.67979575497178146, -10.72451020669898902, 91.66557627198103830 ) ) ;
#170308=CARTESIAN_POINT ( 'NONE',  ( -14.29746914071037622, -8.314922557961029526, 39.16775706135235424 ) ) ;
#170309=CARTESIAN_POINT ( 'NONE',  ( -21.52544592524343514, 5.823673210054127303, 41.04057627198103120 ) ) ;
#170310=CARTESIAN_POINT ( 'NONE',  ( 10.81492255796106328, -18.62759615963255655, 90.41775706135236135 ) ) ;
#170311=CARTESIAN_POINT ( 'NONE',  ( -16.46253265017160317, 9.564922557960807481, 90.83224293864769550 ) ) ;
#170312=CARTESIAN_POINT ( 'NONE',  ( -9.474510206698964154, 16.51473224551069663, 40.41557627198103120 ) ) ;
#170313=CARTESIAN_POINT ( 'NONE',  ( -16.46253265017160317, 9.564922557960807481, 100.8322429386477097 ) ) ;
#170314=CARTESIAN_POINT ( 'NONE',  ( 12.14591786802309770, 12.06949235617756955, 104.3739096053143669 ) ) ;
#170315=CARTESIAN_POINT ( 'NONE',  ( -19.05341960407611168, -5.049401038298163336, 61.45724293864769550 ) ) ;
#170316=CARTESIAN_POINT ( 'NONE',  ( -16.52544592524335698, -4.483927247898792601, 18.95942372801901143 ) ) ;
#170317=CARTESIAN_POINT ( 'NONE',  ( 17.12812012977046905, -6.668231424565697729, 86.14051240676850796 ) ) ;
#170319=CARTESIAN_POINT ( 'NONE',  ( 5.823673210054444382, -21.52544592524334988, 100.2094237280190043 ) ) ;
#170320=CARTESIAN_POINT ( 'NONE',  ( 16.46253265017160672, -9.564922557960803928, 113.3322429386476955 ) ) ;
#170321=CARTESIAN_POINT ( 'NONE',  ( 16.52544592524335698, 4.483927247898782831, 96.45942372801901854 ) ) ;
#170323=CARTESIAN_POINT ( 'NONE',  ( -5.153800228976607833, 19.02544592524334988, 67.70942372801900433 ) ) ;
#170324=CARTESIAN_POINT ( 'NONE',  ( 16.46253265017146816, 9.564922557961045513, 31.66775706135232937 ) ) ;
#170326=CARTESIAN_POINT ( 'NONE',  ( -5.153800228976328057, -19.02544592524343514, 27.29057627198103120 ) ) ;
#170327=CARTESIAN_POINT ( 'NONE',  ( 0.05219959533910956823, 16.53943276465976808, 39.99890960531436690 ) ) ;
#170328=CARTESIAN_POINT ( 'NONE',  ( -17.49999999999999645, -5.500000000000000888, 109.2030961746582847 ) ) ;
#170329=CARTESIAN_POINT ( 'NONE',  ( -16.53943276465976808, 0.05219959533911058130, 31.24890960531435979 ) ) ;
#170330=CARTESIAN_POINT ( 'NONE',  ( 17.26172910966779028, 6.454744622555872446, 66.69353091350777163 ) ) ;
#170331=CARTESIAN_POINT ( 'NONE',  ( -14.34966873604972548, 8.224510206698743886, 93.33442372801901854 ) ) ;
#170332=CARTESIAN_POINT ( 'NONE',  ( -16.51473224551069308, -9.474510206698971260, 41.66557627198103120 ) ) ;
#170333=CARTESIAN_POINT ( 'NONE',  ( -21.53943276465977519, -0.05219959533937600094, 108.7510903946857042 ) ) ;
#170334=CARTESIAN_POINT ( 'NONE',  ( -0.05219959533936034679, 19.03943276465977164, 112.5010903946856757 ) ) ;
#170335=CARTESIAN_POINT ( 'NONE',  ( -5.719274019375665041, -21.55341960407619695, 74.79275706135234714 ) ) ;
#170336=CARTESIAN_POINT ( 'NONE',  ( -9.564922557961040184, 16.46253265017147172, 52.91775706135233293 ) ) ;
#170337=CARTESIAN_POINT ( 'NONE',  ( 16.51473224551069308, 9.474510206698969483, 94.16557627198103830 ) ) ;
#170338=CARTESIAN_POINT ( 'NONE',  ( 19.05341960407611168, 5.049401038298154454, 68.95724293864769550 ) ) ;
#170339=CARTESIAN_POINT ( 'NONE',  ( 16.81555441253552274, 7.025013491695500711, 71.86314554665747778 ) ) ;
#170340=CARTESIAN_POINT ( 'NONE',  ( -15.72974639402197994, 15.80617190586746368, 95.62390960531436690 ) ) ;
#170342=CARTESIAN_POINT ( 'NONE',  ( -16.53943276465976808, 0.05219959533911058130, 66.24890960531436690 ) ) ;
#170343=CARTESIAN_POINT ( 'NONE',  ( -18.67979575497178146, -10.72451020669898902, 61.66557627198103120 ) ) ;
#170344=CARTESIAN_POINT ( 'NONE',  ( -19.03943276465977164, 0.05219959533909376836, 66.24890960531436690 ) ) ;
#170345=CARTESIAN_POINT ( 'NONE',  ( -18.67979575497178146, -10.72451020669898902, 81.66557627198103830 ) ) ;
#170346=CARTESIAN_POINT ( 'NONE',  ( -4.483927247898782831, 16.52544592524335698, 72.70942372801901854 ) ) ;
#170348=CARTESIAN_POINT ( 'NONE',  ( -19.02544592524342804, 5.153800228976336051, 41.04057627198103120 ) ) ;
#170349=CARTESIAN_POINT ( 'NONE',  ( -16.53943276465976808, 0.05219959533911058130, 76.24890960531435269 ) ) ;
#170351=CARTESIAN_POINT ( 'NONE',  ( -16.46253265017160317, 9.564922557960807481, 50.83224293864770260 ) ) ;
#170352=CARTESIAN_POINT ( 'NONE',  ( 4.379528057220339221, -16.55341960407611168, 112.7072429386476955 ) ) ;
#170353=CARTESIAN_POINT ( 'NONE',  ( 13.97604488694548053, -13.89961937509957401, 60.62609039468564731 ) ) ;
#170354=CARTESIAN_POINT ( 'NONE',  ( -4.483927247898539470, -16.52544592524342804, 87.29057627198103830 ) ) ;
#170355=CARTESIAN_POINT ( 'NONE',  ( -10.81492255796105439, 18.62759615963255655, 42.91775706135235424 ) ) ;
#170356=CARTESIAN_POINT ( 'NONE',  ( 19.05341960407611168, 5.049401038298154454, 38.95724293864767418 ) ) ;
#170357=CARTESIAN_POINT ( 'NONE',  ( -5.823673210054116645, -21.52544592524344225, 102.2905762719810383 ) ) ;
#170358=CARTESIAN_POINT ( 'NONE',  ( 12.14591786802309770, 12.06949235617756955, 89.37390960531435269 ) ) ;
#170360=CARTESIAN_POINT ( 'NONE',  ( 16.51473224551069308, 9.474510206698969483, 49.16557627198102409 ) ) ;
#170362=CARTESIAN_POINT ( 'NONE',  ( 9.564922557961047289, -16.46253265017146816, 95.41775706135233293 ) ) ;
#170363=CARTESIAN_POINT ( 'NONE',  ( 19.02544592524343514, -5.153800228976328945, 93.54057627198102409 ) ) ;
#170364=CARTESIAN_POINT ( 'NONE',  ( -5.719274019375665041, -21.55341960407619695, 29.79275706135234358 ) ) ;
#170365=CARTESIAN_POINT ( 'NONE',  ( 13.89961937509977652, -13.97604488694527269, 88.12390960531438111 ) ) ;
#170366=CARTESIAN_POINT ( 'NONE',  ( 0.05219959533936267826, -19.03943276465977164, 75.00109039468566152 ) ) ;
#170367=CARTESIAN_POINT ( 'NONE',  ( 13.97604488694527802, 13.89961937509977652, 44.37390960531435269 ) ) ;
#170368=CARTESIAN_POINT ( 'NONE',  ( -8.314922557960811034, -14.29746914071050412, 72.08224293864769550 ) ) ;
#170369=CARTESIAN_POINT ( 'NONE',  ( 16.53943276465976808, -0.05219959533910856209, 68.74890960531435269 ) ) ;
#170370=CARTESIAN_POINT ( 'NONE',  ( 13.97604488694527802, 13.89961937509977652, 89.37390960531436690 ) ) ;
#170371=CARTESIAN_POINT ( 'NONE',  ( -15.80617190586745835, -15.72974639402198527, 96.87390960531436690 ) ) ;
#170372=CARTESIAN_POINT ( 'NONE',  ( 9.564922557960805705, 16.46253265017160317, 69.58224293864770971 ) ) ;
#170374=CARTESIAN_POINT ( 'NONE',  ( 19.02544592524334988, 5.153800228976608722, 26.45942372801899722 ) ) ;
#170375=CARTESIAN_POINT ( 'NONE',  ( 16.46253265017160672, -9.564922557960803928, 38.33224293864768839 ) ) ;
#170376=CARTESIAN_POINT ( 'NONE',  ( -8.224510206698948167, 14.34966873604960824, 25.41557627198103120 ) ) ;
#170377=CARTESIAN_POINT ( 'NONE',  ( 16.52544592524342804, -4.483927247898539470, 113.5405762719810383 ) ) ;
#170378=CARTESIAN_POINT ( 'NONE',  ( 16.46253265017146816, 9.564922557961045513, 111.6677570613523329 ) ) ;
#170380=CARTESIAN_POINT ( 'NONE',  ( -15.80617190586768217, 15.72974639402176855, 28.12609039468568284 ) ) ;
#170381=CARTESIAN_POINT ( 'NONE',  ( -19.05341960407617563, 5.049401038297882671, 68.54275706135230450 ) ) ;
#170382=CARTESIAN_POINT ( 'NONE',  ( 8.224510206698953496, -14.34966873604960469, 27.91557627198103830 ) ) ;
#170383=CARTESIAN_POINT ( 'NONE',  ( 15.72974639402199770, -15.80617190586745480, 88.12390960531436690 ) ) ;
#170384=CARTESIAN_POINT ( 'NONE',  ( -19.03943276465977164, 0.05219959533909376836, 111.2489096053143669 ) ) ;
#170385=CARTESIAN_POINT ( 'NONE',  ( 8.224510206698953496, -14.34966873604960469, 62.91557627198102409 ) ) ;
#170386=CARTESIAN_POINT ( 'NONE',  ( -16.46253265017160317, 9.564922557960807481, 30.83224293864769550 ) ) ;
#170387=CARTESIAN_POINT ( 'NONE',  ( 5.049401038297881783, 19.05341960407617563, 32.29275706135233293 ) ) ;
#170388=CARTESIAN_POINT ( 'NONE',  ( -8.224510206698735004, -14.34966873604973081, 84.58442372801903275 ) ) ;
#170389=CARTESIAN_POINT ( 'NONE',  ( 14.29746914071037800, 8.314922557961029526, 61.66775706135235424 ) ) ;
#170390=CARTESIAN_POINT ( 'NONE',  ( -0.05219959533909027116, -19.03943276465977164, 112.4989096053143669 ) ) ;
#170391=CARTESIAN_POINT ( 'NONE',  ( -18.62759615963255300, -10.81492255796106328, 109.1677570613523613 ) ) ;
#170392=CARTESIAN_POINT ( 'NONE',  ( 5.049401038298161559, -19.05341960407611168, 77.70724293864765286 ) ) ;
#170393=CARTESIAN_POINT ( 'NONE',  ( 0.05219959533934541429, -16.53943276465976808, 55.00109039468568284 ) ) ;
#170394=CARTESIAN_POINT ( 'NONE',  ( 19.02544592524343514, -5.153800228976328945, 28.54057627198102409 ) ) ;
#170395=CARTESIAN_POINT ( 'NONE',  ( -16.55341960407611168, -4.379528057220339221, 31.45724293864769550 ) ) ;
#170396=DIRECTION ( 'NONE',  ( -0.000000000000000000, -0.000000000000000000, 1.000000000000000000 ) ) ;
#170397=CARTESIAN_POINT ( 'NONE',  ( 5.823673210054444382, -21.52544592524334988, 75.20942372801901854 ) ) ;
#170398=CARTESIAN_POINT ( 'NONE',  ( 13.89961937509977652, -13.97604488694527269, 108.1239096053143669 ) ) ;
#170399=CARTESIAN_POINT ( 'NONE',  ( -9.474510206698964154, 16.51473224551069663, 75.41557627198103830 ) ) ;
#170400=CARTESIAN_POINT ( 'NONE',  ( 9.564922557960805705, 16.46253265017160317, 114.5822429386476955 ) ) ;
#170401=CARTESIAN_POINT ( 'NONE',  ( 16.52544592524342804, -4.483927247898539470, 53.54057627198103120 ) ) ;
#170402=CARTESIAN_POINT ( 'NONE',  ( 0.05219959533910956823, 16.53943276465976808, 34.99890960531435979 ) ) ;
#170403=CARTESIAN_POINT ( 'NONE',  ( -14.34966873604960291, -8.224510206698953496, 56.66557627198103830 ) ) ;
#170404=CARTESIAN_POINT ( 'NONE',  ( -8.314922557961024197, 14.29746914071037800, 37.91775706135235424 ) ) ;
#170405=CARTESIAN_POINT ( 'NONE',  ( 5.153800228976617603, -19.02544592524335343, 60.20942372801899722 ) ) ;
#170406=CARTESIAN_POINT ( 'NONE',  ( -16.46253265017146816, -9.564922557961047289, 49.16775706135233293 ) ) ;
#170407=CARTESIAN_POINT ( 'NONE',  ( -9.474510206698964154, 16.51473224551069663, 70.41557627198102409 ) ) ;
#170408=CARTESIAN_POINT ( 'NONE',  ( 13.97604488694548053, -13.89961937509957401, 55.62609039468566863 ) ) ;
#170409=CARTESIAN_POINT ( 'NONE',  ( 16.46253265017146816, 9.564922557961045513, 51.66775706135233293 ) ) ;
#170410=CARTESIAN_POINT ( 'NONE',  ( -5.153800228976607833, 19.02544592524334988, 92.70942372801901854 ) ) ;
#170411=CARTESIAN_POINT ( 'NONE',  ( -16.55341960407617563, 4.379528057220093196, 88.54275706135236135 ) ) ;
#170413=CARTESIAN_POINT ( 'NONE',  ( -5.153800228976328057, -19.02544592524343514, 22.29057627198102765 ) ) ;
#170414=CARTESIAN_POINT ( 'NONE',  ( 9.474510206698971260, -16.51473224551069308, 97.91557627198102409 ) ) ;
#170415=CARTESIAN_POINT ( 'NONE',  ( 21.53943276465977519, 0.05219959533937863772, 41.25109039468568284 ) ) ;
#170416=CARTESIAN_POINT ( 'NONE',  ( -19.05341960407617563, 5.049401038297882671, 103.5427570613523329 ) ) ;
#170418=CARTESIAN_POINT ( 'NONE',  ( -16.46253265017160317, 9.564922557960807481, 60.83224293864769550 ) ) ;
#170419=CARTESIAN_POINT ( 'NONE',  ( -13.89961937509977652, 13.97604488694528158, 105.6239096053143527 ) ) ;
#170420=CARTESIAN_POINT ( 'NONE',  ( 12.06949235617757843, -12.14591786802309237, 58.12390960531435979 ) ) ;
#170421=CARTESIAN_POINT ( 'NONE',  ( 19.02544592524343514, -5.153800228976328945, 68.54057627198103830 ) ) ;
#170422=CARTESIAN_POINT ( 'NONE',  ( -9.564922557960796823, -16.46253265017161027, 57.08224293864769550 ) ) ;
#170423=CARTESIAN_POINT ( 'NONE',  ( 5.049401038297881783, 19.05341960407617563, 77.29275706135231871 ) ) ;
#170424=CARTESIAN_POINT ( 'NONE',  ( 21.53943276465977519, -0.05219959533907433946, 53.74890960531437401 ) ) ;
#170425=CARTESIAN_POINT ( 'NONE',  ( -19.03943276465977164, -0.05219959533935918106, 43.75109039468566863 ) ) ;
#170426=CARTESIAN_POINT ( 'NONE',  ( -13.89961937509977652, 13.97604488694528158, 80.62390960531436690 ) ) ;
#170427=CARTESIAN_POINT ( 'NONE',  ( -15.80617190586745835, -15.72974639402198527, 76.87390960531439532 ) ) ;
#170428=CARTESIAN_POINT ( 'NONE',  ( -12.14591786802309592, -12.06949235617757132, 81.87390960531435269 ) ) ;
#170429=CARTESIAN_POINT ( 'NONE',  ( 5.049401038297881783, 19.05341960407617563, 37.29275706135232582 ) ) ;
#170430=CARTESIAN_POINT ( 'NONE',  ( 5.823673210054125526, 21.52544592524343514, 44.79057627198103120 ) ) ;
#170431=CARTESIAN_POINT ( 'NONE',  ( -18.67979575497178146, -10.72451020669898902, 36.66557627198103120 ) ) ;
#170432=CARTESIAN_POINT ( 'NONE',  ( 0.05219959533909260263, 19.03943276465977164, 59.99890960531436690 ) ) ;
#170433=CARTESIAN_POINT ( 'NONE',  ( 9.474510206698971260, -16.51473224551069308, 47.91557627198102409 ) ) ;
#170434=CARTESIAN_POINT ( 'NONE',  ( 19.03943276465977164, -0.05219959533909143690, 23.74890960531435269 ) ) ;
#170436=CARTESIAN_POINT ( 'NONE',  ( -0.05219959533937732626, 21.53943276465977519, 27.50109039468567929 ) ) ;
#170437=CARTESIAN_POINT ( 'NONE',  ( -19.02544592524342804, 5.153800228976336051, 116.0405762719810383 ) ) ;
#170438=CARTESIAN_POINT ( 'NONE',  ( 10.81492255796106328, -18.62759615963255655, 45.41775706135234003 ) ) ;
#170439=CARTESIAN_POINT ( 'NONE',  ( 5.153800228976335163, 19.02544592524342804, 39.79057627198100988 ) ) ;
#170440=CARTESIAN_POINT ( 'NONE',  ( 5.719274019375991003, -21.55341960407610458, 112.7072429386476955 ) ) ;
#170441=CARTESIAN_POINT ( 'NONE',  ( 19.03943276465977164, 0.05219959533936151252, 46.25109039468566863 ) ) ;
#170442=CARTESIAN_POINT ( 'NONE',  ( -5.049401038298153566, 19.05341960407611168, 25.20724293864768484 ) ) ;
#170443=CARTESIAN_POINT ( 'NONE',  ( -0.05219959533909027116, -19.03943276465977164, 22.49890960531436690 ) ) ;
#170445=CARTESIAN_POINT ( 'NONE',  ( -12.06949235617739369, -12.14591786802326823, 54.37609039468568994 ) ) ;
#170446=CARTESIAN_POINT ( 'NONE',  ( 19.02544592524343514, -5.153800228976328945, 23.54057627198102054 ) ) ;
#170448=CARTESIAN_POINT ( 'NONE',  ( 19.05341960407611168, 5.049401038298154454, 73.95724293864768129 ) ) ;
#170449=CARTESIAN_POINT ( 'NONE',  ( -4.483927247898539470, -16.52544592524342804, 112.2905762719810241 ) ) ;
#170450=CARTESIAN_POINT ( 'NONE',  ( 21.55341960407610458, 5.719274019375980345, 58.95724293864770971 ) ) ;
#170451=CARTESIAN_POINT ( 'NONE',  ( 16.52544592524342804, -4.483927247898539470, 73.54057627198102409 ) ) ;
#170452=CARTESIAN_POINT ( 'NONE',  ( 14.29746914071037800, 8.314922557961029526, 31.66775706135234358 ) ) ;
#170453=CARTESIAN_POINT ( 'NONE',  ( 18.67979575497194134, -10.72451020669871369, 90.83442372801901854 ) ) ;
#170454=CARTESIAN_POINT ( 'NONE',  ( -19.05341960407611168, -5.049401038298163336, 26.45724293864769550 ) ) ;
#170455=CARTESIAN_POINT ( 'NONE',  ( 8.314922557960818139, 14.29746914071049879, 24.58224293864768839 ) ) ;
#170456=CARTESIAN_POINT ( 'NONE',  ( 8.314922557960818139, 14.29746914071049879, 54.58224293864769550 ) ) ;
#170457=CARTESIAN_POINT ( 'NONE',  ( -9.474510206698964154, 16.51473224551069663, 50.41557627198102409 ) ) ;
#170458=CARTESIAN_POINT ( 'NONE',  ( 15.80617190586769283, -15.72974639402175789, 90.62609039468567573 ) ) ;
#170459=CARTESIAN_POINT ( 'NONE',  ( 18.62759615963271287, -10.81492255796078972, 103.3322429386476955 ) ) ;
#170460=CARTESIAN_POINT ( 'NONE',  ( -21.55341960407619339, 5.719274019375674811, 78.54275706135236135 ) ) ;
#170461=CARTESIAN_POINT ( 'NONE',  ( -8.314922557961024197, 14.29746914071037800, 47.91775706135234714 ) ) ;
#170462=CARTESIAN_POINT ( 'NONE',  ( 8.314922557960818139, 14.29746914071049879, 74.58224293864768129 ) ) ;
#170463=CARTESIAN_POINT ( 'NONE',  ( 0.05219959533937995610, -21.53943276465977519, 90.00109039468567573 ) ) ;
#170465=CARTESIAN_POINT ( 'NONE',  ( -4.483927247898782831, 16.52544592524335698, 107.7094237280190328 ) ) ;
#170467=CARTESIAN_POINT ( 'NONE',  ( -4.483927247898782831, 16.52544592524335698, 42.70942372801901854 ) ) ;
#170468=CARTESIAN_POINT ( 'NONE',  ( 8.224510206698953496, -14.34966873604960469, 47.91557627198102409 ) ) ;
#170469=CARTESIAN_POINT ( 'NONE',  ( -16.52544592524335698, -4.483927247898792601, 88.95942372801901854 ) ) ;
#170470=CARTESIAN_POINT ( 'NONE',  ( 0.05219959533909260263, 19.03943276465977164, 99.99890960531436690 ) ) ;
#170471=CARTESIAN_POINT ( 'NONE',  ( 0.05219959533909260263, 19.03943276465977164, 114.9989096053143669 ) ) ;
#170472=CARTESIAN_POINT ( 'NONE',  ( -0.05219959533937732626, 21.53943276465977519, 102.5010903946856899 ) ) ;
#170473=CARTESIAN_POINT ( 'NONE',  ( -16.53943276465976808, -0.05219959533934237506, 103.7510903946857042 ) ) ;
#170474=CARTESIAN_POINT ( 'NONE',  ( -16.52544592524342804, 4.483927247898546575, 76.04057627198102409 ) ) ;
#170475=CARTESIAN_POINT ( 'NONE',  ( -13.89961937509977652, 13.97604488694528158, 75.62390960531438111 ) ) ;
#170477=CARTESIAN_POINT ( 'NONE',  ( -0.05219959533934338120, 16.53943276465976808, 27.50109039468567929 ) ) ;
#170478=CARTESIAN_POINT ( 'NONE',  ( -9.474510206698964154, 16.51473224551069663, 25.41557627198103120 ) ) ;
#170479=CARTESIAN_POINT ( 'NONE',  ( 16.46253265017160672, -9.564922557960803928, 93.33224293864769550 ) ) ;
#170480=CARTESIAN_POINT ( 'NONE',  ( -12.14591786802326823, 12.06949235617739902, 28.12609039468568284 ) ) ;
#170482=CARTESIAN_POINT ( 'NONE',  ( 9.564922557961047289, -16.46253265017146816, 40.41775706135234003 ) ) ;
#170483=CARTESIAN_POINT ( 'NONE',  ( 8.314922557961029526, -14.29746914071037800, 100.4177570613523471 ) ) ;
#170484=CARTESIAN_POINT ( 'NONE',  ( 13.97604488694527802, 13.89961937509977652, 39.37390960531435269 ) ) ;
#170485=CARTESIAN_POINT ( 'NONE',  ( -4.379528057220086978, -16.55341960407618274, 84.79275706135234714 ) ) ;
#170486=CARTESIAN_POINT ( 'NONE',  ( 0.05219959533934541429, -16.53943276465976808, 65.00109039468568994 ) ) ;
#170487=CARTESIAN_POINT ( 'NONE',  ( -5.153800228976607833, 19.02544592524334988, 87.70942372801897591 ) ) ;
#170488=CARTESIAN_POINT ( 'NONE',  ( 21.55341960407619695, -5.719274019375665929, 111.0427570613523613 ) ) ;
#170489=CARTESIAN_POINT ( 'NONE',  ( 16.51473224551069308, 9.474510206698969483, 49.16557627198102409 ) ) ;
#170490=CARTESIAN_POINT ( 'NONE',  ( 16.46253265017160672, -9.564922557960803928, 93.33224293864769550 ) ) ;
#170491=CARTESIAN_POINT ( 'NONE',  ( -14.29746914071049879, 8.314922557960819915, 85.83224293864768129 ) ) ;
#170493=CARTESIAN_POINT ( 'NONE',  ( 0.05219959533936267826, -19.03943276465977164, 50.00109039468566863 ) ) ;
#170494=CARTESIAN_POINT ( 'NONE',  ( 10.81492255796078972, 18.62759615963270932, 44.58224293864769550 ) ) ;
#170495=CARTESIAN_POINT ( 'NONE',  ( 13.89961937509957401, 13.97604488694547697, 26.87609039468566507 ) ) ;
#170496=CARTESIAN_POINT ( 'NONE',  ( -9.474510206698964154, 16.51473224551069663, 85.41557627198102409 ) ) ;
#170497=CARTESIAN_POINT ( 'NONE',  ( 15.80617190586746368, 15.72974639402197994, 79.37390960531436690 ) ) ;
#170498=CARTESIAN_POINT ( 'NONE',  ( -19.03943276465977164, 0.05219959533909376836, 111.2489096053143669 ) ) ;
#170499=CARTESIAN_POINT ( 'NONE',  ( -13.89961937509957401, -13.97604488694547875, 94.37609039468566152 ) ) ;
#170500=CARTESIAN_POINT ( 'NONE',  ( -5.049401038298153566, 19.05341960407611168, 115.2072429386477097 ) ) ;
#170501=CARTESIAN_POINT ( 'NONE',  ( 13.89961937509957401, 13.97604488694547697, 111.8760903946856757 ) ) ;
#170502=CARTESIAN_POINT ( 'NONE',  ( 19.02544592524343514, -5.153800228976328945, 28.54057627198102409 ) ) ;
#170503=CARTESIAN_POINT ( 'NONE',  ( -16.46253265017160317, 9.564922557960807481, 100.8322429386477097 ) ) ;
#170504=CARTESIAN_POINT ( 'NONE',  ( -21.55341960407610458, -5.719274019375992779, 76.45724293864769550 ) ) ;
#170505=CARTESIAN_POINT ( 'NONE',  ( -16.55341960407617563, 4.379528057220093196, 48.54275706135234714 ) ) ;
#170506=CARTESIAN_POINT ( 'NONE',  ( -10.81492255796105439, 18.62759615963255655, 47.91775706135234714 ) ) ;
#170507=CARTESIAN_POINT ( 'NONE',  ( 16.46253265017146816, 9.564922557961045513, 96.66775706135233293 ) ) ;
#170508=CARTESIAN_POINT ( 'NONE',  ( -15.72974639402176322, -15.80617190586768395, 99.37609039468568994 ) ) ;
#170509=CARTESIAN_POINT ( 'NONE',  ( -0.05219959533934338120, 16.53943276465976808, 102.5010903946856899 ) ) ;
#170511=CARTESIAN_POINT ( 'NONE',  ( 13.89961937509977652, -13.97604488694527269, 103.1239096053143527 ) ) ;
#170512=CARTESIAN_POINT ( 'NONE',  ( 8.314922557960818139, 14.29746914071049879, 89.58224293864768129 ) ) ;
#170513=CARTESIAN_POINT ( 'NONE',  ( -12.06949235617756955, 12.14591786802309770, 40.62390960531435269 ) ) ;
#170514=CARTESIAN_POINT ( 'NONE',  ( -19.03943276465977164, -0.05219959533935918106, 68.75109039468566152 ) ) ;
#170516=CARTESIAN_POINT ( 'NONE',  ( -10.81492255796105439, 18.62759615963255655, 62.91775706135236135 ) ) ;
#170517=CARTESIAN_POINT ( 'NONE',  ( 9.474510206698729675, 16.51473224551082808, 27.08442372801900433 ) ) ;
#170518=CARTESIAN_POINT ( 'NONE',  ( -16.53943276465976808, 0.05219959533911058130, 111.2489096053143669 ) ) ;
#170519=CARTESIAN_POINT ( 'NONE',  ( -15.72974639402197994, 15.80617190586746368, 30.62390960531436335 ) ) ;
#170520=CARTESIAN_POINT ( 'NONE',  ( -14.29746914071049879, 8.314922557960819915, 25.83224293864769194 ) ) ;
#170521=CARTESIAN_POINT ( 'NONE',  ( -15.80617190586768217, 15.72974639402176855, 98.12609039468570415 ) ) ;
#170522=CARTESIAN_POINT ( 'NONE',  ( 8.314922557961029526, -14.29746914071037800, 55.41775706135234714 ) ) ;
#170523=CARTESIAN_POINT ( 'NONE',  ( 4.483927247898545687, 16.52544592524342804, 29.79057627198102409 ) ) ;
#170524=CARTESIAN_POINT ( 'NONE',  ( -15.80617190586768217, 15.72974639402176855, 63.12609039468568994 ) ) ;
#170525=CARTESIAN_POINT ( 'NONE',  ( 10.72451020669871369, 18.67979575497193778, 57.08442372801901854 ) ) ;
#170527=CARTESIAN_POINT ( 'NONE',  ( -21.52544592524334988, -5.823673210054445271, 23.95942372801901143 ) ) ;
#170528=CARTESIAN_POINT ( 'NONE',  ( 8.314922557960818139, 14.29746914071049879, 104.5822429386477097 ) ) ;
#170529=CARTESIAN_POINT ( 'NONE',  ( 16.46253265017160672, -9.564922557960803928, 23.33224293864769194 ) ) ;
#170530=CARTESIAN_POINT ( 'NONE',  ( 8.314922557960818139, 14.29746914071049879, 79.58224293864769550 ) ) ;
#170531=CARTESIAN_POINT ( 'NONE',  ( -13.97604488694527625, -13.89961937509977652, 66.87390960531436690 ) ) ;
#170532=CARTESIAN_POINT ( 'NONE',  ( 16.52544592524335698, 4.483927247898782831, 101.4594237280190185 ) ) ;
#170533=CARTESIAN_POINT ( 'NONE',  ( -5.719274019375978568, 21.55341960407610458, 50.20724293864769550 ) ) ;
#170534=CARTESIAN_POINT ( 'NONE',  ( -4.483927247898539470, -16.52544592524342804, 87.29057627198103830 ) ) ;
#170535=CARTESIAN_POINT ( 'NONE',  ( 18.67979575497178502, 10.72451020669898547, 94.16557627198103830 ) ) ;
#170536=CARTESIAN_POINT ( 'NONE',  ( 19.05341960407611168, 5.049401038298154454, 98.95724293864766707 ) ) ;
#170537=CARTESIAN_POINT ( 'NONE',  ( -9.564922557960796823, -16.46253265017161027, 57.08224293864769550 ) ) ;
#170538=CARTESIAN_POINT ( 'NONE',  ( -16.51473224551082808, 9.474510206698731452, 108.3344237280190043 ) ) ;
#170539=CARTESIAN_POINT ( 'NONE',  ( -15.72974639402197994, 15.80617190586746368, 45.62390960531436690 ) ) ;
#170540=CARTESIAN_POINT ( 'NONE',  ( 18.62759615963255655, 10.81492255796105972, 71.66775706135234714 ) ) ;
#170541=CARTESIAN_POINT ( 'NONE',  ( 9.474510206698971260, -16.51473224551069308, 62.91557627198102409 ) ) ;
#170542=CARTESIAN_POINT ( 'NONE',  ( 16.51473224551069308, 9.474510206698969483, 99.16557627198102409 ) ) ;
#170543=CARTESIAN_POINT ( 'NONE',  ( 4.379528057220092307, 16.55341960407617563, 67.29275706135234714 ) ) ;
#170544=CARTESIAN_POINT ( 'NONE',  ( 18.62759615963255655, 10.81492255796105972, 56.66775706135235424 ) ) ;
#170545=CARTESIAN_POINT ( 'NONE',  ( -10.72451020669870658, -18.67979575497194134, 89.58442372801901854 ) ) ;
#170546=CARTESIAN_POINT ( 'NONE',  ( -10.72451020669898014, 18.67979575497178502, 95.41557627198102409 ) ) ;
#170547=CARTESIAN_POINT ( 'NONE',  ( 5.823673210054444382, -21.52544592524334988, 40.20942372801901854 ) ) ;
#170548=CARTESIAN_POINT ( 'NONE',  ( -8.314922557961024197, 14.29746914071037800, 82.91775706135234714 ) ) ;
#170550=CARTESIAN_POINT ( 'NONE',  ( 21.53943276465977519, -0.05219959533907433946, 78.74890960531436690 ) ) ;
#170551=CARTESIAN_POINT ( 'NONE',  ( -19.03943276465977164, -0.05219959533935918106, 28.75109039468566507 ) ) ;
#170552=CARTESIAN_POINT ( 'NONE',  ( -16.46253265017160317, 9.564922557960807481, 85.83224293864769550 ) ) ;
#170553=CARTESIAN_POINT ( 'NONE',  ( -0.05219959533910754901, -16.53943276465976808, 22.49890960531436335 ) ) ;
#170555=CARTESIAN_POINT ( 'NONE',  ( 9.564922557960805705, 16.46253265017160317, 99.58224293864770971 ) ) ;
#170556=CARTESIAN_POINT ( 'NONE',  ( 17.60691670004651144, 5.500000000000063061, 81.63333313366442212 ) ) ;
#170557=CARTESIAN_POINT ( 'NONE',  ( 9.474510206698729675, 16.51473224551082808, 92.08442372801900433 ) ) ;
#170558=CARTESIAN_POINT ( 'NONE',  ( -10.72451020669898014, 18.67979575497178502, 70.41557627198102409 ) ) ;
#170559=CARTESIAN_POINT ( 'NONE',  ( -12.06949235617756955, 12.14591786802309770, 40.62390960531435269 ) ) ;
#170560=CARTESIAN_POINT ( 'NONE',  ( 13.89961937509957401, 13.97604488694547697, 106.8760903946856757 ) ) ;
#170561=CARTESIAN_POINT ( 'NONE',  ( -19.05341960407611168, -5.049401038298163336, 36.45724293864766707 ) ) ;
#170562=CARTESIAN_POINT ( 'NONE',  ( 14.29746914071037800, 8.314922557961029526, 21.66775706135235069 ) ) ;
#170563=CARTESIAN_POINT ( 'NONE',  ( 10.72451020669898902, -18.67979575497178502, 97.91557627198103830 ) ) ;
#170564=CARTESIAN_POINT ( 'NONE',  ( -9.564922557961040184, 16.46253265017147172, 77.91775706135234714 ) ) ;
#170565=CARTESIAN_POINT ( 'NONE',  ( -4.379528057220086978, -16.55341960407618274, 79.79275706135236135 ) ) ;
#170566=CARTESIAN_POINT ( 'NONE',  ( 13.97604488694527802, 13.89961937509977652, 74.37390960531436690 ) ) ;
#170567=CARTESIAN_POINT ( 'NONE',  ( 14.29746914071049879, -8.314922557960816363, 78.33224293864770971 ) ) ;
#170568=CARTESIAN_POINT ( 'NONE',  ( -5.049401038298153566, 19.05341960407611168, 60.20724293864768129 ) ) ;
#170569=CARTESIAN_POINT ( 'NONE',  ( -16.52544592524342804, 4.483927247898546575, 66.04057627198103830 ) ) ;
#170572=CARTESIAN_POINT ( 'NONE',  ( 12.06949235617757843, -12.14591786802309237, 38.12390960531436690 ) ) ;
#170573=CARTESIAN_POINT ( 'NONE',  ( -13.97604488694527625, -13.89961937509977652, 76.87390960531433848 ) ) ;
#170575=CARTESIAN_POINT ( 'NONE',  ( -5.153800228976607833, 19.02544592524334988, 57.70942372801899012 ) ) ;
#170576=CARTESIAN_POINT ( 'NONE',  ( -14.34966873604972548, 8.224510206698743886, 58.33442372801901143 ) ) ;
#170577=CARTESIAN_POINT ( 'NONE',  ( 18.67979575497178502, 10.72451020669898547, 64.16557627198102409 ) ) ;
#170578=CARTESIAN_POINT ( 'NONE',  ( 19.02544592524334988, 5.153800228976608722, 21.45942372801899012 ) ) ;
#170579=CARTESIAN_POINT ( 'NONE',  ( -16.51473224551069308, -9.474510206698971260, 81.66557627198103830 ) ) ;
#170581=CARTESIAN_POINT ( 'NONE',  ( -13.97604488694527625, -13.89961937509977652, 106.8739096053143669 ) ) ;
#170582=CARTESIAN_POINT ( 'NONE',  ( -13.97604488694527625, -13.89961937509977652, 56.87390960531434558 ) ) ;
#170583=CARTESIAN_POINT ( 'NONE',  ( 21.55341960407619695, -5.719274019375665929, 36.04275706135234714 ) ) ;
#170584=CARTESIAN_POINT ( 'NONE',  ( -4.379528057220328563, 16.55341960407611168, 100.2072429386476955 ) ) ;
#170586=CARTESIAN_POINT ( 'NONE',  ( 0.05219959533907565091, 21.53943276465977519, 104.9989096053143669 ) ) ;
#170587=CARTESIAN_POINT ( 'NONE',  ( -19.03943276465977164, 0.05219959533909376836, 101.2489096053143669 ) ) ;
#170589=CARTESIAN_POINT ( 'NONE',  ( 5.823673210054444382, -21.52544592524334988, 25.20942372801901854 ) ) ;
#170590=ORIENTED_EDGE ( 'NONE', *, *, #43224, .T. ) ;
#170591=CARTESIAN_POINT ( 'NONE',  ( 19.02544592524343514, -5.153800228976328945, 83.54057627198100988 ) ) ;
#170593=CARTESIAN_POINT ( 'NONE',  ( -18.62759615963270932, 10.81492255796079327, 95.83224293864770971 ) ) ;
#170594=CARTESIAN_POINT ( 'NONE',  ( -5.153800228976328057, -19.02544592524343514, 52.29057627198100988 ) ) ;
#170595=CARTESIAN_POINT ( 'NONE',  ( 5.153800228976615827, -19.02544592524334988, 105.2094237280190185 ) ) ;
#170597=CARTESIAN_POINT ( 'NONE',  ( -13.97604488694527625, -13.89961937509977652, 26.87390960531434558 ) ) ;
#170598=CARTESIAN_POINT ( 'NONE',  ( 18.67979575497194134, -10.72451020669871369, 90.83442372801901854 ) ) ;
#170599=CARTESIAN_POINT ( 'NONE',  ( 5.049401038298161559, -19.05341960407611168, 72.70724293864768129 ) ) ;
#170600=CARTESIAN_POINT ( 'NONE',  ( -10.81492255796105439, 18.62759615963255655, 52.91775706135235424 ) ) ;
#170601=CARTESIAN_POINT ( 'NONE',  ( -10.72451020669870658, -18.67979575497194134, 24.58442372801901499 ) ) ;
#170603=CARTESIAN_POINT ( 'NONE',  ( -5.153800228976328057, -19.02544592524343514, 102.2905762719810383 ) ) ;
#170604=CARTESIAN_POINT ( 'NONE',  ( 19.39720447994796615, 5.499999999999970690, 62.16317477297180716 ) ) ;
#170605=CARTESIAN_POINT ( 'NONE',  ( -16.55341960407617563, 4.379528057220093196, 43.54275706135235424 ) ) ;
#170606=CARTESIAN_POINT ( 'NONE',  ( 5.719274019375991003, -21.55341960407610458, 42.70724293864770260 ) ) ;
#170607=CARTESIAN_POINT ( 'NONE',  ( 18.62759615963255655, 10.81492255796105972, 41.66775706135235424 ) ) ;
#170608=CARTESIAN_POINT ( 'NONE',  ( 15.72974639402176855, 15.80617190586768217, 71.87609039468568994 ) ) ;
#170609=CARTESIAN_POINT ( 'NONE',  ( 18.22780087662119897, -5.500000000000146549, 38.51763182126893525 ) ) ;
#170610=CARTESIAN_POINT ( 'NONE',  ( 19.02544592524334988, 5.153800228976608722, 111.4594237280190043 ) ) ;
#170611=CARTESIAN_POINT ( 'NONE',  ( 9.564922557960805705, 16.46253265017160317, 59.58224293864769550 ) ) ;
#170612=CARTESIAN_POINT ( 'NONE',  ( -19.05341960407611168, -5.049401038298163336, 96.45724293864769550 ) ) ;
#170613=VECTOR ( 'NONE', #179634, 1000.000000000000000 ) ;
#170614=CARTESIAN_POINT ( 'NONE',  ( 14.34966873604960469, 8.224510206698951720, 114.1655762719810383 ) ) ;
#170615=CARTESIAN_POINT ( 'NONE',  ( -4.483927247898539470, -16.52544592524342804, 107.2905762719810525 ) ) ;
#170616=CARTESIAN_POINT ( 'NONE',  ( -10.72451020669898014, 18.67979575497178502, 25.41557627198103120 ) ) ;
#170617=CARTESIAN_POINT ( 'NONE',  ( 14.34966873604972726, -8.224510206698740333, 80.83442372801901854 ) ) ;
#170618=CARTESIAN_POINT ( 'NONE',  ( 0.05219959533910956823, 16.53943276465976808, 69.99890960531435269 ) ) ;
#170619=CARTESIAN_POINT ( 'NONE',  ( -9.564922557960796823, -16.46253265017161027, 52.08224293864768839 ) ) ;
#170620=CARTESIAN_POINT ( 'NONE',  ( 18.62759615963255655, 10.81492255796105972, 71.66775706135234714 ) ) ;
#170621=CARTESIAN_POINT ( 'NONE',  ( -5.823673210054431948, 21.52544592524334988, 77.70942372801900433 ) ) ;
#170622=CARTESIAN_POINT ( 'NONE',  ( -9.564922557961040184, 16.46253265017147172, 112.9177570613523329 ) ) ;
#170623=CARTESIAN_POINT ( 'NONE',  ( -8.314922557960811034, -14.29746914071050412, 57.08224293864769550 ) ) ;
#170624=CARTESIAN_POINT ( 'NONE',  ( -5.719274019375665041, -21.55341960407619695, 24.79275706135235779 ) ) ;
#170625=CARTESIAN_POINT ( 'NONE',  ( 0.05219959533907565091, 21.53943276465977519, 54.99890960531435269 ) ) ;
#170626=CARTESIAN_POINT ( 'NONE',  ( -17.50000000000000000, -5.500000000000000000, 106.2823096230357010 ) ) ;
#170628=CARTESIAN_POINT ( 'NONE',  ( 0.05219959533909260263, 19.03943276465977164, 64.99890960531436690 ) ) ;
#170629=CARTESIAN_POINT ( 'NONE',  ( -4.379528057220328563, 16.55341960407611168, 40.20724293864769550 ) ) ;
#170630=CARTESIAN_POINT ( 'NONE',  ( -16.55341960407617563, 4.379528057220093196, 113.5427570613523756 ) ) ;
#170631=CARTESIAN_POINT ( 'NONE',  ( 4.379528057220092307, 16.55341960407617563, 97.29275706135234714 ) ) ;
#170632=CARTESIAN_POINT ( 'NONE',  ( 9.474510206698729675, 16.51473224551082808, 57.08442372801900433 ) ) ;
#170634=CARTESIAN_POINT ( 'NONE',  ( 9.474510206698971260, -16.51473224551069308, 107.9155762719810383 ) ) ;
#170635=CARTESIAN_POINT ( 'NONE',  ( 14.34966873604960469, 8.224510206698951720, 69.16557627198102409 ) ) ;
#170636=CARTESIAN_POINT ( 'NONE',  ( -19.03943276465977164, -0.05219959533935918106, 43.75109039468566863 ) ) ;
#170637=CARTESIAN_POINT ( 'NONE',  ( 19.02544592524343514, -5.153800228976328945, 33.54057627198102409 ) ) ;
#170638=CARTESIAN_POINT ( 'NONE',  ( 18.67979575497178502, 10.72451020669898547, 34.16557627198102409 ) ) ;
#170639=CARTESIAN_POINT ( 'NONE',  ( -21.53943276465977519, 0.05219959533907696930, 56.24890960531436690 ) ) ;
#170641=CARTESIAN_POINT ( 'NONE',  ( 14.34966873604960469, 8.224510206698951720, 99.16557627198100988 ) ) ;
#170642=CARTESIAN_POINT ( 'NONE',  ( 14.34966873604972726, -8.224510206698740333, 50.83442372801901143 ) ) ;
#170643=CARTESIAN_POINT ( 'NONE',  ( -16.53943276465976808, 0.05219959533911058130, 96.24890960531435269 ) ) ;
#170645=CARTESIAN_POINT ( 'NONE',  ( -17.44279575226823198, 5.990770900252468500, 50.83557567514321818 ) ) ;
#170646=CARTESIAN_POINT ( 'NONE',  ( -5.049401038298153566, 19.05341960407611168, 115.2072429386477097 ) ) ;
#170650=CARTESIAN_POINT ( 'NONE',  ( -12.14591786802326823, 12.06949235617739902, 43.12609039468568284 ) ) ;
#170651=CARTESIAN_POINT ( 'NONE',  ( 14.34966873604960469, 8.224510206698951720, 24.16557627198103120 ) ) ;
#170652=CARTESIAN_POINT ( 'NONE',  ( -18.67979575497178146, -10.72451020669898902, 51.66557627198102409 ) ) ;
#170653=CARTESIAN_POINT ( 'NONE',  ( -13.97604488694547697, 13.89961937509957934, 83.12609039468564731 ) ) ;
#170654=CARTESIAN_POINT ( 'NONE',  ( 5.823673210054125526, 21.52544592524343514, 54.79057627198104541 ) ) ;
#170655=CARTESIAN_POINT ( 'NONE',  ( 5.823673210054444382, -21.52544592524334988, 75.20942372801901854 ) ) ;
#170656=DIRECTION ( 'NONE',  ( 0.000000000000000000, 0.000000000000000000, -1.000000000000000000 ) ) ;
#170657=CARTESIAN_POINT ( 'NONE',  ( 4.483927247898790824, -16.52544592524335698, 50.20942372801901854 ) ) ;
#170658=CARTESIAN_POINT ( 'NONE',  ( 19.02544592524343514, -5.153800228976328945, 33.54057627198102409 ) ) ;
#170659=CARTESIAN_POINT ( 'NONE',  ( 0.05219959533909260263, 19.03943276465977164, 104.9989096053143669 ) ) ;
#170660=CARTESIAN_POINT ( 'NONE',  ( 13.97604488694527802, 13.89961937509977652, 29.37390960531435979 ) ) ;
#170661=CARTESIAN_POINT ( 'NONE',  ( -16.55341960407611168, -4.379528057220339221, 96.45724293864770971 ) ) ;
#170663=CARTESIAN_POINT ( 'NONE',  ( 0.05219959533909260263, 19.03943276465977164, 104.9989096053143669 ) ) ;
#170665=CARTESIAN_POINT ( 'NONE',  ( 12.06949235617739724, 12.14591786802326823, 56.87609039468568994 ) ) ;
#170666=CARTESIAN_POINT ( 'NONE',  ( 21.55341960407610458, 5.719274019375980345, 93.95724293864770971 ) ) ;
#170667=CARTESIAN_POINT ( 'NONE',  ( -9.474510206698964154, 16.51473224551069663, 60.41557627198102409 ) ) ;
#170668=CARTESIAN_POINT ( 'NONE',  ( 5.823673210054444382, -21.52544592524334988, 25.20942372801901854 ) ) ;
#170669=CARTESIAN_POINT ( 'NONE',  ( -16.46253265017160317, 9.564922557960807481, 85.83224293864769550 ) ) ;
#170671=ORIENTED_EDGE ( 'NONE', *, *, #10239, .T. ) ;
#170672=CARTESIAN_POINT ( 'NONE',  ( -18.62759615963255300, -10.81492255796106328, 19.16775706135234714 ) ) ;
#170673=CARTESIAN_POINT ( 'NONE',  ( 5.049401038298161559, -19.05341960407611168, 27.70724293864769550 ) ) ;
#170674=CARTESIAN_POINT ( 'NONE',  ( -9.474510206698964154, 16.51473224551069663, 105.4155762719810383 ) ) ;
#170675=CARTESIAN_POINT ( 'NONE',  ( 16.46253265017146816, 9.564922557961045513, 71.66775706135233293 ) ) ;
#170676=CARTESIAN_POINT ( 'NONE',  ( -19.03943276465977164, -0.05219959533935918106, 33.75109039468566863 ) ) ;
#170677=CARTESIAN_POINT ( 'NONE',  ( 21.55341960407610458, 5.719274019375980345, 98.95724293864770971 ) ) ;
#170678=CARTESIAN_POINT ( 'NONE',  ( -19.02544592524334988, -5.153800228976617603, 33.95942372801897591 ) ) ;
#170679=CARTESIAN_POINT ( 'NONE',  ( 8.224510206698742110, 14.34966873604972548, 72.08442372801899012 ) ) ;
#170680=CARTESIAN_POINT ( 'NONE',  ( -19.05341960407611168, -5.049401038298163336, 111.4572429386476671 ) ) ;
#170681=CARTESIAN_POINT ( 'NONE',  ( -9.474510206698964154, 16.51473224551069663, 55.41557627198103120 ) ) ;
#170682=CARTESIAN_POINT ( 'NONE',  ( 18.62759615963255655, 10.81492255796105972, 66.66775706135234714 ) ) ;
#170683=CARTESIAN_POINT ( 'NONE',  ( -21.55341960407619339, 5.719274019375674811, 78.54275706135236135 ) ) ;
#170684=CARTESIAN_POINT ( 'NONE',  ( 19.02544592524343514, -5.153800228976328945, 73.54057627198103830 ) ) ;
#170685=CARTESIAN_POINT ( 'NONE',  ( 15.80617190586769283, -15.72974639402175789, 50.62609039468568994 ) ) ;
#170686=CARTESIAN_POINT ( 'NONE',  ( -19.05341960407617563, 5.049401038297882671, 83.54275706135233293 ) ) ;
#170687=CARTESIAN_POINT ( 'NONE',  ( 13.89961937509977652, -13.97604488694527269, 58.12390960531436690 ) ) ;
#170688=CARTESIAN_POINT ( 'NONE',  ( 13.97604488694527802, 13.89961937509977652, 104.3739096053143385 ) ) ;
#170689=CARTESIAN_POINT ( 'NONE',  ( -16.51473224551069308, -9.474510206698971260, 61.66557627198103120 ) ) ;
#170690=CARTESIAN_POINT ( 'NONE',  ( 19.05341960407611168, 5.049401038298154454, 113.9572429386477097 ) ) ;
#170691=CARTESIAN_POINT ( 'NONE',  ( 5.153800228976335163, 19.02544592524342804, 49.79057627198100988 ) ) ;
#170692=CARTESIAN_POINT ( 'NONE',  ( -0.05219959533907301413, -21.53943276465977519, 97.49890960531436690 ) ) ;
#170693=CARTESIAN_POINT ( 'NONE',  ( 4.483927247898790824, -16.52544592524335698, 80.20942372801901854 ) ) ;
#170695=CARTESIAN_POINT ( 'NONE',  ( -13.97604488694547697, 13.89961937509957934, 43.12609039468566152 ) ) ;
#170696=CARTESIAN_POINT ( 'NONE',  ( 16.46253265017160672, -9.564922557960803928, 68.33224293864770971 ) ) ;
#170697=CARTESIAN_POINT ( 'NONE',  ( -4.483927247898539470, -16.52544592524342804, 62.29057627198102409 ) ) ;
#170698=CARTESIAN_POINT ( 'NONE',  ( 16.52544592524342804, -4.483927247898539470, 88.54057627198103830 ) ) ;
#170699=CARTESIAN_POINT ( 'NONE',  ( 5.153800228976335163, 19.02544592524342804, 99.79057627198102409 ) ) ;
#170700=CARTESIAN_POINT ( 'NONE',  ( 5.153800228976335163, 19.02544592524342804, 89.79057627198102409 ) ) ;
#170701=CARTESIAN_POINT ( 'NONE',  ( -9.564922557960796823, -16.46253265017161027, 102.0822429386477097 ) ) ;
#170702=CARTESIAN_POINT ( 'NONE',  ( 5.719274019375673035, 21.55341960407619339, 107.2927570613523471 ) ) ;
#170703=CARTESIAN_POINT ( 'NONE',  ( -0.05219959533934338120, 16.53943276465976808, 97.50109039468567573 ) ) ;
#170704=CARTESIAN_POINT ( 'NONE',  ( -19.02544592524342804, 5.153800228976336051, 81.04057627198103830 ) ) ;
#170705=CARTESIAN_POINT ( 'NONE',  ( -5.719274019375665041, -21.55341960407619695, 44.79275706135234714 ) ) ;
#170706=CARTESIAN_POINT ( 'NONE',  ( -10.81492255796078084, -18.62759615963271287, 27.08224293864769550 ) ) ;
#170707=CARTESIAN_POINT ( 'NONE',  ( -10.72451020669898014, 18.67979575497178502, 105.4155762719810383 ) ) ;
#170708=CARTESIAN_POINT ( 'NONE',  ( -16.53943276465976808, 0.05219959533911058130, 61.24890960531435979 ) ) ;
#170709=CARTESIAN_POINT ( 'NONE',  ( -9.474510206698964154, 16.51473224551069663, 50.41557627198102409 ) ) ;
#170710=CARTESIAN_POINT ( 'NONE',  ( -8.224510206698948167, 14.34966873604960824, 85.41557627198102409 ) ) ;
#170711=CARTESIAN_POINT ( 'NONE',  ( 5.153800228976615827, -19.02544592524334988, 45.20942372801901143 ) ) ;
#170712=CARTESIAN_POINT ( 'NONE',  ( -12.14591786802309592, -12.06949235617757132, 106.8739096053143811 ) ) ;
#170713=CARTESIAN_POINT ( 'NONE',  ( 4.379528057220092307, 16.55341960407617563, 62.29275706135236845 ) ) ;
#170714=CARTESIAN_POINT ( 'NONE',  ( -5.153800228976328057, -19.02544592524343514, 67.29057627198102409 ) ) ;
#170716=CARTESIAN_POINT ( 'NONE',  ( 12.06949235617757843, -12.14591786802309237, 93.12390960531436690 ) ) ;
#170717=CARTESIAN_POINT ( 'NONE',  ( -15.72974639402197994, 15.80617190586746368, 35.62390960531437401 ) ) ;
#170718=CARTESIAN_POINT ( 'NONE',  ( 8.314922557961029526, -14.29746914071037800, 100.4177570613523471 ) ) ;
#170719=CARTESIAN_POINT ( 'NONE',  ( 16.52544592524335698, 4.483927247898782831, 26.45942372801901854 ) ) ;
#170720=CARTESIAN_POINT ( 'NONE',  ( -21.52544592524334988, -5.823673210054445271, 93.95942372801903275 ) ) ;
#170721=CARTESIAN_POINT ( 'NONE',  ( -19.05341960407611168, -5.049401038298163336, 81.45724293864769550 ) ) ;
#170722=CARTESIAN_POINT ( 'NONE',  ( 15.80617190586769283, -15.72974639402175789, 25.62609039468567929 ) ) ;
#170723=CARTESIAN_POINT ( 'NONE',  ( 16.46253265017160672, -9.564922557960803928, 28.33224293864769550 ) ) ;
#170724=CARTESIAN_POINT ( 'NONE',  ( 14.34966873604972726, -8.224510206698740333, 25.83442372801901499 ) ) ;
#170725=CARTESIAN_POINT ( 'NONE',  ( 0.05219959533936267826, -19.03943276465977164, 90.00109039468567573 ) ) ;
#170726=CARTESIAN_POINT ( 'NONE',  ( -5.823673210054116645, -21.52544592524344225, 87.29057627198103830 ) ) ;
#170727=CARTESIAN_POINT ( 'NONE',  ( 16.51473224551083163, -9.474510206698727899, 70.83442372801900433 ) ) ;
#170728=CARTESIAN_POINT ( 'NONE',  ( -17.72560187377285246, -5.500000000000056843, 64.07814504131322053 ) ) ;
#170729=CARTESIAN_POINT ( 'NONE',  ( -18.62759615963255300, -10.81492255796106328, 19.16775706135234714 ) ) ;
#170730=PLANE ( 'NONE',  #37014 ) ;
#170731=CARTESIAN_POINT ( 'NONE',  ( 16.51473224551069308, 9.474510206698969483, 79.16557627198103830 ) ) ;
#170732=CARTESIAN_POINT ( 'NONE',  ( 16.52544592524335698, 4.483927247898782831, 36.45942372801901143 ) ) ;
#170733=CARTESIAN_POINT ( 'NONE',  ( -17.72517630441458891, 5.499999999999979572, 100.9217571925760097 ) ) ;
#170734=CARTESIAN_POINT ( 'NONE',  ( 16.51473224551083163, -9.474510206698727899, 60.83442372801900433 ) ) ;
#170735=CARTESIAN_POINT ( 'NONE',  ( 21.55341960407610458, 5.719274019375980345, 113.9572429386477239 ) ) ;
#170736=CARTESIAN_POINT ( 'NONE',  ( 8.224510206698953496, -14.34966873604960469, 72.91557627198103830 ) ) ;
#170737=CARTESIAN_POINT ( 'NONE',  ( -16.51473224551069308, -9.474510206698971260, 86.66557627198102409 ) ) ;
#170739=CARTESIAN_POINT ( 'NONE',  ( 16.55341960407618274, -4.379528057220086978, 41.04275706135236135 ) ) ;
#170740=CARTESIAN_POINT ( 'NONE',  ( 0.05219959533936267826, -19.03943276465977164, 50.00109039468566863 ) ) ;
#170741=CARTESIAN_POINT ( 'NONE',  ( 18.67979575497194134, -10.72451020669871369, 65.83442372801900433 ) ) ;
#170742=CARTESIAN_POINT ( 'NONE',  ( 14.29746914071037800, 8.314922557961029526, 21.66775706135235069 ) ) ;
#170743=CARTESIAN_POINT ( 'NONE',  ( 16.51473224551069308, 9.474510206698969483, 59.16557627198102409 ) ) ;
#170745=CARTESIAN_POINT ( 'NONE',  ( -13.97604488694547697, 13.89961937509957934, 78.12609039468567573 ) ) ;
#170746=CARTESIAN_POINT ( 'NONE',  ( -8.224510206698735004, -14.34966873604973081, 59.58442372801901854 ) ) ;
#170747=CARTESIAN_POINT ( 'NONE',  ( 21.53943276465977519, 0.05219959533937863772, 101.2510903946856757 ) ) ;
#170748=CARTESIAN_POINT ( 'NONE',  ( -13.89961937509957401, -13.97604488694547875, 69.37609039468564731 ) ) ;
#170749=CARTESIAN_POINT ( 'NONE',  ( -19.02544592524342804, 5.153800228976336051, 51.04057627198103120 ) ) ;
#170750=CARTESIAN_POINT ( 'NONE',  ( -0.05219959533907301413, -21.53943276465977519, 77.49890960531433848 ) ) ;
#170751=CARTESIAN_POINT ( 'NONE',  ( 8.224510206698953496, -14.34966873604960469, 62.91557627198102409 ) ) ;
#170752=CARTESIAN_POINT ( 'NONE',  ( -9.564922557961040184, 16.46253265017147172, 82.91775706135233293 ) ) ;
#170753=CARTESIAN_POINT ( 'NONE',  ( -19.01529144963335582, -5.500000000000083489, 71.23431955728437970 ) ) ;
#170754=CARTESIAN_POINT ( 'NONE',  ( 5.153800228976615827, -19.02544592524334988, 40.20942372801898301 ) ) ;
#170755=CARTESIAN_POINT ( 'NONE',  ( -8.314922557961024197, 14.29746914071037800, 97.91775706135236135 ) ) ;
#170756=CARTESIAN_POINT ( 'NONE',  ( -16.53943276465976808, 0.05219959533911058130, 71.24890960531435269 ) ) ;
#170757=CARTESIAN_POINT ( 'NONE',  ( -18.67979575497193778, 10.72451020669871902, 98.33442372801901854 ) ) ;
#170759=CARTESIAN_POINT ( 'NONE',  ( -15.72974639402197994, 15.80617190586746368, 90.62390960531436690 ) ) ;
#170760=CARTESIAN_POINT ( 'NONE',  ( 19.02544592524343514, -5.153800228976328945, 58.54057627198102409 ) ) ;
#170761=CARTESIAN_POINT ( 'NONE',  ( 15.80617190586769283, -15.72974639402175789, 65.62609039468568994 ) ) ;
#170762=CARTESIAN_POINT ( 'NONE',  ( -16.51473224551069308, -9.474510206698971260, 46.66557627198102409 ) ) ;
#170763=VERTEX_POINT ( 'NONE', #97998 ) ;
#170764=CARTESIAN_POINT ( 'NONE',  ( -9.564922557960796823, -16.46253265017161027, 72.08224293864770971 ) ) ;
#170765=CARTESIAN_POINT ( 'NONE',  ( -16.52544592524342804, 4.483927247898546575, 116.0405762719810383 ) ) ;
#170766=CARTESIAN_POINT ( 'NONE',  ( 13.89961937509977652, -13.97604488694527269, 108.1239096053143669 ) ) ;
#170767=CARTESIAN_POINT ( 'NONE',  ( 4.379528057220339221, -16.55341960407611168, 62.70724293864769550 ) ) ;
#170768=CARTESIAN_POINT ( 'NONE',  ( -13.97604488694527625, -13.89961937509977652, 36.87390960531436690 ) ) ;
#170769=CARTESIAN_POINT ( 'NONE',  ( 16.55341960407611168, 4.379528057220329451, 88.95724293864769550 ) ) ;
#170770=CARTESIAN_POINT ( 'NONE',  ( 15.72974639402199770, -15.80617190586745480, 93.12390960531436690 ) ) ;
#170771=CARTESIAN_POINT ( 'NONE',  ( 15.80617190586769283, -15.72974639402175789, 35.62609039468568994 ) ) ;
#170773=CARTESIAN_POINT ( 'NONE',  ( -0.05219959533934338120, 16.53943276465976808, 52.50109039468567573 ) ) ;
#170774=CARTESIAN_POINT ( 'NONE',  ( 18.62759615963271287, -10.81492255796078972, 78.33224293864770971 ) ) ;
#170775=CARTESIAN_POINT ( 'NONE',  ( 19.05341960407617918, -5.049401038297876454, 31.04275706135232227 ) ) ;
#170776=CARTESIAN_POINT ( 'NONE',  ( -19.03943276465977164, 0.05219959533909376836, 101.2489096053143669 ) ) ;
#170777=CARTESIAN_POINT ( 'NONE',  ( 15.80617190586769283, -15.72974639402175789, 40.62609039468567573 ) ) ;
#170778=CARTESIAN_POINT ( 'NONE',  ( 5.719274019375991003, -21.55341960407610458, 42.70724293864770260 ) ) ;
#170779=CARTESIAN_POINT ( 'NONE',  ( -4.379528057220328563, 16.55341960407611168, 30.20724293864769550 ) ) ;
#170780=CARTESIAN_POINT ( 'NONE',  ( -10.81492255796105439, 18.62759615963255655, 67.91775706135234714 ) ) ;
#170781=CARTESIAN_POINT ( 'NONE',  ( -21.55341960407619339, 5.719274019375674811, 93.54275706135234714 ) ) ;
#170782=CARTESIAN_POINT ( 'NONE',  ( 13.97604488694548053, -13.89961937509957401, 25.62609039468566507 ) ) ;
#170783=CARTESIAN_POINT ( 'NONE',  ( 14.29746914071037800, 8.314922557961029526, 91.66775706135234714 ) ) ;
#170784=CARTESIAN_POINT ( 'NONE',  ( -10.81492255796105439, 18.62759615963255655, 57.91775706135234714 ) ) ;
#170785=CARTESIAN_POINT ( 'NONE',  ( 9.564922557960805705, 16.46253265017160317, 39.58224293864768839 ) ) ;
#170786=CARTESIAN_POINT ( 'NONE',  ( 16.46253265017146816, 9.564922557961045513, 21.66775706135233648 ) ) ;
#170787=CARTESIAN_POINT ( 'NONE',  ( 10.72451020669898902, -18.67979575497178502, 27.91557627198103830 ) ) ;
#170788=CARTESIAN_POINT ( 'NONE',  ( 15.72974639402199770, -15.80617190586745480, 113.1239096053143953 ) ) ;
#170789=CARTESIAN_POINT ( 'NONE',  ( -10.72451020669898014, 18.67979575497178502, 80.41557627198103830 ) ) ;
#170790=CARTESIAN_POINT ( 'NONE',  ( 12.14591786802327356, -12.06949235617739191, 45.62609039468567573 ) ) ;
#170791=DIRECTION ( 'NONE',  ( 0.000000000000000000, -1.000000000000000000, 0.000000000000000000 ) ) ;
#170792=CARTESIAN_POINT ( 'NONE',  ( -0.05219959533907301413, -21.53943276465977519, 82.49890960531436690 ) ) ;
#170793=CARTESIAN_POINT ( 'NONE',  ( 14.29746914071037800, 8.314922557961029526, 61.66775706135235424 ) ) ;
#170794=CARTESIAN_POINT ( 'NONE',  ( 16.53943276465976808, -0.05219959533910856209, 58.74890960531436690 ) ) ;
#170796=CARTESIAN_POINT ( 'NONE',  ( 13.89961937509957401, 13.97604488694547697, 91.87609039468567573 ) ) ;
#170798=CARTESIAN_POINT ( 'NONE',  ( -16.53943276465976808, -0.05219959533934237506, 38.75109039468567573 ) ) ;
#170799=CARTESIAN_POINT ( 'NONE',  ( 21.53943276465977519, -0.05219959533907433946, 113.7489096053143527 ) ) ;
#170800=CARTESIAN_POINT ( 'NONE',  ( -18.62759615963270932, 10.81492255796079327, 80.83224293864769550 ) ) ;
#170801=CARTESIAN_POINT ( 'NONE',  ( -18.67979575497178146, -10.72451020669898902, 36.66557627198103120 ) ) ;
#170802=CARTESIAN_POINT ( 'NONE',  ( -12.06949235617739369, -12.14591786802326823, 59.37609039468568284 ) ) ;
#170803=CARTESIAN_POINT ( 'NONE',  ( 13.97604488694527802, 13.89961937509977652, 74.37390960531436690 ) ) ;
#170804=CARTESIAN_POINT ( 'NONE',  ( -5.823673210054431948, 21.52544592524334988, 47.70942372801902565 ) ) ;
#170805=CARTESIAN_POINT ( 'NONE',  ( -5.049401038297874678, -19.05341960407617918, 104.7927570613523471 ) ) ;
#170806=CARTESIAN_POINT ( 'NONE',  ( 21.53943276465977519, -0.05219959533907433946, 28.74890960531435624 ) ) ;
#170807=CARTESIAN_POINT ( 'NONE',  ( -9.474510206698720793, -16.51473224551083518, 24.58442372801900078 ) ) ;
#170808=CARTESIAN_POINT ( 'NONE',  ( 16.55341960407618274, -4.379528057220086978, 41.04275706135236135 ) ) ;
#170809=CARTESIAN_POINT ( 'NONE',  ( -13.97604488694527625, -13.89961937509977652, 101.8739096053143811 ) ) ;
#170810=CARTESIAN_POINT ( 'NONE',  ( -21.53943276465977519, 0.05219959533907696930, 101.2489096053143669 ) ) ;
#170811=CARTESIAN_POINT ( 'NONE',  ( 19.02544592524343514, -5.153800228976328945, 68.54057627198103830 ) ) ;
#170812=CARTESIAN_POINT ( 'NONE',  ( -16.21995358207306737, 7.366697692864093483, 24.93551001512159360 ) ) ;
#170813=CARTESIAN_POINT ( 'NONE',  ( 16.55341960407611168, 4.379528057220329451, 83.95724293864770971 ) ) ;
#170814=B_SPLINE_CURVE_WITH_KNOTS ( 'NONE', 3,
 ( #183919, #11103, #45404, #152572, #10102, #135446, #105091, #103101, #133432, #151599, #163784, #134448, #89917, #74755, #121239, #71762, #120248, #150614, #12110, #195121, #60553, #43422, #137404, #136418, #182933, #59564, #29254, #198098, #196133, #149605, #122228, #180956 ),
 .UNSPECIFIED., .F., .F.,
 ( 4, 2, 2, 2, 2, 2, 2, 2, 2, 2, 2, 2, 2, 2, 2, 4 ),
 ( 2.602085213965210256E-18, 0.0003712461730036788090, 0.0007424923460073550160, 0.001113738519011031386, 0.001484984692014707430, 0.002227477038022071879, 0.002598723211025736213, 0.002969969384029400548, 0.003341215557033064883, 0.003712461730036728785, 0.004083707903040393120, 0.004454954076044057888, 0.004826200249047722657, 0.005197446422051386558, 0.005568692595055051327, 0.005939938768058715228 ),
 .UNSPECIFIED. ) ;
#170815=CARTESIAN_POINT ( 'NONE',  ( -18.62759615963270932, 10.81492255796079327, 25.83224293864769194 ) ) ;
#170816=CARTESIAN_POINT ( 'NONE',  ( -17.05587630539785238, 6.762274262135689717, 35.74180309037312497 ) ) ;
#170817=CARTESIAN_POINT ( 'NONE',  ( 18.62759615963271287, -10.81492255796078972, 103.3322429386476955 ) ) ;
#170818=CARTESIAN_POINT ( 'NONE',  ( -19.03943276465977164, -0.05219959533935918106, 68.75109039468566152 ) ) ;
#170819=CARTESIAN_POINT ( 'NONE',  ( 10.72451020669898902, -18.67979575497178502, 37.91557627198102409 ) ) ;
#170820=CARTESIAN_POINT ( 'NONE',  ( 16.46253265017160672, -9.564922557960803928, 23.33224293864769194 ) ) ;
#170821=CARTESIAN_POINT ( 'NONE',  ( 10.72451020669898902, -18.67979575497178502, 67.91557627198102409 ) ) ;
#170822=CARTESIAN_POINT ( 'NONE',  ( -19.05341960407611168, -5.049401038298163336, 101.4572429386476955 ) ) ;
#170823=CARTESIAN_POINT ( 'NONE',  ( -15.80617190586768217, 15.72974639402176855, 88.12609039468570415 ) ) ;
#170824=CARTESIAN_POINT ( 'NONE',  ( 5.049401038298161559, -19.05341960407611168, 52.70724293864767418 ) ) ;
#170826=CARTESIAN_POINT ( 'NONE',  ( -14.34966873604960291, -8.224510206698953496, 86.66557627198102409 ) ) ;
#170827=CARTESIAN_POINT ( 'NONE',  ( 16.53943276465976808, 0.05219959533934440121, 31.25109039468568639 ) ) ;
#170828=CARTESIAN_POINT ( 'NONE',  ( 16.46253265017160672, -9.564922557960803928, 63.33224293864769550 ) ) ;
#170829=CARTESIAN_POINT ( 'NONE',  ( -21.55341960407619339, 5.719274019375674811, 73.54275706135234714 ) ) ;
#170830=VERTEX_POINT ( 'NONE', #140316 ) ;
#170831=CARTESIAN_POINT ( 'NONE',  ( -19.03943276465977164, -0.05219959533935918106, 23.75109039468566152 ) ) ;
#170832=CARTESIAN_POINT ( 'NONE',  ( 9.564922557961047289, -16.46253265017146816, 45.41775706135232582 ) ) ;
#170833=CARTESIAN_POINT ( 'NONE',  ( 10.81492255796106328, -18.62759615963255655, 40.41775706135234714 ) ) ;
#170835=CARTESIAN_POINT ( 'NONE',  ( -19.05341960407617563, 5.049401038297882671, 38.54275706135233293 ) ) ;
#170836=CARTESIAN_POINT ( 'NONE',  ( -19.03943276465977164, 0.05219959533909376836, 81.24890960531436690 ) ) ;
#170837=CARTESIAN_POINT ( 'NONE',  ( 19.02544592524343514, -5.153800228976328945, 68.54057627198103830 ) ) ;
#170838=CARTESIAN_POINT ( 'NONE',  ( -16.52544592524342804, 4.483927247898546575, 26.04057627198103475 ) ) ;
#170839=CARTESIAN_POINT ( 'NONE',  ( -9.474510206698964154, 16.51473224551069663, 110.4155762719810383 ) ) ;
#170840=CARTESIAN_POINT ( 'NONE',  ( -10.72451020669870658, -18.67979575497194134, 89.58442372801901854 ) ) ;
#170844=CARTESIAN_POINT ( 'NONE',  ( -5.719274019375665041, -21.55341960407619695, 79.79275706135236135 ) ) ;
#170845=CARTESIAN_POINT ( 'NONE',  ( 16.21995358207306737, -7.366697692864084601, 42.43551001512160781 ) ) ;
#170846=CARTESIAN_POINT ( 'NONE',  ( 9.474510206698971260, -16.51473224551069308, 97.91557627198102409 ) ) ;
#170848=CARTESIAN_POINT ( 'NONE',  ( 10.72451020669898902, -18.67979575497178502, 72.91557627198103830 ) ) ;
#170849=CARTESIAN_POINT ( 'NONE',  ( -14.34966873604960291, -8.224510206698953496, 21.66557627198102409 ) ) ;
#170850=CARTESIAN_POINT ( 'NONE',  ( -14.34966873604960291, -8.224510206698953496, 111.6655762719810525 ) ) ;
#170851=CARTESIAN_POINT ( 'NONE',  ( 16.51473224551069308, 9.474510206698969483, 99.16557627198102409 ) ) ;
#170852=CARTESIAN_POINT ( 'NONE',  ( -9.564922557961040184, 16.46253265017147172, 27.91775706135232582 ) ) ;
#170853=CARTESIAN_POINT ( 'NONE',  ( 8.314922557960818139, 14.29746914071049879, 109.5822429386476955 ) ) ;
#170854=CARTESIAN_POINT ( 'NONE',  ( -21.55341960407619339, 5.719274019375674811, 63.54275706135234003 ) ) ;
#170855=CARTESIAN_POINT ( 'NONE',  ( -13.89961937509977652, 13.97604488694528158, 110.6239096053143243 ) ) ;
#170856=CARTESIAN_POINT ( 'NONE',  ( 12.14591786802327356, -12.06949235617739191, 110.6260903946857042 ) ) ;
#170857=CARTESIAN_POINT ( 'NONE',  ( 13.89961937509957401, 13.97604488694547697, 66.87609039468567573 ) ) ;
#170858=CARTESIAN_POINT ( 'NONE',  ( 9.474510206698729675, 16.51473224551082808, 67.08442372801900433 ) ) ;
#170859=CARTESIAN_POINT ( 'NONE',  ( 0.05219959533909260263, 19.03943276465977164, 104.9989096053143669 ) ) ;
#170860=CARTESIAN_POINT ( 'NONE',  ( 16.53943276465976808, -0.05219959533910856209, 93.74890960531436690 ) ) ;
#170861=CARTESIAN_POINT ( 'NONE',  ( 19.05341960407617918, -5.049401038297876454, 56.04275706135234714 ) ) ;
#170862=CARTESIAN_POINT ( 'NONE',  ( -19.03943276465977164, 0.05219959533909376836, 81.24890960531436690 ) ) ;
#170863=CARTESIAN_POINT ( 'NONE',  ( 12.06949235617757843, -12.14591786802309237, 58.12390960531435979 ) ) ;
#170864=CARTESIAN_POINT ( 'NONE',  ( -9.564922557961040184, 16.46253265017147172, 97.91775706135233293 ) ) ;
#170865=CARTESIAN_POINT ( 'NONE',  ( 18.62759615963271287, -10.81492255796078972, 48.33224293864770260 ) ) ;
#170867=CARTESIAN_POINT ( 'NONE',  ( -8.224510206698948167, 14.34966873604960824, 115.4155762719810241 ) ) ;
#170868=CARTESIAN_POINT ( 'NONE',  ( -17.49999999999999289, -5.622605283950893984, 31.31207310596114013 ) ) ;
#170869=CARTESIAN_POINT ( 'NONE',  ( -0.05219959533909027116, -19.03943276465977164, 67.49890960531436690 ) ) ;
#170870=CARTESIAN_POINT ( 'NONE',  ( 0.05219959533907565091, 21.53943276465977519, 74.99890960531435269 ) ) ;
#170871=CARTESIAN_POINT ( 'NONE',  ( -16.52544592524335698, -4.483927247898792601, 88.95942372801901854 ) ) ;
#170872=CARTESIAN_POINT ( 'NONE',  ( 5.049401038298161559, -19.05341960407611168, 67.70724293864769550 ) ) ;
#170873=CARTESIAN_POINT ( 'NONE',  ( -5.153800228976607833, 19.02544592524334988, 72.70942372801900433 ) ) ;
#170874=CARTESIAN_POINT ( 'NONE',  ( 21.52544592524334988, 5.823673210054432836, 81.45942372801900433 ) ) ;
#170875=CARTESIAN_POINT ( 'NONE',  ( 10.81492255796078972, 18.62759615963270932, 69.58224293864769550 ) ) ;
#170876=CARTESIAN_POINT ( 'NONE',  ( -10.81492255796078084, -18.62759615963271287, 22.08224293864769194 ) ) ;
#170877=CARTESIAN_POINT ( 'NONE',  ( -19.02544592524342804, 5.153800228976336051, 31.04057627198102409 ) ) ;
#170878=CARTESIAN_POINT ( 'NONE',  ( -8.314922557961024197, 14.29746914071037800, 97.91775706135236135 ) ) ;
#170879=CARTESIAN_POINT ( 'NONE',  ( -16.53943276465976808, -0.05219959533934237506, 23.75109039468567929 ) ) ;
#170880=CARTESIAN_POINT ( 'NONE',  ( 17.31747979337948706, 6.344076630961017038, 53.87944868065186199 ) ) ;
#170881=CARTESIAN_POINT ( 'NONE',  ( -18.62759615963255300, -10.81492255796106328, 94.16775706135237556 ) ) ;
#170882=ORIENTED_EDGE ( 'NONE', *, *, #135545, .T. ) ;
#170883=CARTESIAN_POINT ( 'NONE',  ( 16.52544592524342804, -4.483927247898539470, 53.54057627198103120 ) ) ;
#170884=CARTESIAN_POINT ( 'NONE',  ( -21.52544592524343514, 5.823673210054127303, 91.04057627198103830 ) ) ;
#170885=CARTESIAN_POINT ( 'NONE',  ( 21.52544592524344225, -5.823673210054117533, 103.5405762719810383 ) ) ;
#170886=CARTESIAN_POINT ( 'NONE',  ( 21.52544592524344225, -5.823673210054117533, 43.54057627198103830 ) ) ;
#170887=CARTESIAN_POINT ( 'NONE',  ( 0.05219959533934541429, -16.53943276465976808, 75.00109039468568994 ) ) ;
#170888=CARTESIAN_POINT ( 'NONE',  ( -12.06949235617756955, 12.14591786802309770, 85.62390960531436690 ) ) ;
#170889=CARTESIAN_POINT ( 'NONE',  ( -13.97604488694527625, -13.89961937509977652, 51.87390960531436690 ) ) ;
#170891=CARTESIAN_POINT ( 'NONE',  ( 8.224510206698953496, -14.34966873604960469, 22.91557627198102765 ) ) ;
#170892=CARTESIAN_POINT ( 'NONE',  ( -10.72451020669870658, -18.67979575497194134, 29.58442372801901854 ) ) ;
#170893=CARTESIAN_POINT ( 'NONE',  ( -5.153800228976328057, -19.02544592524343514, 92.29057627198099567 ) ) ;
#170894=CARTESIAN_POINT ( 'NONE',  ( 21.52544592524334988, 5.823673210054432836, 71.45942372801901854 ) ) ;
#170896=CARTESIAN_POINT ( 'NONE',  ( -19.03943276465977164, 0.05219959533909376836, 26.24890960531435624 ) ) ;
#170897=ORIENTED_EDGE ( 'NONE', *, *, #154166, .F. ) ;
#170898=CARTESIAN_POINT ( 'NONE',  ( -5.823673210054431948, 21.52544592524334988, 52.70942372801902565 ) ) ;
#170899=CARTESIAN_POINT ( 'NONE',  ( 19.03943276465977164, -0.05219959533909143690, 48.74890960531435979 ) ) ;
#170900=CARTESIAN_POINT ( 'NONE',  ( -19.03943276465977164, 0.05219959533909376836, 111.2489096053143669 ) ) ;
#170901=CARTESIAN_POINT ( 'NONE',  ( 0.05219959533909260263, 19.03943276465977164, 84.99890960531436690 ) ) ;
#170902=CARTESIAN_POINT ( 'NONE',  ( -0.05219959533936034679, 19.03943276465977164, 67.50109039468566152 ) ) ;
#170903=CARTESIAN_POINT ( 'NONE',  ( -5.719274019375665041, -21.55341960407619695, 44.79275706135234714 ) ) ;
#170904=CARTESIAN_POINT ( 'NONE',  ( -13.97604488694547697, 13.89961937509957934, 63.12609039468566152 ) ) ;
#170905=CARTESIAN_POINT ( 'NONE',  ( -19.05341960407611168, -5.049401038298163336, 36.45724293864766707 ) ) ;
#170906=CARTESIAN_POINT ( 'NONE',  ( -4.379528057220086978, -16.55341960407618274, 104.7927570613523898 ) ) ;
#170907=CARTESIAN_POINT ( 'NONE',  ( -19.03943276465977164, -0.05219959533935918106, 73.75109039468566152 ) ) ;
#170908=CARTESIAN_POINT ( 'NONE',  ( -14.34966873604960291, -8.224510206698953496, 26.66557627198103475 ) ) ;
#170909=CARTESIAN_POINT ( 'NONE',  ( -19.02544592524334988, -5.153800228976617603, 48.95942372801900433 ) ) ;
#170910=CARTESIAN_POINT ( 'NONE',  ( -21.52544592524334988, -5.823673210054445271, 103.9594237280190185 ) ) ;
#170911=CARTESIAN_POINT ( 'NONE',  ( 13.89961937509957401, 13.97604488694547697, 31.87609039468566863 ) ) ;
#170912=CARTESIAN_POINT ( 'NONE',  ( 0.05219959533909260263, 19.03943276465977164, 29.99890960531435979 ) ) ;
#170913=CARTESIAN_POINT ( 'NONE',  ( 0.05219959533937995610, -21.53943276465977519, 95.00109039468568994 ) ) ;
#170914=CARTESIAN_POINT ( 'NONE',  ( 16.52544592524335698, 4.483927247898782831, 26.45942372801901854 ) ) ;
#170915=CARTESIAN_POINT ( 'NONE',  ( -19.05341960407611168, -5.049401038298163336, 86.45724293864769550 ) ) ;
#170918=CARTESIAN_POINT ( 'NONE',  ( -9.474510206698964154, 16.51473224551069663, 80.41557627198103830 ) ) ;
#170920=CARTESIAN_POINT ( 'NONE',  ( -19.05341960407617563, 5.049401038297882671, 78.54275706135233293 ) ) ;
#170921=B_SPLINE_CURVE_WITH_KNOTS ( 'NONE', 3,
 ( #6694, #22883, #193743, #190736, #161391, #145212, #114883, #98700, #130024, #84529, #82534, #20876, #68372, #177579, #39046, #8717, #191723, #129035, #144216, #131046 ),
 .UNSPECIFIED., .F., .F.,
 ( 4, 2, 2, 2, 2, 2, 2, 2, 2, 4 ),
 ( 0.004000878361811951306, 0.004499404418915963801, 0.004997930476019976295, 0.005496456533123988790, 0.005994982590228001285, 0.006244245618779987149, 0.006493508647331973013, 0.006992034704435948211, 0.007490560761539923409, 0.007989086818643898608 ),
 .UNSPECIFIED. ) ;
#170922=CARTESIAN_POINT ( 'NONE',  ( -13.97604488694527625, -13.89961937509977652, 111.8739096053143243 ) ) ;
#170923=CARTESIAN_POINT ( 'NONE',  ( 18.67979575497194134, -10.72451020669871369, 105.8344237280190328 ) ) ;
#170924=CARTESIAN_POINT ( 'NONE',  ( 0.05219959533910956823, 16.53943276465976808, 99.99890960531436690 ) ) ;
#170926=CARTESIAN_POINT ( 'NONE',  ( -10.72451020669898014, 18.67979575497178502, 55.41557627198102409 ) ) ;
#170927=CARTESIAN_POINT ( 'NONE',  ( -10.81492255796078084, -18.62759615963271287, 32.08224293864769550 ) ) ;
#170928=CARTESIAN_POINT ( 'NONE',  ( 19.05341960407611168, 5.049401038298154454, 28.95724293864769550 ) ) ;
#170930=CARTESIAN_POINT ( 'NONE',  ( 19.03943276465977164, 0.05219959533936151252, 56.25109039468566863 ) ) ;
#170931=CARTESIAN_POINT ( 'NONE',  ( 8.224510206698953496, -14.34966873604960469, 42.91557627198103120 ) ) ;
#170932=CARTESIAN_POINT ( 'NONE',  ( 19.02544592524343514, -5.153800228976328945, 113.5405762719810241 ) ) ;
#170933=CARTESIAN_POINT ( 'NONE',  ( -21.52544592524334988, -5.823673210054445271, 73.95942372801901854 ) ) ;
#170934=CARTESIAN_POINT ( 'NONE',  ( 5.719274019375991003, -21.55341960407610458, 67.70724293864769550 ) ) ;
#170935=CARTESIAN_POINT ( 'NONE',  ( 15.80617190586769283, -15.72974639402175789, 45.62609039468567573 ) ) ;
#170936=CARTESIAN_POINT ( 'NONE',  ( 18.67979575497178502, 10.72451020669898547, 94.16557627198103830 ) ) ;
#170937=CARTESIAN_POINT ( 'NONE',  ( 0.05219959533937995610, -21.53943276465977519, 45.00109039468568284 ) ) ;
#170938=CARTESIAN_POINT ( 'NONE',  ( 5.153800228976335163, 19.02544592524342804, 29.79057627198102409 ) ) ;
#170939=CARTESIAN_POINT ( 'NONE',  ( 13.89961937509977652, -13.97604488694527269, 83.12390960531436690 ) ) ;
#170940=CARTESIAN_POINT ( 'NONE',  ( 16.52544592524335698, 4.483927247898782831, 76.45942372801901854 ) ) ;
#170941=CARTESIAN_POINT ( 'NONE',  ( 8.314922557960818139, 14.29746914071049879, 104.5822429386477097 ) ) ;
#170942=CARTESIAN_POINT ( 'NONE',  ( -19.03943276465977164, 0.05219959533909376836, 116.2489096053143669 ) ) ;
#170943=CARTESIAN_POINT ( 'NONE',  ( 16.53943276465976808, -0.05219959533910856209, 48.74890960531435979 ) ) ;
#170944=CARTESIAN_POINT ( 'NONE',  ( 8.224510206698742110, 14.34966873604972548, 107.0844237280190043 ) ) ;
#170945=CARTESIAN_POINT ( 'NONE',  ( -19.02544592524342804, 5.153800228976336051, 66.04057627198103830 ) ) ;
#170946=CARTESIAN_POINT ( 'NONE',  ( 13.89961937509977652, -13.97604488694527269, 33.12390960531434558 ) ) ;
#170947=CARTESIAN_POINT ( 'NONE',  ( 10.72451020669898902, -18.67979575497178502, 42.91557627198103120 ) ) ;
#170948=CARTESIAN_POINT ( 'NONE',  ( -0.05219959533936034679, 19.03943276465977164, 42.50109039468566152 ) ) ;
#170950=CARTESIAN_POINT ( 'NONE',  ( 12.06949235617757843, -12.14591786802309237, 38.12390960531436690 ) ) ;
#170951=CARTESIAN_POINT ( 'NONE',  ( 5.719274019375991003, -21.55341960407610458, 27.70724293864769905 ) ) ;
#170952=CARTESIAN_POINT ( 'NONE',  ( 21.53943276465977519, 0.05219959533937863772, 61.25109039468567573 ) ) ;
#170954=CARTESIAN_POINT ( 'NONE',  ( -8.224510206698735004, -14.34966873604973081, 69.58442372801900433 ) ) ;
#170955=CARTESIAN_POINT ( 'NONE',  ( -19.03943276465977164, -0.05219959533935918106, 63.75109039468566863 ) ) ;
#170956=CARTESIAN_POINT ( 'NONE',  ( -14.29746914071049879, 8.314922557960819915, 40.83224293864769550 ) ) ;
#170957=CARTESIAN_POINT ( 'NONE',  ( -19.49671883438226416, -5.500000000000082601, 74.89279849105685116 ) ) ;
#170958=CARTESIAN_POINT ( 'NONE',  ( 0.05219959533910956823, 16.53943276465976808, 24.99890960531435624 ) ) ;
#170959=CARTESIAN_POINT ( 'NONE',  ( 9.474510206698971260, -16.51473224551069308, 37.91557627198102409 ) ) ;
#170960=CARTESIAN_POINT ( 'NONE',  ( -19.02544592524342804, 5.153800228976336051, 56.04057627198100988 ) ) ;
#170961=CARTESIAN_POINT ( 'NONE',  ( 0.05219959533910956823, 16.53943276465976808, 114.9989096053143669 ) ) ;
#170962=CARTESIAN_POINT ( 'NONE',  ( -18.67979575497193778, 10.72451020669871902, 33.33442372801900433 ) ) ;
#170963=CARTESIAN_POINT ( 'NONE',  ( 0.05219959533909260263, 19.03943276465977164, 54.99890960531435979 ) ) ;
#170964=CARTESIAN_POINT ( 'NONE',  ( 17.50000000000000000, -5.499999999999992895, 81.21769037696435589 ) ) ;
#170965=CARTESIAN_POINT ( 'NONE',  ( 19.03943276465977164, -0.05219959533909143690, 43.74890960531435979 ) ) ;
#170966=CARTESIAN_POINT ( 'NONE',  ( 5.823673210054125526, 21.52544592524343514, 34.79057627198103120 ) ) ;
#170968=CARTESIAN_POINT ( 'NONE',  ( -10.72451020669870658, -18.67979575497194134, 59.58442372801901854 ) ) ;
#170969=CARTESIAN_POINT ( 'NONE',  ( -14.34966873604960291, -8.224510206698953496, 111.6655762719810525 ) ) ;
#170970=CARTESIAN_POINT ( 'NONE',  ( 15.72974639402199770, -15.80617190586745480, 28.12390960531435979 ) ) ;
#170971=CARTESIAN_POINT ( 'NONE',  ( 8.224510206698742110, 14.34966873604972548, 97.08442372801904696 ) ) ;
#170972=CARTESIAN_POINT ( 'NONE',  ( -15.80617190586768217, 15.72974639402176855, 108.1260903946856757 ) ) ;
#170973=CARTESIAN_POINT ( 'NONE',  ( 4.483927247898790824, -16.52544592524335698, 70.20942372801904696 ) ) ;
#170974=CARTESIAN_POINT ( 'NONE',  ( -9.474510206698964154, 16.51473224551069663, 105.4155762719810383 ) ) ;
#170975=CARTESIAN_POINT ( 'NONE',  ( -16.55341960407617563, 4.379528057220093196, 58.54275706135235424 ) ) ;
#170976=CARTESIAN_POINT ( 'NONE',  ( -12.06949235617739369, -12.14591786802326823, 24.37609039468567573 ) ) ;
#170977=CARTESIAN_POINT ( 'NONE',  ( 4.483927247898790824, -16.52544592524335698, 90.20942372801903275 ) ) ;
#170978=CARTESIAN_POINT ( 'NONE',  ( -5.823673210054431948, 21.52544592524334988, 47.70942372801902565 ) ) ;
#170979=CARTESIAN_POINT ( 'NONE',  ( -13.97604488694547697, 13.89961937509957934, 113.1260903946856757 ) ) ;
#170980=CARTESIAN_POINT ( 'NONE',  ( -15.80617190586745835, -15.72974639402198527, 111.8739096053143669 ) ) ;
#170981=CARTESIAN_POINT ( 'NONE',  ( 16.55341960407618274, -4.379528057220086978, 26.04275706135235779 ) ) ;
#170982=CARTESIAN_POINT ( 'NONE',  ( -12.06949235617739369, -12.14591786802326823, 89.37609039468568994 ) ) ;
#170984=CARTESIAN_POINT ( 'NONE',  ( 0.05219959533937995610, -21.53943276465977519, 85.00109039468568994 ) ) ;
#170985=CARTESIAN_POINT ( 'NONE',  ( -9.564922557961040184, 16.46253265017147172, 82.91775706135233293 ) ) ;
#170986=CARTESIAN_POINT ( 'NONE',  ( 8.314922557960818139, 14.29746914071049879, 49.58224293864769550 ) ) ;
#170987=CARTESIAN_POINT ( 'NONE',  ( 16.55341960407611168, 4.379528057220329451, 43.95724293864769550 ) ) ;
#170988=CARTESIAN_POINT ( 'NONE',  ( 16.53943276465976808, -0.05219959533910856209, 108.7489096053143669 ) ) ;
#170989=CARTESIAN_POINT ( 'NONE',  ( 5.049401038297881783, 19.05341960407617563, 47.29275706135231161 ) ) ;
#170990=CARTESIAN_POINT ( 'NONE',  ( 18.22780087662123805, 5.499999999999960032, 96.48236817873105053 ) ) ;
#170991=CARTESIAN_POINT ( 'NONE',  ( -15.80617190586768217, 15.72974639402176855, 53.12609039468568284 ) ) ;
#170992=CARTESIAN_POINT ( 'NONE',  ( -4.379528057220086978, -16.55341960407618274, 19.79275706135235069 ) ) ;
#170994=CARTESIAN_POINT ( 'NONE',  ( 16.51473224551069308, 9.474510206698969483, 99.16557627198102409 ) ) ;
#170995=CARTESIAN_POINT ( 'NONE',  ( -18.62759615963270932, 10.81492255796079327, 65.83224293864769550 ) ) ;
#170996=CARTESIAN_POINT ( 'NONE',  ( 5.153800228976615827, -19.02544592524334988, 95.20942372801897591 ) ) ;
#170998=CARTESIAN_POINT ( 'NONE',  ( 0.05219959533909260263, 19.03943276465977164, 84.99890960531436690 ) ) ;
#170999=CARTESIAN_POINT ( 'NONE',  ( -21.52544592524343514, 5.823673210054127303, 56.04057627198102409 ) ) ;
#171000=CARTESIAN_POINT ( 'NONE',  ( -4.379528057220328563, 16.55341960407611168, 105.2072429386477097 ) ) ;
#171001=CARTESIAN_POINT ( 'NONE',  ( 16.51473224551069308, 9.474510206698969483, 64.16557627198102409 ) ) ;
#171002=CARTESIAN_POINT ( 'NONE',  ( -16.46253265017160317, 9.564922557960807481, 25.83224293864769194 ) ) ;
#171003=CARTESIAN_POINT ( 'NONE',  ( -21.53943276465977519, -0.05219959533937600094, 33.75109039468568284 ) ) ;
#171005=CARTESIAN_POINT ( 'NONE',  ( 21.55341960407619695, -5.719274019375665929, 81.04275706135236135 ) ) ;
#171006=CARTESIAN_POINT ( 'NONE',  ( -16.55341960407617563, 4.379528057220093196, 93.54275706135234714 ) ) ;
#171008=CARTESIAN_POINT ( 'NONE',  ( 21.53943276465977519, 0.05219959533937863772, 26.25109039468567573 ) ) ;
#171009=CARTESIAN_POINT ( 'NONE',  ( -5.719274019375665041, -21.55341960407619695, 39.79275706135235424 ) ) ;
#171010=CARTESIAN_POINT ( 'NONE',  ( 16.51473224551083163, -9.474510206698727899, 70.83442372801900433 ) ) ;
#171011=CARTESIAN_POINT ( 'NONE',  ( -19.03943276465977164, 0.05219959533909376836, 81.24890960531436690 ) ) ;
#171012=CARTESIAN_POINT ( 'NONE',  ( -21.52544592524334988, -5.823673210054445271, 78.95942372801901854 ) ) ;
#171013=CARTESIAN_POINT ( 'NONE',  ( -18.62759615963270932, 10.81492255796079327, 80.83224293864769550 ) ) ;
#171014=CARTESIAN_POINT ( 'NONE',  ( 4.483927247898545687, 16.52544592524342804, 69.79057627198102409 ) ) ;
#171015=CARTESIAN_POINT ( 'NONE',  ( 18.62759615963255655, 10.81492255796105972, 101.6677570613523613 ) ) ;
#171016=CARTESIAN_POINT ( 'NONE',  ( -8.224510206698948167, 14.34966873604960824, 80.41557627198103830 ) ) ;
#171017=CARTESIAN_POINT ( 'NONE',  ( 0.05219959533909260263, 19.03943276465977164, 39.99890960531436690 ) ) ;
#171018=CARTESIAN_POINT ( 'NONE',  ( 16.46253265017146816, 9.564922557961045513, 71.66775706135233293 ) ) ;
#171019=CARTESIAN_POINT ( 'NONE',  ( 12.06949235617757843, -12.14591786802309237, 38.12390960531436690 ) ) ;
#171020=CARTESIAN_POINT ( 'NONE',  ( -10.72451020669870658, -18.67979575497194134, 89.58442372801901854 ) ) ;
#171021=CARTESIAN_POINT ( 'NONE',  ( -5.049401038298153566, 19.05341960407611168, 95.20724293864770971 ) ) ;
#171022=CARTESIAN_POINT ( 'NONE',  ( -13.97604488694547697, 13.89961937509957934, 63.12609039468566152 ) ) ;
#171023=CARTESIAN_POINT ( 'NONE',  ( -21.55341960407610458, -5.719274019375992779, 66.45724293864768129 ) ) ;
#171024=CARTESIAN_POINT ( 'NONE',  ( -5.719274019375665041, -21.55341960407619695, 19.79275706135235069 ) ) ;
#171025=CARTESIAN_POINT ( 'NONE',  ( -19.03943276465977164, -0.05219959533935918106, 113.7510903946856757 ) ) ;
#171026=CARTESIAN_POINT ( 'NONE',  ( 16.55341960407618274, -4.379528057220086978, 81.04275706135236135 ) ) ;
#171028=CARTESIAN_POINT ( 'NONE',  ( -21.52544592524343514, 5.823673210054127303, 116.0405762719810383 ) ) ;
#171029=CARTESIAN_POINT ( 'NONE',  ( 14.29746914071049879, -8.314922557960816363, 98.33224293864769550 ) ) ;
#171031=CARTESIAN_POINT ( 'NONE',  ( 4.483927247898790824, -16.52544592524335698, 50.20942372801901854 ) ) ;
#171032=CARTESIAN_POINT ( 'NONE',  ( 10.81492255796078972, 18.62759615963270932, 64.58224293864769550 ) ) ;
#171033=CARTESIAN_POINT ( 'NONE',  ( 16.55341960407618274, -4.379528057220086978, 111.0427570613523613 ) ) ;
#171034=CARTESIAN_POINT ( 'NONE',  ( 16.52544592524335698, 4.483927247898782831, 31.45942372801901854 ) ) ;
#171035=CARTESIAN_POINT ( 'NONE',  ( -9.474510206698964154, 16.51473224551069663, 25.41557627198103120 ) ) ;
#171036=CARTESIAN_POINT ( 'NONE',  ( 14.34966873604972726, -8.224510206698740333, 85.83442372801901854 ) ) ;
#171037=CARTESIAN_POINT ( 'NONE',  ( -5.049401038297874678, -19.05341960407617918, 79.79275706135233293 ) ) ;
#171038=CARTESIAN_POINT ( 'NONE',  ( 21.52544592524344225, -5.823673210054117533, 68.54057627198103830 ) ) ;
#171039=CARTESIAN_POINT ( 'NONE',  ( -8.314922557961024197, 14.29746914071037800, 97.91775706135236135 ) ) ;
#171040=CARTESIAN_POINT ( 'NONE',  ( 10.72451020669871369, 18.67979575497193778, 82.08442372801901854 ) ) ;
#171041=CARTESIAN_POINT ( 'NONE',  ( -10.72451020669898014, 18.67979575497178502, 65.41557627198102409 ) ) ;
#171042=CARTESIAN_POINT ( 'NONE',  ( 21.53943276465977519, -0.05219959533907433946, 48.74890960531435979 ) ) ;
#171044=CARTESIAN_POINT ( 'NONE',  ( 12.06949235617739724, 12.14591786802326823, 81.87609039468568994 ) ) ;
#171045=CARTESIAN_POINT ( 'NONE',  ( 18.62759615963271287, -10.81492255796078972, 48.33224293864770260 ) ) ;
#171047=CARTESIAN_POINT ( 'NONE',  ( 21.52544592524344225, -5.823673210054117533, 23.54057627198102765 ) ) ;
#171049=CARTESIAN_POINT ( 'NONE',  ( -19.05341960407611168, -5.049401038298163336, 21.45724293864768839 ) ) ;
#171050=CARTESIAN_POINT ( 'NONE',  ( -10.81492255796078084, -18.62759615963271287, 57.08224293864769550 ) ) ;
#171051=CARTESIAN_POINT ( 'NONE',  ( 4.483927247898790824, -16.52544592524335698, 110.2094237280190185 ) ) ;
#171052=CARTESIAN_POINT ( 'NONE',  ( 21.55341960407619695, -5.719274019375665929, 41.04275706135236135 ) ) ;
#171053=CARTESIAN_POINT ( 'NONE',  ( -13.89961937509957401, -13.97604488694547875, 99.37609039468567573 ) ) ;
#171054=CARTESIAN_POINT ( 'NONE',  ( 19.05341960407611168, 5.049401038298154454, 23.95724293864769194 ) ) ;
#171055=CARTESIAN_POINT ( 'NONE',  ( -16.53943276465976808, -0.05219959533934237506, 18.75109039468568639 ) ) ;
#171056=CARTESIAN_POINT ( 'NONE',  ( 5.049401038298161559, -19.05341960407611168, 42.70724293864767418 ) ) ;
#171058=CARTESIAN_POINT ( 'NONE',  ( 19.05341960407611168, 5.049401038298154454, 93.95724293864769550 ) ) ;
#171059=CARTESIAN_POINT ( 'NONE',  ( -4.379528057220086978, -16.55341960407618274, 79.79275706135236135 ) ) ;
#171060=CARTESIAN_POINT ( 'NONE',  ( -16.51473224551082808, 9.474510206698731452, 73.33442372801900433 ) ) ;
#171061=CARTESIAN_POINT ( 'NONE',  ( 5.049401038297881783, 19.05341960407617563, 27.29275706135232937 ) ) ;
#171062=CARTESIAN_POINT ( 'NONE',  ( -18.67979575497178146, -10.72451020669898902, 61.66557627198103120 ) ) ;
#171063=CARTESIAN_POINT ( 'NONE',  ( 8.224510206698742110, 14.34966873604972548, 82.08442372801901854 ) ) ;
#171064=CARTESIAN_POINT ( 'NONE',  ( -19.05341960407617563, 5.049401038297882671, 78.54275706135233293 ) ) ;
#171065=CARTESIAN_POINT ( 'NONE',  ( -13.89961937509977652, 13.97604488694528158, 40.62390960531435979 ) ) ;
#171066=CARTESIAN_POINT ( 'NONE',  ( 16.46253265017160672, -9.564922557960803928, 73.33224293864769550 ) ) ;
#171067=CARTESIAN_POINT ( 'NONE',  ( -15.72974639402176322, -15.80617190586768395, 54.37609039468568994 ) ) ;
#171068=CARTESIAN_POINT ( 'NONE',  ( -16.46253265017160317, 9.564922557960807481, 40.83224293864769550 ) ) ;
#171069=CARTESIAN_POINT ( 'NONE',  ( -13.97604488694547697, 13.89961937509957934, 73.12609039468568994 ) ) ;
#171071=CARTESIAN_POINT ( 'NONE',  ( 19.03943276465977164, -0.05219959533909143690, 108.7489096053143527 ) ) ;
#171072=CARTESIAN_POINT ( 'NONE',  ( 8.314922557960818139, 14.29746914071049879, 59.58224293864770260 ) ) ;
#171073=CARTESIAN_POINT ( 'NONE',  ( 15.80617190586746368, 15.72974639402197994, 64.37390960531435269 ) ) ;
#171075=CARTESIAN_POINT ( 'NONE',  ( -5.049401038297874678, -19.05341960407617918, 39.79275706135232582 ) ) ;
#171077=CARTESIAN_POINT ( 'NONE',  ( 0.05219959533909260263, 19.03943276465977164, 59.99890960531436690 ) ) ;
#171078=CARTESIAN_POINT ( 'NONE',  ( 19.05341960407611168, 5.049401038298154454, 68.95724293864769550 ) ) ;
#171079=CARTESIAN_POINT ( 'NONE',  ( -8.224510206698735004, -14.34966873604973081, 54.58442372801901143 ) ) ;
#171080=CARTESIAN_POINT ( 'NONE',  ( 17.59860650958994555, -7.585241751806880650, 80.92337014262491834 ) ) ;
#171082=CARTESIAN_POINT ( 'NONE',  ( 8.314922557961029526, -14.29746914071037800, 90.41775706135236135 ) ) ;
#171083=CARTESIAN_POINT ( 'NONE',  ( -17.72696623605158806, 5.500000000000047962, 78.59811031808416715 ) ) ;
#171084=CARTESIAN_POINT ( 'NONE',  ( -12.14591786802326823, 12.06949235617739902, 68.12609039468567573 ) ) ;
#171085=CARTESIAN_POINT ( 'NONE',  ( 8.314922557961029526, -14.29746914071037800, 45.41775706135234003 ) ) ;
#171086=CARTESIAN_POINT ( 'NONE',  ( -19.02544592524334988, -5.153800228976617603, 23.95942372801900078 ) ) ;
#171087=CARTESIAN_POINT ( 'NONE',  ( 19.02544592524343514, -5.153800228976328945, 48.54057627198103120 ) ) ;
#171089=CARTESIAN_POINT ( 'NONE',  ( -18.67979575497193778, 10.72451020669871902, 53.33442372801901854 ) ) ;
#171090=CARTESIAN_POINT ( 'NONE',  ( 19.03943276465977164, 0.05219959533936151252, 66.25109039468567573 ) ) ;
#171091=CARTESIAN_POINT ( 'NONE',  ( 5.823673210054444382, -21.52544592524334988, 105.2094237280190328 ) ) ;
#171092=CARTESIAN_POINT ( 'NONE',  ( -13.97604488694527625, -13.89961937509977652, 26.87390960531434558 ) ) ;
#171094=CARTESIAN_POINT ( 'NONE',  ( 18.67979575497178502, 10.72451020669898547, 54.16557627198103120 ) ) ;
#171095=CARTESIAN_POINT ( 'NONE',  ( -10.72451020669898014, 18.67979575497178502, 25.41557627198103120 ) ) ;
#171096=CARTESIAN_POINT ( 'NONE',  ( -8.314922557960811034, -14.29746914071050412, 97.08224293864770971 ) ) ;
#171097=CARTESIAN_POINT ( 'NONE',  ( 14.34966873604972726, -8.224510206698740333, 40.83442372801901854 ) ) ;
#171098=CARTESIAN_POINT ( 'NONE',  ( 14.34966873604960469, 8.224510206698951720, 34.16557627198102409 ) ) ;
#171100=CARTESIAN_POINT ( 'NONE',  ( -5.719274019375665041, -21.55341960407619695, 24.79275706135235779 ) ) ;
#171101=CARTESIAN_POINT ( 'NONE',  ( -8.224510206698948167, 14.34966873604960824, 40.41557627198103120 ) ) ;
#171102=CARTESIAN_POINT ( 'NONE',  ( 13.97604488694527802, 13.89961937509977652, 109.3739096053143669 ) ) ;
#171103=CARTESIAN_POINT ( 'NONE',  ( 9.564922557961047289, -16.46253265017146816, 105.4177570613523471 ) ) ;
#171104=CARTESIAN_POINT ( 'NONE',  ( 0.05219959533936267826, -19.03943276465977164, 20.00109039468567218 ) ) ;
#171105=CARTESIAN_POINT ( 'NONE',  ( 4.379528057220339221, -16.55341960407611168, 27.70724293864769905 ) ) ;
#171106=CARTESIAN_POINT ( 'NONE',  ( 10.72451020669898902, -18.67979575497178502, 107.9155762719810241 ) ) ;
#171108=CARTESIAN_POINT ( 'NONE',  ( 16.81555441253550853, 7.025013491695496270, 31.86314554665743870 ) ) ;
#171109=CARTESIAN_POINT ( 'NONE',  ( 18.67979575497178502, 10.72451020669898547, 64.16557627198102409 ) ) ;
#171110=CARTESIAN_POINT ( 'NONE',  ( 13.89961937509977652, -13.97604488694527269, 83.12390960531436690 ) ) ;
#171111=CARTESIAN_POINT ( 'NONE',  ( 16.53943276465976808, -0.05219959533910856209, 48.74890960531435979 ) ) ;
#171112=CARTESIAN_POINT ( 'NONE',  ( 13.89961937509977652, -13.97604488694527269, 88.12390960531438111 ) ) ;
#171114=CARTESIAN_POINT ( 'NONE',  ( -18.22780087662123805, 5.499999999999981348, 81.01763182126896368 ) ) ;
#171115=CARTESIAN_POINT ( 'NONE',  ( 13.97604488694548053, -13.89961937509957401, 55.62609039468566863 ) ) ;
#171116=CARTESIAN_POINT ( 'NONE',  ( -10.81492255796078084, -18.62759615963271287, 97.08224293864770971 ) ) ;
#171117=CARTESIAN_POINT ( 'NONE',  ( 4.483927247898545687, 16.52544592524342804, 104.7905762719810241 ) ) ;
#171118=CARTESIAN_POINT ( 'NONE',  ( -15.80617190586768217, 15.72974639402176855, 43.12609039468568284 ) ) ;
#171121=CARTESIAN_POINT ( 'NONE',  ( 8.224510206698953496, -14.34966873604960469, 27.91557627198103830 ) ) ;
#171122=CARTESIAN_POINT ( 'NONE',  ( -9.564922557960796823, -16.46253265017161027, 32.08224293864769550 ) ) ;
#171123=CARTESIAN_POINT ( 'NONE',  ( 5.153800228976335163, 19.02544592524342804, 79.79057627198102409 ) ) ;
#171124=CARTESIAN_POINT ( 'NONE',  ( 18.67979575497178502, 10.72451020669898547, 64.16557627198102409 ) ) ;
#171125=CARTESIAN_POINT ( 'NONE',  ( -18.22780087662121673, -5.500000000000063061, 61.48459894673894155 ) ) ;
#171126=CARTESIAN_POINT ( 'NONE',  ( 5.153800228976335163, 19.02544592524342804, 29.79057627198102409 ) ) ;
#171127=CARTESIAN_POINT ( 'NONE',  ( 10.72451020669898902, -18.67979575497178502, 47.91557627198102409 ) ) ;
#171128=CARTESIAN_POINT ( 'NONE',  ( 0.05219959533937995610, -21.53943276465977519, 75.00109039468568994 ) ) ;
#171130=CARTESIAN_POINT ( 'NONE',  ( 4.379528057220092307, 16.55341960407617563, 72.29275706135236135 ) ) ;
#171131=CARTESIAN_POINT ( 'NONE',  ( 19.02544592524343514, -5.153800228976328945, 58.54057627198102409 ) ) ;
#171132=CARTESIAN_POINT ( 'NONE',  ( -5.153800228976328057, -19.02544592524343514, 67.29057627198102409 ) ) ;
#171134=CARTESIAN_POINT ( 'NONE',  ( 15.72974639402176855, 15.80617190586768217, 106.8760903946856899 ) ) ;
#171135=CARTESIAN_POINT ( 'NONE',  ( -0.05219959533934338120, 16.53943276465976808, 72.50109039468568994 ) ) ;
#171136=CARTESIAN_POINT ( 'NONE',  ( -15.80617190586768217, 15.72974639402176855, 93.12609039468568994 ) ) ;
#171137=CARTESIAN_POINT ( 'NONE',  ( -16.51473224551069308, -9.474510206698971260, 81.66557627198103830 ) ) ;
#171138=CARTESIAN_POINT ( 'NONE',  ( -21.53943276465977519, 0.05219959533907696930, 31.24890960531435979 ) ) ;
#171139=CARTESIAN_POINT ( 'NONE',  ( -5.153800228976607833, 19.02544592524334988, 107.7094237280189759 ) ) ;
#171140=CARTESIAN_POINT ( 'NONE',  ( 21.53943276465977519, 0.05219959533937863772, 81.25109039468568994 ) ) ;
#171141=CARTESIAN_POINT ( 'NONE',  ( 8.314922557961029526, -14.29746914071037800, 50.41775706135235424 ) ) ;
#171142=CARTESIAN_POINT ( 'NONE',  ( -10.72451020669898014, 18.67979575497178502, 105.4155762719810383 ) ) ;
#171143=CARTESIAN_POINT ( 'NONE',  ( -9.474510206698720793, -16.51473224551083518, 109.5844237280190043 ) ) ;
#171144=CARTESIAN_POINT ( 'NONE',  ( -19.03943276465977164, 0.05219959533909376836, 76.24890960531435269 ) ) ;
#171145=CARTESIAN_POINT ( 'NONE',  ( -5.153800228976607833, 19.02544592524334988, 112.7094237280190043 ) ) ;
#171146=CARTESIAN_POINT ( 'NONE',  ( -5.049401038298153566, 19.05341960407611168, 40.20724293864768839 ) ) ;
#171148=CARTESIAN_POINT ( 'NONE',  ( 9.474510206698729675, 16.51473224551082808, 112.0844237280190043 ) ) ;
#171149=CARTESIAN_POINT ( 'NONE',  ( -8.224510206698948167, 14.34966873604960824, 65.41557627198102409 ) ) ;
#171150=CARTESIAN_POINT ( 'NONE',  ( 0.05219959533934541429, -16.53943276465976808, 70.00109039468568994 ) ) ;
#171151=CARTESIAN_POINT ( 'NONE',  ( 10.81492255796106328, -18.62759615963255655, 25.41775706135235779 ) ) ;
#171152=CARTESIAN_POINT ( 'NONE',  ( -13.89961937509977652, 13.97604488694528158, 45.62390960531433848 ) ) ;
#171153=CARTESIAN_POINT ( 'NONE',  ( 19.05341960407611168, 5.049401038298154454, 73.95724293864768129 ) ) ;
#171154=CARTESIAN_POINT ( 'NONE',  ( -8.314922557961024197, 14.29746914071037800, 67.91775706135234714 ) ) ;
#171155=ADVANCED_FACE ( 'NONE', ( #108989 ), #122905, .T. ) ;
#171159=CARTESIAN_POINT ( 'NONE',  ( -5.719274019375665041, -21.55341960407619695, 109.7927570613523613 ) ) ;
#171160=CARTESIAN_POINT ( 'NONE',  ( -19.02544592524342804, 5.153800228976336051, 41.04057627198103120 ) ) ;
#171161=CARTESIAN_POINT ( 'NONE',  ( -19.05341960407611168, -5.049401038298163336, 96.45724293864769550 ) ) ;
#171163=CARTESIAN_POINT ( 'NONE',  ( -4.379528057220086978, -16.55341960407618274, 29.79275706135234358 ) ) ;
#171164=CARTESIAN_POINT ( 'NONE',  ( -16.51473224551082808, 9.474510206698731452, 43.33442372801900433 ) ) ;
#171165=CARTESIAN_POINT ( 'NONE',  ( 12.06949235617739724, 12.14591786802326823, 36.87609039468568994 ) ) ;
#171166=CARTESIAN_POINT ( 'NONE',  ( -9.564922557960796823, -16.46253265017161027, 47.08224293864769550 ) ) ;
#171167=CARTESIAN_POINT ( 'NONE',  ( -5.049401038298153566, 19.05341960407611168, 110.2072429386476671 ) ) ;
#171168=CARTESIAN_POINT ( 'NONE',  ( 16.46253265017160672, -9.564922557960803928, 63.33224293864769550 ) ) ;
#171169=CARTESIAN_POINT ( 'NONE',  ( 21.53943276465977519, -0.05219959533907433946, 103.7489096053143669 ) ) ;
#171170=CARTESIAN_POINT ( 'NONE',  ( -19.02544592524342804, 5.153800228976336051, 91.04057627198100988 ) ) ;
#171172=CARTESIAN_POINT ( 'NONE',  ( -16.46253265017160317, 9.564922557960807481, 60.83224293864769550 ) ) ;
#171173=CARTESIAN_POINT ( 'NONE',  ( 4.379528057220339221, -16.55341960407611168, 27.70724293864769905 ) ) ;
#171174=DIRECTION ( 'NONE',  ( 0.000000000000000000, 0.000000000000000000, -1.000000000000000000 ) ) ;
#171175=CARTESIAN_POINT ( 'NONE',  ( -0.05219959533936034679, 19.03943276465977164, 97.50109039468567573 ) ) ;
#171176=CARTESIAN_POINT ( 'NONE',  ( -13.89961937509957401, -13.97604488694547875, 29.37609039468565797 ) ) ;
#171177=CARTESIAN_POINT ( 'NONE',  ( 14.29746914071049879, -8.314922557960816363, 63.33224293864770260 ) ) ;
#171178=CARTESIAN_POINT ( 'NONE',  ( -10.72451020669870658, -18.67979575497194134, 104.5844237280190185 ) ) ;
#171179=CARTESIAN_POINT ( 'NONE',  ( 5.153800228976335163, 19.02544592524342804, 29.79057627198102409 ) ) ;
#171180=CARTESIAN_POINT ( 'NONE',  ( -0.05219959533910754901, -16.53943276465976808, 22.49890960531436335 ) ) ;
#171181=CARTESIAN_POINT ( 'NONE',  ( -21.53943276465977519, -0.05219959533937600094, 93.75109039468567573 ) ) ;
#171182=CARTESIAN_POINT ( 'NONE',  ( -16.46253265017160317, 9.564922557960807481, 75.83224293864769550 ) ) ;
#171183=CARTESIAN_POINT ( 'NONE',  ( -9.474510206698964154, 16.51473224551069663, 95.41557627198102409 ) ) ;
#171184=CARTESIAN_POINT ( 'NONE',  ( -4.483927247898539470, -16.52544592524342804, 97.29057627198105251 ) ) ;
#171185=CARTESIAN_POINT ( 'NONE',  ( -0.05219959533910754901, -16.53943276465976808, 62.49890960531436690 ) ) ;
#171186=CARTESIAN_POINT ( 'NONE',  ( 21.55341960407610458, 5.719274019375980345, 73.95724293864769550 ) ) ;
#171187=CARTESIAN_POINT ( 'NONE',  ( 9.564922557960805705, 16.46253265017160317, 79.58224293864769550 ) ) ;
#171188=CARTESIAN_POINT ( 'NONE',  ( -18.67979575497178146, -10.72451020669898902, 86.66557627198102409 ) ) ;
#171189=CARTESIAN_POINT ( 'NONE',  ( 5.049401038297881783, 19.05341960407617563, 82.29275706135229029 ) ) ;
#171190=CARTESIAN_POINT ( 'NONE',  ( -9.564922557961040184, 16.46253265017147172, 32.91775706135233293 ) ) ;
#171191=CARTESIAN_POINT ( 'NONE',  ( -16.53943276465976808, 0.05219959533911058130, 86.24890960531436690 ) ) ;
#171192=CARTESIAN_POINT ( 'NONE',  ( -0.05219959533909027116, -19.03943276465977164, 57.49890960531435979 ) ) ;
#171193=CARTESIAN_POINT ( 'NONE',  ( -18.67979575497178146, -10.72451020669898902, 61.66557627198103120 ) ) ;
#171194=CARTESIAN_POINT ( 'NONE',  ( 17.13100169013300444, -6.664070546373151771, 28.26789835699850428 ) ) ;
#171195=CARTESIAN_POINT ( 'NONE',  ( -16.52544592524335698, -4.483927247898792601, 108.9594237280190185 ) ) ;
#171197=CARTESIAN_POINT ( 'NONE',  ( -16.51473224551082808, 9.474510206698731452, 108.3344237280190043 ) ) ;
#171198=CARTESIAN_POINT ( 'NONE',  ( 4.483927247898545687, 16.52544592524342804, 84.79057627198102409 ) ) ;
#171200=CARTESIAN_POINT ( 'NONE',  ( 5.153800228976335163, 19.02544592524342804, 74.79057627198103830 ) ) ;
#171201=CARTESIAN_POINT ( 'NONE',  ( -19.03943276465977164, 0.05219959533909376836, 36.24890960531436690 ) ) ;
#171202=CARTESIAN_POINT ( 'NONE',  ( 16.55341960407611168, 4.379528057220329451, 63.95724293864770260 ) ) ;
#171203=CARTESIAN_POINT ( 'NONE',  ( 13.89961937509977652, -13.97604488694527269, 98.12390960531433848 ) ) ;
#171204=CARTESIAN_POINT ( 'NONE',  ( -16.51473224551082808, 9.474510206698731452, 93.33442372801900433 ) ) ;
#171205=CARTESIAN_POINT ( 'NONE',  ( 5.049401038298161559, -19.05341960407611168, 67.70724293864769550 ) ) ;
#171206=CARTESIAN_POINT ( 'NONE',  ( -13.97604488694527625, -13.89961937509977652, 91.87390960531432427 ) ) ;
#171207=CARTESIAN_POINT ( 'NONE',  ( 18.67979575497178502, 10.72451020669898547, 74.16557627198102409 ) ) ;
#171208=CARTESIAN_POINT ( 'NONE',  ( 16.52544592524335698, 4.483927247898782831, 71.45942372801901854 ) ) ;
#171209=CARTESIAN_POINT ( 'NONE',  ( -5.153800228976607833, 19.02544592524335343, 112.7094237280190043 ) ) ;
#171210=CARTESIAN_POINT ( 'NONE',  ( -0.05219959533909027116, -19.03943276465977164, 67.49890960531436690 ) ) ;
#171211=CARTESIAN_POINT ( 'NONE',  ( -5.719274019375978568, 21.55341960407610458, 70.20724293864769550 ) ) ;
#171212=CARTESIAN_POINT ( 'NONE',  ( -5.049401038297874678, -19.05341960407617918, 89.79275706135230450 ) ) ;
#171213=CARTESIAN_POINT ( 'NONE',  ( 8.224510206698953496, -14.34966873604960469, 42.91557627198103120 ) ) ;
#171214=CARTESIAN_POINT ( 'NONE',  ( -21.53943276465977519, -0.05219959533937600094, 48.75109039468568284 ) ) ;
#171216=CARTESIAN_POINT ( 'NONE',  ( 8.314922557961029526, -14.29746914071037800, 75.41775706135233293 ) ) ;
#171217=CARTESIAN_POINT ( 'NONE',  ( -13.97604488694527625, -13.89961937509977652, 111.8739096053143243 ) ) ;
#171218=CARTESIAN_POINT ( 'NONE',  ( 16.46253265017160672, -9.564922557960803928, 108.3322429386476955 ) ) ;
#171219=CARTESIAN_POINT ( 'NONE',  ( -17.26058549869092218, 6.457015423128486198, 78.62254162523936429 ) ) ;
#171220=CARTESIAN_POINT ( 'NONE',  ( 12.06949235617739724, 12.14591786802326823, 96.87609039468568994 ) ) ;
#171221=CARTESIAN_POINT ( 'NONE',  ( 8.224510206698742110, 14.34966873604972548, 42.08442372801901854 ) ) ;
#171222=CARTESIAN_POINT ( 'NONE',  ( 16.46253265017160672, -9.564922557960803928, 53.33224293864768839 ) ) ;
#171223=CARTESIAN_POINT ( 'NONE',  ( 5.049401038298161559, -19.05341960407611168, 57.70724293864769550 ) ) ;
#171224=CARTESIAN_POINT ( 'NONE',  ( -5.823673210054431948, 21.52544592524334988, 47.70942372801902565 ) ) ;
#171225=CARTESIAN_POINT ( 'NONE',  ( -0.05219959533934338120, 16.53943276465976808, 62.50109039468568284 ) ) ;
#171226=CARTESIAN_POINT ( 'NONE',  ( -16.52544592524342804, 4.483927247898546575, 31.04057627198102409 ) ) ;
#171227=CARTESIAN_POINT ( 'NONE',  ( 16.51473224551069308, 9.474510206698969483, 44.16557627198103120 ) ) ;
#171228=CARTESIAN_POINT ( 'NONE',  ( -0.05219959533909027116, -19.03943276465977164, 32.49890960531435979 ) ) ;
#171229=CARTESIAN_POINT ( 'NONE',  ( 8.224510206698742110, 14.34966873604972548, 27.08442372801901854 ) ) ;
#171230=CARTESIAN_POINT ( 'NONE',  ( -19.03943276465977164, -0.05219959533935918106, 88.75109039468567573 ) ) ;
#171231=CARTESIAN_POINT ( 'NONE',  ( 14.29746914071049879, -8.314922557960816363, 83.33224293864769550 ) ) ;
#171232=CARTESIAN_POINT ( 'NONE',  ( -5.153800228976328057, -19.02544592524343514, 57.29057627198103120 ) ) ;
#171233=CARTESIAN_POINT ( 'NONE',  ( 0.05219959533936267826, -19.03943276465977164, 90.00109039468567573 ) ) ;
#171234=CARTESIAN_POINT ( 'NONE',  ( 17.44279575226823198, -5.990770900252456066, 93.33557567514314712 ) ) ;
#171235=CARTESIAN_POINT ( 'NONE',  ( -10.72451020669870658, -18.67979575497194134, 89.58442372801901854 ) ) ;
#171236=CARTESIAN_POINT ( 'NONE',  ( -4.379528057220086978, -16.55341960407618274, 59.79275706135234714 ) ) ;
#171237=CARTESIAN_POINT ( 'NONE',  ( 17.44279575226823553, 5.990770900252484488, 36.66442432485683156 ) ) ;
#171238=CARTESIAN_POINT ( 'NONE',  ( 15.80617190586746368, 15.72974639402197994, 49.37390960531436690 ) ) ;
#171239=CARTESIAN_POINT ( 'NONE',  ( -14.29746914071037622, -8.314922557961029526, 44.16775706135234714 ) ) ;
#171240=CARTESIAN_POINT ( 'NONE',  ( -19.03943276465977164, 0.05219959533909376836, 21.24890960531436335 ) ) ;
#171241=CARTESIAN_POINT ( 'NONE',  ( -13.89961937509957401, -13.97604488694547875, 34.37609039468566863 ) ) ;
#171242=CARTESIAN_POINT ( 'NONE',  ( -16.46253265017160317, 9.564922557960807481, 70.83224293864770971 ) ) ;
#171244=CARTESIAN_POINT ( 'NONE',  ( -13.89961937509977652, 13.97604488694528158, 55.62390960531434558 ) ) ;
#171246=CARTESIAN_POINT ( 'NONE',  ( -5.049401038298153566, 19.05341960407611168, 75.20724293864769550 ) ) ;
#171247=CARTESIAN_POINT ( 'NONE',  ( -19.19724070472091881, -5.500000000000170530, 56.06193348274384647 ) ) ;
#171249=CARTESIAN_POINT ( 'NONE',  ( 19.03943276465977164, 0.05219959533936151252, 31.25109039468566863 ) ) ;
#171250=CARTESIAN_POINT ( 'NONE',  ( -0.05219959533937732626, 21.53943276465977519, 107.5010903946856899 ) ) ;
#171251=CARTESIAN_POINT ( 'NONE',  ( -4.483927247898539470, -16.52544592524342804, 42.29057627198103120 ) ) ;
#171252=CARTESIAN_POINT ( 'NONE',  ( 13.89961937509977652, -13.97604488694527269, 43.12390960531434558 ) ) ;
#171254=CARTESIAN_POINT ( 'NONE',  ( -16.51473224551069308, -9.474510206698971260, 101.6655762719810241 ) ) ;
#171255=CARTESIAN_POINT ( 'NONE',  ( -15.80617190586768217, 15.72974639402176855, 73.12609039468567573 ) ) ;
#171256=CARTESIAN_POINT ( 'NONE',  ( -0.05219959533909027116, -19.03943276465977164, 47.49890960531435979 ) ) ;
#171257=CARTESIAN_POINT ( 'NONE',  ( -21.52544592524334988, -5.823673210054445271, 78.95942372801901854 ) ) ;
#171258=CARTESIAN_POINT ( 'NONE',  ( -5.823673210054116645, -21.52544592524344225, 22.29057627198102765 ) ) ;
#171259=CARTESIAN_POINT ( 'NONE',  ( -0.05219959533909027116, -19.03943276465977164, 32.49890960531435979 ) ) ;
#171260=CARTESIAN_POINT ( 'NONE',  ( 0.05219959533937995610, -21.53943276465977519, 20.00109039468568639 ) ) ;
#171261=CARTESIAN_POINT ( 'NONE',  ( -13.89961937509957401, -13.97604488694547875, 54.37609039468565442 ) ) ;
#171262=CARTESIAN_POINT ( 'NONE',  ( -13.89961937509977652, 13.97604488694528158, 30.62390960531435269 ) ) ;
#171263=CARTESIAN_POINT ( 'NONE',  ( 9.564922557960805705, 16.46253265017160317, 74.58224293864769550 ) ) ;
#171264=CARTESIAN_POINT ( 'NONE',  ( -9.564922557961040184, 16.46253265017147172, 107.9177570613523471 ) ) ;
#171265=CARTESIAN_POINT ( 'NONE',  ( -0.05219959533910754901, -16.53943276465976808, 77.49890960531433848 ) ) ;
#171266=CARTESIAN_POINT ( 'NONE',  ( 10.81492255796078972, 18.62759615963270932, 39.58224293864769550 ) ) ;
#171267=CARTESIAN_POINT ( 'NONE',  ( 19.05341960407617918, -5.049401038297876454, 101.0427570613523045 ) ) ;
#171268=CARTESIAN_POINT ( 'NONE',  ( 15.72974639402199770, -15.80617190586745480, 103.1239096053143811 ) ) ;
#171269=CARTESIAN_POINT ( 'NONE',  ( -0.05219959533937732626, 21.53943276465977519, 57.50109039468568994 ) ) ;
#171270=CARTESIAN_POINT ( 'NONE',  ( 16.55341960407618274, -4.379528057220086978, 51.04275706135234714 ) ) ;
#171271=CARTESIAN_POINT ( 'NONE',  ( -12.14591786802326823, 12.06949235617739902, 53.12609039468568284 ) ) ;
#171272=CARTESIAN_POINT ( 'NONE',  ( 18.62759615963271287, -10.81492255796078972, 63.33224293864770260 ) ) ;
#171273=CARTESIAN_POINT ( 'NONE',  ( 5.049401038298161559, -19.05341960407611168, 52.70724293864767418 ) ) ;
#171274=CARTESIAN_POINT ( 'NONE',  ( -8.314922557961024197, 14.29746914071037800, 82.91775706135234714 ) ) ;
#171275=CARTESIAN_POINT ( 'NONE',  ( -5.719274019375978568, 21.55341960407610458, 105.2072429386477097 ) ) ;
#171276=CARTESIAN_POINT ( 'NONE',  ( -14.29746914071049879, 8.314922557960819915, 45.83224293864769550 ) ) ;
#171277=CARTESIAN_POINT ( 'NONE',  ( 9.564922557960805705, 16.46253265017160317, 74.58224293864769550 ) ) ;
#171278=CARTESIAN_POINT ( 'NONE',  ( 12.14591786802327356, -12.06949235617739191, 80.62609039468567573 ) ) ;
#171279=CARTESIAN_POINT ( 'NONE',  ( -8.224510206698735004, -14.34966873604973081, 19.58442372801901143 ) ) ;
#171280=CARTESIAN_POINT ( 'NONE',  ( 21.55341960407610458, 5.719274019375980345, 108.9572429386476955 ) ) ;
#171281=CARTESIAN_POINT ( 'NONE',  ( -8.314922557960811034, -14.29746914071050412, 42.08224293864769550 ) ) ;
#171284=CARTESIAN_POINT ( 'NONE',  ( -16.31925111598454592, 7.325300261831593218, 70.16424538967251578 ) ) ;
#171285=CARTESIAN_POINT ( 'NONE',  ( -21.53943276465977519, 0.05219959533907696930, 91.24890960531436690 ) ) ;
#171286=CARTESIAN_POINT ( 'NONE',  ( 4.483927247898545687, 16.52544592524342804, 29.79057627198102409 ) ) ;
#171288=CARTESIAN_POINT ( 'NONE',  ( -16.21995358207306381, -7.366697692864128122, 55.06448998487843483 ) ) ;
#171289=CARTESIAN_POINT ( 'NONE',  ( 21.53943276465977519, 0.05219959533937863772, 21.25109039468567218 ) ) ;
#171290=CARTESIAN_POINT ( 'NONE',  ( -5.049401038298153566, 19.05341960407611168, 115.2072429386477097 ) ) ;
#171291=CARTESIAN_POINT ( 'NONE',  ( 0.05219959533937995610, -21.53943276465977519, 20.00109039468568639 ) ) ;
#171292=CARTESIAN_POINT ( 'NONE',  ( 12.06949235617757843, -12.14591786802309237, 53.12390960531436690 ) ) ;
#171293=CARTESIAN_POINT ( 'NONE',  ( 4.483927247898790824, -16.52544592524335698, 45.20942372801901854 ) ) ;
#171295=CARTESIAN_POINT ( 'NONE',  ( -16.51473224551069308, -9.474510206698971260, 56.66557627198103120 ) ) ;
#171296=CARTESIAN_POINT ( 'NONE',  ( -19.05341960407617563, 5.049401038297882671, 58.54275706135234003 ) ) ;
#171297=CARTESIAN_POINT ( 'NONE',  ( 19.02544592524343514, -5.153800228976328945, 78.54057627198099567 ) ) ;
#171298=CARTESIAN_POINT ( 'NONE',  ( 0.05219959533907565091, 21.53943276465977519, 39.99890960531436690 ) ) ;
#171300=CARTESIAN_POINT ( 'NONE',  ( -16.46253265017160317, 9.564922557960807481, 40.83224293864769550 ) ) ;
#171301=CARTESIAN_POINT ( 'NONE',  ( 8.314922557961029526, -14.29746914071037800, 20.41775706135234714 ) ) ;
#171302=CARTESIAN_POINT ( 'NONE',  ( 16.46253265017146816, 9.564922557961045513, 61.66775706135234003 ) ) ;
#171303=CARTESIAN_POINT ( 'NONE',  ( -18.67979575497178146, -10.72451020669898902, 106.6655762719810383 ) ) ;
#171304=CARTESIAN_POINT ( 'NONE',  ( 12.06949235617757843, -12.14591786802309237, 28.12390960531435979 ) ) ;
#171305=CARTESIAN_POINT ( 'NONE',  ( 0.05219959533909260263, 19.03943276465977164, 89.99890960531436690 ) ) ;
#171306=CARTESIAN_POINT ( 'NONE',  ( -18.67979575497178146, -10.72451020669898902, 61.66557627198103120 ) ) ;
#171307=CARTESIAN_POINT ( 'NONE',  ( 10.72451020669898902, -18.67979575497178502, 97.91557627198103830 ) ) ;
#171308=CARTESIAN_POINT ( 'NONE',  ( -14.29746914071037622, -8.314922557961029526, 24.16775706135235424 ) ) ;
#171309=CARTESIAN_POINT ( 'NONE',  ( -15.80617190586745835, -15.72974639402198527, 36.87390960531435979 ) ) ;
#171310=CARTESIAN_POINT ( 'NONE',  ( 21.52544592524334988, 5.823673210054432836, 91.45942372801901854 ) ) ;
#171311=CARTESIAN_POINT ( 'NONE',  ( 13.89961937509977652, -13.97604488694527269, 83.12390960531436690 ) ) ;
#171312=CARTESIAN_POINT ( 'NONE',  ( 16.51473224551069308, 9.474510206698969483, 34.16557627198102409 ) ) ;
#171313=CARTESIAN_POINT ( 'NONE',  ( 13.97604488694527802, 13.89961937509977652, 84.37390960531433848 ) ) ;
#171314=CARTESIAN_POINT ( 'NONE',  ( -12.06949235617756955, 12.14591786802309770, 110.6239096053143669 ) ) ;
#171315=CARTESIAN_POINT ( 'NONE',  ( 0.05219959533909260263, 19.03943276465977164, 64.99890960531436690 ) ) ;
#171316=CARTESIAN_POINT ( 'NONE',  ( -8.224510206698735004, -14.34966873604973081, 19.58442372801901143 ) ) ;
#171318=CARTESIAN_POINT ( 'NONE',  ( -21.53943276465977519, -0.05219959533937600094, 103.7510903946857042 ) ) ;
#171319=CARTESIAN_POINT ( 'NONE',  ( -10.81492255796078084, -18.62759615963271287, 22.08224293864769194 ) ) ;
#171320=CARTESIAN_POINT ( 'NONE',  ( -12.06949235617739369, -12.14591786802326823, 94.37609039468568994 ) ) ;
#171322=CARTESIAN_POINT ( 'NONE',  ( 19.03943276465977164, 0.05219959533936151252, 66.25109039468567573 ) ) ;
#171323=CARTESIAN_POINT ( 'NONE',  ( -5.153800228976607833, 19.02544592524334988, 27.70942372801899722 ) ) ;
#171325=CARTESIAN_POINT ( 'NONE',  ( -16.51473224551069308, -9.474510206698971260, 26.66557627198103120 ) ) ;
#171326=CARTESIAN_POINT ( 'NONE',  ( -16.53943276465976808, 0.05219959533911058130, 31.24890960531435979 ) ) ;
#171327=CARTESIAN_POINT ( 'NONE',  ( 0.05219959533909260263, 19.03943276465977164, 24.99890960531435269 ) ) ;
#171328=CARTESIAN_POINT ( 'NONE',  ( 8.314922557960818139, 14.29746914071049879, 24.58224293864768839 ) ) ;
#171330=CARTESIAN_POINT ( 'NONE',  ( -16.52544592524335698, -4.483927247898792601, 93.95942372801903275 ) ) ;
#171331=CARTESIAN_POINT ( 'NONE',  ( -16.46253265017160317, 9.564922557960807481, 30.83224293864769550 ) ) ;
#171332=CARTESIAN_POINT ( 'NONE',  ( 0.05219959533937995610, -21.53943276465977519, 90.00109039468567573 ) ) ;
#171333=CARTESIAN_POINT ( 'NONE',  ( -13.97604488694547697, 13.89961937509957934, 98.12609039468566152 ) ) ;
#171334=CARTESIAN_POINT ( 'NONE',  ( 5.719274019375673035, 21.55341960407619339, 82.29275706135234714 ) ) ;
#171335=CARTESIAN_POINT ( 'NONE',  ( -9.474510206698720793, -16.51473224551083518, 54.58442372801899722 ) ) ;
#171336=CARTESIAN_POINT ( 'NONE',  ( 0.05219959533909260263, 19.03943276465977164, 89.99890960531436690 ) ) ;
#171337=CARTESIAN_POINT ( 'NONE',  ( -5.153800228976328057, -19.02544592524343514, 67.29057627198102409 ) ) ;
#171339=CARTESIAN_POINT ( 'NONE',  ( 12.06949235617757843, -12.14591786802309237, 68.12390960531436690 ) ) ;
#171340=CARTESIAN_POINT ( 'NONE',  ( -5.719274019375978568, 21.55341960407610458, 60.20724293864768839 ) ) ;
#171341=CARTESIAN_POINT ( 'NONE',  ( -19.02544592524342804, 5.153800228976336051, 51.04057627198103120 ) ) ;
#171342=CARTESIAN_POINT ( 'NONE',  ( 5.719274019375991003, -21.55341960407610458, 82.70724293864770971 ) ) ;
#171343=CARTESIAN_POINT ( 'NONE',  ( -8.314922557961024197, 14.29746914071037800, 77.91775706135231871 ) ) ;
#171345=CARTESIAN_POINT ( 'NONE',  ( -16.51473224551069308, -9.474510206698971260, 46.66557627198102409 ) ) ;
#171346=CARTESIAN_POINT ( 'NONE',  ( 4.379528057220339221, -16.55341960407611168, 82.70724293864770971 ) ) ;
#171348=CARTESIAN_POINT ( 'NONE',  ( -19.02544592524342804, 5.153800228976336051, 46.04057627198101699 ) ) ;
#171349=CARTESIAN_POINT ( 'NONE',  ( -0.05219959533909027116, -19.03943276465977164, 27.49890960531435624 ) ) ;
#171350=CARTESIAN_POINT ( 'NONE',  ( 19.03943276465977164, 0.05219959533936151252, 71.25109039468566152 ) ) ;
#171351=CARTESIAN_POINT ( 'NONE',  ( 8.314922557960818139, 14.29746914071049879, 64.58224293864769550 ) ) ;
#171352=CARTESIAN_POINT ( 'NONE',  ( -21.52544592524334988, -5.823673210054445271, 38.95942372801901854 ) ) ;
#171354=CARTESIAN_POINT ( 'NONE',  ( -16.46253265017160317, 9.564922557960807481, 40.83224293864769550 ) ) ;
#171355=CARTESIAN_POINT ( 'NONE',  ( 18.67979575497178502, 10.72451020669898547, 104.1655762719810241 ) ) ;
#171357=CARTESIAN_POINT ( 'NONE',  ( 12.06949235617757843, -12.14591786802309237, 93.12390960531436690 ) ) ;
#171359=CARTESIAN_POINT ( 'NONE',  ( 5.049401038298161559, -19.05341960407611168, 52.70724293864767418 ) ) ;
#171360=CARTESIAN_POINT ( 'NONE',  ( 17.44270441346517231, 5.991230190323030946, 113.8633507926423079 ) ) ;
#171361=CARTESIAN_POINT ( 'NONE',  ( -13.89961937509957401, -13.97604488694547875, 94.37609039468566152 ) ) ;
#171362=CARTESIAN_POINT ( 'NONE',  ( 5.153800228976335163, 19.02544592524342804, 99.79057627198102409 ) ) ;
#171363=CARTESIAN_POINT ( 'NONE',  ( -5.719274019375665041, -21.55341960407619695, 39.79275706135235424 ) ) ;
#171364=CARTESIAN_POINT ( 'NONE',  ( -5.049401038298153566, 19.05341960407611168, 80.20724293864769550 ) ) ;
#171365=CARTESIAN_POINT ( 'NONE',  ( -9.474510206698720793, -16.51473224551083518, 69.58442372801901854 ) ) ;
#171366=CARTESIAN_POINT ( 'NONE',  ( 16.46253265017160672, -9.564922557960803928, 38.33224293864768839 ) ) ;
#171367=CARTESIAN_POINT ( 'NONE',  ( -14.34966873604960291, -8.224510206698953496, 66.66557627198102409 ) ) ;
#171368=CARTESIAN_POINT ( 'NONE',  ( 16.52544592524342804, -4.483927247898539470, 73.54057627198102409 ) ) ;
#171369=CARTESIAN_POINT ( 'NONE',  ( -13.89961937509977652, 13.97604488694528158, 75.62390960531438111 ) ) ;
#171370=CARTESIAN_POINT ( 'NONE',  ( 0.05219959533907565091, 21.53943276465977519, 99.99890960531436690 ) ) ;
#171371=CARTESIAN_POINT ( 'NONE',  ( -19.05341960407611168, -5.049401038298163336, 66.45724293864769550 ) ) ;
#171373=CARTESIAN_POINT ( 'NONE',  ( 15.72974639402176855, 15.80617190586768217, 111.8760903946856615 ) ) ;
#171374=CARTESIAN_POINT ( 'NONE',  ( -19.03943276465977164, 0.05219959533909376836, 36.24890960531436690 ) ) ;
#171375=CARTESIAN_POINT ( 'NONE',  ( 8.224510206698742110, 14.34966873604972548, 107.0844237280190043 ) ) ;
#171376=CARTESIAN_POINT ( 'NONE',  ( -4.379528057220328563, 16.55341960407611168, 110.2072429386477239 ) ) ;
#171377=CARTESIAN_POINT ( 'NONE',  ( 19.03943276465977164, 0.05219959533936151252, 111.2510903946856757 ) ) ;
#171379=CARTESIAN_POINT ( 'NONE',  ( 21.55341960407619695, -5.719274019375665929, 26.04275706135235779 ) ) ;
#171380=CARTESIAN_POINT ( 'NONE',  ( 9.474510206698729675, 16.51473224551082808, 72.08442372801900433 ) ) ;
#171381=CARTESIAN_POINT ( 'NONE',  ( 8.314922557961029526, -14.29746914071037800, 110.4177570613523756 ) ) ;
#171382=CARTESIAN_POINT ( 'NONE',  ( 15.72974639402199770, -15.80617190586745480, 78.12390960531436690 ) ) ;
#171383=CARTESIAN_POINT ( 'NONE',  ( 9.474510206698971260, -16.51473224551069308, 112.9155762719810383 ) ) ;
#171384=CARTESIAN_POINT ( 'NONE',  ( -16.53943276465976808, 0.05219959533911058130, 51.24890960531436690 ) ) ;
#171385=CARTESIAN_POINT ( 'NONE',  ( -9.564922557960796823, -16.46253265017161027, 32.08224293864769550 ) ) ;
#171386=CARTESIAN_POINT ( 'NONE',  ( 16.46253265017160672, -9.564922557960803928, 43.33224293864769550 ) ) ;
#171387=CARTESIAN_POINT ( 'NONE',  ( -13.97604488694547697, 13.89961937509957934, 28.12609039468565797 ) ) ;
#171388=CARTESIAN_POINT ( 'NONE',  ( -16.53943276465976808, -0.05219959533934237506, 88.75109039468567573 ) ) ;
#171389=CARTESIAN_POINT ( 'NONE',  ( -4.483927247898782831, 16.52544592524335698, 57.70942372801901143 ) ) ;
#171390=CARTESIAN_POINT ( 'NONE',  ( 19.03943276465977164, -0.05219959533909143690, 113.7489096053143669 ) ) ;
#171391=CARTESIAN_POINT ( 'NONE',  ( 9.474510206698971260, -16.51473224551069308, 47.91557627198102409 ) ) ;
#171392=CARTESIAN_POINT ( 'NONE',  ( 10.81492255796106328, -18.62759615963255655, 110.4177570613523756 ) ) ;
#171393=CARTESIAN_POINT ( 'NONE',  ( -9.564922557960796823, -16.46253265017161027, 77.08224293864769550 ) ) ;
#171394=CARTESIAN_POINT ( 'NONE',  ( 4.379528057220092307, 16.55341960407617563, 57.29275706135234714 ) ) ;
#171395=CARTESIAN_POINT ( 'NONE',  ( 0.05219959533910956823, 16.53943276465976808, 104.9989096053143669 ) ) ;
#171396=CARTESIAN_POINT ( 'NONE',  ( 8.224510206698953496, -14.34966873604960469, 22.91557627198102765 ) ) ;
#171398=CARTESIAN_POINT ( 'NONE',  ( -10.72451020669870658, -18.67979575497194134, 64.58442372801900433 ) ) ;
#171399=CARTESIAN_POINT ( 'NONE',  ( -16.46253265017160317, 9.564922557960807481, 95.83224293864769550 ) ) ;
#171400=CARTESIAN_POINT ( 'NONE',  ( -16.46253265017160317, 9.564922557960807481, 75.83224293864769550 ) ) ;
#171401=CARTESIAN_POINT ( 'NONE',  ( -16.46253265017160317, 9.564922557960807481, 105.8322429386476955 ) ) ;
#171402=CARTESIAN_POINT ( 'NONE',  ( -0.05219959533910754901, -16.53943276465976808, 52.49890960531435979 ) ) ;
#171403=CARTESIAN_POINT ( 'NONE',  ( -16.53943276465976808, -0.05219959533934237506, 113.7510903946856757 ) ) ;
#171405=CARTESIAN_POINT ( 'NONE',  ( 16.55341960407611168, 4.379528057220329451, 43.95724293864769550 ) ) ;
#171406=CARTESIAN_POINT ( 'NONE',  ( 8.224510206698742110, 14.34966873604972548, 42.08442372801901854 ) ) ;
#171408=CARTESIAN_POINT ( 'NONE',  ( -13.89961937509957401, -13.97604488694547875, 39.37609039468566152 ) ) ;
#171409=CARTESIAN_POINT ( 'NONE',  ( -19.05341960407611168, -5.049401038298163336, 81.45724293864769550 ) ) ;
#171410=CARTESIAN_POINT ( 'NONE',  ( 16.51473224551083163, -9.474510206698727899, 45.83442372801900433 ) ) ;
#171411=CARTESIAN_POINT ( 'NONE',  ( -19.02544592524334988, -5.153800228976617603, 53.95942372801898301 ) ) ;
#171412=CARTESIAN_POINT ( 'NONE',  ( 19.05341960407617918, -5.049401038297876454, 96.04275706135231871 ) ) ;
#171413=CARTESIAN_POINT ( 'NONE',  ( 8.314922557961029526, -14.29746914071037800, 80.41775706135234714 ) ) ;
#171414=CARTESIAN_POINT ( 'NONE',  ( -13.97604488694527625, -13.89961937509977652, 31.87390960531435979 ) ) ;
#171415=CARTESIAN_POINT ( 'NONE',  ( -5.153800228976328057, -19.02544592524343514, 102.2905762719810383 ) ) ;
#171416=CARTESIAN_POINT ( 'NONE',  ( 10.81492255796106328, -18.62759615963255655, 35.41775706135234003 ) ) ;
#171417=CARTESIAN_POINT ( 'NONE',  ( -16.46253265017146816, -9.564922557961047289, 84.16775706135233293 ) ) ;
#171418=CARTESIAN_POINT ( 'NONE',  ( 17.50000000000002487, 4.262806489437421575, 23.40424424251102664 ) ) ;
#171419=CARTESIAN_POINT ( 'NONE',  ( -19.03943276465977164, 0.05219959533909376836, 56.24890960531435979 ) ) ;
#171420=CARTESIAN_POINT ( 'NONE',  ( 16.51473224551069308, 9.474510206698969483, 109.1655762719810383 ) ) ;
#171421=CARTESIAN_POINT ( 'NONE',  ( 14.34966873604960469, 8.224510206698951720, 59.16557627198103120 ) ) ;
#171422=CARTESIAN_POINT ( 'NONE',  ( -9.564922557960796823, -16.46253265017161027, 47.08224293864769550 ) ) ;
#171423=CARTESIAN_POINT ( 'NONE',  ( -9.474510206698964154, 16.51473224551069663, 65.41557627198102409 ) ) ;
#171424=CARTESIAN_POINT ( 'NONE',  ( 5.153800228976615827, -19.02544592524334988, 65.20942372801900433 ) ) ;
#171425=CARTESIAN_POINT ( 'NONE',  ( 0.05219959533936267826, -19.03943276465977164, 50.00109039468566863 ) ) ;
#171426=CARTESIAN_POINT ( 'NONE',  ( 16.51473224551069308, 9.474510206698969483, 79.16557627198103830 ) ) ;
#171427=CARTESIAN_POINT ( 'NONE',  ( 15.72974639402199770, -15.80617190586745480, 78.12390960531436690 ) ) ;
#171428=CARTESIAN_POINT ( 'NONE',  ( -14.29746914071049879, 8.314922557960819915, 70.83224293864770971 ) ) ;
#171429=CARTESIAN_POINT ( 'NONE',  ( -5.049401038297874678, -19.05341960407617918, 34.79275706135233293 ) ) ;
#171430=CARTESIAN_POINT ( 'NONE',  ( -15.72974639402197994, 15.80617190586746368, 40.62390960531435269 ) ) ;
#171431=CARTESIAN_POINT ( 'NONE',  ( 15.72974639402199770, -15.80617190586745480, 43.12390960531435269 ) ) ;
#171432=CARTESIAN_POINT ( 'NONE',  ( -5.153800228976328057, -19.02544592524343514, 72.29057627198102409 ) ) ;
#171433=CARTESIAN_POINT ( 'NONE',  ( -19.02544592524342804, 5.153800228976336051, 41.04057627198103120 ) ) ;
#171434=CARTESIAN_POINT ( 'NONE',  ( 19.05341960407611168, 5.049401038298154454, 23.95724293864769194 ) ) ;
#171435=CARTESIAN_POINT ( 'NONE',  ( -18.67979575497193778, 10.72451020669871902, 23.33442372801901499 ) ) ;
#171436=CARTESIAN_POINT ( 'NONE',  ( -16.46253265017160317, 9.564922557960807481, 115.8322429386477097 ) ) ;
#171437=CARTESIAN_POINT ( 'NONE',  ( 21.55341960407619695, -5.719274019375665929, 21.04275706135234714 ) ) ;
#171438=CARTESIAN_POINT ( 'NONE',  ( -16.51473224551069308, -9.474510206698971260, 36.66557627198102409 ) ) ;
#171439=CARTESIAN_POINT ( 'NONE',  ( -5.719274019375978568, 21.55341960407610458, 100.2072429386476955 ) ) ;
#171440=CARTESIAN_POINT ( 'NONE',  ( 13.97604488694548053, -13.89961937509957401, 45.62609039468566863 ) ) ;
#171441=CARTESIAN_POINT ( 'NONE',  ( 5.153800228976335163, 19.02544592524342804, 24.79057627198102765 ) ) ;
#171442=CARTESIAN_POINT ( 'NONE',  ( 19.05341960407611168, 5.049401038298154454, 23.95724293864769194 ) ) ;
#171443=CARTESIAN_POINT ( 'NONE',  ( 16.86227489769508026, -6.785021502584605457, 21.28941672232436488 ) ) ;
#171444=CARTESIAN_POINT ( 'NONE',  ( 14.34966873604972726, -8.224510206698740333, 55.83442372801901854 ) ) ;
#171445=CARTESIAN_POINT ( 'NONE',  ( -19.05341960407611168, -5.049401038298163336, 26.45724293864769550 ) ) ;
#171447=CARTESIAN_POINT ( 'NONE',  ( -16.46253265017160317, 9.564922557960807481, 70.83224293864770971 ) ) ;
#171448=CARTESIAN_POINT ( 'NONE',  ( -12.14591786802309592, -12.06949235617757132, 106.8739096053143811 ) ) ;
#171449=CARTESIAN_POINT ( 'NONE',  ( -15.80617190586745835, -15.72974639402198527, 41.87390960531435979 ) ) ;
#171450=CARTESIAN_POINT ( 'NONE',  ( -0.05219959533910754901, -16.53943276465976808, 72.49890960531435269 ) ) ;
#171451=CARTESIAN_POINT ( 'NONE',  ( -8.224510206698735004, -14.34966873604973081, 39.58442372801901143 ) ) ;
#171452=CARTESIAN_POINT ( 'NONE',  ( 18.62759615963255655, 10.81492255796105972, 81.66775706135236135 ) ) ;
#171453=CARTESIAN_POINT ( 'NONE',  ( -0.05219959533909027116, -19.03943276465977164, 32.49890960531435979 ) ) ;
#171454=CARTESIAN_POINT ( 'NONE',  ( -14.34966873604972548, 8.224510206698743886, 108.3344237280190185 ) ) ;
#171455=CARTESIAN_POINT ( 'NONE',  ( -0.05219959533910754901, -16.53943276465976808, 52.49890960531435979 ) ) ;
#171456=CARTESIAN_POINT ( 'NONE',  ( -16.46253265017160317, 9.564922557960807481, 55.83224293864769550 ) ) ;
#171457=CARTESIAN_POINT ( 'NONE',  ( 21.55341960407619695, -5.719274019375665929, 101.0427570613523756 ) ) ;
#171458=CARTESIAN_POINT ( 'NONE',  ( 21.52544592524344225, -5.823673210054117533, 113.5405762719810383 ) ) ;
#171459=CARTESIAN_POINT ( 'NONE',  ( -15.72974639402176322, -15.80617190586768395, 74.37609039468568994 ) ) ;
#171460=CARTESIAN_POINT ( 'NONE',  ( -4.483927247898782831, 16.52544592524335698, 42.70942372801901854 ) ) ;
#171461=CARTESIAN_POINT ( 'NONE',  ( 16.55341960407611168, 4.379528057220329451, 78.95724293864769550 ) ) ;
#171462=CARTESIAN_POINT ( 'NONE',  ( 21.53943276465977519, 0.05219959533937863772, 81.25109039468568994 ) ) ;
#171463=CARTESIAN_POINT ( 'NONE',  ( -14.29746914071049879, 8.314922557960819915, 25.83224293864769194 ) ) ;
#171464=CARTESIAN_POINT ( 'NONE',  ( 17.97182807773873137, -5.500000000000077272, 61.03038844047286915 ) ) ;
#171465=CARTESIAN_POINT ( 'NONE',  ( -12.14591786802326823, 12.06949235617739902, 38.12609039468567573 ) ) ;
#171466=CARTESIAN_POINT ( 'NONE',  ( -8.224510206698948167, 14.34966873604960824, 45.41557627198103830 ) ) ;
#171467=CARTESIAN_POINT ( 'NONE',  ( -16.55341960407617563, 4.379528057220093196, 93.54275706135234714 ) ) ;
#171468=CARTESIAN_POINT ( 'NONE',  ( -16.46253265017160317, 9.564922557960807481, 95.83224293864769550 ) ) ;
#171469=CARTESIAN_POINT ( 'NONE',  ( -13.97604488694527625, -13.89961937509977652, 106.8739096053143669 ) ) ;
#171470=CARTESIAN_POINT ( 'NONE',  ( -18.67979575497193778, 10.72451020669871902, 93.33442372801901854 ) ) ;
#171471=CARTESIAN_POINT ( 'NONE',  ( -16.52544592524335698, -4.483927247898792601, 103.9594237280190185 ) ) ;
#171472=CARTESIAN_POINT ( 'NONE',  ( 14.34966873604960469, 8.224510206698951720, 79.16557627198103830 ) ) ;
#171473=CARTESIAN_POINT ( 'NONE',  ( 5.049401038298161559, -19.05341960407611168, 77.70724293864765286 ) ) ;
#171475=CARTESIAN_POINT ( 'NONE',  ( 12.14591786802327356, -12.06949235617739191, 20.62609039468568639 ) ) ;
#171476=CARTESIAN_POINT ( 'NONE',  ( 9.474510206698971260, -16.51473224551069308, 27.91557627198103120 ) ) ;
#171477=CARTESIAN_POINT ( 'NONE',  ( 5.153800228976335163, 19.02544592524342804, 94.79057627198103830 ) ) ;
#171478=CARTESIAN_POINT ( 'NONE',  ( 4.379528057220092307, 16.55341960407617563, 32.29275706135235424 ) ) ;
#171480=CARTESIAN_POINT ( 'NONE',  ( -5.049401038297874678, -19.05341960407617918, 34.79275706135233293 ) ) ;
#171481=CARTESIAN_POINT ( 'NONE',  ( 12.06949235617739724, 12.14591786802326823, 91.87609039468568994 ) ) ;
#171482=CARTESIAN_POINT ( 'NONE',  ( 16.51473224551083163, -9.474510206698727899, 110.8344237280190043 ) ) ;
#171483=CARTESIAN_POINT ( 'NONE',  ( 0.05219959533909260263, 19.03943276465977164, 34.99890960531435979 ) ) ;
#171484=CARTESIAN_POINT ( 'NONE',  ( 8.224510206698742110, 14.34966873604972548, 82.08442372801901854 ) ) ;
#171485=CARTESIAN_POINT ( 'NONE',  ( 14.34966873604972726, -8.224510206698740333, 65.83442372801900433 ) ) ;
#171486=CARTESIAN_POINT ( 'NONE',  ( -19.02544592524342804, 5.153800228976336051, 36.04057627198100988 ) ) ;
#171487=CARTESIAN_POINT ( 'NONE',  ( -0.05219959533936034679, 19.03943276465977164, 72.50109039468566152 ) ) ;
#171488=CARTESIAN_POINT ( 'NONE',  ( -19.03943276465977164, -0.05219959533935918106, 18.75109039468567218 ) ) ;
#171489=CARTESIAN_POINT ( 'NONE',  ( -13.89961937509977652, 13.97604488694528158, 45.62390960531433848 ) ) ;
#171490=CARTESIAN_POINT ( 'NONE',  ( -5.153800228976328057, -19.02544592524343514, 92.29057627198099567 ) ) ;
#171491=CARTESIAN_POINT ( 'NONE',  ( -14.34966873604960291, -8.224510206698953496, 81.66557627198103830 ) ) ;
#171493=CARTESIAN_POINT ( 'NONE',  ( -19.05341960407617563, 5.049401038297882671, 48.54275706135233293 ) ) ;
#171494=CARTESIAN_POINT ( 'NONE',  ( -10.72451020669898014, 18.67979575497178502, 55.41557627198102409 ) ) ;
#171495=CARTESIAN_POINT ( 'NONE',  ( -21.52544592524334988, -5.823673210054445271, 103.9594237280190185 ) ) ;
#171496=CARTESIAN_POINT ( 'NONE',  ( 9.564922557960805705, 16.46253265017160317, 84.58224293864769550 ) ) ;
#171497=CARTESIAN_POINT ( 'NONE',  ( -19.02544592524334988, -5.153800228976617603, 18.95942372801899722 ) ) ;
#171498=CARTESIAN_POINT ( 'NONE',  ( 10.81492255796078972, 18.62759615963270932, 69.58224293864769550 ) ) ;
#171499=CARTESIAN_POINT ( 'NONE',  ( -19.02544592524342804, 5.153800228976336051, 106.0405762719810241 ) ) ;
#171500=CARTESIAN_POINT ( 'NONE',  ( 9.474510206698729675, 16.51473224551082808, 87.08442372801900433 ) ) ;
#171501=CARTESIAN_POINT ( 'NONE',  ( -17.49999999999999289, 3.850315288878825903, 109.2662913060345460 ) ) ;
#171502=CARTESIAN_POINT ( 'NONE',  ( 16.51473224551083163, -9.474510206698727899, 105.8344237280190043 ) ) ;
#171503=CARTESIAN_POINT ( 'NONE',  ( 16.52544592524342804, -4.483927247898539470, 113.5405762719810383 ) ) ;
#171504=CARTESIAN_POINT ( 'NONE',  ( 19.03943276465977164, -0.05219959533909143690, 98.74890960531436690 ) ) ;
#171505=CARTESIAN_POINT ( 'NONE',  ( -18.67979575497178146, -10.72451020669898902, 81.66557627198103830 ) ) ;
#171506=CARTESIAN_POINT ( 'NONE',  ( -8.314922557961024197, 14.29746914071037800, 42.91775706135235424 ) ) ;
#171507=CARTESIAN_POINT ( 'NONE',  ( 15.72974639402176855, 15.80617190586768217, 46.87609039468568994 ) ) ;
#171508=CARTESIAN_POINT ( 'NONE',  ( 5.719274019375673035, 21.55341960407619339, 92.29275706135236135 ) ) ;
#171509=CARTESIAN_POINT ( 'NONE',  ( 8.314922557961029526, -14.29746914071037800, 90.41775706135236135 ) ) ;
#171510=CARTESIAN_POINT ( 'NONE',  ( -16.51473224551069308, -9.474510206698971260, 86.66557627198102409 ) ) ;
#171511=CARTESIAN_POINT ( 'NONE',  ( -4.483927247898539470, -16.52544592524342804, 92.29057627198103830 ) ) ;
#171512=CARTESIAN_POINT ( 'NONE',  ( 8.314922557960818139, 14.29746914071049879, 39.58224293864769550 ) ) ;
#171513=CARTESIAN_POINT ( 'NONE',  ( 0.05219959533936267826, -19.03943276465977164, 65.00109039468567573 ) ) ;
#171514=CARTESIAN_POINT ( 'NONE',  ( 21.53943276465977519, 0.05219959533937863772, 51.25109039468568994 ) ) ;
#171515=CARTESIAN_POINT ( 'NONE',  ( 9.564922557961047289, -16.46253265017146816, 20.41775706135233293 ) ) ;
#171516=CARTESIAN_POINT ( 'NONE',  ( 8.314922557960818139, 14.29746914071049879, 94.58224293864769550 ) ) ;
#171517=CARTESIAN_POINT ( 'NONE',  ( -21.53943276465977519, 0.05219959533907696930, 36.24890960531435979 ) ) ;
#171518=CARTESIAN_POINT ( 'NONE',  ( 4.483927247898790824, -16.52544592524335698, 110.2094237280190185 ) ) ;
#171519=CARTESIAN_POINT ( 'NONE',  ( 18.62759615963255655, 10.81492255796105972, 81.66775706135236135 ) ) ;
#171520=CARTESIAN_POINT ( 'NONE',  ( 16.53943276465976808, 0.05219959533934440121, 56.25109039468568284 ) ) ;
#171521=CARTESIAN_POINT ( 'NONE',  ( -16.52544592524335698, -4.483927247898792601, 108.9594237280190185 ) ) ;
#171522=CARTESIAN_POINT ( 'NONE',  ( -5.823673210054431948, 21.52544592524334988, 52.70942372801902565 ) ) ;
#171524=ORIENTED_EDGE ( 'NONE', *, *, #84815, .F. ) ;
#171525=CARTESIAN_POINT ( 'NONE',  ( -21.55341960407619339, 5.719274019375674811, 33.54275706135234714 ) ) ;
#171526=CARTESIAN_POINT ( 'NONE',  ( 16.52544592524342804, -4.483927247898539470, 98.54057627198105251 ) ) ;
#171527=CARTESIAN_POINT ( 'NONE',  ( -9.474510206698964154, 16.51473224551069663, 25.41557627198103120 ) ) ;
#171528=CARTESIAN_POINT ( 'NONE',  ( 4.483927247898545687, 16.52544592524342804, 64.79057627198103830 ) ) ;
#171529=CARTESIAN_POINT ( 'NONE',  ( -19.05341960407611168, -5.049401038298163336, 71.45724293864766707 ) ) ;
#171530=CARTESIAN_POINT ( 'NONE',  ( 14.34966873604972726, -8.224510206698740333, 105.8344237280190328 ) ) ;
#171531=CARTESIAN_POINT ( 'NONE',  ( 5.719274019375991003, -21.55341960407610458, 52.70724293864769550 ) ) ;
#171532=CARTESIAN_POINT ( 'NONE',  ( -12.06949235617756955, 12.14591786802309770, 90.62390960531436690 ) ) ;
#171533=CARTESIAN_POINT ( 'NONE',  ( 5.823673210054125526, 21.52544592524343514, 99.79057627198103830 ) ) ;
#171534=CARTESIAN_POINT ( 'NONE',  ( 9.564922557960805705, 16.46253265017160317, 99.58224293864770971 ) ) ;
#171535=CARTESIAN_POINT ( 'NONE',  ( -5.153800228976328057, -19.02544592524343514, 57.29057627198103120 ) ) ;
#171536=CARTESIAN_POINT ( 'NONE',  ( 5.049401038297881783, 19.05341960407617563, 102.2927570613523045 ) ) ;
#171537=CARTESIAN_POINT ( 'NONE',  ( -10.81492255796078084, -18.62759615963271287, 47.08224293864770260 ) ) ;
#171538=CARTESIAN_POINT ( 'NONE',  ( -10.72451020669870658, -18.67979575497194134, 64.58442372801900433 ) ) ;
#171539=CARTESIAN_POINT ( 'NONE',  ( 9.474510206698971260, -16.51473224551069308, 67.91557627198102409 ) ) ;
#171540=CARTESIAN_POINT ( 'NONE',  ( -16.51473224551069308, -9.474510206698971260, 81.66557627198103830 ) ) ;
#171541=CARTESIAN_POINT ( 'NONE',  ( -4.379528057220086978, -16.55341960407618274, 69.79275706135234714 ) ) ;
#171542=CARTESIAN_POINT ( 'NONE',  ( -15.80617190586768217, 15.72974639402176855, 48.12609039468568284 ) ) ;
#171543=CARTESIAN_POINT ( 'NONE',  ( 0.05219959533937995610, -21.53943276465977519, 90.00109039468567573 ) ) ;
#171544=CARTESIAN_POINT ( 'NONE',  ( 10.81492255796078972, 18.62759615963270932, 99.58224293864770971 ) ) ;
#171545=CARTESIAN_POINT ( 'NONE',  ( 15.72974639402176855, 15.80617190586768217, 36.87609039468568994 ) ) ;
#171546=CARTESIAN_POINT ( 'NONE',  ( -12.14591786802326823, 12.06949235617739902, 78.12609039468570415 ) ) ;
#171547=CARTESIAN_POINT ( 'NONE',  ( 21.55341960407610458, 5.719274019375980345, 73.95724293864769550 ) ) ;
#171548=CARTESIAN_POINT ( 'NONE',  ( -5.153800228976607833, 19.02544592524334988, 27.70942372801899722 ) ) ;
#171549=CARTESIAN_POINT ( 'NONE',  ( -5.153800228976328057, -19.02544592524343514, 72.29057627198102409 ) ) ;
#171550=CARTESIAN_POINT ( 'NONE',  ( -12.06949235617756955, 12.14591786802309770, 25.62390960531435624 ) ) ;
#171552=CARTESIAN_POINT ( 'NONE',  ( 9.564922557960805705, 16.46253265017160317, 104.5822429386476955 ) ) ;
#171553=CARTESIAN_POINT ( 'NONE',  ( -16.51473224551082808, 9.474510206698731452, 88.33442372801900433 ) ) ;
#171554=CARTESIAN_POINT ( 'NONE',  ( -10.81492255796078084, -18.62759615963271287, 57.08224293864769550 ) ) ;
#171555=CARTESIAN_POINT ( 'NONE',  ( 8.224510206698953496, -14.34966873604960469, 42.91557627198103120 ) ) ;
#171556=CARTESIAN_POINT ( 'NONE',  ( 19.02544592524334988, 5.153800228976608722, 111.4594237280190043 ) ) ;
#171557=CARTESIAN_POINT ( 'NONE',  ( 5.049401038298161559, -19.05341960407611168, 37.70724293864768839 ) ) ;
#171558=CARTESIAN_POINT ( 'NONE',  ( -19.03943276465977164, -0.05219959533935918106, 103.7510903946856757 ) ) ;
#171559=CARTESIAN_POINT ( 'NONE',  ( 0.05219959533907565091, 21.53943276465977519, 99.99890960531436690 ) ) ;
#171560=CARTESIAN_POINT ( 'NONE',  ( -16.46253265017146816, -9.564922557961047289, 74.16775706135234714 ) ) ;
#171561=CARTESIAN_POINT ( 'NONE',  ( -8.224510206698735004, -14.34966873604973081, 79.58442372801903275 ) ) ;
#171562=CARTESIAN_POINT ( 'NONE',  ( -13.97604488694527625, -13.89961937509977652, 61.87390960531435979 ) ) ;
#171563=CARTESIAN_POINT ( 'NONE',  ( -16.53943276465976808, 0.05219959533911058130, 76.24890960531435269 ) ) ;
#171565=CARTESIAN_POINT ( 'NONE',  ( -13.89961937509977652, 13.97604488694528158, 55.62390960531434558 ) ) ;
#171566=CARTESIAN_POINT ( 'NONE',  ( -0.05219959533910754901, -16.53943276465976808, 62.49890960531436690 ) ) ;
#171567=FACE_BOUND ( 'NONE', #53787, .T. ) ;
#171569=CARTESIAN_POINT ( 'NONE',  ( -16.53943276465976808, 0.05219959533911058130, 46.24890960531435979 ) ) ;
#171570=CARTESIAN_POINT ( 'NONE',  ( 16.46253265017160672, -9.564922557960803928, 78.33224293864769550 ) ) ;
#171572=CARTESIAN_POINT ( 'NONE',  ( 19.02544592524334988, 5.153800228976608722, 41.45942372801900433 ) ) ;
#171573=CARTESIAN_POINT ( 'NONE',  ( 12.06949235617739724, 12.14591786802326823, 41.87609039468568284 ) ) ;
#171574=CARTESIAN_POINT ( 'NONE',  ( -18.67979575497178146, -10.72451020669898902, 61.66557627198103120 ) ) ;
#171575=CARTESIAN_POINT ( 'NONE',  ( -0.05219959533936034679, 19.03943276465977164, 27.50109039468566507 ) ) ;
#171576=CARTESIAN_POINT ( 'NONE',  ( 5.153800228976335163, 19.02544592524342804, 79.79057627198102409 ) ) ;
#171578=CARTESIAN_POINT ( 'NONE',  ( -0.05219959533909027116, -19.03943276465977164, 112.4989096053143669 ) ) ;
#171579=CARTESIAN_POINT ( 'NONE',  ( -19.02544592524342804, 5.153800228976336051, 56.04057627198100988 ) ) ;
#171580=CARTESIAN_POINT ( 'NONE',  ( 21.52544592524334988, 5.823673210054432836, 41.45942372801901143 ) ) ;
#171581=CARTESIAN_POINT ( 'NONE',  ( 4.379528057220339221, -16.55341960407611168, 102.7072429386476955 ) ) ;
#171582=CARTESIAN_POINT ( 'NONE',  ( -5.823673210054116645, -21.52544592524344225, 107.2905762719810525 ) ) ;
#171583=CARTESIAN_POINT ( 'NONE',  ( -0.05219959533909027116, -19.03943276465977164, 82.49890960531436690 ) ) ;
#171584=ORIENTED_EDGE ( 'NONE', *, *, #60477, .T. ) ;
#171585=CARTESIAN_POINT ( 'NONE',  ( 5.823673210054444382, -21.52544592524334988, 30.20942372801902565 ) ) ;
#171587=CARTESIAN_POINT ( 'NONE',  ( -9.474510206698964154, 16.51473224551069663, 85.41557627198102409 ) ) ;
#171589=CARTESIAN_POINT ( 'NONE',  ( 21.55341960407610458, 5.719274019375980345, 93.95724293864770971 ) ) ;
#171590=CARTESIAN_POINT ( 'NONE',  ( 9.564922557960805705, 16.46253265017160317, 39.58224293864768839 ) ) ;
#171591=CARTESIAN_POINT ( 'NONE',  ( 13.97604488694548053, -13.89961937509957401, 100.6260903946856615 ) ) ;
#171593=CARTESIAN_POINT ( 'NONE',  ( -9.474510206698964154, 16.51473224551069663, 35.41557627198102409 ) ) ;
#171594=CARTESIAN_POINT ( 'NONE',  ( -15.72974639402176322, -15.80617190586768395, 79.37609039468567573 ) ) ;
#171595=CARTESIAN_POINT ( 'NONE',  ( -16.51473224551069308, -9.474510206698971260, 71.66557627198102409 ) ) ;
#171596=CARTESIAN_POINT ( 'NONE',  ( 15.80617190586769283, -15.72974639402175789, 50.62609039468568994 ) ) ;
#171597=CARTESIAN_POINT ( 'NONE',  ( 10.72451020669871369, 18.67979575497193778, 22.08442372801901143 ) ) ;
#171599=CARTESIAN_POINT ( 'NONE',  ( 9.564922557960805705, 16.46253265017160317, 89.58224293864769550 ) ) ;
#171601=CARTESIAN_POINT ( 'NONE',  ( -8.224510206698735004, -14.34966873604973081, 34.58442372801900433 ) ) ;
#171602=CARTESIAN_POINT ( 'NONE',  ( 21.53943276465977519, -0.05219959533907433946, 43.74890960531435979 ) ) ;
#171603=CARTESIAN_POINT ( 'NONE',  ( -0.05219959533937732626, 21.53943276465977519, 42.50109039468567573 ) ) ;
#171604=CARTESIAN_POINT ( 'NONE',  ( 10.81492255796106328, -18.62759615963255655, 70.41775706135236135 ) ) ;
#171605=CARTESIAN_POINT ( 'NONE',  ( 17.50000000000000000, -5.499999999999992895, 38.29690382534171533 ) ) ;
#171606=CARTESIAN_POINT ( 'NONE',  ( 16.46253265017146816, 9.564922557961045513, 106.6677570613523471 ) ) ;
#171607=CARTESIAN_POINT ( 'NONE',  ( -19.03943276465977164, 0.05219959533909376836, 56.24890960531435979 ) ) ;
#171608=CARTESIAN_POINT ( 'NONE',  ( 19.05341960407611168, 5.049401038298154454, 78.95724293864769550 ) ) ;
#171609=CARTESIAN_POINT ( 'NONE',  ( -16.53943276465976808, 0.05219959533911058130, 111.2489096053143669 ) ) ;
#171610=CARTESIAN_POINT ( 'NONE',  ( 14.34966873604960469, 8.224510206698951720, 99.16557627198100988 ) ) ;
#171611=CARTESIAN_POINT ( 'NONE',  ( -19.02544592524342804, 5.153800228976336051, 111.0405762719810099 ) ) ;
#171612=CARTESIAN_POINT ( 'NONE',  ( 4.483927247898790824, -16.52544592524335698, 85.20942372801901854 ) ) ;
#171613=CARTESIAN_POINT ( 'NONE',  ( 16.55341960407611168, 4.379528057220329451, 68.95724293864769550 ) ) ;
#171614=CARTESIAN_POINT ( 'NONE',  ( 0.05219959533909260263, 19.03943276465977164, 49.99890960531435979 ) ) ;
#171615=CARTESIAN_POINT ( 'NONE',  ( 21.52544592524334988, 5.823673210054432836, 76.45942372801901854 ) ) ;
#171616=CARTESIAN_POINT ( 'NONE',  ( 15.80617190586769283, -15.72974639402175789, 75.62609039468567573 ) ) ;
#171617=CARTESIAN_POINT ( 'NONE',  ( -13.97604488694547697, 13.89961937509957934, 113.1260903946856757 ) ) ;
#171618=CARTESIAN_POINT ( 'NONE',  ( -8.314922557960811034, -14.29746914071050412, 62.08224293864769550 ) ) ;
#171619=CARTESIAN_POINT ( 'NONE',  ( 21.52544592524344225, -5.823673210054117533, 108.5405762719810241 ) ) ;
#171620=CARTESIAN_POINT ( 'NONE',  ( -5.719274019375978568, 21.55341960407610458, 60.20724293864768839 ) ) ;
#171621=CARTESIAN_POINT ( 'NONE',  ( -17.05587630539787369, -6.762274262135686165, 104.2581969096269319 ) ) ;
#171623=CARTESIAN_POINT ( 'NONE',  ( 9.564922557960805705, 16.46253265017160317, 69.58224293864770971 ) ) ;
#171624=CARTESIAN_POINT ( 'NONE',  ( -14.29746914071049879, 8.314922557960819915, 35.83224293864768839 ) ) ;
#171625=CARTESIAN_POINT ( 'NONE',  ( -16.53943276465976808, 0.05219959533911058130, 26.24890960531435624 ) ) ;
#171626=CARTESIAN_POINT ( 'NONE',  ( 4.379528057220092307, 16.55341960407617563, 92.29275706135236135 ) ) ;
#171627=CARTESIAN_POINT ( 'NONE',  ( 5.153800228976615827, -19.02544592524334988, 50.20942372801897591 ) ) ;
#171628=CARTESIAN_POINT ( 'NONE',  ( 16.61371651742604882, 7.165104196376036683, 48.64584930007006136 ) ) ;
#171629=CARTESIAN_POINT ( 'NONE',  ( -19.03943276465977164, 0.05219959533909376836, 106.2489096053143669 ) ) ;
#171630=CARTESIAN_POINT ( 'NONE',  ( -4.379528057220328563, 16.55341960407611168, 65.20724293864768129 ) ) ;
#171631=CARTESIAN_POINT ( 'NONE',  ( 17.44279575226826395, -5.990770900252401887, 103.3355756751432040 ) ) ;
#171632=CARTESIAN_POINT ( 'NONE',  ( 5.049401038298161559, -19.05341960407611168, 112.7072429386476813 ) ) ;
#171633=CARTESIAN_POINT ( 'NONE',  ( 21.55341960407610458, 5.719274019375980345, 48.95724293864770971 ) ) ;
#171634=CARTESIAN_POINT ( 'NONE',  ( -12.06949235617756955, 12.14591786802309770, 95.62390960531436690 ) ) ;
#171635=CARTESIAN_POINT ( 'NONE',  ( -0.05219959533934338120, 16.53943276465976808, 57.50109039468568994 ) ) ;
#171636=CARTESIAN_POINT ( 'NONE',  ( 16.55341960407611168, 4.379528057220329451, 88.95724293864769550 ) ) ;
#171638=CARTESIAN_POINT ( 'NONE',  ( 19.05341960407617918, -5.049401038297876454, 71.04275706135234714 ) ) ;
#171639=CARTESIAN_POINT ( 'NONE',  ( -19.03943276465977164, 0.05219959533909376836, 116.2489096053143669 ) ) ;
#171642=CARTESIAN_POINT ( 'NONE',  ( -8.224510206698735004, -14.34966873604973081, 49.58442372801901143 ) ) ;
#171643=CARTESIAN_POINT ( 'NONE',  ( -4.379528057220328563, 16.55341960407611168, 35.20724293864768839 ) ) ;
#171644=CARTESIAN_POINT ( 'NONE',  ( -15.72974639402197994, 15.80617190586746368, 60.62390960531437401 ) ) ;
#171645=CARTESIAN_POINT ( 'NONE',  ( -13.89961937509957401, -13.97604488694547875, 89.37609039468563310 ) ) ;
#171646=CARTESIAN_POINT ( 'NONE',  ( 15.72974639402199770, -15.80617190586745480, 48.12390960531436690 ) ) ;
#171647=CARTESIAN_POINT ( 'NONE',  ( -10.72451020669870658, -18.67979575497194134, 79.58442372801903275 ) ) ;
#171649=CARTESIAN_POINT ( 'NONE',  ( -8.224510206698735004, -14.34966873604973081, 39.58442372801901143 ) ) ;
#171650=CARTESIAN_POINT ( 'NONE',  ( 0.05219959533909260263, 19.03943276465977164, 34.99890960531435979 ) ) ;
#171651=CARTESIAN_POINT ( 'NONE',  ( -19.03943276465977164, 0.05219959533909376836, 101.2489096053143669 ) ) ;
#171652=EDGE_CURVE ( 'NONE', #170830, #129803, #60662, .T. ) ;
#171653=CARTESIAN_POINT ( 'NONE',  ( -9.564922557960796823, -16.46253265017161027, 37.08224293864768839 ) ) ;
#171654=CARTESIAN_POINT ( 'NONE',  ( -16.53943276465976808, 0.05219959533911058130, 96.24890960531435269 ) ) ;
#171656=CARTESIAN_POINT ( 'NONE',  ( -16.46253265017160317, 9.564922557960807481, 100.8322429386477097 ) ) ;
#171658=CARTESIAN_POINT ( 'NONE',  ( 4.483927247898790824, -16.52544592524335698, 50.20942372801901854 ) ) ;
#171659=CARTESIAN_POINT ( 'NONE',  ( 10.72451020669898902, -18.67979575497178502, 87.91557627198103830 ) ) ;
#171660=CARTESIAN_POINT ( 'NONE',  ( 16.46253265017160672, -9.564922557960803928, 43.33224293864769550 ) ) ;
#171661=CARTESIAN_POINT ( 'NONE',  ( -0.05219959533937732626, 21.53943276465977519, 32.50109039468568284 ) ) ;
#171662=CARTESIAN_POINT ( 'NONE',  ( -19.05341960407611168, -5.049401038298163336, 81.45724293864769550 ) ) ;
#171665=CARTESIAN_POINT ( 'NONE',  ( -4.483927247898782831, 16.52544592524335698, 52.70942372801902565 ) ) ;
#171666=CARTESIAN_POINT ( 'NONE',  ( 18.67979575497178502, 10.72451020669898547, 114.1655762719810383 ) ) ;
#171667=CARTESIAN_POINT ( 'NONE',  ( 19.02544592524343514, -5.153800228976328945, 28.54057627198102409 ) ) ;
#171668=CARTESIAN_POINT ( 'NONE',  ( -5.049401038298153566, 19.05341960407611168, 100.2072429386476955 ) ) ;
#171669=CARTESIAN_POINT ( 'NONE',  ( 16.46253265017146816, 9.564922557961045513, 81.66775706135233293 ) ) ;
#171670=CARTESIAN_POINT ( 'NONE',  ( 5.153800228976615827, -19.02544592524334988, 25.20942372801900433 ) ) ;
#171671=CARTESIAN_POINT ( 'NONE',  ( 21.52544592524344225, -5.823673210054117533, 83.54057627198102409 ) ) ;
#171672=CARTESIAN_POINT ( 'NONE',  ( 19.03943276465977164, 0.05219959533936151252, 31.25109039468566863 ) ) ;
#171673=CARTESIAN_POINT ( 'NONE',  ( 8.224510206698742110, 14.34966873604972548, 82.08442372801901854 ) ) ;
#171674=CARTESIAN_POINT ( 'NONE',  ( 19.05341960407611168, 5.049401038298154454, 108.9572429386477097 ) ) ;
#171675=CARTESIAN_POINT ( 'NONE',  ( -9.564922557960796823, -16.46253265017161027, 57.08224293864769550 ) ) ;
#171676=CARTESIAN_POINT ( 'NONE',  ( -10.72451020669870658, -18.67979575497194134, 64.58442372801900433 ) ) ;
#171677=CARTESIAN_POINT ( 'NONE',  ( 10.81492255796106328, -18.62759615963255655, 70.41775706135236135 ) ) ;
#171678=CARTESIAN_POINT ( 'NONE',  ( 19.03943276465977164, -0.05219959533909143690, 78.74890960531436690 ) ) ;
#171679=CARTESIAN_POINT ( 'NONE',  ( -10.72451020669870658, -18.67979575497194134, 44.58442372801901854 ) ) ;
#171680=CARTESIAN_POINT ( 'NONE',  ( 5.153800228976615827, -19.02544592524334988, 85.20942372801900433 ) ) ;
#171682=CARTESIAN_POINT ( 'NONE',  ( 9.474510206698971260, -16.51473224551069308, 52.91557627198102409 ) ) ;
#171683=CARTESIAN_POINT ( 'NONE',  ( -19.03943276465977164, 0.05219959533909376836, 96.24890960531436690 ) ) ;
#171684=CARTESIAN_POINT ( 'NONE',  ( -0.05219959533909027116, -19.03943276465977164, 67.49890960531436690 ) ) ;
#171685=CARTESIAN_POINT ( 'NONE',  ( -5.049401038298153566, 19.05341960407611168, 110.2072429386476671 ) ) ;
#171686=CARTESIAN_POINT ( 'NONE',  ( 13.89961937509977652, -13.97604488694527269, 53.12390960531434558 ) ) ;
#171687=CARTESIAN_POINT ( 'NONE',  ( 0.05219959533907565091, 21.53943276465977519, 104.9989096053143669 ) ) ;
#171688=CARTESIAN_POINT ( 'NONE',  ( 14.29746914071037800, 8.314922557961029526, 71.66775706135234714 ) ) ;
#171690=CARTESIAN_POINT ( 'NONE',  ( 5.049401038297881783, 19.05341960407617563, 27.29275706135232937 ) ) ;
#171691=CARTESIAN_POINT ( 'NONE',  ( -9.564922557960796823, -16.46253265017161027, 67.08224293864769550 ) ) ;
#171692=CARTESIAN_POINT ( 'NONE',  ( 14.34966873604960469, 8.224510206698951720, 59.16557627198103120 ) ) ;
#171693=CARTESIAN_POINT ( 'NONE',  ( 16.53943276465976808, -0.05219959533910856209, 98.74890960531438111 ) ) ;
#171694=CARTESIAN_POINT ( 'NONE',  ( 19.02544592524343514, -5.153800228976328945, 103.5405762719809957 ) ) ;
#171695=CARTESIAN_POINT ( 'NONE',  ( 19.03943276465977164, -0.05219959533909143690, 93.74890960531435269 ) ) ;
#171696=CARTESIAN_POINT ( 'NONE',  ( -10.72451020669870658, -18.67979575497194134, 54.58442372801901143 ) ) ;
#171697=CARTESIAN_POINT ( 'NONE',  ( -9.564922557960796823, -16.46253265017161027, 107.0822429386476955 ) ) ;
#171698=CARTESIAN_POINT ( 'NONE',  ( -21.53943276465977519, -0.05219959533937600094, 108.7510903946857042 ) ) ;
#171699=CARTESIAN_POINT ( 'NONE',  ( -8.224510206698735004, -14.34966873604973081, 84.58442372801903275 ) ) ;
#171700=CARTESIAN_POINT ( 'NONE',  ( -10.72451020669870658, -18.67979575497194134, 39.58442372801901143 ) ) ;
#171701=CARTESIAN_POINT ( 'NONE',  ( -21.52544592524343514, 5.823673210054127303, 26.04057627198103475 ) ) ;
#171702=CARTESIAN_POINT ( 'NONE',  ( -18.62759615963270932, 10.81492255796079327, 100.8322429386477097 ) ) ;
#171703=CARTESIAN_POINT ( 'NONE',  ( -8.314922557960811034, -14.29746914071050412, 67.08224293864770971 ) ) ;
#171704=CARTESIAN_POINT ( 'NONE',  ( 19.05341960407611168, 5.049401038298154454, 53.95724293864770260 ) ) ;
#171705=CARTESIAN_POINT ( 'NONE',  ( -12.06949235617756955, 12.14591786802309770, 80.62390960531438111 ) ) ;
#171706=CARTESIAN_POINT ( 'NONE',  ( 21.53943276465977519, -0.05219959533907433946, 38.74890960531435979 ) ) ;
#171707=CARTESIAN_POINT ( 'NONE',  ( 9.474510206698729675, 16.51473224551082808, 47.08442372801900433 ) ) ;
#171708=CARTESIAN_POINT ( 'NONE',  ( -14.29746914071049879, 8.314922557960819915, 115.8322429386477097 ) ) ;
#171709=ORIENTED_EDGE ( 'NONE', *, *, #153149, .T. ) ;
#171710=CARTESIAN_POINT ( 'NONE',  ( 0.05219959533934541429, -16.53943276465976808, 70.00109039468568994 ) ) ;
#171711=CARTESIAN_POINT ( 'NONE',  ( -16.51473224551069308, -9.474510206698971260, 66.66557627198102409 ) ) ;
#171713=CARTESIAN_POINT ( 'NONE',  ( 4.483927247898545687, 16.52544592524342804, 84.79057627198102409 ) ) ;
#171714=CARTESIAN_POINT ( 'NONE',  ( 15.72974639402199770, -15.80617190586745480, 33.12390960531435979 ) ) ;
#171716=CARTESIAN_POINT ( 'NONE',  ( -12.14591786802326823, 12.06949235617739902, 108.1260903946856757 ) ) ;
#171717=CARTESIAN_POINT ( 'NONE',  ( -14.34966873604972548, 8.224510206698743886, 23.33442372801901499 ) ) ;
#171718=CARTESIAN_POINT ( 'NONE',  ( 18.67979575497194134, -10.72451020669871369, 95.83442372801903275 ) ) ;
#171719=CARTESIAN_POINT ( 'NONE',  ( 19.03943276465977164, -0.05219959533909143690, 83.74890960531436690 ) ) ;
#171720=CARTESIAN_POINT ( 'NONE',  ( -18.62759615963270932, 10.81492255796079327, 105.8322429386476955 ) ) ;
#171721=CARTESIAN_POINT ( 'NONE',  ( 12.14591786802327356, -12.06949235617739191, 50.62609039468568994 ) ) ;
#171722=CARTESIAN_POINT ( 'NONE',  ( -9.474510206698964154, 16.51473224551069663, 35.41557627198102409 ) ) ;
#171724=CARTESIAN_POINT ( 'NONE',  ( -16.55341960407617563, 4.379528057220093196, 28.54275706135234358 ) ) ;
#171725=CARTESIAN_POINT ( 'NONE',  ( 13.97604488694548053, -13.89961937509957401, 100.6260903946856615 ) ) ;
#171726=CARTESIAN_POINT ( 'NONE',  ( -5.823673210054116645, -21.52544592524344225, 92.29057627198103830 ) ) ;
#171727=CARTESIAN_POINT ( 'NONE',  ( -19.02544592524334988, -5.153800228976617603, 73.95942372801900433 ) ) ;
#171728=CARTESIAN_POINT ( 'NONE',  ( 18.56197773271728124, -5.500000000000076383, 86.05066217314454491 ) ) ;
#171729=CARTESIAN_POINT ( 'NONE',  ( 21.52544592524344225, -5.823673210054117533, 108.5405762719810241 ) ) ;
#171731=CARTESIAN_POINT ( 'NONE',  ( -13.89961937509977652, 13.97604488694528158, 80.62390960531436690 ) ) ;
#171732=CARTESIAN_POINT ( 'NONE',  ( 4.379528057220092307, 16.55341960407617563, 32.29275706135235424 ) ) ;
#171734=CARTESIAN_POINT ( 'NONE',  ( -13.97604488694547697, 13.89961937509957934, 58.12609039468566863 ) ) ;
#171735=CARTESIAN_POINT ( 'NONE',  ( 0.05219959533937995610, -21.53943276465977519, 25.00109039468567218 ) ) ;
#171736=CARTESIAN_POINT ( 'NONE',  ( -0.05219959533910754901, -16.53943276465976808, 72.49890960531435269 ) ) ;
#171737=CARTESIAN_POINT ( 'NONE',  ( 16.51473224551069308, 9.474510206698969483, 89.16557627198103830 ) ) ;
#171738=CARTESIAN_POINT ( 'NONE',  ( -8.314922557961024197, 14.29746914071037800, 32.91775706135234714 ) ) ;
#171739=CARTESIAN_POINT ( 'NONE',  ( 5.049401038297881783, 19.05341960407617563, 42.29275706135234003 ) ) ;
#171740=CARTESIAN_POINT ( 'NONE',  ( -0.05219959533937732626, 21.53943276465977519, 52.50109039468567573 ) ) ;
#171741=CARTESIAN_POINT ( 'NONE',  ( -16.51473224551082808, 9.474510206698731452, 108.3344237280190043 ) ) ;
#171742=CARTESIAN_POINT ( 'NONE',  ( 19.05341960407611168, 5.049401038298154454, 53.95724293864770260 ) ) ;
#171743=CARTESIAN_POINT ( 'NONE',  ( -0.05219959533936034679, 19.03943276465977164, 77.50109039468566152 ) ) ;
#171744=CARTESIAN_POINT ( 'NONE',  ( 4.379528057220092307, 16.55341960407617563, 52.29275706135236135 ) ) ;
#171745=CARTESIAN_POINT ( 'NONE',  ( -15.80617190586768217, 15.72974639402176855, 103.1260903946856757 ) ) ;
#171746=CARTESIAN_POINT ( 'NONE',  ( 19.05341960407617918, -5.049401038297876454, 66.04275706135233293 ) ) ;
#171747=CARTESIAN_POINT ( 'NONE',  ( -5.153800228976328057, -19.02544592524343514, 32.29057627198102409 ) ) ;
#171748=CARTESIAN_POINT ( 'NONE',  ( -18.67979575497178146, -10.72451020669898902, 76.66557627198103830 ) ) ;
#171749=CARTESIAN_POINT ( 'NONE',  ( -8.314922557960811034, -14.29746914071050412, 67.08224293864770971 ) ) ;
#171750=CARTESIAN_POINT ( 'NONE',  ( -19.03943276465977164, -0.05219959533935918106, 68.75109039468566152 ) ) ;
#171752=CARTESIAN_POINT ( 'NONE',  ( 9.474510206698729675, 16.51473224551082808, 47.08442372801900433 ) ) ;
#171753=CARTESIAN_POINT ( 'NONE',  ( -4.379528057220086978, -16.55341960407618274, 104.7927570613523898 ) ) ;
#171754=CARTESIAN_POINT ( 'NONE',  ( 12.14591786802309770, 12.06949235617756955, 49.37390960531436690 ) ) ;
#171755=CARTESIAN_POINT ( 'NONE',  ( -10.81492255796105439, 18.62759615963255655, 92.91775706135236135 ) ) ;
#171757=CARTESIAN_POINT ( 'NONE',  ( -18.67979575497178146, -10.72451020669898902, 96.66557627198102409 ) ) ;
#171758=CARTESIAN_POINT ( 'NONE',  ( -19.02544592524342804, 5.153800228976336051, 56.04057627198100988 ) ) ;
#171759=CARTESIAN_POINT ( 'NONE',  ( 5.823673210054444382, -21.52544592524334988, 75.20942372801901854 ) ) ;
#171760=CARTESIAN_POINT ( 'NONE',  ( -19.02544592524342804, 5.153800228976336051, 51.04057627198103120 ) ) ;
#171761=CARTESIAN_POINT ( 'NONE',  ( 9.564922557960805705, 16.46253265017160317, 59.58224293864769550 ) ) ;
#171762=CARTESIAN_POINT ( 'NONE',  ( 4.483927247898545687, 16.52544592524342804, 99.79057627198103830 ) ) ;
#171763=CARTESIAN_POINT ( 'NONE',  ( 13.97604488694527802, 13.89961937509977652, 114.3739096053143669 ) ) ;
#171764=CARTESIAN_POINT ( 'NONE',  ( 8.314922557960818139, 14.29746914071049879, 54.58224293864769550 ) ) ;
#171765=CARTESIAN_POINT ( 'NONE',  ( -19.03943276465977164, 0.05219959533909376836, 31.24890960531435979 ) ) ;
#171766=CARTESIAN_POINT ( 'NONE',  ( -4.483927247898539470, -16.52544592524342804, 87.29057627198103830 ) ) ;
#171767=CARTESIAN_POINT ( 'NONE',  ( -18.62759615963270932, 10.81492255796079327, 95.83224293864770971 ) ) ;
#171768=CARTESIAN_POINT ( 'NONE',  ( 0.05219959533937995610, -21.53943276465977519, 30.00109039468568284 ) ) ;
#171769=CARTESIAN_POINT ( 'NONE',  ( 19.03943276465977164, -0.05219959533909143690, 23.74890960531435269 ) ) ;
#171770=CARTESIAN_POINT ( 'NONE',  ( -4.379528057220086978, -16.55341960407618274, 44.79275706135234714 ) ) ;
#171771=CARTESIAN_POINT ( 'NONE',  ( 21.55341960407610458, 5.719274019375980345, 88.95724293864769550 ) ) ;
#171772=CARTESIAN_POINT ( 'NONE',  ( 18.62759615963255655, 10.81492255796105972, 111.6677570613523613 ) ) ;
#171773=CARTESIAN_POINT ( 'NONE',  ( 19.03943276465977164, -0.05219959533909143690, 108.7489096053143527 ) ) ;
#171774=CARTESIAN_POINT ( 'NONE',  ( -21.52544592524334988, -5.823673210054445271, 43.95942372801902565 ) ) ;
#171775=CARTESIAN_POINT ( 'NONE',  ( 10.72451020669898902, -18.67979575497178502, 37.91557627198102409 ) ) ;
#171776=CARTESIAN_POINT ( 'NONE',  ( -0.05219959533934338120, 16.53943276465976808, 97.50109039468567573 ) ) ;
#171778=CARTESIAN_POINT ( 'NONE',  ( -18.67979575497193778, 10.72451020669871902, 58.33442372801901143 ) ) ;
#171779=CARTESIAN_POINT ( 'NONE',  ( -10.72451020669870658, -18.67979575497194134, 89.58442372801901854 ) ) ;
#171780=CARTESIAN_POINT ( 'NONE',  ( 9.564922557961047289, -16.46253265017146816, 30.41775706135232937 ) ) ;
#171781=CARTESIAN_POINT ( 'NONE',  ( 12.06949235617739724, 12.14591786802326823, 91.87609039468568994 ) ) ;
#171782=CARTESIAN_POINT ( 'NONE',  ( 5.719274019375673035, 21.55341960407619339, 47.29275706135234003 ) ) ;
#171783=CARTESIAN_POINT ( 'NONE',  ( -13.89961937509977652, 13.97604488694528158, 45.62390960531433848 ) ) ;
#171784=CARTESIAN_POINT ( 'NONE',  ( 13.89961937509957401, 13.97604488694547697, 26.87609039468566507 ) ) ;
#171785=CARTESIAN_POINT ( 'NONE',  ( 18.62759615963271287, -10.81492255796078972, 28.33224293864769550 ) ) ;
#171786=CARTESIAN_POINT ( 'NONE',  ( -21.52544592524334988, -5.823673210054445271, 18.95942372801901143 ) ) ;
#171787=CARTESIAN_POINT ( 'NONE',  ( 15.80617190586746368, 15.72974639402197994, 69.37390960531436690 ) ) ;
#171789=CARTESIAN_POINT ( 'NONE',  ( 18.62759615963271287, -10.81492255796078972, 78.33224293864770971 ) ) ;
#171790=CARTESIAN_POINT ( 'NONE',  ( -8.224510206698735004, -14.34966873604973081, 59.58442372801901854 ) ) ;
#171791=CARTESIAN_POINT ( 'NONE',  ( 0.05219959533910956823, 16.53943276465976808, 59.99890960531436690 ) ) ;
#171793=CARTESIAN_POINT ( 'NONE',  ( 19.02544592524334988, 5.153800228976608722, 91.45942372801900433 ) ) ;
#171795=CARTESIAN_POINT ( 'NONE',  ( -0.05219959533934338120, 16.53943276465976808, 42.50109039468567573 ) ) ;
#171796=CARTESIAN_POINT ( 'NONE',  ( 10.81492255796078972, 18.62759615963270932, 99.58224293864770971 ) ) ;
#171797=CARTESIAN_POINT ( 'NONE',  ( 18.62759615963271287, -10.81492255796078972, 78.33224293864770971 ) ) ;
#171798=CARTESIAN_POINT ( 'NONE',  ( -19.03943276465977164, 0.05219959533909376836, 111.2489096053143669 ) ) ;
#171799=CARTESIAN_POINT ( 'NONE',  ( 14.29746914071037800, 8.314922557961029526, 61.66775706135235424 ) ) ;
#171800=CARTESIAN_POINT ( 'NONE',  ( 16.51473224551069308, 9.474510206698969483, 69.16557627198102409 ) ) ;
#171801=CARTESIAN_POINT ( 'NONE',  ( 21.53943276465977519, 0.05219959533937863772, 41.25109039468568284 ) ) ;
#171802=CARTESIAN_POINT ( 'NONE',  ( -5.153800228976607833, 19.02544592524334988, 112.7094237280190043 ) ) ;
#171803=CARTESIAN_POINT ( 'NONE',  ( 0.05219959533909260263, 19.03943276465977164, 104.9989096053143669 ) ) ;
#171804=CARTESIAN_POINT ( 'NONE',  ( 9.564922557961047289, -16.46253265017146816, 30.41775706135232937 ) ) ;
#171805=CARTESIAN_POINT ( 'NONE',  ( -16.55341960407617563, 4.379528057220093196, 38.54275706135234714 ) ) ;
#171806=CARTESIAN_POINT ( 'NONE',  ( 5.049401038298161559, -19.05341960407611168, 107.7072429386476955 ) ) ;
#171807=CARTESIAN_POINT ( 'NONE',  ( -15.72974639402197994, 15.80617190586746368, 105.6239096053143669 ) ) ;
#171808=CARTESIAN_POINT ( 'NONE',  ( -9.474510206698964154, 16.51473224551069663, 65.41557627198102409 ) ) ;
#171809=CARTESIAN_POINT ( 'NONE',  ( -16.88567814943165502, 6.947325034625575491, 23.70998877347416922 ) ) ;
#171810=CARTESIAN_POINT ( 'NONE',  ( -0.05219959533910754901, -16.53943276465976808, 77.49890960531433848 ) ) ;
#171811=CARTESIAN_POINT ( 'NONE',  ( 19.05341960407611168, 5.049401038298154454, 113.9572429386477097 ) ) ;
#171812=CARTESIAN_POINT ( 'NONE',  ( 16.46253265017160672, -9.564922557960803928, 23.33224293864769194 ) ) ;
#171813=CARTESIAN_POINT ( 'NONE',  ( -0.05219959533907301413, -21.53943276465977519, 107.4989096053143669 ) ) ;
#171814=CARTESIAN_POINT ( 'NONE',  ( 13.97604488694548053, -13.89961937509957401, 60.62609039468564731 ) ) ;
#171815=CARTESIAN_POINT ( 'NONE',  ( 0.05219959533909260263, 19.03943276465977164, 109.9989096053143669 ) ) ;
#171816=CARTESIAN_POINT ( 'NONE',  ( -5.153800228976328057, -19.02544592524343514, 22.29057627198102765 ) ) ;
#171817=CARTESIAN_POINT ( 'NONE',  ( -5.823673210054116645, -21.52544592524344225, 57.29057627198103120 ) ) ;
#171818=CARTESIAN_POINT ( 'NONE',  ( -9.564922557960796823, -16.46253265017161027, 97.08224293864769550 ) ) ;
#171819=CARTESIAN_POINT ( 'NONE',  ( -21.52544592524334988, -5.823673210054445271, 73.95942372801901854 ) ) ;
#171820=CARTESIAN_POINT ( 'NONE',  ( 13.89961937509977652, -13.97604488694527269, 53.12390960531434558 ) ) ;
#171821=CARTESIAN_POINT ( 'NONE',  ( -14.29746914071049879, 8.314922557960819915, 85.83224293864768129 ) ) ;
#171822=CARTESIAN_POINT ( 'NONE',  ( -12.06949235617739369, -12.14591786802326823, 29.37609039468568284 ) ) ;
#171823=CARTESIAN_POINT ( 'NONE',  ( -18.67979575497193778, 10.72451020669871902, 63.33442372801900433 ) ) ;
#171825=CARTESIAN_POINT ( 'NONE',  ( 19.05341960407617918, -5.049401038297876454, 21.04275706135232582 ) ) ;
#171826=CARTESIAN_POINT ( 'NONE',  ( -19.03943276465977164, -0.05219959533935918106, 78.75109039468567573 ) ) ;
#171827=CARTESIAN_POINT ( 'NONE',  ( -5.153800228976607833, 19.02544592524334988, 42.70942372801901143 ) ) ;
#171828=DIRECTION ( 'NONE',  ( 0.000000000000000000, 1.000000000000000000, 0.000000000000000000 ) ) ;
#171829=CARTESIAN_POINT ( 'NONE',  ( -15.72974639402176322, -15.80617190586768395, 39.37609039468567573 ) ) ;
#171830=CARTESIAN_POINT ( 'NONE',  ( -19.05341960407617563, 5.049401038297882671, 28.54275706135232937 ) ) ;
#171831=CARTESIAN_POINT ( 'NONE',  ( -16.46253265017160317, 9.564922557960807481, 70.83224293864770971 ) ) ;
#171832=CARTESIAN_POINT ( 'NONE',  ( -12.14591786802309592, -12.06949235617757132, 21.87390960531436690 ) ) ;
#171833=CARTESIAN_POINT ( 'NONE',  ( -16.46253265017160317, 9.564922557960807481, 115.8322429386477097 ) ) ;
#171834=CARTESIAN_POINT ( 'NONE',  ( 15.80617190586769283, -15.72974639402175789, 85.62609039468568994 ) ) ;
#171835=B_SPLINE_CURVE_WITH_KNOTS ( 'NONE', 3,
 ( #187094, #33386, #156734, #155725, #77884, #19216 ),
 .UNSPECIFIED., .F., .F.,
 ( 4, 2, 4 ),
 ( 0.000000000000000000, 0.0003837532665554015815, 0.0007675065331108031630 ),
 .UNSPECIFIED. ) ;
#171838=CARTESIAN_POINT ( 'NONE',  ( 15.80617190586769283, -15.72974639402175789, 90.62609039468567573 ) ) ;
#171839=CARTESIAN_POINT ( 'NONE',  ( 17.26172910966779384, -6.454744622555847577, 43.30646908649224258 ) ) ;
#171840=CARTESIAN_POINT ( 'NONE',  ( -5.049401038298153566, 19.05341960407611168, 100.2072429386476955 ) ) ;
#171842=CARTESIAN_POINT ( 'NONE',  ( 19.05341960407611168, 5.049401038298154454, 53.95724293864770260 ) ) ;
#171843=CARTESIAN_POINT ( 'NONE',  ( 5.719274019375991003, -21.55341960407610458, 62.70724293864769550 ) ) ;
#171844=CARTESIAN_POINT ( 'NONE',  ( -12.14591786802326823, 12.06949235617739902, 113.1260903946856899 ) ) ;
#171845=CARTESIAN_POINT ( 'NONE',  ( -19.05341960407611168, -5.049401038298163336, 21.45724293864768839 ) ) ;
#171846=CARTESIAN_POINT ( 'NONE',  ( 9.564922557960805705, 16.46253265017160317, 94.58224293864769550 ) ) ;
#171847=CARTESIAN_POINT ( 'NONE',  ( 13.89961937509957401, 13.97604488694547697, 26.87609039468566507 ) ) ;
#171848=CARTESIAN_POINT ( 'NONE',  ( -0.05219959533910754901, -16.53943276465976808, 102.4989096053143811 ) ) ;
#171849=CARTESIAN_POINT ( 'NONE',  ( -15.72974639402176322, -15.80617190586768395, 74.37609039468568994 ) ) ;
#171851=CARTESIAN_POINT ( 'NONE',  ( 16.52544592524335698, 4.483927247898782831, 106.4594237280190328 ) ) ;
#171852=CARTESIAN_POINT ( 'NONE',  ( -9.474510206698720793, -16.51473224551083518, 59.58442372801900433 ) ) ;
#171854=CARTESIAN_POINT ( 'NONE',  ( 16.46253265017160672, -9.564922557960803928, 113.3322429386476955 ) ) ;
#171855=CARTESIAN_POINT ( 'NONE',  ( -14.34966873604960291, -8.224510206698953496, 81.66557627198103830 ) ) ;
#171856=CARTESIAN_POINT ( 'NONE',  ( -16.51473224551082808, 9.474510206698731452, 53.33442372801900433 ) ) ;
#171857=CARTESIAN_POINT ( 'NONE',  ( 0.05219959533909260263, 19.03943276465977164, 59.99890960531436690 ) ) ;
#171858=CARTESIAN_POINT ( 'NONE',  ( -0.05219959533910754901, -16.53943276465976808, 57.49890960531435979 ) ) ;
#171859=CARTESIAN_POINT ( 'NONE',  ( -0.05219959533936034679, 19.03943276465977164, 87.50109039468567573 ) ) ;
#171860=CARTESIAN_POINT ( 'NONE',  ( 18.62759615963271287, -10.81492255796078972, 53.33224293864769550 ) ) ;
#171862=CARTESIAN_POINT ( 'NONE',  ( 4.483927247898545687, 16.52544592524342804, 109.7905762719810383 ) ) ;
#171863=CARTESIAN_POINT ( 'NONE',  ( 16.46253265017160672, -9.564922557960803928, 63.33224293864769550 ) ) ;
#171864=CARTESIAN_POINT ( 'NONE',  ( -18.62759615963270932, 10.81492255796079327, 60.83224293864769550 ) ) ;
#171865=CARTESIAN_POINT ( 'NONE',  ( 14.29746914071037800, 8.314922557961029526, 96.66775706135234714 ) ) ;
#171866=CARTESIAN_POINT ( 'NONE',  ( -13.97604488694527625, -13.89961937509977652, 76.87390960531433848 ) ) ;
#171867=CARTESIAN_POINT ( 'NONE',  ( 19.03943276465977164, 0.05219959533936151252, 51.25109039468567573 ) ) ;
#171868=CARTESIAN_POINT ( 'NONE',  ( -5.823673210054431948, 21.52544592524334988, 82.70942372801900433 ) ) ;
#171869=CARTESIAN_POINT ( 'NONE',  ( 5.719274019375991003, -21.55341960407610458, 67.70724293864769550 ) ) ;
#171870=CARTESIAN_POINT ( 'NONE',  ( -0.05219959533909027116, -19.03943276465977164, 112.4989096053143669 ) ) ;
#171871=CARTESIAN_POINT ( 'NONE',  ( 19.02544592524343514, -5.153800228976328945, 43.54057627198103120 ) ) ;
#171872=CARTESIAN_POINT ( 'NONE',  ( 16.53943276465976808, 0.05219959533934440121, 96.25109039468568994 ) ) ;
#171873=CARTESIAN_POINT ( 'NONE',  ( -19.05341960407617563, 5.049401038297882671, 113.5427570613523471 ) ) ;
#171874=CARTESIAN_POINT ( 'NONE',  ( 17.40861289039002813, 6.110651285853275994, 53.87232470827435549 ) ) ;
#171875=CARTESIAN_POINT ( 'NONE',  ( 5.823673210054444382, -21.52544592524334988, 90.20942372801903275 ) ) ;
#171877=CARTESIAN_POINT ( 'NONE',  ( 16.55341960407611168, 4.379528057220329451, 58.95724293864770971 ) ) ;
#171878=CARTESIAN_POINT ( 'NONE',  ( -14.34966873604960291, -8.224510206698953496, 71.66557627198100988 ) ) ;
#171879=CARTESIAN_POINT ( 'NONE',  ( 21.55341960407610458, 5.719274019375980345, 88.95724293864769550 ) ) ;
#171880=CARTESIAN_POINT ( 'NONE',  ( -21.52544592524343514, 5.823673210054127303, 91.04057627198103830 ) ) ;
#171881=CARTESIAN_POINT ( 'NONE',  ( 16.21995358207302473, -7.366697692864217828, 97.43551001512156517 ) ) ;
#171882=CARTESIAN_POINT ( 'NONE',  ( 5.719274019375991003, -21.55341960407610458, 52.70724293864769550 ) ) ;
#171884=CARTESIAN_POINT ( 'NONE',  ( 12.14591786802327356, -12.06949235617739191, 65.62609039468568994 ) ) ;
#171885=CARTESIAN_POINT ( 'NONE',  ( -4.483927247898539470, -16.52544592524342804, 97.29057627198105251 ) ) ;
#171886=CARTESIAN_POINT ( 'NONE',  ( -5.153800228976328057, -19.02544592524343514, 47.29057627198102409 ) ) ;
#171887=( NAMED_UNIT ( * ) SI_UNIT ( $, .STERADIAN. ) SOLID_ANGLE_UNIT ( ) );
#171888=CARTESIAN_POINT ( 'NONE',  ( 15.50000000000000178, -5.500000000000000888, 118.0000000000000142 ) ) ;
#171889=CARTESIAN_POINT ( 'NONE',  ( 16.55341960407618274, -4.379528057220086978, 101.0427570613523756 ) ) ;
#171890=CARTESIAN_POINT ( 'NONE',  ( -21.52544592524334988, -5.823673210054445271, 33.95942372801901143 ) ) ;
#171891=CARTESIAN_POINT ( 'NONE',  ( 13.89961937509977652, -13.97604488694527269, 103.1239096053143527 ) ) ;
#171892=CARTESIAN_POINT ( 'NONE',  ( 21.52544592524334988, 5.823673210054432836, 61.45942372801901854 ) ) ;
#171894=CARTESIAN_POINT ( 'NONE',  ( -9.564922557960796823, -16.46253265017161027, 22.08224293864768839 ) ) ;
#171896=CARTESIAN_POINT ( 'NONE',  ( -21.53943276465977519, -0.05219959533937600094, 53.75109039468568994 ) ) ;
#171897=CARTESIAN_POINT ( 'NONE',  ( 5.153800228976335163, 19.02544592524342804, 44.79057627198103830 ) ) ;
#171899=CARTESIAN_POINT ( 'NONE',  ( 9.564922557960805705, 16.46253265017160317, 94.58224293864769550 ) ) ;
#171900=CARTESIAN_POINT ( 'NONE',  ( 16.46253265017146816, 9.564922557961045513, 71.66775706135233293 ) ) ;
#171901=CARTESIAN_POINT ( 'NONE',  ( 18.62759615963255655, 10.81492255796105972, 26.66775706135235424 ) ) ;
#171902=CARTESIAN_POINT ( 'NONE',  ( 13.97604488694548053, -13.89961937509957401, 55.62609039468566863 ) ) ;
#171903=CARTESIAN_POINT ( 'NONE',  ( 9.474510206698971260, -16.51473224551069308, 32.91557627198102409 ) ) ;
#171904=CARTESIAN_POINT ( 'NONE',  ( 16.52544592524335698, 4.483927247898782831, 106.4594237280190328 ) ) ;
#171905=CARTESIAN_POINT ( 'NONE',  ( 13.97604488694548053, -13.89961937509957401, 70.62609039468567573 ) ) ;
#171906=CARTESIAN_POINT ( 'NONE',  ( -8.224510206698948167, 14.34966873604960824, 25.41557627198103120 ) ) ;
#171907=CARTESIAN_POINT ( 'NONE',  ( -0.05219959533936034679, 19.03943276465977164, 47.50109039468566863 ) ) ;
#171908=CARTESIAN_POINT ( 'NONE',  ( -13.97604488694527625, -13.89961937509977652, 101.8739096053143811 ) ) ;
#171909=CARTESIAN_POINT ( 'NONE',  ( -0.05219959533937732626, 21.53943276465977519, 102.5010903946856899 ) ) ;
#171910=CARTESIAN_POINT ( 'NONE',  ( 9.564922557961047289, -16.46253265017146816, 20.41775706135233293 ) ) ;
#171911=CARTESIAN_POINT ( 'NONE',  ( 9.564922557960805705, 16.46253265017160317, 29.58224293864769550 ) ) ;
#171912=CARTESIAN_POINT ( 'NONE',  ( -5.823673210054431948, 21.52544592524334988, 92.70942372801901854 ) ) ;
#171913=CARTESIAN_POINT ( 'NONE',  ( 12.14591786802327356, -12.06949235617739191, 35.62609039468568994 ) ) ;
#171914=CARTESIAN_POINT ( 'NONE',  ( -9.474510206698964154, 16.51473224551069663, 90.41557627198103830 ) ) ;
#171916=CARTESIAN_POINT ( 'NONE',  ( 16.46253265017160672, -9.564922557960803928, 78.33224293864769550 ) ) ;
#171918=CARTESIAN_POINT ( 'NONE',  ( 19.03943276465977164, 0.05219959533936151252, 66.25109039468567573 ) ) ;
#171919=CARTESIAN_POINT ( 'NONE',  ( 5.153800228976335163, 19.02544592524342804, 99.79057627198102409 ) ) ;
#171920=CARTESIAN_POINT ( 'NONE',  ( 21.52544592524334988, 5.823673210054432836, 96.45942372801901854 ) ) ;
#171921=CARTESIAN_POINT ( 'NONE',  ( -16.55341960407611168, -4.379528057220339221, 96.45724293864770971 ) ) ;
#171922=CARTESIAN_POINT ( 'NONE',  ( 5.719274019375991003, -21.55341960407610458, 42.70724293864770260 ) ) ;
#171923=( BOUNDED_SURFACE ( )  B_SPLINE_SURFACE ( 3, 2, ( 
 ( #35458, #69787, #67786, #100114, #98094, #114278, #113284, #131455, #160802, #101107, #174975, #36439, #97109, #159792, #193142, #6105, #37449, #20281, #177979, #162793, #82944, #175981, #145621, #5103, #9128, #21287, #22290, #144622, #7100, #83941, #81927, #129443, #24302, #130439, #192138, #161797, #23292, #84936, #147639, #146617, #166802, #11129, #197140, #108831, #196159, #104122, #88948, #155343, #180982, #86954, #1648, #148638, #42458, #10128, #644, #71789, #133458, #195148, #12135, #31007, #62314, #92656, #123984, #170511, #43448, #63326, #58607, #27301, #32001, #119299, #134474, #179995, #73799, #149631, #77497, #56629, #135472, #93658, #102126, #139167, #118303, #120273, #47172, #178985, #57633, #150639, #25312, #41462, #72804, #165804, #105116, #103127, #181965, #154345, #164808, #15838, #87943, #185682, #16832, #40452, #78483, #163810, #140156, #26303, #143134, #65309, #18828, #34977, #48170, #2649, #5619, #126969, #175485, #96630, #33989, #145133, #19806, #160313, #128957, #50157, #172502, #35962, #83455, #158318, #21803, #142146, #64326, #17833, #4613, #111816, #6616, #66305, #36957, #109827, #127965, #125004, #144137, #98619, #186699, #189668, #173504, #141160, #171510, #32999, #97609, #188677, #49161, #80473, #3630, #159298, #125993, #51141, #94653, #52133, #156333, #112802, #81447, #79491, #67298, #174495, #187691, #20794, #110820, #95645, #157333, #82449, #190657, #113790, #86470, #150157, #84452, #39964, #22806, #87471, #164332, #178497, #117817, #161312, #101634, #25826, #68295, #7616, #195678, #70310, #26820, #40978, #100629, #148155, #116805, #24821, #53125, #146130, #69300, #103650, #9647, #179510, #176496, #132976, #193664, #55135, #114803, #10648, #149158, #129946, #130966, #192656, #71313, #191646, #56136, #194666, #102647, #72310, #133987, #57149, #118827, #163325, #180511, #41984, #165328, #88461, #37972, #99630, #54139, #115813, #38972, #177503, #162310, #23811, #85461, #147150, #8638, #131979, #184457, #119811, #166326, #107592, #15603, #76267, #181496, #135978, #13616, #154110, #92424, #12644, #43962, #42974, #89465, #169270, #46936, #183470, #185446, #91419, #121777, #151154, #90449, #29783, #168287, #137945, #77261, #122768, #27823, #199628, #104639, #196674, #74311, #93415, #61095, #410, #153106, #11658, #197649, #44955, #59115, #30777, #138930, #106612, #45937, #120781, #14610, #62083, #73324, #182481, #123747, #75283, #170273, #108596, #105624, #31766, #60109, #134995, #58143, #167312, #28808, #152133, #136954, #198643, #63084, #19574, #80236, #141907, #1405, #97377, #112567, #16595, #156093, #171273, #173262, #155102, #142898, #81217, #111578, #35730, #20557, #4380, #50909, #188434, #143899, #3398, #159063, #174262, #5381, #49913, #65073, #175248, #125756, #34737, #32761, #187456, #82208, #36713, #124763, #67064, #127731, #186460, #109590, #128722, #190419, #66065, #47938, #79250, #157093, #51895, #113554, #17590, #48924, #94413, #140922, #78243, #139915, #126731, #2408, #96395, #158082, #64087, #33749, #189433, #110578, #172259, #95407, #18589, #10404, #83220, #178259, #195429, #117567, #148915, #160073, #163076, #85216, #114559, #180269, #98376, #9404, #162072, #22567, #53902, #192420, #132736, #37727, #24579, #56905, #25588, #144895, #86228, #115577, #52884, #40732, #100394, #177265, #23568, #8396, #72061, #146907, #6377, #118579, #68057, #70071, #129711, #179268, #191408, #176256, #99389, #131739, #147918, #102402, #71070, #164089, #87232, #194424, #21560, #116570, #193421, #133735, #38736, #54896, #161072, #39720, #69061, #55894, #84213, #101383, #145893, #7376, #130728, #134750, #75043, #107349, #123509, #120542, #151889, #88218, #57902, #74068, #135739, #106365, #196432, #121534, #44710, #181257, #182235, #150912, #43720, #59867, #103403, #136709, #61839, #184216, #26575, #183229, #105381, #197410, #13379, #165081, #119574, #122526, #167068, #92180 ),
 ( #166078, #28569, #45698, #169022, #42734, #58876, #149902, #104396, #199387, #77018, #198390, #15362, #168048, #29545, #27581, #90206, #91178, #152867, #14362, #30527, #76027, #153864, #11409, #137702, #138690, #60851, #171, #73078, #41739, #89219, #12406, #66822, #185202, #96164, #48688, #109347, #140678, #79004, #19344, #124521, #111337, #81964, #112334, #170033, #173027, #2170, #4146, #16359, #78007, #154861, #18353, #34506, #65825, #157853, #127494, #174024, #49673, #46693, #3168, #33511, #35495, #125521, #63850, #186216, #80008, #155851, #80992, #139674, #141677, #97145, #108354, #142667, #1162, #64841, #50674, #31523, #187218, #95170, #93176, #62837, #17348, #110341, #189199, #47697, #126503, #188201, #171029, #172022, #94172, #156858, #158828, #32520, #20316, #5140, #143656, #113320, #146654, #68821, #22327, #38496, #51656, #6142, #9165, #130480, #179022, #100152, #37487, #148677, #23328, #163848, #132500, #53658, #176018, #39482, #86990, #161833, #25349, #145657, #67824, #21325, #8148, #115335, #10165, #69825, #191178, #7138, #159830, #24338, #177026, #194189, #144659, #82983, #190181, #129479, #162829, #99149, #192177, #128485, #147677, #85988, #160838, #84971, #131492, #98133, #102162, #52652, #193179, #83977, #54652, #116326, #175012, #178015, #70832, #36476, #114316, #101143, #55654, #117326, #40490, #42497, #59629, #104161, #89979, #199148, #88985, #197179, #182003, #45464, #73838, #180032, #91936, #41501, #135509, #103165, #164845, #90946, #26341, #87981, #149669, #105153, #121303, #152633, #182995, #14123, #60614, #136479, #153629, #151660, #120310, #122289, #12173, #27339, #72842, #166839, #165842, #167817, #11167, #28340, #183978, #195185, #29316, #134512, #13154, #137468, #71825, #150675, #43486, #118339, #196198, #58644, #74817, #198159, #57670, #44478, #106133, #119337, #75790, #181023, #107118, #168789, #133493, #30291, #56666, #157615, #200138, #33279, #155620, #109115, #125288, #138457, #92939, #95930, #17116, #65592, #186985, #124279, #35257, #110113, #50441, #19106, #140444, #62601, #126272, #173790, #48456, #112100, #32286, #154627, #108111, #94938, #1934, #96911, #156623, #77777, #93941, #46451, #111100, #63613, #80756, #31288, #169795, #76786, #16122, #49439, #185975, #78767, #15124, #34271, #172790, #47459, #171791, #18118, #184967, #188965, #139445, #79773, #170794, #141443, #2930, #61607, #64609, #142433, #123276, #927, #187969, #3912, #127252, #8917, #129237, #146407, #190933, #176778, #85743, #175767, #83733, #68572, #132254, #160593, #66584, #178774, #128248, #22082, #51420, #38250, #174772, #114069, #70585, #52410, #7897, #37243, #99905, #147430, #98899, #145412, #130229, #193945, #6894, #189945, #40240, #113080, #191924, #36238, #177774, #97890, #159582, #21079, #53408, #69582, #39244, #131248, #100900, #55408, #23084, #158594, #161590, #115086, #117078, #84729, #192937, #82735, #54414, #116086, #162584, #144416, #24088, #20083, #81728, #143413, #5902, #4901, #67579, #183742, #180780, #11930, #148426, #118094, #134265, #195952, #166597, #56414, #181760, #104909, #41253, #42255, #10918, #103917, #120072, #163598, #196938, #122051, #44237, #86741, #43242, #165597, #57425, #73594, #25099, #179784, #182753, #27095, #88741, #90714, #194938, #102915, #71580, #197915, #74573, #9921, #164599, #59385, #105894, #28097, #133246, #26093, #150435, #167581, #29075, #87737, #119098, #149422, #72591, #121059, #137226, #135267, #75550, #89736, #58406, #151422, #12909, #136241, #152397, #13883, #198911, #60379, #101916, #30054, #125044, #142188, #64366, #95688, #106883, #109865, #32043, #61370, #127010, #45229, #156372, #108873, #169551, #686, #155383, #91695, #123041, #77539, #139211, #171550, #199906, #186740, #48211, #184727, #185726, #154386, #47215, #63367, #168556, #140197, #65350, #187731, #153387, #33039, #170553, #62357, #16872, #14887, #46211, #126035, #93700 ),
 ( #124027, #107865, #138224, #94694, #78523, #76548, #17876, #31049, #1691, #92698, #141200, #79530, #49202, #15881, #2689, #110860, #172545, #34030, #157376, #18869, #80515, #3672, #25613, #36002, #128999, #98660, #158359, #165111, #128008, #190697, #97649, #160354, #67337, #50202, #82492, #10432, #88246, #81488, #71094, #4655, #144175, #41766, #159338, #179295, #20835, #9429, #118608, #5661, #113829, #21844, #26603, #52172, #96671, #11438, #19847, #175524, #143175, #72090, #66346, #189710, #51183, #86253, #40759, #133764, #102428, #195459, #180298, #55919, #73109, #132761, #36999, #103431, #147943, #194448, #112843, #117594, #164115, #87257, #174535, #148942, #149931, #111857, #56934, #188718, #173547, #35016, #16390, #13407, #150942, #167096, #28597, #199417, #89250, #14392, #137733, #74098, #75071, #43749, #136737, #152895, #196461, #29574, #154892, #77050, #119602, #76058, #198421, #90235, #44739, #57931, #12436, #15393, #59896, #105412, #104425, #183258, #107382, #91205, #170065, #138721, #121563, #182266, #45730, #93207, #168077, #31556, #151918, #135768, #27610, #60881, #106395, #134779, #122558, #197439, #184248, #166108, #30561, #169054, #202, #58905, #120572, #181285, #92212, #153898, #61871, #123541, #42763, #185234, #46726, #108388, #18386, #188231, #47726, #51690, #17379, #80037, #187249, #49704, #156890, #139706, #172053, #97174, #175044, #171059, #157884, #94202, #33540, #128516, #48718, #65855, #110371, #96195, #5171, #95203, #3197, #111370, #113352, #141706, #186248, #98164, #109378, #64871, #32549, #158859, #155882, #79035, #140710, #173059, #127526, #20348, #189230, #81996, #66854, #142698, #159864, #19373, #126532, #190211, #34536, #81022, #2200, #4177, #50708, #174057, #63881, #112366, #36509, #1193, #35526, #125552, #143689, #78037, #62870, #124551, #131528, #67854, #10198, #161867, #177059, #22360, #54686, #192210, #117361, #52684, #116359, #71858, #144689, #179057, #114347, #178048, #87025, #103199, #100185, #193212, #129509, #37519, #53693, #115370, #86023, #176052, #101176, #24372, #160870, #23361, #130514, #85006, #39516, #83014, #162864, #41535, #163885, #6174, #147712, #146687, #38529, #9200, #191209, #99181, #102197, #8183, #69859, #84012, #70865, #194222, #132533, #56700, #25382, #55687, #68855, #40526, #180067, #148710, #118373, #133527, #145690, #7172, #195219, #21357, #46484, #44510, #27370, #182036, #196233, #60647, #90010, #168820, #181054, #119371, #26375, #42530, #199181, #135540, #166871, #164880, #184013, #122321, #12207, #105184, #74847, #134544, #138488, #104193, #28372, #73870, #136510, #43518, #88014, #58674, #45495, #61639, #57702, #106166, #165874, #120341, #15157, #197211, #152665, #151694, #183027, #91967, #13184, #198191, #59661, #200170, #121334, #72876, #185000, #89017, #167849, #150708, #107150, #29349, #90978, #14155, #75823, #137501, #30325, #153661, #76817, #123307, #149702, #11200, #126302, #156654, #18150, #157646, #959, #141476, #65621, #189975, #47491, #35286, #110143, #66614, #80786, #140478, #187998, #79804, #64640, #92973, #62635, #124311, #143445, #49468, #19135, #16154, #172820, #33310, #94970, #154658, #50470, #127281, #169828, #109148, #186009, #111131, #108144, #95962, #34300, #142464, #188994, #173821, #3942, #112130, #2960, #96942, #158623, #20114, #81758, #4931, #128278, #31321, #77808, #78800, #139477, #48489, #170827, #32319, #93972, #155652, #17147, #1966, #63646, #125321, #187018, #171822, #84760, #97922, #52440, #145443, #100932, #39275, #129269, #98931, #159615, #5932, #116116, #132285, #115116, #70619, #161621, #53441, #67608, #83763, #23115, #38281, #146438, #162616, #131279, #8951, #174801, #7929, #193977, #177805, #147461, #51450, #69613, #191955, #190963, #113111, #36267, #24121, #99935, #22113, #130259, #68603, #85774, #37274, #55439, #21111, #117110, #114098, #82766, #176809, #175801, #144447, #160622 ),
 ( #6925, #192967, #54446, #35935, #51114, #82420, #126941, #80445, #52103, #2621, #65282, #172473, #20765, #124975, #171482, #1619, #127937, #4585, #140128, #186672, #189639, #97581, #96601, #63295, #156304, #33960, #174466, #112773, #32971, #64298, #48142, #109799, #159269, #67269, #3603, #5589, #111788, #142118, #94625, #110792, #50128, #188649, #158290, #144109, #143106, #128927, #16804, #173476, #190628, #113760, #31974, #93630, #19779, #18800, #17805, #155315, #78454, #66278, #95618, #79462, #187663, #125965, #141131, #49134, #81420, #157303, #34949, #160283, #101602, #192627, #129915, #117785, #177472, #191615, #163290, #6585, #21774, #53094, #57119, #24791, #164302, #193633, #175456, #114772, #147121, #176466, #194634, #71281, #85430, #86439, #68264, #8608, #132946, #36927, #37939, #102616, #38941, #133955, #148125, #7584, #55105, #23780, #131949, #83425, #99600, #161280, #10617, #116775, #9616, #145102, #39933, #100598, #162280, #22775, #179479, #56104, #98589, #84423, #146100, #178466, #69270, #40944, #25795, #87441, #149126, #72278, #195646, #130936, #70281, #54109, #115783, #83767, #64644, #37278, #145447, #65625, #188002, #141480, #128282, #173826, #130263, #189979, #111135, #127285, #79808, #144451, #35290, #52444, #126306, #2964, #110147, #49472, #82770, #19139, #50474, #48493, #67612, #5936, #95966, #188998, #158627, #18154, #22117, #172824, #112134, #157650, #20118, #96946, #171826, #142468, #129273, #6929, #34304, #51454, #80790, #3946, #98935, #81762, #36271, #143449, #66618, #175805, #4935, #113115, #174805, #68607, #97926, #156658, #33314, #159619, #21115, #190967, #114102, #160626, #94974, #161625, #25135, #41287, #72625, #102949, #134300, #183532, #56450, #76332, #9955, #40278, #45016, #132289, #147465, #192971, #86777, #162620, #87770, #23119, #148462, #106676, #115120, #149455, #84764, #71614, #60169, #191959, #70623, #101951, #38285, #7933, #24126, #85778, #118129, #146441, #133280, #194971, #131283, #193981, #100936, #55443, #179817, #53445, #164633, #14671, #195986, #176813, #26128, #117114, #8955, #163632, #99939, #69617, #121838, #178808, #10951, #54450, #168349, #29845, #91482, #153169, #116120, #177809, #39279, #65135, #122830, #64152, #155166, #92486, #80297, #139979, #154175, #125816, #169331, #184519, #15666, #19635, #187519, #126792, #156155, #138009, #77325, #109653, #138993, #157156, #33810, #47999, #48985, #30839, #171335, #95470, #199693, #472, #188498, #1468, #96456, #110640, #170336, #17653, #186525, #94474, #45999, #62146, #123810, #173326, #79313, #172321, #107654, #2470, #63146, #124825, #185508, #141969, #18651, #61158, #46999, #108658, #140982, #31829, #3458, #49977, #111641, #34801, #158143, #93479, #16658, #32823, #78306, #129769, #85277, #100453, #131802, #176317, #191465, #101446, #51955, #114617, #21623, #70130, #174321, #20619, #50970, #177325, #53961, #189492, #115636, #68117, #112629, #35791, #97438, #5441, #83280, #23629, #162133, #82269, #113615, #159123, #143961, #38796, #116630, #52943, #54958, #161131, #37787, #67125, #160135, #99451, #22627, #7436, #146968, #192478, #193481, #66127, #84274, #178319, #8457, #39782, #142959, #145955, #69120, #128783, #163137, #81277, #4439, #144954, #190483, #36775, #175309, #127792, #98440, #130786, #6435, #103467, #134815, #71131, #40794, #56967, #118640, #89285, #179330, #104460, #27645, #164151, #165146, #133801, #26637, #42798, #86289, #119636, #44773, #167131, #9468, #166143, #88280, #180332, #196495, #147979, #102463, #105447, #149968, #195492, #194484, #73145, #197473, #181319, #59928, #28631, #11474, #182302, #121596, #25648, #13440, #183291, #41800, #87293, #117632, #150976, #57965, #106426, #12470, #148977, #74131, #55956, #120608, #135802, #90268, #10466, #72127, #132797, #58939, #43782, #151951, #75104, #24641, #136771, #198457, #15425, #108418, #78068, #137763, #141736, #107414 ),
 ( #138753, #155916, #235, #186279, #95234, #185268, #93238, #139736, #3226, #170094, #76087, #188261, #199447, #31588, #60915, #187280, #122591, #184279, #45762, #1225, #17411, #48750, #79068, #110403, #156920, #32582, #18417, #124583, #80066, #64900, #154923, #126561, #140741, #61902, #47758, #16421, #109412, #152926, #169087, #30593, #49735, #171091, #2230, #168107, #62903, #92245, #29604, #153931, #94235, #77084, #172085, #123573, #46760, #63912, #125582, #33572, #91236, #14423, #192242, #100215, #6203, #67883, #8214, #161895, #23391, #51717, #66882, #112395, #144717, #82025, #7200, #142727, #129536, #85037, #34567, #68884, #4207, #191236, #177087, #193243, #190240, #21383, #157912, #127559, #143721, #5200, #176078, #65885, #52710, #114374, #50736, #113380, #20378, #175070, #37546, #173088, #99210, #131558, #53722, #96223, #160898, #36536, #128543, #83042, #19402, #189260, #115399, #98192, #159895, #81051, #22390, #84040, #145719, #146718, #38558, #130544, #69889, #111403, #174086, #35555, #97202, #158888, #194251, #147741, #134574, #180096, #136538, #196261, #117390, #71887, #86052, #150735, #41564, #58700, #70895, #9228, #116388, #132562, #89045, #25412, #56732, #54716, #73897, #12235, #102227, #195248, #164909, #24403, #28399, #55718, #118402, #163916, #26403, #133557, #178078, #148739, #135567, #151720, #179089, #57730, #40558, #10227, #105212, #87054, #42558, #103227, #72905, #182063, #88042, #149730, #11231, #119400, #197239, #181083, #120370, #104221, #165902, #39545, #27400, #43546, #166899, #90038, #101204, #13213, #74876, #162894, #138516, #108175, #167878, #171849, #137528, #46876, #107178, #169856, #76845, #59691, #91996, #17174, #94997, #91008, #77837, #14183, #153690, #48516, #168849, #186037, #30354, #16182, #125349, #15186, #123336, #31350, #33337, #61667, #106194, #18177, #29377, #185029, #152694, #78828, #75852, #199210, #60677, #93001, #47519, #140506, #109175, #1995, #187046, #154687, #139504, #156683, #110170, #79834, #46516, #987, #122352, #62662, #124341, #93998, #184041, #170854, #198219, #121362, #155679, #45524, #32345, #63674, #183055, #44539, #51481, #188026, #157676, #173851, #35317, #5962, #95991, #21141, #144478, #80815, #81788, #50498, #143475, #159645, #2989, #36298, #161653, #83795, #126329, #82796, #4959, #96971, #113143, #64667, #19166, #22145, #66644, #112162, #111160, #190007, #114130, #97953, #176843, #145475, #128307, #98963, #38314, #142493, #130292, #99969, #158652, #3971, #34330, #67640, #174833, #23149, #129299, #65651, #20143, #141504, #49498, #190995, #172849, #160653, #127313, #189024, #52471, #175831, #37304, #6956, #68636, #191986, #53473, #115150, #41320, #181828, #135331, #73659, #25168, #40309, #85810, #118159, #55476, #180844, #116150, #179849, #197004, #7964, #42321, #177841, #102980, #150499, #166662, #163666, #195003, #131313, #100968, #117146, #178841, #149488, #39309, #164665, #87802, #24159, #86810, #194013, #148496, #26161, #146472, #10984, #104975, #27159, #69647, #72657, #9987, #101985, #56481, #193003, #162653, #165661, #71647, #133314, #54480, #134332, #57492, #196016, #120137, #88806, #119161, #103982, #43307, #147496, #58470, #84793, #11996, #8987, #70655, #132321, #153456, #109937, #107937, #90780, #45296, #59453, #124100, #14954, #32113, #44303, #182821, #89805, #105962, #62428, #198977, #30121, #28163, #47287, #185799, #75616, #168621, #138292, #197983, #1760, #167647, #91762, #137295, #199973, #106948, #151487, #122119, #108943, #125114, #121126, #169623, #29143, #183808, #78595, #60444, #15950, #76614, #46281, #155451, #61438, #123110, #184795, #63438, #31120, #136308, #170624, #92768, #154458, #12978, #93770, #16941, #77609, #139280, #757, #152464, #186812, #13950, #140268, #48282, #74642, #50269, #33107, #65417, #190763, #68400, #64433, #51250, #187799, #127078, #21911, #142256, #159409, #3740, #189778, #98728 ),
 ( #49268, #143241, #126103, #52238, #67407, #81555, #20904, #110926, #112910, #160422, #128075, #83562, #145241, #173613, #130052, #144244, #188786, #174604, #19913, #36070, #156445, #172612, #34099, #6722, #97719, #82562, #79598, #5728, #96736, #158425, #17944, #113895, #129062, #94763, #95757, #157442, #175593, #171619, #37069, #191752, #53235, #141267, #2757, #18937, #80582, #4724, #111927, #66413, #35083, #134094, #165433, #9751, #163431, #135100, #85570, #148258, #55242, #103754, #7722, #54246, #84557, #10753, #87574, #22911, #149261, #101743, #146235, #69408, #131074, #39076, #116910, #57257, #195784, #115918, #147256, #192763, #177608, #72417, #150268, #86574, #88570, #194769, #24929, #100733, #193773, #133079, #99735, #56243, #11762, #118931, #26928, #176605, #179613, #71415, #162414, #196776, #114911, #25931, #178603, #23916, #70417, #8747, #180616, #132084, #41086, #73429, #42089, #161419, #102749, #40066, #117924, #38079, #164437, #74412, #184562, #89571, #43075, #12747, #140026, #46043, #47047, #76378, #58244, #136078, #29888, #197752, #77371, #154221, #168393, #107698, #151257, #138055, #185553, #14718, #108704, #170383, #60213, #16702, #30885, #90553, #199736, #106719, #61202, #104742, #59219, #120888, #93528, #122874, #169377, #166433, #92532, #183576, #45061, #27928, #519, #15711, #119912, #182587, #44070, #139039, #181598, #62191, #123855, #31874, #155213, #78352, #105730, #167417, #91526, #28913, #153213, #152235, #13720, #75386, #137058, #198748, #121883, #172365, #34844, #142014, #193273, #94519, #141029, #171382, #100243, #177117, #109700, #38587, #188544, #32869, #156201, #17701, #125863, #3503, #146749, #85067, #2516, #33855, #79358, #64196, #161925, #39576, #173374, #178108, #81321, #111687, #187563, #80342, #19679, #158189, #127834, #8244, #112673, #116419, #101235, #96499, #162924, #143004, #4482, #49030, #65179, #66172, #189540, #51012, #69922, #23419, #24432, #186571, #131588, #86080, #54746, #1515, #63192, #124872, #50022, #110685, #48044, #95515, #157201, #126838, #18695, #103258, #41594, #182094, #87083, #73928, #44570, #74906, #132591, #135597, #164940, #102258, #90068, #149759, #163945, #197269, #179119, #194280, #25443, #29409, #58731, #136570, #165934, #147771, #148768, #119430, #10257, #166930, #43578, #57760, #120401, #40587, #27432, #198250, #104251, #59725, #121395, #11263, #106225, #105242, #180126, #89076, #196290, #150767, #55747, #71916, #133588, #183087, #12264, #28431, #117421, #151750, #72935, #134604, #195279, #13243, #167909, #9258, #56761, #118433, #70924, #26433, #88074, #181114, #42588, #171882, #156719, #155711, #187080, #124376, #79869, #139537, #95029, #110203, #141538, #186071, #1021, #111194, #61700, #47554, #31385, #3027, #184073, #30386, #60709, #48549, #63708, #199243, #125383, #77870, #122384, #45557, #107211, #15219, #93034, #33371, #18211, #92033, #123369, #168881, #153723, #64703, #62694, #169891, #152726, #185062, #126365, #188061, #76878, #170886, #138548, #46550, #49531, #108212, #78860, #154722, #109207, #172885, #16215, #32378, #94031, #91039, #17207, #26, #14216, #140540, #2028, #75885, #137560, #65685, #127348, #4006, #67677, #83829, #115184, #145510, #176877, #23184, #129335, #191030, #131348, #84827, #146507, #174868, #190042, #35355, #52505, #4996, #130326, #189062, #114165, #7997, #157712, #192023, #50534, #175868, #100002, #116185, #113178, #144513, #80851, #112196, #66681, #128343, #98998, #173886, #37340, #160687, #97006, #36334, #143510, #97987, #22179, #96026, #6991, #54513, #38346, #19202, #68672, #159681, #51516, #5998, #142528, #158688, #161689, #21177, #82832, #20177, #53507, #69681, #193036, #34365, #81823, #103018, #135367, #13012, #194049, #166695, #74676, #195040, #117183, #70691, #57526, #164701, #59487, #119195, #40345, #56517, #9022, #73695, #26197, #181862, #55513, #132357, #39344, #178878, #12032 ),
 ( #87836, #85844, #102020, #147534, #163703, #179886, #120171, #58505, #25205, #10023, #86847, #148532, #197038, #136343, #149522, #151521, #180880, #11019, #71682, #118195, #196051, #134367, #104017, #43341, #88840, #89840, #162688, #42355, #198018, #105009, #28198, #101003, #165695, #72692, #133349, #177876, #24194, #150532, #41354, #27193, #76647, #14987, #155484, #60476, #47323, #17979, #48317, #105994, #108978, #138325, #75650, #63474, #123144, #137328, #170659, #152496, #167680, #199009, #2791, #32147, #109972, #139313, #121161, #122152, #92803, #183841, #140305, #16976, #31155, #93804, #13984, #792, #171651, #77644, #33141, #94799, #184831, #79633, #78630, #153491, #62464, #169659, #124137, #29177, #45330, #106980, #156478, #185836, #1796, #90813, #125149, #46317, #107972, #168654, #186848, #141301, #182854, #30154, #91797, #44337, #200007, #61473, #154491, #15985, #145275, #130088, #129096, #160454, #97754, #53268, #112944, #68435, #83595, #114946, #159442, #174637, #84591, #35117, #20937, #4757, #176639, #157477, #3773, #34132, #21945, #37102, #172644, #98761, #36102, #161454, #126137, #190796, #51283, #80616, #146271, #64470, #175628, #128107, #188819, #19947, #158458, #6756, #65450, #52270, #22945, #191787, #49301, #113928, #81588, #18970, #38114, #66446, #142293, #99769, #95791, #110960, #127112, #187832, #50302, #111959, #82594, #173648, #96769, #144276, #143274, #189811, #5763, #67439, #57287, #100765, #25961, #135132, #164467, #196806, #58274, #9784, #166464, #180647, #40098, #87604, #56273, #149290, #192797, #162447, #23948, #43108, #10784, #118961, #115952, #72451, #133111, #194800, #54279, #150299, #165464, #69441, #8779, #85602, #134126, #7757, #195815, #42122, #103784, #88603, #73459, #26960, #11795, #41116, #119943, #117956, #181628, #104776, #27961, #102780, #179647, #89602, #178635, #131109, #148290, #177641, #147289, #70448, #39109, #132114, #193807, #55273, #116942, #101776, #163463, #24961, #86607, #71446, #153251, #93563, #31910, #152269, #183612, #59253, #28947, #108742, #186607, #122910, #124909, #30920, #61238, #90588, #29923, #169415, #107733, #77406, #155249, #62225, #63229, #136111, #138090, #140063, #91563, #106753, #13754, #184598, #121919, #47081, #182621, #46079, #1554, #74444, #170418, #44106, #92568, #16738, #32905, #14753, #154256, #197787, #167450, #45096, #168428, #15747, #105764, #139076, #554, #75422, #76414, #60248, #199771, #123893, #12779, #185591, #171419, #78387, #120922, #48079, #109735, #151290, #137096, #198782, #172406, #175390, #96535, #3538, #64235, #143041, #67205, #189576, #129851, #98525, #19715, #52037, #191550, #110725, #83362, #53027, #111724, #33895, #187600, #174402, #81357, #176401, #35872, #157239, #173410, #125900, #190563, #4519, #160218, #95552, #49069, #156238, #18732, #128863, #65216, #158225, #94559, #113694, #36858, #159205, #68199, #80380, #51048, #114708, #142052, #66212, #126876, #127872, #34881, #17740, #188582, #21708, #79397, #50063, #97518, #112710, #20699, #145038, #82355, #144043, #5525, #6520, #141067, #2553, #163220, #148056, #11558, #39863, #146036, #58042, #7519, #101529, #69204, #57048, #130872, #192562, #54045, #71213, #87373, #118722, #149058, #180411, #26720, #132876, #194565, #134895, #88359, #162214, #24722, #41883, #103550, #38878, #70215, #115719, #177407, #195575, #73224, #9547, #196571, #117713, #56035, #100535, #116709, #179409, #40873, #164230, #165225, #10546, #150052, #22711, #86371, #23713, #102547, #119712, #99534, #25727, #72210, #85360, #37876, #161216, #133884, #84358, #147053, #193567, #131882, #8536, #55039, #178399, #78146, #108495, #166220, #107490, #198538, #135878, #123647, #183371, #197549, #169168, #12544, #27721, #59017, #62980, #30672, #170174, #199528, #181396, #120684, #153006, #182383, #313, #77163, #91314, #92325, #74209, #60996, #31667, #137847, #93317, #155001, #44853, #139814 ) ),
 .UNSPECIFIED., .T., .F., .F. ) 
 B_SPLINE_SURFACE_WITH_KNOTS ( ( 4, 3, 4 ),
 ( 3, 2, 2, 2, 2, 2, 2, 2, 2, 2, 2, 2, 2, 2, 2, 2, 2, 2, 2, 2, 2, 2, 2, 2, 2, 2, 2, 2, 2, 2, 2, 2, 2, 2, 2, 2, 2, 2, 2, 2, 2, 2, 2, 2, 2, 2, 2, 2, 2, 2, 2, 2, 2, 2, 2, 2, 2, 2, 2, 2, 2, 2, 2, 2, 2, 2, 2, 2, 2, 2, 2, 2, 2, 2, 2, 2, 2, 2, 2, 2, 2, 2, 2, 2, 2, 2, 2, 2, 2, 2, 2, 2, 2, 2, 2, 2, 2, 2, 2, 2, 2, 2, 2, 2, 2, 2, 2, 2, 2, 2, 2, 2, 2, 2, 2, 2, 2, 2, 2, 2, 2, 2, 2, 2, 2, 2, 2, 2, 2, 2, 2, 2, 2, 2, 2, 2, 2, 2, 2, 2, 2, 2, 2, 2, 2, 2, 2, 2, 2, 2, 2, 2, 2, 2, 2, 2, 2, 2, 2, 2, 2, 2, 2, 2, 2, 2, 2, 2, 2, 2, 2, 2, 2, 2, 2, 2, 2, 2, 2, 2, 2, 2, 2, 2, 2, 2, 2, 2, 2, 2, 2, 2, 2, 2, 2, 2, 2, 2, 2, 2, 2, 2, 2, 2, 2, 2, 2, 2, 2, 2, 2, 2, 2, 2, 2, 2, 2, 2, 2, 2, 2, 2, 2, 2, 2, 2, 2, 2, 3 ),
 ( 0.000000000000000000, 0.5000000000000000000, 1.000000000000000000 ),
 ( 0.000000000000000000, 0.004385964912280701511, 0.008771929824561403022, 0.01315789473684210453, 0.01754385964912280604, 0.02192982456140350755, 0.02631578947368420907, 0.03070175438596491058, 0.03508771929824561209, 0.03947368421052631360, 0.04385964912280701511, 0.04824561403508771662, 0.05263157894736841813, 0.05701754385964911964, 0.06140350877192982115, 0.06578947368421052266, 0.07017543859649122417, 0.07456140350877192569, 0.07894736842105262720, 0.08333333333333332871, 0.08771929824561403022, 0.09210526315789473173, 0.09649122807017543324, 0.1008771929824561348, 0.1052631578947368363, 0.1096491228070175378, 0.1140350877192982393, 0.1184210526315789408, 0.1228070175438596423, 0.1271929824561403577, 0.1315789473684210453, 0.1359649122807017607, 0.1403508771929824483, 0.1447368421052631637, 0.1491228070175438514, 0.1535087719298245668, 0.1578947368421052544, 0.1622807017543859698, 0.1666666666666666574, 0.1710526315789473728, 0.1754385964912280604, 0.1798245614035087758, 0.1842105263157894635, 0.1885964912280701788, 0.1929824561403508665, 0.1973684210526315819, 0.2017543859649122695, 0.2061403508771929849, 0.2105263157894736725, 0.2149122807017543879, 0.2192982456140350755, 0.2236842105263157909, 0.2280701754385964786, 0.2324561403508771940, 0.2368421052631578816, 0.2412280701754385970, 0.2456140350877192846, 0.2500000000000000000, 0.2543859649122807154, 0.2587719298245614308, 0.2631578947368420907, 0.2675438596491228060, 0.2719298245614035214, 0.2763157894736842368, 0.2807017543859648967, 0.2850877192982456121, 0.2894736842105263275, 0.2938596491228070429, 0.2982456140350877027, 0.3026315789473684181, 0.3070175438596491335, 0.3114035087719298489, 0.3157894736842105088, 0.3201754385964912242, 0.3245614035087719396, 0.3289473684210526550, 0.3333333333333333148, 0.3377192982456140302, 0.3421052631578947456, 0.3464912280701754610, 0.3508771929824561209, 0.3552631578947368363, 0.3596491228070175517, 0.3640350877192982670, 0.3684210526315789269, 0.3728070175438596423, 0.3771929824561403577, 0.3815789473684210731, 0.3859649122807017330, 0.3903508771929824483, 0.3947368421052631637, 0.3991228070175438791, 0.4035087719298245390, 0.4078947368421052544, 0.4122807017543859698, 0.4166666666666666852, 0.4210526315789473450, 0.4254385964912280604, 0.4298245614035087758, 0.4342105263157894912, 0.4385964912280701511, 0.4429824561403508665, 0.4473684210526315819, 0.4517543859649122973, 0.4561403508771929571, 0.4605263157894736725, 0.4649122807017543879, 0.4692982456140351033, 0.4736842105263157632, 0.4780701754385964786, 0.4824561403508771940, 0.4868421052631579093, 0.4912280701754385692, 0.4956140350877192846, 0.5000000000000000000, 0.5043859649122807154, 0.5087719298245614308, 0.5131578947368421462, 0.5175438596491228616, 0.5219298245614034659, 0.5263157894736841813, 0.5307017543859648967, 0.5350877192982456121, 0.5394736842105263275, 0.5438596491228070429, 0.5482456140350877583, 0.5526315789473684736, 0.5570175438596490780, 0.5614035087719297934, 0.5657894736842105088, 0.5701754385964912242, 0.5745614035087719396, 0.5789473684210526550, 0.5833333333333333703, 0.5877192982456140857, 0.5921052631578946901, 0.5964912280701754055, 0.6008771929824561209, 0.6052631578947368363, 0.6096491228070175517, 0.6140350877192982670, 0.6184210526315789824, 0.6228070175438596978, 0.6271929824561403022, 0.6315789473684210176, 0.6359649122807017330, 0.6403508771929824483, 0.6447368421052631637, 0.6491228070175438791, 0.6535087719298245945, 0.6578947368421053099, 0.6622807017543859143, 0.6666666666666666297, 0.6710526315789473450, 0.6754385964912280604, 0.6798245614035087758, 0.6842105263157894912, 0.6885964912280702066, 0.6929824561403509220, 0.6973684210526315264, 0.7017543859649122417, 0.7061403508771929571, 0.7105263157894736725, 0.7149122807017543879, 0.7192982456140351033, 0.7236842105263158187, 0.7280701754385965341, 0.7324561403508771384, 0.7368421052631578538, 0.7412280701754385692, 0.7456140350877192846, 0.7500000000000000000, 0.7543859649122807154, 0.7587719298245614308, 0.7631578947368421462, 0.7675438596491228616, 0.7719298245614034659, 0.7763157894736841813, 0.7807017543859648967, 0.7850877192982456121, 0.7894736842105263275, 0.7938596491228070429, 0.7982456140350877583, 0.8026315789473684736, 0.8070175438596490780, 0.8114035087719297934, 0.8157894736842105088, 0.8201754385964912242, 0.8245614035087719396, 0.8289473684210526550, 0.8333333333333333703, 0.8377192982456140857, 0.8421052631578946901, 0.8464912280701754055, 0.8508771929824561209, 0.8552631578947368363, 0.8596491228070175517, 0.8640350877192982670, 0.8684210526315789824, 0.8728070175438596978, 0.8771929824561403022, 0.8815789473684210176, 0.8859649122807017330, 0.8903508771929824483, 0.8947368421052631637, 0.8991228070175438791, 0.9035087719298245945, 0.9078947368421053099, 0.9122807017543859143, 0.9166666666666666297, 0.9210526315789473450, 0.9254385964912280604, 0.9298245614035087758, 0.9342105263157894912, 0.9385964912280702066, 0.9429824561403509220, 0.9473684210526315264, 0.9517543859649122417, 0.9561403508771929571, 0.9605263157894736725, 0.9649122807017543879, 0.9692982456140351033, 0.9736842105263158187, 0.9780701754385965341, 0.9824561403508771384, 0.9868421052631578538, 0.9912280701754385692, 0.9956140350877192846, 1.000000000000000000 ),
 .UNSPECIFIED. ) 
 GEOMETRIC_REPRESENTATION_ITEM ( )  RATIONAL_B_SPLINE_SURFACE ( (
 ( 1.000000000000000000, 0.9659258262890683122, 1.000000000000000000, 0.9659258262890683122, 1.000000000000000000, 0.9659258262890683122, 1.000000000000000000, 0.9659258262890683122, 1.000000000000000000, 0.9659258262890683122, 1.000000000000000000, 0.9659258262890683122, 1.000000000000000000, 0.9659258262890683122, 1.000000000000000000, 0.9659258262890683122, 1.000000000000000000, 0.9659258262890683122, 1.000000000000000000, 0.9659258262890683122, 1.000000000000000000, 0.9659258262890683122, 1.000000000000000000, 0.9659258262890683122, 1.000000000000000000, 0.9659258262890683122, 1.000000000000000000, 0.9659258262890683122, 1.000000000000000000, 0.9659258262890683122, 1.000000000000000000, 0.9659258262890683122, 1.000000000000000000, 0.9659258262890683122, 1.000000000000000000, 0.9659258262890683122, 1.000000000000000000, 0.9659258262890683122, 1.000000000000000000, 0.9659258262890683122, 1.000000000000000000, 0.9659258262890683122, 1.000000000000000000, 0.9659258262890683122, 1.000000000000000000, 0.9659258262890683122, 1.000000000000000000, 0.9659258262890683122, 1.000000000000000000, 0.9659258262890683122, 1.000000000000000000, 0.9659258262890683122, 1.000000000000000000, 0.9659258262890683122, 1.000000000000000000, 0.9659258262890683122, 1.000000000000000000, 0.9659258262890683122, 1.000000000000000000, 0.9659258262890683122, 1.000000000000000000, 0.9659258262890683122, 1.000000000000000000, 0.9659258262890683122, 1.000000000000000000, 0.9659258262890683122, 1.000000000000000000, 0.9659258262890683122, 1.000000000000000000, 0.9659258262890683122, 1.000000000000000000, 0.9659258262890683122, 1.000000000000000000, 0.9659258262890683122, 1.000000000000000000, 0.9659258262890683122, 1.000000000000000000, 0.9659258262890683122, 1.000000000000000000, 0.9659258262890683122, 1.000000000000000000, 0.9659258262890683122, 1.000000000000000000, 0.9659258262890683122, 1.000000000000000000, 0.9659258262890683122, 1.000000000000000000, 0.9659258262890683122, 1.000000000000000000, 0.9659258262890683122, 1.000000000000000000, 0.9659258262890683122, 1.000000000000000000, 0.9659258262890683122, 1.000000000000000000, 0.9659258262890683122, 1.000000000000000000, 0.9659258262890683122, 1.000000000000000000, 0.9659258262890683122, 1.000000000000000000, 0.9659258262890683122, 1.000000000000000000, 0.9659258262890683122, 1.000000000000000000, 0.9659258262890683122, 1.000000000000000000, 0.9659258262890683122, 1.000000000000000000, 0.9659258262890683122, 1.000000000000000000, 0.9659258262890683122, 1.000000000000000000, 0.9659258262890683122, 1.000000000000000000, 0.9659258262890683122, 1.000000000000000000, 0.9659258262890683122, 1.000000000000000000, 0.9659258262890683122, 1.000000000000000000, 0.9659258262890683122, 1.000000000000000000, 0.9659258262890683122, 1.000000000000000000, 0.9659258262890683122, 1.000000000000000000, 0.9659258262890683122, 1.000000000000000000, 0.9659258262890683122, 1.000000000000000000, 0.9659258262890683122, 1.000000000000000000, 0.9659258262890683122, 1.000000000000000000, 0.9659258262890683122, 1.000000000000000000, 0.9659258262890683122, 1.000000000000000000, 0.9659258262890683122, 1.000000000000000000, 0.9659258262890683122, 1.000000000000000000, 0.9659258262890683122, 1.000000000000000000, 0.9659258262890683122, 1.000000000000000000, 0.9659258262890683122, 1.000000000000000000, 0.9659258262890683122, 1.000000000000000000, 0.9659258262890683122, 1.000000000000000000, 0.9659258262890683122, 1.000000000000000000, 0.9659258262890683122, 1.000000000000000000, 0.9659258262890683122, 1.000000000000000000, 0.9659258262890683122, 1.000000000000000000, 0.9659258262890683122, 1.000000000000000000, 0.9659258262890683122, 1.000000000000000000, 0.9659258262890683122, 1.000000000000000000, 0.9659258262890683122, 1.000000000000000000, 0.9659258262890683122, 1.000000000000000000, 0.9659258262890683122, 1.000000000000000000, 0.9659258262890683122, 1.000000000000000000, 0.9659258262890683122, 1.000000000000000000, 0.9659258262890683122, 1.000000000000000000, 0.9659258262890683122, 1.000000000000000000, 0.9659258262890683122, 1.000000000000000000, 0.9659258262890683122, 1.000000000000000000, 0.9659258262890683122, 1.000000000000000000, 0.9659258262890683122, 1.000000000000000000, 0.9659258262890683122, 1.000000000000000000, 0.9659258262890683122, 1.000000000000000000, 0.9659258262890683122, 1.000000000000000000, 0.9659258262890683122, 1.000000000000000000, 0.9659258262890683122, 1.000000000000000000, 0.9659258262890683122, 1.000000000000000000, 0.9659258262890683122, 1.000000000000000000, 0.9659258262890683122, 1.000000000000000000, 0.9659258262890683122, 1.000000000000000000, 0.9659258262890683122, 1.000000000000000000, 0.9659258262890683122, 1.000000000000000000, 0.9659258262890683122, 1.000000000000000000, 0.9659258262890683122, 1.000000000000000000, 0.9659258262890683122, 1.000000000000000000, 0.9659258262890683122, 1.000000000000000000, 0.9659258262890683122, 1.000000000000000000, 0.9659258262890683122, 1.000000000000000000, 0.9659258262890683122, 1.000000000000000000, 0.9659258262890683122, 1.000000000000000000, 0.9659258262890683122, 1.000000000000000000, 0.9659258262890683122, 1.000000000000000000, 0.9659258262890683122, 1.000000000000000000, 0.9659258262890683122, 1.000000000000000000, 0.9659258262890683122, 1.000000000000000000, 0.9659258262890683122, 1.000000000000000000, 0.9659258262890683122, 1.000000000000000000, 0.9659258262890683122, 1.000000000000000000, 0.9659258262890683122, 1.000000000000000000, 0.9659258262890683122, 1.000000000000000000, 0.9659258262890683122, 1.000000000000000000, 0.9659258262890683122, 1.000000000000000000, 0.9659258262890683122, 1.000000000000000000, 0.9659258262890683122, 1.000000000000000000, 0.9659258262890683122, 1.000000000000000000, 0.9659258262890683122, 1.000000000000000000, 0.9659258262890683122, 1.000000000000000000, 0.9659258262890683122, 1.000000000000000000, 0.9659258262890683122, 1.000000000000000000, 0.9659258262890683122, 1.000000000000000000, 0.9659258262890683122, 1.000000000000000000, 0.9659258262890683122, 1.000000000000000000, 0.9659258262890683122, 1.000000000000000000, 0.9659258262890683122, 1.000000000000000000, 0.9659258262890683122, 1.000000000000000000, 0.9659258262890683122, 1.000000000000000000, 0.9659258262890683122, 1.000000000000000000, 0.9659258262890683122, 1.000000000000000000, 0.9659258262890683122, 1.000000000000000000, 0.9659258262890683122, 1.000000000000000000, 0.9659258262890683122, 1.000000000000000000, 0.9659258262890683122, 1.000000000000000000, 0.9659258262890683122, 1.000000000000000000, 0.9659258262890683122, 1.000000000000000000, 0.9659258262890683122, 1.000000000000000000, 0.9659258262890683122, 1.000000000000000000, 0.9659258262890683122, 1.000000000000000000, 0.9659258262890683122, 1.000000000000000000, 0.9659258262890683122, 1.000000000000000000, 0.9659258262890683122, 1.000000000000000000, 0.9659258262890683122, 1.000000000000000000, 0.9659258262890683122, 1.000000000000000000, 0.9659258262890683122, 1.000000000000000000, 0.9659258262890683122, 1.000000000000000000, 0.9659258262890683122, 1.000000000000000000, 0.9659258262890683122, 1.000000000000000000, 0.9659258262890683122, 1.000000000000000000, 0.9659258262890683122, 1.000000000000000000, 0.9659258262890683122, 1.000000000000000000, 0.9659258262890683122, 1.000000000000000000, 0.9659258262890683122, 1.000000000000000000, 0.9659258262890683122, 1.000000000000000000, 0.9659258262890683122, 1.000000000000000000, 0.9659258262890683122, 1.000000000000000000, 0.9659258262890683122, 1.000000000000000000, 0.9659258262890683122, 1.000000000000000000, 0.9659258262890683122, 1.000000000000000000, 0.9659258262890683122, 1.000000000000000000, 0.9659258262890683122, 1.000000000000000000, 0.9659258262890683122, 1.000000000000000000, 0.9659258262890683122, 1.000000000000000000, 0.9659258262890683122, 1.000000000000000000, 0.9659258262890683122, 1.000000000000000000, 0.9659258262890683122, 1.000000000000000000, 0.9659258262890683122, 1.000000000000000000, 0.9659258262890683122, 1.000000000000000000, 0.9659258262890683122, 1.000000000000000000, 0.9659258262890683122, 1.000000000000000000, 0.9659258262890683122, 1.000000000000000000, 0.9659258262890683122, 1.000000000000000000, 0.9659258262890683122, 1.000000000000000000, 0.9659258262890683122, 1.000000000000000000, 0.9659258262890683122, 1.000000000000000000, 0.9659258262890683122, 1.000000000000000000, 0.9659258262890683122, 1.000000000000000000, 0.9659258262890683122, 1.000000000000000000, 0.9659258262890683122, 1.000000000000000000, 0.9659258262890683122, 1.000000000000000000, 0.9659258262890683122, 1.000000000000000000, 0.9659258262890683122, 1.000000000000000000, 0.9659258262890683122, 1.000000000000000000, 0.9659258262890683122, 1.000000000000000000, 0.9659258262890683122, 1.000000000000000000, 0.9659258262890683122, 1.000000000000000000, 0.9659258262890683122, 1.000000000000000000, 0.9659258262890683122, 1.000000000000000000, 0.9659258262890683122, 1.000000000000000000, 0.9659258262890683122, 1.000000000000000000, 0.9659258262890683122, 1.000000000000000000, 0.9659258262890683122, 1.000000000000000000, 0.9659258262890683122, 1.000000000000000000, 0.9659258262890683122, 1.000000000000000000, 0.9659258262890683122, 1.000000000000000000, 0.9659258262890683122, 1.000000000000000000, 0.9659258262890683122, 1.000000000000000000, 0.9659258262890683122, 1.000000000000000000, 0.9659258262890683122, 1.000000000000000000, 0.9659258262890683122, 1.000000000000000000, 0.9659258262890683122, 1.000000000000000000, 0.9659258262890683122, 1.000000000000000000, 0.9659258262890683122, 1.000000000000000000, 0.9659258262890683122, 1.000000000000000000, 0.9659258262890683122, 1.000000000000000000, 0.9659258262890683122, 1.000000000000000000, 0.9659258262890683122, 1.000000000000000000, 0.9659258262890683122, 1.000000000000000000, 0.9659258262890683122, 1.000000000000000000, 0.9659258262890683122, 1.000000000000000000, 0.9659258262890683122, 1.000000000000000000, 0.9659258262890683122, 1.000000000000000000, 0.9659258262890683122, 1.000000000000000000, 0.9659258262890683122, 1.000000000000000000, 0.9659258262890683122, 1.000000000000000000, 0.9659258262890683122, 1.000000000000000000, 0.9659258262890683122, 1.000000000000000000),
 ( 0.3333333333333333703, 0.3219752754296894559, 0.3333333333333333703, 0.3219752754296894559, 0.3333333333333333703, 0.3219752754296894559, 0.3333333333333333703, 0.3219752754296894559, 0.3333333333333333703, 0.3219752754296894559, 0.3333333333333333703, 0.3219752754296894559, 0.3333333333333333703, 0.3219752754296894559, 0.3333333333333333703, 0.3219752754296894559, 0.3333333333333333703, 0.3219752754296894559, 0.3333333333333333703, 0.3219752754296894559, 0.3333333333333333703, 0.3219752754296894559, 0.3333333333333333703, 0.3219752754296894559, 0.3333333333333333703, 0.3219752754296894559, 0.3333333333333333703, 0.3219752754296894559, 0.3333333333333333703, 0.3219752754296894559, 0.3333333333333333703, 0.3219752754296894559, 0.3333333333333333703, 0.3219752754296894559, 0.3333333333333333703, 0.3219752754296894559, 0.3333333333333333703, 0.3219752754296894559, 0.3333333333333333703, 0.3219752754296894559, 0.3333333333333333703, 0.3219752754296894559, 0.3333333333333333703, 0.3219752754296894559, 0.3333333333333333703, 0.3219752754296894559, 0.3333333333333333703, 0.3219752754296894559, 0.3333333333333333703, 0.3219752754296894559, 0.3333333333333333703, 0.3219752754296894559, 0.3333333333333333703, 0.3219752754296894559, 0.3333333333333333703, 0.3219752754296894559, 0.3333333333333333703, 0.3219752754296894559, 0.3333333333333333703, 0.3219752754296894559, 0.3333333333333333703, 0.3219752754296894559, 0.3333333333333333703, 0.3219752754296894559, 0.3333333333333333703, 0.3219752754296894559, 0.3333333333333333703, 0.3219752754296894559, 0.3333333333333333703, 0.3219752754296894559, 0.3333333333333333703, 0.3219752754296894559, 0.3333333333333333703, 0.3219752754296894559, 0.3333333333333333703, 0.3219752754296894559, 0.3333333333333333703, 0.3219752754296894559, 0.3333333333333333703, 0.3219752754296894559, 0.3333333333333333703, 0.3219752754296894559, 0.3333333333333333703, 0.3219752754296894559, 0.3333333333333333703, 0.3219752754296894559, 0.3333333333333333703, 0.3219752754296894559, 0.3333333333333333703, 0.3219752754296894559, 0.3333333333333333703, 0.3219752754296894559, 0.3333333333333333703, 0.3219752754296894559, 0.3333333333333333703, 0.3219752754296894559, 0.3333333333333333703, 0.3219752754296894559, 0.3333333333333333703, 0.3219752754296894559, 0.3333333333333333703, 0.3219752754296894559, 0.3333333333333333703, 0.3219752754296894559, 0.3333333333333333703, 0.3219752754296894559, 0.3333333333333333703, 0.3219752754296894559, 0.3333333333333333703, 0.3219752754296894559, 0.3333333333333333703, 0.3219752754296894559, 0.3333333333333333703, 0.3219752754296894559, 0.3333333333333333703, 0.3219752754296894559, 0.3333333333333333703, 0.3219752754296894559, 0.3333333333333333703, 0.3219752754296894559, 0.3333333333333333703, 0.3219752754296894559, 0.3333333333333333703, 0.3219752754296894559, 0.3333333333333333703, 0.3219752754296894559, 0.3333333333333333703, 0.3219752754296894559, 0.3333333333333333703, 0.3219752754296894559, 0.3333333333333333703, 0.3219752754296894559, 0.3333333333333333703, 0.3219752754296894559, 0.3333333333333333703, 0.3219752754296894559, 0.3333333333333333703, 0.3219752754296894559, 0.3333333333333333703, 0.3219752754296894559, 0.3333333333333333703, 0.3219752754296894559, 0.3333333333333333703, 0.3219752754296894559, 0.3333333333333333703, 0.3219752754296894559, 0.3333333333333333703, 0.3219752754296894559, 0.3333333333333333703, 0.3219752754296894559, 0.3333333333333333703, 0.3219752754296894559, 0.3333333333333333703, 0.3219752754296894559, 0.3333333333333333703, 0.3219752754296894559, 0.3333333333333333703, 0.3219752754296894559, 0.3333333333333333703, 0.3219752754296894559, 0.3333333333333333703, 0.3219752754296894559, 0.3333333333333333703, 0.3219752754296894559, 0.3333333333333333703, 0.3219752754296894559, 0.3333333333333333703, 0.3219752754296894559, 0.3333333333333333703, 0.3219752754296894559, 0.3333333333333333703, 0.3219752754296894559, 0.3333333333333333703, 0.3219752754296894559, 0.3333333333333333703, 0.3219752754296894559, 0.3333333333333333703, 0.3219752754296894559, 0.3333333333333333703, 0.3219752754296894559, 0.3333333333333333703, 0.3219752754296894559, 0.3333333333333333703, 0.3219752754296894559, 0.3333333333333333703, 0.3219752754296894559, 0.3333333333333333703, 0.3219752754296894559, 0.3333333333333333703, 0.3219752754296894559, 0.3333333333333333703, 0.3219752754296894559, 0.3333333333333333703, 0.3219752754296894559, 0.3333333333333333703, 0.3219752754296894559, 0.3333333333333333703, 0.3219752754296894559, 0.3333333333333333703, 0.3219752754296894559, 0.3333333333333333703, 0.3219752754296894559, 0.3333333333333333703, 0.3219752754296894559, 0.3333333333333333703, 0.3219752754296894559, 0.3333333333333333703, 0.3219752754296894559, 0.3333333333333333703, 0.3219752754296894559, 0.3333333333333333703, 0.3219752754296894559, 0.3333333333333333703, 0.3219752754296894559, 0.3333333333333333703, 0.3219752754296894559, 0.3333333333333333703, 0.3219752754296894559, 0.3333333333333333703, 0.3219752754296894559, 0.3333333333333333703, 0.3219752754296894559, 0.3333333333333333703, 0.3219752754296894559, 0.3333333333333333703, 0.3219752754296894559, 0.3333333333333333703, 0.3219752754296894559, 0.3333333333333333703, 0.3219752754296894559, 0.3333333333333333703, 0.3219752754296894559, 0.3333333333333333703, 0.3219752754296894559, 0.3333333333333333703, 0.3219752754296894559, 0.3333333333333333703, 0.3219752754296894559, 0.3333333333333333703, 0.3219752754296894559, 0.3333333333333333703, 0.3219752754296894559, 0.3333333333333333703, 0.3219752754296894559, 0.3333333333333333703, 0.3219752754296894559, 0.3333333333333333703, 0.3219752754296894559, 0.3333333333333333703, 0.3219752754296894559, 0.3333333333333333703, 0.3219752754296894559, 0.3333333333333333703, 0.3219752754296894559, 0.3333333333333333703, 0.3219752754296894559, 0.3333333333333333703, 0.3219752754296894559, 0.3333333333333333703, 0.3219752754296894559, 0.3333333333333333703, 0.3219752754296894559, 0.3333333333333333703, 0.3219752754296894559, 0.3333333333333333703, 0.3219752754296894559, 0.3333333333333333703, 0.3219752754296894559, 0.3333333333333333703, 0.3219752754296894559, 0.3333333333333333703, 0.3219752754296894559, 0.3333333333333333703, 0.3219752754296894559, 0.3333333333333333703, 0.3219752754296894559, 0.3333333333333333703, 0.3219752754296894559, 0.3333333333333333703, 0.3219752754296894559, 0.3333333333333333703, 0.3219752754296894559, 0.3333333333333333703, 0.3219752754296894559, 0.3333333333333333703, 0.3219752754296894559, 0.3333333333333333703, 0.3219752754296894559, 0.3333333333333333703, 0.3219752754296894559, 0.3333333333333333703, 0.3219752754296894559, 0.3333333333333333703, 0.3219752754296894559, 0.3333333333333333703, 0.3219752754296894559, 0.3333333333333333703, 0.3219752754296894559, 0.3333333333333333703, 0.3219752754296894559, 0.3333333333333333703, 0.3219752754296894559, 0.3333333333333333703, 0.3219752754296894559, 0.3333333333333333703, 0.3219752754296894559, 0.3333333333333333703, 0.3219752754296894559, 0.3333333333333333703, 0.3219752754296894559, 0.3333333333333333703, 0.3219752754296894559, 0.3333333333333333703, 0.3219752754296894559, 0.3333333333333333703, 0.3219752754296894559, 0.3333333333333333703, 0.3219752754296894559, 0.3333333333333333703, 0.3219752754296894559, 0.3333333333333333703, 0.3219752754296894559, 0.3333333333333333703, 0.3219752754296894559, 0.3333333333333333703, 0.3219752754296894559, 0.3333333333333333703, 0.3219752754296894559, 0.3333333333333333703, 0.3219752754296894559, 0.3333333333333333703, 0.3219752754296894559, 0.3333333333333333703, 0.3219752754296894559, 0.3333333333333333703, 0.3219752754296894559, 0.3333333333333333703, 0.3219752754296894559, 0.3333333333333333703, 0.3219752754296894559, 0.3333333333333333703, 0.3219752754296894559, 0.3333333333333333703, 0.3219752754296894559, 0.3333333333333333703, 0.3219752754296894559, 0.3333333333333333703, 0.3219752754296894559, 0.3333333333333333703, 0.3219752754296894559, 0.3333333333333333703, 0.3219752754296894559, 0.3333333333333333703, 0.3219752754296894559, 0.3333333333333333703, 0.3219752754296894559, 0.3333333333333333703, 0.3219752754296894559, 0.3333333333333333703, 0.3219752754296894559, 0.3333333333333333703, 0.3219752754296894559, 0.3333333333333333703, 0.3219752754296894559, 0.3333333333333333703, 0.3219752754296894559, 0.3333333333333333703, 0.3219752754296894559, 0.3333333333333333703, 0.3219752754296894559, 0.3333333333333333703, 0.3219752754296894559, 0.3333333333333333703, 0.3219752754296894559, 0.3333333333333333703, 0.3219752754296894559, 0.3333333333333333703, 0.3219752754296894559, 0.3333333333333333703, 0.3219752754296894559, 0.3333333333333333703, 0.3219752754296894559, 0.3333333333333333703, 0.3219752754296894559, 0.3333333333333333703, 0.3219752754296894559, 0.3333333333333333703, 0.3219752754296894559, 0.3333333333333333703, 0.3219752754296894559, 0.3333333333333333703, 0.3219752754296894559, 0.3333333333333333703, 0.3219752754296894559, 0.3333333333333333703, 0.3219752754296894559, 0.3333333333333333703, 0.3219752754296894559, 0.3333333333333333703, 0.3219752754296894559, 0.3333333333333333703, 0.3219752754296894559, 0.3333333333333333703, 0.3219752754296894559, 0.3333333333333333703, 0.3219752754296894559, 0.3333333333333333703, 0.3219752754296894559, 0.3333333333333333703, 0.3219752754296894559, 0.3333333333333333703, 0.3219752754296894559, 0.3333333333333333703, 0.3219752754296894559, 0.3333333333333333703, 0.3219752754296894559, 0.3333333333333333703, 0.3219752754296894559, 0.3333333333333333703, 0.3219752754296894559, 0.3333333333333333703, 0.3219752754296894559, 0.3333333333333333703, 0.3219752754296894559, 0.3333333333333333703, 0.3219752754296894559, 0.3333333333333333703, 0.3219752754296894559, 0.3333333333333333703, 0.3219752754296894559, 0.3333333333333333703, 0.3219752754296894559, 0.3333333333333333703, 0.3219752754296894559, 0.3333333333333333703, 0.3219752754296894559, 0.3333333333333333703, 0.3219752754296894559, 0.3333333333333333703, 0.3219752754296894559, 0.3333333333333333703, 0.3219752754296894559, 0.3333333333333333703, 0.3219752754296894559, 0.3333333333333333703, 0.3219752754296894559, 0.3333333333333333703, 0.3219752754296894559, 0.3333333333333333703, 0.3219752754296894559, 0.3333333333333333703, 0.3219752754296894559, 0.3333333333333333703, 0.3219752754296894559, 0.3333333333333333703, 0.3219752754296894559, 0.3333333333333333703),
 ( 0.3333333333333333703, 0.3219752754296894559, 0.3333333333333333703, 0.3219752754296894559, 0.3333333333333333703, 0.3219752754296894559, 0.3333333333333333703, 0.3219752754296894559, 0.3333333333333333703, 0.3219752754296894559, 0.3333333333333333703, 0.3219752754296894559, 0.3333333333333333703, 0.3219752754296894559, 0.3333333333333333703, 0.3219752754296894559, 0.3333333333333333703, 0.3219752754296894559, 0.3333333333333333703, 0.3219752754296894559, 0.3333333333333333703, 0.3219752754296894559, 0.3333333333333333703, 0.3219752754296894559, 0.3333333333333333703, 0.3219752754296894559, 0.3333333333333333703, 0.3219752754296894559, 0.3333333333333333703, 0.3219752754296894559, 0.3333333333333333703, 0.3219752754296894559, 0.3333333333333333703, 0.3219752754296894559, 0.3333333333333333703, 0.3219752754296894559, 0.3333333333333333703, 0.3219752754296894559, 0.3333333333333333703, 0.3219752754296894559, 0.3333333333333333703, 0.3219752754296894559, 0.3333333333333333703, 0.3219752754296894559, 0.3333333333333333703, 0.3219752754296894559, 0.3333333333333333703, 0.3219752754296894559, 0.3333333333333333703, 0.3219752754296894559, 0.3333333333333333703, 0.3219752754296894559, 0.3333333333333333703, 0.3219752754296894559, 0.3333333333333333703, 0.3219752754296894559, 0.3333333333333333703, 0.3219752754296894559, 0.3333333333333333703, 0.3219752754296894559, 0.3333333333333333703, 0.3219752754296894559, 0.3333333333333333703, 0.3219752754296894559, 0.3333333333333333703, 0.3219752754296894559, 0.3333333333333333703, 0.3219752754296894559, 0.3333333333333333703, 0.3219752754296894559, 0.3333333333333333703, 0.3219752754296894559, 0.3333333333333333703, 0.3219752754296894559, 0.3333333333333333703, 0.3219752754296894559, 0.3333333333333333703, 0.3219752754296894559, 0.3333333333333333703, 0.3219752754296894559, 0.3333333333333333703, 0.3219752754296894559, 0.3333333333333333703, 0.3219752754296894559, 0.3333333333333333703, 0.3219752754296894559, 0.3333333333333333703, 0.3219752754296894559, 0.3333333333333333703, 0.3219752754296894559, 0.3333333333333333703, 0.3219752754296894559, 0.3333333333333333703, 0.3219752754296894559, 0.3333333333333333703, 0.3219752754296894559, 0.3333333333333333703, 0.3219752754296894559, 0.3333333333333333703, 0.3219752754296894559, 0.3333333333333333703, 0.3219752754296894559, 0.3333333333333333703, 0.3219752754296894559, 0.3333333333333333703, 0.3219752754296894559, 0.3333333333333333703, 0.3219752754296894559, 0.3333333333333333703, 0.3219752754296894559, 0.3333333333333333703, 0.3219752754296894559, 0.3333333333333333703, 0.3219752754296894559, 0.3333333333333333703, 0.3219752754296894559, 0.3333333333333333703, 0.3219752754296894559, 0.3333333333333333703, 0.3219752754296894559, 0.3333333333333333703, 0.3219752754296894559, 0.3333333333333333703, 0.3219752754296894559, 0.3333333333333333703, 0.3219752754296894559, 0.3333333333333333703, 0.3219752754296894559, 0.3333333333333333703, 0.3219752754296894559, 0.3333333333333333703, 0.3219752754296894559, 0.3333333333333333703, 0.3219752754296894559, 0.3333333333333333703, 0.3219752754296894559, 0.3333333333333333703, 0.3219752754296894559, 0.3333333333333333703, 0.3219752754296894559, 0.3333333333333333703, 0.3219752754296894559, 0.3333333333333333703, 0.3219752754296894559, 0.3333333333333333703, 0.3219752754296894559, 0.3333333333333333703, 0.3219752754296894559, 0.3333333333333333703, 0.3219752754296894559, 0.3333333333333333703, 0.3219752754296894559, 0.3333333333333333703, 0.3219752754296894559, 0.3333333333333333703, 0.3219752754296894559, 0.3333333333333333703, 0.3219752754296894559, 0.3333333333333333703, 0.3219752754296894559, 0.3333333333333333703, 0.3219752754296894559, 0.3333333333333333703, 0.3219752754296894559, 0.3333333333333333703, 0.3219752754296894559, 0.3333333333333333703, 0.3219752754296894559, 0.3333333333333333703, 0.3219752754296894559, 0.3333333333333333703, 0.3219752754296894559, 0.3333333333333333703, 0.3219752754296894559, 0.3333333333333333703, 0.3219752754296894559, 0.3333333333333333703, 0.3219752754296894559, 0.3333333333333333703, 0.3219752754296894559, 0.3333333333333333703, 0.3219752754296894559, 0.3333333333333333703, 0.3219752754296894559, 0.3333333333333333703, 0.3219752754296894559, 0.3333333333333333703, 0.3219752754296894559, 0.3333333333333333703, 0.3219752754296894559, 0.3333333333333333703, 0.3219752754296894559, 0.3333333333333333703, 0.3219752754296894559, 0.3333333333333333703, 0.3219752754296894559, 0.3333333333333333703, 0.3219752754296894559, 0.3333333333333333703, 0.3219752754296894559, 0.3333333333333333703, 0.3219752754296894559, 0.3333333333333333703, 0.3219752754296894559, 0.3333333333333333703, 0.3219752754296894559, 0.3333333333333333703, 0.3219752754296894559, 0.3333333333333333703, 0.3219752754296894559, 0.3333333333333333703, 0.3219752754296894559, 0.3333333333333333703, 0.3219752754296894559, 0.3333333333333333703, 0.3219752754296894559, 0.3333333333333333703, 0.3219752754296894559, 0.3333333333333333703, 0.3219752754296894559, 0.3333333333333333703, 0.3219752754296894559, 0.3333333333333333703, 0.3219752754296894559, 0.3333333333333333703, 0.3219752754296894559, 0.3333333333333333703, 0.3219752754296894559, 0.3333333333333333703, 0.3219752754296894559, 0.3333333333333333703, 0.3219752754296894559, 0.3333333333333333703, 0.3219752754296894559, 0.3333333333333333703, 0.3219752754296894559, 0.3333333333333333703, 0.3219752754296894559, 0.3333333333333333703, 0.3219752754296894559, 0.3333333333333333703, 0.3219752754296894559, 0.3333333333333333703, 0.3219752754296894559, 0.3333333333333333703, 0.3219752754296894559, 0.3333333333333333703, 0.3219752754296894559, 0.3333333333333333703, 0.3219752754296894559, 0.3333333333333333703, 0.3219752754296894559, 0.3333333333333333703, 0.3219752754296894559, 0.3333333333333333703, 0.3219752754296894559, 0.3333333333333333703, 0.3219752754296894559, 0.3333333333333333703, 0.3219752754296894559, 0.3333333333333333703, 0.3219752754296894559, 0.3333333333333333703, 0.3219752754296894559, 0.3333333333333333703, 0.3219752754296894559, 0.3333333333333333703, 0.3219752754296894559, 0.3333333333333333703, 0.3219752754296894559, 0.3333333333333333703, 0.3219752754296894559, 0.3333333333333333703, 0.3219752754296894559, 0.3333333333333333703, 0.3219752754296894559, 0.3333333333333333703, 0.3219752754296894559, 0.3333333333333333703, 0.3219752754296894559, 0.3333333333333333703, 0.3219752754296894559, 0.3333333333333333703, 0.3219752754296894559, 0.3333333333333333703, 0.3219752754296894559, 0.3333333333333333703, 0.3219752754296894559, 0.3333333333333333703, 0.3219752754296894559, 0.3333333333333333703, 0.3219752754296894559, 0.3333333333333333703, 0.3219752754296894559, 0.3333333333333333703, 0.3219752754296894559, 0.3333333333333333703, 0.3219752754296894559, 0.3333333333333333703, 0.3219752754296894559, 0.3333333333333333703, 0.3219752754296894559, 0.3333333333333333703, 0.3219752754296894559, 0.3333333333333333703, 0.3219752754296894559, 0.3333333333333333703, 0.3219752754296894559, 0.3333333333333333703, 0.3219752754296894559, 0.3333333333333333703, 0.3219752754296894559, 0.3333333333333333703, 0.3219752754296894559, 0.3333333333333333703, 0.3219752754296894559, 0.3333333333333333703, 0.3219752754296894559, 0.3333333333333333703, 0.3219752754296894559, 0.3333333333333333703, 0.3219752754296894559, 0.3333333333333333703, 0.3219752754296894559, 0.3333333333333333703, 0.3219752754296894559, 0.3333333333333333703, 0.3219752754296894559, 0.3333333333333333703, 0.3219752754296894559, 0.3333333333333333703, 0.3219752754296894559, 0.3333333333333333703, 0.3219752754296894559, 0.3333333333333333703, 0.3219752754296894559, 0.3333333333333333703, 0.3219752754296894559, 0.3333333333333333703, 0.3219752754296894559, 0.3333333333333333703, 0.3219752754296894559, 0.3333333333333333703, 0.3219752754296894559, 0.3333333333333333703, 0.3219752754296894559, 0.3333333333333333703, 0.3219752754296894559, 0.3333333333333333703, 0.3219752754296894559, 0.3333333333333333703, 0.3219752754296894559, 0.3333333333333333703, 0.3219752754296894559, 0.3333333333333333703, 0.3219752754296894559, 0.3333333333333333703, 0.3219752754296894559, 0.3333333333333333703, 0.3219752754296894559, 0.3333333333333333703, 0.3219752754296894559, 0.3333333333333333703, 0.3219752754296894559, 0.3333333333333333703, 0.3219752754296894559, 0.3333333333333333703, 0.3219752754296894559, 0.3333333333333333703, 0.3219752754296894559, 0.3333333333333333703, 0.3219752754296894559, 0.3333333333333333703, 0.3219752754296894559, 0.3333333333333333703, 0.3219752754296894559, 0.3333333333333333703, 0.3219752754296894559, 0.3333333333333333703, 0.3219752754296894559, 0.3333333333333333703, 0.3219752754296894559, 0.3333333333333333703, 0.3219752754296894559, 0.3333333333333333703, 0.3219752754296894559, 0.3333333333333333703, 0.3219752754296894559, 0.3333333333333333703, 0.3219752754296894559, 0.3333333333333333703, 0.3219752754296894559, 0.3333333333333333703, 0.3219752754296894559, 0.3333333333333333703, 0.3219752754296894559, 0.3333333333333333703, 0.3219752754296894559, 0.3333333333333333703, 0.3219752754296894559, 0.3333333333333333703, 0.3219752754296894559, 0.3333333333333333703, 0.3219752754296894559, 0.3333333333333333703, 0.3219752754296894559, 0.3333333333333333703, 0.3219752754296894559, 0.3333333333333333703, 0.3219752754296894559, 0.3333333333333333703, 0.3219752754296894559, 0.3333333333333333703, 0.3219752754296894559, 0.3333333333333333703, 0.3219752754296894559, 0.3333333333333333703, 0.3219752754296894559, 0.3333333333333333703, 0.3219752754296894559, 0.3333333333333333703, 0.3219752754296894559, 0.3333333333333333703, 0.3219752754296894559, 0.3333333333333333703, 0.3219752754296894559, 0.3333333333333333703, 0.3219752754296894559, 0.3333333333333333703, 0.3219752754296894559, 0.3333333333333333703, 0.3219752754296894559, 0.3333333333333333703, 0.3219752754296894559, 0.3333333333333333703, 0.3219752754296894559, 0.3333333333333333703, 0.3219752754296894559, 0.3333333333333333703, 0.3219752754296894559, 0.3333333333333333703, 0.3219752754296894559, 0.3333333333333333703, 0.3219752754296894559, 0.3333333333333333703, 0.3219752754296894559, 0.3333333333333333703, 0.3219752754296894559, 0.3333333333333333703, 0.3219752754296894559, 0.3333333333333333703, 0.3219752754296894559, 0.3333333333333333703, 0.3219752754296894559, 0.3333333333333333703, 0.3219752754296894559, 0.3333333333333333703),
 ( 1.000000000000000000, 0.9659258262890683122, 1.000000000000000000, 0.9659258262890683122, 1.000000000000000000, 0.9659258262890683122, 1.000000000000000000, 0.9659258262890683122, 1.000000000000000000, 0.9659258262890683122, 1.000000000000000000, 0.9659258262890683122, 1.000000000000000000, 0.9659258262890683122, 1.000000000000000000, 0.9659258262890683122, 1.000000000000000000, 0.9659258262890683122, 1.000000000000000000, 0.9659258262890683122, 1.000000000000000000, 0.9659258262890683122, 1.000000000000000000, 0.9659258262890683122, 1.000000000000000000, 0.9659258262890683122, 1.000000000000000000, 0.9659258262890683122, 1.000000000000000000, 0.9659258262890683122, 1.000000000000000000, 0.9659258262890683122, 1.000000000000000000, 0.9659258262890683122, 1.000000000000000000, 0.9659258262890683122, 1.000000000000000000, 0.9659258262890683122, 1.000000000000000000, 0.9659258262890683122, 1.000000000000000000, 0.9659258262890683122, 1.000000000000000000, 0.9659258262890683122, 1.000000000000000000, 0.9659258262890683122, 1.000000000000000000, 0.9659258262890683122, 1.000000000000000000, 0.9659258262890683122, 1.000000000000000000, 0.9659258262890683122, 1.000000000000000000, 0.9659258262890683122, 1.000000000000000000, 0.9659258262890683122, 1.000000000000000000, 0.9659258262890683122, 1.000000000000000000, 0.9659258262890683122, 1.000000000000000000, 0.9659258262890683122, 1.000000000000000000, 0.9659258262890683122, 1.000000000000000000, 0.9659258262890683122, 1.000000000000000000, 0.9659258262890683122, 1.000000000000000000, 0.9659258262890683122, 1.000000000000000000, 0.9659258262890683122, 1.000000000000000000, 0.9659258262890683122, 1.000000000000000000, 0.9659258262890683122, 1.000000000000000000, 0.9659258262890683122, 1.000000000000000000, 0.9659258262890683122, 1.000000000000000000, 0.9659258262890683122, 1.000000000000000000, 0.9659258262890683122, 1.000000000000000000, 0.9659258262890683122, 1.000000000000000000, 0.9659258262890683122, 1.000000000000000000, 0.9659258262890683122, 1.000000000000000000, 0.9659258262890683122, 1.000000000000000000, 0.9659258262890683122, 1.000000000000000000, 0.9659258262890683122, 1.000000000000000000, 0.9659258262890683122, 1.000000000000000000, 0.9659258262890683122, 1.000000000000000000, 0.9659258262890683122, 1.000000000000000000, 0.9659258262890683122, 1.000000000000000000, 0.9659258262890683122, 1.000000000000000000, 0.9659258262890683122, 1.000000000000000000, 0.9659258262890683122, 1.000000000000000000, 0.9659258262890683122, 1.000000000000000000, 0.9659258262890683122, 1.000000000000000000, 0.9659258262890683122, 1.000000000000000000, 0.9659258262890683122, 1.000000000000000000, 0.9659258262890683122, 1.000000000000000000, 0.9659258262890683122, 1.000000000000000000, 0.9659258262890683122, 1.000000000000000000, 0.9659258262890683122, 1.000000000000000000, 0.9659258262890683122, 1.000000000000000000, 0.9659258262890683122, 1.000000000000000000, 0.9659258262890683122, 1.000000000000000000, 0.9659258262890683122, 1.000000000000000000, 0.9659258262890683122, 1.000000000000000000, 0.9659258262890683122, 1.000000000000000000, 0.9659258262890683122, 1.000000000000000000, 0.9659258262890683122, 1.000000000000000000, 0.9659258262890683122, 1.000000000000000000, 0.9659258262890683122, 1.000000000000000000, 0.9659258262890683122, 1.000000000000000000, 0.9659258262890683122, 1.000000000000000000, 0.9659258262890683122, 1.000000000000000000, 0.9659258262890683122, 1.000000000000000000, 0.9659258262890683122, 1.000000000000000000, 0.9659258262890683122, 1.000000000000000000, 0.9659258262890683122, 1.000000000000000000, 0.9659258262890683122, 1.000000000000000000, 0.9659258262890683122, 1.000000000000000000, 0.9659258262890683122, 1.000000000000000000, 0.9659258262890683122, 1.000000000000000000, 0.9659258262890683122, 1.000000000000000000, 0.9659258262890683122, 1.000000000000000000, 0.9659258262890683122, 1.000000000000000000, 0.9659258262890683122, 1.000000000000000000, 0.9659258262890683122, 1.000000000000000000, 0.9659258262890683122, 1.000000000000000000, 0.9659258262890683122, 1.000000000000000000, 0.9659258262890683122, 1.000000000000000000, 0.9659258262890683122, 1.000000000000000000, 0.9659258262890683122, 1.000000000000000000, 0.9659258262890683122, 1.000000000000000000, 0.9659258262890683122, 1.000000000000000000, 0.9659258262890683122, 1.000000000000000000, 0.9659258262890683122, 1.000000000000000000, 0.9659258262890683122, 1.000000000000000000, 0.9659258262890683122, 1.000000000000000000, 0.9659258262890683122, 1.000000000000000000, 0.9659258262890683122, 1.000000000000000000, 0.9659258262890683122, 1.000000000000000000, 0.9659258262890683122, 1.000000000000000000, 0.9659258262890683122, 1.000000000000000000, 0.9659258262890683122, 1.000000000000000000, 0.9659258262890683122, 1.000000000000000000, 0.9659258262890683122, 1.000000000000000000, 0.9659258262890683122, 1.000000000000000000, 0.9659258262890683122, 1.000000000000000000, 0.9659258262890683122, 1.000000000000000000, 0.9659258262890683122, 1.000000000000000000, 0.9659258262890683122, 1.000000000000000000, 0.9659258262890683122, 1.000000000000000000, 0.9659258262890683122, 1.000000000000000000, 0.9659258262890683122, 1.000000000000000000, 0.9659258262890683122, 1.000000000000000000, 0.9659258262890683122, 1.000000000000000000, 0.9659258262890683122, 1.000000000000000000, 0.9659258262890683122, 1.000000000000000000, 0.9659258262890683122, 1.000000000000000000, 0.9659258262890683122, 1.000000000000000000, 0.9659258262890683122, 1.000000000000000000, 0.9659258262890683122, 1.000000000000000000, 0.9659258262890683122, 1.000000000000000000, 0.9659258262890683122, 1.000000000000000000, 0.9659258262890683122, 1.000000000000000000, 0.9659258262890683122, 1.000000000000000000, 0.9659258262890683122, 1.000000000000000000, 0.9659258262890683122, 1.000000000000000000, 0.9659258262890683122, 1.000000000000000000, 0.9659258262890683122, 1.000000000000000000, 0.9659258262890683122, 1.000000000000000000, 0.9659258262890683122, 1.000000000000000000, 0.9659258262890683122, 1.000000000000000000, 0.9659258262890683122, 1.000000000000000000, 0.9659258262890683122, 1.000000000000000000, 0.9659258262890683122, 1.000000000000000000, 0.9659258262890683122, 1.000000000000000000, 0.9659258262890683122, 1.000000000000000000, 0.9659258262890683122, 1.000000000000000000, 0.9659258262890683122, 1.000000000000000000, 0.9659258262890683122, 1.000000000000000000, 0.9659258262890683122, 1.000000000000000000, 0.9659258262890683122, 1.000000000000000000, 0.9659258262890683122, 1.000000000000000000, 0.9659258262890683122, 1.000000000000000000, 0.9659258262890683122, 1.000000000000000000, 0.9659258262890683122, 1.000000000000000000, 0.9659258262890683122, 1.000000000000000000, 0.9659258262890683122, 1.000000000000000000, 0.9659258262890683122, 1.000000000000000000, 0.9659258262890683122, 1.000000000000000000, 0.9659258262890683122, 1.000000000000000000, 0.9659258262890683122, 1.000000000000000000, 0.9659258262890683122, 1.000000000000000000, 0.9659258262890683122, 1.000000000000000000, 0.9659258262890683122, 1.000000000000000000, 0.9659258262890683122, 1.000000000000000000, 0.9659258262890683122, 1.000000000000000000, 0.9659258262890683122, 1.000000000000000000, 0.9659258262890683122, 1.000000000000000000, 0.9659258262890683122, 1.000000000000000000, 0.9659258262890683122, 1.000000000000000000, 0.9659258262890683122, 1.000000000000000000, 0.9659258262890683122, 1.000000000000000000, 0.9659258262890683122, 1.000000000000000000, 0.9659258262890683122, 1.000000000000000000, 0.9659258262890683122, 1.000000000000000000, 0.9659258262890683122, 1.000000000000000000, 0.9659258262890683122, 1.000000000000000000, 0.9659258262890683122, 1.000000000000000000, 0.9659258262890683122, 1.000000000000000000, 0.9659258262890683122, 1.000000000000000000, 0.9659258262890683122, 1.000000000000000000, 0.9659258262890683122, 1.000000000000000000, 0.9659258262890683122, 1.000000000000000000, 0.9659258262890683122, 1.000000000000000000, 0.9659258262890683122, 1.000000000000000000, 0.9659258262890683122, 1.000000000000000000, 0.9659258262890683122, 1.000000000000000000, 0.9659258262890683122, 1.000000000000000000, 0.9659258262890683122, 1.000000000000000000, 0.9659258262890683122, 1.000000000000000000, 0.9659258262890683122, 1.000000000000000000, 0.9659258262890683122, 1.000000000000000000, 0.9659258262890683122, 1.000000000000000000, 0.9659258262890683122, 1.000000000000000000, 0.9659258262890683122, 1.000000000000000000, 0.9659258262890683122, 1.000000000000000000, 0.9659258262890683122, 1.000000000000000000, 0.9659258262890683122, 1.000000000000000000, 0.9659258262890683122, 1.000000000000000000, 0.9659258262890683122, 1.000000000000000000, 0.9659258262890683122, 1.000000000000000000, 0.9659258262890683122, 1.000000000000000000, 0.9659258262890683122, 1.000000000000000000, 0.9659258262890683122, 1.000000000000000000, 0.9659258262890683122, 1.000000000000000000, 0.9659258262890683122, 1.000000000000000000, 0.9659258262890683122, 1.000000000000000000, 0.9659258262890683122, 1.000000000000000000, 0.9659258262890683122, 1.000000000000000000, 0.9659258262890683122, 1.000000000000000000, 0.9659258262890683122, 1.000000000000000000, 0.9659258262890683122, 1.000000000000000000, 0.9659258262890683122, 1.000000000000000000, 0.9659258262890683122, 1.000000000000000000, 0.9659258262890683122, 1.000000000000000000, 0.9659258262890683122, 1.000000000000000000, 0.9659258262890683122, 1.000000000000000000, 0.9659258262890683122, 1.000000000000000000, 0.9659258262890683122, 1.000000000000000000, 0.9659258262890683122, 1.000000000000000000, 0.9659258262890683122, 1.000000000000000000, 0.9659258262890683122, 1.000000000000000000, 0.9659258262890683122, 1.000000000000000000, 0.9659258262890683122, 1.000000000000000000, 0.9659258262890683122, 1.000000000000000000, 0.9659258262890683122, 1.000000000000000000, 0.9659258262890683122, 1.000000000000000000, 0.9659258262890683122, 1.000000000000000000, 0.9659258262890683122, 1.000000000000000000, 0.9659258262890683122, 1.000000000000000000, 0.9659258262890683122, 1.000000000000000000, 0.9659258262890683122, 1.000000000000000000, 0.9659258262890683122, 1.000000000000000000, 0.9659258262890683122, 1.000000000000000000),
 ( 0.3333333333333333703, 0.3219752754296894559, 0.3333333333333333703, 0.3219752754296894559, 0.3333333333333333703, 0.3219752754296894559, 0.3333333333333333703, 0.3219752754296894559, 0.3333333333333333703, 0.3219752754296894559, 0.3333333333333333703, 0.3219752754296894559, 0.3333333333333333703, 0.3219752754296894559, 0.3333333333333333703, 0.3219752754296894559, 0.3333333333333333703, 0.3219752754296894559, 0.3333333333333333703, 0.3219752754296894559, 0.3333333333333333703, 0.3219752754296894559, 0.3333333333333333703, 0.3219752754296894559, 0.3333333333333333703, 0.3219752754296894559, 0.3333333333333333703, 0.3219752754296894559, 0.3333333333333333703, 0.3219752754296894559, 0.3333333333333333703, 0.3219752754296894559, 0.3333333333333333703, 0.3219752754296894559, 0.3333333333333333703, 0.3219752754296894559, 0.3333333333333333703, 0.3219752754296894559, 0.3333333333333333703, 0.3219752754296894559, 0.3333333333333333703, 0.3219752754296894559, 0.3333333333333333703, 0.3219752754296894559, 0.3333333333333333703, 0.3219752754296894559, 0.3333333333333333703, 0.3219752754296894559, 0.3333333333333333703, 0.3219752754296894559, 0.3333333333333333703, 0.3219752754296894559, 0.3333333333333333703, 0.3219752754296894559, 0.3333333333333333703, 0.3219752754296894559, 0.3333333333333333703, 0.3219752754296894559, 0.3333333333333333703, 0.3219752754296894559, 0.3333333333333333703, 0.3219752754296894559, 0.3333333333333333703, 0.3219752754296894559, 0.3333333333333333703, 0.3219752754296894559, 0.3333333333333333703, 0.3219752754296894559, 0.3333333333333333703, 0.3219752754296894559, 0.3333333333333333703, 0.3219752754296894559, 0.3333333333333333703, 0.3219752754296894559, 0.3333333333333333703, 0.3219752754296894559, 0.3333333333333333703, 0.3219752754296894559, 0.3333333333333333703, 0.3219752754296894559, 0.3333333333333333703, 0.3219752754296894559, 0.3333333333333333703, 0.3219752754296894559, 0.3333333333333333703, 0.3219752754296894559, 0.3333333333333333703, 0.3219752754296894559, 0.3333333333333333703, 0.3219752754296894559, 0.3333333333333333703, 0.3219752754296894559, 0.3333333333333333703, 0.3219752754296894559, 0.3333333333333333703, 0.3219752754296894559, 0.3333333333333333703, 0.3219752754296894559, 0.3333333333333333703, 0.3219752754296894559, 0.3333333333333333703, 0.3219752754296894559, 0.3333333333333333703, 0.3219752754296894559, 0.3333333333333333703, 0.3219752754296894559, 0.3333333333333333703, 0.3219752754296894559, 0.3333333333333333703, 0.3219752754296894559, 0.3333333333333333703, 0.3219752754296894559, 0.3333333333333333703, 0.3219752754296894559, 0.3333333333333333703, 0.3219752754296894559, 0.3333333333333333703, 0.3219752754296894559, 0.3333333333333333703, 0.3219752754296894559, 0.3333333333333333703, 0.3219752754296894559, 0.3333333333333333703, 0.3219752754296894559, 0.3333333333333333703, 0.3219752754296894559, 0.3333333333333333703, 0.3219752754296894559, 0.3333333333333333703, 0.3219752754296894559, 0.3333333333333333703, 0.3219752754296894559, 0.3333333333333333703, 0.3219752754296894559, 0.3333333333333333703, 0.3219752754296894559, 0.3333333333333333703, 0.3219752754296894559, 0.3333333333333333703, 0.3219752754296894559, 0.3333333333333333703, 0.3219752754296894559, 0.3333333333333333703, 0.3219752754296894559, 0.3333333333333333703, 0.3219752754296894559, 0.3333333333333333703, 0.3219752754296894559, 0.3333333333333333703, 0.3219752754296894559, 0.3333333333333333703, 0.3219752754296894559, 0.3333333333333333703, 0.3219752754296894559, 0.3333333333333333703, 0.3219752754296894559, 0.3333333333333333703, 0.3219752754296894559, 0.3333333333333333703, 0.3219752754296894559, 0.3333333333333333703, 0.3219752754296894559, 0.3333333333333333703, 0.3219752754296894559, 0.3333333333333333703, 0.3219752754296894559, 0.3333333333333333703, 0.3219752754296894559, 0.3333333333333333703, 0.3219752754296894559, 0.3333333333333333703, 0.3219752754296894559, 0.3333333333333333703, 0.3219752754296894559, 0.3333333333333333703, 0.3219752754296894559, 0.3333333333333333703, 0.3219752754296894559, 0.3333333333333333703, 0.3219752754296894559, 0.3333333333333333703, 0.3219752754296894559, 0.3333333333333333703, 0.3219752754296894559, 0.3333333333333333703, 0.3219752754296894559, 0.3333333333333333703, 0.3219752754296894559, 0.3333333333333333703, 0.3219752754296894559, 0.3333333333333333703, 0.3219752754296894559, 0.3333333333333333703, 0.3219752754296894559, 0.3333333333333333703, 0.3219752754296894559, 0.3333333333333333703, 0.3219752754296894559, 0.3333333333333333703, 0.3219752754296894559, 0.3333333333333333703, 0.3219752754296894559, 0.3333333333333333703, 0.3219752754296894559, 0.3333333333333333703, 0.3219752754296894559, 0.3333333333333333703, 0.3219752754296894559, 0.3333333333333333703, 0.3219752754296894559, 0.3333333333333333703, 0.3219752754296894559, 0.3333333333333333703, 0.3219752754296894559, 0.3333333333333333703, 0.3219752754296894559, 0.3333333333333333703, 0.3219752754296894559, 0.3333333333333333703, 0.3219752754296894559, 0.3333333333333333703, 0.3219752754296894559, 0.3333333333333333703, 0.3219752754296894559, 0.3333333333333333703, 0.3219752754296894559, 0.3333333333333333703, 0.3219752754296894559, 0.3333333333333333703, 0.3219752754296894559, 0.3333333333333333703, 0.3219752754296894559, 0.3333333333333333703, 0.3219752754296894559, 0.3333333333333333703, 0.3219752754296894559, 0.3333333333333333703, 0.3219752754296894559, 0.3333333333333333703, 0.3219752754296894559, 0.3333333333333333703, 0.3219752754296894559, 0.3333333333333333703, 0.3219752754296894559, 0.3333333333333333703, 0.3219752754296894559, 0.3333333333333333703, 0.3219752754296894559, 0.3333333333333333703, 0.3219752754296894559, 0.3333333333333333703, 0.3219752754296894559, 0.3333333333333333703, 0.3219752754296894559, 0.3333333333333333703, 0.3219752754296894559, 0.3333333333333333703, 0.3219752754296894559, 0.3333333333333333703, 0.3219752754296894559, 0.3333333333333333703, 0.3219752754296894559, 0.3333333333333333703, 0.3219752754296894559, 0.3333333333333333703, 0.3219752754296894559, 0.3333333333333333703, 0.3219752754296894559, 0.3333333333333333703, 0.3219752754296894559, 0.3333333333333333703, 0.3219752754296894559, 0.3333333333333333703, 0.3219752754296894559, 0.3333333333333333703, 0.3219752754296894559, 0.3333333333333333703, 0.3219752754296894559, 0.3333333333333333703, 0.3219752754296894559, 0.3333333333333333703, 0.3219752754296894559, 0.3333333333333333703, 0.3219752754296894559, 0.3333333333333333703, 0.3219752754296894559, 0.3333333333333333703, 0.3219752754296894559, 0.3333333333333333703, 0.3219752754296894559, 0.3333333333333333703, 0.3219752754296894559, 0.3333333333333333703, 0.3219752754296894559, 0.3333333333333333703, 0.3219752754296894559, 0.3333333333333333703, 0.3219752754296894559, 0.3333333333333333703, 0.3219752754296894559, 0.3333333333333333703, 0.3219752754296894559, 0.3333333333333333703, 0.3219752754296894559, 0.3333333333333333703, 0.3219752754296894559, 0.3333333333333333703, 0.3219752754296894559, 0.3333333333333333703, 0.3219752754296894559, 0.3333333333333333703, 0.3219752754296894559, 0.3333333333333333703, 0.3219752754296894559, 0.3333333333333333703, 0.3219752754296894559, 0.3333333333333333703, 0.3219752754296894559, 0.3333333333333333703, 0.3219752754296894559, 0.3333333333333333703, 0.3219752754296894559, 0.3333333333333333703, 0.3219752754296894559, 0.3333333333333333703, 0.3219752754296894559, 0.3333333333333333703, 0.3219752754296894559, 0.3333333333333333703, 0.3219752754296894559, 0.3333333333333333703, 0.3219752754296894559, 0.3333333333333333703, 0.3219752754296894559, 0.3333333333333333703, 0.3219752754296894559, 0.3333333333333333703, 0.3219752754296894559, 0.3333333333333333703, 0.3219752754296894559, 0.3333333333333333703, 0.3219752754296894559, 0.3333333333333333703, 0.3219752754296894559, 0.3333333333333333703, 0.3219752754296894559, 0.3333333333333333703, 0.3219752754296894559, 0.3333333333333333703, 0.3219752754296894559, 0.3333333333333333703, 0.3219752754296894559, 0.3333333333333333703, 0.3219752754296894559, 0.3333333333333333703, 0.3219752754296894559, 0.3333333333333333703, 0.3219752754296894559, 0.3333333333333333703, 0.3219752754296894559, 0.3333333333333333703, 0.3219752754296894559, 0.3333333333333333703, 0.3219752754296894559, 0.3333333333333333703, 0.3219752754296894559, 0.3333333333333333703, 0.3219752754296894559, 0.3333333333333333703, 0.3219752754296894559, 0.3333333333333333703, 0.3219752754296894559, 0.3333333333333333703, 0.3219752754296894559, 0.3333333333333333703, 0.3219752754296894559, 0.3333333333333333703, 0.3219752754296894559, 0.3333333333333333703, 0.3219752754296894559, 0.3333333333333333703, 0.3219752754296894559, 0.3333333333333333703, 0.3219752754296894559, 0.3333333333333333703, 0.3219752754296894559, 0.3333333333333333703, 0.3219752754296894559, 0.3333333333333333703, 0.3219752754296894559, 0.3333333333333333703, 0.3219752754296894559, 0.3333333333333333703, 0.3219752754296894559, 0.3333333333333333703, 0.3219752754296894559, 0.3333333333333333703, 0.3219752754296894559, 0.3333333333333333703, 0.3219752754296894559, 0.3333333333333333703, 0.3219752754296894559, 0.3333333333333333703, 0.3219752754296894559, 0.3333333333333333703, 0.3219752754296894559, 0.3333333333333333703, 0.3219752754296894559, 0.3333333333333333703, 0.3219752754296894559, 0.3333333333333333703, 0.3219752754296894559, 0.3333333333333333703, 0.3219752754296894559, 0.3333333333333333703, 0.3219752754296894559, 0.3333333333333333703, 0.3219752754296894559, 0.3333333333333333703, 0.3219752754296894559, 0.3333333333333333703, 0.3219752754296894559, 0.3333333333333333703, 0.3219752754296894559, 0.3333333333333333703, 0.3219752754296894559, 0.3333333333333333703, 0.3219752754296894559, 0.3333333333333333703, 0.3219752754296894559, 0.3333333333333333703, 0.3219752754296894559, 0.3333333333333333703, 0.3219752754296894559, 0.3333333333333333703, 0.3219752754296894559, 0.3333333333333333703, 0.3219752754296894559, 0.3333333333333333703, 0.3219752754296894559, 0.3333333333333333703, 0.3219752754296894559, 0.3333333333333333703, 0.3219752754296894559, 0.3333333333333333703, 0.3219752754296894559, 0.3333333333333333703, 0.3219752754296894559, 0.3333333333333333703, 0.3219752754296894559, 0.3333333333333333703, 0.3219752754296894559, 0.3333333333333333703, 0.3219752754296894559, 0.3333333333333333703, 0.3219752754296894559, 0.3333333333333333703),
 ( 0.3333333333333333703, 0.3219752754296894559, 0.3333333333333333703, 0.3219752754296894559, 0.3333333333333333703, 0.3219752754296894559, 0.3333333333333333703, 0.3219752754296894559, 0.3333333333333333703, 0.3219752754296894559, 0.3333333333333333703, 0.3219752754296894559, 0.3333333333333333703, 0.3219752754296894559, 0.3333333333333333703, 0.3219752754296894559, 0.3333333333333333703, 0.3219752754296894559, 0.3333333333333333703, 0.3219752754296894559, 0.3333333333333333703, 0.3219752754296894559, 0.3333333333333333703, 0.3219752754296894559, 0.3333333333333333703, 0.3219752754296894559, 0.3333333333333333703, 0.3219752754296894559, 0.3333333333333333703, 0.3219752754296894559, 0.3333333333333333703, 0.3219752754296894559, 0.3333333333333333703, 0.3219752754296894559, 0.3333333333333333703, 0.3219752754296894559, 0.3333333333333333703, 0.3219752754296894559, 0.3333333333333333703, 0.3219752754296894559, 0.3333333333333333703, 0.3219752754296894559, 0.3333333333333333703, 0.3219752754296894559, 0.3333333333333333703, 0.3219752754296894559, 0.3333333333333333703, 0.3219752754296894559, 0.3333333333333333703, 0.3219752754296894559, 0.3333333333333333703, 0.3219752754296894559, 0.3333333333333333703, 0.3219752754296894559, 0.3333333333333333703, 0.3219752754296894559, 0.3333333333333333703, 0.3219752754296894559, 0.3333333333333333703, 0.3219752754296894559, 0.3333333333333333703, 0.3219752754296894559, 0.3333333333333333703, 0.3219752754296894559, 0.3333333333333333703, 0.3219752754296894559, 0.3333333333333333703, 0.3219752754296894559, 0.3333333333333333703, 0.3219752754296894559, 0.3333333333333333703, 0.3219752754296894559, 0.3333333333333333703, 0.3219752754296894559, 0.3333333333333333703, 0.3219752754296894559, 0.3333333333333333703, 0.3219752754296894559, 0.3333333333333333703, 0.3219752754296894559, 0.3333333333333333703, 0.3219752754296894559, 0.3333333333333333703, 0.3219752754296894559, 0.3333333333333333703, 0.3219752754296894559, 0.3333333333333333703, 0.3219752754296894559, 0.3333333333333333703, 0.3219752754296894559, 0.3333333333333333703, 0.3219752754296894559, 0.3333333333333333703, 0.3219752754296894559, 0.3333333333333333703, 0.3219752754296894559, 0.3333333333333333703, 0.3219752754296894559, 0.3333333333333333703, 0.3219752754296894559, 0.3333333333333333703, 0.3219752754296894559, 0.3333333333333333703, 0.3219752754296894559, 0.3333333333333333703, 0.3219752754296894559, 0.3333333333333333703, 0.3219752754296894559, 0.3333333333333333703, 0.3219752754296894559, 0.3333333333333333703, 0.3219752754296894559, 0.3333333333333333703, 0.3219752754296894559, 0.3333333333333333703, 0.3219752754296894559, 0.3333333333333333703, 0.3219752754296894559, 0.3333333333333333703, 0.3219752754296894559, 0.3333333333333333703, 0.3219752754296894559, 0.3333333333333333703, 0.3219752754296894559, 0.3333333333333333703, 0.3219752754296894559, 0.3333333333333333703, 0.3219752754296894559, 0.3333333333333333703, 0.3219752754296894559, 0.3333333333333333703, 0.3219752754296894559, 0.3333333333333333703, 0.3219752754296894559, 0.3333333333333333703, 0.3219752754296894559, 0.3333333333333333703, 0.3219752754296894559, 0.3333333333333333703, 0.3219752754296894559, 0.3333333333333333703, 0.3219752754296894559, 0.3333333333333333703, 0.3219752754296894559, 0.3333333333333333703, 0.3219752754296894559, 0.3333333333333333703, 0.3219752754296894559, 0.3333333333333333703, 0.3219752754296894559, 0.3333333333333333703, 0.3219752754296894559, 0.3333333333333333703, 0.3219752754296894559, 0.3333333333333333703, 0.3219752754296894559, 0.3333333333333333703, 0.3219752754296894559, 0.3333333333333333703, 0.3219752754296894559, 0.3333333333333333703, 0.3219752754296894559, 0.3333333333333333703, 0.3219752754296894559, 0.3333333333333333703, 0.3219752754296894559, 0.3333333333333333703, 0.3219752754296894559, 0.3333333333333333703, 0.3219752754296894559, 0.3333333333333333703, 0.3219752754296894559, 0.3333333333333333703, 0.3219752754296894559, 0.3333333333333333703, 0.3219752754296894559, 0.3333333333333333703, 0.3219752754296894559, 0.3333333333333333703, 0.3219752754296894559, 0.3333333333333333703, 0.3219752754296894559, 0.3333333333333333703, 0.3219752754296894559, 0.3333333333333333703, 0.3219752754296894559, 0.3333333333333333703, 0.3219752754296894559, 0.3333333333333333703, 0.3219752754296894559, 0.3333333333333333703, 0.3219752754296894559, 0.3333333333333333703, 0.3219752754296894559, 0.3333333333333333703, 0.3219752754296894559, 0.3333333333333333703, 0.3219752754296894559, 0.3333333333333333703, 0.3219752754296894559, 0.3333333333333333703, 0.3219752754296894559, 0.3333333333333333703, 0.3219752754296894559, 0.3333333333333333703, 0.3219752754296894559, 0.3333333333333333703, 0.3219752754296894559, 0.3333333333333333703, 0.3219752754296894559, 0.3333333333333333703, 0.3219752754296894559, 0.3333333333333333703, 0.3219752754296894559, 0.3333333333333333703, 0.3219752754296894559, 0.3333333333333333703, 0.3219752754296894559, 0.3333333333333333703, 0.3219752754296894559, 0.3333333333333333703, 0.3219752754296894559, 0.3333333333333333703, 0.3219752754296894559, 0.3333333333333333703, 0.3219752754296894559, 0.3333333333333333703, 0.3219752754296894559, 0.3333333333333333703, 0.3219752754296894559, 0.3333333333333333703, 0.3219752754296894559, 0.3333333333333333703, 0.3219752754296894559, 0.3333333333333333703, 0.3219752754296894559, 0.3333333333333333703, 0.3219752754296894559, 0.3333333333333333703, 0.3219752754296894559, 0.3333333333333333703, 0.3219752754296894559, 0.3333333333333333703, 0.3219752754296894559, 0.3333333333333333703, 0.3219752754296894559, 0.3333333333333333703, 0.3219752754296894559, 0.3333333333333333703, 0.3219752754296894559, 0.3333333333333333703, 0.3219752754296894559, 0.3333333333333333703, 0.3219752754296894559, 0.3333333333333333703, 0.3219752754296894559, 0.3333333333333333703, 0.3219752754296894559, 0.3333333333333333703, 0.3219752754296894559, 0.3333333333333333703, 0.3219752754296894559, 0.3333333333333333703, 0.3219752754296894559, 0.3333333333333333703, 0.3219752754296894559, 0.3333333333333333703, 0.3219752754296894559, 0.3333333333333333703, 0.3219752754296894559, 0.3333333333333333703, 0.3219752754296894559, 0.3333333333333333703, 0.3219752754296894559, 0.3333333333333333703, 0.3219752754296894559, 0.3333333333333333703, 0.3219752754296894559, 0.3333333333333333703, 0.3219752754296894559, 0.3333333333333333703, 0.3219752754296894559, 0.3333333333333333703, 0.3219752754296894559, 0.3333333333333333703, 0.3219752754296894559, 0.3333333333333333703, 0.3219752754296894559, 0.3333333333333333703, 0.3219752754296894559, 0.3333333333333333703, 0.3219752754296894559, 0.3333333333333333703, 0.3219752754296894559, 0.3333333333333333703, 0.3219752754296894559, 0.3333333333333333703, 0.3219752754296894559, 0.3333333333333333703, 0.3219752754296894559, 0.3333333333333333703, 0.3219752754296894559, 0.3333333333333333703, 0.3219752754296894559, 0.3333333333333333703, 0.3219752754296894559, 0.3333333333333333703, 0.3219752754296894559, 0.3333333333333333703, 0.3219752754296894559, 0.3333333333333333703, 0.3219752754296894559, 0.3333333333333333703, 0.3219752754296894559, 0.3333333333333333703, 0.3219752754296894559, 0.3333333333333333703, 0.3219752754296894559, 0.3333333333333333703, 0.3219752754296894559, 0.3333333333333333703, 0.3219752754296894559, 0.3333333333333333703, 0.3219752754296894559, 0.3333333333333333703, 0.3219752754296894559, 0.3333333333333333703, 0.3219752754296894559, 0.3333333333333333703, 0.3219752754296894559, 0.3333333333333333703, 0.3219752754296894559, 0.3333333333333333703, 0.3219752754296894559, 0.3333333333333333703, 0.3219752754296894559, 0.3333333333333333703, 0.3219752754296894559, 0.3333333333333333703, 0.3219752754296894559, 0.3333333333333333703, 0.3219752754296894559, 0.3333333333333333703, 0.3219752754296894559, 0.3333333333333333703, 0.3219752754296894559, 0.3333333333333333703, 0.3219752754296894559, 0.3333333333333333703, 0.3219752754296894559, 0.3333333333333333703, 0.3219752754296894559, 0.3333333333333333703, 0.3219752754296894559, 0.3333333333333333703, 0.3219752754296894559, 0.3333333333333333703, 0.3219752754296894559, 0.3333333333333333703, 0.3219752754296894559, 0.3333333333333333703, 0.3219752754296894559, 0.3333333333333333703, 0.3219752754296894559, 0.3333333333333333703, 0.3219752754296894559, 0.3333333333333333703, 0.3219752754296894559, 0.3333333333333333703, 0.3219752754296894559, 0.3333333333333333703, 0.3219752754296894559, 0.3333333333333333703, 0.3219752754296894559, 0.3333333333333333703, 0.3219752754296894559, 0.3333333333333333703, 0.3219752754296894559, 0.3333333333333333703, 0.3219752754296894559, 0.3333333333333333703, 0.3219752754296894559, 0.3333333333333333703, 0.3219752754296894559, 0.3333333333333333703, 0.3219752754296894559, 0.3333333333333333703, 0.3219752754296894559, 0.3333333333333333703, 0.3219752754296894559, 0.3333333333333333703, 0.3219752754296894559, 0.3333333333333333703, 0.3219752754296894559, 0.3333333333333333703, 0.3219752754296894559, 0.3333333333333333703, 0.3219752754296894559, 0.3333333333333333703, 0.3219752754296894559, 0.3333333333333333703, 0.3219752754296894559, 0.3333333333333333703, 0.3219752754296894559, 0.3333333333333333703, 0.3219752754296894559, 0.3333333333333333703, 0.3219752754296894559, 0.3333333333333333703, 0.3219752754296894559, 0.3333333333333333703, 0.3219752754296894559, 0.3333333333333333703, 0.3219752754296894559, 0.3333333333333333703, 0.3219752754296894559, 0.3333333333333333703, 0.3219752754296894559, 0.3333333333333333703, 0.3219752754296894559, 0.3333333333333333703, 0.3219752754296894559, 0.3333333333333333703, 0.3219752754296894559, 0.3333333333333333703, 0.3219752754296894559, 0.3333333333333333703, 0.3219752754296894559, 0.3333333333333333703, 0.3219752754296894559, 0.3333333333333333703, 0.3219752754296894559, 0.3333333333333333703, 0.3219752754296894559, 0.3333333333333333703, 0.3219752754296894559, 0.3333333333333333703, 0.3219752754296894559, 0.3333333333333333703, 0.3219752754296894559, 0.3333333333333333703, 0.3219752754296894559, 0.3333333333333333703, 0.3219752754296894559, 0.3333333333333333703, 0.3219752754296894559, 0.3333333333333333703, 0.3219752754296894559, 0.3333333333333333703, 0.3219752754296894559, 0.3333333333333333703, 0.3219752754296894559, 0.3333333333333333703, 0.3219752754296894559, 0.3333333333333333703, 0.3219752754296894559, 0.3333333333333333703),
 ( 1.000000000000000000, 0.9659258262890683122, 1.000000000000000000, 0.9659258262890683122, 1.000000000000000000, 0.9659258262890683122, 1.000000000000000000, 0.9659258262890683122, 1.000000000000000000, 0.9659258262890683122, 1.000000000000000000, 0.9659258262890683122, 1.000000000000000000, 0.9659258262890683122, 1.000000000000000000, 0.9659258262890683122, 1.000000000000000000, 0.9659258262890683122, 1.000000000000000000, 0.9659258262890683122, 1.000000000000000000, 0.9659258262890683122, 1.000000000000000000, 0.9659258262890683122, 1.000000000000000000, 0.9659258262890683122, 1.000000000000000000, 0.9659258262890683122, 1.000000000000000000, 0.9659258262890683122, 1.000000000000000000, 0.9659258262890683122, 1.000000000000000000, 0.9659258262890683122, 1.000000000000000000, 0.9659258262890683122, 1.000000000000000000, 0.9659258262890683122, 1.000000000000000000, 0.9659258262890683122, 1.000000000000000000, 0.9659258262890683122, 1.000000000000000000, 0.9659258262890683122, 1.000000000000000000, 0.9659258262890683122, 1.000000000000000000, 0.9659258262890683122, 1.000000000000000000, 0.9659258262890683122, 1.000000000000000000, 0.9659258262890683122, 1.000000000000000000, 0.9659258262890683122, 1.000000000000000000, 0.9659258262890683122, 1.000000000000000000, 0.9659258262890683122, 1.000000000000000000, 0.9659258262890683122, 1.000000000000000000, 0.9659258262890683122, 1.000000000000000000, 0.9659258262890683122, 1.000000000000000000, 0.9659258262890683122, 1.000000000000000000, 0.9659258262890683122, 1.000000000000000000, 0.9659258262890683122, 1.000000000000000000, 0.9659258262890683122, 1.000000000000000000, 0.9659258262890683122, 1.000000000000000000, 0.9659258262890683122, 1.000000000000000000, 0.9659258262890683122, 1.000000000000000000, 0.9659258262890683122, 1.000000000000000000, 0.9659258262890683122, 1.000000000000000000, 0.9659258262890683122, 1.000000000000000000, 0.9659258262890683122, 1.000000000000000000, 0.9659258262890683122, 1.000000000000000000, 0.9659258262890683122, 1.000000000000000000, 0.9659258262890683122, 1.000000000000000000, 0.9659258262890683122, 1.000000000000000000, 0.9659258262890683122, 1.000000000000000000, 0.9659258262890683122, 1.000000000000000000, 0.9659258262890683122, 1.000000000000000000, 0.9659258262890683122, 1.000000000000000000, 0.9659258262890683122, 1.000000000000000000, 0.9659258262890683122, 1.000000000000000000, 0.9659258262890683122, 1.000000000000000000, 0.9659258262890683122, 1.000000000000000000, 0.9659258262890683122, 1.000000000000000000, 0.9659258262890683122, 1.000000000000000000, 0.9659258262890683122, 1.000000000000000000, 0.9659258262890683122, 1.000000000000000000, 0.9659258262890683122, 1.000000000000000000, 0.9659258262890683122, 1.000000000000000000, 0.9659258262890683122, 1.000000000000000000, 0.9659258262890683122, 1.000000000000000000, 0.9659258262890683122, 1.000000000000000000, 0.9659258262890683122, 1.000000000000000000, 0.9659258262890683122, 1.000000000000000000, 0.9659258262890683122, 1.000000000000000000, 0.9659258262890683122, 1.000000000000000000, 0.9659258262890683122, 1.000000000000000000, 0.9659258262890683122, 1.000000000000000000, 0.9659258262890683122, 1.000000000000000000, 0.9659258262890683122, 1.000000000000000000, 0.9659258262890683122, 1.000000000000000000, 0.9659258262890683122, 1.000000000000000000, 0.9659258262890683122, 1.000000000000000000, 0.9659258262890683122, 1.000000000000000000, 0.9659258262890683122, 1.000000000000000000, 0.9659258262890683122, 1.000000000000000000, 0.9659258262890683122, 1.000000000000000000, 0.9659258262890683122, 1.000000000000000000, 0.9659258262890683122, 1.000000000000000000, 0.9659258262890683122, 1.000000000000000000, 0.9659258262890683122, 1.000000000000000000, 0.9659258262890683122, 1.000000000000000000, 0.9659258262890683122, 1.000000000000000000, 0.9659258262890683122, 1.000000000000000000, 0.9659258262890683122, 1.000000000000000000, 0.9659258262890683122, 1.000000000000000000, 0.9659258262890683122, 1.000000000000000000, 0.9659258262890683122, 1.000000000000000000, 0.9659258262890683122, 1.000000000000000000, 0.9659258262890683122, 1.000000000000000000, 0.9659258262890683122, 1.000000000000000000, 0.9659258262890683122, 1.000000000000000000, 0.9659258262890683122, 1.000000000000000000, 0.9659258262890683122, 1.000000000000000000, 0.9659258262890683122, 1.000000000000000000, 0.9659258262890683122, 1.000000000000000000, 0.9659258262890683122, 1.000000000000000000, 0.9659258262890683122, 1.000000000000000000, 0.9659258262890683122, 1.000000000000000000, 0.9659258262890683122, 1.000000000000000000, 0.9659258262890683122, 1.000000000000000000, 0.9659258262890683122, 1.000000000000000000, 0.9659258262890683122, 1.000000000000000000, 0.9659258262890683122, 1.000000000000000000, 0.9659258262890683122, 1.000000000000000000, 0.9659258262890683122, 1.000000000000000000, 0.9659258262890683122, 1.000000000000000000, 0.9659258262890683122, 1.000000000000000000, 0.9659258262890683122, 1.000000000000000000, 0.9659258262890683122, 1.000000000000000000, 0.9659258262890683122, 1.000000000000000000, 0.9659258262890683122, 1.000000000000000000, 0.9659258262890683122, 1.000000000000000000, 0.9659258262890683122, 1.000000000000000000, 0.9659258262890683122, 1.000000000000000000, 0.9659258262890683122, 1.000000000000000000, 0.9659258262890683122, 1.000000000000000000, 0.9659258262890683122, 1.000000000000000000, 0.9659258262890683122, 1.000000000000000000, 0.9659258262890683122, 1.000000000000000000, 0.9659258262890683122, 1.000000000000000000, 0.9659258262890683122, 1.000000000000000000, 0.9659258262890683122, 1.000000000000000000, 0.9659258262890683122, 1.000000000000000000, 0.9659258262890683122, 1.000000000000000000, 0.9659258262890683122, 1.000000000000000000, 0.9659258262890683122, 1.000000000000000000, 0.9659258262890683122, 1.000000000000000000, 0.9659258262890683122, 1.000000000000000000, 0.9659258262890683122, 1.000000000000000000, 0.9659258262890683122, 1.000000000000000000, 0.9659258262890683122, 1.000000000000000000, 0.9659258262890683122, 1.000000000000000000, 0.9659258262890683122, 1.000000000000000000, 0.9659258262890683122, 1.000000000000000000, 0.9659258262890683122, 1.000000000000000000, 0.9659258262890683122, 1.000000000000000000, 0.9659258262890683122, 1.000000000000000000, 0.9659258262890683122, 1.000000000000000000, 0.9659258262890683122, 1.000000000000000000, 0.9659258262890683122, 1.000000000000000000, 0.9659258262890683122, 1.000000000000000000, 0.9659258262890683122, 1.000000000000000000, 0.9659258262890683122, 1.000000000000000000, 0.9659258262890683122, 1.000000000000000000, 0.9659258262890683122, 1.000000000000000000, 0.9659258262890683122, 1.000000000000000000, 0.9659258262890683122, 1.000000000000000000, 0.9659258262890683122, 1.000000000000000000, 0.9659258262890683122, 1.000000000000000000, 0.9659258262890683122, 1.000000000000000000, 0.9659258262890683122, 1.000000000000000000, 0.9659258262890683122, 1.000000000000000000, 0.9659258262890683122, 1.000000000000000000, 0.9659258262890683122, 1.000000000000000000, 0.9659258262890683122, 1.000000000000000000, 0.9659258262890683122, 1.000000000000000000, 0.9659258262890683122, 1.000000000000000000, 0.9659258262890683122, 1.000000000000000000, 0.9659258262890683122, 1.000000000000000000, 0.9659258262890683122, 1.000000000000000000, 0.9659258262890683122, 1.000000000000000000, 0.9659258262890683122, 1.000000000000000000, 0.9659258262890683122, 1.000000000000000000, 0.9659258262890683122, 1.000000000000000000, 0.9659258262890683122, 1.000000000000000000, 0.9659258262890683122, 1.000000000000000000, 0.9659258262890683122, 1.000000000000000000, 0.9659258262890683122, 1.000000000000000000, 0.9659258262890683122, 1.000000000000000000, 0.9659258262890683122, 1.000000000000000000, 0.9659258262890683122, 1.000000000000000000, 0.9659258262890683122, 1.000000000000000000, 0.9659258262890683122, 1.000000000000000000, 0.9659258262890683122, 1.000000000000000000, 0.9659258262890683122, 1.000000000000000000, 0.9659258262890683122, 1.000000000000000000, 0.9659258262890683122, 1.000000000000000000, 0.9659258262890683122, 1.000000000000000000, 0.9659258262890683122, 1.000000000000000000, 0.9659258262890683122, 1.000000000000000000, 0.9659258262890683122, 1.000000000000000000, 0.9659258262890683122, 1.000000000000000000, 0.9659258262890683122, 1.000000000000000000, 0.9659258262890683122, 1.000000000000000000, 0.9659258262890683122, 1.000000000000000000, 0.9659258262890683122, 1.000000000000000000, 0.9659258262890683122, 1.000000000000000000, 0.9659258262890683122, 1.000000000000000000, 0.9659258262890683122, 1.000000000000000000, 0.9659258262890683122, 1.000000000000000000, 0.9659258262890683122, 1.000000000000000000, 0.9659258262890683122, 1.000000000000000000, 0.9659258262890683122, 1.000000000000000000, 0.9659258262890683122, 1.000000000000000000, 0.9659258262890683122, 1.000000000000000000, 0.9659258262890683122, 1.000000000000000000, 0.9659258262890683122, 1.000000000000000000, 0.9659258262890683122, 1.000000000000000000, 0.9659258262890683122, 1.000000000000000000, 0.9659258262890683122, 1.000000000000000000, 0.9659258262890683122, 1.000000000000000000, 0.9659258262890683122, 1.000000000000000000, 0.9659258262890683122, 1.000000000000000000, 0.9659258262890683122, 1.000000000000000000, 0.9659258262890683122, 1.000000000000000000, 0.9659258262890683122, 1.000000000000000000, 0.9659258262890683122, 1.000000000000000000, 0.9659258262890683122, 1.000000000000000000, 0.9659258262890683122, 1.000000000000000000, 0.9659258262890683122, 1.000000000000000000, 0.9659258262890683122, 1.000000000000000000, 0.9659258262890683122, 1.000000000000000000, 0.9659258262890683122, 1.000000000000000000, 0.9659258262890683122, 1.000000000000000000, 0.9659258262890683122, 1.000000000000000000, 0.9659258262890683122, 1.000000000000000000, 0.9659258262890683122, 1.000000000000000000, 0.9659258262890683122, 1.000000000000000000, 0.9659258262890683122, 1.000000000000000000, 0.9659258262890683122, 1.000000000000000000, 0.9659258262890683122, 1.000000000000000000, 0.9659258262890683122, 1.000000000000000000, 0.9659258262890683122, 1.000000000000000000, 0.9659258262890683122, 1.000000000000000000, 0.9659258262890683122, 1.000000000000000000) ) ) 
 REPRESENTATION_ITEM ( '' )  SURFACE ( )  );
#171924=CARTESIAN_POINT ( 'NONE',  ( 5.719274019375991003, -21.55341960407610458, 42.70724293864770260 ) ) ;
#171925=CARTESIAN_POINT ( 'NONE',  ( -4.379528057220328563, 16.55341960407611168, 110.2072429386477239 ) ) ;
#171927=CARTESIAN_POINT ( 'NONE',  ( 5.049401038297881783, 19.05341960407617563, 62.29275706135234003 ) ) ;
#171928=CARTESIAN_POINT ( 'NONE',  ( 16.53943276465976808, -0.05219959533910856209, 38.74890960531435979 ) ) ;
#171929=CARTESIAN_POINT ( 'NONE',  ( -19.02544592524342804, 5.153800228976336051, 111.0405762719810099 ) ) ;
#171930=CARTESIAN_POINT ( 'NONE',  ( -10.72451020669870658, -18.67979575497194134, 84.58442372801903275 ) ) ;
#171931=CARTESIAN_POINT ( 'NONE',  ( 5.719274019375991003, -21.55341960407610458, 72.70724293864769550 ) ) ;
#171932=CARTESIAN_POINT ( 'NONE',  ( 21.55341960407619695, -5.719274019375665929, 41.04275706135236135 ) ) ;
#171933=CARTESIAN_POINT ( 'NONE',  ( -15.80617190586745835, -15.72974639402198527, 96.87390960531436690 ) ) ;
#171934=CARTESIAN_POINT ( 'NONE',  ( -18.62759615963255300, -10.81492255796106328, 54.16775706135235424 ) ) ;
#171935=CARTESIAN_POINT ( 'NONE',  ( -0.05219959533909027116, -19.03943276465977164, 22.49890960531436690 ) ) ;
#171936=CARTESIAN_POINT ( 'NONE',  ( 0.05219959533909260263, 19.03943276465977164, 84.99890960531436690 ) ) ;
#171937=CARTESIAN_POINT ( 'NONE',  ( -8.314922557961024197, 14.29746914071037800, 82.91775706135234714 ) ) ;
#171938=CARTESIAN_POINT ( 'NONE',  ( -14.29746914071049879, 8.314922557960819915, 110.8322429386476955 ) ) ;
#171939=CARTESIAN_POINT ( 'NONE',  ( -16.51473224551069308, -9.474510206698971260, 106.6655762719810383 ) ) ;
#171940=CARTESIAN_POINT ( 'NONE',  ( -14.29746914071049879, 8.314922557960819915, 60.83224293864769550 ) ) ;
#171941=CARTESIAN_POINT ( 'NONE',  ( -16.53943276465976808, 0.05219959533911058130, 26.24890960531435624 ) ) ;
#171942=CARTESIAN_POINT ( 'NONE',  ( -0.05219959533909027116, -19.03943276465977164, 67.49890960531436690 ) ) ;
#171943=CARTESIAN_POINT ( 'NONE',  ( 19.02544592524343514, -5.153800228976328945, 28.54057627198102409 ) ) ;
#171944=CARTESIAN_POINT ( 'NONE',  ( -21.53943276465977519, 0.05219959533907696930, 46.24890960531435979 ) ) ;
#171945=CARTESIAN_POINT ( 'NONE',  ( 5.049401038297881783, 19.05341960407617563, 42.29275706135234003 ) ) ;
#171947=CARTESIAN_POINT ( 'NONE',  ( -0.05219959533910754901, -16.53943276465976808, 32.49890960531435979 ) ) ;
#171948=CARTESIAN_POINT ( 'NONE',  ( -5.153800228976328057, -19.02544592524343514, 102.2905762719810383 ) ) ;
#171949=CARTESIAN_POINT ( 'NONE',  ( -21.55341960407619339, 5.719274019375674811, 53.54275706135234714 ) ) ;
#171950=CARTESIAN_POINT ( 'NONE',  ( 13.89961937509977652, -13.97604488694527269, 113.1239096053143527 ) ) ;
#171951=CARTESIAN_POINT ( 'NONE',  ( 14.29746914071037800, 8.314922557961029526, 56.66775706135235424 ) ) ;
#171953=CARTESIAN_POINT ( 'NONE',  ( -0.05219959533936034679, 19.03943276465977164, 62.50109039468566863 ) ) ;
#171954=CARTESIAN_POINT ( 'NONE',  ( 12.14591786802309770, 12.06949235617756955, 34.37390960531435979 ) ) ;
#171955=CARTESIAN_POINT ( 'NONE',  ( -19.39056639909674828, -5.499999999999968026, 75.78948781074343799 ) ) ;
#171956=CARTESIAN_POINT ( 'NONE',  ( 12.06949235617739724, 12.14591786802326823, 106.8760903946856899 ) ) ;
#171957=CARTESIAN_POINT ( 'NONE',  ( -9.474510206698964154, 16.51473224551069663, 35.41557627198102409 ) ) ;
#171958=CARTESIAN_POINT ( 'NONE',  ( -13.97604488694527625, -13.89961937509977652, 61.87390960531435979 ) ) ;
#171959=CARTESIAN_POINT ( 'NONE',  ( 13.97604488694527802, 13.89961937509977652, 24.37390960531435624 ) ) ;
#171960=CARTESIAN_POINT ( 'NONE',  ( 18.62759615963255655, 10.81492255796105972, 31.66775706135234358 ) ) ;
#171961=CARTESIAN_POINT ( 'NONE',  ( -19.03943276465977164, 0.05219959533909376836, 46.24890960531435979 ) ) ;
#171963=CARTESIAN_POINT ( 'NONE',  ( -13.97604488694527625, -13.89961937509977652, 51.87390960531436690 ) ) ;
#171964=CARTESIAN_POINT ( 'NONE',  ( 10.81492255796078972, 18.62759615963270932, 24.58224293864768839 ) ) ;
#171966=CARTESIAN_POINT ( 'NONE',  ( -10.81492255796105439, 18.62759615963255655, 52.91775706135235424 ) ) ;
#171967=CARTESIAN_POINT ( 'NONE',  ( 9.474510206698971260, -16.51473224551069308, 27.91557627198103120 ) ) ;
#171968=CARTESIAN_POINT ( 'NONE',  ( 10.81492255796078972, 18.62759615963270932, 34.58224293864770260 ) ) ;
#171969=CARTESIAN_POINT ( 'NONE',  ( -12.14591786802326823, 12.06949235617739902, 73.12609039468567573 ) ) ;
#171970=CARTESIAN_POINT ( 'NONE',  ( -10.72451020669870658, -18.67979575497194134, 109.5844237280190328 ) ) ;
#171971=CARTESIAN_POINT ( 'NONE',  ( -12.14591786802326823, 12.06949235617739902, 53.12609039468568284 ) ) ;
#171972=CARTESIAN_POINT ( 'NONE',  ( -19.05341960407611168, -5.049401038298163336, 91.45724293864766707 ) ) ;
#171973=CARTESIAN_POINT ( 'NONE',  ( 8.224510206698742110, 14.34966873604972548, 47.08442372801901854 ) ) ;
#171974=CARTESIAN_POINT ( 'NONE',  ( 16.55341960407618274, -4.379528057220086978, 21.04275706135234714 ) ) ;
#171975=CARTESIAN_POINT ( 'NONE',  ( 0.05219959533934541429, -16.53943276465976808, 90.00109039468567573 ) ) ;
#171976=CARTESIAN_POINT ( 'NONE',  ( 18.67979575497194134, -10.72451020669871369, 50.83442372801901143 ) ) ;
#171977=CARTESIAN_POINT ( 'NONE',  ( 9.474510206698729675, 16.51473224551082808, 102.0844237280190043 ) ) ;
#171978=CARTESIAN_POINT ( 'NONE',  ( -15.72974639402176322, -15.80617190586768395, 19.37609039468568639 ) ) ;
#171979=CARTESIAN_POINT ( 'NONE',  ( -8.224510206698948167, 14.34966873604960824, 100.4155762719810241 ) ) ;
#171980=CARTESIAN_POINT ( 'NONE',  ( -16.51473224551082808, 9.474510206698731452, 103.3344237280190043 ) ) ;
#171981=CARTESIAN_POINT ( 'NONE',  ( 4.483927247898790824, -16.52544592524335698, 85.20942372801901854 ) ) ;
#171983=CARTESIAN_POINT ( 'NONE',  ( 16.46253265017146816, 9.564922557961045513, 86.66775706135233293 ) ) ;
#171984=CARTESIAN_POINT ( 'NONE',  ( 4.379528057220339221, -16.55341960407611168, 47.70724293864770260 ) ) ;
#171985=CARTESIAN_POINT ( 'NONE',  ( -4.483927247898539470, -16.52544592524342804, 42.29057627198103120 ) ) ;
#171986=CARTESIAN_POINT ( 'NONE',  ( -16.55341960407611168, -4.379528057220339221, 106.4572429386477097 ) ) ;
#171987=CARTESIAN_POINT ( 'NONE',  ( -16.46253265017146816, -9.564922557961047289, 39.16775706135234003 ) ) ;
#171988=CARTESIAN_POINT ( 'NONE',  ( -17.49999999999999645, 5.499999999999992895, 88.71769037696435589 ) ) ;
#171989=CARTESIAN_POINT ( 'NONE',  ( 21.53943276465977519, 0.05219959533937863772, 41.25109039468568284 ) ) ;
#171990=CARTESIAN_POINT ( 'NONE',  ( 5.153800228976615827, -19.02544592524334988, 105.2094237280190185 ) ) ;
#171992=CARTESIAN_POINT ( 'NONE',  ( -19.02544592524342804, 5.153800228976336051, 91.04057627198100988 ) ) ;
#171993=CARTESIAN_POINT ( 'NONE',  ( 16.46253265017160672, -9.564922557960803928, 83.33224293864768129 ) ) ;
#171994=CARTESIAN_POINT ( 'NONE',  ( 5.823673210054125526, 21.52544592524343514, 59.79057627198103120 ) ) ;
#171995=CARTESIAN_POINT ( 'NONE',  ( -8.224510206698948167, 14.34966873604960824, 95.41557627198102409 ) ) ;
#171996=CARTESIAN_POINT ( 'NONE',  ( -5.049401038298153566, 19.05341960407611168, 65.20724293864765286 ) ) ;
#171997=CARTESIAN_POINT ( 'NONE',  ( -19.03943276465977164, 0.05219959533909376836, 36.24890960531436690 ) ) ;
#171998=CARTESIAN_POINT ( 'NONE',  ( -5.823673210054431948, 21.52544592524334988, 42.70942372801901854 ) ) ;
#171999=CARTESIAN_POINT ( 'NONE',  ( 21.53943276465977519, 0.05219959533937863772, 71.25109039468568994 ) ) ;
#172000=CARTESIAN_POINT ( 'NONE',  ( 4.483927247898790824, -16.52544592524335698, 95.20942372801903275 ) ) ;
#172001=CARTESIAN_POINT ( 'NONE',  ( 21.55341960407619695, -5.719274019375665929, 26.04275706135235779 ) ) ;
#172002=CARTESIAN_POINT ( 'NONE',  ( 10.72451020669871369, 18.67979575497193778, 22.08442372801901143 ) ) ;
#172003=CARTESIAN_POINT ( 'NONE',  ( -9.474510206698720793, -16.51473224551083518, 59.58442372801900433 ) ) ;
#172004=CARTESIAN_POINT ( 'NONE',  ( -5.153800228976328057, -19.02544592524343514, 82.29057627198103830 ) ) ;
#172005=CARTESIAN_POINT ( 'NONE',  ( -18.67979575497193778, 10.72451020669871902, 83.33442372801903275 ) ) ;
#172006=CARTESIAN_POINT ( 'NONE',  ( -21.55341960407610458, -5.719274019375992779, 81.45724293864769550 ) ) ;
#172007=CARTESIAN_POINT ( 'NONE',  ( -12.14591786802309592, -12.06949235617757132, 56.87390960531436690 ) ) ;
#172008=CARTESIAN_POINT ( 'NONE',  ( 21.52544592524334988, 5.823673210054432836, 106.4594237280190328 ) ) ;
#172009=CARTESIAN_POINT ( 'NONE',  ( -16.52544592524342804, 4.483927247898546575, 66.04057627198103830 ) ) ;
#172010=CARTESIAN_POINT ( 'NONE',  ( -0.05219959533909027116, -19.03943276465977164, 27.49890960531435624 ) ) ;
#172011=CARTESIAN_POINT ( 'NONE',  ( 19.03943276465977164, 0.05219959533936151252, 76.25109039468566152 ) ) ;
#172012=CARTESIAN_POINT ( 'NONE',  ( 8.224510206698953496, -14.34966873604960469, 32.91557627198102409 ) ) ;
#172013=CARTESIAN_POINT ( 'NONE',  ( 15.72974639402176855, 15.80617190586768217, 81.87609039468568994 ) ) ;
#172014=CARTESIAN_POINT ( 'NONE',  ( -19.02544592524342804, 5.153800228976336051, 86.04057627198103830 ) ) ;
#172015=CARTESIAN_POINT ( 'NONE',  ( -13.97604488694547697, 13.89961937509957934, 58.12609039468566863 ) ) ;
#172016=CARTESIAN_POINT ( 'NONE',  ( -10.81492255796078084, -18.62759615963271287, 62.08224293864769550 ) ) ;
#172017=CARTESIAN_POINT ( 'NONE',  ( -18.62759615963270932, 10.81492255796079327, 110.8322429386476955 ) ) ;
#172018=CARTESIAN_POINT ( 'NONE',  ( 12.14591786802327356, -12.06949235617739191, 20.62609039468568639 ) ) ;
#172019=CARTESIAN_POINT ( 'NONE',  ( 8.314922557961029526, -14.29746914071037800, 85.41775706135236135 ) ) ;
#172020=CARTESIAN_POINT ( 'NONE',  ( 16.36317988757058117, 7.306389748694948949, 63.40210391636776421 ) ) ;
#172021=CARTESIAN_POINT ( 'NONE',  ( -18.67979575497193778, 10.72451020669871902, 28.33442372801902209 ) ) ;
#172022=CARTESIAN_POINT ( 'NONE',  ( 12.06949235617757843, -12.14591786802309237, 98.12390960531436690 ) ) ;
#172024=CARTESIAN_POINT ( 'NONE',  ( 8.224510206698742110, 14.34966873604972548, 42.08442372801901854 ) ) ;
#172025=APPLICATION_CONTEXT ( 'automotive_design' ) ;
#172026=CARTESIAN_POINT ( 'NONE',  ( -21.53943276465977519, 0.05219959533907696930, 56.24890960531436690 ) ) ;
#172027=CARTESIAN_POINT ( 'NONE',  ( -8.224510206698735004, -14.34966873604973081, 109.5844237280190328 ) ) ;
#172028=CARTESIAN_POINT ( 'NONE',  ( 12.14591786802327356, -12.06949235617739191, 40.62609039468567573 ) ) ;
#172029=CARTESIAN_POINT ( 'NONE',  ( 16.51473224551069308, 9.474510206698969483, 34.16557627198102409 ) ) ;
#172030=CARTESIAN_POINT ( 'NONE',  ( -0.05219959533934338120, 16.53943276465976808, 82.50109039468568994 ) ) ;
#172031=CARTESIAN_POINT ( 'NONE',  ( 9.474510206698729675, 16.51473224551082808, 77.08442372801900433 ) ) ;
#172032=CARTESIAN_POINT ( 'NONE',  ( 15.72974639402199770, -15.80617190586745480, 63.12390960531435979 ) ) ;
#172033=CARTESIAN_POINT ( 'NONE',  ( 14.29746914071037800, 8.314922557961029526, 96.66775706135234714 ) ) ;
#172034=CARTESIAN_POINT ( 'NONE',  ( 21.53943276465977519, 0.05219959533937863772, 81.25109039468568994 ) ) ;
#172035=CARTESIAN_POINT ( 'NONE',  ( 18.67979575497178502, 10.72451020669898547, 59.16557627198103120 ) ) ;
#172036=CARTESIAN_POINT ( 'NONE',  ( -10.72451020669898014, 18.67979575497178502, 45.41557627198103830 ) ) ;
#172038=CARTESIAN_POINT ( 'NONE',  ( -16.55341960407617563, 4.379528057220093196, 83.54275706135234714 ) ) ;
#172039=CARTESIAN_POINT ( 'NONE',  ( -15.72974639402197994, 15.80617190586746368, 45.62390960531436690 ) ) ;
#172041=CARTESIAN_POINT ( 'NONE',  ( -19.02544592524342804, 5.153800228976336051, 96.04057627198103830 ) ) ;
#172043=CARTESIAN_POINT ( 'NONE',  ( -16.51473224551069308, -9.474510206698971260, 21.66557627198102765 ) ) ;
#172044=CARTESIAN_POINT ( 'NONE',  ( 5.823673210054125526, 21.52544592524343514, 64.79057627198103830 ) ) ;
#172045=CARTESIAN_POINT ( 'NONE',  ( -8.314922557961024197, 14.29746914071037800, 97.91775706135236135 ) ) ;
#172046=CARTESIAN_POINT ( 'NONE',  ( -10.72451020669870658, -18.67979575497194134, 44.58442372801901854 ) ) ;
#172047=CARTESIAN_POINT ( 'NONE',  ( 5.049401038297881783, 19.05341960407617563, 97.29275706135233293 ) ) ;
#172048=CARTESIAN_POINT ( 'NONE',  ( 8.314922557960818139, 14.29746914071049879, 104.5822429386477097 ) ) ;
#172049=CARTESIAN_POINT ( 'NONE',  ( 5.049401038297881783, 19.05341960407617563, 107.2927570613523187 ) ) ;
#172050=CARTESIAN_POINT ( 'NONE',  ( 16.46253265017160672, -9.564922557960803928, 43.33224293864769550 ) ) ;
#172052=CARTESIAN_POINT ( 'NONE',  ( -9.474510206698964154, 16.51473224551069663, 95.41557627198102409 ) ) ;
#172053=CARTESIAN_POINT ( 'NONE',  ( 8.314922557961029526, -14.29746914071037800, 80.41775706135234714 ) ) ;
#172054=CARTESIAN_POINT ( 'NONE',  ( -9.564922557961040184, 16.46253265017147172, 72.91775706135233293 ) ) ;
#172055=CARTESIAN_POINT ( 'NONE',  ( -10.81492255796105439, 18.62759615963255655, 102.9177570613523756 ) ) ;
#172056=CARTESIAN_POINT ( 'NONE',  ( -18.62759615963270932, 10.81492255796079327, 65.83224293864769550 ) ) ;
#172057=EDGE_CURVE ( 'NONE', #72076, #27411, #63892, .T. ) ;
#172058=CARTESIAN_POINT ( 'NONE',  ( -4.379528057220086978, -16.55341960407618274, 84.79275706135234714 ) ) ;
#172059=CARTESIAN_POINT ( 'NONE',  ( 16.46253265017146816, 9.564922557961045513, 76.66775706135234714 ) ) ;
#172060=CARTESIAN_POINT ( 'NONE',  ( -13.97604488694527625, -13.89961937509977652, 31.87390960531435979 ) ) ;
#172061=CARTESIAN_POINT ( 'NONE',  ( -13.97604488694527625, -13.89961937509977652, 71.87390960531433848 ) ) ;
#172062=CARTESIAN_POINT ( 'NONE',  ( -18.67979575497193778, 10.72451020669871902, 53.33442372801901854 ) ) ;
#172063=CARTESIAN_POINT ( 'NONE',  ( 13.97604488694527802, 13.89961937509977652, 49.37390960531434558 ) ) ;
#172064=CARTESIAN_POINT ( 'NONE',  ( -5.153800228976607833, 19.02544592524334988, 67.70942372801900433 ) ) ;
#172066=CARTESIAN_POINT ( 'NONE',  ( 13.89961937509977652, -13.97604488694527269, 108.1239096053143669 ) ) ;
#172067=CARTESIAN_POINT ( 'NONE',  ( -16.55341960407611168, -4.379528057220339221, 66.45724293864768129 ) ) ;
#172068=CARTESIAN_POINT ( 'NONE',  ( -5.823673210054116645, -21.52544592524344225, 57.29057627198103120 ) ) ;
#172070=CARTESIAN_POINT ( 'NONE',  ( 19.03943276465977164, 0.05219959533936151252, 36.25109039468567573 ) ) ;
#172072=CARTESIAN_POINT ( 'NONE',  ( 19.02544592524343514, -5.153800228976328945, 63.54057627198103830 ) ) ;
#172073=CARTESIAN_POINT ( 'NONE',  ( 13.89961937509977652, -13.97604488694527269, 78.12390960531433848 ) ) ;
#172074=CARTESIAN_POINT ( 'NONE',  ( -14.34966873604972548, 8.224510206698743886, 53.33442372801901854 ) ) ;
#172076=CARTESIAN_POINT ( 'NONE',  ( -17.05587630539787725, 6.762274262135673730, 110.7418030903731534 ) ) ;
#172077=CARTESIAN_POINT ( 'NONE',  ( 12.14591786802327356, -12.06949235617739191, 90.62609039468567573 ) ) ;
#172079=CARTESIAN_POINT ( 'NONE',  ( -0.05219959533934338120, 16.53943276465976808, 62.50109039468568284 ) ) ;
#172080=CARTESIAN_POINT ( 'NONE',  ( 12.06949235617739724, 12.14591786802326823, 36.87609039468568994 ) ) ;
#172081=CARTESIAN_POINT ( 'NONE',  ( -19.05341960407611168, -5.049401038298163336, 56.45724293864768129 ) ) ;
#172083=CARTESIAN_POINT ( 'NONE',  ( -10.81492255796105439, 18.62759615963255655, 47.91775706135234714 ) ) ;
#172084=CARTESIAN_POINT ( 'NONE',  ( 19.05341960407617918, -5.049401038297876454, 61.04275706135232582 ) ) ;
#172085=CARTESIAN_POINT ( 'NONE',  ( -18.67979575497193778, 10.72451020669871902, 103.3344237280190043 ) ) ;
#172086=CARTESIAN_POINT ( 'NONE',  ( -9.474510206698964154, 16.51473224551069663, 35.41557627198102409 ) ) ;
#172088=CARTESIAN_POINT ( 'NONE',  ( 18.62759615963271287, -10.81492255796078972, 48.33224293864770260 ) ) ;
#172089=CARTESIAN_POINT ( 'NONE',  ( -13.97604488694527625, -13.89961937509977652, 111.8739096053143243 ) ) ;
#172090=CARTESIAN_POINT ( 'NONE',  ( -12.06949235617756955, 12.14591786802309770, 95.62390960531436690 ) ) ;
#172091=CARTESIAN_POINT ( 'NONE',  ( -4.379528057220086978, -16.55341960407618274, 39.79275706135235424 ) ) ;
#172092=CARTESIAN_POINT ( 'NONE',  ( 0.05219959533910956823, 16.53943276465976808, 34.99890960531435979 ) ) ;
#172093=ORIENTED_EDGE ( 'NONE', *, *, #41117, .F. ) ;
#172094=CARTESIAN_POINT ( 'NONE',  ( 21.52544592524344225, -5.823673210054117533, 103.5405762719810383 ) ) ;
#172096=CARTESIAN_POINT ( 'NONE',  ( 14.34966873604960469, 8.224510206698951720, 34.16557627198102409 ) ) ;
#172098=CARTESIAN_POINT ( 'NONE',  ( -9.564922557961040184, 16.46253265017147172, 92.91775706135233293 ) ) ;
#172099=CARTESIAN_POINT ( 'NONE',  ( -9.564922557961040184, 16.46253265017147172, 27.91775706135232582 ) ) ;
#172100=CARTESIAN_POINT ( 'NONE',  ( 0.05219959533910956823, 16.53943276465976808, 29.99890960531435979 ) ) ;
#172101=CARTESIAN_POINT ( 'NONE',  ( 10.72451020669898902, -18.67979575497178502, 97.91557627198103830 ) ) ;
#172102=CARTESIAN_POINT ( 'NONE',  ( -18.62759615963270932, 10.81492255796079327, 55.83224293864770260 ) ) ;
#172103=CARTESIAN_POINT ( 'NONE',  ( 19.03943276465977164, -0.05219959533909143690, 78.74890960531436690 ) ) ;
#172104=CARTESIAN_POINT ( 'NONE',  ( -16.53943276465976808, 0.05219959533911058130, 46.24890960531435979 ) ) ;
#172105=CARTESIAN_POINT ( 'NONE',  ( 5.153800228976335163, 19.02544592524342804, 94.79057627198103830 ) ) ;
#172108=CARTESIAN_POINT ( 'NONE',  ( 16.51473224551083163, -9.474510206698727899, 35.83442372801899722 ) ) ;
#172109=CARTESIAN_POINT ( 'NONE',  ( 10.81492255796078972, 18.62759615963270932, 99.58224293864770971 ) ) ;
#172110=CARTESIAN_POINT ( 'NONE',  ( 4.483927247898545687, 16.52544592524342804, 94.79057627198105251 ) ) ;
#172111=CARTESIAN_POINT ( 'NONE',  ( 10.72451020669871369, 18.67979575497193778, 32.08442372801901854 ) ) ;
#172114=CARTESIAN_POINT ( 'NONE',  ( 12.14591786802327356, -12.06949235617739191, 100.6260903946857184 ) ) ;
#172115=CARTESIAN_POINT ( 'NONE',  ( -13.89961937509977652, 13.97604488694528158, 30.62390960531435269 ) ) ;
#172116=CARTESIAN_POINT ( 'NONE',  ( -19.02544592524342804, 5.153800228976336051, 86.04057627198103830 ) ) ;
#172118=CARTESIAN_POINT ( 'NONE',  ( -19.05341960407611168, -5.049401038298163336, 36.45724293864766707 ) ) ;
#172119=CARTESIAN_POINT ( 'NONE',  ( -14.29746914071049879, 8.314922557960819915, 40.83224293864769550 ) ) ;
#172120=CARTESIAN_POINT ( 'NONE',  ( -15.72974639402176322, -15.80617190586768395, 69.37609039468567573 ) ) ;
#172122=CARTESIAN_POINT ( 'NONE',  ( 12.06949235617739724, 12.14591786802326823, 71.87609039468568994 ) ) ;
#172123=CARTESIAN_POINT ( 'NONE',  ( 16.46253265017160672, -9.564922557960803928, 58.33224293864769550 ) ) ;
#172124=CARTESIAN_POINT ( 'NONE',  ( -5.049401038298153566, 19.05341960407611168, 65.20724293864765286 ) ) ;
#172126=CARTESIAN_POINT ( 'NONE',  ( 0.05219959533937995610, -21.53943276465977519, 105.0010903946856757 ) ) ;
#172127=CARTESIAN_POINT ( 'NONE',  ( 4.483927247898790824, -16.52544592524335698, 75.20942372801901854 ) ) ;
#172128=CARTESIAN_POINT ( 'NONE',  ( -18.62759615963255300, -10.81492255796106328, 104.1677570613523471 ) ) ;
#172129=CARTESIAN_POINT ( 'NONE',  ( -0.05219959533909027116, -19.03943276465977164, 67.49890960531436690 ) ) ;
#172130=CARTESIAN_POINT ( 'NONE',  ( -21.55341960407610458, -5.719274019375992779, 41.45724293864769550 ) ) ;
#172131=CARTESIAN_POINT ( 'NONE',  ( -9.474510206698720793, -16.51473224551083518, 104.5844237280190043 ) ) ;
#172132=CARTESIAN_POINT ( 'NONE',  ( 10.72451020669871369, 18.67979575497193778, 87.08442372801901854 ) ) ;
#172133=CARTESIAN_POINT ( 'NONE',  ( -16.52544592524335698, -4.483927247898792601, 53.95942372801900433 ) ) ;
#172134=CARTESIAN_POINT ( 'NONE',  ( 0.05219959533907565091, 21.53943276465977519, 104.9989096053143669 ) ) ;
#172135=CARTESIAN_POINT ( 'NONE',  ( 16.46253265017146816, 9.564922557961045513, 96.66775706135233293 ) ) ;
#172136=CARTESIAN_POINT ( 'NONE',  ( 19.05341960407611168, 5.049401038298154454, 78.95724293864769550 ) ) ;
#172137=CARTESIAN_POINT ( 'NONE',  ( -0.05219959533936034679, 19.03943276465977164, 112.5010903946856757 ) ) ;
#172138=CARTESIAN_POINT ( 'NONE',  ( 16.52544592524335698, 4.483927247898782831, 26.45942372801901854 ) ) ;
#172139=CARTESIAN_POINT ( 'NONE',  ( 0.05219959533910956823, 16.53943276465976808, 64.99890960531435269 ) ) ;
#172140=CARTESIAN_POINT ( 'NONE',  ( 12.14591786802327356, -12.06949235617739191, 80.62609039468567573 ) ) ;
#172141=CARTESIAN_POINT ( 'NONE',  ( -18.62759615963270932, 10.81492255796079327, 115.8322429386477097 ) ) ;
#172142=CARTESIAN_POINT ( 'NONE',  ( 9.474510206698971260, -16.51473224551069308, 47.91557627198102409 ) ) ;
#172143=CARTESIAN_POINT ( 'NONE',  ( 16.51473224551069308, 9.474510206698969483, 64.16557627198102409 ) ) ;
#172145=CARTESIAN_POINT ( 'NONE',  ( 14.29746914071037800, 8.314922557961029526, 76.66775706135234714 ) ) ;
#172147=ORIENTED_EDGE ( 'NONE', *, *, #113016, .T. ) ;
#172148=CARTESIAN_POINT ( 'NONE',  ( 18.62759615963255655, 10.81492255796105972, 106.6677570613523756 ) ) ;
#172149=CARTESIAN_POINT ( 'NONE',  ( -19.05341960407611168, -5.049401038298163336, 36.45724293864766707 ) ) ;
#172150=ORIENTED_EDGE ( 'NONE', *, *, #185592, .F. ) ;
#172151=CARTESIAN_POINT ( 'NONE',  ( 8.224510206698742110, 14.34966873604972548, 32.08442372801901854 ) ) ;
#172152=CARTESIAN_POINT ( 'NONE',  ( 19.05341960407617918, -5.049401038297876454, 41.04275706135233293 ) ) ;
#172153=CARTESIAN_POINT ( 'NONE',  ( 8.314922557961029526, -14.29746914071037800, 35.41775706135234003 ) ) ;
#172154=CARTESIAN_POINT ( 'NONE',  ( -0.05219959533909027116, -19.03943276465977164, 42.49890960531435269 ) ) ;
#172155=CARTESIAN_POINT ( 'NONE',  ( -0.05219959533909027116, -19.03943276465977164, 62.49890960531435979 ) ) ;
#172156=CARTESIAN_POINT ( 'NONE',  ( -15.80617190586745835, -15.72974639402198527, 81.87390960531435269 ) ) ;
#172157=CARTESIAN_POINT ( 'NONE',  ( 19.02544592524343514, -5.153800228976328945, 78.54057627198099567 ) ) ;
#172158=CARTESIAN_POINT ( 'NONE',  ( -16.51473224551069308, -9.474510206698971260, 106.6655762719810383 ) ) ;
#172160=CARTESIAN_POINT ( 'NONE',  ( -19.03943276465977164, 0.05219959533909376836, 51.24890960531436690 ) ) ;
#172162=CARTESIAN_POINT ( 'NONE',  ( -5.049401038297874678, -19.05341960407617918, 99.79275706135234714 ) ) ;
#172163=CARTESIAN_POINT ( 'NONE',  ( 21.52544592524344225, -5.823673210054117533, 78.54057627198103830 ) ) ;
#172164=CARTESIAN_POINT ( 'NONE',  ( -16.46253265017146816, -9.564922557961047289, 19.16775706135233293 ) ) ;
#172165=CARTESIAN_POINT ( 'NONE',  ( 12.14591786802309770, 12.06949235617756955, 64.37390960531435269 ) ) ;
#172166=CARTESIAN_POINT ( 'NONE',  ( 10.72451020669871369, 18.67979575497193778, 87.08442372801901854 ) ) ;
#172167=CARTESIAN_POINT ( 'NONE',  ( 0.05219959533910956823, 16.53943276465976808, 114.9989096053143669 ) ) ;
#172168=CARTESIAN_POINT ( 'NONE',  ( 14.34966873604960469, 8.224510206698951720, 24.16557627198103120 ) ) ;
#172169=CARTESIAN_POINT ( 'NONE',  ( 15.72974639402176855, 15.80617190586768217, 91.87609039468568994 ) ) ;
#172170=CARTESIAN_POINT ( 'NONE',  ( -16.51473224551069308, -9.474510206698971260, 81.66557627198103830 ) ) ;
#172171=CARTESIAN_POINT ( 'NONE',  ( -21.53943276465977519, -0.05219959533937600094, 43.75109039468568284 ) ) ;
#172172=CARTESIAN_POINT ( 'NONE',  ( -16.46253265017160317, 9.564922557960807481, 80.83224293864769550 ) ) ;
#172173=CARTESIAN_POINT ( 'NONE',  ( 16.53943276465976808, -0.05219959533910856209, 98.74890960531438111 ) ) ;
#172174=CARTESIAN_POINT ( 'NONE',  ( 14.34966873604960469, 8.224510206698951720, 64.16557627198102409 ) ) ;
#172175=CARTESIAN_POINT ( 'NONE',  ( -5.823673210054116645, -21.52544592524344225, 72.29057627198102409 ) ) ;
#172176=CARTESIAN_POINT ( 'NONE',  ( 9.564922557960805705, 16.46253265017160317, 69.58224293864770971 ) ) ;
#172177=CARTESIAN_POINT ( 'NONE',  ( 18.67979575497178502, 10.72451020669898547, 89.16557627198102409 ) ) ;
#172178=CARTESIAN_POINT ( 'NONE',  ( -19.05341960407617563, 5.049401038297882671, 78.54275706135233293 ) ) ;
#172179=CARTESIAN_POINT ( 'NONE',  ( -5.153800228976607833, 19.02544592524335343, 32.70942372801899012 ) ) ;
#172180=CARTESIAN_POINT ( 'NONE',  ( -4.483927247898539470, -16.52544592524342804, 77.29057627198102409 ) ) ;
#172181=CARTESIAN_POINT ( 'NONE',  ( 21.55341960407610458, 5.719274019375980345, 53.95724293864770260 ) ) ;
#172182=CARTESIAN_POINT ( 'NONE',  ( 16.62475595723697808, -7.163666690055227271, 28.02713351810468723 ) ) ;
#172183=CARTESIAN_POINT ( 'NONE',  ( -16.53943276465976808, -0.05219959533934237506, 103.7510903946857042 ) ) ;
#172185=CARTESIAN_POINT ( 'NONE',  ( -19.05341960407617563, 5.049401038297882671, 108.5427570613523187 ) ) ;
#172186=CARTESIAN_POINT ( 'NONE',  ( -0.05219959533910754901, -16.53943276465976808, 77.49890960531433848 ) ) ;
#172188=CARTESIAN_POINT ( 'NONE',  ( -9.474510206698964154, 16.51473224551069663, 75.41557627198103830 ) ) ;
#172189=CARTESIAN_POINT ( 'NONE',  ( 13.89961937509977652, -13.97604488694527269, 38.12390960531436690 ) ) ;
#172190=CARTESIAN_POINT ( 'NONE',  ( -16.52544592524342804, 4.483927247898546575, 51.04057627198103120 ) ) ;
#172191=CARTESIAN_POINT ( 'NONE',  ( -13.97604488694527625, -13.89961937509977652, 101.8739096053143811 ) ) ;
#172192=CARTESIAN_POINT ( 'NONE',  ( -19.05341960407617563, 5.049401038297882671, 88.54275706135230450 ) ) ;
#172193=CARTESIAN_POINT ( 'NONE',  ( -5.153800228976328057, -19.02544592524343514, 67.29057627198102409 ) ) ;
#172194=CARTESIAN_POINT ( 'NONE',  ( 14.34966873604972726, -8.224510206698740333, 25.83442372801901499 ) ) ;
#172195=CARTESIAN_POINT ( 'NONE',  ( -13.89961937509977652, 13.97604488694528158, 85.62390960531433848 ) ) ;
#172196=CARTESIAN_POINT ( 'NONE',  ( 21.53943276465977519, -0.05219959533907433946, 68.74890960531435269 ) ) ;
#172197=CARTESIAN_POINT ( 'NONE',  ( 16.55341960407618274, -4.379528057220086978, 56.04275706135235424 ) ) ;
#172198=CARTESIAN_POINT ( 'NONE',  ( -13.89961937509957401, -13.97604488694547697, 109.3760903946856615 ) ) ;
#172199=CARTESIAN_POINT ( 'NONE',  ( -9.564922557960796823, -16.46253265017161027, 67.08224293864769550 ) ) ;
#172200=CARTESIAN_POINT ( 'NONE',  ( -5.719274019375978568, 21.55341960407610458, 65.20724293864768129 ) ) ;
#172201=CARTESIAN_POINT ( 'NONE',  ( 9.564922557961047289, -16.46253265017146816, 90.41775706135234714 ) ) ;
#172202=CARTESIAN_POINT ( 'NONE',  ( 12.06949235617739724, 12.14591786802326823, 111.8760903946856615 ) ) ;
#172203=CARTESIAN_POINT ( 'NONE',  ( 0.05219959533937995610, -21.53943276465977519, 45.00109039468568284 ) ) ;
#172205=CARTESIAN_POINT ( 'NONE',  ( 8.224510206698742110, 14.34966873604972548, 77.08442372801901854 ) ) ;
#172206=CARTESIAN_POINT ( 'NONE',  ( 13.89961937509977652, -13.97604488694527269, 108.1239096053143669 ) ) ;
#172207=CARTESIAN_POINT ( 'NONE',  ( 19.35633801406903842, -5.499999999999758415, 41.63373818172757979 ) ) ;
#172209=CARTESIAN_POINT ( 'NONE',  ( 8.224510206698742110, 14.34966873604972548, 97.08442372801904696 ) ) ;
#172210=CARTESIAN_POINT ( 'NONE',  ( -16.55341960407617563, 4.379528057220093196, 38.54275706135234714 ) ) ;
#172211=CARTESIAN_POINT ( 'NONE',  ( -16.46253265017160317, 9.564922557960807481, 45.83224293864769550 ) ) ;
#172212=CARTESIAN_POINT ( 'NONE',  ( -16.51473224551069308, -9.474510206698971260, 56.66557627198103120 ) ) ;
#172213=CARTESIAN_POINT ( 'NONE',  ( 9.564922557960805705, 16.46253265017160317, 54.58224293864769550 ) ) ;
#172214=CARTESIAN_POINT ( 'NONE',  ( -0.05219959533937732626, 21.53943276465977519, 47.50109039468568994 ) ) ;
#172215=CARTESIAN_POINT ( 'NONE',  ( 4.379528057220092307, 16.55341960407617563, 52.29275706135236135 ) ) ;
#172216=CARTESIAN_POINT ( 'NONE',  ( -14.34966873604960291, -8.224510206698953496, 31.66557627198102054 ) ) ;
#172217=CARTESIAN_POINT ( 'NONE',  ( -13.97604488694527625, -13.89961937509977652, 46.87390960531435979 ) ) ;
#172218=CARTESIAN_POINT ( 'NONE',  ( 13.89961937509977652, -13.97604488694527269, 38.12390960531436690 ) ) ;
#172219=CARTESIAN_POINT ( 'NONE',  ( -12.14591786802326823, 12.06949235617739902, 33.12609039468569705 ) ) ;
#172220=CARTESIAN_POINT ( 'NONE',  ( -9.474510206698720793, -16.51473224551083518, 84.58442372801900433 ) ) ;
#172221=CARTESIAN_POINT ( 'NONE',  ( 8.314922557960818139, 14.29746914071049879, 84.58224293864769550 ) ) ;
#172222=CARTESIAN_POINT ( 'NONE',  ( -9.564922557960796823, -16.46253265017161027, 57.08224293864769550 ) ) ;
#172223=CARTESIAN_POINT ( 'NONE',  ( -0.05219959533936034679, 19.03943276465977164, 87.50109039468567573 ) ) ;
#172225=CARTESIAN_POINT ( 'NONE',  ( 21.55341960407619695, -5.719274019375665929, 71.04275706135234714 ) ) ;
#172226=CARTESIAN_POINT ( 'NONE',  ( -12.06949235617739369, -12.14591786802326823, 54.37609039468568994 ) ) ;
#172227=CARTESIAN_POINT ( 'NONE',  ( 17.48847506799968698, 5.747544572773807481, 36.67302562156721990 ) ) ;
#172228=CARTESIAN_POINT ( 'NONE',  ( -18.62759615963270932, 10.81492255796079327, 45.83224293864769550 ) ) ;
#172229=CARTESIAN_POINT ( 'NONE',  ( -4.483927247898782831, 16.52544592524335698, 37.70942372801900433 ) ) ;
#172230=CARTESIAN_POINT ( 'NONE',  ( -9.564922557960796823, -16.46253265017161027, 22.08224293864768839 ) ) ;
#172231=CARTESIAN_POINT ( 'NONE',  ( -16.46253265017146816, -9.564922557961047289, 29.16775706135232937 ) ) ;
#172233=CARTESIAN_POINT ( 'NONE',  ( 9.564922557960805705, 16.46253265017160317, 54.58224293864769550 ) ) ;
#172235=CARTESIAN_POINT ( 'NONE',  ( 19.02544592524343514, -5.153800228976328945, 73.54057627198103830 ) ) ;
#172236=CARTESIAN_POINT ( 'NONE',  ( -19.49149378614659511, 5.499999999999674039, 99.43757513605360998 ) ) ;
#172237=CARTESIAN_POINT ( 'NONE',  ( 21.52544592524334988, 5.823673210054432836, 111.4594237280190328 ) ) ;
#172238=CARTESIAN_POINT ( 'NONE',  ( 4.379528057220339221, -16.55341960407611168, 32.70724293864770260 ) ) ;
#172239=CARTESIAN_POINT ( 'NONE',  ( -13.97604488694527625, -13.89961937509977652, 46.87390960531435979 ) ) ;
#172240=CARTESIAN_POINT ( 'NONE',  ( 9.474510206698971260, -16.51473224551069308, 107.9155762719810383 ) ) ;
#172241=CARTESIAN_POINT ( 'NONE',  ( 18.62759615963255655, 10.81492255796105972, 66.66775706135234714 ) ) ;
#172242=CARTESIAN_POINT ( 'NONE',  ( -9.474510206698964154, 16.51473224551069663, 45.41557627198103120 ) ) ;
#172243=CARTESIAN_POINT ( 'NONE',  ( -21.53943276465977519, -0.05219959533937600094, 63.75109039468568284 ) ) ;
#172244=CARTESIAN_POINT ( 'NONE',  ( 16.51473224551069308, 9.474510206698969483, 114.1655762719810241 ) ) ;
#172245=CARTESIAN_POINT ( 'NONE',  ( -13.89961937509977652, 13.97604488694528158, 30.62390960531435269 ) ) ;
#172246=CARTESIAN_POINT ( 'NONE',  ( 10.72451020669871369, 18.67979575497193778, 22.08442372801901143 ) ) ;
#172247=CARTESIAN_POINT ( 'NONE',  ( -19.05341960407617563, 5.049401038297882671, 43.54275706135232582 ) ) ;
#172248=CARTESIAN_POINT ( 'NONE',  ( -19.05341960407611168, -5.049401038298163336, 26.45724293864769550 ) ) ;
#172249=CARTESIAN_POINT ( 'NONE',  ( -16.46253265017160317, 9.564922557960807481, 60.83224293864769550 ) ) ;
#172250=CARTESIAN_POINT ( 'NONE',  ( -5.049401038297874678, -19.05341960407617918, 109.7927570613523187 ) ) ;
#172251=CARTESIAN_POINT ( 'NONE',  ( 14.34966873604960469, 8.224510206698951720, 69.16557627198102409 ) ) ;
#172252=CARTESIAN_POINT ( 'NONE',  ( -15.80617190586745835, -15.72974639402198527, 41.87390960531435979 ) ) ;
#172253=CARTESIAN_POINT ( 'NONE',  ( 13.97604488694548053, -13.89961937509957401, 105.6260903946856757 ) ) ;
#172254=CARTESIAN_POINT ( 'NONE',  ( -21.53943276465977519, 0.05219959533907696930, 101.2489096053143669 ) ) ;
#172255=CARTESIAN_POINT ( 'NONE',  ( -15.80617190586768217, 15.72974639402176855, 53.12609039468568284 ) ) ;
#172256=CARTESIAN_POINT ( 'NONE',  ( -0.05219959533934338120, 16.53943276465976808, 52.50109039468567573 ) ) ;
#172257=CARTESIAN_POINT ( 'NONE',  ( -12.14591786802326823, 12.06949235617739902, 58.12609039468568994 ) ) ;
#172258=CARTESIAN_POINT ( 'NONE',  ( -0.05219959533907301413, -21.53943276465977519, 62.49890960531436690 ) ) ;
#172259=CARTESIAN_POINT ( 'NONE',  ( -13.97604488694527625, -13.89961937509977652, 41.87390960531435979 ) ) ;
#172260=CARTESIAN_POINT ( 'NONE',  ( -0.05219959533934338120, 16.53943276465976808, 72.50109039468568994 ) ) ;
#172261=CARTESIAN_POINT ( 'NONE',  ( -10.81492255796078084, -18.62759615963271287, 97.08224293864770971 ) ) ;
#172262=CARTESIAN_POINT ( 'NONE',  ( -8.314922557960811034, -14.29746914071050412, 52.08224293864768839 ) ) ;
#172263=CARTESIAN_POINT ( 'NONE',  ( 16.46253265017160672, -9.564922557960803928, 78.33224293864769550 ) ) ;
#172264=CARTESIAN_POINT ( 'NONE',  ( -16.55341960407617563, 4.379528057220093196, 73.54275706135234714 ) ) ;
#172265=CARTESIAN_POINT ( 'NONE',  ( 19.05341960407617918, -5.049401038297876454, 111.0427570613523329 ) ) ;
#172266=CARTESIAN_POINT ( 'NONE',  ( -5.719274019375665041, -21.55341960407619695, 19.79275706135235069 ) ) ;
#172267=CARTESIAN_POINT ( 'NONE',  ( 12.14591786802309770, 12.06949235617756955, 49.37390960531436690 ) ) ;
#172269=CARTESIAN_POINT ( 'NONE',  ( -16.88567814943163370, 6.947325034625699836, 68.70998877347419409 ) ) ;
#172270=CARTESIAN_POINT ( 'NONE',  ( -10.72451020669898014, 18.67979575497178502, 90.41557627198103830 ) ) ;
#172272=CARTESIAN_POINT ( 'NONE',  ( -16.55341960407611168, -4.379528057220339221, 21.45724293864769550 ) ) ;
#172274=CARTESIAN_POINT ( 'NONE',  ( -17.48853670773242541, -5.747243402303178428, 56.33328700250010002 ) ) ;
#172275=CARTESIAN_POINT ( 'NONE',  ( 15.72974639402199770, -15.80617190586745480, 98.12390960531436690 ) ) ;
#172276=CARTESIAN_POINT ( 'NONE',  ( -13.89961937509977652, 13.97604488694528158, 115.6239096053143669 ) ) ;
#172277=CARTESIAN_POINT ( 'NONE',  ( 0.05219959533907565091, 21.53943276465977519, 114.9989096053143669 ) ) ;
#172278=CARTESIAN_POINT ( 'NONE',  ( 4.379528057220339221, -16.55341960407611168, 47.70724293864770260 ) ) ;
#172279=CARTESIAN_POINT ( 'NONE',  ( -8.224510206698735004, -14.34966873604973081, 54.58442372801901143 ) ) ;
#172280=CARTESIAN_POINT ( 'NONE',  ( -13.89961937509977652, 13.97604488694528158, 55.62390960531434558 ) ) ;
#172281=CARTESIAN_POINT ( 'NONE',  ( 9.564922557961047289, -16.46253265017146816, 50.41775706135233293 ) ) ;
#172282=CARTESIAN_POINT ( 'NONE',  ( -13.89961937509977652, 13.97604488694528158, 85.62390960531433848 ) ) ;
#172283=CARTESIAN_POINT ( 'NONE',  ( -21.55341960407610458, -5.719274019375992779, 41.45724293864769550 ) ) ;
#172284=CARTESIAN_POINT ( 'NONE',  ( 13.97604488694527802, 13.89961937509977830, 64.37390960531436690 ) ) ;
#172285=CARTESIAN_POINT ( 'NONE',  ( -16.52544592524335698, -4.483927247898792601, 23.95942372801901143 ) ) ;
#172286=CARTESIAN_POINT ( 'NONE',  ( 16.51473224551083163, -9.474510206698727899, 70.83442372801900433 ) ) ;
#172287=CARTESIAN_POINT ( 'NONE',  ( -10.72451020669898014, 18.67979575497178502, 100.4155762719810241 ) ) ;
#172289=CARTESIAN_POINT ( 'NONE',  ( -12.14591786802309592, -12.06949235617757132, 31.87390960531435979 ) ) ;
#172290=CARTESIAN_POINT ( 'NONE',  ( 13.97604488694527802, 13.89961937509977652, 79.37390960531435269 ) ) ;
#172291=CARTESIAN_POINT ( 'NONE',  ( -21.53943276465977519, 0.05219959533907696930, 61.24890960531435979 ) ) ;
#172292=CARTESIAN_POINT ( 'NONE',  ( 5.719274019375991003, -21.55341960407610458, 97.70724293864772392 ) ) ;
#172293=CARTESIAN_POINT ( 'NONE',  ( 16.53943276465976808, 0.05219959533934440121, 21.25109039468567218 ) ) ;
#172294=CARTESIAN_POINT ( 'NONE',  ( 5.719274019375991003, -21.55341960407610458, 22.70724293864769194 ) ) ;
#172295=CARTESIAN_POINT ( 'NONE',  ( 5.823673210054444382, -21.52544592524334988, 95.20942372801903275 ) ) ;
#172296=CARTESIAN_POINT ( 'NONE',  ( 13.89961937509977652, -13.97604488694527269, 93.12390960531436690 ) ) ;
#172297=CARTESIAN_POINT ( 'NONE',  ( -16.46253265017160317, 9.564922557960807481, 30.83224293864769550 ) ) ;
#172298=CARTESIAN_POINT ( 'NONE',  ( 9.474510206698971260, -16.51473224551069308, 77.91557627198103830 ) ) ;
#172299=CARTESIAN_POINT ( 'NONE',  ( -14.34966873604960291, -8.224510206698953496, 106.6655762719810383 ) ) ;
#172300=CARTESIAN_POINT ( 'NONE',  ( 13.89961937509977652, -13.97604488694527269, 68.12390960531436690 ) ) ;
#172301=CARTESIAN_POINT ( 'NONE',  ( -12.14591786802326823, 12.06949235617739902, 23.12609039468567573 ) ) ;
#172302=CARTESIAN_POINT ( 'NONE',  ( 17.50000000000015987, 3.417042746626929528, 32.32619603767522420 ) ) ;
#172303=CARTESIAN_POINT ( 'NONE',  ( -9.564922557960796823, -16.46253265017161027, 67.08224293864769550 ) ) ;
#172304=CARTESIAN_POINT ( 'NONE',  ( 18.62759615963255655, 10.81492255796105972, 96.66775706135234714 ) ) ;
#172305=CARTESIAN_POINT ( 'NONE',  ( 9.564922557960805705, 16.46253265017160317, 114.5822429386476955 ) ) ;
#172306=CARTESIAN_POINT ( 'NONE',  ( 4.483927247898790824, -16.52544592524335698, 90.20942372801903275 ) ) ;
#172308=CARTESIAN_POINT ( 'NONE',  ( 13.97604488694548053, -13.89961937509957401, 65.62609039468567573 ) ) ;
#172309=CARTESIAN_POINT ( 'NONE',  ( 19.02544592524334988, 5.153800228976608722, 21.45942372801899012 ) ) ;
#172311=CARTESIAN_POINT ( 'NONE',  ( 5.153800228976335163, 19.02544592524342804, 24.79057627198102765 ) ) ;
#172312=CARTESIAN_POINT ( 'NONE',  ( -14.34966873604960291, -8.224510206698953496, 31.66557627198102054 ) ) ;
#172314=CARTESIAN_POINT ( 'NONE',  ( 16.55341960407618274, -4.379528057220086978, 106.0427570613523471 ) ) ;
#172315=DIRECTION ( 'NONE',  ( 0.000000000000000000, 1.000000000000000000, 0.000000000000000000 ) ) ;
#172316=CARTESIAN_POINT ( 'NONE',  ( -14.29746914071037622, -8.314922557961029526, 84.16775706135234714 ) ) ;
#172317=CARTESIAN_POINT ( 'NONE',  ( 9.474510206698971260, -16.51473224551069308, 32.91557627198102409 ) ) ;
#172318=CARTESIAN_POINT ( 'NONE',  ( -15.72974639402176322, -15.80617190586768395, 94.37609039468568994 ) ) ;
#172319=CARTESIAN_POINT ( 'NONE',  ( 5.049401038297881783, 19.05341960407617563, 107.2927570613523187 ) ) ;
#172320=CARTESIAN_POINT ( 'NONE',  ( 18.62759615963255655, 10.81492255796105972, 76.66775706135234714 ) ) ;
#172321=CARTESIAN_POINT ( 'NONE',  ( 19.05341960407617918, -5.049401038297876454, 51.04275706135231871 ) ) ;
#172322=CARTESIAN_POINT ( 'NONE',  ( 9.564922557960805705, 16.46253265017160317, 84.58224293864769550 ) ) ;
#172323=CARTESIAN_POINT ( 'NONE',  ( -13.97604488694527625, -13.89961937509977652, 76.87390960531433848 ) ) ;
#172325=CARTESIAN_POINT ( 'NONE',  ( 14.34966873604960469, 8.224510206698951720, 64.16557627198102409 ) ) ;
#172326=CARTESIAN_POINT ( 'NONE',  ( 18.67979575497178502, 10.72451020669898547, 64.16557627198102409 ) ) ;
#172327=CARTESIAN_POINT ( 'NONE',  ( 19.02544592524343514, -5.153800228976328945, 48.54057627198103120 ) ) ;
#172328=CARTESIAN_POINT ( 'NONE',  ( -10.72451020669898014, 18.67979575497178502, 90.41557627198103830 ) ) ;
#172329=CARTESIAN_POINT ( 'NONE',  ( -14.29746914071037622, -8.314922557961029526, 79.16775706135234714 ) ) ;
#172331=CARTESIAN_POINT ( 'NONE',  ( 19.02544592524343514, -5.153800228976328945, 53.54057627198102409 ) ) ;
#172332=CARTESIAN_POINT ( 'NONE',  ( 12.06949235617757843, -12.14591786802309237, 83.12390960531436690 ) ) ;
#172334=CARTESIAN_POINT ( 'NONE',  ( -5.153800228976328057, -19.02544592524343514, 57.29057627198103120 ) ) ;
#172335=CARTESIAN_POINT ( 'NONE',  ( 8.224510206698953496, -14.34966873604960469, 112.9155762719810383 ) ) ;
#172336=CARTESIAN_POINT ( 'NONE',  ( -19.02544592524334988, -5.153800228976617603, 63.95942372801899012 ) ) ;
#172337=CARTESIAN_POINT ( 'NONE',  ( 12.06949235617757843, -12.14591786802309237, 68.12390960531436690 ) ) ;
#172338=CARTESIAN_POINT ( 'NONE',  ( 10.81492255796106328, -18.62759615963255655, 40.41775706135234714 ) ) ;
#172339=CARTESIAN_POINT ( 'NONE',  ( 0.05219959533909260263, 19.03943276465977164, 34.99890960531435979 ) ) ;
#172340=CARTESIAN_POINT ( 'NONE',  ( 0.05219959533907565091, 21.53943276465977519, 104.9989096053143669 ) ) ;
#172341=CARTESIAN_POINT ( 'NONE',  ( -9.474510206698964154, 16.51473224551069663, 115.4155762719810241 ) ) ;
#172342=CARTESIAN_POINT ( 'NONE',  ( -8.314922557960811034, -14.29746914071050412, 82.08224293864768129 ) ) ;
#172344=CARTESIAN_POINT ( 'NONE',  ( 19.05341960407611168, 5.049401038298154454, 43.95724293864769550 ) ) ;
#172346=CARTESIAN_POINT ( 'NONE',  ( -5.153800228976607833, 19.02544592524334988, 82.70942372801897591 ) ) ;
#172347=CARTESIAN_POINT ( 'NONE',  ( -15.80617190586768217, 15.72974639402176855, 38.12609039468567573 ) ) ;
#172348=CARTESIAN_POINT ( 'NONE',  ( -0.05219959533909027116, -19.03943276465977164, 72.49890960531435269 ) ) ;
#172349=CARTESIAN_POINT ( 'NONE',  ( 5.049401038297881783, 19.05341960407617563, 62.29275706135234003 ) ) ;
#172350=CARTESIAN_POINT ( 'NONE',  ( -19.02544592524342804, 5.153800228976336051, 46.04057627198101699 ) ) ;
#172351=CARTESIAN_POINT ( 'NONE',  ( 12.14591786802309770, 12.06949235617756955, 59.37390960531436690 ) ) ;
#172352=CARTESIAN_POINT ( 'NONE',  ( -8.314922557960811034, -14.29746914071050412, 62.08224293864769550 ) ) ;
#172353=CARTESIAN_POINT ( 'NONE',  ( 0.05219959533909260263, 19.03943276465977164, 69.99890960531435269 ) ) ;
#172354=CARTESIAN_POINT ( 'NONE',  ( -5.823673210054116645, -21.52544592524344225, 102.2905762719810383 ) ) ;
#172355=CARTESIAN_POINT ( 'NONE',  ( -19.03943276465977164, 0.05219959533909376836, 76.24890960531435269 ) ) ;
#172356=CARTESIAN_POINT ( 'NONE',  ( 5.719274019375673035, 21.55341960407619339, 107.2927570613523471 ) ) ;
#172357=CARTESIAN_POINT ( 'NONE',  ( 5.049401038298161559, -19.05341960407611168, 42.70724293864767418 ) ) ;
#172358=CARTESIAN_POINT ( 'NONE',  ( 16.53943276465976808, 0.05219959533934440121, 111.2510903946856899 ) ) ;
#172359=CARTESIAN_POINT ( 'NONE',  ( -4.483927247898539470, -16.52544592524342804, 97.29057627198105251 ) ) ;
#172360=CARTESIAN_POINT ( 'NONE',  ( 5.049401038297881783, 19.05341960407617563, 112.2927570613523471 ) ) ;
#172362=CARTESIAN_POINT ( 'NONE',  ( -21.55341960407619339, 5.719274019375674811, 33.54275706135234714 ) ) ;
#172363=CARTESIAN_POINT ( 'NONE',  ( -5.049401038297874678, -19.05341960407617918, 49.79275706135231871 ) ) ;
#172364=CARTESIAN_POINT ( 'NONE',  ( -8.314922557961024197, 14.29746914071037800, 112.9177570613523329 ) ) ;
#172365=CARTESIAN_POINT ( 'NONE',  ( 15.80617190586746368, 15.72974639402197994, 79.37390960531436690 ) ) ;
#172366=CARTESIAN_POINT ( 'NONE',  ( 9.564922557960805705, 16.46253265017160317, 104.5822429386476955 ) ) ;
#172367=CARTESIAN_POINT ( 'NONE',  ( -14.29746914071049879, 8.314922557960819915, 55.83224293864770260 ) ) ;
#172368=CARTESIAN_POINT ( 'NONE',  ( -19.02544592524342804, 5.153800228976336051, 31.04057627198102409 ) ) ;
#172369=CARTESIAN_POINT ( 'NONE',  ( -5.153800228976328057, -19.02544592524343514, 32.29057627198102409 ) ) ;
#172370=CARTESIAN_POINT ( 'NONE',  ( 19.03943276465977164, 0.05219959533936151252, 26.25109039468566507 ) ) ;
#172371=CARTESIAN_POINT ( 'NONE',  ( -14.29746914071037622, -8.314922557961029526, 89.16775706135236135 ) ) ;
#172372=CARTESIAN_POINT ( 'NONE',  ( 10.72451020669871369, 18.67979575497193778, 37.08442372801901143 ) ) ;
#172373=CARTESIAN_POINT ( 'NONE',  ( -0.05219959533934338120, 16.53943276465976808, 37.50109039468568284 ) ) ;
#172374=CARTESIAN_POINT ( 'NONE',  ( 9.564922557960805705, 16.46253265017160317, 114.5822429386476955 ) ) ;
#172375=CARTESIAN_POINT ( 'NONE',  ( -9.474510206698964154, 16.51473224551069663, 55.41557627198103120 ) ) ;
#172376=CARTESIAN_POINT ( 'NONE',  ( -15.72974639402176322, -15.80617190586768395, 94.37609039468568994 ) ) ;
#172377=CARTESIAN_POINT ( 'NONE',  ( -19.03943276465977164, 0.05219959533909376836, 76.24890960531435269 ) ) ;
#172378=CARTESIAN_POINT ( 'NONE',  ( -8.224510206698735004, -14.34966873604973081, 59.58442372801901854 ) ) ;
#172379=CARTESIAN_POINT ( 'NONE',  ( -8.314922557960811034, -14.29746914071050412, 102.0822429386476955 ) ) ;
#172380=CARTESIAN_POINT ( 'NONE',  ( -12.06949235617756955, 12.14591786802309770, 25.62390960531435624 ) ) ;
#172381=LINE ( 'NONE', #17716, #186378 ) ;
#172382=CARTESIAN_POINT ( 'NONE',  ( 0.05219959533937995610, -21.53943276465977519, 70.00109039468568994 ) ) ;
#172383=CARTESIAN_POINT ( 'NONE',  ( -19.02544592524342804, 5.153800228976336051, 86.04057627198103830 ) ) ;
#172384=CARTESIAN_POINT ( 'NONE',  ( 19.05341960407611168, 5.049401038298154454, 78.95724293864769550 ) ) ;
#172385=CARTESIAN_POINT ( 'NONE',  ( -19.03943276465977164, 0.05219959533909376836, 106.2489096053143669 ) ) ;
#172386=ADVANCED_FACE ( 'NONE', ( #71867 ), #60897, .T. ) ;
#172387=CARTESIAN_POINT ( 'NONE',  ( -14.29746914071049879, 8.314922557960819915, 55.83224293864770260 ) ) ;
#172388=CARTESIAN_POINT ( 'NONE',  ( -14.29746914071049879, 8.314922557960819915, 25.83224293864769194 ) ) ;
#172391=CARTESIAN_POINT ( 'NONE',  ( 4.379528057220339221, -16.55341960407611168, 42.70724293864770260 ) ) ;
#172392=CARTESIAN_POINT ( 'NONE',  ( 16.55341960407618274, -4.379528057220086978, 36.04275706135234714 ) ) ;
#172394=CARTESIAN_POINT ( 'NONE',  ( 5.049401038297881783, 19.05341960407617563, 42.29275706135234003 ) ) ;
#172395=CARTESIAN_POINT ( 'NONE',  ( 16.46253265017160672, -9.564922557960803928, 78.33224293864769550 ) ) ;
#172396=CARTESIAN_POINT ( 'NONE',  ( -13.89961937509957401, -13.97604488694547875, 49.37609039468567573 ) ) ;
#172399=CARTESIAN_POINT ( 'NONE',  ( -9.564922557961040184, 16.46253265017147172, 87.91775706135233293 ) ) ;
#172400=CARTESIAN_POINT ( 'NONE',  ( 12.06949235617739724, 12.14591786802326823, 86.87609039468568994 ) ) ;
#172401=CARTESIAN_POINT ( 'NONE',  ( 19.02544592524343514, -5.153800228976328945, 28.54057627198102409 ) ) ;
#172402=CARTESIAN_POINT ( 'NONE',  ( -16.46253265017160317, 9.564922557960807481, 100.8322429386477097 ) ) ;
#172403=CARTESIAN_POINT ( 'NONE',  ( -18.62759615963255300, -10.81492255796106328, 24.16775706135235424 ) ) ;
#172404=CARTESIAN_POINT ( 'NONE',  ( 16.46253265017146816, 9.564922557961045513, 91.66775706135234714 ) ) ;
#172405=CARTESIAN_POINT ( 'NONE',  ( 17.50000000000000000, 5.622605283950890431, 88.81207310596111881 ) ) ;
#172406=CARTESIAN_POINT ( 'NONE',  ( 9.564922557960805705, 16.46253265017160317, 54.58224293864769550 ) ) ;
#172407=CARTESIAN_POINT ( 'NONE',  ( -13.97604488694527625, -13.89961937509977652, 101.8739096053143811 ) ) ;
#172408=CARTESIAN_POINT ( 'NONE',  ( 4.379528057220339221, -16.55341960407611168, 57.70724293864770260 ) ) ;
#172409=CARTESIAN_POINT ( 'NONE',  ( -0.05219959533909027116, -19.03943276465977164, 52.49890960531436690 ) ) ;
#172410=CARTESIAN_POINT ( 'NONE',  ( 13.97604488694527802, 13.89961937509977652, 64.37390960531436690 ) ) ;
#172411=CARTESIAN_POINT ( 'NONE',  ( 16.46253265017146816, 9.564922557961045513, 66.66775706135233293 ) ) ;
#172413=CARTESIAN_POINT ( 'NONE',  ( -16.46253265017146816, -9.564922557961047289, 34.16775706135233293 ) ) ;
#172414=CARTESIAN_POINT ( 'NONE',  ( -19.02544592524342804, 5.153800228976336051, 71.04057627198099567 ) ) ;
#172415=CARTESIAN_POINT ( 'NONE',  ( -18.67979575497178146, -10.72451020669898902, 81.66557627198103830 ) ) ;
#172416=CARTESIAN_POINT ( 'NONE',  ( 0.05219959533910956823, 16.53943276465976808, 69.99890960531435269 ) ) ;
#172417=CARTESIAN_POINT ( 'NONE',  ( 13.97604488694548053, -13.89961937509957401, 30.62609039468566863 ) ) ;
#172419=CARTESIAN_POINT ( 'NONE',  ( 15.72974639402199770, -15.80617190586745480, 53.12390960531436690 ) ) ;
#172420=CARTESIAN_POINT ( 'NONE',  ( -15.80617190586745835, -15.72974639402198527, 31.87390960531435979 ) ) ;
#172421=CARTESIAN_POINT ( 'NONE',  ( 19.02544592524343514, -5.153800228976328945, 68.54057627198103830 ) ) ;
#172422=CARTESIAN_POINT ( 'NONE',  ( 5.049401038298161559, -19.05341960407611168, 37.70724293864768839 ) ) ;
#172423=CARTESIAN_POINT ( 'NONE',  ( -8.314922557960811034, -14.29746914071050412, 107.0822429386476955 ) ) ;
#172424=CARTESIAN_POINT ( 'NONE',  ( 18.67979575497178502, 10.72451020669898547, 114.1655762719810383 ) ) ;
#172425=CARTESIAN_POINT ( 'NONE',  ( -19.03943276465977164, 0.05219959533909376836, 116.2489096053143669 ) ) ;
#172426=CARTESIAN_POINT ( 'NONE',  ( -10.81492255796105439, 18.62759615963255655, 32.91775706135234714 ) ) ;
#172427=CARTESIAN_POINT ( 'NONE',  ( -5.049401038298153566, 19.05341960407611168, 25.20724293864768484 ) ) ;
#172428=CARTESIAN_POINT ( 'NONE',  ( -10.81492255796078084, -18.62759615963271287, 107.0822429386476955 ) ) ;
#172429=CARTESIAN_POINT ( 'NONE',  ( -16.51473224551082808, 9.474510206698731452, 43.33442372801900433 ) ) ;
#172431=CARTESIAN_POINT ( 'NONE',  ( -19.05341960407611168, -5.049401038298163336, 26.45724293864769550 ) ) ;
#172433=CARTESIAN_POINT ( 'NONE',  ( -14.34966873604972548, 8.224510206698743886, 43.33442372801901143 ) ) ;
#172434=CARTESIAN_POINT ( 'NONE',  ( -16.52544592524342804, 4.483927247898546575, 116.0405762719810383 ) ) ;
#172437=CARTESIAN_POINT ( 'NONE',  ( 9.564922557960805705, 16.46253265017160317, 69.58224293864770971 ) ) ;
#172438=CARTESIAN_POINT ( 'NONE',  ( 4.483927247898545687, 16.52544592524342804, 104.7905762719810241 ) ) ;
#172439=CARTESIAN_POINT ( 'NONE',  ( 21.55341960407610458, 5.719274019375980345, 43.95724293864769550 ) ) ;
#172440=CARTESIAN_POINT ( 'NONE',  ( -12.06949235617756955, 12.14591786802309770, 75.62390960531439532 ) ) ;
#172441=CARTESIAN_POINT ( 'NONE',  ( -16.53943276465976808, -0.05219959533934237506, 33.75109039468568284 ) ) ;
#172442=CARTESIAN_POINT ( 'NONE',  ( -5.719274019375665041, -21.55341960407619695, 89.79275706135236135 ) ) ;
#172443=CARTESIAN_POINT ( 'NONE',  ( 19.03943276465977164, -0.05219959533909143690, 28.74890960531435624 ) ) ;
#172444=CARTESIAN_POINT ( 'NONE',  ( -16.53943276465976808, -0.05219959533934237506, 113.7510903946856757 ) ) ;
#172445=CARTESIAN_POINT ( 'NONE',  ( -12.06949235617756955, 12.14591786802309770, 45.62390960531436690 ) ) ;
#172446=CARTESIAN_POINT ( 'NONE',  ( 5.049401038298161559, -19.05341960407611168, 47.70724293864770260 ) ) ;
#172447=CARTESIAN_POINT ( 'NONE',  ( -10.81492255796105439, 18.62759615963255655, 102.9177570613523756 ) ) ;
#172448=CARTESIAN_POINT ( 'NONE',  ( 5.719274019375991003, -21.55341960407610458, 107.7072429386476955 ) ) ;
#172450=CARTESIAN_POINT ( 'NONE',  ( -21.55341960407619339, 5.719274019375674811, 68.54275706135234714 ) ) ;
#172451=CARTESIAN_POINT ( 'NONE',  ( 14.29746914071037800, 8.314922557961029526, 41.66775706135235424 ) ) ;
#172452=CARTESIAN_POINT ( 'NONE',  ( -4.483927247898539470, -16.52544592524342804, 77.29057627198102409 ) ) ;
#172453=CARTESIAN_POINT ( 'NONE',  ( 15.72974639402176855, 15.80617190586768217, 81.87609039468568994 ) ) ;
#172454=CARTESIAN_POINT ( 'NONE',  ( 4.379528057220092307, 16.55341960407617563, 112.2927570613523471 ) ) ;
#172456=CARTESIAN_POINT ( 'NONE',  ( -19.39056639909674118, -5.500000000000057732, 65.78948781074339536 ) ) ;
#172457=CARTESIAN_POINT ( 'NONE',  ( 14.29746914071049879, -8.314922557960816363, 38.33224293864768839 ) ) ;
#172458=CARTESIAN_POINT ( 'NONE',  ( -4.379528057220086978, -16.55341960407618274, 74.79275706135234714 ) ) ;
#172459=CARTESIAN_POINT ( 'NONE',  ( -19.05341960407611168, -5.049401038298163336, 86.45724293864769550 ) ) ;
#172460=CARTESIAN_POINT ( 'NONE',  ( 13.89961937509977652, -13.97604488694527269, 98.12390960531433848 ) ) ;
#172461=CARTESIAN_POINT ( 'NONE',  ( 21.53943276465977519, 0.05219959533937863772, 101.2510903946856757 ) ) ;
#172462=CARTESIAN_POINT ( 'NONE',  ( 0.05219959533934541429, -16.53943276465976808, 105.0010903946856757 ) ) ;
#172463=CARTESIAN_POINT ( 'NONE',  ( 4.379528057220339221, -16.55341960407611168, 67.70724293864769550 ) ) ;
#172464=CARTESIAN_POINT ( 'NONE',  ( 16.46253265017160672, -9.564922557960803928, 88.33224293864769550 ) ) ;
#172466=CARTESIAN_POINT ( 'NONE',  ( 4.379528057220092307, 16.55341960407617563, 27.29275706135234358 ) ) ;
#172467=CARTESIAN_POINT ( 'NONE',  ( 9.564922557960805705, 16.46253265017160317, 24.58224293864769194 ) ) ;
#172468=CARTESIAN_POINT ( 'NONE',  ( 19.02544592524343514, -5.153800228976328945, 93.54057627198102409 ) ) ;
#172469=CARTESIAN_POINT ( 'NONE',  ( 16.55341960407618274, -4.379528057220086978, 36.04275706135234714 ) ) ;
#172471=CARTESIAN_POINT ( 'NONE',  ( -18.67979575497193778, 10.72451020669871902, 113.3344237280190328 ) ) ;
#172472=CARTESIAN_POINT ( 'NONE',  ( 4.379528057220092307, 16.55341960407617563, 92.29275706135236135 ) ) ;
#172473=CARTESIAN_POINT ( 'NONE',  ( 19.02544592524334988, 5.153800228976608722, 111.4594237280190043 ) ) ;
#172474=CARTESIAN_POINT ( 'NONE',  ( 16.46253265017160672, -9.564922557960803928, 33.33224293864770260 ) ) ;
#172475=CARTESIAN_POINT ( 'NONE',  ( 8.314922557961029526, -14.29746914071037800, 80.41775706135234714 ) ) ;
#172476=CARTESIAN_POINT ( 'NONE',  ( -8.314922557961024197, 14.29746914071037800, 67.91775706135234714 ) ) ;
#172477=CARTESIAN_POINT ( 'NONE',  ( 5.049401038298161559, -19.05341960407611168, 27.70724293864769550 ) ) ;
#172478=CARTESIAN_POINT ( 'NONE',  ( 9.474510206698729675, 16.51473224551082808, 72.08442372801900433 ) ) ;
#172479=CARTESIAN_POINT ( 'NONE',  ( 10.81492255796106328, -18.62759615963255655, 105.4177570613523613 ) ) ;
#172480=CARTESIAN_POINT ( 'NONE',  ( -9.474510206698964154, 16.51473224551069663, 50.41557627198102409 ) ) ;
#172481=CARTESIAN_POINT ( 'NONE',  ( 16.46253265017160672, -9.564922557960803928, 98.33224293864769550 ) ) ;
#172482=CARTESIAN_POINT ( 'NONE',  ( 14.34966873604960469, 8.224510206698951720, 79.16557627198103830 ) ) ;
#172484=CARTESIAN_POINT ( 'NONE',  ( -16.46253265017146816, -9.564922557961047289, 54.16775706135234003 ) ) ;
#172485=CARTESIAN_POINT ( 'NONE',  ( 15.80617190586746368, 15.72974639402197994, 54.37390960531435979 ) ) ;
#172486=CARTESIAN_POINT ( 'NONE',  ( 0.05219959533937995610, -21.53943276465977519, 105.0010903946856757 ) ) ;
#172487=CARTESIAN_POINT ( 'NONE',  ( 16.51473224551069308, 9.474510206698969483, 89.16557627198103830 ) ) ;
#172488=CARTESIAN_POINT ( 'NONE',  ( 21.52544592524334988, 5.823673210054432836, 106.4594237280190328 ) ) ;
#172489=CARTESIAN_POINT ( 'NONE',  ( -5.719274019375978568, 21.55341960407610458, 70.20724293864769550 ) ) ;
#172490=CARTESIAN_POINT ( 'NONE',  ( -9.564922557960796823, -16.46253265017161027, 107.0822429386476955 ) ) ;
#172491=CARTESIAN_POINT ( 'NONE',  ( -5.153800228976607833, 19.02544592524334988, 82.70942372801897591 ) ) ;
#172492=CARTESIAN_POINT ( 'NONE',  ( -0.05219959533909027116, -19.03943276465977164, 112.4989096053143669 ) ) ;
#172494=CARTESIAN_POINT ( 'NONE',  ( -9.564922557961040184, 16.46253265017147172, 107.9177570613523471 ) ) ;
#172495=CARTESIAN_POINT ( 'NONE',  ( 19.02544592524343514, -5.153800228976328945, 23.54057627198102054 ) ) ;
#172496=CARTESIAN_POINT ( 'NONE',  ( -5.153800228976328057, -19.02544592524343514, 82.29057627198103830 ) ) ;
#172497=CARTESIAN_POINT ( 'NONE',  ( 0.05219959533907565091, 21.53943276465977519, 79.99890960531435269 ) ) ;
#172498=CARTESIAN_POINT ( 'NONE',  ( 8.314922557961029526, -14.29746914071037800, 40.41775706135234714 ) ) ;
#172499=CARTESIAN_POINT ( 'NONE',  ( -18.62759615963255300, -10.81492255796106328, 49.16775706135234003 ) ) ;
#172500=CARTESIAN_POINT ( 'NONE',  ( -10.72451020669870658, -18.67979575497194134, 94.58442372801901854 ) ) ;
#172501=CARTESIAN_POINT ( 'NONE',  ( -4.483927247898782831, 16.52544592524335698, 97.70942372801904696 ) ) ;
#172502=CARTESIAN_POINT ( 'NONE',  ( -19.03943276465977164, 0.05219959533909376836, 91.24890960531436690 ) ) ;
#172503=CARTESIAN_POINT ( 'NONE',  ( -14.34966873604960291, -8.224510206698953496, 96.66557627198102409 ) ) ;
#172504=CARTESIAN_POINT ( 'NONE',  ( -8.224510206698948167, 14.34966873604960824, 30.41557627198101699 ) ) ;
#172505=CARTESIAN_POINT ( 'NONE',  ( 19.05341960407617918, -5.049401038297876454, 71.04275706135234714 ) ) ;
#172506=CARTESIAN_POINT ( 'NONE',  ( 10.72451020669871369, 18.67979575497193778, 47.08442372801901854 ) ) ;
#172507=CARTESIAN_POINT ( 'NONE',  ( -0.05219959533936034679, 19.03943276465977164, 27.50109039468566507 ) ) ;
#172510=CARTESIAN_POINT ( 'NONE',  ( -12.14591786802309592, -12.06949235617757132, 86.87390960531438111 ) ) ;
#172511=CARTESIAN_POINT ( 'NONE',  ( 21.55341960407610458, 5.719274019375980345, 23.95724293864769550 ) ) ;
#172512=CARTESIAN_POINT ( 'NONE',  ( -4.483927247898539470, -16.52544592524342804, 22.29057627198102765 ) ) ;
#172513=CARTESIAN_POINT ( 'NONE',  ( 18.67979575497194134, -10.72451020669871369, 80.83442372801901854 ) ) ;
#172514=CARTESIAN_POINT ( 'NONE',  ( -8.314922557961024197, 14.29746914071037800, 52.91775706135235424 ) ) ;
#172515=CARTESIAN_POINT ( 'NONE',  ( 14.34966873604972726, -8.224510206698740333, 100.8344237280190185 ) ) ;
#172516=CARTESIAN_POINT ( 'NONE',  ( -5.823673210054431948, 21.52544592524334988, 47.70942372801902565 ) ) ;
#172518=CARTESIAN_POINT ( 'NONE',  ( 5.823673210054444382, -21.52544592524334988, 35.20942372801901854 ) ) ;
#172519=CARTESIAN_POINT ( 'NONE',  ( -16.53943276465976808, 0.05219959533911058130, 106.2489096053143811 ) ) ;
#172520=CARTESIAN_POINT ( 'NONE',  ( -13.97604488694527625, -13.89961937509977652, 31.87390960531435979 ) ) ;
#172521=CARTESIAN_POINT ( 'NONE',  ( -0.05219959533910754901, -16.53943276465976808, 72.49890960531435269 ) ) ;
#172522=CARTESIAN_POINT ( 'NONE',  ( -9.564922557960796823, -16.46253265017161027, 72.08224293864770971 ) ) ;
#172523=CARTESIAN_POINT ( 'NONE',  ( -8.224510206698735004, -14.34966873604973081, 109.5844237280190328 ) ) ;
#172524=CARTESIAN_POINT ( 'NONE',  ( 9.564922557960805705, 16.46253265017160317, 34.58224293864770260 ) ) ;
#172525=CARTESIAN_POINT ( 'NONE',  ( -5.823673210054116645, -21.52544592524344225, 57.29057627198103120 ) ) ;
#172526=CARTESIAN_POINT ( 'NONE',  ( 12.14591786802309770, 12.06949235617756955, 94.37390960531436690 ) ) ;
#172527=CARTESIAN_POINT ( 'NONE',  ( 18.67979575497178502, 10.72451020669898547, 99.16557627198100988 ) ) ;
#172528=CARTESIAN_POINT ( 'NONE',  ( 19.03943276465977164, -0.05219959533909143690, 98.74890960531436690 ) ) ;
#172529=CARTESIAN_POINT ( 'NONE',  ( -19.03943276465977164, 0.05219959533909376836, 51.24890960531436690 ) ) ;
#172530=CARTESIAN_POINT ( 'NONE',  ( 9.474510206698729675, 16.51473224551082808, 97.08442372801900433 ) ) ;
#172531=CARTESIAN_POINT ( 'NONE',  ( 10.81492255796078972, 18.62759615963270932, 49.58224293864769550 ) ) ;
#172532=CARTESIAN_POINT ( 'NONE',  ( 21.53943276465977519, 0.05219959533937863772, 66.25109039468567573 ) ) ;
#172533=CARTESIAN_POINT ( 'NONE',  ( -16.51473224551069308, -9.474510206698971260, 56.66557627198103120 ) ) ;
#172534=CARTESIAN_POINT ( 'NONE',  ( -13.89961937509977652, 13.97604488694528158, 80.62390960531436690 ) ) ;
#172535=CARTESIAN_POINT ( 'NONE',  ( -16.55341960407617563, 4.379528057220093196, 63.54275706135234003 ) ) ;
#172536=CARTESIAN_POINT ( 'NONE',  ( -21.53943276465977519, -0.05219959533937600094, 38.75109039468567573 ) ) ;
#172537=EDGE_CURVE ( 'NONE', #135811, #159561, #131108, .T. ) ;
#172538=CARTESIAN_POINT ( 'NONE',  ( -18.67979575497193778, 10.72451020669871902, 88.33442372801901854 ) ) ;
#172539=CARTESIAN_POINT ( 'NONE',  ( -10.81492255796078084, -18.62759615963271287, 97.08224293864770971 ) ) ;
#172540=CARTESIAN_POINT ( 'NONE',  ( 18.67979575497194134, -10.72451020669871369, 40.83442372801901854 ) ) ;
#172541=CARTESIAN_POINT ( 'NONE',  ( 4.483927247898790824, -16.52544592524335698, 65.20942372801901854 ) ) ;
#172542=CARTESIAN_POINT ( 'NONE',  ( 18.62759615963271287, -10.81492255796078972, 68.33224293864769550 ) ) ;
#172543=CARTESIAN_POINT ( 'NONE',  ( 9.474510206698729675, 16.51473224551082808, 37.08442372801899722 ) ) ;
#172544=CARTESIAN_POINT ( 'NONE',  ( -9.474510206698964154, 16.51473224551069663, 65.41557627198102409 ) ) ;
#172545=CARTESIAN_POINT ( 'NONE',  ( 8.314922557961029526, -14.29746914071037800, 110.4177570613523756 ) ) ;
#172547=CARTESIAN_POINT ( 'NONE',  ( 16.51473224551069308, 9.474510206698969483, 99.16557627198102409 ) ) ;
#172549=CARTESIAN_POINT ( 'NONE',  ( -9.474510206698720793, -16.51473224551083518, 79.58442372801899012 ) ) ;
#172550=CARTESIAN_POINT ( 'NONE',  ( 21.55341960407610458, 5.719274019375980345, 58.95724293864770971 ) ) ;
#172551=CARTESIAN_POINT ( 'NONE',  ( -4.483927247898539470, -16.52544592524342804, 37.29057627198102409 ) ) ;
#172552=CARTESIAN_POINT ( 'NONE',  ( -16.53943276465976808, -0.05219959533934237506, 23.75109039468567929 ) ) ;
#172553=CARTESIAN_POINT ( 'NONE',  ( -0.05219959533909027116, -19.03943276465977164, 32.49890960531435979 ) ) ;
#172554=CARTESIAN_POINT ( 'NONE',  ( -19.02544592524334988, -5.153800228976617603, 108.9594237280189759 ) ) ;
#172555=CARTESIAN_POINT ( 'NONE',  ( -15.72974639402197994, 15.80617190586746368, 90.62390960531436690 ) ) ;
#172556=CARTESIAN_POINT ( 'NONE',  ( -16.46253265017146816, -9.564922557961047289, 69.16775706135233293 ) ) ;
#172557=CARTESIAN_POINT ( 'NONE',  ( 16.55341960407618274, -4.379528057220086978, 86.04275706135236135 ) ) ;
#172558=CARTESIAN_POINT ( 'NONE',  ( 19.03943276465977164, -0.05219959533909143690, 73.74890960531435269 ) ) ;
#172559=CARTESIAN_POINT ( 'NONE',  ( -4.483927247898539470, -16.52544592524342804, 77.29057627198102409 ) ) ;
#172560=CARTESIAN_POINT ( 'NONE',  ( -9.564922557960796823, -16.46253265017161027, 42.08224293864769550 ) ) ;
#172561=CARTESIAN_POINT ( 'NONE',  ( 4.483927247898545687, 16.52544592524342804, 54.79057627198104541 ) ) ;
#172564=CARTESIAN_POINT ( 'NONE',  ( 16.53943276465976808, -0.05219959533910856209, 23.74890960531435269 ) ) ;
#172565=CARTESIAN_POINT ( 'NONE',  ( -13.97604488694527625, -13.89961937509977652, 81.87390960531436690 ) ) ;
#172567=CARTESIAN_POINT ( 'NONE',  ( -13.89961937509957401, -13.97604488694547875, 44.37609039468566863 ) ) ;
#172568=CARTESIAN_POINT ( 'NONE',  ( -8.314922557961024197, 14.29746914071037800, 42.91775706135235424 ) ) ;
#172569=CARTESIAN_POINT ( 'NONE',  ( 21.52544592524344225, -5.823673210054117533, 58.54057627198103120 ) ) ;
#172570=CARTESIAN_POINT ( 'NONE',  ( 0.05219959533936267826, -19.03943276465977164, 30.00109039468566863 ) ) ;
#172571=CARTESIAN_POINT ( 'NONE',  ( 16.46253265017160672, -9.564922557960803928, 68.33224293864770971 ) ) ;
#172573=CARTESIAN_POINT ( 'NONE',  ( 19.02544592524343514, -5.153800228976328945, 113.5405762719810241 ) ) ;
#172574=CARTESIAN_POINT ( 'NONE',  ( -21.53943276465977519, -0.05219959533937600094, 33.75109039468568284 ) ) ;
#172575=CARTESIAN_POINT ( 'NONE',  ( -16.55341960407611168, -4.379528057220339221, 106.4572429386477097 ) ) ;
#172576=CARTESIAN_POINT ( 'NONE',  ( 21.52544592524344225, -5.823673210054117533, 103.5405762719810383 ) ) ;
#172577=CARTESIAN_POINT ( 'NONE',  ( -16.46253265017160317, 9.564922557960807481, 75.83224293864769550 ) ) ;
#172578=CARTESIAN_POINT ( 'NONE',  ( 18.22780087662119897, -5.500000000000096811, 68.51763182126893525 ) ) ;
#172579=CARTESIAN_POINT ( 'NONE',  ( -10.72451020669870658, -18.67979575497194134, 24.58442372801901499 ) ) ;
#172581=CARTESIAN_POINT ( 'NONE',  ( -19.03943276465977164, 0.05219959533909376836, 86.24890960531436690 ) ) ;
#172583=CARTESIAN_POINT ( 'NONE',  ( 16.46253265017160672, -9.564922557960803928, 38.33224293864768839 ) ) ;
#172584=CARTESIAN_POINT ( 'NONE',  ( 0.05219959533936267826, -19.03943276465977164, 110.0010903946856757 ) ) ;
#172587=CARTESIAN_POINT ( 'NONE',  ( -12.14591786802309592, -12.06949235617757132, 111.8739096053143669 ) ) ;
#172588=CARTESIAN_POINT ( 'NONE',  ( -5.719274019375665041, -21.55341960407619695, 84.79275706135234714 ) ) ;
#172589=CARTESIAN_POINT ( 'NONE',  ( 0.05219959533909260263, 19.03943276465977164, 74.99890960531435269 ) ) ;
#172590=CARTESIAN_POINT ( 'NONE',  ( 21.52544592524334988, 5.823673210054432836, 46.45942372801901854 ) ) ;
#172591=CARTESIAN_POINT ( 'NONE',  ( 5.719274019375673035, 21.55341960407619339, 22.29275706135235069 ) ) ;
#172593=CARTESIAN_POINT ( 'NONE',  ( -0.05219959533909027116, -19.03943276465977164, 82.49890960531436690 ) ) ;
#172594=CARTESIAN_POINT ( 'NONE',  ( 19.25918095147781983, 5.499999999999580780, 61.95284276293936898 ) ) ;
#172595=CARTESIAN_POINT ( 'NONE',  ( 4.483927247898790824, -16.52544592524335698, 45.20942372801901854 ) ) ;
#172596=CARTESIAN_POINT ( 'NONE',  ( 5.823673210054125526, 21.52544592524343514, 39.79057627198103830 ) ) ;
#172597=CARTESIAN_POINT ( 'NONE',  ( 18.62759615963255655, 10.81492255796105972, 76.66775706135234714 ) ) ;
#172598=CARTESIAN_POINT ( 'NONE',  ( 17.60689202196055447, -5.500000000000023981, 38.36665076390895024 ) ) ;
#172599=CARTESIAN_POINT ( 'NONE',  ( -9.564922557961040184, 16.46253265017147172, 107.9177570613523471 ) ) ;
#172600=CARTESIAN_POINT ( 'NONE',  ( -5.049401038298153566, 19.05341960407611168, 55.20724293864769550 ) ) ;
#172601=CARTESIAN_POINT ( 'NONE',  ( 16.46253265017160672, -9.564922557960803928, 78.33224293864769550 ) ) ;
#172602=CARTESIAN_POINT ( 'NONE',  ( -12.06949235617756955, 12.14591786802309770, 105.6239096053143669 ) ) ;
#172603=CARTESIAN_POINT ( 'NONE',  ( 12.06949235617757843, -12.14591786802309237, 108.1239096053143811 ) ) ;
#172604=CARTESIAN_POINT ( 'NONE',  ( 5.153800228976335163, 19.02544592524342804, 114.7905762719810241 ) ) ;
#172605=CARTESIAN_POINT ( 'NONE',  ( 0.05219959533934541429, -16.53943276465976808, 80.00109039468568994 ) ) ;
#172606=CARTESIAN_POINT ( 'NONE',  ( 8.224510206698953496, -14.34966873604960469, 62.91557627198102409 ) ) ;
#172607=CARTESIAN_POINT ( 'NONE',  ( 16.51473224551069308, 9.474510206698969483, 59.16557627198102409 ) ) ;
#172608=CARTESIAN_POINT ( 'NONE',  ( 0.05219959533937995610, -21.53943276465977519, 80.00109039468568994 ) ) ;
#172609=CARTESIAN_POINT ( 'NONE',  ( -0.05219959533937732626, 21.53943276465977519, 72.50109039468568994 ) ) ;
#172610=CARTESIAN_POINT ( 'NONE',  ( -13.89961937509957401, -13.97604488694547875, 89.37609039468563310 ) ) ;
#172611=CARTESIAN_POINT ( 'NONE',  ( 12.06949235617757843, -12.14591786802309237, 63.12390960531435979 ) ) ;
#172612=CARTESIAN_POINT ( 'NONE',  ( -15.80617190586745835, -15.72974639402198527, 111.8739096053143669 ) ) ;
#172613=CARTESIAN_POINT ( 'NONE',  ( 21.55341960407610458, 5.719274019375980345, 63.95724293864770260 ) ) ;
#172616=CARTESIAN_POINT ( 'NONE',  ( 9.474510206698971260, -16.51473224551069308, 72.91557627198102409 ) ) ;
#172617=CARTESIAN_POINT ( 'NONE',  ( 16.52544592524342804, -4.483927247898539470, 38.54057627198103120 ) ) ;
#172619=CARTESIAN_POINT ( 'NONE',  ( 8.314922557961029526, -14.29746914071037800, 110.4177570613523756 ) ) ;
#172620=CARTESIAN_POINT ( 'NONE',  ( 16.53943276465976808, 0.05219959533934440121, 86.25109039468568994 ) ) ;
#172621=CARTESIAN_POINT ( 'NONE',  ( -0.05219959533936034679, 19.03943276465977164, 37.50109039468567573 ) ) ;
#172622=CARTESIAN_POINT ( 'NONE',  ( -9.474510206698964154, 16.51473224551069663, 95.41557627198102409 ) ) ;
#172623=CARTESIAN_POINT ( 'NONE',  ( -16.53943276465976808, 0.05219959533911058130, 61.24890960531435979 ) ) ;
#172624=CARTESIAN_POINT ( 'NONE',  ( 19.03943276465977164, -0.05219959533909143690, 23.74890960531435269 ) ) ;
#172625=CARTESIAN_POINT ( 'NONE',  ( -18.62759615963270932, 10.81492255796079327, 25.83224293864769194 ) ) ;
#172626=CARTESIAN_POINT ( 'NONE',  ( -21.52544592524343514, 5.823673210054127303, 56.04057627198102409 ) ) ;
#172627=CARTESIAN_POINT ( 'NONE',  ( 16.53943276465976808, -0.05219959533910856209, 103.7489096053143669 ) ) ;
#172628=CARTESIAN_POINT ( 'NONE',  ( 14.29746914071037800, 8.314922557961029526, 51.66775706135234714 ) ) ;
#172629=CARTESIAN_POINT ( 'NONE',  ( 16.53943276465976808, -0.05219959533910856209, 83.74890960531435269 ) ) ;
#172630=CARTESIAN_POINT ( 'NONE',  ( -18.56197773271732032, 5.499999999999902300, 63.55066217314450938 ) ) ;
#172631=CARTESIAN_POINT ( 'NONE',  ( 9.474510206698729675, 16.51473224551082808, 77.08442372801900433 ) ) ;
#172632=CARTESIAN_POINT ( 'NONE',  ( -10.72451020669898014, 18.67979575497178502, 25.41557627198103120 ) ) ;
#172634=CARTESIAN_POINT ( 'NONE',  ( 9.474510206698971260, -16.51473224551069308, 42.91557627198103120 ) ) ;
#172635=CARTESIAN_POINT ( 'NONE',  ( -12.14591786802326823, 12.06949235617739902, 33.12609039468569705 ) ) ;
#172636=CARTESIAN_POINT ( 'NONE',  ( -8.224510206698948167, 14.34966873604960824, 35.41557627198102409 ) ) ;
#172637=CARTESIAN_POINT ( 'NONE',  ( -0.05219959533907301413, -21.53943276465977519, 52.49890960531435979 ) ) ;
#172638=CARTESIAN_POINT ( 'NONE',  ( -19.02544592524334988, -5.153800228976617603, 88.95942372801897591 ) ) ;
#172639=CARTESIAN_POINT ( 'NONE',  ( 5.823673210054125526, 21.52544592524343514, 44.79057627198103120 ) ) ;
#172640=CARTESIAN_POINT ( 'NONE',  ( -21.53943276465977519, -0.05219959533937600094, 83.75109039468568994 ) ) ;
#172642=CARTESIAN_POINT ( 'NONE',  ( 14.34966873604972726, -8.224510206698740333, 35.83442372801901143 ) ) ;
#172643=CARTESIAN_POINT ( 'NONE',  ( -13.97604488694527625, -13.89961937509977652, 41.87390960531435979 ) ) ;
#172644=CARTESIAN_POINT ( 'NONE',  ( 0.05219959533909260263, 19.03943276465977164, 89.99890960531436690 ) ) ;
#172645=CARTESIAN_POINT ( 'NONE',  ( -13.97604488694527625, -13.89961937509977652, 31.87390960531435979 ) ) ;
#172646=CARTESIAN_POINT ( 'NONE',  ( 4.379528057220339221, -16.55341960407611168, 102.7072429386476955 ) ) ;
#172648=CARTESIAN_POINT ( 'NONE',  ( 19.02544592524343514, -5.153800228976328945, 103.5405762719809957 ) ) ;
#172650=CARTESIAN_POINT ( 'NONE',  ( 16.53943276465976808, 0.05219959533934440121, 61.25109039468567573 ) ) ;
#172651=CARTESIAN_POINT ( 'NONE',  ( 5.823673210054125526, 21.52544592524343514, 84.79057627198102409 ) ) ;
#172652=CARTESIAN_POINT ( 'NONE',  ( 19.05341960407611168, 5.049401038298154454, 38.95724293864767418 ) ) ;
#172653=CARTESIAN_POINT ( 'NONE',  ( -19.05341960407617563, 5.049401038297882671, 78.54275706135233293 ) ) ;
#172654=CARTESIAN_POINT ( 'NONE',  ( -15.72974639402176322, -15.80617190586768395, 34.37609039468568284 ) ) ;
#172655=CARTESIAN_POINT ( 'NONE',  ( 19.02544592524343514, -5.153800228976328945, 88.54057627198102409 ) ) ;
#172656=CARTESIAN_POINT ( 'NONE',  ( -19.03943276465977164, 0.05219959533909376836, 106.2489096053143669 ) ) ;
#172657=EDGE_CURVE ( 'NONE', #66839, #46248, #24914, .T. ) ;
#172659=CARTESIAN_POINT ( 'NONE',  ( 8.224510206698742110, 14.34966873604972548, 37.08442372801901143 ) ) ;
#172660=CARTESIAN_POINT ( 'NONE',  ( -10.72451020669898014, 18.67979575497178502, 110.4155762719810383 ) ) ;
#172661=CARTESIAN_POINT ( 'NONE',  ( -0.05219959533910754901, -16.53943276465976808, 102.4989096053143811 ) ) ;
#172662=CARTESIAN_POINT ( 'NONE',  ( -16.46253265017160317, 9.564922557960807481, 90.83224293864769550 ) ) ;
#172663=CARTESIAN_POINT ( 'NONE',  ( -9.474510206698720793, -16.51473224551083518, 79.58442372801899012 ) ) ;
#172664=CARTESIAN_POINT ( 'NONE',  ( 5.153800228976615827, -19.02544592524334988, 30.20942372801900433 ) ) ;
#172665=CARTESIAN_POINT ( 'NONE',  ( 5.719274019375991003, -21.55341960407610458, 87.70724293864769550 ) ) ;
#172666=CARTESIAN_POINT ( 'NONE',  ( -5.049401038297874678, -19.05341960407617918, 19.79275706135233293 ) ) ;
#172667=CARTESIAN_POINT ( 'NONE',  ( 16.52544592524335698, 4.483927247898782831, 76.45942372801901854 ) ) ;
#172669=CARTESIAN_POINT ( 'NONE',  ( 5.049401038298161559, -19.05341960407611168, 107.7072429386476955 ) ) ;
#172670=CARTESIAN_POINT ( 'NONE',  ( -5.153800228976328057, -19.02544592524343514, 52.29057627198100988 ) ) ;
#172671=CARTESIAN_POINT ( 'NONE',  ( -18.62759615963255300, -10.81492255796106328, 59.16775706135234714 ) ) ;
#172672=CARTESIAN_POINT ( 'NONE',  ( -21.55341960407619339, 5.719274019375674811, 73.54275706135234714 ) ) ;
#172673=CARTESIAN_POINT ( 'NONE',  ( 5.153800228976335163, 19.02544592524342804, 69.79057627198103830 ) ) ;
#172674=CARTESIAN_POINT ( 'NONE',  ( 5.719274019375673035, 21.55341960407619339, 52.29275706135236135 ) ) ;
#172675=CARTESIAN_POINT ( 'NONE',  ( 19.02544592524334988, 5.153800228976608722, 91.45942372801900433 ) ) ;
#172676=CARTESIAN_POINT ( 'NONE',  ( 5.049401038298161559, -19.05341960407611168, 47.70724293864770260 ) ) ;
#172677=CARTESIAN_POINT ( 'NONE',  ( 16.52544592524335698, 4.483927247898782831, 91.45942372801901854 ) ) ;
#172678=CARTESIAN_POINT ( 'NONE',  ( 19.05341960407611168, 5.049401038298154454, 68.95724293864769550 ) ) ;
#172679=CARTESIAN_POINT ( 'NONE',  ( -16.46253265017160317, 9.564922557960807481, 115.8322429386477097 ) ) ;
#172680=CARTESIAN_POINT ( 'NONE',  ( 19.05341960407611168, 5.049401038298154454, 48.95724293864768129 ) ) ;
#172682=CARTESIAN_POINT ( 'NONE',  ( 5.719274019375991003, -21.55341960407610458, 87.70724293864769550 ) ) ;
#172683=CARTESIAN_POINT ( 'NONE',  ( 16.52544592524335698, 4.483927247898782831, 71.45942372801901854 ) ) ;
#172685=CARTESIAN_POINT ( 'NONE',  ( -19.05341960407617563, 5.049401038297882671, 33.54275706135231871 ) ) ;
#172686=CARTESIAN_POINT ( 'NONE',  ( 5.049401038298161559, -19.05341960407611168, 72.70724293864768129 ) ) ;
#172687=CARTESIAN_POINT ( 'NONE',  ( -4.483927247898539470, -16.52544592524342804, 57.29057627198103120 ) ) ;
#172688=CARTESIAN_POINT ( 'NONE',  ( -16.53943276465976808, 0.05219959533911058130, 96.24890960531435269 ) ) ;
#172689=CARTESIAN_POINT ( 'NONE',  ( -16.46253265017160317, 9.564922557960807481, 105.8322429386476955 ) ) ;
#172690=CARTESIAN_POINT ( 'NONE',  ( 13.97604488694527802, 13.89961937509977652, 89.37390960531436690 ) ) ;
#172691=CARTESIAN_POINT ( 'NONE',  ( -15.72974639402176322, -15.80617190586768395, 44.37609039468567573 ) ) ;
#172692=CARTESIAN_POINT ( 'NONE',  ( 5.153800228976335163, 19.02544592524342804, 99.79057627198102409 ) ) ;
#172693=CARTESIAN_POINT ( 'NONE',  ( -19.02544592524334988, -5.153800228976617603, 23.95942372801900078 ) ) ;
#172694=CARTESIAN_POINT ( 'NONE',  ( -16.55341960407617563, 4.379528057220093196, 73.54275706135234714 ) ) ;
#172695=CARTESIAN_POINT ( 'NONE',  ( -21.53943276465977519, -0.05219959533937600094, 38.75109039468567573 ) ) ;
#172696=CARTESIAN_POINT ( 'NONE',  ( 18.62759615963271287, -10.81492255796078972, 23.33224293864769194 ) ) ;
#172697=CARTESIAN_POINT ( 'NONE',  ( -21.55341960407610458, -5.719274019375992779, 96.45724293864770971 ) ) ;
#172698=CARTESIAN_POINT ( 'NONE',  ( 4.483927247898545687, 16.52544592524342804, 64.79057627198103830 ) ) ;
#172700=CARTESIAN_POINT ( 'NONE',  ( -0.05219959533909027116, -19.03943276465977164, 57.49890960531435979 ) ) ;
#172701=CARTESIAN_POINT ( 'NONE',  ( -14.29746914071049879, 8.314922557960819915, 75.83224293864769550 ) ) ;
#172702=CARTESIAN_POINT ( 'NONE',  ( 10.72451020669898902, -18.67979575497178502, 42.91557627198103120 ) ) ;
#172703=CARTESIAN_POINT ( 'NONE',  ( -16.46253265017146816, -9.564922557961047289, 39.16775706135234003 ) ) ;
#172704=CARTESIAN_POINT ( 'NONE',  ( 16.51473224551069308, 9.474510206698969483, 24.16557627198102765 ) ) ;
#172706=CARTESIAN_POINT ( 'NONE',  ( 16.52544592524335698, 4.483927247898782831, 71.45942372801901854 ) ) ;
#172707=CARTESIAN_POINT ( 'NONE',  ( 5.153800228976335163, 19.02544592524342804, 74.79057627198103830 ) ) ;
#172709=CARTESIAN_POINT ( 'NONE',  ( 8.314922557960818139, 14.29746914071049879, 89.58224293864768129 ) ) ;
#172710=CARTESIAN_POINT ( 'NONE',  ( -10.72451020669898014, 18.67979575497178502, 35.41557627198102409 ) ) ;
#172712=CARTESIAN_POINT ( 'NONE',  ( 14.34966873604972726, -8.224510206698740333, 105.8344237280190328 ) ) ;
#172713=CARTESIAN_POINT ( 'NONE',  ( -13.97604488694547697, 13.89961937509957934, 103.1260903946856473 ) ) ;
#172714=CARTESIAN_POINT ( 'NONE',  ( -5.719274019375665041, -21.55341960407619695, 84.79275706135234714 ) ) ;
#172715=CARTESIAN_POINT ( 'NONE',  ( -16.46253265017160317, 9.564922557960807481, 90.83224293864769550 ) ) ;
#172716=CARTESIAN_POINT ( 'NONE',  ( 5.823673210054125526, 21.52544592524343514, 104.7905762719810241 ) ) ;
#172717=CARTESIAN_POINT ( 'NONE',  ( -14.34966873604972548, 8.224510206698743886, 53.33442372801901854 ) ) ;
#172719=CARTESIAN_POINT ( 'NONE',  ( -13.89961937509977652, 13.97604488694528158, 25.62390960531434558 ) ) ;
#172720=CARTESIAN_POINT ( 'NONE',  ( 4.483927247898790824, -16.52544592524335698, 30.20942372801902565 ) ) ;
#172721=CARTESIAN_POINT ( 'NONE',  ( 9.474510206698729675, 16.51473224551082808, 97.08442372801900433 ) ) ;
#172722=CARTESIAN_POINT ( 'NONE',  ( 21.55341960407610458, 5.719274019375980345, 93.95724293864770971 ) ) ;
#172723=CARTESIAN_POINT ( 'NONE',  ( -9.564922557961040184, 16.46253265017147172, 57.91775706135233293 ) ) ;
#172725=CARTESIAN_POINT ( 'NONE',  ( -5.719274019375978568, 21.55341960407610458, 100.2072429386476955 ) ) ;
#172727=CARTESIAN_POINT ( 'NONE',  ( -19.02544592524342804, 5.153800228976336051, 81.04057627198103830 ) ) ;
#172729=CARTESIAN_POINT ( 'NONE',  ( 16.53943276465976808, 0.05219959533934440121, 36.25109039468567573 ) ) ;
#172731=CARTESIAN_POINT ( 'NONE',  ( -19.05341960407617563, 5.049401038297882671, 63.54275706135234003 ) ) ;
#172732=CARTESIAN_POINT ( 'NONE',  ( -18.67979575497193778, 10.72451020669871902, 23.33442372801901499 ) ) ;
#172733=CARTESIAN_POINT ( 'NONE',  ( -4.379528057220328563, 16.55341960407611168, 60.20724293864768839 ) ) ;
#172734=CARTESIAN_POINT ( 'NONE',  ( -19.03943276465977164, 0.05219959533909376836, 71.24890960531435269 ) ) ;
#172736=CARTESIAN_POINT ( 'NONE',  ( 4.379528057220092307, 16.55341960407617563, 42.29275706135235424 ) ) ;
#172737=CARTESIAN_POINT ( 'NONE',  ( -13.97604488694547697, 13.89961937509957934, 38.12609039468566152 ) ) ;
#172738=CARTESIAN_POINT ( 'NONE',  ( -0.05219959533937732626, 21.53943276465977519, 57.50109039468568994 ) ) ;
#172739=CARTESIAN_POINT ( 'NONE',  ( -9.564922557961040184, 16.46253265017147172, 112.9177570613523329 ) ) ;
#172740=CARTESIAN_POINT ( 'NONE',  ( 19.05341960407611168, 5.049401038298154454, 48.95724293864768129 ) ) ;
#172741=CARTESIAN_POINT ( 'NONE',  ( -19.05341960407617563, 5.049401038297882671, 78.54275706135233293 ) ) ;
#172742=CARTESIAN_POINT ( 'NONE',  ( 15.80617190586769283, -15.72974639402175789, 85.62609039468568994 ) ) ;
#172743=CARTESIAN_POINT ( 'NONE',  ( -13.97604488694547697, 13.89961937509957934, 68.12609039468563310 ) ) ;
#172744=CARTESIAN_POINT ( 'NONE',  ( -9.474510206698964154, 16.51473224551069663, 40.41557627198103120 ) ) ;
#172745=CARTESIAN_POINT ( 'NONE',  ( 21.53943276465977519, -0.05219959533907433946, 63.74890960531435979 ) ) ;
#172746=CARTESIAN_POINT ( 'NONE',  ( 12.14591786802309770, 12.06949235617756955, 64.37390960531435269 ) ) ;
#172747=CARTESIAN_POINT ( 'NONE',  ( -5.049401038297874678, -19.05341960407617918, 69.79275706135233293 ) ) ;
#172749=CARTESIAN_POINT ( 'NONE',  ( 5.153800228976615827, -19.02544592524334988, 35.20942372801899722 ) ) ;
#172750=CARTESIAN_POINT ( 'NONE',  ( 14.29746914071037800, 8.314922557961029526, 101.6677570613523613 ) ) ;
#172751=CARTESIAN_POINT ( 'NONE',  ( 12.06949235617757843, -12.14591786802309237, 53.12390960531436690 ) ) ;
#172752=CARTESIAN_POINT ( 'NONE',  ( 18.67979575497194134, -10.72451020669871369, 95.83442372801903275 ) ) ;
#172754=CARTESIAN_POINT ( 'NONE',  ( -10.72451020669898014, 18.67979575497178502, 95.41557627198102409 ) ) ;
#172756=CARTESIAN_POINT ( 'NONE',  ( -19.03943276465977164, 0.05219959533909376836, 46.24890960531435979 ) ) ;
#172757=CARTESIAN_POINT ( 'NONE',  ( 21.53943276465977519, 0.05219959533937863772, 71.25109039468568994 ) ) ;
#172758=CARTESIAN_POINT ( 'NONE',  ( 13.89961937509977652, -13.97604488694527269, 43.12390960531434558 ) ) ;
#172760=CARTESIAN_POINT ( 'NONE',  ( -9.474510206698964154, 16.51473224551069663, 65.41557627198102409 ) ) ;
#172761=CARTESIAN_POINT ( 'NONE',  ( -8.224510206698948167, 14.34966873604960824, 110.4155762719810383 ) ) ;
#172762=CARTESIAN_POINT ( 'NONE',  ( -13.97604488694527625, -13.89961937509977652, 106.8739096053143669 ) ) ;
#172763=CARTESIAN_POINT ( 'NONE',  ( -14.29746914071049879, 8.314922557960819915, 50.83224293864770971 ) ) ;
#172764=CARTESIAN_POINT ( 'NONE',  ( 16.51473224551069308, 9.474510206698969483, 29.16557627198103475 ) ) ;
#172765=CARTESIAN_POINT ( 'NONE',  ( 14.29746914071049879, -8.314922557960816363, 83.33224293864769550 ) ) ;
#172767=CARTESIAN_POINT ( 'NONE',  ( -21.55341960407610458, -5.719274019375992779, 96.45724293864770971 ) ) ;
#172768=CARTESIAN_POINT ( 'NONE',  ( -21.52544592524334988, -5.823673210054445271, 38.95942372801901854 ) ) ;
#172769=CARTESIAN_POINT ( 'NONE',  ( -19.03943276465977164, 0.05219959533909376836, 21.24890960531436335 ) ) ;
#172770=CARTESIAN_POINT ( 'NONE',  ( 14.34966873604972726, -8.224510206698740333, 40.83442372801901854 ) ) ;
#172771=CARTESIAN_POINT ( 'NONE',  ( 15.72974639402199770, -15.80617190586745480, 78.12390960531436690 ) ) ;
#172772=CARTESIAN_POINT ( 'NONE',  ( -18.67979575497193778, 10.72451020669871902, 113.3344237280190328 ) ) ;
#172773=CARTESIAN_POINT ( 'NONE',  ( 19.02544592524343514, -5.153800228976328945, 88.54057627198102409 ) ) ;
#172774=CARTESIAN_POINT ( 'NONE',  ( 21.52544592524334988, 5.823673210054432836, 46.45942372801901854 ) ) ;
#172775=CARTESIAN_POINT ( 'NONE',  ( 15.72974639402199770, -15.80617190586745480, 28.12390960531435979 ) ) ;
#172776=CARTESIAN_POINT ( 'NONE',  ( 0.05219959533934541429, -16.53943276465976808, 100.0010903946857042 ) ) ;
#172777=CARTESIAN_POINT ( 'NONE',  ( 18.62759615963255655, 10.81492255796105972, 56.66775706135235424 ) ) ;
#172778=CARTESIAN_POINT ( 'NONE',  ( 5.823673210054444382, -21.52544592524334988, 80.20942372801901854 ) ) ;
#172779=CARTESIAN_POINT ( 'NONE',  ( -5.153800228976607833, 19.02544592524334988, 27.70942372801899722 ) ) ;
#172780=CARTESIAN_POINT ( 'NONE',  ( -16.53943276465976808, -0.05219959533934237506, 88.75109039468567573 ) ) ;
#172781=CARTESIAN_POINT ( 'NONE',  ( 21.53943276465977519, 0.05219959533937863772, 46.25109039468567573 ) ) ;
#172782=CARTESIAN_POINT ( 'NONE',  ( 5.153800228976335163, 19.02544592524342804, 49.79057627198100988 ) ) ;
#172783=CARTESIAN_POINT ( 'NONE',  ( -15.72974639402176322, -15.80617190586768395, 99.37609039468568994 ) ) ;
#172784=CARTESIAN_POINT ( 'NONE',  ( -19.02544592524342804, 5.153800228976336051, 101.0405762719810241 ) ) ;
#172785=CARTESIAN_POINT ( 'NONE',  ( -21.52544592524343514, 5.823673210054127303, 106.0405762719810525 ) ) ;
#172786=CARTESIAN_POINT ( 'NONE',  ( -21.52544592524343514, 5.823673210054127303, 81.04057627198102409 ) ) ;
#172788=CARTESIAN_POINT ( 'NONE',  ( -21.53943276465977519, 0.05219959533907696930, 71.24890960531435269 ) ) ;
#172789=CARTESIAN_POINT ( 'NONE',  ( 4.379528057220092307, 16.55341960407617563, 52.29275706135236135 ) ) ;
#172790=CARTESIAN_POINT ( 'NONE',  ( -8.224510206698948167, 14.34966873604960824, 60.41557627198102409 ) ) ;
#172792=CARTESIAN_POINT ( 'NONE',  ( 0.05219959533936267826, -19.03943276465977164, 95.00109039468567573 ) ) ;
#172794=CARTESIAN_POINT ( 'NONE',  ( 8.224510206698742110, 14.34966873604972548, 22.08442372801901143 ) ) ;
#172795=CARTESIAN_POINT ( 'NONE',  ( 18.67979575497178502, 10.72451020669898547, 94.16557627198103830 ) ) ;
#172796=CARTESIAN_POINT ( 'NONE',  ( -15.72974639402197994, 15.80617190586746368, 80.62390960531438111 ) ) ;
#172797=CARTESIAN_POINT ( 'NONE',  ( -10.81492255796078084, -18.62759615963271287, 22.08224293864769194 ) ) ;
#172798=CARTESIAN_POINT ( 'NONE',  ( 12.14591786802327356, -12.06949235617739191, 55.62609039468568284 ) ) ;
#172799=CARTESIAN_POINT ( 'NONE',  ( -9.474510206698964154, 16.51473224551069663, 65.41557627198102409 ) ) ;
#172800=CARTESIAN_POINT ( 'NONE',  ( -18.67979575497193778, 10.72451020669871902, 38.33442372801900433 ) ) ;
#172801=CARTESIAN_POINT ( 'NONE',  ( 9.474510206698729675, 16.51473224551082808, 107.0844237280190043 ) ) ;
#172802=CARTESIAN_POINT ( 'NONE',  ( 5.153800228976335163, 19.02544592524342804, 104.7905762719809957 ) ) ;
#172803=CARTESIAN_POINT ( 'NONE',  ( 16.46253265017160672, -9.564922557960803928, 98.33224293864769550 ) ) ;
#172804=CARTESIAN_POINT ( 'NONE',  ( -0.05219959533907301413, -21.53943276465977519, 102.4989096053143811 ) ) ;
#172805=CARTESIAN_POINT ( 'NONE',  ( 16.46253265017160672, -9.564922557960803928, 53.33224293864768839 ) ) ;
#172806=CARTESIAN_POINT ( 'NONE',  ( -17.40861289039003523, 6.110651285853257342, 23.62767529172569070 ) ) ;
#172807=CARTESIAN_POINT ( 'NONE',  ( 4.379528057220339221, -16.55341960407611168, 82.70724293864770971 ) ) ;
#172808=CARTESIAN_POINT ( 'NONE',  ( 15.72974639402199770, -15.80617190586745480, 23.12390960531436335 ) ) ;
#172809=CARTESIAN_POINT ( 'NONE',  ( -16.38665767535054130, 7.295008042176027274, 35.26400864214546260 ) ) ;
#172811=CARTESIAN_POINT ( 'NONE',  ( 0.05219959533907565091, 21.53943276465977519, 99.99890960531436690 ) ) ;
#172812=CARTESIAN_POINT ( 'NONE',  ( -0.05219959533936034679, 19.03943276465977164, 67.50109039468566152 ) ) ;
#172813=CARTESIAN_POINT ( 'NONE',  ( 5.719274019375991003, -21.55341960407610458, 22.70724293864769194 ) ) ;
#172814=CARTESIAN_POINT ( 'NONE',  ( 9.474510206698971260, -16.51473224551069308, 22.91557627198102765 ) ) ;
#172815=CARTESIAN_POINT ( 'NONE',  ( 21.55341960407610458, 5.719274019375980345, 48.95724293864770971 ) ) ;
#172816=CARTESIAN_POINT ( 'NONE',  ( 19.03943276465977164, -0.05219959533909143690, 103.7489096053143669 ) ) ;
#172817=CARTESIAN_POINT ( 'NONE',  ( 5.719274019375673035, 21.55341960407619339, 72.29275706135236135 ) ) ;
#172818=CARTESIAN_POINT ( 'NONE',  ( 19.05341960407611168, 5.049401038298154454, 53.95724293864770260 ) ) ;
#172819=CARTESIAN_POINT ( 'NONE',  ( 16.53943276465976808, -0.05219959533910856209, 83.74890960531435269 ) ) ;
#172820=CARTESIAN_POINT ( 'NONE',  ( -0.05219959533934338120, 16.53943276465976808, 37.50109039468568284 ) ) ;
#172821=CARTESIAN_POINT ( 'NONE',  ( 18.67979575497194134, -10.72451020669871369, 70.83442372801901854 ) ) ;
#172823=CARTESIAN_POINT ( 'NONE',  ( 19.02544592524334988, 5.153800228976608722, 31.45942372801900433 ) ) ;
#172824=CARTESIAN_POINT ( 'NONE',  ( -5.049401038297874678, -19.05341960407617918, 79.79275706135233293 ) ) ;
#172826=CARTESIAN_POINT ( 'NONE',  ( -19.03943276465977164, -0.05219959533935918106, 43.75109039468566863 ) ) ;
#172827=LINE ( 'NONE', #144452, #144018 ) ;
#172828=CARTESIAN_POINT ( 'NONE',  ( -21.52544592524334988, -5.823673210054445271, 33.95942372801901143 ) ) ;
#172830=CARTESIAN_POINT ( 'NONE',  ( 19.02544592524334988, 5.153800228976608722, 31.45942372801900433 ) ) ;
#172831=CARTESIAN_POINT ( 'NONE',  ( 13.97604488694527802, 13.89961937509977652, 54.37390960531435979 ) ) ;
#172832=CARTESIAN_POINT ( 'NONE',  ( 19.03943276465977164, 0.05219959533936151252, 31.25109039468566863 ) ) ;
#172833=CARTESIAN_POINT ( 'NONE',  ( 0.05219959533934541429, -16.53943276465976808, 110.0010903946856757 ) ) ;
#172834=CARTESIAN_POINT ( 'NONE',  ( 21.53943276465977519, -0.05219959533907433946, 23.74890960531435269 ) ) ;
#172835=CARTESIAN_POINT ( 'NONE',  ( 0.05219959533937995610, -21.53943276465977519, 80.00109039468568994 ) ) ;
#172838=CARTESIAN_POINT ( 'NONE',  ( 21.53943276465977519, 0.05219959533937863772, 86.25109039468568994 ) ) ;
#172840=CARTESIAN_POINT ( 'NONE',  ( 5.153800228976335163, 19.02544592524342804, 94.79057627198103830 ) ) ;
#172842=CARTESIAN_POINT ( 'NONE',  ( 16.46253265017160672, -9.564922557960803928, 53.33224293864768839 ) ) ;
#172843=CARTESIAN_POINT ( 'NONE',  ( -5.719274019375978568, 21.55341960407610458, 50.20724293864769550 ) ) ;
#172844=CARTESIAN_POINT ( 'NONE',  ( -16.53943276465976808, -0.05219959533934237506, 113.7510903946856757 ) ) ;
#172845=CARTESIAN_POINT ( 'NONE',  ( -0.05219959533910754901, -16.53943276465976808, 97.49890960531436690 ) ) ;
#172846=CARTESIAN_POINT ( 'NONE',  ( 13.97604488694527802, 13.89961937509977652, 99.37390960531436690 ) ) ;
#172847=CARTESIAN_POINT ( 'NONE',  ( 19.05341960407617918, -5.049401038297876454, 21.04275706135232582 ) ) ;
#172848=CARTESIAN_POINT ( 'NONE',  ( -0.05219959533910754901, -16.53943276465976808, 107.4989096053143669 ) ) ;
#172849=CARTESIAN_POINT ( 'NONE',  ( 18.67979575497194134, -10.72451020669871369, 50.83442372801901143 ) ) ;
#172850=CARTESIAN_POINT ( 'NONE',  ( 16.52544592524335698, 4.483927247898782831, 101.4594237280190185 ) ) ;
#172851=CARTESIAN_POINT ( 'NONE',  ( -9.474510206698720793, -16.51473224551083518, 64.58442372801900433 ) ) ;
#172852=CYLINDRICAL_SURFACE ( 'NONE', #39963, 2.000000000000000000 ) ;
#172853=CARTESIAN_POINT ( 'NONE',  ( -5.049401038298153566, 19.05341960407611168, 115.2072429386477097 ) ) ;
#172854=CARTESIAN_POINT ( 'NONE',  ( 4.483927247898545687, 16.52544592524342804, 79.79057627198102409 ) ) ;
#172856=CARTESIAN_POINT ( 'NONE',  ( -19.03943276465977164, -0.05219959533935918106, 58.75109039468566863 ) ) ;
#172857=CARTESIAN_POINT ( 'NONE',  ( 19.02544592524343514, -5.153800228976328945, 63.54057627198103830 ) ) ;
#172858=CARTESIAN_POINT ( 'NONE',  ( 4.483927247898545687, 16.52544592524342804, 64.79057627198103830 ) ) ;
#172859=CARTESIAN_POINT ( 'NONE',  ( -16.51473224551082808, 9.474510206698731452, 98.33442372801900433 ) ) ;
#172860=CARTESIAN_POINT ( 'NONE',  ( -21.53943276465977519, 0.05219959533907696930, 31.24890960531435979 ) ) ;
#172862=CARTESIAN_POINT ( 'NONE',  ( -12.14591786802309592, -12.06949235617757132, 96.87390960531436690 ) ) ;
#172864=CARTESIAN_POINT ( 'NONE',  ( -13.89961937509977652, 13.97604488694528158, 65.62390960531436690 ) ) ;
#172865=CARTESIAN_POINT ( 'NONE',  ( -10.81492255796078084, -18.62759615963271287, 67.08224293864770971 ) ) ;
#172866=CARTESIAN_POINT ( 'NONE',  ( -9.564922557960796823, -16.46253265017161027, 47.08224293864769550 ) ) ;
#172867=CARTESIAN_POINT ( 'NONE',  ( 0.05219959533934541429, -16.53943276465976808, 95.00109039468568994 ) ) ;
#172868=CARTESIAN_POINT ( 'NONE',  ( 19.02544592524343514, -5.153800228976328945, 68.54057627198103830 ) ) ;
#172869=CARTESIAN_POINT ( 'NONE',  ( 19.02544592524334988, 5.153800228976608722, 51.45942372801900433 ) ) ;
#172870=CARTESIAN_POINT ( 'NONE',  ( -18.62759615963255300, -10.81492255796106328, 84.16775706135234714 ) ) ;
#172871=CARTESIAN_POINT ( 'NONE',  ( 15.80617190586746368, 15.72974639402197994, 54.37390960531435979 ) ) ;
#172872=CARTESIAN_POINT ( 'NONE',  ( -19.03943276465977164, 0.05219959533909376836, 111.2489096053143669 ) ) ;
#172873=CARTESIAN_POINT ( 'NONE',  ( 5.153800228976335163, 19.02544592524342804, 24.79057627198102765 ) ) ;
#172874=CARTESIAN_POINT ( 'NONE',  ( -14.29746914071037622, -8.314922557961029526, 84.16775706135234714 ) ) ;
#172875=CARTESIAN_POINT ( 'NONE',  ( -19.05341960407617563, 5.049401038297882671, 108.5427570613523187 ) ) ;
#172876=CARTESIAN_POINT ( 'NONE',  ( 9.564922557960805705, 16.46253265017160317, 24.58224293864769194 ) ) ;
#172877=CARTESIAN_POINT ( 'NONE',  ( 17.60728821186566861, -5.500000000000026645, 43.36690927743004664 ) ) ;
#172878=CARTESIAN_POINT ( 'NONE',  ( -0.05219959533937732626, 21.53943276465977519, 102.5010903946856899 ) ) ;
#172880=CARTESIAN_POINT ( 'NONE',  ( 12.06949235617757843, -12.14591786802309237, 58.12390960531435979 ) ) ;
#172881=CARTESIAN_POINT ( 'NONE',  ( -14.34966873604960291, -8.224510206698953496, 66.66557627198102409 ) ) ;
#172882=CARTESIAN_POINT ( 'NONE',  ( 18.62759615963271287, -10.81492255796078972, 98.33224293864769550 ) ) ;
#172883=CARTESIAN_POINT ( 'NONE',  ( -15.80617190586745835, -15.72974639402198527, 91.87390960531436690 ) ) ;
#172884=CARTESIAN_POINT ( 'NONE',  ( 16.18388926212238133, -7.379444403734519042, 97.06046848633849322 ) ) ;
#172885=CARTESIAN_POINT ( 'NONE',  ( -15.80617190586745835, -15.72974639402198527, 41.87390960531435979 ) ) ;
#172886=CARTESIAN_POINT ( 'NONE',  ( -12.06949235617739369, -12.14591786802326823, 64.37609039468568994 ) ) ;
#172888=CARTESIAN_POINT ( 'NONE',  ( 14.29746914071049879, -8.314922557960816363, 93.33224293864769550 ) ) ;
#172889=CARTESIAN_POINT ( 'NONE',  ( 13.97604488694527802, 13.89961937509977652, 44.37390960531435269 ) ) ;
#172890=( LENGTH_UNIT ( ) NAMED_UNIT ( * ) SI_UNIT ( .MILLI., .METRE. ) );
#172892=CARTESIAN_POINT ( 'NONE',  ( 14.29746914071037800, 8.314922557961029526, 91.66775706135234714 ) ) ;
#172893=CARTESIAN_POINT ( 'NONE',  ( -15.80617190586768217, 15.72974639402176855, 28.12609039468568284 ) ) ;
#172894=CARTESIAN_POINT ( 'NONE',  ( 19.02544592524343514, -5.153800228976328945, 83.54057627198100988 ) ) ;
#172895=CARTESIAN_POINT ( 'NONE',  ( 18.62759615963255655, 10.81492255796105972, 66.66775706135234714 ) ) ;
#172897=CARTESIAN_POINT ( 'NONE',  ( 0.05219959533909260263, 19.03943276465977164, 29.99890960531435979 ) ) ;
#172900=CARTESIAN_POINT ( 'NONE',  ( -21.55341960407619339, 5.719274019375674811, 58.54275706135235424 ) ) ;
#172901=CARTESIAN_POINT ( 'NONE',  ( -19.03943276465977164, 0.05219959533909376836, 31.24890960531435979 ) ) ;
#172902=CARTESIAN_POINT ( 'NONE',  ( -16.51473224551069308, -9.474510206698971260, 111.6655762719810383 ) ) ;
#172903=CARTESIAN_POINT ( 'NONE',  ( -19.03943276465977164, 0.05219959533909376836, 96.24890960531436690 ) ) ;
#172904=CARTESIAN_POINT ( 'NONE',  ( 9.474510206698729675, 16.51473224551082808, 62.08442372801899722 ) ) ;
#172905=CARTESIAN_POINT ( 'NONE',  ( -18.67979575497193778, 10.72451020669871902, 23.33442372801901499 ) ) ;
#172906=CARTESIAN_POINT ( 'NONE',  ( -16.51473224551082808, 9.474510206698731452, 53.33442372801900433 ) ) ;
#172907=CARTESIAN_POINT ( 'NONE',  ( -13.89961937509977652, 13.97604488694528158, 40.62390960531435979 ) ) ;
#172908=CARTESIAN_POINT ( 'NONE',  ( 4.483927247898790824, -16.52544592524335698, 105.2094237280190328 ) ) ;
#172909=CARTESIAN_POINT ( 'NONE',  ( 9.474510206698729675, 16.51473224551082808, 67.08442372801900433 ) ) ;
#172910=CARTESIAN_POINT ( 'NONE',  ( -16.55341960407611168, -4.379528057220339221, 31.45724293864769550 ) ) ;
#172911=CARTESIAN_POINT ( 'NONE',  ( 19.02544592524334988, 5.153800228976608722, 51.45942372801900433 ) ) ;
#172913=CARTESIAN_POINT ( 'NONE',  ( -13.89961937509977652, 13.97604488694528158, 95.62390960531436690 ) ) ;
#172914=CARTESIAN_POINT ( 'NONE',  ( -0.05219959533937732626, 21.53943276465977519, 112.5010903946857042 ) ) ;
#172915=CARTESIAN_POINT ( 'NONE',  ( -5.823673210054431948, 21.52544592524334988, 102.7094237280190185 ) ) ;
#172917=CARTESIAN_POINT ( 'NONE',  ( -18.67979575497193778, 10.72451020669871902, 83.33442372801903275 ) ) ;
#172918=CARTESIAN_POINT ( 'NONE',  ( 12.06949235617739724, 12.14591786802326823, 26.87609039468567218 ) ) ;
#172919=CARTESIAN_POINT ( 'NONE',  ( 9.564922557960805705, 16.46253265017160317, 89.58224293864769550 ) ) ;
#172921=CARTESIAN_POINT ( 'NONE',  ( 19.05341960407611168, 5.049401038298154454, 73.95724293864768129 ) ) ;
#172923=CARTESIAN_POINT ( 'NONE',  ( -16.46253265017146816, -9.564922557961047289, 69.16775706135233293 ) ) ;
#172924=CARTESIAN_POINT ( 'NONE',  ( -0.05219959533909027116, -19.03943276465977164, 107.4989096053143527 ) ) ;
#172925=CARTESIAN_POINT ( 'NONE',  ( 18.62759615963255655, 10.81492255796105972, 106.6677570613523756 ) ) ;
#172926=CARTESIAN_POINT ( 'NONE',  ( 14.29746914071049879, -8.314922557960816363, 93.33224293864769550 ) ) ;
#172927=CARTESIAN_POINT ( 'NONE',  ( -10.81492255796078084, -18.62759615963271287, 47.08224293864770260 ) ) ;
#172928=CARTESIAN_POINT ( 'NONE',  ( -21.52544592524343514, 5.823673210054127303, 41.04057627198103120 ) ) ;
#172929=CARTESIAN_POINT ( 'NONE',  ( -12.06949235617756955, 12.14591786802309770, 105.6239096053143669 ) ) ;
#172931=CARTESIAN_POINT ( 'NONE',  ( -13.97604488694547697, 13.89961937509957934, 53.12609039468565442 ) ) ;
#172932=CARTESIAN_POINT ( 'NONE',  ( -0.05219959533910754901, -16.53943276465976808, 32.49890960531435979 ) ) ;
#172933=CARTESIAN_POINT ( 'NONE',  ( 9.474510206698971260, -16.51473224551069308, 97.91557627198102409 ) ) ;
#172934=CARTESIAN_POINT ( 'NONE',  ( 10.81492255796106328, -18.62759615963255655, 85.41775706135236135 ) ) ;
#172935=CARTESIAN_POINT ( 'NONE',  ( -0.05219959533907301413, -21.53943276465977519, 72.49890960531435269 ) ) ;
#172936=CARTESIAN_POINT ( 'NONE',  ( -18.67979575497193778, 10.72451020669871902, 48.33442372801902565 ) ) ;
#172937=CARTESIAN_POINT ( 'NONE',  ( -10.72451020669898014, 18.67979575497178502, 100.4155762719810241 ) ) ;
#172938=CARTESIAN_POINT ( 'NONE',  ( -5.823673210054431948, 21.52544592524334988, 57.70942372801901143 ) ) ;
#172939=CARTESIAN_POINT ( 'NONE',  ( 13.97604488694527802, 13.89961937509977652, 29.37390960531435979 ) ) ;
#172940=CARTESIAN_POINT ( 'NONE',  ( -5.153800228976328057, -19.02544592524343514, 82.29057627198103830 ) ) ;
#172941=CARTESIAN_POINT ( 'NONE',  ( -8.224510206698735004, -14.34966873604973081, 79.58442372801903275 ) ) ;
#172942=CARTESIAN_POINT ( 'NONE',  ( 14.34966873604960469, 8.224510206698951720, 104.1655762719810241 ) ) ;
#172943=CARTESIAN_POINT ( 'NONE',  ( 9.474510206698971260, -16.51473224551069308, 102.9155762719810241 ) ) ;
#172945=CARTESIAN_POINT ( 'NONE',  ( 8.224510206698953496, -14.34966873604960469, 52.91557627198103830 ) ) ;
#172946=CARTESIAN_POINT ( 'NONE',  ( -8.314922557961024197, 14.29746914071037800, 107.9177570613523471 ) ) ;
#172947=CARTESIAN_POINT ( 'NONE',  ( 9.474510206698971260, -16.51473224551069308, 57.91557627198103120 ) ) ;
#172948=CARTESIAN_POINT ( 'NONE',  ( -9.474510206698964154, 16.51473224551069663, 40.41557627198103120 ) ) ;
#172949=CARTESIAN_POINT ( 'NONE',  ( 10.81492255796078972, 18.62759615963270932, 39.58224293864769550 ) ) ;
#172950=CARTESIAN_POINT ( 'NONE',  ( 0.05219959533936267826, -19.03943276465977164, 25.00109039468566152 ) ) ;
#172952=CARTESIAN_POINT ( 'NONE',  ( -4.379528057220328563, 16.55341960407611168, 35.20724293864768839 ) ) ;
#172953=CARTESIAN_POINT ( 'NONE',  ( 10.81492255796106328, -18.62759615963255655, 40.41775706135234714 ) ) ;
#172955=CARTESIAN_POINT ( 'NONE',  ( 8.314922557961029526, -14.29746914071037800, 60.41775706135235424 ) ) ;
#172956=CARTESIAN_POINT ( 'NONE',  ( -16.51473224551082808, 9.474510206698731452, 63.33442372801900433 ) ) ;
#172957=CARTESIAN_POINT ( 'NONE',  ( 8.224510206698953496, -14.34966873604960469, 22.91557627198102765 ) ) ;
#172958=CARTESIAN_POINT ( 'NONE',  ( -19.01529144963334872, -5.500000000000082601, 76.23431955728440812 ) ) ;
#172959=CARTESIAN_POINT ( 'NONE',  ( 16.52544592524335698, 4.483927247898782831, 111.4594237280190328 ) ) ;
#172960=CARTESIAN_POINT ( 'NONE',  ( -13.89961937509977652, 13.97604488694528158, 35.62390960531435269 ) ) ;
#172961=CARTESIAN_POINT ( 'NONE',  ( -9.474510206698964154, 16.51473224551069663, 60.41557627198102409 ) ) ;
#172962=CARTESIAN_POINT ( 'NONE',  ( -9.564922557960796823, -16.46253265017161027, 22.08224293864768839 ) ) ;
#172963=CARTESIAN_POINT ( 'NONE',  ( 21.52544592524334988, 5.823673210054432836, 31.45942372801901854 ) ) ;
#172964=CARTESIAN_POINT ( 'NONE',  ( -19.05341960407611168, -5.049401038298163336, 51.45724293864770260 ) ) ;
#172966=CARTESIAN_POINT ( 'NONE',  ( -16.51473224551069308, -9.474510206698971260, 51.66557627198102409 ) ) ;
#172967=CARTESIAN_POINT ( 'NONE',  ( -19.03943276465977164, 0.05219959533909376836, 116.2489096053143669 ) ) ;
#172968=CARTESIAN_POINT ( 'NONE',  ( 18.62759615963255655, 10.81492255796105972, 56.66775706135235424 ) ) ;
#172969=CARTESIAN_POINT ( 'NONE',  ( -8.224510206698948167, 14.34966873604960824, 105.4155762719810383 ) ) ;
#172970=CARTESIAN_POINT ( 'NONE',  ( 19.02544592524343514, -5.153800228976328945, 113.5405762719810241 ) ) ;
#172971=CARTESIAN_POINT ( 'NONE',  ( -12.14591786802326823, 12.06949235617739902, 83.12609039468568994 ) ) ;
#172972=CARTESIAN_POINT ( 'NONE',  ( 21.55341960407619695, -5.719274019375665929, 91.04275706135236135 ) ) ;
#172973=CARTESIAN_POINT ( 'NONE',  ( 8.314922557961029526, -14.29746914071037800, 55.41775706135234714 ) ) ;
#172974=CARTESIAN_POINT ( 'NONE',  ( 19.02544592524343514, -5.153800228976328945, 93.54057627198102409 ) ) ;
#172975=CARTESIAN_POINT ( 'NONE',  ( 4.379528057220092307, 16.55341960407617563, 37.29275706135235424 ) ) ;
#172976=CARTESIAN_POINT ( 'NONE',  ( -16.53943276465976808, -0.05219959533934237506, 28.75109039468567929 ) ) ;
#172977=CARTESIAN_POINT ( 'NONE',  ( 14.34966873604972726, -8.224510206698740333, 95.83442372801903275 ) ) ;
#172978=CARTESIAN_POINT ( 'NONE',  ( -15.80617190586768217, 15.72974639402176855, 58.12609039468568994 ) ) ;
#172979=CARTESIAN_POINT ( 'NONE',  ( 0.05219959533936267826, -19.03943276465977164, 100.0010903946856757 ) ) ;
#172980=CARTESIAN_POINT ( 'NONE',  ( -5.719274019375978568, 21.55341960407610458, 115.2072429386476955 ) ) ;
#172981=CARTESIAN_POINT ( 'NONE',  ( 12.06949235617757843, -12.14591786802309237, 103.1239096053143811 ) ) ;
#172982=CARTESIAN_POINT ( 'NONE',  ( -9.564922557961040184, 16.46253265017147172, 107.9177570613523471 ) ) ;
#172983=CARTESIAN_POINT ( 'NONE',  ( 4.483927247898790824, -16.52544592524335698, 75.20942372801901854 ) ) ;
#172985=CARTESIAN_POINT ( 'NONE',  ( -0.05219959533936034679, 19.03943276465977164, 67.50109039468566152 ) ) ;
#172986=CARTESIAN_POINT ( 'NONE',  ( 8.314922557960818139, 14.29746914071049879, 39.58224293864769550 ) ) ;
#172987=CARTESIAN_POINT ( 'NONE',  ( 16.52544592524342804, -4.483927247898539470, 38.54057627198103120 ) ) ;
#172988=CARTESIAN_POINT ( 'NONE',  ( 8.314922557960818139, 14.29746914071049879, 94.58224293864769550 ) ) ;
#172989=CARTESIAN_POINT ( 'NONE',  ( -19.02544592524334988, -5.153800228976617603, 28.95942372801900433 ) ) ;
#172990=CARTESIAN_POINT ( 'NONE',  ( -17.31728774477273447, 6.344390552232388458, 90.81906651689320142 ) ) ;
#172991=CARTESIAN_POINT ( 'NONE',  ( 21.53943276465977519, 0.05219959533937863772, 36.25109039468567573 ) ) ;
#172992=CARTESIAN_POINT ( 'NONE',  ( 5.049401038297881783, 19.05341960407617563, 97.29275706135233293 ) ) ;
#172994=CARTESIAN_POINT ( 'NONE',  ( -19.02544592524342804, 5.153800228976336051, 86.04057627198103830 ) ) ;
#172995=CARTESIAN_POINT ( 'NONE',  ( -9.564922557960796823, -16.46253265017161027, 87.08224293864769550 ) ) ;
#172996=CARTESIAN_POINT ( 'NONE',  ( 10.72451020669898902, -18.67979575497178502, 62.91557627198102409 ) ) ;
#172997=CARTESIAN_POINT ( 'NONE',  ( 0.05219959533910956823, 16.53943276465976808, 89.99890960531438111 ) ) ;
#172998=CARTESIAN_POINT ( 'NONE',  ( -0.05219959533909027116, -19.03943276465977164, 72.49890960531435269 ) ) ;
#172999=CARTESIAN_POINT ( 'NONE',  ( -19.02544592524342804, 5.153800228976336051, 36.04057627198100988 ) ) ;
#173000=CARTESIAN_POINT ( 'NONE',  ( 0.05219959533937995610, -21.53943276465977519, 45.00109039468568284 ) ) ;
#173001=CARTESIAN_POINT ( 'NONE',  ( -10.72451020669870658, -18.67979575497194134, 69.58442372801900433 ) ) ;
#173002=CARTESIAN_POINT ( 'NONE',  ( -5.153800228976328057, -19.02544592524343514, 62.29057627198100988 ) ) ;
#173003=CARTESIAN_POINT ( 'NONE',  ( 12.14591786802327356, -12.06949235617739191, 85.62609039468568994 ) ) ;
#173004=CARTESIAN_POINT ( 'NONE',  ( 21.53943276465977519, 0.05219959533937863772, 31.25109039468568639 ) ) ;
#173005=CARTESIAN_POINT ( 'NONE',  ( -18.62759615963255300, -10.81492255796106328, 29.16775706135234003 ) ) ;
#173006=CARTESIAN_POINT ( 'NONE',  ( -5.049401038297874678, -19.05341960407617918, 49.79275706135231871 ) ) ;
#173007=CARTESIAN_POINT ( 'NONE',  ( 13.97604488694527802, 13.89961937509977652, 74.37390960531436690 ) ) ;
#173008=CARTESIAN_POINT ( 'NONE',  ( -19.03943276465977164, -0.05219959533935918106, 28.75109039468566507 ) ) ;
#173009=CARTESIAN_POINT ( 'NONE',  ( -18.62759615963255300, -10.81492255796106328, 79.16775706135234714 ) ) ;
#173010=CARTESIAN_POINT ( 'NONE',  ( -5.719274019375978568, 21.55341960407610458, 75.20724293864769550 ) ) ;
#173011=CARTESIAN_POINT ( 'NONE',  ( -4.379528057220328563, 16.55341960407611168, 45.20724293864769550 ) ) ;
#173012=CARTESIAN_POINT ( 'NONE',  ( -18.62759615963255300, -10.81492255796106328, 104.1677570613523471 ) ) ;
#173013=CARTESIAN_POINT ( 'NONE',  ( -5.153800228976607833, 19.02544592524334988, 27.70942372801899722 ) ) ;
#173014=CARTESIAN_POINT ( 'NONE',  ( -16.55341960407611168, -4.379528057220339221, 76.45724293864769550 ) ) ;
#173015=CARTESIAN_POINT ( 'NONE',  ( -12.14591786802309592, -12.06949235617757132, 111.8739096053143669 ) ) ;
#173016=CARTESIAN_POINT ( 'NONE',  ( 13.89961937509957401, 13.97604488694547697, 71.87609039468567573 ) ) ;
#173017=CARTESIAN_POINT ( 'NONE',  ( 14.29746914071049879, -8.314922557960816363, 33.33224293864769550 ) ) ;
#173018=CARTESIAN_POINT ( 'NONE',  ( -21.52544592524334988, -5.823673210054445271, 83.95942372801900433 ) ) ;
#173019=CARTESIAN_POINT ( 'NONE',  ( 5.153800228976335163, 19.02544592524342804, 74.79057627198103830 ) ) ;
#173020=CARTESIAN_POINT ( 'NONE',  ( 0.05219959533936267826, -19.03943276465977164, 50.00109039468566863 ) ) ;
#173021=CARTESIAN_POINT ( 'NONE',  ( -10.72451020669898014, 18.67979575497178502, 60.41557627198102409 ) ) ;
#173022=CARTESIAN_POINT ( 'NONE',  ( 21.52544592524334988, 5.823673210054432836, 21.45942372801901499 ) ) ;
#173023=CARTESIAN_POINT ( 'NONE',  ( 9.474510206698729675, 16.51473224551082808, 107.0844237280190043 ) ) ;
#173024=CARTESIAN_POINT ( 'NONE',  ( 8.224510206698742110, 14.34966873604972548, 72.08442372801899012 ) ) ;
#173026=CARTESIAN_POINT ( 'NONE',  ( 0.05219959533907565091, 21.53943276465977519, 104.9989096053143669 ) ) ;
#173027=CARTESIAN_POINT ( 'NONE',  ( -8.314922557960811034, -14.29746914071050412, 107.0822429386476955 ) ) ;
#173028=CARTESIAN_POINT ( 'NONE',  ( -17.49999999999999645, -4.013004640162675329, 29.55394279005589198 ) ) ;
#173029=CARTESIAN_POINT ( 'NONE',  ( -8.224510206698735004, -14.34966873604973081, 39.58442372801901143 ) ) ;
#173031=CARTESIAN_POINT ( 'NONE',  ( 21.53943276465977519, -0.05219959533907433946, 58.74890960531436690 ) ) ;
#173032=CARTESIAN_POINT ( 'NONE',  ( -16.52544592524335698, -4.483927247898792601, 103.9594237280190185 ) ) ;
#173033=CARTESIAN_POINT ( 'NONE',  ( -5.049401038298153566, 19.05341960407611168, 35.20724293864768839 ) ) ;
#173034=CARTESIAN_POINT ( 'NONE',  ( 8.224510206698742110, 14.34966873604972548, 72.08442372801899012 ) ) ;
#173035=CARTESIAN_POINT ( 'NONE',  ( 16.46253265017146816, 9.564922557961045513, 66.66775706135233293 ) ) ;
#173036=CARTESIAN_POINT ( 'NONE',  ( -21.55341960407619339, 5.719274019375674811, 43.54275706135235424 ) ) ;
#173037=CARTESIAN_POINT ( 'NONE',  ( -21.55341960407610458, -5.719274019375992779, 61.45724293864770260 ) ) ;
#173038=CARTESIAN_POINT ( 'NONE',  ( -4.379528057220086978, -16.55341960407618274, 99.79275706135234714 ) ) ;
#173039=CARTESIAN_POINT ( 'NONE',  ( -10.72451020669870658, -18.67979575497194134, 89.58442372801901854 ) ) ;
#173040=CARTESIAN_POINT ( 'NONE',  ( -21.53943276465977519, 0.05219959533907696930, 51.24890960531436690 ) ) ;
#173041=CARTESIAN_POINT ( 'NONE',  ( -5.719274019375978568, 21.55341960407610458, 30.20724293864769550 ) ) ;
#173042=ORIENTED_EDGE ( 'NONE', *, *, #192356, .F. ) ;
#173043=CARTESIAN_POINT ( 'NONE',  ( -8.314922557961024197, 14.29746914071037800, 82.91775706135234714 ) ) ;
#173044=CARTESIAN_POINT ( 'NONE',  ( -21.53943276465977519, 0.05219959533907696930, 46.24890960531435979 ) ) ;
#173046=CARTESIAN_POINT ( 'NONE',  ( -5.049401038298153566, 19.05341960407611168, 95.20724293864770971 ) ) ;
#173048=CARTESIAN_POINT ( 'NONE',  ( -9.564922557960796823, -16.46253265017161027, 32.08224293864769550 ) ) ;
#173049=CARTESIAN_POINT ( 'NONE',  ( -21.53943276465977519, 0.05219959533907696930, 56.24890960531436690 ) ) ;
#173050=CARTESIAN_POINT ( 'NONE',  ( -16.53943276465976808, -0.05219959533934237506, 88.75109039468567573 ) ) ;
#173051=CARTESIAN_POINT ( 'NONE',  ( 5.719274019375673035, 21.55341960407619339, 42.29275706135235424 ) ) ;
#173052=CARTESIAN_POINT ( 'NONE',  ( -5.049401038297874678, -19.05341960407617918, 99.79275706135234714 ) ) ;
#173053=CARTESIAN_POINT ( 'NONE',  ( -14.34966873604960291, -8.224510206698953496, 96.66557627198102409 ) ) ;
#173054=CARTESIAN_POINT ( 'NONE',  ( 14.29746914071037800, 8.314922557961029526, 21.66775706135235069 ) ) ;
#173056=CARTESIAN_POINT ( 'NONE',  ( -5.049401038298153566, 19.05341960407611168, 45.20724293864769550 ) ) ;
#173058=CARTESIAN_POINT ( 'NONE',  ( -5.049401038298153566, 19.05341960407611168, 95.20724293864770971 ) ) ;
#173059=CARTESIAN_POINT ( 'NONE',  ( -4.379528057220086978, -16.55341960407618274, 74.79275706135234714 ) ) ;
#173060=CARTESIAN_POINT ( 'NONE',  ( -5.719274019375665041, -21.55341960407619695, 104.7927570613523898 ) ) ;
#173061=CARTESIAN_POINT ( 'NONE',  ( -15.72974639402197994, 15.80617190586746368, 60.62390960531437401 ) ) ;
#173062=CARTESIAN_POINT ( 'NONE',  ( -14.34966873604972548, 8.224510206698743886, 93.33442372801901854 ) ) ;
#173063=CARTESIAN_POINT ( 'NONE',  ( -16.46253265017146816, -9.564922557961047289, 74.16775706135234714 ) ) ;
#173064=CARTESIAN_POINT ( 'NONE',  ( -19.05341960407611168, -5.049401038298163336, 36.45724293864766707 ) ) ;
#173065=CARTESIAN_POINT ( 'NONE',  ( 19.03943276465977164, -0.05219959533909143690, 78.74890960531436690 ) ) ;
#173066=CARTESIAN_POINT ( 'NONE',  ( 19.05341960407611168, 5.049401038298154454, 33.95724293864769550 ) ) ;
#173067=CARTESIAN_POINT ( 'NONE',  ( 16.51473224551083163, -9.474510206698727899, 70.83442372801900433 ) ) ;
#173069=CARTESIAN_POINT ( 'NONE',  ( 16.51473224551069308, 9.474510206698969483, 114.1655762719810241 ) ) ;
#173070=CARTESIAN_POINT ( 'NONE',  ( -16.52544592524342804, 4.483927247898546575, 61.04057627198103120 ) ) ;
#173071=CARTESIAN_POINT ( 'NONE',  ( 10.72451020669898902, -18.67979575497178502, 57.91557627198103120 ) ) ;
#173073=CARTESIAN_POINT ( 'NONE',  ( 13.97604488694548053, -13.89961937509957401, 35.62609039468567573 ) ) ;
#173075=CARTESIAN_POINT ( 'NONE',  ( 5.049401038298161559, -19.05341960407611168, 62.70724293864769550 ) ) ;
#173076=CARTESIAN_POINT ( 'NONE',  ( 5.153800228976335163, 19.02544592524342804, 69.79057627198103830 ) ) ;
#173077=CARTESIAN_POINT ( 'NONE',  ( -0.05219959533934338120, 16.53943276465976808, 47.50109039468568994 ) ) ;
#173078=CARTESIAN_POINT ( 'NONE',  ( -19.20446147854527297, -5.499999999999958256, 99.38999695167676407 ) ) ;
#173080=CARTESIAN_POINT ( 'NONE',  ( 14.29746914071037800, 8.314922557961029526, 81.66775706135236135 ) ) ;
#173081=CARTESIAN_POINT ( 'NONE',  ( -17.60769864724390388, 5.499999999999982236, 78.65024842019167295 ) ) ;
#173082=CARTESIAN_POINT ( 'NONE',  ( 16.52544592524335698, 4.483927247898782831, 61.45942372801901854 ) ) ;
#173083=CARTESIAN_POINT ( 'NONE',  ( 0.05219959533934541429, -16.53943276465976808, 35.00109039468568284 ) ) ;
#173084=CARTESIAN_POINT ( 'NONE',  ( -5.153800228976328057, -19.02544592524343514, 57.29057627198103120 ) ) ;
#173086=CARTESIAN_POINT ( 'NONE',  ( -10.72451020669870658, -18.67979575497194134, 59.58442372801901854 ) ) ;
#173087=CARTESIAN_POINT ( 'NONE',  ( -16.46253265017146816, -9.564922557961047289, 59.16775706135233293 ) ) ;
#173088=CARTESIAN_POINT ( 'NONE',  ( -21.52544592524334988, -5.823673210054445271, 93.95942372801903275 ) ) ;
#173090=CARTESIAN_POINT ( 'NONE',  ( -16.51473224551069308, -9.474510206698971260, 31.66557627198102054 ) ) ;
#173092=CARTESIAN_POINT ( 'NONE',  ( 21.55341960407610458, 5.719274019375980345, 58.95724293864770971 ) ) ;
#173093=CARTESIAN_POINT ( 'NONE',  ( 19.03943276465977164, -0.05219959533909143690, 103.7489096053143669 ) ) ;
#173094=CARTESIAN_POINT ( 'NONE',  ( 8.314922557960818139, 14.29746914071049879, 99.58224293864770971 ) ) ;
#173095=CARTESIAN_POINT ( 'NONE',  ( 16.52544592524335698, 4.483927247898782831, 36.45942372801901143 ) ) ;
#173097=CARTESIAN_POINT ( 'NONE',  ( -16.55341960407611168, -4.379528057220339221, 36.45724293864768839 ) ) ;
#173099=CARTESIAN_POINT ( 'NONE',  ( -15.72974639402197994, 15.80617190586746368, 100.6239096053143811 ) ) ;
#173100=CARTESIAN_POINT ( 'NONE',  ( 8.314922557960818139, 14.29746914071049879, 34.58224293864770260 ) ) ;
#173101=CARTESIAN_POINT ( 'NONE',  ( 0.05219959533909260263, 19.03943276465977164, 114.9989096053143669 ) ) ;
#173102=CARTESIAN_POINT ( 'NONE',  ( -19.02544592524334988, -5.153800228976617603, 88.95942372801897591 ) ) ;
#173103=CARTESIAN_POINT ( 'NONE',  ( 19.05341960407617918, -5.049401038297876454, 26.04275706135233293 ) ) ;
#173104=CARTESIAN_POINT ( 'NONE',  ( -4.483927247898539470, -16.52544592524342804, 37.29057627198102409 ) ) ;
#173105=CARTESIAN_POINT ( 'NONE',  ( 10.81492255796078972, 18.62759615963270932, 99.58224293864770971 ) ) ;
#173106=CARTESIAN_POINT ( 'NONE',  ( -18.67979575497178146, -10.72451020669898902, 46.66557627198102409 ) ) ;
#173107=CARTESIAN_POINT ( 'NONE',  ( -9.474510206698964154, 16.51473224551069663, 80.41557627198103830 ) ) ;
#173108=CARTESIAN_POINT ( 'NONE',  ( -4.483927247898539470, -16.52544592524342804, 37.29057627198102409 ) ) ;
#173109=CARTESIAN_POINT ( 'NONE',  ( 16.46253265017160672, -9.564922557960803928, 88.33224293864769550 ) ) ;
#173111=CARTESIAN_POINT ( 'NONE',  ( 19.49671883438229969, 5.499999999999974243, 57.39279849105685827 ) ) ;
#173112=CARTESIAN_POINT ( 'NONE',  ( 16.46253265017146816, 9.564922557961045513, 41.66775706135234003 ) ) ;
#173113=CARTESIAN_POINT ( 'NONE',  ( -18.67979575497178146, -10.72451020669898902, 86.66557627198102409 ) ) ;
#173114=CARTESIAN_POINT ( 'NONE',  ( 12.06949235617757843, -12.14591786802309237, 103.1239096053143811 ) ) ;
#173116=CARTESIAN_POINT ( 'NONE',  ( -5.823673210054431948, 21.52544592524334988, 37.70942372801900433 ) ) ;
#173118=CARTESIAN_POINT ( 'NONE',  ( 12.06949235617739724, 12.14591786802326823, 111.8760903946856615 ) ) ;
#173119=CARTESIAN_POINT ( 'NONE',  ( -16.46253265017160317, 9.564922557960807481, 40.83224293864769550 ) ) ;
#173120=CARTESIAN_POINT ( 'NONE',  ( -9.474510206698964154, 16.51473224551069663, 80.41557627198103830 ) ) ;
#173121=CARTESIAN_POINT ( 'NONE',  ( -18.39635199886966532, 5.500000000000103029, 46.01967076360001840 ) ) ;
#173122=CARTESIAN_POINT ( 'NONE',  ( -16.51473224551069308, -9.474510206698971260, 36.66557627198102409 ) ) ;
#173123=CARTESIAN_POINT ( 'NONE',  ( -8.314922557960811034, -14.29746914071050412, 37.08224293864768129 ) ) ;
#173124=CARTESIAN_POINT ( 'NONE',  ( -5.719274019375665041, -21.55341960407619695, 69.79275706135234714 ) ) ;
#173126=CARTESIAN_POINT ( 'NONE',  ( -0.05219959533934338120, 16.53943276465976808, 67.50109039468568994 ) ) ;
#173127=CARTESIAN_POINT ( 'NONE',  ( -16.46253265017160317, 9.564922557960807481, 55.83224293864769550 ) ) ;
#173128=CARTESIAN_POINT ( 'NONE',  ( -13.89961937509977652, 13.97604488694528158, 70.62390960531432427 ) ) ;
#173130=CARTESIAN_POINT ( 'NONE',  ( 21.55341960407619695, -5.719274019375665929, 111.0427570613523613 ) ) ;
#173131=CARTESIAN_POINT ( 'NONE',  ( -8.224510206698735004, -14.34966873604973081, 79.58442372801903275 ) ) ;
#173132=CARTESIAN_POINT ( 'NONE',  ( 18.67979575497194134, -10.72451020669871369, 95.83442372801903275 ) ) ;
#173133=CARTESIAN_POINT ( 'NONE',  ( 13.89961937509977652, -13.97604488694527269, 58.12390960531436690 ) ) ;
#173134=CARTESIAN_POINT ( 'NONE',  ( 15.80617190586746368, 15.72974639402197994, 29.37390960531435269 ) ) ;
#173135=CARTESIAN_POINT ( 'NONE',  ( -19.03943276465977164, -0.05219959533935918106, 103.7510903946856757 ) ) ;
#173136=CARTESIAN_POINT ( 'NONE',  ( 0.05219959533937995610, -21.53943276465977519, 70.00109039468568994 ) ) ;
#173137=CARTESIAN_POINT ( 'NONE',  ( 12.14591786802327356, -12.06949235617739191, 55.62609039468568284 ) ) ;
#173138=CARTESIAN_POINT ( 'NONE',  ( -0.05219959533907301413, -21.53943276465977519, 97.49890960531436690 ) ) ;
#173139=CARTESIAN_POINT ( 'NONE',  ( -16.46253265017146816, -9.564922557961047289, 94.16775706135233293 ) ) ;
#173140=CARTESIAN_POINT ( 'NONE',  ( 9.564922557960805705, 16.46253265017160317, 84.58224293864769550 ) ) ;
#173141=CARTESIAN_POINT ( 'NONE',  ( 0.05219959533936267826, -19.03943276465977164, 110.0010903946856757 ) ) ;
#173142=CARTESIAN_POINT ( 'NONE',  ( -13.97604488694547697, 13.89961937509957934, 113.1260903946856757 ) ) ;
#173143=CARTESIAN_POINT ( 'NONE',  ( -8.314922557960811034, -14.29746914071050412, 72.08224293864769550 ) ) ;
#173144=CARTESIAN_POINT ( 'NONE',  ( 16.53943276465976808, 0.05219959533934440121, 76.25109039468568994 ) ) ;
#173145=CARTESIAN_POINT ( 'NONE',  ( -21.53943276465977519, 0.05219959533907696930, 111.2489096053143669 ) ) ;
#173146=CARTESIAN_POINT ( 'NONE',  ( 13.97604488694527802, 13.89961937509977652, 54.37390960531435979 ) ) ;
#173147=CARTESIAN_POINT ( 'NONE',  ( -16.51473224551069308, -9.474510206698971260, 51.66557627198102409 ) ) ;
#173148=CARTESIAN_POINT ( 'NONE',  ( 16.52544592524335698, 4.483927247898782831, 66.45942372801903275 ) ) ;
#173151=CARTESIAN_POINT ( 'NONE',  ( -10.81492255796105439, 18.62759615963255655, 112.9177570613523329 ) ) ;
#173152=CARTESIAN_POINT ( 'NONE',  ( 13.97604488694527802, 13.89961937509977652, 34.37390960531436690 ) ) ;
#173154=CARTESIAN_POINT ( 'NONE',  ( 5.049401038297881783, 19.05341960407617563, 107.2927570613523187 ) ) ;
#173155=CARTESIAN_POINT ( 'NONE',  ( -19.02544592524334988, -5.153800228976617603, 38.95942372801900433 ) ) ;
#173156=CARTESIAN_POINT ( 'NONE',  ( 4.379528057220092307, 16.55341960407617563, 27.29275706135234358 ) ) ;
#173157=CARTESIAN_POINT ( 'NONE',  ( 13.97604488694527802, 13.89961937509977652, 49.37390960531434558 ) ) ;
#173158=CARTESIAN_POINT ( 'NONE',  ( 9.474510206698971260, -16.51473224551069308, 62.91557627198102409 ) ) ;
#173159=CARTESIAN_POINT ( 'NONE',  ( 10.81492255796078972, 18.62759615963270932, 79.58224293864769550 ) ) ;
#173160=CARTESIAN_POINT ( 'NONE',  ( -0.05219959533909027116, -19.03943276465977164, 112.4989096053143669 ) ) ;
#173161=CARTESIAN_POINT ( 'NONE',  ( -13.97604488694527625, -13.89961937509977652, 51.87390960531436690 ) ) ;
#173163=CARTESIAN_POINT ( 'NONE',  ( 9.474510206698729675, 16.51473224551082808, 92.08442372801900433 ) ) ;
#173164=CARTESIAN_POINT ( 'NONE',  ( 8.314922557960818139, 14.29746914071049879, 69.58224293864769550 ) ) ;
#173165=CARTESIAN_POINT ( 'NONE',  ( -9.474510206698720793, -16.51473224551083518, 24.58442372801900078 ) ) ;
#173166=CARTESIAN_POINT ( 'NONE',  ( 16.52544592524342804, -4.483927247898539470, 58.54057627198103120 ) ) ;
#173167=CARTESIAN_POINT ( 'NONE',  ( 5.719274019375673035, 21.55341960407619339, 87.29275706135236135 ) ) ;
#173168=CARTESIAN_POINT ( 'NONE',  ( -9.564922557960796823, -16.46253265017161027, 27.08224293864769550 ) ) ;
#173169=CARTESIAN_POINT ( 'NONE',  ( 18.62759615963255655, 10.81492255796105972, 86.66775706135234714 ) ) ;
#173170=CARTESIAN_POINT ( 'NONE',  ( -16.55341960407611168, -4.379528057220339221, 31.45724293864769550 ) ) ;
#173171=CARTESIAN_POINT ( 'NONE',  ( -0.05219959533937732626, 21.53943276465977519, 72.50109039468568994 ) ) ;
#173172=CARTESIAN_POINT ( 'NONE',  ( -19.05341960407611168, -5.049401038298163336, 81.45724293864769550 ) ) ;
#173173=CARTESIAN_POINT ( 'NONE',  ( -5.823673210054431948, 21.52544592524334988, 37.70942372801900433 ) ) ;
#173174=CARTESIAN_POINT ( 'NONE',  ( -9.474510206698964154, 16.51473224551069663, 75.41557627198103830 ) ) ;
#173175=CARTESIAN_POINT ( 'NONE',  ( -14.34966873604960291, -8.224510206698953496, 91.66557627198103830 ) ) ;
#173176=CARTESIAN_POINT ( 'NONE',  ( -0.05219959533910754901, -16.53943276465976808, 57.49890960531435979 ) ) ;
#173177=CARTESIAN_POINT ( 'NONE',  ( 21.52544592524344225, -5.823673210054117533, 68.54057627198103830 ) ) ;
#173178=CARTESIAN_POINT ( 'NONE',  ( -19.05341960407611168, -5.049401038298163336, 71.45724293864766707 ) ) ;
#173179=CARTESIAN_POINT ( 'NONE',  ( -5.719274019375978568, 21.55341960407610458, 90.20724293864770971 ) ) ;
#173180=CARTESIAN_POINT ( 'NONE',  ( -5.049401038297874678, -19.05341960407617918, 74.79275706135231871 ) ) ;
#173182=CARTESIAN_POINT ( 'NONE',  ( -18.89770734986048240, -5.500000000000011546, 89.10214472496642202 ) ) ;
#173183=CARTESIAN_POINT ( 'NONE',  ( -14.34966873604960291, -8.224510206698953496, 76.66557627198103830 ) ) ;
#173184=CARTESIAN_POINT ( 'NONE',  ( -5.719274019375978568, 21.55341960407610458, 55.20724293864770260 ) ) ;
#173186=CARTESIAN_POINT ( 'NONE',  ( -8.224510206698735004, -14.34966873604973081, 94.58442372801901854 ) ) ;
#173188=CARTESIAN_POINT ( 'NONE',  ( 9.564922557961047289, -16.46253265017146816, 105.4177570613523471 ) ) ;
#173189=CARTESIAN_POINT ( 'NONE',  ( 14.34966873604960469, 8.224510206698951720, 74.16557627198102409 ) ) ;
#173190=CARTESIAN_POINT ( 'NONE',  ( -19.52851543214743657, -5.499999999999989342, 95.39357721762576148 ) ) ;
#173191=CARTESIAN_POINT ( 'NONE',  ( -9.474510206698964154, 16.51473224551069663, 65.41557627198102409 ) ) ;
#173192=CARTESIAN_POINT ( 'NONE',  ( 8.314922557960818139, 14.29746914071049879, 49.58224293864769550 ) ) ;
#173193=CARTESIAN_POINT ( 'NONE',  ( -5.153800228976328057, -19.02544592524343514, 97.29057627198099567 ) ) ;
#173194=CARTESIAN_POINT ( 'NONE',  ( 19.03943276465977164, 0.05219959533936151252, 91.25109039468566152 ) ) ;
#173195=CARTESIAN_POINT ( 'NONE',  ( 5.049401038298161559, -19.05341960407611168, 72.70724293864768129 ) ) ;
#173196=CARTESIAN_POINT ( 'NONE',  ( 0.05219959533909260263, 19.03943276465977164, 79.99890960531436690 ) ) ;
#173197=CARTESIAN_POINT ( 'NONE',  ( -16.51473224551069308, -9.474510206698971260, 81.66557627198103830 ) ) ;
#173198=CARTESIAN_POINT ( 'NONE',  ( 18.62759615963271287, -10.81492255796078972, 58.33224293864768839 ) ) ;
#173199=CARTESIAN_POINT ( 'NONE',  ( 4.483927247898790824, -16.52544592524335698, 55.20942372801902565 ) ) ;
#173200=CARTESIAN_POINT ( 'NONE',  ( -0.05219959533936034679, 19.03943276465977164, 102.5010903946856757 ) ) ;
#173201=CARTESIAN_POINT ( 'NONE',  ( -13.97604488694527625, -13.89961937509977652, 66.87390960531436690 ) ) ;
#173202=CARTESIAN_POINT ( 'NONE',  ( -15.72974639402197994, 15.80617190586746368, 70.62390960531436690 ) ) ;
#173203=CARTESIAN_POINT ( 'NONE',  ( -9.474510206698720793, -16.51473224551083518, 94.58442372801900433 ) ) ;
#173205=CARTESIAN_POINT ( 'NONE',  ( -0.05219959533910754901, -16.53943276465976808, 22.49890960531436335 ) ) ;
#173206=CARTESIAN_POINT ( 'NONE',  ( -18.67979575497193778, 10.72451020669871902, 43.33442372801901143 ) ) ;
#173207=CARTESIAN_POINT ( 'NONE',  ( 5.049401038297881783, 19.05341960407617563, 42.29275706135234003 ) ) ;
#173208=CARTESIAN_POINT ( 'NONE',  ( 4.379528057220092307, 16.55341960407617563, 57.29275706135234714 ) ) ;
#173209=CARTESIAN_POINT ( 'NONE',  ( -12.14591786802326823, 12.06949235617739902, 93.12609039468568994 ) ) ;
#173211=CARTESIAN_POINT ( 'NONE',  ( 4.379528057220092307, 16.55341960407617563, 82.29275706135234714 ) ) ;
#173212=CARTESIAN_POINT ( 'NONE',  ( -0.05219959533934338120, 16.53943276465976808, 37.50109039468568284 ) ) ;
#173213=CARTESIAN_POINT ( 'NONE',  ( -0.05219959533909027116, -19.03943276465977164, 47.49890960531435979 ) ) ;
#173214=CARTESIAN_POINT ( 'NONE',  ( -13.97604488694527625, -13.89961937509977652, 51.87390960531436690 ) ) ;
#173215=CARTESIAN_POINT ( 'NONE',  ( -16.46253265017160317, 9.564922557960807481, 60.83224293864769550 ) ) ;
#173216=CARTESIAN_POINT ( 'NONE',  ( -5.719274019375665041, -21.55341960407619695, 54.79275706135235424 ) ) ;
#173217=CARTESIAN_POINT ( 'NONE',  ( -4.483927247898782831, 16.52544592524335698, 47.70942372801902565 ) ) ;
#173218=CARTESIAN_POINT ( 'NONE',  ( 8.224510206698953496, -14.34966873604960469, 22.91557627198102765 ) ) ;
#173219=CARTESIAN_POINT ( 'NONE',  ( 19.02544592524343514, -5.153800228976328945, 33.54057627198102409 ) ) ;
#173220=CARTESIAN_POINT ( 'NONE',  ( -21.53943276465977519, -0.05219959533937600094, 113.7510903946856757 ) ) ;
#173221=CARTESIAN_POINT ( 'NONE',  ( -14.29746914071037622, -8.314922557961029526, 24.16775706135235424 ) ) ;
#173222=CARTESIAN_POINT ( 'NONE',  ( 19.05341960407617918, -5.049401038297876454, 81.04275706135231871 ) ) ;
#173223=CARTESIAN_POINT ( 'NONE',  ( 4.483927247898545687, 16.52544592524342804, 84.79057627198102409 ) ) ;
#173224=CARTESIAN_POINT ( 'NONE',  ( 9.474510206698971260, -16.51473224551069308, 42.91557627198103120 ) ) ;
#173225=CARTESIAN_POINT ( 'NONE',  ( -5.153800228976607833, 19.02544592524334988, 77.70942372801900433 ) ) ;
#173226=CARTESIAN_POINT ( 'NONE',  ( 16.21995358207304250, -7.366697692864150326, 92.43551001512157939 ) ) ;
#173227=CARTESIAN_POINT ( 'NONE',  ( -18.62759615963255300, -10.81492255796106328, 74.16775706135231871 ) ) ;
#173228=CARTESIAN_POINT ( 'NONE',  ( 14.34966873604972726, -8.224510206698740333, 35.83442372801901143 ) ) ;
#173229=CARTESIAN_POINT ( 'NONE',  ( -17.49999999999998579, 3.850315288878732201, 24.26629130603454954 ) ) ;
#173230=CARTESIAN_POINT ( 'NONE',  ( -5.719274019375978568, 21.55341960407610458, 40.20724293864769550 ) ) ;
#173231=CARTESIAN_POINT ( 'NONE',  ( 8.314922557961029526, -14.29746914071037800, 20.41775706135234714 ) ) ;
#173232=CARTESIAN_POINT ( 'NONE',  ( 5.049401038298163336, -19.05341960407611168, 27.70724293864769550 ) ) ;
#173233=CARTESIAN_POINT ( 'NONE',  ( 5.049401038297881783, 19.05341960407617563, 32.29275706135233293 ) ) ;
#173235=CARTESIAN_POINT ( 'NONE',  ( 19.02544592524343514, -5.153800228976328945, 43.54057627198103120 ) ) ;
#173236=CARTESIAN_POINT ( 'NONE',  ( -18.22780087662122028, 5.500000000000031086, 58.51540105326107977 ) ) ;
#173237=CARTESIAN_POINT ( 'NONE',  ( 0.05219959533909260263, 19.03943276465977164, 69.99890960531435269 ) ) ;
#173239=CARTESIAN_POINT ( 'NONE',  ( -18.56197773271729190, 5.499999999999996447, 98.55066217314453070 ) ) ;
#173240=CARTESIAN_POINT ( 'NONE',  ( -15.72974639402176322, -15.80617190586768395, 109.3760903946857042 ) ) ;
#173241=CARTESIAN_POINT ( 'NONE',  ( 16.55341960407611168, 4.379528057220329451, 43.95724293864769550 ) ) ;
#173242=CARTESIAN_POINT ( 'NONE',  ( -19.03943276465977164, 0.05219959533909376836, 46.24890960531435979 ) ) ;
#173243=CARTESIAN_POINT ( 'NONE',  ( -16.46253265017160317, 9.564922557960807481, 85.83224293864769550 ) ) ;
#173244=CARTESIAN_POINT ( 'NONE',  ( -10.72451020669870658, -18.67979575497194134, 64.58442372801900433 ) ) ;
#173245=CARTESIAN_POINT ( 'NONE',  ( -5.049401038298153566, 19.05341960407611168, 45.20724293864769550 ) ) ;
#173246=CARTESIAN_POINT ( 'NONE',  ( -15.80617190586768217, 15.72974639402176855, 73.12609039468567573 ) ) ;
#173247=CARTESIAN_POINT ( 'NONE',  ( 21.52544592524344225, -5.823673210054117533, 23.54057627198102765 ) ) ;
#173248=CARTESIAN_POINT ( 'NONE',  ( -16.46253265017160317, 9.564922557960807481, 40.83224293864769550 ) ) ;
#173249=CARTESIAN_POINT ( 'NONE',  ( 15.72974639402176855, 15.80617190586768217, 21.87609039468567573 ) ) ;
#173250=CARTESIAN_POINT ( 'NONE',  ( -13.97604488694547697, 13.89961937509957934, 48.12609039468566863 ) ) ;
#173251=CARTESIAN_POINT ( 'NONE',  ( -0.05219959533910754901, -16.53943276465976808, 112.4989096053143669 ) ) ;
#173252=CARTESIAN_POINT ( 'NONE',  ( -13.97604488694527625, -13.89961937509977652, 56.87390960531434558 ) ) ;
#173253=CARTESIAN_POINT ( 'NONE',  ( 13.97604488694548053, -13.89961937509957401, 110.6260903946856615 ) ) ;
#173254=CARTESIAN_POINT ( 'NONE',  ( -12.14591786802309592, -12.06949235617757132, 81.87390960531435269 ) ) ;
#173255=CARTESIAN_POINT ( 'NONE',  ( -10.81492255796078084, -18.62759615963271287, 27.08224293864769550 ) ) ;
#173256=CARTESIAN_POINT ( 'NONE',  ( -19.03943276465977164, -0.05219959533935918106, 103.7510903946856757 ) ) ;
#173257=CARTESIAN_POINT ( 'NONE',  ( 18.62759615963271287, -10.81492255796078972, 108.3322429386477097 ) ) ;
#173258=CARTESIAN_POINT ( 'NONE',  ( 21.53943276465977519, 0.05219959533937863772, 56.25109039468568284 ) ) ;
#173259=CARTESIAN_POINT ( 'NONE',  ( -8.314922557961024197, 14.29746914071037800, 62.91775706135236135 ) ) ;
#173260=CARTESIAN_POINT ( 'NONE',  ( -14.29746914071037622, -8.314922557961029526, 54.16775706135235424 ) ) ;
#173261=CARTESIAN_POINT ( 'NONE',  ( 21.52544592524344225, -5.823673210054117533, 53.54057627198103120 ) ) ;
#173262=CARTESIAN_POINT ( 'NONE',  ( -0.05219959533909027116, -19.03943276465977164, 52.49890960531436690 ) ) ;
#173263=CARTESIAN_POINT ( 'NONE',  ( -16.53943276465976808, -0.05219959533934237506, 73.75109039468567573 ) ) ;
#173265=CARTESIAN_POINT ( 'NONE',  ( 21.55341960407610458, 5.719274019375980345, 103.9572429386476813 ) ) ;
#173266=CARTESIAN_POINT ( 'NONE',  ( -14.29746914071049879, 8.314922557960819915, 55.83224293864770260 ) ) ;
#173267=CARTESIAN_POINT ( 'NONE',  ( -9.564922557960796823, -16.46253265017161027, 67.08224293864769550 ) ) ;
#173268=CARTESIAN_POINT ( 'NONE',  ( 16.55341960407618274, -4.379528057220086978, 76.04275706135237556 ) ) ;
#173269=CARTESIAN_POINT ( 'NONE',  ( -8.314922557961024197, 14.29746914071037800, 22.91775706135235069 ) ) ;
#173270=CARTESIAN_POINT ( 'NONE',  ( 18.62759615963271287, -10.81492255796078972, 98.33224293864769550 ) ) ;
#173271=CARTESIAN_POINT ( 'NONE',  ( -14.34966873604960291, -8.224510206698953496, 46.66557627198102409 ) ) ;
#173273=CARTESIAN_POINT ( 'NONE',  ( -16.52216118717207749, 7.221426719304494313, 73.92400978953011759 ) ) ;
#173274=CARTESIAN_POINT ( 'NONE',  ( 0.05219959533907565091, 21.53943276465977519, 89.99890960531438111 ) ) ;
#173276=CARTESIAN_POINT ( 'NONE',  ( -0.05219959533910754901, -16.53943276465976808, 27.49890960531435269 ) ) ;
#173278=CARTESIAN_POINT ( 'NONE',  ( -16.88567814943164436, -6.947325034625596807, 56.29001122652586986 ) ) ;
#173279=CARTESIAN_POINT ( 'NONE',  ( 18.67979575497178502, 10.72451020669898547, 104.1655762719810241 ) ) ;
#173280=CARTESIAN_POINT ( 'NONE',  ( -13.89961937509977652, 13.97604488694528158, 95.62390960531436690 ) ) ;
#173281=CARTESIAN_POINT ( 'NONE',  ( -15.80617190586768217, 15.72974639402176855, 28.12609039468568284 ) ) ;
#173282=CARTESIAN_POINT ( 'NONE',  ( -16.52544592524342804, 4.483927247898546575, 36.04057627198102409 ) ) ;
#173283=CARTESIAN_POINT ( 'NONE',  ( -16.55341960407617563, 4.379528057220093196, 43.54275706135235424 ) ) ;
#173284=CARTESIAN_POINT ( 'NONE',  ( 16.46253265017160672, -9.564922557960803928, 48.33224293864769550 ) ) ;
#173285=CARTESIAN_POINT ( 'NONE',  ( 0.05219959533936267826, -19.03943276465977164, 55.00109039468566863 ) ) ;
#173286=CARTESIAN_POINT ( 'NONE',  ( -13.97604488694527625, -13.89961937509977652, 86.87390960531436690 ) ) ;
#173287=ORIENTED_EDGE ( 'NONE', *, *, #34324, .F. ) ;
#173289=CARTESIAN_POINT ( 'NONE',  ( -5.823673210054116645, -21.52544592524344225, 37.29057627198102409 ) ) ;
#173291=CARTESIAN_POINT ( 'NONE',  ( -16.55341960407617563, 4.379528057220093196, 28.54275706135234358 ) ) ;
#173292=CARTESIAN_POINT ( 'NONE',  ( -0.05219959533936034679, 19.03943276465977164, 52.50109039468566863 ) ) ;
#173293=CARTESIAN_POINT ( 'NONE',  ( -10.72451020669898014, 18.67979575497178502, 105.4155762719810383 ) ) ;
#173294=CARTESIAN_POINT ( 'NONE',  ( -4.379528057220328563, 16.55341960407611168, 30.20724293864769550 ) ) ;
#173295=CARTESIAN_POINT ( 'NONE',  ( 19.02544592524343514, -5.153800228976328945, 73.54057627198103830 ) ) ;
#173296=CARTESIAN_POINT ( 'NONE',  ( 0.05219959533907565091, 21.53943276465977519, 54.99890960531435269 ) ) ;
#173297=CARTESIAN_POINT ( 'NONE',  ( 10.81492255796078972, 18.62759615963270932, 89.58224293864768129 ) ) ;
#173298=CARTESIAN_POINT ( 'NONE',  ( -16.55341960407617563, 4.379528057220093196, 23.54275706135235424 ) ) ;
#173299=CARTESIAN_POINT ( 'NONE',  ( -0.05219959533907301413, -21.53943276465977519, 27.49890960531435269 ) ) ;
#173300=CARTESIAN_POINT ( 'NONE',  ( 10.81492255796106328, -18.62759615963255655, 85.41775706135236135 ) ) ;
#173301=CARTESIAN_POINT ( 'NONE',  ( -5.049401038298153566, 19.05341960407611168, 75.20724293864769550 ) ) ;
#173302=CARTESIAN_POINT ( 'NONE',  ( -19.03943276465977164, 0.05219959533909376836, 26.24890960531435624 ) ) ;
#173303=CARTESIAN_POINT ( 'NONE',  ( -5.049401038298153566, 19.05341960407611168, 85.20724293864766707 ) ) ;
#173304=CARTESIAN_POINT ( 'NONE',  ( 0.05219959533910956823, 16.53943276465976808, 109.9989096053143527 ) ) ;
#173305=CARTESIAN_POINT ( 'NONE',  ( -9.564922557960796823, -16.46253265017161027, 62.08224293864769550 ) ) ;
#173306=CARTESIAN_POINT ( 'NONE',  ( 19.05341960407617918, -5.049401038297876454, 101.0427570613523045 ) ) ;
#173308=CARTESIAN_POINT ( 'NONE',  ( 13.89961937509977652, -13.97604488694527269, 73.12390960531436690 ) ) ;
#173309=CARTESIAN_POINT ( 'NONE',  ( -10.72451020669870658, -18.67979575497194134, 99.58442372801900433 ) ) ;
#173310=CARTESIAN_POINT ( 'NONE',  ( -5.049401038298153566, 19.05341960407611168, 115.2072429386477097 ) ) ;
#173311=CARTESIAN_POINT ( 'NONE',  ( -8.314922557961024197, 14.29746914071037800, 92.91775706135236135 ) ) ;
#173312=CARTESIAN_POINT ( 'NONE',  ( -17.31728774477273447, -6.344390552232371583, 74.18093348310682700 ) ) ;
#173313=CARTESIAN_POINT ( 'NONE',  ( 5.049401038297881783, 19.05341960407617563, 62.29275706135234003 ) ) ;
#173314=CARTESIAN_POINT ( 'NONE',  ( -13.97604488694547697, 13.89961937509957934, 23.12609039468565442 ) ) ;
#173315=CARTESIAN_POINT ( 'NONE',  ( -16.36317988757056696, -7.306389748694947173, 45.90210391636773579 ) ) ;
#173316=CARTESIAN_POINT ( 'NONE',  ( 19.05341960407611168, 5.049401038298154454, 33.95724293864769550 ) ) ;
#173317=CARTESIAN_POINT ( 'NONE',  ( -0.05219959533910754901, -16.53943276465976808, 22.49890960531436335 ) ) ;
#173319=CARTESIAN_POINT ( 'NONE',  ( -16.52544592524335698, -4.483927247898792601, 108.9594237280190185 ) ) ;
#173321=CARTESIAN_POINT ( 'NONE',  ( 4.483927247898790824, -16.52544592524335698, 75.20942372801901854 ) ) ;
#173322=CARTESIAN_POINT ( 'NONE',  ( -13.97604488694527625, -13.89961937509977652, 36.87390960531436690 ) ) ;
#173323=CARTESIAN_POINT ( 'NONE',  ( -10.72451020669870658, -18.67979575497194134, 89.58442372801901854 ) ) ;
#173324=CARTESIAN_POINT ( 'NONE',  ( 19.03943276465977164, 0.05219959533936151252, 101.2510903946856757 ) ) ;
#173325=CARTESIAN_POINT ( 'NONE',  ( -0.05219959533937732626, 21.53943276465977519, 67.50109039468568994 ) ) ;
#173326=CARTESIAN_POINT ( 'NONE',  ( 19.02544592524334988, 5.153800228976608722, 51.45942372801900433 ) ) ;
#173327=CARTESIAN_POINT ( 'NONE',  ( -0.05219959533909027116, -19.03943276465977164, 72.49890960531435269 ) ) ;
#173328=CARTESIAN_POINT ( 'NONE',  ( -19.05341960407611168, -5.049401038298163336, 71.45724293864766707 ) ) ;
#173329=CARTESIAN_POINT ( 'NONE',  ( 16.19135201231366139, 7.376712067591956412, 72.68680854052027485 ) ) ;
#173331=CARTESIAN_POINT ( 'NONE',  ( -8.314922557960811034, -14.29746914071050412, 52.08224293864768839 ) ) ;
#173332=CARTESIAN_POINT ( 'NONE',  ( -21.53943276465977519, 0.05219959533907696930, 46.24890960531435979 ) ) ;
#173333=CARTESIAN_POINT ( 'NONE',  ( 16.46253265017160672, -9.564922557960803928, 43.33224293864769550 ) ) ;
#173334=CARTESIAN_POINT ( 'NONE',  ( -21.55341960407610458, -5.719274019375992779, 81.45724293864769550 ) ) ;
#173335=CARTESIAN_POINT ( 'NONE',  ( -16.52544592524335698, -4.483927247898792601, 83.95942372801900433 ) ) ;
#173338=CARTESIAN_POINT ( 'NONE',  ( 4.483927247898545687, 16.52544592524342804, 84.79057627198102409 ) ) ;
#173340=CARTESIAN_POINT ( 'NONE',  ( -0.05219959533934338120, 16.53943276465976808, 32.50109039468568284 ) ) ;
#173341=CARTESIAN_POINT ( 'NONE',  ( -19.03943276465977164, 0.05219959533909376836, 26.24890960531435624 ) ) ;
#173342=CARTESIAN_POINT ( 'NONE',  ( 16.51473224551083163, -9.474510206698727899, 70.83442372801900433 ) ) ;
#173344=CARTESIAN_POINT ( 'NONE',  ( -14.34966873604960291, -8.224510206698953496, 76.66557627198103830 ) ) ;
#173345=CARTESIAN_POINT ( 'NONE',  ( 5.719274019375673035, 21.55341960407619339, 47.29275706135234003 ) ) ;
#173346=CARTESIAN_POINT ( 'NONE',  ( 9.564922557960805705, 16.46253265017160317, 24.58224293864769194 ) ) ;
#173347=CARTESIAN_POINT ( 'NONE',  ( 10.81492255796078972, 18.62759615963270932, 89.58224293864768129 ) ) ;
#173348=CARTESIAN_POINT ( 'NONE',  ( -0.05219959533909027116, -19.03943276465977164, 112.4989096053143669 ) ) ;
#173349=CARTESIAN_POINT ( 'NONE',  ( 4.483927247898545687, 16.52544592524342804, 89.79057627198103830 ) ) ;
#173351=CARTESIAN_POINT ( 'NONE',  ( -5.153800228976328057, -19.02544592524343514, 42.29057627198101699 ) ) ;
#173353=CARTESIAN_POINT ( 'NONE',  ( -13.97604488694547697, 13.89961937509957934, 78.12609039468567573 ) ) ;
#173354=CARTESIAN_POINT ( 'NONE',  ( -5.823673210054431948, 21.52544592524334988, 22.70942372801901499 ) ) ;
#173355=CARTESIAN_POINT ( 'NONE',  ( 16.51473224551069308, 9.474510206698969483, 74.16557627198103830 ) ) ;
#173356=B_SPLINE_CURVE_WITH_KNOTS ( 'NONE', 3,
 ( #96851, #98838, #115025, #146348, #176718, #7835 ),
 .UNSPECIFIED., .F., .F.,
 ( 4, 2, 4 ),
 ( 0.003989672132298079273, 0.004372778065220507722, 0.004755883998142936171 ),
 .UNSPECIFIED. ) ;
#173357=CARTESIAN_POINT ( 'NONE',  ( -19.05341960407617563, 5.049401038297882671, 53.54275706135231871 ) ) ;
#173358=CARTESIAN_POINT ( 'NONE',  ( 5.153800228976335163, 19.02544592524342804, 44.79057627198103830 ) ) ;
#173359=CARTESIAN_POINT ( 'NONE',  ( 4.483927247898545687, 16.52544592524342804, 59.79057627198103120 ) ) ;
#173360=CARTESIAN_POINT ( 'NONE',  ( -8.314922557960811034, -14.29746914071050412, 57.08224293864769550 ) ) ;
#173361=CARTESIAN_POINT ( 'NONE',  ( -13.97604488694527625, -13.89961937509977652, 81.87390960531436690 ) ) ;
#173362=CARTESIAN_POINT ( 'NONE',  ( 18.67979575497178502, 10.72451020669898547, 104.1655762719810241 ) ) ;
#173363=CARTESIAN_POINT ( 'NONE',  ( 16.46253265017160672, -9.564922557960803928, 73.33224293864769550 ) ) ;
#173364=CARTESIAN_POINT ( 'NONE',  ( -21.52544592524343514, 5.823673210054127303, 81.04057627198102409 ) ) ;
#173365=CARTESIAN_POINT ( 'NONE',  ( -10.72451020669870658, -18.67979575497194134, 109.5844237280190328 ) ) ;
#173366=CARTESIAN_POINT ( 'NONE',  ( 19.02544592524343514, -5.153800228976328945, 38.54057627198103120 ) ) ;
#173367=CARTESIAN_POINT ( 'NONE',  ( 14.29746914071049879, -8.314922557960816363, 23.33224293864769194 ) ) ;
#173368=CARTESIAN_POINT ( 'NONE',  ( -14.34966873604960291, -8.224510206698953496, 101.6655762719810383 ) ) ;
#173369=CARTESIAN_POINT ( 'NONE',  ( 9.474510206698729675, 16.51473224551082808, 112.0844237280190043 ) ) ;
#173371=CARTESIAN_POINT ( 'NONE',  ( 5.719274019375673035, 21.55341960407619339, 37.29275706135235424 ) ) ;
#173372=CARTESIAN_POINT ( 'NONE',  ( -16.51473224551082808, 9.474510206698731452, 53.33442372801900433 ) ) ;
#173373=CARTESIAN_POINT ( 'NONE',  ( -16.55341960407617563, 4.379528057220093196, 108.5427570613523756 ) ) ;
#173374=CARTESIAN_POINT ( 'NONE',  ( 18.67979575497178502, 10.72451020669898547, 74.16557627198102409 ) ) ;
#173375=CARTESIAN_POINT ( 'NONE',  ( 0.05219959533909260263, 19.03943276465977164, 104.9989096053143669 ) ) ;
#173376=CARTESIAN_POINT ( 'NONE',  ( 0.05219959533910956823, 16.53943276465976808, 54.99890960531435269 ) ) ;
#173377=CARTESIAN_POINT ( 'NONE',  ( 13.89961937509977652, -13.97604488694527269, 28.12390960531435624 ) ) ;
#173378=CARTESIAN_POINT ( 'NONE',  ( -16.46253265017160317, 9.564922557960807481, 35.83224293864768839 ) ) ;
#173379=CARTESIAN_POINT ( 'NONE',  ( 18.67979575497194134, -10.72451020669871369, 105.8344237280190328 ) ) ;
#173380=CARTESIAN_POINT ( 'NONE',  ( -8.314922557961024197, 14.29746914071037800, 87.91775706135234714 ) ) ;
#173381=CARTESIAN_POINT ( 'NONE',  ( -0.05219959533937732626, 21.53943276465977519, 47.50109039468568994 ) ) ;
#173382=CARTESIAN_POINT ( 'NONE',  ( 4.379528057220092307, 16.55341960407617563, 47.29275706135234003 ) ) ;
#173383=CARTESIAN_POINT ( 'NONE',  ( -10.81492255796078084, -18.62759615963271287, 27.08224293864769550 ) ) ;
#173384=CARTESIAN_POINT ( 'NONE',  ( 13.97604488694527802, 13.89961937509977652, 59.37390960531434558 ) ) ;
#173385=CARTESIAN_POINT ( 'NONE',  ( -9.474510206698964154, 16.51473224551069663, 60.41557627198102409 ) ) ;
#173386=CARTESIAN_POINT ( 'NONE',  ( -4.483927247898782831, 16.52544592524335698, 62.70942372801902565 ) ) ;
#173387=CARTESIAN_POINT ( 'NONE',  ( -8.224510206698948167, 14.34966873604960824, 100.4155762719810241 ) ) ;
#173388=CARTESIAN_POINT ( 'NONE',  ( 4.379528057220339221, -16.55341960407611168, 27.70724293864769905 ) ) ;
#173390=CARTESIAN_POINT ( 'NONE',  ( 15.80617190586769283, -15.72974639402175789, 60.62609039468567573 ) ) ;
#173391=CARTESIAN_POINT ( 'NONE',  ( -13.89961937509977652, 13.97604488694528158, 90.62390960531432427 ) ) ;
#173392=CARTESIAN_POINT ( 'NONE',  ( 5.049401038298161559, -19.05341960407611168, 82.70724293864770971 ) ) ;
#173393=CARTESIAN_POINT ( 'NONE',  ( 9.474510206698971260, -16.51473224551069308, 107.9155762719810383 ) ) ;
#173394=CARTESIAN_POINT ( 'NONE',  ( 16.53943276465976808, -0.05219959533910856209, 48.74890960531435979 ) ) ;
#173395=CARTESIAN_POINT ( 'NONE',  ( -16.55341960407617563, 4.379528057220093196, 108.5427570613523756 ) ) ;
#173396=CARTESIAN_POINT ( 'NONE',  ( 16.52544592524342804, -4.483927247898539470, 38.54057627198103120 ) ) ;
#173398=CARTESIAN_POINT ( 'NONE',  ( -16.46253265017146816, -9.564922557961047289, 34.16775706135233293 ) ) ;
#173399=CARTESIAN_POINT ( 'NONE',  ( -19.02544592524342804, 5.153800228976336051, 76.04057627198102409 ) ) ;
#173400=CARTESIAN_POINT ( 'NONE',  ( 13.89961937509957401, 13.97604488694547697, 51.87609039468566863 ) ) ;
#173403=CARTESIAN_POINT ( 'NONE',  ( 19.05341960407617918, -5.049401038297876454, 86.04275706135233293 ) ) ;
#173404=CARTESIAN_POINT ( 'NONE',  ( 0.05219959533934541429, -16.53943276465976808, 75.00109039468568994 ) ) ;
#173405=CARTESIAN_POINT ( 'NONE',  ( 17.50000000000000000, 5.499999999999992895, 91.70309617465828467 ) ) ;
#173406=CARTESIAN_POINT ( 'NONE',  ( -19.05341960407611168, -5.049401038298163336, 101.4572429386476955 ) ) ;
#173407=CARTESIAN_POINT ( 'NONE',  ( 5.719274019375673035, 21.55341960407619339, 22.29275706135235069 ) ) ;
#173408=CARTESIAN_POINT ( 'NONE',  ( 16.46253265017146816, 9.564922557961045513, 96.66775706135233293 ) ) ;
#173409=CARTESIAN_POINT ( 'NONE',  ( -19.02544592524342804, 5.153800228976336051, 116.0405762719810383 ) ) ;
#173410=CARTESIAN_POINT ( 'NONE',  ( 9.564922557960805705, 16.46253265017160317, 49.58224293864770260 ) ) ;
#173411=CARTESIAN_POINT ( 'NONE',  ( -19.02544592524342804, 5.153800228976336051, 91.04057627198100988 ) ) ;
#173412=CARTESIAN_POINT ( 'NONE',  ( 14.29746914071049879, -8.314922557960816363, 58.33224293864768839 ) ) ;
#173413=CARTESIAN_POINT ( 'NONE',  ( 19.02544592524343514, -5.153800228976328945, 53.54057627198102409 ) ) ;
#173414=CARTESIAN_POINT ( 'NONE',  ( -19.03943276465977164, 0.05219959533909376836, 61.24890960531436690 ) ) ;
#173415=CARTESIAN_POINT ( 'NONE',  ( -19.02544592524334988, -5.153800228976617603, 68.95942372801896170 ) ) ;
#173416=ORIENTED_EDGE ( 'NONE', *, *, #53677, .F. ) ;
#173417=CARTESIAN_POINT ( 'NONE',  ( 5.049401038297881783, 19.05341960407617563, 27.29275706135232937 ) ) ;
#173418=CARTESIAN_POINT ( 'NONE',  ( 5.049401038298161559, -19.05341960407611168, 67.70724293864769550 ) ) ;
#173419=CARTESIAN_POINT ( 'NONE',  ( -10.81492255796078084, -18.62759615963271287, 62.08224293864769550 ) ) ;
#173420=CARTESIAN_POINT ( 'NONE',  ( 16.53943276465976808, -0.05219959533910856209, 63.74890960531435979 ) ) ;
#173421=CARTESIAN_POINT ( 'NONE',  ( -19.03943276465977164, -0.05219959533935918106, 33.75109039468566863 ) ) ;
#173422=CARTESIAN_POINT ( 'NONE',  ( 5.153800228976335163, 19.02544592524342804, 114.7905762719810241 ) ) ;
#173423=CARTESIAN_POINT ( 'NONE',  ( -21.53943276465977519, 0.05219959533907696930, 46.24890960531435979 ) ) ;
#173424=CARTESIAN_POINT ( 'NONE',  ( -5.719274019375978568, 21.55341960407610458, 25.20724293864769550 ) ) ;
#173425=CARTESIAN_POINT ( 'NONE',  ( -13.97604488694527625, -13.89961937509977652, 51.87390960531436690 ) ) ;
#173426=CARTESIAN_POINT ( 'NONE',  ( 16.46253265017160672, -9.564922557960803928, 43.33224293864769550 ) ) ;
#173427=CARTESIAN_POINT ( 'NONE',  ( -4.379528057220328563, 16.55341960407611168, 100.2072429386476955 ) ) ;
#173428=CARTESIAN_POINT ( 'NONE',  ( -21.52544592524343514, 5.823673210054127303, 116.0405762719810383 ) ) ;
#173430=CARTESIAN_POINT ( 'NONE',  ( 10.81492255796106328, -18.62759615963255655, 30.41775706135234358 ) ) ;
#173431=CARTESIAN_POINT ( 'NONE',  ( 16.52544592524342804, -4.483927247898539470, 113.5405762719810383 ) ) ;
#173432=CARTESIAN_POINT ( 'NONE',  ( 15.80617190586769283, -15.72974639402175789, 75.62609039468567573 ) ) ;
#173433=CARTESIAN_POINT ( 'NONE',  ( -5.719274019375978568, 21.55341960407610458, 95.20724293864769550 ) ) ;
#173434=CARTESIAN_POINT ( 'NONE',  ( 5.153800228976615827, -19.02544592524334988, 35.20942372801899722 ) ) ;
#173435=CARTESIAN_POINT ( 'NONE',  ( 5.153800228976335163, 19.02544592524342804, 29.79057627198102409 ) ) ;
#173438=CARTESIAN_POINT ( 'NONE',  ( -0.05219959533934338120, 16.53943276465976808, 47.50109039468568994 ) ) ;
#173439=CARTESIAN_POINT ( 'NONE',  ( 12.14591786802309770, 12.06949235617756955, 104.3739096053143669 ) ) ;
#173441=CARTESIAN_POINT ( 'NONE',  ( -19.03943276465977164, 0.05219959533909376836, 66.24890960531436690 ) ) ;
#173442=CARTESIAN_POINT ( 'NONE',  ( -16.55341960407611168, -4.379528057220339221, 91.45724293864769550 ) ) ;
#173443=ADVANCED_FACE ( 'NONE', ( #56272 ), #166463, .F. ) ;
#173444=CARTESIAN_POINT ( 'NONE',  ( -21.52544592524343514, 5.823673210054127303, 46.04057627198103830 ) ) ;
#173445=CARTESIAN_POINT ( 'NONE',  ( 4.483927247898545687, 16.52544592524342804, 64.79057627198103830 ) ) ;
#173446=CARTESIAN_POINT ( 'NONE',  ( 16.52544592524335698, 4.483927247898782831, 31.45942372801901854 ) ) ;
#173447=CARTESIAN_POINT ( 'NONE',  ( -21.52544592524334988, -5.823673210054445271, 88.95942372801901854 ) ) ;
#173449=CARTESIAN_POINT ( 'NONE',  ( 4.379528057220092307, 16.55341960407617563, 97.29275706135234714 ) ) ;
#173450=CARTESIAN_POINT ( 'NONE',  ( 14.29746914071049879, -8.314922557960816363, 43.33224293864769550 ) ) ;
#173451=CARTESIAN_POINT ( 'NONE',  ( -5.153800228976328057, -19.02544592524343514, 42.29057627198101699 ) ) ;
#173452=CARTESIAN_POINT ( 'NONE',  ( 21.52544592524334988, 5.823673210054432836, 96.45942372801901854 ) ) ;
#173453=CARTESIAN_POINT ( 'NONE',  ( 0.05219959533907565091, 21.53943276465977519, 109.9989096053143527 ) ) ;
#173454=CARTESIAN_POINT ( 'NONE',  ( 18.67979575497194134, -10.72451020669871369, 60.83442372801901854 ) ) ;
#173455=CARTESIAN_POINT ( 'NONE',  ( -8.224510206698735004, -14.34966873604973081, 39.58442372801901143 ) ) ;
#173456=CARTESIAN_POINT ( 'NONE',  ( 12.14591786802309770, 12.06949235617756955, 64.37390960531435269 ) ) ;
#173457=CARTESIAN_POINT ( 'NONE',  ( -21.55341960407619339, 5.719274019375674811, 83.54275706135234714 ) ) ;
#173458=CARTESIAN_POINT ( 'NONE',  ( 4.379528057220339221, -16.55341960407611168, 22.70724293864769194 ) ) ;
#173460=CARTESIAN_POINT ( 'NONE',  ( 4.483927247898545687, 16.52544592524342804, 29.79057627198102409 ) ) ;
#173461=CARTESIAN_POINT ( 'NONE',  ( -16.52544592524335698, -4.483927247898792601, 73.95942372801901854 ) ) ;
#173462=CARTESIAN_POINT ( 'NONE',  ( 0.05219959533909260263, 19.03943276465977164, 79.99890960531436690 ) ) ;
#173463=CARTESIAN_POINT ( 'NONE',  ( 9.564922557960805705, 16.46253265017160317, 104.5822429386476955 ) ) ;
#173464=CARTESIAN_POINT ( 'NONE',  ( 15.80617190586769283, -15.72974639402175789, 80.62609039468567573 ) ) ;
#173465=CARTESIAN_POINT ( 'NONE',  ( -12.14591786802326823, 12.06949235617739902, 83.12609039468568994 ) ) ;
#173466=CARTESIAN_POINT ( 'NONE',  ( 8.224510206698953496, -14.34966873604960469, 72.91557627198103830 ) ) ;
#173467=CARTESIAN_POINT ( 'NONE',  ( -5.049401038298153566, 19.05341960407611168, 65.20724293864765286 ) ) ;
#173469=CARTESIAN_POINT ( 'NONE',  ( 14.34966873604972726, -8.224510206698740333, 30.83442372801902209 ) ) ;
#173470=CARTESIAN_POINT ( 'NONE',  ( -13.97604488694527625, -13.89961937509977652, 21.87390960531435979 ) ) ;
#173471=CARTESIAN_POINT ( 'NONE',  ( -5.153800228976328057, -19.02544592524343514, 92.29057627198099567 ) ) ;
#173472=CARTESIAN_POINT ( 'NONE',  ( -16.55341960407617563, 4.379528057220093196, 23.54275706135235424 ) ) ;
#173474=CARTESIAN_POINT ( 'NONE',  ( -13.97604488694547697, 13.89961937509957934, 28.12609039468565797 ) ) ;
#173475=CARTESIAN_POINT ( 'NONE',  ( 0.05219959533934541429, -16.53943276465976808, 100.0010903946857042 ) ) ;
#173476=CARTESIAN_POINT ( 'NONE',  ( -19.02544592524334988, -5.153800228976617603, 103.9594237280190043 ) ) ;
#173477=CARTESIAN_POINT ( 'NONE',  ( -12.06949235617756955, 12.14591786802309770, 115.6239096053143669 ) ) ;
#173478=CARTESIAN_POINT ( 'NONE',  ( 4.379528057220092307, 16.55341960407617563, 67.29275706135234714 ) ) ;
#173479=CARTESIAN_POINT ( 'NONE',  ( -16.53943276465976808, -0.05219959533934237506, 53.75109039468568994 ) ) ;
#173481=CARTESIAN_POINT ( 'NONE',  ( 9.564922557961047289, -16.46253265017146816, 65.41775706135233293 ) ) ;
#173482=CARTESIAN_POINT ( 'NONE',  ( 21.53943276465977519, 0.05219959533937863772, 111.2510903946856899 ) ) ;
#173483=CARTESIAN_POINT ( 'NONE',  ( -19.05341960407611168, -5.049401038298163336, 46.45724293864768129 ) ) ;
#173484=CARTESIAN_POINT ( 'NONE',  ( 5.153800228976335163, 19.02544592524342804, 84.79057627198099567 ) ) ;
#173485=CARTESIAN_POINT ( 'NONE',  ( -12.14591786802309592, -12.06949235617757132, 66.87390960531436690 ) ) ;
#173486=VECTOR ( 'NONE', #131539, 1000.000000000000000 ) ;
#173487=CARTESIAN_POINT ( 'NONE',  ( -5.049401038297874678, -19.05341960407617918, 54.79275706135234003 ) ) ;
#173488=CARTESIAN_POINT ( 'NONE',  ( -18.62759615963270932, 10.81492255796079327, 45.83224293864769550 ) ) ;
#173489=CARTESIAN_POINT ( 'NONE',  ( -18.67979575497193778, 10.72451020669871902, 103.3344237280190043 ) ) ;
#173490=CARTESIAN_POINT ( 'NONE',  ( -0.05219959533909027116, -19.03943276465977164, 97.49890960531436690 ) ) ;
#173491=CARTESIAN_POINT ( 'NONE',  ( -21.55341960407619339, 5.719274019375674811, 108.5427570613523756 ) ) ;
#173492=CARTESIAN_POINT ( 'NONE',  ( 5.719274019375991003, -21.55341960407610458, 62.70724293864769550 ) ) ;
#173493=CARTESIAN_POINT ( 'NONE',  ( 13.97604488694527802, 13.89961937509977652, 94.37390960531436690 ) ) ;
#173494=CARTESIAN_POINT ( 'NONE',  ( -5.049401038297874678, -19.05341960407617918, 94.79275706135230450 ) ) ;
#173495=CARTESIAN_POINT ( 'NONE',  ( 19.05341960407611168, 5.049401038298154454, 108.9572429386477097 ) ) ;
#173496=CARTESIAN_POINT ( 'NONE',  ( -5.153800228976607833, 19.02544592524334988, 112.7094237280190043 ) ) ;
#173497=CARTESIAN_POINT ( 'NONE',  ( 16.55341960407611168, 4.379528057220329451, 108.9572429386476955 ) ) ;
#173498=CARTESIAN_POINT ( 'NONE',  ( 5.153800228976335163, 19.02544592524342804, 89.79057627198102409 ) ) ;
#173499=CARTESIAN_POINT ( 'NONE',  ( -10.72451020669898014, 18.67979575497178502, 65.41557627198102409 ) ) ;
#173500=CARTESIAN_POINT ( 'NONE',  ( 16.52544592524335698, 4.483927247898782831, 51.45942372801901854 ) ) ;
#173501=CARTESIAN_POINT ( 'NONE',  ( 21.52544592524334988, 5.823673210054432836, 41.45942372801901143 ) ) ;
#173502=CARTESIAN_POINT ( 'NONE',  ( 18.67979575497194134, -10.72451020669871369, 100.8344237280190185 ) ) ;
#173503=CARTESIAN_POINT ( 'NONE',  ( 16.53943276465976808, 0.05219959533934440121, 101.2510903946856757 ) ) ;
#173504=CARTESIAN_POINT ( 'NONE',  ( -9.564922557960796823, -16.46253265017161027, 87.08224293864769550 ) ) ;
#173505=CARTESIAN_POINT ( 'NONE',  ( -16.53943276465976808, 0.05219959533911058130, 86.24890960531436690 ) ) ;
#173506=CARTESIAN_POINT ( 'NONE',  ( 0.05219959533910956823, 16.53943276465976808, 24.99890960531435624 ) ) ;
#173507=CARTESIAN_POINT ( 'NONE',  ( -5.153800228976607833, 19.02544592524334988, 67.70942372801900433 ) ) ;
#173508=CARTESIAN_POINT ( 'NONE',  ( 15.80617190586769283, -15.72974639402175789, 40.62609039468567573 ) ) ;
#173509=CARTESIAN_POINT ( 'NONE',  ( -16.53943276465976808, 0.05219959533911058130, 86.24890960531436690 ) ) ;
#173510=CARTESIAN_POINT ( 'NONE',  ( -0.05219959533909027116, -19.03943276465977164, 107.4989096053143527 ) ) ;
#173511=CARTESIAN_POINT ( 'NONE',  ( -8.314922557960811034, -14.29746914071050412, 22.08224293864769194 ) ) ;
#173512=CARTESIAN_POINT ( 'NONE',  ( -15.80617190586768217, 15.72974639402176855, 88.12609039468570415 ) ) ;
#173513=CARTESIAN_POINT ( 'NONE',  ( 8.224510206698742110, 14.34966873604972548, 52.08442372801901854 ) ) ;
#173514=CARTESIAN_POINT ( 'NONE',  ( 10.81492255796106328, -18.62759615963255655, 45.41775706135234003 ) ) ;
#173516=CARTESIAN_POINT ( 'NONE',  ( -10.72451020669870658, -18.67979575497194134, 29.58442372801901854 ) ) ;
#173517=CARTESIAN_POINT ( 'NONE',  ( -4.483927247898539470, -16.52544592524342804, 107.2905762719810525 ) ) ;
#173519=CARTESIAN_POINT ( 'NONE',  ( -19.05341960407611168, -5.049401038298163336, 31.45724293864769550 ) ) ;
#173520=CARTESIAN_POINT ( 'NONE',  ( -12.06949235617756955, 12.14591786802309770, 65.62390960531436690 ) ) ;
#173521=CARTESIAN_POINT ( 'NONE',  ( 13.97604488694527802, 13.89961937509977652, 59.37390960531434558 ) ) ;
#173522=CARTESIAN_POINT ( 'NONE',  ( -16.53943276465976808, -0.05219959533934237506, 108.7510903946857042 ) ) ;
#173523=CARTESIAN_POINT ( 'NONE',  ( 19.03943276465977164, -0.05219959533909143690, 43.74890960531435979 ) ) ;
#173524=CARTESIAN_POINT ( 'NONE',  ( 18.62759615963271287, -10.81492255796078972, 38.33224293864768839 ) ) ;
#173525=CARTESIAN_POINT ( 'NONE',  ( 14.29746914071049879, -8.314922557960816363, 73.33224293864769550 ) ) ;
#173527=CARTESIAN_POINT ( 'NONE',  ( 18.67979575497178502, 10.72451020669898547, 89.16557627198102409 ) ) ;
#173528=CARTESIAN_POINT ( 'NONE',  ( -5.153800228976328057, -19.02544592524343514, 92.29057627198099567 ) ) ;
#173529=CARTESIAN_POINT ( 'NONE',  ( -0.05219959533909027116, -19.03943276465977164, 52.49890960531436690 ) ) ;
#173530=CARTESIAN_POINT ( 'NONE',  ( 13.97604488694548053, -13.89961937509957401, 90.62609039468567573 ) ) ;
#173531=EDGE_CURVE ( 'NONE', #159561, #16134, #496, .T. ) ;
#173532=CARTESIAN_POINT ( 'NONE',  ( -21.53943276465977519, 0.05219959533907696930, 46.24890960531435979 ) ) ;
#173533=CARTESIAN_POINT ( 'NONE',  ( -0.05219959533937732626, 21.53943276465977519, 72.50109039468568994 ) ) ;
#173534=CARTESIAN_POINT ( 'NONE',  ( -5.153800228976328057, -19.02544592524343514, 57.29057627198103120 ) ) ;
#173535=CARTESIAN_POINT ( 'NONE',  ( 19.03943276465977164, -0.05219959533909143690, 78.74890960531436690 ) ) ;
#173537=CARTESIAN_POINT ( 'NONE',  ( -16.55341960407617563, 4.379528057220093196, 68.54275706135234714 ) ) ;
#173538=CARTESIAN_POINT ( 'NONE',  ( 10.72451020669871369, 18.67979575497193778, 42.08442372801901854 ) ) ;
#173539=CARTESIAN_POINT ( 'NONE',  ( -21.52544592524334988, -5.823673210054445271, 78.95942372801901854 ) ) ;
#173540=CARTESIAN_POINT ( 'NONE',  ( -18.67979575497178146, -10.72451020669898902, 26.66557627198103475 ) ) ;
#173541=CARTESIAN_POINT ( 'NONE',  ( 21.55341960407610458, 5.719274019375980345, 93.95724293864770971 ) ) ;
#173542=CARTESIAN_POINT ( 'NONE',  ( 5.823673210054444382, -21.52544592524334988, 35.20942372801901854 ) ) ;
#173543=CARTESIAN_POINT ( 'NONE',  ( -12.06949235617739369, -12.14591786802326823, 64.37609039468568994 ) ) ;
#173544=CARTESIAN_POINT ( 'NONE',  ( 21.53943276465977519, -0.05219959533907433946, 58.74890960531436690 ) ) ;
#173545=CARTESIAN_POINT ( 'NONE',  ( -19.02544592524334988, -5.153800228976617603, 33.95942372801897591 ) ) ;
#173546=CARTESIAN_POINT ( 'NONE',  ( 19.02544592524343514, -5.153800228976328945, 68.54057627198103830 ) ) ;
#173547=CARTESIAN_POINT ( 'NONE',  ( 16.53943276465976808, 0.05219959533934440121, 96.25109039468568994 ) ) ;
#173549=CARTESIAN_POINT ( 'NONE',  ( 16.46253265017160672, -9.564922557960803928, 103.3322429386476955 ) ) ;
#173551=CARTESIAN_POINT ( 'NONE',  ( 13.89961937509957401, 13.97604488694547697, 81.87609039468564731 ) ) ;
#173552=CARTESIAN_POINT ( 'NONE',  ( 5.719274019375991003, -21.55341960407610458, 62.70724293864769550 ) ) ;
#173553=CARTESIAN_POINT ( 'NONE',  ( 4.379528057220339221, -16.55341960407611168, 37.70724293864769550 ) ) ;
#173554=CARTESIAN_POINT ( 'NONE',  ( -16.51473224551082808, 9.474510206698731452, 98.33442372801900433 ) ) ;
#173555=CARTESIAN_POINT ( 'NONE',  ( -9.564922557960796823, -16.46253265017161027, 27.08224293864769550 ) ) ;
#173556=CARTESIAN_POINT ( 'NONE',  ( 16.55341960407618274, -4.379528057220086978, 21.04275706135234714 ) ) ;
#173557=CARTESIAN_POINT ( 'NONE',  ( 21.53943276465977519, -0.05219959533907433946, 83.74890960531435269 ) ) ;
#173558=CARTESIAN_POINT ( 'NONE',  ( 9.474510206698729675, 16.51473224551082808, 62.08442372801899722 ) ) ;
#173559=CARTESIAN_POINT ( 'NONE',  ( -8.224510206698735004, -14.34966873604973081, 84.58442372801903275 ) ) ;
#173560=CARTESIAN_POINT ( 'NONE',  ( 5.153800228976335163, 19.02544592524342804, 64.79057627198100988 ) ) ;
#173561=CARTESIAN_POINT ( 'NONE',  ( -12.14591786802309592, -12.06949235617757132, 71.87390960531438111 ) ) ;
#173562=CARTESIAN_POINT ( 'NONE',  ( 13.97604488694527802, 13.89961937509977652, 54.37390960531435979 ) ) ;
#173563=CARTESIAN_POINT ( 'NONE',  ( -16.52544592524342804, 4.483927247898546575, 56.04057627198102409 ) ) ;
#173566=CARTESIAN_POINT ( 'NONE',  ( -4.483927247898539470, -16.52544592524342804, 22.29057627198102765 ) ) ;
#173567=CARTESIAN_POINT ( 'NONE',  ( -16.51473224551069308, -9.474510206698971260, 71.66557627198102409 ) ) ;
#173569=CARTESIAN_POINT ( 'NONE',  ( -9.564922557961040184, 16.46253265017147172, 42.91775706135234003 ) ) ;
#173570=CARTESIAN_POINT ( 'NONE',  ( 14.29746914071037800, 8.314922557961029526, 51.66775706135234714 ) ) ;
#173571=CARTESIAN_POINT ( 'NONE',  ( 21.52544592524344225, -5.823673210054117533, 48.54057627198103120 ) ) ;
#173572=CARTESIAN_POINT ( 'NONE',  ( 0.05219959533936267826, -19.03943276465977164, 25.00109039468566152 ) ) ;
#173573=CARTESIAN_POINT ( 'NONE',  ( -19.05341960407611168, -5.049401038298163336, 76.45724293864769550 ) ) ;
#173575=CARTESIAN_POINT ( 'NONE',  ( -9.564922557960796823, -16.46253265017161027, 107.0822429386476955 ) ) ;
#173576=CARTESIAN_POINT ( 'NONE',  ( -15.80617190586768217, 15.72974639402176855, 43.12609039468568284 ) ) ;
#173577=CARTESIAN_POINT ( 'NONE',  ( -8.314922557960811034, -14.29746914071050412, 107.0822429386476955 ) ) ;
#173578=CARTESIAN_POINT ( 'NONE',  ( -5.823673210054116645, -21.52544592524344225, 82.29057627198103830 ) ) ;
#173579=CARTESIAN_POINT ( 'NONE',  ( 5.153800228976335163, 19.02544592524342804, 79.79057627198102409 ) ) ;
#173581=CARTESIAN_POINT ( 'NONE',  ( -18.62759615963255300, -10.81492255796106328, 24.16775706135235424 ) ) ;
#173583=CARTESIAN_POINT ( 'NONE',  ( 19.03943276465977164, -0.05219959533909143690, 88.74890960531436690 ) ) ;
#173584=CARTESIAN_POINT ( 'NONE',  ( -17.60779699588843883, -5.499999999999954703, 76.34981316670108242 ) ) ;
#173585=CARTESIAN_POINT ( 'NONE',  ( -4.379528057220328563, 16.55341960407611168, 115.2072429386476955 ) ) ;
#173586=CARTESIAN_POINT ( 'NONE',  ( 19.05341960407611168, 5.049401038298154454, 33.95724293864769550 ) ) ;
#173587=CARTESIAN_POINT ( 'NONE',  ( -19.02544592524334988, -5.153800228976617603, 108.9594237280189759 ) ) ;
#173589=CARTESIAN_POINT ( 'NONE',  ( 4.379528057220339221, -16.55341960407611168, 107.7072429386476955 ) ) ;
#173590=CARTESIAN_POINT ( 'NONE',  ( 5.823673210054444382, -21.52544592524334988, 90.20942372801903275 ) ) ;
#173591=CARTESIAN_POINT ( 'NONE',  ( 0.05219959533909260263, 19.03943276465977164, 64.99890960531436690 ) ) ;
#173592=CARTESIAN_POINT ( 'NONE',  ( -15.72974639402176322, -15.80617190586768395, 34.37609039468568284 ) ) ;
#173593=CARTESIAN_POINT ( 'NONE',  ( 15.80617190586769283, -15.72974639402175789, 20.62609039468568639 ) ) ;
#173595=CARTESIAN_POINT ( 'NONE',  ( -16.51473224551069308, -9.474510206698971260, 81.66557627198103830 ) ) ;
#173597=CARTESIAN_POINT ( 'NONE',  ( 16.53943276465976808, 0.05219959533934440121, 26.25109039468567573 ) ) ;
#173598=CARTESIAN_POINT ( 'NONE',  ( 21.53943276465977519, -0.05219959533907433946, 48.74890960531435979 ) ) ;
#173599=CARTESIAN_POINT ( 'NONE',  ( -10.72451020669870658, -18.67979575497194134, 74.58442372801901854 ) ) ;
#173600=CARTESIAN_POINT ( 'NONE',  ( -9.474510206698964154, 16.51473224551069663, 115.4155762719810241 ) ) ;
#173601=CARTESIAN_POINT ( 'NONE',  ( 5.049401038297881783, 19.05341960407617563, 102.2927570613523045 ) ) ;
#173602=CARTESIAN_POINT ( 'NONE',  ( 16.46253265017160672, -9.564922557960803928, 58.33224293864769550 ) ) ;
#173603=CARTESIAN_POINT ( 'NONE',  ( 19.03943276465977164, -0.05219959533909143690, 83.74890960531436690 ) ) ;
#173604=CARTESIAN_POINT ( 'NONE',  ( -8.224510206698948167, 14.34966873604960824, 90.41557627198103830 ) ) ;
#173605=CARTESIAN_POINT ( 'NONE',  ( -12.06949235617756955, 12.14591786802309770, 100.6239096053143811 ) ) ;
#173606=CARTESIAN_POINT ( 'NONE',  ( 0.05219959533909260263, 19.03943276465977164, 104.9989096053143669 ) ) ;
#173607=CARTESIAN_POINT ( 'NONE',  ( 8.314922557961029526, -14.29746914071037800, 75.41775706135233293 ) ) ;
#173608=CARTESIAN_POINT ( 'NONE',  ( 16.55341960407611168, 4.379528057220329451, 53.95724293864770260 ) ) ;
#173609=CARTESIAN_POINT ( 'NONE',  ( 9.564922557960805705, 16.46253265017160317, 39.58224293864768839 ) ) ;
#173610=CARTESIAN_POINT ( 'NONE',  ( 21.55341960407619695, -5.719274019375665929, 66.04275706135236135 ) ) ;
#173611=CARTESIAN_POINT ( 'NONE',  ( -13.89961937509957401, -13.97604488694547875, 94.37609039468566152 ) ) ;
#173612=CARTESIAN_POINT ( 'NONE',  ( 12.14591786802309770, 12.06949235617756955, 59.37390960531436690 ) ) ;
#173613=CARTESIAN_POINT ( 'NONE',  ( 21.52544592524344225, -5.823673210054117533, 113.5405762719810383 ) ) ;
#173614=CARTESIAN_POINT ( 'NONE',  ( 21.53943276465977519, -0.05219959533907433946, 43.74890960531435979 ) ) ;
#173615=DIRECTION ( 'NONE',  ( -0.000000000000000000, -0.000000000000000000, 1.000000000000000000 ) ) ;
#173617=CARTESIAN_POINT ( 'NONE',  ( 19.03943276465977164, -0.05219959533909143690, 68.74890960531436690 ) ) ;
#173618=CARTESIAN_POINT ( 'NONE',  ( 4.483927247898545687, 16.52544592524342804, 34.79057627198103120 ) ) ;
#173620=CARTESIAN_POINT ( 'NONE',  ( 12.14591786802327356, -12.06949235617739191, 110.6260903946857042 ) ) ;
#173621=CARTESIAN_POINT ( 'NONE',  ( -4.379528057220086978, -16.55341960407618274, 84.79275706135234714 ) ) ;
#173622=CARTESIAN_POINT ( 'NONE',  ( -16.46253265017146816, -9.564922557961047289, 34.16775706135233293 ) ) ;
#173624=CARTESIAN_POINT ( 'NONE',  ( -16.51473224551069308, -9.474510206698971260, 91.66557627198103830 ) ) ;
#173625=CARTESIAN_POINT ( 'NONE',  ( 9.564922557960805705, 16.46253265017160317, 44.58224293864769550 ) ) ;
#173626=CARTESIAN_POINT ( 'NONE',  ( -16.52544592524342804, 4.483927247898546575, 66.04057627198103830 ) ) ;
#173627=CARTESIAN_POINT ( 'NONE',  ( 17.60728821187776916, -5.500000000000037303, 48.36690927743607915 ) ) ;
#173628=CARTESIAN_POINT ( 'NONE',  ( -0.05219959533907301413, -21.53943276465977519, 27.49890960531435269 ) ) ;
#173629=CARTESIAN_POINT ( 'NONE',  ( -10.81492255796078084, -18.62759615963271287, 57.08224293864769550 ) ) ;
#173630=CARTESIAN_POINT ( 'NONE',  ( 4.483927247898545687, 16.52544592524342804, 89.79057627198103830 ) ) ;
#173631=CARTESIAN_POINT ( 'NONE',  ( -4.483927247898782831, 16.52544592524335698, 42.70942372801901854 ) ) ;
#173633=CARTESIAN_POINT ( 'NONE',  ( 12.14591786802309770, 12.06949235617756955, 74.37390960531436690 ) ) ;
#173636=CARTESIAN_POINT ( 'NONE',  ( -5.153800228976607833, 19.02544592524334988, 77.70942372801900433 ) ) ;
#173637=CARTESIAN_POINT ( 'NONE',  ( -10.81492255796078084, -18.62759615963271287, 22.08224293864769194 ) ) ;
#173639=CARTESIAN_POINT ( 'NONE',  ( 17.50000000000000000, -5.500000000000000888, 28.29690382534172244 ) ) ;
#173640=CARTESIAN_POINT ( 'NONE',  ( 14.29746914071037800, 8.314922557961029526, 26.66775706135235424 ) ) ;
#173641=CARTESIAN_POINT ( 'NONE',  ( -12.14591786802326823, 12.06949235617739902, 113.1260903946856899 ) ) ;
#173642=CARTESIAN_POINT ( 'NONE',  ( 16.51473224551083163, -9.474510206698727899, 65.83442372801900433 ) ) ;
#173643=CARTESIAN_POINT ( 'NONE',  ( -0.05219959533907301413, -21.53943276465977519, 52.49890960531435979 ) ) ;
#173644=CARTESIAN_POINT ( 'NONE',  ( 5.823673210054444382, -21.52544592524334988, 65.20942372801901854 ) ) ;
#173646=CARTESIAN_POINT ( 'NONE',  ( 12.14591786802327356, -12.06949235617739191, 35.62609039468568994 ) ) ;
#173647=CARTESIAN_POINT ( 'NONE',  ( 13.89961937509977652, -13.97604488694527269, 23.12390960531436335 ) ) ;
#173648=CARTESIAN_POINT ( 'NONE',  ( 5.049401038298161559, -19.05341960407611168, 82.70724293864770971 ) ) ;
#173650=CARTESIAN_POINT ( 'NONE',  ( 13.89961937509977652, -13.97604488694527269, 28.12390960531435624 ) ) ;
#173651=CARTESIAN_POINT ( 'NONE',  ( 8.224510206698953496, -14.34966873604960469, 107.9155762719810241 ) ) ;
#173654=CARTESIAN_POINT ( 'NONE',  ( -19.02544592524342804, 5.153800228976336051, 106.0405762719810241 ) ) ;
#173656=CARTESIAN_POINT ( 'NONE',  ( -16.52544592524335698, -4.483927247898792601, 53.95942372801900433 ) ) ;
#173657=CARTESIAN_POINT ( 'NONE',  ( 5.049401038297881783, 19.05341960407617563, 107.2927570613523187 ) ) ;
#173658=CARTESIAN_POINT ( 'NONE',  ( -0.05219959533907301413, -21.53943276465977519, 72.49890960531435269 ) ) ;
#173659=CARTESIAN_POINT ( 'NONE',  ( 19.02544592524343514, -5.153800228976328945, 43.54057627198103120 ) ) ;
#173660=CARTESIAN_POINT ( 'NONE',  ( 5.153800228976615827, -19.02544592524334988, 70.20942372801899012 ) ) ;
#173661=CARTESIAN_POINT ( 'NONE',  ( 21.52544592524344225, -5.823673210054117533, 113.5405762719810383 ) ) ;
#173662=CARTESIAN_POINT ( 'NONE',  ( 5.153800228976335163, 19.02544592524342804, 74.79057627198103830 ) ) ;
#173663=CARTESIAN_POINT ( 'NONE',  ( 0.05219959533909260263, 19.03943276465977164, 99.99890960531436690 ) ) ;
#173665=CARTESIAN_POINT ( 'NONE',  ( -14.34966873604972548, 8.224510206698743886, 33.33442372801900433 ) ) ;
#173666=CARTESIAN_POINT ( 'NONE',  ( 18.67979575497178502, 10.72451020669898547, 109.1655762719810383 ) ) ;
#173667=CARTESIAN_POINT ( 'NONE',  ( 4.379528057220339221, -16.55341960407611168, 107.7072429386476955 ) ) ;
#173668=CARTESIAN_POINT ( 'NONE',  ( -16.51473224551069308, -9.474510206698971260, 96.66557627198102409 ) ) ;
#173669=CARTESIAN_POINT ( 'NONE',  ( 0.05219959533936267826, -19.03943276465977164, 80.00109039468567573 ) ) ;
#173670=CARTESIAN_POINT ( 'NONE',  ( -10.72451020669898014, 18.67979575497178502, 80.41557627198103830 ) ) ;
#173671=CARTESIAN_POINT ( 'NONE',  ( -16.53943276465976808, 0.05219959533911058130, 51.24890960531436690 ) ) ;
#173672=CARTESIAN_POINT ( 'NONE',  ( 16.51473224551083163, -9.474510206698727899, 25.83442372801900078 ) ) ;
#173673=CARTESIAN_POINT ( 'NONE',  ( 16.53943276465976808, 0.05219959533934440121, 71.25109039468568994 ) ) ;
#173674=CARTESIAN_POINT ( 'NONE',  ( 9.474510206698971260, -16.51473224551069308, 87.91557627198102409 ) ) ;
#173675=CARTESIAN_POINT ( 'NONE',  ( -16.51473224551069308, -9.474510206698971260, 51.66557627198102409 ) ) ;
#173676=CARTESIAN_POINT ( 'NONE',  ( 21.53943276465977519, 0.05219959533937863772, 56.25109039468568284 ) ) ;
#173677=CARTESIAN_POINT ( 'NONE',  ( 21.55341960407619695, -5.719274019375665929, 66.04275706135236135 ) ) ;
#173678=CARTESIAN_POINT ( 'NONE',  ( 19.02544592524343514, -5.153800228976328945, 58.54057627198102409 ) ) ;
#173679=CARTESIAN_POINT ( 'NONE',  ( 0.05219959533937995610, -21.53943276465977519, 40.00109039468567573 ) ) ;
#173680=CARTESIAN_POINT ( 'NONE',  ( -9.474510206698720793, -16.51473224551083518, 69.58442372801901854 ) ) ;
#173681=CARTESIAN_POINT ( 'NONE',  ( 16.51473224551069308, 9.474510206698969483, 39.16557627198103120 ) ) ;
#173682=CARTESIAN_POINT ( 'NONE',  ( -16.55341960407617563, 4.379528057220093196, 83.54275706135234714 ) ) ;
#173683=CARTESIAN_POINT ( 'NONE',  ( -19.03943276465977164, 0.05219959533909376836, 71.24890960531435269 ) ) ;
#173684=CARTESIAN_POINT ( 'NONE',  ( -5.049401038298153566, 19.05341960407611168, 115.2072429386477097 ) ) ;
#173685=CARTESIAN_POINT ( 'NONE',  ( -16.46253265017160317, 9.564922557960807481, 35.83224293864768839 ) ) ;
#173686=ADVANCED_FACE ( 'NONE', ( #28946 ), #79396, .T. ) ;
#173687=CARTESIAN_POINT ( 'NONE',  ( -10.72451020669898014, 18.67979575497178502, 85.41557627198102409 ) ) ;
#173688=CARTESIAN_POINT ( 'NONE',  ( -16.52544592524335698, -4.483927247898792601, 68.95942372801901854 ) ) ;
#173690=CARTESIAN_POINT ( 'NONE',  ( -13.97604488694547697, 13.89961937509957934, 28.12609039468565797 ) ) ;
#173691=CARTESIAN_POINT ( 'NONE',  ( 13.89961937509977652, -13.97604488694527269, 63.12390960531435979 ) ) ;
#173692=CARTESIAN_POINT ( 'NONE',  ( 16.52544592524342804, -4.483927247898539470, 38.54057627198103120 ) ) ;
#173693=CARTESIAN_POINT ( 'NONE',  ( -16.52544592524342804, 4.483927247898546575, 81.04057627198102409 ) ) ;
#173694=CARTESIAN_POINT ( 'NONE',  ( 9.474510206698971260, -16.51473224551069308, 107.9155762719810383 ) ) ;
#173695=CARTESIAN_POINT ( 'NONE',  ( 19.05341960407611168, 5.049401038298154454, 93.95724293864769550 ) ) ;
#173696=CARTESIAN_POINT ( 'NONE',  ( -15.80617190586768217, 15.72974639402176855, 53.12609039468568284 ) ) ;
#173697=CARTESIAN_POINT ( 'NONE',  ( -0.05219959533909027116, -19.03943276465977164, 107.4989096053143527 ) ) ;
#173698=CARTESIAN_POINT ( 'NONE',  ( -18.67979575497193778, 10.72451020669871902, 98.33442372801901854 ) ) ;
#173699=CARTESIAN_POINT ( 'NONE',  ( -14.34966873604972548, 8.224510206698743886, 73.33442372801901854 ) ) ;
#173700=CARTESIAN_POINT ( 'NONE',  ( 21.52544592524334988, 5.823673210054432836, 26.45942372801901854 ) ) ;
#173701=CARTESIAN_POINT ( 'NONE',  ( -0.05219959533909027116, -19.03943276465977164, 107.4989096053143527 ) ) ;
#173702=CARTESIAN_POINT ( 'NONE',  ( 10.81492255796078972, 18.62759615963270932, 99.58224293864770971 ) ) ;
#173703=CARTESIAN_POINT ( 'NONE',  ( 16.52544592524342804, -4.483927247898539470, 63.54057627198103830 ) ) ;
#173704=CARTESIAN_POINT ( 'NONE',  ( -16.51473224551069308, -9.474510206698971260, 46.66557627198102409 ) ) ;
#173705=CARTESIAN_POINT ( 'NONE',  ( -4.379528057220328563, 16.55341960407611168, 75.20724293864769550 ) ) ;
#173706=CARTESIAN_POINT ( 'NONE',  ( -18.67979575497178146, -10.72451020669898902, 31.66557627198102054 ) ) ;
#173707=CARTESIAN_POINT ( 'NONE',  ( 13.97604488694548053, -13.89961937509957401, 25.62609039468566507 ) ) ;
#173708=CARTESIAN_POINT ( 'NONE',  ( 14.34966873604960469, 8.224510206698951720, 109.1655762719810383 ) ) ;
#173709=ORIENTED_EDGE ( 'NONE', *, *, #182333, .T. ) ;
#173710=CARTESIAN_POINT ( 'NONE',  ( 16.52544592524335698, 4.483927247898782831, 66.45942372801903275 ) ) ;
#173711=CARTESIAN_POINT ( 'NONE',  ( 19.05341960407611168, 5.049401038298154454, 73.95724293864768129 ) ) ;
#173713=CARTESIAN_POINT ( 'NONE',  ( 12.06949235617757843, -12.14591786802309237, 88.12390960531436690 ) ) ;
#173714=CARTESIAN_POINT ( 'NONE',  ( -18.62759615963270932, 10.81492255796079327, 35.83224293864768839 ) ) ;
#173716=CARTESIAN_POINT ( 'NONE',  ( 12.06949235617739724, 12.14591786802326823, 111.8760903946856615 ) ) ;
#173717=CARTESIAN_POINT ( 'NONE',  ( -19.02544592524334988, -5.153800228976617603, 108.9594237280189759 ) ) ;
#173718=CARTESIAN_POINT ( 'NONE',  ( -18.67979575497193778, 10.72451020669871902, 83.33442372801903275 ) ) ;
#173719=CARTESIAN_POINT ( 'NONE',  ( -0.05219959533909027116, -19.03943276465977164, 82.49890960531436690 ) ) ;
#173720=CARTESIAN_POINT ( 'NONE',  ( -21.53943276465977519, 0.05219959533907696930, 106.2489096053143811 ) ) ;
#173721=CARTESIAN_POINT ( 'NONE',  ( -8.224510206698735004, -14.34966873604973081, 54.58442372801901143 ) ) ;
#173722=CARTESIAN_POINT ( 'NONE',  ( 5.049401038298161559, -19.05341960407611168, 27.70724293864769550 ) ) ;
#173723=CARTESIAN_POINT ( 'NONE',  ( 16.55341960407618274, -4.379528057220086978, 26.04275706135235779 ) ) ;
#173724=CARTESIAN_POINT ( 'NONE',  ( 9.474510206698729675, 16.51473224551082808, 92.08442372801900433 ) ) ;
#173725=CARTESIAN_POINT ( 'NONE',  ( -10.81492255796078084, -18.62759615963271287, 92.08224293864769550 ) ) ;
#173726=CARTESIAN_POINT ( 'NONE',  ( 9.474510206698729675, 16.51473224551082808, 52.08442372801900433 ) ) ;
#173727=CARTESIAN_POINT ( 'NONE',  ( 18.56453257813364388, -5.500000000000048850, 88.49000423690685579 ) ) ;
#173728=CARTESIAN_POINT ( 'NONE',  ( -0.05219959533907301413, -21.53943276465977519, 107.4989096053143669 ) ) ;
#173729=CARTESIAN_POINT ( 'NONE',  ( 17.50000000000000000, 5.499999999999997335, 26.70309617465829888 ) ) ;
#173730=CARTESIAN_POINT ( 'NONE',  ( -13.97604488694527625, -13.89961937509977652, 81.87390960531436690 ) ) ;
#173732=CARTESIAN_POINT ( 'NONE',  ( 16.55341960407618274, -4.379528057220086978, 36.04275706135234714 ) ) ;
#173734=CARTESIAN_POINT ( 'NONE',  ( 15.72974639402199770, -15.80617190586745480, 113.1239096053143953 ) ) ;
#173735=CARTESIAN_POINT ( 'NONE',  ( -8.224510206698948167, 14.34966873604960824, 65.41557627198102409 ) ) ;
#173736=CARTESIAN_POINT ( 'NONE',  ( -5.153800228976328057, -19.02544592524343514, 72.29057627198102409 ) ) ;
#173737=CARTESIAN_POINT ( 'NONE',  ( 14.34966873604972726, -8.224510206698740333, 35.83442372801901143 ) ) ;
#173738=CARTESIAN_POINT ( 'NONE',  ( -5.153800228976607833, 19.02544592524334988, 47.70942372801900433 ) ) ;
#173739=CARTESIAN_POINT ( 'NONE',  ( -15.72974639402176322, -15.80617190586768395, 54.37609039468568994 ) ) ;
#173740=CARTESIAN_POINT ( 'NONE',  ( -0.05219959533936034679, 19.03943276465977164, 107.5010903946856615 ) ) ;
#173741=CARTESIAN_POINT ( 'NONE',  ( -16.46253265017160317, 9.564922557960807481, 55.83224293864769550 ) ) ;
#173742=CARTESIAN_POINT ( 'NONE',  ( 13.97604488694548053, -13.89961937509957401, 80.62609039468567573 ) ) ;
#173743=CARTESIAN_POINT ( 'NONE',  ( -15.72974639402176322, -15.80617190586768395, 84.37609039468570415 ) ) ;
#173744=CARTESIAN_POINT ( 'NONE',  ( 16.51473224551083163, -9.474510206698727899, 60.83442372801900433 ) ) ;
#173745=CARTESIAN_POINT ( 'NONE',  ( -16.51473224551069308, -9.474510206698971260, 36.66557627198102409 ) ) ;
#173746=CARTESIAN_POINT ( 'NONE',  ( -10.81492255796078084, -18.62759615963271287, 57.08224293864769550 ) ) ;
#173747=CARTESIAN_POINT ( 'NONE',  ( 16.55341960407611168, 4.379528057220329451, 63.95724293864770260 ) ) ;
#173748=CARTESIAN_POINT ( 'NONE',  ( -5.153800228976607833, 19.02544592524334988, 67.70942372801900433 ) ) ;
#173750=CARTESIAN_POINT ( 'NONE',  ( 16.51473224551083163, -9.474510206698727899, 35.83442372801899722 ) ) ;
#173751=CARTESIAN_POINT ( 'NONE',  ( 8.224510206698742110, 14.34966873604972548, 97.08442372801904696 ) ) ;
#173752=CARTESIAN_POINT ( 'NONE',  ( 4.379528057220339221, -16.55341960407611168, 52.70724293864769550 ) ) ;
#173753=CARTESIAN_POINT ( 'NONE',  ( -18.62759615963255300, -10.81492255796106328, 89.16775706135236135 ) ) ;
#173755=CARTESIAN_POINT ( 'NONE',  ( -21.52544592524334988, -5.823673210054445271, 88.95942372801901854 ) ) ;
#173756=CARTESIAN_POINT ( 'NONE',  ( 15.80617190586746368, 15.72974639402197994, 89.37390960531435269 ) ) ;
#173757=CARTESIAN_POINT ( 'NONE',  ( 19.02544592524343514, -5.153800228976328945, 48.54057627198103120 ) ) ;
#173758=CARTESIAN_POINT ( 'NONE',  ( 15.72974639402176855, 15.80617190586768217, 71.87609039468568994 ) ) ;
#173759=CARTESIAN_POINT ( 'NONE',  ( -13.97604488694527625, -13.89961937509977652, 46.87390960531435979 ) ) ;
#173761=CARTESIAN_POINT ( 'NONE',  ( -0.05219959533909027116, -19.03943276465977164, 67.49890960531436690 ) ) ;
#173762=CARTESIAN_POINT ( 'NONE',  ( -12.14591786802309592, -12.06949235617757132, 101.8739096053143811 ) ) ;
#173763=CARTESIAN_POINT ( 'NONE',  ( 5.049401038298161559, -19.05341960407611168, 107.7072429386476955 ) ) ;
#173764=CARTESIAN_POINT ( 'NONE',  ( 14.34966873604960469, 8.224510206698951720, 54.16557627198103120 ) ) ;
#173765=CARTESIAN_POINT ( 'NONE',  ( -16.46253265017160317, 9.564922557960807481, 30.83224293864769550 ) ) ;
#173766=CARTESIAN_POINT ( 'NONE',  ( 12.06949235617757843, -12.14591786802309237, 78.12390960531436690 ) ) ;
#173768=CARTESIAN_POINT ( 'NONE',  ( 10.72451020669898902, -18.67979575497178502, 92.91557627198103830 ) ) ;
#173769=CARTESIAN_POINT ( 'NONE',  ( 5.823673210054444382, -21.52544592524334988, 40.20942372801901854 ) ) ;
#173770=CARTESIAN_POINT ( 'NONE',  ( 30.00000000000000000, 5.499999999999992895, 102.5000000000000142 ) ) ;
#173771=CARTESIAN_POINT ( 'NONE',  ( -4.483927247898782831, 16.52544592524335698, 32.70942372801900433 ) ) ;
#173772=CARTESIAN_POINT ( 'NONE',  ( -5.719274019375978568, 21.55341960407610458, 85.20724293864770971 ) ) ;
#173773=CARTESIAN_POINT ( 'NONE',  ( -21.53943276465977519, -0.05219959533937600094, 103.7510903946857042 ) ) ;
#173774=CARTESIAN_POINT ( 'NONE',  ( -5.153800228976328057, -19.02544592524343514, 92.29057627198099567 ) ) ;
#173775=CARTESIAN_POINT ( 'NONE',  ( -18.62759615963255300, -10.81492255796106328, 44.16775706135234714 ) ) ;
#173776=CARTESIAN_POINT ( 'NONE',  ( -10.72451020669898014, 18.67979575497178502, 35.41557627198102409 ) ) ;
#173777=CARTESIAN_POINT ( 'NONE',  ( 12.06949235617739724, 12.14591786802326823, 106.8760903946856899 ) ) ;
#173778=CARTESIAN_POINT ( 'NONE',  ( 21.55341960407619695, -5.719274019375665929, 46.04275706135234714 ) ) ;
#173779=CARTESIAN_POINT ( 'NONE',  ( -15.72974639402176322, -15.80617190586768395, 84.37609039468570415 ) ) ;
#173780=CARTESIAN_POINT ( 'NONE',  ( -21.52544592524334988, -5.823673210054445271, 108.9594237280190185 ) ) ;
#173781=CARTESIAN_POINT ( 'NONE',  ( -14.34966873604972548, 8.224510206698743886, 88.33442372801901854 ) ) ;
#173782=CARTESIAN_POINT ( 'NONE',  ( 18.67979575497194134, -10.72451020669871369, 45.83442372801901854 ) ) ;
#173783=CARTESIAN_POINT ( 'NONE',  ( -19.03943276465977164, 0.05219959533909376836, 36.24890960531436690 ) ) ;
#173784=CARTESIAN_POINT ( 'NONE',  ( -21.52544592524334988, -5.823673210054445271, 98.95942372801903275 ) ) ;
#173785=CARTESIAN_POINT ( 'NONE',  ( 9.474510206698971260, -16.51473224551069308, 112.9155762719810383 ) ) ;
#173786=CARTESIAN_POINT ( 'NONE',  ( 21.52544592524344225, -5.823673210054117533, 108.5405762719810241 ) ) ;
#173788=CARTESIAN_POINT ( 'NONE',  ( -15.72974639402197994, 15.80617190586746368, 70.62390960531436690 ) ) ;
#173789=CARTESIAN_POINT ( 'NONE',  ( -8.314922557961024197, 14.29746914071037800, 52.91775706135235424 ) ) ;
#173790=CARTESIAN_POINT ( 'NONE',  ( -12.06949235617756955, 12.14591786802309770, 65.62390960531436690 ) ) ;
#173791=CARTESIAN_POINT ( 'NONE',  ( 19.53392245597579802, -5.499999999999960032, 102.1255887859039291 ) ) ;
#173792=CARTESIAN_POINT ( 'NONE',  ( 5.049401038297881783, 19.05341960407617563, 92.29275706135234714 ) ) ;
#173795=CARTESIAN_POINT ( 'NONE',  ( -4.483927247898782831, 16.52544592524335698, 32.70942372801900433 ) ) ;
#173796=CARTESIAN_POINT ( 'NONE',  ( -10.81492255796078084, -18.62759615963271287, 102.0822429386476955 ) ) ;
#173797=CARTESIAN_POINT ( 'NONE',  ( -5.823673210054116645, -21.52544592524344225, 77.29057627198102409 ) ) ;
#173798=CARTESIAN_POINT ( 'NONE',  ( 5.719274019375991003, -21.55341960407610458, 22.70724293864769194 ) ) ;
#173799=CARTESIAN_POINT ( 'NONE',  ( -0.05219959533934338120, 16.53943276465976808, 52.50109039468567573 ) ) ;
#173800=CARTESIAN_POINT ( 'NONE',  ( 0.05219959533909260263, 19.03943276465977164, 74.99890960531435269 ) ) ;
#173801=CARTESIAN_POINT ( 'NONE',  ( 21.53943276465977519, 0.05219959533937863772, 36.25109039468567573 ) ) ;
#173802=CARTESIAN_POINT ( 'NONE',  ( -13.89961937509957401, -13.97604488694547875, 99.37609039468567573 ) ) ;
#173804=CARTESIAN_POINT ( 'NONE',  ( 13.97604488694527802, 13.89961937509977652, 109.3739096053143669 ) ) ;
#173805=CARTESIAN_POINT ( 'NONE',  ( 16.51473224551069308, 9.474510206698969483, 89.16557627198103830 ) ) ;
#173806=CARTESIAN_POINT ( 'NONE',  ( 21.53943276465977519, -0.05219959533907433946, 83.74890960531435269 ) ) ;
#173807=CARTESIAN_POINT ( 'NONE',  ( -16.46253265017160317, 9.564922557960807481, 55.83224293864769550 ) ) ;
#173808=CARTESIAN_POINT ( 'NONE',  ( -17.49999999999999645, 5.499999999999992895, 78.71769037696437010 ) ) ;
#173809=CARTESIAN_POINT ( 'NONE',  ( 12.06949235617757843, -12.14591786802309237, 63.12390960531435979 ) ) ;
#173810=CARTESIAN_POINT ( 'NONE',  ( -15.80617190586745835, -15.72974639402198527, 26.87390960531435979 ) ) ;
#173812=CARTESIAN_POINT ( 'NONE',  ( 21.53943276465977519, -0.05219959533907433946, 103.7489096053143669 ) ) ;
#173813=CARTESIAN_POINT ( 'NONE',  ( -13.89961937509957401, -13.97604488694547875, 64.37609039468567573 ) ) ;
#173814=CARTESIAN_POINT ( 'NONE',  ( -13.89961937509977652, 13.97604488694528158, 110.6239096053143243 ) ) ;
#173815=SURFACE_SIDE_STYLE ('',( #24113 ) ) ;
#173816=CARTESIAN_POINT ( 'NONE',  ( -18.62759615963270932, 10.81492255796079327, 55.83224293864770260 ) ) ;
#173817=CARTESIAN_POINT ( 'NONE',  ( -16.51473224551069308, -9.474510206698971260, 86.66557627198102409 ) ) ;
#173818=CARTESIAN_POINT ( 'NONE',  ( 15.72974639402176855, 15.80617190586768217, 76.87609039468567573 ) ) ;
#173819=CARTESIAN_POINT ( 'NONE',  ( -19.05341960407611168, -5.049401038298163336, 51.45724293864770260 ) ) ;
#173820=CARTESIAN_POINT ( 'NONE',  ( -16.55341960407611168, -4.379528057220339221, 86.45724293864770971 ) ) ;
#173821=CARTESIAN_POINT ( 'NONE',  ( -12.06949235617739369, -12.14591786802326823, 34.37609039468568284 ) ) ;
#173822=B_SPLINE_CURVE_WITH_KNOTS ( 'NONE', 3,
 ( #4656, #186741, #35017, #34031, #97650, #94695 ),
 .UNSPECIFIED., .F., .F.,
 ( 4, 2, 4 ),
 ( 0.000000000000000000, 0.0003837532665635174311, 0.0007675065331270348621 ),
 .UNSPECIFIED. ) ;
#173823=CARTESIAN_POINT ( 'NONE',  ( -10.81492255796105439, 18.62759615963255655, 67.91775706135234714 ) ) ;
#173825=CARTESIAN_POINT ( 'NONE',  ( 16.46253265017146816, 9.564922557961045513, 21.66775706135233648 ) ) ;
#173826=CARTESIAN_POINT ( 'NONE',  ( -5.049401038297874678, -19.05341960407617918, 84.79275706135233293 ) ) ;
#173828=CARTESIAN_POINT ( 'NONE',  ( 15.80617190586769283, -15.72974639402175789, 40.62609039468567573 ) ) ;
#173830=CARTESIAN_POINT ( 'NONE',  ( -13.97604488694547697, 13.89961937509957934, 38.12609039468566152 ) ) ;
#173831=CARTESIAN_POINT ( 'NONE',  ( -9.474510206698964154, 16.51473224551069663, 60.41557627198102409 ) ) ;
#173832=CARTESIAN_POINT ( 'NONE',  ( 16.46253265017146816, 9.564922557961045513, 26.66775706135234003 ) ) ;
#173833=CARTESIAN_POINT ( 'NONE',  ( -12.06949235617739369, -12.14591786802326823, 99.37609039468568994 ) ) ;
#173834=CARTESIAN_POINT ( 'NONE',  ( -19.02544592524342804, 5.153800228976336051, 101.0405762719810241 ) ) ;
#173835=CARTESIAN_POINT ( 'NONE',  ( -21.53943276465977519, -0.05219959533937600094, 88.75109039468567573 ) ) ;
#173837=CARTESIAN_POINT ( 'NONE',  ( -17.49999999999999289, -4.013004640162506576, 34.55394279005599145 ) ) ;
#173838=CARTESIAN_POINT ( 'NONE',  ( 0.05219959533937995610, -21.53943276465977519, 85.00109039468568994 ) ) ;
#173839=CARTESIAN_POINT ( 'NONE',  ( 16.88567814943166923, -6.947325034625572826, 41.20998877347414435 ) ) ;
#173840=CARTESIAN_POINT ( 'NONE',  ( 0.05219959533909260263, 19.03943276465977164, 94.99890960531436690 ) ) ;
#173843=CARTESIAN_POINT ( 'NONE',  ( -19.05341960407611168, -5.049401038298163336, 51.45724293864770260 ) ) ;
#173844=CARTESIAN_POINT ( 'NONE',  ( -21.55341960407610458, -5.719274019375992779, 56.45724293864768839 ) ) ;
#173845=CARTESIAN_POINT ( 'NONE',  ( 12.14591786802309770, 12.06949235617756955, 29.37390960531435269 ) ) ;
#173846=CARTESIAN_POINT ( 'NONE',  ( 14.29746914071049879, -8.314922557960816363, 93.33224293864769550 ) ) ;
#173847=CARTESIAN_POINT ( 'NONE',  ( -19.05341960407611168, -5.049401038298163336, 76.45724293864769550 ) ) ;
#173848=CARTESIAN_POINT ( 'NONE',  ( 9.564922557961047289, -16.46253265017146816, 20.41775706135233293 ) ) ;
#173849=CARTESIAN_POINT ( 'NONE',  ( 5.049401038298161559, -19.05341960407611168, 32.70724293864768129 ) ) ;
#173850=CARTESIAN_POINT ( 'NONE',  ( 8.224510206698953496, -14.34966873604960469, 97.91557627198103830 ) ) ;
#173851=CARTESIAN_POINT ( 'NONE',  ( 21.55341960407619695, -5.719274019375665929, 61.04275706135234714 ) ) ;
#173852=CARTESIAN_POINT ( 'NONE',  ( -5.719274019375978568, 21.55341960407610458, 85.20724293864770971 ) ) ;
#173853=CARTESIAN_POINT ( 'NONE',  ( 16.46253265017146816, 9.564922557961045513, 66.66775706135233293 ) ) ;
#173855=CARTESIAN_POINT ( 'NONE',  ( -0.05219959533909027116, -19.03943276465977164, 112.4989096053143669 ) ) ;
#173856=CARTESIAN_POINT ( 'NONE',  ( 0.05219959533910956823, 16.53943276465976808, 79.99890960531435269 ) ) ;
#173857=CARTESIAN_POINT ( 'NONE',  ( -13.97604488694547697, 13.89961937509957934, 48.12609039468566863 ) ) ;
#173858=CARTESIAN_POINT ( 'NONE',  ( -9.564922557960796823, -16.46253265017161027, 67.08224293864769550 ) ) ;
#173859=CARTESIAN_POINT ( 'NONE',  ( 8.224510206698953496, -14.34966873604960469, 62.91557627198102409 ) ) ;
#173860=CARTESIAN_POINT ( 'NONE',  ( -19.05341960407617563, 5.049401038297882671, 78.54275706135233293 ) ) ;
#173861=CARTESIAN_POINT ( 'NONE',  ( -21.52544592524343514, 5.823673210054127303, 41.04057627198103120 ) ) ;
#173863=CARTESIAN_POINT ( 'NONE',  ( -8.224510206698948167, 14.34966873604960824, 105.4155762719810383 ) ) ;
#173864=CARTESIAN_POINT ( 'NONE',  ( -17.50000000000001066, -5.068104630630400287, 24.27181594659972319 ) ) ;
#173865=CARTESIAN_POINT ( 'NONE',  ( 16.46253265017160672, -9.564922557960803928, 53.33224293864768839 ) ) ;
#173866=CARTESIAN_POINT ( 'NONE',  ( -5.823673210054116645, -21.52544592524344225, 57.29057627198103120 ) ) ;
#173867=CARTESIAN_POINT ( 'NONE',  ( 5.049401038298161559, -19.05341960407611168, 37.70724293864768839 ) ) ;
#173868=CARTESIAN_POINT ( 'NONE',  ( -4.379528057220086978, -16.55341960407618274, 79.79275706135236135 ) ) ;
#173869=CARTESIAN_POINT ( 'NONE',  ( -5.049401038298153566, 19.05341960407611168, 70.20724293864769550 ) ) ;
#173870=CARTESIAN_POINT ( 'NONE',  ( -16.46253265017146816, -9.564922557961047289, 49.16775706135233293 ) ) ;
#173871=CARTESIAN_POINT ( 'NONE',  ( -10.72451020669870658, -18.67979575497194134, 64.58442372801900433 ) ) ;
#173872=CARTESIAN_POINT ( 'NONE',  ( -10.81492255796078084, -18.62759615963271287, 47.08224293864770260 ) ) ;
#173873=CARTESIAN_POINT ( 'NONE',  ( 0.05219959533909260263, 19.03943276465977164, 24.99890960531435269 ) ) ;
#173874=CARTESIAN_POINT ( 'NONE',  ( 14.34966873604972726, -8.224510206698740333, 80.83442372801901854 ) ) ;
#173875=CARTESIAN_POINT ( 'NONE',  ( 13.97604488694548053, -13.89961937509957401, 105.6260903946856757 ) ) ;
#173878=CARTESIAN_POINT ( 'NONE',  ( 10.81492255796106328, -18.62759615963255655, 100.4177570613523471 ) ) ;
#173880=CARTESIAN_POINT ( 'NONE',  ( -4.483927247898539470, -16.52544592524342804, 47.29057627198103120 ) ) ;
#173881=CARTESIAN_POINT ( 'NONE',  ( -12.06949235617756955, 12.14591786802309770, 75.62390960531439532 ) ) ;
#173882=CARTESIAN_POINT ( 'NONE',  ( -15.80617190586745835, -15.72974639402198527, 96.87390960531436690 ) ) ;
#173883=CARTESIAN_POINT ( 'NONE',  ( -0.05219959533907301413, -21.53943276465977519, 92.49890960531436690 ) ) ;
#173886=CARTESIAN_POINT ( 'NONE',  ( -15.80617190586745835, -15.72974639402198527, 31.87390960531435979 ) ) ;
#173887=CARTESIAN_POINT ( 'NONE',  ( -14.29746914071037622, -8.314922557961029526, 69.16775706135234714 ) ) ;
#173888=CARTESIAN_POINT ( 'NONE',  ( -4.483927247898539470, -16.52544592524342804, 87.29057627198103830 ) ) ;
#173889=CARTESIAN_POINT ( 'NONE',  ( -19.05341960407611168, -5.049401038298163336, 51.45724293864770260 ) ) ;
#173890=DIRECTION ( 'NONE',  ( 1.000000000000000000, 0.000000000000000000, 0.000000000000000000 ) ) ;
#173891=CARTESIAN_POINT ( 'NONE',  ( 8.314922557961029526, -14.29746914071037800, 95.41775706135234714 ) ) ;
#173892=CARTESIAN_POINT ( 'NONE',  ( -15.72974639402176322, -15.80617190586768395, 29.37609039468568284 ) ) ;
#173893=CARTESIAN_POINT ( 'NONE',  ( -9.474510206698964154, 16.51473224551069663, 80.41557627198103830 ) ) ;
#173894=CARTESIAN_POINT ( 'NONE',  ( 21.55341960407619695, -5.719274019375665929, 66.04275706135236135 ) ) ;
#173895=CARTESIAN_POINT ( 'NONE',  ( 19.03943276465977164, -0.05219959533909143690, 113.7489096053143669 ) ) ;
#173897=EDGE_LOOP ( 'NONE', ( #116140, #55438, #142522 ) ) ;
#173898=CARTESIAN_POINT ( 'NONE',  ( 21.55341960407619695, -5.719274019375665929, 56.04275706135235424 ) ) ;
#173899=CARTESIAN_POINT ( 'NONE',  ( 13.89961937509977652, -13.97604488694527269, 33.12390960531434558 ) ) ;
#173901=CARTESIAN_POINT ( 'NONE',  ( 16.51473224551083163, -9.474510206698727899, 70.83442372801900433 ) ) ;
#173902=CARTESIAN_POINT ( 'NONE',  ( -21.53943276465977519, -0.05219959533937600094, 23.75109039468567929 ) ) ;
#173903=CARTESIAN_POINT ( 'NONE',  ( 5.153800228976615827, -19.02544592524334988, 60.20942372801899012 ) ) ;
#173904=CARTESIAN_POINT ( 'NONE',  ( 19.03943276465977164, -0.05219959533909143690, 23.74890960531435269 ) ) ;
#173905=CARTESIAN_POINT ( 'NONE',  ( 8.314922557961029526, -14.29746914071037800, 90.41775706135236135 ) ) ;
#173906=CARTESIAN_POINT ( 'NONE',  ( 19.03943276465977164, 0.05219959533936151252, 66.25109039468567573 ) ) ;
#173907=CARTESIAN_POINT ( 'NONE',  ( 8.314922557960818139, 14.29746914071049879, 24.58224293864768839 ) ) ;
#173910=CARTESIAN_POINT ( 'NONE',  ( -13.89961937509977652, 13.97604488694528158, 85.62390960531433848 ) ) ;
#173911=CARTESIAN_POINT ( 'NONE',  ( 21.55341960407619695, -5.719274019375665929, 91.04275706135236135 ) ) ;
#173912=CARTESIAN_POINT ( 'NONE',  ( -18.62759615963255300, -10.81492255796106328, 104.1677570613523471 ) ) ;
#173913=CARTESIAN_POINT ( 'NONE',  ( -5.153800228976328057, -19.02544592524343514, 22.29057627198102765 ) ) ;
#173914=CARTESIAN_POINT ( 'NONE',  ( 21.53943276465977519, 0.05219959533937863772, 81.25109039468568994 ) ) ;
#173915=CARTESIAN_POINT ( 'NONE',  ( -16.55341960407617563, 4.379528057220093196, 28.54275706135234358 ) ) ;
#173916=CARTESIAN_POINT ( 'NONE',  ( 13.97604488694527802, 13.89961937509977652, 84.37390960531433848 ) ) ;
#173917=CARTESIAN_POINT ( 'NONE',  ( 21.53943276465977519, -0.05219959533907433946, 23.74890960531435269 ) ) ;
#173919=CARTESIAN_POINT ( 'NONE',  ( -16.51473224551069308, -9.474510206698971260, 76.66557627198103830 ) ) ;
#173920=CARTESIAN_POINT ( 'NONE',  ( -17.31747979337959720, 6.344076630960796770, 98.62055131934816643 ) ) ;
#173921=CARTESIAN_POINT ( 'NONE',  ( 19.05341960407617918, -5.049401038297876454, 71.04275706135234714 ) ) ;
#173922=CARTESIAN_POINT ( 'NONE',  ( -13.97604488694527625, -13.89961937509977652, 106.8739096053143669 ) ) ;
#173923=CARTESIAN_POINT ( 'NONE',  ( 15.80617190586769283, -15.72974639402175789, 100.6260903946857184 ) ) ;
#173924=CARTESIAN_POINT ( 'NONE',  ( 16.55341960407611168, 4.379528057220329451, 103.9572429386476813 ) ) ;
#173925=CARTESIAN_POINT ( 'NONE',  ( 15.80617190586746368, 15.72974639402197994, 49.37390960531436690 ) ) ;
#173926=CARTESIAN_POINT ( 'NONE',  ( -15.80617190586745835, -15.72974639402198527, 31.87390960531435979 ) ) ;
#173927=CARTESIAN_POINT ( 'NONE',  ( -16.52544592524342804, 4.483927247898546575, 106.0405762719810525 ) ) ;
#173929=CARTESIAN_POINT ( 'NONE',  ( -13.89961937509957401, -13.97604488694547875, 54.37609039468565442 ) ) ;
#173930=CARTESIAN_POINT ( 'NONE',  ( 8.224510206698953496, -14.34966873604960469, 27.91557627198103830 ) ) ;
#173932=CARTESIAN_POINT ( 'NONE',  ( -13.89961937509977652, 13.97604488694528158, 95.62390960531436690 ) ) ;
#173933=CARTESIAN_POINT ( 'NONE',  ( -21.55341960407619339, 5.719274019375674811, 83.54275706135234714 ) ) ;
#173934=CARTESIAN_POINT ( 'NONE',  ( -5.719274019375978568, 21.55341960407610458, 55.20724293864770260 ) ) ;
#173935=CARTESIAN_POINT ( 'NONE',  ( -0.05219959533937732626, 21.53943276465977519, 47.50109039468568994 ) ) ;
#173936=CARTESIAN_POINT ( 'NONE',  ( 18.62759615963271287, -10.81492255796078972, 98.33224293864769550 ) ) ;
#173937=CARTESIAN_POINT ( 'NONE',  ( -18.62759615963255300, -10.81492255796106328, 44.16775706135234714 ) ) ;
#173938=CARTESIAN_POINT ( 'NONE',  ( 13.89961937509977652, -13.97604488694527269, 23.12390960531436335 ) ) ;
#173939=CARTESIAN_POINT ( 'NONE',  ( 13.89961937509977652, -13.97604488694527269, 88.12390960531438111 ) ) ;
#173941=CARTESIAN_POINT ( 'NONE',  ( 12.06949235617757843, -12.14591786802309237, 108.1239096053143811 ) ) ;
#173942=CARTESIAN_POINT ( 'NONE',  ( -16.51473224551069308, -9.474510206698971260, 111.6655762719810383 ) ) ;
#173943=CARTESIAN_POINT ( 'NONE',  ( 8.314922557960818139, 14.29746914071049879, 54.58224293864769550 ) ) ;
#173944=CARTESIAN_POINT ( 'NONE',  ( 4.379528057220339221, -16.55341960407611168, 22.70724293864769194 ) ) ;
#173945=CARTESIAN_POINT ( 'NONE',  ( -5.153800228976328057, -19.02544592524343514, 47.29057627198102409 ) ) ;
#173946=CARTESIAN_POINT ( 'NONE',  ( -13.97604488694527625, -13.89961937509977652, 21.87390960531435979 ) ) ;
#173947=CARTESIAN_POINT ( 'NONE',  ( 5.719274019375991003, -21.55341960407610458, 47.70724293864770260 ) ) ;
#173948=CARTESIAN_POINT ( 'NONE',  ( 5.153800228976615827, -19.02544592524334988, 20.20942372801899722 ) ) ;
#173950=CARTESIAN_POINT ( 'NONE',  ( 4.483927247898545687, 16.52544592524342804, 39.79057627198103830 ) ) ;
#173951=CARTESIAN_POINT ( 'NONE',  ( -0.05219959533937732626, 21.53943276465977519, 52.50109039468567573 ) ) ;
#173952=CARTESIAN_POINT ( 'NONE',  ( 9.564922557960805705, 16.46253265017160317, 114.5822429386476955 ) ) ;
#173953=CARTESIAN_POINT ( 'NONE',  ( -4.379528057220086978, -16.55341960407618274, 59.79275706135234714 ) ) ;
#173954=CARTESIAN_POINT ( 'NONE',  ( 5.153800228976615827, -19.02544592524334988, 65.20942372801900433 ) ) ;
#173955=CARTESIAN_POINT ( 'NONE',  ( 16.52544592524342804, -4.483927247898539470, 33.54057627198102409 ) ) ;
#173956=CARTESIAN_POINT ( 'NONE',  ( 16.53943276465976808, 0.05219959533934440121, 111.2510903946856899 ) ) ;
#173957=CARTESIAN_POINT ( 'NONE',  ( -0.05219959533909027116, -19.03943276465977164, 42.49890960531435269 ) ) ;
#173958=CARTESIAN_POINT ( 'NONE',  ( -5.049401038298153566, 19.05341960407611168, 65.20724293864765286 ) ) ;
#173959=CARTESIAN_POINT ( 'NONE',  ( 19.02544592524343514, -5.153800228976328945, 28.54057627198102409 ) ) ;
#173960=CARTESIAN_POINT ( 'NONE',  ( 15.80617190586769283, -15.72974639402175789, 35.62609039468568994 ) ) ;
#173961=CARTESIAN_POINT ( 'NONE',  ( -5.049401038298153566, 19.05341960407611168, 45.20724293864769550 ) ) ;
#173962=CARTESIAN_POINT ( 'NONE',  ( 13.97604488694527802, 13.89961937509977652, 114.3739096053143669 ) ) ;
#173963=CARTESIAN_POINT ( 'NONE',  ( -5.049401038298153566, 19.05341960407611168, 50.20724293864770260 ) ) ;
#173964=CARTESIAN_POINT ( 'NONE',  ( 19.03943276465977164, -0.05219959533909143690, 113.7489096053143669 ) ) ;
#173965=CARTESIAN_POINT ( 'NONE',  ( 21.52544592524334988, 5.823673210054432836, 56.45942372801902565 ) ) ;
#173966=CARTESIAN_POINT ( 'NONE',  ( 0.05219959533910956823, 16.53943276465976808, 109.9989096053143527 ) ) ;
#173967=CARTESIAN_POINT ( 'NONE',  ( -19.03943276465977164, 0.05219959533909376836, 106.2489096053143669 ) ) ;
#173968=CARTESIAN_POINT ( 'NONE',  ( 16.55341960407618274, -4.379528057220086978, 81.04275706135236135 ) ) ;
#173969=CARTESIAN_POINT ( 'NONE',  ( 21.55341960407619695, -5.719274019375665929, 86.04275706135236135 ) ) ;
#173970=CARTESIAN_POINT ( 'NONE',  ( -8.314922557961024197, 14.29746914071037800, 47.91775706135234714 ) ) ;
#173971=CARTESIAN_POINT ( 'NONE',  ( 16.51473224551069308, 9.474510206698969483, 94.16557627198103830 ) ) ;
#173972=CARTESIAN_POINT ( 'NONE',  ( 4.379528057220092307, 16.55341960407617563, 47.29275706135234003 ) ) ;
#173973=CARTESIAN_POINT ( 'NONE',  ( -12.14591786802326823, 12.06949235617739902, 33.12609039468569705 ) ) ;
#173974=CARTESIAN_POINT ( 'NONE',  ( -14.34966873604972548, 8.224510206698743886, 83.33442372801903275 ) ) ;
#173975=CARTESIAN_POINT ( 'NONE',  ( -16.51473224551082808, 9.474510206698731452, 108.3344237280190043 ) ) ;
#173976=CARTESIAN_POINT ( 'NONE',  ( -10.81492255796078084, -18.62759615963271287, 92.08224293864769550 ) ) ;
#173977=CARTESIAN_POINT ( 'NONE',  ( 8.314922557960818139, 14.29746914071049879, 104.5822429386477097 ) ) ;
#173978=CARTESIAN_POINT ( 'NONE',  ( -0.05219959533936034679, 19.03943276465977164, 107.5010903946856615 ) ) ;
#173979=CARTESIAN_POINT ( 'NONE',  ( -14.29746914071037622, -8.314922557961029526, 79.16775706135234714 ) ) ;
#173980=CARTESIAN_POINT ( 'NONE',  ( -17.26058549869106429, 6.457015423128173559, 43.62254162523933587 ) ) ;
#173981=CARTESIAN_POINT ( 'NONE',  ( -9.474510206698720793, -16.51473224551083518, 64.58442372801900433 ) ) ;
#173982=CARTESIAN_POINT ( 'NONE',  ( 14.29746914071049879, -8.314922557960816363, 43.33224293864769550 ) ) ;
#173983=CARTESIAN_POINT ( 'NONE',  ( -8.314922557960811034, -14.29746914071050412, 32.08224293864769550 ) ) ;
#173984=CARTESIAN_POINT ( 'NONE',  ( -8.224510206698948167, 14.34966873604960824, 90.41557627198103830 ) ) ;
#173985=CARTESIAN_POINT ( 'NONE',  ( 16.51473224551083163, -9.474510206698727899, 30.83442372801900433 ) ) ;
#173986=CARTESIAN_POINT ( 'NONE',  ( -19.25663599770060941, 5.499999999999449329, 88.99419308057201761 ) ) ;
#173987=CARTESIAN_POINT ( 'NONE',  ( 15.72974639402176855, 15.80617190586768217, 31.87609039468567929 ) ) ;
#173988=CARTESIAN_POINT ( 'NONE',  ( 16.46253265017146816, 9.564922557961045513, 101.6677570613523329 ) ) ;
#173990=CARTESIAN_POINT ( 'NONE',  ( -9.474510206698964154, 16.51473224551069663, 90.41557627198103830 ) ) ;
#173991=CARTESIAN_POINT ( 'NONE',  ( -19.02544592524342804, 5.153800228976336051, 96.04057627198103830 ) ) ;
#173992=CARTESIAN_POINT ( 'NONE',  ( -10.81492255796078084, -18.62759615963271287, 62.08224293864769550 ) ) ;
#173993=CARTESIAN_POINT ( 'NONE',  ( -14.29746914071049879, 8.314922557960819915, 95.83224293864770971 ) ) ;
#173994=CARTESIAN_POINT ( 'NONE',  ( 5.049401038298161559, -19.05341960407611168, 67.70724293864769550 ) ) ;
#173995=CARTESIAN_POINT ( 'NONE',  ( 16.53943276465976808, -0.05219959533910856209, 113.7489096053143527 ) ) ;
#173996=CARTESIAN_POINT ( 'NONE',  ( 10.81492255796106328, -18.62759615963255655, 40.41775706135234714 ) ) ;
#173997=CARTESIAN_POINT ( 'NONE',  ( 0.05219959533937995610, -21.53943276465977519, 80.00109039468568994 ) ) ;
#173998=CARTESIAN_POINT ( 'NONE',  ( 13.89961937509977652, -13.97604488694527269, 63.12390960531435979 ) ) ;
#173999=CARTESIAN_POINT ( 'NONE',  ( 16.53943276465976808, 0.05219959533934440121, 81.25109039468568994 ) ) ;
#174000=CARTESIAN_POINT ( 'NONE',  ( 21.52544592524334988, 5.823673210054432836, 26.45942372801901854 ) ) ;
#174001=CARTESIAN_POINT ( 'NONE',  ( -15.72974639402176322, -15.80617190586768395, 24.37609039468567573 ) ) ;
#174002=CARTESIAN_POINT ( 'NONE',  ( -0.05219959533936034679, 19.03943276465977164, 57.50109039468566863 ) ) ;
#174003=CARTESIAN_POINT ( 'NONE',  ( 16.46253265017160672, -9.564922557960803928, 73.33224293864769550 ) ) ;
#174004=CARTESIAN_POINT ( 'NONE',  ( -13.97604488694547697, 13.89961937509957934, 28.12609039468565797 ) ) ;
#174005=CARTESIAN_POINT ( 'NONE',  ( -21.53943276465977519, -0.05219959533937600094, 83.75109039468568994 ) ) ;
#174006=CARTESIAN_POINT ( 'NONE',  ( -18.67979575497178146, -10.72451020669898902, 66.66557627198102409 ) ) ;
#174007=CARTESIAN_POINT ( 'NONE',  ( 8.314922557960818139, 14.29746914071049879, 54.58224293864769550 ) ) ;
#174008=CARTESIAN_POINT ( 'NONE',  ( 15.80617190586769283, -15.72974639402175789, 90.62609039468567573 ) ) ;
#174009=CARTESIAN_POINT ( 'NONE',  ( 9.564922557961047289, -16.46253265017146816, 35.41775706135233293 ) ) ;
#174010=CARTESIAN_POINT ( 'NONE',  ( 8.314922557960818139, 14.29746914071049879, 64.58224293864769550 ) ) ;
#174011=CARTESIAN_POINT ( 'NONE',  ( 5.153800228976335163, 19.02544592524342804, 24.79057627198102765 ) ) ;
#174012=CARTESIAN_POINT ( 'NONE',  ( -13.97604488694547697, 13.89961937509957934, 68.12609039468563310 ) ) ;
#174013=CARTESIAN_POINT ( 'NONE',  ( -14.29746914071049879, 8.314922557960819915, 35.83224293864768839 ) ) ;
#174014=CARTESIAN_POINT ( 'NONE',  ( 10.72451020669871369, 18.67979575497193778, 87.08442372801901854 ) ) ;
#174015=CARTESIAN_POINT ( 'NONE',  ( -13.89961937509977652, 13.97604488694528158, 80.62390960531436690 ) ) ;
#174016=CARTESIAN_POINT ( 'NONE',  ( -16.46253265017146816, -9.564922557961047289, 54.16775706135234003 ) ) ;
#174017=CARTESIAN_POINT ( 'NONE',  ( 10.81492255796078972, 18.62759615963270932, 49.58224293864769550 ) ) ;
#174018=CARTESIAN_POINT ( 'NONE',  ( -15.80617190586768217, 15.72974639402176855, 48.12609039468568284 ) ) ;
#174019=CARTESIAN_POINT ( 'NONE',  ( -15.80617190586745835, -15.72974639402198527, 96.87390960531436690 ) ) ;
#174020=CARTESIAN_POINT ( 'NONE',  ( 5.153800228976615827, -19.02544592524334988, 95.20942372801897591 ) ) ;
#174021=CARTESIAN_POINT ( 'NONE',  ( -4.379528057220086978, -16.55341960407618274, 64.79275706135234714 ) ) ;
#174023=CARTESIAN_POINT ( 'NONE',  ( -18.67979575497178146, -10.72451020669898902, 101.6655762719810383 ) ) ;
#174024=CARTESIAN_POINT ( 'NONE',  ( 4.483927247898545687, 16.52544592524342804, 104.7905762719810241 ) ) ;
#174026=CARTESIAN_POINT ( 'NONE',  ( 8.314922557961029526, -14.29746914071037800, 35.41775706135234003 ) ) ;
#174027=CARTESIAN_POINT ( 'NONE',  ( -15.72974639402197994, 15.80617190586746368, 60.62390960531437401 ) ) ;
#174028=CARTESIAN_POINT ( 'NONE',  ( -14.29746914071037622, -8.314922557961029526, 104.1677570613523471 ) ) ;
#174029=CARTESIAN_POINT ( 'NONE',  ( 0.05219959533909260263, 19.03943276465977164, 29.99890960531435979 ) ) ;
#174030=CARTESIAN_POINT ( 'NONE',  ( -12.06949235617739369, -12.14591786802326823, 69.37609039468567573 ) ) ;
#174031=CARTESIAN_POINT ( 'NONE',  ( -5.153800228976607833, 19.02544592524334988, 57.70942372801899012 ) ) ;
#174032=CARTESIAN_POINT ( 'NONE',  ( 18.67979575497194134, -10.72451020669871369, 45.83442372801901854 ) ) ;
#174033=CARTESIAN_POINT ( 'NONE',  ( 15.80617190586746368, 15.72974639402197994, 54.37390960531435979 ) ) ;
#174034=CARTESIAN_POINT ( 'NONE',  ( 12.14591786802327356, -12.06949235617739191, 95.62609039468568994 ) ) ;
#174035=CARTESIAN_POINT ( 'NONE',  ( -18.62759615963255300, -10.81492255796106328, 69.16775706135234714 ) ) ;
#174036=EDGE_CURVE ( 'NONE', #179099, #64402, #43853, .T. ) ;
#174037=CARTESIAN_POINT ( 'NONE',  ( 15.80617190586746368, 15.72974639402197994, 54.37390960531435979 ) ) ;
#174038=CARTESIAN_POINT ( 'NONE',  ( 5.823673210054125526, 21.52544592524343514, 29.79057627198102409 ) ) ;
#174041=CARTESIAN_POINT ( 'NONE',  ( -0.05219959533934338120, 16.53943276465976808, 77.50109039468567573 ) ) ;
#174042=CARTESIAN_POINT ( 'NONE',  ( -21.55341960407610458, -5.719274019375992779, 31.45724293864769550 ) ) ;
#174044=CARTESIAN_POINT ( 'NONE',  ( -5.153800228976328057, -19.02544592524343514, 97.29057627198099567 ) ) ;
#174045=CARTESIAN_POINT ( 'NONE',  ( -14.34966873604960291, -8.224510206698953496, 26.66557627198103475 ) ) ;
#174047=CARTESIAN_POINT ( 'NONE',  ( 8.314922557960818139, 14.29746914071049879, 104.5822429386477097 ) ) ;
#174048=CARTESIAN_POINT ( 'NONE',  ( 10.72451020669898902, -18.67979575497178502, 67.91557627198102409 ) ) ;
#174049=CARTESIAN_POINT ( 'NONE',  ( -16.55341960407617563, 4.379528057220093196, 93.54275706135234714 ) ) ;
#174050=CARTESIAN_POINT ( 'NONE',  ( 21.52544592524334988, 5.823673210054432836, 41.45942372801901143 ) ) ;
#174051=CARTESIAN_POINT ( 'NONE',  ( 19.03943276465977164, 0.05219959533936151252, 101.2510903946856757 ) ) ;
#174052=CARTESIAN_POINT ( 'NONE',  ( 14.29746914071049879, -8.314922557960816363, 108.3322429386477097 ) ) ;
#174053=CARTESIAN_POINT ( 'NONE',  ( 8.314922557961029526, -14.29746914071037800, 20.41775706135234714 ) ) ;
#174054=CARTESIAN_POINT ( 'NONE',  ( 0.05219959533909260263, 19.03943276465977164, 29.99890960531435979 ) ) ;
#174056=CARTESIAN_POINT ( 'NONE',  ( -0.05219959533909027116, -19.03943276465977164, 87.49890960531436690 ) ) ;
#174057=CARTESIAN_POINT ( 'NONE',  ( 16.52544592524335698, 4.483927247898782831, 71.45942372801901854 ) ) ;
#174058=CARTESIAN_POINT ( 'NONE',  ( 10.81492255796106328, -18.62759615963255655, 105.4177570613523613 ) ) ;
#174059=CARTESIAN_POINT ( 'NONE',  ( 15.72974639402199770, -15.80617190586745480, 58.12390960531435979 ) ) ;
#174060=CARTESIAN_POINT ( 'NONE',  ( -16.52544592524335698, -4.483927247898792601, 83.95942372801900433 ) ) ;
#174061=B_SPLINE_CURVE_WITH_KNOTS ( 'NONE', 3,
 ( #178439, #149099, #10589, #13555, #72250, #133928, #195618, #134934, #32699, #183408, #107529, #29721, #63022, #108534, #91353, #106548, #125695, #350, #17526, #139852, #168224, #92362, #154048, #121715, #153045, #48862, #31706, #93355, #94350, #77201, #185383, #109527 ),
 .UNSPECIFIED., .F., .F.,
 ( 4, 2, 2, 2, 2, 2, 2, 2, 2, 2, 2, 2, 2, 2, 2, 4 ),
 ( 1.652208230918760859E-15, 0.0003712461730052253150, 0.0007424923460087984144, 0.001113738519012371459, 0.001484984692015944505, 0.002227477038023091029, 0.002598723211026663857, 0.002969969384030237119, 0.003341215557033810381, 0.003712461730037383209, 0.004083707903040956037, 0.004454954076044529733, 0.004826200249048102561, 0.005197446422051675390, 0.005568692595055249085, 0.005939938768058821913 ),
 .UNSPECIFIED. ) ;
#174062=CARTESIAN_POINT ( 'NONE',  ( -16.51473224551082808, 9.474510206698731452, 78.33442372801900433 ) ) ;
#174063=CARTESIAN_POINT ( 'NONE',  ( -5.049401038298153566, 19.05341960407611168, 30.20724293864768839 ) ) ;
#174064=CARTESIAN_POINT ( 'NONE',  ( -5.153800228976328057, -19.02544592524343514, 82.29057627198103830 ) ) ;
#174065=CARTESIAN_POINT ( 'NONE',  ( 16.46253265017160672, -9.564922557960803928, 33.33224293864770260 ) ) ;
#174066=CARTESIAN_POINT ( 'NONE',  ( -16.51473224551082808, 9.474510206698731452, 78.33442372801900433 ) ) ;
#174068=CARTESIAN_POINT ( 'NONE',  ( 0.05219959533909260263, 19.03943276465977164, 99.99890960531436690 ) ) ;
#174069=CARTESIAN_POINT ( 'NONE',  ( 16.52544592524342804, -4.483927247898539470, 53.54057627198103120 ) ) ;
#174070=CARTESIAN_POINT ( 'NONE',  ( 21.52544592524344225, -5.823673210054117533, 63.54057627198103830 ) ) ;
#174072=CARTESIAN_POINT ( 'NONE',  ( -0.05219959533936034679, 19.03943276465977164, 27.50109039468566507 ) ) ;
#174074=CARTESIAN_POINT ( 'NONE',  ( 16.51473224551069308, 9.474510206698969483, 49.16557627198102409 ) ) ;
#174075=CARTESIAN_POINT ( 'NONE',  ( -0.05219959533909027116, -19.03943276465977164, 77.49890960531435269 ) ) ;
#174076=CARTESIAN_POINT ( 'NONE',  ( 12.14591786802327356, -12.06949235617739191, 40.62609039468567573 ) ) ;
#174079=CARTESIAN_POINT ( 'NONE',  ( 0.05219959533934541429, -16.53943276465976808, 70.00109039468568994 ) ) ;
#174080=CARTESIAN_POINT ( 'NONE',  ( -10.81492255796078084, -18.62759615963271287, 92.08224293864769550 ) ) ;
#174081=CARTESIAN_POINT ( 'NONE',  ( -4.483927247898782831, 16.52544592524335698, 42.70942372801901854 ) ) ;
#174082=CARTESIAN_POINT ( 'NONE',  ( 9.474510206698971260, -16.51473224551069308, 42.91557627198103120 ) ) ;
#174084=CARTESIAN_POINT ( 'NONE',  ( 0.05219959533937995610, -21.53943276465977519, 50.00109039468568994 ) ) ;
#174085=CARTESIAN_POINT ( 'NONE',  ( 5.049401038297881783, 19.05341960407617563, 67.29275706135234714 ) ) ;
#174086=CARTESIAN_POINT ( 'NONE',  ( -18.62759615963255300, -10.81492255796106328, 89.16775706135236135 ) ) ;
#174087=CARTESIAN_POINT ( 'NONE',  ( 17.48847506799968698, 5.747544572773780835, 96.67302562156719148 ) ) ;
#174089=CARTESIAN_POINT ( 'NONE',  ( 21.52544592524344225, -5.823673210054117533, 58.54057627198103120 ) ) ;
#174091=CARTESIAN_POINT ( 'NONE',  ( 5.049401038298161559, -19.05341960407611168, 97.70724293864766707 ) ) ;
#174092=CARTESIAN_POINT ( 'NONE',  ( -14.34966873604960291, -8.224510206698953496, 101.6655762719810383 ) ) ;
#174093=CARTESIAN_POINT ( 'NONE',  ( -16.53943276465976808, -0.05219959533934237506, 23.75109039468567929 ) ) ;
#174094=CARTESIAN_POINT ( 'NONE',  ( 16.55341960407618274, -4.379528057220086978, 106.0427570613523471 ) ) ;
#174096=CARTESIAN_POINT ( 'NONE',  ( -21.53943276465977519, 0.05219959533907696930, 101.2489096053143669 ) ) ;
#174097=CARTESIAN_POINT ( 'NONE',  ( 0.05219959533910956823, 16.53943276465976808, 44.99890960531435979 ) ) ;
#174098=CARTESIAN_POINT ( 'NONE',  ( -13.89961937509977652, 13.97604488694528158, 115.6239096053143669 ) ) ;
#174099=CARTESIAN_POINT ( 'NONE',  ( -9.564922557961040184, 16.46253265017147172, 87.91775706135233293 ) ) ;
#174100=CARTESIAN_POINT ( 'NONE',  ( -18.62759615963255300, -10.81492255796106328, 104.1677570613523471 ) ) ;
#174101=CARTESIAN_POINT ( 'NONE',  ( 14.29746914071049879, -8.314922557960816363, 33.33224293864769550 ) ) ;
#174102=CARTESIAN_POINT ( 'NONE',  ( -5.719274019375978568, 21.55341960407610458, 90.20724293864770971 ) ) ;
#174103=CARTESIAN_POINT ( 'NONE',  ( -21.52544592524343514, 5.823673210054127303, 51.04057627198103120 ) ) ;
#174104=CARTESIAN_POINT ( 'NONE',  ( 19.02544592524343514, -5.153800228976328945, 68.54057627198103830 ) ) ;
#174105=CARTESIAN_POINT ( 'NONE',  ( 4.379528057220339221, -16.55341960407611168, 32.70724293864770260 ) ) ;
#174106=CARTESIAN_POINT ( 'NONE',  ( -9.564922557960796823, -16.46253265017161027, 92.08224293864769550 ) ) ;
#174107=ORIENTED_EDGE ( 'NONE', *, *, #121605, .F. ) ;
#174108=CARTESIAN_POINT ( 'NONE',  ( 19.35633801406910237, -5.499999999999588773, 61.63373818172762952 ) ) ;
#174109=CARTESIAN_POINT ( 'NONE',  ( 0.05219959533936267826, -19.03943276465977164, 45.00109039468566863 ) ) ;
#174110=CARTESIAN_POINT ( 'NONE',  ( 5.823673210054125526, 21.52544592524343514, 74.79057627198105251 ) ) ;
#174111=CARTESIAN_POINT ( 'NONE',  ( 16.55341960407611168, 4.379528057220329451, 103.9572429386476813 ) ) ;
#174112=CARTESIAN_POINT ( 'NONE',  ( 10.81492255796106328, -18.62759615963255655, 40.41775706135234714 ) ) ;
#174114=CARTESIAN_POINT ( 'NONE',  ( 12.14591786802327356, -12.06949235617739191, 105.6260903946856899 ) ) ;
#174115=CARTESIAN_POINT ( 'NONE',  ( 19.02544592524343514, -5.153800228976328945, 33.54057627198102409 ) ) ;
#174116=CARTESIAN_POINT ( 'NONE',  ( 9.474510206698971260, -16.51473224551069308, 82.91557627198103830 ) ) ;
#174117=CARTESIAN_POINT ( 'NONE',  ( -19.02544592524342804, 5.153800228976336051, 26.04057627198103120 ) ) ;
#174118=CARTESIAN_POINT ( 'NONE',  ( 12.06949235617757843, -12.14591786802309237, 38.12390960531436690 ) ) ;
#174119=CARTESIAN_POINT ( 'NONE',  ( -21.55341960407619339, 5.719274019375674811, 78.54275706135236135 ) ) ;
#174121=CARTESIAN_POINT ( 'NONE',  ( 12.06949235617739724, 12.14591786802326823, 66.87609039468568994 ) ) ;
#174122=CARTESIAN_POINT ( 'NONE',  ( 19.03943276465977164, -0.05219959533909143690, 43.74890960531435979 ) ) ;
#174123=CARTESIAN_POINT ( 'NONE',  ( -9.564922557960796823, -16.46253265017161027, 47.08224293864769550 ) ) ;
#174124=ORIENTED_EDGE ( 'NONE', *, *, #91138, .F. ) ;
#174125=CARTESIAN_POINT ( 'NONE',  ( 21.55341960407619695, -5.719274019375665929, 106.0427570613523471 ) ) ;
#174126=CARTESIAN_POINT ( 'NONE',  ( -14.29746914071037622, -8.314922557961029526, 64.16775706135234714 ) ) ;
#174127=CARTESIAN_POINT ( 'NONE',  ( 5.823673210054444382, -21.52544592524334988, 100.2094237280190043 ) ) ;
#174128=CARTESIAN_POINT ( 'NONE',  ( 21.52544592524344225, -5.823673210054117533, 33.54057627198102409 ) ) ;
#174129=CARTESIAN_POINT ( 'NONE',  ( -5.153800228976607833, 19.02544592524334988, 112.7094237280190043 ) ) ;
#174130=CARTESIAN_POINT ( 'NONE',  ( 5.823673210054444382, -21.52544592524334988, 65.20942372801901854 ) ) ;
#174131=CARTESIAN_POINT ( 'NONE',  ( 12.06949235617739724, 12.14591786802326823, 41.87609039468568284 ) ) ;
#174132=CARTESIAN_POINT ( 'NONE',  ( 5.719274019375991003, -21.55341960407610458, 102.7072429386476955 ) ) ;
#174133=CARTESIAN_POINT ( 'NONE',  ( -9.474510206698720793, -16.51473224551083518, 99.58442372801900433 ) ) ;
#174134=CARTESIAN_POINT ( 'NONE',  ( 19.03943276465977164, -0.05219959533909143690, 63.74890960531435979 ) ) ;
#174135=CARTESIAN_POINT ( 'NONE',  ( -12.06949235617739369, -12.14591786802326823, 19.37609039468568639 ) ) ;
#174136=CARTESIAN_POINT ( 'NONE',  ( -19.05341960407617563, 5.049401038297882671, 108.5427570613523187 ) ) ;
#174137=CARTESIAN_POINT ( 'NONE',  ( 16.52544592524342804, -4.483927247898539470, 63.54057627198103830 ) ) ;
#174138=CARTESIAN_POINT ( 'NONE',  ( -12.06949235617739369, -12.14591786802326823, 74.37609039468568994 ) ) ;
#174139=CARTESIAN_POINT ( 'NONE',  ( 10.72451020669898902, -18.67979575497178502, 112.9155762719810383 ) ) ;
#174140=CARTESIAN_POINT ( 'NONE',  ( -5.049401038298153566, 19.05341960407611168, 50.20724293864770260 ) ) ;
#174141=CARTESIAN_POINT ( 'NONE',  ( -19.03943276465977164, 0.05219959533909376836, 56.24890960531435979 ) ) ;
#174142=CARTESIAN_POINT ( 'NONE',  ( 4.379528057220092307, 16.55341960407617563, 72.29275706135236135 ) ) ;
#174145=ORIENTED_EDGE ( 'NONE', *, *, #149169, .T. ) ;
#174146=CARTESIAN_POINT ( 'NONE',  ( -18.67979575497193778, 10.72451020669871902, 108.3344237280190185 ) ) ;
#174147=CARTESIAN_POINT ( 'NONE',  ( 13.89961937509977652, -13.97604488694527269, 28.12390960531435624 ) ) ;
#174149=CARTESIAN_POINT ( 'NONE',  ( -5.049401038297874678, -19.05341960407617918, 104.7927570613523471 ) ) ;
#174151=CARTESIAN_POINT ( 'NONE',  ( -15.80617190586745835, -15.72974639402198527, 46.87390960531435979 ) ) ;
#174152=CARTESIAN_POINT ( 'NONE',  ( 13.97604488694548053, -13.89961937509957401, 45.62609039468566863 ) ) ;
#174153=CARTESIAN_POINT ( 'NONE',  ( 14.34966873604972726, -8.224510206698740333, 25.83442372801901499 ) ) ;
#174154=CARTESIAN_POINT ( 'NONE',  ( -13.89961937509977652, 13.97604488694528158, 45.62390960531433848 ) ) ;
#174155=CARTESIAN_POINT ( 'NONE',  ( -19.03943276465977164, 0.05219959533909376836, 56.24890960531435979 ) ) ;
#174156=CARTESIAN_POINT ( 'NONE',  ( -21.53943276465977519, 0.05219959533907696930, 81.24890960531436690 ) ) ;
#174157=CARTESIAN_POINT ( 'NONE',  ( -13.97604488694527625, -13.89961937509977652, 106.8739096053143669 ) ) ;
#174158=EDGE_CURVE ( 'NONE', #142736, #127046, #199309, .T. ) ;
#174159=CARTESIAN_POINT ( 'NONE',  ( -13.89961937509977652, 13.97604488694528158, 45.62390960531433848 ) ) ;
#174160=DIRECTION ( 'NONE',  ( 0.000000000000000000, 0.000000000000000000, -1.000000000000000000 ) ) ;
#174161=CARTESIAN_POINT ( 'NONE',  ( 19.05341960407617918, -5.049401038297876454, 101.0427570613523045 ) ) ;
#174162=CARTESIAN_POINT ( 'NONE',  ( 12.06949235617757843, -12.14591786802309237, 63.12390960531435979 ) ) ;
#174163=CARTESIAN_POINT ( 'NONE',  ( 16.51473224551083163, -9.474510206698727899, 30.83442372801900433 ) ) ;
#174164=CARTESIAN_POINT ( 'NONE',  ( -10.81492255796078084, -18.62759615963271287, 97.08224293864770971 ) ) ;
#174165=CARTESIAN_POINT ( 'NONE',  ( 10.81492255796106328, -18.62759615963255655, 80.41775706135234714 ) ) ;
#174166=CARTESIAN_POINT ( 'NONE',  ( 0.05219959533909260263, 19.03943276465977164, 24.99890960531435269 ) ) ;
#174167=CARTESIAN_POINT ( 'NONE',  ( 5.823673210054444382, -21.52544592524334988, 75.20942372801901854 ) ) ;
#174168=CARTESIAN_POINT ( 'NONE',  ( -4.483927247898539470, -16.52544592524342804, 22.29057627198102765 ) ) ;
#174169=CARTESIAN_POINT ( 'NONE',  ( 21.55341960407619695, -5.719274019375665929, 81.04275706135236135 ) ) ;
#174170=CARTESIAN_POINT ( 'NONE',  ( 5.049401038298161559, -19.05341960407611168, 67.70724293864769550 ) ) ;
#174171=CARTESIAN_POINT ( 'NONE',  ( 5.719274019375673035, 21.55341960407619339, 47.29275706135234003 ) ) ;
#174172=CARTESIAN_POINT ( 'NONE',  ( 13.89961937509977652, -13.97604488694527269, 83.12390960531436690 ) ) ;
#174173=CARTESIAN_POINT ( 'NONE',  ( 8.314922557960818139, 14.29746914071049879, 99.58224293864770971 ) ) ;
#174174=CARTESIAN_POINT ( 'NONE',  ( -16.52544592524342804, 4.483927247898546575, 56.04057627198102409 ) ) ;
#174175=CARTESIAN_POINT ( 'NONE',  ( -18.62759615963270932, 10.81492255796079327, 65.83224293864769550 ) ) ;
#174176=CARTESIAN_POINT ( 'NONE',  ( 5.153800228976335163, 19.02544592524342804, 79.79057627198102409 ) ) ;
#174177=CARTESIAN_POINT ( 'NONE',  ( -15.80617190586745835, -15.72974639402198527, 81.87390960531435269 ) ) ;
#174178=CARTESIAN_POINT ( 'NONE',  ( -19.03943276465977164, -0.05219959533935918106, 63.75109039468566863 ) ) ;
#174179=CARTESIAN_POINT ( 'NONE',  ( -19.05341960407617918, 5.049401038297883559, 33.54275706135232582 ) ) ;
#174180=CARTESIAN_POINT ( 'NONE',  ( -16.52544592524342804, 4.483927247898546575, 71.04057627198103830 ) ) ;
#174181=CARTESIAN_POINT ( 'NONE',  ( 10.81492255796078972, 18.62759615963270932, 49.58224293864769550 ) ) ;
#174184=CARTESIAN_POINT ( 'NONE',  ( 14.29746914071037800, 8.314922557961029526, 101.6677570613523613 ) ) ;
#174186=CARTESIAN_POINT ( 'NONE',  ( 9.474510206698729675, 16.51473224551082808, 102.0844237280190043 ) ) ;
#174187=CARTESIAN_POINT ( 'NONE',  ( -16.52544592524342804, 4.483927247898546575, 71.04057627198103830 ) ) ;
#174188=CARTESIAN_POINT ( 'NONE',  ( -17.49999999999996447, 3.805241302050396346, 35.37352472782593082 ) ) ;
#174189=CARTESIAN_POINT ( 'NONE',  ( 19.03943276465977164, -0.05219959533909143690, 58.74890960531435979 ) ) ;
#174190=CARTESIAN_POINT ( 'NONE',  ( 4.379528057220339221, -16.55341960407611168, 47.70724293864770260 ) ) ;
#174191=CARTESIAN_POINT ( 'NONE',  ( 9.564922557960805705, 16.46253265017160317, 104.5822429386476955 ) ) ;
#174192=CARTESIAN_POINT ( 'NONE',  ( 13.89961937509957401, 13.97604488694547697, 81.87609039468564731 ) ) ;
#174193=CARTESIAN_POINT ( 'NONE',  ( 19.02544592524343514, -5.153800228976328945, 63.54057627198103830 ) ) ;
#174194=CARTESIAN_POINT ( 'NONE',  ( -16.46253265017160317, 9.564922557960807481, 80.83224293864769550 ) ) ;
#174195=CARTESIAN_POINT ( 'NONE',  ( 5.049401038298161559, -19.05341960407611168, 87.70724293864769550 ) ) ;
#174196=CARTESIAN_POINT ( 'NONE',  ( -21.52544592524343514, 5.823673210054127303, 66.04057627198103830 ) ) ;
#174197=CARTESIAN_POINT ( 'NONE',  ( 16.52544592524335698, 4.483927247898782831, 61.45942372801901854 ) ) ;
#174198=CARTESIAN_POINT ( 'NONE',  ( 16.46253265017146816, 9.564922557961045513, 101.6677570613523329 ) ) ;
#174199=CARTESIAN_POINT ( 'NONE',  ( 13.97604488694527802, 13.89961937509977652, 54.37390960531435979 ) ) ;
#174200=CARTESIAN_POINT ( 'NONE',  ( -0.05219959533907301413, -21.53943276465977519, 57.49890960531435979 ) ) ;
#174201=CARTESIAN_POINT ( 'NONE',  ( -13.89961937509957401, -13.97604488694547875, 94.37609039468566152 ) ) ;
#174202=CARTESIAN_POINT ( 'NONE',  ( 16.53943276465976808, -0.05219959533910856209, 23.74890960531435269 ) ) ;
#174203=CARTESIAN_POINT ( 'NONE',  ( -0.05219959533937732626, 21.53943276465977519, 42.50109039468567573 ) ) ;
#174204=CARTESIAN_POINT ( 'NONE',  ( -9.474510206698720793, -16.51473224551083518, 34.58442372801899722 ) ) ;
#174205=CARTESIAN_POINT ( 'NONE',  ( 16.52544592524335698, 4.483927247898782831, 56.45942372801902565 ) ) ;
#174206=CARTESIAN_POINT ( 'NONE',  ( 16.55341960407618274, -4.379528057220086978, 96.04275706135236135 ) ) ;
#174208=CARTESIAN_POINT ( 'NONE',  ( -4.379528057220086978, -16.55341960407618274, 74.79275706135234714 ) ) ;
#174209=CARTESIAN_POINT ( 'NONE',  ( 0.05219959533907565091, 21.53943276465977519, 24.99890960531435624 ) ) ;
#174210=CARTESIAN_POINT ( 'NONE',  ( 14.29746914071037800, 8.314922557961029526, 31.66775706135234358 ) ) ;
#174211=CARTESIAN_POINT ( 'NONE',  ( -13.97604488694527625, -13.89961937509977652, 41.87390960531435979 ) ) ;
#174212=CARTESIAN_POINT ( 'NONE',  ( -0.05219959533909027116, -19.03943276465977164, 52.49890960531436690 ) ) ;
#174213=CARTESIAN_POINT ( 'NONE',  ( 19.05341960407611168, 5.049401038298154454, 58.95724293864768129 ) ) ;
#174214=CARTESIAN_POINT ( 'NONE',  ( 15.72974639402176855, 15.80617190586768217, 41.87609039468568284 ) ) ;
#174215=CARTESIAN_POINT ( 'NONE',  ( 12.14591786802327356, -12.06949235617739191, 45.62609039468567573 ) ) ;
#174216=CARTESIAN_POINT ( 'NONE',  ( 16.52544592524335698, 4.483927247898782831, 111.4594237280190328 ) ) ;
#174217=CARTESIAN_POINT ( 'NONE',  ( -9.564922557960796823, -16.46253265017161027, 32.08224293864769550 ) ) ;
#174218=CARTESIAN_POINT ( 'NONE',  ( -15.80617190586768217, 15.72974639402176855, 108.1260903946856757 ) ) ;
#174219=CARTESIAN_POINT ( 'NONE',  ( 13.89961937509957401, 13.97604488694547697, 111.8760903946856757 ) ) ;
#174220=CARTESIAN_POINT ( 'NONE',  ( -13.89961937509957401, -13.97604488694547875, 74.37609039468566152 ) ) ;
#174221=CARTESIAN_POINT ( 'NONE',  ( 12.14591786802309770, 12.06949235617756955, 69.37390960531436690 ) ) ;
#174222=CARTESIAN_POINT ( 'NONE',  ( 5.049401038298161559, -19.05341960407611168, 37.70724293864768839 ) ) ;
#174223=CARTESIAN_POINT ( 'NONE',  ( -9.564922557961040184, 16.46253265017147172, 77.91775706135234714 ) ) ;
#174225=CARTESIAN_POINT ( 'NONE',  ( -21.55341960407619339, 5.719274019375674811, 73.54275706135234714 ) ) ;
#174226=CARTESIAN_POINT ( 'NONE',  ( -12.14591786802326823, 12.06949235617739902, 38.12609039468567573 ) ) ;
#174227=CARTESIAN_POINT ( 'NONE',  ( 16.36317988757058828, 7.306389748694952502, 38.40210391636775711 ) ) ;
#174228=CARTESIAN_POINT ( 'NONE',  ( 10.81492255796078972, 18.62759615963270932, 34.58224293864770260 ) ) ;
#174229=CARTESIAN_POINT ( 'NONE',  ( 0.05219959533934541429, -16.53943276465976808, 20.00109039468568639 ) ) ;
#174231=CARTESIAN_POINT ( 'NONE',  ( -0.05219959533936034679, 19.03943276465977164, 27.50109039468566507 ) ) ;
#174233=CARTESIAN_POINT ( 'NONE',  ( -5.049401038298153566, 19.05341960407611168, 45.20724293864769550 ) ) ;
#174235=CARTESIAN_POINT ( 'NONE',  ( 5.153800228976335163, 19.02544592524342804, 64.79057627198100988 ) ) ;
#174236=CARTESIAN_POINT ( 'NONE',  ( -19.36337904590693526, 5.499999999999952927, 100.4149413749561859 ) ) ;
#174238=CARTESIAN_POINT ( 'NONE',  ( -16.46253265017146816, -9.564922557961047289, 19.16775706135233293 ) ) ;
#174239=CARTESIAN_POINT ( 'NONE',  ( -14.34966873604972548, 8.224510206698743886, 113.3344237280190328 ) ) ;
#174240=CARTESIAN_POINT ( 'NONE',  ( -19.05341960407611168, -5.049401038298163336, 36.45724293864766707 ) ) ;
#174241=CARTESIAN_POINT ( 'NONE',  ( 19.05341960407611168, 5.049401038298154454, 98.95724293864766707 ) ) ;
#174242=CARTESIAN_POINT ( 'NONE',  ( -21.53943276465977519, -0.05219959533937600094, 73.75109039468567573 ) ) ;
#174243=CARTESIAN_POINT ( 'NONE',  ( 13.97604488694527802, 13.89961937509977652, 44.37390960531435269 ) ) ;
#174244=CARTESIAN_POINT ( 'NONE',  ( 0.05219959533937995610, -21.53943276465977519, 60.00109039468568284 ) ) ;
#174245=CARTESIAN_POINT ( 'NONE',  ( -0.05219959533936034679, 19.03943276465977164, 97.50109039468567573 ) ) ;
#174246=CARTESIAN_POINT ( 'NONE',  ( 18.67979575497178502, 10.72451020669898547, 24.16557627198103120 ) ) ;
#174247=CARTESIAN_POINT ( 'NONE',  ( 13.89961937509977652, -13.97604488694527269, 38.12390960531436690 ) ) ;
#174248=CARTESIAN_POINT ( 'NONE',  ( 18.62759615963271287, -10.81492255796078972, 108.3322429386477097 ) ) ;
#174249=CARTESIAN_POINT ( 'NONE',  ( 13.97604488694548053, -13.89961937509957401, 40.62609039468564731 ) ) ;
#174250=CARTESIAN_POINT ( 'NONE',  ( 4.379528057220339221, -16.55341960407611168, 107.7072429386476955 ) ) ;
#174251=CARTESIAN_POINT ( 'NONE',  ( 5.153800228976335163, 19.02544592524342804, 64.79057627198100988 ) ) ;
#174252=CARTESIAN_POINT ( 'NONE',  ( -4.379528057220086978, -16.55341960407618274, 19.79275706135235069 ) ) ;
#174253=CARTESIAN_POINT ( 'NONE',  ( 16.53943276465976808, -0.05219959533910856209, 73.74890960531433848 ) ) ;
#174254=CARTESIAN_POINT ( 'NONE',  ( 13.97604488694527802, 13.89961937509977652, 114.3739096053143669 ) ) ;
#174255=CARTESIAN_POINT ( 'NONE',  ( 16.46253265017146816, 9.564922557961045513, 91.66775706135234714 ) ) ;
#174256=CARTESIAN_POINT ( 'NONE',  ( 5.719274019375991003, -21.55341960407610458, 87.70724293864769550 ) ) ;
#174257=CARTESIAN_POINT ( 'NONE',  ( -21.55341960407619339, 5.719274019375674811, 58.54275706135235424 ) ) ;
#174258=CARTESIAN_POINT ( 'NONE',  ( -12.14591786802326823, 12.06949235617739902, 53.12609039468568284 ) ) ;
#174259=CARTESIAN_POINT ( 'NONE',  ( -12.06949235617739369, -12.14591786802326823, 54.37609039468568994 ) ) ;
#174260=CARTESIAN_POINT ( 'NONE',  ( 18.67979575497194134, -10.72451020669871369, 45.83442372801901854 ) ) ;
#174261=CARTESIAN_POINT ( 'NONE',  ( 21.52544592524344225, -5.823673210054117533, 58.54057627198103120 ) ) ;
#174262=CARTESIAN_POINT ( 'NONE',  ( 5.153800228976335163, 19.02544592524342804, 49.79057627198100988 ) ) ;
#174264=CARTESIAN_POINT ( 'NONE',  ( -8.314922557961024197, 14.29746914071037800, 72.91775706135234714 ) ) ;
#174265=CARTESIAN_POINT ( 'NONE',  ( -0.05219959533907301413, -21.53943276465977519, 107.4989096053143669 ) ) ;
#174266=CARTESIAN_POINT ( 'NONE',  ( -4.379528057220328563, 16.55341960407611168, 55.20724293864770260 ) ) ;
#174267=CARTESIAN_POINT ( 'NONE',  ( -16.52544592524335698, -4.483927247898792601, 58.95942372801902565 ) ) ;
#174268=CARTESIAN_POINT ( 'NONE',  ( 9.474510206698729675, 16.51473224551082808, 97.08442372801900433 ) ) ;
#174269=CARTESIAN_POINT ( 'NONE',  ( 10.81492255796078972, 18.62759615963270932, 94.58224293864769550 ) ) ;
#174270=CARTESIAN_POINT ( 'NONE',  ( 0.05219959533910956823, 16.53943276465976808, 44.99890960531435979 ) ) ;
#174272=CARTESIAN_POINT ( 'NONE',  ( 18.22780087662122384, -5.500000000000022204, 91.01540105326107266 ) ) ;
#174273=CARTESIAN_POINT ( 'NONE',  ( 18.67979575497178502, 10.72451020669898547, 74.16557627198102409 ) ) ;
#174274=CARTESIAN_POINT ( 'NONE',  ( 12.14591786802309770, 12.06949235617756955, 29.37390960531435269 ) ) ;
#174275=VERTEX_POINT ( 'NONE', #33894 ) ;
#174276=CARTESIAN_POINT ( 'NONE',  ( -17.49999999999998934, -5.500000000000015987, 56.28230962303566542 ) ) ;
#174277=CARTESIAN_POINT ( 'NONE',  ( -0.05219959533907301413, -21.53943276465977519, 107.4989096053143669 ) ) ;
#174278=CARTESIAN_POINT ( 'NONE',  ( -21.52544592524334988, -5.823673210054445271, 23.95942372801901143 ) ) ;
#174279=CARTESIAN_POINT ( 'NONE',  ( -14.29746914071049879, 8.314922557960819915, 35.83224293864768839 ) ) ;
#174280=CARTESIAN_POINT ( 'NONE',  ( -4.379528057220086978, -16.55341960407618274, 44.79275706135234714 ) ) ;
#174281=CARTESIAN_POINT ( 'NONE',  ( -19.02544592524342804, 5.153800228976336051, 51.04057627198103120 ) ) ;
#174282=CARTESIAN_POINT ( 'NONE',  ( -5.153800228976328057, -19.02544592524343514, 77.29057627198099567 ) ) ;
#174283=CARTESIAN_POINT ( 'NONE',  ( 21.55341960407610458, 5.719274019375980345, 28.95724293864769905 ) ) ;
#174285=CARTESIAN_POINT ( 'NONE',  ( -8.224510206698735004, -14.34966873604973081, 29.58442372801901854 ) ) ;
#174286=CARTESIAN_POINT ( 'NONE',  ( -5.049401038297874678, -19.05341960407617918, 49.79275706135231871 ) ) ;
#174287=CARTESIAN_POINT ( 'NONE',  ( -18.62759615963270932, 10.81492255796079327, 95.83224293864770971 ) ) ;
#174288=CARTESIAN_POINT ( 'NONE',  ( 8.314922557960818139, 14.29746914071049879, 29.58224293864769905 ) ) ;
#174289=CARTESIAN_POINT ( 'NONE',  ( 9.474510206698971260, -16.51473224551069308, 82.91557627198103830 ) ) ;
#174290=CARTESIAN_POINT ( 'NONE',  ( -10.81492255796078084, -18.62759615963271287, 62.08224293864769550 ) ) ;
#174291=CARTESIAN_POINT ( 'NONE',  ( 15.72974639402199770, -15.80617190586745480, 88.12390960531436690 ) ) ;
#174292=CARTESIAN_POINT ( 'NONE',  ( 14.29746914071037800, 8.314922557961029526, 21.66775706135235069 ) ) ;
#174293=CARTESIAN_POINT ( 'NONE',  ( 0.05219959533907565091, 21.53943276465977519, 24.99890960531435624 ) ) ;
#174294=CARTESIAN_POINT ( 'NONE',  ( -21.55341960407619339, 5.719274019375674811, 73.54275706135234714 ) ) ;
#174295=CARTESIAN_POINT ( 'NONE',  ( 16.51473224551069308, 9.474510206698969483, 74.16557627198103830 ) ) ;
#174297=CARTESIAN_POINT ( 'NONE',  ( 13.89961937509977652, -13.97604488694527269, 23.12390960531436335 ) ) ;
#174298=CARTESIAN_POINT ( 'NONE',  ( -16.46253265017160317, 9.564922557960807481, 80.83224293864769550 ) ) ;
#174299=CARTESIAN_POINT ( 'NONE',  ( -16.55341960407611168, -4.379528057220339221, 96.45724293864770971 ) ) ;
#174301=CARTESIAN_POINT ( 'NONE',  ( -19.02544592524334988, -5.153800228976617603, 98.95942372801900433 ) ) ;
#174303=CARTESIAN_POINT ( 'NONE',  ( 13.97604488694527802, 13.89961937509977652, 79.37390960531435269 ) ) ;
#174304=CARTESIAN_POINT ( 'NONE',  ( -18.67979575497193778, 10.72451020669871902, 83.33442372801903275 ) ) ;
#174305=CARTESIAN_POINT ( 'NONE',  ( 13.89961937509977652, -13.97604488694527269, 113.1239096053143527 ) ) ;
#174306=CARTESIAN_POINT ( 'NONE',  ( 8.314922557961029526, -14.29746914071037800, 80.41775706135234714 ) ) ;
#174308=CARTESIAN_POINT ( 'NONE',  ( 5.153800228976615827, -19.02544592524334988, 60.20942372801899012 ) ) ;
#174309=CARTESIAN_POINT ( 'NONE',  ( -9.474510206698720793, -16.51473224551083518, 19.58442372801899722 ) ) ;
#174311=CARTESIAN_POINT ( 'NONE',  ( 13.89961937509977652, -13.97604488694527269, 28.12390960531435624 ) ) ;
#174312=CARTESIAN_POINT ( 'NONE',  ( 8.314922557960818139, 14.29746914071049879, 29.58224293864769905 ) ) ;
#174314=CARTESIAN_POINT ( 'NONE',  ( 8.314922557961029526, -14.29746914071037800, 100.4177570613523471 ) ) ;
#174316=CARTESIAN_POINT ( 'NONE',  ( 8.224510206698742110, 14.34966873604972548, 87.08442372801901854 ) ) ;
#174317=CARTESIAN_POINT ( 'NONE',  ( -16.51473224551069308, -9.474510206698971260, 21.66557627198102765 ) ) ;
#174318=CARTESIAN_POINT ( 'NONE',  ( 15.72974639402176855, 15.80617190586768217, 96.87609039468568994 ) ) ;
#174319=CARTESIAN_POINT ( 'NONE',  ( -19.05341960407617563, 5.049401038297882671, 103.5427570613523329 ) ) ;
#174320=CARTESIAN_POINT ( 'NONE',  ( 21.53943276465977519, 0.05219959533937863772, 71.25109039468568994 ) ) ;
#174321=CARTESIAN_POINT ( 'NONE',  ( -16.46253265017146816, -9.564922557961047289, 44.16775706135232582 ) ) ;
#174322=CARTESIAN_POINT ( 'NONE',  ( -19.05341960407611168, -5.049401038298163336, 81.45724293864769550 ) ) ;
#174323=CARTESIAN_POINT ( 'NONE',  ( 5.153800228976335163, 19.02544592524342804, 74.79057627198103830 ) ) ;
#174326=CARTESIAN_POINT ( 'NONE',  ( -10.81492255796078084, -18.62759615963271287, 42.08224293864769550 ) ) ;
#174327=CARTESIAN_POINT ( 'NONE',  ( -19.05341960407611168, -5.049401038298163336, 46.45724293864768129 ) ) ;
#174328=CARTESIAN_POINT ( 'NONE',  ( -4.483927247898782831, 16.52544592524335698, 82.70942372801900433 ) ) ;
#174330=CARTESIAN_POINT ( 'NONE',  ( 14.29746914071049879, -8.314922557960816363, 83.33224293864769550 ) ) ;
#174332=CARTESIAN_POINT ( 'NONE',  ( -8.224510206698735004, -14.34966873604973081, 34.58442372801900433 ) ) ;
#174333=CARTESIAN_POINT ( 'NONE',  ( 16.55341960407611168, 4.379528057220329451, 108.9572429386476955 ) ) ;
#174334=CARTESIAN_POINT ( 'NONE',  ( -13.97604488694547697, 13.89961937509957934, 73.12609039468568994 ) ) ;
#174335=CARTESIAN_POINT ( 'NONE',  ( -14.29746914071049879, 8.314922557960819915, 75.83224293864769550 ) ) ;
#174336=CARTESIAN_POINT ( 'NONE',  ( -15.80617190586768217, 15.72974639402176855, 28.12609039468568284 ) ) ;
#174338=CARTESIAN_POINT ( 'NONE',  ( -10.72451020669898014, 18.67979575497178502, 95.41557627198102409 ) ) ;
#174339=CARTESIAN_POINT ( 'NONE',  ( 0.05219959533909260263, 19.03943276465977164, 109.9989096053143669 ) ) ;
#174340=CARTESIAN_POINT ( 'NONE',  ( 16.53943276465976808, -0.05219959533910856209, 73.74890960531433848 ) ) ;
#174342=CARTESIAN_POINT ( 'NONE',  ( -19.02544592524342804, 5.153800228976336051, 41.04057627198103120 ) ) ;
#174344=CARTESIAN_POINT ( 'NONE',  ( 19.03943276465977164, 0.05219959533936151252, 81.25109039468567573 ) ) ;
#174345=CARTESIAN_POINT ( 'NONE',  ( -15.72974639402176322, -15.80617190586768395, 19.37609039468568639 ) ) ;
#174346=CARTESIAN_POINT ( 'NONE',  ( -16.46253265017160317, 9.564922557960807481, 75.83224293864769550 ) ) ;
#174347=CARTESIAN_POINT ( 'NONE',  ( -13.89961937509957401, -13.97604488694547875, 54.37609039468565442 ) ) ;
#174348=CARTESIAN_POINT ( 'NONE',  ( -16.51473224551069308, -9.474510206698971260, 46.66557627198102409 ) ) ;
#174349=CARTESIAN_POINT ( 'NONE',  ( 16.52544592524342804, -4.483927247898539470, 63.54057627198103830 ) ) ;
#174350=CARTESIAN_POINT ( 'NONE',  ( 12.06949235617757843, -12.14591786802309237, 48.12390960531436690 ) ) ;
#174351=CARTESIAN_POINT ( 'NONE',  ( 9.474510206698971260, -16.51473224551069308, 77.91557627198103830 ) ) ;
#174352=CARTESIAN_POINT ( 'NONE',  ( -15.80617190586745835, -15.72974639402198527, 81.87390960531435269 ) ) ;
#174353=B_SPLINE_CURVE_WITH_KNOTS ( 'NONE', 3,
 ( #98391, #36729, #113569, #64103, #158097, #4395, #160089, #47953, #140936, #125770, #21576, #81232, #112582, #171288, #127745, #188448, #49928, #109604, #128738, #82223, #32775, #187470, #173278, #83234, #80251, #19589, #110592, #142913, #63099, #172274, #143913, #174276 ),
 .UNSPECIFIED., .F., .F.,
 ( 4, 2, 2, 2, 2, 2, 2, 2, 2, 2, 2, 2, 2, 2, 2, 4 ),
 ( 2.969368287472575283E-17, 0.0003712461730037064562, 0.0007424923460073832053, 0.001113738519011060009, 0.001484984692014736703, 0.002227477038022087925, 0.002598723211025753127, 0.002969969384029418763, 0.003341215557033083098, 0.003712461730036748734, 0.004083707903040413069, 0.004454954076044077838, 0.004826200249047743474, 0.005197446422051408242, 0.005568692595055073011, 0.005939938768058737779 ),
 .UNSPECIFIED. ) ;
#174354=CARTESIAN_POINT ( 'NONE',  ( 16.51473224551069308, 9.474510206698969483, 69.16557627198102409 ) ) ;
#174355=CARTESIAN_POINT ( 'NONE',  ( -5.823673210054116645, -21.52544592524344225, 77.29057627198102409 ) ) ;
#174356=CARTESIAN_POINT ( 'NONE',  ( 18.62759615963255655, 10.81492255796105972, 111.6677570613523613 ) ) ;
#174357=CARTESIAN_POINT ( 'NONE',  ( -19.05341960407611168, -5.049401038298163336, 21.45724293864768839 ) ) ;
#174358=CARTESIAN_POINT ( 'NONE',  ( 14.29746914071037800, 8.314922557961029526, 111.6677570613523613 ) ) ;
#174359=CARTESIAN_POINT ( 'NONE',  ( -4.379528057220328563, 16.55341960407611168, 90.20724293864770971 ) ) ;
#174360=CARTESIAN_POINT ( 'NONE',  ( -5.153800228976607833, 19.02544592524334988, 102.7094237280189759 ) ) ;
#174362=CARTESIAN_POINT ( 'NONE',  ( -5.823673210054431948, 21.52544592524334988, 22.70942372801901499 ) ) ;
#174363=CARTESIAN_POINT ( 'NONE',  ( 19.03943276465977164, 0.05219959533936151252, 51.25109039468567573 ) ) ;
#174364=CARTESIAN_POINT ( 'NONE',  ( -0.05219959533934338120, 16.53943276465976808, 112.5010903946857042 ) ) ;
#174365=CARTESIAN_POINT ( 'NONE',  ( -19.05341960407617563, 5.049401038297882671, 48.54275706135233293 ) ) ;
#174366=CARTESIAN_POINT ( 'NONE',  ( -9.474510206698964154, 16.51473224551069663, 105.4155762719810383 ) ) ;
#174367=CARTESIAN_POINT ( 'NONE',  ( -12.06949235617756955, 12.14591786802309770, 60.62390960531437401 ) ) ;
#174368=CARTESIAN_POINT ( 'NONE',  ( 17.50000000000000000, -5.500000000000000888, 120.0000000000000142 ) ) ;
#174369=CARTESIAN_POINT ( 'NONE',  ( 5.049401038298161559, -19.05341960407611168, 37.70724293864768839 ) ) ;
#174370=CARTESIAN_POINT ( 'NONE',  ( -10.81492255796105439, 18.62759615963255655, 112.9177570613523329 ) ) ;
#174371=CARTESIAN_POINT ( 'NONE',  ( -16.55341960407617563, 4.379528057220093196, 93.54275706135234714 ) ) ;
#174372=CARTESIAN_POINT ( 'NONE',  ( 10.81492255796106328, -18.62759615963255655, 45.41775706135234003 ) ) ;
#174373=CARTESIAN_POINT ( 'NONE',  ( 4.379528057220092307, 16.55341960407617563, 37.29275706135235424 ) ) ;
#174374=CARTESIAN_POINT ( 'NONE',  ( 18.67979575497178502, 10.72451020669898547, 24.16557627198103120 ) ) ;
#174375=CARTESIAN_POINT ( 'NONE',  ( 19.02544592524343514, -5.153800228976328945, 58.54057627198102409 ) ) ;
#174376=CARTESIAN_POINT ( 'NONE',  ( 0.05219959533909260263, 19.03943276465977164, 59.99890960531436690 ) ) ;
#174377=CARTESIAN_POINT ( 'NONE',  ( -0.05219959533934338120, 16.53943276465976808, 52.50109039468567573 ) ) ;
#174378=CARTESIAN_POINT ( 'NONE',  ( 8.314922557960818139, 14.29746914071049879, 99.58224293864770971 ) ) ;
#174379=CARTESIAN_POINT ( 'NONE',  ( 14.29746914071049879, -8.314922557960816363, 23.33224293864769194 ) ) ;
#174381=CARTESIAN_POINT ( 'NONE',  ( -21.53943276465977519, -0.05219959533937600094, 58.75109039468568994 ) ) ;
#174382=CARTESIAN_POINT ( 'NONE',  ( -16.51473224551069308, -9.474510206698971260, 91.66557627198103830 ) ) ;
#174383=CARTESIAN_POINT ( 'NONE',  ( -13.97604488694527625, -13.89961937509977652, 76.87390960531433848 ) ) ;
#174384=CARTESIAN_POINT ( 'NONE',  ( -19.02544592524342804, 5.153800228976336051, 96.04057627198103830 ) ) ;
#174385=CARTESIAN_POINT ( 'NONE',  ( -12.06949235617756955, 12.14591786802309770, 40.62390960531435269 ) ) ;
#174386=CARTESIAN_POINT ( 'NONE',  ( -12.14591786802326823, 12.06949235617739902, 108.1260903946856757 ) ) ;
#174387=CARTESIAN_POINT ( 'NONE',  ( -0.05219959533910754901, -16.53943276465976808, 32.49890960531435979 ) ) ;
#174389=DIRECTION ( 'NONE',  ( -0.000000000000000000, -0.000000000000000000, 1.000000000000000000 ) ) ;
#174390=CARTESIAN_POINT ( 'NONE',  ( -16.51473224551082808, 9.474510206698731452, 43.33442372801900433 ) ) ;
#174391=CARTESIAN_POINT ( 'NONE',  ( 19.02544592524343514, -5.153800228976328945, 68.54057627198103830 ) ) ;
#174392=CARTESIAN_POINT ( 'NONE',  ( -19.03943276465977164, -0.05219959533935918106, 58.75109039468566863 ) ) ;
#174395=CARTESIAN_POINT ( 'NONE',  ( 19.03943276465977164, 0.05219959533936151252, 86.25109039468567573 ) ) ;
#174396=CARTESIAN_POINT ( 'NONE',  ( -16.52544592524335698, -4.483927247898792601, 63.95942372801901854 ) ) ;
#174397=CARTESIAN_POINT ( 'NONE',  ( 17.12812012977026654, 6.668231424565988164, 93.85948759323144941 ) ) ;
#174398=CARTESIAN_POINT ( 'NONE',  ( 5.153800228976335163, 19.02544592524342804, 99.79057627198102409 ) ) ;
#174399=CARTESIAN_POINT ( 'NONE',  ( 0.05219959533937995610, -21.53943276465977519, 35.00109039468568284 ) ) ;
#174400=CARTESIAN_POINT ( 'NONE',  ( -13.97604488694547697, 13.89961937509957934, 93.12609039468566152 ) ) ;
#174401=CARTESIAN_POINT ( 'NONE',  ( 19.02544592524343514, -5.153800228976328945, 113.5405762719810241 ) ) ;
#174402=CARTESIAN_POINT ( 'NONE',  ( -13.89961937509977652, 13.97604488694528158, 50.62390960531435979 ) ) ;
#174403=EDGE_CURVE ( 'NONE', #194062, #91449, #147333, .T. ) ;
#174404=CARTESIAN_POINT ( 'NONE',  ( -5.049401038298153566, 19.05341960407611168, 90.20724293864766707 ) ) ;
#174405=CARTESIAN_POINT ( 'NONE',  ( 16.53943276465976808, -0.05219959533910856209, 53.74890960531437401 ) ) ;
#174406=CARTESIAN_POINT ( 'NONE',  ( 13.97604488694527802, 13.89961937509977652, 49.37390960531434558 ) ) ;
#174407=CARTESIAN_POINT ( 'NONE',  ( 16.51473224551083163, -9.474510206698727899, 60.83442372801900433 ) ) ;
#174408=CARTESIAN_POINT ( 'NONE',  ( -9.564922557961040184, 16.46253265017147172, 27.91775706135232582 ) ) ;
#174409=CARTESIAN_POINT ( 'NONE',  ( -0.05219959533909027116, -19.03943276465977164, 72.49890960531435269 ) ) ;
#174410=CARTESIAN_POINT ( 'NONE',  ( 21.52544592524344225, -5.823673210054117533, 58.54057627198103120 ) ) ;
#174411=CARTESIAN_POINT ( 'NONE',  ( 4.483927247898545687, 16.52544592524342804, 64.79057627198103830 ) ) ;
#174412=CARTESIAN_POINT ( 'NONE',  ( 21.52544592524334988, 5.823673210054432836, 111.4594237280190328 ) ) ;
#174414=CARTESIAN_POINT ( 'NONE',  ( -0.05219959533907301413, -21.53943276465977519, 32.49890960531435979 ) ) ;
#174415=CARTESIAN_POINT ( 'NONE',  ( -9.474510206698964154, 16.51473224551069663, 50.41557627198102409 ) ) ;
#174416=CARTESIAN_POINT ( 'NONE',  ( -19.05341960407611168, -5.049401038298163336, 36.45724293864766707 ) ) ;
#174417=CARTESIAN_POINT ( 'NONE',  ( -4.483927247898539470, -16.52544592524342804, 102.2905762719810383 ) ) ;
#174418=CARTESIAN_POINT ( 'NONE',  ( 15.80617190586746368, 15.72974639402197994, 109.3739096053143811 ) ) ;
#174419=CARTESIAN_POINT ( 'NONE',  ( 19.02544592524343514, -5.153800228976328945, 113.5405762719810241 ) ) ;
#174420=CARTESIAN_POINT ( 'NONE',  ( -10.72451020669870658, -18.67979575497194134, 24.58442372801901499 ) ) ;
#174421=CARTESIAN_POINT ( 'NONE',  ( -16.46253265017160317, 9.564922557960807481, 105.8322429386476955 ) ) ;
#174422=CARTESIAN_POINT ( 'NONE',  ( -16.46253265017160317, 9.564922557960807481, 25.83224293864769194 ) ) ;
#174423=CARTESIAN_POINT ( 'NONE',  ( -18.67979575497193778, 10.72451020669871902, 73.33442372801901854 ) ) ;
#174424=CARTESIAN_POINT ( 'NONE',  ( -21.52544592524343514, 5.823673210054127303, 96.04057627198102409 ) ) ;
#174425=CARTESIAN_POINT ( 'NONE',  ( 16.19135201231366139, -7.376712067591912003, 107.3131914594796825 ) ) ;
#174426=CARTESIAN_POINT ( 'NONE',  ( 16.46253265017160672, -9.564922557960803928, 53.33224293864768839 ) ) ;
#174428=CARTESIAN_POINT ( 'NONE',  ( -4.379528057220086978, -16.55341960407618274, 44.79275706135234714 ) ) ;
#174429=CARTESIAN_POINT ( 'NONE',  ( 4.379528057220339221, -16.55341960407611168, 107.7072429386476955 ) ) ;
#174431=CARTESIAN_POINT ( 'NONE',  ( -19.03943276465977164, 0.05219959533909376836, 56.24890960531435979 ) ) ;
#174432=CARTESIAN_POINT ( 'NONE',  ( -12.14591786802309592, -12.06949235617757132, 96.87390960531436690 ) ) ;
#174433=CARTESIAN_POINT ( 'NONE',  ( -18.62759615963270932, 10.81492255796079327, 45.83224293864769550 ) ) ;
#174434=CARTESIAN_POINT ( 'NONE',  ( 4.379528057220339221, -16.55341960407611168, 67.70724293864769550 ) ) ;
#174435=CARTESIAN_POINT ( 'NONE',  ( -5.049401038297874678, -19.05341960407617918, 109.7927570613523187 ) ) ;
#174436=CARTESIAN_POINT ( 'NONE',  ( -21.55341960407619339, 5.719274019375674811, 88.54275706135236135 ) ) ;
#174437=CARTESIAN_POINT ( 'NONE',  ( 16.79531203550647689, -7.028104445595604766, 76.24755011779559766 ) ) ;
#174438=CARTESIAN_POINT ( 'NONE',  ( -12.06949235617739369, -12.14591786802326823, 94.37609039468568994 ) ) ;
#174439=CARTESIAN_POINT ( 'NONE',  ( 4.379528057220339221, -16.55341960407611168, 42.70724293864770260 ) ) ;
#174440=VECTOR ( 'NONE', #104694, 1000.000000000000000 ) ;
#174441=CARTESIAN_POINT ( 'NONE',  ( -5.049401038298153566, 19.05341960407611168, 35.20724293864768839 ) ) ;
#174442=CARTESIAN_POINT ( 'NONE',  ( 16.46253265017160672, -9.564922557960803928, 93.33224293864769550 ) ) ;
#174443=CARTESIAN_POINT ( 'NONE',  ( -15.80617190586745835, -15.72974639402198527, 91.87390960531436690 ) ) ;
#174444=CARTESIAN_POINT ( 'NONE',  ( -16.53943276465976808, -0.05219959533934237506, 33.75109039468568284 ) ) ;
#174445=CARTESIAN_POINT ( 'NONE',  ( -14.34966873604960291, -8.224510206698953496, 71.66557627198100988 ) ) ;
#174446=CARTESIAN_POINT ( 'NONE',  ( 0.05219959533937995610, -21.53943276465977519, 80.00109039468568994 ) ) ;
#174447=CARTESIAN_POINT ( 'NONE',  ( 8.224510206698742110, 14.34966873604972548, 97.08442372801904696 ) ) ;
#174449=CARTESIAN_POINT ( 'NONE',  ( -19.34837522270365895, -5.499999999999739764, 65.86337684832577111 ) ) ;
#174450=CARTESIAN_POINT ( 'NONE',  ( -16.53943276465976808, 0.05219959533911058130, 26.24890960531435624 ) ) ;
#174451=CARTESIAN_POINT ( 'NONE',  ( 0.05219959533934541429, -16.53943276465976808, 70.00109039468568994 ) ) ;
#174452=CARTESIAN_POINT ( 'NONE',  ( 16.46253265017160672, -9.564922557960803928, 83.33224293864768129 ) ) ;
#174453=CARTESIAN_POINT ( 'NONE',  ( 19.05341960407611168, 5.049401038298154454, 103.9572429386476671 ) ) ;
#174454=CARTESIAN_POINT ( 'NONE',  ( 10.72451020669871369, 18.67979575497193778, 92.08442372801901854 ) ) ;
#174455=CARTESIAN_POINT ( 'NONE',  ( -16.55341960407617563, 4.379528057220093196, 88.54275706135236135 ) ) ;
#174456=CARTESIAN_POINT ( 'NONE',  ( 8.314922557960818139, 14.29746914071049879, 59.58224293864770260 ) ) ;
#174457=CARTESIAN_POINT ( 'NONE',  ( 19.05341960407611168, 5.049401038298154454, 63.95724293864769550 ) ) ;
#174459=CARTESIAN_POINT ( 'NONE',  ( -16.51473224551082808, 9.474510206698731452, 103.3344237280190043 ) ) ;
#174460=CARTESIAN_POINT ( 'NONE',  ( 16.51473224551069308, 9.474510206698969483, 29.16557627198103475 ) ) ;
#174461=CARTESIAN_POINT ( 'NONE',  ( 16.51473224551069308, 9.474510206698969483, 84.16557627198102409 ) ) ;
#174462=CARTESIAN_POINT ( 'NONE',  ( 9.564922557961047289, -16.46253265017146816, 110.4177570613523471 ) ) ;
#174464=CARTESIAN_POINT ( 'NONE',  ( -5.049401038297874678, -19.05341960407617918, 19.79275706135233293 ) ) ;
#174465=CARTESIAN_POINT ( 'NONE',  ( 14.34966873604972726, -8.224510206698740333, 75.83442372801900433 ) ) ;
#174466=CARTESIAN_POINT ( 'NONE',  ( -16.51473224551082808, 9.474510206698731452, 108.3344237280190043 ) ) ;
#174467=CARTESIAN_POINT ( 'NONE',  ( 4.379528057220339221, -16.55341960407611168, 112.7072429386476955 ) ) ;
#174468=CARTESIAN_POINT ( 'NONE',  ( 14.34966873604972726, -8.224510206698740333, 65.83442372801900433 ) ) ;
#174469=CARTESIAN_POINT ( 'NONE',  ( -16.53943276465976808, -0.05219959533934237506, 48.75109039468568284 ) ) ;
#174470=CARTESIAN_POINT ( 'NONE',  ( -9.564922557960796823, -16.46253265017161027, 22.08224293864768839 ) ) ;
#174471=CARTESIAN_POINT ( 'NONE',  ( 19.02544592524334988, 5.153800228976608722, 71.45942372801900433 ) ) ;
#174472=CARTESIAN_POINT ( 'NONE',  ( 15.80617190586769283, -15.72974639402175789, 105.6260903946856899 ) ) ;
#174473=CARTESIAN_POINT ( 'NONE',  ( 5.153800228976335163, 19.02544592524342804, 29.79057627198102409 ) ) ;
#174474=CARTESIAN_POINT ( 'NONE',  ( -5.049401038298153566, 19.05341960407611168, 75.20724293864769550 ) ) ;
#174475=CARTESIAN_POINT ( 'NONE',  ( 12.14591786802309770, 12.06949235617756955, 69.37390960531436690 ) ) ;
#174478=CARTESIAN_POINT ( 'NONE',  ( 9.474510206698729675, 16.51473224551082808, 37.08442372801899722 ) ) ;
#174479=CARTESIAN_POINT ( 'NONE',  ( 18.67979575497178502, 10.72451020669898547, 39.16557627198102409 ) ) ;
#174480=CARTESIAN_POINT ( 'NONE',  ( 5.153800228976615827, -19.02544592524334988, 20.20942372801899722 ) ) ;
#174481=CARTESIAN_POINT ( 'NONE',  ( -9.564922557960796823, -16.46253265017161027, 92.08224293864769550 ) ) ;
#174482=CARTESIAN_POINT ( 'NONE',  ( 10.72451020669871369, 18.67979575497193778, 102.0844237280190185 ) ) ;
#174483=CARTESIAN_POINT ( 'NONE',  ( -5.823673210054116645, -21.52544592524344225, 57.29057627198103120 ) ) ;
#174484=CARTESIAN_POINT ( 'NONE',  ( -19.05341960407611168, -5.049401038298163336, 91.45724293864766707 ) ) ;
#174485=CARTESIAN_POINT ( 'NONE',  ( 16.51473224551083163, -9.474510206698727899, 75.83442372801900433 ) ) ;
#174486=CARTESIAN_POINT ( 'NONE',  ( 16.46253265017160672, -9.564922557960803928, 98.33224293864769550 ) ) ;
#174487=CARTESIAN_POINT ( 'NONE',  ( -16.46253265017146816, -9.564922557961047289, 94.16775706135233293 ) ) ;
#174488=CARTESIAN_POINT ( 'NONE',  ( 5.049401038298161559, -19.05341960407611168, 22.70724293864769194 ) ) ;
#174489=CARTESIAN_POINT ( 'NONE',  ( 16.46253265017160672, -9.564922557960803928, 83.33224293864768129 ) ) ;
#174490=CARTESIAN_POINT ( 'NONE',  ( -10.72451020669898014, 18.67979575497178502, 60.41557627198102409 ) ) ;
#174491=CARTESIAN_POINT ( 'NONE',  ( 8.314922557961029526, -14.29746914071037800, 30.41775706135234358 ) ) ;
#174492=CARTESIAN_POINT ( 'NONE',  ( 18.67979575497194134, -10.72451020669871369, 50.83442372801901143 ) ) ;
#174493=CARTESIAN_POINT ( 'NONE',  ( -21.53943276465977519, -0.05219959533937600094, 93.75109039468567573 ) ) ;
#174494=CARTESIAN_POINT ( 'NONE',  ( 8.224510206698742110, 14.34966873604972548, 102.0844237280190185 ) ) ;
#174495=CARTESIAN_POINT ( 'NONE',  ( 13.89961937509977652, -13.97604488694527269, 83.12390960531436690 ) ) ;
#174496=CARTESIAN_POINT ( 'NONE',  ( -16.55341960407611168, -4.379528057220339221, 91.45724293864769550 ) ) ;
#174497=CARTESIAN_POINT ( 'NONE',  ( -8.314922557961024197, 14.29746914071037800, 112.9177570613523329 ) ) ;
#174498=CARTESIAN_POINT ( 'NONE',  ( 16.51473224551083163, -9.474510206698727899, 70.83442372801900433 ) ) ;
#174499=CARTESIAN_POINT ( 'NONE',  ( -15.72974639402176322, -15.80617190586768395, 39.37609039468567573 ) ) ;
#174500=CARTESIAN_POINT ( 'NONE',  ( 14.34966873604960469, 8.224510206698951720, 89.16557627198102409 ) ) ;
#174501=CARTESIAN_POINT ( 'NONE',  ( -19.02544592524342804, 5.153800228976336051, 116.0405762719810383 ) ) ;
#174502=CARTESIAN_POINT ( 'NONE',  ( -0.05219959533910754901, -16.53943276465976808, 27.49890960531435269 ) ) ;
#174503=CARTESIAN_POINT ( 'NONE',  ( 15.80617190586769283, -15.72974639402175789, 85.62609039468568994 ) ) ;
#174504=CARTESIAN_POINT ( 'NONE',  ( 16.53943276465976808, 0.05219959533934440121, 51.25109039468568994 ) ) ;
#174505=CARTESIAN_POINT ( 'NONE',  ( 21.55341960407619695, -5.719274019375665929, 36.04275706135234714 ) ) ;
#174506=EDGE_LOOP ( 'NONE', ( #27124, #165401, #14999, #91106, #143447, #43736, #145162, #80126 ) ) ;
#174507=CARTESIAN_POINT ( 'NONE',  ( 21.52544592524344225, -5.823673210054117533, 113.5405762719810383 ) ) ;
#174508=CARTESIAN_POINT ( 'NONE',  ( 16.55341960407611168, 4.379528057220329451, 88.95724293864769550 ) ) ;
#174509=CARTESIAN_POINT ( 'NONE',  ( -18.89770734986052148, -5.499999999999913847, 49.10214472496641491 ) ) ;
#174510=CARTESIAN_POINT ( 'NONE',  ( 16.55341960407611168, 4.379528057220329451, 68.95724293864769550 ) ) ;
#174511=CARTESIAN_POINT ( 'NONE',  ( -16.51473224551069308, -9.474510206698971260, 61.66557627198103120 ) ) ;
#174512=CARTESIAN_POINT ( 'NONE',  ( 14.29746914071037800, 8.314922557961029526, 101.6677570613523613 ) ) ;
#174513=CARTESIAN_POINT ( 'NONE',  ( -19.05341960407611168, -5.049401038298163336, 36.45724293864766707 ) ) ;
#174514=CARTESIAN_POINT ( 'NONE',  ( -0.05219959533907301413, -21.53943276465977519, 47.49890960531435979 ) ) ;
#174515=CARTESIAN_POINT ( 'NONE',  ( -12.06949235617756955, 12.14591786802309770, 75.62390960531439532 ) ) ;
#174516=CARTESIAN_POINT ( 'NONE',  ( -15.72974639402197994, 15.80617190586746368, 85.62390960531436690 ) ) ;
#174517=CARTESIAN_POINT ( 'NONE',  ( -19.02544592524342804, 5.153800228976336051, 91.04057627198100988 ) ) ;
#174518=CARTESIAN_POINT ( 'NONE',  ( 19.03943276465977164, -0.05219959533909143690, 33.74890960531435979 ) ) ;
#174519=CARTESIAN_POINT ( 'NONE',  ( -16.51473224551082808, 9.474510206698731452, 98.33442372801900433 ) ) ;
#174520=CARTESIAN_POINT ( 'NONE',  ( 0.05219959533907565091, 21.53943276465977519, 44.99890960531435979 ) ) ;
#174521=CARTESIAN_POINT ( 'NONE',  ( 10.81492255796106328, -18.62759615963255655, 70.41775706135236135 ) ) ;
#174522=CARTESIAN_POINT ( 'NONE',  ( -19.02544592524342804, 5.153800228976336051, 51.04057627198103120 ) ) ;
#174523=CARTESIAN_POINT ( 'NONE',  ( -19.03943276465977164, 0.05219959533909376836, 91.24890960531436690 ) ) ;
#174524=ORIENTED_EDGE ( 'NONE', *, *, #134338, .F. ) ;
#174525=CARTESIAN_POINT ( 'NONE',  ( -8.224510206698735004, -14.34966873604973081, 59.58442372801901854 ) ) ;
#174526=CARTESIAN_POINT ( 'NONE',  ( -18.67979575497193778, 10.72451020669871902, 43.33442372801901143 ) ) ;
#174527=CARTESIAN_POINT ( 'NONE',  ( 18.67979575497194134, -10.72451020669871369, 75.83442372801900433 ) ) ;
#174528=CARTESIAN_POINT ( 'NONE',  ( -15.80617190586745835, -15.72974639402198527, 26.87390960531435979 ) ) ;
#174529=CARTESIAN_POINT ( 'NONE',  ( 5.719274019375991003, -21.55341960407610458, 102.7072429386476955 ) ) ;
#174530=CARTESIAN_POINT ( 'NONE',  ( 0.05219959533937995610, -21.53943276465977519, 40.00109039468567573 ) ) ;
#174531=CARTESIAN_POINT ( 'NONE',  ( 14.34966873604972726, -8.224510206698740333, 60.83442372801901854 ) ) ;
#174532=CARTESIAN_POINT ( 'NONE',  ( -0.05219959533907301413, -21.53943276465977519, 67.49890960531436690 ) ) ;
#174533=CARTESIAN_POINT ( 'NONE',  ( 5.049401038297881783, 19.05341960407617563, 27.29275706135232937 ) ) ;
#174534=CARTESIAN_POINT ( 'NONE',  ( -13.89961937509977652, 13.97604488694528158, 70.62390960531432427 ) ) ;
#174535=CARTESIAN_POINT ( 'NONE',  ( -0.05219959533934338120, 16.53943276465976808, 97.50109039468567573 ) ) ;
#174537=CARTESIAN_POINT ( 'NONE',  ( 19.03943276465977164, -0.05219959533909143690, 103.7489096053143669 ) ) ;
#174539=CARTESIAN_POINT ( 'NONE',  ( -0.05219959533936034679, 19.03943276465977164, 82.50109039468567573 ) ) ;
#174540=CARTESIAN_POINT ( 'NONE',  ( -21.55341960407610458, -5.719274019375992779, 61.45724293864770260 ) ) ;
#174541=CARTESIAN_POINT ( 'NONE',  ( 8.314922557960818139, 14.29746914071049879, 39.58224293864769550 ) ) ;
#174542=CARTESIAN_POINT ( 'NONE',  ( -0.05219959533936034679, 19.03943276465977164, 102.5010903946856757 ) ) ;
#174544=CARTESIAN_POINT ( 'NONE',  ( 19.05341960407617918, -5.049401038297876454, 101.0427570613523045 ) ) ;
#174545=CARTESIAN_POINT ( 'NONE',  ( -18.62759615963270932, 10.81492255796079327, 80.83224293864769550 ) ) ;
#174546=CARTESIAN_POINT ( 'NONE',  ( 5.153800228976615827, -19.02544592524334988, 60.20942372801899012 ) ) ;
#174547=CARTESIAN_POINT ( 'NONE',  ( 17.50000000000000000, 5.499999999999997335, 106.7030961746582847 ) ) ;
#174548=CARTESIAN_POINT ( 'NONE',  ( 5.049401038298161559, -19.05341960407611168, 62.70724293864769550 ) ) ;
#174549=CARTESIAN_POINT ( 'NONE',  ( -12.06949235617756955, 12.14591786802309770, 60.62390960531437401 ) ) ;
#174550=CARTESIAN_POINT ( 'NONE',  ( 16.46253265017160672, -9.564922557960803928, 53.33224293864768839 ) ) ;
#174551=CARTESIAN_POINT ( 'NONE',  ( -0.05219959533910754901, -16.53943276465976808, 47.49890960531435979 ) ) ;
#174552=CARTESIAN_POINT ( 'NONE',  ( -9.474510206698964154, 16.51473224551069663, 25.41557627198103120 ) ) ;
#174554=CARTESIAN_POINT ( 'NONE',  ( 14.29746914071049879, -8.314922557960816363, 33.33224293864769550 ) ) ;
#174555=CARTESIAN_POINT ( 'NONE',  ( 9.474510206698971260, -16.51473224551069308, 67.91557627198102409 ) ) ;
#174556=CARTESIAN_POINT ( 'NONE',  ( -17.97161686093721400, 5.500000000000146549, 50.99637206859166838 ) ) ;
#174557=CARTESIAN_POINT ( 'NONE',  ( -16.51473224551082808, 9.474510206698731452, 33.33442372801899722 ) ) ;
#174558=CARTESIAN_POINT ( 'NONE',  ( -14.29746914071037622, -8.314922557961029526, 49.16775706135234003 ) ) ;
#174559=CARTESIAN_POINT ( 'NONE',  ( -5.719274019375978568, 21.55341960407610458, 45.20724293864769550 ) ) ;
#174560=CARTESIAN_POINT ( 'NONE',  ( 10.72451020669871369, 18.67979575497193778, 107.0844237280190043 ) ) ;
#174561=CARTESIAN_POINT ( 'NONE',  ( -16.46253265017160317, 9.564922557960807481, 75.83224293864769550 ) ) ;
#174562=CARTESIAN_POINT ( 'NONE',  ( 13.89961937509977652, -13.97604488694527269, 113.1239096053143527 ) ) ;
#174563=CARTESIAN_POINT ( 'NONE',  ( 0.05219959533909260263, 19.03943276465977164, 109.9989096053143669 ) ) ;
#174565=CARTESIAN_POINT ( 'NONE',  ( -0.05219959533937732626, 21.53943276465977519, 37.50109039468568284 ) ) ;
#174567=CARTESIAN_POINT ( 'NONE',  ( 0.05219959533910956823, 16.53943276465976808, 99.99890960531436690 ) ) ;
#174568=CARTESIAN_POINT ( 'NONE',  ( 21.53943276465977519, -0.05219959533907433946, 93.74890960531436690 ) ) ;
#174569=CARTESIAN_POINT ( 'NONE',  ( 5.049401038298161559, -19.05341960407611168, 77.70724293864765286 ) ) ;
#174570=CARTESIAN_POINT ( 'NONE',  ( 17.72517630440430025, -5.500000000000136779, 68.42175719257211597 ) ) ;
#174571=CARTESIAN_POINT ( 'NONE',  ( 9.474510206698971260, -16.51473224551069308, 92.91557627198103830 ) ) ;
#174572=CARTESIAN_POINT ( 'NONE',  ( -15.80617190586768217, 15.72974639402176855, 28.12609039468568284 ) ) ;
#174574=CARTESIAN_POINT ( 'NONE',  ( -19.02544592524342804, 5.153800228976336051, 91.04057627198100988 ) ) ;
#174575=ADVANCED_FACE ( 'NONE', ( #51047 ), #116416, .T. ) ;
#174577=CARTESIAN_POINT ( 'NONE',  ( 14.34966873604960469, 8.224510206698951720, 114.1655762719810383 ) ) ;
#174578=CARTESIAN_POINT ( 'NONE',  ( -9.564922557960796823, -16.46253265017161027, 32.08224293864769550 ) ) ;
#174579=CARTESIAN_POINT ( 'NONE',  ( -16.46253265017146816, -9.564922557961047289, 109.1677570613523471 ) ) ;
#174581=CARTESIAN_POINT ( 'NONE',  ( -16.52544592524342804, 4.483927247898546575, 116.0405762719810383 ) ) ;
#174582=CARTESIAN_POINT ( 'NONE',  ( 21.53943276465977519, 0.05219959533937863772, 81.25109039468568994 ) ) ;
#174583=CARTESIAN_POINT ( 'NONE',  ( -19.03943276465977164, 0.05219959533909376836, 66.24890960531436690 ) ) ;
#174584=CARTESIAN_POINT ( 'NONE',  ( 18.62759615963255655, 10.81492255796105972, 26.66775706135235424 ) ) ;
#174585=CARTESIAN_POINT ( 'NONE',  ( 15.80617190586746368, 15.72974639402197994, 109.3739096053143811 ) ) ;
#174587=CARTESIAN_POINT ( 'NONE',  ( 19.03943276465977164, -0.05219959533909143690, 83.74890960531436690 ) ) ;
#174589=CARTESIAN_POINT ( 'NONE',  ( 4.483927247898790824, -16.52544592524335698, 20.20942372801900788 ) ) ;
#174590=CARTESIAN_POINT ( 'NONE',  ( -15.72974639402197994, 15.80617190586746368, 40.62390960531435269 ) ) ;
#174591=CARTESIAN_POINT ( 'NONE',  ( -21.52544592524334988, -5.823673210054445271, 58.95942372801902565 ) ) ;
#174592=CARTESIAN_POINT ( 'NONE',  ( 16.51473224551069308, 9.474510206698969483, 109.1655762719810383 ) ) ;
#174593=CARTESIAN_POINT ( 'NONE',  ( -16.51473224551082808, 9.474510206698731452, 93.33442372801900433 ) ) ;
#174594=CARTESIAN_POINT ( 'NONE',  ( -13.89961937509977652, 13.97604488694528158, 65.62390960531436690 ) ) ;
#174595=CARTESIAN_POINT ( 'NONE',  ( -13.89961937509977652, 13.97604488694528158, 90.62390960531432427 ) ) ;
#174596=CARTESIAN_POINT ( 'NONE',  ( -14.29746914071049879, 8.314922557960819915, 100.8322429386477097 ) ) ;
#174597=CARTESIAN_POINT ( 'NONE',  ( 4.379528057220339221, -16.55341960407611168, 87.70724293864769550 ) ) ;
#174598=CARTESIAN_POINT ( 'NONE',  ( -5.049401038298153566, 19.05341960407611168, 115.2072429386477097 ) ) ;
#174599=CARTESIAN_POINT ( 'NONE',  ( 16.53943276465976808, -0.05219959533910856209, 53.74890960531437401 ) ) ;
#174600=CARTESIAN_POINT ( 'NONE',  ( -5.153800228976328057, -19.02544592524343514, 42.29057627198101699 ) ) ;
#174601=CARTESIAN_POINT ( 'NONE',  ( -15.80617190586768217, 15.72974639402176855, 73.12609039468567573 ) ) ;
#174602=CARTESIAN_POINT ( 'NONE',  ( 5.049401038297881783, 19.05341960407617563, 87.29275706135234714 ) ) ;
#174603=CARTESIAN_POINT ( 'NONE',  ( -16.53943276465976808, 0.05219959533911058130, 56.24890960531436690 ) ) ;
#174604=CARTESIAN_POINT ( 'NONE',  ( 5.719274019375991003, -21.55341960407610458, 112.7072429386476955 ) ) ;
#174605=CARTESIAN_POINT ( 'NONE',  ( -21.53943276465977519, 0.05219959533907696930, 41.24890960531435269 ) ) ;
#174606=CARTESIAN_POINT ( 'NONE',  ( 19.39056639909673407, 5.500000000000047962, 73.28948781074340957 ) ) ;
#174608=CARTESIAN_POINT ( 'NONE',  ( -5.153800228976328057, -19.02544592524343514, 62.29057627198100988 ) ) ;
#174609=CARTESIAN_POINT ( 'NONE',  ( -4.483927247898539470, -16.52544592524342804, 42.29057627198103120 ) ) ;
#174610=ADVANCED_FACE ( 'NONE', ( #102668 ), #130573, .T. ) ;
#174611=CARTESIAN_POINT ( 'NONE',  ( -14.34966873604972548, 8.224510206698743886, 98.33442372801901854 ) ) ;
#174612=CARTESIAN_POINT ( 'NONE',  ( -8.314922557961024197, 14.29746914071037800, 77.91775706135231871 ) ) ;
#174613=CARTESIAN_POINT ( 'NONE',  ( -19.03943276465977164, -0.05219959533935918106, 43.75109039468566863 ) ) ;
#174614=CARTESIAN_POINT ( 'NONE',  ( -17.49999999999999289, 5.624438216177594541, 70.81670344914645909 ) ) ;
#174615=CARTESIAN_POINT ( 'NONE',  ( 9.564922557960805705, 16.46253265017160317, 94.58224293864769550 ) ) ;
#174616=CARTESIAN_POINT ( 'NONE',  ( -19.02544592524342804, 5.153800228976336051, 46.04057627198101699 ) ) ;
#174617=CARTESIAN_POINT ( 'NONE',  ( 8.224510206698953496, -14.34966873604960469, 62.91557627198102409 ) ) ;
#174618=CARTESIAN_POINT ( 'NONE',  ( 17.05116617787825106, -6.768360034955805737, 101.1567555325920011 ) ) ;
#174619=CARTESIAN_POINT ( 'NONE',  ( -21.55341960407610458, -5.719274019375992779, 26.45724293864768839 ) ) ;
#174620=CARTESIAN_POINT ( 'NONE',  ( 18.67979575497178502, 10.72451020669898547, 44.16557627198103120 ) ) ;
#174621=CARTESIAN_POINT ( 'NONE',  ( 8.314922557960818139, 14.29746914071049879, 79.58224293864769550 ) ) ;
#174622=CARTESIAN_POINT ( 'NONE',  ( 14.34966873604972726, -8.224510206698740333, 35.83442372801901143 ) ) ;
#174623=CARTESIAN_POINT ( 'NONE',  ( -14.29746914071049879, 8.314922557960819915, 75.83224293864769550 ) ) ;
#174624=CARTESIAN_POINT ( 'NONE',  ( -18.22780087662119541, 5.500000000000102141, 66.01763182126894947 ) ) ;
#174625=CARTESIAN_POINT ( 'NONE',  ( 9.564922557961047289, -16.46253265017146816, 75.41775706135234714 ) ) ;
#174626=CARTESIAN_POINT ( 'NONE',  ( -18.67979575497178146, -10.72451020669898902, 21.66557627198102409 ) ) ;
#174629=CARTESIAN_POINT ( 'NONE',  ( 8.224510206698742110, 14.34966873604972548, 32.08442372801901854 ) ) ;
#174630=CARTESIAN_POINT ( 'NONE',  ( -12.14591786802326823, 12.06949235617739902, 108.1260903946856757 ) ) ;
#174631=CARTESIAN_POINT ( 'NONE',  ( 5.153800228976615827, -19.02544592524334988, 65.20942372801900433 ) ) ;
#174632=CARTESIAN_POINT ( 'NONE',  ( -18.62759615963270932, 10.81492255796079327, 50.83224293864770971 ) ) ;
#174633=CARTESIAN_POINT ( 'NONE',  ( -0.05219959533937732626, 21.53943276465977519, 72.50109039468568994 ) ) ;
#174635=CARTESIAN_POINT ( 'NONE',  ( -16.53943276465976808, -0.05219959533934237506, 28.75109039468567929 ) ) ;
#174636=CARTESIAN_POINT ( 'NONE',  ( -19.03943276465977164, 0.05219959533909376836, 21.24890960531436335 ) ) ;
#174637=CARTESIAN_POINT ( 'NONE',  ( -5.153800228976328057, -19.02544592524343514, 92.29057627198099567 ) ) ;
#174638=CARTESIAN_POINT ( 'NONE',  ( -5.153800228976328057, -19.02544592524343514, 27.29057627198103120 ) ) ;
#174639=CARTESIAN_POINT ( 'NONE',  ( -8.314922557960811034, -14.29746914071050412, 92.08224293864769550 ) ) ;
#174641=CARTESIAN_POINT ( 'NONE',  ( -19.05341960407611168, -5.049401038298163336, 96.45724293864769550 ) ) ;
#174643=CARTESIAN_POINT ( 'NONE',  ( -16.46253265017146816, -9.564922557961047289, 99.16775706135233293 ) ) ;
#174644=CARTESIAN_POINT ( 'NONE',  ( 5.823673210054125526, 21.52544592524343514, 79.79057627198102409 ) ) ;
#174645=CARTESIAN_POINT ( 'NONE',  ( -9.474510206698964154, 16.51473224551069663, 45.41557627198103120 ) ) ;
#174646=CARTESIAN_POINT ( 'NONE',  ( -9.474510206698720793, -16.51473224551083518, 64.58442372801900433 ) ) ;
#174647=CARTESIAN_POINT ( 'NONE',  ( -21.53943276465977519, 0.05219959533907696930, 116.2489096053143669 ) ) ;
#174648=CARTESIAN_POINT ( 'NONE',  ( 19.05341960407611168, 5.049401038298154454, 63.95724293864769550 ) ) ;
#174649=CARTESIAN_POINT ( 'NONE',  ( 13.97604488694527802, 13.89961937509977652, 104.3739096053143385 ) ) ;
#174651=CARTESIAN_POINT ( 'NONE',  ( -0.05219959533934338120, 16.53943276465976808, 32.50109039468568284 ) ) ;
#174652=CARTESIAN_POINT ( 'NONE',  ( -5.823673210054116645, -21.52544592524344225, 97.29057627198105251 ) ) ;
#174653=CARTESIAN_POINT ( 'NONE',  ( 14.29746914071049879, -8.314922557960816363, 108.3322429386477097 ) ) ;
#174654=CARTESIAN_POINT ( 'NONE',  ( 16.46253265017160672, -9.564922557960803928, 93.33224293864769550 ) ) ;
#174655=CARTESIAN_POINT ( 'NONE',  ( 16.46253265017146816, 9.564922557961045513, 56.66775706135233293 ) ) ;
#174656=CARTESIAN_POINT ( 'NONE',  ( 15.80617190586746368, 15.72974639402197994, 84.37390960531438111 ) ) ;
#174657=CARTESIAN_POINT ( 'NONE',  ( 12.06949235617757843, -12.14591786802309237, 43.12390960531435269 ) ) ;
#174658=CARTESIAN_POINT ( 'NONE',  ( 19.05341960407617918, -5.049401038297876454, 21.04275706135232582 ) ) ;
#174659=CARTESIAN_POINT ( 'NONE',  ( 8.224510206698742110, 14.34966873604972548, 67.08442372801901854 ) ) ;
#174660=CARTESIAN_POINT ( 'NONE',  ( -19.05341960407611168, -5.049401038298163336, 91.45724293864766707 ) ) ;
#174661=CARTESIAN_POINT ( 'NONE',  ( 9.474510206698971260, -16.51473224551069308, 42.91557627198103120 ) ) ;
#174662=CARTESIAN_POINT ( 'NONE',  ( -10.81492255796105439, 18.62759615963255655, 57.91775706135234714 ) ) ;
#174663=CARTESIAN_POINT ( 'NONE',  ( 18.67979575497194134, -10.72451020669871369, 70.83442372801901854 ) ) ;
#174664=CARTESIAN_POINT ( 'NONE',  ( -13.97604488694527625, -13.89961937509977652, 56.87390960531434558 ) ) ;
#174665=CARTESIAN_POINT ( 'NONE',  ( -21.55341960407619339, 5.719274019375674811, 38.54275706135234714 ) ) ;
#174666=CARTESIAN_POINT ( 'NONE',  ( -5.049401038297874678, -19.05341960407617918, 69.79275706135233293 ) ) ;
#174668=CARTESIAN_POINT ( 'NONE',  ( 13.97604488694527802, 13.89961937509977652, 34.37390960531436690 ) ) ;
#174669=CARTESIAN_POINT ( 'NONE',  ( -14.29746914071037622, -8.314922557961029526, 84.16775706135234714 ) ) ;
#174670=CARTESIAN_POINT ( 'NONE',  ( -9.474510206698964154, 16.51473224551069663, 50.41557627198102409 ) ) ;
#174671=CARTESIAN_POINT ( 'NONE',  ( -13.97604488694527625, -13.89961937509977652, 21.87390960531435979 ) ) ;
#174672=CARTESIAN_POINT ( 'NONE',  ( 9.474510206698971260, -16.51473224551069308, 112.9155762719810383 ) ) ;
#174673=CARTESIAN_POINT ( 'NONE',  ( 19.02544592524343514, -5.153800228976328945, 33.54057627198102409 ) ) ;
#174674=CARTESIAN_POINT ( 'NONE',  ( -21.55341960407610458, -5.719274019375992779, 86.45724293864770971 ) ) ;
#174675=CARTESIAN_POINT ( 'NONE',  ( 12.14591786802327356, -12.06949235617739191, 75.62609039468567573 ) ) ;
#174677=CARTESIAN_POINT ( 'NONE',  ( -5.153800228976607833, 19.02544592524334988, 37.70942372801899722 ) ) ;
#174678=CARTESIAN_POINT ( 'NONE',  ( -9.564922557960796823, -16.46253265017161027, 47.08224293864769550 ) ) ;
#174679=CARTESIAN_POINT ( 'NONE',  ( -16.55341960407611168, -4.379528057220339221, 46.45724293864769550 ) ) ;
#174680=CARTESIAN_POINT ( 'NONE',  ( -4.379528057220328563, 16.55341960407611168, 75.20724293864769550 ) ) ;
#174681=CARTESIAN_POINT ( 'NONE',  ( 9.474510206698971260, -16.51473224551069308, 97.91557627198102409 ) ) ;
#174682=CARTESIAN_POINT ( 'NONE',  ( -13.89961937509977652, 13.97604488694528158, 80.62390960531436690 ) ) ;
#174683=CARTESIAN_POINT ( 'NONE',  ( -21.53943276465977519, -0.05219959533937600094, 48.75109039468568284 ) ) ;
#174684=CARTESIAN_POINT ( 'NONE',  ( 16.51473224551069308, 9.474510206698969483, 94.16557627198103830 ) ) ;
#174686=CARTESIAN_POINT ( 'NONE',  ( -18.62759615963255300, -10.81492255796106328, 104.1677570613523471 ) ) ;
#174687=CARTESIAN_POINT ( 'NONE',  ( 12.06949235617739724, 12.14591786802326823, 76.87609039468567573 ) ) ;
#174688=CARTESIAN_POINT ( 'NONE',  ( -5.719274019375665041, -21.55341960407619695, 24.79275706135235779 ) ) ;
#174689=CARTESIAN_POINT ( 'NONE',  ( -15.72974639402197994, 15.80617190586746368, 100.6239096053143811 ) ) ;
#174690=CARTESIAN_POINT ( 'NONE',  ( 8.314922557960818139, 14.29746914071049879, 49.58224293864769550 ) ) ;
#174691=CARTESIAN_POINT ( 'NONE',  ( -19.03943276465977164, 0.05219959533909376836, 46.24890960531435979 ) ) ;
#174692=CARTESIAN_POINT ( 'NONE',  ( 8.314922557960818139, 14.29746914071049879, 74.58224293864768129 ) ) ;
#174693=CARTESIAN_POINT ( 'NONE',  ( 15.72974639402199770, -15.80617190586745480, 33.12390960531435979 ) ) ;
#174694=CARTESIAN_POINT ( 'NONE',  ( -19.02544592524334988, -5.153800228976617603, 23.95942372801900078 ) ) ;
#174695=CARTESIAN_POINT ( 'NONE',  ( 8.314922557960818139, 14.29746914071049879, 99.58224293864770971 ) ) ;
#174697=CARTESIAN_POINT ( 'NONE',  ( -12.14591786802326823, 12.06949235617739902, 73.12609039468567573 ) ) ;
#174698=CARTESIAN_POINT ( 'NONE',  ( 19.02544592524343514, -5.153800228976328945, 73.54057627198103830 ) ) ;
#174699=CARTESIAN_POINT ( 'NONE',  ( -16.66605195848753240, -6.777442124193050255, 20.99343749471847786 ) ) ;
#174700=CARTESIAN_POINT ( 'NONE',  ( 10.81492255796078972, 18.62759615963270932, 39.58224293864769550 ) ) ;
#174701=CARTESIAN_POINT ( 'NONE',  ( 0.05219959533934541429, -16.53943276465976808, 100.0010903946857042 ) ) ;
#174702=CARTESIAN_POINT ( 'NONE',  ( 16.51473224551083163, -9.474510206698727899, 110.8344237280190043 ) ) ;
#174703=CARTESIAN_POINT ( 'NONE',  ( 5.823673210054444382, -21.52544592524334988, 85.20942372801901854 ) ) ;
#174704=CARTESIAN_POINT ( 'NONE',  ( 16.46253265017160672, -9.564922557960803928, 68.33224293864770971 ) ) ;
#174705=CARTESIAN_POINT ( 'NONE',  ( -5.719274019375978568, 21.55341960407610458, 105.2072429386477097 ) ) ;
#174706=CARTESIAN_POINT ( 'NONE',  ( -8.224510206698735004, -14.34966873604973081, 59.58442372801901854 ) ) ;
#174707=CARTESIAN_POINT ( 'NONE',  ( -9.564922557960796823, -16.46253265017161027, 22.08224293864768839 ) ) ;
#174708=CARTESIAN_POINT ( 'NONE',  ( -14.29746914071037622, -8.314922557961029526, 24.16775706135235424 ) ) ;
#174709=CARTESIAN_POINT ( 'NONE',  ( 19.05341960407617918, -5.049401038297876454, 86.04275706135233293 ) ) ;
#174710=CARTESIAN_POINT ( 'NONE',  ( -10.72451020669898014, 18.67979575497178502, 75.41557627198102409 ) ) ;
#174711=CARTESIAN_POINT ( 'NONE',  ( 9.564922557961047289, -16.46253265017146816, 60.41775706135233293 ) ) ;
#174713=CARTESIAN_POINT ( 'NONE',  ( 10.81492255796078972, 18.62759615963270932, 99.58224293864770971 ) ) ;
#174714=DIRECTION ( 'NONE',  ( -0.000000000000000000, 1.000000000000000000, -0.000000000000000000 ) ) ;
#174715=CARTESIAN_POINT ( 'NONE',  ( 13.97604488694527802, 13.89961937509977652, 79.37390960531435269 ) ) ;
#174716=CARTESIAN_POINT ( 'NONE',  ( -19.03943276465977164, -0.05219959533935946555, 113.7510903946856757 ) ) ;
#174717=CARTESIAN_POINT ( 'NONE',  ( -12.14591786802326823, 12.06949235617739902, 28.12609039468568284 ) ) ;
#174718=CARTESIAN_POINT ( 'NONE',  ( -18.22780087662119541, 5.500000000000102141, 51.01763182126894947 ) ) ;
#174719=CARTESIAN_POINT ( 'NONE',  ( -0.05219959533907301413, -21.53943276465977519, 102.4989096053143811 ) ) ;
#174720=CARTESIAN_POINT ( 'NONE',  ( -8.314922557960811034, -14.29746914071050412, 67.08224293864770971 ) ) ;
#174721=CARTESIAN_POINT ( 'NONE',  ( -5.049401038298153566, 19.05341960407611168, 65.20724293864765286 ) ) ;
#174722=CARTESIAN_POINT ( 'NONE',  ( -21.52544592524334988, -5.823673210054445271, 88.95942372801901854 ) ) ;
#174723=CARTESIAN_POINT ( 'NONE',  ( 12.06949235617739724, 12.14591786802326823, 36.87609039468568994 ) ) ;
#174724=CARTESIAN_POINT ( 'NONE',  ( -16.51473224551082808, 9.474510206698731452, 43.33442372801900433 ) ) ;
#174725=CARTESIAN_POINT ( 'NONE',  ( -10.72451020669870658, -18.67979575497194134, 49.58442372801901143 ) ) ;
#174726=CARTESIAN_POINT ( 'NONE',  ( 5.719274019375991003, -21.55341960407610458, 52.70724293864769550 ) ) ;
#174727=CARTESIAN_POINT ( 'NONE',  ( -19.05341960407617563, 5.049401038297882671, 103.5427570613523329 ) ) ;
#174728=CARTESIAN_POINT ( 'NONE',  ( -16.51473224551069308, -9.474510206698971260, 51.66557627198102409 ) ) ;
#174729=CARTESIAN_POINT ( 'NONE',  ( 13.89961937509957401, 13.97604488694547697, 66.87609039468567573 ) ) ;
#174730=CARTESIAN_POINT ( 'NONE',  ( -18.67979575497193778, 10.72451020669871902, 83.33442372801903275 ) ) ;
#174731=CARTESIAN_POINT ( 'NONE',  ( 5.049401038297881783, 19.05341960407617563, 62.29275706135234003 ) ) ;
#174732=CARTESIAN_POINT ( 'NONE',  ( -13.97604488694527625, -13.89961937509977652, 41.87390960531435979 ) ) ;
#174733=CARTESIAN_POINT ( 'NONE',  ( 5.719274019375991003, -21.55341960407610458, 57.70724293864770260 ) ) ;
#174734=CARTESIAN_POINT ( 'NONE',  ( -4.483927247898539470, -16.52544592524342804, 57.29057627198103120 ) ) ;
#174736=CARTESIAN_POINT ( 'NONE',  ( 5.049401038297881783, 19.05341960407617563, 27.29275706135232937 ) ) ;
#174737=CARTESIAN_POINT ( 'NONE',  ( 14.34966873604972726, -8.224510206698740333, 100.8344237280190185 ) ) ;
#174738=CARTESIAN_POINT ( 'NONE',  ( 8.314922557960818139, 14.29746914071049879, 49.58224293864769550 ) ) ;
#174739=CARTESIAN_POINT ( 'NONE',  ( -15.72974639402176322, -15.80617190586768395, 89.37609039468568994 ) ) ;
#174740=CARTESIAN_POINT ( 'NONE',  ( 18.62759615963255655, 10.81492255796105972, 81.66775706135236135 ) ) ;
#174741=CARTESIAN_POINT ( 'NONE',  ( -10.72451020669898014, 18.67979575497178502, 100.4155762719810241 ) ) ;
#174742=CARTESIAN_POINT ( 'NONE',  ( -19.05341960407611168, -5.049401038298163336, 51.45724293864770260 ) ) ;
#174743=CARTESIAN_POINT ( 'NONE',  ( 15.80617190586769283, -15.72974639402175789, 70.62609039468567573 ) ) ;
#174744=CARTESIAN_POINT ( 'NONE',  ( -0.05219959533909027116, -19.03943276465977164, 42.49890960531435269 ) ) ;
#174745=CARTESIAN_POINT ( 'NONE',  ( -19.05341960407611168, -5.049401038298163336, 66.45724293864769550 ) ) ;
#174746=CARTESIAN_POINT ( 'NONE',  ( -8.314922557960811034, -14.29746914071050412, 112.0822429386477097 ) ) ;
#174747=CARTESIAN_POINT ( 'NONE',  ( -9.474510206698964154, 16.51473224551069663, 100.4155762719810241 ) ) ;
#174748=CARTESIAN_POINT ( 'NONE',  ( -4.379528057220328563, 16.55341960407611168, 55.20724293864770260 ) ) ;
#174749=CARTESIAN_POINT ( 'NONE',  ( -16.55341960407611168, -4.379528057220339221, 111.4572429386476813 ) ) ;
#174750=CARTESIAN_POINT ( 'NONE',  ( -15.80617190586745835, -15.72974639402198527, 86.87390960531438111 ) ) ;
#174751=CARTESIAN_POINT ( 'NONE',  ( 0.05219959533937995610, -21.53943276465977519, 40.00109039468567573 ) ) ;
#174753=CARTESIAN_POINT ( 'NONE',  ( 12.14591786802327356, -12.06949235617739191, 40.62609039468567573 ) ) ;
#174754=CARTESIAN_POINT ( 'NONE',  ( 0.05219959533907565091, 21.53943276465977519, 79.99890960531435269 ) ) ;
#174755=CARTESIAN_POINT ( 'NONE',  ( 10.72451020669871369, 18.67979575497193778, 102.0844237280190185 ) ) ;
#174756=CARTESIAN_POINT ( 'NONE',  ( 5.049401038298161559, -19.05341960407611168, 92.70724293864769550 ) ) ;
#174757=CARTESIAN_POINT ( 'NONE',  ( 5.823673210054444382, -21.52544592524334988, 30.20942372801902565 ) ) ;
#174758=CARTESIAN_POINT ( 'NONE',  ( 18.67979575497178502, 10.72451020669898547, 34.16557627198102409 ) ) ;
#174759=CARTESIAN_POINT ( 'NONE',  ( -16.53943276465976808, -0.05219959533934237506, 103.7510903946857042 ) ) ;
#174760=CARTESIAN_POINT ( 'NONE',  ( -10.72451020669870658, -18.67979575497194134, 49.58442372801901143 ) ) ;
#174761=CARTESIAN_POINT ( 'NONE',  ( -15.72974639402176322, -15.80617190586768395, 79.37609039468567573 ) ) ;
#174762=CARTESIAN_POINT ( 'NONE',  ( 9.474510206698729675, 16.51473224551082808, 22.08442372801899722 ) ) ;
#174763=CARTESIAN_POINT ( 'NONE',  ( -8.314922557961024197, 14.29746914071037800, 77.91775706135231871 ) ) ;
#174764=CARTESIAN_POINT ( 'NONE',  ( 5.719274019375673035, 21.55341960407619339, 37.29275706135235424 ) ) ;
#174765=CARTESIAN_POINT ( 'NONE',  ( -19.05341960407611168, -5.049401038298163336, 31.45724293864769550 ) ) ;
#174766=CARTESIAN_POINT ( 'NONE',  ( 5.823673210054444382, -21.52544592524334988, 105.2094237280190328 ) ) ;
#174767=CARTESIAN_POINT ( 'NONE',  ( -16.51473224551069308, -9.474510206698971260, 101.6655762719810241 ) ) ;
#174768=CARTESIAN_POINT ( 'NONE',  ( 5.823673210054125526, 21.52544592524343514, 104.7905762719810241 ) ) ;
#174770=CARTESIAN_POINT ( 'NONE',  ( -15.72974639402197994, 15.80617190586746368, 65.62390960531436690 ) ) ;
#174771=CARTESIAN_POINT ( 'NONE',  ( 8.314922557961029526, -14.29746914071037800, 45.41775706135234003 ) ) ;
#174772=CARTESIAN_POINT ( 'NONE',  ( 8.224510206698953496, -14.34966873604960469, 52.91557627198103830 ) ) ;
#174774=CARTESIAN_POINT ( 'NONE',  ( -9.564922557961040184, 16.46253265017147172, 92.91775706135233293 ) ) ;
#174776=CARTESIAN_POINT ( 'NONE',  ( -4.379528057220086978, -16.55341960407618274, 24.79275706135235779 ) ) ;
#174777=CARTESIAN_POINT ( 'NONE',  ( 18.67979575497178502, 10.72451020669898547, 99.16557627198100988 ) ) ;
#174778=CARTESIAN_POINT ( 'NONE',  ( 0.05219959533907565091, 21.53943276465977519, 69.99890960531435269 ) ) ;
#174779=CARTESIAN_POINT ( 'NONE',  ( 9.474510206698971260, -16.51473224551069308, 112.9155762719810383 ) ) ;
#174780=CARTESIAN_POINT ( 'NONE',  ( 12.14591786802327356, -12.06949235617739191, 40.62609039468567573 ) ) ;
#174781=CARTESIAN_POINT ( 'NONE',  ( 9.564922557960805705, 16.46253265017160317, 64.58224293864769550 ) ) ;
#174782=CARTESIAN_POINT ( 'NONE',  ( -10.72451020669870658, -18.67979575497194134, 29.58442372801901854 ) ) ;
#174783=CARTESIAN_POINT ( 'NONE',  ( -19.02544592524334988, -5.153800228976617603, 103.9594237280190043 ) ) ;
#174784=CARTESIAN_POINT ( 'NONE',  ( -16.46253265017160317, 9.564922557960807481, 105.8322429386476955 ) ) ;
#174785=CARTESIAN_POINT ( 'NONE',  ( 9.474510206698971260, -16.51473224551069308, 92.91557627198103830 ) ) ;
#174786=CARTESIAN_POINT ( 'NONE',  ( 15.72974639402199770, -15.80617190586745480, 93.12390960531436690 ) ) ;
#174787=CARTESIAN_POINT ( 'NONE',  ( -0.05219959533909027116, -19.03943276465977164, 62.49890960531435979 ) ) ;
#174788=CARTESIAN_POINT ( 'NONE',  ( -17.48853670773243252, -5.747243402303183757, 61.33328700250010002 ) ) ;
#174789=CARTESIAN_POINT ( 'NONE',  ( -4.483927247898539470, -16.52544592524342804, 72.29057627198102409 ) ) ;
#174790=CARTESIAN_POINT ( 'NONE',  ( 18.62759615963271287, -10.81492255796078972, 23.33224293864769194 ) ) ;
#174792=CARTESIAN_POINT ( 'NONE',  ( -10.72451020669898014, 18.67979575497178502, 90.41557627198103830 ) ) ;
#174793=CARTESIAN_POINT ( 'NONE',  ( 19.02544592524334988, 5.153800228976608722, 51.45942372801900433 ) ) ;
#174794=CARTESIAN_POINT ( 'NONE',  ( -19.05341960407611168, -5.049401038298163336, 111.4572429386476671 ) ) ;
#174796=CARTESIAN_POINT ( 'NONE',  ( 0.05219959533907565091, 21.53943276465977519, 59.99890960531436690 ) ) ;
#174797=CARTESIAN_POINT ( 'NONE',  ( 5.153800228976335163, 19.02544592524342804, 79.79057627198102409 ) ) ;
#174798=CARTESIAN_POINT ( 'NONE',  ( -21.52544592524334988, -5.823673210054445271, 83.95942372801900433 ) ) ;
#174799=CARTESIAN_POINT ( 'NONE',  ( 9.474510206698971260, -16.51473224551069308, 37.91557627198102409 ) ) ;
#174800=CARTESIAN_POINT ( 'NONE',  ( 0.05219959533910956823, 16.53943276465976808, 74.99890960531435269 ) ) ;
#174801=CARTESIAN_POINT ( 'NONE',  ( -14.29746914071037622, -8.314922557961029526, 24.16775706135235424 ) ) ;
#174802=CARTESIAN_POINT ( 'NONE',  ( -10.81492255796105439, 18.62759615963255655, 62.91775706135236135 ) ) ;
#174804=CARTESIAN_POINT ( 'NONE',  ( 9.474510206698729675, 16.51473224551082808, 27.08442372801900433 ) ) ;
#174805=CARTESIAN_POINT ( 'NONE',  ( 9.564922557961047289, -16.46253265017146816, 75.41775706135234714 ) ) ;
#174808=CARTESIAN_POINT ( 'NONE',  ( 21.53943276465977519, 0.05219959533937863772, 21.25109039468567218 ) ) ;
#174810=CARTESIAN_POINT ( 'NONE',  ( -18.62759615963255300, -10.81492255796106328, 109.1677570613523613 ) ) ;
#174811=CARTESIAN_POINT ( 'NONE',  ( -16.46253265017160317, 9.564922557960807481, 55.83224293864769550 ) ) ;
#174812=CARTESIAN_POINT ( 'NONE',  ( 0.05219959533936267826, -19.03943276465977164, 30.00109039468566863 ) ) ;
#174813=CARTESIAN_POINT ( 'NONE',  ( -0.05219959533934338120, 16.53943276465976808, 107.5010903946856899 ) ) ;
#174814=CARTESIAN_POINT ( 'NONE',  ( -16.51473224551069308, -9.474510206698971260, 101.6655762719810241 ) ) ;
#174815=CARTESIAN_POINT ( 'NONE',  ( 5.823673210054444382, -21.52544592524334988, 70.20942372801904696 ) ) ;
#174817=CARTESIAN_POINT ( 'NONE',  ( -17.49999999999999645, -5.500000000000000888, 34.20309617465829177 ) ) ;
#174818=CARTESIAN_POINT ( 'NONE',  ( 5.719274019375673035, 21.55341960407619339, 87.29275706135236135 ) ) ;
#174819=CARTESIAN_POINT ( 'NONE',  ( -5.823673210054431948, 21.52544592524334988, 102.7094237280190185 ) ) ;
#174820=CARTESIAN_POINT ( 'NONE',  ( 17.50000000000001066, -5.622605283950867339, 41.18792689403890250 ) ) ;
#174821=CARTESIAN_POINT ( 'NONE',  ( 5.049401038298161559, -19.05341960407611168, 102.7072429386476955 ) ) ;
#174822=CARTESIAN_POINT ( 'NONE',  ( 5.049401038297881783, 19.05341960407617563, 22.29275706135233648 ) ) ;
#174823=B_SPLINE_CURVE_WITH_KNOTS ( 'NONE', 3,
 ( #35895, #130896, #38901, #161240, #189598, #192586, #177430, #23737, #163246, #53052, #193591, #146059, #116734, #54069, #174425, #55062, #22734, #83385, #145062, #68223, #129875, #84382, #100558, #115743, #70239, #191574, #159228, #162237, #114732, #85386, #131907, #190586 ),
 .UNSPECIFIED., .F., .F.,
 ( 4, 2, 2, 2, 2, 2, 2, 2, 2, 2, 2, 2, 2, 2, 2, 4 ),
 ( 2.602085213965210642E-18, 0.0003712461730036887837, 0.0007424923460073749653, 0.001113738519011061310, 0.001484984692014747329, 0.002227477038022114813, 0.002598723211025784352, 0.002969969384029453891, 0.003341215557033123430, 0.003712461730036792969, 0.004083707903040462509, 0.004454954076044132481, 0.004826200249047802454, 0.005197446422051472427, 0.005568692595055141532, 0.005939938768058811505 ),
 .UNSPECIFIED. ) ;
#174825=CARTESIAN_POINT ( 'NONE',  ( -19.03943276465977164, 0.05219959533909376836, 41.24890960531435269 ) ) ;
#174826=CARTESIAN_POINT ( 'NONE',  ( -18.62759615963270932, 10.81492255796079327, 60.83224293864769550 ) ) ;
#174827=CARTESIAN_POINT ( 'NONE',  ( -16.55341960407611168, -4.379528057220339221, 21.45724293864769550 ) ) ;
#174828=CARTESIAN_POINT ( 'NONE',  ( -14.29746914071049879, 8.314922557960819915, 90.83224293864769550 ) ) ;
#174829=CARTESIAN_POINT ( 'NONE',  ( -0.05219959533909027116, -19.03943276465977164, 87.49890960531436690 ) ) ;
#174830=CARTESIAN_POINT ( 'NONE',  ( -21.52544592524334988, -5.823673210054445271, 98.95942372801903275 ) ) ;
#174831=CARTESIAN_POINT ( 'NONE',  ( -9.564922557960796823, -16.46253265017161027, 42.08224293864769550 ) ) ;
#174832=CARTESIAN_POINT ( 'NONE',  ( 16.52544592524342804, -4.483927247898539470, 98.54057627198105251 ) ) ;
#174833=CARTESIAN_POINT ( 'NONE',  ( -0.05219959533937732626, 21.53943276465977519, 52.50109039468567573 ) ) ;
#174834=CARTESIAN_POINT ( 'NONE',  ( -18.67979575497178146, -10.72451020669898902, 91.66557627198103830 ) ) ;
#174835=CARTESIAN_POINT ( 'NONE',  ( 19.05341960407617918, -5.049401038297876454, 56.04275706135234714 ) ) ;
#174837=CARTESIAN_POINT ( 'NONE',  ( -9.474510206698964154, 16.51473224551069663, 115.4155762719810241 ) ) ;
#174838=CARTESIAN_POINT ( 'NONE',  ( 14.34966873604960469, 8.224510206698951720, 74.16557627198102409 ) ) ;
#174839=CARTESIAN_POINT ( 'NONE',  ( -19.05341960407617563, 5.049401038297882671, 38.54275706135233293 ) ) ;
#174840=CARTESIAN_POINT ( 'NONE',  ( -0.05219959533909027116, -19.03943276465977164, 62.49890960531435979 ) ) ;
#174841=CARTESIAN_POINT ( 'NONE',  ( 16.53943276465976808, -0.05219959533910856209, 48.74890960531435979 ) ) ;
#174842=CARTESIAN_POINT ( 'NONE',  ( -0.05219959533936034679, 19.03943276465977164, 77.50109039468566152 ) ) ;
#174844=CARTESIAN_POINT ( 'NONE',  ( -15.72974639402197994, 15.80617190586746368, 35.62390960531437401 ) ) ;
#174845=CARTESIAN_POINT ( 'NONE',  ( 8.224510206698953496, -14.34966873604960469, 97.91557627198103830 ) ) ;
#174847=CARTESIAN_POINT ( 'NONE',  ( -5.153800228976328057, -19.02544592524343514, 62.29057627198100988 ) ) ;
#174848=CARTESIAN_POINT ( 'NONE',  ( 10.72451020669898902, -18.67979575497178502, 62.91557627198102409 ) ) ;
#174849=CARTESIAN_POINT ( 'NONE',  ( 5.153800228976335163, 19.02544592524342804, 24.79057627198102765 ) ) ;
#174850=CARTESIAN_POINT ( 'NONE',  ( -8.224510206698735004, -14.34966873604973081, 74.58442372801901854 ) ) ;
#174851=CARTESIAN_POINT ( 'NONE',  ( -9.564922557960796823, -16.46253265017161027, 62.08224293864769550 ) ) ;
#174852=CARTESIAN_POINT ( 'NONE',  ( 16.51473224551083163, -9.474510206698727899, 50.83442372801899722 ) ) ;
#174853=CARTESIAN_POINT ( 'NONE',  ( 10.72451020669871369, 18.67979575497193778, 67.08442372801901854 ) ) ;
#174854=CARTESIAN_POINT ( 'NONE',  ( 21.53943276465977519, -0.05219959533907433946, 43.74890960531435979 ) ) ;
#174855=CARTESIAN_POINT ( 'NONE',  ( -4.483927247898539470, -16.52544592524342804, 112.2905762719810241 ) ) ;
#174856=CARTESIAN_POINT ( 'NONE',  ( -8.314922557961024197, 14.29746914071037800, 92.91775706135236135 ) ) ;
#174857=CARTESIAN_POINT ( 'NONE',  ( 0.05219959533936267826, -19.03943276465977164, 105.0010903946856615 ) ) ;
#174859=CARTESIAN_POINT ( 'NONE',  ( 17.49999999999999645, 5.500000000000010658, 53.78230962303567964 ) ) ;
#174860=CARTESIAN_POINT ( 'NONE',  ( 10.72451020669898902, -18.67979575497178502, 62.91557627198102409 ) ) ;
#174861=CARTESIAN_POINT ( 'NONE',  ( -5.823673210054431948, 21.52544592524334988, 97.70942372801904696 ) ) ;
#174862=CARTESIAN_POINT ( 'NONE',  ( 8.224510206698953496, -14.34966873604960469, 52.91557627198103830 ) ) ;
#174864=CARTESIAN_POINT ( 'NONE',  ( -14.29746914071049879, 8.314922557960819915, 60.83224293864769550 ) ) ;
#174865=CARTESIAN_POINT ( 'NONE',  ( 10.72451020669898902, -18.67979575497178502, 92.91557627198103830 ) ) ;
#174866=CARTESIAN_POINT ( 'NONE',  ( -15.80617190586745835, -15.72974639402198527, 86.87390960531438111 ) ) ;
#174868=CARTESIAN_POINT ( 'NONE',  ( -21.55341960407610458, -5.719274019375992779, 36.45724293864768839 ) ) ;
#174869=CARTESIAN_POINT ( 'NONE',  ( 12.14591786802327356, -12.06949235617739191, 70.62609039468567573 ) ) ;
#174870=CARTESIAN_POINT ( 'NONE',  ( 8.314922557960818139, 14.29746914071049879, 74.58224293864768129 ) ) ;
#174871=CARTESIAN_POINT ( 'NONE',  ( 9.564922557960805705, 16.46253265017160317, 49.58224293864770260 ) ) ;
#174874=CARTESIAN_POINT ( 'NONE',  ( -16.55341960407617563, 4.379528057220093196, 93.54275706135234714 ) ) ;
#174875=CARTESIAN_POINT ( 'NONE',  ( 21.52544592524334988, 5.823673210054432836, 21.45942372801901499 ) ) ;
#174876=CARTESIAN_POINT ( 'NONE',  ( -19.02544592524342804, 5.153800228976336051, 81.04057627198103830 ) ) ;
#174877=CARTESIAN_POINT ( 'NONE',  ( 18.67979575497194134, -10.72451020669871369, 60.83442372801901854 ) ) ;
#174878=CARTESIAN_POINT ( 'NONE',  ( -19.02544592524342804, 5.153800228976336051, 111.0405762719810099 ) ) ;
#174881=CARTESIAN_POINT ( 'NONE',  ( 15.80617190586769283, -15.72974639402175789, 45.62609039468567573 ) ) ;
#174882=CARTESIAN_POINT ( 'NONE',  ( 16.51473224551069308, 9.474510206698969483, 44.16557627198103120 ) ) ;
#174883=CARTESIAN_POINT ( 'NONE',  ( -13.97604488694527625, -13.89961937509977652, 111.8739096053143243 ) ) ;
#174884=CARTESIAN_POINT ( 'NONE',  ( -16.46253265017146816, -9.564922557961047289, 59.16775706135233293 ) ) ;
#174885=CARTESIAN_POINT ( 'NONE',  ( 15.72974639402176855, 15.80617190586768217, 31.87609039468567929 ) ) ;
#174886=CARTESIAN_POINT ( 'NONE',  ( -16.46253265017146816, -9.564922557961047289, 59.16775706135233293 ) ) ;
#174887=CARTESIAN_POINT ( 'NONE',  ( -16.51473224551069308, -9.474510206698971260, 26.66557627198103120 ) ) ;
#174888=CARTESIAN_POINT ( 'NONE',  ( 8.224510206698742110, 14.34966873604972548, 87.08442372801901854 ) ) ;
#174889=CARTESIAN_POINT ( 'NONE',  ( -9.564922557961040184, 16.46253265017147172, 57.91775706135233293 ) ) ;
#174890=CARTESIAN_POINT ( 'NONE',  ( -12.14591786802326823, 12.06949235617739902, 103.1260903946856757 ) ) ;
#174892=CARTESIAN_POINT ( 'NONE',  ( -19.03943276465977164, 0.05219959533909376836, 91.24890960531436690 ) ) ;
#174893=CARTESIAN_POINT ( 'NONE',  ( 15.72974639402176855, 15.80617190586768217, 86.87609039468568994 ) ) ;
#174894=CARTESIAN_POINT ( 'NONE',  ( 10.72451020669871369, 18.67979575497193778, 102.0844237280190185 ) ) ;
#174896=CARTESIAN_POINT ( 'NONE',  ( -13.97604488694527625, -13.89961937509977652, 101.8739096053143811 ) ) ;
#174897=CARTESIAN_POINT ( 'NONE',  ( 15.80617190586769283, -15.72974639402175789, 70.62609039468567573 ) ) ;
#174898=CARTESIAN_POINT ( 'NONE',  ( -0.05219959533934338120, 16.53943276465976808, 22.50109039468567573 ) ) ;
#174900=CARTESIAN_POINT ( 'NONE',  ( 19.02544592524343514, -5.153800228976328945, 83.54057627198100988 ) ) ;
#174901=CARTESIAN_POINT ( 'NONE',  ( 15.72974639402199770, -15.80617190586745480, 28.12390960531435979 ) ) ;
#174902=CARTESIAN_POINT ( 'NONE',  ( 19.02544592524343514, -5.153800228976328945, 88.54057627198102409 ) ) ;
#174905=CARTESIAN_POINT ( 'NONE',  ( -5.153800228976328057, -19.02544592524343514, 72.29057627198102409 ) ) ;
#174906=CARTESIAN_POINT ( 'NONE',  ( 16.53943276465976808, 0.05219959533934440121, 111.2510903946856899 ) ) ;
#174907=CARTESIAN_POINT ( 'NONE',  ( -16.79531203550684282, 7.028104445595293015, 98.74755011779544134 ) ) ;
#174908=CARTESIAN_POINT ( 'NONE',  ( -19.02544592524334988, -5.153800228976617603, 73.95942372801900433 ) ) ;
#174909=CARTESIAN_POINT ( 'NONE',  ( 16.51473224551069308, 9.474510206698969483, 99.16557627198102409 ) ) ;
#174910=CARTESIAN_POINT ( 'NONE',  ( -4.483927247898539470, -16.52544592524342804, 87.29057627198103830 ) ) ;
#174911=CARTESIAN_POINT ( 'NONE',  ( -10.72451020669898014, 18.67979575497178502, 45.41557627198103830 ) ) ;
#174912=CARTESIAN_POINT ( 'NONE',  ( -15.72974639402197994, 15.80617190586746368, 25.62390960531435624 ) ) ;
#174913=CARTESIAN_POINT ( 'NONE',  ( -16.55341960407611168, -4.379528057220339221, 111.4572429386476813 ) ) ;
#174914=CARTESIAN_POINT ( 'NONE',  ( -17.49999999999999289, 5.624438216177590100, 55.81670344914646620 ) ) ;
#174915=CARTESIAN_POINT ( 'NONE',  ( 9.564922557961047289, -16.46253265017146816, 50.41775706135233293 ) ) ;
#174916=CARTESIAN_POINT ( 'NONE',  ( 4.379528057220339221, -16.55341960407611168, 27.70724293864769905 ) ) ;
#174917=CARTESIAN_POINT ( 'NONE',  ( -16.51473224551069308, -9.474510206698971260, 106.6655762719810383 ) ) ;
#174918=CARTESIAN_POINT ( 'NONE',  ( -15.72974639402176322, -15.80617190586768395, 64.37609039468568994 ) ) ;
#174919=CARTESIAN_POINT ( 'NONE',  ( 10.72451020669898902, -18.67979575497178502, 52.91557627198103830 ) ) ;
#174920=CARTESIAN_POINT ( 'NONE',  ( 5.719274019375673035, 21.55341960407619339, 42.29275706135235424 ) ) ;
#174921=CARTESIAN_POINT ( 'NONE',  ( -15.72974639402197994, 15.80617190586746368, 100.6239096053143811 ) ) ;
#174922=CARTESIAN_POINT ( 'NONE',  ( 10.72451020669871369, 18.67979575497193778, 37.08442372801901143 ) ) ;
#174923=CARTESIAN_POINT ( 'NONE',  ( -12.14591786802309592, -12.06949235617757132, 106.8739096053143811 ) ) ;
#174925=CARTESIAN_POINT ( 'NONE',  ( 13.97604488694548053, -13.89961937509957401, 75.62609039468564731 ) ) ;
#174926=CARTESIAN_POINT ( 'NONE',  ( -19.05341960407611168, -5.049401038298163336, 51.45724293864770260 ) ) ;
#174927=CARTESIAN_POINT ( 'NONE',  ( 14.34966873604960469, 8.224510206698951720, 109.1655762719810383 ) ) ;
#174928=CARTESIAN_POINT ( 'NONE',  ( -19.02544592524342804, 5.153800228976336051, 106.0405762719810241 ) ) ;
#174929=CARTESIAN_POINT ( 'NONE',  ( 0.05219959533910956823, 16.53943276465976808, 39.99890960531436690 ) ) ;
#174930=CARTESIAN_POINT ( 'NONE',  ( -4.483927247898539470, -16.52544592524342804, 27.29057627198103120 ) ) ;
#174931=CARTESIAN_POINT ( 'NONE',  ( -9.474510206698964154, 16.51473224551069663, 55.41557627198103120 ) ) ;
#174932=CARTESIAN_POINT ( 'NONE',  ( 14.29746914071049879, -8.314922557960816363, 113.3322429386476955 ) ) ;
#174933=CARTESIAN_POINT ( 'NONE',  ( 9.564922557961047289, -16.46253265017146816, 30.41775706135232937 ) ) ;
#174934=CARTESIAN_POINT ( 'NONE',  ( -17.26058549869088665, -6.457015423128629195, 41.37745837476068544 ) ) ;
#174935=CARTESIAN_POINT ( 'NONE',  ( -14.29746914071049879, 8.314922557960819915, 30.83224293864770260 ) ) ;
#174936=CARTESIAN_POINT ( 'NONE',  ( -21.55341960407619339, 5.719274019375674811, 43.54275706135235424 ) ) ;
#174938=CARTESIAN_POINT ( 'NONE',  ( -14.34966873604972548, 8.224510206698743886, 63.33442372801900433 ) ) ;
#174939=CARTESIAN_POINT ( 'NONE',  ( -16.53943276465976808, 0.05219959533911058130, 26.24890960531435624 ) ) ;
#174940=CARTESIAN_POINT ( 'NONE',  ( -4.379528057220086978, -16.55341960407618274, 104.7927570613523898 ) ) ;
#174942=CARTESIAN_POINT ( 'NONE',  ( 16.53943276465976808, 0.05219959533934440121, 21.25109039468567218 ) ) ;
#174943=CARTESIAN_POINT ( 'NONE',  ( -9.564922557960796823, -16.46253265017161027, 42.08224293864769550 ) ) ;
#174944=CARTESIAN_POINT ( 'NONE',  ( 19.03943276465977164, -0.05219959533909143690, 28.74890960531435624 ) ) ;
#174945=CARTESIAN_POINT ( 'NONE',  ( -15.72974639402176322, -15.80617190586768395, 29.37609039468568284 ) ) ;
#174946=CARTESIAN_POINT ( 'NONE',  ( 9.474510206698971260, -16.51473224551069308, 47.91557627198102409 ) ) ;
#174947=VECTOR ( 'NONE', #89111, 1000.000000000000000 ) ;
#174948=CARTESIAN_POINT ( 'NONE',  ( -13.89961937509977652, 13.97604488694528158, 115.6239096053143669 ) ) ;
#174949=CARTESIAN_POINT ( 'NONE',  ( 9.564922557960805705, 16.46253265017160317, 34.58224293864770260 ) ) ;
#174950=CARTESIAN_POINT ( 'NONE',  ( -21.52544592524343514, 5.823673210054127303, 26.04057627198103475 ) ) ;
#174951=CARTESIAN_POINT ( 'NONE',  ( -21.53943276465977519, -0.05219959533937600094, 48.75109039468568284 ) ) ;
#174952=CARTESIAN_POINT ( 'NONE',  ( 4.483927247898545687, 16.52544592524342804, 109.7905762719810383 ) ) ;
#174953=CARTESIAN_POINT ( 'NONE',  ( 9.564922557960805705, 16.46253265017160317, 104.5822429386476955 ) ) ;
#174954=CARTESIAN_POINT ( 'NONE',  ( 12.06949235617739724, 12.14591786802326823, 76.87609039468567573 ) ) ;
#174955=CARTESIAN_POINT ( 'NONE',  ( 21.53943276465977519, 0.05219959533937863772, 96.25109039468568994 ) ) ;
#174956=CARTESIAN_POINT ( 'NONE',  ( -8.224510206698735004, -14.34966873604973081, 59.58442372801901854 ) ) ;
#174957=CARTESIAN_POINT ( 'NONE',  ( -5.153800228976328057, -19.02544592524343514, 92.29057627198099567 ) ) ;
#174958=CARTESIAN_POINT ( 'NONE',  ( -14.34966873604972548, 8.224510206698743886, 43.33442372801901143 ) ) ;
#174959=CARTESIAN_POINT ( 'NONE',  ( 16.55341960407618274, -4.379528057220086978, 26.04275706135235779 ) ) ;
#174960=CARTESIAN_POINT ( 'NONE',  ( -16.52544592524335698, -4.483927247898792601, 83.95942372801900433 ) ) ;
#174961=CARTESIAN_POINT ( 'NONE',  ( -19.02544592524334988, -5.153800228976617603, 103.9594237280190043 ) ) ;
#174962=CARTESIAN_POINT ( 'NONE',  ( -16.46253265017160317, 9.564922557960807481, 75.83224293864769550 ) ) ;
#174963=CARTESIAN_POINT ( 'NONE',  ( 21.53943276465977519, -0.05219959533907433946, 93.74890960531436690 ) ) ;
#174964=CARTESIAN_POINT ( 'NONE',  ( 0.05219959533910956823, 16.53943276465976808, 99.99890960531436690 ) ) ;
#174965=CARTESIAN_POINT ( 'NONE',  ( -9.564922557961040184, 16.46253265017147172, 102.9177570613523329 ) ) ;
#174966=CARTESIAN_POINT ( 'NONE',  ( 8.314922557961029526, -14.29746914071037800, 70.41775706135236135 ) ) ;
#174968=CARTESIAN_POINT ( 'NONE',  ( 19.03943276465977164, 0.05219959533936151252, 66.25109039468567573 ) ) ;
#174969=CARTESIAN_POINT ( 'NONE',  ( -12.06949235617756955, 12.14591786802309770, 50.62390960531435979 ) ) ;
#174970=CARTESIAN_POINT ( 'NONE',  ( -0.05219959533910754901, -16.53943276465976808, 97.49890960531436690 ) ) ;
#174971=CARTESIAN_POINT ( 'NONE',  ( -0.05219959533936034679, 19.03943276465977164, 37.50109039468567573 ) ) ;
#174972=CARTESIAN_POINT ( 'NONE',  ( -17.49999999999998579, 5.500000000000031974, 90.79690382534171533 ) ) ;
#174973=CARTESIAN_POINT ( 'NONE',  ( -21.52544592524334988, -5.823673210054445271, 38.95942372801901854 ) ) ;
#174974=CARTESIAN_POINT ( 'NONE',  ( -5.049401038297874678, -19.05341960407617918, 94.79275706135230450 ) ) ;
#174975=CARTESIAN_POINT ( 'NONE',  ( 16.51473224551069308, 9.474510206698969483, 114.1655762719810241 ) ) ;
#174976=CARTESIAN_POINT ( 'NONE',  ( -19.05341960407611168, -5.049401038298163336, 91.45724293864766707 ) ) ;
#174977=CARTESIAN_POINT ( 'NONE',  ( -9.474510206698720793, -16.51473224551083518, 19.58442372801899722 ) ) ;
#174978=CARTESIAN_POINT ( 'NONE',  ( -13.89961937509977652, 13.97604488694528158, 85.62390960531433848 ) ) ;
#174979=CARTESIAN_POINT ( 'NONE',  ( -0.05219959533907301413, -21.53943276465977519, 37.49890960531436690 ) ) ;
#174980=CARTESIAN_POINT ( 'NONE',  ( 14.34966873604960469, 8.224510206698951720, 94.16557627198103830 ) ) ;
#174981=CARTESIAN_POINT ( 'NONE',  ( 5.153800228976335163, 19.02544592524342804, 59.79057627198100988 ) ) ;
#174982=CARTESIAN_POINT ( 'NONE',  ( -19.05341960407611168, -5.049401038298163336, 21.45724293864768839 ) ) ;
#174983=CARTESIAN_POINT ( 'NONE',  ( 18.67979575497194134, -10.72451020669871369, 25.83442372801901499 ) ) ;
#174984=CARTESIAN_POINT ( 'NONE',  ( -5.823673210054431948, 21.52544592524334988, 77.70942372801900433 ) ) ;
#174985=CARTESIAN_POINT ( 'NONE',  ( 19.02544592524343514, -5.153800228976328945, 43.54057627198103120 ) ) ;
#174986=CARTESIAN_POINT ( 'NONE',  ( -12.14591786802326823, 12.06949235617739902, 78.12609039468570415 ) ) ;
#174987=CARTESIAN_POINT ( 'NONE',  ( 5.719274019375991003, -21.55341960407610458, 112.7072429386476955 ) ) ;
#174988=CARTESIAN_POINT ( 'NONE',  ( -10.72451020669870658, -18.67979575497194134, 24.58442372801901499 ) ) ;
#174989=CARTESIAN_POINT ( 'NONE',  ( -19.02544592524334988, -5.153800228976617603, 58.95942372801900433 ) ) ;
#174990=CARTESIAN_POINT ( 'NONE',  ( -5.153800228976328057, -19.02544592524343514, 72.29057627198102409 ) ) ;
#174991=CARTESIAN_POINT ( 'NONE',  ( 13.97604488694548053, -13.89961937509957401, 25.62609039468566507 ) ) ;
#174992=CARTESIAN_POINT ( 'NONE',  ( 18.62759615963255655, 10.81492255796105972, 66.66775706135234714 ) ) ;
#174993=CARTESIAN_POINT ( 'NONE',  ( -15.80617190586745835, -15.72974639402198527, 71.87390960531438111 ) ) ;
#174994=CARTESIAN_POINT ( 'NONE',  ( 16.55341960407611168, 4.379528057220329451, 48.95724293864770971 ) ) ;
#174995=CARTESIAN_POINT ( 'NONE',  ( 21.53943276465977519, 0.05219959533937863772, 96.25109039468568994 ) ) ;
#174996=CARTESIAN_POINT ( 'NONE',  ( -9.564922557961040184, 16.46253265017147172, 22.91775706135233648 ) ) ;
#174997=CARTESIAN_POINT ( 'NONE',  ( -16.53943276465976808, 0.05219959533911058130, 71.24890960531435269 ) ) ;
#174998=CARTESIAN_POINT ( 'NONE',  ( 13.89961937509977652, -13.97604488694527269, 28.12390960531435624 ) ) ;
#174999=CARTESIAN_POINT ( 'NONE',  ( -13.89961937509957401, -13.97604488694547875, 54.37609039468565442 ) ) ;
#175000=CARTESIAN_POINT ( 'NONE',  ( -4.483927247898539470, -16.52544592524342804, 27.29057627198103120 ) ) ;
#175001=CARTESIAN_POINT ( 'NONE',  ( -10.81492255796105439, 18.62759615963255655, 82.91775706135234714 ) ) ;
#175003=CARTESIAN_POINT ( 'NONE',  ( 9.474510206698971260, -16.51473224551069308, 77.91557627198103830 ) ) ;
#175004=CARTESIAN_POINT ( 'NONE',  ( -19.05341960407617563, 5.049401038297882671, 48.54275706135233293 ) ) ;
#175005=CARTESIAN_POINT ( 'NONE',  ( -15.72974639402197994, 15.80617190586746368, 45.62390960531436690 ) ) ;
#175006=CARTESIAN_POINT ( 'NONE',  ( 10.72451020669871369, 18.67979575497193778, 52.08442372801901854 ) ) ;
#175007=CARTESIAN_POINT ( 'NONE',  ( -21.52544592524343514, 5.823673210054127303, 101.0405762719810383 ) ) ;
#175008=CARTESIAN_POINT ( 'NONE',  ( -9.564922557961040184, 16.46253265017147172, 92.91775706135233293 ) ) ;
#175009=CARTESIAN_POINT ( 'NONE',  ( -0.05219959533934338120, 16.53943276465976808, 72.50109039468568994 ) ) ;
#175011=CARTESIAN_POINT ( 'NONE',  ( -10.72451020669898014, 18.67979575497178502, 110.4155762719810383 ) ) ;
#175012=CARTESIAN_POINT ( 'NONE',  ( 0.05219959533910956823, 16.53943276465976808, 84.99890960531436690 ) ) ;
#175013=CARTESIAN_POINT ( 'NONE',  ( -17.48847506799967277, -5.747544572773784388, 99.17302562156720569 ) ) ;
#175014=CARTESIAN_POINT ( 'NONE',  ( 8.314922557961029526, -14.29746914071037800, 30.41775706135234358 ) ) ;
#175015=CARTESIAN_POINT ( 'NONE',  ( -18.62759615963270932, 10.81492255796079327, 60.83224293864769550 ) ) ;
#175016=CARTESIAN_POINT ( 'NONE',  ( 16.52544592524335698, 4.483927247898782831, 91.45942372801901854 ) ) ;
#175017=CARTESIAN_POINT ( 'NONE',  ( -13.97604488694527625, -13.89961937509977652, 26.87390960531434558 ) ) ;
#175019=CARTESIAN_POINT ( 'NONE',  ( -12.14591786802326823, 12.06949235617739902, 73.12609039468567573 ) ) ;
#175020=CARTESIAN_POINT ( 'NONE',  ( 13.97604488694548053, -13.89961937509957401, 60.62609039468564731 ) ) ;
#175021=CARTESIAN_POINT ( 'NONE',  ( 5.823673210054444382, -21.52544592524334988, 40.20942372801901854 ) ) ;
#175022=CARTESIAN_POINT ( 'NONE',  ( -0.05219959533907301413, -21.53943276465977519, 62.49890960531436690 ) ) ;
#175023=CARTESIAN_POINT ( 'NONE',  ( -4.483927247898782831, 16.52544592524335698, 77.70942372801900433 ) ) ;
#175024=CARTESIAN_POINT ( 'NONE',  ( 21.52544592524334988, 5.823673210054432836, 66.45942372801903275 ) ) ;
#175025=CARTESIAN_POINT ( 'NONE',  ( 15.80617190586746368, 15.72974639402197994, 59.37390960531436690 ) ) ;
#175026=CARTESIAN_POINT ( 'NONE',  ( 5.823673210054125526, 21.52544592524343514, 34.79057627198103120 ) ) ;
#175027=CARTESIAN_POINT ( 'NONE',  ( 14.34966873604972726, -8.224510206698740333, 65.83442372801900433 ) ) ;
#175028=CARTESIAN_POINT ( 'NONE',  ( 5.719274019375991003, -21.55341960407610458, 32.70724293864770260 ) ) ;
#175029=ORIENTED_EDGE ( 'NONE', *, *, #119720, .F. ) ;
#175030=CARTESIAN_POINT ( 'NONE',  ( 9.564922557960805705, 16.46253265017160317, 104.5822429386476955 ) ) ;
#175031=CARTESIAN_POINT ( 'NONE',  ( 4.379528057220092307, 16.55341960407617563, 107.2927570613523471 ) ) ;
#175033=CARTESIAN_POINT ( 'NONE',  ( -8.314922557960811034, -14.29746914071050412, 102.0822429386476955 ) ) ;
#175034=CARTESIAN_POINT ( 'NONE',  ( -5.719274019375978568, 21.55341960407610458, 60.20724293864768839 ) ) ;
#175035=CARTESIAN_POINT ( 'NONE',  ( 0.05219959533909260263, 19.03943276465977164, 39.99890960531436690 ) ) ;
#175036=CARTESIAN_POINT ( 'NONE',  ( -8.224510206698735004, -14.34966873604973081, 94.58442372801901854 ) ) ;
#175037=CARTESIAN_POINT ( 'NONE',  ( -5.823673210054431948, 21.52544592524334988, 32.70942372801900433 ) ) ;
#175038=CARTESIAN_POINT ( 'NONE',  ( 19.02544592524334988, 5.153800228976608722, 101.4594237280189759 ) ) ;
#175039=CARTESIAN_POINT ( 'NONE',  ( -0.05219959533910754901, -16.53943276465976808, 102.4989096053143811 ) ) ;
#175040=CARTESIAN_POINT ( 'NONE',  ( -19.02544592524342804, 5.153800228976336051, 51.04057627198103120 ) ) ;
#175041=CARTESIAN_POINT ( 'NONE',  ( 0.05219959533909260263, 19.03943276465977164, 24.99890960531435269 ) ) ;
#175042=CARTESIAN_POINT ( 'NONE',  ( 17.44279575226824264, -5.990770900252460507, 38.33557567514319686 ) ) ;
#175043=CARTESIAN_POINT ( 'NONE',  ( -19.02544592524342804, 5.153800228976336051, 96.04057627198103830 ) ) ;
#175044=CARTESIAN_POINT ( 'NONE',  ( 0.05219959533934541429, -16.53943276465976808, 80.00109039468568994 ) ) ;
#175045=CARTESIAN_POINT ( 'NONE',  ( 0.05219959533937995610, -21.53943276465977519, 100.0010903946857042 ) ) ;
#175046=CARTESIAN_POINT ( 'NONE',  ( 15.72974639402199770, -15.80617190586745480, 53.12390960531436690 ) ) ;
#175047=CARTESIAN_POINT ( 'NONE',  ( 16.53943276465976808, 0.05219959533934440121, 71.25109039468568994 ) ) ;
#175048=CARTESIAN_POINT ( 'NONE',  ( 19.05341960407617918, -5.049401038297876454, 76.04275706135230450 ) ) ;
#175050=CARTESIAN_POINT ( 'NONE',  ( -13.89961937509977652, 13.97604488694528158, 35.62390960531435269 ) ) ;
#175051=CARTESIAN_POINT ( 'NONE',  ( 19.05341960407611168, 5.049401038298154454, 73.95724293864768129 ) ) ;
#175052=CARTESIAN_POINT ( 'NONE',  ( -19.03943276465977164, 0.05219959533909376836, 36.24890960531436690 ) ) ;
#175053=CARTESIAN_POINT ( 'NONE',  ( -5.153800228976607833, 19.02544592524334988, 72.70942372801900433 ) ) ;
#175054=CARTESIAN_POINT ( 'NONE',  ( -9.564922557960796823, -16.46253265017161027, 112.0822429386476955 ) ) ;
#175055=CARTESIAN_POINT ( 'NONE',  ( -16.51473224551069308, -9.474510206698971260, 96.66557627198102409 ) ) ;
#175056=CARTESIAN_POINT ( 'NONE',  ( 12.14591786802309770, 12.06949235617756955, 54.37390960531435979 ) ) ;
#175057=CARTESIAN_POINT ( 'NONE',  ( -18.67979575497178146, -10.72451020669898902, 51.66557627198102409 ) ) ;
#175059=CARTESIAN_POINT ( 'NONE',  ( -13.89961937509957401, -13.97604488694547875, 29.37609039468565797 ) ) ;
#175060=CARTESIAN_POINT ( 'NONE',  ( -13.89961937509977652, 13.97604488694528158, 45.62390960531433848 ) ) ;
#175061=CARTESIAN_POINT ( 'NONE',  ( -8.224510206698735004, -14.34966873604973081, 34.58442372801900433 ) ) ;
#175064=CARTESIAN_POINT ( 'NONE',  ( -14.34966873604972548, 8.224510206698743886, 78.33442372801901854 ) ) ;
#175065=CARTESIAN_POINT ( 'NONE',  ( -10.72451020669898014, 18.67979575497178502, 95.41557627198102409 ) ) ;
#175066=CARTESIAN_POINT ( 'NONE',  ( 19.02544592524343514, -5.153800228976328945, 38.54057627198103120 ) ) ;
#175068=CARTESIAN_POINT ( 'NONE',  ( -10.81492255796105439, 18.62759615963255655, 42.91775706135235424 ) ) ;
#175069=CARTESIAN_POINT ( 'NONE',  ( -13.89961937509957401, -13.97604488694547875, 54.37609039468565442 ) ) ;
#175070=CARTESIAN_POINT ( 'NONE',  ( -15.72974639402176322, -15.80617190586768395, 94.37609039468568994 ) ) ;
#175071=CARTESIAN_POINT ( 'NONE',  ( 17.26172910966779739, 6.454744622555850242, 96.69353091350775742 ) ) ;
#175072=CARTESIAN_POINT ( 'NONE',  ( 16.52544592524342804, -4.483927247898539470, 38.54057627198103120 ) ) ;
#175074=CARTESIAN_POINT ( 'NONE',  ( 5.823673210054125526, 21.52544592524343514, 49.79057627198102409 ) ) ;
#175076=CARTESIAN_POINT ( 'NONE',  ( -9.474510206698964154, 16.51473224551069663, 105.4155762719810383 ) ) ;
#175077=CARTESIAN_POINT ( 'NONE',  ( 12.06949235617757843, -12.14591786802309237, 98.12390960531436690 ) ) ;
#175078=CARTESIAN_POINT ( 'NONE',  ( -9.564922557961040184, 16.46253265017147172, 112.9177570613523329 ) ) ;
#175079=CARTESIAN_POINT ( 'NONE',  ( 16.52544592524335698, 4.483927247898782831, 106.4594237280190328 ) ) ;
#175081=CARTESIAN_POINT ( 'NONE',  ( 13.89961937509977652, -13.97604488694527269, 98.12390960531433848 ) ) ;
#175082=CARTESIAN_POINT ( 'NONE',  ( 21.53943276465977519, -0.05219959533907433946, 108.7489096053143669 ) ) ;
#175083=CARTESIAN_POINT ( 'NONE',  ( 14.34966873604960469, 8.224510206698951720, 24.16557627198103120 ) ) ;
#175084=CARTESIAN_POINT ( 'NONE',  ( -9.474510206698964154, 16.51473224551069663, 100.4155762719810241 ) ) ;
#175085=CARTESIAN_POINT ( 'NONE',  ( 5.049401038297881783, 19.05341960407617563, 92.29275706135234714 ) ) ;
#175086=CARTESIAN_POINT ( 'NONE',  ( 5.823673210054444382, -21.52544592524334988, 110.2094237280190185 ) ) ;
#175087=CARTESIAN_POINT ( 'NONE',  ( 5.823673210054125526, 21.52544592524343514, 84.79057627198102409 ) ) ;
#175088=CARTESIAN_POINT ( 'NONE',  ( -5.823673210054116645, -21.52544592524344225, 52.29057627198102409 ) ) ;
#175089=CARTESIAN_POINT ( 'NONE',  ( 9.564922557960805705, 16.46253265017160317, 59.58224293864769550 ) ) ;
#175090=CARTESIAN_POINT ( 'NONE',  ( -16.53943276465976808, 0.05219959533911058130, 36.24890960531435979 ) ) ;
#175091=CARTESIAN_POINT ( 'NONE',  ( 19.03943276465977164, -0.05219959533909143690, 78.74890960531436690 ) ) ;
#175093=CARTESIAN_POINT ( 'NONE',  ( 19.03943276465977164, 0.05219959533936151252, 46.25109039468566863 ) ) ;
#175094=CARTESIAN_POINT ( 'NONE',  ( 18.67979575497178502, 10.72451020669898547, 84.16557627198103830 ) ) ;
#175095=B_SPLINE_CURVE_WITH_KNOTS ( 'NONE', 3,
 ( #154010, #29682, #28709, #152030, #13516, #15506, #14505, #136853, #60009, #121676 ),
 .UNSPECIFIED., .F., .F.,
 ( 4, 2, 2, 2, 4 ),
 ( 8.673617379884035472E-19, 0.001083413406193705275, 0.001625120109290555202, 0.001895973460838981358, 0.002166826812387407080 ),
 .UNSPECIFIED. ) ;
#175096=CARTESIAN_POINT ( 'NONE',  ( -4.483927247898539470, -16.52544592524342804, 87.29057627198103830 ) ) ;
#175097=CARTESIAN_POINT ( 'NONE',  ( 0.05219959533937995610, -21.53943276465977519, 35.00109039468568284 ) ) ;
#175099=CARTESIAN_POINT ( 'NONE',  ( -12.14591786802326823, 12.06949235617739902, 108.1260903946856757 ) ) ;
#175100=CARTESIAN_POINT ( 'NONE',  ( -9.564922557960796823, -16.46253265017161027, 22.08224293864768839 ) ) ;
#175101=CARTESIAN_POINT ( 'NONE',  ( -5.049401038298153566, 19.05341960407611168, 85.20724293864766707 ) ) ;
#175102=CARTESIAN_POINT ( 'NONE',  ( 5.153800228976335163, 19.02544592524342804, 24.79057627198102765 ) ) ;
#175103=CARTESIAN_POINT ( 'NONE',  ( -8.224510206698948167, 14.34966873604960824, 40.41557627198103120 ) ) ;
#175104=CARTESIAN_POINT ( 'NONE',  ( 15.80617190586769283, -15.72974639402175789, 55.62609039468568284 ) ) ;
#175106=CARTESIAN_POINT ( 'NONE',  ( -16.51473224551069308, -9.474510206698971260, 46.66557627198102409 ) ) ;
#175107=CARTESIAN_POINT ( 'NONE',  ( -5.153800228976328057, -19.02544592524343514, 52.29057627198100988 ) ) ;
#175108=( BOUNDED_SURFACE ( )  B_SPLINE_SURFACE ( 3, 2, ( 
 ( #185335, #78136, #75172, #14495, #90336, #30663, #42865, #44843, #93306, #106499, #136844, #151045, #59999, #92316, #104530, #121666, #154001, #77153, #183361, #168176, #12535, #199518, #91304, #74200, #152021, #76157, #154991, #138824, #170164, #137837, #304, #135869, #61972, #123638, #46825, #31657, #197540, #120675, #43851, #182374, #192054, #54540, #144542, #131376, #6027, #146534, #24222, #68700, #23214, #160717, #37369, #94302, #83858, #129364, #155980, #47826, #7018, #38377, #113208, #99027, #32648, #53536, #130355, #21207, #115213, #193064, #100033, #175897, #69709, #174896, #128372, #109477, #36362, #176906, #145539, #67706, #85872, #51544, #98014, #161719, #116213, #17477, #191060, #84857, #22209, #8027, #186346, #66711, #177904, #162716, #39372, #101031, #147561, #9046, #70716, #171161, #79134, #52532, #114193, #159708, #190068, #143539, #5026, #82864, #73721, #102047, #151548, #28226, #164728, #182881, #120198, #181888, #167708, #56546, #163731, #42380, #118223, #179914, #89866, #59511, #104043, #105038, #25232, #86873, #57551, #103046, #12059, #121188, #135394, #88867, #41380, #87862, #148557, #150560, #44364, #13038, #74704, #136368, #198045, #197064, #71708, #119220, #43366, #26222, #11045, #166722, #58532, #149550, #106021, #132384, #72721, #178905, #40373, #29204, #134394, #55540, #10048, #90838, #180905, #196080, #133376, #152522, #165723, #195066, #14010, #194077, #117212, #27219, #122179, #124162, #109998, #153517, #48344, #32173, #46341, #64496, #75676, #154515, #183871, #45356, #171678, #200033, #199034, #30181, #140331, #62491, #107997, #15014, #186874, #109005, #168681, #79660, #126163, #187858, #60504, #107008, #185863, #33168, #76675, #92830, #94827, #110988, #155509, #156504, #47349, #170684, #91824, #93829, #16012, #138351, #137355, #17004, #125177, #61501, #78656, #123170, #1821, #63502, #169684, #18006, #141329, #2817, #49327, #172673, #184858, #31179, #77669, #139338, #34158, #95819, #817, #157504, #81617, #66476, #130118, #84620, #50331, #36129, #113955, #5793, #176668, #18997, #96799, #37129, #192825, #190823, #7787, #177667, #146299, #69470, #191815, #68464, #20964, #82621, #128138, #158486, #127140, #98789, #161484, #160483, #188847, #38144, #114975, #51311, #131137, #6785, #53296, #54306, #143300, #111987, #129125, #4786, #189838, #99798, #115978, #52298, #22972, #173678, #35145, #144303, #112972, #21973, #39135, #83625, #175655, #174664, #97781, #19974, #145302, #100790, #80643, #142320, #3800, #65478, #159469, #67466, #149314, #11819, #71471, #41143, #102806, #196829, #44128, #165487, #26983, #147316, #117982, #9810, #118987, #180670, #89625, #182644, #74468, #25985, #151313, #164492, #42147, #135156, #134151, #163489, #73484, #88628, #8806, #87628, #150324, #57312, #24987, #103807, #59275, #162473, #178661, #58297, #70475, #86632, #119965, #43130, #116970, #104799, #136133, #181651, #55298, #166488, #133136, #132141, #195839, #23975, #120945, #101802, #27986, #197809, #12802, #10808, #40124, #193834, #85630, #148315, #194827, #56300, #179672, #72478, #2573, #107755, #156258, #169438, #76436, #28968, #122931, #170439, #64254, #199794, #123913, #93584, #46100, #184618, #125921, #62244, #92589, #187619, #168450, #77428, #17761, #140083, #171438, #15768, #108762, #79417, #185612, #29946, #91584, #78407, #90610, #138113, #106775, #152291, #31930, #32925, #61261, #48098, #139099, #1575, #153275, #105787, #186627, #141087, #30942, #75443, #167473, #155270, #573, #47101, #13775, #94580, #154278, #14776, #109754, #16759, #137118, #63250, #124929, #198804, #60269, #121942, #183635, #45117, #98546, #49089, #161237, #110746, #22731, #189595, #19734, #190583, #4538, #176422, #174422, #37897, #160239, #172427, #84379, #33916, #127892, #83382, #130893, #52059, #113715, #95573, #66232, #96556, #5546, #67225, #99555, #69225, #146056, #112729, #7540, #51068, #128883 ),
 ( #6540, #157259, #175412, #145059, #20720, #97538, #18754, #144065, #35891, #80400, #142072, #36880, #21729, #173431, #159225, #3558, #68220, #129872, #81375, #191570, #53049, #114729, #82377, #65236, #34901, #188602, #126896, #158243, #50083, #111743, #143060, #89384, #55059, #39884, #103571, #58062, #23734, #9568, #87394, #179430, #150073, #192583, #70236, #10567, #166241, #164253, #181416, #151073, #119733, #42894, #165246, #41905, #194586, #56056, #101551, #131904, #100555, #72231, #134915, #133906, #162234, #11578, #88379, #24743, #104559, #180432, #26740, #27742, #116731, #85383, #102568, #178420, #163243, #73244, #12564, #25748, #196592, #147076, #8560, #117735, #86393, #195597, #74230, #57069, #149079, #148077, #71234, #54066, #115740, #177427, #38898, #132897, #193588, #118744, #40895, #60030, #93337, #63003, #107512, #108516, #28730, #105546, #61017, #106530, #15526, #124681, #138853, #92346, #44874, #91335, #90367, #154031, #47856, #155022, #16518, #78166, #139834, #333, #75203, #122689, #185364, #168207, #14527, #170194, #77183, #29704, #186377, #135898, #76188, #182403, #43882, #31688, #121696, #59037, #152052, #62001, #184378, #153027, #13537, #46856, #169188, #136874, #1323, #109509, #171191, #120704, #167232, #45859, #32680, #198560, #137867, #94333, #156011, #123667, #17508, #30695, #197570, #183392, #199547, #19495, #187375, #140837, #97297, #128642, #3321, #127653, #125677, #82125, #158983, #111497, #20475, #21479, #190336, #65983, #159992, #64994, #18509, #2325, #126652, #143818, #35649, #34658, #176174, #141828, #188355, #51813, #113472, #172180, #5299, #37644, #173183, #66982, #175167, #81140, #96317, #99307, #36633, #189353, #160992, #49833, #50830, #129631, #98290, #144815, #112487, #83139, #52804, #6298, #158003, #142821, #67977, #64007, #4301, #80157, #191326, #114471, #48844, #174180, #79166, #110498, #33665, #95327, #157012, #104317, #38656, #148836, #7296, #85136, #10326, #103325, #177183, #165005, #134671, #87153, #115495, #71982, #193341, #68980, #194348, #22486, #181178, #161991, #26499, #57824, #55816, #9327, #100312, #130645, #88141, #196356, #54815, #117489, #8315, #25509, #119496, #24499, #73002, #178179, #133657, #56827, #23487, #195347, #42655, #116490, #40654, #118502, #162994, #39644, #84134, #179186, #70992, #145813, #146820, #102323, #192339, #180192, #149826, #132660, #41662, #53821, #164013, #69991, #131659, #11331, #101305, #86151, #147841, #89143, #168946, #31447, #121458, #108277, #137626, #61764, #13303, #186138, #46616, #77933, #91104, #135662, #47617, #92100, #75952, #107275, #150832, #93100, #152792, #74968, #169955, #30453, #139600, #106287, #136630, #153788, #183150, #154784, #14284, #16281, #15284, #166001, #1086, #27501, #44635, #94, #12328, #76943, #138612, #73993, #167972, #198312, #122449, #184141, #62762, #197334, #124442, #29471, #58797, #199311, #45623, #123432, #60777, #166992, #185125, #120465, #182157, #43641, #105304, #28494, #59790, #90128, #151812, #21247, #34430, #78927, #129402, #35417, #19269, #50599, #32442, #36398, #96090, #18277, #51580, #112258, #82901, #49597, #79931, #173950, #64766, #98052, #157778, #159752, #158751, #109271, #144580, #170950, #188126, #143581, #191098, #97069, #20240, #94096, #126429, #156784, #65749, #127418, #6066, #155775, #67744, #172952, #17273, #111261, #189127, #81888, #80915, #110266, #5063, #66748, #140603, #142592, #128409, #4072, #171947, #190105, #2093, #63774, #125446, #113244, #187142, #33436, #174935, #48614, #95095, #141603, #3090, #117251, #145580, #102085, #23253, #37410, #24262, #134433, #11086, #192095, #195105, #87902, #85911, #39408, #7057, #160757, #56588, #26261, #84896, #147599, #38416, #55577, #149588, #54577, #103085, #8070, #178943, #86912, #68739, #40414, #72763, #146575, #70754, #163769, #193103, #69746, #52573, #9085, #101068, #114233, #115254, #132422, #164766 ),
 ( #194113, #148595, #100073, #175939, #133416, #99068, #177941, #22248, #83897, #25270, #162753, #10087, #130397, #179952, #71745, #161758, #118262, #41419, #53577, #116249, #131415, #176947, #154311, #125954, #123946, #187652, #48131, #198838, #110781, #60302, #77461, #32960, #80434, #1608, #63284, #183668, #15800, #46134, #155304, #16793, #49123, #18789, #172462, #62278, #33949, #139131, #78443, #171471, #170473, #199828, #109788, #124964, #45153, #185644, #186661, #93618, #61295, #140117, #95607, #121977, #14809, #94614, #106809, #122965, #156293, #79450, #153308, #141120, #157292, #17794, #91620, #2610, #169472, #168483, #31963, #29981, #76470, #138147, #64287, #184652, #107787, #47136, #30973, #92620, #608, #108794, #112762, #113749, #127926, #145091, #38930, #144098, #192616, #97570, #6574, #176455, #34938, #68253, #100587, #35924, #160272, #129904, #82409, #159258, #162269, #98578, #128916, #23769, #4574, #175445, #54098, #37928, #7573, #52092, #191604, #115772, #21763, #66267, #189628, #114761, #65270, #174455, #143095, #126930, #53083, #69259, #20754, #84412, #5578, #142107, #51102, #67258, #96590, #177461, #190617, #83414, #36915, #99589, #161269, #3592, #19768, #22763, #188638, #146089, #130925, #50117, #111777, #173465, #158279, #81409, #87429, #149114, #194621, #24780, #193622, #165282, #27777, #26775, #55094, #104593, #181451, #117773, #135934, #73280, #134950, #120737, #9604, #116764, #195633, #71269, #132934, #42929, #12600, #57106, #58097, #178455, #39922, #10605, #56092, #88417, #74264, #150111, #41940, #179467, #40932, #101591, #103606, #197604, #166280, #89419, #151108, #59070, #11612, #86427, #72266, #196628, #102604, #164290, #119767, #182436, #25783, #43916, #85419, #133943, #131938, #163279, #105578, #118780, #8596, #148113, #167264, #180468, #147110, #70270, #139869, #62037, #121731, #32714, #79203, #140872, #13570, #75237, #77217, #63037, #106564, #45893, #186413, #64042, #108550, #124715, #366, #138886, #136908, #123701, #169222, #198595, #90400, #46890, #78199, #153061, #185399, #60063, #31722, #170229, #61050, #93370, #171225, #1358, #15559, #109543, #14563, #168241, #152085, #76221, #155057, #16552, #47890, #94366, #125712, #137900, #183423, #156045, #199582, #122722, #17542, #2361, #187411, #48879, #44907, #29737, #154064, #184412, #110534, #28763, #91370, #107546, #30731, #92378, #126685, #128676, #84166, #129663, #191359, #114506, #176208, #36667, #111532, #159017, #21513, #81173, #50863, #144848, #190373, #142855, #161025, #172215, #112521, #18544, #80191, #6331, #96350, #95362, #188389, #98326, #20510, #4334, #49866, #83174, #5333, #65029, #37677, #22519, #145846, #157047, #141863, #82158, #68011, #173217, #189386, #52837, #7328, #51848, #99342, #143854, #67017, #3354, #113507, #174215, #34693, #33699, #175202, #69012, #158037, #160026, #19528, #130678, #192372, #66018, #53855, #127686, #35683, #97331, #196388, #39675, #54849, #177217, #163026, #56860, #72016, #71024, #12360, #178211, #24532, #70023, #150866, #102355, #118535, #10359, #164044, #73033, #115529, #193373, #133689, #89174, #87187, #104349, #74023, #181212, #166033, #26530, #165037, #117521, #179219, #86183, #116523, #23521, #195382, #57857, #180224, #85167, #134705, #11363, #147873, #27533, #9359, #41694, #103359, #132692, #135693, #101337, #194380, #131692, #197365, #25543, #88174, #149858, #148868, #119529, #38690, #55847, #42688, #100346, #162025, #146855, #8348, #40685, #109302, #169986, #108306, #60807, #122480, #168004, #198345, #167023, #138644, #1117, #125, #28524, #77962, #154814, #91133, #170981, #46646, #31477, #94127, #183183, #90160, #168976, #44665, #106318, #16312, #186169, #30481, #93129, #151843, #13333, #184171, #29500, #61794, #47651, #123464, #15314, #152823, #14317, #74998, #76973, #32474, #139629, #62791, #124472, #155806, #185156, #59819, #45653, #17304, #75982, #137655 ),
 ( #78959, #199342, #140634, #58830, #92132, #121489, #120497, #182188, #43673, #107304, #105335, #153819, #136663, #20270, #99100, #83931, #18308, #128437, #187175, #64798, #190134, #82934, #156816, #144612, #114267, #66776, #95126, #51609, #172982, #48646, #173978, #2124, #160792, #141633, #6097, #37440, #35446, #189154, #79964, #110298, #67776, #175971, #34460, #97098, #126459, #81916, #22280, #63806, #3123, #113273, #171980, #188157, #174965, #129433, #49630, #191131, #125479, #36429, #111293, #98084, #96119, #33468, #158782, #157807, #19298, #80946, #52605, #142621, #143609, #50627, #4100, #65779, #127448, #112288, #5093, #159782, #21277, #148629, #42450, #147630, #196150, #101098, #10119, #179985, #38449, #71779, #104114, #39438, #163801, #133449, #85941, #162784, #165796, #102116, #132453, #27293, #8100, #117282, #57622, #41453, #11120, #55608, #195139, #119290, #25303, #69778, #131446, #118294, #68772, #116280, #146607, #130430, #56620, #72795, #24292, #87935, #178976, #103118, #193133, #145612, #26294, #180973, #70785, #115286, #7091, #164799, #40443, #86945, #192129, #134465, #194144, #54606, #149622, #53610, #176979, #9118, #177970, #100104, #161788, #23283, #84927, #77737, #138417, #88940, #885, #150631, #167774, #123234, #170752, #91892, #153583, #73791, #44434, #136435, #45421, #107074, #16079, #109073, #62560, #152589, #139403, #29272, #168745, #61565, #60570, #89935, #200097, #15081, #135463, #14080, #76742, #184925, #183936, #151616, #30249, #185932, #12127, #105108, #46409, #197132, #13108, #108068, #169752, #43439, #31247, #124236, #92897, #181957, #154583, #59583, #58599, #122246, #120265, #47417, #28295, #166794, #74773, #198116, #75746, #121257, #182951, #106088, #90903, #137423, #199103, #48414, #111059, #50400, #156581, #127208, #33239, #172747, #157573, #140402, #34228, #112060, #171750, #126232, #95890, #18076, #94897, #173748, #187927, #141400, #32241, #186943, #64567, #188922, #19066, #65549, #49396, #80713, #93899, #142391, #110070, #79731, #3870, #17072, #2888, #155577, #1890, #78726, #63571, #125245, #155240, #184589, #108732, #60239, #32897, #93554, #124900, #138081, #182612, #94549, #139067, #122900, #154247, #136102, #140054, #199762, #121910, #16730, #15738, #186599, #153241, #183603, #77397, #168419, #1544, #61229, #63220, #62216, #12771, #48071, #74435, #91554, #47072, #197778, #545, #123884, #59244, #29914, #45087, #169405, #30911, #109727, #120913, #171411, #76405, #44097, #106744, #90579, #185582, #46070, #105755, #78378, #167441, #28938, #170409, #31901, #152260, #13745, #75413, #137085, #107724, #198773, #14744, #92559, #94219, #138736, #217, #120590, #91220, #183274, #92227, #153913, #62887, #139721, #78052, #61886, #106410, #76071, #15408, #108403, #107397, #136754, #185251, #123556, #182285, #60898, #46744, #30576, #198439, #77065, #32566, #17396, #151934, #170080, #43765, #59911, #31571, #16406, #90251, #1209, #47742, #93222, #28613, #154907, #168091, #105429, #169070, #135785, #155899, #75087, #124567, #171075, #186264, #122573, #13423, #167112, #109395, #197456, #29589, #58922, #121579, #44754, #152911, #137747, #14407, #199431, #184263, #45745, #172070, #143707, #176067, #173073, #97188, #66868, #19387, #96209, #99197, #35541, #65870, #160885, #141721, #50722, #129524, #113367, #144703, #189244, #82011, #52698, #158874, #3211, #64885, #51704, #2216, #49720, #80052, #63897, #5187, #6189, #34550, #21371, #112380, #175059, #126546, #79053, #159882, #191224, #4192, #48734, #140726, #128531, #174072, #20364, #125568, #67869, #127544, #188246, #83029, #190226, #114362, #81036, #111387, #36524, #142712, #157898, #18402, #187265, #98178, #37534, #110388, #33557, #95219, #156905, #54702, #72891, #10212, #71872, #57716, #146703, #53709, #132548, #8200, #69875, #180081, #149716, #194236, #195232, #115386, #192228, #147726, #193228, #102212, #11215, #25397 ),
 ( #133541, #87039, #56715, #118387, #119386, #116375, #134559, #22376, #101190, #68871, #130530, #41550, #131544, #177074, #38545, #39531, #100201, #178063, #161883, #103213, #55702, #23377, #26389, #196247, #181069, #7187, #85023, #70880, #164895, #162880, #24389, #88028, #42544, #163901, #104207, #117375, #179072, #86039, #40542, #9213, #148724, #84027, #145705, #15174, #90024, #14170, #12221, #168837, #184029, #198206, #45511, #108162, #76833, #152681, #46502, #151707, #105198, #27385, #13200, #107166, #122338, #121349, #62651, #28386, #74863, #120356, #975, #75838, #30342, #60665, #137516, #123323, #165888, #43533, #91983, #139493, #199197, #154675, #124328, #31338, #16170, #138505, #200186, #167864, #153677, #73884, #61655, #106181, #135554, #89031, #185016, #169844, #136525, #92989, #197226, #77824, #186026, #59677, #47508, #150722, #58688, #182050, #166885, #183042, #44525, #29364, #90995, #50486, #65638, #64656, #5948, #171838, #156671, #63664, #144463, #95980, #112146, #3959, #157664, #66630, #109164, #187035, #127298, #82782, #80803, #97938, #67625, #174818, #159631, #20130, #158639, #111148, #172838, #18166, #48505, #17164, #189011, #51467, #173838, #78817, #128294, #4946, #141493, #21127, #96959, #81774, #129285, #33325, #140496, #19154, #94986, #79822, #189992, #36283, #142481, #143461, #1984, #125337, #34317, #2977, #35304, #190980, #113128, #170844, #126318, #188015, #110159, #32335, #93988, #155668, #49485, #194987, #56465, #117130, #191972, #39294, #101968, #55459, #163649, #148480, #87786, #23133, #41303, #52457, #131298, #98949, #160639, #25151, #176827, #83781, #145460, #69632, #22130, #84778, #130277, #86793, #85794, #6942, #118143, #102964, #164649, #37290, #68621, #100951, #9971, #53459, #192987, #71631, #149471, #132305, #133297, #24142, #99953, #8970, #70639, #179833, #26144, #10966, #178823, #146456, #54465, #193997, #72640, #147480, #115135, #134315, #40294, #38299, #177824, #114114, #175817, #161639, #7949, #116135, #162635, #11978, #122103, #180827, #58453, #183793, #76599, #150483, #138275, #107921, #60429, #88790, #45280, #166645, #42305, #167630, #77593, #154440, #135314, #199958, #31104, #29127, #182804, #73643, #103966, #61423, #169606, #28147, #90765, #181812, #198962, #92752, #197967, #46266, #151472, #106933, #30106, #196987, #168606, #15934, #89787, #13934, #91746, #136291, #12961, #196001, #152448, #44287, #57474, #120121, #75601, #119146, #153441, #123094, #105945, #14939, #165645, #137280, #43290, #104959, #184780, #27143, #74625, #59437, #121110, #144965, #7446, #94747, #84285, #113624, #37798, #186795, #162143, #22638, #53972, #67135, #108927, #23639, #68127, #51965, #83289, #62412, #69130, #128793, #48266, #145964, #6446, #115645, #82279, #109920, #129778, #156427, #130797, #190493, #192489, #191475, #139264, #177335, #740, #99461, #52953, #100464, #114629, #176328, #124082, #17928, #161141, #185783, #171603, #140252, #47270, #38806, #170607, #143972, #32097, #175319, #93754, #33091, #155435, #16925, #78578, #36785, #1744, #63422, #125097, #98451, #5452, #160144, #21635, #72136, #194493, #27655, #88290, #58949, #25658, #55966, #26647, #40803, #12479, #10476, #74140, #134825, #85287, #197482, #146979, #42807, #196504, #43793, #149978, #11484, #70140, #102473, #132807, #41809, #103477, #135812, #89295, #150987, #73155, #117643, #87303, #165155, #57974, #56976, #86299, #119646, #181328, #131811, #133812, #104469, #180341, #147988, #166154, #182313, #167142, #101456, #120617, #193490, #9477, #105456, #8466, #39792, #54969, #116639, #178329, #163147, #24650, #179340, #71141, #118650, #164160, #148986, #195503, #171100, #63922, #244, #15435, #183301, #136781, #32593, #2239, #199459, #61912, #14435, #31598, #125591, #30603, #79078, #184290, #93247, #62913, #121606, #154933, #187288, #122600, #46769, #16430, #169096, #45771, #48759, #185277, #77094, #110413 ),
 ( #1234, #152936, #59938, #44783, #107423, #75113, #60926, #106436, #139746, #123582, #168117, #94245, #140751, #28641, #13449, #198467, #138763, #124593, #29613, #92256, #186288, #90277, #108428, #47768, #170104, #78078, #91245, #109421, #153940, #76098, #151961, #155925, #17421, #137773, #20389, #18426, #175082, #190252, #4216, #51729, #114388, #21397, #158899, #52722, #96233, #111413, #33581, #19411, #113392, #128557, #127569, #68897, #34576, #81060, #126570, #7213, #82037, #36549, #66894, #143734, #129548, #172094, #49744, #98204, #145732, #5213, #160910, #130557, #37560, #22403, #83055, #144729, #174096, #35565, #142737, #173099, #80076, #159908, #176090, #6216, #141745, #191248, #67895, #65895, #84054, #99223, #192255, #53737, #157921, #3235, #95244, #189270, #50746, #156929, #64909, #188270, #112404, #97213, #85050, #40571, #86065, #195262, #42572, #118417, #71900, #24416, #70908, #69906, #133571, #27414, #72920, #134589, #57744, #119414, #180110, #54730, #102241, #164924, #41578, #26417, #11246, #150751, #147755, #104235, #115411, #194264, #56746, #103242, #165917, #181098, #89060, #88057, #9241, #55731, #149744, #196275, #87067, #116402, #12249, #73911, #100227, #163929, #135581, #10241, #178091, #197253, #177100, #38571, #131572, #161909, #23403, #39561, #146732, #8228, #193256, #101218, #162908, #132576, #117404, #179102, #25426, #148752, #30369, #140522, #17190, #198233, #1003, #94014, #92013, #45539, #13227, #166914, #62677, #32361, #29392, #153706, #44553, #61683, #155695, #60691, #109191, #14198, #123352, #93017, #151734, #185045, #78844, #152708, #76861, #46532, #199226, #75867, #58715, #15202, #107193, #120384, #121378, #138531, #170870, #154705, #124358, #168864, #108192, #182077, #9, #183070, #106208, #31367, #43561, #91022, #59705, #105226, #169874, #186053, #137543, #47537, #16198, #77853, #167892, #28415, #139520, #90052, #184056, #74890, #136553, #122367, #112178, #143491, #125366, #129314, #189040, #111175, #144494, #4976, #175847, #142508, #172865, #66662, #157691, #191010, #127328, #52486, #51498, #2012, #114146, #63691, #159660, #113158, #160668, #128325, #190024, #187062, #19182, #49512, #141520, #50515, #174848, #36314, #97968, #21157, #37320, #34346, #98978, #48532, #80831, #110186, #171864, #82812, #126345, #33353, #95012, #3986, #156700, #96007, #79851, #5977, #35334, #18194, #67657, #22160, #83811, #3007, #64683, #173866, #188042, #65666, #96987, #158669, #20159, #81804, #179864, #117160, #194027, #53488, #40322, #85824, #115165, #6971, #163680, #195019, #69661, #55490, #192002, #148511, #25183, #177855, #86825, #87816, #56495, #132336, #26175, #131328, #84807, #68651, #193016, #10001, #101998, #100983, #42336, #7977, #54493, #99983, #180860, #178856, #71661, #133328, #118173, #102995, #145491, #23164, #41334, #119175, #164681, #134348, #103997, #10999, #196030, #149502, #72671, #147512, #9002, #116165, #146486, #176858, #57506, #165675, #27174, #38327, #130307, #161668, #39324, #162667, #24173, #70669, #124115, #12993, #120152, #198991, #74656, #136323, #46295, #15964, #60459, #61454, #181842, #58485, #13965, #59468, #168635, #77624, #91778, #45311, #197998, #44317, #43322, #106961, #771, #107952, #169639, #31135, #92783, #153472, #185815, #75632, #30135, #183821, #137310, #154472, #88821, #166677, #14968, #62441, #76628, #122134, #170638, #151501, #138306, #139294, #123124, #47302, #199987, #184809, #108959, #150514, #121141, #182835, #12012, #73673, #105976, #89820, #135345, #197019, #104989, #167661, #28178, #29157, #90794, #152478, #52252, #112924, #144258, #157456, #1775, #113909, #158440, #142271, #173628, #155465, #159423, #18950, #141281, #174619, #35098, #5745, #172625, #2771, #96750, #187812, #20919, #80596, #82577, #81569, #32127, #67421, #93784, #189793, #143255, #190777, #19928, #4739, #16955, #49281, #79612, #188800, #50283, #129076, #36084 ),
 ( #78609, #3753, #66428, #109952, #110939, #51264, #140283, #111941, #128089, #65430, #127091, #63453, #97734, #34113, #125130, #186827, #48296, #171632, #156459, #33120, #94777, #17958, #64447, #126117, #95770, #117939, #24942, #162428, #56256, #99751, #114928, #37084, #22927, #116923, #132096, #131090, #72431, #38096, #84573, #130068, #21926, #83577, #148273, #161435, #6737, #68415, #192778, #145256, #146251, #53250, #86590, #8761, #191767, #179628, #25945, #87588, #160436, #176621, #23929, #9765, #7737, #54261, #133093, #10767, #55255, #71429, #147270, #85584, #69423, #70430, #115933, #177623, #98743, #193786, #194783, #39091, #178616, #100747, #40079, #101757, #163445, #41099, #102764, #164451, #149274, #134109, #195798, #57270, #175608, #166446, #60228, #75401, #74425, #15726, #181611, #27942, #73442, #154236, #105744, #121897, #13734, #167431, #76393, #118945, #28927, #29902, #153228, #77386, #107712, #139054, #184576, #169391, #91540, #168407, #120901, #182601, #89584, #58257, #26941, #198762, #61216, #183590, #88583, #138069, #14732, #151270, #30900, #106733, #199750, #534, #43089, #150281, #90567, #104756, #12760, #122888, #46057, #152249, #92547, #11778, #135113, #44086, #136091, #45075, #180630, #42103, #137072, #197766, #59232, #196789, #103767, #165446, #119926, #19697, #4500, #66191, #126857, #1531, #49049, #111706, #65198, #173392, #158207, #97499, #32887, #51030, #62206, #141048, #3522, #18714, #17719, #159185, #124890, #109717, #16718, #20680, #110704, #188563, #157221, #172384, #81339, #123870, #33875, #34862, #96517, #82335, #112691, #144025, #127853, #174383, #143022, #189558, #64215, #125881, #171400, #63210, #170399, #142034, #35853, #50042, #31890, #185568, #47062, #94537, #108722, #93544, #155229, #78368, #186589, #140042, #95534, #48061, #156219, #79377, #2534, #80361, #187581, #98504, #175371, #130851, #176382, #85341, #132858, #8518, #162195, #114687, #161196, #160199, #23693, #117695, #163200, #24704, #148039, #9528, #70196, #145019, #192543, #55020, #131863, #116690, #101510, #40855, #37856, #194546, #5506, #84339, #52018, #113677, #178380, #129832, #36839, #21689, #22692, #83342, #99515, #6500, #39844, #38859, #68180, #71194, #56017, #179392, #190544, #191531, #54026, #86353, #53008, #146018, #102529, #164212, #147034, #25709, #177388, #115699, #7501, #100516, #69185, #193547, #67188, #87354, #128845, #73207, #40, #195556, #154735, #169905, #184088, #31398, #94046, #1035, #138562, #32391, #134878, #88341, #10528, #199257, #62708, #16231, #124390, #47568, #187093, #122398, #140553, #149040, #30401, #57030, #118703, #186085, #60724, #180394, #41865, #168895, #103531, #45571, #26701, #109220, #185075, #165206, #155724, #2041, #63721, #133865, #150032, #61715, #170899, #11539, #92047, #17222, #48563, #93048, #78874, #123383, #46564, #107224, #108225, #153736, #15232, #72191, #77883, #125396, #76891, #139551, #110216, #171897, #33385, #127364, #174882, #37354, #144527, #81836, #175883, #19215, #34379, #156733, #142541, #36348, #51530, #50549, #192040, #157726, #4020, #49546, #130341, #143524, #98001, #190054, #5012, #52518, #95044, #66694, #6013, #129350, #53521, #83843, #115199, #160703, #145525, #67692, #191045, #97020, #158701, #65698, #96039, #3040, #159695, #99012, #21192, #64716, #114179, #22194, #189076, #7004, #82848, #68686, #176891, #80865, #126378, #128358, #112209, #173899, #18226, #79882, #113193, #141551, #188075, #111209, #20190, #35368, #172901, #165710, #41367, #195054, #147546, #194064, #193051, #56532, #150546, #196066, #57539, #180893, #42368, #103033, #177890, #25219, #27207, #86861, #9034, #104031, #164715, #12045, #178891, #70703, #179901, #55525, #88853, #163717, #73709, #87849, #38362, #135381, #100017, #119208, #149537, #197051, #26210, #11032, #23200, #117199, #85857, #118210, #72708, #58519, #120185, #161704, #134380, #132371, #40359 ) ),
 .UNSPECIFIED., .T., .F., .T. ) 
 B_SPLINE_SURFACE_WITH_KNOTS ( ( 4, 3, 4 ),
 ( 3, 2, 2, 2, 2, 2, 2, 2, 2, 2, 2, 2, 2, 2, 2, 2, 2, 2, 2, 2, 2, 2, 2, 2, 2, 2, 2, 2, 2, 2, 2, 2, 2, 2, 2, 2, 2, 2, 2, 2, 2, 2, 2, 2, 2, 2, 2, 2, 2, 2, 2, 2, 2, 2, 2, 2, 2, 2, 2, 2, 2, 2, 2, 2, 2, 2, 2, 2, 2, 2, 2, 2, 2, 2, 2, 2, 2, 2, 2, 2, 2, 2, 2, 2, 2, 2, 2, 2, 2, 2, 2, 2, 2, 2, 2, 2, 2, 2, 2, 2, 2, 2, 2, 2, 2, 2, 2, 2, 2, 2, 2, 2, 2, 2, 2, 2, 2, 2, 2, 2, 2, 2, 2, 2, 2, 2, 2, 2, 2, 2, 2, 2, 2, 2, 2, 2, 2, 2, 2, 2, 2, 2, 2, 2, 2, 2, 2, 2, 2, 2, 2, 2, 2, 2, 2, 2, 2, 2, 2, 2, 2, 2, 2, 2, 2, 2, 2, 2, 2, 2, 2, 2, 2, 2, 2, 2, 2, 2, 2, 2, 2, 2, 2, 2, 2, 2, 2, 2, 2, 2, 2, 2, 2, 2, 2, 2, 2, 2, 2, 2, 2, 2, 2, 2, 2, 2, 2, 2, 2, 2, 2, 2, 2, 2, 2, 2, 2, 2, 2, 2, 2, 2, 2, 2, 2, 2, 2, 2, 3 ),
 ( 0.000000000000000000, 0.5000000000000000000, 1.000000000000000000 ),
 ( 0.000000000000000000, 0.004385964912280701511, 0.008771929824561403022, 0.01315789473684210453, 0.01754385964912280604, 0.02192982456140350755, 0.02631578947368420907, 0.03070175438596491058, 0.03508771929824561209, 0.03947368421052631360, 0.04385964912280701511, 0.04824561403508771662, 0.05263157894736841813, 0.05701754385964911964, 0.06140350877192982115, 0.06578947368421052266, 0.07017543859649122417, 0.07456140350877192569, 0.07894736842105262720, 0.08333333333333332871, 0.08771929824561403022, 0.09210526315789473173, 0.09649122807017543324, 0.1008771929824561348, 0.1052631578947368363, 0.1096491228070175378, 0.1140350877192982393, 0.1184210526315789408, 0.1228070175438596423, 0.1271929824561403577, 0.1315789473684210453, 0.1359649122807017607, 0.1403508771929824483, 0.1447368421052631637, 0.1491228070175438514, 0.1535087719298245668, 0.1578947368421052544, 0.1622807017543859698, 0.1666666666666666574, 0.1710526315789473728, 0.1754385964912280604, 0.1798245614035087758, 0.1842105263157894635, 0.1885964912280701788, 0.1929824561403508665, 0.1973684210526315819, 0.2017543859649122695, 0.2061403508771929849, 0.2105263157894736725, 0.2149122807017543879, 0.2192982456140350755, 0.2236842105263157909, 0.2280701754385964786, 0.2324561403508771940, 0.2368421052631578816, 0.2412280701754385970, 0.2456140350877192846, 0.2500000000000000000, 0.2543859649122807154, 0.2587719298245614308, 0.2631578947368420907, 0.2675438596491228060, 0.2719298245614035214, 0.2763157894736842368, 0.2807017543859648967, 0.2850877192982456121, 0.2894736842105263275, 0.2938596491228070429, 0.2982456140350877027, 0.3026315789473684181, 0.3070175438596491335, 0.3114035087719298489, 0.3157894736842105088, 0.3201754385964912242, 0.3245614035087719396, 0.3289473684210526550, 0.3333333333333333148, 0.3377192982456140302, 0.3421052631578947456, 0.3464912280701754610, 0.3508771929824561209, 0.3552631578947368363, 0.3596491228070175517, 0.3640350877192982670, 0.3684210526315789269, 0.3728070175438596423, 0.3771929824561403577, 0.3815789473684210731, 0.3859649122807017330, 0.3903508771929824483, 0.3947368421052631637, 0.3991228070175438791, 0.4035087719298245390, 0.4078947368421052544, 0.4122807017543859698, 0.4166666666666666852, 0.4210526315789473450, 0.4254385964912280604, 0.4298245614035087758, 0.4342105263157894912, 0.4385964912280701511, 0.4429824561403508665, 0.4473684210526315819, 0.4517543859649122973, 0.4561403508771929571, 0.4605263157894736725, 0.4649122807017543879, 0.4692982456140351033, 0.4736842105263157632, 0.4780701754385964786, 0.4824561403508771940, 0.4868421052631579093, 0.4912280701754385692, 0.4956140350877192846, 0.5000000000000000000, 0.5043859649122807154, 0.5087719298245614308, 0.5131578947368421462, 0.5175438596491228616, 0.5219298245614034659, 0.5263157894736841813, 0.5307017543859648967, 0.5350877192982456121, 0.5394736842105263275, 0.5438596491228070429, 0.5482456140350877583, 0.5526315789473684736, 0.5570175438596490780, 0.5614035087719297934, 0.5657894736842105088, 0.5701754385964912242, 0.5745614035087719396, 0.5789473684210526550, 0.5833333333333333703, 0.5877192982456140857, 0.5921052631578946901, 0.5964912280701754055, 0.6008771929824561209, 0.6052631578947368363, 0.6096491228070175517, 0.6140350877192982670, 0.6184210526315789824, 0.6228070175438596978, 0.6271929824561403022, 0.6315789473684210176, 0.6359649122807017330, 0.6403508771929824483, 0.6447368421052631637, 0.6491228070175438791, 0.6535087719298245945, 0.6578947368421053099, 0.6622807017543859143, 0.6666666666666666297, 0.6710526315789473450, 0.6754385964912280604, 0.6798245614035087758, 0.6842105263157894912, 0.6885964912280702066, 0.6929824561403509220, 0.6973684210526315264, 0.7017543859649122417, 0.7061403508771929571, 0.7105263157894736725, 0.7149122807017543879, 0.7192982456140351033, 0.7236842105263158187, 0.7280701754385965341, 0.7324561403508771384, 0.7368421052631578538, 0.7412280701754385692, 0.7456140350877192846, 0.7500000000000000000, 0.7543859649122807154, 0.7587719298245614308, 0.7631578947368421462, 0.7675438596491228616, 0.7719298245614034659, 0.7763157894736841813, 0.7807017543859648967, 0.7850877192982456121, 0.7894736842105263275, 0.7938596491228070429, 0.7982456140350877583, 0.8026315789473684736, 0.8070175438596490780, 0.8114035087719297934, 0.8157894736842105088, 0.8201754385964912242, 0.8245614035087719396, 0.8289473684210526550, 0.8333333333333333703, 0.8377192982456140857, 0.8421052631578946901, 0.8464912280701754055, 0.8508771929824561209, 0.8552631578947368363, 0.8596491228070175517, 0.8640350877192982670, 0.8684210526315789824, 0.8728070175438596978, 0.8771929824561403022, 0.8815789473684210176, 0.8859649122807017330, 0.8903508771929824483, 0.8947368421052631637, 0.8991228070175438791, 0.9035087719298245945, 0.9078947368421053099, 0.9122807017543859143, 0.9166666666666666297, 0.9210526315789473450, 0.9254385964912280604, 0.9298245614035087758, 0.9342105263157894912, 0.9385964912280702066, 0.9429824561403509220, 0.9473684210526315264, 0.9517543859649122417, 0.9561403508771929571, 0.9605263157894736725, 0.9649122807017543879, 0.9692982456140351033, 0.9736842105263158187, 0.9780701754385965341, 0.9824561403508771384, 0.9868421052631578538, 0.9912280701754385692, 0.9956140350877192846, 1.000000000000000000 ),
 .UNSPECIFIED. ) 
 GEOMETRIC_REPRESENTATION_ITEM ( )  RATIONAL_B_SPLINE_SURFACE ( (
 ( 1.000000000000000000, 0.9659258262890683122, 1.000000000000000000, 0.9659258262890683122, 1.000000000000000000, 0.9659258262890683122, 1.000000000000000000, 0.9659258262890683122, 1.000000000000000000, 0.9659258262890683122, 1.000000000000000000, 0.9659258262890683122, 1.000000000000000000, 0.9659258262890683122, 1.000000000000000000, 0.9659258262890683122, 1.000000000000000000, 0.9659258262890683122, 1.000000000000000000, 0.9659258262890683122, 1.000000000000000000, 0.9659258262890683122, 1.000000000000000000, 0.9659258262890683122, 1.000000000000000000, 0.9659258262890683122, 1.000000000000000000, 0.9659258262890683122, 1.000000000000000000, 0.9659258262890683122, 1.000000000000000000, 0.9659258262890683122, 1.000000000000000000, 0.9659258262890683122, 1.000000000000000000, 0.9659258262890683122, 1.000000000000000000, 0.9659258262890683122, 1.000000000000000000, 0.9659258262890683122, 1.000000000000000000, 0.9659258262890683122, 1.000000000000000000, 0.9659258262890683122, 1.000000000000000000, 0.9659258262890683122, 1.000000000000000000, 0.9659258262890683122, 1.000000000000000000, 0.9659258262890683122, 1.000000000000000000, 0.9659258262890683122, 1.000000000000000000, 0.9659258262890683122, 1.000000000000000000, 0.9659258262890683122, 1.000000000000000000, 0.9659258262890683122, 1.000000000000000000, 0.9659258262890683122, 1.000000000000000000, 0.9659258262890683122, 1.000000000000000000, 0.9659258262890683122, 1.000000000000000000, 0.9659258262890683122, 1.000000000000000000, 0.9659258262890683122, 1.000000000000000000, 0.9659258262890683122, 1.000000000000000000, 0.9659258262890683122, 1.000000000000000000, 0.9659258262890683122, 1.000000000000000000, 0.9659258262890683122, 1.000000000000000000, 0.9659258262890683122, 1.000000000000000000, 0.9659258262890683122, 1.000000000000000000, 0.9659258262890683122, 1.000000000000000000, 0.9659258262890683122, 1.000000000000000000, 0.9659258262890683122, 1.000000000000000000, 0.9659258262890683122, 1.000000000000000000, 0.9659258262890683122, 1.000000000000000000, 0.9659258262890683122, 1.000000000000000000, 0.9659258262890683122, 1.000000000000000000, 0.9659258262890683122, 1.000000000000000000, 0.9659258262890683122, 1.000000000000000000, 0.9659258262890683122, 1.000000000000000000, 0.9659258262890683122, 1.000000000000000000, 0.9659258262890683122, 1.000000000000000000, 0.9659258262890683122, 1.000000000000000000, 0.9659258262890683122, 1.000000000000000000, 0.9659258262890683122, 1.000000000000000000, 0.9659258262890683122, 1.000000000000000000, 0.9659258262890683122, 1.000000000000000000, 0.9659258262890683122, 1.000000000000000000, 0.9659258262890683122, 1.000000000000000000, 0.9659258262890683122, 1.000000000000000000, 0.9659258262890683122, 1.000000000000000000, 0.9659258262890683122, 1.000000000000000000, 0.9659258262890683122, 1.000000000000000000, 0.9659258262890683122, 1.000000000000000000, 0.9659258262890683122, 1.000000000000000000, 0.9659258262890683122, 1.000000000000000000, 0.9659258262890683122, 1.000000000000000000, 0.9659258262890683122, 1.000000000000000000, 0.9659258262890683122, 1.000000000000000000, 0.9659258262890683122, 1.000000000000000000, 0.9659258262890683122, 1.000000000000000000, 0.9659258262890683122, 1.000000000000000000, 0.9659258262890683122, 1.000000000000000000, 0.9659258262890683122, 1.000000000000000000, 0.9659258262890683122, 1.000000000000000000, 0.9659258262890683122, 1.000000000000000000, 0.9659258262890683122, 1.000000000000000000, 0.9659258262890683122, 1.000000000000000000, 0.9659258262890683122, 1.000000000000000000, 0.9659258262890683122, 1.000000000000000000, 0.9659258262890683122, 1.000000000000000000, 0.9659258262890683122, 1.000000000000000000, 0.9659258262890683122, 1.000000000000000000, 0.9659258262890683122, 1.000000000000000000, 0.9659258262890683122, 1.000000000000000000, 0.9659258262890683122, 1.000000000000000000, 0.9659258262890683122, 1.000000000000000000, 0.9659258262890683122, 1.000000000000000000, 0.9659258262890683122, 1.000000000000000000, 0.9659258262890683122, 1.000000000000000000, 0.9659258262890683122, 1.000000000000000000, 0.9659258262890683122, 1.000000000000000000, 0.9659258262890683122, 1.000000000000000000, 0.9659258262890683122, 1.000000000000000000, 0.9659258262890683122, 1.000000000000000000, 0.9659258262890683122, 1.000000000000000000, 0.9659258262890683122, 1.000000000000000000, 0.9659258262890683122, 1.000000000000000000, 0.9659258262890683122, 1.000000000000000000, 0.9659258262890683122, 1.000000000000000000, 0.9659258262890683122, 1.000000000000000000, 0.9659258262890683122, 1.000000000000000000, 0.9659258262890683122, 1.000000000000000000, 0.9659258262890683122, 1.000000000000000000, 0.9659258262890683122, 1.000000000000000000, 0.9659258262890683122, 1.000000000000000000, 0.9659258262890683122, 1.000000000000000000, 0.9659258262890683122, 1.000000000000000000, 0.9659258262890683122, 1.000000000000000000, 0.9659258262890683122, 1.000000000000000000, 0.9659258262890683122, 1.000000000000000000, 0.9659258262890683122, 1.000000000000000000, 0.9659258262890683122, 1.000000000000000000, 0.9659258262890683122, 1.000000000000000000, 0.9659258262890683122, 1.000000000000000000, 0.9659258262890683122, 1.000000000000000000, 0.9659258262890683122, 1.000000000000000000, 0.9659258262890683122, 1.000000000000000000, 0.9659258262890683122, 1.000000000000000000, 0.9659258262890683122, 1.000000000000000000, 0.9659258262890683122, 1.000000000000000000, 0.9659258262890683122, 1.000000000000000000, 0.9659258262890683122, 1.000000000000000000, 0.9659258262890683122, 1.000000000000000000, 0.9659258262890683122, 1.000000000000000000, 0.9659258262890683122, 1.000000000000000000, 0.9659258262890683122, 1.000000000000000000, 0.9659258262890683122, 1.000000000000000000, 0.9659258262890683122, 1.000000000000000000, 0.9659258262890683122, 1.000000000000000000, 0.9659258262890683122, 1.000000000000000000, 0.9659258262890683122, 1.000000000000000000, 0.9659258262890683122, 1.000000000000000000, 0.9659258262890683122, 1.000000000000000000, 0.9659258262890683122, 1.000000000000000000, 0.9659258262890683122, 1.000000000000000000, 0.9659258262890683122, 1.000000000000000000, 0.9659258262890683122, 1.000000000000000000, 0.9659258262890683122, 1.000000000000000000, 0.9659258262890683122, 1.000000000000000000, 0.9659258262890683122, 1.000000000000000000, 0.9659258262890683122, 1.000000000000000000, 0.9659258262890683122, 1.000000000000000000, 0.9659258262890683122, 1.000000000000000000, 0.9659258262890683122, 1.000000000000000000, 0.9659258262890683122, 1.000000000000000000, 0.9659258262890683122, 1.000000000000000000, 0.9659258262890683122, 1.000000000000000000, 0.9659258262890683122, 1.000000000000000000, 0.9659258262890683122, 1.000000000000000000, 0.9659258262890683122, 1.000000000000000000, 0.9659258262890683122, 1.000000000000000000, 0.9659258262890683122, 1.000000000000000000, 0.9659258262890683122, 1.000000000000000000, 0.9659258262890683122, 1.000000000000000000, 0.9659258262890683122, 1.000000000000000000, 0.9659258262890683122, 1.000000000000000000, 0.9659258262890683122, 1.000000000000000000, 0.9659258262890683122, 1.000000000000000000, 0.9659258262890683122, 1.000000000000000000, 0.9659258262890683122, 1.000000000000000000, 0.9659258262890683122, 1.000000000000000000, 0.9659258262890683122, 1.000000000000000000, 0.9659258262890683122, 1.000000000000000000, 0.9659258262890683122, 1.000000000000000000, 0.9659258262890683122, 1.000000000000000000, 0.9659258262890683122, 1.000000000000000000, 0.9659258262890683122, 1.000000000000000000, 0.9659258262890683122, 1.000000000000000000, 0.9659258262890683122, 1.000000000000000000, 0.9659258262890683122, 1.000000000000000000, 0.9659258262890683122, 1.000000000000000000, 0.9659258262890683122, 1.000000000000000000, 0.9659258262890683122, 1.000000000000000000, 0.9659258262890683122, 1.000000000000000000, 0.9659258262890683122, 1.000000000000000000, 0.9659258262890683122, 1.000000000000000000, 0.9659258262890683122, 1.000000000000000000, 0.9659258262890683122, 1.000000000000000000, 0.9659258262890683122, 1.000000000000000000, 0.9659258262890683122, 1.000000000000000000, 0.9659258262890683122, 1.000000000000000000, 0.9659258262890683122, 1.000000000000000000, 0.9659258262890683122, 1.000000000000000000, 0.9659258262890683122, 1.000000000000000000, 0.9659258262890683122, 1.000000000000000000, 0.9659258262890683122, 1.000000000000000000, 0.9659258262890683122, 1.000000000000000000, 0.9659258262890683122, 1.000000000000000000, 0.9659258262890683122, 1.000000000000000000, 0.9659258262890683122, 1.000000000000000000, 0.9659258262890683122, 1.000000000000000000, 0.9659258262890683122, 1.000000000000000000, 0.9659258262890683122, 1.000000000000000000, 0.9659258262890683122, 1.000000000000000000, 0.9659258262890683122, 1.000000000000000000, 0.9659258262890683122, 1.000000000000000000, 0.9659258262890683122, 1.000000000000000000, 0.9659258262890683122, 1.000000000000000000, 0.9659258262890683122, 1.000000000000000000, 0.9659258262890683122, 1.000000000000000000, 0.9659258262890683122, 1.000000000000000000, 0.9659258262890683122, 1.000000000000000000, 0.9659258262890683122, 1.000000000000000000, 0.9659258262890683122, 1.000000000000000000, 0.9659258262890683122, 1.000000000000000000, 0.9659258262890683122, 1.000000000000000000, 0.9659258262890683122, 1.000000000000000000, 0.9659258262890683122, 1.000000000000000000, 0.9659258262890683122, 1.000000000000000000, 0.9659258262890683122, 1.000000000000000000, 0.9659258262890683122, 1.000000000000000000, 0.9659258262890683122, 1.000000000000000000, 0.9659258262890683122, 1.000000000000000000, 0.9659258262890683122, 1.000000000000000000, 0.9659258262890683122, 1.000000000000000000, 0.9659258262890683122, 1.000000000000000000, 0.9659258262890683122, 1.000000000000000000, 0.9659258262890683122, 1.000000000000000000, 0.9659258262890683122, 1.000000000000000000, 0.9659258262890683122, 1.000000000000000000, 0.9659258262890683122, 1.000000000000000000, 0.9659258262890683122, 1.000000000000000000, 0.9659258262890683122, 1.000000000000000000, 0.9659258262890683122, 1.000000000000000000, 0.9659258262890683122, 1.000000000000000000, 0.9659258262890683122, 1.000000000000000000, 0.9659258262890683122, 1.000000000000000000),
 ( 0.3333333333333333703, 0.3219752754296894559, 0.3333333333333333703, 0.3219752754296894559, 0.3333333333333333703, 0.3219752754296894559, 0.3333333333333333703, 0.3219752754296894559, 0.3333333333333333703, 0.3219752754296894559, 0.3333333333333333703, 0.3219752754296894559, 0.3333333333333333703, 0.3219752754296894559, 0.3333333333333333703, 0.3219752754296894559, 0.3333333333333333703, 0.3219752754296894559, 0.3333333333333333703, 0.3219752754296894559, 0.3333333333333333703, 0.3219752754296894559, 0.3333333333333333703, 0.3219752754296894559, 0.3333333333333333703, 0.3219752754296894559, 0.3333333333333333703, 0.3219752754296894559, 0.3333333333333333703, 0.3219752754296894559, 0.3333333333333333703, 0.3219752754296894559, 0.3333333333333333703, 0.3219752754296894559, 0.3333333333333333703, 0.3219752754296894559, 0.3333333333333333703, 0.3219752754296894559, 0.3333333333333333703, 0.3219752754296894559, 0.3333333333333333703, 0.3219752754296894559, 0.3333333333333333703, 0.3219752754296894559, 0.3333333333333333703, 0.3219752754296894559, 0.3333333333333333703, 0.3219752754296894559, 0.3333333333333333703, 0.3219752754296894559, 0.3333333333333333703, 0.3219752754296894559, 0.3333333333333333703, 0.3219752754296894559, 0.3333333333333333703, 0.3219752754296894559, 0.3333333333333333703, 0.3219752754296894559, 0.3333333333333333703, 0.3219752754296894559, 0.3333333333333333703, 0.3219752754296894559, 0.3333333333333333703, 0.3219752754296894559, 0.3333333333333333703, 0.3219752754296894559, 0.3333333333333333703, 0.3219752754296894559, 0.3333333333333333703, 0.3219752754296894559, 0.3333333333333333703, 0.3219752754296894559, 0.3333333333333333703, 0.3219752754296894559, 0.3333333333333333703, 0.3219752754296894559, 0.3333333333333333703, 0.3219752754296894559, 0.3333333333333333703, 0.3219752754296894559, 0.3333333333333333703, 0.3219752754296894559, 0.3333333333333333703, 0.3219752754296894559, 0.3333333333333333703, 0.3219752754296894559, 0.3333333333333333703, 0.3219752754296894559, 0.3333333333333333703, 0.3219752754296894559, 0.3333333333333333703, 0.3219752754296894559, 0.3333333333333333703, 0.3219752754296894559, 0.3333333333333333703, 0.3219752754296894559, 0.3333333333333333703, 0.3219752754296894559, 0.3333333333333333703, 0.3219752754296894559, 0.3333333333333333703, 0.3219752754296894559, 0.3333333333333333703, 0.3219752754296894559, 0.3333333333333333703, 0.3219752754296894559, 0.3333333333333333703, 0.3219752754296894559, 0.3333333333333333703, 0.3219752754296894559, 0.3333333333333333703, 0.3219752754296894559, 0.3333333333333333703, 0.3219752754296894559, 0.3333333333333333703, 0.3219752754296894559, 0.3333333333333333703, 0.3219752754296894559, 0.3333333333333333703, 0.3219752754296894559, 0.3333333333333333703, 0.3219752754296894559, 0.3333333333333333703, 0.3219752754296894559, 0.3333333333333333703, 0.3219752754296894559, 0.3333333333333333703, 0.3219752754296894559, 0.3333333333333333703, 0.3219752754296894559, 0.3333333333333333703, 0.3219752754296894559, 0.3333333333333333703, 0.3219752754296894559, 0.3333333333333333703, 0.3219752754296894559, 0.3333333333333333703, 0.3219752754296894559, 0.3333333333333333703, 0.3219752754296894559, 0.3333333333333333703, 0.3219752754296894559, 0.3333333333333333703, 0.3219752754296894559, 0.3333333333333333703, 0.3219752754296894559, 0.3333333333333333703, 0.3219752754296894559, 0.3333333333333333703, 0.3219752754296894559, 0.3333333333333333703, 0.3219752754296894559, 0.3333333333333333703, 0.3219752754296894559, 0.3333333333333333703, 0.3219752754296894559, 0.3333333333333333703, 0.3219752754296894559, 0.3333333333333333703, 0.3219752754296894559, 0.3333333333333333703, 0.3219752754296894559, 0.3333333333333333703, 0.3219752754296894559, 0.3333333333333333703, 0.3219752754296894559, 0.3333333333333333703, 0.3219752754296894559, 0.3333333333333333703, 0.3219752754296894559, 0.3333333333333333703, 0.3219752754296894559, 0.3333333333333333703, 0.3219752754296894559, 0.3333333333333333703, 0.3219752754296894559, 0.3333333333333333703, 0.3219752754296894559, 0.3333333333333333703, 0.3219752754296894559, 0.3333333333333333703, 0.3219752754296894559, 0.3333333333333333703, 0.3219752754296894559, 0.3333333333333333703, 0.3219752754296894559, 0.3333333333333333703, 0.3219752754296894559, 0.3333333333333333703, 0.3219752754296894559, 0.3333333333333333703, 0.3219752754296894559, 0.3333333333333333703, 0.3219752754296894559, 0.3333333333333333703, 0.3219752754296894559, 0.3333333333333333703, 0.3219752754296894559, 0.3333333333333333703, 0.3219752754296894559, 0.3333333333333333703, 0.3219752754296894559, 0.3333333333333333703, 0.3219752754296894559, 0.3333333333333333703, 0.3219752754296894559, 0.3333333333333333703, 0.3219752754296894559, 0.3333333333333333703, 0.3219752754296894559, 0.3333333333333333703, 0.3219752754296894559, 0.3333333333333333703, 0.3219752754296894559, 0.3333333333333333703, 0.3219752754296894559, 0.3333333333333333703, 0.3219752754296894559, 0.3333333333333333703, 0.3219752754296894559, 0.3333333333333333703, 0.3219752754296894559, 0.3333333333333333703, 0.3219752754296894559, 0.3333333333333333703, 0.3219752754296894559, 0.3333333333333333703, 0.3219752754296894559, 0.3333333333333333703, 0.3219752754296894559, 0.3333333333333333703, 0.3219752754296894559, 0.3333333333333333703, 0.3219752754296894559, 0.3333333333333333703, 0.3219752754296894559, 0.3333333333333333703, 0.3219752754296894559, 0.3333333333333333703, 0.3219752754296894559, 0.3333333333333333703, 0.3219752754296894559, 0.3333333333333333703, 0.3219752754296894559, 0.3333333333333333703, 0.3219752754296894559, 0.3333333333333333703, 0.3219752754296894559, 0.3333333333333333703, 0.3219752754296894559, 0.3333333333333333703, 0.3219752754296894559, 0.3333333333333333703, 0.3219752754296894559, 0.3333333333333333703, 0.3219752754296894559, 0.3333333333333333703, 0.3219752754296894559, 0.3333333333333333703, 0.3219752754296894559, 0.3333333333333333703, 0.3219752754296894559, 0.3333333333333333703, 0.3219752754296894559, 0.3333333333333333703, 0.3219752754296894559, 0.3333333333333333703, 0.3219752754296894559, 0.3333333333333333703, 0.3219752754296894559, 0.3333333333333333703, 0.3219752754296894559, 0.3333333333333333703, 0.3219752754296894559, 0.3333333333333333703, 0.3219752754296894559, 0.3333333333333333703, 0.3219752754296894559, 0.3333333333333333703, 0.3219752754296894559, 0.3333333333333333703, 0.3219752754296894559, 0.3333333333333333703, 0.3219752754296894559, 0.3333333333333333703, 0.3219752754296894559, 0.3333333333333333703, 0.3219752754296894559, 0.3333333333333333703, 0.3219752754296894559, 0.3333333333333333703, 0.3219752754296894559, 0.3333333333333333703, 0.3219752754296894559, 0.3333333333333333703, 0.3219752754296894559, 0.3333333333333333703, 0.3219752754296894559, 0.3333333333333333703, 0.3219752754296894559, 0.3333333333333333703, 0.3219752754296894559, 0.3333333333333333703, 0.3219752754296894559, 0.3333333333333333703, 0.3219752754296894559, 0.3333333333333333703, 0.3219752754296894559, 0.3333333333333333703, 0.3219752754296894559, 0.3333333333333333703, 0.3219752754296894559, 0.3333333333333333703, 0.3219752754296894559, 0.3333333333333333703, 0.3219752754296894559, 0.3333333333333333703, 0.3219752754296894559, 0.3333333333333333703, 0.3219752754296894559, 0.3333333333333333703, 0.3219752754296894559, 0.3333333333333333703, 0.3219752754296894559, 0.3333333333333333703, 0.3219752754296894559, 0.3333333333333333703, 0.3219752754296894559, 0.3333333333333333703, 0.3219752754296894559, 0.3333333333333333703, 0.3219752754296894559, 0.3333333333333333703, 0.3219752754296894559, 0.3333333333333333703, 0.3219752754296894559, 0.3333333333333333703, 0.3219752754296894559, 0.3333333333333333703, 0.3219752754296894559, 0.3333333333333333703, 0.3219752754296894559, 0.3333333333333333703, 0.3219752754296894559, 0.3333333333333333703, 0.3219752754296894559, 0.3333333333333333703, 0.3219752754296894559, 0.3333333333333333703, 0.3219752754296894559, 0.3333333333333333703, 0.3219752754296894559, 0.3333333333333333703, 0.3219752754296894559, 0.3333333333333333703, 0.3219752754296894559, 0.3333333333333333703, 0.3219752754296894559, 0.3333333333333333703, 0.3219752754296894559, 0.3333333333333333703, 0.3219752754296894559, 0.3333333333333333703, 0.3219752754296894559, 0.3333333333333333703, 0.3219752754296894559, 0.3333333333333333703, 0.3219752754296894559, 0.3333333333333333703, 0.3219752754296894559, 0.3333333333333333703, 0.3219752754296894559, 0.3333333333333333703, 0.3219752754296894559, 0.3333333333333333703, 0.3219752754296894559, 0.3333333333333333703, 0.3219752754296894559, 0.3333333333333333703, 0.3219752754296894559, 0.3333333333333333703, 0.3219752754296894559, 0.3333333333333333703, 0.3219752754296894559, 0.3333333333333333703, 0.3219752754296894559, 0.3333333333333333703, 0.3219752754296894559, 0.3333333333333333703, 0.3219752754296894559, 0.3333333333333333703, 0.3219752754296894559, 0.3333333333333333703, 0.3219752754296894559, 0.3333333333333333703, 0.3219752754296894559, 0.3333333333333333703, 0.3219752754296894559, 0.3333333333333333703, 0.3219752754296894559, 0.3333333333333333703, 0.3219752754296894559, 0.3333333333333333703, 0.3219752754296894559, 0.3333333333333333703, 0.3219752754296894559, 0.3333333333333333703, 0.3219752754296894559, 0.3333333333333333703, 0.3219752754296894559, 0.3333333333333333703, 0.3219752754296894559, 0.3333333333333333703, 0.3219752754296894559, 0.3333333333333333703, 0.3219752754296894559, 0.3333333333333333703, 0.3219752754296894559, 0.3333333333333333703, 0.3219752754296894559, 0.3333333333333333703, 0.3219752754296894559, 0.3333333333333333703, 0.3219752754296894559, 0.3333333333333333703, 0.3219752754296894559, 0.3333333333333333703, 0.3219752754296894559, 0.3333333333333333703, 0.3219752754296894559, 0.3333333333333333703, 0.3219752754296894559, 0.3333333333333333703, 0.3219752754296894559, 0.3333333333333333703, 0.3219752754296894559, 0.3333333333333333703, 0.3219752754296894559, 0.3333333333333333703, 0.3219752754296894559, 0.3333333333333333703, 0.3219752754296894559, 0.3333333333333333703, 0.3219752754296894559, 0.3333333333333333703, 0.3219752754296894559, 0.3333333333333333703, 0.3219752754296894559, 0.3333333333333333703, 0.3219752754296894559, 0.3333333333333333703, 0.3219752754296894559, 0.3333333333333333703, 0.3219752754296894559, 0.3333333333333333703, 0.3219752754296894559, 0.3333333333333333703),
 ( 0.3333333333333333703, 0.3219752754296894559, 0.3333333333333333703, 0.3219752754296894559, 0.3333333333333333703, 0.3219752754296894559, 0.3333333333333333703, 0.3219752754296894559, 0.3333333333333333703, 0.3219752754296894559, 0.3333333333333333703, 0.3219752754296894559, 0.3333333333333333703, 0.3219752754296894559, 0.3333333333333333703, 0.3219752754296894559, 0.3333333333333333703, 0.3219752754296894559, 0.3333333333333333703, 0.3219752754296894559, 0.3333333333333333703, 0.3219752754296894559, 0.3333333333333333703, 0.3219752754296894559, 0.3333333333333333703, 0.3219752754296894559, 0.3333333333333333703, 0.3219752754296894559, 0.3333333333333333703, 0.3219752754296894559, 0.3333333333333333703, 0.3219752754296894559, 0.3333333333333333703, 0.3219752754296894559, 0.3333333333333333703, 0.3219752754296894559, 0.3333333333333333703, 0.3219752754296894559, 0.3333333333333333703, 0.3219752754296894559, 0.3333333333333333703, 0.3219752754296894559, 0.3333333333333333703, 0.3219752754296894559, 0.3333333333333333703, 0.3219752754296894559, 0.3333333333333333703, 0.3219752754296894559, 0.3333333333333333703, 0.3219752754296894559, 0.3333333333333333703, 0.3219752754296894559, 0.3333333333333333703, 0.3219752754296894559, 0.3333333333333333703, 0.3219752754296894559, 0.3333333333333333703, 0.3219752754296894559, 0.3333333333333333703, 0.3219752754296894559, 0.3333333333333333703, 0.3219752754296894559, 0.3333333333333333703, 0.3219752754296894559, 0.3333333333333333703, 0.3219752754296894559, 0.3333333333333333703, 0.3219752754296894559, 0.3333333333333333703, 0.3219752754296894559, 0.3333333333333333703, 0.3219752754296894559, 0.3333333333333333703, 0.3219752754296894559, 0.3333333333333333703, 0.3219752754296894559, 0.3333333333333333703, 0.3219752754296894559, 0.3333333333333333703, 0.3219752754296894559, 0.3333333333333333703, 0.3219752754296894559, 0.3333333333333333703, 0.3219752754296894559, 0.3333333333333333703, 0.3219752754296894559, 0.3333333333333333703, 0.3219752754296894559, 0.3333333333333333703, 0.3219752754296894559, 0.3333333333333333703, 0.3219752754296894559, 0.3333333333333333703, 0.3219752754296894559, 0.3333333333333333703, 0.3219752754296894559, 0.3333333333333333703, 0.3219752754296894559, 0.3333333333333333703, 0.3219752754296894559, 0.3333333333333333703, 0.3219752754296894559, 0.3333333333333333703, 0.3219752754296894559, 0.3333333333333333703, 0.3219752754296894559, 0.3333333333333333703, 0.3219752754296894559, 0.3333333333333333703, 0.3219752754296894559, 0.3333333333333333703, 0.3219752754296894559, 0.3333333333333333703, 0.3219752754296894559, 0.3333333333333333703, 0.3219752754296894559, 0.3333333333333333703, 0.3219752754296894559, 0.3333333333333333703, 0.3219752754296894559, 0.3333333333333333703, 0.3219752754296894559, 0.3333333333333333703, 0.3219752754296894559, 0.3333333333333333703, 0.3219752754296894559, 0.3333333333333333703, 0.3219752754296894559, 0.3333333333333333703, 0.3219752754296894559, 0.3333333333333333703, 0.3219752754296894559, 0.3333333333333333703, 0.3219752754296894559, 0.3333333333333333703, 0.3219752754296894559, 0.3333333333333333703, 0.3219752754296894559, 0.3333333333333333703, 0.3219752754296894559, 0.3333333333333333703, 0.3219752754296894559, 0.3333333333333333703, 0.3219752754296894559, 0.3333333333333333703, 0.3219752754296894559, 0.3333333333333333703, 0.3219752754296894559, 0.3333333333333333703, 0.3219752754296894559, 0.3333333333333333703, 0.3219752754296894559, 0.3333333333333333703, 0.3219752754296894559, 0.3333333333333333703, 0.3219752754296894559, 0.3333333333333333703, 0.3219752754296894559, 0.3333333333333333703, 0.3219752754296894559, 0.3333333333333333703, 0.3219752754296894559, 0.3333333333333333703, 0.3219752754296894559, 0.3333333333333333703, 0.3219752754296894559, 0.3333333333333333703, 0.3219752754296894559, 0.3333333333333333703, 0.3219752754296894559, 0.3333333333333333703, 0.3219752754296894559, 0.3333333333333333703, 0.3219752754296894559, 0.3333333333333333703, 0.3219752754296894559, 0.3333333333333333703, 0.3219752754296894559, 0.3333333333333333703, 0.3219752754296894559, 0.3333333333333333703, 0.3219752754296894559, 0.3333333333333333703, 0.3219752754296894559, 0.3333333333333333703, 0.3219752754296894559, 0.3333333333333333703, 0.3219752754296894559, 0.3333333333333333703, 0.3219752754296894559, 0.3333333333333333703, 0.3219752754296894559, 0.3333333333333333703, 0.3219752754296894559, 0.3333333333333333703, 0.3219752754296894559, 0.3333333333333333703, 0.3219752754296894559, 0.3333333333333333703, 0.3219752754296894559, 0.3333333333333333703, 0.3219752754296894559, 0.3333333333333333703, 0.3219752754296894559, 0.3333333333333333703, 0.3219752754296894559, 0.3333333333333333703, 0.3219752754296894559, 0.3333333333333333703, 0.3219752754296894559, 0.3333333333333333703, 0.3219752754296894559, 0.3333333333333333703, 0.3219752754296894559, 0.3333333333333333703, 0.3219752754296894559, 0.3333333333333333703, 0.3219752754296894559, 0.3333333333333333703, 0.3219752754296894559, 0.3333333333333333703, 0.3219752754296894559, 0.3333333333333333703, 0.3219752754296894559, 0.3333333333333333703, 0.3219752754296894559, 0.3333333333333333703, 0.3219752754296894559, 0.3333333333333333703, 0.3219752754296894559, 0.3333333333333333703, 0.3219752754296894559, 0.3333333333333333703, 0.3219752754296894559, 0.3333333333333333703, 0.3219752754296894559, 0.3333333333333333703, 0.3219752754296894559, 0.3333333333333333703, 0.3219752754296894559, 0.3333333333333333703, 0.3219752754296894559, 0.3333333333333333703, 0.3219752754296894559, 0.3333333333333333703, 0.3219752754296894559, 0.3333333333333333703, 0.3219752754296894559, 0.3333333333333333703, 0.3219752754296894559, 0.3333333333333333703, 0.3219752754296894559, 0.3333333333333333703, 0.3219752754296894559, 0.3333333333333333703, 0.3219752754296894559, 0.3333333333333333703, 0.3219752754296894559, 0.3333333333333333703, 0.3219752754296894559, 0.3333333333333333703, 0.3219752754296894559, 0.3333333333333333703, 0.3219752754296894559, 0.3333333333333333703, 0.3219752754296894559, 0.3333333333333333703, 0.3219752754296894559, 0.3333333333333333703, 0.3219752754296894559, 0.3333333333333333703, 0.3219752754296894559, 0.3333333333333333703, 0.3219752754296894559, 0.3333333333333333703, 0.3219752754296894559, 0.3333333333333333703, 0.3219752754296894559, 0.3333333333333333703, 0.3219752754296894559, 0.3333333333333333703, 0.3219752754296894559, 0.3333333333333333703, 0.3219752754296894559, 0.3333333333333333703, 0.3219752754296894559, 0.3333333333333333703, 0.3219752754296894559, 0.3333333333333333703, 0.3219752754296894559, 0.3333333333333333703, 0.3219752754296894559, 0.3333333333333333703, 0.3219752754296894559, 0.3333333333333333703, 0.3219752754296894559, 0.3333333333333333703, 0.3219752754296894559, 0.3333333333333333703, 0.3219752754296894559, 0.3333333333333333703, 0.3219752754296894559, 0.3333333333333333703, 0.3219752754296894559, 0.3333333333333333703, 0.3219752754296894559, 0.3333333333333333703, 0.3219752754296894559, 0.3333333333333333703, 0.3219752754296894559, 0.3333333333333333703, 0.3219752754296894559, 0.3333333333333333703, 0.3219752754296894559, 0.3333333333333333703, 0.3219752754296894559, 0.3333333333333333703, 0.3219752754296894559, 0.3333333333333333703, 0.3219752754296894559, 0.3333333333333333703, 0.3219752754296894559, 0.3333333333333333703, 0.3219752754296894559, 0.3333333333333333703, 0.3219752754296894559, 0.3333333333333333703, 0.3219752754296894559, 0.3333333333333333703, 0.3219752754296894559, 0.3333333333333333703, 0.3219752754296894559, 0.3333333333333333703, 0.3219752754296894559, 0.3333333333333333703, 0.3219752754296894559, 0.3333333333333333703, 0.3219752754296894559, 0.3333333333333333703, 0.3219752754296894559, 0.3333333333333333703, 0.3219752754296894559, 0.3333333333333333703, 0.3219752754296894559, 0.3333333333333333703, 0.3219752754296894559, 0.3333333333333333703, 0.3219752754296894559, 0.3333333333333333703, 0.3219752754296894559, 0.3333333333333333703, 0.3219752754296894559, 0.3333333333333333703, 0.3219752754296894559, 0.3333333333333333703, 0.3219752754296894559, 0.3333333333333333703, 0.3219752754296894559, 0.3333333333333333703, 0.3219752754296894559, 0.3333333333333333703, 0.3219752754296894559, 0.3333333333333333703, 0.3219752754296894559, 0.3333333333333333703, 0.3219752754296894559, 0.3333333333333333703, 0.3219752754296894559, 0.3333333333333333703, 0.3219752754296894559, 0.3333333333333333703, 0.3219752754296894559, 0.3333333333333333703, 0.3219752754296894559, 0.3333333333333333703, 0.3219752754296894559, 0.3333333333333333703, 0.3219752754296894559, 0.3333333333333333703, 0.3219752754296894559, 0.3333333333333333703, 0.3219752754296894559, 0.3333333333333333703, 0.3219752754296894559, 0.3333333333333333703, 0.3219752754296894559, 0.3333333333333333703, 0.3219752754296894559, 0.3333333333333333703, 0.3219752754296894559, 0.3333333333333333703, 0.3219752754296894559, 0.3333333333333333703, 0.3219752754296894559, 0.3333333333333333703, 0.3219752754296894559, 0.3333333333333333703, 0.3219752754296894559, 0.3333333333333333703, 0.3219752754296894559, 0.3333333333333333703, 0.3219752754296894559, 0.3333333333333333703, 0.3219752754296894559, 0.3333333333333333703, 0.3219752754296894559, 0.3333333333333333703, 0.3219752754296894559, 0.3333333333333333703, 0.3219752754296894559, 0.3333333333333333703, 0.3219752754296894559, 0.3333333333333333703, 0.3219752754296894559, 0.3333333333333333703, 0.3219752754296894559, 0.3333333333333333703, 0.3219752754296894559, 0.3333333333333333703, 0.3219752754296894559, 0.3333333333333333703, 0.3219752754296894559, 0.3333333333333333703, 0.3219752754296894559, 0.3333333333333333703, 0.3219752754296894559, 0.3333333333333333703, 0.3219752754296894559, 0.3333333333333333703, 0.3219752754296894559, 0.3333333333333333703, 0.3219752754296894559, 0.3333333333333333703, 0.3219752754296894559, 0.3333333333333333703, 0.3219752754296894559, 0.3333333333333333703, 0.3219752754296894559, 0.3333333333333333703, 0.3219752754296894559, 0.3333333333333333703, 0.3219752754296894559, 0.3333333333333333703, 0.3219752754296894559, 0.3333333333333333703, 0.3219752754296894559, 0.3333333333333333703, 0.3219752754296894559, 0.3333333333333333703, 0.3219752754296894559, 0.3333333333333333703, 0.3219752754296894559, 0.3333333333333333703, 0.3219752754296894559, 0.3333333333333333703, 0.3219752754296894559, 0.3333333333333333703),
 ( 1.000000000000000000, 0.9659258262890683122, 1.000000000000000000, 0.9659258262890683122, 1.000000000000000000, 0.9659258262890683122, 1.000000000000000000, 0.9659258262890683122, 1.000000000000000000, 0.9659258262890683122, 1.000000000000000000, 0.9659258262890683122, 1.000000000000000000, 0.9659258262890683122, 1.000000000000000000, 0.9659258262890683122, 1.000000000000000000, 0.9659258262890683122, 1.000000000000000000, 0.9659258262890683122, 1.000000000000000000, 0.9659258262890683122, 1.000000000000000000, 0.9659258262890683122, 1.000000000000000000, 0.9659258262890683122, 1.000000000000000000, 0.9659258262890683122, 1.000000000000000000, 0.9659258262890683122, 1.000000000000000000, 0.9659258262890683122, 1.000000000000000000, 0.9659258262890683122, 1.000000000000000000, 0.9659258262890683122, 1.000000000000000000, 0.9659258262890683122, 1.000000000000000000, 0.9659258262890683122, 1.000000000000000000, 0.9659258262890683122, 1.000000000000000000, 0.9659258262890683122, 1.000000000000000000, 0.9659258262890683122, 1.000000000000000000, 0.9659258262890683122, 1.000000000000000000, 0.9659258262890683122, 1.000000000000000000, 0.9659258262890683122, 1.000000000000000000, 0.9659258262890683122, 1.000000000000000000, 0.9659258262890683122, 1.000000000000000000, 0.9659258262890683122, 1.000000000000000000, 0.9659258262890683122, 1.000000000000000000, 0.9659258262890683122, 1.000000000000000000, 0.9659258262890683122, 1.000000000000000000, 0.9659258262890683122, 1.000000000000000000, 0.9659258262890683122, 1.000000000000000000, 0.9659258262890683122, 1.000000000000000000, 0.9659258262890683122, 1.000000000000000000, 0.9659258262890683122, 1.000000000000000000, 0.9659258262890683122, 1.000000000000000000, 0.9659258262890683122, 1.000000000000000000, 0.9659258262890683122, 1.000000000000000000, 0.9659258262890683122, 1.000000000000000000, 0.9659258262890683122, 1.000000000000000000, 0.9659258262890683122, 1.000000000000000000, 0.9659258262890683122, 1.000000000000000000, 0.9659258262890683122, 1.000000000000000000, 0.9659258262890683122, 1.000000000000000000, 0.9659258262890683122, 1.000000000000000000, 0.9659258262890683122, 1.000000000000000000, 0.9659258262890683122, 1.000000000000000000, 0.9659258262890683122, 1.000000000000000000, 0.9659258262890683122, 1.000000000000000000, 0.9659258262890683122, 1.000000000000000000, 0.9659258262890683122, 1.000000000000000000, 0.9659258262890683122, 1.000000000000000000, 0.9659258262890683122, 1.000000000000000000, 0.9659258262890683122, 1.000000000000000000, 0.9659258262890683122, 1.000000000000000000, 0.9659258262890683122, 1.000000000000000000, 0.9659258262890683122, 1.000000000000000000, 0.9659258262890683122, 1.000000000000000000, 0.9659258262890683122, 1.000000000000000000, 0.9659258262890683122, 1.000000000000000000, 0.9659258262890683122, 1.000000000000000000, 0.9659258262890683122, 1.000000000000000000, 0.9659258262890683122, 1.000000000000000000, 0.9659258262890683122, 1.000000000000000000, 0.9659258262890683122, 1.000000000000000000, 0.9659258262890683122, 1.000000000000000000, 0.9659258262890683122, 1.000000000000000000, 0.9659258262890683122, 1.000000000000000000, 0.9659258262890683122, 1.000000000000000000, 0.9659258262890683122, 1.000000000000000000, 0.9659258262890683122, 1.000000000000000000, 0.9659258262890683122, 1.000000000000000000, 0.9659258262890683122, 1.000000000000000000, 0.9659258262890683122, 1.000000000000000000, 0.9659258262890683122, 1.000000000000000000, 0.9659258262890683122, 1.000000000000000000, 0.9659258262890683122, 1.000000000000000000, 0.9659258262890683122, 1.000000000000000000, 0.9659258262890683122, 1.000000000000000000, 0.9659258262890683122, 1.000000000000000000, 0.9659258262890683122, 1.000000000000000000, 0.9659258262890683122, 1.000000000000000000, 0.9659258262890683122, 1.000000000000000000, 0.9659258262890683122, 1.000000000000000000, 0.9659258262890683122, 1.000000000000000000, 0.9659258262890683122, 1.000000000000000000, 0.9659258262890683122, 1.000000000000000000, 0.9659258262890683122, 1.000000000000000000, 0.9659258262890683122, 1.000000000000000000, 0.9659258262890683122, 1.000000000000000000, 0.9659258262890683122, 1.000000000000000000, 0.9659258262890683122, 1.000000000000000000, 0.9659258262890683122, 1.000000000000000000, 0.9659258262890683122, 1.000000000000000000, 0.9659258262890683122, 1.000000000000000000, 0.9659258262890683122, 1.000000000000000000, 0.9659258262890683122, 1.000000000000000000, 0.9659258262890683122, 1.000000000000000000, 0.9659258262890683122, 1.000000000000000000, 0.9659258262890683122, 1.000000000000000000, 0.9659258262890683122, 1.000000000000000000, 0.9659258262890683122, 1.000000000000000000, 0.9659258262890683122, 1.000000000000000000, 0.9659258262890683122, 1.000000000000000000, 0.9659258262890683122, 1.000000000000000000, 0.9659258262890683122, 1.000000000000000000, 0.9659258262890683122, 1.000000000000000000, 0.9659258262890683122, 1.000000000000000000, 0.9659258262890683122, 1.000000000000000000, 0.9659258262890683122, 1.000000000000000000, 0.9659258262890683122, 1.000000000000000000, 0.9659258262890683122, 1.000000000000000000, 0.9659258262890683122, 1.000000000000000000, 0.9659258262890683122, 1.000000000000000000, 0.9659258262890683122, 1.000000000000000000, 0.9659258262890683122, 1.000000000000000000, 0.9659258262890683122, 1.000000000000000000, 0.9659258262890683122, 1.000000000000000000, 0.9659258262890683122, 1.000000000000000000, 0.9659258262890683122, 1.000000000000000000, 0.9659258262890683122, 1.000000000000000000, 0.9659258262890683122, 1.000000000000000000, 0.9659258262890683122, 1.000000000000000000, 0.9659258262890683122, 1.000000000000000000, 0.9659258262890683122, 1.000000000000000000, 0.9659258262890683122, 1.000000000000000000, 0.9659258262890683122, 1.000000000000000000, 0.9659258262890683122, 1.000000000000000000, 0.9659258262890683122, 1.000000000000000000, 0.9659258262890683122, 1.000000000000000000, 0.9659258262890683122, 1.000000000000000000, 0.9659258262890683122, 1.000000000000000000, 0.9659258262890683122, 1.000000000000000000, 0.9659258262890683122, 1.000000000000000000, 0.9659258262890683122, 1.000000000000000000, 0.9659258262890683122, 1.000000000000000000, 0.9659258262890683122, 1.000000000000000000, 0.9659258262890683122, 1.000000000000000000, 0.9659258262890683122, 1.000000000000000000, 0.9659258262890683122, 1.000000000000000000, 0.9659258262890683122, 1.000000000000000000, 0.9659258262890683122, 1.000000000000000000, 0.9659258262890683122, 1.000000000000000000, 0.9659258262890683122, 1.000000000000000000, 0.9659258262890683122, 1.000000000000000000, 0.9659258262890683122, 1.000000000000000000, 0.9659258262890683122, 1.000000000000000000, 0.9659258262890683122, 1.000000000000000000, 0.9659258262890683122, 1.000000000000000000, 0.9659258262890683122, 1.000000000000000000, 0.9659258262890683122, 1.000000000000000000, 0.9659258262890683122, 1.000000000000000000, 0.9659258262890683122, 1.000000000000000000, 0.9659258262890683122, 1.000000000000000000, 0.9659258262890683122, 1.000000000000000000, 0.9659258262890683122, 1.000000000000000000, 0.9659258262890683122, 1.000000000000000000, 0.9659258262890683122, 1.000000000000000000, 0.9659258262890683122, 1.000000000000000000, 0.9659258262890683122, 1.000000000000000000, 0.9659258262890683122, 1.000000000000000000, 0.9659258262890683122, 1.000000000000000000, 0.9659258262890683122, 1.000000000000000000, 0.9659258262890683122, 1.000000000000000000, 0.9659258262890683122, 1.000000000000000000, 0.9659258262890683122, 1.000000000000000000, 0.9659258262890683122, 1.000000000000000000, 0.9659258262890683122, 1.000000000000000000, 0.9659258262890683122, 1.000000000000000000, 0.9659258262890683122, 1.000000000000000000, 0.9659258262890683122, 1.000000000000000000, 0.9659258262890683122, 1.000000000000000000, 0.9659258262890683122, 1.000000000000000000, 0.9659258262890683122, 1.000000000000000000, 0.9659258262890683122, 1.000000000000000000, 0.9659258262890683122, 1.000000000000000000, 0.9659258262890683122, 1.000000000000000000, 0.9659258262890683122, 1.000000000000000000, 0.9659258262890683122, 1.000000000000000000, 0.9659258262890683122, 1.000000000000000000, 0.9659258262890683122, 1.000000000000000000, 0.9659258262890683122, 1.000000000000000000, 0.9659258262890683122, 1.000000000000000000, 0.9659258262890683122, 1.000000000000000000, 0.9659258262890683122, 1.000000000000000000, 0.9659258262890683122, 1.000000000000000000, 0.9659258262890683122, 1.000000000000000000, 0.9659258262890683122, 1.000000000000000000, 0.9659258262890683122, 1.000000000000000000, 0.9659258262890683122, 1.000000000000000000, 0.9659258262890683122, 1.000000000000000000, 0.9659258262890683122, 1.000000000000000000, 0.9659258262890683122, 1.000000000000000000, 0.9659258262890683122, 1.000000000000000000, 0.9659258262890683122, 1.000000000000000000, 0.9659258262890683122, 1.000000000000000000, 0.9659258262890683122, 1.000000000000000000, 0.9659258262890683122, 1.000000000000000000, 0.9659258262890683122, 1.000000000000000000, 0.9659258262890683122, 1.000000000000000000, 0.9659258262890683122, 1.000000000000000000, 0.9659258262890683122, 1.000000000000000000, 0.9659258262890683122, 1.000000000000000000, 0.9659258262890683122, 1.000000000000000000, 0.9659258262890683122, 1.000000000000000000, 0.9659258262890683122, 1.000000000000000000, 0.9659258262890683122, 1.000000000000000000, 0.9659258262890683122, 1.000000000000000000, 0.9659258262890683122, 1.000000000000000000, 0.9659258262890683122, 1.000000000000000000, 0.9659258262890683122, 1.000000000000000000, 0.9659258262890683122, 1.000000000000000000, 0.9659258262890683122, 1.000000000000000000, 0.9659258262890683122, 1.000000000000000000, 0.9659258262890683122, 1.000000000000000000, 0.9659258262890683122, 1.000000000000000000, 0.9659258262890683122, 1.000000000000000000, 0.9659258262890683122, 1.000000000000000000, 0.9659258262890683122, 1.000000000000000000, 0.9659258262890683122, 1.000000000000000000, 0.9659258262890683122, 1.000000000000000000, 0.9659258262890683122, 1.000000000000000000, 0.9659258262890683122, 1.000000000000000000, 0.9659258262890683122, 1.000000000000000000, 0.9659258262890683122, 1.000000000000000000, 0.9659258262890683122, 1.000000000000000000),
 ( 0.3333333333333333703, 0.3219752754296894559, 0.3333333333333333703, 0.3219752754296894559, 0.3333333333333333703, 0.3219752754296894559, 0.3333333333333333703, 0.3219752754296894559, 0.3333333333333333703, 0.3219752754296894559, 0.3333333333333333703, 0.3219752754296894559, 0.3333333333333333703, 0.3219752754296894559, 0.3333333333333333703, 0.3219752754296894559, 0.3333333333333333703, 0.3219752754296894559, 0.3333333333333333703, 0.3219752754296894559, 0.3333333333333333703, 0.3219752754296894559, 0.3333333333333333703, 0.3219752754296894559, 0.3333333333333333703, 0.3219752754296894559, 0.3333333333333333703, 0.3219752754296894559, 0.3333333333333333703, 0.3219752754296894559, 0.3333333333333333703, 0.3219752754296894559, 0.3333333333333333703, 0.3219752754296894559, 0.3333333333333333703, 0.3219752754296894559, 0.3333333333333333703, 0.3219752754296894559, 0.3333333333333333703, 0.3219752754296894559, 0.3333333333333333703, 0.3219752754296894559, 0.3333333333333333703, 0.3219752754296894559, 0.3333333333333333703, 0.3219752754296894559, 0.3333333333333333703, 0.3219752754296894559, 0.3333333333333333703, 0.3219752754296894559, 0.3333333333333333703, 0.3219752754296894559, 0.3333333333333333703, 0.3219752754296894559, 0.3333333333333333703, 0.3219752754296894559, 0.3333333333333333703, 0.3219752754296894559, 0.3333333333333333703, 0.3219752754296894559, 0.3333333333333333703, 0.3219752754296894559, 0.3333333333333333703, 0.3219752754296894559, 0.3333333333333333703, 0.3219752754296894559, 0.3333333333333333703, 0.3219752754296894559, 0.3333333333333333703, 0.3219752754296894559, 0.3333333333333333703, 0.3219752754296894559, 0.3333333333333333703, 0.3219752754296894559, 0.3333333333333333703, 0.3219752754296894559, 0.3333333333333333703, 0.3219752754296894559, 0.3333333333333333703, 0.3219752754296894559, 0.3333333333333333703, 0.3219752754296894559, 0.3333333333333333703, 0.3219752754296894559, 0.3333333333333333703, 0.3219752754296894559, 0.3333333333333333703, 0.3219752754296894559, 0.3333333333333333703, 0.3219752754296894559, 0.3333333333333333703, 0.3219752754296894559, 0.3333333333333333703, 0.3219752754296894559, 0.3333333333333333703, 0.3219752754296894559, 0.3333333333333333703, 0.3219752754296894559, 0.3333333333333333703, 0.3219752754296894559, 0.3333333333333333703, 0.3219752754296894559, 0.3333333333333333703, 0.3219752754296894559, 0.3333333333333333703, 0.3219752754296894559, 0.3333333333333333703, 0.3219752754296894559, 0.3333333333333333703, 0.3219752754296894559, 0.3333333333333333703, 0.3219752754296894559, 0.3333333333333333703, 0.3219752754296894559, 0.3333333333333333703, 0.3219752754296894559, 0.3333333333333333703, 0.3219752754296894559, 0.3333333333333333703, 0.3219752754296894559, 0.3333333333333333703, 0.3219752754296894559, 0.3333333333333333703, 0.3219752754296894559, 0.3333333333333333703, 0.3219752754296894559, 0.3333333333333333703, 0.3219752754296894559, 0.3333333333333333703, 0.3219752754296894559, 0.3333333333333333703, 0.3219752754296894559, 0.3333333333333333703, 0.3219752754296894559, 0.3333333333333333703, 0.3219752754296894559, 0.3333333333333333703, 0.3219752754296894559, 0.3333333333333333703, 0.3219752754296894559, 0.3333333333333333703, 0.3219752754296894559, 0.3333333333333333703, 0.3219752754296894559, 0.3333333333333333703, 0.3219752754296894559, 0.3333333333333333703, 0.3219752754296894559, 0.3333333333333333703, 0.3219752754296894559, 0.3333333333333333703, 0.3219752754296894559, 0.3333333333333333703, 0.3219752754296894559, 0.3333333333333333703, 0.3219752754296894559, 0.3333333333333333703, 0.3219752754296894559, 0.3333333333333333703, 0.3219752754296894559, 0.3333333333333333703, 0.3219752754296894559, 0.3333333333333333703, 0.3219752754296894559, 0.3333333333333333703, 0.3219752754296894559, 0.3333333333333333703, 0.3219752754296894559, 0.3333333333333333703, 0.3219752754296894559, 0.3333333333333333703, 0.3219752754296894559, 0.3333333333333333703, 0.3219752754296894559, 0.3333333333333333703, 0.3219752754296894559, 0.3333333333333333703, 0.3219752754296894559, 0.3333333333333333703, 0.3219752754296894559, 0.3333333333333333703, 0.3219752754296894559, 0.3333333333333333703, 0.3219752754296894559, 0.3333333333333333703, 0.3219752754296894559, 0.3333333333333333703, 0.3219752754296894559, 0.3333333333333333703, 0.3219752754296894559, 0.3333333333333333703, 0.3219752754296894559, 0.3333333333333333703, 0.3219752754296894559, 0.3333333333333333703, 0.3219752754296894559, 0.3333333333333333703, 0.3219752754296894559, 0.3333333333333333703, 0.3219752754296894559, 0.3333333333333333703, 0.3219752754296894559, 0.3333333333333333703, 0.3219752754296894559, 0.3333333333333333703, 0.3219752754296894559, 0.3333333333333333703, 0.3219752754296894559, 0.3333333333333333703, 0.3219752754296894559, 0.3333333333333333703, 0.3219752754296894559, 0.3333333333333333703, 0.3219752754296894559, 0.3333333333333333703, 0.3219752754296894559, 0.3333333333333333703, 0.3219752754296894559, 0.3333333333333333703, 0.3219752754296894559, 0.3333333333333333703, 0.3219752754296894559, 0.3333333333333333703, 0.3219752754296894559, 0.3333333333333333703, 0.3219752754296894559, 0.3333333333333333703, 0.3219752754296894559, 0.3333333333333333703, 0.3219752754296894559, 0.3333333333333333703, 0.3219752754296894559, 0.3333333333333333703, 0.3219752754296894559, 0.3333333333333333703, 0.3219752754296894559, 0.3333333333333333703, 0.3219752754296894559, 0.3333333333333333703, 0.3219752754296894559, 0.3333333333333333703, 0.3219752754296894559, 0.3333333333333333703, 0.3219752754296894559, 0.3333333333333333703, 0.3219752754296894559, 0.3333333333333333703, 0.3219752754296894559, 0.3333333333333333703, 0.3219752754296894559, 0.3333333333333333703, 0.3219752754296894559, 0.3333333333333333703, 0.3219752754296894559, 0.3333333333333333703, 0.3219752754296894559, 0.3333333333333333703, 0.3219752754296894559, 0.3333333333333333703, 0.3219752754296894559, 0.3333333333333333703, 0.3219752754296894559, 0.3333333333333333703, 0.3219752754296894559, 0.3333333333333333703, 0.3219752754296894559, 0.3333333333333333703, 0.3219752754296894559, 0.3333333333333333703, 0.3219752754296894559, 0.3333333333333333703, 0.3219752754296894559, 0.3333333333333333703, 0.3219752754296894559, 0.3333333333333333703, 0.3219752754296894559, 0.3333333333333333703, 0.3219752754296894559, 0.3333333333333333703, 0.3219752754296894559, 0.3333333333333333703, 0.3219752754296894559, 0.3333333333333333703, 0.3219752754296894559, 0.3333333333333333703, 0.3219752754296894559, 0.3333333333333333703, 0.3219752754296894559, 0.3333333333333333703, 0.3219752754296894559, 0.3333333333333333703, 0.3219752754296894559, 0.3333333333333333703, 0.3219752754296894559, 0.3333333333333333703, 0.3219752754296894559, 0.3333333333333333703, 0.3219752754296894559, 0.3333333333333333703, 0.3219752754296894559, 0.3333333333333333703, 0.3219752754296894559, 0.3333333333333333703, 0.3219752754296894559, 0.3333333333333333703, 0.3219752754296894559, 0.3333333333333333703, 0.3219752754296894559, 0.3333333333333333703, 0.3219752754296894559, 0.3333333333333333703, 0.3219752754296894559, 0.3333333333333333703, 0.3219752754296894559, 0.3333333333333333703, 0.3219752754296894559, 0.3333333333333333703, 0.3219752754296894559, 0.3333333333333333703, 0.3219752754296894559, 0.3333333333333333703, 0.3219752754296894559, 0.3333333333333333703, 0.3219752754296894559, 0.3333333333333333703, 0.3219752754296894559, 0.3333333333333333703, 0.3219752754296894559, 0.3333333333333333703, 0.3219752754296894559, 0.3333333333333333703, 0.3219752754296894559, 0.3333333333333333703, 0.3219752754296894559, 0.3333333333333333703, 0.3219752754296894559, 0.3333333333333333703, 0.3219752754296894559, 0.3333333333333333703, 0.3219752754296894559, 0.3333333333333333703, 0.3219752754296894559, 0.3333333333333333703, 0.3219752754296894559, 0.3333333333333333703, 0.3219752754296894559, 0.3333333333333333703, 0.3219752754296894559, 0.3333333333333333703, 0.3219752754296894559, 0.3333333333333333703, 0.3219752754296894559, 0.3333333333333333703, 0.3219752754296894559, 0.3333333333333333703, 0.3219752754296894559, 0.3333333333333333703, 0.3219752754296894559, 0.3333333333333333703, 0.3219752754296894559, 0.3333333333333333703, 0.3219752754296894559, 0.3333333333333333703, 0.3219752754296894559, 0.3333333333333333703, 0.3219752754296894559, 0.3333333333333333703, 0.3219752754296894559, 0.3333333333333333703, 0.3219752754296894559, 0.3333333333333333703, 0.3219752754296894559, 0.3333333333333333703, 0.3219752754296894559, 0.3333333333333333703, 0.3219752754296894559, 0.3333333333333333703, 0.3219752754296894559, 0.3333333333333333703, 0.3219752754296894559, 0.3333333333333333703, 0.3219752754296894559, 0.3333333333333333703, 0.3219752754296894559, 0.3333333333333333703, 0.3219752754296894559, 0.3333333333333333703, 0.3219752754296894559, 0.3333333333333333703, 0.3219752754296894559, 0.3333333333333333703, 0.3219752754296894559, 0.3333333333333333703, 0.3219752754296894559, 0.3333333333333333703, 0.3219752754296894559, 0.3333333333333333703, 0.3219752754296894559, 0.3333333333333333703, 0.3219752754296894559, 0.3333333333333333703, 0.3219752754296894559, 0.3333333333333333703, 0.3219752754296894559, 0.3333333333333333703, 0.3219752754296894559, 0.3333333333333333703, 0.3219752754296894559, 0.3333333333333333703, 0.3219752754296894559, 0.3333333333333333703, 0.3219752754296894559, 0.3333333333333333703, 0.3219752754296894559, 0.3333333333333333703, 0.3219752754296894559, 0.3333333333333333703, 0.3219752754296894559, 0.3333333333333333703, 0.3219752754296894559, 0.3333333333333333703, 0.3219752754296894559, 0.3333333333333333703, 0.3219752754296894559, 0.3333333333333333703, 0.3219752754296894559, 0.3333333333333333703, 0.3219752754296894559, 0.3333333333333333703, 0.3219752754296894559, 0.3333333333333333703, 0.3219752754296894559, 0.3333333333333333703, 0.3219752754296894559, 0.3333333333333333703, 0.3219752754296894559, 0.3333333333333333703, 0.3219752754296894559, 0.3333333333333333703, 0.3219752754296894559, 0.3333333333333333703, 0.3219752754296894559, 0.3333333333333333703, 0.3219752754296894559, 0.3333333333333333703, 0.3219752754296894559, 0.3333333333333333703, 0.3219752754296894559, 0.3333333333333333703, 0.3219752754296894559, 0.3333333333333333703, 0.3219752754296894559, 0.3333333333333333703, 0.3219752754296894559, 0.3333333333333333703, 0.3219752754296894559, 0.3333333333333333703),
 ( 0.3333333333333333703, 0.3219752754296894559, 0.3333333333333333703, 0.3219752754296894559, 0.3333333333333333703, 0.3219752754296894559, 0.3333333333333333703, 0.3219752754296894559, 0.3333333333333333703, 0.3219752754296894559, 0.3333333333333333703, 0.3219752754296894559, 0.3333333333333333703, 0.3219752754296894559, 0.3333333333333333703, 0.3219752754296894559, 0.3333333333333333703, 0.3219752754296894559, 0.3333333333333333703, 0.3219752754296894559, 0.3333333333333333703, 0.3219752754296894559, 0.3333333333333333703, 0.3219752754296894559, 0.3333333333333333703, 0.3219752754296894559, 0.3333333333333333703, 0.3219752754296894559, 0.3333333333333333703, 0.3219752754296894559, 0.3333333333333333703, 0.3219752754296894559, 0.3333333333333333703, 0.3219752754296894559, 0.3333333333333333703, 0.3219752754296894559, 0.3333333333333333703, 0.3219752754296894559, 0.3333333333333333703, 0.3219752754296894559, 0.3333333333333333703, 0.3219752754296894559, 0.3333333333333333703, 0.3219752754296894559, 0.3333333333333333703, 0.3219752754296894559, 0.3333333333333333703, 0.3219752754296894559, 0.3333333333333333703, 0.3219752754296894559, 0.3333333333333333703, 0.3219752754296894559, 0.3333333333333333703, 0.3219752754296894559, 0.3333333333333333703, 0.3219752754296894559, 0.3333333333333333703, 0.3219752754296894559, 0.3333333333333333703, 0.3219752754296894559, 0.3333333333333333703, 0.3219752754296894559, 0.3333333333333333703, 0.3219752754296894559, 0.3333333333333333703, 0.3219752754296894559, 0.3333333333333333703, 0.3219752754296894559, 0.3333333333333333703, 0.3219752754296894559, 0.3333333333333333703, 0.3219752754296894559, 0.3333333333333333703, 0.3219752754296894559, 0.3333333333333333703, 0.3219752754296894559, 0.3333333333333333703, 0.3219752754296894559, 0.3333333333333333703, 0.3219752754296894559, 0.3333333333333333703, 0.3219752754296894559, 0.3333333333333333703, 0.3219752754296894559, 0.3333333333333333703, 0.3219752754296894559, 0.3333333333333333703, 0.3219752754296894559, 0.3333333333333333703, 0.3219752754296894559, 0.3333333333333333703, 0.3219752754296894559, 0.3333333333333333703, 0.3219752754296894559, 0.3333333333333333703, 0.3219752754296894559, 0.3333333333333333703, 0.3219752754296894559, 0.3333333333333333703, 0.3219752754296894559, 0.3333333333333333703, 0.3219752754296894559, 0.3333333333333333703, 0.3219752754296894559, 0.3333333333333333703, 0.3219752754296894559, 0.3333333333333333703, 0.3219752754296894559, 0.3333333333333333703, 0.3219752754296894559, 0.3333333333333333703, 0.3219752754296894559, 0.3333333333333333703, 0.3219752754296894559, 0.3333333333333333703, 0.3219752754296894559, 0.3333333333333333703, 0.3219752754296894559, 0.3333333333333333703, 0.3219752754296894559, 0.3333333333333333703, 0.3219752754296894559, 0.3333333333333333703, 0.3219752754296894559, 0.3333333333333333703, 0.3219752754296894559, 0.3333333333333333703, 0.3219752754296894559, 0.3333333333333333703, 0.3219752754296894559, 0.3333333333333333703, 0.3219752754296894559, 0.3333333333333333703, 0.3219752754296894559, 0.3333333333333333703, 0.3219752754296894559, 0.3333333333333333703, 0.3219752754296894559, 0.3333333333333333703, 0.3219752754296894559, 0.3333333333333333703, 0.3219752754296894559, 0.3333333333333333703, 0.3219752754296894559, 0.3333333333333333703, 0.3219752754296894559, 0.3333333333333333703, 0.3219752754296894559, 0.3333333333333333703, 0.3219752754296894559, 0.3333333333333333703, 0.3219752754296894559, 0.3333333333333333703, 0.3219752754296894559, 0.3333333333333333703, 0.3219752754296894559, 0.3333333333333333703, 0.3219752754296894559, 0.3333333333333333703, 0.3219752754296894559, 0.3333333333333333703, 0.3219752754296894559, 0.3333333333333333703, 0.3219752754296894559, 0.3333333333333333703, 0.3219752754296894559, 0.3333333333333333703, 0.3219752754296894559, 0.3333333333333333703, 0.3219752754296894559, 0.3333333333333333703, 0.3219752754296894559, 0.3333333333333333703, 0.3219752754296894559, 0.3333333333333333703, 0.3219752754296894559, 0.3333333333333333703, 0.3219752754296894559, 0.3333333333333333703, 0.3219752754296894559, 0.3333333333333333703, 0.3219752754296894559, 0.3333333333333333703, 0.3219752754296894559, 0.3333333333333333703, 0.3219752754296894559, 0.3333333333333333703, 0.3219752754296894559, 0.3333333333333333703, 0.3219752754296894559, 0.3333333333333333703, 0.3219752754296894559, 0.3333333333333333703, 0.3219752754296894559, 0.3333333333333333703, 0.3219752754296894559, 0.3333333333333333703, 0.3219752754296894559, 0.3333333333333333703, 0.3219752754296894559, 0.3333333333333333703, 0.3219752754296894559, 0.3333333333333333703, 0.3219752754296894559, 0.3333333333333333703, 0.3219752754296894559, 0.3333333333333333703, 0.3219752754296894559, 0.3333333333333333703, 0.3219752754296894559, 0.3333333333333333703, 0.3219752754296894559, 0.3333333333333333703, 0.3219752754296894559, 0.3333333333333333703, 0.3219752754296894559, 0.3333333333333333703, 0.3219752754296894559, 0.3333333333333333703, 0.3219752754296894559, 0.3333333333333333703, 0.3219752754296894559, 0.3333333333333333703, 0.3219752754296894559, 0.3333333333333333703, 0.3219752754296894559, 0.3333333333333333703, 0.3219752754296894559, 0.3333333333333333703, 0.3219752754296894559, 0.3333333333333333703, 0.3219752754296894559, 0.3333333333333333703, 0.3219752754296894559, 0.3333333333333333703, 0.3219752754296894559, 0.3333333333333333703, 0.3219752754296894559, 0.3333333333333333703, 0.3219752754296894559, 0.3333333333333333703, 0.3219752754296894559, 0.3333333333333333703, 0.3219752754296894559, 0.3333333333333333703, 0.3219752754296894559, 0.3333333333333333703, 0.3219752754296894559, 0.3333333333333333703, 0.3219752754296894559, 0.3333333333333333703, 0.3219752754296894559, 0.3333333333333333703, 0.3219752754296894559, 0.3333333333333333703, 0.3219752754296894559, 0.3333333333333333703, 0.3219752754296894559, 0.3333333333333333703, 0.3219752754296894559, 0.3333333333333333703, 0.3219752754296894559, 0.3333333333333333703, 0.3219752754296894559, 0.3333333333333333703, 0.3219752754296894559, 0.3333333333333333703, 0.3219752754296894559, 0.3333333333333333703, 0.3219752754296894559, 0.3333333333333333703, 0.3219752754296894559, 0.3333333333333333703, 0.3219752754296894559, 0.3333333333333333703, 0.3219752754296894559, 0.3333333333333333703, 0.3219752754296894559, 0.3333333333333333703, 0.3219752754296894559, 0.3333333333333333703, 0.3219752754296894559, 0.3333333333333333703, 0.3219752754296894559, 0.3333333333333333703, 0.3219752754296894559, 0.3333333333333333703, 0.3219752754296894559, 0.3333333333333333703, 0.3219752754296894559, 0.3333333333333333703, 0.3219752754296894559, 0.3333333333333333703, 0.3219752754296894559, 0.3333333333333333703, 0.3219752754296894559, 0.3333333333333333703, 0.3219752754296894559, 0.3333333333333333703, 0.3219752754296894559, 0.3333333333333333703, 0.3219752754296894559, 0.3333333333333333703, 0.3219752754296894559, 0.3333333333333333703, 0.3219752754296894559, 0.3333333333333333703, 0.3219752754296894559, 0.3333333333333333703, 0.3219752754296894559, 0.3333333333333333703, 0.3219752754296894559, 0.3333333333333333703, 0.3219752754296894559, 0.3333333333333333703, 0.3219752754296894559, 0.3333333333333333703, 0.3219752754296894559, 0.3333333333333333703, 0.3219752754296894559, 0.3333333333333333703, 0.3219752754296894559, 0.3333333333333333703, 0.3219752754296894559, 0.3333333333333333703, 0.3219752754296894559, 0.3333333333333333703, 0.3219752754296894559, 0.3333333333333333703, 0.3219752754296894559, 0.3333333333333333703, 0.3219752754296894559, 0.3333333333333333703, 0.3219752754296894559, 0.3333333333333333703, 0.3219752754296894559, 0.3333333333333333703, 0.3219752754296894559, 0.3333333333333333703, 0.3219752754296894559, 0.3333333333333333703, 0.3219752754296894559, 0.3333333333333333703, 0.3219752754296894559, 0.3333333333333333703, 0.3219752754296894559, 0.3333333333333333703, 0.3219752754296894559, 0.3333333333333333703, 0.3219752754296894559, 0.3333333333333333703, 0.3219752754296894559, 0.3333333333333333703, 0.3219752754296894559, 0.3333333333333333703, 0.3219752754296894559, 0.3333333333333333703, 0.3219752754296894559, 0.3333333333333333703, 0.3219752754296894559, 0.3333333333333333703, 0.3219752754296894559, 0.3333333333333333703, 0.3219752754296894559, 0.3333333333333333703, 0.3219752754296894559, 0.3333333333333333703, 0.3219752754296894559, 0.3333333333333333703, 0.3219752754296894559, 0.3333333333333333703, 0.3219752754296894559, 0.3333333333333333703, 0.3219752754296894559, 0.3333333333333333703, 0.3219752754296894559, 0.3333333333333333703, 0.3219752754296894559, 0.3333333333333333703, 0.3219752754296894559, 0.3333333333333333703, 0.3219752754296894559, 0.3333333333333333703, 0.3219752754296894559, 0.3333333333333333703, 0.3219752754296894559, 0.3333333333333333703, 0.3219752754296894559, 0.3333333333333333703, 0.3219752754296894559, 0.3333333333333333703, 0.3219752754296894559, 0.3333333333333333703, 0.3219752754296894559, 0.3333333333333333703, 0.3219752754296894559, 0.3333333333333333703, 0.3219752754296894559, 0.3333333333333333703, 0.3219752754296894559, 0.3333333333333333703, 0.3219752754296894559, 0.3333333333333333703, 0.3219752754296894559, 0.3333333333333333703, 0.3219752754296894559, 0.3333333333333333703, 0.3219752754296894559, 0.3333333333333333703, 0.3219752754296894559, 0.3333333333333333703, 0.3219752754296894559, 0.3333333333333333703, 0.3219752754296894559, 0.3333333333333333703, 0.3219752754296894559, 0.3333333333333333703, 0.3219752754296894559, 0.3333333333333333703, 0.3219752754296894559, 0.3333333333333333703, 0.3219752754296894559, 0.3333333333333333703, 0.3219752754296894559, 0.3333333333333333703, 0.3219752754296894559, 0.3333333333333333703, 0.3219752754296894559, 0.3333333333333333703, 0.3219752754296894559, 0.3333333333333333703, 0.3219752754296894559, 0.3333333333333333703, 0.3219752754296894559, 0.3333333333333333703, 0.3219752754296894559, 0.3333333333333333703, 0.3219752754296894559, 0.3333333333333333703, 0.3219752754296894559, 0.3333333333333333703, 0.3219752754296894559, 0.3333333333333333703, 0.3219752754296894559, 0.3333333333333333703, 0.3219752754296894559, 0.3333333333333333703, 0.3219752754296894559, 0.3333333333333333703, 0.3219752754296894559, 0.3333333333333333703, 0.3219752754296894559, 0.3333333333333333703, 0.3219752754296894559, 0.3333333333333333703, 0.3219752754296894559, 0.3333333333333333703),
 ( 1.000000000000000000, 0.9659258262890683122, 1.000000000000000000, 0.9659258262890683122, 1.000000000000000000, 0.9659258262890683122, 1.000000000000000000, 0.9659258262890683122, 1.000000000000000000, 0.9659258262890683122, 1.000000000000000000, 0.9659258262890683122, 1.000000000000000000, 0.9659258262890683122, 1.000000000000000000, 0.9659258262890683122, 1.000000000000000000, 0.9659258262890683122, 1.000000000000000000, 0.9659258262890683122, 1.000000000000000000, 0.9659258262890683122, 1.000000000000000000, 0.9659258262890683122, 1.000000000000000000, 0.9659258262890683122, 1.000000000000000000, 0.9659258262890683122, 1.000000000000000000, 0.9659258262890683122, 1.000000000000000000, 0.9659258262890683122, 1.000000000000000000, 0.9659258262890683122, 1.000000000000000000, 0.9659258262890683122, 1.000000000000000000, 0.9659258262890683122, 1.000000000000000000, 0.9659258262890683122, 1.000000000000000000, 0.9659258262890683122, 1.000000000000000000, 0.9659258262890683122, 1.000000000000000000, 0.9659258262890683122, 1.000000000000000000, 0.9659258262890683122, 1.000000000000000000, 0.9659258262890683122, 1.000000000000000000, 0.9659258262890683122, 1.000000000000000000, 0.9659258262890683122, 1.000000000000000000, 0.9659258262890683122, 1.000000000000000000, 0.9659258262890683122, 1.000000000000000000, 0.9659258262890683122, 1.000000000000000000, 0.9659258262890683122, 1.000000000000000000, 0.9659258262890683122, 1.000000000000000000, 0.9659258262890683122, 1.000000000000000000, 0.9659258262890683122, 1.000000000000000000, 0.9659258262890683122, 1.000000000000000000, 0.9659258262890683122, 1.000000000000000000, 0.9659258262890683122, 1.000000000000000000, 0.9659258262890683122, 1.000000000000000000, 0.9659258262890683122, 1.000000000000000000, 0.9659258262890683122, 1.000000000000000000, 0.9659258262890683122, 1.000000000000000000, 0.9659258262890683122, 1.000000000000000000, 0.9659258262890683122, 1.000000000000000000, 0.9659258262890683122, 1.000000000000000000, 0.9659258262890683122, 1.000000000000000000, 0.9659258262890683122, 1.000000000000000000, 0.9659258262890683122, 1.000000000000000000, 0.9659258262890683122, 1.000000000000000000, 0.9659258262890683122, 1.000000000000000000, 0.9659258262890683122, 1.000000000000000000, 0.9659258262890683122, 1.000000000000000000, 0.9659258262890683122, 1.000000000000000000, 0.9659258262890683122, 1.000000000000000000, 0.9659258262890683122, 1.000000000000000000, 0.9659258262890683122, 1.000000000000000000, 0.9659258262890683122, 1.000000000000000000, 0.9659258262890683122, 1.000000000000000000, 0.9659258262890683122, 1.000000000000000000, 0.9659258262890683122, 1.000000000000000000, 0.9659258262890683122, 1.000000000000000000, 0.9659258262890683122, 1.000000000000000000, 0.9659258262890683122, 1.000000000000000000, 0.9659258262890683122, 1.000000000000000000, 0.9659258262890683122, 1.000000000000000000, 0.9659258262890683122, 1.000000000000000000, 0.9659258262890683122, 1.000000000000000000, 0.9659258262890683122, 1.000000000000000000, 0.9659258262890683122, 1.000000000000000000, 0.9659258262890683122, 1.000000000000000000, 0.9659258262890683122, 1.000000000000000000, 0.9659258262890683122, 1.000000000000000000, 0.9659258262890683122, 1.000000000000000000, 0.9659258262890683122, 1.000000000000000000, 0.9659258262890683122, 1.000000000000000000, 0.9659258262890683122, 1.000000000000000000, 0.9659258262890683122, 1.000000000000000000, 0.9659258262890683122, 1.000000000000000000, 0.9659258262890683122, 1.000000000000000000, 0.9659258262890683122, 1.000000000000000000, 0.9659258262890683122, 1.000000000000000000, 0.9659258262890683122, 1.000000000000000000, 0.9659258262890683122, 1.000000000000000000, 0.9659258262890683122, 1.000000000000000000, 0.9659258262890683122, 1.000000000000000000, 0.9659258262890683122, 1.000000000000000000, 0.9659258262890683122, 1.000000000000000000, 0.9659258262890683122, 1.000000000000000000, 0.9659258262890683122, 1.000000000000000000, 0.9659258262890683122, 1.000000000000000000, 0.9659258262890683122, 1.000000000000000000, 0.9659258262890683122, 1.000000000000000000, 0.9659258262890683122, 1.000000000000000000, 0.9659258262890683122, 1.000000000000000000, 0.9659258262890683122, 1.000000000000000000, 0.9659258262890683122, 1.000000000000000000, 0.9659258262890683122, 1.000000000000000000, 0.9659258262890683122, 1.000000000000000000, 0.9659258262890683122, 1.000000000000000000, 0.9659258262890683122, 1.000000000000000000, 0.9659258262890683122, 1.000000000000000000, 0.9659258262890683122, 1.000000000000000000, 0.9659258262890683122, 1.000000000000000000, 0.9659258262890683122, 1.000000000000000000, 0.9659258262890683122, 1.000000000000000000, 0.9659258262890683122, 1.000000000000000000, 0.9659258262890683122, 1.000000000000000000, 0.9659258262890683122, 1.000000000000000000, 0.9659258262890683122, 1.000000000000000000, 0.9659258262890683122, 1.000000000000000000, 0.9659258262890683122, 1.000000000000000000, 0.9659258262890683122, 1.000000000000000000, 0.9659258262890683122, 1.000000000000000000, 0.9659258262890683122, 1.000000000000000000, 0.9659258262890683122, 1.000000000000000000, 0.9659258262890683122, 1.000000000000000000, 0.9659258262890683122, 1.000000000000000000, 0.9659258262890683122, 1.000000000000000000, 0.9659258262890683122, 1.000000000000000000, 0.9659258262890683122, 1.000000000000000000, 0.9659258262890683122, 1.000000000000000000, 0.9659258262890683122, 1.000000000000000000, 0.9659258262890683122, 1.000000000000000000, 0.9659258262890683122, 1.000000000000000000, 0.9659258262890683122, 1.000000000000000000, 0.9659258262890683122, 1.000000000000000000, 0.9659258262890683122, 1.000000000000000000, 0.9659258262890683122, 1.000000000000000000, 0.9659258262890683122, 1.000000000000000000, 0.9659258262890683122, 1.000000000000000000, 0.9659258262890683122, 1.000000000000000000, 0.9659258262890683122, 1.000000000000000000, 0.9659258262890683122, 1.000000000000000000, 0.9659258262890683122, 1.000000000000000000, 0.9659258262890683122, 1.000000000000000000, 0.9659258262890683122, 1.000000000000000000, 0.9659258262890683122, 1.000000000000000000, 0.9659258262890683122, 1.000000000000000000, 0.9659258262890683122, 1.000000000000000000, 0.9659258262890683122, 1.000000000000000000, 0.9659258262890683122, 1.000000000000000000, 0.9659258262890683122, 1.000000000000000000, 0.9659258262890683122, 1.000000000000000000, 0.9659258262890683122, 1.000000000000000000, 0.9659258262890683122, 1.000000000000000000, 0.9659258262890683122, 1.000000000000000000, 0.9659258262890683122, 1.000000000000000000, 0.9659258262890683122, 1.000000000000000000, 0.9659258262890683122, 1.000000000000000000, 0.9659258262890683122, 1.000000000000000000, 0.9659258262890683122, 1.000000000000000000, 0.9659258262890683122, 1.000000000000000000, 0.9659258262890683122, 1.000000000000000000, 0.9659258262890683122, 1.000000000000000000, 0.9659258262890683122, 1.000000000000000000, 0.9659258262890683122, 1.000000000000000000, 0.9659258262890683122, 1.000000000000000000, 0.9659258262890683122, 1.000000000000000000, 0.9659258262890683122, 1.000000000000000000, 0.9659258262890683122, 1.000000000000000000, 0.9659258262890683122, 1.000000000000000000, 0.9659258262890683122, 1.000000000000000000, 0.9659258262890683122, 1.000000000000000000, 0.9659258262890683122, 1.000000000000000000, 0.9659258262890683122, 1.000000000000000000, 0.9659258262890683122, 1.000000000000000000, 0.9659258262890683122, 1.000000000000000000, 0.9659258262890683122, 1.000000000000000000, 0.9659258262890683122, 1.000000000000000000, 0.9659258262890683122, 1.000000000000000000, 0.9659258262890683122, 1.000000000000000000, 0.9659258262890683122, 1.000000000000000000, 0.9659258262890683122, 1.000000000000000000, 0.9659258262890683122, 1.000000000000000000, 0.9659258262890683122, 1.000000000000000000, 0.9659258262890683122, 1.000000000000000000, 0.9659258262890683122, 1.000000000000000000, 0.9659258262890683122, 1.000000000000000000, 0.9659258262890683122, 1.000000000000000000, 0.9659258262890683122, 1.000000000000000000, 0.9659258262890683122, 1.000000000000000000, 0.9659258262890683122, 1.000000000000000000, 0.9659258262890683122, 1.000000000000000000, 0.9659258262890683122, 1.000000000000000000, 0.9659258262890683122, 1.000000000000000000, 0.9659258262890683122, 1.000000000000000000, 0.9659258262890683122, 1.000000000000000000, 0.9659258262890683122, 1.000000000000000000, 0.9659258262890683122, 1.000000000000000000, 0.9659258262890683122, 1.000000000000000000, 0.9659258262890683122, 1.000000000000000000, 0.9659258262890683122, 1.000000000000000000, 0.9659258262890683122, 1.000000000000000000, 0.9659258262890683122, 1.000000000000000000, 0.9659258262890683122, 1.000000000000000000, 0.9659258262890683122, 1.000000000000000000, 0.9659258262890683122, 1.000000000000000000, 0.9659258262890683122, 1.000000000000000000, 0.9659258262890683122, 1.000000000000000000, 0.9659258262890683122, 1.000000000000000000, 0.9659258262890683122, 1.000000000000000000, 0.9659258262890683122, 1.000000000000000000, 0.9659258262890683122, 1.000000000000000000, 0.9659258262890683122, 1.000000000000000000, 0.9659258262890683122, 1.000000000000000000, 0.9659258262890683122, 1.000000000000000000, 0.9659258262890683122, 1.000000000000000000, 0.9659258262890683122, 1.000000000000000000, 0.9659258262890683122, 1.000000000000000000, 0.9659258262890683122, 1.000000000000000000, 0.9659258262890683122, 1.000000000000000000, 0.9659258262890683122, 1.000000000000000000, 0.9659258262890683122, 1.000000000000000000, 0.9659258262890683122, 1.000000000000000000, 0.9659258262890683122, 1.000000000000000000, 0.9659258262890683122, 1.000000000000000000, 0.9659258262890683122, 1.000000000000000000, 0.9659258262890683122, 1.000000000000000000, 0.9659258262890683122, 1.000000000000000000, 0.9659258262890683122, 1.000000000000000000, 0.9659258262890683122, 1.000000000000000000, 0.9659258262890683122, 1.000000000000000000, 0.9659258262890683122, 1.000000000000000000, 0.9659258262890683122, 1.000000000000000000, 0.9659258262890683122, 1.000000000000000000, 0.9659258262890683122, 1.000000000000000000, 0.9659258262890683122, 1.000000000000000000, 0.9659258262890683122, 1.000000000000000000, 0.9659258262890683122, 1.000000000000000000) ) ) 
 REPRESENTATION_ITEM ( '' )  SURFACE ( )  );
#175110=CARTESIAN_POINT ( 'NONE',  ( -18.67979575497193778, 10.72451020669871902, 113.3344237280190328 ) ) ;
#175111=CARTESIAN_POINT ( 'NONE',  ( 12.06949235617739724, 12.14591786802326823, 61.87609039468568284 ) ) ;
#175112=CARTESIAN_POINT ( 'NONE',  ( 18.62759615963255655, 10.81492255796105972, 91.66775706135234714 ) ) ;
#175113=CARTESIAN_POINT ( 'NONE',  ( -18.67979575497178146, -10.72451020669898902, 21.66557627198102409 ) ) ;
#175114=CARTESIAN_POINT ( 'NONE',  ( -0.05219959533936034679, 19.03943276465977164, 97.50109039468567573 ) ) ;
#175115=CARTESIAN_POINT ( 'NONE',  ( 0.05219959533937995610, -21.53943276465977519, 65.00109039468568994 ) ) ;
#175116=CARTESIAN_POINT ( 'NONE',  ( 12.14591786802327356, -12.06949235617739191, 30.62609039468567929 ) ) ;
#175117=CARTESIAN_POINT ( 'NONE',  ( 15.80617190586746368, 15.72974639402197994, 84.37390960531438111 ) ) ;
#175118=CARTESIAN_POINT ( 'NONE',  ( 5.153800228976615827, -19.02544592524334988, 95.20942372801897591 ) ) ;
#175119=CARTESIAN_POINT ( 'NONE',  ( -13.97604488694527625, -13.89961937509977652, 61.87390960531435979 ) ) ;
#175120=CARTESIAN_POINT ( 'NONE',  ( -16.46253265017146816, -9.564922557961047289, 109.1677570613523471 ) ) ;
#175121=CARTESIAN_POINT ( 'NONE',  ( 0.05219959533936267826, -19.03943276465977164, 100.0010903946856757 ) ) ;
#175122=CARTESIAN_POINT ( 'NONE',  ( 4.379528057220339221, -16.55341960407611168, 57.70724293864770260 ) ) ;
#175124=CARTESIAN_POINT ( 'NONE',  ( -0.05219959533936034679, 19.03943276465977164, 82.50109039468567573 ) ) ;
#175125=CARTESIAN_POINT ( 'NONE',  ( 16.53943276465976808, 0.05219959533934440121, 56.25109039468568284 ) ) ;
#175126=CARTESIAN_POINT ( 'NONE',  ( -10.81492255796078084, -18.62759615963271287, 112.0822429386477097 ) ) ;
#175127=CARTESIAN_POINT ( 'NONE',  ( -0.05219959533909027116, -19.03943276465977164, 32.49890960531435979 ) ) ;
#175128=CARTESIAN_POINT ( 'NONE',  ( -13.89961937509977652, 13.97604488694528158, 50.62390960531435979 ) ) ;
#175129=CARTESIAN_POINT ( 'NONE',  ( 8.224510206698742110, 14.34966873604972548, 62.08442372801901143 ) ) ;
#175132=CARTESIAN_POINT ( 'NONE',  ( -19.05341960407611168, -5.049401038298163336, 101.4572429386476955 ) ) ;
#175133=CARTESIAN_POINT ( 'NONE',  ( 16.46253265017160672, -9.564922557960803928, 23.33224293864769194 ) ) ;
#175135=CARTESIAN_POINT ( 'NONE',  ( -9.474510206698720793, -16.51473224551083518, 109.5844237280190043 ) ) ;
#175136=CARTESIAN_POINT ( 'NONE',  ( 5.823673210054125526, 21.52544592524343514, 44.79057627198103120 ) ) ;
#175137=CARTESIAN_POINT ( 'NONE',  ( -5.049401038297874678, -19.05341960407617918, 49.79275706135231871 ) ) ;
#175138=CARTESIAN_POINT ( 'NONE',  ( -8.314922557961024197, 14.29746914071037800, 27.91775706135234358 ) ) ;
#175139=CARTESIAN_POINT ( 'NONE',  ( -16.51473224551069308, -9.474510206698971260, 26.66557627198103120 ) ) ;
#175140=CARTESIAN_POINT ( 'NONE',  ( 16.46253265017160672, -9.564922557960803928, 53.33224293864768839 ) ) ;
#175141=CARTESIAN_POINT ( 'NONE',  ( -10.72451020669898014, 18.67979575497178502, 85.41557627198102409 ) ) ;
#175142=CARTESIAN_POINT ( 'NONE',  ( -13.89961937509977652, 13.97604488694528158, 105.6239096053143527 ) ) ;
#175143=CARTESIAN_POINT ( 'NONE',  ( -16.51473224551069308, -9.474510206698971260, 56.66557627198103120 ) ) ;
#175145=CARTESIAN_POINT ( 'NONE',  ( -5.049401038297874678, -19.05341960407617918, 79.79275706135233293 ) ) ;
#175146=CARTESIAN_POINT ( 'NONE',  ( -0.05219959533910754901, -16.53943276465976808, 62.49890960531436690 ) ) ;
#175147=CARTESIAN_POINT ( 'NONE',  ( 15.72974639402176855, 15.80617190586768217, 101.8760903946857042 ) ) ;
#175148=CARTESIAN_POINT ( 'NONE',  ( -15.80617190586745835, -15.72974639402198527, 91.87390960531436690 ) ) ;
#175149=CARTESIAN_POINT ( 'NONE',  ( 21.53943276465977519, 0.05219959533937863772, 91.25109039468568994 ) ) ;
#175150=CARTESIAN_POINT ( 'NONE',  ( -19.03943276465977164, 0.05219959533909376836, 21.24890960531436335 ) ) ;
#175151=CARTESIAN_POINT ( 'NONE',  ( -15.80617190586768217, 15.72974639402176855, 73.12609039468567573 ) ) ;
#175152=EDGE_CURVE ( 'NONE', #147783, #5512, #112676, .T. ) ;
#175153=CARTESIAN_POINT ( 'NONE',  ( -9.564922557960796823, -16.46253265017161027, 112.0822429386476955 ) ) ;
#175154=CARTESIAN_POINT ( 'NONE',  ( -14.29746914071049879, 8.314922557960819915, 30.83224293864770260 ) ) ;
#175155=CARTESIAN_POINT ( 'NONE',  ( -10.72451020669870658, -18.67979575497194134, 79.58442372801903275 ) ) ;
#175156=CARTESIAN_POINT ( 'NONE',  ( 5.049401038298161559, -19.05341960407611168, 62.70724293864769550 ) ) ;
#175157=CARTESIAN_POINT ( 'NONE',  ( 15.80617190586769283, -15.72974639402175789, 45.62609039468567573 ) ) ;
#175158=CARTESIAN_POINT ( 'NONE',  ( -19.03943276465977164, 0.05219959533909376836, 76.24890960531435269 ) ) ;
#175159=CARTESIAN_POINT ( 'NONE',  ( -8.224510206698948167, 14.34966873604960824, 90.41557627198103830 ) ) ;
#175160=CARTESIAN_POINT ( 'NONE',  ( -16.52544592524342804, 4.483927247898546575, 61.04057627198103120 ) ) ;
#175161=CARTESIAN_POINT ( 'NONE',  ( -15.80617190586745835, -15.72974639402198527, 71.87390960531438111 ) ) ;
#175162=EDGE_CURVE ( 'NONE', #59793, #93191, #98945, .T. ) ;
#175163=CARTESIAN_POINT ( 'NONE',  ( -19.02544592524342804, 5.153800228976336051, 61.04057627198103120 ) ) ;
#175164=CARTESIAN_POINT ( 'NONE',  ( -5.719274019375978568, 21.55341960407610458, 75.20724293864769550 ) ) ;
#175165=CARTESIAN_POINT ( 'NONE',  ( -9.474510206698720793, -16.51473224551083518, 59.58442372801900433 ) ) ;
#175166=CARTESIAN_POINT ( 'NONE',  ( -9.474510206698720793, -16.51473224551083518, 29.58442372801900433 ) ) ;
#175167=CARTESIAN_POINT ( 'NONE',  ( -16.53943276465976808, 0.05219959533911058130, 76.24890960531435269 ) ) ;
#175168=CARTESIAN_POINT ( 'NONE',  ( -15.80617190586745835, -15.72974639402198527, 56.87390960531436690 ) ) ;
#175169=CARTESIAN_POINT ( 'NONE',  ( -17.60779699588837843, -5.500000000000011546, 41.34981316670104690 ) ) ;
#175170=CARTESIAN_POINT ( 'NONE',  ( -14.29746914071037622, -8.314922557961029526, 94.16775706135237556 ) ) ;
#175172=CARTESIAN_POINT ( 'NONE',  ( -9.564922557961040184, 16.46253265017147172, 97.91775706135233293 ) ) ;
#175173=CARTESIAN_POINT ( 'NONE',  ( 12.14591786802309770, 12.06949235617756955, 69.37390960531436690 ) ) ;
#175175=CARTESIAN_POINT ( 'NONE',  ( 13.97604488694527802, 13.89961937509977652, 59.37390960531434558 ) ) ;
#175176=CARTESIAN_POINT ( 'NONE',  ( -16.55341960407611168, -4.379528057220339221, 56.45724293864768839 ) ) ;
#175177=CARTESIAN_POINT ( 'NONE',  ( -9.564922557960796823, -16.46253265017161027, 102.0822429386477097 ) ) ;
#175178=CARTESIAN_POINT ( 'NONE',  ( 5.049401038297881783, 19.05341960407617563, 82.29275706135229029 ) ) ;
#175179=CARTESIAN_POINT ( 'NONE',  ( 19.03943276465977164, -0.05219959533909143690, 63.74890960531435979 ) ) ;
#175180=CARTESIAN_POINT ( 'NONE',  ( 9.564922557960805705, 16.46253265017160317, 89.58224293864769550 ) ) ;
#175181=CARTESIAN_POINT ( 'NONE',  ( 13.97604488694527802, 13.89961937509977652, 69.37390960531436690 ) ) ;
#175182=CARTESIAN_POINT ( 'NONE',  ( 10.81492255796078972, 18.62759615963270932, 64.58224293864769550 ) ) ;
#175183=CARTESIAN_POINT ( 'NONE',  ( -12.06949235617739369, -12.14591786802326823, 54.37609039468568994 ) ) ;
#175184=B_SPLINE_CURVE_WITH_KNOTS ( 'NONE', 3,
 ( #146753, #112426, #98225, #116424, #159928, #54750 ),
 .UNSPECIFIED., .F., .F.,
 ( 4, 2, 4 ),
 ( 0.003239945802372313274, 0.003620412082092175007, 0.004000878361812037175 ),
 .UNSPECIFIED. ) ;
#175185=CARTESIAN_POINT ( 'NONE',  ( 16.51473224551083163, -9.474510206698727899, 105.8344237280190043 ) ) ;
#175186=CARTESIAN_POINT ( 'NONE',  ( 9.474510206698971260, -16.51473224551069308, 47.91557627198102409 ) ) ;
#175187=CARTESIAN_POINT ( 'NONE',  ( -10.72451020669898014, 18.67979575497178502, 60.41557627198102409 ) ) ;
#175188=CARTESIAN_POINT ( 'NONE',  ( -16.46253265017146816, -9.564922557961047289, 84.16775706135233293 ) ) ;
#175189=CARTESIAN_POINT ( 'NONE',  ( 12.06949235617757843, -12.14591786802309237, 28.12390960531435979 ) ) ;
#175190=CARTESIAN_POINT ( 'NONE',  ( -18.67979575497193778, 10.72451020669871902, 33.33442372801900433 ) ) ;
#175191=CARTESIAN_POINT ( 'NONE',  ( 0.05219959533936267826, -19.03943276465977164, 40.00109039468566152 ) ) ;
#175192=CARTESIAN_POINT ( 'NONE',  ( -16.53943276465976808, -0.05219959533934237506, 63.75109039468568284 ) ) ;
#175193=CARTESIAN_POINT ( 'NONE',  ( -4.483927247898782831, 16.52544592524335698, 87.70942372801901854 ) ) ;
#175194=CARTESIAN_POINT ( 'NONE',  ( 18.22780087662119897, -5.500000000000096811, 43.51763182126894236 ) ) ;
#175195=CARTESIAN_POINT ( 'NONE',  ( 14.34966873604972726, -8.224510206698740333, 75.83442372801900433 ) ) ;
#175196=CARTESIAN_POINT ( 'NONE',  ( -0.05219959533907301413, -21.53943276465977519, 22.49890960531436335 ) ) ;
#175197=CARTESIAN_POINT ( 'NONE',  ( -4.379528057220086978, -16.55341960407618274, 39.79275706135235424 ) ) ;
#175198=CARTESIAN_POINT ( 'NONE',  ( 19.03943276465977164, -0.05219959533909143690, 43.74890960531435979 ) ) ;
#175199=CARTESIAN_POINT ( 'NONE',  ( -13.89961937509977652, 13.97604488694528158, 50.62390960531435979 ) ) ;
#175200=CARTESIAN_POINT ( 'NONE',  ( -5.049401038298153566, 19.05341960407611168, 60.20724293864768129 ) ) ;
#175201=CARTESIAN_POINT ( 'NONE',  ( 21.52544592524334988, 5.823673210054432836, 36.45942372801901143 ) ) ;
#175202=CARTESIAN_POINT ( 'NONE',  ( 0.05219959533934541429, -16.53943276465976808, 45.00109039468568284 ) ) ;
#175203=CARTESIAN_POINT ( 'NONE',  ( 16.52544592524342804, -4.483927247898539470, 23.54057627198102765 ) ) ;
#175204=CARTESIAN_POINT ( 'NONE',  ( 0.05219959533909260263, 19.03943276465977164, 29.99890960531435979 ) ) ;
#175205=CARTESIAN_POINT ( 'NONE',  ( 21.55341960407619695, -5.719274019375665929, 111.0427570613523613 ) ) ;
#175206=CARTESIAN_POINT ( 'NONE',  ( 8.314922557961029526, -14.29746914071037800, 20.41775706135234714 ) ) ;
#175207=CARTESIAN_POINT ( 'NONE',  ( -5.153800228976607833, 19.02544592524334988, 67.70942372801900433 ) ) ;
#175208=CARTESIAN_POINT ( 'NONE',  ( 14.29746914071049879, -8.314922557960816363, 73.33224293864769550 ) ) ;
#175209=CARTESIAN_POINT ( 'NONE',  ( 9.474510206698971260, -16.51473224551069308, 32.91557627198102409 ) ) ;
#175210=CARTESIAN_POINT ( 'NONE',  ( -5.049401038297874678, -19.05341960407617918, 74.79275706135231871 ) ) ;
#175211=CARTESIAN_POINT ( 'NONE',  ( 17.48847506799967988, 5.747544572773808369, 76.67302562156720569 ) ) ;
#175212=CARTESIAN_POINT ( 'NONE',  ( 5.823673210054444382, -21.52544592524334988, 75.20942372801901854 ) ) ;
#175213=CARTESIAN_POINT ( 'NONE',  ( 8.314922557961029526, -14.29746914071037800, 40.41775706135234714 ) ) ;
#175214=CARTESIAN_POINT ( 'NONE',  ( 15.50000000000000178, -7.500000000000000888, 22.00000000000000711 ) ) ;
#175215=CARTESIAN_POINT ( 'NONE',  ( -0.05219959533907301413, -21.53943276465977519, 37.49890960531436690 ) ) ;
#175216=CARTESIAN_POINT ( 'NONE',  ( -14.34966873604972548, 8.224510206698743886, 28.33442372801902209 ) ) ;
#175217=CARTESIAN_POINT ( 'NONE',  ( -16.46253265017160317, 9.564922557960807481, 25.83224293864769194 ) ) ;
#175218=CARTESIAN_POINT ( 'NONE',  ( -5.049401038297874678, -19.05341960407617918, 29.79275706135232227 ) ) ;
#175220=CARTESIAN_POINT ( 'NONE',  ( -0.05219959533909027116, -19.03943276465977164, 32.49890960531435979 ) ) ;
#175222=CARTESIAN_POINT ( 'NONE',  ( 19.03943276465977164, -0.05219959533909143690, 58.74890960531435979 ) ) ;
#175223=CARTESIAN_POINT ( 'NONE',  ( -19.48894818550245844, 5.499999999999918288, 100.1030731043523616 ) ) ;
#175224=CARTESIAN_POINT ( 'NONE',  ( 19.05341960407617918, -5.049401038297876454, 21.04275706135232582 ) ) ;
#175225=CARTESIAN_POINT ( 'NONE',  ( 14.34966873604972726, -8.224510206698740333, 110.8344237280190043 ) ) ;
#175226=CARTESIAN_POINT ( 'NONE',  ( -19.03943276465977164, 0.05219959533909376836, 26.24890960531435624 ) ) ;
#175227=CARTESIAN_POINT ( 'NONE',  ( 9.564922557960805705, 16.46253265017160317, 89.58224293864769550 ) ) ;
#175228=CARTESIAN_POINT ( 'NONE',  ( -21.53943276465977519, -0.05219959533937600094, 63.75109039468568284 ) ) ;
#175229=CARTESIAN_POINT ( 'NONE',  ( -13.97604488694527625, -13.89961937509977652, 41.87390960531435979 ) ) ;
#175230=CARTESIAN_POINT ( 'NONE',  ( -21.53943276465977519, -0.05219959533937600094, 68.75109039468568994 ) ) ;
#175231=CARTESIAN_POINT ( 'NONE',  ( -9.564922557961040184, 16.46253265017147172, 92.91775706135233293 ) ) ;
#175232=CARTESIAN_POINT ( 'NONE',  ( -13.97604488694527625, -13.89961937509977652, 101.8739096053143811 ) ) ;
#175233=CARTESIAN_POINT ( 'NONE',  ( -0.05219959533909027116, -19.03943276465977164, 37.49890960531436690 ) ) ;
#175234=CARTESIAN_POINT ( 'NONE',  ( 15.80617190586746368, 15.72974639402197994, 104.3739096053143669 ) ) ;
#175235=CARTESIAN_POINT ( 'NONE',  ( -13.89961937509957401, -13.97604488694547875, 34.37609039468566863 ) ) ;
#175236=CARTESIAN_POINT ( 'NONE',  ( 4.379528057220339221, -16.55341960407611168, 112.7072429386476955 ) ) ;
#175237=CARTESIAN_POINT ( 'NONE',  ( 5.049401038298161559, -19.05341960407611168, 67.70724293864769550 ) ) ;
#175238=CARTESIAN_POINT ( 'NONE',  ( 9.474510206698729675, 16.51473224551082808, 92.08442372801900433 ) ) ;
#175239=CARTESIAN_POINT ( 'NONE',  ( -16.52544592524342804, 4.483927247898546575, 71.04057627198103830 ) ) ;
#175240=CARTESIAN_POINT ( 'NONE',  ( -15.80617190586745835, -15.72974639402198527, 26.87390960531435979 ) ) ;
#175241=CARTESIAN_POINT ( 'NONE',  ( 13.89961937509957401, 13.97604488694547697, 81.87609039468564731 ) ) ;
#175242=CARTESIAN_POINT ( 'NONE',  ( -15.72974639402197994, 15.80617190586746368, 95.62390960531436690 ) ) ;
#175243=CARTESIAN_POINT ( 'NONE',  ( 21.55341960407619695, -5.719274019375665929, 41.04275706135236135 ) ) ;
#175244=CARTESIAN_POINT ( 'NONE',  ( -8.224510206698735004, -14.34966873604973081, 44.58442372801901854 ) ) ;
#175245=CARTESIAN_POINT ( 'NONE',  ( -16.52544592524335698, -4.483927247898792601, 48.95942372801902565 ) ) ;
#175246=CARTESIAN_POINT ( 'NONE',  ( -0.05219959533937732626, 21.53943276465977519, 52.50109039468567573 ) ) ;
#175247=CARTESIAN_POINT ( 'NONE',  ( 5.823673210054125526, 21.52544592524343514, 59.79057627198103120 ) ) ;
#175248=CARTESIAN_POINT ( 'NONE',  ( 19.05341960407611168, 5.049401038298154454, 48.95724293864768129 ) ) ;
#175250=CARTESIAN_POINT ( 'NONE',  ( 8.224510206698742110, 14.34966873604972548, 72.08442372801899012 ) ) ;
#175251=CARTESIAN_POINT ( 'NONE',  ( -21.55341960407610458, -5.719274019375992779, 96.45724293864770971 ) ) ;
#175252=CARTESIAN_POINT ( 'NONE',  ( 16.55341960407611168, 4.379528057220329451, 38.95724293864768839 ) ) ;
#175253=CARTESIAN_POINT ( 'NONE',  ( -4.379528057220086978, -16.55341960407618274, 64.79275706135234714 ) ) ;
#175254=CARTESIAN_POINT ( 'NONE',  ( -0.05219959533936034679, 19.03943276465977164, 102.5010903946856757 ) ) ;
#175255=CARTESIAN_POINT ( 'NONE',  ( -21.55341960407610458, -5.719274019375992779, 96.45724293864770971 ) ) ;
#175256=CARTESIAN_POINT ( 'NONE',  ( -12.14591786802309592, -12.06949235617757132, 26.87390960531435979 ) ) ;
#175258=CARTESIAN_POINT ( 'NONE',  ( -14.34966873604972548, 8.224510206698743886, 73.33442372801901854 ) ) ;
#175260=CARTESIAN_POINT ( 'NONE',  ( -15.80617190586745835, -15.72974639402198527, 76.87390960531439532 ) ) ;
#175261=CARTESIAN_POINT ( 'NONE',  ( -12.06949235617739369, -12.14591786802326823, 104.3760903946856899 ) ) ;
#175263=CARTESIAN_POINT ( 'NONE',  ( 17.50000000000000000, -5.500000000000000888, 120.0000000000000142 ) ) ;
#175264=CARTESIAN_POINT ( 'NONE',  ( 15.80617190586746368, 15.72974639402197994, 99.37390960531436690 ) ) ;
#175265=CARTESIAN_POINT ( 'NONE',  ( 21.53943276465977519, -0.05219959533907433946, 108.7489096053143669 ) ) ;
#175266=CARTESIAN_POINT ( 'NONE',  ( -12.14591786802309592, -12.06949235617757132, 31.87390960531435979 ) ) ;
#175267=CARTESIAN_POINT ( 'NONE',  ( -12.14591786802326823, 12.06949235617739902, 43.12609039468568284 ) ) ;
#175268=CARTESIAN_POINT ( 'NONE',  ( -16.46253265017160317, 9.564922557960807481, 50.83224293864770260 ) ) ;
#175269=CARTESIAN_POINT ( 'NONE',  ( 16.46253265017160672, -9.564922557960803928, 68.33224293864770971 ) ) ;
#175270=VERTEX_POINT ( 'NONE', #92038 ) ;
#175271=CARTESIAN_POINT ( 'NONE',  ( 18.67979575497178502, 10.72451020669898547, 24.16557627198103120 ) ) ;
#175273=CARTESIAN_POINT ( 'NONE',  ( 19.05341960407617918, -5.049401038297876454, 106.0427570613523471 ) ) ;
#175274=CARTESIAN_POINT ( 'NONE',  ( -16.51473224551082808, 9.474510206698731452, 48.33442372801900433 ) ) ;
#175275=CARTESIAN_POINT ( 'NONE',  ( -15.72974639402197994, 15.80617190586746368, 90.62390960531436690 ) ) ;
#175276=CARTESIAN_POINT ( 'NONE',  ( -16.53943276465976808, -0.05219959533934237506, 108.7510903946857042 ) ) ;
#175277=AXIS2_PLACEMENT_3D ( 'NONE', #192094, #132421, #100072 ) ;
#175278=CARTESIAN_POINT ( 'NONE',  ( 16.51473224551069308, 9.474510206698969483, 74.16557627198103830 ) ) ;
#175279=CARTESIAN_POINT ( 'NONE',  ( -15.72974639402197994, 15.80617190586746368, 40.62390960531435269 ) ) ;
#175280=CARTESIAN_POINT ( 'NONE',  ( 15.72974639402199770, -15.80617190586745480, 78.12390960531436690 ) ) ;
#175281=CARTESIAN_POINT ( 'NONE',  ( 12.14591786802327356, -12.06949235617739191, 30.62609039468567929 ) ) ;
#175282=CARTESIAN_POINT ( 'NONE',  ( -15.72974639402197994, 15.80617190586746368, 25.62390960531435624 ) ) ;
#175283=CARTESIAN_POINT ( 'NONE',  ( 18.67979575497194134, -10.72451020669871369, 75.83442372801900433 ) ) ;
#175284=CARTESIAN_POINT ( 'NONE',  ( 0.05219959533909260263, 19.03943276465977164, 79.99890960531436690 ) ) ;
#175285=CARTESIAN_POINT ( 'NONE',  ( 5.049401038298161559, -19.05341960407611168, 22.70724293864769194 ) ) ;
#175286=CARTESIAN_POINT ( 'NONE',  ( -5.153800228976328057, -19.02544592524343514, 67.29057627198102409 ) ) ;
#175287=CARTESIAN_POINT ( 'NONE',  ( 14.29746914071049879, -8.314922557960816363, 93.33224293864769550 ) ) ;
#175288=ORIENTED_EDGE ( 'NONE', *, *, #26049, .F. ) ;
#175289=CARTESIAN_POINT ( 'NONE',  ( -16.46253265017146816, -9.564922557961047289, 99.16775706135233293 ) ) ;
#175290=CARTESIAN_POINT ( 'NONE',  ( 17.40805194822031865, -6.112264579159332634, 83.33371272510612471 ) ) ;
#175291=CARTESIAN_POINT ( 'NONE',  ( -9.474510206698964154, 16.51473224551069663, 75.41557627198103830 ) ) ;
#175292=CARTESIAN_POINT ( 'NONE',  ( 10.81492255796106328, -18.62759615963255655, 85.41775706135236135 ) ) ;
#175293=CARTESIAN_POINT ( 'NONE',  ( 19.03943276465977164, -0.05219959533909143690, 98.74890960531436690 ) ) ;
#175294=CARTESIAN_POINT ( 'NONE',  ( -12.06949235617739369, -12.14591786802326823, 74.37609039468568994 ) ) ;
#175296=CARTESIAN_POINT ( 'NONE',  ( 19.02544592524334988, 5.153800228976608722, 51.45942372801900433 ) ) ;
#175297=CARTESIAN_POINT ( 'NONE',  ( -0.05219959533937732626, 21.53943276465977519, 112.5010903946857042 ) ) ;
#175301=CARTESIAN_POINT ( 'NONE',  ( -16.55341960407617563, 4.379528057220093196, 113.5427570613523756 ) ) ;
#175302=CARTESIAN_POINT ( 'NONE',  ( 30.00000000000000000, 5.499999999999992895, 102.5000000000000142 ) ) ;
#175303=CARTESIAN_POINT ( 'NONE',  ( 16.53943276465976808, 0.05219959533934440121, 111.2510903946856899 ) ) ;
#175305=CARTESIAN_POINT ( 'NONE',  ( -16.55341960407617563, 4.379528057220093196, 78.54275706135236135 ) ) ;
#175306=CARTESIAN_POINT ( 'NONE',  ( 21.53943276465977519, 0.05219959533937863772, 81.25109039468568994 ) ) ;
#175307=CARTESIAN_POINT ( 'NONE',  ( 16.51473224551083163, -9.474510206698727899, 105.8344237280190043 ) ) ;
#175308=CARTESIAN_POINT ( 'NONE',  ( 18.62759615963255655, 10.81492255796105972, 71.66775706135234714 ) ) ;
#175309=CARTESIAN_POINT ( 'NONE',  ( -16.46253265017146816, -9.564922557961047289, 34.16775706135233293 ) ) ;
#175310=CARTESIAN_POINT ( 'NONE',  ( -19.03943276465977164, 0.05219959533909376836, 76.24890960531435269 ) ) ;
#175311=CARTESIAN_POINT ( 'NONE',  ( -19.02544592524342804, 5.153800228976336051, 61.04057627198103120 ) ) ;
#175313=CARTESIAN_POINT ( 'NONE',  ( 5.823673210054125526, 21.52544592524343514, 94.79057627198105251 ) ) ;
#175314=CARTESIAN_POINT ( 'NONE',  ( -0.05219959533907301413, -21.53943276465977519, 47.49890960531435979 ) ) ;
#175315=CARTESIAN_POINT ( 'NONE',  ( 13.89961937509977652, -13.97604488694527269, 53.12390960531434558 ) ) ;
#175316=CARTESIAN_POINT ( 'NONE',  ( -12.06949235617739369, -12.14591786802326823, 59.37609039468568284 ) ) ;
#175319=CARTESIAN_POINT ( 'NONE',  ( 21.55341960407619695, -5.719274019375665929, 41.04275706135236135 ) ) ;
#175320=CARTESIAN_POINT ( 'NONE',  ( 12.06949235617757843, -12.14591786802309237, 68.12390960531436690 ) ) ;
#175322=CARTESIAN_POINT ( 'NONE',  ( -12.06949235617739369, -12.14591786802326823, 34.37609039468568284 ) ) ;
#175323=CARTESIAN_POINT ( 'NONE',  ( 8.224510206698953496, -14.34966873604960469, 97.91557627198103830 ) ) ;
#175324=CARTESIAN_POINT ( 'NONE',  ( -5.153800228976607833, 19.02544592524334988, 47.70942372801900433 ) ) ;
#175325=CARTESIAN_POINT ( 'NONE',  ( -8.224510206698948167, 14.34966873604960824, 70.41557627198102409 ) ) ;
#175326=CARTESIAN_POINT ( 'NONE',  ( -10.72451020669870658, -18.67979575497194134, 34.58442372801900433 ) ) ;
#175327=CARTESIAN_POINT ( 'NONE',  ( -5.049401038298153566, 19.05341960407611168, 25.20724293864768484 ) ) ;
#175328=CARTESIAN_POINT ( 'NONE',  ( -0.05219959533907301413, -21.53943276465977519, 87.49890960531436690 ) ) ;
#175329=CARTESIAN_POINT ( 'NONE',  ( -9.564922557960796823, -16.46253265017161027, 102.0822429386477097 ) ) ;
#175330=CARTESIAN_POINT ( 'NONE',  ( -16.55341960407611168, -4.379528057220339221, 71.45724293864769550 ) ) ;
#175333=CARTESIAN_POINT ( 'NONE',  ( -9.474510206698720793, -16.51473224551083518, 79.58442372801899012 ) ) ;
#175334=CARTESIAN_POINT ( 'NONE',  ( -0.05219959533937732626, 21.53943276465977519, 27.50109039468567929 ) ) ;
#175335=CARTESIAN_POINT ( 'NONE',  ( -16.46253265017160317, 9.564922557960807481, 65.83224293864769550 ) ) ;
#175336=CARTESIAN_POINT ( 'NONE',  ( -19.02544592524334988, -5.153800228976617603, 53.95942372801898301 ) ) ;
#175337=CARTESIAN_POINT ( 'NONE',  ( 9.564922557960805705, 16.46253265017160317, 34.58224293864770260 ) ) ;
#175338=CARTESIAN_POINT ( 'NONE',  ( -16.53943276465976808, 0.05219959533911058130, 61.24890960531435979 ) ) ;
#175339=CARTESIAN_POINT ( 'NONE',  ( -0.05219959533910754901, -16.53943276465976808, 57.49890960531435979 ) ) ;
#175340=CARTESIAN_POINT ( 'NONE',  ( 9.474510206698971260, -16.51473224551069308, 62.91557627198102409 ) ) ;
#175341=CARTESIAN_POINT ( 'NONE',  ( 15.72974639402199770, -15.80617190586745480, 93.12390960531436690 ) ) ;
#175342=CARTESIAN_POINT ( 'NONE',  ( 0.05219959533909260263, 19.03943276465977164, 59.99890960531436690 ) ) ;
#175343=CARTESIAN_POINT ( 'NONE',  ( 15.80617190586746368, 15.72974639402197994, 84.37390960531438111 ) ) ;
#175344=CARTESIAN_POINT ( 'NONE',  ( 5.823673210054444382, -21.52544592524334988, 110.2094237280190185 ) ) ;
#175345=CARTESIAN_POINT ( 'NONE',  ( 9.474510206698971260, -16.51473224551069308, 27.91557627198103120 ) ) ;
#175346=CARTESIAN_POINT ( 'NONE',  ( 4.379528057220092307, 16.55341960407617563, 107.2927570613523471 ) ) ;
#175347=CARTESIAN_POINT ( 'NONE',  ( -12.14591786802309592, -12.06949235617757132, 96.87390960531436690 ) ) ;
#175348=CARTESIAN_POINT ( 'NONE',  ( 19.02544592524334988, 5.153800228976608722, 86.45942372801900433 ) ) ;
#175350=CARTESIAN_POINT ( 'NONE',  ( -21.52544592524343514, 5.823673210054127303, 116.0405762719810383 ) ) ;
#175351=CARTESIAN_POINT ( 'NONE',  ( -5.153800228976607833, 19.02544592524334988, 47.70942372801900433 ) ) ;
#175352=CARTESIAN_POINT ( 'NONE',  ( 16.55341960407618274, -4.379528057220086978, 106.0427570613523471 ) ) ;
#175353=CARTESIAN_POINT ( 'NONE',  ( -19.03943276465977164, -0.05219959533935918106, 38.75109039468566152 ) ) ;
#175354=CARTESIAN_POINT ( 'NONE',  ( -19.02544592524342804, 5.153800228976336051, 106.0405762719810241 ) ) ;
#175355=CARTESIAN_POINT ( 'NONE',  ( -10.81492255796078084, -18.62759615963271287, 62.08224293864769550 ) ) ;
#175357=CARTESIAN_POINT ( 'NONE',  ( 13.97604488694527802, 13.89961937509977652, 39.37390960531435269 ) ) ;
#175358=CARTESIAN_POINT ( 'NONE',  ( 15.72974639402176855, 15.80617190586768217, 111.8760903946856615 ) ) ;
#175359=CARTESIAN_POINT ( 'NONE',  ( 8.224510206698742110, 14.34966873604972548, 72.08442372801899012 ) ) ;
#175360=CARTESIAN_POINT ( 'NONE',  ( -5.823673210054431948, 21.52544592524334988, 32.70942372801900433 ) ) ;
#175361=CARTESIAN_POINT ( 'NONE',  ( -0.05219959533934338120, 16.53943276465976808, 47.50109039468568994 ) ) ;
#175362=CARTESIAN_POINT ( 'NONE',  ( 19.03943276465977164, -0.05219959533909143690, 108.7489096053143527 ) ) ;
#175363=CARTESIAN_POINT ( 'NONE',  ( 16.46253265017160672, -9.564922557960803928, 53.33224293864768839 ) ) ;
#175364=CARTESIAN_POINT ( 'NONE',  ( 19.02544592524343514, -5.153800228976328945, 63.54057627198103830 ) ) ;
#175365=CARTESIAN_POINT ( 'NONE',  ( -8.224510206698735004, -14.34966873604973081, 49.58442372801901143 ) ) ;
#175366=CARTESIAN_POINT ( 'NONE',  ( -0.05219959533910754901, -16.53943276465976808, 107.4989096053143669 ) ) ;
#175367=CARTESIAN_POINT ( 'NONE',  ( 4.483927247898790824, -16.52544592524335698, 110.2094237280190185 ) ) ;
#175368=CARTESIAN_POINT ( 'NONE',  ( 17.50000000000000000, -5.499999999999992895, 86.21769037696435589 ) ) ;
#175369=CARTESIAN_POINT ( 'NONE',  ( 10.72451020669871369, 18.67979575497193778, 57.08442372801901854 ) ) ;
#175370=CARTESIAN_POINT ( 'NONE',  ( 16.46253265017160672, -9.564922557960803928, 73.33224293864769550 ) ) ;
#175371=CARTESIAN_POINT ( 'NONE',  ( -16.46253265017160317, 9.564922557960807481, 70.83224293864770971 ) ) ;
#175372=CARTESIAN_POINT ( 'NONE',  ( -16.51473224551069308, -9.474510206698971260, 91.66557627198103830 ) ) ;
#175373=CARTESIAN_POINT ( 'NONE',  ( 8.224510206698953496, -14.34966873604960469, 47.91557627198102409 ) ) ;
#175374=CARTESIAN_POINT ( 'NONE',  ( 16.52544592524335698, 4.483927247898782831, 106.4594237280190328 ) ) ;
#175375=CARTESIAN_POINT ( 'NONE',  ( -8.314922557960811034, -14.29746914071050412, 42.08224293864769550 ) ) ;
#175376=ORIENTED_EDGE ( 'NONE', *, *, #22002, .F. ) ;
#175378=CARTESIAN_POINT ( 'NONE',  ( -5.153800228976328057, -19.02544592524343514, 62.29057627198100988 ) ) ;
#175379=CARTESIAN_POINT ( 'NONE',  ( -5.049401038297874678, -19.05341960407617918, 44.79275706135232582 ) ) ;
#175381=CARTESIAN_POINT ( 'NONE',  ( 5.049401038298163336, -19.05341960407611168, 67.70724293864768129 ) ) ;
#175382=CARTESIAN_POINT ( 'NONE',  ( 16.51473224551083163, -9.474510206698727899, 80.83442372801899012 ) ) ;
#175383=CARTESIAN_POINT ( 'NONE',  ( -16.53943276465976808, -0.05219959533934237506, 68.75109039468568994 ) ) ;
#175385=CARTESIAN_POINT ( 'NONE',  ( 0.05219959533909260263, 19.03943276465977164, 94.99890960531436690 ) ) ;
#175386=CARTESIAN_POINT ( 'NONE',  ( 18.62759615963255655, 10.81492255796105972, 31.66775706135234358 ) ) ;
#175388=CARTESIAN_POINT ( 'NONE',  ( 13.89961937509957401, 13.97604488694547697, 71.87609039468567573 ) ) ;
#175389=CARTESIAN_POINT ( 'NONE',  ( 16.52216118717209525, 7.221426719304533393, 88.57599021046995347 ) ) ;
#175390=CARTESIAN_POINT ( 'NONE',  ( 13.97604488694527802, 13.89961937509977652, 54.37390960531435979 ) ) ;
#175391=CARTESIAN_POINT ( 'NONE',  ( 9.564922557960805705, 16.46253265017160317, 84.58224293864769550 ) ) ;
#175392=CARTESIAN_POINT ( 'NONE',  ( -16.55341960407611168, -4.379528057220339221, 41.45724293864769550 ) ) ;
#175393=CARTESIAN_POINT ( 'NONE',  ( -5.049401038298153566, 19.05341960407611168, 50.20724293864770260 ) ) ;
#175394=CARTESIAN_POINT ( 'NONE',  ( -0.05219959533936034679, 19.03943276465977164, 62.50109039468566863 ) ) ;
#175396=CARTESIAN_POINT ( 'NONE',  ( -8.314922557960811034, -14.29746914071050412, 92.08224293864769550 ) ) ;
#175397=CARTESIAN_POINT ( 'NONE',  ( 5.049401038297881783, 19.05341960407617563, 32.29275706135233293 ) ) ;
#175398=CARTESIAN_POINT ( 'NONE',  ( -19.03943276465977164, 0.05219959533909376836, 61.24890960531436690 ) ) ;
#175400=CARTESIAN_POINT ( 'NONE',  ( 5.719274019375991003, -21.55341960407610458, 57.70724293864770260 ) ) ;
#175401=CARTESIAN_POINT ( 'NONE',  ( -16.55341960407611168, -4.379528057220339221, 61.45724293864770260 ) ) ;
#175402=CARTESIAN_POINT ( 'NONE',  ( -19.03943276465977164, -0.05219959533935918106, 23.75109039468566152 ) ) ;
#175403=CARTESIAN_POINT ( 'NONE',  ( -19.03943276465977164, 0.05219959533909376836, 111.2489096053143669 ) ) ;
#175404=CARTESIAN_POINT ( 'NONE',  ( 10.72451020669898902, -18.67979575497178502, 32.91557627198102409 ) ) ;
#175405=CARTESIAN_POINT ( 'NONE',  ( 0.05219959533909260263, 19.03943276465977164, 54.99890960531435979 ) ) ;
#175406=CARTESIAN_POINT ( 'NONE',  ( -5.049401038298153566, 19.05341960407611168, 45.20724293864769550 ) ) ;
#175407=CARTESIAN_POINT ( 'NONE',  ( 14.34966873604960469, 8.224510206698951720, 99.16557627198100988 ) ) ;
#175408=CARTESIAN_POINT ( 'NONE',  ( 0.05219959533907565091, 21.53943276465977519, 109.9989096053143527 ) ) ;
#175409=CARTESIAN_POINT ( 'NONE',  ( 5.153800228976335163, 19.02544592524342804, 99.79057627198102409 ) ) ;
#175410=CARTESIAN_POINT ( 'NONE',  ( -5.823673210054431948, 21.52544592524334988, 22.70942372801901499 ) ) ;
#175411=CARTESIAN_POINT ( 'NONE',  ( -13.89961937509977652, 13.97604488694528158, 100.6239096053143669 ) ) ;
#175412=CARTESIAN_POINT ( 'NONE',  ( -14.29746914071049879, 8.314922557960819915, 115.8322429386477097 ) ) ;
#175413=CARTESIAN_POINT ( 'NONE',  ( -21.55341960407619339, 5.719274019375674811, 78.54275706135236135 ) ) ;
#175414=CARTESIAN_POINT ( 'NONE',  ( 21.53943276465977519, -0.05219959533907433946, 98.74890960531438111 ) ) ;
#175418=CARTESIAN_POINT ( 'NONE',  ( 16.52544592524335698, 4.483927247898782831, 51.45942372801901854 ) ) ;
#175419=CARTESIAN_POINT ( 'NONE',  ( 12.06949235617757843, -12.14591786802309237, 113.1239096053143953 ) ) ;
#175420=CARTESIAN_POINT ( 'NONE',  ( 19.36337904590688197, -5.500000000000146549, 52.91494137495617878 ) ) ;
#175421=CARTESIAN_POINT ( 'NONE',  ( -9.474510206698964154, 16.51473224551069663, 60.41557627198102409 ) ) ;
#175422=CARTESIAN_POINT ( 'NONE',  ( -8.314922557960811034, -14.29746914071050412, 92.08224293864769550 ) ) ;
#175424=CARTESIAN_POINT ( 'NONE',  ( 15.72974639402199770, -15.80617190586745480, 48.12390960531436690 ) ) ;
#175425=CARTESIAN_POINT ( 'NONE',  ( -16.53943276465976808, 0.05219959533911058130, 66.24890960531436690 ) ) ;
#175426=CARTESIAN_POINT ( 'NONE',  ( -16.55341960407617563, 4.379528057220093196, 23.54275706135235424 ) ) ;
#175427=CARTESIAN_POINT ( 'NONE',  ( 5.719274019375673035, 21.55341960407619339, 72.29275706135236135 ) ) ;
#175428=CARTESIAN_POINT ( 'NONE',  ( 18.22780087662126647, 5.499999999999818812, 61.48236817873107896 ) ) ;
#175429=CARTESIAN_POINT ( 'NONE',  ( -0.05219959533934338120, 16.53943276465976808, 92.50109039468567573 ) ) ;
#175430=CARTESIAN_POINT ( 'NONE',  ( -0.05219959533910754901, -16.53943276465976808, 47.49890960531435979 ) ) ;
#175431=CARTESIAN_POINT ( 'NONE',  ( -16.46253265017160317, 9.564922557960807481, 40.83224293864769550 ) ) ;
#175432=CARTESIAN_POINT ( 'NONE',  ( -19.03943276465977164, 0.05219959533909376836, 86.24890960531436690 ) ) ;
#175433=CARTESIAN_POINT ( 'NONE',  ( -18.62759615963270932, 10.81492255796079327, 95.83224293864770971 ) ) ;
#175434=CARTESIAN_POINT ( 'NONE',  ( 8.224510206698742110, 14.34966873604972548, 42.08442372801901854 ) ) ;
#175435=CARTESIAN_POINT ( 'NONE',  ( 16.53943276465976808, -0.05219959533910856209, 68.74890960531435269 ) ) ;
#175436=CARTESIAN_POINT ( 'NONE',  ( 10.81492255796106328, -18.62759615963255655, 70.41775706135236135 ) ) ;
#175437=CARTESIAN_POINT ( 'NONE',  ( 14.34966873604972726, -8.224510206698740333, 100.8344237280190185 ) ) ;
#175438=CARTESIAN_POINT ( 'NONE',  ( 17.44270441346523981, -5.991230190322817784, 46.13664920735775610 ) ) ;
#175440=CARTESIAN_POINT ( 'NONE',  ( 14.34966873604960469, 8.224510206698951720, 29.16557627198103120 ) ) ;
#175441=CARTESIAN_POINT ( 'NONE',  ( -16.52544592524335698, -4.483927247898792601, 68.95942372801901854 ) ) ;
#175442=CARTESIAN_POINT ( 'NONE',  ( 5.153800228976335163, 19.02544592524342804, 89.79057627198102409 ) ) ;
#175443=CARTESIAN_POINT ( 'NONE',  ( 13.89961937509977652, -13.97604488694527269, 103.1239096053143527 ) ) ;
#175444=CARTESIAN_POINT ( 'NONE',  ( 10.72451020669871369, 18.67979575497193778, 82.08442372801901854 ) ) ;
#175445=CARTESIAN_POINT ( 'NONE',  ( 16.55341960407618274, -4.379528057220086978, 91.04275706135236135 ) ) ;
#175446=CARTESIAN_POINT ( 'NONE',  ( -4.483927247898539470, -16.52544592524342804, 62.29057627198102409 ) ) ;
#175447=CARTESIAN_POINT ( 'NONE',  ( -16.46253265017160317, 9.564922557960807481, 70.83224293864770971 ) ) ;
#175449=CARTESIAN_POINT ( 'NONE',  ( -16.46253265017146816, -9.564922557961047289, 109.1677570613523471 ) ) ;
#175450=CARTESIAN_POINT ( 'NONE',  ( -19.05341960407611168, -5.049401038298163336, 21.45724293864768839 ) ) ;
#175451=CARTESIAN_POINT ( 'NONE',  ( -9.474510206698964154, 16.51473224551069663, 80.41557627198103830 ) ) ;
#175452=CARTESIAN_POINT ( 'NONE',  ( -19.03943276465977164, -0.05219959533935918106, 108.7510903946856615 ) ) ;
#175454=CARTESIAN_POINT ( 'NONE',  ( 16.51473224551083163, -9.474510206698727899, 25.83442372801900078 ) ) ;
#175455=CARTESIAN_POINT ( 'NONE',  ( 16.52544592524335698, 4.483927247898782831, 81.45942372801900433 ) ) ;
#175456=CARTESIAN_POINT ( 'NONE',  ( 16.46253265017146816, 9.564922557961045513, 96.66775706135233293 ) ) ;
#175457=CARTESIAN_POINT ( 'NONE',  ( 8.314922557960818139, 14.29746914071049879, 109.5822429386476955 ) ) ;
#175458=CARTESIAN_POINT ( 'NONE',  ( -4.379528057220086978, -16.55341960407618274, 69.79275706135234714 ) ) ;
#175459=CARTESIAN_POINT ( 'NONE',  ( -12.06949235617739369, -12.14591786802326823, 59.37609039468568284 ) ) ;
#175461=CARTESIAN_POINT ( 'NONE',  ( -16.51473224551082808, 9.474510206698731452, 68.33442372801900433 ) ) ;
#175462=CARTESIAN_POINT ( 'NONE',  ( 5.823673210054444382, -21.52544592524334988, 95.20942372801903275 ) ) ;
#175463=CARTESIAN_POINT ( 'NONE',  ( -19.02544592524342804, 5.153800228976336051, 41.04057627198103120 ) ) ;
#175464=CARTESIAN_POINT ( 'NONE',  ( -5.153800228976328057, -19.02544592524343514, 72.29057627198102409 ) ) ;
#175465=CARTESIAN_POINT ( 'NONE',  ( -8.224510206698948167, 14.34966873604960824, 70.41557627198102409 ) ) ;
#175466=CARTESIAN_POINT ( 'NONE',  ( -15.72974639402176322, -15.80617190586768395, 89.37609039468568994 ) ) ;
#175467=CARTESIAN_POINT ( 'NONE',  ( -9.474510206698720793, -16.51473224551083518, 44.58442372801900433 ) ) ;
#175468=CARTESIAN_POINT ( 'NONE',  ( -15.72974639402197994, 15.80617190586746368, 30.62390960531436335 ) ) ;
#175469=CARTESIAN_POINT ( 'NONE',  ( -10.81492255796105439, 18.62759615963255655, 112.9177570613523329 ) ) ;
#175470=CARTESIAN_POINT ( 'NONE',  ( 19.05341960407611168, 5.049401038298154454, 78.95724293864769550 ) ) ;
#175471=CARTESIAN_POINT ( 'NONE',  ( 0.05219959533937995610, -21.53943276465977519, 100.0010903946857042 ) ) ;
#175472=CARTESIAN_POINT ( 'NONE',  ( -10.72451020669898014, 18.67979575497178502, 65.41557627198102409 ) ) ;
#175473=CARTESIAN_POINT ( 'NONE',  ( -5.153800228976328057, -19.02544592524343514, 102.2905762719810383 ) ) ;
#175474=CARTESIAN_POINT ( 'NONE',  ( 19.02544592524334988, 5.153800228976608722, 71.45942372801900433 ) ) ;
#175475=CARTESIAN_POINT ( 'NONE',  ( -13.97604488694527625, -13.89961937509977652, 96.87390960531433848 ) ) ;
#175476=CARTESIAN_POINT ( 'NONE',  ( -5.153800228976607833, 19.02544592524334988, 102.7094237280189759 ) ) ;
#175477=CARTESIAN_POINT ( 'NONE',  ( 8.314922557961029526, -14.29746914071037800, 55.41775706135234714 ) ) ;
#175478=CARTESIAN_POINT ( 'NONE',  ( -5.049401038298153566, 19.05341960407611168, 25.20724293864768484 ) ) ;
#175479=CARTESIAN_POINT ( 'NONE',  ( 16.51473224551069308, 9.474510206698969483, 84.16557627198102409 ) ) ;
#175480=CARTESIAN_POINT ( 'NONE',  ( -18.67979575497178146, -10.72451020669898902, 61.66557627198103120 ) ) ;
#175481=CARTESIAN_POINT ( 'NONE',  ( -8.314922557961024197, 14.29746914071037800, 27.91775706135234358 ) ) ;
#175482=CARTESIAN_POINT ( 'NONE',  ( -15.72974639402176322, -15.80617190586768395, 34.37609039468568284 ) ) ;
#175483=CARTESIAN_POINT ( 'NONE',  ( -21.55341960407619339, 5.719274019375674811, 88.54275706135236135 ) ) ;
#175484=CARTESIAN_POINT ( 'NONE',  ( 14.34966873604972726, -8.224510206698740333, 85.83442372801901854 ) ) ;
#175485=CARTESIAN_POINT ( 'NONE',  ( 9.474510206698971260, -16.51473224551069308, 92.91557627198103830 ) ) ;
#175486=CARTESIAN_POINT ( 'NONE',  ( 16.55341960407611168, 4.379528057220329451, 73.95724293864769550 ) ) ;
#175487=CARTESIAN_POINT ( 'NONE',  ( -14.34966873604960291, -8.224510206698953496, 21.66557627198102409 ) ) ;
#175488=CARTESIAN_POINT ( 'NONE',  ( 16.51473224551083163, -9.474510206698727899, 55.83442372801899722 ) ) ;
#175489=CARTESIAN_POINT ( 'NONE',  ( -21.55341960407619339, 5.719274019375674811, 38.54275706135234714 ) ) ;
#175490=CARTESIAN_POINT ( 'NONE',  ( -4.379528057220328563, 16.55341960407611168, 90.20724293864770971 ) ) ;
#175491=CARTESIAN_POINT ( 'NONE',  ( 18.67979575497178502, 10.72451020669898547, 24.16557627198103120 ) ) ;
#175492=CARTESIAN_POINT ( 'NONE',  ( 0.05219959533934541429, -16.53943276465976808, 100.0010903946857042 ) ) ;
#175493=CARTESIAN_POINT ( 'NONE',  ( 15.72974639402176855, 15.80617190586768217, 81.87609039468568994 ) ) ;
#175494=CARTESIAN_POINT ( 'NONE',  ( 12.06949235617739724, 12.14591786802326823, 41.87609039468568284 ) ) ;
#175495=CARTESIAN_POINT ( 'NONE',  ( 5.823673210054444382, -21.52544592524334988, 35.20942372801901854 ) ) ;
#175497=CARTESIAN_POINT ( 'NONE',  ( 10.72451020669898902, -18.67979575497178502, 107.9155762719810241 ) ) ;
#175498=CARTESIAN_POINT ( 'NONE',  ( 8.314922557960818139, 14.29746914071049879, 89.58224293864768129 ) ) ;
#175499=CARTESIAN_POINT ( 'NONE',  ( 17.50000000000148148, -3.254303733634558160, 27.52395893071405908 ) ) ;
#175500=CARTESIAN_POINT ( 'NONE',  ( -8.224510206698948167, 14.34966873604960824, 60.41557627198102409 ) ) ;
#175501=CARTESIAN_POINT ( 'NONE',  ( -4.379528057220086978, -16.55341960407618274, 99.79275706135234714 ) ) ;
#175502=CARTESIAN_POINT ( 'NONE',  ( -5.049401038298153566, 19.05341960407611168, 45.20724293864769550 ) ) ;
#175503=CARTESIAN_POINT ( 'NONE',  ( -18.67979575497178146, -10.72451020669898902, 46.66557627198102409 ) ) ;
#175504=CARTESIAN_POINT ( 'NONE',  ( 16.53943276465976808, -0.05219959533910856209, 83.74890960531435269 ) ) ;
#175505=CARTESIAN_POINT ( 'NONE',  ( -5.823673210054116645, -21.52544592524344225, 77.29057627198102409 ) ) ;
#175506=CARTESIAN_POINT ( 'NONE',  ( -0.05219959533909027116, -19.03943276465977164, 92.49890960531436690 ) ) ;
#175507=CARTESIAN_POINT ( 'NONE',  ( 13.89961937509977652, -13.97604488694527269, 38.12390960531436690 ) ) ;
#175508=CARTESIAN_POINT ( 'NONE',  ( -13.89961937509957401, -13.97604488694547875, 89.37609039468563310 ) ) ;
#175509=CARTESIAN_POINT ( 'NONE',  ( 21.53943276465977519, -0.05219959533907433946, 28.74890960531435624 ) ) ;
#175510=CARTESIAN_POINT ( 'NONE',  ( -0.05219959533937732626, 21.53943276465977519, 57.50109039468568994 ) ) ;
#175511=CARTESIAN_POINT ( 'NONE',  ( -16.46253265017160317, 9.564922557960807481, 55.83224293864769550 ) ) ;
#175512=CARTESIAN_POINT ( 'NONE',  ( 5.153800228976335163, 19.02544592524342804, 84.79057627198099567 ) ) ;
#175513=ORIENTED_EDGE ( 'NONE', *, *, #44938, .F. ) ;
#175514=CARTESIAN_POINT ( 'NONE',  ( 14.29746914071037800, 8.314922557961029526, 46.66775706135234714 ) ) ;
#175515=CARTESIAN_POINT ( 'NONE',  ( -5.823673210054431948, 21.52544592524334988, 47.70942372801902565 ) ) ;
#175516=CARTESIAN_POINT ( 'NONE',  ( -15.80617190586768217, 15.72974639402176855, 78.12609039468570415 ) ) ;
#175517=CARTESIAN_POINT ( 'NONE',  ( -0.05219959533907301413, -21.53943276465977519, 27.49890960531435269 ) ) ;
#175518=CARTESIAN_POINT ( 'NONE',  ( 21.52544592524344225, -5.823673210054117533, 83.54057627198102409 ) ) ;
#175519=CARTESIAN_POINT ( 'NONE',  ( 5.823673210054444382, -21.52544592524334988, 20.20942372801900788 ) ) ;
#175520=CARTESIAN_POINT ( 'NONE',  ( -12.14591786802326823, 12.06949235617739902, 63.12609039468568994 ) ) ;
#175521=CARTESIAN_POINT ( 'NONE',  ( -10.72451020669898014, 18.67979575497178502, 65.41557627198102409 ) ) ;
#175522=CARTESIAN_POINT ( 'NONE',  ( -18.67979575497193778, 10.72451020669871902, 113.3344237280190328 ) ) ;
#175523=CARTESIAN_POINT ( 'NONE',  ( -16.51473224551069308, -9.474510206698971260, 71.66557627198102409 ) ) ;
#175524=CARTESIAN_POINT ( 'NONE',  ( 4.379528057220092307, 16.55341960407617563, 102.2927570613523613 ) ) ;
#175526=CARTESIAN_POINT ( 'NONE',  ( 9.564922557960805705, 16.46253265017160317, 84.58224293864769550 ) ) ;
#175527=CARTESIAN_POINT ( 'NONE',  ( 17.50000000000000355, 5.499999999999989342, 103.7823096230356867 ) ) ;
#175529=CARTESIAN_POINT ( 'NONE',  ( -13.97604488694547697, 13.89961937509957934, 83.12609039468564731 ) ) ;
#175530=CARTESIAN_POINT ( 'NONE',  ( -10.72451020669898014, 18.67979575497178502, 55.41557627198102409 ) ) ;
#175531=CARTESIAN_POINT ( 'NONE',  ( -4.483927247898782831, 16.52544592524335698, 112.7094237280190328 ) ) ;
#175532=CARTESIAN_POINT ( 'NONE',  ( 5.153800228976615827, -19.02544592524334988, 105.2094237280190185 ) ) ;
#175534=CARTESIAN_POINT ( 'NONE',  ( 13.89961937509957401, 13.97604488694547697, 96.87609039468566152 ) ) ;
#175535=CARTESIAN_POINT ( 'NONE',  ( -15.80617190586745835, -15.72974639402198527, 91.87390960531436690 ) ) ;
#175536=CARTESIAN_POINT ( 'NONE',  ( 19.05341960407617918, -5.049401038297876454, 56.04275706135234714 ) ) ;
#175538=CARTESIAN_POINT ( 'NONE',  ( -0.05219959533909027116, -19.03943276465977164, 57.49890960531435979 ) ) ;
#175539=CARTESIAN_POINT ( 'NONE',  ( -8.314922557960811034, -14.29746914071050412, 57.08224293864769550 ) ) ;
#175540=CARTESIAN_POINT ( 'NONE',  ( -5.049401038298153566, 19.05341960407611168, 50.20724293864770260 ) ) ;
#175541=CARTESIAN_POINT ( 'NONE',  ( 4.379528057220339221, -16.55341960407611168, 57.70724293864770260 ) ) ;
#175544=CARTESIAN_POINT ( 'NONE',  ( -4.379528057220328563, 16.55341960407611168, 30.20724293864769550 ) ) ;
#175545=CARTESIAN_POINT ( 'NONE',  ( -9.564922557960796823, -16.46253265017161027, 57.08224293864769550 ) ) ;
#175547=CARTESIAN_POINT ( 'NONE',  ( -19.02544592524334988, -5.153800228976617603, 38.95942372801900433 ) ) ;
#175548=CARTESIAN_POINT ( 'NONE',  ( 8.314922557961029526, -14.29746914071037800, 45.41775706135234003 ) ) ;
#175549=CARTESIAN_POINT ( 'NONE',  ( -15.80617190586745835, -15.72974639402198527, 56.87390960531436690 ) ) ;
#175550=CARTESIAN_POINT ( 'NONE',  ( 21.52544592524334988, 5.823673210054432836, 106.4594237280190328 ) ) ;
#175551=CARTESIAN_POINT ( 'NONE',  ( -0.05219959533909027116, -19.03943276465977164, 72.49890960531435269 ) ) ;
#175553=CARTESIAN_POINT ( 'NONE',  ( -19.03943276465977164, 0.05219959533909376836, 91.24890960531436690 ) ) ;
#175555=CARTESIAN_POINT ( 'NONE',  ( -10.72451020669870658, -18.67979575497194134, 29.58442372801901854 ) ) ;
#175556=CARTESIAN_POINT ( 'NONE',  ( 12.06949235617757843, -12.14591786802309237, 88.12390960531436690 ) ) ;
#175557=CARTESIAN_POINT ( 'NONE',  ( -5.719274019375978568, 21.55341960407610458, 90.20724293864770971 ) ) ;
#175558=CARTESIAN_POINT ( 'NONE',  ( -19.05341960407611168, -5.049401038298163336, 86.45724293864769550 ) ) ;
#175559=CARTESIAN_POINT ( 'NONE',  ( 19.03943276465977164, -0.05219959533909143690, 83.74890960531436690 ) ) ;
#175560=CARTESIAN_POINT ( 'NONE',  ( 15.80617190586746368, 15.72974639402197994, 114.3739096053143527 ) ) ;
#175561=ORIENTED_EDGE ( 'NONE', *, *, #93872, .T. ) ;
#175562=CARTESIAN_POINT ( 'NONE',  ( -0.05219959533909027116, -19.03943276465977164, 77.49890960531435269 ) ) ;
#175565=CARTESIAN_POINT ( 'NONE',  ( -5.153800228976328057, -19.02544592524343514, 22.29057627198102765 ) ) ;
#175566=CARTESIAN_POINT ( 'NONE',  ( 0.05219959533909260263, 19.03943276465977164, 34.99890960531435979 ) ) ;
#175567=CARTESIAN_POINT ( 'NONE',  ( 16.51473224551083163, -9.474510206698727899, 95.83442372801900433 ) ) ;
#175568=CARTESIAN_POINT ( 'NONE',  ( -12.14591786802309592, -12.06949235617757132, 106.8739096053143811 ) ) ;
#175569=CARTESIAN_POINT ( 'NONE',  ( -0.05219959533937732626, 21.53943276465977519, 67.50109039468568994 ) ) ;
#175570=CARTESIAN_POINT ( 'NONE',  ( -19.02544592524342804, 5.153800228976336051, 61.04057627198103120 ) ) ;
#175571=CARTESIAN_POINT ( 'NONE',  ( 18.67979575497194134, -10.72451020669871369, 35.83442372801901143 ) ) ;
#175572=CARTESIAN_POINT ( 'NONE',  ( 15.72974639402199770, -15.80617190586745480, 113.1239096053143953 ) ) ;
#175574=CARTESIAN_POINT ( 'NONE',  ( 0.05219959533909260263, 19.03943276465977164, 84.99890960531436690 ) ) ;
#175576=CARTESIAN_POINT ( 'NONE',  ( 12.14591786802327356, -12.06949235617739191, 25.62609039468567929 ) ) ;
#175577=CARTESIAN_POINT ( 'NONE',  ( -15.72974639402197994, 15.80617190586746368, 25.62390960531435624 ) ) ;
#175578=CARTESIAN_POINT ( 'NONE',  ( -10.72451020669870658, -18.67979575497194134, 64.58442372801900433 ) ) ;
#175579=CARTESIAN_POINT ( 'NONE',  ( -5.049401038298153566, 19.05341960407611168, 110.2072429386476671 ) ) ;
#175580=CARTESIAN_POINT ( 'NONE',  ( 19.05341960407617918, -5.049401038297876454, 96.04275706135231871 ) ) ;
#175581=CARTESIAN_POINT ( 'NONE',  ( 5.049401038298161559, -19.05341960407611168, 42.70724293864767418 ) ) ;
#175582=CARTESIAN_POINT ( 'NONE',  ( -19.02544592524342804, 5.153800228976336051, 81.04057627198103830 ) ) ;
#175584=CARTESIAN_POINT ( 'NONE',  ( 16.53943276465976808, -0.05219959533910856209, 88.74890960531436690 ) ) ;
#175585=CARTESIAN_POINT ( 'NONE',  ( 19.02544592524343514, -5.153800228976328945, 113.5405762719810241 ) ) ;
#175586=CARTESIAN_POINT ( 'NONE',  ( 14.34966873604960469, 8.224510206698951720, 94.16557627198103830 ) ) ;
#175587=CARTESIAN_POINT ( 'NONE',  ( -5.153800228976328057, -19.02544592524343514, 112.2905762719810099 ) ) ;
#175588=CARTESIAN_POINT ( 'NONE',  ( -8.224510206698948167, 14.34966873604960824, 55.41557627198102409 ) ) ;
#175589=CARTESIAN_POINT ( 'NONE',  ( -16.51473224551069308, -9.474510206698971260, 46.66557627198102409 ) ) ;
#175590=CARTESIAN_POINT ( 'NONE',  ( -15.80617190586768217, 15.72974639402176855, 58.12609039468568994 ) ) ;
#175591=CARTESIAN_POINT ( 'NONE',  ( -16.46253265017146816, -9.564922557961047289, 99.16775706135233293 ) ) ;
#175592=CARTESIAN_POINT ( 'NONE',  ( 12.06949235617757843, -12.14591786802309237, 53.12390960531436690 ) ) ;
#175593=CARTESIAN_POINT ( 'NONE',  ( 21.53943276465977519, -0.05219959533907433946, 108.7489096053143669 ) ) ;
#175594=CARTESIAN_POINT ( 'NONE',  ( 18.62759615963271287, -10.81492255796078972, 48.33224293864770260 ) ) ;
#175595=CARTESIAN_POINT ( 'NONE',  ( 5.153800228976335163, 19.02544592524342804, 114.7905762719810241 ) ) ;
#175597=CARTESIAN_POINT ( 'NONE',  ( -9.564922557960796823, -16.46253265017161027, 52.08224293864768839 ) ) ;
#175598=CARTESIAN_POINT ( 'NONE',  ( 12.06949235617739724, 12.14591786802326823, 111.8760903946856615 ) ) ;
#175599=CARTESIAN_POINT ( 'NONE',  ( 8.224510206698742110, 14.34966873604972548, 107.0844237280190043 ) ) ;
#175600=CARTESIAN_POINT ( 'NONE',  ( -12.06949235617739369, -12.14591786802326823, 89.37609039468568994 ) ) ;
#175601=CARTESIAN_POINT ( 'NONE',  ( 13.89961937509957401, 13.97604488694547697, 41.87609039468566152 ) ) ;
#175602=CARTESIAN_POINT ( 'NONE',  ( -17.31728774477273447, 6.344390552232387570, 70.81906651689320142 ) ) ;
#175603=CARTESIAN_POINT ( 'NONE',  ( -5.049401038298153566, 19.05341960407611168, 90.20724293864766707 ) ) ;
#175604=CARTESIAN_POINT ( 'NONE',  ( -5.049401038298153566, 19.05341960407611168, 50.20724293864770260 ) ) ;
#175606=CARTESIAN_POINT ( 'NONE',  ( -16.55341960407611168, -4.379528057220339221, 66.45724293864768129 ) ) ;
#175607=CARTESIAN_POINT ( 'NONE',  ( 17.12812012977028076, -6.668231424565989052, 101.1405124067685932 ) ) ;
#175608=CARTESIAN_POINT ( 'NONE',  ( 9.474510206698971260, -16.51473224551069308, 97.91557627198102409 ) ) ;
#175609=CARTESIAN_POINT ( 'NONE',  ( 18.62759615963271287, -10.81492255796078972, 38.33224293864768839 ) ) ;
#175610=CARTESIAN_POINT ( 'NONE',  ( -4.483927247898539470, -16.52544592524342804, 87.29057627198103830 ) ) ;
#175611=CARTESIAN_POINT ( 'NONE',  ( -12.14591786802326823, 12.06949235617739902, 43.12609039468568284 ) ) ;
#175612=CARTESIAN_POINT ( 'NONE',  ( 16.55341960407611168, 4.379528057220329451, 78.95724293864769550 ) ) ;
#175614=CARTESIAN_POINT ( 'NONE',  ( -5.049401038297874678, -19.05341960407617918, 79.79275706135233293 ) ) ;
#175615=CARTESIAN_POINT ( 'NONE',  ( 5.049401038298161559, -19.05341960407611168, 97.70724293864766707 ) ) ;
#175616=CARTESIAN_POINT ( 'NONE',  ( -16.46253265017146816, -9.564922557961047289, 79.16775706135234714 ) ) ;
#175618=CARTESIAN_POINT ( 'NONE',  ( 18.22780087662123805, 5.499999999999960032, 101.4823681787310647 ) ) ;
#175619=CARTESIAN_POINT ( 'NONE',  ( 8.314922557961029526, -14.29746914071037800, 35.41775706135234003 ) ) ;
#175620=CARTESIAN_POINT ( 'NONE',  ( 16.55341960407618274, -4.379528057220086978, 111.0427570613523613 ) ) ;
#175622=CARTESIAN_POINT ( 'NONE',  ( -5.049401038297874678, -19.05341960407617918, 74.79275706135231871 ) ) ;
#175623=CARTESIAN_POINT ( 'NONE',  ( -15.72974639402197994, 15.80617190586746368, 35.62390960531437401 ) ) ;
#175624=CARTESIAN_POINT ( 'NONE',  ( -21.53943276465977519, -0.05219959533937600094, 63.75109039468568284 ) ) ;
#175626=CARTESIAN_POINT ( 'NONE',  ( 8.224510206698742110, 14.34966873604972548, 32.08442372801901854 ) ) ;
#175627=CARTESIAN_POINT ( 'NONE',  ( -19.02544592524342804, 5.153800228976336051, 26.04057627198103120 ) ) ;
#175628=CARTESIAN_POINT ( 'NONE',  ( 9.474510206698971260, -16.51473224551069308, 87.91557627198102409 ) ) ;
#175630=CARTESIAN_POINT ( 'NONE',  ( 14.29746914071049879, -8.314922557960816363, 83.33224293864769550 ) ) ;
#175631=CARTESIAN_POINT ( 'NONE',  ( -19.02544592524342804, 5.153800228976336051, 86.04057627198103830 ) ) ;
#175633=CARTESIAN_POINT ( 'NONE',  ( -19.02544592524334988, -5.153800228976617603, 103.9594237280190043 ) ) ;
#175634=CARTESIAN_POINT ( 'NONE',  ( -21.55341960407610458, -5.719274019375992779, 71.45724293864769550 ) ) ;
#175635=CARTESIAN_POINT ( 'NONE',  ( -19.05341960407611168, -5.049401038298163336, 46.45724293864768129 ) ) ;
#175636=CARTESIAN_POINT ( 'NONE',  ( 19.05341960407617918, -5.049401038297876454, 76.04275706135230450 ) ) ;
#175637=CARTESIAN_POINT ( 'NONE',  ( 18.67979575497178502, 10.72451020669898547, 114.1655762719810383 ) ) ;
#175638=CARTESIAN_POINT ( 'NONE',  ( 19.05341960407611168, 5.049401038298154454, 73.95724293864768129 ) ) ;
#175639=CARTESIAN_POINT ( 'NONE',  ( 19.05341960407611168, 5.049401038298154454, 108.9572429386477097 ) ) ;
#175641=CARTESIAN_POINT ( 'NONE',  ( -4.379528057220086978, -16.55341960407618274, 34.79275706135235424 ) ) ;
#175642=CARTESIAN_POINT ( 'NONE',  ( -21.52544592524343514, 5.823673210054127303, 106.0405762719810525 ) ) ;
#175643=CARTESIAN_POINT ( 'NONE',  ( 4.379528057220339221, -16.55341960407611168, 112.7072429386476955 ) ) ;
#175644=CARTESIAN_POINT ( 'NONE',  ( -0.05219959533909027116, -19.03943276465977164, 97.49890960531436690 ) ) ;
#175645=CARTESIAN_POINT ( 'NONE',  ( 5.153800228976615827, -19.02544592524334988, 65.20942372801900433 ) ) ;
#175646=CARTESIAN_POINT ( 'NONE',  ( -15.80617190586745835, -15.72974639402198527, 91.87390960531436690 ) ) ;
#175647=CARTESIAN_POINT ( 'NONE',  ( 0.05219959533910956823, 16.53943276465976808, 44.99890960531435979 ) ) ;
#175648=CARTESIAN_POINT ( 'NONE',  ( 9.564922557961047289, -16.46253265017146816, 20.41775706135233293 ) ) ;
#175649=CARTESIAN_POINT ( 'NONE',  ( -4.483927247898782831, 16.52544592524335698, 62.70942372801902565 ) ) ;
#175650=CARTESIAN_POINT ( 'NONE',  ( -9.564922557960796823, -16.46253265017161027, 87.08224293864769550 ) ) ;
#175651=CARTESIAN_POINT ( 'NONE',  ( -16.46253265017160317, 9.564922557960807481, 40.83224293864769550 ) ) ;
#175653=CARTESIAN_POINT ( 'NONE',  ( -21.52544592524334988, -5.823673210054445271, 48.95942372801902565 ) ) ;
#175654=CARTESIAN_POINT ( 'NONE',  ( -15.72974639402176322, -15.80617190586768395, 69.37609039468567573 ) ) ;
#175655=CARTESIAN_POINT ( 'NONE',  ( -9.564922557960796823, -16.46253265017161027, 57.08224293864769550 ) ) ;
#175656=CARTESIAN_POINT ( 'NONE',  ( 5.823673210054444382, -21.52544592524334988, 30.20942372801902565 ) ) ;
#175657=CARTESIAN_POINT ( 'NONE',  ( 9.564922557961047289, -16.46253265017146816, 80.41775706135234714 ) ) ;
#175658=CARTESIAN_POINT ( 'NONE',  ( -9.474510206698720793, -16.51473224551083518, 79.58442372801899012 ) ) ;
#175659=CARTESIAN_POINT ( 'NONE',  ( 0.05219959533909260263, 19.03943276465977164, 44.99890960531435979 ) ) ;
#175660=CARTESIAN_POINT ( 'NONE',  ( -8.224510206698735004, -14.34966873604973081, 89.58442372801901854 ) ) ;
#175661=CARTESIAN_POINT ( 'NONE',  ( 16.46253265017160672, -9.564922557960803928, 58.33224293864769550 ) ) ;
#175663=CARTESIAN_POINT ( 'NONE',  ( -9.474510206698964154, 16.51473224551069663, 100.4155762719810241 ) ) ;
#175664=CARTESIAN_POINT ( 'NONE',  ( 16.46253265017160672, -9.564922557960803928, 33.33224293864770260 ) ) ;
#175665=CARTESIAN_POINT ( 'NONE',  ( 21.53943276465977519, -0.05219959533907433946, 83.74890960531435269 ) ) ;
#175666=CARTESIAN_POINT ( 'NONE',  ( 16.53943276465976808, 0.05219959533934440121, 56.25109039468568284 ) ) ;
#175667=CARTESIAN_POINT ( 'NONE',  ( -9.564922557961040184, 16.46253265017147172, 37.91775706135233293 ) ) ;
#175668=CARTESIAN_POINT ( 'NONE',  ( 5.049401038298161559, -19.05341960407611168, 52.70724293864767418 ) ) ;
#175669=CARTESIAN_POINT ( 'NONE',  ( -16.52544592524342804, 4.483927247898546575, 51.04057627198103120 ) ) ;
#175670=CARTESIAN_POINT ( 'NONE',  ( 12.14591786802309770, 12.06949235617756955, 79.37390960531436690 ) ) ;
#175671=CARTESIAN_POINT ( 'NONE',  ( -0.05219959533909027116, -19.03943276465977164, 87.49890960531436690 ) ) ;
#175672=CARTESIAN_POINT ( 'NONE',  ( -9.474510206698964154, 16.51473224551069663, 75.41557627198103830 ) ) ;
#175673=CARTESIAN_POINT ( 'NONE',  ( -21.52544592524334988, -5.823673210054445271, 38.95942372801901854 ) ) ;
#175674=CARTESIAN_POINT ( 'NONE',  ( -19.03943276465977164, 0.05219959533909376836, 96.24890960531436690 ) ) ;
#175675=CARTESIAN_POINT ( 'NONE',  ( -5.719274019375665041, -21.55341960407619695, 104.7927570613523898 ) ) ;
#175676=CARTESIAN_POINT ( 'NONE',  ( -12.06949235617739369, -12.14591786802326823, 84.37609039468570415 ) ) ;
#175677=CARTESIAN_POINT ( 'NONE',  ( -15.80617190586768217, 15.72974639402176855, 33.12609039468569705 ) ) ;
#175678=CARTESIAN_POINT ( 'NONE',  ( 21.55341960407610458, 5.719274019375980345, 93.95724293864770971 ) ) ;
#175679=CARTESIAN_POINT ( 'NONE',  ( 16.52544592524342804, -4.483927247898539470, 53.54057627198103120 ) ) ;
#175680=CARTESIAN_POINT ( 'NONE',  ( 19.02544592524343514, -5.153800228976328945, 38.54057627198103120 ) ) ;
#175681=CARTESIAN_POINT ( 'NONE',  ( -16.52544592524342804, 4.483927247898546575, 66.04057627198103830 ) ) ;
#175682=CARTESIAN_POINT ( 'NONE',  ( 21.55341960407610458, 5.719274019375980345, 28.95724293864769905 ) ) ;
#175683=CARTESIAN_POINT ( 'NONE',  ( 19.05341960407617918, -5.049401038297876454, 36.04275706135234003 ) ) ;
#175684=CARTESIAN_POINT ( 'NONE',  ( 14.29746914071049879, -8.314922557960816363, 103.3322429386476955 ) ) ;
#175685=CARTESIAN_POINT ( 'NONE',  ( -16.51473224551069308, -9.474510206698971260, 111.6655762719810383 ) ) ;
#175686=ORIENTED_EDGE ( 'NONE', *, *, #197763, .F. ) ;
#175687=CARTESIAN_POINT ( 'NONE',  ( -16.52544592524335698, -4.483927247898792601, 48.95942372801902565 ) ) ;
#175688=CARTESIAN_POINT ( 'NONE',  ( -16.46253265017160317, 9.564922557960807481, 55.83224293864769550 ) ) ;
#175689=CARTESIAN_POINT ( 'NONE',  ( -16.63550798202463099, -6.755536848170410558, 20.93280403780605781 ) ) ;
#175690=CARTESIAN_POINT ( 'NONE',  ( -12.14591786802326823, 12.06949235617739902, 93.12609039468568994 ) ) ;
#175691=CARTESIAN_POINT ( 'NONE',  ( -14.29746914071037622, -8.314922557961029526, 19.16775706135234714 ) ) ;
#175692=CARTESIAN_POINT ( 'NONE',  ( 15.72974639402176855, 15.80617190586768217, 76.87609039468567573 ) ) ;
#175693=CARTESIAN_POINT ( 'NONE',  ( 0.05219959533909260263, 19.03943276465977164, 79.99890960531436690 ) ) ;
#175694=CARTESIAN_POINT ( 'NONE',  ( 18.67979575497178502, 10.72451020669898547, 104.1655762719810241 ) ) ;
#175695=CARTESIAN_POINT ( 'NONE',  ( -4.379528057220086978, -16.55341960407618274, 54.79275706135235424 ) ) ;
#175696=CARTESIAN_POINT ( 'NONE',  ( 8.224510206698953496, -14.34966873604960469, 107.9155762719810241 ) ) ;
#175697=CARTESIAN_POINT ( 'NONE',  ( 12.14591786802327356, -12.06949235617739191, 20.62609039468568639 ) ) ;
#175698=CARTESIAN_POINT ( 'NONE',  ( 19.05341960407617918, -5.049401038297876454, 81.04275706135231871 ) ) ;
#175699=CARTESIAN_POINT ( 'NONE',  ( 0.05219959533907565091, 21.53943276465977519, 79.99890960531435269 ) ) ;
#175700=CARTESIAN_POINT ( 'NONE',  ( 13.89961937509957401, 13.97604488694547697, 51.87609039468566863 ) ) ;
#175701=CARTESIAN_POINT ( 'NONE',  ( 19.46398650005389896, -5.499999999999943157, 87.68269651486372140 ) ) ;
#175702=CARTESIAN_POINT ( 'NONE',  ( -21.53943276465977519, 0.05219959533907696930, 101.2489096053143669 ) ) ;
#175703=DIRECTION ( 'NONE',  ( 0.000000000000000000, 0.000000000000000000, -1.000000000000000000 ) ) ;
#175704=CARTESIAN_POINT ( 'NONE',  ( 19.05341960407611168, 5.049401038298154454, 68.95724293864769550 ) ) ;
#175706=CARTESIAN_POINT ( 'NONE',  ( -14.34966873604972548, 8.224510206698743886, 23.33442372801901499 ) ) ;
#175708=CARTESIAN_POINT ( 'NONE',  ( 21.53943276465977519, -0.05219959533907433946, 103.7489096053143669 ) ) ;
#175709=CARTESIAN_POINT ( 'NONE',  ( -8.224510206698948167, 14.34966873604960824, 70.41557627198102409 ) ) ;
#175710=CARTESIAN_POINT ( 'NONE',  ( -13.89961937509977652, 13.97604488694528158, 75.62390960531438111 ) ) ;
#175711=CARTESIAN_POINT ( 'NONE',  ( -21.55341960407619339, 5.719274019375674811, 68.54275706135234714 ) ) ;
#175712=CARTESIAN_POINT ( 'NONE',  ( 4.483927247898790824, -16.52544592524335698, 25.20942372801901854 ) ) ;
#175713=CARTESIAN_POINT ( 'NONE',  ( -19.02544592524334988, -5.153800228976617603, 23.95942372801900078 ) ) ;
#175714=CARTESIAN_POINT ( 'NONE',  ( 10.81492255796106328, -18.62759615963255655, 55.41775706135234714 ) ) ;
#175715=CARTESIAN_POINT ( 'NONE',  ( 15.80617190586746368, 15.72974639402197994, 109.3739096053143811 ) ) ;
#175716=CARTESIAN_POINT ( 'NONE',  ( 10.72451020669898902, -18.67979575497178502, 62.91557627198102409 ) ) ;
#175717=CARTESIAN_POINT ( 'NONE',  ( -16.52544592524335698, -4.483927247898792601, 18.95942372801901143 ) ) ;
#175718=CARTESIAN_POINT ( 'NONE',  ( 5.049401038298161559, -19.05341960407611168, 47.70724293864770260 ) ) ;
#175719=CARTESIAN_POINT ( 'NONE',  ( -5.153800228976607833, 19.02544592524334988, 67.70942372801900433 ) ) ;
#175720=CARTESIAN_POINT ( 'NONE',  ( -10.81492255796105439, 18.62759615963255655, 77.91775706135231871 ) ) ;
#175721=CARTESIAN_POINT ( 'NONE',  ( 19.05341960407617918, -5.049401038297876454, 56.04275706135234714 ) ) ;
#175722=CARTESIAN_POINT ( 'NONE',  ( 9.564922557960805705, 16.46253265017160317, 39.58224293864768839 ) ) ;
#175723=CARTESIAN_POINT ( 'NONE',  ( -5.719274019375978568, 21.55341960407610458, 55.20724293864770260 ) ) ;
#175724=CARTESIAN_POINT ( 'NONE',  ( -16.53943276465976808, 0.05219959533911058130, 56.24890960531436690 ) ) ;
#175725=CARTESIAN_POINT ( 'NONE',  ( -17.50000000000000711, -5.624438216177558125, 24.18329655085356933 ) ) ;
#175726=CARTESIAN_POINT ( 'NONE',  ( 13.89961937509957401, 13.97604488694547697, 26.87609039468566507 ) ) ;
#175727=CARTESIAN_POINT ( 'NONE',  ( 0.05219959533934541429, -16.53943276465976808, 90.00109039468567573 ) ) ;
#175728=CARTESIAN_POINT ( 'NONE',  ( 0.05219959533910956823, 16.53943276465976808, 59.99890960531436690 ) ) ;
#175729=CARTESIAN_POINT ( 'NONE',  ( -18.62759615963255300, -10.81492255796106328, 84.16775706135234714 ) ) ;
#175730=CARTESIAN_POINT ( 'NONE',  ( 21.53943276465977519, 0.05219959533937863772, 76.25109039468568994 ) ) ;
#175731=CARTESIAN_POINT ( 'NONE',  ( -15.72974639402197994, 15.80617190586746368, 80.62390960531438111 ) ) ;
#175732=VECTOR ( 'NONE', #175703, 1000.000000000000000 ) ;
#175733=CARTESIAN_POINT ( 'NONE',  ( -16.46253265017160317, 9.564922557960807481, 45.83224293864769550 ) ) ;
#175734=CARTESIAN_POINT ( 'NONE',  ( -21.55341960407619339, 5.719274019375674811, 58.54275706135235424 ) ) ;
#175735=CARTESIAN_POINT ( 'NONE',  ( 13.89961937509977652, -13.97604488694527269, 33.12390960531434558 ) ) ;
#175736=ORIENTED_EDGE ( 'NONE', *, *, #163855, .T. ) ;
#175737=CARTESIAN_POINT ( 'NONE',  ( 9.564922557960805705, 16.46253265017160317, 54.58224293864769550 ) ) ;
#175738=CARTESIAN_POINT ( 'NONE',  ( -14.34966873604960291, -8.224510206698953496, 111.6655762719810525 ) ) ;
#175739=CARTESIAN_POINT ( 'NONE',  ( 5.153800228976335163, 19.02544592524342804, 99.79057627198102409 ) ) ;
#175740=CARTESIAN_POINT ( 'NONE',  ( -4.379528057220328563, 16.55341960407611168, 50.20724293864769550 ) ) ;
#175741=CARTESIAN_POINT ( 'NONE',  ( -16.53943276465976808, 0.05219959533911058130, 106.2489096053143811 ) ) ;
#175742=CARTESIAN_POINT ( 'NONE',  ( 21.52544592524344225, -5.823673210054117533, 88.54057627198103830 ) ) ;
#175743=CARTESIAN_POINT ( 'NONE',  ( 10.72451020669871369, 18.67979575497193778, 27.08442372801901854 ) ) ;
#175745=CARTESIAN_POINT ( 'NONE',  ( 16.53943276465976808, 0.05219959533934440121, 36.25109039468567573 ) ) ;
#175747=CARTESIAN_POINT ( 'NONE',  ( 0.05219959533907565091, 21.53943276465977519, 69.99890960531435269 ) ) ;
#175749=CARTESIAN_POINT ( 'NONE',  ( -5.823673210054431948, 21.52544592524334988, 102.7094237280190185 ) ) ;
#175750=CARTESIAN_POINT ( 'NONE',  ( -16.51473224551069308, -9.474510206698971260, 91.66557627198103830 ) ) ;
#175751=CARTESIAN_POINT ( 'NONE',  ( 21.52544592524334988, 5.823673210054432836, 26.45942372801901854 ) ) ;
#175752=CARTESIAN_POINT ( 'NONE',  ( 10.81492255796078972, 18.62759615963270932, 29.58224293864769905 ) ) ;
#175753=CARTESIAN_POINT ( 'NONE',  ( -16.52544592524335698, -4.483927247898792601, 108.9594237280190185 ) ) ;
#175754=CARTESIAN_POINT ( 'NONE',  ( 21.55341960407619695, -5.719274019375665929, 56.04275706135235424 ) ) ;
#175755=CARTESIAN_POINT ( 'NONE',  ( -18.67979575497193778, 10.72451020669871902, 83.33442372801903275 ) ) ;
#175756=CARTESIAN_POINT ( 'NONE',  ( 15.72974639402176855, 15.80617190586768217, 106.8760903946856899 ) ) ;
#175757=CARTESIAN_POINT ( 'NONE',  ( -16.52544592524335698, -4.483927247898792601, 68.95942372801901854 ) ) ;
#175758=CARTESIAN_POINT ( 'NONE',  ( -18.62759615963255300, -10.81492255796106328, 34.16775706135234714 ) ) ;
#175760=CARTESIAN_POINT ( 'NONE',  ( 0.05219959533909260263, 19.03943276465977164, 34.99890960531435979 ) ) ;
#175761=CARTESIAN_POINT ( 'NONE',  ( 21.55341960407619695, -5.719274019375665929, 101.0427570613523756 ) ) ;
#175762=CARTESIAN_POINT ( 'NONE',  ( -5.153800228976328057, -19.02544592524343514, 107.2905762719810383 ) ) ;
#175763=CARTESIAN_POINT ( 'NONE',  ( 21.55341960407610458, 5.719274019375980345, 103.9572429386476813 ) ) ;
#175765=CARTESIAN_POINT ( 'NONE',  ( 21.53943276465977519, -0.05219959533907433946, 63.74890960531435979 ) ) ;
#175766=CARTESIAN_POINT ( 'NONE',  ( -14.29746914071037622, -8.314922557961029526, 54.16775706135235424 ) ) ;
#175767=CARTESIAN_POINT ( 'NONE',  ( -4.379528057220328563, 16.55341960407611168, 55.20724293864770260 ) ) ;
#175769=CARTESIAN_POINT ( 'NONE',  ( -19.03943276465977164, -0.05219959533935918106, 73.75109039468566152 ) ) ;
#175773=CARTESIAN_POINT ( 'NONE',  ( 4.379528057220092307, 16.55341960407617563, 27.29275706135234358 ) ) ;
#175774=CARTESIAN_POINT ( 'NONE',  ( -21.53943276465977519, 0.05219959533907696930, 96.24890960531435269 ) ) ;
#175775=CARTESIAN_POINT ( 'NONE',  ( -12.14591786802309592, -12.06949235617757132, 71.87390960531438111 ) ) ;
#175776=CARTESIAN_POINT ( 'NONE',  ( -0.05219959533909027116, -19.03943276465977164, 112.4989096053143669 ) ) ;
#175777=CARTESIAN_POINT ( 'NONE',  ( -16.53943276465976808, -0.05219959533934237506, 43.75109039468568284 ) ) ;
#175778=CARTESIAN_POINT ( 'NONE',  ( -19.05341960407611168, -5.049401038298163336, 56.45724293864768129 ) ) ;
#175779=CARTESIAN_POINT ( 'NONE',  ( 18.67979575497194134, -10.72451020669871369, 25.83442372801901499 ) ) ;
#175780=CARTESIAN_POINT ( 'NONE',  ( -13.89961937509957401, -13.97604488694547875, 104.3760903946856757 ) ) ;
#175781=CARTESIAN_POINT ( 'NONE',  ( 19.02544592524343514, -5.153800228976328945, 88.54057627198102409 ) ) ;
#175782=CARTESIAN_POINT ( 'NONE',  ( -5.153800228976328057, -19.02544592524343514, 92.29057627198099567 ) ) ;
#175783=CARTESIAN_POINT ( 'NONE',  ( -18.62759615963270932, 10.81492255796079327, 90.83224293864769550 ) ) ;
#175784=CARTESIAN_POINT ( 'NONE',  ( -13.97604488694527625, -13.89961937509977652, 56.87390960531434558 ) ) ;
#175785=CARTESIAN_POINT ( 'NONE',  ( -17.05587630539785238, -6.762274262135718139, 59.25819690962690345 ) ) ;
#175786=CARTESIAN_POINT ( 'NONE',  ( 12.06949235617757843, -12.14591786802309237, 73.12390960531436690 ) ) ;
#175787=CARTESIAN_POINT ( 'NONE',  ( 13.89961937509977652, -13.97604488694527269, 98.12390960531433848 ) ) ;
#175789=CARTESIAN_POINT ( 'NONE',  ( -9.564922557961040184, 16.46253265017147172, 77.91775706135234714 ) ) ;
#175790=CARTESIAN_POINT ( 'NONE',  ( 18.67979575497178502, 10.72451020669898547, 94.16557627198103830 ) ) ;
#175791=CARTESIAN_POINT ( 'NONE',  ( -19.02544592524334988, -5.153800228976617603, 53.95942372801898301 ) ) ;
#175792=CARTESIAN_POINT ( 'NONE',  ( -9.474510206698964154, 16.51473224551069663, 110.4155762719810383 ) ) ;
#175794=CARTESIAN_POINT ( 'NONE',  ( -15.72974639402197994, 15.80617190586746368, 50.62390960531435979 ) ) ;
#175796=CARTESIAN_POINT ( 'NONE',  ( 5.049401038298161559, -19.05341960407611168, 92.70724293864769550 ) ) ;
#175797=CARTESIAN_POINT ( 'NONE',  ( -18.67979575497193778, 10.72451020669871902, 78.33442372801901854 ) ) ;
#175798=CARTESIAN_POINT ( 'NONE',  ( 19.03943276465977164, -0.05219959533909143690, 43.74890960531435979 ) ) ;
#175800=CARTESIAN_POINT ( 'NONE',  ( -0.05219959533910754901, -16.53943276465976808, 67.49890960531436690 ) ) ;
#175801=CARTESIAN_POINT ( 'NONE',  ( -14.29746914071037622, -8.314922557961029526, 19.16775706135234714 ) ) ;
#175802=CARTESIAN_POINT ( 'NONE',  ( 5.719274019375673035, 21.55341960407619339, 67.29275706135234714 ) ) ;
#175804=CARTESIAN_POINT ( 'NONE',  ( 19.05341960407611168, 5.049401038298154454, 108.9572429386477097 ) ) ;
#175805=CARTESIAN_POINT ( 'NONE',  ( 19.05341960407617918, -5.049401038297876454, 76.04275706135230450 ) ) ;
#175807=CARTESIAN_POINT ( 'NONE',  ( 10.81492255796078972, 18.62759615963270932, 114.5822429386477097 ) ) ;
#175809=CARTESIAN_POINT ( 'NONE',  ( 13.97604488694548053, -13.89961937509957401, 25.62609039468566507 ) ) ;
#175810=CARTESIAN_POINT ( 'NONE',  ( -9.564922557960796823, -16.46253265017161027, 57.08224293864769550 ) ) ;
#175811=CARTESIAN_POINT ( 'NONE',  ( -19.02544592524334988, -5.153800228976617603, 18.95942372801899722 ) ) ;
#175812=CARTESIAN_POINT ( 'NONE',  ( 12.14591786802327356, -12.06949235617739191, 110.6260903946857042 ) ) ;
#175813=CARTESIAN_POINT ( 'NONE',  ( -19.02544592524342804, 5.153800228976336051, 106.0405762719810241 ) ) ;
#175814=CARTESIAN_POINT ( 'NONE',  ( 18.62759615963255655, 10.81492255796105972, 71.66775706135234714 ) ) ;
#175816=CARTESIAN_POINT ( 'NONE',  ( -17.60769864724391098, 5.499999999999987566, 98.65024842019163032 ) ) ;
#175817=CARTESIAN_POINT ( 'NONE',  ( 18.67979575497194134, -10.72451020669871369, 65.83442372801900433 ) ) ;
#175818=CARTESIAN_POINT ( 'NONE',  ( -10.72451020669870658, -18.67979575497194134, 104.5844237280190185 ) ) ;
#175819=CARTESIAN_POINT ( 'NONE',  ( 17.26058549869090797, -6.457015423128605214, 41.12254162523932877 ) ) ;
#175820=CARTESIAN_POINT ( 'NONE',  ( 16.46253265017160672, -9.564922557960803928, 93.33224293864769550 ) ) ;
#175821=CARTESIAN_POINT ( 'NONE',  ( 9.564922557961047289, -16.46253265017146816, 25.41775706135234003 ) ) ;
#175823=CARTESIAN_POINT ( 'NONE',  ( -16.46253265017160317, 9.564922557960807481, 40.83224293864769550 ) ) ;
#175824=CARTESIAN_POINT ( 'NONE',  ( -5.823673210054116645, -21.52544592524344225, 57.29057627198103120 ) ) ;
#175825=CARTESIAN_POINT ( 'NONE',  ( 12.06949235617739724, 12.14591786802326823, 101.8760903946857042 ) ) ;
#175826=CARTESIAN_POINT ( 'NONE',  ( -16.53943276465976808, 0.05219959533911058130, 101.2489096053143669 ) ) ;
#175827=CARTESIAN_POINT ( 'NONE',  ( 13.89961937509977652, -13.97604488694527269, 83.12390960531436690 ) ) ;
#175828=CARTESIAN_POINT ( 'NONE',  ( 10.72451020669871369, 18.67979575497193778, 107.0844237280190043 ) ) ;
#175829=CARTESIAN_POINT ( 'NONE',  ( -13.89961937509977652, 13.97604488694528158, 40.62390960531435979 ) ) ;
#175830=CARTESIAN_POINT ( 'NONE',  ( 0.05219959533910956823, 16.53943276465976808, 104.9989096053143669 ) ) ;
#175831=CARTESIAN_POINT ( 'NONE',  ( -5.719274019375665041, -21.55341960407619695, 49.79275706135234714 ) ) ;
#175832=CARTESIAN_POINT ( 'NONE',  ( -21.53943276465977519, 0.05219959533907696930, 86.24890960531436690 ) ) ;
#175833=CARTESIAN_POINT ( 'NONE',  ( 19.05341960407617918, -5.049401038297876454, 51.04275706135231871 ) ) ;
#175834=CARTESIAN_POINT ( 'NONE',  ( 13.89961937509978007, -13.97604488694527269, 48.12390960531435979 ) ) ;
#175835=CARTESIAN_POINT ( 'NONE',  ( 0.05219959533909260263, 19.03943276465977164, 99.99890960531436690 ) ) ;
#175836=CARTESIAN_POINT ( 'NONE',  ( 4.483927247898545687, 16.52544592524342804, 74.79057627198105251 ) ) ;
#175837=CARTESIAN_POINT ( 'NONE',  ( 19.03943276465977164, 0.05219959533936151252, 51.25109039468567573 ) ) ;
#175838=CARTESIAN_POINT ( 'NONE',  ( 19.02544592524343514, -5.153800228976328945, 58.54057627198102409 ) ) ;
#175839=CARTESIAN_POINT ( 'NONE',  ( 8.314922557960818139, 14.29746914071049879, 44.58224293864769550 ) ) ;
#175840=CARTESIAN_POINT ( 'NONE',  ( -13.89961937509957401, -13.97604488694547875, 79.37609039468567573 ) ) ;
#175841=CARTESIAN_POINT ( 'NONE',  ( -19.25663599770060941, 5.499999999999451994, 83.99419308057203182 ) ) ;
#175842=CARTESIAN_POINT ( 'NONE',  ( -10.81492255796078084, -18.62759615963271287, 37.08224293864768129 ) ) ;
#175843=EDGE_CURVE ( 'NONE', #98417, #3830, #99409, .T. ) ;
#175844=CARTESIAN_POINT ( 'NONE',  ( 12.14591786802309770, 12.06949235617756955, 104.3739096053143669 ) ) ;
#175845=CARTESIAN_POINT ( 'NONE',  ( -17.50000000000000355, -3.345213924137174555, 25.41231376905639294 ) ) ;
#175846=CARTESIAN_POINT ( 'NONE',  ( -19.03943276465977164, 0.05219959533909376836, 61.24890960531436690 ) ) ;
#175847=CARTESIAN_POINT ( 'NONE',  ( -0.05219959533907301413, -21.53943276465977519, 67.49890960531436690 ) ) ;
#175848=CARTESIAN_POINT ( 'NONE',  ( 0.05219959533909260263, 19.03943276465977164, 24.99890960531435269 ) ) ;
#175849=CARTESIAN_POINT ( 'NONE',  ( 0.05219959533934541429, -16.53943276465976808, 75.00109039468568994 ) ) ;
#175850=CARTESIAN_POINT ( 'NONE',  ( 9.474510206698971260, -16.51473224551069308, 57.91557627198103120 ) ) ;
#175851=CARTESIAN_POINT ( 'NONE',  ( -16.51473224551082808, 9.474510206698731452, 53.33442372801900433 ) ) ;
#175853=CARTESIAN_POINT ( 'NONE',  ( -5.823673210054431948, 21.52544592524334988, 67.70942372801901854 ) ) ;
#175854=CARTESIAN_POINT ( 'NONE',  ( -21.55341960407610458, -5.719274019375992779, 46.45724293864769550 ) ) ;
#175855=CARTESIAN_POINT ( 'NONE',  ( 13.97604488694527802, 13.89961937509977652, 24.37390960531435624 ) ) ;
#175856=CARTESIAN_POINT ( 'NONE',  ( -16.53943276465976808, -0.05219959533934237506, 83.75109039468568994 ) ) ;
#175857=CARTESIAN_POINT ( 'NONE',  ( 19.03943276465977164, 0.05219959533936151252, 101.2510903946856757 ) ) ;
#175858=CARTESIAN_POINT ( 'NONE',  ( -13.89961937509977652, 13.97604488694528158, 25.62390960531434558 ) ) ;
#175860=CARTESIAN_POINT ( 'NONE',  ( 15.72974639402199770, -15.80617190586745480, 48.12390960531436690 ) ) ;
#175861=CARTESIAN_POINT ( 'NONE',  ( 15.80617190586769283, -15.72974639402175789, 85.62609039468568994 ) ) ;
#175862=CARTESIAN_POINT ( 'NONE',  ( -8.224510206698948167, 14.34966873604960824, 45.41557627198103830 ) ) ;
#175863=CARTESIAN_POINT ( 'NONE',  ( 14.29746914071049879, -8.314922557960816363, 53.33224293864769550 ) ) ;
#175864=CARTESIAN_POINT ( 'NONE',  ( 21.53943276465977519, -0.05219959533907433946, 78.74890960531436690 ) ) ;
#175866=CARTESIAN_POINT ( 'NONE',  ( -21.55341960407610458, -5.719274019375992779, 91.45724293864769550 ) ) ;
#175868=CARTESIAN_POINT ( 'NONE',  ( 21.55341960407610458, 5.719274019375980345, 33.95724293864769550 ) ) ;
#175869=CARTESIAN_POINT ( 'NONE',  ( -4.379528057220086978, -16.55341960407618274, 64.79275706135234714 ) ) ;
#175870=CARTESIAN_POINT ( 'NONE',  ( -8.224510206698948167, 14.34966873604960824, 75.41557627198102409 ) ) ;
#175871=CARTESIAN_POINT ( 'NONE',  ( -9.474510206698964154, 16.51473224551069663, 30.41557627198102054 ) ) ;
#175873=CARTESIAN_POINT ( 'NONE',  ( 17.50000000000000000, -7.500000000000000888, 37.49999999999999289 ) ) ;
#175874=CARTESIAN_POINT ( 'NONE',  ( -14.34966873604972548, 8.224510206698743886, 98.33442372801901854 ) ) ;
#175875=CARTESIAN_POINT ( 'NONE',  ( 18.67979575497194134, -10.72451020669871369, 20.83442372801901143 ) ) ;
#175876=CARTESIAN_POINT ( 'NONE',  ( -9.474510206698964154, 16.51473224551069663, 85.41557627198102409 ) ) ;
#175877=CARTESIAN_POINT ( 'NONE',  ( 15.80617190586769283, -15.72974639402175789, 60.62609039468567573 ) ) ;
#175878=CARTESIAN_POINT ( 'NONE',  ( -5.049401038298153566, 19.05341960407611168, 115.2072429386477097 ) ) ;
#175882=CARTESIAN_POINT ( 'NONE',  ( 21.55341960407619695, -5.719274019375665929, 41.04275706135236135 ) ) ;
#175883=CARTESIAN_POINT ( 'NONE',  ( 16.46253265017160672, -9.564922557960803928, 43.33224293864769550 ) ) ;
#175884=CARTESIAN_POINT ( 'NONE',  ( -0.05219959533909027116, -19.03943276465977164, 102.4989096053143669 ) ) ;
#175885=CARTESIAN_POINT ( 'NONE',  ( -19.03943276465977164, -0.05219959533935918106, 48.75109039468566863 ) ) ;
#175886=CARTESIAN_POINT ( 'NONE',  ( -21.52544592524334988, -5.823673210054445271, 28.95942372801902209 ) ) ;
#175887=CARTESIAN_POINT ( 'NONE',  ( -16.46253265017146816, -9.564922557961047289, 49.16775706135233293 ) ) ;
#175888=CARTESIAN_POINT ( 'NONE',  ( -19.02544592524342804, 5.153800228976336051, 26.04057627198103120 ) ) ;
#175889=CARTESIAN_POINT ( 'NONE',  ( 4.379528057220092307, 16.55341960407617563, 97.29275706135234714 ) ) ;
#175890=CARTESIAN_POINT ( 'NONE',  ( -13.89961937509957401, -13.97604488694547875, 64.37609039468567573 ) ) ;
#175891=CARTESIAN_POINT ( 'NONE',  ( -8.224510206698735004, -14.34966873604973081, 99.58442372801900433 ) ) ;
#175893=CARTESIAN_POINT ( 'NONE',  ( -13.89961937509977652, 13.97604488694528158, 90.62390960531432427 ) ) ;
#175894=CARTESIAN_POINT ( 'NONE',  ( -15.72974639402176322, -15.80617190586768395, 94.37609039468568994 ) ) ;
#175895=CARTESIAN_POINT ( 'NONE',  ( 10.72451020669871369, 18.67979575497193778, 112.0844237280190185 ) ) ;
#175897=CARTESIAN_POINT ( 'NONE',  ( -5.153800228976328057, -19.02544592524343514, 102.2905762719810383 ) ) ;
#175898=CARTESIAN_POINT ( 'NONE',  ( -15.80617190586768217, 15.72974639402176855, 78.12609039468570415 ) ) ;
#175899=CARTESIAN_POINT ( 'NONE',  ( -8.314922557961024197, 14.29746914071037800, 22.91775706135235069 ) ) ;
#175901=CARTESIAN_POINT ( 'NONE',  ( 19.05341960407611168, 5.049401038298154454, 73.95724293864768129 ) ) ;
#175902=CARTESIAN_POINT ( 'NONE',  ( 18.62759615963271287, -10.81492255796078972, 33.33224293864769550 ) ) ;
#175903=CARTESIAN_POINT ( 'NONE',  ( 9.564922557960805705, 16.46253265017160317, 94.58224293864769550 ) ) ;
#175904=CARTESIAN_POINT ( 'NONE',  ( -17.50000000000000000, -5.624438216177582106, 89.18329655085356933 ) ) ;
#175905=CARTESIAN_POINT ( 'NONE',  ( 5.049401038298161559, -19.05341960407611168, 72.70724293864768129 ) ) ;
#175906=CARTESIAN_POINT ( 'NONE',  ( -16.46253265017160317, 9.564922557960807481, 70.83224293864770971 ) ) ;
#175907=CARTESIAN_POINT ( 'NONE',  ( 12.06949235617739724, 12.14591786802326823, 106.8760903946856899 ) ) ;
#175908=CARTESIAN_POINT ( 'NONE',  ( -17.48853670773246805, 5.747243402303015003, 98.66671299749995683 ) ) ;
#175910=CARTESIAN_POINT ( 'NONE',  ( -9.564922557961040184, 16.46253265017147172, 67.91775706135233293 ) ) ;
#175911=CARTESIAN_POINT ( 'NONE',  ( -19.05341960407611168, -5.049401038298163336, 91.45724293864766707 ) ) ;
#175912=CARTESIAN_POINT ( 'NONE',  ( -8.224510206698948167, 14.34966873604960824, 80.41557627198103830 ) ) ;
#175913=CARTESIAN_POINT ( 'NONE',  ( 21.52544592524344225, -5.823673210054117533, 28.54057627198103120 ) ) ;
#175914=CARTESIAN_POINT ( 'NONE',  ( -21.55341960407610458, -5.719274019375992779, 21.45724293864769550 ) ) ;
#175915=CARTESIAN_POINT ( 'NONE',  ( 4.483927247898545687, 16.52544592524342804, 104.7905762719810241 ) ) ;
#175916=CARTESIAN_POINT ( 'NONE',  ( -17.49999999999999645, 5.499999999999992895, 53.71769037696436300 ) ) ;
#175917=CARTESIAN_POINT ( 'NONE',  ( -9.564922557961040184, 16.46253265017147172, 37.91775706135233293 ) ) ;
#175918=CARTESIAN_POINT ( 'NONE',  ( -4.483927247898539470, -16.52544592524342804, 32.29057627198102409 ) ) ;
#175919=CARTESIAN_POINT ( 'NONE',  ( -0.05219959533909027116, -19.03943276465977164, 97.49890960531436690 ) ) ;
#175920=CARTESIAN_POINT ( 'NONE',  ( 10.81492255796106328, -18.62759615963255655, 60.41775706135235424 ) ) ;
#175921=CARTESIAN_POINT ( 'NONE',  ( 10.72451020669898902, -18.67979575497178502, 57.91557627198103120 ) ) ;
#175922=CARTESIAN_POINT ( 'NONE',  ( 21.55341960407619695, -5.719274019375665929, 36.04275706135234714 ) ) ;
#175923=CARTESIAN_POINT ( 'NONE',  ( -15.80617190586745835, -15.72974639402198527, 81.87390960531435269 ) ) ;
#175924=CARTESIAN_POINT ( 'NONE',  ( 21.53943276465977519, 0.05219959533937863772, 41.25109039468568284 ) ) ;
#175925=CARTESIAN_POINT ( 'NONE',  ( 4.483927247898545687, 16.52544592524342804, 109.7905762719810383 ) ) ;
#175926=CARTESIAN_POINT ( 'NONE',  ( -5.153800228976607833, 19.02544592524334988, 67.70942372801900433 ) ) ;
#175927=CARTESIAN_POINT ( 'NONE',  ( -13.97604488694527625, -13.89961937509977652, 46.87390960531435979 ) ) ;
#175928=CARTESIAN_POINT ( 'NONE',  ( 12.14591786802309770, 12.06949235617756955, 94.37390960531436690 ) ) ;
#175929=CARTESIAN_POINT ( 'NONE',  ( -9.474510206698964154, 16.51473224551069663, 95.41557627198102409 ) ) ;
#175930=CARTESIAN_POINT ( 'NONE',  ( 0.05219959533909260263, 19.03943276465977164, 109.9989096053143669 ) ) ;
#175931=CARTESIAN_POINT ( 'NONE',  ( -13.89961937509977652, 13.97604488694528158, 30.62390960531435269 ) ) ;
#175932=CARTESIAN_POINT ( 'NONE',  ( -14.34966873604960291, -8.224510206698953496, 46.66557627198102409 ) ) ;
#175933=CARTESIAN_POINT ( 'NONE',  ( 16.53943276465976808, 0.05219959533934440121, 96.25109039468568994 ) ) ;
#175934=CARTESIAN_POINT ( 'NONE',  ( -13.89961937509977652, 13.97604488694528158, 50.62390960531435979 ) ) ;
#175935=CARTESIAN_POINT ( 'NONE',  ( 4.483927247898545687, 16.52544592524342804, 114.7905762719810383 ) ) ;
#175936=CARTESIAN_POINT ( 'NONE',  ( 9.474510206698729675, 16.51473224551082808, 22.08442372801899722 ) ) ;
#175938=CARTESIAN_POINT ( 'NONE',  ( -13.97604488694527625, -13.89961937509977652, 111.8739096053143243 ) ) ;
#175939=CARTESIAN_POINT ( 'NONE',  ( -12.14591786802326823, 12.06949235617739902, 113.1260903946856899 ) ) ;
#175940=CARTESIAN_POINT ( 'NONE',  ( 10.72451020669871369, 18.67979575497193778, 52.08442372801901854 ) ) ;
#175942=CARTESIAN_POINT ( 'NONE',  ( -8.314922557961024197, 14.29746914071037800, 52.91775706135235424 ) ) ;
#175943=CARTESIAN_POINT ( 'NONE',  ( -8.314922557960811034, -14.29746914071050412, 22.08224293864769194 ) ) ;
#175944=CARTESIAN_POINT ( 'NONE',  ( 4.379528057220092307, 16.55341960407617563, 112.2927570613523471 ) ) ;
#175945=CARTESIAN_POINT ( 'NONE',  ( -12.14591786802326823, 12.06949235617739902, 23.12609039468567573 ) ) ;
#175947=CARTESIAN_POINT ( 'NONE',  ( -9.564922557960796823, -16.46253265017161027, 47.08224293864769550 ) ) ;
#175948=CARTESIAN_POINT ( 'NONE',  ( 16.52544592524342804, -4.483927247898539470, 113.5405762719810383 ) ) ;
#175949=CARTESIAN_POINT ( 'NONE',  ( -0.05219959533937732626, 21.53943276465977519, 22.50109039468567573 ) ) ;
#175950=CARTESIAN_POINT ( 'NONE',  ( 13.97604488694527802, 13.89961937509977652, 49.37390960531434558 ) ) ;
#175952=CARTESIAN_POINT ( 'NONE',  ( -13.97604488694527625, -13.89961937509977652, 26.87390960531434558 ) ) ;
#175953=CARTESIAN_POINT ( 'NONE',  ( 5.719274019375991003, -21.55341960407610458, 22.70724293864769194 ) ) ;
#175954=CARTESIAN_POINT ( 'NONE',  ( -17.50000000000000711, -5.499999999999956479, 36.28230962303565121 ) ) ;
#175955=CARTESIAN_POINT ( 'NONE',  ( -5.049401038298153566, 19.05341960407611168, 95.20724293864770971 ) ) ;
#175956=CARTESIAN_POINT ( 'NONE',  ( 21.52544592524334988, 5.823673210054432836, 41.45942372801901143 ) ) ;
#175957=CARTESIAN_POINT ( 'NONE',  ( 8.224510206698953496, -14.34966873604960469, 102.9155762719810383 ) ) ;
#175958=CARTESIAN_POINT ( 'NONE',  ( -0.05219959533909027116, -19.03943276465977164, 112.4989096053143669 ) ) ;
#175960=CARTESIAN_POINT ( 'NONE',  ( -14.34966873604972548, 8.224510206698743886, 83.33442372801903275 ) ) ;
#175961=CARTESIAN_POINT ( 'NONE',  ( 10.81492255796106328, -18.62759615963255655, 90.41775706135236135 ) ) ;
#175962=CARTESIAN_POINT ( 'NONE',  ( 0.05219959533934541429, -16.53943276465976808, 60.00109039468568284 ) ) ;
#175963=CARTESIAN_POINT ( 'NONE',  ( 19.03943276465977164, -0.05219959533909143690, 98.74890960531436690 ) ) ;
#175964=CARTESIAN_POINT ( 'NONE',  ( -4.483927247898782831, 16.52544592524335698, 42.70942372801901854 ) ) ;
#175965=CARTESIAN_POINT ( 'NONE',  ( -0.05219959533936034679, 19.03943276465977164, 112.5010903946856757 ) ) ;
#175966=CARTESIAN_POINT ( 'NONE',  ( 8.224510206698742110, 14.34966873604972548, 77.08442372801901854 ) ) ;
#175967=CARTESIAN_POINT ( 'NONE',  ( 19.02544592524334988, 5.153800228976608722, 96.45942372801897591 ) ) ;
#175968=CARTESIAN_POINT ( 'NONE',  ( -19.03943276465977164, 0.05219959533909376836, 71.24890960531435269 ) ) ;
#175969=CARTESIAN_POINT ( 'NONE',  ( -21.55341960407610458, -5.719274019375992779, 96.45724293864770971 ) ) ;
#175970=CARTESIAN_POINT ( 'NONE',  ( -8.224510206698948167, 14.34966873604960824, 95.41557627198102409 ) ) ;
#175971=CARTESIAN_POINT ( 'NONE',  ( 5.153800228976615827, -19.02544592524334988, 105.2094237280190185 ) ) ;
#175972=CARTESIAN_POINT ( 'NONE',  ( -12.14591786802326823, 12.06949235617739902, 73.12609039468567573 ) ) ;
#175974=CARTESIAN_POINT ( 'NONE',  ( 16.46253265017146816, 9.564922557961045513, 71.66775706135233293 ) ) ;
#175975=CARTESIAN_POINT ( 'NONE',  ( -14.34966873604960291, -8.224510206698953496, 36.66557627198103120 ) ) ;
#175976=CARTESIAN_POINT ( 'NONE',  ( 16.52544592524342804, -4.483927247898539470, 98.54057627198105251 ) ) ;
#175977=CARTESIAN_POINT ( 'NONE',  ( 0.05219959533936267826, -19.03943276465977164, 30.00109039468566863 ) ) ;
#175978=CARTESIAN_POINT ( 'NONE',  ( -17.48847506799967988, 5.747544572773787941, 90.82697437843279431 ) ) ;
#175979=CARTESIAN_POINT ( 'NONE',  ( -10.72451020669870658, -18.67979575497194134, 19.58442372801901143 ) ) ;
#175980=CARTESIAN_POINT ( 'NONE',  ( 13.89961937509957401, 13.97604488694547697, 96.87609039468566152 ) ) ;
#175981=CARTESIAN_POINT ( 'NONE',  ( -13.97604488694527625, -13.89961937509977652, 111.8739096053143243 ) ) ;
#175982=CARTESIAN_POINT ( 'NONE',  ( -5.153800228976328057, -19.02544592524343514, 87.29057627198103830 ) ) ;
#175983=CARTESIAN_POINT ( 'NONE',  ( -10.72451020669870658, -18.67979575497194134, 99.58442372801900433 ) ) ;
#175984=CARTESIAN_POINT ( 'NONE',  ( 16.51473224551069308, 9.474510206698969483, 74.16557627198103830 ) ) ;
#175985=CARTESIAN_POINT ( 'NONE',  ( -10.72451020669898014, 18.67979575497178502, 40.41557627198103120 ) ) ;
#175986=CARTESIAN_POINT ( 'NONE',  ( -16.55341960407611168, -4.379528057220339221, 91.45724293864769550 ) ) ;
#175987=CARTESIAN_POINT ( 'NONE',  ( -5.153800228976328057, -19.02544592524343514, 57.29057627198103120 ) ) ;
#175988=CARTESIAN_POINT ( 'NONE',  ( -8.224510206698948167, 14.34966873604960824, 115.4155762719810241 ) ) ;
#175989=CARTESIAN_POINT ( 'NONE',  ( 10.81492255796106328, -18.62759615963255655, 25.41775706135235779 ) ) ;
#175990=CARTESIAN_POINT ( 'NONE',  ( 18.67979575497194134, -10.72451020669871369, 65.83442372801900433 ) ) ;
#175991=CARTESIAN_POINT ( 'NONE',  ( 19.03943276465977164, -0.05219959533909143690, 43.74890960531435979 ) ) ;
#175992=CARTESIAN_POINT ( 'NONE',  ( 4.379528057220092307, 16.55341960407617563, 82.29275706135234714 ) ) ;
#175993=CARTESIAN_POINT ( 'NONE',  ( 10.81492255796106328, -18.62759615963255655, 20.41775706135234714 ) ) ;
#175995=CARTESIAN_POINT ( 'NONE',  ( -21.52544592524343514, 5.823673210054127303, 106.0405762719810525 ) ) ;
#175996=CARTESIAN_POINT ( 'NONE',  ( -19.02544592524334988, -5.153800228976617603, 48.95942372801900433 ) ) ;
#175997=CARTESIAN_POINT ( 'NONE',  ( 19.05341960407611168, 5.049401038298154454, 63.95724293864769550 ) ) ;
#175998=CARTESIAN_POINT ( 'NONE',  ( 5.049401038297881783, 19.05341960407617563, 37.29275706135232582 ) ) ;
#175999=CARTESIAN_POINT ( 'NONE',  ( 18.67979575497194134, -10.72451020669871369, 75.83442372801900433 ) ) ;
#176000=VECTOR ( 'NONE', #147572, 1000.000000000000000 ) ;
#176001=CARTESIAN_POINT ( 'NONE',  ( -18.67979575497178146, -10.72451020669898902, 76.66557627198103830 ) ) ;
#176002=CARTESIAN_POINT ( 'NONE',  ( -16.52544592524342804, 4.483927247898546575, 51.04057627198103120 ) ) ;
#176003=CARTESIAN_POINT ( 'NONE',  ( -18.67979575497193778, 10.72451020669871902, 88.33442372801901854 ) ) ;
#176004=CARTESIAN_POINT ( 'NONE',  ( 19.02544592524334988, 5.153800228976608722, 26.45942372801899722 ) ) ;
#176005=CARTESIAN_POINT ( 'NONE',  ( 0.05219959533910956823, 16.53943276465976808, 74.99890960531435269 ) ) ;
#176006=CARTESIAN_POINT ( 'NONE',  ( 8.314922557960818139, 14.29746914071049879, 114.5822429386477097 ) ) ;
#176007=CARTESIAN_POINT ( 'NONE',  ( 5.049401038297881783, 19.05341960407617563, 52.29275706135234003 ) ) ;
#176008=CARTESIAN_POINT ( 'NONE',  ( 8.314922557961029526, -14.29746914071037800, 110.4177570613523756 ) ) ;
#176009=CARTESIAN_POINT ( 'NONE',  ( 21.52544592524334988, 5.823673210054432836, 76.45942372801901854 ) ) ;
#176010=CARTESIAN_POINT ( 'NONE',  ( -5.153800228976607833, 19.02544592524334988, 42.70942372801901143 ) ) ;
#176011=CARTESIAN_POINT ( 'NONE',  ( -0.05219959533907301413, -21.53943276465977519, 57.49890960531435979 ) ) ;
#176012=CARTESIAN_POINT ( 'NONE',  ( 10.81492255796106328, -18.62759615963255655, 50.41775706135235424 ) ) ;
#176013=CARTESIAN_POINT ( 'NONE',  ( -21.55341960407610458, -5.719274019375992779, 101.4572429386476955 ) ) ;
#176014=CARTESIAN_POINT ( 'NONE',  ( 13.89961937509957401, 13.97604488694547697, 91.87609039468567573 ) ) ;
#176015=CARTESIAN_POINT ( 'NONE',  ( 14.29746914071037800, 8.314922557961029526, 66.66775706135234714 ) ) ;
#176017=CARTESIAN_POINT ( 'NONE',  ( -21.52544592524343514, 5.823673210054127303, 111.0405762719810525 ) ) ;
#176018=CARTESIAN_POINT ( 'NONE',  ( 8.224510206698953496, -14.34966873604960469, 92.91557627198103830 ) ) ;
#176020=CARTESIAN_POINT ( 'NONE',  ( -4.379528057220086978, -16.55341960407618274, 34.79275706135235424 ) ) ;
#176021=CARTESIAN_POINT ( 'NONE',  ( -21.52544592524343514, 5.823673210054127303, 51.04057627198103120 ) ) ;
#176022=CARTESIAN_POINT ( 'NONE',  ( -0.05219959533934338120, 16.53943276465976808, 87.50109039468568994 ) ) ;
#176024=CARTESIAN_POINT ( 'NONE',  ( 14.34966873604972726, -8.224510206698740333, 70.83442372801901854 ) ) ;
#176025=CARTESIAN_POINT ( 'NONE',  ( -15.80617190586768217, 15.72974639402176855, 38.12609039468567573 ) ) ;
#176027=CARTESIAN_POINT ( 'NONE',  ( -15.72974639402197994, 15.80617190586746368, 55.62390960531436690 ) ) ;
#176028=CARTESIAN_POINT ( 'NONE',  ( -12.14591786802326823, 12.06949235617739902, 78.12609039468570415 ) ) ;
#176029=CARTESIAN_POINT ( 'NONE',  ( 21.55341960407619695, -5.719274019375665929, 76.04275706135237556 ) ) ;
#176030=CARTESIAN_POINT ( 'NONE',  ( 15.72974639402199770, -15.80617190586745480, 48.12390960531436690 ) ) ;
#176031=CARTESIAN_POINT ( 'NONE',  ( 15.80617190586746368, 15.72974639402197994, 34.37390960531435979 ) ) ;
#176032=VERTEX_POINT ( 'NONE', #140544 ) ;
#176033=CARTESIAN_POINT ( 'NONE',  ( 8.314922557961029526, -14.29746914071037800, 70.41775706135236135 ) ) ;
#176034=CARTESIAN_POINT ( 'NONE',  ( -15.80617190586745835, -15.72974639402198527, 31.87390960531435979 ) ) ;
#176036=CARTESIAN_POINT ( 'NONE',  ( 0.05219959533909260263, 19.03943276465977164, 99.99890960531436690 ) ) ;
#176037=CARTESIAN_POINT ( 'NONE',  ( -16.53943276465976808, 0.05219959533911058130, 26.24890960531435624 ) ) ;
#176038=CARTESIAN_POINT ( 'NONE',  ( 17.60779699588839264, 5.500000000000008882, 73.84981316670106821 ) ) ;
#176039=CARTESIAN_POINT ( 'NONE',  ( -8.224510206698948167, 14.34966873604960824, 110.4155762719810383 ) ) ;
#176040=CARTESIAN_POINT ( 'NONE',  ( 15.72974639402199770, -15.80617190586745480, 43.12390960531435269 ) ) ;
#176041=CARTESIAN_POINT ( 'NONE',  ( 19.05341960407611168, 5.049401038298154454, 43.95724293864769550 ) ) ;
#176042=CARTESIAN_POINT ( 'NONE',  ( 16.55341960407618274, -4.379528057220086978, 91.04275706135236135 ) ) ;
#176043=CARTESIAN_POINT ( 'NONE',  ( -21.55341960407619339, 5.719274019375674811, 28.54275706135234358 ) ) ;
#176044=CARTESIAN_POINT ( 'NONE',  ( 19.02544592524334988, 5.153800228976608722, 96.45942372801897591 ) ) ;
#176045=CARTESIAN_POINT ( 'NONE',  ( -8.314922557960811034, -14.29746914071050412, 97.08224293864770971 ) ) ;
#176046=CARTESIAN_POINT ( 'NONE',  ( 9.474510206698971260, -16.51473224551069308, 57.91557627198103120 ) ) ;
#176048=CARTESIAN_POINT ( 'NONE',  ( 13.89961937509977652, -13.97604488694527269, 28.12390960531435624 ) ) ;
#176049=CARTESIAN_POINT ( 'NONE',  ( 17.72517630440434644, -5.499999999999995559, 63.42175719257210886 ) ) ;
#176050=CARTESIAN_POINT ( 'NONE',  ( 19.03943276465977164, -0.05219959533909143690, 83.74890960531436690 ) ) ;
#176052=CARTESIAN_POINT ( 'NONE',  ( -16.52544592524335698, -4.483927247898792601, 63.95942372801901854 ) ) ;
#176053=CARTESIAN_POINT ( 'NONE',  ( 5.823673210054444382, -21.52544592524334988, 100.2094237280190043 ) ) ;
#176054=CARTESIAN_POINT ( 'NONE',  ( -10.72451020669898014, 18.67979575497178502, 50.41557627198103120 ) ) ;
#176055=CARTESIAN_POINT ( 'NONE',  ( 4.379528057220092307, 16.55341960407617563, 72.29275706135236135 ) ) ;
#176056=CARTESIAN_POINT ( 'NONE',  ( -0.05219959533936034679, 19.03943276465977164, 67.50109039468566152 ) ) ;
#176057=CARTESIAN_POINT ( 'NONE',  ( -15.80617190586768217, 15.72974639402176855, 58.12609039468568994 ) ) ;
#176058=CARTESIAN_POINT ( 'NONE',  ( 13.89961937509977652, -13.97604488694527269, 63.12390960531435979 ) ) ;
#176060=CARTESIAN_POINT ( 'NONE',  ( 19.02544592524343514, -5.153800228976328945, 33.54057627198102409 ) ) ;
#176061=CARTESIAN_POINT ( 'NONE',  ( 19.03943276465977164, 0.05219959533936151252, 56.25109039468566863 ) ) ;
#176062=CARTESIAN_POINT ( 'NONE',  ( 19.03943276465977164, -0.05219959533909143690, 108.7489096053143527 ) ) ;
#176063=CARTESIAN_POINT ( 'NONE',  ( -13.89961937509977652, 13.97604488694528158, 100.6239096053143669 ) ) ;
#176064=CARTESIAN_POINT ( 'NONE',  ( 8.314922557960818139, 14.29746914071049879, 54.58224293864769550 ) ) ;
#176065=CARTESIAN_POINT ( 'NONE',  ( -15.72974639402197994, 15.80617190586746368, 45.62390960531436690 ) ) ;
#176066=DIRECTION ( 'NONE',  ( 1.000000000000000000, -0.000000000000000000, 0.000000000000000000 ) ) ;
#176067=CARTESIAN_POINT ( 'NONE',  ( 16.51473224551083163, -9.474510206698727899, 35.83442372801899722 ) ) ;
#176068=CARTESIAN_POINT ( 'NONE',  ( -13.89961937509977652, 13.97604488694528158, 55.62390960531434558 ) ) ;
#176070=CARTESIAN_POINT ( 'NONE',  ( -17.49999999999999645, 5.622605283950888655, 108.6879268940389096 ) ) ;
#176071=CARTESIAN_POINT ( 'NONE',  ( -16.53943276465976808, -0.05219959533934237506, 73.75109039468567573 ) ) ;
#176072=CARTESIAN_POINT ( 'NONE',  ( 18.62759615963271287, -10.81492255796078972, 98.33224293864769550 ) ) ;
#176073=CARTESIAN_POINT ( 'NONE',  ( -5.153800228976328057, -19.02544592524343514, 47.29057627198102409 ) ) ;
#176075=CARTESIAN_POINT ( 'NONE',  ( -21.52544592524334988, -5.823673210054445271, 38.95942372801901854 ) ) ;
#176076=CARTESIAN_POINT ( 'NONE',  ( -9.564922557961040184, 16.46253265017147172, 42.91775706135234003 ) ) ;
#176077=CARTESIAN_POINT ( 'NONE',  ( 16.51473224551069308, 9.474510206698969483, 44.16557627198103120 ) ) ;
#176078=CARTESIAN_POINT ( 'NONE',  ( 18.67979575497194134, -10.72451020669871369, 95.83442372801903275 ) ) ;
#176080=CARTESIAN_POINT ( 'NONE',  ( -16.52544592524342804, 4.483927247898546575, 46.04057627198103830 ) ) ;
#176081=CARTESIAN_POINT ( 'NONE',  ( 19.52851543214742591, 5.500000000000025757, 42.89357721762583253 ) ) ;
#176082=CARTESIAN_POINT ( 'NONE',  ( -10.81492255796078084, -18.62759615963271287, 37.08224293864768129 ) ) ;
#176084=CARTESIAN_POINT ( 'NONE',  ( 16.51473224551069308, 9.474510206698969483, 104.1655762719810241 ) ) ;
#176085=CARTESIAN_POINT ( 'NONE',  ( 12.14591786802309770, 12.06949235617756955, 94.37390960531436690 ) ) ;
#176086=CARTESIAN_POINT ( 'NONE',  ( 8.314922557961029526, -14.29746914071037800, 20.41775706135234714 ) ) ;
#176087=CARTESIAN_POINT ( 'NONE',  ( -12.14591786802326823, 12.06949235617739902, 103.1260903946856757 ) ) ;
#176089=CARTESIAN_POINT ( 'NONE',  ( -13.89961937509977652, 13.97604488694528158, 95.62390960531436690 ) ) ;
#176090=CARTESIAN_POINT ( 'NONE',  ( 0.05219959533907565091, 21.53943276465977519, 99.99890960531436690 ) ) ;
#176091=CARTESIAN_POINT ( 'NONE',  ( -12.14591786802326823, 12.06949235617739902, 113.1260903946856899 ) ) ;
#176092=CARTESIAN_POINT ( 'NONE',  ( -16.46253265017160317, 9.564922557960807481, 95.83224293864769550 ) ) ;
#176093=CARTESIAN_POINT ( 'NONE',  ( 13.97604488694548053, -13.89961937509957401, 95.62609039468563310 ) ) ;
#176094=CARTESIAN_POINT ( 'NONE',  ( 21.52544592524334988, 5.823673210054432836, 111.4594237280190328 ) ) ;
#176095=CARTESIAN_POINT ( 'NONE',  ( 21.53943276465977519, -0.05219959533907433946, 83.74890960531435269 ) ) ;
#176096=CARTESIAN_POINT ( 'NONE',  ( -5.719274019375978568, 21.55341960407610458, 45.20724293864769550 ) ) ;
#176097=CARTESIAN_POINT ( 'NONE',  ( 16.51473224551069308, 9.474510206698969483, 59.16557627198102409 ) ) ;
#176098=CARTESIAN_POINT ( 'NONE',  ( -8.224510206698948167, 14.34966873604960824, 40.41557627198103120 ) ) ;
#176099=CARTESIAN_POINT ( 'NONE',  ( 9.564922557960805705, 16.46253265017160317, 74.58224293864769550 ) ) ;
#176101=CARTESIAN_POINT ( 'NONE',  ( 18.56453257813367586, -5.499999999999872102, 63.49000423690685579 ) ) ;
#176102=CARTESIAN_POINT ( 'NONE',  ( -5.049401038297874678, -19.05341960407617918, 39.79275706135232582 ) ) ;
#176103=CARTESIAN_POINT ( 'NONE',  ( -16.55341960407611168, -4.379528057220339221, 81.45724293864769550 ) ) ;
#176104=CARTESIAN_POINT ( 'NONE',  ( -21.53943276465977519, -0.05219959533937600094, 28.75109039468567929 ) ) ;
#176106=CARTESIAN_POINT ( 'NONE',  ( 14.34966873604972726, -8.224510206698740333, 105.8344237280190328 ) ) ;
#176107=CARTESIAN_POINT ( 'NONE',  ( 13.97604488694527802, 13.89961937509977652, 29.37390960531435979 ) ) ;
#176108=CARTESIAN_POINT ( 'NONE',  ( -19.03943276465977164, 0.05219959533909376836, 66.24890960531436690 ) ) ;
#176110=CARTESIAN_POINT ( 'NONE',  ( 19.02544592524343514, -5.153800228976328945, 23.54057627198102054 ) ) ;
#176111=CARTESIAN_POINT ( 'NONE',  ( -16.55341960407611168, -4.379528057220339221, 46.45724293864769550 ) ) ;
#176112=CARTESIAN_POINT ( 'NONE',  ( 0.05219959533937995610, -21.53943276465977519, 55.00109039468568284 ) ) ;
#176114=CARTESIAN_POINT ( 'NONE',  ( 15.80617190586769283, -15.72974639402175789, 100.6260903946857184 ) ) ;
#176115=CARTESIAN_POINT ( 'NONE',  ( -9.564922557960796823, -16.46253265017161027, 37.08224293864768839 ) ) ;
#176116=CARTESIAN_POINT ( 'NONE',  ( -9.474510206698964154, 16.51473224551069663, 45.41557627198103120 ) ) ;
#176117=ORIENTED_EDGE ( 'NONE', *, *, #95241, .F. ) ;
#176118=CARTESIAN_POINT ( 'NONE',  ( 5.719274019375673035, 21.55341960407619339, 92.29275706135236135 ) ) ;
#176119=CARTESIAN_POINT ( 'NONE',  ( -4.483927247898782831, 16.52544592524335698, 57.70942372801901143 ) ) ;
#176120=CARTESIAN_POINT ( 'NONE',  ( 21.53943276465977519, 0.05219959533937863772, 86.25109039468568994 ) ) ;
#176121=CARTESIAN_POINT ( 'NONE',  ( -21.55341960407610458, -5.719274019375992779, 26.45724293864768839 ) ) ;
#176122=CARTESIAN_POINT ( 'NONE',  ( 16.51473224551083163, -9.474510206698727899, 95.83442372801900433 ) ) ;
#176123=CARTESIAN_POINT ( 'NONE',  ( -21.55341960407619339, 5.719274019375674811, 68.54275706135234714 ) ) ;
#176124=CARTESIAN_POINT ( 'NONE',  ( -14.29746914071037622, -8.314922557961029526, 39.16775706135235424 ) ) ;
#176126=CARTESIAN_POINT ( 'NONE',  ( -5.719274019375978568, 21.55341960407610458, 85.20724293864770971 ) ) ;
#176127=CARTESIAN_POINT ( 'NONE',  ( 13.89961937509957401, 13.97604488694547697, 91.87609039468567573 ) ) ;
#176128=CARTESIAN_POINT ( 'NONE',  ( 13.89961937509977652, -13.97604488694527269, 63.12390960531435979 ) ) ;
#176129=CARTESIAN_POINT ( 'NONE',  ( -5.153800228976607833, 19.02544592524334988, 102.7094237280189759 ) ) ;
#176130=CARTESIAN_POINT ( 'NONE',  ( -19.02544592524334988, -5.153800228976617603, 103.9594237280190043 ) ) ;
#176131=CARTESIAN_POINT ( 'NONE',  ( -12.14591786802309592, -12.06949235617757132, 56.87390960531436690 ) ) ;
#176132=CARTESIAN_POINT ( 'NONE',  ( 19.03943276465977164, 0.05219959533936151252, 81.25109039468567573 ) ) ;
#176133=CARTESIAN_POINT ( 'NONE',  ( 14.34966873604972726, -8.224510206698740333, 65.83442372801900433 ) ) ;
#176134=CARTESIAN_POINT ( 'NONE',  ( 15.80617190586746368, 15.72974639402197994, 114.3739096053143527 ) ) ;
#176135=CARTESIAN_POINT ( 'NONE',  ( -16.46253265017160317, 9.564922557960807481, 35.83224293864768839 ) ) ;
#176136=CARTESIAN_POINT ( 'NONE',  ( 9.474510206698971260, -16.51473224551069308, 52.91557627198102409 ) ) ;
#176137=CARTESIAN_POINT ( 'NONE',  ( 4.379528057220092307, 16.55341960407617563, 62.29275706135236845 ) ) ;
#176139=FACE_OUTER_BOUND ( 'NONE', #145043, .T. ) ;
#176140=CARTESIAN_POINT ( 'NONE',  ( 13.97604488694527802, 13.89961937509977652, 99.37390960531436690 ) ) ;
#176141=EDGE_CURVE ( 'NONE', #144387, #24966, #47762, .T. ) ;
#176142=CARTESIAN_POINT ( 'NONE',  ( 9.474510206698971260, -16.51473224551069308, 22.91557627198102765 ) ) ;
#176143=CARTESIAN_POINT ( 'NONE',  ( -9.564922557961040184, 16.46253265017147172, 107.9177570613523471 ) ) ;
#176144=CARTESIAN_POINT ( 'NONE',  ( -10.72451020669898014, 18.67979575497178502, 40.41557627198103120 ) ) ;
#176145=CARTESIAN_POINT ( 'NONE',  ( 19.05341960407617918, -5.049401038297876454, 26.04275706135233293 ) ) ;
#176146=CARTESIAN_POINT ( 'NONE',  ( -0.05219959533934338120, 16.53943276465976808, 27.50109039468567929 ) ) ;
#176147=CARTESIAN_POINT ( 'NONE',  ( 9.564922557960805705, 16.46253265017160317, 29.58224293864769550 ) ) ;
#176148=CARTESIAN_POINT ( 'NONE',  ( 16.46253265017160672, -9.564922557960803928, 48.33224293864769550 ) ) ;
#176149=CARTESIAN_POINT ( 'NONE',  ( -21.55341960407610458, -5.719274019375992779, 81.45724293864769550 ) ) ;
#176150=CARTESIAN_POINT ( 'NONE',  ( 19.02544592524343514, -5.153800228976328945, 103.5405762719809957 ) ) ;
#176151=CARTESIAN_POINT ( 'NONE',  ( -19.02544592524342804, 5.153800228976336051, 46.04057627198101699 ) ) ;
#176153=CARTESIAN_POINT ( 'NONE',  ( -19.02544592524334988, -5.153800228976617603, 78.95942372801900433 ) ) ;
#176154=CARTESIAN_POINT ( 'NONE',  ( 16.53943276465976808, -0.05219959533910856209, 68.74890960531435269 ) ) ;
#176155=CARTESIAN_POINT ( 'NONE',  ( -21.52544592524334988, -5.823673210054445271, 103.9594237280190185 ) ) ;
#176157=CARTESIAN_POINT ( 'NONE',  ( 15.80617190586746368, 15.72974639402197994, 99.37390960531436690 ) ) ;
#176158=CARTESIAN_POINT ( 'NONE',  ( -18.62759615963255300, -10.81492255796106328, 79.16775706135234714 ) ) ;
#176159=CARTESIAN_POINT ( 'NONE',  ( 15.80617190586769283, -15.72974639402175789, 75.62609039468567573 ) ) ;
#176160=CARTESIAN_POINT ( 'NONE',  ( 5.049401038298161559, -19.05341960407611168, 112.7072429386476813 ) ) ;
#176161=CARTESIAN_POINT ( 'NONE',  ( -8.314922557961024197, 14.29746914071037800, 112.9177570613523329 ) ) ;
#176162=CARTESIAN_POINT ( 'NONE',  ( -21.52544592524334988, -5.823673210054445271, 78.95942372801901854 ) ) ;
#176163=CARTESIAN_POINT ( 'NONE',  ( -13.89961937509977652, 13.97604488694528158, 60.62390960531436690 ) ) ;
#176164=CARTESIAN_POINT ( 'NONE',  ( -10.72451020669870658, -18.67979575497194134, 29.58442372801901854 ) ) ;
#176165=CARTESIAN_POINT ( 'NONE',  ( -19.02544592524342804, 5.153800228976336051, 86.04057627198103830 ) ) ;
#176166=CARTESIAN_POINT ( 'NONE',  ( 14.29746914071049879, -8.314922557960816363, 78.33224293864770971 ) ) ;
#176167=CARTESIAN_POINT ( 'NONE',  ( -4.483927247898539470, -16.52544592524342804, 47.29057627198103120 ) ) ;
#176168=CARTESIAN_POINT ( 'NONE',  ( -10.72451020669898014, 18.67979575497178502, 60.41557627198102409 ) ) ;
#176169=CARTESIAN_POINT ( 'NONE',  ( 0.05219959533909260263, 19.03943276465977164, 54.99890960531435979 ) ) ;
#176170=CARTESIAN_POINT ( 'NONE',  ( -21.53943276465977519, 0.05219959533907696930, 66.24890960531436690 ) ) ;
#176172=CARTESIAN_POINT ( 'NONE',  ( -16.51473224551082808, 9.474510206698731452, 63.33442372801900433 ) ) ;
#176173=CARTESIAN_POINT ( 'NONE',  ( 16.51473224551083163, -9.474510206698727899, 25.83442372801900078 ) ) ;
#176174=CARTESIAN_POINT ( 'NONE',  ( 14.29746914071049879, -8.314922557960816363, 78.33224293864770971 ) ) ;
#176175=CARTESIAN_POINT ( 'NONE',  ( 21.53943276465977519, -0.05219959533907433946, 53.74890960531437401 ) ) ;
#176178=CARTESIAN_POINT ( 'NONE',  ( 4.483927247898790824, -16.52544592524335698, 100.2094237280190043 ) ) ;
#176180=CARTESIAN_POINT ( 'NONE',  ( 16.51473224551083163, -9.474510206698727899, 90.83442372801900433 ) ) ;
#176181=CARTESIAN_POINT ( 'NONE',  ( 16.53943276465976808, -0.05219959533910856209, 63.74890960531435979 ) ) ;
#176183=CARTESIAN_POINT ( 'NONE',  ( 5.153800228976335163, 19.02544592524342804, 64.79057627198100988 ) ) ;
#176184=CARTESIAN_POINT ( 'NONE',  ( 16.55341960407611168, 4.379528057220329451, 58.95724293864770971 ) ) ;
#176186=CARTESIAN_POINT ( 'NONE',  ( 19.03943276465977164, -0.05219959533909143690, 88.74890960531436690 ) ) ;
#176187=CARTESIAN_POINT ( 'NONE',  ( -0.05219959533936034679, 19.03943276465977164, 77.50109039468566152 ) ) ;
#176188=CARTESIAN_POINT ( 'NONE',  ( 19.02544592524343514, -5.153800228976328945, 58.54057627198102409 ) ) ;
#176189=CARTESIAN_POINT ( 'NONE',  ( 9.564922557960805705, 16.46253265017160317, 84.58224293864769550 ) ) ;
#176190=CARTESIAN_POINT ( 'NONE',  ( -9.474510206698964154, 16.51473224551069663, 75.41557627198103830 ) ) ;
#176191=CARTESIAN_POINT ( 'NONE',  ( -10.72451020669898014, 18.67979575497178502, 60.41557627198102409 ) ) ;
#176192=CARTESIAN_POINT ( 'NONE',  ( 0.05219959533934541429, -16.53943276465976808, 60.00109039468568284 ) ) ;
#176193=CARTESIAN_POINT ( 'NONE',  ( 18.22780087662123805, 5.499999999999960032, 101.4823681787310647 ) ) ;
#176194=CARTESIAN_POINT ( 'NONE',  ( -9.564922557960796823, -16.46253265017161027, 52.08224293864768839 ) ) ;
#176195=CARTESIAN_POINT ( 'NONE',  ( -21.52544592524343514, 5.823673210054127303, 51.04057627198103120 ) ) ;
#176196=CARTESIAN_POINT ( 'NONE',  ( 0.05219959533936267826, -19.03943276465977164, 75.00109039468566152 ) ) ;
#176197=CARTESIAN_POINT ( 'NONE',  ( -16.52544592524342804, 4.483927247898546575, 26.04057627198103475 ) ) ;
#176198=CARTESIAN_POINT ( 'NONE',  ( 5.153800228976615827, -19.02544592524334988, 35.20942372801899722 ) ) ;
#176199=CARTESIAN_POINT ( 'NONE',  ( -16.55341960407617563, 4.379528057220093196, 58.54275706135235424 ) ) ;
#176200=CARTESIAN_POINT ( 'NONE',  ( 16.53943276465976808, 0.05219959533934440121, 91.25109039468568994 ) ) ;
#176201=CARTESIAN_POINT ( 'NONE',  ( -18.22780087662123805, -5.499999999999968026, 93.98236817873105053 ) ) ;
#176202=CARTESIAN_POINT ( 'NONE',  ( -16.55341960407617563, 4.379528057220093196, 83.54275706135234714 ) ) ;
#176203=CARTESIAN_POINT ( 'NONE',  ( -19.02544592524342804, 5.153800228976336051, 116.0405762719810383 ) ) ;
#176204=CARTESIAN_POINT ( 'NONE',  ( 0.05219959533909260263, 19.03943276465977164, 39.99890960531436690 ) ) ;
#176205=CARTESIAN_POINT ( 'NONE',  ( 16.51473224551069308, 9.474510206698969483, 44.16557627198103120 ) ) ;
#176206=CARTESIAN_POINT ( 'NONE',  ( -19.03943276465977164, 0.05219959533909376836, 41.24890960531435269 ) ) ;
#176207=CARTESIAN_POINT ( 'NONE',  ( -21.52544592524334988, -5.823673210054445271, 33.95942372801901143 ) ) ;
#176208=CARTESIAN_POINT ( 'NONE',  ( -8.224510206698735004, -14.34966873604973081, 54.58442372801901143 ) ) ;
#176209=CARTESIAN_POINT ( 'NONE',  ( 8.224510206698742110, 14.34966873604972548, 112.0844237280190185 ) ) ;
#176210=CARTESIAN_POINT ( 'NONE',  ( -16.46253265017160317, 9.564922557960807481, 30.83224293864769550 ) ) ;
#176211=CARTESIAN_POINT ( 'NONE',  ( -21.55341960407619339, 5.719274019375674811, 113.5427570613523756 ) ) ;
#176212=CARTESIAN_POINT ( 'NONE',  ( -9.564922557961040184, 16.46253265017147172, 107.9177570613523471 ) ) ;
#176213=CARTESIAN_POINT ( 'NONE',  ( -16.46253265017146816, -9.564922557961047289, 74.16775706135234714 ) ) ;
#176214=CARTESIAN_POINT ( 'NONE',  ( -16.55341960407611168, -4.379528057220339221, 71.45724293864769550 ) ) ;
#176215=CARTESIAN_POINT ( 'NONE',  ( -9.564922557960796823, -16.46253265017161027, 37.08224293864768839 ) ) ;
#176216=CARTESIAN_POINT ( 'NONE',  ( -0.05219959533936034679, 19.03943276465977164, 77.50109039468566152 ) ) ;
#176218=CARTESIAN_POINT ( 'NONE',  ( -21.52544592524334988, -5.823673210054445271, 78.95942372801901854 ) ) ;
#176219=CARTESIAN_POINT ( 'NONE',  ( 14.29746914071037800, 8.314922557961029526, 41.66775706135235424 ) ) ;
#176220=CARTESIAN_POINT ( 'NONE',  ( 18.22780087662122384, -5.500000000000022204, 56.01540105326107977 ) ) ;
#176221=CARTESIAN_POINT ( 'NONE',  ( -5.719274019375978568, 21.55341960407610458, 35.20724293864768839 ) ) ;
#176222=CARTESIAN_POINT ( 'NONE',  ( -4.483927247898782831, 16.52544592524335698, 32.70942372801900433 ) ) ;
#176224=CARTESIAN_POINT ( 'NONE',  ( -21.55341960407619339, 5.719274019375674811, 108.5427570613523756 ) ) ;
#176226=CARTESIAN_POINT ( 'NONE',  ( -9.474510206698964154, 16.51473224551069663, 40.41557627198103120 ) ) ;
#176227=CARTESIAN_POINT ( 'NONE',  ( 9.474510206698729675, 16.51473224551082808, 57.08442372801900433 ) ) ;
#176228=CARTESIAN_POINT ( 'NONE',  ( -19.02544592524342804, 5.153800228976336051, 56.04057627198100988 ) ) ;
#176229=CARTESIAN_POINT ( 'NONE',  ( 10.81492255796106328, -18.62759615963255655, 60.41775706135235424 ) ) ;
#176230=CARTESIAN_POINT ( 'NONE',  ( 19.03943276465977164, 0.05219959533936151252, 26.25109039468566507 ) ) ;
#176231=CARTESIAN_POINT ( 'NONE',  ( -14.34966873604960291, -8.224510206698953496, 21.66557627198102409 ) ) ;
#176232=CARTESIAN_POINT ( 'NONE',  ( 5.153800228976335163, 19.02544592524342804, 34.79057627198102409 ) ) ;
#176233=CARTESIAN_POINT ( 'NONE',  ( 5.049401038298161559, -19.05341960407611168, 87.70724293864769550 ) ) ;
#176234=CARTESIAN_POINT ( 'NONE',  ( 18.67979575497194134, -10.72451020669871369, 55.83442372801901854 ) ) ;
#176235=CARTESIAN_POINT ( 'NONE',  ( 5.153800228976335163, 19.02544592524342804, 39.79057627198100988 ) ) ;
#176236=CARTESIAN_POINT ( 'NONE',  ( -0.05219959533937732626, 21.53943276465977519, 72.50109039468568994 ) ) ;
#176237=CARTESIAN_POINT ( 'NONE',  ( -16.46253265017146816, -9.564922557961047289, 89.16775706135234714 ) ) ;
#176238=CARTESIAN_POINT ( 'NONE',  ( -0.05219959533909027116, -19.03943276465977164, 107.4989096053143527 ) ) ;
#176239=CARTESIAN_POINT ( 'NONE',  ( -16.52544592524342804, 4.483927247898546575, 111.0405762719810525 ) ) ;
#176240=CARTESIAN_POINT ( 'NONE',  ( 15.80617190586746368, 15.72974639402197994, 109.3739096053143811 ) ) ;
#176241=CARTESIAN_POINT ( 'NONE',  ( 19.05341960407617918, -5.049401038297876454, 41.04275706135233293 ) ) ;
#176242=CARTESIAN_POINT ( 'NONE',  ( 12.14591786802309770, 12.06949235617756955, 109.3739096053143811 ) ) ;
#176243=CARTESIAN_POINT ( 'NONE',  ( 9.564922557960805705, 16.46253265017160317, 69.58224293864770971 ) ) ;
#176244=CARTESIAN_POINT ( 'NONE',  ( -5.049401038297874678, -19.05341960407617918, 99.79275706135234714 ) ) ;
#176245=CARTESIAN_POINT ( 'NONE',  ( -0.05219959533910754901, -16.53943276465976808, 62.49890960531436690 ) ) ;
#176246=CARTESIAN_POINT ( 'NONE',  ( -13.89961937509957401, -13.97604488694547875, 24.37609039468565442 ) ) ;
#176247=CARTESIAN_POINT ( 'NONE',  ( 21.52544592524344225, -5.823673210054117533, 23.54057627198102765 ) ) ;
#176248=CARTESIAN_POINT ( 'NONE',  ( 5.049401038297881783, 19.05341960407617563, 92.29275706135234714 ) ) ;
#176249=CARTESIAN_POINT ( 'NONE',  ( -18.67979575497178146, -10.72451020669898902, 96.66557627198102409 ) ) ;
#176250=CARTESIAN_POINT ( 'NONE',  ( -21.55341960407619339, 5.719274019375674811, 43.54275706135235424 ) ) ;
#176251=CARTESIAN_POINT ( 'NONE',  ( 12.14591786802327356, -12.06949235617739191, 40.62609039468567573 ) ) ;
#176252=CARTESIAN_POINT ( 'NONE',  ( -4.379528057220086978, -16.55341960407618274, 109.7927570613523613 ) ) ;
#176253=CARTESIAN_POINT ( 'NONE',  ( 8.224510206698742110, 14.34966873604972548, 37.08442372801901143 ) ) ;
#176254=CARTESIAN_POINT ( 'NONE',  ( 18.62759615963255655, 10.81492255796105972, 46.66775706135234714 ) ) ;
#176255=CARTESIAN_POINT ( 'NONE',  ( -18.62759615963270932, 10.81492255796079327, 60.83224293864769550 ) ) ;
#176256=CARTESIAN_POINT ( 'NONE',  ( 9.474510206698971260, -16.51473224551069308, 32.91557627198102409 ) ) ;
#176258=CARTESIAN_POINT ( 'NONE',  ( -8.224510206698735004, -14.34966873604973081, 69.58442372801900433 ) ) ;
#176259=CARTESIAN_POINT ( 'NONE',  ( 18.62759615963271287, -10.81492255796078972, 88.33224293864769550 ) ) ;
#176260=CARTESIAN_POINT ( 'NONE',  ( -8.314922557960811034, -14.29746914071050412, 37.08224293864768129 ) ) ;
#176261=CARTESIAN_POINT ( 'NONE',  ( 8.224510206698742110, 14.34966873604972548, 62.08442372801901143 ) ) ;
#176262=CARTESIAN_POINT ( 'NONE',  ( -5.049401038297874678, -19.05341960407617918, 94.79275706135230450 ) ) ;
#176263=CARTESIAN_POINT ( 'NONE',  ( 21.53943276465977519, -0.05219959533907433946, 98.74890960531438111 ) ) ;
#176264=CARTESIAN_POINT ( 'NONE',  ( -16.53943276465976808, 0.05219959533911058130, 26.24890960531435624 ) ) ;
#176266=CARTESIAN_POINT ( 'NONE',  ( -0.05219959533934338120, 16.53943276465976808, 82.50109039468568994 ) ) ;
#176268=CARTESIAN_POINT ( 'NONE',  ( 10.72451020669898902, -18.67979575497178502, 72.91557627198103830 ) ) ;
#176270=CARTESIAN_POINT ( 'NONE',  ( 12.14591786802327356, -12.06949235617739191, 100.6260903946857184 ) ) ;
#176271=ORIENTED_EDGE ( 'NONE', *, *, #109281, .T. ) ;
#176273=CARTESIAN_POINT ( 'NONE',  ( 5.719274019375991003, -21.55341960407610458, 102.7072429386476955 ) ) ;
#176275=CARTESIAN_POINT ( 'NONE',  ( -21.55341960407610458, -5.719274019375992779, 111.4572429386476813 ) ) ;
#176276=CARTESIAN_POINT ( 'NONE',  ( 8.314922557960818139, 14.29746914071049879, 44.58224293864769550 ) ) ;
#176277=CARTESIAN_POINT ( 'NONE',  ( 14.29746914071037800, 8.314922557961029526, 31.66775706135234358 ) ) ;
#176278=CARTESIAN_POINT ( 'NONE',  ( 16.51473224551069308, 9.474510206698969483, 54.16557627198103120 ) ) ;
#176279=CARTESIAN_POINT ( 'NONE',  ( -19.02544592524342804, 5.153800228976336051, 61.04057627198103120 ) ) ;
#176280=CARTESIAN_POINT ( 'NONE',  ( 10.72451020669898902, -18.67979575497178502, 22.91557627198102765 ) ) ;
#176281=CARTESIAN_POINT ( 'NONE',  ( 17.50000000000000355, 5.500000000000011546, 78.78230962303567253 ) ) ;
#176282=CARTESIAN_POINT ( 'NONE',  ( -9.474510206698720793, -16.51473224551083518, 99.58442372801900433 ) ) ;
#176283=CARTESIAN_POINT ( 'NONE',  ( -19.03943276465977164, -0.05219959533935918106, 53.75109039468566863 ) ) ;
#176284=CARTESIAN_POINT ( 'NONE',  ( -5.823673210054116645, -21.52544592524344225, 82.29057627198103830 ) ) ;
#176285=CARTESIAN_POINT ( 'NONE',  ( -16.52544592524342804, 4.483927247898546575, 26.04057627198103475 ) ) ;
#176286=CARTESIAN_POINT ( 'NONE',  ( -18.67979575497178146, -10.72451020669898902, 41.66557627198103120 ) ) ;
#176287=CARTESIAN_POINT ( 'NONE',  ( 15.80617190586746368, 15.72974639402197994, 79.37390960531436690 ) ) ;
#176288=CARTESIAN_POINT ( 'NONE',  ( 16.51473224551083163, -9.474510206698727899, 100.8344237280190043 ) ) ;
#176289=CARTESIAN_POINT ( 'NONE',  ( -16.46253265017160317, 9.564922557960807481, 110.8322429386476955 ) ) ;
#176290=CARTESIAN_POINT ( 'NONE',  ( 21.55341960407619695, -5.719274019375665929, 81.04275706135236135 ) ) ;
#176291=CARTESIAN_POINT ( 'NONE',  ( 5.049401038298161559, -19.05341960407611168, 77.70724293864765286 ) ) ;
#176293=CARTESIAN_POINT ( 'NONE',  ( -16.46253265017160317, 9.564922557960807481, 75.83224293864769550 ) ) ;
#176294=CARTESIAN_POINT ( 'NONE',  ( 4.483927247898545687, 16.52544592524342804, 94.79057627198105251 ) ) ;
#176296=CARTESIAN_POINT ( 'NONE',  ( -5.153800228976607833, 19.02544592524334988, 107.7094237280189759 ) ) ;
#176298=CARTESIAN_POINT ( 'NONE',  ( 19.03943276465977164, -0.05219959533909143690, 78.74890960531436690 ) ) ;
#176299=CARTESIAN_POINT ( 'NONE',  ( 21.53943276465977519, 0.05219959533937863772, 86.25109039468568994 ) ) ;
#176300=CARTESIAN_POINT ( 'NONE',  ( 16.51473224551069308, 9.474510206698969483, 94.16557627198103830 ) ) ;
#176301=CARTESIAN_POINT ( 'NONE',  ( 14.29746914071037800, 8.314922557961029526, 76.66775706135234714 ) ) ;
#176303=CARTESIAN_POINT ( 'NONE',  ( 16.51473224551083163, -9.474510206698727899, 55.83442372801899722 ) ) ;
#176304=CARTESIAN_POINT ( 'NONE',  ( -19.02544592524334988, -5.153800228976617603, 18.95942372801899722 ) ) ;
#176308=CARTESIAN_POINT ( 'NONE',  ( 8.224510206698742110, 14.34966873604972548, 112.0844237280190185 ) ) ;
#176311=CARTESIAN_POINT ( 'NONE',  ( -16.53943276465976808, -0.05219959533934237506, 103.7510903946857042 ) ) ;
#176312=CARTESIAN_POINT ( 'NONE',  ( 17.49999999999999645, 5.622605283950886879, 68.81207310596114723 ) ) ;
#176313=( BOUNDED_SURFACE ( )  B_SPLINE_SURFACE ( 3, 2, ( 
 ( #85033, #131554, #86048, #160894, #84036, #5197, #70891, #66879, #181079, #197235, #13209, #89041, #56728, #10223, #44535, #75849, #72901, #73893, #88038, #105208, #199207, #104217, #152690, #165898, #134570, #25408, #119396, #196257, #42554, #27396, #29373, #166895, #106190, #198215, #57726, #58696, #150731, #184038, #164905, #135563, #14179, #136534, #167874, #121358, #71883, #133553, #148735, #41560, #91004, #12231, #120366, #182059, #103223, #87050, #28395, #137525, #43542, #60674, #90034, #151716, #122349, #59687, #74872, #102223, #183051, #195244, #163912, #118398, #180092, #26399, #149726, #11227, #140503, #107175, #93995, #126326, #49495, #127309, #186034, #187043, #984, #172846, #170851, #109172, #123333, #65647, #188023, #111157, #62659, #1992, #34327, #48513, #110167, #30351, #124338, #76842, #45521, #185026, #33334, #168846, #157673, #32342, #95988, #142489, #171846, #91993, #47516, #15183, #19162, #80810, #94994, #3967, #155676, #153687, #17171, #138513, #92029, #154684, #61664, #156680, #46513, #108172, #18174, #79831, #169853, #77834, #31347, #78825, #92998, #63671, #16179, #141501, #139501, #2985, #125345, #64664, #130288, #5958, #174829, #68632, #23145, #160649, #37300, #189020, #51477, #115146, #112158, #84789, #98959, #162649, #22141, #131309, #24155, #38310, #144474, #83791, #176839, #129295, #145471, #175827, #69643, #113139, #128303, #50494, #36293, #191982, #6952, #67636, #85806, #97949, #159641, #99965, #54476, #20139, #190991, #52467, #158647, #147492, #53469, #161649, #146468, #192999, #190003, #177837, #8983, #116146, #39305, #7960, #100964, #114125, #70651, #173847, #35313, #96967, #81784, #143471, #4955, #21137, #66640, #82792, #164661, #182816, #120132, #181823, #167642, #56477, #163661, #148492, #55472, #26156, #73654, #59448, #103977, #104970, #25164, #194009, #29138, #117142, #178837, #40305, #87798, #121121, #101981, #44298, #194999, #196999, #118155, #89800, #151482, #74637, #136303, #43302, #86806, #9983, #166657, #90775, #197978, #105957, #102976, #149483, #152459, #132317, #10979, #165656, #179845, #13945, #88801, #71643, #133310, #58465, #119157, #41316, #72652, #134327, #42316, #196012, #57487, #180839, #28158, #12973, #27154, #150494, #135326, #11991, #60439, #31115, #106943, #75611, #14949, #63433, #95752, #187794, #139275, #64428, #172607, #78590, #198972, #154453, #45291, #79593, #110921, #140263, #126098, #92763, #34094, #47282, #49263, #168616, #184790, #157437, #1755, #122114, #138287, #125109, #186807, #137290, #107932, #183803, #108938, #30116, #93765, #153451, #48277, #169618, #91757, #141262, #76609, #15945, #170619, #109932, #62423, #199968, #61433, #17939, #123105, #46276, #32108, #77604, #171614, #752, #124095, #185794, #155446, #16936, #33102, #94758, #156440, #2752, #20900, #146231, #83558, #22907, #114907, #189774, #175589, #5724, #100728, #81551, #190759, #69404, #53231, #84553, #38075, #188782, #50265, #65413, #158421, #7718, #51246, #36066, #112906, #19909, #142251, #21907, #131070, #174600, #161415, #52234, #82558, #177603, #176601, #37065, #192759, #144240, #111923, #39071, #35079, #113891, #173609, #96732, #145237, #98724, #80577, #67403, #99731, #54242, #18932, #159405, #160418, #97715, #115913, #129058, #6718, #143237, #3736, #127074, #4720, #68396, #130048, #66409, #191748, #128071, #180611, #40061, #165428, #56238, #23911, #166428, #59214, #41081, #57252, #73424, #149256, #116905, #70412, #104737, #136073, #133074, #134089, #148253, #26923, #120883, #164432, #12742, #25926, #194764, #85565, #179608, #117919, #102744, #87569, #89566, #88565, #27923, #58239, #10748, #118926, #72412, #44065, #24924, #195779, #74407, #196771, #151252, #181593, #132079, #193768, #8742, #101738, #197747, #42084, #103749, #150263, #163426, #147251, #11757, #182582, #135095, #162409, #119907, #43070, #55237, #178598, #86569, #9746, #71410, #75381 ),
 ( #47041, #61197, #32863, #30880, #169372, #183571, #125857, #48038, #186565, #122869, #513, #109694, #108698, #170377, #90548, #184557, #137053, #105725, #45056, #93522, #187557, #17695, #92527, #94513, #2510, #31868, #28908, #46038, #198743, #171376, #141023, #155207, #156195, #107693, #64190, #77366, #79352, #60208, #14713, #167412, #16696, #152230, #168388, #78346, #140020, #13715, #1509, #63186, #121878, #29883, #106714, #91521, #153208, #199731, #124866, #76373, #139034, #138050, #154216, #15706, #62185, #123849, #185547, #157195, #4476, #176358, #33849, #37831, #111681, #113653, #173368, #6476, #68156, #191507, #52983, #160174, #18689, #3497, #36815, #7477, #114662, #99491, #19673, #81315, #161171, #49024, #127828, #82310, #96493, #69161, #5481, #172359, #65173, #175347, #35829, #22668, #50016, #84315, #159161, #34838, #145994, #158183, #98481, #21664, #142998, #144995, #130828, #66166, #190520, #189534, #51006, #128821, #83318, #20656, #97475, #110679, #112667, #129808, #95509, #80336, #144000, #142008, #67164, #126832, #188538, #174359, #51994, #164189, #118680, #132836, #25687, #179370, #73186, #116667, #131840, #54002, #39822, #133843, #149018, #148017, #89325, #54998, #101488, #103509, #58005, #23670, #9506, #55995, #162172, #27684, #40832, #87332, #195533, #134857, #193523, #181358, #151017, #119675, #42837, #165185, #41841, #194523, #117673, #12508, #26680, #88320, #104502, #166183, #102505, #178358, #10506, #150010, #24681, #74172, #115676, #71172, #85318, #196535, #192519, #57007, #177364, #72168, #38835, #180372, #100493, #147010, #163177, #8495, #11516, #70172, #86330, #64699, #188057, #112192, #168146, #173881, #110199, #97002, #156715, #13478, #141534, #29643, #197511, #142524, #35351, #14465, #33367, #49527, #125379, #90306, #43822, #80847, #158684, #106467, #171878, #121636, #3023, #20173, #137805, #189058, #199489, #91275, #58979, #152966, #76127, #63704, #187076, #65681, #126361, #4002, #34361, #48545, #95025, #18207, #135842, #198498, #79865, #50530, #172881, #127344, #157708, #105486, #167172, #182344, #75143, #120646, #111190, #96022, #19198, #136814, #28671, #151992, #59969, #183331, #44812, #53503, #83825, #40340, #116181, #99998, #194044, #6987, #51512, #102015, #97983, #115180, #174864, #36330, #84823, #176873, #143506, #130322, #162684, #85840, #163697, #22175, #23180, #37336, #9018, #68667, #145506, #159677, #81819, #24190, #147530, #98994, #38342, #70686, #146503, #7993, #66677, #160683, #113174, #4992, #21173, #69677, #128339, #55508, #192019, #132352, #178873, #131344, #175863, #190038, #117178, #82828, #161683, #193032, #54509, #177872, #144509, #5994, #67673, #129331, #52501, #39340, #191026, #100999, #114161, #27188, #75645, #88835, #196046, #148527, #42350, #57521, #165690, #150528, #152491, #89835, #29172, #121156, #119190, #181857, #12027, #106974, #87831, #197033, #137323, #59482, #90808, #44332, #195035, #56512, #71677, #164696, #13978, #180874, #104012, #73690, #26191, #10018, #28193, #199004, #135362, #167675, #58500, #120166, #183835, #182849, #43336, #60470, #105004, #118190, #45324, #41349, #166690, #179881, #103012, #151516, #13007, #86842, #74671, #105989, #122146, #25199, #136338, #198012, #133344, #149517, #11014, #72687, #134362, #188811, #110951, #49293, #124129, #63466, #172636, #171643, #33133, #153484, #185828, #200000, #168648, #107964, #156470, #50295, #80608, #32139, #157469, #65442, #94790, #91790, #47315, #138318, #34124, #3765, #17971, #18962, #108970, #127103, #140297, #142285, #61466, #77636, #30147, #79625, #14980, #31147, #141293, #2783, #76640, #784, #123137, #1788, #184823, #186840, #46308, #64461, #95783, #126129, #169651, #187824, #139305, #125141, #155476, #92795, #154483, #48309, #15977, #62455, #170651, #93796, #16968, #78621, #109964, #51276, #115945, #144269, #129089, #82588, #112937, #35110, #114939, #177635, #67432 ),
 ( #66439, #176632, #6749, #173641, #160447, #192790, #39102, #193799, #52263, #53262, #190789, #100758, #37095, #175620, #189804, #132107, #54272, #162440, #113921, #68428, #23941, #38107, #99762, #96762, #98754, #143266, #111952, #174630, #161447, #158451, #85595, #21937, #147282, #8772, #22938, #19940, #83588, #81581, #70441, #4750, #84584, #128100, #145268, #36095, #130081, #97747, #159434, #20930, #5756, #146264, #191779, #7748, #69434, #131102, #28940, #87598, #90581, #26954, #13747, #73453, #133105, #58268, #149284, #116935, #59246, #152262, #134120, #150293, #166458, #42116, #9778, #163456, #197780, #75415, #25955, #88596, #41110, #119937, #137087, #57281, #105757, #118955, #10778, #178628, #72444, #195809, #180641, #103778, #120915, #182614, #165457, #11789, #44099, #55266, #135126, #196800, #102774, #40091, #181622, #101769, #71440, #43102, #104770, #167443, #56267, #24954, #27955, #117950, #86601, #164461, #89596, #151283, #12773, #74437, #148284, #136104, #194794, #179640, #184591, #78380, #32899, #170411, #47074, #198775, #61231, #124902, #121912, #94551, #108734, #172400, #31903, #141061, #33890, #48073, #154249, #93556, #186601, #139069, #155242, #185584, #79391, #122902, #138083, #60241, #46072, #140056, #16732, #15740, #95546, #107726, #169407, #109729, #64229, #29916, #77399, #62218, #168421, #157234, #1546, #63222, #171413, #2547, #199764, #187594, #18726, #125894, #49063, #156232, #17733, #547, #123886, #80373, #110718, #183605, #45089, #106746, #91556, #30913, #153243, #14746, #92561, #76407, #129845, #191544, #177401, #66204, #173404, #158219, #65210, #35866, #83356, #69198, #113688, #114702, #34875, #3533, #38873, #126869, #188576, #50056, #97512, #130866, #111718, #192556, #4513, #6514, #127866, #99528, #161210, #84352, #146030, #53021, #96529, #19709, #176395, #100529, #175383, #190557, #142046, #189570, #68193, #81351, #37869, #52030, #115713, #36852, #7513, #162208, #22705, #159198, #98519, #54039, #82348, #160212, #128857, #23706, #51042, #143035, #112704, #174396, #145032, #21702, #20693, #144037, #5519, #67199, #196565, #151048, #116703, #102541, #149052, #55033, #120678, #133878, #57042, #26714, #27715, #86365, #74203, #43855, #12538, #135872, #58036, #134889, #87367, #10540, #182377, #119706, #181389, #197543, #59011, #25721, #9540, #118716, #42868, #117707, #105520, #73218, #104533, #167205, #71207, #178393, #101523, #8531, #179403, #88353, #85354, #180405, #166214, #39857, #147047, #70209, #131876, #193561, #163214, #40867, #24716, #148050, #132870, #194559, #150046, #56029, #89358, #164224, #72204, #195569, #41877, #103544, #165219, #11552, #187348, #94306, #155984, #199522, #60990, #17481, #28703, #107485, #61976, #76161, #48818, #185339, #152024, #183365, #93311, #15501, #79138, #29676, #140809, #138828, #91308, #63981, #137841, #16491, #154995, #14499, #124654, #110471, #122664, #170168, #45834, #184352, #108489, #62974, #169163, #2299, #90339, #30667, #123642, #92320, #13510, #46829, #75175, #44847, #78140, #77158, #125651, #153000, #136847, #308, #154005, #198532, #31661, #139808, #1296, #186350, #47830, #60003, #109482, #171165, #32652, #121670, #106503, #168180, #143790, #20447, #172153, #34631, #98262, #95301, #67950, #82098, #145786, #5273, #114445, #7268, #21451, #127626, #66954, #159964, #112461, #128616, #158957, #52776, #96290, #111471, #33639, #19469, #113445, #190309, #189326, #68952, #157977, #81114, #83112, #37616, #3295, #50803, #35624, #141802, #130615, #51785, #175138, #36605, #176146, #173156, #160965, #192311, #99278, #22459, #144789, #6272, #174153, #97269, #53791, #129604, #191300, #84107, #156985, #18483, #142794, #80132, #64967, #4274, #126626, #188327, #49806, #65955, #39616, #146792, #131629, #38628, #9298, #56801, #42627, #87124, #88115, #8285, #177155, #150805, #100285, #161963, #23459, #70964, #104291, #85106, #165972 ),
 ( #10299, #119469, #69963, #11305, #25482, #89117, #148809, #57798, #12301, #164978, #132632, #71956, #41634, #55788, #133629, #102296, #196330, #101275, #54787, #193313, #162965, #118474, #195321, #194320, #73967, #178151, #24471, #26473, #181152, #116462, #117459, #179158, #86121, #135636, #163985, #180164, #103299, #27474, #147812, #197306, #115466, #40626, #149799, #72975, #134644, #167947, #29445, #46589, #107250, #92074, #138587, #68, #106263, #136606, #75925, #153763, #121432, #61739, #45597, #168921, #185100, #74943, #105279, #90104, #120438, #183125, #60750, #123407, #14254, #30427, #166967, #58770, #169930, #43615, #28469, #151788, #91077, #108250, #13279, #182131, #137600, #198286, #199283, #59764, #44608, #152764, #122423, #184115, #15258, #76916, #76663, #166710, #90827, #59501, #182870, #44351, #164716, #135382, #11033, #179902, #119209, #167696, #200022, #91814, #43355, #168670, #138342, #106010, #103034, #58520, #149538, #183858, #15003, #29193, #30170, #197052, #61490, #151537, #153506, #72709, #88854, #41368, #152510, #26211, #42369, #13999, #75666, #87850, #12046, #134381, #120186, #13026, #137343, #181876, #74691, #28214, #60492, #104032, #180894, #196067, #27208, #121176, #136357, #105026, #57540, #165711, #150547, #199023, #45345, #73710, #89854, #198033, #122168, #106997, #171669, #94817, #64486, #65468, #124153, #111977, #81607, #188837, #173669, #34150, #172663, #125166, #186865, #19965, #95809, #18988, #50322, #35136, #63490, #47339, #156495, #80634, #155500, #96788, #110978, #157495, #158477, #108994, #154506, #139329, #46332, #16993, #126153, #143291, #17997, #142311, #16002, #184848, #4777, #107987, #169674, #31170, #78647, #123160, #92820, #77660, #185852, #187849, #170675, #3791, #127131, #808, #62481, #32163, #93820, #140322, #1812, #48334, #109989, #33158, #79650, #141319, #2808, #49318, #145292, #99787, #113946, #86622, #22962, #189829, #20955, #131126, #53285, #193823, #67457, #55288, #176657, #129115, #101791, #175645, #54296, #192814, #52289, #162463, #148305, #37119, #7776, #83614, #98778, #146289, #100780, #38134, #114964, #66465, #190814, #115968, #51301, #23964, #161473, #40113, #84610, #8795, #163479, #177656, #116960, #39125, #85619, #68454, #130108, #24976, #147306, #70465, #132130, #178651, #6775, #160472, #69459, #128127, #21963, #112962, #174655, #36120, #97772, #191804, #159459, #82612, #144293, #5783, #151304, #137108, #181642, #182634, #102796, #71461, #45108, #133126, #194816, #117971, #165478, #198794, #56289, #60260, #72468, #74458, #134141, #167464, #28959, #152282, #13766, #120935, #179662, #164482, #197800, #183626, #149305, #90600, #119956, #180661, #121931, #9799, #88617, #43121, #57301, #29936, #166477, #41132, #25976, #136124, #196820, #106765, #10799, #168440, #104789, #195830, #91575, #118978, #59266, #44118, #42137, #105777, #87619, #103798, #12793, #26974, #150314, #89615, #75434, #27976, #58287, #11810, #73474, #135147, #76426, #49079, #63240, #126886, #186617, #95562, #188592, #2563, #108753, #124920, #79407, #93575, #48089, #140074, #33905, #77418, #92580, #14765, #565, #94571, #109745, #170429, #50073, #15759, #62236, #64245, #18743, #184610, #31921, #16750, #122922, #111734, #1565, #171429, #156249, #157249, #154268, #142062, #173421, #80390, #34891, #123904, #141078, #125912, #139090, #110736, #153264, #185603, #17751, #155260, #47092, #32916, #187610, #172417, #3548, #138102, #78398, #65226, #199783, #61251, #46091, #107746, #169427, #30932, #70225, #146046, #52049, #68210, #22721, #36870, #129862, #83372, #177417, #20710, #35881, #158234, #144054, #37887, #53039, #113705, #193577, #159215, #5536, #7530, #162224, #127881, #175402, #160228, #66221, #131893, #145049, #191560, #99545, #38888, #97528, #85372, #55049, #23723, #147065, #69215, #130883, #98535, #21719, #116720, #192572, #54056, #8548, #178409, #6530, #82366, #114719 ),
 ( #176411, #115730, #189585, #19725, #96547, #81366, #143050, #4529, #161227, #51057, #112719, #174412, #67215, #84369, #128873, #100545, #190573, #182392, #43870, #151062, #9557, #194575, #27730, #13526, #179419, #197559, #150062, #10556, #28719, #39873, #118733, #73233, #87383, #60019, #196581, #163232, #56045, #104548, #26729, #167221, #40884, #90356, #11567, #102557, #134904, #105535, #75192, #89373, #195586, #58051, #166230, #180421, #119722, #88368, #120693, #164242, #25737, #101540, #149068, #181405, #42883, #57058, #136863, #72220, #133895, #12553, #152041, #71223, #41894, #103560, #132886, #198549, #74219, #135887, #59026, #121686, #165235, #24732, #86382, #148066, #117724, #94322, #32669, #185354, #46845, #80146, #156000, #79154, #48833, #110486, #123657, #107502, #16508, #140825, #15516, #33654, #171181, #17497, #18498, #169178, #14516, #199537, #106519, #77173, #124670, #172169, #155012, #2314, #76177, #44864, #141817, #168197, #29694, #91325, #138843, #95315, #153017, #157000, #45849, #47846, #30684, #63996, #125666, #187364, #3310, #64983, #137857, #61007, #183382, #122679, #184368, #92335, #93327, #154021, #323, #61991, #108505, #78156, #170184, #31678, #139824, #1313, #62992, #109499, #186367, #53808, #127641, #115483, #36622, #189341, #161979, #35639, #114460, #52792, #112476, #22475, #146808, #174169, #67966, #143805, #97285, #6287, #160981, #98279, #175155, #126641, #50819, #176162, #49822, #84123, #159980, #100301, #65971, #145802, #21466, #158972, #177171, #188343, #5288, #83128, #20464, #8302, #144804, #111486, #81129, #191315, #113461, #38644, #82114, #23475, #129620, #66971, #85124, #128631, #37632, #99295, #190325, #7285, #173171, #51802, #68969, #130633, #192327, #34647, #96306, #157992, #19484, #142810, #4290, #196345, #193329, #165989, #180181, #43631, #103314, #12317, #105294, #119485, #25497, #41650, #57813, #10314, #164994, #56816, #150820, #194336, #9315, #131647, #117476, #11320, #26488, #87140, #166982, #132648, #179174, #181167, #135651, #101292, #148824, #133645, #39632, #28485, #118490, #88130, #72990, #73982, #70980, #58785, #90119, #197322, #120454, #42644, #104306, #71971, #195336, #151803, #27489, #89132, #182147, #69979, #149814, #55804, #134659, #54803, #102311, #116478, #178167, #162982, #24487, #40642, #86138, #147829, #164001, #110015, #157521, #143317, #187875, #188865, #106277, #74959, #51330, #136621, #198302, #121448, #171696, #4804, #59779, #66493, #75941, #80661, #137616, #173696, #35164, #158504, #19991, #127157, #183140, #167962, #3817, #189856, #18024, #79677, #112990, #65495, #112007, #81634, #128156, #156525, #199300, #49343, #96819, #48361, #174683, #50348, #36148, #97800, #60767, #44624, #29461, #91093, #33185, #19015, #13294, #111005, #152781, #14272, #122439, #184131, #94844, #141348, #2835, #64513, #126180, #172691, #34176, #95837, #142337, #83643, #116987, #178680, #101820, #163508, #70492, #129144, #113975, #147336, #133155, #98806, #40143, #69489, #130136, #148334, #159489, #38161, #192843, #6803, #179691, #115995, #82639, #175673, #23992, #146316, #86650, #160500, #9829, #131154, #21990, #194846, #68481, #8823, #85649, #145320, #55316, #41163, #191833, #100808, #176686, #53314, #39152, #193851, #54323, #7805, #20982, #114992, #132159, #144322, #25006, #177684, #56319, #162491, #71489, #118002, #5811, #99816, #67486, #190841, #161501, #52317, #37147, #22991, #84639, #42166, #164512, #150343, #44147, #59295, #58316, #199813, #165506, #11839, #13797, #168469, #134171, #119984, #166507, #72497, #138132, #151333, #74488, #105806, #45138, #103826, #91605, #61281, #29967, #153294, #75462, #152311, #43149, #136154, #89645, #183654, #27002, #88647, #26005, #73504, #167493, #120964, #181670, #122951, #135176, #196850, #137136, #14795, #195859, #104818, #28005, #57331, #184639, #12822, #197829, #28989, #106795, #182663, #76455, #102826, #87647 ),
 ( #90629, #198823, #149333, #60288, #10827, #121961, #119007, #180690, #48118, #4561, #80421, #64274, #158266, #171458, #15787, #66253, #62265, #79436, #139118, #594, #49109, #141107, #107773, #94601, #126917, #50104, #127913, #186647, #187639, #1595, #173453, #32946, #109775, #123933, #46120, #188623, #143082, #156280, #157278, #125941, #110767, #172448, #30960, #63270, #77447, #169459, #185631, #33936, #92607, #19755, #17781, #34921, #154297, #95594, #47123, #124951, #108781, #111764, #81396, #18774, #96577, #2595, #170459, #142094, #31950, #93605, #155290, #16780, #3579, #78429, #140104, #65257, #38918, #163265, #21750, #24767, #161257, #148099, #7561, #67245, #192603, #83401, #51089, #193609, #86414, #68239, #55081, #9591, #129892, #84400, #100575, #176443, #144085, #97558, #131925, #71256, #160260, #22751, #175433, #54086, #189615, #191592, #39909, #53071, #145079, #112749, #6561, #114749, #37916, #99575, #116751, #115760, #178441, #85406, #146076, #69247, #130913, #174443, #52080, #177448, #101575, #23756, #35912, #8583, #159246, #20741, #82397, #128904, #5566, #162257, #147098, #70257, #190604, #113736, #36902, #98566, #88402, #75223, #104581, #134936, #91355, #167252, #151096, #44893, #58084, #102591, #153047, #149101, #166265, #25770, #87416, #135921, #27764, #194607, #181437, #13557, #136895, #14548, #73267, #74252, #150096, #60050, #119754, #196614, #10591, #132920, #198582, #29723, #42915, #43903, #12587, #197592, #59058, #117760, #11599, #164275, #56079, #72252, #120725, #179452, #106550, #89407, #121717, #40918, #182425, #133930, #105566, #195620, #183410, #168226, #28751, #57092, #90387, #118766, #152072, #180455, #41927, #103593, #165268, #26762, #61036, #138872, #2346, #125697, #49852, #108536, #111517, #47876, #34678, #94352, #154050, #79187, #170215, #137886, #15545, #140857, #31708, #199567, #80177, #173202, #155043, #171211, #187396, #63024, #30716, #184398, #18530, #96336, #46875, #109529, #62022, #64027, #158023, #78185, #126671, #139854, #93357, #122708, #16538, #1343, #124702, #186399, #3340, #48864, #141849, #172200, #32701, #156031, #17528, #76207, #352, #110519, #188375, #33685, #65014, #95348, #45878, #107531, #169208, #77203, #92364, #157032, #123686, #185385, #20495, #142841, #22506, #85155, #175187, #162011, #191346, #21499, #178198, #53842, #37664, #131679, #144834, #189372, #39663, #35668, #52824, #112506, #174200, #84153, #114493, #81159, #67997, #100333, #23507, #101324, #160011, #161012, #36653, #146841, #6318, #83160, #97316, #19514, #8334, #116510, #129650, #130665, #99329, #145832, #7314, #4320, #98311, #50849, #66003, #159002, #68999, #127672, #193360, #176195, #70010, #82143, #192359, #143839, #115516, #5318, #54836, #67002, #177204, #128661, #38677, #190356, #51833, #113492, #194368, #72002, #121478, #89162, #147861, #25530, #150853, #12347, #136650, #195367, #198332, #134691, #183171, #181199, #87174, #74011, #86171, #58817, #73021, #59808, #196376, #105324, #44654, #135681, #118522, #57845, #197353, #103345, #119517, #149846, #43662, #148855, #102343, #24520, #10346, #104337, #42676, #180211, #163013, #133676, #56846, #120485, #28513, #55835, #41681, #26517, #132680, #9347, #11350, #166021, #27521, #167012, #164032, #151832, #71012, #90148, #13322, #182176, #74987, #165024, #88161, #117508, #179205, #40673, #171968, #33455, #46635, #30470, #139618, #2112, #138633, #156803, #94116, #155795, #141621, #92120, #137644, #122468, #29489, #114, #47637, #95114, #77951, #78946, #199331, #167992, #3110, #91122, #152811, #14304, #61783, #18296, #75971, #79951, #168964, #170970, #153808, #63793, #125466, #48634, #110286, #17292, #60796, #184160, #140622, #64786, #45641, #187163, #16301, #76962, #126447, #106307, #185144, #1104, #15302, #188145, #62780, #107293, #123452, #32463, #93118, #108295, #169974, #31466, #124461, #154803, #186158, #109291, #37427 ),
 ( #52592, #34448, #5082, #80934, #49617, #189143, #99087, #69765, #161776, #113261, #38436, #146594, #114252, #172970, #128425, #19287, #53597, #84915, #175958, #100092, #66764, #8088, #21265, #23271, #142610, #158770, #131434, #160778, #96107, #112275, #22267, #83917, #111280, #81905, #157796, #82921, #4089, #67763, #127437, #145599, #143598, #65767, #115273, #50616, #190121, #144598, #7078, #36416, #173967, #35435, #192115, #97087, #20259, #6084, #51597, #68759, #174953, #98070, #159770, #129420, #191118, #130416, #176966, #25289, #133436, #195125, #120252, #57608, #197119, #88926, #163788, #149609, #179972, #74760, #55595, #164786, #43426, #27278, #58586, #12114, #162771, #24280, #39426, #132441, #181943, #86932, #10106, #148615, #194132, #116268, #196137, #105095, #71766, #135450, #26280, #56607, #151603, #150618, #11107, #166781, #118281, #85929, #13094, #9105, #87922, #147618, #70772, #119277, #72782, #54594, #41438, #73777, #28282, #193120, #103105, #134452, #180960, #89921, #42437, #104100, #117270, #177958, #101086, #178963, #165783, #40432, #102103, #139390, #46396, #137409, #171737, #45408, #124222, #62547, #122232, #32228, #156566, #183923, #77724, #153570, #107061, #16066, #170737, #108054, #184911, #136422, #199089, #185919, #59568, #93886, #169739, #110057, #31234, #78713, #33225, #47404, #91878, #92883, #109060, #76728, #154570, #123221, #17058, #60557, #75733, #198102, #168732, #872, #155564, #15067, #94885, #30236, #138403, #140389, #1877, #167760, #200084, #61552, #106073, #18064, #63558, #125232, #186930, #48400, #121243, #182937, #44420, #29258, #90890, #152576, #14066, #81674, #143357, #176726, #129182, #175710, #145360, #6842, #20032, #3857, #113029, #37188, #112048, #130175, #67525, #190880, #115033, #65536, #111047, #95878, #2876, #173736, #21023, #68521, #51368, #52356, #172734, #141388, #38199, #64555, #126219, #187915, #35205, #191872, #49384, #53355, #142378, #144362, #127196, #98846, #160541, #22030, #83682, #114012, #34215, #157561, #99855, #161539, #19054, #79719, #189893, #50388, #80701, #188908, #158542, #174721, #96858, #4846, #36184, #66532, #128195, #5849, #97838, #159526, #82678, #14591, #28788, #91398, #181475, #168267, #197628, #27802, #184438, #60089, #43942, #137925, #151133, #192884, #45918, #39192, #59094, #116034, #177723, #90427, #120760, #84677, #74289, #106591, #29764, #107572, #166306, #167291, #42953, #153087, #12624, #89443, #103631, #23032, #76247, #122747, #135958, #136934, #105604, #152113, #13596, #7843, #104617, #54362, #146356, #165307, #75263, #69529, #199609, #182461, #61075, #131194, #198623, #26801, #121757, #88442, #150137, #11638, #183450, #73305, #44934, #134976, #196653, #58122, #119791, #78224, #127710, #95387, #154090, #31748, #157073, #18569, #142878, #1384, #4358, #140901, #189411, #187436, #46917, #172239, #63065, #30757, #173242, #66043, #47916, #64066, #80216, #156071, #123728, #77242, #111557, #50887, #139895, #2387, #155083, #33724, #169249, #171252, #19553, #32740, #124744, #92404, #186440, #109570, #94392, #17569, #96375, #141887, #34717, #65053, #79230, #125736, #48903, #15584, #93396, #110558, #81197, #3378, #158062, #188413, #138910, #390, #62063, #108577, #185426, #126709, #49890, #170254, #16577, #174240, #35708, #51873, #69036, #130701, #131715, #98351, #193396, #176232, #54872, #161048, #67041, #84189, #160050, #112545, #8372, #97355, #191384, #145869, #38712, #99365, #190397, #5358, #70047, #178234, #144872, #22542, #21538, #192396, #159041, #114531, #116546, #37702, #6355, #143877, #52860, #68035, #7352, #53878, #20534, #177240, #82182, #128700, #115552, #100369, #162048, #113532, #23544, #85191, #175226, #36691, #83198, #129687, #146880, #124391, #139552, #32392, #97021, #125397, #110217, #63722, #94047, #16232, #96040, #158702, #48564, #35369, #64717, #95045, #51531, #127365, #111210, #5013, #18227 ) ),
 .UNSPECIFIED., .T., .F., .T. ) 
 B_SPLINE_SURFACE_WITH_KNOTS ( ( 4, 3, 4 ),
 ( 3, 2, 2, 2, 2, 2, 2, 2, 2, 2, 2, 2, 2, 2, 2, 2, 2, 2, 2, 2, 2, 2, 2, 2, 2, 2, 2, 2, 2, 2, 2, 2, 2, 2, 2, 2, 2, 2, 2, 2, 2, 2, 2, 2, 2, 2, 2, 2, 2, 2, 2, 2, 2, 2, 2, 2, 2, 2, 2, 2, 2, 2, 2, 2, 2, 2, 2, 2, 2, 2, 2, 2, 2, 2, 2, 2, 2, 2, 2, 2, 2, 2, 2, 2, 2, 2, 2, 2, 2, 2, 2, 2, 2, 2, 2, 2, 2, 2, 2, 2, 2, 2, 2, 2, 2, 2, 2, 2, 2, 2, 2, 2, 2, 2, 2, 2, 2, 2, 2, 2, 2, 2, 2, 2, 2, 2, 2, 2, 2, 2, 2, 2, 2, 2, 2, 2, 2, 2, 2, 2, 2, 2, 2, 2, 2, 2, 2, 2, 2, 2, 2, 2, 2, 2, 2, 2, 2, 2, 2, 2, 2, 2, 2, 2, 2, 2, 2, 2, 2, 2, 2, 2, 2, 2, 2, 2, 2, 2, 2, 2, 2, 2, 2, 2, 2, 2, 2, 2, 2, 2, 2, 2, 2, 2, 2, 2, 2, 2, 2, 2, 2, 2, 2, 2, 2, 2, 2, 2, 2, 2, 2, 2, 2, 2, 2, 2, 2, 2, 2, 2, 2, 2, 2, 2, 2, 2, 2, 2, 3 ),
 ( 0.000000000000000000, 0.5000000000000000000, 1.000000000000000000 ),
 ( 0.000000000000000000, 0.004385964912280701511, 0.008771929824561403022, 0.01315789473684210453, 0.01754385964912280604, 0.02192982456140350755, 0.02631578947368420907, 0.03070175438596491058, 0.03508771929824561209, 0.03947368421052631360, 0.04385964912280701511, 0.04824561403508771662, 0.05263157894736841813, 0.05701754385964911964, 0.06140350877192982115, 0.06578947368421052266, 0.07017543859649122417, 0.07456140350877192569, 0.07894736842105262720, 0.08333333333333332871, 0.08771929824561403022, 0.09210526315789473173, 0.09649122807017543324, 0.1008771929824561348, 0.1052631578947368363, 0.1096491228070175378, 0.1140350877192982393, 0.1184210526315789408, 0.1228070175438596423, 0.1271929824561403577, 0.1315789473684210453, 0.1359649122807017607, 0.1403508771929824483, 0.1447368421052631637, 0.1491228070175438514, 0.1535087719298245668, 0.1578947368421052544, 0.1622807017543859698, 0.1666666666666666574, 0.1710526315789473728, 0.1754385964912280604, 0.1798245614035087758, 0.1842105263157894635, 0.1885964912280701788, 0.1929824561403508665, 0.1973684210526315819, 0.2017543859649122695, 0.2061403508771929849, 0.2105263157894736725, 0.2149122807017543879, 0.2192982456140350755, 0.2236842105263157909, 0.2280701754385964786, 0.2324561403508771940, 0.2368421052631578816, 0.2412280701754385970, 0.2456140350877192846, 0.2500000000000000000, 0.2543859649122807154, 0.2587719298245614308, 0.2631578947368420907, 0.2675438596491228060, 0.2719298245614035214, 0.2763157894736842368, 0.2807017543859648967, 0.2850877192982456121, 0.2894736842105263275, 0.2938596491228070429, 0.2982456140350877027, 0.3026315789473684181, 0.3070175438596491335, 0.3114035087719298489, 0.3157894736842105088, 0.3201754385964912242, 0.3245614035087719396, 0.3289473684210526550, 0.3333333333333333148, 0.3377192982456140302, 0.3421052631578947456, 0.3464912280701754610, 0.3508771929824561209, 0.3552631578947368363, 0.3596491228070175517, 0.3640350877192982670, 0.3684210526315789269, 0.3728070175438596423, 0.3771929824561403577, 0.3815789473684210731, 0.3859649122807017330, 0.3903508771929824483, 0.3947368421052631637, 0.3991228070175438791, 0.4035087719298245390, 0.4078947368421052544, 0.4122807017543859698, 0.4166666666666666852, 0.4210526315789473450, 0.4254385964912280604, 0.4298245614035087758, 0.4342105263157894912, 0.4385964912280701511, 0.4429824561403508665, 0.4473684210526315819, 0.4517543859649122973, 0.4561403508771929571, 0.4605263157894736725, 0.4649122807017543879, 0.4692982456140351033, 0.4736842105263157632, 0.4780701754385964786, 0.4824561403508771940, 0.4868421052631579093, 0.4912280701754385692, 0.4956140350877192846, 0.5000000000000000000, 0.5043859649122807154, 0.5087719298245614308, 0.5131578947368421462, 0.5175438596491228616, 0.5219298245614034659, 0.5263157894736841813, 0.5307017543859648967, 0.5350877192982456121, 0.5394736842105263275, 0.5438596491228070429, 0.5482456140350877583, 0.5526315789473684736, 0.5570175438596490780, 0.5614035087719297934, 0.5657894736842105088, 0.5701754385964912242, 0.5745614035087719396, 0.5789473684210526550, 0.5833333333333333703, 0.5877192982456140857, 0.5921052631578946901, 0.5964912280701754055, 0.6008771929824561209, 0.6052631578947368363, 0.6096491228070175517, 0.6140350877192982670, 0.6184210526315789824, 0.6228070175438596978, 0.6271929824561403022, 0.6315789473684210176, 0.6359649122807017330, 0.6403508771929824483, 0.6447368421052631637, 0.6491228070175438791, 0.6535087719298245945, 0.6578947368421053099, 0.6622807017543859143, 0.6666666666666666297, 0.6710526315789473450, 0.6754385964912280604, 0.6798245614035087758, 0.6842105263157894912, 0.6885964912280702066, 0.6929824561403509220, 0.6973684210526315264, 0.7017543859649122417, 0.7061403508771929571, 0.7105263157894736725, 0.7149122807017543879, 0.7192982456140351033, 0.7236842105263158187, 0.7280701754385965341, 0.7324561403508771384, 0.7368421052631578538, 0.7412280701754385692, 0.7456140350877192846, 0.7500000000000000000, 0.7543859649122807154, 0.7587719298245614308, 0.7631578947368421462, 0.7675438596491228616, 0.7719298245614034659, 0.7763157894736841813, 0.7807017543859648967, 0.7850877192982456121, 0.7894736842105263275, 0.7938596491228070429, 0.7982456140350877583, 0.8026315789473684736, 0.8070175438596490780, 0.8114035087719297934, 0.8157894736842105088, 0.8201754385964912242, 0.8245614035087719396, 0.8289473684210526550, 0.8333333333333333703, 0.8377192982456140857, 0.8421052631578946901, 0.8464912280701754055, 0.8508771929824561209, 0.8552631578947368363, 0.8596491228070175517, 0.8640350877192982670, 0.8684210526315789824, 0.8728070175438596978, 0.8771929824561403022, 0.8815789473684210176, 0.8859649122807017330, 0.8903508771929824483, 0.8947368421052631637, 0.8991228070175438791, 0.9035087719298245945, 0.9078947368421053099, 0.9122807017543859143, 0.9166666666666666297, 0.9210526315789473450, 0.9254385964912280604, 0.9298245614035087758, 0.9342105263157894912, 0.9385964912280702066, 0.9429824561403509220, 0.9473684210526315264, 0.9517543859649122417, 0.9561403508771929571, 0.9605263157894736725, 0.9649122807017543879, 0.9692982456140351033, 0.9736842105263158187, 0.9780701754385965341, 0.9824561403508771384, 0.9868421052631578538, 0.9912280701754385692, 0.9956140350877192846, 1.000000000000000000 ),
 .UNSPECIFIED. ) 
 GEOMETRIC_REPRESENTATION_ITEM ( )  RATIONAL_B_SPLINE_SURFACE ( (
 ( 1.000000000000000000, 0.9659258262890683122, 1.000000000000000000, 0.9659258262890683122, 1.000000000000000000, 0.9659258262890683122, 1.000000000000000000, 0.9659258262890683122, 1.000000000000000000, 0.9659258262890683122, 1.000000000000000000, 0.9659258262890683122, 1.000000000000000000, 0.9659258262890683122, 1.000000000000000000, 0.9659258262890683122, 1.000000000000000000, 0.9659258262890683122, 1.000000000000000000, 0.9659258262890683122, 1.000000000000000000, 0.9659258262890683122, 1.000000000000000000, 0.9659258262890683122, 1.000000000000000000, 0.9659258262890683122, 1.000000000000000000, 0.9659258262890683122, 1.000000000000000000, 0.9659258262890683122, 1.000000000000000000, 0.9659258262890683122, 1.000000000000000000, 0.9659258262890683122, 1.000000000000000000, 0.9659258262890683122, 1.000000000000000000, 0.9659258262890683122, 1.000000000000000000, 0.9659258262890683122, 1.000000000000000000, 0.9659258262890683122, 1.000000000000000000, 0.9659258262890683122, 1.000000000000000000, 0.9659258262890683122, 1.000000000000000000, 0.9659258262890683122, 1.000000000000000000, 0.9659258262890683122, 1.000000000000000000, 0.9659258262890683122, 1.000000000000000000, 0.9659258262890683122, 1.000000000000000000, 0.9659258262890683122, 1.000000000000000000, 0.9659258262890683122, 1.000000000000000000, 0.9659258262890683122, 1.000000000000000000, 0.9659258262890683122, 1.000000000000000000, 0.9659258262890683122, 1.000000000000000000, 0.9659258262890683122, 1.000000000000000000, 0.9659258262890683122, 1.000000000000000000, 0.9659258262890683122, 1.000000000000000000, 0.9659258262890683122, 1.000000000000000000, 0.9659258262890683122, 1.000000000000000000, 0.9659258262890683122, 1.000000000000000000, 0.9659258262890683122, 1.000000000000000000, 0.9659258262890683122, 1.000000000000000000, 0.9659258262890683122, 1.000000000000000000, 0.9659258262890683122, 1.000000000000000000, 0.9659258262890683122, 1.000000000000000000, 0.9659258262890683122, 1.000000000000000000, 0.9659258262890683122, 1.000000000000000000, 0.9659258262890683122, 1.000000000000000000, 0.9659258262890683122, 1.000000000000000000, 0.9659258262890683122, 1.000000000000000000, 0.9659258262890683122, 1.000000000000000000, 0.9659258262890683122, 1.000000000000000000, 0.9659258262890683122, 1.000000000000000000, 0.9659258262890683122, 1.000000000000000000, 0.9659258262890683122, 1.000000000000000000, 0.9659258262890683122, 1.000000000000000000, 0.9659258262890683122, 1.000000000000000000, 0.9659258262890683122, 1.000000000000000000, 0.9659258262890683122, 1.000000000000000000, 0.9659258262890683122, 1.000000000000000000, 0.9659258262890683122, 1.000000000000000000, 0.9659258262890683122, 1.000000000000000000, 0.9659258262890683122, 1.000000000000000000, 0.9659258262890683122, 1.000000000000000000, 0.9659258262890683122, 1.000000000000000000, 0.9659258262890683122, 1.000000000000000000, 0.9659258262890683122, 1.000000000000000000, 0.9659258262890683122, 1.000000000000000000, 0.9659258262890683122, 1.000000000000000000, 0.9659258262890683122, 1.000000000000000000, 0.9659258262890683122, 1.000000000000000000, 0.9659258262890683122, 1.000000000000000000, 0.9659258262890683122, 1.000000000000000000, 0.9659258262890683122, 1.000000000000000000, 0.9659258262890683122, 1.000000000000000000, 0.9659258262890683122, 1.000000000000000000, 0.9659258262890683122, 1.000000000000000000, 0.9659258262890683122, 1.000000000000000000, 0.9659258262890683122, 1.000000000000000000, 0.9659258262890683122, 1.000000000000000000, 0.9659258262890683122, 1.000000000000000000, 0.9659258262890683122, 1.000000000000000000, 0.9659258262890683122, 1.000000000000000000, 0.9659258262890683122, 1.000000000000000000, 0.9659258262890683122, 1.000000000000000000, 0.9659258262890683122, 1.000000000000000000, 0.9659258262890683122, 1.000000000000000000, 0.9659258262890683122, 1.000000000000000000, 0.9659258262890683122, 1.000000000000000000, 0.9659258262890683122, 1.000000000000000000, 0.9659258262890683122, 1.000000000000000000, 0.9659258262890683122, 1.000000000000000000, 0.9659258262890683122, 1.000000000000000000, 0.9659258262890683122, 1.000000000000000000, 0.9659258262890683122, 1.000000000000000000, 0.9659258262890683122, 1.000000000000000000, 0.9659258262890683122, 1.000000000000000000, 0.9659258262890683122, 1.000000000000000000, 0.9659258262890683122, 1.000000000000000000, 0.9659258262890683122, 1.000000000000000000, 0.9659258262890683122, 1.000000000000000000, 0.9659258262890683122, 1.000000000000000000, 0.9659258262890683122, 1.000000000000000000, 0.9659258262890683122, 1.000000000000000000, 0.9659258262890683122, 1.000000000000000000, 0.9659258262890683122, 1.000000000000000000, 0.9659258262890683122, 1.000000000000000000, 0.9659258262890683122, 1.000000000000000000, 0.9659258262890683122, 1.000000000000000000, 0.9659258262890683122, 1.000000000000000000, 0.9659258262890683122, 1.000000000000000000, 0.9659258262890683122, 1.000000000000000000, 0.9659258262890683122, 1.000000000000000000, 0.9659258262890683122, 1.000000000000000000, 0.9659258262890683122, 1.000000000000000000, 0.9659258262890683122, 1.000000000000000000, 0.9659258262890683122, 1.000000000000000000, 0.9659258262890683122, 1.000000000000000000, 0.9659258262890683122, 1.000000000000000000, 0.9659258262890683122, 1.000000000000000000, 0.9659258262890683122, 1.000000000000000000, 0.9659258262890683122, 1.000000000000000000, 0.9659258262890683122, 1.000000000000000000, 0.9659258262890683122, 1.000000000000000000, 0.9659258262890683122, 1.000000000000000000, 0.9659258262890683122, 1.000000000000000000, 0.9659258262890683122, 1.000000000000000000, 0.9659258262890683122, 1.000000000000000000, 0.9659258262890683122, 1.000000000000000000, 0.9659258262890683122, 1.000000000000000000, 0.9659258262890683122, 1.000000000000000000, 0.9659258262890683122, 1.000000000000000000, 0.9659258262890683122, 1.000000000000000000, 0.9659258262890683122, 1.000000000000000000, 0.9659258262890683122, 1.000000000000000000, 0.9659258262890683122, 1.000000000000000000, 0.9659258262890683122, 1.000000000000000000, 0.9659258262890683122, 1.000000000000000000, 0.9659258262890683122, 1.000000000000000000, 0.9659258262890683122, 1.000000000000000000, 0.9659258262890683122, 1.000000000000000000, 0.9659258262890683122, 1.000000000000000000, 0.9659258262890683122, 1.000000000000000000, 0.9659258262890683122, 1.000000000000000000, 0.9659258262890683122, 1.000000000000000000, 0.9659258262890683122, 1.000000000000000000, 0.9659258262890683122, 1.000000000000000000, 0.9659258262890683122, 1.000000000000000000, 0.9659258262890683122, 1.000000000000000000, 0.9659258262890683122, 1.000000000000000000, 0.9659258262890683122, 1.000000000000000000, 0.9659258262890683122, 1.000000000000000000, 0.9659258262890683122, 1.000000000000000000, 0.9659258262890683122, 1.000000000000000000, 0.9659258262890683122, 1.000000000000000000, 0.9659258262890683122, 1.000000000000000000, 0.9659258262890683122, 1.000000000000000000, 0.9659258262890683122, 1.000000000000000000, 0.9659258262890683122, 1.000000000000000000, 0.9659258262890683122, 1.000000000000000000, 0.9659258262890683122, 1.000000000000000000, 0.9659258262890683122, 1.000000000000000000, 0.9659258262890683122, 1.000000000000000000, 0.9659258262890683122, 1.000000000000000000, 0.9659258262890683122, 1.000000000000000000, 0.9659258262890683122, 1.000000000000000000, 0.9659258262890683122, 1.000000000000000000, 0.9659258262890683122, 1.000000000000000000, 0.9659258262890683122, 1.000000000000000000, 0.9659258262890683122, 1.000000000000000000, 0.9659258262890683122, 1.000000000000000000, 0.9659258262890683122, 1.000000000000000000, 0.9659258262890683122, 1.000000000000000000, 0.9659258262890683122, 1.000000000000000000, 0.9659258262890683122, 1.000000000000000000, 0.9659258262890683122, 1.000000000000000000, 0.9659258262890683122, 1.000000000000000000, 0.9659258262890683122, 1.000000000000000000, 0.9659258262890683122, 1.000000000000000000, 0.9659258262890683122, 1.000000000000000000, 0.9659258262890683122, 1.000000000000000000, 0.9659258262890683122, 1.000000000000000000, 0.9659258262890683122, 1.000000000000000000, 0.9659258262890683122, 1.000000000000000000, 0.9659258262890683122, 1.000000000000000000, 0.9659258262890683122, 1.000000000000000000, 0.9659258262890683122, 1.000000000000000000, 0.9659258262890683122, 1.000000000000000000, 0.9659258262890683122, 1.000000000000000000, 0.9659258262890683122, 1.000000000000000000, 0.9659258262890683122, 1.000000000000000000, 0.9659258262890683122, 1.000000000000000000, 0.9659258262890683122, 1.000000000000000000, 0.9659258262890683122, 1.000000000000000000, 0.9659258262890683122, 1.000000000000000000, 0.9659258262890683122, 1.000000000000000000, 0.9659258262890683122, 1.000000000000000000, 0.9659258262890683122, 1.000000000000000000, 0.9659258262890683122, 1.000000000000000000, 0.9659258262890683122, 1.000000000000000000, 0.9659258262890683122, 1.000000000000000000, 0.9659258262890683122, 1.000000000000000000, 0.9659258262890683122, 1.000000000000000000, 0.9659258262890683122, 1.000000000000000000, 0.9659258262890683122, 1.000000000000000000, 0.9659258262890683122, 1.000000000000000000, 0.9659258262890683122, 1.000000000000000000, 0.9659258262890683122, 1.000000000000000000, 0.9659258262890683122, 1.000000000000000000, 0.9659258262890683122, 1.000000000000000000, 0.9659258262890683122, 1.000000000000000000, 0.9659258262890683122, 1.000000000000000000, 0.9659258262890683122, 1.000000000000000000, 0.9659258262890683122, 1.000000000000000000, 0.9659258262890683122, 1.000000000000000000, 0.9659258262890683122, 1.000000000000000000, 0.9659258262890683122, 1.000000000000000000, 0.9659258262890683122, 1.000000000000000000, 0.9659258262890683122, 1.000000000000000000, 0.9659258262890683122, 1.000000000000000000, 0.9659258262890683122, 1.000000000000000000, 0.9659258262890683122, 1.000000000000000000, 0.9659258262890683122, 1.000000000000000000, 0.9659258262890683122, 1.000000000000000000, 0.9659258262890683122, 1.000000000000000000, 0.9659258262890683122, 1.000000000000000000, 0.9659258262890683122, 1.000000000000000000, 0.9659258262890683122, 1.000000000000000000, 0.9659258262890683122, 1.000000000000000000, 0.9659258262890683122, 1.000000000000000000),
 ( 0.3333333333333333703, 0.3219752754296894559, 0.3333333333333333703, 0.3219752754296894559, 0.3333333333333333703, 0.3219752754296894559, 0.3333333333333333703, 0.3219752754296894559, 0.3333333333333333703, 0.3219752754296894559, 0.3333333333333333703, 0.3219752754296894559, 0.3333333333333333703, 0.3219752754296894559, 0.3333333333333333703, 0.3219752754296894559, 0.3333333333333333703, 0.3219752754296894559, 0.3333333333333333703, 0.3219752754296894559, 0.3333333333333333703, 0.3219752754296894559, 0.3333333333333333703, 0.3219752754296894559, 0.3333333333333333703, 0.3219752754296894559, 0.3333333333333333703, 0.3219752754296894559, 0.3333333333333333703, 0.3219752754296894559, 0.3333333333333333703, 0.3219752754296894559, 0.3333333333333333703, 0.3219752754296894559, 0.3333333333333333703, 0.3219752754296894559, 0.3333333333333333703, 0.3219752754296894559, 0.3333333333333333703, 0.3219752754296894559, 0.3333333333333333703, 0.3219752754296894559, 0.3333333333333333703, 0.3219752754296894559, 0.3333333333333333703, 0.3219752754296894559, 0.3333333333333333703, 0.3219752754296894559, 0.3333333333333333703, 0.3219752754296894559, 0.3333333333333333703, 0.3219752754296894559, 0.3333333333333333703, 0.3219752754296894559, 0.3333333333333333703, 0.3219752754296894559, 0.3333333333333333703, 0.3219752754296894559, 0.3333333333333333703, 0.3219752754296894559, 0.3333333333333333703, 0.3219752754296894559, 0.3333333333333333703, 0.3219752754296894559, 0.3333333333333333703, 0.3219752754296894559, 0.3333333333333333703, 0.3219752754296894559, 0.3333333333333333703, 0.3219752754296894559, 0.3333333333333333703, 0.3219752754296894559, 0.3333333333333333703, 0.3219752754296894559, 0.3333333333333333703, 0.3219752754296894559, 0.3333333333333333703, 0.3219752754296894559, 0.3333333333333333703, 0.3219752754296894559, 0.3333333333333333703, 0.3219752754296894559, 0.3333333333333333703, 0.3219752754296894559, 0.3333333333333333703, 0.3219752754296894559, 0.3333333333333333703, 0.3219752754296894559, 0.3333333333333333703, 0.3219752754296894559, 0.3333333333333333703, 0.3219752754296894559, 0.3333333333333333703, 0.3219752754296894559, 0.3333333333333333703, 0.3219752754296894559, 0.3333333333333333703, 0.3219752754296894559, 0.3333333333333333703, 0.3219752754296894559, 0.3333333333333333703, 0.3219752754296894559, 0.3333333333333333703, 0.3219752754296894559, 0.3333333333333333703, 0.3219752754296894559, 0.3333333333333333703, 0.3219752754296894559, 0.3333333333333333703, 0.3219752754296894559, 0.3333333333333333703, 0.3219752754296894559, 0.3333333333333333703, 0.3219752754296894559, 0.3333333333333333703, 0.3219752754296894559, 0.3333333333333333703, 0.3219752754296894559, 0.3333333333333333703, 0.3219752754296894559, 0.3333333333333333703, 0.3219752754296894559, 0.3333333333333333703, 0.3219752754296894559, 0.3333333333333333703, 0.3219752754296894559, 0.3333333333333333703, 0.3219752754296894559, 0.3333333333333333703, 0.3219752754296894559, 0.3333333333333333703, 0.3219752754296894559, 0.3333333333333333703, 0.3219752754296894559, 0.3333333333333333703, 0.3219752754296894559, 0.3333333333333333703, 0.3219752754296894559, 0.3333333333333333703, 0.3219752754296894559, 0.3333333333333333703, 0.3219752754296894559, 0.3333333333333333703, 0.3219752754296894559, 0.3333333333333333703, 0.3219752754296894559, 0.3333333333333333703, 0.3219752754296894559, 0.3333333333333333703, 0.3219752754296894559, 0.3333333333333333703, 0.3219752754296894559, 0.3333333333333333703, 0.3219752754296894559, 0.3333333333333333703, 0.3219752754296894559, 0.3333333333333333703, 0.3219752754296894559, 0.3333333333333333703, 0.3219752754296894559, 0.3333333333333333703, 0.3219752754296894559, 0.3333333333333333703, 0.3219752754296894559, 0.3333333333333333703, 0.3219752754296894559, 0.3333333333333333703, 0.3219752754296894559, 0.3333333333333333703, 0.3219752754296894559, 0.3333333333333333703, 0.3219752754296894559, 0.3333333333333333703, 0.3219752754296894559, 0.3333333333333333703, 0.3219752754296894559, 0.3333333333333333703, 0.3219752754296894559, 0.3333333333333333703, 0.3219752754296894559, 0.3333333333333333703, 0.3219752754296894559, 0.3333333333333333703, 0.3219752754296894559, 0.3333333333333333703, 0.3219752754296894559, 0.3333333333333333703, 0.3219752754296894559, 0.3333333333333333703, 0.3219752754296894559, 0.3333333333333333703, 0.3219752754296894559, 0.3333333333333333703, 0.3219752754296894559, 0.3333333333333333703, 0.3219752754296894559, 0.3333333333333333703, 0.3219752754296894559, 0.3333333333333333703, 0.3219752754296894559, 0.3333333333333333703, 0.3219752754296894559, 0.3333333333333333703, 0.3219752754296894559, 0.3333333333333333703, 0.3219752754296894559, 0.3333333333333333703, 0.3219752754296894559, 0.3333333333333333703, 0.3219752754296894559, 0.3333333333333333703, 0.3219752754296894559, 0.3333333333333333703, 0.3219752754296894559, 0.3333333333333333703, 0.3219752754296894559, 0.3333333333333333703, 0.3219752754296894559, 0.3333333333333333703, 0.3219752754296894559, 0.3333333333333333703, 0.3219752754296894559, 0.3333333333333333703, 0.3219752754296894559, 0.3333333333333333703, 0.3219752754296894559, 0.3333333333333333703, 0.3219752754296894559, 0.3333333333333333703, 0.3219752754296894559, 0.3333333333333333703, 0.3219752754296894559, 0.3333333333333333703, 0.3219752754296894559, 0.3333333333333333703, 0.3219752754296894559, 0.3333333333333333703, 0.3219752754296894559, 0.3333333333333333703, 0.3219752754296894559, 0.3333333333333333703, 0.3219752754296894559, 0.3333333333333333703, 0.3219752754296894559, 0.3333333333333333703, 0.3219752754296894559, 0.3333333333333333703, 0.3219752754296894559, 0.3333333333333333703, 0.3219752754296894559, 0.3333333333333333703, 0.3219752754296894559, 0.3333333333333333703, 0.3219752754296894559, 0.3333333333333333703, 0.3219752754296894559, 0.3333333333333333703, 0.3219752754296894559, 0.3333333333333333703, 0.3219752754296894559, 0.3333333333333333703, 0.3219752754296894559, 0.3333333333333333703, 0.3219752754296894559, 0.3333333333333333703, 0.3219752754296894559, 0.3333333333333333703, 0.3219752754296894559, 0.3333333333333333703, 0.3219752754296894559, 0.3333333333333333703, 0.3219752754296894559, 0.3333333333333333703, 0.3219752754296894559, 0.3333333333333333703, 0.3219752754296894559, 0.3333333333333333703, 0.3219752754296894559, 0.3333333333333333703, 0.3219752754296894559, 0.3333333333333333703, 0.3219752754296894559, 0.3333333333333333703, 0.3219752754296894559, 0.3333333333333333703, 0.3219752754296894559, 0.3333333333333333703, 0.3219752754296894559, 0.3333333333333333703, 0.3219752754296894559, 0.3333333333333333703, 0.3219752754296894559, 0.3333333333333333703, 0.3219752754296894559, 0.3333333333333333703, 0.3219752754296894559, 0.3333333333333333703, 0.3219752754296894559, 0.3333333333333333703, 0.3219752754296894559, 0.3333333333333333703, 0.3219752754296894559, 0.3333333333333333703, 0.3219752754296894559, 0.3333333333333333703, 0.3219752754296894559, 0.3333333333333333703, 0.3219752754296894559, 0.3333333333333333703, 0.3219752754296894559, 0.3333333333333333703, 0.3219752754296894559, 0.3333333333333333703, 0.3219752754296894559, 0.3333333333333333703, 0.3219752754296894559, 0.3333333333333333703, 0.3219752754296894559, 0.3333333333333333703, 0.3219752754296894559, 0.3333333333333333703, 0.3219752754296894559, 0.3333333333333333703, 0.3219752754296894559, 0.3333333333333333703, 0.3219752754296894559, 0.3333333333333333703, 0.3219752754296894559, 0.3333333333333333703, 0.3219752754296894559, 0.3333333333333333703, 0.3219752754296894559, 0.3333333333333333703, 0.3219752754296894559, 0.3333333333333333703, 0.3219752754296894559, 0.3333333333333333703, 0.3219752754296894559, 0.3333333333333333703, 0.3219752754296894559, 0.3333333333333333703, 0.3219752754296894559, 0.3333333333333333703, 0.3219752754296894559, 0.3333333333333333703, 0.3219752754296894559, 0.3333333333333333703, 0.3219752754296894559, 0.3333333333333333703, 0.3219752754296894559, 0.3333333333333333703, 0.3219752754296894559, 0.3333333333333333703, 0.3219752754296894559, 0.3333333333333333703, 0.3219752754296894559, 0.3333333333333333703, 0.3219752754296894559, 0.3333333333333333703, 0.3219752754296894559, 0.3333333333333333703, 0.3219752754296894559, 0.3333333333333333703, 0.3219752754296894559, 0.3333333333333333703, 0.3219752754296894559, 0.3333333333333333703, 0.3219752754296894559, 0.3333333333333333703, 0.3219752754296894559, 0.3333333333333333703, 0.3219752754296894559, 0.3333333333333333703, 0.3219752754296894559, 0.3333333333333333703, 0.3219752754296894559, 0.3333333333333333703, 0.3219752754296894559, 0.3333333333333333703, 0.3219752754296894559, 0.3333333333333333703, 0.3219752754296894559, 0.3333333333333333703, 0.3219752754296894559, 0.3333333333333333703, 0.3219752754296894559, 0.3333333333333333703, 0.3219752754296894559, 0.3333333333333333703, 0.3219752754296894559, 0.3333333333333333703, 0.3219752754296894559, 0.3333333333333333703, 0.3219752754296894559, 0.3333333333333333703, 0.3219752754296894559, 0.3333333333333333703, 0.3219752754296894559, 0.3333333333333333703, 0.3219752754296894559, 0.3333333333333333703, 0.3219752754296894559, 0.3333333333333333703, 0.3219752754296894559, 0.3333333333333333703, 0.3219752754296894559, 0.3333333333333333703, 0.3219752754296894559, 0.3333333333333333703, 0.3219752754296894559, 0.3333333333333333703, 0.3219752754296894559, 0.3333333333333333703, 0.3219752754296894559, 0.3333333333333333703, 0.3219752754296894559, 0.3333333333333333703, 0.3219752754296894559, 0.3333333333333333703, 0.3219752754296894559, 0.3333333333333333703, 0.3219752754296894559, 0.3333333333333333703, 0.3219752754296894559, 0.3333333333333333703, 0.3219752754296894559, 0.3333333333333333703, 0.3219752754296894559, 0.3333333333333333703, 0.3219752754296894559, 0.3333333333333333703, 0.3219752754296894559, 0.3333333333333333703, 0.3219752754296894559, 0.3333333333333333703, 0.3219752754296894559, 0.3333333333333333703, 0.3219752754296894559, 0.3333333333333333703, 0.3219752754296894559, 0.3333333333333333703, 0.3219752754296894559, 0.3333333333333333703, 0.3219752754296894559, 0.3333333333333333703, 0.3219752754296894559, 0.3333333333333333703, 0.3219752754296894559, 0.3333333333333333703, 0.3219752754296894559, 0.3333333333333333703, 0.3219752754296894559, 0.3333333333333333703, 0.3219752754296894559, 0.3333333333333333703, 0.3219752754296894559, 0.3333333333333333703),
 ( 0.3333333333333333703, 0.3219752754296894559, 0.3333333333333333703, 0.3219752754296894559, 0.3333333333333333703, 0.3219752754296894559, 0.3333333333333333703, 0.3219752754296894559, 0.3333333333333333703, 0.3219752754296894559, 0.3333333333333333703, 0.3219752754296894559, 0.3333333333333333703, 0.3219752754296894559, 0.3333333333333333703, 0.3219752754296894559, 0.3333333333333333703, 0.3219752754296894559, 0.3333333333333333703, 0.3219752754296894559, 0.3333333333333333703, 0.3219752754296894559, 0.3333333333333333703, 0.3219752754296894559, 0.3333333333333333703, 0.3219752754296894559, 0.3333333333333333703, 0.3219752754296894559, 0.3333333333333333703, 0.3219752754296894559, 0.3333333333333333703, 0.3219752754296894559, 0.3333333333333333703, 0.3219752754296894559, 0.3333333333333333703, 0.3219752754296894559, 0.3333333333333333703, 0.3219752754296894559, 0.3333333333333333703, 0.3219752754296894559, 0.3333333333333333703, 0.3219752754296894559, 0.3333333333333333703, 0.3219752754296894559, 0.3333333333333333703, 0.3219752754296894559, 0.3333333333333333703, 0.3219752754296894559, 0.3333333333333333703, 0.3219752754296894559, 0.3333333333333333703, 0.3219752754296894559, 0.3333333333333333703, 0.3219752754296894559, 0.3333333333333333703, 0.3219752754296894559, 0.3333333333333333703, 0.3219752754296894559, 0.3333333333333333703, 0.3219752754296894559, 0.3333333333333333703, 0.3219752754296894559, 0.3333333333333333703, 0.3219752754296894559, 0.3333333333333333703, 0.3219752754296894559, 0.3333333333333333703, 0.3219752754296894559, 0.3333333333333333703, 0.3219752754296894559, 0.3333333333333333703, 0.3219752754296894559, 0.3333333333333333703, 0.3219752754296894559, 0.3333333333333333703, 0.3219752754296894559, 0.3333333333333333703, 0.3219752754296894559, 0.3333333333333333703, 0.3219752754296894559, 0.3333333333333333703, 0.3219752754296894559, 0.3333333333333333703, 0.3219752754296894559, 0.3333333333333333703, 0.3219752754296894559, 0.3333333333333333703, 0.3219752754296894559, 0.3333333333333333703, 0.3219752754296894559, 0.3333333333333333703, 0.3219752754296894559, 0.3333333333333333703, 0.3219752754296894559, 0.3333333333333333703, 0.3219752754296894559, 0.3333333333333333703, 0.3219752754296894559, 0.3333333333333333703, 0.3219752754296894559, 0.3333333333333333703, 0.3219752754296894559, 0.3333333333333333703, 0.3219752754296894559, 0.3333333333333333703, 0.3219752754296894559, 0.3333333333333333703, 0.3219752754296894559, 0.3333333333333333703, 0.3219752754296894559, 0.3333333333333333703, 0.3219752754296894559, 0.3333333333333333703, 0.3219752754296894559, 0.3333333333333333703, 0.3219752754296894559, 0.3333333333333333703, 0.3219752754296894559, 0.3333333333333333703, 0.3219752754296894559, 0.3333333333333333703, 0.3219752754296894559, 0.3333333333333333703, 0.3219752754296894559, 0.3333333333333333703, 0.3219752754296894559, 0.3333333333333333703, 0.3219752754296894559, 0.3333333333333333703, 0.3219752754296894559, 0.3333333333333333703, 0.3219752754296894559, 0.3333333333333333703, 0.3219752754296894559, 0.3333333333333333703, 0.3219752754296894559, 0.3333333333333333703, 0.3219752754296894559, 0.3333333333333333703, 0.3219752754296894559, 0.3333333333333333703, 0.3219752754296894559, 0.3333333333333333703, 0.3219752754296894559, 0.3333333333333333703, 0.3219752754296894559, 0.3333333333333333703, 0.3219752754296894559, 0.3333333333333333703, 0.3219752754296894559, 0.3333333333333333703, 0.3219752754296894559, 0.3333333333333333703, 0.3219752754296894559, 0.3333333333333333703, 0.3219752754296894559, 0.3333333333333333703, 0.3219752754296894559, 0.3333333333333333703, 0.3219752754296894559, 0.3333333333333333703, 0.3219752754296894559, 0.3333333333333333703, 0.3219752754296894559, 0.3333333333333333703, 0.3219752754296894559, 0.3333333333333333703, 0.3219752754296894559, 0.3333333333333333703, 0.3219752754296894559, 0.3333333333333333703, 0.3219752754296894559, 0.3333333333333333703, 0.3219752754296894559, 0.3333333333333333703, 0.3219752754296894559, 0.3333333333333333703, 0.3219752754296894559, 0.3333333333333333703, 0.3219752754296894559, 0.3333333333333333703, 0.3219752754296894559, 0.3333333333333333703, 0.3219752754296894559, 0.3333333333333333703, 0.3219752754296894559, 0.3333333333333333703, 0.3219752754296894559, 0.3333333333333333703, 0.3219752754296894559, 0.3333333333333333703, 0.3219752754296894559, 0.3333333333333333703, 0.3219752754296894559, 0.3333333333333333703, 0.3219752754296894559, 0.3333333333333333703, 0.3219752754296894559, 0.3333333333333333703, 0.3219752754296894559, 0.3333333333333333703, 0.3219752754296894559, 0.3333333333333333703, 0.3219752754296894559, 0.3333333333333333703, 0.3219752754296894559, 0.3333333333333333703, 0.3219752754296894559, 0.3333333333333333703, 0.3219752754296894559, 0.3333333333333333703, 0.3219752754296894559, 0.3333333333333333703, 0.3219752754296894559, 0.3333333333333333703, 0.3219752754296894559, 0.3333333333333333703, 0.3219752754296894559, 0.3333333333333333703, 0.3219752754296894559, 0.3333333333333333703, 0.3219752754296894559, 0.3333333333333333703, 0.3219752754296894559, 0.3333333333333333703, 0.3219752754296894559, 0.3333333333333333703, 0.3219752754296894559, 0.3333333333333333703, 0.3219752754296894559, 0.3333333333333333703, 0.3219752754296894559, 0.3333333333333333703, 0.3219752754296894559, 0.3333333333333333703, 0.3219752754296894559, 0.3333333333333333703, 0.3219752754296894559, 0.3333333333333333703, 0.3219752754296894559, 0.3333333333333333703, 0.3219752754296894559, 0.3333333333333333703, 0.3219752754296894559, 0.3333333333333333703, 0.3219752754296894559, 0.3333333333333333703, 0.3219752754296894559, 0.3333333333333333703, 0.3219752754296894559, 0.3333333333333333703, 0.3219752754296894559, 0.3333333333333333703, 0.3219752754296894559, 0.3333333333333333703, 0.3219752754296894559, 0.3333333333333333703, 0.3219752754296894559, 0.3333333333333333703, 0.3219752754296894559, 0.3333333333333333703, 0.3219752754296894559, 0.3333333333333333703, 0.3219752754296894559, 0.3333333333333333703, 0.3219752754296894559, 0.3333333333333333703, 0.3219752754296894559, 0.3333333333333333703, 0.3219752754296894559, 0.3333333333333333703, 0.3219752754296894559, 0.3333333333333333703, 0.3219752754296894559, 0.3333333333333333703, 0.3219752754296894559, 0.3333333333333333703, 0.3219752754296894559, 0.3333333333333333703, 0.3219752754296894559, 0.3333333333333333703, 0.3219752754296894559, 0.3333333333333333703, 0.3219752754296894559, 0.3333333333333333703, 0.3219752754296894559, 0.3333333333333333703, 0.3219752754296894559, 0.3333333333333333703, 0.3219752754296894559, 0.3333333333333333703, 0.3219752754296894559, 0.3333333333333333703, 0.3219752754296894559, 0.3333333333333333703, 0.3219752754296894559, 0.3333333333333333703, 0.3219752754296894559, 0.3333333333333333703, 0.3219752754296894559, 0.3333333333333333703, 0.3219752754296894559, 0.3333333333333333703, 0.3219752754296894559, 0.3333333333333333703, 0.3219752754296894559, 0.3333333333333333703, 0.3219752754296894559, 0.3333333333333333703, 0.3219752754296894559, 0.3333333333333333703, 0.3219752754296894559, 0.3333333333333333703, 0.3219752754296894559, 0.3333333333333333703, 0.3219752754296894559, 0.3333333333333333703, 0.3219752754296894559, 0.3333333333333333703, 0.3219752754296894559, 0.3333333333333333703, 0.3219752754296894559, 0.3333333333333333703, 0.3219752754296894559, 0.3333333333333333703, 0.3219752754296894559, 0.3333333333333333703, 0.3219752754296894559, 0.3333333333333333703, 0.3219752754296894559, 0.3333333333333333703, 0.3219752754296894559, 0.3333333333333333703, 0.3219752754296894559, 0.3333333333333333703, 0.3219752754296894559, 0.3333333333333333703, 0.3219752754296894559, 0.3333333333333333703, 0.3219752754296894559, 0.3333333333333333703, 0.3219752754296894559, 0.3333333333333333703, 0.3219752754296894559, 0.3333333333333333703, 0.3219752754296894559, 0.3333333333333333703, 0.3219752754296894559, 0.3333333333333333703, 0.3219752754296894559, 0.3333333333333333703, 0.3219752754296894559, 0.3333333333333333703, 0.3219752754296894559, 0.3333333333333333703, 0.3219752754296894559, 0.3333333333333333703, 0.3219752754296894559, 0.3333333333333333703, 0.3219752754296894559, 0.3333333333333333703, 0.3219752754296894559, 0.3333333333333333703, 0.3219752754296894559, 0.3333333333333333703, 0.3219752754296894559, 0.3333333333333333703, 0.3219752754296894559, 0.3333333333333333703, 0.3219752754296894559, 0.3333333333333333703, 0.3219752754296894559, 0.3333333333333333703, 0.3219752754296894559, 0.3333333333333333703, 0.3219752754296894559, 0.3333333333333333703, 0.3219752754296894559, 0.3333333333333333703, 0.3219752754296894559, 0.3333333333333333703, 0.3219752754296894559, 0.3333333333333333703, 0.3219752754296894559, 0.3333333333333333703, 0.3219752754296894559, 0.3333333333333333703, 0.3219752754296894559, 0.3333333333333333703, 0.3219752754296894559, 0.3333333333333333703, 0.3219752754296894559, 0.3333333333333333703, 0.3219752754296894559, 0.3333333333333333703, 0.3219752754296894559, 0.3333333333333333703, 0.3219752754296894559, 0.3333333333333333703, 0.3219752754296894559, 0.3333333333333333703, 0.3219752754296894559, 0.3333333333333333703, 0.3219752754296894559, 0.3333333333333333703, 0.3219752754296894559, 0.3333333333333333703, 0.3219752754296894559, 0.3333333333333333703, 0.3219752754296894559, 0.3333333333333333703, 0.3219752754296894559, 0.3333333333333333703, 0.3219752754296894559, 0.3333333333333333703, 0.3219752754296894559, 0.3333333333333333703, 0.3219752754296894559, 0.3333333333333333703, 0.3219752754296894559, 0.3333333333333333703, 0.3219752754296894559, 0.3333333333333333703, 0.3219752754296894559, 0.3333333333333333703, 0.3219752754296894559, 0.3333333333333333703, 0.3219752754296894559, 0.3333333333333333703, 0.3219752754296894559, 0.3333333333333333703, 0.3219752754296894559, 0.3333333333333333703, 0.3219752754296894559, 0.3333333333333333703, 0.3219752754296894559, 0.3333333333333333703, 0.3219752754296894559, 0.3333333333333333703, 0.3219752754296894559, 0.3333333333333333703, 0.3219752754296894559, 0.3333333333333333703, 0.3219752754296894559, 0.3333333333333333703, 0.3219752754296894559, 0.3333333333333333703, 0.3219752754296894559, 0.3333333333333333703, 0.3219752754296894559, 0.3333333333333333703, 0.3219752754296894559, 0.3333333333333333703, 0.3219752754296894559, 0.3333333333333333703, 0.3219752754296894559, 0.3333333333333333703),
 ( 1.000000000000000000, 0.9659258262890683122, 1.000000000000000000, 0.9659258262890683122, 1.000000000000000000, 0.9659258262890683122, 1.000000000000000000, 0.9659258262890683122, 1.000000000000000000, 0.9659258262890683122, 1.000000000000000000, 0.9659258262890683122, 1.000000000000000000, 0.9659258262890683122, 1.000000000000000000, 0.9659258262890683122, 1.000000000000000000, 0.9659258262890683122, 1.000000000000000000, 0.9659258262890683122, 1.000000000000000000, 0.9659258262890683122, 1.000000000000000000, 0.9659258262890683122, 1.000000000000000000, 0.9659258262890683122, 1.000000000000000000, 0.9659258262890683122, 1.000000000000000000, 0.9659258262890683122, 1.000000000000000000, 0.9659258262890683122, 1.000000000000000000, 0.9659258262890683122, 1.000000000000000000, 0.9659258262890683122, 1.000000000000000000, 0.9659258262890683122, 1.000000000000000000, 0.9659258262890683122, 1.000000000000000000, 0.9659258262890683122, 1.000000000000000000, 0.9659258262890683122, 1.000000000000000000, 0.9659258262890683122, 1.000000000000000000, 0.9659258262890683122, 1.000000000000000000, 0.9659258262890683122, 1.000000000000000000, 0.9659258262890683122, 1.000000000000000000, 0.9659258262890683122, 1.000000000000000000, 0.9659258262890683122, 1.000000000000000000, 0.9659258262890683122, 1.000000000000000000, 0.9659258262890683122, 1.000000000000000000, 0.9659258262890683122, 1.000000000000000000, 0.9659258262890683122, 1.000000000000000000, 0.9659258262890683122, 1.000000000000000000, 0.9659258262890683122, 1.000000000000000000, 0.9659258262890683122, 1.000000000000000000, 0.9659258262890683122, 1.000000000000000000, 0.9659258262890683122, 1.000000000000000000, 0.9659258262890683122, 1.000000000000000000, 0.9659258262890683122, 1.000000000000000000, 0.9659258262890683122, 1.000000000000000000, 0.9659258262890683122, 1.000000000000000000, 0.9659258262890683122, 1.000000000000000000, 0.9659258262890683122, 1.000000000000000000, 0.9659258262890683122, 1.000000000000000000, 0.9659258262890683122, 1.000000000000000000, 0.9659258262890683122, 1.000000000000000000, 0.9659258262890683122, 1.000000000000000000, 0.9659258262890683122, 1.000000000000000000, 0.9659258262890683122, 1.000000000000000000, 0.9659258262890683122, 1.000000000000000000, 0.9659258262890683122, 1.000000000000000000, 0.9659258262890683122, 1.000000000000000000, 0.9659258262890683122, 1.000000000000000000, 0.9659258262890683122, 1.000000000000000000, 0.9659258262890683122, 1.000000000000000000, 0.9659258262890683122, 1.000000000000000000, 0.9659258262890683122, 1.000000000000000000, 0.9659258262890683122, 1.000000000000000000, 0.9659258262890683122, 1.000000000000000000, 0.9659258262890683122, 1.000000000000000000, 0.9659258262890683122, 1.000000000000000000, 0.9659258262890683122, 1.000000000000000000, 0.9659258262890683122, 1.000000000000000000, 0.9659258262890683122, 1.000000000000000000, 0.9659258262890683122, 1.000000000000000000, 0.9659258262890683122, 1.000000000000000000, 0.9659258262890683122, 1.000000000000000000, 0.9659258262890683122, 1.000000000000000000, 0.9659258262890683122, 1.000000000000000000, 0.9659258262890683122, 1.000000000000000000, 0.9659258262890683122, 1.000000000000000000, 0.9659258262890683122, 1.000000000000000000, 0.9659258262890683122, 1.000000000000000000, 0.9659258262890683122, 1.000000000000000000, 0.9659258262890683122, 1.000000000000000000, 0.9659258262890683122, 1.000000000000000000, 0.9659258262890683122, 1.000000000000000000, 0.9659258262890683122, 1.000000000000000000, 0.9659258262890683122, 1.000000000000000000, 0.9659258262890683122, 1.000000000000000000, 0.9659258262890683122, 1.000000000000000000, 0.9659258262890683122, 1.000000000000000000, 0.9659258262890683122, 1.000000000000000000, 0.9659258262890683122, 1.000000000000000000, 0.9659258262890683122, 1.000000000000000000, 0.9659258262890683122, 1.000000000000000000, 0.9659258262890683122, 1.000000000000000000, 0.9659258262890683122, 1.000000000000000000, 0.9659258262890683122, 1.000000000000000000, 0.9659258262890683122, 1.000000000000000000, 0.9659258262890683122, 1.000000000000000000, 0.9659258262890683122, 1.000000000000000000, 0.9659258262890683122, 1.000000000000000000, 0.9659258262890683122, 1.000000000000000000, 0.9659258262890683122, 1.000000000000000000, 0.9659258262890683122, 1.000000000000000000, 0.9659258262890683122, 1.000000000000000000, 0.9659258262890683122, 1.000000000000000000, 0.9659258262890683122, 1.000000000000000000, 0.9659258262890683122, 1.000000000000000000, 0.9659258262890683122, 1.000000000000000000, 0.9659258262890683122, 1.000000000000000000, 0.9659258262890683122, 1.000000000000000000, 0.9659258262890683122, 1.000000000000000000, 0.9659258262890683122, 1.000000000000000000, 0.9659258262890683122, 1.000000000000000000, 0.9659258262890683122, 1.000000000000000000, 0.9659258262890683122, 1.000000000000000000, 0.9659258262890683122, 1.000000000000000000, 0.9659258262890683122, 1.000000000000000000, 0.9659258262890683122, 1.000000000000000000, 0.9659258262890683122, 1.000000000000000000, 0.9659258262890683122, 1.000000000000000000, 0.9659258262890683122, 1.000000000000000000, 0.9659258262890683122, 1.000000000000000000, 0.9659258262890683122, 1.000000000000000000, 0.9659258262890683122, 1.000000000000000000, 0.9659258262890683122, 1.000000000000000000, 0.9659258262890683122, 1.000000000000000000, 0.9659258262890683122, 1.000000000000000000, 0.9659258262890683122, 1.000000000000000000, 0.9659258262890683122, 1.000000000000000000, 0.9659258262890683122, 1.000000000000000000, 0.9659258262890683122, 1.000000000000000000, 0.9659258262890683122, 1.000000000000000000, 0.9659258262890683122, 1.000000000000000000, 0.9659258262890683122, 1.000000000000000000, 0.9659258262890683122, 1.000000000000000000, 0.9659258262890683122, 1.000000000000000000, 0.9659258262890683122, 1.000000000000000000, 0.9659258262890683122, 1.000000000000000000, 0.9659258262890683122, 1.000000000000000000, 0.9659258262890683122, 1.000000000000000000, 0.9659258262890683122, 1.000000000000000000, 0.9659258262890683122, 1.000000000000000000, 0.9659258262890683122, 1.000000000000000000, 0.9659258262890683122, 1.000000000000000000, 0.9659258262890683122, 1.000000000000000000, 0.9659258262890683122, 1.000000000000000000, 0.9659258262890683122, 1.000000000000000000, 0.9659258262890683122, 1.000000000000000000, 0.9659258262890683122, 1.000000000000000000, 0.9659258262890683122, 1.000000000000000000, 0.9659258262890683122, 1.000000000000000000, 0.9659258262890683122, 1.000000000000000000, 0.9659258262890683122, 1.000000000000000000, 0.9659258262890683122, 1.000000000000000000, 0.9659258262890683122, 1.000000000000000000, 0.9659258262890683122, 1.000000000000000000, 0.9659258262890683122, 1.000000000000000000, 0.9659258262890683122, 1.000000000000000000, 0.9659258262890683122, 1.000000000000000000, 0.9659258262890683122, 1.000000000000000000, 0.9659258262890683122, 1.000000000000000000, 0.9659258262890683122, 1.000000000000000000, 0.9659258262890683122, 1.000000000000000000, 0.9659258262890683122, 1.000000000000000000, 0.9659258262890683122, 1.000000000000000000, 0.9659258262890683122, 1.000000000000000000, 0.9659258262890683122, 1.000000000000000000, 0.9659258262890683122, 1.000000000000000000, 0.9659258262890683122, 1.000000000000000000, 0.9659258262890683122, 1.000000000000000000, 0.9659258262890683122, 1.000000000000000000, 0.9659258262890683122, 1.000000000000000000, 0.9659258262890683122, 1.000000000000000000, 0.9659258262890683122, 1.000000000000000000, 0.9659258262890683122, 1.000000000000000000, 0.9659258262890683122, 1.000000000000000000, 0.9659258262890683122, 1.000000000000000000, 0.9659258262890683122, 1.000000000000000000, 0.9659258262890683122, 1.000000000000000000, 0.9659258262890683122, 1.000000000000000000, 0.9659258262890683122, 1.000000000000000000, 0.9659258262890683122, 1.000000000000000000, 0.9659258262890683122, 1.000000000000000000, 0.9659258262890683122, 1.000000000000000000, 0.9659258262890683122, 1.000000000000000000, 0.9659258262890683122, 1.000000000000000000, 0.9659258262890683122, 1.000000000000000000, 0.9659258262890683122, 1.000000000000000000, 0.9659258262890683122, 1.000000000000000000, 0.9659258262890683122, 1.000000000000000000, 0.9659258262890683122, 1.000000000000000000, 0.9659258262890683122, 1.000000000000000000, 0.9659258262890683122, 1.000000000000000000, 0.9659258262890683122, 1.000000000000000000, 0.9659258262890683122, 1.000000000000000000, 0.9659258262890683122, 1.000000000000000000, 0.9659258262890683122, 1.000000000000000000, 0.9659258262890683122, 1.000000000000000000, 0.9659258262890683122, 1.000000000000000000, 0.9659258262890683122, 1.000000000000000000, 0.9659258262890683122, 1.000000000000000000, 0.9659258262890683122, 1.000000000000000000, 0.9659258262890683122, 1.000000000000000000, 0.9659258262890683122, 1.000000000000000000, 0.9659258262890683122, 1.000000000000000000, 0.9659258262890683122, 1.000000000000000000, 0.9659258262890683122, 1.000000000000000000, 0.9659258262890683122, 1.000000000000000000, 0.9659258262890683122, 1.000000000000000000, 0.9659258262890683122, 1.000000000000000000, 0.9659258262890683122, 1.000000000000000000, 0.9659258262890683122, 1.000000000000000000, 0.9659258262890683122, 1.000000000000000000, 0.9659258262890683122, 1.000000000000000000, 0.9659258262890683122, 1.000000000000000000, 0.9659258262890683122, 1.000000000000000000, 0.9659258262890683122, 1.000000000000000000, 0.9659258262890683122, 1.000000000000000000, 0.9659258262890683122, 1.000000000000000000, 0.9659258262890683122, 1.000000000000000000, 0.9659258262890683122, 1.000000000000000000, 0.9659258262890683122, 1.000000000000000000, 0.9659258262890683122, 1.000000000000000000, 0.9659258262890683122, 1.000000000000000000, 0.9659258262890683122, 1.000000000000000000, 0.9659258262890683122, 1.000000000000000000, 0.9659258262890683122, 1.000000000000000000, 0.9659258262890683122, 1.000000000000000000, 0.9659258262890683122, 1.000000000000000000, 0.9659258262890683122, 1.000000000000000000, 0.9659258262890683122, 1.000000000000000000, 0.9659258262890683122, 1.000000000000000000, 0.9659258262890683122, 1.000000000000000000, 0.9659258262890683122, 1.000000000000000000, 0.9659258262890683122, 1.000000000000000000),
 ( 0.3333333333333333703, 0.3219752754296894559, 0.3333333333333333703, 0.3219752754296894559, 0.3333333333333333703, 0.3219752754296894559, 0.3333333333333333703, 0.3219752754296894559, 0.3333333333333333703, 0.3219752754296894559, 0.3333333333333333703, 0.3219752754296894559, 0.3333333333333333703, 0.3219752754296894559, 0.3333333333333333703, 0.3219752754296894559, 0.3333333333333333703, 0.3219752754296894559, 0.3333333333333333703, 0.3219752754296894559, 0.3333333333333333703, 0.3219752754296894559, 0.3333333333333333703, 0.3219752754296894559, 0.3333333333333333703, 0.3219752754296894559, 0.3333333333333333703, 0.3219752754296894559, 0.3333333333333333703, 0.3219752754296894559, 0.3333333333333333703, 0.3219752754296894559, 0.3333333333333333703, 0.3219752754296894559, 0.3333333333333333703, 0.3219752754296894559, 0.3333333333333333703, 0.3219752754296894559, 0.3333333333333333703, 0.3219752754296894559, 0.3333333333333333703, 0.3219752754296894559, 0.3333333333333333703, 0.3219752754296894559, 0.3333333333333333703, 0.3219752754296894559, 0.3333333333333333703, 0.3219752754296894559, 0.3333333333333333703, 0.3219752754296894559, 0.3333333333333333703, 0.3219752754296894559, 0.3333333333333333703, 0.3219752754296894559, 0.3333333333333333703, 0.3219752754296894559, 0.3333333333333333703, 0.3219752754296894559, 0.3333333333333333703, 0.3219752754296894559, 0.3333333333333333703, 0.3219752754296894559, 0.3333333333333333703, 0.3219752754296894559, 0.3333333333333333703, 0.3219752754296894559, 0.3333333333333333703, 0.3219752754296894559, 0.3333333333333333703, 0.3219752754296894559, 0.3333333333333333703, 0.3219752754296894559, 0.3333333333333333703, 0.3219752754296894559, 0.3333333333333333703, 0.3219752754296894559, 0.3333333333333333703, 0.3219752754296894559, 0.3333333333333333703, 0.3219752754296894559, 0.3333333333333333703, 0.3219752754296894559, 0.3333333333333333703, 0.3219752754296894559, 0.3333333333333333703, 0.3219752754296894559, 0.3333333333333333703, 0.3219752754296894559, 0.3333333333333333703, 0.3219752754296894559, 0.3333333333333333703, 0.3219752754296894559, 0.3333333333333333703, 0.3219752754296894559, 0.3333333333333333703, 0.3219752754296894559, 0.3333333333333333703, 0.3219752754296894559, 0.3333333333333333703, 0.3219752754296894559, 0.3333333333333333703, 0.3219752754296894559, 0.3333333333333333703, 0.3219752754296894559, 0.3333333333333333703, 0.3219752754296894559, 0.3333333333333333703, 0.3219752754296894559, 0.3333333333333333703, 0.3219752754296894559, 0.3333333333333333703, 0.3219752754296894559, 0.3333333333333333703, 0.3219752754296894559, 0.3333333333333333703, 0.3219752754296894559, 0.3333333333333333703, 0.3219752754296894559, 0.3333333333333333703, 0.3219752754296894559, 0.3333333333333333703, 0.3219752754296894559, 0.3333333333333333703, 0.3219752754296894559, 0.3333333333333333703, 0.3219752754296894559, 0.3333333333333333703, 0.3219752754296894559, 0.3333333333333333703, 0.3219752754296894559, 0.3333333333333333703, 0.3219752754296894559, 0.3333333333333333703, 0.3219752754296894559, 0.3333333333333333703, 0.3219752754296894559, 0.3333333333333333703, 0.3219752754296894559, 0.3333333333333333703, 0.3219752754296894559, 0.3333333333333333703, 0.3219752754296894559, 0.3333333333333333703, 0.3219752754296894559, 0.3333333333333333703, 0.3219752754296894559, 0.3333333333333333703, 0.3219752754296894559, 0.3333333333333333703, 0.3219752754296894559, 0.3333333333333333703, 0.3219752754296894559, 0.3333333333333333703, 0.3219752754296894559, 0.3333333333333333703, 0.3219752754296894559, 0.3333333333333333703, 0.3219752754296894559, 0.3333333333333333703, 0.3219752754296894559, 0.3333333333333333703, 0.3219752754296894559, 0.3333333333333333703, 0.3219752754296894559, 0.3333333333333333703, 0.3219752754296894559, 0.3333333333333333703, 0.3219752754296894559, 0.3333333333333333703, 0.3219752754296894559, 0.3333333333333333703, 0.3219752754296894559, 0.3333333333333333703, 0.3219752754296894559, 0.3333333333333333703, 0.3219752754296894559, 0.3333333333333333703, 0.3219752754296894559, 0.3333333333333333703, 0.3219752754296894559, 0.3333333333333333703, 0.3219752754296894559, 0.3333333333333333703, 0.3219752754296894559, 0.3333333333333333703, 0.3219752754296894559, 0.3333333333333333703, 0.3219752754296894559, 0.3333333333333333703, 0.3219752754296894559, 0.3333333333333333703, 0.3219752754296894559, 0.3333333333333333703, 0.3219752754296894559, 0.3333333333333333703, 0.3219752754296894559, 0.3333333333333333703, 0.3219752754296894559, 0.3333333333333333703, 0.3219752754296894559, 0.3333333333333333703, 0.3219752754296894559, 0.3333333333333333703, 0.3219752754296894559, 0.3333333333333333703, 0.3219752754296894559, 0.3333333333333333703, 0.3219752754296894559, 0.3333333333333333703, 0.3219752754296894559, 0.3333333333333333703, 0.3219752754296894559, 0.3333333333333333703, 0.3219752754296894559, 0.3333333333333333703, 0.3219752754296894559, 0.3333333333333333703, 0.3219752754296894559, 0.3333333333333333703, 0.3219752754296894559, 0.3333333333333333703, 0.3219752754296894559, 0.3333333333333333703, 0.3219752754296894559, 0.3333333333333333703, 0.3219752754296894559, 0.3333333333333333703, 0.3219752754296894559, 0.3333333333333333703, 0.3219752754296894559, 0.3333333333333333703, 0.3219752754296894559, 0.3333333333333333703, 0.3219752754296894559, 0.3333333333333333703, 0.3219752754296894559, 0.3333333333333333703, 0.3219752754296894559, 0.3333333333333333703, 0.3219752754296894559, 0.3333333333333333703, 0.3219752754296894559, 0.3333333333333333703, 0.3219752754296894559, 0.3333333333333333703, 0.3219752754296894559, 0.3333333333333333703, 0.3219752754296894559, 0.3333333333333333703, 0.3219752754296894559, 0.3333333333333333703, 0.3219752754296894559, 0.3333333333333333703, 0.3219752754296894559, 0.3333333333333333703, 0.3219752754296894559, 0.3333333333333333703, 0.3219752754296894559, 0.3333333333333333703, 0.3219752754296894559, 0.3333333333333333703, 0.3219752754296894559, 0.3333333333333333703, 0.3219752754296894559, 0.3333333333333333703, 0.3219752754296894559, 0.3333333333333333703, 0.3219752754296894559, 0.3333333333333333703, 0.3219752754296894559, 0.3333333333333333703, 0.3219752754296894559, 0.3333333333333333703, 0.3219752754296894559, 0.3333333333333333703, 0.3219752754296894559, 0.3333333333333333703, 0.3219752754296894559, 0.3333333333333333703, 0.3219752754296894559, 0.3333333333333333703, 0.3219752754296894559, 0.3333333333333333703, 0.3219752754296894559, 0.3333333333333333703, 0.3219752754296894559, 0.3333333333333333703, 0.3219752754296894559, 0.3333333333333333703, 0.3219752754296894559, 0.3333333333333333703, 0.3219752754296894559, 0.3333333333333333703, 0.3219752754296894559, 0.3333333333333333703, 0.3219752754296894559, 0.3333333333333333703, 0.3219752754296894559, 0.3333333333333333703, 0.3219752754296894559, 0.3333333333333333703, 0.3219752754296894559, 0.3333333333333333703, 0.3219752754296894559, 0.3333333333333333703, 0.3219752754296894559, 0.3333333333333333703, 0.3219752754296894559, 0.3333333333333333703, 0.3219752754296894559, 0.3333333333333333703, 0.3219752754296894559, 0.3333333333333333703, 0.3219752754296894559, 0.3333333333333333703, 0.3219752754296894559, 0.3333333333333333703, 0.3219752754296894559, 0.3333333333333333703, 0.3219752754296894559, 0.3333333333333333703, 0.3219752754296894559, 0.3333333333333333703, 0.3219752754296894559, 0.3333333333333333703, 0.3219752754296894559, 0.3333333333333333703, 0.3219752754296894559, 0.3333333333333333703, 0.3219752754296894559, 0.3333333333333333703, 0.3219752754296894559, 0.3333333333333333703, 0.3219752754296894559, 0.3333333333333333703, 0.3219752754296894559, 0.3333333333333333703, 0.3219752754296894559, 0.3333333333333333703, 0.3219752754296894559, 0.3333333333333333703, 0.3219752754296894559, 0.3333333333333333703, 0.3219752754296894559, 0.3333333333333333703, 0.3219752754296894559, 0.3333333333333333703, 0.3219752754296894559, 0.3333333333333333703, 0.3219752754296894559, 0.3333333333333333703, 0.3219752754296894559, 0.3333333333333333703, 0.3219752754296894559, 0.3333333333333333703, 0.3219752754296894559, 0.3333333333333333703, 0.3219752754296894559, 0.3333333333333333703, 0.3219752754296894559, 0.3333333333333333703, 0.3219752754296894559, 0.3333333333333333703, 0.3219752754296894559, 0.3333333333333333703, 0.3219752754296894559, 0.3333333333333333703, 0.3219752754296894559, 0.3333333333333333703, 0.3219752754296894559, 0.3333333333333333703, 0.3219752754296894559, 0.3333333333333333703, 0.3219752754296894559, 0.3333333333333333703, 0.3219752754296894559, 0.3333333333333333703, 0.3219752754296894559, 0.3333333333333333703, 0.3219752754296894559, 0.3333333333333333703, 0.3219752754296894559, 0.3333333333333333703, 0.3219752754296894559, 0.3333333333333333703, 0.3219752754296894559, 0.3333333333333333703, 0.3219752754296894559, 0.3333333333333333703, 0.3219752754296894559, 0.3333333333333333703, 0.3219752754296894559, 0.3333333333333333703, 0.3219752754296894559, 0.3333333333333333703, 0.3219752754296894559, 0.3333333333333333703, 0.3219752754296894559, 0.3333333333333333703, 0.3219752754296894559, 0.3333333333333333703, 0.3219752754296894559, 0.3333333333333333703, 0.3219752754296894559, 0.3333333333333333703, 0.3219752754296894559, 0.3333333333333333703, 0.3219752754296894559, 0.3333333333333333703, 0.3219752754296894559, 0.3333333333333333703, 0.3219752754296894559, 0.3333333333333333703, 0.3219752754296894559, 0.3333333333333333703, 0.3219752754296894559, 0.3333333333333333703, 0.3219752754296894559, 0.3333333333333333703, 0.3219752754296894559, 0.3333333333333333703, 0.3219752754296894559, 0.3333333333333333703, 0.3219752754296894559, 0.3333333333333333703, 0.3219752754296894559, 0.3333333333333333703, 0.3219752754296894559, 0.3333333333333333703, 0.3219752754296894559, 0.3333333333333333703, 0.3219752754296894559, 0.3333333333333333703, 0.3219752754296894559, 0.3333333333333333703, 0.3219752754296894559, 0.3333333333333333703, 0.3219752754296894559, 0.3333333333333333703, 0.3219752754296894559, 0.3333333333333333703, 0.3219752754296894559, 0.3333333333333333703, 0.3219752754296894559, 0.3333333333333333703, 0.3219752754296894559, 0.3333333333333333703, 0.3219752754296894559, 0.3333333333333333703, 0.3219752754296894559, 0.3333333333333333703, 0.3219752754296894559, 0.3333333333333333703, 0.3219752754296894559, 0.3333333333333333703, 0.3219752754296894559, 0.3333333333333333703),
 ( 0.3333333333333333703, 0.3219752754296894559, 0.3333333333333333703, 0.3219752754296894559, 0.3333333333333333703, 0.3219752754296894559, 0.3333333333333333703, 0.3219752754296894559, 0.3333333333333333703, 0.3219752754296894559, 0.3333333333333333703, 0.3219752754296894559, 0.3333333333333333703, 0.3219752754296894559, 0.3333333333333333703, 0.3219752754296894559, 0.3333333333333333703, 0.3219752754296894559, 0.3333333333333333703, 0.3219752754296894559, 0.3333333333333333703, 0.3219752754296894559, 0.3333333333333333703, 0.3219752754296894559, 0.3333333333333333703, 0.3219752754296894559, 0.3333333333333333703, 0.3219752754296894559, 0.3333333333333333703, 0.3219752754296894559, 0.3333333333333333703, 0.3219752754296894559, 0.3333333333333333703, 0.3219752754296894559, 0.3333333333333333703, 0.3219752754296894559, 0.3333333333333333703, 0.3219752754296894559, 0.3333333333333333703, 0.3219752754296894559, 0.3333333333333333703, 0.3219752754296894559, 0.3333333333333333703, 0.3219752754296894559, 0.3333333333333333703, 0.3219752754296894559, 0.3333333333333333703, 0.3219752754296894559, 0.3333333333333333703, 0.3219752754296894559, 0.3333333333333333703, 0.3219752754296894559, 0.3333333333333333703, 0.3219752754296894559, 0.3333333333333333703, 0.3219752754296894559, 0.3333333333333333703, 0.3219752754296894559, 0.3333333333333333703, 0.3219752754296894559, 0.3333333333333333703, 0.3219752754296894559, 0.3333333333333333703, 0.3219752754296894559, 0.3333333333333333703, 0.3219752754296894559, 0.3333333333333333703, 0.3219752754296894559, 0.3333333333333333703, 0.3219752754296894559, 0.3333333333333333703, 0.3219752754296894559, 0.3333333333333333703, 0.3219752754296894559, 0.3333333333333333703, 0.3219752754296894559, 0.3333333333333333703, 0.3219752754296894559, 0.3333333333333333703, 0.3219752754296894559, 0.3333333333333333703, 0.3219752754296894559, 0.3333333333333333703, 0.3219752754296894559, 0.3333333333333333703, 0.3219752754296894559, 0.3333333333333333703, 0.3219752754296894559, 0.3333333333333333703, 0.3219752754296894559, 0.3333333333333333703, 0.3219752754296894559, 0.3333333333333333703, 0.3219752754296894559, 0.3333333333333333703, 0.3219752754296894559, 0.3333333333333333703, 0.3219752754296894559, 0.3333333333333333703, 0.3219752754296894559, 0.3333333333333333703, 0.3219752754296894559, 0.3333333333333333703, 0.3219752754296894559, 0.3333333333333333703, 0.3219752754296894559, 0.3333333333333333703, 0.3219752754296894559, 0.3333333333333333703, 0.3219752754296894559, 0.3333333333333333703, 0.3219752754296894559, 0.3333333333333333703, 0.3219752754296894559, 0.3333333333333333703, 0.3219752754296894559, 0.3333333333333333703, 0.3219752754296894559, 0.3333333333333333703, 0.3219752754296894559, 0.3333333333333333703, 0.3219752754296894559, 0.3333333333333333703, 0.3219752754296894559, 0.3333333333333333703, 0.3219752754296894559, 0.3333333333333333703, 0.3219752754296894559, 0.3333333333333333703, 0.3219752754296894559, 0.3333333333333333703, 0.3219752754296894559, 0.3333333333333333703, 0.3219752754296894559, 0.3333333333333333703, 0.3219752754296894559, 0.3333333333333333703, 0.3219752754296894559, 0.3333333333333333703, 0.3219752754296894559, 0.3333333333333333703, 0.3219752754296894559, 0.3333333333333333703, 0.3219752754296894559, 0.3333333333333333703, 0.3219752754296894559, 0.3333333333333333703, 0.3219752754296894559, 0.3333333333333333703, 0.3219752754296894559, 0.3333333333333333703, 0.3219752754296894559, 0.3333333333333333703, 0.3219752754296894559, 0.3333333333333333703, 0.3219752754296894559, 0.3333333333333333703, 0.3219752754296894559, 0.3333333333333333703, 0.3219752754296894559, 0.3333333333333333703, 0.3219752754296894559, 0.3333333333333333703, 0.3219752754296894559, 0.3333333333333333703, 0.3219752754296894559, 0.3333333333333333703, 0.3219752754296894559, 0.3333333333333333703, 0.3219752754296894559, 0.3333333333333333703, 0.3219752754296894559, 0.3333333333333333703, 0.3219752754296894559, 0.3333333333333333703, 0.3219752754296894559, 0.3333333333333333703, 0.3219752754296894559, 0.3333333333333333703, 0.3219752754296894559, 0.3333333333333333703, 0.3219752754296894559, 0.3333333333333333703, 0.3219752754296894559, 0.3333333333333333703, 0.3219752754296894559, 0.3333333333333333703, 0.3219752754296894559, 0.3333333333333333703, 0.3219752754296894559, 0.3333333333333333703, 0.3219752754296894559, 0.3333333333333333703, 0.3219752754296894559, 0.3333333333333333703, 0.3219752754296894559, 0.3333333333333333703, 0.3219752754296894559, 0.3333333333333333703, 0.3219752754296894559, 0.3333333333333333703, 0.3219752754296894559, 0.3333333333333333703, 0.3219752754296894559, 0.3333333333333333703, 0.3219752754296894559, 0.3333333333333333703, 0.3219752754296894559, 0.3333333333333333703, 0.3219752754296894559, 0.3333333333333333703, 0.3219752754296894559, 0.3333333333333333703, 0.3219752754296894559, 0.3333333333333333703, 0.3219752754296894559, 0.3333333333333333703, 0.3219752754296894559, 0.3333333333333333703, 0.3219752754296894559, 0.3333333333333333703, 0.3219752754296894559, 0.3333333333333333703, 0.3219752754296894559, 0.3333333333333333703, 0.3219752754296894559, 0.3333333333333333703, 0.3219752754296894559, 0.3333333333333333703, 0.3219752754296894559, 0.3333333333333333703, 0.3219752754296894559, 0.3333333333333333703, 0.3219752754296894559, 0.3333333333333333703, 0.3219752754296894559, 0.3333333333333333703, 0.3219752754296894559, 0.3333333333333333703, 0.3219752754296894559, 0.3333333333333333703, 0.3219752754296894559, 0.3333333333333333703, 0.3219752754296894559, 0.3333333333333333703, 0.3219752754296894559, 0.3333333333333333703, 0.3219752754296894559, 0.3333333333333333703, 0.3219752754296894559, 0.3333333333333333703, 0.3219752754296894559, 0.3333333333333333703, 0.3219752754296894559, 0.3333333333333333703, 0.3219752754296894559, 0.3333333333333333703, 0.3219752754296894559, 0.3333333333333333703, 0.3219752754296894559, 0.3333333333333333703, 0.3219752754296894559, 0.3333333333333333703, 0.3219752754296894559, 0.3333333333333333703, 0.3219752754296894559, 0.3333333333333333703, 0.3219752754296894559, 0.3333333333333333703, 0.3219752754296894559, 0.3333333333333333703, 0.3219752754296894559, 0.3333333333333333703, 0.3219752754296894559, 0.3333333333333333703, 0.3219752754296894559, 0.3333333333333333703, 0.3219752754296894559, 0.3333333333333333703, 0.3219752754296894559, 0.3333333333333333703, 0.3219752754296894559, 0.3333333333333333703, 0.3219752754296894559, 0.3333333333333333703, 0.3219752754296894559, 0.3333333333333333703, 0.3219752754296894559, 0.3333333333333333703, 0.3219752754296894559, 0.3333333333333333703, 0.3219752754296894559, 0.3333333333333333703, 0.3219752754296894559, 0.3333333333333333703, 0.3219752754296894559, 0.3333333333333333703, 0.3219752754296894559, 0.3333333333333333703, 0.3219752754296894559, 0.3333333333333333703, 0.3219752754296894559, 0.3333333333333333703, 0.3219752754296894559, 0.3333333333333333703, 0.3219752754296894559, 0.3333333333333333703, 0.3219752754296894559, 0.3333333333333333703, 0.3219752754296894559, 0.3333333333333333703, 0.3219752754296894559, 0.3333333333333333703, 0.3219752754296894559, 0.3333333333333333703, 0.3219752754296894559, 0.3333333333333333703, 0.3219752754296894559, 0.3333333333333333703, 0.3219752754296894559, 0.3333333333333333703, 0.3219752754296894559, 0.3333333333333333703, 0.3219752754296894559, 0.3333333333333333703, 0.3219752754296894559, 0.3333333333333333703, 0.3219752754296894559, 0.3333333333333333703, 0.3219752754296894559, 0.3333333333333333703, 0.3219752754296894559, 0.3333333333333333703, 0.3219752754296894559, 0.3333333333333333703, 0.3219752754296894559, 0.3333333333333333703, 0.3219752754296894559, 0.3333333333333333703, 0.3219752754296894559, 0.3333333333333333703, 0.3219752754296894559, 0.3333333333333333703, 0.3219752754296894559, 0.3333333333333333703, 0.3219752754296894559, 0.3333333333333333703, 0.3219752754296894559, 0.3333333333333333703, 0.3219752754296894559, 0.3333333333333333703, 0.3219752754296894559, 0.3333333333333333703, 0.3219752754296894559, 0.3333333333333333703, 0.3219752754296894559, 0.3333333333333333703, 0.3219752754296894559, 0.3333333333333333703, 0.3219752754296894559, 0.3333333333333333703, 0.3219752754296894559, 0.3333333333333333703, 0.3219752754296894559, 0.3333333333333333703, 0.3219752754296894559, 0.3333333333333333703, 0.3219752754296894559, 0.3333333333333333703, 0.3219752754296894559, 0.3333333333333333703, 0.3219752754296894559, 0.3333333333333333703, 0.3219752754296894559, 0.3333333333333333703, 0.3219752754296894559, 0.3333333333333333703, 0.3219752754296894559, 0.3333333333333333703, 0.3219752754296894559, 0.3333333333333333703, 0.3219752754296894559, 0.3333333333333333703, 0.3219752754296894559, 0.3333333333333333703, 0.3219752754296894559, 0.3333333333333333703, 0.3219752754296894559, 0.3333333333333333703, 0.3219752754296894559, 0.3333333333333333703, 0.3219752754296894559, 0.3333333333333333703, 0.3219752754296894559, 0.3333333333333333703, 0.3219752754296894559, 0.3333333333333333703, 0.3219752754296894559, 0.3333333333333333703, 0.3219752754296894559, 0.3333333333333333703, 0.3219752754296894559, 0.3333333333333333703, 0.3219752754296894559, 0.3333333333333333703, 0.3219752754296894559, 0.3333333333333333703, 0.3219752754296894559, 0.3333333333333333703, 0.3219752754296894559, 0.3333333333333333703, 0.3219752754296894559, 0.3333333333333333703, 0.3219752754296894559, 0.3333333333333333703, 0.3219752754296894559, 0.3333333333333333703, 0.3219752754296894559, 0.3333333333333333703, 0.3219752754296894559, 0.3333333333333333703, 0.3219752754296894559, 0.3333333333333333703, 0.3219752754296894559, 0.3333333333333333703, 0.3219752754296894559, 0.3333333333333333703, 0.3219752754296894559, 0.3333333333333333703, 0.3219752754296894559, 0.3333333333333333703, 0.3219752754296894559, 0.3333333333333333703, 0.3219752754296894559, 0.3333333333333333703, 0.3219752754296894559, 0.3333333333333333703, 0.3219752754296894559, 0.3333333333333333703, 0.3219752754296894559, 0.3333333333333333703, 0.3219752754296894559, 0.3333333333333333703, 0.3219752754296894559, 0.3333333333333333703, 0.3219752754296894559, 0.3333333333333333703, 0.3219752754296894559, 0.3333333333333333703, 0.3219752754296894559, 0.3333333333333333703, 0.3219752754296894559, 0.3333333333333333703, 0.3219752754296894559, 0.3333333333333333703, 0.3219752754296894559, 0.3333333333333333703),
 ( 1.000000000000000000, 0.9659258262890683122, 1.000000000000000000, 0.9659258262890683122, 1.000000000000000000, 0.9659258262890683122, 1.000000000000000000, 0.9659258262890683122, 1.000000000000000000, 0.9659258262890683122, 1.000000000000000000, 0.9659258262890683122, 1.000000000000000000, 0.9659258262890683122, 1.000000000000000000, 0.9659258262890683122, 1.000000000000000000, 0.9659258262890683122, 1.000000000000000000, 0.9659258262890683122, 1.000000000000000000, 0.9659258262890683122, 1.000000000000000000, 0.9659258262890683122, 1.000000000000000000, 0.9659258262890683122, 1.000000000000000000, 0.9659258262890683122, 1.000000000000000000, 0.9659258262890683122, 1.000000000000000000, 0.9659258262890683122, 1.000000000000000000, 0.9659258262890683122, 1.000000000000000000, 0.9659258262890683122, 1.000000000000000000, 0.9659258262890683122, 1.000000000000000000, 0.9659258262890683122, 1.000000000000000000, 0.9659258262890683122, 1.000000000000000000, 0.9659258262890683122, 1.000000000000000000, 0.9659258262890683122, 1.000000000000000000, 0.9659258262890683122, 1.000000000000000000, 0.9659258262890683122, 1.000000000000000000, 0.9659258262890683122, 1.000000000000000000, 0.9659258262890683122, 1.000000000000000000, 0.9659258262890683122, 1.000000000000000000, 0.9659258262890683122, 1.000000000000000000, 0.9659258262890683122, 1.000000000000000000, 0.9659258262890683122, 1.000000000000000000, 0.9659258262890683122, 1.000000000000000000, 0.9659258262890683122, 1.000000000000000000, 0.9659258262890683122, 1.000000000000000000, 0.9659258262890683122, 1.000000000000000000, 0.9659258262890683122, 1.000000000000000000, 0.9659258262890683122, 1.000000000000000000, 0.9659258262890683122, 1.000000000000000000, 0.9659258262890683122, 1.000000000000000000, 0.9659258262890683122, 1.000000000000000000, 0.9659258262890683122, 1.000000000000000000, 0.9659258262890683122, 1.000000000000000000, 0.9659258262890683122, 1.000000000000000000, 0.9659258262890683122, 1.000000000000000000, 0.9659258262890683122, 1.000000000000000000, 0.9659258262890683122, 1.000000000000000000, 0.9659258262890683122, 1.000000000000000000, 0.9659258262890683122, 1.000000000000000000, 0.9659258262890683122, 1.000000000000000000, 0.9659258262890683122, 1.000000000000000000, 0.9659258262890683122, 1.000000000000000000, 0.9659258262890683122, 1.000000000000000000, 0.9659258262890683122, 1.000000000000000000, 0.9659258262890683122, 1.000000000000000000, 0.9659258262890683122, 1.000000000000000000, 0.9659258262890683122, 1.000000000000000000, 0.9659258262890683122, 1.000000000000000000, 0.9659258262890683122, 1.000000000000000000, 0.9659258262890683122, 1.000000000000000000, 0.9659258262890683122, 1.000000000000000000, 0.9659258262890683122, 1.000000000000000000, 0.9659258262890683122, 1.000000000000000000, 0.9659258262890683122, 1.000000000000000000, 0.9659258262890683122, 1.000000000000000000, 0.9659258262890683122, 1.000000000000000000, 0.9659258262890683122, 1.000000000000000000, 0.9659258262890683122, 1.000000000000000000, 0.9659258262890683122, 1.000000000000000000, 0.9659258262890683122, 1.000000000000000000, 0.9659258262890683122, 1.000000000000000000, 0.9659258262890683122, 1.000000000000000000, 0.9659258262890683122, 1.000000000000000000, 0.9659258262890683122, 1.000000000000000000, 0.9659258262890683122, 1.000000000000000000, 0.9659258262890683122, 1.000000000000000000, 0.9659258262890683122, 1.000000000000000000, 0.9659258262890683122, 1.000000000000000000, 0.9659258262890683122, 1.000000000000000000, 0.9659258262890683122, 1.000000000000000000, 0.9659258262890683122, 1.000000000000000000, 0.9659258262890683122, 1.000000000000000000, 0.9659258262890683122, 1.000000000000000000, 0.9659258262890683122, 1.000000000000000000, 0.9659258262890683122, 1.000000000000000000, 0.9659258262890683122, 1.000000000000000000, 0.9659258262890683122, 1.000000000000000000, 0.9659258262890683122, 1.000000000000000000, 0.9659258262890683122, 1.000000000000000000, 0.9659258262890683122, 1.000000000000000000, 0.9659258262890683122, 1.000000000000000000, 0.9659258262890683122, 1.000000000000000000, 0.9659258262890683122, 1.000000000000000000, 0.9659258262890683122, 1.000000000000000000, 0.9659258262890683122, 1.000000000000000000, 0.9659258262890683122, 1.000000000000000000, 0.9659258262890683122, 1.000000000000000000, 0.9659258262890683122, 1.000000000000000000, 0.9659258262890683122, 1.000000000000000000, 0.9659258262890683122, 1.000000000000000000, 0.9659258262890683122, 1.000000000000000000, 0.9659258262890683122, 1.000000000000000000, 0.9659258262890683122, 1.000000000000000000, 0.9659258262890683122, 1.000000000000000000, 0.9659258262890683122, 1.000000000000000000, 0.9659258262890683122, 1.000000000000000000, 0.9659258262890683122, 1.000000000000000000, 0.9659258262890683122, 1.000000000000000000, 0.9659258262890683122, 1.000000000000000000, 0.9659258262890683122, 1.000000000000000000, 0.9659258262890683122, 1.000000000000000000, 0.9659258262890683122, 1.000000000000000000, 0.9659258262890683122, 1.000000000000000000, 0.9659258262890683122, 1.000000000000000000, 0.9659258262890683122, 1.000000000000000000, 0.9659258262890683122, 1.000000000000000000, 0.9659258262890683122, 1.000000000000000000, 0.9659258262890683122, 1.000000000000000000, 0.9659258262890683122, 1.000000000000000000, 0.9659258262890683122, 1.000000000000000000, 0.9659258262890683122, 1.000000000000000000, 0.9659258262890683122, 1.000000000000000000, 0.9659258262890683122, 1.000000000000000000, 0.9659258262890683122, 1.000000000000000000, 0.9659258262890683122, 1.000000000000000000, 0.9659258262890683122, 1.000000000000000000, 0.9659258262890683122, 1.000000000000000000, 0.9659258262890683122, 1.000000000000000000, 0.9659258262890683122, 1.000000000000000000, 0.9659258262890683122, 1.000000000000000000, 0.9659258262890683122, 1.000000000000000000, 0.9659258262890683122, 1.000000000000000000, 0.9659258262890683122, 1.000000000000000000, 0.9659258262890683122, 1.000000000000000000, 0.9659258262890683122, 1.000000000000000000, 0.9659258262890683122, 1.000000000000000000, 0.9659258262890683122, 1.000000000000000000, 0.9659258262890683122, 1.000000000000000000, 0.9659258262890683122, 1.000000000000000000, 0.9659258262890683122, 1.000000000000000000, 0.9659258262890683122, 1.000000000000000000, 0.9659258262890683122, 1.000000000000000000, 0.9659258262890683122, 1.000000000000000000, 0.9659258262890683122, 1.000000000000000000, 0.9659258262890683122, 1.000000000000000000, 0.9659258262890683122, 1.000000000000000000, 0.9659258262890683122, 1.000000000000000000, 0.9659258262890683122, 1.000000000000000000, 0.9659258262890683122, 1.000000000000000000, 0.9659258262890683122, 1.000000000000000000, 0.9659258262890683122, 1.000000000000000000, 0.9659258262890683122, 1.000000000000000000, 0.9659258262890683122, 1.000000000000000000, 0.9659258262890683122, 1.000000000000000000, 0.9659258262890683122, 1.000000000000000000, 0.9659258262890683122, 1.000000000000000000, 0.9659258262890683122, 1.000000000000000000, 0.9659258262890683122, 1.000000000000000000, 0.9659258262890683122, 1.000000000000000000, 0.9659258262890683122, 1.000000000000000000, 0.9659258262890683122, 1.000000000000000000, 0.9659258262890683122, 1.000000000000000000, 0.9659258262890683122, 1.000000000000000000, 0.9659258262890683122, 1.000000000000000000, 0.9659258262890683122, 1.000000000000000000, 0.9659258262890683122, 1.000000000000000000, 0.9659258262890683122, 1.000000000000000000, 0.9659258262890683122, 1.000000000000000000, 0.9659258262890683122, 1.000000000000000000, 0.9659258262890683122, 1.000000000000000000, 0.9659258262890683122, 1.000000000000000000, 0.9659258262890683122, 1.000000000000000000, 0.9659258262890683122, 1.000000000000000000, 0.9659258262890683122, 1.000000000000000000, 0.9659258262890683122, 1.000000000000000000, 0.9659258262890683122, 1.000000000000000000, 0.9659258262890683122, 1.000000000000000000, 0.9659258262890683122, 1.000000000000000000, 0.9659258262890683122, 1.000000000000000000, 0.9659258262890683122, 1.000000000000000000, 0.9659258262890683122, 1.000000000000000000, 0.9659258262890683122, 1.000000000000000000, 0.9659258262890683122, 1.000000000000000000, 0.9659258262890683122, 1.000000000000000000, 0.9659258262890683122, 1.000000000000000000, 0.9659258262890683122, 1.000000000000000000, 0.9659258262890683122, 1.000000000000000000, 0.9659258262890683122, 1.000000000000000000, 0.9659258262890683122, 1.000000000000000000, 0.9659258262890683122, 1.000000000000000000, 0.9659258262890683122, 1.000000000000000000, 0.9659258262890683122, 1.000000000000000000, 0.9659258262890683122, 1.000000000000000000, 0.9659258262890683122, 1.000000000000000000, 0.9659258262890683122, 1.000000000000000000, 0.9659258262890683122, 1.000000000000000000, 0.9659258262890683122, 1.000000000000000000, 0.9659258262890683122, 1.000000000000000000, 0.9659258262890683122, 1.000000000000000000, 0.9659258262890683122, 1.000000000000000000, 0.9659258262890683122, 1.000000000000000000, 0.9659258262890683122, 1.000000000000000000, 0.9659258262890683122, 1.000000000000000000, 0.9659258262890683122, 1.000000000000000000, 0.9659258262890683122, 1.000000000000000000, 0.9659258262890683122, 1.000000000000000000, 0.9659258262890683122, 1.000000000000000000, 0.9659258262890683122, 1.000000000000000000, 0.9659258262890683122, 1.000000000000000000, 0.9659258262890683122, 1.000000000000000000, 0.9659258262890683122, 1.000000000000000000, 0.9659258262890683122, 1.000000000000000000, 0.9659258262890683122, 1.000000000000000000, 0.9659258262890683122, 1.000000000000000000, 0.9659258262890683122, 1.000000000000000000, 0.9659258262890683122, 1.000000000000000000, 0.9659258262890683122, 1.000000000000000000, 0.9659258262890683122, 1.000000000000000000, 0.9659258262890683122, 1.000000000000000000, 0.9659258262890683122, 1.000000000000000000, 0.9659258262890683122, 1.000000000000000000, 0.9659258262890683122, 1.000000000000000000, 0.9659258262890683122, 1.000000000000000000, 0.9659258262890683122, 1.000000000000000000, 0.9659258262890683122, 1.000000000000000000, 0.9659258262890683122, 1.000000000000000000, 0.9659258262890683122, 1.000000000000000000, 0.9659258262890683122, 1.000000000000000000, 0.9659258262890683122, 1.000000000000000000) ) ) 
 REPRESENTATION_ITEM ( '' )  SURFACE ( )  );
#176314=CARTESIAN_POINT ( 'NONE',  ( -14.34966873604972548, 8.224510206698743886, 78.33442372801901854 ) ) ;
#176315=CARTESIAN_POINT ( 'NONE',  ( -21.55341960407619339, 5.719274019375674811, 78.54275706135236135 ) ) ;
#176316=CARTESIAN_POINT ( 'NONE',  ( -13.89961937509957401, -13.97604488694547875, 94.37609039468566152 ) ) ;
#176317=CARTESIAN_POINT ( 'NONE',  ( 13.97604488694548053, -13.89961937509957401, 45.62609039468566863 ) ) ;
#176318=CARTESIAN_POINT ( 'NONE',  ( 13.97604488694527802, 13.89961937509977652, 79.37390960531435269 ) ) ;
#176319=CARTESIAN_POINT ( 'NONE',  ( -9.564922557960796823, -16.46253265017161027, 62.08224293864769550 ) ) ;
#176322=CARTESIAN_POINT ( 'NONE',  ( 17.58332526062529411, -7.635886036038496805, 88.42334959558466778 ) ) ;
#176323=CARTESIAN_POINT ( 'NONE',  ( -10.72451020669898014, 18.67979575497178502, 95.41557627198102409 ) ) ;
#176324=CARTESIAN_POINT ( 'NONE',  ( -18.62759615963270932, 10.81492255796079327, 45.83224293864769550 ) ) ;
#176325=CARTESIAN_POINT ( 'NONE',  ( -5.153800228976328057, -19.02544592524343514, 27.29057627198103120 ) ) ;
#176326=CARTESIAN_POINT ( 'NONE',  ( 0.05219959533934541429, -16.53943276465976808, 60.00109039468568284 ) ) ;
#176328=CARTESIAN_POINT ( 'NONE',  ( -21.55341960407619339, 5.719274019375674811, 43.54275706135235424 ) ) ;
#176329=CARTESIAN_POINT ( 'NONE',  ( -12.14591786802309592, -12.06949235617757132, 61.87390960531436690 ) ) ;
#176331=CARTESIAN_POINT ( 'NONE',  ( -8.314922557961024197, 14.29746914071037800, 32.91775706135234714 ) ) ;
#176332=CARTESIAN_POINT ( 'NONE',  ( -16.52544592524342804, 4.483927247898546575, 101.0405762719810383 ) ) ;
#176333=CARTESIAN_POINT ( 'NONE',  ( -9.564922557961040184, 16.46253265017147172, 52.91775706135233293 ) ) ;
#176334=CARTESIAN_POINT ( 'NONE',  ( 4.379528057220339221, -16.55341960407611168, 57.70724293864770260 ) ) ;
#176335=CARTESIAN_POINT ( 'NONE',  ( 15.72974639402176855, 15.80617190586768217, 31.87609039468567929 ) ) ;
#176336=CARTESIAN_POINT ( 'NONE',  ( 5.049401038298161559, -19.05341960407611168, 22.70724293864769194 ) ) ;
#176337=CARTESIAN_POINT ( 'NONE',  ( 10.81492255796078972, 18.62759615963270932, 84.58224293864769550 ) ) ;
#176338=CARTESIAN_POINT ( 'NONE',  ( -0.05219959533909027116, -19.03943276465977164, 107.4989096053143527 ) ) ;
#176339=CARTESIAN_POINT ( 'NONE',  ( 8.314922557960818139, 14.29746914071049879, 79.58224293864769550 ) ) ;
#176340=CARTESIAN_POINT ( 'NONE',  ( 5.049401038298161559, -19.05341960407611168, 112.7072429386476813 ) ) ;
#176342=CARTESIAN_POINT ( 'NONE',  ( 0.05219959533936267826, -19.03943276465977164, 85.00109039468567573 ) ) ;
#176343=CARTESIAN_POINT ( 'NONE',  ( -5.823673210054431948, 21.52544592524334988, 27.70942372801901854 ) ) ;
#176344=CARTESIAN_POINT ( 'NONE',  ( 13.89961937509977652, -13.97604488694527269, 73.12390960531436690 ) ) ;
#176345=CARTESIAN_POINT ( 'NONE',  ( -19.03943276465977164, -0.05219959533935918106, 53.75109039468566863 ) ) ;
#176346=CARTESIAN_POINT ( 'NONE',  ( -19.03943276465977164, 0.05219959533909376836, 36.24890960531436690 ) ) ;
#176347=CARTESIAN_POINT ( 'NONE',  ( -5.823673210054431948, 21.52544592524334988, 67.70942372801901854 ) ) ;
#176349=CARTESIAN_POINT ( 'NONE',  ( 8.314922557960818139, 14.29746914071049879, 59.58224293864770260 ) ) ;
#176350=CARTESIAN_POINT ( 'NONE',  ( 16.51473224551069308, 9.474510206698969483, 69.16557627198102409 ) ) ;
#176351=CARTESIAN_POINT ( 'NONE',  ( -21.53943276465977519, 0.05219959533907696930, 86.24890960531436690 ) ) ;
#176352=CARTESIAN_POINT ( 'NONE',  ( 13.89961937509977652, -13.97604488694527269, 53.12390960531434558 ) ) ;
#176354=CARTESIAN_POINT ( 'NONE',  ( 18.62759615963271287, -10.81492255796078972, 83.33224293864769550 ) ) ;
#176355=CARTESIAN_POINT ( 'NONE',  ( 21.55341960407619695, -5.719274019375665929, 96.04275706135236135 ) ) ;
#176356=CARTESIAN_POINT ( 'NONE',  ( -13.97604488694527625, -13.89961937509977652, 26.87390960531434558 ) ) ;
#176357=CARTESIAN_POINT ( 'NONE',  ( -8.224510206698735004, -14.34966873604973081, 94.58442372801901854 ) ) ;
#176358=CARTESIAN_POINT ( 'NONE',  ( 4.379528057220339221, -16.55341960407611168, 102.7072429386476955 ) ) ;
#176359=CARTESIAN_POINT ( 'NONE',  ( -0.05219959533936034679, 19.03943276465977164, 97.50109039468567573 ) ) ;
#176360=ORIENTED_EDGE ( 'NONE', *, *, #164865, .F. ) ;
#176361=CARTESIAN_POINT ( 'NONE',  ( 21.53943276465977519, 0.05219959533937863772, 21.25109039468567218 ) ) ;
#176362=CARTESIAN_POINT ( 'NONE',  ( -0.05219959533936034679, 19.03943276465977164, 57.50109039468566863 ) ) ;
#176363=CARTESIAN_POINT ( 'NONE',  ( 14.29746914071037800, 8.314922557961029526, 106.6677570613523756 ) ) ;
#176364=CARTESIAN_POINT ( 'NONE',  ( 9.474510206698729675, 16.51473224551082808, 27.08442372801900433 ) ) ;
#176365=CARTESIAN_POINT ( 'NONE',  ( -9.474510206698964154, 16.51473224551069663, 100.4155762719810241 ) ) ;
#176366=CARTESIAN_POINT ( 'NONE',  ( -0.05219959533907301413, -21.53943276465977519, 57.49890960531435979 ) ) ;
#176368=CARTESIAN_POINT ( 'NONE',  ( -8.224510206698948167, 14.34966873604960824, 115.4155762719810241 ) ) ;
#176369=CARTESIAN_POINT ( 'NONE',  ( 9.564922557961047289, -16.46253265017146816, 20.41775706135233293 ) ) ;
#176370=CARTESIAN_POINT ( 'NONE',  ( 0.05219959533934541429, -16.53943276465976808, 70.00109039468568994 ) ) ;
#176371=CARTESIAN_POINT ( 'NONE',  ( 21.52544592524334988, 5.823673210054432836, 31.45942372801901854 ) ) ;
#176372=CARTESIAN_POINT ( 'NONE',  ( 16.52544592524335698, 4.483927247898782831, 46.45942372801901854 ) ) ;
#176373=CARTESIAN_POINT ( 'NONE',  ( 19.03943276465977164, -0.05219959533909143690, 98.74890960531436690 ) ) ;
#176374=CARTESIAN_POINT ( 'NONE',  ( 5.153800228976335163, 19.02544592524342804, 44.79057627198103830 ) ) ;
#176375=CARTESIAN_POINT ( 'NONE',  ( -0.05219959533909027116, -19.03943276465977164, 62.49890960531435979 ) ) ;
#176376=CARTESIAN_POINT ( 'NONE',  ( 16.53943276465976808, 0.05219959533934440121, 46.25109039468567573 ) ) ;
#176377=CARTESIAN_POINT ( 'NONE',  ( -12.14591786802309592, -12.06949235617757132, 96.87390960531436690 ) ) ;
#176378=CARTESIAN_POINT ( 'NONE',  ( -14.29746914071037622, -8.314922557961029526, 99.16775706135234714 ) ) ;
#176380=CARTESIAN_POINT ( 'NONE',  ( -5.823673210054431948, 21.52544592524334988, 52.70942372801902565 ) ) ;
#176381=CARTESIAN_POINT ( 'NONE',  ( -5.049401038298153566, 19.05341960407611168, 75.20724293864769550 ) ) ;
#176382=CARTESIAN_POINT ( 'NONE',  ( -9.474510206698964154, 16.51473224551069663, 70.41557627198102409 ) ) ;
#176383=CARTESIAN_POINT ( 'NONE',  ( -19.05341960407611168, -5.049401038298163336, 96.45724293864769550 ) ) ;
#176384=CARTESIAN_POINT ( 'NONE',  ( -16.52544592524342804, 4.483927247898546575, 51.04057627198103120 ) ) ;
#176385=CARTESIAN_POINT ( 'NONE',  ( -8.224510206698735004, -14.34966873604973081, 99.58442372801900433 ) ) ;
#176386=CARTESIAN_POINT ( 'NONE',  ( -14.34966873604960291, -8.224510206698953496, 21.66557627198102409 ) ) ;
#176387=ORIENTED_EDGE ( 'NONE', *, *, #82183, .F. ) ;
#176388=CARTESIAN_POINT ( 'NONE',  ( 9.564922557961047289, -16.46253265017146816, 45.41775706135232582 ) ) ;
#176389=CARTESIAN_POINT ( 'NONE',  ( -9.564922557960796823, -16.46253265017161027, 112.0822429386476955 ) ) ;
#176390=CARTESIAN_POINT ( 'NONE',  ( 13.97604488694527802, 13.89961937509977652, 59.37390960531434558 ) ) ;
#176391=CARTESIAN_POINT ( 'NONE',  ( -5.153800228976607833, 19.02544592524334988, 37.70942372801899722 ) ) ;
#176394=CARTESIAN_POINT ( 'NONE',  ( -13.89961937509957401, -13.97604488694547875, 84.37609039468567573 ) ) ;
#176395=CARTESIAN_POINT ( 'NONE',  ( -14.29746914071037622, -8.314922557961029526, 69.16775706135234714 ) ) ;
#176396=CARTESIAN_POINT ( 'NONE',  ( 17.13100169013300444, 6.664070546373150883, 91.73210164300154190 ) ) ;
#176397=CARTESIAN_POINT ( 'NONE',  ( -16.46253265017160317, 9.564922557960807481, 85.83224293864769550 ) ) ;
#176398=CARTESIAN_POINT ( 'NONE',  ( 21.52544592524334988, 5.823673210054432836, 26.45942372801901854 ) ) ;
#176399=CARTESIAN_POINT ( 'NONE',  ( 19.05341960407617918, -5.049401038297876454, 71.04275706135234714 ) ) ;
#176400=CARTESIAN_POINT ( 'NONE',  ( 16.81555441253551209, 7.025013491695498047, 86.86314554665750620 ) ) ;
#176401=CARTESIAN_POINT ( 'NONE',  ( -5.049401038298153566, 19.05341960407611168, 50.20724293864770260 ) ) ;
#176402=CARTESIAN_POINT ( 'NONE',  ( -9.474510206698964154, 16.51473224551069663, 90.41557627198103830 ) ) ;
#176403=CARTESIAN_POINT ( 'NONE',  ( 8.314922557960818139, 14.29746914071049879, 44.58224293864769550 ) ) ;
#176404=CARTESIAN_POINT ( 'NONE',  ( -5.153800228976328057, -19.02544592524343514, 37.29057627198102409 ) ) ;
#176405=CARTESIAN_POINT ( 'NONE',  ( -16.46253265017146816, -9.564922557961047289, 54.16775706135234003 ) ) ;
#176406=CARTESIAN_POINT ( 'NONE',  ( -0.05219959533910754901, -16.53943276465976808, 82.49890960531436690 ) ) ;
#176407=CARTESIAN_POINT ( 'NONE',  ( -5.049401038297874678, -19.05341960407617918, 29.79275706135232227 ) ) ;
#176408=CARTESIAN_POINT ( 'NONE',  ( 16.46253265017160672, -9.564922557960803928, 63.33224293864769550 ) ) ;
#176409=CARTESIAN_POINT ( 'NONE',  ( -0.05219959533907301413, -21.53943276465977519, 62.49890960531436690 ) ) ;
#176410=CARTESIAN_POINT ( 'NONE',  ( 14.34966873604960469, 8.224510206698951720, 54.16557627198103120 ) ) ;
#176411=CARTESIAN_POINT ( 'NONE',  ( -21.53943276465977519, -0.05219959533937600094, 113.7510903946856757 ) ) ;
#176412=CARTESIAN_POINT ( 'NONE',  ( -5.153800228976328057, -19.02544592524343514, 107.2905762719810383 ) ) ;
#176414=CARTESIAN_POINT ( 'NONE',  ( 10.72451020669898902, -18.67979575497178502, 22.91557627198102765 ) ) ;
#176415=CARTESIAN_POINT ( 'NONE',  ( -19.03943276465977164, 0.05219959533909376836, 51.24890960531436690 ) ) ;
#176416=CARTESIAN_POINT ( 'NONE',  ( -19.03943276465977164, 0.05219959533909376836, 31.24890960531435979 ) ) ;
#176417=CARTESIAN_POINT ( 'NONE',  ( -16.53943276465976808, 0.05219959533911058130, 96.24890960531435269 ) ) ;
#176418=CARTESIAN_POINT ( 'NONE',  ( -10.72451020669898014, 18.67979575497178502, 105.4155762719810383 ) ) ;
#176419=CARTESIAN_POINT ( 'NONE',  ( -9.474510206698964154, 16.51473224551069663, 95.41557627198102409 ) ) ;
#176420=CARTESIAN_POINT ( 'NONE',  ( -21.55341960407610458, -5.719274019375992779, 106.4572429386477097 ) ) ;
#176421=CARTESIAN_POINT ( 'NONE',  ( 13.89961937509977652, -13.97604488694527269, 108.1239096053143669 ) ) ;
#176422=CARTESIAN_POINT ( 'NONE',  ( -19.02544592524342804, 5.153800228976336051, 26.04057627198103120 ) ) ;
#176424=CARTESIAN_POINT ( 'NONE',  ( 15.72974639402176855, 15.80617190586768217, 76.87609039468567573 ) ) ;
#176425=CARTESIAN_POINT ( 'NONE',  ( 15.80617190586746368, 15.72974639402197994, 89.37390960531435269 ) ) ;
#176429=CARTESIAN_POINT ( 'NONE',  ( -0.05219959533934338120, 16.53943276465976808, 42.50109039468567573 ) ) ;
#176430=CARTESIAN_POINT ( 'NONE',  ( -16.55341960407611168, -4.379528057220339221, 106.4572429386477097 ) ) ;
#176432=CARTESIAN_POINT ( 'NONE',  ( -13.97604488694527625, -13.89961937509977652, 56.87390960531434558 ) ) ;
#176433=CARTESIAN_POINT ( 'NONE',  ( 16.52544592524342804, -4.483927247898539470, 98.54057627198105251 ) ) ;
#176434=CARTESIAN_POINT ( 'NONE',  ( -21.53943276465977519, 0.05219959533907696930, 36.24890960531435979 ) ) ;
#176435=CARTESIAN_POINT ( 'NONE',  ( -4.483927247898539470, -16.52544592524342804, 67.29057627198103830 ) ) ;
#176436=CARTESIAN_POINT ( 'NONE',  ( -14.29746914071037622, -8.314922557961029526, 24.16775706135235424 ) ) ;
#176437=CARTESIAN_POINT ( 'NONE',  ( 18.67979575497194134, -10.72451020669871369, 70.83442372801901854 ) ) ;
#176438=CARTESIAN_POINT ( 'NONE',  ( 9.474510206698729675, 16.51473224551082808, 62.08442372801899722 ) ) ;
#176439=CARTESIAN_POINT ( 'NONE',  ( 14.29746914071037800, 8.314922557961029526, 91.66775706135234714 ) ) ;
#176440=CARTESIAN_POINT ( 'NONE',  ( 4.379528057220339221, -16.55341960407611168, 37.70724293864769550 ) ) ;
#176441=CARTESIAN_POINT ( 'NONE',  ( 16.51473224551069308, 9.474510206698969483, 44.16557627198103120 ) ) ;
#176442=CARTESIAN_POINT ( 'NONE',  ( -13.97604488694527625, -13.89961937509977652, 91.87390960531432427 ) ) ;
#176443=CARTESIAN_POINT ( 'NONE',  ( -5.823673210054116645, -21.52544592524344225, 97.29057627198105251 ) ) ;
#176444=CARTESIAN_POINT ( 'NONE',  ( 16.55341960407618274, -4.379528057220086978, 31.04275706135234714 ) ) ;
#176445=CARTESIAN_POINT ( 'NONE',  ( 8.314922557960818139, 14.29746914071049879, 59.58224293864770260 ) ) ;
#176446=CARTESIAN_POINT ( 'NONE',  ( -21.55341960407619339, 5.719274019375674811, 68.54275706135234714 ) ) ;
#176447=CARTESIAN_POINT ( 'NONE',  ( 12.14591786802327356, -12.06949235617739191, 100.6260903946857184 ) ) ;
#176448=CARTESIAN_POINT ( 'NONE',  ( 16.81555441253551564, 7.025013491695498935, 26.86314554665745646 ) ) ;
#176449=CARTESIAN_POINT ( 'NONE',  ( -18.22780087662126647, -5.499999999999827693, 63.98236817873107185 ) ) ;
#176450=CARTESIAN_POINT ( 'NONE',  ( 14.29746914071049879, -8.314922557960816363, 33.33224293864769550 ) ) ;
#176451=CARTESIAN_POINT ( 'NONE',  ( -0.05219959533934338120, 16.53943276465976808, 72.50109039468568994 ) ) ;
#176452=CARTESIAN_POINT ( 'NONE',  ( -19.03943276465977164, 0.05219959533909376836, 81.24890960531436690 ) ) ;
#176453=CARTESIAN_POINT ( 'NONE',  ( -16.51473224551069308, -9.474510206698971260, 81.66557627198103830 ) ) ;
#176454=CARTESIAN_POINT ( 'NONE',  ( 5.719274019375673035, 21.55341960407619339, 82.29275706135234714 ) ) ;
#176455=CARTESIAN_POINT ( 'NONE',  ( -16.52544592524335698, -4.483927247898792601, 93.95942372801903275 ) ) ;
#176456=CARTESIAN_POINT ( 'NONE',  ( -8.314922557960811034, -14.29746914071050412, 62.08224293864769550 ) ) ;
#176457=CARTESIAN_POINT ( 'NONE',  ( -5.153800228976328057, -19.02544592524343514, 62.29057627198100988 ) ) ;
#176458=ORIENTED_EDGE ( 'NONE', *, *, #165982, .F. ) ;
#176459=CARTESIAN_POINT ( 'NONE',  ( 13.89961937509957401, 13.97604488694547697, 111.8760903946856757 ) ) ;
#176460=CARTESIAN_POINT ( 'NONE',  ( -4.379528057220328563, 16.55341960407611168, 105.2072429386477097 ) ) ;
#176461=CARTESIAN_POINT ( 'NONE',  ( 5.153800228976335163, 19.02544592524342804, 84.79057627198099567 ) ) ;
#176462=CARTESIAN_POINT ( 'NONE',  ( 9.474510206698729675, 16.51473224551082808, 112.0844237280190043 ) ) ;
#176464=CARTESIAN_POINT ( 'NONE',  ( 0.05219959533936267826, -19.03943276465977164, 25.00109039468566152 ) ) ;
#176465=CARTESIAN_POINT ( 'NONE',  ( 0.05219959533934541429, -16.53943276465976808, 85.00109039468568994 ) ) ;
#176466=CARTESIAN_POINT ( 'NONE',  ( 19.05341960407617918, -5.049401038297876454, 96.04275706135231871 ) ) ;
#176467=CARTESIAN_POINT ( 'NONE',  ( 16.51473224551069308, 9.474510206698969483, 24.16557627198102765 ) ) ;
#176468=CARTESIAN_POINT ( 'NONE',  ( 16.53943276465976808, 0.05219959533934440121, 61.25109039468567573 ) ) ;
#176469=CARTESIAN_POINT ( 'NONE',  ( 12.14591786802327356, -12.06949235617739191, 55.62609039468568284 ) ) ;
#176470=CARTESIAN_POINT ( 'NONE',  ( 13.97604488694527802, 13.89961937509977652, 24.37390960531435624 ) ) ;
#176471=CARTESIAN_POINT ( 'NONE',  ( -9.564922557961040184, 16.46253265017147172, 52.91775706135233293 ) ) ;
#176472=CARTESIAN_POINT ( 'NONE',  ( -0.05219959533937732626, 21.53943276465977519, 102.5010903946856899 ) ) ;
#176473=CARTESIAN_POINT ( 'NONE',  ( -9.564922557960796823, -16.46253265017161027, 37.08224293864768839 ) ) ;
#176474=CARTESIAN_POINT ( 'NONE',  ( 5.153800228976335163, 19.02544592524342804, 79.79057627198102409 ) ) ;
#176475=CARTESIAN_POINT ( 'NONE',  ( 16.55341960407611168, 4.379528057220329451, 78.95724293864769550 ) ) ;
#176476=CARTESIAN_POINT ( 'NONE',  ( 21.52544592524334988, 5.823673210054432836, 86.45942372801901854 ) ) ;
#176477=CARTESIAN_POINT ( 'NONE',  ( -16.46253265017146816, -9.564922557961047289, 59.16775706135233293 ) ) ;
#176478=CARTESIAN_POINT ( 'NONE',  ( -13.89961937509957401, -13.97604488694547875, 44.37609039468566863 ) ) ;
#176479=CARTESIAN_POINT ( 'NONE',  ( -10.72451020669898014, 18.67979575497178502, 35.41557627198102409 ) ) ;
#176480=CARTESIAN_POINT ( 'NONE',  ( 0.05219959533937995610, -21.53943276465977519, 100.0010903946857042 ) ) ;
#176481=CARTESIAN_POINT ( 'NONE',  ( -19.02544592524342804, 5.153800228976336051, 71.04057627198099567 ) ) ;
#176482=CARTESIAN_POINT ( 'NONE',  ( -5.823673210054431948, 21.52544592524334988, 102.7094237280190185 ) ) ;
#176483=CARTESIAN_POINT ( 'NONE',  ( 5.719274019375991003, -21.55341960407610458, 52.70724293864769550 ) ) ;
#176484=CARTESIAN_POINT ( 'NONE',  ( 13.97604488694527802, 13.89961937509977652, 99.37390960531436690 ) ) ;
#176485=CARTESIAN_POINT ( 'NONE',  ( 19.05341960407617918, -5.049401038297876454, 81.04275706135231871 ) ) ;
#176486=CARTESIAN_POINT ( 'NONE',  ( -5.153800228976328057, -19.02544592524343514, 102.2905762719810383 ) ) ;
#176487=CARTESIAN_POINT ( 'NONE',  ( -5.049401038297874678, -19.05341960407617918, 99.79275706135234714 ) ) ;
#176488=CARTESIAN_POINT ( 'NONE',  ( -16.52544592524335698, -4.483927247898792601, 38.95942372801901854 ) ) ;
#176489=CARTESIAN_POINT ( 'NONE',  ( -14.29746914071049879, 8.314922557960819915, 105.8322429386476955 ) ) ;
#176490=CARTESIAN_POINT ( 'NONE',  ( 19.05341960407611168, 5.049401038298154454, 88.95724293864769550 ) ) ;
#176491=CARTESIAN_POINT ( 'NONE',  ( 21.53943276465977519, -0.05219959533907433946, 68.74890960531435269 ) ) ;
#176492=CARTESIAN_POINT ( 'NONE',  ( -12.06949235617739369, -12.14591786802326823, 39.37609039468567573 ) ) ;
#176493=CARTESIAN_POINT ( 'NONE',  ( 15.80617190586769283, -15.72974639402175789, 40.62609039468567573 ) ) ;
#176494=CARTESIAN_POINT ( 'NONE',  ( 18.67979575497194134, -10.72451020669871369, 85.83442372801901854 ) ) ;
#176495=CARTESIAN_POINT ( 'NONE',  ( -16.52544592524335698, -4.483927247898792601, 78.95942372801901854 ) ) ;
#176496=CARTESIAN_POINT ( 'NONE',  ( -9.474510206698964154, 16.51473224551069663, 75.41557627198103830 ) ) ;
#176497=CARTESIAN_POINT ( 'NONE',  ( -12.14591786802309592, -12.06949235617757132, 81.87390960531435269 ) ) ;
#176498=CARTESIAN_POINT ( 'NONE',  ( 16.53943276465976808, -0.05219959533910856209, 28.74890960531435624 ) ) ;
#176499=CARTESIAN_POINT ( 'NONE',  ( 9.474510206698729675, 16.51473224551082808, 52.08442372801900433 ) ) ;
#176500=CARTESIAN_POINT ( 'NONE',  ( -10.81492255796105439, 18.62759615963255655, 37.91775706135235424 ) ) ;
#176501=CARTESIAN_POINT ( 'NONE',  ( -8.314922557960811034, -14.29746914071050412, 82.08224293864768129 ) ) ;
#176502=CARTESIAN_POINT ( 'NONE',  ( 5.153800228976335163, 19.02544592524342804, 114.7905762719810241 ) ) ;
#176503=CARTESIAN_POINT ( 'NONE',  ( -8.314922557961024197, 14.29746914071037800, 102.9177570613523756 ) ) ;
#176504=CARTESIAN_POINT ( 'NONE',  ( 21.52544592524334988, 5.823673210054432836, 76.45942372801901854 ) ) ;
#176505=CARTESIAN_POINT ( 'NONE',  ( 14.34966873604972726, -8.224510206698740333, 40.83442372801901854 ) ) ;
#176506=CARTESIAN_POINT ( 'NONE',  ( -21.52544592524334988, -5.823673210054445271, 38.95942372801901854 ) ) ;
#176508=CARTESIAN_POINT ( 'NONE',  ( -15.80617190586745835, -15.72974639402198527, 111.8739096053143669 ) ) ;
#176509=CARTESIAN_POINT ( 'NONE',  ( -4.379528057220328563, 16.55341960407611168, 85.20724293864770971 ) ) ;
#176510=CARTESIAN_POINT ( 'NONE',  ( 17.50000000000148503, -3.202012800152207461, 27.42822416027260246 ) ) ;
#176511=CARTESIAN_POINT ( 'NONE',  ( -8.314922557960811034, -14.29746914071050412, 57.08224293864769550 ) ) ;
#176512=CARTESIAN_POINT ( 'NONE',  ( 12.06949235617739724, 12.14591786802326823, 91.87609039468568994 ) ) ;
#176513=CARTESIAN_POINT ( 'NONE',  ( -13.97604488694527625, -13.89961937509977652, 26.87390960531434558 ) ) ;
#176514=CARTESIAN_POINT ( 'NONE',  ( 21.55341960407610458, 5.719274019375980345, 43.95724293864769550 ) ) ;
#176515=CARTESIAN_POINT ( 'NONE',  ( -16.52544592524342804, 4.483927247898546575, 76.04057627198102409 ) ) ;
#176517=CARTESIAN_POINT ( 'NONE',  ( 18.62759615963271287, -10.81492255796078972, 73.33224293864769550 ) ) ;
#176518=CARTESIAN_POINT ( 'NONE',  ( -0.05219959533909027116, -19.03943276465977164, 87.49890960531436690 ) ) ;
#176520=CARTESIAN_POINT ( 'NONE',  ( -5.153800228976328057, -19.02544592524343514, 42.29057627198101699 ) ) ;
#176521=CARTESIAN_POINT ( 'NONE',  ( 19.02544592524334988, 5.153800228976608722, 91.45942372801900433 ) ) ;
#176522=CARTESIAN_POINT ( 'NONE',  ( 10.72451020669898902, -18.67979575497178502, 32.91557627198102409 ) ) ;
#176523=CARTESIAN_POINT ( 'NONE',  ( 10.81492255796106328, -18.62759615963255655, 50.41775706135235424 ) ) ;
#176524=CARTESIAN_POINT ( 'NONE',  ( -10.81492255796078084, -18.62759615963271287, 57.08224293864769550 ) ) ;
#176525=CARTESIAN_POINT ( 'NONE',  ( 16.46253265017160672, -9.564922557960803928, 38.33224293864768839 ) ) ;
#176526=CARTESIAN_POINT ( 'NONE',  ( 13.89961937509977652, -13.97604488694527269, 78.12390960531433848 ) ) ;
#176528=CARTESIAN_POINT ( 'NONE',  ( -14.29746914071037622, -8.314922557961029526, 44.16775706135234714 ) ) ;
#176529=CARTESIAN_POINT ( 'NONE',  ( -10.72451020669870658, -18.67979575497194134, 29.58442372801901854 ) ) ;
#176530=CARTESIAN_POINT ( 'NONE',  ( -10.72451020669870658, -18.67979575497194134, 74.58442372801901854 ) ) ;
#176531=CARTESIAN_POINT ( 'NONE',  ( 16.46253265017160672, -9.564922557960803928, 113.3322429386476955 ) ) ;
#176532=CARTESIAN_POINT ( 'NONE',  ( -10.81492255796078084, -18.62759615963271287, 92.08224293864769550 ) ) ;
#176533=CARTESIAN_POINT ( 'NONE',  ( -21.55341960407619339, 5.719274019375674811, 23.54275706135235424 ) ) ;
#176534=CARTESIAN_POINT ( 'NONE',  ( 0.05219959533934541429, -16.53943276465976808, 55.00109039468568284 ) ) ;
#176535=CARTESIAN_POINT ( 'NONE',  ( -15.80617190586745835, -15.72974639402198527, 56.87390960531436690 ) ) ;
#176536=CARTESIAN_POINT ( 'NONE',  ( -5.049401038297874678, -19.05341960407617918, 24.79275706135233648 ) ) ;
#176537=CARTESIAN_POINT ( 'NONE',  ( -16.46253265017160317, 9.564922557960807481, 50.83224293864770260 ) ) ;
#176538=CARTESIAN_POINT ( 'NONE',  ( -19.02544592524342804, 5.153800228976336051, 116.0405762719810383 ) ) ;
#176539=CARTESIAN_POINT ( 'NONE',  ( 5.153800228976335163, 19.02544592524342804, 94.79057627198103830 ) ) ;
#176540=CARTESIAN_POINT ( 'NONE',  ( 17.50000000000000355, 3.210308386893693466, 102.5489375733106812 ) ) ;
#176541=CARTESIAN_POINT ( 'NONE',  ( -5.153800228976607833, 19.02544592524334988, 72.70942372801900433 ) ) ;
#176542=CARTESIAN_POINT ( 'NONE',  ( 15.80617190586746368, 15.72974639402197994, 39.37390960531436690 ) ) ;
#176543=CARTESIAN_POINT ( 'NONE',  ( -8.314922557961024197, 14.29746914071037800, 112.9177570613523329 ) ) ;
#176544=CARTESIAN_POINT ( 'NONE',  ( 13.89961937509957401, 13.97604488694547697, 96.87609039468566152 ) ) ;
#176545=CARTESIAN_POINT ( 'NONE',  ( 13.97604488694527802, 13.89961937509977652, 24.37390960531435624 ) ) ;
#176546=CARTESIAN_POINT ( 'NONE',  ( 9.564922557961047289, -16.46253265017146816, 25.41775706135234003 ) ) ;
#176547=CARTESIAN_POINT ( 'NONE',  ( 13.97604488694548053, -13.89961937509957401, 100.6260903946856615 ) ) ;
#176548=CARTESIAN_POINT ( 'NONE',  ( 21.53943276465977519, -0.05219959533907433946, 88.74890960531436690 ) ) ;
#176549=CARTESIAN_POINT ( 'NONE',  ( -19.03943276465977164, -0.05219959533935918106, 53.75109039468566863 ) ) ;
#176550=CARTESIAN_POINT ( 'NONE',  ( 16.20579543436677739, 7.371946100355104114, 108.0652083417187583 ) ) ;
#176551=CARTESIAN_POINT ( 'NONE',  ( 5.153800228976335163, 19.02544592524342804, 59.79057627198100988 ) ) ;
#176552=CARTESIAN_POINT ( 'NONE',  ( -16.52544592524342804, 4.483927247898546575, 66.04057627198103830 ) ) ;
#176553=EDGE_CURVE ( 'NONE', #24966, #119129, #95033, .T. ) ;
#176554=CARTESIAN_POINT ( 'NONE',  ( -0.05219959533909027116, -19.03943276465977164, 42.49890960531435269 ) ) ;
#176555=CARTESIAN_POINT ( 'NONE',  ( 8.314922557960818139, 14.29746914071049879, 54.58224293864769550 ) ) ;
#176556=DIRECTION ( 'NONE',  ( 0.000000000000000000, 0.000000000000000000, 1.000000000000000000 ) ) ;
#176557=CARTESIAN_POINT ( 'NONE',  ( 12.14591786802309770, 12.06949235617756955, 29.37390960531435269 ) ) ;
#176558=CARTESIAN_POINT ( 'NONE',  ( -5.049401038298153566, 19.05341960407611168, 60.20724293864768129 ) ) ;
#176559=CARTESIAN_POINT ( 'NONE',  ( -5.049401038297874678, -19.05341960407617918, 29.79275706135232227 ) ) ;
#176560=CARTESIAN_POINT ( 'NONE',  ( -16.52544592524335698, -4.483927247898792601, 28.95942372801902209 ) ) ;
#176561=CARTESIAN_POINT ( 'NONE',  ( -21.52544592524343514, 5.823673210054127303, 51.04057627198103120 ) ) ;
#176562=CARTESIAN_POINT ( 'NONE',  ( -21.52544592524334988, -5.823673210054445271, 98.95942372801903275 ) ) ;
#176563=ORIENTED_EDGE ( 'NONE', *, *, #121704, .F. ) ;
#176564=CARTESIAN_POINT ( 'NONE',  ( -19.02544592524342804, 5.153800228976336051, 66.04057627198103830 ) ) ;
#176566=CARTESIAN_POINT ( 'NONE',  ( -9.474510206698964154, 16.51473224551069663, 95.41557627198102409 ) ) ;
#176567=CARTESIAN_POINT ( 'NONE',  ( -17.49999999999999645, -5.499999999999992895, 44.20309617465829888 ) ) ;
#176568=CARTESIAN_POINT ( 'NONE',  ( 21.53943276465977519, 0.05219959533937863772, 31.25109039468568639 ) ) ;
#176570=CARTESIAN_POINT ( 'NONE',  ( 4.379528057220339221, -16.55341960407611168, 97.70724293864772392 ) ) ;
#176571=CARTESIAN_POINT ( 'NONE',  ( -21.53943276465977519, 0.05219959533907696930, 86.24890960531436690 ) ) ;
#176572=CARTESIAN_POINT ( 'NONE',  ( 5.049401038298161559, -19.05341960407611168, 67.70724293864769550 ) ) ;
#176573=CARTESIAN_POINT ( 'NONE',  ( 5.049401038298161559, -19.05341960407611168, 82.70724293864770971 ) ) ;
#176574=CARTESIAN_POINT ( 'NONE',  ( -21.53943276465977519, 0.05219959533907696930, 116.2489096053143669 ) ) ;
#176576=CARTESIAN_POINT ( 'NONE',  ( 5.049401038298161559, -19.05341960407611168, 72.70724293864768129 ) ) ;
#176578=CARTESIAN_POINT ( 'NONE',  ( -14.34966873604960291, -8.224510206698953496, 101.6655762719810383 ) ) ;
#176580=CARTESIAN_POINT ( 'NONE',  ( 19.05341960407617918, -5.049401038297876454, 96.04275706135231871 ) ) ;
#176581=CARTESIAN_POINT ( 'NONE',  ( 8.314922557960818139, 14.29746914071049879, 114.5822429386477097 ) ) ;
#176582=CARTESIAN_POINT ( 'NONE',  ( -15.72974639402176322, -15.80617190586768395, 74.37609039468568994 ) ) ;
#176583=CARTESIAN_POINT ( 'NONE',  ( 9.564922557960805705, 16.46253265017160317, 64.58224293864769550 ) ) ;
#176584=CARTESIAN_POINT ( 'NONE',  ( -5.719274019375665041, -21.55341960407619695, 34.79275706135235424 ) ) ;
#176585=CARTESIAN_POINT ( 'NONE',  ( -15.72974639402197994, 15.80617190586746368, 110.6239096053143669 ) ) ;
#176587=CARTESIAN_POINT ( 'NONE',  ( 13.89961937509977652, -13.97604488694527269, 68.12390960531436690 ) ) ;
#176589=CARTESIAN_POINT ( 'NONE',  ( 8.224510206698742110, 14.34966873604972548, 27.08442372801901854 ) ) ;
#176590=CARTESIAN_POINT ( 'NONE',  ( 5.719274019375991003, -21.55341960407610458, 27.70724293864769905 ) ) ;
#176591=CARTESIAN_POINT ( 'NONE',  ( 18.67979575497194134, -10.72451020669871369, 65.83442372801900433 ) ) ;
#176592=CARTESIAN_POINT ( 'NONE',  ( -9.564922557960796823, -16.46253265017161027, 112.0822429386476955 ) ) ;
#176593=CARTESIAN_POINT ( 'NONE',  ( 13.97604488694548053, -13.89961937509957401, 90.62609039468567573 ) ) ;
#176594=CARTESIAN_POINT ( 'NONE',  ( -5.153800228976328057, -19.02544592524343514, 52.29057627198100988 ) ) ;
#176595=CARTESIAN_POINT ( 'NONE',  ( -0.05219959533909027116, -19.03943276465977164, 72.49890960531435269 ) ) ;
#176596=CARTESIAN_POINT ( 'NONE',  ( -4.379528057220328563, 16.55341960407611168, 100.2072429386476955 ) ) ;
#176597=CARTESIAN_POINT ( 'NONE',  ( -13.89961937509977652, 13.97604488694528158, 100.6239096053143669 ) ) ;
#176598=CARTESIAN_POINT ( 'NONE',  ( -14.29746914071049879, 8.314922557960819915, 95.83224293864770971 ) ) ;
#176599=CARTESIAN_POINT ( 'NONE',  ( -9.474510206698964154, 16.51473224551069663, 100.4155762719810241 ) ) ;
#176600=CARTESIAN_POINT ( 'NONE',  ( 4.379528057220339221, -16.55341960407611168, 57.70724293864770260 ) ) ;
#176601=CARTESIAN_POINT ( 'NONE',  ( -19.03943276465977164, 0.05219959533909376836, 41.24890960531435269 ) ) ;
#176602=CARTESIAN_POINT ( 'NONE',  ( 10.72451020669871369, 18.67979575497193778, 52.08442372801901854 ) ) ;
#176603=CARTESIAN_POINT ( 'NONE',  ( 9.474510206698729675, 16.51473224551082808, 92.08442372801900433 ) ) ;
#176604=CARTESIAN_POINT ( 'NONE',  ( -4.379528057220328563, 16.55341960407611168, 45.20724293864769550 ) ) ;
#176605=CARTESIAN_POINT ( 'NONE',  ( -5.823673210054116645, -21.52544592524344225, 97.29057627198105251 ) ) ;
#176606=CARTESIAN_POINT ( 'NONE',  ( 5.719274019375991003, -21.55341960407610458, 47.70724293864770260 ) ) ;
#176607=CARTESIAN_POINT ( 'NONE',  ( 19.25918095147778786, 5.499999999999571898, 71.95284276293934056 ) ) ;
#176608=CARTESIAN_POINT ( 'NONE',  ( 4.379528057220339221, -16.55341960407611168, 87.70724293864769550 ) ) ;
#176610=CARTESIAN_POINT ( 'NONE',  ( 5.153800228976335163, 19.02544592524342804, 59.79057627198100988 ) ) ;
#176611=CARTESIAN_POINT ( 'NONE',  ( 0.05219959533934541429, -16.53943276465976808, 110.0010903946856757 ) ) ;
#176612=CARTESIAN_POINT ( 'NONE',  ( 0.05219959533934541429, -16.53943276465976808, 95.00109039468568994 ) ) ;
#176613=CARTESIAN_POINT ( 'NONE',  ( 12.14591786802327356, -12.06949235617739191, 85.62609039468568994 ) ) ;
#176614=CARTESIAN_POINT ( 'NONE',  ( -5.049401038297874678, -19.05341960407617918, 39.79275706135232582 ) ) ;
#176615=CARTESIAN_POINT ( 'NONE',  ( -17.50000000001357847, 5.500000000000046185, 45.79690382535059001 ) ) ;
#176616=CARTESIAN_POINT ( 'NONE',  ( -9.564922557960796823, -16.46253265017161027, 112.0822429386476955 ) ) ;
#176617=CARTESIAN_POINT ( 'NONE',  ( -5.153800228976328057, -19.02544592524343514, 87.29057627198103830 ) ) ;
#176618=CARTESIAN_POINT ( 'NONE',  ( 5.049401038298161559, -19.05341960407611168, 37.70724293864768839 ) ) ;
#176619=CARTESIAN_POINT ( 'NONE',  ( 14.34966873604960469, 8.224510206698951720, 54.16557627198103120 ) ) ;
#176620=CARTESIAN_POINT ( 'NONE',  ( -5.049401038298153566, 19.05341960407611168, 115.2072429386477097 ) ) ;
#176621=CARTESIAN_POINT ( 'NONE',  ( 13.97604488694527802, 13.89961937509977652, 104.3739096053143385 ) ) ;
#176622=CARTESIAN_POINT ( 'NONE',  ( -21.55341960407610458, -5.719274019375992779, 46.45724293864769550 ) ) ;
#176623=CARTESIAN_POINT ( 'NONE',  ( 16.52544592524342804, -4.483927247898539470, 88.54057627198103830 ) ) ;
#176624=CARTESIAN_POINT ( 'NONE',  ( 14.29746914071037800, 8.314922557961029526, 41.66775706135235424 ) ) ;
#176625=CARTESIAN_POINT ( 'NONE',  ( 16.53943276465976808, -0.05219959533910856209, 73.74890960531433848 ) ) ;
#176626=LINE ( 'NONE', #177628, #170613 ) ;
#176627=CARTESIAN_POINT ( 'NONE',  ( -13.97604488694547697, 13.89961937509957934, 63.12609039468566152 ) ) ;
#176628=CARTESIAN_POINT ( 'NONE',  ( -13.97604488694527625, -13.89961937509977652, 96.87390960531433848 ) ) ;
#176629=CARTESIAN_POINT ( 'NONE',  ( 19.05341960407617918, -5.049401038297876454, 81.04275706135231871 ) ) ;
#176631=CARTESIAN_POINT ( 'NONE',  ( 0.05219959533934541429, -16.53943276465976808, 30.00109039468568284 ) ) ;
#176632=CARTESIAN_POINT ( 'NONE',  ( -16.55341960407617563, 4.379528057220093196, 113.5427570613523756 ) ) ;
#176633=CARTESIAN_POINT ( 'NONE',  ( 19.02544592524334988, 5.153800228976608722, 76.45942372801897591 ) ) ;
#176634=CARTESIAN_POINT ( 'NONE',  ( -10.81492255796078084, -18.62759615963271287, 42.08224293864769550 ) ) ;
#176635=CARTESIAN_POINT ( 'NONE',  ( -21.52544592524334988, -5.823673210054445271, 68.95942372801901854 ) ) ;
#176637=CARTESIAN_POINT ( 'NONE',  ( -16.55341960407617563, 4.379528057220093196, 23.54275706135235424 ) ) ;
#176638=CARTESIAN_POINT ( 'NONE',  ( -16.51473224551069308, -9.474510206698971260, 26.66557627198103120 ) ) ;
#176639=CARTESIAN_POINT ( 'NONE',  ( -19.03943276465977164, 0.05219959533909376836, 91.24890960531436690 ) ) ;
#176640=CARTESIAN_POINT ( 'NONE',  ( 16.46253265017160672, -9.564922557960803928, 28.33224293864769550 ) ) ;
#176641=CARTESIAN_POINT ( 'NONE',  ( -14.29746914071049879, 8.314922557960819915, 85.83224293864768129 ) ) ;
#176642=CARTESIAN_POINT ( 'NONE',  ( -16.46253265017160317, 9.564922557960807481, 75.83224293864769550 ) ) ;
#176643=SHAPE_DEFINITION_REPRESENTATION ( #61400, #65015 ) ;
#176644=CARTESIAN_POINT ( 'NONE',  ( -13.89961937509977652, 13.97604488694528158, 90.62390960531432427 ) ) ;
#176646=CARTESIAN_POINT ( 'NONE',  ( -19.03943276465977164, -0.05219959533935918106, 93.75109039468566152 ) ) ;
#176647=CARTESIAN_POINT ( 'NONE',  ( 15.80617190586746368, 15.72974639402197994, 74.37390960531436690 ) ) ;
#176648=CARTESIAN_POINT ( 'NONE',  ( -13.89961937509977652, 13.97604488694528158, 35.62390960531435269 ) ) ;
#176649=CARTESIAN_POINT ( 'NONE',  ( -13.89961937509957401, -13.97604488694547875, 74.37609039468566152 ) ) ;
#176650=CARTESIAN_POINT ( 'NONE',  ( -5.719274019375978568, 21.55341960407610458, 115.2072429386476955 ) ) ;
#176651=CARTESIAN_POINT ( 'NONE',  ( 16.51473224551069308, 9.474510206698969483, 74.16557627198103830 ) ) ;
#176652=CARTESIAN_POINT ( 'NONE',  ( 9.474510206698971260, -16.51473224551069308, 107.9155762719810383 ) ) ;
#176653=VERTEX_POINT ( 'NONE', #53512 ) ;
#176654=CARTESIAN_POINT ( 'NONE',  ( -21.53943276465977519, 0.05219959533907696930, 101.2489096053143669 ) ) ;
#176655=CARTESIAN_POINT ( 'NONE',  ( -14.34966873604960291, -8.224510206698953496, 111.6655762719810525 ) ) ;
#176656=CARTESIAN_POINT ( 'NONE',  ( -9.564922557960796823, -16.46253265017161027, 82.08224293864768129 ) ) ;
#176657=CARTESIAN_POINT ( 'NONE',  ( 16.51473224551083163, -9.474510206698727899, 65.83442372801900433 ) ) ;
#176658=CARTESIAN_POINT ( 'NONE',  ( 21.52544592524344225, -5.823673210054117533, 88.54057627198103830 ) ) ;
#176659=CARTESIAN_POINT ( 'NONE',  ( -10.72451020669898014, 18.67979575497178502, 75.41557627198102409 ) ) ;
#176660=CARTESIAN_POINT ( 'NONE',  ( 16.53943276465976808, -0.05219959533910856209, 43.74890960531435979 ) ) ;
#176661=CARTESIAN_POINT ( 'NONE',  ( 21.53943276465977519, 0.05219959533937863772, 111.2510903946856899 ) ) ;
#176662=CARTESIAN_POINT ( 'NONE',  ( 12.06949235617739724, 12.14591786802326823, 71.87609039468568994 ) ) ;
#176663=CARTESIAN_POINT ( 'NONE',  ( 16.46253265017160672, -9.564922557960803928, 93.33224293864769550 ) ) ;
#176664=CARTESIAN_POINT ( 'NONE',  ( -19.03943276465977164, 0.05219959533909376836, 46.24890960531435979 ) ) ;
#176666=CARTESIAN_POINT ( 'NONE',  ( 18.62759615963255655, 10.81492255796105972, 51.66775706135234714 ) ) ;
#176667=CARTESIAN_POINT ( 'NONE',  ( -21.52544592524334988, -5.823673210054445271, 53.95942372801900433 ) ) ;
#176668=CARTESIAN_POINT ( 'NONE',  ( -19.03943276465977164, 0.05219959533909376836, 66.24890960531436690 ) ) ;
#176669=CARTESIAN_POINT ( 'NONE',  ( -18.62759615963255300, -10.81492255796106328, 34.16775706135234714 ) ) ;
#176670=CARTESIAN_POINT ( 'NONE',  ( -16.46253265017146816, -9.564922557961047289, 79.16775706135234714 ) ) ;
#176671=CARTESIAN_POINT ( 'NONE',  ( -19.03943276465977164, -0.05219959533935918106, 73.75109039468566152 ) ) ;
#176672=CARTESIAN_POINT ( 'NONE',  ( -13.97604488694527625, -13.89961937509977652, 41.87390960531435979 ) ) ;
#176673=CARTESIAN_POINT ( 'NONE',  ( 12.14591786802327356, -12.06949235617739191, 80.62609039468567573 ) ) ;
#176674=CARTESIAN_POINT ( 'NONE',  ( -5.153800228976328057, -19.02544592524343514, 57.29057627198103120 ) ) ;
#176676=CARTESIAN_POINT ( 'NONE',  ( 13.97604488694527802, 13.89961937509977652, 94.37390960531436690 ) ) ;
#176677=CARTESIAN_POINT ( 'NONE',  ( -9.564922557960796823, -16.46253265017161027, 42.08224293864769550 ) ) ;
#176678=CARTESIAN_POINT ( 'NONE',  ( -21.55341960407610458, -5.719274019375992779, 81.45724293864769550 ) ) ;
#176679=CARTESIAN_POINT ( 'NONE',  ( -14.29746914071037622, -8.314922557961029526, 54.16775706135235424 ) ) ;
#176681=CARTESIAN_POINT ( 'NONE',  ( -16.51473224551082808, 9.474510206698731452, 23.33442372801900078 ) ) ;
#176682=CARTESIAN_POINT ( 'NONE',  ( -16.51473224551069308, -9.474510206698971260, 51.66557627198102409 ) ) ;
#176683=CARTESIAN_POINT ( 'NONE',  ( 8.314922557960818139, 14.29746914071049879, 49.58224293864769550 ) ) ;
#176684=CARTESIAN_POINT ( 'NONE',  ( 4.379528057220339221, -16.55341960407611168, 82.70724293864770971 ) ) ;
#176685=CARTESIAN_POINT ( 'NONE',  ( 5.049401038298161559, -19.05341960407611168, 72.70724293864768129 ) ) ;
#176686=CARTESIAN_POINT ( 'NONE',  ( 10.81492255796106328, -18.62759615963255655, 35.41775706135234003 ) ) ;
#176687=CARTESIAN_POINT ( 'NONE',  ( 16.51473224551069308, 9.474510206698969483, 89.16557627198103830 ) ) ;
#176688=CARTESIAN_POINT ( 'NONE',  ( -5.719274019375665041, -21.55341960407619695, 94.79275706135234714 ) ) ;
#176689=CARTESIAN_POINT ( 'NONE',  ( 12.14591786802327356, -12.06949235617739191, 65.62609039468568994 ) ) ;
#176690=EDGE_CURVE ( 'NONE', #47139, #27411, #55647, .T. ) ;
#176691=CARTESIAN_POINT ( 'NONE',  ( -18.67979575497193778, 10.72451020669871902, 28.33442372801902209 ) ) ;
#176692=CARTESIAN_POINT ( 'NONE',  ( -19.02544592524342804, 5.153800228976336051, 111.0405762719810099 ) ) ;
#176693=CARTESIAN_POINT ( 'NONE',  ( -18.62759615963270932, 10.81492255796079327, 95.83224293864770971 ) ) ;
#176694=CARTESIAN_POINT ( 'NONE',  ( -12.14591786802309592, -12.06949235617757132, 51.87390960531437401 ) ) ;
#176695=CARTESIAN_POINT ( 'NONE',  ( 13.97604488694527802, 13.89961937509977652, 39.37390960531435269 ) ) ;
#176696=CARTESIAN_POINT ( 'NONE',  ( -12.14591786802309592, -12.06949235617757132, 71.87390960531438111 ) ) ;
#176697=CARTESIAN_POINT ( 'NONE',  ( -5.719274019375978568, 21.55341960407610458, 25.20724293864769550 ) ) ;
#176698=CARTESIAN_POINT ( 'NONE',  ( -0.05219959533936034679, 19.03943276465977164, 32.50109039468566863 ) ) ;
#176699=CARTESIAN_POINT ( 'NONE',  ( -8.224510206698948167, 14.34966873604960824, 100.4155762719810241 ) ) ;
#176700=CARTESIAN_POINT ( 'NONE',  ( 19.05341960407611168, 5.049401038298154454, 113.9572429386477097 ) ) ;
#176702=CARTESIAN_POINT ( 'NONE',  ( -14.34966873604972548, 8.224510206698743886, 48.33442372801902565 ) ) ;
#176703=CARTESIAN_POINT ( 'NONE',  ( -19.03943276465977164, 0.05219959533909376836, 61.24890960531436690 ) ) ;
#176705=CARTESIAN_POINT ( 'NONE',  ( 14.34966873604972726, -8.224510206698740333, 90.83442372801901854 ) ) ;
#176706=CARTESIAN_POINT ( 'NONE',  ( 16.46253265017146816, 9.564922557961045513, 96.66775706135233293 ) ) ;
#176707=CARTESIAN_POINT ( 'NONE',  ( 10.81492255796106328, -18.62759615963255655, 75.41775706135233293 ) ) ;
#176708=CARTESIAN_POINT ( 'NONE',  ( -5.153800228976328057, -19.02544592524343514, 72.29057627198102409 ) ) ;
#176709=CARTESIAN_POINT ( 'NONE',  ( 5.719274019375991003, -21.55341960407610458, 87.70724293864769550 ) ) ;
#176710=CARTESIAN_POINT ( 'NONE',  ( 14.29746914071037800, 8.314922557961029526, 41.66775706135235424 ) ) ;
#176711=CARTESIAN_POINT ( 'NONE',  ( 14.29746914071049879, -8.314922557960816363, 108.3322429386477097 ) ) ;
#176713=CARTESIAN_POINT ( 'NONE',  ( -16.51473224551082808, 9.474510206698731452, 78.33442372801900433 ) ) ;
#176714=CARTESIAN_POINT ( 'NONE',  ( -21.52544592524343514, 5.823673210054127303, 81.04057627198102409 ) ) ;
#176715=CARTESIAN_POINT ( 'NONE',  ( -19.05341960407617563, 5.049401038297882671, 48.54275706135233293 ) ) ;
#176716=CARTESIAN_POINT ( 'NONE',  ( -19.02544592524342804, 5.153800228976336051, 111.0405762719810099 ) ) ;
#176717=CARTESIAN_POINT ( 'NONE',  ( 10.81492255796078972, 18.62759615963270932, 84.58224293864769550 ) ) ;
#176718=CARTESIAN_POINT ( 'NONE',  ( 17.60691670004651499, 5.500000000000063061, 61.63333313366440080 ) ) ;
#176719=CARTESIAN_POINT ( 'NONE',  ( 16.51473224551069308, 9.474510206698969483, 64.16557627198102409 ) ) ;
#176721=CARTESIAN_POINT ( 'NONE',  ( -13.89961937509957401, -13.97604488694547875, 109.3760903946856331 ) ) ;
#176723=CARTESIAN_POINT ( 'NONE',  ( -15.72974639402176322, -15.80617190586768395, 59.37609039468568284 ) ) ;
#176724=CARTESIAN_POINT ( 'NONE',  ( 21.52544592524344225, -5.823673210054117533, 108.5405762719810241 ) ) ;
#176725=CARTESIAN_POINT ( 'NONE',  ( -12.06949235617756955, 12.14591786802309770, 65.62390960531436690 ) ) ;
#176726=CARTESIAN_POINT ( 'NONE',  ( -19.02544592524342804, 5.153800228976336051, 76.04057627198102409 ) ) ;
#176727=CARTESIAN_POINT ( 'NONE',  ( 21.55341960407619695, -5.719274019375665929, 71.04275706135234714 ) ) ;
#176728=CARTESIAN_POINT ( 'NONE',  ( -16.52544592524335698, -4.483927247898792601, 18.95942372801901143 ) ) ;
#176729=CARTESIAN_POINT ( 'NONE',  ( 9.564922557961047289, -16.46253265017146816, 35.41775706135233293 ) ) ;
#176730=CARTESIAN_POINT ( 'NONE',  ( 21.53943276465977519, 0.05219959533937863772, 41.25109039468568284 ) ) ;
#176731=CARTESIAN_POINT ( 'NONE',  ( 5.719274019375991003, -21.55341960407610458, 107.7072429386476955 ) ) ;
#176732=CARTESIAN_POINT ( 'NONE',  ( -15.72974639402197994, 15.80617190586746368, 55.62390960531436690 ) ) ;
#176733=CARTESIAN_POINT ( 'NONE',  ( 13.89961937509957401, 13.97604488694547697, 91.87609039468567573 ) ) ;
#176734=CARTESIAN_POINT ( 'NONE',  ( -19.05341960407617563, 5.049401038297882671, 63.54275706135234003 ) ) ;
#176735=CARTESIAN_POINT ( 'NONE',  ( 10.72451020669871369, 18.67979575497193778, 87.08442372801901854 ) ) ;
#176736=CARTESIAN_POINT ( 'NONE',  ( -13.97604488694547697, 13.89961937509957934, 58.12609039468566863 ) ) ;
#176737=CARTESIAN_POINT ( 'NONE',  ( -19.05341960407611168, -5.049401038298163336, 26.45724293864769550 ) ) ;
#176738=CARTESIAN_POINT ( 'NONE',  ( -18.67979575497178146, -10.72451020669898902, 56.66557627198103830 ) ) ;
#176739=CARTESIAN_POINT ( 'NONE',  ( 4.483927247898545687, 16.52544592524342804, 44.79057627198103120 ) ) ;
#176740=CARTESIAN_POINT ( 'NONE',  ( -16.36317988757060959, -7.306389748694900099, 25.90210391636776777 ) ) ;
#176741=CARTESIAN_POINT ( 'NONE',  ( 9.564922557961047289, -16.46253265017146816, 35.41775706135233293 ) ) ;
#176742=CARTESIAN_POINT ( 'NONE',  ( 16.55341960407618274, -4.379528057220086978, 91.04275706135236135 ) ) ;
#176743=CARTESIAN_POINT ( 'NONE',  ( -16.52544592524342804, 4.483927247898546575, 41.04057627198103120 ) ) ;
#176744=CARTESIAN_POINT ( 'NONE',  ( 15.72974639402176855, 15.80617190586768217, 76.87609039468567573 ) ) ;
#176745=CARTESIAN_POINT ( 'NONE',  ( 5.719274019375673035, 21.55341960407619339, 77.29275706135234714 ) ) ;
#176746=CARTESIAN_POINT ( 'NONE',  ( 0.05219959533907565091, 21.53943276465977519, 74.99890960531435269 ) ) ;
#176747=CARTESIAN_POINT ( 'NONE',  ( -16.51473224551069308, -9.474510206698971260, 41.66557627198103120 ) ) ;
#176748=CARTESIAN_POINT ( 'NONE',  ( 15.80617190586769283, -15.72974639402175789, 50.62609039468568994 ) ) ;
#176749=CARTESIAN_POINT ( 'NONE',  ( -19.05341960407611168, -5.049401038298163336, 36.45724293864766707 ) ) ;
#176750=EDGE_LOOP ( 'NONE', ( #89231, #40110, #75167 ) ) ;
#176751=CARTESIAN_POINT ( 'NONE',  ( -19.02544592524342804, 5.153800228976336051, 46.04057627198101699 ) ) ;
#176752=CARTESIAN_POINT ( 'NONE',  ( -16.55341960407611168, -4.379528057220339221, 96.45724293864770971 ) ) ;
#176753=CARTESIAN_POINT ( 'NONE',  ( -19.03943276465977164, 0.05219959533909376836, 101.2489096053143669 ) ) ;
#176754=CARTESIAN_POINT ( 'NONE',  ( -16.53943276465976808, 0.05219959533911058130, 36.24890960531435979 ) ) ;
#176755=CARTESIAN_POINT ( 'NONE',  ( 14.34966873604960469, 8.224510206698951720, 114.1655762719810383 ) ) ;
#176756=CARTESIAN_POINT ( 'NONE',  ( 15.80617190586746368, 15.72974639402197994, 84.37390960531438111 ) ) ;
#176757=CARTESIAN_POINT ( 'NONE',  ( 15.80617190586769283, -15.72974639402175789, 25.62609039468567929 ) ) ;
#176760=CARTESIAN_POINT ( 'NONE',  ( -16.53943276465976808, -0.05219959533934237506, 33.75109039468568284 ) ) ;
#176761=CARTESIAN_POINT ( 'NONE',  ( 15.80617190586746368, 15.72974639402197994, 64.37390960531435269 ) ) ;
#176762=CARTESIAN_POINT ( 'NONE',  ( -18.62759615963255300, -10.81492255796106328, 99.16775706135234714 ) ) ;
#176763=CARTESIAN_POINT ( 'NONE',  ( -9.564922557960796823, -16.46253265017161027, 97.08224293864769550 ) ) ;
#176764=CARTESIAN_POINT ( 'NONE',  ( 18.62759615963255655, 10.81492255796105972, 31.66775706135234358 ) ) ;
#176765=CARTESIAN_POINT ( 'NONE',  ( -5.823673210054116645, -21.52544592524344225, 32.29057627198102409 ) ) ;
#176766=CARTESIAN_POINT ( 'NONE',  ( -16.55341960407617563, 4.379528057220093196, 93.54275706135234714 ) ) ;
#176767=CARTESIAN_POINT ( 'NONE',  ( 21.52544592524334988, 5.823673210054432836, 66.45942372801903275 ) ) ;
#176768=CARTESIAN_POINT ( 'NONE',  ( 15.72974639402176855, 15.80617190586768217, 111.8760903946856615 ) ) ;
#176769=CARTESIAN_POINT ( 'NONE',  ( -14.29746914071037622, -8.314922557961029526, 74.16775706135231871 ) ) ;
#176770=CARTESIAN_POINT ( 'NONE',  ( 15.72974639402176855, 15.80617190586768217, 21.87609039468567573 ) ) ;
#176771=CARTESIAN_POINT ( 'NONE',  ( -5.049401038298153566, 19.05341960407611168, 30.20724293864768839 ) ) ;
#176772=CARTESIAN_POINT ( 'NONE',  ( -21.55341960407619339, 5.719274019375674811, 108.5427570613523756 ) ) ;
#176773=CARTESIAN_POINT ( 'NONE',  ( 19.02544592524343514, -5.153800228976328945, 113.5405762719810241 ) ) ;
#176774=CARTESIAN_POINT ( 'NONE',  ( -0.05219959533907301413, -21.53943276465977519, 97.49890960531436690 ) ) ;
#176776=CARTESIAN_POINT ( 'NONE',  ( -21.52544592524343514, 5.823673210054127303, 61.04057627198103120 ) ) ;
#176777=CARTESIAN_POINT ( 'NONE',  ( 8.314922557961029526, -14.29746914071037800, 55.41775706135234714 ) ) ;
#176778=CARTESIAN_POINT ( 'NONE',  ( -12.06949235617756955, 12.14591786802309770, 55.62390960531436690 ) ) ;
#176780=CARTESIAN_POINT ( 'NONE',  ( -5.153800228976607833, 19.02544592524334988, 82.70942372801897591 ) ) ;
#176781=CARTESIAN_POINT ( 'NONE',  ( -17.48847506799968698, 5.747544572773742644, 105.8269743784328227 ) ) ;
#176782=CARTESIAN_POINT ( 'NONE',  ( -16.46253265017146816, -9.564922557961047289, 109.1677570613523471 ) ) ;
#176783=CARTESIAN_POINT ( 'NONE',  ( -21.52544592524343514, 5.823673210054127303, 81.04057627198102409 ) ) ;
#176784=CARTESIAN_POINT ( 'NONE',  ( -4.483927247898539470, -16.52544592524342804, 62.29057627198102409 ) ) ;
#176785=CARTESIAN_POINT ( 'NONE',  ( -9.564922557960796823, -16.46253265017161027, 102.0822429386477097 ) ) ;
#176786=CARTESIAN_POINT ( 'NONE',  ( -16.53943276465976808, -0.05219959533934237506, 48.75109039468568284 ) ) ;
#176787=CARTESIAN_POINT ( 'NONE',  ( 13.97604488694527802, 13.89961937509977652, 64.37390960531436690 ) ) ;
#176788=CARTESIAN_POINT ( 'NONE',  ( -10.72451020669870658, -18.67979575497194134, 34.58442372801900433 ) ) ;
#176789=CARTESIAN_POINT ( 'NONE',  ( -9.564922557961040184, 16.46253265017147172, 92.91775706135233293 ) ) ;
#176790=CARTESIAN_POINT ( 'NONE',  ( 16.51473224551069308, 9.474510206698969483, 99.16557627198102409 ) ) ;
#176791=CARTESIAN_POINT ( 'NONE',  ( 5.049401038298161559, -19.05341960407611168, 92.70724293864769550 ) ) ;
#176792=CARTESIAN_POINT ( 'NONE',  ( -18.67979575497178146, -10.72451020669898902, 86.66557627198102409 ) ) ;
#176793=CARTESIAN_POINT ( 'NONE',  ( 16.46253265017160672, -9.564922557960803928, 43.33224293864769550 ) ) ;
#176794=CARTESIAN_POINT ( 'NONE',  ( -16.36317988757058473, -7.306389748694956054, 60.90210391636778553 ) ) ;
#176795=CARTESIAN_POINT ( 'NONE',  ( -12.06949235617756955, 12.14591786802309770, 65.62390960531436690 ) ) ;
#176796=CARTESIAN_POINT ( 'NONE',  ( 13.97604488694527802, 13.89961937509977652, 104.3739096053143385 ) ) ;
#176798=CARTESIAN_POINT ( 'NONE',  ( -19.05341960407617563, 5.049401038297882671, 68.54275706135230450 ) ) ;
#176799=CARTESIAN_POINT ( 'NONE',  ( 10.81492255796078972, 18.62759615963270932, 89.58224293864768129 ) ) ;
#176800=CARTESIAN_POINT ( 'NONE',  ( -19.05341960407617563, 5.049401038297882671, 48.54275706135233293 ) ) ;
#176801=CARTESIAN_POINT ( 'NONE',  ( 13.97604488694527802, 13.89961937509977652, 99.37390960531436690 ) ) ;
#176802=( LENGTH_UNIT ( ) NAMED_UNIT ( * ) SI_UNIT ( .MILLI., .METRE. ) );
#176803=CARTESIAN_POINT ( 'NONE',  ( 15.72974639402199770, -15.80617190586745480, 38.12390960531436690 ) ) ;
#176805=CARTESIAN_POINT ( 'NONE',  ( 0.05219959533909260263, 19.03943276465977164, 79.99890960531436690 ) ) ;
#176806=CARTESIAN_POINT ( 'NONE',  ( -18.67979575497193778, 10.72451020669871902, 63.33442372801900433 ) ) ;
#176807=CARTESIAN_POINT ( 'NONE',  ( 5.049401038298161559, -19.05341960407611168, 32.70724293864768129 ) ) ;
#176808=CARTESIAN_POINT ( 'NONE',  ( 4.379528057220339221, -16.55341960407611168, 77.70724293864770971 ) ) ;
#176809=CARTESIAN_POINT ( 'NONE',  ( -12.06949235617739369, -12.14591786802326823, 19.37609039468568639 ) ) ;
#176810=CARTESIAN_POINT ( 'NONE',  ( 10.81492255796106328, -18.62759615963255655, 50.41775706135235424 ) ) ;
#176813=CARTESIAN_POINT ( 'NONE',  ( -19.05341960407617563, 5.049401038297882671, 63.54275706135234003 ) ) ;
#176815=CARTESIAN_POINT ( 'NONE',  ( -10.81492255796105439, 18.62759615963255655, 22.91775706135235069 ) ) ;
#176817=CARTESIAN_POINT ( 'NONE',  ( 16.51473224551083163, -9.474510206698727899, 25.83442372801900078 ) ) ;
#176818=CARTESIAN_POINT ( 'NONE',  ( 19.02544592524343514, -5.153800228976328945, 58.54057627198102409 ) ) ;
#176819=CARTESIAN_POINT ( 'NONE',  ( 13.89961937509957401, 13.97604488694547697, 21.87609039468566152 ) ) ;
#176820=CARTESIAN_POINT ( 'NONE',  ( -4.379528057220086978, -16.55341960407618274, 109.7927570613523613 ) ) ;
#176821=CARTESIAN_POINT ( 'NONE',  ( 5.153800228976335163, 19.02544592524342804, 104.7905762719809957 ) ) ;
#176822=CARTESIAN_POINT ( 'NONE',  ( -15.72974639402176322, -15.80617190586768395, 79.37609039468567573 ) ) ;
#176824=CARTESIAN_POINT ( 'NONE',  ( 9.474510206698971260, -16.51473224551069308, 112.9155762719810383 ) ) ;
#176826=CARTESIAN_POINT ( 'NONE',  ( 14.29746914071037800, 8.314922557961029526, 61.66775706135235424 ) ) ;
#176827=CARTESIAN_POINT ( 'NONE',  ( -10.72451020669870658, -18.67979575497194134, 74.58442372801901854 ) ) ;
#176828=CARTESIAN_POINT ( 'NONE',  ( -15.72974639402176322, -15.80617190586768395, 109.3760903946857042 ) ) ;
#176830=CARTESIAN_POINT ( 'NONE',  ( 9.564922557960805705, 16.46253265017160317, 84.58224293864769550 ) ) ;
#176831=CARTESIAN_POINT ( 'NONE',  ( -0.05219959533909027116, -19.03943276465977164, 107.4989096053143527 ) ) ;
#176835=CARTESIAN_POINT ( 'NONE',  ( -19.05341960407611168, -5.049401038298163336, 41.45724293864769550 ) ) ;
#176836=CARTESIAN_POINT ( 'NONE',  ( 5.823673210054125526, 21.52544592524343514, 39.79057627198103830 ) ) ;
#176837=CARTESIAN_POINT ( 'NONE',  ( -0.05219959533934338120, 16.53943276465976808, 112.5010903946857042 ) ) ;
#176838=CARTESIAN_POINT ( 'NONE',  ( 14.29746914071049879, -8.314922557960816363, 103.3322429386476955 ) ) ;
#176839=CARTESIAN_POINT ( 'NONE',  ( 19.03943276465977164, -0.05219959533909143690, 83.74890960531436690 ) ) ;
#176840=CARTESIAN_POINT ( 'NONE',  ( -21.53943276465977519, -0.05219959533937600094, 108.7510903946857042 ) ) ;
#176841=CARTESIAN_POINT ( 'NONE',  ( 5.153800228976335163, 19.02544592524342804, 34.79057627198102409 ) ) ;
#176842=CARTESIAN_POINT ( 'NONE',  ( 14.34966873604960469, 8.224510206698951720, 94.16557627198103830 ) ) ;
#176843=CARTESIAN_POINT ( 'NONE',  ( 0.05219959533937995610, -21.53943276465977519, 55.00109039468568284 ) ) ;
#176844=CARTESIAN_POINT ( 'NONE',  ( 21.53943276465977519, -0.05219959533907433946, 93.74890960531436690 ) ) ;
#176845=CARTESIAN_POINT ( 'NONE',  ( 13.97604488694548053, -13.89961937509957401, 45.62609039468566863 ) ) ;
#176846=CARTESIAN_POINT ( 'NONE',  ( -17.59860650958989936, -7.585241751807033417, 46.57662985737508166 ) ) ;
#176847=CARTESIAN_POINT ( 'NONE',  ( -19.02544592524342804, 5.153800228976336051, 91.04057627198100988 ) ) ;
#176848=CARTESIAN_POINT ( 'NONE',  ( -16.53943276465976808, 0.05219959533911058130, 66.24890960531436690 ) ) ;
#176849=CARTESIAN_POINT ( 'NONE',  ( 19.03943276465977164, 0.05219959533936151252, 41.25109039468566152 ) ) ;
#176851=CARTESIAN_POINT ( 'NONE',  ( 4.379528057220339221, -16.55341960407611168, 42.70724293864770260 ) ) ;
#176852=CARTESIAN_POINT ( 'NONE',  ( -13.97604488694547697, 13.89961937509957934, 78.12609039468567573 ) ) ;
#176853=CARTESIAN_POINT ( 'NONE',  ( -19.35633801406909527, 5.499999999999579892, 84.13373818172762242 ) ) ;
#176854=CARTESIAN_POINT ( 'NONE',  ( -21.53943276465977519, 0.05219959533907696930, 36.24890960531435979 ) ) ;
#176855=CARTESIAN_POINT ( 'NONE',  ( -16.53943276465976808, 0.05219959533911058130, 96.24890960531435269 ) ) ;
#176856=CARTESIAN_POINT ( 'NONE',  ( -17.49999999999997158, -3.189878218039251756, 25.12948562571230227 ) ) ;
#176857=CARTESIAN_POINT ( 'NONE',  ( -19.03943276465977164, 0.05219959533909376836, 46.24890960531435979 ) ) ;
#176858=CARTESIAN_POINT ( 'NONE',  ( 5.823673210054125526, 21.52544592524343514, 44.79057627198103120 ) ) ;
#176859=CARTESIAN_POINT ( 'NONE',  ( 9.564922557960805705, 16.46253265017160317, 34.58224293864770260 ) ) ;
#176860=CARTESIAN_POINT ( 'NONE',  ( -12.06949235617739369, -12.14591786802326823, 74.37609039468568994 ) ) ;
#176861=CARTESIAN_POINT ( 'NONE',  ( -0.05219959533909027116, -19.03943276465977164, 57.49890960531435979 ) ) ;
#176862=CARTESIAN_POINT ( 'NONE',  ( 9.474510206698729675, 16.51473224551082808, 42.08442372801900433 ) ) ;
#176863=CARTESIAN_POINT ( 'NONE',  ( 18.67979575497194134, -10.72451020669871369, 65.83442372801900433 ) ) ;
#176864=CARTESIAN_POINT ( 'NONE',  ( 15.72974639402199770, -15.80617190586745480, 53.12390960531436690 ) ) ;
#176865=CARTESIAN_POINT ( 'NONE',  ( 14.34966873604960469, 8.224510206698951720, 114.1655762719810383 ) ) ;
#176866=CARTESIAN_POINT ( 'NONE',  ( -19.05341960407617563, 5.049401038297882671, 98.54275706135233293 ) ) ;
#176867=CARTESIAN_POINT ( 'NONE',  ( 19.03943276465977164, -0.05219959533909143690, 23.74890960531435269 ) ) ;
#176869=CARTESIAN_POINT ( 'NONE',  ( 18.67979575497178502, 10.72451020669898547, 54.16557627198103120 ) ) ;
#176870=CARTESIAN_POINT ( 'NONE',  ( 16.88567814943165857, -6.947325034625565721, 66.20998877347417988 ) ) ;
#176871=CARTESIAN_POINT ( 'NONE',  ( 21.55341960407619695, -5.719274019375665929, 81.04275706135236135 ) ) ;
#176872=CARTESIAN_POINT ( 'NONE',  ( -4.379528057220328563, 16.55341960407611168, 50.20724293864769550 ) ) ;
#176873=CARTESIAN_POINT ( 'NONE',  ( -4.379528057220328563, 16.55341960407611168, 60.20724293864768839 ) ) ;
#176874=CARTESIAN_POINT ( 'NONE',  ( 10.72451020669898902, -18.67979575497178502, 82.91557627198103830 ) ) ;
#176875=CARTESIAN_POINT ( 'NONE',  ( 18.67979575497178502, 10.72451020669898547, 79.16557627198103830 ) ) ;
#176876=CARTESIAN_POINT ( 'NONE',  ( -18.22780087662119541, 5.500000000000102141, 61.01763182126894947 ) ) ;
#176877=CARTESIAN_POINT ( 'NONE',  ( 10.72451020669898902, -18.67979575497178502, 37.91557627198102409 ) ) ;
#176878=CARTESIAN_POINT ( 'NONE',  ( -16.55341960407617563, 4.379528057220093196, 53.54275706135234714 ) ) ;
#176879=CARTESIAN_POINT ( 'NONE',  ( -0.05219959533910754901, -16.53943276465976808, 77.49890960531433848 ) ) ;
#176880=CARTESIAN_POINT ( 'NONE',  ( 5.153800228976335163, 19.02544592524342804, 59.79057627198100988 ) ) ;
#176881=CARTESIAN_POINT ( 'NONE',  ( 16.51473224551069308, 9.474510206698969483, 39.16557627198103120 ) ) ;
#176882=CARTESIAN_POINT ( 'NONE',  ( -17.49999999999999289, 5.500000000000036415, 75.79690382534175797 ) ) ;
#176883=CARTESIAN_POINT ( 'NONE',  ( 16.52544592524335698, 4.483927247898782831, 81.45942372801900433 ) ) ;
#176884=CARTESIAN_POINT ( 'NONE',  ( 10.81492255796106328, -18.62759615963255655, 25.41775706135235779 ) ) ;
#176885=CARTESIAN_POINT ( 'NONE',  ( 5.153800228976335163, 19.02544592524342804, 79.79057627198102409 ) ) ;
#176886=CARTESIAN_POINT ( 'NONE',  ( -15.72974639402176322, -15.80617190586768395, 59.37609039468568284 ) ) ;
#176887=CARTESIAN_POINT ( 'NONE',  ( 13.89961937509977652, -13.97604488694527269, 108.1239096053143669 ) ) ;
#176890=CARTESIAN_POINT ( 'NONE',  ( -10.72451020669870658, -18.67979575497194134, 39.58442372801901143 ) ) ;
#176891=CARTESIAN_POINT ( 'NONE',  ( 16.51473224551069308, 9.474510206698969483, 34.16557627198102409 ) ) ;
#176892=CARTESIAN_POINT ( 'NONE',  ( 19.02544592524343514, -5.153800228976328945, 103.5405762719809957 ) ) ;
#176893=CARTESIAN_POINT ( 'NONE',  ( -5.049401038297874678, -19.05341960407617918, 49.79275706135231871 ) ) ;
#176894=CARTESIAN_POINT ( 'NONE',  ( -5.719274019375978568, 21.55341960407610458, 110.2072429386477239 ) ) ;
#176895=CARTESIAN_POINT ( 'NONE',  ( 13.97604488694548053, -13.89961937509957401, 50.62609039468566152 ) ) ;
#176896=CARTESIAN_POINT ( 'NONE',  ( -16.51473224551069308, -9.474510206698971260, 21.66557627198102765 ) ) ;
#176897=CARTESIAN_POINT ( 'NONE',  ( 14.29746914071037800, 8.314922557961029526, 91.66775706135234714 ) ) ;
#176898=CARTESIAN_POINT ( 'NONE',  ( 16.46253265017146816, 9.564922557961045513, 56.66775706135233293 ) ) ;
#176899=CARTESIAN_POINT ( 'NONE',  ( 12.06949235617739724, 12.14591786802326823, 101.8760903946857042 ) ) ;
#176902=CARTESIAN_POINT ( 'NONE',  ( -19.05341960407611168, -5.049401038298163336, 91.45724293864766707 ) ) ;
#176903=CARTESIAN_POINT ( 'NONE',  ( -18.62759615963255300, -10.81492255796106328, 94.16775706135237556 ) ) ;
#176904=CARTESIAN_POINT ( 'NONE',  ( 21.52544592524334988, 5.823673210054432836, 106.4594237280190328 ) ) ;
#176905=CARTESIAN_POINT ( 'NONE',  ( -19.03943276465977164, 0.05219959533909376836, 21.24890960531436335 ) ) ;
#176906=CARTESIAN_POINT ( 'NONE',  ( -19.02544592524342804, 5.153800228976336051, 101.0405762719810241 ) ) ;
#176907=CARTESIAN_POINT ( 'NONE',  ( 21.55341960407619695, -5.719274019375665929, 76.04275706135237556 ) ) ;
#176908=CARTESIAN_POINT ( 'NONE',  ( -16.52544592524335698, -4.483927247898792601, 23.95942372801901143 ) ) ;
#176909=CARTESIAN_POINT ( 'NONE',  ( 9.564922557960805705, 16.46253265017160317, 84.58224293864769550 ) ) ;
#176910=CARTESIAN_POINT ( 'NONE',  ( -18.62759615963270932, 10.81492255796079327, 35.83224293864768839 ) ) ;
#176911=CARTESIAN_POINT ( 'NONE',  ( -13.97604488694527625, -13.89961937509977652, 96.87390960531433848 ) ) ;
#176912=CARTESIAN_POINT ( 'NONE',  ( -16.19135201231366850, -7.376712067591933319, 90.18680854052031748 ) ) ;
#176913=CARTESIAN_POINT ( 'NONE',  ( -13.89961937509977652, 13.97604488694528158, 75.62390960531438111 ) ) ;
#176914=CARTESIAN_POINT ( 'NONE',  ( 19.03943276465977164, -0.05219959533909143690, 68.74890960531436690 ) ) ;
#176915=CARTESIAN_POINT ( 'NONE',  ( -4.379528057220086978, -16.55341960407618274, 94.79275706135234714 ) ) ;
#176917=CARTESIAN_POINT ( 'NONE',  ( -9.474510206698720793, -16.51473224551083518, 59.58442372801900433 ) ) ;
#176918=CARTESIAN_POINT ( 'NONE',  ( 13.97604488694527802, 13.89961937509977652, 99.37390960531436690 ) ) ;
#176919=CARTESIAN_POINT ( 'NONE',  ( 16.52544592524342804, -4.483927247898539470, 78.54057627198103830 ) ) ;
#176920=CARTESIAN_POINT ( 'NONE',  ( 21.55341960407610458, 5.719274019375980345, 28.95724293864769905 ) ) ;
#176921=CARTESIAN_POINT ( 'NONE',  ( -5.049401038298153566, 19.05341960407611168, 115.2072429386477097 ) ) ;
#176922=CARTESIAN_POINT ( 'NONE',  ( 14.34966873604960469, 8.224510206698951720, 94.16557627198103830 ) ) ;
#176923=CARTESIAN_POINT ( 'NONE',  ( -17.13100169013299023, 6.664070546373147330, 55.76789835699847941 ) ) ;
#176924=CARTESIAN_POINT ( 'NONE',  ( -5.049401038297874678, -19.05341960407617918, 49.79275706135231871 ) ) ;
#176925=CARTESIAN_POINT ( 'NONE',  ( -16.55341960407611168, -4.379528057220339221, 21.45724293864769550 ) ) ;
#176926=CARTESIAN_POINT ( 'NONE',  ( -9.474510206698964154, 16.51473224551069663, 100.4155762719810241 ) ) ;
#176928=CARTESIAN_POINT ( 'NONE',  ( 10.72451020669871369, 18.67979575497193778, 62.08442372801901143 ) ) ;
#176929=CARTESIAN_POINT ( 'NONE',  ( -18.62759615963270932, 10.81492255796079327, 55.83224293864770260 ) ) ;
#176930=CARTESIAN_POINT ( 'NONE',  ( -18.67979575497193778, 10.72451020669871902, 38.33442372801900433 ) ) ;
#176931=CARTESIAN_POINT ( 'NONE',  ( -21.55341960407610458, -5.719274019375992779, 81.45724293864769550 ) ) ;
#176932=CARTESIAN_POINT ( 'NONE',  ( -5.719274019375665041, -21.55341960407619695, 39.79275706135235424 ) ) ;
#176933=CARTESIAN_POINT ( 'NONE',  ( 14.34966873604960469, 8.224510206698951720, 114.1655762719810383 ) ) ;
#176934=CARTESIAN_POINT ( 'NONE',  ( 16.51473224551083163, -9.474510206698727899, 65.83442372801900433 ) ) ;
#176935=CARTESIAN_POINT ( 'NONE',  ( 19.03943276465977164, -0.05219959533909143690, 38.74890960531436690 ) ) ;
#176936=CARTESIAN_POINT ( 'NONE',  ( -8.224510206698948167, 14.34966873604960824, 90.41557627198103830 ) ) ;
#176937=CARTESIAN_POINT ( 'NONE',  ( -13.89961937509977652, 13.97604488694528158, 90.62390960531432427 ) ) ;
#176938=CARTESIAN_POINT ( 'NONE',  ( 13.97604488694527802, 13.89961937509977652, 99.37390960531436690 ) ) ;
#176939=CARTESIAN_POINT ( 'NONE',  ( -9.474510206698964154, 16.51473224551069663, 25.41557627198103120 ) ) ;
#176940=CARTESIAN_POINT ( 'NONE',  ( -12.06949235617756955, 12.14591786802309770, 35.62390960531437401 ) ) ;
#176941=CARTESIAN_POINT ( 'NONE',  ( -16.52544592524335698, -4.483927247898792601, 103.9594237280190185 ) ) ;
#176942=CARTESIAN_POINT ( 'NONE',  ( -5.049401038298153566, 19.05341960407611168, 55.20724293864769550 ) ) ;
#176943=CARTESIAN_POINT ( 'NONE',  ( -5.049401038298153566, 19.05341960407611168, 25.20724293864768484 ) ) ;
#176944=CARTESIAN_POINT ( 'NONE',  ( 0.05219959533936267826, -19.03943276465977164, 30.00109039468566863 ) ) ;
#176947=CARTESIAN_POINT ( 'NONE',  ( -12.06949235617739369, -12.14591786802326823, 109.3760903946857042 ) ) ;
#176948=CARTESIAN_POINT ( 'NONE',  ( -5.823673210054431948, 21.52544592524334988, 52.70942372801902565 ) ) ;
#176949=CARTESIAN_POINT ( 'NONE',  ( -19.05341960407611168, -5.049401038298163336, 101.4572429386476955 ) ) ;
#176950=CARTESIAN_POINT ( 'NONE',  ( -16.53943276465976808, -0.05219959533934237506, 43.75109039468568284 ) ) ;
#176951=CARTESIAN_POINT ( 'NONE',  ( 16.53943276465976808, 0.05219959533934440121, 106.2510903946856757 ) ) ;
#176952=CARTESIAN_POINT ( 'NONE',  ( 9.474510206698971260, -16.51473224551069308, 47.91557627198102409 ) ) ;
#176953=CARTESIAN_POINT ( 'NONE',  ( -8.314922557961024197, 14.29746914071037800, 87.91775706135234714 ) ) ;
#176954=CARTESIAN_POINT ( 'NONE',  ( 8.224510206698742110, 14.34966873604972548, 27.08442372801901854 ) ) ;
#176955=CARTESIAN_POINT ( 'NONE',  ( 16.51473224551069308, 9.474510206698969483, 49.16557627198102409 ) ) ;
#176956=CARTESIAN_POINT ( 'NONE',  ( 4.483927247898545687, 16.52544592524342804, 104.7905762719810241 ) ) ;
#176957=CARTESIAN_POINT ( 'NONE',  ( -15.72974639402197994, 15.80617190586746368, 110.6239096053143669 ) ) ;
#176958=CARTESIAN_POINT ( 'NONE',  ( 19.05341960407611168, 5.049401038298154454, 33.95724293864769550 ) ) ;
#176959=CARTESIAN_POINT ( 'NONE',  ( -5.049401038298153566, 19.05341960407611168, 100.2072429386476955 ) ) ;
#176960=CARTESIAN_POINT ( 'NONE',  ( -16.51473224551069308, -9.474510206698971260, 31.66557627198102054 ) ) ;
#176961=CARTESIAN_POINT ( 'NONE',  ( -5.153800228976328057, -19.02544592524343514, 102.2905762719810383 ) ) ;
#176963=CARTESIAN_POINT ( 'NONE',  ( 9.474510206698971260, -16.51473224551069308, 92.91557627198103830 ) ) ;
#176964=CARTESIAN_POINT ( 'NONE',  ( 5.719274019375673035, 21.55341960407619339, 42.29275706135235424 ) ) ;
#176965=CARTESIAN_POINT ( 'NONE',  ( -16.55341960407611168, -4.379528057220339221, 101.4572429386476955 ) ) ;
#176966=CARTESIAN_POINT ( 'NONE',  ( 16.46253265017160672, -9.564922557960803928, 103.3322429386476955 ) ) ;
#176968=CARTESIAN_POINT ( 'NONE',  ( 4.483927247898790824, -16.52544592524335698, 70.20942372801904696 ) ) ;
#176969=CARTESIAN_POINT ( 'NONE',  ( 15.80617190586769283, -15.72974639402175789, 95.62609039468568994 ) ) ;
#176971=CARTESIAN_POINT ( 'NONE',  ( 12.06949235617739724, 12.14591786802326823, 36.87609039468568994 ) ) ;
#176972=CARTESIAN_POINT ( 'NONE',  ( 13.97604488694527802, 13.89961937509977652, 84.37390960531433848 ) ) ;
#176973=CARTESIAN_POINT ( 'NONE',  ( -5.049401038297874678, -19.05341960407617918, 109.7927570613523187 ) ) ;
#176974=CARTESIAN_POINT ( 'NONE',  ( 14.29746914071037800, 8.314922557961029526, 76.66775706135234714 ) ) ;
#176975=CARTESIAN_POINT ( 'NONE',  ( -13.97604488694547697, 13.89961937509957934, 88.12609039468563310 ) ) ;
#176976=CARTESIAN_POINT ( 'NONE',  ( 19.03943276465977164, -0.05219959533909143690, 78.74890960531436690 ) ) ;
#176977=CARTESIAN_POINT ( 'NONE',  ( 21.55341960407610458, 5.719274019375980345, 98.95724293864770971 ) ) ;
#176978=CARTESIAN_POINT ( 'NONE',  ( -12.14591786802309592, -12.06949235617757132, 91.87390960531436690 ) ) ;
#176979=CARTESIAN_POINT ( 'NONE',  ( 16.51473224551083163, -9.474510206698727899, 85.83442372801900433 ) ) ;
#176980=CARTESIAN_POINT ( 'NONE',  ( -8.314922557961024197, 14.29746914071037800, 77.91775706135231871 ) ) ;
#176981=CARTESIAN_POINT ( 'NONE',  ( -18.87075004821565472, 5.500000000000083489, 78.67408112101043116 ) ) ;
#176982=CARTESIAN_POINT ( 'NONE',  ( 0.05219959533936267826, -19.03943276465977164, 70.00109039468566152 ) ) ;
#176983=CARTESIAN_POINT ( 'NONE',  ( 16.55341960407611168, 4.379528057220329451, 33.95724293864769550 ) ) ;
#176984=CARTESIAN_POINT ( 'NONE',  ( -8.314922557960811034, -14.29746914071050412, 92.08224293864769550 ) ) ;
#176985=CARTESIAN_POINT ( 'NONE',  ( -19.03943276465977164, -0.05219959533935918106, 23.75109039468566152 ) ) ;
#176986=CARTESIAN_POINT ( 'NONE',  ( -16.46253265017146816, -9.564922557961047289, 44.16775706135232582 ) ) ;
#176987=CARTESIAN_POINT ( 'NONE',  ( 10.81492255796106328, -18.62759615963255655, 30.41775706135234358 ) ) ;
#176989=CARTESIAN_POINT ( 'NONE',  ( -16.51473224551069308, -9.474510206698971260, 76.66557627198103830 ) ) ;
#176990=CARTESIAN_POINT ( 'NONE',  ( 15.80617190586769283, -15.72974639402175789, 100.6260903946857184 ) ) ;
#176991=CARTESIAN_POINT ( 'NONE',  ( 5.049401038298161559, -19.05341960407611168, 82.70724293864770971 ) ) ;
#176992=CARTESIAN_POINT ( 'NONE',  ( -15.72974639402197994, 15.80617190586746368, 40.62390960531435269 ) ) ;
#176993=CARTESIAN_POINT ( 'NONE',  ( -0.05219959533910754901, -16.53943276465976808, 82.49890960531436690 ) ) ;
#176994=CARTESIAN_POINT ( 'NONE',  ( -5.153800228976328057, -19.02544592524343514, 52.29057627198100988 ) ) ;
#176995=CARTESIAN_POINT ( 'NONE',  ( 0.05219959533910956823, 16.53943276465976808, 104.9989096053143669 ) ) ;
#176996=CARTESIAN_POINT ( 'NONE',  ( -21.53943276465977519, -0.05219959533937600094, 28.75109039468567929 ) ) ;
#176997=CARTESIAN_POINT ( 'NONE',  ( -5.823673210054431948, 21.52544592524334988, 57.70942372801901143 ) ) ;
#176998=CARTESIAN_POINT ( 'NONE',  ( 13.89961937509977652, -13.97604488694527269, 43.12390960531434558 ) ) ;
#177000=CARTESIAN_POINT ( 'NONE',  ( -8.224510206698735004, -14.34966873604973081, 74.58442372801901854 ) ) ;
#177001=CARTESIAN_POINT ( 'NONE',  ( -21.52544592524334988, -5.823673210054445271, 18.95942372801901143 ) ) ;
#177003=CARTESIAN_POINT ( 'NONE',  ( 18.62759615963271287, -10.81492255796078972, 113.3322429386476955 ) ) ;
#177004=CARTESIAN_POINT ( 'NONE',  ( -5.153800228976607833, 19.02544592524334988, 37.70942372801899722 ) ) ;
#177005=CARTESIAN_POINT ( 'NONE',  ( -9.474510206698964154, 16.51473224551069663, 65.41557627198102409 ) ) ;
#177006=CARTESIAN_POINT ( 'NONE',  ( -9.474510206698720793, -16.51473224551083518, 29.58442372801900433 ) ) ;
#177007=CARTESIAN_POINT ( 'NONE',  ( -15.72974639402176322, -15.80617190586768395, 74.37609039468568994 ) ) ;
#177008=CARTESIAN_POINT ( 'NONE',  ( -18.62759615963270932, 10.81492255796079327, 65.83224293864769550 ) ) ;
#177009=CARTESIAN_POINT ( 'NONE',  ( 8.224510206698953496, -14.34966873604960469, 42.91557627198103120 ) ) ;
#177010=CARTESIAN_POINT ( 'NONE',  ( 21.52544592524334988, 5.823673210054432836, 96.45942372801901854 ) ) ;
#177011=CARTESIAN_POINT ( 'NONE',  ( -16.51473224551082808, 9.474510206698731452, 28.33442372801900433 ) ) ;
#177012=CARTESIAN_POINT ( 'NONE',  ( -0.05219959533910754901, -16.53943276465976808, 62.49890960531436690 ) ) ;
#177013=CARTESIAN_POINT ( 'NONE',  ( -12.14591786802309592, -12.06949235617757132, 106.8739096053143811 ) ) ;
#177014=CARTESIAN_POINT ( 'NONE',  ( 5.153800228976615827, -19.02544592524334988, 55.20942372801899722 ) ) ;
#177015=CARTESIAN_POINT ( 'NONE',  ( -8.314922557960811034, -14.29746914071050412, 27.08224293864769550 ) ) ;
#177016=CARTESIAN_POINT ( 'NONE',  ( -18.62759615963255300, -10.81492255796106328, 64.16775706135234714 ) ) ;
#177017=CARTESIAN_POINT ( 'NONE',  ( 13.97604488694527802, 13.89961937509977652, 79.37390960531435269 ) ) ;
#177018=CARTESIAN_POINT ( 'NONE',  ( 9.564922557961047289, -16.46253265017146816, 50.41775706135233293 ) ) ;
#177019=CARTESIAN_POINT ( 'NONE',  ( -5.719274019375978568, 21.55341960407610458, 50.20724293864769550 ) ) ;
#177020=CARTESIAN_POINT ( 'NONE',  ( 5.719274019375673035, 21.55341960407619339, 47.29275706135234003 ) ) ;
#177021=CARTESIAN_POINT ( 'NONE',  ( -5.823673210054116645, -21.52544592524344225, 102.2905762719810383 ) ) ;
#177022=CARTESIAN_POINT ( 'NONE',  ( 9.564922557961047289, -16.46253265017146816, 95.41775706135233293 ) ) ;
#177023=CARTESIAN_POINT ( 'NONE',  ( -12.06949235617739369, -12.14591786802326823, 64.37609039468568994 ) ) ;
#177025=CARTESIAN_POINT ( 'NONE',  ( 10.81492255796078972, 18.62759615963270932, 104.5822429386477097 ) ) ;
#177026=CARTESIAN_POINT ( 'NONE',  ( 8.314922557960818139, 14.29746914071049879, 89.58224293864768129 ) ) ;
#177027=CARTESIAN_POINT ( 'NONE',  ( -16.21995358207305316, -7.366697692864184965, 100.0644899848783922 ) ) ;
#177028=CARTESIAN_POINT ( 'NONE',  ( -12.06949235617739369, -12.14591786802326823, 19.37609039468568639 ) ) ;
#177029=CARTESIAN_POINT ( 'NONE',  ( 10.72451020669898902, -18.67979575497178502, 42.91557627198103120 ) ) ;
#177030=CARTESIAN_POINT ( 'NONE',  ( 4.379528057220092307, 16.55341960407617563, 92.29275706135236135 ) ) ;
#177032=CARTESIAN_POINT ( 'NONE',  ( 4.379528057220092307, 16.55341960407617563, 72.29275706135236135 ) ) ;
#177033=CARTESIAN_POINT ( 'NONE',  ( -10.72451020669870658, -18.67979575497194134, 34.58442372801900433 ) ) ;
#177034=CARTESIAN_POINT ( 'NONE',  ( -21.55341960407610458, -5.719274019375992779, 41.45724293864769550 ) ) ;
#177035=CARTESIAN_POINT ( 'NONE',  ( 0.05219959533934541429, -16.53943276465976808, 90.00109039468567573 ) ) ;
#177036=CARTESIAN_POINT ( 'NONE',  ( -9.564922557960796823, -16.46253265017161027, 92.08224293864769550 ) ) ;
#177037=CARTESIAN_POINT ( 'NONE',  ( 21.55341960407619695, -5.719274019375665929, 66.04275706135236135 ) ) ;
#177038=CARTESIAN_POINT ( 'NONE',  ( 5.823673210054125526, 21.52544592524343514, 34.79057627198103120 ) ) ;
#177039=CARTESIAN_POINT ( 'NONE',  ( 5.719274019375991003, -21.55341960407610458, 37.70724293864769550 ) ) ;
#177041=CARTESIAN_POINT ( 'NONE',  ( 5.049401038297881783, 19.05341960407617563, 47.29275706135231161 ) ) ;
#177042=CARTESIAN_POINT ( 'NONE',  ( 12.06949235617739724, 12.14591786802326823, 61.87609039468568284 ) ) ;
#177043=CARTESIAN_POINT ( 'NONE',  ( 0.05219959533907565091, 21.53943276465977519, 29.99890960531435979 ) ) ;
#177045=CARTESIAN_POINT ( 'NONE',  ( -19.02544592524342804, 5.153800228976336051, 91.04057627198100988 ) ) ;
#177046=CARTESIAN_POINT ( 'NONE',  ( -12.14591786802309592, -12.06949235617757132, 26.87390960531435979 ) ) ;
#177048=CARTESIAN_POINT ( 'NONE',  ( -8.314922557960811034, -14.29746914071050412, 107.0822429386476955 ) ) ;
#177049=CARTESIAN_POINT ( 'NONE',  ( 10.72451020669898902, -18.67979575497178502, 47.91557627198102409 ) ) ;
#177050=CARTESIAN_POINT ( 'NONE',  ( 9.474510206698971260, -16.51473224551069308, 47.91557627198102409 ) ) ;
#177051=CARTESIAN_POINT ( 'NONE',  ( 16.52544592524335698, 4.483927247898782831, 71.45942372801901854 ) ) ;
#177052=CARTESIAN_POINT ( 'NONE',  ( 5.719274019375673035, 21.55341960407619339, 27.29275706135234358 ) ) ;
#177053=CARTESIAN_POINT ( 'NONE',  ( 16.51473224551083163, -9.474510206698727899, 90.83442372801900433 ) ) ;
#177054=CARTESIAN_POINT ( 'NONE',  ( 14.29746914071049879, -8.314922557960816363, 88.33224293864769550 ) ) ;
#177055=CARTESIAN_POINT ( 'NONE',  ( -9.474510206698964154, 16.51473224551069663, 55.41557627198103120 ) ) ;
#177056=CARTESIAN_POINT ( 'NONE',  ( -19.02544592524342804, 5.153800228976336051, 26.04057627198103120 ) ) ;
#177057=CARTESIAN_POINT ( 'NONE',  ( -15.80617190586768217, 15.72974639402176855, 103.1260903946856757 ) ) ;
#177058=CARTESIAN_POINT ( 'NONE',  ( 5.049401038298161559, -19.05341960407611168, 82.70724293864770971 ) ) ;
#177059=CARTESIAN_POINT ( 'NONE',  ( -14.34966873604972548, 8.224510206698743886, 68.33442372801900433 ) ) ;
#177060=CARTESIAN_POINT ( 'NONE',  ( 10.72451020669871369, 18.67979575497193778, 87.08442372801901854 ) ) ;
#177061=CARTESIAN_POINT ( 'NONE',  ( 15.80617190586746368, 15.72974639402197994, 44.37390960531435979 ) ) ;
#177062=CARTESIAN_POINT ( 'NONE',  ( 16.53943276465976808, 0.05219959533934440121, 76.25109039468568994 ) ) ;
#177063=CARTESIAN_POINT ( 'NONE',  ( 9.474510206698729675, 16.51473224551082808, 57.08442372801900433 ) ) ;
#177064=CARTESIAN_POINT ( 'NONE',  ( 19.02544592524334988, 5.153800228976608722, 71.45942372801900433 ) ) ;
#177065=CARTESIAN_POINT ( 'NONE',  ( 10.72451020669871369, 18.67979575497193778, 57.08442372801901854 ) ) ;
#177066=CARTESIAN_POINT ( 'NONE',  ( 5.049401038298161559, -19.05341960407611168, 62.70724293864769550 ) ) ;
#177067=CARTESIAN_POINT ( 'NONE',  ( 0.05219959533909260263, 19.03943276465977164, 29.99890960531435979 ) ) ;
#177068=CARTESIAN_POINT ( 'NONE',  ( -9.474510206698720793, -16.51473224551083518, 64.58442372801900433 ) ) ;
#177069=CARTESIAN_POINT ( 'NONE',  ( 0.05219959533909260263, 19.03943276465977164, 114.9989096053143669 ) ) ;
#177070=CARTESIAN_POINT ( 'NONE',  ( 16.51473224551069308, 9.474510206698969483, 94.16557627198103830 ) ) ;
#177071=CARTESIAN_POINT ( 'NONE',  ( -4.483927247898539470, -16.52544592524342804, 52.29057627198102409 ) ) ;
#177072=CARTESIAN_POINT ( 'NONE',  ( -10.72451020669898014, 18.67979575497178502, 45.41557627198103830 ) ) ;
#177073=CARTESIAN_POINT ( 'NONE',  ( 18.10062525802554134, -5.500000000000022204, 91.01383468041920821 ) ) ;
#177074=CARTESIAN_POINT ( 'NONE',  ( 21.55341960407619695, -5.719274019375665929, 111.0427570613523613 ) ) ;
#177075=CARTESIAN_POINT ( 'NONE',  ( -16.79531203550646268, -7.028104445595595884, 81.25244988220444498 ) ) ;
#177076=CARTESIAN_POINT ( 'NONE',  ( -9.564922557960796823, -16.46253265017161027, 47.08224293864769550 ) ) ;
#177077=CARTESIAN_POINT ( 'NONE',  ( -19.01529144963336293, -5.500000000000031086, 101.2343195572844081 ) ) ;
#177078=CARTESIAN_POINT ( 'NONE',  ( -17.44270441346516876, 5.991230190323032723, 108.6366492073577632 ) ) ;
#177079=CARTESIAN_POINT ( 'NONE',  ( -12.06949235617739369, -12.14591786802326823, 74.37609039468568994 ) ) ;
#177080=CARTESIAN_POINT ( 'NONE',  ( 5.719274019375991003, -21.55341960407610458, 92.70724293864770971 ) ) ;
#177081=CARTESIAN_POINT ( 'NONE',  ( -0.05219959533910754901, -16.53943276465976808, 52.49890960531435979 ) ) ;
#177082=CARTESIAN_POINT ( 'NONE',  ( 5.153800228976335163, 19.02544592524342804, 44.79057627198103830 ) ) ;
#177084=CARTESIAN_POINT ( 'NONE',  ( -10.72451020669870658, -18.67979575497194134, 44.58442372801901854 ) ) ;
#177085=CARTESIAN_POINT ( 'NONE',  ( -13.97604488694547697, 13.89961937509957934, 53.12609039468565442 ) ) ;
#177086=CARTESIAN_POINT ( 'NONE',  ( -9.474510206698964154, 16.51473224551069663, 35.41557627198102409 ) ) ;
#177087=CARTESIAN_POINT ( 'NONE',  ( -0.05219959533937732626, 21.53943276465977519, 97.50109039468567573 ) ) ;
#177089=CARTESIAN_POINT ( 'NONE',  ( 8.224510206698953496, -14.34966873604960469, 37.91557627198102409 ) ) ;
#177091=CARTESIAN_POINT ( 'NONE',  ( -18.67979575497178146, -10.72451020669898902, 41.66557627198103120 ) ) ;
#177093=CARTESIAN_POINT ( 'NONE',  ( -9.474510206698964154, 16.51473224551069663, 95.41557627198102409 ) ) ;
#177094=CARTESIAN_POINT ( 'NONE',  ( 14.29746914071049879, -8.314922557960816363, 93.33224293864769550 ) ) ;
#177095=CARTESIAN_POINT ( 'NONE',  ( 4.379528057220092307, 16.55341960407617563, 27.29275706135234358 ) ) ;
#177096=CARTESIAN_POINT ( 'NONE',  ( -12.14591786802309592, -12.06949235617757132, 21.87390960531436690 ) ) ;
#177097=ORIENTED_EDGE ( 'NONE', *, *, #47442, .T. ) ;
#177098=EDGE_CURVE ( 'NONE', #86773, #102413, #25209, .T. ) ;
#177099=CARTESIAN_POINT ( 'NONE',  ( 5.153800228976335163, 19.02544592524342804, 104.7905762719809957 ) ) ;
#177100=CARTESIAN_POINT ( 'NONE',  ( -18.62759615963270932, 10.81492255796079327, 85.83224293864768129 ) ) ;
#177101=CARTESIAN_POINT ( 'NONE',  ( -4.379528057220328563, 16.55341960407611168, 25.20724293864769550 ) ) ;
#177102=CARTESIAN_POINT ( 'NONE',  ( -5.049401038298153566, 19.05341960407611168, 95.20724293864770971 ) ) ;
#177103=CARTESIAN_POINT ( 'NONE',  ( 5.153800228976615827, -19.02544592524334988, 75.20942372801896170 ) ) ;
#177104=CARTESIAN_POINT ( 'NONE',  ( -18.67979575497193778, 10.72451020669871902, 113.3344237280190328 ) ) ;
#177105=CARTESIAN_POINT ( 'NONE',  ( -18.67979575497178146, -10.72451020669898902, 91.66557627198103830 ) ) ;
#177106=CARTESIAN_POINT ( 'NONE',  ( 5.823673210054125526, 21.52544592524343514, 39.79057627198103830 ) ) ;
#177107=CARTESIAN_POINT ( 'NONE',  ( 19.03943276465977164, -0.05219959533909143690, 63.74890960531435979 ) ) ;
#177108=CARTESIAN_POINT ( 'NONE',  ( -16.53943276465976808, 0.05219959533911058130, 31.24890960531435979 ) ) ;
#177109=CARTESIAN_POINT ( 'NONE',  ( -13.89961937509977652, 13.97604488694528158, 75.62390960531438111 ) ) ;
#177112=CARTESIAN_POINT ( 'NONE',  ( -5.153800228976607833, 19.02544592524334988, 27.70942372801899722 ) ) ;
#177113=CARTESIAN_POINT ( 'NONE',  ( -14.34966873604960291, -8.224510206698953496, 86.66557627198102409 ) ) ;
#177114=CARTESIAN_POINT ( 'NONE',  ( -21.52544592524334988, -5.823673210054445271, 23.95942372801901143 ) ) ;
#177117=CARTESIAN_POINT ( 'NONE',  ( 5.719274019375991003, -21.55341960407610458, 77.70724293864770971 ) ) ;
#177118=CARTESIAN_POINT ( 'NONE',  ( 8.314922557961029526, -14.29746914071037800, 95.41775706135234714 ) ) ;
#177119=CARTESIAN_POINT ( 'NONE',  ( -5.153800228976328057, -19.02544592524343514, 22.29057627198102765 ) ) ;
#177120=CARTESIAN_POINT ( 'NONE',  ( -9.474510206698964154, 16.51473224551069663, 70.41557627198102409 ) ) ;
#177122=CARTESIAN_POINT ( 'NONE',  ( -0.05219959533910754901, -16.53943276465976808, 27.49890960531435269 ) ) ;
#177123=CARTESIAN_POINT ( 'NONE',  ( 21.52544592524334988, 5.823673210054432836, 66.45942372801903275 ) ) ;
#177125=CARTESIAN_POINT ( 'NONE',  ( 5.823673210054444382, -21.52544592524334988, 100.2094237280190043 ) ) ;
#177126=CARTESIAN_POINT ( 'NONE',  ( 16.46253265017160672, -9.564922557960803928, 48.33224293864769550 ) ) ;
#177127=CARTESIAN_POINT ( 'NONE',  ( -13.97604488694527625, -13.89961937509977652, 56.87390960531434558 ) ) ;
#177129=CARTESIAN_POINT ( 'NONE',  ( -21.52544592524334988, -5.823673210054445271, 93.95942372801903275 ) ) ;
#177130=CARTESIAN_POINT ( 'NONE',  ( -14.34966873604972548, 8.224510206698743886, 58.33442372801901143 ) ) ;
#177131=CARTESIAN_POINT ( 'NONE',  ( -15.72974639402176322, -15.80617190586768395, 84.37609039468570415 ) ) ;
#177132=CARTESIAN_POINT ( 'NONE',  ( -13.89961937509977652, 13.97604488694528158, 110.6239096053143243 ) ) ;
#177133=CARTESIAN_POINT ( 'NONE',  ( -0.05219959533936034679, 19.03943276465977164, 87.50109039468567573 ) ) ;
#177134=CARTESIAN_POINT ( 'NONE',  ( 15.72974639402176855, 15.80617190586768217, 71.87609039468568994 ) ) ;
#177135=CARTESIAN_POINT ( 'NONE',  ( 8.314922557961029526, -14.29746914071037800, 35.41775706135234003 ) ) ;
#177136=CARTESIAN_POINT ( 'NONE',  ( -21.52544592524343514, 5.823673210054127303, 86.04057627198102409 ) ) ;
#177137=CARTESIAN_POINT ( 'NONE',  ( -13.89961937509957401, -13.97604488694547875, 89.37609039468563310 ) ) ;
#177138=CARTESIAN_POINT ( 'NONE',  ( -19.02544592524342804, 5.153800228976336051, 66.04057627198103830 ) ) ;
#177139=CARTESIAN_POINT ( 'NONE',  ( 19.02544592524334988, 5.153800228976608722, 91.45942372801900433 ) ) ;
#177140=CARTESIAN_POINT ( 'NONE',  ( -16.51473224551082808, 9.474510206698731452, 103.3344237280190043 ) ) ;
#177141=CARTESIAN_POINT ( 'NONE',  ( -8.314922557960811034, -14.29746914071050412, 47.08224293864770260 ) ) ;
#177142=CARTESIAN_POINT ( 'NONE',  ( 9.474510206698729675, 16.51473224551082808, 82.08442372801899012 ) ) ;
#177143=CARTESIAN_POINT ( 'NONE',  ( 14.34966873604972726, -8.224510206698740333, 60.83442372801901854 ) ) ;
#177144=CARTESIAN_POINT ( 'NONE',  ( -13.97604488694527625, -13.89961937509977652, 41.87390960531435979 ) ) ;
#177145=CARTESIAN_POINT ( 'NONE',  ( -19.05341960407611168, -5.049401038298163336, 61.45724293864769550 ) ) ;
#177146=CARTESIAN_POINT ( 'NONE',  ( 14.34966873604972726, -8.224510206698740333, 55.83442372801901854 ) ) ;
#177149=CARTESIAN_POINT ( 'NONE',  ( 0.05219959533909260263, 19.03943276465977164, 109.9989096053143669 ) ) ;
#177150=CARTESIAN_POINT ( 'NONE',  ( -19.03943276465977164, -1.327063459122257427E-13, 115.0000000000000142 ) ) ;
#177151=ORIENTED_EDGE ( 'NONE', *, *, #109880, .F. ) ;
#177152=CARTESIAN_POINT ( 'NONE',  ( -0.05219959533936034679, 19.03943276465977164, 112.5010903946856757 ) ) ;
#177153=CARTESIAN_POINT ( 'NONE',  ( -18.67979575497178146, -10.72451020669898902, 31.66557627198102054 ) ) ;
#177154=CARTESIAN_POINT ( 'NONE',  ( -19.05341960407617563, 5.049401038297882671, 28.54275706135232937 ) ) ;
#177155=CARTESIAN_POINT ( 'NONE',  ( 8.314922557961029526, -14.29746914071037800, 20.41775706135234714 ) ) ;
#177156=CARTESIAN_POINT ( 'NONE',  ( -16.46253265017160317, 9.564922557960807481, 35.83224293864768839 ) ) ;
#177157=CARTESIAN_POINT ( 'NONE',  ( 13.89961937509977652, -13.97604488694527269, 53.12390960531434558 ) ) ;
#177158=CARTESIAN_POINT ( 'NONE',  ( 21.52544592524344225, -5.823673210054117533, 73.54057627198102409 ) ) ;
#177159=CARTESIAN_POINT ( 'NONE',  ( -5.153800228976328057, -19.02544592524343514, 102.2905762719810383 ) ) ;
#177160=CARTESIAN_POINT ( 'NONE',  ( 19.02544592524343514, -5.153800228976328945, 38.54057627198103120 ) ) ;
#177162=CARTESIAN_POINT ( 'NONE',  ( -9.564922557961040184, 16.46253265017147172, 82.91775706135233293 ) ) ;
#177163=CARTESIAN_POINT ( 'NONE',  ( 14.34966873604960469, 8.224510206698951720, 64.16557627198102409 ) ) ;
#177164=CARTESIAN_POINT ( 'NONE',  ( 21.53943276465977519, -0.05219959533907433946, 48.74890960531435979 ) ) ;
#177165=CARTESIAN_POINT ( 'NONE',  ( -21.53943276465977519, -0.05219959533937600094, 108.7510903946857042 ) ) ;
#177166=CARTESIAN_POINT ( 'NONE',  ( 10.81492255796078972, 18.62759615963270932, 99.58224293864770971 ) ) ;
#177167=CARTESIAN_POINT ( 'NONE',  ( -5.719274019375665041, -21.55341960407619695, 69.79275706135234714 ) ) ;
#177168=CARTESIAN_POINT ( 'NONE',  ( 21.52544592524334988, 5.823673210054432836, 76.45942372801901854 ) ) ;
#177169=CARTESIAN_POINT ( 'NONE',  ( 5.153800228976335163, 19.02544592524342804, 104.7905762719809957 ) ) ;
#177170=CARTESIAN_POINT ( 'NONE',  ( 0.05219959533934541429, -16.53943276465976808, 105.0010903946856757 ) ) ;
#177171=CARTESIAN_POINT ( 'NONE',  ( 10.72451020669871369, 18.67979575497193778, 77.08442372801901854 ) ) ;
#177172=CARTESIAN_POINT ( 'NONE',  ( -19.02544592524342804, 5.153800228976336051, 71.04057627198099567 ) ) ;
#177173=CARTESIAN_POINT ( 'NONE',  ( 19.03943276465977164, 0.05219959533936151252, 36.25109039468567573 ) ) ;
#177174=CARTESIAN_POINT ( 'NONE',  ( 5.719274019375673035, 21.55341960407619339, 27.29275706135234358 ) ) ;
#177175=CARTESIAN_POINT ( 'NONE',  ( 19.03943276465977164, -0.05219959533909143690, 68.74890960531436690 ) ) ;
#177176=CARTESIAN_POINT ( 'NONE',  ( -14.34966873604960291, -8.224510206698953496, 81.66557627198103830 ) ) ;
#177177=CARTESIAN_POINT ( 'NONE',  ( -8.224510206698948167, 14.34966873604960824, 45.41557627198103830 ) ) ;
#177178=CARTESIAN_POINT ( 'NONE',  ( -21.53943276465977519, 0.05219959533907696930, 56.24890960531436690 ) ) ;
#177179=CARTESIAN_POINT ( 'NONE',  ( 16.46253265017160672, -9.564922557960803928, 58.33224293864769550 ) ) ;
#177180=CARTESIAN_POINT ( 'NONE',  ( 21.53943276465977519, -0.05219959533907433946, 73.74890960531433848 ) ) ;
#177181=CARTESIAN_POINT ( 'NONE',  ( -16.51473224551082808, 9.474510206698731452, 58.33442372801900433 ) ) ;
#177182=CARTESIAN_POINT ( 'NONE',  ( 9.564922557961047289, -16.46253265017146816, 25.41775706135234003 ) ) ;
#177183=CARTESIAN_POINT ( 'NONE',  ( 14.29746914071049879, -8.314922557960816363, 68.33224293864769550 ) ) ;
#177184=CARTESIAN_POINT ( 'NONE',  ( -21.55341960407610458, -5.719274019375992779, 36.45724293864768839 ) ) ;
#177185=ORIENTED_EDGE ( 'NONE', *, *, #31131, .F. ) ;
#177187=CARTESIAN_POINT ( 'NONE',  ( 16.55341960407618274, -4.379528057220086978, 91.04275706135236135 ) ) ;
#177189=CARTESIAN_POINT ( 'NONE',  ( -19.05341960407617563, 5.049401038297882671, 83.54275706135233293 ) ) ;
#177191=CARTESIAN_POINT ( 'NONE',  ( -4.483927247898539470, -16.52544592524342804, 67.29057627198103830 ) ) ;
#177192=CARTESIAN_POINT ( 'NONE',  ( -17.50000000000000355, 5.076555817581239971, 33.82048507950225513 ) ) ;
#177193=CARTESIAN_POINT ( 'NONE',  ( -19.02544592524342804, 5.153800228976336051, 56.04057627198100988 ) ) ;
#177194=CARTESIAN_POINT ( 'NONE',  ( -4.483927247898539470, -16.52544592524342804, 42.29057627198103120 ) ) ;
#177195=CARTESIAN_POINT ( 'NONE',  ( -5.153800228976328057, -19.02544592524343514, 87.29057627198103830 ) ) ;
#177196=CARTESIAN_POINT ( 'NONE',  ( 9.564922557961047289, -16.46253265017146816, 80.41775706135234714 ) ) ;
#177197=CARTESIAN_POINT ( 'NONE',  ( 16.46253265017160672, -9.564922557960803928, 48.33224293864769550 ) ) ;
#177198=CARTESIAN_POINT ( 'NONE',  ( 21.53943276465977519, 0.05219959533937863772, 56.25109039468568284 ) ) ;
#177199=CARTESIAN_POINT ( 'NONE',  ( 19.05341960407611168, 5.049401038298154454, 88.95724293864769550 ) ) ;
#177200=CARTESIAN_POINT ( 'NONE',  ( -5.049401038298153566, 19.05341960407611168, 25.20724293864768484 ) ) ;
#177201=CARTESIAN_POINT ( 'NONE',  ( 9.564922557960805705, 16.46253265017160317, 74.58224293864769550 ) ) ;
#177202=CARTESIAN_POINT ( 'NONE',  ( -5.719274019375978568, 21.55341960407610458, 45.20724293864769550 ) ) ;
#177203=CARTESIAN_POINT ( 'NONE',  ( -0.05219959533909027116, -19.03943276465977164, 47.49890960531435979 ) ) ;
#177204=CARTESIAN_POINT ( 'NONE',  ( 18.67979575497178502, 10.72451020669898547, 49.16557627198102409 ) ) ;
#177205=CARTESIAN_POINT ( 'NONE',  ( -5.049401038297874678, -19.05341960407617918, 74.79275706135231871 ) ) ;
#177206=CARTESIAN_POINT ( 'NONE',  ( 4.483927247898790824, -16.52544592524335698, 105.2094237280190328 ) ) ;
#177207=CARTESIAN_POINT ( 'NONE',  ( 13.89961937509957401, 13.97604488694547697, 31.87609039468566863 ) ) ;
#177208=CARTESIAN_POINT ( 'NONE',  ( -4.379528057220086978, -16.55341960407618274, 59.79275706135234714 ) ) ;
#177209=CARTESIAN_POINT ( 'NONE',  ( 12.06949235617739724, 12.14591786802326823, 91.87609039468568994 ) ) ;
#177211=CARTESIAN_POINT ( 'NONE',  ( 16.52544592524335698, 4.483927247898782831, 76.45942372801901854 ) ) ;
#177212=CARTESIAN_POINT ( 'NONE',  ( 18.62759615963271287, -10.81492255796078972, 28.33224293864769550 ) ) ;
#177213=CARTESIAN_POINT ( 'NONE',  ( 0.05219959533909260263, 19.03943276465977164, 34.99890960531435979 ) ) ;
#177214=CARTESIAN_POINT ( 'NONE',  ( 12.06949235617739724, 12.14591786802326823, 31.87609039468567929 ) ) ;
#177215=CARTESIAN_POINT ( 'NONE',  ( -19.02544592524342804, 5.153800228976336051, 46.04057627198101699 ) ) ;
#177216=CARTESIAN_POINT ( 'NONE',  ( 0.05219959533937995610, -21.53943276465977519, 40.00109039468567573 ) ) ;
#177217=CARTESIAN_POINT ( 'NONE',  ( 12.06949235617739724, 12.14591786802326823, 41.87609039468568284 ) ) ;
#177218=CARTESIAN_POINT ( 'NONE',  ( -4.483927247898782831, 16.52544592524335698, 107.7094237280190328 ) ) ;
#177219=CARTESIAN_POINT ( 'NONE',  ( -5.153800228976328057, -19.02544592524343514, 32.29057627198102409 ) ) ;
#177220=CARTESIAN_POINT ( 'NONE',  ( -13.97604488694547697, 13.89961937509957934, 23.12609039468565442 ) ) ;
#177221=CARTESIAN_POINT ( 'NONE',  ( 16.46253265017146816, 9.564922557961045513, 111.6677570613523329 ) ) ;
#177222=CARTESIAN_POINT ( 'NONE',  ( 9.474510206698729675, 16.51473224551082808, 72.08442372801900433 ) ) ;
#177223=CARTESIAN_POINT ( 'NONE',  ( -4.379528057220328563, 16.55341960407611168, 65.20724293864768129 ) ) ;
#177224=CARTESIAN_POINT ( 'NONE',  ( -5.153800228976328057, -19.02544592524343514, 37.29057627198102409 ) ) ;
#177225=CARTESIAN_POINT ( 'NONE',  ( 5.153800228976615827, -19.02544592524334988, 75.20942372801896170 ) ) ;
#177227=CARTESIAN_POINT ( 'NONE',  ( 21.52544592524334988, 5.823673210054432836, 66.45942372801903275 ) ) ;
#177228=CARTESIAN_POINT ( 'NONE',  ( -16.55341960407617563, 4.379528057220093196, 38.54275706135234714 ) ) ;
#177229=CARTESIAN_POINT ( 'NONE',  ( 17.60728821187777271, -5.500000000000039968, 73.36690927743606494 ) ) ;
#177230=CARTESIAN_POINT ( 'NONE',  ( 0.05219959533907565091, 21.53943276465977519, 39.99890960531436690 ) ) ;
#177231=CARTESIAN_POINT ( 'NONE',  ( 8.224510206698742110, 14.34966873604972548, 22.08442372801901143 ) ) ;
#177232=CARTESIAN_POINT ( 'NONE',  ( 19.02544592524343514, -5.153800228976328945, 113.5405762719810241 ) ) ;
#177234=CARTESIAN_POINT ( 'NONE',  ( -19.03943276465977164, 0.05219959533909376836, 41.24890960531435269 ) ) ;
#177235=CARTESIAN_POINT ( 'NONE',  ( 5.823673210054444382, -21.52544592524334988, 110.2094237280190185 ) ) ;
#177236=CARTESIAN_POINT ( 'NONE',  ( -5.049401038298153566, 19.05341960407611168, 60.20724293864768129 ) ) ;
#177237=CARTESIAN_POINT ( 'NONE',  ( -21.52544592524334988, -5.823673210054445271, 58.95942372801902565 ) ) ;
#177238=CARTESIAN_POINT ( 'NONE',  ( 15.72974639402176855, 15.80617190586768217, 106.8760903946856899 ) ) ;
#177239=CARTESIAN_POINT ( 'NONE',  ( 4.379528057220339221, -16.55341960407611168, 27.70724293864769905 ) ) ;
#177240=CARTESIAN_POINT ( 'NONE',  ( 13.89961937509977652, -13.97604488694527269, 28.12390960531435624 ) ) ;
#177241=CARTESIAN_POINT ( 'NONE',  ( 13.97604488694527802, 13.89961937509977652, 89.37390960531436690 ) ) ;
#177242=CARTESIAN_POINT ( 'NONE',  ( 0.05219959533937995610, -21.53943276465977519, 50.00109039468568994 ) ) ;
#177243=CARTESIAN_POINT ( 'NONE',  ( -16.51473224551069308, -9.474510206698971260, 31.66557627198102054 ) ) ;
#177244=CARTESIAN_POINT ( 'NONE',  ( -5.823673210054431948, 21.52544592524334988, 57.70942372801901143 ) ) ;
#177245=CARTESIAN_POINT ( 'NONE',  ( -19.03943276465977164, -0.05219959533935918106, 88.75109039468567573 ) ) ;
#177246=CARTESIAN_POINT ( 'NONE',  ( -9.474510206698964154, 16.51473224551069663, 100.4155762719810241 ) ) ;
#177247=CARTESIAN_POINT ( 'NONE',  ( 5.049401038298161559, -19.05341960407611168, 22.70724293864769194 ) ) ;
#177248=CARTESIAN_POINT ( 'NONE',  ( -10.81492255796078084, -18.62759615963271287, 112.0822429386477097 ) ) ;
#177249=CARTESIAN_POINT ( 'NONE',  ( 16.46253265017146816, 9.564922557961045513, 41.66775706135234003 ) ) ;
#177250=CARTESIAN_POINT ( 'NONE',  ( 12.14591786802309770, 12.06949235617756955, 114.3739096053143527 ) ) ;
#177251=CARTESIAN_POINT ( 'NONE',  ( -19.02544592524342804, 5.153800228976336051, 56.04057627198100988 ) ) ;
#177252=CARTESIAN_POINT ( 'NONE',  ( 9.564922557961047289, -16.46253265017146816, 95.41775706135233293 ) ) ;
#177253=CARTESIAN_POINT ( 'NONE',  ( 8.314922557960818139, 14.29746914071049879, 64.58224293864769550 ) ) ;
#177254=CARTESIAN_POINT ( 'NONE',  ( -10.81492255796105439, 18.62759615963255655, 107.9177570613523471 ) ) ;
#177255=CARTESIAN_POINT ( 'NONE',  ( -15.80617190586745835, -15.72974639402198527, 21.87390960531436690 ) ) ;
#177256=CARTESIAN_POINT ( 'NONE',  ( 13.89961937509957401, 13.97604488694547697, 86.87609039468567573 ) ) ;
#177257=CARTESIAN_POINT ( 'NONE',  ( -5.823673210054116645, -21.52544592524344225, 92.29057627198103830 ) ) ;
#177258=CARTESIAN_POINT ( 'NONE',  ( -18.67979575497193778, 10.72451020669871902, 43.33442372801901143 ) ) ;
#177259=CARTESIAN_POINT ( 'NONE',  ( 16.53943276465976808, 0.05219959533934440121, 41.25109039468568284 ) ) ;
#177260=CARTESIAN_POINT ( 'NONE',  ( -14.29746914071037622, -8.314922557961029526, 109.1677570613523613 ) ) ;
#177261=CARTESIAN_POINT ( 'NONE',  ( -14.29746914071037622, -8.314922557961029526, 39.16775706135235424 ) ) ;
#177262=CARTESIAN_POINT ( 'NONE',  ( 10.81492255796106328, -18.62759615963255655, 45.41775706135234003 ) ) ;
#177263=CARTESIAN_POINT ( 'NONE',  ( 0.05219959533907565091, 21.53943276465977519, 54.99890960531435269 ) ) ;
#177265=CARTESIAN_POINT ( 'NONE',  ( -9.474510206698964154, 16.51473224551069663, 35.41557627198102409 ) ) ;
#177267=CARTESIAN_POINT ( 'NONE',  ( -8.314922557961024197, 14.29746914071037800, 57.91775706135234714 ) ) ;
#177268=CARTESIAN_POINT ( 'NONE',  ( -10.81492255796078084, -18.62759615963271287, 87.08224293864769550 ) ) ;
#177269=CARTESIAN_POINT ( 'NONE',  ( -16.53943276465976808, 0.05219959533911058130, 41.24890960531435269 ) ) ;
#177270=CARTESIAN_POINT ( 'NONE',  ( 4.379528057220092307, 16.55341960407617563, 57.29275706135234714 ) ) ;
#177271=CARTESIAN_POINT ( 'NONE',  ( 19.05341960407617918, -5.049401038297876454, 101.0427570613523045 ) ) ;
#177272=CARTESIAN_POINT ( 'NONE',  ( 5.823673210054125526, 21.52544592524343514, 104.7905762719810241 ) ) ;
#177273=CARTESIAN_POINT ( 'NONE',  ( 12.06949235617757843, -12.14591786802309237, 38.12390960531436690 ) ) ;
#177274=ORIENTED_EDGE ( 'NONE', *, *, #88626, .T. ) ;
#177275=CARTESIAN_POINT ( 'NONE',  ( 8.224510206698742110, 14.34966873604972548, 72.08442372801899012 ) ) ;
#177277=CARTESIAN_POINT ( 'NONE',  ( 21.52544592524344225, -5.823673210054117533, 73.54057627198102409 ) ) ;
#177279=CARTESIAN_POINT ( 'NONE',  ( -14.29746914071037622, -8.314922557961029526, 99.16775706135234714 ) ) ;
#177281=CARTESIAN_POINT ( 'NONE',  ( 19.49190055781010500, 5.500000000000051514, 88.06116087098783396 ) ) ;
#177282=CARTESIAN_POINT ( 'NONE',  ( 5.823673210054125526, 21.52544592524343514, 89.79057627198103830 ) ) ;
#177283=CARTESIAN_POINT ( 'NONE',  ( 10.81492255796078972, 18.62759615963270932, 114.5822429386477097 ) ) ;
#177284=CARTESIAN_POINT ( 'NONE',  ( 16.53943276465976808, -0.05219959533910856209, 38.74890960531435979 ) ) ;
#177285=CARTESIAN_POINT ( 'NONE',  ( 12.14591786802327356, -12.06949235617739191, 30.62609039468567929 ) ) ;
#177286=CARTESIAN_POINT ( 'NONE',  ( -13.97604488694527625, -13.89961937509977652, 36.87390960531436690 ) ) ;
#177288=CARTESIAN_POINT ( 'NONE',  ( -19.03943276465977164, 0.05219959533909376836, 71.24890960531435269 ) ) ;
#177289=CARTESIAN_POINT ( 'NONE',  ( 21.55341960407610458, 5.719274019375980345, 23.95724293864769550 ) ) ;
#177290=CARTESIAN_POINT ( 'NONE',  ( 13.97604488694527802, 13.89961937509977652, 114.3739096053143669 ) ) ;
#177291=CARTESIAN_POINT ( 'NONE',  ( -13.97604488694547697, 13.89961937509957934, 103.1260903946856473 ) ) ;
#177292=CARTESIAN_POINT ( 'NONE',  ( 13.89961937509957401, 13.97604488694547697, 56.87609039468564731 ) ) ;
#177293=CARTESIAN_POINT ( 'NONE',  ( 21.55341960407610458, 5.719274019375980345, 88.95724293864769550 ) ) ;
#177294=CARTESIAN_POINT ( 'NONE',  ( -14.34966873604972548, 8.224510206698743886, 113.3344237280190328 ) ) ;
#177295=CARTESIAN_POINT ( 'NONE',  ( 21.53943276465977519, -0.05219959533907433946, 48.74890960531435979 ) ) ;
#177296=CARTESIAN_POINT ( 'NONE',  ( 0.05219959533907565091, 21.53943276465977519, 84.99890960531436690 ) ) ;
#177297=CARTESIAN_POINT ( 'NONE',  ( 13.89961937509957401, 13.97604488694547697, 106.8760903946856757 ) ) ;
#177298=CARTESIAN_POINT ( 'NONE',  ( -13.89961937509977652, 13.97604488694528158, 105.6239096053143527 ) ) ;
#177299=CARTESIAN_POINT ( 'NONE',  ( -21.52544592524334988, -5.823673210054445271, 78.95942372801901854 ) ) ;
#177300=CARTESIAN_POINT ( 'NONE',  ( -19.05341960407611168, -5.049401038298163336, 76.45724293864769550 ) ) ;
#177301=CARTESIAN_POINT ( 'NONE',  ( -8.224510206698948167, 14.34966873604960824, 105.4155762719810383 ) ) ;
#177303=CARTESIAN_POINT ( 'NONE',  ( -19.02544592524342804, 5.153800228976336051, 66.04057627198103830 ) ) ;
#177304=CARTESIAN_POINT ( 'NONE',  ( -16.55341960407611168, -4.379528057220339221, 91.45724293864769550 ) ) ;
#177306=CARTESIAN_POINT ( 'NONE',  ( 5.049401038297881783, 19.05341960407617563, 102.2927570613523045 ) ) ;
#177307=CARTESIAN_POINT ( 'NONE',  ( 16.21995358207301763, -7.366697692864224045, 82.43551001512155096 ) ) ;
#177308=CARTESIAN_POINT ( 'NONE',  ( -9.474510206698964154, 16.51473224551069663, 55.41557627198103120 ) ) ;
#177309=CARTESIAN_POINT ( 'NONE',  ( -10.72451020669870658, -18.67979575497194134, 89.58442372801901854 ) ) ;
#177310=CARTESIAN_POINT ( 'NONE',  ( -16.51473224551069308, -9.474510206698971260, 101.6655762719810241 ) ) ;
#177311=CARTESIAN_POINT ( 'NONE',  ( 4.379528057220092307, 16.55341960407617563, 82.29275706135234714 ) ) ;
#177312=EDGE_CURVE ( 'NONE', #73688, #165524, #193041, .T. ) ;
#177314=CARTESIAN_POINT ( 'NONE',  ( -9.474510206698720793, -16.51473224551083518, 54.58442372801899722 ) ) ;
#177315=CARTESIAN_POINT ( 'NONE',  ( -21.52544592524334988, -5.823673210054445271, 93.95942372801903275 ) ) ;
#177318=CARTESIAN_POINT ( 'NONE',  ( 14.29746914071049879, -8.314922557960816363, 28.33224293864769550 ) ) ;
#177320=CARTESIAN_POINT ( 'NONE',  ( -8.224510206698735004, -14.34966873604973081, 89.58442372801901854 ) ) ;
#177322=CARTESIAN_POINT ( 'NONE',  ( -14.34966873604972548, 8.224510206698743886, 68.33442372801900433 ) ) ;
#177323=CARTESIAN_POINT ( 'NONE',  ( -21.52544592524334988, -5.823673210054445271, 83.95942372801900433 ) ) ;
#177324=CARTESIAN_POINT ( 'NONE',  ( -19.05341960407617563, 5.049401038297882671, 88.54275706135230450 ) ) ;
#177325=CARTESIAN_POINT ( 'NONE',  ( -19.05341960407617563, 5.049401038297882671, 43.54275706135232582 ) ) ;
#177326=CARTESIAN_POINT ( 'NONE',  ( 13.97604488694527802, 13.89961937509977652, 59.37390960531434558 ) ) ;
#177327=CARTESIAN_POINT ( 'NONE',  ( -5.153800228976328057, -19.02544592524343514, 52.29057627198100988 ) ) ;
#177329=CARTESIAN_POINT ( 'NONE',  ( 21.53943276465977519, -0.05219959533907433946, 78.74890960531436690 ) ) ;
#177330=CARTESIAN_POINT ( 'NONE',  ( 18.62759615963271287, -10.81492255796078972, 43.33224293864769550 ) ) ;
#177331=CARTESIAN_POINT ( 'NONE',  ( 16.46253265017160672, -9.564922557960803928, 38.33224293864768839 ) ) ;
#177332=CARTESIAN_POINT ( 'NONE',  ( 4.483927247898790824, -16.52544592524335698, 65.20942372801901854 ) ) ;
#177333=EDGE_LOOP ( 'NONE', ( #149014, #106644, #64400, #32078 ) ) ;
#177334=EDGE_CURVE ( 'NONE', #30166, #158898, #111, .T. ) ;
#177335=CARTESIAN_POINT ( 'NONE',  ( -5.719274019375665041, -21.55341960407619695, 44.79275706135234714 ) ) ;
#177336=CARTESIAN_POINT ( 'NONE',  ( -8.314922557960811034, -14.29746914071050412, 62.08224293864769550 ) ) ;
#177338=CARTESIAN_POINT ( 'NONE',  ( 16.55341960407618274, -4.379528057220086978, 36.04275706135234714 ) ) ;
#177339=CARTESIAN_POINT ( 'NONE',  ( -9.474510206698720793, -16.51473224551083518, 49.58442372801899722 ) ) ;
#177340=CARTESIAN_POINT ( 'NONE',  ( -16.52544592524342804, 4.483927247898546575, 56.04057627198102409 ) ) ;
#177341=CARTESIAN_POINT ( 'NONE',  ( 5.719274019375673035, 21.55341960407619339, 27.29275706135234358 ) ) ;
#177343=CARTESIAN_POINT ( 'NONE',  ( 10.81492255796078972, 18.62759615963270932, 94.58224293864769550 ) ) ;
#177344=CARTESIAN_POINT ( 'NONE',  ( 9.564922557960805705, 16.46253265017160317, 104.5822429386476955 ) ) ;
#177345=CARTESIAN_POINT ( 'NONE',  ( 12.14591786802309770, 12.06949235617756955, 79.37390960531436690 ) ) ;
#177349=CARTESIAN_POINT ( 'NONE',  ( 13.89961937509957401, 13.97604488694547697, 71.87609039468567573 ) ) ;
#177350=CARTESIAN_POINT ( 'NONE',  ( 5.823673210054125526, 21.52544592524343514, 114.7905762719810383 ) ) ;
#177351=CARTESIAN_POINT ( 'NONE',  ( 9.564922557960805705, 16.46253265017160317, 54.58224293864769550 ) ) ;
#177352=CARTESIAN_POINT ( 'NONE',  ( -5.049401038297874678, -19.05341960407617918, 44.79275706135232582 ) ) ;
#177353=CARTESIAN_POINT ( 'NONE',  ( 5.049401038298161559, -19.05341960407611168, 32.70724293864768129 ) ) ;
#177354=CARTESIAN_POINT ( 'NONE',  ( 0.05219959533937995610, -21.53943276465977519, 70.00109039468568994 ) ) ;
#177355=CARTESIAN_POINT ( 'NONE',  ( -16.19135201231366139, -7.376712067591931543, 70.18680854052036011 ) ) ;
#177356=CARTESIAN_POINT ( 'NONE',  ( 16.52544592524342804, -4.483927247898539470, 58.54057627198103120 ) ) ;
#177357=CARTESIAN_POINT ( 'NONE',  ( 9.564922557960805705, 16.46253265017160317, 59.58224293864769550 ) ) ;
#177358=CARTESIAN_POINT ( 'NONE',  ( -15.72974639402197994, 15.80617190586746368, 90.62390960531436690 ) ) ;
#177359=CARTESIAN_POINT ( 'NONE',  ( 19.02544592524343514, -5.153800228976328945, 53.54057627198102409 ) ) ;
#177360=CARTESIAN_POINT ( 'NONE',  ( -15.72974639402197994, 15.80617190586746368, 70.62390960531436690 ) ) ;
#177361=CARTESIAN_POINT ( 'NONE',  ( -10.81492255796105439, 18.62759615963255655, 97.91775706135236135 ) ) ;
#177362=CARTESIAN_POINT ( 'NONE',  ( -16.46253265017160317, 9.564922557960807481, 25.83224293864769194 ) ) ;
#177363=CARTESIAN_POINT ( 'NONE',  ( 4.379528057220092307, 16.55341960407617563, 92.29275706135236135 ) ) ;
#177364=CARTESIAN_POINT ( 'NONE',  ( 16.53943276465976808, -0.05219959533910856209, 78.74890960531436690 ) ) ;
#177365=CARTESIAN_POINT ( 'NONE',  ( -9.564922557961040184, 16.46253265017147172, 92.91775706135233293 ) ) ;
#177367=CARTESIAN_POINT ( 'NONE',  ( -0.05219959533937732626, 21.53943276465977519, 22.50109039468567573 ) ) ;
#177368=CARTESIAN_POINT ( 'NONE',  ( 16.51473224551083163, -9.474510206698727899, 35.83442372801899722 ) ) ;
#177369=CARTESIAN_POINT ( 'NONE',  ( -0.05219959533934338120, 16.53943276465976808, 107.5010903946856899 ) ) ;
#177370=CARTESIAN_POINT ( 'NONE',  ( 19.02544592524334988, 5.153800228976608722, 31.45942372801900433 ) ) ;
#177371=CARTESIAN_POINT ( 'NONE',  ( 9.474510206698971260, -16.51473224551069308, 87.91557627198102409 ) ) ;
#177372=CARTESIAN_POINT ( 'NONE',  ( -15.80617190586745835, -15.72974639402198527, 56.87390960531436690 ) ) ;
#177373=CARTESIAN_POINT ( 'NONE',  ( -19.03943276465977164, 0.05219959533909376836, 21.24890960531436335 ) ) ;
#177374=CARTESIAN_POINT ( 'NONE',  ( 13.89961937509977652, -13.97604488694527269, 23.12390960531436335 ) ) ;
#177375=CARTESIAN_POINT ( 'NONE',  ( -15.80617190586768217, 15.72974639402176855, 113.1260903946856899 ) ) ;
#177376=CARTESIAN_POINT ( 'NONE',  ( -4.483927247898782831, 16.52544592524335698, 82.70942372801900433 ) ) ;
#177377=CARTESIAN_POINT ( 'NONE',  ( 15.72974639402176855, 15.80617190586768217, 21.87609039468567573 ) ) ;
#177378=CARTESIAN_POINT ( 'NONE',  ( 16.53943276465976808, 0.05219959533934440121, 31.25109039468568639 ) ) ;
#177379=CARTESIAN_POINT ( 'NONE',  ( -13.89961937509977652, 13.97604488694528158, 110.6239096053143243 ) ) ;
#177380=CARTESIAN_POINT ( 'NONE',  ( 19.02544592524343514, -5.153800228976328945, 38.54057627198103120 ) ) ;
#177381=CARTESIAN_POINT ( 'NONE',  ( 19.05341960407611168, 5.049401038298154454, 68.95724293864769550 ) ) ;
#177382=VECTOR ( 'NONE', #105379, 1000.000000000000000 ) ;
#177383=CARTESIAN_POINT ( 'NONE',  ( -4.483927247898782831, 16.52544592524335698, 42.70942372801901854 ) ) ;
#177384=CARTESIAN_POINT ( 'NONE',  ( -16.55341960407611168, -4.379528057220339221, 86.45724293864770971 ) ) ;
#177385=CARTESIAN_POINT ( 'NONE',  ( -8.314922557961024197, 14.29746914071037800, 97.91775706135236135 ) ) ;
#177386=CARTESIAN_POINT ( 'NONE',  ( 15.80617190586769283, -15.72974639402175789, 55.62609039468568284 ) ) ;
#177387=CARTESIAN_POINT ( 'NONE',  ( -13.89961937509977652, 13.97604488694528158, 75.62390960531438111 ) ) ;
#177388=CARTESIAN_POINT ( 'NONE',  ( 9.564922557960805705, 16.46253265017160317, 59.58224293864769550 ) ) ;
#177389=CARTESIAN_POINT ( 'NONE',  ( 19.03943276465977164, -0.05219959533909143690, 98.74890960531436690 ) ) ;
#177390=CARTESIAN_POINT ( 'NONE',  ( 8.314922557960818139, 14.29746914071049879, 39.58224293864769550 ) ) ;
#177391=CARTESIAN_POINT ( 'NONE',  ( -4.379528057220086978, -16.55341960407618274, 99.79275706135234714 ) ) ;
#177393=CARTESIAN_POINT ( 'NONE',  ( 19.05341960407617918, -5.049401038297876454, 41.04275706135233293 ) ) ;
#177394=CARTESIAN_POINT ( 'NONE',  ( 16.51473224551069308, 9.474510206698969483, 109.1655762719810383 ) ) ;
#177395=CARTESIAN_POINT ( 'NONE',  ( -5.049401038298153566, 19.05341960407611168, 60.20724293864768129 ) ) ;
#177396=CARTESIAN_POINT ( 'NONE',  ( 0.05219959533936267826, -19.03943276465977164, 40.00109039468566152 ) ) ;
#177398=CARTESIAN_POINT ( 'NONE',  ( -17.40861289039003168, -6.110651285853283987, 66.37232470827431996 ) ) ;
#177399=CARTESIAN_POINT ( 'NONE',  ( 16.52544592524335698, 4.483927247898782831, 51.45942372801901854 ) ) ;
#177400=CARTESIAN_POINT ( 'NONE',  ( -5.153800228976607833, 19.02544592524334988, 72.70942372801900433 ) ) ;
#177401=CARTESIAN_POINT ( 'NONE',  ( 8.314922557961029526, -14.29746914071037800, 75.41775706135233293 ) ) ;
#177403=CARTESIAN_POINT ( 'NONE',  ( -9.474510206698964154, 16.51473224551069663, 95.41557627198102409 ) ) ;
#177404=CARTESIAN_POINT ( 'NONE',  ( 10.81492255796106328, -18.62759615963255655, 20.41775706135234714 ) ) ;
#177405=CARTESIAN_POINT ( 'NONE',  ( 19.03943276465977164, 0.05219959533936151252, 76.25109039468566152 ) ) ;
#177406=CARTESIAN_POINT ( 'NONE',  ( 5.153800228976335163, 19.02544592524342804, 99.79057627198102409 ) ) ;
#177407=CARTESIAN_POINT ( 'NONE',  ( 0.05219959533909260263, 19.03943276465977164, 34.99890960531435979 ) ) ;
#177408=CARTESIAN_POINT ( 'NONE',  ( -19.03943276465977164, 0.05219959533909376836, 96.24890960531436690 ) ) ;
#177409=CARTESIAN_POINT ( 'NONE',  ( -14.29746914071049879, 8.314922557960819915, 50.83224293864770971 ) ) ;
#177410=CARTESIAN_POINT ( 'NONE',  ( 19.03943276465977164, -0.05219959533909143690, 38.74890960531436690 ) ) ;
#177411=CARTESIAN_POINT ( 'NONE',  ( 0.05219959533936267826, -19.03943276465977164, 45.00109039468566863 ) ) ;
#177412=CARTESIAN_POINT ( 'NONE',  ( 14.29746914071049879, -8.314922557960816363, 93.33224293864769550 ) ) ;
#177413=CARTESIAN_POINT ( 'NONE',  ( 13.97604488694548053, -13.89961937509957401, 20.62609039468567573 ) ) ;
#177414=CARTESIAN_POINT ( 'NONE',  ( 16.51473224551069308, 9.474510206698969483, 54.16557627198103120 ) ) ;
#177415=CARTESIAN_POINT ( 'NONE',  ( 21.53943276465977519, -0.05219959533907433946, 63.74890960531435979 ) ) ;
#177416=CARTESIAN_POINT ( 'NONE',  ( 16.52544592524342804, -4.483927247898539470, 48.54057627198103120 ) ) ;
#177417=CARTESIAN_POINT ( 'NONE',  ( 16.46253265017146816, 9.564922557961045513, 26.66775706135234003 ) ) ;
#177418=CARTESIAN_POINT ( 'NONE',  ( -16.46253265017160317, 9.564922557960807481, 110.8322429386476955 ) ) ;
#177419=CARTESIAN_POINT ( 'NONE',  ( 5.049401038298161559, -19.05341960407611168, 107.7072429386476955 ) ) ;
#177420=CARTESIAN_POINT ( 'NONE',  ( -13.97604488694527625, -13.89961937509977652, 36.87390960531436690 ) ) ;
#177421=CARTESIAN_POINT ( 'NONE',  ( 13.97604488694527802, 13.89961937509977652, 29.37390960531435979 ) ) ;
#177422=CARTESIAN_POINT ( 'NONE',  ( 12.14591786802309770, 12.06949235617756955, 84.37390960531438111 ) ) ;
#177423=CARTESIAN_POINT ( 'NONE',  ( 0.05219959533907565091, 21.53943276465977519, 94.99890960531436690 ) ) ;
#177424=CARTESIAN_POINT ( 'NONE',  ( -9.564922557960796823, -16.46253265017161027, 97.08224293864769550 ) ) ;
#177425=CARTESIAN_POINT ( 'NONE',  ( -0.05219959533907301413, -21.53943276465977519, 112.4989096053143669 ) ) ;
#177426=CARTESIAN_POINT ( 'NONE',  ( -5.049401038298153566, 19.05341960407611168, 110.2072429386476671 ) ) ;
#177427=CARTESIAN_POINT ( 'NONE',  ( 4.379528057220339221, -16.55341960407611168, 97.70724293864772392 ) ) ;
#177428=CARTESIAN_POINT ( 'NONE',  ( 0.05219959533937995610, -21.53943276465977519, 80.00109039468568994 ) ) ;
#177429=CARTESIAN_POINT ( 'NONE',  ( 5.719274019375991003, -21.55341960407610458, 77.70724293864770971 ) ) ;
#177430=CARTESIAN_POINT ( 'NONE',  ( 17.26172910966779739, -6.454744622555833367, 108.3064690864922284 ) ) ;
#177431=DIRECTION ( 'NONE',  ( 0.000000000000000000, -0.04175967627138118393, -0.9991276842514721368 ) ) ;
#177433=CARTESIAN_POINT ( 'NONE',  ( -0.05219959533934338120, 16.53943276465976808, 37.50109039468568284 ) ) ;
#177435=CARTESIAN_POINT ( 'NONE',  ( 16.53943276465976808, -0.05219959533910856209, 113.7489096053143527 ) ) ;
#177436=CARTESIAN_POINT ( 'NONE',  ( -17.49999999999997513, -4.013004640162659342, 109.5539427900558991 ) ) ;
#177437=CARTESIAN_POINT ( 'NONE',  ( 19.05341960407611168, 5.049401038298154454, 58.95724293864768129 ) ) ;
#177438=CARTESIAN_POINT ( 'NONE',  ( 16.53943276465976808, -0.05219959533910856209, 88.74890960531436690 ) ) ;
#177439=CARTESIAN_POINT ( 'NONE',  ( 18.62759615963271287, -10.81492255796078972, 33.33224293864769550 ) ) ;
#177440=CARTESIAN_POINT ( 'NONE',  ( 16.52544592524342804, -4.483927247898539470, 68.54057627198103830 ) ) ;
#177441=CARTESIAN_POINT ( 'NONE',  ( 4.379528057220092307, 16.55341960407617563, 22.29275706135235069 ) ) ;
#177442=CARTESIAN_POINT ( 'NONE',  ( -5.719274019375665041, -21.55341960407619695, 79.79275706135236135 ) ) ;
#177444=CARTESIAN_POINT ( 'NONE',  ( -13.89961937509977652, 13.97604488694528158, 110.6239096053143243 ) ) ;
#177445=CARTESIAN_POINT ( 'NONE',  ( -16.53943276465976808, -0.05219959533934237506, 98.75109039468568994 ) ) ;
#177446=CARTESIAN_POINT ( 'NONE',  ( 9.564922557960805705, 16.46253265017160317, 34.58224293864770260 ) ) ;
#177447=CARTESIAN_POINT ( 'NONE',  ( 19.03943276465977164, -0.05219959533909143690, 83.74890960531436690 ) ) ;
#177448=CARTESIAN_POINT ( 'NONE',  ( -21.55341960407610458, -5.719274019375992779, 91.45724293864769550 ) ) ;
#177449=CARTESIAN_POINT ( 'NONE',  ( 4.483927247898790824, -16.52544592524335698, 25.20942372801901854 ) ) ;
#177450=CARTESIAN_POINT ( 'NONE',  ( -0.05219959533910754901, -16.53943276465976808, 67.49890960531436690 ) ) ;
#177451=CARTESIAN_POINT ( 'NONE',  ( 18.62759615963255655, 10.81492255796105972, 66.66775706135234714 ) ) ;
#177452=CARTESIAN_POINT ( 'NONE',  ( 16.53943276465976808, 0.05219959533934440121, 106.2510903946856757 ) ) ;
#177453=CARTESIAN_POINT ( 'NONE',  ( 16.62475595723611477, -7.163666690055880082, 48.02713351810404419 ) ) ;
#177454=CARTESIAN_POINT ( 'NONE',  ( -17.49999999999999289, 5.500000000000037303, 80.79690382534172954 ) ) ;
#177455=CARTESIAN_POINT ( 'NONE',  ( 16.52544592524342804, -4.483927247898539470, 33.54057627198102409 ) ) ;
#177456=CARTESIAN_POINT ( 'NONE',  ( 16.53943276465976808, 0.05219959533934440121, 56.25109039468568284 ) ) ;
#177457=CARTESIAN_POINT ( 'NONE',  ( -19.02544592524342804, 5.153800228976336051, 76.04057627198102409 ) ) ;
#177458=CARTESIAN_POINT ( 'NONE',  ( 16.46253265017160672, -9.564922557960803928, 88.33224293864769550 ) ) ;
#177459=CARTESIAN_POINT ( 'NONE',  ( -15.80617190586768217, 15.72974639402176855, 83.12609039468568994 ) ) ;
#177461=CARTESIAN_POINT ( 'NONE',  ( 16.55341960407618274, -4.379528057220086978, 86.04275706135236135 ) ) ;
#177462=CARTESIAN_POINT ( 'NONE',  ( 12.14591786802309770, 12.06949235617756955, 54.37390960531435979 ) ) ;
#177463=CARTESIAN_POINT ( 'NONE',  ( -19.02544592524342804, 5.153800228976336051, 66.04057627198103830 ) ) ;
#177465=CARTESIAN_POINT ( 'NONE',  ( -19.03943276465977164, -0.05219959533935918106, 113.7510903946856757 ) ) ;
#177466=CARTESIAN_POINT ( 'NONE',  ( -12.06949235617756955, 12.14591786802309770, 115.6239096053143669 ) ) ;
#177467=CARTESIAN_POINT ( 'NONE',  ( -16.46253265017160317, 9.564922557960807481, 75.83224293864769550 ) ) ;
#177468=CARTESIAN_POINT ( 'NONE',  ( 4.483927247898790824, -16.52544592524335698, 20.20942372801900788 ) ) ;
#177470=CARTESIAN_POINT ( 'NONE',  ( 10.72451020669871369, 18.67979575497193778, 107.0844237280190043 ) ) ;
#177471=CARTESIAN_POINT ( 'NONE',  ( 14.29746914071037800, 8.314922557961029526, 76.66775706135234714 ) ) ;
#177472=CARTESIAN_POINT ( 'NONE',  ( -19.03943276465977164, -0.05219959533935918106, 98.75109039468567573 ) ) ;
#177473=CARTESIAN_POINT ( 'NONE',  ( 19.05341960407611168, 5.049401038298154454, 23.95724293864769194 ) ) ;
#177474=CARTESIAN_POINT ( 'NONE',  ( -14.34966873604972548, 8.224510206698743886, 68.33442372801900433 ) ) ;
#177476=CARTESIAN_POINT ( 'NONE',  ( -13.89961937509957401, -13.97604488694547875, 49.37609039468567573 ) ) ;
#177477=CARTESIAN_POINT ( 'NONE',  ( -21.52544592524334988, -5.823673210054445271, 103.9594237280190185 ) ) ;
#177478=CARTESIAN_POINT ( 'NONE',  ( -13.89961937509977652, 13.97604488694528158, 40.62390960531435979 ) ) ;
#177479=CARTESIAN_POINT ( 'NONE',  ( -19.02544592524342804, 5.153800228976336051, 76.04057627198102409 ) ) ;
#177480=CARTESIAN_POINT ( 'NONE',  ( -0.05219959533910754901, -16.53943276465976808, 67.49890960531436690 ) ) ;
#177481=CARTESIAN_POINT ( 'NONE',  ( -18.62759615963255300, -10.81492255796106328, 84.16775706135234714 ) ) ;
#177483=CARTESIAN_POINT ( 'NONE',  ( 9.474510206698729675, 16.51473224551082808, 47.08442372801900433 ) ) ;
#177484=CARTESIAN_POINT ( 'NONE',  ( -19.02544592524334988, -5.153800228976617603, 38.95942372801900433 ) ) ;
#177485=CARTESIAN_POINT ( 'NONE',  ( 0.05219959533907565091, 21.53943276465977519, 39.99890960531436690 ) ) ;
#177486=CARTESIAN_POINT ( 'NONE',  ( -18.62759615963255300, -10.81492255796106328, 99.16775706135234714 ) ) ;
#177487=CARTESIAN_POINT ( 'NONE',  ( -9.474510206698964154, 16.51473224551069663, 80.41557627198103830 ) ) ;
#177488=CARTESIAN_POINT ( 'NONE',  ( -15.80617190586768217, 15.72974639402176855, 88.12609039468570415 ) ) ;
#177489=CARTESIAN_POINT ( 'NONE',  ( 18.67979575497178502, 10.72451020669898547, 54.16557627198103120 ) ) ;
#177490=CARTESIAN_POINT ( 'NONE',  ( -13.97604488694527625, -13.89961937509977652, 101.8739096053143811 ) ) ;
#177491=CARTESIAN_POINT ( 'NONE',  ( -16.51473224551082808, 9.474510206698731452, 78.33442372801900433 ) ) ;
#177492=CARTESIAN_POINT ( 'NONE',  ( 9.564922557960805705, 16.46253265017160317, 99.58224293864770971 ) ) ;
#177493=CARTESIAN_POINT ( 'NONE',  ( -16.51473224551082808, 9.474510206698731452, 93.33442372801900433 ) ) ;
#177494=CARTESIAN_POINT ( 'NONE',  ( -14.34966873604972548, 8.224510206698743886, 38.33442372801900433 ) ) ;
#177495=CARTESIAN_POINT ( 'NONE',  ( -16.53943276465976808, 0.05219959533911058130, 96.24890960531435269 ) ) ;
#177496=CARTESIAN_POINT ( 'NONE',  ( 0.05219959533909260263, 19.03943276465977164, 69.99890960531435269 ) ) ;
#177497=CARTESIAN_POINT ( 'NONE',  ( -0.05219959533907301413, -21.53943276465977519, 67.49890960531436690 ) ) ;
#177499=CARTESIAN_POINT ( 'NONE',  ( 14.29746914071037800, 8.314922557961029526, 36.66775706135234714 ) ) ;
#177500=CARTESIAN_POINT ( 'NONE',  ( -15.72974639402176322, -15.80617190586768395, 39.37609039468567573 ) ) ;
#177501=CARTESIAN_POINT ( 'NONE',  ( 0.05219959533937995610, -21.53943276465977519, 90.00109039468567573 ) ) ;
#177502=CARTESIAN_POINT ( 'NONE',  ( 12.06949235617739724, 12.14591786802326823, 76.87609039468567573 ) ) ;
#177503=CARTESIAN_POINT ( 'NONE',  ( 13.97604488694527802, 13.89961937509977652, 69.37390960531436690 ) ) ;
#177504=CARTESIAN_POINT ( 'NONE',  ( -4.483927247898539470, -16.52544592524342804, 72.29057627198102409 ) ) ;
#177505=CARTESIAN_POINT ( 'NONE',  ( 16.53943276465976808, 0.05219959533934440121, 101.2510903946856757 ) ) ;
#177506=CARTESIAN_POINT ( 'NONE',  ( 13.97604488694548053, -13.89961937509957401, 50.62609039468566152 ) ) ;
#177507=CARTESIAN_POINT ( 'NONE',  ( 10.81492255796106328, -18.62759615963255655, 30.41775706135234358 ) ) ;
#177508=CARTESIAN_POINT ( 'NONE',  ( 0.05219959533910956823, 16.53943276465976808, 74.99890960531435269 ) ) ;
#177509=CARTESIAN_POINT ( 'NONE',  ( 19.02544592524343514, -5.153800228976328945, 98.54057627198100988 ) ) ;
#177510=CARTESIAN_POINT ( 'NONE',  ( 16.55341960407618274, -4.379528057220086978, 101.0427570613523756 ) ) ;
#177511=CARTESIAN_POINT ( 'NONE',  ( 15.80617190586769283, -15.72974639402175789, 65.62609039468568994 ) ) ;
#177512=CARTESIAN_POINT ( 'NONE',  ( -8.224510206698735004, -14.34966873604973081, 44.58442372801901854 ) ) ;
#177513=CARTESIAN_POINT ( 'NONE',  ( 15.72974639402176855, 15.80617190586768217, 41.87609039468568284 ) ) ;
#177514=CARTESIAN_POINT ( 'NONE',  ( -16.53943276465976808, 0.05219959533911058130, 76.24890960531435269 ) ) ;
#177516=CARTESIAN_POINT ( 'NONE',  ( -21.53943276465977519, 0.05219959533907696930, 116.2489096053143669 ) ) ;
#177517=CARTESIAN_POINT ( 'NONE',  ( 17.50000000000001421, -3.471454075611625445, 26.98332581144362052 ) ) ;
#177518=CARTESIAN_POINT ( 'NONE',  ( 16.55341960407611168, 4.379528057220329451, 48.95724293864770971 ) ) ;
#177519=CARTESIAN_POINT ( 'NONE',  ( -16.51473224551069308, -9.474510206698971260, 21.66557627198102765 ) ) ;
#177520=CARTESIAN_POINT ( 'NONE',  ( 10.81492255796078972, 18.62759615963270932, 44.58224293864769550 ) ) ;
#177521=CARTESIAN_POINT ( 'NONE',  ( -4.483927247898539470, -16.52544592524342804, 82.29057627198103830 ) ) ;
#177523=CARTESIAN_POINT ( 'NONE',  ( 5.719274019375991003, -21.55341960407610458, 82.70724293864770971 ) ) ;
#177524=CARTESIAN_POINT ( 'NONE',  ( 16.46253265017160672, -9.564922557960803928, 88.33224293864769550 ) ) ;
#177525=CARTESIAN_POINT ( 'NONE',  ( 5.049401038298161559, -19.05341960407611168, 42.70724293864767418 ) ) ;
#177526=CARTESIAN_POINT ( 'NONE',  ( 9.564922557961047289, -16.46253265017146816, 80.41775706135234714 ) ) ;
#177527=CARTESIAN_POINT ( 'NONE',  ( -5.823673210054431948, 21.52544592524334988, 57.70942372801901143 ) ) ;
#177528=CARTESIAN_POINT ( 'NONE',  ( -5.823673210054116645, -21.52544592524344225, 67.29057627198103830 ) ) ;
#177529=CARTESIAN_POINT ( 'NONE',  ( -19.05341960407611168, -5.049401038298163336, 36.45724293864766707 ) ) ;
#177530=CARTESIAN_POINT ( 'NONE',  ( 9.564922557960805705, 16.46253265017160317, 74.58224293864769550 ) ) ;
#177532=CARTESIAN_POINT ( 'NONE',  ( 0.05219959533934541429, -16.53943276465976808, 55.00109039468568284 ) ) ;
#177533=CARTESIAN_POINT ( 'NONE',  ( -21.52544592524334988, -5.823673210054445271, 33.95942372801901143 ) ) ;
#177534=CARTESIAN_POINT ( 'NONE',  ( 21.55341960407619695, -5.719274019375665929, 76.04275706135237556 ) ) ;
#177535=CARTESIAN_POINT ( 'NONE',  ( -16.46253265017160317, 9.564922557960807481, 100.8322429386477097 ) ) ;
#177536=CARTESIAN_POINT ( 'NONE',  ( 18.62759615963271287, -10.81492255796078972, 83.33224293864769550 ) ) ;
#177537=CARTESIAN_POINT ( 'NONE',  ( -18.62759615963255300, -10.81492255796106328, 24.16775706135235424 ) ) ;
#177538=CARTESIAN_POINT ( 'NONE',  ( -8.314922557961024197, 14.29746914071037800, 52.91775706135235424 ) ) ;
#177540=CARTESIAN_POINT ( 'NONE',  ( -15.72974639402197994, 15.80617190586746368, 45.62390960531436690 ) ) ;
#177541=CARTESIAN_POINT ( 'NONE',  ( 9.564922557961047289, -16.46253265017146816, 25.41775706135234003 ) ) ;
#177542=CARTESIAN_POINT ( 'NONE',  ( 19.02544592524343514, -5.153800228976328945, 48.54057627198103120 ) ) ;
#177543=CARTESIAN_POINT ( 'NONE',  ( 19.03943276465977164, -0.05219959533909143690, 108.7489096053143527 ) ) ;
#177544=CARTESIAN_POINT ( 'NONE',  ( 13.97604488694527802, 13.89961937509977652, 94.37390960531436690 ) ) ;
#177546=CARTESIAN_POINT ( 'NONE',  ( -0.05219959533936034679, 19.03943276465977164, 67.50109039468566152 ) ) ;
#177547=CARTESIAN_POINT ( 'NONE',  ( 0.05219959533907565091, 21.53943276465977519, 39.99890960531436690 ) ) ;
#177548=CARTESIAN_POINT ( 'NONE',  ( 12.14591786802309770, 12.06949235617756955, 24.37390960531435979 ) ) ;
#177549=CARTESIAN_POINT ( 'NONE',  ( -19.03943276465977164, -0.05219959533935918106, 103.7510903946856757 ) ) ;
#177551=CARTESIAN_POINT ( 'NONE',  ( -15.80617190586768217, 15.72974639402176855, 113.1260903946856899 ) ) ;
#177552=CARTESIAN_POINT ( 'NONE',  ( -5.049401038297874678, -19.05341960407617918, 94.79275706135230450 ) ) ;
#177553=CARTESIAN_POINT ( 'NONE',  ( -13.97604488694547697, 13.89961937509957934, 63.12609039468566152 ) ) ;
#177554=CARTESIAN_POINT ( 'NONE',  ( 17.50000000000000000, -5.499999999999992895, 91.21769037696437010 ) ) ;
#177555=CARTESIAN_POINT ( 'NONE',  ( 9.564922557960805705, 16.46253265017160317, 54.58224293864769550 ) ) ;
#177556=CARTESIAN_POINT ( 'NONE',  ( -4.379528057220328563, 16.55341960407611168, 65.20724293864768129 ) ) ;
#177557=CARTESIAN_POINT ( 'NONE',  ( 16.46253265017160672, -9.564922557960803928, 38.33224293864768839 ) ) ;
#177558=CARTESIAN_POINT ( 'NONE',  ( -8.224510206698948167, 14.34966873604960824, 35.41557627198102409 ) ) ;
#177559=DIRECTION ( 'NONE',  ( 6.716189716306310304E-15, -0.9991276842514723588, 0.04175967627138119781 ) ) ;
#177560=CARTESIAN_POINT ( 'NONE',  ( -14.34966873604972548, 8.224510206698743886, 103.3344237280190043 ) ) ;
#177561=CARTESIAN_POINT ( 'NONE',  ( -5.153800228976328057, -19.02544592524343514, 67.29057627198102409 ) ) ;
#177562=CARTESIAN_POINT ( 'NONE',  ( -16.46253265017146816, -9.564922557961047289, 24.16775706135233648 ) ) ;
#177563=CARTESIAN_POINT ( 'NONE',  ( -16.55341960407617563, 4.379528057220093196, 28.54275706135234358 ) ) ;
#177564=CARTESIAN_POINT ( 'NONE',  ( 5.719274019375991003, -21.55341960407610458, 52.70724293864769550 ) ) ;
#177565=CARTESIAN_POINT ( 'NONE',  ( -10.81492255796105439, 18.62759615963255655, 102.9177570613523756 ) ) ;
#177566=VERTEX_POINT ( 'NONE', #23190 ) ;
#177567=CARTESIAN_POINT ( 'NONE',  ( 0.05219959533909260263, 19.03943276465977164, 64.99890960531436690 ) ) ;
#177569=CARTESIAN_POINT ( 'NONE',  ( -19.02544592524342804, 5.153800228976336051, 101.0405762719810241 ) ) ;
#177571=CARTESIAN_POINT ( 'NONE',  ( -5.823673210054431948, 21.52544592524334988, 27.70942372801901854 ) ) ;
#177572=CARTESIAN_POINT ( 'NONE',  ( -0.05219959533910754901, -16.53943276465976808, 92.49890960531436690 ) ) ;
#177573=CARTESIAN_POINT ( 'NONE',  ( 0.05219959533907565091, 21.53943276465977519, 84.99890960531436690 ) ) ;
#177574=CARTESIAN_POINT ( 'NONE',  ( 9.474510206698971260, -16.51473224551069308, 62.91557627198102409 ) ) ;
#177575=CARTESIAN_POINT ( 'NONE',  ( 16.46253265017160672, -9.564922557960803928, 78.33224293864769550 ) ) ;
#177576=CARTESIAN_POINT ( 'NONE',  ( 10.81492255796078972, 18.62759615963270932, 114.5822429386477097 ) ) ;
#177577=ORIENTED_EDGE ( 'NONE', *, *, #136064, .F. ) ;
#177578=CARTESIAN_POINT ( 'NONE',  ( -19.02544592524342804, 5.153800228976336051, 71.04057627198099567 ) ) ;
#177579=CARTESIAN_POINT ( 'NONE',  ( 19.36337904590688552, -5.500000000000036415, 97.91494137495618588 ) ) ;
#177580=CARTESIAN_POINT ( 'NONE',  ( -12.06949235617756955, 12.14591786802309770, 105.6239096053143669 ) ) ;
#177582=CARTESIAN_POINT ( 'NONE',  ( -13.89961937509957401, -13.97604488694547875, 94.37609039468566152 ) ) ;
#177583=CARTESIAN_POINT ( 'NONE',  ( -12.14591786802309592, -12.06949235617757132, 91.87390960531436690 ) ) ;
#177584=CARTESIAN_POINT ( 'NONE',  ( 0.05219959533937995610, -21.53943276465977519, 70.00109039468568994 ) ) ;
#177585=CARTESIAN_POINT ( 'NONE',  ( -16.46253265017160317, 9.564922557960807481, 60.83224293864769550 ) ) ;
#177586=CARTESIAN_POINT ( 'NONE',  ( -15.72974639402176322, -15.80617190586768395, 29.37609039468568284 ) ) ;
#177587=CARTESIAN_POINT ( 'NONE',  ( -10.72451020669898014, 18.67979575497178502, 110.4155762719810383 ) ) ;
#177589=CARTESIAN_POINT ( 'NONE',  ( -0.05219959533909027116, -19.03943276465977164, 67.49890960531436690 ) ) ;
#177591=CARTESIAN_POINT ( 'NONE',  ( -14.34966873604972548, 8.224510206698743886, 23.33442372801901499 ) ) ;
#177592=CARTESIAN_POINT ( 'NONE',  ( -18.67979575497178146, -10.72451020669898902, 36.66557627198103120 ) ) ;
#177593=CARTESIAN_POINT ( 'NONE',  ( -10.81492255796105439, 18.62759615963255655, 57.91775706135234714 ) ) ;
#177594=CARTESIAN_POINT ( 'NONE',  ( 16.51473224551069308, 9.474510206698969483, 104.1655762719810241 ) ) ;
#177595=CARTESIAN_POINT ( 'NONE',  ( -16.46253265017146816, -9.564922557961047289, 99.16775706135233293 ) ) ;
#177596=CARTESIAN_POINT ( 'NONE',  ( -16.46253265017160317, 9.564922557960807481, 45.83224293864769550 ) ) ;
#177597=CARTESIAN_POINT ( 'NONE',  ( 13.89961937509977652, -13.97604488694527269, 73.12390960531436690 ) ) ;
#177598=CARTESIAN_POINT ( 'NONE',  ( 4.483927247898545687, 16.52544592524342804, 99.79057627198103830 ) ) ;
#177599=CARTESIAN_POINT ( 'NONE',  ( 19.03943276465977164, -0.05219959533909143690, 98.74890960531436690 ) ) ;
#177600=CARTESIAN_POINT ( 'NONE',  ( -0.05219959533910754901, -16.53943276465976808, 92.49890960531436690 ) ) ;
#177601=CARTESIAN_POINT ( 'NONE',  ( -19.02544592524342804, 5.153800228976336051, 96.04057627198103830 ) ) ;
#177602=CARTESIAN_POINT ( 'NONE',  ( -4.379528057220328563, 16.55341960407611168, 45.20724293864769550 ) ) ;
#177603=CARTESIAN_POINT ( 'NONE',  ( -19.05341960407611168, -5.049401038298163336, 41.45724293864769550 ) ) ;
#177605=CARTESIAN_POINT ( 'NONE',  ( 21.52544592524334988, 5.823673210054432836, 51.45942372801901854 ) ) ;
#177606=CARTESIAN_POINT ( 'NONE',  ( -19.02544592524334988, -5.153800228976617603, 83.95942372801901854 ) ) ;
#177607=CARTESIAN_POINT ( 'NONE',  ( 16.55341960407611168, 4.379528057220329451, 53.95724293864770260 ) ) ;
#177608=CARTESIAN_POINT ( 'NONE',  ( -10.72451020669898014, 18.67979575497178502, 100.4155762719810241 ) ) ;
#177609=CARTESIAN_POINT ( 'NONE',  ( 21.53943276465977519, -0.05219959533907433946, 53.74890960531437401 ) ) ;
#177610=CARTESIAN_POINT ( 'NONE',  ( 5.049401038298161559, -19.05341960407611168, 107.7072429386476955 ) ) ;
#177611=CARTESIAN_POINT ( 'NONE',  ( 12.06949235617757843, -12.14591786802309237, 78.12390960531436690 ) ) ;
#177612=CARTESIAN_POINT ( 'NONE',  ( -13.97604488694527625, -13.89961937509977652, 56.87390960531434558 ) ) ;
#177613=CARTESIAN_POINT ( 'NONE',  ( 12.06949235617757843, -12.14591786802309237, 28.12390960531435979 ) ) ;
#177614=CARTESIAN_POINT ( 'NONE',  ( -16.53943276465976808, -0.05219959533934237506, 98.75109039468568994 ) ) ;
#177615=CARTESIAN_POINT ( 'NONE',  ( -16.53943276465976808, -0.05219959533934237506, 73.75109039468567573 ) ) ;
#177616=CARTESIAN_POINT ( 'NONE',  ( 9.564922557961047289, -16.46253265017146816, 30.41775706135232937 ) ) ;
#177618=CARTESIAN_POINT ( 'NONE',  ( -16.46253265017160317, 9.564922557960807481, 110.8322429386476955 ) ) ;
#177619=CARTESIAN_POINT ( 'NONE',  ( -0.05219959533909027116, -19.03943276465977164, 72.49890960531435269 ) ) ;
#177620=CARTESIAN_POINT ( 'NONE',  ( -9.564922557960796823, -16.46253265017161027, 37.08224293864768839 ) ) ;
#177621=CARTESIAN_POINT ( 'NONE',  ( 16.55341960407611168, 4.379528057220329451, 43.95724293864769550 ) ) ;
#177622=CARTESIAN_POINT ( 'NONE',  ( -5.153800228976328057, -19.02544592524343514, 112.2905762719810099 ) ) ;
#177623=CARTESIAN_POINT ( 'NONE',  ( -19.05341960407611168, -5.049401038298163336, 101.4572429386476955 ) ) ;
#177624=CARTESIAN_POINT ( 'NONE',  ( -18.67979575497178146, -10.72451020669898902, 46.66557627198102409 ) ) ;
#177625=CARTESIAN_POINT ( 'NONE',  ( 12.14591786802309770, 12.06949235617756955, 84.37390960531438111 ) ) ;
#177626=CARTESIAN_POINT ( 'NONE',  ( 12.14591786802327356, -12.06949235617739191, 35.62609039468568994 ) ) ;
#177627=CARTESIAN_POINT ( 'NONE',  ( -4.379528057220328563, 16.55341960407611168, 65.20724293864768129 ) ) ;
#177628=CARTESIAN_POINT ( 'NONE',  ( -17.49999999999999645, -5.499999999999992895, 120.0000000000000142 ) ) ;
#177629=CARTESIAN_POINT ( 'NONE',  ( 0.05219959533936267826, -19.03943276465977164, 60.00109039468566863 ) ) ;
#177630=CARTESIAN_POINT ( 'NONE',  ( -16.51473224551069308, -9.474510206698971260, 101.6655762719810241 ) ) ;
#177631=CARTESIAN_POINT ( 'NONE',  ( 16.51473224551083163, -9.474510206698727899, 75.83442372801900433 ) ) ;
#177634=CARTESIAN_POINT ( 'NONE',  ( -9.474510206698720793, -16.51473224551083518, 109.5844237280190043 ) ) ;
#177635=CARTESIAN_POINT ( 'NONE',  ( -16.55341960407611168, -4.379528057220339221, 21.45724293864769550 ) ) ;
#177636=CARTESIAN_POINT ( 'NONE',  ( 13.97604488694548053, -13.89961937509957401, 75.62609039468564731 ) ) ;
#177637=CARTESIAN_POINT ( 'NONE',  ( -18.62759615963270932, 10.81492255796079327, 30.83224293864770260 ) ) ;
#177638=CARTESIAN_POINT ( 'NONE',  ( -5.823673210054431948, 21.52544592524334988, 72.70942372801901854 ) ) ;
#177639=CARTESIAN_POINT ( 'NONE',  ( 19.08440550902512811, 5.499999999999857003, 38.67052153706850959 ) ) ;
#177640=CARTESIAN_POINT ( 'NONE',  ( -9.564922557961040184, 16.46253265017147172, 112.9177570613523329 ) ) ;
#177641=CARTESIAN_POINT ( 'NONE',  ( -13.89961937509977652, 13.97604488694528158, 70.62390960531432427 ) ) ;
#177643=CARTESIAN_POINT ( 'NONE',  ( -14.34966873604960291, -8.224510206698953496, 81.66557627198103830 ) ) ;
#177644=CARTESIAN_POINT ( 'NONE',  ( -13.89961937509977652, 13.97604488694528158, 80.62390960531436690 ) ) ;
#177645=CARTESIAN_POINT ( 'NONE',  ( -9.474510206698964154, 16.51473224551069663, 90.41557627198103830 ) ) ;
#177646=CARTESIAN_POINT ( 'NONE',  ( 13.97604488694548053, -13.89961937509957401, 90.62609039468567573 ) ) ;
#177647=CARTESIAN_POINT ( 'NONE',  ( -18.62759615963270932, 10.81492255796079327, 80.83224293864769550 ) ) ;
#177648=CARTESIAN_POINT ( 'NONE',  ( -9.474510206698964154, 16.51473224551069663, 25.41557627198103120 ) ) ;
#177649=CARTESIAN_POINT ( 'NONE',  ( 16.46253265017146816, 9.564922557961045513, 51.66775706135233293 ) ) ;
#177650=CARTESIAN_POINT ( 'NONE',  ( 16.51473224551069308, 9.474510206698969483, 59.16557627198102409 ) ) ;
#177651=CARTESIAN_POINT ( 'NONE',  ( -19.03943276465977164, 0.05219959533909376836, 96.24890960531436690 ) ) ;
#177653=CARTESIAN_POINT ( 'NONE',  ( -10.81492255796078084, -18.62759615963271287, 102.0822429386476955 ) ) ;
#177654=CARTESIAN_POINT ( 'NONE',  ( 8.224510206698953496, -14.34966873604960469, 87.91557627198103830 ) ) ;
#177655=CARTESIAN_POINT ( 'NONE',  ( 19.05341960407611168, 5.049401038298154454, 83.95724293864766707 ) ) ;
#177656=CARTESIAN_POINT ( 'NONE',  ( 5.153800228976615827, -19.02544592524334988, 60.20942372801899012 ) ) ;
#177657=CARTESIAN_POINT ( 'NONE',  ( 21.55341960407610458, 5.719274019375980345, 88.95724293864769550 ) ) ;
#177658=CARTESIAN_POINT ( 'NONE',  ( -0.05219959533907301413, -21.53943276465977519, 67.49890960531436690 ) ) ;
#177659=CARTESIAN_POINT ( 'NONE',  ( 8.314922557960818139, 14.29746914071049879, 39.58224293864769550 ) ) ;
#177660=CARTESIAN_POINT ( 'NONE',  ( -5.719274019375665041, -21.55341960407619695, 104.7927570613523898 ) ) ;
#177661=CARTESIAN_POINT ( 'NONE',  ( 16.52544592524335698, 4.483927247898782831, 66.45942372801903275 ) ) ;
#177662=CARTESIAN_POINT ( 'NONE',  ( -9.564922557960796823, -16.46253265017161027, 97.08224293864769550 ) ) ;
#177663=CARTESIAN_POINT ( 'NONE',  ( 0.05219959533909260263, 19.03943276465977164, 34.99890960531435979 ) ) ;
#177664=CARTESIAN_POINT ( 'NONE',  ( -0.05219959533937732626, 21.53943276465977519, 37.50109039468568284 ) ) ;
#177666=CARTESIAN_POINT ( 'NONE',  ( 5.823673210054444382, -21.52544592524334988, 50.20942372801901854 ) ) ;
#177667=CARTESIAN_POINT ( 'NONE',  ( 5.153800228976335163, 19.02544592524342804, 64.79057627198100988 ) ) ;
#177668=CARTESIAN_POINT ( 'NONE',  ( 21.52544592524334988, 5.823673210054432836, 41.45942372801901143 ) ) ;
#177669=CARTESIAN_POINT ( 'NONE',  ( -19.03943276465977164, -0.05219959533935918106, 73.75109039468566152 ) ) ;
#177670=CARTESIAN_POINT ( 'NONE',  ( -13.89961937509957401, -13.97604488694547875, 79.37609039468567573 ) ) ;
#177671=CARTESIAN_POINT ( 'NONE',  ( -5.153800228976328057, -19.02544592524343514, 42.29057627198101699 ) ) ;
#177672=CARTESIAN_POINT ( 'NONE',  ( -8.314922557961024197, 14.29746914071037800, 72.91775706135234714 ) ) ;
#177673=CARTESIAN_POINT ( 'NONE',  ( 19.02544592524343514, -5.153800228976328945, 53.54057627198102409 ) ) ;
#177674=LINE ( 'NONE', #7795, #141800 ) ;
#177675=CARTESIAN_POINT ( 'NONE',  ( 16.46253265017160672, -9.564922557960803928, 93.33224293864769550 ) ) ;
#177676=CARTESIAN_POINT ( 'NONE',  ( 13.97604488694527802, 13.89961937509977652, 39.37390960531435269 ) ) ;
#177677=CARTESIAN_POINT ( 'NONE',  ( 15.72974639402199770, -15.80617190586745480, 78.12390960531436690 ) ) ;
#177678=CARTESIAN_POINT ( 'NONE',  ( 12.06949235617739724, 12.14591786802326823, 66.87609039468568994 ) ) ;
#177679=CARTESIAN_POINT ( 'NONE',  ( -10.81492255796105439, 18.62759615963255655, 112.9177570613523329 ) ) ;
#177680=CARTESIAN_POINT ( 'NONE',  ( 5.049401038298161559, -19.05341960407611168, 47.70724293864770260 ) ) ;
#177681=CARTESIAN_POINT ( 'NONE',  ( -12.14591786802309592, -12.06949235617757132, 41.87390960531435979 ) ) ;
#177682=CARTESIAN_POINT ( 'NONE',  ( -14.29746914071049879, 8.314922557960819915, 75.83224293864769550 ) ) ;
#177683=CARTESIAN_POINT ( 'NONE',  ( 9.564922557960805705, 16.46253265017160317, 84.58224293864769550 ) ) ;
#177684=CARTESIAN_POINT ( 'NONE',  ( -15.80617190586768217, 15.72974639402176855, 33.12609039468569705 ) ) ;
#177685=CARTESIAN_POINT ( 'NONE',  ( 19.05341960407611168, 5.049401038298154454, 88.95724293864769550 ) ) ;
#177686=CARTESIAN_POINT ( 'NONE',  ( 15.80617190586769283, -15.72974639402175789, 105.6260903946856899 ) ) ;
#177687=CARTESIAN_POINT ( 'NONE',  ( -8.224510206698735004, -14.34966873604973081, 64.58442372801900433 ) ) ;
#177688=CARTESIAN_POINT ( 'NONE',  ( 9.564922557960805705, 16.46253265017160317, 109.5822429386476955 ) ) ;
#177689=CARTESIAN_POINT ( 'NONE',  ( 18.67979575497178502, 10.72451020669898547, 89.16557627198102409 ) ) ;
#177690=CARTESIAN_POINT ( 'NONE',  ( 16.55341960407611168, 4.379528057220329451, 48.95724293864770971 ) ) ;
#177691=CARTESIAN_POINT ( 'NONE',  ( -13.97604488694527625, -13.89961937509977652, 41.87390960531435979 ) ) ;
#177692=CARTESIAN_POINT ( 'NONE',  ( -4.379528057220328563, 16.55341960407611168, 70.20724293864769550 ) ) ;
#177693=CARTESIAN_POINT ( 'NONE',  ( -15.80617190586745835, -15.72974639402198527, 36.87390960531435979 ) ) ;
#177694=CARTESIAN_POINT ( 'NONE',  ( 21.55341960407610458, 5.719274019375980345, 28.95724293864769905 ) ) ;
#177695=CARTESIAN_POINT ( 'NONE',  ( -0.05219959533936034679, 19.03943276465977164, 27.50109039468566507 ) ) ;
#177697=CARTESIAN_POINT ( 'NONE',  ( 16.55341960407611168, 4.379528057220329451, 98.95724293864770971 ) ) ;
#177698=CARTESIAN_POINT ( 'NONE',  ( 16.51473224551069308, 9.474510206698969483, 104.1655762719810241 ) ) ;
#177700=CARTESIAN_POINT ( 'NONE',  ( 16.52544592524335698, 4.483927247898782831, 51.45942372801901854 ) ) ;
#177701=CARTESIAN_POINT ( 'NONE',  ( -16.46253265017160317, 9.564922557960807481, 60.83224293864769550 ) ) ;
#177703=CARTESIAN_POINT ( 'NONE',  ( -13.97604488694547697, 13.89961937509957934, 58.12609039468566863 ) ) ;
#177704=CARTESIAN_POINT ( 'NONE',  ( 4.379528057220092307, 16.55341960407617563, 87.29275706135236135 ) ) ;
#177705=CARTESIAN_POINT ( 'NONE',  ( -0.05219959533936034679, 19.03943276465977164, 92.50109039468566152 ) ) ;
#177706=CARTESIAN_POINT ( 'NONE',  ( -18.67979575497193778, 10.72451020669871902, 63.33442372801900433 ) ) ;
#177707=CARTESIAN_POINT ( 'NONE',  ( 19.05341960407611168, 5.049401038298154454, 78.95724293864769550 ) ) ;
#177708=CARTESIAN_POINT ( 'NONE',  ( 10.72451020669898902, -18.67979575497178502, 92.91557627198103830 ) ) ;
#177709=CARTESIAN_POINT ( 'NONE',  ( 14.29746914071049879, -8.314922557960816363, 113.3322429386476955 ) ) ;
#177710=CARTESIAN_POINT ( 'NONE',  ( 16.51473224551083163, -9.474510206698727899, 75.83442372801900433 ) ) ;
#177711=CARTESIAN_POINT ( 'NONE',  ( 10.72451020669898902, -18.67979575497178502, 72.91557627198103830 ) ) ;
#177712=CARTESIAN_POINT ( 'NONE',  ( 9.474510206698729675, 16.51473224551082808, 47.08442372801900433 ) ) ;
#177713=CARTESIAN_POINT ( 'NONE',  ( 18.87255363501904526, 5.500000000000004441, 98.82513748171830059 ) ) ;
#177714=CARTESIAN_POINT ( 'NONE',  ( 18.62759615963271287, -10.81492255796078972, 93.33224293864769550 ) ) ;
#177715=CARTESIAN_POINT ( 'NONE',  ( 17.50000000000003553, 4.049696124445843814, 28.31960329334057391 ) ) ;
#177716=CARTESIAN_POINT ( 'NONE',  ( -19.03943276465977164, 0.05219959533909376836, 66.24890960531436690 ) ) ;
#177717=DIRECTION ( 'NONE',  ( 0.000000000000000000, 1.000000000000000000, 0.000000000000000000 ) ) ;
#177718=CARTESIAN_POINT ( 'NONE',  ( 19.03943276465977164, 0.05219959533936151252, 111.2510903946856757 ) ) ;
#177720=CARTESIAN_POINT ( 'NONE',  ( -16.51473224551069308, -9.474510206698971260, 46.66557627198102409 ) ) ;
#177721=CARTESIAN_POINT ( 'NONE',  ( -5.823673210054116645, -21.52544592524344225, 102.2905762719810383 ) ) ;
#177722=CARTESIAN_POINT ( 'NONE',  ( -16.55341960407611168, -4.379528057220339221, 51.45724293864770260 ) ) ;
#177723=CARTESIAN_POINT ( 'NONE',  ( 9.564922557960805705, 16.46253265017160317, 59.58224293864769550 ) ) ;
#177724=CARTESIAN_POINT ( 'NONE',  ( 5.719274019375673035, 21.55341960407619339, 72.29275706135236135 ) ) ;
#177725=CARTESIAN_POINT ( 'NONE',  ( -0.05219959533934338120, 16.53943276465976808, 22.50109039468567573 ) ) ;
#177726=CARTESIAN_POINT ( 'NONE',  ( 16.46253265017146816, 9.564922557961045513, 26.66775706135234003 ) ) ;
#177727=CARTESIAN_POINT ( 'NONE',  ( 8.314922557960818139, 14.29746914071049879, 24.58224293864768839 ) ) ;
#177728=CARTESIAN_POINT ( 'NONE',  ( -15.80617190586768217, 15.72974639402176855, 43.12609039468568284 ) ) ;
#177729=CARTESIAN_POINT ( 'NONE',  ( -10.72451020669870658, -18.67979575497194134, 19.58442372801901143 ) ) ;
#177730=CARTESIAN_POINT ( 'NONE',  ( 10.81492255796078972, 18.62759615963270932, 59.58224293864770260 ) ) ;
#177731=CARTESIAN_POINT ( 'NONE',  ( 16.51473224551083163, -9.474510206698727899, 95.83442372801900433 ) ) ;
#177732=CARTESIAN_POINT ( 'NONE',  ( -16.51473224551082808, 9.474510206698731452, 73.33442372801900433 ) ) ;
#177733=CARTESIAN_POINT ( 'NONE',  ( 21.53943276465977519, 0.05219959533937863772, 66.25109039468567573 ) ) ;
#177734=CARTESIAN_POINT ( 'NONE',  ( -19.03943276465977164, -0.05219959533935918106, 58.75109039468566863 ) ) ;
#177735=CARTESIAN_POINT ( 'NONE',  ( -14.29746914071049879, 8.314922557960819915, 115.8322429386477097 ) ) ;
#177736=CARTESIAN_POINT ( 'NONE',  ( -10.72451020669898014, 18.67979575497178502, 45.41557627198103830 ) ) ;
#177737=CARTESIAN_POINT ( 'NONE',  ( 16.53943276465976808, -0.05219959533910856209, 53.74890960531437401 ) ) ;
#177738=CARTESIAN_POINT ( 'NONE',  ( -19.01533133064923575, 5.499999999999444000, 93.76586590595742621 ) ) ;
#177739=CARTESIAN_POINT ( 'NONE',  ( 18.67979575497194134, -10.72451020669871369, 110.8344237280190043 ) ) ;
#177740=CARTESIAN_POINT ( 'NONE',  ( -12.06949235617739369, -12.14591786802326823, 89.37609039468568994 ) ) ;
#177741=CARTESIAN_POINT ( 'NONE',  ( 16.53943276465976808, -0.05219959533910856209, 43.74890960531435979 ) ) ;
#177742=CARTESIAN_POINT ( 'NONE',  ( 15.80617190586769283, -15.72974639402175789, 80.62609039468567573 ) ) ;
#177743=CARTESIAN_POINT ( 'NONE',  ( -5.719274019375665041, -21.55341960407619695, 84.79275706135234714 ) ) ;
#177744=CARTESIAN_POINT ( 'NONE',  ( -18.62759615963270932, 10.81492255796079327, 80.83224293864769550 ) ) ;
#177745=CARTESIAN_POINT ( 'NONE',  ( 16.46253265017160672, -9.564922557960803928, 33.33224293864770260 ) ) ;
#177746=CARTESIAN_POINT ( 'NONE',  ( -18.62759615963255300, -10.81492255796106328, 59.16775706135234714 ) ) ;
#177747=CARTESIAN_POINT ( 'NONE',  ( 5.153800228976335163, 19.02544592524342804, 39.79057627198100988 ) ) ;
#177748=CARTESIAN_POINT ( 'NONE',  ( 0.05219959533909260263, 19.03943276465977164, 54.99890960531435979 ) ) ;
#177749=CARTESIAN_POINT ( 'NONE',  ( 12.14591786802309770, 12.06949235617756955, 89.37390960531435269 ) ) ;
#177750=CARTESIAN_POINT ( 'NONE',  ( 0.05219959533909260263, 19.03943276465977164, 99.99890960531436690 ) ) ;
#177751=CARTESIAN_POINT ( 'NONE',  ( 16.55341960407611168, 4.379528057220329451, 38.95724293864768839 ) ) ;
#177752=CARTESIAN_POINT ( 'NONE',  ( -12.06949235617756955, 12.14591786802309770, 115.6239096053143669 ) ) ;
#177753=CARTESIAN_POINT ( 'NONE',  ( 10.72451020669898902, -18.67979575497178502, 77.91557627198102409 ) ) ;
#177754=CARTESIAN_POINT ( 'NONE',  ( 5.719274019375673035, 21.55341960407619339, 22.29275706135235069 ) ) ;
#177756=CARTESIAN_POINT ( 'NONE',  ( 12.06949235617739724, 12.14591786802326823, 26.87609039468567218 ) ) ;
#177757=CARTESIAN_POINT ( 'NONE',  ( -10.81492255796078084, -18.62759615963271287, 72.08224293864769550 ) ) ;
#177758=CARTESIAN_POINT ( 'NONE',  ( 15.72974639402176855, 15.80617190586768217, 96.87609039468568994 ) ) ;
#177759=CARTESIAN_POINT ( 'NONE',  ( -16.51473224551069308, -9.474510206698971260, 76.66557627198103830 ) ) ;
#177760=CARTESIAN_POINT ( 'NONE',  ( 18.67979575497194134, -10.72451020669871369, 35.83442372801901143 ) ) ;
#177761=CARTESIAN_POINT ( 'NONE',  ( -16.51473224551069308, -9.474510206698971260, 111.6655762719810383 ) ) ;
#177762=CARTESIAN_POINT ( 'NONE',  ( 4.483927247898790824, -16.52544592524335698, 95.20942372801903275 ) ) ;
#177763=CARTESIAN_POINT ( 'NONE',  ( -15.72974639402176322, -15.80617190586768395, 69.37609039468567573 ) ) ;
#177764=CARTESIAN_POINT ( 'NONE',  ( -13.97604488694547697, 13.89961937509957934, 23.12609039468565442 ) ) ;
#177765=CARTESIAN_POINT ( 'NONE',  ( -4.379528057220086978, -16.55341960407618274, 69.79275706135234714 ) ) ;
#177766=CARTESIAN_POINT ( 'NONE',  ( -15.72974639402176322, -15.80617190586768395, 29.37609039468568284 ) ) ;
#177767=CARTESIAN_POINT ( 'NONE',  ( 9.474510206698971260, -16.51473224551069308, 37.91557627198102409 ) ) ;
#177768=CARTESIAN_POINT ( 'NONE',  ( 15.80617190586769283, -15.72974639402175789, 95.62609039468568994 ) ) ;
#177769=CARTESIAN_POINT ( 'NONE',  ( 19.05341960407611168, 5.049401038298154454, 88.95724293864769550 ) ) ;
#177770=CARTESIAN_POINT ( 'NONE',  ( 18.67979575497178502, 10.72451020669898547, 94.16557627198103830 ) ) ;
#177772=CARTESIAN_POINT ( 'NONE',  ( 5.823673210054125526, 21.52544592524343514, 49.79057627198102409 ) ) ;
#177773=CARTESIAN_POINT ( 'NONE',  ( 13.97604488694527802, 13.89961937509977652, 94.37390960531436690 ) ) ;
#177774=CARTESIAN_POINT ( 'NONE',  ( 14.34966873604960469, 8.224510206698951720, 49.16557627198102409 ) ) ;
#177776=CARTESIAN_POINT ( 'NONE',  ( -13.97604488694547697, 13.89961937509957934, 83.12609039468564731 ) ) ;
#177777=CARTESIAN_POINT ( 'NONE',  ( -17.40805194822031510, 6.112264579159328193, 105.8337127251061105 ) ) ;
#177778=CARTESIAN_POINT ( 'NONE',  ( -13.97604488694547697, 13.89961937509957934, 108.1260903946856331 ) ) ;
#177779=CARTESIAN_POINT ( 'NONE',  ( 10.81492255796078972, 18.62759615963270932, 79.58224293864769550 ) ) ;
#177780=CARTESIAN_POINT ( 'NONE',  ( -16.52544592524342804, 4.483927247898546575, 61.04057627198103120 ) ) ;
#177781=CARTESIAN_POINT ( 'NONE',  ( 9.474510206698971260, -16.51473224551069308, 102.9155762719810241 ) ) ;
#177782=CARTESIAN_POINT ( 'NONE',  ( 8.224510206698742110, 14.34966873604972548, 47.08442372801901854 ) ) ;
#177783=CARTESIAN_POINT ( 'NONE',  ( -13.97604488694527625, -13.89961937509977652, 61.87390960531435979 ) ) ;
#177784=CARTESIAN_POINT ( 'NONE',  ( -18.62759615963255300, -10.81492255796106328, 29.16775706135234003 ) ) ;
#177785=CARTESIAN_POINT ( 'NONE',  ( -13.89961937509957401, -13.97604488694547875, 94.37609039468566152 ) ) ;
#177786=CARTESIAN_POINT ( 'NONE',  ( 19.03943276465977164, -0.05219959533909143690, 93.74890960531435269 ) ) ;
#177787=CARTESIAN_POINT ( 'NONE',  ( 5.049401038298161559, -19.05341960407611168, 82.70724293864770971 ) ) ;
#177788=CARTESIAN_POINT ( 'NONE',  ( 21.52544592524344225, -5.823673210054117533, 73.54057627198102409 ) ) ;
#177789=CARTESIAN_POINT ( 'NONE',  ( 5.153800228976335163, 19.02544592524342804, 49.79057627198100988 ) ) ;
#177791=CARTESIAN_POINT ( 'NONE',  ( -12.14591786802309592, -12.06949235617757132, 71.87390960531438111 ) ) ;
#177792=CARTESIAN_POINT ( 'NONE',  ( -5.049401038298153566, 19.05341960407611168, 100.2072429386476955 ) ) ;
#177794=CARTESIAN_POINT ( 'NONE',  ( -16.46253265017146816, -9.564922557961047289, 69.16775706135233293 ) ) ;
#177795=CARTESIAN_POINT ( 'NONE',  ( -5.823673210054116645, -21.52544592524344225, 92.29057627198103830 ) ) ;
#177796=CARTESIAN_POINT ( 'NONE',  ( -9.564922557961040184, 16.46253265017147172, 47.91775706135233293 ) ) ;
#177797=CARTESIAN_POINT ( 'NONE',  ( -19.03943276465977164, 0.05219959533909376836, 96.24890960531436690 ) ) ;
#177798=CARTESIAN_POINT ( 'NONE',  ( 19.39056639909674473, 5.500000000000053291, 68.28948781074343799 ) ) ;
#177799=CARTESIAN_POINT ( 'NONE',  ( -5.823673210054116645, -21.52544592524344225, 47.29057627198103120 ) ) ;
#177801=CARTESIAN_POINT ( 'NONE',  ( -9.474510206698964154, 16.51473224551069663, 90.41557627198103830 ) ) ;
#177802=CARTESIAN_POINT ( 'NONE',  ( 21.52544592524334988, 5.823673210054432836, 66.45942372801903275 ) ) ;
#177803=CARTESIAN_POINT ( 'NONE',  ( -9.564922557960796823, -16.46253265017161027, 42.08224293864769550 ) ) ;
#177804=CARTESIAN_POINT ( 'NONE',  ( 16.52544592524342804, -4.483927247898539470, 68.54057627198103830 ) ) ;
#177805=CARTESIAN_POINT ( 'NONE',  ( -16.55341960407617563, 4.379528057220093196, 23.54275706135235424 ) ) ;
#177806=CARTESIAN_POINT ( 'NONE',  ( -0.05219959533937732626, 21.53943276465977519, 57.50109039468568994 ) ) ;
#177808=CARTESIAN_POINT ( 'NONE',  ( -5.153800228976328057, -19.02544592524343514, 112.2905762719810099 ) ) ;
#177809=CARTESIAN_POINT ( 'NONE',  ( 5.153800228976615827, -19.02544592524334988, 60.20942372801899012 ) ) ;
#177811=CARTESIAN_POINT ( 'NONE',  ( 18.67979575497194134, -10.72451020669871369, 25.83442372801901499 ) ) ;
#177812=CARTESIAN_POINT ( 'NONE',  ( -9.474510206698964154, 16.51473224551069663, 55.41557627198103120 ) ) ;
#177814=CARTESIAN_POINT ( 'NONE',  ( -5.049401038297874678, -19.05341960407617918, 19.79275706135233293 ) ) ;
#177815=CARTESIAN_POINT ( 'NONE',  ( -19.02544592524342804, 5.153800228976336051, 46.04057627198101699 ) ) ;
#177816=CARTESIAN_POINT ( 'NONE',  ( 15.80617190586769283, -15.72974639402175789, 105.6260903946856899 ) ) ;
#177817=CARTESIAN_POINT ( 'NONE',  ( 4.379528057220092307, 16.55341960407617563, 97.29275706135234714 ) ) ;
#177818=CARTESIAN_POINT ( 'NONE',  ( -9.474510206698964154, 16.51473224551069663, 100.4155762719810241 ) ) ;
#177819=CARTESIAN_POINT ( 'NONE',  ( 15.80617190586769283, -15.72974639402175789, 75.62609039468567573 ) ) ;
#177821=CARTESIAN_POINT ( 'NONE',  ( -5.153800228976328057, -19.02544592524343514, 107.2905762719810383 ) ) ;
#177823=CARTESIAN_POINT ( 'NONE',  ( 14.29746914071037800, 8.314922557961029526, 66.66775706135234714 ) ) ;
#177824=CARTESIAN_POINT ( 'NONE',  ( 21.53943276465977519, 0.05219959533937863772, 66.25109039468567573 ) ) ;
#177825=CARTESIAN_POINT ( 'NONE',  ( 0.05219959533937995610, -21.53943276465977519, 100.0010903946857042 ) ) ;
#177827=CARTESIAN_POINT ( 'NONE',  ( 4.379528057220092307, 16.55341960407617563, 47.29275706135234003 ) ) ;
#177828=CARTESIAN_POINT ( 'NONE',  ( -16.51473224551069308, -9.474510206698971260, 86.66557627198102409 ) ) ;
#177830=CARTESIAN_POINT ( 'NONE',  ( -5.049401038298153566, 19.05341960407611168, 115.2072429386477097 ) ) ;
#177832=DIRECTION ( 'NONE',  ( 0.000000000000000000, 0.000000000000000000, 1.000000000000000000 ) ) ;
#177833=CARTESIAN_POINT ( 'NONE',  ( -9.564922557960796823, -16.46253265017161027, 42.08224293864769550 ) ) ;
#177834=CARTESIAN_POINT ( 'NONE',  ( -5.719274019375978568, 21.55341960407610458, 45.20724293864769550 ) ) ;
#177835=CARTESIAN_POINT ( 'NONE',  ( -8.224510206698735004, -14.34966873604973081, 99.58442372801900433 ) ) ;
#177836=CARTESIAN_POINT ( 'NONE',  ( -0.05219959533910754901, -16.53943276465976808, 82.49890960531436690 ) ) ;
#177837=CARTESIAN_POINT ( 'NONE',  ( 13.89961937509977652, -13.97604488694527269, 78.12390960531433848 ) ) ;
#177838=CARTESIAN_POINT ( 'NONE',  ( 10.72451020669871369, 18.67979575497193778, 102.0844237280190185 ) ) ;
#177839=CARTESIAN_POINT ( 'NONE',  ( -0.05219959533909027116, -19.03943276465977164, 32.49890960531435979 ) ) ;
#177840=CARTESIAN_POINT ( 'NONE',  ( 16.53943276465976808, -0.05219959533910856209, 88.74890960531436690 ) ) ;
#177841=CARTESIAN_POINT ( 'NONE',  ( 5.823673210054444382, -21.52544592524334988, 45.20942372801901854 ) ) ;
#177842=CARTESIAN_POINT ( 'NONE',  ( 5.823673210054125526, 21.52544592524343514, 89.79057627198103830 ) ) ;
#177843=CARTESIAN_POINT ( 'NONE',  ( -16.51473224551082808, 9.474510206698731452, 48.33442372801900433 ) ) ;
#177845=CARTESIAN_POINT ( 'NONE',  ( -9.474510206698964154, 16.51473224551069663, 95.41557627198102409 ) ) ;
#177846=CARTESIAN_POINT ( 'NONE',  ( 4.379528057220339221, -16.55341960407611168, 57.70724293864770260 ) ) ;
#177847=CARTESIAN_POINT ( 'NONE',  ( 14.29746914071049879, -8.314922557960816363, 53.33224293864769550 ) ) ;
#177848=CARTESIAN_POINT ( 'NONE',  ( 16.53943276465976808, -0.05219959533910856209, 28.74890960531435624 ) ) ;
#177849=CARTESIAN_POINT ( 'NONE',  ( 19.02544592524334988, 5.153800228976608722, 76.45942372801897591 ) ) ;
#177850=CARTESIAN_POINT ( 'NONE',  ( -19.02130022317637525, 5.499999999999802824, 85.78188669246577547 ) ) ;
#177851=CARTESIAN_POINT ( 'NONE',  ( 21.53943276465977519, -0.05219959533907433946, 28.74890960531435624 ) ) ;
#177852=CARTESIAN_POINT ( 'NONE',  ( -8.224510206698948167, 14.34966873604960824, 90.41557627198103830 ) ) ;
#177853=CARTESIAN_POINT ( 'NONE',  ( -17.50000000000004619, -4.049696124445705259, 25.81960329334050641 ) ) ;
#177854=CARTESIAN_POINT ( 'NONE',  ( -19.02544592524342804, 5.153800228976336051, 46.04057627198101699 ) ) ;
#177855=CARTESIAN_POINT ( 'NONE',  ( 5.719274019375991003, -21.55341960407610458, 52.70724293864769550 ) ) ;
#177856=CARTESIAN_POINT ( 'NONE',  ( -9.564922557960796823, -16.46253265017161027, 32.08224293864769550 ) ) ;
#177857=CARTESIAN_POINT ( 'NONE',  ( 0.05219959533934541429, -16.53943276465976808, 80.00109039468568994 ) ) ;
#177858=CARTESIAN_POINT ( 'NONE',  ( 9.564922557960805705, 16.46253265017160317, 59.58224293864769550 ) ) ;
#177859=CARTESIAN_POINT ( 'NONE',  ( -19.02544592524334988, -5.153800228976617603, 33.95942372801897591 ) ) ;
#177860=CARTESIAN_POINT ( 'NONE',  ( 5.823673210054444382, -21.52544592524334988, 65.20942372801901854 ) ) ;
#177861=CARTESIAN_POINT ( 'NONE',  ( 0.05219959533907565091, 21.53943276465977519, 29.99890960531435979 ) ) ;
#177862=CARTESIAN_POINT ( 'NONE',  ( -8.314922557960811034, -14.29746914071050412, 112.0822429386477097 ) ) ;
#177863=CARTESIAN_POINT ( 'NONE',  ( 0.05219959533936267826, -19.03943276465977164, 90.00109039468567573 ) ) ;
#177866=CARTESIAN_POINT ( 'NONE',  ( 5.823673210054125526, 21.52544592524343514, 49.79057627198102409 ) ) ;
#177867=CARTESIAN_POINT ( 'NONE',  ( 9.564922557960805705, 16.46253265017160317, 24.58224293864769194 ) ) ;
#177868=CARTESIAN_POINT ( 'NONE',  ( -18.62759615963255300, -10.81492255796106328, 84.16775706135234714 ) ) ;
#177870=CARTESIAN_POINT ( 'NONE',  ( -14.34966873604960291, -8.224510206698953496, 51.66557627198102409 ) ) ;
#177871=CARTESIAN_POINT ( 'NONE',  ( 14.34966873604972726, -8.224510206698740333, 65.83442372801900433 ) ) ;
#177872=CARTESIAN_POINT ( 'NONE',  ( -12.14591786802309592, -12.06949235617757132, 51.87390960531437401 ) ) ;
#177873=CARTESIAN_POINT ( 'NONE',  ( -10.81492255796078084, -18.62759615963271287, 77.08224293864769550 ) ) ;
#177874=CARTESIAN_POINT ( 'NONE',  ( -10.81492255796078084, -18.62759615963271287, 77.08224293864769550 ) ) ;
#177876=CARTESIAN_POINT ( 'NONE',  ( 19.05341960407611168, 5.049401038298154454, 108.9572429386477097 ) ) ;
#177877=CARTESIAN_POINT ( 'NONE',  ( -8.314922557960811034, -14.29746914071050412, 77.08224293864769550 ) ) ;
#177878=CARTESIAN_POINT ( 'NONE',  ( -0.05219959533909027116, -19.03943276465977164, 62.49890960531435979 ) ) ;
#177879=CARTESIAN_POINT ( 'NONE',  ( -19.02544592524342804, 5.153800228976336051, 36.04057627198100988 ) ) ;
#177882=CARTESIAN_POINT ( 'NONE',  ( 16.52544592524335698, 4.483927247898782831, 76.45942372801901854 ) ) ;
#177883=CARTESIAN_POINT ( 'NONE',  ( -10.72451020669898014, 18.67979575497178502, 115.4155762719810241 ) ) ;
#177884=CARTESIAN_POINT ( 'NONE',  ( -16.46253265017160317, 9.564922557960807481, 70.83224293864770971 ) ) ;
#177885=CARTESIAN_POINT ( 'NONE',  ( -18.67979575497193778, 10.72451020669871902, 58.33442372801901143 ) ) ;
#177886=CARTESIAN_POINT ( 'NONE',  ( -19.05341960407611168, -5.049401038298163336, 111.4572429386476671 ) ) ;
#177889=CARTESIAN_POINT ( 'NONE',  ( 15.72974639402176855, 15.80617190586768217, 46.87609039468568994 ) ) ;
#177890=CARTESIAN_POINT ( 'NONE',  ( 16.46253265017160672, -9.564922557960803928, 28.33224293864769550 ) ) ;
#177891=CARTESIAN_POINT ( 'NONE',  ( 9.474510206698971260, -16.51473224551069308, 107.9155762719810383 ) ) ;
#177892=CARTESIAN_POINT ( 'NONE',  ( -13.97604488694547697, 13.89961937509957934, 53.12609039468565442 ) ) ;
#177893=CARTESIAN_POINT ( 'NONE',  ( 18.62759615963271287, -10.81492255796078972, 113.3322429386476955 ) ) ;
#177894=CARTESIAN_POINT ( 'NONE',  ( 0.05219959533936267826, -19.03943276465977164, 40.00109039468566152 ) ) ;
#177895=CARTESIAN_POINT ( 'NONE',  ( 16.51473224551083163, -9.474510206698727899, 50.83442372801899722 ) ) ;
#177896=CARTESIAN_POINT ( 'NONE',  ( 8.314922557961029526, -14.29746914071037800, 100.4177570613523471 ) ) ;
#177898=ORIENTED_EDGE ( 'NONE', *, *, #149044, .T. ) ;
#177899=CARTESIAN_POINT ( 'NONE',  ( -5.153800228976328057, -19.02544592524343514, 82.29057627198103830 ) ) ;
#177900=CARTESIAN_POINT ( 'NONE',  ( -18.67979575497193778, 10.72451020669871902, 73.33442372801901854 ) ) ;
#177901=CARTESIAN_POINT ( 'NONE',  ( -15.80617190586768217, 15.72974639402176855, 88.12609039468570415 ) ) ;
#177904=CARTESIAN_POINT ( 'NONE',  ( 9.474510206698971260, -16.51473224551069308, 97.91557627198102409 ) ) ;
#177905=CARTESIAN_POINT ( 'NONE',  ( 21.55341960407619695, -5.719274019375665929, 71.04275706135234714 ) ) ;
#177906=CARTESIAN_POINT ( 'NONE',  ( -14.29746914071037622, -8.314922557961029526, 24.16775706135235424 ) ) ;
#177907=CARTESIAN_POINT ( 'NONE',  ( -19.03943276465977164, 0.05219959533909376836, 76.24890960531435269 ) ) ;
#177908=CARTESIAN_POINT ( 'NONE',  ( -5.719274019375978568, 21.55341960407610458, 25.20724293864769550 ) ) ;
#177909=CARTESIAN_POINT ( 'NONE',  ( 19.05341960407611168, 5.049401038298154454, 98.95724293864766707 ) ) ;
#177910=CARTESIAN_POINT ( 'NONE',  ( 9.474510206698729675, 16.51473224551082808, 87.08442372801900433 ) ) ;
#177911=CARTESIAN_POINT ( 'NONE',  ( -9.564922557960796823, -16.46253265017161027, 77.08224293864769550 ) ) ;
#177912=CARTESIAN_POINT ( 'NONE',  ( 9.564922557960805705, 16.46253265017160317, 64.58224293864769550 ) ) ;
#177913=CARTESIAN_POINT ( 'NONE',  ( 18.62759615963271287, -10.81492255796078972, 108.3322429386477097 ) ) ;
#177914=CARTESIAN_POINT ( 'NONE',  ( 16.53943276465976808, 0.05219959533934440121, 96.25109039468568994 ) ) ;
#177916=CARTESIAN_POINT ( 'NONE',  ( 13.89961937509957401, 13.97604488694547697, 51.87609039468566863 ) ) ;
#177917=CARTESIAN_POINT ( 'NONE',  ( -0.05219959533909027116, -19.03943276465977164, 97.49890960531436690 ) ) ;
#177918=CARTESIAN_POINT ( 'NONE',  ( -16.52544592524342804, 4.483927247898546575, 91.04057627198103830 ) ) ;
#177919=CARTESIAN_POINT ( 'NONE',  ( 15.72974639402199770, -15.80617190586745480, 33.12390960531435979 ) ) ;
#177920=CARTESIAN_POINT ( 'NONE',  ( -0.05219959533907301413, -21.53943276465977519, 27.49890960531435269 ) ) ;
#177921=CARTESIAN_POINT ( 'NONE',  ( -12.14591786802309592, -12.06949235617757132, 91.87390960531436690 ) ) ;
#177922=CARTESIAN_POINT ( 'NONE',  ( -16.36317988757058473, 7.306389748694923192, 54.09789608363225000 ) ) ;
#177923=CARTESIAN_POINT ( 'NONE',  ( -19.03943276465977164, -0.05219959533935918106, 38.75109039468566152 ) ) ;
#177924=CARTESIAN_POINT ( 'NONE',  ( -8.224510206698735004, -14.34966873604973081, 104.5844237280190185 ) ) ;
#177925=CARTESIAN_POINT ( 'NONE',  ( 5.153800228976335163, 19.02544592524342804, 84.79057627198099567 ) ) ;
#177926=CARTESIAN_POINT ( 'NONE',  ( -18.67979575497193778, 10.72451020669871902, 68.33442372801900433 ) ) ;
#177927=CARTESIAN_POINT ( 'NONE',  ( 10.72451020669898902, -18.67979575497178502, 62.91557627198102409 ) ) ;
#177928=CARTESIAN_POINT ( 'NONE',  ( 21.52544592524334988, 5.823673210054432836, 36.45942372801901143 ) ) ;
#177930=CARTESIAN_POINT ( 'NONE',  ( 21.55341960407610458, 5.719274019375980345, 83.95724293864770971 ) ) ;
#177931=CARTESIAN_POINT ( 'NONE',  ( 14.29746914071049879, -8.314922557960816363, 103.3322429386476955 ) ) ;
#177932=CARTESIAN_POINT ( 'NONE',  ( -16.46253265017146816, -9.564922557961047289, 74.16775706135234714 ) ) ;
#177933=CARTESIAN_POINT ( 'NONE',  ( -19.03943276465977164, 0.05219959533909376836, 51.24890960531436690 ) ) ;
#177934=CARTESIAN_POINT ( 'NONE',  ( -16.51473224551069308, -9.474510206698971260, 101.6655762719810241 ) ) ;
#177935=CARTESIAN_POINT ( 'NONE',  ( -19.02544592524342804, 5.153800228976336051, 91.04057627198100988 ) ) ;
#177936=CARTESIAN_POINT ( 'NONE',  ( -16.51473224551069308, -9.474510206698971260, 21.66557627198102765 ) ) ;
#177937=CARTESIAN_POINT ( 'NONE',  ( -0.05219959533910754901, -16.53943276465976808, 37.49890960531436690 ) ) ;
#177938=CARTESIAN_POINT ( 'NONE',  ( 16.53943276465976808, 0.05219959533934440121, 46.25109039468567573 ) ) ;
#177939=CARTESIAN_POINT ( 'NONE',  ( 15.72974639402176855, 15.80617190586768217, 101.8760903946857042 ) ) ;
#177940=CARTESIAN_POINT ( 'NONE',  ( 19.02544592524343514, -5.153800228976328945, 113.5405762719810241 ) ) ;
#177941=CARTESIAN_POINT ( 'NONE',  ( -0.05219959533934338120, 16.53943276465976808, 112.5010903946857042 ) ) ;
#177942=CARTESIAN_POINT ( 'NONE',  ( -10.81492255796105439, 18.62759615963255655, 32.91775706135234714 ) ) ;
#177943=CARTESIAN_POINT ( 'NONE',  ( 19.03943276465977164, -0.05219959533909143690, 98.74890960531436690 ) ) ;
#177944=CARTESIAN_POINT ( 'NONE',  ( 16.52544592524335698, 4.483927247898782831, 101.4594237280190185 ) ) ;
#177945=CARTESIAN_POINT ( 'NONE',  ( -14.29746914071037622, -8.314922557961029526, 99.16775706135234714 ) ) ;
#177946=CARTESIAN_POINT ( 'NONE',  ( 12.06949235617739724, 12.14591786802326823, 26.87609039468567218 ) ) ;
#177947=CARTESIAN_POINT ( 'NONE',  ( 19.02544592524343514, -5.153800228976328945, 48.54057627198103120 ) ) ;
#177948=CARTESIAN_POINT ( 'NONE',  ( -14.29746914071049879, 8.314922557960819915, 105.8322429386476955 ) ) ;
#177949=CARTESIAN_POINT ( 'NONE',  ( -21.52544592524343514, 5.823673210054127303, 116.0405762719810383 ) ) ;
#177950=CARTESIAN_POINT ( 'NONE',  ( -13.97604488694527625, -13.89961937509977652, 26.87390960531434558 ) ) ;
#177951=CARTESIAN_POINT ( 'NONE',  ( -13.89961937509977652, 13.97604488694528158, 110.6239096053143243 ) ) ;
#177952=CARTESIAN_POINT ( 'NONE',  ( -13.89961937509977652, 13.97604488694528158, 30.62390960531435269 ) ) ;
#177953=CARTESIAN_POINT ( 'NONE',  ( 19.03943276465977164, -0.05219959533909143690, 103.7489096053143669 ) ) ;
#177954=CARTESIAN_POINT ( 'NONE',  ( -17.48847506799970120, -5.747544572773717775, 34.17302562156721990 ) ) ;
#177955=CARTESIAN_POINT ( 'NONE',  ( -9.474510206698964154, 16.51473224551069663, 100.4155762719810241 ) ) ;
#177956=CARTESIAN_POINT ( 'NONE',  ( -10.72451020669870658, -18.67979575497194134, 49.58442372801901143 ) ) ;
#177957=CARTESIAN_POINT ( 'NONE',  ( -8.314922557960811034, -14.29746914071050412, 92.08224293864769550 ) ) ;
#177958=CARTESIAN_POINT ( 'NONE',  ( -19.02544592524342804, 5.153800228976336051, 91.04057627198100988 ) ) ;
#177960=CARTESIAN_POINT ( 'NONE',  ( 4.379528057220092307, 16.55341960407617563, 62.29275706135236845 ) ) ;
#177961=CARTESIAN_POINT ( 'NONE',  ( -21.55341960407619339, 5.719274019375674811, 78.54275706135236135 ) ) ;
#177962=CARTESIAN_POINT ( 'NONE',  ( -14.34966873604972548, 8.224510206698743886, 43.33442372801901143 ) ) ;
#177963=CARTESIAN_POINT ( 'NONE',  ( 0.05219959533909260263, 19.03943276465977164, 84.99890960531436690 ) ) ;
#177964=CARTESIAN_POINT ( 'NONE',  ( -13.97604488694547697, 13.89961937509957934, 113.1260903946856757 ) ) ;
#177965=CARTESIAN_POINT ( 'NONE',  ( 14.29746914071037800, 8.314922557961029526, 86.66775706135234714 ) ) ;
#177966=CARTESIAN_POINT ( 'NONE',  ( 16.51473224551083163, -9.474510206698727899, 95.83442372801900433 ) ) ;
#177967=CARTESIAN_POINT ( 'NONE',  ( -0.05219959533909027116, -19.03943276465977164, 62.49890960531435979 ) ) ;
#177968=CARTESIAN_POINT ( 'NONE',  ( 10.72451020669898902, -18.67979575497178502, 102.9155762719810383 ) ) ;
#177969=CARTESIAN_POINT ( 'NONE',  ( -12.06949235617756955, 12.14591786802309770, 90.62390960531436690 ) ) ;
#177970=CARTESIAN_POINT ( 'NONE',  ( 9.564922557961047289, -16.46253265017146816, 85.41775706135233293 ) ) ;
#177971=CARTESIAN_POINT ( 'NONE',  ( 8.224510206698742110, 14.34966873604972548, 57.08442372801901854 ) ) ;
#177973=CARTESIAN_POINT ( 'NONE',  ( -9.474510206698720793, -16.51473224551083518, 59.58442372801900433 ) ) ;
#177974=CARTESIAN_POINT ( 'NONE',  ( -14.29746914071049879, 8.314922557960819915, 25.83224293864769194 ) ) ;
#177975=CARTESIAN_POINT ( 'NONE',  ( -16.53943276465976808, 0.05219959533911058130, 81.24890960531436690 ) ) ;
#177976=CARTESIAN_POINT ( 'NONE',  ( 21.53943276465977519, 0.05219959533937863772, 111.2510903946856899 ) ) ;
#177977=CARTESIAN_POINT ( 'NONE',  ( -18.39635199886970085, 5.499999999999980460, 91.01967076360000419 ) ) ;
#177978=CARTESIAN_POINT ( 'NONE',  ( 21.52544592524334988, 5.823673210054432836, 26.45942372801901854 ) ) ;
#177979=CARTESIAN_POINT ( 'NONE',  ( -0.05219959533909027116, -19.03943276465977164, 112.4989096053143669 ) ) ;
#177980=CARTESIAN_POINT ( 'NONE',  ( 5.153800228976335163, 19.02544592524342804, 74.79057627198103830 ) ) ;
#177981=CARTESIAN_POINT ( 'NONE',  ( 0.05219959533937995610, -21.53943276465977519, 100.0010903946857042 ) ) ;
#177982=CARTESIAN_POINT ( 'NONE',  ( -19.05341960407611168, -5.049401038298163336, 76.45724293864769550 ) ) ;
#177983=CARTESIAN_POINT ( 'NONE',  ( -0.05219959533907301413, -21.53943276465977519, 47.49890960531435979 ) ) ;
#177984=CARTESIAN_POINT ( 'NONE',  ( 16.55341960407611168, 4.379528057220329451, 83.95724293864770971 ) ) ;
#177985=CARTESIAN_POINT ( 'NONE',  ( -19.03943276465977164, 0.05219959533909376836, 51.24890960531436690 ) ) ;
#177986=CARTESIAN_POINT ( 'NONE',  ( 8.314922557960818139, 14.29746914071049879, 114.5822429386477097 ) ) ;
#177987=CARTESIAN_POINT ( 'NONE',  ( 21.55341960407619695, -5.719274019375665929, 26.04275706135235779 ) ) ;
#177988=CARTESIAN_POINT ( 'NONE',  ( 21.53943276465977519, 0.05219959533937863772, 61.25109039468567573 ) ) ;
#177989=CARTESIAN_POINT ( 'NONE',  ( 16.46253265017160672, -9.564922557960803928, 43.33224293864769550 ) ) ;
#177990=CARTESIAN_POINT ( 'NONE',  ( -12.06949235617739369, -12.14591786802326823, 79.37609039468567573 ) ) ;
#177991=CARTESIAN_POINT ( 'NONE',  ( -18.62759615963255300, -10.81492255796106328, 19.16775706135234714 ) ) ;
#177992=CARTESIAN_POINT ( 'NONE',  ( -21.52544592524343514, 5.823673210054127303, 116.0405762719810383 ) ) ;
#177993=CARTESIAN_POINT ( 'NONE',  ( -19.02544592524334988, -5.153800228976617603, 33.95942372801897591 ) ) ;
#177994=CARTESIAN_POINT ( 'NONE',  ( -16.46253265017160317, 9.564922557960807481, 60.83224293864769550 ) ) ;
#177996=CARTESIAN_POINT ( 'NONE',  ( 10.81492255796106328, -18.62759615963255655, 75.41775706135233293 ) ) ;
#177997=CARTESIAN_POINT ( 'NONE',  ( -21.52544592524343514, 5.823673210054127303, 61.04057627198103120 ) ) ;
#177998=CARTESIAN_POINT ( 'NONE',  ( -0.05219959533910754901, -16.53943276465976808, 37.49890960531436690 ) ) ;
#177999=CARTESIAN_POINT ( 'NONE',  ( -21.55341960407619339, 5.719274019375674811, 78.54275706135236135 ) ) ;
#178000=CARTESIAN_POINT ( 'NONE',  ( 10.72451020669871369, 18.67979575497193778, 107.0844237280190043 ) ) ;
#178001=CARTESIAN_POINT ( 'NONE',  ( -4.379528057220328563, 16.55341960407611168, 55.20724293864770260 ) ) ;
#178002=CARTESIAN_POINT ( 'NONE',  ( -8.224510206698948167, 14.34966873604960824, 100.4155762719810241 ) ) ;
#178003=CARTESIAN_POINT ( 'NONE',  ( 9.564922557961047289, -16.46253265017146816, 60.41775706135233293 ) ) ;
#178004=CARTESIAN_POINT ( 'NONE',  ( 16.53943276465976808, -0.05219959533910856209, 23.74890960531435269 ) ) ;
#178005=CARTESIAN_POINT ( 'NONE',  ( -15.72974639402176322, -15.80617190586768395, 64.37609039468568994 ) ) ;
#178006=CARTESIAN_POINT ( 'NONE',  ( -13.89961937509977652, 13.97604488694528158, 70.62390960531432427 ) ) ;
#178007=CARTESIAN_POINT ( 'NONE',  ( 13.97604488694548053, -13.89961937509957401, 30.62609039468566863 ) ) ;
#178008=CARTESIAN_POINT ( 'NONE',  ( 5.719274019375991003, -21.55341960407610458, 57.70724293864770260 ) ) ;
#178009=CARTESIAN_POINT ( 'NONE',  ( 21.52544592524334988, 5.823673210054432836, 41.45942372801901143 ) ) ;
#178010=CARTESIAN_POINT ( 'NONE',  ( -15.72974639402197994, 15.80617190586746368, 105.6239096053143669 ) ) ;
#178011=CARTESIAN_POINT ( 'NONE',  ( -19.02544592524334988, -5.153800228976617603, 98.95942372801900433 ) ) ;
#178012=CARTESIAN_POINT ( 'NONE',  ( -8.224510206698735004, -14.34966873604973081, 49.58442372801901143 ) ) ;
#178014=CARTESIAN_POINT ( 'NONE',  ( -21.53943276465977519, 0.05219959533907696930, 96.24890960531435269 ) ) ;
#178015=CARTESIAN_POINT ( 'NONE',  ( 4.483927247898545687, 16.52544592524342804, 84.79057627198102409 ) ) ;
#178017=CARTESIAN_POINT ( 'NONE',  ( 14.34966873604972726, -8.224510206698740333, 25.83442372801901499 ) ) ;
#178018=CARTESIAN_POINT ( 'NONE',  ( -15.80617190586745835, -15.72974639402198527, 51.87390960531437401 ) ) ;
#178019=CARTESIAN_POINT ( 'NONE',  ( 12.06949235617739724, 12.14591786802326823, 96.87609039468568994 ) ) ;
#178021=CARTESIAN_POINT ( 'NONE',  ( 12.14591786802327356, -12.06949235617739191, 50.62609039468568994 ) ) ;
#178022=CARTESIAN_POINT ( 'NONE',  ( 18.62759615963255655, 10.81492255796105972, 21.66775706135235069 ) ) ;
#178023=CARTESIAN_POINT ( 'NONE',  ( 21.55341960407610458, 5.719274019375980345, 38.95724293864768839 ) ) ;
#178024=CARTESIAN_POINT ( 'NONE',  ( -14.34966873604972548, 8.224510206698743886, 88.33442372801901854 ) ) ;
#178025=CARTESIAN_POINT ( 'NONE',  ( -19.02544592524342804, 5.153800228976336051, 101.0405762719810241 ) ) ;
#178026=CARTESIAN_POINT ( 'NONE',  ( -21.52544592524334988, -5.823673210054445271, 63.95942372801901854 ) ) ;
#178027=CARTESIAN_POINT ( 'NONE',  ( 15.80617190586746368, 15.72974639402197994, 34.37390960531435979 ) ) ;
#178028=CARTESIAN_POINT ( 'NONE',  ( -5.823673210054116645, -21.52544592524344225, 22.29057627198102765 ) ) ;
#178030=CARTESIAN_POINT ( 'NONE',  ( 19.02544592524334988, 5.153800228976608722, 46.45942372801899012 ) ) ;
#178031=CARTESIAN_POINT ( 'NONE',  ( -8.224510206698735004, -14.34966873604973081, 69.58442372801900433 ) ) ;
#178032=CARTESIAN_POINT ( 'NONE',  ( -5.823673210054116645, -21.52544592524344225, 27.29057627198103120 ) ) ;
#178034=CARTESIAN_POINT ( 'NONE',  ( -16.46253265017160317, 9.564922557960807481, 80.83224293864769550 ) ) ;
#178035=CARTESIAN_POINT ( 'NONE',  ( -16.55341960407617563, 4.379528057220093196, 108.5427570613523756 ) ) ;
#178037=CARTESIAN_POINT ( 'NONE',  ( -8.314922557960811034, -14.29746914071050412, 112.0822429386477097 ) ) ;
#178038=CARTESIAN_POINT ( 'NONE',  ( 15.72974639402199770, -15.80617190586745480, 53.12390960531436690 ) ) ;
#178039=CARTESIAN_POINT ( 'NONE',  ( -16.51473224551069308, -9.474510206698971260, 51.66557627198102409 ) ) ;
#178040=CARTESIAN_POINT ( 'NONE',  ( 16.55341960407618274, -4.379528057220086978, 81.04275706135236135 ) ) ;
#178041=CARTESIAN_POINT ( 'NONE',  ( -10.72451020669870658, -18.67979575497194134, 34.58442372801900433 ) ) ;
#178042=CARTESIAN_POINT ( 'NONE',  ( -16.51473224551082808, 9.474510206698731452, 88.33442372801900433 ) ) ;
#178043=CARTESIAN_POINT ( 'NONE',  ( 12.06949235617757843, -12.14591786802309237, 93.12390960531436690 ) ) ;
#178044=CARTESIAN_POINT ( 'NONE',  ( -19.02544592524342804, 5.153800228976336051, 56.04057627198100988 ) ) ;
#178045=CARTESIAN_POINT ( 'NONE',  ( -13.97604488694527625, -13.89961937509977652, 31.87390960531435979 ) ) ;
#178046=CARTESIAN_POINT ( 'NONE',  ( -21.53943276465977519, -0.05219959533937600094, 98.75109039468568994 ) ) ;
#178047=CARTESIAN_POINT ( 'NONE',  ( -16.46253265017160317, 9.564922557960807481, 80.83224293864769550 ) ) ;
#178048=CARTESIAN_POINT ( 'NONE',  ( 16.55341960407618274, -4.379528057220086978, 66.04275706135236135 ) ) ;
#178049=CARTESIAN_POINT ( 'NONE',  ( -18.67979575497193778, 10.72451020669871902, 98.33442372801901854 ) ) ;
#178050=CARTESIAN_POINT ( 'NONE',  ( -21.52544592524343514, 5.823673210054127303, 51.04057627198103120 ) ) ;
#178051=CARTESIAN_POINT ( 'NONE',  ( 12.06949235617739724, 12.14591786802326823, 71.87609039468568994 ) ) ;
#178052=CARTESIAN_POINT ( 'NONE',  ( 5.049401038297881783, 19.05341960407617563, 52.29275706135234003 ) ) ;
#178053=CARTESIAN_POINT ( 'NONE',  ( 19.03943276465977164, 0.05219959533936151252, 71.25109039468566152 ) ) ;
#178054=CARTESIAN_POINT ( 'NONE',  ( 10.81492255796106328, -18.62759615963255655, 60.41775706135235424 ) ) ;
#178055=CARTESIAN_POINT ( 'NONE',  ( 16.51473224551069308, 9.474510206698969483, 69.16557627198102409 ) ) ;
#178056=CARTESIAN_POINT ( 'NONE',  ( 19.02544592524343514, -5.153800228976328945, 23.54057627198102054 ) ) ;
#178057=CARTESIAN_POINT ( 'NONE',  ( -19.02544592524334988, -5.153800228976617603, 53.95942372801898301 ) ) ;
#178059=CARTESIAN_POINT ( 'NONE',  ( 9.564922557960805705, 16.46253265017160317, 99.58224293864770971 ) ) ;
#178060=CARTESIAN_POINT ( 'NONE',  ( -16.53943276465976808, 0.05219959533911058130, 51.24890960531436690 ) ) ;
#178061=CARTESIAN_POINT ( 'NONE',  ( 0.05219959533907565091, 21.53943276465977519, 49.99890960531437401 ) ) ;
#178063=CARTESIAN_POINT ( 'NONE',  ( 5.823673210054444382, -21.52544592524334988, 110.2094237280190185 ) ) ;
#178065=CARTESIAN_POINT ( 'NONE',  ( -13.97604488694527625, -13.89961937509977652, 46.87390960531435979 ) ) ;
#178066=CARTESIAN_POINT ( 'NONE',  ( -19.03943276465977164, 0.05219959533909376836, 26.24890960531435624 ) ) ;
#178070=CARTESIAN_POINT ( 'NONE',  ( 8.224510206698742110, 14.34966873604972548, 62.08442372801901143 ) ) ;
#178071=CARTESIAN_POINT ( 'NONE',  ( -21.55341960407610458, -5.719274019375992779, 81.45724293864769550 ) ) ;
#178072=CARTESIAN_POINT ( 'NONE',  ( 4.379528057220339221, -16.55341960407611168, 52.70724293864769550 ) ) ;
#178073=CARTESIAN_POINT ( 'NONE',  ( 5.049401038298161559, -19.05341960407611168, 37.70724293864768839 ) ) ;
#178075=CARTESIAN_POINT ( 'NONE',  ( -15.72974639402176322, -15.80617190586768395, 44.37609039468567573 ) ) ;
#178076=CARTESIAN_POINT ( 'NONE',  ( -16.51473224551082808, 9.474510206698731452, 48.33442372801900433 ) ) ;
#178077=CARTESIAN_POINT ( 'NONE',  ( -13.89961937509977652, 13.97604488694528158, 30.62390960531435269 ) ) ;
#178078=CARTESIAN_POINT ( 'NONE',  ( 18.62759615963255655, 10.81492255796105972, 81.66775706135236135 ) ) ;
#178079=CARTESIAN_POINT ( 'NONE',  ( 19.02544592524343514, -5.153800228976328945, 23.54057627198102054 ) ) ;
#178080=CARTESIAN_POINT ( 'NONE',  ( -8.224510206698948167, 14.34966873604960824, 35.41557627198102409 ) ) ;
#178081=CARTESIAN_POINT ( 'NONE',  ( 17.49999999999999645, 3.189878218039145619, 112.6294856257125900 ) ) ;
#178082=CARTESIAN_POINT ( 'NONE',  ( -15.72974639402197994, 15.80617190586746368, 40.62390960531435269 ) ) ;
#178084=CARTESIAN_POINT ( 'NONE',  ( 5.049401038298161559, -19.05341960407611168, 92.70724293864769550 ) ) ;
#178085=CARTESIAN_POINT ( 'NONE',  ( 8.314922557960818139, 14.29746914071049879, 89.58224293864768129 ) ) ;
#178086=CARTESIAN_POINT ( 'NONE',  ( -14.29746914071037622, -8.314922557961029526, 29.16775706135234003 ) ) ;
#178087=CARTESIAN_POINT ( 'NONE',  ( -12.14591786802326823, 12.06949235617739902, 113.1260903946856899 ) ) ;
#178088=ORIENTED_EDGE ( 'NONE', *, *, #149044, .F. ) ;
#178089=CARTESIAN_POINT ( 'NONE',  ( 19.05341960407611168, 5.049401038298154454, 28.95724293864769550 ) ) ;
#178090=CARTESIAN_POINT ( 'NONE',  ( 0.05219959533909260263, 19.03943276465977164, 89.99890960531436690 ) ) ;
#178091=CARTESIAN_POINT ( 'NONE',  ( -21.53943276465977519, 0.05219959533907696930, 86.24890960531436690 ) ) ;
#178092=CARTESIAN_POINT ( 'NONE',  ( 4.379528057220339221, -16.55341960407611168, 22.70724293864769194 ) ) ;
#178093=CARTESIAN_POINT ( 'NONE',  ( 19.05341960407611168, 5.049401038298154454, 103.9572429386476671 ) ) ;
#178094=CARTESIAN_POINT ( 'NONE',  ( 16.46253265017146816, 9.564922557961045513, 81.66775706135233293 ) ) ;
#178095=CARTESIAN_POINT ( 'NONE',  ( -5.823673210054431948, 21.52544592524334988, 107.7094237280190328 ) ) ;
#178096=CARTESIAN_POINT ( 'NONE',  ( 15.80617190586746368, 15.72974639402197994, 89.37390960531435269 ) ) ;
#178097=CARTESIAN_POINT ( 'NONE',  ( -15.80617190586745835, -15.72974639402198527, 41.87390960531435979 ) ) ;
#178098=CARTESIAN_POINT ( 'NONE',  ( 5.049401038298161559, -19.05341960407611168, 67.70724293864769550 ) ) ;
#178099=CARTESIAN_POINT ( 'NONE',  ( -12.06949235617756955, 12.14591786802309770, 25.62390960531435624 ) ) ;
#178100=CARTESIAN_POINT ( 'NONE',  ( -19.02544592524342804, 5.153800228976336051, 81.04057627198103830 ) ) ;
#178104=CARTESIAN_POINT ( 'NONE',  ( 9.474510206698729675, 16.51473224551082808, 22.08442372801899722 ) ) ;
#178105=CARTESIAN_POINT ( 'NONE',  ( -4.483927247898539470, -16.52544592524342804, 92.29057627198103830 ) ) ;
#178106=CARTESIAN_POINT ( 'NONE',  ( -18.62759615963255300, -10.81492255796106328, 29.16775706135234003 ) ) ;
#178108=CARTESIAN_POINT ( 'NONE',  ( 21.55341960407610458, 5.719274019375980345, 73.95724293864769550 ) ) ;
#178109=CARTESIAN_POINT ( 'NONE',  ( 4.379528057220092307, 16.55341960407617563, 92.29275706135236135 ) ) ;
#178110=CARTESIAN_POINT ( 'NONE',  ( 4.483927247898545687, 16.52544592524342804, 114.7905762719810383 ) ) ;
#178111=CARTESIAN_POINT ( 'NONE',  ( -0.05219959533909027116, -19.03943276465977164, 77.49890960531435269 ) ) ;
#178112=CARTESIAN_POINT ( 'NONE',  ( 13.89961937509957579, 13.97604488694547520, 91.87609039468566152 ) ) ;
#178114=CARTESIAN_POINT ( 'NONE',  ( -16.53943276465976808, 0.05219959533911058130, 26.24890960531435624 ) ) ;
#178115=CARTESIAN_POINT ( 'NONE',  ( 5.823673210054444382, -21.52544592524334988, 60.20942372801902565 ) ) ;
#178116=CARTESIAN_POINT ( 'NONE',  ( 5.153800228976335163, 19.02544592524342804, 104.7905762719809957 ) ) ;
#178117=CARTESIAN_POINT ( 'NONE',  ( 18.67979575497194134, -10.72451020669871369, 90.83442372801901854 ) ) ;
#178118=CARTESIAN_POINT ( 'NONE',  ( 13.89961937509977652, -13.97604488694527269, 38.12390960531436690 ) ) ;
#178119=CARTESIAN_POINT ( 'NONE',  ( 9.564922557960805705, 16.46253265017160317, 49.58224293864770260 ) ) ;
#178120=ORIENTED_EDGE ( 'NONE', *, *, #100803, .T. ) ;
#178121=CARTESIAN_POINT ( 'NONE',  ( -0.05219959533937732626, 21.53943276465977519, 92.50109039468567573 ) ) ;
#178122=CARTESIAN_POINT ( 'NONE',  ( 4.483927247898790824, -16.52544592524335698, 55.20942372801902565 ) ) ;
#178123=CARTESIAN_POINT ( 'NONE',  ( 15.72974639402176855, 15.80617190586768217, 91.87609039468568994 ) ) ;
#178124=CARTESIAN_POINT ( 'NONE',  ( 19.05341960407611168, 5.049401038298154454, 113.9572429386477097 ) ) ;
#178126=CARTESIAN_POINT ( 'NONE',  ( -5.049401038297874678, -19.05341960407617918, 94.79275706135230450 ) ) ;
#178127=CARTESIAN_POINT ( 'NONE',  ( -10.81492255796105439, 18.62759615963255655, 57.91775706135234714 ) ) ;
#178128=CARTESIAN_POINT ( 'NONE',  ( -4.483927247898782831, 16.52544592524335698, 32.70942372801900433 ) ) ;
#178129=CARTESIAN_POINT ( 'NONE',  ( -5.823673210054116645, -21.52544592524344225, 87.29057627198103830 ) ) ;
#178130=CARTESIAN_POINT ( 'NONE',  ( -9.564922557961040184, 16.46253265017147172, 82.91775706135233293 ) ) ;
#178131=CARTESIAN_POINT ( 'NONE',  ( 5.153800228976335163, 19.02544592524342804, 69.79057627198103830 ) ) ;
#178132=CARTESIAN_POINT ( 'NONE',  ( -5.153800228976607833, 19.02544592524334988, 92.70942372801901854 ) ) ;
#178133=CARTESIAN_POINT ( 'NONE',  ( 13.89961937509957401, 13.97604488694547697, 101.8760903946856331 ) ) ;
#178134=CARTESIAN_POINT ( 'NONE',  ( 8.224510206698953496, -14.34966873604960469, 52.91557627198103830 ) ) ;
#178135=CARTESIAN_POINT ( 'NONE',  ( -13.97604488694547697, 13.89961937509957934, 83.12609039468564731 ) ) ;
#178136=CARTESIAN_POINT ( 'NONE',  ( -8.224510206698735004, -14.34966873604973081, 64.58442372801900433 ) ) ;
#178137=CARTESIAN_POINT ( 'NONE',  ( -19.05341960407617563, 5.049401038297882671, 43.54275706135232582 ) ) ;
#178138=ADVANCED_FACE ( 'NONE', ( #165700, #92808, #183845, #166699, #46321, #107976, #77648, #89843, #59490, #180883, #167685, #152499, #29182, #28202 ), #157753, .T. ) ;
#178139=CARTESIAN_POINT ( 'NONE',  ( -5.153800228976328057, -19.02544592524343514, 37.29057627198102409 ) ) ;
#178140=CARTESIAN_POINT ( 'NONE',  ( 9.474510206698971260, -16.51473224551069308, 37.91557627198102409 ) ) ;
#178141=CARTESIAN_POINT ( 'NONE',  ( 8.314922557961029526, -14.29746914071037800, 60.41775706135235424 ) ) ;
#178144=CARTESIAN_POINT ( 'NONE',  ( -13.97604488694527625, -13.89961937509977652, 106.8739096053143669 ) ) ;
#178147=CARTESIAN_POINT ( 'NONE',  ( -9.564922557961040184, 16.46253265017147172, 97.91775706135233293 ) ) ;
#178149=CARTESIAN_POINT ( 'NONE',  ( 15.72974639402199770, -15.80617190586745480, 33.12390960531435979 ) ) ;
#178150=CARTESIAN_POINT ( 'NONE',  ( 19.03943276465977164, 0.05219959533936151252, 26.25109039468566507 ) ) ;
#178151=CARTESIAN_POINT ( 'NONE',  ( -19.05341960407617563, 5.049401038297882671, 108.5427570613523187 ) ) ;
#178152=CARTESIAN_POINT ( 'NONE',  ( -5.153800228976328057, -19.02544592524343514, 27.29057627198103120 ) ) ;
#178153=CARTESIAN_POINT ( 'NONE',  ( -5.049401038298153566, 19.05341960407611168, 55.20724293864769550 ) ) ;
#178154=CARTESIAN_POINT ( 'NONE',  ( -5.823673210054116645, -21.52544592524344225, 67.29057627198103830 ) ) ;
#178155=CARTESIAN_POINT ( 'NONE',  ( -13.97604488694527625, -13.89961937509977652, 101.8739096053143811 ) ) ;
#178156=CARTESIAN_POINT ( 'NONE',  ( -16.46253265017160317, 9.564922557960807481, 40.83224293864769550 ) ) ;
#178158=CARTESIAN_POINT ( 'NONE',  ( -19.05341960407617563, 5.049401038297882671, 88.54275706135230450 ) ) ;
#178159=CARTESIAN_POINT ( 'NONE',  ( -12.06949235617756955, 12.14591786802309770, 50.62390960531435979 ) ) ;
#178160=CARTESIAN_POINT ( 'NONE',  ( 15.72974639402199770, -15.80617190586745480, 28.12390960531435979 ) ) ;
#178161=CARTESIAN_POINT ( 'NONE',  ( 15.72974639402176855, 15.80617190586768217, 106.8760903946856899 ) ) ;
#178162=CARTESIAN_POINT ( 'NONE',  ( -10.72451020669898014, 18.67979575497178502, 95.41557627198102409 ) ) ;
#178163=CARTESIAN_POINT ( 'NONE',  ( 0.05219959533937995610, -21.53943276465977519, 75.00109039468568994 ) ) ;
#178164=CARTESIAN_POINT ( 'NONE',  ( -21.53943276465977519, -0.05219959533937600094, 78.75109039468568994 ) ) ;
#178165=CARTESIAN_POINT ( 'NONE',  ( 5.153800228976335163, 19.02544592524342804, 114.7905762719810241 ) ) ;
#178166=CARTESIAN_POINT ( 'NONE',  ( 8.224510206698742110, 14.34966873604972548, 102.0844237280190185 ) ) ;
#178167=CARTESIAN_POINT ( 'NONE',  ( -18.67979575497193778, 10.72451020669871902, 58.33442372801901143 ) ) ;
#178168=CARTESIAN_POINT ( 'NONE',  ( 13.97604488694527802, 13.89961937509977652, 64.37390960531436690 ) ) ;
#178169=CARTESIAN_POINT ( 'NONE',  ( -19.03943276465977164, -0.05219959533935918106, 38.75109039468566152 ) ) ;
#178170=CARTESIAN_POINT ( 'NONE',  ( -18.62759615963255300, -10.81492255796106328, 29.16775706135234003 ) ) ;
#178171=CARTESIAN_POINT ( 'NONE',  ( 19.03943276465977164, -0.05219959533909143690, 63.74890960531435979 ) ) ;
#178172=CARTESIAN_POINT ( 'NONE',  ( 0.05219959533910956823, 16.53943276465976808, 84.99890960531436690 ) ) ;
#178173=CARTESIAN_POINT ( 'NONE',  ( -8.224510206698948167, 14.34966873604960824, 50.41557627198103120 ) ) ;
#178174=CARTESIAN_POINT ( 'NONE',  ( -21.53943276465977519, 0.05219959533907696930, 51.24890960531436690 ) ) ;
#178175=CARTESIAN_POINT ( 'NONE',  ( 16.51473224551069308, 9.474510206698969483, 64.16557627198102409 ) ) ;
#178176=CARTESIAN_POINT ( 'NONE',  ( -10.81492255796078084, -18.62759615963271287, 77.08224293864769550 ) ) ;
#178177=CARTESIAN_POINT ( 'NONE',  ( -9.564922557961040184, 16.46253265017147172, 67.91775706135233293 ) ) ;
#178178=CARTESIAN_POINT ( 'NONE',  ( 19.03943276465977164, 0.05219959533936151252, 21.25109039468565797 ) ) ;
#178179=CARTESIAN_POINT ( 'NONE',  ( 4.379528057220339221, -16.55341960407611168, 62.70724293864769550 ) ) ;
#178180=CARTESIAN_POINT ( 'NONE',  ( -21.52544592524343514, 5.823673210054127303, 36.04057627198102409 ) ) ;
#178183=CARTESIAN_POINT ( 'NONE',  ( 12.14591786802327356, -12.06949235617739191, 90.62609039468567573 ) ) ;
#178185=CARTESIAN_POINT ( 'NONE',  ( 5.049401038297881783, 19.05341960407617563, 87.29275706135234714 ) ) ;
#178186=CARTESIAN_POINT ( 'NONE',  ( 16.52544592524342804, -4.483927247898539470, 53.54057627198103120 ) ) ;
#178188=CARTESIAN_POINT ( 'NONE',  ( 16.46253265017160672, -9.564922557960803928, 48.33224293864769550 ) ) ;
#178189=CARTESIAN_POINT ( 'NONE',  ( 14.29746914071049879, -8.314922557960816363, 38.33224293864768839 ) ) ;
#178190=CARTESIAN_POINT ( 'NONE',  ( -19.02544592524342804, 5.153800228976336051, 91.04057627198100988 ) ) ;
#178191=CARTESIAN_POINT ( 'NONE',  ( 0.05219959533909260263, 19.03943276465977164, 54.99890960531435979 ) ) ;
#178192=CARTESIAN_POINT ( 'NONE',  ( 15.72974639402176855, 15.80617190586768217, 61.87609039468568284 ) ) ;
#178193=CARTESIAN_POINT ( 'NONE',  ( 19.02544592524343514, -5.153800228976328945, 73.54057627198103830 ) ) ;
#178195=CARTESIAN_POINT ( 'NONE',  ( -16.51473224551069308, -9.474510206698971260, 71.66557627198102409 ) ) ;
#178196=CARTESIAN_POINT ( 'NONE',  ( 15.72974639402199770, -15.80617190586745480, 48.12390960531436690 ) ) ;
#178197=CARTESIAN_POINT ( 'NONE',  ( 19.02544592524343514, -5.153800228976328945, 38.54057627198103120 ) ) ;
#178198=CARTESIAN_POINT ( 'NONE',  ( 10.81492255796078972, 18.62759615963270932, 59.58224293864770260 ) ) ;
#178199=CARTESIAN_POINT ( 'NONE',  ( -13.97604488694547697, 13.89961937509957934, 78.12609039468567573 ) ) ;
#178200=CARTESIAN_POINT ( 'NONE',  ( -16.53943276465976808, -0.05219959533934237506, 108.7510903946857042 ) ) ;
#178201=CARTESIAN_POINT ( 'NONE',  ( 19.02544592524334988, 5.153800228976608722, 21.45942372801899012 ) ) ;
#178202=CARTESIAN_POINT ( 'NONE',  ( 14.34966873604972726, -8.224510206698740333, 50.83442372801901143 ) ) ;
#178203=CARTESIAN_POINT ( 'NONE',  ( 14.29746914071037800, 8.314922557961029526, 81.66775706135236135 ) ) ;
#178204=CARTESIAN_POINT ( 'NONE',  ( -19.03943276465977164, 0.05219959533909376836, 116.2489096053143669 ) ) ;
#178205=CARTESIAN_POINT ( 'NONE',  ( -16.52544592524335698, -4.483927247898792601, 63.95942372801901854 ) ) ;
#178206=CARTESIAN_POINT ( 'NONE',  ( -21.55341960407610458, -5.719274019375992779, 31.45724293864769550 ) ) ;
#178207=CARTESIAN_POINT ( 'NONE',  ( 13.89961937509977652, -13.97604488694527269, 28.12390960531435624 ) ) ;
#178208=CARTESIAN_POINT ( 'NONE',  ( -8.314922557961024197, 14.29746914071037800, 42.91775706135235424 ) ) ;
#178209=CARTESIAN_POINT ( 'NONE',  ( -9.474510206698964154, 16.51473224551069663, 50.41557627198102409 ) ) ;
#178210=CARTESIAN_POINT ( 'NONE',  ( 21.53943276465977519, 0.05219959533937863772, 36.25109039468567573 ) ) ;
#178211=CARTESIAN_POINT ( 'NONE',  ( 12.14591786802327356, -12.06949235617739191, 40.62609039468567573 ) ) ;
#178212=CARTESIAN_POINT ( 'NONE',  ( 14.29746914071037800, 8.314922557961029526, 96.66775706135234714 ) ) ;
#178214=CARTESIAN_POINT ( 'NONE',  ( -18.67979575497193778, 10.72451020669871902, 103.3344237280190043 ) ) ;
#178215=CARTESIAN_POINT ( 'NONE',  ( 14.34966873604972726, -8.224510206698740333, 20.83442372801901143 ) ) ;
#178216=CARTESIAN_POINT ( 'NONE',  ( -16.51473224551082808, 9.474510206698731452, 68.33442372801900433 ) ) ;
#178217=CARTESIAN_POINT ( 'NONE',  ( -4.379528057220328563, 16.55341960407611168, 75.20724293864769550 ) ) ;
#178218=CARTESIAN_POINT ( 'NONE',  ( -16.51473224551069308, -9.474510206698971260, 26.66557627198103120 ) ) ;
#178219=CARTESIAN_POINT ( 'NONE',  ( 19.02544592524334988, 5.153800228976608722, 66.45942372801899012 ) ) ;
#178220=CARTESIAN_POINT ( 'NONE',  ( 16.61371651742640765, -7.165104196375916779, 56.35415069992969705 ) ) ;
#178221=CARTESIAN_POINT ( 'NONE',  ( 5.823673210054444382, -21.52544592524334988, 65.20942372801901854 ) ) ;
#178222=CARTESIAN_POINT ( 'NONE',  ( -0.05219959533934338120, 16.53943276465976808, 27.50109039468567929 ) ) ;
#178223=CARTESIAN_POINT ( 'NONE',  ( 17.50000000001358913, -5.500000000000039968, 73.29690382535059712 ) ) ;
#178224=CARTESIAN_POINT ( 'NONE',  ( 18.62759615963271287, -10.81492255796078972, 23.33224293864769194 ) ) ;
#178225=CARTESIAN_POINT ( 'NONE',  ( 19.02544592524334988, 5.153800228976608722, 111.4594237280190043 ) ) ;
#178226=CARTESIAN_POINT ( 'NONE',  ( -16.46253265017160317, 9.564922557960807481, 110.8322429386476955 ) ) ;
#178228=CARTESIAN_POINT ( 'NONE',  ( 19.05341960407611168, 5.049401038298154454, 23.95724293864769194 ) ) ;
#178229=CARTESIAN_POINT ( 'NONE',  ( 18.67979575497194134, -10.72451020669871369, 105.8344237280190328 ) ) ;
#178230=CARTESIAN_POINT ( 'NONE',  ( -5.049401038298153566, 19.05341960407611168, 50.20724293864770260 ) ) ;
#178231=CARTESIAN_POINT ( 'NONE',  ( 15.80617190586769283, -15.72974639402175789, 70.62609039468567573 ) ) ;
#178232=CARTESIAN_POINT ( 'NONE',  ( -10.81492255796105439, 18.62759615963255655, 102.9177570613523756 ) ) ;
#178233=CARTESIAN_POINT ( 'NONE',  ( -8.314922557960811034, -14.29746914071050412, 22.08224293864769194 ) ) ;
#178234=CARTESIAN_POINT ( 'NONE',  ( -19.05341960407611168, -5.049401038298163336, 31.45724293864769550 ) ) ;
#178235=CARTESIAN_POINT ( 'NONE',  ( -13.97604488694527625, -13.89961937509977652, 81.87390960531436690 ) ) ;
#178236=CARTESIAN_POINT ( 'NONE',  ( 10.81492255796106328, -18.62759615963255655, 60.41775706135235424 ) ) ;
#178237=CARTESIAN_POINT ( 'NONE',  ( 19.02544592524343514, -5.153800228976328945, 38.54057627198103120 ) ) ;
#178239=CARTESIAN_POINT ( 'NONE',  ( 21.53943276465977519, 0.05219959533937863772, 51.25109039468568994 ) ) ;
#178240=CARTESIAN_POINT ( 'NONE',  ( -5.049401038297874678, -19.05341960407617918, 84.79275706135233293 ) ) ;
#178241=CARTESIAN_POINT ( 'NONE',  ( -19.02544592524342804, 5.153800228976336051, 106.0405762719810241 ) ) ;
#178242=CARTESIAN_POINT ( 'NONE',  ( -0.05219959533909027116, -19.03943276465977164, 27.49890960531435624 ) ) ;
#178243=CARTESIAN_POINT ( 'NONE',  ( -18.62759615963270932, 10.81492255796079327, 105.8322429386476955 ) ) ;
#178244=CARTESIAN_POINT ( 'NONE',  ( 5.153800228976615827, -19.02544592524334988, 35.20942372801899722 ) ) ;
#178245=CARTESIAN_POINT ( 'NONE',  ( -16.53943276465976808, 0.05219959533911058130, 91.24890960531436690 ) ) ;
#178246=CARTESIAN_POINT ( 'NONE',  ( 19.03943276465977164, -0.05219959533909143690, 43.74890960531435979 ) ) ;
#178247=CARTESIAN_POINT ( 'NONE',  ( 16.51473224551083163, -9.474510206698727899, 95.83442372801900433 ) ) ;
#178248=CARTESIAN_POINT ( 'NONE',  ( 12.14591786802309770, 12.06949235617756955, 59.37390960531436690 ) ) ;
#178249=CARTESIAN_POINT ( 'NONE',  ( 5.823673210054444382, -21.52544592524334988, 105.2094237280190328 ) ) ;
#178250=CARTESIAN_POINT ( 'NONE',  ( 19.03943276465977164, -0.05219959533909143690, 103.7489096053143669 ) ) ;
#178251=CARTESIAN_POINT ( 'NONE',  ( -16.51473224551082808, 9.474510206698731452, 88.33442372801900433 ) ) ;
#178252=CARTESIAN_POINT ( 'NONE',  ( 10.72451020669898902, -18.67979575497178502, 97.91557627198103830 ) ) ;
#178253=CARTESIAN_POINT ( 'NONE',  ( 18.67979575497194134, -10.72451020669871369, 40.83442372801901854 ) ) ;
#178254=CARTESIAN_POINT ( 'NONE',  ( 12.06949235617739724, 12.14591786802326823, 41.87609039468568284 ) ) ;
#178255=CARTESIAN_POINT ( 'NONE',  ( 12.06949235617739724, 12.14591786802326823, 106.8760903946856899 ) ) ;
#178256=CARTESIAN_POINT ( 'NONE',  ( 8.314922557961029526, -14.29746914071037800, 45.41775706135234003 ) ) ;
#178257=CARTESIAN_POINT ( 'NONE',  ( 0.05219959533937995610, -21.53943276465977519, 35.00109039468568284 ) ) ;
#178258=CARTESIAN_POINT ( 'NONE',  ( -0.05219959533907301413, -21.53943276465977519, 47.49890960531435979 ) ) ;
#178259=CARTESIAN_POINT ( 'NONE',  ( -16.46253265017160317, 9.564922557960807481, 40.83224293864769550 ) ) ;
#178261=CARTESIAN_POINT ( 'NONE',  ( 14.29746914071037800, 8.314922557961029526, 61.66775706135235424 ) ) ;
#178262=CARTESIAN_POINT ( 'NONE',  ( -21.52544592524343514, 5.823673210054127303, 86.04057627198102409 ) ) ;
#178263=CARTESIAN_POINT ( 'NONE',  ( -12.14591786802309592, -12.06949235617757132, 36.87390960531435979 ) ) ;
#178264=CARTESIAN_POINT ( 'NONE',  ( 14.34966873604972726, -8.224510206698740333, 60.83442372801901854 ) ) ;
#178265=CARTESIAN_POINT ( 'NONE',  ( -5.153800228976328057, -19.02544592524343514, 57.29057627198103120 ) ) ;
#178266=CARTESIAN_POINT ( 'NONE',  ( 0.05219959533936267826, -19.03943276465977164, 100.0010903946856757 ) ) ;
#178267=CARTESIAN_POINT ( 'NONE',  ( 10.81492255796078972, 18.62759615963270932, 79.58224293864769550 ) ) ;
#178268=CARTESIAN_POINT ( 'NONE',  ( -8.224510206698948167, 14.34966873604960824, 30.41557627198101699 ) ) ;
#178271=CARTESIAN_POINT ( 'NONE',  ( -10.81492255796078084, -18.62759615963271287, 77.08224293864769550 ) ) ;
#178272=CARTESIAN_POINT ( 'NONE',  ( -4.483927247898782831, 16.52544592524335698, 107.7094237280190328 ) ) ;
#178274=CARTESIAN_POINT ( 'NONE',  ( 17.49999999999999645, -3.556738311674189301, 102.7527116387158941 ) ) ;
#178275=CARTESIAN_POINT ( 'NONE',  ( 21.55341960407610458, 5.719274019375980345, 88.95724293864769550 ) ) ;
#178276=CARTESIAN_POINT ( 'NONE',  ( 21.52544592524344225, -5.823673210054117533, 103.5405762719810383 ) ) ;
#178277=CARTESIAN_POINT ( 'NONE',  ( -4.379528057220328563, 16.55341960407611168, 25.20724293864769550 ) ) ;
#178278=CARTESIAN_POINT ( 'NONE',  ( -0.05219959533934338120, 16.53943276465976808, 37.50109039468568284 ) ) ;
#178279=CARTESIAN_POINT ( 'NONE',  ( 19.05341960407611168, 5.049401038298154454, 28.95724293864769550 ) ) ;
#178280=CARTESIAN_POINT ( 'NONE',  ( -19.02544592524342804, 5.153800228976336051, 66.04057627198103830 ) ) ;
#178282=CARTESIAN_POINT ( 'NONE',  ( -21.53943276465977519, 0.05219959533907696930, 26.24890960531435624 ) ) ;
#178284=CARTESIAN_POINT ( 'NONE',  ( -5.049401038297874678, -19.05341960407617918, 104.7927570613523471 ) ) ;
#178285=CARTESIAN_POINT ( 'NONE',  ( 13.97604488694548053, -13.89961937509957401, 40.62609039468564731 ) ) ;
#178286=CARTESIAN_POINT ( 'NONE',  ( 10.81492255796078972, 18.62759615963270932, 84.58224293864769550 ) ) ;
#178287=CARTESIAN_POINT ( 'NONE',  ( 16.53943276465976808, 0.05219959533934440121, 111.2510903946856899 ) ) ;
#178288=CARTESIAN_POINT ( 'NONE',  ( 15.72974639402199770, -15.80617190586745480, 43.12390960531435269 ) ) ;
#178289=CARTESIAN_POINT ( 'NONE',  ( 18.62759615963271287, -10.81492255796078972, 78.33224293864770971 ) ) ;
#178290=CARTESIAN_POINT ( 'NONE',  ( 16.46253265017146816, 9.564922557961045513, 111.6677570613523329 ) ) ;
#178291=CARTESIAN_POINT ( 'NONE',  ( -19.03943276465977164, 0.05219959533909376836, 106.2489096053143669 ) ) ;
#178292=CARTESIAN_POINT ( 'NONE',  ( 5.719274019375673035, 21.55341960407619339, 72.29275706135236135 ) ) ;
#178293=CARTESIAN_POINT ( 'NONE',  ( -16.51473224551069308, -9.474510206698971260, 56.66557627198103120 ) ) ;
#178294=CARTESIAN_POINT ( 'NONE',  ( -12.14591786802309592, -12.06949235617757132, 96.87390960531436690 ) ) ;
#178296=CARTESIAN_POINT ( 'NONE',  ( -19.02544592524342804, 5.153800228976336051, 76.04057627198102409 ) ) ;
#178297=CARTESIAN_POINT ( 'NONE',  ( 14.29746914071049879, -8.314922557960816363, 88.33224293864769550 ) ) ;
#178299=CARTESIAN_POINT ( 'NONE',  ( 19.05341960407617918, -5.049401038297876454, 91.04275706135234714 ) ) ;
#178301=CARTESIAN_POINT ( 'NONE',  ( 16.51473224551069308, 9.474510206698969483, 64.16557627198102409 ) ) ;
#178302=CARTESIAN_POINT ( 'NONE',  ( -15.80617190586768217, 15.72974639402176855, 78.12609039468570415 ) ) ;
#178303=CARTESIAN_POINT ( 'NONE',  ( -5.049401038298153566, 19.05341960407611168, 100.2072429386476955 ) ) ;
#178305=CARTESIAN_POINT ( 'NONE',  ( -4.483927247898782831, 16.52544592524335698, 77.70942372801900433 ) ) ;
#178306=CARTESIAN_POINT ( 'NONE',  ( -16.38665767535054485, -7.295008042176060137, 49.73599135785455161 ) ) ;
#178307=CARTESIAN_POINT ( 'NONE',  ( -9.564922557961040184, 16.46253265017147172, 47.91775706135233293 ) ) ;
#178308=CARTESIAN_POINT ( 'NONE',  ( -21.53943276465977519, -0.05219959533937600094, 93.75109039468567573 ) ) ;
#178309=CARTESIAN_POINT ( 'NONE',  ( 17.50000000000000000, 5.499999999999997335, 23.78230962303566542 ) ) ;
#178311=CARTESIAN_POINT ( 'NONE',  ( -16.55341960407617563, 4.379528057220093196, 98.54275706135234714 ) ) ;
#178313=CARTESIAN_POINT ( 'NONE',  ( -12.14591786802326823, 12.06949235617739902, 88.12609039468570415 ) ) ;
#178314=CARTESIAN_POINT ( 'NONE',  ( 16.52216118717207038, 7.221426719304515629, 68.57599021046993926 ) ) ;
#178315=CARTESIAN_POINT ( 'NONE',  ( 4.379528057220092307, 16.55341960407617563, 62.29275706135236845 ) ) ;
#178317=CARTESIAN_POINT ( 'NONE',  ( -15.72974639402176322, -15.80617190586768395, 84.37609039468570415 ) ) ;
#178318=CARTESIAN_POINT ( 'NONE',  ( -16.46253265017146816, -9.564922557961047289, 84.16775706135233293 ) ) ;
#178319=CARTESIAN_POINT ( 'NONE',  ( 13.89961937509957401, 13.97604488694547697, 36.87609039468565442 ) ) ;
#178320=CARTESIAN_POINT ( 'NONE',  ( -19.02544592524342804, 5.153800228976336051, 61.04057627198103120 ) ) ;
#178321=CARTESIAN_POINT ( 'NONE',  ( 9.564922557960805705, 16.46253265017160317, 54.58224293864769550 ) ) ;
#178322=CARTESIAN_POINT ( 'NONE',  ( 18.22780087662119897, -5.500000000000146549, 38.51763182126893525 ) ) ;
#178323=CARTESIAN_POINT ( 'NONE',  ( -10.72451020669898014, 18.67979575497178502, 75.41557627198102409 ) ) ;
#178324=CARTESIAN_POINT ( 'NONE',  ( 10.81492255796078972, 18.62759615963270932, 39.58224293864769550 ) ) ;
#178325=CARTESIAN_POINT ( 'NONE',  ( 5.049401038298161559, -19.05341960407611168, 37.70724293864768839 ) ) ;
#178326=CARTESIAN_POINT ( 'NONE',  ( 8.224510206698742110, 14.34966873604972548, 62.08442372801901143 ) ) ;
#178327=ADVANCED_FACE ( 'NONE', ( #70170 ), #82308, .F. ) ;
#178329=CARTESIAN_POINT ( 'NONE',  ( 18.62759615963255655, 10.81492255796105972, 26.66775706135235424 ) ) ;
#178330=CARTESIAN_POINT ( 'NONE',  ( -8.224510206698948167, 14.34966873604960824, 65.41557627198102409 ) ) ;
#178332=CARTESIAN_POINT ( 'NONE',  ( 4.379528057220092307, 16.55341960407617563, 22.29275706135235069 ) ) ;
#178333=CARTESIAN_POINT ( 'NONE',  ( 19.03943276465977164, 0.05219959533936151252, 51.25109039468567573 ) ) ;
#178334=CARTESIAN_POINT ( 'NONE',  ( 8.224510206698953496, -14.34966873604960469, 57.91557627198103120 ) ) ;
#178335=CARTESIAN_POINT ( 'NONE',  ( 18.67979575497194134, -10.72451020669871369, 30.83442372801902209 ) ) ;
#178336=CARTESIAN_POINT ( 'NONE',  ( 16.51473224551069308, 9.474510206698969483, 99.16557627198102409 ) ) ;
#178337=CARTESIAN_POINT ( 'NONE',  ( -21.52544592524343514, 5.823673210054127303, 81.04057627198102409 ) ) ;
#178338=CARTESIAN_POINT ( 'NONE',  ( 13.89961937509977652, -13.97604488694527269, 108.1239096053143669 ) ) ;
#178339=CARTESIAN_POINT ( 'NONE',  ( 8.224510206698953496, -14.34966873604960469, 77.91557627198102409 ) ) ;
#178342=CARTESIAN_POINT ( 'NONE',  ( -19.02544592524334988, -5.153800228976617603, 68.95942372801896170 ) ) ;
#178343=CARTESIAN_POINT ( 'NONE',  ( 15.80617190586746368, 15.72974639402197994, 109.3739096053143811 ) ) ;
#178344=CARTESIAN_POINT ( 'NONE',  ( 5.153800228976335163, 19.02544592524342804, 54.79057627198103120 ) ) ;
#178345=CARTESIAN_POINT ( 'NONE',  ( -19.03943276465977164, -0.05219959533935918106, 48.75109039468566863 ) ) ;
#178346=CARTESIAN_POINT ( 'NONE',  ( 5.049401038298161559, -19.05341960407611168, 27.70724293864769550 ) ) ;
#178347=CARTESIAN_POINT ( 'NONE',  ( -5.719274019375665041, -21.55341960407619695, 64.79275706135234714 ) ) ;
#178349=CARTESIAN_POINT ( 'NONE',  ( 12.14591786802309770, 12.06949235617756955, 39.37390960531436690 ) ) ;
#178350=CARTESIAN_POINT ( 'NONE',  ( -9.564922557960796823, -16.46253265017161027, 67.08224293864769550 ) ) ;
#178351=CARTESIAN_POINT ( 'NONE',  ( 5.719274019375991003, -21.55341960407610458, 87.70724293864769550 ) ) ;
#178352=CARTESIAN_POINT ( 'NONE',  ( -16.51473224551069308, -9.474510206698971260, 56.66557627198103120 ) ) ;
#178353=ORIENTED_EDGE ( 'NONE', *, *, #172057, .F. ) ;
#178354=CARTESIAN_POINT ( 'NONE',  ( -5.719274019375978568, 21.55341960407610458, 60.20724293864768839 ) ) ;
#178355=CARTESIAN_POINT ( 'NONE',  ( -21.55341960407619339, 5.719274019375674811, 103.5427570613523613 ) ) ;
#178357=CARTESIAN_POINT ( 'NONE',  ( 4.483927247898790824, -16.52544592524335698, 90.20942372801903275 ) ) ;
#178358=CARTESIAN_POINT ( 'NONE',  ( -16.52544592524342804, 4.483927247898546575, 81.04057627198102409 ) ) ;
#178359=CARTESIAN_POINT ( 'NONE',  ( -9.474510206698720793, -16.51473224551083518, 94.58442372801900433 ) ) ;
#178360=ORIENTED_EDGE ( 'NONE', *, *, #175162, .F. ) ;
#178361=CARTESIAN_POINT ( 'NONE',  ( -13.89961937509957401, -13.97604488694547875, 34.37609039468566863 ) ) ;
#178362=CARTESIAN_POINT ( 'NONE',  ( 8.314922557961029526, -14.29746914071037800, 95.41775706135234714 ) ) ;
#178363=CARTESIAN_POINT ( 'NONE',  ( -0.05219959533936034679, 19.03943276465977164, 32.50109039468566863 ) ) ;
#178364=CARTESIAN_POINT ( 'NONE',  ( 9.564922557960805705, 16.46253265017160317, 84.58224293864769550 ) ) ;
#178365=CARTESIAN_POINT ( 'NONE',  ( -18.62759615963270932, 10.81492255796079327, 60.83224293864769550 ) ) ;
#178367=CARTESIAN_POINT ( 'NONE',  ( -4.483927247898539470, -16.52544592524342804, 112.2905762719810241 ) ) ;
#178368=CARTESIAN_POINT ( 'NONE',  ( 10.72451020669871369, 18.67979575497193778, 97.08442372801904696 ) ) ;
#178369=CARTESIAN_POINT ( 'NONE',  ( 14.34966873604972726, -8.224510206698740333, 80.83442372801901854 ) ) ;
#178370=CARTESIAN_POINT ( 'NONE',  ( 5.719274019375673035, 21.55341960407619339, 32.29275706135235424 ) ) ;
#178371=CARTESIAN_POINT ( 'NONE',  ( -14.29746914071037622, -8.314922557961029526, 34.16775706135234714 ) ) ;
#178372=CARTESIAN_POINT ( 'NONE',  ( -16.46253265017160317, 9.564922557960807481, 105.8322429386476955 ) ) ;
#178373=CARTESIAN_POINT ( 'NONE',  ( 19.02544592524343514, -5.153800228976328945, 43.54057627198103120 ) ) ;
#178374=CARTESIAN_POINT ( 'NONE',  ( 13.89961937509977652, -13.97604488694527269, 58.12390960531436690 ) ) ;
#178375=CARTESIAN_POINT ( 'NONE',  ( -12.14591786802326823, 12.06949235617739902, 43.12609039468568284 ) ) ;
#178376=CARTESIAN_POINT ( 'NONE',  ( -16.53943276465976808, 0.05219959533911058130, 86.24890960531436690 ) ) ;
#178377=CARTESIAN_POINT ( 'NONE',  ( -8.314922557961024197, 14.29746914071037800, 102.9177570613523756 ) ) ;
#178378=CARTESIAN_POINT ( 'NONE',  ( 21.55341960407619695, -5.719274019375665929, 46.04275706135234714 ) ) ;
#178379=CARTESIAN_POINT ( 'NONE',  ( 13.89961937509977652, -13.97604488694527269, 83.12390960531436690 ) ) ;
#178380=CARTESIAN_POINT ( 'NONE',  ( 9.564922557960805705, 16.46253265017160317, 64.58224293864769550 ) ) ;
#178381=CARTESIAN_POINT ( 'NONE',  ( -9.474510206698964154, 16.51473224551069663, 95.41557627198102409 ) ) ;
#178382=CARTESIAN_POINT ( 'NONE',  ( 12.14591786802309770, 12.06949235617756955, 29.37390960531435269 ) ) ;
#178383=CARTESIAN_POINT ( 'NONE',  ( -14.34966873604972548, 8.224510206698743886, 98.33442372801901854 ) ) ;
#178385=CARTESIAN_POINT ( 'NONE',  ( -5.153800228976607833, 19.02544592524334988, 42.70942372801901143 ) ) ;
#178386=CARTESIAN_POINT ( 'NONE',  ( -9.474510206698964154, 16.51473224551069663, 115.4155762719810241 ) ) ;
#178387=CARTESIAN_POINT ( 'NONE',  ( -13.89961937509977652, 13.97604488694528158, 65.62390960531436690 ) ) ;
#178388=CARTESIAN_POINT ( 'NONE',  ( -0.05219959533936034679, 19.03943276465977164, 37.50109039468567573 ) ) ;
#178390=CARTESIAN_POINT ( 'NONE',  ( 19.46398650005391673, -5.499999999999944933, 72.68269651486370719 ) ) ;
#178391=CARTESIAN_POINT ( 'NONE',  ( -4.483927247898782831, 16.52544592524335698, 47.70942372801902565 ) ) ;
#178392=CARTESIAN_POINT ( 'NONE',  ( 19.05341960407617918, -5.049401038297876454, 66.04275706135233293 ) ) ;
#178393=CARTESIAN_POINT ( 'NONE',  ( 4.483927247898790824, -16.52544592524335698, 55.20942372801902565 ) ) ;
#178394=CARTESIAN_POINT ( 'NONE',  ( 9.564922557960805705, 16.46253265017160317, 114.5822429386476955 ) ) ;
#178395=CARTESIAN_POINT ( 'NONE',  ( -19.03943276465977164, 0.05219959533909376836, 91.24890960531436690 ) ) ;
#178396=CARTESIAN_POINT ( 'NONE',  ( -5.719274019375978568, 21.55341960407610458, 115.2072429386476955 ) ) ;
#178397=CARTESIAN_POINT ( 'NONE',  ( -5.153800228976607833, 19.02544592524334988, 77.70942372801900433 ) ) ;
#178398=CARTESIAN_POINT ( 'NONE',  ( -19.02544592524342804, 5.153800228976336051, 111.0405762719810099 ) ) ;
#178399=CARTESIAN_POINT ( 'NONE',  ( 13.89961937509977652, -13.97604488694527269, 28.12390960531435624 ) ) ;
#178400=CARTESIAN_POINT ( 'NONE',  ( 19.03943276465977164, -0.05219959533909143690, 78.74890960531436690 ) ) ;
#178401=CARTESIAN_POINT ( 'NONE',  ( -4.379528057220328563, 16.55341960407611168, 45.20724293864769550 ) ) ;
#178402=CARTESIAN_POINT ( 'NONE',  ( 16.46253265017160672, -9.564922557960803928, 38.33224293864768839 ) ) ;
#178403=CARTESIAN_POINT ( 'NONE',  ( 9.474510206698729675, 16.51473224551082808, 57.08442372801900433 ) ) ;
#178404=CARTESIAN_POINT ( 'NONE',  ( -8.224510206698948167, 14.34966873604960824, 90.41557627198103830 ) ) ;
#178405=CARTESIAN_POINT ( 'NONE',  ( 21.55341960407619695, -5.719274019375665929, 106.0427570613523471 ) ) ;
#178406=CARTESIAN_POINT ( 'NONE',  ( -13.97604488694527625, -13.89961937509977652, 51.87390960531436690 ) ) ;
#178407=CARTESIAN_POINT ( 'NONE',  ( 5.719274019375991003, -21.55341960407610458, 52.70724293864769550 ) ) ;
#178408=CARTESIAN_POINT ( 'NONE',  ( 16.52544592524342804, -4.483927247898539470, 58.54057627198103120 ) ) ;
#178409=CARTESIAN_POINT ( 'NONE',  ( -13.89961937509957401, -13.97604488694547875, 19.37609039468566507 ) ) ;
#178410=CARTESIAN_POINT ( 'NONE',  ( -13.89961937509977652, 13.97604488694528158, 100.6239096053143669 ) ) ;
#178411=CARTESIAN_POINT ( 'NONE',  ( -19.03943276465977164, 0.05219959533909376836, 111.2489096053143669 ) ) ;
#178412=CARTESIAN_POINT ( 'NONE',  ( 9.564922557960805705, 16.46253265017160317, 34.58224293864770260 ) ) ;
#178413=CARTESIAN_POINT ( 'NONE',  ( -19.05341960407611168, -5.049401038298163336, 31.45724293864769550 ) ) ;
#178414=CARTESIAN_POINT ( 'NONE',  ( -14.34966873604960291, -8.224510206698953496, 86.66557627198102409 ) ) ;
#178415=CARTESIAN_POINT ( 'NONE',  ( 18.67979575497178502, 10.72451020669898547, 94.16557627198103830 ) ) ;
#178416=CARTESIAN_POINT ( 'NONE',  ( 5.049401038298161559, -19.05341960407611168, 97.70724293864766707 ) ) ;
#178417=CARTESIAN_POINT ( 'NONE',  ( 18.67979575497194134, -10.72451020669871369, 20.83442372801901143 ) ) ;
#178418=CARTESIAN_POINT ( 'NONE',  ( -13.89961937509977652, 13.97604488694528158, 110.6239096053143243 ) ) ;
#178420=CARTESIAN_POINT ( 'NONE',  ( -16.55341960407611168, -4.379528057220339221, 101.4572429386476955 ) ) ;
#178421=CARTESIAN_POINT ( 'NONE',  ( -5.153800228976328057, -19.02544592524343514, 77.29057627198099567 ) ) ;
#178422=CARTESIAN_POINT ( 'NONE',  ( 21.52544592524344225, -5.823673210054117533, 83.54057627198102409 ) ) ;
#178425=CARTESIAN_POINT ( 'NONE',  ( -18.67979575497178146, -10.72451020669898902, 26.66557627198103475 ) ) ;
#178427=CARTESIAN_POINT ( 'NONE',  ( 4.379528057220092307, 16.55341960407617563, 32.29275706135235424 ) ) ;
#178428=CARTESIAN_POINT ( 'NONE',  ( -16.52544592524342804, 4.483927247898546575, 91.04057627198103830 ) ) ;
#178430=CARTESIAN_POINT ( 'NONE',  ( 5.153800228976335163, 19.02544592524342804, 59.79057627198100988 ) ) ;
#178431=CARTESIAN_POINT ( 'NONE',  ( 4.379528057220339221, -16.55341960407611168, 82.70724293864770971 ) ) ;
#178432=CARTESIAN_POINT ( 'NONE',  ( -18.67979575497178146, -10.72451020669898902, 36.66557627198103120 ) ) ;
#178433=CARTESIAN_POINT ( 'NONE',  ( 8.314922557960818139, 14.29746914071049879, 54.58224293864769550 ) ) ;
#178434=CARTESIAN_POINT ( 'NONE',  ( 5.153800228976615827, -19.02544592524334988, 110.2094237280189901 ) ) ;
#178435=CARTESIAN_POINT ( 'NONE',  ( 10.81492255796106328, -18.62759615963255655, 70.41775706135236135 ) ) ;
#178437=CARTESIAN_POINT ( 'NONE',  ( -9.564922557960796823, -16.46253265017161027, 112.0822429386476955 ) ) ;
#178438=CARTESIAN_POINT ( 'NONE',  ( -16.55341960407617563, 4.379528057220093196, 78.54275706135236135 ) ) ;
#178439=CARTESIAN_POINT ( 'NONE',  ( -17.50000000001354294, 5.500000000000027534, 95.79690382535056870 ) ) ;
#178440=CARTESIAN_POINT ( 'NONE',  ( -16.51473224551069308, -9.474510206698971260, 91.66557627198103830 ) ) ;
#178441=CARTESIAN_POINT ( 'NONE',  ( 10.72451020669898902, -18.67979575497178502, 92.91557627198103830 ) ) ;
#178443=CARTESIAN_POINT ( 'NONE',  ( 16.52544592524335698, 4.483927247898782831, 31.45942372801901854 ) ) ;
#178444=CARTESIAN_POINT ( 'NONE',  ( -4.379528057220328563, 16.55341960407611168, 55.20724293864770260 ) ) ;
#178445=CARTESIAN_POINT ( 'NONE',  ( 21.53943276465977519, 0.05219959533937863772, 71.25109039468568994 ) ) ;
#178446=CARTESIAN_POINT ( 'NONE',  ( 14.29746914071037800, 8.314922557961029526, 101.6677570613523613 ) ) ;
#178447=CARTESIAN_POINT ( 'NONE',  ( -18.67979575497178146, -10.72451020669898902, 21.66557627198102409 ) ) ;
#178448=CARTESIAN_POINT ( 'NONE',  ( -16.46253265017160317, 9.564922557960807481, 115.8322429386477097 ) ) ;
#178450=CARTESIAN_POINT ( 'NONE',  ( -14.29746914071037622, -8.314922557961029526, 109.1677570613523613 ) ) ;
#178451=CARTESIAN_POINT ( 'NONE',  ( -14.29746914071037622, -8.314922557961029526, 54.16775706135235424 ) ) ;
#178452=CARTESIAN_POINT ( 'NONE',  ( -16.51473224551069308, -9.474510206698971260, 76.66557627198103830 ) ) ;
#178453=CARTESIAN_POINT ( 'NONE',  ( 13.89961937509977652, -13.97604488694527269, 83.12390960531436690 ) ) ;
#178454=CARTESIAN_POINT ( 'NONE',  ( 5.823673210054444382, -21.52544592524334988, 70.20942372801904696 ) ) ;
#178455=CARTESIAN_POINT ( 'NONE',  ( 4.379528057220092307, 16.55341960407617563, 77.29275706135234714 ) ) ;
#178456=CARTESIAN_POINT ( 'NONE',  ( 12.06949235617757843, -12.14591786802309237, 48.12390960531436690 ) ) ;
#178457=CARTESIAN_POINT ( 'NONE',  ( 16.51473224551069308, 9.474510206698969483, 49.16557627198102409 ) ) ;
#178458=VERTEX_POINT ( 'NONE', #52981 ) ;
#178459=CARTESIAN_POINT ( 'NONE',  ( -9.474510206698720793, -16.51473224551083518, 104.5844237280190043 ) ) ;
#178460=CARTESIAN_POINT ( 'NONE',  ( -12.06949235617756955, 12.14591786802309770, 105.6239096053143669 ) ) ;
#178461=CARTESIAN_POINT ( 'NONE',  ( 13.97604488694527802, 13.89961937509977652, 74.37390960531436690 ) ) ;
#178462=CARTESIAN_POINT ( 'NONE',  ( 5.049401038297881783, 19.05341960407617563, 97.29275706135233293 ) ) ;
#178464=CARTESIAN_POINT ( 'NONE',  ( -15.80617190586768217, 15.72974639402176855, 98.12609039468570415 ) ) ;
#178465=CARTESIAN_POINT ( 'NONE',  ( -8.314922557961024197, 14.29746914071037800, 77.91775706135231871 ) ) ;
#178466=CARTESIAN_POINT ( 'NONE',  ( -19.02544592524334988, -5.153800228976617603, 88.95942372801897591 ) ) ;
#178467=CARTESIAN_POINT ( 'NONE',  ( -0.05219959533907301413, -21.53943276465977519, 67.49890960531436690 ) ) ;
#178468=CARTESIAN_POINT ( 'NONE',  ( -12.14591786802326823, 12.06949235617739902, 58.12609039468568994 ) ) ;
#178470=CARTESIAN_POINT ( 'NONE',  ( -9.564922557961040184, 16.46253265017147172, 57.91775706135233293 ) ) ;
#178471=CARTESIAN_POINT ( 'NONE',  ( -10.81492255796105439, 18.62759615963255655, 92.91775706135236135 ) ) ;
#178472=CARTESIAN_POINT ( 'NONE',  ( 5.049401038298161559, -19.05341960407611168, 32.70724293864768129 ) ) ;
#178473=CARTESIAN_POINT ( 'NONE',  ( 9.564922557960805705, 16.46253265017160317, 69.58224293864770971 ) ) ;
#178474=CARTESIAN_POINT ( 'NONE',  ( 4.483927247898545687, 16.52544592524342804, 59.79057627198103120 ) ) ;
#178475=CARTESIAN_POINT ( 'NONE',  ( -21.55341960407619339, 5.719274019375674811, 88.54275706135236135 ) ) ;
#178476=CARTESIAN_POINT ( 'NONE',  ( -9.564922557961040184, 16.46253265017147172, 47.91775706135233293 ) ) ;
#178477=CARTESIAN_POINT ( 'NONE',  ( 5.049401038297881783, 19.05341960407617563, 22.29275706135233648 ) ) ;
#178478=CARTESIAN_POINT ( 'NONE',  ( -15.80617190586745835, -15.72974639402198527, 36.87390960531435979 ) ) ;
#178479=CARTESIAN_POINT ( 'NONE',  ( 21.52544592524334988, 5.823673210054432836, 91.45942372801901854 ) ) ;
#178480=CARTESIAN_POINT ( 'NONE',  ( 13.97604488694527802, 13.89961937509977652, 79.37390960531435269 ) ) ;
#178482=CARTESIAN_POINT ( 'NONE',  ( 15.80617190586769283, -15.72974639402175789, 95.62609039468568994 ) ) ;
#178483=CARTESIAN_POINT ( 'NONE',  ( 5.719274019375991003, -21.55341960407610458, 47.70724293864770260 ) ) ;
#178484=CARTESIAN_POINT ( 'NONE',  ( -19.02544592524342804, 5.153800228976336051, 86.04057627198103830 ) ) ;
#178485=CARTESIAN_POINT ( 'NONE',  ( 9.564922557961047289, -16.46253265017146816, 75.41775706135234714 ) ) ;
#178486=CARTESIAN_POINT ( 'NONE',  ( -19.05341960407611168, -5.049401038298163336, 91.45724293864766707 ) ) ;
#178487=CARTESIAN_POINT ( 'NONE',  ( -16.46253265017146816, -9.564922557961047289, 99.16775706135233293 ) ) ;
#178488=CARTESIAN_POINT ( 'NONE',  ( -4.379528057220086978, -16.55341960407618274, 39.79275706135235424 ) ) ;
#178489=CARTESIAN_POINT ( 'NONE',  ( -16.52544592524342804, 4.483927247898546575, 106.0405762719810525 ) ) ;
#178490=CARTESIAN_POINT ( 'NONE',  ( -0.05219959533909027116, -19.03943276465977164, 77.49890960531435269 ) ) ;
#178491=CARTESIAN_POINT ( 'NONE',  ( -21.52544592524343514, 5.823673210054127303, 56.04057627198102409 ) ) ;
#178492=B_SPLINE_CURVE_WITH_KNOTS ( 'NONE', 3,
 ( #166367, #41020, #91462, #57192, #43013, #74349, #44996, #183513, #105666, #90490, #152172, #181534, #104680, #13655, #42024, #75322, #27864, #106656, #25867, #29825, #9688, #118867, #180551, #103689, #170317, #63128, #49958, #47981, #30818, #155147, #16640, #33791 ),
 .UNSPECIFIED., .F., .F.,
 ( 4, 2, 2, 2, 2, 2, 2, 2, 2, 2, 2, 2, 2, 2, 2, 4 ),
 ( 1.643959876789974123E-15, 0.0003712461730052138767, 0.0007424923460087837776, 0.001113738519012353462, 0.001484984692015923471, 0.002227477038023074982, 0.002598723211026647811, 0.002969969384030220205, 0.003341215557033792600, 0.003712461730037365428, 0.004083707903040937823, 0.004454954076044509784, 0.004826200249048082612, 0.005197446422051654573, 0.005568692595055228269, 0.005939938768058800229 ),
 .UNSPECIFIED. ) ;
#178493=CARTESIAN_POINT ( 'NONE',  ( 4.379528057220092307, 16.55341960407617563, 37.29275706135235424 ) ) ;
#178494=CARTESIAN_POINT ( 'NONE',  ( 21.53943276465977519, 0.05219959533937863772, 31.25109039468568639 ) ) ;
#178495=CARTESIAN_POINT ( 'NONE',  ( 18.67979575497194134, -10.72451020669871369, 80.83442372801901854 ) ) ;
#178496=CARTESIAN_POINT ( 'NONE',  ( -12.06949235617739369, -12.14591786802326823, 89.37609039468568994 ) ) ;
#178497=CARTESIAN_POINT ( 'NONE',  ( 5.153800228976335163, 19.02544592524342804, 79.79057627198102409 ) ) ;
#178498=CARTESIAN_POINT ( 'NONE',  ( 8.314922557960818139, 14.29746914071049879, 74.58224293864768129 ) ) ;
#178499=CARTESIAN_POINT ( 'NONE',  ( -8.314922557961024197, 14.29746914071037800, 107.9177570613523471 ) ) ;
#178500=CARTESIAN_POINT ( 'NONE',  ( 19.03943276465977164, 0.05219959533936151252, 61.25109039468566863 ) ) ;
#178501=CARTESIAN_POINT ( 'NONE',  ( 15.72974639402176855, 15.80617190586768217, 36.87609039468568994 ) ) ;
#178502=CARTESIAN_POINT ( 'NONE',  ( -16.53943276465976808, 0.05219959533911058130, 76.24890960531435269 ) ) ;
#178503=CARTESIAN_POINT ( 'NONE',  ( -0.05219959533909027116, -19.03943276465977164, 102.4989096053143669 ) ) ;
#178504=CARTESIAN_POINT ( 'NONE',  ( 14.29746914071037800, 8.314922557961029526, 96.66775706135234714 ) ) ;
#178505=CARTESIAN_POINT ( 'NONE',  ( 10.72451020669871369, 18.67979575497193778, 72.08442372801899012 ) ) ;
#178506=CARTESIAN_POINT ( 'NONE',  ( 12.14591786802327356, -12.06949235617739191, 45.62609039468567573 ) ) ;
#178507=CARTESIAN_POINT ( 'NONE',  ( 15.72974639402176855, 15.80617190586768217, 26.87609039468567218 ) ) ;
#178508=CARTESIAN_POINT ( 'NONE',  ( -16.55341960407611168, -4.379528057220339221, 76.45724293864769550 ) ) ;
#178510=CARTESIAN_POINT ( 'NONE',  ( -21.53943276465977519, 0.05219959533907696930, 111.2489096053143669 ) ) ;
#178511=CARTESIAN_POINT ( 'NONE',  ( -0.05219959533910754901, -16.53943276465976808, 52.49890960531435979 ) ) ;
#178512=FACE_OUTER_BOUND ( 'NONE', #15434, .T. ) ;
#178513=CARTESIAN_POINT ( 'NONE',  ( -0.05219959533907301413, -21.53943276465977519, 32.49890960531435979 ) ) ;
#178514=CARTESIAN_POINT ( 'NONE',  ( -16.53943276465976808, 0.05219959533911058130, 61.24890960531435979 ) ) ;
#178515=CARTESIAN_POINT ( 'NONE',  ( 10.81492255796078972, 18.62759615963270932, 84.58224293864769550 ) ) ;
#178516=CARTESIAN_POINT ( 'NONE',  ( -9.564922557960796823, -16.46253265017161027, 72.08224293864770971 ) ) ;
#178517=CARTESIAN_POINT ( 'NONE',  ( 0.05219959533909260263, 19.03943276465977164, 44.99890960531435979 ) ) ;
#178518=CARTESIAN_POINT ( 'NONE',  ( 0.05219959533936267826, -19.03943276465977164, 75.00109039468566152 ) ) ;
#178519=CARTESIAN_POINT ( 'NONE',  ( 21.53943276465977519, 0.05219959533937863772, 61.25109039468567573 ) ) ;
#178520=CARTESIAN_POINT ( 'NONE',  ( -21.52544592524343514, 5.823673210054127303, 56.04057627198102409 ) ) ;
#178521=CARTESIAN_POINT ( 'NONE',  ( -5.049401038298153566, 19.05341960407611168, 45.20724293864769550 ) ) ;
#178522=CARTESIAN_POINT ( 'NONE',  ( 9.474510206698971260, -16.51473224551069308, 67.91557627198102409 ) ) ;
#178523=ORIENTED_EDGE ( 'NONE', *, *, #94296, .F. ) ;
#178524=CARTESIAN_POINT ( 'NONE',  ( -14.29746914071037622, -8.314922557961029526, 49.16775706135234003 ) ) ;
#178525=CARTESIAN_POINT ( 'NONE',  ( 21.52544592524334988, 5.823673210054432836, 31.45942372801901854 ) ) ;
#178526=CARTESIAN_POINT ( 'NONE',  ( -0.05219959533937732626, 21.53943276465977519, 57.50109039468568994 ) ) ;
#178527=CARTESIAN_POINT ( 'NONE',  ( 19.03943276465977164, -0.05219959533909143690, 103.7489096053143669 ) ) ;
#178528=CARTESIAN_POINT ( 'NONE',  ( 18.62759615963271287, -10.81492255796078972, 88.33224293864769550 ) ) ;
#178529=CARTESIAN_POINT ( 'NONE',  ( 15.72974639402176855, 15.80617190586768217, 26.87609039468567218 ) ) ;
#178530=CARTESIAN_POINT ( 'NONE',  ( -14.34966873604972548, 8.224510206698743886, 48.33442372801902565 ) ) ;
#178531=CARTESIAN_POINT ( 'NONE',  ( 5.719274019375991003, -21.55341960407610458, 52.70724293864769550 ) ) ;
#178532=CARTESIAN_POINT ( 'NONE',  ( -5.153800228976607833, 19.02544592524334988, 22.70942372801899012 ) ) ;
#178533=CARTESIAN_POINT ( 'NONE',  ( 5.153800228976335163, 19.02544592524342804, 49.79057627198100988 ) ) ;
#178534=FACE_OUTER_BOUND ( 'NONE', #26501, .T. ) ;
#178535=CARTESIAN_POINT ( 'NONE',  ( -16.51473224551069308, -9.474510206698971260, 86.66557627198102409 ) ) ;
#178538=CARTESIAN_POINT ( 'NONE',  ( -19.02544592524334988, -5.153800228976617603, 68.95942372801896170 ) ) ;
#178539=CARTESIAN_POINT ( 'NONE',  ( -21.53943276465977519, 0.05219959533907696930, 51.24890960531436690 ) ) ;
#178540=CARTESIAN_POINT ( 'NONE',  ( 16.55341960407611168, 4.379528057220329451, 28.95724293864769905 ) ) ;
#178541=CARTESIAN_POINT ( 'NONE',  ( 13.89961937509957401, 13.97604488694547697, 86.87609039468567573 ) ) ;
#178542=CARTESIAN_POINT ( 'NONE',  ( 17.50000000000000000, -5.499999999999992895, 51.21769037696435589 ) ) ;
#178543=CARTESIAN_POINT ( 'NONE',  ( 18.67979575497194134, -10.72451020669871369, 110.8344237280190043 ) ) ;
#178544=CARTESIAN_POINT ( 'NONE',  ( -19.05341960407617563, 5.049401038297882671, 103.5427570613523329 ) ) ;
#178545=CARTESIAN_POINT ( 'NONE',  ( 9.564922557961047289, -16.46253265017146816, 50.41775706135233293 ) ) ;
#178546=CARTESIAN_POINT ( 'NONE',  ( 16.18388926212239198, 7.379444403734514601, 107.9395315136615920 ) ) ;
#178547=CARTESIAN_POINT ( 'NONE',  ( 9.474510206698971260, -16.51473224551069308, 52.91557627198102409 ) ) ;
#178548=CARTESIAN_POINT ( 'NONE',  ( 14.29746914071049879, -8.314922557960816363, 68.33224293864769550 ) ) ;
#178549=CARTESIAN_POINT ( 'NONE',  ( 0.05219959533909260263, 19.03943276465977164, 34.99890960531435979 ) ) ;
#178550=CARTESIAN_POINT ( 'NONE',  ( -14.29746914071049879, 8.314922557960819915, 40.83224293864769550 ) ) ;
#178552=CARTESIAN_POINT ( 'NONE',  ( 12.06949235617739724, 12.14591786802326823, 101.8760903946857042 ) ) ;
#178553=CARTESIAN_POINT ( 'NONE',  ( 5.153800228976335163, 19.02544592524342804, 69.79057627198103830 ) ) ;
#178554=CARTESIAN_POINT ( 'NONE',  ( -9.474510206698720793, -16.51473224551083518, 24.58442372801900078 ) ) ;
#178555=CARTESIAN_POINT ( 'NONE',  ( 4.379528057220092307, 16.55341960407617563, 32.29275706135235424 ) ) ;
#178556=CARTESIAN_POINT ( 'NONE',  ( -5.823673210054116645, -21.52544592524344225, 42.29057627198103120 ) ) ;
#178557=CARTESIAN_POINT ( 'NONE',  ( 5.719274019375673035, 21.55341960407619339, 102.2927570613523613 ) ) ;
#178559=CARTESIAN_POINT ( 'NONE',  ( 19.03943276465977164, -0.05219959533909143690, 63.74890960531435979 ) ) ;
#178560=CARTESIAN_POINT ( 'NONE',  ( 9.474510206698971260, -16.51473224551069308, 102.9155762719810241 ) ) ;
#178561=CARTESIAN_POINT ( 'NONE',  ( -5.049401038298153566, 19.05341960407611168, 100.2072429386476955 ) ) ;
#178563=CARTESIAN_POINT ( 'NONE',  ( 15.80617190586769283, -15.72974639402175789, 25.62609039468567929 ) ) ;
#178564=CARTESIAN_POINT ( 'NONE',  ( -16.52544592524342804, 4.483927247898546575, 96.04057627198102409 ) ) ;
#178565=CARTESIAN_POINT ( 'NONE',  ( 5.823673210054125526, 21.52544592524343514, 69.79057627198102409 ) ) ;
#178566=CARTESIAN_POINT ( 'NONE',  ( -5.049401038298153566, 19.05341960407611168, 70.20724293864769550 ) ) ;
#178567=CARTESIAN_POINT ( 'NONE',  ( 13.97604488694527802, 13.89961937509977652, 79.37390960531435269 ) ) ;
#178568=CARTESIAN_POINT ( 'NONE',  ( -0.05219959533907301413, -21.53943276465977519, 112.4989096053143669 ) ) ;
#178569=EDGE_CURVE ( 'NONE', #122302, #107085, #144786, .T. ) ;
#178571=CARTESIAN_POINT ( 'NONE',  ( 5.049401038298161559, -19.05341960407611168, 77.70724293864765286 ) ) ;
#178573=CARTESIAN_POINT ( 'NONE',  ( 16.52544592524342804, -4.483927247898539470, 103.5405762719810383 ) ) ;
#178575=CARTESIAN_POINT ( 'NONE',  ( 13.97604488694527802, 13.89961937509977652, 64.37390960531436690 ) ) ;
#178576=CARTESIAN_POINT ( 'NONE',  ( -19.03943276465977164, -0.05219959533935918106, 88.75109039468567573 ) ) ;
#178577=CARTESIAN_POINT ( 'NONE',  ( -16.52544592524342804, 4.483927247898546575, 96.04057627198102409 ) ) ;
#178578=CARTESIAN_POINT ( 'NONE',  ( -15.72974639402176322, -15.80617190586768395, 69.37609039468567573 ) ) ;
#178579=CARTESIAN_POINT ( 'NONE',  ( -0.05219959533909027116, -19.03943276465977164, 52.49890960531436690 ) ) ;
#178580=CARTESIAN_POINT ( 'NONE',  ( 21.55341960407619695, -5.719274019375665929, 21.04275706135234714 ) ) ;
#178581=CARTESIAN_POINT ( 'NONE',  ( 5.719274019375991003, -21.55341960407610458, 112.7072429386476955 ) ) ;
#178583=CARTESIAN_POINT ( 'NONE',  ( -19.03943276465977164, 0.05219959533909376836, 76.24890960531435269 ) ) ;
#178584=CARTESIAN_POINT ( 'NONE',  ( 17.40805194822031865, 6.112264579159319311, 111.6662872748938895 ) ) ;
#178585=CARTESIAN_POINT ( 'NONE',  ( -16.51473224551082808, 9.474510206698731452, 113.3344237280190043 ) ) ;
#178586=CARTESIAN_POINT ( 'NONE',  ( -15.72974639402197994, 15.80617190586746368, 35.62390960531437401 ) ) ;
#178587=CARTESIAN_POINT ( 'NONE',  ( -21.53943276465977519, -0.05219959533937600094, 63.75109039468568284 ) ) ;
#178588=CARTESIAN_POINT ( 'NONE',  ( -0.05219959533909027116, -19.03943276465977164, 102.4989096053143669 ) ) ;
#178589=CARTESIAN_POINT ( 'NONE',  ( -5.049401038297874678, -19.05341960407617918, 89.79275706135230450 ) ) ;
#178591=CARTESIAN_POINT ( 'NONE',  ( 19.03943276465977164, -0.05219959533909143690, 48.74890960531435979 ) ) ;
#178592=CARTESIAN_POINT ( 'NONE',  ( 5.153800228976335163, 19.02544592524342804, 69.79057627198103830 ) ) ;
#178593=CARTESIAN_POINT ( 'NONE',  ( 14.34966873604960469, 8.224510206698951720, 84.16557627198103830 ) ) ;
#178594=CARTESIAN_POINT ( 'NONE',  ( 9.474510206698971260, -16.51473224551069308, 107.9155762719810383 ) ) ;
#178595=CARTESIAN_POINT ( 'NONE',  ( 16.52544592524342804, -4.483927247898539470, 98.54057627198105251 ) ) ;
#178596=CARTESIAN_POINT ( 'NONE',  ( 9.474510206698971260, -16.51473224551069308, 97.91557627198102409 ) ) ;
#178597=CARTESIAN_POINT ( 'NONE',  ( 16.53943276465976808, -0.05219959533910856209, 43.74890960531435979 ) ) ;
#178598=CARTESIAN_POINT ( 'NONE',  ( -9.564922557960796823, -16.46253265017161027, 22.08224293864768839 ) ) ;
#178600=CARTESIAN_POINT ( 'NONE',  ( -0.05219959533937732626, 21.53943276465977519, 62.50109039468568284 ) ) ;
#178601=CARTESIAN_POINT ( 'NONE',  ( -16.46253265017146816, -9.564922557961047289, 74.16775706135234714 ) ) ;
#178602=CARTESIAN_POINT ( 'NONE',  ( 14.29746914071049879, -8.314922557960816363, 43.33224293864769550 ) ) ;
#178603=CARTESIAN_POINT ( 'NONE',  ( -18.62759615963270932, 10.81492255796079327, 95.83224293864770971 ) ) ;
#178604=CARTESIAN_POINT ( 'NONE',  ( -21.53943276465977519, 0.05219959533907696930, 31.24890960531435979 ) ) ;
#178605=CARTESIAN_POINT ( 'NONE',  ( -12.06949235617756955, 12.14591786802309770, 85.62390960531436690 ) ) ;
#178606=CARTESIAN_POINT ( 'NONE',  ( -13.97604488694527625, -13.89961937509977652, 51.87390960531436690 ) ) ;
#178607=CARTESIAN_POINT ( 'NONE',  ( 16.53943276465976808, -0.05219959533910856209, 23.74890960531435269 ) ) ;
#178608=CARTESIAN_POINT ( 'NONE',  ( 14.29746914071037800, 8.314922557961029526, 96.66775706135234714 ) ) ;
#178609=CARTESIAN_POINT ( 'NONE',  ( -14.34966873604972548, 8.224510206698743886, 73.33442372801901854 ) ) ;
#178610=CARTESIAN_POINT ( 'NONE',  ( 16.51473224551083163, -9.474510206698727899, 25.83442372801900078 ) ) ;
#178611=CARTESIAN_POINT ( 'NONE',  ( 9.564922557960805705, 16.46253265017160317, 99.58224293864770971 ) ) ;
#178612=CARTESIAN_POINT ( 'NONE',  ( 9.474510206698971260, -16.51473224551069308, 77.91557627198103830 ) ) ;
#178613=CARTESIAN_POINT ( 'NONE',  ( -9.474510206698964154, 16.51473224551069663, 35.41557627198102409 ) ) ;
#178614=CARTESIAN_POINT ( 'NONE',  ( -14.29746914071049879, 8.314922557960819915, 45.83224293864769550 ) ) ;
#178615=CARTESIAN_POINT ( 'NONE',  ( 9.564922557960805705, 16.46253265017160317, 114.5822429386476955 ) ) ;
#178616=CARTESIAN_POINT ( 'NONE',  ( -9.474510206698964154, 16.51473224551069663, 100.4155762719810241 ) ) ;
#178617=CARTESIAN_POINT ( 'NONE',  ( -10.81492255796078084, -18.62759615963271287, 37.08224293864768129 ) ) ;
#178618=CARTESIAN_POINT ( 'NONE',  ( 8.224510206698953496, -14.34966873604960469, 72.91557627198103830 ) ) ;
#178619=CARTESIAN_POINT ( 'NONE',  ( -16.53943276465976808, -0.05219959533934237506, 23.75109039468567929 ) ) ;
#178621=CARTESIAN_POINT ( 'NONE',  ( -12.14591786802309592, -12.06949235617757132, 66.87390960531436690 ) ) ;
#178623=CARTESIAN_POINT ( 'NONE',  ( 13.89961937509957401, 13.97604488694547697, 61.87609039468566863 ) ) ;
#178624=CARTESIAN_POINT ( 'NONE',  ( -19.02544592524342804, 5.153800228976336051, 101.0405762719810241 ) ) ;
#178625=CARTESIAN_POINT ( 'NONE',  ( -5.153800228976607833, 19.02544592524334988, 82.70942372801897591 ) ) ;
#178626=CARTESIAN_POINT ( 'NONE',  ( -9.474510206698720793, -16.51473224551083518, 94.58442372801900433 ) ) ;
#178627=CARTESIAN_POINT ( 'NONE',  ( 14.34966873604972726, -8.224510206698740333, 20.83442372801901143 ) ) ;
#178628=CARTESIAN_POINT ( 'NONE',  ( 16.52544592524335698, 4.483927247898782831, 96.45942372801901854 ) ) ;
#178629=CARTESIAN_POINT ( 'NONE',  ( 19.03943276465977164, -0.05219959533909143690, 38.74890960531436690 ) ) ;
#178630=CARTESIAN_POINT ( 'NONE',  ( -10.72451020669898014, 18.67979575497178502, 30.41557627198101699 ) ) ;
#178631=CARTESIAN_POINT ( 'NONE',  ( 0.05219959533937995610, -21.53943276465977519, 50.00109039468568994 ) ) ;
#178632=CARTESIAN_POINT ( 'NONE',  ( 19.53392245597576604, 5.500000000000095035, 37.87441121409608513 ) ) ;
#178633=CARTESIAN_POINT ( 'NONE',  ( 14.34966873604972726, -8.224510206698740333, 20.83442372801901143 ) ) ;
#178634=CARTESIAN_POINT ( 'NONE',  ( 17.49999999999998934, 3.215008338131321697, 22.54447599092367227 ) ) ;
#178635=CARTESIAN_POINT ( 'NONE',  ( -19.03943276465977164, 0.05219959533909376836, 71.24890960531435269 ) ) ;
#178637=CARTESIAN_POINT ( 'NONE',  ( -14.29746914071049879, 8.314922557960819915, 90.83224293864769550 ) ) ;
#178638=CARTESIAN_POINT ( 'NONE',  ( -9.564922557960796823, -16.46253265017161027, 82.08224293864768129 ) ) ;
#178639=CARTESIAN_POINT ( 'NONE',  ( 9.474510206698971260, -16.51473224551069308, 82.91557627198103830 ) ) ;
#178641=CARTESIAN_POINT ( 'NONE',  ( 19.03943276465977164, 0.05219959533936151252, 86.25109039468567573 ) ) ;
#178642=CARTESIAN_POINT ( 'NONE',  ( -10.81492255796078084, -18.62759615963271287, 62.08224293864769550 ) ) ;
#178643=CARTESIAN_POINT ( 'NONE',  ( 19.03943276465977164, -0.05219959533909143690, 23.74890960531435269 ) ) ;
#178644=CARTESIAN_POINT ( 'NONE',  ( 19.02544592524334988, 5.153800228976608722, 51.45942372801900433 ) ) ;
#178645=CARTESIAN_POINT ( 'NONE',  ( -19.02544592524342804, 5.153800228976336051, 56.04057627198100988 ) ) ;
#178646=CARTESIAN_POINT ( 'NONE',  ( 19.05341960407611168, 5.049401038298154454, 93.95724293864769550 ) ) ;
#178648=CARTESIAN_POINT ( 'NONE',  ( -5.719274019375978568, 21.55341960407610458, 90.20724293864770971 ) ) ;
#178649=CARTESIAN_POINT ( 'NONE',  ( 16.53943276465976808, -0.05219959533910856209, 93.74890960531436690 ) ) ;
#178650=CARTESIAN_POINT ( 'NONE',  ( 13.89961937509977652, -13.97604488694527269, 83.12390960531436690 ) ) ;
#178651=CARTESIAN_POINT ( 'NONE',  ( -13.97604488694547697, 13.89961937509957934, 58.12609039468566863 ) ) ;
#178652=CARTESIAN_POINT ( 'NONE',  ( -21.53943276465977519, 0.05219959533907696930, 86.24890960531436690 ) ) ;
#178653=CARTESIAN_POINT ( 'NONE',  ( -0.05219959533907301413, -21.53943276465977519, 72.49890960531435269 ) ) ;
#178654=CARTESIAN_POINT ( 'NONE',  ( 14.34966873604960469, 8.224510206698951720, 29.16557627198103120 ) ) ;
#178655=CARTESIAN_POINT ( 'NONE',  ( 18.67979575497194134, -10.72451020669871369, 110.8344237280190043 ) ) ;
#178656=CARTESIAN_POINT ( 'NONE',  ( -14.34966873604972548, 8.224510206698743886, 58.33442372801901143 ) ) ;
#178657=CARTESIAN_POINT ( 'NONE',  ( -9.474510206698964154, 16.51473224551069663, 75.41557627198103830 ) ) ;
#178658=CARTESIAN_POINT ( 'NONE',  ( -0.05219959533909027116, -19.03943276465977164, 27.49890960531435624 ) ) ;
#178659=CARTESIAN_POINT ( 'NONE',  ( 18.67979575497194134, -10.72451020669871369, 45.83442372801901854 ) ) ;
#178660=CARTESIAN_POINT ( 'NONE',  ( 15.72974639402176855, 15.80617190586768217, 51.87609039468568284 ) ) ;
#178661=CARTESIAN_POINT ( 'NONE',  ( -0.05219959533909027116, -19.03943276465977164, 47.49890960531435979 ) ) ;
#178662=CARTESIAN_POINT ( 'NONE',  ( -18.62759615963270932, 10.81492255796079327, 115.8322429386477097 ) ) ;
#178663=CARTESIAN_POINT ( 'NONE',  ( 13.97604488694548053, -13.89961937509957401, 65.62609039468567573 ) ) ;
#178664=CARTESIAN_POINT ( 'NONE',  ( -5.049401038297874678, -19.05341960407617918, 69.79275706135233293 ) ) ;
#178665=CARTESIAN_POINT ( 'NONE',  ( 12.06949235617739724, 12.14591786802326823, 31.87609039468567929 ) ) ;
#178666=CARTESIAN_POINT ( 'NONE',  ( -9.474510206698964154, 16.51473224551069663, 25.41557627198103120 ) ) ;
#178667=CARTESIAN_POINT ( 'NONE',  ( -8.314922557961024197, 14.29746914071037800, 67.91775706135234714 ) ) ;
#178668=CARTESIAN_POINT ( 'NONE',  ( 16.51473224551069308, 9.474510206698969483, 49.16557627198102409 ) ) ;
#178670=CARTESIAN_POINT ( 'NONE',  ( -19.02544592524342804, 5.153800228976336051, 96.04057627198103830 ) ) ;
#178671=CARTESIAN_POINT ( 'NONE',  ( 5.153800228976335163, 19.02544592524342804, 29.79057627198102409 ) ) ;
#178672=CARTESIAN_POINT ( 'NONE',  ( -18.67979575497178146, -10.72451020669898902, 66.66557627198102409 ) ) ;
#178673=CARTESIAN_POINT ( 'NONE',  ( 16.55341960407618274, -4.379528057220086978, 66.04275706135236135 ) ) ;
#178674=CARTESIAN_POINT ( 'NONE',  ( -5.049401038297874678, -19.05341960407617918, 19.79275706135233293 ) ) ;
#178675=EDGE_CURVE ( 'NONE', #14026, #15707, #154274, .T. ) ;
#178676=CARTESIAN_POINT ( 'NONE',  ( -5.153800228976328057, -19.02544592524343514, 47.29057627198102409 ) ) ;
#178677=CARTESIAN_POINT ( 'NONE',  ( -0.05219959533910754901, -16.53943276465976808, 32.49890960531435979 ) ) ;
#178678=CARTESIAN_POINT ( 'NONE',  ( -14.34966873604960291, -8.224510206698953496, 66.66557627198102409 ) ) ;
#178679=CARTESIAN_POINT ( 'NONE',  ( 13.97604488694527802, 13.89961937509977652, 74.37390960531436690 ) ) ;
#178680=CARTESIAN_POINT ( 'NONE',  ( -15.80617190586768217, 15.72974639402176855, 43.12609039468568284 ) ) ;
#178681=CARTESIAN_POINT ( 'NONE',  ( -19.05341960407611168, -5.049401038298163336, 91.45724293864766707 ) ) ;
#178683=CARTESIAN_POINT ( 'NONE',  ( 21.53943276465977519, 0.05219959533937863772, 86.25109039468568994 ) ) ;
#178684=CARTESIAN_POINT ( 'NONE',  ( 8.314922557961029526, -14.29746914071037800, 60.41775706135235424 ) ) ;
#178685=CARTESIAN_POINT ( 'NONE',  ( -0.05219959533909027116, -19.03943276465977164, 107.4989096053143527 ) ) ;
#178687=CARTESIAN_POINT ( 'NONE',  ( 21.53943276465977519, -0.05219959533907433946, 88.74890960531436690 ) ) ;
#178688=CARTESIAN_POINT ( 'NONE',  ( 12.06949235617757843, -12.14591786802309237, 43.12390960531435269 ) ) ;
#178689=CARTESIAN_POINT ( 'NONE',  ( 19.05341960407611168, 5.049401038298154454, 28.95724293864769550 ) ) ;
#178690=CARTESIAN_POINT ( 'NONE',  ( 4.379528057220092307, 16.55341960407617563, 52.29275706135236135 ) ) ;
#178691=CARTESIAN_POINT ( 'NONE',  ( -12.06949235617756955, 12.14591786802309770, 70.62390960531436690 ) ) ;
#178692=CARTESIAN_POINT ( 'NONE',  ( 18.62759615963271287, -10.81492255796078972, 23.33224293864769194 ) ) ;
#178693=CARTESIAN_POINT ( 'NONE',  ( 21.55341960407610458, 5.719274019375980345, 33.95724293864769550 ) ) ;
#178694=CARTESIAN_POINT ( 'NONE',  ( -5.823673210054431948, 21.52544592524334988, 112.7094237280190328 ) ) ;
#178695=CARTESIAN_POINT ( 'NONE',  ( 16.52544592524342804, -4.483927247898539470, 98.54057627198105251 ) ) ;
#178696=CARTESIAN_POINT ( 'NONE',  ( -0.05219959533909027116, -19.03943276465977164, 107.4989096053143527 ) ) ;
#178698=CARTESIAN_POINT ( 'NONE',  ( 4.483927247898790824, -16.52544592524335698, 50.20942372801901854 ) ) ;
#178699=CARTESIAN_POINT ( 'NONE',  ( 19.02544592524343514, -5.153800228976328945, 53.54057627198102409 ) ) ;
#178700=CARTESIAN_POINT ( 'NONE',  ( -30.00000000000000000, -1.163414459189985801E-14, 95.00000000000000000 ) ) ;
#178701=CARTESIAN_POINT ( 'NONE',  ( 9.564922557961047289, -16.46253265017146816, 45.41775706135232582 ) ) ;
#178702=CARTESIAN_POINT ( 'NONE',  ( -16.52544592524335698, -4.483927247898792601, 93.95942372801903275 ) ) ;
#178703=CARTESIAN_POINT ( 'NONE',  ( -13.89961937509957401, -13.97604488694547875, 89.37609039468563310 ) ) ;
#178704=CARTESIAN_POINT ( 'NONE',  ( 18.62759615963255655, 10.81492255796105972, 71.66775706135234714 ) ) ;
#178705=CARTESIAN_POINT ( 'NONE',  ( 19.05341960407611168, 5.049401038298154454, 68.95724293864769550 ) ) ;
#178706=CARTESIAN_POINT ( 'NONE',  ( -15.80617190586745835, -15.72974639402198527, 96.87390960531436690 ) ) ;
#178707=CARTESIAN_POINT ( 'NONE',  ( -0.05219959533909027116, -19.03943276465977164, 22.49890960531436690 ) ) ;
#178708=CARTESIAN_POINT ( 'NONE',  ( -0.05219959533936034679, 19.03943276465977164, 77.50109039468566152 ) ) ;
#178709=CARTESIAN_POINT ( 'NONE',  ( -0.05219959533907301413, -21.53943276465977519, 72.49890960531435269 ) ) ;
#178710=CARTESIAN_POINT ( 'NONE',  ( 5.049401038297881783, 19.05341960407617563, 37.29275706135232582 ) ) ;
#178711=CARTESIAN_POINT ( 'NONE',  ( 19.19724070472095434, 5.500000000000029310, 98.56193348274383936 ) ) ;
#178713=CARTESIAN_POINT ( 'NONE',  ( 15.80617190586746368, 15.72974639402197994, 84.37390960531438111 ) ) ;
#178714=CARTESIAN_POINT ( 'NONE',  ( 13.89961937509977652, -13.97604488694527269, 68.12390960531436690 ) ) ;
#178715=CARTESIAN_POINT ( 'NONE',  ( -18.22780087662123094, -5.499999999999984901, 91.48459894673894155 ) ) ;
#178716=CARTESIAN_POINT ( 'NONE',  ( 0.05219959533934541429, -16.53943276465976808, 25.00109039468567218 ) ) ;
#178717=CARTESIAN_POINT ( 'NONE',  ( -0.05219959533936034679, 19.03943276465977164, 97.50109039468567573 ) ) ;
#178718=CARTESIAN_POINT ( 'NONE',  ( 13.89961937509977652, -13.97604488694527269, 43.12390960531434558 ) ) ;
#178719=CARTESIAN_POINT ( 'NONE',  ( 9.564922557960805705, 16.46253265017160317, 109.5822429386476955 ) ) ;
#178720=CARTESIAN_POINT ( 'NONE',  ( 15.72974639402199770, -15.80617190586745480, 108.1239096053143811 ) ) ;
#178721=CARTESIAN_POINT ( 'NONE',  ( 4.483927247898545687, 16.52544592524342804, 44.79057627198103120 ) ) ;
#178722=CARTESIAN_POINT ( 'NONE',  ( 15.72974639402176855, 15.80617190586768217, 71.87609039468568994 ) ) ;
#178723=CARTESIAN_POINT ( 'NONE',  ( -8.224510206698735004, -14.34966873604973081, 24.58442372801901499 ) ) ;
#178724=CARTESIAN_POINT ( 'NONE',  ( 9.474510206698729675, 16.51473224551082808, 27.08442372801900433 ) ) ;
#178725=CARTESIAN_POINT ( 'NONE',  ( -12.14591786802309592, -12.06949235617757132, 31.87390960531435979 ) ) ;
#178726=CARTESIAN_POINT ( 'NONE',  ( -15.80617190586745835, -15.72974639402198527, 111.8739096053143669 ) ) ;
#178727=CARTESIAN_POINT ( 'NONE',  ( -8.314922557960811034, -14.29746914071050412, 52.08224293864768839 ) ) ;
#178728=CARTESIAN_POINT ( 'NONE',  ( -19.03943276465977164, -0.05219959533935918106, 93.75109039468566152 ) ) ;
#178729=CARTESIAN_POINT ( 'NONE',  ( 5.049401038297881783, 19.05341960407617563, 67.29275706135234714 ) ) ;
#178730=CARTESIAN_POINT ( 'NONE',  ( 15.80617190586769283, -15.72974639402175789, 65.62609039468568994 ) ) ;
#178731=CARTESIAN_POINT ( 'NONE',  ( 13.89961937509957401, 13.97604488694547697, 56.87609039468564731 ) ) ;
#178732=CARTESIAN_POINT ( 'NONE',  ( 16.53943276465976808, -0.05219959533910856209, 113.7489096053143527 ) ) ;
#178733=CARTESIAN_POINT ( 'NONE',  ( -5.719274019375978568, 21.55341960407610458, 40.20724293864769550 ) ) ;
#178734=CARTESIAN_POINT ( 'NONE',  ( 16.55341960407611168, 4.379528057220329451, 48.95724293864770971 ) ) ;
#178735=CARTESIAN_POINT ( 'NONE',  ( -17.50000000000003197, -5.622605283950793620, 26.31207310596111171 ) ) ;
#178736=CARTESIAN_POINT ( 'NONE',  ( -19.05341960407617563, 5.049401038297882671, 23.54275706135233648 ) ) ;
#178737=CARTESIAN_POINT ( 'NONE',  ( -8.224510206698735004, -14.34966873604973081, 79.58442372801903275 ) ) ;
#178738=CARTESIAN_POINT ( 'NONE',  ( 16.55341960407611168, 4.379528057220329451, 33.95724293864769550 ) ) ;
#178739=CARTESIAN_POINT ( 'NONE',  ( 10.72451020669871369, 18.67979575497193778, 82.08442372801901854 ) ) ;
#178740=CARTESIAN_POINT ( 'NONE',  ( 21.55341960407619695, -5.719274019375665929, 81.04275706135236135 ) ) ;
#178741=CARTESIAN_POINT ( 'NONE',  ( 18.67979575497178502, 10.72451020669898547, 84.16557627198103830 ) ) ;
#178742=CARTESIAN_POINT ( 'NONE',  ( 13.89961937509977652, -13.97604488694527269, 38.12390960531436690 ) ) ;
#178743=CARTESIAN_POINT ( 'NONE',  ( -5.719274019375665041, -21.55341960407619695, 59.79275706135234714 ) ) ;
#178744=CARTESIAN_POINT ( 'NONE',  ( 16.46253265017160672, -9.564922557960803928, 38.33224293864768839 ) ) ;
#178745=CARTESIAN_POINT ( 'NONE',  ( 19.05341960407611168, 5.049401038298154454, 53.95724293864770260 ) ) ;
#178746=CARTESIAN_POINT ( 'NONE',  ( 8.314922557960818139, 14.29746914071049879, 89.58224293864768129 ) ) ;
#178747=CARTESIAN_POINT ( 'NONE',  ( 19.03943276465977164, -0.05219959533909143690, 93.74890960531435269 ) ) ;
#178748=CARTESIAN_POINT ( 'NONE',  ( -4.483927247898539470, -16.52544592524342804, 42.29057627198103120 ) ) ;
#178749=CARTESIAN_POINT ( 'NONE',  ( 16.53943276465976808, -0.05219959533910856209, 113.7489096053143527 ) ) ;
#178750=CARTESIAN_POINT ( 'NONE',  ( 0.05219959533907565091, 21.53943276465977519, 84.99890960531436690 ) ) ;
#178751=CARTESIAN_POINT ( 'NONE',  ( -21.55341960407619339, 5.719274019375674811, 28.54275706135234358 ) ) ;
#178753=CARTESIAN_POINT ( 'NONE',  ( 19.02544592524343514, -5.153800228976328945, 78.54057627198099567 ) ) ;
#178754=CARTESIAN_POINT ( 'NONE',  ( -16.51473224551082808, 9.474510206698731452, 113.3344237280190043 ) ) ;
#178755=CARTESIAN_POINT ( 'NONE',  ( 21.53943276465977519, -0.05219959533907433946, 73.74890960531433848 ) ) ;
#178756=CARTESIAN_POINT ( 'NONE',  ( 21.55341960407619695, -5.719274019375665929, 91.04275706135236135 ) ) ;
#178757=CARTESIAN_POINT ( 'NONE',  ( -13.89961937509977652, 13.97604488694528158, 75.62390960531438111 ) ) ;
#178758=CARTESIAN_POINT ( 'NONE',  ( -18.67979575497193778, 10.72451020669871902, 28.33442372801902209 ) ) ;
#178760=CARTESIAN_POINT ( 'NONE',  ( -0.05219959533909027116, -19.03943276465977164, 112.4989096053143669 ) ) ;
#178761=CARTESIAN_POINT ( 'NONE',  ( 8.314922557961029526, -14.29746914071037800, 95.41775706135234714 ) ) ;
#178762=CARTESIAN_POINT ( 'NONE',  ( 5.719274019375673035, 21.55341960407619339, 77.29275706135234714 ) ) ;
#178763=CARTESIAN_POINT ( 'NONE',  ( -5.719274019375665041, -21.55341960407619695, 104.7927570613523898 ) ) ;
#178764=CARTESIAN_POINT ( 'NONE',  ( -8.224510206698735004, -14.34966873604973081, 74.58442372801901854 ) ) ;
#178765=CARTESIAN_POINT ( 'NONE',  ( 21.53943276465977519, 0.05219959533937863772, 31.25109039468568639 ) ) ;
#178766=CARTESIAN_POINT ( 'NONE',  ( -19.02544592524342804, 5.153800228976336051, 116.0405762719810383 ) ) ;
#178767=CARTESIAN_POINT ( 'NONE',  ( 21.55341960407619695, -5.719274019375665929, 96.04275706135236135 ) ) ;
#178768=CARTESIAN_POINT ( 'NONE',  ( -5.049401038298153566, 19.05341960407611168, 90.20724293864766707 ) ) ;
#178769=CARTESIAN_POINT ( 'NONE',  ( -18.62759615963270932, 10.81492255796079327, 95.83224293864770971 ) ) ;
#178770=CARTESIAN_POINT ( 'NONE',  ( -16.46253265017146816, -9.564922557961047289, 64.16775706135233293 ) ) ;
#178771=CARTESIAN_POINT ( 'NONE',  ( 19.49190055781010855, 5.500000000000050626, 83.06116087098779133 ) ) ;
#178772=CARTESIAN_POINT ( 'NONE',  ( -5.823673210054116645, -21.52544592524344225, 47.29057627198103120 ) ) ;
#178773=CARTESIAN_POINT ( 'NONE',  ( -19.02544592524342804, 5.153800228976336051, 101.0405762719810241 ) ) ;
#178774=CARTESIAN_POINT ( 'NONE',  ( 16.55341960407611168, 4.379528057220329451, 53.95724293864770260 ) ) ;
#178776=CARTESIAN_POINT ( 'NONE',  ( 13.97604488694548053, -13.89961937509957401, 80.62609039468567573 ) ) ;
#178778=CARTESIAN_POINT ( 'NONE',  ( -19.02544592524334988, -5.153800228976617603, 103.9594237280190043 ) ) ;
#178779=CARTESIAN_POINT ( 'NONE',  ( 18.62759615963271287, -10.81492255796078972, 83.33224293864769550 ) ) ;
#178780=CARTESIAN_POINT ( 'NONE',  ( -4.379528057220328563, 16.55341960407611168, 65.20724293864768129 ) ) ;
#178781=CARTESIAN_POINT ( 'NONE',  ( -19.05341960407611168, -5.049401038298163336, 101.4572429386476955 ) ) ;
#178782=CARTESIAN_POINT ( 'NONE',  ( -8.314922557961024197, 14.29746914071037800, 32.91775706135234714 ) ) ;
#178783=CARTESIAN_POINT ( 'NONE',  ( -5.049401038298153566, 19.05341960407611168, 55.20724293864769550 ) ) ;
#178784=CARTESIAN_POINT ( 'NONE',  ( 10.72451020669898902, -18.67979575497178502, 112.9155762719810383 ) ) ;
#178785=CARTESIAN_POINT ( 'NONE',  ( 19.03943276465977164, 0.05219959533936151252, 86.25109039468567573 ) ) ;
#178786=CARTESIAN_POINT ( 'NONE',  ( -9.564922557960796823, -16.46253265017161027, 92.08224293864769550 ) ) ;
#178787=CARTESIAN_POINT ( 'NONE',  ( -19.05341960407611168, -5.049401038298163336, 71.45724293864766707 ) ) ;
#178788=CARTESIAN_POINT ( 'NONE',  ( 5.719274019375991003, -21.55341960407610458, 72.70724293864769550 ) ) ;
#178789=CARTESIAN_POINT ( 'NONE',  ( 9.564922557960805705, 16.46253265017160317, 49.58224293864770260 ) ) ;
#178791=CARTESIAN_POINT ( 'NONE',  ( 4.483927247898545687, 16.52544592524342804, 54.79057627198104541 ) ) ;
#178792=CARTESIAN_POINT ( 'NONE',  ( -9.474510206698964154, 16.51473224551069663, 100.4155762719810241 ) ) ;
#178794=CARTESIAN_POINT ( 'NONE',  ( 13.97604488694548053, -13.89961937509957401, 65.62609039468567573 ) ) ;
#178795=CARTESIAN_POINT ( 'NONE',  ( 21.52544592524344225, -5.823673210054117533, 93.54057627198103830 ) ) ;
#178796=CARTESIAN_POINT ( 'NONE',  ( 16.51473224551083163, -9.474510206698727899, 55.83442372801899722 ) ) ;
#178797=CARTESIAN_POINT ( 'NONE',  ( -19.03943276465977164, 0.05219959533909376836, 101.2489096053143669 ) ) ;
#178798=CARTESIAN_POINT ( 'NONE',  ( -17.50000000000003197, 4.658240926743175692, 113.9447041781680667 ) ) ;
#178799=CARTESIAN_POINT ( 'NONE',  ( 18.67979575497178502, 10.72451020669898547, 44.16557627198103120 ) ) ;
#178800=CARTESIAN_POINT ( 'NONE',  ( 0.05219959533909260263, 19.03943276465977164, 69.99890960531435269 ) ) ;
#178801=CARTESIAN_POINT ( 'NONE',  ( -21.53943276465977519, -0.05219959533937600094, 58.75109039468568994 ) ) ;
#178802=CARTESIAN_POINT ( 'NONE',  ( 9.564922557960805705, 16.46253265017160317, 34.58224293864770260 ) ) ;
#178803=CARTESIAN_POINT ( 'NONE',  ( -16.55341960407611168, -4.379528057220339221, 76.45724293864769550 ) ) ;
#178804=VERTEX_POINT ( 'NONE', #40830 ) ;
#178805=CARTESIAN_POINT ( 'NONE',  ( 21.55341960407619695, -5.719274019375665929, 51.04275706135234714 ) ) ;
#178807=CARTESIAN_POINT ( 'NONE',  ( 5.153800228976335163, 19.02544592524342804, 109.7905762719810099 ) ) ;
#178808=CARTESIAN_POINT ( 'NONE',  ( 13.89961937509957401, 13.97604488694547697, 61.87609039468566863 ) ) ;
#178810=CARTESIAN_POINT ( 'NONE',  ( -21.52544592524334988, -5.823673210054445271, 18.95942372801901143 ) ) ;
#178811=CARTESIAN_POINT ( 'NONE',  ( 16.46253265017160672, -9.564922557960803928, 63.33224293864769550 ) ) ;
#178812=CARTESIAN_POINT ( 'NONE',  ( -12.14591786802326823, 12.06949235617739902, 43.12609039468568284 ) ) ;
#178814=CARTESIAN_POINT ( 'NONE',  ( 19.05341960407617918, -5.049401038297876454, 21.04275706135232582 ) ) ;
#178815=CARTESIAN_POINT ( 'NONE',  ( -19.03943276465977164, 0.05219959533909376836, 41.24890960531435269 ) ) ;
#178816=CARTESIAN_POINT ( 'NONE',  ( -15.80617190586768217, 15.72974639402176855, 113.1260903946856899 ) ) ;
#178817=CARTESIAN_POINT ( 'NONE',  ( -14.29746914071037622, -8.314922557961029526, 94.16775706135237556 ) ) ;
#178818=CARTESIAN_POINT ( 'NONE',  ( 0.05219959533909260263, 19.03943276465977164, 84.99890960531436690 ) ) ;
#178819=CARTESIAN_POINT ( 'NONE',  ( 15.72974639402176855, 15.80617190586768217, 71.87609039468568994 ) ) ;
#178821=CARTESIAN_POINT ( 'NONE',  ( 5.049401038298161559, -19.05341960407611168, 112.7072429386476813 ) ) ;
#178822=CARTESIAN_POINT ( 'NONE',  ( -12.14591786802326823, 12.06949235617739902, 58.12609039468568994 ) ) ;
#178823=CARTESIAN_POINT ( 'NONE',  ( -18.67979575497193778, 10.72451020669871902, 68.33442372801900433 ) ) ;
#178824=CARTESIAN_POINT ( 'NONE',  ( 10.72451020669871369, 18.67979575497193778, 97.08442372801904696 ) ) ;
#178827=CARTESIAN_POINT ( 'NONE',  ( 16.53943276465976808, 0.05219959533934440121, 26.25109039468567573 ) ) ;
#178828=CARTESIAN_POINT ( 'NONE',  ( 0.05219959533909260263, 19.03943276465977164, 89.99890960531436690 ) ) ;
#178832=CARTESIAN_POINT ( 'NONE',  ( 5.049401038298161559, -19.05341960407611168, 32.70724293864768129 ) ) ;
#178833=CARTESIAN_POINT ( 'NONE',  ( -21.55341960407610458, -5.719274019375992779, 36.45724293864768839 ) ) ;
#178835=CARTESIAN_POINT ( 'NONE',  ( -16.52544592524335698, -4.483927247898792601, 103.9594237280190185 ) ) ;
#178836=CARTESIAN_POINT ( 'NONE',  ( 14.29746914071049879, -8.314922557960816363, 83.33224293864769550 ) ) ;
#178837=CARTESIAN_POINT ( 'NONE',  ( -16.46253265017160317, 9.564922557960807481, 70.83224293864770971 ) ) ;
#178838=CARTESIAN_POINT ( 'NONE',  ( 15.80617190586769283, -15.72974639402175789, 105.6260903946856899 ) ) ;
#178839=CARTESIAN_POINT ( 'NONE',  ( 12.14591786802327356, -12.06949235617739191, 30.62609039468567929 ) ) ;
#178840=CARTESIAN_POINT ( 'NONE',  ( -14.34966873604960291, -8.224510206698953496, 91.66557627198103830 ) ) ;
#178841=CARTESIAN_POINT ( 'NONE',  ( -18.67979575497193778, 10.72451020669871902, 43.33442372801901143 ) ) ;
#178842=CARTESIAN_POINT ( 'NONE',  ( 15.72974639402199770, -15.80617190586745480, 68.12390960531436690 ) ) ;
#178843=CARTESIAN_POINT ( 'NONE',  ( 9.564922557961047289, -16.46253265017146816, 50.41775706135233293 ) ) ;
#178845=CARTESIAN_POINT ( 'NONE',  ( -13.97604488694527625, -13.89961937509977652, 101.8739096053143811 ) ) ;
#178846=CARTESIAN_POINT ( 'NONE',  ( -16.53943276465976808, 0.05219959533911058130, 61.24890960531435979 ) ) ;
#178848=CARTESIAN_POINT ( 'NONE',  ( 12.06949235617757843, -12.14591786802309237, 48.12390960531436690 ) ) ;
#178849=CARTESIAN_POINT ( 'NONE',  ( 14.29746914071037800, 8.314922557961029526, 106.6677570613523756 ) ) ;
#178850=CARTESIAN_POINT ( 'NONE',  ( -0.05219959533936034679, 19.03943276465977164, 72.50109039468566152 ) ) ;
#178852=CARTESIAN_POINT ( 'NONE',  ( -0.05219959533909027116, -19.03943276465977164, 112.4989096053143669 ) ) ;
#178853=CARTESIAN_POINT ( 'NONE',  ( -4.379528057220328563, 16.55341960407611168, 85.20724293864770971 ) ) ;
#178855=CARTESIAN_POINT ( 'NONE',  ( 16.51473224551069308, 9.474510206698969483, 39.16557627198103120 ) ) ;
#178856=CARTESIAN_POINT ( 'NONE',  ( 21.55341960407610458, 5.719274019375980345, 48.95724293864770971 ) ) ;
#178857=CARTESIAN_POINT ( 'NONE',  ( 21.52544592524344225, -5.823673210054117533, 83.54057627198102409 ) ) ;
#178858=CARTESIAN_POINT ( 'NONE',  ( 16.51473224551069308, 9.474510206698969483, 24.16557627198102765 ) ) ;
#178859=CARTESIAN_POINT ( 'NONE',  ( 16.52544592524335698, 4.483927247898782831, 66.45942372801903275 ) ) ;
#178860=CARTESIAN_POINT ( 'NONE',  ( -19.05341960407611168, -5.049401038298163336, 56.45724293864768129 ) ) ;
#178861=CARTESIAN_POINT ( 'NONE',  ( 19.02544592524334988, 5.153800228976608722, 46.45942372801899012 ) ) ;
#178862=CARTESIAN_POINT ( 'NONE',  ( -21.52544592524334988, -5.823673210054445271, 48.95942372801902565 ) ) ;
#178863=CARTESIAN_POINT ( 'NONE',  ( -15.80617190586745835, -15.72974639402198527, 41.87390960531435979 ) ) ;
#178864=CARTESIAN_POINT ( 'NONE',  ( 14.34966873604960469, 8.224510206698951720, 104.1655762719810241 ) ) ;
#178865=CARTESIAN_POINT ( 'NONE',  ( -19.05341960407617563, 5.049401038297882671, 88.54275706135230450 ) ) ;
#178868=CARTESIAN_POINT ( 'NONE',  ( -5.719274019375978568, 21.55341960407610458, 45.20724293864769550 ) ) ;
#178869=CARTESIAN_POINT ( 'NONE',  ( 13.97604488694527802, 13.89961937509977652, 24.37390960531435624 ) ) ;
#178870=CARTESIAN_POINT ( 'NONE',  ( -0.05219959533937732626, 21.53943276465977519, 82.50109039468568994 ) ) ;
#178871=CARTESIAN_POINT ( 'NONE',  ( -16.55341960407611168, -4.379528057220339221, 36.45724293864768839 ) ) ;
#178872=CARTESIAN_POINT ( 'NONE',  ( 4.483927247898790824, -16.52544592524335698, 60.20942372801902565 ) ) ;
#178873=CARTESIAN_POINT ( 'NONE',  ( 16.53943276465976808, -0.05219959533910856209, 53.74890960531437401 ) ) ;
#178874=CARTESIAN_POINT ( 'NONE',  ( -15.80617190586745835, -15.72974639402198527, 76.87390960531439532 ) ) ;
#178875=CARTESIAN_POINT ( 'NONE',  ( 21.55341960407610458, 5.719274019375980345, 73.95724293864769550 ) ) ;
#178877=CARTESIAN_POINT ( 'NONE',  ( 13.89961937509957401, 13.97604488694547697, 81.87609039468564731 ) ) ;
#178878=CARTESIAN_POINT ( 'NONE',  ( -21.55341960407610458, -5.719274019375992779, 21.45724293864769550 ) ) ;
#178879=CARTESIAN_POINT ( 'NONE',  ( -13.89961937509977652, 13.97604488694528158, 65.62390960531436690 ) ) ;
#178880=CARTESIAN_POINT ( 'NONE',  ( 9.474510206698971260, -16.51473224551069308, 27.91557627198103120 ) ) ;
#178883=CARTESIAN_POINT ( 'NONE',  ( 16.52544592524335698, 4.483927247898782831, 86.45942372801901854 ) ) ;
#178884=CARTESIAN_POINT ( 'NONE',  ( 0.05219959533907565091, 21.53943276465977519, 114.9989096053143669 ) ) ;
#178885=CARTESIAN_POINT ( 'NONE',  ( 13.97604488694527802, 13.89961937509977652, 74.37390960531436690 ) ) ;
#178886=CARTESIAN_POINT ( 'NONE',  ( 18.62759615963255655, 10.81492255796105972, 41.66775706135235424 ) ) ;
#178887=CARTESIAN_POINT ( 'NONE',  ( 13.89961937509977652, -13.97604488694527269, 103.1239096053143527 ) ) ;
#178889=ORIENTED_EDGE ( 'NONE', *, *, #82905, .F. ) ;
#178890=CARTESIAN_POINT ( 'NONE',  ( -18.67979575497193778, 10.72451020669871902, 48.33442372801902565 ) ) ;
#178891=CARTESIAN_POINT ( 'NONE',  ( -16.51473224551069308, -9.474510206698971260, 26.66557627198103120 ) ) ;
#178892=CARTESIAN_POINT ( 'NONE',  ( 5.153800228976335163, 19.02544592524342804, 104.7905762719809957 ) ) ;
#178893=CARTESIAN_POINT ( 'NONE',  ( 5.049401038297881783, 19.05341960407617563, 47.29275706135231161 ) ) ;
#178894=CARTESIAN_POINT ( 'NONE',  ( 10.81492255796106328, -18.62759615963255655, 20.41775706135234714 ) ) ;
#178895=CARTESIAN_POINT ( 'NONE',  ( 9.474510206698729675, 16.51473224551082808, 52.08442372801900433 ) ) ;
#178896=CARTESIAN_POINT ( 'NONE',  ( -19.02544592524334988, -5.153800228976617603, 53.95942372801898301 ) ) ;
#178897=CARTESIAN_POINT ( 'NONE',  ( 14.29746914071037800, 8.314922557961029526, 106.6677570613523756 ) ) ;
#178901=CARTESIAN_POINT ( 'NONE',  ( -5.049401038298153566, 19.05341960407611168, 70.20724293864769550 ) ) ;
#178902=CARTESIAN_POINT ( 'NONE',  ( -10.72451020669870658, -18.67979575497194134, 74.58442372801901854 ) ) ;
#178903=CARTESIAN_POINT ( 'NONE',  ( 0.05219959533937995610, -21.53943276465977519, 95.00109039468568994 ) ) ;
#178905=CARTESIAN_POINT ( 'NONE',  ( 5.153800228976335163, 19.02544592524342804, 84.79057627198099567 ) ) ;
#178906=CARTESIAN_POINT ( 'NONE',  ( -21.55341960407619339, 5.719274019375674811, 58.54275706135235424 ) ) ;
#178907=CARTESIAN_POINT ( 'NONE',  ( -16.51473224551082808, 9.474510206698731452, 108.3344237280190043 ) ) ;
#178908=CARTESIAN_POINT ( 'NONE',  ( 13.97604488694527802, 13.89961937509977652, 69.37390960531436690 ) ) ;
#178909=CARTESIAN_POINT ( 'NONE',  ( -18.67979575497178146, -10.72451020669898902, 21.66557627198102409 ) ) ;
#178910=AXIS2_PLACEMENT_3D ( 'NONE', #104534, #25722, #166215 ) ;
#178911=CARTESIAN_POINT ( 'NONE',  ( 13.89961937509977652, -13.97604488694527269, 88.12390960531438111 ) ) ;
#178913=CARTESIAN_POINT ( 'NONE',  ( 19.05341960407611168, 5.049401038298154454, 83.95724293864766707 ) ) ;
#178914=CARTESIAN_POINT ( 'NONE',  ( -19.02544592524342804, 5.153800228976336051, 71.04057627198099567 ) ) ;
#178915=CARTESIAN_POINT ( 'NONE',  ( -21.53943276465977519, 0.05219959533907696930, 116.2489096053143669 ) ) ;
#178916=CARTESIAN_POINT ( 'NONE',  ( 16.55341960407618274, -4.379528057220086978, 101.0427570613523756 ) ) ;
#178918=CARTESIAN_POINT ( 'NONE',  ( -13.97604488694547697, 13.89961937509957934, 58.12609039468566863 ) ) ;
#178919=CARTESIAN_POINT ( 'NONE',  ( -16.46253265017160317, 9.564922557960807481, 95.83224293864769550 ) ) ;
#178920=CARTESIAN_POINT ( 'NONE',  ( 12.06949235617757843, -12.14591786802309237, 83.12390960531436690 ) ) ;
#178921=CARTESIAN_POINT ( 'NONE',  ( 4.379528057220339221, -16.55341960407611168, 107.7072429386476955 ) ) ;
#178922=CARTESIAN_POINT ( 'NONE',  ( 21.53943276465977519, -0.05219959533907433946, 38.74890960531435979 ) ) ;
#178923=CARTESIAN_POINT ( 'NONE',  ( -5.823673210054116645, -21.52544592524344225, 22.29057627198102765 ) ) ;
#178924=CARTESIAN_POINT ( 'NONE',  ( -16.52544592524342804, 4.483927247898546575, 91.04057627198103830 ) ) ;
#178925=CARTESIAN_POINT ( 'NONE',  ( -17.40805194822031865, 6.112264579159341515, 55.83371272510613181 ) ) ;
#178926=CARTESIAN_POINT ( 'NONE',  ( -9.564922557961040184, 16.46253265017147172, 42.91775706135234003 ) ) ;
#178927=CARTESIAN_POINT ( 'NONE',  ( 0.05219959533934541429, -16.53943276465976808, 110.0010903946856757 ) ) ;
#178928=CARTESIAN_POINT ( 'NONE',  ( 5.153800228976335163, 19.02544592524342804, 89.79057627198102409 ) ) ;
#178929=CARTESIAN_POINT ( 'NONE',  ( -21.52544592524334988, -5.823673210054445271, 68.95942372801901854 ) ) ;
#178930=CARTESIAN_POINT ( 'NONE',  ( -21.53943276465977519, 0.05219959533907696930, 46.24890960531435979 ) ) ;
#178931=CARTESIAN_POINT ( 'NONE',  ( -15.72974639402176322, -15.80617190586768395, 29.37609039468568284 ) ) ;
#178932=CARTESIAN_POINT ( 'NONE',  ( -18.67979575497178146, -10.72451020669898902, 81.66557627198103830 ) ) ;
#178933=CARTESIAN_POINT ( 'NONE',  ( -12.06949235617756955, 12.14591786802309770, 105.6239096053143669 ) ) ;
#178934=CARTESIAN_POINT ( 'NONE',  ( -9.474510206698720793, -16.51473224551083518, 74.58442372801900433 ) ) ;
#178935=CARTESIAN_POINT ( 'NONE',  ( -9.474510206698964154, 16.51473224551069663, 45.41557627198103120 ) ) ;
#178936=CARTESIAN_POINT ( 'NONE',  ( 9.564922557960805705, 16.46253265017160317, 99.58224293864770971 ) ) ;
#178937=CARTESIAN_POINT ( 'NONE',  ( -16.46253265017160317, 9.564922557960807481, 90.83224293864769550 ) ) ;
#178938=CARTESIAN_POINT ( 'NONE',  ( 5.049401038298161559, -19.05341960407611168, 22.70724293864769194 ) ) ;
#178939=CARTESIAN_POINT ( 'NONE',  ( -8.224510206698948167, 14.34966873604960824, 40.41557627198103120 ) ) ;
#178940=CARTESIAN_POINT ( 'NONE',  ( -4.483927247898782831, 16.52544592524335698, 42.70942372801901854 ) ) ;
#178941=CARTESIAN_POINT ( 'NONE',  ( 10.72451020669871369, 18.67979575497193778, 107.0844237280190043 ) ) ;
#178942=CARTESIAN_POINT ( 'NONE',  ( -13.89961937509977652, 13.97604488694528158, 115.6239096053143669 ) ) ;
#178943=CARTESIAN_POINT ( 'NONE',  ( 8.314922557960818139, 14.29746914071049879, 24.58224293864768839 ) ) ;
#178944=CARTESIAN_POINT ( 'NONE',  ( -21.55341960407619339, 5.719274019375674811, 33.54275706135234714 ) ) ;
#178945=CARTESIAN_POINT ( 'NONE',  ( -5.049401038298153566, 19.05341960407611168, 100.2072429386476955 ) ) ;
#178946=CARTESIAN_POINT ( 'NONE',  ( -8.314922557961024197, 14.29746914071037800, 102.9177570613523756 ) ) ;
#178947=CARTESIAN_POINT ( 'NONE',  ( -8.314922557961024197, 14.29746914071037800, 97.91775706135236135 ) ) ;
#178948=CIRCLE ( 'NONE', #127670, 2.500000000000002220 ) ;
#178949=CARTESIAN_POINT ( 'NONE',  ( -12.06949235617739369, -12.14591786802326823, 24.37609039468567573 ) ) ;
#178950=CARTESIAN_POINT ( 'NONE',  ( 19.05341960407611168, 5.049401038298154454, 43.95724293864769550 ) ) ;
#178951=CARTESIAN_POINT ( 'NONE',  ( -12.14591786802309592, -12.06949235617757132, 101.8739096053143811 ) ) ;
#178952=CARTESIAN_POINT ( 'NONE',  ( 0.05219959533937995610, -21.53943276465977519, 25.00109039468567218 ) ) ;
#178953=CARTESIAN_POINT ( 'NONE',  ( -13.89961937509977652, 13.97604488694528158, 25.62390960531434558 ) ) ;
#178954=CARTESIAN_POINT ( 'NONE',  ( -5.049401038298153566, 19.05341960407611168, 110.2072429386476671 ) ) ;
#178955=CARTESIAN_POINT ( 'NONE',  ( 10.81492255796106328, -18.62759615963255655, 35.41775706135234003 ) ) ;
#178957=CARTESIAN_POINT ( 'NONE',  ( 9.564922557960805705, 16.46253265017160317, 104.5822429386476955 ) ) ;
#178959=CARTESIAN_POINT ( 'NONE',  ( -17.12812012977028076, -6.668231424566004151, 36.35948759323144941 ) ) ;
#178960=CARTESIAN_POINT ( 'NONE',  ( -19.02544592524342804, 5.153800228976336051, 101.0405762719810241 ) ) ;
#178961=CARTESIAN_POINT ( 'NONE',  ( -0.05219959533937732626, 21.53943276465977519, 47.50109039468568994 ) ) ;
#178962=CARTESIAN_POINT ( 'NONE',  ( -4.483927247898539470, -16.52544592524342804, 92.29057627198103830 ) ) ;
#178963=CARTESIAN_POINT ( 'NONE',  ( -13.89961937509977652, 13.97604488694528158, 90.62390960531432427 ) ) ;
#178966=CARTESIAN_POINT ( 'NONE',  ( 12.14591786802327356, -12.06949235617739191, 65.62609039468568994 ) ) ;
#178967=CARTESIAN_POINT ( 'NONE',  ( 21.52544592524334988, 5.823673210054432836, 76.45942372801901854 ) ) ;
#178968=CARTESIAN_POINT ( 'NONE',  ( 14.34966873604972726, -8.224510206698740333, 45.83442372801901854 ) ) ;
#178969=CARTESIAN_POINT ( 'NONE',  ( -16.46253265017160317, 9.564922557960807481, 80.83224293864769550 ) ) ;
#178970=CARTESIAN_POINT ( 'NONE',  ( 16.46253265017146816, 9.564922557961045513, 106.6677570613523471 ) ) ;
#178971=CARTESIAN_POINT ( 'NONE',  ( 16.52544592524335698, 4.483927247898782831, 71.45942372801901854 ) ) ;
#178972=CARTESIAN_POINT ( 'NONE',  ( -0.05219959533936034679, 19.03943276465977164, 92.50109039468566152 ) ) ;
#178973=CARTESIAN_POINT ( 'NONE',  ( -13.97604488694527625, -13.89961937509977652, 66.87390960531436690 ) ) ;
#178974=CARTESIAN_POINT ( 'NONE',  ( 18.67979575497178502, 10.72451020669898547, 84.16557627198103830 ) ) ;
#178975=CARTESIAN_POINT ( 'NONE',  ( 0.05219959533910956823, 16.53943276465976808, 94.99890960531436690 ) ) ;
#178976=CARTESIAN_POINT ( 'NONE',  ( -9.474510206698720793, -16.51473224551083518, 89.58442372801900433 ) ) ;
#178977=CARTESIAN_POINT ( 'NONE',  ( 4.379528057220092307, 16.55341960407617563, 57.29275706135234714 ) ) ;
#178978=CARTESIAN_POINT ( 'NONE',  ( 17.44279575226826751, -5.990770900252369024, 63.33557567514322528 ) ) ;
#178979=CARTESIAN_POINT ( 'NONE',  ( -16.46253265017146816, -9.564922557961047289, 54.16775706135234003 ) ) ;
#178980=CARTESIAN_POINT ( 'NONE',  ( -8.224510206698948167, 14.34966873604960824, 35.41557627198102409 ) ) ;
#178981=CARTESIAN_POINT ( 'NONE',  ( 12.06949235617757843, -12.14591786802309237, 78.12390960531436690 ) ) ;
#178982=CARTESIAN_POINT ( 'NONE',  ( 18.67979575497194134, -10.72451020669871369, 110.8344237280190043 ) ) ;
#178983=CARTESIAN_POINT ( 'NONE',  ( -18.22780087662123805, 5.499999999999981348, 91.01763182126894947 ) ) ;
#178984=CARTESIAN_POINT ( 'NONE',  ( -21.53943276465977519, -0.05219959533937600094, 28.75109039468567929 ) ) ;
#178985=CARTESIAN_POINT ( 'NONE',  ( 19.05341960407611168, 5.049401038298154454, 98.95724293864766707 ) ) ;
#178986=CARTESIAN_POINT ( 'NONE',  ( 5.049401038298161559, -19.05341960407611168, 72.70724293864768129 ) ) ;
#178987=CARTESIAN_POINT ( 'NONE',  ( 21.53943276465977519, 0.05219959533937863772, 91.25109039468568994 ) ) ;
#178988=CARTESIAN_POINT ( 'NONE',  ( -13.97604488694527625, -13.89961937509977652, 81.87390960531436690 ) ) ;
#178989=CARTESIAN_POINT ( 'NONE',  ( -10.81492255796078084, -18.62759615963271287, 42.08224293864769550 ) ) ;
#178990=CARTESIAN_POINT ( 'NONE',  ( -14.29746914071049879, 8.314922557960819915, 75.83224293864769550 ) ) ;
#178991=CARTESIAN_POINT ( 'NONE',  ( -13.97604488694527625, -13.89961937509977652, 51.87390960531436690 ) ) ;
#178992=CARTESIAN_POINT ( 'NONE',  ( -0.05219959533910754901, -16.53943276465976808, 92.49890960531436690 ) ) ;
#178994=CARTESIAN_POINT ( 'NONE',  ( -21.52544592524334988, -5.823673210054445271, 28.95942372801902209 ) ) ;
#178995=CARTESIAN_POINT ( 'NONE',  ( 21.55341960407619695, -5.719274019375665929, 61.04275706135234714 ) ) ;
#178996=CARTESIAN_POINT ( 'NONE',  ( -19.02544592524342804, 5.153800228976336051, 41.04057627198103120 ) ) ;
#178997=CARTESIAN_POINT ( 'NONE',  ( -0.05219959533934338120, 16.53943276465976808, 62.50109039468568284 ) ) ;
#178998=CARTESIAN_POINT ( 'NONE',  ( -5.719274019375978568, 21.55341960407610458, 110.2072429386477239 ) ) ;
#178999=CARTESIAN_POINT ( 'NONE',  ( -10.81492255796078084, -18.62759615963271287, 112.0822429386477097 ) ) ;
#179000=CARTESIAN_POINT ( 'NONE',  ( 5.153800228976615827, -19.02544592524334988, 45.20942372801901143 ) ) ;
#179001=CARTESIAN_POINT ( 'NONE',  ( -19.03943276465977164, 0.05219959533909376836, 66.24890960531436690 ) ) ;
#179002=DIRECTION ( 'NONE',  ( 0.000000000000000000, 0.000000000000000000, -1.000000000000000000 ) ) ;
#179003=CARTESIAN_POINT ( 'NONE',  ( 18.62759615963255655, 10.81492255796105972, 76.66775706135234714 ) ) ;
#179004=CARTESIAN_POINT ( 'NONE',  ( -21.53943276465977519, 0.05219959533907696930, 51.24890960531436690 ) ) ;
#179005=CARTESIAN_POINT ( 'NONE',  ( 16.55341960407611168, 4.379528057220329451, 38.95724293864768839 ) ) ;
#179006=CARTESIAN_POINT ( 'NONE',  ( -18.67979575497193778, 10.72451020669871902, 78.33442372801901854 ) ) ;
#179007=CARTESIAN_POINT ( 'NONE',  ( -5.049401038297874678, -19.05341960407617918, 19.79275706135233293 ) ) ;
#179008=CARTESIAN_POINT ( 'NONE',  ( -16.55341960407611168, -4.379528057220339221, 56.45724293864768839 ) ) ;
#179009=CARTESIAN_POINT ( 'NONE',  ( 16.55341960407611168, 4.379528057220329451, 98.95724293864770971 ) ) ;
#179010=CARTESIAN_POINT ( 'NONE',  ( 5.049401038297881783, 19.05341960407617563, 57.29275706135231871 ) ) ;
#179011=CARTESIAN_POINT ( 'NONE',  ( 16.53943276465976808, 0.05219959533934440121, 111.2510903946856899 ) ) ;
#179012=CARTESIAN_POINT ( 'NONE',  ( 0.05219959533937995610, -21.53943276465977519, 70.00109039468568994 ) ) ;
#179013=CARTESIAN_POINT ( 'NONE',  ( -9.564922557960796823, -16.46253265017161027, 57.08224293864769550 ) ) ;
#179014=CARTESIAN_POINT ( 'NONE',  ( 9.564922557961047289, -16.46253265017146816, 35.41775706135233293 ) ) ;
#179015=CARTESIAN_POINT ( 'NONE',  ( -21.55341960407610458, -5.719274019375992779, 41.45724293864769550 ) ) ;
#179016=CARTESIAN_POINT ( 'NONE',  ( -5.823673210054431948, 21.52544592524334988, 37.70942372801900433 ) ) ;
#179017=CARTESIAN_POINT ( 'NONE',  ( -10.72451020669898014, 18.67979575497178502, 90.41557627198103830 ) ) ;
#179018=CARTESIAN_POINT ( 'NONE',  ( 16.46253265017146816, 9.564922557961045513, 81.66775706135233293 ) ) ;
#179019=CARTESIAN_POINT ( 'NONE',  ( -0.05219959533934338120, 16.53943276465976808, 47.50109039468568994 ) ) ;
#179021=CARTESIAN_POINT ( 'NONE',  ( 21.52544592524344225, -5.823673210054117533, 88.54057627198103830 ) ) ;
#179022=CARTESIAN_POINT ( 'NONE',  ( 8.314922557960818139, 14.29746914071049879, 94.58224293864769550 ) ) ;
#179024=CARTESIAN_POINT ( 'NONE',  ( -12.06949235617739369, -12.14591786802326823, 24.37609039468567573 ) ) ;
#179025=CARTESIAN_POINT ( 'NONE',  ( 15.72974639402199770, -15.80617190586745480, 53.12390960531436690 ) ) ;
#179026=CARTESIAN_POINT ( 'NONE',  ( -8.314922557961024197, 14.29746914071037800, 97.91775706135236135 ) ) ;
#179027=CARTESIAN_POINT ( 'NONE',  ( -19.03943276465977164, 0.05219959533909376836, 21.24890960531436335 ) ) ;
#179028=CARTESIAN_POINT ( 'NONE',  ( 14.29746914071037800, 8.314922557961029526, 46.66775706135234714 ) ) ;
#179030=CARTESIAN_POINT ( 'NONE',  ( -18.62759615963255300, -10.81492255796106328, 24.16775706135235424 ) ) ;
#179031=CARTESIAN_POINT ( 'NONE',  ( -21.52544592524343514, 5.823673210054127303, 51.04057627198103120 ) ) ;
#179032=CARTESIAN_POINT ( 'NONE',  ( -16.55341960407617563, 4.379528057220093196, 83.54275706135234714 ) ) ;
#179033=B_SPLINE_CURVE_WITH_KNOTS ( 'NONE', 3,
 ( #57624, #24294, #69780, #178978, #54608, #116282, #194146, #55610, #117284, #102118, #167775, #138418, #154584, #32242, #109074, #184926, #62561, #73792, #92898, #31248, #197133, #90904, #886, #14081, #152590, #60571, #200098, #108069, #75747, #137424, #44435, #29273 ),
 .UNSPECIFIED., .F., .F.,
 ( 4, 2, 2, 2, 2, 2, 2, 2, 2, 2, 2, 2, 2, 2, 2, 4 ),
 ( 8.184972452126140780E-17, 0.0003712461730037761704, 0.0007424923460074704835, 0.001113738519011164526, 0.001484984692014859001, 0.002227477038022250121, 0.002598723211025934406, 0.002969969384029600909, 0.003341215557033246162, 0.003712461730036892282, 0.004083707903040537102, 0.004454954076044181921, 0.004826200249047828475, 0.005197446422051473294, 0.005568692595055118981, 0.005939938768058764668 ),
 .UNSPECIFIED. ) ;
#179034=CARTESIAN_POINT ( 'NONE',  ( -16.51473224551069308, -9.474510206698971260, 101.6655762719810241 ) ) ;
#179035=CARTESIAN_POINT ( 'NONE',  ( 0.05219959533937995610, -21.53943276465977519, 50.00109039468568994 ) ) ;
#179036=CARTESIAN_POINT ( 'NONE',  ( 18.67979575497178502, 10.72451020669898547, 39.16557627198102409 ) ) ;
#179037=CARTESIAN_POINT ( 'NONE',  ( -5.049401038298153566, 19.05341960407611168, 110.2072429386476671 ) ) ;
#179039=CARTESIAN_POINT ( 'NONE',  ( -19.05341960407617563, 5.049401038297882671, 33.54275706135231871 ) ) ;
#179040=CARTESIAN_POINT ( 'NONE',  ( 14.34966873604972726, -8.224510206698740333, 60.83442372801901854 ) ) ;
#179041=CARTESIAN_POINT ( 'NONE',  ( -9.564922557960796823, -16.46253265017161027, 112.0822429386476955 ) ) ;
#179042=ORIENTED_EDGE ( 'NONE', *, *, #160526, .F. ) ;
#179043=CARTESIAN_POINT ( 'NONE',  ( 5.153800228976335163, 19.02544592524342804, 79.79057627198102409 ) ) ;
#179044=CARTESIAN_POINT ( 'NONE',  ( -8.314922557961024197, 14.29746914071037800, 97.91775706135236135 ) ) ;
#179046=CARTESIAN_POINT ( 'NONE',  ( -8.314922557960811034, -14.29746914071050412, 92.08224293864769550 ) ) ;
#179047=CARTESIAN_POINT ( 'NONE',  ( 10.81492255796078972, 18.62759615963270932, 54.58224293864769550 ) ) ;
#179048=CARTESIAN_POINT ( 'NONE',  ( 0.05219959533909260263, 19.03943276465977164, 29.99890960531435979 ) ) ;
#179049=CARTESIAN_POINT ( 'NONE',  ( 8.314922557961029526, -14.29746914071037800, 80.41775706135234714 ) ) ;
#179050=CARTESIAN_POINT ( 'NONE',  ( -21.55341960407619339, 5.719274019375674811, 33.54275706135234714 ) ) ;
#179051=CARTESIAN_POINT ( 'NONE',  ( 9.474510206698729675, 16.51473224551082808, 87.08442372801900433 ) ) ;
#179052=CARTESIAN_POINT ( 'NONE',  ( -12.06949235617756955, 12.14591786802309770, 95.62390960531436690 ) ) ;
#179053=CARTESIAN_POINT ( 'NONE',  ( 13.97604488694527802, 13.89961937509977652, 39.37390960531435269 ) ) ;
#179054=CARTESIAN_POINT ( 'NONE',  ( 16.46253265017160672, -9.564922557960803928, 108.3322429386476955 ) ) ;
#179055=CARTESIAN_POINT ( 'NONE',  ( 15.80617190586769283, -15.72974639402175789, 110.6260903946857042 ) ) ;
#179056=CARTESIAN_POINT ( 'NONE',  ( 16.46253265017160672, -9.564922557960803928, 73.33224293864769550 ) ) ;
#179057=CARTESIAN_POINT ( 'NONE',  ( 16.52544592524335698, 4.483927247898782831, 66.45942372801903275 ) ) ;
#179058=CARTESIAN_POINT ( 'NONE',  ( 5.719274019375673035, 21.55341960407619339, 97.29275706135234714 ) ) ;
#179059=CARTESIAN_POINT ( 'NONE',  ( -14.29746914071037622, -8.314922557961029526, 74.16775706135231871 ) ) ;
#179060=CARTESIAN_POINT ( 'NONE',  ( -19.03943276465977164, -0.05219959533935918106, 53.75109039468566863 ) ) ;
#179061=CARTESIAN_POINT ( 'NONE',  ( -5.049401038297874678, -19.05341960407617918, 69.79275706135233293 ) ) ;
#179062=ORIENTED_EDGE ( 'NONE', *, *, #50316, .T. ) ;
#179063=CARTESIAN_POINT ( 'NONE',  ( -21.55341960407619339, 5.719274019375674811, 58.54275706135235424 ) ) ;
#179064=CARTESIAN_POINT ( 'NONE',  ( 19.03943276465977164, -0.05219959533909143690, 68.74890960531436690 ) ) ;
#179065=CARTESIAN_POINT ( 'NONE',  ( 16.51473224551069308, 9.474510206698969483, 24.16557627198102765 ) ) ;
#179066=CARTESIAN_POINT ( 'NONE',  ( -19.03943276465977164, -0.05219959533935918106, 53.75109039468566863 ) ) ;
#179067=CARTESIAN_POINT ( 'NONE',  ( -19.03943276465977164, 0.05219959533909376836, 111.2489096053143669 ) ) ;
#179068=CARTESIAN_POINT ( 'NONE',  ( -5.153800228976328057, -19.02544592524343514, 82.29057627198103830 ) ) ;
#179069=CARTESIAN_POINT ( 'NONE',  ( 0.05219959533910956823, 16.53943276465976808, 34.99890960531435979 ) ) ;
#179070=CARTESIAN_POINT ( 'NONE',  ( 21.52544592524344225, -5.823673210054117533, 43.54057627198103830 ) ) ;
#179072=CARTESIAN_POINT ( 'NONE',  ( 21.53943276465977519, 0.05219959533937863772, 106.2510903946856757 ) ) ;
#179073=CARTESIAN_POINT ( 'NONE',  ( -16.36317988757057762, -7.306389748694919639, 80.90210391636773579 ) ) ;
#179074=CARTESIAN_POINT ( 'NONE',  ( 13.89961937509977652, -13.97604488694527269, 43.12390960531434558 ) ) ;
#179077=CARTESIAN_POINT ( 'NONE',  ( 21.52544592524334988, 5.823673210054432836, 71.45942372801901854 ) ) ;
#179079=CARTESIAN_POINT ( 'NONE',  ( 4.379528057220092307, 16.55341960407617563, 62.29275706135236845 ) ) ;
#179080=CARTESIAN_POINT ( 'NONE',  ( -15.80617190586745835, -15.72974639402198527, 81.87390960531435269 ) ) ;
#179083=CARTESIAN_POINT ( 'NONE',  ( -12.06949235617756955, 12.14591786802309770, 50.62390960531435979 ) ) ;
#179084=CARTESIAN_POINT ( 'NONE',  ( 5.049401038298161559, -19.05341960407611168, 27.70724293864769550 ) ) ;
#179086=CARTESIAN_POINT ( 'NONE',  ( 21.52544592524334988, 5.823673210054432836, 36.45942372801901143 ) ) ;
#179087=CARTESIAN_POINT ( 'NONE',  ( -16.46253265017146816, -9.564922557961047289, 44.16775706135232582 ) ) ;
#179088=CARTESIAN_POINT ( 'NONE',  ( -5.049401038298153566, 19.05341960407611168, 35.20724293864768839 ) ) ;
#179089=CARTESIAN_POINT ( 'NONE',  ( 18.67979575497194134, -10.72451020669871369, 80.83442372801901854 ) ) ;
#179091=CARTESIAN_POINT ( 'NONE',  ( -14.29746914071049879, 8.314922557960819915, 45.83224293864769550 ) ) ;
#179093=CARTESIAN_POINT ( 'NONE',  ( 18.62759615963271287, -10.81492255796078972, 43.33224293864769550 ) ) ;
#179094=CARTESIAN_POINT ( 'NONE',  ( -18.22780087662126647, -5.499999999999827693, 38.98236817873107185 ) ) ;
#179095=CARTESIAN_POINT ( 'NONE',  ( -19.05341960407611168, -5.049401038298163336, 96.45724293864769550 ) ) ;
#179096=CARTESIAN_POINT ( 'NONE',  ( -8.314922557960811034, -14.29746914071050412, 82.08224293864768129 ) ) ;
#179097=CARTESIAN_POINT ( 'NONE',  ( -9.564922557961040184, 16.46253265017147172, 102.9177570613523329 ) ) ;
#179098=CARTESIAN_POINT ( 'NONE',  ( 21.52544592524344225, -5.823673210054117533, 58.54057627198103120 ) ) ;
#179099=VERTEX_POINT ( 'NONE', #196533 ) ;
#179100=CARTESIAN_POINT ( 'NONE',  ( 16.46253265017160672, -9.564922557960803928, 33.33224293864770260 ) ) ;
#179101=CARTESIAN_POINT ( 'NONE',  ( -19.02544592524342804, 5.153800228976336051, 91.04057627198100988 ) ) ;
#179102=CARTESIAN_POINT ( 'NONE',  ( 15.72974639402199770, -15.80617190586745480, 83.12390960531436690 ) ) ;
#179103=CARTESIAN_POINT ( 'NONE',  ( -4.483927247898539470, -16.52544592524342804, 27.29057627198103120 ) ) ;
#179104=CARTESIAN_POINT ( 'NONE',  ( -16.46253265017160317, 9.564922557960807481, 105.8322429386476955 ) ) ;
#179105=CARTESIAN_POINT ( 'NONE',  ( 5.153800228976615827, -19.02544592524334988, 85.20942372801900433 ) ) ;
#179106=CARTESIAN_POINT ( 'NONE',  ( -15.80617190586768217, 15.72974639402176855, 93.12609039468568994 ) ) ;
#179107=CARTESIAN_POINT ( 'NONE',  ( -21.55341960407610458, -5.719274019375992779, 76.45724293864769550 ) ) ;
#179108=CARTESIAN_POINT ( 'NONE',  ( -18.67979575497178146, -10.72451020669898902, 31.66557627198102054 ) ) ;
#179110=CARTESIAN_POINT ( 'NONE',  ( 9.474510206698971260, -16.51473224551069308, 47.91557627198102409 ) ) ;
#179111=CARTESIAN_POINT ( 'NONE',  ( 12.14591786802327356, -12.06949235617739191, 110.6260903946857042 ) ) ;
#179112=CARTESIAN_POINT ( 'NONE',  ( 13.89961937509977652, -13.97604488694527269, 83.12390960531436690 ) ) ;
#179115=CARTESIAN_POINT ( 'NONE',  ( -19.02544592524334988, -5.153800228976617603, 33.95942372801897591 ) ) ;
#179116=CARTESIAN_POINT ( 'NONE',  ( -16.53943276465976808, 0.05219959533911058130, 91.24890960531436690 ) ) ;
#179117=CARTESIAN_POINT ( 'NONE',  ( -21.52544592524334988, -5.823673210054445271, 18.95942372801901143 ) ) ;
#179119=CARTESIAN_POINT ( 'NONE',  ( 10.72451020669898902, -18.67979575497178502, 62.91557627198102409 ) ) ;
#179120=CARTESIAN_POINT ( 'NONE',  ( -16.55341960407617563, 4.379528057220093196, 93.54275706135234714 ) ) ;
#179121=CARTESIAN_POINT ( 'NONE',  ( 5.049401038298161559, -19.05341960407611168, 22.70724293864769194 ) ) ;
#179122=CARTESIAN_POINT ( 'NONE',  ( -16.51473224551069308, -9.474510206698971260, 76.66557627198103830 ) ) ;
#179124=CARTESIAN_POINT ( 'NONE',  ( -8.314922557960811034, -14.29746914071050412, 32.08224293864769550 ) ) ;
#179125=CARTESIAN_POINT ( 'NONE',  ( 18.62759615963255655, 10.81492255796105972, 61.66775706135235424 ) ) ;
#179126=CARTESIAN_POINT ( 'NONE',  ( 0.05219959533909260263, 19.03943276465977164, 104.9989096053143669 ) ) ;
#179127=CARTESIAN_POINT ( 'NONE',  ( -10.81492255796105439, 18.62759615963255655, 97.91775706135236135 ) ) ;
#179128=CARTESIAN_POINT ( 'NONE',  ( -5.049401038298153566, 19.05341960407611168, 25.20724293864768484 ) ) ;
#179129=CARTESIAN_POINT ( 'NONE',  ( 19.05341960407611168, 5.049401038298154454, 33.95724293864769550 ) ) ;
#179130=ORIENTED_EDGE ( 'NONE', *, *, #120571, .F. ) ;
#179131=CARTESIAN_POINT ( 'NONE',  ( 5.823673210054444382, -21.52544592524334988, 100.2094237280190043 ) ) ;
#179132=CARTESIAN_POINT ( 'NONE',  ( -12.14591786802326823, 12.06949235617739902, 48.12609039468568284 ) ) ;
#179133=CARTESIAN_POINT ( 'NONE',  ( -10.81492255796105439, 18.62759615963255655, 87.91775706135234714 ) ) ;
#179134=CARTESIAN_POINT ( 'NONE',  ( 21.52544592524344225, -5.823673210054117533, 23.54057627198102765 ) ) ;
#179135=CARTESIAN_POINT ( 'NONE',  ( 19.02544592524334988, 5.153800228976608722, 96.45942372801897591 ) ) ;
#179136=CARTESIAN_POINT ( 'NONE',  ( 21.55341960407619695, -5.719274019375665929, 56.04275706135235424 ) ) ;
#179137=CARTESIAN_POINT ( 'NONE',  ( 16.53943276465976808, 0.05219959533934440121, 21.25109039468567218 ) ) ;
#179138=CARTESIAN_POINT ( 'NONE',  ( 9.564922557961047289, -16.46253265017146816, 90.41775706135234714 ) ) ;
#179139=CARTESIAN_POINT ( 'NONE',  ( 16.51473224551069308, 9.474510206698969483, 49.16557627198102409 ) ) ;
#179140=CARTESIAN_POINT ( 'NONE',  ( -16.51473224551082808, 9.474510206698731452, 103.3344237280190043 ) ) ;
#179142=CARTESIAN_POINT ( 'NONE',  ( 19.02544592524334988, 5.153800228976608722, 86.45942372801900433 ) ) ;
#179143=CARTESIAN_POINT ( 'NONE',  ( -14.29746914071049879, 8.314922557960819915, 50.83224293864770971 ) ) ;
#179144=CARTESIAN_POINT ( 'NONE',  ( -19.05341960407617563, 5.049401038297882671, 78.54275706135233293 ) ) ;
#179145=CARTESIAN_POINT ( 'NONE',  ( 12.14591786802327356, -12.06949235617739191, 65.62609039468568994 ) ) ;
#179146=CARTESIAN_POINT ( 'NONE',  ( 13.97604488694548053, -13.89961937509957401, 30.62609039468566863 ) ) ;
#179147=CARTESIAN_POINT ( 'NONE',  ( -16.46253265017160317, 9.564922557960807481, 40.83224293864769550 ) ) ;
#179148=CARTESIAN_POINT ( 'NONE',  ( -9.564922557960796823, -16.46253265017161027, 42.08224293864769550 ) ) ;
#179149=CARTESIAN_POINT ( 'NONE',  ( 14.29746914071037800, 8.314922557961029526, 56.66775706135235424 ) ) ;
#179152=CARTESIAN_POINT ( 'NONE',  ( 19.03943276465977164, -0.05219959533909143690, 108.7489096053143527 ) ) ;
#179153=CARTESIAN_POINT ( 'NONE',  ( -17.49999999999999645, -5.499999999999992895, 69.20309617465828467 ) ) ;
#179155=CARTESIAN_POINT ( 'NONE',  ( 9.474510206698729675, 16.51473224551082808, 92.08442372801900433 ) ) ;
#179156=CARTESIAN_POINT ( 'NONE',  ( 21.52544592524344225, -5.823673210054117533, 33.54057627198102409 ) ) ;
#179157=CARTESIAN_POINT ( 'NONE',  ( -13.89961937509957401, -13.97604488694547875, 34.37609039468566863 ) ) ;
#179158=CARTESIAN_POINT ( 'NONE',  ( 5.049401038297881783, 19.05341960407617563, 107.2927570613523187 ) ) ;
#179159=CARTESIAN_POINT ( 'NONE',  ( -16.51473224551069308, -9.474510206698971260, 31.66557627198102054 ) ) ;
#179160=CARTESIAN_POINT ( 'NONE',  ( -19.03943276465977164, 0.05219959533909376836, 31.24890960531435979 ) ) ;
#179161=CARTESIAN_POINT ( 'NONE',  ( 18.62759615963271287, -10.81492255796078972, 68.33224293864769550 ) ) ;
#179162=CARTESIAN_POINT ( 'NONE',  ( -5.049401038298153566, 19.05341960407611168, 105.2072429386476671 ) ) ;
#179163=CARTESIAN_POINT ( 'NONE',  ( -13.97604488694527625, -13.89961937509977652, 31.87390960531435979 ) ) ;
#179165=CARTESIAN_POINT ( 'NONE',  ( -19.03943276465977164, -0.05219959533935918106, 88.75109039468567573 ) ) ;
#179166=CARTESIAN_POINT ( 'NONE',  ( 14.29746914071049879, -8.314922557960816363, 53.33224293864769550 ) ) ;
#179167=CARTESIAN_POINT ( 'NONE',  ( 5.719274019375991003, -21.55341960407610458, 37.70724293864769550 ) ) ;
#179168=CARTESIAN_POINT ( 'NONE',  ( 10.81492255796106328, -18.62759615963255655, 110.4177570613523756 ) ) ;
#179169=CARTESIAN_POINT ( 'NONE',  ( 18.62759615963271287, -10.81492255796078972, 83.33224293864769550 ) ) ;
#179170=CARTESIAN_POINT ( 'NONE',  ( -10.81492255796105439, 18.62759615963255655, 72.91775706135234714 ) ) ;
#179171=CARTESIAN_POINT ( 'NONE',  ( 15.72974639402176855, 15.80617190586768217, 61.87609039468568284 ) ) ;
#179172=CARTESIAN_POINT ( 'NONE',  ( 13.89961937509977652, -13.97604488694527269, 108.1239096053143669 ) ) ;
#179173=CARTESIAN_POINT ( 'NONE',  ( -12.14591786802326823, 12.06949235617739902, 108.1260903946856757 ) ) ;
#179174=CARTESIAN_POINT ( 'NONE',  ( 0.05219959533937995610, -21.53943276465977519, 65.00109039468568994 ) ) ;
#179175=CARTESIAN_POINT ( 'NONE',  ( 16.46253265017160672, -9.564922557960803928, 58.33224293864769550 ) ) ;
#179176=CARTESIAN_POINT ( 'NONE',  ( -9.564922557961040184, 16.46253265017147172, 32.91775706135233293 ) ) ;
#179177=CARTESIAN_POINT ( 'NONE',  ( -5.719274019375665041, -21.55341960407619695, 24.79275706135235779 ) ) ;
#179178=CARTESIAN_POINT ( 'NONE',  ( 16.46253265017160672, -9.564922557960803928, 68.33224293864770971 ) ) ;
#179179=CARTESIAN_POINT ( 'NONE',  ( -16.53943276465976808, 0.05219959533911058130, 86.24890960531436690 ) ) ;
#179180=CARTESIAN_POINT ( 'NONE',  ( -16.52544592524342804, 4.483927247898546575, 46.04057627198103830 ) ) ;
#179181=CARTESIAN_POINT ( 'NONE',  ( -21.53943276465977519, 0.05219959533907696930, 61.24890960531435979 ) ) ;
#179182=CARTESIAN_POINT ( 'NONE',  ( -13.97604488694527625, -13.89961937509977652, 61.87390960531435979 ) ) ;
#179183=CARTESIAN_POINT ( 'NONE',  ( -5.823673210054116645, -21.52544592524344225, 72.29057627198102409 ) ) ;
#179184=CARTESIAN_POINT ( 'NONE',  ( -16.51473224551082808, 9.474510206698731452, 53.33442372801900433 ) ) ;
#179186=CARTESIAN_POINT ( 'NONE',  ( -4.379528057220328563, 16.55341960407611168, 60.20724293864768839 ) ) ;
#179187=CARTESIAN_POINT ( 'NONE',  ( 10.81492255796078972, 18.62759615963270932, 34.58224293864770260 ) ) ;
#179190=CARTESIAN_POINT ( 'NONE',  ( 8.224510206698742110, 14.34966873604972548, 87.08442372801901854 ) ) ;
#179192=CARTESIAN_POINT ( 'NONE',  ( -13.89961937509957401, -13.97604488694547875, 89.37609039468563310 ) ) ;
#179193=CARTESIAN_POINT ( 'NONE',  ( 4.379528057220339221, -16.55341960407611168, 57.70724293864770260 ) ) ;
#179195=CARTESIAN_POINT ( 'NONE',  ( -5.049401038298153566, 19.05341960407611168, 45.20724293864769550 ) ) ;
#179196=CARTESIAN_POINT ( 'NONE',  ( 16.52544592524342804, -4.483927247898539470, 38.54057627198103120 ) ) ;
#179197=CARTESIAN_POINT ( 'NONE',  ( -16.51473224551069308, -9.474510206698971260, 91.66557627198103830 ) ) ;
#179198=CARTESIAN_POINT ( 'NONE',  ( 5.049401038298161559, -19.05341960407611168, 52.70724293864767418 ) ) ;
#179199=CARTESIAN_POINT ( 'NONE',  ( -10.72451020669870658, -18.67979575497194134, 54.58442372801901143 ) ) ;
#179200=CARTESIAN_POINT ( 'NONE',  ( 19.05341960407611168, 5.049401038298154454, 68.95724293864769550 ) ) ;
#179201=CARTESIAN_POINT ( 'NONE',  ( -13.97604488694527625, -13.89961937509977652, 26.87390960531434558 ) ) ;
#179202=CARTESIAN_POINT ( 'NONE',  ( -19.02544592524342804, 5.153800228976336051, 71.04057627198099567 ) ) ;
#179203=CARTESIAN_POINT ( 'NONE',  ( 21.53943276465977519, -0.05219959533907433946, 43.74890960531435979 ) ) ;
#179204=CARTESIAN_POINT ( 'NONE',  ( -13.97604488694527625, -13.89961937509977652, 36.87390960531436690 ) ) ;
#179205=CARTESIAN_POINT ( 'NONE',  ( 0.05219959533907565091, 21.53943276465977519, 34.99890960531435979 ) ) ;
#179206=CARTESIAN_POINT ( 'NONE',  ( -4.379528057220086978, -16.55341960407618274, 109.7927570613523613 ) ) ;
#179208=CARTESIAN_POINT ( 'NONE',  ( 19.02544592524334988, 5.153800228976608722, 26.45942372801899722 ) ) ;
#179209=CARTESIAN_POINT ( 'NONE',  ( -14.34966873604972548, 8.224510206698743886, 43.33442372801901143 ) ) ;
#179210=CARTESIAN_POINT ( 'NONE',  ( -4.379528057220086978, -16.55341960407618274, 84.79275706135234714 ) ) ;
#179211=CARTESIAN_POINT ( 'NONE',  ( -17.72560187377285601, -5.500000000000015987, 94.07814504131322053 ) ) ;
#179212=CARTESIAN_POINT ( 'NONE',  ( 14.29746914071037800, 8.314922557961029526, 61.66775706135235424 ) ) ;
#179213=CARTESIAN_POINT ( 'NONE',  ( -16.51473224551069308, -9.474510206698971260, 106.6655762719810383 ) ) ;
#179215=CARTESIAN_POINT ( 'NONE',  ( -16.46253265017160317, 9.564922557960807481, 35.83224293864768839 ) ) ;
#179216=CARTESIAN_POINT ( 'NONE',  ( -14.34966873604972548, 8.224510206698743886, 33.33442372801900433 ) ) ;
#179217=CARTESIAN_POINT ( 'NONE',  ( 16.46253265017160672, -9.564922557960803928, 43.33224293864769550 ) ) ;
#179218=CARTESIAN_POINT ( 'NONE',  ( 0.05219959533937995610, -21.53943276465977519, 30.00109039468568284 ) ) ;
#179219=CARTESIAN_POINT ( 'NONE',  ( 16.53943276465976808, 0.05219959533934440121, 36.25109039468567573 ) ) ;
#179220=CARTESIAN_POINT ( 'NONE',  ( -16.53943276465976808, -0.05219959533934237506, 93.75109039468567573 ) ) ;
#179222=CARTESIAN_POINT ( 'NONE',  ( 18.67979575497194134, -10.72451020669871369, 105.8344237280190328 ) ) ;
#179223=CARTESIAN_POINT ( 'NONE',  ( -5.049401038297874678, -19.05341960407617918, 99.79275706135234714 ) ) ;
#179224=CARTESIAN_POINT ( 'NONE',  ( -13.97604488694547697, 13.89961937509957934, 58.12609039468566863 ) ) ;
#179225=CARTESIAN_POINT ( 'NONE',  ( 14.34966873604960469, 8.224510206698951720, 59.16557627198103120 ) ) ;
#179226=CARTESIAN_POINT ( 'NONE',  ( 14.34966873604960469, 8.224510206698951720, 114.1655762719810383 ) ) ;
#179227=CARTESIAN_POINT ( 'NONE',  ( 19.03943276465977164, 0.05219959533936151252, 61.25109039468566863 ) ) ;
#179228=CARTESIAN_POINT ( 'NONE',  ( 17.50000000000000355, -5.624438216177559902, 58.31670344914645909 ) ) ;
#179229=CARTESIAN_POINT ( 'NONE',  ( 21.55341960407619695, -5.719274019375665929, 66.04275706135236135 ) ) ;
#179230=CARTESIAN_POINT ( 'NONE',  ( 14.29746914071037800, 8.314922557961029526, 21.66775706135235069 ) ) ;
#179232=CARTESIAN_POINT ( 'NONE',  ( 21.52544592524344225, -5.823673210054117533, 23.54057627198102765 ) ) ;
#179233=CARTESIAN_POINT ( 'NONE',  ( -9.564922557961040184, 16.46253265017147172, 107.9177570613523471 ) ) ;
#179234=CARTESIAN_POINT ( 'NONE',  ( 17.50000000000000000, -5.500000000000031086, 98.29690382534174375 ) ) ;
#179236=CARTESIAN_POINT ( 'NONE',  ( 12.14591786802309770, 12.06949235617756955, 114.3739096053143527 ) ) ;
#179237=CARTESIAN_POINT ( 'NONE',  ( -21.55341960407619339, 5.719274019375674811, 108.5427570613523756 ) ) ;
#179238=CARTESIAN_POINT ( 'NONE',  ( -13.97604488694527625, -13.89961937509977652, 51.87390960531436690 ) ) ;
#179239=STYLED_ITEM ( 'NONE', ( #53434 ), #143056 ) ;
#179240=CARTESIAN_POINT ( 'NONE',  ( 0.05219959533937995610, -21.53943276465977519, 60.00109039468568284 ) ) ;
#179241=CARTESIAN_POINT ( 'NONE',  ( -21.52544592524334988, -5.823673210054445271, 98.95942372801903275 ) ) ;
#179242=CARTESIAN_POINT ( 'NONE',  ( 16.52544592524335698, 4.483927247898782831, 106.4594237280190328 ) ) ;
#179243=CARTESIAN_POINT ( 'NONE',  ( 13.89961937509977652, -13.97604488694527269, 73.12390960531436690 ) ) ;
#179244=B_SPLINE_CURVE_WITH_KNOTS ( 'NONE', 3,
 ( #154039, #182411, #42902, #15534, #75211, #104567 ),
 .UNSPECIFIED., .F., .F.,
 ( 4, 2, 4 ),
 ( 0.007228050697041515406, 0.007608510107494982286, 0.007988969517948450033 ),
 .UNSPECIFIED. ) ;
#179245=CARTESIAN_POINT ( 'NONE',  ( -21.55341960407619339, 5.719274019375674811, 58.54275706135235424 ) ) ;
#179246=CARTESIAN_POINT ( 'NONE',  ( 15.72974639402176855, 15.80617190586768217, 51.87609039468568284 ) ) ;
#179247=CARTESIAN_POINT ( 'NONE',  ( 16.51473224551083163, -9.474510206698727899, 85.83442372801900433 ) ) ;
#179248=CARTESIAN_POINT ( 'NONE',  ( 13.89961937509977652, -13.97604488694527269, 103.1239096053143527 ) ) ;
#179249=CARTESIAN_POINT ( 'NONE',  ( -5.153800228976328057, -19.02544592524343514, 22.29057627198102765 ) ) ;
#179250=CARTESIAN_POINT ( 'NONE',  ( 21.52544592524344225, -5.823673210054117533, 93.54057627198103830 ) ) ;
#179251=CARTESIAN_POINT ( 'NONE',  ( 19.05341960407617918, -5.049401038297876454, 26.04275706135233293 ) ) ;
#179252=CARTESIAN_POINT ( 'NONE',  ( -8.314922557960811034, -14.29746914071050412, 102.0822429386476955 ) ) ;
#179253=CARTESIAN_POINT ( 'NONE',  ( 9.564922557960805705, 16.46253265017160317, 44.58224293864769550 ) ) ;
#179254=CARTESIAN_POINT ( 'NONE',  ( -13.97604488694547697, 13.89961937509957934, 98.12609039468566152 ) ) ;
#179255=VECTOR ( 'NONE', #29709, 1000.000000000000000 ) ;
#179256=CARTESIAN_POINT ( 'NONE',  ( -4.483927247898539470, -16.52544592524342804, 62.29057627198102409 ) ) ;
#179257=CARTESIAN_POINT ( 'NONE',  ( -0.05219959533937732626, 21.53943276465977519, 107.5010903946856899 ) ) ;
#179258=CARTESIAN_POINT ( 'NONE',  ( -9.564922557960796823, -16.46253265017161027, 107.0822429386476955 ) ) ;
#179259=CARTESIAN_POINT ( 'NONE',  ( -16.51473224551082808, 9.474510206698731452, 78.33442372801900433 ) ) ;
#179260=CARTESIAN_POINT ( 'NONE',  ( 18.67979575497178502, 10.72451020669898547, 84.16557627198103830 ) ) ;
#179261=CARTESIAN_POINT ( 'NONE',  ( -5.719274019375665041, -21.55341960407619695, 34.79275706135235424 ) ) ;
#179262=CARTESIAN_POINT ( 'NONE',  ( -8.314922557961024197, 14.29746914071037800, 42.91775706135235424 ) ) ;
#179263=CARTESIAN_POINT ( 'NONE',  ( 8.224510206698742110, 14.34966873604972548, 87.08442372801901854 ) ) ;
#179264=CARTESIAN_POINT ( 'NONE',  ( -8.314922557961024197, 14.29746914071037800, 37.91775706135235424 ) ) ;
#179265=CARTESIAN_POINT ( 'NONE',  ( 21.53943276465977519, 0.05219959533937863772, 31.25109039468568639 ) ) ;
#179266=CARTESIAN_POINT ( 'NONE',  ( -15.80617190586745835, -15.72974639402198527, 41.87390960531435979 ) ) ;
#179268=CARTESIAN_POINT ( 'NONE',  ( 16.46253265017160672, -9.564922557960803928, 33.33224293864770260 ) ) ;
#179270=CARTESIAN_POINT ( 'NONE',  ( 12.06949235617739724, 12.14591786802326823, 66.87609039468568994 ) ) ;
#179271=CARTESIAN_POINT ( 'NONE',  ( -0.05219959533907301413, -21.53943276465977519, 87.49890960531436690 ) ) ;
#179272=CARTESIAN_POINT ( 'NONE',  ( 0.05219959533910956823, 16.53943276465976808, 44.99890960531435979 ) ) ;
#179273=CARTESIAN_POINT ( 'NONE',  ( 0.05219959533934541429, -16.53943276465976808, 55.00109039468568284 ) ) ;
#179274=CARTESIAN_POINT ( 'NONE',  ( 9.474510206698971260, -16.51473224551069308, 57.91557627198103120 ) ) ;
#179275=CARTESIAN_POINT ( 'NONE',  ( 9.474510206698729675, 16.51473224551082808, 82.08442372801899012 ) ) ;
#179276=CARTESIAN_POINT ( 'NONE',  ( 21.55341960407610458, 5.719274019375980345, 88.95724293864769550 ) ) ;
#179277=CARTESIAN_POINT ( 'NONE',  ( 14.34966873604960469, 8.224510206698951720, 34.16557627198102409 ) ) ;
#179281=CARTESIAN_POINT ( 'NONE',  ( -15.80617190586745835, -15.72974639402198527, 61.87390960531436690 ) ) ;
#179282=CARTESIAN_POINT ( 'NONE',  ( -8.314922557961024197, 14.29746914071037800, 102.9177570613523756 ) ) ;
#179284=CARTESIAN_POINT ( 'NONE',  ( 17.50000000000000000, -5.500000000000000888, 103.2969038253417153 ) ) ;
#179285=CARTESIAN_POINT ( 'NONE',  ( 15.80617190586746368, 15.72974639402197994, 84.37390960531438111 ) ) ;
#179286=CARTESIAN_POINT ( 'NONE',  ( 14.29746914071049879, -8.314922557960816363, 28.33224293864769550 ) ) ;
#179288=CARTESIAN_POINT ( 'NONE',  ( -4.379528057220086978, -16.55341960407618274, 29.79275706135234358 ) ) ;
#179289=CARTESIAN_POINT ( 'NONE',  ( -9.564922557960796823, -16.46253265017161027, 32.08224293864769550 ) ) ;
#179290=CARTESIAN_POINT ( 'NONE',  ( 19.05341960407611168, 5.049401038298154454, 63.95724293864769550 ) ) ;
#179293=CARTESIAN_POINT ( 'NONE',  ( -15.80617190586745835, -15.72974639402198527, 21.87390960531436690 ) ) ;
#179294=DIRECTION ( 'NONE',  ( 0.000000000000000000, 0.000000000000000000, -1.000000000000000000 ) ) ;
#179295=CARTESIAN_POINT ( 'NONE',  ( -4.379528057220086978, -16.55341960407618274, 104.7927570613523898 ) ) ;
#179296=CARTESIAN_POINT ( 'NONE',  ( 9.564922557961047289, -16.46253265017146816, 105.4177570613523471 ) ) ;
#179297=CARTESIAN_POINT ( 'NONE',  ( -19.02544592524334988, -5.153800228976617603, 38.95942372801900433 ) ) ;
#179298=CARTESIAN_POINT ( 'NONE',  ( -18.62759615963270932, 10.81492255796079327, 85.83224293864768129 ) ) ;
#179299=CARTESIAN_POINT ( 'NONE',  ( -4.483927247898539470, -16.52544592524342804, 22.29057627198102765 ) ) ;
#179300=CARTESIAN_POINT ( 'NONE',  ( -10.81492255796078084, -18.62759615963271287, 37.08224293864768129 ) ) ;
#179301=CARTESIAN_POINT ( 'NONE',  ( 9.564922557961047289, -16.46253265017146816, 105.4177570613523471 ) ) ;
#179302=CARTESIAN_POINT ( 'NONE',  ( -16.46253265017160317, 9.564922557960807481, 105.8322429386476955 ) ) ;
#179303=CARTESIAN_POINT ( 'NONE',  ( 21.53943276465977519, 0.05219959533937863772, 61.25109039468567573 ) ) ;
#179304=CARTESIAN_POINT ( 'NONE',  ( -0.05219959533909027116, -19.03943276465977164, 57.49890960531435979 ) ) ;
#179305=CARTESIAN_POINT ( 'NONE',  ( -16.53943276465976808, 0.05219959533911058130, 106.2489096053143811 ) ) ;
#179307=CARTESIAN_POINT ( 'NONE',  ( 0.05219959533909260263, 19.03943276465977164, 74.99890960531435269 ) ) ;
#179308=CARTESIAN_POINT ( 'NONE',  ( 4.379528057220339221, -16.55341960407611168, 77.70724293864770971 ) ) ;
#179309=VERTEX_POINT ( 'NONE', #57005 ) ;
#179310=CARTESIAN_POINT ( 'NONE',  ( 5.049401038297881783, 19.05341960407617563, 97.29275706135233293 ) ) ;
#179311=CARTESIAN_POINT ( 'NONE',  ( 17.48853670773246449, -5.747243402303036319, 81.16671299749991420 ) ) ;
#179312=CARTESIAN_POINT ( 'NONE',  ( 9.564922557960805705, 16.46253265017160317, 64.58224293864769550 ) ) ;
#179314=CARTESIAN_POINT ( 'NONE',  ( -9.564922557960796823, -16.46253265017161027, 77.08224293864769550 ) ) ;
#179315=CARTESIAN_POINT ( 'NONE',  ( -13.97604488694527625, -13.89961937509977652, 101.8739096053143811 ) ) ;
#179316=CARTESIAN_POINT ( 'NONE',  ( -8.224510206698735004, -14.34966873604973081, 64.58442372801900433 ) ) ;
#179318=CARTESIAN_POINT ( 'NONE',  ( -5.049401038297874678, -19.05341960407617918, 44.79275706135232582 ) ) ;
#179319=CARTESIAN_POINT ( 'NONE',  ( -15.80617190586768217, 15.72974639402176855, 98.12609039468570415 ) ) ;
#179321=CARTESIAN_POINT ( 'NONE',  ( 5.153800228976335163, 19.02544592524342804, 114.7905762719810241 ) ) ;
#179322=CARTESIAN_POINT ( 'NONE',  ( 4.379528057220092307, 16.55341960407617563, 97.29275706135234714 ) ) ;
#179324=CARTESIAN_POINT ( 'NONE',  ( -0.05219959533934338120, 16.53943276465976808, 87.50109039468568994 ) ) ;
#179326=CARTESIAN_POINT ( 'NONE',  ( -16.55341960407617563, 4.379528057220093196, 73.54275706135234714 ) ) ;
#179327=ORIENTED_EDGE ( 'NONE', *, *, #109403, .T. ) ;
#179328=CARTESIAN_POINT ( 'NONE',  ( -18.67979575497193778, 10.72451020669871902, 78.33442372801901854 ) ) ;
#179329=CARTESIAN_POINT ( 'NONE',  ( -16.51473224551082808, 9.474510206698731452, 88.33442372801900433 ) ) ;
#179330=CARTESIAN_POINT ( 'NONE',  ( 16.46253265017146816, 9.564922557961045513, 31.66775706135232937 ) ) ;
#179331=VECTOR ( 'NONE', #153121, 1000.000000000000000 ) ;
#179332=CARTESIAN_POINT ( 'NONE',  ( 9.474510206698971260, -16.51473224551069308, 62.91557627198102409 ) ) ;
#179333=CARTESIAN_POINT ( 'NONE',  ( -19.03943276465977164, 0.05219959533909376836, 61.24890960531436690 ) ) ;
#179335=CARTESIAN_POINT ( 'NONE',  ( -21.55341960407610458, -5.719274019375992779, 86.45724293864770971 ) ) ;
#179336=CARTESIAN_POINT ( 'NONE',  ( 18.67979575497178502, 10.72451020669898547, 29.16557627198103120 ) ) ;
#179337=CARTESIAN_POINT ( 'NONE',  ( -9.564922557960796823, -16.46253265017161027, 32.08224293864769550 ) ) ;
#179338=CARTESIAN_POINT ( 'NONE',  ( 12.14591786802327356, -12.06949235617739191, 70.62609039468567573 ) ) ;
#179339=ORIENTED_EDGE ( 'NONE', *, *, #89272, .F. ) ;
#179340=CARTESIAN_POINT ( 'NONE',  ( 21.55341960407619695, -5.719274019375665929, 26.04275706135235779 ) ) ;
#179341=CARTESIAN_POINT ( 'NONE',  ( 12.14591786802309770, 12.06949235617756955, 64.37390960531435269 ) ) ;
#179343=CARTESIAN_POINT ( 'NONE',  ( 8.314922557961029526, -14.29746914071037800, 20.41775706135234714 ) ) ;
#179344=CARTESIAN_POINT ( 'NONE',  ( -19.03943276465977164, -0.05219959533935918106, 53.75109039468566863 ) ) ;
#179345=CARTESIAN_POINT ( 'NONE',  ( -14.34966873604960291, -8.224510206698953496, 51.66557627198102409 ) ) ;
#179346=CARTESIAN_POINT ( 'NONE',  ( -21.55341960407619339, 5.719274019375674811, 23.54275706135235424 ) ) ;
#179347=CARTESIAN_POINT ( 'NONE',  ( 18.22780087662122384, 5.500000000000018652, 98.98459894673892734 ) ) ;
#179348=CARTESIAN_POINT ( 'NONE',  ( 21.55341960407610458, 5.719274019375980345, 78.95724293864769550 ) ) ;
#179349=CARTESIAN_POINT ( 'NONE',  ( 5.049401038298161559, -19.05341960407611168, 92.70724293864769550 ) ) ;
#179350=CARTESIAN_POINT ( 'NONE',  ( -14.34966873604960291, -8.224510206698953496, 56.66557627198103830 ) ) ;
#179353=CARTESIAN_POINT ( 'NONE',  ( 9.474510206698729675, 16.51473224551082808, 72.08442372801900433 ) ) ;
#179354=CARTESIAN_POINT ( 'NONE',  ( -5.823673210054116645, -21.52544592524344225, 107.2905762719810525 ) ) ;
#179355=CARTESIAN_POINT ( 'NONE',  ( 19.02544592524343514, -5.153800228976328945, 53.54057627198102409 ) ) ;
#179356=CARTESIAN_POINT ( 'NONE',  ( -16.46253265017146816, -9.564922557961047289, 39.16775706135234003 ) ) ;
#179357=CARTESIAN_POINT ( 'NONE',  ( -9.564922557960796823, -16.46253265017161027, 32.08224293864769550 ) ) ;
#179358=CARTESIAN_POINT ( 'NONE',  ( 0.05219959533937995610, -21.53943276465977519, 60.00109039468568284 ) ) ;
#179360=CARTESIAN_POINT ( 'NONE',  ( -16.52544592524342804, 4.483927247898546575, 46.04057627198103830 ) ) ;
#179361=CARTESIAN_POINT ( 'NONE',  ( 19.02544592524343514, -5.153800228976328945, 68.54057627198103830 ) ) ;
#179362=CARTESIAN_POINT ( 'NONE',  ( -21.52544592524343514, 5.823673210054127303, 71.04057627198103830 ) ) ;
#179363=CARTESIAN_POINT ( 'NONE',  ( -16.46253265017160317, 9.564922557960807481, 55.83224293864769550 ) ) ;
#179365=CARTESIAN_POINT ( 'NONE',  ( -18.67979575497178146, -10.72451020669898902, 66.66557627198102409 ) ) ;
#179366=VERTEX_POINT ( 'NONE', #74170 ) ;
#179367=CARTESIAN_POINT ( 'NONE',  ( 0.05219959533937995610, -21.53943276465977519, 95.00109039468568994 ) ) ;
#179369=CARTESIAN_POINT ( 'NONE',  ( 8.224510206698742110, 14.34966873604972548, 102.0844237280190185 ) ) ;
#179370=CARTESIAN_POINT ( 'NONE',  ( 16.55341960407611168, 4.379528057220329451, 88.95724293864769550 ) ) ;
#179371=CARTESIAN_POINT ( 'NONE',  ( -16.46253265017146816, -9.564922557961047289, 89.16775706135234714 ) ) ;
#179373=CARTESIAN_POINT ( 'NONE',  ( 5.049401038297881783, 19.05341960407617563, 37.29275706135232582 ) ) ;
#179374=CARTESIAN_POINT ( 'NONE',  ( 8.224510206698742110, 14.34966873604972548, 97.08442372801904696 ) ) ;
#179375=CARTESIAN_POINT ( 'NONE',  ( -0.05219959533936034679, 19.03943276465977164, 27.50109039468566507 ) ) ;
#179376=CARTESIAN_POINT ( 'NONE',  ( 5.049401038298161559, -19.05341960407611168, 87.70724293864769550 ) ) ;
#179377=CARTESIAN_POINT ( 'NONE',  ( 10.81492255796078972, 18.62759615963270932, 64.58224293864769550 ) ) ;
#179379=CARTESIAN_POINT ( 'NONE',  ( -16.53943276465976808, 0.05219959533911058130, 116.2489096053143669 ) ) ;
#179380=CARTESIAN_POINT ( 'NONE',  ( -5.719274019375665041, -21.55341960407619695, 89.79275706135236135 ) ) ;
#179381=CARTESIAN_POINT ( 'NONE',  ( 4.379528057220092307, 16.55341960407617563, 82.29275706135234714 ) ) ;
#179382=CARTESIAN_POINT ( 'NONE',  ( -15.80617190586768217, 15.72974639402176855, 28.12609039468568284 ) ) ;
#179383=CARTESIAN_POINT ( 'NONE',  ( 12.14591786802327356, -12.06949235617739191, 25.62609039468567929 ) ) ;
#179384=CARTESIAN_POINT ( 'NONE',  ( -13.89961937509977652, 13.97604488694528158, 105.6239096053143527 ) ) ;
#179385=CARTESIAN_POINT ( 'NONE',  ( -19.02544592524342804, 5.153800228976336051, 46.04057627198101699 ) ) ;
#179386=CARTESIAN_POINT ( 'NONE',  ( -13.89961937509977652, 13.97604488694528158, 50.62390960531435979 ) ) ;
#179387=CARTESIAN_POINT ( 'NONE',  ( -8.314922557961024197, 14.29746914071037800, 32.91775706135234714 ) ) ;
#179388=CARTESIAN_POINT ( 'NONE',  ( 8.224510206698953496, -14.34966873604960469, 97.91557627198103830 ) ) ;
#179389=CARTESIAN_POINT ( 'NONE',  ( 4.483927247898790824, -16.52544592524335698, 100.2094237280190043 ) ) ;
#179390=CARTESIAN_POINT ( 'NONE',  ( -0.05219959533937732626, 21.53943276465977519, 37.50109039468568284 ) ) ;
#179391=CARTESIAN_POINT ( 'NONE',  ( 13.97604488694527802, 13.89961937509977652, 84.37390960531433848 ) ) ;
#179392=CARTESIAN_POINT ( 'NONE',  ( -13.97604488694527625, -13.89961937509977652, 61.87390960531435979 ) ) ;
#179393=CARTESIAN_POINT ( 'NONE',  ( 13.97604488694527802, 13.89961937509977652, 84.37390960531433848 ) ) ;
#179394=CARTESIAN_POINT ( 'NONE',  ( 4.379528057220339221, -16.55341960407611168, 27.70724293864769905 ) ) ;
#179395=CARTESIAN_POINT ( 'NONE',  ( 12.06949235617739724, 12.14591786802326823, 101.8760903946857042 ) ) ;
#179397=CARTESIAN_POINT ( 'NONE',  ( -9.564922557961040184, 16.46253265017147172, 37.91775706135233293 ) ) ;
#179398=CARTESIAN_POINT ( 'NONE',  ( -13.97604488694527625, -13.89961937509977652, 46.87390960531435979 ) ) ;
#179399=CARTESIAN_POINT ( 'NONE',  ( 9.564922557961047289, -16.46253265017146816, 35.41775706135233293 ) ) ;
#179401=CARTESIAN_POINT ( 'NONE',  ( -16.52544592524335698, -4.483927247898792601, 38.95942372801901854 ) ) ;
#179402=CARTESIAN_POINT ( 'NONE',  ( -13.97604488694547697, 13.89961937509957934, 68.12609039468563310 ) ) ;
#179403=CARTESIAN_POINT ( 'NONE',  ( -8.224510206698735004, -14.34966873604973081, 54.58442372801901143 ) ) ;
#179404=CARTESIAN_POINT ( 'NONE',  ( 19.02544592524343514, -5.153800228976328945, 113.5405762719810241 ) ) ;
#179405=CARTESIAN_POINT ( 'NONE',  ( -5.153800228976328057, -19.02544592524343514, 87.29057627198103830 ) ) ;
#179406=CARTESIAN_POINT ( 'NONE',  ( 21.55341960407619695, -5.719274019375665929, 21.04275706135234714 ) ) ;
#179407=CARTESIAN_POINT ( 'NONE',  ( -9.564922557961040184, 16.46253265017147172, 82.91775706135233293 ) ) ;
#179408=CARTESIAN_POINT ( 'NONE',  ( 16.51473224551069308, 9.474510206698969483, 99.16557627198102409 ) ) ;
#179409=CARTESIAN_POINT ( 'NONE',  ( 13.89961937509977652, -13.97604488694527269, 33.12390960531434558 ) ) ;
#179410=CARTESIAN_POINT ( 'NONE',  ( 9.474510206698971260, -16.51473224551069308, 77.91557627198103830 ) ) ;
#179411=CARTESIAN_POINT ( 'NONE',  ( -4.379528057220328563, 16.55341960407611168, 30.20724293864769550 ) ) ;
#179412=CARTESIAN_POINT ( 'NONE',  ( -5.153800228976328057, -19.02544592524343514, 32.29057627198102409 ) ) ;
#179413=CARTESIAN_POINT ( 'NONE',  ( 19.05341960407617918, -5.049401038297876454, 51.04275706135231871 ) ) ;
#179414=CARTESIAN_POINT ( 'NONE',  ( -14.34966873604960291, -8.224510206698953496, 81.66557627198103830 ) ) ;
#179415=CARTESIAN_POINT ( 'NONE',  ( -21.53943276465977519, -0.05219959533937600094, 108.7510903946857042 ) ) ;
#179416=CARTESIAN_POINT ( 'NONE',  ( 16.46253265017160672, -9.564922557960803928, 53.33224293864768839 ) ) ;
#179417=CARTESIAN_POINT ( 'NONE',  ( -10.72451020669898014, 18.67979575497178502, 45.41557627198103830 ) ) ;
#179418=CARTESIAN_POINT ( 'NONE',  ( 12.14591786802309770, 12.06949235617756955, 54.37390960531435979 ) ) ;
#179419=CARTESIAN_POINT ( 'NONE',  ( -21.53943276465977519, -0.05219959533937600094, 108.7510903946857042 ) ) ;
#179420=CARTESIAN_POINT ( 'NONE',  ( -19.02544592524342804, 5.153800228976336051, 96.04057627198103830 ) ) ;
#179421=CARTESIAN_POINT ( 'NONE',  ( -5.153800228976328057, -19.02544592524343514, 112.2905762719810099 ) ) ;
#179422=CARTESIAN_POINT ( 'NONE',  ( 13.89961937509977652, -13.97604488694527269, 33.12390960531434558 ) ) ;
#179423=CARTESIAN_POINT ( 'NONE',  ( 19.03943276465977164, -0.05219959533909143690, 28.74890960531435624 ) ) ;
#179424=CARTESIAN_POINT ( 'NONE',  ( -16.52544592524342804, 4.483927247898546575, 86.04057627198102409 ) ) ;
#179425=CARTESIAN_POINT ( 'NONE',  ( -18.62759615963270932, 10.81492255796079327, 90.83224293864769550 ) ) ;
#179426=CARTESIAN_POINT ( 'NONE',  ( 9.474510206698971260, -16.51473224551069308, 102.9155762719810241 ) ) ;
#179427=CARTESIAN_POINT ( 'NONE',  ( 15.72974639402199770, -15.80617190586745480, 108.1239096053143811 ) ) ;
#179428=CARTESIAN_POINT ( 'NONE',  ( 9.474510206698971260, -16.51473224551069308, 92.91557627198103830 ) ) ;
#179430=CARTESIAN_POINT ( 'NONE',  ( 12.06949235617757843, -12.14591786802309237, 108.1239096053143811 ) ) ;
#179431=CARTESIAN_POINT ( 'NONE',  ( -16.46253265017160317, 9.564922557960807481, 75.83224293864769550 ) ) ;
#179432=CARTESIAN_POINT ( 'NONE',  ( 18.67979575497178502, 10.72451020669898547, 74.16557627198102409 ) ) ;
#179435=CARTESIAN_POINT ( 'NONE',  ( 5.719274019375991003, -21.55341960407610458, 27.70724293864769905 ) ) ;
#179436=LINE ( 'NONE', #93342, #146893 ) ;
#179437=CARTESIAN_POINT ( 'NONE',  ( 4.483927247898790824, -16.52544592524335698, 35.20942372801901854 ) ) ;
#179438=CARTESIAN_POINT ( 'NONE',  ( -16.52544592524342804, 4.483927247898546575, 101.0405762719810383 ) ) ;
#179439=CARTESIAN_POINT ( 'NONE',  ( 19.48894818550245489, -5.499999999999918288, 52.60307310435240424 ) ) ;
#179440=CARTESIAN_POINT ( 'NONE',  ( 9.474510206698971260, -16.51473224551069308, 92.91557627198103830 ) ) ;
#179441=CARTESIAN_POINT ( 'NONE',  ( 5.049401038298161559, -19.05341960407611168, 47.70724293864770260 ) ) ;
#179442=CARTESIAN_POINT ( 'NONE',  ( 4.483927247898545687, 16.52544592524342804, 74.79057627198105251 ) ) ;
#179443=CARTESIAN_POINT ( 'NONE',  ( -5.823673210054116645, -21.52544592524344225, 27.29057627198103120 ) ) ;
#179444=CARTESIAN_POINT ( 'NONE',  ( 8.224510206698953496, -14.34966873604960469, 52.91557627198103830 ) ) ;
#179445=CARTESIAN_POINT ( 'NONE',  ( 19.02544592524334988, 5.153800228976608722, 106.4594237280190185 ) ) ;
#179446=CARTESIAN_POINT ( 'NONE',  ( -21.52544592524334988, -5.823673210054445271, 68.95942372801901854 ) ) ;
#179448=CARTESIAN_POINT ( 'NONE',  ( -16.51473224551069308, -9.474510206698971260, 111.6655762719810383 ) ) ;
#179449=CARTESIAN_POINT ( 'NONE',  ( 16.52544592524335698, 4.483927247898782831, 81.45942372801900433 ) ) ;
#179450=CARTESIAN_POINT ( 'NONE',  ( 9.474510206698971260, -16.51473224551069308, 27.91557627198103120 ) ) ;
#179451=CARTESIAN_POINT ( 'NONE',  ( 19.02544592524343514, -5.153800228976328945, 73.54057627198103830 ) ) ;
#179452=CARTESIAN_POINT ( 'NONE',  ( 21.55341960407610458, 5.719274019375980345, 78.95724293864769550 ) ) ;
#179453=CARTESIAN_POINT ( 'NONE',  ( -8.224510206698735004, -14.34966873604973081, 29.58442372801901854 ) ) ;
#179454=CARTESIAN_POINT ( 'NONE',  ( 4.379528057220339221, -16.55341960407611168, 57.70724293864770260 ) ) ;
#179455=CARTESIAN_POINT ( 'NONE',  ( -18.67979575497193778, 10.72451020669871902, 73.33442372801901854 ) ) ;
#179457=CARTESIAN_POINT ( 'NONE',  ( -12.14591786802326823, 12.06949235617739902, 93.12609039468568994 ) ) ;
#179458=CARTESIAN_POINT ( 'NONE',  ( -10.72451020669898014, 18.67979575497178502, 30.41557627198101699 ) ) ;
#179459=CARTESIAN_POINT ( 'NONE',  ( 9.564922557960805705, 16.46253265017160317, 114.5822429386476955 ) ) ;
#179461=CARTESIAN_POINT ( 'NONE',  ( -0.05219959533934338120, 16.53943276465976808, 102.5010903946856899 ) ) ;
#179462=CARTESIAN_POINT ( 'NONE',  ( -4.379528057220086978, -16.55341960407618274, 64.79275706135234714 ) ) ;
#179463=CARTESIAN_POINT ( 'NONE',  ( 13.89961937509977652, -13.97604488694527269, 73.12390960531436690 ) ) ;
#179465=CARTESIAN_POINT ( 'NONE',  ( 9.564922557960805705, 16.46253265017160317, 89.58224293864769550 ) ) ;
#179466=CARTESIAN_POINT ( 'NONE',  ( 15.72974639402176855, 15.80617190586768217, 71.87609039468568994 ) ) ;
#179467=CARTESIAN_POINT ( 'NONE',  ( 12.14591786802327356, -12.06949235617739191, 75.62609039468567573 ) ) ;
#179468=CARTESIAN_POINT ( 'NONE',  ( -14.29746914071049879, 8.314922557960819915, 40.83224293864769550 ) ) ;
#179469=CARTESIAN_POINT ( 'NONE',  ( -16.46253265017160317, 9.564922557960807481, 55.83224293864769550 ) ) ;
#179470=CARTESIAN_POINT ( 'NONE',  ( 16.46253265017160672, -9.564922557960803928, 43.33224293864769550 ) ) ;
#179472=CARTESIAN_POINT ( 'NONE',  ( 19.05341960407617918, -5.049401038297876454, 101.0427570613523045 ) ) ;
#179473=CARTESIAN_POINT ( 'NONE',  ( -8.224510206698948167, 14.34966873604960824, 110.4155762719810383 ) ) ;
#179474=CARTESIAN_POINT ( 'NONE',  ( -0.05219959533909027116, -19.03943276465977164, 62.49890960531435979 ) ) ;
#179475=CARTESIAN_POINT ( 'NONE',  ( -13.97604488694547697, 13.89961937509957934, 103.1260903946856473 ) ) ;
#179477=CARTESIAN_POINT ( 'NONE',  ( 5.719274019375673035, 21.55341960407619339, 97.29275706135234714 ) ) ;
#179478=CARTESIAN_POINT ( 'NONE',  ( -12.14591786802326823, 12.06949235617739902, 63.12609039468568994 ) ) ;
#179479=CARTESIAN_POINT ( 'NONE',  ( 0.05219959533936267826, -19.03943276465977164, 90.00109039468567573 ) ) ;
#179480=CARTESIAN_POINT ( 'NONE',  ( -18.67979575497178146, -10.72451020669898902, 56.66557627198103830 ) ) ;
#179481=CARTESIAN_POINT ( 'NONE',  ( -14.29746914071037622, -8.314922557961029526, 59.16775706135234714 ) ) ;
#179483=CARTESIAN_POINT ( 'NONE',  ( -9.474510206698720793, -16.51473224551083518, 59.58442372801900433 ) ) ;
#179485=CARTESIAN_POINT ( 'NONE',  ( -5.719274019375665041, -21.55341960407619695, 94.79275706135234714 ) ) ;
#179486=CARTESIAN_POINT ( 'NONE',  ( 19.05341960407611168, 5.049401038298154454, 23.95724293864769194 ) ) ;
#179487=CARTESIAN_POINT ( 'NONE',  ( 13.97604488694527802, 13.89961937509977652, 64.37390960531436690 ) ) ;
#179488=CARTESIAN_POINT ( 'NONE',  ( 16.52544592524342804, -4.483927247898539470, 63.54057627198103830 ) ) ;
#179489=CARTESIAN_POINT ( 'NONE',  ( -15.80617190586768217, 15.72974639402176855, 88.12609039468570415 ) ) ;
#179490=CARTESIAN_POINT ( 'NONE',  ( -19.02544592524334988, -5.153800228976617603, 48.95942372801900433 ) ) ;
#179491=CARTESIAN_POINT ( 'NONE',  ( 9.564922557961047289, -16.46253265017146816, 25.41775706135234003 ) ) ;
#179492=CARTESIAN_POINT ( 'NONE',  ( 5.153800228976335163, 19.02544592524342804, 114.7905762719810241 ) ) ;
#179493=CARTESIAN_POINT ( 'NONE',  ( -5.823673210054431948, 21.52544592524334988, 102.7094237280190185 ) ) ;
#179494=CARTESIAN_POINT ( 'NONE',  ( 5.049401038298161559, -19.05341960407611168, 72.70724293864768129 ) ) ;
#179495=CARTESIAN_POINT ( 'NONE',  ( -18.62759615963255300, -10.81492255796106328, 89.16775706135236135 ) ) ;
#179496=CARTESIAN_POINT ( 'NONE',  ( 0.05219959533907565091, 21.53943276465977519, 54.99890960531435269 ) ) ;
#179497=CARTESIAN_POINT ( 'NONE',  ( -9.564922557960796823, -16.46253265017161027, 87.08224293864769550 ) ) ;
#179498=CARTESIAN_POINT ( 'NONE',  ( 13.89961937509957401, 13.97604488694547697, 66.87609039468567573 ) ) ;
#179499=CARTESIAN_POINT ( 'NONE',  ( -13.97604488694527625, -13.89961937509977652, 36.87390960531436690 ) ) ;
#179500=CARTESIAN_POINT ( 'NONE',  ( -13.97604488694527625, -13.89961937509977652, 91.87390960531432427 ) ) ;
#179501=CARTESIAN_POINT ( 'NONE',  ( -16.46253265017146816, -9.564922557961047289, 84.16775706135233293 ) ) ;
#179502=CARTESIAN_POINT ( 'NONE',  ( 16.55341960407618274, -4.379528057220086978, 46.04275706135234714 ) ) ;
#179503=CARTESIAN_POINT ( 'NONE',  ( 4.379528057220339221, -16.55341960407611168, 102.7072429386476955 ) ) ;
#179504=CARTESIAN_POINT ( 'NONE',  ( -13.89961937509977652, 13.97604488694528158, 75.62390960531438111 ) ) ;
#179505=CARTESIAN_POINT ( 'NONE',  ( 5.719274019375991003, -21.55341960407610458, 52.70724293864769550 ) ) ;
#179506=CARTESIAN_POINT ( 'NONE',  ( 16.52544592524335698, 4.483927247898782831, 21.45942372801901499 ) ) ;
#179507=CARTESIAN_POINT ( 'NONE',  ( -18.62759615963270932, 10.81492255796079327, 115.8322429386477097 ) ) ;
#179508=CARTESIAN_POINT ( 'NONE',  ( 21.53943276465977519, 0.05219959533937863772, 86.25109039468568994 ) ) ;
#179509=CARTESIAN_POINT ( 'NONE',  ( -12.14591786802326823, 12.06949235617739902, 83.12609039468568994 ) ) ;
#179510=CARTESIAN_POINT ( 'NONE',  ( -13.89961937509977652, 13.97604488694528158, 75.62390960531438111 ) ) ;
#179511=CARTESIAN_POINT ( 'NONE',  ( 16.53943276465976808, 0.05219959533934440121, 96.25109039468568994 ) ) ;
#179512=CARTESIAN_POINT ( 'NONE',  ( 13.97604488694548053, -13.89961937509957401, 55.62609039468566863 ) ) ;
#179513=CARTESIAN_POINT ( 'NONE',  ( -10.72451020669870658, -18.67979575497194134, 34.58442372801900433 ) ) ;
#179514=CARTESIAN_POINT ( 'NONE',  ( -14.29746914071049879, 8.314922557960819915, 80.83224293864769550 ) ) ;
#179515=CARTESIAN_POINT ( 'NONE',  ( 13.97604488694527802, 13.89961937509977652, 104.3739096053143385 ) ) ;
#179516=CARTESIAN_POINT ( 'NONE',  ( 14.34966873604972726, -8.224510206698740333, 90.83442372801901854 ) ) ;
#179517=CARTESIAN_POINT ( 'NONE',  ( 10.81492255796106328, -18.62759615963255655, 75.41775706135233293 ) ) ;
#179518=CARTESIAN_POINT ( 'NONE',  ( 16.53943276465976808, 0.05219959533934440121, 31.25109039468568639 ) ) ;
#179519=CARTESIAN_POINT ( 'NONE',  ( -10.81492255796105439, 18.62759615963255655, 27.91775706135234358 ) ) ;
#179520=CARTESIAN_POINT ( 'NONE',  ( -0.05219959533910754901, -16.53943276465976808, 67.49890960531436690 ) ) ;
#179522=CARTESIAN_POINT ( 'NONE',  ( 0.05219959533907565091, 21.53943276465977519, 104.9989096053143669 ) ) ;
#179523=CARTESIAN_POINT ( 'NONE',  ( 4.379528057220339221, -16.55341960407611168, 57.70724293864770260 ) ) ;
#179525=CARTESIAN_POINT ( 'NONE',  ( 13.89961937509977652, -13.97604488694527269, 28.12390960531435624 ) ) ;
#179526=CARTESIAN_POINT ( 'NONE',  ( 5.823673210054125526, 21.52544592524343514, 24.79057627198103120 ) ) ;
#179527=CARTESIAN_POINT ( 'NONE',  ( 5.823673210054444382, -21.52544592524334988, 55.20942372801902565 ) ) ;
#179528=CARTESIAN_POINT ( 'NONE',  ( 16.55341960407611168, 4.379528057220329451, 58.95724293864770971 ) ) ;
#179529=CARTESIAN_POINT ( 'NONE',  ( -21.53943276465977519, 0.05219959533907696930, 71.24890960531435269 ) ) ;
#179530=CARTESIAN_POINT ( 'NONE',  ( -19.02544592524342804, 5.153800228976336051, 71.04057627198099567 ) ) ;
#179531=CARTESIAN_POINT ( 'NONE',  ( -0.05219959533909027116, -19.03943276465977164, 27.49890960531435624 ) ) ;
#179532=CARTESIAN_POINT ( 'NONE',  ( 9.474510206698729675, 16.51473224551082808, 82.08442372801899012 ) ) ;
#179534=CARTESIAN_POINT ( 'NONE',  ( -10.72451020669898014, 18.67979575497178502, 55.41557627198102409 ) ) ;
#179535=CARTESIAN_POINT ( 'NONE',  ( -13.97604488694527625, -13.89961937509977652, 41.87390960531435979 ) ) ;
#179536=CARTESIAN_POINT ( 'NONE',  ( -16.46253265017160317, 9.564922557960807481, 65.83224293864769550 ) ) ;
#179537=ORIENTED_EDGE ( 'NONE', *, *, #158923, .F. ) ;
#179538=CARTESIAN_POINT ( 'NONE',  ( 16.52544592524335698, 4.483927247898782831, 51.45942372801901854 ) ) ;
#179539=CARTESIAN_POINT ( 'NONE',  ( 10.72451020669871369, 18.67979575497193778, 27.08442372801901854 ) ) ;
#179540=CARTESIAN_POINT ( 'NONE',  ( 10.81492255796106328, -18.62759615963255655, 65.41775706135234714 ) ) ;
#179541=CARTESIAN_POINT ( 'NONE',  ( 19.02544592524343514, -5.153800228976328945, 98.54057627198100988 ) ) ;
#179542=CARTESIAN_POINT ( 'NONE',  ( -21.55341960407610458, -5.719274019375992779, 81.45724293864769550 ) ) ;
#179543=CARTESIAN_POINT ( 'NONE',  ( -21.53943276465977519, -0.05219959533937600094, 23.75109039468567929 ) ) ;
#179544=CARTESIAN_POINT ( 'NONE',  ( 16.55341960407618274, -4.379528057220086978, 56.04275706135235424 ) ) ;
#179545=CARTESIAN_POINT ( 'NONE',  ( 15.80617190586746368, 15.72974639402197994, 54.37390960531435979 ) ) ;
#179546=CARTESIAN_POINT ( 'NONE',  ( -13.89961937509957401, -13.97604488694547875, 24.37609039468565442 ) ) ;
#179547=CARTESIAN_POINT ( 'NONE',  ( -19.02544592524342804, 5.153800228976336051, 56.04057627198100988 ) ) ;
#179548=CARTESIAN_POINT ( 'NONE',  ( 0.05219959533909260263, 19.03943276465977164, 109.9989096053143669 ) ) ;
#179549=CARTESIAN_POINT ( 'NONE',  ( 16.46253265017160672, -9.564922557960803928, 93.33224293864769550 ) ) ;
#179551=CARTESIAN_POINT ( 'NONE',  ( 13.89961937509957401, 13.97604488694547697, 66.87609039468567573 ) ) ;
#179552=CARTESIAN_POINT ( 'NONE',  ( 10.72451020669898902, -18.67979575497178502, 42.91557627198103120 ) ) ;
#179553=CARTESIAN_POINT ( 'NONE',  ( 14.34966873604960469, 8.224510206698951720, 24.16557627198103120 ) ) ;
#179554=CARTESIAN_POINT ( 'NONE',  ( 9.474510206698729675, 16.51473224551082808, 82.08442372801899012 ) ) ;
#179555=CARTESIAN_POINT ( 'NONE',  ( -17.50000000000001776, 5.622605283950873556, 58.68792689403890250 ) ) ;
#179556=CARTESIAN_POINT ( 'NONE',  ( -19.03943276465977164, -0.05219959533935918106, 23.75109039468566152 ) ) ;
#179557=CARTESIAN_POINT ( 'NONE',  ( 5.153800228976615827, -19.02544592524334988, 80.20942372801901854 ) ) ;
#179558=CARTESIAN_POINT ( 'NONE',  ( -13.89961937509957401, -13.97604488694547875, 44.37609039468566863 ) ) ;
#179559=CARTESIAN_POINT ( 'NONE',  ( -15.49999999999999822, 5.499999999999998224, 120.0000000000000142 ) ) ;
#179560=CARTESIAN_POINT ( 'NONE',  ( -0.05219959533909027116, -19.03943276465977164, 52.49890960531436690 ) ) ;
#179561=CARTESIAN_POINT ( 'NONE',  ( 0.05219959533910956823, 16.53943276465976808, 44.99890960531435979 ) ) ;
#179562=CARTESIAN_POINT ( 'NONE',  ( 0.05219959533909260263, 19.03943276465977164, 39.99890960531436690 ) ) ;
#179563=CARTESIAN_POINT ( 'NONE',  ( 16.55341960407611168, 4.379528057220329451, 43.95724293864769550 ) ) ;
#179564=CARTESIAN_POINT ( 'NONE',  ( 17.60769864724391098, -5.499999999999977796, 56.15024842019168005 ) ) ;
#179565=CARTESIAN_POINT ( 'NONE',  ( 12.14591786802327356, -12.06949235617739191, 110.6260903946857042 ) ) ;
#179566=CARTESIAN_POINT ( 'NONE',  ( 19.03943276465977164, -0.05219959533909143690, 43.74890960531435979 ) ) ;
#179567=CARTESIAN_POINT ( 'NONE',  ( 16.51473224551083163, -9.474510206698727899, 25.83442372801900078 ) ) ;
#179568=CARTESIAN_POINT ( 'NONE',  ( 16.53943276465976808, 0.05219959533934440121, 31.25109039468568639 ) ) ;
#179569=CARTESIAN_POINT ( 'NONE',  ( 21.55341960407610458, 5.719274019375980345, 33.95724293864769550 ) ) ;
#179570=CARTESIAN_POINT ( 'NONE',  ( -15.72974639402176322, -15.80617190586768395, 89.37609039468568994 ) ) ;
#179571=ORIENTED_EDGE ( 'NONE', *, *, #109656, .T. ) ;
#179572=CARTESIAN_POINT ( 'NONE',  ( -5.153800228976328057, -19.02544592524343514, 62.29057627198100988 ) ) ;
#179573=CARTESIAN_POINT ( 'NONE',  ( -5.153800228976328057, -19.02544592524343514, 112.2905762719810099 ) ) ;
#179574=CARTESIAN_POINT ( 'NONE',  ( -13.89961937509977652, 13.97604488694528158, 100.6239096053143669 ) ) ;
#179576=CARTESIAN_POINT ( 'NONE',  ( 10.72451020669871369, 18.67979575497193778, 27.08442372801901854 ) ) ;
#179577=CARTESIAN_POINT ( 'NONE',  ( 4.483927247898545687, 16.52544592524342804, 74.79057627198105251 ) ) ;
#179578=CARTESIAN_POINT ( 'NONE',  ( 21.52544592524344225, -5.823673210054117533, 78.54057627198103830 ) ) ;
#179579=CARTESIAN_POINT ( 'NONE',  ( 9.474510206698971260, -16.51473224551069308, 72.91557627198102409 ) ) ;
#179580=CARTESIAN_POINT ( 'NONE',  ( 9.474510206698971260, -16.51473224551069308, 72.91557627198102409 ) ) ;
#179581=CARTESIAN_POINT ( 'NONE',  ( -5.719274019375978568, 21.55341960407610458, 105.2072429386477097 ) ) ;
#179583=CARTESIAN_POINT ( 'NONE',  ( -16.46253265017160317, 9.564922557960807481, 75.83224293864769550 ) ) ;
#179584=CARTESIAN_POINT ( 'NONE',  ( -12.06949235617756955, 12.14591786802309770, 100.6239096053143811 ) ) ;
#179585=CARTESIAN_POINT ( 'NONE',  ( -16.51473224551069308, -9.474510206698971260, 26.66557627198103120 ) ) ;
#179586=CARTESIAN_POINT ( 'NONE',  ( -13.97604488694527625, -13.89961937509977652, 66.87390960531436690 ) ) ;
#179587=CARTESIAN_POINT ( 'NONE',  ( -5.049401038297874678, -19.05341960407617918, 99.79275706135234714 ) ) ;
#179588=CARTESIAN_POINT ( 'NONE',  ( -4.483927247898539470, -16.52544592524342804, 97.29057627198105251 ) ) ;
#179589=CARTESIAN_POINT ( 'NONE',  ( 15.80617190586769283, -15.72974639402175789, 60.62609039468567573 ) ) ;
#179590=CARTESIAN_POINT ( 'NONE',  ( -0.05219959533909027116, -19.03943276465977164, 47.49890960531435979 ) ) ;
#179591=CARTESIAN_POINT ( 'NONE',  ( 21.53943276465977519, 0.05219959533937863772, 26.25109039468567573 ) ) ;
#179592=CARTESIAN_POINT ( 'NONE',  ( -4.379528057220328563, 16.55341960407611168, 100.2072429386476955 ) ) ;
#179594=CARTESIAN_POINT ( 'NONE',  ( -9.474510206698964154, 16.51473224551069663, 75.41557627198103830 ) ) ;
#179595=CARTESIAN_POINT ( 'NONE',  ( 17.05587630539788080, 6.762274262135663960, 111.7581969096268892 ) ) ;
#179596=CARTESIAN_POINT ( 'NONE',  ( 16.51473224551083163, -9.474510206698727899, 110.8344237280190043 ) ) ;
#179597=CARTESIAN_POINT ( 'NONE',  ( 21.55341960407610458, 5.719274019375980345, 28.95724293864769905 ) ) ;
#179598=CARTESIAN_POINT ( 'NONE',  ( -0.05219959533937732626, 21.53943276465977519, 52.50109039468567573 ) ) ;
#179599=CARTESIAN_POINT ( 'NONE',  ( -13.97604488694527625, -13.89961937509977652, 101.8739096053143811 ) ) ;
#179600=CARTESIAN_POINT ( 'NONE',  ( -9.474510206698720793, -16.51473224551083518, 89.58442372801900433 ) ) ;
#179601=CARTESIAN_POINT ( 'NONE',  ( 16.51473224551069308, 9.474510206698969483, 69.16557627198102409 ) ) ;
#179602=CARTESIAN_POINT ( 'NONE',  ( -4.483927247898539470, -16.52544592524342804, 77.29057627198102409 ) ) ;
#179603=CARTESIAN_POINT ( 'NONE',  ( -0.05219959533909027116, -19.03943276465977164, 102.4989096053143669 ) ) ;
#179604=CARTESIAN_POINT ( 'NONE',  ( -16.55341960407611168, -4.379528057220339221, 81.45724293864769550 ) ) ;
#179605=CARTESIAN_POINT ( 'NONE',  ( -13.97604488694527625, -13.89961937509977652, 96.87390960531433848 ) ) ;
#179606=CARTESIAN_POINT ( 'NONE',  ( -9.474510206698964154, 16.51473224551069663, 50.41557627198102409 ) ) ;
#179607=CARTESIAN_POINT ( 'NONE',  ( -0.05219959533910754901, -16.53943276465976808, 47.49890960531435979 ) ) ;
#179608=CARTESIAN_POINT ( 'NONE',  ( 13.97604488694527802, 13.89961937509977652, 29.37390960531435979 ) ) ;
#179609=EDGE_LOOP ( 'NONE', ( #42934, #12510, #73908, #132776 ) ) ;
#179610=CARTESIAN_POINT ( 'NONE',  ( -5.823673210054431948, 21.52544592524334988, 42.70942372801901854 ) ) ;
#179611=CARTESIAN_POINT ( 'NONE',  ( 16.46253265017146816, 9.564922557961045513, 81.66775706135233293 ) ) ;
#179612=CARTESIAN_POINT ( 'NONE',  ( -12.14591786802309592, -12.06949235617757132, 46.87390960531435979 ) ) ;
#179613=CARTESIAN_POINT ( 'NONE',  ( -10.81492255796078084, -18.62759615963271287, 97.08224293864770971 ) ) ;
#179614=CARTESIAN_POINT ( 'NONE',  ( 21.53943276465977519, -0.05219959533907433946, 33.74890960531436690 ) ) ;
#179615=AXIS2_PLACEMENT_3D ( 'NONE', #104539, #43861, #61981 ) ;
#179616=CARTESIAN_POINT ( 'NONE',  ( -16.55341960407611168, -4.379528057220339221, 81.45724293864769550 ) ) ;
#179617=CARTESIAN_POINT ( 'NONE',  ( 13.89961937509977652, -13.97604488694527269, 38.12390960531436690 ) ) ;
#179618=CARTESIAN_POINT ( 'NONE',  ( -4.483927247898782831, 16.52544592524335698, 112.7094237280190328 ) ) ;
#179619=CARTESIAN_POINT ( 'NONE',  ( -16.52544592524335698, -4.483927247898792601, 88.95942372801901854 ) ) ;
#179620=CARTESIAN_POINT ( 'NONE',  ( -8.314922557961024197, 14.29746914071037800, 72.91775706135234714 ) ) ;
#179621=CARTESIAN_POINT ( 'NONE',  ( 19.05341960407617918, -5.049401038297876454, 21.04275706135232582 ) ) ;
#179622=CARTESIAN_POINT ( 'NONE',  ( 13.89961937509977652, -13.97604488694527269, 93.12390960531436690 ) ) ;
#179623=CARTESIAN_POINT ( 'NONE',  ( 9.474510206698971260, -16.51473224551069308, 82.91557627198103830 ) ) ;
#179624=CARTESIAN_POINT ( 'NONE',  ( 4.379528057220092307, 16.55341960407617563, 92.29275706135236135 ) ) ;
#179625=CARTESIAN_POINT ( 'NONE',  ( 16.46253265017160672, -9.564922557960803928, 38.33224293864768839 ) ) ;
#179626=CARTESIAN_POINT ( 'NONE',  ( 0.05219959533910956823, 16.53943276465976808, 44.99890960531435979 ) ) ;
#179628=CARTESIAN_POINT ( 'NONE',  ( -5.049401038298153566, 19.05341960407611168, 105.2072429386476671 ) ) ;
#179629=CARTESIAN_POINT ( 'NONE',  ( -10.81492255796078084, -18.62759615963271287, 27.08224293864769550 ) ) ;
#179630=CARTESIAN_POINT ( 'NONE',  ( 16.52544592524342804, -4.483927247898539470, 68.54057627198103830 ) ) ;
#179631=B_SPLINE_CURVE_WITH_KNOTS ( 'NONE', 3,
 ( #66121, #19629, #94468, #3452, #65129, #126786, #127786, #112623, #50964, #47993, #155160, #188492, #78299, #124819, #35785, #187513, #97432, #62140, #109647, #15660 ),
 .UNSPECIFIED., .F., .F.,
 ( 4, 2, 2, 2, 2, 2, 2, 2, 2, 4 ),
 ( 0.000000000000000000, 0.0004987090165372566565, 0.0009974180330745133129, 0.001246772541343138009, 0.001496127049611762488, 0.001994836066149011881, 0.002493545082686261273, 0.002742899590954883584, 0.002992254099223505895, 0.003989672132298080140 ),
 .UNSPECIFIED. ) ;
#179633=CARTESIAN_POINT ( 'NONE',  ( -8.314922557960811034, -14.29746914071050412, 67.08224293864770971 ) ) ;
#179634=DIRECTION ( 'NONE',  ( 0.000000000000000000, 0.000000000000000000, -1.000000000000000000 ) ) ;
#179635=CARTESIAN_POINT ( 'NONE',  ( 16.46253265017146816, 9.564922557961045513, 66.66775706135233293 ) ) ;
#179636=CARTESIAN_POINT ( 'NONE',  ( -0.05219959533909027116, -19.03943276465977164, 102.4989096053143669 ) ) ;
#179637=CARTESIAN_POINT ( 'NONE',  ( 19.02544592524334988, 5.153800228976608722, 76.45942372801897591 ) ) ;
#179639=CARTESIAN_POINT ( 'NONE',  ( 14.29746914071037800, 8.314922557961029526, 21.66775706135235069 ) ) ;
#179640=CARTESIAN_POINT ( 'NONE',  ( -12.06949235617739369, -12.14591786802326823, 89.37609039468568994 ) ) ;
#179641=CARTESIAN_POINT ( 'NONE',  ( -13.89961937509977652, 13.97604488694528158, 40.62390960531435979 ) ) ;
#179643=CARTESIAN_POINT ( 'NONE',  ( -18.62759615963270932, 10.81492255796079327, 35.83224293864768839 ) ) ;
#179644=CARTESIAN_POINT ( 'NONE',  ( 15.72974639402176855, 15.80617190586768217, 56.87609039468568994 ) ) ;
#179645=CARTESIAN_POINT ( 'NONE',  ( -5.153800228976607833, 19.02544592524334988, 112.7094237280190043 ) ) ;
#179647=CARTESIAN_POINT ( 'NONE',  ( -16.51473224551069308, -9.474510206698971260, 71.66557627198102409 ) ) ;
#179648=CARTESIAN_POINT ( 'NONE',  ( 19.05341960407611168, 5.049401038298154454, 113.9572429386477097 ) ) ;
#179649=CARTESIAN_POINT ( 'NONE',  ( 16.53943276465976808, -0.05219959533910856209, 73.74890960531433848 ) ) ;
#179650=CARTESIAN_POINT ( 'NONE',  ( -19.05341960407611168, -5.049401038298163336, 81.45724293864769550 ) ) ;
#179651=CARTESIAN_POINT ( 'NONE',  ( -19.05341960407611168, -5.049401038298163336, 91.45724293864766707 ) ) ;
#179653=CARTESIAN_POINT ( 'NONE',  ( -19.05341960407617563, 5.049401038297882671, 93.54275706135234714 ) ) ;
#179654=CARTESIAN_POINT ( 'NONE',  ( 21.55341960407610458, 5.719274019375980345, 58.95724293864770971 ) ) ;
#179655=CARTESIAN_POINT ( 'NONE',  ( -9.564922557960796823, -16.46253265017161027, 27.08224293864769550 ) ) ;
#179656=CARTESIAN_POINT ( 'NONE',  ( -0.05219959533936034679, 19.03943276465977164, 57.50109039468566863 ) ) ;
#179657=CARTESIAN_POINT ( 'NONE',  ( -0.05219959533909027116, -19.03943276465977164, 62.49890960531435979 ) ) ;
#179658=CARTESIAN_POINT ( 'NONE',  ( 5.153800228976335163, 19.02544592524342804, 94.79057627198103830 ) ) ;
#179660=CARTESIAN_POINT ( 'NONE',  ( -21.52544592524343514, 5.823673210054127303, 96.04057627198102409 ) ) ;
#179661=CARTESIAN_POINT ( 'NONE',  ( -14.34966873604960291, -8.224510206698953496, 96.66557627198102409 ) ) ;
#179662=CARTESIAN_POINT ( 'NONE',  ( 9.564922557961047289, -16.46253265017146816, 50.41775706135233293 ) ) ;
#179663=CARTESIAN_POINT ( 'NONE',  ( 5.719274019375991003, -21.55341960407610458, 92.70724293864770971 ) ) ;
#179664=CARTESIAN_POINT ( 'NONE',  ( 21.55341960407610458, 5.719274019375980345, 73.95724293864769550 ) ) ;
#179665=CARTESIAN_POINT ( 'NONE',  ( 12.14591786802309770, 12.06949235617756955, 29.37390960531435269 ) ) ;
#179666=CARTESIAN_POINT ( 'NONE',  ( -21.52544592524334988, -5.823673210054445271, 108.9594237280190185 ) ) ;
#179667=CARTESIAN_POINT ( 'NONE',  ( -14.29746914071037622, -8.314922557961029526, 49.16775706135234003 ) ) ;
#179668=CARTESIAN_POINT ( 'NONE',  ( -13.89961937509977652, 13.97604488694528158, 75.62390960531438111 ) ) ;
#179669=CARTESIAN_POINT ( 'NONE',  ( 19.05341960407611168, 5.049401038298154454, 33.95724293864769550 ) ) ;
#179670=CARTESIAN_POINT ( 'NONE',  ( 10.72451020669871369, 18.67979575497193778, 42.08442372801901854 ) ) ;
#179671=CARTESIAN_POINT ( 'NONE',  ( -10.81492255796105439, 18.62759615963255655, 52.91775706135235424 ) ) ;
#179672=CARTESIAN_POINT ( 'NONE',  ( -16.51473224551069308, -9.474510206698971260, 41.66557627198103120 ) ) ;
#179673=CARTESIAN_POINT ( 'NONE',  ( 18.67979575497194134, -10.72451020669871369, 25.83442372801901499 ) ) ;
#179674=CARTESIAN_POINT ( 'NONE',  ( -13.97604488694547697, 13.89961937509957934, 63.12609039468566152 ) ) ;
#179675=CARTESIAN_POINT ( 'NONE',  ( 0.05219959533936267826, -19.03943276465977164, 80.00109039468567573 ) ) ;
#179676=CARTESIAN_POINT ( 'NONE',  ( -4.379528057220086978, -16.55341960407618274, 29.79275706135234358 ) ) ;
#179677=CARTESIAN_POINT ( 'NONE',  ( 9.564922557960805705, 16.46253265017160317, 24.58224293864769194 ) ) ;
#179678=CARTESIAN_POINT ( 'NONE',  ( -0.05219959533934338120, 16.53943276465976808, 67.50109039468568994 ) ) ;
#179679=CARTESIAN_POINT ( 'NONE',  ( 19.02544592524343514, -5.153800228976328945, 38.54057627198103120 ) ) ;
#179681=CARTESIAN_POINT ( 'NONE',  ( -13.97604488694527625, -13.89961937509977652, 101.8739096053143811 ) ) ;
#179682=CARTESIAN_POINT ( 'NONE',  ( -9.474510206698964154, 16.51473224551069663, 30.41557627198102054 ) ) ;
#179683=CARTESIAN_POINT ( 'NONE',  ( -0.05219959533907301413, -21.53943276465977519, 72.49890960531435269 ) ) ;
#179684=CARTESIAN_POINT ( 'NONE',  ( -12.14591786802326823, 12.06949235617739902, 63.12609039468568994 ) ) ;
#179685=CARTESIAN_POINT ( 'NONE',  ( -5.823673210054431948, 21.52544592524334988, 107.7094237280190328 ) ) ;
#179686=CARTESIAN_POINT ( 'NONE',  ( 5.049401038298161559, -19.05341960407611168, 42.70724293864767418 ) ) ;
#179687=CARTESIAN_POINT ( 'NONE',  ( 12.14591786802309770, 12.06949235617756955, 34.37390960531435979 ) ) ;
#179688=CARTESIAN_POINT ( 'NONE',  ( -16.55341960407611168, -4.379528057220339221, 71.45724293864769550 ) ) ;
#179689=CARTESIAN_POINT ( 'NONE',  ( -0.05219959533909027116, -19.03943276465977164, 67.49890960531436690 ) ) ;
#179690=CARTESIAN_POINT ( 'NONE',  ( -15.80617190586768217, 15.72974639402176855, 108.1260903946856757 ) ) ;
#179691=CARTESIAN_POINT ( 'NONE',  ( -10.72451020669870658, -18.67979575497194134, 39.58442372801901143 ) ) ;
#179692=CARTESIAN_POINT ( 'NONE',  ( -13.89961937509977652, 13.97604488694528158, 75.62390960531438111 ) ) ;
#179693=CARTESIAN_POINT ( 'NONE',  ( 21.53943276465977519, 0.05219959533937863772, 81.25109039468568994 ) ) ;
#179694=CARTESIAN_POINT ( 'NONE',  ( -16.52544592524335698, -4.483927247898792601, 63.95942372801901854 ) ) ;
#179695=CARTESIAN_POINT ( 'NONE',  ( 19.05341960407611168, 5.049401038298154454, 113.9572429386477097 ) ) ;
#179696=CARTESIAN_POINT ( 'NONE',  ( 14.29746914071049879, -8.314922557960816363, 28.33224293864769550 ) ) ;
#179697=CARTESIAN_POINT ( 'NONE',  ( 19.05341960407611168, 5.049401038298154454, 23.95724293864769194 ) ) ;
#179698=CARTESIAN_POINT ( 'NONE',  ( -14.29746914071037622, -8.314922557961029526, 54.16775706135235424 ) ) ;
#179699=CARTESIAN_POINT ( 'NONE',  ( 16.55341960407611168, 4.379528057220329451, 58.95724293864770971 ) ) ;
#179700=CARTESIAN_POINT ( 'NONE',  ( 16.51473224551069308, 9.474510206698969483, 109.1655762719810383 ) ) ;
#179701=CARTESIAN_POINT ( 'NONE',  ( 18.62759615963271287, -10.81492255796078972, 33.33224293864769550 ) ) ;
#179702=CARTESIAN_POINT ( 'NONE',  ( 10.72451020669871369, 18.67979575497193778, 107.0844237280190043 ) ) ;
#179703=CARTESIAN_POINT ( 'NONE',  ( -12.06949235617756955, 12.14591786802309770, 90.62390960531436690 ) ) ;
#179704=CARTESIAN_POINT ( 'NONE',  ( 16.51473224551069308, 9.474510206698969483, 99.16557627198102409 ) ) ;
#179706=CARTESIAN_POINT ( 'NONE',  ( -14.29746914071037622, -8.314922557961029526, 54.16775706135235424 ) ) ;
#179707=CARTESIAN_POINT ( 'NONE',  ( -5.049401038298153566, 19.05341960407611168, 50.20724293864770260 ) ) ;
#179709=CARTESIAN_POINT ( 'NONE',  ( 5.049401038297881783, 19.05341960407617563, 42.29275706135234003 ) ) ;
#179711=CARTESIAN_POINT ( 'NONE',  ( 12.06949235617739724, 12.14591786802326823, 81.87609039468568994 ) ) ;
#179712=CARTESIAN_POINT ( 'NONE',  ( 19.02544592524334988, 5.153800228976608722, 96.45942372801897591 ) ) ;
#179713=CARTESIAN_POINT ( 'NONE',  ( 0.05219959533937995610, -21.53943276465977519, 70.00109039468568994 ) ) ;
#179714=CARTESIAN_POINT ( 'NONE',  ( -19.02544592524342804, 5.153800228976336051, 61.04057627198103120 ) ) ;
#179715=CARTESIAN_POINT ( 'NONE',  ( 18.62759615963271287, -10.81492255796078972, 88.33224293864769550 ) ) ;
#179716=CARTESIAN_POINT ( 'NONE',  ( 12.14591786802309770, 12.06949235617756955, 104.3739096053143669 ) ) ;
#179718=ADVANCED_FACE ( 'NONE', ( #35591 ), #46743, .T. ) ;
#179719=CARTESIAN_POINT ( 'NONE',  ( -5.153800228976607833, 19.02544592524334988, 72.70942372801900433 ) ) ;
#179720=CARTESIAN_POINT ( 'NONE',  ( 18.62759615963271287, -10.81492255796078972, 58.33224293864768839 ) ) ;
#179721=CARTESIAN_POINT ( 'NONE',  ( -16.51473224551082808, 9.474510206698731452, 38.33442372801899722 ) ) ;
#179722=CARTESIAN_POINT ( 'NONE',  ( 19.02544592524343514, -5.153800228976328945, 113.5405762719810241 ) ) ;
#179723=CARTESIAN_POINT ( 'NONE',  ( 15.80617190586746368, 15.72974639402197994, 89.37390960531435269 ) ) ;
#179726=CARTESIAN_POINT ( 'NONE',  ( -19.02544592524334988, -5.153800228976617603, 108.9594237280189759 ) ) ;
#179728=CARTESIAN_POINT ( 'NONE',  ( -16.55341960407617563, 4.379528057220093196, 28.54275706135234358 ) ) ;
#179729=CARTESIAN_POINT ( 'NONE',  ( 19.05341960407611168, 5.049401038298154454, 48.95724293864768129 ) ) ;
#179730=CARTESIAN_POINT ( 'NONE',  ( -19.03943276465977164, 0.05219959533909376836, 106.2489096053143669 ) ) ;
#179731=CARTESIAN_POINT ( 'NONE',  ( 10.81492255796078972, 18.62759615963270932, 84.58224293864769550 ) ) ;
#179732=CARTESIAN_POINT ( 'NONE',  ( -4.483927247898539470, -16.52544592524342804, 52.29057627198102409 ) ) ;
#179733=CARTESIAN_POINT ( 'NONE',  ( 18.67979575497194134, -10.72451020669871369, 75.83442372801900433 ) ) ;
#179734=CARTESIAN_POINT ( 'NONE',  ( 8.314922557961029526, -14.29746914071037800, 20.41775706135234714 ) ) ;
#179735=CARTESIAN_POINT ( 'NONE',  ( -13.97604488694547697, 13.89961937509957934, 28.12609039468565797 ) ) ;
#179736=CARTESIAN_POINT ( 'NONE',  ( -16.55341960407611168, -4.379528057220339221, 36.45724293864768839 ) ) ;
#179737=CARTESIAN_POINT ( 'NONE',  ( -0.05219959533937732626, 21.53943276465977519, 22.50109039468567573 ) ) ;
#179738=CARTESIAN_POINT ( 'NONE',  ( -14.29746914071049879, 8.314922557960819915, 45.83224293864769550 ) ) ;
#179739=CARTESIAN_POINT ( 'NONE',  ( -0.05219959533936034679, 19.03943276465977164, 97.50109039468567573 ) ) ;
#179740=CARTESIAN_POINT ( 'NONE',  ( 16.46253265017146816, 9.564922557961045513, 61.66775706135234003 ) ) ;
#179741=CARTESIAN_POINT ( 'NONE',  ( 5.719274019375673035, 21.55341960407619339, 77.29275706135234714 ) ) ;
#179742=CARTESIAN_POINT ( 'NONE',  ( -16.46253265017146816, -9.564922557961047289, 49.16775706135233293 ) ) ;
#179743=CARTESIAN_POINT ( 'NONE',  ( -16.51473224551069308, -9.474510206698971260, 26.66557627198103120 ) ) ;
#179744=CARTESIAN_POINT ( 'NONE',  ( -18.67979575497178146, -10.72451020669898902, 46.66557627198102409 ) ) ;
#179745=CARTESIAN_POINT ( 'NONE',  ( 16.52544592524342804, -4.483927247898539470, 53.54057627198103120 ) ) ;
#179747=CARTESIAN_POINT ( 'NONE',  ( -19.02544592524334988, -5.153800228976617603, 18.95942372801899722 ) ) ;
#179748=CARTESIAN_POINT ( 'NONE',  ( -8.224510206698735004, -14.34966873604973081, 74.58442372801901854 ) ) ;
#179749=CARTESIAN_POINT ( 'NONE',  ( 14.34966873604960469, 8.224510206698951720, 39.16557627198102409 ) ) ;
#179750=CARTESIAN_POINT ( 'NONE',  ( -21.52544592524334988, -5.823673210054445271, 78.95942372801901854 ) ) ;
#179751=CARTESIAN_POINT ( 'NONE',  ( 21.52544592524334988, 5.823673210054432836, 66.45942372801903275 ) ) ;
#179752=CARTESIAN_POINT ( 'NONE',  ( -21.53943276465977519, 0.05219959533907696930, 76.24890960531435269 ) ) ;
#179753=CARTESIAN_POINT ( 'NONE',  ( -5.049401038298153566, 19.05341960407611168, 40.20724293864768839 ) ) ;
#179754=CARTESIAN_POINT ( 'NONE',  ( -5.719274019375665041, -21.55341960407619695, 54.79275706135235424 ) ) ;
#179755=CARTESIAN_POINT ( 'NONE',  ( 19.03943276465977164, -0.05219959533909143690, 28.74890960531435624 ) ) ;
#179756=CARTESIAN_POINT ( 'NONE',  ( 16.46253265017160672, -9.564922557960803928, 58.33224293864769550 ) ) ;
#179757=CARTESIAN_POINT ( 'NONE',  ( -8.224510206698948167, 14.34966873604960824, 90.41557627198103830 ) ) ;
#179758=CARTESIAN_POINT ( 'NONE',  ( -5.049401038298153566, 19.05341960407611168, 80.20724293864769550 ) ) ;
#179759=CARTESIAN_POINT ( 'NONE',  ( -16.55341960407611168, -4.379528057220339221, 41.45724293864769550 ) ) ;
#179760=CARTESIAN_POINT ( 'NONE',  ( 12.14591786802309770, 12.06949235617756955, 99.37390960531436690 ) ) ;
#179761=CARTESIAN_POINT ( 'NONE',  ( -21.53943276465977519, 0.05219959533907696930, 76.24890960531435269 ) ) ;
#179763=CARTESIAN_POINT ( 'NONE',  ( 10.81492255796078972, 18.62759615963270932, 114.5822429386477097 ) ) ;
#179765=CARTESIAN_POINT ( 'NONE',  ( 13.97604488694527802, 13.89961937509977652, 64.37390960531436690 ) ) ;
#179766=CARTESIAN_POINT ( 'NONE',  ( -12.06949235617739369, -12.14591786802326823, 29.37609039468568284 ) ) ;
#179767=CARTESIAN_POINT ( 'NONE',  ( -5.719274019375978568, 21.55341960407610458, 70.20724293864769550 ) ) ;
#179768=CARTESIAN_POINT ( 'NONE',  ( 10.81492255796106328, -18.62759615963255655, 90.41775706135236135 ) ) ;
#179769=CARTESIAN_POINT ( 'NONE',  ( -19.02544592524342804, 5.153800228976336051, 86.04057627198103830 ) ) ;
#179770=CARTESIAN_POINT ( 'NONE',  ( 21.52544592524344225, -5.823673210054117533, 113.5405762719810383 ) ) ;
#179771=CARTESIAN_POINT ( 'NONE',  ( 13.89961937509977652, -13.97604488694527269, 108.1239096053143669 ) ) ;
#179772=CARTESIAN_POINT ( 'NONE',  ( -16.55341960407617563, 4.379528057220093196, 88.54275706135236135 ) ) ;
#179773=CARTESIAN_POINT ( 'NONE',  ( -18.67979575497193778, 10.72451020669871902, 68.33442372801900433 ) ) ;
#179774=CARTESIAN_POINT ( 'NONE',  ( -18.67979575497193778, 10.72451020669871902, 93.33442372801901854 ) ) ;
#179775=CARTESIAN_POINT ( 'NONE',  ( 16.53943276465976808, 0.05219959533934440121, 56.25109039468568284 ) ) ;
#179776=CARTESIAN_POINT ( 'NONE',  ( -21.53943276465977519, -0.05219959533937600094, 33.75109039468568284 ) ) ;
#179777=CARTESIAN_POINT ( 'NONE',  ( 0.05219959533909260263, 19.03943276465977164, 24.99890960531435269 ) ) ;
#179778=CARTESIAN_POINT ( 'NONE',  ( 21.52544592524334988, 5.823673210054432836, 91.45942372801901854 ) ) ;
#179779=CARTESIAN_POINT ( 'NONE',  ( -19.05341960407611168, -5.049401038298163336, 96.45724293864769550 ) ) ;
#179780=CARTESIAN_POINT ( 'NONE',  ( 15.72974639402199770, -15.80617190586745480, 88.12390960531436690 ) ) ;
#179781=CARTESIAN_POINT ( 'NONE',  ( 19.02544592524334988, 5.153800228976608722, 56.45942372801898301 ) ) ;
#179782=CARTESIAN_POINT ( 'NONE',  ( -18.67979575497178146, -10.72451020669898902, 56.66557627198103830 ) ) ;
#179783=CARTESIAN_POINT ( 'NONE',  ( 5.049401038298161559, -19.05341960407611168, 97.70724293864766707 ) ) ;
#179784=CARTESIAN_POINT ( 'NONE',  ( 4.379528057220339221, -16.55341960407611168, 37.70724293864769550 ) ) ;
#179786=CARTESIAN_POINT ( 'NONE',  ( -13.89961937509957401, -13.97604488694547875, 79.37609039468567573 ) ) ;
#179787=CARTESIAN_POINT ( 'NONE',  ( -19.35543954521082810, -5.499999999999488409, 79.58901960356450900 ) ) ;
#179788=CARTESIAN_POINT ( 'NONE',  ( -5.049401038297874678, -19.05341960407617918, 109.7927570613523187 ) ) ;
#179789=CARTESIAN_POINT ( 'NONE',  ( -15.72974639402197994, 15.80617190586746368, 90.62390960531436690 ) ) ;
#179790=CARTESIAN_POINT ( 'NONE',  ( 0.05219959533910956823, 16.53943276465976808, 59.99890960531436690 ) ) ;
#179791=CARTESIAN_POINT ( 'NONE',  ( -8.224510206698735004, -14.34966873604973081, 34.58442372801900433 ) ) ;
#179792=CARTESIAN_POINT ( 'NONE',  ( -13.97604488694527625, -13.89961937509977652, 46.87390960531435979 ) ) ;
#179793=CARTESIAN_POINT ( 'NONE',  ( 0.05219959533907565091, 21.53943276465977519, 114.9989096053143669 ) ) ;
#179794=CARTESIAN_POINT ( 'NONE',  ( -19.05341960407617563, 5.049401038297882671, 78.54275706135233293 ) ) ;
#179795=CARTESIAN_POINT ( 'NONE',  ( 5.049401038298161559, -19.05341960407611168, 97.70724293864766707 ) ) ;
#179796=CARTESIAN_POINT ( 'NONE',  ( 5.049401038298161559, -19.05341960407611168, 77.70724293864765286 ) ) ;
#179797=CARTESIAN_POINT ( 'NONE',  ( -5.719274019375978568, 21.55341960407610458, 70.20724293864769550 ) ) ;
#179798=CARTESIAN_POINT ( 'NONE',  ( 19.05341960407611168, 5.049401038298154454, 43.95724293864769550 ) ) ;
#179800=CARTESIAN_POINT ( 'NONE',  ( 16.55341960407611168, 4.379528057220329451, 48.95724293864770971 ) ) ;
#179801=CARTESIAN_POINT ( 'NONE',  ( -9.564922557960796823, -16.46253265017161027, 107.0822429386476955 ) ) ;
#179803=CARTESIAN_POINT ( 'NONE',  ( 5.153800228976615827, -19.02544592524334988, 65.20942372801900433 ) ) ;
#179804=CARTESIAN_POINT ( 'NONE',  ( 21.55341960407610458, 5.719274019375980345, 73.95724293864769550 ) ) ;
#179805=CARTESIAN_POINT ( 'NONE',  ( -0.05219959533936034679, 19.03943276465977164, 42.50109039468566152 ) ) ;
#179806=CARTESIAN_POINT ( 'NONE',  ( 5.049401038298161559, -19.05341960407611168, 107.7072429386476955 ) ) ;
#179807=CARTESIAN_POINT ( 'NONE',  ( -18.22780087662124160, -5.499999999999927169, 73.98236817873106475 ) ) ;
#179808=CARTESIAN_POINT ( 'NONE',  ( 10.72451020669898902, -18.67979575497178502, 37.91557627198102409 ) ) ;
#179809=CARTESIAN_POINT ( 'NONE',  ( -13.97604488694527625, -13.89961937509977652, 66.87390960531436690 ) ) ;
#179810=CARTESIAN_POINT ( 'NONE',  ( 21.52544592524334988, 5.823673210054432836, 61.45942372801901854 ) ) ;
#179811=CARTESIAN_POINT ( 'NONE',  ( 8.314922557960818139, 14.29746914071049879, 114.5822429386477097 ) ) ;
#179812=CARTESIAN_POINT ( 'NONE',  ( 21.53943276465977519, -0.05219959533907433946, 108.7489096053143669 ) ) ;
#179813=VERTEX_POINT ( 'NONE', #147683 ) ;
#179814=CARTESIAN_POINT ( 'NONE',  ( -21.53943276465977519, -0.05219959533937600094, 58.75109039468568994 ) ) ;
#179817=CARTESIAN_POINT ( 'NONE',  ( -9.474510206698720793, -16.51473224551083518, 64.58442372801900433 ) ) ;
#179819=CARTESIAN_POINT ( 'NONE',  ( 18.67979575497178502, 10.72451020669898547, 109.1655762719810383 ) ) ;
#179820=CARTESIAN_POINT ( 'NONE',  ( -16.46253265017160317, 9.564922557960807481, 60.83224293864769550 ) ) ;
#179821=CARTESIAN_POINT ( 'NONE',  ( -12.14591786802326823, 12.06949235617739902, 33.12609039468569705 ) ) ;
#179822=EDGE_CURVE ( 'NONE', #129974, #63497, #56671, .T. ) ;
#179824=CARTESIAN_POINT ( 'NONE',  ( -10.81492255796105439, 18.62759615963255655, 107.9177570613523471 ) ) ;
#179825=CARTESIAN_POINT ( 'NONE',  ( -5.049401038298153566, 19.05341960407611168, 40.20724293864768839 ) ) ;
#179826=CARTESIAN_POINT ( 'NONE',  ( -21.52544592524334988, -5.823673210054445271, 108.9594237280190185 ) ) ;
#179827=CARTESIAN_POINT ( 'NONE',  ( 5.153800228976335163, 19.02544592524342804, 89.79057627198102409 ) ) ;
#179828=CARTESIAN_POINT ( 'NONE',  ( -0.05219959533937732626, 21.53943276465977519, 57.50109039468568994 ) ) ;
#179830=CARTESIAN_POINT ( 'NONE',  ( 9.564922557960805705, 16.46253265017160317, 109.5822429386476955 ) ) ;
#179832=CARTESIAN_POINT ( 'NONE',  ( -12.06949235617739369, -12.14591786802326823, 49.37609039468569705 ) ) ;
#179833=CARTESIAN_POINT ( 'NONE',  ( -21.52544592524334988, -5.823673210054445271, 68.95942372801901854 ) ) ;
#179834=CARTESIAN_POINT ( 'NONE',  ( 10.81492255796106328, -18.62759615963255655, 90.41775706135236135 ) ) ;
#179836=CARTESIAN_POINT ( 'NONE',  ( -16.55341960407617563, 4.379528057220093196, 23.54275706135235424 ) ) ;
#179837=CARTESIAN_POINT ( 'NONE',  ( 19.03943276465977164, -0.05219959533909143690, 88.74890960531436690 ) ) ;
#179838=CARTESIAN_POINT ( 'NONE',  ( -5.153800228976328057, -19.02544592524343514, 107.2905762719810383 ) ) ;
#179839=EDGE_CURVE ( 'NONE', #175270, #121093, #34897, .T. ) ;
#179840=CARTESIAN_POINT ( 'NONE',  ( 17.44270441346512968, 5.991230190323100224, 43.86335079264229364 ) ) ;
#179841=CARTESIAN_POINT ( 'NONE',  ( -19.02544592524342804, 5.153800228976336051, 26.04057627198103120 ) ) ;
#179842=CARTESIAN_POINT ( 'NONE',  ( -15.80617190586745835, -15.72974639402198527, 46.87390960531435979 ) ) ;
#179843=CARTESIAN_POINT ( 'NONE',  ( 8.224510206698742110, 14.34966873604972548, 112.0844237280190185 ) ) ;
#179844=CARTESIAN_POINT ( 'NONE',  ( 16.53943276465976808, -0.05219959533910856209, 78.74890960531436690 ) ) ;
#179845=CARTESIAN_POINT ( 'NONE',  ( -9.474510206698964154, 16.51473224551069663, 65.41557627198102409 ) ) ;
#179846=CARTESIAN_POINT ( 'NONE',  ( 21.52544592524334988, 5.823673210054432836, 96.45942372801901854 ) ) ;
#179847=CARTESIAN_POINT ( 'NONE',  ( 4.379528057220092307, 16.55341960407617563, 22.29275706135235069 ) ) ;
#179848=CARTESIAN_POINT ( 'NONE',  ( 0.05219959533910956823, 16.53943276465976808, 84.99890960531436690 ) ) ;
#179849=CARTESIAN_POINT ( 'NONE',  ( 21.55341960407619695, -5.719274019375665929, 46.04275706135234714 ) ) ;
#179850=CARTESIAN_POINT ( 'NONE',  ( 5.719274019375991003, -21.55341960407610458, 67.70724293864769550 ) ) ;
#179851=CARTESIAN_POINT ( 'NONE',  ( -16.46253265017146816, -9.564922557961047289, 44.16775706135232582 ) ) ;
#179853=CARTESIAN_POINT ( 'NONE',  ( -13.97604488694527625, -13.89961937509977652, 96.87390960531433848 ) ) ;
#179854=CARTESIAN_POINT ( 'NONE',  ( -8.314922557960811034, -14.29746914071050412, 67.08224293864770971 ) ) ;
#179856=CARTESIAN_POINT ( 'NONE',  ( 12.06949235617757843, -12.14591786802309237, 38.12390960531436690 ) ) ;
#179857=CARTESIAN_POINT ( 'NONE',  ( -0.05219959533934338120, 16.53943276465976808, 112.5010903946857042 ) ) ;
#179858=CARTESIAN_POINT ( 'NONE',  ( 5.153800228976615827, -19.02544592524334988, 65.20942372801900433 ) ) ;
#179859=CARTESIAN_POINT ( 'NONE',  ( 17.58332526062524437, 7.635886036038643354, 76.57665040441536064 ) ) ;
#179860=CARTESIAN_POINT ( 'NONE',  ( -10.81492255796078084, -18.62759615963271287, 27.08224293864769550 ) ) ;
#179861=CARTESIAN_POINT ( 'NONE',  ( -12.14591786802309592, -12.06949235617757132, 81.87390960531435269 ) ) ;
#179863=CARTESIAN_POINT ( 'NONE',  ( 5.049401038298161559, -19.05341960407611168, 42.70724293864767418 ) ) ;
#179864=CARTESIAN_POINT ( 'NONE',  ( -18.62759615963270932, 10.81492255796079327, 55.83224293864770260 ) ) ;
#179865=CARTESIAN_POINT ( 'NONE',  ( 21.52544592524344225, -5.823673210054117533, 78.54057627198103830 ) ) ;
#179866=CARTESIAN_POINT ( 'NONE',  ( 12.06949235617757843, -12.14591786802309237, 108.1239096053143811 ) ) ;
#179867=CARTESIAN_POINT ( 'NONE',  ( 16.53943276465976808, 0.05219959533934440121, 61.25109039468567573 ) ) ;
#179868=CARTESIAN_POINT ( 'NONE',  ( 13.89961937509977652, -13.97604488694527269, 48.12390960531435979 ) ) ;
#179870=CARTESIAN_POINT ( 'NONE',  ( 15.80617190586769283, -15.72974639402175789, 55.62609039468568284 ) ) ;
#179872=CARTESIAN_POINT ( 'NONE',  ( 8.314922557960818139, 14.29746914071049879, 109.5822429386476955 ) ) ;
#179873=CARTESIAN_POINT ( 'NONE',  ( 5.153800228976615827, -19.02544592524334988, 85.20942372801900433 ) ) ;
#179876=CARTESIAN_POINT ( 'NONE',  ( -18.62759615963270932, 10.81492255796079327, 50.83224293864770971 ) ) ;
#179877=CARTESIAN_POINT ( 'NONE',  ( 17.44279575226823908, -5.990770900252462283, 68.33557567514318976 ) ) ;
#179878=CARTESIAN_POINT ( 'NONE',  ( -0.05219959533937732626, 21.53943276465977519, 87.50109039468568994 ) ) ;
#179879=CARTESIAN_POINT ( 'NONE',  ( 16.52544592524342804, -4.483927247898539470, 33.54057627198102409 ) ) ;
#179880=CARTESIAN_POINT ( 'NONE',  ( 14.29746914071037800, 8.314922557961029526, 51.66775706135234714 ) ) ;
#179881=CARTESIAN_POINT ( 'NONE',  ( 4.483927247898545687, 16.52544592524342804, 39.79057627198103830 ) ) ;
#179882=CARTESIAN_POINT ( 'NONE',  ( -21.52544592524343514, 5.823673210054127303, 71.04057627198103830 ) ) ;
#179883=CARTESIAN_POINT ( 'NONE',  ( -21.53943276465977519, 0.05219959533907696930, 71.24890960531435269 ) ) ;
#179885=CARTESIAN_POINT ( 'NONE',  ( 19.02544592524334988, 5.153800228976608722, 81.45942372801897591 ) ) ;
#179886=CARTESIAN_POINT ( 'NONE',  ( -5.049401038298153566, 19.05341960407611168, 115.2072429386477097 ) ) ;
#179887=B_SPLINE_CURVE_WITH_KNOTS ( 'NONE', 3,
 ( #52085, #99581, #22756, #192609, #144090, #5571, #115766, #160265, #80427, #145084, #177453, #142100, #53076, #3585, #189621, #4567, #50110, #128909, #161262, #65263, #38923, #37921, #7566, #97563, #18781, #190610, #35917, #6567, #175438, #21755, #126923, #146082 ),
 .UNSPECIFIED., .F., .F.,
 ( 4, 2, 2, 2, 2, 2, 2, 2, 2, 2, 2, 2, 2, 2, 2, 4 ),
 ( 1.645181051943004889E-15, 0.0003712461730052120336, 0.0007424923460087788987, 0.001113738519012345655, 0.001484984692015912629, 0.002227477038023061105, 0.002598723211026641739, 0.002969969384030222374, 0.003341215557033802575, 0.003712461730037383643, 0.004083707903040963844, 0.004454954076044545346, 0.004826200249048125113, 0.005197446422051706615, 0.005568692595055287249, 0.005939938768058867884 ),
 .UNSPECIFIED. ) ;
#179888=CARTESIAN_POINT ( 'NONE',  ( 5.049401038298161559, -19.05341960407611168, 42.70724293864767418 ) ) ;
#179889=CARTESIAN_POINT ( 'NONE',  ( 19.03943276465977164, -0.05219959533909143690, 28.74890960531435624 ) ) ;
#179892=VERTEX_POINT ( 'NONE', #102167 ) ;
#179893=CARTESIAN_POINT ( 'NONE',  ( -14.29746914071037622, -8.314922557961029526, 84.16775706135234714 ) ) ;
#179894=CARTESIAN_POINT ( 'NONE',  ( 18.62759615963271287, -10.81492255796078972, 103.3322429386476955 ) ) ;
#179895=CARTESIAN_POINT ( 'NONE',  ( -5.049401038298153566, 19.05341960407611168, 75.20724293864769550 ) ) ;
#179896=CARTESIAN_POINT ( 'NONE',  ( 10.81492255796106328, -18.62759615963255655, 35.41775706135234003 ) ) ;
#179897=CARTESIAN_POINT ( 'NONE',  ( 16.51473224551069308, 9.474510206698969483, 99.16557627198102409 ) ) ;
#179900=CARTESIAN_POINT ( 'NONE',  ( 0.05219959533937995610, -21.53943276465977519, 35.00109039468568284 ) ) ;
#179901=CARTESIAN_POINT ( 'NONE',  ( -19.03943276465977164, 0.05219959533909376836, 26.24890960531435624 ) ) ;
#179902=CARTESIAN_POINT ( 'NONE',  ( -13.97604488694547697, 13.89961937509957934, 93.12609039468566152 ) ) ;
#179903=CARTESIAN_POINT ( 'NONE',  ( -13.89961937509957401, -13.97604488694547875, 44.37609039468566863 ) ) ;
#179904=CARTESIAN_POINT ( 'NONE',  ( 5.719274019375991003, -21.55341960407610458, 107.7072429386476955 ) ) ;
#179905=CARTESIAN_POINT ( 'NONE',  ( 5.153800228976615827, -19.02544592524334988, 40.20942372801898301 ) ) ;
#179906=CARTESIAN_POINT ( 'NONE',  ( 13.97604488694548053, -13.89961937509957401, 50.62609039468566152 ) ) ;
#179907=CARTESIAN_POINT ( 'NONE',  ( 0.05219959533934541429, -16.53943276465976808, 95.00109039468568994 ) ) ;
#179908=DIRECTION ( 'NONE',  ( 0.000000000000000000, -1.000000000000000000, 0.000000000000000000 ) ) ;
#179909=VERTEX_POINT ( 'NONE', #37492 ) ;
#179910=CARTESIAN_POINT ( 'NONE',  ( 5.153800228976335163, 19.02544592524342804, 69.79057627198103830 ) ) ;
#179911=CARTESIAN_POINT ( 'NONE',  ( 15.72974639402176855, 15.80617190586768217, 76.87609039468567573 ) ) ;
#179912=CARTESIAN_POINT ( 'NONE',  ( 18.62759615963255655, 10.81492255796105972, 96.66775706135234714 ) ) ;
#179914=CARTESIAN_POINT ( 'NONE',  ( -13.97604488694527625, -13.89961937509977652, 91.87390960531432427 ) ) ;
#179915=CARTESIAN_POINT ( 'NONE',  ( 10.81492255796106328, -18.62759615963255655, 60.41775706135235424 ) ) ;
#179916=CARTESIAN_POINT ( 'NONE',  ( 19.03943276465977164, 0.05219959533936151252, 101.2510903946856757 ) ) ;
#179917=CARTESIAN_POINT ( 'NONE',  ( -19.05341960407611168, -5.049401038298163336, 71.45724293864766707 ) ) ;
#179918=CARTESIAN_POINT ( 'NONE',  ( -19.02544592524342804, 5.153800228976336051, 106.0405762719810241 ) ) ;
#179919=CARTESIAN_POINT ( 'NONE',  ( 9.474510206698971260, -16.51473224551069308, 82.91557627198103830 ) ) ;
#179921=CARTESIAN_POINT ( 'NONE',  ( -19.05341960407611168, -5.049401038298163336, 66.45724293864769550 ) ) ;
#179922=CARTESIAN_POINT ( 'NONE',  ( 0.05219959533909260263, 19.03943276465977164, 49.99890960531435979 ) ) ;
#179923=CARTESIAN_POINT ( 'NONE',  ( 15.80617190586769283, -15.72974639402175789, 20.62609039468568639 ) ) ;
#179924=CARTESIAN_POINT ( 'NONE',  ( 16.53943276465976808, 0.05219959533934440121, 106.2510903946856757 ) ) ;
#179927=CARTESIAN_POINT ( 'NONE',  ( 13.97604488694548053, -13.89961937509957401, 55.62609039468566863 ) ) ;
#179928=CARTESIAN_POINT ( 'NONE',  ( -5.049401038298153566, 19.05341960407611168, 85.20724293864766707 ) ) ;
#179929=CARTESIAN_POINT ( 'NONE',  ( -8.224510206698948167, 14.34966873604960824, 65.41557627198102409 ) ) ;
#179930=CARTESIAN_POINT ( 'NONE',  ( 8.224510206698953496, -14.34966873604960469, 102.9155762719810383 ) ) ;
#179931=CARTESIAN_POINT ( 'NONE',  ( 21.52544592524344225, -5.823673210054117533, 33.54057627198102409 ) ) ;
#179932=CARTESIAN_POINT ( 'NONE',  ( 13.89961937509977652, -13.97604488694527269, 108.1239096053143669 ) ) ;
#179933=CARTESIAN_POINT ( 'NONE',  ( 8.224510206698953496, -14.34966873604960469, 92.91557627198103830 ) ) ;
#179934=CARTESIAN_POINT ( 'NONE',  ( 13.89961937509977652, -13.97604488694527269, 113.1239096053143527 ) ) ;
#179935=CARTESIAN_POINT ( 'NONE',  ( 9.564922557961047289, -16.46253265017146816, 35.41775706135233293 ) ) ;
#179936=CARTESIAN_POINT ( 'NONE',  ( 16.53943276465976808, 0.05219959533934440121, 106.2510903946856757 ) ) ;
#179937=CARTESIAN_POINT ( 'NONE',  ( 9.474510206698971260, -16.51473224551069308, 82.91557627198103830 ) ) ;
#179938=CARTESIAN_POINT ( 'NONE',  ( -5.823673210054431948, 21.52544592524334988, 47.70942372801902565 ) ) ;
#179939=CARTESIAN_POINT ( 'NONE',  ( -21.52544592524343514, 5.823673210054127303, 41.04057627198103120 ) ) ;
#179940=CARTESIAN_POINT ( 'NONE',  ( -0.05219959533937732626, 21.53943276465977519, 32.50109039468568284 ) ) ;
#179941=CARTESIAN_POINT ( 'NONE',  ( -18.62759615963270932, 10.81492255796079327, 85.83224293864768129 ) ) ;
#179942=CARTESIAN_POINT ( 'NONE',  ( 12.06949235617757843, -12.14591786802309237, 93.12390960531436690 ) ) ;
#179943=CARTESIAN_POINT ( 'NONE',  ( -19.05341960407617563, 5.049401038297882671, 63.54275706135234003 ) ) ;
#179944=CARTESIAN_POINT ( 'NONE',  ( -19.03943276465977164, 0.05219959533909376836, 36.24890960531436690 ) ) ;
#179945=CARTESIAN_POINT ( 'NONE',  ( -13.97604488694527625, -13.89961937509977652, 101.8739096053143811 ) ) ;
#179946=CARTESIAN_POINT ( 'NONE',  ( -13.97604488694527625, -13.89961937509977652, 91.87390960531432427 ) ) ;
#179947=CARTESIAN_POINT ( 'NONE',  ( -4.379528057220328563, 16.55341960407611168, 110.2072429386477239 ) ) ;
#179948=CARTESIAN_POINT ( 'NONE',  ( -14.34966873604960291, -8.224510206698953496, 21.66557627198102409 ) ) ;
#179949=CARTESIAN_POINT ( 'NONE',  ( -12.14591786802326823, 12.06949235617739902, 43.12609039468568284 ) ) ;
#179950=CARTESIAN_POINT ( 'NONE',  ( 21.52544592524334988, 5.823673210054432836, 111.4594237280190328 ) ) ;
#179951=CARTESIAN_POINT ( 'NONE',  ( -16.51473224551069308, -9.474510206698971260, 111.6655762719810383 ) ) ;
#179952=CARTESIAN_POINT ( 'NONE',  ( 16.55341960407618274, -4.379528057220086978, 111.0427570613523613 ) ) ;
#179953=CARTESIAN_POINT ( 'NONE',  ( -15.72974639402176322, -15.80617190586768395, 34.37609039468568284 ) ) ;
#179954=CARTESIAN_POINT ( 'NONE',  ( 19.03943276465977164, -0.05219959533909143690, 38.74890960531436690 ) ) ;
#179955=CARTESIAN_POINT ( 'NONE',  ( -8.314922557961024197, 14.29746914071037800, 37.91775706135235424 ) ) ;
#179956=CARTESIAN_POINT ( 'NONE',  ( -16.52544592524335698, -4.483927247898792601, 108.9594237280190185 ) ) ;
#179957=CARTESIAN_POINT ( 'NONE',  ( -8.224510206698735004, -14.34966873604973081, 89.58442372801901854 ) ) ;
#179958=CARTESIAN_POINT ( 'NONE',  ( -0.05219959533936034679, 19.03943276465977164, 107.5010903946856615 ) ) ;
#179959=CARTESIAN_POINT ( 'NONE',  ( 5.153800228976335163, 19.02544592524342804, 29.79057627198102409 ) ) ;
#179960=CARTESIAN_POINT ( 'NONE',  ( 8.224510206698953496, -14.34966873604960469, 112.9155762719810383 ) ) ;
#179961=CARTESIAN_POINT ( 'NONE',  ( 0.05219959533907565091, 21.53943276465977519, 99.99890960531436690 ) ) ;
#179962=CARTESIAN_POINT ( 'NONE',  ( -16.46253265017160317, 9.564922557960807481, 30.83224293864769550 ) ) ;
#179964=CARTESIAN_POINT ( 'NONE',  ( -0.05219959533909027116, -19.03943276465977164, 102.4989096053143669 ) ) ;
#179965=CARTESIAN_POINT ( 'NONE',  ( 18.62759615963255655, 10.81492255796105972, 36.66775706135234714 ) ) ;
#179967=CARTESIAN_POINT ( 'NONE',  ( -16.51473224551069308, -9.474510206698971260, 101.6655762719810241 ) ) ;
#179969=CARTESIAN_POINT ( 'NONE',  ( 19.02544592524343514, -5.153800228976328945, 93.54057627198102409 ) ) ;
#179970=CARTESIAN_POINT ( 'NONE',  ( 21.55341960407619695, -5.719274019375665929, 31.04275706135234714 ) ) ;
#179971=CARTESIAN_POINT ( 'NONE',  ( 16.53943276465976808, -0.05219959533910856209, 88.74890960531436690 ) ) ;
#179972=CARTESIAN_POINT ( 'NONE',  ( -19.03943276465977164, 0.05219959533909376836, 101.2489096053143669 ) ) ;
#179974=CARTESIAN_POINT ( 'NONE',  ( -8.224510206698735004, -14.34966873604973081, 69.58442372801900433 ) ) ;
#179975=CARTESIAN_POINT ( 'NONE',  ( -15.80617190586768217, 15.72974639402176855, 78.12609039468570415 ) ) ;
#179976=CARTESIAN_POINT ( 'NONE',  ( 12.14591786802327356, -12.06949235617739191, 40.62609039468567573 ) ) ;
#179977=CARTESIAN_POINT ( 'NONE',  ( 9.474510206698971260, -16.51473224551069308, 77.91557627198103830 ) ) ;
#179978=CARTESIAN_POINT ( 'NONE',  ( -19.05341960407617563, 5.049401038297882671, 103.5427570613523329 ) ) ;
#179979=CARTESIAN_POINT ( 'NONE',  ( 8.224510206698742110, 14.34966873604972548, 67.08442372801901854 ) ) ;
#179980=CARTESIAN_POINT ( 'NONE',  ( 5.823673210054444382, -21.52544592524334988, 110.2094237280190185 ) ) ;
#179981=CARTESIAN_POINT ( 'NONE',  ( 19.02544592524334988, 5.153800228976608722, 91.45942372801900433 ) ) ;
#179982=CARTESIAN_POINT ( 'NONE',  ( 13.97604488694527802, 13.89961937509977652, 64.37390960531436690 ) ) ;
#179983=CARTESIAN_POINT ( 'NONE',  ( -21.55341960407610458, -5.719274019375992779, 81.45724293864769550 ) ) ;
#179984=CARTESIAN_POINT ( 'NONE',  ( -14.34966873604960291, -8.224510206698953496, 91.66557627198103830 ) ) ;
#179985=CARTESIAN_POINT ( 'NONE',  ( 19.02544592524334988, 5.153800228976608722, 96.45942372801897591 ) ) ;
#179986=CARTESIAN_POINT ( 'NONE',  ( -8.224510206698735004, -14.34966873604973081, 64.58442372801900433 ) ) ;
#179988=CARTESIAN_POINT ( 'NONE',  ( 9.474510206698729675, 16.51473224551082808, 57.08442372801900433 ) ) ;
#179989=EDGE_CURVE ( 'NONE', #115310, #90405, #148682, .T. ) ;
#179990=CARTESIAN_POINT ( 'NONE',  ( 4.379528057220339221, -16.55341960407611168, 32.70724293864770260 ) ) ;
#179991=CARTESIAN_POINT ( 'NONE',  ( -12.14591786802309592, -12.06949235617757132, 81.87390960531435269 ) ) ;
#179992=CARTESIAN_POINT ( 'NONE',  ( 16.51473224551083163, -9.474510206698727899, 25.83442372801900078 ) ) ;
#179993=CARTESIAN_POINT ( 'NONE',  ( 13.97604488694548053, -13.89961937509957401, 45.62609039468566863 ) ) ;
#179994=CARTESIAN_POINT ( 'NONE',  ( -10.81492255796105439, 18.62759615963255655, 27.91775706135234358 ) ) ;
#179995=CARTESIAN_POINT ( 'NONE',  ( -19.05341960407611168, -5.049401038298163336, 101.4572429386476955 ) ) ;
#179996=CARTESIAN_POINT ( 'NONE',  ( 13.89961937509977652, -13.97604488694527269, 83.12390960531436690 ) ) ;
#179997=CARTESIAN_POINT ( 'NONE',  ( 15.80617190586769283, -15.72974639402175789, 95.62609039468568994 ) ) ;
#179998=CARTESIAN_POINT ( 'NONE',  ( -13.97604488694527625, -13.89961937509977652, 76.87390960531433848 ) ) ;
#179999=CARTESIAN_POINT ( 'NONE',  ( 5.823673210054125526, 21.52544592524343514, 34.79057627198103120 ) ) ;
#180000=CARTESIAN_POINT ( 'NONE',  ( -4.379528057220328563, 16.55341960407611168, 85.20724293864770971 ) ) ;
#180001=CARTESIAN_POINT ( 'NONE',  ( 9.474510206698971260, -16.51473224551069308, 37.91557627198102409 ) ) ;
#180002=CARTESIAN_POINT ( 'NONE',  ( -16.53943276465976808, 0.05219959533911058130, 101.2489096053143669 ) ) ;
#180004=CARTESIAN_POINT ( 'NONE',  ( -5.719274019375978568, 21.55341960407610458, 105.2072429386477097 ) ) ;
#180005=CARTESIAN_POINT ( 'NONE',  ( 15.72974639402176855, 15.80617190586768217, 66.87609039468568994 ) ) ;
#180006=CARTESIAN_POINT ( 'NONE',  ( 19.05341960407611168, 5.049401038298154454, 28.95724293864769550 ) ) ;
#180007=CARTESIAN_POINT ( 'NONE',  ( -12.14591786802326823, 12.06949235617739902, 68.12609039468567573 ) ) ;
#180008=CARTESIAN_POINT ( 'NONE',  ( -18.67979575497178146, -10.72451020669898902, 101.6655762719810383 ) ) ;
#180009=CARTESIAN_POINT ( 'NONE',  ( -21.53943276465977519, 0.05219959533907696930, 116.2489096053143669 ) ) ;
#180010=CARTESIAN_POINT ( 'NONE',  ( -5.049401038297874678, -19.05341960407617918, 39.79275706135232582 ) ) ;
#180011=CARTESIAN_POINT ( 'NONE',  ( -9.564922557960796823, -16.46253265017161027, 57.08224293864769550 ) ) ;
#180012=CARTESIAN_POINT ( 'NONE',  ( 9.564922557960805705, 16.46253265017160317, 114.5822429386476955 ) ) ;
#180013=CARTESIAN_POINT ( 'NONE',  ( 15.72974639402176855, 15.80617190586768217, 51.87609039468568284 ) ) ;
#180014=CARTESIAN_POINT ( 'NONE',  ( -18.67979575497178146, -10.72451020669898902, 61.66557627198103120 ) ) ;
#180015=CARTESIAN_POINT ( 'NONE',  ( -0.05219959533910754901, -16.53943276465976808, 42.49890960531435979 ) ) ;
#180016=CARTESIAN_POINT ( 'NONE',  ( -5.823673210054431948, 21.52544592524334988, 72.70942372801901854 ) ) ;
#180017=CARTESIAN_POINT ( 'NONE',  ( 15.72974639402176855, 15.80617190586768217, 106.8760903946856899 ) ) ;
#180018=CARTESIAN_POINT ( 'NONE',  ( -4.483927247898539470, -16.52544592524342804, 57.29057627198103120 ) ) ;
#180019=CARTESIAN_POINT ( 'NONE',  ( -4.483927247898539470, -16.52544592524342804, 107.2905762719810525 ) ) ;
#180020=CARTESIAN_POINT ( 'NONE',  ( -5.153800228976607833, 19.02544592524334988, 42.70942372801901143 ) ) ;
#180021=CARTESIAN_POINT ( 'NONE',  ( 4.379528057220092307, 16.55341960407617563, 102.2927570613523613 ) ) ;
#180022=CARTESIAN_POINT ( 'NONE',  ( 21.52544592524334988, 5.823673210054432836, 71.45942372801901854 ) ) ;
#180023=CARTESIAN_POINT ( 'NONE',  ( 13.97604488694527802, 13.89961937509977652, 59.37390960531434558 ) ) ;
#180024=CARTESIAN_POINT ( 'NONE',  ( -13.89961937509957401, -13.97604488694547875, 34.37609039468566863 ) ) ;
#180025=CARTESIAN_POINT ( 'NONE',  ( -10.81492255796078084, -18.62759615963271287, 42.08224293864769550 ) ) ;
#180026=CARTESIAN_POINT ( 'NONE',  ( -21.53943276465977519, -0.05219959533937600094, 28.75109039468567929 ) ) ;
#180027=CARTESIAN_POINT ( 'NONE',  ( 5.823673210054125526, 21.52544592524343514, 94.79057627198105251 ) ) ;
#180028=CARTESIAN_POINT ( 'NONE',  ( -9.564922557961040184, 16.46253265017147172, 87.91775706135233293 ) ) ;
#180029=CARTESIAN_POINT ( 'NONE',  ( -16.53943276465976808, -0.05219959533934237506, 53.75109039468568994 ) ) ;
#180030=CARTESIAN_POINT ( 'NONE',  ( 17.97214573761831247, 5.500000000000080824, 63.96970049038658601 ) ) ;
#180031=CARTESIAN_POINT ( 'NONE',  ( 18.62759615963271287, -10.81492255796078972, 98.33224293864769550 ) ) ;
#180032=CARTESIAN_POINT ( 'NONE',  ( -16.52544592524342804, 4.483927247898546575, 81.04057627198102409 ) ) ;
#180034=CARTESIAN_POINT ( 'NONE',  ( 19.03943276465977164, 0.05219959533936151252, 111.2510903946856757 ) ) ;
#180035=CARTESIAN_POINT ( 'NONE',  ( -10.72451020669898014, 18.67979575497178502, 50.41557627198103120 ) ) ;
#180037=CARTESIAN_POINT ( 'NONE',  ( 0.05219959533934541429, -16.53943276465976808, 75.00109039468568994 ) ) ;
#180039=CARTESIAN_POINT ( 'NONE',  ( -16.53943276465976808, -0.05219959533934237506, 58.75109039468568994 ) ) ;
#180040=CARTESIAN_POINT ( 'NONE',  ( 15.80617190586769283, -15.72974639402175789, 30.62609039468567929 ) ) ;
#180041=CARTESIAN_POINT ( 'NONE',  ( 21.53943276465977519, -0.05219959533907433946, 43.74890960531435979 ) ) ;
#180042=CARTESIAN_POINT ( 'NONE',  ( 8.224510206698742110, 14.34966873604972548, 72.08442372801899012 ) ) ;
#180043=CARTESIAN_POINT ( 'NONE',  ( 19.03943276465977164, -0.05219959533909143690, 93.74890960531435269 ) ) ;
#180044=CARTESIAN_POINT ( 'NONE',  ( 15.80617190586769283, -15.72974639402175789, 55.62609039468568284 ) ) ;
#180045=CARTESIAN_POINT ( 'NONE',  ( -9.564922557960796823, -16.46253265017161027, 32.08224293864769550 ) ) ;
#180046=CARTESIAN_POINT ( 'NONE',  ( -18.62759615963270932, 10.81492255796079327, 45.83224293864769550 ) ) ;
#180047=CARTESIAN_POINT ( 'NONE',  ( -15.80617190586745835, -15.72974639402198527, 21.87390960531436690 ) ) ;
#180049=CARTESIAN_POINT ( 'NONE',  ( -5.153800228976607833, 19.02544592524334988, 32.70942372801899722 ) ) ;
#180050=CARTESIAN_POINT ( 'NONE',  ( -14.34966873604972548, 8.224510206698743886, 53.33442372801901854 ) ) ;
#180051=CARTESIAN_POINT ( 'NONE',  ( 5.153800228976335163, 19.02544592524342804, 109.7905762719810099 ) ) ;
#180053=CARTESIAN_POINT ( 'NONE',  ( -0.05219959533909027116, -19.03943276465977164, 87.49890960531436690 ) ) ;
#180054=CARTESIAN_POINT ( 'NONE',  ( -14.29746914071037622, -8.314922557961029526, 104.1677570613523471 ) ) ;
#180056=CARTESIAN_POINT ( 'NONE',  ( -12.06949235617756955, 12.14591786802309770, 90.62390960531436690 ) ) ;
#180057=CARTESIAN_POINT ( 'NONE',  ( 18.67979575497178502, 10.72451020669898547, 49.16557627198102409 ) ) ;
#180058=CARTESIAN_POINT ( 'NONE',  ( -9.564922557960796823, -16.46253265017161027, 27.08224293864769550 ) ) ;
#180059=CARTESIAN_POINT ( 'NONE',  ( -4.483927247898782831, 16.52544592524335698, 82.70942372801900433 ) ) ;
#180060=CARTESIAN_POINT ( 'NONE',  ( -5.823673210054431948, 21.52544592524334988, 22.70942372801901499 ) ) ;
#180061=CARTESIAN_POINT ( 'NONE',  ( -13.89961937509957401, -13.97604488694547875, 94.37609039468566152 ) ) ;
#180062=CARTESIAN_POINT ( 'NONE',  ( -0.05219959533909027116, -19.03943276465977164, 42.49890960531435269 ) ) ;
#180064=CARTESIAN_POINT ( 'NONE',  ( -19.05341960407611168, -5.049401038298163336, 106.4572429386476955 ) ) ;
#180065=CARTESIAN_POINT ( 'NONE',  ( -0.05219959533937732626, 21.53943276465977519, 107.5010903946856899 ) ) ;
#180066=CARTESIAN_POINT ( 'NONE',  ( 5.049401038298161559, -19.05341960407611168, 77.70724293864765286 ) ) ;
#180067=CARTESIAN_POINT ( 'NONE',  ( -0.05219959533934338120, 16.53943276465976808, 57.50109039468568994 ) ) ;
#180068=CARTESIAN_POINT ( 'NONE',  ( -18.62759615963255300, -10.81492255796106328, 94.16775706135237556 ) ) ;
#180069=CARTESIAN_POINT ( 'NONE',  ( 19.02544592524334988, 5.153800228976608722, 56.45942372801898301 ) ) ;
#180070=CARTESIAN_POINT ( 'NONE',  ( -16.46253265017146816, -9.564922557961047289, 49.16775706135233293 ) ) ;
#180071=ORIENTED_EDGE ( 'NONE', *, *, #71324, .F. ) ;
#180072=CARTESIAN_POINT ( 'NONE',  ( 15.72974639402176855, 15.80617190586768217, 61.87609039468568284 ) ) ;
#180073=CARTESIAN_POINT ( 'NONE',  ( 0.05219959533909260263, 19.03943276465977164, 24.99890960531435269 ) ) ;
#180074=CARTESIAN_POINT ( 'NONE',  ( -0.05219959533936034679, 19.03943276465977164, 62.50109039468566863 ) ) ;
#180075=CARTESIAN_POINT ( 'NONE',  ( -13.89961937509977652, 13.97604488694528158, 100.6239096053143669 ) ) ;
#180076=CARTESIAN_POINT ( 'NONE',  ( -19.03943276465977164, 0.05219959533909376836, 86.24890960531436690 ) ) ;
#180077=CARTESIAN_POINT ( 'NONE',  ( -4.483927247898539470, -16.52544592524342804, 37.29057627198102409 ) ) ;
#180078=CARTESIAN_POINT ( 'NONE',  ( -10.72451020669898014, 18.67979575497178502, 30.41557627198101699 ) ) ;
#180081=CARTESIAN_POINT ( 'NONE',  ( 16.51473224551083163, -9.474510206698727899, 20.83442372801899722 ) ) ;
#180083=CARTESIAN_POINT ( 'NONE',  ( -19.05341960407611168, -5.049401038298163336, 36.45724293864766707 ) ) ;
#180084=CARTESIAN_POINT ( 'NONE',  ( 5.049401038298161559, -19.05341960407611168, 22.70724293864769194 ) ) ;
#180086=CARTESIAN_POINT ( 'NONE',  ( 0.05219959533937995610, -21.53943276465977519, 70.00109039468568994 ) ) ;
#180088=CARTESIAN_POINT ( 'NONE',  ( -16.52544592524335698, -4.483927247898792601, 58.95942372801902565 ) ) ;
#180089=CARTESIAN_POINT ( 'NONE',  ( -21.52544592524343514, 5.823673210054127303, 81.04057627198102409 ) ) ;
#180090=CARTESIAN_POINT ( 'NONE',  ( 8.224510206698953496, -14.34966873604960469, 47.91557627198102409 ) ) ;
#180091=CARTESIAN_POINT ( 'NONE',  ( 9.474510206698971260, -16.51473224551069308, 22.91557627198102765 ) ) ;
#180092=CARTESIAN_POINT ( 'NONE',  ( -9.564922557960796823, -16.46253265017161027, 102.0822429386477097 ) ) ;
#180093=CARTESIAN_POINT ( 'NONE',  ( -10.72451020669870658, -18.67979575497194134, 29.58442372801901854 ) ) ;
#180094=CARTESIAN_POINT ( 'NONE',  ( 19.05341960407617918, -5.049401038297876454, 31.04275706135232227 ) ) ;
#180095=CARTESIAN_POINT ( 'NONE',  ( -5.049401038298153566, 19.05341960407611168, 30.20724293864768839 ) ) ;
#180096=CARTESIAN_POINT ( 'NONE',  ( -5.823673210054431948, 21.52544592524334988, 87.70942372801901854 ) ) ;
#180098=CARTESIAN_POINT ( 'NONE',  ( 4.379528057220339221, -16.55341960407611168, 32.70724293864770260 ) ) ;
#180100=CARTESIAN_POINT ( 'NONE',  ( -15.80617190586745835, -15.72974639402198527, 41.87390960531435979 ) ) ;
#180101=CARTESIAN_POINT ( 'NONE',  ( -12.06949235617756955, 12.14591786802309770, 100.6239096053143811 ) ) ;
#180103=CARTESIAN_POINT ( 'NONE',  ( 19.02544592524343514, -5.153800228976328945, 88.54057627198102409 ) ) ;
#180104=CARTESIAN_POINT ( 'NONE',  ( -14.34966873604960291, -8.224510206698953496, 86.66557627198102409 ) ) ;
#180105=CARTESIAN_POINT ( 'NONE',  ( -16.51473224551082808, 9.474510206698731452, 103.3344237280190043 ) ) ;
#180106=CARTESIAN_POINT ( 'NONE',  ( -15.72974639402197994, 15.80617190586746368, 60.62390960531437401 ) ) ;
#180108=CARTESIAN_POINT ( 'NONE',  ( 19.05341960407611168, 5.049401038298154454, 38.95724293864767418 ) ) ;
#180109=CARTESIAN_POINT ( 'NONE',  ( -13.89961937509977652, 13.97604488694528158, 85.62390960531433848 ) ) ;
#180110=CARTESIAN_POINT ( 'NONE',  ( -0.05219959533907301413, -21.53943276465977519, 92.49890960531436690 ) ) ;
#180111=CARTESIAN_POINT ( 'NONE',  ( 4.379528057220092307, 16.55341960407617563, 102.2927570613523613 ) ) ;
#180112=CARTESIAN_POINT ( 'NONE',  ( -16.51473224551069308, -9.474510206698971260, 81.66557627198103830 ) ) ;
#180113=CARTESIAN_POINT ( 'NONE',  ( 13.97604488694548053, -13.89961937509957401, 80.62609039468567573 ) ) ;
#180114=CARTESIAN_POINT ( 'NONE',  ( -18.67979575497193778, 10.72451020669871902, 93.33442372801901854 ) ) ;
#180115=CARTESIAN_POINT ( 'NONE',  ( -21.52544592524343514, 5.823673210054127303, 71.04057627198103830 ) ) ;
#180116=CARTESIAN_POINT ( 'NONE',  ( 10.72451020669898902, -18.67979575497178502, 37.91557627198102409 ) ) ;
#180117=CARTESIAN_POINT ( 'NONE',  ( -16.46253265017160317, 9.564922557960807481, 50.83224293864770260 ) ) ;
#180118=CARTESIAN_POINT ( 'NONE',  ( 8.224510206698953496, -14.34966873604960469, 27.91557627198103830 ) ) ;
#180119=CARTESIAN_POINT ( 'NONE',  ( -13.97604488694527625, -13.89961937509977652, 66.87390960531436690 ) ) ;
#180122=CARTESIAN_POINT ( 'NONE',  ( -19.05341960407617563, 5.049401038297882671, 28.54275706135232937 ) ) ;
#180123=CARTESIAN_POINT ( 'NONE',  ( 12.06949235617757843, -12.14591786802309237, 78.12390960531436690 ) ) ;
#180124=CARTESIAN_POINT ( 'NONE',  ( 10.81492255796106328, -18.62759615963255655, 20.41775706135234714 ) ) ;
#180126=CARTESIAN_POINT ( 'NONE',  ( 10.72451020669898902, -18.67979575497178502, 57.91557627198103120 ) ) ;
#180127=CARTESIAN_POINT ( 'NONE',  ( 14.29746914071037800, 8.314922557961029526, 91.66775706135234714 ) ) ;
#180128=CARTESIAN_POINT ( 'NONE',  ( 14.34966873604960469, 8.224510206698951720, 104.1655762719810241 ) ) ;
#180129=CARTESIAN_POINT ( 'NONE',  ( 9.564922557960805705, 16.46253265017160317, 69.58224293864770971 ) ) ;
#180130=CARTESIAN_POINT ( 'NONE',  ( -8.314922557960811034, -14.29746914071050412, 27.08224293864769550 ) ) ;
#180131=CARTESIAN_POINT ( 'NONE',  ( 5.719274019375673035, 21.55341960407619339, 52.29275706135236135 ) ) ;
#180132=CARTESIAN_POINT ( 'NONE',  ( 19.03943276465977164, -0.05219959533909143690, 113.7489096053143669 ) ) ;
#180133=CARTESIAN_POINT ( 'NONE',  ( -21.52544592524334988, -5.823673210054445271, 78.95942372801901854 ) ) ;
#180134=CARTESIAN_POINT ( 'NONE',  ( -16.46253265017160317, 9.564922557960807481, 35.83224293864768839 ) ) ;
#180135=CARTESIAN_POINT ( 'NONE',  ( -9.564922557960796823, -16.46253265017161027, 32.08224293864769550 ) ) ;
#180137=CARTESIAN_POINT ( 'NONE',  ( 0.05219959533937995610, -21.53943276465977519, 100.0010903946857042 ) ) ;
#180138=CARTESIAN_POINT ( 'NONE',  ( 0.05219959533934541429, -16.53943276465976808, 45.00109039468568284 ) ) ;
#180139=CARTESIAN_POINT ( 'NONE',  ( 15.72974639402176855, 15.80617190586768217, 76.87609039468567573 ) ) ;
#180140=CARTESIAN_POINT ( 'NONE',  ( 19.03943276465977164, -0.05219959533909143690, 98.74890960531436690 ) ) ;
#180141=CARTESIAN_POINT ( 'NONE',  ( 16.51473224551083163, -9.474510206698727899, 80.83442372801899012 ) ) ;
#180142=CARTESIAN_POINT ( 'NONE',  ( 18.67979575497194134, -10.72451020669871369, 60.83442372801901854 ) ) ;
#180143=CARTESIAN_POINT ( 'NONE',  ( -16.53943276465976808, -0.05219959533934237506, 23.75109039468567929 ) ) ;
#180144=CARTESIAN_POINT ( 'NONE',  ( 5.049401038297881783, 19.05341960407617563, 82.29275706135229029 ) ) ;
#180145=CARTESIAN_POINT ( 'NONE',  ( -16.46253265017160317, 9.564922557960807481, 45.83224293864769550 ) ) ;
#180146=CARTESIAN_POINT ( 'NONE',  ( -9.564922557961040184, 16.46253265017147172, 92.91775706135233293 ) ) ;
#180148=CARTESIAN_POINT ( 'NONE',  ( 4.379528057220339221, -16.55341960407611168, 27.70724293864769905 ) ) ;
#180149=CARTESIAN_POINT ( 'NONE',  ( -13.97604488694547697, 13.89961937509957934, 83.12609039468564731 ) ) ;
#180150=CARTESIAN_POINT ( 'NONE',  ( -4.379528057220328563, 16.55341960407611168, 45.20724293864769550 ) ) ;
#180151=CARTESIAN_POINT ( 'NONE',  ( 9.564922557961047289, -16.46253265017146816, 70.41775706135233293 ) ) ;
#180152=CARTESIAN_POINT ( 'NONE',  ( 14.34966873604972726, -8.224510206698740333, 45.83442372801901854 ) ) ;
#180153=CARTESIAN_POINT ( 'NONE',  ( -13.89961937509957401, -13.97604488694547875, 29.37609039468565797 ) ) ;
#180154=CARTESIAN_POINT ( 'NONE',  ( 9.474510206698971260, -16.51473224551069308, 27.91557627198103120 ) ) ;
#180155=CARTESIAN_POINT ( 'NONE',  ( 16.51473224551069308, 9.474510206698969483, 39.16557627198103120 ) ) ;
#180156=CARTESIAN_POINT ( 'NONE',  ( -14.29746914071037622, -8.314922557961029526, 44.16775706135234714 ) ) ;
#180159=CARTESIAN_POINT ( 'NONE',  ( 16.46253265017160672, -9.564922557960803928, 88.33224293864769550 ) ) ;
#180161=CARTESIAN_POINT ( 'NONE',  ( -5.153800228976607833, 19.02544592524334988, 97.70942372801900433 ) ) ;
#180162=CARTESIAN_POINT ( 'NONE',  ( -10.81492255796078084, -18.62759615963271287, 32.08224293864769550 ) ) ;
#180163=CARTESIAN_POINT ( 'NONE',  ( 13.89961937509957401, 13.97604488694547697, 36.87609039468565442 ) ) ;
#180164=CARTESIAN_POINT ( 'NONE',  ( 19.02544592524334988, 5.153800228976608722, 106.4594237280190185 ) ) ;
#180165=CARTESIAN_POINT ( 'NONE',  ( -16.52544592524342804, 4.483927247898546575, 106.0405762719810525 ) ) ;
#180166=B_SPLINE_CURVE_WITH_KNOTS ( 'NONE', 3,
 ( #159073, #156103, #187466, #123758, #155113, #109600, #32771, #141917, #31778, #157103, #3408, #78254, #79260, #124774, #48935, #138941, #108607, #94423, #126742, #173273, #111588, #189443, #96406, #50920, #33759, #421, #140932, #64098, #139927, #125766, #112578, #1416 ),
 .UNSPECIFIED., .F., .F.,
 ( 4, 2, 2, 2, 2, 2, 2, 2, 2, 2, 2, 2, 2, 2, 2, 4 ),
 ( 2.711112516444420852E-17, 0.0003712461730036983247, 0.0007424923460073695443, 0.001113738519011040710, 0.001484984692014711984, 0.002227477038022072746, 0.002598723211025739249, 0.002969969384029405319, 0.003341215557033071389, 0.003712461730036737025, 0.004083707903040402661, 0.004454954076044068297, 0.004826200249047734800, 0.005197446422051400436, 0.005568692595055066939, 0.005939938768058731708 ),
 .UNSPECIFIED. ) ;
#180167=CARTESIAN_POINT ( 'NONE',  ( -19.02544592524342804, 5.153800228976336051, 41.04057627198103120 ) ) ;
#180168=CARTESIAN_POINT ( 'NONE',  ( -21.55341960407610458, -5.719274019375992779, 71.45724293864769550 ) ) ;
#180169=CARTESIAN_POINT ( 'NONE',  ( 19.05341960407611168, 5.049401038298154454, 33.95724293864769550 ) ) ;
#180171=CARTESIAN_POINT ( 'NONE',  ( -5.049401038297874678, -19.05341960407617918, 69.79275706135233293 ) ) ;
#180172=CARTESIAN_POINT ( 'NONE',  ( 12.06949235617757843, -12.14591786802309237, 58.12390960531435979 ) ) ;
#180174=CARTESIAN_POINT ( 'NONE',  ( 18.67979575497178502, 10.72451020669898547, 34.16557627198102409 ) ) ;
#180175=CARTESIAN_POINT ( 'NONE',  ( -5.719274019375665041, -21.55341960407619695, 99.79275706135234714 ) ) ;
#180176=CARTESIAN_POINT ( 'NONE',  ( 15.72974639402199770, -15.80617190586745480, 78.12390960531436690 ) ) ;
#180177=CARTESIAN_POINT ( 'NONE',  ( 18.62759615963255655, 10.81492255796105972, 71.66775706135234714 ) ) ;
#180178=CARTESIAN_POINT ( 'NONE',  ( -21.52544592524334988, -5.823673210054445271, 58.95942372801902565 ) ) ;
#180179=CARTESIAN_POINT ( 'NONE',  ( 5.049401038298161559, -19.05341960407611168, 92.70724293864769550 ) ) ;
#180180=CARTESIAN_POINT ( 'NONE',  ( 12.06949235617739724, 12.14591786802326823, 101.8760903946857042 ) ) ;
#180181=CARTESIAN_POINT ( 'NONE',  ( -10.72451020669870658, -18.67979575497194134, 69.58442372801900433 ) ) ;
#180182=CARTESIAN_POINT ( 'NONE',  ( -5.153800228976328057, -19.02544592524343514, 52.29057627198100988 ) ) ;
#180183=CARTESIAN_POINT ( 'NONE',  ( -5.719274019375665041, -21.55341960407619695, 34.79275706135235424 ) ) ;
#180184=CARTESIAN_POINT ( 'NONE',  ( 19.02544592524343514, -5.153800228976328945, 63.54057627198103830 ) ) ;
#180185=CARTESIAN_POINT ( 'NONE',  ( -14.34966873604960291, -8.224510206698953496, 76.66557627198103830 ) ) ;
#180186=CARTESIAN_POINT ( 'NONE',  ( -0.05219959533910754901, -16.53943276465976808, 52.49890960531435979 ) ) ;
#180187=CARTESIAN_POINT ( 'NONE',  ( -5.719274019375978568, 21.55341960407610458, 55.20724293864770260 ) ) ;
#180188=CARTESIAN_POINT ( 'NONE',  ( 5.049401038298161559, -19.05341960407611168, 42.70724293864767418 ) ) ;
#180189=CARTESIAN_POINT ( 'NONE',  ( 21.55341960407610458, 5.719274019375980345, 58.95724293864770971 ) ) ;
#180190=CARTESIAN_POINT ( 'NONE',  ( -5.153800228976607833, 19.02544592524334988, 52.70942372801900433 ) ) ;
#180192=CARTESIAN_POINT ( 'NONE',  ( 16.55341960407611168, 4.379528057220329451, 58.95724293864770971 ) ) ;
#180193=CARTESIAN_POINT ( 'NONE',  ( 10.72451020669898902, -18.67979575497178502, 37.91557627198102409 ) ) ;
#180195=CARTESIAN_POINT ( 'NONE',  ( 17.12812012977026654, 6.668231424565988164, 103.8594875932314068 ) ) ;
#180196=CARTESIAN_POINT ( 'NONE',  ( 8.224510206698742110, 14.34966873604972548, 82.08442372801901854 ) ) ;
#180198=CARTESIAN_POINT ( 'NONE',  ( -9.564922557961040184, 16.46253265017147172, 92.91775706135233293 ) ) ;
#180199=CARTESIAN_POINT ( 'NONE',  ( -12.06949235617756955, 12.14591786802309770, 60.62390960531437401 ) ) ;
#180201=CARTESIAN_POINT ( 'NONE',  ( 0.05219959533909260263, 19.03943276465977164, 44.99890960531435979 ) ) ;
#180202=CARTESIAN_POINT ( 'NONE',  ( 12.14591786802309770, 12.06949235617756955, 44.37390960531435979 ) ) ;
#180203=CARTESIAN_POINT ( 'NONE',  ( -0.05219959533909027116, -19.03943276465977164, 87.49890960531436690 ) ) ;
#180204=CARTESIAN_POINT ( 'NONE',  ( 9.474510206698971260, -16.51473224551069308, 52.91557627198102409 ) ) ;
#180205=CARTESIAN_POINT ( 'NONE',  ( 18.62759615963255655, 10.81492255796105972, 61.66775706135235424 ) ) ;
#180206=CARTESIAN_POINT ( 'NONE',  ( -16.46253265017160317, 9.564922557960807481, 70.83224293864770971 ) ) ;
#180207=CARTESIAN_POINT ( 'NONE',  ( 19.05341960407611168, 5.049401038298154454, 23.95724293864769194 ) ) ;
#180208=CARTESIAN_POINT ( 'NONE',  ( 5.153800228976335163, 19.02544592524342804, 64.79057627198100988 ) ) ;
#180209=CARTESIAN_POINT ( 'NONE',  ( 18.67979575497178502, 10.72451020669898547, 54.16557627198103120 ) ) ;
#180210=CARTESIAN_POINT ( 'NONE',  ( -5.153800228976328057, -19.02544592524343514, 42.29057627198101699 ) ) ;
#180211=CARTESIAN_POINT ( 'NONE',  ( -5.719274019375978568, 21.55341960407610458, 40.20724293864769550 ) ) ;
#180212=CARTESIAN_POINT ( 'NONE',  ( 16.52544592524335698, 4.483927247898782831, 101.4594237280190185 ) ) ;
#180213=CARTESIAN_POINT ( 'NONE',  ( -9.564922557961040184, 16.46253265017147172, 22.91775706135233648 ) ) ;
#180214=CARTESIAN_POINT ( 'NONE',  ( -12.14591786802326823, 12.06949235617739902, 53.12609039468568284 ) ) ;
#180215=CARTESIAN_POINT ( 'NONE',  ( 16.53943276465976808, 0.05219959533934440121, 76.25109039468568994 ) ) ;
#180216=CARTESIAN_POINT ( 'NONE',  ( -18.10062525802553424, 5.500000000000031974, 68.51383468041923663 ) ) ;
#180217=CARTESIAN_POINT ( 'NONE',  ( -14.29746914071037622, -8.314922557961029526, 74.16775706135231871 ) ) ;
#180218=CARTESIAN_POINT ( 'NONE',  ( 14.29746914071037800, 8.314922557961029526, 51.66775706135234714 ) ) ;
#180219=CARTESIAN_POINT ( 'NONE',  ( 16.51473224551069308, 9.474510206698969483, 104.1655762719810241 ) ) ;
#180220=CARTESIAN_POINT ( 'NONE',  ( 5.153800228976335163, 19.02544592524342804, 29.79057627198102409 ) ) ;
#180221=CARTESIAN_POINT ( 'NONE',  ( -0.05219959533934338120, 16.53943276465976808, 37.50109039468568284 ) ) ;
#180222=CARTESIAN_POINT ( 'NONE',  ( -13.97604488694527625, -13.89961937509977652, 51.87390960531436690 ) ) ;
#180223=CARTESIAN_POINT ( 'NONE',  ( 15.72974639402176855, 15.80617190586768217, 21.87609039468567573 ) ) ;
#180224=CARTESIAN_POINT ( 'NONE',  ( 0.05219959533934541429, -16.53943276465976808, 35.00109039468568284 ) ) ;
#180225=CARTESIAN_POINT ( 'NONE',  ( 4.483927247898790824, -16.52544592524335698, 100.2094237280190043 ) ) ;
#180226=CARTESIAN_POINT ( 'NONE',  ( -17.50000000000001421, -5.499999999999944045, 71.28230962303567253 ) ) ;
#180227=CARTESIAN_POINT ( 'NONE',  ( 21.52544592524334988, 5.823673210054432836, 101.4594237280190185 ) ) ;
#180228=CARTESIAN_POINT ( 'NONE',  ( -0.05219959533936034679, 19.03943276465977164, 102.5010903946856757 ) ) ;
#180229=EDGE_CURVE ( 'NONE', #193812, #134824, #10170, .T. ) ;
#180230=CARTESIAN_POINT ( 'NONE',  ( -0.05219959533910754901, -16.53943276465976808, 52.49890960531435979 ) ) ;
#180231=CARTESIAN_POINT ( 'NONE',  ( 19.03943276465977164, -0.05219959533909143690, 28.74890960531435624 ) ) ;
#180232=CARTESIAN_POINT ( 'NONE',  ( 19.03943276465977164, 0.05219959533936151252, 66.25109039468567573 ) ) ;
#180233=CARTESIAN_POINT ( 'NONE',  ( 16.38665767534995865, -7.295008042176402085, 57.76400864214468811 ) ) ;
#180234=CARTESIAN_POINT ( 'NONE',  ( -10.81492255796105439, 18.62759615963255655, 67.91775706135234714 ) ) ;
#180235=CARTESIAN_POINT ( 'NONE',  ( 4.483927247898790824, -16.52544592524335698, 25.20942372801901854 ) ) ;
#180237=CARTESIAN_POINT ( 'NONE',  ( 15.80617190586746368, 15.72974639402197994, 29.37390960531435269 ) ) ;
#180238=CARTESIAN_POINT ( 'NONE',  ( -5.153800228976607833, 19.02544592524334988, 112.7094237280190043 ) ) ;
#180239=CARTESIAN_POINT ( 'NONE',  ( 17.60728821186568638, -5.500000000000035527, 98.36690927743006796 ) ) ;
#180241=CARTESIAN_POINT ( 'NONE',  ( 9.564922557960805705, 16.46253265017160317, 24.58224293864769194 ) ) ;
#180242=CARTESIAN_POINT ( 'NONE',  ( 15.72974639402176855, 15.80617190586768217, 101.8760903946857042 ) ) ;
#180243=CARTESIAN_POINT ( 'NONE',  ( -9.564922557960796823, -16.46253265017161027, 37.08224293864768839 ) ) ;
#180244=CARTESIAN_POINT ( 'NONE',  ( -10.81492255796105439, 18.62759615963255655, 57.91775706135234714 ) ) ;
#180245=CARTESIAN_POINT ( 'NONE',  ( -18.67979575497193778, 10.72451020669871902, 108.3344237280190185 ) ) ;
#180246=CARTESIAN_POINT ( 'NONE',  ( -4.483927247898782831, 16.52544592524335698, 97.70942372801904696 ) ) ;
#180247=CARTESIAN_POINT ( 'NONE',  ( 5.049401038298161559, -19.05341960407611168, 72.70724293864768129 ) ) ;
#180248=CARTESIAN_POINT ( 'NONE',  ( 10.81492255796106328, -18.62759615963255655, 50.41775706135235424 ) ) ;
#180249=CARTESIAN_POINT ( 'NONE',  ( 21.52544592524334988, 5.823673210054432836, 51.45942372801901854 ) ) ;
#180250=CARTESIAN_POINT ( 'NONE',  ( -9.474510206698720793, -16.51473224551083518, 79.58442372801899012 ) ) ;
#180251=CARTESIAN_POINT ( 'NONE',  ( -5.153800228976328057, -19.02544592524343514, 92.29057627198099567 ) ) ;
#180252=CARTESIAN_POINT ( 'NONE',  ( -8.224510206698948167, 14.34966873604960824, 115.4155762719810241 ) ) ;
#180253=CARTESIAN_POINT ( 'NONE',  ( -15.80617190586745835, -15.72974639402198527, 91.87390960531436690 ) ) ;
#180254=CARTESIAN_POINT ( 'NONE',  ( 10.72451020669871369, 18.67979575497193778, 112.0844237280190185 ) ) ;
#180255=CARTESIAN_POINT ( 'NONE',  ( 12.06949235617757843, -12.14591786802309237, 93.12390960531436690 ) ) ;
#180256=CARTESIAN_POINT ( 'NONE',  ( -16.51473224551069308, -9.474510206698971260, 51.66557627198102409 ) ) ;
#180257=CARTESIAN_POINT ( 'NONE',  ( -13.89961937509957401, -13.97604488694547875, 84.37609039468567573 ) ) ;
#180258=CARTESIAN_POINT ( 'NONE',  ( -14.29746914071049879, 8.314922557960819915, 55.83224293864770260 ) ) ;
#180259=CARTESIAN_POINT ( 'NONE',  ( -13.89961937509957401, -13.97604488694547875, 19.37609039468566507 ) ) ;
#180260=CARTESIAN_POINT ( 'NONE',  ( -13.97604488694527625, -13.89961937509977652, 111.8739096053143243 ) ) ;
#180261=CARTESIAN_POINT ( 'NONE',  ( 9.564922557961047289, -16.46253265017146816, 75.41775706135234714 ) ) ;
#180262=CARTESIAN_POINT ( 'NONE',  ( 10.72451020669898902, -18.67979575497178502, 72.91557627198103830 ) ) ;
#180263=CARTESIAN_POINT ( 'NONE',  ( 18.62759615963255655, 10.81492255796105972, 31.66775706135234358 ) ) ;
#180264=CARTESIAN_POINT ( 'NONE',  ( 14.29746914071037800, 8.314922557961029526, 31.66775706135234358 ) ) ;
#180265=CARTESIAN_POINT ( 'NONE',  ( -16.52544592524335698, -4.483927247898792601, 93.95942372801903275 ) ) ;
#180266=CARTESIAN_POINT ( 'NONE',  ( -17.49999999999999645, -7.500000000000000888, 102.5000000000000142 ) ) ;
#180267=CARTESIAN_POINT ( 'NONE',  ( 18.62759615963255655, 10.81492255796105972, 41.66775706135235424 ) ) ;
#180268=CARTESIAN_POINT ( 'NONE',  ( -0.05219959533907301413, -21.53943276465977519, 37.49890960531436690 ) ) ;
#180269=CARTESIAN_POINT ( 'NONE',  ( 16.51473224551069308, 9.474510206698969483, 39.16557627198103120 ) ) ;
#180271=CARTESIAN_POINT ( 'NONE',  ( 4.379528057220092307, 16.55341960407617563, 57.29275706135234714 ) ) ;
#180272=CARTESIAN_POINT ( 'NONE',  ( -16.52544592524342804, 4.483927247898546575, 96.04057627198102409 ) ) ;
#180273=CARTESIAN_POINT ( 'NONE',  ( 5.823673210054125526, 21.52544592524343514, 89.79057627198103830 ) ) ;
#180274=CARTESIAN_POINT ( 'NONE',  ( -14.34966873604960291, -8.224510206698953496, 26.66557627198103475 ) ) ;
#180275=CARTESIAN_POINT ( 'NONE',  ( -16.55341960407617563, 4.379528057220093196, 53.54275706135234714 ) ) ;
#180276=CARTESIAN_POINT ( 'NONE',  ( 5.153800228976335163, 19.02544592524342804, 64.79057627198100988 ) ) ;
#180277=CARTESIAN_POINT ( 'NONE',  ( -16.53943276465976808, -0.05219959533934237506, 93.75109039468567573 ) ) ;
#180278=CARTESIAN_POINT ( 'NONE',  ( 19.05341960407617918, -5.049401038297876454, 86.04275706135233293 ) ) ;
#180279=CARTESIAN_POINT ( 'NONE',  ( -15.80617190586745835, -15.72974639402198527, 86.87390960531438111 ) ) ;
#180280=CARTESIAN_POINT ( 'NONE',  ( -14.34966873604960291, -8.224510206698953496, 21.66557627198102409 ) ) ;
#180281=ORIENTED_EDGE ( 'NONE', *, *, #91586, .F. ) ;
#180283=CARTESIAN_POINT ( 'NONE',  ( -0.05219959533907301413, -21.53943276465977519, 67.49890960531436690 ) ) ;
#180285=CARTESIAN_POINT ( 'NONE',  ( -12.06949235617739369, -12.14591786802326823, 94.37609039468568994 ) ) ;
#180287=CARTESIAN_POINT ( 'NONE',  ( 0.05219959533907565091, 21.53943276465977519, 24.99890960531435624 ) ) ;
#180289=CARTESIAN_POINT ( 'NONE',  ( 5.719274019375991003, -21.55341960407610458, 87.70724293864769550 ) ) ;
#180290=CARTESIAN_POINT ( 'NONE',  ( 4.379528057220339221, -16.55341960407611168, 27.70724293864769905 ) ) ;
#180291=CARTESIAN_POINT ( 'NONE',  ( 16.55341960407618274, -4.379528057220086978, 41.04275706135236135 ) ) ;
#180292=CARTESIAN_POINT ( 'NONE',  ( 19.05341960407611168, 5.049401038298154454, 33.95724293864769550 ) ) ;
#180293=CARTESIAN_POINT ( 'NONE',  ( 0.05219959533934541429, -16.53943276465976808, 25.00109039468567218 ) ) ;
#180294=CARTESIAN_POINT ( 'NONE',  ( -5.049401038298153566, 19.05341960407611168, 50.20724293864770260 ) ) ;
#180296=CARTESIAN_POINT ( 'NONE',  ( -13.89961937509977652, 13.97604488694528158, 105.6239096053143527 ) ) ;
#180297=CARTESIAN_POINT ( 'NONE',  ( 17.72662750342724891, 5.500000000000081712, 78.90179492283748175 ) ) ;
#180298=CARTESIAN_POINT ( 'NONE',  ( 0.05219959533934541429, -16.53943276465976808, 100.0010903946857042 ) ) ;
#180299=CARTESIAN_POINT ( 'NONE',  ( 19.05341960407617918, -5.049401038297876454, 96.04275706135231871 ) ) ;
#180300=CARTESIAN_POINT ( 'NONE',  ( -16.51473224551082808, 9.474510206698731452, 38.33442372801899722 ) ) ;
#180301=CARTESIAN_POINT ( 'NONE',  ( -21.55341960407610458, -5.719274019375992779, 76.45724293864769550 ) ) ;
#180302=CARTESIAN_POINT ( 'NONE',  ( -14.34966873604972548, 8.224510206698743886, 103.3344237280190043 ) ) ;
#180303=CARTESIAN_POINT ( 'NONE',  ( -21.53943276465977519, 0.05219959533907696930, 26.24890960531435624 ) ) ;
#180304=CARTESIAN_POINT ( 'NONE',  ( -13.89961937509957401, -13.97604488694547875, 109.3760903946856331 ) ) ;
#180305=CARTESIAN_POINT ( 'NONE',  ( 19.02544592524343514, -5.153800228976328945, 108.5405762719810383 ) ) ;
#180306=CARTESIAN_POINT ( 'NONE',  ( -15.72974639402176322, -15.80617190586768395, 59.37609039468568284 ) ) ;
#180307=CARTESIAN_POINT ( 'NONE',  ( -16.46253265017160317, 9.564922557960807481, 60.83224293864769550 ) ) ;
#180308=CARTESIAN_POINT ( 'NONE',  ( 14.34966873604960469, 8.224510206698951720, 99.16557627198100988 ) ) ;
#180310=CARTESIAN_POINT ( 'NONE',  ( 16.53943276465976808, -0.05219959533910856209, 83.74890960531435269 ) ) ;
#180311=CARTESIAN_POINT ( 'NONE',  ( -21.52544592524343514, 5.823673210054127303, 76.04057627198102409 ) ) ;
#180312=ORIENTED_EDGE ( 'NONE', *, *, #91138, .T. ) ;
#180313=CARTESIAN_POINT ( 'NONE',  ( -5.153800228976607833, 19.02544592524334988, 97.70942372801900433 ) ) ;
#180314=CARTESIAN_POINT ( 'NONE',  ( 19.01529144963337359, 5.500000000000033751, 93.73431955728439391 ) ) ;
#180315=CARTESIAN_POINT ( 'NONE',  ( -13.97604488694527625, -13.89961937509977652, 56.87390960531434558 ) ) ;
#180316=CARTESIAN_POINT ( 'NONE',  ( 17.26058549869104652, -6.457015423128295240, 71.12254162523932166 ) ) ;
#180317=CARTESIAN_POINT ( 'NONE',  ( -16.51473224551069308, -9.474510206698971260, 81.66557627198103830 ) ) ;
#180318=CARTESIAN_POINT ( 'NONE',  ( 13.97604488694527802, 13.89961937509977652, 89.37390960531436690 ) ) ;
#180319=CARTESIAN_POINT ( 'NONE',  ( 8.224510206698742110, 14.34966873604972548, 67.08442372801901854 ) ) ;
#180320=CARTESIAN_POINT ( 'NONE',  ( -16.81555441253550853, -7.025013491695501600, 49.36314554665745646 ) ) ;
#180321=CARTESIAN_POINT ( 'NONE',  ( 5.049401038297881783, 19.05341960407617563, 37.29275706135232582 ) ) ;
#180323=CARTESIAN_POINT ( 'NONE',  ( -19.03943276465977164, 0.05219959533909376836, 106.2489096053143669 ) ) ;
#180324=CARTESIAN_POINT ( 'NONE',  ( -0.05219959533934338120, 16.53943276465976808, 107.5010903946856899 ) ) ;
#180325=CARTESIAN_POINT ( 'NONE',  ( -18.22780087662124160, -5.499999999999927169, 73.98236817873106475 ) ) ;
#180326=CARTESIAN_POINT ( 'NONE',  ( -12.06949235617739369, -12.14591786802326823, 94.37609039468568994 ) ) ;
#180327=CARTESIAN_POINT ( 'NONE',  ( -16.31925111598457434, 7.325300261831451110, 30.16424538967251578 ) ) ;
#180328=CARTESIAN_POINT ( 'NONE',  ( 4.379528057220092307, 16.55341960407617563, 67.29275706135234714 ) ) ;
#180330=CARTESIAN_POINT ( 'NONE',  ( 5.823673210054444382, -21.52544592524334988, 70.20942372801904696 ) ) ;
#180331=CARTESIAN_POINT ( 'NONE',  ( -9.564922557961040184, 16.46253265017147172, 82.91775706135233293 ) ) ;
#180332=CARTESIAN_POINT ( 'NONE',  ( -19.05341960407617563, 5.049401038297882671, 28.54275706135232937 ) ) ;
#180333=CARTESIAN_POINT ( 'NONE',  ( -5.049401038298153566, 19.05341960407611168, 70.20724293864769550 ) ) ;
#180334=CARTESIAN_POINT ( 'NONE',  ( -9.474510206698964154, 16.51473224551069663, 50.41557627198102409 ) ) ;
#180336=CARTESIAN_POINT ( 'NONE',  ( 5.719274019375991003, -21.55341960407610458, 87.70724293864769550 ) ) ;
#180337=CARTESIAN_POINT ( 'NONE',  ( -21.53943276465977519, 0.05219959533907696930, 41.24890960531435269 ) ) ;
#180338=CARTESIAN_POINT ( 'NONE',  ( 16.46253265017160672, -9.564922557960803928, 28.33224293864769550 ) ) ;
#180339=CARTESIAN_POINT ( 'NONE',  ( -14.34966873604972548, 8.224510206698743886, 53.33442372801901854 ) ) ;
#180341=CARTESIAN_POINT ( 'NONE',  ( -10.72451020669870658, -18.67979575497194134, 29.58442372801901854 ) ) ;
#180342=CARTESIAN_POINT ( 'NONE',  ( 0.05219959533910956823, 16.53943276465976808, 54.99890960531435269 ) ) ;
#180344=CARTESIAN_POINT ( 'NONE',  ( -12.14591786802326823, 12.06949235617739902, 28.12609039468568284 ) ) ;
#180345=CARTESIAN_POINT ( 'NONE',  ( 13.97604488694548053, -13.89961937509957401, 45.62609039468566863 ) ) ;
#180346=CARTESIAN_POINT ( 'NONE',  ( 14.29746914071049879, -8.314922557960816363, 58.33224293864768839 ) ) ;
#180347=CARTESIAN_POINT ( 'NONE',  ( -15.80617190586745835, -15.72974639402198527, 111.8739096053143669 ) ) ;
#180349=CARTESIAN_POINT ( 'NONE',  ( -21.53943276465977519, 0.05219959533907696930, 81.24890960531436690 ) ) ;
#180350=CARTESIAN_POINT ( 'NONE',  ( -19.05341960407611168, -5.049401038298163336, 91.45724293864766707 ) ) ;
#180351=CARTESIAN_POINT ( 'NONE',  ( 0.05219959533910956823, 16.53943276465976808, 59.99890960531436690 ) ) ;
#180352=CARTESIAN_POINT ( 'NONE',  ( -5.153800228976328057, -19.02544592524343514, 102.2905762719810383 ) ) ;
#180354=CARTESIAN_POINT ( 'NONE',  ( 13.97604488694548053, -13.89961937509957401, 65.62609039468567573 ) ) ;
#180355=CARTESIAN_POINT ( 'NONE',  ( 18.67979575497178502, 10.72451020669898547, 109.1655762719810383 ) ) ;
#180356=CARTESIAN_POINT ( 'NONE',  ( 13.97604488694527802, 13.89961937509977652, 54.37390960531435979 ) ) ;
#180357=CARTESIAN_POINT ( 'NONE',  ( 19.02544592524334988, 5.153800228976608722, 46.45942372801899012 ) ) ;
#180358=CARTESIAN_POINT ( 'NONE',  ( 4.379528057220339221, -16.55341960407611168, 107.7072429386476955 ) ) ;
#180360=CARTESIAN_POINT ( 'NONE',  ( -10.72451020669870658, -18.67979575497194134, 59.58442372801901854 ) ) ;
#180361=CARTESIAN_POINT ( 'NONE',  ( -17.40861289039004234, -6.110651285853239578, 71.37232470827430575 ) ) ;
#180362=CARTESIAN_POINT ( 'NONE',  ( -12.06949235617756955, 12.14591786802309770, 45.62390960531436690 ) ) ;
#180363=CARTESIAN_POINT ( 'NONE',  ( -5.049401038298153566, 19.05341960407611168, 55.20724293864769550 ) ) ;
#180364=CARTESIAN_POINT ( 'NONE',  ( -21.52544592524343514, 5.823673210054127303, 76.04057627198102409 ) ) ;
#180366=CARTESIAN_POINT ( 'NONE',  ( -9.564922557960796823, -16.46253265017161027, 42.08224293864769550 ) ) ;
#180368=CARTESIAN_POINT ( 'NONE',  ( -15.80617190586745835, -15.72974639402198527, 66.87390960531436690 ) ) ;
#180369=CARTESIAN_POINT ( 'NONE',  ( 5.823673210054444382, -21.52544592524334988, 90.20942372801903275 ) ) ;
#180371=CARTESIAN_POINT ( 'NONE',  ( -4.379528057220086978, -16.55341960407618274, 94.79275706135234714 ) ) ;
#180372=CARTESIAN_POINT ( 'NONE',  ( 12.06949235617757843, -12.14591786802309237, 78.12390960531436690 ) ) ;
#180373=CARTESIAN_POINT ( 'NONE',  ( -5.153800228976328057, -19.02544592524343514, 72.29057627198102409 ) ) ;
#180375=CARTESIAN_POINT ( 'NONE',  ( 9.564922557961047289, -16.46253265017146816, 45.41775706135232582 ) ) ;
#180376=CARTESIAN_POINT ( 'NONE',  ( -14.34966873604972548, 8.224510206698743886, 88.33442372801901854 ) ) ;
#180377=CARTESIAN_POINT ( 'NONE',  ( -19.02544592524334988, -5.153800228976617603, 28.95942372801900433 ) ) ;
#180378=CARTESIAN_POINT ( 'NONE',  ( -5.153800228976328057, -19.02544592524343514, 92.29057627198099567 ) ) ;
#180379=CARTESIAN_POINT ( 'NONE',  ( -21.55341960407610458, -5.719274019375992779, 51.45724293864770260 ) ) ;
#180381=CARTESIAN_POINT ( 'NONE',  ( 5.049401038298161559, -19.05341960407611168, 22.70724293864769194 ) ) ;
#180382=CARTESIAN_POINT ( 'NONE',  ( -18.62759615963255300, -10.81492255796106328, 89.16775706135236135 ) ) ;
#180383=CARTESIAN_POINT ( 'NONE',  ( 4.483927247898790824, -16.52544592524335698, 60.20942372801902565 ) ) ;
#180384=CARTESIAN_POINT ( 'NONE',  ( 0.05219959533937995610, -21.53943276465977519, 20.00109039468568639 ) ) ;
#180385=CARTESIAN_POINT ( 'NONE',  ( -8.314922557961024197, 14.29746914071037800, 27.91775706135234358 ) ) ;
#180386=CARTESIAN_POINT ( 'NONE',  ( 13.89961937509977652, -13.97604488694527269, 93.12390960531436690 ) ) ;
#180387=CARTESIAN_POINT ( 'NONE',  ( -13.89961937509977652, 13.97604488694528158, 45.62390960531433848 ) ) ;
#180388=CARTESIAN_POINT ( 'NONE',  ( 13.97604488694527802, 13.89961937509977652, 59.37390960531434558 ) ) ;
#180389=CARTESIAN_POINT ( 'NONE',  ( 8.224510206698742110, 14.34966873604972548, 37.08442372801901143 ) ) ;
#180390=CARTESIAN_POINT ( 'NONE',  ( 12.14591786802309770, 12.06949235617756955, 89.37390960531435269 ) ) ;
#180391=CARTESIAN_POINT ( 'NONE',  ( 12.06949235617739724, 12.14591786802326823, 101.8760903946857042 ) ) ;
#180392=CARTESIAN_POINT ( 'NONE',  ( -18.67979575497193778, 10.72451020669871902, 48.33442372801902565 ) ) ;
#180393=CARTESIAN_POINT ( 'NONE',  ( -13.97604488694527625, -13.89961937509977652, 66.87390960531436690 ) ) ;
#180394=CARTESIAN_POINT ( 'NONE',  ( -13.97604488694527625, -13.89961937509977652, 51.87390960531436690 ) ) ;
#180395=CARTESIAN_POINT ( 'NONE',  ( 13.89961937509977652, -13.97604488694527269, 78.12390960531433848 ) ) ;
#180396=CARTESIAN_POINT ( 'NONE',  ( -4.379528057220328563, 16.55341960407611168, 35.20724293864768839 ) ) ;
#180397=CARTESIAN_POINT ( 'NONE',  ( -8.224510206698735004, -14.34966873604973081, 94.58442372801901854 ) ) ;
#180398=CARTESIAN_POINT ( 'NONE',  ( 5.153800228976615827, -19.02544592524334988, 45.20942372801901143 ) ) ;
#180399=CARTESIAN_POINT ( 'NONE',  ( 19.03943276465977164, -0.05219959533909143690, 108.7489096053143527 ) ) ;
#180400=CARTESIAN_POINT ( 'NONE',  ( -13.89961937509977652, 13.97604488694528158, 45.62390960531433848 ) ) ;
#180401=CARTESIAN_POINT ( 'NONE',  ( 5.153800228976615827, -19.02544592524334988, 30.20942372801900433 ) ) ;
#180403=CARTESIAN_POINT ( 'NONE',  ( -8.314922557961024197, 14.29746914071037800, 42.91775706135235424 ) ) ;
#180404=CARTESIAN_POINT ( 'NONE',  ( -16.51473224551082808, 9.474510206698731452, 73.33442372801900433 ) ) ;
#180405=CARTESIAN_POINT ( 'NONE',  ( -16.52544592524335698, -4.483927247898792601, 53.95942372801900433 ) ) ;
#180407=CARTESIAN_POINT ( 'NONE',  ( 19.02544592524343514, -5.153800228976328945, 73.54057627198103830 ) ) ;
#180408=CARTESIAN_POINT ( 'NONE',  ( 10.72451020669898902, -18.67979575497178502, 112.9155762719810383 ) ) ;
#180409=CARTESIAN_POINT ( 'NONE',  ( 13.89961937509957401, 13.97604488694547697, 66.87609039468567573 ) ) ;
#180410=CARTESIAN_POINT ( 'NONE',  ( 5.153800228976335163, 19.02544592524342804, 104.7905762719809957 ) ) ;
#180411=CARTESIAN_POINT ( 'NONE',  ( 5.049401038298161559, -19.05341960407611168, 37.70724293864768839 ) ) ;
#180412=CARTESIAN_POINT ( 'NONE',  ( 19.05341960407611168, 5.049401038298154454, 73.95724293864768129 ) ) ;
#180413=CARTESIAN_POINT ( 'NONE',  ( 16.53943276465976808, -0.05219959533910856209, 38.74890960531435979 ) ) ;
#180414=CARTESIAN_POINT ( 'NONE',  ( -5.049401038298153566, 19.05341960407611168, 30.20724293864768839 ) ) ;
#180415=CARTESIAN_POINT ( 'NONE',  ( -19.03943276465977164, -0.05219959533935918106, 38.75109039468566152 ) ) ;
#180416=CARTESIAN_POINT ( 'NONE',  ( 0.05219959533910956823, 16.53943276465976808, 79.99890960531435269 ) ) ;
#180417=CARTESIAN_POINT ( 'NONE',  ( -21.53943276465977519, -0.05219959533937600094, 113.7510903946856757 ) ) ;
#180418=CARTESIAN_POINT ( 'NONE',  ( -19.02544592524342804, 5.153800228976336051, 56.04057627198100988 ) ) ;
#180419=CARTESIAN_POINT ( 'NONE',  ( 15.80617190586746368, 15.72974639402197994, 44.37390960531435979 ) ) ;
#180420=CARTESIAN_POINT ( 'NONE',  ( -12.06949235617756955, 12.14591786802309770, 50.62390960531435979 ) ) ;
#180421=CARTESIAN_POINT ( 'NONE',  ( -15.80617190586768217, 15.72974639402176855, 103.1260903946856757 ) ) ;
#180422=CARTESIAN_POINT ( 'NONE',  ( -16.46253265017160317, 9.564922557960807481, 90.83224293864769550 ) ) ;
#180423=CARTESIAN_POINT ( 'NONE',  ( 9.474510206698971260, -16.51473224551069308, 107.9155762719810383 ) ) ;
#180424=CARTESIAN_POINT ( 'NONE',  ( -19.02544592524342804, 5.153800228976336051, 46.04057627198101699 ) ) ;
#180425=CARTESIAN_POINT ( 'NONE',  ( 16.51473224551069308, 9.474510206698969483, 29.16557627198103475 ) ) ;
#180426=CARTESIAN_POINT ( 'NONE',  ( 14.29746914071049879, -8.314922557960816363, 88.33224293864769550 ) ) ;
#180427=CARTESIAN_POINT ( 'NONE',  ( 21.52544592524344225, -5.823673210054117533, 98.54057627198105251 ) ) ;
#180428=CARTESIAN_POINT ( 'NONE',  ( -5.153800228976328057, -19.02544592524343514, 82.29057627198103830 ) ) ;
#180429=CARTESIAN_POINT ( 'NONE',  ( -10.81492255796078084, -18.62759615963271287, 112.0822429386477097 ) ) ;
#180430=CARTESIAN_POINT ( 'NONE',  ( -19.02544592524342804, 5.153800228976336051, 86.04057627198103830 ) ) ;
#180432=CARTESIAN_POINT ( 'NONE',  ( 4.379528057220339221, -16.55341960407611168, 102.7072429386476955 ) ) ;
#180433=CARTESIAN_POINT ( 'NONE',  ( -0.05219959533909027116, -19.03943276465977164, 72.49890960531435269 ) ) ;
#180434=CARTESIAN_POINT ( 'NONE',  ( -5.823673210054116645, -21.52544592524344225, 77.29057627198102409 ) ) ;
#180438=CARTESIAN_POINT ( 'NONE',  ( -15.72974639402197994, 15.80617190586746368, 30.62390960531436335 ) ) ;
#180439=CARTESIAN_POINT ( 'NONE',  ( 19.48894818550241581, -5.500000000000102141, 67.60307310435240424 ) ) ;
#180440=CARTESIAN_POINT ( 'NONE',  ( 16.53943276465976808, 0.05219959533934440121, 36.25109039468567573 ) ) ;
#180441=CARTESIAN_POINT ( 'NONE',  ( 14.34966873604960469, 8.224510206698951720, 99.16557627198100988 ) ) ;
#180443=CARTESIAN_POINT ( 'NONE',  ( 0.05219959533909260263, 19.03943276465977164, 84.99890960531436690 ) ) ;
#180444=CARTESIAN_POINT ( 'NONE',  ( -13.89961937509977652, 13.97604488694528158, 40.62390960531435979 ) ) ;
#180445=CARTESIAN_POINT ( 'NONE',  ( 0.05219959533910956823, 16.53943276465976808, 84.99890960531436690 ) ) ;
#180446=CARTESIAN_POINT ( 'NONE',  ( 5.823673210054125526, 21.52544592524343514, 34.79057627198103120 ) ) ;
#180447=CARTESIAN_POINT ( 'NONE',  ( 4.483927247898545687, 16.52544592524342804, 54.79057627198104541 ) ) ;
#180448=CARTESIAN_POINT ( 'NONE',  ( -19.05341960407617563, 5.049401038297882671, 98.54275706135233293 ) ) ;
#180449=CARTESIAN_POINT ( 'NONE',  ( -21.53943276465977519, -0.05219959533937600094, 63.75109039468568284 ) ) ;
#180451=CARTESIAN_POINT ( 'NONE',  ( 0.05219959533909260263, 19.03943276465977164, 94.99890960531436690 ) ) ;
#180452=CARTESIAN_POINT ( 'NONE',  ( -8.224510206698735004, -14.34966873604973081, 79.58442372801903275 ) ) ;
#180453=CARTESIAN_POINT ( 'NONE',  ( -0.05219959533909027116, -19.03943276465977164, 22.49890960531436690 ) ) ;
#180454=CARTESIAN_POINT ( 'NONE',  ( -16.51473224551069308, -9.474510206698971260, 71.66557627198102409 ) ) ;
#180455=CARTESIAN_POINT ( 'NONE',  ( -15.72974639402197994, 15.80617190586746368, 75.62390960531439532 ) ) ;
#180456=CARTESIAN_POINT ( 'NONE',  ( -0.05219959533934338120, 16.53943276465976808, 32.50109039468568284 ) ) ;
#180457=CARTESIAN_POINT ( 'NONE',  ( -16.55341960407611168, -4.379528057220339221, 56.45724293864768839 ) ) ;
#180458=CARTESIAN_POINT ( 'NONE',  ( 15.72974639402176855, 15.80617190586768217, 61.87609039468568284 ) ) ;
#180459=CARTESIAN_POINT ( 'NONE',  ( -16.53943276465976808, -0.05219959533934237506, 83.75109039468568994 ) ) ;
#180460=CARTESIAN_POINT ( 'NONE',  ( -5.823673210054116645, -21.52544592524344225, 27.29057627198103120 ) ) ;
#180462=CARTESIAN_POINT ( 'NONE',  ( -17.26172910966779384, 6.454744622555854683, 80.80646908649224258 ) ) ;
#180463=CARTESIAN_POINT ( 'NONE',  ( 8.314922557961029526, -14.29746914071037800, 105.4177570613523613 ) ) ;
#180464=CARTESIAN_POINT ( 'NONE',  ( -12.14591786802326823, 12.06949235617739902, 63.12609039468568994 ) ) ;
#180465=CARTESIAN_POINT ( 'NONE',  ( -0.05219959533909027116, -19.03943276465977164, 77.49890960531435269 ) ) ;
#180466=CARTESIAN_POINT ( 'NONE',  ( 19.02544592524343514, -5.153800228976328945, 93.54057627198102409 ) ) ;
#180467=CARTESIAN_POINT ( 'NONE',  ( -10.72451020669870658, -18.67979575497194134, 69.58442372801900433 ) ) ;
#180468=CARTESIAN_POINT ( 'NONE',  ( -4.379528057220086978, -16.55341960407618274, 69.79275706135234714 ) ) ;
#180469=CARTESIAN_POINT ( 'NONE',  ( 14.29746914071049879, -8.314922557960816363, 43.33224293864769550 ) ) ;
#180470=CARTESIAN_POINT ( 'NONE',  ( -19.05341960407611168, -5.049401038298163336, 61.45724293864769550 ) ) ;
#180471=CARTESIAN_POINT ( 'NONE',  ( 19.05341960407611168, 5.049401038298154454, 53.95724293864770260 ) ) ;
#180472=CARTESIAN_POINT ( 'NONE',  ( 14.29746914071037800, 8.314922557961029526, 36.66775706135234714 ) ) ;
#180475=CARTESIAN_POINT ( 'NONE',  ( 19.02544592524334988, 5.153800228976608722, 96.45942372801897591 ) ) ;
#180476=CARTESIAN_POINT ( 'NONE',  ( 14.34966873604960469, 8.224510206698951720, 99.16557627198100988 ) ) ;
#180477=CARTESIAN_POINT ( 'NONE',  ( 19.02544592524343514, -5.153800228976328945, 58.54057627198102409 ) ) ;
#180478=CARTESIAN_POINT ( 'NONE',  ( 9.564922557961047289, -16.46253265017146816, 100.4177570613523329 ) ) ;
#180480=CARTESIAN_POINT ( 'NONE',  ( 21.55341960407619695, -5.719274019375665929, 106.0427570613523471 ) ) ;
#180481=CARTESIAN_POINT ( 'NONE',  ( -8.314922557961024197, 14.29746914071037800, 72.91775706135234714 ) ) ;
#180483=CARTESIAN_POINT ( 'NONE',  ( 5.823673210054125526, 21.52544592524343514, 59.79057627198103120 ) ) ;
#180484=CARTESIAN_POINT ( 'NONE',  ( 8.224510206698742110, 14.34966873604972548, 52.08442372801901854 ) ) ;
#180485=CARTESIAN_POINT ( 'NONE',  ( 19.03943276465977164, 0.05219959533936151252, 61.25109039468566863 ) ) ;
#180486=CARTESIAN_POINT ( 'NONE',  ( -5.153800228976328057, -19.02544592524343514, 87.29057627198103830 ) ) ;
#180487=CARTESIAN_POINT ( 'NONE',  ( -4.379528057220328563, 16.55341960407611168, 110.2072429386477239 ) ) ;
#180488=CARTESIAN_POINT ( 'NONE',  ( -19.05341960407611168, -5.049401038298163336, 61.45724293864769550 ) ) ;
#180489=CARTESIAN_POINT ( 'NONE',  ( -8.314922557960811034, -14.29746914071050412, 62.08224293864769550 ) ) ;
#180490=CARTESIAN_POINT ( 'NONE',  ( 15.80617190586769283, -15.72974639402175789, 80.62609039468567573 ) ) ;
#180491=CARTESIAN_POINT ( 'NONE',  ( 19.02544592524334988, 5.153800228976608722, 46.45942372801899012 ) ) ;
#180492=CARTESIAN_POINT ( 'NONE',  ( 19.05341960407617918, -5.049401038297876454, 26.04275706135233293 ) ) ;
#180493=CARTESIAN_POINT ( 'NONE',  ( -15.80617190586745835, -15.72974639402198527, 26.87390960531435979 ) ) ;
#180494=CARTESIAN_POINT ( 'NONE',  ( 15.72974639402176855, 15.80617190586768217, 101.8760903946857042 ) ) ;
#180495=CARTESIAN_POINT ( 'NONE',  ( 16.51473224551069308, 9.474510206698969483, 69.16557627198102409 ) ) ;
#180496=CARTESIAN_POINT ( 'NONE',  ( 10.81492255796106328, -18.62759615963255655, 90.41775706135236135 ) ) ;
#180497=CARTESIAN_POINT ( 'NONE',  ( -10.72451020669898014, 18.67979575497178502, 45.41557627198103830 ) ) ;
#180498=CARTESIAN_POINT ( 'NONE',  ( 19.05341960407611168, 5.049401038298154454, 83.95724293864766707 ) ) ;
#180499=CARTESIAN_POINT ( 'NONE',  ( -13.97604488694547697, 13.89961937509957934, 58.12609039468566863 ) ) ;
#180500=CARTESIAN_POINT ( 'NONE',  ( 19.05341960407611168, 5.049401038298154454, 43.95724293864769550 ) ) ;
#180501=CARTESIAN_POINT ( 'NONE',  ( 9.564922557960805705, 16.46253265017160317, 89.58224293864769550 ) ) ;
#180502=CARTESIAN_POINT ( 'NONE',  ( 19.02544592524334988, 5.153800228976608722, 86.45942372801900433 ) ) ;
#180503=CARTESIAN_POINT ( 'NONE',  ( -14.29746914071037622, -8.314922557961029526, 34.16775706135234714 ) ) ;
#180504=CARTESIAN_POINT ( 'NONE',  ( -8.314922557960811034, -14.29746914071050412, 97.08224293864770971 ) ) ;
#180505=CARTESIAN_POINT ( 'NONE',  ( -5.153800228976328057, -19.02544592524343514, 72.29057627198102409 ) ) ;
#180506=CARTESIAN_POINT ( 'NONE',  ( -10.72451020669898014, 18.67979575497178502, 50.41557627198103120 ) ) ;
#180507=CARTESIAN_POINT ( 'NONE',  ( -13.97604488694547697, 13.89961937509957934, 108.1260903946856331 ) ) ;
#180508=CARTESIAN_POINT ( 'NONE',  ( 18.67979575497178502, 10.72451020669898547, 114.1655762719810383 ) ) ;
#180509=CARTESIAN_POINT ( 'NONE',  ( 15.72974639402176855, 15.80617190586768217, 66.87609039468568994 ) ) ;
#180510=CARTESIAN_POINT ( 'NONE',  ( 14.34966873604972726, -8.224510206698740333, 75.83442372801900433 ) ) ;
#180511=CARTESIAN_POINT ( 'NONE',  ( -19.03943276465977164, 0.05219959533909376836, 71.24890960531435269 ) ) ;
#180512=CARTESIAN_POINT ( 'NONE',  ( 0.05219959533934541429, -16.53943276465976808, 100.0010903946857042 ) ) ;
#180513=CARTESIAN_POINT ( 'NONE',  ( -16.51473224551082808, 9.474510206698731452, 38.33442372801899722 ) ) ;
#180514=CARTESIAN_POINT ( 'NONE',  ( -5.719274019375665041, -21.55341960407619695, 29.79275706135234358 ) ) ;
#180515=CARTESIAN_POINT ( 'NONE',  ( 16.52544592524342804, -4.483927247898539470, 73.54057627198102409 ) ) ;
#180516=CARTESIAN_POINT ( 'NONE',  ( 19.03943276465977164, -0.05219959533909143690, 93.74890960531435269 ) ) ;
#180517=CARTESIAN_POINT ( 'NONE',  ( 16.52544592524335698, 4.483927247898782831, 86.45942372801901854 ) ) ;
#180518=CARTESIAN_POINT ( 'NONE',  ( -15.80617190586768217, 15.72974639402176855, 68.12609039468567573 ) ) ;
#180519=CARTESIAN_POINT ( 'NONE',  ( -12.06949235617739369, -12.14591786802326823, 34.37609039468568284 ) ) ;
#180520=CARTESIAN_POINT ( 'NONE',  ( -21.53943276465977519, -0.05219959533937600094, 28.75109039468567929 ) ) ;
#180521=CARTESIAN_POINT ( 'NONE',  ( 0.05219959533910956823, 16.53943276465976808, 69.99890960531435269 ) ) ;
#180522=EDGE_LOOP ( 'NONE', ( #194350, #75524, #184529, #61478 ) ) ;
#180523=CARTESIAN_POINT ( 'NONE',  ( 21.53943276465977519, -0.05219959533907433946, 98.74890960531438111 ) ) ;
#180524=CARTESIAN_POINT ( 'NONE',  ( 12.14591786802309770, 12.06949235617756955, 49.37390960531436690 ) ) ;
#180525=EDGE_LOOP ( 'NONE', ( #53971, #158699, #144336, #106500, #91949, #150169, #305, #147463, #136580, #39166, #180707, #166429, #124535, #163630 ) ) ;
#180526=CARTESIAN_POINT ( 'NONE',  ( -5.153800228976328057, -19.02544592524343514, 27.29057627198103120 ) ) ;
#180527=CARTESIAN_POINT ( 'NONE',  ( 21.55341960407610458, 5.719274019375980345, 28.95724293864769905 ) ) ;
#180528=CARTESIAN_POINT ( 'NONE',  ( 15.80617190586769283, -15.72974639402175789, 35.62609039468568994 ) ) ;
#180529=CARTESIAN_POINT ( 'NONE',  ( 16.53943276465976808, -0.05219959533910856209, 63.74890960531435979 ) ) ;
#180530=CARTESIAN_POINT ( 'NONE',  ( -15.72974639402197994, 15.80617190586746368, 70.62390960531436690 ) ) ;
#180531=CARTESIAN_POINT ( 'NONE',  ( -9.474510206698964154, 16.51473224551069663, 75.41557627198103830 ) ) ;
#180532=CARTESIAN_POINT ( 'NONE',  ( 0.05219959533909260263, 19.03943276465977164, 29.99890960531435979 ) ) ;
#180533=CARTESIAN_POINT ( 'NONE',  ( 9.564922557961047289, -16.46253265017146816, 75.41775706135234714 ) ) ;
#180534=CARTESIAN_POINT ( 'NONE',  ( -15.80617190586745835, -15.72974639402198527, 56.87390960531436690 ) ) ;
#180535=CARTESIAN_POINT ( 'NONE',  ( -19.02544592524342804, 5.153800228976336051, 36.04057627198100988 ) ) ;
#180536=CARTESIAN_POINT ( 'NONE',  ( 19.03943276465977164, -0.05219959533909143690, 73.74890960531435269 ) ) ;
#180538=CARTESIAN_POINT ( 'NONE',  ( 4.379528057220092307, 16.55341960407617563, 32.29275706135235424 ) ) ;
#180539=CARTESIAN_POINT ( 'NONE',  ( -5.823673210054431948, 21.52544592524334988, 27.70942372801901854 ) ) ;
#180540=CARTESIAN_POINT ( 'NONE',  ( 18.67979575497194134, -10.72451020669871369, 60.83442372801901854 ) ) ;
#180541=CARTESIAN_POINT ( 'NONE',  ( 19.05341960407611168, 5.049401038298154454, 108.9572429386477097 ) ) ;
#180542=CARTESIAN_POINT ( 'NONE',  ( -18.67979575497178146, -10.72451020669898902, 71.66557627198100988 ) ) ;
#180543=CARTESIAN_POINT ( 'NONE',  ( -18.62759615963270932, 10.81492255796079327, 105.8322429386476955 ) ) ;
#180544=CARTESIAN_POINT ( 'NONE',  ( -0.05219959533934338120, 16.53943276465976808, 52.50109039468567573 ) ) ;
#180545=CARTESIAN_POINT ( 'NONE',  ( 21.55341960407610458, 5.719274019375980345, 48.95724293864770971 ) ) ;
#180546=CARTESIAN_POINT ( 'NONE',  ( 21.55341960407619695, -5.719274019375665929, 101.0427570613523756 ) ) ;
#180548=CARTESIAN_POINT ( 'NONE',  ( 16.51473224551069308, 9.474510206698969483, 59.16557627198102409 ) ) ;
#180549=CARTESIAN_POINT ( 'NONE',  ( 9.564922557960805705, 16.46253265017160317, 104.5822429386476955 ) ) ;
#180550=CARTESIAN_POINT ( 'NONE',  ( -13.89961937509977652, 13.97604488694528158, 75.62390960531438111 ) ) ;
#180551=CARTESIAN_POINT ( 'NONE',  ( 16.88567814943193568, -6.947325034625396967, 86.20998877347402356 ) ) ;
#180552=CARTESIAN_POINT ( 'NONE',  ( 5.049401038297881783, 19.05341960407617563, 67.29275706135234714 ) ) ;
#180553=CARTESIAN_POINT ( 'NONE',  ( -0.05219959533936034679, 19.03943276465977164, 22.50109039468566152 ) ) ;
#180554=CARTESIAN_POINT ( 'NONE',  ( 21.53943276465977519, -0.05219959533907433946, 43.74890960531435979 ) ) ;
#180555=CARTESIAN_POINT ( 'NONE',  ( -4.379528057220086978, -16.55341960407618274, 104.7927570613523898 ) ) ;
#180556=CARTESIAN_POINT ( 'NONE',  ( 16.51473224551083163, -9.474510206698727899, 85.83442372801900433 ) ) ;
#180558=CARTESIAN_POINT ( 'NONE',  ( -16.46253265017146816, -9.564922557961047289, 24.16775706135233648 ) ) ;
#180559=CARTESIAN_POINT ( 'NONE',  ( 13.89961937509957401, 13.97604488694547697, 86.87609039468567573 ) ) ;
#180560=CARTESIAN_POINT ( 'NONE',  ( 13.97604488694548053, -13.89961937509957401, 45.62609039468566863 ) ) ;
#180561=CARTESIAN_POINT ( 'NONE',  ( 17.50000000000000355, 5.622605283950878885, 108.8120731059611188 ) ) ;
#180562=CARTESIAN_POINT ( 'NONE',  ( 13.89961937509977652, -13.97604488694527269, 38.12390960531436690 ) ) ;
#180563=CARTESIAN_POINT ( 'NONE',  ( 12.06949235617757843, -12.14591786802309237, 48.12390960531436690 ) ) ;
#180564=CARTESIAN_POINT ( 'NONE',  ( 16.51473224551069308, 9.474510206698969483, 34.16557627198102409 ) ) ;
#180565=CARTESIAN_POINT ( 'NONE',  ( 16.52544592524342804, -4.483927247898539470, 38.54057627198103120 ) ) ;
#180567=CARTESIAN_POINT ( 'NONE',  ( 8.224510206698742110, 14.34966873604972548, 107.0844237280190043 ) ) ;
#180568=CARTESIAN_POINT ( 'NONE',  ( 19.05341960407611168, 5.049401038298154454, 43.95724293864769550 ) ) ;
#180569=CARTESIAN_POINT ( 'NONE',  ( 5.153800228976615827, -19.02544592524334988, 25.20942372801900433 ) ) ;
#180570=CARTESIAN_POINT ( 'NONE',  ( 12.14591786802327356, -12.06949235617739191, 35.62609039468568994 ) ) ;
#180571=CARTESIAN_POINT ( 'NONE',  ( 18.67979575497178502, 10.72451020669898547, 44.16557627198103120 ) ) ;
#180572=CARTESIAN_POINT ( 'NONE',  ( 21.55341960407619695, -5.719274019375665929, 91.04275706135236135 ) ) ;
#180574=CARTESIAN_POINT ( 'NONE',  ( -9.474510206698964154, 16.51473224551069663, 105.4155762719810383 ) ) ;
#180575=CARTESIAN_POINT ( 'NONE',  ( -9.474510206698964154, 16.51473224551069663, 90.41557627198103830 ) ) ;
#180577=CARTESIAN_POINT ( 'NONE',  ( -18.67979575497178146, -10.72451020669898902, 106.6655762719810383 ) ) ;
#180578=CARTESIAN_POINT ( 'NONE',  ( 4.483927247898545687, 16.52544592524342804, 84.79057627198102409 ) ) ;
#180579=CARTESIAN_POINT ( 'NONE',  ( -15.80617190586745835, -15.72974639402198527, 71.87390960531438111 ) ) ;
#180580=CARTESIAN_POINT ( 'NONE',  ( 16.46253265017160672, -9.564922557960803928, 73.33224293864769550 ) ) ;
#180581=CARTESIAN_POINT ( 'NONE',  ( -19.03943276465977164, 0.05219959533909376836, 71.24890960531435269 ) ) ;
#180582=CARTESIAN_POINT ( 'NONE',  ( 5.823673210054125526, 21.52544592524343514, 94.79057627198105251 ) ) ;
#180584=CARTESIAN_POINT ( 'NONE',  ( -13.89961937509977652, 13.97604488694528158, 55.62390960531434558 ) ) ;
#180585=CARTESIAN_POINT ( 'NONE',  ( -12.14591786802309592, -12.06949235617757132, 96.87390960531436690 ) ) ;
#180587=CARTESIAN_POINT ( 'NONE',  ( 5.049401038298161559, -19.05341960407611168, 57.70724293864769550 ) ) ;
#180588=CARTESIAN_POINT ( 'NONE',  ( 16.46253265017146816, 9.564922557961045513, 76.66775706135234714 ) ) ;
#180589=CARTESIAN_POINT ( 'NONE',  ( 4.379528057220339221, -16.55341960407611168, 92.70724293864770971 ) ) ;
#180590=CARTESIAN_POINT ( 'NONE',  ( 5.719274019375673035, 21.55341960407619339, 57.29275706135234714 ) ) ;
#180591=CARTESIAN_POINT ( 'NONE',  ( 0.05219959533909260263, 19.03943276465977164, 44.99890960531435979 ) ) ;
#180592=CARTESIAN_POINT ( 'NONE',  ( 21.53943276465977519, 0.05219959533937863772, 21.25109039468567218 ) ) ;
#180593=CARTESIAN_POINT ( 'NONE',  ( -16.53943276465976808, 0.05219959533911058130, 101.2489096053143669 ) ) ;
#180595=CARTESIAN_POINT ( 'NONE',  ( -0.05219959533909027116, -19.03943276465977164, 72.49890960531435269 ) ) ;
#180596=CARTESIAN_POINT ( 'NONE',  ( 16.19135201231367560, 7.376712067591920885, 112.6868085405202748 ) ) ;
#180597=CARTESIAN_POINT ( 'NONE',  ( -16.52544592524335698, -4.483927247898792601, 18.95942372801901143 ) ) ;
#180598=CARTESIAN_POINT ( 'NONE',  ( 21.52544592524344225, -5.823673210054117533, 23.54057627198102765 ) ) ;
#180599=CARTESIAN_POINT ( 'NONE',  ( -10.72451020669870658, -18.67979575497194134, 49.58442372801901143 ) ) ;
#180600=CARTESIAN_POINT ( 'NONE',  ( 13.89961937509977652, -13.97604488694527269, 93.12390960531436690 ) ) ;
#180601=CARTESIAN_POINT ( 'NONE',  ( -0.05219959533936034679, 19.03943276465977164, 87.50109039468567573 ) ) ;
#180602=CARTESIAN_POINT ( 'NONE',  ( -19.02544592524342804, 5.153800228976336051, 76.04057627198102409 ) ) ;
#180604=CARTESIAN_POINT ( 'NONE',  ( 16.55341960407611168, 4.379528057220329451, 78.95724293864769550 ) ) ;
#180605=CARTESIAN_POINT ( 'NONE',  ( -16.46253265017160317, 9.564922557960807481, 105.8322429386476955 ) ) ;
#180606=CARTESIAN_POINT ( 'NONE',  ( -16.52544592524342804, 4.483927247898546575, 81.04057627198102409 ) ) ;
#180607=CARTESIAN_POINT ( 'NONE',  ( -5.049401038298153566, 19.05341960407611168, 100.2072429386476955 ) ) ;
#180608=CARTESIAN_POINT ( 'NONE',  ( 19.05341960407617918, -5.049401038297876454, 46.04275706135233293 ) ) ;
#180609=CARTESIAN_POINT ( 'NONE',  ( 5.153800228976335163, 19.02544592524342804, 44.79057627198103830 ) ) ;
#180610=CARTESIAN_POINT ( 'NONE',  ( 12.06949235617757843, -12.14591786802309237, 48.12390960531436690 ) ) ;
#180611=CARTESIAN_POINT ( 'NONE',  ( 9.564922557960805705, 16.46253265017160317, 34.58224293864770260 ) ) ;
#180613=CARTESIAN_POINT ( 'NONE',  ( -5.719274019375665041, -21.55341960407619695, 49.79275706135234714 ) ) ;
#180614=CARTESIAN_POINT ( 'NONE',  ( 5.153800228976615827, -19.02544592524334988, 85.20942372801900433 ) ) ;
#180615=CARTESIAN_POINT ( 'NONE',  ( -14.29746914071049879, 8.314922557960819915, 35.83224293864768839 ) ) ;
#180616=CARTESIAN_POINT ( 'NONE',  ( 0.05219959533907565091, 21.53943276465977519, 94.99890960531436690 ) ) ;
#180617=CARTESIAN_POINT ( 'NONE',  ( 10.81492255796078972, 18.62759615963270932, 39.58224293864769550 ) ) ;
#180618=CARTESIAN_POINT ( 'NONE',  ( -8.314922557960811034, -14.29746914071050412, 82.08224293864768129 ) ) ;
#180619=CARTESIAN_POINT ( 'NONE',  ( -19.05341960407611168, -5.049401038298163336, 46.45724293864768129 ) ) ;
#180620=CARTESIAN_POINT ( 'NONE',  ( -8.224510206698735004, -14.34966873604973081, 99.58442372801900433 ) ) ;
#180621=CARTESIAN_POINT ( 'NONE',  ( 16.55341960407618274, -4.379528057220086978, 91.04275706135236135 ) ) ;
#180622=CARTESIAN_POINT ( 'NONE',  ( 12.14591786802327356, -12.06949235617739191, 70.62609039468567573 ) ) ;
#180623=CARTESIAN_POINT ( 'NONE',  ( 16.46253265017146816, 9.564922557961045513, 26.66775706135234003 ) ) ;
#180624=CARTESIAN_POINT ( 'NONE',  ( 9.564922557960805705, 16.46253265017160317, 94.58224293864769550 ) ) ;
#180625=CARTESIAN_POINT ( 'NONE',  ( 16.51473224551069308, 9.474510206698969483, 74.16557627198103830 ) ) ;
#180626=CARTESIAN_POINT ( 'NONE',  ( 12.14591786802327356, -12.06949235617739191, 75.62609039468567573 ) ) ;
#180627=CARTESIAN_POINT ( 'NONE',  ( 16.46253265017160672, -9.564922557960803928, 33.33224293864770260 ) ) ;
#180628=CARTESIAN_POINT ( 'NONE',  ( -0.05219959533910754901, -16.53943276465976808, 47.49890960531435979 ) ) ;
#180630=CARTESIAN_POINT ( 'NONE',  ( -19.03943276465977164, 0.05219959533909376836, 86.24890960531436690 ) ) ;
#180631=CARTESIAN_POINT ( 'NONE',  ( 10.81492255796078972, 18.62759615963270932, 24.58224293864768839 ) ) ;
#180632=CARTESIAN_POINT ( 'NONE',  ( 12.06949235617757843, -12.14591786802309237, 73.12390960531436690 ) ) ;
#180633=CARTESIAN_POINT ( 'NONE',  ( -4.379528057220328563, 16.55341960407611168, 60.20724293864768839 ) ) ;
#180634=CARTESIAN_POINT ( 'NONE',  ( 4.379528057220092307, 16.55341960407617563, 47.29275706135234003 ) ) ;
#180635=CARTESIAN_POINT ( 'NONE',  ( 17.50000000000001776, -4.640572885337594045, 33.13788164548843440 ) ) ;
#180636=CARTESIAN_POINT ( 'NONE',  ( -13.97604488694547697, 13.89961937509957934, 68.12609039468563310 ) ) ;
#180637=CARTESIAN_POINT ( 'NONE',  ( -13.97604488694527625, -13.89961937509977652, 86.87390960531436690 ) ) ;
#180638=CARTESIAN_POINT ( 'NONE',  ( 13.89961937509957401, 13.97604488694547697, 66.87609039468567573 ) ) ;
#180640=CARTESIAN_POINT ( 'NONE',  ( 16.53943276465976808, 0.05219959533934440121, 21.25109039468567218 ) ) ;
#180641=CARTESIAN_POINT ( 'NONE',  ( 14.34966873604972726, -8.224510206698740333, 95.83442372801903275 ) ) ;
#180642=CARTESIAN_POINT ( 'NONE',  ( 19.05341960407611168, 5.049401038298154454, 43.95724293864769550 ) ) ;
#180643=CARTESIAN_POINT ( 'NONE',  ( -0.05219959533907301413, -21.53943276465977519, 27.49890960531435269 ) ) ;
#180644=CARTESIAN_POINT ( 'NONE',  ( 21.55341960407619695, -5.719274019375665929, 51.04275706135234714 ) ) ;
#180645=CARTESIAN_POINT ( 'NONE',  ( 9.474510206698729675, 16.51473224551082808, 112.0844237280190043 ) ) ;
#180646=CARTESIAN_POINT ( 'NONE',  ( -16.46253265017146816, -9.564922557961047289, 54.16775706135234003 ) ) ;
#180647=CARTESIAN_POINT ( 'NONE',  ( 13.97604488694527802, 13.89961937509977652, 79.37390960531435269 ) ) ;
#180648=CARTESIAN_POINT ( 'NONE',  ( -17.50000000000000000, 5.499999999999992895, 23.71769037696436300 ) ) ;
#180649=CARTESIAN_POINT ( 'NONE',  ( 16.55341960407611168, 4.379528057220329451, 78.95724293864769550 ) ) ;
#180650=CARTESIAN_POINT ( 'NONE',  ( 16.46253265017160672, -9.564922557960803928, 73.33224293864769550 ) ) ;
#180651=CARTESIAN_POINT ( 'NONE',  ( 5.153800228976335163, 19.02544592524342804, 69.79057627198103830 ) ) ;
#180652=CARTESIAN_POINT ( 'NONE',  ( -19.02544592524334988, -5.153800228976617603, 88.95942372801897591 ) ) ;
#180653=CARTESIAN_POINT ( 'NONE',  ( 21.53943276465977519, -0.05219959533907433946, 68.74890960531435269 ) ) ;
#180654=CARTESIAN_POINT ( 'NONE',  ( 13.89961937509977652, -13.97604488694527269, 28.12390960531435624 ) ) ;
#180655=CARTESIAN_POINT ( 'NONE',  ( 19.02544592524334988, 5.153800228976608722, 56.45942372801898301 ) ) ;
#180656=CARTESIAN_POINT ( 'NONE',  ( 9.474510206698971260, -16.51473224551069308, 62.91557627198102409 ) ) ;
#180657=CARTESIAN_POINT ( 'NONE',  ( 19.02544592524343514, -5.153800228976328945, 98.54057627198100988 ) ) ;
#180659=CARTESIAN_POINT ( 'NONE',  ( -10.81492255796078084, -18.62759615963271287, 87.08224293864769550 ) ) ;
#180660=CARTESIAN_POINT ( 'NONE',  ( 12.14591786802309770, 12.06949235617756955, 94.37390960531436690 ) ) ;
#180661=CARTESIAN_POINT ( 'NONE',  ( -19.02544592524334988, -5.153800228976617603, 48.95942372801900433 ) ) ;
#180662=CARTESIAN_POINT ( 'NONE',  ( -5.719274019375978568, 21.55341960407610458, 70.20724293864769550 ) ) ;
#180663=CARTESIAN_POINT ( 'NONE',  ( -15.72974639402197994, 15.80617190586746368, 75.62390960531439532 ) ) ;
#180664=CARTESIAN_POINT ( 'NONE',  ( -14.34966873604960291, -8.224510206698953496, 36.66557627198103120 ) ) ;
#180665=CARTESIAN_POINT ( 'NONE',  ( -15.80617190586768217, 15.72974639402176855, 103.1260903946856757 ) ) ;
#180666=CARTESIAN_POINT ( 'NONE',  ( 0.05219959533909260263, 19.03943276465977164, 74.99890960531435269 ) ) ;
#180667=CARTESIAN_POINT ( 'NONE',  ( -16.46253265017160317, 9.564922557960807481, 30.83224293864769550 ) ) ;
#180668=CARTESIAN_POINT ( 'NONE',  ( 15.72974639402176855, 15.80617190586768217, 41.87609039468568284 ) ) ;
#180669=CARTESIAN_POINT ( 'NONE',  ( -21.53943276465977519, -0.05219959533937600094, 58.75109039468568994 ) ) ;
#180670=CARTESIAN_POINT ( 'NONE',  ( -13.97604488694527625, -13.89961937509977652, 51.87390960531436690 ) ) ;
#180671=CARTESIAN_POINT ( 'NONE',  ( -5.719274019375665041, -21.55341960407619695, 24.79275706135235779 ) ) ;
#180673=CARTESIAN_POINT ( 'NONE',  ( -13.89961937509957401, -13.97604488694547875, 59.37609039468566863 ) ) ;
#180674=CARTESIAN_POINT ( 'NONE',  ( 19.03943276465977164, -0.05219959533909143690, 33.74890960531435979 ) ) ;
#180675=CARTESIAN_POINT ( 'NONE',  ( 8.224510206698742110, 14.34966873604972548, 22.08442372801901143 ) ) ;
#180676=CARTESIAN_POINT ( 'NONE',  ( -13.97604488694527625, -13.89961937509977652, 21.87390960531435979 ) ) ;
#180677=CARTESIAN_POINT ( 'NONE',  ( 0.05219959533934541429, -16.53943276465976808, 80.00109039468568994 ) ) ;
#180678=CARTESIAN_POINT ( 'NONE',  ( 13.97604488694527802, 13.89961937509977652, 34.37390960531436690 ) ) ;
#180680=CARTESIAN_POINT ( 'NONE',  ( -19.05341960407611168, -5.049401038298163336, 91.45724293864766707 ) ) ;
#180681=CARTESIAN_POINT ( 'NONE',  ( 19.03943276465977164, -0.05219959533909143690, 23.74890960531435269 ) ) ;
#180682=CARTESIAN_POINT ( 'NONE',  ( 10.72451020669898902, -18.67979575497178502, 72.91557627198103830 ) ) ;
#180683=CARTESIAN_POINT ( 'NONE',  ( 8.224510206698742110, 14.34966873604972548, 52.08442372801901854 ) ) ;
#180684=CARTESIAN_POINT ( 'NONE',  ( -9.474510206698720793, -16.51473224551083518, 24.58442372801900078 ) ) ;
#180685=CARTESIAN_POINT ( 'NONE',  ( 9.564922557960805705, 16.46253265017160317, 39.58224293864768839 ) ) ;
#180686=CARTESIAN_POINT ( 'NONE',  ( -0.05219959533910754901, -16.53943276465976808, 37.49890960531436690 ) ) ;
#180687=CARTESIAN_POINT ( 'NONE',  ( 14.29746914071049879, -8.314922557960816363, 73.33224293864769550 ) ) ;
#180688=CARTESIAN_POINT ( 'NONE',  ( 13.97604488694527802, 13.89961937509977652, 59.37390960531434558 ) ) ;
#180689=CARTESIAN_POINT ( 'NONE',  ( 10.81492255796106328, -18.62759615963255655, 105.4177570613523613 ) ) ;
#180690=CARTESIAN_POINT ( 'NONE',  ( 5.823673210054125526, 21.52544592524343514, 114.7905762719810383 ) ) ;
#180691=CARTESIAN_POINT ( 'NONE',  ( 16.46253265017160672, -9.564922557960803928, 73.33224293864769550 ) ) ;
#180692=CARTESIAN_POINT ( 'NONE',  ( -18.62759615963255300, -10.81492255796106328, 89.16775706135236135 ) ) ;
#180693=CARTESIAN_POINT ( 'NONE',  ( -4.483927247898782831, 16.52544592524335698, 72.70942372801901854 ) ) ;
#180694=CARTESIAN_POINT ( 'NONE',  ( -4.379528057220086978, -16.55341960407618274, 29.79275706135234358 ) ) ;
#180695=CARTESIAN_POINT ( 'NONE',  ( 4.483927247898545687, 16.52544592524342804, 94.79057627198105251 ) ) ;
#180696=CARTESIAN_POINT ( 'NONE',  ( 5.153800228976335163, 19.02544592524342804, 109.7905762719810099 ) ) ;
#180697=CARTESIAN_POINT ( 'NONE',  ( -0.05219959533910754901, -16.53943276465976808, 27.49890960531435269 ) ) ;
#180698=CARTESIAN_POINT ( 'NONE',  ( 19.02544592524343514, -5.153800228976328945, 23.54057627198102054 ) ) ;
#180699=CARTESIAN_POINT ( 'NONE',  ( -14.34966873604972548, 8.224510206698743886, 58.33442372801901143 ) ) ;
#180700=CARTESIAN_POINT ( 'NONE',  ( 16.55341960407611168, 4.379528057220329451, 48.95724293864770971 ) ) ;
#180701=CARTESIAN_POINT ( 'NONE',  ( 14.34966873604972726, -8.224510206698740333, 105.8344237280190328 ) ) ;
#180702=CARTESIAN_POINT ( 'NONE',  ( -5.049401038298153566, 19.05341960407611168, 110.2072429386476671 ) ) ;
#180703=CARTESIAN_POINT ( 'NONE',  ( 5.719274019375991003, -21.55341960407610458, 27.70724293864769905 ) ) ;
#180704=CARTESIAN_POINT ( 'NONE',  ( 18.67979575497194134, -10.72451020669871369, 105.8344237280190328 ) ) ;
#180705=CARTESIAN_POINT ( 'NONE',  ( 16.52544592524342804, -4.483927247898539470, 83.54057627198102409 ) ) ;
#180706=CARTESIAN_POINT ( 'NONE',  ( 16.51473224551069308, 9.474510206698969483, 89.16557627198103830 ) ) ;
#180707=ORIENTED_EDGE ( 'NONE', *, *, #31222, .T. ) ;
#180708=CARTESIAN_POINT ( 'NONE',  ( -16.53943276465976808, -0.05219959533934237506, 43.75109039468568284 ) ) ;
#180709=CARTESIAN_POINT ( 'NONE',  ( -19.02544592524342804, 5.153800228976336051, 41.04057627198103120 ) ) ;
#180710=CARTESIAN_POINT ( 'NONE',  ( -4.379528057220086978, -16.55341960407618274, 39.79275706135235424 ) ) ;
#180712=CARTESIAN_POINT ( 'NONE',  ( 9.474510206698729675, 16.51473224551082808, 47.08442372801900433 ) ) ;
#180713=CARTESIAN_POINT ( 'NONE',  ( -9.474510206698964154, 16.51473224551069663, 50.41557627198102409 ) ) ;
#180714=CARTESIAN_POINT ( 'NONE',  ( -8.314922557961024197, 14.29746914071037800, 77.91775706135231871 ) ) ;
#180715=CARTESIAN_POINT ( 'NONE',  ( 0.05219959533936267826, -19.03943276465977164, 90.00109039468567573 ) ) ;
#180716=CARTESIAN_POINT ( 'NONE',  ( -13.89961937509977652, 13.97604488694528158, 65.62390960531436690 ) ) ;
#180717=CARTESIAN_POINT ( 'NONE',  ( -12.06949235617756955, 12.14591786802309770, 105.6239096053143669 ) ) ;
#180719=CARTESIAN_POINT ( 'NONE',  ( 19.02544592524334988, 5.153800228976608722, 66.45942372801899012 ) ) ;
#180720=CARTESIAN_POINT ( 'NONE',  ( -10.72451020669898014, 18.67979575497178502, 70.41557627198102409 ) ) ;
#180721=CARTESIAN_POINT ( 'NONE',  ( -19.02544592524334988, -5.153800228976617603, 38.95942372801900433 ) ) ;
#180722=CARTESIAN_POINT ( 'NONE',  ( 18.56101223717332971, 5.500000000000004441, 98.94978406935679516 ) ) ;
#180723=CARTESIAN_POINT ( 'NONE',  ( -0.05219959533907301413, -21.53943276465977519, 87.49890960531436690 ) ) ;
#180725=CARTESIAN_POINT ( 'NONE',  ( -13.89961937509957401, -13.97604488694547875, 99.37609039468567573 ) ) ;
#180726=CARTESIAN_POINT ( 'NONE',  ( -18.56453257813359770, 5.500000000000041744, 60.99000423690687711 ) ) ;
#180727=CARTESIAN_POINT ( 'NONE',  ( 0.05219959533934541429, -16.53943276465976808, 30.00109039468568284 ) ) ;
#180728=CARTESIAN_POINT ( 'NONE',  ( -5.153800228976328057, -19.02544592524343514, 47.29057627198102409 ) ) ;
#180729=CARTESIAN_POINT ( 'NONE',  ( -13.97604488694527625, -13.89961937509977652, 111.8739096053143243 ) ) ;
#180730=CARTESIAN_POINT ( 'NONE',  ( -10.72451020669898014, 18.67979575497178502, 95.41557627198102409 ) ) ;
#180731=CARTESIAN_POINT ( 'NONE',  ( 10.72451020669871369, 18.67979575497193778, 57.08442372801901854 ) ) ;
#180732=CARTESIAN_POINT ( 'NONE',  ( -9.564922557961040184, 16.46253265017147172, 102.9177570613523329 ) ) ;
#180733=CARTESIAN_POINT ( 'NONE',  ( 9.474510206698729675, 16.51473224551082808, 22.08442372801899722 ) ) ;
#180734=CARTESIAN_POINT ( 'NONE',  ( -4.483927247898539470, -16.52544592524342804, 32.29057627198102409 ) ) ;
#180735=CARTESIAN_POINT ( 'NONE',  ( -18.62759615963270932, 10.81492255796079327, 95.83224293864770971 ) ) ;
#180736=CARTESIAN_POINT ( 'NONE',  ( 12.06949235617757843, -12.14591786802309237, 48.12390960531436690 ) ) ;
#180737=CARTESIAN_POINT ( 'NONE',  ( 13.97604488694548053, -13.89961937509957401, 90.62609039468567573 ) ) ;
#180738=CARTESIAN_POINT ( 'NONE',  ( 16.46253265017146816, 9.564922557961045513, 56.66775706135233293 ) ) ;
#180739=CARTESIAN_POINT ( 'NONE',  ( 21.55341960407619695, -5.719274019375665929, 71.04275706135234714 ) ) ;
#180740=CARTESIAN_POINT ( 'NONE',  ( 5.049401038297881783, 19.05341960407617563, 42.29275706135234003 ) ) ;
#180741=CARTESIAN_POINT ( 'NONE',  ( 8.314922557960818139, 14.29746914071049879, 114.5822429386477097 ) ) ;
#180742=CARTESIAN_POINT ( 'NONE',  ( -18.62759615963270932, 10.81492255796079327, 50.83224293864770971 ) ) ;
#180743=CARTESIAN_POINT ( 'NONE',  ( -16.55341960407611168, -4.379528057220339221, 41.45724293864769550 ) ) ;
#180744=CARTESIAN_POINT ( 'NONE',  ( 5.719274019375673035, 21.55341960407619339, 107.2927570613523471 ) ) ;
#180745=CARTESIAN_POINT ( 'NONE',  ( -8.224510206698735004, -14.34966873604973081, 69.58442372801900433 ) ) ;
#180746=CARTESIAN_POINT ( 'NONE',  ( -16.52544592524342804, 4.483927247898546575, 36.04057627198102409 ) ) ;
#180747=CARTESIAN_POINT ( 'NONE',  ( 21.53943276465977519, 0.05219959533937863772, 71.25109039468568994 ) ) ;
#180748=CARTESIAN_POINT ( 'NONE',  ( -5.823673210054431948, 21.52544592524334988, 67.70942372801901854 ) ) ;
#180749=CARTESIAN_POINT ( 'NONE',  ( -5.823673210054116645, -21.52544592524344225, 72.29057627198102409 ) ) ;
#180750=CARTESIAN_POINT ( 'NONE',  ( 19.05341960407611168, 5.049401038298154454, 33.95724293864769550 ) ) ;
#180751=CARTESIAN_POINT ( 'NONE',  ( -10.81492255796105439, 18.62759615963255655, 37.91775706135235424 ) ) ;
#180752=CARTESIAN_POINT ( 'NONE',  ( 16.53943276465976808, -0.05219959533910856209, 113.7489096053143527 ) ) ;
#180753=CARTESIAN_POINT ( 'NONE',  ( 19.03943276465977164, -0.05219959533909143690, 38.74890960531436690 ) ) ;
#180754=CARTESIAN_POINT ( 'NONE',  ( -16.53943276465976808, 0.05219959533911058130, 96.24890960531435269 ) ) ;
#180755=CARTESIAN_POINT ( 'NONE',  ( -13.89961937509977652, 13.97604488694528158, 90.62390960531432427 ) ) ;
#180756=CARTESIAN_POINT ( 'NONE',  ( 0.05219959533910956823, 16.53943276465976808, 44.99890960531435979 ) ) ;
#180757=CARTESIAN_POINT ( 'NONE',  ( 12.14591786802309770, 12.06949235617756955, 94.37390960531436690 ) ) ;
#180758=CARTESIAN_POINT ( 'NONE',  ( 5.823673210054125526, 21.52544592524343514, 69.79057627198102409 ) ) ;
#180759=CARTESIAN_POINT ( 'NONE',  ( -21.55341960407610458, -5.719274019375992779, 101.4572429386476955 ) ) ;
#180760=CARTESIAN_POINT ( 'NONE',  ( 13.97604488694527802, 13.89961937509977652, 109.3739096053143669 ) ) ;
#180761=CARTESIAN_POINT ( 'NONE',  ( 13.89961937509977652, -13.97604488694527269, 63.12390960531435979 ) ) ;
#180762=CARTESIAN_POINT ( 'NONE',  ( -8.314922557961024197, 14.29746914071037800, 27.91775706135234358 ) ) ;
#180763=CARTESIAN_POINT ( 'NONE',  ( 18.62759615963271287, -10.81492255796078972, 58.33224293864768839 ) ) ;
#180764=CARTESIAN_POINT ( 'NONE',  ( -10.72451020669870658, -18.67979575497194134, 89.58442372801901854 ) ) ;
#180765=CARTESIAN_POINT ( 'NONE',  ( 5.153800228976335163, 19.02544592524342804, 79.79057627198102409 ) ) ;
#180766=CARTESIAN_POINT ( 'NONE',  ( 15.80617190586746368, 15.72974639402197994, 114.3739096053143527 ) ) ;
#180768=CARTESIAN_POINT ( 'NONE',  ( 16.51473224551069308, 9.474510206698969483, 109.1655762719810383 ) ) ;
#180769=CARTESIAN_POINT ( 'NONE',  ( 14.29746914071037800, 8.314922557961029526, 91.66775706135234714 ) ) ;
#180770=CARTESIAN_POINT ( 'NONE',  ( 5.719274019375673035, 21.55341960407619339, 72.29275706135236135 ) ) ;
#180771=CARTESIAN_POINT ( 'NONE',  ( 21.53943276465977519, 0.05219959533937863772, 96.25109039468568994 ) ) ;
#180772=CARTESIAN_POINT ( 'NONE',  ( 16.55341960407618274, -4.379528057220086978, 56.04275706135235424 ) ) ;
#180773=CARTESIAN_POINT ( 'NONE',  ( -10.72451020669870658, -18.67979575497194134, 19.58442372801901143 ) ) ;
#180774=CARTESIAN_POINT ( 'NONE',  ( -9.474510206698964154, 16.51473224551069663, 25.41557627198103120 ) ) ;
#180775=CARTESIAN_POINT ( 'NONE',  ( 15.72974639402176855, 15.80617190586768217, 91.87609039468568994 ) ) ;
#180776=CARTESIAN_POINT ( 'NONE',  ( -5.823673210054116645, -21.52544592524344225, 92.29057627198103830 ) ) ;
#180777=CARTESIAN_POINT ( 'NONE',  ( -9.474510206698720793, -16.51473224551083518, 49.58442372801899722 ) ) ;
#180778=CARTESIAN_POINT ( 'NONE',  ( 15.80617190586746368, 15.72974639402197994, 54.37390960531435979 ) ) ;
#180779=CARTESIAN_POINT ( 'NONE',  ( 19.05341960407611168, 5.049401038298154454, 98.95724293864766707 ) ) ;
#180780=CARTESIAN_POINT ( 'NONE',  ( 8.224510206698953496, -14.34966873604960469, 42.91557627198103120 ) ) ;
#180783=CARTESIAN_POINT ( 'NONE',  ( -5.153800228976607833, 19.02544592524334988, 102.7094237280189759 ) ) ;
#180784=CARTESIAN_POINT ( 'NONE',  ( -21.53943276465977519, 0.05219959533907696930, 86.24890960531436690 ) ) ;
#180785=CARTESIAN_POINT ( 'NONE',  ( 0.05219959533910956823, 16.53943276465976808, 49.99890960531437401 ) ) ;
#180786=CARTESIAN_POINT ( 'NONE',  ( 8.224510206698742110, 14.34966873604972548, 27.08442372801901854 ) ) ;
#180787=CARTESIAN_POINT ( 'NONE',  ( 13.97604488694527802, 13.89961937509977652, 39.37390960531435269 ) ) ;
#180788=CARTESIAN_POINT ( 'NONE',  ( 18.67979575497178502, 10.72451020669898547, 114.1655762719810383 ) ) ;
#180789=CARTESIAN_POINT ( 'NONE',  ( 19.02544592524334988, 5.153800228976608722, 86.45942372801900433 ) ) ;
#180790=CARTESIAN_POINT ( 'NONE',  ( -5.049401038298153566, 19.05341960407611168, 85.20724293864766707 ) ) ;
#180791=CARTESIAN_POINT ( 'NONE',  ( -19.03943276465977164, 0.05219959533909376836, 76.24890960531435269 ) ) ;
#180792=CARTESIAN_POINT ( 'NONE',  ( -15.80617190586745835, -15.72974639402198527, 76.87390960531439532 ) ) ;
#180793=CARTESIAN_POINT ( 'NONE',  ( 0.05219959533909260263, 19.03943276465977164, 44.99890960531435979 ) ) ;
#180795=CARTESIAN_POINT ( 'NONE',  ( 16.53943276465976808, -0.05219959533910856209, 58.74890960531436690 ) ) ;
#180796=CARTESIAN_POINT ( 'NONE',  ( -9.564922557960796823, -16.46253265017161027, 87.08224293864769550 ) ) ;
#180798=CARTESIAN_POINT ( 'NONE',  ( 19.03943276465977164, 0.05219959533936151252, 61.25109039468566863 ) ) ;
#180799=CARTESIAN_POINT ( 'NONE',  ( 10.81492255796078972, 18.62759615963270932, 79.58224293864769550 ) ) ;
#180800=CARTESIAN_POINT ( 'NONE',  ( 19.02544592524334988, 5.153800228976608722, 31.45942372801900433 ) ) ;
#180801=CARTESIAN_POINT ( 'NONE',  ( -13.97604488694527625, -13.89961937509977652, 96.87390960531433848 ) ) ;
#180802=CARTESIAN_POINT ( 'NONE',  ( -17.50000000000000000, 3.345213924137367734, 114.5876862309434898 ) ) ;
#180803=CARTESIAN_POINT ( 'NONE',  ( -15.72974639402197994, 15.80617190586746368, 35.62390960531437401 ) ) ;
#180804=CARTESIAN_POINT ( 'NONE',  ( -16.46253265017160317, 9.564922557960807481, 75.83224293864769550 ) ) ;
#180805=CARTESIAN_POINT ( 'NONE',  ( -15.72974639402176322, -15.80617190586768395, 69.37609039468567573 ) ) ;
#180806=CARTESIAN_POINT ( 'NONE',  ( -19.02544592524342804, 5.153800228976336051, 31.04057627198102409 ) ) ;
#180807=CARTESIAN_POINT ( 'NONE',  ( 21.55341960407619695, -5.719274019375665929, 21.04275706135234714 ) ) ;
#180809=CARTESIAN_POINT ( 'NONE',  ( 21.53943276465977519, 0.05219959533937863772, 51.25109039468568994 ) ) ;
#180811=CARTESIAN_POINT ( 'NONE',  ( -9.474510206698964154, 16.51473224551069663, 100.4155762719810241 ) ) ;
#180812=CARTESIAN_POINT ( 'NONE',  ( -18.22780087662122028, 5.500000000000031086, 88.51540105326107266 ) ) ;
#180813=CARTESIAN_POINT ( 'NONE',  ( -0.05219959533907301413, -21.53943276465977519, 102.4989096053143811 ) ) ;
#180814=CARTESIAN_POINT ( 'NONE',  ( -13.97604488694527625, -13.89961937509977652, 56.87390960531434558 ) ) ;
#180815=CARTESIAN_POINT ( 'NONE',  ( 0.05219959533934541429, -16.53943276465976808, 40.00109039468567573 ) ) ;
#180817=CARTESIAN_POINT ( 'NONE',  ( 21.53943276465977519, 0.05219959533937863772, 106.2510903946856757 ) ) ;
#180818=CARTESIAN_POINT ( 'NONE',  ( 0.05219959533909260263, 19.03943276465977164, 44.99890960531435979 ) ) ;
#180819=CARTESIAN_POINT ( 'NONE',  ( 18.62759615963255655, 10.81492255796105972, 101.6677570613523613 ) ) ;
#180820=CARTESIAN_POINT ( 'NONE',  ( 16.46253265017160672, -9.564922557960803928, 93.33224293864769550 ) ) ;
#180821=CARTESIAN_POINT ( 'NONE',  ( 21.53943276465977519, 0.05219959533937863772, 66.25109039468567573 ) ) ;
#180824=CARTESIAN_POINT ( 'NONE',  ( 19.02544592524343514, -5.153800228976328945, 108.5405762719810383 ) ) ;
#180826=CARTESIAN_POINT ( 'NONE',  ( -14.34966873604972548, 8.224510206698743886, 58.33442372801901143 ) ) ;
#180827=CARTESIAN_POINT ( 'NONE',  ( -15.72974639402176322, -15.80617190586768395, 64.37609039468568994 ) ) ;
#180828=CARTESIAN_POINT ( 'NONE',  ( 5.823673210054444382, -21.52544592524334988, 95.20942372801903275 ) ) ;
#180831=CARTESIAN_POINT ( 'NONE',  ( -0.05219959533934338120, 16.53943276465976808, 22.50109039468567573 ) ) ;
#180832=CARTESIAN_POINT ( 'NONE',  ( 5.049401038298161559, -19.05341960407611168, 67.70724293864769550 ) ) ;
#180833=CARTESIAN_POINT ( 'NONE',  ( -16.51473224551069308, -9.474510206698971260, 106.6655762719810383 ) ) ;
#180834=CARTESIAN_POINT ( 'NONE',  ( 16.36317988757058828, 7.306389748694951614, 43.40210391636777132 ) ) ;
#180835=CARTESIAN_POINT ( 'NONE',  ( -9.474510206698964154, 16.51473224551069663, 25.41557627198103120 ) ) ;
#180836=CARTESIAN_POINT ( 'NONE',  ( -21.53943276465977519, 0.05219959533907696930, 41.24890960531435269 ) ) ;
#180837=CARTESIAN_POINT ( 'NONE',  ( -12.06949235617739369, -12.14591786802326823, 99.37609039468568994 ) ) ;
#180838=CARTESIAN_POINT ( 'NONE',  ( 12.14591786802309770, 12.06949235617756955, 79.37390960531436690 ) ) ;
#180839=CARTESIAN_POINT ( 'NONE',  ( 5.049401038298161559, -19.05341960407611168, 62.70724293864769550 ) ) ;
#180840=CARTESIAN_POINT ( 'NONE',  ( 0.05219959533937995610, -21.53943276465977519, 95.00109039468568994 ) ) ;
#180842=CARTESIAN_POINT ( 'NONE',  ( -12.14591786802326823, 12.06949235617739902, 28.12609039468568284 ) ) ;
#180843=CARTESIAN_POINT ( 'NONE',  ( 16.53943276465976808, -0.05219959533910856209, 93.74890960531436690 ) ) ;
#180844=CARTESIAN_POINT ( 'NONE',  ( 21.52544592524334988, 5.823673210054432836, 46.45942372801901854 ) ) ;
#180845=CARTESIAN_POINT ( 'NONE',  ( -10.72451020669898014, 18.67979575497178502, 70.41557627198102409 ) ) ;
#180846=CARTESIAN_POINT ( 'NONE',  ( 19.02544592524334988, 5.153800228976608722, 36.45942372801900433 ) ) ;
#180848=CARTESIAN_POINT ( 'NONE',  ( 13.89961937509977652, -13.97604488694527269, 78.12390960531433848 ) ) ;
#180849=CARTESIAN_POINT ( 'NONE',  ( 0.05219959533910956823, 16.53943276465976808, 64.99890960531435269 ) ) ;
#180851=CARTESIAN_POINT ( 'NONE',  ( -14.29746914071049879, 8.314922557960819915, 30.83224293864770260 ) ) ;
#180852=CARTESIAN_POINT ( 'NONE',  ( -16.53943276465976808, -0.05219959533934237506, 113.7510903946856757 ) ) ;
#180853=CARTESIAN_POINT ( 'NONE',  ( -19.05341960407617563, 5.049401038297882671, 68.54275706135230450 ) ) ;
#180854=CARTESIAN_POINT ( 'NONE',  ( 18.22780087662122739, 5.500000000000000888, 76.48236817873106475 ) ) ;
#180855=CARTESIAN_POINT ( 'NONE',  ( -18.67979575497178146, -10.72451020669898902, 21.66557627198102409 ) ) ;
#180857=CARTESIAN_POINT ( 'NONE',  ( 16.55341960407611168, 4.379528057220329451, 83.95724293864770971 ) ) ;
#180859=CARTESIAN_POINT ( 'NONE',  ( -9.474510206698964154, 16.51473224551069663, 40.41557627198103120 ) ) ;
#180860=CARTESIAN_POINT ( 'NONE',  ( 18.67979575497178502, 10.72451020669898547, 49.16557627198102409 ) ) ;
#180861=CARTESIAN_POINT ( 'NONE',  ( 15.72974639402199770, -15.80617190586745480, 68.12390960531436690 ) ) ;
#180862=CARTESIAN_POINT ( 'NONE',  ( 14.29746914071049879, -8.314922557960816363, 108.3322429386477097 ) ) ;
#180863=CARTESIAN_POINT ( 'NONE',  ( -16.52544592524335698, -4.483927247898792601, 58.95942372801902565 ) ) ;
#180864=CARTESIAN_POINT ( 'NONE',  ( -0.05219959533909027116, -19.03943276465977164, 47.49890960531435979 ) ) ;
#180865=CARTESIAN_POINT ( 'NONE',  ( 5.719274019375673035, 21.55341960407619339, 57.29275706135234714 ) ) ;
#180866=CARTESIAN_POINT ( 'NONE',  ( -14.34966873604960291, -8.224510206698953496, 106.6655762719810383 ) ) ;
#180867=CARTESIAN_POINT ( 'NONE',  ( 5.153800228976615827, -19.02544592524334988, 95.20942372801897591 ) ) ;
#180870=CARTESIAN_POINT ( 'NONE',  ( 21.55341960407610458, 5.719274019375980345, 28.95724293864769905 ) ) ;
#180871=CARTESIAN_POINT ( 'NONE',  ( -19.02544592524342804, 5.153800228976336051, 26.04057627198103120 ) ) ;
#180872=CARTESIAN_POINT ( 'NONE',  ( -21.52544592524334988, -5.823673210054445271, 68.95942372801901854 ) ) ;
#180873=CARTESIAN_POINT ( 'NONE',  ( -0.05219959533934338120, 16.53943276465976808, 62.50109039468568284 ) ) ;
#180874=CARTESIAN_POINT ( 'NONE',  ( 16.55341960407611168, 4.379528057220329451, 43.95724293864769550 ) ) ;
#180875=CARTESIAN_POINT ( 'NONE',  ( 21.53943276465977519, -0.05219959533907433946, 63.74890960531435979 ) ) ;
#180877=CARTESIAN_POINT ( 'NONE',  ( 10.81492255796078972, 18.62759615963270932, 74.58224293864768129 ) ) ;
#180879=CARTESIAN_POINT ( 'NONE',  ( -19.02544592524334988, -5.153800228976617603, 88.95942372801897591 ) ) ;
#180880=CARTESIAN_POINT ( 'NONE',  ( 9.474510206698971260, -16.51473224551069308, 112.9155762719810383 ) ) ;
#180881=CARTESIAN_POINT ( 'NONE',  ( 19.03943276465977164, -0.05219959533909143690, 48.74890960531435979 ) ) ;
#180882=CARTESIAN_POINT ( 'NONE',  ( -4.379528057220328563, 16.55341960407611168, 110.2072429386477239 ) ) ;
#180883=FACE_BOUND ( 'NONE', #113801, .T. ) ;
#180885=CARTESIAN_POINT ( 'NONE',  ( -16.52544592524335698, -4.483927247898792601, 63.95942372801901854 ) ) ;
#180886=CARTESIAN_POINT ( 'NONE',  ( -10.72451020669898014, 18.67979575497178502, 100.4155762719810241 ) ) ;
#180887=CARTESIAN_POINT ( 'NONE',  ( 13.97604488694527802, 13.89961937509977652, 64.37390960531436690 ) ) ;
#180888=CARTESIAN_POINT ( 'NONE',  ( 18.62759615963255655, 10.81492255796105972, 36.66775706135234714 ) ) ;
#180889=CARTESIAN_POINT ( 'NONE',  ( -19.02544592524342804, 5.153800228976336051, 91.04057627198100988 ) ) ;
#180892=CARTESIAN_POINT ( 'NONE',  ( -18.62759615963255300, -10.81492255796106328, 29.16775706135234003 ) ) ;
#180893=CARTESIAN_POINT ( 'NONE',  ( 19.05341960407611168, 5.049401038298154454, 28.95724293864769550 ) ) ;
#180894=CARTESIAN_POINT ( 'NONE',  ( 0.05219959533936267826, -19.03943276465977164, 85.00109039468567573 ) ) ;
#180895=CARTESIAN_POINT ( 'NONE',  ( 5.153800228976615827, -19.02544592524334988, 45.20942372801901143 ) ) ;
#180896=CARTESIAN_POINT ( 'NONE',  ( 21.52544592524344225, -5.823673210054117533, 113.5405762719810383 ) ) ;
#180897=CARTESIAN_POINT ( 'NONE',  ( -5.153800228976607833, 19.02544592524334988, 37.70942372801899722 ) ) ;
#180898=CARTESIAN_POINT ( 'NONE',  ( -16.51473224551082808, 9.474510206698731452, 53.33442372801900433 ) ) ;
#180899=CARTESIAN_POINT ( 'NONE',  ( 16.55341960407618274, -4.379528057220086978, 91.04275706135236135 ) ) ;
#180900=ORIENTED_EDGE ( 'NONE', *, *, #184834, .T. ) ;
#180901=CARTESIAN_POINT ( 'NONE',  ( 19.05341960407611168, 5.049401038298154454, 73.95724293864768129 ) ) ;
#180902=CARTESIAN_POINT ( 'NONE',  ( -10.81492255796105439, 18.62759615963255655, 72.91775706135234714 ) ) ;
#180903=CARTESIAN_POINT ( 'NONE',  ( -18.62759615963255300, -10.81492255796106328, 99.16775706135234714 ) ) ;
#180905=CARTESIAN_POINT ( 'NONE',  ( 16.46253265017160672, -9.564922557960803928, 83.33224293864768129 ) ) ;
#180906=CARTESIAN_POINT ( 'NONE',  ( -0.05219959533937732626, 21.53943276465977519, 57.50109039468568994 ) ) ;
#180907=CARTESIAN_POINT ( 'NONE',  ( -5.153800228976607833, 19.02544592524334988, 97.70942372801900433 ) ) ;
#180908=CARTESIAN_POINT ( 'NONE',  ( -19.03943276465977164, 0.05219959533909376836, 66.24890960531436690 ) ) ;
#180909=CARTESIAN_POINT ( 'NONE',  ( 19.03943276465977164, -0.05219959533909143690, 113.7489096053143669 ) ) ;
#180910=CARTESIAN_POINT ( 'NONE',  ( 13.89961937509977652, -13.97604488694527269, 73.12390960531436690 ) ) ;
#180911=CARTESIAN_POINT ( 'NONE',  ( -17.49999999999999645, 5.499999999999992895, 43.71769037696436300 ) ) ;
#180912=CARTESIAN_POINT ( 'NONE',  ( 9.564922557960805705, 16.46253265017160317, 64.58224293864769550 ) ) ;
#180913=CARTESIAN_POINT ( 'NONE',  ( -13.97604488694527625, -13.89961937509977652, 46.87390960531435979 ) ) ;
#180914=CARTESIAN_POINT ( 'NONE',  ( 15.72974639402176855, 15.80617190586768217, 21.87609039468567573 ) ) ;
#180915=CARTESIAN_POINT ( 'NONE',  ( 12.06949235617739724, 12.14591786802326823, 86.87609039468568994 ) ) ;
#180918=CARTESIAN_POINT ( 'NONE',  ( 9.474510206698729675, 16.51473224551082808, 62.08442372801899722 ) ) ;
#180919=CARTESIAN_POINT ( 'NONE',  ( 9.564922557960805705, 16.46253265017160317, 74.58224293864769550 ) ) ;
#180920=CARTESIAN_POINT ( 'NONE',  ( -16.53943276465976808, 0.05219959533911058130, 71.24890960531435269 ) ) ;
#180921=CARTESIAN_POINT ( 'NONE',  ( -4.483927247898539470, -16.52544592524342804, 112.2905762719810241 ) ) ;
#180922=CARTESIAN_POINT ( 'NONE',  ( -9.474510206698964154, 16.51473224551069663, 115.4155762719810241 ) ) ;
#180923=CARTESIAN_POINT ( 'NONE',  ( -5.049401038298153566, 19.05341960407611168, 100.2072429386476955 ) ) ;
#180924=CARTESIAN_POINT ( 'NONE',  ( -0.05219959533910754901, -16.53943276465976808, 87.49890960531436690 ) ) ;
#180926=CARTESIAN_POINT ( 'NONE',  ( -9.474510206698720793, -16.51473224551083518, 29.58442372801900433 ) ) ;
#180927=CARTESIAN_POINT ( 'NONE',  ( 16.52544592524335698, 4.483927247898782831, 111.4594237280190328 ) ) ;
#180928=CARTESIAN_POINT ( 'NONE',  ( -19.05341960407611168, -5.049401038298163336, 86.45724293864769550 ) ) ;
#180929=CARTESIAN_POINT ( 'NONE',  ( 21.55341960407619695, -5.719274019375665929, 56.04275706135235424 ) ) ;
#180930=CARTESIAN_POINT ( 'NONE',  ( 18.62759615963271287, -10.81492255796078972, 38.33224293864768839 ) ) ;
#180931=CARTESIAN_POINT ( 'NONE',  ( 5.719274019375673035, 21.55341960407619339, 22.29275706135235069 ) ) ;
#180932=CARTESIAN_POINT ( 'NONE',  ( -15.72974639402197994, 15.80617190586746368, 65.62390960531436690 ) ) ;
#180933=CARTESIAN_POINT ( 'NONE',  ( 8.314922557960818139, 14.29746914071049879, 89.58224293864768129 ) ) ;
#180934=CARTESIAN_POINT ( 'NONE',  ( 19.02544592524334988, 5.153800228976608722, 51.45942372801900433 ) ) ;
#180935=CARTESIAN_POINT ( 'NONE',  ( -5.153800228976328057, -19.02544592524343514, 27.29057627198103120 ) ) ;
#180936=CARTESIAN_POINT ( 'NONE',  ( 5.153800228976335163, 19.02544592524342804, 89.79057627198102409 ) ) ;
#180937=CARTESIAN_POINT ( 'NONE',  ( 19.03943276465977164, -0.05219959533909143690, 98.74890960531436690 ) ) ;
#180938=CARTESIAN_POINT ( 'NONE',  ( 0.05219959533910956823, 16.53943276465976808, 114.9989096053143669 ) ) ;
#180939=CARTESIAN_POINT ( 'NONE',  ( 4.483927247898545687, 16.52544592524342804, 24.79057627198103120 ) ) ;
#180940=CARTESIAN_POINT ( 'NONE',  ( 12.06949235617739724, 12.14591786802326823, 46.87609039468568994 ) ) ;
#180941=CARTESIAN_POINT ( 'NONE',  ( -5.823673210054431948, 21.52544592524334988, 107.7094237280190328 ) ) ;
#180942=CARTESIAN_POINT ( 'NONE',  ( 13.89961937509977652, -13.97604488694527269, 98.12390960531433848 ) ) ;
#180943=CARTESIAN_POINT ( 'NONE',  ( 21.55341960407619695, -5.719274019375665929, 31.04275706135234714 ) ) ;
#180944=CARTESIAN_POINT ( 'NONE',  ( 9.474510206698971260, -16.51473224551069308, 47.91557627198102409 ) ) ;
#180945=CARTESIAN_POINT ( 'NONE',  ( 12.14591786802327356, -12.06949235617739191, 50.62609039468568994 ) ) ;
#180946=CARTESIAN_POINT ( 'NONE',  ( -16.55341960407617563, 4.379528057220093196, 88.54275706135236135 ) ) ;
#180947=CARTESIAN_POINT ( 'NONE',  ( 19.02544592524334988, 5.153800228976608722, 111.4594237280190043 ) ) ;
#180948=CARTESIAN_POINT ( 'NONE',  ( 19.02544592524343514, -5.153800228976328945, 28.54057627198102409 ) ) ;
#180949=CARTESIAN_POINT ( 'NONE',  ( 8.224510206698953496, -14.34966873604960469, 97.91557627198103830 ) ) ;
#180950=CARTESIAN_POINT ( 'NONE',  ( -18.62759615963270932, 10.81492255796079327, 105.8322429386476955 ) ) ;
#180951=CARTESIAN_POINT ( 'NONE',  ( 9.474510206698971260, -16.51473224551069308, 27.91557627198103120 ) ) ;
#180952=CARTESIAN_POINT ( 'NONE',  ( 16.51473224551069308, 9.474510206698969483, 109.1655762719810383 ) ) ;
#180953=CARTESIAN_POINT ( 'NONE',  ( -21.53943276465977519, -0.05219959533937600094, 28.75109039468567929 ) ) ;
#180955=CARTESIAN_POINT ( 'NONE',  ( -9.474510206698964154, 16.51473224551069663, 100.4155762719810241 ) ) ;
#180956=CARTESIAN_POINT ( 'NONE',  ( 17.50000000000000000, -5.500000000000000000, 111.2176903769643559 ) ) ;
#180957=CARTESIAN_POINT ( 'NONE',  ( -0.05219959533909027116, -19.03943276465977164, 82.49890960531436690 ) ) ;
#180958=CARTESIAN_POINT ( 'NONE',  ( 18.62759615963255655, 10.81492255796105972, 26.66775706135235424 ) ) ;
#180959=CARTESIAN_POINT ( 'NONE',  ( -14.34966873604960291, -8.224510206698953496, 91.66557627198103830 ) ) ;
#180960=CARTESIAN_POINT ( 'NONE',  ( -9.564922557960796823, -16.46253265017161027, 92.08224293864769550 ) ) ;
#180961=CARTESIAN_POINT ( 'NONE',  ( -9.564922557961040184, 16.46253265017147172, 22.91775706135233648 ) ) ;
#180962=CARTESIAN_POINT ( 'NONE',  ( -14.34966873604972548, 8.224510206698743886, 63.33442372801900433 ) ) ;
#180963=CARTESIAN_POINT ( 'NONE',  ( -10.81492255796105439, 18.62759615963255655, 72.91775706135234714 ) ) ;
#180964=CARTESIAN_POINT ( 'NONE',  ( 0.05219959533934541429, -16.53943276465976808, 45.00109039468568284 ) ) ;
#180965=CARTESIAN_POINT ( 'NONE',  ( 13.89961937509977652, -13.97604488694527269, 83.12390960531436690 ) ) ;
#180966=CARTESIAN_POINT ( 'NONE',  ( 13.89961937509957401, 13.97604488694547697, 101.8760903946856331 ) ) ;
#180967=CARTESIAN_POINT ( 'NONE',  ( -8.224510206698735004, -14.34966873604973081, 69.58442372801900433 ) ) ;
#180968=CARTESIAN_POINT ( 'NONE',  ( -18.62759615963255300, -10.81492255796106328, 109.1677570613523613 ) ) ;
#180969=CARTESIAN_POINT ( 'NONE',  ( 16.51473224551083163, -9.474510206698727899, 80.83442372801899012 ) ) ;
#180970=CARTESIAN_POINT ( 'NONE',  ( 0.05219959533909260263, 19.03943276465977164, 59.99890960531436690 ) ) ;
#180971=CARTESIAN_POINT ( 'NONE',  ( 21.53943276465977519, -0.05219959533907433946, 83.74890960531435269 ) ) ;
#180972=CARTESIAN_POINT ( 'NONE',  ( 0.05219959533910956823, 16.53943276465976808, 74.99890960531435269 ) ) ;
#180973=CARTESIAN_POINT ( 'NONE',  ( -19.05341960407617563, 5.049401038297882671, 88.54275706135230450 ) ) ;
#180974=CARTESIAN_POINT ( 'NONE',  ( 4.379528057220092307, 16.55341960407617563, 62.29275706135236845 ) ) ;
#180975=CARTESIAN_POINT ( 'NONE',  ( -19.02130022317636815, 5.499999999999800160, 80.78188669246576126 ) ) ;
#180976=CARTESIAN_POINT ( 'NONE',  ( 0.05219959533936267826, -19.03943276465977164, 55.00109039468566863 ) ) ;
#180977=CARTESIAN_POINT ( 'NONE',  ( -4.483927247898782831, 16.52544592524335698, 107.7094237280190328 ) ) ;
#180978=CARTESIAN_POINT ( 'NONE',  ( -14.34966873604960291, -8.224510206698953496, 76.66557627198103830 ) ) ;
#180979=CARTESIAN_POINT ( 'NONE',  ( 21.52544592524334988, 5.823673210054432836, 111.4594237280190328 ) ) ;
#180980=CARTESIAN_POINT ( 'NONE',  ( -18.56453257813363678, 5.500000000000055067, 90.99000423690687001 ) ) ;
#180981=CARTESIAN_POINT ( 'NONE',  ( 18.62759615963271287, -10.81492255796078972, 113.3322429386476955 ) ) ;
#180982=CARTESIAN_POINT ( 'NONE',  ( -19.03943276465977164, 0.05219959533909376836, 106.2489096053143669 ) ) ;
#180983=CARTESIAN_POINT ( 'NONE',  ( 16.46253265017160672, -9.564922557960803928, 78.33224293864769550 ) ) ;
#180984=CARTESIAN_POINT ( 'NONE',  ( 18.67979575497194134, -10.72451020669871369, 85.83442372801901854 ) ) ;
#180985=CARTESIAN_POINT ( 'NONE',  ( 9.474510206698971260, -16.51473224551069308, 57.91557627198103120 ) ) ;
#180987=CARTESIAN_POINT ( 'NONE',  ( -10.81492255796078084, -18.62759615963271287, 27.08224293864769550 ) ) ;
#180988=CARTESIAN_POINT ( 'NONE',  ( 4.379528057220339221, -16.55341960407611168, 82.70724293864770971 ) ) ;
#180989=CARTESIAN_POINT ( 'NONE',  ( -9.564922557960796823, -16.46253265017161027, 37.08224293864768839 ) ) ;
#180990=CARTESIAN_POINT ( 'NONE',  ( -8.314922557960811034, -14.29746914071050412, 97.08224293864770971 ) ) ;
#180991=CARTESIAN_POINT ( 'NONE',  ( 21.53943276465977519, -0.05219959533907433946, 103.7489096053143669 ) ) ;
#180993=CARTESIAN_POINT ( 'NONE',  ( 10.72451020669871369, 18.67979575497193778, 47.08442372801901854 ) ) ;
#180994=CARTESIAN_POINT ( 'NONE',  ( -19.02544592524342804, 5.153800228976336051, 31.04057627198102409 ) ) ;
#180995=CARTESIAN_POINT ( 'NONE',  ( 12.06949235617739724, 12.14591786802326823, 66.87609039468568994 ) ) ;
#180997=CARTESIAN_POINT ( 'NONE',  ( 10.72451020669898902, -18.67979575497178502, 97.91557627198103830 ) ) ;
#180998=CARTESIAN_POINT ( 'NONE',  ( -21.55341960407610458, -5.719274019375992779, 96.45724293864770971 ) ) ;
#180999=CARTESIAN_POINT ( 'NONE',  ( -5.049401038297874678, -19.05341960407617918, 34.79275706135233293 ) ) ;
#181000=CARTESIAN_POINT ( 'NONE',  ( 13.89961937509977652, -13.97604488694527269, 53.12390960531434558 ) ) ;
#181001=CARTESIAN_POINT ( 'NONE',  ( 5.153800228976335163, 19.02544592524342804, 114.7905762719810241 ) ) ;
#181002=CARTESIAN_POINT ( 'NONE',  ( 10.72451020669871369, 18.67979575497193778, 57.08442372801901854 ) ) ;
#181004=CARTESIAN_POINT ( 'NONE',  ( -21.55341960407610458, -5.719274019375992779, 61.45724293864770260 ) ) ;
#181005=CARTESIAN_POINT ( 'NONE',  ( -16.52544592524342804, 4.483927247898546575, 31.04057627198102409 ) ) ;
#181006=CARTESIAN_POINT ( 'NONE',  ( 10.72451020669871369, 18.67979575497193778, 82.08442372801901854 ) ) ;
#181007=CARTESIAN_POINT ( 'NONE',  ( 0.05219959533937995610, -21.53943276465977519, 110.0010903946856757 ) ) ;
#181008=CARTESIAN_POINT ( 'NONE',  ( 12.14591786802309770, 12.06949235617756955, 59.37390960531436690 ) ) ;
#181009=CARTESIAN_POINT ( 'NONE',  ( -16.55341960407611168, -4.379528057220339221, 101.4572429386476955 ) ) ;
#181010=CARTESIAN_POINT ( 'NONE',  ( 13.97604488694548053, -13.89961937509957401, 45.62609039468566863 ) ) ;
#181011=CARTESIAN_POINT ( 'NONE',  ( 12.06949235617739724, 12.14591786802326823, 106.8760903946856899 ) ) ;
#181012=CARTESIAN_POINT ( 'NONE',  ( -18.67979575497193778, 10.72451020669871902, 73.33442372801901854 ) ) ;
#181013=CARTESIAN_POINT ( 'NONE',  ( -19.03943276465977164, 0.05219959533909376836, 61.24890960531436690 ) ) ;
#181014=CARTESIAN_POINT ( 'NONE',  ( 5.153800228976615827, -19.02544592524334988, 30.20942372801900433 ) ) ;
#181015=CARTESIAN_POINT ( 'NONE',  ( 0.05219959533907565091, 21.53943276465977519, 39.99890960531436690 ) ) ;
#181016=CARTESIAN_POINT ( 'NONE',  ( -5.719274019375665041, -21.55341960407619695, 34.79275706135235424 ) ) ;
#181017=CARTESIAN_POINT ( 'NONE',  ( 21.52544592524344225, -5.823673210054117533, 88.54057627198103830 ) ) ;
#181018=CARTESIAN_POINT ( 'NONE',  ( -9.564922557961040184, 16.46253265017147172, 82.91775706135233293 ) ) ;
#181019=CARTESIAN_POINT ( 'NONE',  ( -12.06949235617739369, -12.14591786802326823, 49.37609039468569705 ) ) ;
#181021=CARTESIAN_POINT ( 'NONE',  ( -0.05219959533907301413, -21.53943276465977519, 92.49890960531436690 ) ) ;
#181022=CARTESIAN_POINT ( 'NONE',  ( 12.14591786802327356, -12.06949235617739191, 75.62609039468567573 ) ) ;
#181023=CARTESIAN_POINT ( 'NONE',  ( -16.52544592524342804, 4.483927247898546575, 71.04057627198103830 ) ) ;
#181025=CARTESIAN_POINT ( 'NONE',  ( 5.153800228976615827, -19.02544592524334988, 105.2094237280190185 ) ) ;
#181026=CARTESIAN_POINT ( 'NONE',  ( 5.719274019375991003, -21.55341960407610458, 32.70724293864770260 ) ) ;
#181027=CARTESIAN_POINT ( 'NONE',  ( -16.46253265017160317, 9.564922557960807481, 95.83224293864769550 ) ) ;
#181028=CARTESIAN_POINT ( 'NONE',  ( -14.34966873604972548, 8.224510206698743886, 58.33442372801901143 ) ) ;
#181029=CARTESIAN_POINT ( 'NONE',  ( 18.62759615963255655, 10.81492255796105972, 26.66775706135235424 ) ) ;
#181030=CARTESIAN_POINT ( 'NONE',  ( 15.72974639402199770, -15.80617190586745480, 43.12390960531435269 ) ) ;
#181031=CARTESIAN_POINT ( 'NONE',  ( -12.06949235617739369, -12.14591786802326823, 64.37609039468568994 ) ) ;
#181032=CARTESIAN_POINT ( 'NONE',  ( 19.02544592524343514, -5.153800228976328945, 83.54057627198100988 ) ) ;
#181033=CARTESIAN_POINT ( 'NONE',  ( -21.55341960407619339, 5.719274019375674811, 58.54275706135235424 ) ) ;
#181034=CARTESIAN_POINT ( 'NONE',  ( -9.564922557960796823, -16.46253265017161027, 27.08224293864769550 ) ) ;
#181035=CARTESIAN_POINT ( 'NONE',  ( -15.72974639402197994, 15.80617190586746368, 40.62390960531435269 ) ) ;
#181036=ORIENTED_EDGE ( 'NONE', *, *, #132905, .F. ) ;
#181037=CARTESIAN_POINT ( 'NONE',  ( -0.05219959533936034679, 19.03943276465977164, 37.50109039468567573 ) ) ;
#181038=CARTESIAN_POINT ( 'NONE',  ( -12.06949235617739369, -12.14591786802326823, 49.37609039468569705 ) ) ;
#181039=CARTESIAN_POINT ( 'NONE',  ( -21.53943276465977519, 0.05219959533907696930, 21.24890960531436690 ) ) ;
#181041=CARTESIAN_POINT ( 'NONE',  ( -13.89961937509977652, 13.97604488694528158, 80.62390960531436690 ) ) ;
#181042=CARTESIAN_POINT ( 'NONE',  ( 4.483927247898790824, -16.52544592524335698, 105.2094237280190328 ) ) ;
#181044=CARTESIAN_POINT ( 'NONE',  ( -12.06949235617756955, 12.14591786802309770, 100.6239096053143811 ) ) ;
#181045=CARTESIAN_POINT ( 'NONE',  ( -10.72451020669898014, 18.67979575497178502, 30.41557627198101699 ) ) ;
#181046=CARTESIAN_POINT ( 'NONE',  ( -16.46253265017160317, 9.564922557960807481, 25.83224293864769194 ) ) ;
#181047=CARTESIAN_POINT ( 'NONE',  ( -16.52544592524335698, -4.483927247898792601, 78.95942372801901854 ) ) ;
#181048=CARTESIAN_POINT ( 'NONE',  ( -18.67979575497178146, -10.72451020669898902, 111.6655762719810525 ) ) ;
#181049=CARTESIAN_POINT ( 'NONE',  ( 16.46253265017146816, 9.564922557961045513, 71.66775706135233293 ) ) ;
#181050=CARTESIAN_POINT ( 'NONE',  ( 13.97604488694527802, 13.89961937509977652, 44.37390960531435269 ) ) ;
#181051=CARTESIAN_POINT ( 'NONE',  ( -13.89961937509977652, 13.97604488694528158, 115.6239096053143669 ) ) ;
#181052=CARTESIAN_POINT ( 'NONE',  ( 15.80617190586769283, -15.72974639402175789, 100.6260903946857184 ) ) ;
#181053=CARTESIAN_POINT ( 'NONE',  ( -5.153800228976328057, -19.02544592524343514, 62.29057627198100988 ) ) ;
#181054=CARTESIAN_POINT ( 'NONE',  ( -14.29746914071037622, -8.314922557961029526, 54.16775706135235424 ) ) ;
#181055=CARTESIAN_POINT ( 'NONE',  ( 10.81492255796106328, -18.62759615963255655, 90.41775706135236135 ) ) ;
#181056=CARTESIAN_POINT ( 'NONE',  ( 19.02544592524334988, 5.153800228976608722, 51.45942372801900433 ) ) ;
#181057=CARTESIAN_POINT ( 'NONE',  ( 5.153800228976615827, -19.02544592524334988, 50.20942372801897591 ) ) ;
#181059=CARTESIAN_POINT ( 'NONE',  ( 21.55341960407619695, -5.719274019375665929, 46.04275706135234714 ) ) ;
#181062=CARTESIAN_POINT ( 'NONE',  ( -19.02544592524334988, -5.153800228976617603, 48.95942372801900433 ) ) ;
#181063=CARTESIAN_POINT ( 'NONE',  ( 5.153800228976335163, 19.02544592524342804, 94.79057627198103830 ) ) ;
#181064=CARTESIAN_POINT ( 'NONE',  ( 19.03943276465977164, -0.05219959533909143690, 88.74890960531436690 ) ) ;
#181065=CARTESIAN_POINT ( 'NONE',  ( 4.379528057220339221, -16.55341960407611168, 42.70724293864770260 ) ) ;
#181066=CARTESIAN_POINT ( 'NONE',  ( 5.823673210054125526, 21.52544592524343514, 34.79057627198103120 ) ) ;
#181069=CARTESIAN_POINT ( 'NONE',  ( -21.53943276465977519, -0.05219959533937600094, 108.7510903946857042 ) ) ;
#181071=CARTESIAN_POINT ( 'NONE',  ( -13.97604488694527625, -13.89961937509977652, 41.87390960531435979 ) ) ;
#181072=CARTESIAN_POINT ( 'NONE',  ( -16.46253265017160317, 9.564922557960807481, 25.83224293864769194 ) ) ;
#181075=CARTESIAN_POINT ( 'NONE',  ( -14.29746914071037622, -8.314922557961029526, 59.16775706135234714 ) ) ;
#181076=CARTESIAN_POINT ( 'NONE',  ( 18.62759615963271287, -10.81492255796078972, 88.33224293864769550 ) ) ;
#181077=CARTESIAN_POINT ( 'NONE',  ( 0.05219959533910956823, 16.53943276465976808, 44.99890960531435979 ) ) ;
#181078=CARTESIAN_POINT ( 'NONE',  ( -19.02544592524342804, 5.153800228976336051, 31.04057627198102409 ) ) ;
#181079=CARTESIAN_POINT ( 'NONE',  ( 9.564922557960805705, 16.46253265017160317, 114.5822429386476955 ) ) ;
#181080=CARTESIAN_POINT ( 'NONE',  ( 10.81492255796106328, -18.62759615963255655, 30.41775706135234358 ) ) ;
#181081=CARTESIAN_POINT ( 'NONE',  ( 5.153800228976615827, -19.02544592524334988, 30.20942372801900433 ) ) ;
#181082=CARTESIAN_POINT ( 'NONE',  ( 19.03943276465977164, -0.05219959533909143690, 33.74890960531435979 ) ) ;
#181083=CARTESIAN_POINT ( 'NONE',  ( -5.823673210054431948, 21.52544592524334988, 77.70942372801900433 ) ) ;
#181084=DIRECTION ( 'NONE',  ( -1.000000000000000000, -0.000000000000000000, -0.000000000000000000 ) ) ;
#181085=CARTESIAN_POINT ( 'NONE',  ( -14.29746914071049879, 8.314922557960819915, 25.83224293864769194 ) ) ;
#181086=CARTESIAN_POINT ( 'NONE',  ( 17.50000000000147793, 3.202012800152207905, 112.5717758397275077 ) ) ;
#181087=CARTESIAN_POINT ( 'NONE',  ( 15.80617190586746368, 15.72974639402197994, 29.37390960531435269 ) ) ;
#181088=CARTESIAN_POINT ( 'NONE',  ( 8.314922557960818139, 14.29746914071049879, 99.58224293864770971 ) ) ;
#181090=CARTESIAN_POINT ( 'NONE',  ( -16.46253265017160317, 9.564922557960807481, 95.83224293864769550 ) ) ;
#181091=CARTESIAN_POINT ( 'NONE',  ( -0.05219959533910754901, -16.53943276465976808, 77.49890960531433848 ) ) ;
#181092=CARTESIAN_POINT ( 'NONE',  ( 0.05219959533936267826, -19.03943276465977164, 105.0010903946856615 ) ) ;
#181093=CARTESIAN_POINT ( 'NONE',  ( -5.823673210054116645, -21.52544592524344225, 57.29057627198103120 ) ) ;
#181095=EDGE_CURVE ( 'NONE', #92863, #102442, #143556, .T. ) ;
#181096=CARTESIAN_POINT ( 'NONE',  ( 13.89961937509977652, -13.97604488694527269, 38.12390960531436690 ) ) ;
#181097=CARTESIAN_POINT ( 'NONE',  ( -19.02544592524342804, 5.153800228976336051, 86.04057627198103830 ) ) ;
#181098=CARTESIAN_POINT ( 'NONE',  ( 15.80617190586746368, 15.72974639402197994, 89.37390960531435269 ) ) ;
#181099=CARTESIAN_POINT ( 'NONE',  ( 16.52544592524335698, 4.483927247898782831, 101.4594237280190185 ) ) ;
#181100=CARTESIAN_POINT ( 'NONE',  ( -19.05341960407611168, -5.049401038298163336, 91.45724293864766707 ) ) ;
#181101=CARTESIAN_POINT ( 'NONE',  ( -19.02544592524334988, -5.153800228976617603, 83.95942372801901854 ) ) ;
#181102=CARTESIAN_POINT ( 'NONE',  ( -21.55341960407619339, 5.719274019375674811, 98.54275706135234714 ) ) ;
#181103=CARTESIAN_POINT ( 'NONE',  ( 15.72974639402199770, -15.80617190586745480, 78.12390960531436690 ) ) ;
#181104=CARTESIAN_POINT ( 'NONE',  ( -5.823673210054116645, -21.52544592524344225, 32.29057627198102409 ) ) ;
#181105=CARTESIAN_POINT ( 'NONE',  ( 19.02544592524343514, -5.153800228976328945, 48.54057627198103120 ) ) ;
#181106=CARTESIAN_POINT ( 'NONE',  ( -8.224510206698948167, 14.34966873604960824, 25.41557627198103120 ) ) ;
#181107=CARTESIAN_POINT ( 'NONE',  ( 19.05341960407611168, 5.049401038298154454, 58.95724293864768129 ) ) ;
#181109=CARTESIAN_POINT ( 'NONE',  ( -13.97604488694547697, 13.89961937509957934, 28.12609039468565797 ) ) ;
#181110=CARTESIAN_POINT ( 'NONE',  ( -8.224510206698948167, 14.34966873604960824, 75.41557627198102409 ) ) ;
#181111=CARTESIAN_POINT ( 'NONE',  ( 10.81492255796078972, 18.62759615963270932, 109.5822429386476955 ) ) ;
#181112=CARTESIAN_POINT ( 'NONE',  ( 10.72451020669898902, -18.67979575497178502, 112.9155762719810383 ) ) ;
#181114=CARTESIAN_POINT ( 'NONE',  ( 15.72974639402199770, -15.80617190586745480, 53.12390960531436690 ) ) ;
#181115=CARTESIAN_POINT ( 'NONE',  ( 4.483927247898790824, -16.52544592524335698, 100.2094237280190043 ) ) ;
#181116=CARTESIAN_POINT ( 'NONE',  ( -16.55341960407611168, -4.379528057220339221, 101.4572429386476955 ) ) ;
#181117=CARTESIAN_POINT ( 'NONE',  ( 19.03943276465977164, -0.05219959533909143690, 63.74890960531435979 ) ) ;
#181118=CARTESIAN_POINT ( 'NONE',  ( -16.55341960407611168, -4.379528057220339221, 26.45724293864768839 ) ) ;
#181120=CARTESIAN_POINT ( 'NONE',  ( 10.81492255796106328, -18.62759615963255655, 40.41775706135234714 ) ) ;
#181121=CARTESIAN_POINT ( 'NONE',  ( -19.03943276465977164, 0.05219959533909376836, 106.2489096053143669 ) ) ;
#181122=CARTESIAN_POINT ( 'NONE',  ( -21.53943276465977519, -0.05219959533937600094, 78.75109039468568994 ) ) ;
#181123=CARTESIAN_POINT ( 'NONE',  ( 13.89961937509977652, -13.97604488694527269, 28.12390960531435624 ) ) ;
#181124=CARTESIAN_POINT ( 'NONE',  ( -13.97604488694527625, -13.89961937509977652, 41.87390960531435979 ) ) ;
#181125=ORIENTED_EDGE ( 'NONE', *, *, #126300, .F. ) ;
#181126=CARTESIAN_POINT ( 'NONE',  ( 18.67979575497194134, -10.72451020669871369, 85.83442372801901854 ) ) ;
#181127=CARTESIAN_POINT ( 'NONE',  ( 14.29746914071037800, 8.314922557961029526, 51.66775706135234714 ) ) ;
#181128=CARTESIAN_POINT ( 'NONE',  ( -21.53943276465977519, -0.05219959533937600094, 68.75109039468568994 ) ) ;
#181129=CARTESIAN_POINT ( 'NONE',  ( 13.97604488694527802, 13.89961937509977652, 104.3739096053143385 ) ) ;
#181130=CARTESIAN_POINT ( 'NONE',  ( 16.46253265017146816, 9.564922557961045513, 81.66775706135233293 ) ) ;
#181131=CARTESIAN_POINT ( 'NONE',  ( 21.52544592524334988, 5.823673210054432836, 61.45942372801901854 ) ) ;
#181132=CARTESIAN_POINT ( 'NONE',  ( 16.53943276465976808, 0.05219959533934440121, 26.25109039468567573 ) ) ;
#181133=CARTESIAN_POINT ( 'NONE',  ( -19.05341960407617563, 5.049401038297882671, 78.54275706135233293 ) ) ;
#181134=CARTESIAN_POINT ( 'NONE',  ( 9.564922557960805705, 16.46253265017160317, 54.58224293864769550 ) ) ;
#181135=CARTESIAN_POINT ( 'NONE',  ( 13.97604488694548053, -13.89961937509957401, 80.62609039468567573 ) ) ;
#181136=CARTESIAN_POINT ( 'NONE',  ( -8.224510206698948167, 14.34966873604960824, 25.41557627198103120 ) ) ;
#181137=CARTESIAN_POINT ( 'NONE',  ( -9.474510206698720793, -16.51473224551083518, 94.58442372801900433 ) ) ;
#181138=CARTESIAN_POINT ( 'NONE',  ( 8.314922557960818139, 14.29746914071049879, 34.58224293864770260 ) ) ;
#181139=CARTESIAN_POINT ( 'NONE',  ( -19.02544592524334988, -5.153800228976617603, 68.95942372801896170 ) ) ;
#181140=CARTESIAN_POINT ( 'NONE',  ( -14.29746914071037622, -8.314922557961029526, 49.16775706135234003 ) ) ;
#181141=CARTESIAN_POINT ( 'NONE',  ( 13.97604488694548053, -13.89961937509957401, 20.62609039468567573 ) ) ;
#181142=CARTESIAN_POINT ( 'NONE',  ( 9.474510206698971260, -16.51473224551069308, 42.91557627198103120 ) ) ;
#181143=CARTESIAN_POINT ( 'NONE',  ( -8.224510206698735004, -14.34966873604973081, 49.58442372801901143 ) ) ;
#181146=CARTESIAN_POINT ( 'NONE',  ( -16.46253265017160317, 9.564922557960807481, 85.83224293864769550 ) ) ;
#181149=CARTESIAN_POINT ( 'NONE',  ( 16.46253265017146816, 9.564922557961045513, 91.66775706135234714 ) ) ;
#181150=CARTESIAN_POINT ( 'NONE',  ( 13.97604488694527802, 13.89961937509977652, 114.3739096053143669 ) ) ;
#181151=CARTESIAN_POINT ( 'NONE',  ( -21.55341960407619339, 5.719274019375674811, 113.5427570613523756 ) ) ;
#181152=CARTESIAN_POINT ( 'NONE',  ( -9.564922557961040184, 16.46253265017147172, 107.9177570613523471 ) ) ;
#181153=CARTESIAN_POINT ( 'NONE',  ( -16.53943276465976808, 0.05219959533911058130, 116.2489096053143669 ) ) ;
#181154=CARTESIAN_POINT ( 'NONE',  ( 19.05341960407611168, 5.049401038298154454, 38.95724293864767418 ) ) ;
#181155=CARTESIAN_POINT ( 'NONE',  ( 15.80617190586746368, 15.72974639402197994, 69.37390960531436690 ) ) ;
#181156=CARTESIAN_POINT ( 'NONE',  ( -19.05341960407611168, -5.049401038298163336, 41.45724293864769550 ) ) ;
#181157=CARTESIAN_POINT ( 'NONE',  ( -9.564922557961040184, 16.46253265017147172, 47.91775706135233293 ) ) ;
#181158=CARTESIAN_POINT ( 'NONE',  ( 19.02544592524334988, 5.153800228976608722, 66.45942372801899012 ) ) ;
#181159=CARTESIAN_POINT ( 'NONE',  ( 0.05219959533910956823, 16.53943276465976808, 49.99890960531437401 ) ) ;
#181160=CARTESIAN_POINT ( 'NONE',  ( 15.80617190586746368, 15.72974639402197994, 34.37390960531435979 ) ) ;
#181161=CARTESIAN_POINT ( 'NONE',  ( -15.80617190586768217, 15.72974639402176855, 88.12609039468570415 ) ) ;
#181162=CARTESIAN_POINT ( 'NONE',  ( -18.67979575497178146, -10.72451020669898902, 81.66557627198103830 ) ) ;
#181163=CARTESIAN_POINT ( 'NONE',  ( -21.52544592524334988, -5.823673210054445271, 53.95942372801900433 ) ) ;
#181164=CARTESIAN_POINT ( 'NONE',  ( -15.80617190586768217, 15.72974639402176855, 68.12609039468567573 ) ) ;
#181165=CARTESIAN_POINT ( 'NONE',  ( -9.564922557960796823, -16.46253265017161027, 97.08224293864769550 ) ) ;
#181166=CARTESIAN_POINT ( 'NONE',  ( -16.55341960407617563, 4.379528057220093196, 98.54275706135234714 ) ) ;
#181167=CARTESIAN_POINT ( 'NONE',  ( -5.719274019375665041, -21.55341960407619695, 64.79275706135234714 ) ) ;
#181168=CARTESIAN_POINT ( 'NONE',  ( 19.02544592524343514, -5.153800228976328945, 58.54057627198102409 ) ) ;
#181169=CARTESIAN_POINT ( 'NONE',  ( -5.153800228976328057, -19.02544592524343514, 27.29057627198103120 ) ) ;
#181170=CARTESIAN_POINT ( 'NONE',  ( -9.564922557960796823, -16.46253265017161027, 72.08224293864770971 ) ) ;
#181171=CARTESIAN_POINT ( 'NONE',  ( -16.52544592524342804, 4.483927247898546575, 71.04057627198103830 ) ) ;
#181172=CARTESIAN_POINT ( 'NONE',  ( 12.06949235617757843, -12.14591786802309237, 38.12390960531436690 ) ) ;
#181173=CARTESIAN_POINT ( 'NONE',  ( -21.53943276465977519, 0.05219959533907696930, 46.24890960531435979 ) ) ;
#181174=CARTESIAN_POINT ( 'NONE',  ( -19.05341960407611168, -5.049401038298163336, 41.45724293864769550 ) ) ;
#181175=CARTESIAN_POINT ( 'NONE',  ( 21.53943276465977519, -0.05219959533907433946, 63.74890960531435979 ) ) ;
#181176=CARTESIAN_POINT ( 'NONE',  ( 13.97604488694548053, -13.89961937509957401, 50.62609039468566152 ) ) ;
#181178=CARTESIAN_POINT ( 'NONE',  ( -16.53943276465976808, 0.05219959533911058130, 66.24890960531436690 ) ) ;
#181179=CARTESIAN_POINT ( 'NONE',  ( -15.80617190586745835, -15.72974639402198527, 41.87390960531435979 ) ) ;
#181180=ORIENTED_EDGE ( 'NONE', *, *, #183592, .F. ) ;
#181183=CARTESIAN_POINT ( 'NONE',  ( -4.483927247898782831, 16.52544592524335698, 82.70942372801900433 ) ) ;
#181184=CARTESIAN_POINT ( 'NONE',  ( -16.51473224551082808, 9.474510206698731452, 78.33442372801900433 ) ) ;
#181185=CARTESIAN_POINT ( 'NONE',  ( -8.224510206698948167, 14.34966873604960824, 60.41557627198102409 ) ) ;
#181187=CARTESIAN_POINT ( 'NONE',  ( 19.05341960407611168, 5.049401038298154454, 53.95724293864770260 ) ) ;
#181188=CARTESIAN_POINT ( 'NONE',  ( -16.52544592524342804, 4.483927247898546575, 41.04057627198103120 ) ) ;
#181189=CARTESIAN_POINT ( 'NONE',  ( -16.51473224551069308, -9.474510206698971260, 51.66557627198102409 ) ) ;
#181190=CARTESIAN_POINT ( 'NONE',  ( -19.05341960407611168, -5.049401038298163336, 76.45724293864769550 ) ) ;
#181191=CARTESIAN_POINT ( 'NONE',  ( -13.97604488694527625, -13.89961937509977652, 36.87390960531436690 ) ) ;
#181192=CARTESIAN_POINT ( 'NONE',  ( 21.52544592524334988, 5.823673210054432836, 41.45942372801901143 ) ) ;
#181193=CARTESIAN_POINT ( 'NONE',  ( -9.564922557960796823, -16.46253265017161027, 67.08224293864769550 ) ) ;
#181194=CARTESIAN_POINT ( 'NONE',  ( -13.89961937509977652, 13.97604488694528158, 30.62390960531435269 ) ) ;
#181195=CARTESIAN_POINT ( 'NONE',  ( -19.02544592524342804, 5.153800228976336051, 66.04057627198103830 ) ) ;
#181197=CARTESIAN_POINT ( 'NONE',  ( -10.81492255796078084, -18.62759615963271287, 47.08224293864770260 ) ) ;
#181198=CARTESIAN_POINT ( 'NONE',  ( -16.51473224551069308, -9.474510206698971260, 36.66557627198102409 ) ) ;
#181199=CARTESIAN_POINT ( 'NONE',  ( -5.719274019375978568, 21.55341960407610458, 45.20724293864769550 ) ) ;
#181200=CARTESIAN_POINT ( 'NONE',  ( -16.55341960407617563, 4.379528057220093196, 98.54275706135234714 ) ) ;
#181201=CARTESIAN_POINT ( 'NONE',  ( -19.03943276465977164, -0.05219959533935918106, 23.75109039468566152 ) ) ;
#181202=CARTESIAN_POINT ( 'NONE',  ( 4.483927247898790824, -16.52544592524335698, 50.20942372801901854 ) ) ;
#181203=CARTESIAN_POINT ( 'NONE',  ( -8.224510206698735004, -14.34966873604973081, 79.58442372801903275 ) ) ;
#181204=FACE_OUTER_BOUND ( 'NONE', #76473, .T. ) ;
#181206=CARTESIAN_POINT ( 'NONE',  ( -0.05219959533934338120, 16.53943276465976808, 72.50109039468568994 ) ) ;
#181207=CARTESIAN_POINT ( 'NONE',  ( 12.14591786802327356, -12.06949235617739191, 45.62609039468567573 ) ) ;
#181208=CARTESIAN_POINT ( 'NONE',  ( -5.153800228976328057, -19.02544592524343514, 102.2905762719810383 ) ) ;
#181209=CARTESIAN_POINT ( 'NONE',  ( -4.483927247898782831, 16.52544592524335698, 37.70942372801900433 ) ) ;
#181210=CARTESIAN_POINT ( 'NONE',  ( -16.51473224551069308, -9.474510206698971260, 31.66557627198102054 ) ) ;
#181211=CARTESIAN_POINT ( 'NONE',  ( -21.53943276465977519, -0.05219959533937600094, 23.75109039468567929 ) ) ;
#181212=CARTESIAN_POINT ( 'NONE',  ( 4.379528057220092307, 16.55341960407617563, 37.29275706135235424 ) ) ;
#181213=CARTESIAN_POINT ( 'NONE',  ( -12.06949235617739369, -12.14591786802326823, 99.37609039468568994 ) ) ;
#181215=CARTESIAN_POINT ( 'NONE',  ( 5.823673210054444382, -21.52544592524334988, 100.2094237280190043 ) ) ;
#181216=CARTESIAN_POINT ( 'NONE',  ( 0.05219959533936267826, -19.03943276465977164, 95.00109039468567573 ) ) ;
#181217=CARTESIAN_POINT ( 'NONE',  ( 4.379528057220339221, -16.55341960407611168, 57.70724293864770260 ) ) ;
#181218=CARTESIAN_POINT ( 'NONE',  ( -19.03943276465977164, 0.05219959533909376836, 21.24890960531436335 ) ) ;
#181219=CARTESIAN_POINT ( 'NONE',  ( -13.97604488694547697, 13.89961937509957934, 63.12609039468566152 ) ) ;
#181220=CARTESIAN_POINT ( 'NONE',  ( 16.20579543436695502, -7.371946100355079246, 56.93479165828049560 ) ) ;
#181221=CARTESIAN_POINT ( 'NONE',  ( -5.719274019375665041, -21.55341960407619695, 59.79275706135234714 ) ) ;
#181222=CARTESIAN_POINT ( 'NONE',  ( -12.06949235617739369, -12.14591786802326823, 29.37609039468568284 ) ) ;
#181224=CARTESIAN_POINT ( 'NONE',  ( -15.80617190586745835, -15.72974639402198527, 26.87390960531435979 ) ) ;
#181225=CARTESIAN_POINT ( 'NONE',  ( 18.67979575497178502, 10.72451020669898547, 74.16557627198102409 ) ) ;
#181226=CARTESIAN_POINT ( 'NONE',  ( 19.02544592524334988, 5.153800228976608722, 106.4594237280190185 ) ) ;
#181227=CARTESIAN_POINT ( 'NONE',  ( 19.03943276465977164, -0.05219959533909143690, 98.74890960531436690 ) ) ;
#181229=CARTESIAN_POINT ( 'NONE',  ( 0.05219959533909260263, 19.03943276465977164, 24.99890960531435269 ) ) ;
#181230=CARTESIAN_POINT ( 'NONE',  ( -18.67979575497193778, 10.72451020669871902, 108.3344237280190185 ) ) ;
#181231=CARTESIAN_POINT ( 'NONE',  ( 19.05341960407611168, 5.049401038298154454, 43.95724293864769550 ) ) ;
#181232=CARTESIAN_POINT ( 'NONE',  ( -18.67979575497193778, 10.72451020669871902, 53.33442372801901854 ) ) ;
#181233=CARTESIAN_POINT ( 'NONE',  ( 21.55341960407619695, -5.719274019375665929, 96.04275706135236135 ) ) ;
#181234=CARTESIAN_POINT ( 'NONE',  ( -0.05219959533934338120, 16.53943276465976808, 102.5010903946856899 ) ) ;
#181235=CARTESIAN_POINT ( 'NONE',  ( 9.564922557960805705, 16.46253265017160317, 84.58224293864769550 ) ) ;
#181236=CARTESIAN_POINT ( 'NONE',  ( -21.53943276465977519, -0.05219959533937600094, 43.75109039468568284 ) ) ;
#181237=CARTESIAN_POINT ( 'NONE',  ( -10.72451020669870658, -18.67979575497194134, 59.58442372801901854 ) ) ;
#181238=CARTESIAN_POINT ( 'NONE',  ( 16.51473224551083163, -9.474510206698727899, 80.83442372801899012 ) ) ;
#181239=CARTESIAN_POINT ( 'NONE',  ( -5.153800228976328057, -19.02544592524343514, 87.29057627198103830 ) ) ;
#181240=CARTESIAN_POINT ( 'NONE',  ( 12.06949235617757843, -12.14591786802309237, 108.1239096053143811 ) ) ;
#181241=CARTESIAN_POINT ( 'NONE',  ( -10.81492255796078084, -18.62759615963271287, 97.08224293864770971 ) ) ;
#181242=CARTESIAN_POINT ( 'NONE',  ( -5.153800228976607833, 19.02544592524334988, 27.70942372801899722 ) ) ;
#181243=CARTESIAN_POINT ( 'NONE',  ( -14.34966873604960291, -8.224510206698953496, 101.6655762719810383 ) ) ;
#181244=CARTESIAN_POINT ( 'NONE',  ( 16.46253265017160672, -9.564922557960803928, 48.33224293864769550 ) ) ;
#181245=CARTESIAN_POINT ( 'NONE',  ( -16.51473224551082808, 9.474510206698731452, 88.33442372801900433 ) ) ;
#181246=CARTESIAN_POINT ( 'NONE',  ( 8.314922557960818139, 14.29746914071049879, 54.58224293864769550 ) ) ;
#181247=CARTESIAN_POINT ( 'NONE',  ( -15.80617190586768217, 15.72974639402176855, 113.1260903946856899 ) ) ;
#181248=CARTESIAN_POINT ( 'NONE',  ( 5.153800228976335163, 19.02544592524342804, 104.7905762719809957 ) ) ;
#181249=CARTESIAN_POINT ( 'NONE',  ( -13.89961937509957401, -13.97604488694547875, 69.37609039468564731 ) ) ;
#181250=CARTESIAN_POINT ( 'NONE',  ( -15.80617190586745835, -15.72974639402198527, 71.87390960531438111 ) ) ;
#181251=CARTESIAN_POINT ( 'NONE',  ( 15.80617190586769283, -15.72974639402175789, 30.62609039468567929 ) ) ;
#181252=CARTESIAN_POINT ( 'NONE',  ( -14.34966873604972548, 8.224510206698743886, 28.33442372801902209 ) ) ;
#181253=CARTESIAN_POINT ( 'NONE',  ( -14.29746914071037622, -8.314922557961029526, 99.16775706135234714 ) ) ;
#181254=CARTESIAN_POINT ( 'NONE',  ( 17.44279575226822843, 5.990770900252482711, 61.66442432485680314 ) ) ;
#181255=CARTESIAN_POINT ( 'NONE',  ( 21.53943276465977519, 0.05219959533937863772, 36.25109039468567573 ) ) ;
#181256=CARTESIAN_POINT ( 'NONE',  ( -18.62759615963270932, 10.81492255796079327, 40.83224293864769550 ) ) ;
#181257=CARTESIAN_POINT ( 'NONE',  ( 0.05219959533909260263, 19.03943276465977164, 24.99890960531435269 ) ) ;
#181259=CARTESIAN_POINT ( 'NONE',  ( 16.52544592524335698, 4.483927247898782831, 56.45942372801902565 ) ) ;
#181260=CARTESIAN_POINT ( 'NONE',  ( 12.06949235617757843, -12.14591786802309237, 93.12390960531436690 ) ) ;
#181261=CARTESIAN_POINT ( 'NONE',  ( 5.719274019375991003, -21.55341960407610458, 77.70724293864770971 ) ) ;
#181262=CARTESIAN_POINT ( 'NONE',  ( -14.29746914071049879, 8.314922557960819915, 25.83224293864769194 ) ) ;
#181263=CARTESIAN_POINT ( 'NONE',  ( -4.483927247898782831, 16.52544592524335698, 42.70942372801901854 ) ) ;
#181264=CARTESIAN_POINT ( 'NONE',  ( 19.05341960407611168, 5.049401038298154454, 43.95724293864769550 ) ) ;
#181265=CARTESIAN_POINT ( 'NONE',  ( -16.55341960407617563, 4.379528057220093196, 98.54275706135234714 ) ) ;
#181266=CARTESIAN_POINT ( 'NONE',  ( 19.03943276465977164, 0.05219959533936151252, 81.25109039468567573 ) ) ;
#181267=CARTESIAN_POINT ( 'NONE',  ( -15.72974639402197994, 15.80617190586746368, 85.62390960531436690 ) ) ;
#181268=CARTESIAN_POINT ( 'NONE',  ( 4.483927247898790824, -16.52544592524335698, 105.2094237280190328 ) ) ;
#181270=CARTESIAN_POINT ( 'NONE',  ( 19.05341960407611168, 5.049401038298154454, 113.9572429386477097 ) ) ;
#181271=CARTESIAN_POINT ( 'NONE',  ( -5.719274019375978568, 21.55341960407610458, 65.20724293864768129 ) ) ;
#181272=CARTESIAN_POINT ( 'NONE',  ( 4.379528057220092307, 16.55341960407617563, 97.29275706135234714 ) ) ;
#181274=CARTESIAN_POINT ( 'NONE',  ( 18.62759615963271287, -10.81492255796078972, 28.33224293864769550 ) ) ;
#181275=CARTESIAN_POINT ( 'NONE',  ( -19.25663599770061651, 5.499999999999451994, 73.99419308057201761 ) ) ;
#181276=CARTESIAN_POINT ( 'NONE',  ( -10.72451020669898014, 18.67979575497178502, 75.41557627198102409 ) ) ;
#181277=CARTESIAN_POINT ( 'NONE',  ( 8.314922557960818139, 14.29746914071049879, 29.58224293864769905 ) ) ;
#181278=CARTESIAN_POINT ( 'NONE',  ( 0.05219959533934541429, -16.53943276465976808, 20.00109039468568639 ) ) ;
#181279=CARTESIAN_POINT ( 'NONE',  ( -19.02544592524342804, 5.153800228976336051, 41.04057627198103120 ) ) ;
#181280=CARTESIAN_POINT ( 'NONE',  ( -16.52544592524335698, -4.483927247898792601, 28.95942372801902209 ) ) ;
#181281=CARTESIAN_POINT ( 'NONE',  ( 16.51473224551069308, 9.474510206698969483, 49.16557627198102409 ) ) ;
#181283=CARTESIAN_POINT ( 'NONE',  ( 9.564922557960805705, 16.46253265017160317, 109.5822429386476955 ) ) ;
#181284=CARTESIAN_POINT ( 'NONE',  ( -5.153800228976328057, -19.02544592524343514, 107.2905762719810383 ) ) ;
#181285=CARTESIAN_POINT ( 'NONE',  ( -12.06949235617739369, -12.14591786802326823, 84.37609039468570415 ) ) ;
#181286=CARTESIAN_POINT ( 'NONE',  ( -5.153800228976607833, 19.02544592524334988, 97.70942372801900433 ) ) ;
#181287=CARTESIAN_POINT ( 'NONE',  ( -19.03943276465977164, -0.05219959533935918106, 38.75109039468566152 ) ) ;
#181288=CARTESIAN_POINT ( 'NONE',  ( -21.53943276465977519, 0.05219959533907696930, 71.24890960531435269 ) ) ;
#181289=CARTESIAN_POINT ( 'NONE',  ( -0.05219959533934338120, 16.53943276465976808, 97.50109039468567573 ) ) ;
#181290=CARTESIAN_POINT ( 'NONE',  ( 21.55341960407610458, 5.719274019375980345, 38.95724293864768839 ) ) ;
#181291=CARTESIAN_POINT ( 'NONE',  ( 19.05341960407617918, -5.049401038297876454, 91.04275706135234714 ) ) ;
#181292=CARTESIAN_POINT ( 'NONE',  ( 19.03943276465977164, -0.05219959533909143690, 48.74890960531435979 ) ) ;
#181293=CARTESIAN_POINT ( 'NONE',  ( -13.89961937509977652, 13.97604488694528158, 90.62390960531432427 ) ) ;
#181294=CARTESIAN_POINT ( 'NONE',  ( 5.823673210054444382, -21.52544592524334988, 60.20942372801902565 ) ) ;
#181295=CARTESIAN_POINT ( 'NONE',  ( 19.05341960407611168, 5.049401038298154454, 58.95724293864768129 ) ) ;
#181296=CARTESIAN_POINT ( 'NONE',  ( 16.55341960407611168, 4.379528057220329451, 98.95724293864770971 ) ) ;
#181298=CARTESIAN_POINT ( 'NONE',  ( 8.314922557960818139, 14.29746914071049879, 74.58224293864768129 ) ) ;
#181299=CARTESIAN_POINT ( 'NONE',  ( 18.62759615963271287, -10.81492255796078972, 68.33224293864769550 ) ) ;
#181300=CARTESIAN_POINT ( 'NONE',  ( 0.05219959533936267826, -19.03943276465977164, 85.00109039468567573 ) ) ;
#181301=CARTESIAN_POINT ( 'NONE',  ( 17.50000000000000000, -5.499999999999992895, 81.21769037696435589 ) ) ;
#181302=CARTESIAN_POINT ( 'NONE',  ( 9.564922557960805705, 16.46253265017160317, 59.58224293864769550 ) ) ;
#181304=CARTESIAN_POINT ( 'NONE',  ( -19.02544592524342804, 5.153800228976336051, 71.04057627198099567 ) ) ;
#181305=CARTESIAN_POINT ( 'NONE',  ( -5.153800228976328057, -19.02544592524343514, 82.29057627198103830 ) ) ;
#181306=CARTESIAN_POINT ( 'NONE',  ( -0.05219959533934338120, 16.53943276465976808, 67.50109039468568994 ) ) ;
#181307=CARTESIAN_POINT ( 'NONE',  ( -16.52216118717205973, -7.221426719304517405, 51.07599021046991083 ) ) ;
#181308=CARTESIAN_POINT ( 'NONE',  ( -5.049401038297874678, -19.05341960407617918, 49.79275706135231871 ) ) ;
#181309=CARTESIAN_POINT ( 'NONE',  ( 17.47980958864297918, 5.499999999999998224, 21.71653220162190934 ) ) ;
#181310=CARTESIAN_POINT ( 'NONE',  ( 9.474510206698971260, -16.51473224551069308, 112.9155762719810383 ) ) ;
#181311=CARTESIAN_POINT ( 'NONE',  ( -12.14591786802326823, 12.06949235617739902, 108.1260903946856757 ) ) ;
#181312=CARTESIAN_POINT ( 'NONE',  ( 5.153800228976617603, -19.02544592524335343, 75.20942372801899012 ) ) ;
#181313=CARTESIAN_POINT ( 'NONE',  ( 14.29746914071037800, 8.314922557961029526, 76.66775706135234714 ) ) ;
#181314=CARTESIAN_POINT ( 'NONE',  ( -17.40805194822031154, 6.112264579159340627, 30.83371272510612826 ) ) ;
#181315=CARTESIAN_POINT ( 'NONE',  ( -12.14591786802326823, 12.06949235617739902, 63.12609039468568994 ) ) ;
#181317=CARTESIAN_POINT ( 'NONE',  ( -21.53943276465977519, -0.05219959533937600094, 63.75109039468568284 ) ) ;
#181318=CARTESIAN_POINT ( 'NONE',  ( 9.474510206698729675, 16.51473224551082808, 77.08442372801900433 ) ) ;
#181319=CARTESIAN_POINT ( 'NONE',  ( 19.02544592524334988, 5.153800228976608722, 26.45942372801899722 ) ) ;
#181320=CARTESIAN_POINT ( 'NONE',  ( 9.564922557960805705, 16.46253265017160317, 59.58224293864769550 ) ) ;
#181321=CARTESIAN_POINT ( 'NONE',  ( 13.97604488694527802, 13.89961937509977652, 49.37390960531434558 ) ) ;
#181323=CARTESIAN_POINT ( 'NONE',  ( -21.53943276465977519, 0.05219959533907696930, 81.24890960531436690 ) ) ;
#181324=CARTESIAN_POINT ( 'NONE',  ( 5.823673210054125526, 21.52544592524343514, 34.79057627198103120 ) ) ;
#181325=CARTESIAN_POINT ( 'NONE',  ( 8.314922557960818139, 14.29746914071049879, 114.5822429386477097 ) ) ;
#181326=CARTESIAN_POINT ( 'NONE',  ( -8.314922557961024197, 14.29746914071037800, 47.91775706135234714 ) ) ;
#181328=CARTESIAN_POINT ( 'NONE',  ( 10.81492255796106328, -18.62759615963255655, 30.41775706135234358 ) ) ;
#181329=CARTESIAN_POINT ( 'NONE',  ( 8.314922557960818139, 14.29746914071049879, 49.58224293864769550 ) ) ;
#181331=CARTESIAN_POINT ( 'NONE',  ( -16.52544592524335698, -4.483927247898792601, 23.95942372801901143 ) ) ;
#181332=CARTESIAN_POINT ( 'NONE',  ( 0.05219959533936267826, -19.03943276465977164, 35.00109039468566863 ) ) ;
#181333=CARTESIAN_POINT ( 'NONE',  ( 12.06949235617757843, -12.14591786802309237, 48.12390960531436690 ) ) ;
#181334=CARTESIAN_POINT ( 'NONE',  ( -18.62759615963255300, -10.81492255796106328, 19.16775706135234714 ) ) ;
#181336=CARTESIAN_POINT ( 'NONE',  ( 10.72451020669898902, -18.67979575497178502, 82.91557627198103830 ) ) ;
#181337=CARTESIAN_POINT ( 'NONE',  ( -5.049401038298153566, 19.05341960407611168, 95.20724293864770971 ) ) ;
#181338=CARTESIAN_POINT ( 'NONE',  ( -16.55341960407611168, -4.379528057220339221, 61.45724293864770260 ) ) ;
#181339=CARTESIAN_POINT ( 'NONE',  ( 9.474510206698971260, -16.51473224551069308, 97.91557627198102409 ) ) ;
#181341=CARTESIAN_POINT ( 'NONE',  ( 9.564922557961047289, -16.46253265017146816, 70.41775706135233293 ) ) ;
#181342=CARTESIAN_POINT ( 'NONE',  ( -15.72974639402197994, 15.80617190586746368, 110.6239096053143669 ) ) ;
#181343=CARTESIAN_POINT ( 'NONE',  ( 16.51473224551069308, 9.474510206698969483, 54.16557627198103120 ) ) ;
#181344=CARTESIAN_POINT ( 'NONE',  ( -12.14591786802309592, -12.06949235617757132, 106.8739096053143811 ) ) ;
#181345=CARTESIAN_POINT ( 'NONE',  ( -21.53943276465977519, -0.05219959533937600094, 48.75109039468568284 ) ) ;
#181347=CARTESIAN_POINT ( 'NONE',  ( -16.52544592524342804, 4.483927247898546575, 36.04057627198102409 ) ) ;
#181348=CARTESIAN_POINT ( 'NONE',  ( 19.03943276465977164, -0.05219959533909143690, 48.74890960531435979 ) ) ;
#181349=CARTESIAN_POINT ( 'NONE',  ( -19.05341960407611168, -5.049401038298163336, 101.4572429386476955 ) ) ;
#181350=CARTESIAN_POINT ( 'NONE',  ( -18.67979575497178146, -10.72451020669898902, 76.66557627198103830 ) ) ;
#181352=CARTESIAN_POINT ( 'NONE',  ( -13.89961937509977652, 13.97604488694528158, 50.62390960531435979 ) ) ;
#181353=CARTESIAN_POINT ( 'NONE',  ( -5.719274019375978568, 21.55341960407610458, 65.20724293864768129 ) ) ;
#181355=CARTESIAN_POINT ( 'NONE',  ( 18.62759615963255655, 10.81492255796105972, 86.66775706135234714 ) ) ;
#181357=CARTESIAN_POINT ( 'NONE',  ( -12.14591786802326823, 12.06949235617739902, 83.12609039468568994 ) ) ;
#181358=CARTESIAN_POINT ( 'NONE',  ( 16.55341960407611168, 4.379528057220329451, 83.95724293864770971 ) ) ;
#181359=CARTESIAN_POINT ( 'NONE',  ( 19.05341960407611168, 5.049401038298154454, 68.95724293864769550 ) ) ;
#181361=CARTESIAN_POINT ( 'NONE',  ( 13.89961937509957401, 13.97604488694547697, 36.87609039468565442 ) ) ;
#181362=CARTESIAN_POINT ( 'NONE',  ( 16.53943276465976808, 0.05219959533934440121, 91.25109039468568994 ) ) ;
#181363=CARTESIAN_POINT ( 'NONE',  ( 18.67979575497194134, -10.72451020669871369, 110.8344237280190043 ) ) ;
#181364=CARTESIAN_POINT ( 'NONE',  ( 0.05219959533909260263, 19.03943276465977164, 94.99890960531436690 ) ) ;
#181365=CARTESIAN_POINT ( 'NONE',  ( 18.67979575497178502, 10.72451020669898547, 44.16557627198103120 ) ) ;
#181366=CARTESIAN_POINT ( 'NONE',  ( 21.52544592524334988, 5.823673210054432836, 96.45942372801901854 ) ) ;
#181367=CARTESIAN_POINT ( 'NONE',  ( -16.55341960407617563, 4.379528057220093196, 63.54275706135234003 ) ) ;
#181368=CARTESIAN_POINT ( 'NONE',  ( 5.719274019375991003, -21.55341960407610458, 107.7072429386476955 ) ) ;
#181369=CARTESIAN_POINT ( 'NONE',  ( -12.14591786802326823, 12.06949235617739902, 28.12609039468568284 ) ) ;
#181370=CARTESIAN_POINT ( 'NONE',  ( -5.153800228976328057, -19.02544592524343514, 87.29057627198103830 ) ) ;
#181371=EDGE_CURVE ( 'NONE', #142224, #14026, #168793, .T. ) ;
#181372=CARTESIAN_POINT ( 'NONE',  ( -12.06949235617739369, -12.14591786802326823, 29.37609039468568284 ) ) ;
#181373=CARTESIAN_POINT ( 'NONE',  ( -13.97604488694527625, -13.89961937509977652, 56.87390960531434558 ) ) ;
#181374=CARTESIAN_POINT ( 'NONE',  ( 12.06949235617739724, 12.14591786802326823, 31.87609039468567929 ) ) ;
#181375=CARTESIAN_POINT ( 'NONE',  ( -16.52544592524342804, 4.483927247898546575, 81.04057627198102409 ) ) ;
#181376=CARTESIAN_POINT ( 'NONE',  ( 16.52544592524335698, 4.483927247898782831, 91.45942372801901854 ) ) ;
#181377=CARTESIAN_POINT ( 'NONE',  ( 5.823673210054444382, -21.52544592524334988, 40.20942372801901854 ) ) ;
#181378=CARTESIAN_POINT ( 'NONE',  ( -16.51473224551069308, -9.474510206698971260, 66.66557627198102409 ) ) ;
#181379=CARTESIAN_POINT ( 'NONE',  ( -13.97604488694527625, -13.89961937509977652, 86.87390960531436690 ) ) ;
#181380=CARTESIAN_POINT ( 'NONE',  ( -12.06949235617756955, 12.14591786802309770, 35.62390960531437401 ) ) ;
#181381=CARTESIAN_POINT ( 'NONE',  ( 0.05219959533934541429, -16.53943276465976808, 80.00109039468568994 ) ) ;
#181383=CARTESIAN_POINT ( 'NONE',  ( 5.153800228976615827, -19.02544592524334988, 25.20942372801900433 ) ) ;
#181384=CARTESIAN_POINT ( 'NONE',  ( -19.03943276465977164, 0.05219959533909376836, 96.24890960531436690 ) ) ;
#181385=CARTESIAN_POINT ( 'NONE',  ( -19.02544592524342804, 5.153800228976336051, 46.04057627198101699 ) ) ;
#181387=CARTESIAN_POINT ( 'NONE',  ( 8.224510206698742110, 14.34966873604972548, 47.08442372801901854 ) ) ;
#181388=CARTESIAN_POINT ( 'NONE',  ( 19.03943276465977164, 0.05219959533936151252, 71.25109039468566152 ) ) ;
#181389=CARTESIAN_POINT ( 'NONE',  ( -8.314922557961024197, 14.29746914071037800, 57.91775706135234714 ) ) ;
#181390=CARTESIAN_POINT ( 'NONE',  ( 9.474510206698971260, -16.51473224551069308, 112.9155762719810383 ) ) ;
#181392=CARTESIAN_POINT ( 'NONE',  ( -13.97604488694527625, -13.89961937509977652, 71.87390960531433848 ) ) ;
#181393=CARTESIAN_POINT ( 'NONE',  ( -21.53943276465977519, -0.05219959533937600094, 18.75109039468568639 ) ) ;
#181394=CARTESIAN_POINT ( 'NONE',  ( -13.97604488694547697, 13.89961937509957934, 68.12609039468563310 ) ) ;
#181395=CARTESIAN_POINT ( 'NONE',  ( -19.03943276465977164, 0.05219959533909376836, 106.2489096053143669 ) ) ;
#181396=CARTESIAN_POINT ( 'NONE',  ( 13.97604488694527802, 13.89961937509977652, 24.37390960531435624 ) ) ;
#181397=CARTESIAN_POINT ( 'NONE',  ( 5.049401038298161559, -19.05341960407611168, 72.70724293864768129 ) ) ;
#181398=CARTESIAN_POINT ( 'NONE',  ( -16.53943276465976808, 0.05219959533911058130, 41.24890960531435269 ) ) ;
#181400=CARTESIAN_POINT ( 'NONE',  ( 5.049401038297881783, 19.05341960407617563, 32.29275706135233293 ) ) ;
#181401=CARTESIAN_POINT ( 'NONE',  ( -14.29746914071049879, 8.314922557960819915, 70.83224293864770971 ) ) ;
#181402=CARTESIAN_POINT ( 'NONE',  ( -5.823673210054431948, 21.52544592524334988, 107.7094237280190328 ) ) ;
#181403=CARTESIAN_POINT ( 'NONE',  ( -5.153800228976328057, -19.02544592524343514, 57.29057627198103120 ) ) ;
#181404=CARTESIAN_POINT ( 'NONE',  ( 0.05219959533910956823, 16.53943276465976808, 39.99890960531436690 ) ) ;
#181405=CARTESIAN_POINT ( 'NONE',  ( 21.52544592524334988, 5.823673210054432836, 101.4594237280190185 ) ) ;
#181406=CARTESIAN_POINT ( 'NONE',  ( 19.02544592524343514, -5.153800228976328945, 88.54057627198102409 ) ) ;
#181407=CARTESIAN_POINT ( 'NONE',  ( -16.46253265017160317, 9.564922557960807481, 110.8322429386476955 ) ) ;
#181408=CARTESIAN_POINT ( 'NONE',  ( -0.05219959533909027116, -19.03943276465977164, 37.49890960531436690 ) ) ;
#181409=CARTESIAN_POINT ( 'NONE',  ( 8.224510206698953496, -14.34966873604960469, 102.9155762719810383 ) ) ;
#181410=CARTESIAN_POINT ( 'NONE',  ( -8.314922557960811034, -14.29746914071050412, 87.08224293864769550 ) ) ;
#181411=CARTESIAN_POINT ( 'NONE',  ( 18.67979575497178502, 10.72451020669898547, 79.16557627198103830 ) ) ;
#181412=CARTESIAN_POINT ( 'NONE',  ( -19.05341960407611168, -5.049401038298163336, 86.45724293864769550 ) ) ;
#181413=CARTESIAN_POINT ( 'NONE',  ( -5.719274019375978568, 21.55341960407610458, 95.20724293864769550 ) ) ;
#181414=CARTESIAN_POINT ( 'NONE',  ( 5.153800228976335163, 19.02544592524342804, 89.79057627198102409 ) ) ;
#181416=CARTESIAN_POINT ( 'NONE',  ( -14.34966873604960291, -8.224510206698953496, 106.6655762719810383 ) ) ;
#181417=CARTESIAN_POINT ( 'NONE',  ( 5.153800228976335163, 19.02544592524342804, 69.79057627198103830 ) ) ;
#181418=CARTESIAN_POINT ( 'NONE',  ( -21.53943276465977519, 0.05219959533907696930, 81.24890960531436690 ) ) ;
#181420=CARTESIAN_POINT ( 'NONE',  ( -18.67979575497178146, -10.72451020669898902, 31.66557627198102054 ) ) ;
#181422=CARTESIAN_POINT ( 'NONE',  ( -16.55341960407617563, 4.379528057220093196, 38.54275706135234714 ) ) ;
#181423=CARTESIAN_POINT ( 'NONE',  ( 8.224510206698953496, -14.34966873604960469, 92.91557627198103830 ) ) ;
#181425=CARTESIAN_POINT ( 'NONE',  ( 13.97604488694527802, 13.89961937509977652, 94.37390960531436690 ) ) ;
#181426=CARTESIAN_POINT ( 'NONE',  ( -19.05341960407611168, -5.049401038298163336, 51.45724293864770260 ) ) ;
#181427=CARTESIAN_POINT ( 'NONE',  ( -16.52544592524342804, 4.483927247898546575, 81.04057627198102409 ) ) ;
#181428=CARTESIAN_POINT ( 'NONE',  ( -15.72974639402197994, 15.80617190586746368, 25.62390960531435624 ) ) ;
#181429=CARTESIAN_POINT ( 'NONE',  ( 12.06949235617757843, -12.14591786802309237, 53.12390960531436690 ) ) ;
#181430=CARTESIAN_POINT ( 'NONE',  ( -5.049401038297874678, -19.05341960407617918, 99.79275706135234714 ) ) ;
#181431=CARTESIAN_POINT ( 'NONE',  ( 15.80617190586769283, -15.72974639402175789, 55.62609039468568284 ) ) ;
#181433=CARTESIAN_POINT ( 'NONE',  ( -9.564922557960796823, -16.46253265017161027, 97.08224293864769550 ) ) ;
#181434=CARTESIAN_POINT ( 'NONE',  ( 12.06949235617739724, 12.14591786802326823, 86.87609039468568994 ) ) ;
#181435=CARTESIAN_POINT ( 'NONE',  ( -16.51473224551069308, -9.474510206698971260, 26.66557627198103120 ) ) ;
#181436=CARTESIAN_POINT ( 'NONE',  ( 13.89961937509977652, -13.97604488694527269, 73.12390960531436690 ) ) ;
#181437=CARTESIAN_POINT ( 'NONE',  ( 18.67979575497178502, 10.72451020669898547, 84.16557627198103830 ) ) ;
#181438=CARTESIAN_POINT ( 'NONE',  ( 5.153800228976615827, -19.02544592524334988, 105.2094237280190185 ) ) ;
#181439=CARTESIAN_POINT ( 'NONE',  ( 8.224510206698953496, -14.34966873604960469, 52.91557627198103830 ) ) ;
#181440=CARTESIAN_POINT ( 'NONE',  ( 18.67979575497194134, -10.72451020669871369, 55.83442372801901854 ) ) ;
#181442=CARTESIAN_POINT ( 'NONE',  ( 14.29746914071037800, 8.314922557961029526, 81.66775706135236135 ) ) ;
#181443=CARTESIAN_POINT ( 'NONE',  ( 5.153800228976335163, 19.02544592524342804, 114.7905762719810241 ) ) ;
#181444=CARTESIAN_POINT ( 'NONE',  ( -16.51473224551069308, -9.474510206698971260, 111.6655762719810383 ) ) ;
#181446=CARTESIAN_POINT ( 'NONE',  ( 16.52544592524335698, 4.483927247898782831, 106.4594237280190328 ) ) ;
#181447=CARTESIAN_POINT ( 'NONE',  ( 16.53943276465976808, 0.05219959533934440121, 66.25109039468567573 ) ) ;
#181448=CARTESIAN_POINT ( 'NONE',  ( -0.05219959533909027116, -19.03943276465977164, 72.49890960531435269 ) ) ;
#181449=CARTESIAN_POINT ( 'NONE',  ( -0.05219959533909027116, -19.03943276465977164, 77.49890960531435269 ) ) ;
#181450=CARTESIAN_POINT ( 'NONE',  ( -18.67979575497193778, 10.72451020669871902, 78.33442372801901854 ) ) ;
#181451=CARTESIAN_POINT ( 'NONE',  ( 8.314922557961029526, -14.29746914071037800, 80.41775706135234714 ) ) ;
#181452=CARTESIAN_POINT ( 'NONE',  ( -12.14591786802309592, -12.06949235617757132, 46.87390960531435979 ) ) ;
#181453=CARTESIAN_POINT ( 'NONE',  ( 19.02544592524343514, -5.153800228976328945, 53.54057627198102409 ) ) ;
#181454=CARTESIAN_POINT ( 'NONE',  ( 5.049401038298161559, -19.05341960407611168, 52.70724293864767418 ) ) ;
#181455=CARTESIAN_POINT ( 'NONE',  ( -12.14591786802326823, 12.06949235617739902, 38.12609039468567573 ) ) ;
#181456=ORIENTED_EDGE ( 'NONE', *, *, #163492, .T. ) ;
#181457=CARTESIAN_POINT ( 'NONE',  ( -9.474510206698720793, -16.51473224551083518, 94.58442372801900433 ) ) ;
#181458=CARTESIAN_POINT ( 'NONE',  ( 14.34966873604960469, 8.224510206698951720, 94.16557627198103830 ) ) ;
#181459=CARTESIAN_POINT ( 'NONE',  ( 5.049401038298161559, -19.05341960407611168, 67.70724293864769550 ) ) ;
#181460=CARTESIAN_POINT ( 'NONE',  ( 9.474510206698729675, 16.51473224551082808, 107.0844237280190043 ) ) ;
#181462=CARTESIAN_POINT ( 'NONE',  ( 21.55341960407619695, -5.719274019375665929, 101.0427570613523756 ) ) ;
#181463=CARTESIAN_POINT ( 'NONE',  ( 14.34966873604972726, -8.224510206698740333, 70.83442372801901854 ) ) ;
#181465=CARTESIAN_POINT ( 'NONE',  ( -10.81492255796078084, -18.62759615963271287, 67.08224293864770971 ) ) ;
#181466=CARTESIAN_POINT ( 'NONE',  ( 8.314922557961029526, -14.29746914071037800, 55.41775706135234714 ) ) ;
#181468=CARTESIAN_POINT ( 'NONE',  ( 16.51473224551083163, -9.474510206698727899, 45.83442372801900433 ) ) ;
#181469=CARTESIAN_POINT ( 'NONE',  ( 19.05341960407611168, 5.049401038298154454, 83.95724293864766707 ) ) ;
#181470=CARTESIAN_POINT ( 'NONE',  ( 13.89961937509977652, -13.97604488694527269, 23.12390960531436335 ) ) ;
#181471=CARTESIAN_POINT ( 'NONE',  ( -16.46253265017160317, 9.564922557960807481, 60.83224293864769550 ) ) ;
#181472=CARTESIAN_POINT ( 'NONE',  ( 18.67979575497194134, -10.72451020669871369, 70.83442372801901854 ) ) ;
#181473=CARTESIAN_POINT ( 'NONE',  ( 13.97604488694548053, -13.89961937509957401, 45.62609039468566863 ) ) ;
#181474=CARTESIAN_POINT ( 'NONE',  ( -16.51473224551082808, 9.474510206698731452, 28.33442372801900433 ) ) ;
#181475=CARTESIAN_POINT ( 'NONE',  ( -0.05219959533909027116, -19.03943276465977164, 62.49890960531435979 ) ) ;
#181476=CARTESIAN_POINT ( 'NONE',  ( -19.02544592524342804, 5.153800228976336051, 116.0405762719810383 ) ) ;
#181477=CARTESIAN_POINT ( 'NONE',  ( -10.81492255796105439, 18.62759615963255655, 82.91775706135234714 ) ) ;
#181478=CARTESIAN_POINT ( 'NONE',  ( -16.46253265017160317, 9.564922557960807481, 70.83224293864770971 ) ) ;
#181479=CARTESIAN_POINT ( 'NONE',  ( -21.55341960407619339, 5.719274019375674811, 88.54275706135236135 ) ) ;
#181480=CARTESIAN_POINT ( 'NONE',  ( 21.52544592524344225, -5.823673210054117533, 38.54057627198103120 ) ) ;
#181481=AXIS2_PLACEMENT_3D ( 'NONE', #74938, #151782, #90100 ) ;
#181482=CARTESIAN_POINT ( 'NONE',  ( 19.02544592524343514, -5.153800228976328945, 88.54057627198102409 ) ) ;
#181483=CARTESIAN_POINT ( 'NONE',  ( 21.52544592524334988, 5.823673210054432836, 41.45942372801901143 ) ) ;
#181484=CARTESIAN_POINT ( 'NONE',  ( 19.02544592524334988, 5.153800228976608722, 61.45942372801900433 ) ) ;
#181485=CARTESIAN_POINT ( 'NONE',  ( 13.89961937509977652, -13.97604488694527269, 48.12390960531435979 ) ) ;
#181486=CARTESIAN_POINT ( 'NONE',  ( 5.153800228976335163, 19.02544592524342804, 89.79057627198102409 ) ) ;
#181487=CARTESIAN_POINT ( 'NONE',  ( 16.52544592524335698, 4.483927247898782831, 26.45942372801901854 ) ) ;
#181488=CARTESIAN_POINT ( 'NONE',  ( 16.52544592524342804, -4.483927247898539470, 88.54057627198103830 ) ) ;
#181489=CARTESIAN_POINT ( 'NONE',  ( -13.89961937509977652, 13.97604488694528158, 65.62390960531436690 ) ) ;
#181490=CARTESIAN_POINT ( 'NONE',  ( -5.823673210054116645, -21.52544592524344225, 52.29057627198102409 ) ) ;
#181491=CARTESIAN_POINT ( 'NONE',  ( -16.55341960407617563, 4.379528057220093196, 23.54275706135235424 ) ) ;
#181492=CARTESIAN_POINT ( 'NONE',  ( -5.823673210054116645, -21.52544592524344225, 112.2905762719810241 ) ) ;
#181493=CARTESIAN_POINT ( 'NONE',  ( -15.72974639402176322, -15.80617190586768395, 69.37609039468567573 ) ) ;
#181494=CARTESIAN_POINT ( 'NONE',  ( 4.483927247898790824, -16.52544592524335698, 75.20942372801901854 ) ) ;
#181495=CARTESIAN_POINT ( 'NONE',  ( -0.05219959533934338120, 16.53943276465976808, 67.50109039468568994 ) ) ;
#181496=CARTESIAN_POINT ( 'NONE',  ( -16.51473224551069308, -9.474510206698971260, 66.66557627198102409 ) ) ;
#181497=CARTESIAN_POINT ( 'NONE',  ( 8.224510206698742110, 14.34966873604972548, 97.08442372801904696 ) ) ;
#181498=CARTESIAN_POINT ( 'NONE',  ( 19.03943276465977164, 0.05219959533936151252, 36.25109039468567573 ) ) ;
#181499=CARTESIAN_POINT ( 'NONE',  ( 21.52544592524334988, 5.823673210054432836, 26.45942372801901854 ) ) ;
#181500=CARTESIAN_POINT ( 'NONE',  ( -8.314922557960811034, -14.29746914071050412, 72.08224293864769550 ) ) ;
#181501=CARTESIAN_POINT ( 'NONE',  ( -19.05341960407611168, -5.049401038298163336, 101.4572429386476955 ) ) ;
#181502=CARTESIAN_POINT ( 'NONE',  ( 16.55341960407618274, -4.379528057220086978, 86.04275706135236135 ) ) ;
#181503=CARTESIAN_POINT ( 'NONE',  ( 0.05219959533937995610, -21.53943276465977519, 55.00109039468568284 ) ) ;
#181504=CARTESIAN_POINT ( 'NONE',  ( 8.314922557961029526, -14.29746914071037800, 25.41775706135235779 ) ) ;
#181505=CARTESIAN_POINT ( 'NONE',  ( 5.719274019375673035, 21.55341960407619339, 22.29275706135235069 ) ) ;
#181506=CARTESIAN_POINT ( 'NONE',  ( -0.05219959533910754901, -16.53943276465976808, 52.49890960531435979 ) ) ;
#181507=ORIENTED_EDGE ( 'NONE', *, *, #143157, .F. ) ;
#181508=CARTESIAN_POINT ( 'NONE',  ( -18.62759615963270932, 10.81492255796079327, 100.8322429386477097 ) ) ;
#181509=CARTESIAN_POINT ( 'NONE',  ( -16.53943276465976808, 0.05219959533911058130, 36.24890960531435979 ) ) ;
#181512=CARTESIAN_POINT ( 'NONE',  ( -15.72974639402197994, 15.80617190586746368, 30.62390960531436335 ) ) ;
#181513=CARTESIAN_POINT ( 'NONE',  ( 18.62759615963255655, 10.81492255796105972, 41.66775706135235424 ) ) ;
#181514=CARTESIAN_POINT ( 'NONE',  ( -16.55341960407611168, -4.379528057220339221, 66.45724293864768129 ) ) ;
#181515=CARTESIAN_POINT ( 'NONE',  ( 0.05219959533907565091, 21.53943276465977519, 59.99890960531436690 ) ) ;
#181516=CARTESIAN_POINT ( 'NONE',  ( -13.97604488694527625, -13.89961937509977652, 76.87390960531433848 ) ) ;
#181517=CARTESIAN_POINT ( 'NONE',  ( -5.153800228976328057, -19.02544592524343514, 27.29057627198103120 ) ) ;
#181518=CARTESIAN_POINT ( 'NONE',  ( -9.564922557961040184, 16.46253265017147172, 72.91775706135233293 ) ) ;
#181519=CARTESIAN_POINT ( 'NONE',  ( 5.719274019375991003, -21.55341960407610458, 42.70724293864770260 ) ) ;
#181520=CARTESIAN_POINT ( 'NONE',  ( 19.03943276465977164, -0.05219959533909143690, 63.74890960531435979 ) ) ;
#181521=ORIENTED_EDGE ( 'NONE', *, *, #145209, .F. ) ;
#181522=CARTESIAN_POINT ( 'NONE',  ( 16.55341960407618274, -4.379528057220086978, 41.04275706135236135 ) ) ;
#181523=CARTESIAN_POINT ( 'NONE',  ( -21.53943276465977519, 0.05219959533907696930, 111.2489096053143669 ) ) ;
#181524=CARTESIAN_POINT ( 'NONE',  ( 4.379528057220339221, -16.55341960407611168, 47.70724293864770260 ) ) ;
#181525=CARTESIAN_POINT ( 'NONE',  ( -19.05341960407611168, -5.049401038298163336, 101.4572429386476955 ) ) ;
#181526=CARTESIAN_POINT ( 'NONE',  ( 10.72451020669898902, -18.67979575497178502, 72.91557627198103830 ) ) ;
#181527=CARTESIAN_POINT ( 'NONE',  ( -5.719274019375978568, 21.55341960407610458, 110.2072429386477239 ) ) ;
#181528=CARTESIAN_POINT ( 'NONE',  ( -4.483927247898782831, 16.52544592524335698, 42.70942372801901854 ) ) ;
#181529=CARTESIAN_POINT ( 'NONE',  ( -21.53943276465977519, 0.05219959533907696930, 51.24890960531436690 ) ) ;
#181530=CARTESIAN_POINT ( 'NONE',  ( 21.53943276465977519, 0.05219959533937863772, 106.2510903946856757 ) ) ;
#181531=CARTESIAN_POINT ( 'NONE',  ( 19.02544592524343514, -5.153800228976328945, 43.54057627198103120 ) ) ;
#181532=CARTESIAN_POINT ( 'NONE',  ( 16.51473224551069308, 9.474510206698969483, 99.16557627198102409 ) ) ;
#181533=CARTESIAN_POINT ( 'NONE',  ( 16.51473224551069308, 9.474510206698969483, 79.16557627198103830 ) ) ;
#181534=CARTESIAN_POINT ( 'NONE',  ( 16.38665767534995155, -7.295008042176409191, 87.76400864214471653 ) ) ;
#181535=CARTESIAN_POINT ( 'NONE',  ( 5.153800228976615827, -19.02544592524334988, 55.20942372801899722 ) ) ;
#181536=CARTESIAN_POINT ( 'NONE',  ( -10.81492255796105439, 18.62759615963255655, 107.9177570613523471 ) ) ;
#181537=CARTESIAN_POINT ( 'NONE',  ( -0.05219959533907301413, -21.53943276465977519, 27.49890960531435269 ) ) ;
#181538=CARTESIAN_POINT ( 'NONE',  ( 14.34966873604972726, -8.224510206698740333, 105.8344237280190328 ) ) ;
#181539=CARTESIAN_POINT ( 'NONE',  ( -0.05219959533936034679, 19.03943276465977164, 82.50109039468567573 ) ) ;
#181540=CARTESIAN_POINT ( 'NONE',  ( -17.05587630539785593, 6.762274262135693270, 60.74180309037313208 ) ) ;
#181541=CARTESIAN_POINT ( 'NONE',  ( 13.97604488694548053, -13.89961937509957401, 80.62609039468567573 ) ) ;
#181542=CARTESIAN_POINT ( 'NONE',  ( 16.46253265017146816, 9.564922557961045513, 46.66775706135233293 ) ) ;
#181543=B_SPLINE_CURVE_WITH_KNOTS ( 'NONE', 3,
 ( #87013, #6162, #70852, #131514, #36497, #144677 ),
 .UNSPECIFIED., .F., .F.,
 ( 4, 2, 4 ),
 ( 0.003989672132298103559, 0.004372778065220524202, 0.004755883998142945712 ),
 .UNSPECIFIED. ) ;
#181544=CARTESIAN_POINT ( 'NONE',  ( -16.62475595723695321, -7.163666690055258357, 44.47286648189535185 ) ) ;
#181545=CARTESIAN_POINT ( 'NONE',  ( -5.153800228976328057, -19.02544592524343514, 42.29057627198101699 ) ) ;
#181546=CARTESIAN_POINT ( 'NONE',  ( -16.53943276465976808, 0.05219959533911058130, 56.24890960531436690 ) ) ;
#181547=CARTESIAN_POINT ( 'NONE',  ( -5.153800228976328057, -19.02544592524343514, 32.29057627198102409 ) ) ;
#181548=CARTESIAN_POINT ( 'NONE',  ( -16.55341960407611168, -4.379528057220339221, 36.45724293864768839 ) ) ;
#181550=CARTESIAN_POINT ( 'NONE',  ( -4.379528057220086978, -16.55341960407618274, 109.7927570613523613 ) ) ;
#181551=CARTESIAN_POINT ( 'NONE',  ( 19.05341960407611168, 5.049401038298154454, 48.95724293864768129 ) ) ;
#181552=CARTESIAN_POINT ( 'NONE',  ( 18.62759615963255655, 10.81492255796105972, 106.6677570613523756 ) ) ;
#181553=CARTESIAN_POINT ( 'NONE',  ( 0.05219959533934541429, -16.53943276465976808, 25.00109039468567218 ) ) ;
#181554=CARTESIAN_POINT ( 'NONE',  ( -10.81492255796078084, -18.62759615963271287, 37.08224293864768129 ) ) ;
#181555=CARTESIAN_POINT ( 'NONE',  ( -5.719274019375665041, -21.55341960407619695, 94.79275706135234714 ) ) ;
#181557=CARTESIAN_POINT ( 'NONE',  ( 9.474510206698971260, -16.51473224551069308, 107.9155762719810383 ) ) ;
#181558=CARTESIAN_POINT ( 'NONE',  ( -9.474510206698964154, 16.51473224551069663, 80.41557627198103830 ) ) ;
#181560=CARTESIAN_POINT ( 'NONE',  ( 15.80617190586746368, 15.72974639402197994, 109.3739096053143811 ) ) ;
#181561=CARTESIAN_POINT ( 'NONE',  ( 0.05219959533910956823, 16.53943276465976808, 84.99890960531436690 ) ) ;
#181562=CARTESIAN_POINT ( 'NONE',  ( 5.823673210054125526, 21.52544592524343514, 74.79057627198105251 ) ) ;
#181563=CARTESIAN_POINT ( 'NONE',  ( 19.03943276465977164, -0.05219959533909143690, 68.74890960531436690 ) ) ;
#181564=CARTESIAN_POINT ( 'NONE',  ( -10.72451020669898014, 18.67979575497178502, 100.4155762719810241 ) ) ;
#181566=CARTESIAN_POINT ( 'NONE',  ( -5.153800228976328057, -19.02544592524343514, 62.29057627198100988 ) ) ;
#181567=CARTESIAN_POINT ( 'NONE',  ( 8.224510206698953496, -14.34966873604960469, 92.91557627198103830 ) ) ;
#181569=CARTESIAN_POINT ( 'NONE',  ( 19.03943276465977164, -0.05219959533909143690, 63.74890960531435979 ) ) ;
#181570=CARTESIAN_POINT ( 'NONE',  ( -16.46253265017146816, -9.564922557961047289, 84.16775706135233293 ) ) ;
#181571=CARTESIAN_POINT ( 'NONE',  ( -16.53943276465976808, 0.05219959533911058130, 91.24890960531436690 ) ) ;
#181572=CARTESIAN_POINT ( 'NONE',  ( 10.81492255796106328, -18.62759615963255655, 65.41775706135234714 ) ) ;
#181573=CARTESIAN_POINT ( 'NONE',  ( -5.049401038298153566, 19.05341960407611168, 55.20724293864769550 ) ) ;
#181574=CARTESIAN_POINT ( 'NONE',  ( -15.80617190586768217, 15.72974639402176855, 23.12609039468567573 ) ) ;
#181575=CARTESIAN_POINT ( 'NONE',  ( -8.314922557960811034, -14.29746914071050412, 97.08224293864770971 ) ) ;
#181577=CARTESIAN_POINT ( 'NONE',  ( -16.46253265017160317, 9.564922557960807481, 65.83224293864769550 ) ) ;
#181579=CARTESIAN_POINT ( 'NONE',  ( -5.049401038297874678, -19.05341960407617918, 104.7927570613523471 ) ) ;
#181580=CARTESIAN_POINT ( 'NONE',  ( -19.02544592524342804, 5.153800228976336051, 116.0405762719810383 ) ) ;
#181581=CARTESIAN_POINT ( 'NONE',  ( -10.81492255796105439, 18.62759615963255655, 52.91775706135235424 ) ) ;
#181582=CARTESIAN_POINT ( 'NONE',  ( 0.05219959533909260263, 19.03943276465977164, 99.99890960531436690 ) ) ;
#181583=CARTESIAN_POINT ( 'NONE',  ( -16.51473224551082808, 9.474510206698731452, 88.33442372801900433 ) ) ;
#181584=CARTESIAN_POINT ( 'NONE',  ( 0.05219959533909260263, 19.03943276465977164, 54.99890960531435979 ) ) ;
#181585=CARTESIAN_POINT ( 'NONE',  ( 16.52544592524342804, -4.483927247898539470, 83.54057627198102409 ) ) ;
#181586=CARTESIAN_POINT ( 'NONE',  ( -5.153800228976328057, -19.02544592524343514, 92.29057627198099567 ) ) ;
#181587=CARTESIAN_POINT ( 'NONE',  ( 4.483927247898545687, 16.52544592524342804, 84.79057627198102409 ) ) ;
#181588=CARTESIAN_POINT ( 'NONE',  ( 16.46253265017160672, -9.564922557960803928, 83.33224293864768129 ) ) ;
#181590=CARTESIAN_POINT ( 'NONE',  ( -13.97604488694547697, 13.89961937509957934, 28.12609039468565797 ) ) ;
#181591=CARTESIAN_POINT ( 'NONE',  ( 16.51473224551069308, 9.474510206698969483, 49.16557627198102409 ) ) ;
#181592=CARTESIAN_POINT ( 'NONE',  ( 16.55341960407611168, 4.379528057220329451, 43.95724293864769550 ) ) ;
#181593=CARTESIAN_POINT ( 'NONE',  ( -16.46253265017160317, 9.564922557960807481, 25.83224293864769194 ) ) ;
#181595=CARTESIAN_POINT ( 'NONE',  ( 21.53943276465977519, 0.05219959533937863772, 41.25109039468568284 ) ) ;
#181596=CARTESIAN_POINT ( 'NONE',  ( -19.03943276465977164, -0.05219959533935918106, 78.75109039468567573 ) ) ;
#181597=CARTESIAN_POINT ( 'NONE',  ( 12.14591786802309770, 12.06949235617756955, 29.37390960531435269 ) ) ;
#181598=CARTESIAN_POINT ( 'NONE',  ( 10.72451020669898902, -18.67979575497178502, 82.91557627198103830 ) ) ;
#181599=CARTESIAN_POINT ( 'NONE',  ( -5.719274019375978568, 21.55341960407610458, 35.20724293864768839 ) ) ;
#181600=CARTESIAN_POINT ( 'NONE',  ( 8.314922557960818139, 14.29746914071049879, 69.58224293864769550 ) ) ;
#181601=CARTESIAN_POINT ( 'NONE',  ( -9.474510206698964154, 16.51473224551069663, 45.41557627198103120 ) ) ;
#181602=CARTESIAN_POINT ( 'NONE',  ( 14.29746914071037800, 8.314922557961029526, 96.66775706135234714 ) ) ;
#181603=CARTESIAN_POINT ( 'NONE',  ( -14.34966873604972548, 8.224510206698743886, 68.33442372801900433 ) ) ;
#181604=CARTESIAN_POINT ( 'NONE',  ( 9.474510206698729675, 16.51473224551082808, 22.08442372801899722 ) ) ;
#181605=CARTESIAN_POINT ( 'NONE',  ( 13.97604488694527802, 13.89961937509977652, 89.37390960531436690 ) ) ;
#181606=CARTESIAN_POINT ( 'NONE',  ( -0.05219959533909027116, -19.03943276465977164, 77.49890960531435269 ) ) ;
#181607=CARTESIAN_POINT ( 'NONE',  ( 14.29746914071037800, 8.314922557961029526, 76.66775706135234714 ) ) ;
#181608=CARTESIAN_POINT ( 'NONE',  ( 9.564922557960805705, 16.46253265017160317, 29.58224293864769550 ) ) ;
#181609=CARTESIAN_POINT ( 'NONE',  ( -8.224510206698948167, 14.34966873604960824, 40.41557627198103120 ) ) ;
#181610=CARTESIAN_POINT ( 'NONE',  ( 16.51473224551069308, 9.474510206698969483, 99.16557627198102409 ) ) ;
#181611=CARTESIAN_POINT ( 'NONE',  ( -16.51473224551069308, -9.474510206698971260, 96.66557627198102409 ) ) ;
#181612=CARTESIAN_POINT ( 'NONE',  ( 21.55341960407610458, 5.719274019375980345, 28.95724293864769905 ) ) ;
#181613=CARTESIAN_POINT ( 'NONE',  ( 0.05219959533910956823, 16.53943276465976808, 74.99890960531435269 ) ) ;
#181614=CARTESIAN_POINT ( 'NONE',  ( 14.29746914071049879, -8.314922557960816363, 63.33224293864770260 ) ) ;
#181615=CARTESIAN_POINT ( 'NONE',  ( -16.55341960407617563, 4.379528057220093196, 58.54275706135235424 ) ) ;
#181616=CARTESIAN_POINT ( 'NONE',  ( -18.22780087662126647, -5.499999999999827693, 58.98236817873108606 ) ) ;
#181617=CARTESIAN_POINT ( 'NONE',  ( 19.03943276465977164, 0.05219959533936151252, 56.25109039468566863 ) ) ;
#181618=CARTESIAN_POINT ( 'NONE',  ( -16.51473224551069308, -9.474510206698971260, 91.66557627198103830 ) ) ;
#181619=CARTESIAN_POINT ( 'NONE',  ( 19.03943276465977164, 0.05219959533936151252, 61.25109039468566863 ) ) ;
#181621=CARTESIAN_POINT ( 'NONE',  ( 9.564922557961047289, -16.46253265017146816, 110.4177570613523471 ) ) ;
#181622=CARTESIAN_POINT ( 'NONE',  ( -14.34966873604972548, 8.224510206698743886, 93.33442372801901854 ) ) ;
#181623=CARTESIAN_POINT ( 'NONE',  ( -19.03943276465977164, 0.05219959533909376836, 41.24890960531435269 ) ) ;
#181624=CARTESIAN_POINT ( 'NONE',  ( 9.564922557960805705, 16.46253265017160317, 114.5822429386476955 ) ) ;
#181625=CARTESIAN_POINT ( 'NONE',  ( -21.55341960407619339, 5.719274019375674811, 58.54275706135235424 ) ) ;
#181626=CARTESIAN_POINT ( 'NONE',  ( -5.049401038297874678, -19.05341960407617918, 104.7927570613523471 ) ) ;
#181627=CARTESIAN_POINT ( 'NONE',  ( -13.89961937509957401, -13.97604488694547697, 54.37609039468566152 ) ) ;
#181628=CARTESIAN_POINT ( 'NONE',  ( -0.05219959533909027116, -19.03943276465977164, 72.49890960531435269 ) ) ;
#181630=CARTESIAN_POINT ( 'NONE',  ( -14.34966873604960291, -8.224510206698953496, 71.66557627198100988 ) ) ;
#181631=CARTESIAN_POINT ( 'NONE',  ( -16.51473224551069308, -9.474510206698971260, 61.66557627198103120 ) ) ;
#181632=CARTESIAN_POINT ( 'NONE',  ( 16.46253265017160672, -9.564922557960803928, 78.33224293864769550 ) ) ;
#181633=CARTESIAN_POINT ( 'NONE',  ( -16.51473224551082808, 9.474510206698731452, 73.33442372801900433 ) ) ;
#181634=CARTESIAN_POINT ( 'NONE',  ( 15.80617190586746368, 15.72974639402197994, 69.37390960531436690 ) ) ;
#181635=CARTESIAN_POINT ( 'NONE',  ( -14.29746914071049879, 8.314922557960819915, 115.8322429386477097 ) ) ;
#181636=CARTESIAN_POINT ( 'NONE',  ( -19.03943276465977164, -0.05219959533935918106, 53.75109039468566863 ) ) ;
#181637=CARTESIAN_POINT ( 'NONE',  ( -19.05341960407611168, -5.049401038298163336, 51.45724293864770260 ) ) ;
#181638=CARTESIAN_POINT ( 'NONE',  ( -9.474510206698964154, 16.51473224551069663, 90.41557627198103830 ) ) ;
#181639=( BOUNDED_SURFACE ( )  B_SPLINE_SURFACE ( 3, 2, ( 
 ( #81295, #141003, #12968, #66146, #172341, #2491, #110661, #28153, #142979, #125837, #33830, #18670, #141989, #4457, #65154, #140000, #126813, #1489, #173348, #188519, #127809, #49996, #89794, #151477, #121116, #111661, #44293, #105952, #63167, #192498, #174339, #144975, #36796, #145974, #7456, #116648, #9486, #101465, #52963, #178338, #193500, #21646, #176338, #68137, #190502, #38815, #53982, #35809, #114640, #115655, #84295, #51976, #39800, #20638, #98461, #147997, #177344, #97455, #113634, #100473, #129788, #130807, #163156, #112647, #162152, #82291, #23648, #160155, #175329, #71150, #159141, #85296, #8475, #83299, #146988, #6456, #37810, #143982, #5463, #131820, #24659, #191485, #161151, #99471, #70150, #86308, #22648, #189514, #69140, #54978, #67145, #50987, #128803, #152945, #88299, #119655, #120626, #73164, #149987, #14444, #89304, #181337, #197491, #42816, #164169, #166163, #182323, #132816, #25667, #136790, #183310, #44792, #117652, #179349, #104479, #167151, #118659, #74149, #11493, #180350, #12488, #28650, #27664, #150996, #106445, #133821, #135821, #58958, #194502, #43802, #105465, #56985, #55975, #168126, #90286, #151970, #165164, #29622, #134834, #196513, #13458, #75122, #41818, #72145, #40812, #103486, #198476, #59948, #57983, #91254, #195512, #26657, #121615, #102482, #87312, #148996, #10485, #30612, #96241, #171110, #153949, #94254, #49753, #47777, #64917, #34584, #141753, #126578, #187296, #125599, #78088, #139756, #173107, #63930, #170113, #156937, #18434, #17429, #45781, #95252, #172103, #108437, #188279, #48768, #110422, #111421, #253, #107433, #186297, #61922, #123592, #33589, #3243, #109430, #80084, #169105, #92265, #1243, #46778, #155934, #60935, #122609, #157929, #32601, #31607, #15445, #79086, #76107, #137783, #199468, #184299, #77103, #140759, #138772, #62922, #185286, #93257, #154942, #16439, #2247, #124602, #8235, #19419, #98212, #65904, #127577, #192262, #143742, #142745, #174104, #193263, #191255, #69913, #178098, #85058, #131579, #130565, #68905, #21404, #83062, #116409, #7220, #113399, #100234, #161916, #160917, #189278, #38578, #115418, #51737, #54737, #53744, #177107, #39568, #5221, #50754, #129555, #66902, #128565, #23410, #146740, #52730, #101226, #112412, #35573, #144736, #190260, #99230, #4225, #97221, #81067, #114396, #175089, #158907, #176097, #20398, #82047, #36557, #159915, #6223, #84061, #67902, #37567, #22410, #145739, #41585, #135588, #119421, #133579, #151741, #162915, #103249, #9248, #70915, #197260, #87074, #86072, #117412, #27422, #149751, #194271, #196282, #12256, #44560, #55738, #166921, #13234, #74897, #147762, #132583, #11254, #58722, #148759, #104242, #180117, #10248, #42579, #120391, #134596, #72927, #136560, #163936, #165925, #57751, #24423, #181105, #73918, #71907, #179110, #198241, #89067, #150758, #195269, #59713, #164931, #26424, #182085, #43568, #56753, #102248, #40578, #118424, #105233, #28422, #88064, #121385, #25433, #90059, #183077, #171871, #137550, #123359, #60698, #122374, #126353, #1010, #184063, #124366, #62684, #61690, #3015, #168871, #153713, #17197, #33360, #199233, #185052, #45546, #107201, #188050, #186061, #30376, #47544, #79859, #77860, #95019, #64692, #156708, #18201, #78851, #155702, #108200, #169881, #106215, #94021, #16, #187069, #48539, #109198, #75874, #125373, #2019, #138538, #141527, #140530, #63698, #167899, #92021, #15209, #16205, #76868, #46540, #110193, #29399, #139527, #91029, #31374, #93024, #154712, #170877, #32368, #152715, #14206, #83818, #159668, #4983, #3994, #5985, #161675, #6978, #68659, #192010, #53495, #114153, #189048, #36321, #98986, #158677, #128332, #22167, #67665, #20166, #38334, #49520, #190031, #96015, #157700, #145498, #173873, #172873, #65674, #175855, #97975, #80839, #82820, #160675, #131335, #142516, #115172, #99990, #23171, #34354, #19190, #21164, #130314, #35343, #191018 ),
 ( #96994, #111183, #84814, #129322, #52493, #81811, #146494, #51505, #113167, #144501, #176865, #143499, #50523, #127336, #66669, #37327, #7985, #112185, #69668, #174855, #177862, #148518, #40330, #149508, #11005, #120158, #13000, #104995, #56503, #181849, #197025, #25190, #179872, #71668, #194035, #42342, #57513, #39331, #118180, #119181, #87822, #55499, #43328, #24181, #102006, #151507, #180866, #100990, #117168, #104004, #133335, #134354, #166683, #116172, #165682, #85831, #27180, #163688, #178864, #74663, #162674, #88827, #12019, #86832, #150520, #10008, #41340, #147521, #9009, #135353, #28185, #195026, #164687, #103002, #196037, #89827, #26182, #193023, #72678, #73680, #70677, #58492, #132343, #54500, #91783, #123130, #124121, #76633, #153477, #156463, #92788, #184815, #17962, #198997, #107957, #186832, #170643, #1780, #198004, #31140, #136330, #90801, #60464, #122139, #108963, #59474, #106966, #137316, #121148, #139298, #63458, #14973, #78614, #169644, #32131, #183826, #182841, #16961, #48300, #61459, #105982, #44324, #62446, #46301, #77629, #167667, #109957, #138311, #199992, #154476, #776, #171636, #15969, #168641, #185820, #47307, #125134, #93789, #33126, #155469, #29164, #94782, #152484, #140288, #13971, #75638, #45317, #30140, #110944, #189797, #65435, #3758, #37088, #6741, #51268, #52256, #172629, #49286, #4743, #50288, #159427, #64452, #126122, #113914, #112929, #35103, #34117, #36088, #191772, #98747, #160440, #21930, #83581, #144262, #18955, #66432, #129081, #188805, #158444, #175612, #97739, #111945, #68421, #79618, #19932, #187817, #95775, #145260, #127096, #2776, #157462, #5749, #128093, #80600, #174623, #190782, #161439, #142277, #130073, #53254, #114932, #173633, #96754, #20923, #176625, #81574, #82581, #143259, #67425, #38100, #99755, #141286, #71434, #73445, #23934, #25948, #56259, #84577, #41103, #72436, #147275, #104761, #58260, #102767, #164454, #55259, #135118, #24947, #101762, #9770, #103770, #8765, #162433, #146257, #70434, #87591, #179633, #178621, #119929, #85588, #132100, #134113, #88587, #54265, #40083, #177627, #39095, #43093, #117943, #100751, #149277, #196792, #194787, #11781, #181614, #150286, #22931, #195801, #57274, #86594, #148277, #7741, #10772, #116928, #165449, #26946, #118948, #192782, #42108, #180633, #163449, #69427, #133098, #193791, #131094, #115937, #12764, #538, #76398, #121902, #120906, #122893, #78372, #123876, #185574, #108726, #170403, #30904, #105748, #153234, #15730, #75406, #45080, #139059, #184581, #137077, #155234, #166450, #106737, #74428, #136095, #62210, #90571, #89588, #182604, #92551, #14737, #197770, #199755, #77390, #48065, #59236, #31895, #16724, #140048, #151274, #44090, #138074, #47066, #152252, #107717, #183595, #13737, #46063, #93548, #61222, #169397, #1537, #167434, #154240, #63214, #27946, #124894, #186593, #198766, #28930, #60232, #168412, #29907, #91546, #21693, #111710, #188568, #96521, #190549, #33879, #49054, #171405, #157226, #51034, #66195, #65202, #6504, #172391, #18718, #20685, #175375, #141052, #126861, #64220, #125885, #129836, #4505, #187585, #127858, #83347, #81343, #98508, #68184, #36844, #160203, #82339, #159189, #173396, #34867, #191535, #97503, #3526, #52022, #113681, #112696, #79383, #128849, #5511, #142038, #145023, #144029, #67192, #109721, #95538, #2538, #19701, #80365, #50047, #32891, #94543, #143027, #156224, #110709, #158211, #189562, #17724, #174387, #35857, #14236, #121416, #106246, #166949, #105263, #57781, #119451, #152746, #43598, #149782, #136589, #198269, #197289, #22696, #74926, #151770, #88096, #167928, #28452, #90088, #91059, #180148, #84343, #165956, #41616, #103281, #13263, #183108, #27457, #59746, #148791, #10281, #181136, #26454, #135618, #37860, #99519, #44590, #89098, #11285, #71939, #12285, #29428, #75908, #137582, #53012, #114691, #120421, #195303, #42610, #176386, #164961, #134627 ),
 ( #161201, #133609, #72958, #104274, #196312, #56784, #118456, #182112, #150789, #73949, #58752, #94053, #61723, #49553, #30409, #108233, #157733, #125403, #184096, #123391, #187100, #77891, #140560, #126385, #122406, #63728, #92056, #48570, #169913, #185083, #19222, #45579, #110223, #18234, #31405, #171904, #46572, #186093, #153745, #107232, #141558, #172908, #93056, #170906, #154743, #2049, #96046, #1043, #111216, #62716, #16239, #168903, #139559, #15240, #80872, #124399, #47575, #33392, #109227, #199265, #155731, #32398, #60733, #17229, #78881, #34386, #95051, #64723, #76899, #156740, #138570, #48, #79888, #3047, #188082, #4026, #128364, #158707, #65704, #175889, #115205, #51536, #192046, #6019, #7010, #5018, #146526, #130347, #100023, #159701, #50555, #8017, #99018, #144533, #114185, #127370, #38368, #36354, #98006, #67698, #37360, #161710, #21198, #190060, #160709, #113199, #176897, #82854, #23206, #22200, #142548, #189082, #173905, #129356, #84849, #112215, #68692, #53527, #20196, #191051, #52524, #83849, #145531, #35374, #97026, #81842, #143530, #66700, #174888, #155394, #109877, #1703, #124039, #172557, #187743, #107877, #48223, #49214, #17888, #185738, #173559, #154398, #32055, #81500, #110872, #169565, #47227, #34043, #63379, #64379, #50215, #46224, #95700, #15893, #157388, #93712, #108886, #143187, #31062, #18881, #142201, #16884, #80527, #170565, #171561, #77551, #92710, #65362, #96683, #78535, #94706, #140209, #126047, #19860, #125056, #35028, #186753, #33051, #139223, #156383, #698, #4667, #79542, #141212, #3684, #2702, #184739, #127023, #188730, #111869, #123053, #158371, #62370, #78687, #81648, #174697, #111020, #126194, #93861, #47379, #143332, #113003, #110032, #172706, #125208, #142351, #36161, #141362, #189869, #2849, #171710, #62521, #156539, #32204, #159502, #94858, #187890, #127171, #79692, #18038, #20998, #95851, #49357, #139367, #1851, #34190, #51343, #173710, #4819, #848, #157535, #124194, #155539, #63533, #186904, #112021, #185894, #33200, #140364, #109034, #3831, #66507, #64527, #128169, #19029, #35178, #48375, #170713, #20005, #97813, #80675, #17033, #65510, #188881, #50362, #96833, #158517, #133172, #23008, #84654, #54339, #85665, #56335, #146331, #53329, #24009, #38176, #9845, #7820, #71504, #132176, #82653, #194862, #144337, #161516, #117003, #164527, #147352, #8840, #67501, #99832, #130151, #39167, #100825, #118017, #102841, #179706, #69504, #41178, #86666, #115008, #131170, #192860, #83658, #193867, #70508, #129158, #116010, #55333, #177700, #145336, #5825, #113989, #191848, #190855, #178698, #52332, #6818, #40160, #162508, #101836, #175687, #37162, #163523, #176702, #98821, #25022, #160515, #22006, #148349, #68496, #13814, #166526, #43169, #46138, #182680, #12840, #107791, #88666, #197847, #76474, #60306, #91624, #87664, #120982, #26020, #180708, #150362, #11858, #198842, #149349, #196868, #27021, #10846, #29007, #153312, #181688, #168487, #59313, #121981, #73523, #72515, #106813, #138151, #151351, #195877, #134190, #152328, #136172, #167511, #57350, #14813, #90646, #44165, #135194, #104836, #42184, #105824, #199832, #183672, #45157, #29985, #61299, #75480, #165525, #74506, #137153, #58334, #28023, #122969, #184656, #120002, #119025, #103844, #89665, #15804, #77465, #142111, #93623, #92624, #123950, #33953, #156297, #612, #2614, #18793, #51106, #62282, #173469, #19772, #81413, #154315, #139135, #17798, #3596, #155308, #110785, #186665, #16797, #49127, #65275, #141124, #79455, #143099, #170477, #172466, #64291, #30977, #187656, #80438, #78447, #169476, #4578, #95611, #157296, #1612, #126934, #111781, #188642, #125958, #50121, #140121, #108798, #185648, #63288, #34942, #96594, #124968, #66271, #31967, #48135, #127930, #94618, #47140, #189632, #158283, #109792, #171475, #32964, #39926, #99593, #21767, #55098, #115776, #86432, #53087, #83418 ),
 ( #177465, #97574, #68257, #160276, #69263, #130929, #101595, #132939, #24784, #176459, #163283, #116768, #145095, #161273, #191608, #113753, #162273, #38934, #159262, #37932, #100591, #7577, #175449, #148118, #144102, #6578, #71274, #23773, #20758, #36919, #85423, #114765, #54102, #9609, #35928, #147114, #5582, #8601, #129908, #98582, #194627, #82413, #70274, #52096, #178459, #112766, #84416, #22768, #67262, #128920, #174459, #190621, #146093, #192620, #131942, #193626, #153066, #58103, #106569, #119773, #26781, #179472, #73286, #149119, #76226, #11618, #42935, #43921, #196634, #134956, #137906, #12606, #104599, #56097, #118786, #27783, #168246, #90406, #121736, #117778, #151114, #40937, #10610, #180475, #41946, #28768, #102609, #88423, #57112, #164295, #59075, #183428, #181457, #198600, #89425, #152091, #103612, #25788, #136913, #165288, #195639, #87434, #150117, #197610, #74270, #166287, #14568, #135940, #120742, #167269, #44913, #72271, #182441, #133948, #105583, #13575, #75242, #60068, #29742, #91377, #171230, #188394, #158043, #65034, #49872, #110539, #48884, #1363, #63042, #96355, #187416, #93376, #80197, #141868, #140877, #169229, #18549, #95367, #31728, #111537, #172220, #33705, #34698, #123708, #30736, #109549, #185405, #46896, #157052, #126690, #32719, #3359, #92383, #154070, #124721, #170234, #79208, #173222, #2367, #156051, #108556, #155062, #15564, #17548, #19533, #81178, #199588, #61055, #122727, #64047, #138891, #186419, #184418, #16557, #78204, #45898, #125717, #139874, #107551, #77222, #47895, #371, #62043, #94371, #67022, #66024, #97336, #7333, #129668, #174220, #176213, #192377, #24538, #35689, #146861, #193378, #54854, #127691, #189391, #191365, #177222, #128681, #84171, #160031, #190378, #22524, #38695, #114512, #52842, #116528, #143859, #145851, #37682, #4339, #161030, #53860, #51853, #142860, #178216, #69018, #130683, #175207, #115534, #85172, #100351, #99347, #23526, #21518, #159022, #20515, #163031, #162030, #82163, #8353, #39680, #70028, #131697, #101342, #50868, #112526, #5338, #113513, #144853, #6336, #36672, #98332, #83179, #68016, #31236, #30238, #55852, #108057, #184914, #121246, #139392, #76730, #138405, #124225, #10364, #117526, #199092, #72021, #133694, #46398, #16068, #60559, #61554, #179224, #40690, #14068, #59571, #168734, #77726, #91881, #45410, #198105, #44423, #102360, #107063, #874, #169741, #92885, #154572, #62549, #153572, #25548, #75735, #200086, #182940, #167763, #123223, #15069, #106076, #185921, #86188, #29261, #132696, #194385, #47406, #90892, #9364, #164049, #109062, #137411, #87192, #122234, #170740, #147878, #148873, #71029, #152578, #183925, #17060, #78715, #80703, #66535, #18066, #173738, #49386, #79721, #112050, #128199, #3859, #142381, #82681, #33227, #35207, #65538, #93888, #50390, #81676, #156571, #114016, #67528, #96860, #158544, #64557, #20034, #174724, #143359, #19056, #113032, #141390, #171739, #155566, #2878, #4851, #188912, #187917, #129185, #94887, #126221, #189896, #97841, #63560, #144365, #140391, #111049, #51371, #32230, #36187, #159529, #1879, #172737, #34217, #21028, #5852, #190883, #52359, #125234, #95880, #186932, #48402, #157563, #127198, #110059, #176729, #25049, #40186, #160544, #100851, #101866, #70534, #38202, #26044, #6845, #84680, #134217, #163549, #22033, #99858, #86692, #54365, #117029, #102866, #98849, #148376, #68524, #9871, #146359, #161542, #195903, #83685, #71531, #115036, #118045, #10870, #147378, #162533, #130178, #145363, #179735, #149374, #7846, #8867, #23035, #178724, #72540, #177726, #87689, #39195, #69533, #191875, #192887, #53359, #57378, #131197, #24037, #133197, #116037, #85692, #175713, #132203, #193894, #37192, #55359, #194888, #56362, #41205, #164551, #180733, #13840, #642, #73548, #43194, #104862, #91652, #42209, #89691, #120027, #103869, #122009, #184685, #74532, #61328, #90673, #14842 ),
 ( #183700, #75507, #28050, #136197, #135221, #137180, #31005, #76505, #138181, #122999, #46168, #45187, #58360, #105851, #92654, #165550, #197872, #153341, #119051, #106841, #168516, #27047, #59339, #166551, #198868, #60335, #107822, #139165, #154343, #182707, #169506, #15836, #151376, #167538, #121009, #181712, #30014, #199863, #88693, #44192, #77495, #150389, #12867, #11885, #196893, #29033, #152355, #188675, #47170, #125002, #50155, #141158, #3628, #189666, #185680, #126966, #155341, #111814, #32997, #48168, #82447, #108829, #173502, #1646, #4611, #97607, #33987, #49159, #16830, #170508, #66303, #35960, #94651, #95643, #109825, #65307, #159295, #64324, #112800, #125991, #156331, #31999, #79489, #78481, #144135, #17831, #110817, #34975, #2647, #187689, #62312, #18826, #172500, #123982, #186697, #157331, #174493, #96628, #127963, #93656, #80471, #140154, #63324, #171508, #142144, #158316, #19804, #81445, #143131, #51139, #20792, #71311, #161310, #148153, #177501, #101632, #53123, #25824, #86468, #117815, #130964, #175483, #87469, #131977, #115811, #147148, #128955, #132974, #192654, #114801, #9645, #8636, #179508, #146128, #176494, #70308, #22804, #194664, #54137, #56133, #55133, #5617, #84450, #67296, #162308, #38970, #190655, #68293, #100626, #40976, #39961, #102645, #52131, #23808, #113788, #160311, #129944, #191643, #178495, #36955, #37970, #6614, #98617, #193662, #164330, #7613, #21801, #85459, #163322, #99628, #83453, #145131, #69298, #116803, #24819, #169267, #75280, #59112, #90445, #72307, #76263, #135975, #58140, #91416, #152130, #122765, #89462, #119808, #13612, #104634, #137941, #74308, #199625, #198639, #149156, #61092, #10646, #27820, #183466, #30773, #136950, #60105, #133985, #166323, #196671, #105621, #167309, #184454, #195676, #45934, #12641, #107589, #153103, #181493, #197646, #151150, #150154, #121773, #44952, #57147, #120777, #106608, #43959, #11655, #118824, #180509, #42971, #41982, #168283, #103648, #73321, #29780, #182478, #14607, #165326, #26818, #88458, #134992, #28805, #63081, #78240, #112562, #15600, #80232, #31763, #34733, #127727, #64082, #79246, #46933, #407, #96391, #66060, #124760, #125752, #139911, #95403, #189429, #94408, #142894, #156089, #186456, #77258, #109586, #185443, #174257, #47932, #140917, #141903, #32757, #171269, #158078, #187452, #188430, #1401, #92420, #173258, #4376, #17586, #62079, #154106, #18585, #2404, #33743, #138927, #19569, #48920, #110574, #81213, #157089, #50904, #172255, #3394, #65069, #126726, #123744, #49908, #108592, #111574, #170269, #93412, #155098, #16592, #70065, #117561, #38730, #100388, #20552, #191402, #83215, #192414, #53896, #163068, #55888, #147912, #99383, #24573, #39714, #68052, #22561, #114551, #36708, #85210, #162066, #82202, #161066, #23562, #130722, #98370, #86222, #67059, #144890, #194418, #146900, #143894, #160068, #8390, #176250, #177258, #9398, #159058, #131733, #128717, #193415, #6372, #21555, #35725, #5375, #54890, #175243, #178253, #71064, #7370, #84207, #190414, #51890, #101377, #132730, #129706, #69055, #52879, #116564, #97372, #37721, #113549, #145887, #115571, #102395, #196426, #72055, #199382, #134744, #166073, #167063, #119568, #57896, #60846, #135734, #27576, #179261, #41733, #150907, #29540, #13374, #44705, #40726, #74063, #164083, #133729, #103397, #165075, #151884, #25582, #149896, #180263, #87226, #182230, #106359, #89214, #181251, #26569, #28564, #43715, #148908, #104390, #105376, #197405, #88212, #91173, #10398, #11403, #137697, #90201, #195422, #73072, #75038, #42728, #120537, #168043, #56899, #136704, #118573, #198385, #12401, #58871, #59862, #121529, #183224, #152862, #14357, #76022, #94167, #109342, #77013, #30522, #64836, #96159, #93171, #155846, #108349, #125516, #19340, #124516, #173022, #186211, #154856, #45693, #139669, #15357, #142662, #78002, #171024, #110336, #62832, #1157, #4141, #78999 ),
 ( #95165, #107344, #16354, #123504, #169017, #187213, #188196, #47692, #126498, #17343, #18348, #170028, #122521, #3163, #34501, #32515, #92174, #184211, #48684, #140673, #63844, #153859, #49668, #2165, #31518, #111332, #172017, #157848, #33506, #156853, #80003, #141672, #80987, #138685, #166, #61834, #185197, #46688, #127489, #144654, #100147, #147672, #68816, #130475, #50669, #21320, #113315, #22322, #83972, #193174, #85983, #178010, #129474, #54647, #69820, #98128, #53653, #159825, #146649, #8143, #7133, #35490, #84967, #161828, #82978, #116321, #115330, #177021, #101138, #190176, #97140, #176013, #51651, #175007, #23323, #39477, #37482, #38491, #158823, #20311, #191173, #36471, #145652, #162824, #192172, #131487, #6137, #67819, #81959, #24333, #65820, #189194, #112329, #174019, #143651, #5135, #66817, #52647, #128480, #114311, #99144, #160833, #165836, #180027, #198153, #9160, #87976, #55649, #117321, #181997, #133488, #132495, #163843, #73832, #196192, #40485, #42491, #58638, #90941, #102157, #13148, #59623, #121297, #194184, #179017, #57664, #43480, #195180, #150669, #26336, #56661, #88979, #105147, #181017, #119331, #182989, #10160, #12167, #104155, #70827, #27333, #120304, #118334, #25344, #44473, #135503, #197173, #41496, #166833, #151654, #28334, #89973, #74811, #103160, #148672, #86985, #164840, #136473, #106128, #149664, #167812, #71820, #11162, #29311, #72836, #134506, #169790, #107113, #168784, #172786, #47454, #30286, #170789, #126268, #124274, #141439, #111096, #18114, #2926, #63608, #1929, #154622, #16116, #49435, #79769, #108106, #94934, #185970, #48452, #200133, #34267, #33275, #64605, #77773, #122284, #152628, #78762, #62596, #93936, #75785, #187965, #139440, #61602, #156619, #155615, #14118, #92934, #123271, #17111, #31283, #137463, #922, #199143, #125284, #60609, #183973, #45459, #109110, #186981, #91931, #140439, #110109, #153623, #32281, #184962, #171787, #15119, #76781, #138452, #46446, #162335, #87494, #102670, #130991, #85485, #177528, #99655, #148179, #163349, #80752, #23836, #24845, #193691, #161339, #149183, #127248, #7641, #57174, #86494, #142429, #22831, #9672, #38997, #39987, #25851, #19102, #71337, #188961, #132999, #69325, #84478, #118851, #3908, #194690, #38000, #41003, #134010, #70336, #147174, #53151, #65588, #164355, #72335, #192683, #132003, #146155, #101658, #195702, #100653, #10671, #8663, #54166, #114830, #115839, #176524, #180534, #55159, #116829, #56160, #178520, #117842, #95926, #179534, #157611, #123772, #104665, #13638, #92448, #76292, #107615, #103673, #136976, #42008, #196696, #166350, #27848, #14633, #165351, #12668, #42998, #26845, #44977, #106637, #88486, #197672, #89489, #198665, #60132, #169293, #62109, #154136, #105646, #30799, #45961, #74335, #28832, #120805, #151180, #91442, #168310, #150181, #167335, #29806, #121800, #136001, #15628, #73348, #59137, #434, #153130, #11682, #182505, #137970, #43985, #183493, #77285, #135021, #199652, #58167, #61118, #90473, #152155, #119834, #181519, #122792, #75305, #184482, #138955, #157117, #172283, #139941, #93440, #127754, #159085, #156117, #18613, #171298, #188458, #82232, #187481, #35753, #48948, #17616, #108620, #2433, #78268, #5403, #140945, #33773, #173289, #125779, #64114, #67087, #141930, #95433, #185471, #47962, #80260, #97398, #19598, #50933, #46961, #3421, #170298, #1431, #109614, #32784, #158106, #31791, #79275, #186486, #155127, #49939, #112591, #110601, #189455, #65097, #81240, #94436, #16620, #66088, #20580, #126755, #63109, #124787, #111604, #34763, #96420, #142921, #174283, #4403, #143922, #71092, #131763, #102426, #69084, #99413, #70094, #84238, #55917, #53925, #117591, #178282, #128746, #40757, #190443, #7400, #163101, #10430, #193445, #164113, #113577, #175271, #177289, #24604, #114583, #54921, #145917, #176280, #8422, #86251, #100417, #38759, #179293, #129733, #116593, #162098 ),
 ( #83242, #36737, #132759, #25611, #161095, #23594, #37752, #39745, #87255, #130751, #148940, #192443, #22590, #51918, #115600, #21584, #98401, #85241, #146932, #101408, #147941, #9427, #160097, #194446, #144918, #6400, #191430, #68081, #52907, #89248, #74096, #72088, #181283, #133762, #41764, #26601, #88244, #150940, #56932, #149929, #165108, #118606, #166106, #197437, #73107, #135766, #42760, #12434, #11436, #195457, #120569, #180296, #27608, #134777, #103429, #196459, #182263, #57929, #104423, #119600, #58903, #161749, #195098, #55570, #26254, #193094, #23244, #194107, #8061, #179945, #177934, #41412, #102077, #52564, #164759, #114224, #131407, #86905, #134426, #117244, #178936, #37400, #69738, #100064, #9077, #70747, #103078, #72755, #87895, #116242, #149581, #56580, #84888, #39401, #54570, #53567, #163762, #40406, #11079, #101061, #175929, #25262, #99059, #160747, #22239, #162746, #148588, #83888, #10080, #71738, #145571, #24254, #146567, #132415, #133409, #7048, #68730, #130388, #85904, #192085, #118254, #147592, #115245, #176937, #38407, #45384, #60532, #180936, #121220, #122208, #90866, #58562, #46370, #27250, #105069, #154546, #183899, #42411, #120228, #107037, #74735, #137384, #123198, #119252, #168709, #88900, #30211, #166754, #181918, #16041, #104074, #91854, #135424, #138380, #31208, #167735, #182910, #150590, #165756, #200061, #169715, #28257, #29233, #43399, #199063, #92859, #198075, #108029, #59542, #89896, #12089, #13068, #73752, #77700, #151579, #44395, #153546, #136398, #106049, #196112, #152551, #14039, #57582, #75705, #15043, #197095, #76704, #61529, #184888, #26681, #195534, #167173, #29645, #28672, #57008, #106469, #183332, #119676, #137807, #75144, #136815, #122631, #11517, #118681, #197512, #73187, #134858, #44814, #14467, #58980, #59970, #180373, #41843, #12509, #58006, #90307, #76129, #151993, #43823, #196536, #42838, #103510, #105487, #199491, #168148, #91277, #74173, #181359, #152968, #13479, #60957, #27685, #104503, #198499, #166184, #184321, #135843, #45802, #121637, #87333, #107454, #149019, #89326, #169129, #10507, #72169, #133844, #165186, #151018, #120647, #88321, #150011, #182345, #50773, #142764, #94274, #19438, #34602, #62941, #17449, #109448, #31627, #80103, #95272, #15468, #155952, #156955, #125619, #93277, #81086, #61944, #139776, #189296, #18452, #77125, #154962, #141771, #171131, #172123, #157947, #153971, #3264, #123611, #64937, #1264, #16458, #112433, #138794, #126596, #170133, #173127, #65924, #2267, #79105, #185306, #275, #96261, #4244, #124621, #63950, #78107, #33609, #127597, #32620, #30634, #140778, #186316, #46797, #47798, #108456, #92287, #187317, #48788, #188298, #110442, #49775, #111440, #130585, #160935, #55756, #36575, #145756, #24441, #8253, #39586, #84077, #177126, #147781, #192280, #98230, #159933, #146759, #97239, #144756, #175106, #158927, #38597, #101245, #129573, #116430, #7238, #69933, #21420, #194290, #54756, #86090, #99248, #143759, #174122, #100253, #68923, #115435, #20416, #162934, #22427, #9267, #23429, #35593, #70933, #82066, #52745, #131597, #5240, #161934, #85076, #66920, #191270, #83080, #53761, #193282, #132600, #128584, #190278, #37586, #51754, #178118, #6241, #113415, #114414, #67920, #176115, #182101, #102267, #42597, #43586, #12272, #180134, #167917, #148778, #26441, #75895, #105252, #163955, #41603, #166938, #196298, #58740, #44578, #40596, #28441, #10267, #90076, #88083, #103268, #137570, #25453, #151759, #56769, #59734, #152735, #89085, #104260, #71926, #87093, #121403, #91048, #149769, #150777, #164948, #120409, #14225, #119438, #29417, #181123, #11271, #133596, #134614, #195288, #199253, #72944, #165943, #13252, #57768, #27443, #117430, #73937, #135606, #179128, #197277, #74915, #118441, #136578, #183097, #198258, #106234, #34375, #78869, #185071, #46559, #33380, #184083, #31394, #61709, #45567, #63717, #126374, #16227 ) ),
 .UNSPECIFIED., .T., .F., .F. ) 
 B_SPLINE_SURFACE_WITH_KNOTS ( ( 4, 3, 4 ),
 ( 3, 2, 2, 2, 2, 2, 2, 2, 2, 2, 2, 2, 2, 2, 2, 2, 2, 2, 2, 2, 2, 2, 2, 2, 2, 2, 2, 2, 2, 2, 2, 2, 2, 2, 2, 2, 2, 2, 2, 2, 2, 2, 2, 2, 2, 2, 2, 2, 2, 2, 2, 2, 2, 2, 2, 2, 2, 2, 2, 2, 2, 2, 2, 2, 2, 2, 2, 2, 2, 2, 2, 2, 2, 2, 2, 2, 2, 2, 2, 2, 2, 2, 2, 2, 2, 2, 2, 2, 2, 2, 2, 2, 2, 2, 2, 2, 2, 2, 2, 2, 2, 2, 2, 2, 2, 2, 2, 2, 2, 2, 2, 2, 2, 2, 2, 2, 2, 2, 2, 2, 2, 2, 2, 2, 2, 2, 2, 2, 2, 2, 2, 2, 2, 2, 2, 2, 2, 2, 2, 2, 2, 2, 2, 2, 2, 2, 2, 2, 2, 2, 2, 2, 2, 2, 2, 2, 2, 2, 2, 2, 2, 2, 2, 2, 2, 2, 2, 2, 2, 2, 2, 2, 2, 2, 2, 2, 2, 2, 2, 2, 2, 2, 2, 2, 2, 2, 2, 2, 2, 2, 2, 2, 2, 2, 2, 2, 2, 2, 2, 2, 2, 2, 2, 2, 2, 2, 2, 2, 2, 2, 2, 2, 2, 2, 2, 2, 2, 2, 2, 2, 2, 2, 2, 2, 2, 2, 2, 2, 3 ),
 ( 0.000000000000000000, 0.5000000000000000000, 1.000000000000000000 ),
 ( 0.000000000000000000, 0.004385964912280701511, 0.008771929824561403022, 0.01315789473684210453, 0.01754385964912280604, 0.02192982456140350755, 0.02631578947368420907, 0.03070175438596491058, 0.03508771929824561209, 0.03947368421052631360, 0.04385964912280701511, 0.04824561403508771662, 0.05263157894736841813, 0.05701754385964911964, 0.06140350877192982115, 0.06578947368421052266, 0.07017543859649122417, 0.07456140350877192569, 0.07894736842105262720, 0.08333333333333332871, 0.08771929824561403022, 0.09210526315789473173, 0.09649122807017543324, 0.1008771929824561348, 0.1052631578947368363, 0.1096491228070175378, 0.1140350877192982393, 0.1184210526315789408, 0.1228070175438596423, 0.1271929824561403577, 0.1315789473684210453, 0.1359649122807017607, 0.1403508771929824483, 0.1447368421052631637, 0.1491228070175438514, 0.1535087719298245668, 0.1578947368421052544, 0.1622807017543859698, 0.1666666666666666574, 0.1710526315789473728, 0.1754385964912280604, 0.1798245614035087758, 0.1842105263157894635, 0.1885964912280701788, 0.1929824561403508665, 0.1973684210526315819, 0.2017543859649122695, 0.2061403508771929849, 0.2105263157894736725, 0.2149122807017543879, 0.2192982456140350755, 0.2236842105263157909, 0.2280701754385964786, 0.2324561403508771940, 0.2368421052631578816, 0.2412280701754385970, 0.2456140350877192846, 0.2500000000000000000, 0.2543859649122807154, 0.2587719298245614308, 0.2631578947368420907, 0.2675438596491228060, 0.2719298245614035214, 0.2763157894736842368, 0.2807017543859648967, 0.2850877192982456121, 0.2894736842105263275, 0.2938596491228070429, 0.2982456140350877027, 0.3026315789473684181, 0.3070175438596491335, 0.3114035087719298489, 0.3157894736842105088, 0.3201754385964912242, 0.3245614035087719396, 0.3289473684210526550, 0.3333333333333333148, 0.3377192982456140302, 0.3421052631578947456, 0.3464912280701754610, 0.3508771929824561209, 0.3552631578947368363, 0.3596491228070175517, 0.3640350877192982670, 0.3684210526315789269, 0.3728070175438596423, 0.3771929824561403577, 0.3815789473684210731, 0.3859649122807017330, 0.3903508771929824483, 0.3947368421052631637, 0.3991228070175438791, 0.4035087719298245390, 0.4078947368421052544, 0.4122807017543859698, 0.4166666666666666852, 0.4210526315789473450, 0.4254385964912280604, 0.4298245614035087758, 0.4342105263157894912, 0.4385964912280701511, 0.4429824561403508665, 0.4473684210526315819, 0.4517543859649122973, 0.4561403508771929571, 0.4605263157894736725, 0.4649122807017543879, 0.4692982456140351033, 0.4736842105263157632, 0.4780701754385964786, 0.4824561403508771940, 0.4868421052631579093, 0.4912280701754385692, 0.4956140350877192846, 0.5000000000000000000, 0.5043859649122807154, 0.5087719298245614308, 0.5131578947368421462, 0.5175438596491228616, 0.5219298245614034659, 0.5263157894736841813, 0.5307017543859648967, 0.5350877192982456121, 0.5394736842105263275, 0.5438596491228070429, 0.5482456140350877583, 0.5526315789473684736, 0.5570175438596490780, 0.5614035087719297934, 0.5657894736842105088, 0.5701754385964912242, 0.5745614035087719396, 0.5789473684210526550, 0.5833333333333333703, 0.5877192982456140857, 0.5921052631578946901, 0.5964912280701754055, 0.6008771929824561209, 0.6052631578947368363, 0.6096491228070175517, 0.6140350877192982670, 0.6184210526315789824, 0.6228070175438596978, 0.6271929824561403022, 0.6315789473684210176, 0.6359649122807017330, 0.6403508771929824483, 0.6447368421052631637, 0.6491228070175438791, 0.6535087719298245945, 0.6578947368421053099, 0.6622807017543859143, 0.6666666666666666297, 0.6710526315789473450, 0.6754385964912280604, 0.6798245614035087758, 0.6842105263157894912, 0.6885964912280702066, 0.6929824561403509220, 0.6973684210526315264, 0.7017543859649122417, 0.7061403508771929571, 0.7105263157894736725, 0.7149122807017543879, 0.7192982456140351033, 0.7236842105263158187, 0.7280701754385965341, 0.7324561403508771384, 0.7368421052631578538, 0.7412280701754385692, 0.7456140350877192846, 0.7500000000000000000, 0.7543859649122807154, 0.7587719298245614308, 0.7631578947368421462, 0.7675438596491228616, 0.7719298245614034659, 0.7763157894736841813, 0.7807017543859648967, 0.7850877192982456121, 0.7894736842105263275, 0.7938596491228070429, 0.7982456140350877583, 0.8026315789473684736, 0.8070175438596490780, 0.8114035087719297934, 0.8157894736842105088, 0.8201754385964912242, 0.8245614035087719396, 0.8289473684210526550, 0.8333333333333333703, 0.8377192982456140857, 0.8421052631578946901, 0.8464912280701754055, 0.8508771929824561209, 0.8552631578947368363, 0.8596491228070175517, 0.8640350877192982670, 0.8684210526315789824, 0.8728070175438596978, 0.8771929824561403022, 0.8815789473684210176, 0.8859649122807017330, 0.8903508771929824483, 0.8947368421052631637, 0.8991228070175438791, 0.9035087719298245945, 0.9078947368421053099, 0.9122807017543859143, 0.9166666666666666297, 0.9210526315789473450, 0.9254385964912280604, 0.9298245614035087758, 0.9342105263157894912, 0.9385964912280702066, 0.9429824561403509220, 0.9473684210526315264, 0.9517543859649122417, 0.9561403508771929571, 0.9605263157894736725, 0.9649122807017543879, 0.9692982456140351033, 0.9736842105263158187, 0.9780701754385965341, 0.9824561403508771384, 0.9868421052631578538, 0.9912280701754385692, 0.9956140350877192846, 1.000000000000000000 ),
 .UNSPECIFIED. ) 
 GEOMETRIC_REPRESENTATION_ITEM ( )  RATIONAL_B_SPLINE_SURFACE ( (
 ( 1.000000000000000000, 0.9659258262890683122, 1.000000000000000000, 0.9659258262890683122, 1.000000000000000000, 0.9659258262890683122, 1.000000000000000000, 0.9659258262890683122, 1.000000000000000000, 0.9659258262890683122, 1.000000000000000000, 0.9659258262890683122, 1.000000000000000000, 0.9659258262890683122, 1.000000000000000000, 0.9659258262890683122, 1.000000000000000000, 0.9659258262890683122, 1.000000000000000000, 0.9659258262890683122, 1.000000000000000000, 0.9659258262890683122, 1.000000000000000000, 0.9659258262890683122, 1.000000000000000000, 0.9659258262890683122, 1.000000000000000000, 0.9659258262890683122, 1.000000000000000000, 0.9659258262890683122, 1.000000000000000000, 0.9659258262890683122, 1.000000000000000000, 0.9659258262890683122, 1.000000000000000000, 0.9659258262890683122, 1.000000000000000000, 0.9659258262890683122, 1.000000000000000000, 0.9659258262890683122, 1.000000000000000000, 0.9659258262890683122, 1.000000000000000000, 0.9659258262890683122, 1.000000000000000000, 0.9659258262890683122, 1.000000000000000000, 0.9659258262890683122, 1.000000000000000000, 0.9659258262890683122, 1.000000000000000000, 0.9659258262890683122, 1.000000000000000000, 0.9659258262890683122, 1.000000000000000000, 0.9659258262890683122, 1.000000000000000000, 0.9659258262890683122, 1.000000000000000000, 0.9659258262890683122, 1.000000000000000000, 0.9659258262890683122, 1.000000000000000000, 0.9659258262890683122, 1.000000000000000000, 0.9659258262890683122, 1.000000000000000000, 0.9659258262890683122, 1.000000000000000000, 0.9659258262890683122, 1.000000000000000000, 0.9659258262890683122, 1.000000000000000000, 0.9659258262890683122, 1.000000000000000000, 0.9659258262890683122, 1.000000000000000000, 0.9659258262890683122, 1.000000000000000000, 0.9659258262890683122, 1.000000000000000000, 0.9659258262890683122, 1.000000000000000000, 0.9659258262890683122, 1.000000000000000000, 0.9659258262890683122, 1.000000000000000000, 0.9659258262890683122, 1.000000000000000000, 0.9659258262890683122, 1.000000000000000000, 0.9659258262890683122, 1.000000000000000000, 0.9659258262890683122, 1.000000000000000000, 0.9659258262890683122, 1.000000000000000000, 0.9659258262890683122, 1.000000000000000000, 0.9659258262890683122, 1.000000000000000000, 0.9659258262890683122, 1.000000000000000000, 0.9659258262890683122, 1.000000000000000000, 0.9659258262890683122, 1.000000000000000000, 0.9659258262890683122, 1.000000000000000000, 0.9659258262890683122, 1.000000000000000000, 0.9659258262890683122, 1.000000000000000000, 0.9659258262890683122, 1.000000000000000000, 0.9659258262890683122, 1.000000000000000000, 0.9659258262890683122, 1.000000000000000000, 0.9659258262890683122, 1.000000000000000000, 0.9659258262890683122, 1.000000000000000000, 0.9659258262890683122, 1.000000000000000000, 0.9659258262890683122, 1.000000000000000000, 0.9659258262890683122, 1.000000000000000000, 0.9659258262890683122, 1.000000000000000000, 0.9659258262890683122, 1.000000000000000000, 0.9659258262890683122, 1.000000000000000000, 0.9659258262890683122, 1.000000000000000000, 0.9659258262890683122, 1.000000000000000000, 0.9659258262890683122, 1.000000000000000000, 0.9659258262890683122, 1.000000000000000000, 0.9659258262890683122, 1.000000000000000000, 0.9659258262890683122, 1.000000000000000000, 0.9659258262890683122, 1.000000000000000000, 0.9659258262890683122, 1.000000000000000000, 0.9659258262890683122, 1.000000000000000000, 0.9659258262890683122, 1.000000000000000000, 0.9659258262890683122, 1.000000000000000000, 0.9659258262890683122, 1.000000000000000000, 0.9659258262890683122, 1.000000000000000000, 0.9659258262890683122, 1.000000000000000000, 0.9659258262890683122, 1.000000000000000000, 0.9659258262890683122, 1.000000000000000000, 0.9659258262890683122, 1.000000000000000000, 0.9659258262890683122, 1.000000000000000000, 0.9659258262890683122, 1.000000000000000000, 0.9659258262890683122, 1.000000000000000000, 0.9659258262890683122, 1.000000000000000000, 0.9659258262890683122, 1.000000000000000000, 0.9659258262890683122, 1.000000000000000000, 0.9659258262890683122, 1.000000000000000000, 0.9659258262890683122, 1.000000000000000000, 0.9659258262890683122, 1.000000000000000000, 0.9659258262890683122, 1.000000000000000000, 0.9659258262890683122, 1.000000000000000000, 0.9659258262890683122, 1.000000000000000000, 0.9659258262890683122, 1.000000000000000000, 0.9659258262890683122, 1.000000000000000000, 0.9659258262890683122, 1.000000000000000000, 0.9659258262890683122, 1.000000000000000000, 0.9659258262890683122, 1.000000000000000000, 0.9659258262890683122, 1.000000000000000000, 0.9659258262890683122, 1.000000000000000000, 0.9659258262890683122, 1.000000000000000000, 0.9659258262890683122, 1.000000000000000000, 0.9659258262890683122, 1.000000000000000000, 0.9659258262890683122, 1.000000000000000000, 0.9659258262890683122, 1.000000000000000000, 0.9659258262890683122, 1.000000000000000000, 0.9659258262890683122, 1.000000000000000000, 0.9659258262890683122, 1.000000000000000000, 0.9659258262890683122, 1.000000000000000000, 0.9659258262890683122, 1.000000000000000000, 0.9659258262890683122, 1.000000000000000000, 0.9659258262890683122, 1.000000000000000000, 0.9659258262890683122, 1.000000000000000000, 0.9659258262890683122, 1.000000000000000000, 0.9659258262890683122, 1.000000000000000000, 0.9659258262890683122, 1.000000000000000000, 0.9659258262890683122, 1.000000000000000000, 0.9659258262890683122, 1.000000000000000000, 0.9659258262890683122, 1.000000000000000000, 0.9659258262890683122, 1.000000000000000000, 0.9659258262890683122, 1.000000000000000000, 0.9659258262890683122, 1.000000000000000000, 0.9659258262890683122, 1.000000000000000000, 0.9659258262890683122, 1.000000000000000000, 0.9659258262890683122, 1.000000000000000000, 0.9659258262890683122, 1.000000000000000000, 0.9659258262890683122, 1.000000000000000000, 0.9659258262890683122, 1.000000000000000000, 0.9659258262890683122, 1.000000000000000000, 0.9659258262890683122, 1.000000000000000000, 0.9659258262890683122, 1.000000000000000000, 0.9659258262890683122, 1.000000000000000000, 0.9659258262890683122, 1.000000000000000000, 0.9659258262890683122, 1.000000000000000000, 0.9659258262890683122, 1.000000000000000000, 0.9659258262890683122, 1.000000000000000000, 0.9659258262890683122, 1.000000000000000000, 0.9659258262890683122, 1.000000000000000000, 0.9659258262890683122, 1.000000000000000000, 0.9659258262890683122, 1.000000000000000000, 0.9659258262890683122, 1.000000000000000000, 0.9659258262890683122, 1.000000000000000000, 0.9659258262890683122, 1.000000000000000000, 0.9659258262890683122, 1.000000000000000000, 0.9659258262890683122, 1.000000000000000000, 0.9659258262890683122, 1.000000000000000000, 0.9659258262890683122, 1.000000000000000000, 0.9659258262890683122, 1.000000000000000000, 0.9659258262890683122, 1.000000000000000000, 0.9659258262890683122, 1.000000000000000000, 0.9659258262890683122, 1.000000000000000000, 0.9659258262890683122, 1.000000000000000000, 0.9659258262890683122, 1.000000000000000000, 0.9659258262890683122, 1.000000000000000000, 0.9659258262890683122, 1.000000000000000000, 0.9659258262890683122, 1.000000000000000000, 0.9659258262890683122, 1.000000000000000000, 0.9659258262890683122, 1.000000000000000000, 0.9659258262890683122, 1.000000000000000000, 0.9659258262890683122, 1.000000000000000000, 0.9659258262890683122, 1.000000000000000000, 0.9659258262890683122, 1.000000000000000000, 0.9659258262890683122, 1.000000000000000000, 0.9659258262890683122, 1.000000000000000000, 0.9659258262890683122, 1.000000000000000000, 0.9659258262890683122, 1.000000000000000000, 0.9659258262890683122, 1.000000000000000000, 0.9659258262890683122, 1.000000000000000000, 0.9659258262890683122, 1.000000000000000000, 0.9659258262890683122, 1.000000000000000000, 0.9659258262890683122, 1.000000000000000000, 0.9659258262890683122, 1.000000000000000000, 0.9659258262890683122, 1.000000000000000000, 0.9659258262890683122, 1.000000000000000000, 0.9659258262890683122, 1.000000000000000000, 0.9659258262890683122, 1.000000000000000000, 0.9659258262890683122, 1.000000000000000000, 0.9659258262890683122, 1.000000000000000000, 0.9659258262890683122, 1.000000000000000000, 0.9659258262890683122, 1.000000000000000000, 0.9659258262890683122, 1.000000000000000000, 0.9659258262890683122, 1.000000000000000000, 0.9659258262890683122, 1.000000000000000000, 0.9659258262890683122, 1.000000000000000000, 0.9659258262890683122, 1.000000000000000000, 0.9659258262890683122, 1.000000000000000000, 0.9659258262890683122, 1.000000000000000000, 0.9659258262890683122, 1.000000000000000000, 0.9659258262890683122, 1.000000000000000000, 0.9659258262890683122, 1.000000000000000000, 0.9659258262890683122, 1.000000000000000000, 0.9659258262890683122, 1.000000000000000000, 0.9659258262890683122, 1.000000000000000000, 0.9659258262890683122, 1.000000000000000000, 0.9659258262890683122, 1.000000000000000000, 0.9659258262890683122, 1.000000000000000000, 0.9659258262890683122, 1.000000000000000000, 0.9659258262890683122, 1.000000000000000000, 0.9659258262890683122, 1.000000000000000000, 0.9659258262890683122, 1.000000000000000000, 0.9659258262890683122, 1.000000000000000000, 0.9659258262890683122, 1.000000000000000000, 0.9659258262890683122, 1.000000000000000000, 0.9659258262890683122, 1.000000000000000000, 0.9659258262890683122, 1.000000000000000000, 0.9659258262890683122, 1.000000000000000000, 0.9659258262890683122, 1.000000000000000000, 0.9659258262890683122, 1.000000000000000000, 0.9659258262890683122, 1.000000000000000000, 0.9659258262890683122, 1.000000000000000000, 0.9659258262890683122, 1.000000000000000000, 0.9659258262890683122, 1.000000000000000000, 0.9659258262890683122, 1.000000000000000000, 0.9659258262890683122, 1.000000000000000000, 0.9659258262890683122, 1.000000000000000000, 0.9659258262890683122, 1.000000000000000000, 0.9659258262890683122, 1.000000000000000000, 0.9659258262890683122, 1.000000000000000000, 0.9659258262890683122, 1.000000000000000000, 0.9659258262890683122, 1.000000000000000000, 0.9659258262890683122, 1.000000000000000000, 0.9659258262890683122, 1.000000000000000000, 0.9659258262890683122, 1.000000000000000000, 0.9659258262890683122, 1.000000000000000000, 0.9659258262890683122, 1.000000000000000000),
 ( 0.3333333333333333703, 0.3219752754296894559, 0.3333333333333333703, 0.3219752754296894559, 0.3333333333333333703, 0.3219752754296894559, 0.3333333333333333703, 0.3219752754296894559, 0.3333333333333333703, 0.3219752754296894559, 0.3333333333333333703, 0.3219752754296894559, 0.3333333333333333703, 0.3219752754296894559, 0.3333333333333333703, 0.3219752754296894559, 0.3333333333333333703, 0.3219752754296894559, 0.3333333333333333703, 0.3219752754296894559, 0.3333333333333333703, 0.3219752754296894559, 0.3333333333333333703, 0.3219752754296894559, 0.3333333333333333703, 0.3219752754296894559, 0.3333333333333333703, 0.3219752754296894559, 0.3333333333333333703, 0.3219752754296894559, 0.3333333333333333703, 0.3219752754296894559, 0.3333333333333333703, 0.3219752754296894559, 0.3333333333333333703, 0.3219752754296894559, 0.3333333333333333703, 0.3219752754296894559, 0.3333333333333333703, 0.3219752754296894559, 0.3333333333333333703, 0.3219752754296894559, 0.3333333333333333703, 0.3219752754296894559, 0.3333333333333333703, 0.3219752754296894559, 0.3333333333333333703, 0.3219752754296894559, 0.3333333333333333703, 0.3219752754296894559, 0.3333333333333333703, 0.3219752754296894559, 0.3333333333333333703, 0.3219752754296894559, 0.3333333333333333703, 0.3219752754296894559, 0.3333333333333333703, 0.3219752754296894559, 0.3333333333333333703, 0.3219752754296894559, 0.3333333333333333703, 0.3219752754296894559, 0.3333333333333333703, 0.3219752754296894559, 0.3333333333333333703, 0.3219752754296894559, 0.3333333333333333703, 0.3219752754296894559, 0.3333333333333333703, 0.3219752754296894559, 0.3333333333333333703, 0.3219752754296894559, 0.3333333333333333703, 0.3219752754296894559, 0.3333333333333333703, 0.3219752754296894559, 0.3333333333333333703, 0.3219752754296894559, 0.3333333333333333703, 0.3219752754296894559, 0.3333333333333333703, 0.3219752754296894559, 0.3333333333333333703, 0.3219752754296894559, 0.3333333333333333703, 0.3219752754296894559, 0.3333333333333333703, 0.3219752754296894559, 0.3333333333333333703, 0.3219752754296894559, 0.3333333333333333703, 0.3219752754296894559, 0.3333333333333333703, 0.3219752754296894559, 0.3333333333333333703, 0.3219752754296894559, 0.3333333333333333703, 0.3219752754296894559, 0.3333333333333333703, 0.3219752754296894559, 0.3333333333333333703, 0.3219752754296894559, 0.3333333333333333703, 0.3219752754296894559, 0.3333333333333333703, 0.3219752754296894559, 0.3333333333333333703, 0.3219752754296894559, 0.3333333333333333703, 0.3219752754296894559, 0.3333333333333333703, 0.3219752754296894559, 0.3333333333333333703, 0.3219752754296894559, 0.3333333333333333703, 0.3219752754296894559, 0.3333333333333333703, 0.3219752754296894559, 0.3333333333333333703, 0.3219752754296894559, 0.3333333333333333703, 0.3219752754296894559, 0.3333333333333333703, 0.3219752754296894559, 0.3333333333333333703, 0.3219752754296894559, 0.3333333333333333703, 0.3219752754296894559, 0.3333333333333333703, 0.3219752754296894559, 0.3333333333333333703, 0.3219752754296894559, 0.3333333333333333703, 0.3219752754296894559, 0.3333333333333333703, 0.3219752754296894559, 0.3333333333333333703, 0.3219752754296894559, 0.3333333333333333703, 0.3219752754296894559, 0.3333333333333333703, 0.3219752754296894559, 0.3333333333333333703, 0.3219752754296894559, 0.3333333333333333703, 0.3219752754296894559, 0.3333333333333333703, 0.3219752754296894559, 0.3333333333333333703, 0.3219752754296894559, 0.3333333333333333703, 0.3219752754296894559, 0.3333333333333333703, 0.3219752754296894559, 0.3333333333333333703, 0.3219752754296894559, 0.3333333333333333703, 0.3219752754296894559, 0.3333333333333333703, 0.3219752754296894559, 0.3333333333333333703, 0.3219752754296894559, 0.3333333333333333703, 0.3219752754296894559, 0.3333333333333333703, 0.3219752754296894559, 0.3333333333333333703, 0.3219752754296894559, 0.3333333333333333703, 0.3219752754296894559, 0.3333333333333333703, 0.3219752754296894559, 0.3333333333333333703, 0.3219752754296894559, 0.3333333333333333703, 0.3219752754296894559, 0.3333333333333333703, 0.3219752754296894559, 0.3333333333333333703, 0.3219752754296894559, 0.3333333333333333703, 0.3219752754296894559, 0.3333333333333333703, 0.3219752754296894559, 0.3333333333333333703, 0.3219752754296894559, 0.3333333333333333703, 0.3219752754296894559, 0.3333333333333333703, 0.3219752754296894559, 0.3333333333333333703, 0.3219752754296894559, 0.3333333333333333703, 0.3219752754296894559, 0.3333333333333333703, 0.3219752754296894559, 0.3333333333333333703, 0.3219752754296894559, 0.3333333333333333703, 0.3219752754296894559, 0.3333333333333333703, 0.3219752754296894559, 0.3333333333333333703, 0.3219752754296894559, 0.3333333333333333703, 0.3219752754296894559, 0.3333333333333333703, 0.3219752754296894559, 0.3333333333333333703, 0.3219752754296894559, 0.3333333333333333703, 0.3219752754296894559, 0.3333333333333333703, 0.3219752754296894559, 0.3333333333333333703, 0.3219752754296894559, 0.3333333333333333703, 0.3219752754296894559, 0.3333333333333333703, 0.3219752754296894559, 0.3333333333333333703, 0.3219752754296894559, 0.3333333333333333703, 0.3219752754296894559, 0.3333333333333333703, 0.3219752754296894559, 0.3333333333333333703, 0.3219752754296894559, 0.3333333333333333703, 0.3219752754296894559, 0.3333333333333333703, 0.3219752754296894559, 0.3333333333333333703, 0.3219752754296894559, 0.3333333333333333703, 0.3219752754296894559, 0.3333333333333333703, 0.3219752754296894559, 0.3333333333333333703, 0.3219752754296894559, 0.3333333333333333703, 0.3219752754296894559, 0.3333333333333333703, 0.3219752754296894559, 0.3333333333333333703, 0.3219752754296894559, 0.3333333333333333703, 0.3219752754296894559, 0.3333333333333333703, 0.3219752754296894559, 0.3333333333333333703, 0.3219752754296894559, 0.3333333333333333703, 0.3219752754296894559, 0.3333333333333333703, 0.3219752754296894559, 0.3333333333333333703, 0.3219752754296894559, 0.3333333333333333703, 0.3219752754296894559, 0.3333333333333333703, 0.3219752754296894559, 0.3333333333333333703, 0.3219752754296894559, 0.3333333333333333703, 0.3219752754296894559, 0.3333333333333333703, 0.3219752754296894559, 0.3333333333333333703, 0.3219752754296894559, 0.3333333333333333703, 0.3219752754296894559, 0.3333333333333333703, 0.3219752754296894559, 0.3333333333333333703, 0.3219752754296894559, 0.3333333333333333703, 0.3219752754296894559, 0.3333333333333333703, 0.3219752754296894559, 0.3333333333333333703, 0.3219752754296894559, 0.3333333333333333703, 0.3219752754296894559, 0.3333333333333333703, 0.3219752754296894559, 0.3333333333333333703, 0.3219752754296894559, 0.3333333333333333703, 0.3219752754296894559, 0.3333333333333333703, 0.3219752754296894559, 0.3333333333333333703, 0.3219752754296894559, 0.3333333333333333703, 0.3219752754296894559, 0.3333333333333333703, 0.3219752754296894559, 0.3333333333333333703, 0.3219752754296894559, 0.3333333333333333703, 0.3219752754296894559, 0.3333333333333333703, 0.3219752754296894559, 0.3333333333333333703, 0.3219752754296894559, 0.3333333333333333703, 0.3219752754296894559, 0.3333333333333333703, 0.3219752754296894559, 0.3333333333333333703, 0.3219752754296894559, 0.3333333333333333703, 0.3219752754296894559, 0.3333333333333333703, 0.3219752754296894559, 0.3333333333333333703, 0.3219752754296894559, 0.3333333333333333703, 0.3219752754296894559, 0.3333333333333333703, 0.3219752754296894559, 0.3333333333333333703, 0.3219752754296894559, 0.3333333333333333703, 0.3219752754296894559, 0.3333333333333333703, 0.3219752754296894559, 0.3333333333333333703, 0.3219752754296894559, 0.3333333333333333703, 0.3219752754296894559, 0.3333333333333333703, 0.3219752754296894559, 0.3333333333333333703, 0.3219752754296894559, 0.3333333333333333703, 0.3219752754296894559, 0.3333333333333333703, 0.3219752754296894559, 0.3333333333333333703, 0.3219752754296894559, 0.3333333333333333703, 0.3219752754296894559, 0.3333333333333333703, 0.3219752754296894559, 0.3333333333333333703, 0.3219752754296894559, 0.3333333333333333703, 0.3219752754296894559, 0.3333333333333333703, 0.3219752754296894559, 0.3333333333333333703, 0.3219752754296894559, 0.3333333333333333703, 0.3219752754296894559, 0.3333333333333333703, 0.3219752754296894559, 0.3333333333333333703, 0.3219752754296894559, 0.3333333333333333703, 0.3219752754296894559, 0.3333333333333333703, 0.3219752754296894559, 0.3333333333333333703, 0.3219752754296894559, 0.3333333333333333703, 0.3219752754296894559, 0.3333333333333333703, 0.3219752754296894559, 0.3333333333333333703, 0.3219752754296894559, 0.3333333333333333703, 0.3219752754296894559, 0.3333333333333333703, 0.3219752754296894559, 0.3333333333333333703, 0.3219752754296894559, 0.3333333333333333703, 0.3219752754296894559, 0.3333333333333333703, 0.3219752754296894559, 0.3333333333333333703, 0.3219752754296894559, 0.3333333333333333703, 0.3219752754296894559, 0.3333333333333333703, 0.3219752754296894559, 0.3333333333333333703, 0.3219752754296894559, 0.3333333333333333703, 0.3219752754296894559, 0.3333333333333333703, 0.3219752754296894559, 0.3333333333333333703, 0.3219752754296894559, 0.3333333333333333703, 0.3219752754296894559, 0.3333333333333333703, 0.3219752754296894559, 0.3333333333333333703, 0.3219752754296894559, 0.3333333333333333703, 0.3219752754296894559, 0.3333333333333333703, 0.3219752754296894559, 0.3333333333333333703, 0.3219752754296894559, 0.3333333333333333703, 0.3219752754296894559, 0.3333333333333333703, 0.3219752754296894559, 0.3333333333333333703, 0.3219752754296894559, 0.3333333333333333703, 0.3219752754296894559, 0.3333333333333333703, 0.3219752754296894559, 0.3333333333333333703, 0.3219752754296894559, 0.3333333333333333703, 0.3219752754296894559, 0.3333333333333333703, 0.3219752754296894559, 0.3333333333333333703, 0.3219752754296894559, 0.3333333333333333703, 0.3219752754296894559, 0.3333333333333333703, 0.3219752754296894559, 0.3333333333333333703, 0.3219752754296894559, 0.3333333333333333703, 0.3219752754296894559, 0.3333333333333333703, 0.3219752754296894559, 0.3333333333333333703, 0.3219752754296894559, 0.3333333333333333703, 0.3219752754296894559, 0.3333333333333333703, 0.3219752754296894559, 0.3333333333333333703, 0.3219752754296894559, 0.3333333333333333703, 0.3219752754296894559, 0.3333333333333333703, 0.3219752754296894559, 0.3333333333333333703, 0.3219752754296894559, 0.3333333333333333703, 0.3219752754296894559, 0.3333333333333333703, 0.3219752754296894559, 0.3333333333333333703, 0.3219752754296894559, 0.3333333333333333703),
 ( 0.3333333333333333703, 0.3219752754296894559, 0.3333333333333333703, 0.3219752754296894559, 0.3333333333333333703, 0.3219752754296894559, 0.3333333333333333703, 0.3219752754296894559, 0.3333333333333333703, 0.3219752754296894559, 0.3333333333333333703, 0.3219752754296894559, 0.3333333333333333703, 0.3219752754296894559, 0.3333333333333333703, 0.3219752754296894559, 0.3333333333333333703, 0.3219752754296894559, 0.3333333333333333703, 0.3219752754296894559, 0.3333333333333333703, 0.3219752754296894559, 0.3333333333333333703, 0.3219752754296894559, 0.3333333333333333703, 0.3219752754296894559, 0.3333333333333333703, 0.3219752754296894559, 0.3333333333333333703, 0.3219752754296894559, 0.3333333333333333703, 0.3219752754296894559, 0.3333333333333333703, 0.3219752754296894559, 0.3333333333333333703, 0.3219752754296894559, 0.3333333333333333703, 0.3219752754296894559, 0.3333333333333333703, 0.3219752754296894559, 0.3333333333333333703, 0.3219752754296894559, 0.3333333333333333703, 0.3219752754296894559, 0.3333333333333333703, 0.3219752754296894559, 0.3333333333333333703, 0.3219752754296894559, 0.3333333333333333703, 0.3219752754296894559, 0.3333333333333333703, 0.3219752754296894559, 0.3333333333333333703, 0.3219752754296894559, 0.3333333333333333703, 0.3219752754296894559, 0.3333333333333333703, 0.3219752754296894559, 0.3333333333333333703, 0.3219752754296894559, 0.3333333333333333703, 0.3219752754296894559, 0.3333333333333333703, 0.3219752754296894559, 0.3333333333333333703, 0.3219752754296894559, 0.3333333333333333703, 0.3219752754296894559, 0.3333333333333333703, 0.3219752754296894559, 0.3333333333333333703, 0.3219752754296894559, 0.3333333333333333703, 0.3219752754296894559, 0.3333333333333333703, 0.3219752754296894559, 0.3333333333333333703, 0.3219752754296894559, 0.3333333333333333703, 0.3219752754296894559, 0.3333333333333333703, 0.3219752754296894559, 0.3333333333333333703, 0.3219752754296894559, 0.3333333333333333703, 0.3219752754296894559, 0.3333333333333333703, 0.3219752754296894559, 0.3333333333333333703, 0.3219752754296894559, 0.3333333333333333703, 0.3219752754296894559, 0.3333333333333333703, 0.3219752754296894559, 0.3333333333333333703, 0.3219752754296894559, 0.3333333333333333703, 0.3219752754296894559, 0.3333333333333333703, 0.3219752754296894559, 0.3333333333333333703, 0.3219752754296894559, 0.3333333333333333703, 0.3219752754296894559, 0.3333333333333333703, 0.3219752754296894559, 0.3333333333333333703, 0.3219752754296894559, 0.3333333333333333703, 0.3219752754296894559, 0.3333333333333333703, 0.3219752754296894559, 0.3333333333333333703, 0.3219752754296894559, 0.3333333333333333703, 0.3219752754296894559, 0.3333333333333333703, 0.3219752754296894559, 0.3333333333333333703, 0.3219752754296894559, 0.3333333333333333703, 0.3219752754296894559, 0.3333333333333333703, 0.3219752754296894559, 0.3333333333333333703, 0.3219752754296894559, 0.3333333333333333703, 0.3219752754296894559, 0.3333333333333333703, 0.3219752754296894559, 0.3333333333333333703, 0.3219752754296894559, 0.3333333333333333703, 0.3219752754296894559, 0.3333333333333333703, 0.3219752754296894559, 0.3333333333333333703, 0.3219752754296894559, 0.3333333333333333703, 0.3219752754296894559, 0.3333333333333333703, 0.3219752754296894559, 0.3333333333333333703, 0.3219752754296894559, 0.3333333333333333703, 0.3219752754296894559, 0.3333333333333333703, 0.3219752754296894559, 0.3333333333333333703, 0.3219752754296894559, 0.3333333333333333703, 0.3219752754296894559, 0.3333333333333333703, 0.3219752754296894559, 0.3333333333333333703, 0.3219752754296894559, 0.3333333333333333703, 0.3219752754296894559, 0.3333333333333333703, 0.3219752754296894559, 0.3333333333333333703, 0.3219752754296894559, 0.3333333333333333703, 0.3219752754296894559, 0.3333333333333333703, 0.3219752754296894559, 0.3333333333333333703, 0.3219752754296894559, 0.3333333333333333703, 0.3219752754296894559, 0.3333333333333333703, 0.3219752754296894559, 0.3333333333333333703, 0.3219752754296894559, 0.3333333333333333703, 0.3219752754296894559, 0.3333333333333333703, 0.3219752754296894559, 0.3333333333333333703, 0.3219752754296894559, 0.3333333333333333703, 0.3219752754296894559, 0.3333333333333333703, 0.3219752754296894559, 0.3333333333333333703, 0.3219752754296894559, 0.3333333333333333703, 0.3219752754296894559, 0.3333333333333333703, 0.3219752754296894559, 0.3333333333333333703, 0.3219752754296894559, 0.3333333333333333703, 0.3219752754296894559, 0.3333333333333333703, 0.3219752754296894559, 0.3333333333333333703, 0.3219752754296894559, 0.3333333333333333703, 0.3219752754296894559, 0.3333333333333333703, 0.3219752754296894559, 0.3333333333333333703, 0.3219752754296894559, 0.3333333333333333703, 0.3219752754296894559, 0.3333333333333333703, 0.3219752754296894559, 0.3333333333333333703, 0.3219752754296894559, 0.3333333333333333703, 0.3219752754296894559, 0.3333333333333333703, 0.3219752754296894559, 0.3333333333333333703, 0.3219752754296894559, 0.3333333333333333703, 0.3219752754296894559, 0.3333333333333333703, 0.3219752754296894559, 0.3333333333333333703, 0.3219752754296894559, 0.3333333333333333703, 0.3219752754296894559, 0.3333333333333333703, 0.3219752754296894559, 0.3333333333333333703, 0.3219752754296894559, 0.3333333333333333703, 0.3219752754296894559, 0.3333333333333333703, 0.3219752754296894559, 0.3333333333333333703, 0.3219752754296894559, 0.3333333333333333703, 0.3219752754296894559, 0.3333333333333333703, 0.3219752754296894559, 0.3333333333333333703, 0.3219752754296894559, 0.3333333333333333703, 0.3219752754296894559, 0.3333333333333333703, 0.3219752754296894559, 0.3333333333333333703, 0.3219752754296894559, 0.3333333333333333703, 0.3219752754296894559, 0.3333333333333333703, 0.3219752754296894559, 0.3333333333333333703, 0.3219752754296894559, 0.3333333333333333703, 0.3219752754296894559, 0.3333333333333333703, 0.3219752754296894559, 0.3333333333333333703, 0.3219752754296894559, 0.3333333333333333703, 0.3219752754296894559, 0.3333333333333333703, 0.3219752754296894559, 0.3333333333333333703, 0.3219752754296894559, 0.3333333333333333703, 0.3219752754296894559, 0.3333333333333333703, 0.3219752754296894559, 0.3333333333333333703, 0.3219752754296894559, 0.3333333333333333703, 0.3219752754296894559, 0.3333333333333333703, 0.3219752754296894559, 0.3333333333333333703, 0.3219752754296894559, 0.3333333333333333703, 0.3219752754296894559, 0.3333333333333333703, 0.3219752754296894559, 0.3333333333333333703, 0.3219752754296894559, 0.3333333333333333703, 0.3219752754296894559, 0.3333333333333333703, 0.3219752754296894559, 0.3333333333333333703, 0.3219752754296894559, 0.3333333333333333703, 0.3219752754296894559, 0.3333333333333333703, 0.3219752754296894559, 0.3333333333333333703, 0.3219752754296894559, 0.3333333333333333703, 0.3219752754296894559, 0.3333333333333333703, 0.3219752754296894559, 0.3333333333333333703, 0.3219752754296894559, 0.3333333333333333703, 0.3219752754296894559, 0.3333333333333333703, 0.3219752754296894559, 0.3333333333333333703, 0.3219752754296894559, 0.3333333333333333703, 0.3219752754296894559, 0.3333333333333333703, 0.3219752754296894559, 0.3333333333333333703, 0.3219752754296894559, 0.3333333333333333703, 0.3219752754296894559, 0.3333333333333333703, 0.3219752754296894559, 0.3333333333333333703, 0.3219752754296894559, 0.3333333333333333703, 0.3219752754296894559, 0.3333333333333333703, 0.3219752754296894559, 0.3333333333333333703, 0.3219752754296894559, 0.3333333333333333703, 0.3219752754296894559, 0.3333333333333333703, 0.3219752754296894559, 0.3333333333333333703, 0.3219752754296894559, 0.3333333333333333703, 0.3219752754296894559, 0.3333333333333333703, 0.3219752754296894559, 0.3333333333333333703, 0.3219752754296894559, 0.3333333333333333703, 0.3219752754296894559, 0.3333333333333333703, 0.3219752754296894559, 0.3333333333333333703, 0.3219752754296894559, 0.3333333333333333703, 0.3219752754296894559, 0.3333333333333333703, 0.3219752754296894559, 0.3333333333333333703, 0.3219752754296894559, 0.3333333333333333703, 0.3219752754296894559, 0.3333333333333333703, 0.3219752754296894559, 0.3333333333333333703, 0.3219752754296894559, 0.3333333333333333703, 0.3219752754296894559, 0.3333333333333333703, 0.3219752754296894559, 0.3333333333333333703, 0.3219752754296894559, 0.3333333333333333703, 0.3219752754296894559, 0.3333333333333333703, 0.3219752754296894559, 0.3333333333333333703, 0.3219752754296894559, 0.3333333333333333703, 0.3219752754296894559, 0.3333333333333333703, 0.3219752754296894559, 0.3333333333333333703, 0.3219752754296894559, 0.3333333333333333703, 0.3219752754296894559, 0.3333333333333333703, 0.3219752754296894559, 0.3333333333333333703, 0.3219752754296894559, 0.3333333333333333703, 0.3219752754296894559, 0.3333333333333333703, 0.3219752754296894559, 0.3333333333333333703, 0.3219752754296894559, 0.3333333333333333703, 0.3219752754296894559, 0.3333333333333333703, 0.3219752754296894559, 0.3333333333333333703, 0.3219752754296894559, 0.3333333333333333703, 0.3219752754296894559, 0.3333333333333333703, 0.3219752754296894559, 0.3333333333333333703, 0.3219752754296894559, 0.3333333333333333703, 0.3219752754296894559, 0.3333333333333333703, 0.3219752754296894559, 0.3333333333333333703, 0.3219752754296894559, 0.3333333333333333703, 0.3219752754296894559, 0.3333333333333333703, 0.3219752754296894559, 0.3333333333333333703, 0.3219752754296894559, 0.3333333333333333703, 0.3219752754296894559, 0.3333333333333333703, 0.3219752754296894559, 0.3333333333333333703, 0.3219752754296894559, 0.3333333333333333703, 0.3219752754296894559, 0.3333333333333333703, 0.3219752754296894559, 0.3333333333333333703, 0.3219752754296894559, 0.3333333333333333703, 0.3219752754296894559, 0.3333333333333333703, 0.3219752754296894559, 0.3333333333333333703, 0.3219752754296894559, 0.3333333333333333703, 0.3219752754296894559, 0.3333333333333333703, 0.3219752754296894559, 0.3333333333333333703, 0.3219752754296894559, 0.3333333333333333703, 0.3219752754296894559, 0.3333333333333333703, 0.3219752754296894559, 0.3333333333333333703, 0.3219752754296894559, 0.3333333333333333703, 0.3219752754296894559, 0.3333333333333333703, 0.3219752754296894559, 0.3333333333333333703, 0.3219752754296894559, 0.3333333333333333703, 0.3219752754296894559, 0.3333333333333333703, 0.3219752754296894559, 0.3333333333333333703, 0.3219752754296894559, 0.3333333333333333703, 0.3219752754296894559, 0.3333333333333333703, 0.3219752754296894559, 0.3333333333333333703, 0.3219752754296894559, 0.3333333333333333703),
 ( 1.000000000000000000, 0.9659258262890683122, 1.000000000000000000, 0.9659258262890683122, 1.000000000000000000, 0.9659258262890683122, 1.000000000000000000, 0.9659258262890683122, 1.000000000000000000, 0.9659258262890683122, 1.000000000000000000, 0.9659258262890683122, 1.000000000000000000, 0.9659258262890683122, 1.000000000000000000, 0.9659258262890683122, 1.000000000000000000, 0.9659258262890683122, 1.000000000000000000, 0.9659258262890683122, 1.000000000000000000, 0.9659258262890683122, 1.000000000000000000, 0.9659258262890683122, 1.000000000000000000, 0.9659258262890683122, 1.000000000000000000, 0.9659258262890683122, 1.000000000000000000, 0.9659258262890683122, 1.000000000000000000, 0.9659258262890683122, 1.000000000000000000, 0.9659258262890683122, 1.000000000000000000, 0.9659258262890683122, 1.000000000000000000, 0.9659258262890683122, 1.000000000000000000, 0.9659258262890683122, 1.000000000000000000, 0.9659258262890683122, 1.000000000000000000, 0.9659258262890683122, 1.000000000000000000, 0.9659258262890683122, 1.000000000000000000, 0.9659258262890683122, 1.000000000000000000, 0.9659258262890683122, 1.000000000000000000, 0.9659258262890683122, 1.000000000000000000, 0.9659258262890683122, 1.000000000000000000, 0.9659258262890683122, 1.000000000000000000, 0.9659258262890683122, 1.000000000000000000, 0.9659258262890683122, 1.000000000000000000, 0.9659258262890683122, 1.000000000000000000, 0.9659258262890683122, 1.000000000000000000, 0.9659258262890683122, 1.000000000000000000, 0.9659258262890683122, 1.000000000000000000, 0.9659258262890683122, 1.000000000000000000, 0.9659258262890683122, 1.000000000000000000, 0.9659258262890683122, 1.000000000000000000, 0.9659258262890683122, 1.000000000000000000, 0.9659258262890683122, 1.000000000000000000, 0.9659258262890683122, 1.000000000000000000, 0.9659258262890683122, 1.000000000000000000, 0.9659258262890683122, 1.000000000000000000, 0.9659258262890683122, 1.000000000000000000, 0.9659258262890683122, 1.000000000000000000, 0.9659258262890683122, 1.000000000000000000, 0.9659258262890683122, 1.000000000000000000, 0.9659258262890683122, 1.000000000000000000, 0.9659258262890683122, 1.000000000000000000, 0.9659258262890683122, 1.000000000000000000, 0.9659258262890683122, 1.000000000000000000, 0.9659258262890683122, 1.000000000000000000, 0.9659258262890683122, 1.000000000000000000, 0.9659258262890683122, 1.000000000000000000, 0.9659258262890683122, 1.000000000000000000, 0.9659258262890683122, 1.000000000000000000, 0.9659258262890683122, 1.000000000000000000, 0.9659258262890683122, 1.000000000000000000, 0.9659258262890683122, 1.000000000000000000, 0.9659258262890683122, 1.000000000000000000, 0.9659258262890683122, 1.000000000000000000, 0.9659258262890683122, 1.000000000000000000, 0.9659258262890683122, 1.000000000000000000, 0.9659258262890683122, 1.000000000000000000, 0.9659258262890683122, 1.000000000000000000, 0.9659258262890683122, 1.000000000000000000, 0.9659258262890683122, 1.000000000000000000, 0.9659258262890683122, 1.000000000000000000, 0.9659258262890683122, 1.000000000000000000, 0.9659258262890683122, 1.000000000000000000, 0.9659258262890683122, 1.000000000000000000, 0.9659258262890683122, 1.000000000000000000, 0.9659258262890683122, 1.000000000000000000, 0.9659258262890683122, 1.000000000000000000, 0.9659258262890683122, 1.000000000000000000, 0.9659258262890683122, 1.000000000000000000, 0.9659258262890683122, 1.000000000000000000, 0.9659258262890683122, 1.000000000000000000, 0.9659258262890683122, 1.000000000000000000, 0.9659258262890683122, 1.000000000000000000, 0.9659258262890683122, 1.000000000000000000, 0.9659258262890683122, 1.000000000000000000, 0.9659258262890683122, 1.000000000000000000, 0.9659258262890683122, 1.000000000000000000, 0.9659258262890683122, 1.000000000000000000, 0.9659258262890683122, 1.000000000000000000, 0.9659258262890683122, 1.000000000000000000, 0.9659258262890683122, 1.000000000000000000, 0.9659258262890683122, 1.000000000000000000, 0.9659258262890683122, 1.000000000000000000, 0.9659258262890683122, 1.000000000000000000, 0.9659258262890683122, 1.000000000000000000, 0.9659258262890683122, 1.000000000000000000, 0.9659258262890683122, 1.000000000000000000, 0.9659258262890683122, 1.000000000000000000, 0.9659258262890683122, 1.000000000000000000, 0.9659258262890683122, 1.000000000000000000, 0.9659258262890683122, 1.000000000000000000, 0.9659258262890683122, 1.000000000000000000, 0.9659258262890683122, 1.000000000000000000, 0.9659258262890683122, 1.000000000000000000, 0.9659258262890683122, 1.000000000000000000, 0.9659258262890683122, 1.000000000000000000, 0.9659258262890683122, 1.000000000000000000, 0.9659258262890683122, 1.000000000000000000, 0.9659258262890683122, 1.000000000000000000, 0.9659258262890683122, 1.000000000000000000, 0.9659258262890683122, 1.000000000000000000, 0.9659258262890683122, 1.000000000000000000, 0.9659258262890683122, 1.000000000000000000, 0.9659258262890683122, 1.000000000000000000, 0.9659258262890683122, 1.000000000000000000, 0.9659258262890683122, 1.000000000000000000, 0.9659258262890683122, 1.000000000000000000, 0.9659258262890683122, 1.000000000000000000, 0.9659258262890683122, 1.000000000000000000, 0.9659258262890683122, 1.000000000000000000, 0.9659258262890683122, 1.000000000000000000, 0.9659258262890683122, 1.000000000000000000, 0.9659258262890683122, 1.000000000000000000, 0.9659258262890683122, 1.000000000000000000, 0.9659258262890683122, 1.000000000000000000, 0.9659258262890683122, 1.000000000000000000, 0.9659258262890683122, 1.000000000000000000, 0.9659258262890683122, 1.000000000000000000, 0.9659258262890683122, 1.000000000000000000, 0.9659258262890683122, 1.000000000000000000, 0.9659258262890683122, 1.000000000000000000, 0.9659258262890683122, 1.000000000000000000, 0.9659258262890683122, 1.000000000000000000, 0.9659258262890683122, 1.000000000000000000, 0.9659258262890683122, 1.000000000000000000, 0.9659258262890683122, 1.000000000000000000, 0.9659258262890683122, 1.000000000000000000, 0.9659258262890683122, 1.000000000000000000, 0.9659258262890683122, 1.000000000000000000, 0.9659258262890683122, 1.000000000000000000, 0.9659258262890683122, 1.000000000000000000, 0.9659258262890683122, 1.000000000000000000, 0.9659258262890683122, 1.000000000000000000, 0.9659258262890683122, 1.000000000000000000, 0.9659258262890683122, 1.000000000000000000, 0.9659258262890683122, 1.000000000000000000, 0.9659258262890683122, 1.000000000000000000, 0.9659258262890683122, 1.000000000000000000, 0.9659258262890683122, 1.000000000000000000, 0.9659258262890683122, 1.000000000000000000, 0.9659258262890683122, 1.000000000000000000, 0.9659258262890683122, 1.000000000000000000, 0.9659258262890683122, 1.000000000000000000, 0.9659258262890683122, 1.000000000000000000, 0.9659258262890683122, 1.000000000000000000, 0.9659258262890683122, 1.000000000000000000, 0.9659258262890683122, 1.000000000000000000, 0.9659258262890683122, 1.000000000000000000, 0.9659258262890683122, 1.000000000000000000, 0.9659258262890683122, 1.000000000000000000, 0.9659258262890683122, 1.000000000000000000, 0.9659258262890683122, 1.000000000000000000, 0.9659258262890683122, 1.000000000000000000, 0.9659258262890683122, 1.000000000000000000, 0.9659258262890683122, 1.000000000000000000, 0.9659258262890683122, 1.000000000000000000, 0.9659258262890683122, 1.000000000000000000, 0.9659258262890683122, 1.000000000000000000, 0.9659258262890683122, 1.000000000000000000, 0.9659258262890683122, 1.000000000000000000, 0.9659258262890683122, 1.000000000000000000, 0.9659258262890683122, 1.000000000000000000, 0.9659258262890683122, 1.000000000000000000, 0.9659258262890683122, 1.000000000000000000, 0.9659258262890683122, 1.000000000000000000, 0.9659258262890683122, 1.000000000000000000, 0.9659258262890683122, 1.000000000000000000, 0.9659258262890683122, 1.000000000000000000, 0.9659258262890683122, 1.000000000000000000, 0.9659258262890683122, 1.000000000000000000, 0.9659258262890683122, 1.000000000000000000, 0.9659258262890683122, 1.000000000000000000, 0.9659258262890683122, 1.000000000000000000, 0.9659258262890683122, 1.000000000000000000, 0.9659258262890683122, 1.000000000000000000, 0.9659258262890683122, 1.000000000000000000, 0.9659258262890683122, 1.000000000000000000, 0.9659258262890683122, 1.000000000000000000, 0.9659258262890683122, 1.000000000000000000, 0.9659258262890683122, 1.000000000000000000, 0.9659258262890683122, 1.000000000000000000, 0.9659258262890683122, 1.000000000000000000, 0.9659258262890683122, 1.000000000000000000, 0.9659258262890683122, 1.000000000000000000, 0.9659258262890683122, 1.000000000000000000, 0.9659258262890683122, 1.000000000000000000, 0.9659258262890683122, 1.000000000000000000, 0.9659258262890683122, 1.000000000000000000, 0.9659258262890683122, 1.000000000000000000, 0.9659258262890683122, 1.000000000000000000, 0.9659258262890683122, 1.000000000000000000, 0.9659258262890683122, 1.000000000000000000, 0.9659258262890683122, 1.000000000000000000, 0.9659258262890683122, 1.000000000000000000, 0.9659258262890683122, 1.000000000000000000, 0.9659258262890683122, 1.000000000000000000, 0.9659258262890683122, 1.000000000000000000, 0.9659258262890683122, 1.000000000000000000, 0.9659258262890683122, 1.000000000000000000, 0.9659258262890683122, 1.000000000000000000, 0.9659258262890683122, 1.000000000000000000, 0.9659258262890683122, 1.000000000000000000, 0.9659258262890683122, 1.000000000000000000, 0.9659258262890683122, 1.000000000000000000, 0.9659258262890683122, 1.000000000000000000, 0.9659258262890683122, 1.000000000000000000, 0.9659258262890683122, 1.000000000000000000, 0.9659258262890683122, 1.000000000000000000, 0.9659258262890683122, 1.000000000000000000, 0.9659258262890683122, 1.000000000000000000, 0.9659258262890683122, 1.000000000000000000, 0.9659258262890683122, 1.000000000000000000, 0.9659258262890683122, 1.000000000000000000, 0.9659258262890683122, 1.000000000000000000, 0.9659258262890683122, 1.000000000000000000, 0.9659258262890683122, 1.000000000000000000, 0.9659258262890683122, 1.000000000000000000, 0.9659258262890683122, 1.000000000000000000, 0.9659258262890683122, 1.000000000000000000, 0.9659258262890683122, 1.000000000000000000, 0.9659258262890683122, 1.000000000000000000, 0.9659258262890683122, 1.000000000000000000),
 ( 0.3333333333333333703, 0.3219752754296894559, 0.3333333333333333703, 0.3219752754296894559, 0.3333333333333333703, 0.3219752754296894559, 0.3333333333333333703, 0.3219752754296894559, 0.3333333333333333703, 0.3219752754296894559, 0.3333333333333333703, 0.3219752754296894559, 0.3333333333333333703, 0.3219752754296894559, 0.3333333333333333703, 0.3219752754296894559, 0.3333333333333333703, 0.3219752754296894559, 0.3333333333333333703, 0.3219752754296894559, 0.3333333333333333703, 0.3219752754296894559, 0.3333333333333333703, 0.3219752754296894559, 0.3333333333333333703, 0.3219752754296894559, 0.3333333333333333703, 0.3219752754296894559, 0.3333333333333333703, 0.3219752754296894559, 0.3333333333333333703, 0.3219752754296894559, 0.3333333333333333703, 0.3219752754296894559, 0.3333333333333333703, 0.3219752754296894559, 0.3333333333333333703, 0.3219752754296894559, 0.3333333333333333703, 0.3219752754296894559, 0.3333333333333333703, 0.3219752754296894559, 0.3333333333333333703, 0.3219752754296894559, 0.3333333333333333703, 0.3219752754296894559, 0.3333333333333333703, 0.3219752754296894559, 0.3333333333333333703, 0.3219752754296894559, 0.3333333333333333703, 0.3219752754296894559, 0.3333333333333333703, 0.3219752754296894559, 0.3333333333333333703, 0.3219752754296894559, 0.3333333333333333703, 0.3219752754296894559, 0.3333333333333333703, 0.3219752754296894559, 0.3333333333333333703, 0.3219752754296894559, 0.3333333333333333703, 0.3219752754296894559, 0.3333333333333333703, 0.3219752754296894559, 0.3333333333333333703, 0.3219752754296894559, 0.3333333333333333703, 0.3219752754296894559, 0.3333333333333333703, 0.3219752754296894559, 0.3333333333333333703, 0.3219752754296894559, 0.3333333333333333703, 0.3219752754296894559, 0.3333333333333333703, 0.3219752754296894559, 0.3333333333333333703, 0.3219752754296894559, 0.3333333333333333703, 0.3219752754296894559, 0.3333333333333333703, 0.3219752754296894559, 0.3333333333333333703, 0.3219752754296894559, 0.3333333333333333703, 0.3219752754296894559, 0.3333333333333333703, 0.3219752754296894559, 0.3333333333333333703, 0.3219752754296894559, 0.3333333333333333703, 0.3219752754296894559, 0.3333333333333333703, 0.3219752754296894559, 0.3333333333333333703, 0.3219752754296894559, 0.3333333333333333703, 0.3219752754296894559, 0.3333333333333333703, 0.3219752754296894559, 0.3333333333333333703, 0.3219752754296894559, 0.3333333333333333703, 0.3219752754296894559, 0.3333333333333333703, 0.3219752754296894559, 0.3333333333333333703, 0.3219752754296894559, 0.3333333333333333703, 0.3219752754296894559, 0.3333333333333333703, 0.3219752754296894559, 0.3333333333333333703, 0.3219752754296894559, 0.3333333333333333703, 0.3219752754296894559, 0.3333333333333333703, 0.3219752754296894559, 0.3333333333333333703, 0.3219752754296894559, 0.3333333333333333703, 0.3219752754296894559, 0.3333333333333333703, 0.3219752754296894559, 0.3333333333333333703, 0.3219752754296894559, 0.3333333333333333703, 0.3219752754296894559, 0.3333333333333333703, 0.3219752754296894559, 0.3333333333333333703, 0.3219752754296894559, 0.3333333333333333703, 0.3219752754296894559, 0.3333333333333333703, 0.3219752754296894559, 0.3333333333333333703, 0.3219752754296894559, 0.3333333333333333703, 0.3219752754296894559, 0.3333333333333333703, 0.3219752754296894559, 0.3333333333333333703, 0.3219752754296894559, 0.3333333333333333703, 0.3219752754296894559, 0.3333333333333333703, 0.3219752754296894559, 0.3333333333333333703, 0.3219752754296894559, 0.3333333333333333703, 0.3219752754296894559, 0.3333333333333333703, 0.3219752754296894559, 0.3333333333333333703, 0.3219752754296894559, 0.3333333333333333703, 0.3219752754296894559, 0.3333333333333333703, 0.3219752754296894559, 0.3333333333333333703, 0.3219752754296894559, 0.3333333333333333703, 0.3219752754296894559, 0.3333333333333333703, 0.3219752754296894559, 0.3333333333333333703, 0.3219752754296894559, 0.3333333333333333703, 0.3219752754296894559, 0.3333333333333333703, 0.3219752754296894559, 0.3333333333333333703, 0.3219752754296894559, 0.3333333333333333703, 0.3219752754296894559, 0.3333333333333333703, 0.3219752754296894559, 0.3333333333333333703, 0.3219752754296894559, 0.3333333333333333703, 0.3219752754296894559, 0.3333333333333333703, 0.3219752754296894559, 0.3333333333333333703, 0.3219752754296894559, 0.3333333333333333703, 0.3219752754296894559, 0.3333333333333333703, 0.3219752754296894559, 0.3333333333333333703, 0.3219752754296894559, 0.3333333333333333703, 0.3219752754296894559, 0.3333333333333333703, 0.3219752754296894559, 0.3333333333333333703, 0.3219752754296894559, 0.3333333333333333703, 0.3219752754296894559, 0.3333333333333333703, 0.3219752754296894559, 0.3333333333333333703, 0.3219752754296894559, 0.3333333333333333703, 0.3219752754296894559, 0.3333333333333333703, 0.3219752754296894559, 0.3333333333333333703, 0.3219752754296894559, 0.3333333333333333703, 0.3219752754296894559, 0.3333333333333333703, 0.3219752754296894559, 0.3333333333333333703, 0.3219752754296894559, 0.3333333333333333703, 0.3219752754296894559, 0.3333333333333333703, 0.3219752754296894559, 0.3333333333333333703, 0.3219752754296894559, 0.3333333333333333703, 0.3219752754296894559, 0.3333333333333333703, 0.3219752754296894559, 0.3333333333333333703, 0.3219752754296894559, 0.3333333333333333703, 0.3219752754296894559, 0.3333333333333333703, 0.3219752754296894559, 0.3333333333333333703, 0.3219752754296894559, 0.3333333333333333703, 0.3219752754296894559, 0.3333333333333333703, 0.3219752754296894559, 0.3333333333333333703, 0.3219752754296894559, 0.3333333333333333703, 0.3219752754296894559, 0.3333333333333333703, 0.3219752754296894559, 0.3333333333333333703, 0.3219752754296894559, 0.3333333333333333703, 0.3219752754296894559, 0.3333333333333333703, 0.3219752754296894559, 0.3333333333333333703, 0.3219752754296894559, 0.3333333333333333703, 0.3219752754296894559, 0.3333333333333333703, 0.3219752754296894559, 0.3333333333333333703, 0.3219752754296894559, 0.3333333333333333703, 0.3219752754296894559, 0.3333333333333333703, 0.3219752754296894559, 0.3333333333333333703, 0.3219752754296894559, 0.3333333333333333703, 0.3219752754296894559, 0.3333333333333333703, 0.3219752754296894559, 0.3333333333333333703, 0.3219752754296894559, 0.3333333333333333703, 0.3219752754296894559, 0.3333333333333333703, 0.3219752754296894559, 0.3333333333333333703, 0.3219752754296894559, 0.3333333333333333703, 0.3219752754296894559, 0.3333333333333333703, 0.3219752754296894559, 0.3333333333333333703, 0.3219752754296894559, 0.3333333333333333703, 0.3219752754296894559, 0.3333333333333333703, 0.3219752754296894559, 0.3333333333333333703, 0.3219752754296894559, 0.3333333333333333703, 0.3219752754296894559, 0.3333333333333333703, 0.3219752754296894559, 0.3333333333333333703, 0.3219752754296894559, 0.3333333333333333703, 0.3219752754296894559, 0.3333333333333333703, 0.3219752754296894559, 0.3333333333333333703, 0.3219752754296894559, 0.3333333333333333703, 0.3219752754296894559, 0.3333333333333333703, 0.3219752754296894559, 0.3333333333333333703, 0.3219752754296894559, 0.3333333333333333703, 0.3219752754296894559, 0.3333333333333333703, 0.3219752754296894559, 0.3333333333333333703, 0.3219752754296894559, 0.3333333333333333703, 0.3219752754296894559, 0.3333333333333333703, 0.3219752754296894559, 0.3333333333333333703, 0.3219752754296894559, 0.3333333333333333703, 0.3219752754296894559, 0.3333333333333333703, 0.3219752754296894559, 0.3333333333333333703, 0.3219752754296894559, 0.3333333333333333703, 0.3219752754296894559, 0.3333333333333333703, 0.3219752754296894559, 0.3333333333333333703, 0.3219752754296894559, 0.3333333333333333703, 0.3219752754296894559, 0.3333333333333333703, 0.3219752754296894559, 0.3333333333333333703, 0.3219752754296894559, 0.3333333333333333703, 0.3219752754296894559, 0.3333333333333333703, 0.3219752754296894559, 0.3333333333333333703, 0.3219752754296894559, 0.3333333333333333703, 0.3219752754296894559, 0.3333333333333333703, 0.3219752754296894559, 0.3333333333333333703, 0.3219752754296894559, 0.3333333333333333703, 0.3219752754296894559, 0.3333333333333333703, 0.3219752754296894559, 0.3333333333333333703, 0.3219752754296894559, 0.3333333333333333703, 0.3219752754296894559, 0.3333333333333333703, 0.3219752754296894559, 0.3333333333333333703, 0.3219752754296894559, 0.3333333333333333703, 0.3219752754296894559, 0.3333333333333333703, 0.3219752754296894559, 0.3333333333333333703, 0.3219752754296894559, 0.3333333333333333703, 0.3219752754296894559, 0.3333333333333333703, 0.3219752754296894559, 0.3333333333333333703, 0.3219752754296894559, 0.3333333333333333703, 0.3219752754296894559, 0.3333333333333333703, 0.3219752754296894559, 0.3333333333333333703, 0.3219752754296894559, 0.3333333333333333703, 0.3219752754296894559, 0.3333333333333333703, 0.3219752754296894559, 0.3333333333333333703, 0.3219752754296894559, 0.3333333333333333703, 0.3219752754296894559, 0.3333333333333333703, 0.3219752754296894559, 0.3333333333333333703, 0.3219752754296894559, 0.3333333333333333703, 0.3219752754296894559, 0.3333333333333333703, 0.3219752754296894559, 0.3333333333333333703, 0.3219752754296894559, 0.3333333333333333703, 0.3219752754296894559, 0.3333333333333333703, 0.3219752754296894559, 0.3333333333333333703, 0.3219752754296894559, 0.3333333333333333703, 0.3219752754296894559, 0.3333333333333333703, 0.3219752754296894559, 0.3333333333333333703, 0.3219752754296894559, 0.3333333333333333703, 0.3219752754296894559, 0.3333333333333333703, 0.3219752754296894559, 0.3333333333333333703, 0.3219752754296894559, 0.3333333333333333703, 0.3219752754296894559, 0.3333333333333333703, 0.3219752754296894559, 0.3333333333333333703, 0.3219752754296894559, 0.3333333333333333703, 0.3219752754296894559, 0.3333333333333333703, 0.3219752754296894559, 0.3333333333333333703, 0.3219752754296894559, 0.3333333333333333703, 0.3219752754296894559, 0.3333333333333333703, 0.3219752754296894559, 0.3333333333333333703, 0.3219752754296894559, 0.3333333333333333703, 0.3219752754296894559, 0.3333333333333333703, 0.3219752754296894559, 0.3333333333333333703, 0.3219752754296894559, 0.3333333333333333703, 0.3219752754296894559, 0.3333333333333333703, 0.3219752754296894559, 0.3333333333333333703, 0.3219752754296894559, 0.3333333333333333703, 0.3219752754296894559, 0.3333333333333333703, 0.3219752754296894559, 0.3333333333333333703, 0.3219752754296894559, 0.3333333333333333703, 0.3219752754296894559, 0.3333333333333333703, 0.3219752754296894559, 0.3333333333333333703),
 ( 0.3333333333333333703, 0.3219752754296894559, 0.3333333333333333703, 0.3219752754296894559, 0.3333333333333333703, 0.3219752754296894559, 0.3333333333333333703, 0.3219752754296894559, 0.3333333333333333703, 0.3219752754296894559, 0.3333333333333333703, 0.3219752754296894559, 0.3333333333333333703, 0.3219752754296894559, 0.3333333333333333703, 0.3219752754296894559, 0.3333333333333333703, 0.3219752754296894559, 0.3333333333333333703, 0.3219752754296894559, 0.3333333333333333703, 0.3219752754296894559, 0.3333333333333333703, 0.3219752754296894559, 0.3333333333333333703, 0.3219752754296894559, 0.3333333333333333703, 0.3219752754296894559, 0.3333333333333333703, 0.3219752754296894559, 0.3333333333333333703, 0.3219752754296894559, 0.3333333333333333703, 0.3219752754296894559, 0.3333333333333333703, 0.3219752754296894559, 0.3333333333333333703, 0.3219752754296894559, 0.3333333333333333703, 0.3219752754296894559, 0.3333333333333333703, 0.3219752754296894559, 0.3333333333333333703, 0.3219752754296894559, 0.3333333333333333703, 0.3219752754296894559, 0.3333333333333333703, 0.3219752754296894559, 0.3333333333333333703, 0.3219752754296894559, 0.3333333333333333703, 0.3219752754296894559, 0.3333333333333333703, 0.3219752754296894559, 0.3333333333333333703, 0.3219752754296894559, 0.3333333333333333703, 0.3219752754296894559, 0.3333333333333333703, 0.3219752754296894559, 0.3333333333333333703, 0.3219752754296894559, 0.3333333333333333703, 0.3219752754296894559, 0.3333333333333333703, 0.3219752754296894559, 0.3333333333333333703, 0.3219752754296894559, 0.3333333333333333703, 0.3219752754296894559, 0.3333333333333333703, 0.3219752754296894559, 0.3333333333333333703, 0.3219752754296894559, 0.3333333333333333703, 0.3219752754296894559, 0.3333333333333333703, 0.3219752754296894559, 0.3333333333333333703, 0.3219752754296894559, 0.3333333333333333703, 0.3219752754296894559, 0.3333333333333333703, 0.3219752754296894559, 0.3333333333333333703, 0.3219752754296894559, 0.3333333333333333703, 0.3219752754296894559, 0.3333333333333333703, 0.3219752754296894559, 0.3333333333333333703, 0.3219752754296894559, 0.3333333333333333703, 0.3219752754296894559, 0.3333333333333333703, 0.3219752754296894559, 0.3333333333333333703, 0.3219752754296894559, 0.3333333333333333703, 0.3219752754296894559, 0.3333333333333333703, 0.3219752754296894559, 0.3333333333333333703, 0.3219752754296894559, 0.3333333333333333703, 0.3219752754296894559, 0.3333333333333333703, 0.3219752754296894559, 0.3333333333333333703, 0.3219752754296894559, 0.3333333333333333703, 0.3219752754296894559, 0.3333333333333333703, 0.3219752754296894559, 0.3333333333333333703, 0.3219752754296894559, 0.3333333333333333703, 0.3219752754296894559, 0.3333333333333333703, 0.3219752754296894559, 0.3333333333333333703, 0.3219752754296894559, 0.3333333333333333703, 0.3219752754296894559, 0.3333333333333333703, 0.3219752754296894559, 0.3333333333333333703, 0.3219752754296894559, 0.3333333333333333703, 0.3219752754296894559, 0.3333333333333333703, 0.3219752754296894559, 0.3333333333333333703, 0.3219752754296894559, 0.3333333333333333703, 0.3219752754296894559, 0.3333333333333333703, 0.3219752754296894559, 0.3333333333333333703, 0.3219752754296894559, 0.3333333333333333703, 0.3219752754296894559, 0.3333333333333333703, 0.3219752754296894559, 0.3333333333333333703, 0.3219752754296894559, 0.3333333333333333703, 0.3219752754296894559, 0.3333333333333333703, 0.3219752754296894559, 0.3333333333333333703, 0.3219752754296894559, 0.3333333333333333703, 0.3219752754296894559, 0.3333333333333333703, 0.3219752754296894559, 0.3333333333333333703, 0.3219752754296894559, 0.3333333333333333703, 0.3219752754296894559, 0.3333333333333333703, 0.3219752754296894559, 0.3333333333333333703, 0.3219752754296894559, 0.3333333333333333703, 0.3219752754296894559, 0.3333333333333333703, 0.3219752754296894559, 0.3333333333333333703, 0.3219752754296894559, 0.3333333333333333703, 0.3219752754296894559, 0.3333333333333333703, 0.3219752754296894559, 0.3333333333333333703, 0.3219752754296894559, 0.3333333333333333703, 0.3219752754296894559, 0.3333333333333333703, 0.3219752754296894559, 0.3333333333333333703, 0.3219752754296894559, 0.3333333333333333703, 0.3219752754296894559, 0.3333333333333333703, 0.3219752754296894559, 0.3333333333333333703, 0.3219752754296894559, 0.3333333333333333703, 0.3219752754296894559, 0.3333333333333333703, 0.3219752754296894559, 0.3333333333333333703, 0.3219752754296894559, 0.3333333333333333703, 0.3219752754296894559, 0.3333333333333333703, 0.3219752754296894559, 0.3333333333333333703, 0.3219752754296894559, 0.3333333333333333703, 0.3219752754296894559, 0.3333333333333333703, 0.3219752754296894559, 0.3333333333333333703, 0.3219752754296894559, 0.3333333333333333703, 0.3219752754296894559, 0.3333333333333333703, 0.3219752754296894559, 0.3333333333333333703, 0.3219752754296894559, 0.3333333333333333703, 0.3219752754296894559, 0.3333333333333333703, 0.3219752754296894559, 0.3333333333333333703, 0.3219752754296894559, 0.3333333333333333703, 0.3219752754296894559, 0.3333333333333333703, 0.3219752754296894559, 0.3333333333333333703, 0.3219752754296894559, 0.3333333333333333703, 0.3219752754296894559, 0.3333333333333333703, 0.3219752754296894559, 0.3333333333333333703, 0.3219752754296894559, 0.3333333333333333703, 0.3219752754296894559, 0.3333333333333333703, 0.3219752754296894559, 0.3333333333333333703, 0.3219752754296894559, 0.3333333333333333703, 0.3219752754296894559, 0.3333333333333333703, 0.3219752754296894559, 0.3333333333333333703, 0.3219752754296894559, 0.3333333333333333703, 0.3219752754296894559, 0.3333333333333333703, 0.3219752754296894559, 0.3333333333333333703, 0.3219752754296894559, 0.3333333333333333703, 0.3219752754296894559, 0.3333333333333333703, 0.3219752754296894559, 0.3333333333333333703, 0.3219752754296894559, 0.3333333333333333703, 0.3219752754296894559, 0.3333333333333333703, 0.3219752754296894559, 0.3333333333333333703, 0.3219752754296894559, 0.3333333333333333703, 0.3219752754296894559, 0.3333333333333333703, 0.3219752754296894559, 0.3333333333333333703, 0.3219752754296894559, 0.3333333333333333703, 0.3219752754296894559, 0.3333333333333333703, 0.3219752754296894559, 0.3333333333333333703, 0.3219752754296894559, 0.3333333333333333703, 0.3219752754296894559, 0.3333333333333333703, 0.3219752754296894559, 0.3333333333333333703, 0.3219752754296894559, 0.3333333333333333703, 0.3219752754296894559, 0.3333333333333333703, 0.3219752754296894559, 0.3333333333333333703, 0.3219752754296894559, 0.3333333333333333703, 0.3219752754296894559, 0.3333333333333333703, 0.3219752754296894559, 0.3333333333333333703, 0.3219752754296894559, 0.3333333333333333703, 0.3219752754296894559, 0.3333333333333333703, 0.3219752754296894559, 0.3333333333333333703, 0.3219752754296894559, 0.3333333333333333703, 0.3219752754296894559, 0.3333333333333333703, 0.3219752754296894559, 0.3333333333333333703, 0.3219752754296894559, 0.3333333333333333703, 0.3219752754296894559, 0.3333333333333333703, 0.3219752754296894559, 0.3333333333333333703, 0.3219752754296894559, 0.3333333333333333703, 0.3219752754296894559, 0.3333333333333333703, 0.3219752754296894559, 0.3333333333333333703, 0.3219752754296894559, 0.3333333333333333703, 0.3219752754296894559, 0.3333333333333333703, 0.3219752754296894559, 0.3333333333333333703, 0.3219752754296894559, 0.3333333333333333703, 0.3219752754296894559, 0.3333333333333333703, 0.3219752754296894559, 0.3333333333333333703, 0.3219752754296894559, 0.3333333333333333703, 0.3219752754296894559, 0.3333333333333333703, 0.3219752754296894559, 0.3333333333333333703, 0.3219752754296894559, 0.3333333333333333703, 0.3219752754296894559, 0.3333333333333333703, 0.3219752754296894559, 0.3333333333333333703, 0.3219752754296894559, 0.3333333333333333703, 0.3219752754296894559, 0.3333333333333333703, 0.3219752754296894559, 0.3333333333333333703, 0.3219752754296894559, 0.3333333333333333703, 0.3219752754296894559, 0.3333333333333333703, 0.3219752754296894559, 0.3333333333333333703, 0.3219752754296894559, 0.3333333333333333703, 0.3219752754296894559, 0.3333333333333333703, 0.3219752754296894559, 0.3333333333333333703, 0.3219752754296894559, 0.3333333333333333703, 0.3219752754296894559, 0.3333333333333333703, 0.3219752754296894559, 0.3333333333333333703, 0.3219752754296894559, 0.3333333333333333703, 0.3219752754296894559, 0.3333333333333333703, 0.3219752754296894559, 0.3333333333333333703, 0.3219752754296894559, 0.3333333333333333703, 0.3219752754296894559, 0.3333333333333333703, 0.3219752754296894559, 0.3333333333333333703, 0.3219752754296894559, 0.3333333333333333703, 0.3219752754296894559, 0.3333333333333333703, 0.3219752754296894559, 0.3333333333333333703, 0.3219752754296894559, 0.3333333333333333703, 0.3219752754296894559, 0.3333333333333333703, 0.3219752754296894559, 0.3333333333333333703, 0.3219752754296894559, 0.3333333333333333703, 0.3219752754296894559, 0.3333333333333333703, 0.3219752754296894559, 0.3333333333333333703, 0.3219752754296894559, 0.3333333333333333703, 0.3219752754296894559, 0.3333333333333333703, 0.3219752754296894559, 0.3333333333333333703, 0.3219752754296894559, 0.3333333333333333703, 0.3219752754296894559, 0.3333333333333333703, 0.3219752754296894559, 0.3333333333333333703, 0.3219752754296894559, 0.3333333333333333703, 0.3219752754296894559, 0.3333333333333333703, 0.3219752754296894559, 0.3333333333333333703, 0.3219752754296894559, 0.3333333333333333703, 0.3219752754296894559, 0.3333333333333333703, 0.3219752754296894559, 0.3333333333333333703, 0.3219752754296894559, 0.3333333333333333703, 0.3219752754296894559, 0.3333333333333333703, 0.3219752754296894559, 0.3333333333333333703, 0.3219752754296894559, 0.3333333333333333703, 0.3219752754296894559, 0.3333333333333333703, 0.3219752754296894559, 0.3333333333333333703, 0.3219752754296894559, 0.3333333333333333703, 0.3219752754296894559, 0.3333333333333333703, 0.3219752754296894559, 0.3333333333333333703, 0.3219752754296894559, 0.3333333333333333703, 0.3219752754296894559, 0.3333333333333333703, 0.3219752754296894559, 0.3333333333333333703, 0.3219752754296894559, 0.3333333333333333703, 0.3219752754296894559, 0.3333333333333333703, 0.3219752754296894559, 0.3333333333333333703, 0.3219752754296894559, 0.3333333333333333703, 0.3219752754296894559, 0.3333333333333333703, 0.3219752754296894559, 0.3333333333333333703, 0.3219752754296894559, 0.3333333333333333703, 0.3219752754296894559, 0.3333333333333333703, 0.3219752754296894559, 0.3333333333333333703),
 ( 1.000000000000000000, 0.9659258262890683122, 1.000000000000000000, 0.9659258262890683122, 1.000000000000000000, 0.9659258262890683122, 1.000000000000000000, 0.9659258262890683122, 1.000000000000000000, 0.9659258262890683122, 1.000000000000000000, 0.9659258262890683122, 1.000000000000000000, 0.9659258262890683122, 1.000000000000000000, 0.9659258262890683122, 1.000000000000000000, 0.9659258262890683122, 1.000000000000000000, 0.9659258262890683122, 1.000000000000000000, 0.9659258262890683122, 1.000000000000000000, 0.9659258262890683122, 1.000000000000000000, 0.9659258262890683122, 1.000000000000000000, 0.9659258262890683122, 1.000000000000000000, 0.9659258262890683122, 1.000000000000000000, 0.9659258262890683122, 1.000000000000000000, 0.9659258262890683122, 1.000000000000000000, 0.9659258262890683122, 1.000000000000000000, 0.9659258262890683122, 1.000000000000000000, 0.9659258262890683122, 1.000000000000000000, 0.9659258262890683122, 1.000000000000000000, 0.9659258262890683122, 1.000000000000000000, 0.9659258262890683122, 1.000000000000000000, 0.9659258262890683122, 1.000000000000000000, 0.9659258262890683122, 1.000000000000000000, 0.9659258262890683122, 1.000000000000000000, 0.9659258262890683122, 1.000000000000000000, 0.9659258262890683122, 1.000000000000000000, 0.9659258262890683122, 1.000000000000000000, 0.9659258262890683122, 1.000000000000000000, 0.9659258262890683122, 1.000000000000000000, 0.9659258262890683122, 1.000000000000000000, 0.9659258262890683122, 1.000000000000000000, 0.9659258262890683122, 1.000000000000000000, 0.9659258262890683122, 1.000000000000000000, 0.9659258262890683122, 1.000000000000000000, 0.9659258262890683122, 1.000000000000000000, 0.9659258262890683122, 1.000000000000000000, 0.9659258262890683122, 1.000000000000000000, 0.9659258262890683122, 1.000000000000000000, 0.9659258262890683122, 1.000000000000000000, 0.9659258262890683122, 1.000000000000000000, 0.9659258262890683122, 1.000000000000000000, 0.9659258262890683122, 1.000000000000000000, 0.9659258262890683122, 1.000000000000000000, 0.9659258262890683122, 1.000000000000000000, 0.9659258262890683122, 1.000000000000000000, 0.9659258262890683122, 1.000000000000000000, 0.9659258262890683122, 1.000000000000000000, 0.9659258262890683122, 1.000000000000000000, 0.9659258262890683122, 1.000000000000000000, 0.9659258262890683122, 1.000000000000000000, 0.9659258262890683122, 1.000000000000000000, 0.9659258262890683122, 1.000000000000000000, 0.9659258262890683122, 1.000000000000000000, 0.9659258262890683122, 1.000000000000000000, 0.9659258262890683122, 1.000000000000000000, 0.9659258262890683122, 1.000000000000000000, 0.9659258262890683122, 1.000000000000000000, 0.9659258262890683122, 1.000000000000000000, 0.9659258262890683122, 1.000000000000000000, 0.9659258262890683122, 1.000000000000000000, 0.9659258262890683122, 1.000000000000000000, 0.9659258262890683122, 1.000000000000000000, 0.9659258262890683122, 1.000000000000000000, 0.9659258262890683122, 1.000000000000000000, 0.9659258262890683122, 1.000000000000000000, 0.9659258262890683122, 1.000000000000000000, 0.9659258262890683122, 1.000000000000000000, 0.9659258262890683122, 1.000000000000000000, 0.9659258262890683122, 1.000000000000000000, 0.9659258262890683122, 1.000000000000000000, 0.9659258262890683122, 1.000000000000000000, 0.9659258262890683122, 1.000000000000000000, 0.9659258262890683122, 1.000000000000000000, 0.9659258262890683122, 1.000000000000000000, 0.9659258262890683122, 1.000000000000000000, 0.9659258262890683122, 1.000000000000000000, 0.9659258262890683122, 1.000000000000000000, 0.9659258262890683122, 1.000000000000000000, 0.9659258262890683122, 1.000000000000000000, 0.9659258262890683122, 1.000000000000000000, 0.9659258262890683122, 1.000000000000000000, 0.9659258262890683122, 1.000000000000000000, 0.9659258262890683122, 1.000000000000000000, 0.9659258262890683122, 1.000000000000000000, 0.9659258262890683122, 1.000000000000000000, 0.9659258262890683122, 1.000000000000000000, 0.9659258262890683122, 1.000000000000000000, 0.9659258262890683122, 1.000000000000000000, 0.9659258262890683122, 1.000000000000000000, 0.9659258262890683122, 1.000000000000000000, 0.9659258262890683122, 1.000000000000000000, 0.9659258262890683122, 1.000000000000000000, 0.9659258262890683122, 1.000000000000000000, 0.9659258262890683122, 1.000000000000000000, 0.9659258262890683122, 1.000000000000000000, 0.9659258262890683122, 1.000000000000000000, 0.9659258262890683122, 1.000000000000000000, 0.9659258262890683122, 1.000000000000000000, 0.9659258262890683122, 1.000000000000000000, 0.9659258262890683122, 1.000000000000000000, 0.9659258262890683122, 1.000000000000000000, 0.9659258262890683122, 1.000000000000000000, 0.9659258262890683122, 1.000000000000000000, 0.9659258262890683122, 1.000000000000000000, 0.9659258262890683122, 1.000000000000000000, 0.9659258262890683122, 1.000000000000000000, 0.9659258262890683122, 1.000000000000000000, 0.9659258262890683122, 1.000000000000000000, 0.9659258262890683122, 1.000000000000000000, 0.9659258262890683122, 1.000000000000000000, 0.9659258262890683122, 1.000000000000000000, 0.9659258262890683122, 1.000000000000000000, 0.9659258262890683122, 1.000000000000000000, 0.9659258262890683122, 1.000000000000000000, 0.9659258262890683122, 1.000000000000000000, 0.9659258262890683122, 1.000000000000000000, 0.9659258262890683122, 1.000000000000000000, 0.9659258262890683122, 1.000000000000000000, 0.9659258262890683122, 1.000000000000000000, 0.9659258262890683122, 1.000000000000000000, 0.9659258262890683122, 1.000000000000000000, 0.9659258262890683122, 1.000000000000000000, 0.9659258262890683122, 1.000000000000000000, 0.9659258262890683122, 1.000000000000000000, 0.9659258262890683122, 1.000000000000000000, 0.9659258262890683122, 1.000000000000000000, 0.9659258262890683122, 1.000000000000000000, 0.9659258262890683122, 1.000000000000000000, 0.9659258262890683122, 1.000000000000000000, 0.9659258262890683122, 1.000000000000000000, 0.9659258262890683122, 1.000000000000000000, 0.9659258262890683122, 1.000000000000000000, 0.9659258262890683122, 1.000000000000000000, 0.9659258262890683122, 1.000000000000000000, 0.9659258262890683122, 1.000000000000000000, 0.9659258262890683122, 1.000000000000000000, 0.9659258262890683122, 1.000000000000000000, 0.9659258262890683122, 1.000000000000000000, 0.9659258262890683122, 1.000000000000000000, 0.9659258262890683122, 1.000000000000000000, 0.9659258262890683122, 1.000000000000000000, 0.9659258262890683122, 1.000000000000000000, 0.9659258262890683122, 1.000000000000000000, 0.9659258262890683122, 1.000000000000000000, 0.9659258262890683122, 1.000000000000000000, 0.9659258262890683122, 1.000000000000000000, 0.9659258262890683122, 1.000000000000000000, 0.9659258262890683122, 1.000000000000000000, 0.9659258262890683122, 1.000000000000000000, 0.9659258262890683122, 1.000000000000000000, 0.9659258262890683122, 1.000000000000000000, 0.9659258262890683122, 1.000000000000000000, 0.9659258262890683122, 1.000000000000000000, 0.9659258262890683122, 1.000000000000000000, 0.9659258262890683122, 1.000000000000000000, 0.9659258262890683122, 1.000000000000000000, 0.9659258262890683122, 1.000000000000000000, 0.9659258262890683122, 1.000000000000000000, 0.9659258262890683122, 1.000000000000000000, 0.9659258262890683122, 1.000000000000000000, 0.9659258262890683122, 1.000000000000000000, 0.9659258262890683122, 1.000000000000000000, 0.9659258262890683122, 1.000000000000000000, 0.9659258262890683122, 1.000000000000000000, 0.9659258262890683122, 1.000000000000000000, 0.9659258262890683122, 1.000000000000000000, 0.9659258262890683122, 1.000000000000000000, 0.9659258262890683122, 1.000000000000000000, 0.9659258262890683122, 1.000000000000000000, 0.9659258262890683122, 1.000000000000000000, 0.9659258262890683122, 1.000000000000000000, 0.9659258262890683122, 1.000000000000000000, 0.9659258262890683122, 1.000000000000000000, 0.9659258262890683122, 1.000000000000000000, 0.9659258262890683122, 1.000000000000000000, 0.9659258262890683122, 1.000000000000000000, 0.9659258262890683122, 1.000000000000000000, 0.9659258262890683122, 1.000000000000000000, 0.9659258262890683122, 1.000000000000000000, 0.9659258262890683122, 1.000000000000000000, 0.9659258262890683122, 1.000000000000000000, 0.9659258262890683122, 1.000000000000000000, 0.9659258262890683122, 1.000000000000000000, 0.9659258262890683122, 1.000000000000000000, 0.9659258262890683122, 1.000000000000000000, 0.9659258262890683122, 1.000000000000000000, 0.9659258262890683122, 1.000000000000000000, 0.9659258262890683122, 1.000000000000000000, 0.9659258262890683122, 1.000000000000000000, 0.9659258262890683122, 1.000000000000000000, 0.9659258262890683122, 1.000000000000000000, 0.9659258262890683122, 1.000000000000000000, 0.9659258262890683122, 1.000000000000000000, 0.9659258262890683122, 1.000000000000000000, 0.9659258262890683122, 1.000000000000000000, 0.9659258262890683122, 1.000000000000000000, 0.9659258262890683122, 1.000000000000000000, 0.9659258262890683122, 1.000000000000000000, 0.9659258262890683122, 1.000000000000000000, 0.9659258262890683122, 1.000000000000000000, 0.9659258262890683122, 1.000000000000000000, 0.9659258262890683122, 1.000000000000000000, 0.9659258262890683122, 1.000000000000000000, 0.9659258262890683122, 1.000000000000000000, 0.9659258262890683122, 1.000000000000000000, 0.9659258262890683122, 1.000000000000000000, 0.9659258262890683122, 1.000000000000000000, 0.9659258262890683122, 1.000000000000000000, 0.9659258262890683122, 1.000000000000000000, 0.9659258262890683122, 1.000000000000000000, 0.9659258262890683122, 1.000000000000000000, 0.9659258262890683122, 1.000000000000000000, 0.9659258262890683122, 1.000000000000000000, 0.9659258262890683122, 1.000000000000000000, 0.9659258262890683122, 1.000000000000000000, 0.9659258262890683122, 1.000000000000000000, 0.9659258262890683122, 1.000000000000000000, 0.9659258262890683122, 1.000000000000000000, 0.9659258262890683122, 1.000000000000000000, 0.9659258262890683122, 1.000000000000000000, 0.9659258262890683122, 1.000000000000000000, 0.9659258262890683122, 1.000000000000000000, 0.9659258262890683122, 1.000000000000000000, 0.9659258262890683122, 1.000000000000000000, 0.9659258262890683122, 1.000000000000000000, 0.9659258262890683122, 1.000000000000000000) ) ) 
 REPRESENTATION_ITEM ( '' )  SURFACE ( )  );
#181640=CARTESIAN_POINT ( 'NONE',  ( 0.05219959533907565091, 21.53943276465977519, 89.99890960531438111 ) ) ;
#181641=CARTESIAN_POINT ( 'NONE',  ( 4.379528057220339221, -16.55341960407611168, 77.70724293864770971 ) ) ;
#181642=CARTESIAN_POINT ( 'NONE',  ( -9.474510206698720793, -16.51473224551083518, 54.58442372801899722 ) ) ;
#181643=CARTESIAN_POINT ( 'NONE',  ( -5.719274019375978568, 21.55341960407610458, 75.20724293864769550 ) ) ;
#181644=CARTESIAN_POINT ( 'NONE',  ( 21.53943276465977519, -0.05219959533907433946, 53.74890960531437401 ) ) ;
#181645=CARTESIAN_POINT ( 'NONE',  ( 12.14591786802309770, 12.06949235617756955, 34.37390960531435979 ) ) ;
#181646=CARTESIAN_POINT ( 'NONE',  ( 0.05219959533937995610, -21.53943276465977519, 100.0010903946857042 ) ) ;
#181647=CARTESIAN_POINT ( 'NONE',  ( -19.02544592524342804, 5.153800228976336051, 76.04057627198102409 ) ) ;
#181648=CARTESIAN_POINT ( 'NONE',  ( -5.049401038298153566, 19.05341960407611168, 35.20724293864768839 ) ) ;
#181649=CARTESIAN_POINT ( 'NONE',  ( -21.55341960407619339, 5.719274019375674811, 43.54275706135235424 ) ) ;
#181650=CARTESIAN_POINT ( 'NONE',  ( -5.823673210054431948, 21.52544592524334988, 42.70942372801901854 ) ) ;
#181651=CARTESIAN_POINT ( 'NONE',  ( -13.89961937509977652, 13.97604488694528158, 45.62390960531433848 ) ) ;
#181652=CARTESIAN_POINT ( 'NONE',  ( -21.53943276465977519, 0.05219959533907696930, 116.2489096053143669 ) ) ;
#181653=CARTESIAN_POINT ( 'NONE',  ( -19.02544592524334988, -5.153800228976617603, 63.95942372801899012 ) ) ;
#181654=CARTESIAN_POINT ( 'NONE',  ( -0.05219959533909027116, -19.03943276465977164, 32.49890960531435979 ) ) ;
#181655=CARTESIAN_POINT ( 'NONE',  ( -4.483927247898782831, 16.52544592524335698, 27.70942372801901854 ) ) ;
#181656=CARTESIAN_POINT ( 'NONE',  ( 19.05341960407611168, 5.049401038298154454, 23.95724293864769194 ) ) ;
#181657=CARTESIAN_POINT ( 'NONE',  ( 14.34966873604972726, -8.224510206698740333, 70.83442372801901854 ) ) ;
#181658=CARTESIAN_POINT ( 'NONE',  ( 19.03943276465977164, -0.05219959533909143690, 38.74890960531436690 ) ) ;
#181660=CARTESIAN_POINT ( 'NONE',  ( 9.474510206698971260, -16.51473224551069308, 87.91557627198102409 ) ) ;
#181661=CARTESIAN_POINT ( 'NONE',  ( -5.153800228976328057, -19.02544592524343514, 22.29057627198102765 ) ) ;
#181662=CARTESIAN_POINT ( 'NONE',  ( -18.62759615963270932, 10.81492255796079327, 75.83224293864769550 ) ) ;
#181663=CARTESIAN_POINT ( 'NONE',  ( -14.34966873604972548, 8.224510206698743886, 43.33442372801901143 ) ) ;
#181664=CARTESIAN_POINT ( 'NONE',  ( -15.72974639402176322, -15.80617190586768395, 104.3760903946856899 ) ) ;
#181665=CARTESIAN_POINT ( 'NONE',  ( 19.05341960407611168, 5.049401038298154454, 43.95724293864769550 ) ) ;
#181666=CARTESIAN_POINT ( 'NONE',  ( 8.314922557960818139, 14.29746914071049879, 34.58224293864770260 ) ) ;
#181667=CARTESIAN_POINT ( 'NONE',  ( -12.06949235617756955, 12.14591786802309770, 70.62390960531436690 ) ) ;
#181668=CARTESIAN_POINT ( 'NONE',  ( -9.474510206698964154, 16.51473224551069663, 60.41557627198102409 ) ) ;
#181669=CARTESIAN_POINT ( 'NONE',  ( -5.823673210054431948, 21.52544592524334988, 112.7094237280190328 ) ) ;
#181670=CARTESIAN_POINT ( 'NONE',  ( -0.05219959533937732626, 21.53943276465977519, 22.50109039468567573 ) ) ;
#181671=CARTESIAN_POINT ( 'NONE',  ( -13.89961937509977652, 13.97604488694528158, 85.62390960531433848 ) ) ;
#181672=CARTESIAN_POINT ( 'NONE',  ( 5.719274019375673035, 21.55341960407619339, 92.29275706135236135 ) ) ;
#181673=CARTESIAN_POINT ( 'NONE',  ( -4.483927247898782831, 16.52544592524335698, 57.70942372801901143 ) ) ;
#181674=CARTESIAN_POINT ( 'NONE',  ( -16.53943276465976808, -0.05219959533934237506, 28.75109039468567929 ) ) ;
#181675=CARTESIAN_POINT ( 'NONE',  ( -14.29746914071049879, 8.314922557960819915, 90.83224293864769550 ) ) ;
#181676=CARTESIAN_POINT ( 'NONE',  ( 18.62759615963255655, 10.81492255796105972, 101.6677570613523613 ) ) ;
#181677=CARTESIAN_POINT ( 'NONE',  ( -0.05219959533910754901, -16.53943276465976808, 37.49890960531436690 ) ) ;
#181678=CARTESIAN_POINT ( 'NONE',  ( -16.46253265017160317, 9.564922557960807481, 30.83224293864769550 ) ) ;
#181679=CARTESIAN_POINT ( 'NONE',  ( -16.53943276465976808, -0.05219959533934237506, 58.75109039468568994 ) ) ;
#181680=CARTESIAN_POINT ( 'NONE',  ( 14.29746914071049879, -8.314922557960816363, 48.33224293864770260 ) ) ;
#181681=CARTESIAN_POINT ( 'NONE',  ( -14.34966873604972548, 8.224510206698743886, 98.33442372801901854 ) ) ;
#181682=CARTESIAN_POINT ( 'NONE',  ( 5.049401038298161559, -19.05341960407611168, 112.7072429386476813 ) ) ;
#181683=CARTESIAN_POINT ( 'NONE',  ( 10.72451020669898902, -18.67979575497178502, 32.91557627198102409 ) ) ;
#181684=CARTESIAN_POINT ( 'NONE',  ( -0.05219959533937732626, 21.53943276465977519, 112.5010903946857042 ) ) ;
#181685=CARTESIAN_POINT ( 'NONE',  ( -14.34966873604960291, -8.224510206698953496, 81.66557627198103830 ) ) ;
#181686=CARTESIAN_POINT ( 'NONE',  ( 19.03943276465977164, -0.05219959533909143690, 98.74890960531436690 ) ) ;
#181687=EDGE_LOOP ( 'NONE', ( #121638, #103041, #56743 ) ) ;
#181688=CARTESIAN_POINT ( 'NONE',  ( 14.29746914071037800, 8.314922557961029526, 41.66775706135235424 ) ) ;
#181689=CARTESIAN_POINT ( 'NONE',  ( 13.97604488694527802, 13.89961937509977652, 39.37390960531435269 ) ) ;
#181690=CARTESIAN_POINT ( 'NONE',  ( 16.52544592524335698, 4.483927247898782831, 51.45942372801901854 ) ) ;
#181691=CARTESIAN_POINT ( 'NONE',  ( 16.51473224551083163, -9.474510206698727899, 45.83442372801900433 ) ) ;
#181692=CARTESIAN_POINT ( 'NONE',  ( -0.05219959533909027116, -19.03943276465977164, 47.49890960531435979 ) ) ;
#181693=CARTESIAN_POINT ( 'NONE',  ( -14.29746914071037622, -8.314922557961029526, 84.16775706135234714 ) ) ;
#181694=CARTESIAN_POINT ( 'NONE',  ( 5.049401038297881783, 19.05341960407617563, 77.29275706135231871 ) ) ;
#181695=CARTESIAN_POINT ( 'NONE',  ( -5.049401038297874678, -19.05341960407617918, 24.79275706135233648 ) ) ;
#181696=CARTESIAN_POINT ( 'NONE',  ( -13.89961937509977652, 13.97604488694528158, 55.62390960531434558 ) ) ;
#181697=CARTESIAN_POINT ( 'NONE',  ( 4.379528057220339221, -16.55341960407611168, 92.70724293864770971 ) ) ;
#181698=CARTESIAN_POINT ( 'NONE',  ( -19.03943276465977164, -0.05219959533935918106, 63.75109039468566863 ) ) ;
#181699=CARTESIAN_POINT ( 'NONE',  ( -5.719274019375978568, 21.55341960407610458, 60.20724293864768839 ) ) ;
#181700=CARTESIAN_POINT ( 'NONE',  ( -19.05341960407617563, 5.049401038297882671, 38.54275706135233293 ) ) ;
#181701=CARTESIAN_POINT ( 'NONE',  ( 19.05341960407611168, 5.049401038298154454, 108.9572429386477097 ) ) ;
#181702=CARTESIAN_POINT ( 'NONE',  ( 21.52544592524344225, -5.823673210054117533, 73.54057627198102409 ) ) ;
#181703=CARTESIAN_POINT ( 'NONE',  ( -16.52216118717208104, 7.221426719304498754, 83.92400978953007495 ) ) ;
#181704=CARTESIAN_POINT ( 'NONE',  ( -16.51473224551082808, 9.474510206698731452, 103.3344237280190043 ) ) ;
#181706=CARTESIAN_POINT ( 'NONE',  ( -8.314922557961024197, 14.29746914071037800, 27.91775706135234358 ) ) ;
#181707=CARTESIAN_POINT ( 'NONE',  ( -19.03943276465977164, 0.05219959533909376836, 31.24890960531435979 ) ) ;
#181708=CARTESIAN_POINT ( 'NONE',  ( -18.67979575497178146, -10.72451020669898902, 21.66557627198102409 ) ) ;
#181709=CARTESIAN_POINT ( 'NONE',  ( -18.62759615963270932, 10.81492255796079327, 85.83224293864768129 ) ) ;
#181710=CARTESIAN_POINT ( 'NONE',  ( 15.80617190586769283, -15.72974639402175789, 55.62609039468568284 ) ) ;
#181711=CARTESIAN_POINT ( 'NONE',  ( -16.51473224551082808, 9.474510206698731452, 103.3344237280190043 ) ) ;
#181712=CARTESIAN_POINT ( 'NONE',  ( 21.52544592524334988, 5.823673210054432836, 106.4594237280190328 ) ) ;
#181713=CARTESIAN_POINT ( 'NONE',  ( 4.379528057220339221, -16.55341960407611168, 22.70724293864769194 ) ) ;
#181714=CARTESIAN_POINT ( 'NONE',  ( 21.55341960407610458, 5.719274019375980345, 93.95724293864770971 ) ) ;
#181715=CARTESIAN_POINT ( 'NONE',  ( 4.379528057220339221, -16.55341960407611168, 52.70724293864769550 ) ) ;
#181716=CARTESIAN_POINT ( 'NONE',  ( -16.51473224551082808, 9.474510206698731452, 78.33442372801900433 ) ) ;
#181718=CARTESIAN_POINT ( 'NONE',  ( -19.02544592524334988, -5.153800228976617603, 53.95942372801898301 ) ) ;
#181719=CARTESIAN_POINT ( 'NONE',  ( -0.05219959533937732626, 21.53943276465977519, 72.50109039468568994 ) ) ;
#181720=CARTESIAN_POINT ( 'NONE',  ( 5.049401038297881783, 19.05341960407617563, 37.29275706135232582 ) ) ;
#181721=CARTESIAN_POINT ( 'NONE',  ( 14.29746914071049879, -8.314922557960816363, 103.3322429386476955 ) ) ;
#181722=CARTESIAN_POINT ( 'NONE',  ( -0.05219959533907301413, -21.53943276465977519, 42.49890960531435979 ) ) ;
#181723=CARTESIAN_POINT ( 'NONE',  ( -8.224510206698948167, 14.34966873604960824, 30.41557627198101699 ) ) ;
#181725=CARTESIAN_POINT ( 'NONE',  ( 15.80617190586769283, -15.72974639402175789, 105.6260903946856899 ) ) ;
#181726=CARTESIAN_POINT ( 'NONE',  ( -4.483927247898782831, 16.52544592524335698, 67.70942372801901854 ) ) ;
#181727=CARTESIAN_POINT ( 'NONE',  ( 4.379528057220339221, -16.55341960407611168, 27.70724293864769905 ) ) ;
#181728=CARTESIAN_POINT ( 'NONE',  ( -21.53943276465977519, -0.05219959533937600094, 68.75109039468568994 ) ) ;
#181729=CARTESIAN_POINT ( 'NONE',  ( -10.72451020669870658, -18.67979575497194134, 69.58442372801900433 ) ) ;
#181730=CARTESIAN_POINT ( 'NONE',  ( 18.62759615963271287, -10.81492255796078972, 68.33224293864769550 ) ) ;
#181732=CARTESIAN_POINT ( 'NONE',  ( -19.05341960407611168, -5.049401038298163336, 26.45724293864769550 ) ) ;
#181733=CARTESIAN_POINT ( 'NONE',  ( -21.53943276465977519, -0.05219959533937600094, 43.75109039468568284 ) ) ;
#181734=CARTESIAN_POINT ( 'NONE',  ( -5.153800228976328057, -19.02544592524343514, 22.29057627198102765 ) ) ;
#181735=CARTESIAN_POINT ( 'NONE',  ( -9.564922557960796823, -16.46253265017161027, 37.08224293864768839 ) ) ;
#181736=CARTESIAN_POINT ( 'NONE',  ( 12.06949235617757843, -12.14591786802309237, 83.12390960531436690 ) ) ;
#181737=CARTESIAN_POINT ( 'NONE',  ( -5.049401038298153566, 19.05341960407611168, 90.20724293864766707 ) ) ;
#181738=CARTESIAN_POINT ( 'NONE',  ( -8.314922557960811034, -14.29746914071050412, 22.08224293864769194 ) ) ;
#181739=CARTESIAN_POINT ( 'NONE',  ( 4.379528057220339221, -16.55341960407611168, 102.7072429386476955 ) ) ;
#181740=CARTESIAN_POINT ( 'NONE',  ( -5.719274019375978568, 21.55341960407610458, 70.20724293864769550 ) ) ;
#181741=CARTESIAN_POINT ( 'NONE',  ( -10.81492255796078084, -18.62759615963271287, 107.0822429386476955 ) ) ;
#181742=CARTESIAN_POINT ( 'NONE',  ( 16.46253265017160672, -9.564922557960803928, 113.3322429386476955 ) ) ;
#181743=CARTESIAN_POINT ( 'NONE',  ( 9.564922557960805705, 16.46253265017160317, 69.58224293864770971 ) ) ;
#181744=CARTESIAN_POINT ( 'NONE',  ( -4.483927247898782831, 16.52544592524335698, 22.70942372801901499 ) ) ;
#181745=CARTESIAN_POINT ( 'NONE',  ( -5.823673210054116645, -21.52544592524344225, 57.29057627198103120 ) ) ;
#181746=CARTESIAN_POINT ( 'NONE',  ( -15.72974639402176322, -15.80617190586768395, 84.37609039468570415 ) ) ;
#181748=CARTESIAN_POINT ( 'NONE',  ( -13.89961937509977652, 13.97604488694528158, 85.62390960531433848 ) ) ;
#181749=CARTESIAN_POINT ( 'NONE',  ( -19.05341960407611168, -5.049401038298163336, 111.4572429386476671 ) ) ;
#181750=CARTESIAN_POINT ( 'NONE',  ( 16.52544592524335698, 4.483927247898782831, 81.45942372801900433 ) ) ;
#181751=CARTESIAN_POINT ( 'NONE',  ( -15.80617190586768217, 15.72974639402176855, 53.12609039468568284 ) ) ;
#181752=CARTESIAN_POINT ( 'NONE',  ( -15.72974639402176322, -15.80617190586768395, 99.37609039468568994 ) ) ;
#181753=CARTESIAN_POINT ( 'NONE',  ( 8.314922557961029526, -14.29746914071037800, 60.41775706135235424 ) ) ;
#181754=CARTESIAN_POINT ( 'NONE',  ( -10.81492255796078084, -18.62759615963271287, 112.0822429386477097 ) ) ;
#181755=CARTESIAN_POINT ( 'NONE',  ( 0.05219959533909260263, 19.03943276465977164, 114.9989096053143669 ) ) ;
#181756=CARTESIAN_POINT ( 'NONE',  ( 0.05219959533907565091, 21.53943276465977519, 89.99890960531438111 ) ) ;
#181757=CARTESIAN_POINT ( 'NONE',  ( -0.05219959533936034679, 19.03943276465977164, 42.50109039468566152 ) ) ;
#181758=CARTESIAN_POINT ( 'NONE',  ( -10.72451020669898014, 18.67979575497178502, 45.41557627198103830 ) ) ;
#181759=CARTESIAN_POINT ( 'NONE',  ( 19.03943276465977164, -0.05219959533909143690, 93.74890960531435269 ) ) ;
#181760=CARTESIAN_POINT ( 'NONE',  ( -16.53943276465976808, 0.05219959533911058130, 41.24890960531435269 ) ) ;
#181763=CARTESIAN_POINT ( 'NONE',  ( -19.49190055781012276, -5.499999999999968026, 80.56116087098781975 ) ) ;
#181764=CARTESIAN_POINT ( 'NONE',  ( 0.05219959533936267826, -19.03943276465977164, 100.0010903946856757 ) ) ;
#181765=CARTESIAN_POINT ( 'NONE',  ( -21.55341960407610458, -5.719274019375992779, 71.45724293864769550 ) ) ;
#181766=CARTESIAN_POINT ( 'NONE',  ( 8.224510206698953496, -14.34966873604960469, 52.91557627198103830 ) ) ;
#181767=CARTESIAN_POINT ( 'NONE',  ( 8.314922557961029526, -14.29746914071037800, 30.41775706135234358 ) ) ;
#181768=CARTESIAN_POINT ( 'NONE',  ( -13.89961937509977652, 13.97604488694528158, 45.62390960531433848 ) ) ;
#181769=CARTESIAN_POINT ( 'NONE',  ( 10.81492255796106328, -18.62759615963255655, 20.41775706135234714 ) ) ;
#181770=CARTESIAN_POINT ( 'NONE',  ( 5.153800228976615827, -19.02544592524334988, 80.20942372801901854 ) ) ;
#181771=CARTESIAN_POINT ( 'NONE',  ( 13.89961937509977652, -13.97604488694527269, 78.12390960531433848 ) ) ;
#181772=CARTESIAN_POINT ( 'NONE',  ( -16.46253265017160317, 9.564922557960807481, 70.83224293864770971 ) ) ;
#181773=CARTESIAN_POINT ( 'NONE',  ( 0.05219959533907565091, 21.53943276465977519, 79.99890960531435269 ) ) ;
#181774=CARTESIAN_POINT ( 'NONE',  ( 19.03943276465977164, -0.05219959533909143690, 28.74890960531435624 ) ) ;
#181776=CARTESIAN_POINT ( 'NONE',  ( -8.224510206698948167, 14.34966873604960824, 60.41557627198102409 ) ) ;
#181777=CARTESIAN_POINT ( 'NONE',  ( -5.153800228976328057, -19.02544592524343514, 92.29057627198099567 ) ) ;
#181778=CARTESIAN_POINT ( 'NONE',  ( -17.49999999999999645, -5.500000000000000888, 120.0000000000000142 ) ) ;
#181779=CARTESIAN_POINT ( 'NONE',  ( 9.564922557961047289, -16.46253265017146816, 50.41775706135233293 ) ) ;
#181780=CARTESIAN_POINT ( 'NONE',  ( -0.05219959533907301413, -21.53943276465977519, 77.49890960531433848 ) ) ;
#181781=CARTESIAN_POINT ( 'NONE',  ( -13.89961937509957401, -13.97604488694547875, 39.37609039468566152 ) ) ;
#181782=CARTESIAN_POINT ( 'NONE',  ( -0.05219959533909027116, -19.03943276465977164, 87.49890960531436690 ) ) ;
#181783=CARTESIAN_POINT ( 'NONE',  ( -17.72560187377286667, -5.499999999999973355, 74.07814504131320632 ) ) ;
#181784=CARTESIAN_POINT ( 'NONE',  ( 5.719274019375991003, -21.55341960407610458, 27.70724293864769905 ) ) ;
#181785=CARTESIAN_POINT ( 'NONE',  ( -16.51473224551069308, -9.474510206698971260, 76.66557627198103830 ) ) ;
#181786=CARTESIAN_POINT ( 'NONE',  ( -18.67979575497193778, 10.72451020669871902, 58.33442372801901143 ) ) ;
#181787=CARTESIAN_POINT ( 'NONE',  ( -19.05341960407611168, -5.049401038298163336, 21.45724293864768839 ) ) ;
#181789=CARTESIAN_POINT ( 'NONE',  ( -21.52544592524343514, 5.823673210054127303, 111.0405762719810525 ) ) ;
#181790=CARTESIAN_POINT ( 'NONE',  ( -5.153800228976328057, -19.02544592524343514, 97.29057627198099567 ) ) ;
#181792=CARTESIAN_POINT ( 'NONE',  ( 15.80617190586769283, -15.72974639402175789, 35.62609039468568994 ) ) ;
#181794=CARTESIAN_POINT ( 'NONE',  ( 16.51473224551069308, 9.474510206698969483, 94.16557627198103830 ) ) ;
#181797=CARTESIAN_POINT ( 'NONE',  ( -21.53943276465977519, 0.05219959533907696930, 101.2489096053143669 ) ) ;
#181798=CARTESIAN_POINT ( 'NONE',  ( -5.049401038298153566, 19.05341960407611168, 65.20724293864765286 ) ) ;
#181799=CARTESIAN_POINT ( 'NONE',  ( -16.51473224551082808, 9.474510206698731452, 113.3344237280190043 ) ) ;
#181801=CARTESIAN_POINT ( 'NONE',  ( 10.81492255796106328, -18.62759615963255655, 105.4177570613523613 ) ) ;
#181802=CARTESIAN_POINT ( 'NONE',  ( 16.51473224551069308, 9.474510206698969483, 49.16557627198102409 ) ) ;
#181803=CARTESIAN_POINT ( 'NONE',  ( 5.823673210054444382, -21.52544592524334988, 105.2094237280190328 ) ) ;
#181805=CARTESIAN_POINT ( 'NONE',  ( -16.46253265017160317, 9.564922557960807481, 85.83224293864769550 ) ) ;
#181806=CARTESIAN_POINT ( 'NONE',  ( -10.72451020669870658, -18.67979575497194134, 64.58442372801900433 ) ) ;
#181808=CARTESIAN_POINT ( 'NONE',  ( 13.97604488694527802, 13.89961937509977652, 104.3739096053143385 ) ) ;
#181809=DIRECTION ( 'NONE',  ( -1.000000000000000000, -0.000000000000000000, -0.000000000000000000 ) ) ;
#181810=CARTESIAN_POINT ( 'NONE',  ( 16.55341960407618274, -4.379528057220086978, 51.04275706135234714 ) ) ;
#181811=CARTESIAN_POINT ( 'NONE',  ( 8.224510206698742110, 14.34966873604972548, 67.08442372801901854 ) ) ;
#181812=CARTESIAN_POINT ( 'NONE',  ( -21.52544592524334988, -5.823673210054445271, 58.95942372801902565 ) ) ;
#181813=CARTESIAN_POINT ( 'NONE',  ( -15.72974639402176322, -15.80617190586768395, 89.37609039468568994 ) ) ;
#181815=CARTESIAN_POINT ( 'NONE',  ( -12.14591786802326823, 12.06949235617739902, 23.12609039468567573 ) ) ;
#181816=CARTESIAN_POINT ( 'NONE',  ( 9.474510206698971260, -16.51473224551069308, 77.91557627198103830 ) ) ;
#181817=CARTESIAN_POINT ( 'NONE',  ( -16.51473224551069308, -9.474510206698971260, 91.66557627198103830 ) ) ;
#181819=CARTESIAN_POINT ( 'NONE',  ( 16.46253265017160672, -9.564922557960803928, 28.33224293864769550 ) ) ;
#181820=CARTESIAN_POINT ( 'NONE',  ( 5.823673210054125526, 21.52544592524343514, 24.79057627198103120 ) ) ;
#181821=CARTESIAN_POINT ( 'NONE',  ( -14.34966873604972548, 8.224510206698743886, 88.33442372801901854 ) ) ;
#181822=CARTESIAN_POINT ( 'NONE',  ( -8.314922557960811034, -14.29746914071050412, 87.08224293864769550 ) ) ;
#181823=CARTESIAN_POINT ( 'NONE',  ( 19.05341960407611168, 5.049401038298154454, 73.95724293864768129 ) ) ;
#181824=CARTESIAN_POINT ( 'NONE',  ( -18.67979575497193778, 10.72451020669871902, 93.33442372801901854 ) ) ;
#181826=CARTESIAN_POINT ( 'NONE',  ( -16.53943276465976808, -0.05219959533934237506, 23.75109039468567929 ) ) ;
#181827=CARTESIAN_POINT ( 'NONE',  ( -16.53943276465976808, 0.05219959533911058130, 71.24890960531435269 ) ) ;
#181828=CARTESIAN_POINT ( 'NONE',  ( -15.80617190586768217, 15.72974639402176855, 48.12609039468568284 ) ) ;
#181829=CARTESIAN_POINT ( 'NONE',  ( -5.719274019375978568, 21.55341960407610458, 80.20724293864769550 ) ) ;
#181830=CARTESIAN_POINT ( 'NONE',  ( -9.564922557961040184, 16.46253265017147172, 42.91775706135234003 ) ) ;
#181832=CARTESIAN_POINT ( 'NONE',  ( -5.049401038298153566, 19.05341960407611168, 85.20724293864766707 ) ) ;
#181833=CARTESIAN_POINT ( 'NONE',  ( -4.483927247898539470, -16.52544592524342804, 47.29057627198103120 ) ) ;
#181834=CARTESIAN_POINT ( 'NONE',  ( -14.34966873604960291, -8.224510206698953496, 31.66557627198102054 ) ) ;
#181835=CARTESIAN_POINT ( 'NONE',  ( -8.314922557961024197, 14.29746914071037800, 107.9177570613523471 ) ) ;
#181836=CARTESIAN_POINT ( 'NONE',  ( 19.02544592524334988, 5.153800228976608722, 61.45942372801900433 ) ) ;
#181838=CARTESIAN_POINT ( 'NONE',  ( -21.55341960407610458, -5.719274019375992779, 21.45724293864769550 ) ) ;
#181839=CARTESIAN_POINT ( 'NONE',  ( -14.29746914071049879, 8.314922557960819915, 85.83224293864768129 ) ) ;
#181841=CARTESIAN_POINT ( 'NONE',  ( 13.89961937509977652, -13.97604488694527269, 28.12390960531435624 ) ) ;
#181842=CARTESIAN_POINT ( 'NONE',  ( -10.72451020669898014, 18.67979575497178502, 40.41557627198103120 ) ) ;
#181843=CARTESIAN_POINT ( 'NONE',  ( 21.55341960407610458, 5.719274019375980345, 73.95724293864769550 ) ) ;
#181844=CARTESIAN_POINT ( 'NONE',  ( 12.06949235617757843, -12.14591786802309237, 113.1239096053143953 ) ) ;
#181845=CARTESIAN_POINT ( 'NONE',  ( -16.53943276465976808, -0.05219959533934237506, 63.75109039468568284 ) ) ;
#181846=CARTESIAN_POINT ( 'NONE',  ( 16.51473224551069308, 9.474510206698969483, 44.16557627198103120 ) ) ;
#181847=CARTESIAN_POINT ( 'NONE',  ( 0.05219959533937995610, -21.53943276465977519, 55.00109039468568284 ) ) ;
#181849=CARTESIAN_POINT ( 'NONE',  ( -4.379528057220328563, 16.55341960407611168, 110.2072429386477239 ) ) ;
#181850=CARTESIAN_POINT ( 'NONE',  ( -5.049401038297874678, -19.05341960407617918, 89.79275706135230450 ) ) ;
#181853=CARTESIAN_POINT ( 'NONE',  ( 15.72974639402199770, -15.80617190586745480, 38.12390960531436690 ) ) ;
#181855=CARTESIAN_POINT ( 'NONE',  ( 15.80617190586769283, -15.72974639402175789, 75.62609039468567573 ) ) ;
#181856=CARTESIAN_POINT ( 'NONE',  ( -8.314922557961024197, 14.29746914071037800, 57.91775706135234714 ) ) ;
#181857=CARTESIAN_POINT ( 'NONE',  ( -12.14591786802309592, -12.06949235617757132, 46.87390960531435979 ) ) ;
#181858=CARTESIAN_POINT ( 'NONE',  ( 10.81492255796078972, 18.62759615963270932, 64.58224293864769550 ) ) ;
#181859=CARTESIAN_POINT ( 'NONE',  ( -21.53943276465977519, 0.05219959533907696930, 61.24890960531435979 ) ) ;
#181861=CARTESIAN_POINT ( 'NONE',  ( 19.05341960407617918, -5.049401038297876454, 81.04275706135231871 ) ) ;
#181862=CARTESIAN_POINT ( 'NONE',  ( -5.823673210054116645, -21.52544592524344225, 22.29057627198102765 ) ) ;
#181863=CARTESIAN_POINT ( 'NONE',  ( 5.049401038298161559, -19.05341960407611168, 52.70724293864767418 ) ) ;
#181864=CARTESIAN_POINT ( 'NONE',  ( -14.34966873604960291, -8.224510206698953496, 111.6655762719810525 ) ) ;
#181865=CARTESIAN_POINT ( 'NONE',  ( 16.46253265017160672, -9.564922557960803928, 108.3322429386476955 ) ) ;
#181867=CARTESIAN_POINT ( 'NONE',  ( 14.34966873604972726, -8.224510206698740333, 65.83442372801900433 ) ) ;
#181868=CARTESIAN_POINT ( 'NONE',  ( -18.67979575497178146, -10.72451020669898902, 101.6655762719810383 ) ) ;
#181869=CARTESIAN_POINT ( 'NONE',  ( 19.05341960407611168, 5.049401038298154454, 73.95724293864768129 ) ) ;
#181870=CARTESIAN_POINT ( 'NONE',  ( -15.80617190586768217, 15.72974639402176855, 43.12609039468568284 ) ) ;
#181871=CARTESIAN_POINT ( 'NONE',  ( -9.564922557960796823, -16.46253265017161027, 97.08224293864769550 ) ) ;
#181874=CARTESIAN_POINT ( 'NONE',  ( -5.719274019375665041, -21.55341960407619695, 29.79275706135234358 ) ) ;
#181875=CARTESIAN_POINT ( 'NONE',  ( -9.564922557960796823, -16.46253265017161027, 102.0822429386477097 ) ) ;
#181876=CARTESIAN_POINT ( 'NONE',  ( 19.05341960407617918, -5.049401038297876454, 86.04275706135233293 ) ) ;
#181877=CARTESIAN_POINT ( 'NONE',  ( 16.51473224551083163, -9.474510206698727899, 45.83442372801900433 ) ) ;
#181878=CARTESIAN_POINT ( 'NONE',  ( 10.81492255796078972, 18.62759615963270932, 94.58224293864769550 ) ) ;
#181879=CARTESIAN_POINT ( 'NONE',  ( 9.474510206698729675, 16.51473224551082808, 32.08442372801900433 ) ) ;
#181880=CARTESIAN_POINT ( 'NONE',  ( 16.46253265017146816, 9.564922557961045513, 51.66775706135233293 ) ) ;
#181881=CARTESIAN_POINT ( 'NONE',  ( 12.06949235617739724, 12.14591786802326823, 86.87609039468568994 ) ) ;
#181884=CARTESIAN_POINT ( 'NONE',  ( 5.049401038298161559, -19.05341960407611168, 77.70724293864765286 ) ) ;
#181885=CARTESIAN_POINT ( 'NONE',  ( 10.81492255796106328, -18.62759615963255655, 80.41775706135234714 ) ) ;
#181886=CARTESIAN_POINT ( 'NONE',  ( 15.80617190586769283, -15.72974639402175789, 80.62609039468567573 ) ) ;
#181888=CARTESIAN_POINT ( 'NONE',  ( 13.89961937509977652, -13.97604488694527269, 93.12390960531436690 ) ) ;
#181889=CARTESIAN_POINT ( 'NONE',  ( -21.55341960407619339, 5.719274019375674811, 63.54275706135234003 ) ) ;
#181890=CARTESIAN_POINT ( 'NONE',  ( 19.05341960407617918, -5.049401038297876454, 101.0427570613523045 ) ) ;
#181891=CARTESIAN_POINT ( 'NONE',  ( 5.049401038298161559, -19.05341960407611168, 72.70724293864768129 ) ) ;
#181892=CARTESIAN_POINT ( 'NONE',  ( 16.51473224551069308, 9.474510206698969483, 109.1655762719810383 ) ) ;
#181893=CARTESIAN_POINT ( 'NONE',  ( -16.51473224551069308, -9.474510206698971260, 81.66557627198103830 ) ) ;
#181895=CARTESIAN_POINT ( 'NONE',  ( 13.97604488694527802, 13.89961937509977652, 69.37390960531436690 ) ) ;
#181896=CARTESIAN_POINT ( 'NONE',  ( -19.05341960407611168, -5.049401038298163336, 56.45724293864768129 ) ) ;
#181897=CARTESIAN_POINT ( 'NONE',  ( -18.67979575497178146, -10.72451020669898902, 111.6655762719810525 ) ) ;
#181898=CARTESIAN_POINT ( 'NONE',  ( 12.06949235617739724, 12.14591786802326823, 91.87609039468568994 ) ) ;
#181900=CARTESIAN_POINT ( 'NONE',  ( -16.51473224551082808, 9.474510206698731452, 48.33442372801900433 ) ) ;
#181901=CARTESIAN_POINT ( 'NONE',  ( 9.564922557960805705, 16.46253265017160317, 84.58224293864769550 ) ) ;
#181902=CARTESIAN_POINT ( 'NONE',  ( 8.224510206698953496, -14.34966873604960469, 72.91557627198103830 ) ) ;
#181903=CARTESIAN_POINT ( 'NONE',  ( -4.379528057220328563, 16.55341960407611168, 110.2072429386477239 ) ) ;
#181904=CARTESIAN_POINT ( 'NONE',  ( -5.719274019375978568, 21.55341960407610458, 25.20724293864769550 ) ) ;
#181905=CARTESIAN_POINT ( 'NONE',  ( 0.05219959533909260263, 19.03943276465977164, 104.9989096053143669 ) ) ;
#181906=CARTESIAN_POINT ( 'NONE',  ( 14.34966873604960469, 8.224510206698951720, 84.16557627198103830 ) ) ;
#181908=CARTESIAN_POINT ( 'NONE',  ( 9.474510206698729675, 16.51473224551082808, 27.08442372801900433 ) ) ;
#181909=CARTESIAN_POINT ( 'NONE',  ( -0.05219959533934338120, 16.53943276465976808, 107.5010903946856899 ) ) ;
#181910=CARTESIAN_POINT ( 'NONE',  ( -5.153800228976328057, -19.02544592524343514, 87.29057627198103830 ) ) ;
#181911=CARTESIAN_POINT ( 'NONE',  ( -21.53943276465977519, -0.05219959533937600094, 58.75109039468568994 ) ) ;
#181912=CARTESIAN_POINT ( 'NONE',  ( -15.80617190586745835, -15.72974639402198527, 46.87390960531435979 ) ) ;
#181913=CARTESIAN_POINT ( 'NONE',  ( 21.55341960407619695, -5.719274019375665929, 21.04275706135234714 ) ) ;
#181914=CARTESIAN_POINT ( 'NONE',  ( -21.52544592524343514, 5.823673210054127303, 71.04057627198103830 ) ) ;
#181915=CARTESIAN_POINT ( 'NONE',  ( -16.55341960407611168, -4.379528057220339221, 91.45724293864769550 ) ) ;
#181916=CARTESIAN_POINT ( 'NONE',  ( -13.89961937509957401, -13.97604488694547875, 54.37609039468565442 ) ) ;
#181917=CARTESIAN_POINT ( 'NONE',  ( 0.05219959533909260263, 19.03943276465977164, 24.99890960531435269 ) ) ;
#181918=CARTESIAN_POINT ( 'NONE',  ( -9.474510206698964154, 16.51473224551069663, 85.41557627198102409 ) ) ;
#181919=CARTESIAN_POINT ( 'NONE',  ( -13.97604488694527625, -13.89961937509977652, 81.87390960531436690 ) ) ;
#181920=CARTESIAN_POINT ( 'NONE',  ( 4.483927247898545687, 16.52544592524342804, 104.7905762719810241 ) ) ;
#181922=CARTESIAN_POINT ( 'NONE',  ( -12.06949235617756955, 12.14591786802309770, 25.62390960531435624 ) ) ;
#181923=CARTESIAN_POINT ( 'NONE',  ( -14.34966873604972548, 8.224510206698743886, 38.33442372801900433 ) ) ;
#181924=CARTESIAN_POINT ( 'NONE',  ( 15.72974639402176855, 15.80617190586768217, 106.8760903946856899 ) ) ;
#181925=CARTESIAN_POINT ( 'NONE',  ( -5.049401038298153566, 19.05341960407611168, 95.20724293864770971 ) ) ;
#181926=CARTESIAN_POINT ( 'NONE',  ( -5.719274019375665041, -21.55341960407619695, 39.79275706135235424 ) ) ;
#181927=CARTESIAN_POINT ( 'NONE',  ( 19.05341960407611168, 5.049401038298154454, 48.95724293864768129 ) ) ;
#181928=CARTESIAN_POINT ( 'NONE',  ( -16.55341960407617563, 4.379528057220093196, 38.54275706135234714 ) ) ;
#181929=CARTESIAN_POINT ( 'NONE',  ( -16.51473224551082808, 9.474510206698731452, 103.3344237280190043 ) ) ;
#181930=CARTESIAN_POINT ( 'NONE',  ( -19.03943276465977164, 0.05219959533909376836, 36.24890960531436690 ) ) ;
#181932=CARTESIAN_POINT ( 'NONE',  ( -12.06949235617756955, 12.14591786802309770, 90.62390960531436690 ) ) ;
#181933=CARTESIAN_POINT ( 'NONE',  ( 21.53943276465977519, -0.05219959533907433946, 108.7489096053143669 ) ) ;
#181934=CARTESIAN_POINT ( 'NONE',  ( 16.51473224551083163, -9.474510206698727899, 85.83442372801900433 ) ) ;
#181935=CARTESIAN_POINT ( 'NONE',  ( -9.564922557960796823, -16.46253265017161027, 92.08224293864769550 ) ) ;
#181936=CARTESIAN_POINT ( 'NONE',  ( 18.62759615963255655, 10.81492255796105972, 26.66775706135235424 ) ) ;
#181937=CARTESIAN_POINT ( 'NONE',  ( 16.51473224551069308, 9.474510206698969483, 24.16557627198102765 ) ) ;
#181938=CARTESIAN_POINT ( 'NONE',  ( -19.05341960407611168, -5.049401038298163336, 96.45724293864769550 ) ) ;
#181940=CARTESIAN_POINT ( 'NONE',  ( 16.51473224551069308, 9.474510206698969483, 84.16557627198102409 ) ) ;
#181941=CARTESIAN_POINT ( 'NONE',  ( -21.52544592524334988, -5.823673210054445271, 33.95942372801901143 ) ) ;
#181942=CARTESIAN_POINT ( 'NONE',  ( 8.314922557960818139, 14.29746914071049879, 84.58224293864769550 ) ) ;
#181943=CARTESIAN_POINT ( 'NONE',  ( 19.03943276465977164, -0.05219959533909143690, 98.74890960531436690 ) ) ;
#181944=CARTESIAN_POINT ( 'NONE',  ( 19.03943276465977164, 0.05219959533936151252, 31.25109039468566863 ) ) ;
#181945=CARTESIAN_POINT ( 'NONE',  ( -12.06949235617739369, -12.14591786802326823, 49.37609039468569705 ) ) ;
#181946=CARTESIAN_POINT ( 'NONE',  ( -0.05219959533937732626, 21.53943276465977519, 77.50109039468567573 ) ) ;
#181947=CARTESIAN_POINT ( 'NONE',  ( 8.314922557961029526, -14.29746914071037800, 30.41775706135234358 ) ) ;
#181948=CARTESIAN_POINT ( 'NONE',  ( 16.51473224551069308, 9.474510206698969483, 74.16557627198103830 ) ) ;
#181950=CARTESIAN_POINT ( 'NONE',  ( 0.05219959533936267826, -19.03943276465977164, 100.0010903946856757 ) ) ;
#181951=CARTESIAN_POINT ( 'NONE',  ( -12.14591786802326823, 12.06949235617739902, 73.12609039468567573 ) ) ;
#181952=CARTESIAN_POINT ( 'NONE',  ( 18.67979575497194134, -10.72451020669871369, 110.8344237280190043 ) ) ;
#181953=CARTESIAN_POINT ( 'NONE',  ( -16.51473224551082808, 9.474510206698731452, 83.33442372801899012 ) ) ;
#181954=CARTESIAN_POINT ( 'NONE',  ( -13.89961937509977652, 13.97604488694528158, 60.62390960531436690 ) ) ;
#181955=CARTESIAN_POINT ( 'NONE',  ( -15.72974639402197994, 15.80617190586746368, 90.62390960531436690 ) ) ;
#181956=CARTESIAN_POINT ( 'NONE',  ( -8.224510206698948167, 14.34966873604960824, 80.41557627198103830 ) ) ;
#181957=CARTESIAN_POINT ( 'NONE',  ( -5.049401038297874678, -19.05341960407617918, 74.79275706135231871 ) ) ;
#181958=CARTESIAN_POINT ( 'NONE',  ( -18.56399227203342761, -5.499999999999928058, 68.97830131249901342 ) ) ;
#181959=CARTESIAN_POINT ( 'NONE',  ( -0.05219959533936034679, 19.03943276465977164, 52.50109039468566863 ) ) ;
#181960=CARTESIAN_POINT ( 'NONE',  ( 14.34966873604972726, -8.224510206698740333, 110.8344237280190043 ) ) ;
#181961=CARTESIAN_POINT ( 'NONE',  ( 4.483927247898545687, 16.52544592524342804, 84.79057627198102409 ) ) ;
#181962=CARTESIAN_POINT ( 'NONE',  ( -10.81492255796105439, 18.62759615963255655, 107.9177570613523471 ) ) ;
#181964=CARTESIAN_POINT ( 'NONE',  ( -0.05219959533907301413, -21.53943276465977519, 102.4989096053143811 ) ) ;
#181965=CARTESIAN_POINT ( 'NONE',  ( -9.564922557960796823, -16.46253265017161027, 97.08224293864769550 ) ) ;
#181966=CARTESIAN_POINT ( 'NONE',  ( 13.89961937509977652, -13.97604488694527269, 63.12390960531435979 ) ) ;
#181967=CARTESIAN_POINT ( 'NONE',  ( -15.80617190586768217, 15.72974639402176855, 83.12609039468568994 ) ) ;
#181968=CARTESIAN_POINT ( 'NONE',  ( 13.89961937509977652, -13.97604488694527269, 58.12390960531436690 ) ) ;
#181970=CARTESIAN_POINT ( 'NONE',  ( 0.05219959533909260263, 19.03943276465977164, 34.99890960531435979 ) ) ;
#181971=CARTESIAN_POINT ( 'NONE',  ( 5.719274019375991003, -21.55341960407610458, 32.70724293864770260 ) ) ;
#181972=CARTESIAN_POINT ( 'NONE',  ( 4.379528057220339221, -16.55341960407611168, 72.70724293864769550 ) ) ;
#181973=CARTESIAN_POINT ( 'NONE',  ( 0.05219959533909260263, 19.03943276465977164, 44.99890960531435979 ) ) ;
#181974=CARTESIAN_POINT ( 'NONE',  ( 8.224510206698953496, -14.34966873604960469, 97.91557627198103830 ) ) ;
#181975=CARTESIAN_POINT ( 'NONE',  ( -18.67979575497178146, -10.72451020669898902, 111.6655762719810525 ) ) ;
#181976=CARTESIAN_POINT ( 'NONE',  ( -18.62759615963255300, -10.81492255796106328, 44.16775706135234714 ) ) ;
#181977=CARTESIAN_POINT ( 'NONE',  ( -16.51473224551069308, -9.474510206698971260, 31.66557627198102054 ) ) ;
#181978=CARTESIAN_POINT ( 'NONE',  ( -0.05219959533934338120, 16.53943276465976808, 67.50109039468568994 ) ) ;
#181980=CARTESIAN_POINT ( 'NONE',  ( -0.05219959533907301413, -21.53943276465977519, 107.4989096053143669 ) ) ;
#181981=CARTESIAN_POINT ( 'NONE',  ( -5.823673210054116645, -21.52544592524344225, 97.29057627198105251 ) ) ;
#181982=CARTESIAN_POINT ( 'NONE',  ( -16.46253265017146816, -9.564922557961047289, 29.16775706135232937 ) ) ;
#181983=CARTESIAN_POINT ( 'NONE',  ( -19.02544592524342804, 5.153800228976336051, 46.04057627198101699 ) ) ;
#181985=CARTESIAN_POINT ( 'NONE',  ( 5.823673210054444382, -21.52544592524334988, 60.20942372801902565 ) ) ;
#181986=CARTESIAN_POINT ( 'NONE',  ( 5.719274019375991003, -21.55341960407610458, 62.70724293864769550 ) ) ;
#181987=CARTESIAN_POINT ( 'NONE',  ( 8.314922557960818139, 14.29746914071049879, 29.58224293864769905 ) ) ;
#181988=CARTESIAN_POINT ( 'NONE',  ( 10.72451020669871369, 18.67979575497193778, 77.08442372801901854 ) ) ;
#181989=CARTESIAN_POINT ( 'NONE',  ( -13.89961937509957401, -13.97604488694547875, 19.37609039468566507 ) ) ;
#181990=CARTESIAN_POINT ( 'NONE',  ( 16.51473224551083163, -9.474510206698727899, 50.83442372801899722 ) ) ;
#181991=CARTESIAN_POINT ( 'NONE',  ( 12.06949235617739724, 12.14591786802326823, 96.87609039468568994 ) ) ;
#181992=CARTESIAN_POINT ( 'NONE',  ( 18.67979575497194134, -10.72451020669871369, 60.83442372801901854 ) ) ;
#181993=CARTESIAN_POINT ( 'NONE',  ( 19.03943276465977164, -0.05219959533909143690, 58.74890960531435979 ) ) ;
#181994=CARTESIAN_POINT ( 'NONE',  ( 19.03943276465977164, 0.05219959533936151252, 36.25109039468567573 ) ) ;
#181995=CARTESIAN_POINT ( 'NONE',  ( -15.72974639402197994, 15.80617190586746368, 40.62390960531435269 ) ) ;
#181996=CARTESIAN_POINT ( 'NONE',  ( -18.62759615963255300, -10.81492255796106328, 34.16775706135234714 ) ) ;
#181997=CARTESIAN_POINT ( 'NONE',  ( 21.52544592524344225, -5.823673210054117533, 93.54057627198103830 ) ) ;
#181998=CARTESIAN_POINT ( 'NONE',  ( 9.474510206698729675, 16.51473224551082808, 87.08442372801900433 ) ) ;
#181999=CARTESIAN_POINT ( 'NONE',  ( -14.29746914071037622, -8.314922557961029526, 49.16775706135234003 ) ) ;
#182001=CARTESIAN_POINT ( 'NONE',  ( 15.80617190586746368, 15.72974639402197994, 89.37390960531435269 ) ) ;
#182002=CARTESIAN_POINT ( 'NONE',  ( -16.55341960407617563, 4.379528057220093196, 83.54275706135234714 ) ) ;
#182003=CARTESIAN_POINT ( 'NONE',  ( -14.34966873604960291, -8.224510206698953496, 81.66557627198103830 ) ) ;
#182005=CARTESIAN_POINT ( 'NONE',  ( -19.03943276465977164, -0.05219959533935918106, 103.7510903946856757 ) ) ;
#182007=CARTESIAN_POINT ( 'NONE',  ( -18.67979575497178146, -10.72451020669898902, 36.66557627198103120 ) ) ;
#182009=CARTESIAN_POINT ( 'NONE',  ( -16.53943276465976808, -0.05219959533934237506, 48.75109039468568284 ) ) ;
#182010=CARTESIAN_POINT ( 'NONE',  ( -18.67979575497193778, 10.72451020669871902, 23.33442372801901499 ) ) ;
#182011=CARTESIAN_POINT ( 'NONE',  ( 21.53943276465977519, -0.05219959533907433946, 28.74890960531435624 ) ) ;
#182012=CARTESIAN_POINT ( 'NONE',  ( -12.14591786802326823, 12.06949235617739902, 73.12609039468567573 ) ) ;
#182013=CARTESIAN_POINT ( 'NONE',  ( -13.89961937509977652, 13.97604488694528158, 80.62390960531436690 ) ) ;
#182014=CARTESIAN_POINT ( 'NONE',  ( -5.719274019375665041, -21.55341960407619695, 54.79275706135235424 ) ) ;
#182015=CARTESIAN_POINT ( 'NONE',  ( -19.02544592524342804, 5.153800228976336051, 26.04057627198103120 ) ) ;
#182016=CARTESIAN_POINT ( 'NONE',  ( -0.05219959533907301413, -21.53943276465977519, 32.49890960531435979 ) ) ;
#182018=CARTESIAN_POINT ( 'NONE',  ( 5.153800228976615827, -19.02544592524334988, 45.20942372801901143 ) ) ;
#182019=CARTESIAN_POINT ( 'NONE',  ( 4.483927247898790824, -16.52544592524335698, 50.20942372801901854 ) ) ;
#182020=CARTESIAN_POINT ( 'NONE',  ( 13.97604488694527802, 13.89961937509977652, 114.3739096053143669 ) ) ;
#182021=CARTESIAN_POINT ( 'NONE',  ( -5.049401038298153566, 19.05341960407611168, 70.20724293864769550 ) ) ;
#182022=CARTESIAN_POINT ( 'NONE',  ( 8.314922557961029526, -14.29746914071037800, 105.4177570613523613 ) ) ;
#182023=CARTESIAN_POINT ( 'NONE',  ( -5.049401038298153566, 19.05341960407611168, 115.2072429386477097 ) ) ;
#182024=CARTESIAN_POINT ( 'NONE',  ( -16.55341960407611168, -4.379528057220339221, 96.45724293864770971 ) ) ;
#182025=CARTESIAN_POINT ( 'NONE',  ( 10.81492255796078972, 18.62759615963270932, 29.58224293864769905 ) ) ;
#182026=CARTESIAN_POINT ( 'NONE',  ( 5.049401038298161559, -19.05341960407611168, 27.70724293864769550 ) ) ;
#182027=CARTESIAN_POINT ( 'NONE',  ( 8.314922557961029526, -14.29746914071037800, 70.41775706135236135 ) ) ;
#182028=CARTESIAN_POINT ( 'NONE',  ( -10.72451020669870658, -18.67979575497194134, 19.58442372801901143 ) ) ;
#182029=CARTESIAN_POINT ( 'NONE',  ( 5.049401038297881783, 19.05341960407617563, 77.29275706135231871 ) ) ;
#182030=CARTESIAN_POINT ( 'NONE',  ( 19.03943276465977164, -0.05219959533909143690, 38.74890960531436690 ) ) ;
#182031=CARTESIAN_POINT ( 'NONE',  ( -18.67979575497178146, -10.72451020669898902, 71.66557627198100988 ) ) ;
#182033=CARTESIAN_POINT ( 'NONE',  ( 0.05219959533937995610, -21.53943276465977519, 90.00109039468567573 ) ) ;
#182034=CARTESIAN_POINT ( 'NONE',  ( 13.97604488694527802, 13.89961937509977652, 69.37390960531436690 ) ) ;
#182036=CARTESIAN_POINT ( 'NONE',  ( 4.483927247898790824, -16.52544592524335698, 55.20942372801902565 ) ) ;
#182037=CARTESIAN_POINT ( 'NONE',  ( 21.52544592524334988, 5.823673210054432836, 76.45942372801901854 ) ) ;
#182038=CARTESIAN_POINT ( 'NONE',  ( 13.97604488694548053, -13.89961937509957401, 45.62609039468566863 ) ) ;
#182039=CARTESIAN_POINT ( 'NONE',  ( 16.46253265017146816, 9.564922557961045513, 56.66775706135233293 ) ) ;
#182040=ORIENTED_EDGE ( 'NONE', *, *, #58394, .T. ) ;
#182041=CARTESIAN_POINT ( 'NONE',  ( -21.52544592524334988, -5.823673210054445271, 48.95942372801902565 ) ) ;
#182043=CARTESIAN_POINT ( 'NONE',  ( -9.564922557961040184, 16.46253265017147172, 47.91775706135233293 ) ) ;
#182044=CARTESIAN_POINT ( 'NONE',  ( 9.474510206698971260, -16.51473224551069308, 102.9155762719810241 ) ) ;
#182045=CARTESIAN_POINT ( 'NONE',  ( 19.03943276465977164, -0.05219959533909143690, 83.74890960531436690 ) ) ;
#182046=CARTESIAN_POINT ( 'NONE',  ( 8.314922557960818139, 14.29746914071049879, 39.58224293864769550 ) ) ;
#182047=CARTESIAN_POINT ( 'NONE',  ( 0.05219959533907565091, 21.53943276465977519, 29.99890960531435979 ) ) ;
#182050=CARTESIAN_POINT ( 'NONE',  ( -5.823673210054431948, 21.52544592524334988, 92.70942372801901854 ) ) ;
#182052=CARTESIAN_POINT ( 'NONE',  ( 9.474510206698971260, -16.51473224551069308, 37.91557627198102409 ) ) ;
#182053=CARTESIAN_POINT ( 'NONE',  ( 5.153800228976335163, 19.02544592524342804, 114.7905762719810241 ) ) ;
#182055=CARTESIAN_POINT ( 'NONE',  ( 16.55341960407618274, -4.379528057220086978, 56.04275706135235424 ) ) ;
#182056=CARTESIAN_POINT ( 'NONE',  ( -21.52544592524343514, 5.823673210054127303, 86.04057627198102409 ) ) ;
#182057=CARTESIAN_POINT ( 'NONE',  ( 4.483927247898545687, 16.52544592524342804, 34.79057627198103120 ) ) ;
#182058=CARTESIAN_POINT ( 'NONE',  ( 16.46253265017160672, -9.564922557960803928, 28.33224293864769550 ) ) ;
#182059=CARTESIAN_POINT ( 'NONE',  ( -13.89961937509977652, 13.97604488694528158, 105.6239096053143527 ) ) ;
#182060=CARTESIAN_POINT ( 'NONE',  ( 21.52544592524334988, 5.823673210054432836, 26.45942372801901854 ) ) ;
#182061=CARTESIAN_POINT ( 'NONE',  ( -16.46253265017146816, -9.564922557961047289, 29.16775706135232937 ) ) ;
#182062=CARTESIAN_POINT ( 'NONE',  ( -16.52544592524342804, 4.483927247898546575, 116.0405762719810383 ) ) ;
#182063=CARTESIAN_POINT ( 'NONE',  ( -21.52544592524334988, -5.823673210054445271, 78.95942372801901854 ) ) ;
#182064=CARTESIAN_POINT ( 'NONE',  ( 16.21995358207306737, -7.366697692864086378, 32.43551001512160781 ) ) ;
#182065=CARTESIAN_POINT ( 'NONE',  ( -16.53943276465976808, 0.05219959533911058130, 21.24890960531436690 ) ) ;
#182066=CARTESIAN_POINT ( 'NONE',  ( 17.50000000000000000, 5.499999999999995559, 113.7823096230356583 ) ) ;
#182067=CARTESIAN_POINT ( 'NONE',  ( -15.80617190586745835, -15.72974639402198527, 21.87390960531436690 ) ) ;
#182068=CARTESIAN_POINT ( 'NONE',  ( -8.224510206698948167, 14.34966873604960824, 90.41557627198103830 ) ) ;
#182070=CARTESIAN_POINT ( 'NONE',  ( 0.05219959533909260263, 19.03943276465977164, 74.99890960531435269 ) ) ;
#182071=CARTESIAN_POINT ( 'NONE',  ( -14.34966873604960291, -8.224510206698953496, 71.66557627198100988 ) ) ;
#182072=CARTESIAN_POINT ( 'NONE',  ( 19.03943276465977164, 0.05219959533936151252, 106.2510903946856615 ) ) ;
#182073=CARTESIAN_POINT ( 'NONE',  ( 5.823673210054125526, 21.52544592524343514, 64.79057627198103830 ) ) ;
#182075=CARTESIAN_POINT ( 'NONE',  ( 19.02544592524343514, -5.153800228976328945, 38.54057627198103120 ) ) ;
#182076=CARTESIAN_POINT ( 'NONE',  ( -5.049401038298153566, 19.05341960407611168, 90.20724293864766707 ) ) ;
#182077=CARTESIAN_POINT ( 'NONE',  ( 21.55341960407610458, 5.719274019375980345, 73.95724293864769550 ) ) ;
#182079=CARTESIAN_POINT ( 'NONE',  ( -16.52544592524335698, -4.483927247898792601, 108.9594237280190185 ) ) ;
#182080=CARTESIAN_POINT ( 'NONE',  ( 19.02544592524343514, -5.153800228976328945, 93.54057627198102409 ) ) ;
#182081=CARTESIAN_POINT ( 'NONE',  ( 16.46253265017146816, 9.564922557961045513, 61.66775706135234003 ) ) ;
#182082=CARTESIAN_POINT ( 'NONE',  ( 5.823673210054444382, -21.52544592524334988, 90.20942372801903275 ) ) ;
#182083=CARTESIAN_POINT ( 'NONE',  ( -5.823673210054116645, -21.52544592524344225, 72.29057627198102409 ) ) ;
#182084=CARTESIAN_POINT ( 'NONE',  ( -13.89961937509977652, 13.97604488694528158, 115.6239096053143669 ) ) ;
#182085=CARTESIAN_POINT ( 'NONE',  ( -19.03943276465977164, 0.05219959533909376836, 46.24890960531435979 ) ) ;
#182086=CARTESIAN_POINT ( 'NONE',  ( -16.53943276465976808, 0.05219959533911058130, 21.24890960531436690 ) ) ;
#182087=CARTESIAN_POINT ( 'NONE',  ( 5.049401038298161559, -19.05341960407611168, 57.70724293864769550 ) ) ;
#182089=CARTESIAN_POINT ( 'NONE',  ( -5.719274019375665041, -21.55341960407619695, 104.7927570613523898 ) ) ;
#182090=CARTESIAN_POINT ( 'NONE',  ( -16.52544592524342804, 4.483927247898546575, 71.04057627198103830 ) ) ;
#182091=CARTESIAN_POINT ( 'NONE',  ( 15.80617190586746368, 15.72974639402197994, 104.3739096053143669 ) ) ;
#182092=CARTESIAN_POINT ( 'NONE',  ( 21.55341960407610458, 5.719274019375980345, 103.9572429386476813 ) ) ;
#182094=CARTESIAN_POINT ( 'NONE',  ( -15.72974639402197994, 15.80617190586746368, 65.62390960531436690 ) ) ;
#182095=CARTESIAN_POINT ( 'NONE',  ( 16.53943276465976808, 0.05219959533934440121, 81.25109039468568994 ) ) ;
#182096=CARTESIAN_POINT ( 'NONE',  ( 16.53943276465976808, -0.05219959533910856209, 108.7489096053143669 ) ) ;
#182097=CARTESIAN_POINT ( 'NONE',  ( 19.02544592524343514, -5.153800228976328945, 53.54057627198102409 ) ) ;
#182098=CARTESIAN_POINT ( 'NONE',  ( -16.53943276465976808, -0.05219959533934237506, 103.7510903946857042 ) ) ;
#182099=CARTESIAN_POINT ( 'NONE',  ( -15.72974639402176322, -15.80617190586768395, 44.37609039468567573 ) ) ;
#182100=CARTESIAN_POINT ( 'NONE',  ( 18.67979575497194134, -10.72451020669871369, 80.83442372801901854 ) ) ;
#182101=CARTESIAN_POINT ( 'NONE',  ( -13.97604488694527625, -13.89961937509977652, 36.87390960531436690 ) ) ;
#182102=CARTESIAN_POINT ( 'NONE',  ( -19.05341960407611168, -5.049401038298163336, 36.45724293864766707 ) ) ;
#182103=ORIENTED_EDGE ( 'NONE', *, *, #15442, .F. ) ;
#182104=CARTESIAN_POINT ( 'NONE',  ( -15.72974639402176322, -15.80617190586768395, 69.37609039468567573 ) ) ;
#182105=CARTESIAN_POINT ( 'NONE',  ( 5.049401038298161559, -19.05341960407611168, 97.70724293864766707 ) ) ;
#182106=CARTESIAN_POINT ( 'NONE',  ( 9.564922557961047289, -16.46253265017146816, 80.41775706135234714 ) ) ;
#182107=CARTESIAN_POINT ( 'NONE',  ( 0.05219959533937995610, -21.53943276465977519, 55.00109039468568284 ) ) ;
#182108=CARTESIAN_POINT ( 'NONE',  ( -16.55341960407617563, 4.379528057220093196, 23.54275706135235424 ) ) ;
#182109=CARTESIAN_POINT ( 'NONE',  ( 16.51473224551083163, -9.474510206698727899, 75.83442372801900433 ) ) ;
#182110=CARTESIAN_POINT ( 'NONE',  ( 9.474510206698971260, -16.51473224551069308, 47.91557627198102409 ) ) ;
#182111=CARTESIAN_POINT ( 'NONE',  ( 13.89961937509957401, 13.97604488694547697, 86.87609039468567573 ) ) ;
#182112=CARTESIAN_POINT ( 'NONE',  ( 4.379528057220092307, 16.55341960407617563, 112.2927570613523471 ) ) ;
#182113=CARTESIAN_POINT ( 'NONE',  ( 9.474510206698729675, 16.51473224551082808, 87.08442372801900433 ) ) ;
#182114=CARTESIAN_POINT ( 'NONE',  ( -12.14591786802309592, -12.06949235617757132, 41.87390960531435979 ) ) ;
#182115=CARTESIAN_POINT ( 'NONE',  ( -9.564922557961040184, 16.46253265017147172, 57.91775706135233293 ) ) ;
#182116=CARTESIAN_POINT ( 'NONE',  ( -8.314922557961024197, 14.29746914071037800, 52.91775706135235424 ) ) ;
#182117=CARTESIAN_POINT ( 'NONE',  ( -9.564922557961040184, 16.46253265017147172, 22.91775706135233648 ) ) ;
#182118=CARTESIAN_POINT ( 'NONE',  ( 5.049401038298161559, -19.05341960407611168, 47.70724293864770260 ) ) ;
#182119=CARTESIAN_POINT ( 'NONE',  ( -17.31728774477271671, -6.344390552232408886, 64.18093348310682700 ) ) ;
#182120=CARTESIAN_POINT ( 'NONE',  ( -12.06949235617739369, -12.14591786802326823, 39.37609039468567573 ) ) ;
#182121=B_SPLINE_CURVE_WITH_KNOTS ( 'NONE', 3,
 ( #93772, #155453, #141269, #16943, #78597, #140270, #1763, #2759, #174606, #39078, #191754, #161421, #129064, #112912, #38081, #176607, #134848, #22913, #103499, #37071 ),
 .UNSPECIFIED., .F., .F.,
 ( 4, 2, 2, 2, 2, 2, 2, 2, 2, 4 ),
 ( 3.469446951953614189E-18, 0.0004987090165372363819, 0.0009974180330744692943, 0.001246772541343085751, 0.001496127049611702207, 0.001994836066148977186, 0.002493545082686252166, 0.002742899590954890089, 0.002992254099223527579, 0.003989672132298154733 ),
 .UNSPECIFIED. ) ;
#182125=CARTESIAN_POINT ( 'NONE',  ( 16.46253265017160672, -9.564922557960803928, 93.33224293864769550 ) ) ;
#182126=CARTESIAN_POINT ( 'NONE',  ( 17.50000000000000355, 3.242565516147348337, 102.5000000000000142 ) ) ;
#182128=CARTESIAN_POINT ( 'NONE',  ( -19.05341960407617563, 5.049401038297882671, 103.5427570613523329 ) ) ;
#182129=CARTESIAN_POINT ( 'NONE',  ( -5.049401038298153566, 19.05341960407611168, 115.2072429386477097 ) ) ;
#182130=CARTESIAN_POINT ( 'NONE',  ( 5.719274019375673035, 21.55341960407619339, 107.2927570613523471 ) ) ;
#182131=CARTESIAN_POINT ( 'NONE',  ( 5.049401038297881783, 19.05341960407617563, 97.29275706135233293 ) ) ;
#182132=CARTESIAN_POINT ( 'NONE',  ( 8.314922557960818139, 14.29746914071049879, 114.5822429386477097 ) ) ;
#182133=CARTESIAN_POINT ( 'NONE',  ( 0.05219959533909260263, 19.03943276465977164, 34.99890960531435979 ) ) ;
#182134=CARTESIAN_POINT ( 'NONE',  ( 0.05219959533907565091, 21.53943276465977519, 64.99890960531435269 ) ) ;
#182135=VECTOR ( 'NONE', #48898, 1000.000000000000000 ) ;
#182136=CARTESIAN_POINT ( 'NONE',  ( 4.379528057220339221, -16.55341960407611168, 112.7072429386476955 ) ) ;
#182138=CARTESIAN_POINT ( 'NONE',  ( 16.46253265017146816, 9.564922557961045513, 76.66775706135234714 ) ) ;
#182139=CARTESIAN_POINT ( 'NONE',  ( -12.14591786802309592, -12.06949235617757132, 46.87390960531435979 ) ) ;
#182140=CARTESIAN_POINT ( 'NONE',  ( 15.80617190586746368, 15.72974639402197994, 29.37390960531435269 ) ) ;
#182141=CARTESIAN_POINT ( 'NONE',  ( -21.55341960407619339, 5.719274019375674811, 88.54275706135236135 ) ) ;
#182142=CARTESIAN_POINT ( 'NONE',  ( -21.53943276465977519, 0.05219959533907696930, 81.24890960531436690 ) ) ;
#182143=CARTESIAN_POINT ( 'NONE',  ( -10.72451020669870658, -18.67979575497194134, 59.58442372801901854 ) ) ;
#182144=CARTESIAN_POINT ( 'NONE',  ( -5.719274019375665041, -21.55341960407619695, 64.79275706135234714 ) ) ;
#182145=CARTESIAN_POINT ( 'NONE',  ( 5.153800228976335163, 19.02544592524342804, 89.79057627198102409 ) ) ;
#182146=CARTESIAN_POINT ( 'NONE',  ( -16.53943276465976808, -0.05219959533934237506, 88.75109039468567573 ) ) ;
#182147=CARTESIAN_POINT ( 'NONE',  ( 0.05219959533937995610, -21.53943276465977519, 60.00109039468568284 ) ) ;
#182148=CARTESIAN_POINT ( 'NONE',  ( -16.53943276465976808, 0.05219959533911058130, 116.2489096053143669 ) ) ;
#182149=CARTESIAN_POINT ( 'NONE',  ( -0.05219959533910754901, -16.53943276465976808, 62.49890960531436690 ) ) ;
#182150=CARTESIAN_POINT ( 'NONE',  ( 14.34966873604960469, 8.224510206698951720, 39.16557627198102409 ) ) ;
#182151=CARTESIAN_POINT ( 'NONE',  ( 5.823673210054125526, 21.52544592524343514, 39.79057627198103830 ) ) ;
#182152=CARTESIAN_POINT ( 'NONE',  ( 0.05219959533909260263, 19.03943276465977164, 49.99890960531435979 ) ) ;
#182153=CARTESIAN_POINT ( 'NONE',  ( -21.52544592524343514, 5.823673210054127303, 56.04057627198102409 ) ) ;
#182154=CARTESIAN_POINT ( 'NONE',  ( 16.51473224551083163, -9.474510206698727899, 45.83442372801900433 ) ) ;
#182156=CARTESIAN_POINT ( 'NONE',  ( -16.31925111598457079, -7.325300261831483084, 39.83575461032750553 ) ) ;
#182157=CARTESIAN_POINT ( 'NONE',  ( 8.314922557960818139, 14.29746914071049879, 44.58224293864769550 ) ) ;
#182158=CARTESIAN_POINT ( 'NONE',  ( -10.81492255796078084, -18.62759615963271287, 22.08224293864769194 ) ) ;
#182162=CARTESIAN_POINT ( 'NONE',  ( -16.55341960407617563, 4.379528057220093196, 78.54275706135236135 ) ) ;
#182163=CARTESIAN_POINT ( 'NONE',  ( -5.153800228976607833, 19.02544592524334988, 77.70942372801900433 ) ) ;
#182164=CARTESIAN_POINT ( 'NONE',  ( 4.379528057220339221, -16.55341960407611168, 52.70724293864769550 ) ) ;
#182165=CARTESIAN_POINT ( 'NONE',  ( 17.13100169013303287, -6.664070546373075388, 53.26789835699850784 ) ) ;
#182166=CARTESIAN_POINT ( 'NONE',  ( -4.483927247898539470, -16.52544592524342804, 22.29057627198102765 ) ) ;
#182167=CARTESIAN_POINT ( 'NONE',  ( -5.049401038298153566, 19.05341960407611168, 50.20724293864770260 ) ) ;
#182168=CARTESIAN_POINT ( 'NONE',  ( -19.03943276465977164, 0.05219959533909376836, 76.24890960531435269 ) ) ;
#182169=CARTESIAN_POINT ( 'NONE',  ( 19.02544592524343514, -5.153800228976328945, 33.54057627198102409 ) ) ;
#182170=CARTESIAN_POINT ( 'NONE',  ( -0.05219959533937732626, 21.53943276465977519, 47.50109039468568994 ) ) ;
#182171=CARTESIAN_POINT ( 'NONE',  ( -16.51473224551069308, -9.474510206698971260, 66.66557627198102409 ) ) ;
#182173=CARTESIAN_POINT ( 'NONE',  ( -9.474510206698964154, 16.51473224551069663, 65.41557627198102409 ) ) ;
#182174=CARTESIAN_POINT ( 'NONE',  ( 21.53943276465977519, -0.05219959533907433946, 33.74890960531436690 ) ) ;
#182175=CARTESIAN_POINT ( 'NONE',  ( -13.97604488694527625, -13.89961937509977652, 31.87390960531435979 ) ) ;
#182176=CARTESIAN_POINT ( 'NONE',  ( -21.52544592524343514, 5.823673210054127303, 36.04057627198102409 ) ) ;
#182177=CARTESIAN_POINT ( 'NONE',  ( 16.53943276465976808, 0.05219959533934440121, 91.25109039468568994 ) ) ;
#182178=CARTESIAN_POINT ( 'NONE',  ( -19.05341960407617563, 5.049401038297882671, 23.54275706135233648 ) ) ;
#182179=CARTESIAN_POINT ( 'NONE',  ( -16.53943276465976808, -0.05219959533934237506, 43.75109039468568284 ) ) ;
#182180=CARTESIAN_POINT ( 'NONE',  ( -16.53943276465976808, -0.05219959533934237506, 73.75109039468567573 ) ) ;
#182181=CARTESIAN_POINT ( 'NONE',  ( -19.05341960407611168, -5.049401038298163336, 106.4572429386476955 ) ) ;
#182182=CARTESIAN_POINT ( 'NONE',  ( -8.314922557961024197, 14.29746914071037800, 72.91775706135234714 ) ) ;
#182183=CARTESIAN_POINT ( 'NONE',  ( 8.314922557961029526, -14.29746914071037800, 35.41775706135234003 ) ) ;
#182184=CARTESIAN_POINT ( 'NONE',  ( 9.474510206698971260, -16.51473224551069308, 107.9155762719810383 ) ) ;
#182185=CARTESIAN_POINT ( 'NONE',  ( 16.53943276465976808, 0.05219959533934440121, 21.25109039468567218 ) ) ;
#182186=CARTESIAN_POINT ( 'NONE',  ( 0.05219959533909260263, 19.03943276465977164, 34.99890960531435979 ) ) ;
#182187=CARTESIAN_POINT ( 'NONE',  ( 18.62759615963255655, 10.81492255796105972, 31.66775706135234358 ) ) ;
#182188=CARTESIAN_POINT ( 'NONE',  ( 5.049401038297881783, 19.05341960407617563, 112.2927570613523471 ) ) ;
#182189=CARTESIAN_POINT ( 'NONE',  ( -14.34966873604972548, 8.224510206698743886, 93.33442372801901854 ) ) ;
#182191=CARTESIAN_POINT ( 'NONE',  ( 15.72974639402176855, 15.80617190586768217, 96.87609039468568994 ) ) ;
#182192=CARTESIAN_POINT ( 'NONE',  ( 9.474510206698729675, 16.51473224551082808, 97.08442372801900433 ) ) ;
#182193=CARTESIAN_POINT ( 'NONE',  ( -8.314922557960811034, -14.29746914071050412, 57.08224293864769550 ) ) ;
#182194=CARTESIAN_POINT ( 'NONE',  ( 9.564922557960805705, 16.46253265017160317, 24.58224293864769194 ) ) ;
#182195=CARTESIAN_POINT ( 'NONE',  ( -13.89961937509957401, -13.97604488694547875, 64.37609039468567573 ) ) ;
#182197=CARTESIAN_POINT ( 'NONE',  ( 10.81492255796106328, -18.62759615963255655, 50.41775706135235424 ) ) ;
#182198=CARTESIAN_POINT ( 'NONE',  ( -8.314922557961024197, 14.29746914071037800, 32.91775706135234714 ) ) ;
#182199=CARTESIAN_POINT ( 'NONE',  ( 16.36317988757058473, 7.306389748694940067, 83.40210391636773579 ) ) ;
#182200=CARTESIAN_POINT ( 'NONE',  ( -5.153800228976328057, -19.02544592524343514, 112.2905762719810099 ) ) ;
#182201=CARTESIAN_POINT ( 'NONE',  ( 5.719274019375991003, -21.55341960407610458, 72.70724293864769550 ) ) ;
#182202=CARTESIAN_POINT ( 'NONE',  ( 5.049401038297881783, 19.05341960407617563, 112.2927570613523471 ) ) ;
#182204=CARTESIAN_POINT ( 'NONE',  ( -13.97604488694527625, -13.89961937509977652, 96.87390960531433848 ) ) ;
#182206=CARTESIAN_POINT ( 'NONE',  ( 16.46253265017160672, -9.564922557960803928, 23.33224293864769194 ) ) ;
#182207=CARTESIAN_POINT ( 'NONE',  ( 21.53943276465977519, 0.05219959533937863772, 96.25109039468568994 ) ) ;
#182208=CARTESIAN_POINT ( 'NONE',  ( 19.05341960407611168, 5.049401038298154454, 38.95724293864767418 ) ) ;
#182209=CARTESIAN_POINT ( 'NONE',  ( 21.52544592524334988, 5.823673210054432836, 46.45942372801901854 ) ) ;
#182210=CARTESIAN_POINT ( 'NONE',  ( -21.53943276465977519, -0.05219959533937600094, 88.75109039468567573 ) ) ;
#182211=CARTESIAN_POINT ( 'NONE',  ( 16.55341960407618274, -4.379528057220086978, 101.0427570613523756 ) ) ;
#182213=CARTESIAN_POINT ( 'NONE',  ( 5.049401038298161559, -19.05341960407611168, 77.70724293864765286 ) ) ;
#182214=CARTESIAN_POINT ( 'NONE',  ( 18.67979575497194134, -10.72451020669871369, 45.83442372801901854 ) ) ;
#182215=CARTESIAN_POINT ( 'NONE',  ( 18.62759615963255655, 10.81492255796105972, 36.66775706135234714 ) ) ;
#182216=CARTESIAN_POINT ( 'NONE',  ( 13.97604488694548053, -13.89961937509957401, 75.62609039468564731 ) ) ;
#182217=CARTESIAN_POINT ( 'NONE',  ( -16.51473224551069308, -9.474510206698971260, 86.66557627198102409 ) ) ;
#182218=CARTESIAN_POINT ( 'NONE',  ( -8.224510206698948167, 14.34966873604960824, 100.4155762719810241 ) ) ;
#182219=CARTESIAN_POINT ( 'NONE',  ( 21.55341960407610458, 5.719274019375980345, 98.95724293864770971 ) ) ;
#182220=CARTESIAN_POINT ( 'NONE',  ( -12.06949235617756955, 12.14591786802309770, 80.62390960531438111 ) ) ;
#182221=CARTESIAN_POINT ( 'NONE',  ( 19.03943276465977164, 0.05219959533936151252, 21.25109039468565797 ) ) ;
#182222=CARTESIAN_POINT ( 'NONE',  ( -4.483927247898539470, -16.52544592524342804, 102.2905762719810383 ) ) ;
#182223=CARTESIAN_POINT ( 'NONE',  ( -9.474510206698964154, 16.51473224551069663, 35.41557627198102409 ) ) ;
#182224=CARTESIAN_POINT ( 'NONE',  ( 0.05219959533936267826, -19.03943276465977164, 85.00109039468567573 ) ) ;
#182225=CARTESIAN_POINT ( 'NONE',  ( 8.224510206698953496, -14.34966873604960469, 42.91557627198103120 ) ) ;
#182226=CARTESIAN_POINT ( 'NONE',  ( -15.72974639402176322, -15.80617190586768395, 94.37609039468568994 ) ) ;
#182227=CARTESIAN_POINT ( 'NONE',  ( -19.05341960407611168, -5.049401038298163336, 111.4572429386476671 ) ) ;
#182228=CARTESIAN_POINT ( 'NONE',  ( 5.153800228976615827, -19.02544592524334988, 70.20942372801899012 ) ) ;
#182229=CARTESIAN_POINT ( 'NONE',  ( 10.81492255796078972, 18.62759615963270932, 79.58224293864769550 ) ) ;
#182230=CARTESIAN_POINT ( 'NONE',  ( 21.53943276465977519, 0.05219959533937863772, 31.25109039468568639 ) ) ;
#182231=CARTESIAN_POINT ( 'NONE',  ( -16.55341960407617563, 4.379528057220093196, 28.54275706135234358 ) ) ;
#182232=CARTESIAN_POINT ( 'NONE',  ( 0.05219959533934541429, -16.53943276465976808, 95.00109039468568994 ) ) ;
#182233=CARTESIAN_POINT ( 'NONE',  ( 16.46253265017160672, -9.564922557960803928, 23.33224293864769194 ) ) ;
#182234=CARTESIAN_POINT ( 'NONE',  ( 21.52544592524334988, 5.823673210054432836, 41.45942372801901143 ) ) ;
#182235=CARTESIAN_POINT ( 'NONE',  ( 5.153800228976335163, 19.02544592524342804, 24.79057627198102765 ) ) ;
#182237=CARTESIAN_POINT ( 'NONE',  ( -16.52544592524335698, -4.483927247898792601, 48.95942372801902565 ) ) ;
#182238=CARTESIAN_POINT ( 'NONE',  ( 8.314922557960818139, 14.29746914071049879, 79.58224293864769550 ) ) ;
#182239=CARTESIAN_POINT ( 'NONE',  ( -18.62759615963270932, 10.81492255796079327, 70.83224293864770971 ) ) ;
#182240=CARTESIAN_POINT ( 'NONE',  ( 12.06949235617739724, 12.14591786802326823, 111.8760903946856615 ) ) ;
#182241=CARTESIAN_POINT ( 'NONE',  ( -4.379528057220086978, -16.55341960407618274, 54.79275706135235424 ) ) ;
#182242=CARTESIAN_POINT ( 'NONE',  ( 19.02544592524343514, -5.153800228976328945, 43.54057627198103120 ) ) ;
#182243=CARTESIAN_POINT ( 'NONE',  ( 14.34966873604972726, -8.224510206698740333, 95.83442372801903275 ) ) ;
#182244=CARTESIAN_POINT ( 'NONE',  ( -19.03943276465977164, -0.05219959533935918106, 88.75109039468567573 ) ) ;
#182245=CARTESIAN_POINT ( 'NONE',  ( 18.67979575497178502, 10.72451020669898547, 89.16557627198102409 ) ) ;
#182246=CARTESIAN_POINT ( 'NONE',  ( 14.29746914071037800, 8.314922557961029526, 111.6677570613523613 ) ) ;
#182250=CARTESIAN_POINT ( 'NONE',  ( -15.72974639402197994, 15.80617190586746368, 60.62390960531437401 ) ) ;
#182252=CARTESIAN_POINT ( 'NONE',  ( 14.34966873604972726, -8.224510206698740333, 85.83442372801901854 ) ) ;
#182254=CARTESIAN_POINT ( 'NONE',  ( 19.03943276465977164, -0.05219959533909143690, 108.7489096053143527 ) ) ;
#182255=CARTESIAN_POINT ( 'NONE',  ( -18.87580814761074777, 5.500000000000058620, 75.87172394265758157 ) ) ;
#182256=CARTESIAN_POINT ( 'NONE',  ( 15.72974639402199770, -15.80617190586745480, 73.12390960531436690 ) ) ;
#182257=CARTESIAN_POINT ( 'NONE',  ( -14.34966873604972548, 8.224510206698743886, 113.3344237280190328 ) ) ;
#182258=CARTESIAN_POINT ( 'NONE',  ( 8.224510206698742110, 14.34966873604972548, 27.08442372801901854 ) ) ;
#182259=CARTESIAN_POINT ( 'NONE',  ( 8.224510206698953496, -14.34966873604960469, 112.9155762719810383 ) ) ;
#182260=CARTESIAN_POINT ( 'NONE',  ( -14.29746914071037622, -8.314922557961029526, 29.16775706135234003 ) ) ;
#182261=CARTESIAN_POINT ( 'NONE',  ( -9.474510206698964154, 16.51473224551069663, 55.41557627198103120 ) ) ;
#182263=CARTESIAN_POINT ( 'NONE',  ( 9.564922557960805705, 16.46253265017160317, 104.5822429386476955 ) ) ;
#182264=CARTESIAN_POINT ( 'NONE',  ( -13.89961937509977652, 13.97604488694528158, 100.6239096053143669 ) ) ;
#182266=CARTESIAN_POINT ( 'NONE',  ( -16.55341960407617563, 4.379528057220093196, 88.54275706135236135 ) ) ;
#182267=CARTESIAN_POINT ( 'NONE',  ( -9.564922557961040184, 16.46253265017147172, 97.91775706135233293 ) ) ;
#182268=CARTESIAN_POINT ( 'NONE',  ( -19.05341960407617563, 5.049401038297882671, 43.54275706135232582 ) ) ;
#182269=CARTESIAN_POINT ( 'NONE',  ( 5.823673210054125526, 21.52544592524343514, 74.79057627198105251 ) ) ;
#182270=CARTESIAN_POINT ( 'NONE',  ( 4.483927247898790824, -16.52544592524335698, 95.20942372801903275 ) ) ;
#182271=CARTESIAN_POINT ( 'NONE',  ( 18.62759615963271287, -10.81492255796078972, 38.33224293864768839 ) ) ;
#182272=CARTESIAN_POINT ( 'NONE',  ( -13.89961937509957401, -13.97604488694547875, 99.37609039468567573 ) ) ;
#182273=CARTESIAN_POINT ( 'NONE',  ( 13.97604488694527802, 13.89961937509977652, 44.37390960531435269 ) ) ;
#182274=CARTESIAN_POINT ( 'NONE',  ( -16.46253265017160317, 9.564922557960807481, 85.83224293864769550 ) ) ;
#182275=CIRCLE ( 'NONE', #66055, 2.500000000000002220 ) ;
#182276=CARTESIAN_POINT ( 'NONE',  ( -15.80617190586768217, 15.72974639402176855, 58.12609039468568994 ) ) ;
#182277=CARTESIAN_POINT ( 'NONE',  ( 0.05219959533909260263, 19.03943276465977164, 64.99890960531436690 ) ) ;
#182278=CARTESIAN_POINT ( 'NONE',  ( 12.14591786802309770, 12.06949235617756955, 89.37390960531435269 ) ) ;
#182279=CARTESIAN_POINT ( 'NONE',  ( -17.50000000000001066, -5.499999999999943157, 86.28230962303568674 ) ) ;
#182280=CARTESIAN_POINT ( 'NONE',  ( -12.06949235617756955, 12.14591786802309770, 80.62390960531438111 ) ) ;
#182281=CARTESIAN_POINT ( 'NONE',  ( -5.719274019375978568, 21.55341960407610458, 70.20724293864769550 ) ) ;
#182282=CARTESIAN_POINT ( 'NONE',  ( 13.89961937509957401, 13.97604488694547697, 96.87609039468566152 ) ) ;
#182285=CARTESIAN_POINT ( 'NONE',  ( 9.564922557961047289, -16.46253265017146816, 45.41775706135232582 ) ) ;
#182286=CARTESIAN_POINT ( 'NONE',  ( 17.31747979337956878, -6.344076630960847396, 71.12055131934816643 ) ) ;
#182287=CARTESIAN_POINT ( 'NONE',  ( -13.97604488694527625, -13.89961937509977652, 81.87390960531436690 ) ) ;
#182288=CARTESIAN_POINT ( 'NONE',  ( 9.564922557960805705, 16.46253265017160317, 84.58224293864769550 ) ) ;
#182289=CARTESIAN_POINT ( 'NONE',  ( 0.05219959533934541429, -16.53943276465976808, 65.00109039468568994 ) ) ;
#182291=CARTESIAN_POINT ( 'NONE',  ( -0.05219959533936034679, 19.03943276465977164, 47.50109039468566863 ) ) ;
#182293=CARTESIAN_POINT ( 'NONE',  ( -13.97604488694527625, -13.89961937509977652, 106.8739096053143669 ) ) ;
#182294=CARTESIAN_POINT ( 'NONE',  ( 14.29746914071037800, 8.314922557961029526, 101.6677570613523613 ) ) ;
#182296=CARTESIAN_POINT ( 'NONE',  ( 12.06949235617739724, 12.14591786802326823, 76.87609039468567573 ) ) ;
#182297=CARTESIAN_POINT ( 'NONE',  ( -17.05587630539785593, 6.762274262135690606, 30.74180309037313563 ) ) ;
#182298=CARTESIAN_POINT ( 'NONE',  ( 0.05219959533934541429, -16.53943276465976808, 60.00109039468568284 ) ) ;
#182300=CARTESIAN_POINT ( 'NONE',  ( 5.719274019375673035, 21.55341960407619339, 72.29275706135236135 ) ) ;
#182301=CARTESIAN_POINT ( 'NONE',  ( -5.049401038297874678, -19.05341960407617918, 69.79275706135233293 ) ) ;
#182302=CARTESIAN_POINT ( 'NONE',  ( 13.97604488694548053, -13.89961937509957401, 25.62609039468566507 ) ) ;
#182303=CARTESIAN_POINT ( 'NONE',  ( 13.89961937509977652, -13.97604488694527269, 58.12390960531436690 ) ) ;
#182304=CARTESIAN_POINT ( 'NONE',  ( 16.51473224551069308, 9.474510206698969483, 44.16557627198103120 ) ) ;
#182306=CARTESIAN_POINT ( 'NONE',  ( -15.72974639402197994, 15.80617190586746368, 70.62390960531436690 ) ) ;
#182307=AXIS2_PLACEMENT_3D ( 'NONE', #13010, #73693, #165693 ) ;
#182308=B_SPLINE_CURVE_WITH_KNOTS ( 'NONE', 3,
 ( #156711, #128336, #190035, #126357, #157704, #19194, #48542, #125376, #96019, #94024, #188054, #80843, #81815, #36325, #159672, #189052, #82824, #158681, #96998, #32371 ),
 .UNSPECIFIED., .F., .F.,
 ( 4, 2, 2, 2, 2, 2, 2, 2, 2, 4 ),
 ( 0.000000000000000000, 0.0004987090165372654385, 0.0009974180330745308770, 0.001246772541343163596, 0.001496127049611796532, 0.001994836066149057851, 0.002493545082686318953, 0.002742899590954949503, 0.002992254099223580488, 0.003989672132298186825 ),
 .UNSPECIFIED. ) ;
#182309=CARTESIAN_POINT ( 'NONE',  ( -5.823673210054116645, -21.52544592524344225, 37.29057627198102409 ) ) ;
#182310=CARTESIAN_POINT ( 'NONE',  ( -16.53943276465976808, 0.05219959533911058130, 111.2489096053143669 ) ) ;
#182311=CARTESIAN_POINT ( 'NONE',  ( 4.483927247898790824, -16.52544592524335698, 50.20942372801901854 ) ) ;
#182313=CARTESIAN_POINT ( 'NONE',  ( -21.52544592524334988, -5.823673210054445271, 28.95942372801902209 ) ) ;
#182314=CARTESIAN_POINT ( 'NONE',  ( 14.34966873604960469, 8.224510206698951720, 54.16557627198103120 ) ) ;
#182316=CARTESIAN_POINT ( 'NONE',  ( 19.05341960407617918, -5.049401038297876454, 101.0427570613523045 ) ) ;
#182317=CARTESIAN_POINT ( 'NONE',  ( 19.02544592524334988, 5.153800228976608722, 41.45942372801900433 ) ) ;
#182318=CARTESIAN_POINT ( 'NONE',  ( 14.29746914071049879, -8.314922557960816363, 43.33224293864769550 ) ) ;
#182319=CARTESIAN_POINT ( 'NONE',  ( -5.823673210054431948, 21.52544592524334988, 22.70942372801901499 ) ) ;
#182322=CARTESIAN_POINT ( 'NONE',  ( -15.80617190586745835, -15.72974639402198527, 81.87390960531435269 ) ) ;
#182323=CARTESIAN_POINT ( 'NONE',  ( 16.51473224551069308, 9.474510206698969483, 94.16557627198103830 ) ) ;
#182324=CARTESIAN_POINT ( 'NONE',  ( 16.53943276465976808, -0.05219959533910856209, 58.74890960531436690 ) ) ;
#182325=CARTESIAN_POINT ( 'NONE',  ( -0.05219959533909027116, -19.03943276465977164, 102.4989096053143669 ) ) ;
#182327=CARTESIAN_POINT ( 'NONE',  ( 5.153800228976615827, -19.02544592524334988, 50.20942372801897591 ) ) ;
#182328=CARTESIAN_POINT ( 'NONE',  ( 15.72974639402199770, -15.80617190586745480, 108.1239096053143811 ) ) ;
#182329=CARTESIAN_POINT ( 'NONE',  ( 19.02544592524343514, -5.153800228976328945, 48.54057627198103120 ) ) ;
#182330=CARTESIAN_POINT ( 'NONE',  ( 8.224510206698953496, -14.34966873604960469, 107.9155762719810241 ) ) ;
#182331=CARTESIAN_POINT ( 'NONE',  ( -5.719274019375665041, -21.55341960407619695, 49.79275706135234714 ) ) ;
#182333=EDGE_CURVE ( 'NONE', #114833, #113576, #195318, .T. ) ;
#182334=CARTESIAN_POINT ( 'NONE',  ( 12.14591786802309770, 12.06949235617756955, 34.37390960531435979 ) ) ;
#182335=CARTESIAN_POINT ( 'NONE',  ( -9.564922557960796823, -16.46253265017161027, 52.08224293864768839 ) ) ;
#182336=CARTESIAN_POINT ( 'NONE',  ( 13.97604488694527802, 13.89961937509977652, 99.37390960531436690 ) ) ;
#182337=CARTESIAN_POINT ( 'NONE',  ( -10.72451020669898014, 18.67979575497178502, 75.41557627198102409 ) ) ;
#182339=CARTESIAN_POINT ( 'NONE',  ( 9.564922557960805705, 16.46253265017160317, 44.58224293864769550 ) ) ;
#182340=CARTESIAN_POINT ( 'NONE',  ( -15.80617190586745835, -15.72974639402198527, 56.87390960531436690 ) ) ;
#182341=CARTESIAN_POINT ( 'NONE',  ( 18.67979575497194134, -10.72451020669871369, 85.83442372801901854 ) ) ;
#182343=CARTESIAN_POINT ( 'NONE',  ( -12.14591786802326823, 12.06949235617739902, 78.12609039468570415 ) ) ;
#182344=CARTESIAN_POINT ( 'NONE',  ( -12.06949235617756955, 12.14591786802309770, 65.62390960531436690 ) ) ;
#182345=CARTESIAN_POINT ( 'NONE',  ( 19.03943276465977164, -0.05219959533909143690, 63.74890960531435979 ) ) ;
#182347=CARTESIAN_POINT ( 'NONE',  ( -19.05341960407617563, 5.049401038297882671, 23.54275706135233648 ) ) ;
#182348=CARTESIAN_POINT ( 'NONE',  ( 12.06949235617739724, 12.14591786802326823, 86.87609039468568994 ) ) ;
#182349=CARTESIAN_POINT ( 'NONE',  ( 21.55341960407619695, -5.719274019375665929, 111.0427570613523613 ) ) ;
#182350=CARTESIAN_POINT ( 'NONE',  ( -9.474510206698964154, 16.51473224551069663, 80.41557627198103830 ) ) ;
#182351=CARTESIAN_POINT ( 'NONE',  ( 10.72451020669898902, -18.67979575497178502, 52.91557627198103830 ) ) ;
#182352=CARTESIAN_POINT ( 'NONE',  ( -8.224510206698735004, -14.34966873604973081, 19.58442372801901143 ) ) ;
#182353=CARTESIAN_POINT ( 'NONE',  ( 10.81492255796106328, -18.62759615963255655, 100.4177570613523471 ) ) ;
#182354=CARTESIAN_POINT ( 'NONE',  ( 14.29746914071037800, 8.314922557961029526, 66.66775706135234714 ) ) ;
#182355=CARTESIAN_POINT ( 'NONE',  ( -10.72451020669898014, 18.67979575497178502, 115.4155762719810241 ) ) ;
#182356=CARTESIAN_POINT ( 'NONE',  ( -19.05341960407617563, 5.049401038297882671, 113.5427570613523471 ) ) ;
#182357=CARTESIAN_POINT ( 'NONE',  ( -16.46253265017160317, 9.564922557960807481, 85.83224293864769550 ) ) ;
#182358=CARTESIAN_POINT ( 'NONE',  ( -12.14591786802326823, 12.06949235617739902, 23.12609039468567573 ) ) ;
#182359=CARTESIAN_POINT ( 'NONE',  ( 16.46253265017160672, -9.564922557960803928, 53.33224293864768839 ) ) ;
#182360=CARTESIAN_POINT ( 'NONE',  ( 16.52544592524335698, 4.483927247898782831, 36.45942372801901143 ) ) ;
#182361=CARTESIAN_POINT ( 'NONE',  ( 14.29746914071049879, -8.314922557960816363, 73.33224293864769550 ) ) ;
#182362=CARTESIAN_POINT ( 'NONE',  ( 8.224510206698742110, 14.34966873604972548, 82.08442372801901854 ) ) ;
#182363=CARTESIAN_POINT ( 'NONE',  ( -21.52544592524334988, -5.823673210054445271, 48.95942372801902565 ) ) ;
#182364=CARTESIAN_POINT ( 'NONE',  ( 19.02544592524343514, -5.153800228976328945, 58.54057627198102409 ) ) ;
#182365=CARTESIAN_POINT ( 'NONE',  ( -0.05219959533909027116, -19.03943276465977164, 82.49890960531436690 ) ) ;
#182366=CARTESIAN_POINT ( 'NONE',  ( -12.14591786802326823, 12.06949235617739902, 83.12609039468568994 ) ) ;
#182370=ORIENTED_EDGE ( 'NONE', *, *, #35450, .T. ) ;
#182371=CARTESIAN_POINT ( 'NONE',  ( 5.153800228976615827, -19.02544592524334988, 35.20942372801899722 ) ) ;
#182372=CARTESIAN_POINT ( 'NONE',  ( -19.02544592524342804, 5.153800228976336051, 96.04057627198103830 ) ) ;
#182373=CARTESIAN_POINT ( 'NONE',  ( 9.474510206698971260, -16.51473224551069308, 52.91557627198102409 ) ) ;
#182374=CARTESIAN_POINT ( 'NONE',  ( 13.89961937509977652, -13.97604488694527269, 108.1239096053143669 ) ) ;
#182375=CARTESIAN_POINT ( 'NONE',  ( -16.55341960407617563, 4.379528057220093196, 38.54275706135234714 ) ) ;
#182376=CARTESIAN_POINT ( 'NONE',  ( 9.564922557961047289, -16.46253265017146816, 60.41775706135233293 ) ) ;
#182377=CARTESIAN_POINT ( 'NONE',  ( -14.34966873604972548, 8.224510206698743886, 58.33442372801901143 ) ) ;
#182378=CARTESIAN_POINT ( 'NONE',  ( 19.03943276465977164, -0.05219959533909143690, 108.7489096053143527 ) ) ;
#182379=CARTESIAN_POINT ( 'NONE',  ( -5.153800228976328057, -19.02544592524343514, 77.29057627198099567 ) ) ;
#182380=CARTESIAN_POINT ( 'NONE',  ( 18.62759615963271287, -10.81492255796078972, 98.33224293864769550 ) ) ;
#182381=CARTESIAN_POINT ( 'NONE',  ( 13.97604488694548053, -13.89961937509957401, 60.62609039468564731 ) ) ;
#182382=CARTESIAN_POINT ( 'NONE',  ( -13.97604488694527625, -13.89961937509977652, 96.87390960531433848 ) ) ;
#182383=CARTESIAN_POINT ( 'NONE',  ( 19.03943276465977164, -0.05219959533909143690, 23.74890960531435269 ) ) ;
#182384=CARTESIAN_POINT ( 'NONE',  ( 16.46253265017160672, -9.564922557960803928, 83.33224293864768129 ) ) ;
#182385=CARTESIAN_POINT ( 'NONE',  ( 14.34966873604960469, 8.224510206698951720, 34.16557627198102409 ) ) ;
#182386=CARTESIAN_POINT ( 'NONE',  ( 16.51473224551069308, 9.474510206698969483, 24.16557627198102765 ) ) ;
#182387=CARTESIAN_POINT ( 'NONE',  ( 5.049401038297881783, 19.05341960407617563, 42.29275706135234003 ) ) ;
#182388=CARTESIAN_POINT ( 'NONE',  ( 4.483927247898545687, 16.52544592524342804, 74.79057627198105251 ) ) ;
#182389=CARTESIAN_POINT ( 'NONE',  ( 18.62759615963255655, 10.81492255796105972, 101.6677570613523613 ) ) ;
#182390=CARTESIAN_POINT ( 'NONE',  ( -19.02544592524342804, 5.153800228976336051, 36.04057627198100988 ) ) ;
#182391=CARTESIAN_POINT ( 'NONE',  ( -14.34966873604960291, -8.224510206698953496, 36.66557627198103120 ) ) ;
#182392=CARTESIAN_POINT ( 'NONE',  ( 5.823673210054444382, -21.52544592524334988, 110.2094237280190185 ) ) ;
#182393=CARTESIAN_POINT ( 'NONE',  ( -9.564922557960796823, -16.46253265017161027, 92.08224293864769550 ) ) ;
#182394=CARTESIAN_POINT ( 'NONE',  ( 16.51473224551069308, 9.474510206698969483, 89.16557627198103830 ) ) ;
#182395=CARTESIAN_POINT ( 'NONE',  ( -19.05341960407611168, -5.049401038298163336, 26.45724293864769550 ) ) ;
#182396=CARTESIAN_POINT ( 'NONE',  ( -16.52544592524342804, 4.483927247898546575, 101.0405762719810383 ) ) ;
#182397=CARTESIAN_POINT ( 'NONE',  ( 4.483927247898545687, 16.52544592524342804, 69.79057627198102409 ) ) ;
#182398=CARTESIAN_POINT ( 'NONE',  ( 15.80617190586746368, 15.72974639402197994, 79.37390960531436690 ) ) ;
#182399=CARTESIAN_POINT ( 'NONE',  ( 13.97604488694527802, 13.89961937509977652, 94.37390960531436690 ) ) ;
#182400=CARTESIAN_POINT ( 'NONE',  ( -21.53943276465977519, 0.05219959533907696930, 101.2489096053143669 ) ) ;
#182401=CARTESIAN_POINT ( 'NONE',  ( 13.97604488694527802, 13.89961937509977652, 84.37390960531433848 ) ) ;
#182402=CARTESIAN_POINT ( 'NONE',  ( -18.87255363501902750, -5.500000000000064837, 91.32513748171830059 ) ) ;
#182403=CARTESIAN_POINT ( 'NONE',  ( 12.14591786802309770, 12.06949235617756955, 89.37390960531435269 ) ) ;
#182404=CARTESIAN_POINT ( 'NONE',  ( -13.89961937509977652, 13.97604488694528158, 65.62390960531436690 ) ) ;
#182405=CARTESIAN_POINT ( 'NONE',  ( -21.55341960407610458, -5.719274019375992779, 61.45724293864770260 ) ) ;
#182407=CARTESIAN_POINT ( 'NONE',  ( -0.05219959533907301413, -21.53943276465977519, 27.49890960531435269 ) ) ;
#182408=DIRECTION ( 'NONE',  ( 0.000000000000000000, 0.000000000000000000, -1.000000000000000000 ) ) ;
#182409=CARTESIAN_POINT ( 'NONE',  ( -4.379528057220086978, -16.55341960407618274, 24.79275706135235779 ) ) ;
#182410=CARTESIAN_POINT ( 'NONE',  ( 12.14591786802309770, 12.06949235617756955, 94.37390960531436690 ) ) ;
#182411=CARTESIAN_POINT ( 'NONE',  ( -17.60779699588840330, -5.500000000000024869, 46.34981316670106111 ) ) ;
#182412=CARTESIAN_POINT ( 'NONE',  ( -13.97604488694527625, -13.89961937509977652, 86.87390960531436690 ) ) ;
#182413=CARTESIAN_POINT ( 'NONE',  ( -16.51473224551069308, -9.474510206698971260, 46.66557627198102409 ) ) ;
#182414=CARTESIAN_POINT ( 'NONE',  ( -8.224510206698948167, 14.34966873604960824, 85.41557627198102409 ) ) ;
#182415=CARTESIAN_POINT ( 'NONE',  ( 19.05341960407611168, 5.049401038298154454, 113.9572429386477097 ) ) ;
#182416=CARTESIAN_POINT ( 'NONE',  ( -5.153800228976607833, 19.02544592524334988, 107.7094237280189759 ) ) ;
#182417=CARTESIAN_POINT ( 'NONE',  ( 21.52544592524334988, 5.823673210054432836, 61.45942372801901854 ) ) ;
#182419=CARTESIAN_POINT ( 'NONE',  ( 13.89961937509977652, -13.97604488694527269, 103.1239096053143527 ) ) ;
#182420=CARTESIAN_POINT ( 'NONE',  ( -21.53943276465977519, 0.05219959533907696930, 86.24890960531436690 ) ) ;
#182421=CARTESIAN_POINT ( 'NONE',  ( 16.55341960407618274, -4.379528057220086978, 86.04275706135236135 ) ) ;
#182423=CARTESIAN_POINT ( 'NONE',  ( 5.049401038298161559, -19.05341960407611168, 22.70724293864769194 ) ) ;
#182424=CARTESIAN_POINT ( 'NONE',  ( -13.97604488694527625, -13.89961937509977652, 71.87390960531433848 ) ) ;
#182425=CARTESIAN_POINT ( 'NONE',  ( 10.72451020669898902, -18.67979575497178502, 77.91557627198102409 ) ) ;
#182426=CARTESIAN_POINT ( 'NONE',  ( -16.51473224551082808, 9.474510206698731452, 108.3344237280190043 ) ) ;
#182427=CARTESIAN_POINT ( 'NONE',  ( 4.483927247898545687, 16.52544592524342804, 39.79057627198103830 ) ) ;
#182428=CARTESIAN_POINT ( 'NONE',  ( 15.72974639402176855, 15.80617190586768217, 56.87609039468568994 ) ) ;
#182429=CARTESIAN_POINT ( 'NONE',  ( -12.14591786802326823, 12.06949235617739902, 83.12609039468568994 ) ) ;
#182430=CARTESIAN_POINT ( 'NONE',  ( 5.719274019375991003, -21.55341960407610458, 27.70724293864769905 ) ) ;
#182432=CARTESIAN_POINT ( 'NONE',  ( 12.06949235617739724, 12.14591786802326823, 101.8760903946857042 ) ) ;
#182433=CARTESIAN_POINT ( 'NONE',  ( -4.379528057220086978, -16.55341960407618274, 49.79275706135234714 ) ) ;
#182434=CARTESIAN_POINT ( 'NONE',  ( 5.153800228976335163, 19.02544592524342804, 64.79057627198100988 ) ) ;
#182435=CARTESIAN_POINT ( 'NONE',  ( -13.97604488694527625, -13.89961937509977652, 71.87390960531433848 ) ) ;
#182436=CARTESIAN_POINT ( 'NONE',  ( 4.379528057220092307, 16.55341960407617563, 72.29275706135236135 ) ) ;
#182437=CARTESIAN_POINT ( 'NONE',  ( -4.483927247898539470, -16.52544592524342804, 52.29057627198102409 ) ) ;
#182438=CARTESIAN_POINT ( 'NONE',  ( 13.89961937509977652, -13.97604488694527269, 58.12390960531436690 ) ) ;
#182439=CARTESIAN_POINT ( 'NONE',  ( 19.02544592524343514, -5.153800228976328945, 48.54057627198103120 ) ) ;
#182440=CARTESIAN_POINT ( 'NONE',  ( 0.05219959533934541429, -16.53943276465976808, 40.00109039468567573 ) ) ;
#182441=CARTESIAN_POINT ( 'NONE',  ( 9.564922557961047289, -16.46253265017146816, 90.41775706135234714 ) ) ;
#182442=CARTESIAN_POINT ( 'NONE',  ( 16.52544592524342804, -4.483927247898539470, 103.5405762719810383 ) ) ;
#182443=CARTESIAN_POINT ( 'NONE',  ( -19.05341960407611168, -5.049401038298163336, 66.45724293864769550 ) ) ;
#182444=CARTESIAN_POINT ( 'NONE',  ( 19.02544592524334988, 5.153800228976608722, 101.4594237280189759 ) ) ;
#182446=CARTESIAN_POINT ( 'NONE',  ( -15.80617190586768217, 15.72974639402176855, 93.12609039468568994 ) ) ;
#182447=CARTESIAN_POINT ( 'NONE',  ( 4.379528057220092307, 16.55341960407617563, 67.29275706135234714 ) ) ;
#182449=CARTESIAN_POINT ( 'NONE',  ( 10.72451020669898902, -18.67979575497178502, 67.91557627198102409 ) ) ;
#182450=CARTESIAN_POINT ( 'NONE',  ( 16.53943276465976808, 0.05219959533934440121, 51.25109039468568994 ) ) ;
#182451=CARTESIAN_POINT ( 'NONE',  ( -18.22780087662123805, 5.499999999999981348, 71.01763182126894947 ) ) ;
#182452=CARTESIAN_POINT ( 'NONE',  ( 19.05341960407617918, -5.049401038297876454, 41.04275706135233293 ) ) ;
#182453=CARTESIAN_POINT ( 'NONE',  ( -13.89961937509977652, 13.97604488694528158, 90.62390960531432427 ) ) ;
#182454=CARTESIAN_POINT ( 'NONE',  ( 12.06949235617757843, -12.14591786802309237, 113.1239096053143953 ) ) ;
#182455=CARTESIAN_POINT ( 'NONE',  ( -9.474510206698964154, 16.51473224551069663, 70.41557627198102409 ) ) ;
#182458=CARTESIAN_POINT ( 'NONE',  ( -10.81492255796105439, 18.62759615963255655, 77.91775706135231871 ) ) ;
#182459=CARTESIAN_POINT ( 'NONE',  ( 13.97604488694548053, -13.89961937509957401, 35.62609039468567573 ) ) ;
#182460=CARTESIAN_POINT ( 'NONE',  ( -5.153800228976607833, 19.02544592524334988, 22.70942372801899012 ) ) ;
#182461=CARTESIAN_POINT ( 'NONE',  ( 13.89961937509977652, -13.97604488694527269, 53.12390960531434558 ) ) ;
#182462=CARTESIAN_POINT ( 'NONE',  ( -21.53943276465977519, 0.05219959533907696930, 26.24890960531435624 ) ) ;
#182463=CARTESIAN_POINT ( 'NONE',  ( 15.72974639402176855, 15.80617190586768217, 86.87609039468568994 ) ) ;
#182464=CARTESIAN_POINT ( 'NONE',  ( -5.153800228976328057, -19.02544592524343514, 67.29057627198102409 ) ) ;
#182465=CARTESIAN_POINT ( 'NONE',  ( -10.72451020669870658, -18.67979575497194134, 84.58442372801903275 ) ) ;
#182466=CARTESIAN_POINT ( 'NONE',  ( 5.719274019375991003, -21.55341960407610458, 37.70724293864769550 ) ) ;
#182467=CARTESIAN_POINT ( 'NONE',  ( -19.03943276465977164, 0.05219959533909376836, 66.24890960531436690 ) ) ;
#182468=CARTESIAN_POINT ( 'NONE',  ( -15.72974639402176322, -15.80617190586768395, 39.37609039468567573 ) ) ;
#182469=CARTESIAN_POINT ( 'NONE',  ( -9.564922557961040184, 16.46253265017147172, 67.91775706135233293 ) ) ;
#182470=CARTESIAN_POINT ( 'NONE',  ( 16.46253265017160672, -9.564922557960803928, 43.33224293864769550 ) ) ;
#182471=CARTESIAN_POINT ( 'NONE',  ( -19.03943276465977164, 0.05219959533909376836, 96.24890960531436690 ) ) ;
#182472=CARTESIAN_POINT ( 'NONE',  ( 8.224510206698742110, 14.34966873604972548, 27.08442372801901854 ) ) ;
#182473=CARTESIAN_POINT ( 'NONE',  ( -12.14591786802309592, -12.06949235617757132, 86.87390960531438111 ) ) ;
#182474=CARTESIAN_POINT ( 'NONE',  ( 19.02544592524343514, -5.153800228976328945, 53.54057627198102409 ) ) ;
#182475=CARTESIAN_POINT ( 'NONE',  ( -21.53943276465977519, 0.05219959533907696930, 46.24890960531435979 ) ) ;
#182476=CARTESIAN_POINT ( 'NONE',  ( -13.97604488694547697, 13.89961937509957934, 113.1260903946856757 ) ) ;
#182477=CARTESIAN_POINT ( 'NONE',  ( -10.72451020669870658, -18.67979575497194134, 19.58442372801901143 ) ) ;
#182478=CARTESIAN_POINT ( 'NONE',  ( 10.81492255796106328, -18.62759615963255655, 65.41775706135234714 ) ) ;
#182479=CARTESIAN_POINT ( 'NONE',  ( 14.29746914071037800, 8.314922557961029526, 66.66775706135234714 ) ) ;
#182480=CARTESIAN_POINT ( 'NONE',  ( -12.06949235617739369, -12.14591786802326823, 69.37609039468567573 ) ) ;
#182481=CARTESIAN_POINT ( 'NONE',  ( 5.049401038298161559, -19.05341960407611168, 57.70724293864769550 ) ) ;
#182482=CARTESIAN_POINT ( 'NONE',  ( 12.14591786802327356, -12.06949235617739191, 95.62609039468568994 ) ) ;
#182483=CARTESIAN_POINT ( 'NONE',  ( 19.02544592524334988, 5.153800228976608722, 41.45942372801900433 ) ) ;
#182484=CARTESIAN_POINT ( 'NONE',  ( 5.823673210054125526, 21.52544592524343514, 109.7905762719810383 ) ) ;
#182485=CARTESIAN_POINT ( 'NONE',  ( 16.52544592524342804, -4.483927247898539470, 63.54057627198103830 ) ) ;
#182486=CARTESIAN_POINT ( 'NONE',  ( -19.02544592524342804, 5.153800228976336051, 86.04057627198103830 ) ) ;
#182487=CARTESIAN_POINT ( 'NONE',  ( -4.379528057220086978, -16.55341960407618274, 89.79275706135236135 ) ) ;
#182488=CARTESIAN_POINT ( 'NONE',  ( -0.05219959533937732626, 21.53943276465977519, 52.50109039468567573 ) ) ;
#182489=CARTESIAN_POINT ( 'NONE',  ( -14.34966873604972548, 8.224510206698743886, 38.33442372801900433 ) ) ;
#182490=CARTESIAN_POINT ( 'NONE',  ( -15.80617190586768217, 15.72974639402176855, 33.12609039468569705 ) ) ;
#182491=CARTESIAN_POINT ( 'NONE',  ( 16.55341960407611168, 4.379528057220329451, 53.95724293864770260 ) ) ;
#182494=CARTESIAN_POINT ( 'NONE',  ( 18.62759615963271287, -10.81492255796078972, 98.33224293864769550 ) ) ;
#182495=CARTESIAN_POINT ( 'NONE',  ( 4.379528057220339221, -16.55341960407611168, 37.70724293864769550 ) ) ;
#182496=VERTEX_POINT ( 'NONE', #119101 ) ;
#182499=CARTESIAN_POINT ( 'NONE',  ( -0.05219959533907301413, -21.53943276465977519, 27.49890960531435269 ) ) ;
#182500=CARTESIAN_POINT ( 'NONE',  ( -21.55341960407619339, 5.719274019375674811, 33.54275706135234714 ) ) ;
#182501=CARTESIAN_POINT ( 'NONE',  ( 14.29746914071049879, -8.314922557960816363, 68.33224293864769550 ) ) ;
#182502=CARTESIAN_POINT ( 'NONE',  ( 19.03943276465977164, -0.05219959533909143690, 78.74890960531436690 ) ) ;
#182503=CARTESIAN_POINT ( 'NONE',  ( -16.46253265017160317, 9.564922557960807481, 30.83224293864769550 ) ) ;
#182504=CARTESIAN_POINT ( 'NONE',  ( -16.51473224551082808, 9.474510206698731452, 68.33442372801900433 ) ) ;
#182505=CARTESIAN_POINT ( 'NONE',  ( -5.719274019375978568, 21.55341960407610458, 45.20724293864769550 ) ) ;
#182507=CARTESIAN_POINT ( 'NONE',  ( -16.51473224551069308, -9.474510206698971260, 61.66557627198103120 ) ) ;
#182508=CARTESIAN_POINT ( 'NONE',  ( 16.52544592524335698, 4.483927247898782831, 41.45942372801901143 ) ) ;
#182509=CARTESIAN_POINT ( 'NONE',  ( 21.55341960407619695, -5.719274019375665929, 21.04275706135234714 ) ) ;
#182510=CARTESIAN_POINT ( 'NONE',  ( -4.483927247898539470, -16.52544592524342804, 42.29057627198103120 ) ) ;
#182513=CARTESIAN_POINT ( 'NONE',  ( 9.474510206698971260, -16.51473224551069308, 87.91557627198102409 ) ) ;
#182514=CARTESIAN_POINT ( 'NONE',  ( -10.72451020669898014, 18.67979575497178502, 70.41557627198102409 ) ) ;
#182515=CARTESIAN_POINT ( 'NONE',  ( 5.719274019375991003, -21.55341960407610458, 112.7072429386476955 ) ) ;
#182516=CARTESIAN_POINT ( 'NONE',  ( 14.34966873604972726, -8.224510206698740333, 35.83442372801901143 ) ) ;
#182517=CARTESIAN_POINT ( 'NONE',  ( -21.53943276465977519, 0.05219959533907696930, 36.24890960531435979 ) ) ;
#182518=CARTESIAN_POINT ( 'NONE',  ( -15.80617190586768217, 15.72974639402176855, 103.1260903946856757 ) ) ;
#182519=CARTESIAN_POINT ( 'NONE',  ( 13.97604488694527802, 13.89961937509977652, 94.37390960531436690 ) ) ;
#182520=CARTESIAN_POINT ( 'NONE',  ( 9.474510206698971260, -16.51473224551069308, 37.91557627198102409 ) ) ;
#182521=CARTESIAN_POINT ( 'NONE',  ( 16.46253265017160672, -9.564922557960803928, 93.33224293864769550 ) ) ;
#182522=CARTESIAN_POINT ( 'NONE',  ( -5.049401038298153566, 19.05341960407611168, 75.20724293864769550 ) ) ;
#182524=CARTESIAN_POINT ( 'NONE',  ( 16.51473224551083163, -9.474510206698727899, 50.83442372801899722 ) ) ;
#182525=CARTESIAN_POINT ( 'NONE',  ( 18.67979575497194134, -10.72451020669871369, 110.8344237280190043 ) ) ;
#182526=CARTESIAN_POINT ( 'NONE',  ( -10.72451020669898014, 18.67979575497178502, 25.41557627198103120 ) ) ;
#182527=CARTESIAN_POINT ( 'NONE',  ( 4.483927247898790824, -16.52544592524335698, 110.2094237280190185 ) ) ;
#182528=CARTESIAN_POINT ( 'NONE',  ( -13.89961937509957401, -13.97604488694547875, 84.37609039468567573 ) ) ;
#182529=CARTESIAN_POINT ( 'NONE',  ( -17.44270441346513323, 5.991230190323084237, 58.63664920735774189 ) ) ;
#182530=CARTESIAN_POINT ( 'NONE',  ( -13.97604488694547697, 13.89961937509957934, 83.12609039468564731 ) ) ;
#182531=CARTESIAN_POINT ( 'NONE',  ( 16.51473224551083163, -9.474510206698727899, 40.83442372801900433 ) ) ;
#182533=CARTESIAN_POINT ( 'NONE',  ( -9.564922557960796823, -16.46253265017161027, 42.08224293864769550 ) ) ;
#182534=CARTESIAN_POINT ( 'NONE',  ( -14.29746914071049879, 8.314922557960819915, 45.83224293864769550 ) ) ;
#182535=CARTESIAN_POINT ( 'NONE',  ( -17.40861289039001392, -6.110651285853327508, 111.3723247082743626 ) ) ;
#182536=CARTESIAN_POINT ( 'NONE',  ( -8.224510206698948167, 14.34966873604960824, 25.41557627198103120 ) ) ;
#182538=CARTESIAN_POINT ( 'NONE',  ( -14.29746914071037622, -8.314922557961029526, 99.16775706135234714 ) ) ;
#182539=CARTESIAN_POINT ( 'NONE',  ( -19.03943276465977164, 0.05219959533909376836, 46.24890960531435979 ) ) ;
#182540=CARTESIAN_POINT ( 'NONE',  ( 10.72451020669871369, 18.67979575497193778, 102.0844237280190185 ) ) ;
#182541=CARTESIAN_POINT ( 'NONE',  ( 5.049401038297881783, 19.05341960407617563, 112.2927570613523471 ) ) ;
#182542=CARTESIAN_POINT ( 'NONE',  ( 10.72451020669871369, 18.67979575497193778, 97.08442372801904696 ) ) ;
#182544=CARTESIAN_POINT ( 'NONE',  ( -13.97604488694527625, -13.89961937509977652, 96.87390960531433848 ) ) ;
#182545=CARTESIAN_POINT ( 'NONE',  ( -16.51473224551069308, -9.474510206698971260, 81.66557627198103830 ) ) ;
#182547=CARTESIAN_POINT ( 'NONE',  ( -0.05219959533907301413, -21.53943276465977519, 107.4989096053143669 ) ) ;
#182549=CARTESIAN_POINT ( 'NONE',  ( -16.53943276465976808, 0.05219959533911058130, 76.24890960531435269 ) ) ;
#182550=CARTESIAN_POINT ( 'NONE',  ( 18.62759615963271287, -10.81492255796078972, 73.33224293864769550 ) ) ;
#182551=CARTESIAN_POINT ( 'NONE',  ( 19.03943276465977164, -0.05219959533909143690, 63.74890960531435979 ) ) ;
#182552=CARTESIAN_POINT ( 'NONE',  ( -5.719274019375978568, 21.55341960407610458, 100.2072429386476955 ) ) ;
#182553=CARTESIAN_POINT ( 'NONE',  ( 12.14591786802327356, -12.06949235617739191, 95.62609039468568994 ) ) ;
#182555=CARTESIAN_POINT ( 'NONE',  ( -19.03943276465977164, 0.05219959533909376836, 61.24890960531436690 ) ) ;
#182556=CARTESIAN_POINT ( 'NONE',  ( 4.379528057220339221, -16.55341960407611168, 97.70724293864772392 ) ) ;
#182558=CARTESIAN_POINT ( 'NONE',  ( -19.05341960407611168, -5.049401038298163336, 66.45724293864769550 ) ) ;
#182559=CARTESIAN_POINT ( 'NONE',  ( 0.05219959533936267826, -19.03943276465977164, 75.00109039468566152 ) ) ;
#182560=CARTESIAN_POINT ( 'NONE',  ( 4.379528057220339221, -16.55341960407611168, 82.70724293864770971 ) ) ;
#182561=CARTESIAN_POINT ( 'NONE',  ( 5.823673210054444382, -21.52544592524334988, 60.20942372801902565 ) ) ;
#182562=CARTESIAN_POINT ( 'NONE',  ( -19.02544592524342804, 5.153800228976336051, 46.04057627198101699 ) ) ;
#182563=CARTESIAN_POINT ( 'NONE',  ( -21.53943276465977519, -0.05219959533937600094, 18.75109039468568639 ) ) ;
#182564=CARTESIAN_POINT ( 'NONE',  ( -14.29746914071049879, 8.314922557960819915, 100.8322429386477097 ) ) ;
#182566=CARTESIAN_POINT ( 'NONE',  ( 13.89961937509977652, -13.97604488694527269, 63.12390960531435979 ) ) ;
#182568=CARTESIAN_POINT ( 'NONE',  ( 9.564922557961047289, -16.46253265017146816, 110.4177570613523471 ) ) ;
#182569=CARTESIAN_POINT ( 'NONE',  ( -21.55341960407610458, -5.719274019375992779, 21.45724293864769550 ) ) ;
#182570=CARTESIAN_POINT ( 'NONE',  ( -5.823673210054431948, 21.52544592524334988, 47.70942372801902565 ) ) ;
#182571=CARTESIAN_POINT ( 'NONE',  ( 5.153800228976335163, 19.02544592524342804, 99.79057627198102409 ) ) ;
#182572=CARTESIAN_POINT ( 'NONE',  ( 13.89961937509957401, 13.97604488694547697, 81.87609039468564731 ) ) ;
#182573=CARTESIAN_POINT ( 'NONE',  ( 5.049401038298161559, -19.05341960407611168, 62.70724293864769550 ) ) ;
#182574=CARTESIAN_POINT ( 'NONE',  ( 4.483927247898545687, 16.52544592524342804, 69.79057627198102409 ) ) ;
#182575=CARTESIAN_POINT ( 'NONE',  ( -14.29746914071049879, 8.314922557960819915, 75.83224293864769550 ) ) ;
#182576=CARTESIAN_POINT ( 'NONE',  ( -19.05341960407611168, -5.049401038298163336, 86.45724293864769550 ) ) ;
#182577=CARTESIAN_POINT ( 'NONE',  ( 0.05219959533910956823, 16.53943276465976808, 79.99890960531435269 ) ) ;
#182578=CARTESIAN_POINT ( 'NONE',  ( 19.05341960407611168, 5.049401038298154454, 88.95724293864769550 ) ) ;
#182579=CARTESIAN_POINT ( 'NONE',  ( 9.474510206698729675, 16.51473224551082808, 37.08442372801899722 ) ) ;
#182580=CARTESIAN_POINT ( 'NONE',  ( -13.89961937509977652, 13.97604488694528158, 50.62390960531435979 ) ) ;
#182581=CARTESIAN_POINT ( 'NONE',  ( 4.483927247898545687, 16.52544592524342804, 24.79057627198103120 ) ) ;
#182582=CARTESIAN_POINT ( 'NONE',  ( 16.46253265017160672, -9.564922557960803928, 23.33224293864769194 ) ) ;
#182583=ORIENTED_EDGE ( 'NONE', *, *, #127855, .F. ) ;
#182584=CARTESIAN_POINT ( 'NONE',  ( 0.05219959533937995610, -21.53943276465977519, 50.00109039468568994 ) ) ;
#182585=CARTESIAN_POINT ( 'NONE',  ( 0.05219959533936267826, -19.03943276465977164, 65.00109039468567573 ) ) ;
#182586=CARTESIAN_POINT ( 'NONE',  ( -8.314922557960811034, -14.29746914071050412, 37.08224293864768129 ) ) ;
#182587=CARTESIAN_POINT ( 'NONE',  ( 21.52544592524344225, -5.823673210054117533, 83.54057627198102409 ) ) ;
#182588=CARTESIAN_POINT ( 'NONE',  ( 21.53943276465977519, -0.05219959533907433946, 28.74890960531435624 ) ) ;
#182589=CARTESIAN_POINT ( 'NONE',  ( -8.224510206698948167, 14.34966873604960824, 70.41557627198102409 ) ) ;
#182590=CARTESIAN_POINT ( 'NONE',  ( 0.05219959533909260263, 19.03943276465977164, 39.99890960531436690 ) ) ;
#182591=CARTESIAN_POINT ( 'NONE',  ( -13.97604488694547697, 13.89961937509957934, 38.12609039468566152 ) ) ;
#182592=CARTESIAN_POINT ( 'NONE',  ( -4.483927247898782831, 16.52544592524335698, 107.7094237280190328 ) ) ;
#182593=CARTESIAN_POINT ( 'NONE',  ( 8.314922557961029526, -14.29746914071037800, 55.41775706135234714 ) ) ;
#182594=CARTESIAN_POINT ( 'NONE',  ( 18.67979575497178502, 10.72451020669898547, 39.16557627198102409 ) ) ;
#182595=CARTESIAN_POINT ( 'NONE',  ( -15.80617190586768217, 15.72974639402176855, 113.1260903946856899 ) ) ;
#182596=CARTESIAN_POINT ( 'NONE',  ( -13.97604488694527625, -13.89961937509977652, 86.87390960531436690 ) ) ;
#182597=CARTESIAN_POINT ( 'NONE',  ( -14.29746914071037622, -8.314922557961029526, 79.16775706135234714 ) ) ;
#182598=CARTESIAN_POINT ( 'NONE',  ( 16.53943276465976808, -0.05219959533910856209, 113.7489096053143527 ) ) ;
#182599=CARTESIAN_POINT ( 'NONE',  ( -4.379528057220328563, 16.55341960407611168, 30.20724293864769550 ) ) ;
#182600=CARTESIAN_POINT ( 'NONE',  ( 13.97604488694527802, 13.89961937509977652, 99.37390960531436690 ) ) ;
#182601=CARTESIAN_POINT ( 'NONE',  ( -5.153800228976328057, -19.02544592524343514, 92.29057627198099567 ) ) ;
#182602=CARTESIAN_POINT ( 'NONE',  ( 15.72974639402199770, -15.80617190586745480, 28.12390960531435979 ) ) ;
#182603=CARTESIAN_POINT ( 'NONE',  ( -12.14591786802309592, -12.06949235617757132, 76.87390960531439532 ) ) ;
#182604=CARTESIAN_POINT ( 'NONE',  ( 8.224510206698953496, -14.34966873604960469, 52.91557627198103830 ) ) ;
#182606=CARTESIAN_POINT ( 'NONE',  ( 4.483927247898790824, -16.52544592524335698, 55.20942372801902565 ) ) ;
#182608=CARTESIAN_POINT ( 'NONE',  ( 9.474510206698729675, 16.51473224551082808, 57.08442372801900433 ) ) ;
#182609=CARTESIAN_POINT ( 'NONE',  ( 13.89961937509977652, -13.97604488694527269, 83.12390960531436690 ) ) ;
#182610=CARTESIAN_POINT ( 'NONE',  ( 16.51473224551083163, -9.474510206698727899, 70.83442372801900433 ) ) ;
#182612=CARTESIAN_POINT ( 'NONE',  ( 19.03943276465977164, 0.05219959533936151252, 61.25109039468566863 ) ) ;
#182613=CARTESIAN_POINT ( 'NONE',  ( 16.51473224551083163, -9.474510206698727899, 95.83442372801900433 ) ) ;
#182614=CARTESIAN_POINT ( 'NONE',  ( 4.483927247898790824, -16.52544592524335698, 95.20942372801903275 ) ) ;
#182616=CARTESIAN_POINT ( 'NONE',  ( -5.049401038298153566, 19.05341960407611168, 45.20724293864769550 ) ) ;
#182617=CARTESIAN_POINT ( 'NONE',  ( -19.03943276465977164, 0.05219959533909376836, 111.2489096053143669 ) ) ;
#182618=CARTESIAN_POINT ( 'NONE',  ( 5.719274019375673035, 21.55341960407619339, 57.29275706135234714 ) ) ;
#182619=CARTESIAN_POINT ( 'NONE',  ( 16.51473224551083163, -9.474510206698727899, 100.8344237280190043 ) ) ;
#182620=DIRECTION ( 'NONE',  ( 0.000000000000000000, 0.000000000000000000, 1.000000000000000000 ) ) ;
#182621=CARTESIAN_POINT ( 'NONE',  ( -16.51473224551069308, -9.474510206698971260, 61.66557627198103120 ) ) ;
#182622=CARTESIAN_POINT ( 'NONE',  ( -9.474510206698964154, 16.51473224551069663, 110.4155762719810383 ) ) ;
#182623=CARTESIAN_POINT ( 'NONE',  ( -8.224510206698948167, 14.34966873604960824, 75.41557627198102409 ) ) ;
#182624=CARTESIAN_POINT ( 'NONE',  ( 5.153800228976335163, 19.02544592524342804, 69.79057627198103830 ) ) ;
#182625=CARTESIAN_POINT ( 'NONE',  ( -9.564922557960796823, -16.46253265017161027, 77.08224293864769550 ) ) ;
#182626=CARTESIAN_POINT ( 'NONE',  ( 19.02544592524334988, 5.153800228976608722, 71.45942372801900433 ) ) ;
#182627=CARTESIAN_POINT ( 'NONE',  ( -21.55341960407610458, -5.719274019375992779, 66.45724293864768129 ) ) ;
#182628=CARTESIAN_POINT ( 'NONE',  ( -19.03943276465977164, 0.05219959533909376836, 21.24890960531436335 ) ) ;
#182629=CARTESIAN_POINT ( 'NONE',  ( 9.474510206698729675, 16.51473224551082808, 42.08442372801900433 ) ) ;
#182630=CARTESIAN_POINT ( 'NONE',  ( 19.03943276465977164, -0.05219959533909143690, 48.74890960531435979 ) ) ;
#182631=CARTESIAN_POINT ( 'NONE',  ( -5.153800228976328057, -19.02544592524343514, 82.29057627198103830 ) ) ;
#182632=CARTESIAN_POINT ( 'NONE',  ( 15.80617190586746368, 15.72974639402197994, 89.37390960531435269 ) ) ;
#182633=CARTESIAN_POINT ( 'NONE',  ( -4.379528057220328563, 16.55341960407611168, 80.20724293864769550 ) ) ;
#182634=CARTESIAN_POINT ( 'NONE',  ( -13.89961937509957401, -13.97604488694547875, 54.37609039468565442 ) ) ;
#182635=CARTESIAN_POINT ( 'NONE',  ( 15.72974639402199770, -15.80617190586745480, 78.12390960531436690 ) ) ;
#182636=B_SPLINE_CURVE_WITH_KNOTS ( 'NONE', 3,
 ( #130074, #82582, #172630, #114933, #33127, #19933, #187818, #4744, #49287, #34118, #36089, #66433, #95777, #142278, #128094, #20924, #189798, #159428, #51270, #174624 ),
 .UNSPECIFIED., .F., .F.,
 ( 4, 2, 2, 2, 2, 2, 2, 2, 2, 4 ),
 ( 0.004000878361811908805, 0.004499404418915909157, 0.004997930476019910376, 0.005496456533123911595, 0.005994982590227911946, 0.006244245618779911688, 0.006493508647331912298, 0.006992034704435916986, 0.007490560761539923409, 0.007989086818643928098 ),
 .UNSPECIFIED. ) ;
#182637=CARTESIAN_POINT ( 'NONE',  ( 15.72974639402199770, -15.80617190586745480, 63.12390960531435979 ) ) ;
#182638=CARTESIAN_POINT ( 'NONE',  ( -5.823673210054116645, -21.52544592524344225, 42.29057627198103120 ) ) ;
#182639=CARTESIAN_POINT ( 'NONE',  ( -21.53943276465977519, -0.05219959533937600094, 88.75109039468567573 ) ) ;
#182640=CARTESIAN_POINT ( 'NONE',  ( -5.153800228976328057, -19.02544592524343514, 77.29057627198099567 ) ) ;
#182641=CARTESIAN_POINT ( 'NONE',  ( -16.53943276465976808, 0.05219959533911058130, 116.2489096053143669 ) ) ;
#182642=CARTESIAN_POINT ( 'NONE',  ( 21.52544592524334988, 5.823673210054432836, 31.45942372801901854 ) ) ;
#182643=CARTESIAN_POINT ( 'NONE',  ( -21.55341960407619339, 5.719274019375674811, 38.54275706135234714 ) ) ;
#182644=CARTESIAN_POINT ( 'NONE',  ( -19.05341960407611168, -5.049401038298163336, 51.45724293864770260 ) ) ;
#182645=CARTESIAN_POINT ( 'NONE',  ( 15.80617190586769283, -15.72974639402175789, 25.62609039468567929 ) ) ;
#182646=CARTESIAN_POINT ( 'NONE',  ( 5.153800228976615827, -19.02544592524334988, 60.20942372801899012 ) ) ;
#182647=CARTESIAN_POINT ( 'NONE',  ( 5.153800228976335163, 19.02544592524342804, 39.79057627198100988 ) ) ;
#182648=CARTESIAN_POINT ( 'NONE',  ( -14.29746914071037622, -8.314922557961029526, 24.16775706135235424 ) ) ;
#182649=CARTESIAN_POINT ( 'NONE',  ( -19.02544592524342804, 5.153800228976336051, 31.04057627198102409 ) ) ;
#182650=CARTESIAN_POINT ( 'NONE',  ( -16.55341960407617563, 4.379528057220093196, 58.54275706135235424 ) ) ;
#182651=CARTESIAN_POINT ( 'NONE',  ( 0.05219959533909260263, 19.03943276465977164, 44.99890960531435979 ) ) ;
#182653=CARTESIAN_POINT ( 'NONE',  ( 0.05219959533909260263, 19.03943276465977164, 84.99890960531436690 ) ) ;
#182654=CARTESIAN_POINT ( 'NONE',  ( -16.46253265017160317, 9.564922557960807481, 25.83224293864769194 ) ) ;
#182655=CARTESIAN_POINT ( 'NONE',  ( -10.81492255796078084, -18.62759615963271287, 57.08224293864769550 ) ) ;
#182656=CARTESIAN_POINT ( 'NONE',  ( 8.314922557961029526, -14.29746914071037800, 50.41775706135235424 ) ) ;
#182657=CARTESIAN_POINT ( 'NONE',  ( -21.55341960407619339, 5.719274019375674811, 93.54275706135234714 ) ) ;
#182658=CARTESIAN_POINT ( 'NONE',  ( 16.46253265017160672, -9.564922557960803928, 38.33224293864768839 ) ) ;
#182659=CARTESIAN_POINT ( 'NONE',  ( -16.53943276465976808, 0.05219959533911058130, 36.24890960531435979 ) ) ;
#182660=CARTESIAN_POINT ( 'NONE',  ( 16.52544592524342804, -4.483927247898539470, 73.54057627198102409 ) ) ;
#182661=CARTESIAN_POINT ( 'NONE',  ( -5.153800228976328057, -19.02544592524343514, 62.29057627198100988 ) ) ;
#182662=CARTESIAN_POINT ( 'NONE',  ( 10.81492255796106328, -18.62759615963255655, 110.4177570613523756 ) ) ;
#182663=CARTESIAN_POINT ( 'NONE',  ( -15.72974639402176322, -15.80617190586768395, 19.37609039468568639 ) ) ;
#182664=CARTESIAN_POINT ( 'NONE',  ( -10.81492255796105439, 18.62759615963255655, 87.91775706135234714 ) ) ;
#182665=CARTESIAN_POINT ( 'NONE',  ( -16.53943276465976808, -0.05219959533934237506, 48.75109039468568284 ) ) ;
#182666=CARTESIAN_POINT ( 'NONE',  ( -16.55341960407617563, 4.379528057220093196, 28.54275706135234358 ) ) ;
#182667=CARTESIAN_POINT ( 'NONE',  ( 4.379528057220339221, -16.55341960407611168, 92.70724293864770971 ) ) ;
#182668=CARTESIAN_POINT ( 'NONE',  ( 5.823673210054444382, -21.52544592524334988, 95.20942372801903275 ) ) ;
#182669=CARTESIAN_POINT ( 'NONE',  ( -8.314922557960811034, -14.29746914071050412, 32.08224293864769550 ) ) ;
#182670=CARTESIAN_POINT ( 'NONE',  ( 5.049401038298161559, -19.05341960407611168, 32.70724293864768129 ) ) ;
#182671=CARTESIAN_POINT ( 'NONE',  ( 8.224510206698742110, 14.34966873604972548, 47.08442372801901854 ) ) ;
#182672=CARTESIAN_POINT ( 'NONE',  ( -16.52544592524342804, 4.483927247898546575, 56.04057627198102409 ) ) ;
#182673=CARTESIAN_POINT ( 'NONE',  ( 8.224510206698742110, 14.34966873604972548, 102.0844237280190185 ) ) ;
#182674=CARTESIAN_POINT ( 'NONE',  ( 19.02544592524343514, -5.153800228976328945, 113.5405762719810241 ) ) ;
#182675=CARTESIAN_POINT ( 'NONE',  ( -0.05219959533909027116, -19.03943276465977164, 107.4989096053143527 ) ) ;
#182676=CARTESIAN_POINT ( 'NONE',  ( -21.55341960407619339, 5.719274019375674811, 113.5427570613523756 ) ) ;
#182677=CARTESIAN_POINT ( 'NONE',  ( -8.224510206698948167, 14.34966873604960824, 85.41557627198102409 ) ) ;
#182678=CARTESIAN_POINT ( 'NONE',  ( 16.46253265017160672, -9.564922557960803928, 93.33224293864769550 ) ) ;
#182680=CARTESIAN_POINT ( 'NONE',  ( 16.55341960407618274, -4.379528057220086978, 46.04275706135234714 ) ) ;
#182681=CARTESIAN_POINT ( 'NONE',  ( -0.05219959533909027116, -19.03943276465977164, 47.49890960531435979 ) ) ;
#182682=CARTESIAN_POINT ( 'NONE',  ( 13.97604488694527802, 13.89961937509977652, 104.3739096053143385 ) ) ;
#182683=CARTESIAN_POINT ( 'NONE',  ( -14.29746914071037622, -8.314922557961029526, 49.16775706135234003 ) ) ;
#182684=CARTESIAN_POINT ( 'NONE',  ( 18.22780087662123805, 5.499999999999960032, 101.4823681787310647 ) ) ;
#182685=CARTESIAN_POINT ( 'NONE',  ( -5.049401038297874678, -19.05341960407617918, 54.79275706135234003 ) ) ;
#182686=CARTESIAN_POINT ( 'NONE',  ( -13.97604488694527625, -13.89961937509977652, 41.87390960531435979 ) ) ;
#182687=CARTESIAN_POINT ( 'NONE',  ( -8.224510206698735004, -14.34966873604973081, 79.58442372801903275 ) ) ;
#182688=CARTESIAN_POINT ( 'NONE',  ( -13.97604488694547697, 13.89961937509957934, 78.12609039468567573 ) ) ;
#182689=CARTESIAN_POINT ( 'NONE',  ( -19.05341960407617563, 5.049401038297882671, 33.54275706135231871 ) ) ;
#182690=CARTESIAN_POINT ( 'NONE',  ( -19.03943276465977164, 0.05219959533909376836, 56.24890960531435979 ) ) ;
#182691=CARTESIAN_POINT ( 'NONE',  ( 8.314922557960818139, 14.29746914071049879, 99.58224293864770971 ) ) ;
#182693=CARTESIAN_POINT ( 'NONE',  ( -16.51473224551082808, 9.474510206698731452, 73.33442372801900433 ) ) ;
#182694=CARTESIAN_POINT ( 'NONE',  ( -10.72451020669898014, 18.67979575497178502, 60.41557627198102409 ) ) ;
#182695=CARTESIAN_POINT ( 'NONE',  ( -9.564922557961040184, 16.46253265017147172, 32.91775706135233293 ) ) ;
#182696=CARTESIAN_POINT ( 'NONE',  ( 5.049401038298161559, -19.05341960407611168, 97.70724293864766707 ) ) ;
#182697=CARTESIAN_POINT ( 'NONE',  ( 10.72451020669898902, -18.67979575497178502, 72.91557627198103830 ) ) ;
#182698=CARTESIAN_POINT ( 'NONE',  ( -17.40861289039003168, 6.110651285853254677, 83.62767529172566583 ) ) ;
#182699=CARTESIAN_POINT ( 'NONE',  ( 19.03943276465977164, 0.05219959533936151252, 96.25109039468567573 ) ) ;
#182700=CARTESIAN_POINT ( 'NONE',  ( -17.49999999999999645, -5.500000000000000888, 120.0000000000000142 ) ) ;
#182701=CARTESIAN_POINT ( 'NONE',  ( -8.224510206698735004, -14.34966873604973081, 29.58442372801901854 ) ) ;
#182702=CARTESIAN_POINT ( 'NONE',  ( -5.153800228976328057, -19.02544592524343514, 27.29057627198103120 ) ) ;
#182703=CARTESIAN_POINT ( 'NONE',  ( 13.97604488694527802, 13.89961937509977652, 114.3739096053143669 ) ) ;
#182704=CARTESIAN_POINT ( 'NONE',  ( -21.53943276465977519, 0.05219959533907696930, 86.24890960531436690 ) ) ;
#182705=CARTESIAN_POINT ( 'NONE',  ( 0.05219959533937995610, -21.53943276465977519, 65.00109039468568994 ) ) ;
#182706=CARTESIAN_POINT ( 'NONE',  ( 13.89961937509957401, 13.97604488694547697, 111.8760903946856757 ) ) ;
#182707=CARTESIAN_POINT ( 'NONE',  ( -5.823673210054431948, 21.52544592524334988, 107.7094237280190328 ) ) ;
#182708=CARTESIAN_POINT ( 'NONE',  ( 12.06949235617739724, 12.14591786802326823, 106.8760903946856899 ) ) ;
#182709=CARTESIAN_POINT ( 'NONE',  ( -18.67979575497178146, -10.72451020669898902, 96.66557627198102409 ) ) ;
#182710=CARTESIAN_POINT ( 'NONE',  ( -4.379528057220328563, 16.55341960407611168, 55.20724293864770260 ) ) ;
#182711=CARTESIAN_POINT ( 'NONE',  ( 19.02544592524334988, 5.153800228976608722, 81.45942372801897591 ) ) ;
#182712=CARTESIAN_POINT ( 'NONE',  ( -16.46253265017146816, -9.564922557961047289, 59.16775706135233293 ) ) ;
#182713=CARTESIAN_POINT ( 'NONE',  ( -18.67979575497193778, 10.72451020669871902, 63.33442372801900433 ) ) ;
#182714=CARTESIAN_POINT ( 'NONE',  ( -16.51473224551082808, 9.474510206698731452, 43.33442372801900433 ) ) ;
#182715=CARTESIAN_POINT ( 'NONE',  ( -12.06949235617756955, 12.14591786802309770, 110.6239096053143669 ) ) ;
#182716=CARTESIAN_POINT ( 'NONE',  ( 15.80617190586746368, 15.72974639402197994, 24.37390960531435979 ) ) ;
#182717=CARTESIAN_POINT ( 'NONE',  ( 8.314922557960818139, 14.29746914071049879, 34.58224293864770260 ) ) ;
#182718=CARTESIAN_POINT ( 'NONE',  ( -5.719274019375665041, -21.55341960407619695, 94.79275706135234714 ) ) ;
#182719=CARTESIAN_POINT ( 'NONE',  ( -4.483927247898782831, 16.52544592524335698, 77.70942372801900433 ) ) ;
#182720=CARTESIAN_POINT ( 'NONE',  ( -4.483927247898539470, -16.52544592524342804, 32.29057627198102409 ) ) ;
#182721=CARTESIAN_POINT ( 'NONE',  ( 18.62759615963255655, 10.81492255796105972, 61.66775706135235424 ) ) ;
#182722=CARTESIAN_POINT ( 'NONE',  ( -21.52544592524334988, -5.823673210054445271, 63.95942372801901854 ) ) ;
#182723=CARTESIAN_POINT ( 'NONE',  ( -15.80617190586745835, -15.72974639402198527, 71.87390960531438111 ) ) ;
#182726=CARTESIAN_POINT ( 'NONE',  ( -19.03943276465977164, 0.05219959533909376836, 31.24890960531435979 ) ) ;
#182727=CARTESIAN_POINT ( 'NONE',  ( -5.719274019375665041, -21.55341960407619695, 49.79275706135234714 ) ) ;
#182728=CARTESIAN_POINT ( 'NONE',  ( -19.02544592524342804, 5.153800228976336051, 26.04057627198103120 ) ) ;
#182729=CARTESIAN_POINT ( 'NONE',  ( -13.97604488694527625, -13.89961937509977652, 36.87390960531436690 ) ) ;
#182730=CARTESIAN_POINT ( 'NONE',  ( -12.06949235617756955, 12.14591786802309770, 75.62390960531439532 ) ) ;
#182731=CARTESIAN_POINT ( 'NONE',  ( -0.05219959533909027116, -19.03943276465977164, 87.49890960531436690 ) ) ;
#182732=CARTESIAN_POINT ( 'NONE',  ( 14.29746914071049879, -8.314922557960816363, 23.33224293864769194 ) ) ;
#182733=CARTESIAN_POINT ( 'NONE',  ( -16.55341960407611168, -4.379528057220339221, 96.45724293864770971 ) ) ;
#182734=CARTESIAN_POINT ( 'NONE',  ( -21.55341960407610458, -5.719274019375992779, 66.45724293864768129 ) ) ;
#182736=CARTESIAN_POINT ( 'NONE',  ( 21.55341960407610458, 5.719274019375980345, 108.9572429386476955 ) ) ;
#182737=CARTESIAN_POINT ( 'NONE',  ( 19.03943276465977164, -0.05219959533909143690, 113.7489096053143669 ) ) ;
#182738=CARTESIAN_POINT ( 'NONE',  ( 19.03943276465977164, -0.05219959533909143690, 63.74890960531435979 ) ) ;
#182739=CARTESIAN_POINT ( 'NONE',  ( -9.564922557961040184, 16.46253265017147172, 107.9177570613523471 ) ) ;
#182740=CARTESIAN_POINT ( 'NONE',  ( 21.53943276465977519, -0.05219959533907433946, 63.74890960531435979 ) ) ;
#182741=CARTESIAN_POINT ( 'NONE',  ( -21.53943276465977519, -0.05219959533937600094, 83.75109039468568994 ) ) ;
#182742=CARTESIAN_POINT ( 'NONE',  ( 13.89961937509977652, -13.97604488694527269, 73.12390960531436690 ) ) ;
#182743=CARTESIAN_POINT ( 'NONE',  ( 19.05341960407611168, 5.049401038298154454, 93.95724293864769550 ) ) ;
#182744=CARTESIAN_POINT ( 'NONE',  ( 8.314922557961029526, -14.29746914071037800, 75.41775706135233293 ) ) ;
#182745=CARTESIAN_POINT ( 'NONE',  ( -10.72451020669870658, -18.67979575497194134, 59.58442372801901854 ) ) ;
#182746=CARTESIAN_POINT ( 'NONE',  ( -10.72451020669870658, -18.67979575497194134, 104.5844237280190185 ) ) ;
#182747=CARTESIAN_POINT ( 'NONE',  ( -5.823673210054116645, -21.52544592524344225, 112.2905762719810241 ) ) ;
#182748=B_SPLINE_CURVE_WITH_KNOTS ( 'NONE', 3,
 ( #63655, #14161, #137507, #199188, #94978, #159622, #68611, #97929, #189983, #65629, #2968, #35294, #95971, #64648, #130267, #19144, #83770, #113119, #156663, #36274 ),
 .UNSPECIFIED., .F., .F.,
 ( 4, 2, 2, 2, 2, 2, 2, 2, 2, 4 ),
 ( 0.000000000000000000, 0.0004987090165372679322, 0.0009974180330745358643, 0.001246772541343169668, 0.001496127049611803905, 0.001994836066149056984, 0.002493545082686310279, 0.002742899590954944733, 0.002992254099223578320, 0.003989672132298099222 ),
 .UNSPECIFIED. ) ;
#182749=CARTESIAN_POINT ( 'NONE',  ( 10.72451020669898902, -18.67979575497178502, 72.91557627198103830 ) ) ;
#182750=CARTESIAN_POINT ( 'NONE',  ( -19.02544592524334988, -5.153800228976617603, 43.95942372801899012 ) ) ;
#182751=CARTESIAN_POINT ( 'NONE',  ( 5.719274019375991003, -21.55341960407610458, 37.70724293864769550 ) ) ;
#182752=CARTESIAN_POINT ( 'NONE',  ( -19.03943276465977164, 0.05219959533909376836, 76.24890960531435269 ) ) ;
#182753=CARTESIAN_POINT ( 'NONE',  ( -0.05219959533910754901, -16.53943276465976808, 37.49890960531436690 ) ) ;
#182754=CARTESIAN_POINT ( 'NONE',  ( -17.44279575226823198, 5.990770900252463171, 65.83557567514320397 ) ) ;
#182756=CARTESIAN_POINT ( 'NONE',  ( -13.89961937509957401, -13.97604488694547875, 94.37609039468566152 ) ) ;
#182757=CARTESIAN_POINT ( 'NONE',  ( -15.72974639402197994, 15.80617190586746368, 75.62390960531439532 ) ) ;
#182758=CARTESIAN_POINT ( 'NONE',  ( -14.34966873604960291, -8.224510206698953496, 56.66557627198103830 ) ) ;
#182759=CARTESIAN_POINT ( 'NONE',  ( -14.29746914071037622, -8.314922557961029526, 29.16775706135234003 ) ) ;
#182760=CARTESIAN_POINT ( 'NONE',  ( 5.153800228976335163, 19.02544592524342804, 49.79057627198100988 ) ) ;
#182761=CARTESIAN_POINT ( 'NONE',  ( -0.05219959533907301413, -21.53943276465977519, 107.4989096053143669 ) ) ;
#182762=CARTESIAN_POINT ( 'NONE',  ( 9.474510206698729675, 16.51473224551082808, 87.08442372801900433 ) ) ;
#182763=CARTESIAN_POINT ( 'NONE',  ( -5.049401038298153566, 19.05341960407611168, 75.20724293864769550 ) ) ;
#182764=CARTESIAN_POINT ( 'NONE',  ( -4.483927247898539470, -16.52544592524342804, 87.29057627198103830 ) ) ;
#182765=CARTESIAN_POINT ( 'NONE',  ( 16.51473224551069308, 9.474510206698969483, 59.16557627198102409 ) ) ;
#182766=CARTESIAN_POINT ( 'NONE',  ( -16.55341960407611168, -4.379528057220339221, 61.45724293864770260 ) ) ;
#182767=CARTESIAN_POINT ( 'NONE',  ( -19.05341960407611168, -5.049401038298163336, 26.45724293864769550 ) ) ;
#182768=CARTESIAN_POINT ( 'NONE',  ( -17.28531771875952572, -5.454187267896333680, 21.09794194731993500 ) ) ;
#182769=CARTESIAN_POINT ( 'NONE',  ( 8.224510206698953496, -14.34966873604960469, 37.91557627198102409 ) ) ;
#182770=CARTESIAN_POINT ( 'NONE',  ( -16.46253265017160317, 9.564922557960807481, 90.83224293864769550 ) ) ;
#182772=CARTESIAN_POINT ( 'NONE',  ( 9.474510206698729675, 16.51473224551082808, 47.08442372801900433 ) ) ;
#182773=CARTESIAN_POINT ( 'NONE',  ( -4.379528057220086978, -16.55341960407618274, 59.79275706135234714 ) ) ;
#182775=CARTESIAN_POINT ( 'NONE',  ( 21.55341960407610458, 5.719274019375980345, 83.95724293864770971 ) ) ;
#182776=CARTESIAN_POINT ( 'NONE',  ( -19.05341960407617563, 5.049401038297882671, 38.54275706135233293 ) ) ;
#182777=CARTESIAN_POINT ( 'NONE',  ( 9.564922557960805705, 16.46253265017160317, 89.58224293864769550 ) ) ;
#182778=CARTESIAN_POINT ( 'NONE',  ( -17.49999999999999645, 3.471454075611698276, 114.4833258114436489 ) ) ;
#182779=CARTESIAN_POINT ( 'NONE',  ( 18.67979575497178502, 10.72451020669898547, 34.16557627198102409 ) ) ;
#182780=CARTESIAN_POINT ( 'NONE',  ( -13.97604488694527625, -13.89961937509977652, 76.87390960531433848 ) ) ;
#182781=CARTESIAN_POINT ( 'NONE',  ( 21.52544592524334988, 5.823673210054432836, 51.45942372801901854 ) ) ;
#182782=CARTESIAN_POINT ( 'NONE',  ( 4.483927247898545687, 16.52544592524342804, 114.7905762719810383 ) ) ;
#182783=CARTESIAN_POINT ( 'NONE',  ( -18.67979575497178146, -10.72451020669898902, 111.6655762719810525 ) ) ;
#182784=CARTESIAN_POINT ( 'NONE',  ( -13.89961937509977652, 13.97604488694528158, 90.62390960531432427 ) ) ;
#182786=CARTESIAN_POINT ( 'NONE',  ( -21.55341960407619339, 5.719274019375674811, 33.54275706135234714 ) ) ;
#182787=EDGE_LOOP ( 'NONE', ( #100776, #166004, #191191 ) ) ;
#182788=CARTESIAN_POINT ( 'NONE',  ( -19.05341960407611168, -5.049401038298163336, 101.4572429386476955 ) ) ;
#182790=CARTESIAN_POINT ( 'NONE',  ( -10.81492255796078084, -18.62759615963271287, 112.0822429386477097 ) ) ;
#182791=CARTESIAN_POINT ( 'NONE',  ( -19.02544592524342804, 5.153800228976336051, 46.04057627198101699 ) ) ;
#182792=CARTESIAN_POINT ( 'NONE',  ( -8.224510206698735004, -14.34966873604973081, 24.58442372801901499 ) ) ;
#182794=CARTESIAN_POINT ( 'NONE',  ( 18.62759615963255655, 10.81492255796105972, 106.6677570613523756 ) ) ;
#182795=CARTESIAN_POINT ( 'NONE',  ( 9.564922557960805705, 16.46253265017160317, 34.58224293864770260 ) ) ;
#182796=CARTESIAN_POINT ( 'NONE',  ( -5.823673210054431948, 21.52544592524334988, 102.7094237280190185 ) ) ;
#182797=CARTESIAN_POINT ( 'NONE',  ( 16.51473224551069308, 9.474510206698969483, 84.16557627198102409 ) ) ;
#182798=CARTESIAN_POINT ( 'NONE',  ( 21.53943276465977519, 0.05219959533937863772, 61.25109039468567573 ) ) ;
#182800=CARTESIAN_POINT ( 'NONE',  ( 19.03943276465977164, -0.05219959533909143690, 98.74890960531436690 ) ) ;
#182801=CARTESIAN_POINT ( 'NONE',  ( -17.49999999999999289, 3.850315288878727316, 29.26629130603453177 ) ) ;
#182802=CARTESIAN_POINT ( 'NONE',  ( -8.224510206698735004, -14.34966873604973081, 59.58442372801901854 ) ) ;
#182803=CARTESIAN_POINT ( 'NONE',  ( 12.06949235617739724, 12.14591786802326823, 61.87609039468568284 ) ) ;
#182804=CARTESIAN_POINT ( 'NONE',  ( 10.81492255796106328, -18.62759615963255655, 60.41775706135235424 ) ) ;
#182805=CARTESIAN_POINT ( 'NONE',  ( 21.55341960407619695, -5.719274019375665929, 96.04275706135236135 ) ) ;
#182807=CARTESIAN_POINT ( 'NONE',  ( -4.483927247898782831, 16.52544592524335698, 27.70942372801901854 ) ) ;
#182808=CARTESIAN_POINT ( 'NONE',  ( 19.03943276465977164, -0.05219959533909143690, 68.74890960531436690 ) ) ;
#182809=CARTESIAN_POINT ( 'NONE',  ( -0.05219959533909027116, -19.03943276465977164, 97.49890960531436690 ) ) ;
#182811=CARTESIAN_POINT ( 'NONE',  ( -16.46253265017160317, 9.564922557960807481, 25.83224293864769194 ) ) ;
#182812=CARTESIAN_POINT ( 'NONE',  ( 21.55341960407610458, 5.719274019375980345, 23.95724293864769550 ) ) ;
#182813=CARTESIAN_POINT ( 'NONE',  ( 16.52544592524335698, 4.483927247898782831, 86.45942372801901854 ) ) ;
#182814=CARTESIAN_POINT ( 'NONE',  ( -14.34966873604960291, -8.224510206698953496, 66.66557627198102409 ) ) ;
#182816=CARTESIAN_POINT ( 'NONE',  ( 13.97604488694527802, 13.89961937509977652, 74.37390960531436690 ) ) ;
#182817=CARTESIAN_POINT ( 'NONE',  ( -15.80617190586768217, 15.72974639402176855, 93.12609039468568994 ) ) ;
#182819=CARTESIAN_POINT ( 'NONE',  ( 16.52544592524335698, 4.483927247898782831, 21.45942372801901499 ) ) ;
#182820=CARTESIAN_POINT ( 'NONE',  ( 14.34966873604960469, 8.224510206698951720, 74.16557627198102409 ) ) ;
#182821=CARTESIAN_POINT ( 'NONE',  ( -10.81492255796105439, 18.62759615963255655, 32.91775706135234714 ) ) ;
#182822=CARTESIAN_POINT ( 'NONE',  ( 15.80617190586746368, 15.72974639402197994, 74.37390960531436690 ) ) ;
#182823=CARTESIAN_POINT ( 'NONE',  ( -13.97604488694547697, 13.89961937509957934, 38.12609039468566152 ) ) ;
#182825=CARTESIAN_POINT ( 'NONE',  ( 13.89961937509977652, -13.97604488694527269, 83.12390960531436690 ) ) ;
#182826=CARTESIAN_POINT ( 'NONE',  ( 16.55341960407611168, 4.379528057220329451, 53.95724293864770260 ) ) ;
#182827=CARTESIAN_POINT ( 'NONE',  ( 16.55341960407611168, 4.379528057220329451, 38.95724293864768839 ) ) ;
#182828=CARTESIAN_POINT ( 'NONE',  ( -12.14591786802326823, 12.06949235617739902, 108.1260903946856757 ) ) ;
#182829=CARTESIAN_POINT ( 'NONE',  ( -0.05219959533936034679, 19.03943276465977164, 62.50109039468566863 ) ) ;
#182831=CARTESIAN_POINT ( 'NONE',  ( 5.049401038298161559, -19.05341960407611168, 102.7072429386476955 ) ) ;
#182832=CARTESIAN_POINT ( 'NONE',  ( -12.14591786802309592, -12.06949235617757132, 76.87390960531439532 ) ) ;
#182834=CARTESIAN_POINT ( 'NONE',  ( -19.05341960407611168, -5.049401038298163336, 26.45724293864769550 ) ) ;
#182835=CARTESIAN_POINT ( 'NONE',  ( -15.80617190586745835, -15.72974639402198527, 31.87390960531435979 ) ) ;
#182836=CARTESIAN_POINT ( 'NONE',  ( 21.53943276465977519, -0.05219959533907433946, 68.74890960531435269 ) ) ;
#182837=CARTESIAN_POINT ( 'NONE',  ( -0.05219959533910754901, -16.53943276465976808, 112.4989096053143669 ) ) ;
#182838=CARTESIAN_POINT ( 'NONE',  ( -4.483927247898782831, 16.52544592524335698, 62.70942372801902565 ) ) ;
#182839=CARTESIAN_POINT ( 'NONE',  ( 13.97604488694527802, 13.89961937509977652, 49.37390960531434558 ) ) ;
#182840=CARTESIAN_POINT ( 'NONE',  ( -21.53943276465977519, -0.05219959533937600094, 58.75109039468568994 ) ) ;
#182841=CARTESIAN_POINT ( 'NONE',  ( -8.314922557960811034, -14.29746914071050412, 92.08224293864769550 ) ) ;
#182842=CARTESIAN_POINT ( 'NONE',  ( 17.12812012977025233, -6.668231424566041454, 36.14051240676857191 ) ) ;
#182844=CARTESIAN_POINT ( 'NONE',  ( -10.72451020669898014, 18.67979575497178502, 30.41557627198101699 ) ) ;
#182845=CARTESIAN_POINT ( 'NONE',  ( 17.97161686093727084, -5.499999999999964473, 78.49637206859165417 ) ) ;
#182846=CARTESIAN_POINT ( 'NONE',  ( 5.823673210054444382, -21.52544592524334988, 70.20942372801904696 ) ) ;
#182847=CARTESIAN_POINT ( 'NONE',  ( -18.10062525802553424, 5.500000000000031086, 43.51383468041920821 ) ) ;
#182848=CARTESIAN_POINT ( 'NONE',  ( -4.379528057220086978, -16.55341960407618274, 59.79275706135234714 ) ) ;
#182849=CARTESIAN_POINT ( 'NONE',  ( -16.55341960407611168, -4.379528057220339221, 41.45724293864769550 ) ) ;
#182850=CARTESIAN_POINT ( 'NONE',  ( 18.67979575497178502, 10.72451020669898547, 69.16557627198102409 ) ) ;
#182851=CARTESIAN_POINT ( 'NONE',  ( -18.67979575497178146, -10.72451020669898902, 56.66557627198103830 ) ) ;
#182853=CARTESIAN_POINT ( 'NONE',  ( 9.474510206698729675, 16.51473224551082808, 82.08442372801899012 ) ) ;
#182854=CARTESIAN_POINT ( 'NONE',  ( -19.03943276465977164, 0.05219959533909376836, 96.24890960531436690 ) ) ;
#182856=CARTESIAN_POINT ( 'NONE',  ( 0.05219959533909260263, 19.03943276465977164, 44.99890960531435979 ) ) ;
#182857=CARTESIAN_POINT ( 'NONE',  ( 16.55341960407611168, 4.379528057220329451, 108.9572429386476955 ) ) ;
#182861=CARTESIAN_POINT ( 'NONE',  ( -12.14591786802326823, 12.06949235617739902, 63.12609039468568994 ) ) ;
#182862=CARTESIAN_POINT ( 'NONE',  ( 10.72451020669898902, -18.67979575497178502, 107.9155762719810241 ) ) ;
#182863=CARTESIAN_POINT ( 'NONE',  ( -13.97604488694527625, -13.89961937509977652, 56.87390960531434558 ) ) ;
#182864=CARTESIAN_POINT ( 'NONE',  ( 10.81492255796106328, -18.62759615963255655, 45.41775706135234003 ) ) ;
#182865=CARTESIAN_POINT ( 'NONE',  ( -9.564922557960796823, -16.46253265017161027, 92.08224293864769550 ) ) ;
#182868=CARTESIAN_POINT ( 'NONE',  ( 21.53943276465977519, 0.05219959533937863772, 36.25109039468567573 ) ) ;
#182869=CARTESIAN_POINT ( 'NONE',  ( -5.153800228976328057, -19.02544592524343514, 112.2905762719810099 ) ) ;
#182870=CARTESIAN_POINT ( 'NONE',  ( -16.46253265017146816, -9.564922557961047289, 94.16775706135233293 ) ) ;
#182871=CARTESIAN_POINT ( 'NONE',  ( 13.97604488694548053, -13.89961937509957401, 35.62609039468567573 ) ) ;
#182872=CARTESIAN_POINT ( 'NONE',  ( 21.55341960407610458, 5.719274019375980345, 93.95724293864770971 ) ) ;
#182873=CARTESIAN_POINT ( 'NONE',  ( 13.89961937509957401, 13.97604488694547697, 36.87609039468565442 ) ) ;
#182874=CARTESIAN_POINT ( 'NONE',  ( -5.049401038297874678, -19.05341960407617918, 34.79275706135233293 ) ) ;
#182875=CARTESIAN_POINT ( 'NONE',  ( -16.55341960407617563, 4.379528057220093196, 88.54275706135236135 ) ) ;
#182876=CARTESIAN_POINT ( 'NONE',  ( -9.474510206698964154, 16.51473224551069663, 115.4155762719810241 ) ) ;
#182877=CARTESIAN_POINT ( 'NONE',  ( -19.03943276465977164, 0.05219959533909376836, 56.24890960531435979 ) ) ;
#182878=CARTESIAN_POINT ( 'NONE',  ( 15.72974639402176855, 15.80617190586768217, 66.87609039468568994 ) ) ;
#182879=CARTESIAN_POINT ( 'NONE',  ( -0.05219959533937732626, 21.53943276465977519, 82.50109039468568994 ) ) ;
#182881=CARTESIAN_POINT ( 'NONE',  ( 19.02544592524343514, -5.153800228976328945, 93.54057627198102409 ) ) ;
#182882=CARTESIAN_POINT ( 'NONE',  ( 21.55341960407619695, -5.719274019375665929, 66.04275706135236135 ) ) ;
#182883=CARTESIAN_POINT ( 'NONE',  ( -19.02544592524334988, -5.153800228976617603, 103.9594237280190043 ) ) ;
#182884=CARTESIAN_POINT ( 'NONE',  ( 5.153800228976335163, 19.02544592524342804, 64.79057627198100988 ) ) ;
#182885=CARTESIAN_POINT ( 'NONE',  ( -19.05341960407611168, -5.049401038298163336, 111.4572429386476671 ) ) ;
#182886=CARTESIAN_POINT ( 'NONE',  ( -13.97604488694527625, -13.89961937509977652, 81.87390960531436690 ) ) ;
#182888=CARTESIAN_POINT ( 'NONE',  ( 0.05219959533909260263, 19.03943276465977164, 69.99890960531435269 ) ) ;
#182889=CARTESIAN_POINT ( 'NONE',  ( 16.46253265017160672, -9.564922557960803928, 58.33224293864769550 ) ) ;
#182890=CARTESIAN_POINT ( 'NONE',  ( 10.81492255796078972, 18.62759615963270932, 94.58224293864769550 ) ) ;
#182891=CARTESIAN_POINT ( 'NONE',  ( -16.52544592524335698, -4.483927247898792601, 93.95942372801903275 ) ) ;
#182892=CARTESIAN_POINT ( 'NONE',  ( -13.89961937509957401, -13.97604488694547875, 39.37609039468566152 ) ) ;
#182893=CARTESIAN_POINT ( 'NONE',  ( 0.05219959533909260263, 19.03943276465977164, 74.99890960531435269 ) ) ;
#182894=CARTESIAN_POINT ( 'NONE',  ( -8.224510206698948167, 14.34966873604960824, 75.41557627198102409 ) ) ;
#182895=CARTESIAN_POINT ( 'NONE',  ( -16.53943276465976808, 0.05219959533911058130, 111.2489096053143669 ) ) ;
#182896=CARTESIAN_POINT ( 'NONE',  ( -19.02544592524342804, 5.153800228976336051, 116.0405762719810383 ) ) ;
#182897=CARTESIAN_POINT ( 'NONE',  ( 9.474510206698971260, -16.51473224551069308, 107.9155762719810383 ) ) ;
#182898=CARTESIAN_POINT ( 'NONE',  ( -4.379528057220328563, 16.55341960407611168, 75.20724293864769550 ) ) ;
#182899=CARTESIAN_POINT ( 'NONE',  ( 17.58332526062529411, -7.635886036038496805, 83.42334959558465357 ) ) ;
#182900=CARTESIAN_POINT ( 'NONE',  ( -19.03943276465977164, -0.05219959533935918106, 33.75109039468566863 ) ) ;
#182901=CARTESIAN_POINT ( 'NONE',  ( -4.483927247898782831, 16.52544592524335698, 97.70942372801904696 ) ) ;
#182902=CARTESIAN_POINT ( 'NONE',  ( 0.05219959533909260263, 19.03943276465977164, 79.99890960531436690 ) ) ;
#182903=CARTESIAN_POINT ( 'NONE',  ( 0.05219959533937995610, -21.53943276465977519, 50.00109039468568994 ) ) ;
#182904=CARTESIAN_POINT ( 'NONE',  ( 21.55341960407610458, 5.719274019375980345, 38.95724293864768839 ) ) ;
#182905=CARTESIAN_POINT ( 'NONE',  ( 10.72451020669871369, 18.67979575497193778, 22.08442372801901143 ) ) ;
#182906=CARTESIAN_POINT ( 'NONE',  ( -21.55341960407610458, -5.719274019375992779, 76.45724293864769550 ) ) ;
#182907=CARTESIAN_POINT ( 'NONE',  ( -8.224510206698948167, 14.34966873604960824, 100.4155762719810241 ) ) ;
#182908=CARTESIAN_POINT ( 'NONE',  ( 19.02544592524334988, 5.153800228976608722, 61.45942372801900433 ) ) ;
#182909=CARTESIAN_POINT ( 'NONE',  ( -5.049401038298153566, 19.05341960407611168, 35.20724293864768839 ) ) ;
#182910=CARTESIAN_POINT ( 'NONE',  ( 19.03943276465977164, -0.05219959533909143690, 83.74890960531436690 ) ) ;
#182911=CARTESIAN_POINT ( 'NONE',  ( 19.02544592524343514, -5.153800228976328945, 83.54057627198100988 ) ) ;
#182912=CARTESIAN_POINT ( 'NONE',  ( 16.55341960407611168, 4.379528057220329451, 103.9572429386476813 ) ) ;
#182915=CARTESIAN_POINT ( 'NONE',  ( 12.06949235617757843, -12.14591786802309237, 23.12390960531436335 ) ) ;
#182916=CARTESIAN_POINT ( 'NONE',  ( 14.34966873604972726, -8.224510206698740333, 30.83442372801902209 ) ) ;
#182917=CARTESIAN_POINT ( 'NONE',  ( 21.53943276465977519, 0.05219959533937863772, 96.25109039468568994 ) ) ;
#182918=CARTESIAN_POINT ( 'NONE',  ( 19.05341960407611168, 5.049401038298154454, 98.95724293864766707 ) ) ;
#182919=CARTESIAN_POINT ( 'NONE',  ( 18.67979575497194134, -10.72451020669871369, 20.83442372801901143 ) ) ;
#182920=CARTESIAN_POINT ( 'NONE',  ( -19.05341960407611168, -5.049401038298163336, 41.45724293864769550 ) ) ;
#182922=EDGE_CURVE ( 'NONE', #72646, #1176, #45594, .T. ) ;
#182923=CARTESIAN_POINT ( 'NONE',  ( 12.14591786802327356, -12.06949235617739191, 45.62609039468567573 ) ) ;
#182924=CARTESIAN_POINT ( 'NONE',  ( -16.51473224551082808, 9.474510206698731452, 113.3344237280190043 ) ) ;
#182925=CARTESIAN_POINT ( 'NONE',  ( 5.049401038298161559, -19.05341960407611168, 32.70724293864768129 ) ) ;
#182926=CARTESIAN_POINT ( 'NONE',  ( 14.29746914071049879, -8.314922557960816363, 93.33224293864769550 ) ) ;
#182927=CARTESIAN_POINT ( 'NONE',  ( 21.55341960407610458, 5.719274019375980345, 98.95724293864770971 ) ) ;
#182928=CARTESIAN_POINT ( 'NONE',  ( -19.03943276465977164, -0.05219959533935918106, 63.75109039468566863 ) ) ;
#182930=CARTESIAN_POINT ( 'NONE',  ( 15.80617190586769283, -15.72974639402175789, 20.62609039468568639 ) ) ;
#182931=CARTESIAN_POINT ( 'NONE',  ( -9.474510206698964154, 16.51473224551069663, 25.41557627198103120 ) ) ;
#182932=CARTESIAN_POINT ( 'NONE',  ( -13.89961937509977652, 13.97604488694528158, 95.62390960531436690 ) ) ;
#182933=CARTESIAN_POINT ( 'NONE',  ( 17.12812012977027010, -6.668231424565989940, 111.1405124067685648 ) ) ;
#182934=CARTESIAN_POINT ( 'NONE',  ( 16.51473224551069308, 9.474510206698969483, 89.16557627198103830 ) ) ;
#182935=CARTESIAN_POINT ( 'NONE',  ( -5.719274019375665041, -21.55341960407619695, 29.79275706135234358 ) ) ;
#182936=CARTESIAN_POINT ( 'NONE',  ( 16.53943276465976808, -0.05219959533910856209, 83.74890960531435269 ) ) ;
#182937=CARTESIAN_POINT ( 'NONE',  ( 5.049401038298161559, -19.05341960407611168, 77.70724293864765286 ) ) ;
#182938=CARTESIAN_POINT ( 'NONE',  ( 13.97604488694548053, -13.89961937509957401, 20.62609039468567573 ) ) ;
#182939=CARTESIAN_POINT ( 'NONE',  ( -8.314922557961024197, 14.29746914071037800, 47.91775706135234714 ) ) ;
#182940=CARTESIAN_POINT ( 'NONE',  ( -19.03943276465977164, -0.05219959533935918106, 53.75109039468566863 ) ) ;
#182941=CARTESIAN_POINT ( 'NONE',  ( -10.81492255796105439, 18.62759615963255655, 62.91775706135236135 ) ) ;
#182942=CARTESIAN_POINT ( 'NONE',  ( -16.52544592524335698, -4.483927247898792601, 28.95942372801902209 ) ) ;
#182943=CARTESIAN_POINT ( 'NONE',  ( 16.46253265017160672, -9.564922557960803928, 63.33224293864769550 ) ) ;
#182944=CARTESIAN_POINT ( 'NONE',  ( -16.51473224551082808, 9.474510206698731452, 98.33442372801900433 ) ) ;
#182945=CARTESIAN_POINT ( 'NONE',  ( -16.52544592524335698, -4.483927247898792601, 63.95942372801901854 ) ) ;
#182946=CARTESIAN_POINT ( 'NONE',  ( 5.719274019375673035, 21.55341960407619339, 97.29275706135234714 ) ) ;
#182947=CARTESIAN_POINT ( 'NONE',  ( 19.05341960407617918, -5.049401038297876454, 86.04275706135233293 ) ) ;
#182948=CARTESIAN_POINT ( 'NONE',  ( -16.46253265017160317, 9.564922557960807481, 55.83224293864769550 ) ) ;
#182949=CARTESIAN_POINT ( 'NONE',  ( -10.72451020669898014, 18.67979575497178502, 80.41557627198103830 ) ) ;
#182950=CARTESIAN_POINT ( 'NONE',  ( -4.483927247898539470, -16.52544592524342804, 82.29057627198103830 ) ) ;
#182951=CARTESIAN_POINT ( 'NONE',  ( 9.474510206698729675, 16.51473224551082808, 72.08442372801900433 ) ) ;
#182953=CARTESIAN_POINT ( 'NONE',  ( -19.02544592524334988, -5.153800228976617603, 43.95942372801899012 ) ) ;
#182954=CARTESIAN_POINT ( 'NONE',  ( -16.55341960407617563, 4.379528057220093196, 113.5427570613523756 ) ) ;
#182955=CARTESIAN_POINT ( 'NONE',  ( -14.29746914071049879, 8.314922557960819915, 70.83224293864770971 ) ) ;
#182956=CARTESIAN_POINT ( 'NONE',  ( -18.62759615963255300, -10.81492255796106328, 104.1677570613523471 ) ) ;
#182958=CARTESIAN_POINT ( 'NONE',  ( 21.55341960407610458, 5.719274019375980345, 113.9572429386477239 ) ) ;
#182959=CARTESIAN_POINT ( 'NONE',  ( -9.564922557960796823, -16.46253265017161027, 62.08224293864769550 ) ) ;
#182960=CARTESIAN_POINT ( 'NONE',  ( 15.80617190586769283, -15.72974639402175789, 80.62609039468567573 ) ) ;
#182961=CARTESIAN_POINT ( 'NONE',  ( -19.03943276465977164, 0.05219959533909376836, 61.24890960531436690 ) ) ;
#182962=ORIENTED_EDGE ( 'NONE', *, *, #164879, .F. ) ;
#182963=CARTESIAN_POINT ( 'NONE',  ( -14.29746914071049879, 8.314922557960819915, 115.8322429386477097 ) ) ;
#182964=CARTESIAN_POINT ( 'NONE',  ( 18.67979575497178502, 10.72451020669898547, 34.16557627198102409 ) ) ;
#182965=CARTESIAN_POINT ( 'NONE',  ( 8.224510206698953496, -14.34966873604960469, 62.91557627198102409 ) ) ;
#182966=CARTESIAN_POINT ( 'NONE',  ( -5.153800228976328057, -19.02544592524343514, 47.29057627198102409 ) ) ;
#182967=CARTESIAN_POINT ( 'NONE',  ( 16.52544592524342804, -4.483927247898539470, 103.5405762719810383 ) ) ;
#182968=CARTESIAN_POINT ( 'NONE',  ( 0.05219959533907565091, 21.53943276465977519, 114.9989096053143669 ) ) ;
#182969=CARTESIAN_POINT ( 'NONE',  ( 21.53943276465977519, 0.05219959533937863772, 51.25109039468568994 ) ) ;
#182970=CARTESIAN_POINT ( 'NONE',  ( 5.153800228976335163, 19.02544592524342804, 29.79057627198102409 ) ) ;
#182971=CARTESIAN_POINT ( 'NONE',  ( 8.314922557961029526, -14.29746914071037800, 60.41775706135235424 ) ) ;
#182972=CARTESIAN_POINT ( 'NONE',  ( 21.52544592524344225, -5.823673210054117533, 103.5405762719810383 ) ) ;
#182973=CARTESIAN_POINT ( 'NONE',  ( -10.72451020669898014, 18.67979575497178502, 100.4155762719810241 ) ) ;
#182974=CARTESIAN_POINT ( 'NONE',  ( 5.153800228976615827, -19.02544592524334988, 20.20942372801899722 ) ) ;
#182975=CARTESIAN_POINT ( 'NONE',  ( 16.51473224551069308, 9.474510206698969483, 54.16557627198103120 ) ) ;
#182976=CARTESIAN_POINT ( 'NONE',  ( -9.564922557960796823, -16.46253265017161027, 102.0822429386477097 ) ) ;
#182977=CARTESIAN_POINT ( 'NONE',  ( -21.52544592524334988, -5.823673210054445271, 63.95942372801901854 ) ) ;
#182978=CARTESIAN_POINT ( 'NONE',  ( -15.80617190586745835, -15.72974639402198527, 46.87390960531435979 ) ) ;
#182979=CARTESIAN_POINT ( 'NONE',  ( 12.14591786802309770, 12.06949235617756955, 24.37390960531435979 ) ) ;
#182980=CARTESIAN_POINT ( 'NONE',  ( -15.80617190586768217, 15.72974639402176855, 58.12609039468568994 ) ) ;
#182981=CARTESIAN_POINT ( 'NONE',  ( 15.80617190586769283, -15.72974639402175789, 95.62609039468568994 ) ) ;
#182982=CARTESIAN_POINT ( 'NONE',  ( 5.049401038297881783, 19.05341960407617563, 42.29275706135234003 ) ) ;
#182983=CARTESIAN_POINT ( 'NONE',  ( 16.55341960407618274, -4.379528057220086978, 106.0427570613523471 ) ) ;
#182984=CARTESIAN_POINT ( 'NONE',  ( -15.72974639402176322, -15.80617190586768395, 49.37609039468569705 ) ) ;
#182985=CARTESIAN_POINT ( 'NONE',  ( -5.049401038298153566, 19.05341960407611168, 60.20724293864768129 ) ) ;
#182986=CARTESIAN_POINT ( 'NONE',  ( 16.46253265017146816, 9.564922557961045513, 26.66775706135234003 ) ) ;
#182987=CARTESIAN_POINT ( 'NONE',  ( -21.53943276465977519, 0.05219959533907696930, 21.24890960531436690 ) ) ;
#182988=CARTESIAN_POINT ( 'NONE',  ( 21.53943276465977519, 0.05219959533937863772, 26.25109039468567573 ) ) ;
#182989=CARTESIAN_POINT ( 'NONE',  ( 15.72974639402199770, -15.80617190586745480, 88.12390960531436690 ) ) ;
#182990=CARTESIAN_POINT ( 'NONE',  ( -19.03943276465977164, -0.05219959533935918106, 88.75109039468567573 ) ) ;
#182991=CARTESIAN_POINT ( 'NONE',  ( 16.55341960407618274, -4.379528057220086978, 41.04275706135236135 ) ) ;
#182992=CARTESIAN_POINT ( 'NONE',  ( 17.50000000000001066, -3.203707223489874689, 37.27319652649031667 ) ) ;
#182993=CARTESIAN_POINT ( 'NONE',  ( -21.55341960407610458, -5.719274019375992779, 76.45724293864769550 ) ) ;
#182994=CARTESIAN_POINT ( 'NONE',  ( -8.314922557961024197, 14.29746914071037800, 62.91775706135236135 ) ) ;
#182995=CARTESIAN_POINT ( 'NONE',  ( 14.29746914071049879, -8.314922557960816363, 78.33224293864770971 ) ) ;
#182997=CARTESIAN_POINT ( 'NONE',  ( -5.049401038297874678, -19.05341960407617918, 109.7927570613523187 ) ) ;
#182998=CARTESIAN_POINT ( 'NONE',  ( 5.823673210054125526, 21.52544592524343514, 34.79057627198103120 ) ) ;
#182999=CARTESIAN_POINT ( 'NONE',  ( 13.97604488694527802, 13.89961937509977830, 94.37390960531436690 ) ) ;
#183000=CARTESIAN_POINT ( 'NONE',  ( 12.06949235617739724, 12.14591786802326823, 36.87609039468568994 ) ) ;
#183001=CARTESIAN_POINT ( 'NONE',  ( -15.80617190586745835, -15.72974639402198527, 106.8739096053143811 ) ) ;
#183002=CARTESIAN_POINT ( 'NONE',  ( -10.81492255796078084, -18.62759615963271287, 27.08224293864769550 ) ) ;
#183003=CARTESIAN_POINT ( 'NONE',  ( 8.314922557961029526, -14.29746914071037800, 65.41775706135234714 ) ) ;
#183004=CARTESIAN_POINT ( 'NONE',  ( -19.02544592524342804, 5.153800228976336051, 81.04057627198103830 ) ) ;
#183005=CARTESIAN_POINT ( 'NONE',  ( -5.719274019375665041, -21.55341960407619695, 59.79275706135234714 ) ) ;
#183006=CARTESIAN_POINT ( 'NONE',  ( 5.153800228976335163, 19.02544592524342804, 29.79057627198102409 ) ) ;
#183007=CARTESIAN_POINT ( 'NONE',  ( -16.46253265017160317, 9.564922557960807481, 115.8322429386477097 ) ) ;
#183009=CARTESIAN_POINT ( 'NONE',  ( 0.05219959533936267826, -19.03943276465977164, 40.00109039468566152 ) ) ;
#183010=CARTESIAN_POINT ( 'NONE',  ( -16.52544592524335698, -4.483927247898792601, 53.95942372801900433 ) ) ;
#183011=CARTESIAN_POINT ( 'NONE',  ( -5.049401038298153566, 19.05341960407611168, 110.2072429386476671 ) ) ;
#183012=CARTESIAN_POINT ( 'NONE',  ( -5.153800228976328057, -19.02544592524343514, 72.29057627198102409 ) ) ;
#183013=CARTESIAN_POINT ( 'NONE',  ( -12.06949235617739369, -12.14591786802326823, 94.37609039468568994 ) ) ;
#183015=CARTESIAN_POINT ( 'NONE',  ( -12.14591786802309592, -12.06949235617757132, 91.87390960531436690 ) ) ;
#183016=CARTESIAN_POINT ( 'NONE',  ( 21.53943276465977519, -0.05219959533907433946, 38.74890960531435979 ) ) ;
#183017=CARTESIAN_POINT ( 'NONE',  ( -13.89961937509977652, 13.97604488694528158, 35.62390960531435269 ) ) ;
#183018=CARTESIAN_POINT ( 'NONE',  ( 14.29746914071037800, 8.314922557961029526, 61.66775706135235424 ) ) ;
#183019=CARTESIAN_POINT ( 'NONE',  ( 21.55341960407619695, -5.719274019375665929, 21.04275706135234714 ) ) ;
#183020=CARTESIAN_POINT ( 'NONE',  ( -19.03943276465977164, -0.05219959533935918106, 73.75109039468566152 ) ) ;
#183021=CARTESIAN_POINT ( 'NONE',  ( 19.02544592524343514, -5.153800228976328945, 38.54057627198103120 ) ) ;
#183022=CARTESIAN_POINT ( 'NONE',  ( -21.53943276465977519, 0.05219959533907696930, 66.24890960531436690 ) ) ;
#183024=CARTESIAN_POINT ( 'NONE',  ( 19.03943276465977164, -0.05219959533909143690, 113.7489096053143669 ) ) ;
#183025=CARTESIAN_POINT ( 'NONE',  ( 21.53943276465977519, 0.05219959533937863772, 91.25109039468568994 ) ) ;
#183026=CARTESIAN_POINT ( 'NONE',  ( -9.474510206698964154, 16.51473224551069663, 65.41557627198102409 ) ) ;
#183027=CARTESIAN_POINT ( 'NONE',  ( -0.05219959533934338120, 16.53943276465976808, 47.50109039468568994 ) ) ;
#183028=CARTESIAN_POINT ( 'NONE',  ( 19.05341960407611168, 5.049401038298154454, 63.95724293864769550 ) ) ;
#183029=CARTESIAN_POINT ( 'NONE',  ( -15.80617190586768217, 15.72974639402176855, 78.12609039468570415 ) ) ;
#183030=CARTESIAN_POINT ( 'NONE',  ( -5.049401038297874678, -19.05341960407617918, 34.79275706135233293 ) ) ;
#183031=CARTESIAN_POINT ( 'NONE',  ( 9.474510206698729675, 16.51473224551082808, 57.08442372801900433 ) ) ;
#183032=CARTESIAN_POINT ( 'NONE',  ( 21.53943276465977519, 0.05219959533937863772, 46.25109039468567573 ) ) ;
#183034=CARTESIAN_POINT ( 'NONE',  ( 16.46253265017146816, 9.564922557961045513, 46.66775706135233293 ) ) ;
#183035=CARTESIAN_POINT ( 'NONE',  ( -9.474510206698964154, 16.51473224551069663, 100.4155762719810241 ) ) ;
#183036=CARTESIAN_POINT ( 'NONE',  ( -9.474510206698964154, 16.51473224551069663, 85.41557627198102409 ) ) ;
#183037=CARTESIAN_POINT ( 'NONE',  ( 16.53943276465976808, -0.05219959533910856209, 33.74890960531436690 ) ) ;
#183038=CARTESIAN_POINT ( 'NONE',  ( -21.52544592524343514, 5.823673210054127303, 31.04057627198102409 ) ) ;
#183039=CARTESIAN_POINT ( 'NONE',  ( -15.80617190586768217, 15.72974639402176855, 103.1260903946856757 ) ) ;
#183041=CARTESIAN_POINT ( 'NONE',  ( 16.29526858892878849, 7.335722546919997811, 58.29670597800210174 ) ) ;
#183042=CARTESIAN_POINT ( 'NONE',  ( 5.719274019375673035, 21.55341960407619339, 92.29275706135236135 ) ) ;
#183044=CARTESIAN_POINT ( 'NONE',  ( -19.03943276465977164, 0.05219959533909376836, 41.24890960531435269 ) ) ;
#183045=CARTESIAN_POINT ( 'NONE',  ( -5.153800228976328057, -19.02544592524343514, 107.2905762719810383 ) ) ;
#183047=CARTESIAN_POINT ( 'NONE',  ( 16.55341960407618274, -4.379528057220086978, 51.04275706135234714 ) ) ;
#183048=CARTESIAN_POINT ( 'NONE',  ( -0.05219959533907301413, -21.53943276465977519, 67.49890960531436690 ) ) ;
#183049=CARTESIAN_POINT ( 'NONE',  ( -16.52544592524342804, 4.483927247898546575, 46.04057627198103830 ) ) ;
#183050=CARTESIAN_POINT ( 'NONE',  ( -13.89961937509977652, 13.97604488694528158, 25.62390960531434558 ) ) ;
#183051=CARTESIAN_POINT ( 'NONE',  ( 9.474510206698971260, -16.51473224551069308, 102.9155762719810241 ) ) ;
#183052=CARTESIAN_POINT ( 'NONE',  ( -15.80617190586768217, 15.72974639402176855, 23.12609039468567573 ) ) ;
#183053=CARTESIAN_POINT ( 'NONE',  ( 5.049401038297881783, 19.05341960407617563, 32.29275706135233293 ) ) ;
#183054=CARTESIAN_POINT ( 'NONE',  ( 14.34966873604960469, 8.224510206698951720, 109.1655762719810383 ) ) ;
#183055=CARTESIAN_POINT ( 'NONE',  ( 10.72451020669871369, 18.67979575497193778, 62.08442372801901143 ) ) ;
#183056=CARTESIAN_POINT ( 'NONE',  ( 30.00000000000000000, -5.499999999999992895, 102.5000000000000142 ) ) ;
#183057=CARTESIAN_POINT ( 'NONE',  ( -4.483927247898539470, -16.52544592524342804, 27.29057627198103120 ) ) ;
#183059=CARTESIAN_POINT ( 'NONE',  ( 21.55341960407610458, 5.719274019375980345, 23.95724293864769550 ) ) ;
#183060=CARTESIAN_POINT ( 'NONE',  ( -14.29746914071049879, 8.314922557960819915, 85.83224293864768129 ) ) ;
#183063=CARTESIAN_POINT ( 'NONE',  ( -0.05219959533909027116, -19.03943276465977164, 72.49890960531435269 ) ) ;
#183064=CARTESIAN_POINT ( 'NONE',  ( -16.55341960407611168, -4.379528057220339221, 71.45724293864769550 ) ) ;
#183065=CARTESIAN_POINT ( 'NONE',  ( -19.03943276465977164, -0.05219959533935918106, 103.7510903946856757 ) ) ;
#183066=CARTESIAN_POINT ( 'NONE',  ( 21.55341960407610458, 5.719274019375980345, 53.95724293864770260 ) ) ;
#183068=CARTESIAN_POINT ( 'NONE',  ( -16.52544592524342804, 4.483927247898546575, 116.0405762719810383 ) ) ;
#183069=CARTESIAN_POINT ( 'NONE',  ( -13.97604488694527625, -13.89961937509977652, 76.87390960531433848 ) ) ;
#183070=CARTESIAN_POINT ( 'NONE',  ( 21.52544592524344225, -5.823673210054117533, 73.54057627198102409 ) ) ;
#183071=CARTESIAN_POINT ( 'NONE',  ( 14.34966873604972726, -8.224510206698740333, 100.8344237280190185 ) ) ;
#183072=CARTESIAN_POINT ( 'NONE',  ( -13.97604488694527625, -13.89961937509977652, 91.87390960531432427 ) ) ;
#183073=CARTESIAN_POINT ( 'NONE',  ( 13.97604488694548053, -13.89961937509957401, 60.62609039468564731 ) ) ;
#183074=CARTESIAN_POINT ( 'NONE',  ( 10.72451020669871369, 18.67979575497193778, 97.08442372801904696 ) ) ;
#183075=CARTESIAN_POINT ( 'NONE',  ( 15.72974639402199770, -15.80617190586745480, 68.12390960531436690 ) ) ;
#183076=CARTESIAN_POINT ( 'NONE',  ( 19.03943276465977164, -0.05219959533909143690, 113.7489096053143669 ) ) ;
#183077=CARTESIAN_POINT ( 'NONE',  ( 19.03943276465977164, -0.05219959533909143690, 43.74890960531435979 ) ) ;
#183078=CARTESIAN_POINT ( 'NONE',  ( 4.379528057220092307, 16.55341960407617563, 102.2927570613523613 ) ) ;
#183079=CARTESIAN_POINT ( 'NONE',  ( -0.05219959533909027116, -19.03943276465977164, 62.49890960531435979 ) ) ;
#183080=CARTESIAN_POINT ( 'NONE',  ( 8.314922557961029526, -14.29746914071037800, 25.41775706135235779 ) ) ;
#183081=CARTESIAN_POINT ( 'NONE',  ( 16.81555441253550853, 7.025013491695498047, 51.86314554665744936 ) ) ;
#183082=CARTESIAN_POINT ( 'NONE',  ( -15.80617190586768217, 15.72974639402176855, 113.1260903946856899 ) ) ;
#183083=CARTESIAN_POINT ( 'NONE',  ( 16.55341960407611168, 4.379528057220329451, 68.95724293864769550 ) ) ;
#183084=CARTESIAN_POINT ( 'NONE',  ( 5.719274019375991003, -21.55341960407610458, 107.7072429386476955 ) ) ;
#183085=CARTESIAN_POINT ( 'NONE',  ( 21.52544592524344225, -5.823673210054117533, 108.5405762719810241 ) ) ;
#183087=CARTESIAN_POINT ( 'NONE',  ( -21.55341960407610458, -5.719274019375992779, 56.45724293864768839 ) ) ;
#183089=CARTESIAN_POINT ( 'NONE',  ( -4.483927247898782831, 16.52544592524335698, 77.70942372801900433 ) ) ;
#183090=CARTESIAN_POINT ( 'NONE',  ( 16.55341960407611168, 4.379528057220329451, 108.9572429386476955 ) ) ;
#183091=CARTESIAN_POINT ( 'NONE',  ( 9.474510206698971260, -16.51473224551069308, 62.91557627198102409 ) ) ;
#183092=( LENGTH_UNIT ( ) NAMED_UNIT ( * ) SI_UNIT ( .MILLI., .METRE. ) );
#183093=CARTESIAN_POINT ( 'NONE',  ( -14.34966873604972548, 8.224510206698743886, 108.3344237280190185 ) ) ;
#183094=CARTESIAN_POINT ( 'NONE',  ( 21.55341960407619695, -5.719274019375665929, 46.04275706135234714 ) ) ;
#183095=CARTESIAN_POINT ( 'NONE',  ( -19.02544592524342804, 5.153800228976336051, 96.04057627198103830 ) ) ;
#183096=CARTESIAN_POINT ( 'NONE',  ( -18.62759615963255300, -10.81492255796106328, 84.16775706135234714 ) ) ;
#183097=CARTESIAN_POINT ( 'NONE',  ( 16.51473224551069308, 9.474510206698969483, 24.16557627198102765 ) ) ;
#183098=CARTESIAN_POINT ( 'NONE',  ( -0.05219959533909027116, -19.03943276465977164, 42.49890960531435269 ) ) ;
#183100=CARTESIAN_POINT ( 'NONE',  ( 21.52544592524334988, 5.823673210054432836, 71.45942372801901854 ) ) ;
#183101=CARTESIAN_POINT ( 'NONE',  ( -19.03943276465977164, 0.05219959533909376836, 106.2489096053143669 ) ) ;
#183102=CARTESIAN_POINT ( 'NONE',  ( 9.474510206698729675, 16.51473224551082808, 82.08442372801899012 ) ) ;
#183103=CARTESIAN_POINT ( 'NONE',  ( -21.55341960407619339, 5.719274019375674811, 38.54275706135234714 ) ) ;
#183104=CARTESIAN_POINT ( 'NONE',  ( -19.03943276465977164, -0.05219959533935918106, 113.7510903946856757 ) ) ;
#183105=CARTESIAN_POINT ( 'NONE',  ( 9.564922557961047289, -16.46253265017146816, 75.41775706135234714 ) ) ;
#183106=CARTESIAN_POINT ( 'NONE',  ( 16.51473224551069308, 9.474510206698969483, 54.16557627198103120 ) ) ;
#183107=CARTESIAN_POINT ( 'NONE',  ( 13.97604488694548053, -13.89961937509957401, 85.62609039468568994 ) ) ;
#183108=CARTESIAN_POINT ( 'NONE',  ( -16.55341960407611168, -4.379528057220339221, 26.45724293864768839 ) ) ;
#183109=CARTESIAN_POINT ( 'NONE',  ( 16.51473224551083163, -9.474510206698727899, 95.83442372801900433 ) ) ;
#183110=CARTESIAN_POINT ( 'NONE',  ( -14.29746914071049879, 8.314922557960819915, 35.83224293864768839 ) ) ;
#183111=CARTESIAN_POINT ( 'NONE',  ( 5.049401038297881783, 19.05341960407617563, 57.29275706135231871 ) ) ;
#183112=CARTESIAN_POINT ( 'NONE',  ( 4.483927247898790824, -16.52544592524335698, 50.20942372801901854 ) ) ;
#183113=CARTESIAN_POINT ( 'NONE',  ( -21.53943276465977519, -0.05219959533937600094, 113.7510903946856757 ) ) ;
#183114=CARTESIAN_POINT ( 'NONE',  ( -5.049401038298153566, 19.05341960407611168, 30.20724293864768839 ) ) ;
#183115=CARTESIAN_POINT ( 'NONE',  ( -17.48853670773242186, -5.747243402303177540, 66.33328700250008580 ) ) ;
#183116=CARTESIAN_POINT ( 'NONE',  ( 8.314922557961029526, -14.29746914071037800, 50.41775706135235424 ) ) ;
#183119=CARTESIAN_POINT ( 'NONE',  ( 5.153800228976335163, 19.02544592524342804, 89.79057627198102409 ) ) ;
#183120=CARTESIAN_POINT ( 'NONE',  ( 17.50000000000000355, 3.242565516147348337, 102.5000000000000142 ) ) ;
#183122=CARTESIAN_POINT ( 'NONE',  ( 9.564922557961047289, -16.46253265017146816, 80.41775706135234714 ) ) ;
#183123=CARTESIAN_POINT ( 'NONE',  ( 15.72974639402199770, -15.80617190586745480, 23.12390960531436335 ) ) ;
#183124=CARTESIAN_POINT ( 'NONE',  ( 5.719274019375673035, 21.55341960407619339, 112.2927570613523471 ) ) ;
#183125=CARTESIAN_POINT ( 'NONE',  ( 5.153800228976615827, -19.02544592524334988, 100.2094237280190043 ) ) ;
#183126=CARTESIAN_POINT ( 'NONE',  ( 12.14591786802309770, 12.06949235617756955, 109.3739096053143811 ) ) ;
#183127=CARTESIAN_POINT ( 'NONE',  ( 16.46253265017160672, -9.564922557960803928, 33.33224293864770260 ) ) ;
#183128=CARTESIAN_POINT ( 'NONE',  ( -0.05219959533907301413, -21.53943276465977519, 62.49890960531436690 ) ) ;
#183129=CARTESIAN_POINT ( 'NONE',  ( 16.46253265017160672, -9.564922557960803928, 28.33224293864769550 ) ) ;
#183131=CARTESIAN_POINT ( 'NONE',  ( 13.89961937509957401, 13.97604488694547697, 66.87609039468567573 ) ) ;
#183132=CARTESIAN_POINT ( 'NONE',  ( -12.06949235617756955, 12.14591786802309770, 35.62390960531437401 ) ) ;
#183133=CARTESIAN_POINT ( 'NONE',  ( 9.564922557960805705, 16.46253265017160317, 109.5822429386476955 ) ) ;
#183134=CARTESIAN_POINT ( 'NONE',  ( -10.72451020669870658, -18.67979575497194134, 99.58442372801900433 ) ) ;
#183135=CARTESIAN_POINT ( 'NONE',  ( -15.72974639402197994, 15.80617190586746368, 90.62390960531436690 ) ) ;
#183136=CARTESIAN_POINT ( 'NONE',  ( 15.80617190586769283, -15.72974639402175789, 55.62609039468568284 ) ) ;
#183137=CARTESIAN_POINT ( 'NONE',  ( 10.72451020669871369, 18.67979575497193778, 62.08442372801901143 ) ) ;
#183138=CARTESIAN_POINT ( 'NONE',  ( 13.89961937509977652, -13.97604488694527269, 93.12390960531436690 ) ) ;
#183139=CARTESIAN_POINT ( 'NONE',  ( -14.34966873604972548, 8.224510206698743886, 93.33442372801901854 ) ) ;
#183140=CARTESIAN_POINT ( 'NONE',  ( 10.72451020669871369, 18.67979575497193778, 52.08442372801901854 ) ) ;
#183141=CARTESIAN_POINT ( 'NONE',  ( 14.29746914071049879, -8.314922557960816363, 113.3322429386476955 ) ) ;
#183142=CARTESIAN_POINT ( 'NONE',  ( 16.55341960407611168, 4.379528057220329451, 73.95724293864769550 ) ) ;
#183143=CARTESIAN_POINT ( 'NONE',  ( -14.29746914071049879, 8.314922557960819915, 40.83224293864769550 ) ) ;
#183144=CARTESIAN_POINT ( 'NONE',  ( -18.67979575497178146, -10.72451020669898902, 46.66557627198102409 ) ) ;
#183145=CARTESIAN_POINT ( 'NONE',  ( 0.05219959533909260263, 19.03943276465977164, 69.99890960531435269 ) ) ;
#183146=CARTESIAN_POINT ( 'NONE',  ( 5.049401038298161559, -19.05341960407611168, 47.70724293864770260 ) ) ;
#183147=CARTESIAN_POINT ( 'NONE',  ( 21.52544592524344225, -5.823673210054117533, 63.54057627198103830 ) ) ;
#183148=CARTESIAN_POINT ( 'NONE',  ( -19.02544592524334988, -5.153800228976617603, 43.95942372801899012 ) ) ;
#183149=CARTESIAN_POINT ( 'NONE',  ( -17.48847506799968343, -5.747544572773810145, 39.17302562156721990 ) ) ;
#183150=CARTESIAN_POINT ( 'NONE',  ( -14.29746914071049879, 8.314922557960819915, 50.83224293864770971 ) ) ;
#183151=CARTESIAN_POINT ( 'NONE',  ( 18.67979575497178502, 10.72451020669898547, 29.16557627198103120 ) ) ;
#183152=ORIENTED_EDGE ( 'NONE', *, *, #141448, .F. ) ;
#183154=LINE ( 'NONE', #153791, #103296 ) ;
#183155=CARTESIAN_POINT ( 'NONE',  ( 12.06949235617739724, 12.14591786802326823, 71.87609039468568994 ) ) ;
#183157=CARTESIAN_POINT ( 'NONE',  ( 5.153800228976615827, -19.02544592524334988, 80.20942372801901854 ) ) ;
#183158=CARTESIAN_POINT ( 'NONE',  ( -16.53943276465976808, 0.05219959533911058130, 41.24890960531435269 ) ) ;
#183159=CARTESIAN_POINT ( 'NONE',  ( -18.89770734986050016, -5.499999999999909406, 59.10214472496638649 ) ) ;
#183160=CARTESIAN_POINT ( 'NONE',  ( 12.14591786802309770, 12.06949235617756955, 29.37390960531435269 ) ) ;
#183161=CARTESIAN_POINT ( 'NONE',  ( -13.89961937509977652, 13.97604488694528158, 45.62390960531433848 ) ) ;
#183162=CARTESIAN_POINT ( 'NONE',  ( -16.46253265017160317, 9.564922557960807481, 80.83224293864769550 ) ) ;
#183163=CARTESIAN_POINT ( 'NONE',  ( 9.474510206698971260, -16.51473224551069308, 32.91557627198102409 ) ) ;
#183164=CARTESIAN_POINT ( 'NONE',  ( 18.67979575497194134, -10.72451020669871369, 45.83442372801901854 ) ) ;
#183165=CARTESIAN_POINT ( 'NONE',  ( 5.049401038298161559, -19.05341960407611168, 52.70724293864767418 ) ) ;
#183166=CARTESIAN_POINT ( 'NONE',  ( 17.72696623605158806, -5.500000000000042633, 81.09811031808415294 ) ) ;
#183168=CARTESIAN_POINT ( 'NONE',  ( 5.153800228976335163, 19.02544592524342804, 54.79057627198103120 ) ) ;
#183169=CARTESIAN_POINT ( 'NONE',  ( -15.80617190586745835, -15.72974639402198527, 31.87390960531435979 ) ) ;
#183170=CARTESIAN_POINT ( 'NONE',  ( -16.53943276465976808, 0.05219959533911058130, 116.2489096053143669 ) ) ;
#183171=CARTESIAN_POINT ( 'NONE',  ( -10.72451020669898014, 18.67979575497178502, 45.41557627198103830 ) ) ;
#183172=CARTESIAN_POINT ( 'NONE',  ( 16.53943276465976808, 0.05219959533934440121, 86.25109039468568994 ) ) ;
#183173=CARTESIAN_POINT ( 'NONE',  ( 5.719274019375673035, 21.55341960407619339, 107.2927570613523471 ) ) ;
#183175=CARTESIAN_POINT ( 'NONE',  ( 0.05219959533934541429, -16.53943276465976808, 65.00109039468568994 ) ) ;
#183176=CARTESIAN_POINT ( 'NONE',  ( 16.51473224551069308, 9.474510206698969483, 109.1655762719810383 ) ) ;
#183177=CARTESIAN_POINT ( 'NONE',  ( 16.55341960407618274, -4.379528057220086978, 51.04275706135234714 ) ) ;
#183178=CARTESIAN_POINT ( 'NONE',  ( -12.06949235617739369, -12.14591786802326823, 34.37609039468568284 ) ) ;
#183179=CARTESIAN_POINT ( 'NONE',  ( 13.89961937509977652, -13.97604488694527269, 113.1239096053143527 ) ) ;
#183180=CARTESIAN_POINT ( 'NONE',  ( -16.52544592524335698, -4.483927247898792601, 18.95942372801901143 ) ) ;
#183181=CARTESIAN_POINT ( 'NONE',  ( -9.564922557960796823, -16.46253265017161027, 37.08224293864768839 ) ) ;
#183182=CARTESIAN_POINT ( 'NONE',  ( 21.53943276465977519, 0.05219959533937863772, 21.25109039468567218 ) ) ;
#183183=CARTESIAN_POINT ( 'NONE',  ( 4.483927247898790824, -16.52544592524335698, 25.20942372801901854 ) ) ;
#183184=CARTESIAN_POINT ( 'NONE',  ( -16.52544592524335698, -4.483927247898792601, 83.95942372801900433 ) ) ;
#183186=CARTESIAN_POINT ( 'NONE',  ( -15.80617190586768217, 15.72974639402176855, 83.12609039468568994 ) ) ;
#183187=CARTESIAN_POINT ( 'NONE',  ( -16.51473224551082808, 9.474510206698731452, 93.33442372801900433 ) ) ;
#183188=CARTESIAN_POINT ( 'NONE',  ( -0.05219959533910754901, -16.53943276465976808, 57.49890960531435979 ) ) ;
#183189=CARTESIAN_POINT ( 'NONE',  ( 8.224510206698953496, -14.34966873604960469, 112.9155762719810383 ) ) ;
#183190=CARTESIAN_POINT ( 'NONE',  ( -19.05341960407617563, 5.049401038297882671, 43.54275706135232582 ) ) ;
#183192=CARTESIAN_POINT ( 'NONE',  ( -10.81492255796105439, 18.62759615963255655, 52.91775706135235424 ) ) ;
#183193=CARTESIAN_POINT ( 'NONE',  ( -16.53943276465976808, -0.05219959533934237506, 18.75109039468568639 ) ) ;
#183195=CARTESIAN_POINT ( 'NONE',  ( 9.474510206698971260, -16.51473224551069308, 102.9155762719810241 ) ) ;
#183196=CARTESIAN_POINT ( 'NONE',  ( -21.52544592524343514, 5.823673210054127303, 66.04057627198103830 ) ) ;
#183197=CARTESIAN_POINT ( 'NONE',  ( -5.049401038297874678, -19.05341960407617918, 99.79275706135234714 ) ) ;
#183198=CARTESIAN_POINT ( 'NONE',  ( 16.46253265017160672, -9.564922557960803928, 98.33224293864769550 ) ) ;
#183200=CARTESIAN_POINT ( 'NONE',  ( 4.379528057220339221, -16.55341960407611168, 107.7072429386476955 ) ) ;
#183201=CARTESIAN_POINT ( 'NONE',  ( -15.80617190586768217, 15.72974639402176855, 93.12609039468568994 ) ) ;
#183202=CARTESIAN_POINT ( 'NONE',  ( 19.03943276465977164, -0.05219959533909143690, 48.74890960531435979 ) ) ;
#183204=CARTESIAN_POINT ( 'NONE',  ( -5.823673210054431948, 21.52544592524334988, 57.70942372801901143 ) ) ;
#183205=CARTESIAN_POINT ( 'NONE',  ( -15.80617190586768217, 15.72974639402176855, 83.12609039468568994 ) ) ;
#183206=CARTESIAN_POINT ( 'NONE',  ( 14.34966873604972726, -8.224510206698740333, 100.8344237280190185 ) ) ;
#183207=CARTESIAN_POINT ( 'NONE',  ( 13.89961937509977652, -13.97604488694527269, 63.12390960531435979 ) ) ;
#183208=CARTESIAN_POINT ( 'NONE',  ( -5.719274019375665041, -21.55341960407619695, 49.79275706135234714 ) ) ;
#183209=CARTESIAN_POINT ( 'NONE',  ( 18.62759615963255655, 10.81492255796105972, 41.66775706135235424 ) ) ;
#183210=CARTESIAN_POINT ( 'NONE',  ( 16.46253265017146816, 9.564922557961045513, 71.66775706135233293 ) ) ;
#183211=CARTESIAN_POINT ( 'NONE',  ( 9.564922557960805705, 16.46253265017160317, 94.58224293864769550 ) ) ;
#183212=CARTESIAN_POINT ( 'NONE',  ( -4.483927247898539470, -16.52544592524342804, 102.2905762719810383 ) ) ;
#183213=CARTESIAN_POINT ( 'NONE',  ( -15.80617190586745835, -15.72974639402198527, 101.8739096053143811 ) ) ;
#183214=CARTESIAN_POINT ( 'NONE',  ( 16.55341960407611168, 4.379528057220329451, 63.95724293864770260 ) ) ;
#183215=CARTESIAN_POINT ( 'NONE',  ( -19.03943276465977164, -0.05219959533935918106, 23.75109039468566152 ) ) ;
#183216=CARTESIAN_POINT ( 'NONE',  ( 4.483927247898545687, 16.52544592524342804, 84.79057627198102409 ) ) ;
#183217=CARTESIAN_POINT ( 'NONE',  ( 5.049401038298161559, -19.05341960407611168, 37.70724293864768839 ) ) ;
#183218=CARTESIAN_POINT ( 'NONE',  ( 19.05341960407617918, -5.049401038297876454, 86.04275706135233293 ) ) ;
#183219=CARTESIAN_POINT ( 'NONE',  ( 16.55341960407611168, 4.379528057220329451, 53.95724293864770260 ) ) ;
#183220=CARTESIAN_POINT ( 'NONE',  ( 18.62759615963255655, 10.81492255796105972, 101.6677570613523613 ) ) ;
#183221=CARTESIAN_POINT ( 'NONE',  ( -19.03943276465977164, 0.05219959533909376836, 86.24890960531436690 ) ) ;
#183222=CARTESIAN_POINT ( 'NONE',  ( -13.97604488694547697, 13.89961937509957934, 68.12609039468563310 ) ) ;
#183223=CARTESIAN_POINT ( 'NONE',  ( -15.80617190586745835, -15.72974639402198527, 81.87390960531435269 ) ) ;
#183224=CARTESIAN_POINT ( 'NONE',  ( -5.719274019375665041, -21.55341960407619695, 24.79275706135235779 ) ) ;
#183225=CARTESIAN_POINT ( 'NONE',  ( -12.14591786802326823, 12.06949235617739902, 33.12609039468569705 ) ) ;
#183226=CARTESIAN_POINT ( 'NONE',  ( 12.14591786802327356, -12.06949235617739191, 95.62609039468568994 ) ) ;
#183227=CARTESIAN_POINT ( 'NONE',  ( 9.474510206698971260, -16.51473224551069308, 22.91557627198102765 ) ) ;
#183228=CARTESIAN_POINT ( 'NONE',  ( -0.05219959533937732626, 21.53943276465977519, 27.50109039468567929 ) ) ;
#183229=CARTESIAN_POINT ( 'NONE',  ( 9.474510206698971260, -16.51473224551069308, 22.91557627198102765 ) ) ;
#183231=CARTESIAN_POINT ( 'NONE',  ( 14.34966873604972726, -8.224510206698740333, 45.83442372801901854 ) ) ;
#183232=CARTESIAN_POINT ( 'NONE',  ( 16.52544592524342804, -4.483927247898539470, 78.54057627198103830 ) ) ;
#183233=CARTESIAN_POINT ( 'NONE',  ( -10.81492255796078084, -18.62759615963271287, 82.08224293864768129 ) ) ;
#183234=CARTESIAN_POINT ( 'NONE',  ( 4.483927247898545687, 16.52544592524342804, 29.79057627198102409 ) ) ;
#183235=CARTESIAN_POINT ( 'NONE',  ( 16.53943276465976808, 0.05219959533934440121, 46.25109039468567573 ) ) ;
#183236=CARTESIAN_POINT ( 'NONE',  ( 19.03943276465977164, -0.05219959533909143690, 48.74890960531435979 ) ) ;
#183237=CARTESIAN_POINT ( 'NONE',  ( 16.53943276465976808, 0.05219959533934440121, 86.25109039468568994 ) ) ;
#183238=CARTESIAN_POINT ( 'NONE',  ( -9.474510206698720793, -16.51473224551083518, 69.58442372801901854 ) ) ;
#183239=CARTESIAN_POINT ( 'NONE',  ( 15.80617190586746368, 15.72974639402197994, 69.37390960531436690 ) ) ;
#183240=CARTESIAN_POINT ( 'NONE',  ( -0.05219959533910754901, -16.53943276465976808, 22.49890960531436335 ) ) ;
#183241=ORIENTED_EDGE ( 'NONE', *, *, #124318, .F. ) ;
#183243=CARTESIAN_POINT ( 'NONE',  ( 15.80617190586746368, 15.72974639402197994, 64.37390960531435269 ) ) ;
#183245=VERTEX_POINT ( 'NONE', #11933 ) ;
#183246=CARTESIAN_POINT ( 'NONE',  ( -16.53943276465976808, -0.05219959533934237506, 93.75109039468567573 ) ) ;
#183248=CARTESIAN_POINT ( 'NONE',  ( 16.51473224551069308, 9.474510206698969483, 114.1655762719810241 ) ) ;
#183249=CARTESIAN_POINT ( 'NONE',  ( -19.02130022317636815, 5.499999999999801048, 75.78188669246573284 ) ) ;
#183250=CARTESIAN_POINT ( 'NONE',  ( 21.55341960407610458, 5.719274019375980345, 68.95724293864769550 ) ) ;
#183251=CARTESIAN_POINT ( 'NONE',  ( -4.379528057220086978, -16.55341960407618274, 104.7927570613523898 ) ) ;
#183252=CARTESIAN_POINT ( 'NONE',  ( 5.049401038297881783, 19.05341960407617563, 112.2927570613523471 ) ) ;
#183253=CARTESIAN_POINT ( 'NONE',  ( -5.049401038298153566, 19.05341960407611168, 25.20724293864768484 ) ) ;
#183254=CARTESIAN_POINT ( 'NONE',  ( 4.483927247898790824, -16.52544592524335698, 25.20942372801901854 ) ) ;
#183255=CARTESIAN_POINT ( 'NONE',  ( 5.049401038298161559, -19.05341960407611168, 57.70724293864769550 ) ) ;
#183257=CARTESIAN_POINT ( 'NONE',  ( -13.89961937509977652, 13.97604488694528158, 110.6239096053143243 ) ) ;
#183258=CARTESIAN_POINT ( 'NONE',  ( -4.379528057220086978, -16.55341960407618274, 89.79275706135236135 ) ) ;
#183259=CARTESIAN_POINT ( 'NONE',  ( 16.46253265017146816, 9.564922557961045513, 86.66775706135233293 ) ) ;
#183260=CARTESIAN_POINT ( 'NONE',  ( 16.51473224551083163, -9.474510206698727899, 30.83442372801900433 ) ) ;
#183261=CARTESIAN_POINT ( 'NONE',  ( -10.72451020669898014, 18.67979575497178502, 75.41557627198102409 ) ) ;
#183263=CARTESIAN_POINT ( 'NONE',  ( -12.14591786802326823, 12.06949235617739902, 103.1260903946856757 ) ) ;
#183264=CARTESIAN_POINT ( 'NONE',  ( -5.049401038297874678, -19.05341960407617918, 99.79275706135234714 ) ) ;
#183265=CARTESIAN_POINT ( 'NONE',  ( 16.51473224551069308, 9.474510206698969483, 49.16557627198102409 ) ) ;
#183266=CARTESIAN_POINT ( 'NONE',  ( -19.05341960407611168, -5.049401038298163336, 91.45724293864766707 ) ) ;
#183267=CARTESIAN_POINT ( 'NONE',  ( 18.67979575497194134, -10.72451020669871369, 55.83442372801901854 ) ) ;
#183268=CARTESIAN_POINT ( 'NONE',  ( 19.05341960407611168, 5.049401038298154454, 48.95724293864768129 ) ) ;
#183269=CARTESIAN_POINT ( 'NONE',  ( -17.05116617787827593, -6.768360034955819948, 86.34324446740804149 ) ) ;
#183270=CARTESIAN_POINT ( 'NONE',  ( -16.55341960407611168, -4.379528057220339221, 81.45724293864769550 ) ) ;
#183271=CARTESIAN_POINT ( 'NONE',  ( 15.80617190586746368, 15.72974639402197994, 79.37390960531436690 ) ) ;
#183272=CARTESIAN_POINT ( 'NONE',  ( 20.02699684519808798, 3.713461942911795433, 102.5000000000000284 ) ) ;
#183274=CARTESIAN_POINT ( 'NONE',  ( -19.05341960407617563, 5.049401038297882671, 48.54275706135233293 ) ) ;
#183275=CARTESIAN_POINT ( 'NONE',  ( 17.50000000000000000, -5.624438216177559902, 73.31670344914644488 ) ) ;
#183276=CARTESIAN_POINT ( 'NONE',  ( -13.97604488694527625, -13.89961937509977652, 71.87390960531433848 ) ) ;
#183277=CARTESIAN_POINT ( 'NONE',  ( -5.049401038298153566, 19.05341960407611168, 90.20724293864766707 ) ) ;
#183278=CARTESIAN_POINT ( 'NONE',  ( 0.05219959533934541429, -16.53943276465976808, 60.00109039468568284 ) ) ;
#183280=CARTESIAN_POINT ( 'NONE',  ( -9.474510206698720793, -16.51473224551083518, 34.58442372801899722 ) ) ;
#183282=CARTESIAN_POINT ( 'NONE',  ( 16.51473224551069308, 9.474510206698969483, 114.1655762719810241 ) ) ;
#183283=CARTESIAN_POINT ( 'NONE',  ( -4.379528057220086978, -16.55341960407618274, 84.79275706135234714 ) ) ;
#183285=CARTESIAN_POINT ( 'NONE',  ( -16.55341960407617563, 4.379528057220093196, 73.54275706135234714 ) ) ;
#183286=CARTESIAN_POINT ( 'NONE',  ( -16.21995358207306737, 7.366697692864089930, 29.93551001512158294 ) ) ;
#183287=CARTESIAN_POINT ( 'NONE',  ( 14.34966873604972726, -8.224510206698740333, 60.83442372801901854 ) ) ;
#183288=CARTESIAN_POINT ( 'NONE',  ( -17.72560187377285246, -5.500000000000056843, 59.07814504131317790 ) ) ;
#183289=CARTESIAN_POINT ( 'NONE',  ( -15.72974639402176322, -15.80617190586768395, 69.37609039468567573 ) ) ;
#183290=CARTESIAN_POINT ( 'NONE',  ( 9.474510206698729675, 16.51473224551082808, 82.08442372801899012 ) ) ;
#183291=CARTESIAN_POINT ( 'NONE',  ( -5.049401038297874678, -19.05341960407617918, 24.79275706135233648 ) ) ;
#183292=CARTESIAN_POINT ( 'NONE',  ( 9.564922557960805705, 16.46253265017160317, 54.58224293864769550 ) ) ;
#183293=CARTESIAN_POINT ( 'NONE',  ( 16.51473224551069308, 9.474510206698969483, 39.16557627198103120 ) ) ;
#183295=CARTESIAN_POINT ( 'NONE',  ( -21.53943276465977519, 0.05219959533907696930, 61.24890960531435979 ) ) ;
#183297=CARTESIAN_POINT ( 'NONE',  ( -21.53943276465977519, 0.05219959533907696930, 26.24890960531435624 ) ) ;
#183298=CARTESIAN_POINT ( 'NONE',  ( 0.05219959533909260263, 19.03943276465977164, 24.99890960531435269 ) ) ;
#183299=CARTESIAN_POINT ( 'NONE',  ( 16.55341960407618274, -4.379528057220086978, 51.04275706135234714 ) ) ;
#183301=CARTESIAN_POINT ( 'NONE',  ( -21.52544592524334988, -5.823673210054445271, 23.95942372801901143 ) ) ;
#183302=CARTESIAN_POINT ( 'NONE',  ( 8.224510206698953496, -14.34966873604960469, 52.91557627198103830 ) ) ;
#183304=CARTESIAN_POINT ( 'NONE',  ( -19.03943276465977164, -0.05219959533935918106, 108.7510903946856615 ) ) ;
#183305=CARTESIAN_POINT ( 'NONE',  ( -5.049401038297874678, -19.05341960407617918, 34.79275706135233293 ) ) ;
#183306=CARTESIAN_POINT ( 'NONE',  ( -12.06949235617756955, 12.14591786802309770, 40.62390960531435269 ) ) ;
#183307=CARTESIAN_POINT ( 'NONE',  ( 15.80617190586769283, -15.72974639402175789, 20.62609039468568639 ) ) ;
#183309=CARTESIAN_POINT ( 'NONE',  ( 10.81492255796078972, 18.62759615963270932, 59.58224293864770260 ) ) ;
#183310=CARTESIAN_POINT ( 'NONE',  ( 16.46253265017160672, -9.564922557960803928, 93.33224293864769550 ) ) ;
#183311=CARTESIAN_POINT ( 'NONE',  ( -14.29746914071049879, 8.314922557960819915, 45.83224293864769550 ) ) ;
#183312=CARTESIAN_POINT ( 'NONE',  ( 9.474510206698971260, -16.51473224551069308, 102.9155762719810241 ) ) ;
#183314=CARTESIAN_POINT ( 'NONE',  ( -16.51473224551082808, 9.474510206698731452, 48.33442372801900433 ) ) ;
#183315=CARTESIAN_POINT ( 'NONE',  ( 21.52544592524344225, -5.823673210054117533, 98.54057627198105251 ) ) ;
#183316=CARTESIAN_POINT ( 'NONE',  ( 0.05219959533909260263, 19.03943276465977164, 44.99890960531435979 ) ) ;
#183317=CARTESIAN_POINT ( 'NONE',  ( 16.53943276465976808, -0.05219959533910856209, 108.7489096053143669 ) ) ;
#183318=CARTESIAN_POINT ( 'NONE',  ( -10.72451020669870658, -18.67979575497194134, 44.58442372801901854 ) ) ;
#183321=CARTESIAN_POINT ( 'NONE',  ( 14.29746914071049879, -8.314922557960816363, 23.33224293864769194 ) ) ;
#183322=CARTESIAN_POINT ( 'NONE',  ( 5.153800228976335163, 19.02544592524342804, 49.79057627198100988 ) ) ;
#183323=CARTESIAN_POINT ( 'NONE',  ( 13.89961937509977652, -13.97604488694527269, 93.12390960531436690 ) ) ;
#183324=CARTESIAN_POINT ( 'NONE',  ( 10.81492255796078972, 18.62759615963270932, 69.58224293864769550 ) ) ;
#183326=CARTESIAN_POINT ( 'NONE',  ( 16.51473224551069308, 9.474510206698969483, 44.16557627198103120 ) ) ;
#183327=CARTESIAN_POINT ( 'NONE',  ( -18.67979575497178146, -10.72451020669898902, 51.66557627198102409 ) ) ;
#183328=CARTESIAN_POINT ( 'NONE',  ( -5.719274019375665041, -21.55341960407619695, 89.79275706135236135 ) ) ;
#183330=CARTESIAN_POINT ( 'NONE',  ( 8.314922557961029526, -14.29746914071037800, 80.41775706135234714 ) ) ;
#183331=CARTESIAN_POINT ( 'NONE',  ( 16.52544592524342804, -4.483927247898539470, 63.54057627198103830 ) ) ;
#183332=CARTESIAN_POINT ( 'NONE',  ( -9.474510206698964154, 16.51473224551069663, 75.41557627198103830 ) ) ;
#183334=CARTESIAN_POINT ( 'NONE',  ( 19.05341960407617918, -5.049401038297876454, 21.04275706135232582 ) ) ;
#183335=CARTESIAN_POINT ( 'NONE',  ( 0.05219959533934541429, -16.53943276465976808, 85.00109039468568994 ) ) ;
#183336=CARTESIAN_POINT ( 'NONE',  ( -19.03943276465977164, -0.05219959533935918106, 18.75109039468567218 ) ) ;
#183337=CARTESIAN_POINT ( 'NONE',  ( 16.51473224551069308, 9.474510206698969483, 69.16557627198102409 ) ) ;
#183338=CARTESIAN_POINT ( 'NONE',  ( -15.80617190586745835, -15.72974639402198527, 51.87390960531437401 ) ) ;
#183339=CARTESIAN_POINT ( 'NONE',  ( 0.05219959533934541429, -16.53943276465976808, 25.00109039468567218 ) ) ;
#183340=CARTESIAN_POINT ( 'NONE',  ( -18.67979575497193778, 10.72451020669871902, 78.33442372801901854 ) ) ;
#183341=CARTESIAN_POINT ( 'NONE',  ( 16.55341960407618274, -4.379528057220086978, 61.04275706135234714 ) ) ;
#183342=CARTESIAN_POINT ( 'NONE',  ( -21.55341960407610458, -5.719274019375992779, 111.4572429386476813 ) ) ;
#183343=CARTESIAN_POINT ( 'NONE',  ( -0.05219959533936034679, 19.03943276465977164, 107.5010903946856615 ) ) ;
#183344=CARTESIAN_POINT ( 'NONE',  ( 5.049401038298161559, -19.05341960407611168, 92.70724293864769550 ) ) ;
#183345=CARTESIAN_POINT ( 'NONE',  ( -4.483927247898782831, 16.52544592524335698, 27.70942372801901854 ) ) ;
#183346=CARTESIAN_POINT ( 'NONE',  ( 5.153800228976335163, 19.02544592524342804, 44.79057627198103830 ) ) ;
#183347=CARTESIAN_POINT ( 'NONE',  ( -12.14591786802326823, 12.06949235617739902, 38.12609039468567573 ) ) ;
#183348=CARTESIAN_POINT ( 'NONE',  ( 0.05219959533910956823, 16.53943276465976808, 79.99890960531435269 ) ) ;
#183349=CARTESIAN_POINT ( 'NONE',  ( -16.52544592524335698, -4.483927247898792601, 88.95942372801901854 ) ) ;
#183350=CARTESIAN_POINT ( 'NONE',  ( -10.72451020669870658, -18.67979575497194134, 34.58442372801900433 ) ) ;
#183351=CARTESIAN_POINT ( 'NONE',  ( 16.46253265017160672, -9.564922557960803928, 63.33224293864769550 ) ) ;
#183352=CARTESIAN_POINT ( 'NONE',  ( -9.564922557960796823, -16.46253265017161027, 87.08224293864769550 ) ) ;
#183354=CARTESIAN_POINT ( 'NONE',  ( -4.483927247898782831, 16.52544592524335698, 82.70942372801900433 ) ) ;
#183357=ORIENTED_EDGE ( 'NONE', *, *, #194116, .F. ) ;
#183358=CARTESIAN_POINT ( 'NONE',  ( -9.564922557961040184, 16.46253265017147172, 32.91775706135233293 ) ) ;
#183359=CARTESIAN_POINT ( 'NONE',  ( 5.049401038298161559, -19.05341960407611168, 97.70724293864766707 ) ) ;
#183360=CARTESIAN_POINT ( 'NONE',  ( -16.46253265017160317, 9.564922557960807481, 45.83224293864769550 ) ) ;
#183361=CARTESIAN_POINT ( 'NONE',  ( -0.05219959533909027116, -19.03943276465977164, 112.4989096053143669 ) ) ;
#183363=CARTESIAN_POINT ( 'NONE',  ( 8.314922557961029526, -14.29746914071037800, 25.41775706135235779 ) ) ;
#183364=CARTESIAN_POINT ( 'NONE',  ( -19.05341960407617563, 5.049401038297882671, 53.54275706135231871 ) ) ;
#183365=CARTESIAN_POINT ( 'NONE',  ( 16.52544592524335698, 4.483927247898782831, 46.45942372801901854 ) ) ;
#183366=CARTESIAN_POINT ( 'NONE',  ( 5.049401038298161559, -19.05341960407611168, 107.7072429386476955 ) ) ;
#183367=CARTESIAN_POINT ( 'NONE',  ( -19.03943276465977164, 0.05219959533909376836, 71.24890960531435269 ) ) ;
#183368=CARTESIAN_POINT ( 'NONE',  ( -5.719274019375978568, 21.55341960407610458, 95.20724293864769550 ) ) ;
#183369=CARTESIAN_POINT ( 'NONE',  ( 0.05219959533936267826, -19.03943276465977164, 60.00109039468566863 ) ) ;
#183370=CARTESIAN_POINT ( 'NONE',  ( 13.89961937509977652, -13.97604488694527269, 93.12390960531436690 ) ) ;
#183371=CARTESIAN_POINT ( 'NONE',  ( -19.05341960407611168, -5.049401038298163336, 26.45724293864769550 ) ) ;
#183373=CARTESIAN_POINT ( 'NONE',  ( -5.153800228976328057, -19.02544592524343514, 67.29057627198102409 ) ) ;
#183374=CARTESIAN_POINT ( 'NONE',  ( 4.483927247898545687, 16.52544592524342804, 29.79057627198102409 ) ) ;
#183375=CARTESIAN_POINT ( 'NONE',  ( -0.05219959533909027116, -19.03943276465977164, 27.49890960531435624 ) ) ;
#183376=CARTESIAN_POINT ( 'NONE',  ( -13.97604488694547697, 13.89961937509957934, 38.12609039468566152 ) ) ;
#183377=CARTESIAN_POINT ( 'NONE',  ( 14.34966873604960469, 8.224510206698951720, 74.16557627198102409 ) ) ;
#183378=CARTESIAN_POINT ( 'NONE',  ( -21.52544592524334988, -5.823673210054445271, 98.95942372801903275 ) ) ;
#183379=CARTESIAN_POINT ( 'NONE',  ( 16.46253265017160672, -9.564922557960803928, 43.33224293864769550 ) ) ;
#183380=CARTESIAN_POINT ( 'NONE',  ( 12.06949235617739724, 12.14591786802326823, 56.87609039468568994 ) ) ;
#183381=CARTESIAN_POINT ( 'NONE',  ( 12.06949235617757843, -12.14591786802309237, 43.12390960531435269 ) ) ;
#183382=CARTESIAN_POINT ( 'NONE',  ( 10.72451020669871369, 18.67979575497193778, 87.08442372801901854 ) ) ;
#183383=CARTESIAN_POINT ( 'NONE',  ( 9.564922557960805705, 16.46253265017160317, 89.58224293864769550 ) ) ;
#183384=CARTESIAN_POINT ( 'NONE',  ( -19.05341960407611168, -5.049401038298163336, 101.4572429386476955 ) ) ;
#183385=CARTESIAN_POINT ( 'NONE',  ( -14.34966873604960291, -8.224510206698953496, 101.6655762719810383 ) ) ;
#183386=CARTESIAN_POINT ( 'NONE',  ( 16.53943276465976808, -0.05219959533910856209, 68.74890960531435269 ) ) ;
#183387=CARTESIAN_POINT ( 'NONE',  ( 18.62759615963271287, -10.81492255796078972, 78.33224293864770971 ) ) ;
#183388=CARTESIAN_POINT ( 'NONE',  ( 16.51473224551069308, 9.474510206698969483, 84.16557627198102409 ) ) ;
#183389=CARTESIAN_POINT ( 'NONE',  ( -18.62759615963270932, 10.81492255796079327, 95.83224293864770971 ) ) ;
#183390=CARTESIAN_POINT ( 'NONE',  ( 19.05341960407611168, 5.049401038298154454, 88.95724293864769550 ) ) ;
#183392=CARTESIAN_POINT ( 'NONE',  ( 16.52544592524342804, -4.483927247898539470, 83.54057627198102409 ) ) ;
#183393=CARTESIAN_POINT ( 'NONE',  ( -19.05341960407611168, -5.049401038298163336, 56.45724293864768129 ) ) ;
#183394=CARTESIAN_POINT ( 'NONE',  ( -15.80617190586745835, -15.72974639402198527, 61.87390960531436690 ) ) ;
#183395=CARTESIAN_POINT ( 'NONE',  ( 16.52216118717208460, -7.221426719304491648, 26.42400978953008561 ) ) ;
#183396=CARTESIAN_POINT ( 'NONE',  ( -16.53943276465976808, -0.05219959533934237506, 113.7510903946856757 ) ) ;
#183397=CARTESIAN_POINT ( 'NONE',  ( 19.02544592524334988, 5.153800228976608722, 111.4594237280190043 ) ) ;
#183398=CARTESIAN_POINT ( 'NONE',  ( -4.379528057220328563, 16.55341960407611168, 85.20724293864770971 ) ) ;
#183399=CARTESIAN_POINT ( 'NONE',  ( -16.62475595723696742, -7.163666690055314312, 94.47286648189535185 ) ) ;
#183400=CARTESIAN_POINT ( 'NONE',  ( 19.05341960407611168, 5.049401038298154454, 73.95724293864768129 ) ) ;
#183401=CARTESIAN_POINT ( 'NONE',  ( 9.564922557960805705, 16.46253265017160317, 44.58224293864769550 ) ) ;
#183402=CARTESIAN_POINT ( 'NONE',  ( -14.29746914071049879, 8.314922557960819915, 60.83224293864769550 ) ) ;
#183403=CARTESIAN_POINT ( 'NONE',  ( 10.72451020669898902, -18.67979575497178502, 22.91557627198102765 ) ) ;
#183404=CARTESIAN_POINT ( 'NONE',  ( -16.51473224551082808, 9.474510206698731452, 103.3344237280190043 ) ) ;
#183405=CARTESIAN_POINT ( 'NONE',  ( 13.97604488694527802, 13.89961937509977652, 99.37390960531436690 ) ) ;
#183406=CARTESIAN_POINT ( 'NONE',  ( 18.62759615963271287, -10.81492255796078972, 73.33224293864769550 ) ) ;
#183407=CARTESIAN_POINT ( 'NONE',  ( 16.53943276465976808, 0.05219959533934440121, 76.25109039468568994 ) ) ;
#183408=CARTESIAN_POINT ( 'NONE',  ( -16.81555441253469851, 7.025013491696157075, 95.63685445334218116 ) ) ;
#183409=CARTESIAN_POINT ( 'NONE',  ( -9.474510206698964154, 16.51473224551069663, 80.41557627198103830 ) ) ;
#183410=CARTESIAN_POINT ( 'NONE',  ( -10.81492255796078084, -18.62759615963271287, 77.08224293864769550 ) ) ;
#183411=CARTESIAN_POINT ( 'NONE',  ( 16.51473224551083163, -9.474510206698727899, 110.8344237280190043 ) ) ;
#183412=CARTESIAN_POINT ( 'NONE',  ( 14.34966873604960469, 8.224510206698951720, 39.16557627198102409 ) ) ;
#183413=CARTESIAN_POINT ( 'NONE',  ( -10.81492255796105439, 18.62759615963255655, 62.91775706135236135 ) ) ;
#183414=CARTESIAN_POINT ( 'NONE',  ( 0.05219959533934541429, -16.53943276465976808, 90.00109039468567573 ) ) ;
#183415=CARTESIAN_POINT ( 'NONE',  ( -19.05341960407611168, -5.049401038298163336, 111.4572429386476671 ) ) ;
#183416=CARTESIAN_POINT ( 'NONE',  ( -18.22780087662122028, -5.500000000000014211, 101.4845989467389273 ) ) ;
#183418=CARTESIAN_POINT ( 'NONE',  ( 14.34966873604972726, -8.224510206698740333, 95.83442372801903275 ) ) ;
#183419=CARTESIAN_POINT ( 'NONE',  ( 8.314922557961029526, -14.29746914071037800, 50.41775706135235424 ) ) ;
#183420=CARTESIAN_POINT ( 'NONE',  ( -0.05219959533909027116, -19.03943276465977164, 62.49890960531435979 ) ) ;
#183421=CARTESIAN_POINT ( 'NONE',  ( -5.153800228976328057, -19.02544592524343514, 77.29057627198099567 ) ) ;
#183422=CARTESIAN_POINT ( 'NONE',  ( 10.72451020669871369, 18.67979575497193778, 67.08442372801901854 ) ) ;
#183423=CARTESIAN_POINT ( 'NONE',  ( -8.224510206698735004, -14.34966873604973081, 59.58442372801901854 ) ) ;
#183424=CARTESIAN_POINT ( 'NONE',  ( 8.314922557960818139, 14.29746914071049879, 39.58224293864769550 ) ) ;
#183425=CARTESIAN_POINT ( 'NONE',  ( 13.97604488694527802, 13.89961937509977652, 44.37390960531435269 ) ) ;
#183426=CARTESIAN_POINT ( 'NONE',  ( 9.564922557960805705, 16.46253265017160317, 44.58224293864769550 ) ) ;
#183427=CARTESIAN_POINT ( 'NONE',  ( 12.14591786802327356, -12.06949235617739191, 35.62609039468568994 ) ) ;
#183428=CARTESIAN_POINT ( 'NONE',  ( -5.049401038297874678, -19.05341960407617918, 94.79275706135230450 ) ) ;
#183429=CARTESIAN_POINT ( 'NONE',  ( -14.29746914071049879, 8.314922557960819915, 95.83224293864770971 ) ) ;
#183430=CARTESIAN_POINT ( 'NONE',  ( -5.049401038298153566, 19.05341960407611168, 70.20724293864769550 ) ) ;
#183431=CARTESIAN_POINT ( 'NONE',  ( 16.51473224551083163, -9.474510206698727899, 85.83442372801900433 ) ) ;
#183433=CARTESIAN_POINT ( 'NONE',  ( -21.52544592524334988, -5.823673210054445271, 88.95942372801901854 ) ) ;
#183434=CARTESIAN_POINT ( 'NONE',  ( -12.06949235617739369, -12.14591786802326823, 69.37609039468567573 ) ) ;
#183436=CARTESIAN_POINT ( 'NONE',  ( 21.53943276465977519, -0.05219959533907433946, 43.74890960531435979 ) ) ;
#183437=CARTESIAN_POINT ( 'NONE',  ( 14.34966873604972726, -8.224510206698740333, 35.83442372801901143 ) ) ;
#183438=CARTESIAN_POINT ( 'NONE',  ( -18.87075004821565472, 5.500000000000079048, 68.67408112101045958 ) ) ;
#183439=CARTESIAN_POINT ( 'NONE',  ( -13.89961937509957401, -13.97604488694547875, 44.37609039468566863 ) ) ;
#183440=CARTESIAN_POINT ( 'NONE',  ( -16.51473224551069308, -9.474510206698971260, 96.66557627198102409 ) ) ;
#183441=CARTESIAN_POINT ( 'NONE',  ( -5.153800228976328057, -19.02544592524343514, 22.29057627198102765 ) ) ;
#183442=CARTESIAN_POINT ( 'NONE',  ( 9.474510206698971260, -16.51473224551069308, 52.91557627198102409 ) ) ;
#183445=CARTESIAN_POINT ( 'NONE',  ( 10.81492255796106328, -18.62759615963255655, 75.41775706135233293 ) ) ;
#183447=CARTESIAN_POINT ( 'NONE',  ( -19.03943276465977164, -0.05219959533935918106, 28.75109039468566507 ) ) ;
#183448=CARTESIAN_POINT ( 'NONE',  ( 21.53943276465977519, 0.05219959533937863772, 111.2510903946856899 ) ) ;
#183449=CARTESIAN_POINT ( 'NONE',  ( 12.14591786802309770, 12.06949235617756955, 49.37390960531436690 ) ) ;
#183450=CARTESIAN_POINT ( 'NONE',  ( -19.03943276465977164, 0.05219959533909376836, 51.24890960531436690 ) ) ;
#183451=CARTESIAN_POINT ( 'NONE',  ( 9.474510206698971260, -16.51473224551069308, 102.9155762719810241 ) ) ;
#183452=CARTESIAN_POINT ( 'NONE',  ( 0.05219959533937995610, -21.53943276465977519, 85.00109039468568994 ) ) ;
#183453=CARTESIAN_POINT ( 'NONE',  ( -16.46253265017160317, 9.564922557960807481, 60.83224293864769550 ) ) ;
#183454=CARTESIAN_POINT ( 'NONE',  ( -18.62759615963255300, -10.81492255796106328, 74.16775706135231871 ) ) ;
#183455=CARTESIAN_POINT ( 'NONE',  ( 0.05219959533907565091, 21.53943276465977519, 39.99890960531436690 ) ) ;
#183456=CARTESIAN_POINT ( 'NONE',  ( 0.05219959533937995610, -21.53943276465977519, 35.00109039468568284 ) ) ;
#183457=CARTESIAN_POINT ( 'NONE',  ( 13.97604488694548053, -13.89961937509957401, 65.62609039468567573 ) ) ;
#183458=CARTESIAN_POINT ( 'NONE',  ( -16.46253265017160317, 9.564922557960807481, 30.83224293864769550 ) ) ;
#183459=CARTESIAN_POINT ( 'NONE',  ( 13.89961937509977652, -13.97604488694527269, 73.12390960531436690 ) ) ;
#183460=CARTESIAN_POINT ( 'NONE',  ( -14.29746914071037622, -8.314922557961029526, 29.16775706135234003 ) ) ;
#183461=CARTESIAN_POINT ( 'NONE',  ( 16.55341960407611168, 4.379528057220329451, 93.95724293864770971 ) ) ;
#183462=CARTESIAN_POINT ( 'NONE',  ( -0.05219959533909027116, -19.03943276465977164, 62.49890960531435979 ) ) ;
#183463=CARTESIAN_POINT ( 'NONE',  ( 5.719274019375991003, -21.55341960407610458, 37.70724293864769550 ) ) ;
#183464=CARTESIAN_POINT ( 'NONE',  ( 19.05341960407617918, -5.049401038297876454, 111.0427570613523329 ) ) ;
#183465=CARTESIAN_POINT ( 'NONE',  ( -21.53943276465977519, -0.05219959533937600094, 23.75109039468567929 ) ) ;
#183466=CARTESIAN_POINT ( 'NONE',  ( -0.05219959533937732626, 21.53943276465977519, 72.50109039468568994 ) ) ;
#183467=CARTESIAN_POINT ( 'NONE',  ( 16.52544592524335698, 4.483927247898782831, 66.45942372801903275 ) ) ;
#183468=CARTESIAN_POINT ( 'NONE',  ( 16.53943276465976808, 0.05219959533934440121, 71.25109039468568994 ) ) ;
#183470=CARTESIAN_POINT ( 'NONE',  ( 13.97604488694527802, 13.89961937509977652, 64.37390960531436690 ) ) ;
#183471=CARTESIAN_POINT ( 'NONE',  ( 16.55341960407618274, -4.379528057220086978, 86.04275706135236135 ) ) ;
#183472=CARTESIAN_POINT ( 'NONE',  ( 16.46253265017146816, 9.564922557961045513, 36.66775706135233293 ) ) ;
#183474=CARTESIAN_POINT ( 'NONE',  ( 21.53943276465977519, 0.05219959533937863772, 21.25109039468567218 ) ) ;
#183475=CARTESIAN_POINT ( 'NONE',  ( 12.14591786802309770, 12.06949235617756955, 59.37390960531436690 ) ) ;
#183476=CARTESIAN_POINT ( 'NONE',  ( 16.46253265017160672, -9.564922557960803928, 83.33224293864768129 ) ) ;
#183477=CARTESIAN_POINT ( 'NONE',  ( 4.379528057220092307, 16.55341960407617563, 87.29275706135236135 ) ) ;
#183478=CARTESIAN_POINT ( 'NONE',  ( -18.62759615963255300, -10.81492255796106328, 54.16775706135235424 ) ) ;
#183479=CARTESIAN_POINT ( 'NONE',  ( -16.53943276465976808, -0.05219959533934237506, 28.75109039468567929 ) ) ;
#183480=CARTESIAN_POINT ( 'NONE',  ( 10.81492255796078972, 18.62759615963270932, 109.5822429386476955 ) ) ;
#183481=CARTESIAN_POINT ( 'NONE',  ( 4.379528057220339221, -16.55341960407611168, 57.70724293864770260 ) ) ;
#183483=CARTESIAN_POINT ( 'NONE',  ( -21.55341960407610458, -5.719274019375992779, 96.45724293864770971 ) ) ;
#183484=CARTESIAN_POINT ( 'NONE',  ( -8.224510206698948167, 14.34966873604960824, 35.41557627198102409 ) ) ;
#183487=CARTESIAN_POINT ( 'NONE',  ( -19.02544592524342804, 5.153800228976336051, 106.0405762719810241 ) ) ;
#183488=CARTESIAN_POINT ( 'NONE',  ( 0.05219959533937995610, -21.53943276465977519, 35.00109039468568284 ) ) ;
#183489=CARTESIAN_POINT ( 'NONE',  ( 4.483927247898545687, 16.52544592524342804, 54.79057627198104541 ) ) ;
#183490=CARTESIAN_POINT ( 'NONE',  ( -5.049401038298153566, 19.05341960407611168, 60.20724293864768129 ) ) ;
#183491=CARTESIAN_POINT ( 'NONE',  ( -13.89961937509957401, -13.97604488694547875, 69.37609039468564731 ) ) ;
#183492=CARTESIAN_POINT ( 'NONE',  ( -5.153800228976328057, -19.02544592524343514, 92.29057627198099567 ) ) ;
#183493=CARTESIAN_POINT ( 'NONE',  ( 10.81492255796078972, 18.62759615963270932, 44.58224293864769550 ) ) ;
#183495=CARTESIAN_POINT ( 'NONE',  ( 19.05341960407611168, 5.049401038298154454, 53.95724293864770260 ) ) ;
#183496=CARTESIAN_POINT ( 'NONE',  ( -0.05219959533934338120, 16.53943276465976808, 32.50109039468568284 ) ) ;
#183497=CARTESIAN_POINT ( 'NONE',  ( 19.03943276465977164, 0.05219959533936151252, 61.25109039468566863 ) ) ;
#183498=CARTESIAN_POINT ( 'NONE',  ( 21.55341960407610458, 5.719274019375980345, 108.9572429386476955 ) ) ;
#183500=CARTESIAN_POINT ( 'NONE',  ( -16.53943276465976808, 0.05219959533911058130, 51.24890960531436690 ) ) ;
#183502=CARTESIAN_POINT ( 'NONE',  ( -9.564922557960796823, -16.46253265017161027, 92.08224293864769550 ) ) ;
#183503=CARTESIAN_POINT ( 'NONE',  ( -15.80617190586745835, -15.72974639402198527, 66.87390960531436690 ) ) ;
#183504=CARTESIAN_POINT ( 'NONE',  ( -18.67979575497178146, -10.72451020669898902, 111.6655762719810525 ) ) ;
#183505=CARTESIAN_POINT ( 'NONE',  ( -16.52544592524335698, -4.483927247898792601, 38.95942372801901854 ) ) ;
#183506=CARTESIAN_POINT ( 'NONE',  ( 21.55341960407610458, 5.719274019375980345, 33.95724293864769550 ) ) ;
#183507=CARTESIAN_POINT ( 'NONE',  ( 0.05219959533937995610, -21.53943276465977519, 100.0010903946857042 ) ) ;
#183508=CARTESIAN_POINT ( 'NONE',  ( -0.05219959533909027116, -19.03943276465977164, 102.4989096053143669 ) ) ;
#183510=CARTESIAN_POINT ( 'NONE',  ( -19.03943276465977164, 0.05219959533909376836, 46.24890960531435979 ) ) ;
#183511=CARTESIAN_POINT ( 'NONE',  ( -9.564922557960796823, -16.46253265017161027, 92.08224293864769550 ) ) ;
#183512=CARTESIAN_POINT ( 'NONE',  ( 9.474510206698971260, -16.51473224551069308, 77.91557627198103830 ) ) ;
#183513=CARTESIAN_POINT ( 'NONE',  ( 17.13100169013223706, -6.664070546374243342, 88.26789835699827336 ) ) ;
#183514=CARTESIAN_POINT ( 'NONE',  ( -16.51473224551082808, 9.474510206698731452, 58.33442372801900433 ) ) ;
#183515=CARTESIAN_POINT ( 'NONE',  ( 18.62759615963255655, 10.81492255796105972, 111.6677570613523613 ) ) ;
#183516=CARTESIAN_POINT ( 'NONE',  ( 0.05219959533907565091, 21.53943276465977519, 34.99890960531435979 ) ) ;
#183517=CARTESIAN_POINT ( 'NONE',  ( 14.29746914071037800, 8.314922557961029526, 101.6677570613523613 ) ) ;
#183518=CARTESIAN_POINT ( 'NONE',  ( -17.26058549869091152, 6.457015423128609655, 58.62254162523934298 ) ) ;
#183519=CARTESIAN_POINT ( 'NONE',  ( 19.05341960407617918, -5.049401038297876454, 86.04275706135233293 ) ) ;
#183520=CARTESIAN_POINT ( 'NONE',  ( 0.05219959533936267826, -19.03943276465977164, 30.00109039468566863 ) ) ;
#183521=CARTESIAN_POINT ( 'NONE',  ( 17.72560187377285246, 5.500000000000046185, 71.57814504131319211 ) ) ;
#183522=CARTESIAN_POINT ( 'NONE',  ( -19.05341960407611168, -5.049401038298163336, 36.45724293864766707 ) ) ;
#183523=CARTESIAN_POINT ( 'NONE',  ( 12.14591786802309770, 12.06949235617756955, 39.37390960531436690 ) ) ;
#183524=CARTESIAN_POINT ( 'NONE',  ( -17.48847506799969409, -5.747544572773738203, 109.1730256215671631 ) ) ;
#183525=CARTESIAN_POINT ( 'NONE',  ( 0.05219959533910956823, 16.53943276465976808, 29.99890960531435979 ) ) ;
#183527=CARTESIAN_POINT ( 'NONE',  ( 16.53943276465976808, 0.05219959533934440121, 91.25109039468568994 ) ) ;
#183528=CARTESIAN_POINT ( 'NONE',  ( 13.89961937509977652, -13.97604488694527269, 53.12390960531434558 ) ) ;
#183529=CARTESIAN_POINT ( 'NONE',  ( -15.80617190586768217, 15.72974639402176855, 103.1260903946856757 ) ) ;
#183530=CARTESIAN_POINT ( 'NONE',  ( -16.46253265017146816, -9.564922557961047289, 109.1677570613523471 ) ) ;
#183531=CARTESIAN_POINT ( 'NONE',  ( -15.80617190586768217, 15.72974639402176855, 88.12609039468570415 ) ) ;
#183532=CARTESIAN_POINT ( 'NONE',  ( 13.89961937509957401, 13.97604488694547697, 71.87609039468567573 ) ) ;
#183533=CARTESIAN_POINT ( 'NONE',  ( 5.049401038298161559, -19.05341960407611168, 87.70724293864769550 ) ) ;
#183534=CARTESIAN_POINT ( 'NONE',  ( -5.153800228976328057, -19.02544592524343514, 87.29057627198103830 ) ) ;
#183536=CARTESIAN_POINT ( 'NONE',  ( 5.823673210054125526, 21.52544592524343514, 109.7905762719810383 ) ) ;
#183537=CARTESIAN_POINT ( 'NONE',  ( -16.53943276465976808, 0.05219959533911058130, 81.24890960531436690 ) ) ;
#183538=CARTESIAN_POINT ( 'NONE',  ( 21.52544592524344225, -5.823673210054117533, 58.54057627198103120 ) ) ;
#183539=CARTESIAN_POINT ( 'NONE',  ( -19.02544592524342804, 5.153800228976336051, 61.04057627198103120 ) ) ;
#183540=CARTESIAN_POINT ( 'NONE',  ( 21.53943276465977519, -0.05219959533907433946, 93.74890960531436690 ) ) ;
#183541=CARTESIAN_POINT ( 'NONE',  ( -4.379528057220086978, -16.55341960407618274, 84.79275706135234714 ) ) ;
#183543=CARTESIAN_POINT ( 'NONE',  ( -5.049401038298153566, 19.05341960407611168, 60.20724293864768129 ) ) ;
#183544=CARTESIAN_POINT ( 'NONE',  ( 14.34966873604960469, 8.224510206698951720, 99.16557627198100988 ) ) ;
#183546=CARTESIAN_POINT ( 'NONE',  ( -13.89961937509977652, 13.97604488694528158, 55.62390960531434558 ) ) ;
#183547=CARTESIAN_POINT ( 'NONE',  ( 19.02544592524334988, 5.153800228976608722, 86.45942372801900433 ) ) ;
#183548=CARTESIAN_POINT ( 'NONE',  ( 16.55341960407611168, 4.379528057220329451, 83.95724293864770971 ) ) ;
#183549=CARTESIAN_POINT ( 'NONE',  ( 15.72974639402176855, 15.80617190586768217, 56.87609039468568994 ) ) ;
#183550=CARTESIAN_POINT ( 'NONE',  ( -13.89961937509977652, 13.97604488694528158, 30.62390960531435269 ) ) ;
#183551=CARTESIAN_POINT ( 'NONE',  ( 21.52544592524344225, -5.823673210054117533, 98.54057627198105251 ) ) ;
#183552=CARTESIAN_POINT ( 'NONE',  ( 14.29746914071049879, -8.314922557960816363, 98.33224293864769550 ) ) ;
#183554=CARTESIAN_POINT ( 'NONE',  ( -0.05219959533909027116, -19.03943276465977164, 57.49890960531435979 ) ) ;
#183556=CARTESIAN_POINT ( 'NONE',  ( 19.03943276465977164, 0.05219959533936151252, 101.2510903946856757 ) ) ;
#183557=CARTESIAN_POINT ( 'NONE',  ( -9.474510206698964154, 16.51473224551069663, 115.4155762719810241 ) ) ;
#183558=CARTESIAN_POINT ( 'NONE',  ( -21.55341960407619339, 5.719274019375674811, 48.54275706135234714 ) ) ;
#183559=CARTESIAN_POINT ( 'NONE',  ( 0.05219959533909260263, 19.03943276465977164, 89.99890960531436690 ) ) ;
#183560=CARTESIAN_POINT ( 'NONE',  ( -0.05219959533936034679, 19.03943276465977164, 67.50109039468566152 ) ) ;
#183561=CARTESIAN_POINT ( 'NONE',  ( -19.05341960407611168, -5.049401038298163336, 56.45724293864768129 ) ) ;
#183563=CARTESIAN_POINT ( 'NONE',  ( -8.224510206698948167, 14.34966873604960824, 80.41557627198103830 ) ) ;
#183564=CARTESIAN_POINT ( 'NONE',  ( -0.05219959533910754901, -16.53943276465976808, 72.49890960531435269 ) ) ;
#183565=CARTESIAN_POINT ( 'NONE',  ( 5.153800228976335163, 19.02544592524342804, 94.79057627198103830 ) ) ;
#183566=CARTESIAN_POINT ( 'NONE',  ( 12.06949235617757843, -12.14591786802309237, 78.12390960531436690 ) ) ;
#183567=CARTESIAN_POINT ( 'NONE',  ( 5.153800228976335163, 19.02544592524342804, 79.79057627198102409 ) ) ;
#183568=CARTESIAN_POINT ( 'NONE',  ( 16.46253265017146816, 9.564922557961045513, 26.66775706135234003 ) ) ;
#183569=CARTESIAN_POINT ( 'NONE',  ( -19.02544592524342804, 5.153800228976336051, 46.04057627198101699 ) ) ;
#183570=CARTESIAN_POINT ( 'NONE',  ( -8.314922557960811034, -14.29746914071050412, 32.08224293864769550 ) ) ;
#183571=CARTESIAN_POINT ( 'NONE',  ( -4.379528057220328563, 16.55341960407611168, 115.2072429386476955 ) ) ;
#183572=ORIENTED_EDGE ( 'NONE', *, *, #147777, .T. ) ;
#183573=CARTESIAN_POINT ( 'NONE',  ( -18.62759615963255300, -10.81492255796106328, 49.16775706135234003 ) ) ;
#183574=CARTESIAN_POINT ( 'NONE',  ( -16.51473224551082808, 9.474510206698731452, 68.33442372801900433 ) ) ;
#183575=CARTESIAN_POINT ( 'NONE',  ( 16.55341960407611168, 4.379528057220329451, 33.95724293864769550 ) ) ;
#183576=CARTESIAN_POINT ( 'NONE',  ( 5.823673210054125526, 21.52544592524343514, 84.79057627198102409 ) ) ;
#183577=CARTESIAN_POINT ( 'NONE',  ( 19.02544592524343514, -5.153800228976328945, 113.5405762719810241 ) ) ;
#183578=CARTESIAN_POINT ( 'NONE',  ( -16.52544592524342804, 4.483927247898546575, 71.04057627198103830 ) ) ;
#183579=CARTESIAN_POINT ( 'NONE',  ( -16.51473224551069308, -9.474510206698971260, 46.66557627198102409 ) ) ;
#183580=CARTESIAN_POINT ( 'NONE',  ( -0.05219959533936034679, 19.03943276465977164, 42.50109039468566152 ) ) ;
#183581=CARTESIAN_POINT ( 'NONE',  ( 12.06949235617739724, 12.14591786802326823, 101.8760903946857042 ) ) ;
#183582=CARTESIAN_POINT ( 'NONE',  ( 16.52544592524335698, 4.483927247898782831, 61.45942372801901854 ) ) ;
#183583=CARTESIAN_POINT ( 'NONE',  ( -18.62759615963270932, 10.81492255796079327, 35.83224293864768839 ) ) ;
#183584=CARTESIAN_POINT ( 'NONE',  ( -10.81492255796105439, 18.62759615963255655, 102.9177570613523756 ) ) ;
#183585=CARTESIAN_POINT ( 'NONE',  ( 5.153800228976335163, 19.02544592524342804, 94.79057627198103830 ) ) ;
#183586=CARTESIAN_POINT ( 'NONE',  ( 8.314922557961029526, -14.29746914071037800, 75.41775706135233293 ) ) ;
#183587=CARTESIAN_POINT ( 'NONE',  ( 16.46253265017160672, -9.564922557960803928, 23.33224293864769194 ) ) ;
#183588=CARTESIAN_POINT ( 'NONE',  ( -12.14591786802309592, -12.06949235617757132, 31.87390960531435979 ) ) ;
#183589=CARTESIAN_POINT ( 'NONE',  ( 0.05219959533909260263, 19.03943276465977164, 109.9989096053143669 ) ) ;
#183590=CARTESIAN_POINT ( 'NONE',  ( -19.02544592524342804, 5.153800228976336051, 91.04057627198100988 ) ) ;
#183591=CARTESIAN_POINT ( 'NONE',  ( 21.52544592524344225, -5.823673210054117533, 28.54057627198103120 ) ) ;
#183592=EDGE_CURVE ( 'NONE', #123077, #1850, #2250, .T. ) ;
#183593=CARTESIAN_POINT ( 'NONE',  ( -16.53943276465976808, 0.05219959533911058130, 56.24890960531436690 ) ) ;
#183594=CARTESIAN_POINT ( 'NONE',  ( -4.483927247898539470, -16.52544592524342804, 37.29057627198102409 ) ) ;
#183595=CARTESIAN_POINT ( 'NONE',  ( 12.14591786802309770, 12.06949235617756955, 49.37390960531436690 ) ) ;
#183597=CARTESIAN_POINT ( 'NONE',  ( 12.14591786802327356, -12.06949235617739191, 50.62609039468568994 ) ) ;
#183598=DIRECTION ( 'NONE',  ( 0.000000000000000000, -0.000000000000000000, 1.000000000000000000 ) ) ;
#183599=CARTESIAN_POINT ( 'NONE',  ( -19.05341960407617563, 5.049401038297882671, 48.54275706135233293 ) ) ;
#183600=CARTESIAN_POINT ( 'NONE',  ( 16.51473224551069308, 9.474510206698969483, 89.16557627198103830 ) ) ;
#183601=CARTESIAN_POINT ( 'NONE',  ( 19.05341960407617918, -5.049401038297876454, 66.04275706135233293 ) ) ;
#183603=CARTESIAN_POINT ( 'NONE',  ( -19.05341960407617563, 5.049401038297882671, 58.54275706135234003 ) ) ;
#183604=CARTESIAN_POINT ( 'NONE',  ( -16.51473224551082808, 9.474510206698731452, 93.33442372801900433 ) ) ;
#183605=CARTESIAN_POINT ( 'NONE',  ( -4.483927247898782831, 16.52544592524335698, 77.70942372801900433 ) ) ;
#183607=CARTESIAN_POINT ( 'NONE',  ( 5.153800228976335163, 19.02544592524342804, 29.79057627198102409 ) ) ;
#183608=CARTESIAN_POINT ( 'NONE',  ( -10.81492255796078084, -18.62759615963271287, 22.08224293864769194 ) ) ;
#183609=CARTESIAN_POINT ( 'NONE',  ( -5.719274019375665041, -21.55341960407619695, 39.79275706135235424 ) ) ;
#183610=CARTESIAN_POINT ( 'NONE',  ( -5.153800228976607833, 19.02544592524334988, 102.7094237280189759 ) ) ;
#183612=CARTESIAN_POINT ( 'NONE',  ( -9.564922557960796823, -16.46253265017161027, 67.08224293864769550 ) ) ;
#183614=CARTESIAN_POINT ( 'NONE',  ( 13.89961937509977652, -13.97604488694527269, 108.1239096053143669 ) ) ;
#183615=CARTESIAN_POINT ( 'NONE',  ( 16.53943276465976808, -0.05219959533910856209, 78.74890960531436690 ) ) ;
#183616=CARTESIAN_POINT ( 'NONE',  ( -9.474510206698964154, 16.51473224551069663, 60.41557627198102409 ) ) ;
#183617=CARTESIAN_POINT ( 'NONE',  ( 9.564922557960805705, 16.46253265017160317, 74.58224293864769550 ) ) ;
#183618=CARTESIAN_POINT ( 'NONE',  ( -16.51473224551082808, 9.474510206698731452, 83.33442372801899012 ) ) ;
#183619=CARTESIAN_POINT ( 'NONE',  ( -15.72974639402197994, 15.80617190586746368, 55.62390960531436690 ) ) ;
#183620=CARTESIAN_POINT ( 'NONE',  ( 13.89961937509977652, -13.97604488694527269, 23.12390960531436335 ) ) ;
#183621=CARTESIAN_POINT ( 'NONE',  ( -19.05341960407617563, 5.049401038297882671, 38.54275706135233293 ) ) ;
#183622=CARTESIAN_POINT ( 'NONE',  ( -16.51473224551069308, -9.474510206698971260, 76.66557627198103830 ) ) ;
#183624=CARTESIAN_POINT ( 'NONE',  ( 5.823673210054125526, 21.52544592524343514, 79.79057627198102409 ) ) ;
#183625=CARTESIAN_POINT ( 'NONE',  ( 0.05219959533910956823, 16.53943276465976808, 84.99890960531436690 ) ) ;
#183626=CARTESIAN_POINT ( 'NONE',  ( -5.049401038297874678, -19.05341960407617918, 49.79275706135231871 ) ) ;
#183627=CARTESIAN_POINT ( 'NONE',  ( -10.72451020669898014, 18.67979575497178502, 75.41557627198102409 ) ) ;
#183628=CARTESIAN_POINT ( 'NONE',  ( -21.53943276465977519, 0.05219959533907696930, 66.24890960531436690 ) ) ;
#183629=CARTESIAN_POINT ( 'NONE',  ( -21.53943276465977519, 0.05219959533907696930, 36.24890960531435979 ) ) ;
#183630=CARTESIAN_POINT ( 'NONE',  ( 21.53943276465977519, 0.05219959533937863772, 86.25109039468568994 ) ) ;
#183631=CARTESIAN_POINT ( 'NONE',  ( -5.049401038298153566, 19.05341960407611168, 65.20724293864765286 ) ) ;
#183632=CARTESIAN_POINT ( 'NONE',  ( -16.52544592524342804, 4.483927247898546575, 116.0405762719810383 ) ) ;
#183633=CARTESIAN_POINT ( 'NONE',  ( 5.823673210054444382, -21.52544592524334988, 30.20942372801902565 ) ) ;
#183634=CARTESIAN_POINT ( 'NONE',  ( 18.67979575497194134, -10.72451020669871369, 45.83442372801901854 ) ) ;
#183635=CARTESIAN_POINT ( 'NONE',  ( 16.46253265017160672, -9.564922557960803928, 28.33224293864769550 ) ) ;
#183636=CARTESIAN_POINT ( 'NONE',  ( 5.823673210054125526, 21.52544592524343514, 109.7905762719810383 ) ) ;
#183637=CARTESIAN_POINT ( 'NONE',  ( 9.474510206698729675, 16.51473224551082808, 47.08442372801900433 ) ) ;
#183638=CARTESIAN_POINT ( 'NONE',  ( -0.05219959533909027116, -19.03943276465977164, 37.49890960531436690 ) ) ;
#183639=CARTESIAN_POINT ( 'NONE',  ( 5.049401038298161559, -19.05341960407611168, 22.70724293864769194 ) ) ;
#183641=CARTESIAN_POINT ( 'NONE',  ( 12.14591786802327356, -12.06949235617739191, 60.62609039468567573 ) ) ;
#183642=CARTESIAN_POINT ( 'NONE',  ( 0.05219959533909260263, 19.03943276465977164, 29.99890960531435979 ) ) ;
#183644=CARTESIAN_POINT ( 'NONE',  ( -13.97604488694527625, -13.89961937509977652, 81.87390960531436690 ) ) ;
#183645=CARTESIAN_POINT ( 'NONE',  ( 4.379528057220339221, -16.55341960407611168, 102.7072429386476955 ) ) ;
#183646=CARTESIAN_POINT ( 'NONE',  ( -0.05219959533907301413, -21.53943276465977519, 57.49890960531435979 ) ) ;
#183647=CARTESIAN_POINT ( 'NONE',  ( 4.379528057220092307, 16.55341960407617563, 47.29275706135234003 ) ) ;
#183648=CARTESIAN_POINT ( 'NONE',  ( -18.62759615963255300, -10.81492255796106328, 104.1677570613523471 ) ) ;
#183649=CARTESIAN_POINT ( 'NONE',  ( -9.474510206698964154, 16.51473224551069663, 35.41557627198102409 ) ) ;
#183650=CARTESIAN_POINT ( 'NONE',  ( 16.55341960407618274, -4.379528057220086978, 111.0427570613523613 ) ) ;
#183651=CARTESIAN_POINT ( 'NONE',  ( 12.06949235617757843, -12.14591786802309237, 58.12390960531435979 ) ) ;
#183652=CARTESIAN_POINT ( 'NONE',  ( 9.474510206698971260, -16.51473224551069308, 62.91557627198102409 ) ) ;
#183653=CARTESIAN_POINT ( 'NONE',  ( -21.52544592524334988, -5.823673210054445271, 103.9594237280190185 ) ) ;
#183654=CARTESIAN_POINT ( 'NONE',  ( -21.52544592524334988, -5.823673210054445271, 23.95942372801901143 ) ) ;
#183655=CARTESIAN_POINT ( 'NONE',  ( -21.52544592524334988, -5.823673210054445271, 68.95942372801901854 ) ) ;
#183656=CARTESIAN_POINT ( 'NONE',  ( 8.224510206698742110, 14.34966873604972548, 52.08442372801901854 ) ) ;
#183657=CARTESIAN_POINT ( 'NONE',  ( -8.314922557961024197, 14.29746914071037800, 27.91775706135234358 ) ) ;
#183658=CARTESIAN_POINT ( 'NONE',  ( -16.53943276465976808, 0.05219959533911058130, 76.24890960531435269 ) ) ;
#183659=CARTESIAN_POINT ( 'NONE',  ( -18.67979575497193778, 10.72451020669871902, 93.33442372801901854 ) ) ;
#183660=CARTESIAN_POINT ( 'NONE',  ( -12.14591786802309592, -12.06949235617757132, 31.87390960531435979 ) ) ;
#183661=CARTESIAN_POINT ( 'NONE',  ( -17.40805194822031510, 6.112264579159310429, 115.8337127251061531 ) ) ;
#183662=CARTESIAN_POINT ( 'NONE',  ( -14.34966873604972548, 8.224510206698743886, 38.33442372801900433 ) ) ;
#183663=CARTESIAN_POINT ( 'NONE',  ( -4.483927247898539470, -16.52544592524342804, 47.29057627198103120 ) ) ;
#183664=CARTESIAN_POINT ( 'NONE',  ( -8.224510206698735004, -14.34966873604973081, 84.58442372801903275 ) ) ;
#183665=CARTESIAN_POINT ( 'NONE',  ( -16.51473224551069308, -9.474510206698971260, 101.6655762719810241 ) ) ;
#183666=CARTESIAN_POINT ( 'NONE',  ( 10.81492255796078972, 18.62759615963270932, 24.58224293864768839 ) ) ;
#183667=CARTESIAN_POINT ( 'NONE',  ( -5.719274019375665041, -21.55341960407619695, 104.7927570613523898 ) ) ;
#183668=CARTESIAN_POINT ( 'NONE',  ( 16.52544592524335698, 4.483927247898782831, 106.4594237280190328 ) ) ;
#183669=CARTESIAN_POINT ( 'NONE',  ( 4.379528057220339221, -16.55341960407611168, 92.70724293864770971 ) ) ;
#183670=CARTESIAN_POINT ( 'NONE',  ( 13.89961937509977652, -13.97604488694527269, 88.12390960531438111 ) ) ;
#183671=ORIENTED_EDGE ( 'NONE', *, *, #175152, .F. ) ;
#183672=CARTESIAN_POINT ( 'NONE',  ( 12.06949235617739724, 12.14591786802326823, 36.87609039468568994 ) ) ;
#183673=CARTESIAN_POINT ( 'NONE',  ( -16.51473224551069308, -9.474510206698971260, 41.66557627198103120 ) ) ;
#183674=CARTESIAN_POINT ( 'NONE',  ( -19.03943276465977164, 0.05219959533909376836, 101.2489096053143669 ) ) ;
#183675=CARTESIAN_POINT ( 'NONE',  ( 16.53943276465976808, 0.05219959533934440121, 51.25109039468568994 ) ) ;
#183677=CARTESIAN_POINT ( 'NONE',  ( -5.049401038297874678, -19.05341960407617918, 29.79275706135232227 ) ) ;
#183678=CARTESIAN_POINT ( 'NONE',  ( -8.224510206698735004, -14.34966873604973081, 104.5844237280190185 ) ) ;
#183679=CARTESIAN_POINT ( 'NONE',  ( -19.05341960407611168, -5.049401038298163336, 46.45724293864768129 ) ) ;
#183680=CARTESIAN_POINT ( 'NONE',  ( -14.34966873604972548, 8.224510206698743886, 83.33442372801903275 ) ) ;
#183681=CARTESIAN_POINT ( 'NONE',  ( 13.97604488694548053, -13.89961937509957401, 85.62609039468568994 ) ) ;
#183682=CARTESIAN_POINT ( 'NONE',  ( -9.564922557961040184, 16.46253265017147172, 22.91775706135233648 ) ) ;
#183683=CARTESIAN_POINT ( 'NONE',  ( -16.46253265017160317, 9.564922557960807481, 65.83224293864769550 ) ) ;
#183684=CARTESIAN_POINT ( 'NONE',  ( -14.29746914071049879, 8.314922557960819915, 95.83224293864770971 ) ) ;
#183685=CARTESIAN_POINT ( 'NONE',  ( -13.97604488694547697, 13.89961937509957934, 63.12609039468566152 ) ) ;
#183686=CARTESIAN_POINT ( 'NONE',  ( 15.72974639402199770, -15.80617190586745480, 58.12390960531435979 ) ) ;
#183687=CARTESIAN_POINT ( 'NONE',  ( 9.474510206698729675, 16.51473224551082808, 27.08442372801900433 ) ) ;
#183688=CARTESIAN_POINT ( 'NONE',  ( 16.46253265017160672, -9.564922557960803928, 103.3322429386476955 ) ) ;
#183689=CARTESIAN_POINT ( 'NONE',  ( -21.53943276465977519, 0.05219959533907696930, 71.24890960531435269 ) ) ;
#183690=CARTESIAN_POINT ( 'NONE',  ( -0.05219959533909027116, -19.03943276465977164, 112.4989096053143669 ) ) ;
#183691=CARTESIAN_POINT ( 'NONE',  ( 13.97604488694548053, -13.89961937509957401, 95.62609039468563310 ) ) ;
#183692=CARTESIAN_POINT ( 'NONE',  ( 19.03943276465977164, -0.05219959533909143690, 113.7489096053143669 ) ) ;
#183694=CARTESIAN_POINT ( 'NONE',  ( -14.34966873604972548, 8.224510206698743886, 23.33442372801901499 ) ) ;
#183695=CARTESIAN_POINT ( 'NONE',  ( 16.51473224551069308, 9.474510206698969483, 29.16557627198103475 ) ) ;
#183696=CARTESIAN_POINT ( 'NONE',  ( -9.474510206698964154, 16.51473224551069663, 95.41557627198102409 ) ) ;
#183697=CARTESIAN_POINT ( 'NONE',  ( -21.55341960407610458, -5.719274019375992779, 86.45724293864770971 ) ) ;
#183698=CARTESIAN_POINT ( 'NONE',  ( 21.53943276465977519, 0.05219959533937863772, 61.25109039468567573 ) ) ;
#183699=CARTESIAN_POINT ( 'NONE',  ( 13.89961937509957401, 13.97604488694547697, 101.8760903946856331 ) ) ;
#183700=CARTESIAN_POINT ( 'NONE',  ( -21.53943276465977519, -0.05219959533937600094, 113.7510903946856757 ) ) ;
#183701=CARTESIAN_POINT ( 'NONE',  ( 12.14591786802327356, -12.06949235617739191, 110.6260903946857042 ) ) ;
#183702=CARTESIAN_POINT ( 'NONE',  ( -5.719274019375978568, 21.55341960407610458, 95.20724293864769550 ) ) ;
#183703=CARTESIAN_POINT ( 'NONE',  ( -8.314922557960811034, -14.29746914071050412, 42.08224293864769550 ) ) ;
#183704=CARTESIAN_POINT ( 'NONE',  ( -9.564922557961040184, 16.46253265017147172, 77.91775706135234714 ) ) ;
#183705=CARTESIAN_POINT ( 'NONE',  ( -5.153800228976607833, 19.02544592524334988, 57.70942372801899012 ) ) ;
#183706=CARTESIAN_POINT ( 'NONE',  ( 18.67979575497194134, -10.72451020669871369, 60.83442372801901854 ) ) ;
#183707=CARTESIAN_POINT ( 'NONE',  ( -5.153800228976607833, 19.02544592524334988, 42.70942372801901143 ) ) ;
#183708=CARTESIAN_POINT ( 'NONE',  ( -8.314922557960811034, -14.29746914071050412, 112.0822429386477097 ) ) ;
#183709=CARTESIAN_POINT ( 'NONE',  ( 5.719274019375991003, -21.55341960407610458, 32.70724293864770260 ) ) ;
#183710=CARTESIAN_POINT ( 'NONE',  ( -12.06949235617756955, 12.14591786802309770, 40.62390960531435269 ) ) ;
#183711=CARTESIAN_POINT ( 'NONE',  ( -0.05219959533937732626, 21.53943276465977519, 92.50109039468567573 ) ) ;
#183712=CARTESIAN_POINT ( 'NONE',  ( -16.52544592524335698, -4.483927247898792601, 73.95942372801901854 ) ) ;
#183713=CARTESIAN_POINT ( 'NONE',  ( -8.224510206698948167, 14.34966873604960824, 30.41557627198101699 ) ) ;
#183714=CARTESIAN_POINT ( 'NONE',  ( -21.55341960407619339, 5.719274019375674811, 68.54275706135234714 ) ) ;
#183715=CARTESIAN_POINT ( 'NONE',  ( -18.67979575497193778, 10.72451020669871902, 73.33442372801901854 ) ) ;
#183717=CARTESIAN_POINT ( 'NONE',  ( 13.97604488694527802, 13.89961937509977652, 24.37390960531435624 ) ) ;
#183718=CARTESIAN_POINT ( 'NONE',  ( 18.67979575497194134, -10.72451020669871369, 40.83442372801901854 ) ) ;
#183719=CARTESIAN_POINT ( 'NONE',  ( -19.05341960407611168, -5.049401038298163336, 26.45724293864769550 ) ) ;
#183720=CARTESIAN_POINT ( 'NONE',  ( -13.97604488694527625, -13.89961937509977652, 41.87390960531435979 ) ) ;
#183721=CARTESIAN_POINT ( 'NONE',  ( 0.05219959533910956823, 16.53943276465976808, 84.99890960531436690 ) ) ;
#183722=CARTESIAN_POINT ( 'NONE',  ( -19.03943276465977164, 0.05219959533909376836, 91.24890960531436690 ) ) ;
#183723=CARTESIAN_POINT ( 'NONE',  ( 8.224510206698953496, -14.34966873604960469, 32.91557627198102409 ) ) ;
#183724=CARTESIAN_POINT ( 'NONE',  ( -18.67979575497178146, -10.72451020669898902, 61.66557627198103120 ) ) ;
#183725=CARTESIAN_POINT ( 'NONE',  ( -5.719274019375978568, 21.55341960407610458, 105.2072429386477097 ) ) ;
#183726=CARTESIAN_POINT ( 'NONE',  ( 9.474510206698971260, -16.51473224551069308, 102.9155762719810241 ) ) ;
#183727=CARTESIAN_POINT ( 'NONE',  ( -19.03943276465977164, 0.05219959533909376836, 71.24890960531435269 ) ) ;
#183728=CARTESIAN_POINT ( 'NONE',  ( 9.564922557961047289, -16.46253265017146816, 100.4177570613523329 ) ) ;
#183729=CARTESIAN_POINT ( 'NONE',  ( 0.05219959533907565091, 21.53943276465977519, 54.99890960531435269 ) ) ;
#183730=CARTESIAN_POINT ( 'NONE',  ( -18.62759615963255300, -10.81492255796106328, 79.16775706135234714 ) ) ;
#183731=CARTESIAN_POINT ( 'NONE',  ( 19.05341960407611168, 5.049401038298154454, 68.95724293864769550 ) ) ;
#183732=CARTESIAN_POINT ( 'NONE',  ( 0.05219959533909260263, 19.03943276465977164, 104.9989096053143669 ) ) ;
#183733=CARTESIAN_POINT ( 'NONE',  ( -16.53943276465976808, -0.05219959533934237506, 78.75109039468568994 ) ) ;
#183734=CARTESIAN_POINT ( 'NONE',  ( -18.67979575497193778, 10.72451020669871902, 58.33442372801901143 ) ) ;
#183735=CARTESIAN_POINT ( 'NONE',  ( 21.53943276465977519, 0.05219959533937863772, 86.25109039468568994 ) ) ;
#183736=CARTESIAN_POINT ( 'NONE',  ( -18.62759615963255300, -10.81492255796106328, 19.16775706135234714 ) ) ;
#183737=CARTESIAN_POINT ( 'NONE',  ( -14.29746914071037622, -8.314922557961029526, 74.16775706135231871 ) ) ;
#183738=CARTESIAN_POINT ( 'NONE',  ( -21.52544592524343514, 5.823673210054127303, 71.04057627198103830 ) ) ;
#183739=CARTESIAN_POINT ( 'NONE',  ( 9.474510206698729675, 16.51473224551082808, 47.08442372801900433 ) ) ;
#183740=CARTESIAN_POINT ( 'NONE',  ( -10.81492255796078084, -18.62759615963271287, 42.08224293864769550 ) ) ;
#183741=CARTESIAN_POINT ( 'NONE',  ( 5.049401038298161559, -19.05341960407611168, 77.70724293864765286 ) ) ;
#183742=CARTESIAN_POINT ( 'NONE',  ( 12.06949235617757843, -12.14591786802309237, 43.12390960531435269 ) ) ;
#183745=CARTESIAN_POINT ( 'NONE',  ( -13.89961937509977652, 13.97604488694528158, 115.6239096053143669 ) ) ;
#183746=CARTESIAN_POINT ( 'NONE',  ( -19.49671883438226772, -5.500000000000084377, 79.89279849105686537 ) ) ;
#183747=CARTESIAN_POINT ( 'NONE',  ( -19.03943276465977164, -0.05219959533935918106, 98.75109039468567573 ) ) ;
#183748=CARTESIAN_POINT ( 'NONE',  ( -18.67979575497178146, -10.72451020669898902, 76.66557627198103830 ) ) ;
#183749=CARTESIAN_POINT ( 'NONE',  ( 16.52544592524342804, -4.483927247898539470, 53.54057627198103120 ) ) ;
#183750=CARTESIAN_POINT ( 'NONE',  ( 4.483927247898790824, -16.52544592524335698, 20.20942372801900788 ) ) ;
#183751=CARTESIAN_POINT ( 'NONE',  ( -9.474510206698964154, 16.51473224551069663, 40.41557627198103120 ) ) ;
#183752=CARTESIAN_POINT ( 'NONE',  ( 10.72451020669898902, -18.67979575497178502, 102.9155762719810383 ) ) ;
#183753=CARTESIAN_POINT ( 'NONE',  ( 13.97604488694548053, -13.89961937509957401, 65.62609039468567573 ) ) ;
#183754=CARTESIAN_POINT ( 'NONE',  ( 16.51473224551069308, 9.474510206698969483, 84.16557627198102409 ) ) ;
#183755=CARTESIAN_POINT ( 'NONE',  ( 14.34966873604960469, 8.224510206698951720, 84.16557627198103830 ) ) ;
#183756=CARTESIAN_POINT ( 'NONE',  ( 5.153800228976335163, 19.02544592524342804, 59.79057627198100988 ) ) ;
#183757=CARTESIAN_POINT ( 'NONE',  ( 4.483927247898545687, 16.52544592524342804, 64.79057627198103830 ) ) ;
#183758=CARTESIAN_POINT ( 'NONE',  ( 19.02544592524343514, -5.153800228976328945, 28.54057627198102409 ) ) ;
#183760=CARTESIAN_POINT ( 'NONE',  ( -12.14591786802309592, -12.06949235617757132, 41.87390960531435979 ) ) ;
#183761=CARTESIAN_POINT ( 'NONE',  ( -9.474510206698964154, 16.51473224551069663, 95.41557627198102409 ) ) ;
#183763=CARTESIAN_POINT ( 'NONE',  ( -9.474510206698720793, -16.51473224551083518, 49.58442372801899722 ) ) ;
#183764=CARTESIAN_POINT ( 'NONE',  ( -12.06949235617739369, -12.14591786802326823, 54.37609039468568994 ) ) ;
#183765=CARTESIAN_POINT ( 'NONE',  ( 5.823673210054125526, 21.52544592524343514, 79.79057627198102409 ) ) ;
#183766=CARTESIAN_POINT ( 'NONE',  ( -19.05341960407617563, 5.049401038297882671, 33.54275706135231871 ) ) ;
#183767=CARTESIAN_POINT ( 'NONE',  ( 5.049401038298161559, -19.05341960407611168, 92.70724293864769550 ) ) ;
#183769=CARTESIAN_POINT ( 'NONE',  ( 5.823673210054125526, 21.52544592524343514, 34.79057627198103120 ) ) ;
#183770=CARTESIAN_POINT ( 'NONE',  ( -5.153800228976328057, -19.02544592524343514, 62.29057627198100988 ) ) ;
#183771=CARTESIAN_POINT ( 'NONE',  ( -0.05219959533937732626, 21.53943276465977519, 52.50109039468567573 ) ) ;
#183772=CARTESIAN_POINT ( 'NONE',  ( 0.05219959533909260263, 19.03943276465977164, 29.99890960531435979 ) ) ;
#183773=CARTESIAN_POINT ( 'NONE',  ( -15.72974639402197994, 15.80617190586746368, 110.6239096053143669 ) ) ;
#183774=CARTESIAN_POINT ( 'NONE',  ( -19.02544592524342804, 5.153800228976336051, 91.04057627198100988 ) ) ;
#183776=CARTESIAN_POINT ( 'NONE',  ( -10.72451020669870658, -18.67979575497194134, 34.58442372801900433 ) ) ;
#183778=CARTESIAN_POINT ( 'NONE',  ( 9.564922557960805705, 16.46253265017160317, 104.5822429386476955 ) ) ;
#183779=CARTESIAN_POINT ( 'NONE',  ( -16.46253265017160317, 9.564922557960807481, 90.83224293864769550 ) ) ;
#183780=CARTESIAN_POINT ( 'NONE',  ( 5.719274019375991003, -21.55341960407610458, 107.7072429386476955 ) ) ;
#183781=CARTESIAN_POINT ( 'NONE',  ( 16.46253265017160672, -9.564922557960803928, 48.33224293864769550 ) ) ;
#183782=CARTESIAN_POINT ( 'NONE',  ( -4.379528057220086978, -16.55341960407618274, 29.79275706135234358 ) ) ;
#183784=CARTESIAN_POINT ( 'NONE',  ( 16.46253265017160672, -9.564922557960803928, 33.33224293864770260 ) ) ;
#183785=CARTESIAN_POINT ( 'NONE',  ( 10.81492255796106328, -18.62759615963255655, 100.4177570613523471 ) ) ;
#183786=CARTESIAN_POINT ( 'NONE',  ( -5.049401038298153566, 19.05341960407611168, 70.20724293864769550 ) ) ;
#183787=CARTESIAN_POINT ( 'NONE',  ( -18.62759615963255300, -10.81492255796106328, 54.16775706135235424 ) ) ;
#183789=CARTESIAN_POINT ( 'NONE',  ( 19.02544592524343514, -5.153800228976328945, 93.54057627198102409 ) ) ;
#183791=CARTESIAN_POINT ( 'NONE',  ( 16.52544592524335698, 4.483927247898782831, 41.45942372801901143 ) ) ;
#183792=CARTESIAN_POINT ( 'NONE',  ( 16.53943276465976808, 0.05219959533934440121, 71.25109039468568994 ) ) ;
#183793=CARTESIAN_POINT ( 'NONE',  ( -21.52544592524334988, -5.823673210054445271, 63.95942372801901854 ) ) ;
#183794=CARTESIAN_POINT ( 'NONE',  ( -15.80617190586768217, 15.72974639402176855, 93.12609039468568994 ) ) ;
#183796=CARTESIAN_POINT ( 'NONE',  ( 9.564922557961047289, -16.46253265017146816, 105.4177570613523471 ) ) ;
#183797=CARTESIAN_POINT ( 'NONE',  ( -5.049401038298153566, 19.05341960407611168, 80.20724293864769550 ) ) ;
#183798=CARTESIAN_POINT ( 'NONE',  ( -9.474510206698964154, 16.51473224551069663, 100.4155762719810241 ) ) ;
#183799=CARTESIAN_POINT ( 'NONE',  ( -16.51473224551069308, -9.474510206698971260, 31.66557627198102054 ) ) ;
#183800=CARTESIAN_POINT ( 'NONE',  ( -10.81492255796078084, -18.62759615963271287, 32.08224293864769550 ) ) ;
#183801=CARTESIAN_POINT ( 'NONE',  ( -16.53943276465976808, -0.05219959533934237506, 93.75109039468567573 ) ) ;
#183802=CARTESIAN_POINT ( 'NONE',  ( 16.53943276465976808, -0.05219959533910856209, 63.74890960531435979 ) ) ;
#183803=CARTESIAN_POINT ( 'NONE',  ( 13.97604488694527802, 13.89961937509977652, 54.37390960531435979 ) ) ;
#183804=CARTESIAN_POINT ( 'NONE',  ( 18.62759615963255655, 10.81492255796105972, 96.66775706135234714 ) ) ;
#183805=CARTESIAN_POINT ( 'NONE',  ( 17.49700485646017256, 4.621336975095707622, 21.88126978150424762 ) ) ;
#183806=CARTESIAN_POINT ( 'NONE',  ( 9.564922557961047289, -16.46253265017146816, 105.4177570613523471 ) ) ;
#183807=CARTESIAN_POINT ( 'NONE',  ( -16.53943276465976808, 0.05219959533911058130, 81.24890960531436690 ) ) ;
#183808=CARTESIAN_POINT ( 'NONE',  ( -0.05219959533937732626, 21.53943276465977519, 27.50109039468567929 ) ) ;
#183809=CARTESIAN_POINT ( 'NONE',  ( 15.72974639402199770, -15.80617190586745480, 58.12390960531435979 ) ) ;
#183810=CARTESIAN_POINT ( 'NONE',  ( 16.51473224551083163, -9.474510206698727899, 40.83442372801900433 ) ) ;
#183811=CARTESIAN_POINT ( 'NONE',  ( 9.564922557960805705, 16.46253265017160317, 89.58224293864769550 ) ) ;
#183812=CARTESIAN_POINT ( 'NONE',  ( 8.314922557960818139, 14.29746914071049879, 49.58224293864769550 ) ) ;
#183813=CARTESIAN_POINT ( 'NONE',  ( -12.14591786802309592, -12.06949235617757132, 36.87390960531435979 ) ) ;
#183814=CARTESIAN_POINT ( 'NONE',  ( 14.34966873604972726, -8.224510206698740333, 100.8344237280190185 ) ) ;
#183815=CARTESIAN_POINT ( 'NONE',  ( -16.51473224551082808, 9.474510206698731452, 48.33442372801900433 ) ) ;
#183816=CARTESIAN_POINT ( 'NONE',  ( -9.564922557961040184, 16.46253265017147172, 77.91775706135234714 ) ) ;
#183817=CARTESIAN_POINT ( 'NONE',  ( 13.89961937509977652, -13.97604488694527269, 103.1239096053143527 ) ) ;
#183818=CARTESIAN_POINT ( 'NONE',  ( -12.06949235617756955, 12.14591786802309770, 70.62390960531436690 ) ) ;
#183819=CARTESIAN_POINT ( 'NONE',  ( -9.564922557961040184, 16.46253265017147172, 47.91775706135233293 ) ) ;
#183820=CARTESIAN_POINT ( 'NONE',  ( 16.51473224551069308, 9.474510206698969483, 34.16557627198102409 ) ) ;
#183821=CARTESIAN_POINT ( 'NONE',  ( -21.52544592524343514, 5.823673210054127303, 36.04057627198102409 ) ) ;
#183822=CARTESIAN_POINT ( 'NONE',  ( -18.67979575497178146, -10.72451020669898902, 71.66557627198100988 ) ) ;
#183823=CARTESIAN_POINT ( 'NONE',  ( 4.483927247898545687, 16.52544592524342804, 114.7905762719810383 ) ) ;
#183824=CARTESIAN_POINT ( 'NONE',  ( 8.224510206698742110, 14.34966873604972548, 52.08442372801901854 ) ) ;
#183825=CARTESIAN_POINT ( 'NONE',  ( -18.62759615963255300, -10.81492255796106328, 39.16775706135235424 ) ) ;
#183826=CARTESIAN_POINT ( 'NONE',  ( -4.483927247898539470, -16.52544592524342804, 92.29057627198103830 ) ) ;
#183828=CARTESIAN_POINT ( 'NONE',  ( 17.31747979337950838, -6.344076630960994834, 36.12055131934817354 ) ) ;
#183830=CARTESIAN_POINT ( 'NONE',  ( 10.81492255796078972, 18.62759615963270932, 34.58224293864770260 ) ) ;
#183831=CARTESIAN_POINT ( 'NONE',  ( 17.48853670773243252, -5.747243402303153559, 66.16671299749991420 ) ) ;
#183833=AXIS2_PLACEMENT_3D ( 'NONE', #147725, #8199, #162879 ) ;
#183834=CARTESIAN_POINT ( 'NONE',  ( 16.53943276465976808, 0.05219959533934440121, 41.25109039468568284 ) ) ;
#183835=CARTESIAN_POINT ( 'NONE',  ( -14.34966873604960291, -8.224510206698953496, 41.66557627198103120 ) ) ;
#183836=CARTESIAN_POINT ( 'NONE',  ( 5.719274019375991003, -21.55341960407610458, 67.70724293864769550 ) ) ;
#183837=CARTESIAN_POINT ( 'NONE',  ( 5.049401038297881783, 19.05341960407617563, 82.29275706135229029 ) ) ;
#183838=CARTESIAN_POINT ( 'NONE',  ( 10.72451020669898902, -18.67979575497178502, 67.91557627198102409 ) ) ;
#183840=CARTESIAN_POINT ( 'NONE',  ( 13.89961937509977652, -13.97604488694527269, 38.12390960531436690 ) ) ;
#183841=CARTESIAN_POINT ( 'NONE',  ( 5.049401038298161559, -19.05341960407611168, 102.7072429386476955 ) ) ;
#183842=CARTESIAN_POINT ( 'NONE',  ( 9.474510206698971260, -16.51473224551069308, 52.91557627198102409 ) ) ;
#183843=CARTESIAN_POINT ( 'NONE',  ( 4.379528057220339221, -16.55341960407611168, 112.7072429386476955 ) ) ;
#183845=FACE_BOUND ( 'NONE', #25927, .T. ) ;
#183847=CARTESIAN_POINT ( 'NONE',  ( 8.224510206698742110, 14.34966873604972548, 67.08442372801901854 ) ) ;
#183848=CARTESIAN_POINT ( 'NONE',  ( 5.719274019375991003, -21.55341960407610458, 97.70724293864772392 ) ) ;
#183849=CARTESIAN_POINT ( 'NONE',  ( -0.05219959533909027116, -19.03943276465977164, 57.49890960531435979 ) ) ;
#183850=CARTESIAN_POINT ( 'NONE',  ( 15.72974639402176855, 15.80617190586768217, 26.87609039468567218 ) ) ;
#183851=CARTESIAN_POINT ( 'NONE',  ( 16.46253265017160672, -9.564922557960803928, 88.33224293864769550 ) ) ;
#183855=CARTESIAN_POINT ( 'NONE',  ( 15.72974639402176855, 15.80617190586768217, 36.87609039468568994 ) ) ;
#183856=CARTESIAN_POINT ( 'NONE',  ( -16.46253265017160317, 9.564922557960807481, 30.83224293864769550 ) ) ;
#183857=CARTESIAN_POINT ( 'NONE',  ( 16.51473224551069308, 9.474510206698969483, 104.1655762719810241 ) ) ;
#183858=CARTESIAN_POINT ( 'NONE',  ( 13.97604488694548053, -13.89961937509957401, 90.62609039468567573 ) ) ;
#183859=CARTESIAN_POINT ( 'NONE',  ( -5.049401038297874678, -19.05341960407617918, 44.79275706135232582 ) ) ;
#183860=CARTESIAN_POINT ( 'NONE',  ( 0.05219959533907565091, 21.53943276465977519, 99.99890960531436690 ) ) ;
#183861=CARTESIAN_POINT ( 'NONE',  ( -19.03943276465977164, -0.05219959533935918106, 38.75109039468566152 ) ) ;
#183862=CARTESIAN_POINT ( 'NONE',  ( -13.97604488694547697, 13.89961937509957934, 33.12609039468566863 ) ) ;
#183863=CARTESIAN_POINT ( 'NONE',  ( 16.53943276465976808, 0.05219959533934440121, 86.25109039468568994 ) ) ;
#183864=CARTESIAN_POINT ( 'NONE',  ( -19.03943276465977164, 0.05219959533909376836, 111.2489096053143669 ) ) ;
#183865=EDGE_LOOP ( 'NONE', ( #159617, #90276 ) ) ;
#183866=CARTESIAN_POINT ( 'NONE',  ( 13.97604488694527802, 13.89961937509977652, 54.37390960531435979 ) ) ;
#183868=CARTESIAN_POINT ( 'NONE',  ( 10.72451020669871369, 18.67979575497193778, 62.08442372801901143 ) ) ;
#183869=CARTESIAN_POINT ( 'NONE',  ( 5.719274019375673035, 21.55341960407619339, 77.29275706135234714 ) ) ;
#183870=CARTESIAN_POINT ( 'NONE',  ( 0.05219959533909260263, 19.03943276465977164, 114.9989096053143669 ) ) ;
#183871=CARTESIAN_POINT ( 'NONE',  ( 16.51473224551069308, 9.474510206698969483, 79.16557627198103830 ) ) ;
#183872=CARTESIAN_POINT ( 'NONE',  ( 10.72451020669871369, 18.67979575497193778, 52.08442372801901854 ) ) ;
#183873=CARTESIAN_POINT ( 'NONE',  ( -16.51473224551082808, 9.474510206698731452, 98.33442372801900433 ) ) ;
#183874=CARTESIAN_POINT ( 'NONE',  ( -16.51473224551069308, -9.474510206698971260, 51.66557627198102409 ) ) ;
#183875=CARTESIAN_POINT ( 'NONE',  ( -9.474510206698964154, 16.51473224551069663, 105.4155762719810383 ) ) ;
#183876=CARTESIAN_POINT ( 'NONE',  ( -9.474510206698964154, 16.51473224551069663, 80.41557627198103830 ) ) ;
#183877=CARTESIAN_POINT ( 'NONE',  ( 9.474510206698971260, -16.51473224551069308, 77.91557627198103830 ) ) ;
#183878=CARTESIAN_POINT ( 'NONE',  ( -5.153800228976328057, -19.02544592524343514, 62.29057627198100988 ) ) ;
#183879=CARTESIAN_POINT ( 'NONE',  ( 0.05219959533907565091, 21.53943276465977519, 94.99890960531436690 ) ) ;
#183880=CARTESIAN_POINT ( 'NONE',  ( -12.14591786802326823, 12.06949235617739902, 83.12609039468568994 ) ) ;
#183882=CARTESIAN_POINT ( 'NONE',  ( -5.049401038297874678, -19.05341960407617918, 39.79275706135232582 ) ) ;
#183883=CARTESIAN_POINT ( 'NONE',  ( -5.153800228976328057, -19.02544592524343514, 82.29057627198103830 ) ) ;
#183884=CARTESIAN_POINT ( 'NONE',  ( -8.314922557960811034, -14.29746914071050412, 57.08224293864769550 ) ) ;
#183885=CARTESIAN_POINT ( 'NONE',  ( -16.55341960407611168, -4.379528057220339221, 96.45724293864770971 ) ) ;
#183886=CARTESIAN_POINT ( 'NONE',  ( 0.05219959533907565091, 21.53943276465977519, 24.99890960531435624 ) ) ;
#183887=CARTESIAN_POINT ( 'NONE',  ( 0.05219959533909260263, 19.03943276465977164, 99.99890960531436690 ) ) ;
#183888=CARTESIAN_POINT ( 'NONE',  ( 0.05219959533909260263, 19.03943276465977164, 114.9989096053143669 ) ) ;
#183889=CARTESIAN_POINT ( 'NONE',  ( 19.05341960407617918, -5.049401038297876454, 36.04275706135234003 ) ) ;
#183890=CARTESIAN_POINT ( 'NONE',  ( -16.52544592524335698, -4.483927247898792601, 98.95942372801903275 ) ) ;
#183891=CARTESIAN_POINT ( 'NONE',  ( 19.03943276465977164, -0.05219959533909143690, 78.74890960531436690 ) ) ;
#183892=CARTESIAN_POINT ( 'NONE',  ( -18.62759615963255300, -10.81492255796106328, 39.16775706135235424 ) ) ;
#183893=CARTESIAN_POINT ( 'NONE',  ( 15.80617190586746368, 15.72974639402197994, 34.37390960531435979 ) ) ;
#183894=CARTESIAN_POINT ( 'NONE',  ( 15.80617190586746368, 15.72974639402197994, 114.3739096053143527 ) ) ;
#183895=CARTESIAN_POINT ( 'NONE',  ( 5.719274019375991003, -21.55341960407610458, 72.70724293864769550 ) ) ;
#183896=CARTESIAN_POINT ( 'NONE',  ( 12.14591786802309770, 12.06949235617756955, 89.37390960531435269 ) ) ;
#183897=CARTESIAN_POINT ( 'NONE',  ( 16.51473224551083163, -9.474510206698727899, 55.83442372801899722 ) ) ;
#183898=CARTESIAN_POINT ( 'NONE',  ( 9.474510206698971260, -16.51473224551069308, 32.91557627198102409 ) ) ;
#183899=CARTESIAN_POINT ( 'NONE',  ( 9.474510206698971260, -16.51473224551069308, 87.91557627198102409 ) ) ;
#183900=CARTESIAN_POINT ( 'NONE',  ( -16.51473224551069308, -9.474510206698971260, 86.66557627198102409 ) ) ;
#183902=CARTESIAN_POINT ( 'NONE',  ( 12.14591786802309770, 12.06949235617756955, 104.3739096053143669 ) ) ;
#183904=CARTESIAN_POINT ( 'NONE',  ( -14.34966873604960291, -8.224510206698953496, 31.66557627198102054 ) ) ;
#183905=CARTESIAN_POINT ( 'NONE',  ( 16.53943276465976808, 0.05219959533934440121, 21.25109039468567218 ) ) ;
#183906=CARTESIAN_POINT ( 'NONE',  ( 21.53943276465977519, 0.05219959533937863772, 91.25109039468568994 ) ) ;
#183907=CARTESIAN_POINT ( 'NONE',  ( 9.474510206698971260, -16.51473224551069308, 102.9155762719810241 ) ) ;
#183908=CARTESIAN_POINT ( 'NONE',  ( -15.80617190586745835, -15.72974639402198527, 111.8739096053143669 ) ) ;
#183909=CARTESIAN_POINT ( 'NONE',  ( 9.474510206698971260, -16.51473224551069308, 42.91557627198103120 ) ) ;
#183910=CARTESIAN_POINT ( 'NONE',  ( 16.55341960407618274, -4.379528057220086978, 46.04275706135234714 ) ) ;
#183911=CARTESIAN_POINT ( 'NONE',  ( -12.06949235617739369, -12.14591786802326823, 19.37609039468568639 ) ) ;
#183912=CARTESIAN_POINT ( 'NONE',  ( -16.52544592524342804, 4.483927247898546575, 91.04057627198103830 ) ) ;
#183913=CARTESIAN_POINT ( 'NONE',  ( -5.823673210054116645, -21.52544592524344225, 107.2905762719810525 ) ) ;
#183914=CARTESIAN_POINT ( 'NONE',  ( -9.564922557961040184, 16.46253265017147172, 72.91775706135233293 ) ) ;
#183916=CARTESIAN_POINT ( 'NONE',  ( 5.719274019375673035, 21.55341960407619339, 22.29275706135235069 ) ) ;
#183918=CARTESIAN_POINT ( 'NONE',  ( 16.46253265017160672, -9.564922557960803928, 93.33224293864769550 ) ) ;
#183919=CARTESIAN_POINT ( 'NONE',  ( 17.50000000000000000, -5.500000000000000888, 113.2969038253417153 ) ) ;
#183920=CARTESIAN_POINT ( 'NONE',  ( 0.05219959533909260263, 19.03943276465977164, 89.99890960531436690 ) ) ;
#183921=CARTESIAN_POINT ( 'NONE',  ( 15.80617190586769283, -15.72974639402175789, 30.62609039468567929 ) ) ;
#183922=CARTESIAN_POINT ( 'NONE',  ( -4.483927247898539470, -16.52544592524342804, 82.29057627198103830 ) ) ;
#183923=CARTESIAN_POINT ( 'NONE',  ( 5.049401038298161559, -19.05341960407611168, 87.70724293864769550 ) ) ;
#183924=CARTESIAN_POINT ( 'NONE',  ( 14.29746914071037800, 8.314922557961029526, 51.66775706135234714 ) ) ;
#183925=CARTESIAN_POINT ( 'NONE',  ( -19.02544592524334988, -5.153800228976617603, 48.95942372801900433 ) ) ;
#183926=CARTESIAN_POINT ( 'NONE',  ( -15.72974639402176322, -15.80617190586768395, 59.37609039468568284 ) ) ;
#183927=CARTESIAN_POINT ( 'NONE',  ( 16.52544592524335698, 4.483927247898782831, 31.45942372801901854 ) ) ;
#183928=CARTESIAN_POINT ( 'NONE',  ( 19.05341960407611168, 5.049401038298154454, 63.95724293864769550 ) ) ;
#183929=CARTESIAN_POINT ( 'NONE',  ( 9.474510206698729675, 16.51473224551082808, 102.0844237280190043 ) ) ;
#183930=CARTESIAN_POINT ( 'NONE',  ( 16.53943276465976808, 0.05219959533934440121, 61.25109039468567573 ) ) ;
#183931=CARTESIAN_POINT ( 'NONE',  ( 0.05219959533937995610, -21.53943276465977519, 95.00109039468568994 ) ) ;
#183932=CARTESIAN_POINT ( 'NONE',  ( -0.05219959533936034679, 19.03943276465977164, 77.50109039468566152 ) ) ;
#183933=CARTESIAN_POINT ( 'NONE',  ( -13.89961937509977652, 13.97604488694528158, 45.62390960531433848 ) ) ;
#183934=CARTESIAN_POINT ( 'NONE',  ( -21.55341960407610458, -5.719274019375992779, 71.45724293864769550 ) ) ;
#183935=CARTESIAN_POINT ( 'NONE',  ( 8.224510206698953496, -14.34966873604960469, 82.91557627198103830 ) ) ;
#183936=CARTESIAN_POINT ( 'NONE',  ( -9.564922557961040184, 16.46253265017147172, 77.91775706135234714 ) ) ;
#183937=CARTESIAN_POINT ( 'NONE',  ( -18.89770734986048950, -5.500000000000011546, 69.10214472496642202 ) ) ;
#183938=CARTESIAN_POINT ( 'NONE',  ( -0.05219959533936034679, 19.03943276465977164, 37.50109039468567573 ) ) ;
#183939=CARTESIAN_POINT ( 'NONE',  ( 8.224510206698953496, -14.34966873604960469, 22.91557627198102765 ) ) ;
#183940=CARTESIAN_POINT ( 'NONE',  ( 14.34966873604960469, 8.224510206698951720, 64.16557627198102409 ) ) ;
#183941=CARTESIAN_POINT ( 'NONE',  ( -18.62759615963255300, -10.81492255796106328, 109.1677570613523613 ) ) ;
#183943=CARTESIAN_POINT ( 'NONE',  ( 5.719274019375991003, -21.55341960407610458, 107.7072429386476955 ) ) ;
#183944=CARTESIAN_POINT ( 'NONE',  ( 9.564922557960805705, 16.46253265017160317, 64.58224293864769550 ) ) ;
#183945=CARTESIAN_POINT ( 'NONE',  ( -5.719274019375665041, -21.55341960407619695, 89.79275706135236135 ) ) ;
#183946=CARTESIAN_POINT ( 'NONE',  ( 19.02544592524343514, -5.153800228976328945, 63.54057627198103830 ) ) ;
#183947=CARTESIAN_POINT ( 'NONE',  ( 4.483927247898545687, 16.52544592524342804, 114.7905762719810383 ) ) ;
#183948=CARTESIAN_POINT ( 'NONE',  ( -5.823673210054116645, -21.52544592524344225, 27.29057627198103120 ) ) ;
#183949=CARTESIAN_POINT ( 'NONE',  ( 8.224510206698953496, -14.34966873604960469, 72.91557627198103830 ) ) ;
#183950=CARTESIAN_POINT ( 'NONE',  ( -5.153800228976328057, -19.02544592524343514, 42.29057627198101699 ) ) ;
#183951=CARTESIAN_POINT ( 'NONE',  ( 16.53943276465976808, -0.05219959533910856209, 83.74890960531435269 ) ) ;
#183952=CARTESIAN_POINT ( 'NONE',  ( -0.05219959533907301413, -21.53943276465977519, 112.4989096053143669 ) ) ;
#183953=CARTESIAN_POINT ( 'NONE',  ( 10.81492255796106328, -18.62759615963255655, 50.41775706135235424 ) ) ;
#183954=CARTESIAN_POINT ( 'NONE',  ( -19.03943276465977164, 0.05219959533909376836, 36.24890960531436690 ) ) ;
#183955=CARTESIAN_POINT ( 'NONE',  ( -8.224510206698735004, -14.34966873604973081, 54.58442372801901143 ) ) ;
#183956=CARTESIAN_POINT ( 'NONE',  ( 5.719274019375991003, -21.55341960407610458, 97.70724293864772392 ) ) ;
#183957=CARTESIAN_POINT ( 'NONE',  ( 13.97604488694548053, -13.89961937509957401, 25.62609039468566507 ) ) ;
#183958=CARTESIAN_POINT ( 'NONE',  ( -19.03943276465977164, 0.05219959533909376836, 51.24890960531436690 ) ) ;
#183959=CARTESIAN_POINT ( 'NONE',  ( 5.049401038298161559, -19.05341960407611168, 102.7072429386476955 ) ) ;
#183960=CARTESIAN_POINT ( 'NONE',  ( 21.53943276465977519, 0.05219959533937863772, 56.25109039468568284 ) ) ;
#183961=CARTESIAN_POINT ( 'NONE',  ( 18.67979575497178502, 10.72451020669898547, 49.16557627198102409 ) ) ;
#183962=CARTESIAN_POINT ( 'NONE',  ( 14.34966873604972726, -8.224510206698740333, 110.8344237280190043 ) ) ;
#183963=CARTESIAN_POINT ( 'NONE',  ( -18.62759615963255300, -10.81492255796106328, 64.16775706135234714 ) ) ;
#183964=CARTESIAN_POINT ( 'NONE',  ( -15.80617190586768217, 15.72974639402176855, 103.1260903946856757 ) ) ;
#183965=CARTESIAN_POINT ( 'NONE',  ( -0.05219959533936034679, 19.03943276465977164, 32.50109039468566863 ) ) ;
#183966=CARTESIAN_POINT ( 'NONE',  ( -4.379528057220086978, -16.55341960407618274, 99.79275706135234714 ) ) ;
#183967=CARTESIAN_POINT ( 'NONE',  ( -0.05219959533937732626, 21.53943276465977519, 57.50109039468568994 ) ) ;
#183968=CARTESIAN_POINT ( 'NONE',  ( 19.03943276465977164, -0.05219959533909143690, 48.74890960531435979 ) ) ;
#183969=CARTESIAN_POINT ( 'NONE',  ( -9.564922557961040184, 16.46253265017147172, 27.91775706135232582 ) ) ;
#183970=CARTESIAN_POINT ( 'NONE',  ( 0.05219959533909260263, 19.03943276465977164, 114.9989096053143669 ) ) ;
#183971=CARTESIAN_POINT ( 'NONE',  ( 18.62759615963255655, 10.81492255796105972, 21.66775706135235069 ) ) ;
#183973=CARTESIAN_POINT ( 'NONE',  ( -21.55341960407610458, -5.719274019375992779, 71.45724293864769550 ) ) ;
#183974=CARTESIAN_POINT ( 'NONE',  ( -16.55341960407617563, 4.379528057220093196, 38.54275706135234714 ) ) ;
#183976=CARTESIAN_POINT ( 'NONE',  ( 15.80617190586746368, 15.72974639402197994, 79.37390960531436690 ) ) ;
#183977=CARTESIAN_POINT ( 'NONE',  ( 4.379528057220092307, 16.55341960407617563, 62.29275706135236845 ) ) ;
#183978=CARTESIAN_POINT ( 'NONE',  ( 0.05219959533910956823, 16.53943276465976808, 74.99890960531435269 ) ) ;
#183980=CARTESIAN_POINT ( 'NONE',  ( -16.51473224551082808, 9.474510206698731452, 103.3344237280190043 ) ) ;
#183982=CARTESIAN_POINT ( 'NONE',  ( -15.72974639402197994, 15.80617190586746368, 30.62390960531436335 ) ) ;
#183984=CARTESIAN_POINT ( 'NONE',  ( -14.29746914071037622, -8.314922557961029526, 44.16775706135234714 ) ) ;
#183985=CARTESIAN_POINT ( 'NONE',  ( 10.81492255796078972, 18.62759615963270932, 114.5822429386477097 ) ) ;
#183986=CARTESIAN_POINT ( 'NONE',  ( 21.55341960407610458, 5.719274019375980345, 28.95724293864769905 ) ) ;
#183987=CARTESIAN_POINT ( 'NONE',  ( -4.483927247898782831, 16.52544592524335698, 72.70942372801901854 ) ) ;
#183988=CARTESIAN_POINT ( 'NONE',  ( 5.049401038298161559, -19.05341960407611168, 87.70724293864769550 ) ) ;
#183989=CARTESIAN_POINT ( 'NONE',  ( -5.719274019375665041, -21.55341960407619695, 44.79275706135234714 ) ) ;
#183990=CARTESIAN_POINT ( 'NONE',  ( -16.52544592524335698, -4.483927247898792601, 18.95942372801901143 ) ) ;
#183991=CARTESIAN_POINT ( 'NONE',  ( -5.823673210054116645, -21.52544592524344225, 32.29057627198102409 ) ) ;
#183993=CARTESIAN_POINT ( 'NONE',  ( -13.97604488694547697, 13.89961937509957934, 23.12609039468565442 ) ) ;
#183994=( BOUNDED_SURFACE ( )  B_SPLINE_SURFACE ( 3, 2, ( 
 ( #139749, #158901, #187290, #174098, #141747, #80078, #173101, #34578, #109423, #82039, #95246, #1236, #190254, #96235, #3237, #157923, #93249, #20392, #156931, #79080, #143736, #5215, #51731, #64911, #31600, #4219, #110415, #170106, #65897, #154935, #127571, #124595, #47770, #171102, #189272, #50748, #32595, #94247, #155928, #17423, #33583, #2241, #63924, #69908, #40573, #71902, #192257, #115413, #129550, #10243, #179104, #161911, #159910, #102243, #68900, #55733, #85053, #23405, #54732, #178093, #52725, #25428, #38573, #83057, #133574, #39563, #146734, #116404, #36552, #163931, #100229, #22405, #117407, #87069, #195264, #8230, #175084, #101221, #130559, #148754, #131574, #113394, #162910, #98206, #21399, #144731, #70910, #24418, #6218, #86067, #147757, #67897, #53739, #160912, #193258, #9243, #191250, #114390, #176092, #132578, #84056, #177102, #194266, #37562, #99225, #145734, #7215, #197255, #88059, #182080, #121380, #151736, #119416, #72922, #150753, #60693, #76863, #183072, #41580, #181100, #44555, #137545, #11248, #199228, #168866, #106210, #149746, #167894, #27416, #103244, #28417, #138533, #15204, #196277, #122369, #92015, #90054, #43563, #134591, #164926, #184058, #30371, #89062, #13229, #42574, #59707, #153708, #58717, #107195, #12251, #29394, #91024, #57746, #152710, #56748, #73913, #74892, #14201, #120386, #45541, #104237, #136555, #105228, #118419, #165920, #198236, #180112, #75869, #26419, #135583, #166916, #158672, #157694, #155697, #3009, #34349, #93019, #64686, #96990, #94016, #18196, #96010, #2014, #3989, #62679, #156702, #187064, #81807, #124360, #171866, #50518, #19185, #65669, #186055, #47539, #20162, #80834, #11, #78846, #63693, #16200, #61685, #127331, #48534, #46535, #189043, #17192, #142511, #33355, #110188, #141522, #126348, #139522, #112181, #125368, #169876, #123354, #188045, #95014, #49515, #185047, #173869, #79853, #109193, #35337, #108194, #31369, #111178, #154707, #172868, #140524, #77855, #1005, #170872, #32363, #143494, #55494, #4979, #100986, #54496, #102002, #146489, #7980, #128328, #98981, #191013, #99986, #161671, #70672, #147515, #85827, #69664, #114149, #83814, #23167, #116168, #115168, #113161, #130310, #145494, #174851, #68654, #131331, #38330, #5980, #159663, #37323, #9005, #163684, #193019, #190027, #67660, #177858, #24176, #97971, #132339, #117164, #39327, #36317, #162670, #175850, #51501, #176861, #25187, #66665, #82815, #194031, #178860, #84810, #192005, #21160, #144497, #40326, #129317, #160671, #52489, #22163, #6974, #53491, #88825, #137314, #136327, #150518, #12016, #73677, #135349, #124876, #28182, #43326, #133332, #197023, #148515, #121145, #71665, #57510, #72675, #198002, #186575, #11003, #118177, #119179, #182839, #167665, #59472, #13969, #58489, #44321, #179868, #56499, #120156, #180864, #166681, #75636, #89824, #104993, #196034, #152482, #42340, #104001, #105980, #29161, #90798, #198995, #63196, #151505, #26179, #181846, #48048, #12997, #109704, #171386, #86829, #165679, #10005, #195023, #27178, #41338, #102999, #164685, #134352, #87820, #149506, #74660, #79362, #3507, #110689, #144010, #66176, #36825, #175357, #187567, #18699, #17705, #141033, #81325, #67174, #98491, #174369, #52994, #19683, #112677, #128831, #4486, #143008, #2520, #127838, #173378, #64200, #94523, #51016, #82320, #157205, #189544, #125867, #35839, #97485, #65183, #159171, #160184, #5491, #20666, #113663, #80346, #172369, #156205, #142018, #190530, #52004, #188548, #129818, #95519, #126842, #49034, #68166, #21674, #83328, #145005, #6486, #191517, #32873, #114672, #33859, #50026, #111691, #34848, #96503, #158193, #72178, #56004, #7487, #194533, #162182, #99501, #39831, #41851, #118689, #192529, #25696, #57016, #101497, #116677, #69171, #22678, #87341, #195542, #23680, #163186, #177374, #9515, #180381, #70182, #133852, #85328, #71181, #117682, #130838, #132845 ),
 ( #179379, #149027, #115686, #38846, #176368, #102514, #37841, #193533, #55007, #54012, #161182, #84325, #86339, #100503, #146004, #40841, #147020, #8504, #131850, #178367, #24690, #164198, #148026, #10515, #64130, #169309, #15644, #171314, #16637, #125795, #173304, #48963, #2448, #155144, #111619, #78284, #139957, #157133, #3436, #65112, #188474, #49955, #110617, #185487, #32801, #95448, #172299, #18628, #141946, #81255, #1447, #34779, #45977, #124804, #92464, #154152, #80275, #170314, #77303, #138972, #63125, #450, #186502, #123788, #126770, #79292, #96435, #158122, #62125, #31807, #30815, #46977, #94453, #19613, #142937, #187497, #66104, #156133, #33788, #4418, #17632, #140961, #108636, #127770, #47978, #93457, #107631, #109631, #143938, #131778, #101424, #53940, #82247, #38776, #160112, #174299, #161110, #71109, #147957, #128761, #193460, #24619, #22606, #176294, #5419, #97414, #54937, #163116, #21600, #84252, #175287, #192457, #86267, #191445, #39761, #144933, #115615, #23610, #67102, #177304, #9444, #83258, #7415, #85256, #52921, #116609, #51933, #145933, #37766, #189470, #113593, #69098, #50948, #146948, #178297, #36752, #98416, #112607, #8437, #35768, #68096, #114597, #190460, #159101, #20595, #99428, #6415, #129748, #130765, #100432, #162113, #70109, #74111, #197452, #72104, #73123, #180310, #120586, #56946, #58918, #42776, #135781, #55933, #59907, #119615, #41778, #75083, #183270, #91216, #104438, #194462, #182280, #88258, #121575, #57944, #44750, #43761, #132775, #106406, #117608, #90247, #105425, #152907, #167108, #28609, #179308, #149945, #103444, #89263, #150955, #168088, #136750, #198434, #151930, #165123, #134792, #12449, #13419, #166122, #102441, #181298, #196473, #164128, #27624, #29585, #14404, #195470, #148955, #26615, #40772, #25626, #87271, #10444, #118620, #133777, #11451, #199428, #45742, #1206, #46739, #155895, #3208, #79049, #32562, #185248, #141718, #108400, #170077, #187262, #33554, #95216, #18398, #80049, #140723, #15405, #62883, #125565, #2213, #48731, #172067, #111382, #31568, #64882, #76068, #154904, #122570, #184260, #110385, #214, #107394, #169067, #93219, #30573, #16403, #153910, #156902, #109392, #126543, #188242, #92224, #61883, #60894, #77062, #124564, #49717, #173070, #17393, #96206, #186261, #63894, #34547, #47739, #171072, #138734, #94216, #78049, #123553, #137744, #157895, #139718, #143702, #67866, #65867, #22373, #37531, #51701, #99194, #161880, #68868, #6186, #100198, #5184, #158871, #81033, #66865, #160882, #176064, #175056, #116372, #82008, #128528, #174069, #54699, #129521, #84024, #114359, #191221, #177071, #19384, #52695, #130527, #53706, #178060, #8197, #39528, #85019, #69872, #192224, #115383, #21368, #83026, #144700, #145702, #101188, #7184, #38542, #127539, #23374, #142709, #146700, #4188, #190222, #113364, #131541, #189241, #36520, #50719, #98175, #193225, #112377, #35538, #97185, #159877, #20360, #198202, #87036, #194233, #133537, #197222, #43529, #12217, #164891, #26385, #181065, #86036, #132544, #88024, #195229, #42540, #90020, #165884, #119382, #71869, #28382, #56710, #118383, #73880, #120351, #182046, #105194, #166881, #27381, #102209, #149712, #135550, #89027, #58684, #151703, #59672, #180077, #13196, #162877, #41546, #9210, #70877, #74859, #148721, #55699, #117372, #103209, #179069, #11211, #40538, #136521, #196243, #121344, #183037, #163898, #10209, #147723, #25394, #72886, #44520, #24385, #104203, #134555, #57712, #150718, #140491, #77819, #154669, #14165, #970, #46496, #75833, #167859, #124323, #155663, #30337, #16165, #152676, #109159, #186021, #138499, #47503, #48500, #17159, #92984, #187029, #91978, #45506, #29359, #153672, #170838, #62646, #61650, #2971, #168832, #15169, #60659, #141488, #139488, #32330, #93983, #78812, #63659, #106176, #1979, #125332, #110154, #64651, #94981, #126313, #171832, #156666, #33320, #18161 ),
 ( #137511, #79817, #199192, #188010, #123318, #90989, #122332, #184024, #107161, #76828, #200181, #108157, #185011, #169839, #31333, #175812, #159626, #190975, #172833, #176820, #36278, #158634, #191966, #99946, #7942, #21121, #111143, #52452, #4941, #38292, #174813, #161632, #98942, #49480, #23126, #34312, #6936, #160633, #69625, #114109, #37285, #95975, #66625, #96954, #5943, #67619, #84771, #53452, #115127, #22124, #20125, #189987, #129280, #83774, #82777, #19148, #97933, #51461, #80798, #144458, #145454, #68615, #112141, #65633, #143456, #146449, #131291, #130271, #157659, #173833, #142476, #3954, #127293, #189006, #50481, #35298, #81769, #128289, #113123, #177817, #167382, #77335, #154185, #132298, #138019, #30849, #28879, #182553, #147473, #100944, #199702, #169340, #163642, #90519, #178817, #198712, #92496, #194980, #46008, #148471, #60179, #29854, #85787, #121848, #15675, #86786, #13685, #91491, #59184, #61168, #55452, #152201, #44035, #192979, #117123, #75352, #107663, #153178, #122839, #40287, #101961, #54458, #14681, #116128, #71624, #120853, #8963, #39287, #184528, #70631, #9964, #162628, #25144, #193990, #106685, #137022, #24135, #133290, #105696, #183541, #45026, #168358, #76343, #173335, #142967, #80305, #159129, #125825, #189499, #174328, #34808, #19642, #93489, #81284, #50975, #3466, #31838, #188506, #109663, #123819, #110648, #20627, #97444, #78314, #4445, #35797, #172329, #187528, #155175, #47009, #66133, #112635, #171343, #33818, #124834, #141978, #139002, #140991, #481, #94482, #65143, #96463, #16666, #126800, #62155, #32831, #157165, #158151, #2479, #127798, #1476, #95478, #48993, #185517, #63155, #18659, #108668, #170346, #139987, #186534, #48007, #156163, #17661, #79321, #64160, #49985, #111649, #179338, #147986, #130794, #128790, #9475, #37795, #24648, #53969, #192487, #23636, #146976, #21631, #22635, #129776, #70138, #6443, #8464, #115643, #85285, #5449, #71139, #69128, #191472, #86297, #132804, #40801, #177332, #143969, #131809, #99458, #194491, #7443, #55963, #193488, #82276, #117640, #67132, #39789, #54966, #102471, #116637, #178326, #190491, #161138, #52951, #38804, #100460, #164158, #51962, #113622, #114626, #176326, #101454, #163145, #175316, #36783, #98448, #160142, #83287, #162140, #144961, #68124, #84281, #145962, #60923, #196502, #14432, #25656, #104467, #72134, #133809, #198465, #149976, #56974, #118648, #42805, #195500, #57972, #103475, #136779, #58947, #29611, #168115, #180339, #11481, #10473, #41807, #74138, #59936, #91243, #167139, #45768, #12477, #120615, #183299, #165153, #119644, #26644, #182311, #166151, #88287, #87301, #43790, #75111, #73152, #135810, #134823, #28638, #105454, #181326, #90275, #152933, #121603, #197480, #106433, #27653, #89292, #148984, #150984, #151959, #13447, #44780, #122597, #76095, #137770, #199455, #184286, #107420, #110409, #63919, #155922, #126567, #169093, #17417, #80073, #3232, #4213, #157918, #127566, #34573, #19408, #141742, #18423, #171097, #32589, #94242, #79075, #65891, #172091, #125588, #15432, #140748, #30600, #64906, #153937, #139742, #154929, #188266, #189267, #93244, #241, #1231, #49741, #111410, #173095, #2236, #187285, #48756, #92253, #138759, #33578, #62910, #95240, #96230, #156926, #81057, #78074, #142734, #50742, #77090, #61908, #31595, #123579, #185274, #46766, #16427, #108425, #170101, #124590, #186285, #47765, #109418, #70903, #69900, #132570, #191244, #114382, #128551, #9236, #178086, #160906, #158896, #39555, #67891, #54724, #84049, #22399, #53732, #177095, #51725, #52718, #159904, #100223, #36544, #38567, #145728, #115407, #35562, #101213, #99218, #21392, #116397, #162902, #194259, #7209, #174093, #161904, #129544, #24411, #37556, #86060, #23398, #112401, #147749, #97210, #131567, #85045, #20386, #146726, #8223, #82033, #176086, #83051, #68893, #130553, #143730, #5209, #66890, #193251, #144725 ),
 ( #6211, #190248, #113388, #98200, #175078, #192250, #151729, #136547, #10235, #198228, #167887, #120379, #148747, #105221, #26412, #40566, #27409, #137538, #14192, #195256, #59700, #91017, #89055, #42567, #71895, #163924, #121372, #29386, #88051, #150745, #41573, #58709, #152703, #57739, #106203, #11240, #182072, #90047, #133566, #43555, #75862, #149739, #181092, #166909, #12244, #118412, #56741, #72914, #183065, #55726, #180105, #117398, #179097, #13222, #44548, #103236, #102236, #25420, #28408, #164918, #74885, #134584, #87062, #73906, #196270, #119409, #104230, #165911, #135576, #197248, #186047, #153700, #107187, #141514, #172859, #169867, #170864, #185039, #2006, #96001, #997, #49506, #154697, #63685, #33347, #92006, #125359, #157685, #93011, #17184, #95006, #62671, #3000, #61677, #155689, #47530, #80824, #123346, #32355, #111169, #156694, #64677, #46526, #108186, #19176, #18188, #199220, #77847, #124352, #15195, #60686, #126339, #109185, #45533, #188036, #16192, #34340, #94008, #78838, #140516, #187056, #138525, #139514, #31361, #48526, #110180, #171859, #79845, #122361, #184050, #168858, #30363, #76854, #3, #193010, #100977, #114139, #3980, #83805, #97962, #69654, #67651, #131321, #191995, #142502, #54487, #65660, #99977, #53481, #162661, #145485, #6965, #127322, #159654, #190017, #98972, #160663, #116159, #146480, #84801, #68645, #113152, #82806, #22154, #115159, #175840, #112172, #129308, #144488, #173860, #130301, #176852, #51491, #7971, #174842, #36307, #38322, #161661, #23158, #177849, #39317, #24167, #81797, #191004, #189034, #50508, #35327, #96980, #158661, #21151, #20152, #143484, #5971, #4969, #66655, #128317, #52480, #37314, #178850, #102988, #132330, #56489, #163674, #197013, #119169, #89814, #28172, #40316, #71655, #70663, #194021, #134341, #120145, #151495, #27168, #105970, #72665, #180853, #43316, #101993, #118167, #55484, #42329, #26169, #117154, #147505, #103990, #135339, #9995, #196025, #25176, #88815, #165669, #179858, #150508, #12987, #58478, #57500, #166670, #133322, #86818, #8995, #195012, #12006, #73667, #41328, #182829, #148505, #164674, #87810, #121135, #181836, #104983, #74650, #136316, #197991, #85818, #59462, #44311, #167655, #149496, #10993, #187807, #94771, #79606, #140277, #78603, #31128, #92777, #154466, #15958, #64441, #170632, #185809, #75625, #77618, #90788, #63447, #13958, #199981, #14962, #1769, #126112, #153465, #60453, #61447, #125123, #109946, #186820, #139288, #765, #47295, #152472, #198985, #62436, #123118, #108952, #156454, #124109, #32121, #93778, #155459, #48290, #29151, #16949, #171627, #33115, #49276, #17953, #110934, #141276, #2765, #137304, #122127, #183815, #45305, #106956, #168629, #30129, #91771, #76622, #138300, #184803, #46289, #107946, #169632, #143249, #158434, #21920, #7730, #96744, #3748, #4733, #6731, #53244, #83571, #174613, #36078, #190771, #95765, #142265, #97727, #66422, #52246, #99744, #175601, #129070, #81563, #38089, #128083, #189787, #145250, #130062, #191761, #114921, #176614, #37078, #111935, #159417, #68409, #98737, #161428, #22920, #69416, #51258, #84566, #172621, #112918, #18945, #80590, #146244, #19921, #65425, #127086, #20913, #188795, #82571, #50277, #131082, #5738, #192771, #54255, #173622, #144252, #157451, #35091, #67415, #34108, #113903, #160430, #136085, #102757, #149268, #73435, #8754, #86582, #23923, #10760, #56250, #85578, #177616, #134102, #165439, #40073, #164444, #162421, #118938, #195792, #148265, #57264, #58250, #26934, #25938, #196782, #101751, #55249, #39084, #163439, #180623, #72424, #71422, #12754, #178610, #24936, #70425, #151264, #132091, #74419, #87581, #42095, #103760, #88576, #135106, #115926, #150274, #11770, #119918, #197759, #104749, #100740, #181604, #166440, #43082, #27935, #117932, #179621, #41093, #89578, #147264, #193780, #116917, #9758, #133086, #194776, #93536, #44079, #29896 ),
 ( #185561, #169385, #527, #182595, #186580, #46051, #168401, #1523, #109709, #17711, #30893, #120895, #62199, #14726, #48053, #184570, #171392, #108712, #59226, #32879, #105738, #16710, #170391, #79368, #123863, #47055, #167425, #76386, #106727, #15719, #77379, #94529, #63201, #124881, #31882, #91534, #199744, #139047, #155221, #92540, #28921, #107706, #61210, #90561, #154229, #78360, #140034, #121891, #75394, #153221, #156211, #141039, #183584, #152243, #13728, #137066, #198756, #60221, #45069, #138063, #122882, #95526, #54755, #176114, #187573, #177125, #87092, #163954, #142025, #147780, #40595, #38596, #192279, #157212, #110696, #9266, #179127, #37585, #100252, #188555, #8252, #102266, #7237, #55755, #160934, #80353, #116429, #161933, #70932, #132599, #18706, #50033, #49041, #172376, #53760, #39585, #194289, #146758, #25452, #115434, #23428, #162933, #3514, #99247, #33866, #85075, #145755, #65190, #64206, #69932, #178117, #126849, #131596, #114413, #193281, #101244, #22426, #24440, #117429, #86089, #2526, #125873, #84076, #68922, #130584, #196297, #90075, #105251, #104259, #45566, #11270, #57767, #103267, #184082, #135605, #151758, #43585, #197276, #106233, #148777, #58739, #59733, #183096, #107219, #137569, #168890, #14224, #199252, #121402, #198257, #150776, #12271, #73936, #120408, #30395, #13251, #166937, #195287, #182100, #10266, #44577, #133595, #119437, #134613, #167916, #71925, #72943, #180133, #181122, #29416, #91047, #152734, #28440, #74914, #136577, #56768, #118440, #75894, #42596, #60719, #122393, #41602, #164947, #165942, #26440, #27442, #89084, #88082, #149768, #49541, #34374, #96034, #156728, #31393, #78868, #141546, #95037, #3035, #188070, #127358, #62702, #80860, #92042, #170894, #138557, #35, #64711, #16226, #123378, #185070, #109215, #61708, #124385, #189071, #154730, #139545, #46558, #50543, #140548, #33379, #187088, #2036, #111203, #153731, #63716, #126373, #172895, #112204, #142536, #173894, #157721, #4015, #19210, #65693, #94041, #155719, #17216, #125391, #15227, #18221, #48558, #108220, #110211, #76886, #169900, #93043, #186080, #77878, #1030, #47562, #32386, #171892, #79877, #100012, #174877, #175877, #82843, #23195, #159689, #161698, #145519, #176886, #158696, #162697, #22189, #144522, #177885, #85852, #194059, #6999, #97015, #38357, #191040, #24203, #160698, #147541, #84838, #35363, #9029, #20185, #193046, #146517, #55520, #8007, #69690, #81831, #52513, #6007, #192034, #53516, #70698, #39354, #101013, #131357, #67687, #37349, #115194, #54523, #68681, #5007, #83837, #99007, #66690, #130336, #116196, #132366, #97996, #51525, #129345, #117193, #143518, #21187, #128352, #190050, #113188, #36343, #114174, #121170, #90821, #43349, #71691, #28207, #149532, #163711, #150540, #60486, #137337, #118205, #182864, #13993, #12040, #165705, #133358, #86856, #44345, #152504, #11027, #73704, #164710, #181870, #120180, #134375, #106003, #104026, #167690, #89848, #178886, #75660, #40354, #136351, #151531, #199017, #105020, #166704, #25214, #196061, #26205, #135376, #197046, #29187, #102029, #148540, #13020, #72702, #119203, #58514, #74685, #198027, #10031, #27202, #180888, #195048, #88848, #59495, #56527, #41362, #179896, #57534, #103028, #87844, #42363, #172654, #157487, #17989, #2800, #76656, #64478, #34142, #186857, #14996, #171661, #92813, #106990, #93813, #3783, #80626, #61482, #126145, #18980, #155493, #108987, #138335, #30163, #187841, #95801, #154500, #16985, #107980, #125158, #142303, #124146, #122161, #77653, #48326, #156487, #200015, #109981, #183850, #15995, #140314, #79642, #185845, #49310, #184841, #78639, #170668, #45338, #46326, #1804, #168663, #141311, #110970, #169668, #31163, #91807, #153499, #123153, #801, #47332, #139321, #62474, #32156, #63482, #33150, #94808, #128118, #81599, #98770, #67449, #37111, #160464, #143283, #159451, #189821, #21955, #4769, #83605 ),
 ( #174647, #51293, #52280, #113938, #38126, #176650, #114957, #145284, #112954, #20947, #175637, #6767, #129107, #173661, #144285, #82604, #35128, #5774, #68446, #130100, #66456, #158469, #36112, #99780, #69452, #97764, #161465, #146282, #191797, #53278, #19957, #22955, #84603, #7769, #96780, #131119, #190806, #188829, #65460, #127123, #50313, #111969, #111675, #78341, #187552, #124861, #18683, #62180, #77361, #199726, #185542, #79347, #94508, #93516, #34832, #508, #47036, #92521, #173362, #186560, #141018, #32858, #48032, #95503, #138045, #109689, #49019, #172354, #96487, #126826, #158177, #3490, #188532, #110674, #33843, #140015, #1503, #63181, #171370, #19667, #2505, #156190, #184552, #17689, #61192, #157189, #122864, #108693, #123844, #169366, #64185, #80330, #46033, #170371, #142002, #65167, #50010, #125851, #107688, #30875, #154211, #15700, #139029, #31863, #155202, #16691, #84308, #37824, #190514, #147002, #51988, #175341, #192511, #38828, #100486, #23662, #85311, #145987, #20650, #68150, #130820, #7470, #53995, #177358, #116660, #113647, #21658, #115669, #129801, #162165, #5475, #82304, #142992, #128815, #22661, #99484, #36808, #178351, #143994, #98475, #35823, #39814, #191500, #69154, #176351, #52976, #8488, #81308, #114654, #70164, #131833, #101480, #193515, #163169, #54991, #4470, #66160, #127822, #83311, #144988, #6469, #161165, #189528, #51000, #112661, #174352, #97469, #159154, #67158, #160168, #195525, #10498, #55989, #134849, #167165, #86323, #56998, #58971, #105478, #74163, #26672, #88313, #42829, #148010, #194515, #150001, #118673, #104494, #151984, #27677, #181350, #133834, #90299, #180364, #41832, #135835, #182337, #43815, #28664, #13472, #89317, #164182, #11507, #197504, #151010, #120639, #75135, #59962, #103500, #136805, #24673, #165177, #71164, #132829, #198489, #149010, #117666, #179362, #73178, #40825, #196527, #102497, #121628, #57998, #183324, #44805, #25680, #72159, #9500, #87325, #119668, #106460, #166176, #12501, #191023, #154955, #1257, #125611, #60948, #138786, #76120, #62934, #108449, #137798, #29635, #186309, #17442, #92278, #16451, #14457, #171124, #47790, #109441, #144506, #79098, #124614, #174860, #110435, #122623, #153962, #152959, #199482, #78100, #2260, #36326, #32613, #52498, #139769, #94267, #187310, #184313, #267, #45794, #155946, #170125, #107446, #91268, #140771, #63943, #15460, #48781, #169120, #97980, #159673, #21169, #5990, #31620, #82825, #67670, #129328, #77116, #30625, #61935, #123604, #168139, #185299, #46790, #93270, #176869, #161679, #68663, #149512, #100994, #55503, #9013, #162679, #71672, #114158, #24185, #25194, #148522, #11009, #103006, #72683, #179876, #164691, #86836, #163692, #116176, #177866, #39335, #85835, #134358, #117173, #70681, #160680, #147525, #175860, #10012, #98991, #84819, #99994, #145502, #132347, #56507, #37332, #146498, #133339, #195030, #118185, #194039, #178868, #40335, #22172, #83822, #102010, #7989, #41344, #26186, #87826, #196042, #23175, #6983, #69672, #131339, #130318, #192015, #53499, #115176, #38338, #193027, #54504, #44327, #106970, #60467, #168644, #153480, #92791, #28189, #46304, #57517, #136333, #104008, #165686, #30143, #181853, #88831, #150524, #74666, #27184, #89831, #135357, #199995, #31143, #151511, #29168, #43332, #122142, #154479, #59477, #107960, #13003, #183830, #91786, #12023, #45320, #15972, #198007, #75641, #14976, #121151, #61462, #120162, #13974, #105986, #139301, #105000, #90804, #169647, #76636, #123133, #166687, #182844, #77632, #138314, #119185, #167670, #152487, #73685, #180870, #184819, #137319, #197029, #199000, #42346, #58496, #3761, #110947, #142280, #65438, #140292, #141289, #48303, #188808, #125137, #127099, #172632, #50291, #124124, #128096, #187820, #109960, #143262, #51272, #159430, #34120, #62450, #111948, #156466, #189800, #126125, #112932, #173637, #779, #174626, #185823, #158447 ),
 ( #171639, #2779, #157465, #35106, #95779, #170646, #49289, #64455, #32134, #18958, #96757, #80603, #63461, #16964, #94785, #4746, #20926, #186835, #36091, #97742, #19935, #81577, #155472, #66435, #82584, #47310, #93792, #108965, #33129, #78617, #1783, #17966, #79621, #162436, #71437, #68424, #132103, #131097, #98750, #52259, #113917, #5752, #23937, #193794, #130076, #192785, #190785, #147278, #85591, #8768, #117946, #84580, #55262, #54268, #24950, #191775, #83584, #67428, #53257, #70437, #100754, #99758, #41106, #6745, #114935, #160443, #179636, #115940, #116931, #39098, #177630, #101765, #144265, #178624, #40087, #163452, #102770, #133101, #164457, #9773, #194790, #86597, #148280, #146260, #7744, #69430, #56263, #25951, #129085, #175615, #37091, #21933, #145263, #176628, #38103, #161442, #22934, #118951, #197775, #29911, #149280, #58264, #121907, #168416, #137082, #89592, #151279, #105752, #10775, #57277, #12768, #119933, #167438, #14741, #90576, #44094, #196796, #153238, #181618, #43097, #198770, #45084, #106741, #91551, #76402, #152257, #26950, #74432, #60236, #13742, #183600, #138078, #122897, #104766, #199759, #87594, #166454, #134116, #195805, #61226, #11785, #180637, #42112, #27951, #103774, #136099, #165453, #184586, #120910, #46067, #107721, #88592, #73449, #72440, #150290, #59241, #169402, #135122, #28935, #182609, #75410, #64224, #188571, #123881, #1542, #139064, #125889, #171409, #142041, #65205, #66198, #19704, #189565, #96524, #81346, #3529, #80368, #32895, #94547, #156228, #17729, #127861, #172395, #187589, #77394, #79387, #92556, #126864, #15735, #63218, #16728, #62213, #141056, #173399, #154244, #124898, #50051, #111713, #34870, #2542, #49058, #110713, #542, #185579, #33884, #186597, #95541, #158214, #157229, #18721, #140052, #143030, #48069, #109725, #4508, #51037, #112699, #30908, #47070, #108730, #170407, #31899, #93552, #155238, #78376, #70203, #9535, #145027, #163207, #174391, #53016, #20688, #82343, #147041, #98513, #5514, #67194, #191539, #144032, #6508, #52025, #85348, #7508, #178387, #116697, #128852, #160207, #159193, #190552, #22700, #8525, #39851, #115707, #194554, #161205, #69192, #131870, #113683, #68188, #175378, #130859, #114696, #36847, #35861, #192550, #23700, #21697, #84347, #83351, #177395, #54033, #38867, #148045, #176390, #193555, #146025, #55027, #129840, #37864, #97507, #99523, #100523, #162202, #101517, #71202, #24711, #86360, #132865, #56024, #104529, #59007, #12534, #166210, #75171, #117702, #27711, #41872, #168175, #152994, #13506, #198528, #72199, #59998, #29671, #182373, #10535, #167201, #88348, #102536, #89354, #199517, #76156, #135868, #44842, #103539, #105516, #151044, #133873, #25716, #121665, #91303, #150041, #74199, #165214, #120674, #14494, #119702, #137836, #73214, #43850, #152020, #195563, #28699, #179398, #11546, #197539, #136843, #181385, #183360, #180400, #90335, #106498, #40862, #26709, #164219, #87362, #149047, #57037, #134885, #196561, #118710, #58032, #42864, #139803, #126622, #125646, #95297, #45829, #31656, #46824, #92315, #171160, #3291, #122659, #93305, #156981, #141797, #110467, #62969, #124649, #79133, #184347, #30662, #186345, #154990, #140805, #188323, #63976, #17476, #170163, #49802, #16486, #78135, #172149, #18479, #80128, #64963, #111467, #187344, #303, #47825, #33635, #48814, #173152, #34627, #96286, #1291, #157972, #60984, #109476, #107480, #169158, #19465, #185334, #154000, #15496, #32646, #77152, #94301, #138823, #81110, #155979, #142790, #61971, #123637, #108484, #2295, #50798, #52771, #38622, #8280, #145781, #24466, #174147, #191295, #144783, #35619, #129599, #68947, #99273, #66949, #20442, #98257, #69958, #86116, #128611, #54782, #39611, #100279, #85101, #158952, #146787, #116457, #130610, #97264, #53786, #175133, #189321, #176142, #4271, #162960, #22453, #131624, #190303, #192306, #114440, #82093 ) ),
 .UNSPECIFIED., .T., .F., .F. ) 
 B_SPLINE_SURFACE_WITH_KNOTS ( ( 4, 3, 4 ),
 ( 3, 2, 2, 2, 2, 2, 2, 2, 2, 2, 2, 2, 2, 2, 2, 2, 2, 2, 2, 2, 2, 2, 2, 2, 2, 2, 2, 2, 2, 2, 2, 2, 2, 2, 2, 2, 2, 2, 2, 2, 2, 2, 2, 2, 2, 2, 2, 2, 2, 2, 2, 2, 2, 2, 2, 2, 2, 2, 2, 2, 2, 2, 2, 2, 2, 2, 2, 2, 2, 2, 2, 2, 2, 2, 2, 2, 2, 2, 2, 2, 2, 2, 2, 2, 2, 2, 2, 2, 2, 2, 2, 2, 2, 2, 2, 2, 2, 2, 2, 2, 2, 2, 2, 2, 2, 2, 2, 2, 2, 2, 2, 2, 2, 2, 2, 2, 2, 2, 2, 2, 2, 2, 2, 2, 2, 2, 2, 2, 2, 2, 2, 2, 2, 2, 2, 2, 2, 2, 2, 2, 2, 2, 2, 2, 2, 2, 2, 2, 2, 2, 2, 2, 2, 2, 2, 2, 2, 2, 2, 2, 2, 2, 2, 2, 2, 2, 2, 2, 2, 2, 2, 2, 2, 2, 2, 2, 2, 2, 2, 2, 2, 2, 2, 2, 2, 2, 2, 2, 2, 2, 2, 2, 2, 2, 2, 2, 2, 2, 2, 2, 2, 2, 2, 2, 2, 2, 2, 2, 2, 2, 2, 2, 2, 2, 2, 2, 2, 2, 2, 2, 2, 2, 2, 2, 2, 2, 2, 2, 3 ),
 ( 0.000000000000000000, 0.5000000000000000000, 1.000000000000000000 ),
 ( 0.000000000000000000, 0.004385964912280701511, 0.008771929824561403022, 0.01315789473684210453, 0.01754385964912280604, 0.02192982456140350755, 0.02631578947368420907, 0.03070175438596491058, 0.03508771929824561209, 0.03947368421052631360, 0.04385964912280701511, 0.04824561403508771662, 0.05263157894736841813, 0.05701754385964911964, 0.06140350877192982115, 0.06578947368421052266, 0.07017543859649122417, 0.07456140350877192569, 0.07894736842105262720, 0.08333333333333332871, 0.08771929824561403022, 0.09210526315789473173, 0.09649122807017543324, 0.1008771929824561348, 0.1052631578947368363, 0.1096491228070175378, 0.1140350877192982393, 0.1184210526315789408, 0.1228070175438596423, 0.1271929824561403577, 0.1315789473684210453, 0.1359649122807017607, 0.1403508771929824483, 0.1447368421052631637, 0.1491228070175438514, 0.1535087719298245668, 0.1578947368421052544, 0.1622807017543859698, 0.1666666666666666574, 0.1710526315789473728, 0.1754385964912280604, 0.1798245614035087758, 0.1842105263157894635, 0.1885964912280701788, 0.1929824561403508665, 0.1973684210526315819, 0.2017543859649122695, 0.2061403508771929849, 0.2105263157894736725, 0.2149122807017543879, 0.2192982456140350755, 0.2236842105263157909, 0.2280701754385964786, 0.2324561403508771940, 0.2368421052631578816, 0.2412280701754385970, 0.2456140350877192846, 0.2500000000000000000, 0.2543859649122807154, 0.2587719298245614308, 0.2631578947368420907, 0.2675438596491228060, 0.2719298245614035214, 0.2763157894736842368, 0.2807017543859648967, 0.2850877192982456121, 0.2894736842105263275, 0.2938596491228070429, 0.2982456140350877027, 0.3026315789473684181, 0.3070175438596491335, 0.3114035087719298489, 0.3157894736842105088, 0.3201754385964912242, 0.3245614035087719396, 0.3289473684210526550, 0.3333333333333333148, 0.3377192982456140302, 0.3421052631578947456, 0.3464912280701754610, 0.3508771929824561209, 0.3552631578947368363, 0.3596491228070175517, 0.3640350877192982670, 0.3684210526315789269, 0.3728070175438596423, 0.3771929824561403577, 0.3815789473684210731, 0.3859649122807017330, 0.3903508771929824483, 0.3947368421052631637, 0.3991228070175438791, 0.4035087719298245390, 0.4078947368421052544, 0.4122807017543859698, 0.4166666666666666852, 0.4210526315789473450, 0.4254385964912280604, 0.4298245614035087758, 0.4342105263157894912, 0.4385964912280701511, 0.4429824561403508665, 0.4473684210526315819, 0.4517543859649122973, 0.4561403508771929571, 0.4605263157894736725, 0.4649122807017543879, 0.4692982456140351033, 0.4736842105263157632, 0.4780701754385964786, 0.4824561403508771940, 0.4868421052631579093, 0.4912280701754385692, 0.4956140350877192846, 0.5000000000000000000, 0.5043859649122807154, 0.5087719298245614308, 0.5131578947368421462, 0.5175438596491228616, 0.5219298245614034659, 0.5263157894736841813, 0.5307017543859648967, 0.5350877192982456121, 0.5394736842105263275, 0.5438596491228070429, 0.5482456140350877583, 0.5526315789473684736, 0.5570175438596490780, 0.5614035087719297934, 0.5657894736842105088, 0.5701754385964912242, 0.5745614035087719396, 0.5789473684210526550, 0.5833333333333333703, 0.5877192982456140857, 0.5921052631578946901, 0.5964912280701754055, 0.6008771929824561209, 0.6052631578947368363, 0.6096491228070175517, 0.6140350877192982670, 0.6184210526315789824, 0.6228070175438596978, 0.6271929824561403022, 0.6315789473684210176, 0.6359649122807017330, 0.6403508771929824483, 0.6447368421052631637, 0.6491228070175438791, 0.6535087719298245945, 0.6578947368421053099, 0.6622807017543859143, 0.6666666666666666297, 0.6710526315789473450, 0.6754385964912280604, 0.6798245614035087758, 0.6842105263157894912, 0.6885964912280702066, 0.6929824561403509220, 0.6973684210526315264, 0.7017543859649122417, 0.7061403508771929571, 0.7105263157894736725, 0.7149122807017543879, 0.7192982456140351033, 0.7236842105263158187, 0.7280701754385965341, 0.7324561403508771384, 0.7368421052631578538, 0.7412280701754385692, 0.7456140350877192846, 0.7500000000000000000, 0.7543859649122807154, 0.7587719298245614308, 0.7631578947368421462, 0.7675438596491228616, 0.7719298245614034659, 0.7763157894736841813, 0.7807017543859648967, 0.7850877192982456121, 0.7894736842105263275, 0.7938596491228070429, 0.7982456140350877583, 0.8026315789473684736, 0.8070175438596490780, 0.8114035087719297934, 0.8157894736842105088, 0.8201754385964912242, 0.8245614035087719396, 0.8289473684210526550, 0.8333333333333333703, 0.8377192982456140857, 0.8421052631578946901, 0.8464912280701754055, 0.8508771929824561209, 0.8552631578947368363, 0.8596491228070175517, 0.8640350877192982670, 0.8684210526315789824, 0.8728070175438596978, 0.8771929824561403022, 0.8815789473684210176, 0.8859649122807017330, 0.8903508771929824483, 0.8947368421052631637, 0.8991228070175438791, 0.9035087719298245945, 0.9078947368421053099, 0.9122807017543859143, 0.9166666666666666297, 0.9210526315789473450, 0.9254385964912280604, 0.9298245614035087758, 0.9342105263157894912, 0.9385964912280702066, 0.9429824561403509220, 0.9473684210526315264, 0.9517543859649122417, 0.9561403508771929571, 0.9605263157894736725, 0.9649122807017543879, 0.9692982456140351033, 0.9736842105263158187, 0.9780701754385965341, 0.9824561403508771384, 0.9868421052631578538, 0.9912280701754385692, 0.9956140350877192846, 1.000000000000000000 ),
 .UNSPECIFIED. ) 
 GEOMETRIC_REPRESENTATION_ITEM ( )  RATIONAL_B_SPLINE_SURFACE ( (
 ( 1.000000000000000000, 0.9659258262890683122, 1.000000000000000000, 0.9659258262890683122, 1.000000000000000000, 0.9659258262890683122, 1.000000000000000000, 0.9659258262890683122, 1.000000000000000000, 0.9659258262890683122, 1.000000000000000000, 0.9659258262890683122, 1.000000000000000000, 0.9659258262890683122, 1.000000000000000000, 0.9659258262890683122, 1.000000000000000000, 0.9659258262890683122, 1.000000000000000000, 0.9659258262890683122, 1.000000000000000000, 0.9659258262890683122, 1.000000000000000000, 0.9659258262890683122, 1.000000000000000000, 0.9659258262890683122, 1.000000000000000000, 0.9659258262890683122, 1.000000000000000000, 0.9659258262890683122, 1.000000000000000000, 0.9659258262890683122, 1.000000000000000000, 0.9659258262890683122, 1.000000000000000000, 0.9659258262890683122, 1.000000000000000000, 0.9659258262890683122, 1.000000000000000000, 0.9659258262890683122, 1.000000000000000000, 0.9659258262890683122, 1.000000000000000000, 0.9659258262890683122, 1.000000000000000000, 0.9659258262890683122, 1.000000000000000000, 0.9659258262890683122, 1.000000000000000000, 0.9659258262890683122, 1.000000000000000000, 0.9659258262890683122, 1.000000000000000000, 0.9659258262890683122, 1.000000000000000000, 0.9659258262890683122, 1.000000000000000000, 0.9659258262890683122, 1.000000000000000000, 0.9659258262890683122, 1.000000000000000000, 0.9659258262890683122, 1.000000000000000000, 0.9659258262890683122, 1.000000000000000000, 0.9659258262890683122, 1.000000000000000000, 0.9659258262890683122, 1.000000000000000000, 0.9659258262890683122, 1.000000000000000000, 0.9659258262890683122, 1.000000000000000000, 0.9659258262890683122, 1.000000000000000000, 0.9659258262890683122, 1.000000000000000000, 0.9659258262890683122, 1.000000000000000000, 0.9659258262890683122, 1.000000000000000000, 0.9659258262890683122, 1.000000000000000000, 0.9659258262890683122, 1.000000000000000000, 0.9659258262890683122, 1.000000000000000000, 0.9659258262890683122, 1.000000000000000000, 0.9659258262890683122, 1.000000000000000000, 0.9659258262890683122, 1.000000000000000000, 0.9659258262890683122, 1.000000000000000000, 0.9659258262890683122, 1.000000000000000000, 0.9659258262890683122, 1.000000000000000000, 0.9659258262890683122, 1.000000000000000000, 0.9659258262890683122, 1.000000000000000000, 0.9659258262890683122, 1.000000000000000000, 0.9659258262890683122, 1.000000000000000000, 0.9659258262890683122, 1.000000000000000000, 0.9659258262890683122, 1.000000000000000000, 0.9659258262890683122, 1.000000000000000000, 0.9659258262890683122, 1.000000000000000000, 0.9659258262890683122, 1.000000000000000000, 0.9659258262890683122, 1.000000000000000000, 0.9659258262890683122, 1.000000000000000000, 0.9659258262890683122, 1.000000000000000000, 0.9659258262890683122, 1.000000000000000000, 0.9659258262890683122, 1.000000000000000000, 0.9659258262890683122, 1.000000000000000000, 0.9659258262890683122, 1.000000000000000000, 0.9659258262890683122, 1.000000000000000000, 0.9659258262890683122, 1.000000000000000000, 0.9659258262890683122, 1.000000000000000000, 0.9659258262890683122, 1.000000000000000000, 0.9659258262890683122, 1.000000000000000000, 0.9659258262890683122, 1.000000000000000000, 0.9659258262890683122, 1.000000000000000000, 0.9659258262890683122, 1.000000000000000000, 0.9659258262890683122, 1.000000000000000000, 0.9659258262890683122, 1.000000000000000000, 0.9659258262890683122, 1.000000000000000000, 0.9659258262890683122, 1.000000000000000000, 0.9659258262890683122, 1.000000000000000000, 0.9659258262890683122, 1.000000000000000000, 0.9659258262890683122, 1.000000000000000000, 0.9659258262890683122, 1.000000000000000000, 0.9659258262890683122, 1.000000000000000000, 0.9659258262890683122, 1.000000000000000000, 0.9659258262890683122, 1.000000000000000000, 0.9659258262890683122, 1.000000000000000000, 0.9659258262890683122, 1.000000000000000000, 0.9659258262890683122, 1.000000000000000000, 0.9659258262890683122, 1.000000000000000000, 0.9659258262890683122, 1.000000000000000000, 0.9659258262890683122, 1.000000000000000000, 0.9659258262890683122, 1.000000000000000000, 0.9659258262890683122, 1.000000000000000000, 0.9659258262890683122, 1.000000000000000000, 0.9659258262890683122, 1.000000000000000000, 0.9659258262890683122, 1.000000000000000000, 0.9659258262890683122, 1.000000000000000000, 0.9659258262890683122, 1.000000000000000000, 0.9659258262890683122, 1.000000000000000000, 0.9659258262890683122, 1.000000000000000000, 0.9659258262890683122, 1.000000000000000000, 0.9659258262890683122, 1.000000000000000000, 0.9659258262890683122, 1.000000000000000000, 0.9659258262890683122, 1.000000000000000000, 0.9659258262890683122, 1.000000000000000000, 0.9659258262890683122, 1.000000000000000000, 0.9659258262890683122, 1.000000000000000000, 0.9659258262890683122, 1.000000000000000000, 0.9659258262890683122, 1.000000000000000000, 0.9659258262890683122, 1.000000000000000000, 0.9659258262890683122, 1.000000000000000000, 0.9659258262890683122, 1.000000000000000000, 0.9659258262890683122, 1.000000000000000000, 0.9659258262890683122, 1.000000000000000000, 0.9659258262890683122, 1.000000000000000000, 0.9659258262890683122, 1.000000000000000000, 0.9659258262890683122, 1.000000000000000000, 0.9659258262890683122, 1.000000000000000000, 0.9659258262890683122, 1.000000000000000000, 0.9659258262890683122, 1.000000000000000000, 0.9659258262890683122, 1.000000000000000000, 0.9659258262890683122, 1.000000000000000000, 0.9659258262890683122, 1.000000000000000000, 0.9659258262890683122, 1.000000000000000000, 0.9659258262890683122, 1.000000000000000000, 0.9659258262890683122, 1.000000000000000000, 0.9659258262890683122, 1.000000000000000000, 0.9659258262890683122, 1.000000000000000000, 0.9659258262890683122, 1.000000000000000000, 0.9659258262890683122, 1.000000000000000000, 0.9659258262890683122, 1.000000000000000000, 0.9659258262890683122, 1.000000000000000000, 0.9659258262890683122, 1.000000000000000000, 0.9659258262890683122, 1.000000000000000000, 0.9659258262890683122, 1.000000000000000000, 0.9659258262890683122, 1.000000000000000000, 0.9659258262890683122, 1.000000000000000000, 0.9659258262890683122, 1.000000000000000000, 0.9659258262890683122, 1.000000000000000000, 0.9659258262890683122, 1.000000000000000000, 0.9659258262890683122, 1.000000000000000000, 0.9659258262890683122, 1.000000000000000000, 0.9659258262890683122, 1.000000000000000000, 0.9659258262890683122, 1.000000000000000000, 0.9659258262890683122, 1.000000000000000000, 0.9659258262890683122, 1.000000000000000000, 0.9659258262890683122, 1.000000000000000000, 0.9659258262890683122, 1.000000000000000000, 0.9659258262890683122, 1.000000000000000000, 0.9659258262890683122, 1.000000000000000000, 0.9659258262890683122, 1.000000000000000000, 0.9659258262890683122, 1.000000000000000000, 0.9659258262890683122, 1.000000000000000000, 0.9659258262890683122, 1.000000000000000000, 0.9659258262890683122, 1.000000000000000000, 0.9659258262890683122, 1.000000000000000000, 0.9659258262890683122, 1.000000000000000000, 0.9659258262890683122, 1.000000000000000000, 0.9659258262890683122, 1.000000000000000000, 0.9659258262890683122, 1.000000000000000000, 0.9659258262890683122, 1.000000000000000000, 0.9659258262890683122, 1.000000000000000000, 0.9659258262890683122, 1.000000000000000000, 0.9659258262890683122, 1.000000000000000000, 0.9659258262890683122, 1.000000000000000000, 0.9659258262890683122, 1.000000000000000000, 0.9659258262890683122, 1.000000000000000000, 0.9659258262890683122, 1.000000000000000000, 0.9659258262890683122, 1.000000000000000000, 0.9659258262890683122, 1.000000000000000000, 0.9659258262890683122, 1.000000000000000000, 0.9659258262890683122, 1.000000000000000000, 0.9659258262890683122, 1.000000000000000000, 0.9659258262890683122, 1.000000000000000000, 0.9659258262890683122, 1.000000000000000000, 0.9659258262890683122, 1.000000000000000000, 0.9659258262890683122, 1.000000000000000000, 0.9659258262890683122, 1.000000000000000000, 0.9659258262890683122, 1.000000000000000000, 0.9659258262890683122, 1.000000000000000000, 0.9659258262890683122, 1.000000000000000000, 0.9659258262890683122, 1.000000000000000000, 0.9659258262890683122, 1.000000000000000000, 0.9659258262890683122, 1.000000000000000000, 0.9659258262890683122, 1.000000000000000000, 0.9659258262890683122, 1.000000000000000000, 0.9659258262890683122, 1.000000000000000000, 0.9659258262890683122, 1.000000000000000000, 0.9659258262890683122, 1.000000000000000000, 0.9659258262890683122, 1.000000000000000000, 0.9659258262890683122, 1.000000000000000000, 0.9659258262890683122, 1.000000000000000000, 0.9659258262890683122, 1.000000000000000000, 0.9659258262890683122, 1.000000000000000000, 0.9659258262890683122, 1.000000000000000000, 0.9659258262890683122, 1.000000000000000000, 0.9659258262890683122, 1.000000000000000000, 0.9659258262890683122, 1.000000000000000000, 0.9659258262890683122, 1.000000000000000000, 0.9659258262890683122, 1.000000000000000000, 0.9659258262890683122, 1.000000000000000000, 0.9659258262890683122, 1.000000000000000000, 0.9659258262890683122, 1.000000000000000000, 0.9659258262890683122, 1.000000000000000000, 0.9659258262890683122, 1.000000000000000000, 0.9659258262890683122, 1.000000000000000000, 0.9659258262890683122, 1.000000000000000000, 0.9659258262890683122, 1.000000000000000000, 0.9659258262890683122, 1.000000000000000000, 0.9659258262890683122, 1.000000000000000000, 0.9659258262890683122, 1.000000000000000000, 0.9659258262890683122, 1.000000000000000000, 0.9659258262890683122, 1.000000000000000000, 0.9659258262890683122, 1.000000000000000000, 0.9659258262890683122, 1.000000000000000000, 0.9659258262890683122, 1.000000000000000000, 0.9659258262890683122, 1.000000000000000000, 0.9659258262890683122, 1.000000000000000000, 0.9659258262890683122, 1.000000000000000000, 0.9659258262890683122, 1.000000000000000000, 0.9659258262890683122, 1.000000000000000000, 0.9659258262890683122, 1.000000000000000000, 0.9659258262890683122, 1.000000000000000000, 0.9659258262890683122, 1.000000000000000000, 0.9659258262890683122, 1.000000000000000000, 0.9659258262890683122, 1.000000000000000000, 0.9659258262890683122, 1.000000000000000000, 0.9659258262890683122, 1.000000000000000000, 0.9659258262890683122, 1.000000000000000000),
 ( 0.3333333333333333703, 0.3219752754296894559, 0.3333333333333333703, 0.3219752754296894559, 0.3333333333333333703, 0.3219752754296894559, 0.3333333333333333703, 0.3219752754296894559, 0.3333333333333333703, 0.3219752754296894559, 0.3333333333333333703, 0.3219752754296894559, 0.3333333333333333703, 0.3219752754296894559, 0.3333333333333333703, 0.3219752754296894559, 0.3333333333333333703, 0.3219752754296894559, 0.3333333333333333703, 0.3219752754296894559, 0.3333333333333333703, 0.3219752754296894559, 0.3333333333333333703, 0.3219752754296894559, 0.3333333333333333703, 0.3219752754296894559, 0.3333333333333333703, 0.3219752754296894559, 0.3333333333333333703, 0.3219752754296894559, 0.3333333333333333703, 0.3219752754296894559, 0.3333333333333333703, 0.3219752754296894559, 0.3333333333333333703, 0.3219752754296894559, 0.3333333333333333703, 0.3219752754296894559, 0.3333333333333333703, 0.3219752754296894559, 0.3333333333333333703, 0.3219752754296894559, 0.3333333333333333703, 0.3219752754296894559, 0.3333333333333333703, 0.3219752754296894559, 0.3333333333333333703, 0.3219752754296894559, 0.3333333333333333703, 0.3219752754296894559, 0.3333333333333333703, 0.3219752754296894559, 0.3333333333333333703, 0.3219752754296894559, 0.3333333333333333703, 0.3219752754296894559, 0.3333333333333333703, 0.3219752754296894559, 0.3333333333333333703, 0.3219752754296894559, 0.3333333333333333703, 0.3219752754296894559, 0.3333333333333333703, 0.3219752754296894559, 0.3333333333333333703, 0.3219752754296894559, 0.3333333333333333703, 0.3219752754296894559, 0.3333333333333333703, 0.3219752754296894559, 0.3333333333333333703, 0.3219752754296894559, 0.3333333333333333703, 0.3219752754296894559, 0.3333333333333333703, 0.3219752754296894559, 0.3333333333333333703, 0.3219752754296894559, 0.3333333333333333703, 0.3219752754296894559, 0.3333333333333333703, 0.3219752754296894559, 0.3333333333333333703, 0.3219752754296894559, 0.3333333333333333703, 0.3219752754296894559, 0.3333333333333333703, 0.3219752754296894559, 0.3333333333333333703, 0.3219752754296894559, 0.3333333333333333703, 0.3219752754296894559, 0.3333333333333333703, 0.3219752754296894559, 0.3333333333333333703, 0.3219752754296894559, 0.3333333333333333703, 0.3219752754296894559, 0.3333333333333333703, 0.3219752754296894559, 0.3333333333333333703, 0.3219752754296894559, 0.3333333333333333703, 0.3219752754296894559, 0.3333333333333333703, 0.3219752754296894559, 0.3333333333333333703, 0.3219752754296894559, 0.3333333333333333703, 0.3219752754296894559, 0.3333333333333333703, 0.3219752754296894559, 0.3333333333333333703, 0.3219752754296894559, 0.3333333333333333703, 0.3219752754296894559, 0.3333333333333333703, 0.3219752754296894559, 0.3333333333333333703, 0.3219752754296894559, 0.3333333333333333703, 0.3219752754296894559, 0.3333333333333333703, 0.3219752754296894559, 0.3333333333333333703, 0.3219752754296894559, 0.3333333333333333703, 0.3219752754296894559, 0.3333333333333333703, 0.3219752754296894559, 0.3333333333333333703, 0.3219752754296894559, 0.3333333333333333703, 0.3219752754296894559, 0.3333333333333333703, 0.3219752754296894559, 0.3333333333333333703, 0.3219752754296894559, 0.3333333333333333703, 0.3219752754296894559, 0.3333333333333333703, 0.3219752754296894559, 0.3333333333333333703, 0.3219752754296894559, 0.3333333333333333703, 0.3219752754296894559, 0.3333333333333333703, 0.3219752754296894559, 0.3333333333333333703, 0.3219752754296894559, 0.3333333333333333703, 0.3219752754296894559, 0.3333333333333333703, 0.3219752754296894559, 0.3333333333333333703, 0.3219752754296894559, 0.3333333333333333703, 0.3219752754296894559, 0.3333333333333333703, 0.3219752754296894559, 0.3333333333333333703, 0.3219752754296894559, 0.3333333333333333703, 0.3219752754296894559, 0.3333333333333333703, 0.3219752754296894559, 0.3333333333333333703, 0.3219752754296894559, 0.3333333333333333703, 0.3219752754296894559, 0.3333333333333333703, 0.3219752754296894559, 0.3333333333333333703, 0.3219752754296894559, 0.3333333333333333703, 0.3219752754296894559, 0.3333333333333333703, 0.3219752754296894559, 0.3333333333333333703, 0.3219752754296894559, 0.3333333333333333703, 0.3219752754296894559, 0.3333333333333333703, 0.3219752754296894559, 0.3333333333333333703, 0.3219752754296894559, 0.3333333333333333703, 0.3219752754296894559, 0.3333333333333333703, 0.3219752754296894559, 0.3333333333333333703, 0.3219752754296894559, 0.3333333333333333703, 0.3219752754296894559, 0.3333333333333333703, 0.3219752754296894559, 0.3333333333333333703, 0.3219752754296894559, 0.3333333333333333703, 0.3219752754296894559, 0.3333333333333333703, 0.3219752754296894559, 0.3333333333333333703, 0.3219752754296894559, 0.3333333333333333703, 0.3219752754296894559, 0.3333333333333333703, 0.3219752754296894559, 0.3333333333333333703, 0.3219752754296894559, 0.3333333333333333703, 0.3219752754296894559, 0.3333333333333333703, 0.3219752754296894559, 0.3333333333333333703, 0.3219752754296894559, 0.3333333333333333703, 0.3219752754296894559, 0.3333333333333333703, 0.3219752754296894559, 0.3333333333333333703, 0.3219752754296894559, 0.3333333333333333703, 0.3219752754296894559, 0.3333333333333333703, 0.3219752754296894559, 0.3333333333333333703, 0.3219752754296894559, 0.3333333333333333703, 0.3219752754296894559, 0.3333333333333333703, 0.3219752754296894559, 0.3333333333333333703, 0.3219752754296894559, 0.3333333333333333703, 0.3219752754296894559, 0.3333333333333333703, 0.3219752754296894559, 0.3333333333333333703, 0.3219752754296894559, 0.3333333333333333703, 0.3219752754296894559, 0.3333333333333333703, 0.3219752754296894559, 0.3333333333333333703, 0.3219752754296894559, 0.3333333333333333703, 0.3219752754296894559, 0.3333333333333333703, 0.3219752754296894559, 0.3333333333333333703, 0.3219752754296894559, 0.3333333333333333703, 0.3219752754296894559, 0.3333333333333333703, 0.3219752754296894559, 0.3333333333333333703, 0.3219752754296894559, 0.3333333333333333703, 0.3219752754296894559, 0.3333333333333333703, 0.3219752754296894559, 0.3333333333333333703, 0.3219752754296894559, 0.3333333333333333703, 0.3219752754296894559, 0.3333333333333333703, 0.3219752754296894559, 0.3333333333333333703, 0.3219752754296894559, 0.3333333333333333703, 0.3219752754296894559, 0.3333333333333333703, 0.3219752754296894559, 0.3333333333333333703, 0.3219752754296894559, 0.3333333333333333703, 0.3219752754296894559, 0.3333333333333333703, 0.3219752754296894559, 0.3333333333333333703, 0.3219752754296894559, 0.3333333333333333703, 0.3219752754296894559, 0.3333333333333333703, 0.3219752754296894559, 0.3333333333333333703, 0.3219752754296894559, 0.3333333333333333703, 0.3219752754296894559, 0.3333333333333333703, 0.3219752754296894559, 0.3333333333333333703, 0.3219752754296894559, 0.3333333333333333703, 0.3219752754296894559, 0.3333333333333333703, 0.3219752754296894559, 0.3333333333333333703, 0.3219752754296894559, 0.3333333333333333703, 0.3219752754296894559, 0.3333333333333333703, 0.3219752754296894559, 0.3333333333333333703, 0.3219752754296894559, 0.3333333333333333703, 0.3219752754296894559, 0.3333333333333333703, 0.3219752754296894559, 0.3333333333333333703, 0.3219752754296894559, 0.3333333333333333703, 0.3219752754296894559, 0.3333333333333333703, 0.3219752754296894559, 0.3333333333333333703, 0.3219752754296894559, 0.3333333333333333703, 0.3219752754296894559, 0.3333333333333333703, 0.3219752754296894559, 0.3333333333333333703, 0.3219752754296894559, 0.3333333333333333703, 0.3219752754296894559, 0.3333333333333333703, 0.3219752754296894559, 0.3333333333333333703, 0.3219752754296894559, 0.3333333333333333703, 0.3219752754296894559, 0.3333333333333333703, 0.3219752754296894559, 0.3333333333333333703, 0.3219752754296894559, 0.3333333333333333703, 0.3219752754296894559, 0.3333333333333333703, 0.3219752754296894559, 0.3333333333333333703, 0.3219752754296894559, 0.3333333333333333703, 0.3219752754296894559, 0.3333333333333333703, 0.3219752754296894559, 0.3333333333333333703, 0.3219752754296894559, 0.3333333333333333703, 0.3219752754296894559, 0.3333333333333333703, 0.3219752754296894559, 0.3333333333333333703, 0.3219752754296894559, 0.3333333333333333703, 0.3219752754296894559, 0.3333333333333333703, 0.3219752754296894559, 0.3333333333333333703, 0.3219752754296894559, 0.3333333333333333703, 0.3219752754296894559, 0.3333333333333333703, 0.3219752754296894559, 0.3333333333333333703, 0.3219752754296894559, 0.3333333333333333703, 0.3219752754296894559, 0.3333333333333333703, 0.3219752754296894559, 0.3333333333333333703, 0.3219752754296894559, 0.3333333333333333703, 0.3219752754296894559, 0.3333333333333333703, 0.3219752754296894559, 0.3333333333333333703, 0.3219752754296894559, 0.3333333333333333703, 0.3219752754296894559, 0.3333333333333333703, 0.3219752754296894559, 0.3333333333333333703, 0.3219752754296894559, 0.3333333333333333703, 0.3219752754296894559, 0.3333333333333333703, 0.3219752754296894559, 0.3333333333333333703, 0.3219752754296894559, 0.3333333333333333703, 0.3219752754296894559, 0.3333333333333333703, 0.3219752754296894559, 0.3333333333333333703, 0.3219752754296894559, 0.3333333333333333703, 0.3219752754296894559, 0.3333333333333333703, 0.3219752754296894559, 0.3333333333333333703, 0.3219752754296894559, 0.3333333333333333703, 0.3219752754296894559, 0.3333333333333333703, 0.3219752754296894559, 0.3333333333333333703, 0.3219752754296894559, 0.3333333333333333703, 0.3219752754296894559, 0.3333333333333333703, 0.3219752754296894559, 0.3333333333333333703, 0.3219752754296894559, 0.3333333333333333703, 0.3219752754296894559, 0.3333333333333333703, 0.3219752754296894559, 0.3333333333333333703, 0.3219752754296894559, 0.3333333333333333703, 0.3219752754296894559, 0.3333333333333333703, 0.3219752754296894559, 0.3333333333333333703, 0.3219752754296894559, 0.3333333333333333703, 0.3219752754296894559, 0.3333333333333333703, 0.3219752754296894559, 0.3333333333333333703, 0.3219752754296894559, 0.3333333333333333703, 0.3219752754296894559, 0.3333333333333333703, 0.3219752754296894559, 0.3333333333333333703, 0.3219752754296894559, 0.3333333333333333703, 0.3219752754296894559, 0.3333333333333333703, 0.3219752754296894559, 0.3333333333333333703, 0.3219752754296894559, 0.3333333333333333703, 0.3219752754296894559, 0.3333333333333333703, 0.3219752754296894559, 0.3333333333333333703, 0.3219752754296894559, 0.3333333333333333703, 0.3219752754296894559, 0.3333333333333333703, 0.3219752754296894559, 0.3333333333333333703, 0.3219752754296894559, 0.3333333333333333703),
 ( 0.3333333333333333703, 0.3219752754296894559, 0.3333333333333333703, 0.3219752754296894559, 0.3333333333333333703, 0.3219752754296894559, 0.3333333333333333703, 0.3219752754296894559, 0.3333333333333333703, 0.3219752754296894559, 0.3333333333333333703, 0.3219752754296894559, 0.3333333333333333703, 0.3219752754296894559, 0.3333333333333333703, 0.3219752754296894559, 0.3333333333333333703, 0.3219752754296894559, 0.3333333333333333703, 0.3219752754296894559, 0.3333333333333333703, 0.3219752754296894559, 0.3333333333333333703, 0.3219752754296894559, 0.3333333333333333703, 0.3219752754296894559, 0.3333333333333333703, 0.3219752754296894559, 0.3333333333333333703, 0.3219752754296894559, 0.3333333333333333703, 0.3219752754296894559, 0.3333333333333333703, 0.3219752754296894559, 0.3333333333333333703, 0.3219752754296894559, 0.3333333333333333703, 0.3219752754296894559, 0.3333333333333333703, 0.3219752754296894559, 0.3333333333333333703, 0.3219752754296894559, 0.3333333333333333703, 0.3219752754296894559, 0.3333333333333333703, 0.3219752754296894559, 0.3333333333333333703, 0.3219752754296894559, 0.3333333333333333703, 0.3219752754296894559, 0.3333333333333333703, 0.3219752754296894559, 0.3333333333333333703, 0.3219752754296894559, 0.3333333333333333703, 0.3219752754296894559, 0.3333333333333333703, 0.3219752754296894559, 0.3333333333333333703, 0.3219752754296894559, 0.3333333333333333703, 0.3219752754296894559, 0.3333333333333333703, 0.3219752754296894559, 0.3333333333333333703, 0.3219752754296894559, 0.3333333333333333703, 0.3219752754296894559, 0.3333333333333333703, 0.3219752754296894559, 0.3333333333333333703, 0.3219752754296894559, 0.3333333333333333703, 0.3219752754296894559, 0.3333333333333333703, 0.3219752754296894559, 0.3333333333333333703, 0.3219752754296894559, 0.3333333333333333703, 0.3219752754296894559, 0.3333333333333333703, 0.3219752754296894559, 0.3333333333333333703, 0.3219752754296894559, 0.3333333333333333703, 0.3219752754296894559, 0.3333333333333333703, 0.3219752754296894559, 0.3333333333333333703, 0.3219752754296894559, 0.3333333333333333703, 0.3219752754296894559, 0.3333333333333333703, 0.3219752754296894559, 0.3333333333333333703, 0.3219752754296894559, 0.3333333333333333703, 0.3219752754296894559, 0.3333333333333333703, 0.3219752754296894559, 0.3333333333333333703, 0.3219752754296894559, 0.3333333333333333703, 0.3219752754296894559, 0.3333333333333333703, 0.3219752754296894559, 0.3333333333333333703, 0.3219752754296894559, 0.3333333333333333703, 0.3219752754296894559, 0.3333333333333333703, 0.3219752754296894559, 0.3333333333333333703, 0.3219752754296894559, 0.3333333333333333703, 0.3219752754296894559, 0.3333333333333333703, 0.3219752754296894559, 0.3333333333333333703, 0.3219752754296894559, 0.3333333333333333703, 0.3219752754296894559, 0.3333333333333333703, 0.3219752754296894559, 0.3333333333333333703, 0.3219752754296894559, 0.3333333333333333703, 0.3219752754296894559, 0.3333333333333333703, 0.3219752754296894559, 0.3333333333333333703, 0.3219752754296894559, 0.3333333333333333703, 0.3219752754296894559, 0.3333333333333333703, 0.3219752754296894559, 0.3333333333333333703, 0.3219752754296894559, 0.3333333333333333703, 0.3219752754296894559, 0.3333333333333333703, 0.3219752754296894559, 0.3333333333333333703, 0.3219752754296894559, 0.3333333333333333703, 0.3219752754296894559, 0.3333333333333333703, 0.3219752754296894559, 0.3333333333333333703, 0.3219752754296894559, 0.3333333333333333703, 0.3219752754296894559, 0.3333333333333333703, 0.3219752754296894559, 0.3333333333333333703, 0.3219752754296894559, 0.3333333333333333703, 0.3219752754296894559, 0.3333333333333333703, 0.3219752754296894559, 0.3333333333333333703, 0.3219752754296894559, 0.3333333333333333703, 0.3219752754296894559, 0.3333333333333333703, 0.3219752754296894559, 0.3333333333333333703, 0.3219752754296894559, 0.3333333333333333703, 0.3219752754296894559, 0.3333333333333333703, 0.3219752754296894559, 0.3333333333333333703, 0.3219752754296894559, 0.3333333333333333703, 0.3219752754296894559, 0.3333333333333333703, 0.3219752754296894559, 0.3333333333333333703, 0.3219752754296894559, 0.3333333333333333703, 0.3219752754296894559, 0.3333333333333333703, 0.3219752754296894559, 0.3333333333333333703, 0.3219752754296894559, 0.3333333333333333703, 0.3219752754296894559, 0.3333333333333333703, 0.3219752754296894559, 0.3333333333333333703, 0.3219752754296894559, 0.3333333333333333703, 0.3219752754296894559, 0.3333333333333333703, 0.3219752754296894559, 0.3333333333333333703, 0.3219752754296894559, 0.3333333333333333703, 0.3219752754296894559, 0.3333333333333333703, 0.3219752754296894559, 0.3333333333333333703, 0.3219752754296894559, 0.3333333333333333703, 0.3219752754296894559, 0.3333333333333333703, 0.3219752754296894559, 0.3333333333333333703, 0.3219752754296894559, 0.3333333333333333703, 0.3219752754296894559, 0.3333333333333333703, 0.3219752754296894559, 0.3333333333333333703, 0.3219752754296894559, 0.3333333333333333703, 0.3219752754296894559, 0.3333333333333333703, 0.3219752754296894559, 0.3333333333333333703, 0.3219752754296894559, 0.3333333333333333703, 0.3219752754296894559, 0.3333333333333333703, 0.3219752754296894559, 0.3333333333333333703, 0.3219752754296894559, 0.3333333333333333703, 0.3219752754296894559, 0.3333333333333333703, 0.3219752754296894559, 0.3333333333333333703, 0.3219752754296894559, 0.3333333333333333703, 0.3219752754296894559, 0.3333333333333333703, 0.3219752754296894559, 0.3333333333333333703, 0.3219752754296894559, 0.3333333333333333703, 0.3219752754296894559, 0.3333333333333333703, 0.3219752754296894559, 0.3333333333333333703, 0.3219752754296894559, 0.3333333333333333703, 0.3219752754296894559, 0.3333333333333333703, 0.3219752754296894559, 0.3333333333333333703, 0.3219752754296894559, 0.3333333333333333703, 0.3219752754296894559, 0.3333333333333333703, 0.3219752754296894559, 0.3333333333333333703, 0.3219752754296894559, 0.3333333333333333703, 0.3219752754296894559, 0.3333333333333333703, 0.3219752754296894559, 0.3333333333333333703, 0.3219752754296894559, 0.3333333333333333703, 0.3219752754296894559, 0.3333333333333333703, 0.3219752754296894559, 0.3333333333333333703, 0.3219752754296894559, 0.3333333333333333703, 0.3219752754296894559, 0.3333333333333333703, 0.3219752754296894559, 0.3333333333333333703, 0.3219752754296894559, 0.3333333333333333703, 0.3219752754296894559, 0.3333333333333333703, 0.3219752754296894559, 0.3333333333333333703, 0.3219752754296894559, 0.3333333333333333703, 0.3219752754296894559, 0.3333333333333333703, 0.3219752754296894559, 0.3333333333333333703, 0.3219752754296894559, 0.3333333333333333703, 0.3219752754296894559, 0.3333333333333333703, 0.3219752754296894559, 0.3333333333333333703, 0.3219752754296894559, 0.3333333333333333703, 0.3219752754296894559, 0.3333333333333333703, 0.3219752754296894559, 0.3333333333333333703, 0.3219752754296894559, 0.3333333333333333703, 0.3219752754296894559, 0.3333333333333333703, 0.3219752754296894559, 0.3333333333333333703, 0.3219752754296894559, 0.3333333333333333703, 0.3219752754296894559, 0.3333333333333333703, 0.3219752754296894559, 0.3333333333333333703, 0.3219752754296894559, 0.3333333333333333703, 0.3219752754296894559, 0.3333333333333333703, 0.3219752754296894559, 0.3333333333333333703, 0.3219752754296894559, 0.3333333333333333703, 0.3219752754296894559, 0.3333333333333333703, 0.3219752754296894559, 0.3333333333333333703, 0.3219752754296894559, 0.3333333333333333703, 0.3219752754296894559, 0.3333333333333333703, 0.3219752754296894559, 0.3333333333333333703, 0.3219752754296894559, 0.3333333333333333703, 0.3219752754296894559, 0.3333333333333333703, 0.3219752754296894559, 0.3333333333333333703, 0.3219752754296894559, 0.3333333333333333703, 0.3219752754296894559, 0.3333333333333333703, 0.3219752754296894559, 0.3333333333333333703, 0.3219752754296894559, 0.3333333333333333703, 0.3219752754296894559, 0.3333333333333333703, 0.3219752754296894559, 0.3333333333333333703, 0.3219752754296894559, 0.3333333333333333703, 0.3219752754296894559, 0.3333333333333333703, 0.3219752754296894559, 0.3333333333333333703, 0.3219752754296894559, 0.3333333333333333703, 0.3219752754296894559, 0.3333333333333333703, 0.3219752754296894559, 0.3333333333333333703, 0.3219752754296894559, 0.3333333333333333703, 0.3219752754296894559, 0.3333333333333333703, 0.3219752754296894559, 0.3333333333333333703, 0.3219752754296894559, 0.3333333333333333703, 0.3219752754296894559, 0.3333333333333333703, 0.3219752754296894559, 0.3333333333333333703, 0.3219752754296894559, 0.3333333333333333703, 0.3219752754296894559, 0.3333333333333333703, 0.3219752754296894559, 0.3333333333333333703, 0.3219752754296894559, 0.3333333333333333703, 0.3219752754296894559, 0.3333333333333333703, 0.3219752754296894559, 0.3333333333333333703, 0.3219752754296894559, 0.3333333333333333703, 0.3219752754296894559, 0.3333333333333333703, 0.3219752754296894559, 0.3333333333333333703, 0.3219752754296894559, 0.3333333333333333703, 0.3219752754296894559, 0.3333333333333333703, 0.3219752754296894559, 0.3333333333333333703, 0.3219752754296894559, 0.3333333333333333703, 0.3219752754296894559, 0.3333333333333333703, 0.3219752754296894559, 0.3333333333333333703, 0.3219752754296894559, 0.3333333333333333703, 0.3219752754296894559, 0.3333333333333333703, 0.3219752754296894559, 0.3333333333333333703, 0.3219752754296894559, 0.3333333333333333703, 0.3219752754296894559, 0.3333333333333333703, 0.3219752754296894559, 0.3333333333333333703, 0.3219752754296894559, 0.3333333333333333703, 0.3219752754296894559, 0.3333333333333333703, 0.3219752754296894559, 0.3333333333333333703, 0.3219752754296894559, 0.3333333333333333703, 0.3219752754296894559, 0.3333333333333333703, 0.3219752754296894559, 0.3333333333333333703, 0.3219752754296894559, 0.3333333333333333703, 0.3219752754296894559, 0.3333333333333333703, 0.3219752754296894559, 0.3333333333333333703, 0.3219752754296894559, 0.3333333333333333703, 0.3219752754296894559, 0.3333333333333333703, 0.3219752754296894559, 0.3333333333333333703, 0.3219752754296894559, 0.3333333333333333703, 0.3219752754296894559, 0.3333333333333333703, 0.3219752754296894559, 0.3333333333333333703, 0.3219752754296894559, 0.3333333333333333703, 0.3219752754296894559, 0.3333333333333333703, 0.3219752754296894559, 0.3333333333333333703, 0.3219752754296894559, 0.3333333333333333703, 0.3219752754296894559, 0.3333333333333333703, 0.3219752754296894559, 0.3333333333333333703, 0.3219752754296894559, 0.3333333333333333703),
 ( 1.000000000000000000, 0.9659258262890683122, 1.000000000000000000, 0.9659258262890683122, 1.000000000000000000, 0.9659258262890683122, 1.000000000000000000, 0.9659258262890683122, 1.000000000000000000, 0.9659258262890683122, 1.000000000000000000, 0.9659258262890683122, 1.000000000000000000, 0.9659258262890683122, 1.000000000000000000, 0.9659258262890683122, 1.000000000000000000, 0.9659258262890683122, 1.000000000000000000, 0.9659258262890683122, 1.000000000000000000, 0.9659258262890683122, 1.000000000000000000, 0.9659258262890683122, 1.000000000000000000, 0.9659258262890683122, 1.000000000000000000, 0.9659258262890683122, 1.000000000000000000, 0.9659258262890683122, 1.000000000000000000, 0.9659258262890683122, 1.000000000000000000, 0.9659258262890683122, 1.000000000000000000, 0.9659258262890683122, 1.000000000000000000, 0.9659258262890683122, 1.000000000000000000, 0.9659258262890683122, 1.000000000000000000, 0.9659258262890683122, 1.000000000000000000, 0.9659258262890683122, 1.000000000000000000, 0.9659258262890683122, 1.000000000000000000, 0.9659258262890683122, 1.000000000000000000, 0.9659258262890683122, 1.000000000000000000, 0.9659258262890683122, 1.000000000000000000, 0.9659258262890683122, 1.000000000000000000, 0.9659258262890683122, 1.000000000000000000, 0.9659258262890683122, 1.000000000000000000, 0.9659258262890683122, 1.000000000000000000, 0.9659258262890683122, 1.000000000000000000, 0.9659258262890683122, 1.000000000000000000, 0.9659258262890683122, 1.000000000000000000, 0.9659258262890683122, 1.000000000000000000, 0.9659258262890683122, 1.000000000000000000, 0.9659258262890683122, 1.000000000000000000, 0.9659258262890683122, 1.000000000000000000, 0.9659258262890683122, 1.000000000000000000, 0.9659258262890683122, 1.000000000000000000, 0.9659258262890683122, 1.000000000000000000, 0.9659258262890683122, 1.000000000000000000, 0.9659258262890683122, 1.000000000000000000, 0.9659258262890683122, 1.000000000000000000, 0.9659258262890683122, 1.000000000000000000, 0.9659258262890683122, 1.000000000000000000, 0.9659258262890683122, 1.000000000000000000, 0.9659258262890683122, 1.000000000000000000, 0.9659258262890683122, 1.000000000000000000, 0.9659258262890683122, 1.000000000000000000, 0.9659258262890683122, 1.000000000000000000, 0.9659258262890683122, 1.000000000000000000, 0.9659258262890683122, 1.000000000000000000, 0.9659258262890683122, 1.000000000000000000, 0.9659258262890683122, 1.000000000000000000, 0.9659258262890683122, 1.000000000000000000, 0.9659258262890683122, 1.000000000000000000, 0.9659258262890683122, 1.000000000000000000, 0.9659258262890683122, 1.000000000000000000, 0.9659258262890683122, 1.000000000000000000, 0.9659258262890683122, 1.000000000000000000, 0.9659258262890683122, 1.000000000000000000, 0.9659258262890683122, 1.000000000000000000, 0.9659258262890683122, 1.000000000000000000, 0.9659258262890683122, 1.000000000000000000, 0.9659258262890683122, 1.000000000000000000, 0.9659258262890683122, 1.000000000000000000, 0.9659258262890683122, 1.000000000000000000, 0.9659258262890683122, 1.000000000000000000, 0.9659258262890683122, 1.000000000000000000, 0.9659258262890683122, 1.000000000000000000, 0.9659258262890683122, 1.000000000000000000, 0.9659258262890683122, 1.000000000000000000, 0.9659258262890683122, 1.000000000000000000, 0.9659258262890683122, 1.000000000000000000, 0.9659258262890683122, 1.000000000000000000, 0.9659258262890683122, 1.000000000000000000, 0.9659258262890683122, 1.000000000000000000, 0.9659258262890683122, 1.000000000000000000, 0.9659258262890683122, 1.000000000000000000, 0.9659258262890683122, 1.000000000000000000, 0.9659258262890683122, 1.000000000000000000, 0.9659258262890683122, 1.000000000000000000, 0.9659258262890683122, 1.000000000000000000, 0.9659258262890683122, 1.000000000000000000, 0.9659258262890683122, 1.000000000000000000, 0.9659258262890683122, 1.000000000000000000, 0.9659258262890683122, 1.000000000000000000, 0.9659258262890683122, 1.000000000000000000, 0.9659258262890683122, 1.000000000000000000, 0.9659258262890683122, 1.000000000000000000, 0.9659258262890683122, 1.000000000000000000, 0.9659258262890683122, 1.000000000000000000, 0.9659258262890683122, 1.000000000000000000, 0.9659258262890683122, 1.000000000000000000, 0.9659258262890683122, 1.000000000000000000, 0.9659258262890683122, 1.000000000000000000, 0.9659258262890683122, 1.000000000000000000, 0.9659258262890683122, 1.000000000000000000, 0.9659258262890683122, 1.000000000000000000, 0.9659258262890683122, 1.000000000000000000, 0.9659258262890683122, 1.000000000000000000, 0.9659258262890683122, 1.000000000000000000, 0.9659258262890683122, 1.000000000000000000, 0.9659258262890683122, 1.000000000000000000, 0.9659258262890683122, 1.000000000000000000, 0.9659258262890683122, 1.000000000000000000, 0.9659258262890683122, 1.000000000000000000, 0.9659258262890683122, 1.000000000000000000, 0.9659258262890683122, 1.000000000000000000, 0.9659258262890683122, 1.000000000000000000, 0.9659258262890683122, 1.000000000000000000, 0.9659258262890683122, 1.000000000000000000, 0.9659258262890683122, 1.000000000000000000, 0.9659258262890683122, 1.000000000000000000, 0.9659258262890683122, 1.000000000000000000, 0.9659258262890683122, 1.000000000000000000, 0.9659258262890683122, 1.000000000000000000, 0.9659258262890683122, 1.000000000000000000, 0.9659258262890683122, 1.000000000000000000, 0.9659258262890683122, 1.000000000000000000, 0.9659258262890683122, 1.000000000000000000, 0.9659258262890683122, 1.000000000000000000, 0.9659258262890683122, 1.000000000000000000, 0.9659258262890683122, 1.000000000000000000, 0.9659258262890683122, 1.000000000000000000, 0.9659258262890683122, 1.000000000000000000, 0.9659258262890683122, 1.000000000000000000, 0.9659258262890683122, 1.000000000000000000, 0.9659258262890683122, 1.000000000000000000, 0.9659258262890683122, 1.000000000000000000, 0.9659258262890683122, 1.000000000000000000, 0.9659258262890683122, 1.000000000000000000, 0.9659258262890683122, 1.000000000000000000, 0.9659258262890683122, 1.000000000000000000, 0.9659258262890683122, 1.000000000000000000, 0.9659258262890683122, 1.000000000000000000, 0.9659258262890683122, 1.000000000000000000, 0.9659258262890683122, 1.000000000000000000, 0.9659258262890683122, 1.000000000000000000, 0.9659258262890683122, 1.000000000000000000, 0.9659258262890683122, 1.000000000000000000, 0.9659258262890683122, 1.000000000000000000, 0.9659258262890683122, 1.000000000000000000, 0.9659258262890683122, 1.000000000000000000, 0.9659258262890683122, 1.000000000000000000, 0.9659258262890683122, 1.000000000000000000, 0.9659258262890683122, 1.000000000000000000, 0.9659258262890683122, 1.000000000000000000, 0.9659258262890683122, 1.000000000000000000, 0.9659258262890683122, 1.000000000000000000, 0.9659258262890683122, 1.000000000000000000, 0.9659258262890683122, 1.000000000000000000, 0.9659258262890683122, 1.000000000000000000, 0.9659258262890683122, 1.000000000000000000, 0.9659258262890683122, 1.000000000000000000, 0.9659258262890683122, 1.000000000000000000, 0.9659258262890683122, 1.000000000000000000, 0.9659258262890683122, 1.000000000000000000, 0.9659258262890683122, 1.000000000000000000, 0.9659258262890683122, 1.000000000000000000, 0.9659258262890683122, 1.000000000000000000, 0.9659258262890683122, 1.000000000000000000, 0.9659258262890683122, 1.000000000000000000, 0.9659258262890683122, 1.000000000000000000, 0.9659258262890683122, 1.000000000000000000, 0.9659258262890683122, 1.000000000000000000, 0.9659258262890683122, 1.000000000000000000, 0.9659258262890683122, 1.000000000000000000, 0.9659258262890683122, 1.000000000000000000, 0.9659258262890683122, 1.000000000000000000, 0.9659258262890683122, 1.000000000000000000, 0.9659258262890683122, 1.000000000000000000, 0.9659258262890683122, 1.000000000000000000, 0.9659258262890683122, 1.000000000000000000, 0.9659258262890683122, 1.000000000000000000, 0.9659258262890683122, 1.000000000000000000, 0.9659258262890683122, 1.000000000000000000, 0.9659258262890683122, 1.000000000000000000, 0.9659258262890683122, 1.000000000000000000, 0.9659258262890683122, 1.000000000000000000, 0.9659258262890683122, 1.000000000000000000, 0.9659258262890683122, 1.000000000000000000, 0.9659258262890683122, 1.000000000000000000, 0.9659258262890683122, 1.000000000000000000, 0.9659258262890683122, 1.000000000000000000, 0.9659258262890683122, 1.000000000000000000, 0.9659258262890683122, 1.000000000000000000, 0.9659258262890683122, 1.000000000000000000, 0.9659258262890683122, 1.000000000000000000, 0.9659258262890683122, 1.000000000000000000, 0.9659258262890683122, 1.000000000000000000, 0.9659258262890683122, 1.000000000000000000, 0.9659258262890683122, 1.000000000000000000, 0.9659258262890683122, 1.000000000000000000, 0.9659258262890683122, 1.000000000000000000, 0.9659258262890683122, 1.000000000000000000, 0.9659258262890683122, 1.000000000000000000, 0.9659258262890683122, 1.000000000000000000, 0.9659258262890683122, 1.000000000000000000, 0.9659258262890683122, 1.000000000000000000, 0.9659258262890683122, 1.000000000000000000, 0.9659258262890683122, 1.000000000000000000, 0.9659258262890683122, 1.000000000000000000, 0.9659258262890683122, 1.000000000000000000, 0.9659258262890683122, 1.000000000000000000, 0.9659258262890683122, 1.000000000000000000, 0.9659258262890683122, 1.000000000000000000, 0.9659258262890683122, 1.000000000000000000, 0.9659258262890683122, 1.000000000000000000, 0.9659258262890683122, 1.000000000000000000, 0.9659258262890683122, 1.000000000000000000, 0.9659258262890683122, 1.000000000000000000, 0.9659258262890683122, 1.000000000000000000, 0.9659258262890683122, 1.000000000000000000, 0.9659258262890683122, 1.000000000000000000, 0.9659258262890683122, 1.000000000000000000, 0.9659258262890683122, 1.000000000000000000, 0.9659258262890683122, 1.000000000000000000, 0.9659258262890683122, 1.000000000000000000, 0.9659258262890683122, 1.000000000000000000, 0.9659258262890683122, 1.000000000000000000, 0.9659258262890683122, 1.000000000000000000, 0.9659258262890683122, 1.000000000000000000, 0.9659258262890683122, 1.000000000000000000, 0.9659258262890683122, 1.000000000000000000, 0.9659258262890683122, 1.000000000000000000, 0.9659258262890683122, 1.000000000000000000, 0.9659258262890683122, 1.000000000000000000),
 ( 0.3333333333333333703, 0.3219752754296894559, 0.3333333333333333703, 0.3219752754296894559, 0.3333333333333333703, 0.3219752754296894559, 0.3333333333333333703, 0.3219752754296894559, 0.3333333333333333703, 0.3219752754296894559, 0.3333333333333333703, 0.3219752754296894559, 0.3333333333333333703, 0.3219752754296894559, 0.3333333333333333703, 0.3219752754296894559, 0.3333333333333333703, 0.3219752754296894559, 0.3333333333333333703, 0.3219752754296894559, 0.3333333333333333703, 0.3219752754296894559, 0.3333333333333333703, 0.3219752754296894559, 0.3333333333333333703, 0.3219752754296894559, 0.3333333333333333703, 0.3219752754296894559, 0.3333333333333333703, 0.3219752754296894559, 0.3333333333333333703, 0.3219752754296894559, 0.3333333333333333703, 0.3219752754296894559, 0.3333333333333333703, 0.3219752754296894559, 0.3333333333333333703, 0.3219752754296894559, 0.3333333333333333703, 0.3219752754296894559, 0.3333333333333333703, 0.3219752754296894559, 0.3333333333333333703, 0.3219752754296894559, 0.3333333333333333703, 0.3219752754296894559, 0.3333333333333333703, 0.3219752754296894559, 0.3333333333333333703, 0.3219752754296894559, 0.3333333333333333703, 0.3219752754296894559, 0.3333333333333333703, 0.3219752754296894559, 0.3333333333333333703, 0.3219752754296894559, 0.3333333333333333703, 0.3219752754296894559, 0.3333333333333333703, 0.3219752754296894559, 0.3333333333333333703, 0.3219752754296894559, 0.3333333333333333703, 0.3219752754296894559, 0.3333333333333333703, 0.3219752754296894559, 0.3333333333333333703, 0.3219752754296894559, 0.3333333333333333703, 0.3219752754296894559, 0.3333333333333333703, 0.3219752754296894559, 0.3333333333333333703, 0.3219752754296894559, 0.3333333333333333703, 0.3219752754296894559, 0.3333333333333333703, 0.3219752754296894559, 0.3333333333333333703, 0.3219752754296894559, 0.3333333333333333703, 0.3219752754296894559, 0.3333333333333333703, 0.3219752754296894559, 0.3333333333333333703, 0.3219752754296894559, 0.3333333333333333703, 0.3219752754296894559, 0.3333333333333333703, 0.3219752754296894559, 0.3333333333333333703, 0.3219752754296894559, 0.3333333333333333703, 0.3219752754296894559, 0.3333333333333333703, 0.3219752754296894559, 0.3333333333333333703, 0.3219752754296894559, 0.3333333333333333703, 0.3219752754296894559, 0.3333333333333333703, 0.3219752754296894559, 0.3333333333333333703, 0.3219752754296894559, 0.3333333333333333703, 0.3219752754296894559, 0.3333333333333333703, 0.3219752754296894559, 0.3333333333333333703, 0.3219752754296894559, 0.3333333333333333703, 0.3219752754296894559, 0.3333333333333333703, 0.3219752754296894559, 0.3333333333333333703, 0.3219752754296894559, 0.3333333333333333703, 0.3219752754296894559, 0.3333333333333333703, 0.3219752754296894559, 0.3333333333333333703, 0.3219752754296894559, 0.3333333333333333703, 0.3219752754296894559, 0.3333333333333333703, 0.3219752754296894559, 0.3333333333333333703, 0.3219752754296894559, 0.3333333333333333703, 0.3219752754296894559, 0.3333333333333333703, 0.3219752754296894559, 0.3333333333333333703, 0.3219752754296894559, 0.3333333333333333703, 0.3219752754296894559, 0.3333333333333333703, 0.3219752754296894559, 0.3333333333333333703, 0.3219752754296894559, 0.3333333333333333703, 0.3219752754296894559, 0.3333333333333333703, 0.3219752754296894559, 0.3333333333333333703, 0.3219752754296894559, 0.3333333333333333703, 0.3219752754296894559, 0.3333333333333333703, 0.3219752754296894559, 0.3333333333333333703, 0.3219752754296894559, 0.3333333333333333703, 0.3219752754296894559, 0.3333333333333333703, 0.3219752754296894559, 0.3333333333333333703, 0.3219752754296894559, 0.3333333333333333703, 0.3219752754296894559, 0.3333333333333333703, 0.3219752754296894559, 0.3333333333333333703, 0.3219752754296894559, 0.3333333333333333703, 0.3219752754296894559, 0.3333333333333333703, 0.3219752754296894559, 0.3333333333333333703, 0.3219752754296894559, 0.3333333333333333703, 0.3219752754296894559, 0.3333333333333333703, 0.3219752754296894559, 0.3333333333333333703, 0.3219752754296894559, 0.3333333333333333703, 0.3219752754296894559, 0.3333333333333333703, 0.3219752754296894559, 0.3333333333333333703, 0.3219752754296894559, 0.3333333333333333703, 0.3219752754296894559, 0.3333333333333333703, 0.3219752754296894559, 0.3333333333333333703, 0.3219752754296894559, 0.3333333333333333703, 0.3219752754296894559, 0.3333333333333333703, 0.3219752754296894559, 0.3333333333333333703, 0.3219752754296894559, 0.3333333333333333703, 0.3219752754296894559, 0.3333333333333333703, 0.3219752754296894559, 0.3333333333333333703, 0.3219752754296894559, 0.3333333333333333703, 0.3219752754296894559, 0.3333333333333333703, 0.3219752754296894559, 0.3333333333333333703, 0.3219752754296894559, 0.3333333333333333703, 0.3219752754296894559, 0.3333333333333333703, 0.3219752754296894559, 0.3333333333333333703, 0.3219752754296894559, 0.3333333333333333703, 0.3219752754296894559, 0.3333333333333333703, 0.3219752754296894559, 0.3333333333333333703, 0.3219752754296894559, 0.3333333333333333703, 0.3219752754296894559, 0.3333333333333333703, 0.3219752754296894559, 0.3333333333333333703, 0.3219752754296894559, 0.3333333333333333703, 0.3219752754296894559, 0.3333333333333333703, 0.3219752754296894559, 0.3333333333333333703, 0.3219752754296894559, 0.3333333333333333703, 0.3219752754296894559, 0.3333333333333333703, 0.3219752754296894559, 0.3333333333333333703, 0.3219752754296894559, 0.3333333333333333703, 0.3219752754296894559, 0.3333333333333333703, 0.3219752754296894559, 0.3333333333333333703, 0.3219752754296894559, 0.3333333333333333703, 0.3219752754296894559, 0.3333333333333333703, 0.3219752754296894559, 0.3333333333333333703, 0.3219752754296894559, 0.3333333333333333703, 0.3219752754296894559, 0.3333333333333333703, 0.3219752754296894559, 0.3333333333333333703, 0.3219752754296894559, 0.3333333333333333703, 0.3219752754296894559, 0.3333333333333333703, 0.3219752754296894559, 0.3333333333333333703, 0.3219752754296894559, 0.3333333333333333703, 0.3219752754296894559, 0.3333333333333333703, 0.3219752754296894559, 0.3333333333333333703, 0.3219752754296894559, 0.3333333333333333703, 0.3219752754296894559, 0.3333333333333333703, 0.3219752754296894559, 0.3333333333333333703, 0.3219752754296894559, 0.3333333333333333703, 0.3219752754296894559, 0.3333333333333333703, 0.3219752754296894559, 0.3333333333333333703, 0.3219752754296894559, 0.3333333333333333703, 0.3219752754296894559, 0.3333333333333333703, 0.3219752754296894559, 0.3333333333333333703, 0.3219752754296894559, 0.3333333333333333703, 0.3219752754296894559, 0.3333333333333333703, 0.3219752754296894559, 0.3333333333333333703, 0.3219752754296894559, 0.3333333333333333703, 0.3219752754296894559, 0.3333333333333333703, 0.3219752754296894559, 0.3333333333333333703, 0.3219752754296894559, 0.3333333333333333703, 0.3219752754296894559, 0.3333333333333333703, 0.3219752754296894559, 0.3333333333333333703, 0.3219752754296894559, 0.3333333333333333703, 0.3219752754296894559, 0.3333333333333333703, 0.3219752754296894559, 0.3333333333333333703, 0.3219752754296894559, 0.3333333333333333703, 0.3219752754296894559, 0.3333333333333333703, 0.3219752754296894559, 0.3333333333333333703, 0.3219752754296894559, 0.3333333333333333703, 0.3219752754296894559, 0.3333333333333333703, 0.3219752754296894559, 0.3333333333333333703, 0.3219752754296894559, 0.3333333333333333703, 0.3219752754296894559, 0.3333333333333333703, 0.3219752754296894559, 0.3333333333333333703, 0.3219752754296894559, 0.3333333333333333703, 0.3219752754296894559, 0.3333333333333333703, 0.3219752754296894559, 0.3333333333333333703, 0.3219752754296894559, 0.3333333333333333703, 0.3219752754296894559, 0.3333333333333333703, 0.3219752754296894559, 0.3333333333333333703, 0.3219752754296894559, 0.3333333333333333703, 0.3219752754296894559, 0.3333333333333333703, 0.3219752754296894559, 0.3333333333333333703, 0.3219752754296894559, 0.3333333333333333703, 0.3219752754296894559, 0.3333333333333333703, 0.3219752754296894559, 0.3333333333333333703, 0.3219752754296894559, 0.3333333333333333703, 0.3219752754296894559, 0.3333333333333333703, 0.3219752754296894559, 0.3333333333333333703, 0.3219752754296894559, 0.3333333333333333703, 0.3219752754296894559, 0.3333333333333333703, 0.3219752754296894559, 0.3333333333333333703, 0.3219752754296894559, 0.3333333333333333703, 0.3219752754296894559, 0.3333333333333333703, 0.3219752754296894559, 0.3333333333333333703, 0.3219752754296894559, 0.3333333333333333703, 0.3219752754296894559, 0.3333333333333333703, 0.3219752754296894559, 0.3333333333333333703, 0.3219752754296894559, 0.3333333333333333703, 0.3219752754296894559, 0.3333333333333333703, 0.3219752754296894559, 0.3333333333333333703, 0.3219752754296894559, 0.3333333333333333703, 0.3219752754296894559, 0.3333333333333333703, 0.3219752754296894559, 0.3333333333333333703, 0.3219752754296894559, 0.3333333333333333703, 0.3219752754296894559, 0.3333333333333333703, 0.3219752754296894559, 0.3333333333333333703, 0.3219752754296894559, 0.3333333333333333703, 0.3219752754296894559, 0.3333333333333333703, 0.3219752754296894559, 0.3333333333333333703, 0.3219752754296894559, 0.3333333333333333703, 0.3219752754296894559, 0.3333333333333333703, 0.3219752754296894559, 0.3333333333333333703, 0.3219752754296894559, 0.3333333333333333703, 0.3219752754296894559, 0.3333333333333333703, 0.3219752754296894559, 0.3333333333333333703, 0.3219752754296894559, 0.3333333333333333703, 0.3219752754296894559, 0.3333333333333333703, 0.3219752754296894559, 0.3333333333333333703, 0.3219752754296894559, 0.3333333333333333703, 0.3219752754296894559, 0.3333333333333333703, 0.3219752754296894559, 0.3333333333333333703, 0.3219752754296894559, 0.3333333333333333703, 0.3219752754296894559, 0.3333333333333333703, 0.3219752754296894559, 0.3333333333333333703, 0.3219752754296894559, 0.3333333333333333703, 0.3219752754296894559, 0.3333333333333333703, 0.3219752754296894559, 0.3333333333333333703, 0.3219752754296894559, 0.3333333333333333703, 0.3219752754296894559, 0.3333333333333333703, 0.3219752754296894559, 0.3333333333333333703, 0.3219752754296894559, 0.3333333333333333703, 0.3219752754296894559, 0.3333333333333333703, 0.3219752754296894559, 0.3333333333333333703, 0.3219752754296894559, 0.3333333333333333703, 0.3219752754296894559, 0.3333333333333333703, 0.3219752754296894559, 0.3333333333333333703, 0.3219752754296894559, 0.3333333333333333703, 0.3219752754296894559, 0.3333333333333333703, 0.3219752754296894559, 0.3333333333333333703),
 ( 0.3333333333333333703, 0.3219752754296894559, 0.3333333333333333703, 0.3219752754296894559, 0.3333333333333333703, 0.3219752754296894559, 0.3333333333333333703, 0.3219752754296894559, 0.3333333333333333703, 0.3219752754296894559, 0.3333333333333333703, 0.3219752754296894559, 0.3333333333333333703, 0.3219752754296894559, 0.3333333333333333703, 0.3219752754296894559, 0.3333333333333333703, 0.3219752754296894559, 0.3333333333333333703, 0.3219752754296894559, 0.3333333333333333703, 0.3219752754296894559, 0.3333333333333333703, 0.3219752754296894559, 0.3333333333333333703, 0.3219752754296894559, 0.3333333333333333703, 0.3219752754296894559, 0.3333333333333333703, 0.3219752754296894559, 0.3333333333333333703, 0.3219752754296894559, 0.3333333333333333703, 0.3219752754296894559, 0.3333333333333333703, 0.3219752754296894559, 0.3333333333333333703, 0.3219752754296894559, 0.3333333333333333703, 0.3219752754296894559, 0.3333333333333333703, 0.3219752754296894559, 0.3333333333333333703, 0.3219752754296894559, 0.3333333333333333703, 0.3219752754296894559, 0.3333333333333333703, 0.3219752754296894559, 0.3333333333333333703, 0.3219752754296894559, 0.3333333333333333703, 0.3219752754296894559, 0.3333333333333333703, 0.3219752754296894559, 0.3333333333333333703, 0.3219752754296894559, 0.3333333333333333703, 0.3219752754296894559, 0.3333333333333333703, 0.3219752754296894559, 0.3333333333333333703, 0.3219752754296894559, 0.3333333333333333703, 0.3219752754296894559, 0.3333333333333333703, 0.3219752754296894559, 0.3333333333333333703, 0.3219752754296894559, 0.3333333333333333703, 0.3219752754296894559, 0.3333333333333333703, 0.3219752754296894559, 0.3333333333333333703, 0.3219752754296894559, 0.3333333333333333703, 0.3219752754296894559, 0.3333333333333333703, 0.3219752754296894559, 0.3333333333333333703, 0.3219752754296894559, 0.3333333333333333703, 0.3219752754296894559, 0.3333333333333333703, 0.3219752754296894559, 0.3333333333333333703, 0.3219752754296894559, 0.3333333333333333703, 0.3219752754296894559, 0.3333333333333333703, 0.3219752754296894559, 0.3333333333333333703, 0.3219752754296894559, 0.3333333333333333703, 0.3219752754296894559, 0.3333333333333333703, 0.3219752754296894559, 0.3333333333333333703, 0.3219752754296894559, 0.3333333333333333703, 0.3219752754296894559, 0.3333333333333333703, 0.3219752754296894559, 0.3333333333333333703, 0.3219752754296894559, 0.3333333333333333703, 0.3219752754296894559, 0.3333333333333333703, 0.3219752754296894559, 0.3333333333333333703, 0.3219752754296894559, 0.3333333333333333703, 0.3219752754296894559, 0.3333333333333333703, 0.3219752754296894559, 0.3333333333333333703, 0.3219752754296894559, 0.3333333333333333703, 0.3219752754296894559, 0.3333333333333333703, 0.3219752754296894559, 0.3333333333333333703, 0.3219752754296894559, 0.3333333333333333703, 0.3219752754296894559, 0.3333333333333333703, 0.3219752754296894559, 0.3333333333333333703, 0.3219752754296894559, 0.3333333333333333703, 0.3219752754296894559, 0.3333333333333333703, 0.3219752754296894559, 0.3333333333333333703, 0.3219752754296894559, 0.3333333333333333703, 0.3219752754296894559, 0.3333333333333333703, 0.3219752754296894559, 0.3333333333333333703, 0.3219752754296894559, 0.3333333333333333703, 0.3219752754296894559, 0.3333333333333333703, 0.3219752754296894559, 0.3333333333333333703, 0.3219752754296894559, 0.3333333333333333703, 0.3219752754296894559, 0.3333333333333333703, 0.3219752754296894559, 0.3333333333333333703, 0.3219752754296894559, 0.3333333333333333703, 0.3219752754296894559, 0.3333333333333333703, 0.3219752754296894559, 0.3333333333333333703, 0.3219752754296894559, 0.3333333333333333703, 0.3219752754296894559, 0.3333333333333333703, 0.3219752754296894559, 0.3333333333333333703, 0.3219752754296894559, 0.3333333333333333703, 0.3219752754296894559, 0.3333333333333333703, 0.3219752754296894559, 0.3333333333333333703, 0.3219752754296894559, 0.3333333333333333703, 0.3219752754296894559, 0.3333333333333333703, 0.3219752754296894559, 0.3333333333333333703, 0.3219752754296894559, 0.3333333333333333703, 0.3219752754296894559, 0.3333333333333333703, 0.3219752754296894559, 0.3333333333333333703, 0.3219752754296894559, 0.3333333333333333703, 0.3219752754296894559, 0.3333333333333333703, 0.3219752754296894559, 0.3333333333333333703, 0.3219752754296894559, 0.3333333333333333703, 0.3219752754296894559, 0.3333333333333333703, 0.3219752754296894559, 0.3333333333333333703, 0.3219752754296894559, 0.3333333333333333703, 0.3219752754296894559, 0.3333333333333333703, 0.3219752754296894559, 0.3333333333333333703, 0.3219752754296894559, 0.3333333333333333703, 0.3219752754296894559, 0.3333333333333333703, 0.3219752754296894559, 0.3333333333333333703, 0.3219752754296894559, 0.3333333333333333703, 0.3219752754296894559, 0.3333333333333333703, 0.3219752754296894559, 0.3333333333333333703, 0.3219752754296894559, 0.3333333333333333703, 0.3219752754296894559, 0.3333333333333333703, 0.3219752754296894559, 0.3333333333333333703, 0.3219752754296894559, 0.3333333333333333703, 0.3219752754296894559, 0.3333333333333333703, 0.3219752754296894559, 0.3333333333333333703, 0.3219752754296894559, 0.3333333333333333703, 0.3219752754296894559, 0.3333333333333333703, 0.3219752754296894559, 0.3333333333333333703, 0.3219752754296894559, 0.3333333333333333703, 0.3219752754296894559, 0.3333333333333333703, 0.3219752754296894559, 0.3333333333333333703, 0.3219752754296894559, 0.3333333333333333703, 0.3219752754296894559, 0.3333333333333333703, 0.3219752754296894559, 0.3333333333333333703, 0.3219752754296894559, 0.3333333333333333703, 0.3219752754296894559, 0.3333333333333333703, 0.3219752754296894559, 0.3333333333333333703, 0.3219752754296894559, 0.3333333333333333703, 0.3219752754296894559, 0.3333333333333333703, 0.3219752754296894559, 0.3333333333333333703, 0.3219752754296894559, 0.3333333333333333703, 0.3219752754296894559, 0.3333333333333333703, 0.3219752754296894559, 0.3333333333333333703, 0.3219752754296894559, 0.3333333333333333703, 0.3219752754296894559, 0.3333333333333333703, 0.3219752754296894559, 0.3333333333333333703, 0.3219752754296894559, 0.3333333333333333703, 0.3219752754296894559, 0.3333333333333333703, 0.3219752754296894559, 0.3333333333333333703, 0.3219752754296894559, 0.3333333333333333703, 0.3219752754296894559, 0.3333333333333333703, 0.3219752754296894559, 0.3333333333333333703, 0.3219752754296894559, 0.3333333333333333703, 0.3219752754296894559, 0.3333333333333333703, 0.3219752754296894559, 0.3333333333333333703, 0.3219752754296894559, 0.3333333333333333703, 0.3219752754296894559, 0.3333333333333333703, 0.3219752754296894559, 0.3333333333333333703, 0.3219752754296894559, 0.3333333333333333703, 0.3219752754296894559, 0.3333333333333333703, 0.3219752754296894559, 0.3333333333333333703, 0.3219752754296894559, 0.3333333333333333703, 0.3219752754296894559, 0.3333333333333333703, 0.3219752754296894559, 0.3333333333333333703, 0.3219752754296894559, 0.3333333333333333703, 0.3219752754296894559, 0.3333333333333333703, 0.3219752754296894559, 0.3333333333333333703, 0.3219752754296894559, 0.3333333333333333703, 0.3219752754296894559, 0.3333333333333333703, 0.3219752754296894559, 0.3333333333333333703, 0.3219752754296894559, 0.3333333333333333703, 0.3219752754296894559, 0.3333333333333333703, 0.3219752754296894559, 0.3333333333333333703, 0.3219752754296894559, 0.3333333333333333703, 0.3219752754296894559, 0.3333333333333333703, 0.3219752754296894559, 0.3333333333333333703, 0.3219752754296894559, 0.3333333333333333703, 0.3219752754296894559, 0.3333333333333333703, 0.3219752754296894559, 0.3333333333333333703, 0.3219752754296894559, 0.3333333333333333703, 0.3219752754296894559, 0.3333333333333333703, 0.3219752754296894559, 0.3333333333333333703, 0.3219752754296894559, 0.3333333333333333703, 0.3219752754296894559, 0.3333333333333333703, 0.3219752754296894559, 0.3333333333333333703, 0.3219752754296894559, 0.3333333333333333703, 0.3219752754296894559, 0.3333333333333333703, 0.3219752754296894559, 0.3333333333333333703, 0.3219752754296894559, 0.3333333333333333703, 0.3219752754296894559, 0.3333333333333333703, 0.3219752754296894559, 0.3333333333333333703, 0.3219752754296894559, 0.3333333333333333703, 0.3219752754296894559, 0.3333333333333333703, 0.3219752754296894559, 0.3333333333333333703, 0.3219752754296894559, 0.3333333333333333703, 0.3219752754296894559, 0.3333333333333333703, 0.3219752754296894559, 0.3333333333333333703, 0.3219752754296894559, 0.3333333333333333703, 0.3219752754296894559, 0.3333333333333333703, 0.3219752754296894559, 0.3333333333333333703, 0.3219752754296894559, 0.3333333333333333703, 0.3219752754296894559, 0.3333333333333333703, 0.3219752754296894559, 0.3333333333333333703, 0.3219752754296894559, 0.3333333333333333703, 0.3219752754296894559, 0.3333333333333333703, 0.3219752754296894559, 0.3333333333333333703, 0.3219752754296894559, 0.3333333333333333703, 0.3219752754296894559, 0.3333333333333333703, 0.3219752754296894559, 0.3333333333333333703, 0.3219752754296894559, 0.3333333333333333703, 0.3219752754296894559, 0.3333333333333333703, 0.3219752754296894559, 0.3333333333333333703, 0.3219752754296894559, 0.3333333333333333703, 0.3219752754296894559, 0.3333333333333333703, 0.3219752754296894559, 0.3333333333333333703, 0.3219752754296894559, 0.3333333333333333703, 0.3219752754296894559, 0.3333333333333333703, 0.3219752754296894559, 0.3333333333333333703, 0.3219752754296894559, 0.3333333333333333703, 0.3219752754296894559, 0.3333333333333333703, 0.3219752754296894559, 0.3333333333333333703, 0.3219752754296894559, 0.3333333333333333703, 0.3219752754296894559, 0.3333333333333333703, 0.3219752754296894559, 0.3333333333333333703, 0.3219752754296894559, 0.3333333333333333703, 0.3219752754296894559, 0.3333333333333333703, 0.3219752754296894559, 0.3333333333333333703, 0.3219752754296894559, 0.3333333333333333703, 0.3219752754296894559, 0.3333333333333333703, 0.3219752754296894559, 0.3333333333333333703, 0.3219752754296894559, 0.3333333333333333703, 0.3219752754296894559, 0.3333333333333333703, 0.3219752754296894559, 0.3333333333333333703, 0.3219752754296894559, 0.3333333333333333703, 0.3219752754296894559, 0.3333333333333333703, 0.3219752754296894559, 0.3333333333333333703, 0.3219752754296894559, 0.3333333333333333703, 0.3219752754296894559, 0.3333333333333333703, 0.3219752754296894559, 0.3333333333333333703, 0.3219752754296894559, 0.3333333333333333703, 0.3219752754296894559, 0.3333333333333333703, 0.3219752754296894559, 0.3333333333333333703),
 ( 1.000000000000000000, 0.9659258262890683122, 1.000000000000000000, 0.9659258262890683122, 1.000000000000000000, 0.9659258262890683122, 1.000000000000000000, 0.9659258262890683122, 1.000000000000000000, 0.9659258262890683122, 1.000000000000000000, 0.9659258262890683122, 1.000000000000000000, 0.9659258262890683122, 1.000000000000000000, 0.9659258262890683122, 1.000000000000000000, 0.9659258262890683122, 1.000000000000000000, 0.9659258262890683122, 1.000000000000000000, 0.9659258262890683122, 1.000000000000000000, 0.9659258262890683122, 1.000000000000000000, 0.9659258262890683122, 1.000000000000000000, 0.9659258262890683122, 1.000000000000000000, 0.9659258262890683122, 1.000000000000000000, 0.9659258262890683122, 1.000000000000000000, 0.9659258262890683122, 1.000000000000000000, 0.9659258262890683122, 1.000000000000000000, 0.9659258262890683122, 1.000000000000000000, 0.9659258262890683122, 1.000000000000000000, 0.9659258262890683122, 1.000000000000000000, 0.9659258262890683122, 1.000000000000000000, 0.9659258262890683122, 1.000000000000000000, 0.9659258262890683122, 1.000000000000000000, 0.9659258262890683122, 1.000000000000000000, 0.9659258262890683122, 1.000000000000000000, 0.9659258262890683122, 1.000000000000000000, 0.9659258262890683122, 1.000000000000000000, 0.9659258262890683122, 1.000000000000000000, 0.9659258262890683122, 1.000000000000000000, 0.9659258262890683122, 1.000000000000000000, 0.9659258262890683122, 1.000000000000000000, 0.9659258262890683122, 1.000000000000000000, 0.9659258262890683122, 1.000000000000000000, 0.9659258262890683122, 1.000000000000000000, 0.9659258262890683122, 1.000000000000000000, 0.9659258262890683122, 1.000000000000000000, 0.9659258262890683122, 1.000000000000000000, 0.9659258262890683122, 1.000000000000000000, 0.9659258262890683122, 1.000000000000000000, 0.9659258262890683122, 1.000000000000000000, 0.9659258262890683122, 1.000000000000000000, 0.9659258262890683122, 1.000000000000000000, 0.9659258262890683122, 1.000000000000000000, 0.9659258262890683122, 1.000000000000000000, 0.9659258262890683122, 1.000000000000000000, 0.9659258262890683122, 1.000000000000000000, 0.9659258262890683122, 1.000000000000000000, 0.9659258262890683122, 1.000000000000000000, 0.9659258262890683122, 1.000000000000000000, 0.9659258262890683122, 1.000000000000000000, 0.9659258262890683122, 1.000000000000000000, 0.9659258262890683122, 1.000000000000000000, 0.9659258262890683122, 1.000000000000000000, 0.9659258262890683122, 1.000000000000000000, 0.9659258262890683122, 1.000000000000000000, 0.9659258262890683122, 1.000000000000000000, 0.9659258262890683122, 1.000000000000000000, 0.9659258262890683122, 1.000000000000000000, 0.9659258262890683122, 1.000000000000000000, 0.9659258262890683122, 1.000000000000000000, 0.9659258262890683122, 1.000000000000000000, 0.9659258262890683122, 1.000000000000000000, 0.9659258262890683122, 1.000000000000000000, 0.9659258262890683122, 1.000000000000000000, 0.9659258262890683122, 1.000000000000000000, 0.9659258262890683122, 1.000000000000000000, 0.9659258262890683122, 1.000000000000000000, 0.9659258262890683122, 1.000000000000000000, 0.9659258262890683122, 1.000000000000000000, 0.9659258262890683122, 1.000000000000000000, 0.9659258262890683122, 1.000000000000000000, 0.9659258262890683122, 1.000000000000000000, 0.9659258262890683122, 1.000000000000000000, 0.9659258262890683122, 1.000000000000000000, 0.9659258262890683122, 1.000000000000000000, 0.9659258262890683122, 1.000000000000000000, 0.9659258262890683122, 1.000000000000000000, 0.9659258262890683122, 1.000000000000000000, 0.9659258262890683122, 1.000000000000000000, 0.9659258262890683122, 1.000000000000000000, 0.9659258262890683122, 1.000000000000000000, 0.9659258262890683122, 1.000000000000000000, 0.9659258262890683122, 1.000000000000000000, 0.9659258262890683122, 1.000000000000000000, 0.9659258262890683122, 1.000000000000000000, 0.9659258262890683122, 1.000000000000000000, 0.9659258262890683122, 1.000000000000000000, 0.9659258262890683122, 1.000000000000000000, 0.9659258262890683122, 1.000000000000000000, 0.9659258262890683122, 1.000000000000000000, 0.9659258262890683122, 1.000000000000000000, 0.9659258262890683122, 1.000000000000000000, 0.9659258262890683122, 1.000000000000000000, 0.9659258262890683122, 1.000000000000000000, 0.9659258262890683122, 1.000000000000000000, 0.9659258262890683122, 1.000000000000000000, 0.9659258262890683122, 1.000000000000000000, 0.9659258262890683122, 1.000000000000000000, 0.9659258262890683122, 1.000000000000000000, 0.9659258262890683122, 1.000000000000000000, 0.9659258262890683122, 1.000000000000000000, 0.9659258262890683122, 1.000000000000000000, 0.9659258262890683122, 1.000000000000000000, 0.9659258262890683122, 1.000000000000000000, 0.9659258262890683122, 1.000000000000000000, 0.9659258262890683122, 1.000000000000000000, 0.9659258262890683122, 1.000000000000000000, 0.9659258262890683122, 1.000000000000000000, 0.9659258262890683122, 1.000000000000000000, 0.9659258262890683122, 1.000000000000000000, 0.9659258262890683122, 1.000000000000000000, 0.9659258262890683122, 1.000000000000000000, 0.9659258262890683122, 1.000000000000000000, 0.9659258262890683122, 1.000000000000000000, 0.9659258262890683122, 1.000000000000000000, 0.9659258262890683122, 1.000000000000000000, 0.9659258262890683122, 1.000000000000000000, 0.9659258262890683122, 1.000000000000000000, 0.9659258262890683122, 1.000000000000000000, 0.9659258262890683122, 1.000000000000000000, 0.9659258262890683122, 1.000000000000000000, 0.9659258262890683122, 1.000000000000000000, 0.9659258262890683122, 1.000000000000000000, 0.9659258262890683122, 1.000000000000000000, 0.9659258262890683122, 1.000000000000000000, 0.9659258262890683122, 1.000000000000000000, 0.9659258262890683122, 1.000000000000000000, 0.9659258262890683122, 1.000000000000000000, 0.9659258262890683122, 1.000000000000000000, 0.9659258262890683122, 1.000000000000000000, 0.9659258262890683122, 1.000000000000000000, 0.9659258262890683122, 1.000000000000000000, 0.9659258262890683122, 1.000000000000000000, 0.9659258262890683122, 1.000000000000000000, 0.9659258262890683122, 1.000000000000000000, 0.9659258262890683122, 1.000000000000000000, 0.9659258262890683122, 1.000000000000000000, 0.9659258262890683122, 1.000000000000000000, 0.9659258262890683122, 1.000000000000000000, 0.9659258262890683122, 1.000000000000000000, 0.9659258262890683122, 1.000000000000000000, 0.9659258262890683122, 1.000000000000000000, 0.9659258262890683122, 1.000000000000000000, 0.9659258262890683122, 1.000000000000000000, 0.9659258262890683122, 1.000000000000000000, 0.9659258262890683122, 1.000000000000000000, 0.9659258262890683122, 1.000000000000000000, 0.9659258262890683122, 1.000000000000000000, 0.9659258262890683122, 1.000000000000000000, 0.9659258262890683122, 1.000000000000000000, 0.9659258262890683122, 1.000000000000000000, 0.9659258262890683122, 1.000000000000000000, 0.9659258262890683122, 1.000000000000000000, 0.9659258262890683122, 1.000000000000000000, 0.9659258262890683122, 1.000000000000000000, 0.9659258262890683122, 1.000000000000000000, 0.9659258262890683122, 1.000000000000000000, 0.9659258262890683122, 1.000000000000000000, 0.9659258262890683122, 1.000000000000000000, 0.9659258262890683122, 1.000000000000000000, 0.9659258262890683122, 1.000000000000000000, 0.9659258262890683122, 1.000000000000000000, 0.9659258262890683122, 1.000000000000000000, 0.9659258262890683122, 1.000000000000000000, 0.9659258262890683122, 1.000000000000000000, 0.9659258262890683122, 1.000000000000000000, 0.9659258262890683122, 1.000000000000000000, 0.9659258262890683122, 1.000000000000000000, 0.9659258262890683122, 1.000000000000000000, 0.9659258262890683122, 1.000000000000000000, 0.9659258262890683122, 1.000000000000000000, 0.9659258262890683122, 1.000000000000000000, 0.9659258262890683122, 1.000000000000000000, 0.9659258262890683122, 1.000000000000000000, 0.9659258262890683122, 1.000000000000000000, 0.9659258262890683122, 1.000000000000000000, 0.9659258262890683122, 1.000000000000000000, 0.9659258262890683122, 1.000000000000000000, 0.9659258262890683122, 1.000000000000000000, 0.9659258262890683122, 1.000000000000000000, 0.9659258262890683122, 1.000000000000000000, 0.9659258262890683122, 1.000000000000000000, 0.9659258262890683122, 1.000000000000000000, 0.9659258262890683122, 1.000000000000000000, 0.9659258262890683122, 1.000000000000000000, 0.9659258262890683122, 1.000000000000000000, 0.9659258262890683122, 1.000000000000000000, 0.9659258262890683122, 1.000000000000000000, 0.9659258262890683122, 1.000000000000000000, 0.9659258262890683122, 1.000000000000000000, 0.9659258262890683122, 1.000000000000000000, 0.9659258262890683122, 1.000000000000000000, 0.9659258262890683122, 1.000000000000000000, 0.9659258262890683122, 1.000000000000000000, 0.9659258262890683122, 1.000000000000000000, 0.9659258262890683122, 1.000000000000000000, 0.9659258262890683122, 1.000000000000000000, 0.9659258262890683122, 1.000000000000000000, 0.9659258262890683122, 1.000000000000000000, 0.9659258262890683122, 1.000000000000000000, 0.9659258262890683122, 1.000000000000000000, 0.9659258262890683122, 1.000000000000000000, 0.9659258262890683122, 1.000000000000000000, 0.9659258262890683122, 1.000000000000000000, 0.9659258262890683122, 1.000000000000000000, 0.9659258262890683122, 1.000000000000000000, 0.9659258262890683122, 1.000000000000000000, 0.9659258262890683122, 1.000000000000000000, 0.9659258262890683122, 1.000000000000000000, 0.9659258262890683122, 1.000000000000000000, 0.9659258262890683122, 1.000000000000000000, 0.9659258262890683122, 1.000000000000000000, 0.9659258262890683122, 1.000000000000000000, 0.9659258262890683122, 1.000000000000000000, 0.9659258262890683122, 1.000000000000000000, 0.9659258262890683122, 1.000000000000000000, 0.9659258262890683122, 1.000000000000000000, 0.9659258262890683122, 1.000000000000000000, 0.9659258262890683122, 1.000000000000000000, 0.9659258262890683122, 1.000000000000000000, 0.9659258262890683122, 1.000000000000000000, 0.9659258262890683122, 1.000000000000000000, 0.9659258262890683122, 1.000000000000000000, 0.9659258262890683122, 1.000000000000000000, 0.9659258262890683122, 1.000000000000000000, 0.9659258262890683122, 1.000000000000000000, 0.9659258262890683122, 1.000000000000000000) ) ) 
 REPRESENTATION_ITEM ( '' )  SURFACE ( )  );
#183995=CARTESIAN_POINT ( 'NONE',  ( -14.29746914071037622, -8.314922557961029526, 49.16775706135234003 ) ) ;
#183996=CARTESIAN_POINT ( 'NONE',  ( -9.564922557960796823, -16.46253265017161027, 97.08224293864769550 ) ) ;
#183997=CARTESIAN_POINT ( 'NONE',  ( 21.53943276465977519, -0.05219959533907433946, 103.7489096053143669 ) ) ;
#183998=CARTESIAN_POINT ( 'NONE',  ( 13.97604488694527802, 13.89961937509977652, 74.37390960531436690 ) ) ;
#184001=CARTESIAN_POINT ( 'NONE',  ( 4.379528057220339221, -16.55341960407611168, 87.70724293864769550 ) ) ;
#184002=CARTESIAN_POINT ( 'NONE',  ( -10.81492255796078084, -18.62759615963271287, 37.08224293864768129 ) ) ;
#184003=CARTESIAN_POINT ( 'NONE',  ( 19.02544592524343514, -5.153800228976328945, 23.54057627198102054 ) ) ;
#184004=CARTESIAN_POINT ( 'NONE',  ( 16.53943276465976808, 0.05219959533934440121, 61.25109039468567573 ) ) ;
#184005=CARTESIAN_POINT ( 'NONE',  ( 0.05219959533907565091, 21.53943276465977519, 114.9989096053143669 ) ) ;
#184006=CARTESIAN_POINT ( 'NONE',  ( 13.97604488694548053, -13.89961937509957401, 75.62609039468564731 ) ) ;
#184007=CARTESIAN_POINT ( 'NONE',  ( -19.02544592524342804, 5.153800228976336051, 26.04057627198103120 ) ) ;
#184008=CARTESIAN_POINT ( 'NONE',  ( 10.72451020669898902, -18.67979575497178502, 62.91557627198102409 ) ) ;
#184010=CARTESIAN_POINT ( 'NONE',  ( 13.89961937509977652, -13.97604488694527269, 103.1239096053143527 ) ) ;
#184011=CARTESIAN_POINT ( 'NONE',  ( 0.05219959533937995610, -21.53943276465977519, 95.00109039468568994 ) ) ;
#184012=CARTESIAN_POINT ( 'NONE',  ( 0.05219959533909260263, 19.03943276465977164, 64.99890960531436690 ) ) ;
#184013=CARTESIAN_POINT ( 'NONE',  ( -0.05219959533934338120, 16.53943276465976808, 52.50109039468567573 ) ) ;
#184014=CARTESIAN_POINT ( 'NONE',  ( -16.51473224551069308, -9.474510206698971260, 56.66557627198103120 ) ) ;
#184015=CARTESIAN_POINT ( 'NONE',  ( 18.62759615963255655, 10.81492255796105972, 81.66775706135236135 ) ) ;
#184017=CARTESIAN_POINT ( 'NONE',  ( -5.153800228976607833, 19.02544592524334988, 42.70942372801901143 ) ) ;
#184018=CARTESIAN_POINT ( 'NONE',  ( -5.049401038297874678, -19.05341960407617918, 59.79275706135231871 ) ) ;
#184019=CARTESIAN_POINT ( 'NONE',  ( -15.72974639402176322, -15.80617190586768395, 54.37609039468568994 ) ) ;
#184021=CARTESIAN_POINT ( 'NONE',  ( -13.97604488694547697, 13.89961937509957934, 43.12609039468566152 ) ) ;
#184022=CARTESIAN_POINT ( 'NONE',  ( -19.05341960407611168, -5.049401038298163336, 101.4572429386476955 ) ) ;
#184023=CARTESIAN_POINT ( 'NONE',  ( 9.474510206698971260, -16.51473224551069308, 72.91557627198102409 ) ) ;
#184024=CARTESIAN_POINT ( 'NONE',  ( 4.379528057220092307, 16.55341960407617563, 112.2927570613523471 ) ) ;
#184025=CARTESIAN_POINT ( 'NONE',  ( -10.81492255796078084, -18.62759615963271287, 37.08224293864768129 ) ) ;
#184026=CARTESIAN_POINT ( 'NONE',  ( 18.62759615963255655, 10.81492255796105972, 96.66775706135234714 ) ) ;
#184028=CARTESIAN_POINT ( 'NONE',  ( 17.44279575226823198, 5.990770900252482711, 56.66442432485683156 ) ) ;
#184029=CARTESIAN_POINT ( 'NONE',  ( -21.53943276465977519, -0.05219959533937600094, 103.7510903946857042 ) ) ;
#184030=CARTESIAN_POINT ( 'NONE',  ( 17.31728774477273447, -6.344390552232384906, 43.31906651689319432 ) ) ;
#184031=CARTESIAN_POINT ( 'NONE',  ( -19.03943276465977164, 0.05219959533909376836, 26.24890960531435624 ) ) ;
#184032=CARTESIAN_POINT ( 'NONE',  ( -5.153800228976328057, -19.02544592524343514, 112.2905762719810099 ) ) ;
#184034=CARTESIAN_POINT ( 'NONE',  ( -16.52544592524335698, -4.483927247898792601, 48.95942372801902565 ) ) ;
#184035=CARTESIAN_POINT ( 'NONE',  ( -15.72974639402197994, 15.80617190586746368, 70.62390960531436690 ) ) ;
#184036=CARTESIAN_POINT ( 'NONE',  ( -8.224510206698948167, 14.34966873604960824, 40.41557627198103120 ) ) ;
#184037=CARTESIAN_POINT ( 'NONE',  ( -16.53943276465976808, 0.05219959533911058130, 106.2489096053143811 ) ) ;
#184038=CARTESIAN_POINT ( 'NONE',  ( 19.02544592524343514, -5.153800228976328945, 108.5405762719810383 ) ) ;
#184039=CARTESIAN_POINT ( 'NONE',  ( -13.89961937509957401, -13.97604488694547875, 39.37609039468566152 ) ) ;
#184040=CARTESIAN_POINT ( 'NONE',  ( 19.05341960407611168, 5.049401038298154454, 23.95724293864769194 ) ) ;
#184041=CARTESIAN_POINT ( 'NONE',  ( -21.53943276465977519, -0.05219959533937600094, 63.75109039468568284 ) ) ;
#184042=CARTESIAN_POINT ( 'NONE',  ( -18.22780087662122028, 5.500000000000031086, 78.51540105326107266 ) ) ;
#184043=CARTESIAN_POINT ( 'NONE',  ( 14.34966873604972726, -8.224510206698740333, 105.8344237280190328 ) ) ;
#184044=CARTESIAN_POINT ( 'NONE',  ( -5.153800228976607833, 19.02544592524335343, 67.70942372801900433 ) ) ;
#184045=CARTESIAN_POINT ( 'NONE',  ( -5.719274019375978568, 21.55341960407610458, 25.20724293864769550 ) ) ;
#184046=CARTESIAN_POINT ( 'NONE',  ( 16.55341960407611168, 4.379528057220329451, 88.95724293864769550 ) ) ;
#184047=CARTESIAN_POINT ( 'NONE',  ( -13.97604488694547697, 13.89961937509957934, 58.12609039468566863 ) ) ;
#184048=CARTESIAN_POINT ( 'NONE',  ( -13.97604488694527625, -13.89961937509977652, 71.87390960531433848 ) ) ;
#184049=CARTESIAN_POINT ( 'NONE',  ( -16.55341960407611168, -4.379528057220339221, 81.45724293864769550 ) ) ;
#184050=CARTESIAN_POINT ( 'NONE',  ( 13.89961937509957401, 13.97604488694547697, 86.87609039468567573 ) ) ;
#184051=CARTESIAN_POINT ( 'NONE',  ( 15.80617190586746368, 15.72974639402197994, 44.37390960531435979 ) ) ;
#184052=ORIENTED_EDGE ( 'NONE', *, *, #121704, .T. ) ;
#184053=CARTESIAN_POINT ( 'NONE',  ( 16.52544592524342804, -4.483927247898539470, 108.5405762719810241 ) ) ;
#184054=CARTESIAN_POINT ( 'NONE',  ( -16.31925111598457789, -7.325300261831485749, 29.83575461032750553 ) ) ;
#184055=CARTESIAN_POINT ( 'NONE',  ( 9.474510206698971260, -16.51473224551069308, 67.91557627198102409 ) ) ;
#184056=CARTESIAN_POINT ( 'NONE',  ( 0.05219959533907565091, 21.53943276465977519, 69.99890960531435269 ) ) ;
#184057=CARTESIAN_POINT ( 'NONE',  ( 14.34966873604972726, -8.224510206698740333, 85.83442372801901854 ) ) ;
#184058=CARTESIAN_POINT ( 'NONE',  ( -9.564922557960796823, -16.46253265017161027, 87.08224293864769550 ) ) ;
#184059=CARTESIAN_POINT ( 'NONE',  ( -16.46253265017146816, -9.564922557961047289, 69.16775706135233293 ) ) ;
#184060=CARTESIAN_POINT ( 'NONE',  ( -5.719274019375665041, -21.55341960407619695, 79.79275706135236135 ) ) ;
#184061=CARTESIAN_POINT ( 'NONE',  ( -21.52544592524343514, 5.823673210054127303, 66.04057627198103830 ) ) ;
#184062=CARTESIAN_POINT ( 'NONE',  ( -0.05219959533907301413, -21.53943276465977519, 22.49890960531436335 ) ) ;
#184063=CARTESIAN_POINT ( 'NONE',  ( -9.564922557960796823, -16.46253265017161027, 42.08224293864769550 ) ) ;
#184064=CARTESIAN_POINT ( 'NONE',  ( 14.29746914071037800, 8.314922557961029526, 106.6677570613523756 ) ) ;
#184065=CARTESIAN_POINT ( 'NONE',  ( -13.89961937509977652, 13.97604488694528158, 60.62390960531436690 ) ) ;
#184066=CARTESIAN_POINT ( 'NONE',  ( -4.483927247898782831, 16.52544592524335698, 27.70942372801901854 ) ) ;
#184068=CARTESIAN_POINT ( 'NONE',  ( -5.823673210054431948, 21.52544592524334988, 107.7094237280190328 ) ) ;
#184069=CARTESIAN_POINT ( 'NONE',  ( 8.314922557960818139, 14.29746914071049879, 79.58224293864769550 ) ) ;
#184070=CARTESIAN_POINT ( 'NONE',  ( -5.719274019375978568, 21.55341960407610458, 110.2072429386477239 ) ) ;
#184071=CARTESIAN_POINT ( 'NONE',  ( -21.55341960407610458, -5.719274019375992779, 101.4572429386476955 ) ) ;
#184073=CARTESIAN_POINT ( 'NONE',  ( 18.67979575497178502, 10.72451020669898547, 49.16557627198102409 ) ) ;
#184074=CARTESIAN_POINT ( 'NONE',  ( 16.55341960407618274, -4.379528057220086978, 76.04275706135237556 ) ) ;
#184075=CARTESIAN_POINT ( 'NONE',  ( 4.379528057220339221, -16.55341960407611168, 107.7072429386476955 ) ) ;
#184076=CARTESIAN_POINT ( 'NONE',  ( -16.51473224551069308, -9.474510206698971260, 61.66557627198103120 ) ) ;
#184078=CARTESIAN_POINT ( 'NONE',  ( -16.55341960407617563, 4.379528057220093196, 108.5427570613523756 ) ) ;
#184080=CARTESIAN_POINT ( 'NONE',  ( 18.67979575497194134, -10.72451020669871369, 50.83442372801901143 ) ) ;
#184081=CARTESIAN_POINT ( 'NONE',  ( 5.049401038298161559, -19.05341960407611168, 92.70724293864769550 ) ) ;
#184082=CARTESIAN_POINT ( 'NONE',  ( 21.55341960407619695, -5.719274019375665929, 86.04275706135236135 ) ) ;
#184083=CARTESIAN_POINT ( 'NONE',  ( -0.05219959533909027116, -19.03943276465977164, 22.49890960531436690 ) ) ;
#184084=CARTESIAN_POINT ( 'NONE',  ( 19.02544592524343514, -5.153800228976328945, 23.54057627198102054 ) ) ;
#184087=CARTESIAN_POINT ( 'NONE',  ( 15.72974639402176855, 15.80617190586768217, 66.87609039468568994 ) ) ;
#184088=CARTESIAN_POINT ( 'NONE',  ( -16.51473224551069308, -9.474510206698971260, 56.66557627198103120 ) ) ;
#184089=CARTESIAN_POINT ( 'NONE',  ( 19.02544592524343514, -5.153800228976328945, 108.5405762719810383 ) ) ;
#184090=CARTESIAN_POINT ( 'NONE',  ( 19.02544592524334988, 5.153800228976608722, 86.45942372801900433 ) ) ;
#184091=CARTESIAN_POINT ( 'NONE',  ( -10.72451020669870658, -18.67979575497194134, 44.58442372801901854 ) ) ;
#184092=CARTESIAN_POINT ( 'NONE',  ( -19.03943276465977164, -0.05219959533935918106, 108.7510903946856615 ) ) ;
#184093=CARTESIAN_POINT ( 'NONE',  ( -13.97604488694547697, 13.89961937509957934, 73.12609039468568994 ) ) ;
#184094=CARTESIAN_POINT ( 'NONE',  ( 13.97604488694527802, 13.89961937509977652, 44.37390960531435269 ) ) ;
#184095=CARTESIAN_POINT ( 'NONE',  ( -13.89961937509957401, -13.97604488694547875, 89.37609039468563310 ) ) ;
#184096=CARTESIAN_POINT ( 'NONE',  ( 0.05219959533934541429, -16.53943276465976808, 110.0010903946856757 ) ) ;
#184097=CARTESIAN_POINT ( 'NONE',  ( 9.474510206698729675, 16.51473224551082808, 77.08442372801900433 ) ) ;
#184098=CARTESIAN_POINT ( 'NONE',  ( 4.379528057220339221, -16.55341960407611168, 32.70724293864770260 ) ) ;
#184099=CARTESIAN_POINT ( 'NONE',  ( -5.049401038297874678, -19.05341960407617918, 64.79275706135233293 ) ) ;
#184100=CARTESIAN_POINT ( 'NONE',  ( -10.81492255796105439, 18.62759615963255655, 102.9177570613523756 ) ) ;
#184101=PRODUCT ( 'Mica Insulated Heating Coil Unit', 'Mica Insulated Heating Coil Unit', '', ( #113931 ) ) ;
#184102=CARTESIAN_POINT ( 'NONE',  ( 19.02544592524334988, 5.153800228976608722, 31.45942372801900433 ) ) ;
#184103=CARTESIAN_POINT ( 'NONE',  ( -16.46253265017160317, 9.564922557960807481, 35.83224293864768839 ) ) ;
#184105=CARTESIAN_POINT ( 'NONE',  ( -16.53943276465976808, -0.05219959533934237506, 43.75109039468568284 ) ) ;
#184109=CARTESIAN_POINT ( 'NONE',  ( 5.153800228976335163, 19.02544592524342804, 94.79057627198103830 ) ) ;
#184111=CARTESIAN_POINT ( 'NONE',  ( -9.474510206698720793, -16.51473224551083518, 79.58442372801899012 ) ) ;
#184112=CIRCLE ( 'NONE', #151785, 1.250000000000006439 ) ;
#184113=CARTESIAN_POINT ( 'NONE',  ( -0.05219959533907301413, -21.53943276465977519, 27.49890960531435269 ) ) ;
#184114=CARTESIAN_POINT ( 'NONE',  ( -16.51473224551082808, 9.474510206698731452, 23.33442372801900078 ) ) ;
#184115=CARTESIAN_POINT ( 'NONE',  ( 13.97604488694548053, -13.89961937509957401, 95.62609039468563310 ) ) ;
#184116=CARTESIAN_POINT ( 'NONE',  ( 16.52544592524342804, -4.483927247898539470, 113.5405762719810383 ) ) ;
#184117=CARTESIAN_POINT ( 'NONE',  ( -16.46253265017160317, 9.564922557960807481, 25.83224293864769194 ) ) ;
#184118=CARTESIAN_POINT ( 'NONE',  ( 5.823673210054125526, 21.52544592524343514, 64.79057627198103830 ) ) ;
#184119=CARTESIAN_POINT ( 'NONE',  ( -15.80617190586745835, -15.72974639402198527, 51.87390960531437401 ) ) ;
#184120=CARTESIAN_POINT ( 'NONE',  ( 5.153800228976335163, 19.02544592524342804, 29.79057627198102409 ) ) ;
#184122=CARTESIAN_POINT ( 'NONE',  ( 9.474510206698729675, 16.51473224551082808, 77.08442372801900433 ) ) ;
#184123=CARTESIAN_POINT ( 'NONE',  ( 16.52544592524342804, -4.483927247898539470, 43.54057627198103830 ) ) ;
#184124=CARTESIAN_POINT ( 'NONE',  ( -19.05341960407611168, -5.049401038298163336, 111.4572429386476671 ) ) ;
#184125=CARTESIAN_POINT ( 'NONE',  ( 5.823673210054444382, -21.52544592524334988, 90.20942372801903275 ) ) ;
#184126=CARTESIAN_POINT ( 'NONE',  ( -10.81492255796078084, -18.62759615963271287, 67.08224293864770971 ) ) ;
#184127=CARTESIAN_POINT ( 'NONE',  ( -5.823673210054431948, 21.52544592524334988, 52.70942372801902565 ) ) ;
#184128=CARTESIAN_POINT ( 'NONE',  ( 10.72451020669871369, 18.67979575497193778, 47.08442372801901854 ) ) ;
#184129=CARTESIAN_POINT ( 'NONE',  ( -16.46253265017160317, 9.564922557960807481, 100.8322429386477097 ) ) ;
#184130=CARTESIAN_POINT ( 'NONE',  ( -12.06949235617739369, -12.14591786802326823, 94.37609039468568994 ) ) ;
#184131=CARTESIAN_POINT ( 'NONE',  ( 15.80617190586769283, -15.72974639402175789, 45.62609039468567573 ) ) ;
#184132=CARTESIAN_POINT ( 'NONE',  ( 5.153800228976335163, 19.02544592524342804, 24.79057627198102765 ) ) ;
#184134=CARTESIAN_POINT ( 'NONE',  ( 8.314922557960818139, 14.29746914071049879, 69.58224293864769550 ) ) ;
#184135=CARTESIAN_POINT ( 'NONE',  ( 4.379528057220339221, -16.55341960407611168, 27.70724293864769905 ) ) ;
#184136=CARTESIAN_POINT ( 'NONE',  ( -5.153800228976328057, -19.02544592524343514, 67.29057627198102409 ) ) ;
#184137=CARTESIAN_POINT ( 'NONE',  ( -5.049401038298153566, 19.05341960407611168, 40.20724293864768839 ) ) ;
#184138=CARTESIAN_POINT ( 'NONE',  ( -5.823673210054116645, -21.52544592524344225, 57.29057627198103120 ) ) ;
#184139=CARTESIAN_POINT ( 'NONE',  ( 0.05219959533936267826, -19.03943276465977164, 40.00109039468566152 ) ) ;
#184141=CARTESIAN_POINT ( 'NONE',  ( -4.483927247898539470, -16.52544592524342804, 47.29057627198103120 ) ) ;
#184142=CARTESIAN_POINT ( 'NONE',  ( 15.72974639402199770, -15.80617190586745480, 28.12390960531435979 ) ) ;
#184143=AXIS2_PLACEMENT_3D ( 'NONE', #51508, #145500, #130316 ) ;
#184146=CARTESIAN_POINT ( 'NONE',  ( -14.34966873604972548, 8.224510206698743886, 78.33442372801901854 ) ) ;
#184147=CARTESIAN_POINT ( 'NONE',  ( -13.97604488694547697, 13.89961937509957934, 73.12609039468568994 ) ) ;
#184148=CARTESIAN_POINT ( 'NONE',  ( -14.34966873604960291, -8.224510206698953496, 41.66557627198103120 ) ) ;
#184149=CARTESIAN_POINT ( 'NONE',  ( 16.62475595723704558, -7.163666690055165098, 53.02713351810471210 ) ) ;
#184150=CARTESIAN_POINT ( 'NONE',  ( -12.06949235617756955, 12.14591786802309770, 30.62390960531436335 ) ) ;
#184151=CARTESIAN_POINT ( 'NONE',  ( 19.05341960407611168, 5.049401038298154454, 53.95724293864770260 ) ) ;
#184152=CARTESIAN_POINT ( 'NONE',  ( -19.02544592524342804, 5.153800228976336051, 81.04057627198103830 ) ) ;
#184153=CARTESIAN_POINT ( 'NONE',  ( 16.46253265017160672, -9.564922557960803928, 38.33224293864768839 ) ) ;
#184154=CARTESIAN_POINT ( 'NONE',  ( -18.67979575497193778, 10.72451020669871902, 43.33442372801901143 ) ) ;
#184155=CARTESIAN_POINT ( 'NONE',  ( 19.03943276465977164, -0.05219959533909143690, 63.74890960531435979 ) ) ;
#184157=CARTESIAN_POINT ( 'NONE',  ( -19.05341960407611168, -5.049401038298163336, 61.45724293864769550 ) ) ;
#184158=CARTESIAN_POINT ( 'NONE',  ( -18.62759615963270932, 10.81492255796079327, 35.83224293864768839 ) ) ;
#184159=CARTESIAN_POINT ( 'NONE',  ( -0.05219959533909027116, -19.03943276465977164, 22.49890960531436690 ) ) ;
#184160=CARTESIAN_POINT ( 'NONE',  ( -21.55341960407610458, -5.719274019375992779, 26.45724293864768839 ) ) ;
#184161=CARTESIAN_POINT ( 'NONE',  ( 14.29746914071037800, 8.314922557961029526, 91.66775706135234714 ) ) ;
#184162=CARTESIAN_POINT ( 'NONE',  ( 10.72451020669871369, 18.67979575497193778, 102.0844237280190185 ) ) ;
#184163=CARTESIAN_POINT ( 'NONE',  ( -16.52544592524335698, -4.483927247898792601, 63.95942372801901854 ) ) ;
#184164=CARTESIAN_POINT ( 'NONE',  ( -5.049401038298153566, 19.05341960407611168, 110.2072429386476671 ) ) ;
#184165=CARTESIAN_POINT ( 'NONE',  ( -8.224510206698735004, -14.34966873604973081, 59.58442372801901854 ) ) ;
#184166=CARTESIAN_POINT ( 'NONE',  ( -0.05219959533934338120, 16.53943276465976808, 42.50109039468567573 ) ) ;
#184167=CARTESIAN_POINT ( 'NONE',  ( -8.314922557961024197, 14.29746914071037800, 92.91775706135236135 ) ) ;
#184168=CARTESIAN_POINT ( 'NONE',  ( -16.55341960407617563, 4.379528057220093196, 23.54275706135235424 ) ) ;
#184169=CARTESIAN_POINT ( 'NONE',  ( 19.03943276465977164, -0.05219959533909143690, 38.74890960531436690 ) ) ;
#184170=CARTESIAN_POINT ( 'NONE',  ( 0.05219959533907565091, 21.53943276465977519, 109.9989096053143527 ) ) ;
#184171=CARTESIAN_POINT ( 'NONE',  ( -8.314922557961024197, 14.29746914071037800, 22.91775706135235069 ) ) ;
#184172=CARTESIAN_POINT ( 'NONE',  ( -16.52544592524335698, -4.483927247898792601, 88.95942372801901854 ) ) ;
#184173=CARTESIAN_POINT ( 'NONE',  ( 18.22780087662121673, 5.500000000000056843, 43.98459894673892734 ) ) ;
#184174=CARTESIAN_POINT ( 'NONE',  ( -0.05219959533937732626, 21.53943276465977519, 82.50109039468568994 ) ) ;
#184175=CARTESIAN_POINT ( 'NONE',  ( 19.05341960407617918, -5.049401038297876454, 81.04275706135231871 ) ) ;
#184176=CARTESIAN_POINT ( 'NONE',  ( -4.483927247898539470, -16.52544592524342804, 62.29057627198102409 ) ) ;
#184177=CARTESIAN_POINT ( 'NONE',  ( 4.483927247898545687, 16.52544592524342804, 49.79057627198102409 ) ) ;
#184178=CARTESIAN_POINT ( 'NONE',  ( -14.34966873604960291, -8.224510206698953496, 101.6655762719810383 ) ) ;
#184179=CARTESIAN_POINT ( 'NONE',  ( 13.89961937509957401, 13.97604488694547697, 41.87609039468566152 ) ) ;
#184180=CARTESIAN_POINT ( 'NONE',  ( 17.60728821186572546, -5.499999999999887201, 53.36690927743005375 ) ) ;
#184181=CARTESIAN_POINT ( 'NONE',  ( 15.80617190586769283, -15.72974639402175789, 45.62609039468567573 ) ) ;
#184182=CARTESIAN_POINT ( 'NONE',  ( -19.02544592524334988, -5.153800228976617603, 108.9594237280189759 ) ) ;
#184184=CARTESIAN_POINT ( 'NONE',  ( -0.05219959533909027116, -19.03943276465977164, 107.4989096053143527 ) ) ;
#184185=CARTESIAN_POINT ( 'NONE',  ( 21.55341960407610458, 5.719274019375980345, 68.95724293864769550 ) ) ;
#184186=CARTESIAN_POINT ( 'NONE',  ( 19.05341960407617918, -5.049401038297876454, 101.0427570613523045 ) ) ;
#184187=CARTESIAN_POINT ( 'NONE',  ( -19.05341960407611168, -5.049401038298163336, 101.4572429386476955 ) ) ;
#184188=CARTESIAN_POINT ( 'NONE',  ( -9.474510206698720793, -16.51473224551083518, 49.58442372801899722 ) ) ;
#184189=CARTESIAN_POINT ( 'NONE',  ( -0.05219959533910754901, -16.53943276465976808, 112.4989096053143669 ) ) ;
#184190=CARTESIAN_POINT ( 'NONE',  ( -21.52544592524334988, -5.823673210054445271, 93.95942372801903275 ) ) ;
#184191=CARTESIAN_POINT ( 'NONE',  ( 5.049401038298161559, -19.05341960407611168, 42.70724293864767418 ) ) ;
#184192=CARTESIAN_POINT ( 'NONE',  ( 15.72974639402176855, 15.80617190586768217, 51.87609039468568284 ) ) ;
#184193=CARTESIAN_POINT ( 'NONE',  ( 18.67979575497194134, -10.72451020669871369, 90.83442372801901854 ) ) ;
#184194=CARTESIAN_POINT ( 'NONE',  ( -12.06949235617739369, -12.14591786802326823, 89.37609039468568994 ) ) ;
#184195=CARTESIAN_POINT ( 'NONE',  ( 5.719274019375673035, 21.55341960407619339, 37.29275706135235424 ) ) ;
#184196=CARTESIAN_POINT ( 'NONE',  ( -18.62759615963255300, -10.81492255796106328, 39.16775706135235424 ) ) ;
#184197=CARTESIAN_POINT ( 'NONE',  ( 0.05219959533936267826, -19.03943276465977164, 65.00109039468567573 ) ) ;
#184198=CARTESIAN_POINT ( 'NONE',  ( 13.89961937509977652, -13.97604488694527269, 93.12390960531436690 ) ) ;
#184199=CARTESIAN_POINT ( 'NONE',  ( -12.14591786802309592, -12.06949235617757132, 106.8739096053143811 ) ) ;
#184200=CARTESIAN_POINT ( 'NONE',  ( -10.72451020669898014, 18.67979575497178502, 85.41557627198102409 ) ) ;
#184201=CARTESIAN_POINT ( 'NONE',  ( -12.14591786802309592, -12.06949235617757132, 61.87390960531436690 ) ) ;
#184202=CARTESIAN_POINT ( 'NONE',  ( 21.53943276465977519, 0.05219959533937863772, 101.2510903946856757 ) ) ;
#184203=CARTESIAN_POINT ( 'NONE',  ( -12.14591786802309592, -12.06949235617757132, 81.87390960531435269 ) ) ;
#184204=CARTESIAN_POINT ( 'NONE',  ( -16.51473224551069308, -9.474510206698971260, 41.66557627198103120 ) ) ;
#184205=CARTESIAN_POINT ( 'NONE',  ( 9.474510206698729675, 16.51473224551082808, 82.08442372801899012 ) ) ;
#184206=CARTESIAN_POINT ( 'NONE',  ( 16.53943276465976808, -0.05219959533910856209, 48.74890960531435979 ) ) ;
#184207=CARTESIAN_POINT ( 'NONE',  ( -5.719274019375665041, -21.55341960407619695, 99.79275706135234714 ) ) ;
#184208=CARTESIAN_POINT ( 'NONE',  ( -13.89961937509977652, 13.97604488694528158, 95.62390960531436690 ) ) ;
#184209=CARTESIAN_POINT ( 'NONE',  ( -0.05219959533936034679, 19.03943276465977164, 57.50109039468566863 ) ) ;
#184210=CARTESIAN_POINT ( 'NONE',  ( 21.52544592524344225, -5.823673210054117533, 68.54057627198103830 ) ) ;
#184211=CARTESIAN_POINT ( 'NONE',  ( 5.719274019375991003, -21.55341960407610458, 112.7072429386476955 ) ) ;
#184212=CARTESIAN_POINT ( 'NONE',  ( 4.483927247898790824, -16.52544592524335698, 25.20942372801901854 ) ) ;
#184213=CARTESIAN_POINT ( 'NONE',  ( 0.05219959533934541429, -16.53943276465976808, 85.00109039468568994 ) ) ;
#184214=LINE ( 'NONE', #180266, #177382 ) ;
#184215=CARTESIAN_POINT ( 'NONE',  ( 10.72451020669871369, 18.67979575497193778, 22.08442372801901143 ) ) ;
#184216=CARTESIAN_POINT ( 'NONE',  ( 16.46253265017160672, -9.564922557960803928, 23.33224293864769194 ) ) ;
#184218=CARTESIAN_POINT ( 'NONE',  ( 12.14591786802327356, -12.06949235617739191, 45.62609039468567573 ) ) ;
#184219=EDGE_CURVE ( 'NONE', #22576, #96464, #95691, .T. ) ;
#184220=CARTESIAN_POINT ( 'NONE',  ( 4.483927247898545687, 16.52544592524342804, 79.79057627198102409 ) ) ;
#184221=CARTESIAN_POINT ( 'NONE',  ( -5.823673210054116645, -21.52544592524344225, 77.29057627198102409 ) ) ;
#184222=CARTESIAN_POINT ( 'NONE',  ( -16.55341960407611168, -4.379528057220339221, 31.45724293864769550 ) ) ;
#184223=CARTESIAN_POINT ( 'NONE',  ( -12.06949235617739369, -12.14591786802326823, 34.37609039468568284 ) ) ;
#184224=CARTESIAN_POINT ( 'NONE',  ( 0.05219959533909260263, 19.03943276465977164, 49.99890960531435979 ) ) ;
#184225=CARTESIAN_POINT ( 'NONE',  ( 14.34966873604972726, -8.224510206698740333, 75.83442372801900433 ) ) ;
#184226=CARTESIAN_POINT ( 'NONE',  ( -16.51473224551082808, 9.474510206698731452, 68.33442372801900433 ) ) ;
#184227=CARTESIAN_POINT ( 'NONE',  ( -5.823673210054116645, -21.52544592524344225, 77.29057627198102409 ) ) ;
#184228=CARTESIAN_POINT ( 'NONE',  ( 16.52544592524335698, 4.483927247898782831, 111.4594237280190328 ) ) ;
#184231=CARTESIAN_POINT ( 'NONE',  ( -10.81492255796078084, -18.62759615963271287, 47.08224293864770260 ) ) ;
#184233=CARTESIAN_POINT ( 'NONE',  ( 16.52544592524335698, 4.483927247898782831, 96.45942372801901854 ) ) ;
#184234=CARTESIAN_POINT ( 'NONE',  ( -10.72451020669898014, 18.67979575497178502, 50.41557627198103120 ) ) ;
#184236=CARTESIAN_POINT ( 'NONE',  ( -16.51473224551069308, -9.474510206698971260, 111.6655762719810383 ) ) ;
#184237=CARTESIAN_POINT ( 'NONE',  ( 17.49999999999998934, 3.305555262949649187, 107.8748284784340541 ) ) ;
#184238=CARTESIAN_POINT ( 'NONE',  ( -16.52544592524342804, 4.483927247898546575, 116.0405762719810383 ) ) ;
#184239=CARTESIAN_POINT ( 'NONE',  ( 0.05219959533907565091, 21.53943276465977519, 69.99890960531435269 ) ) ;
#184240=CARTESIAN_POINT ( 'NONE',  ( -0.05219959533934338120, 16.53943276465976808, 102.5010903946856899 ) ) ;
#184241=CARTESIAN_POINT ( 'NONE',  ( -18.67979575497193778, 10.72451020669871902, 63.33442372801900433 ) ) ;
#184242=CARTESIAN_POINT ( 'NONE',  ( 12.06949235617739724, 12.14591786802326823, 21.87609039468567573 ) ) ;
#184243=CARTESIAN_POINT ( 'NONE',  ( 0.05219959533910956823, 16.53943276465976808, 109.9989096053143527 ) ) ;
#184244=CARTESIAN_POINT ( 'NONE',  ( 8.314922557961029526, -14.29746914071037800, 35.41775706135234003 ) ) ;
#184245=CARTESIAN_POINT ( 'NONE',  ( -5.153800228976328057, -19.02544592524343514, 52.29057627198100988 ) ) ;
#184247=CARTESIAN_POINT ( 'NONE',  ( 0.05219959533909260263, 19.03943276465977164, 109.9989096053143669 ) ) ;
#184248=CARTESIAN_POINT ( 'NONE',  ( 14.34966873604972726, -8.224510206698740333, 85.83442372801901854 ) ) ;
#184249=CARTESIAN_POINT ( 'NONE',  ( -16.46253265017146816, -9.564922557961047289, 94.16775706135233293 ) ) ;
#184250=CARTESIAN_POINT ( 'NONE',  ( -18.67979575497193778, 10.72451020669871902, 113.3344237280190328 ) ) ;
#184251=CARTESIAN_POINT ( 'NONE',  ( 21.52544592524344225, -5.823673210054117533, 78.54057627198103830 ) ) ;
#184252=CARTESIAN_POINT ( 'NONE',  ( 8.224510206698742110, 14.34966873604972548, 102.0844237280190185 ) ) ;
#184253=CARTESIAN_POINT ( 'NONE',  ( -9.564922557961040184, 16.46253265017147172, 97.91775706135233293 ) ) ;
#184254=CARTESIAN_POINT ( 'NONE',  ( -9.474510206698964154, 16.51473224551069663, 50.41557627198102409 ) ) ;
#184255=CARTESIAN_POINT ( 'NONE',  ( 9.474510206698971260, -16.51473224551069308, 97.91557627198102409 ) ) ;
#184256=CARTESIAN_POINT ( 'NONE',  ( 10.81492255796106328, -18.62759615963255655, 50.41775706135235424 ) ) ;
#184257=CARTESIAN_POINT ( 'NONE',  ( 16.46253265017160672, -9.564922557960803928, 43.33224293864769550 ) ) ;
#184258=CARTESIAN_POINT ( 'NONE',  ( -16.61371651742603461, -7.165104196376156587, 86.14584930007006847 ) ) ;
#184259=CARTESIAN_POINT ( 'NONE',  ( -5.153800228976328057, -19.02544592524343514, 112.2905762719810099 ) ) ;
#184260=CARTESIAN_POINT ( 'NONE',  ( 0.05219959533910956823, 16.53943276465976808, 64.99890960531435269 ) ) ;
#184261=CARTESIAN_POINT ( 'NONE',  ( -18.62759615963270932, 10.81492255796079327, 70.83224293864770971 ) ) ;
#184263=CARTESIAN_POINT ( 'NONE',  ( 16.46253265017146816, 9.564922557961045513, 36.66775706135233293 ) ) ;
#184264=CARTESIAN_POINT ( 'NONE',  ( 17.50000000000001776, -3.242565516147306592, 37.50000000000000000 ) ) ;
#184265=CARTESIAN_POINT ( 'NONE',  ( 9.564922557960805705, 16.46253265017160317, 64.58224293864769550 ) ) ;
#184266=CARTESIAN_POINT ( 'NONE',  ( -19.05341960407611168, -5.049401038298163336, 81.45724293864769550 ) ) ;
#184267=CARTESIAN_POINT ( 'NONE',  ( 14.34966873604972726, -8.224510206698740333, 55.83442372801901854 ) ) ;
#184269=CARTESIAN_POINT ( 'NONE',  ( -16.46253265017146816, -9.564922557961047289, 34.16775706135233293 ) ) ;
#184270=CARTESIAN_POINT ( 'NONE',  ( 14.29746914071037800, 8.314922557961029526, 91.66775706135234714 ) ) ;
#184272=CARTESIAN_POINT ( 'NONE',  ( 4.483927247898790824, -16.52544592524335698, 85.20942372801901854 ) ) ;
#184273=CARTESIAN_POINT ( 'NONE',  ( -14.34966873604972548, 8.224510206698743886, 58.33442372801901143 ) ) ;
#184274=CARTESIAN_POINT ( 'NONE',  ( -19.05341960407617563, 5.049401038297882671, 23.54275706135233648 ) ) ;
#184275=CARTESIAN_POINT ( 'NONE',  ( 5.153800228976335163, 19.02544592524342804, 59.79057627198100988 ) ) ;
#184277=CARTESIAN_POINT ( 'NONE',  ( 21.55341960407619695, -5.719274019375665929, 61.04275706135234714 ) ) ;
#184278=CARTESIAN_POINT ( 'NONE',  ( 13.89961937509957401, 13.97604488694547697, 76.87609039468566152 ) ) ;
#184279=CARTESIAN_POINT ( 'NONE',  ( 5.823673210054444382, -21.52544592524334988, 110.2094237280190185 ) ) ;
#184280=CARTESIAN_POINT ( 'NONE',  ( 5.153800228976335163, 19.02544592524342804, 49.79057627198100988 ) ) ;
#184281=CARTESIAN_POINT ( 'NONE',  ( 17.33830594066689912, 6.305085581112166437, 23.88102644207486946 ) ) ;
#184282=CARTESIAN_POINT ( 'NONE',  ( 21.53943276465977519, -0.05219959533907433946, 68.74890960531435269 ) ) ;
#184284=CARTESIAN_POINT ( 'NONE',  ( 15.80617190586746368, 15.72974639402197994, 24.37390960531435979 ) ) ;
#184285=CARTESIAN_POINT ( 'NONE',  ( -12.06949235617756955, 12.14591786802309770, 115.6239096053143669 ) ) ;
#184286=CARTESIAN_POINT ( 'NONE',  ( -12.06949235617739369, -12.14591786802326823, 44.37609039468567573 ) ) ;
#184288=CARTESIAN_POINT ( 'NONE',  ( -4.379528057220328563, 16.55341960407611168, 30.20724293864769550 ) ) ;
#184289=ORIENTED_EDGE ( 'NONE', *, *, #175843, .F. ) ;
#184290=CARTESIAN_POINT ( 'NONE',  ( 18.62759615963255655, 10.81492255796105972, 21.66775706135235069 ) ) ;
#184291=CARTESIAN_POINT ( 'NONE',  ( -14.34966873604960291, -8.224510206698953496, 46.66557627198102409 ) ) ;
#184293=CARTESIAN_POINT ( 'NONE',  ( -9.564922557961040184, 16.46253265017147172, 107.9177570613523471 ) ) ;
#184294=CARTESIAN_POINT ( 'NONE',  ( 0.05219959533936267826, -19.03943276465977164, 45.00109039468566863 ) ) ;
#184295=CARTESIAN_POINT ( 'NONE',  ( -8.314922557960811034, -14.29746914071050412, 47.08224293864770260 ) ) ;
#184296=CARTESIAN_POINT ( 'NONE',  ( -18.67979575497178146, -10.72451020669898902, 101.6655762719810383 ) ) ;
#184298=CARTESIAN_POINT ( 'NONE',  ( -5.823673210054116645, -21.52544592524344225, 67.29057627198103830 ) ) ;
#184299=CARTESIAN_POINT ( 'NONE',  ( -0.05219959533909027116, -19.03943276465977164, 72.49890960531435269 ) ) ;
#184300=CARTESIAN_POINT ( 'NONE',  ( -12.06949235617756955, 12.14591786802309770, 45.62390960531436690 ) ) ;
#184301=CARTESIAN_POINT ( 'NONE',  ( -5.049401038298153566, 19.05341960407611168, 100.2072429386476955 ) ) ;
#184304=CARTESIAN_POINT ( 'NONE',  ( 19.05341960407617918, -5.049401038297876454, 61.04275706135232582 ) ) ;
#184305=CARTESIAN_POINT ( 'NONE',  ( -15.72974639402197994, 15.80617190586746368, 100.6239096053143811 ) ) ;
#184306=CARTESIAN_POINT ( 'NONE',  ( 19.03943276465977164, -0.05219959533909143690, 43.74890960531435979 ) ) ;
#184307=CARTESIAN_POINT ( 'NONE',  ( 9.564922557960805705, 16.46253265017160317, 24.58224293864769194 ) ) ;
#184308=CARTESIAN_POINT ( 'NONE',  ( -21.55341960407619339, 5.719274019375674811, 53.54275706135234714 ) ) ;
#184310=CARTESIAN_POINT ( 'NONE',  ( -16.53943276465976808, -0.05219959533934237506, 113.7510903946856757 ) ) ;
#184311=CARTESIAN_POINT ( 'NONE',  ( -5.153800228976328057, -19.02544592524343514, 47.29057627198102409 ) ) ;
#184312=CARTESIAN_POINT ( 'NONE',  ( -5.049401038298153566, 19.05341960407611168, 100.2072429386476955 ) ) ;
#184313=CARTESIAN_POINT ( 'NONE',  ( 0.05219959533907565091, 21.53943276465977519, 59.99890960531436690 ) ) ;
#184314=CARTESIAN_POINT ( 'NONE',  ( -19.25663599770061651, 5.499999999999455547, 43.99419308057201761 ) ) ;
#184315=CARTESIAN_POINT ( 'NONE',  ( 13.97604488694527802, 13.89961937509977652, 49.37390960531434558 ) ) ;
#184316=CARTESIAN_POINT ( 'NONE',  ( -10.81492255796078084, -18.62759615963271287, 52.08224293864768839 ) ) ;
#184317=CARTESIAN_POINT ( 'NONE',  ( 10.72451020669871369, 18.67979575497193778, 87.08442372801901854 ) ) ;
#184319=CARTESIAN_POINT ( 'NONE',  ( -14.34966873604972548, 8.224510206698743886, 78.33442372801901854 ) ) ;
#184320=CARTESIAN_POINT ( 'NONE',  ( -16.53943276465976808, -0.05219959533934237506, 93.75109039468567573 ) ) ;
#184321=CARTESIAN_POINT ( 'NONE',  ( -5.153800228976328057, -19.02544592524343514, 67.29057627198102409 ) ) ;
#184322=ORIENTED_EDGE ( 'NONE', *, *, #163889, .F. ) ;
#184323=CARTESIAN_POINT ( 'NONE',  ( 9.564922557961047289, -16.46253265017146816, 30.41775706135232937 ) ) ;
#184324=CARTESIAN_POINT ( 'NONE',  ( -16.55341960407617563, 4.379528057220093196, 83.54275706135234714 ) ) ;
#184325=CARTESIAN_POINT ( 'NONE',  ( 18.62759615963255655, 10.81492255796105972, 111.6677570613523613 ) ) ;
#184326=CARTESIAN_POINT ( 'NONE',  ( -13.89961937509977652, 13.97604488694528158, 75.62390960531438111 ) ) ;
#184327=CARTESIAN_POINT ( 'NONE',  ( 18.67979575497178502, 10.72451020669898547, 49.16557627198102409 ) ) ;
#184328=CARTESIAN_POINT ( 'NONE',  ( -4.483927247898782831, 16.52544592524335698, 22.70942372801901499 ) ) ;
#184329=CARTESIAN_POINT ( 'NONE',  ( 18.67979575497194134, -10.72451020669871369, 80.83442372801901854 ) ) ;
#184330=CARTESIAN_POINT ( 'NONE',  ( -16.53943276465976808, -0.05219959533934237506, 63.75109039468568284 ) ) ;
#184331=CARTESIAN_POINT ( 'NONE',  ( -15.72974639402197994, 15.80617190586746368, 115.6239096053143669 ) ) ;
#184332=CARTESIAN_POINT ( 'NONE',  ( 19.05341960407617918, -5.049401038297876454, 111.0427570613523329 ) ) ;
#184333=CARTESIAN_POINT ( 'NONE',  ( 0.05219959533909260263, 19.03943276465977164, 94.99890960531436690 ) ) ;
#184334=CARTESIAN_POINT ( 'NONE',  ( 12.14591786802327356, -12.06949235617739191, 25.62609039468567929 ) ) ;
#184335=CARTESIAN_POINT ( 'NONE',  ( -19.02544592524342804, 5.153800228976336051, 41.04057627198103120 ) ) ;
#184336=CARTESIAN_POINT ( 'NONE',  ( 14.29746914071037800, 8.314922557961029526, 21.66775706135235069 ) ) ;
#184337=CARTESIAN_POINT ( 'NONE',  ( 12.14591786802309770, 12.06949235617756955, 79.37390960531436690 ) ) ;
#184338=CARTESIAN_POINT ( 'NONE',  ( -14.34966873604972548, 8.224510206698743886, 88.33442372801901854 ) ) ;
#184339=CARTESIAN_POINT ( 'NONE',  ( -18.62759615963255300, -10.81492255796106328, 29.16775706135234003 ) ) ;
#184340=CARTESIAN_POINT ( 'NONE',  ( -13.89961937509977652, 13.97604488694528158, 60.62390960531436690 ) ) ;
#184341=CARTESIAN_POINT ( 'NONE',  ( 19.03943276465977164, -0.05219959533909143690, 63.74890960531435979 ) ) ;
#184342=CARTESIAN_POINT ( 'NONE',  ( 16.55341960407618274, -4.379528057220086978, 86.04275706135236135 ) ) ;
#184346=CARTESIAN_POINT ( 'NONE',  ( 5.049401038297881783, 19.05341960407617563, 27.29275706135232937 ) ) ;
#184347=CARTESIAN_POINT ( 'NONE',  ( 19.05341960407611168, 5.049401038298154454, 38.95724293864767418 ) ) ;
#184350=CARTESIAN_POINT ( 'NONE',  ( 16.53943276465976808, 0.05219959533934440121, 31.25109039468568639 ) ) ;
#184351=CARTESIAN_POINT ( 'NONE',  ( 19.05341960407617918, -5.049401038297876454, 61.04275706135232582 ) ) ;
#184352=CARTESIAN_POINT ( 'NONE',  ( -4.483927247898782831, 16.52544592524335698, 42.70942372801901854 ) ) ;
#184353=CARTESIAN_POINT ( 'NONE',  ( 16.51473224551069308, 9.474510206698969483, 109.1655762719810383 ) ) ;
#184354=CARTESIAN_POINT ( 'NONE',  ( -9.474510206698964154, 16.51473224551069663, 80.41557627198103830 ) ) ;
#184355=CARTESIAN_POINT ( 'NONE',  ( -10.72451020669898014, 18.67979575497178502, 100.4155762719810241 ) ) ;
#184356=CARTESIAN_POINT ( 'NONE',  ( -16.46253265017146816, -9.564922557961047289, 64.16775706135233293 ) ) ;
#184357=CARTESIAN_POINT ( 'NONE',  ( 9.474510206698971260, -16.51473224551069308, 97.91557627198102409 ) ) ;
#184359=CARTESIAN_POINT ( 'NONE',  ( 9.564922557960805705, 16.46253265017160317, 64.58224293864769550 ) ) ;
#184360=CARTESIAN_POINT ( 'NONE',  ( -16.55341960407617563, 4.379528057220093196, 113.5427570613523756 ) ) ;
#184361=CARTESIAN_POINT ( 'NONE',  ( 0.05219959533909260263, 19.03943276465977164, 69.99890960531435269 ) ) ;
#184362=CARTESIAN_POINT ( 'NONE',  ( -5.049401038297874678, -19.05341960407617918, 34.79275706135233293 ) ) ;
#184363=CARTESIAN_POINT ( 'NONE',  ( 4.379528057220339221, -16.55341960407611168, 72.70724293864769550 ) ) ;
#184364=CARTESIAN_POINT ( 'NONE',  ( 21.55341960407619695, -5.719274019375665929, 96.04275706135236135 ) ) ;
#184365=CARTESIAN_POINT ( 'NONE',  ( -19.03943276465977164, 0.05219959533909376836, 41.24890960531435269 ) ) ;
#184366=CARTESIAN_POINT ( 'NONE',  ( 16.55341960407618274, -4.379528057220086978, 51.04275706135234714 ) ) ;
#184367=CARTESIAN_POINT ( 'NONE',  ( -16.52544592524342804, 4.483927247898546575, 41.04057627198103120 ) ) ;
#184368=CARTESIAN_POINT ( 'NONE',  ( 18.62759615963255655, 10.81492255796105972, 86.66775706135234714 ) ) ;
#184369=CARTESIAN_POINT ( 'NONE',  ( 16.46253265017160672, -9.564922557960803928, 73.33224293864769550 ) ) ;
#184370=CARTESIAN_POINT ( 'NONE',  ( -19.03943276465977164, 0.05219959533909376836, 101.2489096053143669 ) ) ;
#184371=CARTESIAN_POINT ( 'NONE',  ( 16.55341960407611168, 4.379528057220329451, 103.9572429386476813 ) ) ;
#184372=CARTESIAN_POINT ( 'NONE',  ( 12.06949235617757843, -12.14591786802309237, 73.12390960531436690 ) ) ;
#184373=CARTESIAN_POINT ( 'NONE',  ( 15.80617190586746368, 15.72974639402197994, 89.37390960531435269 ) ) ;
#184374=CARTESIAN_POINT ( 'NONE',  ( -16.51473224551069308, -9.474510206698971260, 86.66557627198102409 ) ) ;
#184375=CARTESIAN_POINT ( 'NONE',  ( -5.823673210054116645, -21.52544592524344225, 97.29057627198105251 ) ) ;
#184376=CARTESIAN_POINT ( 'NONE',  ( -19.03943276465977164, -0.05219959533935918106, 73.75109039468566152 ) ) ;
#184377=CARTESIAN_POINT ( 'NONE',  ( 19.52837319214028611, -5.499999999999893419, 47.10471352585541638 ) ) ;
#184378=CARTESIAN_POINT ( 'NONE',  ( 8.224510206698953496, -14.34966873604960469, 87.91557627198103830 ) ) ;
#184379=CARTESIAN_POINT ( 'NONE',  ( -5.153800228976328057, -19.02544592524343514, 52.29057627198100988 ) ) ;
#184380=CARTESIAN_POINT ( 'NONE',  ( 0.05219959533907565091, 21.53943276465977519, 59.99890960531436690 ) ) ;
#184381=CARTESIAN_POINT ( 'NONE',  ( 16.29526858892873875, -7.335722546920261600, 26.70329402199794444 ) ) ;
#184382=CARTESIAN_POINT ( 'NONE',  ( 16.55341960407618274, -4.379528057220086978, 106.0427570613523471 ) ) ;
#184384=CARTESIAN_POINT ( 'NONE',  ( 8.224510206698742110, 14.34966873604972548, 22.08442372801901143 ) ) ;
#184385=CARTESIAN_POINT ( 'NONE',  ( 4.379528057220339221, -16.55341960407611168, 82.70724293864770971 ) ) ;
#184386=CARTESIAN_POINT ( 'NONE',  ( 18.87580814761078329, -5.499999999999872102, 53.37172394265758868 ) ) ;
#184387=CARTESIAN_POINT ( 'NONE',  ( 19.02544592524343514, -5.153800228976328945, 73.54057627198103830 ) ) ;
#184388=CARTESIAN_POINT ( 'NONE',  ( 13.97604488694527802, 13.89961937509977652, 29.37390960531435979 ) ) ;
#184389=CARTESIAN_POINT ( 'NONE',  ( 14.29746914071049879, -8.314922557960816363, 73.33224293864769550 ) ) ;
#184391=CARTESIAN_POINT ( 'NONE',  ( 16.51473224551069308, 9.474510206698969483, 114.1655762719810241 ) ) ;
#184392=CARTESIAN_POINT ( 'NONE',  ( -9.564922557961040184, 16.46253265017147172, 82.91775706135233293 ) ) ;
#184393=CARTESIAN_POINT ( 'NONE',  ( 9.564922557960805705, 16.46253265017160317, 99.58224293864770971 ) ) ;
#184394=CARTESIAN_POINT ( 'NONE',  ( -0.05219959533907301413, -21.53943276465977519, 72.49890960531435269 ) ) ;
#184395=CARTESIAN_POINT ( 'NONE',  ( 16.52544592524335698, 4.483927247898782831, 66.45942372801903275 ) ) ;
#184396=CARTESIAN_POINT ( 'NONE',  ( 19.03943276465977164, 0.05219959533936151252, 106.2510903946856615 ) ) ;
#184397=CARTESIAN_POINT ( 'NONE',  ( 5.049401038298161559, -19.05341960407611168, 67.70724293864769550 ) ) ;
#184398=CARTESIAN_POINT ( 'NONE',  ( 15.80617190586746368, 15.72974639402197994, 69.37390960531436690 ) ) ;
#184399=CARTESIAN_POINT ( 'NONE',  ( 9.474510206698729675, 16.51473224551082808, 102.0844237280190043 ) ) ;
#184400=CARTESIAN_POINT ( 'NONE',  ( 4.379528057220339221, -16.55341960407611168, 37.70724293864769550 ) ) ;
#184401=CARTESIAN_POINT ( 'NONE',  ( 10.81492255796106328, -18.62759615963255655, 60.41775706135235424 ) ) ;
#184402=CARTESIAN_POINT ( 'NONE',  ( 16.46253265017146816, 9.564922557961045513, 71.66775706135233293 ) ) ;
#184403=CARTESIAN_POINT ( 'NONE',  ( 4.483927247898790824, -16.52544592524335698, 75.20942372801901854 ) ) ;
#184404=CARTESIAN_POINT ( 'NONE',  ( -13.89961937509977652, 13.97604488694528158, 110.6239096053143243 ) ) ;
#184407=CARTESIAN_POINT ( 'NONE',  ( -8.314922557961024197, 14.29746914071037800, 92.91775706135236135 ) ) ;
#184408=CARTESIAN_POINT ( 'NONE',  ( -12.14591786802326823, 12.06949235617739902, 48.12609039468568284 ) ) ;
#184409=CARTESIAN_POINT ( 'NONE',  ( 5.049401038298161559, -19.05341960407611168, 62.70724293864769550 ) ) ;
#184410=CARTESIAN_POINT ( 'NONE',  ( 19.05341960407611168, 5.049401038298154454, 78.95724293864769550 ) ) ;
#184411=CARTESIAN_POINT ( 'NONE',  ( -10.72451020669870658, -18.67979575497194134, 69.58442372801900433 ) ) ;
#184412=CARTESIAN_POINT ( 'NONE',  ( 4.379528057220092307, 16.55341960407617563, 57.29275706135234714 ) ) ;
#184413=CARTESIAN_POINT ( 'NONE',  ( 14.34966873604960469, 8.224510206698951720, 29.16557627198103120 ) ) ;
#184414=CARTESIAN_POINT ( 'NONE',  ( 5.049401038298161559, -19.05341960407611168, 37.70724293864768839 ) ) ;
#184415=CARTESIAN_POINT ( 'NONE',  ( -19.02544592524342804, 5.153800228976336051, 36.04057627198100988 ) ) ;
#184416=CARTESIAN_POINT ( 'NONE',  ( -16.55341960407617563, 4.379528057220093196, 28.54275706135234358 ) ) ;
#184418=CARTESIAN_POINT ( 'NONE',  ( -9.564922557961040184, 16.46253265017147172, 77.91775706135234714 ) ) ;
#184419=CARTESIAN_POINT ( 'NONE',  ( -14.34966873604960291, -8.224510206698953496, 96.66557627198102409 ) ) ;
#184420=CARTESIAN_POINT ( 'NONE',  ( 16.51473224551069308, 9.474510206698969483, 49.16557627198102409 ) ) ;
#184421=CARTESIAN_POINT ( 'NONE',  ( -0.05219959533936034679, 19.03943276465977164, 82.50109039468567573 ) ) ;
#184423=CARTESIAN_POINT ( 'NONE',  ( 0.05219959533937995610, -21.53943276465977519, 85.00109039468568994 ) ) ;
#184424=CARTESIAN_POINT ( 'NONE',  ( 12.06949235617739724, 12.14591786802326823, 51.87609039468568284 ) ) ;
#184426=CARTESIAN_POINT ( 'NONE',  ( 18.62759615963271287, -10.81492255796078972, 53.33224293864769550 ) ) ;
#184427=CARTESIAN_POINT ( 'NONE',  ( -16.52544592524335698, -4.483927247898792601, 33.95942372801901143 ) ) ;
#184428=CARTESIAN_POINT ( 'NONE',  ( 16.51473224551069308, 9.474510206698969483, 34.16557627198102409 ) ) ;
#184429=CARTESIAN_POINT ( 'NONE',  ( -19.05341960407617563, 5.049401038297882671, 43.54275706135232582 ) ) ;
#184430=CARTESIAN_POINT ( 'NONE',  ( -5.153800228976328057, -19.02544592524343514, 92.29057627198099567 ) ) ;
#184431=CARTESIAN_POINT ( 'NONE',  ( -19.05341960407611168, -5.049401038298163336, 51.45724293864770260 ) ) ;
#184433=CARTESIAN_POINT ( 'NONE',  ( 21.52544592524334988, 5.823673210054432836, 76.45942372801901854 ) ) ;
#184435=CARTESIAN_POINT ( 'NONE',  ( 9.564922557961047289, -16.46253265017146816, 35.41775706135233293 ) ) ;
#184436=CARTESIAN_POINT ( 'NONE',  ( 18.67979575497194134, -10.72451020669871369, 105.8344237280190328 ) ) ;
#184437=CARTESIAN_POINT ( 'NONE',  ( 4.483927247898545687, 16.52544592524342804, 34.79057627198103120 ) ) ;
#184438=CARTESIAN_POINT ( 'NONE',  ( -16.51473224551069308, -9.474510206698971260, 61.66557627198103120 ) ) ;
#184439=CARTESIAN_POINT ( 'NONE',  ( 16.51473224551069308, 9.474510206698969483, 109.1655762719810383 ) ) ;
#184440=CARTESIAN_POINT ( 'NONE',  ( 21.53943276465977519, 0.05219959533937863772, 86.25109039468568994 ) ) ;
#184441=CARTESIAN_POINT ( 'NONE',  ( -16.51473224551069308, -9.474510206698971260, 66.66557627198102409 ) ) ;
#184442=CARTESIAN_POINT ( 'NONE',  ( -21.52544592524334988, -5.823673210054445271, 83.95942372801900433 ) ) ;
#184443=CARTESIAN_POINT ( 'NONE',  ( 18.67979575497178502, 10.72451020669898547, 34.16557627198102409 ) ) ;
#184444=CARTESIAN_POINT ( 'NONE',  ( 21.52544592524334988, 5.823673210054432836, 26.45942372801901854 ) ) ;
#184445=CARTESIAN_POINT ( 'NONE',  ( -19.02544592524334988, -5.153800228976617603, 43.95942372801899012 ) ) ;
#184446=CARTESIAN_POINT ( 'NONE',  ( -0.05219959533909027116, -19.03943276465977164, 32.49890960531435979 ) ) ;
#184447=CARTESIAN_POINT ( 'NONE',  ( -13.89961937509977652, 13.97604488694528158, 70.62390960531432427 ) ) ;
#184448=CARTESIAN_POINT ( 'NONE',  ( 12.06949235617739724, 12.14591786802326823, 26.87609039468567218 ) ) ;
#184449=CARTESIAN_POINT ( 'NONE',  ( -12.14591786802309592, -12.06949235617757132, 91.87390960531436690 ) ) ;
#184450=CARTESIAN_POINT ( 'NONE',  ( 19.05341960407611168, 5.049401038298154454, 63.95724293864769550 ) ) ;
#184451=CARTESIAN_POINT ( 'NONE',  ( 18.62759615963271287, -10.81492255796078972, 33.33224293864769550 ) ) ;
#184452=CARTESIAN_POINT ( 'NONE',  ( 19.02544592524334988, 5.153800228976608722, 101.4594237280189759 ) ) ;
#184453=CARTESIAN_POINT ( 'NONE',  ( -15.80617190586745835, -15.72974639402198527, 106.8739096053143811 ) ) ;
#184454=CARTESIAN_POINT ( 'NONE',  ( 15.80617190586769283, -15.72974639402175789, 70.62609039468567573 ) ) ;
#184455=CARTESIAN_POINT ( 'NONE',  ( 4.379528057220092307, 16.55341960407617563, 72.29275706135236135 ) ) ;
#184456=CARTESIAN_POINT ( 'NONE',  ( 12.14591786802327356, -12.06949235617739191, 65.62609039468568994 ) ) ;
#184457=CARTESIAN_POINT ( 'NONE',  ( 9.474510206698971260, -16.51473224551069308, 67.91557627198102409 ) ) ;
#184458=CARTESIAN_POINT ( 'NONE',  ( -14.34966873604972548, 8.224510206698743886, 88.33442372801901854 ) ) ;
#184459=CARTESIAN_POINT ( 'NONE',  ( -19.03943276465977164, -0.05219959533935918106, 43.75109039468566863 ) ) ;
#184461=CARTESIAN_POINT ( 'NONE',  ( -18.62759615963255300, -10.81492255796106328, 19.16775706135234714 ) ) ;
#184462=CARTESIAN_POINT ( 'NONE',  ( -8.314922557960811034, -14.29746914071050412, 67.08224293864770971 ) ) ;
#184463=CARTESIAN_POINT ( 'NONE',  ( -13.89961937509977652, 13.97604488694528158, 85.62390960531433848 ) ) ;
#184464=CARTESIAN_POINT ( 'NONE',  ( 12.06949235617739724, 12.14591786802326823, 71.87609039468568994 ) ) ;
#184465=CARTESIAN_POINT ( 'NONE',  ( -21.52544592524334988, -5.823673210054445271, 63.95942372801901854 ) ) ;
#184466=CARTESIAN_POINT ( 'NONE',  ( 16.55341960407618274, -4.379528057220086978, 21.04275706135234714 ) ) ;
#184467=CARTESIAN_POINT ( 'NONE',  ( -10.72451020669870658, -18.67979575497194134, 19.58442372801901143 ) ) ;
#184468=CARTESIAN_POINT ( 'NONE',  ( -16.55341960407611168, -4.379528057220339221, 61.45724293864770260 ) ) ;
#184470=CARTESIAN_POINT ( 'NONE',  ( -10.81492255796078084, -18.62759615963271287, 92.08224293864769550 ) ) ;
#184471=CARTESIAN_POINT ( 'NONE',  ( -14.34966873604960291, -8.224510206698953496, 41.66557627198103120 ) ) ;
#184472=VERTEX_POINT ( 'NONE', #3675 ) ;
#184474=CARTESIAN_POINT ( 'NONE',  ( -5.823673210054116645, -21.52544592524344225, 112.2905762719810241 ) ) ;
#184475=CARTESIAN_POINT ( 'NONE',  ( -16.51473224551069308, -9.474510206698971260, 106.6655762719810383 ) ) ;
#184476=CARTESIAN_POINT ( 'NONE',  ( 10.81492255796106328, -18.62759615963255655, 30.41775706135234358 ) ) ;
#184477=CARTESIAN_POINT ( 'NONE',  ( -8.314922557960811034, -14.29746914071050412, 57.08224293864769550 ) ) ;
#184478=CARTESIAN_POINT ( 'NONE',  ( -0.05219959533909027116, -19.03943276465977164, 67.49890960531436690 ) ) ;
#184479=CARTESIAN_POINT ( 'NONE',  ( 9.564922557961047289, -16.46253265017146816, 70.41775706135233293 ) ) ;
#184480=CARTESIAN_POINT ( 'NONE',  ( -16.46253265017160317, 9.564922557960807481, 95.83224293864769550 ) ) ;
#184482=CARTESIAN_POINT ( 'NONE',  ( -10.81492255796078084, -18.62759615963271287, 42.08224293864769550 ) ) ;
#184484=CARTESIAN_POINT ( 'NONE',  ( 13.89961937509977652, -13.97604488694527269, 58.12390960531436690 ) ) ;
#184485=CARTESIAN_POINT ( 'NONE',  ( 16.52544592524335698, 4.483927247898782831, 36.45942372801901143 ) ) ;
#184486=CARTESIAN_POINT ( 'NONE',  ( -19.02544592524334988, -5.153800228976617603, 58.95942372801900433 ) ) ;
#184487=CARTESIAN_POINT ( 'NONE',  ( -0.05219959533937732626, 21.53943276465977519, 22.50109039468567573 ) ) ;
#184488=CARTESIAN_POINT ( 'NONE',  ( 14.29746914071049879, -8.314922557960816363, 48.33224293864770260 ) ) ;
#184489=CARTESIAN_POINT ( 'NONE',  ( 5.049401038298161559, -19.05341960407611168, 87.70724293864769550 ) ) ;
#184490=CARTESIAN_POINT ( 'NONE',  ( -21.53943276465977519, 0.05219959533907696930, 66.24890960531436690 ) ) ;
#184491=CARTESIAN_POINT ( 'NONE',  ( 5.719274019375991003, -21.55341960407610458, 107.7072429386476955 ) ) ;
#184492=CARTESIAN_POINT ( 'NONE',  ( -16.52544592524335698, -4.483927247898792601, 43.95942372801902565 ) ) ;
#184493=CARTESIAN_POINT ( 'NONE',  ( 18.67979575497178502, 10.72451020669898547, 39.16557627198102409 ) ) ;
#184494=CARTESIAN_POINT ( 'NONE',  ( 5.719274019375673035, 21.55341960407619339, 102.2927570613523613 ) ) ;
#184495=CARTESIAN_POINT ( 'NONE',  ( -19.03943276465977164, 0.05219959533909376836, 91.24890960531436690 ) ) ;
#184496=CARTESIAN_POINT ( 'NONE',  ( -0.05219959533909027116, -19.03943276465977164, 42.49890960531435269 ) ) ;
#184497=CARTESIAN_POINT ( 'NONE',  ( 5.153800228976335163, 19.02544592524342804, 99.79057627198102409 ) ) ;
#184498=CARTESIAN_POINT ( 'NONE',  ( -19.02544592524342804, 5.153800228976336051, 71.04057627198099567 ) ) ;
#184499=CARTESIAN_POINT ( 'NONE',  ( -16.53943276465976808, -0.05219959533934237506, 28.75109039468567929 ) ) ;
#184501=CARTESIAN_POINT ( 'NONE',  ( 9.474510206698729675, 16.51473224551082808, 52.08442372801900433 ) ) ;
#184502=CARTESIAN_POINT ( 'NONE',  ( -21.55341960407619339, 5.719274019375674811, 113.5427570613523756 ) ) ;
#184503=CARTESIAN_POINT ( 'NONE',  ( -21.52544592524343514, 5.823673210054127303, 31.04057627198102409 ) ) ;
#184504=CARTESIAN_POINT ( 'NONE',  ( -16.52544592524335698, -4.483927247898792601, 93.95942372801903275 ) ) ;
#184506=CARTESIAN_POINT ( 'NONE',  ( 9.564922557961047289, -16.46253265017146816, 65.41775706135233293 ) ) ;
#184507=CARTESIAN_POINT ( 'NONE',  ( 0.05219959533936267826, -19.03943276465977164, 25.00109039468566152 ) ) ;
#184509=CARTESIAN_POINT ( 'NONE',  ( -5.049401038298153566, 19.05341960407611168, 35.20724293864768839 ) ) ;
#184510=CARTESIAN_POINT ( 'NONE',  ( -14.29746914071049879, 8.314922557960819915, 30.83224293864770260 ) ) ;
#184511=CARTESIAN_POINT ( 'NONE',  ( -19.05341960407611168, -5.049401038298163336, 26.45724293864769550 ) ) ;
#184512=CARTESIAN_POINT ( 'NONE',  ( 4.483927247898545687, 16.52544592524342804, 29.79057627198102409 ) ) ;
#184514=CARTESIAN_POINT ( 'NONE',  ( 4.379528057220092307, 16.55341960407617563, 92.29275706135236135 ) ) ;
#184515=CARTESIAN_POINT ( 'NONE',  ( 19.03943276465977164, -0.05219959533909143690, 33.74890960531435979 ) ) ;
#184516=CARTESIAN_POINT ( 'NONE',  ( -21.52544592524334988, -5.823673210054445271, 103.9594237280190185 ) ) ;
#184517=CARTESIAN_POINT ( 'NONE',  ( 16.53943276465976808, 0.05219959533934440121, 21.25109039468567218 ) ) ;
#184518=CARTESIAN_POINT ( 'NONE',  ( -15.80617190586768217, 15.72974639402176855, 73.12609039468567573 ) ) ;
#184519=CARTESIAN_POINT ( 'NONE',  ( -5.153800228976607833, 19.02544592524334988, 57.70942372801899012 ) ) ;
#184520=CARTESIAN_POINT ( 'NONE',  ( 16.46253265017160672, -9.564922557960803928, 93.33224293864769550 ) ) ;
#184521=CARTESIAN_POINT ( 'NONE',  ( -13.89961937509977652, 13.97604488694528158, 80.62390960531436690 ) ) ;
#184522=CARTESIAN_POINT ( 'NONE',  ( 16.38665767535054485, 7.295008042176069019, 72.23599135785453029 ) ) ;
#184523=CARTESIAN_POINT ( 'NONE',  ( 5.823673210054125526, 21.52544592524343514, 104.7905762719810241 ) ) ;
#184524=CARTESIAN_POINT ( 'NONE',  ( 16.52544592524342804, -4.483927247898539470, 68.54057627198103830 ) ) ;
#184525=CARTESIAN_POINT ( 'NONE',  ( -21.52544592524343514, 5.823673210054127303, 56.04057627198102409 ) ) ;
#184526=CARTESIAN_POINT ( 'NONE',  ( -13.97604488694527625, -13.89961937509977652, 61.87390960531435979 ) ) ;
#184527=CARTESIAN_POINT ( 'NONE',  ( -18.67979575497178146, -10.72451020669898902, 91.66557627198103830 ) ) ;
#184528=CARTESIAN_POINT ( 'NONE',  ( 8.224510206698742110, 14.34966873604972548, 87.08442372801901854 ) ) ;
#184529=ORIENTED_EDGE ( 'NONE', *, *, #21229, .F. ) ;
#184530=CARTESIAN_POINT ( 'NONE',  ( -19.05341960407611168, -5.049401038298163336, 56.45724293864768129 ) ) ;
#184531=CARTESIAN_POINT ( 'NONE',  ( 12.06949235617757843, -12.14591786802309237, 98.12390960531436690 ) ) ;
#184533=CARTESIAN_POINT ( 'NONE',  ( 19.03943276465977164, -0.05219959533909143690, 53.74890960531436690 ) ) ;
#184534=CARTESIAN_POINT ( 'NONE',  ( -19.02544592524334988, -5.153800228976617603, 78.95942372801900433 ) ) ;
#184535=CARTESIAN_POINT ( 'NONE',  ( 16.55341960407611168, 4.379528057220329451, 88.95724293864769550 ) ) ;
#184536=CARTESIAN_POINT ( 'NONE',  ( 15.72974639402176855, 15.80617190586768217, 41.87609039468568284 ) ) ;
#184537=CARTESIAN_POINT ( 'NONE',  ( -0.05219959533909027116, -19.03943276465977164, 42.49890960531435269 ) ) ;
#184538=CARTESIAN_POINT ( 'NONE',  ( 15.72974639402199770, -15.80617190586745480, 98.12390960531436690 ) ) ;
#184539=CARTESIAN_POINT ( 'NONE',  ( -4.379528057220328563, 16.55341960407611168, 90.20724293864770971 ) ) ;
#184541=CARTESIAN_POINT ( 'NONE',  ( -9.474510206698964154, 16.51473224551069663, 65.41557627198102409 ) ) ;
#184542=CARTESIAN_POINT ( 'NONE',  ( 18.89770734986051792, 5.499999999999905853, 46.60214472496640781 ) ) ;
#184543=CARTESIAN_POINT ( 'NONE',  ( -13.97604488694547697, 13.89961937509957934, 98.12609039468566152 ) ) ;
#184544=CARTESIAN_POINT ( 'NONE',  ( -13.89961937509977652, 13.97604488694528158, 110.6239096053143243 ) ) ;
#184545=CARTESIAN_POINT ( 'NONE',  ( -0.05219959533937732626, 21.53943276465977519, 32.50109039468568284 ) ) ;
#184546=CARTESIAN_POINT ( 'NONE',  ( -9.564922557960796823, -16.46253265017161027, 82.08224293864768129 ) ) ;
#184547=CARTESIAN_POINT ( 'NONE',  ( 0.05219959533936267826, -19.03943276465977164, 65.00109039468567573 ) ) ;
#184548=CARTESIAN_POINT ( 'NONE',  ( -16.46253265017160317, 9.564922557960807481, 55.83224293864769550 ) ) ;
#184549=CARTESIAN_POINT ( 'NONE',  ( -16.53943276465976808, 0.05219959533911058130, 81.24890960531436690 ) ) ;
#184550=CARTESIAN_POINT ( 'NONE',  ( 4.379528057220339221, -16.55341960407611168, 62.70724293864769550 ) ) ;
#184551=CARTESIAN_POINT ( 'NONE',  ( -19.03943276465977164, 0.05219959533909376836, 86.24890960531436690 ) ) ;
#184552=CARTESIAN_POINT ( 'NONE',  ( 18.67979575497178502, 10.72451020669898547, 99.16557627198100988 ) ) ;
#184553=CARTESIAN_POINT ( 'NONE',  ( 9.474510206698971260, -16.51473224551069308, 87.91557627198102409 ) ) ;
#184554=CARTESIAN_POINT ( 'NONE',  ( -5.049401038297874678, -19.05341960407617918, 29.79275706135232227 ) ) ;
#184555=CARTESIAN_POINT ( 'NONE',  ( -9.474510206698964154, 16.51473224551069663, 40.41557627198103120 ) ) ;
#184556=CARTESIAN_POINT ( 'NONE',  ( -8.224510206698948167, 14.34966873604960824, 35.41557627198102409 ) ) ;
#184557=CARTESIAN_POINT ( 'NONE',  ( 12.06949235617757843, -12.14591786802309237, 113.1239096053143953 ) ) ;
#184558=ORIENTED_EDGE ( 'NONE', *, *, #87010, .T. ) ;
#184559=CARTESIAN_POINT ( 'NONE',  ( 18.67979575497194134, -10.72451020669871369, 35.83442372801901143 ) ) ;
#184560=CARTESIAN_POINT ( 'NONE',  ( 19.03943276465977164, 0.05219959533936151252, 66.25109039468567573 ) ) ;
#184561=CARTESIAN_POINT ( 'NONE',  ( -0.05219959533910754901, -16.53943276465976808, 37.49890960531436690 ) ) ;
#184562=CARTESIAN_POINT ( 'NONE',  ( -0.05219959533907301413, -21.53943276465977519, 92.49890960531436690 ) ) ;
#184563=CARTESIAN_POINT ( 'NONE',  ( -18.67979575497178146, -10.72451020669898902, 21.66557627198102409 ) ) ;
#184564=CARTESIAN_POINT ( 'NONE',  ( 8.224510206698953496, -14.34966873604960469, 67.91557627198102409 ) ) ;
#184565=CARTESIAN_POINT ( 'NONE',  ( -5.049401038298153566, 19.05341960407611168, 30.20724293864768839 ) ) ;
#184566=CARTESIAN_POINT ( 'NONE',  ( -9.564922557961040184, 16.46253265017147172, 22.91775706135233648 ) ) ;
#184567=CARTESIAN_POINT ( 'NONE',  ( -16.55341960407617563, 4.379528057220093196, 103.5427570613523613 ) ) ;
#184568=CARTESIAN_POINT ( 'NONE',  ( 12.06949235617739724, 12.14591786802326823, 56.87609039468568994 ) ) ;
#184569=CARTESIAN_POINT ( 'NONE',  ( -21.55341960407610458, -5.719274019375992779, 36.45724293864768839 ) ) ;
#184570=CARTESIAN_POINT ( 'NONE',  ( 15.80617190586769283, -15.72974639402175789, 110.6260903946857042 ) ) ;
#184571=CARTESIAN_POINT ( 'NONE',  ( 13.97604488694527802, 13.89961937509977652, 74.37390960531436690 ) ) ;
#184572=CARTESIAN_POINT ( 'NONE',  ( 16.53943276465976808, 0.05219959533934440121, 76.25109039468568994 ) ) ;
#184573=CARTESIAN_POINT ( 'NONE',  ( -16.52544592524342804, 4.483927247898546575, 116.0405762719810383 ) ) ;
#184574=CARTESIAN_POINT ( 'NONE',  ( -4.483927247898539470, -16.52544592524342804, 32.29057627198102409 ) ) ;
#184575=CARTESIAN_POINT ( 'NONE',  ( -19.05341960407611168, -5.049401038298163336, 111.4572429386476671 ) ) ;
#184576=CARTESIAN_POINT ( 'NONE',  ( 16.46253265017160672, -9.564922557960803928, 93.33224293864769550 ) ) ;
#184577=CARTESIAN_POINT ( 'NONE',  ( 19.03943276465977164, -0.05219959533909143690, 113.7489096053143669 ) ) ;
#184578=CARTESIAN_POINT ( 'NONE',  ( 0.05219959533910956823, 16.53943276465976808, 59.99890960531436690 ) ) ;
#184579=CARTESIAN_POINT ( 'NONE',  ( 16.52544592524342804, -4.483927247898539470, 28.54057627198103120 ) ) ;
#184581=CARTESIAN_POINT ( 'NONE',  ( 0.05219959533910956823, 16.53943276465976808, 54.99890960531435269 ) ) ;
#184582=VERTEX_POINT ( 'NONE', #123044 ) ;
#184583=CARTESIAN_POINT ( 'NONE',  ( 4.379528057220092307, 16.55341960407617563, 42.29275706135235424 ) ) ;
#184584=CARTESIAN_POINT ( 'NONE',  ( 17.49999999999999289, -3.850315288878723763, 31.76629130603453888 ) ) ;
#184585=CARTESIAN_POINT ( 'NONE',  ( -16.51473224551082808, 9.474510206698731452, 53.33442372801900433 ) ) ;
#184586=CARTESIAN_POINT ( 'NONE',  ( -13.89961937509977652, 13.97604488694528158, 85.62390960531433848 ) ) ;
#184587=CARTESIAN_POINT ( 'NONE',  ( -19.05341960407617563, 5.049401038297882671, 63.54275706135234003 ) ) ;
#184589=CARTESIAN_POINT ( 'NONE',  ( -5.153800228976607833, 19.02544592524334988, 62.70942372801899722 ) ) ;
#184590=CARTESIAN_POINT ( 'NONE',  ( -9.564922557961040184, 16.46253265017147172, 97.91775706135233293 ) ) ;
#184591=CARTESIAN_POINT ( 'NONE',  ( -14.29746914071037622, -8.314922557961029526, 89.16775706135236135 ) ) ;
#184593=CARTESIAN_POINT ( 'NONE',  ( 16.46253265017160672, -9.564922557960803928, 23.33224293864769194 ) ) ;
#184594=CARTESIAN_POINT ( 'NONE',  ( -10.72451020669898014, 18.67979575497178502, 25.41557627198103120 ) ) ;
#184595=CARTESIAN_POINT ( 'NONE',  ( 15.80617190586769283, -15.72974639402175789, 40.62609039468567573 ) ) ;
#184596=CARTESIAN_POINT ( 'NONE',  ( 0.05219959533936267826, -19.03943276465977164, 105.0010903946856615 ) ) ;
#184597=CARTESIAN_POINT ( 'NONE',  ( 17.50000000000002132, -4.658240926743160593, 106.4447041781680383 ) ) ;
#184598=CARTESIAN_POINT ( 'NONE',  ( -5.153800228976328057, -19.02544592524343514, 62.29057627198100988 ) ) ;
#184599=CARTESIAN_POINT ( 'NONE',  ( 5.049401038298161559, -19.05341960407611168, 97.70724293864766707 ) ) ;
#184600=CARTESIAN_POINT ( 'NONE',  ( -8.314922557960811034, -14.29746914071050412, 67.08224293864770971 ) ) ;
#184601=CARTESIAN_POINT ( 'NONE',  ( -9.564922557960796823, -16.46253265017161027, 67.08224293864769550 ) ) ;
#184602=CARTESIAN_POINT ( 'NONE',  ( 13.89961937509977652, -13.97604488694527269, 68.12390960531436690 ) ) ;
#184603=CARTESIAN_POINT ( 'NONE',  ( -5.049401038297874678, -19.05341960407617918, 79.79275706135233293 ) ) ;
#184604=CARTESIAN_POINT ( 'NONE',  ( 21.52544592524344225, -5.823673210054117533, 53.54057627198103120 ) ) ;
#184605=CARTESIAN_POINT ( 'NONE',  ( 5.049401038298161559, -19.05341960407611168, 22.70724293864769194 ) ) ;
#184606=CARTESIAN_POINT ( 'NONE',  ( -5.049401038297874678, -19.05341960407617918, 44.79275706135232582 ) ) ;
#184607=CARTESIAN_POINT ( 'NONE',  ( 0.05219959533909260263, 19.03943276465977164, 84.99890960531436690 ) ) ;
#184608=CARTESIAN_POINT ( 'NONE',  ( -5.719274019375978568, 21.55341960407610458, 70.20724293864769550 ) ) ;
#184609=CARTESIAN_POINT ( 'NONE',  ( -14.29746914071049879, 8.314922557960819915, 75.83224293864769550 ) ) ;
#184610=CARTESIAN_POINT ( 'NONE',  ( 19.05341960407617918, -5.049401038297876454, 36.04275706135234003 ) ) ;
#184611=CARTESIAN_POINT ( 'NONE',  ( 18.62759615963271287, -10.81492255796078972, 63.33224293864770260 ) ) ;
#184612=CARTESIAN_POINT ( 'NONE',  ( -10.72451020669898014, 18.67979575497178502, 45.41557627198103830 ) ) ;
#184613=CARTESIAN_POINT ( 'NONE',  ( 21.55341960407619695, -5.719274019375665929, 96.04275706135236135 ) ) ;
#184614=CARTESIAN_POINT ( 'NONE',  ( -5.153800228976328057, -19.02544592524343514, 67.29057627198102409 ) ) ;
#184615=CARTESIAN_POINT ( 'NONE',  ( 5.049401038298161559, -19.05341960407611168, 22.70724293864769194 ) ) ;
#184616=CARTESIAN_POINT ( 'NONE',  ( -21.53943276465977519, -0.05219959533937600094, 28.75109039468567929 ) ) ;
#184617=CARTESIAN_POINT ( 'NONE',  ( 21.52544592524334988, 5.823673210054432836, 41.45942372801901143 ) ) ;
#184618=CARTESIAN_POINT ( 'NONE',  ( 19.02544592524343514, -5.153800228976328945, 38.54057627198103120 ) ) ;
#184619=CARTESIAN_POINT ( 'NONE',  ( 15.80617190586746368, 15.72974639402197994, 109.3739096053143811 ) ) ;
#184620=CARTESIAN_POINT ( 'NONE',  ( -9.564922557961040184, 16.46253265017147172, 47.91775706135233293 ) ) ;
#184621=CARTESIAN_POINT ( 'NONE',  ( 17.50000000000000000, -5.499999999999992895, 76.21769037696435589 ) ) ;
#184622=CARTESIAN_POINT ( 'NONE',  ( 16.46253265017160672, -9.564922557960803928, 28.33224293864769550 ) ) ;
#184624=CARTESIAN_POINT ( 'NONE',  ( -12.06949235617739369, -12.14591786802326823, 59.37609039468568284 ) ) ;
#184625=CARTESIAN_POINT ( 'NONE',  ( 13.89961937509977652, -13.97604488694527269, 23.12390960531436335 ) ) ;
#184627=CARTESIAN_POINT ( 'NONE',  ( -5.049401038298153566, 19.05341960407611168, 70.20724293864769550 ) ) ;
#184628=CARTESIAN_POINT ( 'NONE',  ( 4.379528057220339221, -16.55341960407611168, 112.7072429386476955 ) ) ;
#184631=CARTESIAN_POINT ( 'NONE',  ( 10.81492255796078972, 18.62759615963270932, 59.58224293864770260 ) ) ;
#184632=CARTESIAN_POINT ( 'NONE',  ( -16.53943276465976808, -0.05219959533934237506, 43.75109039468568284 ) ) ;
#184633=CARTESIAN_POINT ( 'NONE',  ( -21.52544592524334988, -5.823673210054445271, 93.95942372801903275 ) ) ;
#184634=CARTESIAN_POINT ( 'NONE',  ( 13.97604488694527802, 13.89961937509977652, 24.37390960531435624 ) ) ;
#184635=CARTESIAN_POINT ( 'NONE',  ( 4.379528057220092307, 16.55341960407617563, 112.2927570613523471 ) ) ;
#184636=CARTESIAN_POINT ( 'NONE',  ( -14.29746914071049879, 8.314922557960819915, 50.83224293864770971 ) ) ;
#184637=CARTESIAN_POINT ( 'NONE',  ( -19.05341960407611168, -5.049401038298163336, 51.45724293864770260 ) ) ;
#184638=CARTESIAN_POINT ( 'NONE',  ( -15.72974639402176322, -15.80617190586768395, 94.37609039468568994 ) ) ;
#184639=CARTESIAN_POINT ( 'NONE',  ( 10.81492255796106328, -18.62759615963255655, 20.41775706135234714 ) ) ;
#184640=CARTESIAN_POINT ( 'NONE',  ( -21.53943276465977519, -0.05219959533937600094, 68.75109039468568994 ) ) ;
#184641=CARTESIAN_POINT ( 'NONE',  ( 0.05219959533934541429, -16.53943276465976808, 55.00109039468568284 ) ) ;
#184642=CARTESIAN_POINT ( 'NONE',  ( -14.29746914071049879, 8.314922557960819915, 80.83224293864769550 ) ) ;
#184643=CARTESIAN_POINT ( 'NONE',  ( 0.05219959533937995610, -21.53943276465977519, 95.00109039468568994 ) ) ;
#184644=CARTESIAN_POINT ( 'NONE',  ( 16.53943276465976808, -0.05219959533910856209, 23.74890960531435269 ) ) ;
#184646=CARTESIAN_POINT ( 'NONE',  ( -14.29746914071037622, -8.314922557961029526, 34.16775706135234714 ) ) ;
#184647=CARTESIAN_POINT ( 'NONE',  ( 8.224510206698953496, -14.34966873604960469, 42.91557627198103120 ) ) ;
#184648=CARTESIAN_POINT ( 'NONE',  ( 12.06949235617739724, 12.14591786802326823, 86.87609039468568994 ) ) ;
#184649=CARTESIAN_POINT ( 'NONE',  ( 13.89961937509977652, -13.97604488694527269, 98.12390960531433848 ) ) ;
#184650=CARTESIAN_POINT ( 'NONE',  ( -16.51473224551069308, -9.474510206698971260, 111.6655762719810383 ) ) ;
#184651=CARTESIAN_POINT ( 'NONE',  ( -21.53943276465977519, -0.05219959533937600094, 93.75109039468567573 ) ) ;
#184652=CARTESIAN_POINT ( 'NONE',  ( 4.379528057220092307, 16.55341960407617563, 97.29275706135234714 ) ) ;
#184653=CARTESIAN_POINT ( 'NONE',  ( 16.55341960407611168, 4.379528057220329451, 68.95724293864769550 ) ) ;
#184654=CARTESIAN_POINT ( 'NONE',  ( 5.153800228976335163, 19.02544592524342804, 79.79057627198102409 ) ) ;
#184656=CARTESIAN_POINT ( 'NONE',  ( -8.224510206698735004, -14.34966873604973081, 34.58442372801900433 ) ) ;
#184657=CARTESIAN_POINT ( 'NONE',  ( 19.02544592524343514, -5.153800228976328945, 43.54057627198103120 ) ) ;
#184658=CARTESIAN_POINT ( 'NONE',  ( -16.46253265017160317, 9.564922557960807481, 95.83224293864769550 ) ) ;
#184659=CARTESIAN_POINT ( 'NONE',  ( 16.53943276465976808, 0.05219959533934440121, 31.25109039468568639 ) ) ;
#184661=CARTESIAN_POINT ( 'NONE',  ( -9.474510206698720793, -16.51473224551083518, 29.58442372801900433 ) ) ;
#184662=CARTESIAN_POINT ( 'NONE',  ( 8.224510206698742110, 14.34966873604972548, 97.08442372801904696 ) ) ;
#184663=CARTESIAN_POINT ( 'NONE',  ( 19.03943276465977164, -0.05219959533909143690, 33.74890960531435979 ) ) ;
#184664=CARTESIAN_POINT ( 'NONE',  ( 12.14591786802327356, -12.06949235617739191, 85.62609039468568994 ) ) ;
#184665=CARTESIAN_POINT ( 'NONE',  ( -12.06949235617739369, -12.14591786802326823, 69.37609039468567573 ) ) ;
#184666=CARTESIAN_POINT ( 'NONE',  ( 9.474510206698729675, 16.51473224551082808, 87.08442372801900433 ) ) ;
#184667=CARTESIAN_POINT ( 'NONE',  ( 0.05219959533936267826, -19.03943276465977164, 25.00109039468566152 ) ) ;
#184668=CARTESIAN_POINT ( 'NONE',  ( -16.46253265017160317, 9.564922557960807481, 45.83224293864769550 ) ) ;
#184669=CARTESIAN_POINT ( 'NONE',  ( 8.314922557960818139, 14.29746914071049879, 79.58224293864769550 ) ) ;
#184670=CARTESIAN_POINT ( 'NONE',  ( 19.05341960407617918, -5.049401038297876454, 56.04275706135234714 ) ) ;
#184671=CARTESIAN_POINT ( 'NONE',  ( -18.67979575497178146, -10.72451020669898902, 56.66557627198103830 ) ) ;
#184672=CARTESIAN_POINT ( 'NONE',  ( -16.51473224551082808, 9.474510206698731452, 33.33442372801899722 ) ) ;
#184673=CARTESIAN_POINT ( 'NONE',  ( -5.153800228976328057, -19.02544592524343514, 102.2905762719810383 ) ) ;
#184674=CARTESIAN_POINT ( 'NONE',  ( 15.72974639402199770, -15.80617190586745480, 83.12390960531436690 ) ) ;
#184675=CARTESIAN_POINT ( 'NONE',  ( 16.51473224551069308, 9.474510206698969483, 114.1655762719810241 ) ) ;
#184676=CARTESIAN_POINT ( 'NONE',  ( -5.153800228976607833, 19.02544592524334988, 107.7094237280189759 ) ) ;
#184677=CARTESIAN_POINT ( 'NONE',  ( 13.89961937509977652, -13.97604488694527269, 113.1239096053143527 ) ) ;
#184678=CARTESIAN_POINT ( 'NONE',  ( 16.51473224551083163, -9.474510206698727899, 110.8344237280190043 ) ) ;
#184679=CARTESIAN_POINT ( 'NONE',  ( -19.05341960407611168, -5.049401038298163336, 36.45724293864766707 ) ) ;
#184680=CARTESIAN_POINT ( 'NONE',  ( -19.05341960407611168, -5.049401038298163336, 96.45724293864769550 ) ) ;
#184681=CARTESIAN_POINT ( 'NONE',  ( -18.67979575497178146, -10.72451020669898902, 76.66557627198103830 ) ) ;
#184682=CARTESIAN_POINT ( 'NONE',  ( 16.55341960407618274, -4.379528057220086978, 51.04275706135234714 ) ) ;
#184683=CARTESIAN_POINT ( 'NONE',  ( -10.72451020669870658, -18.67979575497194134, 64.58442372801900433 ) ) ;
#184684=CARTESIAN_POINT ( 'NONE',  ( 13.97604488694548053, -13.89961937509957401, 105.6260903946856757 ) ) ;
#184685=CARTESIAN_POINT ( 'NONE',  ( -9.474510206698720793, -16.51473224551083518, 19.58442372801899722 ) ) ;
#184686=CARTESIAN_POINT ( 'NONE',  ( -4.483927247898782831, 16.52544592524335698, 112.7094237280190328 ) ) ;
#184687=CARTESIAN_POINT ( 'NONE',  ( -18.67979575497178146, -10.72451020669898902, 106.6655762719810383 ) ) ;
#184688=CARTESIAN_POINT ( 'NONE',  ( 4.483927247898545687, 16.52544592524342804, 34.79057627198103120 ) ) ;
#184689=CARTESIAN_POINT ( 'NONE',  ( 5.153800228976615827, -19.02544592524334988, 85.20942372801900433 ) ) ;
#184690=CARTESIAN_POINT ( 'NONE',  ( -18.67979575497193778, 10.72451020669871902, 58.33442372801901143 ) ) ;
#184691=CARTESIAN_POINT ( 'NONE',  ( 9.564922557961047289, -16.46253265017146816, 45.41775706135232582 ) ) ;
#184692=CARTESIAN_POINT ( 'NONE',  ( -16.52544592524342804, 4.483927247898546575, 101.0405762719810383 ) ) ;
#184693=CARTESIAN_POINT ( 'NONE',  ( 0.05219959533907565091, 21.53943276465977519, 24.99890960531435624 ) ) ;
#184694=CARTESIAN_POINT ( 'NONE',  ( 12.06949235617757843, -12.14591786802309237, 33.12390960531435979 ) ) ;
#184695=CARTESIAN_POINT ( 'NONE',  ( -15.80617190586768217, 15.72974639402176855, 103.1260903946856757 ) ) ;
#184696=CARTESIAN_POINT ( 'NONE',  ( -4.483927247898782831, 16.52544592524335698, 57.70942372801901143 ) ) ;
#184697=CARTESIAN_POINT ( 'NONE',  ( 12.06949235617757843, -12.14591786802309237, 23.12390960531436335 ) ) ;
#184698=CARTESIAN_POINT ( 'NONE',  ( 10.81492255796106328, -18.62759615963255655, 65.41775706135234714 ) ) ;
#184699=CARTESIAN_POINT ( 'NONE',  ( 0.05219959533937995610, -21.53943276465977519, 60.00109039468568284 ) ) ;
#184700=CARTESIAN_POINT ( 'NONE',  ( -16.51473224551069308, -9.474510206698971260, 21.66557627198102765 ) ) ;
#184701=CARTESIAN_POINT ( 'NONE',  ( 21.55341960407619695, -5.719274019375665929, 26.04275706135235779 ) ) ;
#184702=CARTESIAN_POINT ( 'NONE',  ( -0.05219959533910754901, -16.53943276465976808, 107.4989096053143669 ) ) ;
#184703=CARTESIAN_POINT ( 'NONE',  ( -5.049401038298153566, 19.05341960407611168, 35.20724293864768839 ) ) ;
#184704=CARTESIAN_POINT ( 'NONE',  ( -14.34966873604960291, -8.224510206698953496, 76.66557627198103830 ) ) ;
#184705=CARTESIAN_POINT ( 'NONE',  ( 0.05219959533909260263, 19.03943276465977164, 74.99890960531435269 ) ) ;
#184706=CARTESIAN_POINT ( 'NONE',  ( 4.379528057220339221, -16.55341960407611168, 27.70724293864769905 ) ) ;
#184707=CARTESIAN_POINT ( 'NONE',  ( -15.72974639402197994, 15.80617190586746368, 55.62390960531436690 ) ) ;
#184708=CARTESIAN_POINT ( 'NONE',  ( 8.314922557960818139, 14.29746914071049879, 89.58224293864768129 ) ) ;
#184709=CARTESIAN_POINT ( 'NONE',  ( -5.823673210054116645, -21.52544592524344225, 112.2905762719810241 ) ) ;
#184710=CARTESIAN_POINT ( 'NONE',  ( -5.153800228976328057, -19.02544592524343514, 97.29057627198099567 ) ) ;
#184711=CARTESIAN_POINT ( 'NONE',  ( 19.02544592524343514, -5.153800228976328945, 48.54057627198103120 ) ) ;
#184712=CARTESIAN_POINT ( 'NONE',  ( -19.02544592524334988, -5.153800228976617603, 103.9594237280190043 ) ) ;
#184714=CARTESIAN_POINT ( 'NONE',  ( -0.05219959533907301413, -21.53943276465977519, 62.49890960531436690 ) ) ;
#184715=CARTESIAN_POINT ( 'NONE',  ( 15.72974639402176855, 15.80617190586768217, 86.87609039468568994 ) ) ;
#184716=CARTESIAN_POINT ( 'NONE',  ( 5.049401038298161559, -19.05341960407611168, 67.70724293864769550 ) ) ;
#184717=CARTESIAN_POINT ( 'NONE',  ( 0.05219959533909260263, 19.03943276465977164, 99.99890960531436690 ) ) ;
#184718=CARTESIAN_POINT ( 'NONE',  ( -0.05219959533934338120, 16.53943276465976808, 82.50109039468568994 ) ) ;
#184719=CARTESIAN_POINT ( 'NONE',  ( 18.62759615963255655, 10.81492255796105972, 61.66775706135235424 ) ) ;
#184720=CARTESIAN_POINT ( 'NONE',  ( 18.62759615963255655, 10.81492255796105972, 86.66775706135234714 ) ) ;
#184721=CARTESIAN_POINT ( 'NONE',  ( -21.52544592524343514, 5.823673210054127303, 116.0405762719810383 ) ) ;
#184722=CARTESIAN_POINT ( 'NONE',  ( -8.314922557961024197, 14.29746914071037800, 77.91775706135231871 ) ) ;
#184723=CARTESIAN_POINT ( 'NONE',  ( 15.72974639402199770, -15.80617190586745480, 78.12390960531436690 ) ) ;
#184724=CARTESIAN_POINT ( 'NONE',  ( 19.02544592524334988, 5.153800228976608722, 41.45942372801900433 ) ) ;
#184725=CARTESIAN_POINT ( 'NONE',  ( -0.05219959533907301413, -21.53943276465977519, 37.49890960531436690 ) ) ;
#184726=CARTESIAN_POINT ( 'NONE',  ( -13.97604488694527625, -13.89961937509977652, 81.87390960531436690 ) ) ;
#184727=CARTESIAN_POINT ( 'NONE',  ( 4.483927247898545687, 16.52544592524342804, 24.79057627198103120 ) ) ;
#184728=CARTESIAN_POINT ( 'NONE',  ( -16.52216118717209170, 7.221426719304499642, 63.92400978953008206 ) ) ;
#184729=CARTESIAN_POINT ( 'NONE',  ( 15.80617190586746368, 15.72974639402197994, 24.37390960531435979 ) ) ;
#184731=CARTESIAN_POINT ( 'NONE',  ( 19.03943276465977164, 0.05219959533936151252, 101.2510903946856757 ) ) ;
#184732=CARTESIAN_POINT ( 'NONE',  ( -5.823673210054116645, -21.52544592524344225, 72.29057627198102409 ) ) ;
#184733=CARTESIAN_POINT ( 'NONE',  ( 4.379528057220339221, -16.55341960407611168, 47.70724293864770260 ) ) ;
#184734=CARTESIAN_POINT ( 'NONE',  ( 16.46253265017146816, 9.564922557961045513, 111.6677570613523329 ) ) ;
#184735=CARTESIAN_POINT ( 'NONE',  ( -9.474510206698964154, 16.51473224551069663, 35.41557627198102409 ) ) ;
#184736=CARTESIAN_POINT ( 'NONE',  ( 0.05219959533934541429, -16.53943276465976808, 20.00109039468568639 ) ) ;
#184737=CARTESIAN_POINT ( 'NONE',  ( -10.72451020669898014, 18.67979575497178502, 100.4155762719810241 ) ) ;
#184738=CARTESIAN_POINT ( 'NONE',  ( 16.46253265017146816, 9.564922557961045513, 71.66775706135233293 ) ) ;
#184739=CARTESIAN_POINT ( 'NONE',  ( 0.05219959533934541429, -16.53943276465976808, 75.00109039468568994 ) ) ;
#184740=CARTESIAN_POINT ( 'NONE',  ( -13.97604488694527625, -13.89961937509977652, 81.87390960531436690 ) ) ;
#184741=CARTESIAN_POINT ( 'NONE',  ( -14.34966873604960291, -8.224510206698953496, 71.66557627198100988 ) ) ;
#184742=CARTESIAN_POINT ( 'NONE',  ( 9.564922557960805705, 16.46253265017160317, 64.58224293864769550 ) ) ;
#184743=CARTESIAN_POINT ( 'NONE',  ( 16.52544592524342804, -4.483927247898539470, 68.54057627198103830 ) ) ;
#184744=CARTESIAN_POINT ( 'NONE',  ( -16.51473224551069308, -9.474510206698971260, 36.66557627198102409 ) ) ;
#184746=CARTESIAN_POINT ( 'NONE',  ( 4.379528057220339221, -16.55341960407611168, 42.70724293864770260 ) ) ;
#184747=CARTESIAN_POINT ( 'NONE',  ( -5.049401038298153566, 19.05341960407611168, 75.20724293864769550 ) ) ;
#184748=CARTESIAN_POINT ( 'NONE',  ( -30.00000000000000000, 5.499999999999992895, 102.5000000000000142 ) ) ;
#184749=CARTESIAN_POINT ( 'NONE',  ( 13.89961937509957401, 13.97604488694547697, 56.87609039468564731 ) ) ;
#184750=CARTESIAN_POINT ( 'NONE',  ( 4.483927247898790824, -16.52544592524335698, 60.20942372801902565 ) ) ;
#184751=CARTESIAN_POINT ( 'NONE',  ( 18.62759615963271287, -10.81492255796078972, 58.33224293864768839 ) ) ;
#184752=CARTESIAN_POINT ( 'NONE',  ( -16.51473224551082808, 9.474510206698731452, 28.33442372801900433 ) ) ;
#184753=CARTESIAN_POINT ( 'NONE',  ( 16.51473224551069308, 9.474510206698969483, 94.16557627198103830 ) ) ;
#184755=CARTESIAN_POINT ( 'NONE',  ( -10.81492255796078084, -18.62759615963271287, 32.08224293864769550 ) ) ;
#184756=CARTESIAN_POINT ( 'NONE',  ( -13.89961937509977652, 13.97604488694528158, 65.62390960531436690 ) ) ;
#184757=CARTESIAN_POINT ( 'NONE',  ( 21.52544592524334988, 5.823673210054432836, 56.45942372801902565 ) ) ;
#184758=CARTESIAN_POINT ( 'NONE',  ( 16.55341960407611168, 4.379528057220329451, 108.9572429386476955 ) ) ;
#184759=CARTESIAN_POINT ( 'NONE',  ( -18.67979575497178146, -10.72451020669898902, 106.6655762719810383 ) ) ;
#184760=CARTESIAN_POINT ( 'NONE',  ( 9.564922557960805705, 16.46253265017160317, 99.58224293864770971 ) ) ;
#184762=CARTESIAN_POINT ( 'NONE',  ( -10.81492255796105439, 18.62759615963255655, 42.91775706135235424 ) ) ;
#184764=CARTESIAN_POINT ( 'NONE',  ( -19.02544592524342804, 5.153800228976336051, 101.0405762719810241 ) ) ;
#184766=CARTESIAN_POINT ( 'NONE',  ( -0.05219959533907301413, -21.53943276465977519, 97.49890960531436690 ) ) ;
#184767=CARTESIAN_POINT ( 'NONE',  ( 5.049401038298161559, -19.05341960407611168, 42.70724293864767418 ) ) ;
#184768=CARTESIAN_POINT ( 'NONE',  ( -12.06949235617739369, -12.14591786802326823, 19.37609039468568639 ) ) ;
#184770=CARTESIAN_POINT ( 'NONE',  ( -0.05219959533909027116, -19.03943276465977164, 27.49890960531435624 ) ) ;
#184771=CARTESIAN_POINT ( 'NONE',  ( -21.52544592524334988, -5.823673210054445271, 103.9594237280190185 ) ) ;
#184772=CARTESIAN_POINT ( 'NONE',  ( -9.474510206698964154, 16.51473224551069663, 75.41557627198103830 ) ) ;
#184773=CARTESIAN_POINT ( 'NONE',  ( 18.67979575497194134, -10.72451020669871369, 45.83442372801901854 ) ) ;
#184774=CARTESIAN_POINT ( 'NONE',  ( -21.52544592524334988, -5.823673210054445271, 28.95942372801902209 ) ) ;
#184776=CARTESIAN_POINT ( 'NONE',  ( -13.97604488694527625, -13.89961937509977652, 101.8739096053143811 ) ) ;
#184778=CARTESIAN_POINT ( 'NONE',  ( -16.52544592524335698, -4.483927247898792601, 43.95942372801902565 ) ) ;
#184779=CARTESIAN_POINT ( 'NONE',  ( -0.05219959533934338120, 16.53943276465976808, 72.50109039468568994 ) ) ;
#184780=CARTESIAN_POINT ( 'NONE',  ( -0.05219959533937732626, 21.53943276465977519, 52.50109039468567573 ) ) ;
#184781=CARTESIAN_POINT ( 'NONE',  ( -18.67979575497193778, 10.72451020669871902, 78.33442372801901854 ) ) ;
#184783=CARTESIAN_POINT ( 'NONE',  ( -19.05341960407617563, 5.049401038297882671, 103.5427570613523329 ) ) ;
#184784=CARTESIAN_POINT ( 'NONE',  ( 16.46253265017160672, -9.564922557960803928, 73.33224293864769550 ) ) ;
#184785=CARTESIAN_POINT ( 'NONE',  ( 19.02544592524343514, -5.153800228976328945, 98.54057627198100988 ) ) ;
#184786=CARTESIAN_POINT ( 'NONE',  ( 12.06949235617757843, -12.14591786802309237, 108.1239096053143811 ) ) ;
#184787=CARTESIAN_POINT ( 'NONE',  ( -18.62759615963270932, 10.81492255796079327, 35.83224293864768839 ) ) ;
#184788=CARTESIAN_POINT ( 'NONE',  ( -4.483927247898782831, 16.52544592524335698, 87.70942372801901854 ) ) ;
#184789=CARTESIAN_POINT ( 'NONE',  ( 4.379528057220339221, -16.55341960407611168, 72.70724293864769550 ) ) ;
#184790=CARTESIAN_POINT ( 'NONE',  ( -19.03943276465977164, 0.05219959533909376836, 56.24890960531435979 ) ) ;
#184791=CARTESIAN_POINT ( 'NONE',  ( -21.55341960407619339, 5.719274019375674811, 78.54275706135236135 ) ) ;
#184793=CARTESIAN_POINT ( 'NONE',  ( -16.51473224551082808, 9.474510206698731452, 108.3344237280190043 ) ) ;
#184794=CARTESIAN_POINT ( 'NONE',  ( 8.314922557960818139, 14.29746914071049879, 74.58224293864768129 ) ) ;
#184795=CARTESIAN_POINT ( 'NONE',  ( 15.80617190586769283, -15.72974639402175789, 25.62609039468567929 ) ) ;
#184796=CARTESIAN_POINT ( 'NONE',  ( -10.72451020669898014, 18.67979575497178502, 60.41557627198102409 ) ) ;
#184797=FACE_OUTER_BOUND ( 'NONE', #192721, .T. ) ;
#184799=CARTESIAN_POINT ( 'NONE',  ( -9.474510206698964154, 16.51473224551069663, 85.41557627198102409 ) ) ;
#184800=CARTESIAN_POINT ( 'NONE',  ( -16.53943276465976808, 0.05219959533911058130, 56.24890960531436690 ) ) ;
#184801=CARTESIAN_POINT ( 'NONE',  ( -12.14591786802326823, 12.06949235617739902, 108.1260903946856757 ) ) ;
#184802=CARTESIAN_POINT ( 'NONE',  ( -14.34966873604972548, 8.224510206698743886, 93.33442372801901854 ) ) ;
#184803=CARTESIAN_POINT ( 'NONE',  ( 16.46253265017146816, 9.564922557961045513, 46.66775706135233293 ) ) ;
#184805=CARTESIAN_POINT ( 'NONE',  ( 16.46253265017160672, -9.564922557960803928, 103.3322429386476955 ) ) ;
#184806=CARTESIAN_POINT ( 'NONE',  ( -14.29746914071049879, 8.314922557960819915, 75.83224293864769550 ) ) ;
#184807=CARTESIAN_POINT ( 'NONE',  ( 5.049401038297881783, 19.05341960407617563, 37.29275706135232582 ) ) ;
#184808=CARTESIAN_POINT ( 'NONE',  ( -19.05341960407611168, -5.049401038298163336, 31.45724293864769550 ) ) ;
#184809=CARTESIAN_POINT ( 'NONE',  ( 5.719274019375991003, -21.55341960407610458, 32.70724293864770260 ) ) ;
#184810=CARTESIAN_POINT ( 'NONE',  ( 18.67979575497178502, 10.72451020669898547, 69.16557627198102409 ) ) ;
#184812=CARTESIAN_POINT ( 'NONE',  ( 16.53943276465976808, -0.05219959533910856209, 98.74890960531438111 ) ) ;
#184813=CARTESIAN_POINT ( 'NONE',  ( -14.29746914071037622, -8.314922557961029526, 49.16775706135234003 ) ) ;
#184814=CARTESIAN_POINT ( 'NONE',  ( 21.52544592524334988, 5.823673210054432836, 41.45942372801901143 ) ) ;
#184815=CARTESIAN_POINT ( 'NONE',  ( -4.483927247898539470, -16.52544592524342804, 97.29057627198105251 ) ) ;
#184816=EDGE_CURVE ( 'NONE', #26208, #99459, #81723, .T. ) ;
#184818=CARTESIAN_POINT ( 'NONE',  ( -17.48853670773243252, 5.747243402303158000, 48.66671299749990709 ) ) ;
#184819=CARTESIAN_POINT ( 'NONE',  ( 21.53943276465977519, -0.05219959533907433946, 28.74890960531435624 ) ) ;
#184820=CARTESIAN_POINT ( 'NONE',  ( -17.49999999999999645, -5.500000000000000888, 120.0000000000000142 ) ) ;
#184822=CARTESIAN_POINT ( 'NONE',  ( 4.379528057220092307, 16.55341960407617563, 37.29275706135235424 ) ) ;
#184823=CARTESIAN_POINT ( 'NONE',  ( -0.05219959533910754901, -16.53943276465976808, 27.49890960531435269 ) ) ;
#184824=CARTESIAN_POINT ( 'NONE',  ( 15.72974639402199770, -15.80617190586745480, 58.12390960531435979 ) ) ;
#184825=CARTESIAN_POINT ( 'NONE',  ( 5.153800228976615827, -19.02544592524334988, 80.20942372801901854 ) ) ;
#184826=CARTESIAN_POINT ( 'NONE',  ( 21.55341960407610458, 5.719274019375980345, 63.95724293864770260 ) ) ;
#184827=CARTESIAN_POINT ( 'NONE',  ( -5.823673210054431948, 21.52544592524334988, 77.70942372801900433 ) ) ;
#184828=CYLINDRICAL_SURFACE ( 'NONE', #53104, 2.000000000000000000 ) ;
#184829=CARTESIAN_POINT ( 'NONE',  ( 8.314922557961029526, -14.29746914071037800, 45.41775706135234003 ) ) ;
#184830=CARTESIAN_POINT ( 'NONE',  ( -13.89961937509977652, 13.97604488694528158, 40.62390960531435979 ) ) ;
#184831=CARTESIAN_POINT ( 'NONE',  ( -9.474510206698964154, 16.51473224551069663, 100.4155762719810241 ) ) ;
#184832=CARTESIAN_POINT ( 'NONE',  ( 19.03943276465977164, -0.05219959533909143690, 33.74890960531435979 ) ) ;
#184833=CARTESIAN_POINT ( 'NONE',  ( 16.55341960407611168, 4.379528057220329451, 103.9572429386476813 ) ) ;
#184834=EDGE_CURVE ( 'NONE', #23884, #14621, #88071, .T. ) ;
#184836=CARTESIAN_POINT ( 'NONE',  ( 9.564922557960805705, 16.46253265017160317, 109.5822429386476955 ) ) ;
#184838=CARTESIAN_POINT ( 'NONE',  ( 8.314922557961029526, -14.29746914071037800, 70.41775706135236135 ) ) ;
#184839=CARTESIAN_POINT ( 'NONE',  ( 5.719274019375991003, -21.55341960407610458, 87.70724293864769550 ) ) ;
#184840=CARTESIAN_POINT ( 'NONE',  ( 13.97604488694527802, 13.89961937509977652, 54.37390960531435979 ) ) ;
#184841=CARTESIAN_POINT ( 'NONE',  ( 15.80617190586769283, -15.72974639402175789, 25.62609039468567929 ) ) ;
#184842=CARTESIAN_POINT ( 'NONE',  ( 13.97604488694527802, 13.89961937509977652, 79.37390960531435269 ) ) ;
#184845=CARTESIAN_POINT ( 'NONE',  ( -21.53943276465977519, 0.05219959533907696930, 116.2489096053143669 ) ) ;
#184846=CARTESIAN_POINT ( 'NONE',  ( -13.97604488694527625, -13.89961937509977652, 26.87390960531434558 ) ) ;
#184847=CARTESIAN_POINT ( 'NONE',  ( -13.97604488694527625, -13.89961937509977652, 111.8739096053143243 ) ) ;
#184848=CARTESIAN_POINT ( 'NONE',  ( -19.02544592524334988, -5.153800228976617603, 73.95942372801900433 ) ) ;
#184849=CARTESIAN_POINT ( 'NONE',  ( 19.03943276465977164, 0.05219959533936151252, 26.25109039468566507 ) ) ;
#184850=CARTESIAN_POINT ( 'NONE',  ( -15.80617190586745835, -15.72974639402198527, 96.87390960531436690 ) ) ;
#184851=CARTESIAN_POINT ( 'NONE',  ( -13.97604488694547697, 13.89961937509957934, 38.12609039468566152 ) ) ;
#184852=CARTESIAN_POINT ( 'NONE',  ( -12.06949235617739369, -12.14591786802326823, 79.37609039468567573 ) ) ;
#184853=CARTESIAN_POINT ( 'NONE',  ( -9.564922557960796823, -16.46253265017161027, 107.0822429386476955 ) ) ;
#184854=CARTESIAN_POINT ( 'NONE',  ( 13.89961937509977652, -13.97604488694527269, 53.12390960531434558 ) ) ;
#184855=CARTESIAN_POINT ( 'NONE',  ( 15.80617190586769283, -15.72974639402175789, 65.62609039468568994 ) ) ;
#184856=CARTESIAN_POINT ( 'NONE',  ( -18.62759615963255300, -10.81492255796106328, 84.16775706135234714 ) ) ;
#184858=CARTESIAN_POINT ( 'NONE',  ( 9.564922557960805705, 16.46253265017160317, 69.58224293864770971 ) ) ;
#184859=CARTESIAN_POINT ( 'NONE',  ( -18.67979575497193778, 10.72451020669871902, 43.33442372801901143 ) ) ;
#184860=CARTESIAN_POINT ( 'NONE',  ( 19.03943276465977164, 0.05219959533936151252, 86.25109039468567573 ) ) ;
#184861=CARTESIAN_POINT ( 'NONE',  ( 9.474510206698971260, -16.51473224551069308, 57.91557627198103120 ) ) ;
#184862=CARTESIAN_POINT ( 'NONE',  ( 13.97604488694527802, 13.89961937509977652, 99.37390960531436690 ) ) ;
#184863=CARTESIAN_POINT ( 'NONE',  ( 16.46253265017160672, -9.564922557960803928, 68.33224293864770971 ) ) ;
#184864=CARTESIAN_POINT ( 'NONE',  ( 17.50000000000008882, -3.296979923273363866, 22.57062549986184052 ) ) ;
#184865=CARTESIAN_POINT ( 'NONE',  ( 16.46253265017160672, -9.564922557960803928, 58.33224293864769550 ) ) ;
#184867=CARTESIAN_POINT ( 'NONE',  ( 15.72974639402199770, -15.80617190586745480, 103.1239096053143811 ) ) ;
#184868=CARTESIAN_POINT ( 'NONE',  ( 16.52544592524335698, 4.483927247898782831, 91.45942372801901854 ) ) ;
#184870=CARTESIAN_POINT ( 'NONE',  ( 9.474510206698729675, 16.51473224551082808, 47.08442372801900433 ) ) ;
#184871=CARTESIAN_POINT ( 'NONE',  ( 0.05219959533909260263, 19.03943276465977164, 59.99890960531436690 ) ) ;
#184872=CARTESIAN_POINT ( 'NONE',  ( 0.05219959533910956823, 16.53943276465976808, 64.99890960531435269 ) ) ;
#184873=CARTESIAN_POINT ( 'NONE',  ( -16.52544592524342804, 4.483927247898546575, 91.04057627198103830 ) ) ;
#184874=CARTESIAN_POINT ( 'NONE',  ( 10.81492255796078972, 18.62759615963270932, 24.58224293864768839 ) ) ;
#184875=CARTESIAN_POINT ( 'NONE',  ( -9.474510206698964154, 16.51473224551069663, 95.41557627198102409 ) ) ;
#184876=CARTESIAN_POINT ( 'NONE',  ( 5.049401038298161559, -19.05341960407611168, 102.7072429386476955 ) ) ;
#184877=CARTESIAN_POINT ( 'NONE',  ( -16.46253265017146816, -9.564922557961047289, 24.16775706135233648 ) ) ;
#184878=CARTESIAN_POINT ( 'NONE',  ( -8.314922557961024197, 14.29746914071037800, 87.91775706135234714 ) ) ;
#184879=CARTESIAN_POINT ( 'NONE',  ( -19.03943276465977164, 0.05219959533909376836, 71.24890960531435269 ) ) ;
#184880=CARTESIAN_POINT ( 'NONE',  ( -10.72451020669870658, -18.67979575497194134, 34.58442372801900433 ) ) ;
#184881=CARTESIAN_POINT ( 'NONE',  ( -18.67979575497178146, -10.72451020669898902, 26.66557627198103475 ) ) ;
#184882=CARTESIAN_POINT ( 'NONE',  ( 18.67979575497194134, -10.72451020669871369, 20.83442372801901143 ) ) ;
#184883=CARTESIAN_POINT ( 'NONE',  ( -21.53943276465977519, 0.05219959533907696930, 71.24890960531435269 ) ) ;
#184884=CARTESIAN_POINT ( 'NONE',  ( -19.02544592524342804, 5.153800228976336051, 56.04057627198100988 ) ) ;
#184885=CARTESIAN_POINT ( 'NONE',  ( 8.224510206698953496, -14.34966873604960469, 82.91557627198103830 ) ) ;
#184886=CARTESIAN_POINT ( 'NONE',  ( 5.049401038297881783, 19.05341960407617563, 37.29275706135232582 ) ) ;
#184887=CARTESIAN_POINT ( 'NONE',  ( 14.29746914071049879, -8.314922557960816363, 113.3322429386476955 ) ) ;
#184888=CARTESIAN_POINT ( 'NONE',  ( -9.564922557960796823, -16.46253265017161027, 77.08224293864769550 ) ) ;
#184889=CARTESIAN_POINT ( 'NONE',  ( -13.89961937509977652, 13.97604488694528158, 75.62390960531438111 ) ) ;
#184891=CARTESIAN_POINT ( 'NONE',  ( 16.52544592524342804, -4.483927247898539470, 98.54057627198105251 ) ) ;
#184893=CARTESIAN_POINT ( 'NONE',  ( -16.55341960407617563, 4.379528057220093196, 108.5427570613523756 ) ) ;
#184894=CARTESIAN_POINT ( 'NONE',  ( -0.05219959533934338120, 16.53943276465976808, 22.50109039468567573 ) ) ;
#184895=CARTESIAN_POINT ( 'NONE',  ( 15.72974639402176855, 15.80617190586768217, 86.87609039468568994 ) ) ;
#184896=CARTESIAN_POINT ( 'NONE',  ( 16.51473224551069308, 9.474510206698969483, 99.16557627198102409 ) ) ;
#184897=CARTESIAN_POINT ( 'NONE',  ( -10.81492255796105439, 18.62759615963255655, 22.91775706135235069 ) ) ;
#184898=CARTESIAN_POINT ( 'NONE',  ( 5.153800228976335163, 19.02544592524342804, 34.79057627198102409 ) ) ;
#184899=CARTESIAN_POINT ( 'NONE',  ( -16.52544592524335698, -4.483927247898792601, 33.95942372801901143 ) ) ;
#184900=CARTESIAN_POINT ( 'NONE',  ( -13.97604488694547697, 13.89961937509957934, 98.12609039468566152 ) ) ;
#184901=CARTESIAN_POINT ( 'NONE',  ( -18.67979575497178146, -10.72451020669898902, 91.66557627198103830 ) ) ;
#184902=CARTESIAN_POINT ( 'NONE',  ( -13.89961937509957401, -13.97604488694547875, 64.37609039468567573 ) ) ;
#184903=CARTESIAN_POINT ( 'NONE',  ( -19.05341960407611168, -5.049401038298163336, 21.45724293864768839 ) ) ;
#184904=CARTESIAN_POINT ( 'NONE',  ( -21.55341960407619339, 5.719274019375674811, 23.54275706135235424 ) ) ;
#184905=LINE ( 'NONE', #84669, #175732 ) ;
#184906=CARTESIAN_POINT ( 'NONE',  ( 19.03943276465977164, -0.05219959533909143690, 88.74890960531436690 ) ) ;
#184908=CARTESIAN_POINT ( 'NONE',  ( 13.97604488694527802, 13.89961937509977652, 89.37390960531436690 ) ) ;
#184909=CARTESIAN_POINT ( 'NONE',  ( 10.72451020669898902, -18.67979575497178502, 112.9155762719810383 ) ) ;
#184910=CARTESIAN_POINT ( 'NONE',  ( -4.483927247898539470, -16.52544592524342804, 77.29057627198102409 ) ) ;
#184911=CARTESIAN_POINT ( 'NONE',  ( -19.03943276465977164, 0.05219959533909376836, 86.24890960531436690 ) ) ;
#184912=CARTESIAN_POINT ( 'NONE',  ( 0.05219959533934541429, -16.53943276465976808, 50.00109039468568994 ) ) ;
#184914=CARTESIAN_POINT ( 'NONE',  ( 19.03943276465977164, 0.05219959533936151252, 61.25109039468566863 ) ) ;
#184915=CARTESIAN_POINT ( 'NONE',  ( 21.53943276465977519, 0.05219959533937863772, 61.25109039468567573 ) ) ;
#184916=CARTESIAN_POINT ( 'NONE',  ( 16.53943276465976808, 0.05219959533934440121, 21.25109039468567218 ) ) ;
#184917=CARTESIAN_POINT ( 'NONE',  ( -16.51473224551069308, -9.474510206698971260, 71.66557627198102409 ) ) ;
#184918=CARTESIAN_POINT ( 'NONE',  ( -9.474510206698720793, -16.51473224551083518, 89.58442372801900433 ) ) ;
#184919=CARTESIAN_POINT ( 'NONE',  ( 16.55341960407618274, -4.379528057220086978, 56.04275706135235424 ) ) ;
#184920=CARTESIAN_POINT ( 'NONE',  ( 21.53943276465977519, 0.05219959533937863772, 91.25109039468568994 ) ) ;
#184921=CARTESIAN_POINT ( 'NONE',  ( 9.564922557961047289, -16.46253265017146816, 75.41775706135234714 ) ) ;
#184922=CARTESIAN_POINT ( 'NONE',  ( 5.153800228976335163, 19.02544592524342804, 44.79057627198103830 ) ) ;
#184923=CARTESIAN_POINT ( 'NONE',  ( 18.62759615963271287, -10.81492255796078972, 68.33224293864769550 ) ) ;
#184924=CARTESIAN_POINT ( 'NONE',  ( -16.53943276465976808, 0.05219959533911058130, 71.24890960531435269 ) ) ;
#184925=CARTESIAN_POINT ( 'NONE',  ( -13.97604488694547697, 13.89961937509957934, 78.12609039468567573 ) ) ;
#184926=CARTESIAN_POINT ( 'NONE',  ( 16.18388926212235646, -7.379444403734614077, 62.06046848633851454 ) ) ;
#184927=CARTESIAN_POINT ( 'NONE',  ( -13.97604488694547697, 13.89961937509957934, 48.12609039468566863 ) ) ;
#184928=CARTESIAN_POINT ( 'NONE',  ( -16.53943276465976808, -0.05219959533934237506, 108.7510903946857042 ) ) ;
#184929=CARTESIAN_POINT ( 'NONE',  ( 4.483927247898545687, 16.52544592524342804, 64.79057627198103830 ) ) ;
#184930=CARTESIAN_POINT ( 'NONE',  ( 21.52544592524334988, 5.823673210054432836, 101.4594237280190185 ) ) ;
#184932=CARTESIAN_POINT ( 'NONE',  ( -15.80617190586745835, -15.72974639402198527, 106.8739096053143811 ) ) ;
#184933=CARTESIAN_POINT ( 'NONE',  ( -19.05341960407611168, -5.049401038298163336, 61.45724293864769550 ) ) ;
#184934=CARTESIAN_POINT ( 'NONE',  ( 0.05219959533937995610, -21.53943276465977519, 90.00109039468567573 ) ) ;
#184935=CARTESIAN_POINT ( 'NONE',  ( 19.02544592524343514, -5.153800228976328945, 58.54057627198102409 ) ) ;
#184937=CARTESIAN_POINT ( 'NONE',  ( 13.97604488694527802, 13.89961937509977652, 24.37390960531435624 ) ) ;
#184938=CARTESIAN_POINT ( 'NONE',  ( -19.02544592524342804, 5.153800228976336051, 116.0405762719810383 ) ) ;
#184939=CARTESIAN_POINT ( 'NONE',  ( -16.52544592524342804, 4.483927247898546575, 71.04057627198103830 ) ) ;
#184940=CARTESIAN_POINT ( 'NONE',  ( 5.049401038298161559, -19.05341960407611168, 27.70724293864769550 ) ) ;
#184941=CARTESIAN_POINT ( 'NONE',  ( -4.483927247898539470, -16.52544592524342804, 82.29057627198103830 ) ) ;
#184942=CARTESIAN_POINT ( 'NONE',  ( -10.72451020669898014, 18.67979575497178502, 95.41557627198102409 ) ) ;
#184943=CARTESIAN_POINT ( 'NONE',  ( 15.80617190586769283, -15.72974639402175789, 50.62609039468568994 ) ) ;
#184945=CARTESIAN_POINT ( 'NONE',  ( -12.06949235617739369, -12.14591786802326823, 54.37609039468568994 ) ) ;
#184946=CARTESIAN_POINT ( 'NONE',  ( 15.72974639402199770, -15.80617190586745480, 93.12390960531436690 ) ) ;
#184947=CARTESIAN_POINT ( 'NONE',  ( -19.05341960407617563, 5.049401038297882671, 28.54275706135232937 ) ) ;
#184948=CARTESIAN_POINT ( 'NONE',  ( -13.89961937509977652, 13.97604488694528158, 110.6239096053143243 ) ) ;
#184949=CARTESIAN_POINT ( 'NONE',  ( -15.80617190586768217, 15.72974639402176855, 43.12609039468568284 ) ) ;
#184950=VECTOR ( 'NONE', #143580, 1000.000000000000000 ) ;
#184951=CARTESIAN_POINT ( 'NONE',  ( 0.05219959533907565091, 21.53943276465977519, 44.99890960531435979 ) ) ;
#184952=CARTESIAN_POINT ( 'NONE',  ( -16.53943276465976808, -0.05219959533934237506, 113.7510903946856757 ) ) ;
#184953=CARTESIAN_POINT ( 'NONE',  ( 21.55341960407619695, -5.719274019375665929, 61.04275706135234714 ) ) ;
#184954=CARTESIAN_POINT ( 'NONE',  ( 21.53943276465977519, 0.05219959533937863772, 91.25109039468568994 ) ) ;
#184955=CARTESIAN_POINT ( 'NONE',  ( 19.05341960407617918, -5.049401038297876454, 36.04275706135234003 ) ) ;
#184956=CARTESIAN_POINT ( 'NONE',  ( -4.379528057220086978, -16.55341960407618274, 84.79275706135234714 ) ) ;
#184957=CARTESIAN_POINT ( 'NONE',  ( 5.823673210054444382, -21.52544592524334988, 60.20942372801902565 ) ) ;
#184958=CARTESIAN_POINT ( 'NONE',  ( -9.564922557960796823, -16.46253265017161027, 42.08224293864769550 ) ) ;
#184959=CARTESIAN_POINT ( 'NONE',  ( 19.05341960407617918, -5.049401038297876454, 26.04275706135233293 ) ) ;
#184960=CARTESIAN_POINT ( 'NONE',  ( 0.05219959533907565091, 21.53943276465977519, 29.99890960531435979 ) ) ;
#184961=CARTESIAN_POINT ( 'NONE',  ( 5.823673210054125526, 21.52544592524343514, 114.7905762719810383 ) ) ;
#184962=CARTESIAN_POINT ( 'NONE',  ( 10.81492255796078972, 18.62759615963270932, 69.58224293864769550 ) ) ;
#184963=CARTESIAN_POINT ( 'NONE',  ( 8.314922557961029526, -14.29746914071037800, 45.41775706135234003 ) ) ;
#184965=CARTESIAN_POINT ( 'NONE',  ( 18.67979575497178502, 10.72451020669898547, 84.16557627198103830 ) ) ;
#184966=CARTESIAN_POINT ( 'NONE',  ( 12.06949235617739724, 12.14591786802326823, 71.87609039468568994 ) ) ;
#184967=CARTESIAN_POINT ( 'NONE',  ( 8.314922557960818139, 14.29746914071049879, 59.58224293864770260 ) ) ;
#184969=CARTESIAN_POINT ( 'NONE',  ( -16.46253265017146816, -9.564922557961047289, 99.16775706135233293 ) ) ;
#184970=CARTESIAN_POINT ( 'NONE',  ( -5.823673210054116645, -21.52544592524344225, 37.29057627198102409 ) ) ;
#184972=CARTESIAN_POINT ( 'NONE',  ( -16.52544592524335698, -4.483927247898792601, 38.95942372801901854 ) ) ;
#184973=CARTESIAN_POINT ( 'NONE',  ( -21.53943276465977519, -0.05219959533937600094, 18.75109039468568639 ) ) ;
#184974=CARTESIAN_POINT ( 'NONE',  ( -15.80617190586745835, -15.72974639402198527, 26.87390960531435979 ) ) ;
#184975=CARTESIAN_POINT ( 'NONE',  ( 8.224510206698742110, 14.34966873604972548, 52.08442372801901854 ) ) ;
#184976=CARTESIAN_POINT ( 'NONE',  ( 5.153800228976335163, 19.02544592524342804, 84.79057627198099567 ) ) ;
#184977=CARTESIAN_POINT ( 'NONE',  ( 21.52544592524334988, 5.823673210054432836, 36.45942372801901143 ) ) ;
#184978=CARTESIAN_POINT ( 'NONE',  ( 9.474510206698729675, 16.51473224551082808, 112.0844237280190043 ) ) ;
#184980=CARTESIAN_POINT ( 'NONE',  ( -5.823673210054116645, -21.52544592524344225, 27.29057627198103120 ) ) ;
#184982=CARTESIAN_POINT ( 'NONE',  ( 5.049401038297881783, 19.05341960407617563, 22.29275706135233648 ) ) ;
#184983=CARTESIAN_POINT ( 'NONE',  ( 8.314922557961029526, -14.29746914071037800, 45.41775706135234003 ) ) ;
#184984=CARTESIAN_POINT ( 'NONE',  ( -9.474510206698964154, 16.51473224551069663, 95.41557627198102409 ) ) ;
#184985=CARTESIAN_POINT ( 'NONE',  ( -18.67979575497178146, -10.72451020669898902, 101.6655762719810383 ) ) ;
#184986=CARTESIAN_POINT ( 'NONE',  ( -0.05219959533909027116, -19.03943276465977164, 77.49890960531435269 ) ) ;
#184988=CARTESIAN_POINT ( 'NONE',  ( -12.14591786802309592, -12.06949235617757132, 86.87390960531438111 ) ) ;
#184989=CARTESIAN_POINT ( 'NONE',  ( -10.72451020669898014, 18.67979575497178502, 35.41557627198102409 ) ) ;
#184991=CARTESIAN_POINT ( 'NONE',  ( 14.34966873604972726, -8.224510206698740333, 60.83442372801901854 ) ) ;
#184992=CARTESIAN_POINT ( 'NONE',  ( 18.62759615963271287, -10.81492255796078972, 98.33224293864769550 ) ) ;
#184993=CARTESIAN_POINT ( 'NONE',  ( 19.03943276465977164, 0.05219959533936151252, 81.25109039468567573 ) ) ;
#184995=CARTESIAN_POINT ( 'NONE',  ( 13.89961937509977652, -13.97604488694527269, 23.12390960531436335 ) ) ;
#184996=CARTESIAN_POINT ( 'NONE',  ( 0.05219959533907565091, 21.53943276465977519, 69.99890960531435269 ) ) ;
#184997=CARTESIAN_POINT ( 'NONE',  ( 9.564922557960805705, 16.46253265017160317, 94.58224293864769550 ) ) ;
#184998=CARTESIAN_POINT ( 'NONE',  ( 18.67979575497194134, -10.72451020669871369, 85.83442372801901854 ) ) ;
#184999=CARTESIAN_POINT ( 'NONE',  ( -0.05219959533909027116, -19.03943276465977164, 62.49890960531435979 ) ) ;
#185000=CARTESIAN_POINT ( 'NONE',  ( 14.34966873604972726, -8.224510206698740333, 45.83442372801901854 ) ) ;
#185001=CARTESIAN_POINT ( 'NONE',  ( 9.564922557960805705, 16.46253265017160317, 54.58224293864769550 ) ) ;
#185002=CARTESIAN_POINT ( 'NONE',  ( 10.81492255796106328, -18.62759615963255655, 75.41775706135233293 ) ) ;
#185004=CARTESIAN_POINT ( 'NONE',  ( 19.05341960407617918, -5.049401038297876454, 41.04275706135233293 ) ) ;
#185005=CARTESIAN_POINT ( 'NONE',  ( -9.474510206698720793, -16.51473224551083518, 44.58442372801900433 ) ) ;
#185006=CARTESIAN_POINT ( 'NONE',  ( 18.67979575497194134, -10.72451020669871369, 35.83442372801901143 ) ) ;
#185008=CARTESIAN_POINT ( 'NONE',  ( -13.89961937509957401, -13.97604488694547875, 34.37609039468566863 ) ) ;
#185009=CARTESIAN_POINT ( 'NONE',  ( 9.564922557960805705, 16.46253265017160317, 84.58224293864769550 ) ) ;
#185010=CARTESIAN_POINT ( 'NONE',  ( -19.05341960407611168, -5.049401038298163336, 71.45724293864766707 ) ) ;
#185011=CARTESIAN_POINT ( 'NONE',  ( 16.53943276465976808, 0.05219959533934440121, 111.2510903946856899 ) ) ;
#185012=CARTESIAN_POINT ( 'NONE',  ( -18.62759615963270932, 10.81492255796079327, 25.83224293864769194 ) ) ;
#185013=CARTESIAN_POINT ( 'NONE',  ( -15.80617190586768217, 15.72974639402176855, 88.12609039468570415 ) ) ;
#185015=CARTESIAN_POINT ( 'NONE',  ( 17.12812012977024878, 6.668231424566068100, 58.85948759323144941 ) ) ;
#185016=CARTESIAN_POINT ( 'NONE',  ( 0.05219959533937995610, -21.53943276465977519, 95.00109039468568994 ) ) ;
#185019=CARTESIAN_POINT ( 'NONE',  ( -5.049401038298153566, 19.05341960407611168, 25.20724293864768484 ) ) ;
#185020=CARTESIAN_POINT ( 'NONE',  ( -5.049401038298153566, 19.05341960407611168, 110.2072429386476671 ) ) ;
#185022=CARTESIAN_POINT ( 'NONE',  ( 14.29746914071037800, 8.314922557961029526, 51.66775706135234714 ) ) ;
#185023=CARTESIAN_POINT ( 'NONE',  ( 21.52544592524344225, -5.823673210054117533, 63.54057627198103830 ) ) ;
#185024=CARTESIAN_POINT ( 'NONE',  ( 0.05219959533910956823, 16.53943276465976808, 39.99890960531436690 ) ) ;
#185025=CARTESIAN_POINT ( 'NONE',  ( 12.14591786802309770, 12.06949235617756955, 104.3739096053143669 ) ) ;
#185026=CARTESIAN_POINT ( 'NONE',  ( -19.02544592524342804, 5.153800228976336051, 96.04057627198103830 ) ) ;
#185027=CARTESIAN_POINT ( 'NONE',  ( 19.05341960407617918, -5.049401038297876454, 26.04275706135233293 ) ) ;
#185028=CARTESIAN_POINT ( 'NONE',  ( 5.049401038298161559, -19.05341960407611168, 22.70724293864769194 ) ) ;
#185029=CARTESIAN_POINT ( 'NONE',  ( -21.55341960407619339, 5.719274019375674811, 68.54275706135234714 ) ) ;
#185031=CARTESIAN_POINT ( 'NONE',  ( 8.224510206698742110, 14.34966873604972548, 102.0844237280190185 ) ) ;
#185032=CARTESIAN_POINT ( 'NONE',  ( -0.05219959533936034679, 19.03943276465977164, 62.50109039468566863 ) ) ;
#185034=CARTESIAN_POINT ( 'NONE',  ( 15.80617190586746368, 15.72974639402197994, 34.37390960531435979 ) ) ;
#185035=CARTESIAN_POINT ( 'NONE',  ( -0.05219959533910754901, -16.53943276465976808, 87.49890960531436690 ) ) ;
#185036=CARTESIAN_POINT ( 'NONE',  ( -13.97604488694547697, 13.89961937509957934, 53.12609039468565442 ) ) ;
#185037=CARTESIAN_POINT ( 'NONE',  ( -19.05341960407611168, -5.049401038298163336, 76.45724293864769550 ) ) ;
#185038=CARTESIAN_POINT ( 'NONE',  ( 16.55341960407611168, 4.379528057220329451, 68.95724293864769550 ) ) ;
#185039=CARTESIAN_POINT ( 'NONE',  ( -5.153800228976607833, 19.02544592524334988, 97.70942372801900433 ) ) ;
#185040=CARTESIAN_POINT ( 'NONE',  ( 18.62759615963271287, -10.81492255796078972, 43.33224293864769550 ) ) ;
#185042=CARTESIAN_POINT ( 'NONE',  ( 19.05341960407611168, 5.049401038298154454, 23.95724293864769194 ) ) ;
#185044=CARTESIAN_POINT ( 'NONE',  ( 16.51473224551069308, 9.474510206698969483, 74.16557627198103830 ) ) ;
#185045=CARTESIAN_POINT ( 'NONE',  ( 5.719274019375991003, -21.55341960407610458, 77.70724293864770971 ) ) ;
#185046=CARTESIAN_POINT ( 'NONE',  ( -14.34966873604972548, 8.224510206698743886, 93.33442372801901854 ) ) ;
#185047=CARTESIAN_POINT ( 'NONE',  ( -9.474510206698964154, 16.51473224551069663, 70.41557627198102409 ) ) ;
#185048=CARTESIAN_POINT ( 'NONE',  ( 9.564922557961047289, -16.46253265017146816, 65.41775706135233293 ) ) ;
#185049=CARTESIAN_POINT ( 'NONE',  ( 21.53943276465977519, 0.05219959533937863772, 86.25109039468568994 ) ) ;
#185050=CARTESIAN_POINT ( 'NONE',  ( 21.55341960407610458, 5.719274019375980345, 63.95724293864770260 ) ) ;
#185051=CARTESIAN_POINT ( 'NONE',  ( -18.67979575497178146, -10.72451020669898902, 21.66557627198102409 ) ) ;
#185052=CARTESIAN_POINT ( 'NONE',  ( 0.05219959533909260263, 19.03943276465977164, 39.99890960531436690 ) ) ;
#185053=CARTESIAN_POINT ( 'NONE',  ( -4.379528057220086978, -16.55341960407618274, 99.79275706135234714 ) ) ;
#185054=CARTESIAN_POINT ( 'NONE',  ( -16.46253265017160317, 9.564922557960807481, 55.83224293864769550 ) ) ;
#185055=CARTESIAN_POINT ( 'NONE',  ( 19.05341960407617918, -5.049401038297876454, 111.0427570613523329 ) ) ;
#185056=CARTESIAN_POINT ( 'NONE',  ( 17.26172910966777962, 6.454744622555866229, 51.69353091350778584 ) ) ;
#185057=CARTESIAN_POINT ( 'NONE',  ( 10.72451020669871369, 18.67979575497193778, 107.0844237280190043 ) ) ;
#185058=CARTESIAN_POINT ( 'NONE',  ( -12.06949235617756955, 12.14591786802309770, 65.62390960531436690 ) ) ;
#185059=CARTESIAN_POINT ( 'NONE',  ( -10.81492255796078084, -18.62759615963271287, 102.0822429386476955 ) ) ;
#185060=CARTESIAN_POINT ( 'NONE',  ( 21.53943276465977519, -0.05219959533907433946, 108.7489096053143669 ) ) ;
#185062=CARTESIAN_POINT ( 'NONE',  ( 15.80617190586746368, 15.72974639402197994, 44.37390960531435979 ) ) ;
#185063=CARTESIAN_POINT ( 'NONE',  ( 14.29746914071037800, 8.314922557961029526, 81.66775706135236135 ) ) ;
#185064=CARTESIAN_POINT ( 'NONE',  ( -0.05219959533910754901, -16.53943276465976808, 97.49890960531436690 ) ) ;
#185065=CARTESIAN_POINT ( 'NONE',  ( -16.46253265017160317, 9.564922557960807481, 60.83224293864769550 ) ) ;
#185066=CARTESIAN_POINT ( 'NONE',  ( -18.87580814761073356, 5.500000000000047962, 50.87172394265760289 ) ) ;
#185067=CARTESIAN_POINT ( 'NONE',  ( 4.483927247898790824, -16.52544592524335698, 105.2094237280190328 ) ) ;
#185068=CARTESIAN_POINT ( 'NONE',  ( 5.719274019375673035, 21.55341960407619339, 32.29275706135235424 ) ) ;
#185069=CARTESIAN_POINT ( 'NONE',  ( -19.02544592524342804, 5.153800228976336051, 101.0405762719810241 ) ) ;
#185070=CARTESIAN_POINT ( 'NONE',  ( 5.823673210054444382, -21.52544592524334988, 70.20942372801904696 ) ) ;
#185071=CARTESIAN_POINT ( 'NONE',  ( 13.89961937509977652, -13.97604488694527269, 23.12390960531436335 ) ) ;
#185072=CARTESIAN_POINT ( 'NONE',  ( 13.97604488694527802, 13.89961937509977652, 29.37390960531435979 ) ) ;
#185074=CARTESIAN_POINT ( 'NONE',  ( -21.53943276465977519, -0.05219959533937600094, 63.75109039468568284 ) ) ;
#185075=CARTESIAN_POINT ( 'NONE',  ( -9.474510206698964154, 16.51473224551069663, 50.41557627198102409 ) ) ;
#185076=CARTESIAN_POINT ( 'NONE',  ( -19.02544592524342804, 5.153800228976336051, 96.04057627198103830 ) ) ;
#185077=CARTESIAN_POINT ( 'NONE',  ( -9.564922557961040184, 16.46253265017147172, 72.91775706135233293 ) ) ;
#185078=CARTESIAN_POINT ( 'NONE',  ( 21.53943276465977519, 0.05219959533937863772, 46.25109039468567573 ) ) ;
#185079=CARTESIAN_POINT ( 'NONE',  ( -9.474510206698720793, -16.51473224551083518, 99.58442372801900433 ) ) ;
#185080=CARTESIAN_POINT ( 'NONE',  ( 16.51473224551083163, -9.474510206698727899, 70.83442372801900433 ) ) ;
#185081=CARTESIAN_POINT ( 'NONE',  ( -16.46253265017160317, 9.564922557960807481, 35.83224293864768839 ) ) ;
#185082=CARTESIAN_POINT ( 'NONE',  ( -9.474510206698720793, -16.51473224551083518, 79.58442372801899012 ) ) ;
#185083=CARTESIAN_POINT ( 'NONE',  ( -4.483927247898782831, 16.52544592524335698, 107.7094237280190328 ) ) ;
#185084=CARTESIAN_POINT ( 'NONE',  ( -9.474510206698720793, -16.51473224551083518, 79.58442372801899012 ) ) ;
#185085=CARTESIAN_POINT ( 'NONE',  ( 14.34966873604960469, 8.224510206698951720, 24.16557627198103120 ) ) ;
#185086=CARTESIAN_POINT ( 'NONE',  ( -13.89961937509957401, -13.97604488694547875, 49.37609039468567573 ) ) ;
#185087=CARTESIAN_POINT ( 'NONE',  ( 21.53943276465977519, 0.05219959533937863772, 111.2510903946856899 ) ) ;
#185088=CARTESIAN_POINT ( 'NONE',  ( 13.97604488694548053, -13.89961937509957401, 20.62609039468567573 ) ) ;
#185089=CARTESIAN_POINT ( 'NONE',  ( 5.153800228976335163, 19.02544592524342804, 24.79057627198102765 ) ) ;
#185090=CARTESIAN_POINT ( 'NONE',  ( -21.53943276465977519, -0.05219959533937600094, 93.75109039468567573 ) ) ;
#185091=CARTESIAN_POINT ( 'NONE',  ( -14.34966873604972548, 8.224510206698743886, 28.33442372801902209 ) ) ;
#185092=CARTESIAN_POINT ( 'NONE',  ( 16.46253265017160672, -9.564922557960803928, 88.33224293864769550 ) ) ;
#185093=VECTOR ( 'NONE', #113475, 999.9999999999998863 ) ;
#185095=CARTESIAN_POINT ( 'NONE',  ( 13.97604488694527802, 13.89961937509977652, 74.37390960531436690 ) ) ;
#185096=CARTESIAN_POINT ( 'NONE',  ( -17.50000000001354294, 5.500000000000027534, 95.79690382535056870 ) ) ;
#185097=CARTESIAN_POINT ( 'NONE',  ( 16.46253265017146816, 9.564922557961045513, 86.66775706135233293 ) ) ;
#185098=CARTESIAN_POINT ( 'NONE',  ( 16.51473224551069308, 9.474510206698969483, 114.1655762719810241 ) ) ;
#185099=CARTESIAN_POINT ( 'NONE',  ( -13.89961937509957401, -13.97604488694547875, 24.37609039468565442 ) ) ;
#185100=CARTESIAN_POINT ( 'NONE',  ( 19.03943276465977164, 0.05219959533936151252, 101.2510903946856757 ) ) ;
#185101=CARTESIAN_POINT ( 'NONE',  ( -8.224510206698948167, 14.34966873604960824, 95.41557627198102409 ) ) ;
#185102=CARTESIAN_POINT ( 'NONE',  ( 19.02544592524343514, -5.153800228976328945, 28.54057627198102409 ) ) ;
#185103=CARTESIAN_POINT ( 'NONE',  ( -18.62759615963270932, 10.81492255796079327, 60.83224293864769550 ) ) ;
#185104=CARTESIAN_POINT ( 'NONE',  ( 15.80617190586746368, 15.72974639402197994, 54.37390960531435979 ) ) ;
#185105=CARTESIAN_POINT ( 'NONE',  ( -13.89961937509977652, 13.97604488694528158, 25.62390960531434558 ) ) ;
#185107=CARTESIAN_POINT ( 'NONE',  ( 13.89961937509957401, 13.97604488694547697, 51.87609039468566863 ) ) ;
#185108=CARTESIAN_POINT ( 'NONE',  ( 16.52544592524342804, -4.483927247898539470, 33.54057627198102409 ) ) ;
#185109=CARTESIAN_POINT ( 'NONE',  ( -13.97604488694527625, -13.89961937509977652, 111.8739096053143243 ) ) ;
#185110=CARTESIAN_POINT ( 'NONE',  ( -10.81492255796105439, 18.62759615963255655, 77.91775706135231871 ) ) ;
#185111=CARTESIAN_POINT ( 'NONE',  ( 5.823673210054125526, 21.52544592524343514, 64.79057627198103830 ) ) ;
#185112=CARTESIAN_POINT ( 'NONE',  ( 21.53943276465977519, 0.05219959533937863772, 56.25109039468568284 ) ) ;
#185113=CARTESIAN_POINT ( 'NONE',  ( -10.72451020669870658, -18.67979575497194134, 44.58442372801901854 ) ) ;
#185114=CARTESIAN_POINT ( 'NONE',  ( -5.153800228976328057, -19.02544592524343514, 77.29057627198099567 ) ) ;
#185115=CARTESIAN_POINT ( 'NONE',  ( 12.14591786802327356, -12.06949235617739191, 80.62609039468567573 ) ) ;
#185116=CARTESIAN_POINT ( 'NONE',  ( 5.049401038298161559, -19.05341960407611168, 22.70724293864769194 ) ) ;
#185118=CARTESIAN_POINT ( 'NONE',  ( -16.52544592524342804, 4.483927247898546575, 66.04057627198103830 ) ) ;
#185119=CARTESIAN_POINT ( 'NONE',  ( 8.314922557960818139, 14.29746914071049879, 29.58224293864769905 ) ) ;
#185120=CARTESIAN_POINT ( 'NONE',  ( 0.05219959533909260263, 19.03943276465977164, 59.99890960531436690 ) ) ;
#185121=CARTESIAN_POINT ( 'NONE',  ( 19.03943276465977164, -0.05219959533909143690, 28.74890960531435624 ) ) ;
#185122=CARTESIAN_POINT ( 'NONE',  ( -10.72451020669898014, 18.67979575497178502, 40.41557627198103120 ) ) ;
#185123=CARTESIAN_POINT ( 'NONE',  ( 5.049401038297881783, 19.05341960407617563, 32.29275706135233293 ) ) ;
#185125=CARTESIAN_POINT ( 'NONE',  ( 0.05219959533910956823, 16.53943276465976808, 44.99890960531435979 ) ) ;
#185126=CARTESIAN_POINT ( 'NONE',  ( 15.80617190586746368, 15.72974639402197994, 24.37390960531435979 ) ) ;
#185127=CARTESIAN_POINT ( 'NONE',  ( 17.76566638676855803, 1.079584607093802662, 37.49999999999999289 ) ) ;
#185128=CARTESIAN_POINT ( 'NONE',  ( 0.05219959533934541429, -16.53943276465976808, 75.00109039468568994 ) ) ;
#185129=CARTESIAN_POINT ( 'NONE',  ( -9.474510206698720793, -16.51473224551083518, 74.58442372801900433 ) ) ;
#185130=CARTESIAN_POINT ( 'NONE',  ( 16.52544592524342804, -4.483927247898539470, 43.54057627198103830 ) ) ;
#185132=CARTESIAN_POINT ( 'NONE',  ( -19.53091890409953635, -5.499999999999947597, 75.06097431831420863 ) ) ;
#185133=CARTESIAN_POINT ( 'NONE',  ( 16.52544592524342804, -4.483927247898539470, 28.54057627198103120 ) ) ;
#185134=CARTESIAN_POINT ( 'NONE',  ( -0.05219959533909027116, -19.03943276465977164, 47.49890960531435979 ) ) ;
#185135=CARTESIAN_POINT ( 'NONE',  ( 9.564922557960805705, 16.46253265017160317, 79.58224293864769550 ) ) ;
#185136=CARTESIAN_POINT ( 'NONE',  ( -13.97604488694527625, -13.89961937509977652, 41.87390960531435979 ) ) ;
#185137=CARTESIAN_POINT ( 'NONE',  ( -0.05219959533937732626, 21.53943276465977519, 52.50109039468567573 ) ) ;
#185138=CARTESIAN_POINT ( 'NONE',  ( -5.049401038298153566, 19.05341960407611168, 60.20724293864768129 ) ) ;
#185139=CARTESIAN_POINT ( 'NONE',  ( 17.50000000000000355, 5.499999999999989342, 103.7823096230356867 ) ) ;
#185140=CARTESIAN_POINT ( 'NONE',  ( -0.05219959533909027116, -19.03943276465977164, 42.49890960531435269 ) ) ;
#185141=CARTESIAN_POINT ( 'NONE',  ( -21.53943276465977519, 0.05219959533907696930, 31.24890960531435979 ) ) ;
#185142=CARTESIAN_POINT ( 'NONE',  ( -21.53943276465977519, -0.05219959533937600094, 78.75109039468568994 ) ) ;
#185143=CARTESIAN_POINT ( 'NONE',  ( 4.483927247898545687, 16.52544592524342804, 114.7905762719810383 ) ) ;
#185144=CARTESIAN_POINT ( 'NONE',  ( 10.81492255796078972, 18.62759615963270932, 24.58224293864768839 ) ) ;
#185146=CARTESIAN_POINT ( 'NONE',  ( -12.14591786802326823, 12.06949235617739902, 93.12609039468568994 ) ) ;
#185147=CARTESIAN_POINT ( 'NONE',  ( 18.62759615963255655, 10.81492255796105972, 111.6677570613523613 ) ) ;
#185148=CARTESIAN_POINT ( 'NONE',  ( -0.05219959533934338120, 16.53943276465976808, 72.50109039468568994 ) ) ;
#185149=CARTESIAN_POINT ( 'NONE',  ( 19.05341960407611168, 5.049401038298154454, 103.9572429386476671 ) ) ;
#185150=CARTESIAN_POINT ( 'NONE',  ( -8.224510206698735004, -14.34966873604973081, 54.58442372801901143 ) ) ;
#185151=CARTESIAN_POINT ( 'NONE',  ( 8.224510206698742110, 14.34966873604972548, 37.08442372801901143 ) ) ;
#185152=CARTESIAN_POINT ( 'NONE',  ( 16.55341960407618274, -4.379528057220086978, 91.04275706135236135 ) ) ;
#185153=CARTESIAN_POINT ( 'NONE',  ( 10.72451020669871369, 18.67979575497193778, 57.08442372801901854 ) ) ;
#185154=CARTESIAN_POINT ( 'NONE',  ( -8.224510206698735004, -14.34966873604973081, 19.58442372801901143 ) ) ;
#185155=CARTESIAN_POINT ( 'NONE',  ( 10.81492255796078972, 18.62759615963270932, 109.5822429386476955 ) ) ;
#185156=CARTESIAN_POINT ( 'NONE',  ( -4.379528057220086978, -16.55341960407618274, 19.79275706135235069 ) ) ;
#185157=CARTESIAN_POINT ( 'NONE',  ( 16.55341960407618274, -4.379528057220086978, 81.04275706135236135 ) ) ;
#185159=CARTESIAN_POINT ( 'NONE',  ( 18.62759615963255655, 10.81492255796105972, 91.66775706135234714 ) ) ;
#185160=CARTESIAN_POINT ( 'NONE',  ( 19.03943276465977164, 0.05219959533936151252, 86.25109039468567573 ) ) ;
#185161=CARTESIAN_POINT ( 'NONE',  ( 8.314922557960818139, 14.29746914071049879, 54.58224293864769550 ) ) ;
#185162=CARTESIAN_POINT ( 'NONE',  ( 12.06949235617757843, -12.14591786802309237, 48.12390960531436690 ) ) ;
#185163=CARTESIAN_POINT ( 'NONE',  ( -8.224510206698948167, 14.34966873604960824, 100.4155762719810241 ) ) ;
#185164=CARTESIAN_POINT ( 'NONE',  ( 13.89961937509957401, 13.97604488694547697, 51.87609039468566863 ) ) ;
#185165=LINE ( 'NONE', #113281, #7879 ) ;
#185166=CARTESIAN_POINT ( 'NONE',  ( -18.62759615963255300, -10.81492255796106328, 44.16775706135234714 ) ) ;
#185167=CARTESIAN_POINT ( 'NONE',  ( 16.46253265017146816, 9.564922557961045513, 111.6677570613523329 ) ) ;
#185169=CARTESIAN_POINT ( 'NONE',  ( 0.05219959533909260263, 19.03943276465977164, 109.9989096053143669 ) ) ;
#185170=CARTESIAN_POINT ( 'NONE',  ( -21.53943276465977519, 0.05219959533907696930, 71.24890960531435269 ) ) ;
#185171=CARTESIAN_POINT ( 'NONE',  ( 19.03943276465977164, 0.05219959533936151252, 96.25109039468567573 ) ) ;
#185172=CARTESIAN_POINT ( 'NONE',  ( -9.474510206698964154, 16.51473224551069663, 100.4155762719810241 ) ) ;
#185173=CARTESIAN_POINT ( 'NONE',  ( 16.51473224551083163, -9.474510206698727899, 50.83442372801899722 ) ) ;
#185174=CARTESIAN_POINT ( 'NONE',  ( -16.53943276465976808, 0.05219959533911058130, 106.2489096053143811 ) ) ;
#185175=CARTESIAN_POINT ( 'NONE',  ( 21.52544592524334988, 5.823673210054432836, 91.45942372801901854 ) ) ;
#185176=CARTESIAN_POINT ( 'NONE',  ( -0.05219959533909027116, -19.03943276465977164, 27.49890960531435624 ) ) ;
#185177=CARTESIAN_POINT ( 'NONE',  ( -10.72451020669870658, -18.67979575497194134, 44.58442372801901854 ) ) ;
#185179=CARTESIAN_POINT ( 'NONE',  ( 0.05219959533937995610, -21.53943276465977519, 90.00109039468567573 ) ) ;
#185180=CARTESIAN_POINT ( 'NONE',  ( 12.14591786802327356, -12.06949235617739191, 90.62609039468567573 ) ) ;
#185181=CARTESIAN_POINT ( 'NONE',  ( -5.823673210054431948, 21.52544592524334988, 47.70942372801902565 ) ) ;
#185182=CARTESIAN_POINT ( 'NONE',  ( 15.72974639402176855, 15.80617190586768217, 36.87609039468568994 ) ) ;
#185183=CARTESIAN_POINT ( 'NONE',  ( 19.03943276465977164, 0.05219959533936151252, 71.25109039468566152 ) ) ;
#185184=CARTESIAN_POINT ( 'NONE',  ( -0.05219959533909027116, -19.03943276465977164, 77.49890960531435269 ) ) ;
#185185=CARTESIAN_POINT ( 'NONE',  ( 8.314922557960818139, 14.29746914071049879, 99.58224293864770971 ) ) ;
#185186=CARTESIAN_POINT ( 'NONE',  ( -0.05219959533907301413, -21.53943276465977519, 77.49890960531433848 ) ) ;
#185187=CARTESIAN_POINT ( 'NONE',  ( -4.379528057220328563, 16.55341960407611168, 60.20724293864768839 ) ) ;
#185188=CARTESIAN_POINT ( 'NONE',  ( 15.72974639402176855, 15.80617190586768217, 101.8760903946857042 ) ) ;
#185189=CARTESIAN_POINT ( 'NONE',  ( 14.29746914071049879, -8.314922557960816363, 83.33224293864769550 ) ) ;
#185190=CARTESIAN_POINT ( 'NONE',  ( -13.97604488694527625, -13.89961937509977652, 36.87390960531436690 ) ) ;
#185191=CARTESIAN_POINT ( 'NONE',  ( 9.564922557961047289, -16.46253265017146816, 65.41775706135233293 ) ) ;
#185192=CARTESIAN_POINT ( 'NONE',  ( -16.53943276465976808, 0.05219959533911058130, 31.24890960531435979 ) ) ;
#185193=CARTESIAN_POINT ( 'NONE',  ( 21.52544592524334988, 5.823673210054432836, 96.45942372801901854 ) ) ;
#185194=CARTESIAN_POINT ( 'NONE',  ( -13.97604488694527625, -13.89961937509977652, 86.87390960531436690 ) ) ;
#185195=CARTESIAN_POINT ( 'NONE',  ( 19.03943276465977164, 0.05219959533936151252, 56.25109039468566863 ) ) ;
#185196=CARTESIAN_POINT ( 'NONE',  ( 15.80617190586746368, 15.72974639402197994, 69.37390960531436690 ) ) ;
#185197=CARTESIAN_POINT ( 'NONE',  ( 21.53943276465977519, -0.05219959533907433946, 108.7489096053143669 ) ) ;
#185198=CARTESIAN_POINT ( 'NONE',  ( 0.05219959533936267826, -19.03943276465977164, 110.0010903946856757 ) ) ;
#185199=CARTESIAN_POINT ( 'NONE',  ( 0.05219959533934541429, -16.53943276465976808, 75.00109039468568994 ) ) ;
#185201=CARTESIAN_POINT ( 'NONE',  ( 0.05219959533937995610, -21.53943276465977519, 20.00109039468568639 ) ) ;
#185202=CARTESIAN_POINT ( 'NONE',  ( 8.314922557960818139, 14.29746914071049879, 109.5822429386476955 ) ) ;
#185204=CARTESIAN_POINT ( 'NONE',  ( -4.483927247898782831, 16.52544592524335698, 47.70942372801902565 ) ) ;
#185205=CARTESIAN_POINT ( 'NONE',  ( -4.483927247898539470, -16.52544592524342804, 77.29057627198102409 ) ) ;
#185206=CARTESIAN_POINT ( 'NONE',  ( -21.52544592524343514, 5.823673210054127303, 81.04057627198102409 ) ) ;
#185207=CARTESIAN_POINT ( 'NONE',  ( 16.55341960407618274, -4.379528057220086978, 101.0427570613523756 ) ) ;
#185208=CARTESIAN_POINT ( 'NONE',  ( -14.34966873604972548, 8.224510206698743886, 38.33442372801900433 ) ) ;
#185209=CARTESIAN_POINT ( 'NONE',  ( -13.89961937509977652, 13.97604488694528158, 45.62390960531433848 ) ) ;
#185210=CARTESIAN_POINT ( 'NONE',  ( 8.314922557961029526, -14.29746914071037800, 75.41775706135233293 ) ) ;
#185211=CARTESIAN_POINT ( 'NONE',  ( -16.51473224551082808, 9.474510206698731452, 73.33442372801900433 ) ) ;
#185212=CARTESIAN_POINT ( 'NONE',  ( -0.05219959533907301413, -21.53943276465977519, 77.49890960531433848 ) ) ;
#185213=CARTESIAN_POINT ( 'NONE',  ( -16.55341960407617563, 4.379528057220093196, 103.5427570613523613 ) ) ;
#185214=CARTESIAN_POINT ( 'NONE',  ( -18.67979575497193778, 10.72451020669871902, 83.33442372801903275 ) ) ;
#185216=CARTESIAN_POINT ( 'NONE',  ( 18.62759615963271287, -10.81492255796078972, 63.33224293864770260 ) ) ;
#185217=CARTESIAN_POINT ( 'NONE',  ( -21.55341960407610458, -5.719274019375992779, 41.45724293864769550 ) ) ;
#185219=CARTESIAN_POINT ( 'NONE',  ( -12.06949235617739369, -12.14591786802326823, 84.37609039468570415 ) ) ;
#185220=CARTESIAN_POINT ( 'NONE',  ( 10.72451020669898902, -18.67979575497178502, 47.91557627198102409 ) ) ;
#185222=CARTESIAN_POINT ( 'NONE',  ( 5.049401038298161559, -19.05341960407611168, 112.7072429386476813 ) ) ;
#185224=CARTESIAN_POINT ( 'NONE',  ( 19.02544592524343514, -5.153800228976328945, 23.54057627198102054 ) ) ;
#185225=CARTESIAN_POINT ( 'NONE',  ( 5.719274019375991003, -21.55341960407610458, 77.70724293864770971 ) ) ;
#185226=CARTESIAN_POINT ( 'NONE',  ( 4.483927247898790824, -16.52544592524335698, 100.2094237280190043 ) ) ;
#185227=CARTESIAN_POINT ( 'NONE',  ( -15.72974639402176322, -15.80617190586768395, 64.37609039468568994 ) ) ;
#185228=CARTESIAN_POINT ( 'NONE',  ( 12.14591786802327356, -12.06949235617739191, 20.62609039468568639 ) ) ;
#185229=CARTESIAN_POINT ( 'NONE',  ( -13.89961937509977652, 13.97604488694528158, 25.62390960531434558 ) ) ;
#185230=CARTESIAN_POINT ( 'NONE',  ( -0.05219959533936034679, 19.03943276465977164, 112.5010903946856757 ) ) ;
#185231=CARTESIAN_POINT ( 'NONE',  ( 9.564922557960805705, 16.46253265017160317, 34.58224293864770260 ) ) ;
#185233=CARTESIAN_POINT ( 'NONE',  ( -9.564922557960796823, -16.46253265017161027, 102.0822429386477097 ) ) ;
#185234=CARTESIAN_POINT ( 'NONE',  ( -12.14591786802326823, 12.06949235617739902, 83.12609039468568994 ) ) ;
#185235=CARTESIAN_POINT ( 'NONE',  ( -5.153800228976607833, 19.02544592524334988, 82.70942372801897591 ) ) ;
#185236=CARTESIAN_POINT ( 'NONE',  ( 13.89961937509957401, 13.97604488694547697, 26.87609039468566507 ) ) ;
#185237=CARTESIAN_POINT ( 'NONE',  ( 18.67979575497178502, 10.72451020669898547, 59.16557627198103120 ) ) ;
#185238=CARTESIAN_POINT ( 'NONE',  ( -16.53943276465976808, -0.05219959533934237506, 88.75109039468567573 ) ) ;
#185239=AXIS2_PLACEMENT_3D ( 'NONE', #136055, #120865, #58222 ) ;
#185240=CARTESIAN_POINT ( 'NONE',  ( -16.51473224551082808, 9.474510206698731452, 88.33442372801900433 ) ) ;
#185241=CARTESIAN_POINT ( 'NONE',  ( -16.51473224551069308, -9.474510206698971260, 46.66557627198102409 ) ) ;
#185242=CARTESIAN_POINT ( 'NONE',  ( 16.51473224551069308, 9.474510206698969483, 94.16557627198103830 ) ) ;
#185243=CARTESIAN_POINT ( 'NONE',  ( -15.80617190586768217, 15.72974639402176855, 53.12609039468568284 ) ) ;
#185244=CARTESIAN_POINT ( 'NONE',  ( 5.049401038298161559, -19.05341960407611168, 42.70724293864767418 ) ) ;
#185247=CARTESIAN_POINT ( 'NONE',  ( 5.153800228976335163, 19.02544592524342804, 104.7905762719809957 ) ) ;
#185248=CARTESIAN_POINT ( 'NONE',  ( 8.314922557960818139, 14.29746914071049879, 69.58224293864769550 ) ) ;
#185249=CARTESIAN_POINT ( 'NONE',  ( -10.81492255796078084, -18.62759615963271287, 57.08224293864769550 ) ) ;
#185251=CARTESIAN_POINT ( 'NONE',  ( 16.51473224551083163, -9.474510206698727899, 45.83442372801900433 ) ) ;
#185253=CARTESIAN_POINT ( 'NONE',  ( 13.97604488694527802, 13.89961937509977652, 64.37390960531436690 ) ) ;
#185254=CARTESIAN_POINT ( 'NONE',  ( -5.153800228976328057, -19.02544592524343514, 72.29057627198102409 ) ) ;
#185255=CARTESIAN_POINT ( 'NONE',  ( -0.05219959533934338120, 16.53943276465976808, 57.50109039468568994 ) ) ;
#185256=CARTESIAN_POINT ( 'NONE',  ( 0.05219959533936267826, -19.03943276465977164, 80.00109039468567573 ) ) ;
#185259=CARTESIAN_POINT ( 'NONE',  ( 16.52544592524335698, 4.483927247898782831, 86.45942372801901854 ) ) ;
#185261=CARTESIAN_POINT ( 'NONE',  ( -0.05219959533934338120, 16.53943276465976808, 82.50109039468568994 ) ) ;
#185262=CARTESIAN_POINT ( 'NONE',  ( 16.52544592524335698, 4.483927247898782831, 51.45942372801901854 ) ) ;
#185263=CARTESIAN_POINT ( 'NONE',  ( 16.46253265017146816, 9.564922557961045513, 21.66775706135233648 ) ) ;
#185264=CARTESIAN_POINT ( 'NONE',  ( 9.474510206698971260, -16.51473224551069308, 52.91557627198102409 ) ) ;
#185266=CARTESIAN_POINT ( 'NONE',  ( -5.719274019375665041, -21.55341960407619695, 54.79275706135235424 ) ) ;
#185267=CARTESIAN_POINT ( 'NONE',  ( 5.049401038297881783, 19.05341960407617563, 72.29275706135234714 ) ) ;
#185268=CARTESIAN_POINT ( 'NONE',  ( -5.823673210054431948, 21.52544592524334988, 112.7094237280190328 ) ) ;
#185269=CARTESIAN_POINT ( 'NONE',  ( -16.51473224551069308, -9.474510206698971260, 36.66557627198102409 ) ) ;
#185270=CARTESIAN_POINT ( 'NONE',  ( 16.86294246435915767, 6.972627225432042941, 23.78307040723333543 ) ) ;
#185271=CARTESIAN_POINT ( 'NONE',  ( 21.55341960407610458, 5.719274019375980345, 68.95724293864769550 ) ) ;
#185272=CARTESIAN_POINT ( 'NONE',  ( -16.46253265017160317, 9.564922557960807481, 115.8322429386477097 ) ) ;
#185273=CARTESIAN_POINT ( 'NONE',  ( -12.14591786802309592, -12.06949235617757132, 111.8739096053143669 ) ) ;
#185274=CARTESIAN_POINT ( 'NONE',  ( -0.05219959533934338120, 16.53943276465976808, 32.50109039468568284 ) ) ;
#185275=CARTESIAN_POINT ( 'NONE',  ( 12.14591786802309770, 12.06949235617756955, 24.37390960531435979 ) ) ;
#185276=ORIENTED_EDGE ( 'NONE', *, *, #46382, .F. ) ;
#185277=CARTESIAN_POINT ( 'NONE',  ( -18.62759615963255300, -10.81492255796106328, 19.16775706135234714 ) ) ;
#185278=CARTESIAN_POINT ( 'NONE',  ( 8.314922557960818139, 14.29746914071049879, 44.58224293864769550 ) ) ;
#185280=CARTESIAN_POINT ( 'NONE',  ( 13.97604488694548053, -13.89961937509957401, 105.6260903946856757 ) ) ;
#185281=CARTESIAN_POINT ( 'NONE',  ( 19.05341960407617918, -5.049401038297876454, 21.04275706135232582 ) ) ;
#185282=CARTESIAN_POINT ( 'NONE',  ( 14.34966873604960469, 8.224510206698951720, 39.16557627198102409 ) ) ;
#185283=CARTESIAN_POINT ( 'NONE',  ( 21.55341960407610458, 5.719274019375980345, 108.9572429386476955 ) ) ;
#185285=CARTESIAN_POINT ( 'NONE',  ( 18.67979575497178502, 10.72451020669898547, 69.16557627198102409 ) ) ;
#185286=CARTESIAN_POINT ( 'NONE',  ( -19.05341960407611168, -5.049401038298163336, 71.45724293864766707 ) ) ;
#185287=CARTESIAN_POINT ( 'NONE',  ( 12.06949235617757843, -12.14591786802309237, 43.12390960531435269 ) ) ;
#185288=CARTESIAN_POINT ( 'NONE',  ( -0.05219959533909027116, -19.03943276465977164, 92.49890960531436690 ) ) ;
#185290=CARTESIAN_POINT ( 'NONE',  ( 19.02544592524334988, 5.153800228976608722, 61.45942372801900433 ) ) ;
#185291=CARTESIAN_POINT ( 'NONE',  ( 15.72974639402199770, -15.80617190586745480, 88.12390960531436690 ) ) ;
#185292=CARTESIAN_POINT ( 'NONE',  ( 8.314922557960818139, 14.29746914071049879, 99.58224293864770971 ) ) ;
#185294=CARTESIAN_POINT ( 'NONE',  ( 18.62759615963255655, 10.81492255796105972, 46.66775706135234714 ) ) ;
#185296=CARTESIAN_POINT ( 'NONE',  ( 12.06949235617757843, -12.14591786802309237, 33.12390960531435979 ) ) ;
#185297=CARTESIAN_POINT ( 'NONE',  ( -19.02544592524342804, 5.153800228976336051, 41.04057627198103120 ) ) ;
#185298=CARTESIAN_POINT ( 'NONE',  ( -5.049401038298153566, 19.05341960407611168, 95.20724293864770971 ) ) ;
#185299=CARTESIAN_POINT ( 'NONE',  ( 5.823673210054125526, 21.52544592524343514, 54.79057627198104541 ) ) ;
#185301=CARTESIAN_POINT ( 'NONE',  ( 5.049401038298161559, -19.05341960407611168, 37.70724293864768839 ) ) ;
#185302=CARTESIAN_POINT ( 'NONE',  ( 15.80617190586746368, 15.72974639402197994, 59.37390960531436690 ) ) ;
#185303=CARTESIAN_POINT ( 'NONE',  ( -18.62759615963255300, -10.81492255796106328, 69.16775706135234714 ) ) ;
#185305=CARTESIAN_POINT ( 'NONE',  ( 8.224510206698742110, 14.34966873604972548, 87.08442372801901854 ) ) ;
#185306=CARTESIAN_POINT ( 'NONE',  ( 0.05219959533909260263, 19.03943276465977164, 54.99890960531435979 ) ) ;
#185307=CARTESIAN_POINT ( 'NONE',  ( 16.51473224551069308, 9.474510206698969483, 69.16557627198102409 ) ) ;
#185308=ORIENTED_EDGE ( 'NONE', *, *, #179989, .T. ) ;
#185309=CARTESIAN_POINT ( 'NONE',  ( 16.46253265017146816, 9.564922557961045513, 31.66775706135232937 ) ) ;
#185310=CARTESIAN_POINT ( 'NONE',  ( 16.53943276465976808, 0.05219959533934440121, 76.25109039468568994 ) ) ;
#185311=CARTESIAN_POINT ( 'NONE',  ( -5.719274019375665041, -21.55341960407619695, 94.79275706135234714 ) ) ;
#185312=CARTESIAN_POINT ( 'NONE',  ( -19.02544592524342804, 5.153800228976336051, 81.04057627198103830 ) ) ;
#185313=CARTESIAN_POINT ( 'NONE',  ( 5.823673210054125526, 21.52544592524343514, 34.79057627198103120 ) ) ;
#185314=CARTESIAN_POINT ( 'NONE',  ( -12.14591786802326823, 12.06949235617739902, 28.12609039468568284 ) ) ;
#185315=CARTESIAN_POINT ( 'NONE',  ( -15.72974639402176322, -15.80617190586768395, 84.37609039468570415 ) ) ;
#185316=CARTESIAN_POINT ( 'NONE',  ( -14.29746914071037622, -8.314922557961029526, 54.16775706135235424 ) ) ;
#185317=CARTESIAN_POINT ( 'NONE',  ( -5.719274019375978568, 21.55341960407610458, 105.2072429386477097 ) ) ;
#185318=CARTESIAN_POINT ( 'NONE',  ( 9.564922557961047289, -16.46253265017146816, 110.4177570613523471 ) ) ;
#185319=CARTESIAN_POINT ( 'NONE',  ( 5.153800228976335163, 19.02544592524342804, 79.79057627198102409 ) ) ;
#185320=CARTESIAN_POINT ( 'NONE',  ( 8.224510206698742110, 14.34966873604972548, 27.08442372801901854 ) ) ;
#185321=CARTESIAN_POINT ( 'NONE',  ( -13.97604488694527625, -13.89961937509977652, 36.87390960531436690 ) ) ;
#185323=CARTESIAN_POINT ( 'NONE',  ( 19.05341960407617918, -5.049401038297876454, 111.0427570613523329 ) ) ;
#185324=CARTESIAN_POINT ( 'NONE',  ( 16.52544592524342804, -4.483927247898539470, 78.54057627198103830 ) ) ;
#185325=CARTESIAN_POINT ( 'NONE',  ( 4.483927247898790824, -16.52544592524335698, 85.20942372801901854 ) ) ;
#185326=CARTESIAN_POINT ( 'NONE',  ( -21.53943276465977519, -0.05219959533937600094, 33.75109039468568284 ) ) ;
#185327=CARTESIAN_POINT ( 'NONE',  ( -19.03943276465977164, 0.05219959533909376836, 46.24890960531435979 ) ) ;
#185328=CARTESIAN_POINT ( 'NONE',  ( -9.474510206698964154, 16.51473224551069663, 65.41557627198102409 ) ) ;
#185329=CARTESIAN_POINT ( 'NONE',  ( 16.53943276465976808, 0.05219959533934440121, 86.25109039468568994 ) ) ;
#185332=ORIENTED_EDGE ( 'NONE', *, *, #26831, .T. ) ;
#185333=CARTESIAN_POINT ( 'NONE',  ( -19.03943276465977164, -0.05219959533935918106, 18.75109039468567218 ) ) ;
#185334=CARTESIAN_POINT ( 'NONE',  ( -5.153800228976328057, -19.02544592524343514, 32.29057627198102409 ) ) ;
#185335=CARTESIAN_POINT ( 'NONE',  ( -19.03943276465977164, 0.05219959533909376836, 116.2489096053143669 ) ) ;
#185337=CARTESIAN_POINT ( 'NONE',  ( 14.29746914071037800, 8.314922557961029526, 26.66775706135235424 ) ) ;
#185338=CARTESIAN_POINT ( 'NONE',  ( 16.46253265017146816, 9.564922557961045513, 51.66775706135233293 ) ) ;
#185339=CARTESIAN_POINT ( 'NONE',  ( 12.06949235617739724, 12.14591786802326823, 46.87609039468568994 ) ) ;
#185340=CARTESIAN_POINT ( 'NONE',  ( -13.97604488694527625, -13.89961937509977652, 106.8739096053143669 ) ) ;
#185341=CARTESIAN_POINT ( 'NONE',  ( 5.049401038298161559, -19.05341960407611168, 62.70724293864769550 ) ) ;
#185342=CARTESIAN_POINT ( 'NONE',  ( 0.05219959533907565091, 21.53943276465977519, 94.99890960531436690 ) ) ;
#185343=CARTESIAN_POINT ( 'NONE',  ( 5.153800228976335163, 19.02544592524342804, 89.79057627198102409 ) ) ;
#185346=CARTESIAN_POINT ( 'NONE',  ( 16.46253265017160672, -9.564922557960803928, 68.33224293864770971 ) ) ;
#185347=CARTESIAN_POINT ( 'NONE',  ( 0.05219959533934541429, -16.53943276465976808, 110.0010903946856757 ) ) ;
#185348=CARTESIAN_POINT ( 'NONE',  ( 16.51473224551069308, 9.474510206698969483, 69.16557627198102409 ) ) ;
#185349=CARTESIAN_POINT ( 'NONE',  ( -19.02544592524334988, -5.153800228976617603, 18.95942372801899722 ) ) ;
#185350=CARTESIAN_POINT ( 'NONE',  ( -16.52544592524342804, 4.483927247898546575, 66.04057627198103830 ) ) ;
#185351=CARTESIAN_POINT ( 'NONE',  ( -5.823673210054431948, 21.52544592524334988, 102.7094237280190185 ) ) ;
#185352=CARTESIAN_POINT ( 'NONE',  ( -9.564922557960796823, -16.46253265017161027, 42.08224293864769550 ) ) ;
#185353=CARTESIAN_POINT ( 'NONE',  ( 4.379528057220339221, -16.55341960407611168, 37.70724293864769550 ) ) ;
#185354=CARTESIAN_POINT ( 'NONE',  ( 21.52544592524334988, 5.823673210054432836, 96.45942372801901854 ) ) ;
#185355=CARTESIAN_POINT ( 'NONE',  ( 5.049401038298161559, -19.05341960407611168, 82.70724293864770971 ) ) ;
#185356=CARTESIAN_POINT ( 'NONE',  ( -16.46253265017160317, 9.564922557960807481, 100.8322429386477097 ) ) ;
#185357=CARTESIAN_POINT ( 'NONE',  ( -12.14591786802309592, -12.06949235617757132, 106.8739096053143811 ) ) ;
#185358=CARTESIAN_POINT ( 'NONE',  ( 12.14591786802309770, 12.06949235617756955, 74.37390960531436690 ) ) ;
#185359=CARTESIAN_POINT ( 'NONE',  ( 21.53943276465977519, -0.05219959533907433946, 83.74890960531435269 ) ) ;
#185360=CARTESIAN_POINT ( 'NONE',  ( -9.474510206698964154, 16.51473224551069663, 70.41557627198102409 ) ) ;
#185361=CARTESIAN_POINT ( 'NONE',  ( 21.55341960407610458, 5.719274019375980345, 83.95724293864770971 ) ) ;
#185362=CARTESIAN_POINT ( 'NONE',  ( -19.03943276465977164, -0.05219959533935918106, 83.75109039468567573 ) ) ;
#185363=CARTESIAN_POINT ( 'NONE',  ( 18.56453257813361191, -5.500000000000031974, 48.49000423690687001 ) ) ;
#185364=CARTESIAN_POINT ( 'NONE',  ( -16.53943276465976808, 0.05219959533911058130, 91.24890960531436690 ) ) ;
#185365=CARTESIAN_POINT ( 'NONE',  ( -16.51473224551069308, -9.474510206698971260, 61.66557627198103120 ) ) ;
#185366=CARTESIAN_POINT ( 'NONE',  ( -18.62759615963270932, 10.81492255796079327, 70.83224293864770971 ) ) ;
#185367=CARTESIAN_POINT ( 'NONE',  ( -17.72560187377285956, -5.499999999999973355, 84.07814504131316369 ) ) ;
#185368=CARTESIAN_POINT ( 'NONE',  ( 4.483927247898790824, -16.52544592524335698, 110.2094237280190185 ) ) ;
#185370=CARTESIAN_POINT ( 'NONE',  ( 9.564922557961047289, -16.46253265017146816, 110.4177570613523471 ) ) ;
#185371=CARTESIAN_POINT ( 'NONE',  ( -8.224510206698948167, 14.34966873604960824, 75.41557627198102409 ) ) ;
#185372=CARTESIAN_POINT ( 'NONE',  ( -18.87255363501902750, -5.500000000000005329, 96.32513748171830059 ) ) ;
#185373=CARTESIAN_POINT ( 'NONE',  ( 19.05341960407611168, 5.049401038298154454, 68.95724293864769550 ) ) ;
#185374=CARTESIAN_POINT ( 'NONE',  ( 5.049401038298161559, -19.05341960407611168, 37.70724293864768839 ) ) ;
#185375=CARTESIAN_POINT ( 'NONE',  ( 16.55341960407611168, 4.379528057220329451, 68.95724293864769550 ) ) ;
#185377=CARTESIAN_POINT ( 'NONE',  ( 5.153800228976335163, 19.02544592524342804, 114.7905762719810241 ) ) ;
#185378=CARTESIAN_POINT ( 'NONE',  ( -9.474510206698720793, -16.51473224551083518, 89.58442372801900433 ) ) ;
#185379=CARTESIAN_POINT ( 'NONE',  ( -5.153800228976328057, -19.02544592524343514, 77.29057627198099567 ) ) ;
#185380=CARTESIAN_POINT ( 'NONE',  ( -0.05219959533909027116, -19.03943276465977164, 92.49890960531436690 ) ) ;
#185381=CARTESIAN_POINT ( 'NONE',  ( 5.823673210054125526, 21.52544592524343514, 69.79057627198102409 ) ) ;
#185382=CARTESIAN_POINT ( 'NONE',  ( 12.14591786802327356, -12.06949235617739191, 75.62609039468567573 ) ) ;
#185383=CARTESIAN_POINT ( 'NONE',  ( -17.50000000000000355, 5.622605283950836252, 93.68792689403892382 ) ) ;
#185384=CARTESIAN_POINT ( 'NONE',  ( 16.46253265017160672, -9.564922557960803928, 68.33224293864770971 ) ) ;
#185385=CARTESIAN_POINT ( 'NONE',  ( -21.55341960407610458, -5.719274019375992779, 61.45724293864770260 ) ) ;
#185386=CARTESIAN_POINT ( 'NONE',  ( -5.153800228976607833, 19.02544592524334988, 112.7094237280190043 ) ) ;
#185387=CARTESIAN_POINT ( 'NONE',  ( 16.53943276465976808, -0.05219959533910856209, 38.74890960531435979 ) ) ;
#185388=CARTESIAN_POINT ( 'NONE',  ( 15.80617190586769283, -15.72974639402175789, 40.62609039468567573 ) ) ;
#185390=CARTESIAN_POINT ( 'NONE',  ( -16.55341960407617563, 4.379528057220093196, 73.54275706135234714 ) ) ;
#185391=CARTESIAN_POINT ( 'NONE',  ( 19.03943276465977164, -0.05219959533909143690, 108.7489096053143527 ) ) ;
#185392=CARTESIAN_POINT ( 'NONE',  ( 13.89961937509978007, -13.97604488694527269, 108.1239096053143669 ) ) ;
#185393=DIRECTION ( 'NONE',  ( -6.948002486793210646E-15, 0.9991276842514723588, -0.04175967627138119781 ) ) ;
#185394=CARTESIAN_POINT ( 'NONE',  ( 8.314922557961029526, -14.29746914071037800, 90.41775706135236135 ) ) ;
#185395=CARTESIAN_POINT ( 'NONE',  ( 16.53943276465976808, 0.05219959533934440121, 51.25109039468568994 ) ) ;
#185396=CARTESIAN_POINT ( 'NONE',  ( -5.153800228976328057, -19.02544592524343514, 57.29057627198103120 ) ) ;
#185397=CARTESIAN_POINT ( 'NONE',  ( 13.89961937509977652, -13.97604488694527269, 78.12390960531433848 ) ) ;
#185398=CARTESIAN_POINT ( 'NONE',  ( 10.81492255796106328, -18.62759615963255655, 50.41775706135235424 ) ) ;
#185399=CARTESIAN_POINT ( 'NONE',  ( -16.53943276465976808, -0.05219959533934237506, 63.75109039468568284 ) ) ;
#185400=CARTESIAN_POINT ( 'NONE',  ( -8.314922557960811034, -14.29746914071050412, 27.08224293864769550 ) ) ;
#185401=CARTESIAN_POINT ( 'NONE',  ( -9.474510206698964154, 16.51473224551069663, 35.41557627198102409 ) ) ;
#185402=CARTESIAN_POINT ( 'NONE',  ( 0.05219959533909260263, 19.03943276465977164, 29.99890960531435979 ) ) ;
#185403=CARTESIAN_POINT ( 'NONE',  ( -8.314922557961024197, 14.29746914071037800, 22.91775706135235069 ) ) ;
#185404=CONICAL_SURFACE ( 'NONE', #36867, 2.500000000000002220, 1.029744258676656754 ) ;
#185405=CARTESIAN_POINT ( 'NONE',  ( -16.51473224551082808, 9.474510206698731452, 83.33442372801899012 ) ) ;
#185406=CARTESIAN_POINT ( 'NONE',  ( 4.483927247898545687, 16.52544592524342804, 79.79057627198102409 ) ) ;
#185407=CARTESIAN_POINT ( 'NONE',  ( -13.89961937509977652, 13.97604488694528158, 45.62390960531433848 ) ) ;
#185408=CARTESIAN_POINT ( 'NONE',  ( 5.049401038297881783, 19.05341960407617563, 92.29275706135234714 ) ) ;
#185410=CARTESIAN_POINT ( 'NONE',  ( -5.719274019375665041, -21.55341960407619695, 94.79275706135234714 ) ) ;
#185411=CARTESIAN_POINT ( 'NONE',  ( 16.53943276465976808, 0.05219959533934440121, 51.25109039468568994 ) ) ;
#185412=CARTESIAN_POINT ( 'NONE',  ( 17.05587630539785238, 6.762274262135711922, 36.75819690962688924 ) ) ;
#185413=CARTESIAN_POINT ( 'NONE',  ( 0.05219959533907565091, 21.53943276465977519, 44.99890960531435979 ) ) ;
#185414=CARTESIAN_POINT ( 'NONE',  ( -12.14591786802326823, 12.06949235617739902, 43.12609039468568284 ) ) ;
#185415=CYLINDRICAL_SURFACE ( 'NONE', #34478, 2.000000000000001776 ) ;
#185416=CARTESIAN_POINT ( 'NONE',  ( 13.97604488694548053, -13.89961937509957401, 45.62609039468566863 ) ) ;
#185417=CARTESIAN_POINT ( 'NONE',  ( 9.564922557960805705, 16.46253265017160317, 74.58224293864769550 ) ) ;
#185418=CARTESIAN_POINT ( 'NONE',  ( -13.97604488694527625, -13.89961937509977652, 56.87390960531434558 ) ) ;
#185420=CARTESIAN_POINT ( 'NONE',  ( -19.02544592524342804, 5.153800228976336051, 66.04057627198103830 ) ) ;
#185423=CARTESIAN_POINT ( 'NONE',  ( 0.05219959533936267826, -19.03943276465977164, 30.00109039468566863 ) ) ;
#185424=CARTESIAN_POINT ( 'NONE',  ( 0.05219959533937995610, -21.53943276465977519, 110.0010903946856757 ) ) ;
#185425=CARTESIAN_POINT ( 'NONE',  ( -12.06949235617756955, 12.14591786802309770, 40.62390960531435269 ) ) ;
#185426=CARTESIAN_POINT ( 'NONE',  ( -0.05219959533909027116, -19.03943276465977164, 37.49890960531436690 ) ) ;
#185428=CARTESIAN_POINT ( 'NONE',  ( -13.97604488694527625, -13.89961937509977652, 111.8739096053143243 ) ) ;
#185429=CARTESIAN_POINT ( 'NONE',  ( 15.72974639402176855, 15.80617190586768217, 81.87609039468568994 ) ) ;
#185430=CARTESIAN_POINT ( 'NONE',  ( 19.02544592524343514, -5.153800228976328945, 53.54057627198102409 ) ) ;
#185431=CARTESIAN_POINT ( 'NONE',  ( -5.823673210054431948, 21.52544592524334988, 82.70942372801900433 ) ) ;
#185432=CARTESIAN_POINT ( 'NONE',  ( -18.62759615963270932, 10.81492255796079327, 35.83224293864768839 ) ) ;
#185433=CARTESIAN_POINT ( 'NONE',  ( 15.80617190586769283, -15.72974639402175789, 20.62609039468568639 ) ) ;
#185434=CARTESIAN_POINT ( 'NONE',  ( -0.05219959533936034679, 19.03943276465977164, 47.50109039468566863 ) ) ;
#185435=CARTESIAN_POINT ( 'NONE',  ( 9.474510206698971260, -16.51473224551069308, 32.91557627198102409 ) ) ;
#185436=CARTESIAN_POINT ( 'NONE',  ( 19.03943276465977164, -0.05219959533909143690, 78.74890960531436690 ) ) ;
#185437=CARTESIAN_POINT ( 'NONE',  ( 19.03943276465977164, 0.05219959533936151252, 111.2510903946856757 ) ) ;
#185438=CARTESIAN_POINT ( 'NONE',  ( 4.379528057220339221, -16.55341960407611168, 92.70724293864770971 ) ) ;
#185439=CARTESIAN_POINT ( 'NONE',  ( -9.564922557960796823, -16.46253265017161027, 52.08224293864768839 ) ) ;
#185440=CARTESIAN_POINT ( 'NONE',  ( -0.05219959533907301413, -21.53943276465977519, 32.49890960531435979 ) ) ;
#185441=CARTESIAN_POINT ( 'NONE',  ( 5.153800228976615827, -19.02544592524334988, 105.2094237280190185 ) ) ;
#185442=CARTESIAN_POINT ( 'NONE',  ( -18.62759615963270932, 10.81492255796079327, 100.8322429386477097 ) ) ;
#185443=CARTESIAN_POINT ( 'NONE',  ( -21.53943276465977519, -0.05219959533937600094, 58.75109039468568994 ) ) ;
#185444=CARTESIAN_POINT ( 'NONE',  ( 4.379528057220092307, 16.55341960407617563, 57.29275706135234714 ) ) ;
#185445=CARTESIAN_POINT ( 'NONE',  ( -16.55341960407617563, 4.379528057220093196, 68.54275706135234714 ) ) ;
#185446=CARTESIAN_POINT ( 'NONE',  ( 16.51473224551069308, 9.474510206698969483, 64.16557627198102409 ) ) ;
#185447=CARTESIAN_POINT ( 'NONE',  ( -8.224510206698735004, -14.34966873604973081, 89.58442372801901854 ) ) ;
#185448=CARTESIAN_POINT ( 'NONE',  ( 18.62759615963255655, 10.81492255796105972, 21.66775706135235069 ) ) ;
#185449=CARTESIAN_POINT ( 'NONE',  ( -4.379528057220328563, 16.55341960407611168, 70.20724293864769550 ) ) ;
#185450=CARTESIAN_POINT ( 'NONE',  ( -0.05219959533909027116, -19.03943276465977164, 92.49890960531436690 ) ) ;
#185451=CARTESIAN_POINT ( 'NONE',  ( 16.55341960407618274, -4.379528057220086978, 71.04275706135234714 ) ) ;
#185452=CARTESIAN_POINT ( 'NONE',  ( -10.81492255796105439, 18.62759615963255655, 62.91775706135236135 ) ) ;
#185453=CARTESIAN_POINT ( 'NONE',  ( 5.153800228976615827, -19.02544592524334988, 110.2094237280189901 ) ) ;
#185454=CARTESIAN_POINT ( 'NONE',  ( -15.80617190586745835, -15.72974639402198527, 111.8739096053143669 ) ) ;
#185455=CARTESIAN_POINT ( 'NONE',  ( 12.06949235617757843, -12.14591786802309237, 53.12390960531436690 ) ) ;
#185457=CARTESIAN_POINT ( 'NONE',  ( 19.25663599770062007, -5.499999999999442224, 91.49419308057203182 ) ) ;
#185458=CARTESIAN_POINT ( 'NONE',  ( 5.823673210054125526, 21.52544592524343514, 84.79057627198102409 ) ) ;
#185459=CARTESIAN_POINT ( 'NONE',  ( 4.483927247898545687, 16.52544592524342804, 44.79057627198103120 ) ) ;
#185460=ORIENTED_EDGE ( 'NONE', *, *, #26227, .T. ) ;
#185462=CARTESIAN_POINT ( 'NONE',  ( 0.05219959533937995610, -21.53943276465977519, 20.00109039468568639 ) ) ;
#185463=CARTESIAN_POINT ( 'NONE',  ( -10.81492255796078084, -18.62759615963271287, 22.08224293864769194 ) ) ;
#185464=CARTESIAN_POINT ( 'NONE',  ( -15.72974639402176322, -15.80617190586768395, 24.37609039468567573 ) ) ;
#185465=CARTESIAN_POINT ( 'NONE',  ( 12.14591786802309770, 12.06949235617756955, 49.37390960531436690 ) ) ;
#185467=CARTESIAN_POINT ( 'NONE',  ( -0.05219959533934338120, 16.53943276465976808, 67.50109039468568994 ) ) ;
#185468=CARTESIAN_POINT ( 'NONE',  ( -19.05341960407611168, -5.049401038298163336, 61.45724293864769550 ) ) ;
#185469=CARTESIAN_POINT ( 'NONE',  ( 19.02544592524334988, 5.153800228976608722, 66.45942372801899012 ) ) ;
#185470=CARTESIAN_POINT ( 'NONE',  ( -5.049401038298153566, 19.05341960407611168, 75.20724293864769550 ) ) ;
#185471=CARTESIAN_POINT ( 'NONE',  ( -21.52544592524343514, 5.823673210054127303, 36.04057627198102409 ) ) ;
#185473=CARTESIAN_POINT ( 'NONE',  ( 9.564922557960805705, 16.46253265017160317, 59.58224293864769550 ) ) ;
#185474=CARTESIAN_POINT ( 'NONE',  ( -16.52544592524335698, -4.483927247898792601, 28.95942372801902209 ) ) ;
#185475=CARTESIAN_POINT ( 'NONE',  ( 19.05341960407617918, -5.049401038297876454, 61.04275706135232582 ) ) ;
#185476=CARTESIAN_POINT ( 'NONE',  ( -21.53943276465977519, -0.05219959533937600094, 18.75109039468568639 ) ) ;
#185477=CARTESIAN_POINT ( 'NONE',  ( -14.29746914071049879, 8.314922557960819915, 50.83224293864770971 ) ) ;
#185478=CARTESIAN_POINT ( 'NONE',  ( 9.564922557960805705, 16.46253265017160317, 89.58224293864769550 ) ) ;
#185479=CARTESIAN_POINT ( 'NONE',  ( -21.55341960407610458, -5.719274019375992779, 56.45724293864768839 ) ) ;
#185480=CARTESIAN_POINT ( 'NONE',  ( 21.52544592524344225, -5.823673210054117533, 98.54057627198105251 ) ) ;
#185481=CARTESIAN_POINT ( 'NONE',  ( 8.224510206698742110, 14.34966873604972548, 37.08442372801901143 ) ) ;
#185482=CARTESIAN_POINT ( 'NONE',  ( -0.05219959533907301413, -21.53943276465977519, 42.49890960531435979 ) ) ;
#185483=CARTESIAN_POINT ( 'NONE',  ( 21.52544592524334988, 5.823673210054432836, 86.45942372801901854 ) ) ;
#185484=CARTESIAN_POINT ( 'NONE',  ( 5.049401038298161559, -19.05341960407611168, 87.70724293864769550 ) ) ;
#185485=CARTESIAN_POINT ( 'NONE',  ( -16.51473224551069308, -9.474510206698971260, 36.66557627198102409 ) ) ;
#185486=CARTESIAN_POINT ( 'NONE',  ( -19.02544592524342804, 5.153800228976336051, 91.04057627198100988 ) ) ;
#185487=CARTESIAN_POINT ( 'NONE',  ( -4.483927247898539470, -16.52544592524342804, 107.2905762719810525 ) ) ;
#185488=CARTESIAN_POINT ( 'NONE',  ( 9.564922557960805705, 16.46253265017160317, 59.58224293864769550 ) ) ;
#185489=CARTESIAN_POINT ( 'NONE',  ( -9.564922557961040184, 16.46253265017147172, 112.9177570613523329 ) ) ;
#185491=CARTESIAN_POINT ( 'NONE',  ( -10.81492255796105439, 18.62759615963255655, 92.91775706135236135 ) ) ;
#185492=CARTESIAN_POINT ( 'NONE',  ( -5.823673210054116645, -21.52544592524344225, 32.29057627198102409 ) ) ;
#185493=CARTESIAN_POINT ( 'NONE',  ( 16.52544592524335698, 4.483927247898782831, 86.45942372801901854 ) ) ;
#185494=CARTESIAN_POINT ( 'NONE',  ( -17.49999999999999645, -5.500000000000000888, 120.0000000000000142 ) ) ;
#185495=CARTESIAN_POINT ( 'NONE',  ( -5.049401038297874678, -19.05341960407617918, 69.79275706135233293 ) ) ;
#185496=CARTESIAN_POINT ( 'NONE',  ( 9.474510206698729675, 16.51473224551082808, 32.08442372801900433 ) ) ;
#185498=CARTESIAN_POINT ( 'NONE',  ( 9.564922557960805705, 16.46253265017160317, 29.58224293864769550 ) ) ;
#185499=CARTESIAN_POINT ( 'NONE',  ( 8.314922557960818139, 14.29746914071049879, 34.58224293864770260 ) ) ;
#185500=CARTESIAN_POINT ( 'NONE',  ( -17.05116617787823685, -6.768360034955810178, 111.3432444674080841 ) ) ;
#185501=CARTESIAN_POINT ( 'NONE',  ( -16.53943276465976808, 0.05219959533911058130, 21.24890960531436690 ) ) ;
#185502=CARTESIAN_POINT ( 'NONE',  ( 17.48847506799968698, 5.747544572773809257, 66.67302562156720569 ) ) ;
#185503=CARTESIAN_POINT ( 'NONE',  ( -16.52544592524335698, -4.483927247898792601, 98.95942372801903275 ) ) ;
#185504=CARTESIAN_POINT ( 'NONE',  ( -9.564922557960796823, -16.46253265017161027, 42.08224293864769550 ) ) ;
#185505=CARTESIAN_POINT ( 'NONE',  ( 18.62759615963255655, 10.81492255796105972, 111.6677570613523613 ) ) ;
#185506=CARTESIAN_POINT ( 'NONE',  ( -16.52544592524335698, -4.483927247898792601, 23.95942372801901143 ) ) ;
#185507=CARTESIAN_POINT ( 'NONE',  ( -0.05219959533937732626, 21.53943276465977519, 72.50109039468568994 ) ) ;
#185508=CARTESIAN_POINT ( 'NONE',  ( 0.05219959533936267826, -19.03943276465977164, 50.00109039468566863 ) ) ;
#185509=CARTESIAN_POINT ( 'NONE',  ( 13.89961937509977652, -13.97604488694527269, 88.12390960531438111 ) ) ;
#185510=CARTESIAN_POINT ( 'NONE',  ( 9.564922557960805705, 16.46253265017160317, 69.58224293864770971 ) ) ;
#185511=CARTESIAN_POINT ( 'NONE',  ( -19.53037848336981241, 5.499999999999901412, 39.85532783611445495 ) ) ;
#185512=CARTESIAN_POINT ( 'NONE',  ( -21.53943276465977519, 0.05219959533907696930, 96.24890960531435269 ) ) ;
#185513=CARTESIAN_POINT ( 'NONE',  ( -12.06949235617756955, 12.14591786802309770, 60.62390960531437401 ) ) ;
#185514=CARTESIAN_POINT ( 'NONE',  ( 15.72974639402199770, -15.80617190586745480, 63.12390960531435979 ) ) ;
#185515=CARTESIAN_POINT ( 'NONE',  ( -5.153800228976328057, -19.02544592524343514, 62.29057627198100988 ) ) ;
#185516=CARTESIAN_POINT ( 'NONE',  ( 5.823673210054125526, 21.52544592524343514, 89.79057627198103830 ) ) ;
#185517=CARTESIAN_POINT ( 'NONE',  ( -16.55341960407617563, 4.379528057220093196, 73.54275706135234714 ) ) ;
#185519=CARTESIAN_POINT ( 'NONE',  ( -19.05341960407611168, -5.049401038298163336, 41.45724293864769550 ) ) ;
#185520=CARTESIAN_POINT ( 'NONE',  ( 4.483927247898545687, 16.52544592524342804, 74.79057627198105251 ) ) ;
#185522=CARTESIAN_POINT ( 'NONE',  ( 19.05341960407611168, 5.049401038298154454, 53.95724293864770260 ) ) ;
#185523=CARTESIAN_POINT ( 'NONE',  ( 16.52544592524342804, -4.483927247898539470, 113.5405762719810383 ) ) ;
#185524=CARTESIAN_POINT ( 'NONE',  ( 19.03943276465977164, 0.05219959533936151252, 61.25109039468566863 ) ) ;
#185525=CARTESIAN_POINT ( 'NONE',  ( 0.05219959533910956823, 16.53943276465976808, 84.99890960531436690 ) ) ;
#185526=CARTESIAN_POINT ( 'NONE',  ( -18.62759615963255300, -10.81492255796106328, 44.16775706135234714 ) ) ;
#185527=CARTESIAN_POINT ( 'NONE',  ( 13.97604488694527802, 13.89961937509977652, 29.37390960531435979 ) ) ;
#185528=CARTESIAN_POINT ( 'NONE',  ( 15.80617190586746368, 15.72974639402197994, 99.37390960531436690 ) ) ;
#185529=CARTESIAN_POINT ( 'NONE',  ( 16.52544592524342804, -4.483927247898539470, 83.54057627198102409 ) ) ;
#185531=CARTESIAN_POINT ( 'NONE',  ( -5.153800228976328057, -19.02544592524343514, 57.29057627198103120 ) ) ;
#185533=CARTESIAN_POINT ( 'NONE',  ( 13.97604488694548053, -13.89961937509957401, 95.62609039468563310 ) ) ;
#185534=CARTESIAN_POINT ( 'NONE',  ( 9.564922557960805705, 16.46253265017160317, 99.58224293864770971 ) ) ;
#185535=CARTESIAN_POINT ( 'NONE',  ( -21.55341960407619339, 5.719274019375674811, 33.54275706135234714 ) ) ;
#185536=CARTESIAN_POINT ( 'NONE',  ( 19.05341960407611168, 5.049401038298154454, 88.95724293864769550 ) ) ;
#185537=CARTESIAN_POINT ( 'NONE',  ( 16.46253265017146816, 9.564922557961045513, 66.66775706135233293 ) ) ;
#185538=CARTESIAN_POINT ( 'NONE',  ( 9.564922557960805705, 16.46253265017160317, 54.58224293864769550 ) ) ;
#185539=CARTESIAN_POINT ( 'NONE',  ( 4.483927247898545687, 16.52544592524342804, 74.79057627198105251 ) ) ;
#185540=CARTESIAN_POINT ( 'NONE',  ( 16.53943276465976808, -0.05219959533910856209, 63.74890960531435979 ) ) ;
#185541=CARTESIAN_POINT ( 'NONE',  ( 19.02544592524343514, -5.153800228976328945, 83.54057627198100988 ) ) ;
#185542=CARTESIAN_POINT ( 'NONE',  ( -18.62759615963270932, 10.81492255796079327, 105.8322429386476955 ) ) ;
#185543=CARTESIAN_POINT ( 'NONE',  ( 19.05341960407611168, 5.049401038298154454, 78.95724293864769550 ) ) ;
#185544=CARTESIAN_POINT ( 'NONE',  ( -9.564922557961040184, 16.46253265017147172, 27.91775706135232582 ) ) ;
#185545=CARTESIAN_POINT ( 'NONE',  ( 0.05219959533909260263, 19.03943276465977164, 29.99890960531435979 ) ) ;
#185546=CARTESIAN_POINT ( 'NONE',  ( 8.224510206698953496, -14.34966873604960469, 27.91557627198103830 ) ) ;
#185547=CARTESIAN_POINT ( 'NONE',  ( 14.29746914071049879, -8.314922557960816363, 103.3322429386476955 ) ) ;
#185548=CARTESIAN_POINT ( 'NONE',  ( -0.05219959533936034679, 19.03943276465977164, 102.5010903946856757 ) ) ;
#185550=CARTESIAN_POINT ( 'NONE',  ( -15.72974639402176322, -15.80617190586768395, 29.37609039468568284 ) ) ;
#185551=CARTESIAN_POINT ( 'NONE',  ( 16.51473224551083163, -9.474510206698727899, 70.83442372801900433 ) ) ;
#185552=CARTESIAN_POINT ( 'NONE',  ( -0.05219959533910754901, -16.53943276465976808, 22.49890960531436335 ) ) ;
#185553=CARTESIAN_POINT ( 'NONE',  ( 21.53943276465977519, -0.05219959533907433946, 88.74890960531436690 ) ) ;
#185554=CARTESIAN_POINT ( 'NONE',  ( 19.05341960407611168, 5.049401038298154454, 113.9572429386477097 ) ) ;
#185555=CARTESIAN_POINT ( 'NONE',  ( -0.05219959533910754901, -16.53943276465976808, 72.49890960531435269 ) ) ;
#185556=CARTESIAN_POINT ( 'NONE',  ( 16.46253265017160672, -9.564922557960803928, 23.33224293864769194 ) ) ;
#185557=CARTESIAN_POINT ( 'NONE',  ( 0.05219959533936267826, -19.03943276465977164, 25.00109039468566152 ) ) ;
#185558=CARTESIAN_POINT ( 'NONE',  ( 8.314922557961029526, -14.29746914071037800, 85.41775706135236135 ) ) ;
#185559=CARTESIAN_POINT ( 'NONE',  ( -12.14591786802326823, 12.06949235617739902, 58.12609039468568994 ) ) ;
#185560=CARTESIAN_POINT ( 'NONE',  ( 15.72974639402199770, -15.80617190586745480, 28.12390960531435979 ) ) ;
#185561=CARTESIAN_POINT ( 'NONE',  ( -21.53943276465977519, -0.05219959533937600094, 113.7510903946856757 ) ) ;
#185562=CARTESIAN_POINT ( 'NONE',  ( 13.89961937509977652, -13.97604488694527269, 73.12390960531436690 ) ) ;
#185563=CARTESIAN_POINT ( 'NONE',  ( 12.06949235617739724, 12.14591786802326823, 61.87609039468568284 ) ) ;
#185564=CARTESIAN_POINT ( 'NONE',  ( 16.46253265017160672, -9.564922557960803928, 28.33224293864769550 ) ) ;
#185565=CARTESIAN_POINT ( 'NONE',  ( 14.34966873604960469, 8.224510206698951720, 39.16557627198102409 ) ) ;
#185567=CARTESIAN_POINT ( 'NONE',  ( -5.153800228976328057, -19.02544592524343514, 102.2905762719810383 ) ) ;
#185568=CARTESIAN_POINT ( 'NONE',  ( 13.97604488694527802, 13.89961937509977652, 74.37390960531436690 ) ) ;
#185569=CARTESIAN_POINT ( 'NONE',  ( -9.564922557960796823, -16.46253265017161027, 112.0822429386476955 ) ) ;
#185571=CARTESIAN_POINT ( 'NONE',  ( 16.53943276465976808, -0.05219959533910856209, 58.74890960531436690 ) ) ;
#185572=CARTESIAN_POINT ( 'NONE',  ( 12.06949235617757843, -12.14591786802309237, 33.12390960531435979 ) ) ;
#185573=ORIENTED_EDGE ( 'NONE', *, *, #146110, .F. ) ;
#185574=CARTESIAN_POINT ( 'NONE',  ( -8.314922557960811034, -14.29746914071050412, 57.08224293864769550 ) ) ;
#185575=CARTESIAN_POINT ( 'NONE',  ( 16.53943276465976808, 0.05219959533934440121, 46.25109039468567573 ) ) ;
#185576=CARTESIAN_POINT ( 'NONE',  ( 16.51473224551083163, -9.474510206698727899, 60.83442372801900433 ) ) ;
#185577=VECTOR ( 'NONE', #58068, 1000.000000000000000 ) ;
#185578=CARTESIAN_POINT ( 'NONE',  ( 19.02544592524334988, 5.153800228976608722, 56.45942372801898301 ) ) ;
#185579=CARTESIAN_POINT ( 'NONE',  ( 19.05341960407611168, 5.049401038298154454, 73.95724293864768129 ) ) ;
#185580=CARTESIAN_POINT ( 'NONE',  ( -13.97604488694547697, 13.89961937509957934, 53.12609039468565442 ) ) ;
#185582=CARTESIAN_POINT ( 'NONE',  ( -9.564922557961040184, 16.46253265017147172, 52.91775706135233293 ) ) ;
#185583=CARTESIAN_POINT ( 'NONE',  ( -5.049401038297874678, -19.05341960407617918, 94.79275706135230450 ) ) ;
#185584=CARTESIAN_POINT ( 'NONE',  ( -4.379528057220086978, -16.55341960407618274, 84.79275706135234714 ) ) ;
#185586=CARTESIAN_POINT ( 'NONE',  ( 13.89961937509977652, -13.97604488694527269, 23.12390960531436335 ) ) ;
#185587=CARTESIAN_POINT ( 'NONE',  ( -0.05219959533909027116, -19.03943276465977164, 97.49890960531436690 ) ) ;
#185588=CARTESIAN_POINT ( 'NONE',  ( -5.823673210054431948, 21.52544592524334988, 47.70942372801902565 ) ) ;
#185589=CARTESIAN_POINT ( 'NONE',  ( 9.564922557961047289, -16.46253265017146816, 105.4177570613523471 ) ) ;
#185590=CARTESIAN_POINT ( 'NONE',  ( 17.50000000000000000, -5.500000000000001776, 106.2176903769643417 ) ) ;
#185591=CARTESIAN_POINT ( 'NONE',  ( -19.05341960407611168, -5.049401038298163336, 56.45724293864768129 ) ) ;
#185592=EDGE_CURVE ( 'NONE', #109472, #65144, #178492, .T. ) ;
#185593=CARTESIAN_POINT ( 'NONE',  ( -16.51473224551069308, -9.474510206698971260, 101.6655762719810241 ) ) ;
#185594=CARTESIAN_POINT ( 'NONE',  ( -12.06949235617756955, 12.14591786802309770, 60.62390960531437401 ) ) ;
#185595=CARTESIAN_POINT ( 'NONE',  ( 19.05341960407611168, 5.049401038298154454, 63.95724293864769550 ) ) ;
#185596=CARTESIAN_POINT ( 'NONE',  ( -19.05341960407611168, -5.049401038298163336, 66.45724293864769550 ) ) ;
#185597=CARTESIAN_POINT ( 'NONE',  ( 16.51473224551083163, -9.474510206698727899, 80.83442372801899012 ) ) ;
#185598=CARTESIAN_POINT ( 'NONE',  ( 0.05219959533907565091, 21.53943276465977519, 54.99890960531435269 ) ) ;
#185599=CARTESIAN_POINT ( 'NONE',  ( 13.89961937509957401, 13.97604488694547697, 41.87609039468566152 ) ) ;
#185600=CARTESIAN_POINT ( 'NONE',  ( 0.05219959533909260263, 19.03943276465977164, 74.99890960531435269 ) ) ;
#185601=CARTESIAN_POINT ( 'NONE',  ( 21.53943276465977519, -0.05219959533907433946, 78.74890960531436690 ) ) ;
#185602=CARTESIAN_POINT ( 'NONE',  ( 4.483927247898545687, 16.52544592524342804, 74.79057627198105251 ) ) ;
#185603=CARTESIAN_POINT ( 'NONE',  ( 13.89961937509957401, 13.97604488694547697, 31.87609039468566863 ) ) ;
#185604=CARTESIAN_POINT ( 'NONE',  ( -5.823673210054116645, -21.52544592524344225, 57.29057627198103120 ) ) ;
#185605=CARTESIAN_POINT ( 'NONE',  ( 21.53943276465977519, -0.05219959533907433946, 43.74890960531435979 ) ) ;
#185606=CARTESIAN_POINT ( 'NONE',  ( -19.02544592524342804, 5.153800228976336051, 61.04057627198103120 ) ) ;
#185607=CARTESIAN_POINT ( 'NONE',  ( 12.06949235617757843, -12.14591786802309237, 108.1239096053143811 ) ) ;
#185609=CARTESIAN_POINT ( 'NONE',  ( 10.72451020669871369, 18.67979575497193778, 32.08442372801901854 ) ) ;
#185610=CARTESIAN_POINT ( 'NONE',  ( 9.474510206698971260, -16.51473224551069308, 112.9155762719810383 ) ) ;
#185611=CARTESIAN_POINT ( 'NONE',  ( 21.55341960407619695, -5.719274019375665929, 46.04275706135234714 ) ) ;
#185612=CARTESIAN_POINT ( 'NONE',  ( -16.46253265017160317, 9.564922557960807481, 35.83224293864768839 ) ) ;
#185613=CARTESIAN_POINT ( 'NONE',  ( 5.719274019375991003, -21.55341960407610458, 102.7072429386476955 ) ) ;
#185614=CARTESIAN_POINT ( 'NONE',  ( -19.02544592524334988, -5.153800228976617603, 48.95942372801900433 ) ) ;
#185615=CARTESIAN_POINT ( 'NONE',  ( -13.97604488694527625, -13.89961937509977652, 26.87390960531434558 ) ) ;
#185616=CARTESIAN_POINT ( 'NONE',  ( 19.02544592524343514, -5.153800228976328945, 28.54057627198102409 ) ) ;
#185617=CARTESIAN_POINT ( 'NONE',  ( 16.58166387080255433, -7.087407987291991063, 21.43250955971513250 ) ) ;
#185618=CARTESIAN_POINT ( 'NONE',  ( 8.224510206698742110, 14.34966873604972548, 57.08442372801901854 ) ) ;
#185619=CARTESIAN_POINT ( 'NONE',  ( -5.153800228976328057, -19.02544592524343514, 22.29057627198102765 ) ) ;
#185621=CARTESIAN_POINT ( 'NONE',  ( -5.153800228976328057, -19.02544592524343514, 67.29057627198102409 ) ) ;
#185622=CARTESIAN_POINT ( 'NONE',  ( -12.06949235617756955, 12.14591786802309770, 100.6239096053143811 ) ) ;
#185623=CARTESIAN_POINT ( 'NONE',  ( 15.80617190586746368, 15.72974639402197994, 59.37390960531436690 ) ) ;
#185624=CARTESIAN_POINT ( 'NONE',  ( -4.483927247898782831, 16.52544592524335698, 32.70942372801900433 ) ) ;
#185625=CARTESIAN_POINT ( 'NONE',  ( -5.719274019375665041, -21.55341960407619695, 104.7927570613523898 ) ) ;
#185626=CARTESIAN_POINT ( 'NONE',  ( 9.474510206698971260, -16.51473224551069308, 27.91557627198103120 ) ) ;
#185627=CARTESIAN_POINT ( 'NONE',  ( -8.314922557961024197, 14.29746914071037800, 107.9177570613523471 ) ) ;
#185628=CARTESIAN_POINT ( 'NONE',  ( -4.483927247898539470, -16.52544592524342804, 57.29057627198103120 ) ) ;
#185629=CARTESIAN_POINT ( 'NONE',  ( -0.05219959533909027116, -19.03943276465977164, 57.49890960531435979 ) ) ;
#185630=CARTESIAN_POINT ( 'NONE',  ( 18.62759615963255655, 10.81492255796105972, 91.66775706135234714 ) ) ;
#185631=CARTESIAN_POINT ( 'NONE',  ( -18.67979575497178146, -10.72451020669898902, 106.6655762719810383 ) ) ;
#185632=CARTESIAN_POINT ( 'NONE',  ( -21.53943276465977519, -0.05219959533937600094, 73.75109039468567573 ) ) ;
#185633=CARTESIAN_POINT ( 'NONE',  ( -8.224510206698735004, -14.34966873604973081, 49.58442372801901143 ) ) ;
#185634=CARTESIAN_POINT ( 'NONE',  ( -12.06949235617756955, 12.14591786802309770, 80.62390960531438111 ) ) ;
#185635=CARTESIAN_POINT ( 'NONE',  ( 15.72974639402176855, 15.80617190586768217, 96.87609039468568994 ) ) ;
#185636=CARTESIAN_POINT ( 'NONE',  ( -8.224510206698735004, -14.34966873604973081, 109.5844237280190328 ) ) ;
#185637=CARTESIAN_POINT ( 'NONE',  ( -17.50000000000000000, 5.622605283950884214, 113.6879268940389665 ) ) ;
#185638=CARTESIAN_POINT ( 'NONE',  ( -12.14591786802326823, 12.06949235617739902, 33.12609039468569705 ) ) ;
#185639=CARTESIAN_POINT ( 'NONE',  ( 8.224510206698953496, -14.34966873604960469, 37.91557627198102409 ) ) ;
#185640=CARTESIAN_POINT ( 'NONE',  ( 16.53943276465976808, 0.05219959533934440121, 86.25109039468568994 ) ) ;
#185641=CARTESIAN_POINT ( 'NONE',  ( 13.89961937509977652, -13.97604488694527269, 93.12390960531436690 ) ) ;
#185642=CARTESIAN_POINT ( 'NONE',  ( 19.03943276465977164, -0.05219959533909143690, 108.7489096053143527 ) ) ;
#185643=CARTESIAN_POINT ( 'NONE',  ( -21.55341960407619339, 5.719274019375674811, 93.54275706135234714 ) ) ;
#185644=CARTESIAN_POINT ( 'NONE',  ( -4.483927247898782831, 16.52544592524335698, 102.7094237280190185 ) ) ;
#185645=CARTESIAN_POINT ( 'NONE',  ( -14.34966873604960291, -8.224510206698953496, 76.66557627198103830 ) ) ;
#185646=CARTESIAN_POINT ( 'NONE',  ( -19.02544592524342804, 5.153800228976336051, 76.04057627198102409 ) ) ;
#185648=CARTESIAN_POINT ( 'NONE',  ( -16.55341960407617563, 4.379528057220093196, 23.54275706135235424 ) ) ;
#185649=CARTESIAN_POINT ( 'NONE',  ( -5.049401038298153566, 19.05341960407611168, 25.20724293864768484 ) ) ;
#185650=CARTESIAN_POINT ( 'NONE',  ( -19.03943276465977164, 0.05219959533909376836, 86.24890960531436690 ) ) ;
#185651=CARTESIAN_POINT ( 'NONE',  ( -16.53943276465976808, -0.05219959533934237506, 38.75109039468567573 ) ) ;
#185653=CARTESIAN_POINT ( 'NONE',  ( -13.89961937509957401, -13.97604488694547875, 39.37609039468566152 ) ) ;
#185654=CARTESIAN_POINT ( 'NONE',  ( -14.34966873604972548, 8.224510206698743886, 88.33442372801901854 ) ) ;
#185655=CARTESIAN_POINT ( 'NONE',  ( 5.153800228976335163, 19.02544592524342804, 34.79057627198102409 ) ) ;
#185656=CARTESIAN_POINT ( 'NONE',  ( -16.55341960407617563, 4.379528057220093196, 73.54275706135234714 ) ) ;
#185657=CARTESIAN_POINT ( 'NONE',  ( 12.14591786802327356, -12.06949235617739191, 65.62609039468568994 ) ) ;
#185658=CARTESIAN_POINT ( 'NONE',  ( 5.153800228976615827, -19.02544592524334988, 80.20942372801901854 ) ) ;
#185659=CARTESIAN_POINT ( 'NONE',  ( 19.05341960407617918, -5.049401038297876454, 31.04275706135232227 ) ) ;
#185660=CARTESIAN_POINT ( 'NONE',  ( -13.97604488694527625, -13.89961937509977652, 46.87390960531435979 ) ) ;
#185661=CARTESIAN_POINT ( 'NONE',  ( -9.564922557960796823, -16.46253265017161027, 97.08224293864769550 ) ) ;
#185662=CARTESIAN_POINT ( 'NONE',  ( -16.53943276465976808, 0.05219959533911058130, 81.24890960531436690 ) ) ;
#185663=EDGE_CURVE ( 'NONE', #128521, #13391, #151285, .T. ) ;
#185664=CARTESIAN_POINT ( 'NONE',  ( -0.05219959533936034679, 19.03943276465977164, 52.50109039468566863 ) ) ;
#185665=CARTESIAN_POINT ( 'NONE',  ( -18.67979575497178146, -10.72451020669898902, 51.66557627198102409 ) ) ;
#185666=CARTESIAN_POINT ( 'NONE',  ( 19.02544592524334988, 5.153800228976608722, 31.45942372801900433 ) ) ;
#185667=CARTESIAN_POINT ( 'NONE',  ( -16.46253265017160317, 9.564922557960807481, 100.8322429386477097 ) ) ;
#185668=CARTESIAN_POINT ( 'NONE',  ( 21.53943276465977519, -0.05219959533907433946, 83.74890960531435269 ) ) ;
#185669=CARTESIAN_POINT ( 'NONE',  ( 13.89961937509977652, -13.97604488694527269, 113.1239096053143527 ) ) ;
#185670=CARTESIAN_POINT ( 'NONE',  ( -19.02544592524334988, -5.153800228976617603, 83.95942372801901854 ) ) ;
#185671=CARTESIAN_POINT ( 'NONE',  ( -17.50000000000000711, 4.640572885337571840, 110.6378816454884486 ) ) ;
#185672=CARTESIAN_POINT ( 'NONE',  ( -19.03943276465977164, -0.05219959533935918106, 113.7510903946856757 ) ) ;
#185674=CARTESIAN_POINT ( 'NONE',  ( -13.89961937509977652, 13.97604488694528158, 30.62390960531435269 ) ) ;
#185675=CARTESIAN_POINT ( 'NONE',  ( 13.97604488694527802, 13.89961937509977652, 99.37390960531436690 ) ) ;
#185676=CARTESIAN_POINT ( 'NONE',  ( -18.62759615963270932, 10.81492255796079327, 70.83224293864770971 ) ) ;
#185677=CARTESIAN_POINT ( 'NONE',  ( 14.29746914071037800, 8.314922557961029526, 51.66775706135234714 ) ) ;
#185678=CARTESIAN_POINT ( 'NONE',  ( 5.719274019375673035, 21.55341960407619339, 52.29275706135236135 ) ) ;
#185679=CARTESIAN_POINT ( 'NONE',  ( -13.97604488694547697, 13.89961937509957934, 98.12609039468566152 ) ) ;
#185680=CARTESIAN_POINT ( 'NONE',  ( -0.05219959533937732626, 21.53943276465977519, 102.5010903946856899 ) ) ;
#185681=CARTESIAN_POINT ( 'NONE',  ( -12.14591786802326823, 12.06949235617739902, 113.1260903946856899 ) ) ;
#185682=CARTESIAN_POINT ( 'NONE',  ( -19.02544592524342804, 5.153800228976336051, 96.04057627198103830 ) ) ;
#185683=CARTESIAN_POINT ( 'NONE',  ( 4.483927247898545687, 16.52544592524342804, 94.79057627198105251 ) ) ;
#185684=CARTESIAN_POINT ( 'NONE',  ( 4.379528057220339221, -16.55341960407611168, 37.70724293864769550 ) ) ;
#185685=CARTESIAN_POINT ( 'NONE',  ( 9.564922557961047289, -16.46253265017146816, 70.41775706135233293 ) ) ;
#185686=CARTESIAN_POINT ( 'NONE',  ( 10.72451020669871369, 18.67979575497193778, 62.08442372801901143 ) ) ;
#185687=CARTESIAN_POINT ( 'NONE',  ( -16.46253265017146816, -9.564922557961047289, 29.16775706135232937 ) ) ;
#185688=CARTESIAN_POINT ( 'NONE',  ( 8.224510206698953496, -14.34966873604960469, 102.9155762719810383 ) ) ;
#185689=CARTESIAN_POINT ( 'NONE',  ( -18.62759615963270932, 10.81492255796079327, 35.83224293864768839 ) ) ;
#185690=CARTESIAN_POINT ( 'NONE',  ( -16.53943276465976808, -0.05219959533934237506, 113.7510903946856757 ) ) ;
#185691=CARTESIAN_POINT ( 'NONE',  ( -10.81492255796105439, 18.62759615963255655, 97.91775706135236135 ) ) ;
#185692=CARTESIAN_POINT ( 'NONE',  ( 16.55341960407618274, -4.379528057220086978, 56.04275706135235424 ) ) ;
#185693=CARTESIAN_POINT ( 'NONE',  ( -14.34966873604960291, -8.224510206698953496, 26.66557627198103475 ) ) ;
#185694=CARTESIAN_POINT ( 'NONE',  ( 18.62759615963255655, 10.81492255796105972, 66.66775706135234714 ) ) ;
#185695=CARTESIAN_POINT ( 'NONE',  ( 18.62759615963255655, 10.81492255796105972, 51.66775706135234714 ) ) ;
#185697=CARTESIAN_POINT ( 'NONE',  ( 16.46253265017160672, -9.564922557960803928, 23.33224293864769194 ) ) ;
#185698=CARTESIAN_POINT ( 'NONE',  ( -5.719274019375665041, -21.55341960407619695, 24.79275706135235779 ) ) ;
#185699=CARTESIAN_POINT ( 'NONE',  ( -12.06949235617756955, 12.14591786802309770, 100.6239096053143811 ) ) ;
#185700=CARTESIAN_POINT ( 'NONE',  ( -9.564922557960796823, -16.46253265017161027, 32.08224293864769550 ) ) ;
#185701=CARTESIAN_POINT ( 'NONE',  ( 14.29746914071049879, -8.314922557960816363, 83.33224293864769550 ) ) ;
#185702=CARTESIAN_POINT ( 'NONE',  ( 9.564922557960805705, 16.46253265017160317, 69.58224293864770971 ) ) ;
#185703=CARTESIAN_POINT ( 'NONE',  ( 12.06949235617757843, -12.14591786802309237, 23.12390960531436335 ) ) ;
#185704=CARTESIAN_POINT ( 'NONE',  ( -0.05219959533907301413, -21.53943276465977519, 57.49890960531435979 ) ) ;
#185705=CARTESIAN_POINT ( 'NONE',  ( 8.224510206698953496, -14.34966873604960469, 87.91557627198103830 ) ) ;
#185706=CARTESIAN_POINT ( 'NONE',  ( -10.72451020669898014, 18.67979575497178502, 90.41557627198103830 ) ) ;
#185707=CARTESIAN_POINT ( 'NONE',  ( -13.89961937509977652, 13.97604488694528158, 100.6239096053143669 ) ) ;
#185708=CARTESIAN_POINT ( 'NONE',  ( -16.46253265017160317, 9.564922557960807481, 45.83224293864769550 ) ) ;
#185709=CARTESIAN_POINT ( 'NONE',  ( -0.05219959533936034679, 19.03943276465977164, 102.5010903946856757 ) ) ;
#185710=CARTESIAN_POINT ( 'NONE',  ( 18.62759615963271287, -10.81492255796078972, 43.33224293864769550 ) ) ;
#185711=CARTESIAN_POINT ( 'NONE',  ( 21.52544592524334988, 5.823673210054432836, 81.45942372801900433 ) ) ;
#185712=CARTESIAN_POINT ( 'NONE',  ( 16.46253265017160672, -9.564922557960803928, 63.33224293864769550 ) ) ;
#185713=CARTESIAN_POINT ( 'NONE',  ( -19.03943276465977164, 0.05219959533909376836, 96.24890960531436690 ) ) ;
#185714=CARTESIAN_POINT ( 'NONE',  ( -16.52544592524335698, -4.483927247898792601, 78.95942372801901854 ) ) ;
#185715=CARTESIAN_POINT ( 'NONE',  ( -5.823673210054431948, 21.52544592524334988, 57.70942372801901143 ) ) ;
#185716=CARTESIAN_POINT ( 'NONE',  ( 0.05219959533937995610, -21.53943276465977519, 80.00109039468568994 ) ) ;
#185717=CARTESIAN_POINT ( 'NONE',  ( -5.823673210054116645, -21.52544592524344225, 97.29057627198105251 ) ) ;
#185719=CARTESIAN_POINT ( 'NONE',  ( -21.55341960407619339, 5.719274019375674811, 38.54275706135234714 ) ) ;
#185720=CARTESIAN_POINT ( 'NONE',  ( 4.483927247898790824, -16.52544592524335698, 75.20942372801901854 ) ) ;
#185721=CARTESIAN_POINT ( 'NONE',  ( -10.81492255796078084, -18.62759615963271287, 77.08224293864769550 ) ) ;
#185722=CARTESIAN_POINT ( 'NONE',  ( 5.153800228976615827, -19.02544592524334988, 35.20942372801899722 ) ) ;
#185723=CARTESIAN_POINT ( 'NONE',  ( 5.823673210054125526, 21.52544592524343514, 44.79057627198103120 ) ) ;
#185725=CARTESIAN_POINT ( 'NONE',  ( -19.03943276465977164, 0.05219959533909376836, 86.24890960531436690 ) ) ;
#185726=CARTESIAN_POINT ( 'NONE',  ( 8.314922557960818139, 14.29746914071049879, 24.58224293864768839 ) ) ;
#185728=CARTESIAN_POINT ( 'NONE',  ( -13.97604488694527625, -13.89961937509977652, 101.8739096053143811 ) ) ;
#185730=CARTESIAN_POINT ( 'NONE',  ( 16.51473224551083163, -9.474510206698727899, 100.8344237280190043 ) ) ;
#185731=CARTESIAN_POINT ( 'NONE',  ( 5.719274019375991003, -21.55341960407610458, 77.70724293864770971 ) ) ;
#185732=CARTESIAN_POINT ( 'NONE',  ( 14.29746914071049879, -8.314922557960816363, 43.33224293864769550 ) ) ;
#185733=CARTESIAN_POINT ( 'NONE',  ( 13.97604488694548053, -13.89961937509957401, 110.6260903946856615 ) ) ;
#185734=CARTESIAN_POINT ( 'NONE',  ( -19.03943276465977164, 0.05219959533909376836, 26.24890960531435624 ) ) ;
#185735=CARTESIAN_POINT ( 'NONE',  ( 9.474510206698729675, 16.51473224551082808, 107.0844237280190043 ) ) ;
#185736=CARTESIAN_POINT ( 'NONE',  ( -5.719274019375978568, 21.55341960407610458, 105.2072429386477097 ) ) ;
#185737=CARTESIAN_POINT ( 'NONE',  ( 19.05341960407617918, -5.049401038297876454, 71.04275706135234714 ) ) ;
#185738=CARTESIAN_POINT ( 'NONE',  ( -4.379528057220086978, -16.55341960407618274, 84.79275706135234714 ) ) ;
#185739=CARTESIAN_POINT ( 'NONE',  ( -19.03943276465977164, 0.05219959533909376836, 66.24890960531436690 ) ) ;
#185740=CARTESIAN_POINT ( 'NONE',  ( 14.34966873604960469, 8.224510206698951720, 79.16557627198103830 ) ) ;
#185742=CARTESIAN_POINT ( 'NONE',  ( -19.02544592524342804, 5.153800228976336051, 56.04057627198100988 ) ) ;
#185743=CARTESIAN_POINT ( 'NONE',  ( 16.55341960407611168, 4.379528057220329451, 63.95724293864770260 ) ) ;
#185744=CARTESIAN_POINT ( 'NONE',  ( 0.05219959533909260263, 19.03943276465977164, 24.99890960531435269 ) ) ;
#185746=CARTESIAN_POINT ( 'NONE',  ( 8.314922557960818139, 14.29746914071049879, 39.58224293864769550 ) ) ;
#185747=CARTESIAN_POINT ( 'NONE',  ( -5.153800228976328057, -19.02544592524343514, 72.29057627198102409 ) ) ;
#185749=CARTESIAN_POINT ( 'NONE',  ( 16.51473224551083163, -9.474510206698727899, 45.83442372801900433 ) ) ;
#185750=CARTESIAN_POINT ( 'NONE',  ( -16.53943276465976808, -0.05219959533934237506, 58.75109039468568994 ) ) ;
#185751=CARTESIAN_POINT ( 'NONE',  ( -0.05219959533907301413, -21.53943276465977519, 67.49890960531436690 ) ) ;
#185752=CARTESIAN_POINT ( 'NONE',  ( 5.153800228976615827, -19.02544592524334988, 20.20942372801899722 ) ) ;
#185753=CARTESIAN_POINT ( 'NONE',  ( 5.049401038298161559, -19.05341960407611168, 82.70724293864770971 ) ) ;
#185755=CARTESIAN_POINT ( 'NONE',  ( 21.53943276465977519, -0.05219959533907433946, 33.74890960531436690 ) ) ;
#185757=CARTESIAN_POINT ( 'NONE',  ( -13.89961937509977652, 13.97604488694528158, 60.62390960531436690 ) ) ;
#185758=CARTESIAN_POINT ( 'NONE',  ( -0.05219959533937732626, 21.53943276465977519, 57.50109039468568994 ) ) ;
#185760=CARTESIAN_POINT ( 'NONE',  ( -4.379528057220328563, 16.55341960407611168, 105.2072429386477097 ) ) ;
#185761=CARTESIAN_POINT ( 'NONE',  ( -0.05219959533907301413, -21.53943276465977519, 107.4989096053143669 ) ) ;
#185762=CARTESIAN_POINT ( 'NONE',  ( -19.03943276465977164, 0.05219959533909376836, 96.24890960531436690 ) ) ;
#185764=CARTESIAN_POINT ( 'NONE',  ( 10.72451020669871369, 18.67979575497193778, 37.08442372801901143 ) ) ;
#185766=CARTESIAN_POINT ( 'NONE',  ( -13.97604488694527625, -13.89961937509977652, 91.87390960531432427 ) ) ;
#185768=CARTESIAN_POINT ( 'NONE',  ( -18.22780087662122028, 5.500000000000031086, 63.51540105326107266 ) ) ;
#185769=CARTESIAN_POINT ( 'NONE',  ( 18.62759615963271287, -10.81492255796078972, 93.33224293864769550 ) ) ;
#185770=CARTESIAN_POINT ( 'NONE',  ( 5.049401038298161559, -19.05341960407611168, 52.70724293864767418 ) ) ;
#185771=CARTESIAN_POINT ( 'NONE',  ( 4.483927247898790824, -16.52544592524335698, 30.20942372801902565 ) ) ;
#185773=CARTESIAN_POINT ( 'NONE',  ( 16.51473224551069308, 9.474510206698969483, 34.16557627198102409 ) ) ;
#185774=CARTESIAN_POINT ( 'NONE',  ( 5.719274019375673035, 21.55341960407619339, 82.29275706135234714 ) ) ;
#185775=CARTESIAN_POINT ( 'NONE',  ( 13.97604488694527802, 13.89961937509977652, 69.37390960531436690 ) ) ;
#185776=CARTESIAN_POINT ( 'NONE',  ( -5.823673210054431948, 21.52544592524334988, 42.70942372801901854 ) ) ;
#185777=CARTESIAN_POINT ( 'NONE',  ( -18.67979575497193778, 10.72451020669871902, 23.33442372801901499 ) ) ;
#185779=CARTESIAN_POINT ( 'NONE',  ( -19.02544592524342804, 5.153800228976336051, 106.0405762719810241 ) ) ;
#185781=CARTESIAN_POINT ( 'NONE',  ( 4.379528057220092307, 16.55341960407617563, 37.29275706135235424 ) ) ;
#185782=CARTESIAN_POINT ( 'NONE',  ( 14.29746914071037800, 8.314922557961029526, 71.66775706135234714 ) ) ;
#185783=CARTESIAN_POINT ( 'NONE',  ( -5.823673210054431948, 21.52544592524334988, 42.70942372801901854 ) ) ;
#185784=CARTESIAN_POINT ( 'NONE',  ( 10.72451020669871369, 18.67979575497193778, 72.08442372801899012 ) ) ;
#185786=CARTESIAN_POINT ( 'NONE',  ( -12.06949235617739369, -12.14591786802326823, 19.37609039468568639 ) ) ;
#185787=CARTESIAN_POINT ( 'NONE',  ( 16.51473224551069308, 9.474510206698969483, 59.16557627198102409 ) ) ;
#185788=CARTESIAN_POINT ( 'NONE',  ( 5.153800228976335163, 19.02544592524342804, 94.79057627198103830 ) ) ;
#185789=CARTESIAN_POINT ( 'NONE',  ( -16.52544592524342804, 4.483927247898546575, 111.0405762719810525 ) ) ;
#185790=CARTESIAN_POINT ( 'NONE',  ( 16.53943276465976808, -0.05219959533910856209, 98.74890960531438111 ) ) ;
#185791=CARTESIAN_POINT ( 'NONE',  ( 15.80617190586746368, 15.72974639402197994, 34.37390960531435979 ) ) ;
#185792=CARTESIAN_POINT ( 'NONE',  ( 12.06949235617739724, 12.14591786802326823, 81.87609039468568994 ) ) ;
#185793=CARTESIAN_POINT ( 'NONE',  ( -4.483927247898539470, -16.52544592524342804, 67.29057627198103830 ) ) ;
#185794=CARTESIAN_POINT ( 'NONE',  ( 13.97604488694527802, 13.89961937509977652, 49.37390960531434558 ) ) ;
#185795=CARTESIAN_POINT ( 'NONE',  ( 5.719274019375673035, 21.55341960407619339, 72.29275706135236135 ) ) ;
#185796=CARTESIAN_POINT ( 'NONE',  ( -18.67979575497193778, 10.72451020669871902, 68.33442372801900433 ) ) ;
#185797=CARTESIAN_POINT ( 'NONE',  ( 19.02544592524334988, 5.153800228976608722, 106.4594237280190185 ) ) ;
#185798=CARTESIAN_POINT ( 'NONE',  ( 16.53943276465976808, -0.05219959533910856209, 73.74890960531433848 ) ) ;
#185799=CARTESIAN_POINT ( 'NONE',  ( 21.53943276465977519, 0.05219959533937863772, 31.25109039468568639 ) ) ;
#185800=CARTESIAN_POINT ( 'NONE',  ( 21.53943276465977519, -0.05219959533907433946, 63.74890960531435979 ) ) ;
#185802=CARTESIAN_POINT ( 'NONE',  ( -17.50000000000001421, -5.622605283950884214, 106.3120731059611899 ) ) ;
#185804=CARTESIAN_POINT ( 'NONE',  ( 9.474510206698971260, -16.51473224551069308, 67.91557627198102409 ) ) ;
#185805=CARTESIAN_POINT ( 'NONE',  ( -12.14591786802309592, -12.06949235617757132, 46.87390960531435979 ) ) ;
#185807=CARTESIAN_POINT ( 'NONE',  ( 12.06949235617757843, -12.14591786802309237, 23.12390960531436335 ) ) ;
#185808=CARTESIAN_POINT ( 'NONE',  ( 0.05219959533934541429, -16.53943276465976808, 100.0010903946857042 ) ) ;
#185809=CARTESIAN_POINT ( 'NONE',  ( 13.89961937509957401, 13.97604488694547697, 56.87609039468564731 ) ) ;
#185810=CARTESIAN_POINT ( 'NONE',  ( 16.31925111598458145, 7.325300261831479531, 47.33575461032752685 ) ) ;
#185811=CARTESIAN_POINT ( 'NONE',  ( 5.049401038298161559, -19.05341960407611168, 107.7072429386476955 ) ) ;
#185812=CARTESIAN_POINT ( 'NONE',  ( -14.29746914071049879, 8.314922557960819915, 70.83224293864770971 ) ) ;
#185813=CARTESIAN_POINT ( 'NONE',  ( 5.153800228976615827, -19.02544592524334988, 45.20942372801901143 ) ) ;
#185814=CARTESIAN_POINT ( 'NONE',  ( 0.05219959533909260263, 19.03943276465977164, 29.99890960531435979 ) ) ;
#185815=CARTESIAN_POINT ( 'NONE',  ( -18.67979575497178146, -10.72451020669898902, 36.66557627198103120 ) ) ;
#185816=CARTESIAN_POINT ( 'NONE',  ( -21.53943276465977519, 0.05219959533907696930, 51.24890960531436690 ) ) ;
#185818=CARTESIAN_POINT ( 'NONE',  ( 12.06949235617757843, -12.14591786802309237, 98.12390960531436690 ) ) ;
#185819=CARTESIAN_POINT ( 'NONE',  ( 14.34966873604972726, -8.224510206698740333, 55.83442372801901854 ) ) ;
#185820=CARTESIAN_POINT ( 'NONE',  ( 14.29746914071049879, -8.314922557960816363, 88.33224293864769550 ) ) ;
#185821=CARTESIAN_POINT ( 'NONE',  ( 16.88567814943165502, -6.947325034625567497, 36.20998877347415856 ) ) ;
#185823=CARTESIAN_POINT ( 'NONE',  ( -21.55341960407610458, -5.719274019375992779, 21.45724293864769550 ) ) ;
#185827=CARTESIAN_POINT ( 'NONE',  ( -8.314922557961024197, 14.29746914071037800, 47.91775706135234714 ) ) ;
#185828=CARTESIAN_POINT ( 'NONE',  ( 8.314922557960818139, 14.29746914071049879, 34.58224293864770260 ) ) ;
#185829=CARTESIAN_POINT ( 'NONE',  ( -15.80617190586745835, -15.72974639402198527, 51.87390960531437401 ) ) ;
#185830=CARTESIAN_POINT ( 'NONE',  ( 9.564922557961047289, -16.46253265017146816, 85.41775706135233293 ) ) ;
#185831=CARTESIAN_POINT ( 'NONE',  ( -10.81492255796078084, -18.62759615963271287, 52.08224293864768839 ) ) ;
#185832=CARTESIAN_POINT ( 'NONE',  ( 10.72451020669871369, 18.67979575497193778, 82.08442372801901854 ) ) ;
#185834=CARTESIAN_POINT ( 'NONE',  ( 12.06949235617739724, 12.14591786802326823, 41.87609039468568284 ) ) ;
#185835=CARTESIAN_POINT ( 'NONE',  ( -19.05341960407611168, -5.049401038298163336, 31.45724293864769550 ) ) ;
#185836=CARTESIAN_POINT ( 'NONE',  ( 13.89961937509977652, -13.97604488694527269, 98.12390960531433848 ) ) ;
#185837=CARTESIAN_POINT ( 'NONE',  ( -19.02544592524342804, 5.153800228976336051, 36.04057627198100988 ) ) ;
#185838=CARTESIAN_POINT ( 'NONE',  ( -12.06949235617756955, 12.14591786802309770, 100.6239096053143811 ) ) ;
#185840=CARTESIAN_POINT ( 'NONE',  ( 5.153800228976335163, 19.02544592524342804, 99.79057627198102409 ) ) ;
#185842=CARTESIAN_POINT ( 'NONE',  ( -8.314922557961024197, 14.29746914071037800, 57.91775706135234714 ) ) ;
#185843=CARTESIAN_POINT ( 'NONE',  ( 10.81492255796078972, 18.62759615963270932, 84.58224293864769550 ) ) ;
#185844=CARTESIAN_POINT ( 'NONE',  ( 16.46253265017160672, -9.564922557960803928, 58.33224293864769550 ) ) ;
#185845=CARTESIAN_POINT ( 'NONE',  ( 21.55341960407619695, -5.719274019375665929, 26.04275706135235779 ) ) ;
#185846=CARTESIAN_POINT ( 'NONE',  ( 5.153800228976335163, 19.02544592524342804, 84.79057627198099567 ) ) ;
#185849=CARTESIAN_POINT ( 'NONE',  ( 15.80617190586769283, -15.72974639402175789, 20.62609039468568639 ) ) ;
#185850=CARTESIAN_POINT ( 'NONE',  ( 13.97604488694527802, 13.89961937509977652, 29.37390960531435979 ) ) ;
#185851=CARTESIAN_POINT ( 'NONE',  ( -9.474510206698964154, 16.51473224551069663, 110.4155762719810383 ) ) ;
#185852=CARTESIAN_POINT ( 'NONE',  ( 9.474510206698729675, 16.51473224551082808, 72.08442372801900433 ) ) ;
#185854=CARTESIAN_POINT ( 'NONE',  ( -19.02544592524334988, -5.153800228976617603, 23.95942372801900078 ) ) ;
#185855=CARTESIAN_POINT ( 'NONE',  ( -21.52544592524343514, 5.823673210054127303, 106.0405762719810525 ) ) ;
#185856=CARTESIAN_POINT ( 'NONE',  ( -5.049401038297874678, -19.05341960407617918, 39.79275706135232582 ) ) ;
#185857=CARTESIAN_POINT ( 'NONE',  ( -12.14591786802326823, 12.06949235617739902, 73.12609039468567573 ) ) ;
#185858=CARTESIAN_POINT ( 'NONE',  ( -13.97604488694527625, -13.89961937509977652, 101.8739096053143811 ) ) ;
#185859=CARTESIAN_POINT ( 'NONE',  ( 5.049401038298161559, -19.05341960407611168, 52.70724293864767418 ) ) ;
#185861=CARTESIAN_POINT ( 'NONE',  ( 10.81492255796106328, -18.62759615963255655, 70.41775706135236135 ) ) ;
#185862=CARTESIAN_POINT ( 'NONE',  ( -10.81492255796105439, 18.62759615963255655, 77.91775706135231871 ) ) ;
#185863=CARTESIAN_POINT ( 'NONE',  ( -9.474510206698964154, 16.51473224551069663, 75.41557627198103830 ) ) ;
#185864=CARTESIAN_POINT ( 'NONE',  ( -18.62759615963255300, -10.81492255796106328, 44.16775706135234714 ) ) ;
#185865=CARTESIAN_POINT ( 'NONE',  ( -9.474510206698720793, -16.51473224551083518, 84.58442372801900433 ) ) ;
#185867=CARTESIAN_POINT ( 'NONE',  ( -0.05219959533909027116, -19.03943276465977164, 52.49890960531436690 ) ) ;
#185868=CARTESIAN_POINT ( 'NONE',  ( -13.89961937509977652, 13.97604488694528158, 100.6239096053143669 ) ) ;
#185869=CARTESIAN_POINT ( 'NONE',  ( -5.049401038298153566, 19.05341960407611168, 70.20724293864769550 ) ) ;
#185870=CARTESIAN_POINT ( 'NONE',  ( 19.03943276465977164, -0.05219959533909143690, 108.7489096053143527 ) ) ;
#185871=CARTESIAN_POINT ( 'NONE',  ( 0.05219959533909260263, 19.03943276465977164, 54.99890960531435979 ) ) ;
#185872=CARTESIAN_POINT ( 'NONE',  ( 15.80617190586746368, 15.72974639402197994, 104.3739096053143669 ) ) ;
#185873=CARTESIAN_POINT ( 'NONE',  ( -12.06949235617739369, -12.14591786802326823, 79.37609039468567573 ) ) ;
#185875=CARTESIAN_POINT ( 'NONE',  ( -9.474510206698720793, -16.51473224551083518, 39.58442372801899722 ) ) ;
#185876=CARTESIAN_POINT ( 'NONE',  ( 5.153800228976335163, 19.02544592524342804, 64.79057627198100988 ) ) ;
#185877=CARTESIAN_POINT ( 'NONE',  ( -0.05219959533910754901, -16.53943276465976808, 52.49890960531435979 ) ) ;
#185878=CARTESIAN_POINT ( 'NONE',  ( -0.05219959533910754901, -16.53943276465976808, 92.49890960531436690 ) ) ;
#185880=CARTESIAN_POINT ( 'NONE',  ( -5.049401038298153566, 19.05341960407611168, 95.20724293864770971 ) ) ;
#185881=CARTESIAN_POINT ( 'NONE',  ( -13.89961937509977652, 13.97604488694528158, 85.62390960531433848 ) ) ;
#185882=CARTESIAN_POINT ( 'NONE',  ( 0.05219959533909260263, 19.03943276465977164, 104.9989096053143669 ) ) ;
#185883=CARTESIAN_POINT ( 'NONE',  ( 18.62759615963255655, 10.81492255796105972, 106.6677570613523756 ) ) ;
#185884=CARTESIAN_POINT ( 'NONE',  ( 12.06949235617739724, 12.14591786802326823, 86.87609039468568994 ) ) ;
#185885=CARTESIAN_POINT ( 'NONE',  ( 19.03943276465977164, -0.05219959533909143690, 73.74890960531435269 ) ) ;
#185886=CARTESIAN_POINT ( 'NONE',  ( -5.823673210054431948, 21.52544592524334988, 37.70942372801900433 ) ) ;
#185887=CARTESIAN_POINT ( 'NONE',  ( 5.823673210054125526, 21.52544592524343514, 29.79057627198102409 ) ) ;
#185888=CARTESIAN_POINT ( 'NONE',  ( -15.80617190586745835, -15.72974639402198527, 106.8739096053143811 ) ) ;
#185889=CARTESIAN_POINT ( 'NONE',  ( -16.55341960407611168, -4.379528057220339221, 56.45724293864768839 ) ) ;
#185890=CARTESIAN_POINT ( 'NONE',  ( 16.46253265017160672, -9.564922557960803928, 48.33224293864769550 ) ) ;
#185891=CARTESIAN_POINT ( 'NONE',  ( -14.34966873604960291, -8.224510206698953496, 81.66557627198103830 ) ) ;
#185892=CARTESIAN_POINT ( 'NONE',  ( 9.564922557961047289, -16.46253265017146816, 50.41775706135233293 ) ) ;
#185893=CARTESIAN_POINT ( 'NONE',  ( -4.483927247898539470, -16.52544592524342804, 107.2905762719810525 ) ) ;
#185894=CARTESIAN_POINT ( 'NONE',  ( -8.224510206698735004, -14.34966873604973081, 64.58442372801900433 ) ) ;
#185895=CARTESIAN_POINT ( 'NONE',  ( -9.474510206698964154, 16.51473224551069663, 80.41557627198103830 ) ) ;
#185897=CARTESIAN_POINT ( 'NONE',  ( -8.224510206698948167, 14.34966873604960824, 105.4155762719810383 ) ) ;
#185898=CARTESIAN_POINT ( 'NONE',  ( -0.05219959533907301413, -21.53943276465977519, 37.49890960531436690 ) ) ;
#185899=ORIENTED_EDGE ( 'NONE', *, *, #128937, .T. ) ;
#185900=CARTESIAN_POINT ( 'NONE',  ( 14.34966873604972726, -8.224510206698740333, 100.8344237280190185 ) ) ;
#185901=CARTESIAN_POINT ( 'NONE',  ( 12.14591786802327356, -12.06949235617739191, 25.62609039468567929 ) ) ;
#185902=CARTESIAN_POINT ( 'NONE',  ( -0.05219959533937732626, 21.53943276465977519, 87.50109039468568994 ) ) ;
#185903=CARTESIAN_POINT ( 'NONE',  ( -5.049401038298153566, 19.05341960407611168, 85.20724293864766707 ) ) ;
#185904=CARTESIAN_POINT ( 'NONE',  ( -15.72974639402197994, 15.80617190586746368, 115.6239096053143669 ) ) ;
#185905=CARTESIAN_POINT ( 'NONE',  ( -5.049401038298153566, 19.05341960407611168, 25.20724293864768484 ) ) ;
#185906=CARTESIAN_POINT ( 'NONE',  ( 14.34966873604972726, -8.224510206698740333, 35.83442372801901143 ) ) ;
#185907=CARTESIAN_POINT ( 'NONE',  ( 13.97604488694548053, -13.89961937509957401, 90.62609039468567573 ) ) ;
#185908=CARTESIAN_POINT ( 'NONE',  ( 0.05219959533907565091, 21.53943276465977519, 84.99890960531436690 ) ) ;
#185909=CARTESIAN_POINT ( 'NONE',  ( 19.03943276465977164, 0.05219959533936151252, 66.25109039468567573 ) ) ;
#185911=CARTESIAN_POINT ( 'NONE',  ( -18.62759615963255300, -10.81492255796106328, 24.16775706135235424 ) ) ;
#185912=CARTESIAN_POINT ( 'NONE',  ( 5.049401038298163336, -19.05341960407611168, 72.70724293864769550 ) ) ;
#185913=CARTESIAN_POINT ( 'NONE',  ( -13.89961937509977652, 13.97604488694528158, 90.62390960531432427 ) ) ;
#185914=CARTESIAN_POINT ( 'NONE',  ( 16.53943276465976808, 0.05219959533934440121, 31.25109039468568639 ) ) ;
#185916=CARTESIAN_POINT ( 'NONE',  ( -5.153800228976607833, 19.02544592524334988, 57.70942372801899012 ) ) ;
#185917=CARTESIAN_POINT ( 'NONE',  ( 10.81492255796078972, 18.62759615963270932, 114.5822429386477097 ) ) ;
#185918=CARTESIAN_POINT ( 'NONE',  ( -16.55341960407611168, -4.379528057220339221, 76.45724293864769550 ) ) ;
#185919=CARTESIAN_POINT ( 'NONE',  ( -13.89961937509977652, 13.97604488694528158, 85.62390960531433848 ) ) ;
#185920=CARTESIAN_POINT ( 'NONE',  ( 14.29746914071037800, 8.314922557961029526, 36.66775706135234714 ) ) ;
#185921=CARTESIAN_POINT ( 'NONE',  ( -5.153800228976607833, 19.02544592524334988, 52.70942372801900433 ) ) ;
#185922=CARTESIAN_POINT ( 'NONE',  ( 5.823673210054444382, -21.52544592524334988, 70.20942372801904696 ) ) ;
#185923=CARTESIAN_POINT ( 'NONE',  ( -4.379528057220086978, -16.55341960407618274, 24.79275706135235779 ) ) ;
#185924=CARTESIAN_POINT ( 'NONE',  ( 19.02544592524343514, -5.153800228976328945, 68.54057627198103830 ) ) ;
#185925=CARTESIAN_POINT ( 'NONE',  ( 16.51473224551083163, -9.474510206698727899, 80.83442372801899012 ) ) ;
#185926=CARTESIAN_POINT ( 'NONE',  ( 4.379528057220092307, 16.55341960407617563, 62.29275706135236845 ) ) ;
#185927=CARTESIAN_POINT ( 'NONE',  ( 21.52544592524334988, 5.823673210054432836, 101.4594237280190185 ) ) ;
#185928=CARTESIAN_POINT ( 'NONE',  ( 19.05341960407617918, -5.049401038297876454, 71.04275706135234714 ) ) ;
#185929=CARTESIAN_POINT ( 'NONE',  ( -19.05341960407611168, -5.049401038298163336, 51.45724293864770260 ) ) ;
#185930=CARTESIAN_POINT ( 'NONE',  ( 18.67979575497178502, 10.72451020669898547, 69.16557627198102409 ) ) ;
#185931=CARTESIAN_POINT ( 'NONE',  ( 4.379528057220339221, -16.55341960407611168, 67.70724293864769550 ) ) ;
#185932=CARTESIAN_POINT ( 'NONE',  ( 5.049401038297881783, 19.05341960407617563, 77.29275706135231871 ) ) ;
#185933=LINE ( 'NONE', #106089, #86019 ) ;
#185934=CARTESIAN_POINT ( 'NONE',  ( 16.46253265017146816, 9.564922557961045513, 46.66775706135233293 ) ) ;
#185935=CARTESIAN_POINT ( 'NONE',  ( -16.52544592524335698, -4.483927247898792601, 103.9594237280190185 ) ) ;
#185936=CARTESIAN_POINT ( 'NONE',  ( -4.379528057220328563, 16.55341960407611168, 70.20724293864769550 ) ) ;
#185937=CARTESIAN_POINT ( 'NONE',  ( -21.52544592524334988, -5.823673210054445271, 98.95942372801903275 ) ) ;
#185939=CARTESIAN_POINT ( 'NONE',  ( 10.81492255796078972, 18.62759615963270932, 94.58224293864769550 ) ) ;
#185940=CARTESIAN_POINT ( 'NONE',  ( -5.049401038298153566, 19.05341960407611168, 70.20724293864769550 ) ) ;
#185941=CARTESIAN_POINT ( 'NONE',  ( -18.67979575497193778, 10.72451020669871902, 73.33442372801901854 ) ) ;
#185942=CARTESIAN_POINT ( 'NONE',  ( -13.97604488694527625, -13.89961937509977652, 51.87390960531436690 ) ) ;
#185944=CARTESIAN_POINT ( 'NONE',  ( 13.89961937509977652, -13.97604488694527269, 23.12390960531436335 ) ) ;
#185945=CARTESIAN_POINT ( 'NONE',  ( 9.564922557960805705, 16.46253265017160317, 109.5822429386476955 ) ) ;
#185947=CARTESIAN_POINT ( 'NONE',  ( 16.53943276465976808, -0.05219959533910856209, 63.74890960531435979 ) ) ;
#185948=CARTESIAN_POINT ( 'NONE',  ( 19.03943276465977164, -0.05219959533909143690, 28.74890960531435624 ) ) ;
#185949=CARTESIAN_POINT ( 'NONE',  ( 12.14591786802309770, 12.06949235617756955, 79.37390960531436690 ) ) ;
#185950=CARTESIAN_POINT ( 'NONE',  ( -21.52544592524343514, 5.823673210054127303, 96.04057627198102409 ) ) ;
#185951=CARTESIAN_POINT ( 'NONE',  ( 0.05219959533937995610, -21.53943276465977519, 35.00109039468568284 ) ) ;
#185953=CARTESIAN_POINT ( 'NONE',  ( -4.483927247898782831, 16.52544592524335698, 52.70942372801902565 ) ) ;
#185954=CARTESIAN_POINT ( 'NONE',  ( 10.81492255796078972, 18.62759615963270932, 89.58224293864768129 ) ) ;
#185955=CARTESIAN_POINT ( 'NONE',  ( 9.474510206698729675, 16.51473224551082808, 22.08442372801899722 ) ) ;
#185956=CARTESIAN_POINT ( 'NONE',  ( 19.05341960407611168, 5.049401038298154454, 103.9572429386476671 ) ) ;
#185957=CARTESIAN_POINT ( 'NONE',  ( -5.719274019375665041, -21.55341960407619695, 39.79275706135235424 ) ) ;
#185958=CARTESIAN_POINT ( 'NONE',  ( 10.72451020669898902, -18.67979575497178502, 42.91557627198103120 ) ) ;
#185959=CARTESIAN_POINT ( 'NONE',  ( -0.05219959533910754901, -16.53943276465976808, 22.49890960531436335 ) ) ;
#185960=CARTESIAN_POINT ( 'NONE',  ( 21.53943276465977519, 0.05219959533937863772, 66.25109039468567573 ) ) ;
#185961=CARTESIAN_POINT ( 'NONE',  ( 0.05219959533937995610, -21.53943276465977519, 95.00109039468568994 ) ) ;
#185962=CARTESIAN_POINT ( 'NONE',  ( -5.049401038297874678, -19.05341960407617918, 24.79275706135233648 ) ) ;
#185963=CARTESIAN_POINT ( 'NONE',  ( 14.34966873604972726, -8.224510206698740333, 85.83442372801901854 ) ) ;
#185964=CARTESIAN_POINT ( 'NONE',  ( 21.55341960407619695, -5.719274019375665929, 56.04275706135235424 ) ) ;
#185965=EDGE_CURVE ( 'NONE', #95725, #24895, #40973, .T. ) ;
#185966=CARTESIAN_POINT ( 'NONE',  ( 13.89961937509977652, -13.97604488694527269, 48.12390960531435979 ) ) ;
#185967=CARTESIAN_POINT ( 'NONE',  ( 18.62759615963255655, 10.81492255796105972, 111.6677570613523613 ) ) ;
#185968=CARTESIAN_POINT ( 'NONE',  ( -18.67979575497178146, -10.72451020669898902, 26.66557627198103475 ) ) ;
#185969=CARTESIAN_POINT ( 'NONE',  ( -18.62759615963270932, 10.81492255796079327, 115.8322429386477097 ) ) ;
#185970=CARTESIAN_POINT ( 'NONE',  ( -5.823673210054116645, -21.52544592524344225, 77.29057627198102409 ) ) ;
#185971=CARTESIAN_POINT ( 'NONE',  ( -8.224510206698735004, -14.34966873604973081, 44.58442372801901854 ) ) ;
#185973=CARTESIAN_POINT ( 'NONE',  ( 21.53943276465977519, -0.05219959533907433946, 73.74890960531433848 ) ) ;
#185974=CARTESIAN_POINT ( 'NONE',  ( 4.483927247898790824, -16.52544592524335698, 65.20942372801901854 ) ) ;
#185975=CARTESIAN_POINT ( 'NONE',  ( -16.53943276465976808, 0.05219959533911058130, 61.24890960531435979 ) ) ;
#185977=CARTESIAN_POINT ( 'NONE',  ( 9.474510206698729675, 16.51473224551082808, 97.08442372801900433 ) ) ;
#185980=CARTESIAN_POINT ( 'NONE',  ( 4.483927247898790824, -16.52544592524335698, 35.20942372801901854 ) ) ;
#185981=CARTESIAN_POINT ( 'NONE',  ( 5.719274019375991003, -21.55341960407610458, 112.7072429386476955 ) ) ;
#185982=CARTESIAN_POINT ( 'NONE',  ( 5.719274019375991003, -21.55341960407610458, 77.70724293864770971 ) ) ;
#185983=CARTESIAN_POINT ( 'NONE',  ( -21.53943276465977519, 0.05219959533907696930, 36.24890960531435979 ) ) ;
#185984=CARTESIAN_POINT ( 'NONE',  ( -0.05219959533934338120, 16.53943276465976808, 62.50109039468568284 ) ) ;
#185985=CARTESIAN_POINT ( 'NONE',  ( 16.46253265017160672, -9.564922557960803928, 68.33224293864770971 ) ) ;
#185986=CARTESIAN_POINT ( 'NONE',  ( -10.72451020669870658, -18.67979575497194134, 39.58442372801901143 ) ) ;
#185987=CARTESIAN_POINT ( 'NONE',  ( 19.02544592524334988, 5.153800228976608722, 106.4594237280190185 ) ) ;
#185988=CARTESIAN_POINT ( 'NONE',  ( -10.72451020669898014, 18.67979575497178502, 30.41557627198101699 ) ) ;
#185989=CARTESIAN_POINT ( 'NONE',  ( -19.05341960407617563, 5.049401038297882671, 23.54275706135233648 ) ) ;
#185990=CARTESIAN_POINT ( 'NONE',  ( -14.34966873604972548, 8.224510206698743886, 38.33442372801900433 ) ) ;
#185991=CARTESIAN_POINT ( 'NONE',  ( -5.153800228976328057, -19.02544592524343514, 102.2905762719810383 ) ) ;
#185992=CARTESIAN_POINT ( 'NONE',  ( -5.719274019375978568, 21.55341960407610458, 105.2072429386477097 ) ) ;
#185993=CARTESIAN_POINT ( 'NONE',  ( -16.46253265017160317, 9.564922557960807481, 75.83224293864769550 ) ) ;
#185994=CARTESIAN_POINT ( 'NONE',  ( -16.36317988757058828, 7.306389748694928521, 24.09789608363227487 ) ) ;
#185995=CARTESIAN_POINT ( 'NONE',  ( -8.314922557960811034, -14.29746914071050412, 87.08224293864769550 ) ) ;
#185996=CARTESIAN_POINT ( 'NONE',  ( -16.46253265017160317, 9.564922557960807481, 110.8322429386476955 ) ) ;
#185998=CARTESIAN_POINT ( 'NONE',  ( 12.06949235617739724, 12.14591786802326823, 66.87609039468568994 ) ) ;
#185999=CARTESIAN_POINT ( 'NONE',  ( -10.72451020669898014, 18.67979575497178502, 105.4155762719810383 ) ) ;
#186000=CARTESIAN_POINT ( 'NONE',  ( -5.049401038297874678, -19.05341960407617918, 64.79275706135233293 ) ) ;
#186002=CARTESIAN_POINT ( 'NONE',  ( 21.55341960407610458, 5.719274019375980345, 33.95724293864769550 ) ) ;
#186003=CARTESIAN_POINT ( 'NONE',  ( -13.97604488694527625, -13.89961937509977652, 26.87390960531434558 ) ) ;
#186004=CARTESIAN_POINT ( 'NONE',  ( -15.72974639402197994, 15.80617190586746368, 70.62390960531436690 ) ) ;
#186005=CARTESIAN_POINT ( 'NONE',  ( 19.03943276465977164, -0.05219959533909143690, 93.74890960531435269 ) ) ;
#186006=CARTESIAN_POINT ( 'NONE',  ( -15.80617190586768217, 15.72974639402176855, 93.12609039468568994 ) ) ;
#186007=CARTESIAN_POINT ( 'NONE',  ( 5.049401038298161559, -19.05341960407611168, 47.70724293864770260 ) ) ;
#186008=CARTESIAN_POINT ( 'NONE',  ( 0.05219959533910956823, 16.53943276465976808, 89.99890960531438111 ) ) ;
#186009=CARTESIAN_POINT ( 'NONE',  ( 14.34966873604972726, -8.224510206698740333, 35.83442372801901143 ) ) ;
#186010=CARTESIAN_POINT ( 'NONE',  ( 9.474510206698971260, -16.51473224551069308, 57.91557627198103120 ) ) ;
#186011=CARTESIAN_POINT ( 'NONE',  ( -15.72974639402176322, -15.80617190586768395, 79.37609039468567573 ) ) ;
#186012=EDGE_LOOP ( 'NONE', ( #179537, #63864 ) ) ;
#186013=CARTESIAN_POINT ( 'NONE',  ( -19.02544592524334988, -5.153800228976617603, 28.95942372801900433 ) ) ;
#186015=CARTESIAN_POINT ( 'NONE',  ( 19.03943276465977164, 0.05219959533936151252, 36.25109039468567573 ) ) ;
#186016=CARTESIAN_POINT ( 'NONE',  ( 21.53943276465977519, 0.05219959533937863772, 31.25109039468568639 ) ) ;
#186017=CARTESIAN_POINT ( 'NONE',  ( 9.564922557960805705, 16.46253265017160317, 54.58224293864769550 ) ) ;
#186018=CARTESIAN_POINT ( 'NONE',  ( 16.46253265017146816, 9.564922557961045513, 31.66775706135232937 ) ) ;
#186019=CARTESIAN_POINT ( 'NONE',  ( -19.05341960407611168, -5.049401038298163336, 81.45724293864769550 ) ) ;
#186020=CARTESIAN_POINT ( 'NONE',  ( -16.46253265017160317, 9.564922557960807481, 75.83224293864769550 ) ) ;
#186021=CARTESIAN_POINT ( 'NONE',  ( 14.29746914071049879, -8.314922557960816363, 28.33224293864769550 ) ) ;
#186022=CARTESIAN_POINT ( 'NONE',  ( 19.02544592524343514, -5.153800228976328945, 113.5405762719810241 ) ) ;
#186023=CARTESIAN_POINT ( 'NONE',  ( -10.81492255796105439, 18.62759615963255655, 87.91775706135234714 ) ) ;
#186025=CARTESIAN_POINT ( 'NONE',  ( 16.61371651742604172, 7.165104196376048229, 58.64584930007005426 ) ) ;
#186026=CARTESIAN_POINT ( 'NONE',  ( -21.53943276465977519, -0.05219959533937600094, 93.75109039468567573 ) ) ;
#186028=CARTESIAN_POINT ( 'NONE',  ( 9.564922557960805705, 16.46253265017160317, 109.5822429386476955 ) ) ;
#186030=CARTESIAN_POINT ( 'NONE',  ( 14.34966873604972726, -8.224510206698740333, 45.83442372801901854 ) ) ;
#186031=CARTESIAN_POINT ( 'NONE',  ( 21.53943276465977519, -0.05219959533907433946, 68.74890960531435269 ) ) ;
#186032=CARTESIAN_POINT ( 'NONE',  ( 16.55341960407611168, 4.379528057220329451, 23.95724293864769550 ) ) ;
#186033=CARTESIAN_POINT ( 'NONE',  ( -16.52544592524342804, 4.483927247898546575, 116.0405762719810383 ) ) ;
#186034=CARTESIAN_POINT ( 'NONE',  ( 0.05219959533909260263, 19.03943276465977164, 99.99890960531436690 ) ) ;
#186035=CARTESIAN_POINT ( 'NONE',  ( -21.53943276465977519, -0.05219959533937600094, 113.7510903946856757 ) ) ;
#186036=CARTESIAN_POINT ( 'NONE',  ( -8.314922557960811034, -14.29746914071050412, 112.0822429386477097 ) ) ;
#186037=CARTESIAN_POINT ( 'NONE',  ( 21.55341960407619695, -5.719274019375665929, 71.04275706135234714 ) ) ;
#186038=CARTESIAN_POINT ( 'NONE',  ( -16.55341960407617563, 4.379528057220093196, 108.5427570613523756 ) ) ;
#186039=CARTESIAN_POINT ( 'NONE',  ( 19.03943276465977164, 0.05219959533936151252, 61.25109039468566863 ) ) ;
#186041=CARTESIAN_POINT ( 'NONE',  ( 19.02544592524343514, -5.153800228976328945, 108.5405762719810383 ) ) ;
#186042=CARTESIAN_POINT ( 'NONE',  ( -4.483927247898539470, -16.52544592524342804, 92.29057627198103830 ) ) ;
#186044=CARTESIAN_POINT ( 'NONE',  ( -16.51473224551082808, 9.474510206698731452, 58.33442372801900433 ) ) ;
#186045=CARTESIAN_POINT ( 'NONE',  ( -5.049401038298153566, 19.05341960407611168, 75.20724293864769550 ) ) ;
#186046=CARTESIAN_POINT ( 'NONE',  ( 14.29746914071049879, -8.314922557960816363, 58.33224293864768839 ) ) ;
#186047=CARTESIAN_POINT ( 'NONE',  ( -16.46253265017146816, -9.564922557961047289, 99.16775706135233293 ) ) ;
#186048=CARTESIAN_POINT ( 'NONE',  ( -0.05219959533907301413, -21.53943276465977519, 52.49890960531435979 ) ) ;
#186049=ORIENTED_EDGE ( 'NONE', *, *, #179839, .F. ) ;
#186050=CARTESIAN_POINT ( 'NONE',  ( -0.05219959533910754901, -16.53943276465976808, 112.4989096053143669 ) ) ;
#186052=CARTESIAN_POINT ( 'NONE',  ( 19.03943276465977164, -0.05219959533909143690, 73.74890960531435269 ) ) ;
#186053=CARTESIAN_POINT ( 'NONE',  ( -15.80617190586745835, -15.72974639402198527, 71.87390960531438111 ) ) ;
#186054=CARTESIAN_POINT ( 'NONE',  ( -0.05219959533934338120, 16.53943276465976808, 87.50109039468568994 ) ) ;
#186055=CARTESIAN_POINT ( 'NONE',  ( -19.02544592524342804, 5.153800228976336051, 76.04057627198102409 ) ) ;
#186056=CARTESIAN_POINT ( 'NONE',  ( -13.97604488694547697, 13.89961937509957934, 63.12609039468566152 ) ) ;
#186057=CARTESIAN_POINT ( 'NONE',  ( -21.53943276465977519, -0.05219959533937600094, 83.75109039468568994 ) ) ;
#186059=CARTESIAN_POINT ( 'NONE',  ( 0.05219959533907565091, 21.53943276465977519, 64.99890960531435269 ) ) ;
#186060=CARTESIAN_POINT ( 'NONE',  ( 18.62759615963271287, -10.81492255796078972, 28.33224293864769550 ) ) ;
#186061=CARTESIAN_POINT ( 'NONE',  ( 16.51473224551069308, 9.474510206698969483, 39.16557627198103120 ) ) ;
#186062=CARTESIAN_POINT ( 'NONE',  ( -8.314922557961024197, 14.29746914071037800, 102.9177570613523756 ) ) ;
#186063=CARTESIAN_POINT ( 'NONE',  ( -16.46253265017160317, 9.564922557960807481, 50.83224293864770260 ) ) ;
#186064=CARTESIAN_POINT ( 'NONE',  ( -16.55341960407617563, 4.379528057220093196, 28.54275706135234358 ) ) ;
#186065=CARTESIAN_POINT ( 'NONE',  ( 9.474510206698729675, 16.51473224551082808, 82.08442372801899012 ) ) ;
#186066=CARTESIAN_POINT ( 'NONE',  ( -5.823673210054431948, 21.52544592524334988, 112.7094237280190328 ) ) ;
#186067=CARTESIAN_POINT ( 'NONE',  ( 12.14591786802309770, 12.06949235617756955, 54.37390960531435979 ) ) ;
#186068=CARTESIAN_POINT ( 'NONE',  ( -21.53943276465977519, 0.05219959533907696930, 101.2489096053143669 ) ) ;
#186069=CARTESIAN_POINT ( 'NONE',  ( 18.62759615963271287, -10.81492255796078972, 98.33224293864769550 ) ) ;
#186070=CARTESIAN_POINT ( 'NONE',  ( 16.31925111598454592, -7.325300261831587001, 97.66424538967254421 ) ) ;
#186071=CARTESIAN_POINT ( 'NONE',  ( -15.72974639402197994, 15.80617190586746368, 50.62390960531435979 ) ) ;
#186072=CARTESIAN_POINT ( 'NONE',  ( 4.379528057220092307, 16.55341960407617563, 77.29275706135234714 ) ) ;
#186073=CARTESIAN_POINT ( 'NONE',  ( -16.52544592524342804, 4.483927247898546575, 96.04057627198102409 ) ) ;
#186074=CARTESIAN_POINT ( 'NONE',  ( 16.51473224551069308, 9.474510206698969483, 44.16557627198103120 ) ) ;
#186076=CARTESIAN_POINT ( 'NONE',  ( -19.36337904590692460, 5.499999999999952927, 50.41494137495620009 ) ) ;
#186077=CARTESIAN_POINT ( 'NONE',  ( -16.52544592524335698, -4.483927247898792601, 103.9594237280190185 ) ) ;
#186078=CARTESIAN_POINT ( 'NONE',  ( 15.72974639402176855, 15.80617190586768217, 26.87609039468567218 ) ) ;
#186079=CARTESIAN_POINT ( 'NONE',  ( -19.03943276465977164, 0.05219959533909376836, 91.24890960531436690 ) ) ;
#186080=CARTESIAN_POINT ( 'NONE',  ( -0.05219959533937732626, 21.53943276465977519, 62.50109039468568284 ) ) ;
#186082=CARTESIAN_POINT ( 'NONE',  ( 13.97604488694527802, 13.89961937509977652, 24.37390960531435624 ) ) ;
#186083=ORIENTED_EDGE ( 'NONE', *, *, #116452, .T. ) ;
#186084=CARTESIAN_POINT ( 'NONE',  ( -18.62759615963255300, -10.81492255796106328, 54.16775706135235424 ) ) ;
#186085=CARTESIAN_POINT ( 'NONE',  ( -5.153800228976328057, -19.02544592524343514, 52.29057627198100988 ) ) ;
#186086=CARTESIAN_POINT ( 'NONE',  ( -9.474510206698964154, 16.51473224551069663, 110.4155762719810383 ) ) ;
#186087=CARTESIAN_POINT ( 'NONE',  ( 13.89961937509977652, -13.97604488694527269, 93.12390960531436690 ) ) ;
#186088=CARTESIAN_POINT ( 'NONE',  ( -19.03943276465977164, -0.05219959533935918106, 68.75109039468566152 ) ) ;
#186089=CARTESIAN_POINT ( 'NONE',  ( 21.52544592524334988, 5.823673210054432836, 46.45942372801901854 ) ) ;
#186090=CARTESIAN_POINT ( 'NONE',  ( 16.51473224551083163, -9.474510206698727899, 100.8344237280190043 ) ) ;
#186091=CARTESIAN_POINT ( 'NONE',  ( -5.049401038297874678, -19.05341960407617918, 59.79275706135231871 ) ) ;
#186092=CARTESIAN_POINT ( 'NONE',  ( 5.049401038298161559, -19.05341960407611168, 37.70724293864768839 ) ) ;
#186093=CARTESIAN_POINT ( 'NONE',  ( 16.55341960407618274, -4.379528057220086978, 106.0427570613523471 ) ) ;
#186094=CARTESIAN_POINT ( 'NONE',  ( 16.46253265017146816, 9.564922557961045513, 76.66775706135234714 ) ) ;
#186095=CARTESIAN_POINT ( 'NONE',  ( 4.379528057220339221, -16.55341960407611168, 27.70724293864769905 ) ) ;
#186096=CARTESIAN_POINT ( 'NONE',  ( -5.049401038297874678, -19.05341960407617918, 44.79275706135232582 ) ) ;
#186097=CARTESIAN_POINT ( 'NONE',  ( -10.72451020669870658, -18.67979575497194134, 104.5844237280190185 ) ) ;
#186098=CARTESIAN_POINT ( 'NONE',  ( -19.03943276465977164, -0.05219959533935918106, 23.75109039468566152 ) ) ;
#186099=CARTESIAN_POINT ( 'NONE',  ( 19.05341960407611168, 5.049401038298154454, 23.95724293864769194 ) ) ;
#186100=CARTESIAN_POINT ( 'NONE',  ( -18.67979575497193778, 10.72451020669871902, 93.33442372801901854 ) ) ;
#186101=CARTESIAN_POINT ( 'NONE',  ( -0.05219959533934338120, 16.53943276465976808, 32.50109039468568284 ) ) ;
#186103=CARTESIAN_POINT ( 'NONE',  ( -13.97604488694527625, -13.89961937509977652, 86.87390960531436690 ) ) ;
#186105=CARTESIAN_POINT ( 'NONE',  ( 5.049401038298161559, -19.05341960407611168, 82.70724293864770971 ) ) ;
#186106=CARTESIAN_POINT ( 'NONE',  ( -17.72517630441457470, 5.499999999999976907, 95.92175719257602395 ) ) ;
#186107=CARTESIAN_POINT ( 'NONE',  ( 9.564922557961047289, -16.46253265017146816, 85.41775706135233293 ) ) ;
#186108=CARTESIAN_POINT ( 'NONE',  ( -16.46253265017160317, 9.564922557960807481, 105.8322429386476955 ) ) ;
#186109=CARTESIAN_POINT ( 'NONE',  ( -10.81492255796105439, 18.62759615963255655, 97.91775706135236135 ) ) ;
#186110=CARTESIAN_POINT ( 'NONE',  ( -12.14591786802309592, -12.06949235617757132, 96.87390960531436690 ) ) ;
#186112=CARTESIAN_POINT ( 'NONE',  ( 10.81492255796078972, 18.62759615963270932, 59.58224293864770260 ) ) ;
#186114=CARTESIAN_POINT ( 'NONE',  ( -0.05219959533907301413, -21.53943276465977519, 37.49890960531436690 ) ) ;
#186115=CARTESIAN_POINT ( 'NONE',  ( 8.224510206698953496, -14.34966873604960469, 112.9155762719810383 ) ) ;
#186117=CARTESIAN_POINT ( 'NONE',  ( 19.05341960407617918, -5.049401038297876454, 51.04275706135231871 ) ) ;
#186118=CARTESIAN_POINT ( 'NONE',  ( 0.05219959533910956823, 16.53943276465976808, 44.99890960531435979 ) ) ;
#186119=CARTESIAN_POINT ( 'NONE',  ( 15.72974639402199770, -15.80617190586745480, 23.12390960531436335 ) ) ;
#186120=CARTESIAN_POINT ( 'NONE',  ( -18.62759615963255300, -10.81492255796106328, 74.16775706135231871 ) ) ;
#186121=CARTESIAN_POINT ( 'NONE',  ( -0.05219959533907301413, -21.53943276465977519, 67.49890960531436690 ) ) ;
#186122=CARTESIAN_POINT ( 'NONE',  ( -5.823673210054431948, 21.52544592524334988, 47.70942372801902565 ) ) ;
#186123=CARTESIAN_POINT ( 'NONE',  ( -21.52544592524343514, 5.823673210054127303, 96.04057627198102409 ) ) ;
#186124=CARTESIAN_POINT ( 'NONE',  ( 21.55341960407619695, -5.719274019375665929, 51.04275706135234714 ) ) ;
#186125=CARTESIAN_POINT ( 'NONE',  ( -19.03943276465977164, 0.05219959533909376836, 26.24890960531435624 ) ) ;
#186127=CARTESIAN_POINT ( 'NONE',  ( -13.97604488694527625, -13.89961937509977652, 81.87390960531436690 ) ) ;
#186128=CARTESIAN_POINT ( 'NONE',  ( -14.34966873604972548, 8.224510206698743886, 78.33442372801901854 ) ) ;
#186129=CARTESIAN_POINT ( 'NONE',  ( 14.29746914071049879, -8.314922557960816363, 103.3322429386476955 ) ) ;
#186131=CARTESIAN_POINT ( 'NONE',  ( 4.379528057220339221, -16.55341960407611168, 52.70724293864769550 ) ) ;
#186132=CARTESIAN_POINT ( 'NONE',  ( 12.14591786802327356, -12.06949235617739191, 110.6260903946857042 ) ) ;
#186133=CARTESIAN_POINT ( 'NONE',  ( 16.51473224551069308, 9.474510206698969483, 69.16557627198102409 ) ) ;
#186134=CARTESIAN_POINT ( 'NONE',  ( -5.049401038298153566, 19.05341960407611168, 35.20724293864768839 ) ) ;
#186135=CARTESIAN_POINT ( 'NONE',  ( -5.719274019375978568, 21.55341960407610458, 50.20724293864769550 ) ) ;
#186136=CARTESIAN_POINT ( 'NONE',  ( 16.46253265017146816, 9.564922557961045513, 41.66775706135234003 ) ) ;
#186138=CARTESIAN_POINT ( 'NONE',  ( 4.483927247898545687, 16.52544592524342804, 54.79057627198104541 ) ) ;
#186139=CARTESIAN_POINT ( 'NONE',  ( 21.55341960407610458, 5.719274019375980345, 28.95724293864769905 ) ) ;
#186140=CARTESIAN_POINT ( 'NONE',  ( -18.62759615963255300, -10.81492255796106328, 59.16775706135234714 ) ) ;
#186142=CARTESIAN_POINT ( 'NONE',  ( 12.06949235617739724, 12.14591786802326823, 66.87609039468568994 ) ) ;
#186143=CARTESIAN_POINT ( 'NONE',  ( -5.153800228976607833, 19.02544592524334988, 57.70942372801899012 ) ) ;
#186144=CARTESIAN_POINT ( 'NONE',  ( -8.314922557960811034, -14.29746914071050412, 42.08224293864769550 ) ) ;
#186145=CARTESIAN_POINT ( 'NONE',  ( 17.05116617787822264, -6.768360034955866134, 51.15675553259197983 ) ) ;
#186146=CARTESIAN_POINT ( 'NONE',  ( 4.379528057220339221, -16.55341960407611168, 32.70724293864770260 ) ) ;
#186147=CARTESIAN_POINT ( 'NONE',  ( 19.05341960407611168, 5.049401038298154454, 38.95724293864767418 ) ) ;
#186148=CARTESIAN_POINT ( 'NONE',  ( 19.03943276465977164, -0.05219959533909143690, 63.74890960531435979 ) ) ;
#186149=CARTESIAN_POINT ( 'NONE',  ( -12.06949235617756955, 12.14591786802309770, 115.6239096053143669 ) ) ;
#186150=CARTESIAN_POINT ( 'NONE',  ( -21.55341960407619339, 5.719274019375674811, 33.54275706135234714 ) ) ;
#186151=CARTESIAN_POINT ( 'NONE',  ( -13.97604488694527625, -13.89961937509977652, 56.87390960531434558 ) ) ;
#186152=DIRECTION ( 'NONE',  ( -0.000000000000000000, 0.000000000000000000, 1.000000000000000000 ) ) ;
#186153=CARTESIAN_POINT ( 'NONE',  ( 5.049401038298161559, -19.05341960407611168, 47.70724293864770260 ) ) ;
#186154=CARTESIAN_POINT ( 'NONE',  ( 21.53943276465977519, -0.05219959533907433946, 38.74890960531435979 ) ) ;
#186155=B_SPLINE_CURVE_WITH_KNOTS ( 'NONE', 3,
 ( #10126, #162791, #38456, #72802, #165802, #147637, #25310, #103125, #55615, #23290, #84934, #196157, #27299, #24300, #86952, #193140, #71786, #88946, #9126, #57630, #70792, #119297, #146615, #132460, #8107, #69785, #7098, #148636, #131453, #133456, #116287, #195146 ),
 .UNSPECIFIED., .F., .F.,
 ( 4, 2, 2, 2, 2, 2, 2, 2, 2, 2, 2, 2, 2, 2, 2, 4 ),
 ( 1.644325935668032048E-15, 0.0003712461730052168583, 0.0007424923460087894155, 0.001113738519012361919, 0.001484984692015934530, 0.002227477038023092330, 0.002598723211026664724, 0.002969969384030237119, 0.003341215557033808646, 0.003712461730037381041, 0.004083707903040952568, 0.004454954076044524529, 0.004826200249048096490, 0.005197446422051668451, 0.005568692595055240412, 0.005939938768058812373 ),
 .UNSPECIFIED. ) ;
#186156=CARTESIAN_POINT ( 'NONE',  ( 10.81492255796106328, -18.62759615963255655, 55.41775706135234714 ) ) ;
#186157=CARTESIAN_POINT ( 'NONE',  ( -16.52544592524342804, 4.483927247898546575, 116.0405762719810383 ) ) ;
#186158=CARTESIAN_POINT ( 'NONE',  ( -18.67979575497178146, -10.72451020669898902, 21.66557627198102409 ) ) ;
#186159=CARTESIAN_POINT ( 'NONE',  ( -14.29746914071037622, -8.314922557961029526, 89.16775706135236135 ) ) ;
#186160=CARTESIAN_POINT ( 'NONE',  ( -5.719274019375665041, -21.55341960407619695, 99.79275706135234714 ) ) ;
#186161=CARTESIAN_POINT ( 'NONE',  ( 16.53943276465976808, 0.05219959533934440121, 61.25109039468567573 ) ) ;
#186162=CARTESIAN_POINT ( 'NONE',  ( -13.97604488694527625, -13.89961937509977652, 106.8739096053143669 ) ) ;
#186163=CARTESIAN_POINT ( 'NONE',  ( 16.52544592524335698, 4.483927247898782831, 56.45942372801902565 ) ) ;
#186164=CARTESIAN_POINT ( 'NONE',  ( 16.52544592524335698, 4.483927247898782831, 31.45942372801901854 ) ) ;
#186165=CARTESIAN_POINT ( 'NONE',  ( 12.14591786802327356, -12.06949235617739191, 100.6260903946857184 ) ) ;
#186166=CARTESIAN_POINT ( 'NONE',  ( 21.55341960407619695, -5.719274019375665929, 51.04275706135234714 ) ) ;
#186167=CARTESIAN_POINT ( 'NONE',  ( 4.379528057220092307, 16.55341960407617563, 27.29275706135234358 ) ) ;
#186168=CARTESIAN_POINT ( 'NONE',  ( -5.823673210054116645, -21.52544592524344225, 112.2905762719810241 ) ) ;
#186169=CARTESIAN_POINT ( 'NONE',  ( -16.52544592524335698, -4.483927247898792601, 23.95942372801901143 ) ) ;
#186170=CARTESIAN_POINT ( 'NONE',  ( 14.29746914071037800, 8.314922557961029526, 81.66775706135236135 ) ) ;
#186172=CARTESIAN_POINT ( 'NONE',  ( 21.52544592524334988, 5.823673210054432836, 86.45942372801901854 ) ) ;
#186173=CARTESIAN_POINT ( 'NONE',  ( -9.474510206698720793, -16.51473224551083518, 84.58442372801900433 ) ) ;
#186174=CARTESIAN_POINT ( 'NONE',  ( 14.29746914071049879, -8.314922557960816363, 48.33224293864770260 ) ) ;
#186175=CARTESIAN_POINT ( 'NONE',  ( 4.379528057220339221, -16.55341960407611168, 47.70724293864770260 ) ) ;
#186176=CARTESIAN_POINT ( 'NONE',  ( -0.05219959533910754901, -16.53943276465976808, 102.4989096053143811 ) ) ;
#186177=CARTESIAN_POINT ( 'NONE',  ( -9.474510206698720793, -16.51473224551083518, 49.58442372801899722 ) ) ;
#186178=CARTESIAN_POINT ( 'NONE',  ( 17.26058549869107850, -6.457015423128172671, 56.12254162523934298 ) ) ;
#186179=CARTESIAN_POINT ( 'NONE',  ( -21.53943276465977519, -0.05219959533937600094, 48.75109039468568284 ) ) ;
#186180=CARTESIAN_POINT ( 'NONE',  ( 16.51473224551083163, -9.474510206698727899, 105.8344237280190043 ) ) ;
#186182=CARTESIAN_POINT ( 'NONE',  ( -9.474510206698964154, 16.51473224551069663, 100.4155762719810241 ) ) ;
#186183=CARTESIAN_POINT ( 'NONE',  ( 0.05219959533907565091, 21.53943276465977519, 54.99890960531435269 ) ) ;
#186184=CARTESIAN_POINT ( 'NONE',  ( -5.153800228976607833, 19.02544592524334988, 92.70942372801901854 ) ) ;
#186185=CARTESIAN_POINT ( 'NONE',  ( -13.97604488694527625, -13.89961937509977652, 86.87390960531436690 ) ) ;
#186186=CARTESIAN_POINT ( 'NONE',  ( -5.719274019375978568, 21.55341960407610458, 60.20724293864768839 ) ) ;
#186187=CARTESIAN_POINT ( 'NONE',  ( 4.483927247898545687, 16.52544592524342804, 109.7905762719810383 ) ) ;
#186188=CARTESIAN_POINT ( 'NONE',  ( 5.153800228976335163, 19.02544592524342804, 64.79057627198100988 ) ) ;
#186189=CARTESIAN_POINT ( 'NONE',  ( -13.97604488694527625, -13.89961937509977652, 26.87390960531434558 ) ) ;
#186191=CARTESIAN_POINT ( 'NONE',  ( -18.62759615963255300, -10.81492255796106328, 34.16775706135234714 ) ) ;
#186192=CARTESIAN_POINT ( 'NONE',  ( -15.80617190586768217, 15.72974639402176855, 93.12609039468568994 ) ) ;
#186193=CARTESIAN_POINT ( 'NONE',  ( 8.224510206698742110, 14.34966873604972548, 92.08442372801901854 ) ) ;
#186194=CARTESIAN_POINT ( 'NONE',  ( -18.62759615963255300, -10.81492255796106328, 29.16775706135234003 ) ) ;
#186195=CARTESIAN_POINT ( 'NONE',  ( 18.67979575497194134, -10.72451020669871369, 45.83442372801901854 ) ) ;
#186196=CARTESIAN_POINT ( 'NONE',  ( 9.474510206698729675, 16.51473224551082808, 67.08442372801900433 ) ) ;
#186197=CARTESIAN_POINT ( 'NONE',  ( -9.564922557960796823, -16.46253265017161027, 82.08224293864768129 ) ) ;
#186198=CARTESIAN_POINT ( 'NONE',  ( 10.81492255796106328, -18.62759615963255655, 90.41775706135236135 ) ) ;
#186199=CARTESIAN_POINT ( 'NONE',  ( -18.67979575497178146, -10.72451020669898902, 81.66557627198103830 ) ) ;
#186200=CARTESIAN_POINT ( 'NONE',  ( 16.55341960407611168, 4.379528057220329451, 58.95724293864770971 ) ) ;
#186201=CARTESIAN_POINT ( 'NONE',  ( 5.719274019375673035, 21.55341960407619339, 107.2927570613523471 ) ) ;
#186202=CARTESIAN_POINT ( 'NONE',  ( 12.06949235617757843, -12.14591786802309237, 83.12390960531436690 ) ) ;
#186203=CARTESIAN_POINT ( 'NONE',  ( -16.51473224551069308, -9.474510206698971260, 31.66557627198102054 ) ) ;
#186204=CARTESIAN_POINT ( 'NONE',  ( 13.97604488694548053, -13.89961937509957401, 75.62609039468564731 ) ) ;
#186205=CARTESIAN_POINT ( 'NONE',  ( 12.06949235617757843, -12.14591786802309237, 33.12390960531435979 ) ) ;
#186206=CARTESIAN_POINT ( 'NONE',  ( 18.62759615963255655, 10.81492255796105972, 91.66775706135234714 ) ) ;
#186208=CARTESIAN_POINT ( 'NONE',  ( -5.153800228976328057, -19.02544592524343514, 92.29057627198099567 ) ) ;
#186209=CARTESIAN_POINT ( 'NONE',  ( -19.05341960407617563, 5.049401038297882671, 63.54275706135234003 ) ) ;
#186210=CARTESIAN_POINT ( 'NONE',  ( 10.81492255796078972, 18.62759615963270932, 69.58224293864769550 ) ) ;
#186211=CARTESIAN_POINT ( 'NONE',  ( 21.53943276465977519, 0.05219959533937863772, 21.25109039468567218 ) ) ;
#186212=CARTESIAN_POINT ( 'NONE',  ( 9.564922557961047289, -16.46253265017146816, 105.4177570613523471 ) ) ;
#186213=CARTESIAN_POINT ( 'NONE',  ( -0.05219959533934338120, 16.53943276465976808, 82.50109039468568994 ) ) ;
#186214=DIRECTION ( 'NONE',  ( -1.000000000000000000, -0.000000000000000000, -0.000000000000000000 ) ) ;
#186215=CARTESIAN_POINT ( 'NONE',  ( -21.55341960407619339, 5.719274019375674811, 23.54275706135235424 ) ) ;
#186216=CARTESIAN_POINT ( 'NONE',  ( 12.06949235617757843, -12.14591786802309237, 103.1239096053143811 ) ) ;
#186218=CARTESIAN_POINT ( 'NONE',  ( 4.379528057220092307, 16.55341960407617563, 52.29275706135236135 ) ) ;
#186219=CARTESIAN_POINT ( 'NONE',  ( -18.62759615963270932, 10.81492255796079327, 65.83224293864769550 ) ) ;
#186220=CARTESIAN_POINT ( 'NONE',  ( 12.06949235617739724, 12.14591786802326823, 101.8760903946857042 ) ) ;
#186221=CARTESIAN_POINT ( 'NONE',  ( -8.224510206698735004, -14.34966873604973081, 34.58442372801900433 ) ) ;
#186222=CARTESIAN_POINT ( 'NONE',  ( 19.02544592524343514, -5.153800228976328945, 28.54057627198102409 ) ) ;
#186223=CARTESIAN_POINT ( 'NONE',  ( -16.52544592524335698, -4.483927247898792601, 78.95942372801901854 ) ) ;
#186224=CARTESIAN_POINT ( 'NONE',  ( 9.564922557961047289, -16.46253265017146816, 75.41775706135234714 ) ) ;
#186225=CARTESIAN_POINT ( 'NONE',  ( -21.55341960407610458, -5.719274019375992779, 76.45724293864769550 ) ) ;
#186226=CARTESIAN_POINT ( 'NONE',  ( 16.55341960407618274, -4.379528057220086978, 91.04275706135236135 ) ) ;
#186228=CARTESIAN_POINT ( 'NONE',  ( -15.72974639402176322, -15.80617190586768395, 79.37609039468567573 ) ) ;
#186229=CARTESIAN_POINT ( 'NONE',  ( 5.719274019375991003, -21.55341960407610458, 67.70724293864769550 ) ) ;
#186230=CARTESIAN_POINT ( 'NONE',  ( -10.72451020669898014, 18.67979575497178502, 50.41557627198103120 ) ) ;
#186231=EDGE_LOOP ( 'NONE', ( #30660, #70711, #159906, #101206 ) ) ;
#186232=ORIENTED_EDGE ( 'NONE', *, *, #96707, .T. ) ;
#186233=CARTESIAN_POINT ( 'NONE',  ( 16.52544592524335698, 4.483927247898782831, 76.45942372801901854 ) ) ;
#186234=CARTESIAN_POINT ( 'NONE',  ( 10.72451020669898902, -18.67979575497178502, 42.91557627198103120 ) ) ;
#186236=CARTESIAN_POINT ( 'NONE',  ( 19.03943276465977164, -0.05219959533909143690, 113.7489096053143669 ) ) ;
#186238=CARTESIAN_POINT ( 'NONE',  ( 19.05341960407611168, 5.049401038298154454, 23.95724293864769194 ) ) ;
#186239=CARTESIAN_POINT ( 'NONE',  ( 18.62759615963271287, -10.81492255796078972, 68.33224293864769550 ) ) ;
#186240=CARTESIAN_POINT ( 'NONE',  ( -14.34966873604972548, 8.224510206698743886, 103.3344237280190043 ) ) ;
#186241=CARTESIAN_POINT ( 'NONE',  ( 0.05219959533937995610, -21.53943276465977519, 45.00109039468568284 ) ) ;
#186242=CARTESIAN_POINT ( 'NONE',  ( -16.46253265017146816, -9.564922557961047289, 99.16775706135233293 ) ) ;
#186243=CARTESIAN_POINT ( 'NONE',  ( 9.474510206698971260, -16.51473224551069308, 27.91557627198103120 ) ) ;
#186244=CARTESIAN_POINT ( 'NONE',  ( -14.29746914071037622, -8.314922557961029526, 19.16775706135234714 ) ) ;
#186245=CARTESIAN_POINT ( 'NONE',  ( 19.05341960407611168, 5.049401038298154454, 43.95724293864769550 ) ) ;
#186247=CARTESIAN_POINT ( 'NONE',  ( -0.05219959533909027116, -19.03943276465977164, 92.49890960531436690 ) ) ;
#186248=CARTESIAN_POINT ( 'NONE',  ( 14.29746914071037800, 8.314922557961029526, 76.66775706135234714 ) ) ;
#186249=CARTESIAN_POINT ( 'NONE',  ( -19.05341960407617563, 5.049401038297882671, 73.54275706135233293 ) ) ;
#186250=CARTESIAN_POINT ( 'NONE',  ( -19.05341960407617563, 5.049401038297882671, 23.54275706135233648 ) ) ;
#186251=CARTESIAN_POINT ( 'NONE',  ( -15.72974639402197994, 15.80617190586746368, 65.62390960531436690 ) ) ;
#186252=CARTESIAN_POINT ( 'NONE',  ( 16.52544592524335698, 4.483927247898782831, 81.45942372801900433 ) ) ;
#186253=CARTESIAN_POINT ( 'NONE',  ( -0.05219959533936034679, 19.03943276465977164, 82.50109039468567573 ) ) ;
#186254=CARTESIAN_POINT ( 'NONE',  ( -19.03943276465977164, 0.05219959533909376836, 41.24890960531435269 ) ) ;
#186255=CARTESIAN_POINT ( 'NONE',  ( -19.02544592524342804, 5.153800228976336051, 81.04057627198103830 ) ) ;
#186256=CARTESIAN_POINT ( 'NONE',  ( -21.53943276465977519, -0.05219959533937600094, 53.75109039468568994 ) ) ;
#186257=CARTESIAN_POINT ( 'NONE',  ( -16.51473224551069308, -9.474510206698971260, 51.66557627198102409 ) ) ;
#186258=CARTESIAN_POINT ( 'NONE',  ( 13.97604488694548053, -13.89961937509957401, 75.62609039468564731 ) ) ;
#186260=CARTESIAN_POINT ( 'NONE',  ( 9.564922557960805705, 16.46253265017160317, 104.5822429386476955 ) ) ;
#186261=CARTESIAN_POINT ( 'NONE',  ( -8.224510206698948167, 14.34966873604960824, 60.41557627198102409 ) ) ;
#186262=CARTESIAN_POINT ( 'NONE',  ( 15.80617190586746368, 15.72974639402197994, 54.37390960531435979 ) ) ;
#186263=CARTESIAN_POINT ( 'NONE',  ( 19.50973618000807619, 5.499999999999992895, 102.5000000000000142 ) ) ;
#186264=CARTESIAN_POINT ( 'NONE',  ( -9.474510206698720793, -16.51473224551083518, 39.58442372801899722 ) ) ;
#186265=CARTESIAN_POINT ( 'NONE',  ( -19.02544592524342804, 5.153800228976336051, 66.04057627198103830 ) ) ;
#186266=CARTESIAN_POINT ( 'NONE',  ( -0.05219959533909027116, -19.03943276465977164, 67.49890960531436690 ) ) ;
#186267=CARTESIAN_POINT ( 'NONE',  ( 4.483927247898790824, -16.52544592524335698, 45.20942372801901854 ) ) ;
#186269=CARTESIAN_POINT ( 'NONE',  ( 17.60728821186567217, -5.500000000000025757, 93.36690927743009638 ) ) ;
#186270=CARTESIAN_POINT ( 'NONE',  ( -12.14591786802326823, 12.06949235617739902, 83.12609039468568994 ) ) ;
#186272=CARTESIAN_POINT ( 'NONE',  ( 14.34966873604972726, -8.224510206698740333, 70.83442372801901854 ) ) ;
#186273=CARTESIAN_POINT ( 'NONE',  ( -14.34966873604972548, 8.224510206698743886, 38.33442372801900433 ) ) ;
#186274=CARTESIAN_POINT ( 'NONE',  ( 16.46253265017146816, 9.564922557961045513, 26.66775706135234003 ) ) ;
#186275=CARTESIAN_POINT ( 'NONE',  ( 9.564922557960805705, 16.46253265017160317, 54.58224293864769550 ) ) ;
#186277=CARTESIAN_POINT ( 'NONE',  ( -0.05219959533937732626, 21.53943276465977519, 57.50109039468568994 ) ) ;
#186278=CARTESIAN_POINT ( 'NONE',  ( -19.03943276465977164, -0.05219959533935918106, 63.75109039468566863 ) ) ;
#186279=CARTESIAN_POINT ( 'NONE',  ( -15.80617190586768217, 15.72974639402176855, 113.1260903946856899 ) ) ;
#186280=CARTESIAN_POINT ( 'NONE',  ( -19.03943276465977164, 0.05219959533909376836, 26.24890960531435624 ) ) ;
#186281=CARTESIAN_POINT ( 'NONE',  ( 16.22749556775600865, 7.364991527249977743, 23.15813903950547825 ) ) ;
#186282=CARTESIAN_POINT ( 'NONE',  ( -0.05219959533907301413, -21.53943276465977519, 72.49890960531435269 ) ) ;
#186283=CARTESIAN_POINT ( 'NONE',  ( 21.52544592524344225, -5.823673210054117533, 23.54057627198102765 ) ) ;
#186284=CARTESIAN_POINT ( 'NONE',  ( 8.224510206698953496, -14.34966873604960469, 97.91557627198103830 ) ) ;
#186285=CARTESIAN_POINT ( 'NONE',  ( 16.53943276465976808, 0.05219959533934440121, 31.25109039468568639 ) ) ;
#186286=CARTESIAN_POINT ( 'NONE',  ( 16.52544592524342804, -4.483927247898539470, 28.54057627198103120 ) ) ;
#186288=CARTESIAN_POINT ( 'NONE',  ( -10.81492255796078084, -18.62759615963271287, 112.0822429386477097 ) ) ;
#186289=CARTESIAN_POINT ( 'NONE',  ( -16.55341960407611168, -4.379528057220339221, 36.45724293864768839 ) ) ;
#186291=CARTESIAN_POINT ( 'NONE',  ( 19.05341960407617918, -5.049401038297876454, 111.0427570613523329 ) ) ;
#186292=CARTESIAN_POINT ( 'NONE',  ( 5.153800228976615827, -19.02544592524334988, 20.20942372801899722 ) ) ;
#186293=CARTESIAN_POINT ( 'NONE',  ( -12.06949235617756955, 12.14591786802309770, 25.62390960531435624 ) ) ;
#186294=CARTESIAN_POINT ( 'NONE',  ( -5.719274019375978568, 21.55341960407610458, 100.2072429386476955 ) ) ;
#186295=CARTESIAN_POINT ( 'NONE',  ( 17.48847506799968343, 5.747544572773804816, 31.67302562156722345 ) ) ;
#186296=CARTESIAN_POINT ( 'NONE',  ( -15.72974639402197994, 15.80617190586746368, 65.62390960531436690 ) ) ;
#186297=CARTESIAN_POINT ( 'NONE',  ( -9.564922557960796823, -16.46253265017161027, 77.08224293864769550 ) ) ;
#186298=CARTESIAN_POINT ( 'NONE',  ( -14.34966873604960291, -8.224510206698953496, 51.66557627198102409 ) ) ;
#186299=CARTESIAN_POINT ( 'NONE',  ( 13.97604488694527802, 13.89961937509977652, 84.37390960531433848 ) ) ;
#186301=CARTESIAN_POINT ( 'NONE',  ( -16.51473224551082808, 9.474510206698731452, 58.33442372801900433 ) ) ;
#186302=CARTESIAN_POINT ( 'NONE',  ( 21.53943276465977519, -0.05219959533907433946, 93.74890960531436690 ) ) ;
#186303=CARTESIAN_POINT ( 'NONE',  ( -8.224510206698948167, 14.34966873604960824, 100.4155762719810241 ) ) ;
#186304=CARTESIAN_POINT ( 'NONE',  ( -21.55341960407619339, 5.719274019375674811, 33.54275706135234714 ) ) ;
#186306=CARTESIAN_POINT ( 'NONE',  ( 12.06949235617757843, -12.14591786802309237, 28.12390960531435979 ) ) ;
#186307=CARTESIAN_POINT ( 'NONE',  ( 19.05341960407611168, 5.049401038298154454, 33.95724293864769550 ) ) ;
#186308=CARTESIAN_POINT ( 'NONE',  ( -13.89961937509977652, 13.97604488694528158, 80.62390960531436690 ) ) ;
#186309=CARTESIAN_POINT ( 'NONE',  ( -5.719274019375978568, 21.55341960407610458, 65.20724293864768129 ) ) ;
#186310=CARTESIAN_POINT ( 'NONE',  ( -18.22780087662122028, 5.500000000000031086, 83.51540105326107266 ) ) ;
#186311=CARTESIAN_POINT ( 'NONE',  ( -16.51473224551069308, -9.474510206698971260, 26.66557627198103120 ) ) ;
#186312=CARTESIAN_POINT ( 'NONE',  ( -21.55341960407610458, -5.719274019375992779, 51.45724293864770260 ) ) ;
#186313=CARTESIAN_POINT ( 'NONE',  ( -10.72451020669870658, -18.67979575497194134, 74.58442372801901854 ) ) ;
#186315=CARTESIAN_POINT ( 'NONE',  ( -8.224510206698735004, -14.34966873604973081, 64.58442372801900433 ) ) ;
#186316=CARTESIAN_POINT ( 'NONE',  ( -0.05219959533909027116, -19.03943276465977164, 52.49890960531436690 ) ) ;
#186317=CARTESIAN_POINT ( 'NONE',  ( -16.46253265017160317, 9.564922557960807481, 60.83224293864769550 ) ) ;
#186318=ORIENTED_EDGE ( 'NONE', *, *, #100439, .T. ) ;
#186319=CARTESIAN_POINT ( 'NONE',  ( -19.02544592524334988, -5.153800228976617603, 28.95942372801900433 ) ) ;
#186320=CARTESIAN_POINT ( 'NONE',  ( 14.34966873604972726, -8.224510206698740333, 70.83442372801901854 ) ) ;
#186321=CARTESIAN_POINT ( 'NONE',  ( -18.67979575497193778, 10.72451020669871902, 93.33442372801901854 ) ) ;
#186322=CARTESIAN_POINT ( 'NONE',  ( 5.153800228976335163, 19.02544592524342804, 74.79057627198103830 ) ) ;
#186323=CARTESIAN_POINT ( 'NONE',  ( 10.72451020669898902, -18.67979575497178502, 37.91557627198102409 ) ) ;
#186324=CARTESIAN_POINT ( 'NONE',  ( -19.03943276465977164, -0.05219959533935918106, 113.7510903946856757 ) ) ;
#186325=CARTESIAN_POINT ( 'NONE',  ( -5.823673210054431948, 21.52544592524334988, 87.70942372801901854 ) ) ;
#186326=CARTESIAN_POINT ( 'NONE',  ( -16.55341960407617563, 4.379528057220093196, 43.54275706135235424 ) ) ;
#186327=CARTESIAN_POINT ( 'NONE',  ( -10.81492255796078084, -18.62759615963271287, 102.0822429386476955 ) ) ;
#186328=CARTESIAN_POINT ( 'NONE',  ( -5.049401038297874678, -19.05341960407617918, 109.7927570613523187 ) ) ;
#186329=CARTESIAN_POINT ( 'NONE',  ( -9.474510206698964154, 16.51473224551069663, 75.41557627198103830 ) ) ;
#186330=CARTESIAN_POINT ( 'NONE',  ( -19.05341960407617563, 5.049401038297882671, 113.5427570613523471 ) ) ;
#186331=CARTESIAN_POINT ( 'NONE',  ( 9.474510206698971260, -16.51473224551069308, 42.91557627198103120 ) ) ;
#186333=CARTESIAN_POINT ( 'NONE',  ( -8.314922557961024197, 14.29746914071037800, 22.91775706135235069 ) ) ;
#186334=CARTESIAN_POINT ( 'NONE',  ( -4.483927247898539470, -16.52544592524342804, 67.29057627198103830 ) ) ;
#186335=CARTESIAN_POINT ( 'NONE',  ( 12.14591786802327356, -12.06949235617739191, 70.62609039468567573 ) ) ;
#186336=CARTESIAN_POINT ( 'NONE',  ( -15.72974639402176322, -15.80617190586768395, 29.37609039468568284 ) ) ;
#186337=CARTESIAN_POINT ( 'NONE',  ( 16.51473224551069308, 9.474510206698969483, 54.16557627198103120 ) ) ;
#186338=CARTESIAN_POINT ( 'NONE',  ( -16.51473224551069308, -9.474510206698971260, 66.66557627198102409 ) ) ;
#186339=CARTESIAN_POINT ( 'NONE',  ( 16.53943276465976808, 0.05219959533934440121, 76.25109039468568994 ) ) ;
#186341=ORIENTED_EDGE ( 'NONE', *, *, #121605, .T. ) ;
#186343=CARTESIAN_POINT ( 'NONE',  ( -16.46253265017146816, -9.564922557961047289, 24.16775706135233648 ) ) ;
#186345=CARTESIAN_POINT ( 'NONE',  ( 19.02544592524343514, -5.153800228976328945, 38.54057627198103120 ) ) ;
#186346=CARTESIAN_POINT ( 'NONE',  ( 16.46253265017160672, -9.564922557960803928, 98.33224293864769550 ) ) ;
#186347=VERTEX_POINT ( 'NONE', #98419 ) ;
#186348=CARTESIAN_POINT ( 'NONE',  ( 8.224510206698742110, 14.34966873604972548, 27.08442372801901854 ) ) ;
#186349=CARTESIAN_POINT ( 'NONE',  ( -5.153800228976607833, 19.02544592524334988, 62.70942372801899722 ) ) ;
#186350=CARTESIAN_POINT ( 'NONE',  ( -4.483927247898782831, 16.52544592524335698, 37.70942372801900433 ) ) ;
#186351=CARTESIAN_POINT ( 'NONE',  ( -9.564922557960796823, -16.46253265017161027, 37.08224293864768839 ) ) ;
#186352=CARTESIAN_POINT ( 'NONE',  ( -5.049401038298153566, 19.05341960407611168, 105.2072429386476671 ) ) ;
#186353=CARTESIAN_POINT ( 'NONE',  ( 19.02544592524343514, -5.153800228976328945, 58.54057627198102409 ) ) ;
#186354=CARTESIAN_POINT ( 'NONE',  ( 21.52544592524344225, -5.823673210054117533, 103.5405762719810383 ) ) ;
#186355=CARTESIAN_POINT ( 'NONE',  ( -16.46253265017160317, 9.564922557960807481, 90.83224293864769550 ) ) ;
#186356=CARTESIAN_POINT ( 'NONE',  ( -16.51473224551069308, -9.474510206698971260, 111.6655762719810383 ) ) ;
#186357=CARTESIAN_POINT ( 'NONE',  ( -19.02544592524342804, 5.153800228976336051, 61.04057627198103120 ) ) ;
#186358=CARTESIAN_POINT ( 'NONE',  ( 12.14591786802327356, -12.06949235617739191, 110.6260903946857042 ) ) ;
#186359=CARTESIAN_POINT ( 'NONE',  ( -22.00000000000000000, -1.163414459189985801E-14, 95.00000000000000000 ) ) ;
#186360=CARTESIAN_POINT ( 'NONE',  ( -19.05341960407617563, 5.049401038297882671, 103.5427570613523329 ) ) ;
#186361=CARTESIAN_POINT ( 'NONE',  ( 16.46253265017146816, 9.564922557961045513, 21.66775706135233648 ) ) ;
#186362=CARTESIAN_POINT ( 'NONE',  ( 0.05219959533910956823, 16.53943276465976808, 54.99890960531435269 ) ) ;
#186363=CARTESIAN_POINT ( 'NONE',  ( 18.67979575497194134, -10.72451020669871369, 100.8344237280190185 ) ) ;
#186364=CARTESIAN_POINT ( 'NONE',  ( 19.02544592524343514, -5.153800228976328945, 43.54057627198103120 ) ) ;
#186366=CARTESIAN_POINT ( 'NONE',  ( 16.55341960407611168, 4.379528057220329451, 23.95724293864769550 ) ) ;
#186367=CARTESIAN_POINT ( 'NONE',  ( -21.53943276465977519, -0.05219959533937600094, 83.75109039468568994 ) ) ;
#186368=CARTESIAN_POINT ( 'NONE',  ( 16.46253265017160672, -9.564922557960803928, 78.33224293864769550 ) ) ;
#186369=CARTESIAN_POINT ( 'NONE',  ( -13.97604488694527625, -13.89961937509977652, 91.87390960531432427 ) ) ;
#186370=CARTESIAN_POINT ( 'NONE',  ( -12.14591786802309592, -12.06949235617757132, 96.87390960531436690 ) ) ;
#186371=CARTESIAN_POINT ( 'NONE',  ( 12.14591786802309770, 12.06949235617756955, 54.37390960531435979 ) ) ;
#186372=CARTESIAN_POINT ( 'NONE',  ( -18.62759615963270932, 10.81492255796079327, 70.83224293864770971 ) ) ;
#186373=CARTESIAN_POINT ( 'NONE',  ( 0.05219959533909260263, 19.03943276465977164, 69.99890960531435269 ) ) ;
#186374=CARTESIAN_POINT ( 'NONE',  ( -18.62759615963270932, 10.81492255796079327, 85.83224293864768129 ) ) ;
#186375=CARTESIAN_POINT ( 'NONE',  ( 19.05341960407617918, -5.049401038297876454, 81.04275706135231871 ) ) ;
#186376=CARTESIAN_POINT ( 'NONE',  ( 18.56197773271732387, -5.499999999999896971, 46.05066217314453070 ) ) ;
#186377=CARTESIAN_POINT ( 'NONE',  ( 0.05219959533910956823, 16.53943276465976808, 89.99890960531438111 ) ) ;
#186378=VECTOR ( 'NONE', #28188, 1000.000000000000000 ) ;
#186379=CARTESIAN_POINT ( 'NONE',  ( -16.51473224551069308, -9.474510206698971260, 56.66557627198103120 ) ) ;
#186380=CARTESIAN_POINT ( 'NONE',  ( -0.05219959533907301413, -21.53943276465977519, 72.49890960531435269 ) ) ;
#186381=CARTESIAN_POINT ( 'NONE',  ( 17.48847506799967633, -5.747544572773779059, 28.32697437843280497 ) ) ;
#186382=CARTESIAN_POINT ( 'NONE',  ( 0.05219959533910956823, 16.53943276465976808, 24.99890960531435624 ) ) ;
#186384=CARTESIAN_POINT ( 'NONE',  ( -9.474510206698720793, -16.51473224551083518, 109.5844237280190043 ) ) ;
#186385=CARTESIAN_POINT ( 'NONE',  ( 16.55341960407611168, 4.379528057220329451, 83.95724293864770971 ) ) ;
#186386=B_SPLINE_CURVE_WITH_KNOTS ( 'NONE', 3,
 ( #4190, #160884, #115385, #65869, #177073, #130529 ),
 .UNSPECIFIED., .F., .F.,
 ( 4, 2, 4 ),
 ( 0.003239945802372268171, 0.003620412082092120364, 0.004000878361811972990 ),
 .UNSPECIFIED. ) ;
#186387=CARTESIAN_POINT ( 'NONE',  ( -19.34837522270366250, -5.499999999999798383, 95.86337684832578532 ) ) ;
#186388=CARTESIAN_POINT ( 'NONE',  ( 19.03943276465977164, -0.05219959533909143690, 73.74890960531435269 ) ) ;
#186389=CARTESIAN_POINT ( 'NONE',  ( 16.51473224551069308, 9.474510206698969483, 34.16557627198102409 ) ) ;
#186390=CARTESIAN_POINT ( 'NONE',  ( -16.52544592524342804, 4.483927247898546575, 66.04057627198103830 ) ) ;
#186391=CARTESIAN_POINT ( 'NONE',  ( 5.153800228976335163, 19.02544592524342804, 99.79057627198102409 ) ) ;
#186392=CARTESIAN_POINT ( 'NONE',  ( -19.02544592524334988, -5.153800228976617603, 83.95942372801901854 ) ) ;
#186393=CARTESIAN_POINT ( 'NONE',  ( -5.153800228976328057, -19.02544592524343514, 72.29057627198102409 ) ) ;
#186394=CARTESIAN_POINT ( 'NONE',  ( -16.51473224551069308, -9.474510206698971260, 91.66557627198103830 ) ) ;
#186395=CARTESIAN_POINT ( 'NONE',  ( -10.72451020669898014, 18.67979575497178502, 75.41557627198102409 ) ) ;
#186396=CARTESIAN_POINT ( 'NONE',  ( 4.379528057220092307, 16.55341960407617563, 77.29275706135234714 ) ) ;
#186397=CARTESIAN_POINT ( 'NONE',  ( 9.564922557961047289, -16.46253265017146816, 110.4177570613523471 ) ) ;
#186398=CARTESIAN_POINT ( 'NONE',  ( -19.02544592524342804, 5.153800228976336051, 61.04057627198103120 ) ) ;
#186399=CARTESIAN_POINT ( 'NONE',  ( -21.52544592524343514, 5.823673210054127303, 66.04057627198103830 ) ) ;
#186400=CARTESIAN_POINT ( 'NONE',  ( 13.97604488694548053, -13.89961937509957401, 95.62609039468563310 ) ) ;
#186401=CARTESIAN_POINT ( 'NONE',  ( 4.483927247898545687, 16.52544592524342804, 44.79057627198103120 ) ) ;
#186402=CARTESIAN_POINT ( 'NONE',  ( -10.72451020669870658, -18.67979575497194134, 39.58442372801901143 ) ) ;
#186404=CARTESIAN_POINT ( 'NONE',  ( 4.483927247898790824, -16.52544592524335698, 70.20942372801904696 ) ) ;
#186405=CARTESIAN_POINT ( 'NONE',  ( -5.153800228976328057, -19.02544592524343514, 112.2905762719810099 ) ) ;
#186406=DIRECTION ( 'NONE',  ( -0.000000000000000000, -0.000000000000000000, -1.000000000000000000 ) ) ;
#186408=CARTESIAN_POINT ( 'NONE',  ( -12.14591786802326823, 12.06949235617739902, 88.12609039468570415 ) ) ;
#186409=CARTESIAN_POINT ( 'NONE',  ( 16.53943276465976808, 0.05219959533934440121, 46.25109039468567573 ) ) ;
#186410=CARTESIAN_POINT ( 'NONE',  ( -16.46253265017160317, 9.564922557960807481, 55.83224293864769550 ) ) ;
#186411=CARTESIAN_POINT ( 'NONE',  ( 13.97604488694527802, 13.89961937509977652, 59.37390960531434558 ) ) ;
#186412=CARTESIAN_POINT ( 'NONE',  ( -18.67979575497193778, 10.72451020669871902, 53.33442372801901854 ) ) ;
#186413=CARTESIAN_POINT ( 'NONE',  ( 14.29746914071037800, 8.314922557961029526, 66.66775706135234714 ) ) ;
#186414=CARTESIAN_POINT ( 'NONE',  ( 14.34966873604960469, 8.224510206698951720, 39.16557627198102409 ) ) ;
#186415=CARTESIAN_POINT ( 'NONE',  ( 9.564922557960805705, 16.46253265017160317, 44.58224293864769550 ) ) ;
#186416=CARTESIAN_POINT ( 'NONE',  ( -5.049401038298153566, 19.05341960407611168, 35.20724293864768839 ) ) ;
#186417=CARTESIAN_POINT ( 'NONE',  ( -8.314922557961024197, 14.29746914071037800, 32.91775706135234714 ) ) ;
#186419=CARTESIAN_POINT ( 'NONE',  ( -13.97604488694547697, 13.89961937509957934, 78.12609039468567573 ) ) ;
#186420=CARTESIAN_POINT ( 'NONE',  ( 0.05219959533910956823, 16.53943276465976808, 89.99890960531438111 ) ) ;
#186421=CARTESIAN_POINT ( 'NONE',  ( 19.05341960407611168, 5.049401038298154454, 53.95724293864770260 ) ) ;
#186422=CARTESIAN_POINT ( 'NONE',  ( 16.46253265017146816, 9.564922557961045513, 91.66775706135234714 ) ) ;
#186424=CARTESIAN_POINT ( 'NONE',  ( 15.72974639402176855, 15.80617190586768217, 86.87609039468568994 ) ) ;
#186425=CARTESIAN_POINT ( 'NONE',  ( 14.34966873604972726, -8.224510206698740333, 55.83442372801901854 ) ) ;
#186426=CARTESIAN_POINT ( 'NONE',  ( 16.20579543436681291, 7.371946100354972664, 38.06520834171877965 ) ) ;
#186427=CARTESIAN_POINT ( 'NONE',  ( -15.72974639402197994, 15.80617190586746368, 45.62390960531436690 ) ) ;
#186428=CARTESIAN_POINT ( 'NONE',  ( -16.52544592524335698, -4.483927247898792601, 43.95942372801902565 ) ) ;
#186429=CARTESIAN_POINT ( 'NONE',  ( -5.153800228976328057, -19.02544592524343514, 32.29057627198102409 ) ) ;
#186430=CARTESIAN_POINT ( 'NONE',  ( 9.564922557961047289, -16.46253265017146816, 30.41775706135232937 ) ) ;
#186431=CARTESIAN_POINT ( 'NONE',  ( -13.97604488694527625, -13.89961937509977652, 71.87390960531433848 ) ) ;
#186433=CARTESIAN_POINT ( 'NONE',  ( 0.05219959533909260263, 19.03943276465977164, 54.99890960531435979 ) ) ;
#186435=CARTESIAN_POINT ( 'NONE',  ( -5.153800228976328057, -19.02544592524343514, 67.29057627198102409 ) ) ;
#186436=CARTESIAN_POINT ( 'NONE',  ( -19.39720447994795904, -5.499999999999977796, 54.66317477297177874 ) ) ;
#186437=CARTESIAN_POINT ( 'NONE',  ( 19.02544592524334988, 5.153800228976608722, 36.45942372801900433 ) ) ;
#186438=CARTESIAN_POINT ( 'NONE',  ( -0.05219959533937732626, 21.53943276465977519, 112.5010903946857042 ) ) ;
#186439=CARTESIAN_POINT ( 'NONE',  ( -16.53943276465976808, 0.05219959533911058130, 41.24890960531435269 ) ) ;
#186440=CARTESIAN_POINT ( 'NONE',  ( -9.564922557960796823, -16.46253265017161027, 42.08224293864769550 ) ) ;
#186441=CARTESIAN_POINT ( 'NONE',  ( 9.564922557960805705, 16.46253265017160317, 104.5822429386476955 ) ) ;
#186442=CARTESIAN_POINT ( 'NONE',  ( 15.72974639402176855, 15.80617190586768217, 71.87609039468568994 ) ) ;
#186443=CARTESIAN_POINT ( 'NONE',  ( 16.51473224551069308, 9.474510206698969483, 54.16557627198103120 ) ) ;
#186444=CARTESIAN_POINT ( 'NONE',  ( 10.72451020669871369, 18.67979575497193778, 82.08442372801901854 ) ) ;
#186445=CARTESIAN_POINT ( 'NONE',  ( -15.72974639402197994, 15.80617190586746368, 25.62390960531435624 ) ) ;
#186446=CARTESIAN_POINT ( 'NONE',  ( 13.89961937509977652, -13.97604488694527269, 33.12390960531434558 ) ) ;
#186447=CARTESIAN_POINT ( 'NONE',  ( 18.67979575497194134, -10.72451020669871369, 20.83442372801901143 ) ) ;
#186448=CARTESIAN_POINT ( 'NONE',  ( 5.049401038297881783, 19.05341960407617563, 47.29275706135231161 ) ) ;
#186449=CARTESIAN_POINT ( 'NONE',  ( -0.05219959533909027116, -19.03943276465977164, 27.49890960531435624 ) ) ;
#186450=CARTESIAN_POINT ( 'NONE',  ( 0.05219959533909260263, 19.03943276465977164, 74.99890960531435269 ) ) ;
#186451=CARTESIAN_POINT ( 'NONE',  ( -16.51473224551082808, 9.474510206698731452, 108.3344237280190043 ) ) ;
#186452=CARTESIAN_POINT ( 'NONE',  ( 14.34966873604960469, 8.224510206698951720, 79.16557627198103830 ) ) ;
#186453=CARTESIAN_POINT ( 'NONE',  ( 15.72974639402199770, -15.80617190586745480, 38.12390960531436690 ) ) ;
#186454=CARTESIAN_POINT ( 'NONE',  ( 5.049401038297881783, 19.05341960407617563, 102.2927570613523045 ) ) ;
#186455=CARTESIAN_POINT ( 'NONE',  ( -21.55341960407610458, -5.719274019375992779, 111.4572429386476813 ) ) ;
#186456=CARTESIAN_POINT ( 'NONE',  ( -15.72974639402176322, -15.80617190586768395, 59.37609039468568284 ) ) ;
#186457=CARTESIAN_POINT ( 'NONE',  ( 14.34966873604972726, -8.224510206698740333, 55.83442372801901854 ) ) ;
#186458=CARTESIAN_POINT ( 'NONE',  ( -8.224510206698735004, -14.34966873604973081, 54.58442372801901143 ) ) ;
#186459=CARTESIAN_POINT ( 'NONE',  ( 10.72451020669898902, -18.67979575497178502, 72.91557627198103830 ) ) ;
#186460=CARTESIAN_POINT ( 'NONE',  ( -13.97604488694527625, -13.89961937509977652, 46.87390960531435979 ) ) ;
#186461=CARTESIAN_POINT ( 'NONE',  ( -8.224510206698735004, -14.34966873604973081, 94.58442372801901854 ) ) ;
#186462=B_SPLINE_CURVE_WITH_KNOTS ( 'NONE', 3,
 ( #156390, #182768, #17894, #121074, #13900, #75566, #137242, #122067, #45245, #106899 ),
 .UNSPECIFIED., .F., .F.,
 ( 4, 2, 2, 2, 4 ),
 ( 2.459394992999530923E-17, 0.0001682128350528851516, 0.0003364256701057457459, 0.0005046385051586063132, 0.0006728513402114668805 ),
 .UNSPECIFIED. ) ;
#186463=CARTESIAN_POINT ( 'NONE',  ( -15.72974639402197994, 15.80617190586746368, 100.6239096053143811 ) ) ;
#186464=CARTESIAN_POINT ( 'NONE',  ( -14.29746914071049879, 8.314922557960819915, 50.83224293864770971 ) ) ;
#186465=CARTESIAN_POINT ( 'NONE',  ( -5.153800228976328057, -19.02544592524343514, 82.29057627198103830 ) ) ;
#186466=CARTESIAN_POINT ( 'NONE',  ( 8.224510206698742110, 14.34966873604972548, 82.08442372801901854 ) ) ;
#186467=CARTESIAN_POINT ( 'NONE',  ( 15.72974639402176855, 15.80617190586768217, 51.87609039468568284 ) ) ;
#186468=CARTESIAN_POINT ( 'NONE',  ( -8.224510206698735004, -14.34966873604973081, 24.58442372801901499 ) ) ;
#186469=CARTESIAN_POINT ( 'NONE',  ( 21.55341960407610458, 5.719274019375980345, 113.9572429386477239 ) ) ;
#186470=CARTESIAN_POINT ( 'NONE',  ( -4.379528057220328563, 16.55341960407611168, 50.20724293864769550 ) ) ;
#186472=CARTESIAN_POINT ( 'NONE',  ( 18.56197773271728835, -5.499999999999983125, 91.05066217314453070 ) ) ;
#186473=CARTESIAN_POINT ( 'NONE',  ( 15.72974639402199770, -15.80617190586745480, 93.12390960531436690 ) ) ;
#186474=CARTESIAN_POINT ( 'NONE',  ( 4.379528057220092307, 16.55341960407617563, 112.2927570613523471 ) ) ;
#186477=CARTESIAN_POINT ( 'NONE',  ( -21.52544592524343514, 5.823673210054127303, 111.0405762719810525 ) ) ;
#186478=CARTESIAN_POINT ( 'NONE',  ( -16.51473224551069308, -9.474510206698971260, 111.6655762719810383 ) ) ;
#186479=CARTESIAN_POINT ( 'NONE',  ( -21.52544592524334988, -5.823673210054445271, 18.95942372801901143 ) ) ;
#186480=CARTESIAN_POINT ( 'NONE',  ( 8.224510206698953496, -14.34966873604960469, 57.91557627198103120 ) ) ;
#186481=CARTESIAN_POINT ( 'NONE',  ( 14.29746914071037800, 8.314922557961029526, 66.66775706135234714 ) ) ;
#186483=CARTESIAN_POINT ( 'NONE',  ( 0.05219959533909260263, 19.03943276465977164, 64.99890960531436690 ) ) ;
#186484=CARTESIAN_POINT ( 'NONE',  ( 0.05219959533936267826, -19.03943276465977164, 70.00109039468566152 ) ) ;
#186485=CARTESIAN_POINT ( 'NONE',  ( 19.03943276465977164, -0.05219959533909143690, 78.74890960531436690 ) ) ;
#186486=CARTESIAN_POINT ( 'NONE',  ( 10.72451020669898902, -18.67979575497178502, 32.91557627198102409 ) ) ;
#186488=CARTESIAN_POINT ( 'NONE',  ( 16.51473224551069308, 9.474510206698969483, 44.16557627198103120 ) ) ;
#186489=CARTESIAN_POINT ( 'NONE',  ( -16.53943276465976808, -0.05219959533934237506, 23.75109039468567929 ) ) ;
#186490=CARTESIAN_POINT ( 'NONE',  ( 0.05219959533936267826, -19.03943276465977164, 65.00109039468567573 ) ) ;
#186491=CARTESIAN_POINT ( 'NONE',  ( 21.52544592524344225, -5.823673210054117533, 98.54057627198105251 ) ) ;
#186492=CARTESIAN_POINT ( 'NONE',  ( -4.483927247898539470, -16.52544592524342804, 32.29057627198102409 ) ) ;
#186493=CARTESIAN_POINT ( 'NONE',  ( 5.153800228976335163, 19.02544592524342804, 94.79057627198103830 ) ) ;
#186494=CARTESIAN_POINT ( 'NONE',  ( 21.52544592524344225, -5.823673210054117533, 53.54057627198103120 ) ) ;
#186495=CARTESIAN_POINT ( 'NONE',  ( -15.72974639402197994, 15.80617190586746368, 100.6239096053143811 ) ) ;
#186496=CARTESIAN_POINT ( 'NONE',  ( 16.52544592524335698, 4.483927247898782831, 26.45942372801901854 ) ) ;
#186497=CARTESIAN_POINT ( 'NONE',  ( -5.719274019375978568, 21.55341960407610458, 30.20724293864769550 ) ) ;
#186498=CARTESIAN_POINT ( 'NONE',  ( 15.72974639402176855, 15.80617190586768217, 86.87609039468568994 ) ) ;
#186499=CARTESIAN_POINT ( 'NONE',  ( -19.03943276465977164, 0.05219959533909376836, 86.24890960531436690 ) ) ;
#186500=CARTESIAN_POINT ( 'NONE',  ( -16.51473224551069308, -9.474510206698971260, 21.66557627198102765 ) ) ;
#186501=CARTESIAN_POINT ( 'NONE',  ( 16.46253265017160672, -9.564922557960803928, 88.33224293864769550 ) ) ;
#186502=CARTESIAN_POINT ( 'NONE',  ( 14.29746914071049879, -8.314922557960816363, 103.3322429386476955 ) ) ;
#186503=CARTESIAN_POINT ( 'NONE',  ( -0.05219959533909027116, -19.03943276465977164, 67.49890960531436690 ) ) ;
#186504=CARTESIAN_POINT ( 'NONE',  ( -4.483927247898782831, 16.52544592524335698, 22.70942372801901499 ) ) ;
#186508=CARTESIAN_POINT ( 'NONE',  ( -5.823673210054431948, 21.52544592524334988, 92.70942372801901854 ) ) ;
#186509=CARTESIAN_POINT ( 'NONE',  ( 0.05219959533909260263, 19.03943276465977164, 114.9989096053143669 ) ) ;
#186510=CARTESIAN_POINT ( 'NONE',  ( 8.224510206698742110, 14.34966873604972548, 87.08442372801901854 ) ) ;
#186512=CARTESIAN_POINT ( 'NONE',  ( 0.05219959533936267826, -19.03943276465977164, 75.00109039468566152 ) ) ;
#186513=CARTESIAN_POINT ( 'NONE',  ( 16.51473224551083163, -9.474510206698727899, 35.83442372801899722 ) ) ;
#186514=CARTESIAN_POINT ( 'NONE',  ( -17.12812012977024523, -6.668231424566069876, 46.35948759323146362 ) ) ;
#186515=CARTESIAN_POINT ( 'NONE',  ( -9.564922557960796823, -16.46253265017161027, 32.08224293864769550 ) ) ;
#186516=CARTESIAN_POINT ( 'NONE',  ( -16.55341960407611168, -4.379528057220339221, 36.45724293864768839 ) ) ;
#186517=CARTESIAN_POINT ( 'NONE',  ( 13.89961937509977652, -13.97604488694527269, 23.12390960531436335 ) ) ;
#186518=CARTESIAN_POINT ( 'NONE',  ( 16.52544592524342804, -4.483927247898539470, 33.54057627198102409 ) ) ;
#186520=CARTESIAN_POINT ( 'NONE',  ( 16.55341960407618274, -4.379528057220086978, 96.04275706135236135 ) ) ;
#186521=CARTESIAN_POINT ( 'NONE',  ( 9.474510206698971260, -16.51473224551069308, 42.91557627198103120 ) ) ;
#186522=CARTESIAN_POINT ( 'NONE',  ( 5.719274019375673035, 21.55341960407619339, 97.29275706135234714 ) ) ;
#186523=CARTESIAN_POINT ( 'NONE',  ( -13.89961937509957401, -13.97604488694547875, 104.3760903946856757 ) ) ;
#186524=CARTESIAN_POINT ( 'NONE',  ( -18.67979575497193778, 10.72451020669871902, 83.33442372801903275 ) ) ;
#186525=CARTESIAN_POINT ( 'NONE',  ( -0.05219959533936034679, 19.03943276465977164, 52.50109039468566863 ) ) ;
#186526=CARTESIAN_POINT ( 'NONE',  ( -16.46253265017160317, 9.564922557960807481, 95.83224293864769550 ) ) ;
#186527=CARTESIAN_POINT ( 'NONE',  ( 5.049401038298161559, -19.05341960407611168, 67.70724293864769550 ) ) ;
#186528=CARTESIAN_POINT ( 'NONE',  ( 17.13100169013299023, 6.664070546373165094, 71.73210164300154190 ) ) ;
#186530=CARTESIAN_POINT ( 'NONE',  ( 14.34966873604960469, 8.224510206698951720, 69.16557627198102409 ) ) ;
#186531=CARTESIAN_POINT ( 'NONE',  ( 21.55341960407610458, 5.719274019375980345, 63.95724293864770260 ) ) ;
#186532=CARTESIAN_POINT ( 'NONE',  ( -16.51473224551069308, -9.474510206698971260, 66.66557627198102409 ) ) ;
#186533=CARTESIAN_POINT ( 'NONE',  ( -21.53943276465977519, 0.05219959533907696930, 81.24890960531436690 ) ) ;
#186534=CARTESIAN_POINT ( 'NONE',  ( 4.379528057220092307, 16.55341960407617563, 72.29275706135236135 ) ) ;
#186536=CARTESIAN_POINT ( 'NONE',  ( -5.153800228976328057, -19.02544592524343514, 52.29057627198100988 ) ) ;
#186537=CARTESIAN_POINT ( 'NONE',  ( 8.314922557960818139, 14.29746914071049879, 74.58224293864768129 ) ) ;
#186539=CARTESIAN_POINT ( 'NONE',  ( -16.51473224551069308, -9.474510206698971260, 46.66557627198102409 ) ) ;
#186540=CARTESIAN_POINT ( 'NONE',  ( -16.53943276465976808, 0.05219959533911058130, 111.2489096053143669 ) ) ;
#186541=CARTESIAN_POINT ( 'NONE',  ( -16.51473224551082808, 9.474510206698731452, 68.33442372801900433 ) ) ;
#186542=CARTESIAN_POINT ( 'NONE',  ( -8.224510206698948167, 14.34966873604960824, 85.41557627198102409 ) ) ;
#186543=CARTESIAN_POINT ( 'NONE',  ( -5.719274019375665041, -21.55341960407619695, 39.79275706135235424 ) ) ;
#186544=CARTESIAN_POINT ( 'NONE',  ( -5.153800228976328057, -19.02544592524343514, 32.29057627198102409 ) ) ;
#186545=CARTESIAN_POINT ( 'NONE',  ( 15.72974639402199770, -15.80617190586745480, 108.1239096053143811 ) ) ;
#186547=CARTESIAN_POINT ( 'NONE',  ( 12.14591786802309770, 12.06949235617756955, 94.37390960531436690 ) ) ;
#186549=CARTESIAN_POINT ( 'NONE',  ( 13.89961937509977652, -13.97604488694527269, 43.12390960531434558 ) ) ;
#186551=CARTESIAN_POINT ( 'NONE',  ( 9.564922557961047289, -16.46253265017146816, 100.4177570613523329 ) ) ;
#186552=CARTESIAN_POINT ( 'NONE',  ( 19.03943276465977164, -0.05219959533909143690, 98.74890960531436690 ) ) ;
#186553=CARTESIAN_POINT ( 'NONE',  ( 0.05219959533937995610, -21.53943276465977519, 35.00109039468568284 ) ) ;
#186554=CARTESIAN_POINT ( 'NONE',  ( 16.46253265017160672, -9.564922557960803928, 83.33224293864768129 ) ) ;
#186555=CARTESIAN_POINT ( 'NONE',  ( 19.03943276465977164, 0.05219959533936151252, 71.25109039468566152 ) ) ;
#186556=CARTESIAN_POINT ( 'NONE',  ( 13.89961937509977652, -13.97604488694527269, 43.12390960531434558 ) ) ;
#186557=CARTESIAN_POINT ( 'NONE',  ( 14.34966873604960469, 8.224510206698951720, 79.16557627198103830 ) ) ;
#186558=CARTESIAN_POINT ( 'NONE',  ( 8.314922557960818139, 14.29746914071049879, 69.58224293864769550 ) ) ;
#186559=CARTESIAN_POINT ( 'NONE',  ( -0.05219959533909027116, -19.03943276465977164, 77.49890960531435269 ) ) ;
#186560=CARTESIAN_POINT ( 'NONE',  ( 21.55341960407610458, 5.719274019375980345, 103.9572429386476813 ) ) ;
#186561=CARTESIAN_POINT ( 'NONE',  ( -16.46253265017160317, 9.564922557960807481, 65.83224293864769550 ) ) ;
#186562=CARTESIAN_POINT ( 'NONE',  ( -21.53943276465977519, -0.05219959533937600094, 113.7510903946856757 ) ) ;
#186563=CARTESIAN_POINT ( 'NONE',  ( 13.89961937509977652, -13.97604488694527269, 43.12390960531434558 ) ) ;
#186564=CARTESIAN_POINT ( 'NONE',  ( 12.14591786802309770, 12.06949235617756955, 29.37390960531435269 ) ) ;
#186565=CARTESIAN_POINT ( 'NONE',  ( 8.314922557960818139, 14.29746914071049879, 114.5822429386477097 ) ) ;
#186566=CARTESIAN_POINT ( 'NONE',  ( 16.46253265017146816, 9.564922557961045513, 101.6677570613523329 ) ) ;
#186568=CARTESIAN_POINT ( 'NONE',  ( 5.823673210054444382, -21.52544592524334988, 25.20942372801901854 ) ) ;
#186569=CARTESIAN_POINT ( 'NONE',  ( 19.05341960407617918, -5.049401038297876454, 61.04275706135232582 ) ) ;
#186570=CARTESIAN_POINT ( 'NONE',  ( 16.52544592524342804, -4.483927247898539470, 28.54057627198103120 ) ) ;
#186571=CARTESIAN_POINT ( 'NONE',  ( 21.55341960407610458, 5.719274019375980345, 68.95724293864769550 ) ) ;
#186572=CARTESIAN_POINT ( 'NONE',  ( 5.823673210054125526, 21.52544592524343514, 24.79057627198103120 ) ) ;
#186573=CARTESIAN_POINT ( 'NONE',  ( -8.314922557960811034, -14.29746914071050412, 52.08224293864768839 ) ) ;
#186574=CARTESIAN_POINT ( 'NONE',  ( -16.46253265017160317, 9.564922557960807481, 25.83224293864769194 ) ) ;
#186575=CARTESIAN_POINT ( 'NONE',  ( -5.049401038298153566, 19.05341960407611168, 50.20724293864770260 ) ) ;
#186576=CARTESIAN_POINT ( 'NONE',  ( -9.564922557961040184, 16.46253265017147172, 27.91775706135232582 ) ) ;
#186577=CARTESIAN_POINT ( 'NONE',  ( -4.483927247898782831, 16.52544592524335698, 87.70942372801901854 ) ) ;
#186578=CARTESIAN_POINT ( 'NONE',  ( -8.224510206698735004, -14.34966873604973081, 59.58442372801901854 ) ) ;
#186579=CARTESIAN_POINT ( 'NONE',  ( -15.80617190586745835, -15.72974639402198527, 26.87390960531435979 ) ) ;
#186580=CARTESIAN_POINT ( 'NONE',  ( -10.81492255796105439, 18.62759615963255655, 112.9177570613523329 ) ) ;
#186581=CARTESIAN_POINT ( 'NONE',  ( -5.153800228976328057, -19.02544592524343514, 77.29057627198099567 ) ) ;
#186582=CARTESIAN_POINT ( 'NONE',  ( 12.06949235617739724, 12.14591786802326823, 66.87609039468568994 ) ) ;
#186583=CARTESIAN_POINT ( 'NONE',  ( -8.224510206698948167, 14.34966873604960824, 105.4155762719810383 ) ) ;
#186585=CARTESIAN_POINT ( 'NONE',  ( -16.52544592524335698, -4.483927247898792601, 108.9594237280190185 ) ) ;
#186587=CARTESIAN_POINT ( 'NONE',  ( 21.55341960407619695, -5.719274019375665929, 66.04275706135236135 ) ) ;
#186588=CARTESIAN_POINT ( 'NONE',  ( 5.049401038298161559, -19.05341960407611168, 97.70724293864766707 ) ) ;
#186589=CARTESIAN_POINT ( 'NONE',  ( 9.474510206698971260, -16.51473224551069308, 72.91557627198102409 ) ) ;
#186590=CARTESIAN_POINT ( 'NONE',  ( -0.05219959533909027116, -19.03943276465977164, 107.4989096053143527 ) ) ;
#186591=CARTESIAN_POINT ( 'NONE',  ( -12.06949235617756955, 12.14591786802309770, 55.62390960531436690 ) ) ;
#186592=CARTESIAN_POINT ( 'NONE',  ( 16.52544592524335698, 4.483927247898782831, 111.4594237280190328 ) ) ;
#186593=CARTESIAN_POINT ( 'NONE',  ( -12.14591786802309592, -12.06949235617757132, 46.87390960531435979 ) ) ;
#186594=CARTESIAN_POINT ( 'NONE',  ( 12.06949235617739724, 12.14591786802326823, 46.87609039468568994 ) ) ;
#186596=CARTESIAN_POINT ( 'NONE',  ( 5.153800228976615827, -19.02544592524334988, 35.20942372801899722 ) ) ;
#186597=CARTESIAN_POINT ( 'NONE',  ( 19.02544592524343514, -5.153800228976328945, 73.54057627198103830 ) ) ;
#186598=CARTESIAN_POINT ( 'NONE',  ( -19.05341960407617563, 5.049401038297882671, 48.54275706135233293 ) ) ;
#186599=CARTESIAN_POINT ( 'NONE',  ( -19.02544592524334988, -5.153800228976617603, 58.95942372801900433 ) ) ;
#186600=CARTESIAN_POINT ( 'NONE',  ( -19.02544592524334988, -5.153800228976617603, 103.9594237280190043 ) ) ;
#186601=CARTESIAN_POINT ( 'NONE',  ( 8.314922557961029526, -14.29746914071037800, 85.41775706135236135 ) ) ;
#186602=CARTESIAN_POINT ( 'NONE',  ( -5.153800228976328057, -19.02544592524343514, 27.29057627198103120 ) ) ;
#186603=CARTESIAN_POINT ( 'NONE',  ( -19.05341960407611168, -5.049401038298163336, 106.4572429386476955 ) ) ;
#186604=CARTESIAN_POINT ( 'NONE',  ( 18.67979575497194134, -10.72451020669871369, 35.83442372801901143 ) ) ;
#186605=CARTESIAN_POINT ( 'NONE',  ( 13.97604488694548053, -13.89961937509957401, 95.62609039468563310 ) ) ;
#186606=CARTESIAN_POINT ( 'NONE',  ( 17.50000000000000355, -3.805241302050290209, 107.8735247278259521 ) ) ;
#186607=CARTESIAN_POINT ( 'NONE',  ( -19.03943276465977164, 0.05219959533909376836, 66.24890960531436690 ) ) ;
#186608=CARTESIAN_POINT ( 'NONE',  ( -5.049401038298153566, 19.05341960407611168, 100.2072429386476955 ) ) ;
#186609=CARTESIAN_POINT ( 'NONE',  ( 4.379528057220339221, -16.55341960407611168, 62.70724293864769550 ) ) ;
#186610=CARTESIAN_POINT ( 'NONE',  ( -19.03943276465977164, 0.05219959533909376836, 51.24890960531436690 ) ) ;
#186611=CARTESIAN_POINT ( 'NONE',  ( -19.02544592524342804, 5.153800228976336051, 66.04057627198103830 ) ) ;
#186612=CARTESIAN_POINT ( 'NONE',  ( -19.05341960407617563, 5.049401038297882671, 68.54275706135230450 ) ) ;
#186613=CARTESIAN_POINT ( 'NONE',  ( -5.049401038297874678, -19.05341960407617918, 49.79275706135231871 ) ) ;
#186614=CARTESIAN_POINT ( 'NONE',  ( -9.474510206698964154, 16.51473224551069663, 75.41557627198103830 ) ) ;
#186615=CARTESIAN_POINT ( 'NONE',  ( 10.72451020669898902, -18.67979575497178502, 77.91557627198102409 ) ) ;
#186616=CARTESIAN_POINT ( 'NONE',  ( -8.224510206698948167, 14.34966873604960824, 60.41557627198102409 ) ) ;
#186617=CARTESIAN_POINT ( 'NONE',  ( 16.51473224551083163, -9.474510206698727899, 40.83442372801900433 ) ) ;
#186618=CARTESIAN_POINT ( 'NONE',  ( -5.823673210054116645, -21.52544592524344225, 42.29057627198103120 ) ) ;
#186619=CARTESIAN_POINT ( 'NONE',  ( 5.823673210054125526, 21.52544592524343514, 34.79057627198103120 ) ) ;
#186620=CARTESIAN_POINT ( 'NONE',  ( -19.03943276465977164, 0.05219959533909376836, 71.24890960531435269 ) ) ;
#186621=CARTESIAN_POINT ( 'NONE',  ( 19.05341960407611168, 5.049401038298154454, 58.95724293864768129 ) ) ;
#186622=CARTESIAN_POINT ( 'NONE',  ( 14.29746914071049879, -8.314922557960816363, 108.3322429386477097 ) ) ;
#186624=CARTESIAN_POINT ( 'NONE',  ( 10.81492255796106328, -18.62759615963255655, 20.41775706135234714 ) ) ;
#186625=CARTESIAN_POINT ( 'NONE',  ( 0.05219959533909260263, 19.03943276465977164, 109.9989096053143669 ) ) ;
#186626=CARTESIAN_POINT ( 'NONE',  ( 5.823673210054444382, -21.52544592524334988, 25.20942372801901854 ) ) ;
#186627=CARTESIAN_POINT ( 'NONE',  ( -0.05219959533909027116, -19.03943276465977164, 32.49890960531435979 ) ) ;
#186628=CARTESIAN_POINT ( 'NONE',  ( -21.53943276465977519, 0.05219959533907696930, 101.2489096053143669 ) ) ;
#186629=CARTESIAN_POINT ( 'NONE',  ( 16.46253265017146816, 9.564922557961045513, 46.66775706135233293 ) ) ;
#186631=CARTESIAN_POINT ( 'NONE',  ( -13.89961937509977652, 13.97604488694528158, 25.62390960531434558 ) ) ;
#186632=DIRECTION ( 'NONE',  ( 0.000000000000000000, 0.000000000000000000, -1.000000000000000000 ) ) ;
#186633=CARTESIAN_POINT ( 'NONE',  ( 0.05219959533934541429, -16.53943276465976808, 60.00109039468568284 ) ) ;
#186634=CARTESIAN_POINT ( 'NONE',  ( -14.29746914071049879, 8.314922557960819915, 115.8322429386477097 ) ) ;
#186636=CARTESIAN_POINT ( 'NONE',  ( -13.97604488694527625, -13.89961937509977652, 71.87390960531433848 ) ) ;
#186637=CARTESIAN_POINT ( 'NONE',  ( 8.224510206698953496, -14.34966873604960469, 107.9155762719810241 ) ) ;
#186638=CARTESIAN_POINT ( 'NONE',  ( 21.55341960407610458, 5.719274019375980345, 48.95724293864770971 ) ) ;
#186639=CARTESIAN_POINT ( 'NONE',  ( -14.34966873604960291, -8.224510206698953496, 76.66557627198103830 ) ) ;
#186640=CARTESIAN_POINT ( 'NONE',  ( -8.314922557961024197, 14.29746914071037800, 27.91775706135234358 ) ) ;
#186641=CARTESIAN_POINT ( 'NONE',  ( 10.81492255796106328, -18.62759615963255655, 85.41775706135236135 ) ) ;
#186642=CARTESIAN_POINT ( 'NONE',  ( 16.51473224551069308, 9.474510206698969483, 24.16557627198102765 ) ) ;
#186643=CARTESIAN_POINT ( 'NONE',  ( -8.314922557961024197, 14.29746914071037800, 112.9177570613523329 ) ) ;
#186644=CARTESIAN_POINT ( 'NONE',  ( 0.05219959533910956823, 16.53943276465976808, 59.99890960531436690 ) ) ;
#186645=CARTESIAN_POINT ( 'NONE',  ( -5.049401038298153566, 19.05341960407611168, 50.20724293864770260 ) ) ;
#186646=CARTESIAN_POINT ( 'NONE',  ( 21.53943276465977519, 0.05219959533937863772, 101.2510903946856757 ) ) ;
#186647=CARTESIAN_POINT ( 'NONE',  ( -15.72974639402197994, 15.80617190586746368, 110.6239096053143669 ) ) ;
#186648=CARTESIAN_POINT ( 'NONE',  ( -5.823673210054431948, 21.52544592524334988, 72.70942372801901854 ) ) ;
#186649=CARTESIAN_POINT ( 'NONE',  ( -0.05219959533934338120, 16.53943276465976808, 42.50109039468567573 ) ) ;
#186650=CARTESIAN_POINT ( 'NONE',  ( 12.06949235617757843, -12.14591786802309237, 73.12390960531436690 ) ) ;
#186651=CARTESIAN_POINT ( 'NONE',  ( -5.823673210054431948, 21.52544592524334988, 82.70942372801900433 ) ) ;
#186652=CIRCLE ( 'NONE', #125292, 2.000000000000001776 ) ;
#186653=CARTESIAN_POINT ( 'NONE',  ( -12.06949235617756955, 12.14591786802309770, 25.62390960531435624 ) ) ;
#186654=CARTESIAN_POINT ( 'NONE',  ( 17.60769864724393940, -5.499999999999833022, 61.15024842019166584 ) ) ;
#186655=CARTESIAN_POINT ( 'NONE',  ( -0.05219959533934338120, 16.53943276465976808, 42.50109039468567573 ) ) ;
#186656=CARTESIAN_POINT ( 'NONE',  ( -16.52544592524342804, 4.483927247898546575, 46.04057627198103830 ) ) ;
#186657=CARTESIAN_POINT ( 'NONE',  ( -16.55341960407617563, 4.379528057220093196, 88.54275706135236135 ) ) ;
#186658=CARTESIAN_POINT ( 'NONE',  ( 9.474510206698971260, -16.51473224551069308, 97.91557627198102409 ) ) ;
#186659=CARTESIAN_POINT ( 'NONE',  ( -5.823673210054116645, -21.52544592524344225, 22.29057627198102765 ) ) ;
#186660=CARTESIAN_POINT ( 'NONE',  ( 18.67979575497194134, -10.72451020669871369, 100.8344237280190185 ) ) ;
#186661=CARTESIAN_POINT ( 'NONE',  ( -0.05219959533934338120, 16.53943276465976808, 102.5010903946856899 ) ) ;
#186662=CARTESIAN_POINT ( 'NONE',  ( 14.34966873604960469, 8.224510206698951720, 69.16557627198102409 ) ) ;
#186663=CARTESIAN_POINT ( 'NONE',  ( -5.049401038298153566, 19.05341960407611168, 80.20724293864769550 ) ) ;
#186665=CARTESIAN_POINT ( 'NONE',  ( -16.52544592524335698, -4.483927247898792601, 28.95942372801902209 ) ) ;
#186666=CARTESIAN_POINT ( 'NONE',  ( 5.049401038298161559, -19.05341960407611168, 32.70724293864768129 ) ) ;
#186667=CARTESIAN_POINT ( 'NONE',  ( -13.97604488694527625, -13.89961937509977652, 86.87390960531436690 ) ) ;
#186668=CARTESIAN_POINT ( 'NONE',  ( -14.34966873604972548, 8.224510206698743886, 33.33442372801900433 ) ) ;
#186670=CARTESIAN_POINT ( 'NONE',  ( 13.89961937509957401, 13.97604488694547697, 36.87609039468565442 ) ) ;
#186671=CARTESIAN_POINT ( 'NONE',  ( 8.224510206698742110, 14.34966873604972548, 92.08442372801901854 ) ) ;
#186672=CARTESIAN_POINT ( 'NONE',  ( -5.049401038297874678, -19.05341960407617918, 109.7927570613523187 ) ) ;
#186673=CARTESIAN_POINT ( 'NONE',  ( -0.05219959533909027116, -19.03943276465977164, 27.49890960531435624 ) ) ;
#186674=CARTESIAN_POINT ( 'NONE',  ( -14.29746914071037622, -8.314922557961029526, 74.16775706135231871 ) ) ;
#186675=CARTESIAN_POINT ( 'NONE',  ( -16.55341960407617563, 4.379528057220093196, 68.54275706135234714 ) ) ;
#186676=CARTESIAN_POINT ( 'NONE',  ( 13.97604488694527802, 13.89961937509977652, 34.37390960531436690 ) ) ;
#186677=CARTESIAN_POINT ( 'NONE',  ( -16.51473224551082808, 9.474510206698731452, 73.33442372801900433 ) ) ;
#186678=CARTESIAN_POINT ( 'NONE',  ( -16.46253265017146816, -9.564922557961047289, 19.16775706135233293 ) ) ;
#186679=CARTESIAN_POINT ( 'NONE',  ( -5.153800228976328057, -19.02544592524343514, 47.29057627198102409 ) ) ;
#186680=CARTESIAN_POINT ( 'NONE',  ( 13.89961937509977652, -13.97604488694527269, 98.12390960531433848 ) ) ;
#186681=CARTESIAN_POINT ( 'NONE',  ( -4.483927247898539470, -16.52544592524342804, 87.29057627198103830 ) ) ;
#186682=CARTESIAN_POINT ( 'NONE',  ( -19.02544592524334988, -5.153800228976617603, 48.95942372801900433 ) ) ;
#186683=CARTESIAN_POINT ( 'NONE',  ( 18.62759615963271287, -10.81492255796078972, 53.33224293864769550 ) ) ;
#186684=CARTESIAN_POINT ( 'NONE',  ( -13.89961937509957401, -13.97604488694547875, 34.37609039468566863 ) ) ;
#186685=CARTESIAN_POINT ( 'NONE',  ( 0.05219959533909260263, 19.03943276465977164, 84.99890960531436690 ) ) ;
#186686=CARTESIAN_POINT ( 'NONE',  ( 0.05219959533936267826, -19.03943276465977164, 20.00109039468567218 ) ) ;
#186687=CARTESIAN_POINT ( 'NONE',  ( -5.823673210054116645, -21.52544592524344225, 62.29057627198102409 ) ) ;
#186688=CARTESIAN_POINT ( 'NONE',  ( -19.03943276465977164, 0.05219959533909376836, 106.2489096053143669 ) ) ;
#186689=CARTESIAN_POINT ( 'NONE',  ( 5.153800228976615827, -19.02544592524334988, 90.20942372801900433 ) ) ;
#186690=CARTESIAN_POINT ( 'NONE',  ( 5.153800228976335163, 19.02544592524342804, 109.7905762719810099 ) ) ;
#186691=CARTESIAN_POINT ( 'NONE',  ( -13.97604488694547697, 13.89961937509957934, 113.1260903946856757 ) ) ;
#186692=CARTESIAN_POINT ( 'NONE',  ( -4.379528057220328563, 16.55341960407611168, 115.2072429386476955 ) ) ;
#186693=CARTESIAN_POINT ( 'NONE',  ( -9.474510206698964154, 16.51473224551069663, 100.4155762719810241 ) ) ;
#186694=CARTESIAN_POINT ( 'NONE',  ( 21.53943276465977519, -0.05219959533907433946, 73.74890960531433848 ) ) ;
#186695=CARTESIAN_POINT ( 'NONE',  ( 16.55341960407618274, -4.379528057220086978, 46.04275706135234714 ) ) ;
#186696=CARTESIAN_POINT ( 'NONE',  ( -21.53943276465977519, -0.05219959533937600094, 43.75109039468568284 ) ) ;
#186697=CARTESIAN_POINT ( 'NONE',  ( -18.62759615963255300, -10.81492255796106328, 94.16775706135237556 ) ) ;
#186698=CARTESIAN_POINT ( 'NONE',  ( -14.29746914071037622, -8.314922557961029526, 94.16775706135237556 ) ) ;
#186699=CARTESIAN_POINT ( 'NONE',  ( -0.05219959533909027116, -19.03943276465977164, 87.49890960531436690 ) ) ;
#186700=CARTESIAN_POINT ( 'NONE',  ( 14.29746914071049879, -8.314922557960816363, 93.33224293864769550 ) ) ;
#186701=CARTESIAN_POINT ( 'NONE',  ( -12.14591786802309592, -12.06949235617757132, 31.87390960531435979 ) ) ;
#186702=CARTESIAN_POINT ( 'NONE',  ( 19.03943276465977164, 0.05219959533936151252, 66.25109039468567573 ) ) ;
#186704=CARTESIAN_POINT ( 'NONE',  ( -0.05219959533937732626, 21.53943276465977519, 57.50109039468568994 ) ) ;
#186705=CARTESIAN_POINT ( 'NONE',  ( 19.03943276465977164, 0.05219959533936151252, 21.25109039468565797 ) ) ;
#186706=CARTESIAN_POINT ( 'NONE',  ( -8.224510206698948167, 14.34966873604960824, 90.41557627198103830 ) ) ;
#186707=CARTESIAN_POINT ( 'NONE',  ( 5.823673210054125526, 21.52544592524343514, 24.79057627198103120 ) ) ;
#186708=CARTESIAN_POINT ( 'NONE',  ( 16.55341960407618274, -4.379528057220086978, 111.0427570613523613 ) ) ;
#186709=CARTESIAN_POINT ( 'NONE',  ( 10.72451020669871369, 18.67979575497193778, 97.08442372801904696 ) ) ;
#186710=CARTESIAN_POINT ( 'NONE',  ( -8.224510206698735004, -14.34966873604973081, 54.58442372801901143 ) ) ;
#186711=CARTESIAN_POINT ( 'NONE',  ( 14.34966873604972726, -8.224510206698740333, 105.8344237280190328 ) ) ;
#186712=CARTESIAN_POINT ( 'NONE',  ( -18.67979575497193778, 10.72451020669871902, 48.33442372801902565 ) ) ;
#186713=CARTESIAN_POINT ( 'NONE',  ( -10.72451020669870658, -18.67979575497194134, 59.58442372801901854 ) ) ;
#186715=CARTESIAN_POINT ( 'NONE',  ( 5.719274019375673035, 21.55341960407619339, 27.29275706135234358 ) ) ;
#186716=CARTESIAN_POINT ( 'NONE',  ( 16.52544592524342804, -4.483927247898539470, 103.5405762719810383 ) ) ;
#186717=CARTESIAN_POINT ( 'NONE',  ( -19.05341960407611168, -5.049401038298163336, 26.45724293864769550 ) ) ;
#186718=CARTESIAN_POINT ( 'NONE',  ( -16.55341960407611168, -4.379528057220339221, 66.45724293864768129 ) ) ;
#186719=CARTESIAN_POINT ( 'NONE',  ( -13.89961937509977652, 13.97604488694528158, 65.62390960531436690 ) ) ;
#186720=CARTESIAN_POINT ( 'NONE',  ( -0.05219959533934338120, 16.53943276465976808, 107.5010903946856899 ) ) ;
#186721=CARTESIAN_POINT ( 'NONE',  ( 0.05219959533907565091, 21.53943276465977519, 59.99890960531436690 ) ) ;
#186722=CARTESIAN_POINT ( 'NONE',  ( -14.29746914071049879, 8.314922557960819915, 85.83224293864768129 ) ) ;
#186723=CARTESIAN_POINT ( 'NONE',  ( -21.55341960407610458, -5.719274019375992779, 91.45724293864769550 ) ) ;
#186724=CARTESIAN_POINT ( 'NONE',  ( -16.46253265017160317, 9.564922557960807481, 100.8322429386477097 ) ) ;
#186725=CARTESIAN_POINT ( 'NONE',  ( 19.03943276465977164, -0.05219959533909143690, 53.74890960531436690 ) ) ;
#186726=CARTESIAN_POINT ( 'NONE',  ( -5.153800228976607833, 19.02544592524334988, 102.7094237280189759 ) ) ;
#186727=CARTESIAN_POINT ( 'NONE',  ( -15.80617190586745835, -15.72974639402198527, 46.87390960531435979 ) ) ;
#186728=CARTESIAN_POINT ( 'NONE',  ( -10.72451020669870658, -18.67979575497194134, 74.58442372801901854 ) ) ;
#186729=CARTESIAN_POINT ( 'NONE',  ( 0.05219959533909260263, 19.03943276465977164, 64.99890960531436690 ) ) ;
#186730=CARTESIAN_POINT ( 'NONE',  ( 9.474510206698971260, -16.51473224551069308, 97.91557627198102409 ) ) ;
#186731=CARTESIAN_POINT ( 'NONE',  ( -16.53943276465976808, -0.05219959533934237506, 58.75109039468568994 ) ) ;
#186732=CARTESIAN_POINT ( 'NONE',  ( 15.72974639402176855, 15.80617190586768217, 46.87609039468568994 ) ) ;
#186733=CARTESIAN_POINT ( 'NONE',  ( -5.719274019375665041, -21.55341960407619695, 89.79275706135236135 ) ) ;
#186734=CARTESIAN_POINT ( 'NONE',  ( 15.80617190586746368, 15.72974639402197994, 99.37390960531436690 ) ) ;
#186735=CARTESIAN_POINT ( 'NONE',  ( 15.72974639402176855, 15.80617190586768217, 41.87609039468568284 ) ) ;
#186736=CARTESIAN_POINT ( 'NONE',  ( 16.53943276465976808, 0.05219959533934440121, 81.25109039468568994 ) ) ;
#186737=CARTESIAN_POINT ( 'NONE',  ( -21.55341960407610458, -5.719274019375992779, 81.45724293864769550 ) ) ;
#186738=CARTESIAN_POINT ( 'NONE',  ( -9.474510206698720793, -16.51473224551083518, 34.58442372801899722 ) ) ;
#186739=CARTESIAN_POINT ( 'NONE',  ( 5.153800228976335163, 19.02544592524342804, 79.79057627198102409 ) ) ;
#186740=CARTESIAN_POINT ( 'NONE',  ( -4.379528057220328563, 16.55341960407611168, 25.20724293864769550 ) ) ;
#186741=CARTESIAN_POINT ( 'NONE',  ( 18.09805431107249518, -5.499999999999974243, 83.51606229291887473 ) ) ;
#186742=CARTESIAN_POINT ( 'NONE',  ( -0.05219959533909027116, -19.03943276465977164, 97.49890960531436690 ) ) ;
#186744=EDGE_CURVE ( 'NONE', #61486, #147783, #76724, .T. ) ;
#186745=CARTESIAN_POINT ( 'NONE',  ( -9.564922557961040184, 16.46253265017147172, 82.91775706135233293 ) ) ;
#186746=CARTESIAN_POINT ( 'NONE',  ( 21.55341960407610458, 5.719274019375980345, 63.95724293864770260 ) ) ;
#186747=CARTESIAN_POINT ( 'NONE',  ( -0.05219959533910754901, -16.53943276465976808, 42.49890960531435979 ) ) ;
#186748=CARTESIAN_POINT ( 'NONE',  ( 14.29746914071037800, 8.314922557961029526, 21.66775706135235069 ) ) ;
#186749=CARTESIAN_POINT ( 'NONE',  ( -13.89961937509977652, 13.97604488694528158, 30.62390960531435269 ) ) ;
#186750=CARTESIAN_POINT ( 'NONE',  ( -12.06949235617739369, -12.14591786802326823, 19.37609039468568639 ) ) ;
#186751=CARTESIAN_POINT ( 'NONE',  ( -15.80617190586745835, -15.72974639402198527, 96.87390960531436690 ) ) ;
#186752=CARTESIAN_POINT ( 'NONE',  ( -5.153800228976607833, 19.02544592524334988, 72.70942372801900433 ) ) ;
#186753=CARTESIAN_POINT ( 'NONE',  ( 8.224510206698742110, 14.34966873604972548, 77.08442372801901854 ) ) ;
#186754=CARTESIAN_POINT ( 'NONE',  ( 19.02544592524343514, -5.153800228976328945, 73.54057627198103830 ) ) ;
#186755=CARTESIAN_POINT ( 'NONE',  ( -16.55341960407611168, -4.379528057220339221, 71.45724293864769550 ) ) ;
#186756=CARTESIAN_POINT ( 'NONE',  ( 19.03943276465977164, -0.05219959533909143690, 58.74890960531435979 ) ) ;
#186757=CARTESIAN_POINT ( 'NONE',  ( -8.224510206698948167, 14.34966873604960824, 65.41557627198102409 ) ) ;
#186760=CARTESIAN_POINT ( 'NONE',  ( 12.06949235617757843, -12.14591786802309237, 48.12390960531436690 ) ) ;
#186761=CARTESIAN_POINT ( 'NONE',  ( -19.03943276465977164, 0.05219959533909376836, 76.24890960531435269 ) ) ;
#186763=CARTESIAN_POINT ( 'NONE',  ( 9.564922557961047289, -16.46253265017146816, 35.41775706135233293 ) ) ;
#186764=CARTESIAN_POINT ( 'NONE',  ( 16.53943276465976808, 0.05219959533934440121, 61.25109039468567573 ) ) ;
#186765=CARTESIAN_POINT ( 'NONE',  ( 18.62759615963271287, -10.81492255796078972, 68.33224293864769550 ) ) ;
#186766=CARTESIAN_POINT ( 'NONE',  ( 19.05341960407617918, -5.049401038297876454, 26.04275706135233293 ) ) ;
#186767=CARTESIAN_POINT ( 'NONE',  ( -16.46253265017160317, 9.564922557960807481, 70.83224293864770971 ) ) ;
#186769=CARTESIAN_POINT ( 'NONE',  ( 13.97604488694527802, 13.89961937509977652, 109.3739096053143669 ) ) ;
#186770=CARTESIAN_POINT ( 'NONE',  ( -19.05341960407611168, -5.049401038298163336, 56.45724293864768129 ) ) ;
#186771=CARTESIAN_POINT ( 'NONE',  ( -0.05219959533937732626, 21.53943276465977519, 42.50109039468567573 ) ) ;
#186772=CARTESIAN_POINT ( 'NONE',  ( 8.314922557960818139, 14.29746914071049879, 109.5822429386476955 ) ) ;
#186773=CARTESIAN_POINT ( 'NONE',  ( -5.823673210054116645, -21.52544592524344225, 97.29057627198105251 ) ) ;
#186774=CARTESIAN_POINT ( 'NONE',  ( 0.05219959533909260263, 19.03943276465977164, 84.99890960531436690 ) ) ;
#186776=CARTESIAN_POINT ( 'NONE',  ( 18.62759615963255655, 10.81492255796105972, 26.66775706135235424 ) ) ;
#186779=CARTESIAN_POINT ( 'NONE',  ( -9.564922557960796823, -16.46253265017161027, 82.08224293864768129 ) ) ;
#186781=CARTESIAN_POINT ( 'NONE',  ( -15.80617190586745835, -15.72974639402198527, 96.87390960531436690 ) ) ;
#186782=CARTESIAN_POINT ( 'NONE',  ( -16.46253265017160317, 9.564922557960807481, 40.83224293864769550 ) ) ;
#186783=CARTESIAN_POINT ( 'NONE',  ( 19.02544592524334988, 5.153800228976608722, 101.4594237280189759 ) ) ;
#186785=CARTESIAN_POINT ( 'NONE',  ( -19.03943276465977164, 0.05219959533909376836, 31.24890960531435979 ) ) ;
#186786=CARTESIAN_POINT ( 'NONE',  ( 10.81492255796106328, -18.62759615963255655, 90.41775706135236135 ) ) ;
#186787=CARTESIAN_POINT ( 'NONE',  ( -16.51473224551069308, -9.474510206698971260, 81.66557627198103830 ) ) ;
#186788=CARTESIAN_POINT ( 'NONE',  ( -5.719274019375665041, -21.55341960407619695, 49.79275706135234714 ) ) ;
#186789=CARTESIAN_POINT ( 'NONE',  ( -15.72974639402176322, -15.80617190586768395, 29.37609039468568284 ) ) ;
#186791=CARTESIAN_POINT ( 'NONE',  ( 19.03943276465977164, -0.05219959533909143690, 88.74890960531436690 ) ) ;
#186793=CARTESIAN_POINT ( 'NONE',  ( 8.314922557961029526, -14.29746914071037800, 35.41775706135234003 ) ) ;
#186794=CARTESIAN_POINT ( 'NONE',  ( -5.823673210054116645, -21.52544592524344225, 47.29057627198103120 ) ) ;
#186795=CARTESIAN_POINT ( 'NONE',  ( 5.823673210054444382, -21.52544592524334988, 50.20942372801901854 ) ) ;
#186796=CARTESIAN_POINT ( 'NONE',  ( 18.62759615963255655, 10.81492255796105972, 71.66775706135234714 ) ) ;
#186797=CARTESIAN_POINT ( 'NONE',  ( 17.72566875460847768, -5.500000000000063061, 38.42186708195907130 ) ) ;
#186798=CARTESIAN_POINT ( 'NONE',  ( -0.05219959533936034679, 19.03943276465977164, 107.5010903946856615 ) ) ;
#186799=CARTESIAN_POINT ( 'NONE',  ( 13.97604488694527802, 13.89961937509977652, 59.37390960531434558 ) ) ;
#186800=CARTESIAN_POINT ( 'NONE',  ( 13.89961937509977652, -13.97604488694527269, 83.12390960531436690 ) ) ;
#186802=CARTESIAN_POINT ( 'NONE',  ( 12.06949235617757843, -12.14591786802309237, 103.1239096053143811 ) ) ;
#186803=CARTESIAN_POINT ( 'NONE',  ( 12.14591786802309770, 12.06949235617756955, 99.37390960531436690 ) ) ;
#186804=CARTESIAN_POINT ( 'NONE',  ( 0.05219959533909260263, 19.03943276465977164, 109.9989096053143669 ) ) ;
#186805=CARTESIAN_POINT ( 'NONE',  ( -4.379528057220086978, -16.55341960407618274, 79.79275706135236135 ) ) ;
#186806=CARTESIAN_POINT ( 'NONE',  ( -8.314922557960811034, -14.29746914071050412, 72.08224293864769550 ) ) ;
#186807=CARTESIAN_POINT ( 'NONE',  ( 0.05219959533909260263, 19.03943276465977164, 54.99890960531435979 ) ) ;
#186808=CARTESIAN_POINT ( 'NONE',  ( -21.55341960407619339, 5.719274019375674811, 83.54275706135234714 ) ) ;
#186809=CARTESIAN_POINT ( 'NONE',  ( 10.81492255796106328, -18.62759615963255655, 70.41775706135236135 ) ) ;
#186810=CARTESIAN_POINT ( 'NONE',  ( -9.564922557961040184, 16.46253265017147172, 102.9177570613523329 ) ) ;
#186811=CARTESIAN_POINT ( 'NONE',  ( -16.52544592524342804, 4.483927247898546575, 56.04057627198102409 ) ) ;
#186812=CARTESIAN_POINT ( 'NONE',  ( -5.823673210054431948, 21.52544592524334988, 22.70942372801901499 ) ) ;
#186813=CARTESIAN_POINT ( 'NONE',  ( -15.80617190586745835, -15.72974639402198527, 61.87390960531436690 ) ) ;
#186814=CARTESIAN_POINT ( 'NONE',  ( 17.50000000000000000, 5.499999999999997335, 120.0000000000000142 ) ) ;
#186816=CARTESIAN_POINT ( 'NONE',  ( 19.02544592524343514, -5.153800228976328945, 73.54057627198103830 ) ) ;
#186817=CARTESIAN_POINT ( 'NONE',  ( -12.06949235617756955, 12.14591786802309770, 35.62390960531437401 ) ) ;
#186818=CARTESIAN_POINT ( 'NONE',  ( 14.29746914071049879, -8.314922557960816363, 23.33224293864769194 ) ) ;
#186819=CARTESIAN_POINT ( 'NONE',  ( 4.483927247898790824, -16.52544592524335698, 100.2094237280190043 ) ) ;
#186820=CARTESIAN_POINT ( 'NONE',  ( -19.03943276465977164, -0.05219959533935918106, 53.75109039468566863 ) ) ;
#186822=CARTESIAN_POINT ( 'NONE',  ( -13.97604488694527625, -13.89961937509977652, 101.8739096053143811 ) ) ;
#186824=CARTESIAN_POINT ( 'NONE',  ( -0.05219959533910754901, -16.53943276465976808, 72.49890960531435269 ) ) ;
#186825=CARTESIAN_POINT ( 'NONE',  ( -13.89961937509957401, -13.97604488694547875, 49.37609039468567573 ) ) ;
#186826=CARTESIAN_POINT ( 'NONE',  ( 17.05587630539786659, -6.762274262135694158, 103.2418030903731250 ) ) ;
#186827=CARTESIAN_POINT ( 'NONE',  ( 13.89961937509977652, -13.97604488694527269, 113.1239096053143527 ) ) ;
#186828=CARTESIAN_POINT ( 'NONE',  ( -18.67979575497178146, -10.72451020669898902, 51.66557627198102409 ) ) ;
#186830=CARTESIAN_POINT ( 'NONE',  ( 16.52544592524342804, -4.483927247898539470, 103.5405762719810383 ) ) ;
#186831=CARTESIAN_POINT ( 'NONE',  ( 16.53943276465976808, 0.05219959533934440121, 46.25109039468567573 ) ) ;
#186832=CARTESIAN_POINT ( 'NONE',  ( -16.55341960407611168, -4.379528057220339221, 96.45724293864770971 ) ) ;
#186833=CARTESIAN_POINT ( 'NONE',  ( 16.20579543436675607, -7.371946100355228459, 36.93479165828124167 ) ) ;
#186834=CARTESIAN_POINT ( 'NONE',  ( -16.88567814943165146, 6.947325034625571050, 48.70998877347415856 ) ) ;
#186835=CARTESIAN_POINT ( 'NONE',  ( 5.049401038298161559, -19.05341960407611168, 112.7072429386476813 ) ) ;
#186838=CARTESIAN_POINT ( 'NONE',  ( -18.22780087662122028, 5.500000000000031086, 43.51540105326107977 ) ) ;
#186839=CARTESIAN_POINT ( 'NONE',  ( -16.53943276465976808, -0.05219959533934237506, 48.75109039468568284 ) ) ;
#186840=CARTESIAN_POINT ( 'NONE',  ( -4.483927247898539470, -16.52544592524342804, 27.29057627198103120 ) ) ;
#186841=CARTESIAN_POINT ( 'NONE',  ( 18.67979575497178502, 10.72451020669898547, 54.16557627198103120 ) ) ;
#186842=CARTESIAN_POINT ( 'NONE',  ( 9.474510206698729675, 16.51473224551082808, 82.08442372801899012 ) ) ;
#186843=CARTESIAN_POINT ( 'NONE',  ( 0.05219959533907565091, 21.53943276465977519, 54.99890960531435269 ) ) ;
#186844=CARTESIAN_POINT ( 'NONE',  ( 0.05219959533937995610, -21.53943276465977519, 85.00109039468568994 ) ) ;
#186846=CARTESIAN_POINT ( 'NONE',  ( 16.52544592524335698, 4.483927247898782831, 31.45942372801901854 ) ) ;
#186847=CARTESIAN_POINT ( 'NONE',  ( -5.153800228976328057, -19.02544592524343514, 42.29057627198101699 ) ) ;
#186848=CARTESIAN_POINT ( 'NONE',  ( -16.51473224551069308, -9.474510206698971260, 96.66557627198102409 ) ) ;
#186849=CARTESIAN_POINT ( 'NONE',  ( 19.05341960407611168, 5.049401038298154454, 33.95724293864769550 ) ) ;
#186850=CARTESIAN_POINT ( 'NONE',  ( 12.06949235617757843, -12.14591786802309237, 98.12390960531436690 ) ) ;
#186852=CARTESIAN_POINT ( 'NONE',  ( 5.153800228976335163, 19.02544592524342804, 94.79057627198103830 ) ) ;
#186854=CARTESIAN_POINT ( 'NONE',  ( 12.14591786802327356, -12.06949235617739191, 50.62609039468568994 ) ) ;
#186855=CARTESIAN_POINT ( 'NONE',  ( -21.53943276465977519, 0.05219959533907696930, 91.24890960531436690 ) ) ;
#186856=CARTESIAN_POINT ( 'NONE',  ( -19.03943276465977164, 0.05219959533909376836, 46.24890960531435979 ) ) ;
#186857=CARTESIAN_POINT ( 'NONE',  ( -10.81492255796105439, 18.62759615963255655, 32.91775706135234714 ) ) ;
#186858=CARTESIAN_POINT ( 'NONE',  ( -13.89961937509977652, 13.97604488694528158, 85.62390960531433848 ) ) ;
#186860=ORIENTED_EDGE ( 'NONE', *, *, #193126, .T. ) ;
#186861=CARTESIAN_POINT ( 'NONE',  ( 14.34966873604972726, -8.224510206698740333, 40.83442372801901854 ) ) ;
#186862=CARTESIAN_POINT ( 'NONE',  ( 10.72451020669871369, 18.67979575497193778, 22.08442372801901143 ) ) ;
#186863=CARTESIAN_POINT ( 'NONE',  ( -19.02544592524342804, 5.153800228976336051, 31.04057627198102409 ) ) ;
#186864=CARTESIAN_POINT ( 'NONE',  ( 19.03943276465977164, -0.05219959533909143690, 93.74890960531435269 ) ) ;
#186865=CARTESIAN_POINT ( 'NONE',  ( -16.46253265017146816, -9.564922557961047289, 79.16775706135234714 ) ) ;
#186866=CARTESIAN_POINT ( 'NONE',  ( -16.51473224551082808, 9.474510206698731452, 23.33442372801900078 ) ) ;
#186867=CARTESIAN_POINT ( 'NONE',  ( -5.719274019375978568, 21.55341960407610458, 85.20724293864770971 ) ) ;
#186868=CARTESIAN_POINT ( 'NONE',  ( -5.153800228976607833, 19.02544592524334988, 37.70942372801899722 ) ) ;
#186869=CARTESIAN_POINT ( 'NONE',  ( -4.379528057220086978, -16.55341960407618274, 79.79275706135236135 ) ) ;
#186870=CARTESIAN_POINT ( 'NONE',  ( 9.474510206698971260, -16.51473224551069308, 112.9155762719810383 ) ) ;
#186871=CARTESIAN_POINT ( 'NONE',  ( -13.89961937509977652, 13.97604488694528158, 65.62390960531436690 ) ) ;
#186872=CARTESIAN_POINT ( 'NONE',  ( 15.72974639402176855, 15.80617190586768217, 71.87609039468568994 ) ) ;
#186873=CARTESIAN_POINT ( 'NONE',  ( -0.05219959533937732626, 21.53943276465977519, 62.50109039468568284 ) ) ;
#186874=CARTESIAN_POINT ( 'NONE',  ( -9.564922557960796823, -16.46253265017161027, 77.08224293864769550 ) ) ;
#186875=CARTESIAN_POINT ( 'NONE',  ( 21.55341960407619695, -5.719274019375665929, 46.04275706135234714 ) ) ;
#186876=CARTESIAN_POINT ( 'NONE',  ( -5.153800228976607833, 19.02544592524334988, 87.70942372801897591 ) ) ;
#186877=CARTESIAN_POINT ( 'NONE',  ( -19.02544592524342804, 5.153800228976336051, 56.04057627198100988 ) ) ;
#186878=CARTESIAN_POINT ( 'NONE',  ( -16.51473224551069308, -9.474510206698971260, 101.6655762719810241 ) ) ;
#186879=CARTESIAN_POINT ( 'NONE',  ( -0.05219959533909027116, -19.03943276465977164, 72.49890960531435269 ) ) ;
#186880=CARTESIAN_POINT ( 'NONE',  ( -16.46253265017160317, 9.564922557960807481, 110.8322429386476955 ) ) ;
#186881=CARTESIAN_POINT ( 'NONE',  ( -19.02544592524342804, 5.153800228976336051, 56.04057627198100988 ) ) ;
#186882=CARTESIAN_POINT ( 'NONE',  ( -21.55341960407610458, -5.719274019375992779, 96.45724293864770971 ) ) ;
#186883=CARTESIAN_POINT ( 'NONE',  ( 14.34966873604972726, -8.224510206698740333, 75.83442372801900433 ) ) ;
#186885=CARTESIAN_POINT ( 'NONE',  ( -16.46253265017146816, -9.564922557961047289, 29.16775706135232937 ) ) ;
#186886=CARTESIAN_POINT ( 'NONE',  ( -9.474510206698964154, 16.51473224551069663, 60.41557627198102409 ) ) ;
#186887=CARTESIAN_POINT ( 'NONE',  ( -16.55341960407611168, -4.379528057220339221, 61.45724293864770260 ) ) ;
#186888=CARTESIAN_POINT ( 'NONE',  ( 12.14591786802309770, 12.06949235617756955, 99.37390960531436690 ) ) ;
#186889=CARTESIAN_POINT ( 'NONE',  ( -19.03943276465977164, 0.05219959533909376836, 106.2489096053143669 ) ) ;
#186890=CARTESIAN_POINT ( 'NONE',  ( -16.51473224551069308, -9.474510206698971260, 96.66557627198102409 ) ) ;
#186891=CARTESIAN_POINT ( 'NONE',  ( 5.153800228976335163, 19.02544592524342804, 109.7905762719810099 ) ) ;
#186892=CARTESIAN_POINT ( 'NONE',  ( 21.55341960407619695, -5.719274019375665929, 111.0427570613523613 ) ) ;
#186893=CARTESIAN_POINT ( 'NONE',  ( 4.379528057220092307, 16.55341960407617563, 77.29275706135234714 ) ) ;
#186894=CARTESIAN_POINT ( 'NONE',  ( 18.67979575497194134, -10.72451020669871369, 35.83442372801901143 ) ) ;
#186895=CARTESIAN_POINT ( 'NONE',  ( 15.80617190586746368, 15.72974639402197994, 29.37390960531435269 ) ) ;
#186896=CARTESIAN_POINT ( 'NONE',  ( -10.72451020669898014, 18.67979575497178502, 100.4155762719810241 ) ) ;
#186897=CARTESIAN_POINT ( 'NONE',  ( 8.314922557960818139, 14.29746914071049879, 59.58224293864770260 ) ) ;
#186898=CARTESIAN_POINT ( 'NONE',  ( 9.474510206698971260, -16.51473224551069308, 57.91557627198103120 ) ) ;
#186899=CARTESIAN_POINT ( 'NONE',  ( -0.05219959533910754901, -16.53943276465976808, 82.49890960531436690 ) ) ;
#186900=CARTESIAN_POINT ( 'NONE',  ( -18.67979575497178146, -10.72451020669898902, 41.66557627198103120 ) ) ;
#186901=CARTESIAN_POINT ( 'NONE',  ( -9.474510206698720793, -16.51473224551083518, 44.58442372801900433 ) ) ;
#186902=CARTESIAN_POINT ( 'NONE',  ( 16.55341960407611168, 4.379528057220329451, 113.9572429386477239 ) ) ;
#186904=CARTESIAN_POINT ( 'NONE',  ( 0.05219959533934541429, -16.53943276465976808, 65.00109039468568994 ) ) ;
#186905=CARTESIAN_POINT ( 'NONE',  ( 13.89961937509977652, -13.97604488694527269, 68.12390960531436690 ) ) ;
#186907=CARTESIAN_POINT ( 'NONE',  ( -16.53943276465976808, 0.05219959533911058130, 91.24890960531436690 ) ) ;
#186908=CARTESIAN_POINT ( 'NONE',  ( 21.55341960407610458, 5.719274019375980345, 33.95724293864769550 ) ) ;
#186909=CARTESIAN_POINT ( 'NONE',  ( 0.05219959533934541429, -16.53943276465976808, 105.0010903946856757 ) ) ;
#186910=CARTESIAN_POINT ( 'NONE',  ( 8.224510206698742110, 14.34966873604972548, 22.08442372801901143 ) ) ;
#186911=CARTESIAN_POINT ( 'NONE',  ( 15.80617190586769283, -15.72974639402175789, 90.62609039468567573 ) ) ;
#186912=CARTESIAN_POINT ( 'NONE',  ( -13.97604488694527625, -13.89961937509977652, 91.87390960531432427 ) ) ;
#186913=CARTESIAN_POINT ( 'NONE',  ( 5.823673210054444382, -21.52544592524334988, 25.20942372801901854 ) ) ;
#186914=CARTESIAN_POINT ( 'NONE',  ( -8.314922557961024197, 14.29746914071037800, 52.91775706135235424 ) ) ;
#186915=CARTESIAN_POINT ( 'NONE',  ( 9.564922557960805705, 16.46253265017160317, 29.58224293864769550 ) ) ;
#186916=CARTESIAN_POINT ( 'NONE',  ( 8.314922557961029526, -14.29746914071037800, 30.41775706135234358 ) ) ;
#186917=CARTESIAN_POINT ( 'NONE',  ( -19.02544592524334988, -5.153800228976617603, 88.95942372801897591 ) ) ;
#186919=CARTESIAN_POINT ( 'NONE',  ( -10.72451020669898014, 18.67979575497178502, 95.41557627198102409 ) ) ;
#186920=CARTESIAN_POINT ( 'NONE',  ( 0.05219959533936267826, -19.03943276465977164, 65.00109039468567573 ) ) ;
#186922=CARTESIAN_POINT ( 'NONE',  ( -5.823673210054431948, 21.52544592524334988, 22.70942372801901499 ) ) ;
#186923=CARTESIAN_POINT ( 'NONE',  ( 9.474510206698971260, -16.51473224551069308, 72.91557627198102409 ) ) ;
#186924=CARTESIAN_POINT ( 'NONE',  ( -16.46253265017160317, 9.564922557960807481, 75.83224293864769550 ) ) ;
#186925=CARTESIAN_POINT ( 'NONE',  ( 12.06949235617739724, 12.14591786802326823, 26.87609039468567218 ) ) ;
#186927=CARTESIAN_POINT ( 'NONE',  ( 9.474510206698729675, 16.51473224551082808, 57.08442372801900433 ) ) ;
#186928=CARTESIAN_POINT ( 'NONE',  ( -0.05219959533907301413, -21.53943276465977519, 112.4989096053143669 ) ) ;
#186929=CARTESIAN_POINT ( 'NONE',  ( -16.55341960407611168, -4.379528057220339221, 81.45724293864769550 ) ) ;
#186930=CARTESIAN_POINT ( 'NONE',  ( 16.46253265017160672, -9.564922557960803928, 78.33224293864769550 ) ) ;
#186931=CARTESIAN_POINT ( 'NONE',  ( -14.34966873604972548, 8.224510206698743886, 33.33442372801900433 ) ) ;
#186932=CARTESIAN_POINT ( 'NONE',  ( 19.02544592524334988, 5.153800228976608722, 36.45942372801900433 ) ) ;
#186933=CARTESIAN_POINT ( 'NONE',  ( -15.72974639402176322, -15.80617190586768395, 64.37609039468568994 ) ) ;
#186934=CARTESIAN_POINT ( 'NONE',  ( -4.379528057220086978, -16.55341960407618274, 19.79275706135235069 ) ) ;
#186935=CARTESIAN_POINT ( 'NONE',  ( 19.03943276465977164, -0.05219959533909143690, 53.74890960531436690 ) ) ;
#186936=CARTESIAN_POINT ( 'NONE',  ( -0.05219959533936034679, 19.03943276465977164, 82.50109039468567573 ) ) ;
#186937=CARTESIAN_POINT ( 'NONE',  ( 14.29746914071037800, 8.314922557961029526, 61.66775706135235424 ) ) ;
#186938=CARTESIAN_POINT ( 'NONE',  ( 18.67979575497194134, -10.72451020669871369, 95.83442372801903275 ) ) ;
#186939=CARTESIAN_POINT ( 'NONE',  ( 13.97604488694548053, -13.89961937509957401, 70.62609039468567573 ) ) ;
#186940=CARTESIAN_POINT ( 'NONE',  ( -9.474510206698964154, 16.51473224551069663, 45.41557627198103120 ) ) ;
#186941=CARTESIAN_POINT ( 'NONE',  ( 15.72974639402199770, -15.80617190586745480, 73.12390960531436690 ) ) ;
#186942=CARTESIAN_POINT ( 'NONE',  ( -4.483927247898539470, -16.52544592524342804, 67.29057627198103830 ) ) ;
#186943=CARTESIAN_POINT ( 'NONE',  ( 13.89961937509957401, 13.97604488694547697, 66.87609039468567573 ) ) ;
#186945=CARTESIAN_POINT ( 'NONE',  ( -13.89961937509957401, -13.97604488694547875, 39.37609039468566152 ) ) ;
#186946=CARTESIAN_POINT ( 'NONE',  ( -8.224510206698735004, -14.34966873604973081, 104.5844237280190185 ) ) ;
#186947=CARTESIAN_POINT ( 'NONE',  ( -16.53943276465976808, 0.05219959533911058130, 61.24890960531435979 ) ) ;
#186948=CARTESIAN_POINT ( 'NONE',  ( -21.52544592524334988, -5.823673210054445271, 88.95942372801901854 ) ) ;
#186950=CARTESIAN_POINT ( 'NONE',  ( 5.823673210054125526, 21.52544592524343514, 99.79057627198103830 ) ) ;
#186952=CARTESIAN_POINT ( 'NONE',  ( -5.049401038298153566, 19.05341960407611168, 55.20724293864769550 ) ) ;
#186953=CARTESIAN_POINT ( 'NONE',  ( -21.55341960407619339, 5.719274019375674811, 68.54275706135234714 ) ) ;
#186954=CARTESIAN_POINT ( 'NONE',  ( 19.05341960407611168, 5.049401038298154454, 43.95724293864769550 ) ) ;
#186955=CARTESIAN_POINT ( 'NONE',  ( -5.049401038298153566, 19.05341960407611168, 60.20724293864768129 ) ) ;
#186956=CARTESIAN_POINT ( 'NONE',  ( 19.02544592524343514, -5.153800228976328945, 23.54057627198102054 ) ) ;
#186957=CARTESIAN_POINT ( 'NONE',  ( 5.719274019375991003, -21.55341960407610458, 22.70724293864769194 ) ) ;
#186958=CARTESIAN_POINT ( 'NONE',  ( -16.52544592524342804, 4.483927247898546575, 56.04057627198102409 ) ) ;
#186959=CARTESIAN_POINT ( 'NONE',  ( 0.05219959533909260263, 19.03943276465977164, 24.99890960531435269 ) ) ;
#186960=CARTESIAN_POINT ( 'NONE',  ( 14.34966873604960469, 8.224510206698951720, 84.16557627198103830 ) ) ;
#186962=CARTESIAN_POINT ( 'NONE',  ( -18.67979575497178146, -10.72451020669898902, 101.6655762719810383 ) ) ;
#186963=CARTESIAN_POINT ( 'NONE',  ( 18.67979575497194134, -10.72451020669871369, 30.83442372801902209 ) ) ;
#186965=CARTESIAN_POINT ( 'NONE',  ( 0.05219959533934541429, -16.53943276465976808, 45.00109039468568284 ) ) ;
#186966=CARTESIAN_POINT ( 'NONE',  ( 18.67979575497178502, 10.72451020669898547, 89.16557627198102409 ) ) ;
#186967=CARTESIAN_POINT ( 'NONE',  ( -5.719274019375665041, -21.55341960407619695, 104.7927570613523898 ) ) ;
#186968=CARTESIAN_POINT ( 'NONE',  ( -19.05341960407611168, -5.049401038298163336, 106.4572429386476955 ) ) ;
#186969=CARTESIAN_POINT ( 'NONE',  ( -10.81492255796105439, 18.62759615963255655, 47.91775706135234714 ) ) ;
#186970=CARTESIAN_POINT ( 'NONE',  ( 15.80617190586746368, 15.72974639402197994, 44.37390960531435979 ) ) ;
#186971=CARTESIAN_POINT ( 'NONE',  ( -14.34966873604972548, 8.224510206698743886, 98.33442372801901854 ) ) ;
#186972=CARTESIAN_POINT ( 'NONE',  ( -21.52544592524334988, -5.823673210054445271, 58.95942372801902565 ) ) ;
#186973=CARTESIAN_POINT ( 'NONE',  ( -5.823673210054431948, 21.52544592524334988, 102.7094237280190185 ) ) ;
#186974=CARTESIAN_POINT ( 'NONE',  ( 16.51473224551083163, -9.474510206698727899, 30.83442372801900433 ) ) ;
#186975=CARTESIAN_POINT ( 'NONE',  ( 16.55341960407618274, -4.379528057220086978, 91.04275706135236135 ) ) ;
#186976=CARTESIAN_POINT ( 'NONE',  ( 21.52544592524334988, 5.823673210054432836, 46.45942372801901854 ) ) ;
#186977=CARTESIAN_POINT ( 'NONE',  ( -19.02544592524342804, 5.153800228976336051, 51.04057627198103120 ) ) ;
#186978=CARTESIAN_POINT ( 'NONE',  ( 15.72974639402176855, 15.80617190586768217, 111.8760903946856615 ) ) ;
#186979=CARTESIAN_POINT ( 'NONE',  ( -15.80617190586745835, -15.72974639402198527, 21.87390960531436690 ) ) ;
#186980=CARTESIAN_POINT ( 'NONE',  ( 21.52544592524334988, 5.823673210054432836, 21.45942372801901499 ) ) ;
#186981=CARTESIAN_POINT ( 'NONE',  ( -18.62759615963270932, 10.81492255796079327, 70.83224293864770971 ) ) ;
#186983=CARTESIAN_POINT ( 'NONE',  ( 0.05219959533907565091, 21.53943276465977519, 79.99890960531435269 ) ) ;
#186984=CARTESIAN_POINT ( 'NONE',  ( 12.14591786802327356, -12.06949235617739191, 65.62609039468568994 ) ) ;
#186985=CARTESIAN_POINT ( 'NONE',  ( -0.05219959533910754901, -16.53943276465976808, 67.49890960531436690 ) ) ;
#186987=CARTESIAN_POINT ( 'NONE',  ( -9.474510206698720793, -16.51473224551083518, 94.58442372801900433 ) ) ;
#186989=EDGE_CURVE ( 'NONE', #102442, #93070, #64551, .T. ) ;
#186990=CARTESIAN_POINT ( 'NONE',  ( -16.53943276465976808, -0.05219959533934237506, 43.75109039468568284 ) ) ;
#186991=CARTESIAN_POINT ( 'NONE',  ( -15.80617190586745835, -15.72974639402198527, 96.87390960531436690 ) ) ;
#186992=CARTESIAN_POINT ( 'NONE',  ( 15.72974639402199770, -15.80617190586745480, 73.12390960531436690 ) ) ;
#186993=CARTESIAN_POINT ( 'NONE',  ( -13.97604488694527625, -13.89961937509977652, 111.8739096053143243 ) ) ;
#186994=CARTESIAN_POINT ( 'NONE',  ( 16.52544592524335698, 4.483927247898782831, 56.45942372801902565 ) ) ;
#186995=CARTESIAN_POINT ( 'NONE',  ( -16.46253265017160317, 9.564922557960807481, 70.83224293864770971 ) ) ;
#186996=CARTESIAN_POINT ( 'NONE',  ( 21.55341960407619695, -5.719274019375665929, 41.04275706135236135 ) ) ;
#186997=CARTESIAN_POINT ( 'NONE',  ( -19.03943276465977164, -0.05219959533935918106, 113.7510903946856757 ) ) ;
#186998=CARTESIAN_POINT ( 'NONE',  ( -5.049401038298153566, 19.05341960407611168, 105.2072429386476671 ) ) ;
#186999=CARTESIAN_POINT ( 'NONE',  ( 13.97604488694548053, -13.89961937509957401, 25.62609039468566507 ) ) ;
#187000=CARTESIAN_POINT ( 'NONE',  ( 14.34966873604972726, -8.224510206698740333, 40.83442372801901854 ) ) ;
#187001=CARTESIAN_POINT ( 'NONE',  ( 5.153800228976335163, 19.02544592524342804, 99.79057627198102409 ) ) ;
#187002=CARTESIAN_POINT ( 'NONE',  ( 21.52544592524344225, -5.823673210054117533, 98.54057627198105251 ) ) ;
#187003=CARTESIAN_POINT ( 'NONE',  ( -9.474510206698964154, 16.51473224551069663, 55.41557627198103120 ) ) ;
#187004=CARTESIAN_POINT ( 'NONE',  ( -17.44270441346515099, 5.991230190323086013, 23.63664920735773123 ) ) ;
#187005=CARTESIAN_POINT ( 'NONE',  ( -4.483927247898539470, -16.52544592524342804, 77.29057627198102409 ) ) ;
#187006=CARTESIAN_POINT ( 'NONE',  ( -9.474510206698964154, 16.51473224551069663, 115.4155762719810241 ) ) ;
#187008=CARTESIAN_POINT ( 'NONE',  ( -21.52544592524343514, 5.823673210054127303, 101.0405762719810383 ) ) ;
#187009=CARTESIAN_POINT ( 'NONE',  ( 5.049401038297881783, 19.05341960407617563, 57.29275706135231871 ) ) ;
#187010=CARTESIAN_POINT ( 'NONE',  ( -9.474510206698964154, 16.51473224551069663, 115.4155762719810241 ) ) ;
#187011=CARTESIAN_POINT ( 'NONE',  ( 13.89961937509977652, -13.97604488694527269, 33.12390960531434558 ) ) ;
#187012=CARTESIAN_POINT ( 'NONE',  ( 5.823673210054125526, 21.52544592524343514, 54.79057627198104541 ) ) ;
#187013=CARTESIAN_POINT ( 'NONE',  ( -19.02544592524342804, 5.153800228976336051, 106.0405762719810241 ) ) ;
#187014=CARTESIAN_POINT ( 'NONE',  ( 21.52544592524334988, 5.823673210054432836, 76.45942372801901854 ) ) ;
#187015=CARTESIAN_POINT ( 'NONE',  ( -16.51473224551069308, -9.474510206698971260, 46.66557627198102409 ) ) ;
#187017=CARTESIAN_POINT ( 'NONE',  ( -16.52544592524342804, 4.483927247898546575, 91.04057627198103830 ) ) ;
#187018=CARTESIAN_POINT ( 'NONE',  ( -8.224510206698735004, -14.34966873604973081, 29.58442372801901854 ) ) ;
#187019=CARTESIAN_POINT ( 'NONE',  ( -0.05219959533909027116, -19.03943276465977164, 62.49890960531435979 ) ) ;
#187020=CARTESIAN_POINT ( 'NONE',  ( -21.55341960407619339, 5.719274019375674811, 63.54275706135234003 ) ) ;
#187022=CARTESIAN_POINT ( 'NONE',  ( 5.049401038297881783, 19.05341960407617563, 22.29275706135233648 ) ) ;
#187023=CARTESIAN_POINT ( 'NONE',  ( -19.05341960407617563, 5.049401038297882671, 43.54275706135232582 ) ) ;
#187025=CARTESIAN_POINT ( 'NONE',  ( -10.81492255796105439, 18.62759615963255655, 37.91775706135235424 ) ) ;
#187026=CARTESIAN_POINT ( 'NONE',  ( 0.05219959533909260263, 19.03943276465977164, 54.99890960531435979 ) ) ;
#187027=CARTESIAN_POINT ( 'NONE',  ( 9.564922557961047289, -16.46253265017146816, 35.41775706135233293 ) ) ;
#187028=CARTESIAN_POINT ( 'NONE',  ( 19.03943276465977164, -0.05219959533909143690, 63.74890960531435979 ) ) ;
#187029=CARTESIAN_POINT ( 'NONE',  ( -8.314922557960811034, -14.29746914071050412, 27.08224293864769550 ) ) ;
#187030=CARTESIAN_POINT ( 'NONE',  ( -21.53943276465977519, 0.05219959533907696930, 26.24890960531435624 ) ) ;
#187031=CARTESIAN_POINT ( 'NONE',  ( -10.81492255796105439, 18.62759615963255655, 92.91775706135236135 ) ) ;
#187034=CARTESIAN_POINT ( 'NONE',  ( 17.13100169013299379, 6.664070546373164206, 56.73210164300152059 ) ) ;
#187035=CARTESIAN_POINT ( 'NONE',  ( -21.55341960407619339, 5.719274019375674811, 88.54275706135236135 ) ) ;
#187037=CARTESIAN_POINT ( 'NONE',  ( -16.51473224551069308, -9.474510206698971260, 96.66557627198102409 ) ) ;
#187039=CARTESIAN_POINT ( 'NONE',  ( -0.05219959533909027116, -19.03943276465977164, 47.49890960531435979 ) ) ;
#187040=CARTESIAN_POINT ( 'NONE',  ( 21.52544592524344225, -5.823673210054117533, 73.54057627198102409 ) ) ;
#187041=CARTESIAN_POINT ( 'NONE',  ( 12.06949235617757843, -12.14591786802309237, 33.12390960531435979 ) ) ;
#187042=CARTESIAN_POINT ( 'NONE',  ( -8.224510206698948167, 14.34966873604960824, 115.4155762719810241 ) ) ;
#187043=CARTESIAN_POINT ( 'NONE',  ( 5.153800228976335163, 19.02544592524342804, 99.79057627198102409 ) ) ;
#187044=CARTESIAN_POINT ( 'NONE',  ( 21.55341960407619695, -5.719274019375665929, 111.0427570613523613 ) ) ;
#187045=CARTESIAN_POINT ( 'NONE',  ( 16.52544592524342804, -4.483927247898539470, 103.5405762719810383 ) ) ;
#187046=CARTESIAN_POINT ( 'NONE',  ( 21.53943276465977519, 0.05219959533937863772, 66.25109039468567573 ) ) ;
#187047=CARTESIAN_POINT ( 'NONE',  ( 13.89961937509978007, -13.97604488694527269, 98.12390960531435269 ) ) ;
#187048=CARTESIAN_POINT ( 'NONE',  ( 4.379528057220092307, 16.55341960407617563, 112.2927570613523471 ) ) ;
#187049=CARTESIAN_POINT ( 'NONE',  ( 13.89961937509957401, 13.97604488694547697, 61.87609039468566863 ) ) ;
#187051=CARTESIAN_POINT ( 'NONE',  ( -9.564922557960796823, -16.46253265017161027, 112.0822429386476955 ) ) ;
#187052=CARTESIAN_POINT ( 'NONE',  ( -16.53943276465976808, 0.05219959533911058130, 71.24890960531435269 ) ) ;
#187053=CARTESIAN_POINT ( 'NONE',  ( 5.153800228976615827, -19.02544592524334988, 60.20942372801899012 ) ) ;
#187054=CARTESIAN_POINT ( 'NONE',  ( 9.564922557960805705, 16.46253265017160317, 59.58224293864769550 ) ) ;
#187055=CARTESIAN_POINT ( 'NONE',  ( 16.55341960407611168, 4.379528057220329451, 58.95724293864770971 ) ) ;
#187056=CARTESIAN_POINT ( 'NONE',  ( -19.03943276465977164, -0.05219959533935918106, 88.75109039468567573 ) ) ;
#187057=CARTESIAN_POINT ( 'NONE',  ( -5.719274019375978568, 21.55341960407610458, 50.20724293864769550 ) ) ;
#187059=CARTESIAN_POINT ( 'NONE',  ( 8.224510206698953496, -14.34966873604960469, 112.9155762719810383 ) ) ;
#187060=CARTESIAN_POINT ( 'NONE',  ( -17.44279575226822843, -5.990770900252486264, 29.16442432485682801 ) ) ;
#187061=CARTESIAN_POINT ( 'NONE',  ( -19.02544592524342804, 5.153800228976336051, 76.04057627198102409 ) ) ;
#187062=CARTESIAN_POINT ( 'NONE',  ( 21.55341960407610458, 5.719274019375980345, 63.95724293864770260 ) ) ;
#187063=CARTESIAN_POINT ( 'NONE',  ( 12.06949235617739724, 12.14591786802326823, 91.87609039468568994 ) ) ;
#187064=CARTESIAN_POINT ( 'NONE',  ( -0.05219959533909027116, -19.03943276465977164, 77.49890960531435269 ) ) ;
#187065=CARTESIAN_POINT ( 'NONE',  ( 9.474510206698729675, 16.51473224551082808, 57.08442372801900433 ) ) ;
#187066=CARTESIAN_POINT ( 'NONE',  ( -0.05219959533937732626, 21.53943276465977519, 87.50109039468568994 ) ) ;
#187067=CARTESIAN_POINT ( 'NONE',  ( 18.67979575497178502, 10.72451020669898547, 64.16557627198102409 ) ) ;
#187068=CARTESIAN_POINT ( 'NONE',  ( -19.05341960407611168, -5.049401038298163336, 106.4572429386476955 ) ) ;
#187069=CARTESIAN_POINT ( 'NONE',  ( -16.46253265017160317, 9.564922557960807481, 35.83224293864768839 ) ) ;
#187070=CARTESIAN_POINT ( 'NONE',  ( 4.379528057220092307, 16.55341960407617563, 97.29275706135234714 ) ) ;
#187071=CARTESIAN_POINT ( 'NONE',  ( -16.53943276465976808, -0.05219959533934237506, 18.75109039468568639 ) ) ;
#187073=CARTESIAN_POINT ( 'NONE',  ( 10.81492255796106328, -18.62759615963255655, 95.41775706135234714 ) ) ;
#187075=CARTESIAN_POINT ( 'NONE',  ( 4.483927247898545687, 16.52544592524342804, 59.79057627198103120 ) ) ;
#187076=CARTESIAN_POINT ( 'NONE',  ( 14.34966873604960469, 8.224510206698951720, 69.16557627198102409 ) ) ;
#187077=CARTESIAN_POINT ( 'NONE',  ( 18.62759615963271287, -10.81492255796078972, 93.33224293864769550 ) ) ;
#187078=CARTESIAN_POINT ( 'NONE',  ( -18.62759615963270932, 10.81492255796079327, 85.83224293864768129 ) ) ;
#187079=CARTESIAN_POINT ( 'NONE',  ( 17.31747979337947640, -6.344076630961051677, 96.12055131934815222 ) ) ;
#187080=CARTESIAN_POINT ( 'NONE',  ( -10.81492255796078084, -18.62759615963271287, 52.08224293864768839 ) ) ;
#187081=CARTESIAN_POINT ( 'NONE',  ( -12.14591786802326823, 12.06949235617739902, 73.12609039468567573 ) ) ;
#187082=CARTESIAN_POINT ( 'NONE',  ( 16.53943276465976808, -0.05219959533910856209, 88.74890960531436690 ) ) ;
#187083=CARTESIAN_POINT ( 'NONE',  ( -9.564922557960796823, -16.46253265017161027, 42.08224293864769550 ) ) ;
#187085=CARTESIAN_POINT ( 'NONE',  ( 12.06949235617739724, 12.14591786802326823, 101.8760903946857042 ) ) ;
#187086=CARTESIAN_POINT ( 'NONE',  ( 18.67979575497194134, -10.72451020669871369, 30.83442372801902209 ) ) ;
#187087=CARTESIAN_POINT ( 'NONE',  ( 9.564922557960805705, 16.46253265017160317, 94.58224293864769550 ) ) ;
#187088=CARTESIAN_POINT ( 'NONE',  ( -10.81492255796105439, 18.62759615963255655, 67.91775706135234714 ) ) ;
#187090=CARTESIAN_POINT ( 'NONE',  ( 5.049401038298161559, -19.05341960407611168, 22.70724293864769194 ) ) ;
#187092=CARTESIAN_POINT ( 'NONE',  ( -18.67979575497193778, 10.72451020669871902, 58.33442372801901143 ) ) ;
#187093=CARTESIAN_POINT ( 'NONE',  ( 19.03943276465977164, -0.05219959533909143690, 53.74890960531436690 ) ) ;
#187094=CARTESIAN_POINT ( 'NONE',  ( 18.22780087662119897, -5.500000000000096811, 58.51763182126894947 ) ) ;
#187095=CARTESIAN_POINT ( 'NONE',  ( 19.02544592524343514, -5.153800228976328945, 88.54057627198102409 ) ) ;
#187096=CARTESIAN_POINT ( 'NONE',  ( 19.05341960407617918, -5.049401038297876454, 61.04275706135232582 ) ) ;
#187097=CARTESIAN_POINT ( 'NONE',  ( -21.55341960407619339, 5.719274019375674811, 48.54275706135234714 ) ) ;
#187098=CARTESIAN_POINT ( 'NONE',  ( 16.51473224551083163, -9.474510206698727899, 55.83442372801899722 ) ) ;
#187099=CARTESIAN_POINT ( 'NONE',  ( 5.153800228976335163, 19.02544592524342804, 39.79057627198100988 ) ) ;
#187100=CARTESIAN_POINT ( 'NONE',  ( -8.224510206698735004, -14.34966873604973081, 109.5844237280190328 ) ) ;
#187101=CARTESIAN_POINT ( 'NONE',  ( 5.049401038297881783, 19.05341960407617563, 77.29275706135231871 ) ) ;
#187102=CARTESIAN_POINT ( 'NONE',  ( -8.314922557961024197, 14.29746914071037800, 112.9177570613523329 ) ) ;
#187103=CARTESIAN_POINT ( 'NONE',  ( 13.89961937509957401, 13.97604488694547697, 46.87609039468565442 ) ) ;
#187104=CARTESIAN_POINT ( 'NONE',  ( 5.049401038298161559, -19.05341960407611168, 102.7072429386476955 ) ) ;
#187105=CARTESIAN_POINT ( 'NONE',  ( -10.72451020669870658, -18.67979575497194134, 109.5844237280190328 ) ) ;
#187106=CARTESIAN_POINT ( 'NONE',  ( 13.97604488694548053, -13.89961937509957401, 30.62609039468566863 ) ) ;
#187107=CARTESIAN_POINT ( 'NONE',  ( -5.153800228976328057, -19.02544592524343514, 32.29057627198102409 ) ) ;
#187108=CARTESIAN_POINT ( 'NONE',  ( -21.52544592524334988, -5.823673210054445271, 88.95942372801901854 ) ) ;
#187109=CARTESIAN_POINT ( 'NONE',  ( 16.52544592524335698, 4.483927247898782831, 36.45942372801901143 ) ) ;
#187110=CARTESIAN_POINT ( 'NONE',  ( -19.02544592524342804, 5.153800228976336051, 96.04057627198103830 ) ) ;
#187112=CARTESIAN_POINT ( 'NONE',  ( 9.474510206698971260, -16.51473224551069308, 72.91557627198102409 ) ) ;
#187113=CARTESIAN_POINT ( 'NONE',  ( 0.05219959533936267826, -19.03943276465977164, 75.00109039468566152 ) ) ;
#187114=CARTESIAN_POINT ( 'NONE',  ( -19.05341960407611168, -5.049401038298163336, 101.4572429386476955 ) ) ;
#187115=CARTESIAN_POINT ( 'NONE',  ( -10.72451020669870658, -18.67979575497194134, 99.58442372801900433 ) ) ;
#187116=CARTESIAN_POINT ( 'NONE',  ( 4.483927247898545687, 16.52544592524342804, 94.79057627198105251 ) ) ;
#187117=CARTESIAN_POINT ( 'NONE',  ( 9.564922557960805705, 16.46253265017160317, 29.58224293864769550 ) ) ;
#187118=CARTESIAN_POINT ( 'NONE',  ( 5.823673210054125526, 21.52544592524343514, 44.79057627198103120 ) ) ;
#187119=CARTESIAN_POINT ( 'NONE',  ( 21.55341960407610458, 5.719274019375980345, 38.95724293864768839 ) ) ;
#187120=CARTESIAN_POINT ( 'NONE',  ( 16.55341960407611168, 4.379528057220329451, 103.9572429386476813 ) ) ;
#187122=CARTESIAN_POINT ( 'NONE',  ( -16.46253265017146816, -9.564922557961047289, 59.16775706135233293 ) ) ;
#187123=CARTESIAN_POINT ( 'NONE',  ( -4.483927247898539470, -16.52544592524342804, 37.29057627198102409 ) ) ;
#187124=CARTESIAN_POINT ( 'NONE',  ( -13.89961937509977652, 13.97604488694528158, 115.6239096053143669 ) ) ;
#187125=CARTESIAN_POINT ( 'NONE',  ( -21.53943276465977519, -0.05219959533937600094, 78.75109039468568994 ) ) ;
#187126=CARTESIAN_POINT ( 'NONE',  ( -10.72451020669898014, 18.67979575497178502, 75.41557627198102409 ) ) ;
#187127=CARTESIAN_POINT ( 'NONE',  ( -15.80617190586768217, 15.72974639402176855, 43.12609039468568284 ) ) ;
#187128=CARTESIAN_POINT ( 'NONE',  ( -18.67979575497178146, -10.72451020669898902, 91.66557627198103830 ) ) ;
#187129=CARTESIAN_POINT ( 'NONE',  ( 15.80617190586769283, -15.72974639402175789, 50.62609039468568994 ) ) ;
#187130=CARTESIAN_POINT ( 'NONE',  ( -13.89961937509977652, 13.97604488694528158, 30.62390960531435269 ) ) ;
#187131=CARTESIAN_POINT ( 'NONE',  ( -9.474510206698964154, 16.51473224551069663, 85.41557627198102409 ) ) ;
#187132=CARTESIAN_POINT ( 'NONE',  ( 4.483927247898790824, -16.52544592524335698, 75.20942372801901854 ) ) ;
#187133=CARTESIAN_POINT ( 'NONE',  ( -14.29746914071049879, 8.314922557960819915, 100.8322429386477097 ) ) ;
#187134=CARTESIAN_POINT ( 'NONE',  ( -13.97604488694527625, -13.89961937509977652, 106.8739096053143669 ) ) ;
#187135=CARTESIAN_POINT ( 'NONE',  ( 14.34966873604960469, 8.224510206698951720, 54.16557627198103120 ) ) ;
#187136=CARTESIAN_POINT ( 'NONE',  ( 12.06949235617757843, -12.14591786802309237, 23.12390960531436335 ) ) ;
#187137=CARTESIAN_POINT ( 'NONE',  ( -13.97604488694527625, -13.89961937509977652, 71.87390960531433848 ) ) ;
#187138=CARTESIAN_POINT ( 'NONE',  ( 19.05341960407611168, 5.049401038298154454, 28.95724293864769550 ) ) ;
#187139=CARTESIAN_POINT ( 'NONE',  ( -21.55341960407610458, -5.719274019375992779, 51.45724293864770260 ) ) ;
#187140=CARTESIAN_POINT ( 'NONE',  ( -19.03943276465977164, -0.05219959533935918106, 38.75109039468566152 ) ) ;
#187141=CARTESIAN_POINT ( 'NONE',  ( -17.05116617787826527, -6.768360034955709814, 41.34324446740802017 ) ) ;
#187142=CARTESIAN_POINT ( 'NONE',  ( -16.53943276465976808, 0.05219959533911058130, 31.24890960531435979 ) ) ;
#187143=CARTESIAN_POINT ( 'NONE',  ( -5.049401038298153566, 19.05341960407611168, 110.2072429386476671 ) ) ;
#187144=CARTESIAN_POINT ( 'NONE',  ( -15.72974639402176322, -15.80617190586768395, 59.37609039468568284 ) ) ;
#187145=CARTESIAN_POINT ( 'NONE',  ( 13.97604488694527802, 13.89961937509977652, 114.3739096053143669 ) ) ;
#187146=CARTESIAN_POINT ( 'NONE',  ( -4.379528057220086978, -16.55341960407618274, 64.79275706135234714 ) ) ;
#187147=CARTESIAN_POINT ( 'NONE',  ( -0.05219959533936034679, 19.03943276465977164, 57.50109039468566863 ) ) ;
#187148=CARTESIAN_POINT ( 'NONE',  ( 12.14591786802309770, 12.06949235617756955, 29.37390960531435269 ) ) ;
#187149=CARTESIAN_POINT ( 'NONE',  ( 16.36317988757059538, -7.306389748694852138, 51.59789608363229974 ) ) ;
#187150=CARTESIAN_POINT ( 'NONE',  ( 14.34966873604972726, -8.224510206698740333, 100.8344237280190185 ) ) ;
#187151=CARTESIAN_POINT ( 'NONE',  ( -19.05341960407611168, -5.049401038298163336, 36.45724293864766707 ) ) ;
#187153=CARTESIAN_POINT ( 'NONE',  ( -9.474510206698964154, 16.51473224551069663, 55.41557627198103120 ) ) ;
#187154=CARTESIAN_POINT ( 'NONE',  ( 5.153800228976335163, 19.02544592524342804, 29.79057627198102409 ) ) ;
#187155=CARTESIAN_POINT ( 'NONE',  ( -21.53943276465977519, -0.05219959533937600094, 33.75109039468568284 ) ) ;
#187156=CARTESIAN_POINT ( 'NONE',  ( 5.153800228976335163, 19.02544592524342804, 59.79057627198100988 ) ) ;
#187158=CARTESIAN_POINT ( 'NONE',  ( -9.564922557960796823, -16.46253265017161027, 42.08224293864769550 ) ) ;
#187159=CARTESIAN_POINT ( 'NONE',  ( 15.80617190586746368, 15.72974639402197994, 29.37390960531435269 ) ) ;
#187161=CARTESIAN_POINT ( 'NONE',  ( -21.55341960407619339, 5.719274019375674811, 53.54275706135234714 ) ) ;
#187162=CARTESIAN_POINT ( 'NONE',  ( 16.46253265017160672, -9.564922557960803928, 28.33224293864769550 ) ) ;
#187163=CARTESIAN_POINT ( 'NONE',  ( -15.72974639402197994, 15.80617190586746368, 25.62390960531435624 ) ) ;
#187164=CARTESIAN_POINT ( 'NONE',  ( 0.05219959533934541429, -16.53943276465976808, 75.00109039468568994 ) ) ;
#187165=CARTESIAN_POINT ( 'NONE',  ( 21.55341960407619695, -5.719274019375665929, 106.0427570613523471 ) ) ;
#187166=CARTESIAN_POINT ( 'NONE',  ( -16.52544592524335698, -4.483927247898792601, 53.95942372801900433 ) ) ;
#187167=CARTESIAN_POINT ( 'NONE',  ( -9.474510206698964154, 16.51473224551069663, 90.41557627198103830 ) ) ;
#187168=CARTESIAN_POINT ( 'NONE',  ( 8.224510206698742110, 14.34966873604972548, 37.08442372801901143 ) ) ;
#187169=CARTESIAN_POINT ( 'NONE',  ( 16.53943276465976808, 0.05219959533934440121, 21.25109039468567218 ) ) ;
#187170=CARTESIAN_POINT ( 'NONE',  ( -4.379528057220086978, -16.55341960407618274, 94.79275706135234714 ) ) ;
#187171=CARTESIAN_POINT ( 'NONE',  ( 5.823673210054444382, -21.52544592524334988, 60.20942372801902565 ) ) ;
#187172=CARTESIAN_POINT ( 'NONE',  ( -16.51473224551082808, 9.474510206698731452, 103.3344237280190043 ) ) ;
#187173=CARTESIAN_POINT ( 'NONE',  ( 15.80617190586746368, 15.72974639402197994, 114.3739096053143527 ) ) ;
#187174=CARTESIAN_POINT ( 'NONE',  ( 14.29746914071049879, -8.314922557960816363, 98.33224293864769550 ) ) ;
#187175=CARTESIAN_POINT ( 'NONE',  ( 0.05219959533936267826, -19.03943276465977164, 110.0010903946856757 ) ) ;
#187176=CARTESIAN_POINT ( 'NONE',  ( 16.52544592524335698, 4.483927247898782831, 86.45942372801901854 ) ) ;
#187178=CARTESIAN_POINT ( 'NONE',  ( 16.51473224551083163, -9.474510206698727899, 80.83442372801899012 ) ) ;
#187179=CARTESIAN_POINT ( 'NONE',  ( -0.05219959533910754901, -16.53943276465976808, 47.49890960531435979 ) ) ;
#187180=CARTESIAN_POINT ( 'NONE',  ( 8.314922557960818139, 14.29746914071049879, 44.58224293864769550 ) ) ;
#187181=CARTESIAN_POINT ( 'NONE',  ( -12.14591786802309592, -12.06949235617757132, 106.8739096053143811 ) ) ;
#187182=CARTESIAN_POINT ( 'NONE',  ( 16.46253265017146816, 9.564922557961045513, 51.66775706135233293 ) ) ;
#187183=CARTESIAN_POINT ( 'NONE',  ( -17.49999999999998934, 5.624438216177589211, 90.81670344914643067 ) ) ;
#187184=CARTESIAN_POINT ( 'NONE',  ( 18.67979575497194134, -10.72451020669871369, 30.83442372801902209 ) ) ;
#187185=CARTESIAN_POINT ( 'NONE',  ( 0.05219959533936267826, -19.03943276465977164, 110.0010903946856757 ) ) ;
#187187=CARTESIAN_POINT ( 'NONE',  ( -9.564922557960796823, -16.46253265017161027, 107.0822429386476955 ) ) ;
#187188=CARTESIAN_POINT ( 'NONE',  ( 19.03943276465977164, -0.05219959533909143690, 83.74890960531436690 ) ) ;
#187189=CARTESIAN_POINT ( 'NONE',  ( -18.67979575497178146, -10.72451020669898902, 56.66557627198103830 ) ) ;
#187190=CARTESIAN_POINT ( 'NONE',  ( 8.224510206698953496, -14.34966873604960469, 112.9155762719810383 ) ) ;
#187191=CARTESIAN_POINT ( 'NONE',  ( -13.89961937509977652, 13.97604488694528158, 75.62390960531438111 ) ) ;
#187192=CARTESIAN_POINT ( 'NONE',  ( 5.153800228976335163, 19.02544592524342804, 29.79057627198102409 ) ) ;
#187193=CARTESIAN_POINT ( 'NONE',  ( -18.67979575497193778, 10.72451020669871902, 33.33442372801900433 ) ) ;
#187195=CARTESIAN_POINT ( 'NONE',  ( -18.62759615963255300, -10.81492255796106328, 74.16775706135231871 ) ) ;
#187196=CARTESIAN_POINT ( 'NONE',  ( -16.52544592524335698, -4.483927247898792601, 88.95942372801901854 ) ) ;
#187197=CARTESIAN_POINT ( 'NONE',  ( -21.52544592524334988, -5.823673210054445271, 23.95942372801901143 ) ) ;
#187198=CARTESIAN_POINT ( 'NONE',  ( 5.719274019375673035, 21.55341960407619339, 22.29275706135235069 ) ) ;
#187199=CARTESIAN_POINT ( 'NONE',  ( -0.05219959533936034679, 19.03943276465977164, 67.50109039468566152 ) ) ;
#187200=CARTESIAN_POINT ( 'NONE',  ( 9.474510206698971260, -16.51473224551069308, 82.91557627198103830 ) ) ;
#187201=CARTESIAN_POINT ( 'NONE',  ( 15.80617190586769283, -15.72974639402175789, 90.62609039468567573 ) ) ;
#187202=CARTESIAN_POINT ( 'NONE',  ( -18.67979575497178146, -10.72451020669898902, 86.66557627198102409 ) ) ;
#187203=CARTESIAN_POINT ( 'NONE',  ( -14.29746914071049879, 8.314922557960819915, 70.83224293864770971 ) ) ;
#187204=CARTESIAN_POINT ( 'NONE',  ( -10.81492255796105439, 18.62759615963255655, 97.91775706135236135 ) ) ;
#187205=CARTESIAN_POINT ( 'NONE',  ( 12.14591786802309770, 12.06949235617756955, 79.37390960531436690 ) ) ;
#187206=CARTESIAN_POINT ( 'NONE',  ( -5.153800228976328057, -19.02544592524343514, 22.29057627198102765 ) ) ;
#187207=CARTESIAN_POINT ( 'NONE',  ( -19.02544592524334988, -5.153800228976617603, 73.95942372801900433 ) ) ;
#187208=CARTESIAN_POINT ( 'NONE',  ( -8.314922557960811034, -14.29746914071050412, 42.08224293864769550 ) ) ;
#187209=CARTESIAN_POINT ( 'NONE',  ( 18.62759615963255655, 10.81492255796105972, 81.66775706135236135 ) ) ;
#187210=CARTESIAN_POINT ( 'NONE',  ( 13.89961937509977652, -13.97604488694527269, 93.12390960531436690 ) ) ;
#187211=CARTESIAN_POINT ( 'NONE',  ( 19.03943276465977164, 0.05219959533936151252, 61.25109039468566863 ) ) ;
#187212=CARTESIAN_POINT ( 'NONE',  ( -5.823673210054116645, -21.52544592524344225, 62.29057627198102409 ) ) ;
#187213=CARTESIAN_POINT ( 'NONE',  ( -5.719274019375978568, 21.55341960407610458, 115.2072429386476955 ) ) ;
#187214=CARTESIAN_POINT ( 'NONE',  ( -0.05219959533934338120, 16.53943276465976808, 22.50109039468567573 ) ) ;
#187215=CARTESIAN_POINT ( 'NONE',  ( 4.483927247898790824, -16.52544592524335698, 80.20942372801901854 ) ) ;
#187217=CARTESIAN_POINT ( 'NONE',  ( -15.72974639402176322, -15.80617190586768395, 19.37609039468568639 ) ) ;
#187218=CARTESIAN_POINT ( 'NONE',  ( -8.224510206698948167, 14.34966873604960824, 100.4155762719810241 ) ) ;
#187220=CARTESIAN_POINT ( 'NONE',  ( 16.53943276465976808, 0.05219959533934440121, 31.25109039468568639 ) ) ;
#187221=CARTESIAN_POINT ( 'NONE',  ( 10.72451020669898902, -18.67979575497178502, 67.91557627198102409 ) ) ;
#187222=CARTESIAN_POINT ( 'NONE',  ( -14.34966873604972548, 8.224510206698743886, 103.3344237280190043 ) ) ;
#187223=CARTESIAN_POINT ( 'NONE',  ( -4.483927247898782831, 16.52544592524335698, 37.70942372801900433 ) ) ;
#187224=CARTESIAN_POINT ( 'NONE',  ( 16.46253265017160672, -9.564922557960803928, 28.33224293864769550 ) ) ;
#187225=CARTESIAN_POINT ( 'NONE',  ( -12.14591786802326823, 12.06949235617739902, 83.12609039468568994 ) ) ;
#187226=CARTESIAN_POINT ( 'NONE',  ( -9.564922557961040184, 16.46253265017147172, 72.91775706135233293 ) ) ;
#187227=CARTESIAN_POINT ( 'NONE',  ( 0.05219959533907565091, 21.53943276465977519, 69.99890960531435269 ) ) ;
#187228=CARTESIAN_POINT ( 'NONE',  ( 4.379528057220092307, 16.55341960407617563, 102.2927570613523613 ) ) ;
#187229=CARTESIAN_POINT ( 'NONE',  ( -15.80617190586768217, 15.72974639402176855, 78.12609039468570415 ) ) ;
#187230=CARTESIAN_POINT ( 'NONE',  ( -18.67979575497178146, -10.72451020669898902, 56.66557627198103830 ) ) ;
#187231=CARTESIAN_POINT ( 'NONE',  ( -5.719274019375978568, 21.55341960407610458, 50.20724293864769550 ) ) ;
#187233=CARTESIAN_POINT ( 'NONE',  ( 8.314922557961029526, -14.29746914071037800, 85.41775706135236135 ) ) ;
#187234=CARTESIAN_POINT ( 'NONE',  ( -18.62759615963270932, 10.81492255796079327, 40.83224293864769550 ) ) ;
#187235=ORIENTED_EDGE ( 'NONE', *, *, #17219, .F. ) ;
#187236=CARTESIAN_POINT ( 'NONE',  ( 5.153800228976335163, 19.02544592524342804, 94.79057627198103830 ) ) ;
#187238=CARTESIAN_POINT ( 'NONE',  ( -5.153800228976328057, -19.02544592524343514, 27.29057627198103120 ) ) ;
#187239=CARTESIAN_POINT ( 'NONE',  ( 21.53943276465977519, -0.05219959533907433946, 63.74890960531435979 ) ) ;
#187240=CARTESIAN_POINT ( 'NONE',  ( -12.14591786802326823, 12.06949235617739902, 98.12609039468570415 ) ) ;
#187241=CARTESIAN_POINT ( 'NONE',  ( 21.53943276465977519, 0.05219959533937863772, 51.25109039468568994 ) ) ;
#187242=CARTESIAN_POINT ( 'NONE',  ( 9.474510206698729675, 16.51473224551082808, 107.0844237280190043 ) ) ;
#187243=CARTESIAN_POINT ( 'NONE',  ( 8.224510206698953496, -14.34966873604960469, 107.9155762719810241 ) ) ;
#187244=CARTESIAN_POINT ( 'NONE',  ( -16.46253265017146816, -9.564922557961047289, 109.1677570613523471 ) ) ;
#187245=CARTESIAN_POINT ( 'NONE',  ( -16.51473224551069308, -9.474510206698971260, 41.66557627198103120 ) ) ;
#187247=CARTESIAN_POINT ( 'NONE',  ( -0.05219959533909027116, -19.03943276465977164, 97.49890960531436690 ) ) ;
#187249=CARTESIAN_POINT ( 'NONE',  ( 16.53943276465976808, 0.05219959533934440121, 81.25109039468568994 ) ) ;
#187250=CARTESIAN_POINT ( 'NONE',  ( 5.153800228976615827, -19.02544592524334988, 75.20942372801896170 ) ) ;
#187251=CARTESIAN_POINT ( 'NONE',  ( -21.52544592524334988, -5.823673210054445271, 103.9594237280190185 ) ) ;
#187252=CARTESIAN_POINT ( 'NONE',  ( 15.80617190586746368, 15.72974639402197994, 64.37390960531435269 ) ) ;
#187253=CARTESIAN_POINT ( 'NONE',  ( -12.14591786802326823, 12.06949235617739902, 93.12609039468568994 ) ) ;
#187254=CARTESIAN_POINT ( 'NONE',  ( -19.05341960407617563, 5.049401038297882671, 83.54275706135233293 ) ) ;
#187255=CARTESIAN_POINT ( 'NONE',  ( 13.97604488694527802, 13.89961937509977652, 39.37390960531435269 ) ) ;
#187256=CARTESIAN_POINT ( 'NONE',  ( 9.474510206698971260, -16.51473224551069308, 72.91557627198102409 ) ) ;
#187257=CARTESIAN_POINT ( 'NONE',  ( -21.52544592524334988, -5.823673210054445271, 48.95942372801902565 ) ) ;
#187258=CARTESIAN_POINT ( 'NONE',  ( 19.03943276465977164, -0.05219959533909143690, 43.74890960531435979 ) ) ;
#187259=CARTESIAN_POINT ( 'NONE',  ( -19.03943276465977164, -0.05219959533935918106, 73.75109039468566152 ) ) ;
#187261=CARTESIAN_POINT ( 'NONE',  ( 16.51473224551069308, 9.474510206698969483, 109.1655762719810383 ) ) ;
#187262=CARTESIAN_POINT ( 'NONE',  ( 16.53943276465976808, -0.05219959533910856209, 68.74890960531435269 ) ) ;
#187263=CARTESIAN_POINT ( 'NONE',  ( -0.05219959533907301413, -21.53943276465977519, 57.49890960531435979 ) ) ;
#187265=CARTESIAN_POINT ( 'NONE',  ( -13.89961937509957401, -13.97604488694547875, 24.37609039468565442 ) ) ;
#187267=CARTESIAN_POINT ( 'NONE',  ( -5.049401038298153566, 19.05341960407611168, 65.20724293864765286 ) ) ;
#187268=CARTESIAN_POINT ( 'NONE',  ( 16.46253265017160672, -9.564922557960803928, 68.33224293864770971 ) ) ;
#187269=CARTESIAN_POINT ( 'NONE',  ( 12.06949235617739724, 12.14591786802326823, 51.87609039468568284 ) ) ;
#187270=CARTESIAN_POINT ( 'NONE',  ( 13.97604488694548053, -13.89961937509957401, 80.62609039468567573 ) ) ;
#187272=CARTESIAN_POINT ( 'NONE',  ( 4.379528057220092307, 16.55341960407617563, 92.29275706135236135 ) ) ;
#187274=CARTESIAN_POINT ( 'NONE',  ( -16.55341960407617563, 4.379528057220093196, 63.54275706135234003 ) ) ;
#187275=CARTESIAN_POINT ( 'NONE',  ( 4.379528057220092307, 16.55341960407617563, 37.29275706135235424 ) ) ;
#187276=CARTESIAN_POINT ( 'NONE',  ( 19.03943276465977164, -0.05219959533909143690, 58.74890960531435979 ) ) ;
#187278=CARTESIAN_POINT ( 'NONE',  ( -18.62759615963255300, -10.81492255796106328, 49.16775706135234003 ) ) ;
#187279=CARTESIAN_POINT ( 'NONE',  ( -5.153800228976607833, 19.02544592524334988, 67.70942372801900433 ) ) ;
#187280=CARTESIAN_POINT ( 'NONE',  ( 15.80617190586769283, -15.72974639402175789, 110.6260903946857042 ) ) ;
#187281=CARTESIAN_POINT ( 'NONE',  ( 19.05341960407611168, 5.049401038298154454, 23.95724293864769194 ) ) ;
#187282=CARTESIAN_POINT ( 'NONE',  ( 21.55341960407610458, 5.719274019375980345, 48.95724293864770971 ) ) ;
#187283=CARTESIAN_POINT ( 'NONE',  ( -21.52544592524343514, 5.823673210054127303, 26.04057627198103475 ) ) ;
#187284=CARTESIAN_POINT ( 'NONE',  ( 8.224510206698953496, -14.34966873604960469, 102.9155762719810383 ) ) ;
#187285=CARTESIAN_POINT ( 'NONE',  ( 16.55341960407618274, -4.379528057220086978, 36.04275706135234714 ) ) ;
#187286=CARTESIAN_POINT ( 'NONE',  ( -12.14591786802309592, -12.06949235617757132, 31.87390960531435979 ) ) ;
#187287=ORIENTED_EDGE ( 'NONE', *, *, #172657, .F. ) ;
#187288=CARTESIAN_POINT ( 'NONE',  ( 15.80617190586769283, -15.72974639402175789, 20.62609039468568639 ) ) ;
#187289=CARTESIAN_POINT ( 'NONE',  ( 8.224510206698953496, -14.34966873604960469, 37.91557627198102409 ) ) ;
#187290=CARTESIAN_POINT ( 'NONE',  ( -16.46253265017160317, 9.564922557960807481, 115.8322429386477097 ) ) ;
#187291=CARTESIAN_POINT ( 'NONE',  ( -5.049401038297874678, -19.05341960407617918, 94.79275706135230450 ) ) ;
#187292=CARTESIAN_POINT ( 'NONE',  ( 5.153800228976615827, -19.02544592524334988, 25.20942372801900433 ) ) ;
#187293=CARTESIAN_POINT ( 'NONE',  ( 14.34966873604960469, 8.224510206698951720, 34.16557627198102409 ) ) ;
#187294=CARTESIAN_POINT ( 'NONE',  ( 21.55341960407610458, 5.719274019375980345, 98.95724293864770971 ) ) ;
#187295=CARTESIAN_POINT ( 'NONE',  ( 5.823673210054125526, 21.52544592524343514, 64.79057627198103830 ) ) ;
#187296=CARTESIAN_POINT ( 'NONE',  ( -19.03943276465977164, 0.05219959533909376836, 81.24890960531436690 ) ) ;
#187297=CARTESIAN_POINT ( 'NONE',  ( 16.55341960407611168, 4.379528057220329451, 53.95724293864770260 ) ) ;
#187298=CARTESIAN_POINT ( 'NONE',  ( -9.564922557960796823, -16.46253265017161027, 97.08224293864769550 ) ) ;
#187301=CARTESIAN_POINT ( 'NONE',  ( 19.05341960407617918, -5.049401038297876454, 36.04275706135234003 ) ) ;
#187302=CARTESIAN_POINT ( 'NONE',  ( 10.81492255796078972, 18.62759615963270932, 94.58224293864769550 ) ) ;
#187303=CARTESIAN_POINT ( 'NONE',  ( 12.14591786802309770, 12.06949235617756955, 99.37390960531436690 ) ) ;
#187304=( BOUNDED_CURVE ( )  B_SPLINE_CURVE ( 2, ( #135214, #136190, #117022, #75499, #196886, #193887, #178717, #150381, #120020, #87682, #194881, #58353, #43186 ),
 .UNSPECIFIED., .F., .T. ) 
 B_SPLINE_CURVE_WITH_KNOTS ( ( 3, 2, 2, 2, 2, 2, 3 ),
 ( 0.1603708530912406061, 0.1622807017543859698, 0.1666666666666666574, 0.1710526315789473728, 0.1754385964912280604, 0.1798245614035087758, 0.1817800898887444450 ),
 .UNSPECIFIED. ) 
 CURVE ( )  GEOMETRIC_REPRESENTATION_ITEM ( )  RATIONAL_B_SPLINE_CURVE ( ( 0.9832469066685285419, 0.9851625545550100060, 1.000000000000000000, 0.9659258262890683122, 1.000000000000000000, 0.9659258262890683122, 1.000000000000000000, 0.9659258262890683122, 1.000000000000000000, 0.9659258262890683122, 1.000000000000000000, 0.9848076720550082985, 0.9831626618144004848 ) ) 
 REPRESENTATION_ITEM ( '' )  );
#187305=CARTESIAN_POINT ( 'NONE',  ( -21.53943276465977519, -0.05219959533937600094, 33.75109039468568284 ) ) ;
#187307=CARTESIAN_POINT ( 'NONE',  ( 16.53943276465976808, -0.05219959533910856209, 23.74890960531435269 ) ) ;
#187308=CARTESIAN_POINT ( 'NONE',  ( -13.89961937509977652, 13.97604488694528158, 35.62390960531435269 ) ) ;
#187309=CARTESIAN_POINT ( 'NONE',  ( -16.51473224551069308, -9.474510206698971260, 91.66557627198103830 ) ) ;
#187310=CARTESIAN_POINT ( 'NONE',  ( -5.719274019375978568, 21.55341960407610458, 60.20724293864768839 ) ) ;
#187312=CARTESIAN_POINT ( 'NONE',  ( 13.97604488694527802, 13.89961937509977652, 29.37390960531435979 ) ) ;
#187313=CARTESIAN_POINT ( 'NONE',  ( -16.55341960407611168, -4.379528057220339221, 41.45724293864769550 ) ) ;
#187314=CARTESIAN_POINT ( 'NONE',  ( -5.719274019375665041, -21.55341960407619695, 74.79275706135234714 ) ) ;
#187316=CARTESIAN_POINT ( 'NONE',  ( -14.34966873604972548, 8.224510206698743886, 63.33442372801900433 ) ) ;
#187317=CARTESIAN_POINT ( 'NONE',  ( -19.05341960407611168, -5.049401038298163336, 51.45724293864770260 ) ) ;
#187318=CARTESIAN_POINT ( 'NONE',  ( 19.03943276465977164, -0.05219959533909143690, 68.74890960531436690 ) ) ;
#187320=CARTESIAN_POINT ( 'NONE',  ( -0.05219959533937732626, 21.53943276465977519, 107.5010903946856899 ) ) ;
#187321=CARTESIAN_POINT ( 'NONE',  ( 12.06949235617739724, 12.14591786802326823, 71.87609039468568994 ) ) ;
#187322=CARTESIAN_POINT ( 'NONE',  ( -21.53943276465977519, -0.05219959533937600094, 98.75109039468568994 ) ) ;
#187323=CARTESIAN_POINT ( 'NONE',  ( 19.03943276465977164, -0.05219959533909143690, 58.74890960531435979 ) ) ;
#187324=CARTESIAN_POINT ( 'NONE',  ( 0.05219959533907565091, 21.53943276465977519, 39.99890960531436690 ) ) ;
#187325=CARTESIAN_POINT ( 'NONE',  ( 13.89961937509957401, 13.97604488694547697, 101.8760903946856331 ) ) ;
#187326=CARTESIAN_POINT ( 'NONE',  ( -15.80617190586768217, 15.72974639402176855, 83.12609039468568994 ) ) ;
#187327=CARTESIAN_POINT ( 'NONE',  ( 16.52544592524335698, 4.483927247898782831, 51.45942372801901854 ) ) ;
#187328=CARTESIAN_POINT ( 'NONE',  ( 21.52544592524344225, -5.823673210054117533, 103.5405762719810383 ) ) ;
#187329=CARTESIAN_POINT ( 'NONE',  ( 5.049401038297881783, 19.05341960407617563, 102.2927570613523045 ) ) ;
#187330=CARTESIAN_POINT ( 'NONE',  ( 19.03943276465977164, -0.05219959533909143690, 83.74890960531436690 ) ) ;
#187331=CARTESIAN_POINT ( 'NONE',  ( 16.51473224551083163, -9.474510206698727899, 105.8344237280190043 ) ) ;
#187333=CARTESIAN_POINT ( 'NONE',  ( -16.52544592524335698, -4.483927247898792601, 18.95942372801901143 ) ) ;
#187334=CARTESIAN_POINT ( 'NONE',  ( -14.34966873604960291, -8.224510206698953496, 61.66557627198103120 ) ) ;
#187335=CARTESIAN_POINT ( 'NONE',  ( -16.53943276465976808, -0.05219959533934237506, 68.75109039468568994 ) ) ;
#187336=CARTESIAN_POINT ( 'NONE',  ( 18.67979575497194134, -10.72451020669871369, 25.83442372801901499 ) ) ;
#187337=CARTESIAN_POINT ( 'NONE',  ( 19.03943276465977164, -0.05219959533909143690, 48.74890960531435979 ) ) ;
#187338=CARTESIAN_POINT ( 'NONE',  ( -16.51473224551069308, -9.474510206698971260, 71.66557627198102409 ) ) ;
#187339=CARTESIAN_POINT ( 'NONE',  ( 0.05219959533934541429, -16.53943276465976808, 70.00109039468568994 ) ) ;
#187342=CARTESIAN_POINT ( 'NONE',  ( 10.72451020669871369, 18.67979575497193778, 107.0844237280190043 ) ) ;
#187344=CARTESIAN_POINT ( 'NONE',  ( -9.474510206698964154, 16.51473224551069663, 35.41557627198102409 ) ) ;
#187346=CARTESIAN_POINT ( 'NONE',  ( -16.55341960407617563, 4.379528057220093196, 33.54275706135234714 ) ) ;
#187347=CARTESIAN_POINT ( 'NONE',  ( 5.153800228976615827, -19.02544592524334988, 45.20942372801901143 ) ) ;
#187348=CARTESIAN_POINT ( 'NONE',  ( -14.29746914071037622, -8.314922557961029526, 49.16775706135234003 ) ) ;
#187349=CARTESIAN_POINT ( 'NONE',  ( -16.46253265017160317, 9.564922557960807481, 45.83224293864769550 ) ) ;
#187350=CARTESIAN_POINT ( 'NONE',  ( 13.97604488694527802, 13.89961937509977652, 69.37390960531436690 ) ) ;
#187351=CARTESIAN_POINT ( 'NONE',  ( 21.52544592524344225, -5.823673210054117533, 83.54057627198102409 ) ) ;
#187352=CARTESIAN_POINT ( 'NONE',  ( -16.46253265017160317, 9.564922557960807481, 80.83224293864769550 ) ) ;
#187353=CARTESIAN_POINT ( 'NONE',  ( 5.049401038298161559, -19.05341960407611168, 107.7072429386476955 ) ) ;
#187354=CARTESIAN_POINT ( 'NONE',  ( -0.05219959533909027116, -19.03943276465977164, 67.49890960531436690 ) ) ;
#187356=CARTESIAN_POINT ( 'NONE',  ( 19.02544592524334988, 5.153800228976608722, 101.4594237280189759 ) ) ;
#187357=CARTESIAN_POINT ( 'NONE',  ( -21.52544592524343514, 5.823673210054127303, 81.04057627198102409 ) ) ;
#187358=CARTESIAN_POINT ( 'NONE',  ( -13.97604488694547697, 13.89961937509957934, 23.12609039468565442 ) ) ;
#187360=CARTESIAN_POINT ( 'NONE',  ( -16.55341960407611168, -4.379528057220339221, 66.45724293864768129 ) ) ;
#187361=CARTESIAN_POINT ( 'NONE',  ( -5.719274019375665041, -21.55341960407619695, 89.79275706135236135 ) ) ;
#187362=CARTESIAN_POINT ( 'NONE',  ( -19.03943276465977164, 0.05219959533909376836, 31.24890960531435979 ) ) ;
#187363=CARTESIAN_POINT ( 'NONE',  ( 8.224510206698953496, -14.34966873604960469, 27.91557627198103830 ) ) ;
#187364=CARTESIAN_POINT ( 'NONE',  ( -15.80617190586768217, 15.72974639402176855, 88.12609039468570415 ) ) ;
#187365=CARTESIAN_POINT ( 'NONE',  ( 19.02544592524343514, -5.153800228976328945, 83.54057627198100988 ) ) ;
#187366=CARTESIAN_POINT ( 'NONE',  ( -5.823673210054431948, 21.52544592524334988, 42.70942372801901854 ) ) ;
#187367=CARTESIAN_POINT ( 'NONE',  ( -13.97604488694527625, -13.89961937509977652, 76.87390960531433848 ) ) ;
#187368=CARTESIAN_POINT ( 'NONE',  ( -0.05219959533910754901, -16.53943276465976808, 97.49890960531436690 ) ) ;
#187369=CARTESIAN_POINT ( 'NONE',  ( -4.379528057220328563, 16.55341960407611168, 60.20724293864768839 ) ) ;
#187370=CARTESIAN_POINT ( 'NONE',  ( -21.52544592524343514, 5.823673210054127303, 71.04057627198103830 ) ) ;
#187371=CARTESIAN_POINT ( 'NONE',  ( 19.03943276465977164, -0.05219959533909143690, 73.74890960531435269 ) ) ;
#187372=CARTESIAN_POINT ( 'NONE',  ( -15.80617190586745835, -15.72974639402198527, 91.87390960531436690 ) ) ;
#187373=CARTESIAN_POINT ( 'NONE',  ( -5.153800228976607833, 19.02544592524334988, 82.70942372801897591 ) ) ;
#187374=CARTESIAN_POINT ( 'NONE',  ( 5.153800228976617603, -19.02544592524335343, 35.20942372801899722 ) ) ;
#187375=CARTESIAN_POINT ( 'NONE',  ( 8.224510206698953496, -14.34966873604960469, 82.91557627198103830 ) ) ;
#187376=CARTESIAN_POINT ( 'NONE',  ( -18.62759615963270932, 10.81492255796079327, 55.83224293864770260 ) ) ;
#187377=CARTESIAN_POINT ( 'NONE',  ( 16.31925111598458500, -7.325300261831447557, 27.66424538967253355 ) ) ;
#187378=CARTESIAN_POINT ( 'NONE',  ( -16.53943276465976808, -0.05219959533934237506, 108.7510903946857042 ) ) ;
#187380=CARTESIAN_POINT ( 'NONE',  ( 5.153800228976615827, -19.02544592524334988, 105.2094237280190185 ) ) ;
#187381=CARTESIAN_POINT ( 'NONE',  ( -4.379528057220328563, 16.55341960407611168, 80.20724293864769550 ) ) ;
#187382=CARTESIAN_POINT ( 'NONE',  ( -17.50000000000014566, 3.417042746626901994, 35.17380396232475448 ) ) ;
#187383=CARTESIAN_POINT ( 'NONE',  ( -13.97604488694527625, -13.89961937509977652, 71.87390960531433848 ) ) ;
#187384=CARTESIAN_POINT ( 'NONE',  ( 16.51473224551069308, 9.474510206698969483, 29.16557627198103475 ) ) ;
#187385=CARTESIAN_POINT ( 'NONE',  ( -12.14591786802309592, -12.06949235617757132, 61.87390960531436690 ) ) ;
#187387=CARTESIAN_POINT ( 'NONE',  ( -13.89961937509977652, 13.97604488694528158, 95.62390960531436690 ) ) ;
#187388=CARTESIAN_POINT ( 'NONE',  ( -5.153800228976607833, 19.02544592524334988, 87.70942372801897591 ) ) ;
#187389=CARTESIAN_POINT ( 'NONE',  ( -13.89961937509977652, 13.97604488694528158, 60.62390960531436690 ) ) ;
#187390=CARTESIAN_POINT ( 'NONE',  ( -8.224510206698735004, -14.34966873604973081, 24.58442372801901499 ) ) ;
#187391=CARTESIAN_POINT ( 'NONE',  ( -9.564922557960796823, -16.46253265017161027, 82.08224293864768129 ) ) ;
#187392=CARTESIAN_POINT ( 'NONE',  ( -21.53943276465977519, 0.05219959533907696930, 61.24890960531435979 ) ) ;
#187393=CARTESIAN_POINT ( 'NONE',  ( -4.379528057220086978, -16.55341960407618274, 59.79275706135234714 ) ) ;
#187394=CARTESIAN_POINT ( 'NONE',  ( -13.97604488694547520, 13.89961937509957934, 113.1260903946856757 ) ) ;
#187395=CARTESIAN_POINT ( 'NONE',  ( 19.05341960407611168, 5.049401038298154454, 58.95724293864768129 ) ) ;
#187396=CARTESIAN_POINT ( 'NONE',  ( 0.05219959533907565091, 21.53943276465977519, 69.99890960531435269 ) ) ;
#187397=CARTESIAN_POINT ( 'NONE',  ( -19.05341960407617563, 5.049401038297882671, 98.54275706135233293 ) ) ;
#187398=CARTESIAN_POINT ( 'NONE',  ( -12.06949235617756955, 12.14591786802309770, 30.62390960531436335 ) ) ;
#187399=CARTESIAN_POINT ( 'NONE',  ( 21.55341960407619695, -5.719274019375665929, 51.04275706135234714 ) ) ;
#187401=CARTESIAN_POINT ( 'NONE',  ( -12.06949235617739369, -12.14591786802326823, 69.37609039468567573 ) ) ;
#187402=CARTESIAN_POINT ( 'NONE',  ( 0.05219959533909260263, 19.03943276465977164, 104.9989096053143669 ) ) ;
#187403=CARTESIAN_POINT ( 'NONE',  ( -0.05219959533909027116, -19.03943276465977164, 102.4989096053143669 ) ) ;
#187405=CARTESIAN_POINT ( 'NONE',  ( 8.224510206698742110, 14.34966873604972548, 92.08442372801901854 ) ) ;
#187406=CARTESIAN_POINT ( 'NONE',  ( 12.06949235617739724, 12.14591786802326823, 31.87609039468567929 ) ) ;
#187407=CARTESIAN_POINT ( 'NONE',  ( 5.049401038298161559, -19.05341960407611168, 47.70724293864770260 ) ) ;
#187408=CARTESIAN_POINT ( 'NONE',  ( 16.46253265017160672, -9.564922557960803928, 48.33224293864769550 ) ) ;
#187409=CARTESIAN_POINT ( 'NONE',  ( 5.153800228976335163, 19.02544592524342804, 54.79057627198103120 ) ) ;
#187410=CARTESIAN_POINT ( 'NONE',  ( -10.81492255796105439, 18.62759615963255655, 47.91775706135234714 ) ) ;
#187411=CARTESIAN_POINT ( 'NONE',  ( -14.34966873604972548, 8.224510206698743886, 58.33442372801901143 ) ) ;
#187412=CARTESIAN_POINT ( 'NONE',  ( -12.14591786802309592, -12.06949235617757132, 36.87390960531435979 ) ) ;
#187413=CARTESIAN_POINT ( 'NONE',  ( -19.03943276465977164, 0.05219959533909376836, 41.24890960531435269 ) ) ;
#187414=CARTESIAN_POINT ( 'NONE',  ( 9.474510206698971260, -16.51473224551069308, 37.91557627198102409 ) ) ;
#187415=CARTESIAN_POINT ( 'NONE',  ( -16.53943276465976808, -0.05219959533934237506, 28.75109039468567929 ) ) ;
#187416=CARTESIAN_POINT ( 'NONE',  ( 16.46253265017146816, 9.564922557961045513, 86.66775706135233293 ) ) ;
#187417=CARTESIAN_POINT ( 'NONE',  ( -16.55341960407611168, -4.379528057220339221, 86.45724293864770971 ) ) ;
#187418=CARTESIAN_POINT ( 'NONE',  ( -13.89961937509977652, 13.97604488694528158, 50.62390960531435979 ) ) ;
#187419=CARTESIAN_POINT ( 'NONE',  ( 9.474510206698729675, 16.51473224551082808, 92.08442372801900433 ) ) ;
#187421=CARTESIAN_POINT ( 'NONE',  ( 18.62759615963255655, 10.81492255796105972, 71.66775706135234714 ) ) ;
#187422=CARTESIAN_POINT ( 'NONE',  ( -4.379528057220086978, -16.55341960407618274, 49.79275706135234714 ) ) ;
#187424=CARTESIAN_POINT ( 'NONE',  ( 5.719274019375991003, -21.55341960407610458, 47.70724293864770260 ) ) ;
#187425=CARTESIAN_POINT ( 'NONE',  ( -14.34966873604972548, 8.224510206698743886, 38.33442372801900433 ) ) ;
#187426=CARTESIAN_POINT ( 'NONE',  ( 19.02544592524343514, -5.153800228976328945, 23.54057627198102409 ) ) ;
#187427=CARTESIAN_POINT ( 'NONE',  ( -16.51473224551082808, 9.474510206698731452, 28.33442372801900433 ) ) ;
#187429=CARTESIAN_POINT ( 'NONE',  ( -9.474510206698964154, 16.51473224551069663, 50.41557627198102409 ) ) ;
#187431=CARTESIAN_POINT ( 'NONE',  ( -16.51473224551069308, -9.474510206698971260, 66.66557627198102409 ) ) ;
#187432=CARTESIAN_POINT ( 'NONE',  ( 17.50000000000000711, -3.565345528327973135, 111.9249448680647276 ) ) ;
#187434=CARTESIAN_POINT ( 'NONE',  ( -0.05219959533937732626, 21.53943276465977519, 112.5010903946857042 ) ) ;
#187435=CARTESIAN_POINT ( 'NONE',  ( 12.06949235617757843, -12.14591786802309237, 33.12390960531435979 ) ) ;
#187436=CARTESIAN_POINT ( 'NONE',  ( -5.153800228976328057, -19.02544592524343514, 47.29057627198102409 ) ) ;
#187437=CARTESIAN_POINT ( 'NONE',  ( -5.049401038298153566, 19.05341960407611168, 100.2072429386476955 ) ) ;
#187438=CARTESIAN_POINT ( 'NONE',  ( 18.67979575497194134, -10.72451020669871369, 70.83442372801901854 ) ) ;
#187439=CARTESIAN_POINT ( 'NONE',  ( -5.153800228976328057, -19.02544592524343514, 52.29057627198100988 ) ) ;
#187440=CARTESIAN_POINT ( 'NONE',  ( 21.52544592524334988, 5.823673210054432836, 71.45942372801901854 ) ) ;
#187441=CARTESIAN_POINT ( 'NONE',  ( -0.05219959533907301413, -21.53943276465977519, 22.49890960531436335 ) ) ;
#187442=CARTESIAN_POINT ( 'NONE',  ( -9.474510206698964154, 16.51473224551069663, 35.41557627198102409 ) ) ;
#187443=CARTESIAN_POINT ( 'NONE',  ( 18.67979575497194134, -10.72451020669871369, 25.83442372801901499 ) ) ;
#187444=CARTESIAN_POINT ( 'NONE',  ( 19.03943276465977164, 0.05219959533936151252, 51.25109039468567573 ) ) ;
#187445=CARTESIAN_POINT ( 'NONE',  ( -13.89961937509977652, 13.97604488694528158, 25.62390960531434558 ) ) ;
#187446=CARTESIAN_POINT ( 'NONE',  ( -16.51473224551069308, -9.474510206698971260, 81.66557627198103830 ) ) ;
#187447=CARTESIAN_POINT ( 'NONE',  ( 13.89961937509957401, 13.97604488694547697, 106.8760903946856757 ) ) ;
#187448=CARTESIAN_POINT ( 'NONE',  ( -16.55341960407611168, -4.379528057220339221, 71.45724293864769550 ) ) ;
#187449=CARTESIAN_POINT ( 'NONE',  ( -21.55341960407610458, -5.719274019375992779, 36.45724293864768839 ) ) ;
#187450=CARTESIAN_POINT ( 'NONE',  ( 16.51473224551083163, -9.474510206698727899, 100.8344237280190043 ) ) ;
#187451=CARTESIAN_POINT ( 'NONE',  ( -0.05219959533907301413, -21.53943276465977519, 107.4989096053143669 ) ) ;
#187452=CARTESIAN_POINT ( 'NONE',  ( 10.72451020669871369, 18.67979575497193778, 57.08442372801901854 ) ) ;
#187453=CARTESIAN_POINT ( 'NONE',  ( 8.314922557961029526, -14.29746914071037800, 55.41775706135234714 ) ) ;
#187454=CARTESIAN_POINT ( 'NONE',  ( -14.34966873604972548, 8.224510206698743886, 53.33442372801901854 ) ) ;
#187455=CARTESIAN_POINT ( 'NONE',  ( 10.72451020669898902, -18.67979575497178502, 62.91557627198102409 ) ) ;
#187456=CARTESIAN_POINT ( 'NONE',  ( 13.89961937509977652, -13.97604488694527269, 48.12390960531435979 ) ) ;
#187457=CARTESIAN_POINT ( 'NONE',  ( -4.483927247898782831, 16.52544592524335698, 77.70942372801900433 ) ) ;
#187458=CARTESIAN_POINT ( 'NONE',  ( 0.05219959533907565091, 21.53943276465977519, 104.9989096053143669 ) ) ;
#187459=CARTESIAN_POINT ( 'NONE',  ( -16.55341960407611168, -4.379528057220339221, 51.45724293864770260 ) ) ;
#187460=CARTESIAN_POINT ( 'NONE',  ( -19.05341960407611168, -5.049401038298163336, 76.45724293864769550 ) ) ;
#187461=CARTESIAN_POINT ( 'NONE',  ( -0.05219959533934338120, 16.53943276465976808, 82.50109039468568994 ) ) ;
#187462=CARTESIAN_POINT ( 'NONE',  ( -16.52544592524335698, -4.483927247898792601, 18.95942372801901143 ) ) ;
#187463=CARTESIAN_POINT ( 'NONE',  ( -5.719274019375978568, 21.55341960407610458, 110.2072429386477239 ) ) ;
#187464=CARTESIAN_POINT ( 'NONE',  ( 16.55341960407611168, 4.379528057220329451, 38.95724293864768839 ) ) ;
#187465=VERTEX_POINT ( 'NONE', #95968 ) ;
#187466=CARTESIAN_POINT ( 'NONE',  ( -17.48847506799968343, 5.747544572773787941, 75.82697437843280852 ) ) ;
#187467=CARTESIAN_POINT ( 'NONE',  ( 18.62759615963271287, -10.81492255796078972, 93.33224293864769550 ) ) ;
#187468=CARTESIAN_POINT ( 'NONE',  ( 0.05219959533910956823, 16.53943276465976808, 24.99890960531435624 ) ) ;
#187470=CARTESIAN_POINT ( 'NONE',  ( -16.79531203550650176, -7.028104445595493743, 56.25244988220440945 ) ) ;
#187471=CARTESIAN_POINT ( 'NONE',  ( -10.81492255796078084, -18.62759615963271287, 102.0822429386476955 ) ) ;
#187472=CARTESIAN_POINT ( 'NONE',  ( 0.05219959533909260263, 19.03943276465977164, 104.9989096053143669 ) ) ;
#187473=CARTESIAN_POINT ( 'NONE',  ( 15.80617190586769283, -15.72974639402175789, 20.62609039468568639 ) ) ;
#187474=CARTESIAN_POINT ( 'NONE',  ( 14.29746914071049879, -8.314922557960816363, 48.33224293864770260 ) ) ;
#187475=CARTESIAN_POINT ( 'NONE',  ( 16.55341960407618274, -4.379528057220086978, 51.04275706135234714 ) ) ;
#187477=CARTESIAN_POINT ( 'NONE',  ( 0.05219959533909260263, 19.03943276465977164, 54.99890960531435979 ) ) ;
#187479=CARTESIAN_POINT ( 'NONE',  ( -19.05341960407617563, 5.049401038297882671, 53.54275706135231871 ) ) ;
#187480=CARTESIAN_POINT ( 'NONE',  ( 16.51473224551069308, 9.474510206698969483, 79.16557627198103830 ) ) ;
#187481=CARTESIAN_POINT ( 'NONE',  ( 15.80617190586746368, 15.72974639402197994, 39.37390960531436690 ) ) ;
#187482=CARTESIAN_POINT ( 'NONE',  ( -5.049401038298153566, 19.05341960407611168, 65.20724293864766707 ) ) ;
#187483=CARTESIAN_POINT ( 'NONE',  ( -5.049401038298153566, 19.05341960407611168, 45.20724293864769550 ) ) ;
#187484=CARTESIAN_POINT ( 'NONE',  ( -16.51473224551082808, 9.474510206698731452, 113.3344237280190043 ) ) ;
#187485=CARTESIAN_POINT ( 'NONE',  ( 5.153800228976615827, -19.02544592524334988, 70.20942372801899012 ) ) ;
#187486=CARTESIAN_POINT ( 'NONE',  ( 21.52544592524344225, -5.823673210054117533, 103.5405762719810383 ) ) ;
#187487=CARTESIAN_POINT ( 'NONE',  ( -12.06949235617756955, 12.14591786802309770, 40.62390960531435269 ) ) ;
#187488=CARTESIAN_POINT ( 'NONE',  ( 19.05341960407611168, 5.049401038298154454, 83.95724293864766707 ) ) ;
#187489=CARTESIAN_POINT ( 'NONE',  ( -0.05219959533907301413, -21.53943276465977519, 57.49890960531435979 ) ) ;
#187490=CARTESIAN_POINT ( 'NONE',  ( 21.55341960407610458, 5.719274019375980345, 98.95724293864770971 ) ) ;
#187491=CARTESIAN_POINT ( 'NONE',  ( 8.224510206698742110, 14.34966873604972548, 27.08442372801901854 ) ) ;
#187492=CARTESIAN_POINT ( 'NONE',  ( -15.80617190586745835, -15.72974639402198527, 21.87390960531436690 ) ) ;
#187493=CARTESIAN_POINT ( 'NONE',  ( -18.62759615963255300, -10.81492255796106328, 84.16775706135234714 ) ) ;
#187494=CARTESIAN_POINT ( 'NONE',  ( 19.02544592524343514, -5.153800228976328945, 83.54057627198100988 ) ) ;
#187495=CARTESIAN_POINT ( 'NONE',  ( 19.02544592524343514, -5.153800228976328945, 33.54057627198102409 ) ) ;
#187496=CARTESIAN_POINT ( 'NONE',  ( 19.02544592524343514, -5.153800228976328945, 78.54057627198099567 ) ) ;
#187497=CARTESIAN_POINT ( 'NONE',  ( -12.06949235617756955, 12.14591786802309770, 100.6239096053143811 ) ) ;
#187498=CARTESIAN_POINT ( 'NONE',  ( 16.46253265017160672, -9.564922557960803928, 68.33224293864770971 ) ) ;
#187499=CARTESIAN_POINT ( 'NONE',  ( -0.05219959533936034679, 19.03943276465977164, 112.5010903946856757 ) ) ;
#187500=CARTESIAN_POINT ( 'NONE',  ( 9.474510206698729675, 16.51473224551082808, 42.08442372801900433 ) ) ;
#187501=CARTESIAN_POINT ( 'NONE',  ( -21.53943276465977519, -0.05219959533937600094, 98.75109039468568994 ) ) ;
#187502=CARTESIAN_POINT ( 'NONE',  ( -9.564922557960796823, -16.46253265017161027, 107.0822429386476955 ) ) ;
#187503=CARTESIAN_POINT ( 'NONE',  ( 4.483927247898790824, -16.52544592524335698, 85.20942372801901854 ) ) ;
#187505=CARTESIAN_POINT ( 'NONE',  ( 16.51473224551083163, -9.474510206698727899, 70.83442372801900433 ) ) ;
#187506=CARTESIAN_POINT ( 'NONE',  ( 15.72974639402176855, 15.80617190586768217, 106.8760903946856899 ) ) ;
#187508=CARTESIAN_POINT ( 'NONE',  ( 5.049401038298161559, -19.05341960407611168, 32.70724293864768129 ) ) ;
#187509=CARTESIAN_POINT ( 'NONE',  ( -12.06949235617756955, 12.14591786802309770, 40.62390960531435269 ) ) ;
#187512=CARTESIAN_POINT ( 'NONE',  ( -8.224510206698735004, -14.34966873604973081, 109.5844237280190328 ) ) ;
#187513=CARTESIAN_POINT ( 'NONE',  ( -19.25918095147779852, -5.499999999999484857, 84.45284276293931214 ) ) ;
#187514=CARTESIAN_POINT ( 'NONE',  ( 16.53943276465976808, 0.05219959533934440121, 76.25109039468568994 ) ) ;
#187515=CARTESIAN_POINT ( 'NONE',  ( -16.46253265017160317, 9.564922557960807481, 35.83224293864768839 ) ) ;
#187516=CARTESIAN_POINT ( 'NONE',  ( 21.52544592524334988, 5.823673210054432836, 96.45942372801901854 ) ) ;
#187517=CARTESIAN_POINT ( 'NONE',  ( 13.89961937509957401, 13.97604488694547697, 96.87609039468566152 ) ) ;
#187518=CARTESIAN_POINT ( 'NONE',  ( 15.72974639402176855, 15.80617190586768217, 76.87609039468567573 ) ) ;
#187519=CARTESIAN_POINT ( 'NONE',  ( 9.474510206698729675, 16.51473224551082808, 57.08442372801900433 ) ) ;
#187520=CARTESIAN_POINT ( 'NONE',  ( 13.89961937509977652, -13.97604488694527269, 78.12390960531433848 ) ) ;
#187521=CARTESIAN_POINT ( 'NONE',  ( -19.03943276465977164, 0.05219959533909376836, 66.24890960531436690 ) ) ;
#187522=EDGE_CURVE ( 'NONE', #11857, #11672, #172827, .T. ) ;
#187523=CARTESIAN_POINT ( 'NONE',  ( 17.26058549869091507, 6.457015423128499521, 73.87745837476064992 ) ) ;
#187524=CARTESIAN_POINT ( 'NONE',  ( 4.483927247898545687, 16.52544592524342804, 69.79057627198102409 ) ) ;
#187525=CARTESIAN_POINT ( 'NONE',  ( -21.53943276465977519, 0.05219959533907696930, 66.24890960531436690 ) ) ;
#187526=CARTESIAN_POINT ( 'NONE',  ( -13.89961937509977652, 13.97604488694528158, 45.62390960531433848 ) ) ;
#187527=CARTESIAN_POINT ( 'NONE',  ( 0.05219959533907565091, 21.53943276465977519, 84.99890960531436690 ) ) ;
#187528=CARTESIAN_POINT ( 'NONE',  ( -16.52544592524335698, -4.483927247898792601, 78.95942372801901854 ) ) ;
#187530=CARTESIAN_POINT ( 'NONE',  ( -13.97604488694527625, -13.89961937509977652, 51.87390960531436690 ) ) ;
#187531=CARTESIAN_POINT ( 'NONE',  ( 12.06949235617757843, -12.14591786802309237, 78.12390960531436690 ) ) ;
#187533=CARTESIAN_POINT ( 'NONE',  ( -9.474510206698964154, 16.51473224551069663, 45.41557627198103120 ) ) ;
#187534=CARTESIAN_POINT ( 'NONE',  ( -13.97604488694527625, -13.89961937509977652, 21.87390960531435979 ) ) ;
#187535=CARTESIAN_POINT ( 'NONE',  ( 16.51473224551083163, -9.474510206698727899, 65.83442372801900433 ) ) ;
#187536=CARTESIAN_POINT ( 'NONE',  ( 8.314922557960818139, 14.29746914071049879, 69.58224293864769550 ) ) ;
#187537=CARTESIAN_POINT ( 'NONE',  ( -15.80617190586768217, 15.72974639402176855, 43.12609039468568284 ) ) ;
#187538=CARTESIAN_POINT ( 'NONE',  ( -19.02544592524342804, 5.153800228976336051, 36.04057627198100988 ) ) ;
#187539=CARTESIAN_POINT ( 'NONE',  ( -21.52544592524343514, 5.823673210054127303, 101.0405762719810383 ) ) ;
#187540=CARTESIAN_POINT ( 'NONE',  ( -14.29746914071049879, 8.314922557960819915, 85.83224293864768129 ) ) ;
#187542=CARTESIAN_POINT ( 'NONE',  ( -19.05341960407611168, -5.049401038298163336, 51.45724293864770260 ) ) ;
#187544=CARTESIAN_POINT ( 'NONE',  ( 13.97604488694548053, -13.89961937509957401, 85.62609039468568994 ) ) ;
#187545=CARTESIAN_POINT ( 'NONE',  ( 10.72451020669871369, 18.67979575497193778, 32.08442372801901854 ) ) ;
#187546=CARTESIAN_POINT ( 'NONE',  ( 13.97604488694527802, 13.89961937509977652, 64.37390960531436690 ) ) ;
#187547=CARTESIAN_POINT ( 'NONE',  ( 13.89961937509957401, 13.97604488694547697, 71.87609039468567573 ) ) ;
#187548=CARTESIAN_POINT ( 'NONE',  ( 13.89961937509977652, -13.97604488694527269, 38.12390960531436690 ) ) ;
#187549=CARTESIAN_POINT ( 'NONE',  ( -8.314922557960811034, -14.29746914071050412, 67.08224293864770971 ) ) ;
#187550=CARTESIAN_POINT ( 'NONE',  ( 12.14591786802309770, 12.06949235617756955, 69.37390960531436690 ) ) ;
#187551=CARTESIAN_POINT ( 'NONE',  ( -5.049401038298153566, 19.05341960407611168, 70.20724293864769550 ) ) ;
#187552=CARTESIAN_POINT ( 'NONE',  ( -10.81492255796078084, -18.62759615963271287, 107.0822429386476955 ) ) ;
#187553=CARTESIAN_POINT ( 'NONE',  ( -19.05341960407611168, -5.049401038298163336, 71.45724293864766707 ) ) ;
#187554=CARTESIAN_POINT ( 'NONE',  ( -5.049401038297874678, -19.05341960407617918, 24.79275706135233648 ) ) ;
#187555=CARTESIAN_POINT ( 'NONE',  ( -13.97604488694527625, -13.89961937509977652, 31.87390960531435979 ) ) ;
#187556=CARTESIAN_POINT ( 'NONE',  ( -8.314922557961024197, 14.29746914071037800, 107.9177570613523471 ) ) ;
#187557=CARTESIAN_POINT ( 'NONE',  ( -8.314922557960811034, -14.29746914071050412, 112.0822429386477097 ) ) ;
#187558=CARTESIAN_POINT ( 'NONE',  ( -9.564922557961040184, 16.46253265017147172, 107.9177570613523471 ) ) ;
#187559=EDGE_LOOP ( 'NONE', ( #67073, #10415, #117401 ) ) ;
#187560=CARTESIAN_POINT ( 'NONE',  ( 21.52544592524334988, 5.823673210054432836, 31.45942372801901854 ) ) ;
#187561=CARTESIAN_POINT ( 'NONE',  ( -19.03943276465977164, -0.05219959533935918106, 48.75109039468566863 ) ) ;
#187562=CARTESIAN_POINT ( 'NONE',  ( -14.29746914071037622, -8.314922557961029526, 109.1677570613523613 ) ) ;
#187563=CARTESIAN_POINT ( 'NONE',  ( 18.62759615963271287, -10.81492255796078972, 73.33224293864769550 ) ) ;
#187564=CARTESIAN_POINT ( 'NONE',  ( 19.03943276465977164, -0.05219959533909143690, 108.7489096053143527 ) ) ;
#187565=CARTESIAN_POINT ( 'NONE',  ( 12.06949235617757843, -12.14591786802309237, 53.12390960531436690 ) ) ;
#187566=CARTESIAN_POINT ( 'NONE',  ( -19.03943276465977164, 0.05219959533909376836, 36.24890960531436690 ) ) ;
#187567=CARTESIAN_POINT ( 'NONE',  ( 16.51473224551069308, 9.474510206698969483, 39.16557627198103120 ) ) ;
#187568=CARTESIAN_POINT ( 'NONE',  ( 16.46253265017146816, 9.564922557961045513, 31.66775706135232937 ) ) ;
#187569=CARTESIAN_POINT ( 'NONE',  ( -4.379528057220086978, -16.55341960407618274, 89.79275706135236135 ) ) ;
#187570=CARTESIAN_POINT ( 'NONE',  ( -16.55341960407617563, 4.379528057220093196, 43.54275706135235424 ) ) ;
#187571=CARTESIAN_POINT ( 'NONE',  ( -15.72974639402197994, 15.80617190586746368, 25.62390960531435624 ) ) ;
#187572=CARTESIAN_POINT ( 'NONE',  ( -5.153800228976328057, -19.02544592524343514, 57.29057627198103120 ) ) ;
#187573=CARTESIAN_POINT ( 'NONE',  ( 10.81492255796106328, -18.62759615963255655, 100.4177570613523471 ) ) ;
#187574=CARTESIAN_POINT ( 'NONE',  ( 16.51473224551069308, 9.474510206698969483, 84.16557627198102409 ) ) ;
#187575=CARTESIAN_POINT ( 'NONE',  ( -12.06949235617739369, -12.14591786802326823, 64.37609039468568994 ) ) ;
#187576=CARTESIAN_POINT ( 'NONE',  ( -4.379528057220328563, 16.55341960407611168, 105.2072429386477097 ) ) ;
#187577=CARTESIAN_POINT ( 'NONE',  ( 12.06949235617757843, -12.14591786802309237, 23.12390960531436335 ) ) ;
#187579=CARTESIAN_POINT ( 'NONE',  ( 18.67979575497194134, -10.72451020669871369, 70.83442372801901854 ) ) ;
#187580=CARTESIAN_POINT ( 'NONE',  ( -13.89961937509977652, 13.97604488694528158, 85.62390960531433848 ) ) ;
#187581=CARTESIAN_POINT ( 'NONE',  ( -19.03943276465977164, 0.05219959533909376836, 71.24890960531435269 ) ) ;
#187582=CARTESIAN_POINT ( 'NONE',  ( -13.89961937509977652, 13.97604488694528158, 110.6239096053143243 ) ) ;
#187583=CARTESIAN_POINT ( 'NONE',  ( 12.14591786802309770, 12.06949235617756955, 59.37390960531436690 ) ) ;
#187584=CARTESIAN_POINT ( 'NONE',  ( -4.379528057220086978, -16.55341960407618274, 109.7927570613523613 ) ) ;
#187585=CARTESIAN_POINT ( 'NONE',  ( -12.06949235617756955, 12.14591786802309770, 40.62390960531435269 ) ) ;
#187586=CARTESIAN_POINT ( 'NONE',  ( 14.34966873604972726, -8.224510206698740333, 40.83442372801901854 ) ) ;
#187588=CARTESIAN_POINT ( 'NONE',  ( 9.474510206698729675, 16.51473224551082808, 42.08442372801900433 ) ) ;
#187589=CARTESIAN_POINT ( 'NONE',  ( 13.89961937509977652, -13.97604488694527269, 78.12390960531433848 ) ) ;
#187590=CARTESIAN_POINT ( 'NONE',  ( -5.153800228976607833, 19.02544592524334988, 57.70942372801899012 ) ) ;
#187592=CARTESIAN_POINT ( 'NONE',  ( 18.09918380851992481, 5.500000000000036415, 58.98618307335610211 ) ) ;
#187593=CARTESIAN_POINT ( 'NONE',  ( 19.03943276465977164, 0.05219959533936151252, 81.25109039468567573 ) ) ;
#187594=CARTESIAN_POINT ( 'NONE',  ( -4.379528057220086978, -16.55341960407618274, 79.79275706135236135 ) ) ;
#187596=CARTESIAN_POINT ( 'NONE',  ( 19.02544592524343514, -5.153800228976328945, 108.5405762719810383 ) ) ;
#187597=CARTESIAN_POINT ( 'NONE',  ( -5.823673210054431948, 21.52544592524334988, 42.70942372801901854 ) ) ;
#187598=CARTESIAN_POINT ( 'NONE',  ( -19.03943276465977164, -0.05219959533935918106, 93.75109039468566152 ) ) ;
#187599=CARTESIAN_POINT ( 'NONE',  ( 17.31728774477272736, 6.344390552232407110, 86.68093348310682700 ) ) ;
#187600=CARTESIAN_POINT ( 'NONE',  ( -16.46253265017160317, 9.564922557960807481, 50.83224293864770260 ) ) ;
#187601=CARTESIAN_POINT ( 'NONE',  ( 13.97604488694527802, 13.89961937509977652, 109.3739096053143669 ) ) ;
#187602=CARTESIAN_POINT ( 'NONE',  ( -14.29746914071049879, 8.314922557960819915, 65.83224293864769550 ) ) ;
#187603=CARTESIAN_POINT ( 'NONE',  ( -16.51473224551069308, -9.474510206698971260, 56.66557627198103120 ) ) ;
#187604=CARTESIAN_POINT ( 'NONE',  ( -5.153800228976328057, -19.02544592524343514, 62.29057627198100988 ) ) ;
#187605=CARTESIAN_POINT ( 'NONE',  ( -19.05341960407617563, 5.049401038297882671, 63.54275706135234003 ) ) ;
#187606=CARTESIAN_POINT ( 'NONE',  ( 0.05219959533936267826, -19.03943276465977164, 30.00109039468566863 ) ) ;
#187607=CARTESIAN_POINT ( 'NONE',  ( -16.51473224551069308, -9.474510206698971260, 61.66557627198103120 ) ) ;
#187608=CARTESIAN_POINT ( 'NONE',  ( -15.72974639402197994, 15.80617190586746368, 75.62390960531439532 ) ) ;
#187609=CARTESIAN_POINT ( 'NONE',  ( -0.05219959533910754901, -16.53943276465976808, 67.49890960531436690 ) ) ;
#187610=CARTESIAN_POINT ( 'NONE',  ( 16.51473224551083163, -9.474510206698727899, 30.83442372801900433 ) ) ;
#187611=CARTESIAN_POINT ( 'NONE',  ( 21.55341960407610458, 5.719274019375980345, 43.95724293864769550 ) ) ;
#187612=CARTESIAN_POINT ( 'NONE',  ( -5.823673210054116645, -21.52544592524344225, 32.29057627198102409 ) ) ;
#187613=CARTESIAN_POINT ( 'NONE',  ( 5.049401038298161559, -19.05341960407611168, 72.70724293864768129 ) ) ;
#187614=CARTESIAN_POINT ( 'NONE',  ( -5.153800228976328057, -19.02544592524343514, 42.29057627198101699 ) ) ;
#187615=CARTESIAN_POINT ( 'NONE',  ( 12.14591786802309770, 12.06949235617756955, 94.37390960531436690 ) ) ;
#187616=CARTESIAN_POINT ( 'NONE',  ( 10.81492255796078972, 18.62759615963270932, 114.5822429386477097 ) ) ;
#187618=CARTESIAN_POINT ( 'NONE',  ( -21.52544592524334988, -5.823673210054445271, 28.95942372801902209 ) ) ;
#187619=CARTESIAN_POINT ( 'NONE',  ( 5.049401038298161559, -19.05341960407611168, 37.70724293864768839 ) ) ;
#187620=CARTESIAN_POINT ( 'NONE',  ( -10.72451020669898014, 18.67979575497178502, 105.4155762719810383 ) ) ;
#187621=CARTESIAN_POINT ( 'NONE',  ( 5.049401038297881783, 19.05341960407617563, 47.29275706135231161 ) ) ;
#187622=CARTESIAN_POINT ( 'NONE',  ( 9.474510206698971260, -16.51473224551069308, 22.91557627198102765 ) ) ;
#187623=CARTESIAN_POINT ( 'NONE',  ( 19.01533133064923931, -5.499999999999436895, 76.26586590595739779 ) ) ;
#187625=CARTESIAN_POINT ( 'NONE',  ( 16.52544592524335698, 4.483927247898782831, 46.45942372801901854 ) ) ;
#187626=CARTESIAN_POINT ( 'NONE',  ( -13.97604488694527625, -13.89961937509977652, 21.87390960531435979 ) ) ;
#187628=CARTESIAN_POINT ( 'NONE',  ( 19.05341960407611168, 5.049401038298154454, 68.95724293864769550 ) ) ;
#187629=CARTESIAN_POINT ( 'NONE',  ( 0.05219959533910956823, 16.53943276465976808, 104.9989096053143669 ) ) ;
#187630=CARTESIAN_POINT ( 'NONE',  ( -15.72974639402197994, 15.80617190586746368, 40.62390960531435269 ) ) ;
#187631=CARTESIAN_POINT ( 'NONE',  ( -16.55341960407611168, -4.379528057220339221, 76.45724293864769550 ) ) ;
#187632=CARTESIAN_POINT ( 'NONE',  ( 8.314922557961029526, -14.29746914071037800, 40.41775706135234714 ) ) ;
#187633=CARTESIAN_POINT ( 'NONE',  ( 10.81492255796106328, -18.62759615963255655, 80.41775706135234714 ) ) ;
#187634=CARTESIAN_POINT ( 'NONE',  ( -13.89961937509977652, 13.97604488694528158, 25.62390960531434558 ) ) ;
#187635=CARTESIAN_POINT ( 'NONE',  ( 14.29746914071037800, 8.314922557961029526, 106.6677570613523756 ) ) ;
#187636=CARTESIAN_POINT ( 'NONE',  ( -16.53943276465976808, 0.05219959533911058130, 61.24890960531435979 ) ) ;
#187637=CARTESIAN_POINT ( 'NONE',  ( 16.51473224551069308, 9.474510206698969483, 54.16557627198103120 ) ) ;
#187638=CARTESIAN_POINT ( 'NONE',  ( 21.52544592524334988, 5.823673210054432836, 91.45942372801901854 ) ) ;
#187639=CARTESIAN_POINT ( 'NONE',  ( -10.72451020669898014, 18.67979575497178502, 110.4155762719810383 ) ) ;
#187640=CARTESIAN_POINT ( 'NONE',  ( 10.72451020669871369, 18.67979575497193778, 77.08442372801901854 ) ) ;
#187641=CARTESIAN_POINT ( 'NONE',  ( -0.05219959533934338120, 16.53943276465976808, 37.50109039468568284 ) ) ;
#187642=CARTESIAN_POINT ( 'NONE',  ( -14.34966873604960291, -8.224510206698953496, 81.66557627198103830 ) ) ;
#187643=CARTESIAN_POINT ( 'NONE',  ( 15.72974639402176855, 15.80617190586768217, 91.87609039468568994 ) ) ;
#187644=CARTESIAN_POINT ( 'NONE',  ( -4.483927247898539470, -16.52544592524342804, 22.29057627198102765 ) ) ;
#187647=CARTESIAN_POINT ( 'NONE',  ( -8.224510206698948167, 14.34966873604960824, 35.41557627198102409 ) ) ;
#187648=CARTESIAN_POINT ( 'NONE',  ( 4.379528057220092307, 16.55341960407617563, 87.29275706135236135 ) ) ;
#187649=CARTESIAN_POINT ( 'NONE',  ( -16.51473224551069308, -9.474510206698971260, 91.66557627198103830 ) ) ;
#187650=CARTESIAN_POINT ( 'NONE',  ( 9.474510206698971260, -16.51473224551069308, 97.91557627198102409 ) ) ;
#187651=CARTESIAN_POINT ( 'NONE',  ( 21.52544592524334988, 5.823673210054432836, 96.45942372801901854 ) ) ;
#187652=CARTESIAN_POINT ( 'NONE',  ( -16.55341960407617563, 4.379528057220093196, 108.5427570613523756 ) ) ;
#187653=CARTESIAN_POINT ( 'NONE',  ( 8.224510206698953496, -14.34966873604960469, 67.91557627198102409 ) ) ;
#187654=CARTESIAN_POINT ( 'NONE',  ( -16.51473224551069308, -9.474510206698971260, 81.66557627198103830 ) ) ;
#187656=CARTESIAN_POINT ( 'NONE',  ( 14.29746914071037800, 8.314922557961029526, 26.66775706135235424 ) ) ;
#187657=CARTESIAN_POINT ( 'NONE',  ( -19.05341960407611168, -5.049401038298163336, 26.45724293864769550 ) ) ;
#187658=CARTESIAN_POINT ( 'NONE',  ( -5.153800228976328057, -19.02544592524343514, 87.29057627198103830 ) ) ;
#187659=CARTESIAN_POINT ( 'NONE',  ( -16.55341960407617563, 4.379528057220093196, 28.54275706135234358 ) ) ;
#187661=CARTESIAN_POINT ( 'NONE',  ( 16.46253265017146816, 9.564922557961045513, 41.66775706135234003 ) ) ;
#187662=CARTESIAN_POINT ( 'NONE',  ( -12.06949235617739369, -12.14591786802326823, 94.37609039468568994 ) ) ;
#187663=CARTESIAN_POINT ( 'NONE',  ( 19.03943276465977164, 0.05219959533936151252, 101.2510903946856757 ) ) ;
#187664=CARTESIAN_POINT ( 'NONE',  ( -5.153800228976328057, -19.02544592524343514, 27.29057627198103120 ) ) ;
#187665=B_SPLINE_CURVE_WITH_KNOTS ( 'NONE', 3,
 ( #19371, #144687, #67852, #176049, #36507, #49702 ),
 .UNSPECIFIED., .F., .F.,
 ( 4, 2, 4 ),
 ( 0.000000000000000000, 0.0003837532665635066433, 0.0007675065331270132865 ),
 .UNSPECIFIED. ) ;
#187666=CARTESIAN_POINT ( 'NONE',  ( 12.14591786802327356, -12.06949235617739191, 75.62609039468567573 ) ) ;
#187667=CARTESIAN_POINT ( 'NONE',  ( 14.29746914071037800, 8.314922557961029526, 61.66775706135235424 ) ) ;
#187669=CARTESIAN_POINT ( 'NONE',  ( -16.51473224551082808, 9.474510206698731452, 63.33442372801900433 ) ) ;
#187670=CARTESIAN_POINT ( 'NONE',  ( 21.53943276465977519, 0.05219959533937863772, 106.2510903946856757 ) ) ;
#187671=CARTESIAN_POINT ( 'NONE',  ( 0.05219959533909260263, 19.03943276465977164, 44.99890960531435979 ) ) ;
#187672=CARTESIAN_POINT ( 'NONE',  ( -16.46253265017160317, 9.564922557960807481, 90.83224293864769550 ) ) ;
#187673=CARTESIAN_POINT ( 'NONE',  ( -4.379528057220328563, 16.55341960407611168, 80.20724293864769550 ) ) ;
#187674=CARTESIAN_POINT ( 'NONE',  ( 9.474510206698729675, 16.51473224551082808, 57.08442372801900433 ) ) ;
#187675=CARTESIAN_POINT ( 'NONE',  ( 15.72974639402199770, -15.80617190586745480, 48.12390960531436690 ) ) ;
#187676=CARTESIAN_POINT ( 'NONE',  ( 10.81492255796106328, -18.62759615963255655, 105.4177570613523613 ) ) ;
#187677=CARTESIAN_POINT ( 'NONE',  ( -9.474510206698964154, 16.51473224551069663, 95.41557627198102409 ) ) ;
#187678=CARTESIAN_POINT ( 'NONE',  ( 5.049401038297881783, 19.05341960407617563, 22.29275706135233648 ) ) ;
#187679=CARTESIAN_POINT ( 'NONE',  ( 10.81492255796078972, 18.62759615963270932, 59.58224293864770260 ) ) ;
#187680=CARTESIAN_POINT ( 'NONE',  ( -9.474510206698964154, 16.51473224551069663, 115.4155762719810241 ) ) ;
#187681=CARTESIAN_POINT ( 'NONE',  ( -5.049401038297874678, -19.05341960407617918, 84.79275706135233293 ) ) ;
#187682=CARTESIAN_POINT ( 'NONE',  ( -17.49999999999999645, 3.512728167236898624, 110.2280999518112310 ) ) ;
#187683=CARTESIAN_POINT ( 'NONE',  ( -19.03943276465977164, -0.05219959533935918106, 103.7510903946856757 ) ) ;
#187684=CARTESIAN_POINT ( 'NONE',  ( -19.05341960407611168, -5.049401038298163336, 26.45724293864769550 ) ) ;
#187685=CARTESIAN_POINT ( 'NONE',  ( 0.05219959533909260263, 19.03943276465977164, 94.99890960531436690 ) ) ;
#187686=CARTESIAN_POINT ( 'NONE',  ( -5.719274019375978568, 21.55341960407610458, 75.20724293864769550 ) ) ;
#187687=CARTESIAN_POINT ( 'NONE',  ( -12.06949235617739369, -12.14591786802326823, 49.37609039468569705 ) ) ;
#187688=CARTESIAN_POINT ( 'NONE',  ( -21.53943276465977519, -0.05219959533937600094, 53.75109039468568994 ) ) ;
#187689=CARTESIAN_POINT ( 'NONE',  ( 5.823673210054444382, -21.52544592524334988, 95.20942372801903275 ) ) ;
#187690=CARTESIAN_POINT ( 'NONE',  ( -4.483927247898782831, 16.52544592524335698, 92.70942372801901854 ) ) ;
#187691=CARTESIAN_POINT ( 'NONE',  ( 9.474510206698971260, -16.51473224551069308, 82.91557627198103830 ) ) ;
#187692=CARTESIAN_POINT ( 'NONE',  ( -14.29746914071049879, 8.314922557960819915, 95.83224293864770971 ) ) ;
#187693=CARTESIAN_POINT ( 'NONE',  ( -16.53943276465976808, 0.05219959533911058130, 31.24890960531435979 ) ) ;
#187694=CARTESIAN_POINT ( 'NONE',  ( -9.564922557961040184, 16.46253265017147172, 72.91775706135233293 ) ) ;
#187695=CARTESIAN_POINT ( 'NONE',  ( -0.05219959533937732626, 21.53943276465977519, 47.50109039468568994 ) ) ;
#187696=CARTESIAN_POINT ( 'NONE',  ( 19.03943276465977164, 0.05219959533936151252, 31.25109039468566863 ) ) ;
#187697=CARTESIAN_POINT ( 'NONE',  ( 12.06949235617757843, -12.14591786802309237, 88.12390960531436690 ) ) ;
#187698=CARTESIAN_POINT ( 'NONE',  ( -16.46253265017160317, 9.564922557960807481, 115.8322429386477097 ) ) ;
#187699=CARTESIAN_POINT ( 'NONE',  ( 12.14591786802327356, -12.06949235617739191, 110.6260903946857042 ) ) ;
#187700=CARTESIAN_POINT ( 'NONE',  ( -18.67979575497193778, 10.72451020669871902, 83.33442372801903275 ) ) ;
#187701=CARTESIAN_POINT ( 'NONE',  ( 12.14591786802327356, -12.06949235617739191, 55.62609039468568284 ) ) ;
#187702=CARTESIAN_POINT ( 'NONE',  ( 12.06949235617739724, 12.14591786802326823, 101.8760903946857042 ) ) ;
#187703=CARTESIAN_POINT ( 'NONE',  ( -10.81492255796105439, 18.62759615963255655, 57.91775706135234714 ) ) ;
#187704=CARTESIAN_POINT ( 'NONE',  ( 0.05219959533937995610, -21.53943276465977519, 30.00109039468568284 ) ) ;
#187705=CARTESIAN_POINT ( 'NONE',  ( -8.224510206698948167, 14.34966873604960824, 110.4155762719810383 ) ) ;
#187706=CARTESIAN_POINT ( 'NONE',  ( 20.28939339942064635, 0.9295024462022883904, 37.50000000000002842 ) ) ;
#187707=CARTESIAN_POINT ( 'NONE',  ( -4.483927247898539470, -16.52544592524342804, 72.29057627198102409 ) ) ;
#187708=CARTESIAN_POINT ( 'NONE',  ( -13.97604488694527625, -13.89961937509977652, 76.87390960531433848 ) ) ;
#187709=CARTESIAN_POINT ( 'NONE',  ( -4.483927247898782831, 16.52544592524335698, 112.7094237280190328 ) ) ;
#187710=CARTESIAN_POINT ( 'NONE',  ( 16.51473224551069308, 9.474510206698969483, 39.16557627198103120 ) ) ;
#187711=CARTESIAN_POINT ( 'NONE',  ( -21.52544592524343514, 5.823673210054127303, 51.04057627198103120 ) ) ;
#187712=CARTESIAN_POINT ( 'NONE',  ( -12.06949235617756955, 12.14591786802309770, 95.62390960531436690 ) ) ;
#187713=CARTESIAN_POINT ( 'NONE',  ( -21.53943276465977519, 0.05219959533907696930, 91.24890960531436690 ) ) ;
#187714=CARTESIAN_POINT ( 'NONE',  ( -5.153800228976328057, -19.02544592524343514, 107.2905762719810383 ) ) ;
#187715=ADVANCED_FACE ( 'NONE', ( #19142 ), #18156, .T. ) ;
#187716=CARTESIAN_POINT ( 'NONE',  ( 9.564922557960805705, 16.46253265017160317, 54.58224293864769550 ) ) ;
#187717=CARTESIAN_POINT ( 'NONE',  ( 13.89961937509957401, 13.97604488694547697, 86.87609039468567573 ) ) ;
#187718=CARTESIAN_POINT ( 'NONE',  ( -21.53943276465977519, 0.05219959533907696930, 41.24890960531435269 ) ) ;
#187719=CARTESIAN_POINT ( 'NONE',  ( 15.72974639402176855, 15.80617190586768217, 61.87609039468568284 ) ) ;
#187720=CARTESIAN_POINT ( 'NONE',  ( 0.05219959533909260263, 19.03943276465977164, 54.99890960531435979 ) ) ;
#187721=CARTESIAN_POINT ( 'NONE',  ( -19.02544592524342804, 5.153800228976336051, 86.04057627198103830 ) ) ;
#187722=CARTESIAN_POINT ( 'NONE',  ( 14.29746914071037800, 8.314922557961029526, 66.66775706135234714 ) ) ;
#187723=CARTESIAN_POINT ( 'NONE',  ( -21.53943276465977519, -0.05219959533937600094, 43.75109039468568284 ) ) ;
#187724=CARTESIAN_POINT ( 'NONE',  ( 10.81492255796106328, -18.62759615963255655, 85.41775706135236135 ) ) ;
#187725=CARTESIAN_POINT ( 'NONE',  ( -21.55341960407610458, -5.719274019375992779, 96.45724293864770971 ) ) ;
#187726=CARTESIAN_POINT ( 'NONE',  ( 21.55341960407619695, -5.719274019375665929, 31.04275706135234714 ) ) ;
#187727=CARTESIAN_POINT ( 'NONE',  ( 16.52544592524335698, 4.483927247898782831, 61.45942372801901854 ) ) ;
#187728=CARTESIAN_POINT ( 'NONE',  ( 0.05219959533907565091, 21.53943276465977519, 64.99890960531435269 ) ) ;
#187729=CARTESIAN_POINT ( 'NONE',  ( 13.97604488694548053, -13.89961937509957401, 35.62609039468567573 ) ) ;
#187730=CARTESIAN_POINT ( 'NONE',  ( -9.474510206698964154, 16.51473224551069663, 70.41557627198102409 ) ) ;
#187731=CARTESIAN_POINT ( 'NONE',  ( 12.06949235617757843, -12.14591786802309237, 23.12390960531436335 ) ) ;
#187732=CARTESIAN_POINT ( 'NONE',  ( 30.00000000000000000, -5.499999999999992895, 102.5000000000000142 ) ) ;
#187733=CARTESIAN_POINT ( 'NONE',  ( 9.474510206698971260, -16.51473224551069308, 107.9155762719810383 ) ) ;
#187735=CARTESIAN_POINT ( 'NONE',  ( -5.049401038297874678, -19.05341960407617918, 79.79275706135233293 ) ) ;
#187736=CARTESIAN_POINT ( 'NONE',  ( 21.52544592524344225, -5.823673210054117533, 63.54057627198103830 ) ) ;
#187737=CARTESIAN_POINT ( 'NONE',  ( -12.14591786802309592, -12.06949235617757132, 41.87390960531435979 ) ) ;
#187738=CARTESIAN_POINT ( 'NONE',  ( 8.314922557961029526, -14.29746914071037800, 20.41775706135234714 ) ) ;
#187739=CARTESIAN_POINT ( 'NONE',  ( -13.97604488694527625, -13.89961937509977652, 36.87390960531436690 ) ) ;
#187740=CARTESIAN_POINT ( 'NONE',  ( -13.89961937509957401, -13.97604488694547875, 109.3760903946856331 ) ) ;
#187741=CARTESIAN_POINT ( 'NONE',  ( -18.67979575497178146, -10.72451020669898902, 101.6655762719810383 ) ) ;
#187742=CARTESIAN_POINT ( 'NONE',  ( 19.02544592524334988, 5.153800228976608722, 76.45942372801897591 ) ) ;
#187743=CARTESIAN_POINT ( 'NONE',  ( 14.34966873604972726, -8.224510206698740333, 85.83442372801901854 ) ) ;
#187744=CARTESIAN_POINT ( 'NONE',  ( -16.51473224551069308, -9.474510206698971260, 71.66557627198102409 ) ) ;
#187745=CARTESIAN_POINT ( 'NONE',  ( 0.05219959533910956823, 16.53943276465976808, 69.99890960531435269 ) ) ;
#187747=CARTESIAN_POINT ( 'NONE',  ( -16.46253265017160317, 9.564922557960807481, 45.83224293864769550 ) ) ;
#187748=CARTESIAN_POINT ( 'NONE',  ( -14.34966873604960291, -8.224510206698953496, 56.66557627198103830 ) ) ;
#187751=CARTESIAN_POINT ( 'NONE',  ( 8.314922557960818139, 14.29746914071049879, 24.58224293864768839 ) ) ;
#187752=CARTESIAN_POINT ( 'NONE',  ( 0.05219959533909260263, 19.03943276465977164, 79.99890960531436690 ) ) ;
#187754=CARTESIAN_POINT ( 'NONE',  ( -16.51473224551082808, 9.474510206698731452, 38.33442372801899722 ) ) ;
#187755=CARTESIAN_POINT ( 'NONE',  ( 14.34966873604972726, -8.224510206698740333, 45.83442372801901854 ) ) ;
#187756=CARTESIAN_POINT ( 'NONE',  ( 0.05219959533907565091, 21.53943276465977519, 59.99890960531436690 ) ) ;
#187757=CARTESIAN_POINT ( 'NONE',  ( -5.153800228976607833, 19.02544592524334988, 22.70942372801899012 ) ) ;
#187758=CARTESIAN_POINT ( 'NONE',  ( 16.51473224551069308, 9.474510206698969483, 69.16557627198102409 ) ) ;
#187760=CARTESIAN_POINT ( 'NONE',  ( -19.03943276465977164, 0.05219959533909376836, 116.2489096053143669 ) ) ;
#187761=CARTESIAN_POINT ( 'NONE',  ( -10.81492255796105439, 18.62759615963255655, 37.91775706135235424 ) ) ;
#187762=CARTESIAN_POINT ( 'NONE',  ( -14.34966873604960291, -8.224510206698953496, 111.6655762719810525 ) ) ;
#187763=CARTESIAN_POINT ( 'NONE',  ( -5.719274019375978568, 21.55341960407610458, 95.20724293864769550 ) ) ;
#187764=CARTESIAN_POINT ( 'NONE',  ( -0.05219959533909027116, -19.03943276465977164, 77.49890960531435269 ) ) ;
#187765=ORIENTED_EDGE ( 'NONE', *, *, #294, .T. ) ;
#187766=CARTESIAN_POINT ( 'NONE',  ( -5.719274019375665041, -21.55341960407619695, 24.79275706135235779 ) ) ;
#187767=ORIENTED_EDGE ( 'NONE', *, *, #52301, .F. ) ;
#187768=CARTESIAN_POINT ( 'NONE',  ( 5.049401038298161559, -19.05341960407611168, 87.70724293864769550 ) ) ;
#187770=CARTESIAN_POINT ( 'NONE',  ( 5.049401038298161559, -19.05341960407611168, 27.70724293864769550 ) ) ;
#187771=CARTESIAN_POINT ( 'NONE',  ( 0.05219959533936267826, -19.03943276465977164, 100.0010903946856757 ) ) ;
#187773=CARTESIAN_POINT ( 'NONE',  ( -12.06949235617756955, 12.14591786802309770, 115.6239096053143669 ) ) ;
#187774=CARTESIAN_POINT ( 'NONE',  ( -5.823673210054431948, 21.52544592524334988, 82.70942372801900433 ) ) ;
#187775=CARTESIAN_POINT ( 'NONE',  ( -9.474510206698964154, 16.51473224551069663, 80.41557627198103830 ) ) ;
#187776=CARTESIAN_POINT ( 'NONE',  ( 18.62759615963255655, 10.81492255796105972, 51.66775706135234714 ) ) ;
#187777=CARTESIAN_POINT ( 'NONE',  ( -21.52544592524334988, -5.823673210054445271, 23.95942372801901143 ) ) ;
#187779=CARTESIAN_POINT ( 'NONE',  ( -5.049401038298153566, 19.05341960407611168, 85.20724293864766707 ) ) ;
#187781=CARTESIAN_POINT ( 'NONE',  ( 16.55341960407618274, -4.379528057220086978, 36.04275706135234714 ) ) ;
#187782=CARTESIAN_POINT ( 'NONE',  ( -5.719274019375978568, 21.55341960407610458, 45.20724293864769550 ) ) ;
#187783=CARTESIAN_POINT ( 'NONE',  ( -10.81492255796105439, 18.62759615963255655, 82.91775706135234714 ) ) ;
#187785=CARTESIAN_POINT ( 'NONE',  ( 12.14591786802327356, -12.06949235617739191, 20.62609039468568639 ) ) ;
#187786=CARTESIAN_POINT ( 'NONE',  ( 5.153800228976335163, 19.02544592524342804, 54.79057627198103120 ) ) ;
#187787=CARTESIAN_POINT ( 'NONE',  ( -19.02544592524342804, 5.153800228976336051, 86.04057627198103830 ) ) ;
#187789=CARTESIAN_POINT ( 'NONE',  ( -12.06949235617756955, 12.14591786802309770, 110.6239096053143669 ) ) ;
#187790=CARTESIAN_POINT ( 'NONE',  ( -8.224510206698948167, 14.34966873604960824, 110.4155762719810383 ) ) ;
#187791=CARTESIAN_POINT ( 'NONE',  ( -5.049401038298153566, 19.05341960407611168, 110.2072429386476671 ) ) ;
#187792=CARTESIAN_POINT ( 'NONE',  ( 12.06949235617739724, 12.14591786802326823, 76.87609039468567573 ) ) ;
#187793=CARTESIAN_POINT ( 'NONE',  ( -16.53943276465976808, 0.05219959533911058130, 61.24890960531435979 ) ) ;
#187794=CARTESIAN_POINT ( 'NONE',  ( 5.153800228976335163, 19.02544592524342804, 59.79057627198100988 ) ) ;
#187795=CARTESIAN_POINT ( 'NONE',  ( -18.67979575497193778, 10.72451020669871902, 78.33442372801901854 ) ) ;
#187796=CARTESIAN_POINT ( 'NONE',  ( -10.72451020669870658, -18.67979575497194134, 64.58442372801900433 ) ) ;
#187797=CARTESIAN_POINT ( 'NONE',  ( -19.02544592524334988, -5.153800228976617603, 108.9594237280189759 ) ) ;
#187798=CARTESIAN_POINT ( 'NONE',  ( -12.06949235617756955, 12.14591786802309770, 65.62390960531436690 ) ) ;
#187799=CARTESIAN_POINT ( 'NONE',  ( 5.823673210054444382, -21.52544592524334988, 20.20942372801900788 ) ) ;
#187800=CARTESIAN_POINT ( 'NONE',  ( 21.52544592524344225, -5.823673210054117533, 63.54057627198103830 ) ) ;
#187801=CARTESIAN_POINT ( 'NONE',  ( -16.38665767535054130, -7.295008042176104546, 104.7359913578545587 ) ) ;
#187803=CARTESIAN_POINT ( 'NONE',  ( 19.03943276465977164, -0.05219959533909143690, 73.74890960531435269 ) ) ;
#187804=CARTESIAN_POINT ( 'NONE',  ( 14.29746914071049879, -8.314922557960816363, 33.33224293864769550 ) ) ;
#187805=CARTESIAN_POINT ( 'NONE',  ( 4.379528057220092307, 16.55341960407617563, 112.2927570613523471 ) ) ;
#187806=CARTESIAN_POINT ( 'NONE',  ( 16.52544592524335698, 4.483927247898782831, 96.45942372801901854 ) ) ;
#187807=CARTESIAN_POINT ( 'NONE',  ( -16.46253265017146816, -9.564922557961047289, 59.16775706135233293 ) ) ;
#187809=CARTESIAN_POINT ( 'NONE',  ( -19.02544592524342804, 5.153800228976336051, 86.04057627198103830 ) ) ;
#187810=CARTESIAN_POINT ( 'NONE',  ( -12.06949235617756955, 12.14591786802309770, 65.62390960531436690 ) ) ;
#187811=CARTESIAN_POINT ( 'NONE',  ( 17.50000000000000711, -5.622605283950869115, 101.1879268940388812 ) ) ;
#187812=CARTESIAN_POINT ( 'NONE',  ( -5.719274019375978568, 21.55341960407610458, 25.20724293864769550 ) ) ;
#187813=CARTESIAN_POINT ( 'NONE',  ( 15.72974639402199770, -15.80617190586745480, 48.12390960531436690 ) ) ;
#187815=CARTESIAN_POINT ( 'NONE',  ( 8.224510206698953496, -14.34966873604960469, 92.91557627198103830 ) ) ;
#187816=CARTESIAN_POINT ( 'NONE',  ( 4.483927247898790824, -16.52544592524335698, 50.20942372801901854 ) ) ;
#187817=CARTESIAN_POINT ( 'NONE',  ( 4.379528057220339221, -16.55341960407611168, 77.70724293864770971 ) ) ;
#187818=CARTESIAN_POINT ( 'NONE',  ( -19.35633801406906329, 5.499999999999777955, 64.13373818172762242 ) ) ;
#187819=CARTESIAN_POINT ( 'NONE',  ( 16.46253265017146816, 9.564922557961045513, 76.66775706135234714 ) ) ;
#187820=CARTESIAN_POINT ( 'NONE',  ( 10.81492255796078972, 18.62759615963270932, 24.58224293864768839 ) ) ;
#187822=CARTESIAN_POINT ( 'NONE',  ( -9.564922557960796823, -16.46253265017161027, 42.08224293864769550 ) ) ;
#187823=CARTESIAN_POINT ( 'NONE',  ( 4.379528057220092307, 16.55341960407617563, 42.29275706135235424 ) ) ;
#187824=CARTESIAN_POINT ( 'NONE',  ( -16.52544592524342804, 4.483927247898546575, 26.04057627198103475 ) ) ;
#187825=CARTESIAN_POINT ( 'NONE',  ( 21.55341960407610458, 5.719274019375980345, 58.95724293864770971 ) ) ;
#187826=CARTESIAN_POINT ( 'NONE',  ( 16.51473224551083163, -9.474510206698727899, 85.83442372801900433 ) ) ;
#187827=CARTESIAN_POINT ( 'NONE',  ( 10.72451020669898902, -18.67979575497178502, 42.91557627198103120 ) ) ;
#187828=CARTESIAN_POINT ( 'NONE',  ( -15.72974639402176322, -15.80617190586768395, 79.37609039468567573 ) ) ;
#187830=CARTESIAN_POINT ( 'NONE',  ( 4.483927247898790824, -16.52544592524335698, 30.20942372801902565 ) ) ;
#187831=CARTESIAN_POINT ( 'NONE',  ( -5.049401038298153566, 19.05341960407611168, 40.20724293864768839 ) ) ;
#187832=CARTESIAN_POINT ( 'NONE',  ( 19.02544592524343514, -5.153800228976328945, 83.54057627198100988 ) ) ;
#187833=CARTESIAN_POINT ( 'NONE',  ( -16.46253265017160317, 9.564922557960807481, 30.83224293864769550 ) ) ;
#187834=CARTESIAN_POINT ( 'NONE',  ( 16.52544592524342804, -4.483927247898539470, 103.5405762719810383 ) ) ;
#187836=CARTESIAN_POINT ( 'NONE',  ( 13.97604488694527802, 13.89961937509977652, 104.3739096053143385 ) ) ;
#187838=CARTESIAN_POINT ( 'NONE',  ( -8.224510206698735004, -14.34966873604973081, 49.58442372801901143 ) ) ;
#187839=CARTESIAN_POINT ( 'NONE',  ( -21.53943276465977519, 0.05219959533907696930, 96.24890960531435269 ) ) ;
#187840=CARTESIAN_POINT ( 'NONE',  ( -13.97604488694527625, -13.89961937509977652, 41.87390960531435979 ) ) ;
#187841=CARTESIAN_POINT ( 'NONE',  ( -5.719274019375665041, -21.55341960407619695, 29.79275706135234358 ) ) ;
#187842=CARTESIAN_POINT ( 'NONE',  ( 5.153800228976335163, 19.02544592524342804, 79.79057627198102409 ) ) ;
#187845=CARTESIAN_POINT ( 'NONE',  ( 16.53943276465976808, 0.05219959533934440121, 31.25109039468568639 ) ) ;
#187846=CARTESIAN_POINT ( 'NONE',  ( 18.62759615963271287, -10.81492255796078972, 113.3322429386476955 ) ) ;
#187847=CARTESIAN_POINT ( 'NONE',  ( 8.314922557960818139, 14.29746914071049879, 109.5822429386476955 ) ) ;
#187848=CARTESIAN_POINT ( 'NONE',  ( 5.049401038298161559, -19.05341960407611168, 92.70724293864769550 ) ) ;
#187849=CARTESIAN_POINT ( 'NONE',  ( 13.89961937509957401, 13.97604488694547697, 71.87609039468567573 ) ) ;
#187850=CARTESIAN_POINT ( 'NONE',  ( 13.97604488694548053, -13.89961937509957401, 25.62609039468566507 ) ) ;
#187851=CARTESIAN_POINT ( 'NONE',  ( -21.52544592524343514, 5.823673210054127303, 81.04057627198102409 ) ) ;
#187852=CARTESIAN_POINT ( 'NONE',  ( -16.51473224551082808, 9.474510206698731452, 28.33442372801900433 ) ) ;
#187853=CARTESIAN_POINT ( 'NONE',  ( 16.55341960407618274, -4.379528057220086978, 81.04275706135236135 ) ) ;
#187854=CARTESIAN_POINT ( 'NONE',  ( 0.05219959533909260263, 19.03943276465977164, 104.9989096053143669 ) ) ;
#187855=CARTESIAN_POINT ( 'NONE',  ( 9.564922557960805705, 16.46253265017160317, 49.58224293864770260 ) ) ;
#187856=CARTESIAN_POINT ( 'NONE',  ( -21.53943276465977519, -0.05219959533937600094, 58.75109039468568994 ) ) ;
#187857=CARTESIAN_POINT ( 'NONE',  ( -10.72451020669870658, -18.67979575497194134, 69.58442372801900433 ) ) ;
#187858=CARTESIAN_POINT ( 'NONE',  ( -19.02544592524342804, 5.153800228976336051, 76.04057627198102409 ) ) ;
#187859=CARTESIAN_POINT ( 'NONE',  ( -21.55341960407619339, 5.719274019375674811, 43.54275706135235424 ) ) ;
#187860=CARTESIAN_POINT ( 'NONE',  ( 5.049401038297881783, 19.05341960407617563, 92.29275706135234714 ) ) ;
#187861=CARTESIAN_POINT ( 'NONE',  ( -5.049401038298153566, 19.05341960407611168, 55.20724293864769550 ) ) ;
#187862=CARTESIAN_POINT ( 'NONE',  ( -16.46253265017160317, 9.564922557960807481, 95.83224293864769550 ) ) ;
#187863=CARTESIAN_POINT ( 'NONE',  ( 5.153800228976335163, 19.02544592524342804, 69.79057627198103830 ) ) ;
#187864=CARTESIAN_POINT ( 'NONE',  ( 0.05219959533909260263, 19.03943276465977164, 109.9989096053143669 ) ) ;
#187865=CARTESIAN_POINT ( 'NONE',  ( 9.474510206698971260, -16.51473224551069308, 52.91557627198102409 ) ) ;
#187866=CARTESIAN_POINT ( 'NONE',  ( -21.53943276465977519, 0.05219959533907696930, 91.24890960531436690 ) ) ;
#187867=CARTESIAN_POINT ( 'NONE',  ( -4.483927247898782831, 16.52544592524335698, 72.70942372801901854 ) ) ;
#187869=CARTESIAN_POINT ( 'NONE',  ( 19.05341960407617918, -5.049401038297876454, 26.04275706135233293 ) ) ;
#187870=CARTESIAN_POINT ( 'NONE',  ( -0.05219959533909027116, -19.03943276465977164, 62.49890960531435979 ) ) ;
#187871=CARTESIAN_POINT ( 'NONE',  ( 12.14591786802309770, 12.06949235617756955, 59.37390960531436690 ) ) ;
#187872=CARTESIAN_POINT ( 'NONE',  ( -8.224510206698948167, 14.34966873604960824, 100.4155762719810241 ) ) ;
#187873=CARTESIAN_POINT ( 'NONE',  ( -5.153800228976328057, -19.02544592524343514, 97.29057627198099567 ) ) ;
#187874=CARTESIAN_POINT ( 'NONE',  ( 0.05219959533909260263, 19.03943276465977164, 89.99890960531436690 ) ) ;
#187875=CARTESIAN_POINT ( 'NONE',  ( 21.53943276465977519, 0.05219959533937863772, 56.25109039468568284 ) ) ;
#187876=CARTESIAN_POINT ( 'NONE',  ( -16.46253265017160317, 9.564922557960807481, 100.8322429386477097 ) ) ;
#187877=CARTESIAN_POINT ( 'NONE',  ( -9.474510206698720793, -16.51473224551083518, 19.58442372801899722 ) ) ;
#187878=CARTESIAN_POINT ( 'NONE',  ( -14.29746914071037622, -8.314922557961029526, 74.16775706135231871 ) ) ;
#187880=CARTESIAN_POINT ( 'NONE',  ( 15.80617190586769283, -15.72974639402175789, 45.62609039468567573 ) ) ;
#187881=CARTESIAN_POINT ( 'NONE',  ( 15.80617190586746368, 15.72974639402197994, 24.37390960531435979 ) ) ;
#187882=CARTESIAN_POINT ( 'NONE',  ( 21.52544592524344225, -5.823673210054117533, 98.54057627198105251 ) ) ;
#187883=CARTESIAN_POINT ( 'NONE',  ( -8.224510206698948167, 14.34966873604960824, 60.41557627198102409 ) ) ;
#187884=CARTESIAN_POINT ( 'NONE',  ( -0.05219959533909027116, -19.03943276465977164, 52.49890960531436690 ) ) ;
#187885=CARTESIAN_POINT ( 'NONE',  ( 16.52544592524342804, -4.483927247898539470, 83.54057627198102409 ) ) ;
#187886=CARTESIAN_POINT ( 'NONE',  ( 10.72451020669898902, -18.67979575497178502, 37.91557627198102409 ) ) ;
#187887=CARTESIAN_POINT ( 'NONE',  ( 5.153800228976615827, -19.02544592524334988, 40.20942372801898301 ) ) ;
#187888=CARTESIAN_POINT ( 'NONE',  ( 4.379528057220339221, -16.55341960407611168, 112.7072429386476955 ) ) ;
#187890=CARTESIAN_POINT ( 'NONE',  ( -16.53943276465976808, -0.05219959533934237506, 68.75109039468568994 ) ) ;
#187891=CARTESIAN_POINT ( 'NONE',  ( 16.46253265017160672, -9.564922557960803928, 68.33224293864770971 ) ) ;
#187893=CARTESIAN_POINT ( 'NONE',  ( 16.53943276465976808, -0.05219959533910856209, 88.74890960531436690 ) ) ;
#187894=CARTESIAN_POINT ( 'NONE',  ( 18.67979575497178502, 10.72451020669898547, 44.16557627198103120 ) ) ;
#187895=CARTESIAN_POINT ( 'NONE',  ( -16.55341960407617563, 4.379528057220093196, 113.5427570613523756 ) ) ;
#187896=CARTESIAN_POINT ( 'NONE',  ( -16.46253265017146816, -9.564922557961047289, 104.1677570613523329 ) ) ;
#187897=CARTESIAN_POINT ( 'NONE',  ( -10.81492255796105439, 18.62759615963255655, 82.91775706135234714 ) ) ;
#187898=CARTESIAN_POINT ( 'NONE',  ( -16.46253265017160317, 9.564922557960807481, 85.83224293864769550 ) ) ;
#187899=CARTESIAN_POINT ( 'NONE',  ( 5.719274019375991003, -21.55341960407610458, 102.7072429386476955 ) ) ;
#187900=CARTESIAN_POINT ( 'NONE',  ( -16.52544592524335698, -4.483927247898792601, 53.95942372801900433 ) ) ;
#187901=CARTESIAN_POINT ( 'NONE',  ( -16.51473224551069308, -9.474510206698971260, 26.66557627198103120 ) ) ;
#187902=CARTESIAN_POINT ( 'NONE',  ( 8.224510206698742110, 14.34966873604972548, 32.08442372801901854 ) ) ;
#187903=CARTESIAN_POINT ( 'NONE',  ( 0.05219959533936267826, -19.03943276465977164, 95.00109039468567573 ) ) ;
#187904=CARTESIAN_POINT ( 'NONE',  ( 10.72451020669898902, -18.67979575497178502, 92.91557627198103830 ) ) ;
#187905=CARTESIAN_POINT ( 'NONE',  ( -5.049401038297874678, -19.05341960407617918, 59.79275706135231871 ) ) ;
#187907=CARTESIAN_POINT ( 'NONE',  ( -18.67979575497178146, -10.72451020669898902, 101.6655762719810383 ) ) ;
#187909=CARTESIAN_POINT ( 'NONE',  ( 19.02544592524343514, -5.153800228976328945, 73.54057627198103830 ) ) ;
#187910=CARTESIAN_POINT ( 'NONE',  ( -16.55341960407617563, 4.379528057220093196, 38.54275706135234714 ) ) ;
#187912=CARTESIAN_POINT ( 'NONE',  ( 19.03943276465977164, 0.05219959533936151252, 66.25109039468567573 ) ) ;
#187913=CARTESIAN_POINT ( 'NONE',  ( -21.53943276465977519, 0.05219959533907696930, 116.2489096053143669 ) ) ;
#187914=CARTESIAN_POINT ( 'NONE',  ( -16.53943276465976808, 0.05219959533911058130, 66.24890960531436690 ) ) ;
#187915=CARTESIAN_POINT ( 'NONE',  ( -5.049401038298153566, 19.05341960407611168, 70.20724293864769550 ) ) ;
#187916=CARTESIAN_POINT ( 'NONE',  ( 12.06949235617739724, 12.14591786802326823, 41.87609039468568284 ) ) ;
#187917=CARTESIAN_POINT ( 'NONE',  ( 19.03943276465977164, 0.05219959533936151252, 41.25109039468566152 ) ) ;
#187918=CARTESIAN_POINT ( 'NONE',  ( 10.72451020669871369, 18.67979575497193778, 47.08442372801901854 ) ) ;
#187919=CARTESIAN_POINT ( 'NONE',  ( -16.51473224551082808, 9.474510206698731452, 103.3344237280190043 ) ) ;
#187920=CARTESIAN_POINT ( 'NONE',  ( 5.153800228976335163, 19.02544592524342804, 49.79057627198100988 ) ) ;
#187921=CARTESIAN_POINT ( 'NONE',  ( 5.049401038297881783, 19.05341960407617563, 82.29275706135229029 ) ) ;
#187922=CARTESIAN_POINT ( 'NONE',  ( 15.80617190586769283, -15.72974639402175789, 90.62609039468567573 ) ) ;
#187923=CARTESIAN_POINT ( 'NONE',  ( 19.03943276465977164, 0.05219959533936151252, 71.25109039468566152 ) ) ;
#187924=CARTESIAN_POINT ( 'NONE',  ( 19.05341960407611168, 5.049401038298154454, 33.95724293864769550 ) ) ;
#187925=CARTESIAN_POINT ( 'NONE',  ( 5.823673210054125526, 21.52544592524343514, 74.79057627198105251 ) ) ;
#187926=CARTESIAN_POINT ( 'NONE',  ( 16.52544592524342804, -4.483927247898539470, 58.54057627198103120 ) ) ;
#187927=CARTESIAN_POINT ( 'NONE',  ( -0.05219959533936034679, 19.03943276465977164, 67.50109039468566152 ) ) ;
#187928=CARTESIAN_POINT ( 'NONE',  ( -16.38665767535055195, -7.295008042175997964, 24.73599135785456937 ) ) ;
#187929=CARTESIAN_POINT ( 'NONE',  ( 9.474510206698729675, 16.51473224551082808, 32.08442372801900433 ) ) ;
#187930=CARTESIAN_POINT ( 'NONE',  ( -16.53943276465976808, -0.05219959533934237506, 93.75109039468567573 ) ) ;
#187931=CARTESIAN_POINT ( 'NONE',  ( 14.34966873604960469, 8.224510206698951720, 49.16557627198102409 ) ) ;
#187932=CARTESIAN_POINT ( 'NONE',  ( 15.80617190586769283, -15.72974639402175789, 95.62609039468568994 ) ) ;
#187934=CARTESIAN_POINT ( 'NONE',  ( 21.52544592524344225, -5.823673210054117533, 93.54057627198103830 ) ) ;
#187935=CARTESIAN_POINT ( 'NONE',  ( -19.05341960407611168, -5.049401038298163336, 46.45724293864768129 ) ) ;
#187936=CARTESIAN_POINT ( 'NONE',  ( 0.05219959533937995610, -21.53943276465977519, 65.00109039468568994 ) ) ;
#187937=CARTESIAN_POINT ( 'NONE',  ( 0.05219959533909260263, 19.03943276465977164, 49.99890960531435979 ) ) ;
#187939=CARTESIAN_POINT ( 'NONE',  ( 16.51473224551069308, 9.474510206698969483, 69.16557627198102409 ) ) ;
#187940=CARTESIAN_POINT ( 'NONE',  ( -16.55341960407611168, -4.379528057220339221, 106.4572429386477097 ) ) ;
#187941=CARTESIAN_POINT ( 'NONE',  ( 16.46253265017160672, -9.564922557960803928, 108.3322429386476955 ) ) ;
#187942=CARTESIAN_POINT ( 'NONE',  ( 8.224510206698953496, -14.34966873604960469, 57.91557627198103120 ) ) ;
#187943=CARTESIAN_POINT ( 'NONE',  ( -9.474510206698964154, 16.51473224551069663, 30.41557627198102054 ) ) ;
#187944=CARTESIAN_POINT ( 'NONE',  ( -8.224510206698948167, 14.34966873604960824, 90.41557627198103830 ) ) ;
#187945=CARTESIAN_POINT ( 'NONE',  ( -5.719274019375978568, 21.55341960407610458, 90.20724293864770971 ) ) ;
#187946=CARTESIAN_POINT ( 'NONE',  ( 15.80617190586769283, -15.72974639402175789, 40.62609039468567573 ) ) ;
#187948=EDGE_CURVE ( 'NONE', #127622, #63455, #43099, .T. ) ;
#187949=CARTESIAN_POINT ( 'NONE',  ( -16.53943276465976808, -0.05219959533934237506, 38.75109039468567573 ) ) ;
#187950=CARTESIAN_POINT ( 'NONE',  ( 18.67979575497178502, 10.72451020669898547, 79.16557627198103830 ) ) ;
#187951=CARTESIAN_POINT ( 'NONE',  ( 21.55341960407619695, -5.719274019375665929, 111.0427570613523613 ) ) ;
#187952=CARTESIAN_POINT ( 'NONE',  ( 16.51473224551069308, 9.474510206698969483, 89.16557627198103830 ) ) ;
#187953=CARTESIAN_POINT ( 'NONE',  ( 18.67979575497194134, -10.72451020669871369, 45.83442372801901854 ) ) ;
#187954=CARTESIAN_POINT ( 'NONE',  ( -15.72974639402197994, 15.80617190586746368, 30.62390960531436335 ) ) ;
#187955=CARTESIAN_POINT ( 'NONE',  ( -16.55341960407617563, 4.379528057220093196, 108.5427570613523756 ) ) ;
#187956=CARTESIAN_POINT ( 'NONE',  ( 0.05219959533937995610, -21.53943276465977519, 50.00109039468568994 ) ) ;
#187957=CARTESIAN_POINT ( 'NONE',  ( 0.05219959533937995610, -21.53943276465977519, 85.00109039468568994 ) ) ;
#187958=CARTESIAN_POINT ( 'NONE',  ( 13.89961937509957401, 13.97604488694547697, 31.87609039468566863 ) ) ;
#187959=CARTESIAN_POINT ( 'NONE',  ( -16.55341960407617563, 4.379528057220093196, 88.54275706135236135 ) ) ;
#187960=CARTESIAN_POINT ( 'NONE',  ( -0.05219959533937732626, 21.53943276465977519, 42.50109039468567573 ) ) ;
#187961=CARTESIAN_POINT ( 'NONE',  ( -13.97604488694527625, -13.89961937509977652, 41.87390960531435979 ) ) ;
#187962=CARTESIAN_POINT ( 'NONE',  ( -0.05219959533937732626, 21.53943276465977519, 102.5010903946856899 ) ) ;
#187963=CARTESIAN_POINT ( 'NONE',  ( -19.05341960407611168, -5.049401038298163336, 101.4572429386476955 ) ) ;
#187964=CARTESIAN_POINT ( 'NONE',  ( 21.52544592524344225, -5.823673210054117533, 113.5405762719810383 ) ) ;
#187965=CARTESIAN_POINT ( 'NONE',  ( 10.81492255796078972, 18.62759615963270932, 74.58224293864768129 ) ) ;
#187966=CARTESIAN_POINT ( 'NONE',  ( -17.60779699588839975, -5.500000000000020428, 61.34981316670106821 ) ) ;
#187967=CARTESIAN_POINT ( 'NONE',  ( 5.719274019375991003, -21.55341960407610458, 67.70724293864769550 ) ) ;
#187968=CARTESIAN_POINT ( 'NONE',  ( -14.29746914071037622, -8.314922557961029526, 49.16775706135234003 ) ) ;
#187969=CARTESIAN_POINT ( 'NONE',  ( -8.314922557960811034, -14.29746914071050412, 57.08224293864769550 ) ) ;
#187971=CARTESIAN_POINT ( 'NONE',  ( -13.89961937509957401, -13.97604488694547875, 84.37609039468567573 ) ) ;
#187973=CARTESIAN_POINT ( 'NONE',  ( 16.53943276465976808, 0.05219959533934440121, 31.25109039468568639 ) ) ;
#187974=CARTESIAN_POINT ( 'NONE',  ( 10.72451020669898902, -18.67979575497178502, 92.91557627198103830 ) ) ;
#187975=CARTESIAN_POINT ( 'NONE',  ( 21.53943276465977519, -0.05219959533907433946, 68.74890960531435269 ) ) ;
#187976=CARTESIAN_POINT ( 'NONE',  ( 19.03943276465977164, -0.05219959533909143690, 108.7489096053143527 ) ) ;
#187977=CARTESIAN_POINT ( 'NONE',  ( -14.34966873604972548, 8.224510206698743886, 53.33442372801901854 ) ) ;
#187978=CARTESIAN_POINT ( 'NONE',  ( -13.89961937509977652, 13.97604488694528158, 70.62390960531432427 ) ) ;
#187979=CARTESIAN_POINT ( 'NONE',  ( -21.53943276465977519, -0.05219959533937600094, 48.75109039468568284 ) ) ;
#187980=CARTESIAN_POINT ( 'NONE',  ( -16.51473224551082808, 9.474510206698731452, 113.3344237280190043 ) ) ;
#187981=CARTESIAN_POINT ( 'NONE',  ( 16.46253265017160672, -9.564922557960803928, 108.3322429386476955 ) ) ;
#187982=CARTESIAN_POINT ( 'NONE',  ( -9.474510206698964154, 16.51473224551069663, 100.4155762719810241 ) ) ;
#187983=CARTESIAN_POINT ( 'NONE',  ( 15.72974639402199770, -15.80617190586745480, 98.12390960531436690 ) ) ;
#187984=CARTESIAN_POINT ( 'NONE',  ( 19.03943276465977164, -0.05219959533909143690, 53.74890960531436690 ) ) ;
#187985=CARTESIAN_POINT ( 'NONE',  ( -17.50000000000000000, 5.499999999999992895, 23.71769037696436300 ) ) ;
#187986=CARTESIAN_POINT ( 'NONE',  ( -16.53943276465976808, 0.05219959533911058130, 76.24890960531435269 ) ) ;
#187987=CARTESIAN_POINT ( 'NONE',  ( 21.53943276465977519, -0.05219959533907433946, 23.74890960531435269 ) ) ;
#187989=CARTESIAN_POINT ( 'NONE',  ( -21.55341960407610458, -5.719274019375992779, 101.4572429386476955 ) ) ;
#187990=CARTESIAN_POINT ( 'NONE',  ( 19.05341960407617918, -5.049401038297876454, 61.04275706135232582 ) ) ;
#187991=CARTESIAN_POINT ( 'NONE',  ( 10.81492255796078972, 18.62759615963270932, 24.58224293864768839 ) ) ;
#187992=CARTESIAN_POINT ( 'NONE',  ( 19.03943276465977164, -0.05219959533909143690, 28.74890960531435624 ) ) ;
#187993=CARTESIAN_POINT ( 'NONE',  ( 10.81492255796078972, 18.62759615963270932, 49.58224293864769550 ) ) ;
#187994=CARTESIAN_POINT ( 'NONE',  ( -13.97604488694527625, -13.89961937509977652, 101.8739096053143811 ) ) ;
#187995=CARTESIAN_POINT ( 'NONE',  ( -15.72974639402176322, -15.80617190586768395, 79.37609039468567573 ) ) ;
#187996=CARTESIAN_POINT ( 'NONE',  ( -9.474510206698964154, 16.51473224551069663, 45.41557627198103120 ) ) ;
#187997=CARTESIAN_POINT ( 'NONE',  ( -8.314922557960811034, -14.29746914071050412, 92.08224293864769550 ) ) ;
#187998=CARTESIAN_POINT ( 'NONE',  ( -8.224510206698735004, -14.34966873604973081, 39.58442372801901143 ) ) ;
#187999=CARTESIAN_POINT ( 'NONE',  ( -5.719274019375665041, -21.55341960407619695, 69.79275706135234714 ) ) ;
#188000=ORIENTED_EDGE ( 'NONE', *, *, #165982, .T. ) ;
#188001=CARTESIAN_POINT ( 'NONE',  ( 13.89961937509957401, 13.97604488694547697, 26.87609039468566507 ) ) ;
#188002=CARTESIAN_POINT ( 'NONE',  ( 9.564922557961047289, -16.46253265017146816, 85.41775706135233293 ) ) ;
#188003=CARTESIAN_POINT ( 'NONE',  ( 16.46253265017146816, 9.564922557961045513, 36.66775706135233293 ) ) ;
#188004=DIRECTION ( 'NONE',  ( 0.000000000000000000, 0.000000000000000000, -1.000000000000000000 ) ) ;
#188005=CARTESIAN_POINT ( 'NONE',  ( -21.55341960407619339, 5.719274019375674811, 33.54275706135234714 ) ) ;
#188007=CARTESIAN_POINT ( 'NONE',  ( 13.89961937509957401, 13.97604488694547697, 36.87609039468565442 ) ) ;
#188008=CARTESIAN_POINT ( 'NONE',  ( 9.564922557960805705, 16.46253265017160317, 74.58224293864769550 ) ) ;
#188009=CARTESIAN_POINT ( 'NONE',  ( 13.97604488694548053, -13.89961937509957401, 25.62609039468566507 ) ) ;
#188010=CARTESIAN_POINT ( 'NONE',  ( -12.14591786802326823, 12.06949235617739902, 113.1260903946856899 ) ) ;
#188011=CARTESIAN_POINT ( 'NONE',  ( 21.52544592524344225, -5.823673210054117533, 23.54057627198102765 ) ) ;
#188012=CARTESIAN_POINT ( 'NONE',  ( 21.53943276465977519, 0.05219959533937863772, 81.25109039468568994 ) ) ;
#188015=CARTESIAN_POINT ( 'NONE',  ( -15.72974639402176322, -15.80617190586768395, 79.37609039468567573 ) ) ;
#188016=CARTESIAN_POINT ( 'NONE',  ( 16.38665767535054485, -7.295008042176021945, 42.76400864214548392 ) ) ;
#188017=CARTESIAN_POINT ( 'NONE',  ( -9.474510206698964154, 16.51473224551069663, 100.4155762719810241 ) ) ;
#188019=CARTESIAN_POINT ( 'NONE',  ( -16.51473224551069308, -9.474510206698971260, 46.66557627198102409 ) ) ;
#188020=CARTESIAN_POINT ( 'NONE',  ( 10.72451020669898902, -18.67979575497178502, 62.91557627198102409 ) ) ;
#188021=CARTESIAN_POINT ( 'NONE',  ( 12.06949235617757843, -12.14591786802309237, 23.12390960531436335 ) ) ;
#188022=CARTESIAN_POINT ( 'NONE',  ( 12.06949235617757843, -12.14591786802309237, 103.1239096053143811 ) ) ;
#188023=CARTESIAN_POINT ( 'NONE',  ( 16.46253265017160672, -9.564922557960803928, 98.33224293864769550 ) ) ;
#188024=CARTESIAN_POINT ( 'NONE',  ( 5.049401038297881783, 19.05341960407617563, 22.29275706135233648 ) ) ;
#188025=CARTESIAN_POINT ( 'NONE',  ( -14.29746914071049879, 8.314922557960819915, 95.83224293864770971 ) ) ;
#188026=CARTESIAN_POINT ( 'NONE',  ( 21.52544592524334988, 5.823673210054432836, 61.45942372801901854 ) ) ;
#188028=CARTESIAN_POINT ( 'NONE',  ( 14.29746914071037800, 8.314922557961029526, 111.6677570613523613 ) ) ;
#188029=CARTESIAN_POINT ( 'NONE',  ( 9.564922557961047289, -16.46253265017146816, 70.41775706135233293 ) ) ;
#188031=CARTESIAN_POINT ( 'NONE',  ( -13.89961937509977652, 13.97604488694528158, 115.6239096053143669 ) ) ;
#188032=CARTESIAN_POINT ( 'NONE',  ( -8.224510206698948167, 14.34966873604960824, 80.41557627198103830 ) ) ;
#188033=CARTESIAN_POINT ( 'NONE',  ( 13.89961937509957401, 13.97604488694547697, 61.87609039468566863 ) ) ;
#188034=CARTESIAN_POINT ( 'NONE',  ( -5.153800228976328057, -19.02544592524343514, 57.29057627198103120 ) ) ;
#188035=CARTESIAN_POINT ( 'NONE',  ( -8.224510206698948167, 14.34966873604960824, 55.41557627198102409 ) ) ;
#188036=CARTESIAN_POINT ( 'NONE',  ( 0.05219959533936267826, -19.03943276465977164, 90.00109039468567573 ) ) ;
#188037=CARTESIAN_POINT ( 'NONE',  ( 0.05219959533907565091, 21.53943276465977519, 34.99890960531435979 ) ) ;
#188039=CARTESIAN_POINT ( 'NONE',  ( -4.483927247898539470, -16.52544592524342804, 97.29057627198105251 ) ) ;
#188041=CARTESIAN_POINT ( 'NONE',  ( 13.89961937509977652, -13.97604488694527269, 63.12390960531435979 ) ) ;
#188042=CARTESIAN_POINT ( 'NONE',  ( -10.81492255796078084, -18.62759615963271287, 57.08224293864769550 ) ) ;
#188043=CARTESIAN_POINT ( 'NONE',  ( -19.02544592524342804, 5.153800228976336051, 41.04057627198103120 ) ) ;
#188044=CARTESIAN_POINT ( 'NONE',  ( -8.314922557961024197, 14.29746914071037800, 92.91775706135236135 ) ) ;
#188045=CARTESIAN_POINT ( 'NONE',  ( -19.02544592524342804, 5.153800228976336051, 71.04057627198099567 ) ) ;
#188046=CARTESIAN_POINT ( 'NONE',  ( -19.05341960407617563, 5.049401038297882671, 53.54275706135231871 ) ) ;
#188047=CARTESIAN_POINT ( 'NONE',  ( 18.62759615963255655, 10.81492255796105972, 81.66775706135236135 ) ) ;
#188048=CARTESIAN_POINT ( 'NONE',  ( 10.72451020669898902, -18.67979575497178502, 47.91557627198102409 ) ) ;
#188049=CARTESIAN_POINT ( 'NONE',  ( -19.03943276465977164, 0.05219959533909376836, 106.2489096053143669 ) ) ;
#188050=CARTESIAN_POINT ( 'NONE',  ( 13.97604488694527802, 13.89961937509977652, 39.37390960531435269 ) ) ;
#188051=CARTESIAN_POINT ( 'NONE',  ( 8.314922557961029526, -14.29746914071037800, 85.41775706135236135 ) ) ;
#188052=CARTESIAN_POINT ( 'NONE',  ( 16.51473224551083163, -9.474510206698727899, 105.8344237280190043 ) ) ;
#188053=CARTESIAN_POINT ( 'NONE',  ( -5.153800228976328057, -19.02544592524343514, 22.29057627198102765 ) ) ;
#188054=CARTESIAN_POINT ( 'NONE',  ( 19.52851543214743302, 5.500000000000029310, 77.89357721762580411 ) ) ;
#188055=CARTESIAN_POINT ( 'NONE',  ( 21.55341960407619695, -5.719274019375665929, 96.04275706135236135 ) ) ;
#188056=CARTESIAN_POINT ( 'NONE',  ( 16.53943276465976808, -0.05219959533910856209, 58.74890960531436690 ) ) ;
#188057=CARTESIAN_POINT ( 'NONE',  ( -16.53943276465976808, 0.05219959533911058130, 76.24890960531435269 ) ) ;
#188058=CARTESIAN_POINT ( 'NONE',  ( 5.823673210054125526, 21.52544592524343514, 94.79057627198105251 ) ) ;
#188059=CARTESIAN_POINT ( 'NONE',  ( 21.52544592524344225, -5.823673210054117533, 83.54057627198102409 ) ) ;
#188061=CARTESIAN_POINT ( 'NONE',  ( 21.55341960407610458, 5.719274019375980345, 43.95724293864769550 ) ) ;
#188062=CARTESIAN_POINT ( 'NONE',  ( 12.14591786802327356, -12.06949235617739191, 60.62609039468567573 ) ) ;
#188063=CARTESIAN_POINT ( 'NONE',  ( 12.06949235617757843, -12.14591786802309237, 88.12390960531436690 ) ) ;
#188064=CARTESIAN_POINT ( 'NONE',  ( 13.97604488694527802, 13.89961937509977652, 49.37390960531434558 ) ) ;
#188065=( NAMED_UNIT ( * ) PLANE_ANGLE_UNIT ( ) SI_UNIT ( $, .RADIAN. ) );
#188067=CARTESIAN_POINT ( 'NONE',  ( 4.379528057220092307, 16.55341960407617563, 97.29275706135234714 ) ) ;
#188068=CARTESIAN_POINT ( 'NONE',  ( -18.62759615963255300, -10.81492255796106328, 29.16775706135234003 ) ) ;
#188069=CARTESIAN_POINT ( 'NONE',  ( 5.153800228976335163, 19.02544592524342804, 84.79057627198099567 ) ) ;
#188070=CARTESIAN_POINT ( 'NONE',  ( -0.05219959533937732626, 21.53943276465977519, 72.50109039468568994 ) ) ;
#188072=CARTESIAN_POINT ( 'NONE',  ( 9.564922557960805705, 16.46253265017160317, 24.58224293864769194 ) ) ;
#188074=CARTESIAN_POINT ( 'NONE',  ( 21.52544592524334988, 5.823673210054432836, 61.45942372801901854 ) ) ;
#188075=CARTESIAN_POINT ( 'NONE',  ( -9.564922557960796823, -16.46253265017161027, 32.08224293864769550 ) ) ;
#188076=CARTESIAN_POINT ( 'NONE',  ( -5.153800228976328057, -19.02544592524343514, 112.2905762719810099 ) ) ;
#188077=CARTESIAN_POINT ( 'NONE',  ( 19.03943276465977164, -0.05219959533909143690, 93.74890960531435269 ) ) ;
#188078=CARTESIAN_POINT ( 'NONE',  ( 5.049401038297881783, 19.05341960407617563, 72.29275706135234714 ) ) ;
#188079=CARTESIAN_POINT ( 'NONE',  ( 21.52544592524334988, 5.823673210054432836, 26.45942372801901854 ) ) ;
#188080=CARTESIAN_POINT ( 'NONE',  ( -0.05219959533936034679, 19.03943276465977164, 62.50109039468566863 ) ) ;
#188081=CARTESIAN_POINT ( 'NONE',  ( -9.474510206698964154, 16.51473224551069663, 40.41557627198103120 ) ) ;
#188082=CARTESIAN_POINT ( 'NONE',  ( -14.34966873604972548, 8.224510206698743886, 98.33442372801901854 ) ) ;
#188083=CARTESIAN_POINT ( 'NONE',  ( 13.97604488694548053, -13.89961937509957401, 75.62609039468564731 ) ) ;
#188084=CARTESIAN_POINT ( 'NONE',  ( 0.05219959533910956823, 16.53943276465976808, 24.99890960531435624 ) ) ;
#188085=CARTESIAN_POINT ( 'NONE',  ( 5.153800228976615827, -19.02544592524334988, 55.20942372801899722 ) ) ;
#188086=CARTESIAN_POINT ( 'NONE',  ( -0.05219959533909027116, -19.03943276465977164, 97.49890960531436690 ) ) ;
#188087=CARTESIAN_POINT ( 'NONE',  ( 10.81492255796106328, -18.62759615963255655, 110.4177570613523756 ) ) ;
#188088=CARTESIAN_POINT ( 'NONE',  ( 21.55341960407619695, -5.719274019375665929, 111.0427570613523613 ) ) ;
#188090=CARTESIAN_POINT ( 'NONE',  ( 10.81492255796106328, -18.62759615963255655, 85.41775706135236135 ) ) ;
#188091=CARTESIAN_POINT ( 'NONE',  ( 4.379528057220092307, 16.55341960407617563, 27.29275706135234358 ) ) ;
#188092=CARTESIAN_POINT ( 'NONE',  ( -16.51473224551069308, -9.474510206698971260, 91.66557627198103830 ) ) ;
#188094=CARTESIAN_POINT ( 'NONE',  ( 5.049401038298161559, -19.05341960407611168, 77.70724293864765286 ) ) ;
#188096=CARTESIAN_POINT ( 'NONE',  ( 9.564922557961047289, -16.46253265017146816, 75.41775706135234714 ) ) ;
#188097=CARTESIAN_POINT ( 'NONE',  ( -19.02544592524342804, 5.153800228976336051, 106.0405762719810241 ) ) ;
#188098=CARTESIAN_POINT ( 'NONE',  ( 15.80617190586769283, -15.72974639402175789, 95.62609039468568994 ) ) ;
#188099=CARTESIAN_POINT ( 'NONE',  ( 12.06949235617757843, -12.14591786802309237, 98.12390960531436690 ) ) ;
#188100=CARTESIAN_POINT ( 'NONE',  ( -5.823673210054116645, -21.52544592524344225, 42.29057627198103120 ) ) ;
#188101=CARTESIAN_POINT ( 'NONE',  ( -15.80617190586745835, -15.72974639402198527, 36.87390960531435979 ) ) ;
#188102=CARTESIAN_POINT ( 'NONE',  ( -12.14591786802309592, -12.06949235617757132, 101.8739096053143811 ) ) ;
#188104=CARTESIAN_POINT ( 'NONE',  ( -19.05341960407617563, 5.049401038297882671, 53.54275706135231871 ) ) ;
#188105=CARTESIAN_POINT ( 'NONE',  ( 0.05219959533910956823, 16.53943276465976808, 24.99890960531435624 ) ) ;
#188106=CARTESIAN_POINT ( 'NONE',  ( 16.46253265017160672, -9.564922557960803928, 98.33224293864769550 ) ) ;
#188108=CARTESIAN_POINT ( 'NONE',  ( 5.719274019375673035, 21.55341960407619339, 82.29275706135234714 ) ) ;
#188109=CARTESIAN_POINT ( 'NONE',  ( 21.53943276465977519, -0.05219959533907433946, 68.74890960531435269 ) ) ;
#188110=CARTESIAN_POINT ( 'NONE',  ( 21.52544592524334988, 5.823673210054432836, 46.45942372801901854 ) ) ;
#188111=CARTESIAN_POINT ( 'NONE',  ( -18.62759615963270932, 10.81492255796079327, 100.8322429386477097 ) ) ;
#188112=CARTESIAN_POINT ( 'NONE',  ( -18.67979575497193778, 10.72451020669871902, 48.33442372801902565 ) ) ;
#188113=CARTESIAN_POINT ( 'NONE',  ( -5.049401038298153566, 19.05341960407611168, 25.20724293864768484 ) ) ;
#188114=CARTESIAN_POINT ( 'NONE',  ( -16.46253265017160317, 9.564922557960807481, 80.83224293864769550 ) ) ;
#188115=CARTESIAN_POINT ( 'NONE',  ( -16.52544592524335698, -4.483927247898792601, 78.95942372801901854 ) ) ;
#188116=( BOUNDED_SURFACE ( )  B_SPLINE_SURFACE ( 3, 2, ( 
 ( #170942, #94088, #102572, #133909, #195600, #57073, #140595, #190098, #52565, #128401, #99060, #35409, #129394, #3082, #33428, #4063, #65741, #51573, #113237, #114225, #110258, #112250, #173942, #97061, #50591, #98045, #21239, #191090, #142584, #127409, #175930, #158743, #78918, #143572, #37401, #2085, #20232, #81880, #17265, #63765, #48606, #189118, #159743, #125438, #66740, #187134, #171939, #5054, #95087, #174928, #36391, #156775, #18269, #79922, #82894, #144572, #141595, #64758, #6058, #67736, #126420, #188118, #49589, #111252, #172943, #34422, #96081, #157770, #19261, #80907, #117245, #133410, #132416, #41413, #193095, #192086, #195099, #85905, #25263, #55571, #23245, #176938, #54571, #164760, #180937, #84889, #11080, #196113, #56581, #119253, #145572, #70748, #9078, #86906, #53568, #10081, #131408, #26255, #7049, #68731, #147593, #42412, #102078, #160748, #22240, #87896, #8062, #149582, #194108, #163763, #148589, #57583, #71739, #118255, #116243, #103079, #39402, #179946, #83889, #72756, #134427, #177935, #178937, #130389, #115246, #38408, #162747, #100065, #146568, #161750, #40407, #69739, #101062, #24255, #74736, #89897, #28258, #166755, #151580, #62522, #61530, #169716, #183900, #120229, #31209, #73753, #92860, #60533, #106050, #167736, #13069, #43400, #107038, #90867, #154547, #849, #135425, #182911, #104075, #75706, #59543, #136399, #137385, #44396, #45385, #181919, #124195, #27251, #29234, #16042, #152552, #30212, #185895, #165757, #88901, #108030, #150591, #168710, #122209, #14040, #91855, #123199, #12090, #197096, #46371, #153547, #199064, #58563, #105070, #15044, #198076, #76705, #138381, #200062, #121221, #184889, #77701, #139368, #82654, #172707, #113004, #65511, #36162, #173711, #93862, #174698, #19030, #2850, #18039, #79693, #64528, #141363, #125209, #158518, #80676, #126195, #48376, #97814, #155540, #32205, #17034, #95852, #81649, #51344, #188882, #67502, #34191, #142352, #4820, #140365, #187891, #186905, #110033, #109035, #143333, #170714, #127172, #96834, #171711, #33201, #66508, #128170, #49358, #157536, #3832, #94859, #63534, #1852, #50363, #111021, #189870, #20006, #159503, #20999, #112022, #5826, #156540, #78688, #144338, #129159, #47380, #35179, #8841, #102842, #176703, #6819, #177701, #39168, #101837, #25023, #26021, #83659, #85666, #147353, #70509, #24010, #71505, #194863, #164528, #116011, #100826, #87665, #132177, #52333, #117004, #149350, #113990, #193868, #55334, #72516, #175688, #22007, #162509, #133173, #37163, #40161, #10847, #145337, #98822, #56336, #192861, #178699, #190856, #69505, #160516, #163524, #86667, #68497, #130152, #191849, #148350, #53330, #9846, #118018, #115009, #38177, #99833, #179707, #41179, #161517, #23009, #84655, #146332, #7821, #131171, #54340, #121983, #90647, #30978, #195878, #182681, #58335, #74507, #152329, #106814, #105825, #14814, #166527, #165526, #168488, #59314, #198843, #29008, #196869, #150363, #28024, #138152, #154316, #120003, #184657, #169477, #29986, #92625, #119026, #44166, #167512, #60307, #27022, #183673, #104837, #199833, #180709, #42185, #120983, #15805, #75481, #134191, #57351, #61300, #181689, #122970, #13815, #137154, #45158, #103845, #91625, #153313, #89666, #76475, #12841, #46139, #88667, #107793, #11859, #151352, #73524, #135195, #43170, #136173, #197848, #81414, #140122, #158284, #64292, #189633, #159263, #157297, #48136, #63289, #1613, #124969, #186666, #35929, #34943, #143100, #18794, #93624, #4579, #47141, #66272, #33954, #79456, #141125, #109793, #16798, #80439, #125959, #127931, #174460, #108799, #156298, #77466, #49128, #32965, #171476, #110786, #17799, #142112, #155309, #97575, #613, #187657, #19773, #139136, #126935, #62283, #170478, #185649, #51108, #2615, #172467, #123951, #112767, #31968, #3597, #95612, #65276, #188643, #96595, #78448, #94619, #50122, #111782, #173470, #20759, #175450, #161274 ),
 ( #9610, #71275, #8602, #177466, #117779, #82414, #69264, #145096, #22769, #38935, #193627, #192621, #101596, #53088, #52097, #55099, #146094, #85424, #115777, #83419, #36921, #114766, #24785, #40938, #6579, #132940, #56098, #116769, #179473, #5583, #130930, #54103, #147115, #113754, #70275, #191609, #86433, #67263, #128921, #7578, #102610, #162274, #144103, #190622, #148119, #68258, #194628, #100592, #23774, #131943, #98583, #178460, #39927, #176460, #163284, #99594, #160277, #21768, #129909, #37933, #84417, #182442, #167270, #133949, #60069, #166288, #168247, #26782, #44914, #151115, #76227, #45899, #43922, #134957, #150118, #88424, #11619, #73287, #122728, #121737, #29743, #105584, #180476, #91378, #195640, #153067, #120743, #27784, #89426, #59076, #196635, #41947, #58104, #14569, #184419, #119774, #137907, #199589, #183429, #164296, #149120, #74271, #12607, #28769, #57113, #13576, #181458, #61056, #10611, #72272, #135941, #25789, #90407, #87435, #118787, #103613, #42936, #165289, #197611, #152092, #75243, #104600, #136914, #198601, #106570, #188395, #186420, #48885, #107552, #126691, #19534, #139875, #125718, #110540, #77223, #3360, #109550, #111538, #170235, #49873, #94372, #81179, #189392, #187417, #78205, #93377, #31729, #155063, #16558, #66025, #65035, #173223, #172221, #123709, #34699, #138892, #96356, #64048, #171231, #32720, #1364, #46897, #33706, #156052, #158044, #4340, #372, #47896, #169230, #79209, #63043, #124722, #140878, #17549, #95368, #185406, #127692, #30737, #2368, #142861, #157053, #18550, #92384, #154071, #15565, #80198, #108557, #141869, #62044, #190379, #9365, #50869, #8354, #162031, #71030, #147879, #161031, #178217, #37683, #39681, #101343, #38696, #7334, #132697, #112527, #99348, #175208, #191366, #69019, #23527, #22525, #131698, #83180, #82164, #85173, #176214, #115535, #20516, #146862, #52843, #54855, #113514, #193379, #84172, #163032, #174221, #130684, #21519, #36673, #98333, #160032, #144854, #35690, #70029, #116529, #192378, #67023, #24539, #143860, #86189, #53861, #114513, #145852, #6337, #51854, #177223, #100352, #97337, #159023, #5339, #129669, #128682, #68017, #149863, #41699, #27538, #134710, #135699, #72022, #152828, #117527, #73038, #106323, #42693, #120502, #14322, #55853, #75987, #58835, #133695, #74028, #119534, #195387, #194386, #179225, #151848, #105340, #40691, #91139, #104354, #121494, #181217, #183188, #44670, #182193, #150871, #102361, #164050, #166038, #118540, #196393, #12365, #167027, #89179, #75003, #26535, #25549, #28529, #197370, #43678, #90165, #56865, #10365, #88179, #198350, #87193, #180230, #168009, #29505, #13339, #148874, #103364, #136668, #59824, #165042, #11368, #57862, #108312, #141638, #184177, #122486, #124479, #19303, #78965, #137660, #199347, #3128, #185162, #64803, #186175, #140640, #2130, #34465, #125484, #110303, #93135, #18313, #16318, #63811, #60812, #156821, #49635, #169992, #155812, #187180, #15320, #48651, #170987, #31483, #138650, #126464, #45659, #107310, #168983, #47657, #171985, #188162, #33473, #157813, #109308, #32480, #95131, #30487, #154820, #76979, #131, #92138, #79970, #153825, #17310, #111298, #61800, #123470, #172987, #96124, #77968, #94133, #46653, #139635, #1123, #62797, #163550, #162534, #179736, #56363, #10871, #134218, #25050, #42210, #81921, #4105, #118046, #119052, #194889, #165551, #101867, #195904, #69534, #97103, #70535, #132204, #41206, #102867, #180734, #173983, #178725, #40187, #86693, #117030, #164552, #87690, #57379, #8868, #193895, #103870, #148377, #142626, #9872, #80951, #65784, #71532, #133198, #127453, #189159, #112293, #55360, #26045, #50632, #149375, #35452, #158787, #20275, #72541, #85693, #146360, #7847, #131198, #192888, #54366, #116038, #177727, #39196, #100852, #24038, #147379, #169507, #153342, #75508, #27048, #181713, #167539, #135222, #168517, #138182, #198869, #88694, #30015 ),
 ( #197873, #44193, #59340, #185681, #150390, #184686, #199865, #47171, #123983, #137181, #154344, #13841, #15837, #77496, #14843, #183701, #108830, #11886, #60336, #151377, #29034, #45188, #61329, #122010, #107823, #121010, #58361, #123000, #152356, #91653, #106842, #89692, #43195, #182708, #31006, #73549, #12868, #139166, #62313, #46169, #196894, #120028, #76506, #92655, #643, #104863, #166552, #105852, #28051, #74533, #136198, #90674, #52132, #111815, #170509, #32000, #174494, #17832, #35961, #18827, #173503, #34976, #67297, #158317, #143132, #125992, #51140, #49160, #96629, #93657, #189667, #82448, #2648, #188676, #19805, #140155, #66304, #172501, #97608, #32998, #112801, #157332, #144136, #155342, #50156, #141159, #156332, #94652, #79490, #64325, #128956, #127964, #159296, #81446, #186698, #20793, #1647, #5618, #126967, #33988, #95644, #187690, #109826, #4612, #16831, #190656, #78482, #63325, #125003, #80472, #65308, #48169, #171509, #110818, #142145, #3629, #38971, #178496, #71312, #36956, #160312, #56134, #39962, #162309, #113789, #68294, #54138, #21802, #55134, #24820, #85460, #117816, #101633, #23809, #175484, #129945, #115812, #83454, #116804, #86469, #147149, #98618, #163324, #148154, #9646, #149157, #100628, #179509, #131978, #102646, #132975, #145132, #40977, #8637, #69299, #84451, #146129, #130965, #7614, #191644, #194665, #70309, #192655, #114802, #164331, #6615, #53124, #176495, #193663, #25825, #87470, #10647, #133986, #72308, #195677, #37971, #99629, #177502, #161311, #22805, #118825, #91417, #180510, #75281, #106609, #181494, #42972, #76264, #137942, #12642, #105622, #167310, #196672, #73322, #150155, #136951, #135976, #153104, #29781, #184455, #107590, #198640, #15601, #58141, #41983, #14608, #92421, #168284, #138928, #60106, #169268, #104635, #134993, #43960, #28806, #199626, #61093, #154107, #11656, #152131, #13614, #121774, #90446, #122766, #45935, #30774, #182479, #183467, #77259, #44953, #103649, #57148, #165327, #26819, #88459, #119809, #166324, #27821, #89463, #151152, #74309, #197647, #59113, #120778, #173259, #170270, #66061, #2405, #95404, #159059, #4377, #62080, #3395, #157090, #125753, #65070, #158079, #123745, #46934, #139912, #16593, #93413, #80233, #79247, #96392, #34734, #127728, #50905, #141904, #20553, #1403, #185444, #19570, #35726, #111575, #82203, #18586, #112563, #186457, #78241, #187453, #48921, #81214, #142895, #97373, #155099, #126728, #188431, #49909, #33744, #189430, #174258, #408, #110575, #172256, #108593, #31764, #63082, #124761, #47933, #109587, #171270, #32758, #94409, #156090, #17587, #140918, #64084, #5376, #67060, #39715, #116565, #113550, #9399, #145888, #38731, #102397, #147913, #128718, #146901, #100389, #69056, #8391, #101378, #190415, #51891, #86223, #70066, #192415, #143895, #98371, #84208, #175244, #85211, #54891, #115572, #36709, #131734, #193416, #163069, #179262, #130723, #71065, #162067, #132731, #178254, #160069, #194419, #177259, #99384, #114553, #176251, #161067, #37722, #21556, #24574, #23563, #22562, #144891, #55889, #83216, #6373, #68053, #53897, #117562, #40727, #164084, #25583, #129707, #191403, #52880, #7371, #57897, #165076, #26570, #148909, #121530, #10399, #105377, #136705, #11404, #73073, #106360, #168044, #42729, #135735, #197406, #183225, #91174, #28565, #107345, #74064, #120538, #44706, #180264, #119569, #88213, #149897, #72056, #29541, #133730, #167064, #198386, #134745, #196427, #152863, #14358, #104391, #58872, #182231, #181252, #103398, #41734, #90202, #166074, #76023, #59863, #137698, #199383, #151885, #45694, #27577, #195423, #60847, #122522, #184212, #169018, #13375, #87227, #89215, #150908, #43716, #75039, #56900, #118574, #12402, #123505, #125517, #187214, #48685, #63845, #111333, #34502, #4142, #155847, #17344, #65821, #172018, #92175, #156854, #127490, #153860, #110337, #95166, #112330, #15358, #61835 ),
 ( #171025, #33507, #108350, #189195, #77014, #109343, #142663, #79000, #18349, #50670, #138686, #30523, #80004, #170029, #141673, #140674, #31519, #167, #185198, #188197, #3164, #46689, #93172, #2166, #157849, #64837, #19341, #80988, #126499, #49669, #154857, #16355, #173023, #78003, #32516, #96160, #139670, #1158, #62833, #124517, #186212, #47693, #94168, #38492, #68817, #70828, #83973, #101139, #160834, #162825, #24334, #161829, #130476, #132496, #35491, #22323, #98129, #114312, #192173, #146650, #145653, #54648, #6138, #5136, #8144, #99145, #100148, #53654, #36472, #190177, #67820, #178011, #194185, #159826, #85984, #9161, #69821, #55650, #158824, #7134, #115331, #23324, #66818, #84968, #144655, #39478, #20312, #81960, #177022, #174020, #131488, #97141, #143652, #147673, #21321, #128481, #193175, #116322, #51652, #113316, #175008, #82979, #129475, #191174, #52648, #176014, #37483, #43481, #74812, #103161, #27334, #150670, #25345, #120305, #72837, #28335, #56662, #105148, #57665, #136474, #182990, #88980, #164841, #118335, #180028, #41497, #26337, #121298, #181998, #89974, #12168, #10161, #151655, #86986, #13149, #104156, #134507, #196193, #87977, #133489, #73833, #59624, #149665, #119332, #165837, #11163, #117322, #42492, #181018, #135504, #197174, #58639, #166834, #195181, #179018, #102158, #198154, #40486, #163844, #148673, #71821, #159473, #179675, #162476, #175658, #177670, #22975, #37132, #56303, #97784, #55301, #8809, #117985, #147321, #193837, #133139, #84624, #163493, #115981, #86635, #23978, #144306, #24991, #69474, #53299, #68467, #130122, #114978, #191819, #98792, #70478, #131140, #176671, #160486, #148318, #5796, #82624, #67469, #146302, #132144, #101805, #39138, #20967, #7791, #192828, #116973, #190826, #38147, #21976, #83628, #129128, #178664, #52302, #100793, #40127, #145305, #6788, #9813, #71474, #99801, #54309, #85634, #161487, #113959, #194830, #140386, #124219, #49381, #187912, #146111, #34212, #19051, #1874, #129927, #125229, #111044, #46393, #68276, #161291, #78710, #64552, #172731, #16063, #142375, #48397, #53106, #109057, #191626, #33222, #22786, #130947, #126216, #17055, #32225, #170734, #93883, #155561, #7595, #6597, #114784, #95875, #62544, #176477, #77721, #37953, #2873, #110054, #171734, #63555, #185916, #157558, #69281, #186927, #94882, #80698, #156563, #108051, #18061, #79716, #141385, #99611, #84433, #169736, #47401, #31231, #92880, #154567, #139387, #869, #118805, #151130, #54120, #74287, #57129, #70291, #72288, #117797, #131959, #12622, #192637, #150135, #104615, #24801, #10627, #195658, #162291, #88440, #194644, #196651, #55116, #73303, #179490, #166304, #115793, #133966, #163303, #178476, #116785, #39943, #101614, #177483, #11636, #58120, #180491, #8619, #119789, #23791, #181473, #149137, #56114, #40955, #86450, #193644, #41963, #89441, #148135, #102627, #103629, #71293, #38952, #164312, #9626, #132956, #25805, #87451, #165305, #26799, #100608, #85441, #134974, #27800, #42951, #147131, #94389, #197626, #17566, #387, #13593, #15581, #61072, #75260, #156068, #135956, #93393, #46914, #59092, #32737, #45915, #63062, #122744, #124741, #186437, #123725, #92401, #120758, #182459, #184435, #60086, #76244, #154087, #108574, #107569, #16574, #168264, #167288, #170251, #169246, #62060, #30754, #198620, #152110, #29761, #139892, #43940, #121754, #47913, #171249, #31745, #105601, #28785, #77239, #138907, #185423, #90424, #155080, #106588, #1381, #136931, #183447, #78221, #44931, #109567, #91395, #153084, #14588, #137922, #199606, #157071, #82180, #20532, #176230, #67039, #51871, #34715, #160048, #158060, #143875, #79227, #98349, #96373, #127708, #189409, #18567, #95385, #66041, #64064, #19551, #50885, #113530, #6353, #129685, #159039, #37700, #80214, #2385, #175224, #114529, #190395, #161046, #97353, #191382, #65051, #141885, #112543, #174238, #36689, #21536 ),
 ( #140898, #5356, #99363, #125734, #35706, #128698, #187434, #48901, #110556, #83196, #144870, #172237, #33722, #68033, #52858, #3376, #126707, #81195, #188411, #49888, #111555, #173240, #142876, #4356, #147894, #87208, #180245, #145867, #69034, #165057, #148889, #71045, #22540, #177238, #163048, #130699, #164065, #133710, #194400, #84187, #25564, #72037, #118555, #57878, #9380, #88194, #40708, #11384, #10380, #192394, #149878, #55868, #178232, #193394, #54870, #39696, #116544, #100367, #195403, #117542, #101358, #23542, #73054, #53876, #7350, #115550, #132712, #56881, #26550, #41714, #42709, #179241, #102377, #103379, #38710, #24555, #162046, #85189, #146878, #134726, #8370, #196408, #119550, #70045, #131713, #181233, #104370, #86204, #199364, #59842, #167044, #154837, #12382, #150888, #74044, #14338, #147, #170009, #107326, #186192, #152844, #60828, #123486, #58851, #136684, #43695, #105357, #27555, #61816, #89195, #184193, #15338, #90182, #151865, #185179, #46669, #121510, #76004, #137678, #28545, #182210, #122503, #135715, #44686, #45675, #138667, #93152, #16335, #168999, #124497, #13355, #197386, #108329, #1139, #76995, #47673, #30503, #77984, #75019, #198366, #92154, #153841, #31500, #139651, #62813, #120518, #166054, #183205, #106340, #168025, #29521, #91155, #82954, #34480, #96138, #144631, #50646, #171005, #35468, #6114, #32496, #65798, #173997, #191151, #94149, #140655, #19318, #51629, #155828, #17325, #5112, #81936, #78980, #174984, #111312, #4119, #67797, #113293, #2147, #112307, #127467, #157827, #97117, #66794, #63825, #125497, #36448, #158800, #80965, #109324, #187195, #49649, #48665, #20289, #143627, #142641, #110317, #128457, #190153, #98105, #129452, #189173, #159801, #21296, #171999, #33487, #95145, #156834, #18329, #79984, #141652, #3143, #173001, #64817, #126478, #188176, #101116, #162802, #192148, #68792, #39455, #37459, #131465, #24311, #25321, #180005, #103136, #132472, #11140, #53629, #175990, #86963, #87953, #163820, #134483, #70803, #164818, #38467, #130450, #85960, #147649, #148649, #10137, #149642, #145630, #9137, #194162, #55626, #117299, #133467, #56639, #26313, #177988, #178995, #72814, #40463, #114288, #102135, #52625, #99120, #71798, #195158, #160811, #22299, #83950, #118312, #41472, #7110, #115305, #176997, #100124, #161806, #23301, #54623, #84945, #146627, #8119, #69797, #193151, #116299, #121275, #60589, #153604, #119308, #42470, #138434, #122264, #44453, #196170, #150649, #136452, #104132, #137442, #107093, #167791, #57642, #199121, #45440, #91911, #31265, #182969, #61584, #14097, #184943, #183953, #88959, #29291, #58617, #151633, #166813, #28314, #13128, #89953, #73812, #168763, #90921, #74790, #197152, #46428, #165814, #180993, #27312, #106106, #30266, #200115, #15100, #16097, #152607, #75765, #76760, #12147, #198133, #135482, #120284, #181976, #123252, #43458, #108087, #169771, #105127, #59602, #92916, #154601, #77755, #50420, #21056, #157593, #51399, #125265, #155596, #126250, #187946, #112079, #173769, #174751, #32260, #34248, #95908, #19084, #172768, #20061, #143388, #113059, #64585, #49416, #36215, #80732, #903, #65568, #97868, #62578, #142411, #3889, #139421, #124256, #170771, #111078, #81705, #185951, #47435, #35235, #96889, #109092, #4880, #141420, #127228, #159558, #66562, #93918, #188943, #158572, #128227, #189924, #17091, #78744, #140421, #1911, #63590, #186963, #48433, #110089, #79750, #171768, #33257, #94915, #156601, #18095, #2907, #132230, #178751, #118072, #7875, #148404, #100879, #71559, #85721, #175743, #54393, #145390, #38230, #53387, #115066, #99885, #176757, #160572, #193923, #116066, #161570, #83712, #133224, #129213, #67556, #190911, #131227, #117056, #86719, #24066, #102893, #69561, #177754, #40215, #37221, #23063, #22061, #6872, #144394, #101894, #5879, #162561, #55386, #68551, #130207, #163576, #25076, #84708, #192916, #39223 ),
 ( #147408, #9898, #8895, #194915, #146387, #114045, #56390, #70563, #179763, #41232, #191902, #98877, #164578, #82711, #52388, #150417, #76531, #61353, #122035, #184709, #10896, #136224, #74557, #90698, #119077, #75533, #196920, #30037, #72569, #134244, #12894, #107847, #167565, #26072, #87715, #182736, #152381, #120054, #103896, #29058, #13866, #123024, #137208, #198895, #181741, #106865, #104890, #60363, #149401, #45211, #138207, #58387, #44220, #183725, #195930, #168539, #28079, #91676, #88721, #153368, #197899, #199889, #57405, #105878, #43222, #11912, #73575, #135248, #166579, #46194, #14870, #180759, #42235, #165576, #27075, #89719, #151404, #59368, #121038, #171533, #16855, #108856, #172527, #66327, #63350, #17857, #126018, #48194, #169532, #141183, #125027, #78506, #2672, #109848, #110843, #47196, #127988, #92681, #33021, #81469, #79513, #95670, #189691, #31032, #51163, #34013, #170535, #49185, #94676, #32025, #154369, #15863, #126992, #80497, #77521, #139193, #64349, #96652, #156355, #186723, #187713, #668, #62338, #124008, #185706, #157357, #93683, #18851, #142170, #50181, #173527, #143155, #3654, #65332, #4636, #188699, #155366, #111838, #140179, #1672, #34997, #158339, #19828, #97630, #144156, #22825, #55154, #174516, #35983, #8658, #85480, #82471, #178515, #114824, #7636, #71332, #116824, #159319, #115834, #69320, #37994, #177523, #70331, #20814, #5641, #39981, #38992, #161333, #112824, #67318, #53145, #128979, #54161, #23830, #84471, #190677, #100648, #162329, #131998, #148174, #99649, #101652, #130986, #163344, #147169, #52153, #146149, #175505, #68315, #83476, #145154, #129966, #6637, #113810, #193686, #192678, #191666, #36979, #24840, #98640, #160335, #21824, #86489, #9666, #132994, #194685, #176517, #42994, #89485, #16371, #149179, #26841, #134006, #195697, #117836, #93189, #179529, #74331, #108369, #180530, #42004, #78019, #139688, #11678, #104661, #166346, #57169, #72331, #27844, #40999, #135016, #151175, #31536, #186229, #109359, #135997, #17361, #118847, #102666, #154874, #94184, #170046, #140692, #197668, #171041, #103669, #165347, #12663, #61853, #1174, #62851, #155863, #10667, #123522, #185216, #46707, #124533, #79016, #47709, #164351, #32532, #56155, #25847, #87490, #88481, #150177, #73343, #196693, #58163, #119830, #181515, #63862, #98144, #175025, #172035, #67835, #4158, #97157, #160850, #6155, #125533, #5152, #158840, #127507, #66834, #159843, #187230, #48701, #144670, #128498, #50689, #2182, #156871, #142679, #110353, #143671, #113332, #174037, #33523, #190193, #51669, #21336, #37498, #189211, #129492, #20328, #191189, #36488, #95185, #35507, #64853, #157866, #173040, #34518, #19356, #96177, #80020, #82994, #81977, #81005, #3180, #52665, #18368, #141689, #126515, #112346, #114327, #176030, #99160, #22339, #83990, #188213, #49685, #111350, #65837, #23340, #84985, #7151, #180046, #68834, #163863, #195199, #69837, #131504, #164858, #26354, #101155, #194201, #55666, #146666, #161846, #132512, #130493, #24350, #117340, #118353, #72855, #196212, #25362, #104173, #8161, #192189, #41515, #181035, #56679, #27351, #87003, #57683, #193191, #54664, #179036, #40504, #103178, #87994, #42509, #38508, #102175, #148690, #10178, #71838, #149682, #11180, #119351, #70844, #165855, #133507, #145669, #116338, #53670, #134525, #115348, #177038, #100164, #178027, #39495, #162843, #86001, #147690, #9177, #200150, #123288, #124291, #182016, #183991, #45476, #107131, #122301, #169807, #92952, #62613, #14135, #75802, #185988, #30305, #150688, #15136, #47471, #12186, #168801, #153641, #170806, #73851, #120322, #199160, #31300, #135521, #197192, #184980, #61620, #58656, #154638, #90958, #91948, #109128, #16133, #43499, #76798, #138469, #137480, #46464, #108124, #105165, #166851, #77788, #139457, #60627, #88997, #28353, #29330, #89991, #938, #151673, #13166, #74830, #136491, #198171, #59641 ),
 ( #152645, #121315, #183007, #44491, #106147, #167829, #63626, #4913, #157628, #96924, #127264, #94951, #48468, #126284, #36250, #52422, #156635, #82748, #67591, #128260, #190945, #17128, #142446, #80768, #158606, #125302, #81740, #2942, #97903, #78780, #140457, #19118, #114080, #173804, #32298, #93954, #188977, #20096, #187981, #110125, #35269, #143426, #129250, #66596, #50453, #3924, #189958, #51433, #155632, #1946, #174784, #113092, #65604, #186998, #171803, #172802, #33291, #159594, #21091, #112112, #18131, #144428, #5914, #79785, #141457, #64622, #49450, #111113, #34283, #95943, #68585, #147442, #38263, #131261, #146419, #7910, #192949, #69594, #53421, #86755, #8930, #54428, #176790, #164611, #22095, #160605, #83745, #24101, #9933, #179795, #117091, #195964, #162597, #70598, #133258, #130241, #116098, #115098, #99917, #37255, #71592, #98912, #193957, #25111, #161602, #23096, #194949, #56425, #177786, #85755, #132266, #84742, #191937, #55420, #145424, #39256, #178786, #148438, #102926, #26105, #40255, #134276, #100912, #6907, #118106, #10929, #41264, #57436, #101928, #87748, #163610, #149433, #72602, #175781, #30065, #153400, #154399, #11941, #13894, #75561, #137237, #152407, #199918, #123054, #92711, #44247, #105904, #15894, #60390, #180790, #45240, #77552, #42267, #198921, #183754, #699, #103927, #150445, #29085, #61382, #165607, #27106, #14898, #91706, #88752, #184740, #121069, #122062, #139224, #46225, #73605, #106894, #59395, #168567, #196948, #119109, #135276, #197927, #31063, #167590, #76559, #58416, #120083, #181771, #138235, #43252, #107878, #90724, #104920, #166607, #28107, #169566, #89746, #151432, #12919, #74583, #136251, #182763, #17889, #110873, #159353, #170566, #20849, #124040, #172558, #186754, #2703, #18882, #35029, #34044, #143188, #94707, #93713, #96684, #187744, #127024, #157389, #125057, #78536, #156384, #66360, #82507, #48224, #112857, #97664, #158372, #144189, #47228, #95701, #80528, #188731, #155395, #111870, #33052, #128021, #108887, #32056, #49215, #62371, #3685, #185739, #16885, #142202, #50216, #79543, #140210, #65363, #173560, #1704, #19861, #81501, #141213, #4668, #64380, #189723, #63380, #51196, #174548, #126048, #36015, #109878, #171562, #101686, #7668, #9698, #68347, #86521, #192710, #117870, #87521, #85513, #176551, #191698, #129998, #53181, #114857, #164384, #163375, #71363, #147201, #21857, #133027, #175538, #194717, #162361, #69352, #131021, #38027, #145185, #8692, #102696, #99683, #54193, #23862, #84505, #5675, #177555, #161367, #22858, #83508, #115866, #190711, #146183, #39024, #178547, #56187, #179560, #70362, #25877, #6669, #100679, #132029, #67351, #24872, #41030, #193719, #55187, #116856, #37012, #148205, #40013, #129011, #52184, #113842, #98673, #160367, #30828, #28860, #119860, #135048, #73376, #11709, #196724, #107644, #106665, #14660, #90500, #165379, #76320, #118878, #137998, #105676, #151205, #12693, #58192, #88516, #152182, #45989, #43023, #197699, #167362, #27874, #149209, #120833, #104690, #181545, #182533, #89515, #13666, #26873, #169321, #72363, #74359, #61147, #59165, #75333, #10700, #134037, #195730, #137003, #150212, #198692, #136025, #166378, #57203, #180562, #168338, #60159, #42036, #103700, #44015, #199682, #121828, #183522, #45005, #29834, #91471, #153159, #122819, #184509, #16648, #32813, #48975, #65124, #64142, #173316, #124815, #123800, #126782, #17643, #157146, #187508, #155156, #108648, #186515, #96446, #112619, #78295, #142948, #127782, #188488, #50960, #77315, #2460, #140972, #18641, #185498, #141959, #63136, #158133, #138983, #461, #79303, #174311, #33800, #92476, #95460, #170326, #154164, #15656, #171325, #4429, #125806, #80287, #62136, #46989, #31818, #3448, #93469, #172311, #110630, #139969, #1458, #47989, #49967, #111631, #109642, #189482, #34791, #19625, #81267, #94464, #66117, #156145, #143951, #132788, #97427 ) ),
 .UNSPECIFIED., .T., .F., .T. ) 
 B_SPLINE_SURFACE_WITH_KNOTS ( ( 4, 3, 4 ),
 ( 3, 2, 2, 2, 2, 2, 2, 2, 2, 2, 2, 2, 2, 2, 2, 2, 2, 2, 2, 2, 2, 2, 2, 2, 2, 2, 2, 2, 2, 2, 2, 2, 2, 2, 2, 2, 2, 2, 2, 2, 2, 2, 2, 2, 2, 2, 2, 2, 2, 2, 2, 2, 2, 2, 2, 2, 2, 2, 2, 2, 2, 2, 2, 2, 2, 2, 2, 2, 2, 2, 2, 2, 2, 2, 2, 2, 2, 2, 2, 2, 2, 2, 2, 2, 2, 2, 2, 2, 2, 2, 2, 2, 2, 2, 2, 2, 2, 2, 2, 2, 2, 2, 2, 2, 2, 2, 2, 2, 2, 2, 2, 2, 2, 2, 2, 2, 2, 2, 2, 2, 2, 2, 2, 2, 2, 2, 2, 2, 2, 2, 2, 2, 2, 2, 2, 2, 2, 2, 2, 2, 2, 2, 2, 2, 2, 2, 2, 2, 2, 2, 2, 2, 2, 2, 2, 2, 2, 2, 2, 2, 2, 2, 2, 2, 2, 2, 2, 2, 2, 2, 2, 2, 2, 2, 2, 2, 2, 2, 2, 2, 2, 2, 2, 2, 2, 2, 2, 2, 2, 2, 2, 2, 2, 2, 2, 2, 2, 2, 2, 2, 2, 2, 2, 2, 2, 2, 2, 2, 2, 2, 2, 2, 2, 2, 2, 2, 2, 2, 2, 2, 2, 2, 2, 2, 2, 2, 2, 2, 3 ),
 ( 0.000000000000000000, 0.5000000000000000000, 1.000000000000000000 ),
 ( 0.000000000000000000, 0.004385964912280701511, 0.008771929824561403022, 0.01315789473684210453, 0.01754385964912280604, 0.02192982456140350755, 0.02631578947368420907, 0.03070175438596491058, 0.03508771929824561209, 0.03947368421052631360, 0.04385964912280701511, 0.04824561403508771662, 0.05263157894736841813, 0.05701754385964911964, 0.06140350877192982115, 0.06578947368421052266, 0.07017543859649122417, 0.07456140350877192569, 0.07894736842105262720, 0.08333333333333332871, 0.08771929824561403022, 0.09210526315789473173, 0.09649122807017543324, 0.1008771929824561348, 0.1052631578947368363, 0.1096491228070175378, 0.1140350877192982393, 0.1184210526315789408, 0.1228070175438596423, 0.1271929824561403577, 0.1315789473684210453, 0.1359649122807017607, 0.1403508771929824483, 0.1447368421052631637, 0.1491228070175438514, 0.1535087719298245668, 0.1578947368421052544, 0.1622807017543859698, 0.1666666666666666574, 0.1710526315789473728, 0.1754385964912280604, 0.1798245614035087758, 0.1842105263157894635, 0.1885964912280701788, 0.1929824561403508665, 0.1973684210526315819, 0.2017543859649122695, 0.2061403508771929849, 0.2105263157894736725, 0.2149122807017543879, 0.2192982456140350755, 0.2236842105263157909, 0.2280701754385964786, 0.2324561403508771940, 0.2368421052631578816, 0.2412280701754385970, 0.2456140350877192846, 0.2500000000000000000, 0.2543859649122807154, 0.2587719298245614308, 0.2631578947368420907, 0.2675438596491228060, 0.2719298245614035214, 0.2763157894736842368, 0.2807017543859648967, 0.2850877192982456121, 0.2894736842105263275, 0.2938596491228070429, 0.2982456140350877027, 0.3026315789473684181, 0.3070175438596491335, 0.3114035087719298489, 0.3157894736842105088, 0.3201754385964912242, 0.3245614035087719396, 0.3289473684210526550, 0.3333333333333333148, 0.3377192982456140302, 0.3421052631578947456, 0.3464912280701754610, 0.3508771929824561209, 0.3552631578947368363, 0.3596491228070175517, 0.3640350877192982670, 0.3684210526315789269, 0.3728070175438596423, 0.3771929824561403577, 0.3815789473684210731, 0.3859649122807017330, 0.3903508771929824483, 0.3947368421052631637, 0.3991228070175438791, 0.4035087719298245390, 0.4078947368421052544, 0.4122807017543859698, 0.4166666666666666852, 0.4210526315789473450, 0.4254385964912280604, 0.4298245614035087758, 0.4342105263157894912, 0.4385964912280701511, 0.4429824561403508665, 0.4473684210526315819, 0.4517543859649122973, 0.4561403508771929571, 0.4605263157894736725, 0.4649122807017543879, 0.4692982456140351033, 0.4736842105263157632, 0.4780701754385964786, 0.4824561403508771940, 0.4868421052631579093, 0.4912280701754385692, 0.4956140350877192846, 0.5000000000000000000, 0.5043859649122807154, 0.5087719298245614308, 0.5131578947368421462, 0.5175438596491228616, 0.5219298245614034659, 0.5263157894736841813, 0.5307017543859648967, 0.5350877192982456121, 0.5394736842105263275, 0.5438596491228070429, 0.5482456140350877583, 0.5526315789473684736, 0.5570175438596490780, 0.5614035087719297934, 0.5657894736842105088, 0.5701754385964912242, 0.5745614035087719396, 0.5789473684210526550, 0.5833333333333333703, 0.5877192982456140857, 0.5921052631578946901, 0.5964912280701754055, 0.6008771929824561209, 0.6052631578947368363, 0.6096491228070175517, 0.6140350877192982670, 0.6184210526315789824, 0.6228070175438596978, 0.6271929824561403022, 0.6315789473684210176, 0.6359649122807017330, 0.6403508771929824483, 0.6447368421052631637, 0.6491228070175438791, 0.6535087719298245945, 0.6578947368421053099, 0.6622807017543859143, 0.6666666666666666297, 0.6710526315789473450, 0.6754385964912280604, 0.6798245614035087758, 0.6842105263157894912, 0.6885964912280702066, 0.6929824561403509220, 0.6973684210526315264, 0.7017543859649122417, 0.7061403508771929571, 0.7105263157894736725, 0.7149122807017543879, 0.7192982456140351033, 0.7236842105263158187, 0.7280701754385965341, 0.7324561403508771384, 0.7368421052631578538, 0.7412280701754385692, 0.7456140350877192846, 0.7500000000000000000, 0.7543859649122807154, 0.7587719298245614308, 0.7631578947368421462, 0.7675438596491228616, 0.7719298245614034659, 0.7763157894736841813, 0.7807017543859648967, 0.7850877192982456121, 0.7894736842105263275, 0.7938596491228070429, 0.7982456140350877583, 0.8026315789473684736, 0.8070175438596490780, 0.8114035087719297934, 0.8157894736842105088, 0.8201754385964912242, 0.8245614035087719396, 0.8289473684210526550, 0.8333333333333333703, 0.8377192982456140857, 0.8421052631578946901, 0.8464912280701754055, 0.8508771929824561209, 0.8552631578947368363, 0.8596491228070175517, 0.8640350877192982670, 0.8684210526315789824, 0.8728070175438596978, 0.8771929824561403022, 0.8815789473684210176, 0.8859649122807017330, 0.8903508771929824483, 0.8947368421052631637, 0.8991228070175438791, 0.9035087719298245945, 0.9078947368421053099, 0.9122807017543859143, 0.9166666666666666297, 0.9210526315789473450, 0.9254385964912280604, 0.9298245614035087758, 0.9342105263157894912, 0.9385964912280702066, 0.9429824561403509220, 0.9473684210526315264, 0.9517543859649122417, 0.9561403508771929571, 0.9605263157894736725, 0.9649122807017543879, 0.9692982456140351033, 0.9736842105263158187, 0.9780701754385965341, 0.9824561403508771384, 0.9868421052631578538, 0.9912280701754385692, 0.9956140350877192846, 1.000000000000000000 ),
 .UNSPECIFIED. ) 
 GEOMETRIC_REPRESENTATION_ITEM ( )  RATIONAL_B_SPLINE_SURFACE ( (
 ( 1.000000000000000000, 0.9659258262890683122, 1.000000000000000000, 0.9659258262890683122, 1.000000000000000000, 0.9659258262890683122, 1.000000000000000000, 0.9659258262890683122, 1.000000000000000000, 0.9659258262890683122, 1.000000000000000000, 0.9659258262890683122, 1.000000000000000000, 0.9659258262890683122, 1.000000000000000000, 0.9659258262890683122, 1.000000000000000000, 0.9659258262890683122, 1.000000000000000000, 0.9659258262890683122, 1.000000000000000000, 0.9659258262890683122, 1.000000000000000000, 0.9659258262890683122, 1.000000000000000000, 0.9659258262890683122, 1.000000000000000000, 0.9659258262890683122, 1.000000000000000000, 0.9659258262890683122, 1.000000000000000000, 0.9659258262890683122, 1.000000000000000000, 0.9659258262890683122, 1.000000000000000000, 0.9659258262890683122, 1.000000000000000000, 0.9659258262890683122, 1.000000000000000000, 0.9659258262890683122, 1.000000000000000000, 0.9659258262890683122, 1.000000000000000000, 0.9659258262890683122, 1.000000000000000000, 0.9659258262890683122, 1.000000000000000000, 0.9659258262890683122, 1.000000000000000000, 0.9659258262890683122, 1.000000000000000000, 0.9659258262890683122, 1.000000000000000000, 0.9659258262890683122, 1.000000000000000000, 0.9659258262890683122, 1.000000000000000000, 0.9659258262890683122, 1.000000000000000000, 0.9659258262890683122, 1.000000000000000000, 0.9659258262890683122, 1.000000000000000000, 0.9659258262890683122, 1.000000000000000000, 0.9659258262890683122, 1.000000000000000000, 0.9659258262890683122, 1.000000000000000000, 0.9659258262890683122, 1.000000000000000000, 0.9659258262890683122, 1.000000000000000000, 0.9659258262890683122, 1.000000000000000000, 0.9659258262890683122, 1.000000000000000000, 0.9659258262890683122, 1.000000000000000000, 0.9659258262890683122, 1.000000000000000000, 0.9659258262890683122, 1.000000000000000000, 0.9659258262890683122, 1.000000000000000000, 0.9659258262890683122, 1.000000000000000000, 0.9659258262890683122, 1.000000000000000000, 0.9659258262890683122, 1.000000000000000000, 0.9659258262890683122, 1.000000000000000000, 0.9659258262890683122, 1.000000000000000000, 0.9659258262890683122, 1.000000000000000000, 0.9659258262890683122, 1.000000000000000000, 0.9659258262890683122, 1.000000000000000000, 0.9659258262890683122, 1.000000000000000000, 0.9659258262890683122, 1.000000000000000000, 0.9659258262890683122, 1.000000000000000000, 0.9659258262890683122, 1.000000000000000000, 0.9659258262890683122, 1.000000000000000000, 0.9659258262890683122, 1.000000000000000000, 0.9659258262890683122, 1.000000000000000000, 0.9659258262890683122, 1.000000000000000000, 0.9659258262890683122, 1.000000000000000000, 0.9659258262890683122, 1.000000000000000000, 0.9659258262890683122, 1.000000000000000000, 0.9659258262890683122, 1.000000000000000000, 0.9659258262890683122, 1.000000000000000000, 0.9659258262890683122, 1.000000000000000000, 0.9659258262890683122, 1.000000000000000000, 0.9659258262890683122, 1.000000000000000000, 0.9659258262890683122, 1.000000000000000000, 0.9659258262890683122, 1.000000000000000000, 0.9659258262890683122, 1.000000000000000000, 0.9659258262890683122, 1.000000000000000000, 0.9659258262890683122, 1.000000000000000000, 0.9659258262890683122, 1.000000000000000000, 0.9659258262890683122, 1.000000000000000000, 0.9659258262890683122, 1.000000000000000000, 0.9659258262890683122, 1.000000000000000000, 0.9659258262890683122, 1.000000000000000000, 0.9659258262890683122, 1.000000000000000000, 0.9659258262890683122, 1.000000000000000000, 0.9659258262890683122, 1.000000000000000000, 0.9659258262890683122, 1.000000000000000000, 0.9659258262890683122, 1.000000000000000000, 0.9659258262890683122, 1.000000000000000000, 0.9659258262890683122, 1.000000000000000000, 0.9659258262890683122, 1.000000000000000000, 0.9659258262890683122, 1.000000000000000000, 0.9659258262890683122, 1.000000000000000000, 0.9659258262890683122, 1.000000000000000000, 0.9659258262890683122, 1.000000000000000000, 0.9659258262890683122, 1.000000000000000000, 0.9659258262890683122, 1.000000000000000000, 0.9659258262890683122, 1.000000000000000000, 0.9659258262890683122, 1.000000000000000000, 0.9659258262890683122, 1.000000000000000000, 0.9659258262890683122, 1.000000000000000000, 0.9659258262890683122, 1.000000000000000000, 0.9659258262890683122, 1.000000000000000000, 0.9659258262890683122, 1.000000000000000000, 0.9659258262890683122, 1.000000000000000000, 0.9659258262890683122, 1.000000000000000000, 0.9659258262890683122, 1.000000000000000000, 0.9659258262890683122, 1.000000000000000000, 0.9659258262890683122, 1.000000000000000000, 0.9659258262890683122, 1.000000000000000000, 0.9659258262890683122, 1.000000000000000000, 0.9659258262890683122, 1.000000000000000000, 0.9659258262890683122, 1.000000000000000000, 0.9659258262890683122, 1.000000000000000000, 0.9659258262890683122, 1.000000000000000000, 0.9659258262890683122, 1.000000000000000000, 0.9659258262890683122, 1.000000000000000000, 0.9659258262890683122, 1.000000000000000000, 0.9659258262890683122, 1.000000000000000000, 0.9659258262890683122, 1.000000000000000000, 0.9659258262890683122, 1.000000000000000000, 0.9659258262890683122, 1.000000000000000000, 0.9659258262890683122, 1.000000000000000000, 0.9659258262890683122, 1.000000000000000000, 0.9659258262890683122, 1.000000000000000000, 0.9659258262890683122, 1.000000000000000000, 0.9659258262890683122, 1.000000000000000000, 0.9659258262890683122, 1.000000000000000000, 0.9659258262890683122, 1.000000000000000000, 0.9659258262890683122, 1.000000000000000000, 0.9659258262890683122, 1.000000000000000000, 0.9659258262890683122, 1.000000000000000000, 0.9659258262890683122, 1.000000000000000000, 0.9659258262890683122, 1.000000000000000000, 0.9659258262890683122, 1.000000000000000000, 0.9659258262890683122, 1.000000000000000000, 0.9659258262890683122, 1.000000000000000000, 0.9659258262890683122, 1.000000000000000000, 0.9659258262890683122, 1.000000000000000000, 0.9659258262890683122, 1.000000000000000000, 0.9659258262890683122, 1.000000000000000000, 0.9659258262890683122, 1.000000000000000000, 0.9659258262890683122, 1.000000000000000000, 0.9659258262890683122, 1.000000000000000000, 0.9659258262890683122, 1.000000000000000000, 0.9659258262890683122, 1.000000000000000000, 0.9659258262890683122, 1.000000000000000000, 0.9659258262890683122, 1.000000000000000000, 0.9659258262890683122, 1.000000000000000000, 0.9659258262890683122, 1.000000000000000000, 0.9659258262890683122, 1.000000000000000000, 0.9659258262890683122, 1.000000000000000000, 0.9659258262890683122, 1.000000000000000000, 0.9659258262890683122, 1.000000000000000000, 0.9659258262890683122, 1.000000000000000000, 0.9659258262890683122, 1.000000000000000000, 0.9659258262890683122, 1.000000000000000000, 0.9659258262890683122, 1.000000000000000000, 0.9659258262890683122, 1.000000000000000000, 0.9659258262890683122, 1.000000000000000000, 0.9659258262890683122, 1.000000000000000000, 0.9659258262890683122, 1.000000000000000000, 0.9659258262890683122, 1.000000000000000000, 0.9659258262890683122, 1.000000000000000000, 0.9659258262890683122, 1.000000000000000000, 0.9659258262890683122, 1.000000000000000000, 0.9659258262890683122, 1.000000000000000000, 0.9659258262890683122, 1.000000000000000000, 0.9659258262890683122, 1.000000000000000000, 0.9659258262890683122, 1.000000000000000000, 0.9659258262890683122, 1.000000000000000000, 0.9659258262890683122, 1.000000000000000000, 0.9659258262890683122, 1.000000000000000000, 0.9659258262890683122, 1.000000000000000000, 0.9659258262890683122, 1.000000000000000000, 0.9659258262890683122, 1.000000000000000000, 0.9659258262890683122, 1.000000000000000000, 0.9659258262890683122, 1.000000000000000000, 0.9659258262890683122, 1.000000000000000000, 0.9659258262890683122, 1.000000000000000000, 0.9659258262890683122, 1.000000000000000000, 0.9659258262890683122, 1.000000000000000000, 0.9659258262890683122, 1.000000000000000000, 0.9659258262890683122, 1.000000000000000000, 0.9659258262890683122, 1.000000000000000000, 0.9659258262890683122, 1.000000000000000000, 0.9659258262890683122, 1.000000000000000000, 0.9659258262890683122, 1.000000000000000000, 0.9659258262890683122, 1.000000000000000000, 0.9659258262890683122, 1.000000000000000000, 0.9659258262890683122, 1.000000000000000000, 0.9659258262890683122, 1.000000000000000000, 0.9659258262890683122, 1.000000000000000000, 0.9659258262890683122, 1.000000000000000000, 0.9659258262890683122, 1.000000000000000000, 0.9659258262890683122, 1.000000000000000000, 0.9659258262890683122, 1.000000000000000000, 0.9659258262890683122, 1.000000000000000000, 0.9659258262890683122, 1.000000000000000000, 0.9659258262890683122, 1.000000000000000000, 0.9659258262890683122, 1.000000000000000000, 0.9659258262890683122, 1.000000000000000000, 0.9659258262890683122, 1.000000000000000000, 0.9659258262890683122, 1.000000000000000000, 0.9659258262890683122, 1.000000000000000000, 0.9659258262890683122, 1.000000000000000000, 0.9659258262890683122, 1.000000000000000000, 0.9659258262890683122, 1.000000000000000000, 0.9659258262890683122, 1.000000000000000000, 0.9659258262890683122, 1.000000000000000000, 0.9659258262890683122, 1.000000000000000000, 0.9659258262890683122, 1.000000000000000000, 0.9659258262890683122, 1.000000000000000000, 0.9659258262890683122, 1.000000000000000000, 0.9659258262890683122, 1.000000000000000000, 0.9659258262890683122, 1.000000000000000000, 0.9659258262890683122, 1.000000000000000000, 0.9659258262890683122, 1.000000000000000000, 0.9659258262890683122, 1.000000000000000000, 0.9659258262890683122, 1.000000000000000000, 0.9659258262890683122, 1.000000000000000000, 0.9659258262890683122, 1.000000000000000000, 0.9659258262890683122, 1.000000000000000000, 0.9659258262890683122, 1.000000000000000000, 0.9659258262890683122, 1.000000000000000000, 0.9659258262890683122, 1.000000000000000000, 0.9659258262890683122, 1.000000000000000000, 0.9659258262890683122, 1.000000000000000000, 0.9659258262890683122, 1.000000000000000000, 0.9659258262890683122, 1.000000000000000000, 0.9659258262890683122, 1.000000000000000000, 0.9659258262890683122, 1.000000000000000000, 0.9659258262890683122, 1.000000000000000000, 0.9659258262890683122, 1.000000000000000000, 0.9659258262890683122, 1.000000000000000000),
 ( 0.3333333333333333703, 0.3219752754296894559, 0.3333333333333333703, 0.3219752754296894559, 0.3333333333333333703, 0.3219752754296894559, 0.3333333333333333703, 0.3219752754296894559, 0.3333333333333333703, 0.3219752754296894559, 0.3333333333333333703, 0.3219752754296894559, 0.3333333333333333703, 0.3219752754296894559, 0.3333333333333333703, 0.3219752754296894559, 0.3333333333333333703, 0.3219752754296894559, 0.3333333333333333703, 0.3219752754296894559, 0.3333333333333333703, 0.3219752754296894559, 0.3333333333333333703, 0.3219752754296894559, 0.3333333333333333703, 0.3219752754296894559, 0.3333333333333333703, 0.3219752754296894559, 0.3333333333333333703, 0.3219752754296894559, 0.3333333333333333703, 0.3219752754296894559, 0.3333333333333333703, 0.3219752754296894559, 0.3333333333333333703, 0.3219752754296894559, 0.3333333333333333703, 0.3219752754296894559, 0.3333333333333333703, 0.3219752754296894559, 0.3333333333333333703, 0.3219752754296894559, 0.3333333333333333703, 0.3219752754296894559, 0.3333333333333333703, 0.3219752754296894559, 0.3333333333333333703, 0.3219752754296894559, 0.3333333333333333703, 0.3219752754296894559, 0.3333333333333333703, 0.3219752754296894559, 0.3333333333333333703, 0.3219752754296894559, 0.3333333333333333703, 0.3219752754296894559, 0.3333333333333333703, 0.3219752754296894559, 0.3333333333333333703, 0.3219752754296894559, 0.3333333333333333703, 0.3219752754296894559, 0.3333333333333333703, 0.3219752754296894559, 0.3333333333333333703, 0.3219752754296894559, 0.3333333333333333703, 0.3219752754296894559, 0.3333333333333333703, 0.3219752754296894559, 0.3333333333333333703, 0.3219752754296894559, 0.3333333333333333703, 0.3219752754296894559, 0.3333333333333333703, 0.3219752754296894559, 0.3333333333333333703, 0.3219752754296894559, 0.3333333333333333703, 0.3219752754296894559, 0.3333333333333333703, 0.3219752754296894559, 0.3333333333333333703, 0.3219752754296894559, 0.3333333333333333703, 0.3219752754296894559, 0.3333333333333333703, 0.3219752754296894559, 0.3333333333333333703, 0.3219752754296894559, 0.3333333333333333703, 0.3219752754296894559, 0.3333333333333333703, 0.3219752754296894559, 0.3333333333333333703, 0.3219752754296894559, 0.3333333333333333703, 0.3219752754296894559, 0.3333333333333333703, 0.3219752754296894559, 0.3333333333333333703, 0.3219752754296894559, 0.3333333333333333703, 0.3219752754296894559, 0.3333333333333333703, 0.3219752754296894559, 0.3333333333333333703, 0.3219752754296894559, 0.3333333333333333703, 0.3219752754296894559, 0.3333333333333333703, 0.3219752754296894559, 0.3333333333333333703, 0.3219752754296894559, 0.3333333333333333703, 0.3219752754296894559, 0.3333333333333333703, 0.3219752754296894559, 0.3333333333333333703, 0.3219752754296894559, 0.3333333333333333703, 0.3219752754296894559, 0.3333333333333333703, 0.3219752754296894559, 0.3333333333333333703, 0.3219752754296894559, 0.3333333333333333703, 0.3219752754296894559, 0.3333333333333333703, 0.3219752754296894559, 0.3333333333333333703, 0.3219752754296894559, 0.3333333333333333703, 0.3219752754296894559, 0.3333333333333333703, 0.3219752754296894559, 0.3333333333333333703, 0.3219752754296894559, 0.3333333333333333703, 0.3219752754296894559, 0.3333333333333333703, 0.3219752754296894559, 0.3333333333333333703, 0.3219752754296894559, 0.3333333333333333703, 0.3219752754296894559, 0.3333333333333333703, 0.3219752754296894559, 0.3333333333333333703, 0.3219752754296894559, 0.3333333333333333703, 0.3219752754296894559, 0.3333333333333333703, 0.3219752754296894559, 0.3333333333333333703, 0.3219752754296894559, 0.3333333333333333703, 0.3219752754296894559, 0.3333333333333333703, 0.3219752754296894559, 0.3333333333333333703, 0.3219752754296894559, 0.3333333333333333703, 0.3219752754296894559, 0.3333333333333333703, 0.3219752754296894559, 0.3333333333333333703, 0.3219752754296894559, 0.3333333333333333703, 0.3219752754296894559, 0.3333333333333333703, 0.3219752754296894559, 0.3333333333333333703, 0.3219752754296894559, 0.3333333333333333703, 0.3219752754296894559, 0.3333333333333333703, 0.3219752754296894559, 0.3333333333333333703, 0.3219752754296894559, 0.3333333333333333703, 0.3219752754296894559, 0.3333333333333333703, 0.3219752754296894559, 0.3333333333333333703, 0.3219752754296894559, 0.3333333333333333703, 0.3219752754296894559, 0.3333333333333333703, 0.3219752754296894559, 0.3333333333333333703, 0.3219752754296894559, 0.3333333333333333703, 0.3219752754296894559, 0.3333333333333333703, 0.3219752754296894559, 0.3333333333333333703, 0.3219752754296894559, 0.3333333333333333703, 0.3219752754296894559, 0.3333333333333333703, 0.3219752754296894559, 0.3333333333333333703, 0.3219752754296894559, 0.3333333333333333703, 0.3219752754296894559, 0.3333333333333333703, 0.3219752754296894559, 0.3333333333333333703, 0.3219752754296894559, 0.3333333333333333703, 0.3219752754296894559, 0.3333333333333333703, 0.3219752754296894559, 0.3333333333333333703, 0.3219752754296894559, 0.3333333333333333703, 0.3219752754296894559, 0.3333333333333333703, 0.3219752754296894559, 0.3333333333333333703, 0.3219752754296894559, 0.3333333333333333703, 0.3219752754296894559, 0.3333333333333333703, 0.3219752754296894559, 0.3333333333333333703, 0.3219752754296894559, 0.3333333333333333703, 0.3219752754296894559, 0.3333333333333333703, 0.3219752754296894559, 0.3333333333333333703, 0.3219752754296894559, 0.3333333333333333703, 0.3219752754296894559, 0.3333333333333333703, 0.3219752754296894559, 0.3333333333333333703, 0.3219752754296894559, 0.3333333333333333703, 0.3219752754296894559, 0.3333333333333333703, 0.3219752754296894559, 0.3333333333333333703, 0.3219752754296894559, 0.3333333333333333703, 0.3219752754296894559, 0.3333333333333333703, 0.3219752754296894559, 0.3333333333333333703, 0.3219752754296894559, 0.3333333333333333703, 0.3219752754296894559, 0.3333333333333333703, 0.3219752754296894559, 0.3333333333333333703, 0.3219752754296894559, 0.3333333333333333703, 0.3219752754296894559, 0.3333333333333333703, 0.3219752754296894559, 0.3333333333333333703, 0.3219752754296894559, 0.3333333333333333703, 0.3219752754296894559, 0.3333333333333333703, 0.3219752754296894559, 0.3333333333333333703, 0.3219752754296894559, 0.3333333333333333703, 0.3219752754296894559, 0.3333333333333333703, 0.3219752754296894559, 0.3333333333333333703, 0.3219752754296894559, 0.3333333333333333703, 0.3219752754296894559, 0.3333333333333333703, 0.3219752754296894559, 0.3333333333333333703, 0.3219752754296894559, 0.3333333333333333703, 0.3219752754296894559, 0.3333333333333333703, 0.3219752754296894559, 0.3333333333333333703, 0.3219752754296894559, 0.3333333333333333703, 0.3219752754296894559, 0.3333333333333333703, 0.3219752754296894559, 0.3333333333333333703, 0.3219752754296894559, 0.3333333333333333703, 0.3219752754296894559, 0.3333333333333333703, 0.3219752754296894559, 0.3333333333333333703, 0.3219752754296894559, 0.3333333333333333703, 0.3219752754296894559, 0.3333333333333333703, 0.3219752754296894559, 0.3333333333333333703, 0.3219752754296894559, 0.3333333333333333703, 0.3219752754296894559, 0.3333333333333333703, 0.3219752754296894559, 0.3333333333333333703, 0.3219752754296894559, 0.3333333333333333703, 0.3219752754296894559, 0.3333333333333333703, 0.3219752754296894559, 0.3333333333333333703, 0.3219752754296894559, 0.3333333333333333703, 0.3219752754296894559, 0.3333333333333333703, 0.3219752754296894559, 0.3333333333333333703, 0.3219752754296894559, 0.3333333333333333703, 0.3219752754296894559, 0.3333333333333333703, 0.3219752754296894559, 0.3333333333333333703, 0.3219752754296894559, 0.3333333333333333703, 0.3219752754296894559, 0.3333333333333333703, 0.3219752754296894559, 0.3333333333333333703, 0.3219752754296894559, 0.3333333333333333703, 0.3219752754296894559, 0.3333333333333333703, 0.3219752754296894559, 0.3333333333333333703, 0.3219752754296894559, 0.3333333333333333703, 0.3219752754296894559, 0.3333333333333333703, 0.3219752754296894559, 0.3333333333333333703, 0.3219752754296894559, 0.3333333333333333703, 0.3219752754296894559, 0.3333333333333333703, 0.3219752754296894559, 0.3333333333333333703, 0.3219752754296894559, 0.3333333333333333703, 0.3219752754296894559, 0.3333333333333333703, 0.3219752754296894559, 0.3333333333333333703, 0.3219752754296894559, 0.3333333333333333703, 0.3219752754296894559, 0.3333333333333333703, 0.3219752754296894559, 0.3333333333333333703, 0.3219752754296894559, 0.3333333333333333703, 0.3219752754296894559, 0.3333333333333333703, 0.3219752754296894559, 0.3333333333333333703, 0.3219752754296894559, 0.3333333333333333703, 0.3219752754296894559, 0.3333333333333333703, 0.3219752754296894559, 0.3333333333333333703, 0.3219752754296894559, 0.3333333333333333703, 0.3219752754296894559, 0.3333333333333333703, 0.3219752754296894559, 0.3333333333333333703, 0.3219752754296894559, 0.3333333333333333703, 0.3219752754296894559, 0.3333333333333333703, 0.3219752754296894559, 0.3333333333333333703, 0.3219752754296894559, 0.3333333333333333703, 0.3219752754296894559, 0.3333333333333333703, 0.3219752754296894559, 0.3333333333333333703, 0.3219752754296894559, 0.3333333333333333703, 0.3219752754296894559, 0.3333333333333333703, 0.3219752754296894559, 0.3333333333333333703, 0.3219752754296894559, 0.3333333333333333703, 0.3219752754296894559, 0.3333333333333333703, 0.3219752754296894559, 0.3333333333333333703, 0.3219752754296894559, 0.3333333333333333703, 0.3219752754296894559, 0.3333333333333333703, 0.3219752754296894559, 0.3333333333333333703, 0.3219752754296894559, 0.3333333333333333703, 0.3219752754296894559, 0.3333333333333333703, 0.3219752754296894559, 0.3333333333333333703, 0.3219752754296894559, 0.3333333333333333703, 0.3219752754296894559, 0.3333333333333333703, 0.3219752754296894559, 0.3333333333333333703, 0.3219752754296894559, 0.3333333333333333703, 0.3219752754296894559, 0.3333333333333333703, 0.3219752754296894559, 0.3333333333333333703, 0.3219752754296894559, 0.3333333333333333703, 0.3219752754296894559, 0.3333333333333333703, 0.3219752754296894559, 0.3333333333333333703, 0.3219752754296894559, 0.3333333333333333703, 0.3219752754296894559, 0.3333333333333333703, 0.3219752754296894559, 0.3333333333333333703, 0.3219752754296894559, 0.3333333333333333703, 0.3219752754296894559, 0.3333333333333333703, 0.3219752754296894559, 0.3333333333333333703, 0.3219752754296894559, 0.3333333333333333703, 0.3219752754296894559, 0.3333333333333333703, 0.3219752754296894559, 0.3333333333333333703, 0.3219752754296894559, 0.3333333333333333703),
 ( 0.3333333333333333703, 0.3219752754296894559, 0.3333333333333333703, 0.3219752754296894559, 0.3333333333333333703, 0.3219752754296894559, 0.3333333333333333703, 0.3219752754296894559, 0.3333333333333333703, 0.3219752754296894559, 0.3333333333333333703, 0.3219752754296894559, 0.3333333333333333703, 0.3219752754296894559, 0.3333333333333333703, 0.3219752754296894559, 0.3333333333333333703, 0.3219752754296894559, 0.3333333333333333703, 0.3219752754296894559, 0.3333333333333333703, 0.3219752754296894559, 0.3333333333333333703, 0.3219752754296894559, 0.3333333333333333703, 0.3219752754296894559, 0.3333333333333333703, 0.3219752754296894559, 0.3333333333333333703, 0.3219752754296894559, 0.3333333333333333703, 0.3219752754296894559, 0.3333333333333333703, 0.3219752754296894559, 0.3333333333333333703, 0.3219752754296894559, 0.3333333333333333703, 0.3219752754296894559, 0.3333333333333333703, 0.3219752754296894559, 0.3333333333333333703, 0.3219752754296894559, 0.3333333333333333703, 0.3219752754296894559, 0.3333333333333333703, 0.3219752754296894559, 0.3333333333333333703, 0.3219752754296894559, 0.3333333333333333703, 0.3219752754296894559, 0.3333333333333333703, 0.3219752754296894559, 0.3333333333333333703, 0.3219752754296894559, 0.3333333333333333703, 0.3219752754296894559, 0.3333333333333333703, 0.3219752754296894559, 0.3333333333333333703, 0.3219752754296894559, 0.3333333333333333703, 0.3219752754296894559, 0.3333333333333333703, 0.3219752754296894559, 0.3333333333333333703, 0.3219752754296894559, 0.3333333333333333703, 0.3219752754296894559, 0.3333333333333333703, 0.3219752754296894559, 0.3333333333333333703, 0.3219752754296894559, 0.3333333333333333703, 0.3219752754296894559, 0.3333333333333333703, 0.3219752754296894559, 0.3333333333333333703, 0.3219752754296894559, 0.3333333333333333703, 0.3219752754296894559, 0.3333333333333333703, 0.3219752754296894559, 0.3333333333333333703, 0.3219752754296894559, 0.3333333333333333703, 0.3219752754296894559, 0.3333333333333333703, 0.3219752754296894559, 0.3333333333333333703, 0.3219752754296894559, 0.3333333333333333703, 0.3219752754296894559, 0.3333333333333333703, 0.3219752754296894559, 0.3333333333333333703, 0.3219752754296894559, 0.3333333333333333703, 0.3219752754296894559, 0.3333333333333333703, 0.3219752754296894559, 0.3333333333333333703, 0.3219752754296894559, 0.3333333333333333703, 0.3219752754296894559, 0.3333333333333333703, 0.3219752754296894559, 0.3333333333333333703, 0.3219752754296894559, 0.3333333333333333703, 0.3219752754296894559, 0.3333333333333333703, 0.3219752754296894559, 0.3333333333333333703, 0.3219752754296894559, 0.3333333333333333703, 0.3219752754296894559, 0.3333333333333333703, 0.3219752754296894559, 0.3333333333333333703, 0.3219752754296894559, 0.3333333333333333703, 0.3219752754296894559, 0.3333333333333333703, 0.3219752754296894559, 0.3333333333333333703, 0.3219752754296894559, 0.3333333333333333703, 0.3219752754296894559, 0.3333333333333333703, 0.3219752754296894559, 0.3333333333333333703, 0.3219752754296894559, 0.3333333333333333703, 0.3219752754296894559, 0.3333333333333333703, 0.3219752754296894559, 0.3333333333333333703, 0.3219752754296894559, 0.3333333333333333703, 0.3219752754296894559, 0.3333333333333333703, 0.3219752754296894559, 0.3333333333333333703, 0.3219752754296894559, 0.3333333333333333703, 0.3219752754296894559, 0.3333333333333333703, 0.3219752754296894559, 0.3333333333333333703, 0.3219752754296894559, 0.3333333333333333703, 0.3219752754296894559, 0.3333333333333333703, 0.3219752754296894559, 0.3333333333333333703, 0.3219752754296894559, 0.3333333333333333703, 0.3219752754296894559, 0.3333333333333333703, 0.3219752754296894559, 0.3333333333333333703, 0.3219752754296894559, 0.3333333333333333703, 0.3219752754296894559, 0.3333333333333333703, 0.3219752754296894559, 0.3333333333333333703, 0.3219752754296894559, 0.3333333333333333703, 0.3219752754296894559, 0.3333333333333333703, 0.3219752754296894559, 0.3333333333333333703, 0.3219752754296894559, 0.3333333333333333703, 0.3219752754296894559, 0.3333333333333333703, 0.3219752754296894559, 0.3333333333333333703, 0.3219752754296894559, 0.3333333333333333703, 0.3219752754296894559, 0.3333333333333333703, 0.3219752754296894559, 0.3333333333333333703, 0.3219752754296894559, 0.3333333333333333703, 0.3219752754296894559, 0.3333333333333333703, 0.3219752754296894559, 0.3333333333333333703, 0.3219752754296894559, 0.3333333333333333703, 0.3219752754296894559, 0.3333333333333333703, 0.3219752754296894559, 0.3333333333333333703, 0.3219752754296894559, 0.3333333333333333703, 0.3219752754296894559, 0.3333333333333333703, 0.3219752754296894559, 0.3333333333333333703, 0.3219752754296894559, 0.3333333333333333703, 0.3219752754296894559, 0.3333333333333333703, 0.3219752754296894559, 0.3333333333333333703, 0.3219752754296894559, 0.3333333333333333703, 0.3219752754296894559, 0.3333333333333333703, 0.3219752754296894559, 0.3333333333333333703, 0.3219752754296894559, 0.3333333333333333703, 0.3219752754296894559, 0.3333333333333333703, 0.3219752754296894559, 0.3333333333333333703, 0.3219752754296894559, 0.3333333333333333703, 0.3219752754296894559, 0.3333333333333333703, 0.3219752754296894559, 0.3333333333333333703, 0.3219752754296894559, 0.3333333333333333703, 0.3219752754296894559, 0.3333333333333333703, 0.3219752754296894559, 0.3333333333333333703, 0.3219752754296894559, 0.3333333333333333703, 0.3219752754296894559, 0.3333333333333333703, 0.3219752754296894559, 0.3333333333333333703, 0.3219752754296894559, 0.3333333333333333703, 0.3219752754296894559, 0.3333333333333333703, 0.3219752754296894559, 0.3333333333333333703, 0.3219752754296894559, 0.3333333333333333703, 0.3219752754296894559, 0.3333333333333333703, 0.3219752754296894559, 0.3333333333333333703, 0.3219752754296894559, 0.3333333333333333703, 0.3219752754296894559, 0.3333333333333333703, 0.3219752754296894559, 0.3333333333333333703, 0.3219752754296894559, 0.3333333333333333703, 0.3219752754296894559, 0.3333333333333333703, 0.3219752754296894559, 0.3333333333333333703, 0.3219752754296894559, 0.3333333333333333703, 0.3219752754296894559, 0.3333333333333333703, 0.3219752754296894559, 0.3333333333333333703, 0.3219752754296894559, 0.3333333333333333703, 0.3219752754296894559, 0.3333333333333333703, 0.3219752754296894559, 0.3333333333333333703, 0.3219752754296894559, 0.3333333333333333703, 0.3219752754296894559, 0.3333333333333333703, 0.3219752754296894559, 0.3333333333333333703, 0.3219752754296894559, 0.3333333333333333703, 0.3219752754296894559, 0.3333333333333333703, 0.3219752754296894559, 0.3333333333333333703, 0.3219752754296894559, 0.3333333333333333703, 0.3219752754296894559, 0.3333333333333333703, 0.3219752754296894559, 0.3333333333333333703, 0.3219752754296894559, 0.3333333333333333703, 0.3219752754296894559, 0.3333333333333333703, 0.3219752754296894559, 0.3333333333333333703, 0.3219752754296894559, 0.3333333333333333703, 0.3219752754296894559, 0.3333333333333333703, 0.3219752754296894559, 0.3333333333333333703, 0.3219752754296894559, 0.3333333333333333703, 0.3219752754296894559, 0.3333333333333333703, 0.3219752754296894559, 0.3333333333333333703, 0.3219752754296894559, 0.3333333333333333703, 0.3219752754296894559, 0.3333333333333333703, 0.3219752754296894559, 0.3333333333333333703, 0.3219752754296894559, 0.3333333333333333703, 0.3219752754296894559, 0.3333333333333333703, 0.3219752754296894559, 0.3333333333333333703, 0.3219752754296894559, 0.3333333333333333703, 0.3219752754296894559, 0.3333333333333333703, 0.3219752754296894559, 0.3333333333333333703, 0.3219752754296894559, 0.3333333333333333703, 0.3219752754296894559, 0.3333333333333333703, 0.3219752754296894559, 0.3333333333333333703, 0.3219752754296894559, 0.3333333333333333703, 0.3219752754296894559, 0.3333333333333333703, 0.3219752754296894559, 0.3333333333333333703, 0.3219752754296894559, 0.3333333333333333703, 0.3219752754296894559, 0.3333333333333333703, 0.3219752754296894559, 0.3333333333333333703, 0.3219752754296894559, 0.3333333333333333703, 0.3219752754296894559, 0.3333333333333333703, 0.3219752754296894559, 0.3333333333333333703, 0.3219752754296894559, 0.3333333333333333703, 0.3219752754296894559, 0.3333333333333333703, 0.3219752754296894559, 0.3333333333333333703, 0.3219752754296894559, 0.3333333333333333703, 0.3219752754296894559, 0.3333333333333333703, 0.3219752754296894559, 0.3333333333333333703, 0.3219752754296894559, 0.3333333333333333703, 0.3219752754296894559, 0.3333333333333333703, 0.3219752754296894559, 0.3333333333333333703, 0.3219752754296894559, 0.3333333333333333703, 0.3219752754296894559, 0.3333333333333333703, 0.3219752754296894559, 0.3333333333333333703, 0.3219752754296894559, 0.3333333333333333703, 0.3219752754296894559, 0.3333333333333333703, 0.3219752754296894559, 0.3333333333333333703, 0.3219752754296894559, 0.3333333333333333703, 0.3219752754296894559, 0.3333333333333333703, 0.3219752754296894559, 0.3333333333333333703, 0.3219752754296894559, 0.3333333333333333703, 0.3219752754296894559, 0.3333333333333333703, 0.3219752754296894559, 0.3333333333333333703, 0.3219752754296894559, 0.3333333333333333703, 0.3219752754296894559, 0.3333333333333333703, 0.3219752754296894559, 0.3333333333333333703, 0.3219752754296894559, 0.3333333333333333703, 0.3219752754296894559, 0.3333333333333333703, 0.3219752754296894559, 0.3333333333333333703, 0.3219752754296894559, 0.3333333333333333703, 0.3219752754296894559, 0.3333333333333333703, 0.3219752754296894559, 0.3333333333333333703, 0.3219752754296894559, 0.3333333333333333703, 0.3219752754296894559, 0.3333333333333333703, 0.3219752754296894559, 0.3333333333333333703, 0.3219752754296894559, 0.3333333333333333703, 0.3219752754296894559, 0.3333333333333333703, 0.3219752754296894559, 0.3333333333333333703, 0.3219752754296894559, 0.3333333333333333703, 0.3219752754296894559, 0.3333333333333333703, 0.3219752754296894559, 0.3333333333333333703, 0.3219752754296894559, 0.3333333333333333703, 0.3219752754296894559, 0.3333333333333333703, 0.3219752754296894559, 0.3333333333333333703, 0.3219752754296894559, 0.3333333333333333703, 0.3219752754296894559, 0.3333333333333333703, 0.3219752754296894559, 0.3333333333333333703, 0.3219752754296894559, 0.3333333333333333703, 0.3219752754296894559, 0.3333333333333333703, 0.3219752754296894559, 0.3333333333333333703, 0.3219752754296894559, 0.3333333333333333703, 0.3219752754296894559, 0.3333333333333333703, 0.3219752754296894559, 0.3333333333333333703, 0.3219752754296894559, 0.3333333333333333703),
 ( 1.000000000000000000, 0.9659258262890683122, 1.000000000000000000, 0.9659258262890683122, 1.000000000000000000, 0.9659258262890683122, 1.000000000000000000, 0.9659258262890683122, 1.000000000000000000, 0.9659258262890683122, 1.000000000000000000, 0.9659258262890683122, 1.000000000000000000, 0.9659258262890683122, 1.000000000000000000, 0.9659258262890683122, 1.000000000000000000, 0.9659258262890683122, 1.000000000000000000, 0.9659258262890683122, 1.000000000000000000, 0.9659258262890683122, 1.000000000000000000, 0.9659258262890683122, 1.000000000000000000, 0.9659258262890683122, 1.000000000000000000, 0.9659258262890683122, 1.000000000000000000, 0.9659258262890683122, 1.000000000000000000, 0.9659258262890683122, 1.000000000000000000, 0.9659258262890683122, 1.000000000000000000, 0.9659258262890683122, 1.000000000000000000, 0.9659258262890683122, 1.000000000000000000, 0.9659258262890683122, 1.000000000000000000, 0.9659258262890683122, 1.000000000000000000, 0.9659258262890683122, 1.000000000000000000, 0.9659258262890683122, 1.000000000000000000, 0.9659258262890683122, 1.000000000000000000, 0.9659258262890683122, 1.000000000000000000, 0.9659258262890683122, 1.000000000000000000, 0.9659258262890683122, 1.000000000000000000, 0.9659258262890683122, 1.000000000000000000, 0.9659258262890683122, 1.000000000000000000, 0.9659258262890683122, 1.000000000000000000, 0.9659258262890683122, 1.000000000000000000, 0.9659258262890683122, 1.000000000000000000, 0.9659258262890683122, 1.000000000000000000, 0.9659258262890683122, 1.000000000000000000, 0.9659258262890683122, 1.000000000000000000, 0.9659258262890683122, 1.000000000000000000, 0.9659258262890683122, 1.000000000000000000, 0.9659258262890683122, 1.000000000000000000, 0.9659258262890683122, 1.000000000000000000, 0.9659258262890683122, 1.000000000000000000, 0.9659258262890683122, 1.000000000000000000, 0.9659258262890683122, 1.000000000000000000, 0.9659258262890683122, 1.000000000000000000, 0.9659258262890683122, 1.000000000000000000, 0.9659258262890683122, 1.000000000000000000, 0.9659258262890683122, 1.000000000000000000, 0.9659258262890683122, 1.000000000000000000, 0.9659258262890683122, 1.000000000000000000, 0.9659258262890683122, 1.000000000000000000, 0.9659258262890683122, 1.000000000000000000, 0.9659258262890683122, 1.000000000000000000, 0.9659258262890683122, 1.000000000000000000, 0.9659258262890683122, 1.000000000000000000, 0.9659258262890683122, 1.000000000000000000, 0.9659258262890683122, 1.000000000000000000, 0.9659258262890683122, 1.000000000000000000, 0.9659258262890683122, 1.000000000000000000, 0.9659258262890683122, 1.000000000000000000, 0.9659258262890683122, 1.000000000000000000, 0.9659258262890683122, 1.000000000000000000, 0.9659258262890683122, 1.000000000000000000, 0.9659258262890683122, 1.000000000000000000, 0.9659258262890683122, 1.000000000000000000, 0.9659258262890683122, 1.000000000000000000, 0.9659258262890683122, 1.000000000000000000, 0.9659258262890683122, 1.000000000000000000, 0.9659258262890683122, 1.000000000000000000, 0.9659258262890683122, 1.000000000000000000, 0.9659258262890683122, 1.000000000000000000, 0.9659258262890683122, 1.000000000000000000, 0.9659258262890683122, 1.000000000000000000, 0.9659258262890683122, 1.000000000000000000, 0.9659258262890683122, 1.000000000000000000, 0.9659258262890683122, 1.000000000000000000, 0.9659258262890683122, 1.000000000000000000, 0.9659258262890683122, 1.000000000000000000, 0.9659258262890683122, 1.000000000000000000, 0.9659258262890683122, 1.000000000000000000, 0.9659258262890683122, 1.000000000000000000, 0.9659258262890683122, 1.000000000000000000, 0.9659258262890683122, 1.000000000000000000, 0.9659258262890683122, 1.000000000000000000, 0.9659258262890683122, 1.000000000000000000, 0.9659258262890683122, 1.000000000000000000, 0.9659258262890683122, 1.000000000000000000, 0.9659258262890683122, 1.000000000000000000, 0.9659258262890683122, 1.000000000000000000, 0.9659258262890683122, 1.000000000000000000, 0.9659258262890683122, 1.000000000000000000, 0.9659258262890683122, 1.000000000000000000, 0.9659258262890683122, 1.000000000000000000, 0.9659258262890683122, 1.000000000000000000, 0.9659258262890683122, 1.000000000000000000, 0.9659258262890683122, 1.000000000000000000, 0.9659258262890683122, 1.000000000000000000, 0.9659258262890683122, 1.000000000000000000, 0.9659258262890683122, 1.000000000000000000, 0.9659258262890683122, 1.000000000000000000, 0.9659258262890683122, 1.000000000000000000, 0.9659258262890683122, 1.000000000000000000, 0.9659258262890683122, 1.000000000000000000, 0.9659258262890683122, 1.000000000000000000, 0.9659258262890683122, 1.000000000000000000, 0.9659258262890683122, 1.000000000000000000, 0.9659258262890683122, 1.000000000000000000, 0.9659258262890683122, 1.000000000000000000, 0.9659258262890683122, 1.000000000000000000, 0.9659258262890683122, 1.000000000000000000, 0.9659258262890683122, 1.000000000000000000, 0.9659258262890683122, 1.000000000000000000, 0.9659258262890683122, 1.000000000000000000, 0.9659258262890683122, 1.000000000000000000, 0.9659258262890683122, 1.000000000000000000, 0.9659258262890683122, 1.000000000000000000, 0.9659258262890683122, 1.000000000000000000, 0.9659258262890683122, 1.000000000000000000, 0.9659258262890683122, 1.000000000000000000, 0.9659258262890683122, 1.000000000000000000, 0.9659258262890683122, 1.000000000000000000, 0.9659258262890683122, 1.000000000000000000, 0.9659258262890683122, 1.000000000000000000, 0.9659258262890683122, 1.000000000000000000, 0.9659258262890683122, 1.000000000000000000, 0.9659258262890683122, 1.000000000000000000, 0.9659258262890683122, 1.000000000000000000, 0.9659258262890683122, 1.000000000000000000, 0.9659258262890683122, 1.000000000000000000, 0.9659258262890683122, 1.000000000000000000, 0.9659258262890683122, 1.000000000000000000, 0.9659258262890683122, 1.000000000000000000, 0.9659258262890683122, 1.000000000000000000, 0.9659258262890683122, 1.000000000000000000, 0.9659258262890683122, 1.000000000000000000, 0.9659258262890683122, 1.000000000000000000, 0.9659258262890683122, 1.000000000000000000, 0.9659258262890683122, 1.000000000000000000, 0.9659258262890683122, 1.000000000000000000, 0.9659258262890683122, 1.000000000000000000, 0.9659258262890683122, 1.000000000000000000, 0.9659258262890683122, 1.000000000000000000, 0.9659258262890683122, 1.000000000000000000, 0.9659258262890683122, 1.000000000000000000, 0.9659258262890683122, 1.000000000000000000, 0.9659258262890683122, 1.000000000000000000, 0.9659258262890683122, 1.000000000000000000, 0.9659258262890683122, 1.000000000000000000, 0.9659258262890683122, 1.000000000000000000, 0.9659258262890683122, 1.000000000000000000, 0.9659258262890683122, 1.000000000000000000, 0.9659258262890683122, 1.000000000000000000, 0.9659258262890683122, 1.000000000000000000, 0.9659258262890683122, 1.000000000000000000, 0.9659258262890683122, 1.000000000000000000, 0.9659258262890683122, 1.000000000000000000, 0.9659258262890683122, 1.000000000000000000, 0.9659258262890683122, 1.000000000000000000, 0.9659258262890683122, 1.000000000000000000, 0.9659258262890683122, 1.000000000000000000, 0.9659258262890683122, 1.000000000000000000, 0.9659258262890683122, 1.000000000000000000, 0.9659258262890683122, 1.000000000000000000, 0.9659258262890683122, 1.000000000000000000, 0.9659258262890683122, 1.000000000000000000, 0.9659258262890683122, 1.000000000000000000, 0.9659258262890683122, 1.000000000000000000, 0.9659258262890683122, 1.000000000000000000, 0.9659258262890683122, 1.000000000000000000, 0.9659258262890683122, 1.000000000000000000, 0.9659258262890683122, 1.000000000000000000, 0.9659258262890683122, 1.000000000000000000, 0.9659258262890683122, 1.000000000000000000, 0.9659258262890683122, 1.000000000000000000, 0.9659258262890683122, 1.000000000000000000, 0.9659258262890683122, 1.000000000000000000, 0.9659258262890683122, 1.000000000000000000, 0.9659258262890683122, 1.000000000000000000, 0.9659258262890683122, 1.000000000000000000, 0.9659258262890683122, 1.000000000000000000, 0.9659258262890683122, 1.000000000000000000, 0.9659258262890683122, 1.000000000000000000, 0.9659258262890683122, 1.000000000000000000, 0.9659258262890683122, 1.000000000000000000, 0.9659258262890683122, 1.000000000000000000, 0.9659258262890683122, 1.000000000000000000, 0.9659258262890683122, 1.000000000000000000, 0.9659258262890683122, 1.000000000000000000, 0.9659258262890683122, 1.000000000000000000, 0.9659258262890683122, 1.000000000000000000, 0.9659258262890683122, 1.000000000000000000, 0.9659258262890683122, 1.000000000000000000, 0.9659258262890683122, 1.000000000000000000, 0.9659258262890683122, 1.000000000000000000, 0.9659258262890683122, 1.000000000000000000, 0.9659258262890683122, 1.000000000000000000, 0.9659258262890683122, 1.000000000000000000, 0.9659258262890683122, 1.000000000000000000, 0.9659258262890683122, 1.000000000000000000, 0.9659258262890683122, 1.000000000000000000, 0.9659258262890683122, 1.000000000000000000, 0.9659258262890683122, 1.000000000000000000, 0.9659258262890683122, 1.000000000000000000, 0.9659258262890683122, 1.000000000000000000, 0.9659258262890683122, 1.000000000000000000, 0.9659258262890683122, 1.000000000000000000, 0.9659258262890683122, 1.000000000000000000, 0.9659258262890683122, 1.000000000000000000, 0.9659258262890683122, 1.000000000000000000, 0.9659258262890683122, 1.000000000000000000, 0.9659258262890683122, 1.000000000000000000, 0.9659258262890683122, 1.000000000000000000, 0.9659258262890683122, 1.000000000000000000, 0.9659258262890683122, 1.000000000000000000, 0.9659258262890683122, 1.000000000000000000, 0.9659258262890683122, 1.000000000000000000, 0.9659258262890683122, 1.000000000000000000, 0.9659258262890683122, 1.000000000000000000, 0.9659258262890683122, 1.000000000000000000, 0.9659258262890683122, 1.000000000000000000, 0.9659258262890683122, 1.000000000000000000, 0.9659258262890683122, 1.000000000000000000, 0.9659258262890683122, 1.000000000000000000, 0.9659258262890683122, 1.000000000000000000, 0.9659258262890683122, 1.000000000000000000, 0.9659258262890683122, 1.000000000000000000, 0.9659258262890683122, 1.000000000000000000, 0.9659258262890683122, 1.000000000000000000, 0.9659258262890683122, 1.000000000000000000, 0.9659258262890683122, 1.000000000000000000),
 ( 0.3333333333333333703, 0.3219752754296894559, 0.3333333333333333703, 0.3219752754296894559, 0.3333333333333333703, 0.3219752754296894559, 0.3333333333333333703, 0.3219752754296894559, 0.3333333333333333703, 0.3219752754296894559, 0.3333333333333333703, 0.3219752754296894559, 0.3333333333333333703, 0.3219752754296894559, 0.3333333333333333703, 0.3219752754296894559, 0.3333333333333333703, 0.3219752754296894559, 0.3333333333333333703, 0.3219752754296894559, 0.3333333333333333703, 0.3219752754296894559, 0.3333333333333333703, 0.3219752754296894559, 0.3333333333333333703, 0.3219752754296894559, 0.3333333333333333703, 0.3219752754296894559, 0.3333333333333333703, 0.3219752754296894559, 0.3333333333333333703, 0.3219752754296894559, 0.3333333333333333703, 0.3219752754296894559, 0.3333333333333333703, 0.3219752754296894559, 0.3333333333333333703, 0.3219752754296894559, 0.3333333333333333703, 0.3219752754296894559, 0.3333333333333333703, 0.3219752754296894559, 0.3333333333333333703, 0.3219752754296894559, 0.3333333333333333703, 0.3219752754296894559, 0.3333333333333333703, 0.3219752754296894559, 0.3333333333333333703, 0.3219752754296894559, 0.3333333333333333703, 0.3219752754296894559, 0.3333333333333333703, 0.3219752754296894559, 0.3333333333333333703, 0.3219752754296894559, 0.3333333333333333703, 0.3219752754296894559, 0.3333333333333333703, 0.3219752754296894559, 0.3333333333333333703, 0.3219752754296894559, 0.3333333333333333703, 0.3219752754296894559, 0.3333333333333333703, 0.3219752754296894559, 0.3333333333333333703, 0.3219752754296894559, 0.3333333333333333703, 0.3219752754296894559, 0.3333333333333333703, 0.3219752754296894559, 0.3333333333333333703, 0.3219752754296894559, 0.3333333333333333703, 0.3219752754296894559, 0.3333333333333333703, 0.3219752754296894559, 0.3333333333333333703, 0.3219752754296894559, 0.3333333333333333703, 0.3219752754296894559, 0.3333333333333333703, 0.3219752754296894559, 0.3333333333333333703, 0.3219752754296894559, 0.3333333333333333703, 0.3219752754296894559, 0.3333333333333333703, 0.3219752754296894559, 0.3333333333333333703, 0.3219752754296894559, 0.3333333333333333703, 0.3219752754296894559, 0.3333333333333333703, 0.3219752754296894559, 0.3333333333333333703, 0.3219752754296894559, 0.3333333333333333703, 0.3219752754296894559, 0.3333333333333333703, 0.3219752754296894559, 0.3333333333333333703, 0.3219752754296894559, 0.3333333333333333703, 0.3219752754296894559, 0.3333333333333333703, 0.3219752754296894559, 0.3333333333333333703, 0.3219752754296894559, 0.3333333333333333703, 0.3219752754296894559, 0.3333333333333333703, 0.3219752754296894559, 0.3333333333333333703, 0.3219752754296894559, 0.3333333333333333703, 0.3219752754296894559, 0.3333333333333333703, 0.3219752754296894559, 0.3333333333333333703, 0.3219752754296894559, 0.3333333333333333703, 0.3219752754296894559, 0.3333333333333333703, 0.3219752754296894559, 0.3333333333333333703, 0.3219752754296894559, 0.3333333333333333703, 0.3219752754296894559, 0.3333333333333333703, 0.3219752754296894559, 0.3333333333333333703, 0.3219752754296894559, 0.3333333333333333703, 0.3219752754296894559, 0.3333333333333333703, 0.3219752754296894559, 0.3333333333333333703, 0.3219752754296894559, 0.3333333333333333703, 0.3219752754296894559, 0.3333333333333333703, 0.3219752754296894559, 0.3333333333333333703, 0.3219752754296894559, 0.3333333333333333703, 0.3219752754296894559, 0.3333333333333333703, 0.3219752754296894559, 0.3333333333333333703, 0.3219752754296894559, 0.3333333333333333703, 0.3219752754296894559, 0.3333333333333333703, 0.3219752754296894559, 0.3333333333333333703, 0.3219752754296894559, 0.3333333333333333703, 0.3219752754296894559, 0.3333333333333333703, 0.3219752754296894559, 0.3333333333333333703, 0.3219752754296894559, 0.3333333333333333703, 0.3219752754296894559, 0.3333333333333333703, 0.3219752754296894559, 0.3333333333333333703, 0.3219752754296894559, 0.3333333333333333703, 0.3219752754296894559, 0.3333333333333333703, 0.3219752754296894559, 0.3333333333333333703, 0.3219752754296894559, 0.3333333333333333703, 0.3219752754296894559, 0.3333333333333333703, 0.3219752754296894559, 0.3333333333333333703, 0.3219752754296894559, 0.3333333333333333703, 0.3219752754296894559, 0.3333333333333333703, 0.3219752754296894559, 0.3333333333333333703, 0.3219752754296894559, 0.3333333333333333703, 0.3219752754296894559, 0.3333333333333333703, 0.3219752754296894559, 0.3333333333333333703, 0.3219752754296894559, 0.3333333333333333703, 0.3219752754296894559, 0.3333333333333333703, 0.3219752754296894559, 0.3333333333333333703, 0.3219752754296894559, 0.3333333333333333703, 0.3219752754296894559, 0.3333333333333333703, 0.3219752754296894559, 0.3333333333333333703, 0.3219752754296894559, 0.3333333333333333703, 0.3219752754296894559, 0.3333333333333333703, 0.3219752754296894559, 0.3333333333333333703, 0.3219752754296894559, 0.3333333333333333703, 0.3219752754296894559, 0.3333333333333333703, 0.3219752754296894559, 0.3333333333333333703, 0.3219752754296894559, 0.3333333333333333703, 0.3219752754296894559, 0.3333333333333333703, 0.3219752754296894559, 0.3333333333333333703, 0.3219752754296894559, 0.3333333333333333703, 0.3219752754296894559, 0.3333333333333333703, 0.3219752754296894559, 0.3333333333333333703, 0.3219752754296894559, 0.3333333333333333703, 0.3219752754296894559, 0.3333333333333333703, 0.3219752754296894559, 0.3333333333333333703, 0.3219752754296894559, 0.3333333333333333703, 0.3219752754296894559, 0.3333333333333333703, 0.3219752754296894559, 0.3333333333333333703, 0.3219752754296894559, 0.3333333333333333703, 0.3219752754296894559, 0.3333333333333333703, 0.3219752754296894559, 0.3333333333333333703, 0.3219752754296894559, 0.3333333333333333703, 0.3219752754296894559, 0.3333333333333333703, 0.3219752754296894559, 0.3333333333333333703, 0.3219752754296894559, 0.3333333333333333703, 0.3219752754296894559, 0.3333333333333333703, 0.3219752754296894559, 0.3333333333333333703, 0.3219752754296894559, 0.3333333333333333703, 0.3219752754296894559, 0.3333333333333333703, 0.3219752754296894559, 0.3333333333333333703, 0.3219752754296894559, 0.3333333333333333703, 0.3219752754296894559, 0.3333333333333333703, 0.3219752754296894559, 0.3333333333333333703, 0.3219752754296894559, 0.3333333333333333703, 0.3219752754296894559, 0.3333333333333333703, 0.3219752754296894559, 0.3333333333333333703, 0.3219752754296894559, 0.3333333333333333703, 0.3219752754296894559, 0.3333333333333333703, 0.3219752754296894559, 0.3333333333333333703, 0.3219752754296894559, 0.3333333333333333703, 0.3219752754296894559, 0.3333333333333333703, 0.3219752754296894559, 0.3333333333333333703, 0.3219752754296894559, 0.3333333333333333703, 0.3219752754296894559, 0.3333333333333333703, 0.3219752754296894559, 0.3333333333333333703, 0.3219752754296894559, 0.3333333333333333703, 0.3219752754296894559, 0.3333333333333333703, 0.3219752754296894559, 0.3333333333333333703, 0.3219752754296894559, 0.3333333333333333703, 0.3219752754296894559, 0.3333333333333333703, 0.3219752754296894559, 0.3333333333333333703, 0.3219752754296894559, 0.3333333333333333703, 0.3219752754296894559, 0.3333333333333333703, 0.3219752754296894559, 0.3333333333333333703, 0.3219752754296894559, 0.3333333333333333703, 0.3219752754296894559, 0.3333333333333333703, 0.3219752754296894559, 0.3333333333333333703, 0.3219752754296894559, 0.3333333333333333703, 0.3219752754296894559, 0.3333333333333333703, 0.3219752754296894559, 0.3333333333333333703, 0.3219752754296894559, 0.3333333333333333703, 0.3219752754296894559, 0.3333333333333333703, 0.3219752754296894559, 0.3333333333333333703, 0.3219752754296894559, 0.3333333333333333703, 0.3219752754296894559, 0.3333333333333333703, 0.3219752754296894559, 0.3333333333333333703, 0.3219752754296894559, 0.3333333333333333703, 0.3219752754296894559, 0.3333333333333333703, 0.3219752754296894559, 0.3333333333333333703, 0.3219752754296894559, 0.3333333333333333703, 0.3219752754296894559, 0.3333333333333333703, 0.3219752754296894559, 0.3333333333333333703, 0.3219752754296894559, 0.3333333333333333703, 0.3219752754296894559, 0.3333333333333333703, 0.3219752754296894559, 0.3333333333333333703, 0.3219752754296894559, 0.3333333333333333703, 0.3219752754296894559, 0.3333333333333333703, 0.3219752754296894559, 0.3333333333333333703, 0.3219752754296894559, 0.3333333333333333703, 0.3219752754296894559, 0.3333333333333333703, 0.3219752754296894559, 0.3333333333333333703, 0.3219752754296894559, 0.3333333333333333703, 0.3219752754296894559, 0.3333333333333333703, 0.3219752754296894559, 0.3333333333333333703, 0.3219752754296894559, 0.3333333333333333703, 0.3219752754296894559, 0.3333333333333333703, 0.3219752754296894559, 0.3333333333333333703, 0.3219752754296894559, 0.3333333333333333703, 0.3219752754296894559, 0.3333333333333333703, 0.3219752754296894559, 0.3333333333333333703, 0.3219752754296894559, 0.3333333333333333703, 0.3219752754296894559, 0.3333333333333333703, 0.3219752754296894559, 0.3333333333333333703, 0.3219752754296894559, 0.3333333333333333703, 0.3219752754296894559, 0.3333333333333333703, 0.3219752754296894559, 0.3333333333333333703, 0.3219752754296894559, 0.3333333333333333703, 0.3219752754296894559, 0.3333333333333333703, 0.3219752754296894559, 0.3333333333333333703, 0.3219752754296894559, 0.3333333333333333703, 0.3219752754296894559, 0.3333333333333333703, 0.3219752754296894559, 0.3333333333333333703, 0.3219752754296894559, 0.3333333333333333703, 0.3219752754296894559, 0.3333333333333333703, 0.3219752754296894559, 0.3333333333333333703, 0.3219752754296894559, 0.3333333333333333703, 0.3219752754296894559, 0.3333333333333333703, 0.3219752754296894559, 0.3333333333333333703, 0.3219752754296894559, 0.3333333333333333703, 0.3219752754296894559, 0.3333333333333333703, 0.3219752754296894559, 0.3333333333333333703, 0.3219752754296894559, 0.3333333333333333703, 0.3219752754296894559, 0.3333333333333333703, 0.3219752754296894559, 0.3333333333333333703, 0.3219752754296894559, 0.3333333333333333703, 0.3219752754296894559, 0.3333333333333333703, 0.3219752754296894559, 0.3333333333333333703, 0.3219752754296894559, 0.3333333333333333703, 0.3219752754296894559, 0.3333333333333333703, 0.3219752754296894559, 0.3333333333333333703, 0.3219752754296894559, 0.3333333333333333703, 0.3219752754296894559, 0.3333333333333333703, 0.3219752754296894559, 0.3333333333333333703, 0.3219752754296894559, 0.3333333333333333703, 0.3219752754296894559, 0.3333333333333333703, 0.3219752754296894559, 0.3333333333333333703),
 ( 0.3333333333333333703, 0.3219752754296894559, 0.3333333333333333703, 0.3219752754296894559, 0.3333333333333333703, 0.3219752754296894559, 0.3333333333333333703, 0.3219752754296894559, 0.3333333333333333703, 0.3219752754296894559, 0.3333333333333333703, 0.3219752754296894559, 0.3333333333333333703, 0.3219752754296894559, 0.3333333333333333703, 0.3219752754296894559, 0.3333333333333333703, 0.3219752754296894559, 0.3333333333333333703, 0.3219752754296894559, 0.3333333333333333703, 0.3219752754296894559, 0.3333333333333333703, 0.3219752754296894559, 0.3333333333333333703, 0.3219752754296894559, 0.3333333333333333703, 0.3219752754296894559, 0.3333333333333333703, 0.3219752754296894559, 0.3333333333333333703, 0.3219752754296894559, 0.3333333333333333703, 0.3219752754296894559, 0.3333333333333333703, 0.3219752754296894559, 0.3333333333333333703, 0.3219752754296894559, 0.3333333333333333703, 0.3219752754296894559, 0.3333333333333333703, 0.3219752754296894559, 0.3333333333333333703, 0.3219752754296894559, 0.3333333333333333703, 0.3219752754296894559, 0.3333333333333333703, 0.3219752754296894559, 0.3333333333333333703, 0.3219752754296894559, 0.3333333333333333703, 0.3219752754296894559, 0.3333333333333333703, 0.3219752754296894559, 0.3333333333333333703, 0.3219752754296894559, 0.3333333333333333703, 0.3219752754296894559, 0.3333333333333333703, 0.3219752754296894559, 0.3333333333333333703, 0.3219752754296894559, 0.3333333333333333703, 0.3219752754296894559, 0.3333333333333333703, 0.3219752754296894559, 0.3333333333333333703, 0.3219752754296894559, 0.3333333333333333703, 0.3219752754296894559, 0.3333333333333333703, 0.3219752754296894559, 0.3333333333333333703, 0.3219752754296894559, 0.3333333333333333703, 0.3219752754296894559, 0.3333333333333333703, 0.3219752754296894559, 0.3333333333333333703, 0.3219752754296894559, 0.3333333333333333703, 0.3219752754296894559, 0.3333333333333333703, 0.3219752754296894559, 0.3333333333333333703, 0.3219752754296894559, 0.3333333333333333703, 0.3219752754296894559, 0.3333333333333333703, 0.3219752754296894559, 0.3333333333333333703, 0.3219752754296894559, 0.3333333333333333703, 0.3219752754296894559, 0.3333333333333333703, 0.3219752754296894559, 0.3333333333333333703, 0.3219752754296894559, 0.3333333333333333703, 0.3219752754296894559, 0.3333333333333333703, 0.3219752754296894559, 0.3333333333333333703, 0.3219752754296894559, 0.3333333333333333703, 0.3219752754296894559, 0.3333333333333333703, 0.3219752754296894559, 0.3333333333333333703, 0.3219752754296894559, 0.3333333333333333703, 0.3219752754296894559, 0.3333333333333333703, 0.3219752754296894559, 0.3333333333333333703, 0.3219752754296894559, 0.3333333333333333703, 0.3219752754296894559, 0.3333333333333333703, 0.3219752754296894559, 0.3333333333333333703, 0.3219752754296894559, 0.3333333333333333703, 0.3219752754296894559, 0.3333333333333333703, 0.3219752754296894559, 0.3333333333333333703, 0.3219752754296894559, 0.3333333333333333703, 0.3219752754296894559, 0.3333333333333333703, 0.3219752754296894559, 0.3333333333333333703, 0.3219752754296894559, 0.3333333333333333703, 0.3219752754296894559, 0.3333333333333333703, 0.3219752754296894559, 0.3333333333333333703, 0.3219752754296894559, 0.3333333333333333703, 0.3219752754296894559, 0.3333333333333333703, 0.3219752754296894559, 0.3333333333333333703, 0.3219752754296894559, 0.3333333333333333703, 0.3219752754296894559, 0.3333333333333333703, 0.3219752754296894559, 0.3333333333333333703, 0.3219752754296894559, 0.3333333333333333703, 0.3219752754296894559, 0.3333333333333333703, 0.3219752754296894559, 0.3333333333333333703, 0.3219752754296894559, 0.3333333333333333703, 0.3219752754296894559, 0.3333333333333333703, 0.3219752754296894559, 0.3333333333333333703, 0.3219752754296894559, 0.3333333333333333703, 0.3219752754296894559, 0.3333333333333333703, 0.3219752754296894559, 0.3333333333333333703, 0.3219752754296894559, 0.3333333333333333703, 0.3219752754296894559, 0.3333333333333333703, 0.3219752754296894559, 0.3333333333333333703, 0.3219752754296894559, 0.3333333333333333703, 0.3219752754296894559, 0.3333333333333333703, 0.3219752754296894559, 0.3333333333333333703, 0.3219752754296894559, 0.3333333333333333703, 0.3219752754296894559, 0.3333333333333333703, 0.3219752754296894559, 0.3333333333333333703, 0.3219752754296894559, 0.3333333333333333703, 0.3219752754296894559, 0.3333333333333333703, 0.3219752754296894559, 0.3333333333333333703, 0.3219752754296894559, 0.3333333333333333703, 0.3219752754296894559, 0.3333333333333333703, 0.3219752754296894559, 0.3333333333333333703, 0.3219752754296894559, 0.3333333333333333703, 0.3219752754296894559, 0.3333333333333333703, 0.3219752754296894559, 0.3333333333333333703, 0.3219752754296894559, 0.3333333333333333703, 0.3219752754296894559, 0.3333333333333333703, 0.3219752754296894559, 0.3333333333333333703, 0.3219752754296894559, 0.3333333333333333703, 0.3219752754296894559, 0.3333333333333333703, 0.3219752754296894559, 0.3333333333333333703, 0.3219752754296894559, 0.3333333333333333703, 0.3219752754296894559, 0.3333333333333333703, 0.3219752754296894559, 0.3333333333333333703, 0.3219752754296894559, 0.3333333333333333703, 0.3219752754296894559, 0.3333333333333333703, 0.3219752754296894559, 0.3333333333333333703, 0.3219752754296894559, 0.3333333333333333703, 0.3219752754296894559, 0.3333333333333333703, 0.3219752754296894559, 0.3333333333333333703, 0.3219752754296894559, 0.3333333333333333703, 0.3219752754296894559, 0.3333333333333333703, 0.3219752754296894559, 0.3333333333333333703, 0.3219752754296894559, 0.3333333333333333703, 0.3219752754296894559, 0.3333333333333333703, 0.3219752754296894559, 0.3333333333333333703, 0.3219752754296894559, 0.3333333333333333703, 0.3219752754296894559, 0.3333333333333333703, 0.3219752754296894559, 0.3333333333333333703, 0.3219752754296894559, 0.3333333333333333703, 0.3219752754296894559, 0.3333333333333333703, 0.3219752754296894559, 0.3333333333333333703, 0.3219752754296894559, 0.3333333333333333703, 0.3219752754296894559, 0.3333333333333333703, 0.3219752754296894559, 0.3333333333333333703, 0.3219752754296894559, 0.3333333333333333703, 0.3219752754296894559, 0.3333333333333333703, 0.3219752754296894559, 0.3333333333333333703, 0.3219752754296894559, 0.3333333333333333703, 0.3219752754296894559, 0.3333333333333333703, 0.3219752754296894559, 0.3333333333333333703, 0.3219752754296894559, 0.3333333333333333703, 0.3219752754296894559, 0.3333333333333333703, 0.3219752754296894559, 0.3333333333333333703, 0.3219752754296894559, 0.3333333333333333703, 0.3219752754296894559, 0.3333333333333333703, 0.3219752754296894559, 0.3333333333333333703, 0.3219752754296894559, 0.3333333333333333703, 0.3219752754296894559, 0.3333333333333333703, 0.3219752754296894559, 0.3333333333333333703, 0.3219752754296894559, 0.3333333333333333703, 0.3219752754296894559, 0.3333333333333333703, 0.3219752754296894559, 0.3333333333333333703, 0.3219752754296894559, 0.3333333333333333703, 0.3219752754296894559, 0.3333333333333333703, 0.3219752754296894559, 0.3333333333333333703, 0.3219752754296894559, 0.3333333333333333703, 0.3219752754296894559, 0.3333333333333333703, 0.3219752754296894559, 0.3333333333333333703, 0.3219752754296894559, 0.3333333333333333703, 0.3219752754296894559, 0.3333333333333333703, 0.3219752754296894559, 0.3333333333333333703, 0.3219752754296894559, 0.3333333333333333703, 0.3219752754296894559, 0.3333333333333333703, 0.3219752754296894559, 0.3333333333333333703, 0.3219752754296894559, 0.3333333333333333703, 0.3219752754296894559, 0.3333333333333333703, 0.3219752754296894559, 0.3333333333333333703, 0.3219752754296894559, 0.3333333333333333703, 0.3219752754296894559, 0.3333333333333333703, 0.3219752754296894559, 0.3333333333333333703, 0.3219752754296894559, 0.3333333333333333703, 0.3219752754296894559, 0.3333333333333333703, 0.3219752754296894559, 0.3333333333333333703, 0.3219752754296894559, 0.3333333333333333703, 0.3219752754296894559, 0.3333333333333333703, 0.3219752754296894559, 0.3333333333333333703, 0.3219752754296894559, 0.3333333333333333703, 0.3219752754296894559, 0.3333333333333333703, 0.3219752754296894559, 0.3333333333333333703, 0.3219752754296894559, 0.3333333333333333703, 0.3219752754296894559, 0.3333333333333333703, 0.3219752754296894559, 0.3333333333333333703, 0.3219752754296894559, 0.3333333333333333703, 0.3219752754296894559, 0.3333333333333333703, 0.3219752754296894559, 0.3333333333333333703, 0.3219752754296894559, 0.3333333333333333703, 0.3219752754296894559, 0.3333333333333333703, 0.3219752754296894559, 0.3333333333333333703, 0.3219752754296894559, 0.3333333333333333703, 0.3219752754296894559, 0.3333333333333333703, 0.3219752754296894559, 0.3333333333333333703, 0.3219752754296894559, 0.3333333333333333703, 0.3219752754296894559, 0.3333333333333333703, 0.3219752754296894559, 0.3333333333333333703, 0.3219752754296894559, 0.3333333333333333703, 0.3219752754296894559, 0.3333333333333333703, 0.3219752754296894559, 0.3333333333333333703, 0.3219752754296894559, 0.3333333333333333703, 0.3219752754296894559, 0.3333333333333333703, 0.3219752754296894559, 0.3333333333333333703, 0.3219752754296894559, 0.3333333333333333703, 0.3219752754296894559, 0.3333333333333333703, 0.3219752754296894559, 0.3333333333333333703, 0.3219752754296894559, 0.3333333333333333703, 0.3219752754296894559, 0.3333333333333333703, 0.3219752754296894559, 0.3333333333333333703, 0.3219752754296894559, 0.3333333333333333703, 0.3219752754296894559, 0.3333333333333333703, 0.3219752754296894559, 0.3333333333333333703, 0.3219752754296894559, 0.3333333333333333703, 0.3219752754296894559, 0.3333333333333333703, 0.3219752754296894559, 0.3333333333333333703, 0.3219752754296894559, 0.3333333333333333703, 0.3219752754296894559, 0.3333333333333333703, 0.3219752754296894559, 0.3333333333333333703, 0.3219752754296894559, 0.3333333333333333703, 0.3219752754296894559, 0.3333333333333333703, 0.3219752754296894559, 0.3333333333333333703, 0.3219752754296894559, 0.3333333333333333703, 0.3219752754296894559, 0.3333333333333333703, 0.3219752754296894559, 0.3333333333333333703, 0.3219752754296894559, 0.3333333333333333703, 0.3219752754296894559, 0.3333333333333333703, 0.3219752754296894559, 0.3333333333333333703, 0.3219752754296894559, 0.3333333333333333703, 0.3219752754296894559, 0.3333333333333333703, 0.3219752754296894559, 0.3333333333333333703, 0.3219752754296894559, 0.3333333333333333703, 0.3219752754296894559, 0.3333333333333333703, 0.3219752754296894559, 0.3333333333333333703),
 ( 1.000000000000000000, 0.9659258262890683122, 1.000000000000000000, 0.9659258262890683122, 1.000000000000000000, 0.9659258262890683122, 1.000000000000000000, 0.9659258262890683122, 1.000000000000000000, 0.9659258262890683122, 1.000000000000000000, 0.9659258262890683122, 1.000000000000000000, 0.9659258262890683122, 1.000000000000000000, 0.9659258262890683122, 1.000000000000000000, 0.9659258262890683122, 1.000000000000000000, 0.9659258262890683122, 1.000000000000000000, 0.9659258262890683122, 1.000000000000000000, 0.9659258262890683122, 1.000000000000000000, 0.9659258262890683122, 1.000000000000000000, 0.9659258262890683122, 1.000000000000000000, 0.9659258262890683122, 1.000000000000000000, 0.9659258262890683122, 1.000000000000000000, 0.9659258262890683122, 1.000000000000000000, 0.9659258262890683122, 1.000000000000000000, 0.9659258262890683122, 1.000000000000000000, 0.9659258262890683122, 1.000000000000000000, 0.9659258262890683122, 1.000000000000000000, 0.9659258262890683122, 1.000000000000000000, 0.9659258262890683122, 1.000000000000000000, 0.9659258262890683122, 1.000000000000000000, 0.9659258262890683122, 1.000000000000000000, 0.9659258262890683122, 1.000000000000000000, 0.9659258262890683122, 1.000000000000000000, 0.9659258262890683122, 1.000000000000000000, 0.9659258262890683122, 1.000000000000000000, 0.9659258262890683122, 1.000000000000000000, 0.9659258262890683122, 1.000000000000000000, 0.9659258262890683122, 1.000000000000000000, 0.9659258262890683122, 1.000000000000000000, 0.9659258262890683122, 1.000000000000000000, 0.9659258262890683122, 1.000000000000000000, 0.9659258262890683122, 1.000000000000000000, 0.9659258262890683122, 1.000000000000000000, 0.9659258262890683122, 1.000000000000000000, 0.9659258262890683122, 1.000000000000000000, 0.9659258262890683122, 1.000000000000000000, 0.9659258262890683122, 1.000000000000000000, 0.9659258262890683122, 1.000000000000000000, 0.9659258262890683122, 1.000000000000000000, 0.9659258262890683122, 1.000000000000000000, 0.9659258262890683122, 1.000000000000000000, 0.9659258262890683122, 1.000000000000000000, 0.9659258262890683122, 1.000000000000000000, 0.9659258262890683122, 1.000000000000000000, 0.9659258262890683122, 1.000000000000000000, 0.9659258262890683122, 1.000000000000000000, 0.9659258262890683122, 1.000000000000000000, 0.9659258262890683122, 1.000000000000000000, 0.9659258262890683122, 1.000000000000000000, 0.9659258262890683122, 1.000000000000000000, 0.9659258262890683122, 1.000000000000000000, 0.9659258262890683122, 1.000000000000000000, 0.9659258262890683122, 1.000000000000000000, 0.9659258262890683122, 1.000000000000000000, 0.9659258262890683122, 1.000000000000000000, 0.9659258262890683122, 1.000000000000000000, 0.9659258262890683122, 1.000000000000000000, 0.9659258262890683122, 1.000000000000000000, 0.9659258262890683122, 1.000000000000000000, 0.9659258262890683122, 1.000000000000000000, 0.9659258262890683122, 1.000000000000000000, 0.9659258262890683122, 1.000000000000000000, 0.9659258262890683122, 1.000000000000000000, 0.9659258262890683122, 1.000000000000000000, 0.9659258262890683122, 1.000000000000000000, 0.9659258262890683122, 1.000000000000000000, 0.9659258262890683122, 1.000000000000000000, 0.9659258262890683122, 1.000000000000000000, 0.9659258262890683122, 1.000000000000000000, 0.9659258262890683122, 1.000000000000000000, 0.9659258262890683122, 1.000000000000000000, 0.9659258262890683122, 1.000000000000000000, 0.9659258262890683122, 1.000000000000000000, 0.9659258262890683122, 1.000000000000000000, 0.9659258262890683122, 1.000000000000000000, 0.9659258262890683122, 1.000000000000000000, 0.9659258262890683122, 1.000000000000000000, 0.9659258262890683122, 1.000000000000000000, 0.9659258262890683122, 1.000000000000000000, 0.9659258262890683122, 1.000000000000000000, 0.9659258262890683122, 1.000000000000000000, 0.9659258262890683122, 1.000000000000000000, 0.9659258262890683122, 1.000000000000000000, 0.9659258262890683122, 1.000000000000000000, 0.9659258262890683122, 1.000000000000000000, 0.9659258262890683122, 1.000000000000000000, 0.9659258262890683122, 1.000000000000000000, 0.9659258262890683122, 1.000000000000000000, 0.9659258262890683122, 1.000000000000000000, 0.9659258262890683122, 1.000000000000000000, 0.9659258262890683122, 1.000000000000000000, 0.9659258262890683122, 1.000000000000000000, 0.9659258262890683122, 1.000000000000000000, 0.9659258262890683122, 1.000000000000000000, 0.9659258262890683122, 1.000000000000000000, 0.9659258262890683122, 1.000000000000000000, 0.9659258262890683122, 1.000000000000000000, 0.9659258262890683122, 1.000000000000000000, 0.9659258262890683122, 1.000000000000000000, 0.9659258262890683122, 1.000000000000000000, 0.9659258262890683122, 1.000000000000000000, 0.9659258262890683122, 1.000000000000000000, 0.9659258262890683122, 1.000000000000000000, 0.9659258262890683122, 1.000000000000000000, 0.9659258262890683122, 1.000000000000000000, 0.9659258262890683122, 1.000000000000000000, 0.9659258262890683122, 1.000000000000000000, 0.9659258262890683122, 1.000000000000000000, 0.9659258262890683122, 1.000000000000000000, 0.9659258262890683122, 1.000000000000000000, 0.9659258262890683122, 1.000000000000000000, 0.9659258262890683122, 1.000000000000000000, 0.9659258262890683122, 1.000000000000000000, 0.9659258262890683122, 1.000000000000000000, 0.9659258262890683122, 1.000000000000000000, 0.9659258262890683122, 1.000000000000000000, 0.9659258262890683122, 1.000000000000000000, 0.9659258262890683122, 1.000000000000000000, 0.9659258262890683122, 1.000000000000000000, 0.9659258262890683122, 1.000000000000000000, 0.9659258262890683122, 1.000000000000000000, 0.9659258262890683122, 1.000000000000000000, 0.9659258262890683122, 1.000000000000000000, 0.9659258262890683122, 1.000000000000000000, 0.9659258262890683122, 1.000000000000000000, 0.9659258262890683122, 1.000000000000000000, 0.9659258262890683122, 1.000000000000000000, 0.9659258262890683122, 1.000000000000000000, 0.9659258262890683122, 1.000000000000000000, 0.9659258262890683122, 1.000000000000000000, 0.9659258262890683122, 1.000000000000000000, 0.9659258262890683122, 1.000000000000000000, 0.9659258262890683122, 1.000000000000000000, 0.9659258262890683122, 1.000000000000000000, 0.9659258262890683122, 1.000000000000000000, 0.9659258262890683122, 1.000000000000000000, 0.9659258262890683122, 1.000000000000000000, 0.9659258262890683122, 1.000000000000000000, 0.9659258262890683122, 1.000000000000000000, 0.9659258262890683122, 1.000000000000000000, 0.9659258262890683122, 1.000000000000000000, 0.9659258262890683122, 1.000000000000000000, 0.9659258262890683122, 1.000000000000000000, 0.9659258262890683122, 1.000000000000000000, 0.9659258262890683122, 1.000000000000000000, 0.9659258262890683122, 1.000000000000000000, 0.9659258262890683122, 1.000000000000000000, 0.9659258262890683122, 1.000000000000000000, 0.9659258262890683122, 1.000000000000000000, 0.9659258262890683122, 1.000000000000000000, 0.9659258262890683122, 1.000000000000000000, 0.9659258262890683122, 1.000000000000000000, 0.9659258262890683122, 1.000000000000000000, 0.9659258262890683122, 1.000000000000000000, 0.9659258262890683122, 1.000000000000000000, 0.9659258262890683122, 1.000000000000000000, 0.9659258262890683122, 1.000000000000000000, 0.9659258262890683122, 1.000000000000000000, 0.9659258262890683122, 1.000000000000000000, 0.9659258262890683122, 1.000000000000000000, 0.9659258262890683122, 1.000000000000000000, 0.9659258262890683122, 1.000000000000000000, 0.9659258262890683122, 1.000000000000000000, 0.9659258262890683122, 1.000000000000000000, 0.9659258262890683122, 1.000000000000000000, 0.9659258262890683122, 1.000000000000000000, 0.9659258262890683122, 1.000000000000000000, 0.9659258262890683122, 1.000000000000000000, 0.9659258262890683122, 1.000000000000000000, 0.9659258262890683122, 1.000000000000000000, 0.9659258262890683122, 1.000000000000000000, 0.9659258262890683122, 1.000000000000000000, 0.9659258262890683122, 1.000000000000000000, 0.9659258262890683122, 1.000000000000000000, 0.9659258262890683122, 1.000000000000000000, 0.9659258262890683122, 1.000000000000000000, 0.9659258262890683122, 1.000000000000000000, 0.9659258262890683122, 1.000000000000000000, 0.9659258262890683122, 1.000000000000000000, 0.9659258262890683122, 1.000000000000000000, 0.9659258262890683122, 1.000000000000000000, 0.9659258262890683122, 1.000000000000000000, 0.9659258262890683122, 1.000000000000000000, 0.9659258262890683122, 1.000000000000000000, 0.9659258262890683122, 1.000000000000000000, 0.9659258262890683122, 1.000000000000000000, 0.9659258262890683122, 1.000000000000000000, 0.9659258262890683122, 1.000000000000000000, 0.9659258262890683122, 1.000000000000000000, 0.9659258262890683122, 1.000000000000000000, 0.9659258262890683122, 1.000000000000000000, 0.9659258262890683122, 1.000000000000000000, 0.9659258262890683122, 1.000000000000000000, 0.9659258262890683122, 1.000000000000000000, 0.9659258262890683122, 1.000000000000000000, 0.9659258262890683122, 1.000000000000000000, 0.9659258262890683122, 1.000000000000000000, 0.9659258262890683122, 1.000000000000000000, 0.9659258262890683122, 1.000000000000000000, 0.9659258262890683122, 1.000000000000000000, 0.9659258262890683122, 1.000000000000000000, 0.9659258262890683122, 1.000000000000000000, 0.9659258262890683122, 1.000000000000000000, 0.9659258262890683122, 1.000000000000000000, 0.9659258262890683122, 1.000000000000000000, 0.9659258262890683122, 1.000000000000000000, 0.9659258262890683122, 1.000000000000000000, 0.9659258262890683122, 1.000000000000000000, 0.9659258262890683122, 1.000000000000000000, 0.9659258262890683122, 1.000000000000000000, 0.9659258262890683122, 1.000000000000000000, 0.9659258262890683122, 1.000000000000000000, 0.9659258262890683122, 1.000000000000000000, 0.9659258262890683122, 1.000000000000000000, 0.9659258262890683122, 1.000000000000000000, 0.9659258262890683122, 1.000000000000000000, 0.9659258262890683122, 1.000000000000000000, 0.9659258262890683122, 1.000000000000000000, 0.9659258262890683122, 1.000000000000000000, 0.9659258262890683122, 1.000000000000000000, 0.9659258262890683122, 1.000000000000000000, 0.9659258262890683122, 1.000000000000000000, 0.9659258262890683122, 1.000000000000000000, 0.9659258262890683122, 1.000000000000000000) ) ) 
 REPRESENTATION_ITEM ( '' )  SURFACE ( )  );
#188117=CARTESIAN_POINT ( 'NONE',  ( 4.483927247898545687, 16.52544592524342804, 99.79057627198103830 ) ) ;
#188118=CARTESIAN_POINT ( 'NONE',  ( 19.02544592524343514, -5.153800228976328945, 103.5405762719809957 ) ) ;
#188119=CARTESIAN_POINT ( 'NONE',  ( -14.29746914071049879, 8.314922557960819915, 55.83224293864770260 ) ) ;
#188120=CARTESIAN_POINT ( 'NONE',  ( -16.53943276465976808, -0.05219959533934237506, 108.7510903946857042 ) ) ;
#188121=CARTESIAN_POINT ( 'NONE',  ( 19.02544592524343514, -5.153800228976328945, 53.54057627198102409 ) ) ;
#188122=CARTESIAN_POINT ( 'NONE',  ( -5.153800228976328057, -19.02544592524343514, 37.29057627198102409 ) ) ;
#188123=CARTESIAN_POINT ( 'NONE',  ( 18.62759615963271287, -10.81492255796078972, 43.33224293864769550 ) ) ;
#188124=CARTESIAN_POINT ( 'NONE',  ( -0.05219959533936034679, 19.03943276465977164, 27.50109039468566507 ) ) ;
#188126=CARTESIAN_POINT ( 'NONE',  ( 8.224510206698953496, -14.34966873604960469, 37.91557627198102409 ) ) ;
#188127=CARTESIAN_POINT ( 'NONE',  ( 10.72451020669871369, 18.67979575497193778, 42.08442372801901854 ) ) ;
#188129=CARTESIAN_POINT ( 'NONE',  ( -0.05219959533934338120, 16.53943276465976808, 52.50109039468567573 ) ) ;
#188130=CARTESIAN_POINT ( 'NONE',  ( -19.03943276465977164, -0.05219959533935918106, 58.75109039468566863 ) ) ;
#188132=CARTESIAN_POINT ( 'NONE',  ( 14.29746914071049879, -8.314922557960816363, 23.33224293864769194 ) ) ;
#188133=CARTESIAN_POINT ( 'NONE',  ( -19.34837522270364474, -5.499999999999852562, 75.86337684832575690 ) ) ;
#188134=CARTESIAN_POINT ( 'NONE',  ( 12.14591786802327356, -12.06949235617739191, 110.6260903946857042 ) ) ;
#188135=CARTESIAN_POINT ( 'NONE',  ( 0.05219959533909260263, 19.03943276465977164, 39.99890960531436690 ) ) ;
#188136=CARTESIAN_POINT ( 'NONE',  ( -9.474510206698964154, 16.51473224551069663, 65.41557627198102409 ) ) ;
#188137=CARTESIAN_POINT ( 'NONE',  ( 9.564922557960805705, 16.46253265017160317, 24.58224293864769194 ) ) ;
#188138=CARTESIAN_POINT ( 'NONE',  ( -21.55341960407619339, 5.719274019375674811, 38.54275706135234714 ) ) ;
#188139=CARTESIAN_POINT ( 'NONE',  ( 19.03943276465977164, -0.05219959533909143690, 43.74890960531435979 ) ) ;
#188140=CARTESIAN_POINT ( 'NONE',  ( 17.49999999999999645, 5.500000000000009770, 58.78230962303567253 ) ) ;
#188141=CARTESIAN_POINT ( 'NONE',  ( -16.46253265017160317, 9.564922557960807481, 50.83224293864770260 ) ) ;
#188142=CARTESIAN_POINT ( 'NONE',  ( 10.72451020669898902, -18.67979575497178502, 27.91557627198103830 ) ) ;
#188143=CARTESIAN_POINT ( 'NONE',  ( -0.05219959533937732626, 21.53943276465977519, 62.50109039468568284 ) ) ;
#188144=CARTESIAN_POINT ( 'NONE',  ( 12.14591786802309770, 12.06949235617756955, 99.37390960531436690 ) ) ;
#188145=CARTESIAN_POINT ( 'NONE',  ( 21.55341960407610458, 5.719274019375980345, 23.95724293864769550 ) ) ;
#188146=CARTESIAN_POINT ( 'NONE',  ( 16.53943276465976808, 0.05219959533934440121, 71.25109039468568994 ) ) ;
#188147=CARTESIAN_POINT ( 'NONE',  ( -5.823673210054431948, 21.52544592524334988, 92.70942372801901854 ) ) ;
#188148=CARTESIAN_POINT ( 'NONE',  ( -16.53943276465976808, -0.05219959533934237506, 48.75109039468568284 ) ) ;
#188149=CARTESIAN_POINT ( 'NONE',  ( 16.51473224551069308, 9.474510206698969483, 89.16557627198103830 ) ) ;
#188150=CARTESIAN_POINT ( 'NONE',  ( -8.314922557961024197, 14.29746914071037800, 37.91775706135235424 ) ) ;
#188151=CARTESIAN_POINT ( 'NONE',  ( -12.14591786802326823, 12.06949235617739902, 23.12609039468567573 ) ) ;
#188152=CARTESIAN_POINT ( 'NONE',  ( 16.52544592524335698, 4.483927247898782831, 96.45942372801901854 ) ) ;
#188153=CARTESIAN_POINT ( 'NONE',  ( 21.52544592524334988, 5.823673210054432836, 51.45942372801901854 ) ) ;
#188154=CARTESIAN_POINT ( 'NONE',  ( 13.97604488694548053, -13.89961937509957401, 100.6260903946856615 ) ) ;
#188155=CARTESIAN_POINT ( 'NONE',  ( 0.05219959533907565091, 21.53943276465977519, 114.9989096053143669 ) ) ;
#188156=CARTESIAN_POINT ( 'NONE',  ( -12.14591786802309592, -12.06949235617757132, 106.8739096053143811 ) ) ;
#188157=CARTESIAN_POINT ( 'NONE',  ( -13.97604488694547697, 13.89961937509957934, 103.1260903946856473 ) ) ;
#188158=CARTESIAN_POINT ( 'NONE',  ( 12.14591786802327356, -12.06949235617739191, 75.62609039468567573 ) ) ;
#188159=CARTESIAN_POINT ( 'NONE',  ( -17.50000000000000711, 5.622605283950838029, 43.68792689403891671 ) ) ;
#188160=CARTESIAN_POINT ( 'NONE',  ( 5.153800228976615827, -19.02544592524334988, 90.20942372801900433 ) ) ;
#188161=CARTESIAN_POINT ( 'NONE',  ( 0.05219959533910956823, 16.53943276465976808, 39.99890960531436690 ) ) ;
#188162=CARTESIAN_POINT ( 'NONE',  ( -8.314922557960811034, -14.29746914071050412, 42.08224293864769550 ) ) ;
#188163=CARTESIAN_POINT ( 'NONE',  ( -8.224510206698948167, 14.34966873604960824, 95.41557627198102409 ) ) ;
#188164=CARTESIAN_POINT ( 'NONE',  ( -13.89961937509957401, -13.97604488694547875, 29.37609039468565797 ) ) ;
#188165=CARTESIAN_POINT ( 'NONE',  ( -16.81555441253553695, 7.025013491695484724, 90.63685445334257906 ) ) ;
#188166=CARTESIAN_POINT ( 'NONE',  ( -21.52544592524334988, -5.823673210054445271, 33.95942372801901143 ) ) ;
#188167=CARTESIAN_POINT ( 'NONE',  ( -5.049401038297874678, -19.05341960407617918, 99.79275706135234714 ) ) ;
#188169=CARTESIAN_POINT ( 'NONE',  ( -19.05341960407611168, -5.049401038298163336, 86.45724293864769550 ) ) ;
#188170=CARTESIAN_POINT ( 'NONE',  ( 5.153800228976335163, 19.02544592524342804, 94.79057627198103830 ) ) ;
#188171=CARTESIAN_POINT ( 'NONE',  ( -5.823673210054116645, -21.52544592524344225, 52.29057627198102409 ) ) ;
#188172=CARTESIAN_POINT ( 'NONE',  ( -0.05219959533910754901, -16.53943276465976808, 92.49890960531436690 ) ) ;
#188173=CARTESIAN_POINT ( 'NONE',  ( 19.03943276465977164, -0.05219959533909143690, 73.74890960531435269 ) ) ;
#188174=CARTESIAN_POINT ( 'NONE',  ( -16.46253265017160317, 9.564922557960807481, 30.83224293864769550 ) ) ;
#188175=CARTESIAN_POINT ( 'NONE',  ( -18.67979575497193778, 10.72451020669871902, 38.33442372801900433 ) ) ;
#188176=CARTESIAN_POINT ( 'NONE',  ( -21.52544592524334988, -5.823673210054445271, 68.95942372801901854 ) ) ;
#188178=CARTESIAN_POINT ( 'NONE',  ( 12.06949235617739724, 12.14591786802326823, 86.87609039468568994 ) ) ;
#188179=CARTESIAN_POINT ( 'NONE',  ( 21.55341960407619695, -5.719274019375665929, 36.04275706135234714 ) ) ;
#188180=CARTESIAN_POINT ( 'NONE',  ( -10.81492255796105439, 18.62759615963255655, 32.91775706135234714 ) ) ;
#188181=CARTESIAN_POINT ( 'NONE',  ( 19.05341960407617918, -5.049401038297876454, 51.04275706135231871 ) ) ;
#188182=CARTESIAN_POINT ( 'NONE',  ( -9.564922557960796823, -16.46253265017161027, 77.08224293864769550 ) ) ;
#188183=CARTESIAN_POINT ( 'NONE',  ( 10.81492255796106328, -18.62759615963255655, 80.41775706135234714 ) ) ;
#188184=CARTESIAN_POINT ( 'NONE',  ( 21.53943276465977519, -0.05219959533907433946, 78.74890960531436690 ) ) ;
#188185=CARTESIAN_POINT ( 'NONE',  ( 4.379528057220339221, -16.55341960407611168, 47.70724293864770260 ) ) ;
#188186=CARTESIAN_POINT ( 'NONE',  ( -0.05219959533937732626, 21.53943276465977519, 107.5010903946856899 ) ) ;
#188187=CARTESIAN_POINT ( 'NONE',  ( -19.02544592524334988, -5.153800228976617603, 28.95942372801900433 ) ) ;
#188188=CARTESIAN_POINT ( 'NONE',  ( -4.379528057220328563, 16.55341960407611168, 70.20724293864769550 ) ) ;
#188189=CARTESIAN_POINT ( 'NONE',  ( -4.483927247898539470, -16.52544592524342804, 112.2905762719810241 ) ) ;
#188190=CARTESIAN_POINT ( 'NONE',  ( 9.564922557961047289, -16.46253265017146816, 70.41775706135233293 ) ) ;
#188191=CARTESIAN_POINT ( 'NONE',  ( -16.52544592524342804, 4.483927247898546575, 36.04057627198102409 ) ) ;
#188192=CARTESIAN_POINT ( 'NONE',  ( -0.05219959533937732626, 21.53943276465977519, 77.50109039468567573 ) ) ;
#188193=CARTESIAN_POINT ( 'NONE',  ( -19.05341960407611168, -5.049401038298163336, 81.45724293864769550 ) ) ;
#188194=CARTESIAN_POINT ( 'NONE',  ( 9.474510206698729675, 16.51473224551082808, 42.08442372801900433 ) ) ;
#188195=CARTESIAN_POINT ( 'NONE',  ( 15.80617190586746368, 15.72974639402197994, 64.37390960531435269 ) ) ;
#188196=CARTESIAN_POINT ( 'NONE',  ( 0.05219959533907565091, 21.53943276465977519, 114.9989096053143669 ) ) ;
#188197=CARTESIAN_POINT ( 'NONE',  ( -5.049401038297874678, -19.05341960407617918, 109.7927570613523187 ) ) ;
#188198=CARTESIAN_POINT ( 'NONE',  ( 14.29746914071037800, 8.314922557961029526, 76.66775706135234714 ) ) ;
#188199=CARTESIAN_POINT ( 'NONE',  ( 16.18388926212241685, 7.379444403734408908, 62.93953151366150678 ) ) ;
#188200=CARTESIAN_POINT ( 'NONE',  ( 15.72974639402199770, -15.80617190586745480, 113.1239096053143953 ) ) ;
#188201=CARTESIAN_POINT ( 'NONE',  ( 16.52544592524342804, -4.483927247898539470, 98.54057627198105251 ) ) ;
#188203=CARTESIAN_POINT ( 'NONE',  ( 4.483927247898790824, -16.52544592524335698, 40.20942372801901854 ) ) ;
#188204=CARTESIAN_POINT ( 'NONE',  ( 18.62759615963271287, -10.81492255796078972, 63.33224293864770260 ) ) ;
#188205=CARTESIAN_POINT ( 'NONE',  ( 14.34966873604972726, -8.224510206698740333, 100.8344237280190185 ) ) ;
#188206=CARTESIAN_POINT ( 'NONE',  ( -19.03943276465977164, 0.05219959533909376836, 36.24890960531436690 ) ) ;
#188207=CARTESIAN_POINT ( 'NONE',  ( 12.14591786802327356, -12.06949235617739191, 70.62609039468567573 ) ) ;
#188208=CARTESIAN_POINT ( 'NONE',  ( 13.89961937509957401, 13.97604488694547697, 66.87609039468567573 ) ) ;
#188209=CARTESIAN_POINT ( 'NONE',  ( 21.53943276465977519, 0.05219959533937863772, 46.25109039468567573 ) ) ;
#188210=CARTESIAN_POINT ( 'NONE',  ( -21.53943276465977519, 0.05219959533907696930, 56.24890960531436690 ) ) ;
#188211=CARTESIAN_POINT ( 'NONE',  ( -16.52544592524335698, -4.483927247898792601, 98.95942372801903275 ) ) ;
#188212=CARTESIAN_POINT ( 'NONE',  ( -21.52544592524334988, -5.823673210054445271, 83.95942372801900433 ) ) ;
#188213=CARTESIAN_POINT ( 'NONE',  ( -5.823673210054116645, -21.52544592524344225, 47.29057627198103120 ) ) ;
#188214=CARTESIAN_POINT ( 'NONE',  ( -15.80617190586745835, -15.72974639402198527, 31.87390960531435979 ) ) ;
#188215=ORIENTED_EDGE ( 'NONE', *, *, #153559, .T. ) ;
#188216=CARTESIAN_POINT ( 'NONE',  ( 16.52544592524335698, 4.483927247898782831, 81.45942372801900433 ) ) ;
#188217=CARTESIAN_POINT ( 'NONE',  ( -10.81492255796078084, -18.62759615963271287, 42.08224293864769550 ) ) ;
#188219=CARTESIAN_POINT ( 'NONE',  ( 13.89961937509977652, -13.97604488694527269, 98.12390960531433848 ) ) ;
#188221=CARTESIAN_POINT ( 'NONE',  ( -9.474510206698964154, 16.51473224551069663, 30.41557627198102054 ) ) ;
#188222=CARTESIAN_POINT ( 'NONE',  ( 15.80617190586746368, 15.72974639402197994, 59.37390960531436690 ) ) ;
#188223=CARTESIAN_POINT ( 'NONE',  ( 4.379528057220092307, 16.55341960407617563, 97.29275706135234714 ) ) ;
#188224=CARTESIAN_POINT ( 'NONE',  ( -10.81492255796105439, 18.62759615963255655, 47.91775706135234714 ) ) ;
#188225=CARTESIAN_POINT ( 'NONE',  ( -13.97604488694547697, 13.89961937509957934, 108.1260903946856331 ) ) ;
#188226=CARTESIAN_POINT ( 'NONE',  ( -0.05219959533910754901, -16.53943276465976808, 97.49890960531436690 ) ) ;
#188227=CARTESIAN_POINT ( 'NONE',  ( -16.52544592524335698, -4.483927247898792601, 18.95942372801901143 ) ) ;
#188228=CARTESIAN_POINT ( 'NONE',  ( -0.05219959533909027116, -19.03943276465977164, 37.49890960531436690 ) ) ;
#188230=CARTESIAN_POINT ( 'NONE',  ( 9.564922557960805705, 16.46253265017160317, 94.58224293864769550 ) ) ;
#188231=CARTESIAN_POINT ( 'NONE',  ( 4.379528057220092307, 16.55341960407617563, 82.29275706135234714 ) ) ;
#188232=CARTESIAN_POINT ( 'NONE',  ( 15.80617190586769283, -15.72974639402175789, 100.6260903946857184 ) ) ;
#188233=CARTESIAN_POINT ( 'NONE',  ( 5.719274019375991003, -21.55341960407610458, 67.70724293864769550 ) ) ;
#188234=CARTESIAN_POINT ( 'NONE',  ( -16.52544592524335698, -4.483927247898792601, 88.95942372801901854 ) ) ;
#188235=CARTESIAN_POINT ( 'NONE',  ( -0.05219959533936034679, 19.03943276465977164, 77.50109039468566152 ) ) ;
#188236=CARTESIAN_POINT ( 'NONE',  ( 9.564922557960805705, 16.46253265017160317, 39.58224293864768839 ) ) ;
#188237=CARTESIAN_POINT ( 'NONE',  ( 13.97604488694527802, 13.89961937509977652, 84.37390960531433848 ) ) ;
#188238=CARTESIAN_POINT ( 'NONE',  ( 19.05341960407611168, 5.049401038298154454, 28.95724293864769550 ) ) ;
#188239=CARTESIAN_POINT ( 'NONE',  ( -19.02544592524334988, -5.153800228976617603, 73.95942372801900433 ) ) ;
#188241=CARTESIAN_POINT ( 'NONE',  ( 9.564922557960805705, 16.46253265017160317, 109.5822429386476955 ) ) ;
#188242=CARTESIAN_POINT ( 'NONE',  ( -0.05219959533910754901, -16.53943276465976808, 62.49890960531436690 ) ) ;
#188243=CARTESIAN_POINT ( 'NONE',  ( 21.52544592524344225, -5.823673210054117533, 58.54057627198103120 ) ) ;
#188246=CARTESIAN_POINT ( 'NONE',  ( 19.02544592524334988, 5.153800228976608722, 26.45942372801899722 ) ) ;
#188248=CARTESIAN_POINT ( 'NONE',  ( -13.89961937509977652, 13.97604488694528158, 65.62390960531436690 ) ) ;
#188249=CARTESIAN_POINT ( 'NONE',  ( 5.153800228976335163, 19.02544592524342804, 74.79057627198103830 ) ) ;
#188250=CARTESIAN_POINT ( 'NONE',  ( -8.224510206698735004, -14.34966873604973081, 49.58442372801901143 ) ) ;
#188253=CARTESIAN_POINT ( 'NONE',  ( 4.379528057220092307, 16.55341960407617563, 72.29275706135236135 ) ) ;
#188254=DIRECTION ( 'NONE',  ( 0.000000000000000000, -0.000000000000000000, -1.000000000000000000 ) ) ;
#188255=CARTESIAN_POINT ( 'NONE',  ( 8.224510206698742110, 14.34966873604972548, 72.08442372801899012 ) ) ;
#188256=CARTESIAN_POINT ( 'NONE',  ( 4.483927247898790824, -16.52544592524335698, 35.20942372801901854 ) ) ;
#188257=CARTESIAN_POINT ( 'NONE',  ( -16.46253265017160317, 9.564922557960807481, 55.83224293864769550 ) ) ;
#188259=CARTESIAN_POINT ( 'NONE',  ( 21.53943276465977519, 0.05219959533937863772, 56.25109039468568284 ) ) ;
#188260=CARTESIAN_POINT ( 'NONE',  ( -16.46253265017146816, -9.564922557961047289, 64.16775706135233293 ) ) ;
#188261=CARTESIAN_POINT ( 'NONE',  ( 21.52544592524334988, 5.823673210054432836, 111.4594237280190328 ) ) ;
#188262=CARTESIAN_POINT ( 'NONE',  ( -19.05341960407611168, -5.049401038298163336, 36.45724293864766707 ) ) ;
#188263=CARTESIAN_POINT ( 'NONE',  ( 15.72974639402199770, -15.80617190586745480, 58.12390960531435979 ) ) ;
#188264=CARTESIAN_POINT ( 'NONE',  ( 19.05341960407611168, 5.049401038298154454, 108.9572429386477097 ) ) ;
#188265=CARTESIAN_POINT ( 'NONE',  ( -16.53943276465976808, 0.05219959533911058130, 101.2489096053143669 ) ) ;
#188266=CARTESIAN_POINT ( 'NONE',  ( -8.314922557961024197, 14.29746914071037800, 37.91775706135235424 ) ) ;
#188267=CARTESIAN_POINT ( 'NONE',  ( 8.314922557960818139, 14.29746914071049879, 24.58224293864768839 ) ) ;
#188270=CARTESIAN_POINT ( 'NONE',  ( -21.55341960407610458, -5.719274019375992779, 96.45724293864770971 ) ) ;
#188272=CARTESIAN_POINT ( 'NONE',  ( -16.53943276465976808, 0.05219959533911058130, 41.24890960531435269 ) ) ;
#188274=CARTESIAN_POINT ( 'NONE',  ( -9.474510206698720793, -16.51473224551083518, 89.58442372801900433 ) ) ;
#188275=CARTESIAN_POINT ( 'NONE',  ( 19.02544592524334988, 5.153800228976608722, 21.45942372801899012 ) ) ;
#188276=CARTESIAN_POINT ( 'NONE',  ( -14.29746914071049879, 8.314922557960819915, 25.83224293864769194 ) ) ;
#188277=CARTESIAN_POINT ( 'NONE',  ( 18.67979575497178502, 10.72451020669898547, 109.1655762719810383 ) ) ;
#188278=CARTESIAN_POINT ( 'NONE',  ( 5.719274019375991003, -21.55341960407610458, 52.70724293864769550 ) ) ;
#188279=CARTESIAN_POINT ( 'NONE',  ( 16.46253265017160672, -9.564922557960803928, 78.33224293864769550 ) ) ;
#188280=CARTESIAN_POINT ( 'NONE',  ( -0.05219959533910754901, -16.53943276465976808, 37.49890960531436690 ) ) ;
#188281=CARTESIAN_POINT ( 'NONE',  ( -19.03943276465977164, 0.05219959533909376836, 91.24890960531436690 ) ) ;
#188283=CARTESIAN_POINT ( 'NONE',  ( 5.153800228976335163, 19.02544592524342804, 79.79057627198102409 ) ) ;
#188284=CARTESIAN_POINT ( 'NONE',  ( -13.97604488694547697, 13.89961937509957934, 38.12609039468566152 ) ) ;
#188285=CARTESIAN_POINT ( 'NONE',  ( -5.823673210054116645, -21.52544592524344225, 77.29057627198102409 ) ) ;
#188286=CARTESIAN_POINT ( 'NONE',  ( -14.34966873604960291, -8.224510206698953496, 96.66557627198102409 ) ) ;
#188287=CARTESIAN_POINT ( 'NONE',  ( -5.823673210054431948, 21.52544592524334988, 42.70942372801901854 ) ) ;
#188289=CARTESIAN_POINT ( 'NONE',  ( 16.52544592524335698, 4.483927247898782831, 106.4594237280190328 ) ) ;
#188290=CARTESIAN_POINT ( 'NONE',  ( -19.02544592524342804, 5.153800228976336051, 36.04057627198100988 ) ) ;
#188291=CARTESIAN_POINT ( 'NONE',  ( -16.46253265017160317, 9.564922557960807481, 80.83224293864769550 ) ) ;
#188293=CARTESIAN_POINT ( 'NONE',  ( 13.89961937509977652, -13.97604488694527269, 33.12390960531434558 ) ) ;
#188294=CARTESIAN_POINT ( 'NONE',  ( 0.05219959533910956823, 16.53943276465976808, 49.99890960531437401 ) ) ;
#188295=CARTESIAN_POINT ( 'NONE',  ( 5.719274019375673035, 21.55341960407619339, 72.29275706135236135 ) ) ;
#188297=CARTESIAN_POINT ( 'NONE',  ( -14.29746914071037622, -8.314922557961029526, 74.16775706135231871 ) ) ;
#188298=CARTESIAN_POINT ( 'NONE',  ( -19.02544592524342804, 5.153800228976336051, 51.04057627198103120 ) ) ;
#188299=CARTESIAN_POINT ( 'NONE',  ( -19.03943276465977164, 0.05219959533909376836, 61.24890960531436690 ) ) ;
#188300=EDGE_LOOP ( 'NONE', ( #105928, #46009, #133624, #17992, #91194, #12423, #50758, #177274 ) ) ;
#188301=CARTESIAN_POINT ( 'NONE',  ( -0.05219959533937732626, 21.53943276465977519, 112.5010903946857042 ) ) ;
#188302=CARTESIAN_POINT ( 'NONE',  ( -12.06949235617739369, -12.14591786802326823, 79.37609039468567573 ) ) ;
#188303=CARTESIAN_POINT ( 'NONE',  ( -18.62759615963255300, -10.81492255796106328, 99.16775706135234714 ) ) ;
#188304=CARTESIAN_POINT ( 'NONE',  ( 16.46253265017160672, -9.564922557960803928, 58.33224293864769550 ) ) ;
#188305=CARTESIAN_POINT ( 'NONE',  ( 21.53943276465977519, -0.05219959533907433946, 28.74890960531435624 ) ) ;
#188306=CARTESIAN_POINT ( 'NONE',  ( 13.97604488694548053, -13.89961937509957401, 110.6260903946856615 ) ) ;
#188307=CARTESIAN_POINT ( 'NONE',  ( -21.53943276465977519, -0.05219959533937600094, 63.75109039468568284 ) ) ;
#188308=CARTESIAN_POINT ( 'NONE',  ( 16.55341960407618274, -4.379528057220086978, 46.04275706135234714 ) ) ;
#188309=CARTESIAN_POINT ( 'NONE',  ( 21.53943276465977519, -0.05219959533907433946, 103.7489096053143669 ) ) ;
#188310=CARTESIAN_POINT ( 'NONE',  ( -19.02544592524334988, -5.153800228976617603, 98.95942372801900433 ) ) ;
#188311=CARTESIAN_POINT ( 'NONE',  ( -16.51473224551069308, -9.474510206698971260, 76.66557627198103830 ) ) ;
#188312=CARTESIAN_POINT ( 'NONE',  ( -13.89961937509957401, -13.97604488694547875, 104.3760903946856757 ) ) ;
#188313=CARTESIAN_POINT ( 'NONE',  ( 0.05219959533934541429, -16.53943276465976808, 25.00109039468567218 ) ) ;
#188314=CARTESIAN_POINT ( 'NONE',  ( 12.14591786802309770, 12.06949235617756955, 59.37390960531436690 ) ) ;
#188315=CARTESIAN_POINT ( 'NONE',  ( -4.483927247898782831, 16.52544592524335698, 77.70942372801900433 ) ) ;
#188316=CARTESIAN_POINT ( 'NONE',  ( 5.719274019375991003, -21.55341960407610458, 112.7072429386476955 ) ) ;
#188317=CARTESIAN_POINT ( 'NONE',  ( 19.05341960407611168, 5.049401038298154454, 53.95724293864770260 ) ) ;
#188318=CARTESIAN_POINT ( 'NONE',  ( -13.89961937509977652, 13.97604488694528158, 65.62390960531436690 ) ) ;
#188319=CARTESIAN_POINT ( 'NONE',  ( 16.53943276465976808, 0.05219959533934440121, 66.25109039468567573 ) ) ;
#188322=CARTESIAN_POINT ( 'NONE',  ( 0.05219959533936267826, -19.03943276465977164, 20.00109039468567218 ) ) ;
#188323=CARTESIAN_POINT ( 'NONE',  ( 9.474510206698971260, -16.51473224551069308, 37.91557627198102409 ) ) ;
#188324=VERTEX_POINT ( 'NONE', #83768 ) ;
#188325=CARTESIAN_POINT ( 'NONE',  ( 19.05341960407617918, -5.049401038297876454, 106.0427570613523471 ) ) ;
#188326=CARTESIAN_POINT ( 'NONE',  ( -9.474510206698720793, -16.51473224551083518, 39.58442372801899722 ) ) ;
#188327=CARTESIAN_POINT ( 'NONE',  ( -12.14591786802326823, 12.06949235617739902, 23.12609039468567573 ) ) ;
#188328=CARTESIAN_POINT ( 'NONE',  ( 5.049401038298161559, -19.05341960407611168, 47.70724293864770260 ) ) ;
#188329=CARTESIAN_POINT ( 'NONE',  ( -9.474510206698964154, 16.51473224551069663, 65.41557627198102409 ) ) ;
#188330=CARTESIAN_POINT ( 'NONE',  ( 5.719274019375991003, -21.55341960407610458, 82.70724293864770971 ) ) ;
#188331=CARTESIAN_POINT ( 'NONE',  ( -5.049401038298153566, 19.05341960407611168, 110.2072429386476671 ) ) ;
#188333=CARTESIAN_POINT ( 'NONE',  ( -5.049401038298153566, 19.05341960407611168, 45.20724293864769550 ) ) ;
#188334=CARTESIAN_POINT ( 'NONE',  ( -17.97182807773872781, 5.499999999999960920, 93.53038844047289047 ) ) ;
#188335=CARTESIAN_POINT ( 'NONE',  ( -9.564922557961040184, 16.46253265017147172, 97.91775706135233293 ) ) ;
#188336=CARTESIAN_POINT ( 'NONE',  ( -8.314922557960811034, -14.29746914071050412, 72.08224293864769550 ) ) ;
#188337=CARTESIAN_POINT ( 'NONE',  ( 19.05341960407617918, -5.049401038297876454, 26.04275706135233293 ) ) ;
#188338=CARTESIAN_POINT ( 'NONE',  ( -8.224510206698948167, 14.34966873604960824, 65.41557627198102409 ) ) ;
#188339=CARTESIAN_POINT ( 'NONE',  ( -0.05219959533937732626, 21.53943276465977519, 87.50109039468568994 ) ) ;
#188340=CARTESIAN_POINT ( 'NONE',  ( -0.05219959533909027116, -19.03943276465977164, 32.49890960531435979 ) ) ;
#188341=CARTESIAN_POINT ( 'NONE',  ( 15.80617190586769283, -15.72974639402175789, 85.62609039468568994 ) ) ;
#188342=CARTESIAN_POINT ( 'NONE',  ( -16.53943276465976808, 0.05219959533911058130, 26.24890960531435624 ) ) ;
#188343=CARTESIAN_POINT ( 'NONE',  ( 15.72974639402176855, 15.80617190586768217, 76.87609039468567573 ) ) ;
#188344=CARTESIAN_POINT ( 'NONE',  ( -9.474510206698964154, 16.51473224551069663, 75.41557627198103830 ) ) ;
#188346=CARTESIAN_POINT ( 'NONE',  ( 21.52544592524334988, 5.823673210054432836, 41.45942372801901143 ) ) ;
#188347=CARTESIAN_POINT ( 'NONE',  ( 16.51473224551069308, 9.474510206698969483, 79.16557627198103830 ) ) ;
#188348=CARTESIAN_POINT ( 'NONE',  ( -12.06949235617756955, 12.14591786802309770, 100.6239096053143811 ) ) ;
#188349=CARTESIAN_POINT ( 'NONE',  ( -14.29746914071049879, 8.314922557960819915, 60.83224293864769550 ) ) ;
#188350=CARTESIAN_POINT ( 'NONE',  ( 21.53943276465977519, -0.05219959533907433946, 73.74890960531433848 ) ) ;
#188351=CARTESIAN_POINT ( 'NONE',  ( -19.03943276465977164, 0.05219959533909376836, 81.24890960531436690 ) ) ;
#188352=CARTESIAN_POINT ( 'NONE',  ( -0.05219959533907301413, -21.53943276465977519, 87.49890960531436690 ) ) ;
#188353=CARTESIAN_POINT ( 'NONE',  ( 5.153800228976615827, -19.02544592524334988, 80.20942372801901854 ) ) ;
#188354=CARTESIAN_POINT ( 'NONE',  ( -0.05219959533936034679, 19.03943276465977164, 27.50109039468566507 ) ) ;
#188355=CARTESIAN_POINT ( 'NONE',  ( 8.224510206698953496, -14.34966873604960469, 77.91557627198102409 ) ) ;
#188356=CARTESIAN_POINT ( 'NONE',  ( -10.72451020669898014, 18.67979575497178502, 50.41557627198103120 ) ) ;
#188358=CARTESIAN_POINT ( 'NONE',  ( 14.29746914071037800, 8.314922557961029526, 96.66775706135234714 ) ) ;
#188360=CARTESIAN_POINT ( 'NONE',  ( -9.474510206698720793, -16.51473224551083518, 104.5844237280190043 ) ) ;
#188362=CARTESIAN_POINT ( 'NONE',  ( -8.314922557960811034, -14.29746914071050412, 67.08224293864770971 ) ) ;
#188364=CARTESIAN_POINT ( 'NONE',  ( 5.049401038298161559, -19.05341960407611168, 67.70724293864769550 ) ) ;
#188365=CARTESIAN_POINT ( 'NONE',  ( -8.224510206698948167, 14.34966873604960824, 50.41557627198103120 ) ) ;
#188366=CARTESIAN_POINT ( 'NONE',  ( -9.474510206698964154, 16.51473224551069663, 95.41557627198102409 ) ) ;
#188367=CARTESIAN_POINT ( 'NONE',  ( -16.46253265017146816, -9.564922557961047289, 89.16775706135234714 ) ) ;
#188368=CARTESIAN_POINT ( 'NONE',  ( -5.049401038298153566, 19.05341960407611168, 65.20724293864765286 ) ) ;
#188369=CARTESIAN_POINT ( 'NONE',  ( 13.97604488694527802, 13.89961937509977652, 84.37390960531433848 ) ) ;
#188370=CARTESIAN_POINT ( 'NONE',  ( 5.153800228976335163, 19.02544592524342804, 89.79057627198102409 ) ) ;
#188371=CARTESIAN_POINT ( 'NONE',  ( 21.55341960407610458, 5.719274019375980345, 58.95724293864770971 ) ) ;
#188372=CARTESIAN_POINT ( 'NONE',  ( -8.314922557961024197, 14.29746914071037800, 52.91775706135235424 ) ) ;
#188373=CARTESIAN_POINT ( 'NONE',  ( -5.049401038297874678, -19.05341960407618274, 104.7927570613523471 ) ) ;
#188374=CARTESIAN_POINT ( 'NONE',  ( 9.474510206698971260, -16.51473224551069308, 67.91557627198102409 ) ) ;
#188375=CARTESIAN_POINT ( 'NONE',  ( 21.53943276465977519, -0.05219959533907433946, 63.74890960531435979 ) ) ;
#188376=CARTESIAN_POINT ( 'NONE',  ( 19.05341960407617918, -5.049401038297876454, 96.04275706135231871 ) ) ;
#188377=CARTESIAN_POINT ( 'NONE',  ( -4.379528057220328563, 16.55341960407611168, 25.20724293864769550 ) ) ;
#188378=CARTESIAN_POINT ( 'NONE',  ( 21.52544592524334988, 5.823673210054432836, 51.45942372801901854 ) ) ;
#188379=CARTESIAN_POINT ( 'NONE',  ( -5.153800228976607833, 19.02544592524334988, 42.70942372801901143 ) ) ;
#188380=CARTESIAN_POINT ( 'NONE',  ( -8.224510206698735004, -14.34966873604973081, 74.58442372801901854 ) ) ;
#188381=CARTESIAN_POINT ( 'NONE',  ( -14.29746914071037622, -8.314922557961029526, 99.16775706135234714 ) ) ;
#188383=CARTESIAN_POINT ( 'NONE',  ( 4.483927247898790824, -16.52544592524335698, 85.20942372801901854 ) ) ;
#188384=CARTESIAN_POINT ( 'NONE',  ( 16.53943276465976808, 0.05219959533934440121, 36.25109039468567573 ) ) ;
#188385=CARTESIAN_POINT ( 'NONE',  ( 16.51473224551069308, 9.474510206698969483, 44.16557627198103120 ) ) ;
#188386=CARTESIAN_POINT ( 'NONE',  ( -13.97604488694527625, -13.89961937509977652, 46.87390960531435979 ) ) ;
#188387=CARTESIAN_POINT ( 'NONE',  ( -9.474510206698964154, 16.51473224551069663, 55.41557627198103120 ) ) ;
#188388=CARTESIAN_POINT ( 'NONE',  ( 18.67979575497194134, -10.72451020669871369, 50.83442372801901143 ) ) ;
#188389=CARTESIAN_POINT ( 'NONE',  ( 14.34966873604972726, -8.224510206698740333, 50.83442372801901143 ) ) ;
#188390=CARTESIAN_POINT ( 'NONE',  ( 4.483927247898545687, 16.52544592524342804, 24.79057627198103120 ) ) ;
#188391=CARTESIAN_POINT ( 'NONE',  ( 13.89961937509977652, -13.97604488694527269, 28.12390960531435624 ) ) ;
#188392=CARTESIAN_POINT ( 'NONE',  ( 16.51473224551069308, 9.474510206698969483, 39.16557627198103120 ) ) ;
#188393=CARTESIAN_POINT ( 'NONE',  ( 4.483927247898790824, -16.52544592524335698, 25.20942372801901854 ) ) ;
#188394=CARTESIAN_POINT ( 'NONE',  ( -19.05341960407617563, 5.049401038297882671, 88.54275706135230450 ) ) ;
#188395=CARTESIAN_POINT ( 'NONE',  ( -4.379528057220328563, 16.55341960407611168, 90.20724293864770971 ) ) ;
#188396=CARTESIAN_POINT ( 'NONE',  ( 19.02544592524343514, -5.153800228976328945, 38.54057627198103120 ) ) ;
#188397=CARTESIAN_POINT ( 'NONE',  ( 16.46253265017146816, 9.564922557961045513, 71.66775706135233293 ) ) ;
#188398=CARTESIAN_POINT ( 'NONE',  ( 17.50000000000000000, 5.499999999999997335, 120.0000000000000142 ) ) ;
#188399=CARTESIAN_POINT ( 'NONE',  ( -21.53943276465977519, -0.05219959533937600094, 73.75109039468567573 ) ) ;
#188400=CARTESIAN_POINT ( 'NONE',  ( 8.314922557961029526, -14.29746914071037800, 50.41775706135235424 ) ) ;
#188402=CARTESIAN_POINT ( 'NONE',  ( -15.72974639402197994, 15.80617190586746368, 35.62390960531437401 ) ) ;
#188403=CARTESIAN_POINT ( 'NONE',  ( 12.06949235617739724, 12.14591786802326823, 26.87609039468567218 ) ) ;
#188404=CARTESIAN_POINT ( 'NONE',  ( -5.049401038298153566, 19.05341960407611168, 30.20724293864769194 ) ) ;
#188405=CARTESIAN_POINT ( 'NONE',  ( -19.03943276465977164, -0.05219959533935918106, 28.75109039468566507 ) ) ;
#188407=CARTESIAN_POINT ( 'NONE',  ( -16.51473224551069308, -9.474510206698971260, 36.66557627198102409 ) ) ;
#188409=CARTESIAN_POINT ( 'NONE',  ( -9.474510206698964154, 16.51473224551069663, 70.41557627198102409 ) ) ;
#188410=CARTESIAN_POINT ( 'NONE',  ( 17.49999999999999645, -3.189878218039153168, 112.3705143742875237 ) ) ;
#188411=CARTESIAN_POINT ( 'NONE',  ( 0.05219959533937995610, -21.53943276465977519, 110.0010903946856757 ) ) ;
#188412=CARTESIAN_POINT ( 'NONE',  ( -0.05219959533910754901, -16.53943276465976808, 37.49890960531436690 ) ) ;
#188413=CARTESIAN_POINT ( 'NONE',  ( 19.02544592524343514, -5.153800228976328945, 38.54057627198103120 ) ) ;
#188414=CARTESIAN_POINT ( 'NONE',  ( 5.153800228976335163, 19.02544592524342804, 94.79057627198103830 ) ) ;
#188415=CARTESIAN_POINT ( 'NONE',  ( 15.80617190586769283, -15.72974639402175789, 65.62609039468568994 ) ) ;
#188416=CARTESIAN_POINT ( 'NONE',  ( -9.564922557960796823, -16.46253265017161027, 47.08224293864769550 ) ) ;
#188418=CARTESIAN_POINT ( 'NONE',  ( 18.62759615963255655, 10.81492255796105972, 61.66775706135235424 ) ) ;
#188419=CARTESIAN_POINT ( 'NONE',  ( 18.62759615963271287, -10.81492255796078972, 28.33224293864769550 ) ) ;
#188420=CARTESIAN_POINT ( 'NONE',  ( 0.05219959533909260263, 19.03943276465977164, 29.99890960531435979 ) ) ;
#188421=CARTESIAN_POINT ( 'NONE',  ( 21.55341960407619695, -5.719274019375665929, 26.04275706135235779 ) ) ;
#188422=CARTESIAN_POINT ( 'NONE',  ( 5.049401038297881783, 19.05341960407617563, 52.29275706135234003 ) ) ;
#188423=CARTESIAN_POINT ( 'NONE',  ( 12.06949235617757843, -12.14591786802309237, 113.1239096053143953 ) ) ;
#188424=CARTESIAN_POINT ( 'NONE',  ( 16.46253265017160672, -9.564922557960803928, 63.33224293864769550 ) ) ;
#188425=CARTESIAN_POINT ( 'NONE',  ( 0.05219959533934541429, -16.53943276465976808, 20.00109039468568639 ) ) ;
#188426=CARTESIAN_POINT ( 'NONE',  ( -14.29746914071049879, 8.314922557960819915, 70.83224293864770971 ) ) ;
#188427=CARTESIAN_POINT ( 'NONE',  ( -19.03943276465977164, 0.05219959533909376836, 116.2489096053143669 ) ) ;
#188428=CARTESIAN_POINT ( 'NONE',  ( 9.564922557961047289, -16.46253265017146816, 100.4177570613523329 ) ) ;
#188429=CARTESIAN_POINT ( 'NONE',  ( -10.81492255796078084, -18.62759615963271287, 107.0822429386476955 ) ) ;
#188430=CARTESIAN_POINT ( 'NONE',  ( 15.72974639402176855, 15.80617190586768217, 56.87609039468568994 ) ) ;
#188431=CARTESIAN_POINT ( 'NONE',  ( -16.52544592524335698, -4.483927247898792601, 53.95942372801900433 ) ) ;
#188432=CARTESIAN_POINT ( 'NONE',  ( -16.55341960407617563, 4.379528057220093196, 58.54275706135235424 ) ) ;
#188433=CARTESIAN_POINT ( 'NONE',  ( 10.81492255796078972, 18.62759615963270932, 59.58224293864770260 ) ) ;
#188434=CARTESIAN_POINT ( 'NONE',  ( -13.89961937509977652, 13.97604488694528158, 50.62390960531435979 ) ) ;
#188435=CARTESIAN_POINT ( 'NONE',  ( -8.224510206698735004, -14.34966873604973081, 74.58442372801901854 ) ) ;
#188436=CARTESIAN_POINT ( 'NONE',  ( -15.72974639402197994, 15.80617190586746368, 95.62390960531436690 ) ) ;
#188437=CARTESIAN_POINT ( 'NONE',  ( 14.29746914071049879, -8.314922557960816363, 48.33224293864770260 ) ) ;
#188438=CARTESIAN_POINT ( 'NONE',  ( -5.153800228976328057, -19.02544592524343514, 72.29057627198102409 ) ) ;
#188439=CARTESIAN_POINT ( 'NONE',  ( 16.55341960407618274, -4.379528057220086978, 81.04275706135236135 ) ) ;
#188440=CARTESIAN_POINT ( 'NONE',  ( -4.379528057220086978, -16.55341960407618274, 24.79275706135235779 ) ) ;
#188441=CARTESIAN_POINT ( 'NONE',  ( -21.52544592524343514, 5.823673210054127303, 101.0405762719810383 ) ) ;
#188442=CARTESIAN_POINT ( 'NONE',  ( 16.53943276465976808, -0.05219959533910856209, 38.74890960531435979 ) ) ;
#188444=CARTESIAN_POINT ( 'NONE',  ( 19.53037848336980531, -5.499999999999989342, 92.35532783611446916 ) ) ;
#188445=CARTESIAN_POINT ( 'NONE',  ( 10.72451020669898902, -18.67979575497178502, 82.91557627198103830 ) ) ;
#188446=CARTESIAN_POINT ( 'NONE',  ( -16.55341960407611168, -4.379528057220339221, 26.45724293864768839 ) ) ;
#188448=CARTESIAN_POINT ( 'NONE',  ( -16.18388926212241330, -7.379444403734409796, 55.43953151366151388 ) ) ;
#188449=CARTESIAN_POINT ( 'NONE',  ( 21.53943276465977519, -0.05219959533907433946, 98.74890960531438111 ) ) ;
#188450=CARTESIAN_POINT ( 'NONE',  ( 16.46253265017160672, -9.564922557960803928, 98.33224293864769550 ) ) ;
#188451=CARTESIAN_POINT ( 'NONE',  ( -10.72451020669898014, 18.67979575497178502, 115.4155762719810241 ) ) ;
#188452=CARTESIAN_POINT ( 'NONE',  ( -4.379528057220328563, 16.55341960407611168, 40.20724293864769550 ) ) ;
#188453=CARTESIAN_POINT ( 'NONE',  ( -16.52544592524335698, -4.483927247898792601, 48.95942372801902565 ) ) ;
#188454=CARTESIAN_POINT ( 'NONE',  ( 9.564922557960805705, 16.46253265017160317, 54.58224293864769550 ) ) ;
#188455=CARTESIAN_POINT ( 'NONE',  ( -9.564922557961040184, 16.46253265017147172, 57.91775706135233293 ) ) ;
#188456=CARTESIAN_POINT ( 'NONE',  ( 13.89961937509977652, -13.97604488694527269, 78.12390960531433848 ) ) ;
#188457=VERTEX_POINT ( 'NONE', #146442 ) ;
#188458=CARTESIAN_POINT ( 'NONE',  ( 5.823673210054125526, 21.52544592524343514, 39.79057627198103830 ) ) ;
#188460=CARTESIAN_POINT ( 'NONE',  ( 5.049401038297881783, 19.05341960407617563, 112.2927570613523471 ) ) ;
#188461=CARTESIAN_POINT ( 'NONE',  ( -5.049401038297874678, -19.05341960407617918, 44.79275706135232582 ) ) ;
#188462=CARTESIAN_POINT ( 'NONE',  ( -21.55341960407610458, -5.719274019375992779, 96.45724293864770971 ) ) ;
#188463=CARTESIAN_POINT ( 'NONE',  ( -16.53943276465976808, 0.05219959533911058130, 31.24890960531435979 ) ) ;
#188464=CARTESIAN_POINT ( 'NONE',  ( -19.03943276465977164, 0.05219959533909376836, 81.24890960531436690 ) ) ;
#188465=CARTESIAN_POINT ( 'NONE',  ( -10.72451020669898014, 18.67979575497178502, 55.41557627198102409 ) ) ;
#188466=CARTESIAN_POINT ( 'NONE',  ( -15.80617190586745835, -15.72974639402198527, 96.87390960531436690 ) ) ;
#188467=CARTESIAN_POINT ( 'NONE',  ( 8.314922557961029526, -14.29746914071037800, 30.41775706135234358 ) ) ;
#188469=CARTESIAN_POINT ( 'NONE',  ( -18.67979575497178146, -10.72451020669898902, 26.66557627198103475 ) ) ;
#188470=CARTESIAN_POINT ( 'NONE',  ( 5.823673210054444382, -21.52544592524334988, 85.20942372801901854 ) ) ;
#188471=CARTESIAN_POINT ( 'NONE',  ( -0.05219959533909027116, -19.03943276465977164, 82.49890960531436690 ) ) ;
#188472=CARTESIAN_POINT ( 'NONE',  ( 16.51473224551069308, 9.474510206698969483, 29.16557627198103475 ) ) ;
#188473=CARTESIAN_POINT ( 'NONE',  ( 5.153800228976335163, 19.02544592524342804, 84.79057627198099567 ) ) ;
#188474=CARTESIAN_POINT ( 'NONE',  ( 8.224510206698953496, -14.34966873604960469, 107.9155762719810241 ) ) ;
#188475=CARTESIAN_POINT ( 'NONE',  ( -13.89961937509977652, 13.97604488694528158, 60.62390960531436690 ) ) ;
#188476=CARTESIAN_POINT ( 'NONE',  ( -0.05219959533936034679, 19.03943276465977164, 102.5010903946856757 ) ) ;
#188478=CARTESIAN_POINT ( 'NONE',  ( 17.50000000000000355, 3.237210098469580632, 32.78763012620459705 ) ) ;
#188479=CARTESIAN_POINT ( 'NONE',  ( -19.02544592524342804, 5.153800228976336051, 76.04057627198102409 ) ) ;
#188480=CARTESIAN_POINT ( 'NONE',  ( 21.53943276465977519, 0.05219959533937863772, 101.2510903946856757 ) ) ;
#188481=CARTESIAN_POINT ( 'NONE',  ( -9.474510206698964154, 16.51473224551069663, 115.4155762719810241 ) ) ;
#188482=CARTESIAN_POINT ( 'NONE',  ( 14.29746914071037800, 8.314922557961029526, 91.66775706135234714 ) ) ;
#188485=CARTESIAN_POINT ( 'NONE',  ( 16.51473224551083163, -9.474510206698727899, 75.83442372801900433 ) ) ;
#188486=CARTESIAN_POINT ( 'NONE',  ( -5.049401038297874678, -19.05341960407617918, 19.79275706135233293 ) ) ;
#188488=CARTESIAN_POINT ( 'NONE',  ( -16.46253265017160317, 9.564922557960807481, 30.83224293864769550 ) ) ;
#188489=CARTESIAN_POINT ( 'NONE',  ( 4.483927247898545687, 16.52544592524342804, 24.79057627198103120 ) ) ;
#188491=CARTESIAN_POINT ( 'NONE',  ( -12.06949235617739369, -12.14591786802326823, 104.3760903946856899 ) ) ;
#188492=CARTESIAN_POINT ( 'NONE',  ( -19.53091890409953635, -5.499999999999944933, 85.06097431831423705 ) ) ;
#188493=CARTESIAN_POINT ( 'NONE',  ( 14.34966873604972726, -8.224510206698740333, 75.83442372801900433 ) ) ;
#188494=CARTESIAN_POINT ( 'NONE',  ( -0.05219959533909027116, -19.03943276465977164, 42.49890960531435269 ) ) ;
#188495=CARTESIAN_POINT ( 'NONE',  ( -0.05219959533937732626, 21.53943276465977519, 92.50109039468567573 ) ) ;
#188496=CARTESIAN_POINT ( 'NONE',  ( 13.89961937509957401, 13.97604488694547697, 106.8760903946856757 ) ) ;
#188497=CARTESIAN_POINT ( 'NONE',  ( 18.67979575497194134, -10.72451020669871369, 75.83442372801900433 ) ) ;
#188498=CARTESIAN_POINT ( 'NONE',  ( -19.03943276465977164, -0.05219959533935918106, 53.75109039468566863 ) ) ;
#188499=CARTESIAN_POINT ( 'NONE',  ( -16.46253265017160317, 9.564922557960807481, 75.83224293864769550 ) ) ;
#188500=CARTESIAN_POINT ( 'NONE',  ( -19.05341960407611168, -5.049401038298163336, 66.45724293864769550 ) ) ;
#188502=CARTESIAN_POINT ( 'NONE',  ( -0.05219959533910754901, -16.53943276465976808, 62.49890960531436690 ) ) ;
#188503=CARTESIAN_POINT ( 'NONE',  ( 18.67979575497178502, 10.72451020669898547, 44.16557627198103120 ) ) ;
#188504=CARTESIAN_POINT ( 'NONE',  ( -13.97604488694527625, -13.89961937509977652, 41.87390960531435979 ) ) ;
#188505=CARTESIAN_POINT ( 'NONE',  ( 15.72974639402199770, -15.80617190586745480, 88.12390960531436690 ) ) ;
#188506=CARTESIAN_POINT ( 'NONE',  ( 16.55341960407618274, -4.379528057220086978, 81.04275706135236135 ) ) ;
#188507=B_SPLINE_CURVE_WITH_KNOTS ( 'NONE', 3,
 ( #28502, #134678, #166010, #27510, #57832, #60785, #122456, #182165, #43650, #167000, #184149, #45630, #87162, #76950, #110274, #141609, #64773, #78934, #187149, #126435, #17280, #2100, #153795, #186145, #109278, #108283, #111267, #140610, #31453, #34436, #138620, #63781 ),
 .UNSPECIFIED., .F., .F.,
 ( 4, 2, 2, 2, 2, 2, 2, 2, 2, 2, 2, 2, 2, 2, 2, 4 ),
 ( 8.044049492208757700E-17, 0.0003712461730037431022, 0.0007424923460074057567, 0.001113738519011068248, 0.001484984692014731066, 0.002227477038022061904, 0.002598723211025727540, 0.002969969384029393176, 0.003341215557033058812, 0.003712461730036724014, 0.004083707903040389650, 0.004454954076044054419, 0.004826200249047720055, 0.005197446422051385691, 0.005568692595055050459, 0.005939938768058716095 ),
 .UNSPECIFIED. ) ;
#188510=CARTESIAN_POINT ( 'NONE',  ( 8.224510206698953496, -14.34966873604960469, 82.91557627198103830 ) ) ;
#188512=CARTESIAN_POINT ( 'NONE',  ( 4.379528057220092307, 16.55341960407617563, 37.29275706135235424 ) ) ;
#188513=CARTESIAN_POINT ( 'NONE',  ( 16.55341960407611168, 4.379528057220329451, 113.9572429386477239 ) ) ;
#188514=CARTESIAN_POINT ( 'NONE',  ( -19.03943276465977164, -0.05219959533935918106, 63.75109039468566863 ) ) ;
#188515=CARTESIAN_POINT ( 'NONE',  ( -8.224510206698948167, 14.34966873604960824, 65.41557627198102409 ) ) ;
#188516=CARTESIAN_POINT ( 'NONE',  ( -21.53943276465977519, -0.05219959533937600094, 48.75109039468568284 ) ) ;
#188517=CARTESIAN_POINT ( 'NONE',  ( 19.03943276465977164, -0.05219959533909143690, 28.74890960531435624 ) ) ;
#188518=CARTESIAN_POINT ( 'NONE',  ( -15.80617190586745835, -15.72974639402198527, 91.87390960531436690 ) ) ;
#188519=CARTESIAN_POINT ( 'NONE',  ( -5.153800228976328057, -19.02544592524343514, 112.2905762719810099 ) ) ;
#188520=CARTESIAN_POINT ( 'NONE',  ( -4.483927247898539470, -16.52544592524342804, 92.29057627198103830 ) ) ;
#188522=CARTESIAN_POINT ( 'NONE',  ( 5.153800228976335163, 19.02544592524342804, 49.79057627198100988 ) ) ;
#188524=CARTESIAN_POINT ( 'NONE',  ( 19.03943276465977164, 0.05219959533936151252, 76.25109039468566152 ) ) ;
#188525=CARTESIAN_POINT ( 'NONE',  ( -10.81492255796105439, 18.62759615963255655, 37.91775706135235424 ) ) ;
#188526=CARTESIAN_POINT ( 'NONE',  ( -16.46253265017160317, 9.564922557960807481, 70.83224293864770971 ) ) ;
#188527=CARTESIAN_POINT ( 'NONE',  ( -16.51473224551082808, 9.474510206698731452, 53.33442372801900433 ) ) ;
#188528=CARTESIAN_POINT ( 'NONE',  ( -5.049401038298153566, 19.05341960407611168, 45.20724293864769550 ) ) ;
#188529=CARTESIAN_POINT ( 'NONE',  ( -12.14591786802309592, -12.06949235617757132, 56.87390960531436690 ) ) ;
#188530=CARTESIAN_POINT ( 'NONE',  ( 4.483927247898545687, 16.52544592524342804, 54.79057627198104541 ) ) ;
#188531=CARTESIAN_POINT ( 'NONE',  ( 19.02544592524343514, -5.153800228976328945, 73.54057627198103830 ) ) ;
#188532=CARTESIAN_POINT ( 'NONE',  ( -21.53943276465977519, 0.05219959533907696930, 101.2489096053143669 ) ) ;
#188533=CARTESIAN_POINT ( 'NONE',  ( 19.05341960407611168, 5.049401038298154454, 73.95724293864768129 ) ) ;
#188534=CARTESIAN_POINT ( 'NONE',  ( -21.52544592524343514, 5.823673210054127303, 76.04057627198102409 ) ) ;
#188535=CARTESIAN_POINT ( 'NONE',  ( -10.81492255796105439, 18.62759615963255655, 107.9177570613523471 ) ) ;
#188536=CARTESIAN_POINT ( 'NONE',  ( -13.97604488694527625, -13.89961937509977652, 41.87390960531435979 ) ) ;
#188537=CARTESIAN_POINT ( 'NONE',  ( -16.53943276465976808, -0.05219959533934237506, 103.7510903946857042 ) ) ;
#188538=CARTESIAN_POINT ( 'NONE',  ( -8.224510206698948167, 14.34966873604960824, 90.41557627198103830 ) ) ;
#188539=CARTESIAN_POINT ( 'NONE',  ( 19.02544592524334988, 5.153800228976608722, 101.4594237280189759 ) ) ;
#188541=CARTESIAN_POINT ( 'NONE',  ( -18.62759615963255300, -10.81492255796106328, 29.16775706135234003 ) ) ;
#188542=CARTESIAN_POINT ( 'NONE',  ( -9.474510206698720793, -16.51473224551083518, 54.58442372801899722 ) ) ;
#188543=CARTESIAN_POINT ( 'NONE',  ( 0.05219959533934541429, -16.53943276465976808, 110.0010903946856757 ) ) ;
#188544=CARTESIAN_POINT ( 'NONE',  ( -10.81492255796078084, -18.62759615963271287, 77.08224293864769550 ) ) ;
#188545=CARTESIAN_POINT ( 'NONE',  ( -19.02544592524342804, 5.153800228976336051, 96.04057627198103830 ) ) ;
#188546=CARTESIAN_POINT ( 'NONE',  ( -16.53943276465976808, 0.05219959533911058130, 61.24890960531435979 ) ) ;
#188547=CARTESIAN_POINT ( 'NONE',  ( -5.049401038298153566, 19.05341960407611168, 35.20724293864768839 ) ) ;
#188548=CARTESIAN_POINT ( 'NONE',  ( -19.03943276465977164, 0.05219959533909376836, 31.24890960531435979 ) ) ;
#188549=CARTESIAN_POINT ( 'NONE',  ( -18.67979575497193778, 10.72451020669871902, 108.3344237280190185 ) ) ;
#188550=CARTESIAN_POINT ( 'NONE',  ( -8.224510206698735004, -14.34966873604973081, 89.58442372801901854 ) ) ;
#188551=CARTESIAN_POINT ( 'NONE',  ( 18.67979575497194134, -10.72451020669871369, 35.83442372801901143 ) ) ;
#188552=CARTESIAN_POINT ( 'NONE',  ( 16.53943276465976808, 0.05219959533934440121, 41.25109039468568284 ) ) ;
#188553=CARTESIAN_POINT ( 'NONE',  ( -19.03943276465977164, 0.05219959533909376836, 116.2489096053143669 ) ) ;
#188554=CARTESIAN_POINT ( 'NONE',  ( 5.049401038298161559, -19.05341960407611168, 52.70724293864767418 ) ) ;
#188555=CARTESIAN_POINT ( 'NONE',  ( 5.719274019375673035, 21.55341960407619339, 97.29275706135234714 ) ) ;
#188556=CARTESIAN_POINT ( 'NONE',  ( 9.564922557960805705, 16.46253265017160317, 74.58224293864769550 ) ) ;
#188557=CARTESIAN_POINT ( 'NONE',  ( -14.29746914071037622, -8.314922557961029526, 59.16775706135234714 ) ) ;
#188558=CARTESIAN_POINT ( 'NONE',  ( 8.314922557960818139, 14.29746914071049879, 104.5822429386477097 ) ) ;
#188559=CARTESIAN_POINT ( 'NONE',  ( 4.379528057220092307, 16.55341960407617563, 112.2927570613523471 ) ) ;
#188560=CARTESIAN_POINT ( 'NONE',  ( 13.97604488694527802, 13.89961937509977830, 49.37390960531435269 ) ) ;
#188561=CARTESIAN_POINT ( 'NONE',  ( 21.53943276465977519, 0.05219959533937863772, 51.25109039468568994 ) ) ;
#188562=CARTESIAN_POINT ( 'NONE',  ( 16.51473224551069308, 9.474510206698969483, 94.16557627198103830 ) ) ;
#188563=CARTESIAN_POINT ( 'NONE',  ( 13.97604488694527802, 13.89961937509977652, 79.37390960531435269 ) ) ;
#188564=CARTESIAN_POINT ( 'NONE',  ( 5.049401038298161559, -19.05341960407611168, 112.7072429386476813 ) ) ;
#188565=CARTESIAN_POINT ( 'NONE',  ( 14.34966873604960469, 8.224510206698951720, 44.16557627198103120 ) ) ;
#188566=CARTESIAN_POINT ( 'NONE',  ( -16.55341960407611168, -4.379528057220339221, 26.45724293864768839 ) ) ;
#188568=CARTESIAN_POINT ( 'NONE',  ( 0.05219959533910956823, 16.53943276465976808, 44.99890960531435979 ) ) ;
#188570=CARTESIAN_POINT ( 'NONE',  ( 13.89961937509957401, 13.97604488694547697, 31.87609039468566863 ) ) ;
#188571=CARTESIAN_POINT ( 'NONE',  ( -0.05219959533909027116, -19.03943276465977164, 82.49890960531436690 ) ) ;
#188572=CARTESIAN_POINT ( 'NONE',  ( -13.89961937509957401, -13.97604488694547875, 54.37609039468565442 ) ) ;
#188574=CARTESIAN_POINT ( 'NONE',  ( -13.97604488694527625, -13.89961937509977830, 66.87390960531436690 ) ) ;
#188575=CARTESIAN_POINT ( 'NONE',  ( 16.46253265017146816, 9.564922557961045513, 86.66775706135233293 ) ) ;
#188576=CARTESIAN_POINT ( 'NONE',  ( -0.05219959533934338120, 16.53943276465976808, 72.50109039468568994 ) ) ;
#188577=CARTESIAN_POINT ( 'NONE',  ( 17.44279575226823908, 5.990770900252462283, 91.66442432485682446 ) ) ;
#188578=CARTESIAN_POINT ( 'NONE',  ( 19.03943276465977164, -0.05219959533909143690, 108.7489096053143527 ) ) ;
#188579=CARTESIAN_POINT ( 'NONE',  ( 10.81492255796106328, -18.62759615963255655, 30.41775706135234358 ) ) ;
#188580=CARTESIAN_POINT ( 'NONE',  ( 0.05219959533936267826, -19.03943276465977164, 85.00109039468567573 ) ) ;
#188581=CARTESIAN_POINT ( 'NONE',  ( 16.36317988757060604, 7.306389748694960495, 88.40210391636782106 ) ) ;
#188582=CARTESIAN_POINT ( 'NONE',  ( 16.51473224551069308, 9.474510206698969483, 44.16557627198103120 ) ) ;
#188583=CARTESIAN_POINT ( 'NONE',  ( 19.02544592524343514, -5.153800228976328945, 88.54057627198102409 ) ) ;
#188584=CARTESIAN_POINT ( 'NONE',  ( 14.34966873604960469, 8.224510206698951720, 64.16557627198102409 ) ) ;
#188585=CARTESIAN_POINT ( 'NONE',  ( 19.03943276465977164, -0.05219959533909143690, 48.74890960531435979 ) ) ;
#188586=CARTESIAN_POINT ( 'NONE',  ( 19.05341960407611168, 5.049401038298154454, 58.95724293864768129 ) ) ;
#188587=CARTESIAN_POINT ( 'NONE',  ( -16.46253265017146816, -9.564922557961047289, 64.16775706135233293 ) ) ;
#188588=CARTESIAN_POINT ( 'NONE',  ( 9.564922557961047289, -16.46253265017146816, 30.41775706135232937 ) ) ;
#188589=CARTESIAN_POINT ( 'NONE',  ( -9.474510206698964154, 16.51473224551069663, 70.41557627198102409 ) ) ;
#188590=CARTESIAN_POINT ( 'NONE',  ( -18.62759615963270932, 10.81492255796079327, 65.83224293864769550 ) ) ;
#188591=CARTESIAN_POINT ( 'NONE',  ( 12.06949235617757843, -12.14591786802309237, 68.12390960531436690 ) ) ;
#188592=CARTESIAN_POINT ( 'NONE',  ( 9.564922557961047289, -16.46253265017146816, 40.41775706135234003 ) ) ;
#188594=CARTESIAN_POINT ( 'NONE',  ( 18.67979575497178502, 10.72451020669898547, 44.16557627198103120 ) ) ;
#188595=CARTESIAN_POINT ( 'NONE',  ( 15.80617190586746368, 15.72974639402197994, 24.37390960531435979 ) ) ;
#188596=CARTESIAN_POINT ( 'NONE',  ( -16.51473224551069308, -9.474510206698971260, 51.66557627198102409 ) ) ;
#188597=CARTESIAN_POINT ( 'NONE',  ( 9.474510206698971260, -16.51473224551069308, 42.91557627198103120 ) ) ;
#188598=CARTESIAN_POINT ( 'NONE',  ( -8.224510206698948167, 14.34966873604960824, 100.4155762719810241 ) ) ;
#188599=CARTESIAN_POINT ( 'NONE',  ( -21.53943276465977519, 0.05219959533907696930, 116.2489096053143669 ) ) ;
#188601=CARTESIAN_POINT ( 'NONE',  ( -15.80617190586768217, 15.72974639402176855, 28.12609039468568284 ) ) ;
#188602=CARTESIAN_POINT ( 'NONE',  ( -16.52544592524342804, 4.483927247898546575, 111.0405762719810525 ) ) ;
#188603=CARTESIAN_POINT ( 'NONE',  ( -15.80617190586768217, 15.72974639402176855, 83.12609039468568994 ) ) ;
#188604=CARTESIAN_POINT ( 'NONE',  ( 18.67979575497178502, 10.72451020669898547, 89.16557627198102409 ) ) ;
#188605=CARTESIAN_POINT ( 'NONE',  ( -0.05219959533936034679, 19.03943276465977164, 37.50109039468567573 ) ) ;
#188606=CARTESIAN_POINT ( 'NONE',  ( -0.05219959533909027116, -19.03943276465977164, 22.49890960531436690 ) ) ;
#188607=CARTESIAN_POINT ( 'NONE',  ( 5.049401038298163336, -19.05341960407611168, 52.70724293864768129 ) ) ;
#188609=CARTESIAN_POINT ( 'NONE',  ( 8.314922557961029526, -14.29746914071037800, 45.41775706135234003 ) ) ;
#188610=CARTESIAN_POINT ( 'NONE',  ( -12.06949235617756955, 12.14591786802309770, 105.6239096053143669 ) ) ;
#188612=CARTESIAN_POINT ( 'NONE',  ( 13.97604488694527802, 13.89961937509977652, 74.37390960531436690 ) ) ;
#188613=CARTESIAN_POINT ( 'NONE',  ( 8.314922557960818139, 14.29746914071049879, 94.58224293864769550 ) ) ;
#188614=CARTESIAN_POINT ( 'NONE',  ( -15.80617190586745835, -15.72974639402198527, 46.87390960531435979 ) ) ;
#188615=CARTESIAN_POINT ( 'NONE',  ( -4.483927247898539470, -16.52544592524342804, 82.29057627198103830 ) ) ;
#188616=CARTESIAN_POINT ( 'NONE',  ( -8.224510206698735004, -14.34966873604973081, 29.58442372801901854 ) ) ;
#188617=CARTESIAN_POINT ( 'NONE',  ( -15.80617190586768217, 15.72974639402176855, 93.12609039468568994 ) ) ;
#188618=CARTESIAN_POINT ( 'NONE',  ( 19.02544592524343514, -5.153800228976328945, 28.54057627198102409 ) ) ;
#188619=CARTESIAN_POINT ( 'NONE',  ( 4.379528057220092307, 16.55341960407617563, 102.2927570613523613 ) ) ;
#188620=CARTESIAN_POINT ( 'NONE',  ( -4.483927247898539470, -16.52544592524342804, 42.29057627198103120 ) ) ;
#188621=CARTESIAN_POINT ( 'NONE',  ( -0.05219959533909027116, -19.03943276465977164, 47.49890960531435979 ) ) ;
#188622=CARTESIAN_POINT ( 'NONE',  ( 18.62759615963255655, 10.81492255796105972, 101.6677570613523613 ) ) ;
#188623=CARTESIAN_POINT ( 'NONE',  ( 21.55341960407610458, 5.719274019375980345, 108.9572429386476955 ) ) ;
#188625=CARTESIAN_POINT ( 'NONE',  ( -15.80617190586768217, 15.72974639402176855, 53.12609039468568284 ) ) ;
#188626=CARTESIAN_POINT ( 'NONE',  ( -16.55341960407617563, 4.379528057220093196, 33.54275706135234714 ) ) ;
#188627=CARTESIAN_POINT ( 'NONE',  ( 4.483927247898545687, 16.52544592524342804, 64.79057627198103830 ) ) ;
#188628=CARTESIAN_POINT ( 'NONE',  ( -21.52544592524334988, -5.823673210054445271, 83.95942372801900433 ) ) ;
#188629=CARTESIAN_POINT ( 'NONE',  ( -0.05219959533934338120, 16.53943276465976808, 107.5010903946856899 ) ) ;
#188631=CARTESIAN_POINT ( 'NONE',  ( -19.19724070472091171, -5.500000000000165201, 66.06193348274382515 ) ) ;
#188632=CARTESIAN_POINT ( 'NONE',  ( -14.34966873604960291, -8.224510206698953496, 26.66557627198103475 ) ) ;
#188633=CARTESIAN_POINT ( 'NONE',  ( -12.14591786802326823, 12.06949235617739902, 78.12609039468570415 ) ) ;
#188634=CARTESIAN_POINT ( 'NONE',  ( 13.89961937509977652, -13.97604488694527269, 88.12390960531438111 ) ) ;
#188635=CARTESIAN_POINT ( 'NONE',  ( -13.97604488694527625, -13.89961937509977652, 101.8739096053143811 ) ) ;
#188636=CARTESIAN_POINT ( 'NONE',  ( 18.62759615963255655, 10.81492255796105972, 81.66775706135236135 ) ) ;
#188637=EDGE_CURVE ( 'NONE', #194003, #45948, #148463, .T. ) ;
#188638=CARTESIAN_POINT ( 'NONE',  ( -14.29746914071037622, -8.314922557961029526, 84.16775706135234714 ) ) ;
#188639=CARTESIAN_POINT ( 'NONE',  ( -12.14591786802309592, -12.06949235617757132, 76.87390960531439532 ) ) ;
#188640=CARTESIAN_POINT ( 'NONE',  ( 13.97604488694527802, 13.89961937509977652, 69.37390960531436690 ) ) ;
#188641=VERTEX_POINT ( 'NONE', #52446 ) ;
#188642=CARTESIAN_POINT ( 'NONE',  ( -8.224510206698735004, -14.34966873604973081, 24.58442372801901499 ) ) ;
#188643=CARTESIAN_POINT ( 'NONE',  ( 13.89961937509977652, -13.97604488694527269, 23.12390960531436335 ) ) ;
#188644=CARTESIAN_POINT ( 'NONE',  ( 0.05219959533909260263, 19.03943276465977164, 94.99890960531436690 ) ) ;
#188645=CARTESIAN_POINT ( 'NONE',  ( 12.14591786802327356, -12.06949235617739191, 35.62609039468568994 ) ) ;
#188647=CARTESIAN_POINT ( 'NONE',  ( 19.05341960407617918, -5.049401038297876454, 26.04275706135233293 ) ) ;
#188648=CARTESIAN_POINT ( 'NONE',  ( -16.52544592524335698, -4.483927247898792601, 88.95942372801901854 ) ) ;
#188649=CARTESIAN_POINT ( 'NONE',  ( 5.153800228976615827, -19.02544592524334988, 105.2094237280190185 ) ) ;
#188650=CARTESIAN_POINT ( 'NONE',  ( -19.03943276465977164, 0.05219959533909376836, 21.24890960531436335 ) ) ;
#188651=CARTESIAN_POINT ( 'NONE',  ( -0.05219959533934338120, 16.53943276465976808, 82.50109039468568994 ) ) ;
#188652=CARTESIAN_POINT ( 'NONE',  ( 12.14591786802327356, -12.06949235617739191, 60.62609039468567573 ) ) ;
#188653=CARTESIAN_POINT ( 'NONE',  ( 19.03943276465977164, -0.05219959533909143690, 23.74890960531435269 ) ) ;
#188654=CARTESIAN_POINT ( 'NONE',  ( -19.05341960407617563, 5.049401038297882671, 73.54275706135233293 ) ) ;
#188655=CARTESIAN_POINT ( 'NONE',  ( -18.62759615963255300, -10.81492255796106328, 104.1677570613523471 ) ) ;
#188656=CARTESIAN_POINT ( 'NONE',  ( 19.05341960407611168, 5.049401038298154454, 53.95724293864770260 ) ) ;
#188657=CARTESIAN_POINT ( 'NONE',  ( 9.564922557960805705, 16.46253265017160317, 94.58224293864769550 ) ) ;
#188658=CARTESIAN_POINT ( 'NONE',  ( 0.05219959533910956823, 16.53943276465976808, 79.99890960531435269 ) ) ;
#188660=CARTESIAN_POINT ( 'NONE',  ( 19.05341960407617918, -5.049401038297876454, 51.04275706135231871 ) ) ;
#188661=CARTESIAN_POINT ( 'NONE',  ( -5.719274019375978568, 21.55341960407610458, 50.20724293864769550 ) ) ;
#188662=CARTESIAN_POINT ( 'NONE',  ( 18.67979575497194134, -10.72451020669871369, 110.8344237280190043 ) ) ;
#188663=CARTESIAN_POINT ( 'NONE',  ( 5.153800228976335163, 19.02544592524342804, 94.79057627198103830 ) ) ;
#188664=CARTESIAN_POINT ( 'NONE',  ( -15.80617190586768217, 15.72974639402176855, 108.1260903946856757 ) ) ;
#188665=CARTESIAN_POINT ( 'NONE',  ( 18.62759615963271287, -10.81492255796078972, 58.33224293864768839 ) ) ;
#188666=CARTESIAN_POINT ( 'NONE',  ( -16.51473224551069308, -9.474510206698971260, 101.6655762719810241 ) ) ;
#188667=CARTESIAN_POINT ( 'NONE',  ( -9.474510206698720793, -16.51473224551083518, 89.58442372801900433 ) ) ;
#188668=CARTESIAN_POINT ( 'NONE',  ( 19.03943276465977164, -0.05219959533909143690, 108.7489096053143527 ) ) ;
#188669=CARTESIAN_POINT ( 'NONE',  ( -9.474510206698720793, -16.51473224551083518, 109.5844237280190043 ) ) ;
#188670=CARTESIAN_POINT ( 'NONE',  ( 14.34966873604960469, 8.224510206698951720, 109.1655762719810383 ) ) ;
#188671=CARTESIAN_POINT ( 'NONE',  ( 19.05341960407611168, 5.049401038298154454, 83.95724293864766707 ) ) ;
#188672=CARTESIAN_POINT ( 'NONE',  ( -10.81492255796078084, -18.62759615963271287, 82.08224293864768129 ) ) ;
#188673=CARTESIAN_POINT ( 'NONE',  ( -16.55341960407617563, 4.379528057220093196, 43.54275706135235424 ) ) ;
#188674=CARTESIAN_POINT ( 'NONE',  ( -0.05219959533937732626, 21.53943276465977519, 42.50109039468567573 ) ) ;
#188675=CARTESIAN_POINT ( 'NONE',  ( -21.52544592524334988, -5.823673210054445271, 103.9594237280190185 ) ) ;
#188676=CARTESIAN_POINT ( 'NONE',  ( -16.55341960407617563, 4.379528057220093196, 98.54275706135234714 ) ) ;
#188677=CARTESIAN_POINT ( 'NONE',  ( -19.02544592524342804, 5.153800228976336051, 86.04057627198103830 ) ) ;
#188678=CARTESIAN_POINT ( 'NONE',  ( -16.55341960407611168, -4.379528057220339221, 86.45724293864770971 ) ) ;
#188679=CARTESIAN_POINT ( 'NONE',  ( 16.52544592524342804, -4.483927247898539470, 23.54057627198102765 ) ) ;
#188680=CARTESIAN_POINT ( 'NONE',  ( -0.05219959533936034679, 19.03943276465977164, 72.50109039468566152 ) ) ;
#188681=CARTESIAN_POINT ( 'NONE',  ( 10.81492255796106328, -18.62759615963255655, 45.41775706135234003 ) ) ;
#188683=CARTESIAN_POINT ( 'NONE',  ( 14.29746914071049879, -8.314922557960816363, 93.33224293864769550 ) ) ;
#188684=CARTESIAN_POINT ( 'NONE',  ( 9.474510206698971260, -16.51473224551069308, 107.9155762719810383 ) ) ;
#188685=CARTESIAN_POINT ( 'NONE',  ( 16.52544592524342804, -4.483927247898539470, 28.54057627198103120 ) ) ;
#188686=CARTESIAN_POINT ( 'NONE',  ( 15.80617190586769283, -15.72974639402175789, 90.62609039468567573 ) ) ;
#188687=CARTESIAN_POINT ( 'NONE',  ( -12.06949235617739369, -12.14591786802326823, 64.37609039468568994 ) ) ;
#188688=CARTESIAN_POINT ( 'NONE',  ( -4.379528057220086978, -16.55341960407618274, 99.79275706135234714 ) ) ;
#188689=CARTESIAN_POINT ( 'NONE',  ( 5.823673210054444382, -21.52544592524334988, 45.20942372801901854 ) ) ;
#188690=CARTESIAN_POINT ( 'NONE',  ( -15.72974639402176322, -15.80617190586768395, 24.37609039468567573 ) ) ;
#188691=CARTESIAN_POINT ( 'NONE',  ( -16.55341960407611168, -4.379528057220339221, 111.4572429386476813 ) ) ;
#188692=CARTESIAN_POINT ( 'NONE',  ( -9.474510206698964154, 16.51473224551069663, 30.41557627198102054 ) ) ;
#188693=CARTESIAN_POINT ( 'NONE',  ( 16.52544592524342804, -4.483927247898539470, 68.54057627198103830 ) ) ;
#188694=CARTESIAN_POINT ( 'NONE',  ( 13.89961937509977652, -13.97604488694527269, 78.12390960531433848 ) ) ;
#188695=CARTESIAN_POINT ( 'NONE',  ( 4.483927247898790824, -16.52544592524335698, 100.2094237280190043 ) ) ;
#188696=CARTESIAN_POINT ( 'NONE',  ( 19.02544592524343514, -5.153800228976328945, 43.54057627198103120 ) ) ;
#188697=CARTESIAN_POINT ( 'NONE',  ( 21.53943276465977519, -0.05219959533907433946, 48.74890960531435979 ) ) ;
#188698=CARTESIAN_POINT ( 'NONE',  ( 14.29746914071049879, -8.314922557960816363, 93.33224293864769550 ) ) ;
#188699=CARTESIAN_POINT ( 'NONE',  ( 15.72974639402199770, -15.80617190586745480, 88.12390960531436690 ) ) ;
#188700=CARTESIAN_POINT ( 'NONE',  ( -16.46253265017160317, 9.564922557960807481, 90.83224293864769550 ) ) ;
#188701=CARTESIAN_POINT ( 'NONE',  ( 13.97604488694527802, 13.89961937509977652, 49.37390960531434558 ) ) ;
#188702=CARTESIAN_POINT ( 'NONE',  ( 16.51473224551083163, -9.474510206698727899, 85.83442372801900433 ) ) ;
#188703=CARTESIAN_POINT ( 'NONE',  ( 10.72451020669898902, -18.67979575497178502, 37.91557627198102409 ) ) ;
#188704=CARTESIAN_POINT ( 'NONE',  ( -5.823673210054431948, 21.52544592524334988, 72.70942372801901854 ) ) ;
#188705=CARTESIAN_POINT ( 'NONE',  ( -13.89961937509977652, 13.97604488694528158, 55.62390960531434558 ) ) ;
#188706=CARTESIAN_POINT ( 'NONE',  ( 13.97604488694527802, 13.89961937509977652, 79.37390960531435269 ) ) ;
#188708=CARTESIAN_POINT ( 'NONE',  ( 4.483927247898790824, -16.52544592524335698, 60.20942372801902565 ) ) ;
#188709=CARTESIAN_POINT ( 'NONE',  ( -10.72451020669870658, -18.67979575497194134, 49.58442372801901143 ) ) ;
#188710=CARTESIAN_POINT ( 'NONE',  ( -5.719274019375665041, -21.55341960407619695, 69.79275706135234714 ) ) ;
#188711=CARTESIAN_POINT ( 'NONE',  ( -5.153800228976328057, -19.02544592524343514, 112.2905762719810099 ) ) ;
#188712=CARTESIAN_POINT ( 'NONE',  ( -21.52544592524343514, 5.823673210054127303, 96.04057627198102409 ) ) ;
#188713=CARTESIAN_POINT ( 'NONE',  ( 10.72451020669871369, 18.67979575497193778, 37.08442372801901143 ) ) ;
#188714=CARTESIAN_POINT ( 'NONE',  ( -16.52544592524335698, -4.483927247898792601, 68.95942372801901854 ) ) ;
#188715=CARTESIAN_POINT ( 'NONE',  ( -5.823673210054116645, -21.52544592524344225, 62.29057627198102409 ) ) ;
#188716=CARTESIAN_POINT ( 'NONE',  ( -5.049401038297874678, -19.05341960407617918, 34.79275706135233293 ) ) ;
#188717=CARTESIAN_POINT ( 'NONE',  ( 13.97604488694527802, 13.89961937509977652, 69.37390960531436690 ) ) ;
#188718=CARTESIAN_POINT ( 'NONE',  ( 16.52544592524335698, 4.483927247898782831, 96.45942372801901854 ) ) ;
#188720=CARTESIAN_POINT ( 'NONE',  ( 19.05341960407611168, 5.049401038298154454, 108.9572429386477097 ) ) ;
#188722=CARTESIAN_POINT ( 'NONE',  ( 0.05219959533936267826, -19.03943276465977164, 80.00109039468567573 ) ) ;
#188723=CARTESIAN_POINT ( 'NONE',  ( 10.81492255796078972, 18.62759615963270932, 64.58224293864769550 ) ) ;
#188724=CARTESIAN_POINT ( 'NONE',  ( -4.379528057220328563, 16.55341960407611168, 40.20724293864769550 ) ) ;
#188725=CARTESIAN_POINT ( 'NONE',  ( -13.97604488694547697, 13.89961937509957934, 98.12609039468566152 ) ) ;
#188726=CARTESIAN_POINT ( 'NONE',  ( 19.02544592524343514, -5.153800228976328945, 28.54057627198102409 ) ) ;
#188727=CARTESIAN_POINT ( 'NONE',  ( 19.05341960407617918, -5.049401038297876454, 106.0427570613523471 ) ) ;
#188728=CARTESIAN_POINT ( 'NONE',  ( -10.72451020669898014, 18.67979575497178502, 85.41557627198102409 ) ) ;
#188729=CARTESIAN_POINT ( 'NONE',  ( -16.51473224551082808, 9.474510206698731452, 58.33442372801900433 ) ) ;
#188730=CARTESIAN_POINT ( 'NONE',  ( -8.224510206698735004, -14.34966873604973081, 74.58442372801901854 ) ) ;
#188731=CARTESIAN_POINT ( 'NONE',  ( 16.46253265017160672, -9.564922557960803928, 68.33224293864770971 ) ) ;
#188732=CARTESIAN_POINT ( 'NONE',  ( 4.483927247898545687, 16.52544592524342804, 74.79057627198105251 ) ) ;
#188733=CARTESIAN_POINT ( 'NONE',  ( 16.46253265017160672, -9.564922557960803928, 48.33224293864769550 ) ) ;
#188734=CARTESIAN_POINT ( 'NONE',  ( 0.05219959533910956823, 16.53943276465976808, 49.99890960531437401 ) ) ;
#188735=DIRECTION ( 'NONE',  ( 1.000000000000000000, 0.000000000000000000, 0.000000000000000000 ) ) ;
#188737=CARTESIAN_POINT ( 'NONE',  ( -0.05219959533910754901, -16.53943276465976808, 22.49890960531436335 ) ) ;
#188738=CARTESIAN_POINT ( 'NONE',  ( 13.97604488694527802, 13.89961937509977652, 79.37390960531435269 ) ) ;
#188740=CARTESIAN_POINT ( 'NONE',  ( -5.153800228976607833, 19.02544592524334988, 32.70942372801899722 ) ) ;
#188741=CARTESIAN_POINT ( 'NONE',  ( 0.05219959533934541429, -16.53943276465976808, 45.00109039468568284 ) ) ;
#188742=CARTESIAN_POINT ( 'NONE',  ( -10.81492255796078084, -18.62759615963271287, 67.08224293864770971 ) ) ;
#188743=CARTESIAN_POINT ( 'NONE',  ( -15.80617190586768217, 15.72974639402176855, 113.1260903946856899 ) ) ;
#188744=CARTESIAN_POINT ( 'NONE',  ( 19.03943276465977164, -0.05219959533909143690, 73.74890960531435269 ) ) ;
#188745=CARTESIAN_POINT ( 'NONE',  ( -13.89961937509977652, 13.97604488694528158, 115.6239096053143669 ) ) ;
#188746=CARTESIAN_POINT ( 'NONE',  ( 13.89961937509977652, -13.97604488694527269, 108.1239096053143669 ) ) ;
#188747=CARTESIAN_POINT ( 'NONE',  ( 21.52544592524334988, 5.823673210054432836, 36.45942372801901143 ) ) ;
#188748=CARTESIAN_POINT ( 'NONE',  ( 8.224510206698953496, -14.34966873604960469, 102.9155762719810383 ) ) ;
#188749=CARTESIAN_POINT ( 'NONE',  ( -10.72451020669898014, 18.67979575497178502, 105.4155762719810383 ) ) ;
#188750=CARTESIAN_POINT ( 'NONE',  ( -5.049401038298153566, 19.05341960407611168, 75.20724293864769550 ) ) ;
#188751=VERTEX_POINT ( 'NONE', #147466 ) ;
#188752=CARTESIAN_POINT ( 'NONE',  ( 15.80617190586769283, -15.72974639402175789, 25.62609039468567929 ) ) ;
#188753=ORIENTED_EDGE ( 'NONE', *, *, #52659, .T. ) ;
#188754=CARTESIAN_POINT ( 'NONE',  ( -19.02544592524342804, 5.153800228976336051, 81.04057627198103830 ) ) ;
#188755=CARTESIAN_POINT ( 'NONE',  ( 19.25663599770060586, -5.499999999999437783, 81.49419308057203182 ) ) ;
#188756=CARTESIAN_POINT ( 'NONE',  ( 19.03943276465977164, -0.05219959533909143690, 23.74890960531435269 ) ) ;
#188757=CARTESIAN_POINT ( 'NONE',  ( -9.564922557960796823, -16.46253265017161027, 27.08224293864769550 ) ) ;
#188758=CARTESIAN_POINT ( 'NONE',  ( -13.89961937509957401, -13.97604488694547875, 109.3760903946856331 ) ) ;
#188761=CARTESIAN_POINT ( 'NONE',  ( -4.483927247898539470, -16.52544592524342804, 112.2905762719810241 ) ) ;
#188762=CARTESIAN_POINT ( 'NONE',  ( 10.72451020669871369, 18.67979575497193778, 82.08442372801901854 ) ) ;
#188763=CARTESIAN_POINT ( 'NONE',  ( 19.02544592524343514, -5.153800228976328945, 58.54057627198102409 ) ) ;
#188764=CARTESIAN_POINT ( 'NONE',  ( 0.05219959533937995610, -21.53943276465977519, 40.00109039468567573 ) ) ;
#188765=CARTESIAN_POINT ( 'NONE',  ( -0.05219959533937732626, 21.53943276465977519, 32.50109039468568284 ) ) ;
#188767=CARTESIAN_POINT ( 'NONE',  ( -9.564922557960796823, -16.46253265017161027, 82.08224293864768129 ) ) ;
#188769=CARTESIAN_POINT ( 'NONE',  ( -8.224510206698735004, -14.34966873604973081, 24.58442372801901499 ) ) ;
#188770=CARTESIAN_POINT ( 'NONE',  ( 10.72451020669898902, -18.67979575497178502, 42.91557627198103120 ) ) ;
#188771=CARTESIAN_POINT ( 'NONE',  ( -15.72974639402176322, -15.80617190586768395, 74.37609039468568994 ) ) ;
#188773=CARTESIAN_POINT ( 'NONE',  ( -9.564922557960796823, -16.46253265017161027, 107.0822429386476955 ) ) ;
#188774=CARTESIAN_POINT ( 'NONE',  ( 9.474510206698729675, 16.51473224551082808, 97.08442372801900433 ) ) ;
#188775=CARTESIAN_POINT ( 'NONE',  ( -5.049401038298153566, 19.05341960407611168, 65.20724293864765286 ) ) ;
#188776=CARTESIAN_POINT ( 'NONE',  ( 16.46253265017160672, -9.564922557960803928, 88.33224293864769550 ) ) ;
#188777=CARTESIAN_POINT ( 'NONE',  ( -8.224510206698948167, 14.34966873604960824, 100.4155762719810241 ) ) ;
#188778=CARTESIAN_POINT ( 'NONE',  ( 14.34966873604960469, 8.224510206698951720, 109.1655762719810383 ) ) ;
#188779=CARTESIAN_POINT ( 'NONE',  ( -13.89961937509977652, 13.97604488694528158, 110.6239096053143243 ) ) ;
#188780=CARTESIAN_POINT ( 'NONE',  ( 16.55341960407618274, -4.379528057220086978, 76.04275706135237556 ) ) ;
#188781=CARTESIAN_POINT ( 'NONE',  ( -4.379528057220328563, 16.55341960407611168, 60.20724293864768839 ) ) ;
#188782=CARTESIAN_POINT ( 'NONE',  ( 5.153800228976335163, 19.02544592524342804, 44.79057627198103830 ) ) ;
#188783=CARTESIAN_POINT ( 'NONE',  ( 15.72974639402176855, 15.80617190586768217, 66.87609039468568994 ) ) ;
#188784=CARTESIAN_POINT ( 'NONE',  ( -13.97604488694547697, 13.89961937509957934, 98.12609039468566152 ) ) ;
#188785=CARTESIAN_POINT ( 'NONE',  ( -0.05219959533910754901, -16.53943276465976808, 62.49890960531436690 ) ) ;
#188786=CARTESIAN_POINT ( 'NONE',  ( 10.72451020669898902, -18.67979575497178502, 112.9155762719810383 ) ) ;
#188787=CARTESIAN_POINT ( 'NONE',  ( 18.67979575497178502, 10.72451020669898547, 44.16557627198103120 ) ) ;
#188790=CARTESIAN_POINT ( 'NONE',  ( 5.049401038298161559, -19.05341960407611168, 72.70724293864768129 ) ) ;
#188791=CARTESIAN_POINT ( 'NONE',  ( -0.05219959533910754901, -16.53943276465976808, 37.49890960531436690 ) ) ;
#188793=CARTESIAN_POINT ( 'NONE',  ( 8.224510206698742110, 14.34966873604972548, 112.0844237280190185 ) ) ;
#188794=CARTESIAN_POINT ( 'NONE',  ( 16.53943276465976808, 0.05219959533934440121, 81.25109039468568994 ) ) ;
#188795=CARTESIAN_POINT ( 'NONE',  ( 13.97604488694548053, -13.89961937509957401, 35.62609039468567573 ) ) ;
#188796=CARTESIAN_POINT ( 'NONE',  ( 16.52216118717208460, 7.221426719304526287, 48.57599021046995347 ) ) ;
#188797=CARTESIAN_POINT ( 'NONE',  ( -0.05219959533909027116, -19.03943276465977164, 97.49890960531436690 ) ) ;
#188798=CARTESIAN_POINT ( 'NONE',  ( -8.224510206698948167, 14.34966873604960824, 55.41557627198102409 ) ) ;
#188799=CARTESIAN_POINT ( 'NONE',  ( 16.81555441253553695, -7.025013491695479395, 103.1368544533426075 ) ) ;
#188800=CARTESIAN_POINT ( 'NONE',  ( -15.80617190586745835, -15.72974639402198527, 21.87390960531436690 ) ) ;
#188801=CARTESIAN_POINT ( 'NONE',  ( 5.823673210054125526, 21.52544592524343514, 54.79057627198104541 ) ) ;
#188803=CARTESIAN_POINT ( 'NONE',  ( 4.483927247898545687, 16.52544592524342804, 104.7905762719810241 ) ) ;
#188804=CARTESIAN_POINT ( 'NONE',  ( -12.06949235617739369, -12.14591786802326823, 34.37609039468568284 ) ) ;
#188805=CARTESIAN_POINT ( 'NONE',  ( 12.14591786802309770, 12.06949235617756955, 79.37390960531436690 ) ) ;
#188806=LINE ( 'NONE', #50289, #51093 ) ;
#188807=CARTESIAN_POINT ( 'NONE',  ( 19.02544592524334988, 5.153800228976608722, 81.45942372801897591 ) ) ;
#188808=CARTESIAN_POINT ( 'NONE',  ( -21.52544592524343514, 5.823673210054127303, 26.04057627198103475 ) ) ;
#188810=CARTESIAN_POINT ( 'NONE',  ( -16.53943276465976808, -0.05219959533934237506, 28.75109039468567929 ) ) ;
#188811=CARTESIAN_POINT ( 'NONE',  ( -16.55341960407611168, -4.379528057220339221, 36.45724293864768839 ) ) ;
#188812=CARTESIAN_POINT ( 'NONE',  ( -18.62759615963270932, 10.81492255796079327, 60.83224293864769550 ) ) ;
#188813=CARTESIAN_POINT ( 'NONE',  ( -16.46253265017146816, -9.564922557961047289, 74.16775706135234714 ) ) ;
#188814=CARTESIAN_POINT ( 'NONE',  ( -5.719274019375978568, 21.55341960407610458, 55.20724293864770260 ) ) ;
#188815=CARTESIAN_POINT ( 'NONE',  ( -5.719274019375665041, -21.55341960407619695, 74.79275706135234714 ) ) ;
#188817=CARTESIAN_POINT ( 'NONE',  ( 0.05219959533934541429, -16.53943276465976808, 40.00109039468567573 ) ) ;
#188818=CARTESIAN_POINT ( 'NONE',  ( 19.05341960407611168, 5.049401038298154454, 28.95724293864769550 ) ) ;
#188819=CARTESIAN_POINT ( 'NONE',  ( -0.05219959533909027116, -19.03943276465977164, 87.49890960531436690 ) ) ;
#188820=CARTESIAN_POINT ( 'NONE',  ( -13.89961937509977652, 13.97604488694528158, 30.62390960531435269 ) ) ;
#188821=CARTESIAN_POINT ( 'NONE',  ( -4.379528057220328563, 16.55341960407611168, 100.2072429386476955 ) ) ;
#188823=CARTESIAN_POINT ( 'NONE',  ( -0.05219959533909027116, -19.03943276465977164, 97.49890960531436690 ) ) ;
#188825=CARTESIAN_POINT ( 'NONE',  ( -4.379528057220086978, -16.55341960407618274, 54.79275706135235424 ) ) ;
#188826=CARTESIAN_POINT ( 'NONE',  ( -15.72974639402197994, 15.80617190586746368, 75.62390960531439532 ) ) ;
#188827=CARTESIAN_POINT ( 'NONE',  ( -5.153800228976328057, -19.02544592524343514, 37.29057627198102409 ) ) ;
#188828=CARTESIAN_POINT ( 'NONE',  ( 19.03943276465977164, 0.05219959533936151252, 76.25109039468566152 ) ) ;
#188829=CARTESIAN_POINT ( 'NONE',  ( 21.52544592524344225, -5.823673210054117533, 108.5405762719810241 ) ) ;
#188830=CARTESIAN_POINT ( 'NONE',  ( 5.049401038298161559, -19.05341960407611168, 67.70724293864769550 ) ) ;
#188831=CARTESIAN_POINT ( 'NONE',  ( -16.46253265017160317, 9.564922557960807481, 110.8322429386476955 ) ) ;
#188833=CARTESIAN_POINT ( 'NONE',  ( 14.29746914071037800, 8.314922557961029526, 36.66775706135234714 ) ) ;
#188834=CARTESIAN_POINT ( 'NONE',  ( 21.52544592524344225, -5.823673210054117533, 98.54057627198105251 ) ) ;
#188835=CARTESIAN_POINT ( 'NONE',  ( 12.06949235617757843, -12.14591786802309237, 103.1239096053143811 ) ) ;
#188836=CARTESIAN_POINT ( 'NONE',  ( 19.05341960407611168, 5.049401038298154454, 88.95724293864769550 ) ) ;
#188837=CARTESIAN_POINT ( 'NONE',  ( 5.153800228976615827, -19.02544592524334988, 80.20942372801901854 ) ) ;
#188838=CARTESIAN_POINT ( 'NONE',  ( -18.62759615963270932, 10.81492255796079327, 80.83224293864769550 ) ) ;
#188839=CARTESIAN_POINT ( 'NONE',  ( -8.314922557960811034, -14.29746914071050412, 52.08224293864768839 ) ) ;
#188840=CARTESIAN_POINT ( 'NONE',  ( 19.02544592524334988, 5.153800228976608722, 26.45942372801899722 ) ) ;
#188841=CARTESIAN_POINT ( 'NONE',  ( -14.34966873604972548, 8.224510206698743886, 78.33442372801901854 ) ) ;
#188842=CARTESIAN_POINT ( 'NONE',  ( 13.97604488694527802, 13.89961937509977652, 89.37390960531436690 ) ) ;
#188844=CARTESIAN_POINT ( 'NONE',  ( 19.03943276465977164, -0.05219959533909143690, 43.74890960531435979 ) ) ;
#188845=CARTESIAN_POINT ( 'NONE',  ( -5.823673210054431948, 21.52544592524334988, 57.70942372801901143 ) ) ;
#188846=CARTESIAN_POINT ( 'NONE',  ( 5.719274019375673035, 21.55341960407619339, 72.29275706135236135 ) ) ;
#188847=CARTESIAN_POINT ( 'NONE',  ( -9.564922557960796823, -16.46253265017161027, 62.08224293864769550 ) ) ;
#188848=CARTESIAN_POINT ( 'NONE',  ( -10.72451020669870658, -18.67979575497194134, 34.58442372801900433 ) ) ;
#188849=CARTESIAN_POINT ( 'NONE',  ( 0.05219959533936267826, -19.03943276465977164, 90.00109039468567573 ) ) ;
#188850=CARTESIAN_POINT ( 'NONE',  ( -19.05341960407611168, -5.049401038298163336, 36.45724293864766707 ) ) ;
#188851=CARTESIAN_POINT ( 'NONE',  ( 4.483927247898790824, -16.52544592524335698, 85.20942372801901854 ) ) ;
#188852=CARTESIAN_POINT ( 'NONE',  ( -5.153800228976328057, -19.02544592524343514, 67.29057627198102409 ) ) ;
#188853=CARTESIAN_POINT ( 'NONE',  ( 13.97604488694527802, 13.89961937509977652, 109.3739096053143669 ) ) ;
#188854=CARTESIAN_POINT ( 'NONE',  ( 5.049401038298161559, -19.05341960407611168, 47.70724293864770260 ) ) ;
#188855=VECTOR ( 'NONE', #171174, 1000.000000000000000 ) ;
#188856=CARTESIAN_POINT ( 'NONE',  ( 15.80617190586746368, 15.72974639402197994, 89.37390960531435269 ) ) ;
#188857=CARTESIAN_POINT ( 'NONE',  ( -4.379528057220086978, -16.55341960407618274, 74.79275706135234714 ) ) ;
#188859=CARTESIAN_POINT ( 'NONE',  ( -19.03943276465977164, -0.05219959533935918106, 33.75109039468566863 ) ) ;
#188860=CARTESIAN_POINT ( 'NONE',  ( -19.02544592524342804, 5.153800228976336051, 61.04057627198103120 ) ) ;
#188861=CARTESIAN_POINT ( 'NONE',  ( 0.05219959533910956823, 16.53943276465976808, 49.99890960531437401 ) ) ;
#188862=CARTESIAN_POINT ( 'NONE',  ( 16.52544592524342804, -4.483927247898539470, 83.54057627198102409 ) ) ;
#188863=CARTESIAN_POINT ( 'NONE',  ( 0.05219959533909260263, 19.03943276465977164, 104.9989096053143669 ) ) ;
#188864=CARTESIAN_POINT ( 'NONE',  ( 16.51473224551069308, 9.474510206698969483, 94.16557627198103830 ) ) ;
#188865=CARTESIAN_POINT ( 'NONE',  ( 21.55341960407619695, -5.719274019375665929, 56.04275706135235424 ) ) ;
#188866=CARTESIAN_POINT ( 'NONE',  ( -19.02544592524342804, 5.153800228976336051, 101.0405762719810241 ) ) ;
#188867=CARTESIAN_POINT ( 'NONE',  ( -18.62759615963255300, -10.81492255796106328, 109.1677570613523613 ) ) ;
#188868=CARTESIAN_POINT ( 'NONE',  ( -8.224510206698735004, -14.34966873604973081, 79.58442372801903275 ) ) ;
#188869=CARTESIAN_POINT ( 'NONE',  ( 10.81492255796106328, -18.62759615963255655, 30.41775706135234358 ) ) ;
#188870=CARTESIAN_POINT ( 'NONE',  ( -19.03943276465977164, 0.05219959533909376836, 111.2489096053143669 ) ) ;
#188871=CARTESIAN_POINT ( 'NONE',  ( 18.62759615963271287, -10.81492255796078972, 108.3322429386477097 ) ) ;
#188872=CARTESIAN_POINT ( 'NONE',  ( 16.55341960407611168, 4.379528057220329451, 53.95724293864770260 ) ) ;
#188874=CARTESIAN_POINT ( 'NONE',  ( -19.02544592524342804, 5.153800228976336051, 41.04057627198103120 ) ) ;
#188875=CARTESIAN_POINT ( 'NONE',  ( 16.55341960407611168, 4.379528057220329451, 78.95724293864769550 ) ) ;
#188876=CARTESIAN_POINT ( 'NONE',  ( 18.62759615963271287, -10.81492255796078972, 33.33224293864769550 ) ) ;
#188877=CARTESIAN_POINT ( 'NONE',  ( 0.05219959533936267826, -19.03943276465977164, 50.00109039468566863 ) ) ;
#188879=CARTESIAN_POINT ( 'NONE',  ( 4.483927247898545687, 16.52544592524342804, 114.7905762719810383 ) ) ;
#188881=CARTESIAN_POINT ( 'NONE',  ( 16.55341960407618274, -4.379528057220086978, 61.04275706135234714 ) ) ;
#188882=CARTESIAN_POINT ( 'NONE',  ( 9.564922557960805705, 16.46253265017160317, 69.58224293864770971 ) ) ;
#188884=CARTESIAN_POINT ( 'NONE',  ( -14.34966873604960291, -8.224510206698953496, 86.66557627198102409 ) ) ;
#188885=CARTESIAN_POINT ( 'NONE',  ( 18.62759615963271287, -10.81492255796078972, 38.33224293864768839 ) ) ;
#188886=CARTESIAN_POINT ( 'NONE',  ( 12.14591786802327356, -12.06949235617739191, 105.6260903946856899 ) ) ;
#188887=CARTESIAN_POINT ( 'NONE',  ( -5.153800228976607833, 19.02544592524334988, 102.7094237280189759 ) ) ;
#188888=CARTESIAN_POINT ( 'NONE',  ( 15.72974639402176855, 15.80617190586768217, 81.87609039468568994 ) ) ;
#188889=CARTESIAN_POINT ( 'NONE',  ( 5.153800228976335163, 19.02544592524342804, 89.79057627198102409 ) ) ;
#188890=CARTESIAN_POINT ( 'NONE',  ( 21.52544592524344225, -5.823673210054117533, 98.54057627198105251 ) ) ;
#188891=CARTESIAN_POINT ( 'NONE',  ( -8.314922557961024197, 14.29746914071037800, 57.91775706135234714 ) ) ;
#188893=CARTESIAN_POINT ( 'NONE',  ( -19.05341960407611168, -5.049401038298163336, 36.45724293864766707 ) ) ;
#188894=CARTESIAN_POINT ( 'NONE',  ( -4.483927247898782831, 16.52544592524335698, 37.70942372801900433 ) ) ;
#188895=CARTESIAN_POINT ( 'NONE',  ( 5.153800228976615827, -19.02544592524334988, 100.2094237280190043 ) ) ;
#188896=CARTESIAN_POINT ( 'NONE',  ( 15.80617190586746368, 15.72974639402197994, 89.37390960531435269 ) ) ;
#188897=CARTESIAN_POINT ( 'NONE',  ( -5.153800228976607833, 19.02544592524334988, 52.70942372801900433 ) ) ;
#188899=CARTESIAN_POINT ( 'NONE',  ( -18.62759615963270932, 10.81492255796079327, 100.8322429386477097 ) ) ;
#188900=CARTESIAN_POINT ( 'NONE',  ( 17.50000000000002842, 3.512728167236816912, 27.27190004818877966 ) ) ;
#188901=CARTESIAN_POINT ( 'NONE',  ( 5.153800228976335163, 19.02544592524342804, 74.79057627198103830 ) ) ;
#188904=CARTESIAN_POINT ( 'NONE',  ( -0.05219959533934338120, 16.53943276465976808, 32.50109039468568284 ) ) ;
#188906=CARTESIAN_POINT ( 'NONE',  ( -18.67979575497178146, -10.72451020669898902, 111.6655762719810525 ) ) ;
#188907=CARTESIAN_POINT ( 'NONE',  ( 12.14591786802309770, 12.06949235617756955, 64.37390960531435269 ) ) ;
#188908=CARTESIAN_POINT ( 'NONE',  ( -13.89961937509977652, 13.97604488694528158, 65.62390960531436690 ) ) ;
#188911=CARTESIAN_POINT ( 'NONE',  ( -14.29746914071037622, -8.314922557961029526, 39.16775706135235424 ) ) ;
#188912=CARTESIAN_POINT ( 'NONE',  ( 19.02544592524334988, 5.153800228976608722, 41.45942372801900433 ) ) ;
#188913=CARTESIAN_POINT ( 'NONE',  ( -21.53943276465977519, -0.05219959533937600094, 53.75109039468568994 ) ) ;
#188914=CARTESIAN_POINT ( 'NONE',  ( 9.474510206698729675, 16.51473224551082808, 112.0844237280190043 ) ) ;
#188915=CARTESIAN_POINT ( 'NONE',  ( -13.97604488694527625, -13.89961937509977652, 56.87390960531434558 ) ) ;
#188916=CARTESIAN_POINT ( 'NONE',  ( -16.46253265017146816, -9.564922557961047289, 79.16775706135234714 ) ) ;
#188917=CARTESIAN_POINT ( 'NONE',  ( -21.52544592524334988, -5.823673210054445271, 83.95942372801900433 ) ) ;
#188918=CARTESIAN_POINT ( 'NONE',  ( 9.474510206698729675, 16.51473224551082808, 62.08442372801899722 ) ) ;
#188919=CARTESIAN_POINT ( 'NONE',  ( 9.474510206698971260, -16.51473224551069308, 37.91557627198102409 ) ) ;
#188920=CARTESIAN_POINT ( 'NONE',  ( -21.53943276465977519, 0.05219959533907696930, 61.24890960531435979 ) ) ;
#188921=CARTESIAN_POINT ( 'NONE',  ( -16.52544592524342804, 4.483927247898546575, 61.04057627198103120 ) ) ;
#188922=CARTESIAN_POINT ( 'NONE',  ( 19.02544592524334988, 5.153800228976608722, 66.45942372801899012 ) ) ;
#188923=CARTESIAN_POINT ( 'NONE',  ( -17.72662750342726667, -5.499999999999957367, 101.4017949228374391 ) ) ;
#188924=CARTESIAN_POINT ( 'NONE',  ( -19.03943276465977164, -0.05219959533935918106, 23.75109039468566152 ) ) ;
#188925=CARTESIAN_POINT ( 'NONE',  ( -14.29746914071037622, -8.314922557961029526, 99.16775706135234714 ) ) ;
#188926=CARTESIAN_POINT ( 'NONE',  ( 12.14591786802309770, 12.06949235617756955, 54.37390960531435979 ) ) ;
#188927=CARTESIAN_POINT ( 'NONE',  ( 10.72451020669871369, 18.67979575497193778, 92.08442372801901854 ) ) ;
#188929=CARTESIAN_POINT ( 'NONE',  ( -15.72974639402176322, -15.80617190586768395, 89.37609039468568994 ) ) ;
#188930=CARTESIAN_POINT ( 'NONE',  ( -21.53943276465977519, 0.05219959533907696930, 96.24890960531435269 ) ) ;
#188931=CARTESIAN_POINT ( 'NONE',  ( -16.46253265017160317, 9.564922557960807481, 50.83224293864770260 ) ) ;
#188932=CARTESIAN_POINT ( 'NONE',  ( -21.52544592524334988, -5.823673210054445271, 73.95942372801901854 ) ) ;
#188933=CARTESIAN_POINT ( 'NONE',  ( -16.46253265017160317, 9.564922557960807481, 50.83224293864770260 ) ) ;
#188935=CARTESIAN_POINT ( 'NONE',  ( -19.03943276465977164, 0.05219959533909376836, 66.24890960531436690 ) ) ;
#188936=CARTESIAN_POINT ( 'NONE',  ( -12.14591786802309592, -12.06949235617757132, 111.8739096053143669 ) ) ;
#188937=CARTESIAN_POINT ( 'NONE',  ( 19.03943276465977164, -0.05219959533909143690, 108.7489096053143527 ) ) ;
#188938=CARTESIAN_POINT ( 'NONE',  ( 12.14591786802309770, 12.06949235617756955, 49.37390960531436690 ) ) ;
#188939=CARTESIAN_POINT ( 'NONE',  ( 13.97604488694527802, 13.89961937509977652, 29.37390960531435979 ) ) ;
#188940=CARTESIAN_POINT ( 'NONE',  ( 12.14591786802309770, 12.06949235617756955, 74.37390960531436690 ) ) ;
#188942=CARTESIAN_POINT ( 'NONE',  ( 21.52544592524344225, -5.823673210054117533, 93.54057627198103830 ) ) ;
#188943=CARTESIAN_POINT ( 'NONE',  ( -5.823673210054431948, 21.52544592524334988, 32.70942372801900433 ) ) ;
#188945=CARTESIAN_POINT ( 'NONE',  ( -12.06949235617739369, -12.14591786802326823, 34.37609039468568284 ) ) ;
#188946=CARTESIAN_POINT ( 'NONE',  ( 5.719274019375991003, -21.55341960407610458, 82.70724293864770971 ) ) ;
#188947=CARTESIAN_POINT ( 'NONE',  ( -15.72974639402176322, -15.80617190586768395, 104.3760903946856899 ) ) ;
#188948=CARTESIAN_POINT ( 'NONE',  ( -19.02544592524342804, 5.153800228976336051, 91.04057627198100988 ) ) ;
#188949=CARTESIAN_POINT ( 'NONE',  ( -15.80617190586768217, 15.72974639402176855, 48.12609039468568284 ) ) ;
#188950=CARTESIAN_POINT ( 'NONE',  ( 10.81492255796078972, 18.62759615963270932, 24.58224293864768839 ) ) ;
#188951=CARTESIAN_POINT ( 'NONE',  ( 4.379528057220092307, 16.55341960407617563, 97.29275706135234714 ) ) ;
#188952=CARTESIAN_POINT ( 'NONE',  ( 15.72974639402176855, 15.80617190586768217, 46.87609039468568994 ) ) ;
#188953=CARTESIAN_POINT ( 'NONE',  ( -15.80617190586768217, 15.72974639402176855, 88.12609039468570415 ) ) ;
#188954=CARTESIAN_POINT ( 'NONE',  ( 21.53943276465977519, 0.05219959533937863772, 111.2510903946856899 ) ) ;
#188955=CARTESIAN_POINT ( 'NONE',  ( 8.314922557961029526, -14.29746914071037800, 85.41775706135236135 ) ) ;
#188956=CARTESIAN_POINT ( 'NONE',  ( 21.55341960407619695, -5.719274019375665929, 41.04275706135236135 ) ) ;
#188957=CARTESIAN_POINT ( 'NONE',  ( -16.51473224551069308, -9.474510206698971260, 26.66557627198103120 ) ) ;
#188958=CARTESIAN_POINT ( 'NONE',  ( -10.81492255796105439, 18.62759615963255655, 97.91775706135236135 ) ) ;
#188959=CARTESIAN_POINT ( 'NONE',  ( 13.97604488694527802, 13.89961937509977652, 104.3739096053143385 ) ) ;
#188960=CARTESIAN_POINT ( 'NONE',  ( -5.719274019375978568, 21.55341960407610458, 105.2072429386477097 ) ) ;
#188961=CARTESIAN_POINT ( 'NONE',  ( 5.719274019375991003, -21.55341960407610458, 62.70724293864769550 ) ) ;
#188963=CARTESIAN_POINT ( 'NONE',  ( -21.55341960407610458, -5.719274019375992779, 71.45724293864769550 ) ) ;
#188964=CARTESIAN_POINT ( 'NONE',  ( -8.314922557961024197, 14.29746914071037800, 57.91775706135234714 ) ) ;
#188965=CARTESIAN_POINT ( 'NONE',  ( 12.14591786802309770, 12.06949235617756955, 59.37390960531436690 ) ) ;
#188967=CARTESIAN_POINT ( 'NONE',  ( -19.05341960407617563, 5.049401038297882671, 88.54275706135230450 ) ) ;
#188969=CARTESIAN_POINT ( 'NONE',  ( 14.29746914071037800, 8.314922557961029526, 31.66775706135234358 ) ) ;
#188970=CARTESIAN_POINT ( 'NONE',  ( -15.80617190586745835, -15.72974639402198527, 101.8739096053143811 ) ) ;
#188971=CARTESIAN_POINT ( 'NONE',  ( -21.55341960407610458, -5.719274019375992779, 76.45724293864769550 ) ) ;
#188972=CARTESIAN_POINT ( 'NONE',  ( 18.62759615963271287, -10.81492255796078972, 23.33224293864769194 ) ) ;
#188973=CARTESIAN_POINT ( 'NONE',  ( -16.55341960407617563, 4.379528057220093196, 53.54275706135234714 ) ) ;
#188974=CARTESIAN_POINT ( 'NONE',  ( 0.05219959533909260263, 19.03943276465977164, 69.99890960531435269 ) ) ;
#188975=CARTESIAN_POINT ( 'NONE',  ( -10.72451020669870658, -18.67979575497194134, 24.58442372801901499 ) ) ;
#188976=CARTESIAN_POINT ( 'NONE',  ( -16.46253265017146816, -9.564922557961047289, 104.1677570613523329 ) ) ;
#188977=CARTESIAN_POINT ( 'NONE',  ( 19.03943276465977164, -0.05219959533909143690, 108.7489096053143527 ) ) ;
#188978=CARTESIAN_POINT ( 'NONE',  ( 19.02544592524343514, -5.153800228976328945, 88.54057627198102409 ) ) ;
#188979=CARTESIAN_POINT ( 'NONE',  ( 10.81492255796078972, 18.62759615963270932, 84.58224293864769550 ) ) ;
#188980=CARTESIAN_POINT ( 'NONE',  ( -16.46253265017160317, 9.564922557960807481, 60.83224293864769550 ) ) ;
#188981=CARTESIAN_POINT ( 'NONE',  ( -17.49999999999999645, -5.499999999999992895, 59.20309617465829177 ) ) ;
#188982=CARTESIAN_POINT ( 'NONE',  ( 8.314922557960818139, 14.29746914071049879, 74.58224293864768129 ) ) ;
#188983=CARTESIAN_POINT ( 'NONE',  ( 18.62759615963271287, -10.81492255796078972, 28.33224293864769550 ) ) ;
#188986=CARTESIAN_POINT ( 'NONE',  ( 5.719274019375991003, -21.55341960407610458, 107.7072429386476955 ) ) ;
#188987=CARTESIAN_POINT ( 'NONE',  ( -16.51473224551082808, 9.474510206698731452, 68.33442372801900433 ) ) ;
#188988=CARTESIAN_POINT ( 'NONE',  ( -19.03943276465977164, 0.05219959533909376836, 116.2489096053143669 ) ) ;
#188989=CARTESIAN_POINT ( 'NONE',  ( -10.81492255796078084, -18.62759615963271287, 57.08224293864769550 ) ) ;
#188990=CARTESIAN_POINT ( 'NONE',  ( -19.03943276465977164, 0.05219959533909376836, 91.24890960531436690 ) ) ;
#188991=CARTESIAN_POINT ( 'NONE',  ( 18.62759615963255655, 10.81492255796105972, 81.66775706135236135 ) ) ;
#188992=CARTESIAN_POINT ( 'NONE',  ( 13.97604488694527802, 13.89961937509977652, 49.37390960531434558 ) ) ;
#188993=CARTESIAN_POINT ( 'NONE',  ( 4.483927247898545687, 16.52544592524342804, 89.79057627198103830 ) ) ;
#188994=CARTESIAN_POINT ( 'NONE',  ( -8.224510206698735004, -14.34966873604973081, 34.58442372801900433 ) ) ;
#188995=CARTESIAN_POINT ( 'NONE',  ( -21.52544592524334988, -5.823673210054445271, 63.95942372801901854 ) ) ;
#188997=CARTESIAN_POINT ( 'NONE',  ( 9.474510206698729675, 16.51473224551082808, 32.08442372801900433 ) ) ;
#188998=CARTESIAN_POINT ( 'NONE',  ( 13.97604488694548053, -13.89961937509957401, 80.62609039468567573 ) ) ;
#188999=CARTESIAN_POINT ( 'NONE',  ( 13.89961937509957401, 13.97604488694547697, 41.87609039468566152 ) ) ;
#189001=CARTESIAN_POINT ( 'NONE',  ( -10.72451020669870658, -18.67979575497194134, 39.58442372801901143 ) ) ;
#189003=CARTESIAN_POINT ( 'NONE',  ( -5.049401038297874678, -19.05341960407617918, 34.79275706135233293 ) ) ;
#189004=CARTESIAN_POINT ( 'NONE',  ( 9.564922557960805705, 16.46253265017160317, 59.58224293864769550 ) ) ;
#189005=CARTESIAN_POINT ( 'NONE',  ( 19.02544592524334988, 5.153800228976608722, 26.45942372801899722 ) ) ;
#189006=CARTESIAN_POINT ( 'NONE',  ( -16.55341960407617563, 4.379528057220093196, 98.54275706135234714 ) ) ;
#189007=CARTESIAN_POINT ( 'NONE',  ( -5.823673210054116645, -21.52544592524344225, 27.29057627198103120 ) ) ;
#189008=CARTESIAN_POINT ( 'NONE',  ( -10.72451020669870658, -18.67979575497194134, 84.58442372801903275 ) ) ;
#189010=CARTESIAN_POINT ( 'NONE',  ( -17.50000000000000355, -3.209263204892690791, 35.23803174393751192 ) ) ;
#189011=CARTESIAN_POINT ( 'NONE',  ( 10.81492255796106328, -18.62759615963255655, 85.41775706135236135 ) ) ;
#189013=CARTESIAN_POINT ( 'NONE',  ( -13.97604488694527625, -13.89961937509977652, 106.8739096053143669 ) ) ;
#189016=CARTESIAN_POINT ( 'NONE',  ( 19.05341960407611168, 5.049401038298154454, 58.95724293864768129 ) ) ;
#189017=CARTESIAN_POINT ( 'NONE',  ( 15.80617190586746368, 15.72974639402197994, 59.37390960531436690 ) ) ;
#189018=CARTESIAN_POINT ( 'NONE',  ( -12.14591786802309592, -12.06949235617757132, 21.87390960531436690 ) ) ;
#189019=CARTESIAN_POINT ( 'NONE',  ( 14.34966873604960469, 8.224510206698951720, 94.16557627198103830 ) ) ;
#189020=CARTESIAN_POINT ( 'NONE',  ( -19.05341960407611168, -5.049401038298163336, 86.45724293864769550 ) ) ;
#189021=CARTESIAN_POINT ( 'NONE',  ( 0.05219959533936267826, -19.03943276465977164, 25.00109039468566152 ) ) ;
#189022=CARTESIAN_POINT ( 'NONE',  ( 16.46253265017160672, -9.564922557960803928, 33.33224293864770260 ) ) ;
#189023=CARTESIAN_POINT ( 'NONE',  ( -16.55341960407611168, -4.379528057220339221, 106.4572429386477097 ) ) ;
#189024=CARTESIAN_POINT ( 'NONE',  ( 5.823673210054444382, -21.52544592524334988, 50.20942372801901854 ) ) ;
#189025=CARTESIAN_POINT ( 'NONE',  ( -21.52544592524343514, 5.823673210054127303, 86.04057627198102409 ) ) ;
#189026=CARTESIAN_POINT ( 'NONE',  ( 5.153800228976615827, -19.02544592524334988, 70.20942372801899012 ) ) ;
#189027=DIRECTION ( 'NONE',  ( -1.000000000000000000, 0.000000000000000000, 0.000000000000000000 ) ) ;
#189028=CARTESIAN_POINT ( 'NONE',  ( -0.05219959533909027116, -19.03943276465977164, 107.4989096053143527 ) ) ;
#189029=CARTESIAN_POINT ( 'NONE',  ( 0.05219959533910956823, 16.53943276465976808, 74.99890960531435269 ) ) ;
#189031=CARTESIAN_POINT ( 'NONE',  ( 0.05219959533936267826, -19.03943276465977164, 45.00109039468566863 ) ) ;
#189032=CARTESIAN_POINT ( 'NONE',  ( -13.89961937509977652, 13.97604488694528158, 65.62390960531436690 ) ) ;
#189033=CARTESIAN_POINT ( 'NONE',  ( -0.05219959533910754901, -16.53943276465976808, 67.49890960531436690 ) ) ;
#189034=CARTESIAN_POINT ( 'NONE',  ( 9.564922557961047289, -16.46253265017146816, 75.41775706135234714 ) ) ;
#189035=CARTESIAN_POINT ( 'NONE',  ( 21.55341960407610458, 5.719274019375980345, 38.95724293864768839 ) ) ;
#189037=CARTESIAN_POINT ( 'NONE',  ( -4.483927247898539470, -16.52544592524342804, 107.2905762719810525 ) ) ;
#189039=CARTESIAN_POINT ( 'NONE',  ( 19.02544592524343514, -5.153800228976328945, 53.54057627198102409 ) ) ;
#189040=CARTESIAN_POINT ( 'NONE',  ( 18.62759615963271287, -10.81492255796078972, 68.33224293864769550 ) ) ;
#189041=CARTESIAN_POINT ( 'NONE',  ( -16.51473224551069308, -9.474510206698971260, 41.66557627198103120 ) ) ;
#189042=CARTESIAN_POINT ( 'NONE',  ( -12.14591786802326823, 12.06949235617739902, 78.12609039468570415 ) ) ;
#189043=CARTESIAN_POINT ( 'NONE',  ( 19.02544592524343514, -5.153800228976328945, 73.54057627198103830 ) ) ;
#189044=CARTESIAN_POINT ( 'NONE',  ( -16.51473224551082808, 9.474510206698731452, 58.33442372801900433 ) ) ;
#189045=CARTESIAN_POINT ( 'NONE',  ( 15.80617190586769283, -15.72974639402175789, 65.62609039468568994 ) ) ;
#189046=CARTESIAN_POINT ( 'NONE',  ( -5.719274019375978568, 21.55341960407610458, 50.20724293864769550 ) ) ;
#189047=CARTESIAN_POINT ( 'NONE',  ( -0.05219959533909027116, -19.03943276465977164, 107.4989096053143527 ) ) ;
#189048=CARTESIAN_POINT ( 'NONE',  ( 9.474510206698971260, -16.51473224551069308, 27.91557627198103120 ) ) ;
#189049=CARTESIAN_POINT ( 'NONE',  ( -16.55341960407617563, 4.379528057220093196, 83.54275706135234714 ) ) ;
#189050=CARTESIAN_POINT ( 'NONE',  ( -0.05219959533936034679, 19.03943276465977164, 107.5010903946856615 ) ) ;
#189052=CARTESIAN_POINT ( 'NONE',  ( 19.25918095147779496, 5.499999999999574563, 76.95284276293931214 ) ) ;
#189053=CARTESIAN_POINT ( 'NONE',  ( -10.72451020669870658, -18.67979575497194134, 99.58442372801900433 ) ) ;
#189054=AXIS2_PLACEMENT_3D ( 'NONE', #11984, #101976, #163656 ) ;
#189056=CARTESIAN_POINT ( 'NONE',  ( -12.06949235617756955, 12.14591786802309770, 60.62390960531437401 ) ) ;
#189057=( BOUNDED_CURVE ( )  B_SPLINE_CURVE ( 2, ( #68120, #176322, #85280, #99454, #161134, #84277, #145958, #83283, #69123, #82272, #130790, #100456, #101449 ),
 .UNSPECIFIED., .F., .T. ) 
 B_SPLINE_CURVE_WITH_KNOTS ( ( 3, 2, 2, 2, 2, 2, 3 ),
 ( 0.2919041206375714848, 0.2938596491228070429, 0.2982456140350877027, 0.3026315789473684181, 0.3070175438596491335, 0.3114035087719298489, 0.3133133574350753237 ),
 .UNSPECIFIED. ) 
 CURVE ( )  GEOMETRIC_REPRESENTATION_ITEM ( )  RATIONAL_B_SPLINE_CURVE ( ( 0.9831626618144004848, 0.9848076720550091867, 1.000000000000000000, 0.9659258262890683122, 1.000000000000000000, 0.9659258262890683122, 1.000000000000000000, 0.9659258262890683122, 1.000000000000000000, 0.9659258262890683122, 1.000000000000000000, 0.9851625545550088958, 0.9832469066685279868 ) ) 
 REPRESENTATION_ITEM ( '' )  );
#189058=CARTESIAN_POINT ( 'NONE',  ( -12.06949235617756955, 12.14591786802309770, 70.62390960531436690 ) ) ;
#189059=CARTESIAN_POINT ( 'NONE',  ( -5.823673210054116645, -21.52544592524344225, 97.29057627198105251 ) ) ;
#189060=CARTESIAN_POINT ( 'NONE',  ( -0.05219959533907301413, -21.53943276465977519, 82.49890960531436690 ) ) ;
#189061=CARTESIAN_POINT ( 'NONE',  ( 17.31728774477274158, -6.344390552232389346, 98.31906651689324406 ) ) ;
#189062=CARTESIAN_POINT ( 'NONE',  ( -5.719274019375978568, 21.55341960407610458, 35.20724293864768839 ) ) ;
#189063=CARTESIAN_POINT ( 'NONE',  ( -16.52544592524335698, -4.483927247898792601, 68.95942372801901854 ) ) ;
#189065=CARTESIAN_POINT ( 'NONE',  ( 4.379528057220339221, -16.55341960407611168, 97.70724293864772392 ) ) ;
#189066=CARTESIAN_POINT ( 'NONE',  ( 0.05219959533909260263, 19.03943276465977164, 44.99890960531435979 ) ) ;
#189068=CARTESIAN_POINT ( 'NONE',  ( -8.314922557961024197, 14.29746914071037800, 97.91775706135236135 ) ) ;
#189069=CARTESIAN_POINT ( 'NONE',  ( 10.72451020669871369, 18.67979575497193778, 32.08442372801901854 ) ) ;
#189070=CARTESIAN_POINT ( 'NONE',  ( -5.153800228976328057, -19.02544592524343514, 87.29057627198103830 ) ) ;
#189071=CARTESIAN_POINT ( 'NONE',  ( -15.72974639402176322, -15.80617190586768395, 69.37609039468567573 ) ) ;
#189072=CARTESIAN_POINT ( 'NONE',  ( 5.049401038298161559, -19.05341960407611168, 112.7072429386476813 ) ) ;
#189074=EDGE_LOOP ( 'NONE', ( #102658, #162142, #170882, #115826 ) ) ;
#189075=CARTESIAN_POINT ( 'NONE',  ( 21.53943276465977519, 0.05219959533937863772, 56.25109039468568284 ) ) ;
#189076=CARTESIAN_POINT ( 'NONE',  ( 0.05219959533909260263, 19.03943276465977164, 34.99890960531435979 ) ) ;
#189077=CARTESIAN_POINT ( 'NONE',  ( -19.02544592524342804, 5.153800228976336051, 111.0405762719810099 ) ) ;
#189078=CARTESIAN_POINT ( 'NONE',  ( -5.049401038297874678, -19.05341960407617918, 64.79275706135233293 ) ) ;
#189079=CARTESIAN_POINT ( 'NONE',  ( 10.81492255796106328, -18.62759615963255655, 30.41775706135234358 ) ) ;
#189080=CARTESIAN_POINT ( 'NONE',  ( 16.46253265017146816, 9.564922557961045513, 61.66775706135234003 ) ) ;
#189081=CARTESIAN_POINT ( 'NONE',  ( -19.03943276465977164, 0.05219959533909376836, 26.24890960531435624 ) ) ;
#189082=CARTESIAN_POINT ( 'NONE',  ( 12.14591786802327356, -12.06949235617739191, 90.62609039468567573 ) ) ;
#189083=CARTESIAN_POINT ( 'NONE',  ( 16.51473224551083163, -9.474510206698727899, 60.83442372801900433 ) ) ;
#189084=CARTESIAN_POINT ( 'NONE',  ( 16.53943276465976808, -0.05219959533910856209, 28.74890960531435624 ) ) ;
#189085=CARTESIAN_POINT ( 'NONE',  ( 5.153800228976615827, -19.02544592524334988, 50.20942372801897591 ) ) ;
#189086=CARTESIAN_POINT ( 'NONE',  ( -19.03943276465977164, 0.05219959533909376836, 86.24890960531436690 ) ) ;
#189087=CARTESIAN_POINT ( 'NONE',  ( -18.67979575497193778, 10.72451020669871902, 98.33442372801901854 ) ) ;
#189088=CARTESIAN_POINT ( 'NONE',  ( 21.55341960407619695, -5.719274019375665929, 106.0427570613523471 ) ) ;
#189090=DIRECTION ( 'NONE',  ( -1.000000000000000000, -0.000000000000000000, -0.000000000000000000 ) ) ;
#189091=CARTESIAN_POINT ( 'NONE',  ( -15.80617190586768217, 15.72974639402176855, 88.12609039468570415 ) ) ;
#189092=CARTESIAN_POINT ( 'NONE',  ( -16.53943276465976808, -0.05219959533934237506, 38.75109039468567573 ) ) ;
#189093=CARTESIAN_POINT ( 'NONE',  ( 19.03943276465977164, -0.05219959533909143690, 98.74890960531436690 ) ) ;
#189094=CARTESIAN_POINT ( 'NONE',  ( -0.05219959533907301413, -21.53943276465977519, 27.49890960531435269 ) ) ;
#189096=CARTESIAN_POINT ( 'NONE',  ( 9.474510206698971260, -16.51473224551069308, 77.91557627198103830 ) ) ;
#189097=CARTESIAN_POINT ( 'NONE',  ( -18.56101223717331905, -5.499999999999949374, 41.44978406935677384 ) ) ;
#189098=CARTESIAN_POINT ( 'NONE',  ( 13.89961937509957401, 13.97604488694547697, 76.87609039468566152 ) ) ;
#189099=CARTESIAN_POINT ( 'NONE',  ( -5.153800228976328057, -19.02544592524343514, 112.2905762719810099 ) ) ;
#189100=CARTESIAN_POINT ( 'NONE',  ( -15.80617190586768217, 15.72974639402176855, 103.1260903946856757 ) ) ;
#189101=CARTESIAN_POINT ( 'NONE',  ( 16.53943276465976808, -0.05219959533910856209, 98.74890960531438111 ) ) ;
#189102=CARTESIAN_POINT ( 'NONE',  ( -5.719274019375978568, 21.55341960407610458, 45.20724293864769550 ) ) ;
#189103=CARTESIAN_POINT ( 'NONE',  ( 15.80617190586746368, 15.72974639402197994, 34.37390960531435979 ) ) ;
#189104=CARTESIAN_POINT ( 'NONE',  ( 8.314922557960818139, 14.29746914071049879, 99.58224293864770971 ) ) ;
#189106=CARTESIAN_POINT ( 'NONE',  ( -5.153800228976607833, 19.02544592524334988, 52.70942372801900433 ) ) ;
#189107=CARTESIAN_POINT ( 'NONE',  ( 14.29746914071049879, -8.314922557960816363, 28.33224293864769550 ) ) ;
#189108=CARTESIAN_POINT ( 'NONE',  ( -16.46253265017160317, 9.564922557960807481, 95.83224293864769550 ) ) ;
#189109=CARTESIAN_POINT ( 'NONE',  ( -18.62759615963255300, -10.81492255796106328, 79.16775706135234714 ) ) ;
#189110=CARTESIAN_POINT ( 'NONE',  ( 5.719274019375991003, -21.55341960407610458, 57.70724293864770260 ) ) ;
#189111=CARTESIAN_POINT ( 'NONE',  ( 21.53943276465977519, 0.05219959533937863772, 51.25109039468568994 ) ) ;
#189112=CARTESIAN_POINT ( 'NONE',  ( -0.05219959533907301413, -21.53943276465977519, 92.49890960531436690 ) ) ;
#189113=CARTESIAN_POINT ( 'NONE',  ( -21.55341960407619339, 5.719274019375674811, 33.54275706135234714 ) ) ;
#189114=CARTESIAN_POINT ( 'NONE',  ( -9.474510206698964154, 16.51473224551069663, 25.41557627198103120 ) ) ;
#189115=CARTESIAN_POINT ( 'NONE',  ( 19.03943276465977164, -0.05219959533909143690, 78.74890960531436690 ) ) ;
#189116=CARTESIAN_POINT ( 'NONE',  ( -14.29746914071037622, -8.314922557961029526, 84.16775706135234714 ) ) ;
#189117=CARTESIAN_POINT ( 'NONE',  ( -8.224510206698948167, 14.34966873604960824, 105.4155762719810383 ) ) ;
#189118=CARTESIAN_POINT ( 'NONE',  ( 5.049401038298161559, -19.05341960407611168, 107.7072429386476955 ) ) ;
#189120=CARTESIAN_POINT ( 'NONE',  ( 14.34966873604960469, 8.224510206698951720, 59.16557627198103120 ) ) ;
#189121=CARTESIAN_POINT ( 'NONE',  ( -12.14591786802309592, -12.06949235617757132, 26.87390960531435979 ) ) ;
#189122=CARTESIAN_POINT ( 'NONE',  ( 5.049401038298161559, -19.05341960407611168, 47.70724293864770260 ) ) ;
#189123=CARTESIAN_POINT ( 'NONE',  ( 13.97604488694527802, 13.89961937509977652, 24.37390960531435624 ) ) ;
#189124=CARTESIAN_POINT ( 'NONE',  ( -10.72451020669898014, 18.67979575497178502, 50.41557627198103120 ) ) ;
#189125=CARTESIAN_POINT ( 'NONE',  ( 19.05341960407617918, -5.049401038297876454, 31.04275706135232227 ) ) ;
#189126=CARTESIAN_POINT ( 'NONE',  ( -17.50000000000001066, -5.499999999999943157, 86.28230962303568674 ) ) ;
#189127=CARTESIAN_POINT ( 'NONE',  ( 8.314922557960818139, 14.29746914071049879, 34.58224293864770260 ) ) ;
#189128=CARTESIAN_POINT ( 'NONE',  ( -15.72974639402176322, -15.80617190586768395, 49.37609039468569705 ) ) ;
#189130=CARTESIAN_POINT ( 'NONE',  ( -8.224510206698735004, -14.34966873604973081, 54.58442372801901143 ) ) ;
#189131=CARTESIAN_POINT ( 'NONE',  ( -5.049401038297874678, -19.05341960407617918, 64.79275706135233293 ) ) ;
#189132=CARTESIAN_POINT ( 'NONE',  ( 14.34966873604960469, 8.224510206698951720, 24.16557627198103120 ) ) ;
#189133=CARTESIAN_POINT ( 'NONE',  ( 0.05219959533934541429, -16.53943276465976808, 100.0010903946857042 ) ) ;
#189134=CARTESIAN_POINT ( 'NONE',  ( 13.97604488694527802, 13.89961937509977652, 39.37390960531435269 ) ) ;
#189135=CARTESIAN_POINT ( 'NONE',  ( -13.89961937509977652, 13.97604488694528158, 60.62390960531436690 ) ) ;
#189136=CARTESIAN_POINT ( 'NONE',  ( -5.153800228976328057, -19.02544592524343514, 22.29057627198102765 ) ) ;
#189137=CARTESIAN_POINT ( 'NONE',  ( -0.05219959533937732626, 21.53943276465977519, 37.50109039468568284 ) ) ;
#189138=CARTESIAN_POINT ( 'NONE',  ( 13.97604488694527802, 13.89961937509977652, 44.37390960531435269 ) ) ;
#189139=CARTESIAN_POINT ( 'NONE',  ( 5.153800228976335163, 19.02544592524342804, 39.79057627198100988 ) ) ;
#189140=CARTESIAN_POINT ( 'NONE',  ( -10.72451020669898014, 18.67979575497178502, 25.41557627198103120 ) ) ;
#189141=CARTESIAN_POINT ( 'NONE',  ( -21.53943276465977519, -0.05219959533937600094, 63.75109039468568284 ) ) ;
#189142=CARTESIAN_POINT ( 'NONE',  ( -14.29746914071049879, 8.314922557960819915, 100.8322429386477097 ) ) ;
#189143=CARTESIAN_POINT ( 'NONE',  ( -5.049401038298153566, 19.05341960407611168, 115.2072429386477097 ) ) ;
#189144=CARTESIAN_POINT ( 'NONE',  ( 0.05219959533934541429, -16.53943276465976808, 80.00109039468568994 ) ) ;
#189145=CARTESIAN_POINT ( 'NONE',  ( 21.53943276465977519, 0.05219959533937863772, 86.25109039468568994 ) ) ;
#189146=CARTESIAN_POINT ( 'NONE',  ( -14.29746914071037622, -8.314922557961029526, 59.16775706135234714 ) ) ;
#189147=CARTESIAN_POINT ( 'NONE',  ( 19.02544592524343514, -5.153800228976328945, 98.54057627198100988 ) ) ;
#189148=CARTESIAN_POINT ( 'NONE',  ( -8.224510206698735004, -14.34966873604973081, 34.58442372801900433 ) ) ;
#189149=CARTESIAN_POINT ( 'NONE',  ( 4.379528057220092307, 16.55341960407617563, 22.29275706135235069 ) ) ;
#189150=CARTESIAN_POINT ( 'NONE',  ( -16.55341960407617563, 4.379528057220093196, 83.54275706135234714 ) ) ;
#189151=CARTESIAN_POINT ( 'NONE',  ( -19.03943276465977164, -0.05219959533935918106, 108.7510903946856615 ) ) ;
#189152=CARTESIAN_POINT ( 'NONE',  ( -21.52544592524343514, 5.823673210054127303, 96.04057627198102409 ) ) ;
#189153=CARTESIAN_POINT ( 'NONE',  ( 14.29746914071049879, -8.314922557960816363, 108.3322429386477097 ) ) ;
#189154=CARTESIAN_POINT ( 'NONE',  ( 19.05341960407617918, -5.049401038297876454, 106.0427570613523471 ) ) ;
#189155=CARTESIAN_POINT ( 'NONE',  ( 8.224510206698742110, 14.34966873604972548, 67.08442372801901854 ) ) ;
#189157=CARTESIAN_POINT ( 'NONE',  ( -5.049401038297874678, -19.05341960407617918, 64.79275706135233293 ) ) ;
#189158=CARTESIAN_POINT ( 'NONE',  ( -16.52544592524342804, 4.483927247898546575, 51.04057627198103120 ) ) ;
#189159=CARTESIAN_POINT ( 'NONE',  ( 12.06949235617757843, -12.14591786802309237, 28.12390960531435979 ) ) ;
#189160=CARTESIAN_POINT ( 'NONE',  ( 12.14591786802309770, 12.06949235617756955, 89.37390960531435269 ) ) ;
#189161=CARTESIAN_POINT ( 'NONE',  ( -13.97604488694547697, 13.89961937509957934, 28.12609039468565797 ) ) ;
#189162=CARTESIAN_POINT ( 'NONE',  ( -19.01533133064924641, 5.499999999999447553, 88.76586590595742621 ) ) ;
#189163=CARTESIAN_POINT ( 'NONE',  ( 18.67979575497194134, -10.72451020669871369, 35.83442372801901143 ) ) ;
#189164=CARTESIAN_POINT ( 'NONE',  ( 13.89961937509957401, 13.97604488694547697, 91.87609039468567573 ) ) ;
#189166=CARTESIAN_POINT ( 'NONE',  ( 5.049401038298161559, -19.05341960407611168, 97.70724293864766707 ) ) ;
#189167=CARTESIAN_POINT ( 'NONE',  ( -16.51473224551069308, -9.474510206698971260, 91.66557627198103830 ) ) ;
#189168=CARTESIAN_POINT ( 'NONE',  ( -10.72451020669898014, 18.67979575497178502, 50.41557627198103120 ) ) ;
#189169=CARTESIAN_POINT ( 'NONE',  ( 16.55341960407611168, 4.379528057220329451, 98.95724293864770971 ) ) ;
#189170=CARTESIAN_POINT ( 'NONE',  ( -5.153800228976328057, -19.02544592524343514, 72.29057627198102409 ) ) ;
#189171=CARTESIAN_POINT ( 'NONE',  ( -5.049401038298153566, 19.05341960407611168, 25.20724293864768484 ) ) ;
#189172=CARTESIAN_POINT ( 'NONE',  ( 21.55341960407619695, -5.719274019375665929, 36.04275706135234714 ) ) ;
#189173=CARTESIAN_POINT ( 'NONE',  ( 15.72974639402176855, 15.80617190586768217, 71.87609039468568994 ) ) ;
#189174=CARTESIAN_POINT ( 'NONE',  ( -16.46253265017160317, 9.564922557960807481, 55.83224293864769550 ) ) ;
#189175=CARTESIAN_POINT ( 'NONE',  ( 12.06949235617739724, 12.14591786802326823, 76.87609039468567573 ) ) ;
#189176=CARTESIAN_POINT ( 'NONE',  ( -5.823673210054431948, 21.52544592524334988, 27.70942372801901854 ) ) ;
#189177=CARTESIAN_POINT ( 'NONE',  ( -15.72974639402176322, -15.80617190586768395, 29.37609039468568284 ) ) ;
#189178=CARTESIAN_POINT ( 'NONE',  ( 9.474510206698729675, 16.51473224551082808, 47.08442372801900433 ) ) ;
#189179=CARTESIAN_POINT ( 'NONE',  ( -19.02544592524342804, 5.153800228976336051, 76.04057627198102409 ) ) ;
#189180=CARTESIAN_POINT ( 'NONE',  ( 19.02544592524334988, 5.153800228976608722, 31.45942372801900433 ) ) ;
#189181=CARTESIAN_POINT ( 'NONE',  ( -5.719274019375665041, -21.55341960407619695, 79.79275706135236135 ) ) ;
#189182=CARTESIAN_POINT ( 'NONE',  ( 21.52544592524344225, -5.823673210054117533, 73.54057627198102409 ) ) ;
#189183=CARTESIAN_POINT ( 'NONE',  ( 8.224510206698953496, -14.34966873604960469, 52.91557627198103830 ) ) ;
#189184=CARTESIAN_POINT ( 'NONE',  ( -21.52544592524334988, -5.823673210054445271, 88.95942372801901854 ) ) ;
#189185=CARTESIAN_POINT ( 'NONE',  ( -5.049401038297874678, -19.05341960407617918, 24.79275706135233648 ) ) ;
#189186=CARTESIAN_POINT ( 'NONE',  ( -4.483927247898539470, -16.52544592524342804, 67.29057627198103830 ) ) ;
#189187=CARTESIAN_POINT ( 'NONE',  ( -0.05219959533909027116, -19.03943276465977164, 22.49890960531436690 ) ) ;
#189188=CARTESIAN_POINT ( 'NONE',  ( -0.05219959533936034679, 19.03943276465977164, 72.50109039468566152 ) ) ;
#189189=CARTESIAN_POINT ( 'NONE',  ( 16.55341960407611168, 4.379528057220329451, 33.95724293864769550 ) ) ;
#189190=CARTESIAN_POINT ( 'NONE',  ( 5.823673210054444382, -21.52544592524334988, 80.20942372801901854 ) ) ;
#189191=CARTESIAN_POINT ( 'NONE',  ( -9.564922557960796823, -16.46253265017161027, 82.08224293864768129 ) ) ;
#189192=CARTESIAN_POINT ( 'NONE',  ( 13.97604488694548053, -13.89961937509957401, 50.62609039468566152 ) ) ;
#189193=CARTESIAN_POINT ( 'NONE',  ( -21.52544592524343514, 5.823673210054127303, 56.04057627198102409 ) ) ;
#189194=CARTESIAN_POINT ( 'NONE',  ( -5.823673210054116645, -21.52544592524344225, 97.29057627198105251 ) ) ;
#189195=CARTESIAN_POINT ( 'NONE',  ( -13.97604488694547697, 13.89961937509957934, 113.1260903946856757 ) ) ;
#189196=CARTESIAN_POINT ( 'NONE',  ( 16.52544592524335698, 4.483927247898782831, 66.45942372801903275 ) ) ;
#189197=CARTESIAN_POINT ( 'NONE',  ( 16.29526858892878849, 7.335722546919996034, 63.29670597800208043 ) ) ;
#189198=CARTESIAN_POINT ( 'NONE',  ( 18.62759615963271287, -10.81492255796078972, 108.3322429386477097 ) ) ;
#189199=CARTESIAN_POINT ( 'NONE',  ( 14.34966873604960469, 8.224510206698951720, 99.16557627198100988 ) ) ;
#189200=CARTESIAN_POINT ( 'NONE',  ( -17.49999999999998579, -3.345213924137320216, 30.41231376905646044 ) ) ;
#189201=CARTESIAN_POINT ( 'NONE',  ( 16.53943276465976808, 0.05219959533934440121, 36.25109039468567573 ) ) ;
#189202=CARTESIAN_POINT ( 'NONE',  ( 21.52544592524344225, -5.823673210054117533, 58.54057627198103120 ) ) ;
#189203=CARTESIAN_POINT ( 'NONE',  ( -4.379528057220086978, -16.55341960407618274, 104.7927570613523898 ) ) ;
#189204=CARTESIAN_POINT ( 'NONE',  ( 9.474510206698971260, -16.51473224551069308, 32.91557627198102409 ) ) ;
#189205=CARTESIAN_POINT ( 'NONE',  ( -16.52544592524335698, -4.483927247898792601, 63.95942372801901854 ) ) ;
#189206=CARTESIAN_POINT ( 'NONE',  ( 9.564922557961047289, -16.46253265017146816, 60.41775706135233293 ) ) ;
#189207=CARTESIAN_POINT ( 'NONE',  ( -21.53943276465977519, -0.05219959533937600094, 38.75109039468567573 ) ) ;
#189208=CARTESIAN_POINT ( 'NONE',  ( -21.52544592524343514, 5.823673210054127303, 56.04057627198102409 ) ) ;
#189209=CARTESIAN_POINT ( 'NONE',  ( -12.14591786802326823, 12.06949235617739902, 93.12609039468568994 ) ) ;
#189210=CARTESIAN_POINT ( 'NONE',  ( 15.72974639402176855, 15.80617190586768217, 81.87609039468568994 ) ) ;
#189211=CARTESIAN_POINT ( 'NONE',  ( 15.72974639402199770, -15.80617190586745480, 53.12390960531436690 ) ) ;
#189212=CARTESIAN_POINT ( 'NONE',  ( 21.53943276465977519, -0.05219959533907433946, 28.74890960531435624 ) ) ;
#189213=CARTESIAN_POINT ( 'NONE',  ( -8.224510206698735004, -14.34966873604973081, 84.58442372801903275 ) ) ;
#189214=CARTESIAN_POINT ( 'NONE',  ( -18.67979575497178146, -10.72451020669898902, 36.66557627198103120 ) ) ;
#189216=CARTESIAN_POINT ( 'NONE',  ( 9.564922557960805705, 16.46253265017160317, 99.58224293864770971 ) ) ;
#189217=CARTESIAN_POINT ( 'NONE',  ( -14.34966873604960291, -8.224510206698953496, 21.66557627198102409 ) ) ;
#189219=CARTESIAN_POINT ( 'NONE',  ( -14.34966873604960291, -8.224510206698953496, 106.6655762719810383 ) ) ;
#189220=CARTESIAN_POINT ( 'NONE',  ( 5.719274019375991003, -21.55341960407610458, 57.70724293864770260 ) ) ;
#189221=CARTESIAN_POINT ( 'NONE',  ( 4.483927247898790824, -16.52544592524335698, 85.20942372801901854 ) ) ;
#189222=CARTESIAN_POINT ( 'NONE',  ( 15.80617190586769283, -15.72974639402175789, 40.62609039468567573 ) ) ;
#189223=CARTESIAN_POINT ( 'NONE',  ( -19.03943276465977164, -0.05219959533935918106, 103.7510903946856757 ) ) ;
#189224=CARTESIAN_POINT ( 'NONE',  ( -4.379528057220328563, 16.55341960407611168, 105.2072429386477097 ) ) ;
#189225=CARTESIAN_POINT ( 'NONE',  ( 9.474510206698729675, 16.51473224551082808, 107.0844237280190043 ) ) ;
#189227=CARTESIAN_POINT ( 'NONE',  ( 16.46253265017160672, -9.564922557960803928, 23.33224293864769194 ) ) ;
#189228=FACE_OUTER_BOUND ( 'NONE', #180522, .T. ) ;
#189229=CARTESIAN_POINT ( 'NONE',  ( 19.03943276465977164, -0.05219959533909143690, 93.74890960531435269 ) ) ;
#189230=CARTESIAN_POINT ( 'NONE',  ( -14.29746914071037622, -8.314922557961029526, 74.16775706135231871 ) ) ;
#189231=CARTESIAN_POINT ( 'NONE',  ( 18.67979575497194134, -10.72451020669871369, 100.8344237280190185 ) ) ;
#189232=CARTESIAN_POINT ( 'NONE',  ( 21.53943276465977519, -0.05219959533907433946, 63.74890960531435979 ) ) ;
#189233=CARTESIAN_POINT ( 'NONE',  ( -8.224510206698735004, -14.34966873604973081, 84.58442372801903275 ) ) ;
#189234=CARTESIAN_POINT ( 'NONE',  ( 13.97604488694548053, -13.89961937509957401, 85.62609039468568994 ) ) ;
#189235=CARTESIAN_POINT ( 'NONE',  ( -13.89961937509977652, 13.97604488694528158, 30.62390960531435269 ) ) ;
#189236=CARTESIAN_POINT ( 'NONE',  ( 13.97604488694527802, 13.89961937509977652, 79.37390960531435269 ) ) ;
#189237=CARTESIAN_POINT ( 'NONE',  ( -0.05219959533909027116, -19.03943276465977164, 27.49890960531435624 ) ) ;
#189238=CARTESIAN_POINT ( 'NONE',  ( 13.89961937509957401, 13.97604488694547697, 66.87609039468567573 ) ) ;
#189240=CARTESIAN_POINT ( 'NONE',  ( -19.05341960407611168, -5.049401038298163336, 96.45724293864769550 ) ) ;
#189241=CARTESIAN_POINT ( 'NONE',  ( -14.34966873604960291, -8.224510206698953496, 46.66557627198102409 ) ) ;
#189242=CARTESIAN_POINT ( 'NONE',  ( -21.55341960407610458, -5.719274019375992779, 66.45724293864768129 ) ) ;
#189243=CARTESIAN_POINT ( 'NONE',  ( -17.50000000000000000, 3.237210098469633923, 104.7123698737954385 ) ) ;
#189244=CARTESIAN_POINT ( 'NONE',  ( -5.153800228976607833, 19.02544592524334988, 32.70942372801899722 ) ) ;
#189246=CARTESIAN_POINT ( 'NONE',  ( -9.474510206698964154, 16.51473224551069663, 50.41557627198102409 ) ) ;
#189247=CARTESIAN_POINT ( 'NONE',  ( -9.474510206698964154, 16.51473224551069663, 75.41557627198103830 ) ) ;
#189249=CARTESIAN_POINT ( 'NONE',  ( 14.29746914071037800, 8.314922557961029526, 41.66775706135235424 ) ) ;
#189252=CARTESIAN_POINT ( 'NONE',  ( 16.53943276465976808, 0.05219959533934440121, 71.25109039468568994 ) ) ;
#189253=CARTESIAN_POINT ( 'NONE',  ( 14.34966873604972726, -8.224510206698740333, 65.83442372801900433 ) ) ;
#189254=CARTESIAN_POINT ( 'NONE',  ( -21.55341960407610458, -5.719274019375992779, 91.45724293864769550 ) ) ;
#189255=CARTESIAN_POINT ( 'NONE',  ( 4.379528057220092307, 16.55341960407617563, 42.29275706135235424 ) ) ;
#189256=CARTESIAN_POINT ( 'NONE',  ( -19.02544592524342804, 5.153800228976336051, 46.04057627198101699 ) ) ;
#189258=CARTESIAN_POINT ( 'NONE',  ( -10.81492255796105439, 18.62759615963255655, 52.91775706135235424 ) ) ;
#189259=CARTESIAN_POINT ( 'NONE',  ( -13.97604488694547697, 13.89961937509957934, 63.12609039468566152 ) ) ;
#189260=CARTESIAN_POINT ( 'NONE',  ( 15.72974639402176855, 15.80617190586768217, 91.87609039468568994 ) ) ;
#189262=CARTESIAN_POINT ( 'NONE',  ( -13.89961937509977652, 13.97604488694528158, 25.62390960531434558 ) ) ;
#189264=CARTESIAN_POINT ( 'NONE',  ( -10.81492255796078084, -18.62759615963271287, 52.08224293864768839 ) ) ;
#189265=CARTESIAN_POINT ( 'NONE',  ( 9.564922557960805705, 16.46253265017160317, 99.58224293864770971 ) ) ;
#189266=CARTESIAN_POINT ( 'NONE',  ( 0.05219959533910956823, 16.53943276465976808, 104.9989096053143669 ) ) ;
#189267=CARTESIAN_POINT ( 'NONE',  ( -4.483927247898782831, 16.52544592524335698, 37.70942372801900433 ) ) ;
#189268=CARTESIAN_POINT ( 'NONE',  ( 12.06949235617739724, 12.14591786802326823, 106.8760903946856899 ) ) ;
#189270=CARTESIAN_POINT ( 'NONE',  ( -5.823673210054116645, -21.52544592524344225, 97.29057627198105251 ) ) ;
#189271=CARTESIAN_POINT ( 'NONE',  ( 16.55341960407611168, 4.379528057220329451, 33.95724293864769550 ) ) ;
#189272=CARTESIAN_POINT ( 'NONE',  ( 16.51473224551069308, 9.474510206698969483, 109.1655762719810383 ) ) ;
#189273=CARTESIAN_POINT ( 'NONE',  ( 19.02544592524334988, 5.153800228976608722, 96.45942372801897591 ) ) ;
#189274=CARTESIAN_POINT ( 'NONE',  ( 5.049401038297881783, 19.05341960407617563, 22.29275706135233648 ) ) ;
#189275=CARTESIAN_POINT ( 'NONE',  ( 16.53943276465976808, -0.05219959533910856209, 33.74890960531436690 ) ) ;
#189276=CARTESIAN_POINT ( 'NONE',  ( -21.55341960407610458, -5.719274019375992779, 91.45724293864769550 ) ) ;
#189277=CARTESIAN_POINT ( 'NONE',  ( -5.823673210054116645, -21.52544592524344225, 57.29057627198103120 ) ) ;
#189278=CARTESIAN_POINT ( 'NONE',  ( 0.05219959533909260263, 19.03943276465977164, 64.99890960531436690 ) ) ;
#189279=CARTESIAN_POINT ( 'NONE',  ( 14.34966873604960469, 8.224510206698951720, 34.16557627198102409 ) ) ;
#189280=CARTESIAN_POINT ( 'NONE',  ( -19.02544592524342804, 5.153800228976336051, 91.04057627198100988 ) ) ;
#189281=CARTESIAN_POINT ( 'NONE',  ( -5.049401038298153566, 19.05341960407611168, 80.20724293864769550 ) ) ;
#189282=CARTESIAN_POINT ( 'NONE',  ( -16.46253265017146816, -9.564922557961047289, 39.16775706135234003 ) ) ;
#189283=CARTESIAN_POINT ( 'NONE',  ( 0.05219959533907565091, 21.53943276465977519, 74.99890960531435269 ) ) ;
#189284=CARTESIAN_POINT ( 'NONE',  ( 4.483927247898545687, 16.52544592524342804, 99.79057627198103830 ) ) ;
#189285=CARTESIAN_POINT ( 'NONE',  ( 18.62759615963255655, 10.81492255796105972, 41.66775706135235424 ) ) ;
#189287=CARTESIAN_POINT ( 'NONE',  ( -16.53943276465976808, -0.05219959533934237506, 103.7510903946857042 ) ) ;
#189288=CARTESIAN_POINT ( 'NONE',  ( -5.049401038298153566, 19.05341960407611168, 35.20724293864768839 ) ) ;
#189289=CARTESIAN_POINT ( 'NONE',  ( -13.97604488694527625, -13.89961937509977652, 91.87390960531432427 ) ) ;
#189291=CARTESIAN_POINT ( 'NONE',  ( -16.51473224551069308, -9.474510206698971260, 31.66557627198102054 ) ) ;
#189292=CARTESIAN_POINT ( 'NONE',  ( -16.53943276465976808, 0.05219959533911058130, 46.24890960531435979 ) ) ;
#189293=CARTESIAN_POINT ( 'NONE',  ( 5.719274019375673035, 21.55341960407619339, 77.29275706135234714 ) ) ;
#189295=CARTESIAN_POINT ( 'NONE',  ( -8.224510206698735004, -14.34966873604973081, 74.58442372801901854 ) ) ;
#189296=CARTESIAN_POINT ( 'NONE',  ( 9.564922557960805705, 16.46253265017160317, 59.58224293864769550 ) ) ;
#189297=CARTESIAN_POINT ( 'NONE',  ( 19.05341960407611168, 5.049401038298154454, 53.95724293864770260 ) ) ;
#189299=CARTESIAN_POINT ( 'NONE',  ( 15.80617190586769283, -15.72974639402175789, 110.6260903946857042 ) ) ;
#189300=CARTESIAN_POINT ( 'NONE',  ( 12.14591786802327356, -12.06949235617739191, 75.62609039468567573 ) ) ;
#189301=CARTESIAN_POINT ( 'NONE',  ( 15.80617190586769283, -15.72974639402175789, 95.62609039468568994 ) ) ;
#189302=CARTESIAN_POINT ( 'NONE',  ( 0.05219959533907565091, 21.53943276465977519, 34.99890960531435979 ) ) ;
#189303=CARTESIAN_POINT ( 'NONE',  ( 16.46253265017146816, 9.564922557961045513, 106.6677570613523471 ) ) ;
#189304=CARTESIAN_POINT ( 'NONE',  ( -15.72974639402176322, -15.80617190586768395, 74.37609039468568994 ) ) ;
#189305=CARTESIAN_POINT ( 'NONE',  ( 16.53943276465976808, 0.05219959533934440121, 51.25109039468568994 ) ) ;
#189306=CARTESIAN_POINT ( 'NONE',  ( -15.80617190586745835, -15.72974639402198527, 96.87390960531436690 ) ) ;
#189307=CARTESIAN_POINT ( 'NONE',  ( -9.474510206698720793, -16.51473224551083518, 104.5844237280190043 ) ) ;
#189308=CARTESIAN_POINT ( 'NONE',  ( 16.46253265017160672, -9.564922557960803928, 63.33224293864769550 ) ) ;
#189309=CARTESIAN_POINT ( 'NONE',  ( -5.049401038297874678, -19.05341960407617918, 109.7927570613523187 ) ) ;
#189310=CARTESIAN_POINT ( 'NONE',  ( -9.564922557961040184, 16.46253265017147172, 102.9177570613523329 ) ) ;
#189311=CARTESIAN_POINT ( 'NONE',  ( 0.05219959533910956823, 16.53943276465976808, 69.99890960531435269 ) ) ;
#189312=CARTESIAN_POINT ( 'NONE',  ( 16.52544592524335698, 4.483927247898782831, 76.45942372801901854 ) ) ;
#189314=CARTESIAN_POINT ( 'NONE',  ( -10.72451020669870658, -18.67979575497194134, 19.58442372801901143 ) ) ;
#189315=CARTESIAN_POINT ( 'NONE',  ( -5.153800228976328057, -19.02544592524343514, 52.29057627198100988 ) ) ;
#189316=CARTESIAN_POINT ( 'NONE',  ( -19.02544592524342804, 5.153800228976336051, 56.04057627198100988 ) ) ;
#189317=CARTESIAN_POINT ( 'NONE',  ( -12.14591786802326823, 12.06949235617739902, 68.12609039468567573 ) ) ;
#189320=CARTESIAN_POINT ( 'NONE',  ( -16.46253265017146816, -9.564922557961047289, 19.16775706135233293 ) ) ;
#189321=CARTESIAN_POINT ( 'NONE',  ( 13.89961937509977652, -13.97604488694527269, 23.12390960531436335 ) ) ;
#189322=VERTEX_POINT ( 'NONE', #180812 ) ;
#189323=CARTESIAN_POINT ( 'NONE',  ( 13.97604488694548053, -13.89961937509957401, 105.6260903946856757 ) ) ;
#189324=CARTESIAN_POINT ( 'NONE',  ( 15.80617190586746368, 15.72974639402197994, 54.37390960531435979 ) ) ;
#189325=CARTESIAN_POINT ( 'NONE',  ( -13.97604488694547697, 13.89961937509957934, 48.12609039468566863 ) ) ;
#189326=CARTESIAN_POINT ( 'NONE',  ( 8.314922557961029526, -14.29746914071037800, 30.41775706135234358 ) ) ;
#189327=CARTESIAN_POINT ( 'NONE',  ( -13.97604488694527625, -13.89961937509977652, 41.87390960531435979 ) ) ;
#189328=CARTESIAN_POINT ( 'NONE',  ( 13.97604488694527802, 13.89961937509977652, 49.37390960531434558 ) ) ;
#189329=CARTESIAN_POINT ( 'NONE',  ( 18.62759615963271287, -10.81492255796078972, 83.33224293864769550 ) ) ;
#189330=CARTESIAN_POINT ( 'NONE',  ( -19.05341960407611168, -5.049401038298163336, 111.4572429386476671 ) ) ;
#189331=CARTESIAN_POINT ( 'NONE',  ( -9.564922557960796823, -16.46253265017161027, 47.08224293864769550 ) ) ;
#189332=CARTESIAN_POINT ( 'NONE',  ( -17.49999999999999645, -5.500000000000000888, 118.0000000000000142 ) ) ;
#189333=CARTESIAN_POINT ( 'NONE',  ( 13.89961937509957401, 13.97604488694547697, 96.87609039468566152 ) ) ;
#189334=CARTESIAN_POINT ( 'NONE',  ( -12.06949235617756955, 12.14591786802309770, 65.62390960531436690 ) ) ;
#189335=CARTESIAN_POINT ( 'NONE',  ( -19.05341960407617563, 5.049401038297882671, 28.54275706135232937 ) ) ;
#189336=CARTESIAN_POINT ( 'NONE',  ( -4.483927247898539470, -16.52544592524342804, 57.29057627198103120 ) ) ;
#189337=CARTESIAN_POINT ( 'NONE',  ( 21.55341960407619695, -5.719274019375665929, 81.04275706135236135 ) ) ;
#189338=CARTESIAN_POINT ( 'NONE',  ( -9.564922557960796823, -16.46253265017161027, 32.08224293864769550 ) ) ;
#189339=CARTESIAN_POINT ( 'NONE',  ( 10.81492255796106328, -18.62759615963255655, 95.41775706135234714 ) ) ;
#189340=CARTESIAN_POINT ( 'NONE',  ( 12.06949235617757843, -12.14591786802309237, 23.12390960531436335 ) ) ;
#189341=CARTESIAN_POINT ( 'NONE',  ( -5.823673210054431948, 21.52544592524334988, 82.70942372801900433 ) ) ;
#189342=CARTESIAN_POINT ( 'NONE',  ( -19.03943276465977164, 0.05219959533909376836, 71.24890960531435269 ) ) ;
#189343=CARTESIAN_POINT ( 'NONE',  ( 21.53943276465977519, 0.05219959533937863772, 46.25109039468567573 ) ) ;
#189344=CARTESIAN_POINT ( 'NONE',  ( -5.153800228976328057, -19.02544592524343514, 77.29057627198099567 ) ) ;
#189345=CARTESIAN_POINT ( 'NONE',  ( 16.52544592524342804, -4.483927247898539470, 93.54057627198103830 ) ) ;
#189346=CARTESIAN_POINT ( 'NONE',  ( 16.52544592524342804, -4.483927247898539470, 58.54057627198103120 ) ) ;
#189347=CARTESIAN_POINT ( 'NONE',  ( -21.52544592524343514, 5.823673210054127303, 76.04057627198102409 ) ) ;
#189348=CARTESIAN_POINT ( 'NONE',  ( -13.97604488694527625, -13.89961937509977652, 71.87390960531433848 ) ) ;
#189349=CARTESIAN_POINT ( 'NONE',  ( 5.823673210054125526, 21.52544592524343514, 79.79057627198102409 ) ) ;
#189350=CARTESIAN_POINT ( 'NONE',  ( -19.05341960407617563, 5.049401038297882671, 68.54275706135230450 ) ) ;
#189352=CARTESIAN_POINT ( 'NONE',  ( -5.049401038297874678, -19.05341960407618274, 29.79275706135232582 ) ) ;
#189353=CARTESIAN_POINT ( 'NONE',  ( -4.379528057220328563, 16.55341960407611168, 75.20724293864769550 ) ) ;
#189354=CARTESIAN_POINT ( 'NONE',  ( -0.05219959533907301413, -21.53943276465977519, 52.49890960531435979 ) ) ;
#189356=CARTESIAN_POINT ( 'NONE',  ( -16.52544592524335698, -4.483927247898792601, 98.95942372801903275 ) ) ;
#189358=CARTESIAN_POINT ( 'NONE',  ( 19.03943276465977164, 0.05219959533936151252, 106.2510903946856615 ) ) ;
#189359=CARTESIAN_POINT ( 'NONE',  ( 16.55341960407611168, 4.379528057220329451, 68.95724293864769550 ) ) ;
#189361=CARTESIAN_POINT ( 'NONE',  ( -9.564922557960796823, -16.46253265017161027, 67.08224293864769550 ) ) ;
#189362=CARTESIAN_POINT ( 'NONE',  ( 14.29746914071049879, -8.314922557960816363, 48.33224293864770260 ) ) ;
#189363=CARTESIAN_POINT ( 'NONE',  ( 19.05341960407611168, 5.049401038298154454, 98.95724293864766707 ) ) ;
#189364=CARTESIAN_POINT ( 'NONE',  ( 16.46253265017146816, 9.564922557961045513, 76.66775706135234714 ) ) ;
#189365=CARTESIAN_POINT ( 'NONE',  ( 13.97604488694527802, 13.89961937509977652, 64.37390960531436690 ) ) ;
#189366=CARTESIAN_POINT ( 'NONE',  ( -9.564922557960796823, -16.46253265017161027, 92.08224293864769550 ) ) ;
#189367=CARTESIAN_POINT ( 'NONE',  ( -9.474510206698964154, 16.51473224551069663, 80.41557627198103830 ) ) ;
#189368=CARTESIAN_POINT ( 'NONE',  ( -18.62759615963270932, 10.81492255796079327, 65.83224293864769550 ) ) ;
#189369=CARTESIAN_POINT ( 'NONE',  ( -12.14591786802326823, 12.06949235617739902, 53.12609039468568284 ) ) ;
#189371=CARTESIAN_POINT ( 'NONE',  ( 19.05341960407611168, 5.049401038298154454, 48.95724293864768129 ) ) ;
#189372=CARTESIAN_POINT ( 'NONE',  ( 21.52544592524344225, -5.823673210054117533, 58.54057627198103120 ) ) ;
#189373=CARTESIAN_POINT ( 'NONE',  ( 16.46253265017146816, 9.564922557961045513, 96.66775706135233293 ) ) ;
#189374=CARTESIAN_POINT ( 'NONE',  ( 0.05219959533910956823, 16.53943276465976808, 24.99890960531435624 ) ) ;
#189375=CARTESIAN_POINT ( 'NONE',  ( -21.52544592524334988, -5.823673210054445271, 48.95942372801902565 ) ) ;
#189376=CARTESIAN_POINT ( 'NONE',  ( -0.05219959533936034679, 19.03943276465977164, 37.50109039468567573 ) ) ;
#189377=CARTESIAN_POINT ( 'NONE',  ( -14.29746914071037622, -8.314922557961029526, 64.16775706135234714 ) ) ;
#189378=CARTESIAN_POINT ( 'NONE',  ( 12.14591786802327356, -12.06949235617739191, 90.62609039468567573 ) ) ;
#189379=CARTESIAN_POINT ( 'NONE',  ( -17.60769864724391098, 5.499999999999986677, 53.65024842019163032 ) ) ;
#189380=CARTESIAN_POINT ( 'NONE',  ( -16.52544592524335698, -4.483927247898792601, 83.95942372801900433 ) ) ;
#189381=CARTESIAN_POINT ( 'NONE',  ( -16.53943276465976808, -0.05219959533934237506, 38.75109039468567573 ) ) ;
#189382=CARTESIAN_POINT ( 'NONE',  ( 0.05219959533909260263, 19.03943276465977164, 49.99890960531435979 ) ) ;
#189383=CARTESIAN_POINT ( 'NONE',  ( 0.05219959533909260263, 19.03943276465977164, 49.99890960531435979 ) ) ;
#189384=CARTESIAN_POINT ( 'NONE',  ( -13.97604488694527625, -13.89961937509977652, 61.87390960531435979 ) ) ;
#189385=CARTESIAN_POINT ( 'NONE',  ( -10.72451020669870658, -18.67979575497194134, 39.58442372801901143 ) ) ;
#189386=CARTESIAN_POINT ( 'NONE',  ( -0.05219959533934338120, 16.53943276465976808, 47.50109039468568994 ) ) ;
#189387=CARTESIAN_POINT ( 'NONE',  ( -12.06949235617739369, -12.14591786802326823, 109.3760903946857042 ) ) ;
#189388=CARTESIAN_POINT ( 'NONE',  ( 16.46253265017160672, -9.564922557960803928, 33.33224293864770260 ) ) ;
#189389=CARTESIAN_POINT ( 'NONE',  ( -21.52544592524334988, -5.823673210054445271, 108.9594237280190185 ) ) ;
#189390=CARTESIAN_POINT ( 'NONE',  ( 19.03943276465977164, 0.05219959533936151252, 106.2510903946856615 ) ) ;
#189391=CARTESIAN_POINT ( 'NONE',  ( -0.05219959533936034679, 19.03943276465977164, 72.50109039468566152 ) ) ;
#189392=CARTESIAN_POINT ( 'NONE',  ( -14.34966873604960291, -8.224510206698953496, 86.66557627198102409 ) ) ;
#189393=CARTESIAN_POINT ( 'NONE',  ( 13.97604488694527802, 13.89961937509977652, 34.37390960531436690 ) ) ;
#189394=CARTESIAN_POINT ( 'NONE',  ( 0.05219959533936267826, -19.03943276465977164, 70.00109039468566152 ) ) ;
#189395=CARTESIAN_POINT ( 'NONE',  ( 16.62475595723696387, -7.163666690055295660, 93.02713351810467657 ) ) ;
#189396=CARTESIAN_POINT ( 'NONE',  ( 21.52544592524334988, 5.823673210054432836, 76.45942372801901854 ) ) ;
#189397=CARTESIAN_POINT ( 'NONE',  ( 4.379528057220092307, 16.55341960407617563, 47.29275706135234003 ) ) ;
#189398=CARTESIAN_POINT ( 'NONE',  ( 16.81555441253551209, 7.025013491695498047, 36.86314554665744936 ) ) ;
#189399=CARTESIAN_POINT ( 'NONE',  ( -15.80617190586745835, -15.72974639402198527, 41.87390960531435979 ) ) ;
#189400=CARTESIAN_POINT ( 'NONE',  ( -0.05219959533934338120, 16.53943276465976808, 22.50109039468567573 ) ) ;
#189401=CARTESIAN_POINT ( 'NONE',  ( 5.049401038298163336, -19.05341960407611168, 22.70724293864768839 ) ) ;
#189402=CARTESIAN_POINT ( 'NONE',  ( 16.51473224551083163, -9.474510206698727899, 35.83442372801899722 ) ) ;
#189404=CARTESIAN_POINT ( 'NONE',  ( 16.51473224551069308, 9.474510206698969483, 34.16557627198102409 ) ) ;
#189406=CARTESIAN_POINT ( 'NONE',  ( 9.564922557960805705, 16.46253265017160317, 74.58224293864769550 ) ) ;
#189408=CARTESIAN_POINT ( 'NONE',  ( -17.97161686093721045, 5.500000000000142997, 65.99637206859163996 ) ) ;
#189409=CARTESIAN_POINT ( 'NONE',  ( -19.02544592524334988, -5.153800228976617603, 23.95942372801900078 ) ) ;
#189410=CARTESIAN_POINT ( 'NONE',  ( 4.483927247898545687, 16.52544592524342804, 29.79057627198102409 ) ) ;
#189411=CARTESIAN_POINT ( 'NONE',  ( -0.05219959533909027116, -19.03943276465977164, 47.49890960531435979 ) ) ;
#189412=CARTESIAN_POINT ( 'NONE',  ( -19.05341960407611168, -5.049401038298163336, 96.45724293864769550 ) ) ;
#189413=CARTESIAN_POINT ( 'NONE',  ( 18.67979575497194134, -10.72451020669871369, 65.83442372801900433 ) ) ;
#189414=CARTESIAN_POINT ( 'NONE',  ( 13.89961937509977652, -13.97604488694527269, 48.12390960531435979 ) ) ;
#189415=EDGE_CURVE ( 'NONE', #192521, #187465, #129378, .T. ) ;
#189416=CARTESIAN_POINT ( 'NONE',  ( 18.67979575497194134, -10.72451020669871369, 70.83442372801901854 ) ) ;
#189417=CARTESIAN_POINT ( 'NONE',  ( 5.153800228976615827, -19.02544592524334988, 95.20942372801897591 ) ) ;
#189418=CARTESIAN_POINT ( 'NONE',  ( -10.72451020669898014, 18.67979575497178502, 30.41557627198101699 ) ) ;
#189419=CARTESIAN_POINT ( 'NONE',  ( -19.02544592524342804, 5.153800228976336051, 36.04057627198100988 ) ) ;
#189420=CARTESIAN_POINT ( 'NONE',  ( 5.823673210054125526, 21.52544592524343514, 109.7905762719810383 ) ) ;
#189421=CARTESIAN_POINT ( 'NONE',  ( -19.02544592524334988, -5.153800228976617603, 28.95942372801900433 ) ) ;
#189422=CARTESIAN_POINT ( 'NONE',  ( -12.06949235617756955, 12.14591786802309770, 105.6239096053143669 ) ) ;
#189423=CARTESIAN_POINT ( 'NONE',  ( 16.46253265017160672, -9.564922557960803928, 68.33224293864770971 ) ) ;
#189424=CARTESIAN_POINT ( 'NONE',  ( -4.483927247898782831, 16.52544592524335698, 22.70942372801901499 ) ) ;
#189425=CARTESIAN_POINT ( 'NONE',  ( 16.52544592524342804, -4.483927247898539470, 73.54057627198102409 ) ) ;
#189426=CARTESIAN_POINT ( 'NONE',  ( 15.72974639402199770, -15.80617190586745480, 23.12390960531436335 ) ) ;
#189427=CARTESIAN_POINT ( 'NONE',  ( 19.03943276465977164, 0.05219959533936151252, 86.25109039468567573 ) ) ;
#189428=CARTESIAN_POINT ( 'NONE',  ( 5.719274019375991003, -21.55341960407610458, 97.70724293864772392 ) ) ;
#189429=CARTESIAN_POINT ( 'NONE',  ( 5.823673210054444382, -21.52544592524334988, 60.20942372801902565 ) ) ;
#189430=CARTESIAN_POINT ( 'NONE',  ( -14.34966873604972548, 8.224510206698743886, 53.33442372801901854 ) ) ;
#189431=CARTESIAN_POINT ( 'NONE',  ( -0.05219959533934338120, 16.53943276465976808, 57.50109039468568994 ) ) ;
#189432=CARTESIAN_POINT ( 'NONE',  ( 21.53943276465977519, -0.05219959533907433946, 53.74890960531437401 ) ) ;
#189433=CARTESIAN_POINT ( 'NONE',  ( -5.153800228976328057, -19.02544592524343514, 42.29057627198101699 ) ) ;
#189435=CARTESIAN_POINT ( 'NONE',  ( 8.314922557961029526, -14.29746914071037800, 75.41775706135233293 ) ) ;
#189436=CARTESIAN_POINT ( 'NONE',  ( -18.67979575497178146, -10.72451020669898902, 106.6655762719810383 ) ) ;
#189437=CARTESIAN_POINT ( 'NONE',  ( 8.224510206698953496, -14.34966873604960469, 47.91557627198102409 ) ) ;
#189438=CARTESIAN_POINT ( 'NONE',  ( 8.314922557961029526, -14.29746914071037800, 65.41775706135234714 ) ) ;
#189439=CARTESIAN_POINT ( 'NONE',  ( 13.97604488694548053, -13.89961937509957401, 100.6260903946856615 ) ) ;
#189440=CARTESIAN_POINT ( 'NONE',  ( 15.72974639402199770, -15.80617190586745480, 93.12390960531436690 ) ) ;
#189441=CARTESIAN_POINT ( 'NONE',  ( -4.379528057220328563, 16.55341960407611168, 40.20724293864769550 ) ) ;
#189443=CARTESIAN_POINT ( 'NONE',  ( -16.79531203550646978, 7.028104445595605654, 73.74755011779562608 ) ) ;
#189444=CARTESIAN_POINT ( 'NONE',  ( 15.72974639402199770, -15.80617190586745480, 78.12390960531436690 ) ) ;
#189445=CARTESIAN_POINT ( 'NONE',  ( -4.483927247898539470, -16.52544592524342804, 22.29057627198102765 ) ) ;
#189448=CARTESIAN_POINT ( 'NONE',  ( 5.719274019375991003, -21.55341960407610458, 97.70724293864772392 ) ) ;
#189449=CARTESIAN_POINT ( 'NONE',  ( 18.62759615963255655, 10.81492255796105972, 26.66775706135235424 ) ) ;
#189450=CARTESIAN_POINT ( 'NONE',  ( 16.55341960407611168, 4.379528057220329451, 43.95724293864769550 ) ) ;
#189451=CARTESIAN_POINT ( 'NONE',  ( 8.224510206698742110, 14.34966873604972548, 47.08442372801901854 ) ) ;
#189452=CARTESIAN_POINT ( 'NONE',  ( 9.474510206698971260, -16.51473224551069308, 52.91557627198102409 ) ) ;
#189453=CARTESIAN_POINT ( 'NONE',  ( 19.02544592524343514, -5.153800228976328945, 83.54057627198100988 ) ) ;
#189454=ORIENTED_EDGE ( 'NONE', *, *, #95776, .T. ) ;
#189455=CARTESIAN_POINT ( 'NONE',  ( -15.80617190586745835, -15.72974639402198527, 31.87390960531435979 ) ) ;
#189456=CARTESIAN_POINT ( 'NONE',  ( 0.05219959533909260263, 19.03943276465977164, 64.99890960531436690 ) ) ;
#189457=CARTESIAN_POINT ( 'NONE',  ( 14.29746914071037800, 8.314922557961029526, 21.66775706135235069 ) ) ;
#189458=CARTESIAN_POINT ( 'NONE',  ( -16.46253265017146816, -9.564922557961047289, 49.16775706135233293 ) ) ;
#189459=CARTESIAN_POINT ( 'NONE',  ( -21.52544592524343514, 5.823673210054127303, 96.04057627198102409 ) ) ;
#189460=CARTESIAN_POINT ( 'NONE',  ( -0.05219959533910754901, -16.53943276465976808, 37.49890960531436690 ) ) ;
#189461=CARTESIAN_POINT ( 'NONE',  ( -9.564922557960796823, -16.46253265017161027, 77.08224293864769550 ) ) ;
#189462=CARTESIAN_POINT ( 'NONE',  ( -15.72974639402197994, 15.80617190586746368, 65.62390960531436690 ) ) ;
#189463=CARTESIAN_POINT ( 'NONE',  ( 15.72974639402199770, -15.80617190586745480, 83.12390960531436690 ) ) ;
#189464=CARTESIAN_POINT ( 'NONE',  ( -19.03943276465977164, -0.05219959533935918106, 113.7510903946856757 ) ) ;
#189465=CARTESIAN_POINT ( 'NONE',  ( 5.823673210054125526, 21.52544592524343514, 24.79057627198103120 ) ) ;
#189466=CARTESIAN_POINT ( 'NONE',  ( 10.72451020669871369, 18.67979575497193778, 77.08442372801901854 ) ) ;
#189467=CARTESIAN_POINT ( 'NONE',  ( -5.049401038298153566, 19.05341960407611168, 70.20724293864769550 ) ) ;
#189468=CARTESIAN_POINT ( 'NONE',  ( 9.564922557960805705, 16.46253265017160317, 29.58224293864769550 ) ) ;
#189469=CARTESIAN_POINT ( 'NONE',  ( -16.51473224551069308, -9.474510206698971260, 81.66557627198103830 ) ) ;
#189470=CARTESIAN_POINT ( 'NONE',  ( 12.14591786802309770, 12.06949235617756955, 89.37390960531435269 ) ) ;
#189472=CARTESIAN_POINT ( 'NONE',  ( -16.46253265017146816, -9.564922557961047289, 104.1677570613523329 ) ) ;
#189474=CARTESIAN_POINT ( 'NONE',  ( -9.564922557960796823, -16.46253265017161027, 72.08224293864770971 ) ) ;
#189475=CARTESIAN_POINT ( 'NONE',  ( -21.52544592524334988, -5.823673210054445271, 103.9594237280190185 ) ) ;
#189476=CARTESIAN_POINT ( 'NONE',  ( -19.02544592524342804, 5.153800228976336051, 116.0405762719810383 ) ) ;
#189477=CARTESIAN_POINT ( 'NONE',  ( -16.53943276465976808, -0.05219959533934237506, 73.75109039468567573 ) ) ;
#189479=CARTESIAN_POINT ( 'NONE',  ( -19.05341960407617563, 5.049401038297882671, 58.54275706135234003 ) ) ;
#189480=CARTESIAN_POINT ( 'NONE',  ( -15.80617190586768217, 15.72974639402176855, 113.1260903946856899 ) ) ;
#189482=CARTESIAN_POINT ( 'NONE',  ( 13.89961937509977652, -13.97604488694527269, 23.12390960531436335 ) ) ;
#189483=CARTESIAN_POINT ( 'NONE',  ( 16.52544592524342804, -4.483927247898539470, 23.54057627198102765 ) ) ;
#189485=CARTESIAN_POINT ( 'NONE',  ( 12.14591786802327356, -12.06949235617739191, 110.6260903946857042 ) ) ;
#189487=CARTESIAN_POINT ( 'NONE',  ( 4.483927247898790824, -16.52544592524335698, 85.20942372801901854 ) ) ;
#189488=CARTESIAN_POINT ( 'NONE',  ( -5.153800228976328057, -19.02544592524343514, 22.29057627198102765 ) ) ;
#189489=CARTESIAN_POINT ( 'NONE',  ( -21.55341960407619339, 5.719274019375674811, 88.54275706135236135 ) ) ;
#189490=CARTESIAN_POINT ( 'NONE',  ( 9.564922557961047289, -16.46253265017146816, 105.4177570613523471 ) ) ;
#189491=CARTESIAN_POINT ( 'NONE',  ( -15.72974639402176322, -15.80617190586768395, 64.37609039468568994 ) ) ;
#189492=CARTESIAN_POINT ( 'NONE',  ( -13.97604488694547697, 13.89961937509957934, 43.12609039468566152 ) ) ;
#189493=CARTESIAN_POINT ( 'NONE',  ( -5.153800228976328057, -19.02544592524343514, 82.29057627198103830 ) ) ;
#189494=CARTESIAN_POINT ( 'NONE',  ( 16.51473224551069308, 9.474510206698969483, 64.16557627198102409 ) ) ;
#189497=CARTESIAN_POINT ( 'NONE',  ( -21.55341960407610458, -5.719274019375992779, 41.45724293864769550 ) ) ;
#189498=CARTESIAN_POINT ( 'NONE',  ( -5.049401038298153566, 19.05341960407611168, 45.20724293864769550 ) ) ;
#189499=CARTESIAN_POINT ( 'NONE',  ( -8.314922557961024197, 14.29746914071037800, 82.91775706135234714 ) ) ;
#189503=CARTESIAN_POINT ( 'NONE',  ( -16.53943276465976808, 0.05219959533911058130, 81.24890960531436690 ) ) ;
#189505=CARTESIAN_POINT ( 'NONE',  ( 14.29746914071037800, 8.314922557961029526, 36.66775706135234714 ) ) ;
#189506=CARTESIAN_POINT ( 'NONE',  ( 8.314922557960818139, 14.29746914071049879, 114.5822429386477097 ) ) ;
#189507=CARTESIAN_POINT ( 'NONE',  ( 9.474510206698729675, 16.51473224551082808, 62.08442372801899722 ) ) ;
#189509=CARTESIAN_POINT ( 'NONE',  ( -4.483927247898539470, -16.52544592524342804, 67.29057627198103830 ) ) ;
#189510=CARTESIAN_POINT ( 'NONE',  ( 5.823673210054444382, -21.52544592524334988, 35.20942372801901854 ) ) ;
#189512=CARTESIAN_POINT ( 'NONE',  ( 21.53943276465977519, -0.05219959533907433946, 93.74890960531436690 ) ) ;
#189514=CARTESIAN_POINT ( 'NONE',  ( 13.89961937509977652, -13.97604488694527269, 98.12390960531433848 ) ) ;
#189515=CARTESIAN_POINT ( 'NONE',  ( 12.14591786802309770, 12.06949235617756955, 74.37390960531436690 ) ) ;
#189517=CARTESIAN_POINT ( 'NONE',  ( -13.97604488694527625, -13.89961937509977652, 46.87390960531435979 ) ) ;
#189519=CARTESIAN_POINT ( 'NONE',  ( 0.05219959533936267826, -19.03943276465977164, 75.00109039468566152 ) ) ;
#189520=CARTESIAN_POINT ( 'NONE',  ( 10.81492255796106328, -18.62759615963255655, 20.41775706135234714 ) ) ;
#189521=CARTESIAN_POINT ( 'NONE',  ( -13.97604488694527625, -13.89961937509977652, 66.87390960531436690 ) ) ;
#189522=CARTESIAN_POINT ( 'NONE',  ( 16.46253265017146816, 9.564922557961045513, 56.66775706135233293 ) ) ;
#189523=CARTESIAN_POINT ( 'NONE',  ( -5.049401038298153566, 19.05341960407611168, 50.20724293864770260 ) ) ;
#189525=CARTESIAN_POINT ( 'NONE',  ( -16.55341960407611168, -4.379528057220339221, 66.45724293864768129 ) ) ;
#189526=CARTESIAN_POINT ( 'NONE',  ( -4.379528057220328563, 16.55341960407611168, 50.20724293864769550 ) ) ;
#189527=CARTESIAN_POINT ( 'NONE',  ( -19.05341960407611168, -5.049401038298163336, 81.45724293864769550 ) ) ;
#189528=CARTESIAN_POINT ( 'NONE',  ( -0.05219959533907301413, -21.53943276465977519, 82.49890960531436690 ) ) ;
#189529=CARTESIAN_POINT ( 'NONE',  ( -9.474510206698964154, 16.51473224551069663, 75.41557627198103830 ) ) ;
#189530=CARTESIAN_POINT ( 'NONE',  ( 0.05219959533907565091, 21.53943276465977519, 84.99890960531436690 ) ) ;
#189531=CARTESIAN_POINT ( 'NONE',  ( -16.51473224551082808, 9.474510206698731452, 23.33442372801900078 ) ) ;
#189532=CARTESIAN_POINT ( 'NONE',  ( -13.97604488694527625, -13.89961937509977652, 21.87390960531435979 ) ) ;
#189533=CARTESIAN_POINT ( 'NONE',  ( -16.55341960407617563, 4.379528057220093196, 113.5427570613523756 ) ) ;
#189534=CARTESIAN_POINT ( 'NONE',  ( 16.52544592524342804, -4.483927247898539470, 93.54057627198103830 ) ) ;
#189535=CARTESIAN_POINT ( 'NONE',  ( 19.02544592524334988, 5.153800228976608722, 106.4594237280190185 ) ) ;
#189537=CARTESIAN_POINT ( 'NONE',  ( -5.719274019375978568, 21.55341960407610458, 115.2072429386476955 ) ) ;
#189538=CARTESIAN_POINT ( 'NONE',  ( 13.89961937509957401, 13.97604488694547697, 51.87609039468566863 ) ) ;
#189539=CARTESIAN_POINT ( 'NONE',  ( 14.29746914071037800, 8.314922557961029526, 111.6677570613523613 ) ) ;
#189540=CARTESIAN_POINT ( 'NONE',  ( 0.05219959533907565091, 21.53943276465977519, 69.99890960531435269 ) ) ;
#189541=CARTESIAN_POINT ( 'NONE',  ( 16.51473224551069308, 9.474510206698969483, 99.16557627198102409 ) ) ;
#189542=CARTESIAN_POINT ( 'NONE',  ( -14.34966873604960291, -8.224510206698953496, 56.66557627198103830 ) ) ;
#189543=CARTESIAN_POINT ( 'NONE',  ( -0.05219959533909027116, -19.03943276465977164, 22.49890960531436690 ) ) ;
#189544=CARTESIAN_POINT ( 'NONE',  ( 9.564922557960805705, 16.46253265017160317, 34.58224293864770260 ) ) ;
#189545=CARTESIAN_POINT ( 'NONE',  ( -18.67979575497193778, 10.72451020669871902, 103.3344237280190043 ) ) ;
#189546=CARTESIAN_POINT ( 'NONE',  ( 12.06949235617739724, 12.14591786802326823, 91.87609039468568994 ) ) ;
#189547=CARTESIAN_POINT ( 'NONE',  ( 18.67979575497194134, -10.72451020669871369, 45.83442372801901854 ) ) ;
#189548=CARTESIAN_POINT ( 'NONE',  ( 0.05219959533934541429, -16.53943276465976808, 45.00109039468568284 ) ) ;
#189549=CARTESIAN_POINT ( 'NONE',  ( -0.05219959533907301413, -21.53943276465977519, 27.49890960531435269 ) ) ;
#189550=CARTESIAN_POINT ( 'NONE',  ( -9.564922557960796823, -16.46253265017161027, 47.08224293864769550 ) ) ;
#189551=CARTESIAN_POINT ( 'NONE',  ( 13.89961937509977652, -13.97604488694527269, 63.12390960531435979 ) ) ;
#189552=CARTESIAN_POINT ( 'NONE',  ( -14.29746914071037622, -8.314922557961029526, 49.16775706135234003 ) ) ;
#189553=CARTESIAN_POINT ( 'NONE',  ( 4.379528057220339221, -16.55341960407611168, 107.7072429386476955 ) ) ;
#189554=CARTESIAN_POINT ( 'NONE',  ( -14.29746914071037622, -8.314922557961029526, 109.1677570613523613 ) ) ;
#189555=CARTESIAN_POINT ( 'NONE',  ( 22.00000000000000000, -1.132798289211302014E-14, 97.50000000000000000 ) ) ;
#189556=CARTESIAN_POINT ( 'NONE',  ( 5.823673210054444382, -21.52544592524334988, 50.20942372801901854 ) ) ;
#189557=CARTESIAN_POINT ( 'NONE',  ( -19.03943276465977164, 0.05219959533909376836, 96.24890960531436690 ) ) ;
#189558=CARTESIAN_POINT ( 'NONE',  ( -19.05341960407611168, -5.049401038298163336, 76.45724293864769550 ) ) ;
#189559=CARTESIAN_POINT ( 'NONE',  ( -0.05219959533909027116, -19.03943276465977164, 97.49890960531436690 ) ) ;
#189560=CARTESIAN_POINT ( 'NONE',  ( -14.34966873604960291, -8.224510206698953496, 41.66557627198103120 ) ) ;
#189561=CARTESIAN_POINT ( 'NONE',  ( 14.29746914071049879, -8.314922557960816363, 23.33224293864769194 ) ) ;
#189562=CARTESIAN_POINT ( 'NONE',  ( 8.224510206698953496, -14.34966873604960469, 32.91557627198102409 ) ) ;
#189563=CARTESIAN_POINT ( 'NONE',  ( 17.50000000000000000, 5.499999999999997335, 120.0000000000000142 ) ) ;
#189564=CARTESIAN_POINT ( 'NONE',  ( -5.049401038297874678, -19.05341960407617918, 39.79275706135232582 ) ) ;
#189565=CARTESIAN_POINT ( 'NONE',  ( -9.474510206698964154, 16.51473224551069663, 80.41557627198103830 ) ) ;
#189566=CARTESIAN_POINT ( 'NONE',  ( -9.474510206698720793, -16.51473224551083518, 49.58442372801899722 ) ) ;
#189569=CARTESIAN_POINT ( 'NONE',  ( -19.02544592524334988, -5.153800228976617603, 78.95942372801900433 ) ) ;
#189570=CARTESIAN_POINT ( 'NONE',  ( -12.14591786802326823, 12.06949235617739902, 68.12609039468567573 ) ) ;
#189571=CARTESIAN_POINT ( 'NONE',  ( 16.52216118717206683, 7.221426719304505859, 93.57599021046993926 ) ) ;
#189572=CARTESIAN_POINT ( 'NONE',  ( 16.51473224551069308, 9.474510206698969483, 109.1655762719810383 ) ) ;
#189573=CARTESIAN_POINT ( 'NONE',  ( 10.72451020669871369, 18.67979575497193778, 22.08442372801901143 ) ) ;
#189574=CARTESIAN_POINT ( 'NONE',  ( -13.89961937509957401, -13.97604488694547875, 89.37609039468563310 ) ) ;
#189575=CARTESIAN_POINT ( 'NONE',  ( 17.50000000000000000, 5.499999999999992895, 86.70309617465828467 ) ) ;
#189576=CARTESIAN_POINT ( 'NONE',  ( 13.89961937509977652, -13.97604488694527269, 53.12390960531434558 ) ) ;
#189577=CARTESIAN_POINT ( 'NONE',  ( 16.46253265017160672, -9.564922557960803928, 93.33224293864769550 ) ) ;
#189578=CARTESIAN_POINT ( 'NONE',  ( 16.52544592524342804, -4.483927247898539470, 43.54057627198103830 ) ) ;
#189579=CARTESIAN_POINT ( 'NONE',  ( -13.97604488694527625, -13.89961937509977652, 51.87390960531436690 ) ) ;
#189580=CARTESIAN_POINT ( 'NONE',  ( 19.05341960407617918, -5.049401038297876454, 61.04275706135232582 ) ) ;
#189581=CARTESIAN_POINT ( 'NONE',  ( 13.97604488694548053, -13.89961937509957401, 30.62609039468566863 ) ) ;
#189582=CARTESIAN_POINT ( 'NONE',  ( -19.02544592524342804, 5.153800228976336051, 66.04057627198103830 ) ) ;
#189583=CARTESIAN_POINT ( 'NONE',  ( 15.72974639402199770, -15.80617190586745480, 63.12390960531435979 ) ) ;
#189584=CARTESIAN_POINT ( 'NONE',  ( 14.29746914071049879, -8.314922557960816363, 68.33224293864769550 ) ) ;
#189585=CARTESIAN_POINT ( 'NONE',  ( -18.67979575497193778, 10.72451020669871902, 113.3344237280190328 ) ) ;
#189587=CARTESIAN_POINT ( 'NONE',  ( -5.049401038298153566, 19.05341960407611168, 115.2072429386477097 ) ) ;
#189588=CARTESIAN_POINT ( 'NONE',  ( -19.05341960407611168, -5.049401038298163336, 56.45724293864768129 ) ) ;
#189589=CARTESIAN_POINT ( 'NONE',  ( -16.51473224551069308, -9.474510206698971260, 36.66557627198102409 ) ) ;
#189590=CARTESIAN_POINT ( 'NONE',  ( -12.14591786802309592, -12.06949235617757132, 96.87390960531436690 ) ) ;
#189591=CARTESIAN_POINT ( 'NONE',  ( -5.823673210054116645, -21.52544592524344225, 112.2905762719810241 ) ) ;
#189592=CARTESIAN_POINT ( 'NONE',  ( 19.03943276465977164, -0.05219959533909143690, 113.7489096053143669 ) ) ;
#189593=CARTESIAN_POINT ( 'NONE',  ( -18.67979575497193778, 10.72451020669871902, 33.33442372801900433 ) ) ;
#189594=CARTESIAN_POINT ( 'NONE',  ( 0.05219959533909260263, 19.03943276465977164, 99.99890960531436690 ) ) ;
#189595=CARTESIAN_POINT ( 'NONE',  ( -13.97604488694527625, -13.89961937509977652, 26.87390960531434558 ) ) ;
#189596=CARTESIAN_POINT ( 'NONE',  ( -15.80617190586768217, 15.72974639402176855, 73.12609039468567573 ) ) ;
#189597=CARTESIAN_POINT ( 'NONE',  ( -18.67979575497178146, -10.72451020669898902, 96.66557627198102409 ) ) ;
#189598=CARTESIAN_POINT ( 'NONE',  ( 17.40805194822030799, -6.112264579159321087, 108.3337127251061247 ) ) ;
#189601=CARTESIAN_POINT ( 'NONE',  ( 4.483927247898790824, -16.52544592524335698, 45.20942372801901854 ) ) ;
#189602=CARTESIAN_POINT ( 'NONE',  ( 14.34966873604960469, 8.224510206698951720, 114.1655762719810383 ) ) ;
#189604=CARTESIAN_POINT ( 'NONE',  ( 16.46253265017160672, -9.564922557960803928, 63.33224293864769550 ) ) ;
#189605=CARTESIAN_POINT ( 'NONE',  ( 16.55341960407611168, 4.379528057220329451, 93.95724293864770971 ) ) ;
#189606=CARTESIAN_POINT ( 'NONE',  ( 21.53943276465977519, -0.05219959533907433946, 48.74890960531435979 ) ) ;
#189607=CARTESIAN_POINT ( 'NONE',  ( 8.314922557960818139, 14.29746914071049879, 64.58224293864769550 ) ) ;
#189608=CARTESIAN_POINT ( 'NONE',  ( -12.14591786802326823, 12.06949235617739902, 33.12609039468569705 ) ) ;
#189609=CARTESIAN_POINT ( 'NONE',  ( 15.72974639402176855, 15.80617190586768217, 91.87609039468568994 ) ) ;
#189610=CARTESIAN_POINT ( 'NONE',  ( 16.31925111598455302, -7.325300261831589665, 77.66424538967254421 ) ) ;
#189611=CARTESIAN_POINT ( 'NONE',  ( 16.52544592524335698, 4.483927247898782831, 96.45942372801901854 ) ) ;
#189612=CARTESIAN_POINT ( 'NONE',  ( 12.14591786802309770, 12.06949235617756955, 39.37390960531436690 ) ) ;
#189613=CARTESIAN_POINT ( 'NONE',  ( -16.51473224551069308, -9.474510206698971260, 41.66557627198103120 ) ) ;
#189614=CARTESIAN_POINT ( 'NONE',  ( 13.97604488694527802, 13.89961937509977652, 94.37390960531436690 ) ) ;
#189615=CARTESIAN_POINT ( 'NONE',  ( -10.72451020669898014, 18.67979575497178502, 95.41557627198102409 ) ) ;
#189616=CARTESIAN_POINT ( 'NONE',  ( -18.67979575497193778, 10.72451020669871902, 53.33442372801901854 ) ) ;
#189617=CARTESIAN_POINT ( 'NONE',  ( -8.224510206698735004, -14.34966873604973081, 34.58442372801900433 ) ) ;
#189618=CARTESIAN_POINT ( 'NONE',  ( 16.52544592524342804, -4.483927247898539470, 68.54057627198103830 ) ) ;
#189619=CARTESIAN_POINT ( 'NONE',  ( 10.81492255796106328, -18.62759615963255655, 80.41775706135234714 ) ) ;
#189620=CARTESIAN_POINT ( 'NONE',  ( -8.224510206698735004, -14.34966873604973081, 99.58442372801900433 ) ) ;
#189621=CARTESIAN_POINT ( 'NONE',  ( 16.19135201231351218, -7.376712067592055888, 47.31319145947882276 ) ) ;
#189623=CARTESIAN_POINT ( 'NONE',  ( -8.314922557960811034, -14.29746914071050412, 27.08224293864769550 ) ) ;
#189624=CARTESIAN_POINT ( 'NONE',  ( -12.14591786802326823, 12.06949235617739902, 73.12609039468567573 ) ) ;
#189625=CARTESIAN_POINT ( 'NONE',  ( 13.97604488694527802, 13.89961937509977652, 79.37390960531435269 ) ) ;
#189626=CARTESIAN_POINT ( 'NONE',  ( 19.02544592524343514, -5.153800228976328945, 103.5405762719809957 ) ) ;
#189627=CARTESIAN_POINT ( 'NONE',  ( -18.62759615963255300, -10.81492255796106328, 79.16775706135234714 ) ) ;
#189628=CARTESIAN_POINT ( 'NONE',  ( -14.29746914071037622, -8.314922557961029526, 89.16775706135236135 ) ) ;
#189629=CARTESIAN_POINT ( 'NONE',  ( -16.53943276465976808, 0.05219959533911058130, 56.24890960531436690 ) ) ;
#189630=CARTESIAN_POINT ( 'NONE',  ( 0.05219959533909260263, 19.03943276465977164, 64.99890960531436690 ) ) ;
#189632=CARTESIAN_POINT ( 'NONE',  ( 16.53943276465976808, 0.05219959533934440121, 21.25109039468567218 ) ) ;
#189633=CARTESIAN_POINT ( 'NONE',  ( 16.51473224551069308, 9.474510206698969483, 34.16557627198102409 ) ) ;
#189634=CARTESIAN_POINT ( 'NONE',  ( 5.049401038298161559, -19.05341960407611168, 72.70724293864768129 ) ) ;
#189635=CARTESIAN_POINT ( 'NONE',  ( 13.89961937509957401, 13.97604488694547697, 111.8760903946856757 ) ) ;
#189637=CARTESIAN_POINT ( 'NONE',  ( 19.03943276465977164, 0.05219959533936151252, 21.25109039468565797 ) ) ;
#189638=CARTESIAN_POINT ( 'NONE',  ( -12.14591786802326823, 12.06949235617739902, 78.12609039468570415 ) ) ;
#189639=CARTESIAN_POINT ( 'NONE',  ( -9.474510206698720793, -16.51473224551083518, 109.5844237280190043 ) ) ;
#189640=CARTESIAN_POINT ( 'NONE',  ( 14.34966873604960469, 8.224510206698951720, 114.1655762719810383 ) ) ;
#189641=CARTESIAN_POINT ( 'NONE',  ( 14.29746914071037800, 8.314922557961029526, 61.66775706135235424 ) ) ;
#189642=CARTESIAN_POINT ( 'NONE',  ( -4.483927247898782831, 16.52544592524335698, 52.70942372801902565 ) ) ;
#189643=CARTESIAN_POINT ( 'NONE',  ( 13.89961937509977652, -13.97604488694527269, 28.12390960531435624 ) ) ;
#189644=CARTESIAN_POINT ( 'NONE',  ( 9.564922557961047289, -16.46253265017146816, 75.41775706135234714 ) ) ;
#189645=CARTESIAN_POINT ( 'NONE',  ( 21.52544592524334988, 5.823673210054432836, 106.4594237280190328 ) ) ;
#189646=CARTESIAN_POINT ( 'NONE',  ( 5.153800228976335163, 19.02544592524342804, 34.79057627198102409 ) ) ;
#189647=CARTESIAN_POINT ( 'NONE',  ( -13.97604488694527625, -13.89961937509977652, 76.87390960531433848 ) ) ;
#189648=CARTESIAN_POINT ( 'NONE',  ( -16.53943276465976808, 0.05219959533911058130, 71.24890960531435269 ) ) ;
#189650=CARTESIAN_POINT ( 'NONE',  ( -13.97604488694547697, 13.89961937509957934, 43.12609039468566152 ) ) ;
#189651=CARTESIAN_POINT ( 'NONE',  ( 15.80617190586746368, 15.72974639402197994, 39.37390960531436690 ) ) ;
#189652=CARTESIAN_POINT ( 'NONE',  ( 21.52544592524334988, 5.823673210054432836, 111.4594237280190328 ) ) ;
#189653=CARTESIAN_POINT ( 'NONE',  ( -9.564922557960796823, -16.46253265017161027, 97.08224293864769550 ) ) ;
#189655=CARTESIAN_POINT ( 'NONE',  ( 10.81492255796106328, -18.62759615963255655, 105.4177570613523613 ) ) ;
#189656=CARTESIAN_POINT ( 'NONE',  ( -0.05219959533907301413, -21.53943276465977519, 57.49890960531435979 ) ) ;
#189657=CARTESIAN_POINT ( 'NONE',  ( -9.474510206698964154, 16.51473224551069663, 95.41557627198102409 ) ) ;
#189658=CARTESIAN_POINT ( 'NONE',  ( 0.05219959533936267826, -19.03943276465977164, 90.00109039468567573 ) ) ;
#189659=CARTESIAN_POINT ( 'NONE',  ( 13.97604488694527802, 13.89961937509977652, 99.37390960531436690 ) ) ;
#189660=CARTESIAN_POINT ( 'NONE',  ( 5.153800228976615827, -19.02544592524334988, 95.20942372801897591 ) ) ;
#189661=CARTESIAN_POINT ( 'NONE',  ( -0.05219959533910754901, -16.53943276465976808, 112.4989096053143669 ) ) ;
#189662=CARTESIAN_POINT ( 'NONE',  ( -13.89961937509977652, 13.97604488694528158, 85.62390960531433848 ) ) ;
#189663=CARTESIAN_POINT ( 'NONE',  ( 18.62759615963271287, -10.81492255796078972, 63.33224293864770260 ) ) ;
#189664=CARTESIAN_POINT ( 'NONE',  ( 16.53943276465976808, 0.05219959533934440121, 36.25109039468567573 ) ) ;
#189665=CARTESIAN_POINT ( 'NONE',  ( -18.67979575497193778, 10.72451020669871902, 43.33442372801901143 ) ) ;
#189666=CARTESIAN_POINT ( 'NONE',  ( -5.823673210054431948, 21.52544592524334988, 102.7094237280190185 ) ) ;
#189667=CARTESIAN_POINT ( 'NONE',  ( -14.29746914071037622, -8.314922557961029526, 99.16775706135234714 ) ) ;
#189668=CARTESIAN_POINT ( 'NONE',  ( -5.153800228976328057, -19.02544592524343514, 87.29057627198103830 ) ) ;
#189669=CARTESIAN_POINT ( 'NONE',  ( 14.34966873604960469, 8.224510206698951720, 89.16557627198102409 ) ) ;
#189670=CARTESIAN_POINT ( 'NONE',  ( 16.55341960407618274, -4.379528057220086978, 111.0427570613523613 ) ) ;
#189671=CARTESIAN_POINT ( 'NONE',  ( -5.153800228976607833, 19.02544592524334988, 62.70942372801899722 ) ) ;
#189673=CARTESIAN_POINT ( 'NONE',  ( -5.823673210054431948, 21.52544592524334988, 47.70942372801902565 ) ) ;
#189674=CARTESIAN_POINT ( 'NONE',  ( -16.55341960407611168, -4.379528057220339221, 91.45724293864769550 ) ) ;
#189675=CARTESIAN_POINT ( 'NONE',  ( -19.05341960407611168, -5.049401038298163336, 106.4572429386476955 ) ) ;
#189676=CARTESIAN_POINT ( 'NONE',  ( 8.314922557960818139, 14.29746914071049879, 29.58224293864769905 ) ) ;
#189677=CARTESIAN_POINT ( 'NONE',  ( 5.823673210054444382, -21.52544592524334988, 90.20942372801903275 ) ) ;
#189678=CARTESIAN_POINT ( 'NONE',  ( -0.05219959533934338120, 16.53943276465976808, 42.50109039468567573 ) ) ;
#189679=CARTESIAN_POINT ( 'NONE',  ( 5.823673210054444382, -21.52544592524334988, 40.20942372801901854 ) ) ;
#189680=ORIENTED_EDGE ( 'NONE', *, *, #74286, .F. ) ;
#189681=CARTESIAN_POINT ( 'NONE',  ( 0.05219959533937995610, -21.53943276465977519, 20.00109039468568639 ) ) ;
#189682=CARTESIAN_POINT ( 'NONE',  ( 14.34966873604960469, 8.224510206698951720, 89.16557627198102409 ) ) ;
#189683=CARTESIAN_POINT ( 'NONE',  ( -19.25176906914649066, -5.499999999999738876, 50.99927264242279534 ) ) ;
#189684=CARTESIAN_POINT ( 'NONE',  ( 14.34966873604960469, 8.224510206698951720, 64.16557627198102409 ) ) ;
#189685=CARTESIAN_POINT ( 'NONE',  ( 9.564922557960805705, 16.46253265017160317, 54.58224293864769550 ) ) ;
#189686=CARTESIAN_POINT ( 'NONE',  ( -12.06949235617739369, -12.14591786802326823, 109.3760903946857042 ) ) ;
#189687=CARTESIAN_POINT ( 'NONE',  ( 9.564922557960805705, 16.46253265017160317, 44.58224293864769550 ) ) ;
#189688=CARTESIAN_POINT ( 'NONE',  ( -10.81492255796078084, -18.62759615963271287, 42.08224293864769550 ) ) ;
#189689=CARTESIAN_POINT ( 'NONE',  ( 14.34966873604960469, 8.224510206698951720, 74.16557627198102409 ) ) ;
#189690=VECTOR ( 'NONE', #92719, 1000.000000000000000 ) ;
#189691=CARTESIAN_POINT ( 'NONE',  ( 0.05219959533907565091, 21.53943276465977519, 94.99890960531436690 ) ) ;
#189692=CARTESIAN_POINT ( 'NONE',  ( 5.049401038298161559, -19.05341960407611168, 87.70724293864769550 ) ) ;
#189693=CARTESIAN_POINT ( 'NONE',  ( 16.51473224551069308, 9.474510206698969483, 39.16557627198103120 ) ) ;
#189694=CARTESIAN_POINT ( 'NONE',  ( -16.46253265017146816, -9.564922557961047289, 94.16775706135233293 ) ) ;
#189695=CARTESIAN_POINT ( 'NONE',  ( -15.80617190586745835, -15.72974639402198527, 41.87390960531435979 ) ) ;
#189696=CARTESIAN_POINT ( 'NONE',  ( -10.81492255796105439, 18.62759615963255655, 72.91775706135234714 ) ) ;
#189697=CARTESIAN_POINT ( 'NONE',  ( -16.51473224551069308, -9.474510206698971260, 51.66557627198102409 ) ) ;
#189698=CARTESIAN_POINT ( 'NONE',  ( 9.564922557960805705, 16.46253265017160317, 79.58224293864769550 ) ) ;
#189699=ORIENTED_EDGE ( 'NONE', *, *, #114623, .T. ) ;
#189700=CARTESIAN_POINT ( 'NONE',  ( -8.314922557961024197, 14.29746914071037800, 57.91775706135234714 ) ) ;
#189701=CARTESIAN_POINT ( 'NONE',  ( -21.52544592524334988, -5.823673210054445271, 43.95942372801902565 ) ) ;
#189702=CARTESIAN_POINT ( 'NONE',  ( -0.05219959533937732626, 21.53943276465977519, 77.50109039468567573 ) ) ;
#189703=CARTESIAN_POINT ( 'NONE',  ( -5.049401038298153566, 19.05341960407611168, 115.2072429386477097 ) ) ;
#189704=CARTESIAN_POINT ( 'NONE',  ( -21.53943276465977519, 0.05219959533907696930, 101.2489096053143669 ) ) ;
#189705=CARTESIAN_POINT ( 'NONE',  ( -10.81492255796105439, 18.62759615963255655, 42.91775706135235424 ) ) ;
#189706=CARTESIAN_POINT ( 'NONE',  ( -4.483927247898782831, 16.52544592524335698, 67.70942372801901854 ) ) ;
#189707=CARTESIAN_POINT ( 'NONE',  ( -0.05219959533907301413, -21.53943276465977519, 62.49890960531436690 ) ) ;
#189708=CARTESIAN_POINT ( 'NONE',  ( -19.05341960407617563, 5.049401038297882671, 33.54275706135231871 ) ) ;
#189709=CARTESIAN_POINT ( 'NONE',  ( 13.89961937509977652, -13.97604488694527269, 68.12390960531436690 ) ) ;
#189710=CARTESIAN_POINT ( 'NONE',  ( 16.52544592524335698, 4.483927247898782831, 101.4594237280190185 ) ) ;
#189712=CARTESIAN_POINT ( 'NONE',  ( 5.153800228976335163, 19.02544592524342804, 99.79057627198102409 ) ) ;
#189713=CARTESIAN_POINT ( 'NONE',  ( -9.564922557961040184, 16.46253265017147172, 52.91775706135233293 ) ) ;
#189714=CARTESIAN_POINT ( 'NONE',  ( 13.97604488694548053, -13.89961937509957401, 80.62609039468567573 ) ) ;
#189715=CARTESIAN_POINT ( 'NONE',  ( 15.80617190586746368, 15.72974639402197994, 64.37390960531435269 ) ) ;
#189716=CARTESIAN_POINT ( 'NONE',  ( -4.379528057220328563, 16.55341960407611168, 45.20724293864769550 ) ) ;
#189717=CARTESIAN_POINT ( 'NONE',  ( -9.564922557961040184, 16.46253265017147172, 92.91775706135233293 ) ) ;
#189719=CARTESIAN_POINT ( 'NONE',  ( -0.05219959533936034679, 19.03943276465977164, 102.5010903946856757 ) ) ;
#189720=CARTESIAN_POINT ( 'NONE',  ( -21.52544592524343514, 5.823673210054127303, 81.04057627198102409 ) ) ;
#189721=CARTESIAN_POINT ( 'NONE',  ( 13.97604488694548053, -13.89961937509957401, 55.62609039468566863 ) ) ;
#189723=CARTESIAN_POINT ( 'NONE',  ( 16.46253265017160672, -9.564922557960803928, 63.33224293864769550 ) ) ;
#189724=CARTESIAN_POINT ( 'NONE',  ( -16.53943276465976808, 0.05219959533911058130, 66.24890960531436690 ) ) ;
#189725=CARTESIAN_POINT ( 'NONE',  ( -5.049401038298153566, 19.05341960407611168, 45.20724293864769550 ) ) ;
#189726=CARTESIAN_POINT ( 'NONE',  ( -4.379528057220328563, 16.55341960407611168, 60.20724293864768839 ) ) ;
#189727=CARTESIAN_POINT ( 'NONE',  ( -5.049401038298153566, 19.05341960407611168, 25.20724293864768484 ) ) ;
#189729=CARTESIAN_POINT ( 'NONE',  ( -16.53943276465976808, 0.05219959533911058130, 31.24890960531435979 ) ) ;
#189730=CARTESIAN_POINT ( 'NONE',  ( -5.049401038298153566, 19.05341960407611168, 65.20724293864765286 ) ) ;
#189732=CARTESIAN_POINT ( 'NONE',  ( 13.97604488694548053, -13.89961937509957401, 35.62609039468567573 ) ) ;
#189733=CARTESIAN_POINT ( 'NONE',  ( 14.29746914071037800, 8.314922557961029526, 46.66775706135234714 ) ) ;
#189734=CARTESIAN_POINT ( 'NONE',  ( 5.823673210054125526, 21.52544592524343514, 49.79057627198102409 ) ) ;
#189735=CARTESIAN_POINT ( 'NONE',  ( 21.52544592524334988, 5.823673210054432836, 111.4594237280190328 ) ) ;
#189736=CARTESIAN_POINT ( 'NONE',  ( -5.049401038298153566, 19.05341960407611168, 75.20724293864769550 ) ) ;
#189738=CARTESIAN_POINT ( 'NONE',  ( 0.05219959533909260263, 19.03943276465977164, 104.9989096053143669 ) ) ;
#189739=CARTESIAN_POINT ( 'NONE',  ( 5.823673210054444382, -21.52544592524334988, 40.20942372801901854 ) ) ;
#189740=CARTESIAN_POINT ( 'NONE',  ( 16.52544592524342804, -4.483927247898539470, 98.54057627198105251 ) ) ;
#189741=CARTESIAN_POINT ( 'NONE',  ( 21.53943276465977519, -0.05219959533907433946, 88.74890960531436690 ) ) ;
#189742=CARTESIAN_POINT ( 'NONE',  ( -16.51473224551069308, -9.474510206698971260, 81.66557627198103830 ) ) ;
#189743=VERTEX_POINT ( 'NONE', #30092 ) ;
#189744=CARTESIAN_POINT ( 'NONE',  ( 19.05341960407611168, 5.049401038298154454, 83.95724293864766707 ) ) ;
#189745=CARTESIAN_POINT ( 'NONE',  ( 18.67979575497194134, -10.72451020669871369, 20.83442372801901143 ) ) ;
#189748=CARTESIAN_POINT ( 'NONE',  ( -13.97604488694527625, -13.89961937509977652, 81.87390960531436690 ) ) ;
#189750=CARTESIAN_POINT ( 'NONE',  ( 13.89961937509977652, -13.97604488694527269, 23.12390960531436335 ) ) ;
#189751=CARTESIAN_POINT ( 'NONE',  ( 13.89961937509977652, -13.97604488694527269, 33.12390960531434558 ) ) ;
#189752=CARTESIAN_POINT ( 'NONE',  ( 9.474510206698729675, 16.51473224551082808, 107.0844237280190043 ) ) ;
#189754=CARTESIAN_POINT ( 'NONE',  ( -12.06949235617756955, 12.14591786802309770, 105.6239096053143669 ) ) ;
#189755=CARTESIAN_POINT ( 'NONE',  ( -15.80617190586768217, 15.72974639402176855, 88.12609039468570415 ) ) ;
#189756=CARTESIAN_POINT ( 'NONE',  ( 13.89961937509977652, -13.97604488694527269, 63.12390960531435979 ) ) ;
#189757=CARTESIAN_POINT ( 'NONE',  ( -15.80617190586768217, 15.72974639402176855, 33.12609039468569705 ) ) ;
#189758=CARTESIAN_POINT ( 'NONE',  ( -18.67979575497178146, -10.72451020669898902, 106.6655762719810383 ) ) ;
#189760=CARTESIAN_POINT ( 'NONE',  ( 16.51473224551069308, 9.474510206698969483, 84.16557627198102409 ) ) ;
#189762=CARTESIAN_POINT ( 'NONE',  ( 14.34966873604972726, -8.224510206698740333, 25.83442372801901499 ) ) ;
#189763=CARTESIAN_POINT ( 'NONE',  ( -18.67979575497178146, -10.72451020669898902, 41.66557627198103120 ) ) ;
#189764=CARTESIAN_POINT ( 'NONE',  ( 18.67979575497194134, -10.72451020669871369, 60.83442372801901854 ) ) ;
#189765=CARTESIAN_POINT ( 'NONE',  ( 9.474510206698971260, -16.51473224551069308, 112.9155762719810383 ) ) ;
#189766=CARTESIAN_POINT ( 'NONE',  ( 13.97604488694548053, -13.89961937509957401, 95.62609039468563310 ) ) ;
#189767=CARTESIAN_POINT ( 'NONE',  ( 9.474510206698971260, -16.51473224551069308, 62.91557627198102409 ) ) ;
#189768=CARTESIAN_POINT ( 'NONE',  ( 13.89961937509977652, -13.97604488694527269, 88.12390960531438111 ) ) ;
#189769=CARTESIAN_POINT ( 'NONE',  ( 14.34966873604960469, 8.224510206698951720, 94.16557627198103830 ) ) ;
#189770=CARTESIAN_POINT ( 'NONE',  ( -4.379528057220328563, 16.55341960407611168, 100.2072429386476955 ) ) ;
#189771=CARTESIAN_POINT ( 'NONE',  ( -16.51473224551069308, -9.474510206698971260, 111.6655762719810383 ) ) ;
#189773=CARTESIAN_POINT ( 'NONE',  ( -14.29746914071049879, 8.314922557960819915, 50.83224293864770971 ) ) ;
#189774=CARTESIAN_POINT ( 'NONE',  ( -13.97604488694527625, -13.89961937509977652, 46.87390960531435979 ) ) ;
#189775=CARTESIAN_POINT ( 'NONE',  ( 10.72451020669871369, 18.67979575497193778, 67.08442372801901854 ) ) ;
#189776=CARTESIAN_POINT ( 'NONE',  ( -19.03943276465977164, -0.05219959533935918106, 88.75109039468567573 ) ) ;
#189777=CARTESIAN_POINT ( 'NONE',  ( 16.52544592524342804, -4.483927247898539470, 63.54057627198103830 ) ) ;
#189778=CARTESIAN_POINT ( 'NONE',  ( -21.52544592524334988, -5.823673210054445271, 18.95942372801901143 ) ) ;
#189779=CARTESIAN_POINT ( 'NONE',  ( -21.55341960407610458, -5.719274019375992779, 41.45724293864769550 ) ) ;
#189780=CARTESIAN_POINT ( 'NONE',  ( -9.564922557960796823, -16.46253265017161027, 107.0822429386476955 ) ) ;
#189782=CARTESIAN_POINT ( 'NONE',  ( -0.05219959533909027116, -19.03943276465977164, 67.49890960531436690 ) ) ;
#189783=CARTESIAN_POINT ( 'NONE',  ( -16.55341960407611168, -4.379528057220339221, 41.45724293864769550 ) ) ;
#189785=CARTESIAN_POINT ( 'NONE',  ( -12.14591786802326823, 12.06949235617739902, 103.1260903946856757 ) ) ;
#189786=CARTESIAN_POINT ( 'NONE',  ( 4.483927247898790824, -16.52544592524335698, 80.20942372801901854 ) ) ;
#189787=CARTESIAN_POINT ( 'NONE',  ( 16.51473224551083163, -9.474510206698727899, 40.83442372801900433 ) ) ;
#189788=CARTESIAN_POINT ( 'NONE',  ( -17.50000000001358202, 5.499999999999951150, 100.7969038253505687 ) ) ;
#189789=CARTESIAN_POINT ( 'NONE',  ( 5.049401038298161559, -19.05341960407611168, 97.70724293864766707 ) ) ;
#189790=CARTESIAN_POINT ( 'NONE',  ( 19.03943276465977164, -0.05219959533909143690, 48.74890960531435979 ) ) ;
#189791=CARTESIAN_POINT ( 'NONE',  ( 14.29746914071049879, -8.314922557960816363, 63.33224293864770260 ) ) ;
#189792=CARTESIAN_POINT ( 'NONE',  ( 17.31747979337947996, -6.344076630961053453, 101.1205513193481664 ) ) ;
#189793=CARTESIAN_POINT ( 'NONE',  ( 21.52544592524344225, -5.823673210054117533, 23.54057627198102765 ) ) ;
#189794=CARTESIAN_POINT ( 'NONE',  ( 5.823673210054125526, 21.52544592524343514, 49.79057627198102409 ) ) ;
#189795=CARTESIAN_POINT ( 'NONE',  ( -8.224510206698948167, 14.34966873604960824, 90.41557627198103830 ) ) ;
#189796=CARTESIAN_POINT ( 'NONE',  ( 4.379528057220092307, 16.55341960407617563, 37.29275706135235424 ) ) ;
#189797=CARTESIAN_POINT ( 'NONE',  ( -4.379528057220328563, 16.55341960407611168, 85.20724293864770971 ) ) ;
#189798=CARTESIAN_POINT ( 'NONE',  ( -18.87580814761070513, 5.500000000000040856, 65.87172394265761000 ) ) ;
#189799=CARTESIAN_POINT ( 'NONE',  ( -19.05341960407617563, 5.049401038297882671, 73.54275706135233293 ) ) ;
#189800=CARTESIAN_POINT ( 'NONE',  ( 5.719274019375991003, -21.55341960407610458, 22.70724293864769194 ) ) ;
#189802=CARTESIAN_POINT ( 'NONE',  ( 19.42893418801160621, 5.499999999999992895, 102.2141673858846076 ) ) ;
#189803=CARTESIAN_POINT ( 'NONE',  ( 8.314922557961029526, -14.29746914071037800, 25.41775706135235779 ) ) ;
#189804=CARTESIAN_POINT ( 'NONE',  ( 14.34966873604972726, -8.224510206698740333, 110.8344237280190043 ) ) ;
#189805=CARTESIAN_POINT ( 'NONE',  ( -16.51473224551082808, 9.474510206698731452, 68.33442372801900433 ) ) ;
#189806=CARTESIAN_POINT ( 'NONE',  ( 15.80617190586746368, 15.72974639402197994, 54.37390960531435979 ) ) ;
#189807=CARTESIAN_POINT ( 'NONE',  ( 5.719274019375673035, 21.55341960407619339, 62.29275706135236845 ) ) ;
#189808=CARTESIAN_POINT ( 'NONE',  ( 18.59930490233253408, 5.500000000000118128, 38.94150099494206785 ) ) ;
#189809=CARTESIAN_POINT ( 'NONE',  ( -12.06949235617739369, -12.14591786802326823, 34.37609039468568284 ) ) ;
#189810=CARTESIAN_POINT ( 'NONE',  ( 5.153800228976335163, 19.02544592524342804, 24.79057627198102765 ) ) ;
#189811=CARTESIAN_POINT ( 'NONE',  ( -13.97604488694527625, -13.89961937509977652, 81.87390960531436690 ) ) ;
#189813=CARTESIAN_POINT ( 'NONE',  ( 5.153800228976335163, 19.02544592524342804, 24.79057627198102765 ) ) ;
#189814=CARTESIAN_POINT ( 'NONE',  ( -8.314922557960811034, -14.29746914071050412, 87.08224293864769550 ) ) ;
#189815=CARTESIAN_POINT ( 'NONE',  ( -13.97604488694527625, -13.89961937509977652, 96.87390960531433848 ) ) ;
#189817=CARTESIAN_POINT ( 'NONE',  ( 19.03943276465977164, 0.05219959533936151252, 101.2510903946856757 ) ) ;
#189818=CARTESIAN_POINT ( 'NONE',  ( -15.80617190586745835, -15.72974639402198527, 76.87390960531439532 ) ) ;
#189819=CARTESIAN_POINT ( 'NONE',  ( 19.03943276465977164, -0.05219959533909143690, 48.74890960531435979 ) ) ;
#189820=CARTESIAN_POINT ( 'NONE',  ( 0.05219959533936267826, -19.03943276465977164, 65.00109039468567573 ) ) ;
#189821=CARTESIAN_POINT ( 'NONE',  ( -15.72974639402176322, -15.80617190586768395, 19.37609039468568639 ) ) ;
#189822=CARTESIAN_POINT ( 'NONE',  ( 13.97604488694527802, 13.89961937509977652, 64.37390960531436690 ) ) ;
#189823=CARTESIAN_POINT ( 'NONE',  ( -16.46253265017160317, 9.564922557960807481, 105.8322429386476955 ) ) ;
#189825=CARTESIAN_POINT ( 'NONE',  ( 14.34966873604972726, -8.224510206698740333, 35.83442372801901143 ) ) ;
#189826=CARTESIAN_POINT ( 'NONE',  ( 15.72974639402199770, -15.80617190586745480, 98.12390960531436690 ) ) ;
#189827=CARTESIAN_POINT ( 'NONE',  ( -4.379528057220328563, 16.55341960407611168, 110.2072429386477239 ) ) ;
#189828=CARTESIAN_POINT ( 'NONE',  ( -13.97604488694527625, -13.89961937509977652, 91.87390960531432427 ) ) ;
#189829=CARTESIAN_POINT ( 'NONE',  ( 5.049401038297881783, 19.05341960407617563, 67.29275706135234714 ) ) ;
#189830=CARTESIAN_POINT ( 'NONE',  ( 18.62759615963271287, -10.81492255796078972, 93.33224293864769550 ) ) ;
#189831=CARTESIAN_POINT ( 'NONE',  ( -12.06949235617756955, 12.14591786802309770, 50.62390960531435979 ) ) ;
#189832=CARTESIAN_POINT ( 'NONE',  ( 5.153800228976615827, -19.02544592524334988, 20.20942372801899722 ) ) ;
#189833=CARTESIAN_POINT ( 'NONE',  ( -16.52544592524335698, -4.483927247898792601, 63.95942372801901854 ) ) ;
#189834=CARTESIAN_POINT ( 'NONE',  ( -13.89961937509977652, 13.97604488694528158, 90.62390960531432427 ) ) ;
#189835=CARTESIAN_POINT ( 'NONE',  ( -16.46253265017160317, 9.564922557960807481, 45.83224293864769550 ) ) ;
#189836=CARTESIAN_POINT ( 'NONE',  ( 15.80617190586769283, -15.72974639402175789, 50.62609039468568994 ) ) ;
#189837=CARTESIAN_POINT ( 'NONE',  ( 15.80617190586769283, -15.72974639402175789, 70.62609039468567573 ) ) ;
#189838=CARTESIAN_POINT ( 'NONE',  ( 9.564922557960805705, 16.46253265017160317, 59.58224293864769550 ) ) ;
#189839=CARTESIAN_POINT ( 'NONE',  ( -5.719274019375665041, -21.55341960407619695, 29.79275706135234358 ) ) ;
#189840=CARTESIAN_POINT ( 'NONE',  ( -13.97604488694547697, 13.89961937509957934, 78.12609039468567573 ) ) ;
#189841=CARTESIAN_POINT ( 'NONE',  ( 19.02544592524343514, -5.153800228976328945, 38.54057627198103120 ) ) ;
#189842=CARTESIAN_POINT ( 'NONE',  ( 14.29746914071037800, 8.314922557961029526, 81.66775706135236135 ) ) ;
#189843=CARTESIAN_POINT ( 'NONE',  ( -16.51473224551069308, -9.474510206698971260, 56.66557627198103120 ) ) ;
#189845=CARTESIAN_POINT ( 'NONE',  ( -13.97604488694527625, -13.89961937509977652, 36.87390960531436690 ) ) ;
#189846=CARTESIAN_POINT ( 'NONE',  ( 10.81492255796078972, 18.62759615963270932, 89.58224293864768129 ) ) ;
#189847=CARTESIAN_POINT ( 'NONE',  ( 8.314922557961029526, -14.29746914071037800, 75.41775706135233293 ) ) ;
#189849=CARTESIAN_POINT ( 'NONE',  ( -19.03943276465977164, -0.05219959533935918106, 28.75109039468566507 ) ) ;
#189851=CARTESIAN_POINT ( 'NONE',  ( 19.03943276465977164, -0.05219959533909143690, 58.74890960531435979 ) ) ;
#189852=CARTESIAN_POINT ( 'NONE',  ( -8.224510206698948167, 14.34966873604960824, 45.41557627198103830 ) ) ;
#189853=CARTESIAN_POINT ( 'NONE',  ( -16.53943276465976808, 0.05219959533911058130, 76.24890960531435269 ) ) ;
#189854=CARTESIAN_POINT ( 'NONE',  ( -13.97604488694527625, -13.89961937509977652, 101.8739096053143811 ) ) ;
#189855=CARTESIAN_POINT ( 'NONE',  ( 16.51473224551069308, 9.474510206698969483, 84.16557627198102409 ) ) ;
#189856=CARTESIAN_POINT ( 'NONE',  ( 21.52544592524334988, 5.823673210054432836, 51.45942372801901854 ) ) ;
#189857=CARTESIAN_POINT ( 'NONE',  ( 0.05219959533909260263, 19.03943276465977164, 94.99890960531436690 ) ) ;
#189858=CARTESIAN_POINT ( 'NONE',  ( -21.53943276465977519, -0.05219959533937600094, 98.75109039468568994 ) ) ;
#189859=CARTESIAN_POINT ( 'NONE',  ( -4.379528057220086978, -16.55341960407618274, 84.79275706135234714 ) ) ;
#189860=CARTESIAN_POINT ( 'NONE',  ( -18.67979575497193778, 10.72451020669871902, 23.33442372801901499 ) ) ;
#189861=CARTESIAN_POINT ( 'NONE',  ( -18.62759615963270932, 10.81492255796079327, 105.8322429386476955 ) ) ;
#189862=CARTESIAN_POINT ( 'NONE',  ( -14.34966873604960291, -8.224510206698953496, 66.66557627198102409 ) ) ;
#189863=CARTESIAN_POINT ( 'NONE',  ( -13.97604488694527625, -13.89961937509977652, 36.87390960531436690 ) ) ;
#189864=CARTESIAN_POINT ( 'NONE',  ( -14.29746914071049879, 8.314922557960819915, 70.83224293864770971 ) ) ;
#189865=CARTESIAN_POINT ( 'NONE',  ( 21.52544592524344225, -5.823673210054117533, 28.54057627198103120 ) ) ;
#189866=CARTESIAN_POINT ( 'NONE',  ( -19.05341960407617563, 5.049401038297882671, 33.54275706135231871 ) ) ;
#189867=CARTESIAN_POINT ( 'NONE',  ( -12.06949235617756955, 12.14591786802309770, 105.6239096053143669 ) ) ;
#189869=CARTESIAN_POINT ( 'NONE',  ( 8.314922557961029526, -14.29746914071037800, 70.41775706135236135 ) ) ;
#189870=CARTESIAN_POINT ( 'NONE',  ( 16.51473224551069308, 9.474510206698969483, 64.16557627198102409 ) ) ;
#189871=CARTESIAN_POINT ( 'NONE',  ( -12.14591786802309592, -12.06949235617757132, 86.87390960531438111 ) ) ;
#189872=CARTESIAN_POINT ( 'NONE',  ( -15.72974639402197994, 15.80617190586746368, 40.62390960531435269 ) ) ;
#189873=CARTESIAN_POINT ( 'NONE',  ( 16.55341960407618274, -4.379528057220086978, 96.04275706135236135 ) ) ;
#189874=CARTESIAN_POINT ( 'NONE',  ( -16.52544592524335698, -4.483927247898792601, 18.95942372801901143 ) ) ;
#189875=CARTESIAN_POINT ( 'NONE',  ( 18.62759615963255655, 10.81492255796105972, 81.66775706135236135 ) ) ;
#189876=CARTESIAN_POINT ( 'NONE',  ( -13.97604488694527625, -13.89961937509977652, 81.87390960531436690 ) ) ;
#189877=CARTESIAN_POINT ( 'NONE',  ( -5.823673210054116645, -21.52544592524344225, 102.2905762719810383 ) ) ;
#189878=CARTESIAN_POINT ( 'NONE',  ( 4.379528057220092307, 16.55341960407617563, 52.29275706135236135 ) ) ;
#189879=CARTESIAN_POINT ( 'NONE',  ( -19.05341960407611168, -5.049401038298163336, 21.45724293864768839 ) ) ;
#189880=CARTESIAN_POINT ( 'NONE',  ( -5.153800228976607833, 19.02544592524334988, 112.7094237280190043 ) ) ;
#189881=CARTESIAN_POINT ( 'NONE',  ( -16.51473224551082808, 9.474510206698731452, 83.33442372801899012 ) ) ;
#189882=CARTESIAN_POINT ( 'NONE',  ( 15.80617190586746368, 15.72974639402197994, 79.37390960531436690 ) ) ;
#189883=CARTESIAN_POINT ( 'NONE',  ( 0.05219959533936267826, -19.03943276465977164, 50.00109039468566863 ) ) ;
#189885=CARTESIAN_POINT ( 'NONE',  ( 0.05219959533907565091, 21.53943276465977519, 104.9989096053143669 ) ) ;
#189887=CARTESIAN_POINT ( 'NONE',  ( -5.153800228976328057, -19.02544592524343514, 77.29057627198099567 ) ) ;
#189889=CARTESIAN_POINT ( 'NONE',  ( -16.53943276465976808, -0.05219959533934237506, 28.75109039468567929 ) ) ;
#189891=CARTESIAN_POINT ( 'NONE',  ( 15.72974639402199770, -15.80617190586745480, 98.12390960531436690 ) ) ;
#189892=CARTESIAN_POINT ( 'NONE',  ( 8.314922557960818139, 14.29746914071049879, 69.58224293864769550 ) ) ;
#189893=CARTESIAN_POINT ( 'NONE',  ( -19.03943276465977164, 0.05219959533909376836, 66.24890960531436690 ) ) ;
#189894=CARTESIAN_POINT ( 'NONE',  ( -0.05219959533937732626, 21.53943276465977519, 87.50109039468568994 ) ) ;
#189895=CARTESIAN_POINT ( 'NONE',  ( 16.52544592524335698, 4.483927247898782831, 36.45942372801901143 ) ) ;
#189896=CARTESIAN_POINT ( 'NONE',  ( 9.564922557961047289, -16.46253265017146816, 40.41775706135234003 ) ) ;
#189897=CARTESIAN_POINT ( 'NONE',  ( -18.62759615963255300, -10.81492255796106328, 54.16775706135235424 ) ) ;
#189898=CARTESIAN_POINT ( 'NONE',  ( -10.72451020669898014, 18.67979575497178502, 55.41557627198102409 ) ) ;
#189899=CARTESIAN_POINT ( 'NONE',  ( 16.51473224551083163, -9.474510206698727899, 105.8344237280190043 ) ) ;
#189900=CARTESIAN_POINT ( 'NONE',  ( -13.89961937509977652, 13.97604488694528158, 55.62390960531434558 ) ) ;
#189901=CARTESIAN_POINT ( 'NONE',  ( 19.03943276465977164, 0.05219959533936151252, 86.25109039468567573 ) ) ;
#189902=CARTESIAN_POINT ( 'NONE',  ( -18.62759615963255300, -10.81492255796106328, 84.16775706135234714 ) ) ;
#189903=CARTESIAN_POINT ( 'NONE',  ( -5.049401038297874678, -19.05341960407617918, 69.79275706135233293 ) ) ;
#189904=CARTESIAN_POINT ( 'NONE',  ( 16.46253265017160672, -9.564922557960803928, 33.33224293864770260 ) ) ;
#189905=CARTESIAN_POINT ( 'NONE',  ( -15.80617190586745835, -15.72974639402198527, 56.87390960531436690 ) ) ;
#189906=CARTESIAN_POINT ( 'NONE',  ( 8.224510206698953496, -14.34966873604960469, 57.91557627198103120 ) ) ;
#189908=CARTESIAN_POINT ( 'NONE',  ( 19.02544592524334988, 5.153800228976608722, 36.45942372801900433 ) ) ;
#189909=CARTESIAN_POINT ( 'NONE',  ( -8.224510206698735004, -14.34966873604973081, 94.58442372801901854 ) ) ;
#189910=CARTESIAN_POINT ( 'NONE',  ( -14.29746914071049879, 8.314922557960819915, 55.83224293864770260 ) ) ;
#189911=CARTESIAN_POINT ( 'NONE',  ( 10.81492255796106328, -18.62759615963255655, 85.41775706135236135 ) ) ;
#189912=CARTESIAN_POINT ( 'NONE',  ( 10.72451020669871369, 18.67979575497193778, 82.08442372801901854 ) ) ;
#189913=CARTESIAN_POINT ( 'NONE',  ( 5.719274019375991003, -21.55341960407610458, 97.70724293864772392 ) ) ;
#189914=CARTESIAN_POINT ( 'NONE',  ( -0.05219959533909027116, -19.03943276465977164, 52.49890960531436690 ) ) ;
#189915=CARTESIAN_POINT ( 'NONE',  ( -21.53943276465977519, -0.05219959533937600094, 63.75109039468568284 ) ) ;
#189916=CARTESIAN_POINT ( 'NONE',  ( 19.05341960407611168, 5.049401038298154454, 48.95724293864768129 ) ) ;
#189918=CARTESIAN_POINT ( 'NONE',  ( -16.46253265017160317, 9.564922557960807481, 60.83224293864769550 ) ) ;
#189919=CARTESIAN_POINT ( 'NONE',  ( -4.379528057220328563, 16.55341960407611168, 110.2072429386477239 ) ) ;
#189920=CARTESIAN_POINT ( 'NONE',  ( 0.05219959533909260263, 19.03943276465977164, 94.99890960531436690 ) ) ;
#189921=CARTESIAN_POINT ( 'NONE',  ( -16.53943276465976808, 0.05219959533911058130, 56.24890960531436690 ) ) ;
#189922=CARTESIAN_POINT ( 'NONE',  ( 13.89961937509977652, -13.97604488694527269, 23.12390960531436335 ) ) ;
#189923=CARTESIAN_POINT ( 'NONE',  ( -10.72451020669898014, 18.67979575497178502, 80.41557627198103830 ) ) ;
#189924=CARTESIAN_POINT ( 'NONE',  ( 10.72451020669871369, 18.67979575497193778, 32.08442372801901854 ) ) ;
#189926=CARTESIAN_POINT ( 'NONE',  ( 8.314922557961029526, -14.29746914071037800, 35.41775706135234003 ) ) ;
#189927=CARTESIAN_POINT ( 'NONE',  ( -0.05219959533907301413, -21.53943276465977519, 82.49890960531436690 ) ) ;
#189928=CARTESIAN_POINT ( 'NONE',  ( 5.719274019375673035, 21.55341960407619339, 112.2927570613523471 ) ) ;
#189929=CARTESIAN_POINT ( 'NONE',  ( 16.46253265017160672, -9.564922557960803928, 93.33224293864769550 ) ) ;
#189930=CARTESIAN_POINT ( 'NONE',  ( 21.55341960407619695, -5.719274019375665929, 31.04275706135234714 ) ) ;
#189931=CARTESIAN_POINT ( 'NONE',  ( -21.53943276465977519, 0.05219959533907696930, 31.24890960531435979 ) ) ;
#189932=CARTESIAN_POINT ( 'NONE',  ( -14.34966873604972548, 8.224510206698743886, 108.3344237280190185 ) ) ;
#189933=CARTESIAN_POINT ( 'NONE',  ( -21.55341960407619339, 5.719274019375674811, 48.54275706135234714 ) ) ;
#189934=CARTESIAN_POINT ( 'NONE',  ( -10.72451020669870658, -18.67979575497194134, 79.58442372801903275 ) ) ;
#189935=CARTESIAN_POINT ( 'NONE',  ( 0.05219959533937995610, -21.53943276465977519, 110.0010903946856757 ) ) ;
#189936=CARTESIAN_POINT ( 'NONE',  ( -12.06949235617739369, -12.14591786802326823, 69.37609039468567573 ) ) ;
#189937=CARTESIAN_POINT ( 'NONE',  ( -10.81492255796105439, 18.62759615963255655, 47.91775706135234714 ) ) ;
#189938=CARTESIAN_POINT ( 'NONE',  ( 19.02544592524343514, -5.153800228976328945, 38.54057627198103120 ) ) ;
#189939=CARTESIAN_POINT ( 'NONE',  ( -21.55341960407619339, 5.719274019375674811, 103.5427570613523613 ) ) ;
#189940=CARTESIAN_POINT ( 'NONE',  ( -16.46253265017160317, 9.564922557960807481, 105.8322429386476955 ) ) ;
#189941=CARTESIAN_POINT ( 'NONE',  ( 10.81492255796078972, 18.62759615963270932, 104.5822429386477097 ) ) ;
#189943=CARTESIAN_POINT ( 'NONE',  ( 15.72974639402199770, -15.80617190586745480, 68.12390960531436690 ) ) ;
#189944=CARTESIAN_POINT ( 'NONE',  ( 12.14591786802327356, -12.06949235617739191, 45.62609039468567573 ) ) ;
#189945=CARTESIAN_POINT ( 'NONE',  ( -4.379528057220328563, 16.55341960407611168, 50.20724293864769550 ) ) ;
#189947=CARTESIAN_POINT ( 'NONE',  ( 13.97604488694548053, -13.89961937509957401, 85.62609039468568994 ) ) ;
#189950=CARTESIAN_POINT ( 'NONE',  ( -12.06949235617739369, -12.14591786802326823, 29.37609039468568284 ) ) ;
#189951=CARTESIAN_POINT ( 'NONE',  ( 21.52544592524344225, -5.823673210054117533, 103.5405762719810383 ) ) ;
#189952=CARTESIAN_POINT ( 'NONE',  ( -5.719274019375978568, 21.55341960407610458, 70.20724293864769550 ) ) ;
#189953=CARTESIAN_POINT ( 'NONE',  ( 19.05341960407611168, 5.049401038298154454, 108.9572429386477097 ) ) ;
#189954=CARTESIAN_POINT ( 'NONE',  ( -12.06949235617739369, -12.14591786802326823, 44.37609039468567573 ) ) ;
#189955=CARTESIAN_POINT ( 'NONE',  ( 19.03943276465977164, -0.05219959533909143690, 63.74890960531435979 ) ) ;
#189956=CARTESIAN_POINT ( 'NONE',  ( 10.81492255796106328, -18.62759615963255655, 30.41775706135234358 ) ) ;
#189957=CARTESIAN_POINT ( 'NONE',  ( 16.51473224551083163, -9.474510206698727899, 95.83442372801900433 ) ) ;
#189958=CARTESIAN_POINT ( 'NONE',  ( -16.51473224551069308, -9.474510206698971260, 106.6655762719810383 ) ) ;
#189959=CARTESIAN_POINT ( 'NONE',  ( -9.564922557960796823, -16.46253265017161027, 82.08224293864768129 ) ) ;
#189960=CARTESIAN_POINT ( 'NONE',  ( -21.55341960407610458, -5.719274019375992779, 91.45724293864769550 ) ) ;
#189961=CARTESIAN_POINT ( 'NONE',  ( 16.51473224551069308, 9.474510206698969483, 54.16557627198103120 ) ) ;
#189962=CARTESIAN_POINT ( 'NONE',  ( -16.19135201231369336, -7.376712067591814304, 60.18680854052035301 ) ) ;
#189963=CARTESIAN_POINT ( 'NONE',  ( 8.224510206698953496, -14.34966873604960469, 72.91557627198103830 ) ) ;
#189964=CARTESIAN_POINT ( 'NONE',  ( -13.89961937509977652, 13.97604488694528158, 115.6239096053143669 ) ) ;
#189966=CARTESIAN_POINT ( 'NONE',  ( 21.55341960407610458, 5.719274019375980345, 88.95724293864769550 ) ) ;
#189967=CARTESIAN_POINT ( 'NONE',  ( -9.474510206698720793, -16.51473224551083518, 69.58442372801901854 ) ) ;
#189968=CARTESIAN_POINT ( 'NONE',  ( -21.52544592524343514, 5.823673210054127303, 26.04057627198103475 ) ) ;
#189970=CARTESIAN_POINT ( 'NONE',  ( 10.81492255796078972, 18.62759615963270932, 54.58224293864769550 ) ) ;
#189971=CARTESIAN_POINT ( 'NONE',  ( -19.02544592524342804, 5.153800228976336051, 81.04057627198103830 ) ) ;
#189972=CARTESIAN_POINT ( 'NONE',  ( 21.52544592524334988, 5.823673210054432836, 81.45942372801900433 ) ) ;
#189973=CARTESIAN_POINT ( 'NONE',  ( -9.564922557960796823, -16.46253265017161027, 37.08224293864768839 ) ) ;
#189974=CARTESIAN_POINT ( 'NONE',  ( 8.314922557960818139, 14.29746914071049879, 74.58224293864768129 ) ) ;
#189975=CARTESIAN_POINT ( 'NONE',  ( 16.55341960407618274, -4.379528057220086978, 41.04275706135236135 ) ) ;
#189976=CARTESIAN_POINT ( 'NONE',  ( -0.05219959533937732626, 21.53943276465977519, 72.50109039468568994 ) ) ;
#189978=CARTESIAN_POINT ( 'NONE',  ( -9.474510206698720793, -16.51473224551083518, 29.58442372801900433 ) ) ;
#189979=CARTESIAN_POINT ( 'NONE',  ( -13.89961937509957401, -13.97604488694547875, 84.37609039468567573 ) ) ;
#189981=B_SPLINE_CURVE_WITH_KNOTS ( 'NONE', 3,
 ( #122383, #168880, #30385, #156718, #96025, #189061, #154721, #110202, #112195, #18210, #111193, #31384, #186070, #171881, #139536, #172884, #142527, #3026, #93033, #33370, #109206, #77869, #34364, #140539, #158687, #157711, #187079, #79868, #128342, #1020, #65684, #95028 ),
 .UNSPECIFIED., .F., .F.,
 ( 4, 2, 2, 2, 2, 2, 2, 2, 2, 2, 2, 2, 2, 2, 2, 4 ),
 ( 2.195984522899319715E-17, 0.0003712461730037024989, 0.0007424923460073830968, 0.001113738519011063478, 0.001484984692014744076, 0.002227477038022111777, 0.002598723211025781316, 0.002969969384029451289, 0.003341215557033120395, 0.003712461730036789934, 0.004083707903040459039, 0.004454954076044128145, 0.004826200249047797250, 0.005197446422051466355, 0.005568692595055136328, 0.005939938768058804566 ),
 .UNSPECIFIED. ) ;
#189982=CARTESIAN_POINT ( 'NONE',  ( -15.72974639402176322, -15.80617190586768395, 29.37609039468568284 ) ) ;
#189983=CARTESIAN_POINT ( 'NONE',  ( -19.39056639909672342, -5.500000000000052403, 45.78948781074343088 ) ) ;
#189984=CARTESIAN_POINT ( 'NONE',  ( 15.72974639402176855, 15.80617190586768217, 111.8760903946856615 ) ) ;
#189985=CARTESIAN_POINT ( 'NONE',  ( 0.05219959533909260263, 19.03943276465977164, 59.99890960531436690 ) ) ;
#189986=CARTESIAN_POINT ( 'NONE',  ( 5.153800228976615827, -19.02544592524334988, 30.20942372801900433 ) ) ;
#189987=CARTESIAN_POINT ( 'NONE',  ( -12.14591786802326823, 12.06949235617739902, 103.1260903946856757 ) ) ;
#189988=CARTESIAN_POINT ( 'NONE',  ( 19.03943276465977164, -0.05219959533909143690, 108.7489096053143527 ) ) ;
#189989=CARTESIAN_POINT ( 'NONE',  ( 18.67979575497194134, -10.72451020669871369, 75.83442372801900433 ) ) ;
#189991=CARTESIAN_POINT ( 'NONE',  ( -17.49999999999996092, -3.345213924137635964, 35.41231376905670203 ) ) ;
#189992=CARTESIAN_POINT ( 'NONE',  ( 10.72451020669871369, 18.67979575497193778, 82.08442372801901854 ) ) ;
#189993=CARTESIAN_POINT ( 'NONE',  ( -10.72451020669870658, -18.67979575497194134, 109.5844237280190328 ) ) ;
#189995=CARTESIAN_POINT ( 'NONE',  ( 19.02544592524343514, -5.153800228976328945, 103.5405762719809957 ) ) ;
#189996=CARTESIAN_POINT ( 'NONE',  ( -16.51473224551082808, 9.474510206698731452, 23.33442372801900078 ) ) ;
#189998=CARTESIAN_POINT ( 'NONE',  ( 19.05341960407611168, 5.049401038298154454, 43.95724293864769550 ) ) ;
#189999=CARTESIAN_POINT ( 'NONE',  ( 18.62759615963271287, -10.81492255796078972, 58.33224293864768839 ) ) ;
#190001=CARTESIAN_POINT ( 'NONE',  ( -12.06949235617756955, 12.14591786802309770, 30.62390960531436335 ) ) ;
#190002=CARTESIAN_POINT ( 'NONE',  ( -16.53943276465976808, 0.05219959533911058130, 91.24890960531436690 ) ) ;
#190003=CARTESIAN_POINT ( 'NONE',  ( 16.46253265017160672, -9.564922557960803928, 78.33224293864769550 ) ) ;
#190004=CARTESIAN_POINT ( 'NONE',  ( -18.62759615963255300, -10.81492255796106328, 104.1677570613523471 ) ) ;
#190005=CARTESIAN_POINT ( 'NONE',  ( -5.049401038298153566, 19.05341960407611168, 30.20724293864768839 ) ) ;
#190006=CARTESIAN_POINT ( 'NONE',  ( 0.05219959533910956823, 16.53943276465976808, 99.99890960531436690 ) ) ;
#190007=CARTESIAN_POINT ( 'NONE',  ( 15.80617190586769283, -15.72974639402175789, 55.62609039468568284 ) ) ;
#190008=CARTESIAN_POINT ( 'NONE',  ( -18.62759615963270932, 10.81492255796079327, 85.83224293864768129 ) ) ;
#190009=CARTESIAN_POINT ( 'NONE',  ( -13.89961937509957401, -13.97604488694547875, 49.37609039468567573 ) ) ;
#190011=CARTESIAN_POINT ( 'NONE',  ( 9.564922557960805705, 16.46253265017160317, 104.5822429386476955 ) ) ;
#190012=CARTESIAN_POINT ( 'NONE',  ( -12.06949235617756955, 12.14591786802309770, 80.62390960531438111 ) ) ;
#190013=EDGE_CURVE ( 'NONE', #60746, #179813, #129703, .T. ) ;
#190014=CARTESIAN_POINT ( 'NONE',  ( -19.03943276465977164, -0.05219959533935918106, 38.75109039468566152 ) ) ;
#190015=CARTESIAN_POINT ( 'NONE',  ( -5.153800228976328057, -19.02544592524343514, 62.29057627198100988 ) ) ;
#190016=CARTESIAN_POINT ( 'NONE',  ( -16.55341960407611168, -4.379528057220339221, 61.45724293864770260 ) ) ;
#190017=CARTESIAN_POINT ( 'NONE',  ( 16.46253265017146816, 9.564922557961045513, 81.66775706135233293 ) ) ;
#190019=CARTESIAN_POINT ( 'NONE',  ( 21.53943276465977519, -0.05219959533907433946, 33.74890960531436690 ) ) ;
#190021=CARTESIAN_POINT ( 'NONE',  ( 4.483927247898545687, 16.52544592524342804, 99.79057627198103830 ) ) ;
#190023=CARTESIAN_POINT ( 'NONE',  ( 19.02544592524343514, -5.153800228976328945, 63.54057627198103830 ) ) ;
#190024=CARTESIAN_POINT ( 'NONE',  ( 18.67979575497178502, 10.72451020669898547, 64.16557627198102409 ) ) ;
#190025=CARTESIAN_POINT ( 'NONE',  ( -5.153800228976328057, -19.02544592524343514, 32.29057627198102409 ) ) ;
#190026=CARTESIAN_POINT ( 'NONE',  ( 4.379528057220092307, 16.55341960407617563, 77.29275706135234714 ) ) ;
#190027=CARTESIAN_POINT ( 'NONE',  ( 0.05219959533909260263, 19.03943276465977164, 59.99890960531436690 ) ) ;
#190028=CARTESIAN_POINT ( 'NONE',  ( -5.049401038297874678, -19.05341960407617918, 49.79275706135231871 ) ) ;
#190029=CARTESIAN_POINT ( 'NONE',  ( -0.05219959533937732626, 21.53943276465977519, 62.50109039468568284 ) ) ;
#190030=CARTESIAN_POINT ( 'NONE',  ( 18.62759615963271287, -10.81492255796078972, 53.33224293864769550 ) ) ;
#190031=CARTESIAN_POINT ( 'NONE',  ( -16.46253265017160317, 9.564922557960807481, 25.83224293864769194 ) ) ;
#190032=CARTESIAN_POINT ( 'NONE',  ( -12.06949235617739369, -12.14591786802326823, 89.37609039468568994 ) ) ;
#190033=CARTESIAN_POINT ( 'NONE',  ( 16.51473224551083163, -9.474510206698727899, 100.8344237280190043 ) ) ;
#190034=CARTESIAN_POINT ( 'NONE',  ( 5.153800228976335163, 19.02544592524342804, 24.79057627198102765 ) ) ;
#190035=CARTESIAN_POINT ( 'NONE',  ( 18.56101223717332616, 5.499999999999945821, 78.94978406935679516 ) ) ;
#190036=CARTESIAN_POINT ( 'NONE',  ( 21.53943276465977519, 0.05219959533937863772, 101.2510903946856757 ) ) ;
#190037=CARTESIAN_POINT ( 'NONE',  ( 16.52544592524342804, -4.483927247898539470, 43.54057627198103830 ) ) ;
#190038=CARTESIAN_POINT ( 'NONE',  ( 12.06949235617757843, -12.14591786802309237, 53.12390960531436690 ) ) ;
#190039=CARTESIAN_POINT ( 'NONE',  ( -15.80617190586745835, -15.72974639402198527, 91.87390960531436690 ) ) ;
#190040=CARTESIAN_POINT ( 'NONE',  ( 10.72451020669898902, -18.67979575497178502, 92.91557627198103830 ) ) ;
#190042=CARTESIAN_POINT ( 'NONE',  ( -21.53943276465977519, 0.05219959533907696930, 36.24890960531435979 ) ) ;
#190043=CARTESIAN_POINT ( 'NONE',  ( 14.34966873604972726, -8.224510206698740333, 65.83442372801900433 ) ) ;
#190044=CARTESIAN_POINT ( 'NONE',  ( 0.05219959533910956823, 16.53943276465976808, 79.99890960531435269 ) ) ;
#190045=CARTESIAN_POINT ( 'NONE',  ( -9.474510206698964154, 16.51473224551069663, 50.41557627198102409 ) ) ;
#190047=CARTESIAN_POINT ( 'NONE',  ( -16.53943276465976808, -0.05219959533934237506, 93.75109039468567573 ) ) ;
#190048=CARTESIAN_POINT ( 'NONE',  ( -18.62759615963255300, -10.81492255796106328, 19.16775706135234714 ) ) ;
#190049=CARTESIAN_POINT ( 'NONE',  ( -9.564922557960796823, -16.46253265017161027, 87.08224293864769550 ) ) ;
#190050=CARTESIAN_POINT ( 'NONE',  ( -21.55341960407619339, 5.719274019375674811, 48.54275706135234714 ) ) ;
#190051=CARTESIAN_POINT ( 'NONE',  ( 16.46253265017160672, -9.564922557960803928, 103.3322429386476955 ) ) ;
#190052=VERTEX_POINT ( 'NONE', #185768 ) ;
#190053=CARTESIAN_POINT ( 'NONE',  ( 5.823673210054444382, -21.52544592524334988, 50.20942372801901854 ) ) ;
#190054=CARTESIAN_POINT ( 'NONE',  ( -5.049401038298153566, 19.05341960407611168, 40.20724293864768839 ) ) ;
#190055=CARTESIAN_POINT ( 'NONE',  ( 19.02544592524343514, -5.153800228976328945, 113.5405762719810241 ) ) ;
#190056=CARTESIAN_POINT ( 'NONE',  ( -5.153800228976607833, 19.02544592524334988, 57.70942372801899012 ) ) ;
#190057=CARTESIAN_POINT ( 'NONE',  ( 15.80617190586769283, -15.72974639402175789, 35.62609039468568994 ) ) ;
#190058=CARTESIAN_POINT ( 'NONE',  ( 9.474510206698729675, 16.51473224551082808, 62.08442372801899722 ) ) ;
#190059=CARTESIAN_POINT ( 'NONE',  ( 9.474510206698971260, -16.51473224551069308, 27.91557627198103120 ) ) ;
#190060=CARTESIAN_POINT ( 'NONE',  ( 4.379528057220092307, 16.55341960407617563, 92.29275706135236135 ) ) ;
#190061=CARTESIAN_POINT ( 'NONE',  ( -16.46253265017146816, -9.564922557961047289, 64.16775706135233293 ) ) ;
#190062=CARTESIAN_POINT ( 'NONE',  ( 8.224510206698742110, 14.34966873604972548, 102.0844237280190185 ) ) ;
#190064=CARTESIAN_POINT ( 'NONE',  ( 5.049401038298161559, -19.05341960407611168, 82.70724293864770971 ) ) ;
#190065=CARTESIAN_POINT ( 'NONE',  ( -21.53943276465977519, -0.05219959533937600094, 98.75109039468568994 ) ) ;
#190066=CARTESIAN_POINT ( 'NONE',  ( -10.81492255796105439, 18.62759615963255655, 102.9177570613523756 ) ) ;
#190068=CARTESIAN_POINT ( 'NONE',  ( -9.474510206698964154, 16.51473224551069663, 95.41557627198102409 ) ) ;
#190069=CARTESIAN_POINT ( 'NONE',  ( 21.52544592524334988, 5.823673210054432836, 71.45942372801901854 ) ) ;
#190070=CARTESIAN_POINT ( 'NONE',  ( 14.34966873604972726, -8.224510206698740333, 20.83442372801901143 ) ) ;
#190071=CARTESIAN_POINT ( 'NONE',  ( -19.02544592524342804, 5.153800228976336051, 81.04057627198103830 ) ) ;
#190072=CARTESIAN_POINT ( 'NONE',  ( 0.05219959533907565091, 21.53943276465977519, 29.99890960531435979 ) ) ;
#190073=CARTESIAN_POINT ( 'NONE',  ( 5.153800228976335163, 19.02544592524342804, 94.79057627198103830 ) ) ;
#190075=CARTESIAN_POINT ( 'NONE',  ( 5.153800228976335163, 19.02544592524342804, 69.79057627198103830 ) ) ;
#190076=CARTESIAN_POINT ( 'NONE',  ( -8.314922557961024197, 14.29746914071037800, 112.9177570613523329 ) ) ;
#190077=CARTESIAN_POINT ( 'NONE',  ( -17.49999999999999645, 5.499999999999992895, 98.71769037696435589 ) ) ;
#190078=CARTESIAN_POINT ( 'NONE',  ( 19.03943276465977164, 0.05219959533936151252, 76.25109039468566152 ) ) ;
#190079=CARTESIAN_POINT ( 'NONE',  ( 13.97604488694527802, 13.89961937509977652, 94.37390960531436690 ) ) ;
#190080=CARTESIAN_POINT ( 'NONE',  ( 0.05219959533910956823, 16.53943276465976808, 89.99890960531438111 ) ) ;
#190081=CARTESIAN_POINT ( 'NONE',  ( 5.719274019375991003, -21.55341960407610458, 52.70724293864769550 ) ) ;
#190082=CARTESIAN_POINT ( 'NONE',  ( -15.72974639402197994, 15.80617190586746368, 40.62390960531435269 ) ) ;
#190083=CARTESIAN_POINT ( 'NONE',  ( -4.483927247898539470, -16.52544592524342804, 107.2905762719810525 ) ) ;
#190084=CARTESIAN_POINT ( 'NONE',  ( -16.79531203550650176, 7.028104445595466210, 53.74755011779559766 ) ) ;
#190085=CARTESIAN_POINT ( 'NONE',  ( -19.02544592524334988, -5.153800228976617603, 43.95942372801899012 ) ) ;
#190086=CARTESIAN_POINT ( 'NONE',  ( -12.14591786802309592, -12.06949235617757132, 31.87390960531435979 ) ) ;
#190087=VECTOR ( 'NONE', #174389, 1000.000000000000000 ) ;
#190088=CARTESIAN_POINT ( 'NONE',  ( 5.049401038298161559, -19.05341960407611168, 97.70724293864766707 ) ) ;
#190089=CARTESIAN_POINT ( 'NONE',  ( -21.55341960407619339, 5.719274019375674811, 68.54275706135234714 ) ) ;
#190090=CARTESIAN_POINT ( 'NONE',  ( -15.80617190586745835, -15.72974639402198527, 56.87390960531436690 ) ) ;
#190091=CARTESIAN_POINT ( 'NONE',  ( -21.55341960407619339, 5.719274019375674811, 48.54275706135234714 ) ) ;
#190092=CARTESIAN_POINT ( 'NONE',  ( 18.62759615963271287, -10.81492255796078972, 93.33224293864769550 ) ) ;
#190093=CARTESIAN_POINT ( 'NONE',  ( 15.72974639402176855, 15.80617190586768217, 41.87609039468568284 ) ) ;
#190094=CARTESIAN_POINT ( 'NONE',  ( 14.34966873604960469, 8.224510206698951720, 104.1655762719810241 ) ) ;
#190095=CARTESIAN_POINT ( 'NONE',  ( -13.89961937509957401, -13.97604488694547875, 69.37609039468564731 ) ) ;
#190096=CARTESIAN_POINT ( 'NONE',  ( 0.05219959533909260263, 19.03943276465977164, 59.99890960531436690 ) ) ;
#190097=CARTESIAN_POINT ( 'NONE',  ( -14.34966873604960291, -8.224510206698953496, 106.6655762719810383 ) ) ;
#190098=CARTESIAN_POINT ( 'NONE',  ( 5.153800228976335163, 19.02544592524342804, 114.7905762719810241 ) ) ;
#190099=CARTESIAN_POINT ( 'NONE',  ( 12.14591786802309770, 12.06949235617756955, 54.37390960531435979 ) ) ;
#190100=CARTESIAN_POINT ( 'NONE',  ( 14.29746914071037800, 8.314922557961029526, 111.6677570613523613 ) ) ;
#190101=CARTESIAN_POINT ( 'NONE',  ( 5.153800228976335163, 19.02544592524342804, 54.79057627198103120 ) ) ;
#190102=CARTESIAN_POINT ( 'NONE',  ( -5.153800228976328057, -19.02544592524343514, 27.29057627198103120 ) ) ;
#190103=CARTESIAN_POINT ( 'NONE',  ( 5.049401038297881783, 19.05341960407617563, 22.29275706135233648 ) ) ;
#190104=CARTESIAN_POINT ( 'NONE',  ( 17.60691670004650788, 5.500000000000058620, 51.63333313366440080 ) ) ;
#190105=CARTESIAN_POINT ( 'NONE',  ( -4.483927247898539470, -16.52544592524342804, 32.29057627198102409 ) ) ;
#190106=CARTESIAN_POINT ( 'NONE',  ( 21.53943276465977519, 0.05219959533937863772, 46.25109039468567573 ) ) ;
#190108=CARTESIAN_POINT ( 'NONE',  ( -12.06949235617739369, -12.14591786802326823, 64.37609039468568994 ) ) ;
#190109=CARTESIAN_POINT ( 'NONE',  ( 16.52544592524342804, -4.483927247898539470, 28.54057627198103120 ) ) ;
#190110=CARTESIAN_POINT ( 'NONE',  ( -0.05219959533934338120, 16.53943276465976808, 102.5010903946856899 ) ) ;
#190111=CARTESIAN_POINT ( 'NONE',  ( 19.03943276465977164, -0.05219959533909143690, 43.74890960531435979 ) ) ;
#190112=CARTESIAN_POINT ( 'NONE',  ( 13.97604488694527802, 13.89961937509977652, 44.37390960531435269 ) ) ;
#190113=CARTESIAN_POINT ( 'NONE',  ( -0.05219959533909027116, -19.03943276465977164, 22.49890960531436690 ) ) ;
#190114=CARTESIAN_POINT ( 'NONE',  ( -5.719274019375665041, -21.55341960407619695, 29.79275706135234358 ) ) ;
#190115=CARTESIAN_POINT ( 'NONE',  ( -16.51473224551069308, -9.474510206698971260, 46.66557627198102409 ) ) ;
#190117=CARTESIAN_POINT ( 'NONE',  ( 19.03943276465977164, -0.05219959533909143690, 38.74890960531436690 ) ) ;
#190118=CARTESIAN_POINT ( 'NONE',  ( 18.67979575497178502, 10.72451020669898547, 29.16557627198103120 ) ) ;
#190119=CARTESIAN_POINT ( 'NONE',  ( -21.55341960407619339, 5.719274019375674811, 58.54275706135235424 ) ) ;
#190120=CARTESIAN_POINT ( 'NONE',  ( -16.53943276465976808, 0.05219959533911058130, 106.2489096053143811 ) ) ;
#190121=CARTESIAN_POINT ( 'NONE',  ( -9.564922557960796823, -16.46253265017161027, 107.0822429386476955 ) ) ;
#190122=CARTESIAN_POINT ( 'NONE',  ( 14.34966873604972726, -8.224510206698740333, 75.83442372801900433 ) ) ;
#190124=CARTESIAN_POINT ( 'NONE',  ( 15.72974639402176855, 15.80617190586768217, 91.87609039468568994 ) ) ;
#190125=CARTESIAN_POINT ( 'NONE',  ( 12.14591786802327356, -12.06949235617739191, 50.62609039468568994 ) ) ;
#190126=CARTESIAN_POINT ( 'NONE',  ( 16.51473224551069308, 9.474510206698969483, 99.16557627198102409 ) ) ;
#190127=CARTESIAN_POINT ( 'NONE',  ( -12.06949235617739369, -12.14591786802326823, 44.37609039468567573 ) ) ;
#190128=CARTESIAN_POINT ( 'NONE',  ( -4.483927247898782831, 16.52544592524335698, 32.70942372801900433 ) ) ;
#190129=CARTESIAN_POINT ( 'NONE',  ( -4.379528057220086978, -16.55341960407618274, 79.79275706135236135 ) ) ;
#190130=CARTESIAN_POINT ( 'NONE',  ( -9.564922557961040184, 16.46253265017147172, 107.9177570613523471 ) ) ;
#190131=CARTESIAN_POINT ( 'NONE',  ( 19.02544592524343514, -5.153800228976328945, 78.54057627198099567 ) ) ;
#190132=CARTESIAN_POINT ( 'NONE',  ( 21.53943276465977519, -0.05219959533907433946, 98.74890960531438111 ) ) ;
#190133=CARTESIAN_POINT ( 'NONE',  ( -12.14591786802309592, -12.06949235617757132, 101.8739096053143811 ) ) ;
#190134=CARTESIAN_POINT ( 'NONE',  ( -9.474510206698720793, -16.51473224551083518, 109.5844237280190043 ) ) ;
#190135=CARTESIAN_POINT ( 'NONE',  ( -0.05219959533934338120, 16.53943276465976808, 72.50109039468568994 ) ) ;
#190137=CARTESIAN_POINT ( 'NONE',  ( 19.02544592524334988, 5.153800228976608722, 66.45942372801899012 ) ) ;
#190138=CARTESIAN_POINT ( 'NONE',  ( -4.379528057220328563, 16.55341960407611168, 50.20724293864769550 ) ) ;
#190139=CARTESIAN_POINT ( 'NONE',  ( -4.483927247898539470, -16.52544592524342804, 87.29057627198103830 ) ) ;
#190140=CARTESIAN_POINT ( 'NONE',  ( 19.03943276465977164, 0.05219959533936151252, 36.25109039468567573 ) ) ;
#190141=CARTESIAN_POINT ( 'NONE',  ( -18.67979575497193778, 10.72451020669871902, 38.33442372801900433 ) ) ;
#190142=CARTESIAN_POINT ( 'NONE',  ( -9.474510206698720793, -16.51473224551083518, 94.58442372801900433 ) ) ;
#190144=CARTESIAN_POINT ( 'NONE',  ( -5.153800228976328057, -19.02544592524343514, 92.29057627198099567 ) ) ;
#190145=B_SPLINE_CURVE_WITH_KNOTS ( 'NONE', 3,
 ( #33221, #2872, #64550, #170733, #31230, #138399 ),
 .UNSPECIFIED., .F., .F.,
 ( 4, 2, 4 ),
 ( 0.000000000000000000, 0.0003837532665554268434, 0.0007675065331108536868 ),
 .UNSPECIFIED. ) ;
#190146=CARTESIAN_POINT ( 'NONE',  ( 10.72451020669871369, 18.67979575497193778, 112.0844237280190185 ) ) ;
#190147=CARTESIAN_POINT ( 'NONE',  ( -16.46253265017160317, 9.564922557960807481, 90.83224293864769550 ) ) ;
#190148=CARTESIAN_POINT ( 'NONE',  ( -10.72451020669898014, 18.67979575497178502, 60.41557627198102409 ) ) ;
#190149=CARTESIAN_POINT ( 'NONE',  ( -14.34966873604960291, -8.224510206698953496, 96.66557627198102409 ) ) ;
#190150=CARTESIAN_POINT ( 'NONE',  ( -5.049401038298153566, 19.05341960407611168, 55.20724293864769550 ) ) ;
#190151=CARTESIAN_POINT ( 'NONE',  ( -5.153800228976328057, -19.02544592524343514, 22.29057627198102765 ) ) ;
#190152=CARTESIAN_POINT ( 'NONE',  ( -15.72974639402176322, -15.80617190586768395, 29.37609039468568284 ) ) ;
#190153=CARTESIAN_POINT ( 'NONE',  ( -0.05219959533937732626, 21.53943276465977519, 72.50109039468568994 ) ) ;
#190154=CARTESIAN_POINT ( 'NONE',  ( -16.51473224551069308, -9.474510206698971260, 41.66557627198103120 ) ) ;
#190155=CARTESIAN_POINT ( 'NONE',  ( 14.29746914071037800, 8.314922557961029526, 71.66775706135234714 ) ) ;
#190156=CARTESIAN_POINT ( 'NONE',  ( -5.719274019375665041, -21.55341960407619695, 34.79275706135235424 ) ) ;
#190157=CARTESIAN_POINT ( 'NONE',  ( 5.719274019375673035, 21.55341960407619339, 32.29275706135235424 ) ) ;
#190158=CARTESIAN_POINT ( 'NONE',  ( -13.89961937509957401, -13.97604488694547875, 54.37609039468565442 ) ) ;
#190159=CARTESIAN_POINT ( 'NONE',  ( 13.97604488694527802, 13.89961937509977652, 64.37390960531436690 ) ) ;
#190160=CARTESIAN_POINT ( 'NONE',  ( 19.03943276465977164, 0.05219959533936151252, 26.25109039468566507 ) ) ;
#190161=CARTESIAN_POINT ( 'NONE',  ( -5.719274019375665041, -21.55341960407619695, 89.79275706135236135 ) ) ;
#190162=CARTESIAN_POINT ( 'NONE',  ( 10.81492255796078972, 18.62759615963270932, 64.58224293864769550 ) ) ;
#190163=CARTESIAN_POINT ( 'NONE',  ( -16.55341960407611168, -4.379528057220339221, 51.45724293864770260 ) ) ;
#190164=CARTESIAN_POINT ( 'NONE',  ( 5.719274019375673035, 21.55341960407619339, 87.29275706135236135 ) ) ;
#190165=CARTESIAN_POINT ( 'NONE',  ( -13.97604488694547697, 13.89961937509957934, 28.12609039468565797 ) ) ;
#190166=CARTESIAN_POINT ( 'NONE',  ( -4.483927247898539470, -16.52544592524342804, 72.29057627198102409 ) ) ;
#190167=CARTESIAN_POINT ( 'NONE',  ( -13.97604488694527625, -13.89961937509977652, 26.87390960531434558 ) ) ;
#190168=CARTESIAN_POINT ( 'NONE',  ( -5.153800228976607833, 19.02544592524334988, 62.70942372801899722 ) ) ;
#190169=CARTESIAN_POINT ( 'NONE',  ( 14.34966873604960469, 8.224510206698951720, 24.16557627198103120 ) ) ;
#190170=CARTESIAN_POINT ( 'NONE',  ( -15.80617190586768217, 15.72974639402176855, 78.12609039468570415 ) ) ;
#190171=CARTESIAN_POINT ( 'NONE',  ( -9.564922557960796823, -16.46253265017161027, 72.08224293864770971 ) ) ;
#190172=CARTESIAN_POINT ( 'NONE',  ( 16.51473224551083163, -9.474510206698727899, 45.83442372801900433 ) ) ;
#190173=CARTESIAN_POINT ( 'NONE',  ( -21.52544592524343514, 5.823673210054127303, 46.04057627198103830 ) ) ;
#190174=CARTESIAN_POINT ( 'NONE',  ( 21.55341960407619695, -5.719274019375665929, 51.04275706135234714 ) ) ;
#190176=CARTESIAN_POINT ( 'NONE',  ( -15.80617190586745835, -15.72974639402198527, 101.8739096053143811 ) ) ;
#190177=CARTESIAN_POINT ( 'NONE',  ( -13.89961937509957401, -13.97604488694547875, 99.37609039468567573 ) ) ;
#190178=CARTESIAN_POINT ( 'NONE',  ( 16.53943276465976808, 0.05219959533934440121, 61.25109039468567573 ) ) ;
#190179=CARTESIAN_POINT ( 'NONE',  ( -18.22780087662119541, 5.500000000000102141, 56.01763182126894947 ) ) ;
#190180=CARTESIAN_POINT ( 'NONE',  ( -10.81492255796078084, -18.62759615963271287, 112.0822429386477097 ) ) ;
#190181=CARTESIAN_POINT ( 'NONE',  ( 16.53943276465976808, -0.05219959533910856209, 88.74890960531436690 ) ) ;
#190183=CARTESIAN_POINT ( 'NONE',  ( -16.55341960407617563, 4.379528057220093196, 38.54275706135234714 ) ) ;
#190184=CARTESIAN_POINT ( 'NONE',  ( 15.72974639402199770, -15.80617190586745480, 63.12390960531435979 ) ) ;
#190185=CARTESIAN_POINT ( 'NONE',  ( 4.379528057220092307, 16.55341960407617563, 97.29275706135234714 ) ) ;
#190186=CARTESIAN_POINT ( 'NONE',  ( -0.05219959533909027116, -19.03943276465977164, 27.49890960531435624 ) ) ;
#190187=CARTESIAN_POINT ( 'NONE',  ( 12.14591786802327356, -12.06949235617739191, 60.62609039468567573 ) ) ;
#190188=CARTESIAN_POINT ( 'NONE',  ( 19.05341960407617918, -5.049401038297876454, 66.04275706135233293 ) ) ;
#190189=CARTESIAN_POINT ( 'NONE',  ( -5.719274019375665041, -21.55341960407619695, 44.79275706135234714 ) ) ;
#190190=CARTESIAN_POINT ( 'NONE',  ( -10.72451020669898014, 18.67979575497178502, 60.41557627198102409 ) ) ;
#190191=CARTESIAN_POINT ( 'NONE',  ( -12.14591786802326823, 12.06949235617739902, 83.12609039468568994 ) ) ;
#190192=CARTESIAN_POINT ( 'NONE',  ( -21.53943276465977519, -0.05219959533937600094, 68.75109039468568994 ) ) ;
#190193=CARTESIAN_POINT ( 'NONE',  ( 21.55341960407610458, 5.719274019375980345, 53.95724293864770260 ) ) ;
#190194=CARTESIAN_POINT ( 'NONE',  ( -15.80617190586745835, -15.72974639402198527, 36.87390960531435979 ) ) ;
#190195=CARTESIAN_POINT ( 'NONE',  ( -14.29746914071037622, -8.314922557961029526, 64.16775706135234714 ) ) ;
#190196=CARTESIAN_POINT ( 'NONE',  ( -18.62759615963270932, 10.81492255796079327, 30.83224293864770260 ) ) ;
#190198=CARTESIAN_POINT ( 'NONE',  ( 16.51473224551069308, 9.474510206698969483, 99.16557627198102409 ) ) ;
#190199=CARTESIAN_POINT ( 'NONE',  ( -8.224510206698948167, 14.34966873604960824, 25.41557627198103120 ) ) ;
#190201=CARTESIAN_POINT ( 'NONE',  ( -4.483927247898539470, -16.52544592524342804, 102.2905762719810383 ) ) ;
#190202=CARTESIAN_POINT ( 'NONE',  ( 15.72974639402199770, -15.80617190586745480, 63.12390960531435979 ) ) ;
#190203=CARTESIAN_POINT ( 'NONE',  ( 4.379528057220092307, 16.55341960407617563, 92.29275706135236135 ) ) ;
#190204=CARTESIAN_POINT ( 'NONE',  ( 18.67979575497194134, -10.72451020669871369, 35.83442372801901143 ) ) ;
#190205=CARTESIAN_POINT ( 'NONE',  ( 0.05219959533936267826, -19.03943276465977164, 105.0010903946856615 ) ) ;
#190206=CARTESIAN_POINT ( 'NONE',  ( -12.14591786802309592, -12.06949235617757132, 101.8739096053143811 ) ) ;
#190207=CARTESIAN_POINT ( 'NONE',  ( -19.03943276465977164, 0.05219959533909376836, 51.24890960531436690 ) ) ;
#190208=CARTESIAN_POINT ( 'NONE',  ( 5.049401038298161559, -19.05341960407611168, 22.70724293864769194 ) ) ;
#190210=CARTESIAN_POINT ( 'NONE',  ( -9.564922557960796823, -16.46253265017161027, 87.08224293864769550 ) ) ;
#190211=CARTESIAN_POINT ( 'NONE',  ( -4.483927247898782831, 16.52544592524335698, 72.70942372801901854 ) ) ;
#190212=CARTESIAN_POINT ( 'NONE',  ( -10.72451020669870658, -18.67979575497194134, 109.5844237280190328 ) ) ;
#190213=CARTESIAN_POINT ( 'NONE',  ( -18.62759615963270932, 10.81492255796079327, 45.83224293864769550 ) ) ;
#190214=CARTESIAN_POINT ( 'NONE',  ( -8.224510206698735004, -14.34966873604973081, 74.58442372801901854 ) ) ;
#190215=CARTESIAN_POINT ( 'NONE',  ( 9.474510206698729675, 16.51473224551082808, 82.08442372801899012 ) ) ;
#190216=CARTESIAN_POINT ( 'NONE',  ( 13.89961937509977652, -13.97604488694527269, 33.12390960531434558 ) ) ;
#190217=CARTESIAN_POINT ( 'NONE',  ( -13.89961937509977652, 13.97604488694528158, 75.62390960531438111 ) ) ;
#190218=CARTESIAN_POINT ( 'NONE',  ( -0.05219959533909027116, -19.03943276465977164, 37.49890960531436690 ) ) ;
#190219=CARTESIAN_POINT ( 'NONE',  ( 19.03943276465977164, 0.05219959533936151252, 71.25109039468566152 ) ) ;
#190221=CARTESIAN_POINT ( 'NONE',  ( -16.51473224551069308, -9.474510206698971260, 101.6655762719810241 ) ) ;
#190222=CARTESIAN_POINT ( 'NONE',  ( -4.483927247898539470, -16.52544592524342804, 47.29057627198103120 ) ) ;
#190223=CARTESIAN_POINT ( 'NONE',  ( -18.62759615963270932, 10.81492255796079327, 40.83224293864769550 ) ) ;
#190224=CARTESIAN_POINT ( 'NONE',  ( -17.50000000000014921, 3.292511757969716513, 105.0652027021053954 ) ) ;
#190226=CARTESIAN_POINT ( 'NONE',  ( 19.05341960407617918, -5.049401038297876454, 26.04275706135233293 ) ) ;
#190228=CARTESIAN_POINT ( 'NONE',  ( -16.46253265017160317, 9.564922557960807481, 50.83224293864770260 ) ) ;
#190229=CARTESIAN_POINT ( 'NONE',  ( -0.05219959533934338120, 16.53943276465976808, 37.50109039468568284 ) ) ;
#190231=CARTESIAN_POINT ( 'NONE',  ( -17.49999999999999645, 5.500000000000000888, 108.7176903769643559 ) ) ;
#190232=CARTESIAN_POINT ( 'NONE',  ( 4.379528057220092307, 16.55341960407617563, 77.29275706135234714 ) ) ;
#190233=CARTESIAN_POINT ( 'NONE',  ( -21.53943276465977519, 0.05219959533907696930, 101.2489096053143669 ) ) ;
#190235=CARTESIAN_POINT ( 'NONE',  ( -16.55341960407617563, 4.379528057220093196, 43.54275706135235424 ) ) ;
#190236=CARTESIAN_POINT ( 'NONE',  ( -0.05219959533909027116, -19.03943276465977164, 47.49890960531435979 ) ) ;
#190238=CARTESIAN_POINT ( 'NONE',  ( -21.55341960407619339, 5.719274019375674811, 43.54275706135235424 ) ) ;
#190239=CARTESIAN_POINT ( 'NONE',  ( 16.46253265017146816, 9.564922557961045513, 56.66775706135233293 ) ) ;
#190240=CARTESIAN_POINT ( 'NONE',  ( 10.72451020669871369, 18.67979575497193778, 97.08442372801904696 ) ) ;
#190241=CARTESIAN_POINT ( 'NONE',  ( -17.97182807773869584, 5.499999999999855227, 48.53038844047289757 ) ) ;
#190242=CARTESIAN_POINT ( 'NONE',  ( -4.483927247898539470, -16.52544592524342804, 47.29057627198103120 ) ) ;
#190243=CARTESIAN_POINT ( 'NONE',  ( 19.25176906914648711, 5.499999999999731770, 43.49927264242279534 ) ) ;
#190244=CARTESIAN_POINT ( 'NONE',  ( -5.823673210054116645, -21.52544592524344225, 52.29057627198102409 ) ) ;
#190246=CARTESIAN_POINT ( 'NONE',  ( -0.05219959533909027116, -19.03943276465977164, 97.49890960531436690 ) ) ;
#190247=CARTESIAN_POINT ( 'NONE',  ( -8.314922557960811034, -14.29746914071050412, 107.0822429386476955 ) ) ;
#190248=CARTESIAN_POINT ( 'NONE',  ( -19.05341960407617563, 5.049401038297882671, 113.5427570613523471 ) ) ;
#190249=CARTESIAN_POINT ( 'NONE',  ( -14.34966873604960291, -8.224510206698953496, 21.66557627198102409 ) ) ;
#190251=CARTESIAN_POINT ( 'NONE',  ( -13.97604488694527625, -13.89961937509977652, 96.87390960531433848 ) ) ;
#190252=CARTESIAN_POINT ( 'NONE',  ( 21.52544592524344225, -5.823673210054117533, 108.5405762719810241 ) ) ;
#190253=CARTESIAN_POINT ( 'NONE',  ( -12.14591786802309592, -12.06949235617757132, 26.87390960531435979 ) ) ;
#190254=CARTESIAN_POINT ( 'NONE',  ( 19.03943276465977164, -0.05219959533909143690, 113.7489096053143669 ) ) ;
#190255=CARTESIAN_POINT ( 'NONE',  ( -5.049401038297874678, -19.05341960407617918, 99.79275706135234714 ) ) ;
#190256=CARTESIAN_POINT ( 'NONE',  ( 21.53943276465977519, 0.05219959533937863772, 106.2510903946856757 ) ) ;
#190257=CARTESIAN_POINT ( 'NONE',  ( 16.52544592524342804, -4.483927247898539470, 33.54057627198102409 ) ) ;
#190258=CARTESIAN_POINT ( 'NONE',  ( -21.52544592524343514, 5.823673210054127303, 86.04057627198102409 ) ) ;
#190259=CARTESIAN_POINT ( 'NONE',  ( -5.823673210054116645, -21.52544592524344225, 47.29057627198103120 ) ) ;
#190260=CARTESIAN_POINT ( 'NONE',  ( -16.46253265017160317, 9.564922557960807481, 60.83224293864769550 ) ) ;
#190261=CARTESIAN_POINT ( 'NONE',  ( 12.06949235617757843, -12.14591786802309237, 28.12390960531435979 ) ) ;
#190262=CARTESIAN_POINT ( 'NONE',  ( -5.049401038298153566, 19.05341960407611168, 80.20724293864769550 ) ) ;
#190264=CARTESIAN_POINT ( 'NONE',  ( 19.39056639909671986, 5.500000000000041744, 58.28948781074345220 ) ) ;
#190265=CARTESIAN_POINT ( 'NONE',  ( -16.51473224551082808, 9.474510206698731452, 38.33442372801899722 ) ) ;
#190266=CARTESIAN_POINT ( 'NONE',  ( 0.05219959533907565091, 21.53943276465977519, 79.99890960531435269 ) ) ;
#190267=CARTESIAN_POINT ( 'NONE',  ( -4.483927247898539470, -16.52544592524342804, 82.29057627198103830 ) ) ;
#190268=CARTESIAN_POINT ( 'NONE',  ( 18.62759615963255655, 10.81492255796105972, 36.66775706135234714 ) ) ;
#190270=CARTESIAN_POINT ( 'NONE',  ( 16.53943276465976808, 0.05219959533934440121, 101.2510903946856757 ) ) ;
#190271=CARTESIAN_POINT ( 'NONE',  ( 19.02544592524343514, -5.153800228976328945, 28.54057627198102409 ) ) ;
#190272=CARTESIAN_POINT ( 'NONE',  ( -5.049401038298153566, 19.05341960407611168, 80.20724293864769550 ) ) ;
#190275=CARTESIAN_POINT ( 'NONE',  ( 8.224510206698953496, -14.34966873604960469, 42.91557627198103120 ) ) ;
#190276=CARTESIAN_POINT ( 'NONE',  ( -18.62759615963255300, -10.81492255796106328, 64.16775706135234714 ) ) ;
#190278=CARTESIAN_POINT ( 'NONE',  ( 19.03943276465977164, -0.05219959533909143690, 38.74890960531436690 ) ) ;
#190279=CARTESIAN_POINT ( 'NONE',  ( 16.51473224551069308, 9.474510206698969483, 49.16557627198102409 ) ) ;
#190281=CARTESIAN_POINT ( 'NONE',  ( -21.53943276465977519, -0.05219959533937600094, 103.7510903946857042 ) ) ;
#190282=CARTESIAN_POINT ( 'NONE',  ( 16.55341960407618274, -4.379528057220086978, 61.04275706135234714 ) ) ;
#190283=CARTESIAN_POINT ( 'NONE',  ( -5.719274019375665041, -21.55341960407619695, 84.79275706135234714 ) ) ;
#190284=CARTESIAN_POINT ( 'NONE',  ( -19.05341960407611168, -5.049401038298163336, 111.4572429386476671 ) ) ;
#190285=CARTESIAN_POINT ( 'NONE',  ( 0.05219959533936267826, -19.03943276465977164, 90.00109039468567573 ) ) ;
#190286=CARTESIAN_POINT ( 'NONE',  ( 10.81492255796106328, -18.62759615963255655, 65.41775706135234714 ) ) ;
#190287=CARTESIAN_POINT ( 'NONE',  ( 16.55341960407618274, -4.379528057220086978, 31.04275706135234714 ) ) ;
#190288=CARTESIAN_POINT ( 'NONE',  ( -15.80617190586745835, -15.72974639402198527, 81.87390960531435269 ) ) ;
#190289=CARTESIAN_POINT ( 'NONE',  ( 19.02544592524334988, 5.153800228976608722, 96.45942372801897591 ) ) ;
#190290=CARTESIAN_POINT ( 'NONE',  ( 19.05341960407611168, 5.049401038298154454, 68.95724293864769550 ) ) ;
#190291=CARTESIAN_POINT ( 'NONE',  ( -0.05219959533936034679, 19.03943276465977164, 107.5010903946856615 ) ) ;
#190292=CARTESIAN_POINT ( 'NONE',  ( -19.02544592524334988, -5.153800228976617603, 98.95942372801900433 ) ) ;
#190293=CARTESIAN_POINT ( 'NONE',  ( 8.314922557960818139, 14.29746914071049879, 59.58224293864770260 ) ) ;
#190294=CARTESIAN_POINT ( 'NONE',  ( 19.03943276465977164, 0.05219959533936151252, 76.25109039468566152 ) ) ;
#190295=CARTESIAN_POINT ( 'NONE',  ( -14.29746914071037622, -8.314922557961029526, 79.16775706135234714 ) ) ;
#190296=CARTESIAN_POINT ( 'NONE',  ( 5.719274019375673035, 21.55341960407619339, 22.29275706135235069 ) ) ;
#190297=CARTESIAN_POINT ( 'NONE',  ( 16.51473224551069308, 9.474510206698969483, 44.16557627198103120 ) ) ;
#190298=CARTESIAN_POINT ( 'NONE',  ( -19.03943276465977164, 0.05219959533909376836, 51.24890960531436690 ) ) ;
#190299=CARTESIAN_POINT ( 'NONE',  ( 12.06949235617739724, 12.14591786802326823, 76.87609039468567573 ) ) ;
#190300=CARTESIAN_POINT ( 'NONE',  ( -17.72517630441458181, 5.499999999999974243, 45.92175719257601685 ) ) ;
#190302=CARTESIAN_POINT ( 'NONE',  ( -13.89961937509977652, 13.97604488694528158, 100.6239096053143669 ) ) ;
#190303=CARTESIAN_POINT ( 'NONE',  ( -13.97604488694527625, -13.89961937509977652, 21.87390960531435979 ) ) ;
#190305=CARTESIAN_POINT ( 'NONE',  ( -14.29746914071037622, -8.314922557961029526, 19.16775706135234714 ) ) ;
#190307=CARTESIAN_POINT ( 'NONE',  ( -21.55341960407610458, -5.719274019375992779, 56.45724293864768839 ) ) ;
#190308=CARTESIAN_POINT ( 'NONE',  ( -19.03943276465977164, -0.05219959533935918106, 48.75109039468566863 ) ) ;
#190309=CARTESIAN_POINT ( 'NONE',  ( 12.14591786802327356, -12.06949235617739191, 30.62609039468567929 ) ) ;
#190310=CARTESIAN_POINT ( 'NONE',  ( 13.97604488694527802, 13.89961937509977652, 34.37390960531436690 ) ) ;
#190311=CARTESIAN_POINT ( 'NONE',  ( -19.05341960407611168, -5.049401038298163336, 56.45724293864768129 ) ) ;
#190312=CARTESIAN_POINT ( 'NONE',  ( 21.55341960407610458, 5.719274019375980345, 88.95724293864769550 ) ) ;
#190313=CARTESIAN_POINT ( 'NONE',  ( -0.05219959533909027116, -19.03943276465977164, 107.4989096053143527 ) ) ;
#190314=CARTESIAN_POINT ( 'NONE',  ( 9.474510206698971260, -16.51473224551069308, 52.91557627198102409 ) ) ;
#190316=CARTESIAN_POINT ( 'NONE',  ( 19.05341960407617918, -5.049401038297876454, 91.04275706135234714 ) ) ;
#190317=CARTESIAN_POINT ( 'NONE',  ( 16.55341960407611168, 4.379528057220329451, 68.95724293864769550 ) ) ;
#190318=CARTESIAN_POINT ( 'NONE',  ( 21.53943276465977519, 0.05219959533937863772, 106.2510903946856757 ) ) ;
#190319=CARTESIAN_POINT ( 'NONE',  ( 21.52544592524344225, -5.823673210054117533, 103.5405762719810383 ) ) ;
#190320=CARTESIAN_POINT ( 'NONE',  ( -5.719274019375665041, -21.55341960407619695, 84.79275706135234714 ) ) ;
#190321=CARTESIAN_POINT ( 'NONE',  ( 9.474510206698971260, -16.51473224551069308, 22.91557627198102765 ) ) ;
#190322=CARTESIAN_POINT ( 'NONE',  ( -15.80617190586768217, 15.72974639402176855, 78.12609039468570415 ) ) ;
#190323=CARTESIAN_POINT ( 'NONE',  ( 0.05219959533909260263, 19.03943276465977164, 109.9989096053143669 ) ) ;
#190324=CARTESIAN_POINT ( 'NONE',  ( 8.224510206698953496, -14.34966873604960469, 32.91557627198102409 ) ) ;
#190325=CARTESIAN_POINT ( 'NONE',  ( -10.81492255796105439, 18.62759615963255655, 72.91775706135234714 ) ) ;
#190326=CARTESIAN_POINT ( 'NONE',  ( 19.05341960407611168, 5.049401038298154454, 63.95724293864769550 ) ) ;
#190327=CARTESIAN_POINT ( 'NONE',  ( 18.67979575497194134, -10.72451020669871369, 40.83442372801901854 ) ) ;
#190328=CARTESIAN_POINT ( 'NONE',  ( 9.474510206698971260, -16.51473224551069308, 77.91557627198103830 ) ) ;
#190329=CARTESIAN_POINT ( 'NONE',  ( -4.483927247898539470, -16.52544592524342804, 92.29057627198103830 ) ) ;
#190330=CARTESIAN_POINT ( 'NONE',  ( 16.52544592524342804, -4.483927247898539470, 63.54057627198103830 ) ) ;
#190331=CARTESIAN_POINT ( 'NONE',  ( -10.72451020669898014, 18.67979575497178502, 65.41557627198102409 ) ) ;
#190332=CARTESIAN_POINT ( 'NONE',  ( 13.89961937509977652, -13.97604488694527269, 63.12390960531435979 ) ) ;
#190333=CARTESIAN_POINT ( 'NONE',  ( 21.52544592524344225, -5.823673210054117533, 68.54057627198103830 ) ) ;
#190334=CARTESIAN_POINT ( 'NONE',  ( 5.153800228976615827, -19.02544592524334988, 60.20942372801899012 ) ) ;
#190335=CARTESIAN_POINT ( 'NONE',  ( 19.02544592524335343, 5.153800228976608722, 31.45942372801900788 ) ) ;
#190336=CARTESIAN_POINT ( 'NONE',  ( -8.224510206698948167, 14.34966873604960824, 80.41557627198103830 ) ) ;
#190337=CARTESIAN_POINT ( 'NONE',  ( -10.72451020669898014, 18.67979575497178502, 55.41557627198102409 ) ) ;
#190339=CARTESIAN_POINT ( 'NONE',  ( 17.31728774477274158, 6.344390552232390235, 101.6809334831068270 ) ) ;
#190340=CARTESIAN_POINT ( 'NONE',  ( -16.55341960407617563, 4.379528057220093196, 98.54275706135234714 ) ) ;
#190342=CARTESIAN_POINT ( 'NONE',  ( -13.97604488694547697, 13.89961937509957934, 103.1260903946856473 ) ) ;
#190343=CARTESIAN_POINT ( 'NONE',  ( -4.483927247898539470, -16.52544592524342804, 72.29057627198102409 ) ) ;
#190344=CARTESIAN_POINT ( 'NONE',  ( -30.00000000000000000, -5.499999999999992895, 37.50000000000000000 ) ) ;
#190345=CARTESIAN_POINT ( 'NONE',  ( -13.89961937509977652, 13.97604488694528158, 55.62390960531434558 ) ) ;
#190346=CARTESIAN_POINT ( 'NONE',  ( -12.14591786802309592, -12.06949235617757132, 51.87390960531437401 ) ) ;
#190347=CARTESIAN_POINT ( 'NONE',  ( -5.153800228976328057, -19.02544592524343514, 107.2905762719810383 ) ) ;
#190348=CARTESIAN_POINT ( 'NONE',  ( 9.474510206698729675, 16.51473224551082808, 72.08442372801900433 ) ) ;
#190349=CARTESIAN_POINT ( 'NONE',  ( 0.05219959533909260263, 19.03943276465977164, 69.99890960531435269 ) ) ;
#190350=CARTESIAN_POINT ( 'NONE',  ( -5.049401038298153566, 19.05341960407611168, 85.20724293864766707 ) ) ;
#190351=CARTESIAN_POINT ( 'NONE',  ( 16.46253265017160672, -9.564922557960803928, 68.33224293864770971 ) ) ;
#190352=CARTESIAN_POINT ( 'NONE',  ( 5.823673210054125526, 21.52544592524343514, 64.79057627198103830 ) ) ;
#190353=CARTESIAN_POINT ( 'NONE',  ( -14.29746914071037622, -8.314922557961029526, 64.16775706135234714 ) ) ;
#190355=CARTESIAN_POINT ( 'NONE',  ( 5.153800228976335163, 19.02544592524342804, 49.79057627198100988 ) ) ;
#190356=CARTESIAN_POINT ( 'NONE',  ( 21.52544592524344225, -5.823673210054117533, 48.54057627198103120 ) ) ;
#190357=CARTESIAN_POINT ( 'NONE',  ( 13.89961937509957401, 13.97604488694547697, 76.87609039468566152 ) ) ;
#190358=CARTESIAN_POINT ( 'NONE',  ( -16.53943276465976808, 0.05219959533911058130, 21.24890960531436690 ) ) ;
#190359=CARTESIAN_POINT ( 'NONE',  ( -21.52544592524334988, -5.823673210054445271, 38.95942372801901854 ) ) ;
#190361=CARTESIAN_POINT ( 'NONE',  ( -5.153800228976607833, 19.02544592524334988, 37.70942372801899722 ) ) ;
#190362=CARTESIAN_POINT ( 'NONE',  ( 16.53943276465976808, 0.05219959533934440121, 56.25109039468568284 ) ) ;
#190363=CARTESIAN_POINT ( 'NONE',  ( -8.224510206698735004, -14.34966873604973081, 89.58442372801901854 ) ) ;
#190365=CARTESIAN_POINT ( 'NONE',  ( -4.379528057220086978, -16.55341960407618274, 84.79275706135234714 ) ) ;
#190366=CARTESIAN_POINT ( 'NONE',  ( 21.52544592524344225, -5.823673210054117533, 28.54057627198103120 ) ) ;
#190367=CARTESIAN_POINT ( 'NONE',  ( -16.52544592524335698, -4.483927247898792601, 38.95942372801901854 ) ) ;
#190369=CARTESIAN_POINT ( 'NONE',  ( -19.03943276465977164, 0.05219959533909376836, 46.24890960531435979 ) ) ;
#190370=CARTESIAN_POINT ( 'NONE',  ( 16.51473224551069308, 9.474510206698969483, 49.16557627198102409 ) ) ;
#190371=CARTESIAN_POINT ( 'NONE',  ( -19.05341960407611168, -5.049401038298163336, 66.45724293864769550 ) ) ;
#190372=CARTESIAN_POINT ( 'NONE',  ( -0.05219959533937732626, 21.53943276465977519, 37.50109039468568284 ) ) ;
#190373=CARTESIAN_POINT ( 'NONE',  ( -8.314922557961024197, 14.29746914071037800, 52.91775706135235424 ) ) ;
#190374=CARTESIAN_POINT ( 'NONE',  ( -16.53943276465976808, 0.05219959533911058130, 26.24890960531435624 ) ) ;
#190375=CARTESIAN_POINT ( 'NONE',  ( 5.153800228976335163, 19.02544592524342804, 34.79057627198102409 ) ) ;
#190376=CARTESIAN_POINT ( 'NONE',  ( 18.62759615963255655, 10.81492255796105972, 111.6677570613523613 ) ) ;
#190377=CARTESIAN_POINT ( 'NONE',  ( -16.51473224551082808, 9.474510206698731452, 113.3344237280190043 ) ) ;
#190378=CARTESIAN_POINT ( 'NONE',  ( 19.03943276465977164, 0.05219959533936151252, 71.25109039468566152 ) ) ;
#190379=CARTESIAN_POINT ( 'NONE',  ( -12.14591786802309592, -12.06949235617757132, 76.87390960531439532 ) ) ;
#190380=CARTESIAN_POINT ( 'NONE',  ( 13.97604488694527802, 13.89961937509977652, 39.37390960531435269 ) ) ;
#190381=CARTESIAN_POINT ( 'NONE',  ( -13.89961937509957401, -13.97604488694547875, 79.37609039468567573 ) ) ;
#190382=CARTESIAN_POINT ( 'NONE',  ( 17.40805194822030799, 6.112264579159357503, 76.66628727489388950 ) ) ;
#190383=CARTESIAN_POINT ( 'NONE',  ( -21.55341960407619339, 5.719274019375674811, 78.54275706135236135 ) ) ;
#190384=CARTESIAN_POINT ( 'NONE',  ( 12.06949235617739724, 12.14591786802326823, 41.87609039468568284 ) ) ;
#190386=CARTESIAN_POINT ( 'NONE',  ( 5.823673210054125526, 21.52544592524343514, 29.79057627198102409 ) ) ;
#190387=CARTESIAN_POINT ( 'NONE',  ( -16.53943276465976808, -0.05219959533934237506, 23.75109039468567929 ) ) ;
#190388=CARTESIAN_POINT ( 'NONE',  ( -19.02544592524342804, 5.153800228976336939, 31.04057627198102054 ) ) ;
#190389=CARTESIAN_POINT ( 'NONE',  ( -19.02544592524334988, -5.153800228976617603, 33.95942372801897591 ) ) ;
#190391=CARTESIAN_POINT ( 'NONE',  ( -16.46253265017160317, 9.564922557960807481, 40.83224293864769550 ) ) ;
#190393=CARTESIAN_POINT ( 'NONE',  ( -19.03943276465977164, 0.05219959533909376836, 61.24890960531436690 ) ) ;
#190394=CARTESIAN_POINT ( 'NONE',  ( 17.50000000000014566, -3.417042746626890892, 112.6738039623247545 ) ) ;
#190395=CARTESIAN_POINT ( 'NONE',  ( 13.97604488694548053, -13.89961937509957401, 20.62609039468567573 ) ) ;
#190396=CARTESIAN_POINT ( 'NONE',  ( -0.05219959533934338120, 16.53943276465976808, 112.5010903946857042 ) ) ;
#190397=CARTESIAN_POINT ( 'NONE',  ( -9.564922557960796823, -16.46253265017161027, 32.08224293864769550 ) ) ;
#190398=CARTESIAN_POINT ( 'NONE',  ( -13.97604488694527625, -13.89961937509977652, 91.87390960531432427 ) ) ;
#190399=CARTESIAN_POINT ( 'NONE',  ( 5.823673210054444382, -21.52544592524334988, 65.20942372801901854 ) ) ;
#190400=CARTESIAN_POINT ( 'NONE',  ( -0.05219959533909027116, -19.03943276465977164, 32.49890960531435979 ) ) ;
#190401=CARTESIAN_POINT ( 'NONE',  ( 0.05219959533937995610, -21.53943276465977519, 65.00109039468568994 ) ) ;
#190402=CARTESIAN_POINT ( 'NONE',  ( -19.05341960407617563, 5.049401038297882671, 98.54275706135233293 ) ) ;
#190403=CARTESIAN_POINT ( 'NONE',  ( -13.89961937509977652, 13.97604488694528158, 115.6239096053143669 ) ) ;
#190404=CARTESIAN_POINT ( 'NONE',  ( 0.05219959533909260263, 19.03943276465977164, 39.99890960531436690 ) ) ;
#190405=CARTESIAN_POINT ( 'NONE',  ( 5.823673210054125526, 21.52544592524343514, 104.7905762719810241 ) ) ;
#190406=CARTESIAN_POINT ( 'NONE',  ( -16.51473224551082808, 9.474510206698731452, 38.33442372801899722 ) ) ;
#190407=CARTESIAN_POINT ( 'NONE',  ( 8.314922557960818139, 14.29746914071049879, 109.5822429386476955 ) ) ;
#190408=CARTESIAN_POINT ( 'NONE',  ( 13.97604488694527802, 13.89961937509977652, 69.37390960531436690 ) ) ;
#190409=CARTESIAN_POINT ( 'NONE',  ( -19.02544592524334988, -5.153800228976617603, 98.95942372801900433 ) ) ;
#190410=CARTESIAN_POINT ( 'NONE',  ( -0.05219959533910754901, -16.53943276465976808, 72.49890960531435269 ) ) ;
#190411=CARTESIAN_POINT ( 'NONE',  ( 13.89961937509977652, -13.97604488694527269, 113.1239096053143527 ) ) ;
#190412=CARTESIAN_POINT ( 'NONE',  ( -0.05219959533936034679, 19.03943276465977164, 82.50109039468567573 ) ) ;
#190413=CARTESIAN_POINT ( 'NONE',  ( 21.55341960407610458, 5.719274019375980345, 93.95724293864770971 ) ) ;
#190414=CARTESIAN_POINT ( 'NONE',  ( 0.05219959533937995610, -21.53943276465977519, 40.00109039468567573 ) ) ;
#190415=CARTESIAN_POINT ( 'NONE',  ( 16.53943276465976808, 0.05219959533934440121, 46.25109039468567573 ) ) ;
#190416=CARTESIAN_POINT ( 'NONE',  ( -0.05219959533934338120, 16.53943276465976808, 52.50109039468567573 ) ) ;
#190417=CARTESIAN_POINT ( 'NONE',  ( 10.81492255796106328, -18.62759615963255655, 55.41775706135234714 ) ) ;
#190418=CARTESIAN_POINT ( 'NONE',  ( 18.67979575497178502, 10.72451020669898547, 59.16557627198103120 ) ) ;
#190419=CARTESIAN_POINT ( 'NONE',  ( -19.03943276465977164, 0.05219959533909376836, 46.24890960531435979 ) ) ;
#190421=CARTESIAN_POINT ( 'NONE',  ( -16.52544592524335698, -4.483927247898792601, 73.95942372801901854 ) ) ;
#190422=CARTESIAN_POINT ( 'NONE',  ( 10.72451020669898902, -18.67979575497178502, 97.91557627198103830 ) ) ;
#190423=CARTESIAN_POINT ( 'NONE',  ( 14.29746914071049879, -8.314922557960816363, 53.33224293864769550 ) ) ;
#190424=CARTESIAN_POINT ( 'NONE',  ( 0.05219959533934541429, -16.53943276465976808, 65.00109039468568994 ) ) ;
#190425=CARTESIAN_POINT ( 'NONE',  ( 19.05341960407617918, -5.049401038297876454, 96.04275706135231871 ) ) ;
#190426=CARTESIAN_POINT ( 'NONE',  ( -15.80617190586745835, -15.72974639402198527, 96.87390960531436690 ) ) ;
#190427=CARTESIAN_POINT ( 'NONE',  ( -8.314922557960811034, -14.29746914071050412, 47.08224293864770260 ) ) ;
#190428=ORIENTED_EDGE ( 'NONE', *, *, #176141, .F. ) ;
#190429=CARTESIAN_POINT ( 'NONE',  ( 0.05219959533934541429, -16.53943276465976808, 75.00109039468568994 ) ) ;
#190431=CARTESIAN_POINT ( 'NONE',  ( -21.53943276465977519, 0.05219959533907696930, 71.24890960531435269 ) ) ;
#190432=CARTESIAN_POINT ( 'NONE',  ( -4.379528057220328563, 16.55341960407611168, 25.20724293864769550 ) ) ;
#190435=CARTESIAN_POINT ( 'NONE',  ( -18.62759615963270932, 10.81492255796079327, 100.8322429386477097 ) ) ;
#190436=CARTESIAN_POINT ( 'NONE',  ( -15.80617190586745835, -15.72974639402198527, 111.8739096053143669 ) ) ;
#190437=CARTESIAN_POINT ( 'NONE',  ( -8.224510206698948167, 14.34966873604960824, 40.41557627198103120 ) ) ;
#190438=CARTESIAN_POINT ( 'NONE',  ( -0.05219959533934338120, 16.53943276465976808, 52.50109039468567573 ) ) ;
#190439=CARTESIAN_POINT ( 'NONE',  ( 0.05219959533909260263, 19.03943276465977164, 44.99890960531435979 ) ) ;
#190440=CARTESIAN_POINT ( 'NONE',  ( 19.02544592524343514, -5.153800228976328945, 63.54057627198103830 ) ) ;
#190442=EDGE_CURVE ( 'NONE', #85848, #141234, #21219, .T. ) ;
#190443=CARTESIAN_POINT ( 'NONE',  ( -15.72974639402197994, 15.80617190586746368, 25.62390960531435624 ) ) ;
#190445=CARTESIAN_POINT ( 'NONE',  ( 16.51473224551083163, -9.474510206698727899, 100.8344237280190043 ) ) ;
#190446=CARTESIAN_POINT ( 'NONE',  ( 19.02544592524334988, 5.153800228976608722, 56.45942372801898301 ) ) ;
#190447=CARTESIAN_POINT ( 'NONE',  ( -10.81492255796078084, -18.62759615963271287, 102.0822429386476955 ) ) ;
#190448=CARTESIAN_POINT ( 'NONE',  ( 16.52544592524335698, 4.483927247898782831, 111.4594237280190328 ) ) ;
#190449=CARTESIAN_POINT ( 'NONE',  ( -19.02544592524342804, 5.153800228976336051, 76.04057627198102409 ) ) ;
#190450=CARTESIAN_POINT ( 'NONE',  ( -0.05219959533907301413, -21.53943276465977519, 42.49890960531435979 ) ) ;
#190451=CARTESIAN_POINT ( 'NONE',  ( 18.67979575497178502, 10.72451020669898547, 79.16557627198103830 ) ) ;
#190452=CARTESIAN_POINT ( 'NONE',  ( 14.34966873604972726, -8.224510206698740333, 25.83442372801901499 ) ) ;
#190453=CARTESIAN_POINT ( 'NONE',  ( 9.564922557960805705, 16.46253265017160317, 114.5822429386476955 ) ) ;
#190454=CARTESIAN_POINT ( 'NONE',  ( -5.823673210054431948, 21.52544592524334988, 72.70942372801901854 ) ) ;
#190455=CARTESIAN_POINT ( 'NONE',  ( -5.049401038298153566, 19.05341960407611168, 80.20724293864769550 ) ) ;
#190456=ADVANCED_FACE ( 'NONE', ( #4694 ), #110897, .T. ) ;
#190458=CARTESIAN_POINT ( 'NONE',  ( -13.97604488694527625, -13.89961937509977652, 31.87390960531435979 ) ) ;
#190459=CARTESIAN_POINT ( 'NONE',  ( 9.564922557960805705, 16.46253265017160317, 79.58224293864769550 ) ) ;
#190460=CARTESIAN_POINT ( 'NONE',  ( -14.34966873604960291, -8.224510206698953496, 86.66557627198102409 ) ) ;
#190462=CARTESIAN_POINT ( 'NONE',  ( 0.05219959533936267826, -19.03943276465977164, 100.0010903946856757 ) ) ;
#190464=CARTESIAN_POINT ( 'NONE',  ( 19.03943276465977164, -0.05219959533909143690, 68.74890960531436690 ) ) ;
#190465=CARTESIAN_POINT ( 'NONE',  ( 21.55341960407619695, -5.719274019375665929, 81.04275706135236135 ) ) ;
#190466=CARTESIAN_POINT ( 'NONE',  ( 19.05341960407611168, 5.049401038298154454, 98.95724293864766707 ) ) ;
#190467=CARTESIAN_POINT ( 'NONE',  ( -4.483927247898782831, 16.52544592524335698, 72.70942372801901854 ) ) ;
#190469=CARTESIAN_POINT ( 'NONE',  ( 9.474510206698729675, 16.51473224551082808, 52.08442372801900433 ) ) ;
#190470=CARTESIAN_POINT ( 'NONE',  ( 15.72974639402176855, 15.80617190586768217, 111.8760903946856615 ) ) ;
#190474=CARTESIAN_POINT ( 'NONE',  ( -14.29746914071049879, 8.314922557960819915, 25.83224293864769194 ) ) ;
#190476=CARTESIAN_POINT ( 'NONE',  ( 0.05219959533934541429, -16.53943276465976808, 110.0010903946856757 ) ) ;
#190478=( BOUNDED_CURVE ( )  B_SPLINE_CURVE ( 2, ( #74128, #199444, #136768, #76084, #168104, #42795, #28628, #58936, #153928, #134812, #43779, #122588, #106423 ),
 .UNSPECIFIED., .F., .T. ) 
 B_SPLINE_CURVE_WITH_KNOTS ( ( 3, 2, 2, 2, 2, 2, 3 ),
 ( 0.4234830680059925023, 0.4254385964912280604, 0.4298245614035087758, 0.4342105263157894912, 0.4385964912280701511, 0.4429824561403508665, 0.4448923048034963412 ),
 .UNSPECIFIED. ) 
 CURVE ( )  GEOMETRIC_REPRESENTATION_ITEM ( )  RATIONAL_B_SPLINE_CURVE ( ( 0.9831626618144004848, 0.9848076720550091867, 1.000000000000000000, 0.9659258262890683122, 1.000000000000000000, 0.9659258262890683122, 1.000000000000000000, 0.9659258262890683122, 1.000000000000000000, 0.9659258262890683122, 1.000000000000000000, 0.9851625545550091179, 0.9832469066685282089 ) ) 
 REPRESENTATION_ITEM ( '' )  );
#190479=CARTESIAN_POINT ( 'NONE',  ( 16.52544592524335698, 4.483927247898782831, 81.45942372801900433 ) ) ;
#190480=CARTESIAN_POINT ( 'NONE',  ( 18.62759615963255655, 10.81492255796105972, 96.66775706135234714 ) ) ;
#190481=CARTESIAN_POINT ( 'NONE',  ( 9.564922557961047289, -16.46253265017146816, 100.4177570613523329 ) ) ;
#190482=CARTESIAN_POINT ( 'NONE',  ( -21.53943276465977519, -0.05219959533937600094, 68.75109039468568994 ) ) ;
#190483=CARTESIAN_POINT ( 'NONE',  ( -9.474510206698720793, -16.51473224551083518, 34.58442372801899722 ) ) ;
#190484=CARTESIAN_POINT ( 'NONE',  ( 19.02544592524343514, -5.153800228976328945, 78.54057627198099567 ) ) ;
#190485=CARTESIAN_POINT ( 'NONE',  ( -16.46253265017160317, 9.564922557960807481, 55.83224293864769550 ) ) ;
#190487=CARTESIAN_POINT ( 'NONE',  ( 21.52544592524344225, -5.823673210054117533, 98.54057627198105251 ) ) ;
#190489=CARTESIAN_POINT ( 'NONE',  ( -15.72974639402197994, 15.80617190586746368, 50.62390960531435979 ) ) ;
#190490=CARTESIAN_POINT ( 'NONE',  ( -5.153800228976328057, -19.02544592524343514, 52.29057627198100988 ) ) ;
#190491=CARTESIAN_POINT ( 'NONE',  ( 12.06949235617739724, 12.14591786802326823, 61.87609039468568284 ) ) ;
#190492=ORIENTED_EDGE ( 'NONE', *, *, #26831, .F. ) ;
#190493=CARTESIAN_POINT ( 'NONE',  ( 15.80617190586769283, -15.72974639402175789, 45.62609039468567573 ) ) ;
#190494=CARTESIAN_POINT ( 'NONE',  ( -14.29746914071049879, 8.314922557960819915, 60.83224293864769550 ) ) ;
#190495=CARTESIAN_POINT ( 'NONE',  ( -16.53943276465976808, -0.05219959533934237506, 38.75109039468567573 ) ) ;
#190496=CARTESIAN_POINT ( 'NONE',  ( 16.53943276465976808, -0.05219959533910856209, 103.7489096053143669 ) ) ;
#190497=CARTESIAN_POINT ( 'NONE',  ( -19.03943276465977164, -0.05219959533935918106, 48.75109039468566863 ) ) ;
#190498=CARTESIAN_POINT ( 'NONE',  ( -16.55341960407611168, -4.379528057220339221, 66.45724293864768129 ) ) ;
#190499=CARTESIAN_POINT ( 'NONE',  ( -5.719274019375665041, -21.55341960407619695, 34.79275706135235424 ) ) ;
#190500=CARTESIAN_POINT ( 'NONE',  ( -9.564922557960796823, -16.46253265017161027, 27.08224293864769550 ) ) ;
#190501=CARTESIAN_POINT ( 'NONE',  ( 18.67979575497178502, 10.72451020669898547, 94.16557627198103830 ) ) ;
#190502=CARTESIAN_POINT ( 'NONE',  ( -9.564922557960796823, -16.46253265017161027, 107.0822429386476955 ) ) ;
#190503=CARTESIAN_POINT ( 'NONE',  ( -8.224510206698948167, 14.34966873604960824, 75.41557627198102409 ) ) ;
#190504=CARTESIAN_POINT ( 'NONE',  ( 0.05219959533909260263, 19.03943276465977164, 114.9989096053143669 ) ) ;
#190506=CARTESIAN_POINT ( 'NONE',  ( -16.46253265017146816, -9.564922557961047289, 84.16775706135233293 ) ) ;
#190507=CARTESIAN_POINT ( 'NONE',  ( -21.52544592524334988, -5.823673210054445271, 28.95942372801902209 ) ) ;
#190508=CARTESIAN_POINT ( 'NONE',  ( 19.02544592524343514, -5.153800228976328945, 68.54057627198103830 ) ) ;
#190509=CARTESIAN_POINT ( 'NONE',  ( 19.03943276465977164, 0.05219959533936151252, 56.25109039468566863 ) ) ;
#190510=CARTESIAN_POINT ( 'NONE',  ( 5.153800228976335163, 19.02544592524342804, 24.79057627198102765 ) ) ;
#190511=CARTESIAN_POINT ( 'NONE',  ( 12.06949235617757843, -12.14591786802309237, 58.12390960531435979 ) ) ;
#190512=CARTESIAN_POINT ( 'NONE',  ( -14.34966873604960291, -8.224510206698953496, 51.66557627198102409 ) ) ;
#190513=CARTESIAN_POINT ( 'NONE',  ( 5.049401038298161559, -19.05341960407611168, 72.70724293864768129 ) ) ;
#190514=CARTESIAN_POINT ( 'NONE',  ( 21.53943276465977519, -0.05219959533907433946, 93.74890960531436690 ) ) ;
#190515=CARTESIAN_POINT ( 'NONE',  ( -5.049401038298153566, 19.05341960407611168, 70.20724293864769550 ) ) ;
#190516=CARTESIAN_POINT ( 'NONE',  ( 10.81492255796078972, 18.62759615963270932, 79.58224293864769550 ) ) ;
#190517=CARTESIAN_POINT ( 'NONE',  ( -13.89961937509957401, -13.97604488694547875, 24.37609039468565442 ) ) ;
#190518=CARTESIAN_POINT ( 'NONE',  ( -19.03943276465977164, 0.05219959533909376836, 26.24890960531435624 ) ) ;
#190519=CARTESIAN_POINT ( 'NONE',  ( 4.379528057220339221, -16.55341960407611168, 22.70724293864769194 ) ) ;
#190520=CARTESIAN_POINT ( 'NONE',  ( 16.53943276465976808, -0.05219959533910856209, 93.74890960531436690 ) ) ;
#190521=CARTESIAN_POINT ( 'NONE',  ( 0.05219959533936267826, -19.03943276465977164, 95.00109039468567573 ) ) ;
#190522=VERTEX_POINT ( 'NONE', #66385 ) ;
#190523=CARTESIAN_POINT ( 'NONE',  ( 5.719274019375673035, 21.55341960407619339, 22.29275706135235069 ) ) ;
#190524=CARTESIAN_POINT ( 'NONE',  ( -13.89961937509957401, -13.97604488694547875, 49.37609039468567573 ) ) ;
#190525=CARTESIAN_POINT ( 'NONE',  ( 4.379528057220092307, 16.55341960407617563, 107.2927570613523471 ) ) ;
#190526=CARTESIAN_POINT ( 'NONE',  ( -16.46253265017146816, -9.564922557961047289, 39.16775706135234003 ) ) ;
#190527=CARTESIAN_POINT ( 'NONE',  ( -13.89961937509977652, 13.97604488694528158, 100.6239096053143669 ) ) ;
#190528=CARTESIAN_POINT ( 'NONE',  ( -8.224510206698948167, 14.34966873604960824, 55.41557627198102409 ) ) ;
#190529=CARTESIAN_POINT ( 'NONE',  ( -18.56197773271724571, 5.499999999999873879, 48.55066217314450228 ) ) ;
#190530=CARTESIAN_POINT ( 'NONE',  ( -16.51473224551069308, -9.474510206698971260, 31.66557627198102054 ) ) ;
#190531=CARTESIAN_POINT ( 'NONE',  ( 10.81492255796106328, -18.62759615963255655, 110.4177570613523756 ) ) ;
#190532=CARTESIAN_POINT ( 'NONE',  ( 4.379528057220092307, 16.55341960407617563, 77.29275706135234714 ) ) ;
#190533=CARTESIAN_POINT ( 'NONE',  ( -15.80617190586768217, 15.72974639402176855, 38.12609039468567573 ) ) ;
#190534=CARTESIAN_POINT ( 'NONE',  ( 8.314922557961029526, -14.29746914071037800, 50.41775706135235424 ) ) ;
#190535=CARTESIAN_POINT ( 'NONE',  ( 0.05219959533909260263, 19.03943276465977164, 104.9989096053143669 ) ) ;
#190536=CARTESIAN_POINT ( 'NONE',  ( 16.51473224551069308, 9.474510206698969483, 59.16557627198102409 ) ) ;
#190537=CARTESIAN_POINT ( 'NONE',  ( -16.51473224551069308, -9.474510206698971260, 66.66557627198102409 ) ) ;
#190538=CARTESIAN_POINT ( 'NONE',  ( -4.379528057220086978, -16.55341960407618274, 44.79275706135234714 ) ) ;
#190539=CARTESIAN_POINT ( 'NONE',  ( 14.29746914071049879, -8.314922557960816363, 108.3322429386477097 ) ) ;
#190540=CARTESIAN_POINT ( 'NONE',  ( 16.53943276465976808, -0.05219959533910856209, 23.74890960531435269 ) ) ;
#190542=CARTESIAN_POINT ( 'NONE',  ( 0.05219959533937995610, -21.53943276465977519, 60.00109039468568284 ) ) ;
#190543=CARTESIAN_POINT ( 'NONE',  ( -5.049401038298153566, 19.05341960407611168, 95.20724293864770971 ) ) ;
#190544=CARTESIAN_POINT ( 'NONE',  ( -16.51473224551069308, -9.474510206698971260, 61.66557627198103120 ) ) ;
#190545=CARTESIAN_POINT ( 'NONE',  ( 9.474510206698971260, -16.51473224551069308, 92.91557627198103830 ) ) ;
#190546=CARTESIAN_POINT ( 'NONE',  ( 8.314922557960818139, 14.29746914071049879, 49.58224293864769550 ) ) ;
#190548=CARTESIAN_POINT ( 'NONE',  ( 14.29746914071037800, 8.314922557961029526, 111.6677570613523613 ) ) ;
#190549=CARTESIAN_POINT ( 'NONE',  ( 8.314922557960818139, 14.29746914071049879, 44.58224293864769550 ) ) ;
#190552=CARTESIAN_POINT ( 'NONE',  ( 9.564922557960805705, 16.46253265017160317, 64.58224293864769550 ) ) ;
#190553=CARTESIAN_POINT ( 'NONE',  ( -16.46253265017146816, -9.564922557961047289, 39.16775706135234003 ) ) ;
#190556=CARTESIAN_POINT ( 'NONE',  ( 5.049401038297881783, 19.05341960407617563, 82.29275706135229029 ) ) ;
#190557=CARTESIAN_POINT ( 'NONE',  ( -16.55341960407617563, 4.379528057220093196, 68.54275706135234714 ) ) ;
#190559=CARTESIAN_POINT ( 'NONE',  ( -13.97604488694527625, -13.89961937509977652, 96.87390960531433848 ) ) ;
#190560=CARTESIAN_POINT ( 'NONE',  ( -15.80617190586768217, 15.72974639402176855, 33.12609039468569705 ) ) ;
#190561=CARTESIAN_POINT ( 'NONE',  ( 13.97604488694548053, -13.89961937509957401, 90.62609039468567573 ) ) ;
#190562=CARTESIAN_POINT ( 'NONE',  ( -9.564922557960796823, -16.46253265017161027, 112.0822429386476955 ) ) ;
#190563=CARTESIAN_POINT ( 'NONE',  ( 16.51473224551069308, 9.474510206698969483, 49.16557627198102409 ) ) ;
#190564=CARTESIAN_POINT ( 'NONE',  ( 0.05219959533909260263, 19.03943276465977164, 84.99890960531436690 ) ) ;
#190565=CARTESIAN_POINT ( 'NONE',  ( -12.14591786802309592, -12.06949235617757132, 41.87390960531435979 ) ) ;
#190566=CARTESIAN_POINT ( 'NONE',  ( -9.474510206698964154, 16.51473224551069663, 55.41557627198103120 ) ) ;
#190567=CARTESIAN_POINT ( 'NONE',  ( 16.51473224551083163, -9.474510206698727899, 70.83442372801900433 ) ) ;
#190568=CARTESIAN_POINT ( 'NONE',  ( 8.314922557960818139, 14.29746914071049879, 89.58224293864768129 ) ) ;
#190569=CARTESIAN_POINT ( 'NONE',  ( -19.05341960407617563, 5.049401038297882671, 28.54275706135232937 ) ) ;
#190570=CARTESIAN_POINT ( 'NONE',  ( -19.05341960407611168, -5.049401038298163336, 66.45724293864769550 ) ) ;
#190571=CARTESIAN_POINT ( 'NONE',  ( -15.72974639402197994, 15.80617190586746368, 60.62390960531437401 ) ) ;
#190572=CARTESIAN_POINT ( 'NONE',  ( -0.05219959533910754901, -16.53943276465976808, 62.49890960531436690 ) ) ;
#190573=CARTESIAN_POINT ( 'NONE',  ( 10.81492255796106328, -18.62759615963255655, 110.4177570613523756 ) ) ;
#190574=CARTESIAN_POINT ( 'NONE',  ( 13.97604488694527802, 13.89961937509977652, 104.3739096053143385 ) ) ;
#190575=CARTESIAN_POINT ( 'NONE',  ( -5.823673210054116645, -21.52544592524344225, 27.29057627198103120 ) ) ;
#190576=CARTESIAN_POINT ( 'NONE',  ( 19.05341960407611168, 5.049401038298154454, 53.95724293864770260 ) ) ;
#190577=CARTESIAN_POINT ( 'NONE',  ( 0.05219959533909260263, 19.03943276465977164, 44.99890960531435979 ) ) ;
#190578=CARTESIAN_POINT ( 'NONE',  ( 14.34966873604960469, 8.224510206698951720, 104.1655762719810241 ) ) ;
#190579=CARTESIAN_POINT ( 'NONE',  ( -18.62759615963255300, -10.81492255796106328, 19.16775706135234714 ) ) ;
#190580=CARTESIAN_POINT ( 'NONE',  ( -16.46253265017160317, 9.564922557960807481, 95.83224293864769550 ) ) ;
#190581=CARTESIAN_POINT ( 'NONE',  ( -0.05219959533937732626, 21.53943276465977519, 32.50109039468568284 ) ) ;
#190582=CARTESIAN_POINT ( 'NONE',  ( 19.02544592524343514, -5.153800228976328945, 108.5405762719810383 ) ) ;
#190583=CARTESIAN_POINT ( 'NONE',  ( -19.05341960407611168, -5.049401038298163336, 26.45724293864769550 ) ) ;
#190584=CARTESIAN_POINT ( 'NONE',  ( -0.05219959533937732626, 21.53943276465977519, 82.50109039468568994 ) ) ;
#190585=CARTESIAN_POINT ( 'NONE',  ( 15.80617190586746368, 15.72974639402197994, 99.37390960531436690 ) ) ;
#190586=CARTESIAN_POINT ( 'NONE',  ( 17.50000000000000000, -5.500000000000001776, 106.2176903769643417 ) ) ;
#190588=CARTESIAN_POINT ( 'NONE',  ( -18.22780087662119897, 5.500000000000102141, 61.01763182126894947 ) ) ;
#190589=CARTESIAN_POINT ( 'NONE',  ( 12.14591786802327356, -12.06949235617739191, 45.62609039468567573 ) ) ;
#190590=CARTESIAN_POINT ( 'NONE',  ( -0.05219959533910754901, -16.53943276465976808, 107.4989096053143669 ) ) ;
#190592=CARTESIAN_POINT ( 'NONE',  ( 13.89961937509977652, -13.97604488694527269, 63.12390960531435979 ) ) ;
#190593=CARTESIAN_POINT ( 'NONE',  ( -12.06949235617756955, 12.14591786802309770, 95.62390960531436690 ) ) ;
#190594=CARTESIAN_POINT ( 'NONE',  ( -0.05219959533907301413, -21.53943276465977519, 42.49890960531435979 ) ) ;
#190595=CARTESIAN_POINT ( 'NONE',  ( -14.34966873604960291, -8.224510206698953496, 71.66557627198100988 ) ) ;
#190596=CARTESIAN_POINT ( 'NONE',  ( 16.53943276465976808, 0.05219959533934440121, 21.25109039468567218 ) ) ;
#190597=CARTESIAN_POINT ( 'NONE',  ( 18.67979575497194134, -10.72451020669871369, 75.83442372801900433 ) ) ;
#190598=CARTESIAN_POINT ( 'NONE',  ( 17.50000000000001421, -5.622605283950867339, 76.18792689403886698 ) ) ;
#190599=CARTESIAN_POINT ( 'NONE',  ( 16.53943276465976808, 0.05219959533934440121, 96.25109039468568994 ) ) ;
#190600=CARTESIAN_POINT ( 'NONE',  ( -12.14591786802309592, -12.06949235617757132, 36.87390960531435979 ) ) ;
#190602=CARTESIAN_POINT ( 'NONE',  ( -9.564922557960796823, -16.46253265017161027, 37.08224293864768839 ) ) ;
#190603=CARTESIAN_POINT ( 'NONE',  ( 19.02544592524343514, -5.153800228976328945, 83.54057627198100988 ) ) ;
#190604=CARTESIAN_POINT ( 'NONE',  ( 21.53943276465977519, -0.05219959533907433946, 88.74890960531436690 ) ) ;
#190605=CARTESIAN_POINT ( 'NONE',  ( -16.55341960407617563, 4.379528057220093196, 38.54275706135234714 ) ) ;
#190606=CARTESIAN_POINT ( 'NONE',  ( -4.483927247898539470, -16.52544592524342804, 67.29057627198103830 ) ) ;
#190607=CARTESIAN_POINT ( 'NONE',  ( 0.05219959533937995610, -21.53943276465977519, 75.00109039468568994 ) ) ;
#190609=CARTESIAN_POINT ( 'NONE',  ( -4.379528057220086978, -16.55341960407618274, 99.79275706135234714 ) ) ;
#190610=CARTESIAN_POINT ( 'NONE',  ( 17.26058549869101810, -6.457015423128417808, 46.12254162523932877 ) ) ;
#190611=CARTESIAN_POINT ( 'NONE',  ( -19.35543954521081034, -5.499999999999585221, 64.58901960356450900 ) ) ;
#190612=CARTESIAN_POINT ( 'NONE',  ( 14.29746914071049879, -8.314922557960816363, 23.33224293864769194 ) ) ;
#190613=CARTESIAN_POINT ( 'NONE',  ( -8.314922557961024197, 14.29746914071037800, 67.91775706135234714 ) ) ;
#190614=CARTESIAN_POINT ( 'NONE',  ( -9.474510206698964154, 16.51473224551069663, 90.41557627198103830 ) ) ;
#190615=CARTESIAN_POINT ( 'NONE',  ( -19.02544592524342804, 5.153800228976336051, 106.0405762719810241 ) ) ;
#190616=CARTESIAN_POINT ( 'NONE',  ( 18.67979575497194134, -10.72451020669871369, 85.83442372801901854 ) ) ;
#190617=CARTESIAN_POINT ( 'NONE',  ( 14.34966873604972726, -8.224510206698740333, 85.83442372801901854 ) ) ;
#190618=CARTESIAN_POINT ( 'NONE',  ( -12.14591786802309592, -12.06949235617757132, 56.87390960531436690 ) ) ;
#190619=CARTESIAN_POINT ( 'NONE',  ( 16.46253265017160672, -9.564922557960803928, 68.33224293864770971 ) ) ;
#190621=CARTESIAN_POINT ( 'NONE',  ( -13.97604488694547697, 13.89961937509957934, 103.1260903946856473 ) ) ;
#190622=CARTESIAN_POINT ( 'NONE',  ( -4.483927247898539470, -16.52544592524342804, 107.2905762719810525 ) ) ;
#190623=CARTESIAN_POINT ( 'NONE',  ( 13.97604488694527802, 13.89961937509977652, 79.37390960531435269 ) ) ;
#190624=CARTESIAN_POINT ( 'NONE',  ( -13.89961937509957401, -13.97604488694547875, 109.3760903946856331 ) ) ;
#190626=CARTESIAN_POINT ( 'NONE',  ( -19.02544592524334988, -5.153800228976617603, 18.95942372801899722 ) ) ;
#190627=CARTESIAN_POINT ( 'NONE',  ( -14.29746914071037622, -8.314922557961029526, 74.16775706135231871 ) ) ;
#190628=CARTESIAN_POINT ( 'NONE',  ( -19.03943276465977164, -0.05219959533935918106, 103.7510903946856757 ) ) ;
#190629=CARTESIAN_POINT ( 'NONE',  ( -4.379528057220328563, 16.55341960407611168, 110.2072429386477239 ) ) ;
#190630=CARTESIAN_POINT ( 'NONE',  ( -4.483927247898782831, 16.52544592524335698, 67.70942372801901854 ) ) ;
#190631=CARTESIAN_POINT ( 'NONE',  ( -14.29746914071037622, -8.314922557961029526, 59.16775706135234714 ) ) ;
#190632=CARTESIAN_POINT ( 'NONE',  ( -16.51473224551069308, -9.474510206698971260, 26.66557627198103120 ) ) ;
#190633=CARTESIAN_POINT ( 'NONE',  ( 16.51473224551083163, -9.474510206698727899, 65.83442372801900433 ) ) ;
#190634=CARTESIAN_POINT ( 'NONE',  ( -15.80617190586768217, 15.72974639402176855, 93.12609039468568994 ) ) ;
#190635=CARTESIAN_POINT ( 'NONE',  ( -16.46253265017160317, 9.564922557960807481, 30.83224293864769550 ) ) ;
#190636=CARTESIAN_POINT ( 'NONE',  ( 5.049401038298161559, -19.05341960407611168, 72.70724293864768129 ) ) ;
#190637=CARTESIAN_POINT ( 'NONE',  ( 14.29746914071049879, -8.314922557960816363, 68.33224293864769550 ) ) ;
#190638=EDGE_CURVE ( 'NONE', #110833, #22958, #48250, .T. ) ;
#190639=CARTESIAN_POINT ( 'NONE',  ( -19.03943276465977164, -0.05219959533935918106, 43.75109039468566863 ) ) ;
#190640=CARTESIAN_POINT ( 'NONE',  ( 10.81492255796078972, 18.62759615963270932, 39.58224293864769550 ) ) ;
#190641=CARTESIAN_POINT ( 'NONE',  ( -15.80617190586768217, 15.72974639402176855, 113.1260903946856899 ) ) ;
#190642=CARTESIAN_POINT ( 'NONE',  ( -16.46253265017160317, 9.564922557960807481, 85.83224293864769550 ) ) ;
#190643=CARTESIAN_POINT ( 'NONE',  ( 21.53943276465977519, 0.05219959533937863772, 111.2510903946856899 ) ) ;
#190644=CARTESIAN_POINT ( 'NONE',  ( -15.72974639402197994, 15.80617190586746368, 65.62390960531436690 ) ) ;
#190645=CARTESIAN_POINT ( 'NONE',  ( -13.97604488694527625, -13.89961937509977652, 96.87390960531433848 ) ) ;
#190646=CARTESIAN_POINT ( 'NONE',  ( -19.05341960407617563, 5.049401038297882671, 73.54275706135233293 ) ) ;
#190647=CARTESIAN_POINT ( 'NONE',  ( 16.51473224551069308, 9.474510206698969483, 109.1655762719810383 ) ) ;
#190648=CARTESIAN_POINT ( 'NONE',  ( -9.564922557961040184, 16.46253265017147172, 92.91775706135233293 ) ) ;
#190649=CARTESIAN_POINT ( 'NONE',  ( 16.55341960407618274, -4.379528057220086978, 61.04275706135234714 ) ) ;
#190650=CARTESIAN_POINT ( 'NONE',  ( 5.153800228976335163, 19.02544592524342804, 24.79057627198102765 ) ) ;
#190651=CARTESIAN_POINT ( 'NONE',  ( -13.89961937509977652, 13.97604488694528158, 90.62390960531432427 ) ) ;
#190652=CARTESIAN_POINT ( 'NONE',  ( 21.52544592524344225, -5.823673210054117533, 58.54057627198103120 ) ) ;
#190653=CARTESIAN_POINT ( 'NONE',  ( -14.34966873604972548, 8.224510206698743886, 28.33442372801902209 ) ) ;
#190654=CARTESIAN_POINT ( 'NONE',  ( -18.67979575497193778, 10.72451020669871902, 33.33442372801900433 ) ) ;
#190655=CARTESIAN_POINT ( 'NONE',  ( -18.67979575497193778, 10.72451020669871902, 83.33442372801903275 ) ) ;
#190656=CARTESIAN_POINT ( 'NONE',  ( 12.06949235617739724, 12.14591786802326823, 91.87609039468568994 ) ) ;
#190657=CARTESIAN_POINT ( 'NONE',  ( -16.51473224551069308, -9.474510206698971260, 81.66557627198103830 ) ) ;
#190658=CARTESIAN_POINT ( 'NONE',  ( -16.52544592524342804, 4.483927247898546575, 81.04057627198102409 ) ) ;
#190659=CARTESIAN_POINT ( 'NONE',  ( -4.483927247898539470, -16.52544592524342804, 22.29057627198102765 ) ) ;
#190660=CARTESIAN_POINT ( 'NONE',  ( 13.97604488694548053, -13.89961937509957401, 60.62609039468564731 ) ) ;
#190661=CARTESIAN_POINT ( 'NONE',  ( 0.05219959533937995610, -21.53943276465977519, 45.00109039468568284 ) ) ;
#190662=CARTESIAN_POINT ( 'NONE',  ( -16.53943276465976808, 0.05219959533911058130, 91.24890960531436690 ) ) ;
#190663=CARTESIAN_POINT ( 'NONE',  ( -5.049401038298153566, 19.05341960407611168, 115.2072429386477097 ) ) ;
#190664=CARTESIAN_POINT ( 'NONE',  ( -12.06949235617739369, -12.14591786802326823, 99.37609039468568994 ) ) ;
#190665=CARTESIAN_POINT ( 'NONE',  ( 21.52544592524334988, 5.823673210054432836, 86.45942372801901854 ) ) ;
#190666=CARTESIAN_POINT ( 'NONE',  ( 8.224510206698742110, 14.34966873604972548, 42.08442372801901854 ) ) ;
#190667=CARTESIAN_POINT ( 'NONE',  ( -21.53943276465977519, -0.05219959533937600094, 38.75109039468567573 ) ) ;
#190669=CARTESIAN_POINT ( 'NONE',  ( 15.72974639402199770, -15.80617190586745480, 108.1239096053143811 ) ) ;
#190670=CARTESIAN_POINT ( 'NONE',  ( -8.314922557960811034, -14.29746914071050412, 87.08224293864769550 ) ) ;
#190671=CARTESIAN_POINT ( 'NONE',  ( -19.39720447994795904, -5.499999999999981348, 49.66317477297177163 ) ) ;
#190672=CARTESIAN_POINT ( 'NONE',  ( -16.52544592524342804, 4.483927247898546575, 61.04057627198103120 ) ) ;
#190673=CARTESIAN_POINT ( 'NONE',  ( 12.06949235617739724, 12.14591786802326823, 111.8760903946856615 ) ) ;
#190674=CARTESIAN_POINT ( 'NONE',  ( -13.97604488694527625, -13.89961937509977652, 36.87390960531436690 ) ) ;
#190675=CARTESIAN_POINT ( 'NONE',  ( -21.55341960407610458, -5.719274019375992779, 36.45724293864768839 ) ) ;
#190676=CARTESIAN_POINT ( 'NONE',  ( -14.34966873604960291, -8.224510206698953496, 81.66557627198103830 ) ) ;
#190677=CARTESIAN_POINT ( 'NONE',  ( 5.823673210054125526, 21.52544592524343514, 79.79057627198102409 ) ) ;
#190678=CARTESIAN_POINT ( 'NONE',  ( 16.51473224551069308, 9.474510206698969483, 89.16557627198103830 ) ) ;
#190679=CARTESIAN_POINT ( 'NONE',  ( -9.474510206698964154, 16.51473224551069663, 35.41557627198102409 ) ) ;
#190680=CARTESIAN_POINT ( 'NONE',  ( 19.03943276465977164, 0.05219959533936151252, 91.25109039468566152 ) ) ;
#190681=EDGE_CURVE ( 'NONE', #169831, #132379, #170921, .T. ) ;
#190682=CARTESIAN_POINT ( 'NONE',  ( -15.72974639402197994, 15.80617190586746368, 30.62390960531436335 ) ) ;
#190683=CARTESIAN_POINT ( 'NONE',  ( -5.823673210054431948, 21.52544592524334988, 67.70942372801901854 ) ) ;
#190684=CARTESIAN_POINT ( 'NONE',  ( 9.474510206698971260, -16.51473224551069308, 52.91557627198102409 ) ) ;
#190685=CARTESIAN_POINT ( 'NONE',  ( -5.153800228976328057, -19.02544592524343514, 87.29057627198103830 ) ) ;
#190687=CARTESIAN_POINT ( 'NONE',  ( -0.05219959533934338120, 16.53943276465976808, 62.50109039468568284 ) ) ;
#190688=CARTESIAN_POINT ( 'NONE',  ( 15.80617190586769283, -15.72974639402175789, 45.62609039468567573 ) ) ;
#190689=CARTESIAN_POINT ( 'NONE',  ( -15.80617190586768217, 15.72974639402176855, 73.12609039468567573 ) ) ;
#190690=CARTESIAN_POINT ( 'NONE',  ( -15.80617190586745835, -15.72974639402198527, 21.87390960531436690 ) ) ;
#190691=CARTESIAN_POINT ( 'NONE',  ( -15.72974639402197994, 15.80617190586746368, 85.62390960531436690 ) ) ;
#190692=CARTESIAN_POINT ( 'NONE',  ( 18.62759615963255655, 10.81492255796105972, 26.66775706135235424 ) ) ;
#190693=CARTESIAN_POINT ( 'NONE',  ( 4.379528057220092307, 16.55341960407617563, 62.29275706135236845 ) ) ;
#190694=CARTESIAN_POINT ( 'NONE',  ( -10.72451020669898014, 18.67979575497178502, 60.41557627198102409 ) ) ;
#190695=CARTESIAN_POINT ( 'NONE',  ( 5.153800228976615827, -19.02544592524334988, 20.20942372801899722 ) ) ;
#190696=CARTESIAN_POINT ( 'NONE',  ( 9.474510206698971260, -16.51473224551069308, 62.91557627198102409 ) ) ;
#190697=CARTESIAN_POINT ( 'NONE',  ( -4.483927247898782831, 16.52544592524335698, 107.7094237280190328 ) ) ;
#190698=CARTESIAN_POINT ( 'NONE',  ( -17.50000000000001421, -4.049696124445921086, 105.8196032933405633 ) ) ;
#190699=CARTESIAN_POINT ( 'NONE',  ( -13.89961937509977652, 13.97604488694528158, 85.62390960531433848 ) ) ;
#190700=CARTESIAN_POINT ( 'NONE',  ( 17.50000000000051159, 4.380085919831660846, 103.4503187307105776 ) ) ;
#190701=B_SPLINE_CURVE_WITH_KNOTS ( 'NONE', 3,
 ( #170609, #125099, #32099, #186797, #172598, #171605 ),
 .UNSPECIFIED., .F., .F.,
 ( 4, 2, 4 ),
 ( 0.001769412596444684812, 0.002152742221722617720, 0.002536071847000550411 ),
 .UNSPECIFIED. ) ;
#190702=CARTESIAN_POINT ( 'NONE',  ( -13.97604488694547697, 13.89961937509957934, 88.12609039468563310 ) ) ;
#190703=CARTESIAN_POINT ( 'NONE',  ( -21.52544592524343514, 5.823673210054127303, 56.04057627198102409 ) ) ;
#190704=CARTESIAN_POINT ( 'NONE',  ( -16.53943276465976808, -0.05219959533934237506, 113.7510903946856757 ) ) ;
#190705=CARTESIAN_POINT ( 'NONE',  ( -5.153800228976607833, 19.02544592524334988, 102.7094237280189759 ) ) ;
#190706=CARTESIAN_POINT ( 'NONE',  ( -13.89961937509977830, 13.97604488694528158, 40.62390960531435269 ) ) ;
#190707=CARTESIAN_POINT ( 'NONE',  ( 16.51473224551083163, -9.474510206698727899, 90.83442372801900433 ) ) ;
#190708=CARTESIAN_POINT ( 'NONE',  ( 21.55341960407610458, 5.719274019375980345, 93.95724293864770971 ) ) ;
#190709=CARTESIAN_POINT ( 'NONE',  ( 19.03943276465977164, 0.05219959533936151252, 56.25109039468566863 ) ) ;
#190711=CARTESIAN_POINT ( 'NONE',  ( 19.02544592524343514, -5.153800228976328945, 53.54057627198102409 ) ) ;
#190712=CARTESIAN_POINT ( 'NONE',  ( 4.379528057220339221, -16.55341960407611168, 57.70724293864770260 ) ) ;
#190713=CARTESIAN_POINT ( 'NONE',  ( -16.51473224551069308, -9.474510206698971260, 51.66557627198102409 ) ) ;
#190714=CARTESIAN_POINT ( 'NONE',  ( -16.53943276465976808, 0.05219959533911058130, 56.24890960531436690 ) ) ;
#190717=CARTESIAN_POINT ( 'NONE',  ( 14.34966873604960469, 8.224510206698951720, 29.16557627198103120 ) ) ;
#190718=CARTESIAN_POINT ( 'NONE',  ( 5.049401038298161559, -19.05341960407611168, 67.70724293864769550 ) ) ;
#190719=CARTESIAN_POINT ( 'NONE',  ( -5.153800228976607833, 19.02544592524335343, 72.70942372801900433 ) ) ;
#190720=CARTESIAN_POINT ( 'NONE',  ( -5.049401038297874678, -19.05341960407617918, 39.79275706135232582 ) ) ;
#190721=CARTESIAN_POINT ( 'NONE',  ( 0.05219959533934541429, -16.53943276465976808, 50.00109039468568994 ) ) ;
#190722=CARTESIAN_POINT ( 'NONE',  ( -10.72451020669898014, 18.67979575497178502, 50.41557627198103120 ) ) ;
#190723=CARTESIAN_POINT ( 'NONE',  ( 15.72974639402176855, 15.80617190586768217, 111.8760903946856615 ) ) ;
#190724=CARTESIAN_POINT ( 'NONE',  ( -9.564922557960796823, -16.46253265017161027, 77.08224293864769550 ) ) ;
#190725=CARTESIAN_POINT ( 'NONE',  ( -0.05219959533909027116, -19.03943276465977164, 112.4989096053143669 ) ) ;
#190726=CARTESIAN_POINT ( 'NONE',  ( 9.564922557960805705, 16.46253265017160317, 114.5822429386476955 ) ) ;
#190728=CARTESIAN_POINT ( 'NONE',  ( -21.53943276465977519, -0.05219959533937600094, 18.75109039468568639 ) ) ;
#190729=CARTESIAN_POINT ( 'NONE',  ( 14.29746914071049879, -8.314922557960816363, 93.33224293864769550 ) ) ;
#190730=CARTESIAN_POINT ( 'NONE',  ( 15.80617190586746368, 15.72974639402197994, 94.37390960531436690 ) ) ;
#190731=CARTESIAN_POINT ( 'NONE',  ( 16.46253265017160672, -9.564922557960803928, 83.33224293864768129 ) ) ;
#190732=CARTESIAN_POINT ( 'NONE',  ( 16.51473224551069308, 9.474510206698969483, 89.16557627198103830 ) ) ;
#190733=CARTESIAN_POINT ( 'NONE',  ( -10.72451020669898014, 18.67979575497178502, 110.4155762719810383 ) ) ;
#190735=CARTESIAN_POINT ( 'NONE',  ( 16.51473224551069308, 9.474510206698969483, 74.16557627198103830 ) ) ;
#190736=CARTESIAN_POINT ( 'NONE',  ( 18.87075004821569024, -5.499999999999984013, 96.17408112101044537 ) ) ;
#190737=CARTESIAN_POINT ( 'NONE',  ( 16.51473224551069308, 9.474510206698969483, 29.16557627198103475 ) ) ;
#190738=CARTESIAN_POINT ( 'NONE',  ( -5.049401038298153566, 19.05341960407611168, 40.20724293864768839 ) ) ;
#190739=CARTESIAN_POINT ( 'NONE',  ( -9.474510206698720793, -16.51473224551083518, 99.58442372801900433 ) ) ;
#190740=CARTESIAN_POINT ( 'NONE',  ( 0.05219959533910956823, 16.53943276465976808, 114.9989096053143669 ) ) ;
#190741=CARTESIAN_POINT ( 'NONE',  ( 10.81492255796106328, -18.62759615963255655, 70.41775706135236135 ) ) ;
#190742=CARTESIAN_POINT ( 'NONE',  ( 19.05341960407611168, 5.049401038298154454, 63.95724293864769550 ) ) ;
#190743=CARTESIAN_POINT ( 'NONE',  ( -18.62759615963255300, -10.81492255796106328, 29.16775706135234003 ) ) ;
#190744=CARTESIAN_POINT ( 'NONE',  ( 5.719274019375991003, -21.55341960407610458, 107.7072429386476955 ) ) ;
#190746=CARTESIAN_POINT ( 'NONE',  ( 5.153800228976335163, 19.02544592524342804, 84.79057627198099567 ) ) ;
#190748=CARTESIAN_POINT ( 'NONE',  ( 12.14591786802327356, -12.06949235617739191, 30.62609039468567929 ) ) ;
#190749=CARTESIAN_POINT ( 'NONE',  ( -5.719274019375978568, 21.55341960407610458, 50.20724293864769550 ) ) ;
#190750=CARTESIAN_POINT ( 'NONE',  ( 18.62759615963255655, 10.81492255796105972, 61.66775706135235424 ) ) ;
#190751=CARTESIAN_POINT ( 'NONE',  ( 19.05341960407611168, 5.049401038298154454, 113.9572429386477097 ) ) ;
#190752=CARTESIAN_POINT ( 'NONE',  ( 5.153800228976615827, -19.02544592524334988, 90.20942372801900433 ) ) ;
#190753=CARTESIAN_POINT ( 'NONE',  ( 5.049401038298161559, -19.05341960407611168, 47.70724293864770260 ) ) ;
#190754=CARTESIAN_POINT ( 'NONE',  ( -5.153800228976328057, -19.02544592524343514, 87.29057627198103830 ) ) ;
#190755=CARTESIAN_POINT ( 'NONE',  ( -8.314922557960811034, -14.29746914071050412, 97.08224293864770971 ) ) ;
#190756=CARTESIAN_POINT ( 'NONE',  ( -16.52544592524342804, 4.483927247898546575, 86.04057627198102409 ) ) ;
#190757=CARTESIAN_POINT ( 'NONE',  ( 5.049401038298161559, -19.05341960407611168, 107.7072429386476955 ) ) ;
#190758=CARTESIAN_POINT ( 'NONE',  ( -16.52544592524342804, 4.483927247898546575, 61.04057627198103120 ) ) ;
#190759=CARTESIAN_POINT ( 'NONE',  ( -16.46253265017160317, 9.564922557960807481, 45.83224293864769550 ) ) ;
#190760=CARTESIAN_POINT ( 'NONE',  ( 10.72451020669871369, 18.67979575497193778, 62.08442372801901143 ) ) ;
#190761=CARTESIAN_POINT ( 'NONE',  ( -19.02544592524334988, -5.153800228976617603, 93.95942372801900433 ) ) ;
#190762=CARTESIAN_POINT ( 'NONE',  ( 8.224510206698953496, -14.34966873604960469, 67.91557627198102409 ) ) ;
#190763=CARTESIAN_POINT ( 'NONE',  ( 21.55341960407619695, -5.719274019375665929, 21.04275706135234714 ) ) ;
#190764=CARTESIAN_POINT ( 'NONE',  ( -21.52544592524343514, 5.823673210054127303, 51.04057627198103120 ) ) ;
#190765=CARTESIAN_POINT ( 'NONE',  ( 16.51473224551069308, 9.474510206698969483, 109.1655762719810383 ) ) ;
#190767=CARTESIAN_POINT ( 'NONE',  ( 13.89961937509977652, -13.97604488694527269, 53.12390960531434558 ) ) ;
#190768=CARTESIAN_POINT ( 'NONE',  ( -14.34966873604960291, -8.224510206698953496, 31.66557627198102054 ) ) ;
#190769=CARTESIAN_POINT ( 'NONE',  ( 16.53943276465976808, 0.05219959533934440121, 96.25109039468568994 ) ) ;
#190770=CARTESIAN_POINT ( 'NONE',  ( -16.53943276465976808, -0.05219959533934237506, 78.75109039468568994 ) ) ;
#190771=CARTESIAN_POINT ( 'NONE',  ( -16.51473224551082808, 9.474510206698731452, 43.33442372801900433 ) ) ;
#190772=CARTESIAN_POINT ( 'NONE',  ( -17.44279575226823908, 5.990770900252465836, 70.83557567514318976 ) ) ;
#190773=CARTESIAN_POINT ( 'NONE',  ( 19.03943276465977164, -0.05219959533909143690, 88.74890960531436690 ) ) ;
#190774=CARTESIAN_POINT ( 'NONE',  ( -9.564922557960796823, -16.46253265017161027, 57.08224293864769550 ) ) ;
#190775=CARTESIAN_POINT ( 'NONE',  ( -0.05219959533910754901, -16.53943276465976808, 67.49890960531436690 ) ) ;
#190776=CARTESIAN_POINT ( 'NONE',  ( 5.153800228976335163, 19.02544592524342804, 24.79057627198102765 ) ) ;
#190777=CARTESIAN_POINT ( 'NONE',  ( 15.72974639402199770, -15.80617190586745480, 23.12390960531436335 ) ) ;
#190778=CARTESIAN_POINT ( 'NONE',  ( 5.719274019375991003, -21.55341960407610458, 42.70724293864770260 ) ) ;
#190779=CARTESIAN_POINT ( 'NONE',  ( -8.224510206698948167, 14.34966873604960824, 85.41557627198102409 ) ) ;
#190780=CARTESIAN_POINT ( 'NONE',  ( 16.53943276465976808, 0.05219959533934440121, 41.25109039468568284 ) ) ;
#190782=CARTESIAN_POINT ( 'NONE',  ( -12.06949235617756955, 12.14591786802309770, 75.62390960531439532 ) ) ;
#190784=CARTESIAN_POINT ( 'NONE',  ( -0.05219959533936034679, 19.03943276465977164, 77.50109039468566152 ) ) ;
#190785=CARTESIAN_POINT ( 'NONE',  ( -16.51473224551069308, -9.474510206698971260, 106.6655762719810383 ) ) ;
#190788=CARTESIAN_POINT ( 'NONE',  ( 12.14591786802327356, -12.06949235617739191, 35.62609039468568994 ) ) ;
#190789=CARTESIAN_POINT ( 'NONE',  ( 14.29746914071037800, 8.314922557961029526, 111.6677570613523613 ) ) ;
#190790=CARTESIAN_POINT ( 'NONE',  ( 13.89961937509957401, 13.97604488694547697, 66.87609039468567573 ) ) ;
#190791=CARTESIAN_POINT ( 'NONE',  ( 21.55341960407610458, 5.719274019375980345, 33.95724293864769550 ) ) ;
#190792=CARTESIAN_POINT ( 'NONE',  ( 10.72451020669871369, 18.67979575497193778, 67.08442372801901854 ) ) ;
#190794=CARTESIAN_POINT ( 'NONE',  ( 0.05219959533934541429, -16.53943276465976808, 30.00109039468568284 ) ) ;
#190795=CARTESIAN_POINT ( 'NONE',  ( 19.05341960407611168, 5.049401038298154454, 23.95724293864769194 ) ) ;
#190796=CARTESIAN_POINT ( 'NONE',  ( 19.05341960407611168, 5.049401038298154454, 88.95724293864769550 ) ) ;
#190797=CARTESIAN_POINT ( 'NONE',  ( -16.46253265017160317, 9.564922557960807481, 25.83224293864769194 ) ) ;
#190798=CARTESIAN_POINT ( 'NONE',  ( 8.224510206698953496, -14.34966873604960469, 87.91557627198103830 ) ) ;
#190800=CARTESIAN_POINT ( 'NONE',  ( 5.049401038298161559, -19.05341960407611168, 82.70724293864770971 ) ) ;
#190802=CARTESIAN_POINT ( 'NONE',  ( -5.049401038297874678, -19.05341960407617918, 99.79275706135234714 ) ) ;
#190803=CARTESIAN_POINT ( 'NONE',  ( 15.80617190586746368, 15.72974639402197994, 84.37390960531438111 ) ) ;
#190804=CARTESIAN_POINT ( 'NONE',  ( -19.02544592524342804, 5.153800228976336051, 41.04057627198103120 ) ) ;
#190805=CARTESIAN_POINT ( 'NONE',  ( -19.03943276465977164, -0.05219959533935918106, 63.75109039468566863 ) ) ;
#190806=CARTESIAN_POINT ( 'NONE',  ( 21.53943276465977519, -0.05219959533907433946, 108.7489096053143669 ) ) ;
#190807=CARTESIAN_POINT ( 'NONE',  ( 19.02544592524343514, -5.153800228976328945, 63.54057627198103830 ) ) ;
#190808=CARTESIAN_POINT ( 'NONE',  ( -16.51473224551069308, -9.474510206698971260, 106.6655762719810383 ) ) ;
#190810=CARTESIAN_POINT ( 'NONE',  ( -4.379528057220086978, -16.55341960407618274, 39.79275706135235424 ) ) ;
#190811=CARTESIAN_POINT ( 'NONE',  ( 0.05219959533907565091, 21.53943276465977519, 109.9989096053143527 ) ) ;
#190812=CARTESIAN_POINT ( 'NONE',  ( 4.483927247898545687, 16.52544592524342804, 109.7905762719810383 ) ) ;
#190813=CARTESIAN_POINT ( 'NONE',  ( 16.46253265017160672, -9.564922557960803928, 88.33224293864769550 ) ) ;
#190814=CARTESIAN_POINT ( 'NONE',  ( 9.474510206698729675, 16.51473224551082808, 62.08442372801899722 ) ) ;
#190815=CARTESIAN_POINT ( 'NONE',  ( -5.823673210054116645, -21.52544592524344225, 82.29057627198103830 ) ) ;
#190816=CARTESIAN_POINT ( 'NONE',  ( 12.06949235617757843, -12.14591786802309237, 48.12390960531436690 ) ) ;
#190817=CARTESIAN_POINT ( 'NONE',  ( 10.72451020669871369, 18.67979575497193778, 112.0844237280190185 ) ) ;
#190818=CARTESIAN_POINT ( 'NONE',  ( -16.52544592524335698, -4.483927247898792601, 68.95942372801901854 ) ) ;
#190819=CARTESIAN_POINT ( 'NONE',  ( 16.51473224551069308, 9.474510206698969483, 89.16557627198103830 ) ) ;
#190820=CARTESIAN_POINT ( 'NONE',  ( -13.89961937509977652, 13.97604488694528158, 50.62390960531435979 ) ) ;
#190821=CARTESIAN_POINT ( 'NONE',  ( 18.67979575497194134, -10.72451020669871369, 55.83442372801901854 ) ) ;
#190822=CARTESIAN_POINT ( 'NONE',  ( 0.05219959533937995610, -21.53943276465977519, 65.00109039468568994 ) ) ;
#190823=CARTESIAN_POINT ( 'NONE',  ( -5.049401038298153566, 19.05341960407611168, 65.20724293864765286 ) ) ;
#190824=CARTESIAN_POINT ( 'NONE',  ( 15.72974639402176855, 15.80617190586768217, 31.87609039468567929 ) ) ;
#190825=CARTESIAN_POINT ( 'NONE',  ( -9.564922557961040184, 16.46253265017147172, 67.91775706135233293 ) ) ;
#190826=CARTESIAN_POINT ( 'NONE',  ( 16.51473224551083163, -9.474510206698727899, 70.83442372801900433 ) ) ;
#190827=CARTESIAN_POINT ( 'NONE',  ( 19.05341960407611168, 5.049401038298154454, 38.95724293864767418 ) ) ;
#190828=CARTESIAN_POINT ( 'NONE',  ( 8.314922557961029526, -14.29746914071037800, 90.41775706135236135 ) ) ;
#190829=CARTESIAN_POINT ( 'NONE',  ( -9.564922557960796823, -16.46253265017161027, 47.08224293864769550 ) ) ;
#190830=CARTESIAN_POINT ( 'NONE',  ( -9.564922557960796823, -16.46253265017161027, 22.08224293864768839 ) ) ;
#190831=CARTESIAN_POINT ( 'NONE',  ( 16.46253265017160672, -9.564922557960803928, 98.33224293864769550 ) ) ;
#190832=CARTESIAN_POINT ( 'NONE',  ( -16.46253265017160317, 9.564922557960807481, 40.83224293864769550 ) ) ;
#190833=CARTESIAN_POINT ( 'NONE',  ( 18.67979575497178502, 10.72451020669898547, 84.16557627198103830 ) ) ;
#190834=CARTESIAN_POINT ( 'NONE',  ( 12.06949235617739724, 12.14591786802326823, 61.87609039468568284 ) ) ;
#190835=CARTESIAN_POINT ( 'NONE',  ( -9.564922557961040184, 16.46253265017147172, 27.91775706135232582 ) ) ;
#190836=CARTESIAN_POINT ( 'NONE',  ( 5.049401038298161559, -19.05341960407611168, 57.70724293864769550 ) ) ;
#190837=CARTESIAN_POINT ( 'NONE',  ( -16.52544592524342804, 4.483927247898546575, 41.04057627198103120 ) ) ;
#190838=CARTESIAN_POINT ( 'NONE',  ( 8.224510206698953496, -14.34966873604960469, 82.91557627198103830 ) ) ;
#190839=CARTESIAN_POINT ( 'NONE',  ( 16.51473224551069308, 9.474510206698969483, 94.16557627198103830 ) ) ;
#190840=CARTESIAN_POINT ( 'NONE',  ( -13.89961937509977652, 13.97604488694528158, 75.62390960531438111 ) ) ;
#190841=CARTESIAN_POINT ( 'NONE',  ( 21.52544592524334988, 5.823673210054432836, 31.45942372801901854 ) ) ;
#190842=CARTESIAN_POINT ( 'NONE',  ( 19.02544592524343514, -5.153800228976328945, 93.54057627198102409 ) ) ;
#190843=CARTESIAN_POINT ( 'NONE',  ( 10.72451020669871369, 18.67979575497193778, 102.0844237280190185 ) ) ;
#190844=CARTESIAN_POINT ( 'NONE',  ( -8.314922557961024197, 14.29746914071037800, 72.91775706135234714 ) ) ;
#190845=CARTESIAN_POINT ( 'NONE',  ( 10.72451020669871369, 18.67979575497193778, 22.08442372801901143 ) ) ;
#190846=CARTESIAN_POINT ( 'NONE',  ( 15.80617190586746368, 15.72974639402197994, 94.37390960531436690 ) ) ;
#190847=CARTESIAN_POINT ( 'NONE',  ( 14.34966873604960469, 8.224510206698951720, 44.16557627198103120 ) ) ;
#190848=CARTESIAN_POINT ( 'NONE',  ( 16.51473224551069308, 9.474510206698969483, 44.16557627198103120 ) ) ;
#190849=CARTESIAN_POINT ( 'NONE',  ( 4.483927247898545687, 16.52544592524342804, 74.79057627198105251 ) ) ;
#190850=CARTESIAN_POINT ( 'NONE',  ( -21.53943276465977519, 0.05219959533907696930, 31.24890960531435979 ) ) ;
#190851=CARTESIAN_POINT ( 'NONE',  ( -5.153800228976607833, 19.02544592524334988, 27.70942372801899722 ) ) ;
#190852=CARTESIAN_POINT ( 'NONE',  ( -16.55341960407611168, -4.379528057220339221, 101.4572429386476955 ) ) ;
#190853=CARTESIAN_POINT ( 'NONE',  ( 5.153800228976335163, 19.02544592524342804, 109.7905762719810099 ) ) ;
#190854=ORIENTED_EDGE ( 'NONE', *, *, #109281, .F. ) ;
#190855=CARTESIAN_POINT ( 'NONE',  ( 8.314922557961029526, -14.29746914071037800, 50.41775706135235424 ) ) ;
#190856=CARTESIAN_POINT ( 'NONE',  ( 16.46253265017160672, -9.564922557960803928, 53.33224293864768839 ) ) ;
#190857=CARTESIAN_POINT ( 'NONE',  ( -17.08307644218149690, -6.499664160759800247, 21.28380661205804358 ) ) ;
#190858=CARTESIAN_POINT ( 'NONE',  ( -13.89961937509977652, 13.97604488694528158, 115.6239096053143669 ) ) ;
#190859=CARTESIAN_POINT ( 'NONE',  ( -16.53943276465976808, -0.05219959533934237506, 88.75109039468567573 ) ) ;
#190860=CARTESIAN_POINT ( 'NONE',  ( 13.89961937509957401, 13.97604488694547697, 106.8760903946856757 ) ) ;
#190861=CARTESIAN_POINT ( 'NONE',  ( 18.67979575497194134, -10.72451020669871369, 85.83442372801901854 ) ) ;
#190862=CARTESIAN_POINT ( 'NONE',  ( 13.97604488694527802, 13.89961937509977652, 74.37390960531436690 ) ) ;
#190863=CARTESIAN_POINT ( 'NONE',  ( 5.719274019375991003, -21.55341960407610458, 97.70724293864772392 ) ) ;
#190864=CARTESIAN_POINT ( 'NONE',  ( 0.05219959533934541429, -16.53943276465976808, 55.00109039468568284 ) ) ;
#190865=CARTESIAN_POINT ( 'NONE',  ( 19.02544592524343514, -5.153800228976328945, 23.54057627198102054 ) ) ;
#190866=CARTESIAN_POINT ( 'NONE',  ( 16.55341960407618274, -4.379528057220086978, 21.04275706135234714 ) ) ;
#190868=CARTESIAN_POINT ( 'NONE',  ( -9.474510206698720793, -16.51473224551083518, 84.58442372801900433 ) ) ;
#190869=CARTESIAN_POINT ( 'NONE',  ( 21.53943276465977519, -0.05219959533907433946, 73.74890960531433848 ) ) ;
#190870=CARTESIAN_POINT ( 'NONE',  ( -9.474510206698720793, -16.51473224551083518, 59.58442372801900433 ) ) ;
#190872=CARTESIAN_POINT ( 'NONE',  ( -18.62759615963270932, 10.81492255796079327, 105.8322429386476955 ) ) ;
#190873=CARTESIAN_POINT ( 'NONE',  ( -17.49999999999999645, 5.624438216177591876, 85.81670344914643067 ) ) ;
#190874=CARTESIAN_POINT ( 'NONE',  ( 5.049401038298161559, -19.05341960407611168, 62.70724293864769550 ) ) ;
#190876=CARTESIAN_POINT ( 'NONE',  ( -16.55341960407617563, 4.379528057220093196, 23.54275706135235424 ) ) ;
#190878=CARTESIAN_POINT ( 'NONE',  ( 5.823673210054125526, 21.52544592524343514, 109.7905762719810383 ) ) ;
#190879=CARTESIAN_POINT ( 'NONE',  ( -0.05219959533910754901, -16.53943276465976808, 67.49890960531436690 ) ) ;
#190880=CARTESIAN_POINT ( 'NONE',  ( 19.02544592524343514, -5.153800228976328945, 73.54057627198103830 ) ) ;
#190881=CARTESIAN_POINT ( 'NONE',  ( -18.62759615963255300, -10.81492255796106328, 69.16775706135234714 ) ) ;
#190882=CARTESIAN_POINT ( 'NONE',  ( -4.483927247898782831, 16.52544592524335698, 27.70942372801901854 ) ) ;
#190883=CARTESIAN_POINT ( 'NONE',  ( 5.049401038297881783, 19.05341960407617563, 37.29275706135232582 ) ) ;
#190884=CARTESIAN_POINT ( 'NONE',  ( -10.72451020669870658, -18.67979575497194134, 54.58442372801901143 ) ) ;
#190885=CARTESIAN_POINT ( 'NONE',  ( 21.53943276465977519, -0.05219959533907433946, 113.7489096053143527 ) ) ;
#190886=CARTESIAN_POINT ( 'NONE',  ( -18.67979575497178146, -10.72451020669898902, 56.66557627198103830 ) ) ;
#190887=CARTESIAN_POINT ( 'NONE',  ( 5.049401038297881783, 19.05341960407617563, 107.2927570613523187 ) ) ;
#190888=CARTESIAN_POINT ( 'NONE',  ( -5.049401038298153566, 19.05341960407611168, 50.20724293864770260 ) ) ;
#190889=CARTESIAN_POINT ( 'NONE',  ( -5.049401038297874678, -19.05341960407617918, 69.79275706135233293 ) ) ;
#190890=CARTESIAN_POINT ( 'NONE',  ( -15.80617190586768217, 15.72974639402176855, 88.12609039468570415 ) ) ;
#190891=CARTESIAN_POINT ( 'NONE',  ( -5.153800228976607833, 19.02544592524334988, 47.70942372801900433 ) ) ;
#190892=CARTESIAN_POINT ( 'NONE',  ( 5.049401038298161559, -19.05341960407611168, 32.70724293864768129 ) ) ;
#190893=CARTESIAN_POINT ( 'NONE',  ( 10.81492255796078972, 18.62759615963270932, 59.58224293864770260 ) ) ;
#190894=CARTESIAN_POINT ( 'NONE',  ( -12.14591786802309592, -12.06949235617757132, 51.87390960531437401 ) ) ;
#190896=CARTESIAN_POINT ( 'NONE',  ( -9.474510206698720793, -16.51473224551083518, 29.58442372801900433 ) ) ;
#190897=CARTESIAN_POINT ( 'NONE',  ( 0.05219959533934541429, -16.53943276465976808, 85.00109039468568994 ) ) ;
#190898=CARTESIAN_POINT ( 'NONE',  ( 4.483927247898545687, 16.52544592524342804, 49.79057627198102409 ) ) ;
#190899=CARTESIAN_POINT ( 'NONE',  ( -5.823673210054431948, 21.52544592524334988, 87.70942372801901854 ) ) ;
#190900=CARTESIAN_POINT ( 'NONE',  ( 18.62759615963255655, 10.81492255796105972, 86.66775706135234714 ) ) ;
#190901=CARTESIAN_POINT ( 'NONE',  ( -0.05219959533907301413, -21.53943276465977519, 82.49890960531436690 ) ) ;
#190902=CARTESIAN_POINT ( 'NONE',  ( -13.97604488694527625, -13.89961937509977652, 46.87390960531435979 ) ) ;
#190903=CARTESIAN_POINT ( 'NONE',  ( -21.53943276465977519, -0.05219959533937600094, 53.75109039468568994 ) ) ;
#190904=CARTESIAN_POINT ( 'NONE',  ( 13.97604488694527802, 13.89961937509977652, 34.37390960531436690 ) ) ;
#190905=CARTESIAN_POINT ( 'NONE',  ( 16.51473224551069308, 9.474510206698969483, 49.16557627198102409 ) ) ;
#190906=CARTESIAN_POINT ( 'NONE',  ( -16.55341960407611168, -4.379528057220339221, 101.4572429386476955 ) ) ;
#190907=CARTESIAN_POINT ( 'NONE',  ( -9.564922557960796823, -16.46253265017161027, 92.08224293864769550 ) ) ;
#190908=CARTESIAN_POINT ( 'NONE',  ( -12.14591786802309592, -12.06949235617757132, 56.87390960531436690 ) ) ;
#190909=CARTESIAN_POINT ( 'NONE',  ( 16.52544592524342804, -4.483927247898539470, 113.5405762719810383 ) ) ;
#190910=CARTESIAN_POINT ( 'NONE',  ( 18.67979575497178502, 10.72451020669898547, 89.16557627198102409 ) ) ;
#190911=CARTESIAN_POINT ( 'NONE',  ( -21.53943276465977519, -0.05219959533937600094, 23.75109039468567929 ) ) ;
#190913=CARTESIAN_POINT ( 'NONE',  ( 8.224510206698742110, 14.34966873604972548, 37.08442372801901143 ) ) ;
#190915=CARTESIAN_POINT ( 'NONE',  ( 15.80617190586746368, 15.72974639402197994, 74.37390960531436690 ) ) ;
#190916=CARTESIAN_POINT ( 'NONE',  ( -15.72974639402176322, -15.80617190586768395, 109.3760903946857042 ) ) ;
#190917=CARTESIAN_POINT ( 'NONE',  ( 13.89961937509977652, -13.97604488694527269, 93.12390960531436690 ) ) ;
#190918=CARTESIAN_POINT ( 'NONE',  ( -15.80617190586768217, 15.72974639402176855, 33.12609039468569705 ) ) ;
#190919=CARTESIAN_POINT ( 'NONE',  ( -21.53943276465977519, 0.05219959533907696930, 36.24890960531435979 ) ) ;
#190920=CARTESIAN_POINT ( 'NONE',  ( -16.55341960407617563, 4.379528057220093196, 103.5427570613523613 ) ) ;
#190921=CARTESIAN_POINT ( 'NONE',  ( 5.823673210054444382, -21.52544592524334988, 45.20942372801901854 ) ) ;
#190922=CARTESIAN_POINT ( 'NONE',  ( -10.81492255796105439, 18.62759615963255655, 82.91775706135234714 ) ) ;
#190923=CARTESIAN_POINT ( 'NONE',  ( 10.72451020669871369, 18.67979575497193778, 107.0844237280190043 ) ) ;
#190924=CARTESIAN_POINT ( 'NONE',  ( 8.224510206698742110, 14.34966873604972548, 77.08442372801901854 ) ) ;
#190925=CARTESIAN_POINT ( 'NONE',  ( 18.67979575497194134, -10.72451020669871369, 35.83442372801901143 ) ) ;
#190926=CARTESIAN_POINT ( 'NONE',  ( -19.05341960407611168, -5.049401038298163336, 26.45724293864769550 ) ) ;
#190927=CARTESIAN_POINT ( 'NONE',  ( 21.52544592524334988, 5.823673210054432836, 101.4594237280190185 ) ) ;
#190928=CARTESIAN_POINT ( 'NONE',  ( 19.03943276465977164, -0.05219959533909143690, 108.7489096053143527 ) ) ;
#190929=CARTESIAN_POINT ( 'NONE',  ( 10.81492255796078972, 18.62759615963270932, 109.5822429386476955 ) ) ;
#190931=CARTESIAN_POINT ( 'NONE',  ( 10.81492255796078972, 18.62759615963270932, 64.58224293864769550 ) ) ;
#190932=CARTESIAN_POINT ( 'NONE',  ( -8.224510206698735004, -14.34966873604973081, 49.58442372801901143 ) ) ;
#190933=CARTESIAN_POINT ( 'NONE',  ( -14.29746914071049879, 8.314922557960819915, 55.83224293864770260 ) ) ;
#190935=CARTESIAN_POINT ( 'NONE',  ( -9.564922557961040184, 16.46253265017147172, 82.91775706135233293 ) ) ;
#190936=CARTESIAN_POINT ( 'NONE',  ( -16.81555441253552985, 7.025013491695478507, 105.6368544533425791 ) ) ;
#190937=CARTESIAN_POINT ( 'NONE',  ( -14.34966873604972548, 8.224510206698743886, 23.33442372801901499 ) ) ;
#190938=CARTESIAN_POINT ( 'NONE',  ( 21.55341960407610458, 5.719274019375980345, 103.9572429386476813 ) ) ;
#190939=CARTESIAN_POINT ( 'NONE',  ( -14.34966873604960291, -8.224510206698953496, 71.66557627198100988 ) ) ;
#190940=CARTESIAN_POINT ( 'NONE',  ( -21.55341960407610458, -5.719274019375992779, 21.45724293864769550 ) ) ;
#190941=CARTESIAN_POINT ( 'NONE',  ( -12.14591786802326823, 12.06949235617739902, 38.12609039468567573 ) ) ;
#190942=CARTESIAN_POINT ( 'NONE',  ( -5.153800228976328057, -19.02544592524343514, 52.29057627198100988 ) ) ;
#190943=CARTESIAN_POINT ( 'NONE',  ( 5.823673210054444382, -21.52544592524334988, 30.20942372801902565 ) ) ;
#190944=CARTESIAN_POINT ( 'NONE',  ( 5.153800228976615827, -19.02544592524334988, 100.2094237280190043 ) ) ;
#190945=CARTESIAN_POINT ( 'NONE',  ( -9.564922557960796823, -16.46253265017161027, 112.0822429386476955 ) ) ;
#190946=CARTESIAN_POINT ( 'NONE',  ( 13.97604488694527802, 13.89961937509977652, 89.37390960531436690 ) ) ;
#190947=CARTESIAN_POINT ( 'NONE',  ( 10.81492255796078972, 18.62759615963270932, 89.58224293864768129 ) ) ;
#190948=CARTESIAN_POINT ( 'NONE',  ( 19.03943276465977164, -0.05219959533909143690, 58.74890960531435979 ) ) ;
#190949=DIRECTION ( 'NONE',  ( 0.000000000000000000, 1.000000000000000000, 0.000000000000000000 ) ) ;
#190950=CARTESIAN_POINT ( 'NONE',  ( -14.34966873604960291, -8.224510206698953496, 71.66557627198100988 ) ) ;
#190951=CARTESIAN_POINT ( 'NONE',  ( 16.51473224551069308, 9.474510206698969483, 109.1655762719810383 ) ) ;
#190953=CARTESIAN_POINT ( 'NONE',  ( -16.51473224551082808, 9.474510206698731452, 78.33442372801900433 ) ) ;
#190954=CARTESIAN_POINT ( 'NONE',  ( -21.52544592524343514, 5.823673210054127303, 96.04057627198102409 ) ) ;
#190955=CARTESIAN_POINT ( 'NONE',  ( 0.05219959533936267826, -19.03943276465977164, 45.00109039468566863 ) ) ;
#190956=CARTESIAN_POINT ( 'NONE',  ( -15.80617190586745835, -15.72974639402198527, 21.87390960531436690 ) ) ;
#190957=CARTESIAN_POINT ( 'NONE',  ( 19.49190055781011210, 5.500000000000053291, 68.06116087098781975 ) ) ;
#190958=CARTESIAN_POINT ( 'NONE',  ( -0.05219959533907301413, -21.53943276465977519, 52.49890960531435979 ) ) ;
#190959=CARTESIAN_POINT ( 'NONE',  ( -0.05219959533909027116, -19.03943276465977164, 82.49890960531436690 ) ) ;
#190960=CARTESIAN_POINT ( 'NONE',  ( 15.80617190586769283, -15.72974639402175789, 80.62609039468567573 ) ) ;
#190961=CARTESIAN_POINT ( 'NONE',  ( 16.46253265017160672, -9.564922557960803928, 43.33224293864769550 ) ) ;
#190962=CARTESIAN_POINT ( 'NONE',  ( 4.379528057220339221, -16.55341960407611168, 67.70724293864769550 ) ) ;
#190963=CARTESIAN_POINT ( 'NONE',  ( -0.05219959533934338120, 16.53943276465976808, 22.50109039468567573 ) ) ;
#190964=CARTESIAN_POINT ( 'NONE',  ( 0.05219959533937995610, -21.53943276465977519, 70.00109039468568994 ) ) ;
#190966=CARTESIAN_POINT ( 'NONE',  ( 9.474510206698971260, -16.51473224551069308, 112.9155762719810383 ) ) ;
#190967=CARTESIAN_POINT ( 'NONE',  ( -19.02544592524334988, -5.153800228976617603, 73.95942372801900433 ) ) ;
#190969=CARTESIAN_POINT ( 'NONE',  ( -15.72974639402197994, 15.80617190586746368, 115.6239096053143669 ) ) ;
#190972=CARTESIAN_POINT ( 'NONE',  ( -15.72974639402176322, -15.80617190586768395, 109.3760903946857042 ) ) ;
#190973=CARTESIAN_POINT ( 'NONE',  ( 5.153800228976335163, 19.02544592524342804, 49.79057627198100988 ) ) ;
#190974=CARTESIAN_POINT ( 'NONE',  ( -5.823673210054431948, 21.52544592524334988, 107.7094237280190328 ) ) ;
#190975=CARTESIAN_POINT ( 'NONE',  ( 4.483927247898790824, -16.52544592524335698, 110.2094237280190185 ) ) ;
#190976=CARTESIAN_POINT ( 'NONE',  ( -19.03943276465977164, 0.05219959533909376836, 96.24890960531436690 ) ) ;
#190977=CARTESIAN_POINT ( 'NONE',  ( -21.53943276465977519, -0.05219959533937600094, 78.75109039468568994 ) ) ;
#190979=CARTESIAN_POINT ( 'NONE',  ( -17.50000000000001776, -3.512728167236664145, 34.77190004818887559 ) ) ;
#190980=CARTESIAN_POINT ( 'NONE',  ( 5.823673210054444382, -21.52544592524334988, 80.20942372801901854 ) ) ;
#190981=CARTESIAN_POINT ( 'NONE',  ( -10.72451020669870658, -18.67979575497194134, 99.58442372801900433 ) ) ;
#190983=CARTESIAN_POINT ( 'NONE',  ( 19.02544592524343514, -5.153800228976328945, 88.54057627198102409 ) ) ;
#190984=CARTESIAN_POINT ( 'NONE',  ( -9.564922557961040184, 16.46253265017147172, 22.91775706135233648 ) ) ;
#190985=EDGE_CURVE ( 'NONE', #139245, #110833, #159381, .T. ) ;
#190987=CARTESIAN_POINT ( 'NONE',  ( 5.049401038298161559, -19.05341960407611168, 42.70724293864767418 ) ) ;
#190988=CARTESIAN_POINT ( 'NONE',  ( -0.05219959533907301413, -21.53943276465977519, 57.49890960531435979 ) ) ;
#190989=CARTESIAN_POINT ( 'NONE',  ( -4.379528057220086978, -16.55341960407618274, 109.7927570613523613 ) ) ;
#190990=CARTESIAN_POINT ( 'NONE',  ( -16.52544592524342804, 4.483927247898546575, 96.04057627198102409 ) ) ;
#190991=CARTESIAN_POINT ( 'NONE',  ( 0.05219959533909260263, 19.03943276465977164, 79.99890960531436690 ) ) ;
#190992=CARTESIAN_POINT ( 'NONE',  ( -21.55341960407619339, 5.719274019375674811, 98.54275706135234714 ) ) ;
#190993=CARTESIAN_POINT ( 'NONE',  ( 19.05341960407611168, 5.049401038298154454, 33.95724293864769550 ) ) ;
#190994=CARTESIAN_POINT ( 'NONE',  ( -16.52544592524342804, 4.483927247898546575, 106.0405762719810525 ) ) ;
#190995=CARTESIAN_POINT ( 'NONE',  ( 21.55341960407619695, -5.719274019375665929, 51.04275706135234714 ) ) ;
#190996=CARTESIAN_POINT ( 'NONE',  ( -5.823673210054116645, -21.52544592524344225, 82.29057627198103830 ) ) ;
#190997=CARTESIAN_POINT ( 'NONE',  ( -13.97604488694547697, 13.89961937509957934, 48.12609039468566863 ) ) ;
#190999=CARTESIAN_POINT ( 'NONE',  ( -5.153800228976328057, -19.02544592524343514, 97.29057627198099567 ) ) ;
#191000=CARTESIAN_POINT ( 'NONE',  ( 16.52544592524342804, -4.483927247898539470, 73.54057627198102409 ) ) ;
#191001=CARTESIAN_POINT ( 'NONE',  ( -19.03943276465977164, -0.05219959533935918106, 48.75109039468566863 ) ) ;
#191002=CARTESIAN_POINT ( 'NONE',  ( -9.564922557960796823, -16.46253265017161027, 62.08224293864769550 ) ) ;
#191003=CARTESIAN_POINT ( 'NONE',  ( -16.55341960407611168, -4.379528057220339221, 46.45724293864769550 ) ) ;
#191004=CARTESIAN_POINT ( 'NONE',  ( 13.97604488694548053, -13.89961937509957401, 75.62609039468564731 ) ) ;
#191006=CARTESIAN_POINT ( 'NONE',  ( 5.719274019375991003, -21.55341960407610458, 42.70724293864770260 ) ) ;
#191007=CARTESIAN_POINT ( 'NONE',  ( -16.55341960407611168, -4.379528057220339221, 106.4572429386477097 ) ) ;
#191009=CARTESIAN_POINT ( 'NONE',  ( -0.05219959533909027116, -19.03943276465977164, 62.49890960531435979 ) ) ;
#191010=CARTESIAN_POINT ( 'NONE',  ( -21.55341960407610458, -5.719274019375992779, 66.45724293864768129 ) ) ;
#191011=CARTESIAN_POINT ( 'NONE',  ( -19.03943276465977164, 0.05219959533909376836, 26.24890960531435624 ) ) ;
#191012=CARTESIAN_POINT ( 'NONE',  ( 14.29746914071037800, 8.314922557961029526, 81.66775706135236135 ) ) ;
#191013=CARTESIAN_POINT ( 'NONE',  ( -5.049401038298153566, 19.05341960407611168, 65.20724293864765286 ) ) ;
#191014=CARTESIAN_POINT ( 'NONE',  ( -9.564922557961040184, 16.46253265017147172, 57.91775706135233293 ) ) ;
#191016=CARTESIAN_POINT ( 'NONE',  ( 5.719274019375673035, 21.55341960407619339, 62.29275706135236845 ) ) ;
#191017=CARTESIAN_POINT ( 'NONE',  ( -15.72974639402197994, 15.80617190586746368, 50.62390960531435979 ) ) ;
#191018=CARTESIAN_POINT ( 'NONE',  ( -19.03943276465977164, 0.05219959533909376836, 21.24890960531436335 ) ) ;
#191019=CARTESIAN_POINT ( 'NONE',  ( 16.55341960407618274, -4.379528057220086978, 91.04275706135236135 ) ) ;
#191020=CARTESIAN_POINT ( 'NONE',  ( -13.89961937509957401, -13.97604488694547875, 99.37609039468567573 ) ) ;
#191021=CARTESIAN_POINT ( 'NONE',  ( 19.05341960407611168, 5.049401038298154454, 23.95724293864769194 ) ) ;
#191022=CARTESIAN_POINT ( 'NONE',  ( 16.88567814943165502, 6.947325034625595919, 53.79001122652586986 ) ) ;
#191023=CARTESIAN_POINT ( 'NONE',  ( -0.05219959533907301413, -21.53943276465977519, 67.49890960531436690 ) ) ;
#191024=CARTESIAN_POINT ( 'NONE',  ( -21.55341960407619339, 5.719274019375674811, 88.54275706135236135 ) ) ;
#191025=CARTESIAN_POINT ( 'NONE',  ( -8.314922557960811034, -14.29746914071050412, 47.08224293864770260 ) ) ;
#191026=CARTESIAN_POINT ( 'NONE',  ( -8.224510206698948167, 14.34966873604960824, 50.41557627198103120 ) ) ;
#191027=CARTESIAN_POINT ( 'NONE',  ( -21.55341960407610458, -5.719274019375992779, 81.45724293864769550 ) ) ;
#191028=CARTESIAN_POINT ( 'NONE',  ( 5.823673210054125526, 21.52544592524343514, 94.79057627198105251 ) ) ;
#191030=CARTESIAN_POINT ( 'NONE',  ( -5.823673210054116645, -21.52544592524344225, 37.29057627198102409 ) ) ;
#191031=CARTESIAN_POINT ( 'NONE',  ( 16.53943276465976808, 0.05219959533934440121, 66.25109039468567573 ) ) ;
#191032=CARTESIAN_POINT ( 'NONE',  ( 16.53943276465976808, -0.05219959533910856209, 83.74890960531435269 ) ) ;
#191033=CARTESIAN_POINT ( 'NONE',  ( -9.474510206698964154, 16.51473224551069663, 35.41557627198102409 ) ) ;
#191037=CARTESIAN_POINT ( 'NONE',  ( 12.06949235617739724, 12.14591786802326823, 91.87609039468568994 ) ) ;
#191038=CARTESIAN_POINT ( 'NONE',  ( -15.80617190586745835, -15.72974639402198527, 111.8739096053143669 ) ) ;
#191039=CARTESIAN_POINT ( 'NONE',  ( -5.153800228976328057, -19.02544592524343514, 77.29057627198099567 ) ) ;
#191040=CARTESIAN_POINT ( 'NONE',  ( 10.72451020669871369, 18.67979575497193778, 57.08442372801901854 ) ) ;
#191041=CARTESIAN_POINT ( 'NONE',  ( -5.153800228976328057, -19.02544592524343514, 112.2905762719810099 ) ) ;
#191044=CARTESIAN_POINT ( 'NONE',  ( -0.05219959533937732626, 21.53943276465977519, 47.50109039468568994 ) ) ;
#191045=CARTESIAN_POINT ( 'NONE',  ( -0.05219959533909027116, -19.03943276465977164, 37.49890960531436690 ) ) ;
#191046=CARTESIAN_POINT ( 'NONE',  ( -19.02544592524342804, 5.153800228976336051, 101.0405762719810241 ) ) ;
#191047=CARTESIAN_POINT ( 'NONE',  ( 19.03943276465977164, 0.05219959533936151252, 51.25109039468567573 ) ) ;
#191048=CARTESIAN_POINT ( 'NONE',  ( -21.52544592524334988, -5.823673210054445271, 33.95942372801901143 ) ) ;
#191049=CARTESIAN_POINT ( 'NONE',  ( 9.564922557961047289, -16.46253265017146816, 50.41775706135233293 ) ) ;
#191050=CARTESIAN_POINT ( 'NONE',  ( -9.474510206698964154, 16.51473224551069663, 30.41557627198102054 ) ) ;
#191051=CARTESIAN_POINT ( 'NONE',  ( -16.52544592524335698, -4.483927247898792601, 88.95942372801901854 ) ) ;
#191052=CARTESIAN_POINT ( 'NONE',  ( -5.153800228976607833, 19.02544592524334988, 57.70942372801899012 ) ) ;
#191053=CARTESIAN_POINT ( 'NONE',  ( 16.52544592524335698, 4.483927247898782831, 101.4594237280190185 ) ) ;
#191054=CARTESIAN_POINT ( 'NONE',  ( 17.50000000000000000, 5.499999999999992895, 86.70309617465828467 ) ) ;
#191056=CARTESIAN_POINT ( 'NONE',  ( 9.564922557960805705, 16.46253265017160317, 79.58224293864769550 ) ) ;
#191057=CARTESIAN_POINT ( 'NONE',  ( 21.52544592524334988, 5.823673210054432836, 96.45942372801901854 ) ) ;
#191058=CARTESIAN_POINT ( 'NONE',  ( -0.05219959533937732626, 21.53943276465977519, 102.5010903946856899 ) ) ;
#191059=CARTESIAN_POINT ( 'NONE',  ( 17.72560187377284535, 5.500000000000042633, 66.57814504131322053 ) ) ;
#191060=CARTESIAN_POINT ( 'NONE',  ( 16.51473224551069308, 9.474510206698969483, 99.16557627198102409 ) ) ;
#191061=CARTESIAN_POINT ( 'NONE',  ( 18.67979575497194134, -10.72451020669871369, 75.83442372801900433 ) ) ;
#191062=CARTESIAN_POINT ( 'NONE',  ( 0.05219959533934541429, -16.53943276465976808, 20.00109039468568639 ) ) ;
#191063=CARTESIAN_POINT ( 'NONE',  ( -9.564922557960796823, -16.46253265017161027, 82.08224293864768129 ) ) ;
#191064=CARTESIAN_POINT ( 'NONE',  ( -21.53943276465977519, 0.05219959533907696930, 31.24890960531435979 ) ) ;
#191065=CARTESIAN_POINT ( 'NONE',  ( -5.153800228976328057, -19.02544592524343514, 97.29057627198099567 ) ) ;
#191067=CARTESIAN_POINT ( 'NONE',  ( 5.049401038298161559, -19.05341960407611168, 82.70724293864770971 ) ) ;
#191068=CARTESIAN_POINT ( 'NONE',  ( -9.564922557960796823, -16.46253265017161027, 72.08224293864770971 ) ) ;
#191069=CARTESIAN_POINT ( 'NONE',  ( 4.379528057220092307, 16.55341960407617563, 102.2927570613523613 ) ) ;
#191070=CARTESIAN_POINT ( 'NONE',  ( -17.50000000000001421, 5.622605283950837141, 98.68792689403895224 ) ) ;
#191071=CARTESIAN_POINT ( 'NONE',  ( 16.51473224551083163, -9.474510206698727899, 70.83442372801900433 ) ) ;
#191072=CARTESIAN_POINT ( 'NONE',  ( 13.97604488694527802, 13.89961937509977652, 89.37390960531436690 ) ) ;
#191073=CARTESIAN_POINT ( 'NONE',  ( -4.483927247898539470, -16.52544592524342804, 82.29057627198103830 ) ) ;
#191074=CARTESIAN_POINT ( 'NONE',  ( 5.823673210054125526, 21.52544592524343514, 49.79057627198102409 ) ) ;
#191075=CARTESIAN_POINT ( 'NONE',  ( 15.72974639402199770, -15.80617190586745480, 23.12390960531436335 ) ) ;
#191076=CARTESIAN_POINT ( 'NONE',  ( -8.224510206698948167, 14.34966873604960824, 105.4155762719810383 ) ) ;
#191078=CARTESIAN_POINT ( 'NONE',  ( -5.153800228976607833, 19.02544592524334988, 37.70942372801899722 ) ) ;
#191079=CARTESIAN_POINT ( 'NONE',  ( 12.06949235617757843, -12.14591786802309237, 23.12390960531436335 ) ) ;
#191080=CARTESIAN_POINT ( 'NONE',  ( 9.474510206698971260, -16.51473224551069308, 102.9155762719810241 ) ) ;
#191081=CARTESIAN_POINT ( 'NONE',  ( -0.05219959533937732626, 21.53943276465977519, 62.50109039468568284 ) ) ;
#191082=CARTESIAN_POINT ( 'NONE',  ( 18.67979575497178502, 10.72451020669898547, 54.16557627198103120 ) ) ;
#191083=CARTESIAN_POINT ( 'NONE',  ( 21.55341960407619695, -5.719274019375665929, 31.04275706135234714 ) ) ;
#191084=CARTESIAN_POINT ( 'NONE',  ( -0.05219959533907301413, -21.53943276465977519, 87.49890960531436690 ) ) ;
#191085=CARTESIAN_POINT ( 'NONE',  ( 0.05219959533937995610, -21.53943276465977519, 40.00109039468567573 ) ) ;
#191086=CARTESIAN_POINT ( 'NONE',  ( -8.314922557960811034, -14.29746914071050412, 112.0822429386477097 ) ) ;
#191087=CARTESIAN_POINT ( 'NONE',  ( 5.153800228976615827, -19.02544592524334988, 65.20942372801900433 ) ) ;
#191088=CARTESIAN_POINT ( 'NONE',  ( 19.05341960407611168, 5.049401038298154454, 43.95724293864769550 ) ) ;
#191089=CARTESIAN_POINT ( 'NONE',  ( 4.379528057220339221, -16.55341960407611168, 97.70724293864772392 ) ) ;
#191090=CARTESIAN_POINT ( 'NONE',  ( -13.89961937509977652, 13.97604488694528158, 110.6239096053143243 ) ) ;
#191091=CARTESIAN_POINT ( 'NONE',  ( -19.02544592524342804, 5.153800228976336051, 26.04057627198103120 ) ) ;
#191092=CARTESIAN_POINT ( 'NONE',  ( -8.314922557960811034, -14.29746914071050412, 47.08224293864770260 ) ) ;
#191093=CARTESIAN_POINT ( 'NONE',  ( 12.06949235617739724, 12.14591786802326823, 106.8760903946856899 ) ) ;
#191094=CARTESIAN_POINT ( 'NONE',  ( 19.03943276465977164, -0.05219959533909143690, 58.74890960531435979 ) ) ;
#191095=CARTESIAN_POINT ( 'NONE',  ( 9.564922557960805705, 16.46253265017160317, 24.58224293864769194 ) ) ;
#191096=CARTESIAN_POINT ( 'NONE',  ( 13.97604488694548053, -13.89961937509957401, 20.62609039468567573 ) ) ;
#191097=CARTESIAN_POINT ( 'NONE',  ( -19.05341960407611168, -5.049401038298163336, 111.4572429386476671 ) ) ;
#191098=CARTESIAN_POINT ( 'NONE',  ( -0.05219959533910754901, -16.53943276465976808, 37.49890960531436690 ) ) ;
#191099=CARTESIAN_POINT ( 'NONE',  ( -18.62759615963255300, -10.81492255796106328, 44.16775706135234714 ) ) ;
#191102=CARTESIAN_POINT ( 'NONE',  ( -16.53943276465976808, -0.05219959533934237506, 53.75109039468568994 ) ) ;
#191103=CARTESIAN_POINT ( 'NONE',  ( -0.05219959533910754901, -16.53943276465976808, 22.49890960531436335 ) ) ;
#191104=CARTESIAN_POINT ( 'NONE',  ( 8.224510206698742110, 14.34966873604972548, 112.0844237280190185 ) ) ;
#191105=CARTESIAN_POINT ( 'NONE',  ( -14.29746914071037622, -8.314922557961029526, 29.16775706135234003 ) ) ;
#191106=CARTESIAN_POINT ( 'NONE',  ( -16.46253265017160317, 9.564922557960807481, 50.83224293864770260 ) ) ;
#191107=CARTESIAN_POINT ( 'NONE',  ( 0.05219959533910956823, 16.53943276465976808, 104.9989096053143669 ) ) ;
#191108=CARTESIAN_POINT ( 'NONE',  ( 5.823673210054444382, -21.52544592524334988, 25.20942372801901854 ) ) ;
#191109=CARTESIAN_POINT ( 'NONE',  ( 9.564922557960805705, 16.46253265017160317, 39.58224293864768839 ) ) ;
#191112=CARTESIAN_POINT ( 'NONE',  ( -0.05219959533909027116, -19.03943276465977164, 27.49890960531435624 ) ) ;
#191113=CARTESIAN_POINT ( 'NONE',  ( -5.823673210054116645, -21.52544592524344225, 22.29057627198102765 ) ) ;
#191115=CARTESIAN_POINT ( 'NONE',  ( -19.03943276465977164, 0.05219959533909376836, 96.24890960531436690 ) ) ;
#191116=CARTESIAN_POINT ( 'NONE',  ( -18.67979575497193778, 10.72451020669871902, 48.33442372801902565 ) ) ;
#191117=CARTESIAN_POINT ( 'NONE',  ( 16.53943276465976808, -0.05219959533910856209, 98.74890960531438111 ) ) ;
#191118=CARTESIAN_POINT ( 'NONE',  ( 19.03943276465977164, -0.05219959533909143690, 103.7489096053143669 ) ) ;
#191120=CARTESIAN_POINT ( 'NONE',  ( -8.224510206698735004, -14.34966873604973081, 74.58442372801901854 ) ) ;
#191121=CARTESIAN_POINT ( 'NONE',  ( 5.823673210054444382, -21.52544592524334988, 95.20942372801903275 ) ) ;
#191122=CARTESIAN_POINT ( 'NONE',  ( 4.483927247898790824, -16.52544592524335698, 60.20942372801902565 ) ) ;
#191123=CARTESIAN_POINT ( 'NONE',  ( 5.049401038298161559, -19.05341960407611168, 97.70724293864766707 ) ) ;
#191124=CARTESIAN_POINT ( 'NONE',  ( -16.52544592524335698, -4.483927247898792601, 43.95942372801902565 ) ) ;
#191125=CARTESIAN_POINT ( 'NONE',  ( 5.153800228976615827, -19.02544592524334988, 110.2094237280189901 ) ) ;
#191126=CARTESIAN_POINT ( 'NONE',  ( -8.314922557961024197, 14.29746914071037800, 77.91775706135231871 ) ) ;
#191127=CARTESIAN_POINT ( 'NONE',  ( 19.05341960407617918, -5.049401038297876454, 111.0427570613523329 ) ) ;
#191128=CARTESIAN_POINT ( 'NONE',  ( 16.46253265017160672, -9.564922557960803928, 78.33224293864769550 ) ) ;
#191129=CARTESIAN_POINT ( 'NONE',  ( -21.52544592524343514, 5.823673210054127303, 91.04057627198103830 ) ) ;
#191130=CARTESIAN_POINT ( 'NONE',  ( -16.53943276465976808, 0.05219959533911058130, 106.2489096053143811 ) ) ;
#191131=CARTESIAN_POINT ( 'NONE',  ( 5.049401038297881783, 19.05341960407617563, 102.2927570613523045 ) ) ;
#191132=CARTESIAN_POINT ( 'NONE',  ( -8.224510206698735004, -14.34966873604973081, 74.58442372801901854 ) ) ;
#191134=CARTESIAN_POINT ( 'NONE',  ( 9.474510206698729675, 16.51473224551082808, 67.08442372801900433 ) ) ;
#191136=CARTESIAN_POINT ( 'NONE',  ( 14.29746914071049879, -8.314922557960816363, 38.33224293864768839 ) ) ;
#191137=CARTESIAN_POINT ( 'NONE',  ( -4.483927247898539470, -16.52544592524342804, 92.29057627198103830 ) ) ;
#191138=CARTESIAN_POINT ( 'NONE',  ( -19.02544592524334988, -5.153800228976617603, 33.95942372801897591 ) ) ;
#191139=CARTESIAN_POINT ( 'NONE',  ( -17.44270441346519362, 5.991230190322972327, 88.63664920735774899 ) ) ;
#191140=CARTESIAN_POINT ( 'NONE',  ( 10.72451020669871369, 18.67979575497193778, 32.08442372801901854 ) ) ;
#191141=CARTESIAN_POINT ( 'NONE',  ( 13.97604488694548053, -13.89961937509957401, 95.62609039468563310 ) ) ;
#191143=CARTESIAN_POINT ( 'NONE',  ( -13.97604488694527625, -13.89961937509977652, 96.87390960531433848 ) ) ;
#191144=CARTESIAN_POINT ( 'NONE',  ( -15.80617190586768217, 15.72974639402176855, 103.1260903946856757 ) ) ;
#191145=CARTESIAN_POINT ( 'NONE',  ( -5.153800228976328057, -19.02544592524343514, 77.29057627198099567 ) ) ;
#191146=CARTESIAN_POINT ( 'NONE',  ( 18.62759615963271287, -10.81492255796078972, 38.33224293864768839 ) ) ;
#191147=CARTESIAN_POINT ( 'NONE',  ( -8.314922557960811034, -14.29746914071050412, 92.08224293864769550 ) ) ;
#191148=CARTESIAN_POINT ( 'NONE',  ( -9.564922557960796823, -16.46253265017161027, 52.08224293864768839 ) ) ;
#191149=CARTESIAN_POINT ( 'NONE',  ( 4.379528057220339221, -16.55341960407611168, 107.7072429386476955 ) ) ;
#191150=CARTESIAN_POINT ( 'NONE',  ( 0.05219959533937995610, -21.53943276465977519, 20.00109039468568639 ) ) ;
#191151=CARTESIAN_POINT ( 'NONE',  ( -5.719274019375665041, -21.55341960407619695, 79.79275706135236135 ) ) ;
#191152=CARTESIAN_POINT ( 'NONE',  ( 0.05219959533909260263, 19.03943276465977164, 49.99890960531435979 ) ) ;
#191153=CARTESIAN_POINT ( 'NONE',  ( -14.29746914071037622, -8.314922557961029526, 74.16775706135231871 ) ) ;
#191154=CARTESIAN_POINT ( 'NONE',  ( -0.05219959533907301413, -21.53943276465977519, 112.4989096053143669 ) ) ;
#191156=CARTESIAN_POINT ( 'NONE',  ( -18.67979575497193778, 10.72451020669871902, 28.33442372801902209 ) ) ;
#191157=CARTESIAN_POINT ( 'NONE',  ( -5.153800228976607833, 19.02544592524334988, 52.70942372801900433 ) ) ;
#191158=CARTESIAN_POINT ( 'NONE',  ( 13.97604488694527802, 13.89961937509977652, 59.37390960531434558 ) ) ;
#191159=CARTESIAN_POINT ( 'NONE',  ( 19.05341960407617918, -5.049401038297876454, 36.04275706135234003 ) ) ;
#191160=CARTESIAN_POINT ( 'NONE',  ( -5.823673210054431948, 21.52544592524334988, 72.70942372801901854 ) ) ;
#191161=CARTESIAN_POINT ( 'NONE',  ( -18.67979575497178146, -10.72451020669898902, 71.66557627198100988 ) ) ;
#191162=CARTESIAN_POINT ( 'NONE',  ( -16.52544592524342804, 4.483927247898546575, 56.04057627198102409 ) ) ;
#191163=CARTESIAN_POINT ( 'NONE',  ( 21.55341960407619695, -5.719274019375665929, 86.04275706135236135 ) ) ;
#191164=CARTESIAN_POINT ( 'NONE',  ( -16.46253265017146816, -9.564922557961047289, 29.16775706135232937 ) ) ;
#191165=CARTESIAN_POINT ( 'NONE',  ( -0.05219959533910754901, -16.53943276465976808, 67.49890960531436690 ) ) ;
#191166=CARTESIAN_POINT ( 'NONE',  ( 0.05219959533909260263, 19.03943276465977164, 24.99890960531435269 ) ) ;
#191167=CARTESIAN_POINT ( 'NONE',  ( -13.97604488694547697, 13.89961937509957934, 58.12609039468566863 ) ) ;
#191168=CARTESIAN_POINT ( 'NONE',  ( 4.483927247898790824, -16.52544592524335698, 110.2094237280190185 ) ) ;
#191169=CARTESIAN_POINT ( 'NONE',  ( 5.823673210054444382, -21.52544592524334988, 85.20942372801901854 ) ) ;
#191170=CARTESIAN_POINT ( 'NONE',  ( -16.51473224551082808, 9.474510206698731452, 53.33442372801900433 ) ) ;
#191171=CARTESIAN_POINT ( 'NONE',  ( -10.72451020669898014, 18.67979575497178502, 50.41557627198103120 ) ) ;
#191172=CARTESIAN_POINT ( 'NONE',  ( -10.72451020669870658, -18.67979575497194134, 39.58442372801901143 ) ) ;
#191173=CARTESIAN_POINT ( 'NONE',  ( 10.81492255796078972, 18.62759615963270932, 99.58224293864770971 ) ) ;
#191174=CARTESIAN_POINT ( 'NONE',  ( 5.049401038297881783, 19.05341960407617563, 92.29275706135234714 ) ) ;
#191175=CARTESIAN_POINT ( 'NONE',  ( 4.379528057220092307, 16.55341960407617563, 67.29275706135234714 ) ) ;
#191177=CARTESIAN_POINT ( 'NONE',  ( -21.53943276465977519, 0.05219959533907696930, 106.2489096053143811 ) ) ;
#191178=CARTESIAN_POINT ( 'NONE',  ( -8.224510206698948167, 14.34966873604960824, 90.41557627198103830 ) ) ;
#191179=CARTESIAN_POINT ( 'NONE',  ( -17.40805194822030444, -6.112264579159341515, 99.16628727489390371 ) ) ;
#191180=CARTESIAN_POINT ( 'NONE',  ( 8.314922557961029526, -14.29746914071037800, 40.41775706135234714 ) ) ;
#191181=CARTESIAN_POINT ( 'NONE',  ( -5.823673210054116645, -21.52544592524344225, 52.29057627198102409 ) ) ;
#191182=CARTESIAN_POINT ( 'NONE',  ( 8.224510206698742110, 14.34966873604972548, 92.08442372801901854 ) ) ;
#191183=CARTESIAN_POINT ( 'NONE',  ( -19.05341960407611168, -5.049401038298163336, 21.45724293864768839 ) ) ;
#191184=CARTESIAN_POINT ( 'NONE',  ( 12.14591786802327356, -12.06949235617739191, 65.62609039468568994 ) ) ;
#191185=CARTESIAN_POINT ( 'NONE',  ( -15.80617190586768217, 15.72974639402176855, 43.12609039468568284 ) ) ;
#191186=CARTESIAN_POINT ( 'NONE',  ( 21.52544592524344225, -5.823673210054117533, 58.54057627198103120 ) ) ;
#191187=CARTESIAN_POINT ( 'NONE',  ( -16.55341960407617563, 4.379528057220093196, 78.54275706135236135 ) ) ;
#191188=CARTESIAN_POINT ( 'NONE',  ( 21.55341960407619695, -5.719274019375665929, 71.04275706135234714 ) ) ;
#191189=CARTESIAN_POINT ( 'NONE',  ( -0.05219959533907301413, -21.53943276465977519, 52.49890960531435979 ) ) ;
#191190=CARTESIAN_POINT ( 'NONE',  ( -21.55341960407610458, -5.719274019375992779, 36.45724293864768839 ) ) ;
#191191=ORIENTED_EDGE ( 'NONE', *, *, #193397, .F. ) ;
#191192=CARTESIAN_POINT ( 'NONE',  ( 4.483927247898790824, -16.52544592524335698, 70.20942372801904696 ) ) ;
#191193=CARTESIAN_POINT ( 'NONE',  ( 15.80617190586746368, 15.72974639402197994, 34.37390960531435979 ) ) ;
#191194=ORIENTED_EDGE ( 'NONE', *, *, #82217, .F. ) ;
#191195=CARTESIAN_POINT ( 'NONE',  ( -13.89961937509977652, 13.97604488694528158, 105.6239096053143527 ) ) ;
#191196=CARTESIAN_POINT ( 'NONE',  ( 16.52544592524342804, -4.483927247898539470, 23.54057627198102765 ) ) ;
#191198=CARTESIAN_POINT ( 'NONE',  ( -14.29746914071049879, 8.314922557960819915, 110.8322429386476955 ) ) ;
#191199=CARTESIAN_POINT ( 'NONE',  ( -21.53943276465977519, 0.05219959533907696930, 51.24890960531436690 ) ) ;
#191200=CARTESIAN_POINT ( 'NONE',  ( -9.564922557960796823, -16.46253265017161027, 42.08224293864769550 ) ) ;
#191201=CARTESIAN_POINT ( 'NONE',  ( 0.05219959533934541429, -16.53943276465976808, 95.00109039468568994 ) ) ;
#191202=CARTESIAN_POINT ( 'NONE',  ( -15.72974639402176322, -15.80617190586768395, 39.37609039468567573 ) ) ;
#191203=CARTESIAN_POINT ( 'NONE',  ( -5.049401038297874678, -19.05341960407617918, 84.79275706135233293 ) ) ;
#191204=CARTESIAN_POINT ( 'NONE',  ( -14.29746914071049879, 8.314922557960819915, 100.8322429386477097 ) ) ;
#191205=CARTESIAN_POINT ( 'NONE',  ( -9.564922557960796823, -16.46253265017161027, 57.08224293864769550 ) ) ;
#191207=PLANE ( 'NONE',  #96397 ) ;
#191208=CARTESIAN_POINT ( 'NONE',  ( -5.049401038298153566, 19.05341960407611168, 75.20724293864769550 ) ) ;
#191209=CARTESIAN_POINT ( 'NONE',  ( 8.314922557961029526, -14.29746914071037800, 60.41775706135235424 ) ) ;
#191210=CARTESIAN_POINT ( 'NONE',  ( -18.62759615963255300, -10.81492255796106328, 104.1677570613523471 ) ) ;
#191211=CARTESIAN_POINT ( 'NONE',  ( 0.05219959533907565091, 21.53943276465977519, 54.99890960531435269 ) ) ;
#191212=CARTESIAN_POINT ( 'NONE',  ( 0.05219959533934541429, -16.53943276465976808, 70.00109039468568994 ) ) ;
#191213=CARTESIAN_POINT ( 'NONE',  ( -13.97604488694547697, 13.89961937509957934, 63.12609039468566152 ) ) ;
#191215=CARTESIAN_POINT ( 'NONE',  ( -21.52544592524334988, -5.823673210054445271, 58.95942372801902565 ) ) ;
#191216=CARTESIAN_POINT ( 'NONE',  ( -19.03943276465977164, 0.05219959533909376836, 71.24890960531435269 ) ) ;
#191217=CARTESIAN_POINT ( 'NONE',  ( -9.474510206698964154, 16.51473224551069663, 40.41557627198103120 ) ) ;
#191218=CARTESIAN_POINT ( 'NONE',  ( -9.474510206698720793, -16.51473224551083518, 59.58442372801900433 ) ) ;
#191219=CARTESIAN_POINT ( 'NONE',  ( -17.49999999999999645, 5.499999999999997335, 120.0000000000000142 ) ) ;
#191220=CARTESIAN_POINT ( 'NONE',  ( 5.049401038298161559, -19.05341960407611168, 92.70724293864769550 ) ) ;
#191221=CARTESIAN_POINT ( 'NONE',  ( -0.05219959533910754901, -16.53943276465976808, 52.49890960531435979 ) ) ;
#191222=CARTESIAN_POINT ( 'NONE',  ( 15.72974639402199770, -15.80617190586745480, 43.12390960531435269 ) ) ;
#191223=CARTESIAN_POINT ( 'NONE',  ( -17.50000000000147793, 3.254303733634563933, 105.0239589307140307 ) ) ;
#191224=CARTESIAN_POINT ( 'NONE',  ( -19.05341960407617563, 5.049401038297882671, 28.54275706135232937 ) ) ;
#191226=CARTESIAN_POINT ( 'NONE',  ( -19.02544592524342804, 5.153800228976336051, 51.04057627198103120 ) ) ;
#191227=CARTESIAN_POINT ( 'NONE',  ( -18.22780087662123805, -5.499999999999968026, 98.98236817873106475 ) ) ;
#191229=CARTESIAN_POINT ( 'NONE',  ( 8.224510206698742110, 14.34966873604972548, 77.08442372801901854 ) ) ;
#191230=CARTESIAN_POINT ( 'NONE',  ( 18.62759615963271287, -10.81492255796078972, 93.33224293864769550 ) ) ;
#191231=CARTESIAN_POINT ( 'NONE',  ( -0.05219959533909027116, -19.03943276465977164, 42.49890960531435269 ) ) ;
#191233=CARTESIAN_POINT ( 'NONE',  ( 21.53943276465977519, 0.05219959533937863772, 36.25109039468567573 ) ) ;
#191234=CARTESIAN_POINT ( 'NONE',  ( 5.049401038297881783, 19.05341960407617563, 52.29275706135234003 ) ) ;
#191235=CARTESIAN_POINT ( 'NONE',  ( 16.46253265017160672, -9.564922557960803928, 48.33224293864769550 ) ) ;
#191236=CARTESIAN_POINT ( 'NONE',  ( -5.823673210054431948, 21.52544592524334988, 97.70942372801904696 ) ) ;
#191237=CARTESIAN_POINT ( 'NONE',  ( 17.05116617787825106, 6.768360034955821725, 98.84324446740804149 ) ) ;
#191238=CARTESIAN_POINT ( 'NONE',  ( -14.34966873604960291, -8.224510206698953496, 36.66557627198103120 ) ) ;
#191240=CARTESIAN_POINT ( 'NONE',  ( -10.72451020669898014, 18.67979575497178502, 40.41557627198103120 ) ) ;
#191242=CARTESIAN_POINT ( 'NONE',  ( 19.05341960407611168, 5.049401038298154454, 98.95724293864766707 ) ) ;
#191243=CARTESIAN_POINT ( 'NONE',  ( -12.14591786802309592, -12.06949235617757132, 91.87390960531436690 ) ) ;
#191244=CARTESIAN_POINT ( 'NONE',  ( 0.05219959533934541429, -16.53943276465976808, 30.00109039468568284 ) ) ;
#191245=CARTESIAN_POINT ( 'NONE',  ( -14.34966873604972548, 8.224510206698743886, 103.3344237280190043 ) ) ;
#191247=CARTESIAN_POINT ( 'NONE',  ( -19.03943276465977164, 0.05219959533909376836, 96.24890960531436690 ) ) ;
#191248=CARTESIAN_POINT ( 'NONE',  ( 15.80617190586746368, 15.72974639402197994, 99.37390960531436690 ) ) ;
#191249=CARTESIAN_POINT ( 'NONE',  ( -16.53943276465976808, -0.05219959533934237506, 113.7510903946856757 ) ) ;
#191250=CARTESIAN_POINT ( 'NONE',  ( -19.03943276465977164, 0.05219959533909376836, 96.24890960531436690 ) ) ;
#191251=CARTESIAN_POINT ( 'NONE',  ( -16.46253265017146816, -9.564922557961047289, 94.16775706135233293 ) ) ;
#191252=CARTESIAN_POINT ( 'NONE',  ( 0.05219959533937995610, -21.53943276465977519, 105.0010903946856757 ) ) ;
#191253=CARTESIAN_POINT ( 'NONE',  ( -18.62759615963270932, 10.81492255796079327, 95.83224293864770971 ) ) ;
#191254=CARTESIAN_POINT ( 'NONE',  ( 5.823673210054125526, 21.52544592524343514, 49.79057627198102409 ) ) ;
#191255=CARTESIAN_POINT ( 'NONE',  ( 13.89961937509977652, -13.97604488694527269, 68.12390960531436690 ) ) ;
#191256=CARTESIAN_POINT ( 'NONE',  ( 0.05219959533910956823, 16.53943276465976808, 39.99890960531436690 ) ) ;
#191257=CARTESIAN_POINT ( 'NONE',  ( -16.46253265017160317, 9.564922557960807481, 75.83224293864769550 ) ) ;
#191258=CARTESIAN_POINT ( 'NONE',  ( 19.25176906914649066, 5.499999999999730882, 58.49927264242278824 ) ) ;
#191259=CARTESIAN_POINT ( 'NONE',  ( -9.564922557961040184, 16.46253265017147172, 42.91775706135234003 ) ) ;
#191260=CARTESIAN_POINT ( 'NONE',  ( 4.379528057220339221, -16.55341960407611168, 87.70724293864769550 ) ) ;
#191261=CARTESIAN_POINT ( 'NONE',  ( -10.72451020669870658, -18.67979575497194134, 29.58442372801901854 ) ) ;
#191263=CARTESIAN_POINT ( 'NONE',  ( 16.52544592524335698, 4.483927247898782831, 111.4594237280190328 ) ) ;
#191264=CARTESIAN_POINT ( 'NONE',  ( -4.379528057220328563, 16.55341960407611168, 115.2072429386476955 ) ) ;
#191265=CARTESIAN_POINT ( 'NONE',  ( -16.51473224551069308, -9.474510206698971260, 66.66557627198102409 ) ) ;
#191267=CARTESIAN_POINT ( 'NONE',  ( 16.53943276465976808, -0.05219959533910856209, 38.74890960531435979 ) ) ;
#191268=CARTESIAN_POINT ( 'NONE',  ( 21.52544592524334988, 5.823673210054432836, 61.45942372801901854 ) ) ;
#191270=CARTESIAN_POINT ( 'NONE',  ( 0.05219959533909260263, 19.03943276465977164, 39.99890960531436690 ) ) ;
#191271=CARTESIAN_POINT ( 'NONE',  ( -16.51473224551069308, -9.474510206698971260, 56.66557627198103120 ) ) ;
#191273=CARTESIAN_POINT ( 'NONE',  ( -15.80617190586768217, 15.72974639402176855, 113.1260903946856899 ) ) ;
#191274=CARTESIAN_POINT ( 'NONE',  ( 4.379528057220092307, 16.55341960407617563, 62.29275706135236845 ) ) ;
#191275=CARTESIAN_POINT ( 'NONE',  ( 5.823673210054444382, -21.52544592524334988, 85.20942372801901854 ) ) ;
#191276=CARTESIAN_POINT ( 'NONE',  ( -9.474510206698964154, 16.51473224551069663, 115.4155762719810241 ) ) ;
#191277=CARTESIAN_POINT ( 'NONE',  ( -5.153800228976607833, 19.02544592524334988, 97.70942372801900433 ) ) ;
#191278=CARTESIAN_POINT ( 'NONE',  ( 18.67979575497194134, -10.72451020669871369, 70.83442372801901854 ) ) ;
#191279=CARTESIAN_POINT ( 'NONE',  ( -4.379528057220086978, -16.55341960407618274, 39.79275706135235424 ) ) ;
#191280=CARTESIAN_POINT ( 'NONE',  ( 5.823673210054125526, 21.52544592524343514, 89.79057627198103830 ) ) ;
#191281=CARTESIAN_POINT ( 'NONE',  ( 9.474510206698729675, 16.51473224551082808, 102.0844237280190043 ) ) ;
#191282=CARTESIAN_POINT ( 'NONE',  ( -19.03943276465977164, 0.05219959533909376836, 61.24890960531436690 ) ) ;
#191283=CARTESIAN_POINT ( 'NONE',  ( -16.46253265017146816, -9.564922557961047289, 94.16775706135233293 ) ) ;
#191284=CARTESIAN_POINT ( 'NONE',  ( -0.05219959533936034679, 19.03943276465977164, 102.5010903946856757 ) ) ;
#191285=CARTESIAN_POINT ( 'NONE',  ( -16.55341960407611168, -4.379528057220339221, 56.45724293864768839 ) ) ;
#191286=CARTESIAN_POINT ( 'NONE',  ( 9.474510206698729675, 16.51473224551082808, 72.08442372801900433 ) ) ;
#191287=CARTESIAN_POINT ( 'NONE',  ( 12.06949235617739724, 12.14591786802326823, 56.87609039468568994 ) ) ;
#191288=CARTESIAN_POINT ( 'NONE',  ( 0.05219959533937995610, -21.53943276465977519, 20.00109039468568639 ) ) ;
#191289=CARTESIAN_POINT ( 'NONE',  ( -19.03943276465977164, 0.05219959533909376836, 41.24890960531435269 ) ) ;
#191290=CARTESIAN_POINT ( 'NONE',  ( 16.46253265017160672, -9.564922557960803928, 58.33224293864769550 ) ) ;
#191291=CARTESIAN_POINT ( 'NONE',  ( -0.05219959533934338120, 16.53943276465976808, 62.50109039468568284 ) ) ;
#191293=DIRECTION ( 'NONE',  ( -1.000000000000000000, 0.000000000000000000, 0.000000000000000000 ) ) ;
#191294=CARTESIAN_POINT ( 'NONE',  ( 5.153800228976335163, 19.02544592524342804, 99.79057627198102409 ) ) ;
#191295=CARTESIAN_POINT ( 'NONE',  ( 9.474510206698971260, -16.51473224551069308, 27.91557627198103120 ) ) ;
#191297=CARTESIAN_POINT ( 'NONE',  ( -13.89961937509957401, -13.97604488694547875, 109.3760903946856331 ) ) ;
#191298=CARTESIAN_POINT ( 'NONE',  ( 18.67979575497178502, 10.72451020669898547, 44.16557627198103120 ) ) ;
#191299=CARTESIAN_POINT ( 'NONE',  ( 5.049401038297881783, 19.05341960407617563, 47.29275706135231161 ) ) ;
#191300=CARTESIAN_POINT ( 'NONE',  ( 0.05219959533934541429, -16.53943276465976808, 25.00109039468567218 ) ) ;
#191301=CARTESIAN_POINT ( 'NONE',  ( 0.05219959533909260263, 19.03943276465977164, 34.99890960531435979 ) ) ;
#191302=CARTESIAN_POINT ( 'NONE',  ( 9.474510206698971260, -16.51473224551069308, 47.91557627198102409 ) ) ;
#191303=CARTESIAN_POINT ( 'NONE',  ( 10.81492255796078972, 18.62759615963270932, 84.58224293864769550 ) ) ;
#191304=CARTESIAN_POINT ( 'NONE',  ( -16.46253265017160317, 9.564922557960807481, 100.8322429386477097 ) ) ;
#191305=CARTESIAN_POINT ( 'NONE',  ( 19.02544592524343514, -5.153800228976328945, 48.54057627198103120 ) ) ;
#191307=CARTESIAN_POINT ( 'NONE',  ( 16.46253265017146816, 9.564922557961045513, 81.66775706135233293 ) ) ;
#191308=CARTESIAN_POINT ( 'NONE',  ( -14.34966873604960291, -8.224510206698953496, 66.66557627198102409 ) ) ;
#191309=CARTESIAN_POINT ( 'NONE',  ( 0.05219959533937995610, -21.53943276465977519, 100.0010903946857042 ) ) ;
#191310=CARTESIAN_POINT ( 'NONE',  ( -21.53943276465977519, 0.05219959533907696930, 91.24890960531436690 ) ) ;
#191311=CARTESIAN_POINT ( 'NONE',  ( -5.719274019375665041, -21.55341960407619695, 79.79275706135236135 ) ) ;
#191312=CARTESIAN_POINT ( 'NONE',  ( -18.62759615963255300, -10.81492255796106328, 74.16775706135231871 ) ) ;
#191313=CARTESIAN_POINT ( 'NONE',  ( 0.05219959533909260263, 19.03943276465977164, 114.9989096053143669 ) ) ;
#191314=CARTESIAN_POINT ( 'NONE',  ( -14.29746914071037622, -8.314922557961029526, 109.1677570613523613 ) ) ;
#191315=CARTESIAN_POINT ( 'NONE',  ( 5.823673210054444382, -21.52544592524334988, 75.20942372801901854 ) ) ;
#191316=CARTESIAN_POINT ( 'NONE',  ( -16.46253265017160317, 9.564922557960807481, 65.83224293864769550 ) ) ;
#191317=CARTESIAN_POINT ( 'NONE',  ( -5.823673210054431948, 21.52544592524334988, 47.70942372801902565 ) ) ;
#191318=CARTESIAN_POINT ( 'NONE',  ( 9.564922557960805705, 16.46253265017160317, 79.58224293864769550 ) ) ;
#191319=CARTESIAN_POINT ( 'NONE',  ( -12.06949235617756955, 12.14591786802309770, 75.62390960531439532 ) ) ;
#191320=CARTESIAN_POINT ( 'NONE',  ( 4.483927247898545687, 16.52544592524342804, 49.79057627198102409 ) ) ;
#191321=CARTESIAN_POINT ( 'NONE',  ( -21.52544592524343514, 5.823673210054127303, 61.04057627198103120 ) ) ;
#191322=CARTESIAN_POINT ( 'NONE',  ( -13.89961937509977652, 13.97604488694528158, 65.62390960531436690 ) ) ;
#191323=CARTESIAN_POINT ( 'NONE',  ( 5.719274019375991003, -21.55341960407610458, 67.70724293864769550 ) ) ;
#191324=CARTESIAN_POINT ( 'NONE',  ( -13.89961937509957401, -13.97604488694547875, 69.37609039468564731 ) ) ;
#191325=CARTESIAN_POINT ( 'NONE',  ( -19.02544592524335343, -5.153800228976618492, 28.95942372801900788 ) ) ;
#191326=CARTESIAN_POINT ( 'NONE',  ( -14.34966873604960291, -8.224510206698953496, 71.66557627198100988 ) ) ;
#191327=CARTESIAN_POINT ( 'NONE',  ( 21.55341960407610458, 5.719274019375980345, 48.95724293864770971 ) ) ;
#191329=CARTESIAN_POINT ( 'NONE',  ( 17.13100169013300089, 6.664070546373150883, 101.7321016430015277 ) ) ;
#191330=CARTESIAN_POINT ( 'NONE',  ( -16.52544592524335698, -4.483927247898792601, 103.9594237280190185 ) ) ;
#191332=CARTESIAN_POINT ( 'NONE',  ( 19.02544592524334988, 5.153800228976608722, 106.4594237280190185 ) ) ;
#191333=CARTESIAN_POINT ( 'NONE',  ( 8.314922557960818139, 14.29746914071049879, 69.58224293864769550 ) ) ;
#191335=CARTESIAN_POINT ( 'NONE',  ( -13.89961937509977652, 13.97604488694528158, 60.62390960531436690 ) ) ;
#191336=CARTESIAN_POINT ( 'NONE',  ( -4.483927247898539470, -16.52544592524342804, 52.29057627198102409 ) ) ;
#191337=CARTESIAN_POINT ( 'NONE',  ( -13.89961937509977652, 13.97604488694528158, 85.62390960531433848 ) ) ;
#191338=CARTESIAN_POINT ( 'NONE',  ( 5.153800228976615827, -19.02544592524334988, 80.20942372801901854 ) ) ;
#191339=CARTESIAN_POINT ( 'NONE',  ( -9.564922557960796823, -16.46253265017161027, 52.08224293864768839 ) ) ;
#191340=CARTESIAN_POINT ( 'NONE',  ( 19.02544592524343514, -5.153800228976328945, 88.54057627198102409 ) ) ;
#191341=CARTESIAN_POINT ( 'NONE',  ( 13.97604488694527802, 13.89961937509977652, 79.37390960531435269 ) ) ;
#191342=CARTESIAN_POINT ( 'NONE',  ( -18.67979575497178146, -10.72451020669898902, 61.66557627198103120 ) ) ;
#191343=CARTESIAN_POINT ( 'NONE',  ( 8.224510206698742110, 14.34966873604972548, 62.08442372801901143 ) ) ;
#191344=DIRECTION ( 'NONE',  ( 0.000000000000000000, -3.469446951953611033E-15, -1.000000000000000000 ) ) ;
#191345=CARTESIAN_POINT ( 'NONE',  ( 19.03943276465977164, -0.05219959533909143690, 53.74890960531436690 ) ) ;
#191346=CARTESIAN_POINT ( 'NONE',  ( 0.05219959533907565091, 21.53943276465977519, 59.99890960531436690 ) ) ;
#191347=CARTESIAN_POINT ( 'NONE',  ( 19.05341960407617918, -5.049401038297876454, 81.04275706135231871 ) ) ;
#191348=CARTESIAN_POINT ( 'NONE',  ( -12.14591786802326823, 12.06949235617739902, 113.1260903946856899 ) ) ;
#191349=CARTESIAN_POINT ( 'NONE',  ( -19.05341960407617563, 5.049401038297882671, 38.54275706135233293 ) ) ;
#191350=CARTESIAN_POINT ( 'NONE',  ( 8.314922557961029526, -14.29746914071037800, 60.41775706135235424 ) ) ;
#191351=CARTESIAN_POINT ( 'NONE',  ( 14.29746914071037800, 8.314922557961029526, 91.66775706135234714 ) ) ;
#191352=CARTESIAN_POINT ( 'NONE',  ( 19.52217212775657984, -5.500000000000107470, 42.43993709005258808 ) ) ;
#191353=CARTESIAN_POINT ( 'NONE',  ( 14.29746914071037800, 8.314922557961029526, 86.66775706135234714 ) ) ;
#191354=CARTESIAN_POINT ( 'NONE',  ( -18.67979575497178146, -10.72451020669898902, 21.66557627198102409 ) ) ;
#191355=CARTESIAN_POINT ( 'NONE',  ( -16.46253265017160317, 9.564922557960807481, 40.83224293864769550 ) ) ;
#191356=CARTESIAN_POINT ( 'NONE',  ( 0.05219959533909260263, 19.03943276465977164, 44.99890960531435979 ) ) ;
#191357=CARTESIAN_POINT ( 'NONE',  ( 19.02544592524343514, -5.153800228976328945, 43.54057627198103120 ) ) ;
#191358=CARTESIAN_POINT ( 'NONE',  ( 15.80617190586769283, -15.72974639402175789, 35.62609039468568994 ) ) ;
#191359=CARTESIAN_POINT ( 'NONE',  ( 0.05219959533934541429, -16.53943276465976808, 55.00109039468568284 ) ) ;
#191360=CARTESIAN_POINT ( 'NONE',  ( -4.379528057220328563, 16.55341960407611168, 25.20724293864769550 ) ) ;
#191361=CARTESIAN_POINT ( 'NONE',  ( 0.05219959533909260263, 19.03943276465977164, 24.99890960531435269 ) ) ;
#191362=CARTESIAN_POINT ( 'NONE',  ( 19.02544592524334988, 5.153800228976608722, 21.45942372801899012 ) ) ;
#191363=CARTESIAN_POINT ( 'NONE',  ( -19.03943276465977164, -0.05219959533935918106, 108.7510903946856615 ) ) ;
#191365=CARTESIAN_POINT ( 'NONE',  ( 5.049401038297881783, 19.05341960407617563, 72.29275706135234714 ) ) ;
#191366=CARTESIAN_POINT ( 'NONE',  ( 12.06949235617757843, -12.14591786802309237, 73.12390960531436690 ) ) ;
#191367=CARTESIAN_POINT ( 'NONE',  ( -19.05341960407611168, -5.049401038298163336, 36.45724293864766707 ) ) ;
#191368=CARTESIAN_POINT ( 'NONE',  ( -19.05341960407617563, 5.049401038297882671, 73.54275706135233293 ) ) ;
#191370=CARTESIAN_POINT ( 'NONE',  ( 18.62759615963255655, 10.81492255796105972, 81.66775706135236135 ) ) ;
#191371=CARTESIAN_POINT ( 'NONE',  ( -14.34966873604972548, 8.224510206698743886, 43.33442372801901143 ) ) ;
#191372=CARTESIAN_POINT ( 'NONE',  ( 18.09805431107524498, -5.499999999999975131, 73.51606229291890315 ) ) ;
#191373=CARTESIAN_POINT ( 'NONE',  ( -21.55341960407610458, -5.719274019375992779, 36.45724293864768839 ) ) ;
#191374=CARTESIAN_POINT ( 'NONE',  ( 4.483927247898790824, -16.52544592524335698, 25.20942372801901854 ) ) ;
#191375=CARTESIAN_POINT ( 'NONE',  ( 5.153800228976335163, 19.02544592524342804, 29.79057627198102054 ) ) ;
#191376=CARTESIAN_POINT ( 'NONE',  ( 0.05219959533937995610, -21.53943276465977519, 105.0010903946856757 ) ) ;
#191377=PLANE ( 'NONE',  #168965 ) ;
#191378=CARTESIAN_POINT ( 'NONE',  ( -19.05341960407611168, -5.049401038298163336, 41.45724293864769550 ) ) ;
#191379=LINE ( 'NONE', #52855, #182135 ) ;
#191380=CARTESIAN_POINT ( 'NONE',  ( -19.05341960407611168, -5.049401038298163336, 61.45724293864769550 ) ) ;
#191381=CARTESIAN_POINT ( 'NONE',  ( 21.52544592524334988, 5.823673210054432836, 61.45942372801901854 ) ) ;
#191382=CARTESIAN_POINT ( 'NONE',  ( 0.05219959533936267826, -19.03943276465977164, 20.00109039468567218 ) ) ;
#191383=CARTESIAN_POINT ( 'NONE',  ( -16.52544592524342804, 4.483927247898546575, 26.04057627198103475 ) ) ;
#191384=CARTESIAN_POINT ( 'NONE',  ( 9.474510206698971260, -16.51473224551069308, 32.91557627198102409 ) ) ;
#191385=CARTESIAN_POINT ( 'NONE',  ( 13.89961937509977652, -13.97604488694527269, 88.12390960531438111 ) ) ;
#191386=CARTESIAN_POINT ( 'NONE',  ( -10.72451020669870658, -18.67979575497194134, 54.58442372801901143 ) ) ;
#191387=CARTESIAN_POINT ( 'NONE',  ( -5.049401038298153566, 19.05341960407611168, 35.20724293864768839 ) ) ;
#191388=CARTESIAN_POINT ( 'NONE',  ( 5.823673210054444382, -21.52544592524334988, 70.20942372801904696 ) ) ;
#191389=CARTESIAN_POINT ( 'NONE',  ( 5.153800228976615827, -19.02544592524334988, 90.20942372801900433 ) ) ;
#191390=CARTESIAN_POINT ( 'NONE',  ( -16.46253265017160317, 9.564922557960807481, 105.8322429386476955 ) ) ;
#191391=CARTESIAN_POINT ( 'NONE',  ( -16.53943276465976808, 0.05219959533911058130, 111.2489096053143669 ) ) ;
#191392=CARTESIAN_POINT ( 'NONE',  ( 21.52544592524344225, -5.823673210054117533, 113.5405762719810383 ) ) ;
#191393=CARTESIAN_POINT ( 'NONE',  ( 9.474510206698729675, 16.51473224551082808, 32.08442372801900433 ) ) ;
#191394=CARTESIAN_POINT ( 'NONE',  ( 4.483927247898545687, 16.52544592524342804, 114.7905762719810383 ) ) ;
#191395=CARTESIAN_POINT ( 'NONE',  ( -9.564922557960796823, -16.46253265017161027, 62.08224293864769550 ) ) ;
#191396=CARTESIAN_POINT ( 'NONE',  ( -19.03943276465977164, -0.05219959533935918106, 93.75109039468566152 ) ) ;
#191397=CARTESIAN_POINT ( 'NONE',  ( 14.29746914071049879, -8.314922557960816363, 63.33224293864770260 ) ) ;
#191398=CARTESIAN_POINT ( 'NONE',  ( 9.564922557961047289, -16.46253265017146816, 30.41775706135232937 ) ) ;
#191399=CARTESIAN_POINT ( 'NONE',  ( -5.823673210054116645, -21.52544592524344225, 22.29057627198102765 ) ) ;
#191400=CARTESIAN_POINT ( 'NONE',  ( 19.05341960407617918, -5.049401038297876454, 86.04275706135233293 ) ) ;
#191401=CARTESIAN_POINT ( 'NONE',  ( 5.823673210054125526, 21.52544592524343514, 94.79057627198105251 ) ) ;
#191402=CARTESIAN_POINT ( 'NONE',  ( -10.72451020669870658, -18.67979575497194134, 49.58442372801901143 ) ) ;
#191403=CARTESIAN_POINT ( 'NONE',  ( 12.06949235617739724, 12.14591786802326823, 36.87609039468568994 ) ) ;
#191404=CARTESIAN_POINT ( 'NONE',  ( -12.14591786802326823, 12.06949235617739902, 38.12609039468567573 ) ) ;
#191405=CARTESIAN_POINT ( 'NONE',  ( -15.72974639402176322, -15.80617190586768395, 49.37609039468569705 ) ) ;
#191406=CARTESIAN_POINT ( 'NONE',  ( 21.53943276465977519, -0.05219959533907433946, 58.74890960531436690 ) ) ;
#191408=CARTESIAN_POINT ( 'NONE',  ( 13.89961937509977652, -13.97604488694527269, 33.12390960531434558 ) ) ;
#191410=CARTESIAN_POINT ( 'NONE',  ( 16.53943276465976808, 0.05219959533934440121, 76.25109039468568994 ) ) ;
#191411=CARTESIAN_POINT ( 'NONE',  ( 18.62759615963271287, -10.81492255796078972, 93.33224293864769550 ) ) ;
#191412=CARTESIAN_POINT ( 'NONE',  ( 14.34966873604960469, 8.224510206698951720, 39.16557627198102409 ) ) ;
#191413=CARTESIAN_POINT ( 'NONE',  ( -4.483927247898782831, 16.52544592524335698, 57.70942372801901143 ) ) ;
#191414=CARTESIAN_POINT ( 'NONE',  ( -16.46253265017146816, -9.564922557961047289, 99.16775706135233293 ) ) ;
#191415=CARTESIAN_POINT ( 'NONE',  ( -5.823673210054116645, -21.52544592524344225, 92.29057627198103830 ) ) ;
#191416=CARTESIAN_POINT ( 'NONE',  ( 14.29746914071049879, -8.314922557960816363, 28.33224293864769550 ) ) ;
#191418=CARTESIAN_POINT ( 'NONE',  ( -4.483927247898782831, 16.52544592524335698, 72.70942372801901854 ) ) ;
#191420=CARTESIAN_POINT ( 'NONE',  ( 0.05219959533907565091, 21.53943276465977519, 69.99890960531435269 ) ) ;
#191421=CARTESIAN_POINT ( 'NONE',  ( 16.53943276465976808, 0.05219959533934440121, 106.2510903946856757 ) ) ;
#191424=CARTESIAN_POINT ( 'NONE',  ( 15.72974639402199770, -15.80617190586745480, 108.1239096053143811 ) ) ;
#191425=CARTESIAN_POINT ( 'NONE',  ( 5.823673210054125526, 21.52544592524343514, 109.7905762719810383 ) ) ;
#191426=CARTESIAN_POINT ( 'NONE',  ( -4.483927247898539470, -16.52544592524342804, 42.29057627198103120 ) ) ;
#191427=CARTESIAN_POINT ( 'NONE',  ( -16.55341960407617563, 4.379528057220093196, 33.54275706135234714 ) ) ;
#191428=CARTESIAN_POINT ( 'NONE',  ( -9.564922557960796823, -16.46253265017161027, 47.08224293864769550 ) ) ;
#191429=CARTESIAN_POINT ( 'NONE',  ( -16.51473224551069308, -9.474510206698971260, 61.66557627198103120 ) ) ;
#191430=CARTESIAN_POINT ( 'NONE',  ( -16.46253265017160317, 9.564922557960807481, 110.8322429386476955 ) ) ;
#191432=CARTESIAN_POINT ( 'NONE',  ( -13.89961937509957401, -13.97604488694547875, 104.3760903946856757 ) ) ;
#191433=CARTESIAN_POINT ( 'NONE',  ( -0.05219959533936034679, 19.03943276465977164, 57.50109039468566863 ) ) ;
#191434=CARTESIAN_POINT ( 'NONE',  ( -21.52544592524343514, 5.823673210054127303, 86.04057627198102409 ) ) ;
#191435=CARTESIAN_POINT ( 'NONE',  ( -8.314922557960811034, -14.29746914071050412, 27.08224293864769550 ) ) ;
#191437=CARTESIAN_POINT ( 'NONE',  ( -21.53943276465977519, 0.05219959533907696930, 46.24890960531435979 ) ) ;
#191438=CARTESIAN_POINT ( 'NONE',  ( 5.719274019375991003, -21.55341960407610458, 77.70724293864770971 ) ) ;
#191439=CARTESIAN_POINT ( 'NONE',  ( 9.474510206698729675, 16.51473224551082808, 107.0844237280190043 ) ) ;
#191440=CARTESIAN_POINT ( 'NONE',  ( -13.89961937509977652, 13.97604488694528158, 115.6239096053143669 ) ) ;
#191441=CARTESIAN_POINT ( 'NONE',  ( 21.55341960407619695, -5.719274019375665929, 71.04275706135234714 ) ) ;
#191442=CARTESIAN_POINT ( 'NONE',  ( 16.46253265017160672, -9.564922557960803928, 73.33224293864769550 ) ) ;
#191444=CARTESIAN_POINT ( 'NONE',  ( 13.89961937509977652, -13.97604488694527269, 73.12390960531436690 ) ) ;
#191445=CARTESIAN_POINT ( 'NONE',  ( 4.379528057220339221, -16.55341960407611168, 92.70724293864770971 ) ) ;
#191446=EDGE_LOOP ( 'NONE', ( #2420, #18691, #102472, #171584, #5530, #134616, #108033, #161324, #193042, #67077, #35927, #3234, #34390, #55209 ) ) ;
#191447=CARTESIAN_POINT ( 'NONE',  ( -9.564922557961040184, 16.46253265017147172, 102.9177570613523329 ) ) ;
#191449=CARTESIAN_POINT ( 'NONE',  ( -16.51473224551069308, -9.474510206698971260, 76.66557627198103830 ) ) ;
#191450=CARTESIAN_POINT ( 'NONE',  ( -18.62759615963255300, -10.81492255796106328, 79.16775706135234714 ) ) ;
#191451=CARTESIAN_POINT ( 'NONE',  ( -16.46253265017160317, 9.564922557960807481, 95.83224293864769550 ) ) ;
#191452=CARTESIAN_POINT ( 'NONE',  ( 12.06949235617739724, 12.14591786802326823, 71.87609039468568994 ) ) ;
#191453=CARTESIAN_POINT ( 'NONE',  ( -17.49999999999999289, -5.624438216177582994, 74.18329655085356933 ) ) ;
#191454=CARTESIAN_POINT ( 'NONE',  ( 19.05341960407617918, -5.049401038297876454, 61.04275706135232582 ) ) ;
#191455=CARTESIAN_POINT ( 'NONE',  ( -18.62759615963255300, -10.81492255796106328, 109.1677570613523613 ) ) ;
#191458=CARTESIAN_POINT ( 'NONE',  ( 12.14591786802309770, 12.06949235617756955, 24.37390960531435979 ) ) ;
#191460=CARTESIAN_POINT ( 'NONE',  ( -12.06949235617739369, -12.14591786802326823, 109.3760903946857042 ) ) ;
#191461=CARTESIAN_POINT ( 'NONE',  ( 16.21995358207305671, 7.366697692864118352, 67.56448998487842061 ) ) ;
#191462=CARTESIAN_POINT ( 'NONE',  ( -4.379528057220086978, -16.55341960407618274, 84.79275706135234714 ) ) ;
#191463=CARTESIAN_POINT ( 'NONE',  ( 18.67979575497194134, -10.72451020669871369, 85.83442372801901854 ) ) ;
#191464=CARTESIAN_POINT ( 'NONE',  ( 19.05341960407617918, -5.049401038297876454, 91.04275706135234714 ) ) ;
#191465=CARTESIAN_POINT ( 'NONE',  ( 9.564922557961047289, -16.46253265017146816, 45.41775706135232582 ) ) ;
#191466=CARTESIAN_POINT ( 'NONE',  ( -9.474510206698964154, 16.51473224551069663, 85.41557627198102409 ) ) ;
#191467=CARTESIAN_POINT ( 'NONE',  ( -16.46253265017160317, 9.564922557960807481, 50.83224293864770260 ) ) ;
#191468=CARTESIAN_POINT ( 'NONE',  ( -19.36337904590690684, 5.499999999999948486, 40.41494137495620720 ) ) ;
#191469=CARTESIAN_POINT ( 'NONE',  ( 15.80617190586746368, 15.72974639402197994, 89.37390960531435269 ) ) ;
#191470=CARTESIAN_POINT ( 'NONE',  ( 21.53943276465977519, -0.05219959533907433946, 43.74890960531435979 ) ) ;
#191471=CARTESIAN_POINT ( 'NONE',  ( -16.51473224551069308, -9.474510206698971260, 46.66557627198102409 ) ) ;
#191472=CARTESIAN_POINT ( 'NONE',  ( 16.55341960407618274, -4.379528057220086978, 66.04275706135236135 ) ) ;
#191475=CARTESIAN_POINT ( 'NONE',  ( 5.823673210054444382, -21.52544592524334988, 45.20942372801901854 ) ) ;
#191476=CARTESIAN_POINT ( 'NONE',  ( 12.06949235617757843, -12.14591786802309237, 63.12390960531435979 ) ) ;
#191478=CARTESIAN_POINT ( 'NONE',  ( 0.05219959533934541429, -16.53943276465976808, 35.00109039468568284 ) ) ;
#191479=CARTESIAN_POINT ( 'NONE',  ( 14.29746914071049879, -8.314922557960816363, 103.3322429386476955 ) ) ;
#191480=CARTESIAN_POINT ( 'NONE',  ( -13.89961937509957401, -13.97604488694547875, 54.37609039468565442 ) ) ;
#191481=CARTESIAN_POINT ( 'NONE',  ( -4.379528057220328563, 16.55341960407611168, 70.20724293864769550 ) ) ;
#191482=CARTESIAN_POINT ( 'NONE',  ( -0.05219959533937732626, 21.53943276465977519, 27.50109039468567929 ) ) ;
#191483=CARTESIAN_POINT ( 'NONE',  ( -0.05219959533909027116, -19.03943276465977164, 22.49890960531436690 ) ) ;
#191484=CARTESIAN_POINT ( 'NONE',  ( -5.823673210054116645, -21.52544592524344225, 87.29057627198103830 ) ) ;
#191485=CARTESIAN_POINT ( 'NONE',  ( 13.97604488694527802, 13.89961937509977652, 99.37390960531436690 ) ) ;
#191486=CARTESIAN_POINT ( 'NONE',  ( -16.53943276465976808, 0.05219959533911058130, 71.24890960531435269 ) ) ;
#191487=CARTESIAN_POINT ( 'NONE',  ( -19.03943276465977164, 0.05219959533909376836, 116.2489096053143669 ) ) ;
#191489=CARTESIAN_POINT ( 'NONE',  ( 13.89961937509957401, 13.97604488694547697, 81.87609039468564731 ) ) ;
#191490=CARTESIAN_POINT ( 'NONE',  ( 18.62759615963255655, 10.81492255796105972, 21.66775706135235069 ) ) ;
#191491=CARTESIAN_POINT ( 'NONE',  ( 9.564922557960805705, 16.46253265017160317, 64.58224293864769550 ) ) ;
#191492=CARTESIAN_POINT ( 'NONE',  ( 9.474510206698729675, 16.51473224551082808, 52.08442372801900433 ) ) ;
#191493=CARTESIAN_POINT ( 'NONE',  ( 9.474510206698971260, -16.51473224551069308, 32.91557627198102409 ) ) ;
#191495=EDGE_CURVE ( 'NONE', #133171, #122538, #110382, .T. ) ;
#191496=CARTESIAN_POINT ( 'NONE',  ( 15.80617190586769283, -15.72974639402175789, 75.62609039468567573 ) ) ;
#191497=CARTESIAN_POINT ( 'NONE',  ( 8.224510206698953496, -14.34966873604960469, 62.91557627198102409 ) ) ;
#191498=CARTESIAN_POINT ( 'NONE',  ( 14.29746914071049879, -8.314922557960816363, 58.33224293864768839 ) ) ;
#191499=CARTESIAN_POINT ( 'NONE',  ( 13.89961937509977652, -13.97604488694527269, 68.12390960531436690 ) ) ;
#191500=CARTESIAN_POINT ( 'NONE',  ( -18.67979575497178146, -10.72451020669898902, 86.66557627198102409 ) ) ;
#191501=CARTESIAN_POINT ( 'NONE',  ( -13.97604488694527625, -13.89961937509977652, 56.87390960531434558 ) ) ;
#191503=CARTESIAN_POINT ( 'NONE',  ( -10.72451020669898014, 18.67979575497178502, 80.41557627198103830 ) ) ;
#191504=CARTESIAN_POINT ( 'NONE',  ( -0.05219959533937732626, 21.53943276465977519, 97.50109039468567573 ) ) ;
#191506=CARTESIAN_POINT ( 'NONE',  ( 16.52544592524335698, 4.483927247898782831, 96.45942372801901854 ) ) ;
#191507=CARTESIAN_POINT ( 'NONE',  ( -16.52544592524342804, 4.483927247898546575, 101.0405762719810383 ) ) ;
#191508=CARTESIAN_POINT ( 'NONE',  ( -13.89961937509957401, -13.97604488694547875, 94.37609039468566152 ) ) ;
#191509=ORIENTED_EDGE ( 'NONE', *, *, #141668, .T. ) ;
#191510=CARTESIAN_POINT ( 'NONE',  ( 15.80617190586746368, 15.72974639402197994, 109.3739096053143811 ) ) ;
#191511=CARTESIAN_POINT ( 'NONE',  ( -5.153800228976607833, 19.02544592524334988, 57.70942372801899012 ) ) ;
#191512=CARTESIAN_POINT ( 'NONE',  ( 8.314922557961029526, -14.29746914071037800, 105.4177570613523613 ) ) ;
#191513=CARTESIAN_POINT ( 'NONE',  ( -13.97604488694547697, 13.89961937509957934, 28.12609039468565797 ) ) ;
#191514=CARTESIAN_POINT ( 'NONE',  ( -9.564922557960796823, -16.46253265017161027, 97.08224293864769550 ) ) ;
#191515=CARTESIAN_POINT ( 'NONE',  ( -15.80617190586745835, -15.72974639402198527, 66.87390960531436690 ) ) ;
#191517=CARTESIAN_POINT ( 'NONE',  ( 16.51473224551069308, 9.474510206698969483, 29.16557627198103475 ) ) ;
#191518=CARTESIAN_POINT ( 'NONE',  ( -13.89961937509957401, -13.97604488694547875, 19.37609039468566507 ) ) ;
#191519=CARTESIAN_POINT ( 'NONE',  ( 4.483927247898790824, -16.52544592524335698, 70.20942372801904696 ) ) ;
#191520=CARTESIAN_POINT ( 'NONE',  ( -18.62759615963255300, -10.81492255796106328, 24.16775706135235424 ) ) ;
#191521=CARTESIAN_POINT ( 'NONE',  ( 4.483927247898790824, -16.52544592524335698, 50.20942372801901854 ) ) ;
#191522=CARTESIAN_POINT ( 'NONE',  ( -5.049401038298153566, 19.05341960407611168, 100.2072429386476955 ) ) ;
#191523=CARTESIAN_POINT ( 'NONE',  ( 19.05341960407611168, 5.049401038298154454, 48.95724293864768129 ) ) ;
#191524=CARTESIAN_POINT ( 'NONE',  ( -13.89961937509977652, 13.97604488694528158, 65.62390960531436690 ) ) ;
#191525=CARTESIAN_POINT ( 'NONE',  ( 14.34966873604972726, -8.224510206698740333, 50.83442372801901143 ) ) ;
#191526=CARTESIAN_POINT ( 'NONE',  ( -12.06949235617756955, 12.14591786802309770, 90.62390960531436690 ) ) ;
#191527=CARTESIAN_POINT ( 'NONE',  ( -16.52544592524335698, -4.483927247898792601, 103.9594237280190185 ) ) ;
#191529=CARTESIAN_POINT ( 'NONE',  ( 10.81492255796106328, -18.62759615963255655, 60.41775706135235424 ) ) ;
#191530=CARTESIAN_POINT ( 'NONE',  ( -0.05219959533909027116, -19.03943276465977164, 82.49890960531436690 ) ) ;
#191531=CARTESIAN_POINT ( 'NONE',  ( -19.05341960407611168, -5.049401038298163336, 61.45724293864769550 ) ) ;
#191532=CARTESIAN_POINT ( 'NONE',  ( -9.474510206698964154, 16.51473224551069663, 90.41557627198103830 ) ) ;
#191533=CARTESIAN_POINT ( 'NONE',  ( -14.29746914071049879, 8.314922557960819915, 40.83224293864769550 ) ) ;
#191534=CARTESIAN_POINT ( 'NONE',  ( -14.29746914071037622, -8.314922557961029526, 94.16775706135237556 ) ) ;
#191535=CARTESIAN_POINT ( 'NONE',  ( 12.06949235617757843, -12.14591786802309237, 38.12390960531436690 ) ) ;
#191536=ORIENTED_EDGE ( 'NONE', *, *, #199845, .F. ) ;
#191537=CARTESIAN_POINT ( 'NONE',  ( 16.51473224551083163, -9.474510206698727899, 45.83442372801900433 ) ) ;
#191538=CARTESIAN_POINT ( 'NONE',  ( 16.46253265017160672, -9.564922557960803928, 113.3322429386476955 ) ) ;
#191539=CARTESIAN_POINT ( 'NONE',  ( -13.97604488694527625, -13.89961937509977652, 66.87390960531436690 ) ) ;
#191540=CARTESIAN_POINT ( 'NONE',  ( -9.474510206698720793, -16.51473224551083518, 39.58442372801899722 ) ) ;
#191543=CARTESIAN_POINT ( 'NONE',  ( 9.564922557961047289, -16.46253265017146816, 90.41775706135234714 ) ) ;
#191544=CARTESIAN_POINT ( 'NONE',  ( 12.14591786802327356, -12.06949235617739191, 75.62609039468567573 ) ) ;
#191545=CARTESIAN_POINT ( 'NONE',  ( 16.62475595723697808, 7.163666690055314312, 91.97286648189532343 ) ) ;
#191546=CARTESIAN_POINT ( 'NONE',  ( 9.564922557960805705, 16.46253265017160317, 89.58224293864769550 ) ) ;
#191547=CARTESIAN_POINT ( 'NONE',  ( 21.53943276465977519, 0.05219959533937863772, 26.25109039468567573 ) ) ;
#191548=CARTESIAN_POINT ( 'NONE',  ( 19.03943276465977164, 0.05219959533936151252, 71.25109039468566152 ) ) ;
#191549=CARTESIAN_POINT ( 'NONE',  ( 17.44279575226822132, 5.990770900252481823, 86.66442432485682446 ) ) ;
#191550=CARTESIAN_POINT ( 'NONE',  ( -9.564922557960796823, -16.46253265017161027, 52.08224293864768839 ) ) ;
#191551=CARTESIAN_POINT ( 'NONE',  ( -9.564922557960796823, -16.46253265017161027, 92.08224293864769550 ) ) ;
#191552=CARTESIAN_POINT ( 'NONE',  ( 14.34966873604960469, 8.224510206698951720, 49.16557627198102409 ) ) ;
#191553=CARTESIAN_POINT ( 'NONE',  ( 19.02544592524343514, -5.153800228976328945, 38.54057627198103120 ) ) ;
#191554=CARTESIAN_POINT ( 'NONE',  ( -13.97604488694547697, 13.89961937509957934, 53.12609039468565442 ) ) ;
#191555=CARTESIAN_POINT ( 'NONE',  ( 4.379528057220339221, -16.55341960407611168, 82.70724293864770971 ) ) ;
#191556=CARTESIAN_POINT ( 'NONE',  ( -13.89961937509957401, -13.97604488694547875, 24.37609039468565442 ) ) ;
#191557=CARTESIAN_POINT ( 'NONE',  ( 19.03943276465977164, -0.05219959533909143690, 68.74890960531436690 ) ) ;
#191558=CARTESIAN_POINT ( 'NONE',  ( 15.80617190586746368, 15.72974639402197994, 64.37390960531435269 ) ) ;
#191559=CARTESIAN_POINT ( 'NONE',  ( 8.314922557960818139, 14.29746914071049879, 49.58224293864769550 ) ) ;
#191560=CARTESIAN_POINT ( 'NONE',  ( -5.153800228976607833, 19.02544592524334988, 22.70942372801899012 ) ) ;
#191561=CARTESIAN_POINT ( 'NONE',  ( -5.153800228976328057, -19.02544592524343514, 102.2905762719810383 ) ) ;
#191562=CARTESIAN_POINT ( 'NONE',  ( 10.81492255796078972, 18.62759615963270932, 29.58224293864769905 ) ) ;
#191563=CARTESIAN_POINT ( 'NONE',  ( -9.474510206698964154, 16.51473224551069663, 55.41557627198103120 ) ) ;
#191564=CARTESIAN_POINT ( 'NONE',  ( -5.049401038298153566, 19.05341960407611168, 25.20724293864768484 ) ) ;
#191565=CARTESIAN_POINT ( 'NONE',  ( 14.29746914071049879, -8.314922557960816363, 98.33224293864769550 ) ) ;
#191566=CARTESIAN_POINT ( 'NONE',  ( 15.72974639402199770, -15.80617190586745480, 108.1239096053143811 ) ) ;
#191567=CARTESIAN_POINT ( 'NONE',  ( 13.97604488694527802, 13.89961937509977652, 104.3739096053143385 ) ) ;
#191568=CARTESIAN_POINT ( 'NONE',  ( 5.719274019375991003, -21.55341960407610458, 107.7072429386476955 ) ) ;
#191569=CARTESIAN_POINT ( 'NONE',  ( 16.51473224551069308, 9.474510206698969483, 109.1655762719810383 ) ) ;
#191570=CARTESIAN_POINT ( 'NONE',  ( -4.483927247898539470, -16.52544592524342804, 112.2905762719810241 ) ) ;
#191571=CARTESIAN_POINT ( 'NONE',  ( 10.81492255796106328, -18.62759615963255655, 80.41775706135234714 ) ) ;
#191572=CARTESIAN_POINT ( 'NONE',  ( 0.05219959533907565091, 21.53943276465977519, 89.99890960531438111 ) ) ;
#191574=CARTESIAN_POINT ( 'NONE',  ( 17.26058549869091507, -6.457015423128527942, 106.1225416252393501 ) ) ;
#191575=CARTESIAN_POINT ( 'NONE',  ( 19.48894818550246555, -5.499999999999912070, 77.60307310435240424 ) ) ;
#191576=CARTESIAN_POINT ( 'NONE',  ( 16.51473224551069308, 9.474510206698969483, 59.16557627198102409 ) ) ;
#191577=CARTESIAN_POINT ( 'NONE',  ( 12.06949235617739724, 12.14591786802326823, 41.87609039468568284 ) ) ;
#191578=CARTESIAN_POINT ( 'NONE',  ( -14.34966873604960291, -8.224510206698953496, 106.6655762719810383 ) ) ;
#191580=CARTESIAN_POINT ( 'NONE',  ( -13.89961937509977652, 13.97604488694528158, 60.62390960531436690 ) ) ;
#191581=CARTESIAN_POINT ( 'NONE',  ( -12.14591786802309592, -12.06949235617757132, 91.87390960531436690 ) ) ;
#191583=CARTESIAN_POINT ( 'NONE',  ( -18.62759615963270932, 10.81492255796079327, 30.83224293864770260 ) ) ;
#191584=CARTESIAN_POINT ( 'NONE',  ( -12.06949235617756955, 12.14591786802309770, 65.62390960531436690 ) ) ;
#191585=CARTESIAN_POINT ( 'NONE',  ( -9.564922557961040184, 16.46253265017147172, 112.9177570613523329 ) ) ;
#191586=CARTESIAN_POINT ( 'NONE',  ( -0.05219959533937732626, 21.53943276465977519, 67.50109039468568994 ) ) ;
#191587=CARTESIAN_POINT ( 'NONE',  ( 18.22780087662122739, 5.500000000000000888, 66.48236817873106475 ) ) ;
#191588=CARTESIAN_POINT ( 'NONE',  ( -8.224510206698735004, -14.34966873604973081, 99.58442372801900433 ) ) ;
#191589=CARTESIAN_POINT ( 'NONE',  ( -16.52544592524342804, 4.483927247898546575, 41.04057627198103120 ) ) ;
#191590=CARTESIAN_POINT ( 'NONE',  ( -19.03943276465977164, 0.05219959533909376836, 36.24890960531436690 ) ) ;
#191591=CARTESIAN_POINT ( 'NONE',  ( -13.89961937509977652, 13.97604488694528158, 90.62390960531432427 ) ) ;
#191592=CARTESIAN_POINT ( 'NONE',  ( -5.719274019375978568, 21.55341960407610458, 95.20724293864769550 ) ) ;
#191593=CARTESIAN_POINT ( 'NONE',  ( 12.14591786802327356, -12.06949235617739191, 20.62609039468568639 ) ) ;
#191594=CARTESIAN_POINT ( 'NONE',  ( -16.55341960407611168, -4.379528057220339221, 61.45724293864770260 ) ) ;
#191595=CARTESIAN_POINT ( 'NONE',  ( -18.62759615963255300, -10.81492255796106328, 69.16775706135234714 ) ) ;
#191596=CARTESIAN_POINT ( 'NONE',  ( -0.05219959533934338120, 16.53943276465976808, 102.5010903946856899 ) ) ;
#191597=CARTESIAN_POINT ( 'NONE',  ( 17.44279575226823553, 5.990770900252484488, 26.66442432485683156 ) ) ;
#191598=PLANE ( 'NONE',  #142262 ) ;
#191599=CARTESIAN_POINT ( 'NONE',  ( -4.379528057220328563, 16.55341960407611168, 30.20724293864769550 ) ) ;
#191600=CARTESIAN_POINT ( 'NONE',  ( 16.53943276465976808, 0.05219959533934440121, 71.25109039468568994 ) ) ;
#191601=CARTESIAN_POINT ( 'NONE',  ( 19.03943276465977164, -0.05219959533909143690, 83.74890960531436690 ) ) ;
#191602=CARTESIAN_POINT ( 'NONE',  ( 9.474510206698971260, -16.51473224551069308, 82.91557627198103830 ) ) ;
#191603=CARTESIAN_POINT ( 'NONE',  ( -10.72451020669870658, -18.67979575497194134, 84.58442372801903275 ) ) ;
#191604=CARTESIAN_POINT ( 'NONE',  ( 0.05219959533934541429, -16.53943276465976808, 90.00109039468567573 ) ) ;
#191605=CARTESIAN_POINT ( 'NONE',  ( -12.06949235617756955, 12.14591786802309770, 55.62390960531436690 ) ) ;
#191606=CARTESIAN_POINT ( 'NONE',  ( 5.153800228976335163, 19.02544592524342804, 64.79057627198100988 ) ) ;
#191607=ORIENTED_EDGE ( 'NONE', *, *, #98059, .F. ) ;
#191608=CARTESIAN_POINT ( 'NONE',  ( 16.51473224551083163, -9.474510206698727899, 110.8344237280190043 ) ) ;
#191609=CARTESIAN_POINT ( 'NONE',  ( 16.55341960407611168, 4.379528057220329451, 108.9572429386476955 ) ) ;
#191610=CARTESIAN_POINT ( 'NONE',  ( 9.474510206698971260, -16.51473224551069308, 82.91557627198103830 ) ) ;
#191611=CARTESIAN_POINT ( 'NONE',  ( -16.53943276465976808, -0.05219959533934237506, 18.75109039468568639 ) ) ;
#191613=CARTESIAN_POINT ( 'NONE',  ( 21.55341960407619695, -5.719274019375665929, 111.0427570613523613 ) ) ;
#191614=CARTESIAN_POINT ( 'NONE',  ( 16.53943276465976808, 0.05219959533934440121, 76.25109039468568994 ) ) ;
#191615=CARTESIAN_POINT ( 'NONE',  ( -19.05341960407617563, 5.049401038297882671, 98.54275706135233293 ) ) ;
#191616=CARTESIAN_POINT ( 'NONE',  ( -16.51473224551069308, -9.474510206698971260, 21.66557627198102765 ) ) ;
#191617=CARTESIAN_POINT ( 'NONE',  ( -4.483927247898782831, 16.52544592524335698, 72.70942372801901854 ) ) ;
#191618=CARTESIAN_POINT ( 'NONE',  ( -16.52544592524335698, -4.483927247898792601, 58.95942372801902565 ) ) ;
#191620=CARTESIAN_POINT ( 'NONE',  ( 5.049401038297881783, 19.05341960407617563, 57.29275706135231871 ) ) ;
#191621=CARTESIAN_POINT ( 'NONE',  ( 10.81492255796106328, -18.62759615963255655, 95.41775706135234714 ) ) ;
#191622=CARTESIAN_POINT ( 'NONE',  ( 19.02544592524343514, -5.153800228976328945, 28.54057627198102409 ) ) ;
#191623=CARTESIAN_POINT ( 'NONE',  ( 5.049401038298161559, -19.05341960407611168, 82.70724293864770971 ) ) ;
#191624=CARTESIAN_POINT ( 'NONE',  ( -14.29746914071049879, 8.314922557960819915, 70.83224293864770971 ) ) ;
#191625=CARTESIAN_POINT ( 'NONE',  ( -10.81492255796105439, 18.62759615963255655, 87.91775706135234714 ) ) ;
#191626=CARTESIAN_POINT ( 'NONE',  ( 5.049401038297881783, 19.05341960407617563, 62.29275706135234003 ) ) ;
#191627=CARTESIAN_POINT ( 'NONE',  ( 19.03943276465977164, 0.05219959533936151252, 41.25109039468566152 ) ) ;
#191628=CARTESIAN_POINT ( 'NONE',  ( -5.823673210054116645, -21.52544592524344225, 37.29057627198102409 ) ) ;
#191629=CARTESIAN_POINT ( 'NONE',  ( -18.67979575497193778, 10.72451020669871902, 108.3344237280190185 ) ) ;
#191630=CARTESIAN_POINT ( 'NONE',  ( -16.46253265017160317, 9.564922557960807481, 80.83224293864769550 ) ) ;
#191631=CARTESIAN_POINT ( 'NONE',  ( -5.823673210054431948, 21.52544592524334988, 107.7094237280190328 ) ) ;
#191632=CARTESIAN_POINT ( 'NONE',  ( 15.80617190586746368, 15.72974639402197994, 44.37390960531435979 ) ) ;
#191633=CARTESIAN_POINT ( 'NONE',  ( 19.02544592524343514, -5.153800228976328945, 98.54057627198100988 ) ) ;
#191634=CARTESIAN_POINT ( 'NONE',  ( 13.97604488694548053, -13.89961937509957401, 80.62609039468567573 ) ) ;
#191635=CARTESIAN_POINT ( 'NONE',  ( 5.049401038298161559, -19.05341960407611168, 102.7072429386476955 ) ) ;
#191636=CARTESIAN_POINT ( 'NONE',  ( 9.564922557961047289, -16.46253265017146816, 95.41775706135233293 ) ) ;
#191637=CARTESIAN_POINT ( 'NONE',  ( -4.483927247898782831, 16.52544592524335698, 42.70942372801901854 ) ) ;
#191638=CARTESIAN_POINT ( 'NONE',  ( -16.55341960407611168, -4.379528057220339221, 96.45724293864770971 ) ) ;
#191639=CARTESIAN_POINT ( 'NONE',  ( -9.474510206698964154, 16.51473224551069663, 80.41557627198103830 ) ) ;
#191640=CARTESIAN_POINT ( 'NONE',  ( -5.823673210054116645, -21.52544592524344225, 62.29057627198102409 ) ) ;
#191641=CARTESIAN_POINT ( 'NONE',  ( 16.53943276465976808, 0.05219959533934440121, 26.25109039468567573 ) ) ;
#191642=CARTESIAN_POINT ( 'NONE',  ( 0.05219959533937995610, -21.53943276465977519, 40.00109039468567573 ) ) ;
#191643=CARTESIAN_POINT ( 'NONE',  ( 21.55341960407619695, -5.719274019375665929, 81.04275706135236135 ) ) ;
#191644=CARTESIAN_POINT ( 'NONE',  ( 12.14591786802327356, -12.06949235617739191, 80.62609039468567573 ) ) ;
#191646=CARTESIAN_POINT ( 'NONE',  ( 13.89961937509977652, -13.97604488694527269, 73.12390960531436690 ) ) ;
#191647=CARTESIAN_POINT ( 'NONE',  ( 14.34966873604960469, 8.224510206698951720, 79.16557627198103830 ) ) ;
#191648=CARTESIAN_POINT ( 'NONE',  ( -8.224510206698948167, 14.34966873604960824, 25.41557627198103120 ) ) ;
#191649=CARTESIAN_POINT ( 'NONE',  ( -19.05341960407617563, 5.049401038297882671, 53.54275706135231871 ) ) ;
#191650=CARTESIAN_POINT ( 'NONE',  ( -21.53943276465977519, -0.05219959533937600094, 38.75109039468567573 ) ) ;
#191651=CARTESIAN_POINT ( 'NONE',  ( 8.314922557960818139, 14.29746914071049879, 74.58224293864768129 ) ) ;
#191652=CARTESIAN_POINT ( 'NONE',  ( 5.049401038298161559, -19.05341960407611168, 107.7072429386476955 ) ) ;
#191653=CARTESIAN_POINT ( 'NONE',  ( 8.314922557961029526, -14.29746914071037800, 100.4177570613523471 ) ) ;
#191654=CARTESIAN_POINT ( 'NONE',  ( -21.55341960407619339, 5.719274019375674811, 88.54275706135236135 ) ) ;
#191655=CARTESIAN_POINT ( 'NONE',  ( -16.52544592524335698, -4.483927247898792601, 43.95942372801902565 ) ) ;
#191656=CARTESIAN_POINT ( 'NONE',  ( 5.719274019375673035, 21.55341960407619339, 47.29275706135234003 ) ) ;
#191658=CARTESIAN_POINT ( 'NONE',  ( 18.67979575497194134, -10.72451020669871369, 20.83442372801901143 ) ) ;
#191659=CARTESIAN_POINT ( 'NONE',  ( -16.52544592524342804, 4.483927247898546575, 86.04057627198102409 ) ) ;
#191660=CARTESIAN_POINT ( 'NONE',  ( 17.50000000000015987, -3.417042746626905103, 27.67380396232477580 ) ) ;
#191661=CARTESIAN_POINT ( 'NONE',  ( 4.483927247898545687, 16.52544592524342804, 54.79057627198104541 ) ) ;
#191662=CARTESIAN_POINT ( 'NONE',  ( 12.06949235617739724, 12.14591786802326823, 96.87609039468568994 ) ) ;
#191663=CARTESIAN_POINT ( 'NONE',  ( 5.049401038298161559, -19.05341960407611168, 32.70724293864768129 ) ) ;
#191664=CARTESIAN_POINT ( 'NONE',  ( -5.719274019375978568, 21.55341960407610458, 40.20724293864769550 ) ) ;
#191665=CARTESIAN_POINT ( 'NONE',  ( 16.52544592524342804, -4.483927247898539470, 83.54057627198102409 ) ) ;
#191666=CARTESIAN_POINT ( 'NONE',  ( -10.72451020669898014, 18.67979575497178502, 75.41557627198102409 ) ) ;
#191667=CARTESIAN_POINT ( 'NONE',  ( -5.153800228976328057, -19.02544592524343514, 82.29057627198103830 ) ) ;
#191668=CARTESIAN_POINT ( 'NONE',  ( -9.564922557960796823, -16.46253265017161027, 37.08224293864768839 ) ) ;
#191669=CARTESIAN_POINT ( 'NONE',  ( -19.03943276465977164, -0.05219959533935918106, 88.75109039468567573 ) ) ;
#191670=CARTESIAN_POINT ( 'NONE',  ( 5.719274019375991003, -21.55341960407610458, 32.70724293864770260 ) ) ;
#191671=CARTESIAN_POINT ( 'NONE',  ( -21.52544592524334988, -5.823673210054445271, 58.95942372801902565 ) ) ;
#191672=CARTESIAN_POINT ( 'NONE',  ( -0.05219959533909027116, -19.03943276465977164, 47.49890960531435979 ) ) ;
#191673=CARTESIAN_POINT ( 'NONE',  ( -19.02544592524342804, 5.153800228976336051, 81.04057627198103830 ) ) ;
#191675=CARTESIAN_POINT ( 'NONE',  ( -12.14591786802326823, 12.06949235617739902, 48.12609039468568284 ) ) ;
#191676=CARTESIAN_POINT ( 'NONE',  ( 0.05219959533937995610, -21.53943276465977519, 25.00109039468567218 ) ) ;
#191677=CARTESIAN_POINT ( 'NONE',  ( 21.52544592524334988, 5.823673210054432836, 71.45942372801901854 ) ) ;
#191678=CARTESIAN_POINT ( 'NONE',  ( -13.89961937509977652, 13.97604488694528158, 115.6239096053143669 ) ) ;
#191679=CARTESIAN_POINT ( 'NONE',  ( 5.719274019375991003, -21.55341960407610458, 82.70724293864770971 ) ) ;
#191680=CARTESIAN_POINT ( 'NONE',  ( 0.05219959533937995610, -21.53943276465977519, 30.00109039468568284 ) ) ;
#191681=CARTESIAN_POINT ( 'NONE',  ( -0.05219959533934338120, 16.53943276465976808, 62.50109039468568284 ) ) ;
#191682=CARTESIAN_POINT ( 'NONE',  ( 5.823673210054125526, 21.52544592524343514, 69.79057627198102409 ) ) ;
#191683=CARTESIAN_POINT ( 'NONE',  ( 21.52544592524334988, 5.823673210054432836, 111.4594237280190328 ) ) ;
#191684=CARTESIAN_POINT ( 'NONE',  ( 9.564922557960805705, 16.46253265017160317, 59.58224293864769550 ) ) ;
#191685=CARTESIAN_POINT ( 'NONE',  ( -19.05341960407611168, -5.049401038298163336, 111.4572429386476671 ) ) ;
#191686=CARTESIAN_POINT ( 'NONE',  ( 13.89961937509977652, -13.97604488694527269, 83.12390960531436690 ) ) ;
#191688=CARTESIAN_POINT ( 'NONE',  ( 0.05219959533936267826, -19.03943276465977164, 75.00109039468566152 ) ) ;
#191689=CARTESIAN_POINT ( 'NONE',  ( -21.53943276465977519, 0.05219959533907696930, 41.24890960531435269 ) ) ;
#191690=CARTESIAN_POINT ( 'NONE',  ( 12.06949235617757843, -12.14591786802309237, 23.12390960531436335 ) ) ;
#191691=CARTESIAN_POINT ( 'NONE',  ( -19.05341960407617563, 5.049401038297882671, 103.5427570613523329 ) ) ;
#191692=CARTESIAN_POINT ( 'NONE',  ( 19.05341960407611168, 5.049401038298154454, 23.95724293864769194 ) ) ;
#191693=CARTESIAN_POINT ( 'NONE',  ( -5.153800228976607833, 19.02544592524334988, 22.70942372801899012 ) ) ;
#191694=CARTESIAN_POINT ( 'NONE',  ( 19.02544592524334988, 5.153800228976608722, 96.45942372801897591 ) ) ;
#191695=CARTESIAN_POINT ( 'NONE',  ( 21.55341960407610458, 5.719274019375980345, 88.95724293864769550 ) ) ;
#191696=CARTESIAN_POINT ( 'NONE',  ( 16.46253265017146816, 9.564922557961045513, 51.66775706135233293 ) ) ;
#191698=CARTESIAN_POINT ( 'NONE',  ( 9.564922557960805705, 16.46253265017160317, 59.58224293864769550 ) ) ;
#191699=CARTESIAN_POINT ( 'NONE',  ( 8.224510206698953496, -14.34966873604960469, 67.91557627198102409 ) ) ;
#191700=CARTESIAN_POINT ( 'NONE',  ( 13.97604488694527802, 13.89961937509977652, 49.37390960531434558 ) ) ;
#191701=CARTESIAN_POINT ( 'NONE',  ( -8.314922557960811034, -14.29746914071050412, 52.08224293864768839 ) ) ;
#191703=CARTESIAN_POINT ( 'NONE',  ( -14.29746914071049879, 8.314922557960819915, 25.83224293864769194 ) ) ;
#191704=CARTESIAN_POINT ( 'NONE',  ( -19.05341960407611168, -5.049401038298163336, 61.45724293864769550 ) ) ;
#191705=CARTESIAN_POINT ( 'NONE',  ( 13.89961937509957401, 13.97604488694547697, 21.87609039468566152 ) ) ;
#191706=CARTESIAN_POINT ( 'NONE',  ( -16.52544592524335698, -4.483927247898792601, 48.95942372801902565 ) ) ;
#191707=CARTESIAN_POINT ( 'NONE',  ( 21.55341960407610458, 5.719274019375980345, 53.95724293864770260 ) ) ;
#191708=CARTESIAN_POINT ( 'NONE',  ( -21.55341960407619339, 5.719274019375674811, 108.5427570613523756 ) ) ;
#191710=CARTESIAN_POINT ( 'NONE',  ( 5.153800228976335163, 19.02544592524342804, 64.79057627198100988 ) ) ;
#191712=CARTESIAN_POINT ( 'NONE',  ( 19.05341960407611168, 5.049401038298154454, 93.95724293864769550 ) ) ;
#191714=CARTESIAN_POINT ( 'NONE',  ( -10.81492255796105439, 18.62759615963255655, 27.91775706135234358 ) ) ;
#191715=CARTESIAN_POINT ( 'NONE',  ( 12.14591786802309770, 12.06949235617756955, 94.37390960531436690 ) ) ;
#191716=CARTESIAN_POINT ( 'NONE',  ( 0.05219959533907565091, 21.53943276465977519, 89.99890960531438111 ) ) ;
#191717=CARTESIAN_POINT ( 'NONE',  ( -5.153800228976328057, -19.02544592524343514, 67.29057627198102409 ) ) ;
#191718=CARTESIAN_POINT ( 'NONE',  ( 5.153800228976335163, 19.02544592524342804, 89.79057627198102409 ) ) ;
#191719=CARTESIAN_POINT ( 'NONE',  ( 18.62759615963271287, -10.81492255796078972, 108.3322429386477097 ) ) ;
#191721=CARTESIAN_POINT ( 'NONE',  ( -0.05219959533909027116, -19.03943276465977164, 67.49890960531436690 ) ) ;
#191723=CARTESIAN_POINT ( 'NONE',  ( 18.87580814761077974, -5.499999999999959144, 98.37172394265762421 ) ) ;
#191724=CARTESIAN_POINT ( 'NONE',  ( -16.53943276465976808, 0.05219959533911058130, 106.2489096053143811 ) ) ;
#191725=CARTESIAN_POINT ( 'NONE',  ( 19.03943276465977164, -0.05219959533909143690, 28.74890960531435624 ) ) ;
#191726=CARTESIAN_POINT ( 'NONE',  ( 19.02544592524334988, 5.153800228976608722, 91.45942372801900433 ) ) ;
#191727=CARTESIAN_POINT ( 'NONE',  ( -14.29746914071049879, 8.314922557960819915, 105.8322429386476955 ) ) ;
#191728=CARTESIAN_POINT ( 'NONE',  ( -15.80617190586768217, 15.72974639402176855, 78.12609039468570415 ) ) ;
#191729=CARTESIAN_POINT ( 'NONE',  ( -9.564922557960796823, -16.46253265017161027, 57.08224293864769550 ) ) ;
#191730=CARTESIAN_POINT ( 'NONE',  ( 5.823673210054444382, -21.52544592524334988, 35.20942372801901854 ) ) ;
#191731=CARTESIAN_POINT ( 'NONE',  ( 18.62759615963271287, -10.81492255796078972, 108.3322429386477097 ) ) ;
#191733=CARTESIAN_POINT ( 'NONE',  ( 16.51473224551069308, 9.474510206698969483, 79.16557627198103830 ) ) ;
#191735=CARTESIAN_POINT ( 'NONE',  ( -12.14591786802326823, 12.06949235617739902, 23.12609039468567573 ) ) ;
#191736=CARTESIAN_POINT ( 'NONE',  ( -21.53943276465977519, 0.05219959533907696930, 26.24890960531435624 ) ) ;
#191737=CARTESIAN_POINT ( 'NONE',  ( 10.72451020669871369, 18.67979575497193778, 62.08442372801901143 ) ) ;
#191738=CARTESIAN_POINT ( 'NONE',  ( 16.51473224551069308, 9.474510206698969483, 114.1655762719810241 ) ) ;
#191739=CARTESIAN_POINT ( 'NONE',  ( -13.89961937509957401, -13.97604488694547875, 99.37609039468567573 ) ) ;
#191740=CARTESIAN_POINT ( 'NONE',  ( -13.97604488694527625, -13.89961937509977652, 46.87390960531435979 ) ) ;
#191741=CARTESIAN_POINT ( 'NONE',  ( 19.03943276465977164, -0.05219959533909143690, 73.74890960531435269 ) ) ;
#191743=CARTESIAN_POINT ( 'NONE',  ( 0.05219959533910956823, 16.53943276465976808, 89.99890960531438111 ) ) ;
#191744=CARTESIAN_POINT ( 'NONE',  ( -19.02544592524342804, 5.153800228976336051, 101.0405762719810241 ) ) ;
#191745=CARTESIAN_POINT ( 'NONE',  ( -0.05219959533910754901, -16.53943276465976808, 97.49890960531436690 ) ) ;
#191746=CARTESIAN_POINT ( 'NONE',  ( 16.51473224551069308, 9.474510206698969483, 104.1655762719810241 ) ) ;
#191747=CARTESIAN_POINT ( 'NONE',  ( 12.14591786802309770, 12.06949235617756955, 59.37390960531436690 ) ) ;
#191748=CARTESIAN_POINT ( 'NONE',  ( 0.05219959533909260263, 19.03943276465977164, 34.99890960531435979 ) ) ;
#191749=CARTESIAN_POINT ( 'NONE',  ( -10.72451020669870658, -18.67979575497194134, 54.58442372801901143 ) ) ;
#191750=CARTESIAN_POINT ( 'NONE',  ( -16.46253265017146816, -9.564922557961047289, 94.16775706135233293 ) ) ;
#191751=CARTESIAN_POINT ( 'NONE',  ( -12.06949235617756955, 12.14591786802309770, 50.62390960531435979 ) ) ;
#191752=CARTESIAN_POINT ( 'NONE',  ( 15.72974639402199770, -15.80617190586745480, 108.1239096053143811 ) ) ;
#191753=CARTESIAN_POINT ( 'NONE',  ( -5.823673210054116645, -21.52544592524344225, 52.29057627198102409 ) ) ;
#191754=CARTESIAN_POINT ( 'NONE',  ( 19.52851543214744012, 5.500000000000032863, 72.89357721762576148 ) ) ;
#191755=CARTESIAN_POINT ( 'NONE',  ( -8.224510206698948167, 14.34966873604960824, 85.41557627198102409 ) ) ;
#191757=CARTESIAN_POINT ( 'NONE',  ( 0.05219959533909260263, 19.03943276465977164, 59.99890960531436690 ) ) ;
#191758=CARTESIAN_POINT ( 'NONE',  ( 8.314922557961029526, -14.29746914071037800, 110.4177570613523756 ) ) ;
#191759=CARTESIAN_POINT ( 'NONE',  ( 8.314922557961029526, -14.29746914071037800, 105.4177570613523613 ) ) ;
#191760=CARTESIAN_POINT ( 'NONE',  ( -14.34966873604972548, 8.224510206698743886, 83.33442372801903275 ) ) ;
#191761=CARTESIAN_POINT ( 'NONE',  ( 5.153800228976615827, -19.02544592524334988, 40.20942372801898301 ) ) ;
#191762=CARTESIAN_POINT ( 'NONE',  ( -17.26172910966779028, 6.454744622555852018, 70.80646908649224258 ) ) ;
#191763=CARTESIAN_POINT ( 'NONE',  ( -0.05219959533909027116, -19.03943276465977164, 92.49890960531436690 ) ) ;
#191764=CARTESIAN_POINT ( 'NONE',  ( -13.97604488694527625, -13.89961937509977652, 41.87390960531435979 ) ) ;
#191765=CARTESIAN_POINT ( 'NONE',  ( 4.483927247898545687, 16.52544592524342804, 59.79057627198103120 ) ) ;
#191767=CARTESIAN_POINT ( 'NONE',  ( -9.474510206698964154, 16.51473224551069663, 105.4155762719810383 ) ) ;
#191768=CARTESIAN_POINT ( 'NONE',  ( 18.67979575497178502, 10.72451020669898547, 39.16557627198102409 ) ) ;
#191769=CARTESIAN_POINT ( 'NONE',  ( -16.52544592524342804, 4.483927247898546575, 81.04057627198102409 ) ) ;
#191770=CARTESIAN_POINT ( 'NONE',  ( -16.53943276465976808, -0.05219959533934237506, 43.75109039468568284 ) ) ;
#191772=CARTESIAN_POINT ( 'NONE',  ( -16.53943276465976808, 0.05219959533911058130, 81.24890960531436690 ) ) ;
#191774=CARTESIAN_POINT ( 'NONE',  ( 19.02544592524334988, 5.153800228976608722, 71.45942372801900433 ) ) ;
#191775=CARTESIAN_POINT ( 'NONE',  ( 5.153800228976335163, 19.02544592524342804, 104.7905762719809957 ) ) ;
#191776=CARTESIAN_POINT ( 'NONE',  ( -13.97604488694547697, 13.89961937509957934, 73.12609039468568994 ) ) ;
#191778=CARTESIAN_POINT ( 'NONE',  ( 14.29746914071037800, 8.314922557961029526, 31.66775706135234358 ) ) ;
#191779=CARTESIAN_POINT ( 'NONE',  ( -14.34966873604972548, 8.224510206698743886, 103.3344237280190043 ) ) ;
#191781=CARTESIAN_POINT ( 'NONE',  ( -19.02544592524334988, -5.153800228976617603, 68.95942372801896170 ) ) ;
#191782=CARTESIAN_POINT ( 'NONE',  ( 5.719274019375991003, -21.55341960407610458, 32.70724293864770260 ) ) ;
#191783=CARTESIAN_POINT ( 'NONE',  ( -15.72974639402176322, -15.80617190586768395, 74.37609039468568994 ) ) ;
#191784=CARTESIAN_POINT ( 'NONE',  ( 18.41295718396490955, 5.500000000000055955, 38.98231844820842440 ) ) ;
#191785=CARTESIAN_POINT ( 'NONE',  ( 14.29746914071037800, 8.314922557961029526, 21.66775706135235069 ) ) ;
#191786=CARTESIAN_POINT ( 'NONE',  ( 19.02544592524343514, -5.153800228976328945, 28.54057627198102409 ) ) ;
#191787=CARTESIAN_POINT ( 'NONE',  ( -19.02544592524342804, 5.153800228976336051, 86.04057627198103830 ) ) ;
#191788=CARTESIAN_POINT ( 'NONE',  ( 16.51473224551069308, 9.474510206698969483, 24.16557627198102765 ) ) ;
#191789=CARTESIAN_POINT ( 'NONE',  ( -16.52544592524342804, 4.483927247898546575, 91.04057627198103830 ) ) ;
#191790=CARTESIAN_POINT ( 'NONE',  ( 5.049401038298161559, -19.05341960407611168, 87.70724293864769550 ) ) ;
#191791=CARTESIAN_POINT ( 'NONE',  ( -5.049401038298153566, 19.05341960407611168, 90.20724293864766707 ) ) ;
#191793=CARTESIAN_POINT ( 'NONE',  ( 0.05219959533936267826, -19.03943276465977164, 85.00109039468567573 ) ) ;
#191794=CARTESIAN_POINT ( 'NONE',  ( -5.823673210054116645, -21.52544592524344225, 77.29057627198102409 ) ) ;
#191795=CARTESIAN_POINT ( 'NONE',  ( 16.51473224551069308, 9.474510206698969483, 29.16557627198103475 ) ) ;
#191796=CARTESIAN_POINT ( 'NONE',  ( 13.97604488694548053, -13.89961937509957401, 70.62609039468567573 ) ) ;
#191797=CARTESIAN_POINT ( 'NONE',  ( -10.72451020669898014, 18.67979575497178502, 110.4155762719810383 ) ) ;
#191798=CARTESIAN_POINT ( 'NONE',  ( 19.03943276465977164, -0.05219959533909143690, 68.74890960531436690 ) ) ;
#191799=CARTESIAN_POINT ( 'NONE',  ( 5.049401038298161559, -19.05341960407611168, 102.7072429386476955 ) ) ;
#191801=CARTESIAN_POINT ( 'NONE',  ( -0.05219959533907301413, -21.53943276465977519, 102.4989096053143811 ) ) ;
#191802=CARTESIAN_POINT ( 'NONE',  ( -16.55341960407611168, -4.379528057220339221, 101.4572429386476955 ) ) ;
#191803=CARTESIAN_POINT ( 'NONE',  ( 16.51473224551069308, 9.474510206698969483, 84.16557627198102409 ) ) ;
#191804=CARTESIAN_POINT ( 'NONE',  ( 19.05341960407617918, -5.049401038297876454, 56.04275706135234714 ) ) ;
#191805=CARTESIAN_POINT ( 'NONE',  ( 10.72451020669898902, -18.67979575497178502, 87.91557627198103830 ) ) ;
#191806=CARTESIAN_POINT ( 'NONE',  ( -10.81492255796078084, -18.62759615963271287, 77.08224293864769550 ) ) ;
#191807=CARTESIAN_POINT ( 'NONE',  ( -0.05219959533910754901, -16.53943276465976808, 42.49890960531435979 ) ) ;
#191808=CARTESIAN_POINT ( 'NONE',  ( -16.46253265017146816, -9.564922557961047289, 29.16775706135232937 ) ) ;
#191809=CARTESIAN_POINT ( 'NONE',  ( -0.05219959533934338120, 16.53943276465976808, 67.50109039468568994 ) ) ;
#191810=CARTESIAN_POINT ( 'NONE',  ( -16.51473224551069308, -9.474510206698971260, 96.66557627198102409 ) ) ;
#191811=CARTESIAN_POINT ( 'NONE',  ( -9.474510206698964154, 16.51473224551069663, 40.41557627198103120 ) ) ;
#191812=AXIS2_PLACEMENT_3D ( 'NONE', #128190, #177717, #39185 ) ;
#191813=CARTESIAN_POINT ( 'NONE',  ( -21.52544592524334988, -5.823673210054445271, 58.95942372801902565 ) ) ;
#191814=CARTESIAN_POINT ( 'NONE',  ( -5.719274019375665041, -21.55341960407619695, 49.79275706135234714 ) ) ;
#191815=CARTESIAN_POINT ( 'NONE',  ( 16.51473224551069308, 9.474510206698969483, 64.16557627198102409 ) ) ;
#191816=CARTESIAN_POINT ( 'NONE',  ( 18.67979575497194134, -10.72451020669871369, 40.83442372801901854 ) ) ;
#191817=ADVANCED_FACE ( 'NONE', ( #70039 ), #191377, .F. ) ;
#191818=CARTESIAN_POINT ( 'NONE',  ( 5.153800228976615827, -19.02544592524334988, 80.20942372801901854 ) ) ;
#191819=CARTESIAN_POINT ( 'NONE',  ( -9.474510206698720793, -16.51473224551083518, 74.58442372801900433 ) ) ;
#191820=CARTESIAN_POINT ( 'NONE',  ( 13.89961937509977652, -13.97604488694527269, 43.12390960531434558 ) ) ;
#191821=CARTESIAN_POINT ( 'NONE',  ( 8.224510206698742110, 14.34966873604972548, 82.08442372801901854 ) ) ;
#191822=CARTESIAN_POINT ( 'NONE',  ( 16.46253265017160672, -9.564922557960803928, 48.33224293864769550 ) ) ;
#191824=CARTESIAN_POINT ( 'NONE',  ( -13.89961937509977652, 13.97604488694528158, 100.6239096053143669 ) ) ;
#191825=CARTESIAN_POINT ( 'NONE',  ( -5.153800228976328057, -19.02544592524343514, 42.29057627198101699 ) ) ;
#191826=CARTESIAN_POINT ( 'NONE',  ( 0.05219959533907565091, 21.53943276465977519, 79.99890960531435269 ) ) ;
#191827=CARTESIAN_POINT ( 'NONE',  ( 14.34966873604972726, -8.224510206698740333, 65.83442372801900433 ) ) ;
#191828=CARTESIAN_POINT ( 'NONE',  ( 15.72974639402176855, 15.80617190586768217, 106.8760903946856899 ) ) ;
#191829=CARTESIAN_POINT ( 'NONE',  ( 13.97604488694527802, 13.89961937509977652, 54.37390960531435979 ) ) ;
#191830=CARTESIAN_POINT ( 'NONE',  ( -16.52544592524342804, 4.483927247898546575, 46.04057627198103830 ) ) ;
#191831=CARTESIAN_POINT ( 'NONE',  ( 4.379528057220339221, -16.55341960407611168, 87.70724293864769550 ) ) ;
#191832=CARTESIAN_POINT ( 'NONE',  ( 13.89961937509977652, -13.97604488694527269, 73.12390960531436690 ) ) ;
#191833=CARTESIAN_POINT ( 'NONE',  ( 18.67979575497194134, -10.72451020669871369, 35.83442372801901143 ) ) ;
#191834=CARTESIAN_POINT ( 'NONE',  ( 19.03943276465977164, -0.05219959533909143690, 93.74890960531435269 ) ) ;
#191835=CARTESIAN_POINT ( 'NONE',  ( -5.823673210054431948, 21.52544592524334988, 102.7094237280190185 ) ) ;
#191836=CARTESIAN_POINT ( 'NONE',  ( 16.55341960407618274, -4.379528057220086978, 61.04275706135234714 ) ) ;
#191837=CARTESIAN_POINT ( 'NONE',  ( 15.72974639402176855, 15.80617190586768217, 26.87609039468567218 ) ) ;
#191838=CARTESIAN_POINT ( 'NONE',  ( 19.02544592524343514, -5.153800228976328945, 113.5405762719810241 ) ) ;
#191839=CARTESIAN_POINT ( 'NONE',  ( -21.52544592524343514, 5.823673210054127303, 96.04057627198102409 ) ) ;
#191840=CARTESIAN_POINT ( 'NONE',  ( 16.52544592524342804, -4.483927247898539470, 48.54057627198103120 ) ) ;
#191841=CARTESIAN_POINT ( 'NONE',  ( -0.05219959533909027116, -19.03943276465977164, 42.49890960531435269 ) ) ;
#191842=CARTESIAN_POINT ( 'NONE',  ( 8.224510206698953496, -14.34966873604960469, 62.91557627198102409 ) ) ;
#191843=CARTESIAN_POINT ( 'NONE',  ( -21.52544592524343514, 5.823673210054127303, 26.04057627198103475 ) ) ;
#191844=CARTESIAN_POINT ( 'NONE',  ( 13.89961937509957401, 13.97604488694547697, 36.87609039468565442 ) ) ;
#191845=CARTESIAN_POINT ( 'NONE',  ( 14.34966873604960469, 8.224510206698951720, 104.1655762719810241 ) ) ;
#191846=CARTESIAN_POINT ( 'NONE',  ( 16.51473224551069308, 9.474510206698969483, 109.1655762719810383 ) ) ;
#191848=CARTESIAN_POINT ( 'NONE',  ( 12.14591786802327356, -12.06949235617739191, 50.62609039468568994 ) ) ;
#191849=CARTESIAN_POINT ( 'NONE',  ( -13.97604488694527625, -13.89961937509977652, 51.87390960531436690 ) ) ;
#191851=CARTESIAN_POINT ( 'NONE',  ( 4.483927247898790824, -16.52544592524335698, 90.20942372801903275 ) ) ;
#191852=CARTESIAN_POINT ( 'NONE',  ( -19.02544592524334988, -5.153800228976617603, 103.9594237280190043 ) ) ;
#191853=CARTESIAN_POINT ( 'NONE',  ( 15.80617190586769283, -15.72974639402175789, 75.62609039468567573 ) ) ;
#191854=CARTESIAN_POINT ( 'NONE',  ( -16.46253265017160317, 9.564922557960807481, 75.83224293864769550 ) ) ;
#191855=CARTESIAN_POINT ( 'NONE',  ( -21.52544592524343514, 5.823673210054127303, 106.0405762719810525 ) ) ;
#191856=CARTESIAN_POINT ( 'NONE',  ( -4.379528057220086978, -16.55341960407618274, 39.79275706135235424 ) ) ;
#191857=CARTESIAN_POINT ( 'NONE',  ( -0.05219959533910754901, -16.53943276465976808, 107.4989096053143669 ) ) ;
#191858=CARTESIAN_POINT ( 'NONE',  ( -16.53943276465976808, -0.05219959533934237506, 23.75109039468567929 ) ) ;
#191859=CARTESIAN_POINT ( 'NONE',  ( -9.564922557961040184, 16.46253265017147172, 77.91775706135234714 ) ) ;
#191860=CARTESIAN_POINT ( 'NONE',  ( -10.81492255796078084, -18.62759615963271287, 77.08224293864769550 ) ) ;
#191861=CARTESIAN_POINT ( 'NONE',  ( 13.97604488694548053, -13.89961937509957401, 55.62609039468566863 ) ) ;
#191862=CARTESIAN_POINT ( 'NONE',  ( -19.05341960407611168, -5.049401038298163336, 111.4572429386476671 ) ) ;
#191863=CARTESIAN_POINT ( 'NONE',  ( 5.719274019375991003, -21.55341960407610458, 107.7072429386476955 ) ) ;
#191864=CARTESIAN_POINT ( 'NONE',  ( 17.49999999999999645, 5.068104630630399399, 26.77181594659973030 ) ) ;
#191865=CARTESIAN_POINT ( 'NONE',  ( 5.153800228976335163, 19.02544592524342804, 64.79057627198100988 ) ) ;
#191866=DIRECTION ( 'NONE',  ( -1.000000000000000000, -0.000000000000000000, -0.000000000000000000 ) ) ;
#191867=CARTESIAN_POINT ( 'NONE',  ( -5.049401038297874678, -19.05341960407617918, 109.7927570613523187 ) ) ;
#191869=CARTESIAN_POINT ( 'NONE',  ( -10.72451020669870658, -18.67979575497194134, 59.58442372801901854 ) ) ;
#191870=CARTESIAN_POINT ( 'NONE',  ( 0.05219959533907565091, 21.53943276465977519, 109.9989096053143527 ) ) ;
#191871=CARTESIAN_POINT ( 'NONE',  ( 14.34966873604960469, 8.224510206698951720, 69.16557627198102409 ) ) ;
#191872=CARTESIAN_POINT ( 'NONE',  ( 5.153800228976335163, 19.02544592524342804, 69.79057627198103830 ) ) ;
#191873=CARTESIAN_POINT ( 'NONE',  ( 0.05219959533937995610, -21.53943276465977519, 70.00109039468568994 ) ) ;
#191874=CARTESIAN_POINT ( 'NONE',  ( -8.224510206698735004, -14.34966873604973081, 19.58442372801901143 ) ) ;
#191875=CARTESIAN_POINT ( 'NONE',  ( 16.51473224551083163, -9.474510206698727899, 25.83442372801900078 ) ) ;
#191876=CARTESIAN_POINT ( 'NONE',  ( 5.719274019375673035, 21.55341960407619339, 37.29275706135235424 ) ) ;
#191877=CARTESIAN_POINT ( 'NONE',  ( -18.62759615963255300, -10.81492255796106328, 19.16775706135234714 ) ) ;
#191878=CARTESIAN_POINT ( 'NONE',  ( 5.719274019375991003, -21.55341960407610458, 57.70724293864770260 ) ) ;
#191879=CARTESIAN_POINT ( 'NONE',  ( 9.564922557961047289, -16.46253265017146816, 100.4177570613523329 ) ) ;
#191880=CARTESIAN_POINT ( 'NONE',  ( 9.564922557961047289, -16.46253265017146816, 70.41775706135233293 ) ) ;
#191881=CARTESIAN_POINT ( 'NONE',  ( -5.823673210054431948, 21.52544592524334988, 82.70942372801900433 ) ) ;
#191882=CARTESIAN_POINT ( 'NONE',  ( 9.474510206698729675, 16.51473224551082808, 47.08442372801900433 ) ) ;
#191883=CARTESIAN_POINT ( 'NONE',  ( -13.89961937509977652, 13.97604488694528158, 40.62390960531435979 ) ) ;
#191884=CARTESIAN_POINT ( 'NONE',  ( -21.52544592524343514, 5.823673210054127303, 51.04057627198103120 ) ) ;
#191885=CARTESIAN_POINT ( 'NONE',  ( 4.379528057220339221, -16.55341960407611168, 52.70724293864769550 ) ) ;
#191887=CARTESIAN_POINT ( 'NONE',  ( -13.97604488694547697, 13.89961937509957934, 28.12609039468565797 ) ) ;
#191888=CARTESIAN_POINT ( 'NONE',  ( 14.34966873604972726, -8.224510206698740333, 90.83442372801901854 ) ) ;
#191889=CARTESIAN_POINT ( 'NONE',  ( -14.34966873604960291, -8.224510206698953496, 36.66557627198103120 ) ) ;
#191890=CARTESIAN_POINT ( 'NONE',  ( -15.72974639402176322, -15.80617190586768395, 79.37609039468567573 ) ) ;
#191891=CARTESIAN_POINT ( 'NONE',  ( 21.52544592524334988, 5.823673210054432836, 86.45942372801901854 ) ) ;
#191892=CARTESIAN_POINT ( 'NONE',  ( 21.53943276465977519, -0.05219959533907433946, 78.74890960531436690 ) ) ;
#191893=CARTESIAN_POINT ( 'NONE',  ( -16.51473224551069308, -9.474510206698971260, 36.66557627198102409 ) ) ;
#191894=CARTESIAN_POINT ( 'NONE',  ( -21.53943276465977519, -0.05219959533937600094, 58.75109039468568994 ) ) ;
#191895=CARTESIAN_POINT ( 'NONE',  ( -16.51473224551069308, -9.474510206698971260, 41.66557627198103120 ) ) ;
#191896=CARTESIAN_POINT ( 'NONE',  ( -0.05219959533909027116, -19.03943276465977164, 57.49890960531435979 ) ) ;
#191897=CARTESIAN_POINT ( 'NONE',  ( -4.483927247898539470, -16.52544592524342804, 112.2905762719810241 ) ) ;
#191898=CARTESIAN_POINT ( 'NONE',  ( 5.049401038298161559, -19.05341960407611168, 102.7072429386476955 ) ) ;
#191899=CARTESIAN_POINT ( 'NONE',  ( 8.224510206698953496, -14.34966873604960469, 42.91557627198103120 ) ) ;
#191900=CARTESIAN_POINT ( 'NONE',  ( -13.97604488694527625, -13.89961937509977652, 21.87390960531435979 ) ) ;
#191901=CARTESIAN_POINT ( 'NONE',  ( -18.67979575497178146, -10.72451020669898902, 81.66557627198103830 ) ) ;
#191902=CARTESIAN_POINT ( 'NONE',  ( 18.67979575497178502, 10.72451020669898547, 114.1655762719810383 ) ) ;
#191904=CARTESIAN_POINT ( 'NONE',  ( 16.52544592524335698, 4.483927247898782831, 41.45942372801901143 ) ) ;
#191906=CARTESIAN_POINT ( 'NONE',  ( -10.72451020669898014, 18.67979575497178502, 65.41557627198102409 ) ) ;
#191907=CARTESIAN_POINT ( 'NONE',  ( -10.72451020669870658, -18.67979575497194134, 94.58442372801901854 ) ) ;
#191908=CARTESIAN_POINT ( 'NONE',  ( -9.474510206698964154, 16.51473224551069663, 95.41557627198102409 ) ) ;
#191909=CARTESIAN_POINT ( 'NONE',  ( 10.81492255796106328, -18.62759615963255655, 25.41775706135235779 ) ) ;
#191911=CARTESIAN_POINT ( 'NONE',  ( -15.72974639402197994, 15.80617190586746368, 25.62390960531435624 ) ) ;
#191912=CARTESIAN_POINT ( 'NONE',  ( 0.05219959533934541429, -16.53943276465976808, 85.00109039468568994 ) ) ;
#191913=CARTESIAN_POINT ( 'NONE',  ( -21.55341960407619339, 5.719274019375674811, 68.54275706135234714 ) ) ;
#191914=CARTESIAN_POINT ( 'NONE',  ( -5.823673210054431948, 21.52544592524334988, 112.7094237280190328 ) ) ;
#191915=CARTESIAN_POINT ( 'NONE',  ( -14.34966873604972548, 8.224510206698743886, 78.33442372801901854 ) ) ;
#191916=CARTESIAN_POINT ( 'NONE',  ( 18.67979575497194134, -10.72451020669871369, 25.83442372801901499 ) ) ;
#191918=CARTESIAN_POINT ( 'NONE',  ( 9.564922557960805705, 16.46253265017160317, 29.58224293864769550 ) ) ;
#191919=CARTESIAN_POINT ( 'NONE',  ( -5.719274019375665041, -21.55341960407619695, 99.79275706135234714 ) ) ;
#191920=CARTESIAN_POINT ( 'NONE',  ( -19.03943276465977164, 0.05219959533909376836, 111.2489096053143669 ) ) ;
#191921=CARTESIAN_POINT ( 'NONE',  ( 5.719274019375991003, -21.55341960407610458, 97.70724293864772392 ) ) ;
#191922=CARTESIAN_POINT ( 'NONE',  ( -15.72974639402197994, 15.80617190586746368, 60.62390960531437401 ) ) ;
#191923=CARTESIAN_POINT ( 'NONE',  ( -0.05219959533934338120, 16.53943276465976808, 47.50109039468568994 ) ) ;
#191924=CARTESIAN_POINT ( 'NONE',  ( 8.314922557960818139, 14.29746914071049879, 49.58224293864769550 ) ) ;
#191925=LINE ( 'NONE', #53409, #195241 ) ;
#191926=CARTESIAN_POINT ( 'NONE',  ( -19.03943276465977164, -0.05219959533935918106, 78.75109039468567573 ) ) ;
#191928=CARTESIAN_POINT ( 'NONE',  ( -17.48853670773245739, 5.747243402303086945, 103.6667129974999568 ) ) ;
#191929=CARTESIAN_POINT ( 'NONE',  ( -14.29746914071037622, -8.314922557961029526, 29.16775706135234003 ) ) ;
#191930=CARTESIAN_POINT ( 'NONE',  ( -0.05219959533907301413, -21.53943276465977519, 82.49890960531436690 ) ) ;
#191931=CARTESIAN_POINT ( 'NONE',  ( 16.55341960407611168, 4.379528057220329451, 68.95724293864769550 ) ) ;
#191932=CARTESIAN_POINT ( 'NONE',  ( -9.474510206698964154, 16.51473224551069663, 100.4155762719810241 ) ) ;
#191933=CARTESIAN_POINT ( 'NONE',  ( -8.314922557961024197, 14.29746914071037800, 42.91775706135235424 ) ) ;
#191934=CARTESIAN_POINT ( 'NONE',  ( 19.05341960407611168, 5.049401038298154454, 58.95724293864768129 ) ) ;
#191935=CARTESIAN_POINT ( 'NONE',  ( -15.80617190586768217, 15.72974639402176855, 23.12609039468567573 ) ) ;
#191936=CARTESIAN_POINT ( 'NONE',  ( 19.02544592524334988, 5.153800228976608722, 101.4594237280189759 ) ) ;
#191937=CARTESIAN_POINT ( 'NONE',  ( 9.474510206698971260, -16.51473224551069308, 92.91557627198103830 ) ) ;
#191938=CARTESIAN_POINT ( 'NONE',  ( 0.05219959533909260263, 19.03943276465977164, 84.99890960531436690 ) ) ;
#191939=CARTESIAN_POINT ( 'NONE',  ( 21.53943276465977519, -0.05219959533907433946, 93.74890960531436690 ) ) ;
#191940=CARTESIAN_POINT ( 'NONE',  ( -13.97604488694527625, -13.89961937509977652, 41.87390960531435979 ) ) ;
#191941=CARTESIAN_POINT ( 'NONE',  ( -16.52544592524342804, 4.483927247898546575, 66.04057627198103830 ) ) ;
#191942=CARTESIAN_POINT ( 'NONE',  ( 9.564922557960805705, 16.46253265017160317, 104.5822429386476955 ) ) ;
#191944=CARTESIAN_POINT ( 'NONE',  ( 16.51473224551083163, -9.474510206698727899, 75.83442372801900433 ) ) ;
#191945=CARTESIAN_POINT ( 'NONE',  ( 0.05219959533907565091, 21.53943276465977519, 84.99890960531436690 ) ) ;
#191946=CARTESIAN_POINT ( 'NONE',  ( -19.03943276465977164, -0.05219959533935918106, 43.75109039468566863 ) ) ;
#191947=CARTESIAN_POINT ( 'NONE',  ( -19.02544592524342804, 5.153800228976336051, 106.0405762719810241 ) ) ;
#191949=CARTESIAN_POINT ( 'NONE',  ( -18.67979575497178146, -10.72451020669898902, 46.66557627198102409 ) ) ;
#191951=CARTESIAN_POINT ( 'NONE',  ( -13.89961937509977652, 13.97604488694528158, 80.62390960531436690 ) ) ;
#191952=CARTESIAN_POINT ( 'NONE',  ( -5.719274019375665041, -21.55341960407619695, 69.79275706135234714 ) ) ;
#191953=CARTESIAN_POINT ( 'NONE',  ( 5.049401038298161559, -19.05341960407611168, 42.70724293864767418 ) ) ;
#191954=CARTESIAN_POINT ( 'NONE',  ( -16.52544592524342804, 4.483927247898546575, 71.04057627198103830 ) ) ;
#191955=CARTESIAN_POINT ( 'NONE',  ( -4.483927247898782831, 16.52544592524335698, 22.70942372801901499 ) ) ;
#191956=CARTESIAN_POINT ( 'NONE',  ( 0.05219959533937995610, -21.53943276465977519, 55.00109039468568284 ) ) ;
#191958=CARTESIAN_POINT ( 'NONE',  ( -13.97604488694527625, -13.89961937509977652, 111.8739096053143243 ) ) ;
#191959=CARTESIAN_POINT ( 'NONE',  ( -5.153800228976607833, 19.02544592524334988, 67.70942372801900433 ) ) ;
#191961=CARTESIAN_POINT ( 'NONE',  ( -21.55341960407619339, 5.719274019375674811, 23.54275706135235424 ) ) ;
#191962=CARTESIAN_POINT ( 'NONE',  ( 17.50000000000000000, 5.499999999999997335, 120.0000000000000142 ) ) ;
#191963=CARTESIAN_POINT ( 'NONE',  ( 5.049401038297881783, 19.05341960407617563, 22.29275706135233648 ) ) ;
#191964=CARTESIAN_POINT ( 'NONE',  ( -19.05341960407611168, -5.049401038298163336, 51.45724293864770260 ) ) ;
#191965=CARTESIAN_POINT ( 'NONE',  ( -5.719274019375665041, -21.55341960407619695, 109.7927570613523613 ) ) ;
#191966=CARTESIAN_POINT ( 'NONE',  ( -14.29746914071037622, -8.314922557961029526, 109.1677570613523613 ) ) ;
#191967=CARTESIAN_POINT ( 'NONE',  ( 16.51473224551069308, 9.474510206698969483, 109.1655762719810383 ) ) ;
#191968=CARTESIAN_POINT ( 'NONE',  ( 21.52544592524334988, 5.823673210054432836, 71.45942372801901854 ) ) ;
#191970=CARTESIAN_POINT ( 'NONE',  ( 19.03943276465977164, -0.05219959533909143690, 113.7489096053143669 ) ) ;
#191972=CARTESIAN_POINT ( 'NONE',  ( -0.05219959533937732626, 21.53943276465977519, 77.50109039468567573 ) ) ;
#191973=CARTESIAN_POINT ( 'NONE',  ( 18.62759615963255655, 10.81492255796105972, 96.66775706135234714 ) ) ;
#191975=CARTESIAN_POINT ( 'NONE',  ( -19.03943276465977164, 0.05219959533909376836, 86.24890960531436690 ) ) ;
#191978=CARTESIAN_POINT ( 'NONE',  ( 19.03943276465977164, -0.05219959533909143690, 38.74890960531436690 ) ) ;
#191979=CARTESIAN_POINT ( 'NONE',  ( 5.719274019375991003, -21.55341960407610458, 52.70724293864769550 ) ) ;
#191980=CARTESIAN_POINT ( 'NONE',  ( -8.314922557961024197, 14.29746914071037800, 102.9177570613523756 ) ) ;
#191981=CARTESIAN_POINT ( 'NONE',  ( -8.314922557960811034, -14.29746914071050412, 97.08224293864770971 ) ) ;
#191982=CARTESIAN_POINT ( 'NONE',  ( -13.97604488694527625, -13.89961937509977652, 81.87390960531436690 ) ) ;
#191983=CARTESIAN_POINT ( 'NONE',  ( 18.62759615963255655, 10.81492255796105972, 106.6677570613523756 ) ) ;
#191984=CARTESIAN_POINT ( 'NONE',  ( -0.05219959533909027116, -19.03943276465977164, 37.49890960531436690 ) ) ;
#191985=CARTESIAN_POINT ( 'NONE',  ( 8.224510206698953496, -14.34966873604960469, 87.91557627198103830 ) ) ;
#191986=CARTESIAN_POINT ( 'NONE',  ( -21.52544592524334988, -5.823673210054445271, 48.95942372801902565 ) ) ;
#191987=CARTESIAN_POINT ( 'NONE',  ( -15.72974639402197994, 15.80617190586746368, 90.62390960531436690 ) ) ;
#191988=CARTESIAN_POINT ( 'NONE',  ( -19.03943276465977164, -0.05219959533935918106, 48.75109039468566863 ) ) ;
#191989=CARTESIAN_POINT ( 'NONE',  ( -9.564922557960796823, -16.46253265017161027, 47.08224293864769550 ) ) ;
#191990=CARTESIAN_POINT ( 'NONE',  ( -19.05341960407611168, -5.049401038298163336, 91.45724293864766707 ) ) ;
#191991=CARTESIAN_POINT ( 'NONE',  ( -4.483927247898539470, -16.52544592524342804, 57.29057627198103120 ) ) ;
#191992=CARTESIAN_POINT ( 'NONE',  ( 5.049401038297881783, 19.05341960407617563, 47.29275706135231161 ) ) ;
#191993=CARTESIAN_POINT ( 'NONE',  ( -16.46253265017160317, 9.564922557960807481, 50.83224293864770260 ) ) ;
#191994=CARTESIAN_POINT ( 'NONE',  ( -0.05219959533910754901, -16.53943276465976808, 47.49890960531435979 ) ) ;
#191995=CARTESIAN_POINT ( 'NONE',  ( -19.02544592524334988, -5.153800228976617603, 83.95942372801901854 ) ) ;
#191997=CARTESIAN_POINT ( 'NONE',  ( -15.72974639402197994, 15.80617190586746368, 30.62390960531436335 ) ) ;
#191998=EDGE_CURVE ( 'NONE', #141920, #170763, #72741, .T. ) ;
#191999=CARTESIAN_POINT ( 'NONE',  ( 8.314922557960818139, 14.29746914071049879, 104.5822429386477097 ) ) ;
#192001=CARTESIAN_POINT ( 'NONE',  ( 5.049401038298161559, -19.05341960407611168, 52.70724293864767418 ) ) ;
#192002=CARTESIAN_POINT ( 'NONE',  ( 18.62759615963271287, -10.81492255796078972, 53.33224293864769550 ) ) ;
#192003=CARTESIAN_POINT ( 'NONE',  ( 13.89961937509977652, -13.97604488694527269, 33.12390960531434558 ) ) ;
#192004=CARTESIAN_POINT ( 'NONE',  ( 16.53943276465976808, 0.05219959533934440121, 76.25109039468568994 ) ) ;
#192005=CARTESIAN_POINT ( 'NONE',  ( -19.02544592524342804, 5.153800228976336051, 56.04057627198100988 ) ) ;
#192006=CARTESIAN_POINT ( 'NONE',  ( 13.97604488694548053, -13.89961937509957401, 45.62609039468566863 ) ) ;
#192008=CARTESIAN_POINT ( 'NONE',  ( -5.823673210054431948, 21.52544592524334988, 72.70942372801901854 ) ) ;
#192009=CARTESIAN_POINT ( 'NONE',  ( -21.53943276465977519, 0.05219959533907696930, 56.24890960531436690 ) ) ;
#192010=CARTESIAN_POINT ( 'NONE',  ( 19.02544592524343514, -5.153800228976328945, 28.54057627198102409 ) ) ;
#192012=CARTESIAN_POINT ( 'NONE',  ( -13.89961937509957401, -13.97604488694547875, 104.3760903946856757 ) ) ;
#192015=CARTESIAN_POINT ( 'NONE',  ( -10.81492255796078084, -18.62759615963271287, 42.08224293864769550 ) ) ;
#192016=CARTESIAN_POINT ( 'NONE',  ( 16.61371651742598843, -7.165104196376269385, 66.35415069992994574 ) ) ;
#192017=CARTESIAN_POINT ( 'NONE',  ( -18.67979575497193778, 10.72451020669871902, 78.33442372801901854 ) ) ;
#192018=CARTESIAN_POINT ( 'NONE',  ( 14.29746914071049879, -8.314922557960816363, 48.33224293864770260 ) ) ;
#192019=CARTESIAN_POINT ( 'NONE',  ( 14.34966873604960469, 8.224510206698951720, 54.16557627198103120 ) ) ;
#192020=CARTESIAN_POINT ( 'NONE',  ( 21.52544592524344225, -5.823673210054117533, 83.54057627198102409 ) ) ;
#192021=CARTESIAN_POINT ( 'NONE',  ( -18.67979575497178146, -10.72451020669898902, 71.66557627198100988 ) ) ;
#192023=CARTESIAN_POINT ( 'NONE',  ( 15.80617190586746368, 15.72974639402197994, 34.37390960531435979 ) ) ;
#192024=CARTESIAN_POINT ( 'NONE',  ( -12.06949235617739369, -12.14591786802326823, 54.37609039468568994 ) ) ;
#192025=CARTESIAN_POINT ( 'NONE',  ( 16.53943276465976808, -0.05219959533910856209, 78.74890960531436690 ) ) ;
#192026=CARTESIAN_POINT ( 'NONE',  ( -19.02544592524342804, 5.153800228976336051, 66.04057627198103830 ) ) ;
#192027=CARTESIAN_POINT ( 'NONE',  ( 19.05341960407611168, 5.049401038298154454, 38.95724293864767418 ) ) ;
#192031=CARTESIAN_POINT ( 'NONE',  ( -14.34966873604972548, 8.224510206698743886, 78.33442372801901854 ) ) ;
#192032=CARTESIAN_POINT ( 'NONE',  ( 21.53943276465977519, 0.05219959533937863772, 21.25109039468567218 ) ) ;
#192033=CARTESIAN_POINT ( 'NONE',  ( 13.89961937509977652, -13.97604488694527269, 88.12390960531438111 ) ) ;
#192034=CARTESIAN_POINT ( 'NONE',  ( -21.53943276465977519, -0.05219959533937600094, 53.75109039468568994 ) ) ;
#192035=CARTESIAN_POINT ( 'NONE',  ( -16.46253265017160317, 9.564922557960807481, 110.8322429386476955 ) ) ;
#192039=CARTESIAN_POINT ( 'NONE',  ( 15.80617190586769283, -15.72974639402175789, 40.62609039468567573 ) ) ;
#192040=CARTESIAN_POINT ( 'NONE',  ( -16.51473224551069308, -9.474510206698971260, 41.66557627198103120 ) ) ;
#192041=CARTESIAN_POINT ( 'NONE',  ( 16.51473224551069308, 9.474510206698969483, 104.1655762719810241 ) ) ;
#192042=CARTESIAN_POINT ( 'NONE',  ( -16.51473224551082808, 9.474510206698731452, 53.33442372801900433 ) ) ;
#192043=CARTESIAN_POINT ( 'NONE',  ( -21.55341960407610458, -5.719274019375992779, 111.4572429386476813 ) ) ;
#192044=CARTESIAN_POINT ( 'NONE',  ( 5.049401038297881783, 19.05341960407617563, 42.29275706135234003 ) ) ;
#192045=CARTESIAN_POINT ( 'NONE',  ( -19.05341960407611168, -5.049401038298163336, 31.45724293864769550 ) ) ;
#192046=CARTESIAN_POINT ( 'NONE',  ( 14.29746914071037800, 8.314922557961029526, 96.66775706135234714 ) ) ;
#192047=CARTESIAN_POINT ( 'NONE',  ( 13.97604488694548053, -13.89961937509957401, 60.62609039468564731 ) ) ;
#192048=CARTESIAN_POINT ( 'NONE',  ( 16.53943276465976808, 0.05219959533934440121, 106.2510903946856757 ) ) ;
#192050=CARTESIAN_POINT ( 'NONE',  ( 19.02544592524343514, -5.153800228976328945, 83.54057627198100988 ) ) ;
#192051=CARTESIAN_POINT ( 'NONE',  ( 0.05219959533937995610, -21.53943276465977519, 95.00109039468568994 ) ) ;
#192052=CARTESIAN_POINT ( 'NONE',  ( 15.72974639402176855, 15.80617190586768217, 106.8760903946856899 ) ) ;
#192054=CARTESIAN_POINT ( 'NONE',  ( 9.474510206698971260, -16.51473224551069308, 107.9155762719810383 ) ) ;
#192055=CARTESIAN_POINT ( 'NONE',  ( 21.55341960407619695, -5.719274019375665929, 81.04275706135236135 ) ) ;
#192056=CARTESIAN_POINT ( 'NONE',  ( 19.02544592524334988, 5.153800228976608722, 111.4594237280190043 ) ) ;
#192057=CARTESIAN_POINT ( 'NONE',  ( -9.474510206698964154, 16.51473224551069663, 80.41557627198103830 ) ) ;
#192058=CARTESIAN_POINT ( 'NONE',  ( 5.823673210054125526, 21.52544592524343514, 24.79057627198103120 ) ) ;
#192059=CARTESIAN_POINT ( 'NONE',  ( -13.97604488694527625, -13.89961937509977652, 86.87390960531436690 ) ) ;
#192060=CARTESIAN_POINT ( 'NONE',  ( -16.79531203550648755, -7.028104445595603877, 91.25244988220444498 ) ) ;
#192061=CARTESIAN_POINT ( 'NONE',  ( 5.153800228976335163, 19.02544592524342804, 84.79057627198099567 ) ) ;
#192062=CARTESIAN_POINT ( 'NONE',  ( 13.89961937509977652, -13.97604488694527269, 68.12390960531436690 ) ) ;
#192063=CARTESIAN_POINT ( 'NONE',  ( -16.52544592524335698, -4.483927247898792601, 98.95942372801903275 ) ) ;
#192065=CARTESIAN_POINT ( 'NONE',  ( 19.02544592524334988, 5.153800228976608722, 61.45942372801900433 ) ) ;
#192066=CARTESIAN_POINT ( 'NONE',  ( -9.564922557960796823, -16.46253265017161027, 87.08224293864769550 ) ) ;
#192067=CARTESIAN_POINT ( 'NONE',  ( 12.14591786802309770, 12.06949235617756955, 79.37390960531436690 ) ) ;
#192068=CARTESIAN_POINT ( 'NONE',  ( -0.05219959533907301413, -21.53943276465977519, 37.49890960531436690 ) ) ;
#192070=CARTESIAN_POINT ( 'NONE',  ( 19.02544592524343514, -5.153800228976328945, 113.5405762719810241 ) ) ;
#192071=CARTESIAN_POINT ( 'NONE',  ( -14.34966873604960291, -8.224510206698953496, 86.66557627198102409 ) ) ;
#192073=CARTESIAN_POINT ( 'NONE',  ( -9.564922557961040184, 16.46253265017147172, 47.91775706135233293 ) ) ;
#192074=CARTESIAN_POINT ( 'NONE',  ( 16.52544592524342804, -4.483927247898539470, 28.54057627198103120 ) ) ;
#192075=CARTESIAN_POINT ( 'NONE',  ( -13.89961937509977652, 13.97604488694528158, 100.6239096053143669 ) ) ;
#192076=CARTESIAN_POINT ( 'NONE',  ( 21.53943276465977519, 0.05219959533937863772, 66.25109039468567573 ) ) ;
#192077=CARTESIAN_POINT ( 'NONE',  ( -5.823673210054116645, -21.52544592524344225, 52.29057627198102409 ) ) ;
#192078=CARTESIAN_POINT ( 'NONE',  ( 18.62759615963255655, 10.81492255796105972, 31.66775706135234358 ) ) ;
#192079=CARTESIAN_POINT ( 'NONE',  ( 18.62759615963271287, -10.81492255796078972, 83.33224293864769550 ) ) ;
#192080=CARTESIAN_POINT ( 'NONE',  ( -10.81492255796105439, 18.62759615963255655, 42.91775706135235424 ) ) ;
#192081=CARTESIAN_POINT ( 'NONE',  ( 0.05219959533910956823, 16.53943276465976808, 109.9989096053143527 ) ) ;
#192082=CARTESIAN_POINT ( 'NONE',  ( 13.97604488694548053, -13.89961937509957401, 70.62609039468567573 ) ) ;
#192083=CARTESIAN_POINT ( 'NONE',  ( 13.89961937509977652, -13.97604488694527269, 48.12390960531435979 ) ) ;
#192084=CARTESIAN_POINT ( 'NONE',  ( 14.29746914071049879, -8.314922557960816363, 98.33224293864769550 ) ) ;
#192085=CARTESIAN_POINT ( 'NONE',  ( -19.05341960407611168, -5.049401038298163336, 91.45724293864766707 ) ) ;
#192086=CARTESIAN_POINT ( 'NONE',  ( -13.89961937509977652, 13.97604488694528158, 100.6239096053143669 ) ) ;
#192087=CARTESIAN_POINT ( 'NONE',  ( -4.483927247898539470, -16.52544592524342804, 112.2905762719810241 ) ) ;
#192088=CARTESIAN_POINT ( 'NONE',  ( -16.52544592524342804, 4.483927247898546575, 36.04057627198102409 ) ) ;
#192089=CARTESIAN_POINT ( 'NONE',  ( 12.14591786802327356, -12.06949235617739191, 105.6260903946856899 ) ) ;
#192090=CARTESIAN_POINT ( 'NONE',  ( -0.05219959533909027116, -19.03943276465977164, 57.49890960531435979 ) ) ;
#192091=CARTESIAN_POINT ( 'NONE',  ( -16.53943276465976808, 0.05219959533911058130, 116.2489096053143669 ) ) ;
#192092=CARTESIAN_POINT ( 'NONE',  ( -21.55341960407619339, 5.719274019375674811, 113.5427570613523756 ) ) ;
#192094=CARTESIAN_POINT ( 'NONE',  ( -15.49999999999999822, 5.499999999999998224, 118.0000000000000142 ) ) ;
#192095=CARTESIAN_POINT ( 'NONE',  ( 12.06949235617757843, -12.14591786802309237, 28.12390960531435979 ) ) ;
#192096=CARTESIAN_POINT ( 'NONE',  ( 18.67979575497194134, -10.72451020669871369, 50.83442372801901143 ) ) ;
#192097=CARTESIAN_POINT ( 'NONE',  ( -5.153800228976328057, -19.02544592524343514, 102.2905762719810383 ) ) ;
#192098=CARTESIAN_POINT ( 'NONE',  ( -4.379528057220086978, -16.55341960407618274, 44.79275706135234714 ) ) ;
#192099=CARTESIAN_POINT ( 'NONE',  ( 8.224510206698742110, 14.34966873604972548, 102.0844237280190185 ) ) ;
#192100=CARTESIAN_POINT ( 'NONE',  ( -16.46253265017160317, 9.564922557960807481, 45.83224293864769550 ) ) ;
#192101=CARTESIAN_POINT ( 'NONE',  ( -12.14591786802326823, 12.06949235617739902, 88.12609039468570415 ) ) ;
#192102=CARTESIAN_POINT ( 'NONE',  ( -4.483927247898782831, 16.52544592524335698, 32.70942372801900433 ) ) ;
#192103=CARTESIAN_POINT ( 'NONE',  ( 19.02544592524343514, -5.153800228976328945, 53.54057627198102409 ) ) ;
#192104=CARTESIAN_POINT ( 'NONE',  ( -12.14591786802309592, -12.06949235617757132, 111.8739096053143669 ) ) ;
#192105=CARTESIAN_POINT ( 'NONE',  ( -21.52544592524343514, 5.823673210054127303, 111.0405762719810525 ) ) ;
#192106=CARTESIAN_POINT ( 'NONE',  ( -19.03943276465977164, 0.05219959533909376836, 31.24890960531435979 ) ) ;
#192107=CARTESIAN_POINT ( 'NONE',  ( 5.049401038298161559, -19.05341960407611168, 102.7072429386476955 ) ) ;
#192108=CARTESIAN_POINT ( 'NONE',  ( -5.049401038298153566, 19.05341960407611168, 35.20724293864768839 ) ) ;
#192110=CARTESIAN_POINT ( 'NONE',  ( -19.03943276465977164, 0.05219959533909376836, 106.2489096053143669 ) ) ;
#192112=CARTESIAN_POINT ( 'NONE',  ( -13.89961937509977652, 13.97604488694528158, 100.6239096053143669 ) ) ;
#192113=CARTESIAN_POINT ( 'NONE',  ( -18.62759615963255300, -10.81492255796106328, 39.16775706135235424 ) ) ;
#192114=CARTESIAN_POINT ( 'NONE',  ( -14.34966873604960291, -8.224510206698953496, 106.6655762719810383 ) ) ;
#192115=CARTESIAN_POINT ( 'NONE',  ( -16.46253265017160317, 9.564922557960807481, 105.8322429386476955 ) ) ;
#192117=CARTESIAN_POINT ( 'NONE',  ( -16.53943276465976808, -0.05219959533934237506, 58.75109039468568994 ) ) ;
#192118=CARTESIAN_POINT ( 'NONE',  ( 10.72451020669871369, 18.67979575497193778, 87.08442372801901854 ) ) ;
#192119=CARTESIAN_POINT ( 'NONE',  ( 16.52544592524335698, 4.483927247898782831, 36.45942372801901143 ) ) ;
#192120=CARTESIAN_POINT ( 'NONE',  ( -5.049401038298153566, 19.05341960407611168, 85.20724293864766707 ) ) ;
#192122=CARTESIAN_POINT ( 'NONE',  ( -14.34966873604972548, 8.224510206698743886, 33.33442372801900433 ) ) ;
#192123=CARTESIAN_POINT ( 'NONE',  ( -13.97604488694547697, 13.89961937509957934, 108.1260903946856331 ) ) ;
#192124=CARTESIAN_POINT ( 'NONE',  ( -12.06949235617739369, -12.14591786802326823, 84.37609039468570415 ) ) ;
#192125=CARTESIAN_POINT ( 'NONE',  ( -5.049401038297874678, -19.05341960407617918, 94.79275706135230450 ) ) ;
#192126=CARTESIAN_POINT ( 'NONE',  ( -19.02544592524342804, 5.153800228976336051, 76.04057627198102409 ) ) ;
#192127=CARTESIAN_POINT ( 'NONE',  ( -18.62759615963270932, 10.81492255796079327, 100.8322429386477097 ) ) ;
#192128=CARTESIAN_POINT ( 'NONE',  ( 12.14591786802309770, 12.06949235617756955, 84.37390960531438111 ) ) ;
#192129=CARTESIAN_POINT ( 'NONE',  ( 9.474510206698729675, 16.51473224551082808, 87.08442372801900433 ) ) ;
#192130=CARTESIAN_POINT ( 'NONE',  ( -12.06949235617739369, -12.14591786802326823, 69.37609039468567573 ) ) ;
#192131=CARTESIAN_POINT ( 'NONE',  ( 22.00000000000000000, -5.204748896376250896E-15, 47.50000000000000000 ) ) ;
#192132=CARTESIAN_POINT ( 'NONE',  ( -13.97604488694547697, 13.89961937509957934, 73.12609039468568994 ) ) ;
#192133=CARTESIAN_POINT ( 'NONE',  ( -4.379528057220328563, 16.55341960407611168, 35.20724293864768839 ) ) ;
#192134=CARTESIAN_POINT ( 'NONE',  ( 16.55341960407611168, 4.379528057220329451, 88.95724293864769550 ) ) ;
#192135=CARTESIAN_POINT ( 'NONE',  ( -19.05341960407617563, 5.049401038297882671, 33.54275706135231871 ) ) ;
#192136=CARTESIAN_POINT ( 'NONE',  ( -9.474510206698720793, -16.51473224551083518, 44.58442372801900433 ) ) ;
#192137=CARTESIAN_POINT ( 'NONE',  ( -21.52544592524334988, -5.823673210054445271, 28.95942372801902209 ) ) ;
#192138=CARTESIAN_POINT ( 'NONE',  ( 16.51473224551069308, 9.474510206698969483, 109.1655762719810383 ) ) ;
#192139=CARTESIAN_POINT ( 'NONE',  ( -0.05219959533909027116, -19.03943276465977164, 72.49890960531435269 ) ) ;
#192140=CARTESIAN_POINT ( 'NONE',  ( 10.72451020669871369, 18.67979575497193778, 102.0844237280190185 ) ) ;
#192141=CARTESIAN_POINT ( 'NONE',  ( -19.05341960407611168, -5.049401038298163336, 81.45724293864769550 ) ) ;
#192142=CARTESIAN_POINT ( 'NONE',  ( -5.719274019375978568, 21.55341960407610458, 40.20724293864769550 ) ) ;
#192144=CARTESIAN_POINT ( 'NONE',  ( 16.53943276465976808, -0.05219959533910856209, 93.74890960531436690 ) ) ;
#192145=CARTESIAN_POINT ( 'NONE',  ( -9.474510206698964154, 16.51473224551069663, 55.41557627198103120 ) ) ;
#192146=CARTESIAN_POINT ( 'NONE',  ( 16.52544592524342804, -4.483927247898539470, 108.5405762719810241 ) ) ;
#192147=CARTESIAN_POINT ( 'NONE',  ( 10.72451020669871369, 18.67979575497193778, 27.08442372801901854 ) ) ;
#192148=CARTESIAN_POINT ( 'NONE',  ( -18.67979575497193778, 10.72451020669871902, 68.33442372801900433 ) ) ;
#192149=CARTESIAN_POINT ( 'NONE',  ( -5.049401038298153566, 19.05341960407611168, 45.20724293864769550 ) ) ;
#192150=CARTESIAN_POINT ( 'NONE',  ( -8.224510206698735004, -14.34966873604973081, 79.58442372801903275 ) ) ;
#192151=CARTESIAN_POINT ( 'NONE',  ( 10.81492255796078972, 18.62759615963270932, 109.5822429386476955 ) ) ;
#192152=ORIENTED_EDGE ( 'NONE', *, *, #96611, .F. ) ;
#192153=CARTESIAN_POINT ( 'NONE',  ( -10.72451020669898014, 18.67979575497178502, 105.4155762719810383 ) ) ;
#192154=CARTESIAN_POINT ( 'NONE',  ( 13.89961937509957401, 13.97604488694547697, 36.87609039468565442 ) ) ;
#192155=CARTESIAN_POINT ( 'NONE',  ( -5.049401038298153566, 19.05341960407611168, 60.20724293864768129 ) ) ;
#192156=CARTESIAN_POINT ( 'NONE',  ( 16.46253265017146816, 9.564922557961045513, 36.66775706135233293 ) ) ;
#192157=CARTESIAN_POINT ( 'NONE',  ( 21.53943276465977519, 0.05219959533937863772, 76.25109039468568994 ) ) ;
#192158=EDGE_CURVE ( 'NONE', #179309, #127046, #52443, .T. ) ;
#192159=CARTESIAN_POINT ( 'NONE',  ( -15.80617190586745835, -15.72974639402198527, 66.87390960531436690 ) ) ;
#192160=CARTESIAN_POINT ( 'NONE',  ( -8.224510206698948167, 14.34966873604960824, 35.41557627198102409 ) ) ;
#192161=CARTESIAN_POINT ( 'NONE',  ( 21.53943276465977519, 0.05219959533937863772, 91.25109039468568994 ) ) ;
#192162=CARTESIAN_POINT ( 'NONE',  ( 19.05341960407617918, -5.049401038297876454, 31.04275706135232227 ) ) ;
#192163=CARTESIAN_POINT ( 'NONE',  ( 8.314922557960818139, 14.29746914071049879, 74.58224293864768129 ) ) ;
#192164=CARTESIAN_POINT ( 'NONE',  ( 14.29746914071049879, -8.314922557960816363, 103.3322429386476955 ) ) ;
#192165=CARTESIAN_POINT ( 'NONE',  ( 5.153800228976615827, -19.02544592524334988, 60.20942372801899012 ) ) ;
#192166=CARTESIAN_POINT ( 'NONE',  ( -16.55341960407617563, 4.379528057220093196, 113.5427570613523756 ) ) ;
#192167=CARTESIAN_POINT ( 'NONE',  ( 15.72974639402176855, 15.80617190586768217, 66.87609039468568994 ) ) ;
#192168=CARTESIAN_POINT ( 'NONE',  ( 9.474510206698971260, -16.51473224551069308, 77.91557627198103830 ) ) ;
#192169=CARTESIAN_POINT ( 'NONE',  ( -16.46253265017146816, -9.564922557961047289, 49.16775706135233293 ) ) ;
#192170=CARTESIAN_POINT ( 'NONE',  ( -18.67979575497178146, -10.72451020669898902, 56.66557627198103830 ) ) ;
#192171=CARTESIAN_POINT ( 'NONE',  ( 10.72451020669871369, 18.67979575497193778, 42.08442372801901854 ) ) ;
#192172=CARTESIAN_POINT ( 'NONE',  ( 21.53943276465977519, -0.05219959533907433946, 98.74890960531438111 ) ) ;
#192173=CARTESIAN_POINT ( 'NONE',  ( 16.46253265017146816, 9.564922557961045513, 101.6677570613523329 ) ) ;
#192174=CARTESIAN_POINT ( 'NONE',  ( -14.34966873604972548, 8.224510206698743886, 68.33442372801900433 ) ) ;
#192176=CARTESIAN_POINT ( 'NONE',  ( -5.719274019375978568, 21.55341960407610458, 110.2072429386477239 ) ) ;
#192177=CARTESIAN_POINT ( 'NONE',  ( 8.224510206698953496, -14.34966873604960469, 87.91557627198103830 ) ) ;
#192178=CARTESIAN_POINT ( 'NONE',  ( -17.50000000000001776, -4.049696124445835821, 30.81960329334054549 ) ) ;
#192179=CARTESIAN_POINT ( 'NONE',  ( -4.379528057220086978, -16.55341960407618274, 19.79275706135235069 ) ) ;
#192180=CARTESIAN_POINT ( 'NONE',  ( 10.81492255796078972, 18.62759615963270932, 49.58224293864769550 ) ) ;
#192181=CARTESIAN_POINT ( 'NONE',  ( 14.29746914071037800, 8.314922557961029526, 86.66775706135234714 ) ) ;
#192183=CARTESIAN_POINT ( 'NONE',  ( 8.224510206698742110, 14.34966873604972548, 67.08442372801901854 ) ) ;
#192184=CARTESIAN_POINT ( 'NONE',  ( 5.719274019375673035, 21.55341960407619339, 42.29275706135235424 ) ) ;
#192185=CARTESIAN_POINT ( 'NONE',  ( 0.05219959533907565091, 21.53943276465977519, 44.99890960531435979 ) ) ;
#192186=CARTESIAN_POINT ( 'NONE',  ( -8.224510206698735004, -14.34966873604973081, 79.58442372801903275 ) ) ;
#192187=CARTESIAN_POINT ( 'NONE',  ( -19.03943276465977164, 0.05219959533909376836, 101.2489096053143669 ) ) ;
#192188=CARTESIAN_POINT ( 'NONE',  ( -21.55341960407619339, 5.719274019375674811, 68.54275706135234714 ) ) ;
#192189=CARTESIAN_POINT ( 'NONE',  ( -21.52544592524343514, 5.823673210054127303, 41.04057627198103120 ) ) ;
#192190=CARTESIAN_POINT ( 'NONE',  ( -10.72451020669898014, 18.67979575497178502, 30.41557627198101699 ) ) ;
#192192=CARTESIAN_POINT ( 'NONE',  ( -13.97604488694547697, 13.89961937509957934, 53.12609039468565442 ) ) ;
#192193=CARTESIAN_POINT ( 'NONE',  ( -4.379528057220086978, -16.55341960407618274, 64.79275706135234714 ) ) ;
#192194=CARTESIAN_POINT ( 'NONE',  ( -5.823673210054116645, -21.52544592524344225, 32.29057627198102409 ) ) ;
#192196=CARTESIAN_POINT ( 'NONE',  ( 9.564922557960805705, 16.46253265017160317, 84.58224293864769550 ) ) ;
#192197=CARTESIAN_POINT ( 'NONE',  ( -16.53943276465976808, 0.05219959533911058130, 21.24890960531436690 ) ) ;
#192199=CARTESIAN_POINT ( 'NONE',  ( 12.14591786802309770, 12.06949235617756955, 114.3739096053143527 ) ) ;
#192200=CARTESIAN_POINT ( 'NONE',  ( 5.823673210054125526, 21.52544592524343514, 44.79057627198103120 ) ) ;
#192201=CARTESIAN_POINT ( 'NONE',  ( -19.03943276465977164, 0.05219959533909376836, 51.24890960531436690 ) ) ;
#192202=CARTESIAN_POINT ( 'NONE',  ( -16.53943276465976808, -0.05219959533934237506, 93.75109039468567573 ) ) ;
#192203=CARTESIAN_POINT ( 'NONE',  ( -5.823673210054431948, 21.52544592524334988, 27.70942372801901854 ) ) ;
#192204=CARTESIAN_POINT ( 'NONE',  ( 5.153800228976615827, -19.02544592524334988, 95.20942372801897591 ) ) ;
#192205=CARTESIAN_POINT ( 'NONE',  ( -16.52544592524342804, 4.483927247898546575, 91.04057627198103830 ) ) ;
#192206=CARTESIAN_POINT ( 'NONE',  ( -5.049401038298153566, 19.05341960407611168, 55.20724293864769550 ) ) ;
#192207=CARTESIAN_POINT ( 'NONE',  ( 16.51473224551069308, 9.474510206698969483, 29.16557627198103475 ) ) ;
#192208=CARTESIAN_POINT ( 'NONE',  ( 21.52544592524334988, 5.823673210054432836, 111.4594237280190328 ) ) ;
#192209=CARTESIAN_POINT ( 'NONE',  ( -13.89961937509977652, 13.97604488694528158, 80.62390960531436690 ) ) ;
#192210=CARTESIAN_POINT ( 'NONE',  ( -4.483927247898782831, 16.52544592524335698, 67.70942372801901854 ) ) ;
#192211=CARTESIAN_POINT ( 'NONE',  ( 21.52544592524334988, 5.823673210054432836, 91.45942372801901854 ) ) ;
#192212=CARTESIAN_POINT ( 'NONE',  ( 21.52544592524344225, -5.823673210054117533, 48.54057627198103120 ) ) ;
#192213=CARTESIAN_POINT ( 'NONE',  ( -4.379528057220086978, -16.55341960407618274, 74.79275706135234714 ) ) ;
#192214=CARTESIAN_POINT ( 'NONE',  ( -19.02544592524334988, -5.153800228976617603, 48.95942372801900433 ) ) ;
#192215=CARTESIAN_POINT ( 'NONE',  ( 19.05341960407617918, -5.049401038297876454, 71.04275706135234714 ) ) ;
#192216=ORIENTED_EDGE ( 'NONE', *, *, #22880, .T. ) ;
#192217=CARTESIAN_POINT ( 'NONE',  ( 18.62759615963255655, 10.81492255796105972, 61.66775706135235424 ) ) ;
#192218=CARTESIAN_POINT ( 'NONE',  ( -13.89961937509977652, 13.97604488694528158, 60.62390960531436690 ) ) ;
#192220=CARTESIAN_POINT ( 'NONE',  ( -16.46253265017160317, 9.564922557960807481, 30.83224293864769550 ) ) ;
#192221=CARTESIAN_POINT ( 'NONE',  ( 13.89961937509957401, 13.97604488694547697, 56.87609039468564731 ) ) ;
#192222=CARTESIAN_POINT ( 'NONE',  ( 19.05341960407611168, 5.049401038298154454, 108.9572429386477097 ) ) ;
#192223=CARTESIAN_POINT ( 'NONE',  ( -13.97604488694527625, -13.89961937509977652, 96.87390960531433848 ) ) ;
#192224=CARTESIAN_POINT ( 'NONE',  ( -4.379528057220328563, 16.55341960407611168, 50.20724293864769550 ) ) ;
#192225=CARTESIAN_POINT ( 'NONE',  ( -21.52544592524343514, 5.823673210054127303, 46.04057627198103830 ) ) ;
#192228=CARTESIAN_POINT ( 'NONE',  ( -5.049401038297874678, -19.05341960407617918, 19.79275706135233293 ) ) ;
#192229=CARTESIAN_POINT ( 'NONE',  ( -16.61371651742599909, -7.165104196376135270, 81.14584930007002583 ) ) ;
#192230=CARTESIAN_POINT ( 'NONE',  ( -5.049401038298153566, 19.05341960407611168, 55.20724293864769550 ) ) ;
#192232=CARTESIAN_POINT ( 'NONE',  ( -17.40861289039002813, 6.110651285853322179, 108.6276752917256943 ) ) ;
#192233=CARTESIAN_POINT ( 'NONE',  ( -16.52544592524335698, -4.483927247898792601, 78.95942372801901854 ) ) ;
#192234=CARTESIAN_POINT ( 'NONE',  ( 10.72451020669898902, -18.67979575497178502, 92.91557627198103830 ) ) ;
#192236=CARTESIAN_POINT ( 'NONE',  ( -14.29746914071049879, 8.314922557960819915, 50.83224293864770971 ) ) ;
#192237=CARTESIAN_POINT ( 'NONE',  ( -9.474510206698964154, 16.51473224551069663, 35.41557627198102409 ) ) ;
#192239=CARTESIAN_POINT ( 'NONE',  ( 18.62759615963255655, 10.81492255796105972, 36.66775706135234714 ) ) ;
#192240=CARTESIAN_POINT ( 'NONE',  ( 5.049401038297881783, 19.05341960407617563, 42.29275706135234003 ) ) ;
#192241=CARTESIAN_POINT ( 'NONE',  ( 0.05219959533909260263, 19.03943276465977164, 39.99890960531436690 ) ) ;
#192242=CARTESIAN_POINT ( 'NONE',  ( 18.62759615963255655, 10.81492255796105972, 101.6677570613523613 ) ) ;
#192243=CARTESIAN_POINT ( 'NONE',  ( -19.05341960407611168, -5.049401038298163336, 21.45724293864768839 ) ) ;
#192244=CARTESIAN_POINT ( 'NONE',  ( 16.53943276465976808, -0.05219959533910856209, 38.74890960531435979 ) ) ;
#192246=CARTESIAN_POINT ( 'NONE',  ( 15.80617190586746368, 15.72974639402197994, 39.37390960531436690 ) ) ;
#192248=CARTESIAN_POINT ( 'NONE',  ( -16.46253265017160317, 9.564922557960807481, 105.8322429386476955 ) ) ;
#192249=CARTESIAN_POINT ( 'NONE',  ( 12.14591786802309770, 12.06949235617756955, 84.37390960531438111 ) ) ;
#192250=CARTESIAN_POINT ( 'NONE',  ( -5.153800228976607833, 19.02544592524334988, 112.7094237280190043 ) ) ;
#192251=CARTESIAN_POINT ( 'NONE',  ( -14.29746914071037622, -8.314922557961029526, 109.1677570613523613 ) ) ;
#192253=ADVANCED_FACE ( 'NONE', ( #99938 ), #114014, .T. ) ;
#192254=CARTESIAN_POINT ( 'NONE',  ( 13.89961937509977652, -13.97604488694527269, 93.12390960531436690 ) ) ;
#192255=CARTESIAN_POINT ( 'NONE',  ( 18.62759615963271287, -10.81492255796078972, 98.33224293864769550 ) ) ;
#192256=CARTESIAN_POINT ( 'NONE',  ( -16.52544592524342804, 4.483927247898546575, 31.04057627198102409 ) ) ;
#192257=CARTESIAN_POINT ( 'NONE',  ( -16.51473224551069308, -9.474510206698971260, 106.6655762719810383 ) ) ;
#192258=CARTESIAN_POINT ( 'NONE',  ( -19.03943276465977164, -0.05219959533935918106, 83.75109039468567573 ) ) ;
#192259=CARTESIAN_POINT ( 'NONE',  ( -10.81492255796105439, 18.62759615963255655, 112.9177570613523329 ) ) ;
#192260=CARTESIAN_POINT ( 'NONE',  ( -5.719274019375978568, 21.55341960407610458, 85.20724293864770971 ) ) ;
#192261=CARTESIAN_POINT ( 'NONE',  ( 18.67979575497178502, 10.72451020669898547, 54.16557627198103120 ) ) ;
#192262=CARTESIAN_POINT ( 'NONE',  ( 16.51473224551069308, 9.474510206698969483, 69.16557627198102409 ) ) ;
#192263=CARTESIAN_POINT ( 'NONE',  ( -16.55341960407611168, -4.379528057220339221, 31.45724293864769550 ) ) ;
#192264=CARTESIAN_POINT ( 'NONE',  ( -0.05219959533909027116, -19.03943276465977164, 77.49890960531435269 ) ) ;
#192265=ORIENTED_EDGE ( 'NONE', *, *, #95479, .F. ) ;
#192267=CARTESIAN_POINT ( 'NONE',  ( -19.03943276465977164, -0.05219959533935918106, 23.75109039468566152 ) ) ;
#192268=CARTESIAN_POINT ( 'NONE',  ( -8.314922557960811034, -14.29746914071050412, 87.08224293864769550 ) ) ;
#192269=CARTESIAN_POINT ( 'NONE',  ( -18.62759615963255300, -10.81492255796106328, 24.16775706135235424 ) ) ;
#192271=CARTESIAN_POINT ( 'NONE',  ( -0.05219959533934338120, 16.53943276465976808, 97.50109039468567573 ) ) ;
#192272=CARTESIAN_POINT ( 'NONE',  ( -4.483927247898539470, -16.52544592524342804, 112.2905762719810241 ) ) ;
#192273=CARTESIAN_POINT ( 'NONE',  ( 0.05219959533909260263, 19.03943276465977164, 74.99890960531435269 ) ) ;
#192274=CARTESIAN_POINT ( 'NONE',  ( 16.51473224551069308, 9.474510206698969483, 24.16557627198102765 ) ) ;
#192275=CARTESIAN_POINT ( 'NONE',  ( 14.34966873604960469, 8.224510206698951720, 29.16557627198103120 ) ) ;
#192276=EDGE_CURVE ( 'NONE', #90870, #160624, #37871, .T. ) ;
#192277=CARTESIAN_POINT ( 'NONE',  ( -18.62759615963255300, -10.81492255796106328, 54.16775706135235424 ) ) ;
#192279=CARTESIAN_POINT ( 'NONE',  ( -21.53943276465977519, -0.05219959533937600094, 98.75109039468568994 ) ) ;
#192280=CARTESIAN_POINT ( 'NONE',  ( 9.474510206698971260, -16.51473224551069308, 47.91557627198102409 ) ) ;
#192281=CARTESIAN_POINT ( 'NONE',  ( -5.049401038298153566, 19.05341960407611168, 50.20724293864770260 ) ) ;
#192283=CARTESIAN_POINT ( 'NONE',  ( 5.823673210054444382, -21.52544592524334988, 95.20942372801903275 ) ) ;
#192284=CARTESIAN_POINT ( 'NONE',  ( -8.314922557961024197, 14.29746914071037800, 57.91775706135234714 ) ) ;
#192286=CARTESIAN_POINT ( 'NONE',  ( -5.823673210054431948, 21.52544592524334988, 87.70942372801901854 ) ) ;
#192287=CARTESIAN_POINT ( 'NONE',  ( -10.81492255796078084, -18.62759615963271287, 22.08224293864769194 ) ) ;
#192288=CARTESIAN_POINT ( 'NONE',  ( -9.564922557961040184, 16.46253265017147172, 87.91775706135233293 ) ) ;
#192289=CARTESIAN_POINT ( 'NONE',  ( -10.72451020669870658, -18.67979575497194134, 69.58442372801900433 ) ) ;
#192290=CARTESIAN_POINT ( 'NONE',  ( 14.34966873604972726, -8.224510206698740333, 35.83442372801901143 ) ) ;
#192291=AXIS2_PLACEMENT_3D ( 'NONE', #135947, #42942, #104606 ) ;
#192292=CARTESIAN_POINT ( 'NONE',  ( -15.72974639402197994, 15.80617190586746368, 90.62390960531436690 ) ) ;
#192293=CARTESIAN_POINT ( 'NONE',  ( 19.02544592524334988, 5.153800228976608722, 91.45942372801900433 ) ) ;
#192294=CARTESIAN_POINT ( 'NONE',  ( 5.153800228976335163, 19.02544592524342804, 59.79057627198100988 ) ) ;
#192295=CARTESIAN_POINT ( 'NONE',  ( -19.03943276465977164, -0.05219959533935918106, 98.75109039468567573 ) ) ;
#192296=CARTESIAN_POINT ( 'NONE',  ( -19.03943276465977164, -0.05219959533935918106, 103.7510903946856757 ) ) ;
#192297=CARTESIAN_POINT ( 'NONE',  ( 0.05219959533910956823, 16.53943276465976808, 49.99890960531437401 ) ) ;
#192298=CARTESIAN_POINT ( 'NONE',  ( -0.05219959533936034679, 19.03943276465977164, 77.50109039468566152 ) ) ;
#192299=CARTESIAN_POINT ( 'NONE',  ( 4.483927247898790824, -16.52544592524335698, 60.20942372801902565 ) ) ;
#192300=CARTESIAN_POINT ( 'NONE',  ( 16.51473224551069308, 9.474510206698969483, 34.16557627198102409 ) ) ;
#192301=CARTESIAN_POINT ( 'NONE',  ( -16.46253265017160317, 9.564922557960807481, 55.83224293864769550 ) ) ;
#192302=CARTESIAN_POINT ( 'NONE',  ( -16.53943276465976808, -0.05219959533934237506, 58.75109039468568994 ) ) ;
#192305=CARTESIAN_POINT ( 'NONE',  ( 9.474510206698971260, -16.51473224551069308, 107.9155762719810383 ) ) ;
#192306=CARTESIAN_POINT ( 'NONE',  ( -16.51473224551069308, -9.474510206698971260, 21.66557627198102765 ) ) ;
#192308=CARTESIAN_POINT ( 'NONE',  ( 19.03943276465977164, 0.05219959533936151252, 106.2510903946856615 ) ) ;
#192309=CARTESIAN_POINT ( 'NONE',  ( -21.53943276465977519, 0.05219959533907696930, 41.24890960531435269 ) ) ;
#192310=CARTESIAN_POINT ( 'NONE',  ( 19.03943276465977164, 0.05219959533936151252, 31.25109039468566863 ) ) ;
#192311=CARTESIAN_POINT ( 'NONE',  ( 12.06949235617739724, 12.14591786802326823, 26.87609039468567218 ) ) ;
#192312=CARTESIAN_POINT ( 'NONE',  ( -19.05341960407611168, -5.049401038298163336, 31.45724293864769550 ) ) ;
#192313=CARTESIAN_POINT ( 'NONE',  ( -16.51473224551069308, -9.474510206698971260, 56.66557627198103120 ) ) ;
#192314=CARTESIAN_POINT ( 'NONE',  ( -10.72451020669898014, 18.67979575497178502, 75.41557627198102409 ) ) ;
#192315=CARTESIAN_POINT ( 'NONE',  ( -19.05341960407611168, -5.049401038298163336, 96.45724293864769550 ) ) ;
#192316=CARTESIAN_POINT ( 'NONE',  ( 0.05219959533909260263, 19.03943276465977164, 44.99890960531435979 ) ) ;
#192318=CARTESIAN_POINT ( 'NONE',  ( 0.05219959533936267826, -19.03943276465977164, 80.00109039468567573 ) ) ;
#192319=CARTESIAN_POINT ( 'NONE',  ( 12.14591786802309770, 12.06949235617756955, 64.37390960531435269 ) ) ;
#192320=CARTESIAN_POINT ( 'NONE',  ( 21.52544592524344225, -5.823673210054117533, 43.54057627198103830 ) ) ;
#192321=CARTESIAN_POINT ( 'NONE',  ( 21.52544592524334988, 5.823673210054432836, 106.4594237280190328 ) ) ;
#192322=CARTESIAN_POINT ( 'NONE',  ( -10.72451020669898014, 18.67979575497178502, 100.4155762719810241 ) ) ;
#192323=CARTESIAN_POINT ( 'NONE',  ( 15.80617190586769283, -15.72974639402175789, 75.62609039468567573 ) ) ;
#192324=CARTESIAN_POINT ( 'NONE',  ( -5.823673210054431948, 21.52544592524334988, 77.70942372801900433 ) ) ;
#192325=CARTESIAN_POINT ( 'NONE',  ( -19.05341960407611168, -5.049401038298163336, 111.4572429386476671 ) ) ;
#192326=CARTESIAN_POINT ( 'NONE',  ( 8.224510206698742110, 14.34966873604972548, 112.0844237280190185 ) ) ;
#192327=CARTESIAN_POINT ( 'NONE',  ( 18.62759615963255655, 10.81492255796105972, 71.66775706135234714 ) ) ;
#192328=CARTESIAN_POINT ( 'NONE',  ( 0.05219959533909260263, 19.03943276465977164, 64.99890960531436690 ) ) ;
#192329=CARTESIAN_POINT ( 'NONE',  ( 16.46253265017146816, 9.564922557961045513, 31.66775706135232937 ) ) ;
#192330=CARTESIAN_POINT ( 'NONE',  ( -10.81492255796105439, 18.62759615963255655, 32.91775706135234714 ) ) ;
#192331=CARTESIAN_POINT ( 'NONE',  ( 9.474510206698971260, -16.51473224551069308, 67.91557627198102409 ) ) ;
#192332=CARTESIAN_POINT ( 'NONE',  ( 12.06949235617757843, -12.14591786802309237, 78.12390960531436690 ) ) ;
#192333=CARTESIAN_POINT ( 'NONE',  ( 8.224510206698953496, -14.34966873604960469, 42.91557627198103120 ) ) ;
#192334=CARTESIAN_POINT ( 'NONE',  ( 10.72451020669898902, -18.67979575497178502, 52.91557627198103830 ) ) ;
#192335=CARTESIAN_POINT ( 'NONE',  ( -19.03943276465977164, 0.05219959533909376836, 66.24890960531436690 ) ) ;
#192336=CARTESIAN_POINT ( 'NONE',  ( -15.72974639402197994, 15.80617190586746368, 65.62390960531436690 ) ) ;
#192337=CARTESIAN_POINT ( 'NONE',  ( -19.03943276465977164, -0.05219959533935918106, 68.75109039468566152 ) ) ;
#192339=CARTESIAN_POINT ( 'NONE',  ( 14.34966873604960469, 8.224510206698951720, 59.16557627198103120 ) ) ;
#192340=CARTESIAN_POINT ( 'NONE',  ( 10.81492255796078972, 18.62759615963270932, 44.58224293864769550 ) ) ;
#192342=CARTESIAN_POINT ( 'NONE',  ( -17.49999999999999289, 5.500000000000036415, 65.79690382534171533 ) ) ;
#192343=CARTESIAN_POINT ( 'NONE',  ( 8.314922557961029526, -14.29746914071037800, 85.41775706135236135 ) ) ;
#192345=CARTESIAN_POINT ( 'NONE',  ( -13.89961937509957401, -13.97604488694547875, 94.37609039468566152 ) ) ;
#192346=CARTESIAN_POINT ( 'NONE',  ( 16.52544592524342804, -4.483927247898539470, 73.54057627198102409 ) ) ;
#192348=CARTESIAN_POINT ( 'NONE',  ( 5.049401038298161559, -19.05341960407611168, 62.70724293864769550 ) ) ;
#192349=CARTESIAN_POINT ( 'NONE',  ( -12.06949235617756955, 12.14591786802309770, 50.62390960531435979 ) ) ;
#192350=CARTESIAN_POINT ( 'NONE',  ( -9.564922557960796823, -16.46253265017161027, 82.08224293864768129 ) ) ;
#192351=CARTESIAN_POINT ( 'NONE',  ( -19.05341960407617563, 5.049401038297882671, 73.54275706135233293 ) ) ;
#192352=CARTESIAN_POINT ( 'NONE',  ( 5.153800228976335163, 19.02544592524342804, 49.79057627198100988 ) ) ;
#192353=CARTESIAN_POINT ( 'NONE',  ( -5.049401038298153566, 19.05341960407611168, 80.20724293864769550 ) ) ;
#192354=CARTESIAN_POINT ( 'NONE',  ( -19.05341960407611168, -5.049401038298163336, 31.45724293864769550 ) ) ;
#192355=CARTESIAN_POINT ( 'NONE',  ( -19.03943276465977164, 0.05219959533909376836, 66.24890960531436690 ) ) ;
#192356=EDGE_CURVE ( 'NONE', #199940, #148926, #78623, .T. ) ;
#192357=CARTESIAN_POINT ( 'NONE',  ( -15.72974639402197994, 15.80617190586746368, 55.62390960531436690 ) ) ;
#192358=CARTESIAN_POINT ( 'NONE',  ( -13.89961937509977652, 13.97604488694528158, 55.62390960531434558 ) ) ;
#192359=CARTESIAN_POINT ( 'NONE',  ( -10.72451020669898014, 18.67979575497178502, 50.41557627198103120 ) ) ;
#192360=CARTESIAN_POINT ( 'NONE',  ( -16.46253265017146816, -9.564922557961047289, 79.16775706135234714 ) ) ;
#192361=CARTESIAN_POINT ( 'NONE',  ( -12.14591786802326823, 12.06949235617739902, 103.1260903946856757 ) ) ;
#192362=CARTESIAN_POINT ( 'NONE',  ( -13.97604488694547697, 13.89961937509957934, 43.12609039468566152 ) ) ;
#192363=CARTESIAN_POINT ( 'NONE',  ( -16.55341960407617563, 4.379528057220093196, 63.54275706135234003 ) ) ;
#192364=CARTESIAN_POINT ( 'NONE',  ( 4.379528057220092307, 16.55341960407617563, 92.29275706135236135 ) ) ;
#192365=CARTESIAN_POINT ( 'NONE',  ( -17.49999999999999645, -5.499999999999992895, 94.20309617465827046 ) ) ;
#192366=CARTESIAN_POINT ( 'NONE',  ( 16.53943276465976808, 0.05219959533934440121, 81.25109039468568994 ) ) ;
#192367=CARTESIAN_POINT ( 'NONE',  ( 10.72451020669898902, -18.67979575497178502, 27.91557627198103830 ) ) ;
#192368=CARTESIAN_POINT ( 'NONE',  ( -9.474510206698964154, 16.51473224551069663, 35.41557627198102409 ) ) ;
#192369=CARTESIAN_POINT ( 'NONE',  ( -4.483927247898782831, 16.52544592524335698, 32.70942372801900433 ) ) ;
#192370=CARTESIAN_POINT ( 'NONE',  ( 5.049401038298161559, -19.05341960407611168, 52.70724293864767418 ) ) ;
#192371=CARTESIAN_POINT ( 'NONE',  ( -5.823673210054431948, 21.52544592524334988, 37.70942372801900433 ) ) ;
#192372=CARTESIAN_POINT ( 'NONE',  ( -16.53943276465976808, -0.05219959533934237506, 43.75109039468568284 ) ) ;
#192373=CARTESIAN_POINT ( 'NONE',  ( 16.53943276465976808, 0.05219959533934440121, 111.2510903946856899 ) ) ;
#192374=CARTESIAN_POINT ( 'NONE',  ( -19.05341960407611168, -5.049401038298163336, 31.45724293864769550 ) ) ;
#192375=CARTESIAN_POINT ( 'NONE',  ( 9.474510206698729675, 16.51473224551082808, 22.08442372801899722 ) ) ;
#192376=CARTESIAN_POINT ( 'NONE',  ( -0.05219959533936034679, 19.03943276465977164, 107.5010903946856615 ) ) ;
#192377=CARTESIAN_POINT ( 'NONE',  ( -19.02544592524334988, -5.153800228976617603, 73.95942372801900433 ) ) ;
#192378=CARTESIAN_POINT ( 'NONE',  ( -4.483927247898539470, -16.52544592524342804, 67.29057627198103830 ) ) ;
#192379=CARTESIAN_POINT ( 'NONE',  ( -9.474510206698964154, 16.51473224551069663, 40.41557627198103120 ) ) ;
#192380=CARTESIAN_POINT ( 'NONE',  ( 9.564922557961047289, -16.46253265017146816, 80.41775706135234714 ) ) ;
#192381=CARTESIAN_POINT ( 'NONE',  ( 17.44270441346516876, -5.991230190323020288, 91.13664920735770636 ) ) ;
#192382=CARTESIAN_POINT ( 'NONE',  ( 15.72974639402176855, 15.80617190586768217, 61.87609039468568284 ) ) ;
#192383=CARTESIAN_POINT ( 'NONE',  ( 14.34966873604972726, -8.224510206698740333, 45.83442372801901854 ) ) ;
#192384=CARTESIAN_POINT ( 'NONE',  ( 18.39635199886966888, -5.500000000000096811, 58.51967076359999709 ) ) ;
#192385=CARTESIAN_POINT ( 'NONE',  ( 10.72451020669898902, -18.67979575497178502, 42.91557627198103120 ) ) ;
#192386=CARTESIAN_POINT ( 'NONE',  ( 14.29746914071037800, 8.314922557961029526, 26.66775706135235424 ) ) ;
#192389=CARTESIAN_POINT ( 'NONE',  ( 19.02544592524343514, -5.153800228976328945, 38.54057627198103120 ) ) ;
#192390=CARTESIAN_POINT ( 'NONE',  ( 21.55341960407619695, -5.719274019375665929, 106.0427570613523471 ) ) ;
#192391=CARTESIAN_POINT ( 'NONE',  ( -19.05341960407611168, -5.049401038298163336, 51.45724293864770260 ) ) ;
#192393=CARTESIAN_POINT ( 'NONE',  ( 15.72974639402176855, 15.80617190586768217, 71.87609039468568994 ) ) ;
#192394=CARTESIAN_POINT ( 'NONE',  ( -21.55341960407619339, 5.719274019375674811, 103.5427570613523613 ) ) ;
#192395=CARTESIAN_POINT ( 'NONE',  ( 8.224510206698742110, 14.34966873604972548, 112.0844237280190185 ) ) ;
#192396=CARTESIAN_POINT ( 'NONE',  ( -13.89961937509977652, 13.97604488694528158, 30.62390960531435269 ) ) ;
#192397=CARTESIAN_POINT ( 'NONE',  ( 0.05219959533909260263, 19.03943276465977164, 94.99890960531436690 ) ) ;
#192398=CARTESIAN_POINT ( 'NONE',  ( 21.53943276465977519, 0.05219959533937863772, 61.25109039468567573 ) ) ;
#192399=CARTESIAN_POINT ( 'NONE',  ( -9.564922557960796823, -16.46253265017161027, 37.08224293864768839 ) ) ;
#192400=CARTESIAN_POINT ( 'NONE',  ( -5.823673210054431948, 21.52544592524334988, 47.70942372801902565 ) ) ;
#192401=CARTESIAN_POINT ( 'NONE',  ( -13.89961937509957401, -13.97604488694547875, 89.37609039468563310 ) ) ;
#192402=CARTESIAN_POINT ( 'NONE',  ( -19.03943276465977164, 0.05219959533909376836, 101.2489096053143669 ) ) ;
#192403=CARTESIAN_POINT ( 'NONE',  ( -5.153800228976328057, -19.02544592524343514, 27.29057627198103120 ) ) ;
#192404=CARTESIAN_POINT ( 'NONE',  ( 0.05219959533907565091, 21.53943276465977519, 109.9989096053143527 ) ) ;
#192405=CARTESIAN_POINT ( 'NONE',  ( 5.153800228976615827, -19.02544592524334988, 30.20942372801900433 ) ) ;
#192406=CARTESIAN_POINT ( 'NONE',  ( 8.224510206698953496, -14.34966873604960469, 112.9155762719810383 ) ) ;
#192407=CARTESIAN_POINT ( 'NONE',  ( -16.46253265017160317, 9.564922557960807481, 65.83224293864769550 ) ) ;
#192408=CARTESIAN_POINT ( 'NONE',  ( -19.05341960407617563, 5.049401038297882671, 103.5427570613523329 ) ) ;
#192409=CARTESIAN_POINT ( 'NONE',  ( 12.06949235617757843, -12.14591786802309237, 68.12390960531436690 ) ) ;
#192410=CARTESIAN_POINT ( 'NONE',  ( 13.97604488694548053, -13.89961937509957401, 20.62609039468567573 ) ) ;
#192411=CARTESIAN_POINT ( 'NONE',  ( -21.55341960407610458, -5.719274019375992779, 26.45724293864768839 ) ) ;
#192412=CARTESIAN_POINT ( 'NONE',  ( 19.05341960407617918, -5.049401038297876454, 91.04275706135234714 ) ) ;
#192413=CARTESIAN_POINT ( 'NONE',  ( 15.80617190586746368, 15.72974639402197994, 94.37390960531436690 ) ) ;
#192414=CARTESIAN_POINT ( 'NONE',  ( -18.62759615963255300, -10.81492255796106328, 49.16775706135234003 ) ) ;
#192415=CARTESIAN_POINT ( 'NONE',  ( 8.314922557961029526, -14.29746914071037800, 45.41775706135234003 ) ) ;
#192416=CARTESIAN_POINT ( 'NONE',  ( 4.379528057220092307, 16.55341960407617563, 102.2927570613523613 ) ) ;
#192417=CARTESIAN_POINT ( 'NONE',  ( -8.224510206698735004, -14.34966873604973081, 44.58442372801901854 ) ) ;
#192418=CARTESIAN_POINT ( 'NONE',  ( -21.55341960407619339, 5.719274019375674811, 43.54275706135235424 ) ) ;
#192419=CARTESIAN_POINT ( 'NONE',  ( 10.72451020669898902, -18.67979575497178502, 52.91557627198103830 ) ) ;
#192420=CARTESIAN_POINT ( 'NONE',  ( 9.474510206698971260, -16.51473224551069308, 37.91557627198102409 ) ) ;
#192422=CARTESIAN_POINT ( 'NONE',  ( -16.52544592524335698, -4.483927247898792601, 63.95942372801901854 ) ) ;
#192423=CARTESIAN_POINT ( 'NONE',  ( 5.719274019375991003, -21.55341960407610458, 87.70724293864769550 ) ) ;
#192424=CARTESIAN_POINT ( 'NONE',  ( 14.29746914071049879, -8.314922557960816363, 33.33224293864769550 ) ) ;
#192425=CARTESIAN_POINT ( 'NONE',  ( -8.314922557961024197, 14.29746914071037800, 57.91775706135234714 ) ) ;
#192426=CARTESIAN_POINT ( 'NONE',  ( -16.51473224551082808, 9.474510206698731452, 103.3344237280190043 ) ) ;
#192427=CARTESIAN_POINT ( 'NONE',  ( -15.72974639402197994, 15.80617190586746368, 95.62390960531436690 ) ) ;
#192428=CARTESIAN_POINT ( 'NONE',  ( -4.483927247898539470, -16.52544592524342804, 32.29057627198102409 ) ) ;
#192430=CARTESIAN_POINT ( 'NONE',  ( -8.314922557961024197, 14.29746914071037800, 72.91775706135234714 ) ) ;
#192432=CARTESIAN_POINT ( 'NONE',  ( -15.72974639402197994, 15.80617190586746368, 75.62390960531439532 ) ) ;
#192433=CARTESIAN_POINT ( 'NONE',  ( -12.06949235617739369, -12.14591786802326823, 99.37609039468568994 ) ) ;
#192435=CARTESIAN_POINT ( 'NONE',  ( 18.89770734986049305, 5.499999999999896083, 86.60214472496637939 ) ) ;
#192436=CARTESIAN_POINT ( 'NONE',  ( -21.52544592524343514, 5.823673210054127303, 86.04057627198102409 ) ) ;
#192438=CARTESIAN_POINT ( 'NONE',  ( 18.67979575497178502, 10.72451020669898547, 104.1655762719810241 ) ) ;
#192439=CARTESIAN_POINT ( 'NONE',  ( -0.05219959533910754901, -16.53943276465976808, 37.49890960531436690 ) ) ;
#192440=CARTESIAN_POINT ( 'NONE',  ( 12.06949235617739724, 12.14591786802326823, 36.87609039468568994 ) ) ;
#192441=CARTESIAN_POINT ( 'NONE',  ( -9.474510206698964154, 16.51473224551069663, 50.41557627198102409 ) ) ;
#192442=CARTESIAN_POINT ( 'NONE',  ( 5.049401038298161559, -19.05341960407611168, 72.70724293864768129 ) ) ;
#192443=CARTESIAN_POINT ( 'NONE',  ( 19.05341960407611168, 5.049401038298154454, 113.9572429386477097 ) ) ;
#192444=CARTESIAN_POINT ( 'NONE',  ( -9.564922557960796823, -16.46253265017161027, 112.0822429386476955 ) ) ;
#192445=CARTESIAN_POINT ( 'NONE',  ( -9.474510206698720793, -16.51473224551083518, 109.5844237280190043 ) ) ;
#192446=CARTESIAN_POINT ( 'NONE',  ( 19.02544592524334988, 5.153800228976608722, 46.45942372801899012 ) ) ;
#192447=CARTESIAN_POINT ( 'NONE',  ( 18.67979575497178502, 10.72451020669898547, 89.16557627198102409 ) ) ;
#192448=CARTESIAN_POINT ( 'NONE',  ( -4.483927247898539470, -16.52544592524342804, 27.29057627198103120 ) ) ;
#192449=CARTESIAN_POINT ( 'NONE',  ( 0.05219959533907565091, 21.53943276465977519, 39.99890960531436690 ) ) ;
#192450=CARTESIAN_POINT ( 'NONE',  ( -21.53943276465977519, 0.05219959533907696930, 86.24890960531436690 ) ) ;
#192451=CARTESIAN_POINT ( 'NONE',  ( -9.564922557961040184, 16.46253265017147172, 112.9177570613523329 ) ) ;
#192452=CARTESIAN_POINT ( 'NONE',  ( -5.049401038298153566, 19.05341960407611168, 100.2072429386476955 ) ) ;
#192453=CARTESIAN_POINT ( 'NONE',  ( 21.52544592524334988, 5.823673210054432836, 81.45942372801900433 ) ) ;
#192454=CARTESIAN_POINT ( 'NONE',  ( 9.474510206698971260, -16.51473224551069308, 67.91557627198102409 ) ) ;
#192456=CARTESIAN_POINT ( 'NONE',  ( 13.97604488694527802, 13.89961937509977652, 69.37390960531436690 ) ) ;
#192457=CARTESIAN_POINT ( 'NONE',  ( 12.06949235617757843, -12.14591786802309237, 93.12390960531436690 ) ) ;
#192458=VERTEX_POINT ( 'NONE', #195225 ) ;
#192459=CARTESIAN_POINT ( 'NONE',  ( -19.02544592524334988, -5.153800228976617603, 103.9594237280190043 ) ) ;
#192460=CARTESIAN_POINT ( 'NONE',  ( 16.20579543436679160, -7.371946100355085463, 81.93479165828128430 ) ) ;
#192461=CARTESIAN_POINT ( 'NONE',  ( -13.89961937509977652, 13.97604488694528158, 60.62390960531436690 ) ) ;
#192462=CARTESIAN_POINT ( 'NONE',  ( 18.62759615963255655, 10.81492255796105972, 86.66775706135234714 ) ) ;
#192463=CARTESIAN_POINT ( 'NONE',  ( -19.05341960407611168, -5.049401038298163336, 106.4572429386476955 ) ) ;
#192464=CARTESIAN_POINT ( 'NONE',  ( -8.314922557961024197, 14.29746914071037800, 82.91775706135234714 ) ) ;
#192466=CARTESIAN_POINT ( 'NONE',  ( -13.89961937509957401, -13.97604488694547875, 59.37609039468566863 ) ) ;
#192467=CARTESIAN_POINT ( 'NONE',  ( -0.05219959533937732626, 21.53943276465977519, 97.50109039468567573 ) ) ;
#192471=CARTESIAN_POINT ( 'NONE',  ( -8.224510206698735004, -14.34966873604973081, 109.5844237280190328 ) ) ;
#192472=CARTESIAN_POINT ( 'NONE',  ( -5.049401038297874678, -19.05341960407618274, 74.79275706135231871 ) ) ;
#192473=CARTESIAN_POINT ( 'NONE',  ( 16.55341960407618274, -4.379528057220086978, 91.04275706135236135 ) ) ;
#192474=FACE_OUTER_BOUND ( 'NONE', #116927, .T. ) ;
#192475=CARTESIAN_POINT ( 'NONE',  ( 4.379528057220092307, 16.55341960407617563, 72.29275706135236135 ) ) ;
#192476=CARTESIAN_POINT ( 'NONE',  ( -10.81492255796105439, 18.62759615963255655, 82.91775706135234714 ) ) ;
#192477=CARTESIAN_POINT ( 'NONE',  ( -16.46253265017146816, -9.564922557961047289, 89.16775706135234714 ) ) ;
#192478=CARTESIAN_POINT ( 'NONE',  ( -5.153800228976607833, 19.02544592524334988, 37.70942372801899722 ) ) ;
#192479=CARTESIAN_POINT ( 'NONE',  ( 13.89961937509977652, -13.97604488694527269, 63.12390960531435979 ) ) ;
#192480=CARTESIAN_POINT ( 'NONE',  ( 9.474510206698971260, -16.51473224551069308, 52.91557627198102409 ) ) ;
#192483=CARTESIAN_POINT ( 'NONE',  ( 15.80617190586746368, 15.72974639402197994, 84.37390960531438111 ) ) ;
#192485=CARTESIAN_POINT ( 'NONE',  ( 0.05219959533907565091, 21.53943276465977519, 44.99890960531435979 ) ) ;
#192486=CARTESIAN_POINT ( 'NONE',  ( -13.97604488694527625, -13.89961937509977652, 26.87390960531434558 ) ) ;
#192487=CARTESIAN_POINT ( 'NONE',  ( -16.52544592524335698, -4.483927247898792601, 68.95942372801901854 ) ) ;
#192488=ORIENTED_EDGE ( 'NONE', *, *, #129099, .T. ) ;
#192489=CARTESIAN_POINT ( 'NONE',  ( 10.81492255796106328, -18.62759615963255655, 45.41775706135234003 ) ) ;
#192490=CARTESIAN_POINT ( 'NONE',  ( 4.483927247898545687, 16.52544592524342804, 59.79057627198103120 ) ) ;
#192492=CARTESIAN_POINT ( 'NONE',  ( 12.14591786802327356, -12.06949235617739191, 35.62609039468568994 ) ) ;
#192493=CARTESIAN_POINT ( 'NONE',  ( 9.564922557961047289, -16.46253265017146816, 55.41775706135234003 ) ) ;
#192494=CARTESIAN_POINT ( 'NONE',  ( 12.06949235617757843, -12.14591786802309237, 53.12390960531436690 ) ) ;
#192495=CARTESIAN_POINT ( 'NONE',  ( 10.81492255796106328, -18.62759615963255655, 30.41775706135234358 ) ) ;
#192496=CARTESIAN_POINT ( 'NONE',  ( -19.03943276465977164, 0.05219959533909376836, 26.24890960531435624 ) ) ;
#192497=CARTESIAN_POINT ( 'NONE',  ( -10.72451020669898014, 18.67979575497178502, 90.41557627198103830 ) ) ;
#192498=CARTESIAN_POINT ( 'NONE',  ( -5.049401038298153566, 19.05341960407611168, 110.2072429386476671 ) ) ;
#192499=CARTESIAN_POINT ( 'NONE',  ( 16.52544592524342804, -4.483927247898539470, 78.54057627198103830 ) ) ;
#192500=CARTESIAN_POINT ( 'NONE',  ( 19.02544592524343514, -5.153800228976328945, 113.5405762719810241 ) ) ;
#192502=CARTESIAN_POINT ( 'NONE',  ( -13.89961937509957401, -13.97604488694547875, 64.37609039468567573 ) ) ;
#192503=CARTESIAN_POINT ( 'NONE',  ( -21.53943276465977519, 0.05219959533907696930, 116.2489096053143669 ) ) ;
#192504=CARTESIAN_POINT ( 'NONE',  ( -16.46253265017160317, 9.564922557960807481, 60.83224293864769550 ) ) ;
#192505=CARTESIAN_POINT ( 'NONE',  ( 9.564922557961047289, -16.46253265017146816, 45.41775706135232582 ) ) ;
#192506=CARTESIAN_POINT ( 'NONE',  ( 16.46253265017160672, -9.564922557960803928, 28.33224293864769550 ) ) ;
#192507=CARTESIAN_POINT ( 'NONE',  ( -21.53943276465977519, -0.05219959533937600094, 68.75109039468568994 ) ) ;
#192509=CARTESIAN_POINT ( 'NONE',  ( -16.55341960407611168, -4.379528057220339221, 51.45724293864770260 ) ) ;
#192510=CARTESIAN_POINT ( 'NONE',  ( 19.03943276465977164, -0.05219959533909143690, 63.74890960531435979 ) ) ;
#192511=CARTESIAN_POINT ( 'NONE',  ( 10.72451020669898902, -18.67979575497178502, 92.91557627198103830 ) ) ;
#192512=CARTESIAN_POINT ( 'NONE',  ( -13.97604488694527625, -13.89961937509977652, 61.87390960531435979 ) ) ;
#192514=CARTESIAN_POINT ( 'NONE',  ( -21.52544592524343514, 5.823673210054127303, 86.04057627198102409 ) ) ;
#192516=CARTESIAN_POINT ( 'NONE',  ( 18.62759615963255655, 10.81492255796105972, 101.6677570613523613 ) ) ;
#192518=CARTESIAN_POINT ( 'NONE',  ( -8.314922557961024197, 14.29746914071037800, 92.91775706135236135 ) ) ;
#192519=CARTESIAN_POINT ( 'NONE',  ( 14.34966873604960469, 8.224510206698951720, 79.16557627198103830 ) ) ;
#192520=CARTESIAN_POINT ( 'NONE',  ( 16.46253265017146816, 9.564922557961045513, 96.66775706135233293 ) ) ;
#192521=VERTEX_POINT ( 'NONE', #131537 ) ;
#192522=CARTESIAN_POINT ( 'NONE',  ( -21.52544592524334988, -5.823673210054445271, 18.95942372801901143 ) ) ;
#192523=CARTESIAN_POINT ( 'NONE',  ( 16.51473224551083163, -9.474510206698727899, 45.83442372801900433 ) ) ;
#192524=CARTESIAN_POINT ( 'NONE',  ( 4.483927247898790824, -16.52544592524335698, 100.2094237280190043 ) ) ;
#192525=CARTESIAN_POINT ( 'NONE',  ( 13.97604488694548053, -13.89961937509957401, 30.62609039468566863 ) ) ;
#192526=CARTESIAN_POINT ( 'NONE',  ( -16.51473224551069308, -9.474510206698971260, 91.66557627198103830 ) ) ;
#192527=CARTESIAN_POINT ( 'NONE',  ( 10.72451020669898902, -18.67979575497178502, 57.91557627198103120 ) ) ;
#192529=CARTESIAN_POINT ( 'NONE',  ( -9.474510206698964154, 16.51473224551069663, 25.41557627198103120 ) ) ;
#192530=CARTESIAN_POINT ( 'NONE',  ( 10.72451020669871369, 18.67979575497193778, 112.0844237280190185 ) ) ;
#192531=CARTESIAN_POINT ( 'NONE',  ( 16.55341960407618274, -4.379528057220086978, 76.04275706135237556 ) ) ;
#192532=CARTESIAN_POINT ( 'NONE',  ( 5.719274019375673035, 21.55341960407619339, 22.29275706135235069 ) ) ;
#192533=CARTESIAN_POINT ( 'NONE',  ( 12.06949235617739724, 12.14591786802326823, 31.87609039468567929 ) ) ;
#192534=CARTESIAN_POINT ( 'NONE',  ( 16.51473224551069308, 9.474510206698969483, 104.1655762719810241 ) ) ;
#192535=CARTESIAN_POINT ( 'NONE',  ( -16.51473224551069308, -9.474510206698971260, 46.66557627198102409 ) ) ;
#192536=CARTESIAN_POINT ( 'NONE',  ( 5.153800228976335163, 19.02544592524342804, 64.79057627198100988 ) ) ;
#192538=CARTESIAN_POINT ( 'NONE',  ( 0.05219959533934541429, -16.53943276465976808, 45.00109039468568284 ) ) ;
#192539=CARTESIAN_POINT ( 'NONE',  ( 12.06949235617757843, -12.14591786802309237, 88.12390960531436690 ) ) ;
#192540=CARTESIAN_POINT ( 'NONE',  ( 14.34966873604972726, -8.224510206698740333, 95.83442372801903275 ) ) ;
#192541=CARTESIAN_POINT ( 'NONE',  ( -5.823673210054431948, 21.52544592524334988, 62.70942372801902565 ) ) ;
#192542=CARTESIAN_POINT ( 'NONE',  ( -9.474510206698964154, 16.51473224551069663, 75.41557627198103830 ) ) ;
#192543=CARTESIAN_POINT ( 'NONE',  ( -9.564922557960796823, -16.46253265017161027, 67.08224293864769550 ) ) ;
#192544=CARTESIAN_POINT ( 'NONE',  ( -16.51473224551069308, -9.474510206698971260, 96.66557627198102409 ) ) ;
#192545=CARTESIAN_POINT ( 'NONE',  ( -16.55341960407611168, -4.379528057220339221, 41.45724293864769550 ) ) ;
#192546=CARTESIAN_POINT ( 'NONE',  ( -14.34966873604972548, 8.224510206698743886, 93.33442372801901854 ) ) ;
#192548=CARTESIAN_POINT ( 'NONE',  ( -9.474510206698720793, -16.51473224551083518, 49.58442372801899722 ) ) ;
#192550=CARTESIAN_POINT ( 'NONE',  ( -19.03943276465977164, 0.05219959533909376836, 61.24890960531436690 ) ) ;
#192551=CARTESIAN_POINT ( 'NONE',  ( -16.51473224551082808, 9.474510206698731452, 43.33442372801900433 ) ) ;
#192554=CARTESIAN_POINT ( 'NONE',  ( 14.34966873604972726, -8.224510206698740333, 55.83442372801901854 ) ) ;
#192555=CARTESIAN_POINT ( 'NONE',  ( -19.03943276465977164, -0.05219959533935918106, 68.75109039468566152 ) ) ;
#192556=CARTESIAN_POINT ( 'NONE',  ( 16.52544592524335698, 4.483927247898782831, 71.45942372801901854 ) ) ;
#192557=CARTESIAN_POINT ( 'NONE',  ( 17.31747979337948351, 6.344076630961057006, 93.87944868065186199 ) ) ;
#192558=CARTESIAN_POINT ( 'NONE',  ( 19.02544592524343514, -5.153800228976328945, 93.54057627198102409 ) ) ;
#192559=CARTESIAN_POINT ( 'NONE',  ( 5.719274019375673035, 21.55341960407619339, 27.29275706135234358 ) ) ;
#192560=CARTESIAN_POINT ( 'NONE',  ( 16.51473224551083163, -9.474510206698727899, 75.83442372801900433 ) ) ;
#192561=CARTESIAN_POINT ( 'NONE',  ( -19.03943276465977164, 0.05219959533909376836, 111.2489096053143669 ) ) ;
#192562=CARTESIAN_POINT ( 'NONE',  ( 19.05341960407611168, 5.049401038298154454, 38.95724293864767418 ) ) ;
#192563=CARTESIAN_POINT ( 'NONE',  ( -13.97604488694527625, -13.89961937509977652, 96.87390960531433848 ) ) ;
#192564=CARTESIAN_POINT ( 'NONE',  ( 4.379528057220339221, -16.55341960407611168, 42.70724293864770260 ) ) ;
#192565=CARTESIAN_POINT ( 'NONE',  ( -9.564922557960796823, -16.46253265017161027, 37.08224293864768839 ) ) ;
#192566=CARTESIAN_POINT ( 'NONE',  ( 5.049401038297881783, 19.05341960407617563, 57.29275706135231871 ) ) ;
#192567=CARTESIAN_POINT ( 'NONE',  ( 12.06949235617757843, -12.14591786802309237, 93.12390960531436690 ) ) ;
#192568=CARTESIAN_POINT ( 'NONE',  ( -9.564922557961040184, 16.46253265017147172, 22.91775706135233648 ) ) ;
#192569=CARTESIAN_POINT ( 'NONE',  ( 5.153800228976335163, 19.02544592524342804, 54.79057627198103120 ) ) ;
#192570=CARTESIAN_POINT ( 'NONE',  ( 21.52544592524344225, -5.823673210054117533, 68.54057627198103830 ) ) ;
#192571=CARTESIAN_POINT ( 'NONE',  ( 16.55341960407611168, 4.379528057220329451, 48.95724293864770971 ) ) ;
#192572=CARTESIAN_POINT ( 'NONE',  ( 0.05219959533936267826, -19.03943276465977164, 20.00109039468567218 ) ) ;
#192573=CARTESIAN_POINT ( 'NONE',  ( -19.05341960407611168, -5.049401038298163336, 101.4572429386476955 ) ) ;
#192575=CARTESIAN_POINT ( 'NONE',  ( -13.97604488694527625, -13.89961937509977652, 111.8739096053143243 ) ) ;
#192576=CARTESIAN_POINT ( 'NONE',  ( -13.89961937509977652, 13.97604488694528158, 55.62390960531434558 ) ) ;
#192577=CARTESIAN_POINT ( 'NONE',  ( 5.153800228976335163, 19.02544592524342804, 24.79057627198102765 ) ) ;
#192578=CARTESIAN_POINT ( 'NONE',  ( 12.14591786802309770, 12.06949235617756955, 89.37390960531435269 ) ) ;
#192579=CARTESIAN_POINT ( 'NONE',  ( -0.05219959533907301413, -21.53943276465977519, 92.49890960531436690 ) ) ;
#192580=CARTESIAN_POINT ( 'NONE',  ( -19.02544592524342804, 5.153800228976336051, 106.0405762719810241 ) ) ;
#192581=CARTESIAN_POINT ( 'NONE',  ( 18.67979575497178502, 10.72451020669898547, 109.1655762719810383 ) ) ;
#192582=CARTESIAN_POINT ( 'NONE',  ( -5.153800228976328057, -19.02544592524343514, 107.2905762719810383 ) ) ;
#192583=CARTESIAN_POINT ( 'NONE',  ( 4.379528057220339221, -16.55341960407611168, 107.7072429386476955 ) ) ;
#192584=CARTESIAN_POINT ( 'NONE',  ( 21.55341960407619695, -5.719274019375665929, 76.04275706135237556 ) ) ;
#192585=CARTESIAN_POINT ( 'NONE',  ( 21.53943276465977519, -0.05219959533907433946, 88.74890960531436690 ) ) ;
#192586=CARTESIAN_POINT ( 'NONE',  ( 17.31728774477274158, -6.344390552232372471, 108.3190665168931730 ) ) ;
#192587=CARTESIAN_POINT ( 'NONE',  ( 19.46398650005391318, -5.499999999999944045, 77.68269651486370719 ) ) ;
#192589=CARTESIAN_POINT ( 'NONE',  ( 16.53943276465976808, 0.05219959533934440121, 31.25109039468568639 ) ) ;
#192590=CARTESIAN_POINT ( 'NONE',  ( 14.29746914071049879, -8.314922557960816363, 113.3322429386476955 ) ) ;
#192591=CARTESIAN_POINT ( 'NONE',  ( 18.22780087662125226, -5.499999999999864997, 51.01540105326108687 ) ) ;
#192592=CARTESIAN_POINT ( 'NONE',  ( -5.049401038298153566, 19.05341960407611168, 55.20724293864769550 ) ) ;
#192593=CARTESIAN_POINT ( 'NONE',  ( -4.483927247898539470, -16.52544592524342804, 97.29057627198105251 ) ) ;
#192594=CARTESIAN_POINT ( 'NONE',  ( 21.53943276465977519, -0.05219959533907433946, 28.74890960531435624 ) ) ;
#192595=CARTESIAN_POINT ( 'NONE',  ( 8.314922557960818139, 14.29746914071049879, 69.58224293864769550 ) ) ;
#192596=CARTESIAN_POINT ( 'NONE',  ( 13.97604488694548053, -13.89961937509957401, 110.6260903946856615 ) ) ;
#192597=CARTESIAN_POINT ( 'NONE',  ( -21.53943276465977519, -0.05219959533937600094, 68.75109039468568994 ) ) ;
#192598=CARTESIAN_POINT ( 'NONE',  ( 16.52216118717207749, -7.221426719304491648, 76.42400978953006074 ) ) ;
#192599=CARTESIAN_POINT ( 'NONE',  ( -13.97604488694527625, -13.89961937509977652, 106.8739096053143669 ) ) ;
#192600=CARTESIAN_POINT ( 'NONE',  ( -8.314922557961024197, 14.29746914071037800, 97.91775706135236135 ) ) ;
#192601=CARTESIAN_POINT ( 'NONE',  ( -19.02544592524342804, 5.153800228976336051, 41.04057627198103120 ) ) ;
#192602=CARTESIAN_POINT ( 'NONE',  ( 13.89961937509977652, -13.97604488694527269, 93.12390960531436690 ) ) ;
#192603=CARTESIAN_POINT ( 'NONE',  ( 10.81492255796078972, 18.62759615963270932, 99.58224293864770971 ) ) ;
#192605=CARTESIAN_POINT ( 'NONE',  ( 12.14591786802327356, -12.06949235617739191, 25.62609039468567929 ) ) ;
#192606=CARTESIAN_POINT ( 'NONE',  ( 14.34966873604960469, 8.224510206698951720, 59.16557627198103120 ) ) ;
#192607=CARTESIAN_POINT ( 'NONE',  ( 15.72974639402176855, 15.80617190586768217, 66.87609039468568994 ) ) ;
#192608=CARTESIAN_POINT ( 'NONE',  ( 14.29746914071037800, 8.314922557961029526, 96.66775706135234714 ) ) ;
#192609=CARTESIAN_POINT ( 'NONE',  ( 17.44279575226787671, -5.990770900253883369, 48.33557567514320397 ) ) ;
#192611=CARTESIAN_POINT ( 'NONE',  ( 0.05219959533910956823, 16.53943276465976808, 24.99890960531435624 ) ) ;
#192612=CARTESIAN_POINT ( 'NONE',  ( -8.314922557961024197, 14.29746914071037800, 62.91775706135236135 ) ) ;
#192613=CARTESIAN_POINT ( 'NONE',  ( 0.05219959533909260263, 19.03943276465977164, 69.99890960531435269 ) ) ;
#192614=CARTESIAN_POINT ( 'NONE',  ( 16.46253265017160672, -9.564922557960803928, 83.33224293864768129 ) ) ;
#192615=CARTESIAN_POINT ( 'NONE',  ( 21.53943276465977519, 0.05219959533937863772, 81.25109039468568994 ) ) ;
#192616=CARTESIAN_POINT ( 'NONE',  ( -8.224510206698735004, -14.34966873604973081, 94.58442372801901854 ) ) ;
#192617=CARTESIAN_POINT ( 'NONE',  ( 14.29746914071049879, -8.314922557960816363, 58.33224293864768839 ) ) ;
#192618=CARTESIAN_POINT ( 'NONE',  ( -16.51473224551069308, -9.474510206698971260, 66.66557627198102409 ) ) ;
#192620=CARTESIAN_POINT ( 'NONE',  ( -5.153800228976607833, 19.02544592524334988, 102.7094237280189759 ) ) ;
#192621=CARTESIAN_POINT ( 'NONE',  ( 16.55341960407611168, 4.379528057220329451, 113.9572429386477239 ) ) ;
#192622=CARTESIAN_POINT ( 'NONE',  ( -0.05219959533909027116, -19.03943276465977164, 82.49890960531436690 ) ) ;
#192623=CARTESIAN_POINT ( 'NONE',  ( 0.05219959533934541429, -16.53943276465976808, 25.00109039468567218 ) ) ;
#192625=CARTESIAN_POINT ( 'NONE',  ( 9.564922557961047289, -16.46253265017146816, 20.41775706135233293 ) ) ;
#192626=CARTESIAN_POINT ( 'NONE',  ( -4.483927247898782831, 16.52544592524335698, 77.70942372801900433 ) ) ;
#192627=CARTESIAN_POINT ( 'NONE',  ( -13.89961937509957401, -13.97604488694547875, 99.37609039468567573 ) ) ;
#192628=CARTESIAN_POINT ( 'NONE',  ( -4.483927247898539470, -16.52544592524342804, 112.2905762719810241 ) ) ;
#192629=CARTESIAN_POINT ( 'NONE',  ( 16.52544592524335698, 4.483927247898782831, 66.45942372801903275 ) ) ;
#192631=CARTESIAN_POINT ( 'NONE',  ( 16.51473224551083163, -9.474510206698727899, 55.83442372801899722 ) ) ;
#192632=CARTESIAN_POINT ( 'NONE',  ( 15.72974639402176855, 15.80617190586768217, 101.8760903946857042 ) ) ;
#192633=CARTESIAN_POINT ( 'NONE',  ( 13.97604488694527802, 13.89961937509977652, 34.37390960531436690 ) ) ;
#192634=CARTESIAN_POINT ( 'NONE',  ( -19.02544592524342804, 5.153800228976336051, 81.04057627198103830 ) ) ;
#192635=CARTESIAN_POINT ( 'NONE',  ( 4.379528057220339221, -16.55341960407611168, 77.70724293864770971 ) ) ;
#192636=CARTESIAN_POINT ( 'NONE',  ( 5.823673210054444382, -21.52544592524334988, 95.20942372801903275 ) ) ;
#192637=CARTESIAN_POINT ( 'NONE',  ( 19.02544592524334988, 5.153800228976608722, 51.45942372801900433 ) ) ;
#192638=CARTESIAN_POINT ( 'NONE',  ( 19.05341960407617918, -5.049401038297876454, 46.04275706135233293 ) ) ;
#192639=CARTESIAN_POINT ( 'NONE',  ( 18.62759615963271287, -10.81492255796078972, 43.33224293864769550 ) ) ;
#192640=CARTESIAN_POINT ( 'NONE',  ( -18.62759615963255300, -10.81492255796106328, 94.16775706135237556 ) ) ;
#192641=CARTESIAN_POINT ( 'NONE',  ( 19.03943276465977164, -0.05219959533909143690, 73.74890960531435269 ) ) ;
#192642=CARTESIAN_POINT ( 'NONE',  ( -15.80617190586768217, 15.72974639402176855, 113.1260903946856899 ) ) ;
#192643=CARTESIAN_POINT ( 'NONE',  ( 10.72451020669898902, -18.67979575497178502, 52.91557627198103830 ) ) ;
#192644=CARTESIAN_POINT ( 'NONE',  ( 9.564922557960805705, 16.46253265017160317, 94.58224293864769550 ) ) ;
#192645=CARTESIAN_POINT ( 'NONE',  ( -13.89961937509957401, -13.97604488694547875, 74.37609039468566152 ) ) ;
#192646=CARTESIAN_POINT ( 'NONE',  ( -5.049401038298153566, 19.05341960407611168, 100.2072429386476955 ) ) ;
#192647=CARTESIAN_POINT ( 'NONE',  ( -19.03943276465977164, -0.05219959533935918106, 98.75109039468567573 ) ) ;
#192648=CARTESIAN_POINT ( 'NONE',  ( -14.34966873604972548, 8.224510206698743886, 43.33442372801901143 ) ) ;
#192649=CARTESIAN_POINT ( 'NONE',  ( 12.14591786802309770, 12.06949235617756955, 104.3739096053143669 ) ) ;
#192650=CARTESIAN_POINT ( 'NONE',  ( -16.46253265017160317, 9.564922557960807481, 90.83224293864769550 ) ) ;
#192651=CARTESIAN_POINT ( 'NONE',  ( -18.67979575497178146, -10.72451020669898902, 66.66557627198102409 ) ) ;
#192652=CARTESIAN_POINT ( 'NONE',  ( -4.483927247898782831, 16.52544592524335698, 32.70942372801900433 ) ) ;
#192653=CARTESIAN_POINT ( 'NONE',  ( 15.80617190586769283, -15.72974639402175789, 35.62609039468568994 ) ) ;
#192654=CARTESIAN_POINT ( 'NONE',  ( 10.72451020669871369, 18.67979575497193778, 87.08442372801901854 ) ) ;
#192655=CARTESIAN_POINT ( 'NONE',  ( 0.05219959533934541429, -16.53943276465976808, 80.00109039468568994 ) ) ;
#192656=CARTESIAN_POINT ( 'NONE',  ( 19.02544592524343514, -5.153800228976328945, 73.54057627198103830 ) ) ;
#192657=CARTESIAN_POINT ( 'NONE',  ( 0.05219959533910956823, 16.53943276465976808, 74.99890960531435269 ) ) ;
#192658=CARTESIAN_POINT ( 'NONE',  ( -12.14591786802309592, -12.06949235617757132, 26.87390960531435979 ) ) ;
#192659=CARTESIAN_POINT ( 'NONE',  ( -5.153800228976607833, 19.02544592524334988, 57.70942372801899012 ) ) ;
#192661=CARTESIAN_POINT ( 'NONE',  ( -21.52544592524334988, -5.823673210054445271, 33.95942372801901143 ) ) ;
#192662=CARTESIAN_POINT ( 'NONE',  ( -8.224510206698948167, 14.34966873604960824, 80.41557627198103830 ) ) ;
#192663=CARTESIAN_POINT ( 'NONE',  ( -16.46253265017160317, 9.564922557960807481, 100.8322429386477097 ) ) ;
#192664=CARTESIAN_POINT ( 'NONE',  ( -14.34966873604972548, 8.224510206698743886, 103.3344237280190043 ) ) ;
#192665=CARTESIAN_POINT ( 'NONE',  ( 21.55341960407619695, -5.719274019375665929, 66.04275706135236135 ) ) ;
#192666=CARTESIAN_POINT ( 'NONE',  ( -4.379528057220086978, -16.55341960407618274, 44.79275706135234714 ) ) ;
#192667=CARTESIAN_POINT ( 'NONE',  ( -15.80617190586768217, 15.72974639402176855, 38.12609039468567573 ) ) ;
#192668=CARTESIAN_POINT ( 'NONE',  ( -12.14591786802309592, -12.06949235617757132, 76.87390960531439532 ) ) ;
#192670=CARTESIAN_POINT ( 'NONE',  ( -0.05219959533937732626, 21.53943276465977519, 22.50109039468567573 ) ) ;
#192671=CARTESIAN_POINT ( 'NONE',  ( -16.53943276465976808, 0.05219959533911058130, 86.24890960531436690 ) ) ;
#192672=CARTESIAN_POINT ( 'NONE',  ( 17.50000000000005329, -4.658240926743120625, 26.44470417816803121 ) ) ;
#192673=CARTESIAN_POINT ( 'NONE',  ( 16.55341960407611168, 4.379528057220329451, 53.95724293864770260 ) ) ;
#192674=CARTESIAN_POINT ( 'NONE',  ( 19.03943276465977164, -0.05219959533909143690, 28.74890960531435624 ) ) ;
#192675=CARTESIAN_POINT ( 'NONE',  ( 10.81492255796078972, 18.62759615963270932, 39.58224293864769550 ) ) ;
#192676=CARTESIAN_POINT ( 'NONE',  ( 12.14591786802309770, 12.06949235617756955, 79.37390960531436690 ) ) ;
#192678=CARTESIAN_POINT ( 'NONE',  ( -15.72974639402197994, 15.80617190586746368, 75.62390960531439532 ) ) ;
#192679=CARTESIAN_POINT ( 'NONE',  ( -13.97604488694527625, -13.89961937509977652, 81.87390960531436690 ) ) ;
#192680=CARTESIAN_POINT ( 'NONE',  ( -19.03943276465977164, 0.05219959533909376836, 41.24890960531435269 ) ) ;
#192681=CARTESIAN_POINT ( 'NONE',  ( 13.97604488694548053, -13.89961937509957401, 85.62609039468568994 ) ) ;
#192682=CARTESIAN_POINT ( 'NONE',  ( -10.72451020669870658, -18.67979575497194134, 59.58442372801901854 ) ) ;
#192683=CARTESIAN_POINT ( 'NONE',  ( 15.80617190586746368, 15.72974639402197994, 59.37390960531436690 ) ) ;
#192684=CARTESIAN_POINT ( 'NONE',  ( -5.049401038298153566, 19.05341960407611168, 35.20724293864768839 ) ) ;
#192685=CARTESIAN_POINT ( 'NONE',  ( 16.46253265017160672, -9.564922557960803928, 73.33224293864769550 ) ) ;
#192686=VERTEX_POINT ( 'NONE', #196239 ) ;
#192687=CARTESIAN_POINT ( 'NONE',  ( -14.34966873604972548, 8.224510206698743886, 53.33442372801901854 ) ) ;
#192688=CARTESIAN_POINT ( 'NONE',  ( 18.67979575497194134, -10.72451020669871369, 30.83442372801902209 ) ) ;
#192689=CARTESIAN_POINT ( 'NONE',  ( -15.80617190586768217, 15.72974639402176855, 68.12609039468567573 ) ) ;
#192690=CARTESIAN_POINT ( 'NONE',  ( 0.05219959533909260263, 19.03943276465977164, 104.9989096053143669 ) ) ;
#192691=CARTESIAN_POINT ( 'NONE',  ( 15.72974639402199770, -15.80617190586745480, 88.12390960531436690 ) ) ;
#192692=CARTESIAN_POINT ( 'NONE',  ( -15.72974639402197994, 15.80617190586746368, 115.6239096053143669 ) ) ;
#192693=CARTESIAN_POINT ( 'NONE',  ( -0.05219959533934338120, 16.53943276465976808, 47.50109039468568994 ) ) ;
#192694=CARTESIAN_POINT ( 'NONE',  ( 5.823673210054125526, 21.52544592524343514, 49.79057627198102409 ) ) ;
#192695=CARTESIAN_POINT ( 'NONE',  ( 15.80617190586769283, -15.72974639402175789, 110.6260903946857042 ) ) ;
#192696=CARTESIAN_POINT ( 'NONE',  ( -9.564922557960796823, -16.46253265017161027, 57.08224293864769550 ) ) ;
#192697=CARTESIAN_POINT ( 'NONE',  ( -0.05219959533909027116, -19.03943276465977164, 107.4989096053143527 ) ) ;
#192698=CARTESIAN_POINT ( 'NONE',  ( -16.46253265017160317, 9.564922557960807481, 95.83224293864769550 ) ) ;
#192700=CARTESIAN_POINT ( 'NONE',  ( -5.153800228976607833, 19.02544592524334988, 62.70942372801899722 ) ) ;
#192701=CARTESIAN_POINT ( 'NONE',  ( 5.823673210054125526, 21.52544592524343514, 49.79057627198102409 ) ) ;
#192702=CARTESIAN_POINT ( 'NONE',  ( -14.34966873604960291, -8.224510206698953496, 31.66557627198102054 ) ) ;
#192703=CARTESIAN_POINT ( 'NONE',  ( -5.049401038297874678, -19.05341960407617918, 94.79275706135230450 ) ) ;
#192704=CARTESIAN_POINT ( 'NONE',  ( 18.10062525802556621, -5.499999999999864997, 51.01383468041923663 ) ) ;
#192705=CARTESIAN_POINT ( 'NONE',  ( -0.05219959533936034679, 19.03943276465977164, 27.50109039468566507 ) ) ;
#192706=CARTESIAN_POINT ( 'NONE',  ( 9.474510206698729675, 16.51473224551082808, 92.08442372801900433 ) ) ;
#192707=CARTESIAN_POINT ( 'NONE',  ( -21.53943276465977519, 0.05219959533907696930, 81.24890960531436690 ) ) ;
#192708=CARTESIAN_POINT ( 'NONE',  ( 5.049401038297881783, 19.05341960407617563, 52.29275706135234003 ) ) ;
#192709=CARTESIAN_POINT ( 'NONE',  ( 16.31925111598457789, 7.325300261831552362, 107.3357546103274558 ) ) ;
#192710=CARTESIAN_POINT ( 'NONE',  ( -13.89961937509977652, 13.97604488694528158, 60.62390960531436690 ) ) ;
#192711=CARTESIAN_POINT ( 'NONE',  ( -14.34966873604960291, -8.224510206698953496, 66.66557627198102409 ) ) ;
#192712=CARTESIAN_POINT ( 'NONE',  ( -5.049401038298153566, 19.05341960407611168, 35.20724293864768839 ) ) ;
#192713=CARTESIAN_POINT ( 'NONE',  ( -12.06949235617756955, 12.14591786802309770, 35.62390960531437401 ) ) ;
#192714=CARTESIAN_POINT ( 'NONE',  ( 18.10062525802553779, -5.500000000000022204, 56.01383468041922242 ) ) ;
#192715=CARTESIAN_POINT ( 'NONE',  ( 12.14591786802327356, -12.06949235617739191, 105.6260903946856899 ) ) ;
#192716=CARTESIAN_POINT ( 'NONE',  ( -5.049401038298153566, 19.05341960407611168, 70.20724293864769550 ) ) ;
#192717=CARTESIAN_POINT ( 'NONE',  ( 16.46253265017146816, 9.564922557961045513, 31.66775706135232937 ) ) ;
#192718=CARTESIAN_POINT ( 'NONE',  ( 14.34966873604972726, -8.224510206698740333, 35.83442372801901143 ) ) ;
#192719=CARTESIAN_POINT ( 'NONE',  ( -15.80617190586745835, -15.72974639402198527, 51.87390960531437401 ) ) ;
#192720=CARTESIAN_POINT ( 'NONE',  ( -10.72451020669870658, -18.67979575497194134, 104.5844237280190185 ) ) ;
#192721=EDGE_LOOP ( 'NONE', ( #44399, #166449, #133750 ) ) ;
#192722=CARTESIAN_POINT ( 'NONE',  ( -16.46253265017160317, 9.564922557960807481, 60.83224293864769550 ) ) ;
#192724=CARTESIAN_POINT ( 'NONE',  ( -13.97604488694527625, -13.89961937509977652, 91.87390960531432427 ) ) ;
#192726=CARTESIAN_POINT ( 'NONE',  ( -18.67979575497193778, 10.72451020669871902, 23.33442372801901499 ) ) ;
#192728=CARTESIAN_POINT ( 'NONE',  ( 4.483927247898545687, 16.52544592524342804, 99.79057627198103830 ) ) ;
#192729=EDGE_CURVE ( 'NONE', #10184, #107085, #30198, .T. ) ;
#192730=CARTESIAN_POINT ( 'NONE',  ( 18.62759615963271287, -10.81492255796078972, 83.33224293864769550 ) ) ;
#192731=CARTESIAN_POINT ( 'NONE',  ( 19.05341960407611168, 5.049401038298154454, 63.95724293864769550 ) ) ;
#192732=CARTESIAN_POINT ( 'NONE',  ( 13.89961937509977652, -13.97604488694527269, 68.12390960531436690 ) ) ;
#192733=CARTESIAN_POINT ( 'NONE',  ( 18.67979575497178502, 10.72451020669898547, 104.1655762719810241 ) ) ;
#192735=CARTESIAN_POINT ( 'NONE',  ( -19.05341960407611168, -5.049401038298163336, 71.45724293864766707 ) ) ;
#192737=CARTESIAN_POINT ( 'NONE',  ( 0.05219959533910956823, 16.53943276465976808, 99.99890960531436690 ) ) ;
#192738=CARTESIAN_POINT ( 'NONE',  ( 19.05341960407611168, 5.049401038298154454, 23.95724293864769194 ) ) ;
#192739=CARTESIAN_POINT ( 'NONE',  ( -19.02544592524334988, -5.153800228976617603, 88.95942372801897591 ) ) ;
#192740=CARTESIAN_POINT ( 'NONE',  ( -4.483927247898539470, -16.52544592524342804, 92.29057627198103830 ) ) ;
#192741=CARTESIAN_POINT ( 'NONE',  ( -10.72451020669870658, -18.67979575497194134, 74.58442372801901854 ) ) ;
#192742=CARTESIAN_POINT ( 'NONE',  ( -13.89961937509977652, 13.97604488694528158, 65.62390960531436690 ) ) ;
#192743=CARTESIAN_POINT ( 'NONE',  ( 21.55341960407619695, -5.719274019375665929, 36.04275706135234714 ) ) ;
#192744=CARTESIAN_POINT ( 'NONE',  ( 21.53943276465977519, -0.05219959533907433946, 108.7489096053143669 ) ) ;
#192745=CARTESIAN_POINT ( 'NONE',  ( -5.049401038298153566, 19.05341960407611168, 75.20724293864769550 ) ) ;
#192747=CARTESIAN_POINT ( 'NONE',  ( 4.483927247898790824, -16.52544592524335698, 30.20942372801902565 ) ) ;
#192748=CARTESIAN_POINT ( 'NONE',  ( -10.72451020669898014, 18.67979575497178502, 30.41557627198101699 ) ) ;
#192749=CARTESIAN_POINT ( 'NONE',  ( 5.823673210054444382, -21.52544592524334988, 60.20942372801902565 ) ) ;
#192750=CARTESIAN_POINT ( 'NONE',  ( 13.97604488694527802, 13.89961937509977652, 104.3739096053143385 ) ) ;
#192751=CARTESIAN_POINT ( 'NONE',  ( 19.03943276465977164, 0.05219959533936151252, 96.25109039468567573 ) ) ;
#192752=CARTESIAN_POINT ( 'NONE',  ( 5.153800228976335163, 19.02544592524342804, 44.79057627198103830 ) ) ;
#192753=CARTESIAN_POINT ( 'NONE',  ( -13.97604488694527625, -13.89961937509977652, 76.87390960531433848 ) ) ;
#192754=CARTESIAN_POINT ( 'NONE',  ( 12.14591786802309770, 12.06949235617756955, 99.37390960531436690 ) ) ;
#192755=CARTESIAN_POINT ( 'NONE',  ( 16.51473224551069308, 9.474510206698969483, 109.1655762719810383 ) ) ;
#192756=CARTESIAN_POINT ( 'NONE',  ( -4.483927247898539470, -16.52544592524342804, 87.29057627198103830 ) ) ;
#192757=CARTESIAN_POINT ( 'NONE',  ( -19.03943276465977164, 0.05219959533909376836, 101.2489096053143669 ) ) ;
#192758=CARTESIAN_POINT ( 'NONE',  ( 4.379528057220339221, -16.55341960407611168, 47.70724293864770260 ) ) ;
#192759=CARTESIAN_POINT ( 'NONE',  ( -16.46253265017160317, 9.564922557960807481, 40.83224293864769550 ) ) ;
#192760=CARTESIAN_POINT ( 'NONE',  ( 18.62759615963255655, 10.81492255796105972, 51.66775706135234714 ) ) ;
#192761=CARTESIAN_POINT ( 'NONE',  ( 9.474510206698729675, 16.51473224551082808, 77.08442372801900433 ) ) ;
#192762=CARTESIAN_POINT ( 'NONE',  ( -16.53943276465976808, 0.05219959533911058130, 51.24890960531436690 ) ) ;
#192763=CARTESIAN_POINT ( 'NONE',  ( -15.72974639402197994, 15.80617190586746368, 100.6239096053143811 ) ) ;
#192764=CARTESIAN_POINT ( 'NONE',  ( -5.719274019375978568, 21.55341960407610458, 50.20724293864769550 ) ) ;
#192765=CARTESIAN_POINT ( 'NONE',  ( 16.46253265017160672, -9.564922557960803928, 108.3322429386476955 ) ) ;
#192766=CARTESIAN_POINT ( 'NONE',  ( -14.34966873604960291, -8.224510206698953496, 81.66557627198103830 ) ) ;
#192767=CARTESIAN_POINT ( 'NONE',  ( -5.153800228976328057, -19.02544592524343514, 52.29057627198100988 ) ) ;
#192768=CARTESIAN_POINT ( 'NONE',  ( 14.34966873604960469, 8.224510206698951720, 29.16557627198103120 ) ) ;
#192769=CARTESIAN_POINT ( 'NONE',  ( -8.314922557961024197, 14.29746914071037800, 102.9177570613523756 ) ) ;
#192770=CARTESIAN_POINT ( 'NONE',  ( -16.55341960407617563, 4.379528057220093196, 78.54275706135236135 ) ) ;
#192771=CARTESIAN_POINT ( 'NONE',  ( -9.474510206698720793, -16.51473224551083518, 34.58442372801899722 ) ) ;
#192773=CARTESIAN_POINT ( 'NONE',  ( 19.03943276465977164, -0.05219959533909143690, 103.7489096053143669 ) ) ;
#192774=CARTESIAN_POINT ( 'NONE',  ( -19.02544592524342804, 5.153800228976336051, 81.04057627198103830 ) ) ;
#192775=CARTESIAN_POINT ( 'NONE',  ( -13.97604488694527625, -13.89961937509977652, 31.87390960531435979 ) ) ;
#192776=CARTESIAN_POINT ( 'NONE',  ( 16.55341960407611168, 4.379528057220329451, 48.95724293864770971 ) ) ;
#192777=CARTESIAN_POINT ( 'NONE',  ( 5.049401038298161559, -19.05341960407611168, 112.7072429386476813 ) ) ;
#192778=CARTESIAN_POINT ( 'NONE',  ( -16.51473224551069308, -9.474510206698971260, 106.6655762719810383 ) ) ;
#192779=CARTESIAN_POINT ( 'NONE',  ( 5.823673210054125526, 21.52544592524343514, 44.79057627198103120 ) ) ;
#192780=CARTESIAN_POINT ( 'NONE',  ( -16.53943276465976808, 0.05219959533911058130, 86.24890960531436690 ) ) ;
#192781=CARTESIAN_POINT ( 'NONE',  ( 8.314922557961029526, -14.29746914071037800, 40.41775706135234714 ) ) ;
#192782=CARTESIAN_POINT ( 'NONE',  ( -12.06949235617756955, 12.14591786802309770, 60.62390960531437401 ) ) ;
#192783=CARTESIAN_POINT ( 'NONE',  ( 18.22780087662122384, -5.500000000000022204, 86.01540105326108687 ) ) ;
#192784=CARTESIAN_POINT ( 'NONE',  ( 0.05219959533936267826, -19.03943276465977164, 65.00109039468567573 ) ) ;
#192785=CARTESIAN_POINT ( 'NONE',  ( -13.97604488694527625, -13.89961937509977652, 106.8739096053143669 ) ) ;
#192786=CARTESIAN_POINT ( 'NONE',  ( 0.05219959533936267826, -19.03943276465977164, 85.00109039468567573 ) ) ;
#192789=CARTESIAN_POINT ( 'NONE',  ( 4.379528057220092307, 16.55341960407617563, 32.29275706135235424 ) ) ;
#192790=CARTESIAN_POINT ( 'NONE',  ( -4.483927247898782831, 16.52544592524335698, 112.7094237280190328 ) ) ;
#192791=CARTESIAN_POINT ( 'NONE',  ( 16.46253265017146816, 9.564922557961045513, 71.66775706135233293 ) ) ;
#192792=CARTESIAN_POINT ( 'NONE',  ( -0.05219959533907301413, -21.53943276465977519, 37.49890960531436690 ) ) ;
#192793=CARTESIAN_POINT ( 'NONE',  ( 18.62759615963255655, 10.81492255796105972, 66.66775706135234714 ) ) ;
#192794=CARTESIAN_POINT ( 'NONE',  ( 19.50973618000806198, 5.499999999999992895, 37.50000000000000000 ) ) ;
#192795=CARTESIAN_POINT ( 'NONE',  ( 13.97604488694548053, -13.89961937509957401, 110.6260903946856615 ) ) ;
#192796=CARTESIAN_POINT ( 'NONE',  ( 17.50000000000000000, 7.499999999999999112, 22.00000000000000711 ) ) ;
#192797=CARTESIAN_POINT ( 'NONE',  ( 16.46253265017160672, -9.564922557960803928, 78.33224293864769550 ) ) ;
#192798=CARTESIAN_POINT ( 'NONE',  ( -9.564922557960796823, -16.46253265017161027, 27.08224293864769550 ) ) ;
#192799=CARTESIAN_POINT ( 'NONE',  ( 14.29746914071049879, -8.314922557960816363, 88.33224293864769550 ) ) ;
#192800=CARTESIAN_POINT ( 'NONE',  ( 16.46253265017160672, -9.564922557960803928, 83.33224293864768129 ) ) ;
#192801=CARTESIAN_POINT ( 'NONE',  ( -13.97604488694527625, -13.89961937509977652, 81.87390960531436690 ) ) ;
#192803=CARTESIAN_POINT ( 'NONE',  ( 16.46253265017146816, 9.564922557961045513, 96.66775706135233293 ) ) ;
#192804=B_SPLINE_CURVE_WITH_KNOTS ( 'NONE', 3,
 ( #7190, #67873, #35546, #128535, #177077, #49725, #34555, #111393, #115389, #129527, #20368, #36528, #52701, #113371, #160888, #112385, #173078, #114364, #5191, #191227 ),
 .UNSPECIFIED., .F., .F.,
 ( 4, 2, 2, 2, 2, 2, 2, 2, 2, 4 ),
 ( 3.469446951953614189E-18, 0.0004987090165372534039, 0.0009974180330745033383, 0.001246772541343131938, 0.001496127049611760537, 0.001994836066149021855, 0.002493545082686283391, 0.002742899590954914375, 0.002992254099223544492, 0.003989672132298145192 ),
 .UNSPECIFIED. ) ;
#192805=CARTESIAN_POINT ( 'NONE',  ( -21.53943276465977519, 0.05219959533907696930, 76.24890960531435269 ) ) ;
#192806=CARTESIAN_POINT ( 'NONE',  ( -19.03943276465977164, 0.05219959533909376836, 26.24890960531435624 ) ) ;
#192807=CARTESIAN_POINT ( 'NONE',  ( 16.51473224551083163, -9.474510206698727899, 65.83442372801900433 ) ) ;
#192808=CARTESIAN_POINT ( 'NONE',  ( -19.05341960407611168, -5.049401038298163336, 76.45724293864769550 ) ) ;
#192809=CARTESIAN_POINT ( 'NONE',  ( 16.51473224551069308, 9.474510206698969483, 99.16557627198102409 ) ) ;
#192811=CARTESIAN_POINT ( 'NONE',  ( 18.62759615963271287, -10.81492255796078972, 98.33224293864769550 ) ) ;
#192812=CARTESIAN_POINT ( 'NONE',  ( 12.06949235617757843, -12.14591786802309237, 88.12390960531436690 ) ) ;
#192813=CARTESIAN_POINT ( 'NONE',  ( -16.51473224551069308, -9.474510206698971260, 81.66557627198103830 ) ) ;
#192814=CARTESIAN_POINT ( 'NONE',  ( -5.049401038297874678, -19.05341960407617918, 64.79275706135233293 ) ) ;
#192815=CARTESIAN_POINT ( 'NONE',  ( 15.72974639402199770, -15.80617190586745480, 83.12390960531436690 ) ) ;
#192816=CARTESIAN_POINT ( 'NONE',  ( 10.81492255796078972, 18.62759615963270932, 79.58224293864769550 ) ) ;
#192817=CARTESIAN_POINT ( 'NONE',  ( 4.483927247898545687, 16.52544592524342804, 39.79057627198103830 ) ) ;
#192818=CARTESIAN_POINT ( 'NONE',  ( 10.81492255796106328, -18.62759615963255655, 105.4177570613523613 ) ) ;
#192819=CARTESIAN_POINT ( 'NONE',  ( -4.379528057220086978, -16.55341960407618274, 69.79275706135234714 ) ) ;
#192820=CARTESIAN_POINT ( 'NONE',  ( -5.049401038298153566, 19.05341960407611168, 90.20724293864766707 ) ) ;
#192821=CARTESIAN_POINT ( 'NONE',  ( -9.564922557960796823, -16.46253265017161027, 32.08224293864769550 ) ) ;
#192823=CARTESIAN_POINT ( 'NONE',  ( 18.67979575497194134, -10.72451020669871369, 35.83442372801901143 ) ) ;
#192824=CARTESIAN_POINT ( 'NONE',  ( -0.05219959533937732626, 21.53943276465977519, 52.50109039468567573 ) ) ;
#192825=CARTESIAN_POINT ( 'NONE',  ( -9.474510206698964154, 16.51473224551069663, 65.41557627198102409 ) ) ;
#192826=CARTESIAN_POINT ( 'NONE',  ( 10.81492255796106328, -18.62759615963255655, 35.41775706135234003 ) ) ;
#192827=CARTESIAN_POINT ( 'NONE',  ( 16.51473224551083163, -9.474510206698727899, 75.83442372801900433 ) ) ;
#192828=CARTESIAN_POINT ( 'NONE',  ( 19.03943276465977164, 0.05219959533936151252, 71.25109039468566152 ) ) ;
#192829=CARTESIAN_POINT ( 'NONE',  ( -19.05341960407611168, -5.049401038298163336, 41.45724293864769550 ) ) ;
#192830=CARTESIAN_POINT ( 'NONE',  ( 4.483927247898790824, -16.52544592524335698, 70.20942372801904696 ) ) ;
#192831=CARTESIAN_POINT ( 'NONE',  ( 9.564922557960805705, 16.46253265017160317, 49.58224293864770260 ) ) ;
#192833=CARTESIAN_POINT ( 'NONE',  ( 13.89961937509977652, -13.97604488694527269, 93.12390960531436690 ) ) ;
#192834=CARTESIAN_POINT ( 'NONE',  ( 13.97604488694527802, 13.89961937509977652, 44.37390960531435269 ) ) ;
#192835=CARTESIAN_POINT ( 'NONE',  ( 18.62759615963271287, -10.81492255796078972, 68.33224293864769550 ) ) ;
#192836=CARTESIAN_POINT ( 'NONE',  ( -8.224510206698735004, -14.34966873604973081, 64.58442372801900433 ) ) ;
#192838=CARTESIAN_POINT ( 'NONE',  ( 16.46253265017146816, 9.564922557961045513, 21.66775706135233648 ) ) ;
#192839=CARTESIAN_POINT ( 'NONE',  ( -19.02544592524342804, 5.153800228976336051, 56.04057627198100988 ) ) ;
#192840=CARTESIAN_POINT ( 'NONE',  ( 4.483927247898545687, 16.52544592524342804, 44.79057627198103120 ) ) ;
#192841=CARTESIAN_POINT ( 'NONE',  ( 16.53943276465976808, -0.05219959533910856209, 78.74890960531436690 ) ) ;
#192842=CARTESIAN_POINT ( 'NONE',  ( -19.05341960407611168, -5.049401038298163336, 76.45724293864769550 ) ) ;
#192843=CARTESIAN_POINT ( 'NONE',  ( 0.05219959533937995610, -21.53943276465977519, 40.00109039468567573 ) ) ;
#192844=CARTESIAN_POINT ( 'NONE',  ( -5.153800228976328057, -19.02544592524343514, 97.29057627198099567 ) ) ;
#192845=CARTESIAN_POINT ( 'NONE',  ( -5.719274019375665041, -21.55341960407619695, 99.79275706135234714 ) ) ;
#192846=CARTESIAN_POINT ( 'NONE',  ( -16.55341960407617563, 4.379528057220093196, 68.54275706135234714 ) ) ;
#192847=CARTESIAN_POINT ( 'NONE',  ( -21.55341960407619339, 5.719274019375674811, 28.54275706135234358 ) ) ;
#192848=CARTESIAN_POINT ( 'NONE',  ( -16.46253265017160317, 9.564922557960807481, 110.8322429386476955 ) ) ;
#192850=CARTESIAN_POINT ( 'NONE',  ( -10.81492255796078084, -18.62759615963271287, 92.08224293864769550 ) ) ;
#192851=CARTESIAN_POINT ( 'NONE',  ( 12.14591786802309770, 12.06949235617756955, 44.37390960531435979 ) ) ;
#192852=CARTESIAN_POINT ( 'NONE',  ( 0.05219959533909260263, 19.03943276465977164, 34.99890960531435979 ) ) ;
#192853=CARTESIAN_POINT ( 'NONE',  ( -4.483927247898539470, -16.52544592524342804, 62.29057627198102409 ) ) ;
#192854=CARTESIAN_POINT ( 'NONE',  ( -15.80617190586745835, -15.72974639402198527, 26.87390960531435979 ) ) ;
#192855=CARTESIAN_POINT ( 'NONE',  ( -5.823673210054116645, -21.52544592524344225, 27.29057627198103120 ) ) ;
#192856=CARTESIAN_POINT ( 'NONE',  ( 0.05219959533936267826, -19.03943276465977164, 35.00109039468566863 ) ) ;
#192857=CARTESIAN_POINT ( 'NONE',  ( 4.379528057220339221, -16.55341960407611168, 97.70724293864772392 ) ) ;
#192858=CARTESIAN_POINT ( 'NONE',  ( 5.153800228976335163, 19.02544592524342804, 104.7905762719809957 ) ) ;
#192860=CARTESIAN_POINT ( 'NONE',  ( -8.314922557961024197, 14.29746914071037800, 52.91775706135235424 ) ) ;
#192861=CARTESIAN_POINT ( 'NONE',  ( 19.03943276465977164, -0.05219959533909143690, 53.74890960531436690 ) ) ;
#192862=CARTESIAN_POINT ( 'NONE',  ( -16.80344708052379232, -6.753205037831589763, 21.14260904372344285 ) ) ;
#192863=CARTESIAN_POINT ( 'NONE',  ( -9.474510206698720793, -16.51473224551083518, 59.58442372801900433 ) ) ;
#192864=CARTESIAN_POINT ( 'NONE',  ( 16.53943276465976808, 0.05219959533934440121, 96.25109039468568994 ) ) ;
#192865=CARTESIAN_POINT ( 'NONE',  ( 9.474510206698729675, 16.51473224551082808, 102.0844237280190043 ) ) ;
#192866=CARTESIAN_POINT ( 'NONE',  ( -5.719274019375665041, -21.55341960407619695, 64.79275706135234714 ) ) ;
#192867=CARTESIAN_POINT ( 'NONE',  ( 16.46253265017160672, -9.564922557960803928, 78.33224293864769550 ) ) ;
#192868=CARTESIAN_POINT ( 'NONE',  ( 5.823673210054125526, 21.52544592524343514, 94.79057627198105251 ) ) ;
#192869=CARTESIAN_POINT ( 'NONE',  ( 4.483927247898545687, 16.52544592524342804, 109.7905762719810383 ) ) ;
#192871=CARTESIAN_POINT ( 'NONE',  ( 19.03943276465977164, 0.05219959533936151252, 76.25109039468566152 ) ) ;
#192872=CARTESIAN_POINT ( 'NONE',  ( -18.67979575497178146, -10.72451020669898902, 71.66557627198100988 ) ) ;
#192873=CARTESIAN_POINT ( 'NONE',  ( 9.474510206698729675, 16.51473224551082808, 42.08442372801900433 ) ) ;
#192874=CARTESIAN_POINT ( 'NONE',  ( 19.25918095147779141, 5.499999999999523936, 96.95284276293932635 ) ) ;
#192875=CARTESIAN_POINT ( 'NONE',  ( 21.53943276465977519, -0.05219959533907433946, 93.74890960531436690 ) ) ;
#192876=CARTESIAN_POINT ( 'NONE',  ( 17.50000000000003197, 3.565345528327901636, 28.07505513193531854 ) ) ;
#192877=CARTESIAN_POINT ( 'NONE',  ( 13.97604488694527802, 13.89961937509977652, 64.37390960531436690 ) ) ;
#192878=CARTESIAN_POINT ( 'NONE',  ( -17.50000000000000000, 5.499999999999992895, 33.71769037696435589 ) ) ;
#192879=CARTESIAN_POINT ( 'NONE',  ( 5.049401038297881783, 19.05341960407617563, 112.2927570613523471 ) ) ;
#192881=CARTESIAN_POINT ( 'NONE',  ( 19.02544592524343514, -5.153800228976328945, 43.54057627198103120 ) ) ;
#192882=CARTESIAN_POINT ( 'NONE',  ( 21.55341960407610458, 5.719274019375980345, 103.9572429386476813 ) ) ;
#192883=CARTESIAN_POINT ( 'NONE',  ( -8.314922557960811034, -14.29746914071050412, 57.08224293864769550 ) ) ;
#192884=CARTESIAN_POINT ( 'NONE',  ( -13.89961937509977652, 13.97604488694528158, 60.62390960531436690 ) ) ;
#192885=CARTESIAN_POINT ( 'NONE',  ( -0.05219959533937732626, 21.53943276465977519, 72.50109039468568994 ) ) ;
#192886=CARTESIAN_POINT ( 'NONE',  ( -13.97604488694547697, 13.89961937509957934, 113.1260903946856757 ) ) ;
#192887=CARTESIAN_POINT ( 'NONE',  ( 13.97604488694548053, -13.89961937509957401, 25.62609039468566507 ) ) ;
#192888=CARTESIAN_POINT ( 'NONE',  ( -4.379528057220328563, 16.55341960407611168, 25.20724293864769550 ) ) ;
#192889=CARTESIAN_POINT ( 'NONE',  ( -21.52544592524334988, -5.823673210054445271, 43.95942372801902565 ) ) ;
#192890=CARTESIAN_POINT ( 'NONE',  ( 5.719274019375673035, 21.55341960407619339, 22.29275706135235069 ) ) ;
#192891=CARTESIAN_POINT ( 'NONE',  ( -18.62759615963270932, 10.81492255796079327, 60.83224293864769550 ) ) ;
#192892=CARTESIAN_POINT ( 'NONE',  ( 16.51473224551083163, -9.474510206698727899, 90.83442372801900433 ) ) ;
#192894=CARTESIAN_POINT ( 'NONE',  ( 16.46253265017146816, 9.564922557961045513, 71.66775706135233293 ) ) ;
#192895=CARTESIAN_POINT ( 'NONE',  ( 0.05219959533937995610, -21.53943276465977519, 75.00109039468568994 ) ) ;
#192896=CARTESIAN_POINT ( 'NONE',  ( -19.02544592524334988, -5.153800228976617603, 48.95942372801900433 ) ) ;
#192897=CARTESIAN_POINT ( 'NONE',  ( 13.89961937509977652, -13.97604488694527269, 28.12390960531435624 ) ) ;
#192898=CARTESIAN_POINT ( 'NONE',  ( -0.05219959533907301413, -21.53943276465977519, 47.49890960531435979 ) ) ;
#192899=CARTESIAN_POINT ( 'NONE',  ( 8.224510206698953496, -14.34966873604960469, 52.91557627198103830 ) ) ;
#192900=CARTESIAN_POINT ( 'NONE',  ( -19.49149378614659511, 5.499999999999677591, 94.43757513605362419 ) ) ;
#192901=CARTESIAN_POINT ( 'NONE',  ( 15.72974639402176855, 15.80617190586768217, 111.8760903946856615 ) ) ;
#192902=CARTESIAN_POINT ( 'NONE',  ( 4.379528057220092307, 16.55341960407617563, 82.29275706135234714 ) ) ;
#192903=CARTESIAN_POINT ( 'NONE',  ( 12.14591786802309770, 12.06949235617756955, 44.37390960531435979 ) ) ;
#192904=CARTESIAN_POINT ( 'NONE',  ( -18.67979575497193778, 10.72451020669871902, 73.33442372801901854 ) ) ;
#192905=CARTESIAN_POINT ( 'NONE',  ( 0.05219959533937995610, -21.53943276465977519, 75.00109039468568994 ) ) ;
#192906=CARTESIAN_POINT ( 'NONE',  ( 15.72974639402199770, -15.80617190586745480, 88.12390960531436690 ) ) ;
#192907=CARTESIAN_POINT ( 'NONE',  ( 19.03943276465977164, -0.05219959533909143690, 33.74890960531435979 ) ) ;
#192908=CARTESIAN_POINT ( 'NONE',  ( 18.67979575497194134, -10.72451020669871369, 55.83442372801901854 ) ) ;
#192909=CARTESIAN_POINT ( 'NONE',  ( -19.05341960407611168, -5.049401038298163336, 31.45724293864769550 ) ) ;
#192910=CARTESIAN_POINT ( 'NONE',  ( 9.474510206698971260, -16.51473224551069308, 57.91557627198103120 ) ) ;
#192911=CARTESIAN_POINT ( 'NONE',  ( 14.34966873604960469, 8.224510206698951720, 89.16557627198102409 ) ) ;
#192912=CARTESIAN_POINT ( 'NONE',  ( -19.02544592524342804, 5.153800228976336051, 101.0405762719810241 ) ) ;
#192913=CARTESIAN_POINT ( 'NONE',  ( -8.224510206698948167, 14.34966873604960824, 40.41557627198103120 ) ) ;
#192914=CARTESIAN_POINT ( 'NONE',  ( -0.05219959533910754901, -16.53943276465976808, 107.4989096053143669 ) ) ;
#192915=CARTESIAN_POINT ( 'NONE',  ( 18.62759615963271287, -10.81492255796078972, 78.33224293864770971 ) ) ;
#192916=CARTESIAN_POINT ( 'NONE',  ( -21.52544592524334988, -5.823673210054445271, 18.95942372801901143 ) ) ;
#192918=CARTESIAN_POINT ( 'NONE',  ( 16.53943276465976808, 0.05219959533934440121, 26.25109039468567573 ) ) ;
#192919=CARTESIAN_POINT ( 'NONE',  ( 5.719274019375991003, -21.55341960407610458, 67.70724293864769550 ) ) ;
#192920=CARTESIAN_POINT ( 'NONE',  ( 18.62759615963255655, 10.81492255796105972, 91.66775706135234714 ) ) ;
#192921=CARTESIAN_POINT ( 'NONE',  ( 16.46253265017160672, -9.564922557960803928, 83.33224293864768129 ) ) ;
#192922=CARTESIAN_POINT ( 'NONE',  ( -21.53943276465977519, -0.05219959533937600094, 33.75109039468568284 ) ) ;
#192923=CARTESIAN_POINT ( 'NONE',  ( 10.72451020669898902, -18.67979575497178502, 22.91557627198102765 ) ) ;
#192924=CARTESIAN_POINT ( 'NONE',  ( 4.379528057220092307, 16.55341960407617563, 87.29275706135236135 ) ) ;
#192925=CARTESIAN_POINT ( 'NONE',  ( 18.67979575497194134, -10.72451020669871369, 65.83442372801900433 ) ) ;
#192926=CARTESIAN_POINT ( 'NONE',  ( -19.05341960407617563, 5.049401038297882671, 23.54275706135233648 ) ) ;
#192927=CARTESIAN_POINT ( 'NONE',  ( 4.483927247898790824, -16.52544592524335698, 75.20942372801901854 ) ) ;
#192928=CARTESIAN_POINT ( 'NONE',  ( 10.72451020669871369, 18.67979575497193778, 27.08442372801901854 ) ) ;
#192929=CARTESIAN_POINT ( 'NONE',  ( -9.474510206698964154, 16.51473224551069663, 30.41557627198102054 ) ) ;
#192930=CARTESIAN_POINT ( 'NONE',  ( -15.80617190586768217, 15.72974639402176855, 88.12609039468570415 ) ) ;
#192931=CARTESIAN_POINT ( 'NONE',  ( -19.02544592524342804, 5.153800228976336051, 91.04057627198100988 ) ) ;
#192932=B_SPLINE_CURVE_WITH_KNOTS ( 'NONE', 3,
 ( #181309, #9457, #13430, #11464, #134805, #196485, #58929, #75094, #57955, #10456 ),
 .UNSPECIFIED., .F., .F.,
 ( 4, 2, 2, 2, 4 ),
 ( 9.540979117872437479E-18, 0.0004927478742826785652, 0.0009854957485653475895, 0.001478243622848016614, 0.001970991497130685638 ),
 .UNSPECIFIED. ) ;
#192933=CARTESIAN_POINT ( 'NONE',  ( -5.823673210054116645, -21.52544592524344225, 102.2905762719810383 ) ) ;
#192934=CARTESIAN_POINT ( 'NONE',  ( 19.49671883438228548, 5.499999999999966249, 82.39279849105678011 ) ) ;
#192935=CARTESIAN_POINT ( 'NONE',  ( 21.52544592524344225, -5.823673210054117533, 53.54057627198103120 ) ) ;
#192936=CARTESIAN_POINT ( 'NONE',  ( -13.89961937509977652, 13.97604488694528158, 95.62390960531436690 ) ) ;
#192937=CARTESIAN_POINT ( 'NONE',  ( -14.29746914071049879, 8.314922557960819915, 45.83224293864769550 ) ) ;
#192939=CARTESIAN_POINT ( 'NONE',  ( 13.97604488694548053, -13.89961937509957401, 75.62609039468564731 ) ) ;
#192940=CARTESIAN_POINT ( 'NONE',  ( -16.52216118717205262, 7.221426719304517405, 103.9240097895301318 ) ) ;
#192941=CARTESIAN_POINT ( 'NONE',  ( 0.05219959533936267826, -19.03943276465977164, 110.0010903946856757 ) ) ;
#192942=CARTESIAN_POINT ( 'NONE',  ( 21.53943276465977519, -0.05219959533907433946, 83.74890960531435269 ) ) ;
#192943=CARTESIAN_POINT ( 'NONE',  ( 14.34966873604960469, 8.224510206698951720, 64.16557627198102409 ) ) ;
#192944=CARTESIAN_POINT ( 'NONE',  ( -5.153800228976328057, -19.02544592524343514, 97.29057627198099567 ) ) ;
#192945=CARTESIAN_POINT ( 'NONE',  ( -16.53943276465976808, -0.05219959533934237506, 38.75109039468567573 ) ) ;
#192946=CARTESIAN_POINT ( 'NONE',  ( -0.05219959533909027116, -19.03943276465977164, 62.49890960531435979 ) ) ;
#192947=CARTESIAN_POINT ( 'NONE',  ( 21.53943276465977519, 0.05219959533937863772, 26.25109039468567573 ) ) ;
#192948=CARTESIAN_POINT ( 'NONE',  ( 5.153800228976615827, -19.02544592524334988, 95.20942372801897591 ) ) ;
#192949=CARTESIAN_POINT ( 'NONE',  ( -9.474510206698964154, 16.51473224551069663, 100.4155762719810241 ) ) ;
#192950=CARTESIAN_POINT ( 'NONE',  ( 13.97604488694527802, 13.89961937509977652, 84.37390960531433848 ) ) ;
#192951=CARTESIAN_POINT ( 'NONE',  ( 0.05219959533907565091, 21.53943276465977519, 89.99890960531438111 ) ) ;
#192952=CARTESIAN_POINT ( 'NONE',  ( 9.564922557960805705, 16.46253265017160317, 44.58224293864769550 ) ) ;
#192953=CARTESIAN_POINT ( 'NONE',  ( -17.49999999999999645, -5.500000000000020428, 61.28230962303567964 ) ) ;
#192954=CARTESIAN_POINT ( 'NONE',  ( 12.06949235617757843, -12.14591786802309237, 68.12390960531436690 ) ) ;
#192955=CARTESIAN_POINT ( 'NONE',  ( -19.03943276465977164, 0.05219959533909376836, 101.2489096053143669 ) ) ;
#192957=CARTESIAN_POINT ( 'NONE',  ( -16.46253265017146816, -9.564922557961047289, 64.16775706135233293 ) ) ;
#192958=CARTESIAN_POINT ( 'NONE',  ( 5.719274019375991003, -21.55341960407610458, 87.70724293864769550 ) ) ;
#192959=CARTESIAN_POINT ( 'NONE',  ( -5.153800228976607833, 19.02544592524334988, 47.70942372801900433 ) ) ;
#192960=CARTESIAN_POINT ( 'NONE',  ( -16.51473224551069308, -9.474510206698971260, 96.66557627198102409 ) ) ;
#192961=CARTESIAN_POINT ( 'NONE',  ( -5.719274019375978568, 21.55341960407610458, 40.20724293864769550 ) ) ;
#192962=CARTESIAN_POINT ( 'NONE',  ( -19.03943276465977164, 0.05219959533909376836, 86.24890960531436690 ) ) ;
#192963=CARTESIAN_POINT ( 'NONE',  ( 5.823673210054444382, -21.52544592524334988, 70.20942372801904696 ) ) ;
#192964=CARTESIAN_POINT ( 'NONE',  ( -16.46253265017160317, 9.564922557960807481, 40.83224293864769550 ) ) ;
#192966=CARTESIAN_POINT ( 'NONE',  ( 16.55341960407611168, 4.379528057220329451, 73.95724293864769550 ) ) ;
#192967=CARTESIAN_POINT ( 'NONE',  ( -19.05341960407617563, 5.049401038297882671, 113.5427570613523471 ) ) ;
#192968=CARTESIAN_POINT ( 'NONE',  ( -5.719274019375665041, -21.55341960407619695, 49.79275706135234714 ) ) ;
#192970=CARTESIAN_POINT ( 'NONE',  ( 16.46253265017160672, -9.564922557960803928, 113.3322429386476955 ) ) ;
#192971=CARTESIAN_POINT ( 'NONE',  ( 5.153800228976615827, -19.02544592524334988, 70.20942372801899012 ) ) ;
#192973=CARTESIAN_POINT ( 'NONE',  ( -15.72974639402176322, -15.80617190586768395, 19.37609039468568639 ) ) ;
#192974=CARTESIAN_POINT ( 'NONE',  ( -19.05341960407611168, -5.049401038298163336, 61.45724293864769550 ) ) ;
#192976=CARTESIAN_POINT ( 'NONE',  ( -13.97604488694547697, 13.89961937509957934, 23.12609039468565442 ) ) ;
#192977=CARTESIAN_POINT ( 'NONE',  ( -5.153800228976328057, -19.02544592524343514, 42.29057627198101699 ) ) ;
#192978=CARTESIAN_POINT ( 'NONE',  ( -0.05219959533937732626, 21.53943276465977519, 107.5010903946856899 ) ) ;
#192979=CARTESIAN_POINT ( 'NONE',  ( 4.483927247898790824, -16.52544592524335698, 90.20942372801903275 ) ) ;
#192981=CARTESIAN_POINT ( 'NONE',  ( 13.89961937509977652, -13.97604488694527269, 108.1239096053143669 ) ) ;
#192982=CARTESIAN_POINT ( 'NONE',  ( 21.53943276465977519, 0.05219959533937863772, 71.25109039468568994 ) ) ;
#192984=CARTESIAN_POINT ( 'NONE',  ( 16.51473224551069308, 9.474510206698969483, 109.1655762719810383 ) ) ;
#192986=CARTESIAN_POINT ( 'NONE',  ( -4.379528057220086978, -16.55341960407618274, 69.79275706135234714 ) ) ;
#192987=CARTESIAN_POINT ( 'NONE',  ( 18.67979575497194134, -10.72451020669871369, 70.83442372801901854 ) ) ;
#192988=CARTESIAN_POINT ( 'NONE',  ( 10.81492255796106328, -18.62759615963255655, 100.4177570613523471 ) ) ;
#192990=CARTESIAN_POINT ( 'NONE',  ( -16.46253265017160317, 9.564922557960807481, 80.83224293864769550 ) ) ;
#192991=CARTESIAN_POINT ( 'NONE',  ( 16.46253265017160672, -9.564922557960803928, 113.3322429386476955 ) ) ;
#192995=CARTESIAN_POINT ( 'NONE',  ( -13.97604488694527625, -13.89961937509977652, 36.87390960531436690 ) ) ;
#192996=CARTESIAN_POINT ( 'NONE',  ( -21.53943276465977519, 0.05219959533907696930, 46.24890960531435979 ) ) ;
#192997=CARTESIAN_POINT ( 'NONE',  ( -16.55341960407617563, 4.379528057220093196, 103.5427570613523613 ) ) ;
#192998=CARTESIAN_POINT ( 'NONE',  ( 14.29746914071049879, -8.314922557960816363, 78.33224293864770971 ) ) ;
#192999=CARTESIAN_POINT ( 'NONE',  ( 19.02544592524343514, -5.153800228976328945, 78.54057627198099567 ) ) ;
#193000=CARTESIAN_POINT ( 'NONE',  ( -18.62759615963255300, -10.81492255796106328, 109.1677570613523613 ) ) ;
#193001=CARTESIAN_POINT ( 'NONE',  ( -9.564922557960796823, -16.46253265017161027, 32.08224293864769550 ) ) ;
#193002=CARTESIAN_POINT ( 'NONE',  ( -8.224510206698948167, 14.34966873604960824, 85.41557627198102409 ) ) ;
#193003=CARTESIAN_POINT ( 'NONE',  ( -15.72974639402176322, -15.80617190586768395, 39.37609039468567573 ) ) ;
#193004=CARTESIAN_POINT ( 'NONE',  ( 5.719274019375991003, -21.55341960407610458, 82.70724293864770971 ) ) ;
#193005=CARTESIAN_POINT ( 'NONE',  ( 16.46253265017146816, 9.564922557961045513, 51.66775706135233293 ) ) ;
#193007=CARTESIAN_POINT ( 'NONE',  ( 5.049401038298161559, -19.05341960407611168, 97.70724293864766707 ) ) ;
#193008=CARTESIAN_POINT ( 'NONE',  ( -12.06949235617756955, 12.14591786802309770, 65.62390960531436690 ) ) ;
#193009=CARTESIAN_POINT ( 'NONE',  ( -12.14591786802309592, -12.06949235617757132, 46.87390960531435979 ) ) ;
#193010=CARTESIAN_POINT ( 'NONE',  ( 16.51473224551083163, -9.474510206698727899, 85.83442372801900433 ) ) ;
#193012=CARTESIAN_POINT ( 'NONE',  ( -21.53943276465977519, 0.05219959533907696930, 21.24890960531436690 ) ) ;
#193013=CARTESIAN_POINT ( 'NONE',  ( 8.314922557960818139, 14.29746914071049879, 89.58224293864768129 ) ) ;
#193015=CARTESIAN_POINT ( 'NONE',  ( 16.46253265017160672, -9.564922557960803928, 48.33224293864769550 ) ) ;
#193016=CARTESIAN_POINT ( 'NONE',  ( -18.62759615963270932, 10.81492255796079327, 50.83224293864770971 ) ) ;
#193017=CARTESIAN_POINT ( 'NONE',  ( -19.05341960407611168, -5.049401038298163336, 36.45724293864766707 ) ) ;
#193018=CARTESIAN_POINT ( 'NONE',  ( -4.379528057220086978, -16.55341960407618274, 84.79275706135234714 ) ) ;
#193019=CARTESIAN_POINT ( 'NONE',  ( -5.049401038298153566, 19.05341960407611168, 60.20724293864768129 ) ) ;
#193020=CARTESIAN_POINT ( 'NONE',  ( 9.564922557961047289, -16.46253265017146816, 40.41775706135234003 ) ) ;
#193021=CARTESIAN_POINT ( 'NONE',  ( -18.67979575497193778, 10.72451020669871902, 73.33442372801901854 ) ) ;
#193022=CARTESIAN_POINT ( 'NONE',  ( -0.05219959533907301413, -21.53943276465977519, 42.49890960531435979 ) ) ;
#193023=CARTESIAN_POINT ( 'NONE',  ( -4.379528057220328563, 16.55341960407611168, 100.2072429386476955 ) ) ;
#193024=CARTESIAN_POINT ( 'NONE',  ( 5.049401038297881783, 19.05341960407617563, 87.29275706135234714 ) ) ;
#193027=CARTESIAN_POINT ( 'NONE',  ( -21.53943276465977519, 0.05219959533907696930, 41.24890960531435269 ) ) ;
#193028=CARTESIAN_POINT ( 'NONE',  ( 17.05116617787826883, -6.768360034955673399, 66.15675553259198693 ) ) ;
#193029=CARTESIAN_POINT ( 'NONE',  ( 15.72974639402176855, 15.80617190586768217, 76.87609039468567573 ) ) ;
#193030=CARTESIAN_POINT ( 'NONE',  ( 4.483927247898545687, 16.52544592524342804, 44.79057627198103120 ) ) ;
#193031=CARTESIAN_POINT ( 'NONE',  ( 8.224510206698742110, 14.34966873604972548, 72.08442372801899012 ) ) ;
#193032=CARTESIAN_POINT ( 'NONE',  ( -4.483927247898539470, -16.52544592524342804, 52.29057627198102409 ) ) ;
#193033=CARTESIAN_POINT ( 'NONE',  ( -0.05219959533907301413, -21.53943276465977519, 87.49890960531436690 ) ) ;
#193034=CARTESIAN_POINT ( 'NONE',  ( 5.823673210054125526, 21.52544592524343514, 74.79057627198105251 ) ) ;
#193036=CARTESIAN_POINT ( 'NONE',  ( -18.67979575497178146, -10.72451020669898902, 26.66557627198103475 ) ) ;
#193037=CARTESIAN_POINT ( 'NONE',  ( 12.14591786802327356, -12.06949235617739191, 55.62609039468568284 ) ) ;
#193038=CARTESIAN_POINT ( 'NONE',  ( -12.06949235617756955, 12.14591786802309770, 75.62390960531439532 ) ) ;
#193039=CARTESIAN_POINT ( 'NONE',  ( 0.05219959533909260263, 19.03943276465977164, 64.99890960531436690 ) ) ;
#193040=CARTESIAN_POINT ( 'NONE',  ( 16.46253265017160672, -9.564922557960803928, 33.33224293864770260 ) ) ;
#193041=LINE ( 'NONE', #175873, #125263 ) ;
#193042=ORIENTED_EDGE ( 'NONE', *, *, #143824, .T. ) ;
#193043=CARTESIAN_POINT ( 'NONE',  ( 12.14591786802327356, -12.06949235617739191, 80.62609039468567573 ) ) ;
#193044=CARTESIAN_POINT ( 'NONE',  ( 21.52544592524344225, -5.823673210054117533, 113.5405762719810383 ) ) ;
#193045=CARTESIAN_POINT ( 'NONE',  ( -19.03943276465977164, 0.05219959533909376836, 71.24890960531435269 ) ) ;
#193046=CARTESIAN_POINT ( 'NONE',  ( 10.81492255796106328, -18.62759615963255655, 55.41775706135234714 ) ) ;
#193047=CARTESIAN_POINT ( 'NONE',  ( -9.474510206698964154, 16.51473224551069663, 110.4155762719810383 ) ) ;
#193050=CARTESIAN_POINT ( 'NONE',  ( 21.53943276465977519, 0.05219959533937863772, 51.25109039468568994 ) ) ;
#193051=CARTESIAN_POINT ( 'NONE',  ( 0.05219959533909260263, 19.03943276465977164, 29.99890960531435979 ) ) ;
#193052=CARTESIAN_POINT ( 'NONE',  ( -16.51473224551069308, -9.474510206698971260, 101.6655762719810241 ) ) ;
#193053=CARTESIAN_POINT ( 'NONE',  ( 19.02544592524334988, 5.153800228976608722, 56.45942372801898301 ) ) ;
#193054=CARTESIAN_POINT ( 'NONE',  ( 18.67979575497194134, -10.72451020669871369, 20.83442372801901143 ) ) ;
#193055=CARTESIAN_POINT ( 'NONE',  ( 16.46253265017146816, 9.564922557961045513, 41.66775706135234003 ) ) ;
#193056=CARTESIAN_POINT ( 'NONE',  ( -19.05341960407617563, 5.049401038297882671, 53.54275706135231871 ) ) ;
#193057=CARTESIAN_POINT ( 'NONE',  ( 12.06949235617739724, 12.14591786802326823, 106.8760903946856899 ) ) ;
#193060=CARTESIAN_POINT ( 'NONE',  ( 16.46253265017160672, -9.564922557960803928, 83.33224293864768129 ) ) ;
#193061=CARTESIAN_POINT ( 'NONE',  ( 21.53943276465977519, 0.05219959533937863772, 96.25109039468568994 ) ) ;
#193062=CARTESIAN_POINT ( 'NONE',  ( -5.719274019375665041, -21.55341960407619695, 89.79275706135236135 ) ) ;
#193064=CARTESIAN_POINT ( 'NONE',  ( 5.049401038298161559, -19.05341960407611168, 102.7072429386476955 ) ) ;
#193065=CARTESIAN_POINT ( 'NONE',  ( -5.719274019375665041, -21.55341960407619695, 74.79275706135234714 ) ) ;
#193066=CARTESIAN_POINT ( 'NONE',  ( -16.55341960407617563, 4.379528057220093196, 23.54275706135235424 ) ) ;
#193067=CARTESIAN_POINT ( 'NONE',  ( 16.46253265017160672, -9.564922557960803928, 83.33224293864768129 ) ) ;
#193068=CARTESIAN_POINT ( 'NONE',  ( -15.72974639402197994, 15.80617190586746368, 25.62390960531435624 ) ) ;
#193070=CARTESIAN_POINT ( 'NONE',  ( -19.02544592524342804, 5.153800228976336051, 96.04057627198103830 ) ) ;
#193071=CARTESIAN_POINT ( 'NONE',  ( -18.22780087662123805, -5.499999999999968026, 98.98236817873106475 ) ) ;
#193072=CARTESIAN_POINT ( 'NONE',  ( -5.153800228976328057, -19.02544592524343514, 77.29057627198099567 ) ) ;
#193073=CARTESIAN_POINT ( 'NONE',  ( 19.05341960407611168, 5.049401038298154454, 68.95724293864769550 ) ) ;
#193074=CARTESIAN_POINT ( 'NONE',  ( 21.55341960407610458, 5.719274019375980345, 108.9572429386476955 ) ) ;
#193075=CARTESIAN_POINT ( 'NONE',  ( 8.224510206698742110, 14.34966873604972548, 107.0844237280190043 ) ) ;
#193076=CARTESIAN_POINT ( 'NONE',  ( -16.36317988757099329, 7.306389748694731345, 99.09789608363170998 ) ) ;
#193077=CARTESIAN_POINT ( 'NONE',  ( -19.02544592524334988, -5.153800228976617603, 53.95942372801898301 ) ) ;
#193078=CARTESIAN_POINT ( 'NONE',  ( -13.97604488694527625, -13.89961937509977652, 91.87390960531432427 ) ) ;
#193079=CARTESIAN_POINT ( 'NONE',  ( 14.29746914071049879, -8.314922557960816363, 83.33224293864769550 ) ) ;
#193080=CARTESIAN_POINT ( 'NONE',  ( -15.80617190586745835, -15.72974639402198527, 26.87390960531435979 ) ) ;
#193081=CARTESIAN_POINT ( 'NONE',  ( 21.55341960407610458, 5.719274019375980345, 28.95724293864769905 ) ) ;
#193082=CARTESIAN_POINT ( 'NONE',  ( 14.29746914071049879, -8.314922557960816363, 98.33224293864769550 ) ) ;
#193083=CARTESIAN_POINT ( 'NONE',  ( -17.12812012977024168, 6.668231424566045895, 53.64051240676857191 ) ) ;
#193084=CARTESIAN_POINT ( 'NONE',  ( -9.474510206698720793, -16.51473224551083518, 49.58442372801899722 ) ) ;
#193085=CARTESIAN_POINT ( 'NONE',  ( -12.14591786802326823, 12.06949235617739902, 108.1260903946856757 ) ) ;
#193086=CARTESIAN_POINT ( 'NONE',  ( 9.564922557960805705, 16.46253265017160317, 94.58224293864769550 ) ) ;
#193087=CARTESIAN_POINT ( 'NONE',  ( 5.823673210054444382, -21.52544592524334988, 65.20942372801901854 ) ) ;
#193088=CARTESIAN_POINT ( 'NONE',  ( -21.52544592524343514, 5.823673210054127303, 51.04057627198103120 ) ) ;
#193089=CARTESIAN_POINT ( 'NONE',  ( 21.52544592524334988, 5.823673210054432836, 26.45942372801901854 ) ) ;
#193090=CARTESIAN_POINT ( 'NONE',  ( -5.823673210054116645, -21.52544592524344225, 87.29057627198103830 ) ) ;
#193091=CARTESIAN_POINT ( 'NONE',  ( 8.224510206698953496, -14.34966873604960469, 112.9155762719810383 ) ) ;
#193092=CARTESIAN_POINT ( 'NONE',  ( 9.564922557961047289, -16.46253265017146816, 70.41775706135233293 ) ) ;
#193093=CARTESIAN_POINT ( 'NONE',  ( 19.03943276465977164, -0.05219959533909143690, 43.74890960531435979 ) ) ;
#193094=CARTESIAN_POINT ( 'NONE',  ( 5.049401038298161559, -19.05341960407611168, 102.7072429386476955 ) ) ;
#193095=CARTESIAN_POINT ( 'NONE',  ( -16.46253265017160317, 9.564922557960807481, 100.8322429386477097 ) ) ;
#193096=CARTESIAN_POINT ( 'NONE',  ( -16.52544592524342804, 4.483927247898546575, 111.0405762719810525 ) ) ;
#193097=CARTESIAN_POINT ( 'NONE',  ( -0.05219959533910754901, -16.53943276465976808, 42.49890960531435979 ) ) ;
#193098=CARTESIAN_POINT ( 'NONE',  ( -14.34966873604972548, 8.224510206698743886, 43.33442372801901143 ) ) ;
#193099=CARTESIAN_POINT ( 'NONE',  ( 8.314922557960818139, 14.29746914071049879, 114.5822429386477097 ) ) ;
#193100=CARTESIAN_POINT ( 'NONE',  ( 0.05219959533937995610, -21.53943276465977519, 100.0010903946857042 ) ) ;
#193102=CARTESIAN_POINT ( 'NONE',  ( 13.89961937509977652, -13.97604488694527269, 108.1239096053143669 ) ) ;
#193103=CARTESIAN_POINT ( 'NONE',  ( 8.224510206698953496, -14.34966873604960469, 22.91557627198102765 ) ) ;
#193104=CARTESIAN_POINT ( 'NONE',  ( 15.80617190586769283, -15.72974639402175789, 35.62609039468568994 ) ) ;
#193105=CARTESIAN_POINT ( 'NONE',  ( 19.05341960407611168, 5.049401038298154454, 103.9572429386476671 ) ) ;
#193106=CARTESIAN_POINT ( 'NONE',  ( -0.05219959533934338120, 16.53943276465976808, 112.5010903946857042 ) ) ;
#193107=CARTESIAN_POINT ( 'NONE',  ( 14.29746914071037800, 8.314922557961029526, 86.66775706135234714 ) ) ;
#193108=CARTESIAN_POINT ( 'NONE',  ( -16.55341960407617563, 4.379528057220093196, 28.54275706135234358 ) ) ;
#193109=CARTESIAN_POINT ( 'NONE',  ( 5.049401038298161559, -19.05341960407611168, 47.70724293864770260 ) ) ;
#193110=CARTESIAN_POINT ( 'NONE',  ( -4.483927247898539470, -16.52544592524342804, 107.2905762719810525 ) ) ;
#193111=CARTESIAN_POINT ( 'NONE',  ( 5.719274019375991003, -21.55341960407610458, 112.7072429386476955 ) ) ;
#193112=CARTESIAN_POINT ( 'NONE',  ( -0.05219959533909027116, -19.03943276465977164, 27.49890960531435624 ) ) ;
#193113=CARTESIAN_POINT ( 'NONE',  ( 19.05341960407611168, 5.049401038298154454, 98.95724293864766707 ) ) ;
#193114=CARTESIAN_POINT ( 'NONE',  ( -19.02544592524342804, 5.153800228976336051, 31.04057627198102409 ) ) ;
#193115=CARTESIAN_POINT ( 'NONE',  ( 16.51473224551069308, 9.474510206698969483, 99.16557627198102409 ) ) ;
#193117=CARTESIAN_POINT ( 'NONE',  ( 16.46253265017160672, -9.564922557960803928, 93.33224293864769550 ) ) ;
#193118=CARTESIAN_POINT ( 'NONE',  ( -5.719274019375665041, -21.55341960407619695, 49.79275706135234714 ) ) ;
#193119=CARTESIAN_POINT ( 'NONE',  ( 12.06949235617757843, -12.14591786802309237, 93.12390960531436690 ) ) ;
#193120=CARTESIAN_POINT ( 'NONE',  ( 5.049401038298161559, -19.05341960407611168, 92.70724293864769550 ) ) ;
#193122=CARTESIAN_POINT ( 'NONE',  ( -16.55341960407617563, 4.379528057220093196, 68.54275706135234714 ) ) ;
#193123=CARTESIAN_POINT ( 'NONE',  ( -18.67979575497193778, 10.72451020669871902, 83.33442372801903275 ) ) ;
#193124=CARTESIAN_POINT ( 'NONE',  ( -16.52544592524335698, -4.483927247898792601, 33.95942372801901143 ) ) ;
#193125=CARTESIAN_POINT ( 'NONE',  ( 19.05341960407611168, 5.049401038298154454, 83.95724293864766707 ) ) ;
#193126=EDGE_CURVE ( 'NONE', #188751, #111352, #1975, .T. ) ;
#193127=CARTESIAN_POINT ( 'NONE',  ( -13.89961937509957401, -13.97604488694547875, 104.3760903946856757 ) ) ;
#193128=CARTESIAN_POINT ( 'NONE',  ( 16.55341960407618274, -4.379528057220086978, 81.04275706135236135 ) ) ;
#193129=CARTESIAN_POINT ( 'NONE',  ( -19.03943276465977164, -0.05219959533935918106, 93.75109039468566152 ) ) ;
#193130=CARTESIAN_POINT ( 'NONE',  ( 5.049401038298161559, -19.05341960407611168, 57.70724293864769550 ) ) ;
#193131=CARTESIAN_POINT ( 'NONE',  ( -15.80617190586745835, -15.72974639402198527, 91.87390960531436690 ) ) ;
#193132=CARTESIAN_POINT ( 'NONE',  ( 16.52544592524342804, -4.483927247898539470, 93.54057627198103830 ) ) ;
#193133=CARTESIAN_POINT ( 'NONE',  ( -16.46253265017146816, -9.564922557961047289, 89.16775706135234714 ) ) ;
#193134=CARTESIAN_POINT ( 'NONE',  ( -16.53943276465976808, -0.05219959533934237506, 58.75109039468568994 ) ) ;
#193136=CARTESIAN_POINT ( 'NONE',  ( -5.153800228976607833, 19.02544592524334988, 57.70942372801899012 ) ) ;
#193137=CARTESIAN_POINT ( 'NONE',  ( -12.14591786802309592, -12.06949235617757132, 31.87390960531435979 ) ) ;
#193138=CARTESIAN_POINT ( 'NONE',  ( 14.34966873604960469, 8.224510206698951720, 74.16557627198102409 ) ) ;
#193139=CARTESIAN_POINT ( 'NONE',  ( -10.81492255796105439, 18.62759615963255655, 112.9177570613523329 ) ) ;
#193140=CARTESIAN_POINT ( 'NONE',  ( -16.18388926212246304, 7.379444403734580327, 39.56046848633771873 ) ) ;
#193141=CARTESIAN_POINT ( 'NONE',  ( -5.719274019375978568, 21.55341960407610458, 115.2072429386476955 ) ) ;
#193142=CARTESIAN_POINT ( 'NONE',  ( 16.46253265017160672, -9.564922557960803928, 113.3322429386476955 ) ) ;
#193143=CARTESIAN_POINT ( 'NONE',  ( 19.03943276465977164, -0.05219959533909143690, 78.74890960531436690 ) ) ;
#193144=CARTESIAN_POINT ( 'NONE',  ( -18.62759615963255300, -10.81492255796106328, 94.16775706135237556 ) ) ;
#193145=CARTESIAN_POINT ( 'NONE',  ( -0.05219959533909027116, -19.03943276465977164, 82.49890960531436690 ) ) ;
#193146=CARTESIAN_POINT ( 'NONE',  ( 21.55341960407610458, 5.719274019375980345, 38.95724293864768839 ) ) ;
#193147=CARTESIAN_POINT ( 'NONE',  ( 16.55341960407611168, 4.379528057220329451, 78.95724293864769550 ) ) ;
#193148=CARTESIAN_POINT ( 'NONE',  ( -13.89961937509977652, 13.97604488694528158, 55.62390960531434558 ) ) ;
#193149=CARTESIAN_POINT ( 'NONE',  ( -12.06949235617756955, 12.14591786802309770, 105.6239096053143669 ) ) ;
#193150=CARTESIAN_POINT ( 'NONE',  ( -21.55341960407619339, 5.719274019375674811, 28.54275706135234358 ) ) ;
#193151=CARTESIAN_POINT ( 'NONE',  ( 18.67979575497194134, -10.72451020669871369, 55.83442372801901854 ) ) ;
#193152=CARTESIAN_POINT ( 'NONE',  ( 5.153800228976335163, 19.02544592524342804, 39.79057627198100988 ) ) ;
#193153=CARTESIAN_POINT ( 'NONE',  ( 14.34966873604972726, -8.224510206698740333, 70.83442372801901854 ) ) ;
#193154=EDGE_CURVE ( 'NONE', #178458, #66658, #182748, .T. ) ;
#193155=CARTESIAN_POINT ( 'NONE',  ( 0.05219959533937995610, -21.53943276465977519, 20.00109039468568639 ) ) ;
#193156=CARTESIAN_POINT ( 'NONE',  ( 5.719274019375991003, -21.55341960407610458, 107.7072429386476955 ) ) ;
#193157=CARTESIAN_POINT ( 'NONE',  ( 19.03943276465977164, 0.05219959533936151252, 36.25109039468567573 ) ) ;
#193158=CARTESIAN_POINT ( 'NONE',  ( 9.564922557960805705, 16.46253265017160317, 59.58224293864769550 ) ) ;
#193159=CARTESIAN_POINT ( 'NONE',  ( -19.02544592524334988, -5.153800228976617603, 28.95942372801900433 ) ) ;
#193160=CARTESIAN_POINT ( 'NONE',  ( -21.53943276465977519, -0.05219959533937600094, 73.75109039468567573 ) ) ;
#193161=CARTESIAN_POINT ( 'NONE',  ( -21.55341960407610458, -5.719274019375992779, 76.45724293864769550 ) ) ;
#193162=CARTESIAN_POINT ( 'NONE',  ( -4.483927247898539470, -16.52544592524342804, 32.29057627198102409 ) ) ;
#193163=CARTESIAN_POINT ( 'NONE',  ( -5.719274019375665041, -21.55341960407619695, 94.79275706135234714 ) ) ;
#193164=CARTESIAN_POINT ( 'NONE',  ( 18.67979575497194134, -10.72451020669871369, 110.8344237280190043 ) ) ;
#193165=CARTESIAN_POINT ( 'NONE',  ( 14.29746914071049879, -8.314922557960816363, 58.33224293864768839 ) ) ;
#193166=CARTESIAN_POINT ( 'NONE',  ( -14.29746914071049879, 8.314922557960819915, 100.8322429386477097 ) ) ;
#193167=CARTESIAN_POINT ( 'NONE',  ( -13.89961937509957401, -13.97604488694547875, 64.37609039468567573 ) ) ;
#193168=CARTESIAN_POINT ( 'NONE',  ( -8.314922557960811034, -14.29746914071050412, 22.08224293864769194 ) ) ;
#193169=CARTESIAN_POINT ( 'NONE',  ( -5.719274019375665041, -21.55341960407619695, 74.79275706135234714 ) ) ;
#193170=CARTESIAN_POINT ( 'NONE',  ( 0.05219959533909260263, 19.03943276465977164, 74.99890960531435269 ) ) ;
#193171=CARTESIAN_POINT ( 'NONE',  ( 19.02544592524334988, 5.153800228976608722, 31.45942372801900433 ) ) ;
#193172=CARTESIAN_POINT ( 'NONE',  ( 5.719274019375991003, -21.55341960407610458, 52.70724293864769550 ) ) ;
#193173=CARTESIAN_POINT ( 'NONE',  ( -21.52544592524334988, -5.823673210054445271, 43.95942372801902565 ) ) ;
#193174=CARTESIAN_POINT ( 'NONE',  ( -21.52544592524343514, 5.823673210054127303, 106.0405762719810525 ) ) ;
#193175=CARTESIAN_POINT ( 'NONE',  ( -19.03943276465977164, -0.05219959533935918106, 93.75109039468566152 ) ) ;
#193176=CARTESIAN_POINT ( 'NONE',  ( 16.55341960407618274, -4.379528057220086978, 66.04275706135236135 ) ) ;
#193178=CARTESIAN_POINT ( 'NONE',  ( 18.67979575497178502, 10.72451020669898547, 99.16557627198100988 ) ) ;
#193179=CARTESIAN_POINT ( 'NONE',  ( -14.29746914071049879, 8.314922557960819915, 85.83224293864768129 ) ) ;
#193180=CARTESIAN_POINT ( 'NONE',  ( -16.88567814943161949, -6.947325034625704276, 101.2900112265258343 ) ) ;
#193181=CARTESIAN_POINT ( 'NONE',  ( -14.34966873604972548, 8.224510206698743886, 23.33442372801901499 ) ) ;
#193182=CARTESIAN_POINT ( 'NONE',  ( -18.67979575497178146, -10.72451020669898902, 46.66557627198102409 ) ) ;
#193183=CARTESIAN_POINT ( 'NONE',  ( -16.52544592524335698, -4.483927247898792601, 88.95942372801901854 ) ) ;
#193185=CARTESIAN_POINT ( 'NONE',  ( 16.52544592524335698, 4.483927247898782831, 51.45942372801901854 ) ) ;
#193186=CARTESIAN_POINT ( 'NONE',  ( 21.52544592524334988, 5.823673210054432836, 26.45942372801901854 ) ) ;
#193187=CARTESIAN_POINT ( 'NONE',  ( 15.80617190586746368, 15.72974639402197994, 39.37390960531436690 ) ) ;
#193188=CARTESIAN_POINT ( 'NONE',  ( 14.34966873604972726, -8.224510206698740333, 80.83442372801901854 ) ) ;
#193189=CARTESIAN_POINT ( 'NONE',  ( -0.05219959533909027116, -19.03943276465977164, 92.49890960531436690 ) ) ;
#193190=CARTESIAN_POINT ( 'NONE',  ( -0.05219959533937732626, 21.53943276465977519, 72.50109039468568994 ) ) ;
#193191=CARTESIAN_POINT ( 'NONE',  ( 10.81492255796078972, 18.62759615963270932, 39.58224293864769550 ) ) ;
#193192=CARTESIAN_POINT ( 'NONE',  ( -21.55341960407610458, -5.719274019375992779, 26.45724293864768839 ) ) ;
#193194=CARTESIAN_POINT ( 'NONE',  ( -16.46253265017146816, -9.564922557961047289, 49.16775706135233293 ) ) ;
#193195=CARTESIAN_POINT ( 'NONE',  ( 16.53943276465976808, 0.05219959533934440121, 71.25109039468568994 ) ) ;
#193196=CARTESIAN_POINT ( 'NONE',  ( -0.05219959533907301413, -21.53943276465977519, 32.49890960531435979 ) ) ;
#193197=ORIENTED_EDGE ( 'NONE', *, *, #127302, .T. ) ;
#193198=CARTESIAN_POINT ( 'NONE',  ( -9.474510206698964154, 16.51473224551069663, 85.41557627198102409 ) ) ;
#193199=CARTESIAN_POINT ( 'NONE',  ( -8.224510206698735004, -14.34966873604973081, 109.5844237280190328 ) ) ;
#193201=CARTESIAN_POINT ( 'NONE',  ( -4.379528057220328563, 16.55341960407611168, 115.2072429386476955 ) ) ;
#193202=CARTESIAN_POINT ( 'NONE',  ( -15.80617190586745835, -15.72974639402198527, 41.87390960531435979 ) ) ;
#193203=CARTESIAN_POINT ( 'NONE',  ( 16.46253265017160672, -9.564922557960803928, 43.33224293864769550 ) ) ;
#193204=CARTESIAN_POINT ( 'NONE',  ( -8.314922557961024197, 14.29746914071037800, 82.91775706135234714 ) ) ;
#193205=CARTESIAN_POINT ( 'NONE',  ( 18.62759615963255655, 10.81492255796105972, 26.66775706135235424 ) ) ;
#193206=CARTESIAN_POINT ( 'NONE',  ( -5.049401038297874678, -19.05341960407617918, 94.79275706135230450 ) ) ;
#193207=CARTESIAN_POINT ( 'NONE',  ( 12.14591786802309770, 12.06949235617756955, 84.37390960531438111 ) ) ;
#193208=CARTESIAN_POINT ( 'NONE',  ( 9.474510206698971260, -16.51473224551069308, 47.91557627198102409 ) ) ;
#193209=CARTESIAN_POINT ( 'NONE',  ( -5.153800228976328057, -19.02544592524343514, 27.29057627198103120 ) ) ;
#193210=CARTESIAN_POINT ( 'NONE',  ( 18.67979575497194134, -10.72451020669871369, 100.8344237280190185 ) ) ;
#193211=CARTESIAN_POINT ( 'NONE',  ( -0.05219959533909027116, -19.03943276465977164, 82.49890960531436690 ) ) ;
#193212=CARTESIAN_POINT ( 'NONE',  ( 4.483927247898790824, -16.52544592524335698, 65.20942372801901854 ) ) ;
#193213=CARTESIAN_POINT ( 'NONE',  ( 5.719274019375673035, 21.55341960407619339, 92.29275706135236135 ) ) ;
#193214=CARTESIAN_POINT ( 'NONE',  ( 21.55341960407610458, 5.719274019375980345, 53.95724293864770260 ) ) ;
#193215=CARTESIAN_POINT ( 'NONE',  ( 12.14591786802327356, -12.06949235617739191, 75.62609039468567573 ) ) ;
#193216=CARTESIAN_POINT ( 'NONE',  ( 9.564922557961047289, -16.46253265017146816, 55.41775706135234003 ) ) ;
#193217=CARTESIAN_POINT ( 'NONE',  ( 9.564922557961047289, -16.46253265017146816, 60.41775706135233293 ) ) ;
#193219=CARTESIAN_POINT ( 'NONE',  ( -15.72974639402176322, -15.80617190586768395, 64.37609039468568994 ) ) ;
#193220=CARTESIAN_POINT ( 'NONE',  ( 13.89961937509977652, -13.97604488694527269, 68.12390960531436690 ) ) ;
#193221=CARTESIAN_POINT ( 'NONE',  ( -19.02544592524342804, 5.153800228976336051, 26.04057627198103120 ) ) ;
#193222=CARTESIAN_POINT ( 'NONE',  ( 19.05341960407617918, -5.049401038297876454, 61.04275706135232582 ) ) ;
#193224=CARTESIAN_POINT ( 'NONE',  ( -19.02544592524342804, 5.153800228976336051, 101.0405762719810241 ) ) ;
#193225=CARTESIAN_POINT ( 'NONE',  ( -14.29746914071049879, 8.314922557960819915, 45.83224293864769550 ) ) ;
#193226=CARTESIAN_POINT ( 'NONE',  ( -21.53943276465977519, 0.05219959533907696930, 41.24890960531435269 ) ) ;
#193228=CARTESIAN_POINT ( 'NONE',  ( -13.89961937509957401, -13.97604488694547875, 19.37609039468566507 ) ) ;
#193230=CARTESIAN_POINT ( 'NONE',  ( 13.89961937509977652, -13.97604488694527269, 53.12390960531434558 ) ) ;
#193231=B_SPLINE_CURVE_WITH_KNOTS ( 'NONE', 3,
 ( #79054, #141722, #109396, #94220, #140727, #64886 ),
 .UNSPECIFIED., .F., .F.,
 ( 4, 2, 4 ),
 ( 0.003239945802372282482, 0.003620412082092132073, 0.004000878361811981664 ),
 .UNSPECIFIED. ) ;
#193232=CARTESIAN_POINT ( 'NONE',  ( -16.51473224551069308, -9.474510206698971260, 26.66557627198103120 ) ) ;
#193235=CARTESIAN_POINT ( 'NONE',  ( 8.314922557961029526, -14.29746914071037800, 60.41775706135235424 ) ) ;
#193236=CARTESIAN_POINT ( 'NONE',  ( 15.72974639402199770, -15.80617190586745480, 88.12390960531436690 ) ) ;
#193237=CARTESIAN_POINT ( 'NONE',  ( 8.224510206698953496, -14.34966873604960469, 52.91557627198103830 ) ) ;
#193238=CARTESIAN_POINT ( 'NONE',  ( -9.564922557960796823, -16.46253265017161027, 37.08224293864768839 ) ) ;
#193240=CARTESIAN_POINT ( 'NONE',  ( 18.62759615963255655, 10.81492255796105972, 46.66775706135234714 ) ) ;
#193241=CARTESIAN_POINT ( 'NONE',  ( -16.51473224551082808, 9.474510206698731452, 53.33442372801900433 ) ) ;
#193242=CARTESIAN_POINT ( 'NONE',  ( -9.564922557960796823, -16.46253265017161027, 32.08224293864769550 ) ) ;
#193243=CARTESIAN_POINT ( 'NONE',  ( 5.719274019375673035, 21.55341960407619339, 97.29275706135234714 ) ) ;
#193244=CARTESIAN_POINT ( 'NONE',  ( -18.10062525802547029, 5.499999999999999112, 48.51383468041923663 ) ) ;
#193245=CARTESIAN_POINT ( 'NONE',  ( -4.379528057220328563, 16.55341960407611168, 40.20724293864769550 ) ) ;
#193247=CARTESIAN_POINT ( 'NONE',  ( 18.67979575497178502, 10.72451020669898547, 39.16557627198102409 ) ) ;
#193249=CARTESIAN_POINT ( 'NONE',  ( 5.049401038298161559, -19.05341960407611168, 87.70724293864769550 ) ) ;
#193250=CARTESIAN_POINT ( 'NONE',  ( -0.05219959533910754901, -16.53943276465976808, 82.49890960531436690 ) ) ;
#193251=CARTESIAN_POINT ( 'NONE',  ( -16.52544592524335698, -4.483927247898792601, 18.95942372801901143 ) ) ;
#193252=CARTESIAN_POINT ( 'NONE',  ( -14.34966873604972548, 8.224510206698743886, 108.3344237280190185 ) ) ;
#193253=ORIENTED_EDGE ( 'NONE', *, *, #155903, .F. ) ;
#193254=CARTESIAN_POINT ( 'NONE',  ( 13.97604488694527802, 13.89961937509977652, 49.37390960531434558 ) ) ;
#193255=CARTESIAN_POINT ( 'NONE',  ( 19.02544592524343514, -5.153800228976328945, 83.54057627198100988 ) ) ;
#193256=CARTESIAN_POINT ( 'NONE',  ( 18.67979575497178502, 10.72451020669898547, 84.16557627198103830 ) ) ;
#193257=CARTESIAN_POINT ( 'NONE',  ( 12.06949235617757843, -12.14591786802309237, 23.12390960531436335 ) ) ;
#193258=CARTESIAN_POINT ( 'NONE',  ( -16.51473224551069308, -9.474510206698971260, 96.66557627198102409 ) ) ;
#193259=CARTESIAN_POINT ( 'NONE',  ( -9.474510206698720793, -16.51473224551083518, 74.58442372801900433 ) ) ;
#193260=CARTESIAN_POINT ( 'NONE',  ( -15.72974639402176322, -15.80617190586768395, 104.3760903946856899 ) ) ;
#193261=CARTESIAN_POINT ( 'NONE',  ( 18.62759615963271287, -10.81492255796078972, 93.33224293864769550 ) ) ;
#193262=CARTESIAN_POINT ( 'NONE',  ( 18.67979575497178502, 10.72451020669898547, 34.16557627198102409 ) ) ;
#193263=CARTESIAN_POINT ( 'NONE',  ( 16.46253265017160672, -9.564922557960803928, 68.33224293864770971 ) ) ;
#193264=CARTESIAN_POINT ( 'NONE',  ( -12.14591786802326823, 12.06949235617739902, 108.1260903946856757 ) ) ;
#193265=CARTESIAN_POINT ( 'NONE',  ( -16.51473224551069308, -9.474510206698971260, 81.66557627198103830 ) ) ;
#193267=CARTESIAN_POINT ( 'NONE',  ( 17.71576930673726480, 5.500000000000005329, 38.91742649432649159 ) ) ;
#193268=CARTESIAN_POINT ( 'NONE',  ( 5.049401038297881783, 19.05341960407617563, 27.29275706135232937 ) ) ;
#193269=CARTESIAN_POINT ( 'NONE',  ( 16.53943276465976808, -0.05219959533910856209, 88.74890960531436690 ) ) ;
#193270=CARTESIAN_POINT ( 'NONE',  ( -0.05219959533937732626, 21.53943276465977519, 27.50109039468567929 ) ) ;
#193273=CARTESIAN_POINT ( 'NONE',  ( 21.53943276465977519, -0.05219959533907433946, 78.74890960531436690 ) ) ;
#193274=CARTESIAN_POINT ( 'NONE',  ( 0.05219959533934541429, -16.53943276465976808, 95.00109039468568994 ) ) ;
#193275=CARTESIAN_POINT ( 'NONE',  ( 5.153800228976335163, 19.02544592524342804, 24.79057627198102765 ) ) ;
#193276=CARTESIAN_POINT ( 'NONE',  ( -13.89961937509977652, 13.97604488694528158, 75.62390960531438111 ) ) ;
#193277=CARTESIAN_POINT ( 'NONE',  ( -17.49999999999999645, -5.500000000000000888, 120.0000000000000142 ) ) ;
#193278=CARTESIAN_POINT ( 'NONE',  ( 8.224510206698953496, -14.34966873604960469, 27.91557627198103830 ) ) ;
#193279=CARTESIAN_POINT ( 'NONE',  ( -18.67979575497193778, 10.72451020669871902, 63.33442372801900433 ) ) ;
#193280=CARTESIAN_POINT ( 'NONE',  ( -16.51473224551069308, -9.474510206698971260, 106.6655762719810383 ) ) ;
#193281=CARTESIAN_POINT ( 'NONE',  ( 0.05219959533937995610, -21.53943276465977519, 90.00109039468567573 ) ) ;
#193282=CARTESIAN_POINT ( 'NONE',  ( 13.97604488694527802, 13.89961937509977652, 39.37390960531435269 ) ) ;
#193283=CARTESIAN_POINT ( 'NONE',  ( -9.564922557960796823, -16.46253265017161027, 52.08224293864768839 ) ) ;
#193285=CARTESIAN_POINT ( 'NONE',  ( 18.62759615963255655, 10.81492255796105972, 96.66775706135234714 ) ) ;
#193286=CARTESIAN_POINT ( 'NONE',  ( -16.55341960407617563, 4.379528057220093196, 58.54275706135235424 ) ) ;
#193287=CARTESIAN_POINT ( 'NONE',  ( 0.05219959533937995610, -21.53943276465977519, 90.00109039468567573 ) ) ;
#193288=CARTESIAN_POINT ( 'NONE',  ( 15.80617190586746368, 15.72974639402197994, 24.37390960531435979 ) ) ;
#193289=CARTESIAN_POINT ( 'NONE',  ( -9.564922557961040184, 16.46253265017147172, 97.91775706135233293 ) ) ;
#193290=CARTESIAN_POINT ( 'NONE',  ( 18.62759615963255655, 10.81492255796105972, 51.66775706135234714 ) ) ;
#193291=CARTESIAN_POINT ( 'NONE',  ( -16.53943276465976808, -0.05219959533934237506, 33.75109039468568284 ) ) ;
#193292=CARTESIAN_POINT ( 'NONE',  ( -5.823673210054116645, -21.52544592524344225, 92.29057627198103830 ) ) ;
#193293=CARTESIAN_POINT ( 'NONE',  ( 9.474510206698729675, 16.51473224551082808, 87.08442372801900433 ) ) ;
#193294=CARTESIAN_POINT ( 'NONE',  ( 9.564922557960805705, 16.46253265017160317, 59.58224293864769550 ) ) ;
#193295=CARTESIAN_POINT ( 'NONE',  ( -19.02544592524334988, -5.153800228976617603, 93.95942372801900433 ) ) ;
#193296=CARTESIAN_POINT ( 'NONE',  ( -19.03943276465977164, -0.05219959533935918106, 98.75109039468567573 ) ) ;
#193297=CARTESIAN_POINT ( 'NONE',  ( 14.29746914071049879, -8.314922557960816363, 58.33224293864768839 ) ) ;
#193298=CARTESIAN_POINT ( 'NONE',  ( 16.46253265017146816, 9.564922557961045513, 76.66775706135234714 ) ) ;
#193299=CARTESIAN_POINT ( 'NONE',  ( 16.52544592524335698, 4.483927247898782831, 56.45942372801902565 ) ) ;
#193300=CARTESIAN_POINT ( 'NONE',  ( -19.05341960407617563, 5.049401038297882671, 38.54275706135233293 ) ) ;
#193301=CARTESIAN_POINT ( 'NONE',  ( 9.564922557960805705, 16.46253265017160317, 34.58224293864770260 ) ) ;
#193302=CARTESIAN_POINT ( 'NONE',  ( 5.153800228976335163, 19.02544592524342804, 54.79057627198103120 ) ) ;
#193303=CARTESIAN_POINT ( 'NONE',  ( -4.483927247898782831, 16.52544592524335698, 57.70942372801901143 ) ) ;
#193307=CARTESIAN_POINT ( 'NONE',  ( -0.05219959533909027116, -19.03943276465977164, 107.4989096053143527 ) ) ;
#193310=CARTESIAN_POINT ( 'NONE',  ( -9.474510206698720793, -16.51473224551083518, 104.5844237280190043 ) ) ;
#193311=CARTESIAN_POINT ( 'NONE',  ( 15.80617190586746368, 15.72974639402197994, 44.37390960531435979 ) ) ;
#193312=CARTESIAN_POINT ( 'NONE',  ( -13.89961937509957401, -13.97604488694547875, 29.37609039468565797 ) ) ;
#193313=CARTESIAN_POINT ( 'NONE',  ( -5.049401038297874678, -19.05341960407617918, 109.7927570613523187 ) ) ;
#193314=CARTESIAN_POINT ( 'NONE',  ( -16.46253265017160317, 9.564922557960807481, 30.83224293864769550 ) ) ;
#193315=CARTESIAN_POINT ( 'NONE',  ( -16.46253265017160317, 9.564922557960807481, 55.83224293864769550 ) ) ;
#193316=CARTESIAN_POINT ( 'NONE',  ( -10.72451020669898014, 18.67979575497178502, 70.41557627198102409 ) ) ;
#193317=CARTESIAN_POINT ( 'NONE',  ( 0.05219959533909260263, 19.03943276465977164, 99.99890960531436690 ) ) ;
#193318=CARTESIAN_POINT ( 'NONE',  ( 19.03943276465977164, -0.05219959533909143690, 33.74890960531435979 ) ) ;
#193320=CARTESIAN_POINT ( 'NONE',  ( 19.05341960407617918, -5.049401038297876454, 86.04275706135233293 ) ) ;
#193321=CARTESIAN_POINT ( 'NONE',  ( -8.314922557960811034, -14.29746914071050412, 57.08224293864769550 ) ) ;
#193322=CARTESIAN_POINT ( 'NONE',  ( -0.05219959533907301413, -21.53943276465977519, 42.49890960531435979 ) ) ;
#193323=CARTESIAN_POINT ( 'NONE',  ( -5.823673210054431948, 21.52544592524334988, 112.7094237280190328 ) ) ;
#193324=CARTESIAN_POINT ( 'NONE',  ( 18.62759615963271287, -10.81492255796078972, 103.3322429386476955 ) ) ;
#193325=CARTESIAN_POINT ( 'NONE',  ( 21.55341960407619695, -5.719274019375665929, 66.04275706135236135 ) ) ;
#193326=CARTESIAN_POINT ( 'NONE',  ( -18.67979575497193778, 10.72451020669871902, 83.33442372801903275 ) ) ;
#193327=CARTESIAN_POINT ( 'NONE',  ( -0.05219959533909027116, -19.03943276465977164, 107.4989096053143527 ) ) ;
#193328=CARTESIAN_POINT ( 'NONE',  ( -0.05219959533934338120, 16.53943276465976808, 102.5010903946856899 ) ) ;
#193329=CARTESIAN_POINT ( 'NONE',  ( 0.05219959533937995610, -21.53943276465977519, 70.00109039468568994 ) ) ;
#193330=CARTESIAN_POINT ( 'NONE',  ( -9.474510206698964154, 16.51473224551069663, 65.41557627198102409 ) ) ;
#193331=CARTESIAN_POINT ( 'NONE',  ( 9.564922557961047289, -16.46253265017146816, 30.41775706135232937 ) ) ;
#193332=CARTESIAN_POINT ( 'NONE',  ( -15.80617190586768217, 15.72974639402176855, 28.12609039468568284 ) ) ;
#193333=CARTESIAN_POINT ( 'NONE',  ( -9.474510206698964154, 16.51473224551069663, 70.41557627198102409 ) ) ;
#193334=CARTESIAN_POINT ( 'NONE',  ( -14.29746914071049879, 8.314922557960819915, 85.83224293864768129 ) ) ;
#193335=CARTESIAN_POINT ( 'NONE',  ( 16.52544592524342804, -4.483927247898539470, 48.54057627198103120 ) ) ;
#193336=CARTESIAN_POINT ( 'NONE',  ( -15.80617190586745835, -15.72974639402198527, 51.87390960531437401 ) ) ;
#193337=CARTESIAN_POINT ( 'NONE',  ( 13.97604488694527802, 13.89961937509977652, 64.37390960531436690 ) ) ;
#193338=CARTESIAN_POINT ( 'NONE',  ( 5.719274019375991003, -21.55341960407610458, 77.70724293864770971 ) ) ;
#193339=CARTESIAN_POINT ( 'NONE',  ( -19.05341960407617563, 5.049401038297882671, 63.54275706135234003 ) ) ;
#193340=CARTESIAN_POINT ( 'NONE',  ( -16.46253265017146816, -9.564922557961047289, 24.16775706135233648 ) ) ;
#193341=CARTESIAN_POINT ( 'NONE',  ( -8.314922557960811034, -14.29746914071050412, 67.08224293864770971 ) ) ;
#193342=CARTESIAN_POINT ( 'NONE',  ( 18.62759615963271287, -10.81492255796078972, 33.33224293864769550 ) ) ;
#193345=CARTESIAN_POINT ( 'NONE',  ( 4.483927247898790824, -16.52544592524335698, 80.20942372801901854 ) ) ;
#193347=CARTESIAN_POINT ( 'NONE',  ( 9.474510206698729675, 16.51473224551082808, 82.08442372801899012 ) ) ;
#193348=CARTESIAN_POINT ( 'NONE',  ( -8.314922557960811034, -14.29746914071050412, 57.08224293864769550 ) ) ;
#193350=CARTESIAN_POINT ( 'NONE',  ( -5.049401038298153566, 19.05341960407611168, 50.20724293864770260 ) ) ;
#193351=CARTESIAN_POINT ( 'NONE',  ( 4.483927247898545687, 16.52544592524342804, 39.79057627198103830 ) ) ;
#193352=CARTESIAN_POINT ( 'NONE',  ( 9.564922557960805705, 16.46253265017160317, 84.58224293864769550 ) ) ;
#193353=CARTESIAN_POINT ( 'NONE',  ( -16.51473224551069308, -9.474510206698971260, 46.66557627198102409 ) ) ;
#193354=CARTESIAN_POINT ( 'NONE',  ( 15.80617190586769283, -15.72974639402175789, 60.62609039468567573 ) ) ;
#193355=CARTESIAN_POINT ( 'NONE',  ( -13.97604488694527625, -13.89961937509977652, 76.87390960531433848 ) ) ;
#193356=CARTESIAN_POINT ( 'NONE',  ( -16.51473224551069308, -9.474510206698971260, 26.66557627198103120 ) ) ;
#193357=CARTESIAN_POINT ( 'NONE',  ( 19.03943276465977164, -0.05219959533909143690, 78.74890960531436690 ) ) ;
#193358=CARTESIAN_POINT ( 'NONE',  ( -0.05219959533907301413, -21.53943276465977519, 52.49890960531435979 ) ) ;
#193359=CARTESIAN_POINT ( 'NONE',  ( 9.474510206698971260, -16.51473224551069308, 42.91557627198103120 ) ) ;
#193360=CARTESIAN_POINT ( 'NONE',  ( -21.53943276465977519, 0.05219959533907696930, 51.24890960531436690 ) ) ;
#193361=CARTESIAN_POINT ( 'NONE',  ( -13.89961937509957401, -13.97604488694547875, 84.37609039468567573 ) ) ;
#193362=CARTESIAN_POINT ( 'NONE',  ( 16.53943276465976808, 0.05219959533934440121, 101.2510903946856757 ) ) ;
#193363=CARTESIAN_POINT ( 'NONE',  ( 5.153800228976615827, -19.02544592524334988, 30.20942372801900433 ) ) ;
#193364=CARTESIAN_POINT ( 'NONE',  ( 16.52544592524335698, 4.483927247898782831, 61.45942372801901854 ) ) ;
#193365=CARTESIAN_POINT ( 'NONE',  ( -8.314922557961024197, 14.29746914071037800, 77.91775706135231871 ) ) ;
#193367=CARTESIAN_POINT ( 'NONE',  ( -12.14591786802326823, 12.06949235617739902, 73.12609039468567573 ) ) ;
#193368=CARTESIAN_POINT ( 'NONE',  ( 5.823673210054125526, 21.52544592524343514, 29.79057627198102409 ) ) ;
#193369=CARTESIAN_POINT ( 'NONE',  ( -19.03943276465977164, 0.05219959533909376836, 31.24890960531435979 ) ) ;
#193370=CARTESIAN_POINT ( 'NONE',  ( -16.53943276465976808, -0.05219959533934237506, 43.75109039468568284 ) ) ;
#193371=CARTESIAN_POINT ( 'NONE',  ( 9.564922557960805705, 16.46253265017160317, 49.58224293864770260 ) ) ;
#193372=CARTESIAN_POINT ( 'NONE',  ( -21.53943276465977519, -0.05219959533937600094, 38.75109039468567573 ) ) ;
#193373=CARTESIAN_POINT ( 'NONE',  ( -16.55341960407617563, 4.379528057220093196, 38.54275706135234714 ) ) ;
#193374=CARTESIAN_POINT ( 'NONE',  ( -4.379528057220086978, -16.55341960407618274, 104.7927570613523898 ) ) ;
#193376=CARTESIAN_POINT ( 'NONE',  ( 5.153800228976615827, -19.02544592524334988, 25.20942372801900433 ) ) ;
#193377=CARTESIAN_POINT ( 'NONE',  ( -5.049401038297874678, -19.05341960407617918, 104.7927570613523471 ) ) ;
#193378=CARTESIAN_POINT ( 'NONE',  ( -13.97604488694547697, 13.89961937509957934, 73.12609039468568994 ) ) ;
#193379=CARTESIAN_POINT ( 'NONE',  ( 0.05219959533910956823, 16.53943276465976808, 69.99890960531435269 ) ) ;
#193380=CARTESIAN_POINT ( 'NONE',  ( -4.379528057220328563, 16.55341960407611168, 115.2072429386476955 ) ) ;
#193381=CARTESIAN_POINT ( 'NONE',  ( -13.89961937509957401, -13.97604488694547875, 59.37609039468566863 ) ) ;
#193382=CARTESIAN_POINT ( 'NONE',  ( 16.29526858892907626, -7.335722546920041331, 56.70329402199735824 ) ) ;
#193383=CARTESIAN_POINT ( 'NONE',  ( -5.719274019375665041, -21.55341960407619695, 69.79275706135234714 ) ) ;
#193384=CARTESIAN_POINT ( 'NONE',  ( 12.06949235617739724, 12.14591786802326823, 26.87609039468567218 ) ) ;
#193386=CARTESIAN_POINT ( 'NONE',  ( -18.67979575497178146, -10.72451020669898902, 26.66557627198103475 ) ) ;
#193387=CARTESIAN_POINT ( 'NONE',  ( -0.05219959533936034679, 19.03943276465977164, 102.5010903946856757 ) ) ;
#193388=CARTESIAN_POINT ( 'NONE',  ( 19.05341960407611168, 5.049401038298154454, 113.9572429386477097 ) ) ;
#193390=CARTESIAN_POINT ( 'NONE',  ( -19.05341960407611168, -5.049401038298163336, 31.45724293864769550 ) ) ;
#193391=CARTESIAN_POINT ( 'NONE',  ( -18.67979575497193778, 10.72451020669871902, 103.3344237280190043 ) ) ;
#193392=CARTESIAN_POINT ( 'NONE',  ( -16.46253265017160317, 9.564922557960807481, 50.83224293864770260 ) ) ;
#193393=CARTESIAN_POINT ( 'NONE',  ( 0.05219959533937995610, -21.53943276465977519, 70.00109039468568994 ) ) ;
#193394=CARTESIAN_POINT ( 'NONE',  ( -5.823673210054431948, 21.52544592524334988, 102.7094237280190185 ) ) ;
#193395=CARTESIAN_POINT ( 'NONE',  ( 16.52544592524342804, -4.483927247898539470, 28.54057627198103120 ) ) ;
#193396=CARTESIAN_POINT ( 'NONE',  ( 0.05219959533909260263, 19.03943276465977164, 34.99890960531435979 ) ) ;
#193397=EDGE_CURVE ( 'NONE', #98417, #179309, #59296, .T. ) ;
#193398=CARTESIAN_POINT ( 'NONE',  ( 0.05219959533909260263, 19.03943276465977164, 74.99890960531435269 ) ) ;
#193399=CARTESIAN_POINT ( 'NONE',  ( 18.62759615963255655, 10.81492255796105972, 56.66775706135235424 ) ) ;
#193400=CARTESIAN_POINT ( 'NONE',  ( -19.05341960407611168, -5.049401038298163336, 31.45724293864769550 ) ) ;
#193401=CARTESIAN_POINT ( 'NONE',  ( 21.55341960407619695, -5.719274019375665929, 56.04275706135235424 ) ) ;
#193402=CARTESIAN_POINT ( 'NONE',  ( -19.02544592524334988, -5.153800228976617603, 83.95942372801901854 ) ) ;
#193403=CARTESIAN_POINT ( 'NONE',  ( 19.05341960407611168, 5.049401038298154454, 108.9572429386477097 ) ) ;
#193404=CARTESIAN_POINT ( 'NONE',  ( -13.97604488694527625, -13.89961937509977652, 21.87390960531435979 ) ) ;
#193405=CARTESIAN_POINT ( 'NONE',  ( -21.53943276465977519, 0.05219959533907696930, 111.2489096053143669 ) ) ;
#193406=CARTESIAN_POINT ( 'NONE',  ( 5.153800228976615827, -19.02544592524334988, 40.20942372801898301 ) ) ;
#193407=CARTESIAN_POINT ( 'NONE',  ( -0.05219959533910754901, -16.53943276465976808, 92.49890960531436690 ) ) ;
#193408=CARTESIAN_POINT ( 'NONE',  ( 5.049401038298161559, -19.05341960407611168, 52.70724293864767418 ) ) ;
#193409=CARTESIAN_POINT ( 'NONE',  ( 19.02544592524334988, 5.153800228976608722, 101.4594237280189759 ) ) ;
#193410=CARTESIAN_POINT ( 'NONE',  ( 14.29746914071049879, -8.314922557960816363, 58.33224293864768839 ) ) ;
#193411=CARTESIAN_POINT ( 'NONE',  ( -15.80617190586768217, 15.72974639402176855, 108.1260903946856757 ) ) ;
#193412=CARTESIAN_POINT ( 'NONE',  ( 16.51473224551069308, 9.474510206698969483, 104.1655762719810241 ) ) ;
#193413=CARTESIAN_POINT ( 'NONE',  ( -9.564922557961040184, 16.46253265017147172, 92.91775706135233293 ) ) ;
#193414=CARTESIAN_POINT ( 'NONE',  ( 15.80617190586746368, 15.72974639402197994, 89.37390960531435269 ) ) ;
#193415=CARTESIAN_POINT ( 'NONE',  ( 5.719274019375673035, 21.55341960407619339, 42.29275706135235424 ) ) ;
#193416=CARTESIAN_POINT ( 'NONE',  ( -14.34966873604972548, 8.224510206698743886, 43.33442372801901143 ) ) ;
#193417=CARTESIAN_POINT ( 'NONE',  ( 4.379528057220092307, 16.55341960407617563, 107.2927570613523471 ) ) ;
#193418=CARTESIAN_POINT ( 'NONE',  ( -14.29746914071037622, -8.314922557961029526, 44.16775706135234714 ) ) ;
#193419=CARTESIAN_POINT ( 'NONE',  ( 10.72451020669871369, 18.67979575497193778, 47.08442372801901854 ) ) ;
#193420=CARTESIAN_POINT ( 'NONE',  ( -0.05219959533907301413, -21.53943276465977519, 42.49890960531435979 ) ) ;
#193421=CARTESIAN_POINT ( 'NONE',  ( -13.89961937509977652, 13.97604488694528158, 30.62390960531435269 ) ) ;
#193423=CARTESIAN_POINT ( 'NONE',  ( -8.224510206698735004, -14.34966873604973081, 64.58442372801900433 ) ) ;
#193424=CARTESIAN_POINT ( 'NONE',  ( 10.72451020669898902, -18.67979575497178502, 82.91557627198103830 ) ) ;
#193425=CARTESIAN_POINT ( 'NONE',  ( 12.06949235617757843, -12.14591786802309237, 33.12390960531435979 ) ) ;
#193426=CARTESIAN_POINT ( 'NONE',  ( 16.55341960407618274, -4.379528057220086978, 61.04275706135234714 ) ) ;
#193427=CARTESIAN_POINT ( 'NONE',  ( 16.51473224551069308, 9.474510206698969483, 64.16557627198102409 ) ) ;
#193428=CARTESIAN_POINT ( 'NONE',  ( 5.153800228976615827, -19.02544592524334988, 95.20942372801897591 ) ) ;
#193429=CARTESIAN_POINT ( 'NONE',  ( 0.05219959533907565091, 21.53943276465977519, 84.99890960531436690 ) ) ;
#193430=CARTESIAN_POINT ( 'NONE',  ( -4.483927247898539470, -16.52544592524342804, 37.29057627198102409 ) ) ;
#193433=( BOUNDED_CURVE ( )  B_SPLINE_CURVE ( 2, ( #60702, #28425, #124370, #166924, #46544, #92025, #90062, #16209, #186065, #61694, #47548, #150761, #137554 ),
 .UNSPECIFIED., .F., .F. ) 
 B_SPLINE_CURVE_WITH_KNOTS ( ( 3, 2, 2, 2, 2, 2, 3 ),
 ( 0.3182655899333458605, 0.3201754385964912242, 0.3245614035087719396, 0.3289473684210526550, 0.3333333333333333148, 0.3377192982456140302, 0.3396748267308496994 ),
 .UNSPECIFIED. ) 
 CURVE ( )  GEOMETRIC_REPRESENTATION_ITEM ( )  RATIONAL_B_SPLINE_CURVE ( ( 0.9832469066685285419, 0.9851625545550100060, 1.000000000000000000, 0.9659258262890683122, 1.000000000000000000, 0.9659258262890683122, 1.000000000000000000, 0.9659258262890683122, 1.000000000000000000, 0.9659258262890683122, 1.000000000000000000, 0.9848076720550082985, 0.9831626618144002627 ) ) 
 REPRESENTATION_ITEM ( '' )  );
#193434=CARTESIAN_POINT ( 'NONE',  ( 21.52544592524344225, -5.823673210054117533, 68.54057627198103830 ) ) ;
#193435=CARTESIAN_POINT ( 'NONE',  ( 12.06949235617739724, 12.14591786802326823, 106.8760903946856899 ) ) ;
#193438=CARTESIAN_POINT ( 'NONE',  ( 21.52544592524344225, -5.823673210054117533, 93.54057627198103830 ) ) ;
#193439=CARTESIAN_POINT ( 'NONE',  ( -21.55341960407610458, -5.719274019375992779, 106.4572429386477097 ) ) ;
#193440=CARTESIAN_POINT ( 'NONE',  ( -16.53943276465976808, 0.05219959533911058130, 26.24890960531435624 ) ) ;
#193441=CARTESIAN_POINT ( 'NONE',  ( -4.379528057220086978, -16.55341960407618274, 39.79275706135235424 ) ) ;
#193442=CARTESIAN_POINT ( 'NONE',  ( -19.03943276465977164, 0.05219959533909376836, 36.24890960531436690 ) ) ;
#193443=CARTESIAN_POINT ( 'NONE',  ( -19.05341960407611168, -5.049401038298163336, 66.45724293864769550 ) ) ;
#193445=CARTESIAN_POINT ( 'NONE',  ( 5.823673210054125526, 21.52544592524343514, 24.79057627198103120 ) ) ;
#193446=CARTESIAN_POINT ( 'NONE',  ( 17.60779699588839264, 5.500000000000007105, 78.84981316670105400 ) ) ;
#193447=CARTESIAN_POINT ( 'NONE',  ( 19.05341960407617918, -5.049401038297876454, 111.0427570613523329 ) ) ;
#193448=CARTESIAN_POINT ( 'NONE',  ( -16.46253265017146816, -9.564922557961047289, 39.16775706135234003 ) ) ;
#193449=CARTESIAN_POINT ( 'NONE',  ( -5.719274019375978568, 21.55341960407610458, 85.20724293864770971 ) ) ;
#193450=CARTESIAN_POINT ( 'NONE',  ( -16.55341960407617563, 4.379528057220093196, 108.5427570613523756 ) ) ;
#193451=CARTESIAN_POINT ( 'NONE',  ( 21.55341960407610458, 5.719274019375980345, 43.95724293864769550 ) ) ;
#193452=CARTESIAN_POINT ( 'NONE',  ( -0.05219959533907301413, -21.53943276465977519, 82.49890960531436690 ) ) ;
#193453=CARTESIAN_POINT ( 'NONE',  ( -9.564922557961040184, 16.46253265017147172, 107.9177570613523471 ) ) ;
#193454=CARTESIAN_POINT ( 'NONE',  ( -9.564922557960796823, -16.46253265017161027, 102.0822429386477097 ) ) ;
#193455=CARTESIAN_POINT ( 'NONE',  ( 21.52544592524334988, 5.823673210054432836, 76.45942372801901854 ) ) ;
#193456=CARTESIAN_POINT ( 'NONE',  ( 9.564922557960805705, 16.46253265017160317, 79.58224293864769550 ) ) ;
#193457=CARTESIAN_POINT ( 'NONE',  ( 8.224510206698953496, -14.34966873604960469, 102.9155762719810383 ) ) ;
#193459=CARTESIAN_POINT ( 'NONE',  ( 5.049401038298161559, -19.05341960407611168, 67.70724293864769550 ) ) ;
#193460=CARTESIAN_POINT ( 'NONE',  ( -8.224510206698948167, 14.34966873604960824, 95.41557627198102409 ) ) ;
#193462=CARTESIAN_POINT ( 'NONE',  ( -13.97604488694547697, 13.89961937509957934, 88.12609039468563310 ) ) ;
#193463=CARTESIAN_POINT ( 'NONE',  ( 17.13100169013300444, -6.664070546373146442, 83.26789835699850073 ) ) ;
#193464=CARTESIAN_POINT ( 'NONE',  ( 5.049401038298161559, -19.05341960407611168, 57.70724293864769550 ) ) ;
#193465=CARTESIAN_POINT ( 'NONE',  ( 18.62759615963255655, 10.81492255796105972, 81.66775706135236135 ) ) ;
#193466=CARTESIAN_POINT ( 'NONE',  ( -5.153800228976328057, -19.02544592524343514, 102.2905762719810383 ) ) ;
#193467=CARTESIAN_POINT ( 'NONE',  ( -8.224510206698735004, -14.34966873604973081, 84.58442372801903275 ) ) ;
#193469=CARTESIAN_POINT ( 'NONE',  ( 0.05219959533936267826, -19.03943276465977164, 60.00109039468566863 ) ) ;
#193470=CARTESIAN_POINT ( 'NONE',  ( -21.52544592524334988, -5.823673210054445271, 98.95942372801903275 ) ) ;
#193473=CARTESIAN_POINT ( 'NONE',  ( 8.224510206698742110, 14.34966873604972548, 102.0844237280190185 ) ) ;
#193475=CARTESIAN_POINT ( 'NONE',  ( -16.53943276465976808, -0.05219959533934237506, 88.75109039468567573 ) ) ;
#193477=CARTESIAN_POINT ( 'NONE',  ( -16.55341960407617563, 4.379528057220093196, 63.54275706135234003 ) ) ;
#193479=CARTESIAN_POINT ( 'NONE',  ( 15.72974639402176855, 15.80617190586768217, 86.87609039468568994 ) ) ;
#193480=CARTESIAN_POINT ( 'NONE',  ( -9.474510206698720793, -16.51473224551083518, 84.58442372801900433 ) ) ;
#193481=CARTESIAN_POINT ( 'NONE',  ( -0.05219959533936034679, 19.03943276465977164, 37.50109039468567573 ) ) ;
#193482=CARTESIAN_POINT ( 'NONE',  ( 19.03943276465977164, -0.05219959533909143690, 63.74890960531435979 ) ) ;
#193483=CARTESIAN_POINT ( 'NONE',  ( 9.474510206698971260, -16.51473224551069308, 57.91557627198103120 ) ) ;
#193485=CARTESIAN_POINT ( 'NONE',  ( -18.62759615963270932, 10.81492255796079327, 75.83224293864769550 ) ) ;
#193486=CARTESIAN_POINT ( 'NONE',  ( 15.80617190586746368, 15.72974639402197994, 39.37390960531436690 ) ) ;
#193487=CARTESIAN_POINT ( 'NONE',  ( 19.02544592524343514, -5.153800228976328945, 38.54057627198103120 ) ) ;
#193488=CARTESIAN_POINT ( 'NONE',  ( -16.53943276465976808, -0.05219959533934237506, 63.75109039468568284 ) ) ;
#193489=ORIENTED_EDGE ( 'NONE', *, *, #17219, .T. ) ;
#193490=CARTESIAN_POINT ( 'NONE',  ( -15.80617190586768217, 15.72974639402176855, 28.12609039468568284 ) ) ;
#193491=CARTESIAN_POINT ( 'NONE',  ( -14.34966873604960291, -8.224510206698953496, 71.66557627198100988 ) ) ;
#193493=CARTESIAN_POINT ( 'NONE',  ( -14.29746914071037622, -8.314922557961029526, 29.16775706135234003 ) ) ;
#193494=CARTESIAN_POINT ( 'NONE',  ( -13.97604488694547697, 13.89961937509957934, 53.12609039468565442 ) ) ;
#193495=CARTESIAN_POINT ( 'NONE',  ( 14.29746914071049879, -8.314922557960816363, 53.33224293864769550 ) ) ;
#193496=CARTESIAN_POINT ( 'NONE',  ( -5.823673210054431948, 21.52544592524334988, 37.70942372801900433 ) ) ;
#193499=CARTESIAN_POINT ( 'NONE',  ( -21.52544592524343514, 5.823673210054127303, 71.04057627198103830 ) ) ;
#193500=CARTESIAN_POINT ( 'NONE',  ( 9.474510206698971260, -16.51473224551069308, 107.9155762719810383 ) ) ;
#193501=CARTESIAN_POINT ( 'NONE',  ( 8.314922557960818139, 14.29746914071049879, 74.58224293864768129 ) ) ;
#193504=CARTESIAN_POINT ( 'NONE',  ( 17.49999999999999289, 5.500000000000009770, 43.78230962303566542 ) ) ;
#193505=CARTESIAN_POINT ( 'NONE',  ( -16.46253265017146816, -9.564922557961047289, 64.16775706135233293 ) ) ;
#193506=CARTESIAN_POINT ( 'NONE',  ( 10.72451020669898902, -18.67979575497178502, 112.9155762719810383 ) ) ;
#193507=CARTESIAN_POINT ( 'NONE',  ( -5.153800228976328057, -19.02544592524343514, 57.29057627198103120 ) ) ;
#193508=CARTESIAN_POINT ( 'NONE',  ( 19.03943276465977164, 0.05219959533936151252, 41.25109039468566152 ) ) ;
#193509=CARTESIAN_POINT ( 'NONE',  ( -13.89961937509977652, 13.97604488694528158, 30.62390960531435269 ) ) ;
#193510=CARTESIAN_POINT ( 'NONE',  ( 10.81492255796106328, -18.62759615963255655, 70.41775706135236135 ) ) ;
#193512=EDGE_CURVE ( 'NONE', #68126, #20566, #51457, .T. ) ;
#193513=CARTESIAN_POINT ( 'NONE',  ( -16.55341960407611168, -4.379528057220339221, 46.45724293864769550 ) ) ;
#193514=CARTESIAN_POINT ( 'NONE',  ( 13.97604488694527802, 13.89961937509977652, 64.37390960531436690 ) ) ;
#193515=CARTESIAN_POINT ( 'NONE',  ( 10.81492255796078972, 18.62759615963270932, 84.58224293864769550 ) ) ;
#193516=CARTESIAN_POINT ( 'NONE',  ( 13.97604488694527802, 13.89961937509977652, 59.37390960531434558 ) ) ;
#193518=CARTESIAN_POINT ( 'NONE',  ( -15.80617190586745835, -15.72974639402198527, 61.87390960531436690 ) ) ;
#193519=ORIENTED_EDGE ( 'NONE', *, *, #186989, .F. ) ;
#193520=CARTESIAN_POINT ( 'NONE',  ( 5.719274019375673035, 21.55341960407619339, 102.2927570613523613 ) ) ;
#193521=CARTESIAN_POINT ( 'NONE',  ( 19.03943276465977164, -0.05219959533909143690, 23.74890960531435269 ) ) ;
#193522=CARTESIAN_POINT ( 'NONE',  ( 14.34966873604972726, -8.224510206698740333, 90.83442372801901854 ) ) ;
#193523=CARTESIAN_POINT ( 'NONE',  ( 14.34966873604960469, 8.224510206698951720, 84.16557627198103830 ) ) ;
#193524=CARTESIAN_POINT ( 'NONE',  ( -19.03943276465977164, -0.05219959533935918106, 98.75109039468567573 ) ) ;
#193526=CARTESIAN_POINT ( 'NONE',  ( 10.81492255796106328, -18.62759615963255655, 20.41775706135234714 ) ) ;
#193527=CARTESIAN_POINT ( 'NONE',  ( -13.97604488694547697, 13.89961937509957934, 43.12609039468566152 ) ) ;
#193528=CARTESIAN_POINT ( 'NONE',  ( 16.53943276465976808, 0.05219959533934440121, 96.25109039468568994 ) ) ;
#193529=CARTESIAN_POINT ( 'NONE',  ( 13.89961937509957401, 13.97604488694547697, 31.87609039468566863 ) ) ;
#193530=CARTESIAN_POINT ( 'NONE',  ( -13.89961937509977652, 13.97604488694528158, 85.62390960531433848 ) ) ;
#193531=CARTESIAN_POINT ( 'NONE',  ( -15.72974639402197994, 15.80617190586746368, 60.62390960531437401 ) ) ;
#193533=CARTESIAN_POINT ( 'NONE',  ( 4.483927247898545687, 16.52544592524342804, 114.7905762719810383 ) ) ;
#193534=CARTESIAN_POINT ( 'NONE',  ( -18.62759615963255300, -10.81492255796106328, 99.16775706135234714 ) ) ;
#193535=CARTESIAN_POINT ( 'NONE',  ( -16.55341960407617563, 4.379528057220093196, 73.54275706135234714 ) ) ;
#193536=CARTESIAN_POINT ( 'NONE',  ( -21.52544592524334988, -5.823673210054445271, 23.95942372801901143 ) ) ;
#193537=CARTESIAN_POINT ( 'NONE',  ( 14.29746914071037800, 8.314922557961029526, 26.66775706135235424 ) ) ;
#193538=CARTESIAN_POINT ( 'NONE',  ( 19.05341960407611168, 5.049401038298154454, 98.95724293864766707 ) ) ;
#193539=CARTESIAN_POINT ( 'NONE',  ( -5.153800228976328057, -19.02544592524343514, 37.29057627198102409 ) ) ;
#193540=CARTESIAN_POINT ( 'NONE',  ( 9.564922557960805705, 16.46253265017160317, 69.58224293864770971 ) ) ;
#193541=AXIS2_PLACEMENT_3D ( 'NONE', #22325, #145655, #82981 ) ;
#193542=CARTESIAN_POINT ( 'NONE',  ( 4.483927247898790824, -16.52544592524335698, 45.20942372801901854 ) ) ;
#193543=CARTESIAN_POINT ( 'NONE',  ( -16.52544592524342804, 4.483927247898546575, 96.04057627198102409 ) ) ;
#193544=CARTESIAN_POINT ( 'NONE',  ( -8.224510206698735004, -14.34966873604973081, 94.58442372801901854 ) ) ;
#193545=CARTESIAN_POINT ( 'NONE',  ( 18.67979575497194134, -10.72451020669871369, 40.83442372801901854 ) ) ;
#193546=CARTESIAN_POINT ( 'NONE',  ( -9.474510206698964154, 16.51473224551069663, 80.41557627198103830 ) ) ;
#193547=CARTESIAN_POINT ( 'NONE',  ( 19.02544592524343514, -5.153800228976328945, 58.54057627198102409 ) ) ;
#193548=CARTESIAN_POINT ( 'NONE',  ( -19.05341960407611168, -5.049401038298163336, 101.4572429386476955 ) ) ;
#193549=CARTESIAN_POINT ( 'NONE',  ( -16.53943276465976808, 0.05219959533911058130, 31.24890960531435979 ) ) ;
#193550=CARTESIAN_POINT ( 'NONE',  ( 8.314922557961029526, -14.29746914071037800, 100.4177570613523471 ) ) ;
#193553=CARTESIAN_POINT ( 'NONE',  ( 5.049401038297881783, 19.05341960407617563, 47.29275706135231161 ) ) ;
#193554=CARTESIAN_POINT ( 'NONE',  ( -13.89961937509977652, 13.97604488694528158, 115.6239096053143669 ) ) ;
#193555=CARTESIAN_POINT ( 'NONE',  ( 16.51473224551069308, 9.474510206698969483, 59.16557627198102409 ) ) ;
#193556=CARTESIAN_POINT ( 'NONE',  ( 19.02544592524334988, 5.153800228976608722, 41.45942372801900433 ) ) ;
#193558=CARTESIAN_POINT ( 'NONE',  ( -17.31747979337949062, -6.344076630961018815, 66.37944868065184778 ) ) ;
#193559=CARTESIAN_POINT ( 'NONE',  ( -14.29746914071037622, -8.314922557961029526, 39.16775706135235424 ) ) ;
#193560=CARTESIAN_POINT ( 'NONE',  ( 13.89961937509957401, 13.97604488694547697, 66.87609039468567573 ) ) ;
#193561=CARTESIAN_POINT ( 'NONE',  ( -4.483927247898782831, 16.52544592524335698, 52.70942372801902565 ) ) ;
#193563=CARTESIAN_POINT ( 'NONE',  ( 5.153800228976335163, 19.02544592524342804, 94.79057627198103830 ) ) ;
#193564=CARTESIAN_POINT ( 'NONE',  ( -5.823673210054116645, -21.52544592524344225, 107.2905762719810525 ) ) ;
#193565=CARTESIAN_POINT ( 'NONE',  ( -9.564922557961040184, 16.46253265017147172, 72.91775706135233293 ) ) ;
#193566=CARTESIAN_POINT ( 'NONE',  ( -13.89961937509977652, 13.97604488694528158, 105.6239096053143527 ) ) ;
#193567=CARTESIAN_POINT ( 'NONE',  ( 19.05341960407611168, 5.049401038298154454, 28.95724293864769550 ) ) ;
#193568=CARTESIAN_POINT ( 'NONE',  ( 19.02544592524343514, -5.153800228976328945, 73.54057627198103830 ) ) ;
#193569=CARTESIAN_POINT ( 'NONE',  ( -8.314922557960811034, -14.29746914071050412, 47.08224293864770260 ) ) ;
#193570=CARTESIAN_POINT ( 'NONE',  ( 16.46253265017160672, -9.564922557960803928, 43.33224293864769550 ) ) ;
#193571=CARTESIAN_POINT ( 'NONE',  ( 9.564922557961047289, -16.46253265017146816, 55.41775706135234003 ) ) ;
#193572=CARTESIAN_POINT ( 'NONE',  ( 12.14591786802309770, 12.06949235617756955, 89.37390960531435269 ) ) ;
#193573=CARTESIAN_POINT ( 'NONE',  ( 18.62759615963255655, 10.81492255796105972, 106.6677570613523756 ) ) ;
#193574=CARTESIAN_POINT ( 'NONE',  ( 5.153800228976335163, 19.02544592524342804, 49.79057627198100988 ) ) ;
#193575=CARTESIAN_POINT ( 'NONE',  ( -21.55341960407610458, -5.719274019375992779, 56.45724293864768839 ) ) ;
#193576=CARTESIAN_POINT ( 'NONE',  ( 16.53943276465976808, -0.05219959533910856209, 53.74890960531437401 ) ) ;
#193577=CARTESIAN_POINT ( 'NONE',  ( 0.05219959533936267826, -19.03943276465977164, 25.00109039468566152 ) ) ;
#193578=CARTESIAN_POINT ( 'NONE',  ( 19.02544592524343514, -5.153800228976328945, 108.5405762719810383 ) ) ;
#193579=CARTESIAN_POINT ( 'NONE',  ( 9.474510206698971260, -16.51473224551069308, 102.9155762719810241 ) ) ;
#193580=CARTESIAN_POINT ( 'NONE',  ( -16.46253265017160317, 9.564922557960807481, 40.83224293864769550 ) ) ;
#193581=CARTESIAN_POINT ( 'NONE',  ( 0.05219959533909260263, 19.03943276465977164, 29.99890960531435979 ) ) ;
#193582=CARTESIAN_POINT ( 'NONE',  ( -4.483927247898539470, -16.52544592524342804, 87.29057627198103830 ) ) ;
#193583=CARTESIAN_POINT ( 'NONE',  ( -21.55341960407610458, -5.719274019375992779, 91.45724293864769550 ) ) ;
#193584=CARTESIAN_POINT ( 'NONE',  ( 5.049401038298161559, -19.05341960407611168, 102.7072429386476955 ) ) ;
#193585=CARTESIAN_POINT ( 'NONE',  ( -21.53943276465977519, 0.05219959533907696930, 106.2489096053143811 ) ) ;
#193586=CARTESIAN_POINT ( 'NONE',  ( 19.02544592524343514, -5.153800228976328945, 103.5405762719809957 ) ) ;
#193588=CARTESIAN_POINT ( 'NONE',  ( -8.314922557960811034, -14.29746914071050412, 97.08224293864770971 ) ) ;
#193589=CARTESIAN_POINT ( 'NONE',  ( 19.05341960407611168, 5.049401038298154454, 73.95724293864768129 ) ) ;
#193590=CARTESIAN_POINT ( 'NONE',  ( 18.62759615963271287, -10.81492255796078972, 83.33224293864769550 ) ) ;
#193591=CARTESIAN_POINT ( 'NONE',  ( 16.62475595723699939, -7.163666690055295660, 108.0271335181047050 ) ) ;
#193593=CARTESIAN_POINT ( 'NONE',  ( 10.81492255796078972, 18.62759615963270932, 24.58224293864768839 ) ) ;
#193595=CARTESIAN_POINT ( 'NONE',  ( 16.52544592524335698, 4.483927247898782831, 31.45942372801901854 ) ) ;
#193596=CARTESIAN_POINT ( 'NONE',  ( -12.14591786802309592, -12.06949235617757132, 96.87390960531436690 ) ) ;
#193597=CARTESIAN_POINT ( 'NONE',  ( 19.25663599770058454, -5.499999999999650946, 51.49419308057199629 ) ) ;
#193598=CARTESIAN_POINT ( 'NONE',  ( -5.153800228976328057, -19.02544592524343514, 62.29057627198100988 ) ) ;
#193599=CARTESIAN_POINT ( 'NONE',  ( -14.34966873604960291, -8.224510206698953496, 86.66557627198102409 ) ) ;
#193600=CARTESIAN_POINT ( 'NONE',  ( 10.81492255796078972, 18.62759615963270932, 39.58224293864769550 ) ) ;
#193601=CARTESIAN_POINT ( 'NONE',  ( -16.55341960407611168, -4.379528057220339221, 71.45724293864769550 ) ) ;
#193602=CARTESIAN_POINT ( 'NONE',  ( 16.46253265017146816, 9.564922557961045513, 111.6677570613523329 ) ) ;
#193603=CARTESIAN_POINT ( 'NONE',  ( -18.62759615963255300, -10.81492255796106328, 74.16775706135231871 ) ) ;
#193605=CARTESIAN_POINT ( 'NONE',  ( 21.52544592524344225, -5.823673210054117533, 23.54057627198102765 ) ) ;
#193606=CARTESIAN_POINT ( 'NONE',  ( -12.06949235617739369, -12.14591786802326823, 79.37609039468567573 ) ) ;
#193607=CARTESIAN_POINT ( 'NONE',  ( 19.05341960407611168, 5.049401038298154454, 33.95724293864769550 ) ) ;
#193608=CARTESIAN_POINT ( 'NONE',  ( 16.46253265017160672, -9.564922557960803928, 88.33224293864769550 ) ) ;
#193609=CARTESIAN_POINT ( 'NONE',  ( 21.55341960407610458, 5.719274019375980345, 98.95724293864770971 ) ) ;
#193610=CARTESIAN_POINT ( 'NONE',  ( -14.29746914071037622, -8.314922557961029526, 29.16775706135234003 ) ) ;
#193611=CARTESIAN_POINT ( 'NONE',  ( -12.14591786802309592, -12.06949235617757132, 56.87390960531436690 ) ) ;
#193612=CARTESIAN_POINT ( 'NONE',  ( 21.53943276465977519, 0.05219959533937863772, 76.25109039468568994 ) ) ;
#193613=CARTESIAN_POINT ( 'NONE',  ( 0.05219959533934541429, -16.53943276465976808, 105.0010903946856757 ) ) ;
#193614=CARTESIAN_POINT ( 'NONE',  ( 9.474510206698971260, -16.51473224551069308, 112.9155762719810383 ) ) ;
#193615=CARTESIAN_POINT ( 'NONE',  ( -17.05587630539786659, 6.762274262135700376, 80.74180309037312497 ) ) ;
#193616=CARTESIAN_POINT ( 'NONE',  ( 14.29746914071037800, 8.314922557961029526, 111.6677570613523613 ) ) ;
#193617=CARTESIAN_POINT ( 'NONE',  ( 12.06949235617739724, 12.14591786802326823, 61.87609039468568284 ) ) ;
#193618=CARTESIAN_POINT ( 'NONE',  ( 5.049401038298161559, -19.05341960407611168, 67.70724293864769550 ) ) ;
#193620=CARTESIAN_POINT ( 'NONE',  ( -5.153800228976328057, -19.02544592524343514, 92.29057627198099567 ) ) ;
#193621=CARTESIAN_POINT ( 'NONE',  ( -21.55341960407619339, 5.719274019375674811, 73.54275706135234714 ) ) ;
#193622=CARTESIAN_POINT ( 'NONE',  ( 14.29746914071037800, 8.314922557961029526, 81.66775706135236135 ) ) ;
#193623=CARTESIAN_POINT ( 'NONE',  ( 16.52544592524342804, -4.483927247898539470, 63.54057627198103830 ) ) ;
#193624=CARTESIAN_POINT ( 'NONE',  ( 9.474510206698971260, -16.51473224551069308, 57.91557627198103120 ) ) ;
#193626=CARTESIAN_POINT ( 'NONE',  ( 5.049401038297881783, 19.05341960407617563, 102.2927570613523045 ) ) ;
#193627=CARTESIAN_POINT ( 'NONE',  ( 14.34966873604960469, 8.224510206698951720, 114.1655762719810383 ) ) ;
#193628=CARTESIAN_POINT ( 'NONE',  ( 9.564922557960805705, 16.46253265017160317, 79.58224293864769550 ) ) ;
#193629=CARTESIAN_POINT ( 'NONE',  ( -8.224510206698735004, -14.34966873604973081, 19.58442372801901143 ) ) ;
#193631=CARTESIAN_POINT ( 'NONE',  ( -21.52544592524334988, -5.823673210054445271, 98.95942372801903275 ) ) ;
#193632=CARTESIAN_POINT ( 'NONE',  ( 0.05219959533934541429, -16.53943276465976808, 75.00109039468568994 ) ) ;
#193633=CARTESIAN_POINT ( 'NONE',  ( 13.89961937509957401, 13.97604488694547697, 96.87609039468566152 ) ) ;
#193634=CARTESIAN_POINT ( 'NONE',  ( -0.05219959533907301413, -21.53943276465977519, 57.49890960531435979 ) ) ;
#193635=CARTESIAN_POINT ( 'NONE',  ( 14.29746914071037800, 8.314922557961029526, 71.66775706135234714 ) ) ;
#193637=CARTESIAN_POINT ( 'NONE',  ( -0.05219959533936034679, 19.03943276465977164, 52.50109039468566863 ) ) ;
#193638=CARTESIAN_POINT ( 'NONE',  ( 5.719274019375673035, 21.55341960407619339, 102.2927570613523613 ) ) ;
#193639=CARTESIAN_POINT ( 'NONE',  ( 9.474510206698971260, -16.51473224551069308, 37.91557627198102409 ) ) ;
#193640=CARTESIAN_POINT ( 'NONE',  ( 5.153800228976335163, 19.02544592524342804, 59.79057627198100988 ) ) ;
#193641=CARTESIAN_POINT ( 'NONE',  ( 8.224510206698953496, -14.34966873604960469, 67.91557627198102409 ) ) ;
#193643=CARTESIAN_POINT ( 'NONE',  ( -0.05219959533937732626, 21.53943276465977519, 92.50109039468567573 ) ) ;
#193644=CARTESIAN_POINT ( 'NONE',  ( -9.474510206698720793, -16.51473224551083518, 44.58442372801900433 ) ) ;
#193645=CARTESIAN_POINT ( 'NONE',  ( -5.153800228976607833, 19.02544592524334988, 47.70942372801900433 ) ) ;
#193646=CARTESIAN_POINT ( 'NONE',  ( 18.67979575497178502, 10.72451020669898547, 34.16557627198102409 ) ) ;
#193647=CARTESIAN_POINT ( 'NONE',  ( -15.80617190586768217, 15.72974639402176855, 98.12609039468570415 ) ) ;
#193648=CARTESIAN_POINT ( 'NONE',  ( 5.153800228976335163, 19.02544592524342804, 79.79057627198102409 ) ) ;
#193649=CARTESIAN_POINT ( 'NONE',  ( -18.67979575497193778, 10.72451020669871902, 88.33442372801901854 ) ) ;
#193650=CARTESIAN_POINT ( 'NONE',  ( -21.55341960407610458, -5.719274019375992779, 56.45724293864768839 ) ) ;
#193651=CARTESIAN_POINT ( 'NONE',  ( -19.02544592524342804, 5.153800228976336051, 81.04057627198103830 ) ) ;
#193652=CARTESIAN_POINT ( 'NONE',  ( 13.97604488694548053, -13.89961937509957401, 75.62609039468564731 ) ) ;
#193653=CARTESIAN_POINT ( 'NONE',  ( 19.02544592524343514, -5.153800228976328945, 88.54057627198102409 ) ) ;
#193654=CARTESIAN_POINT ( 'NONE',  ( 9.564922557961047289, -16.46253265017146816, 90.41775706135234714 ) ) ;
#193655=CARTESIAN_POINT ( 'NONE',  ( 12.06949235617739724, 12.14591786802326823, 41.87609039468568284 ) ) ;
#193656=CARTESIAN_POINT ( 'NONE',  ( -12.06949235617756955, 12.14591786802309770, 95.62390960531436690 ) ) ;
#193657=CARTESIAN_POINT ( 'NONE',  ( 5.153800228976335163, 19.02544592524342804, 64.79057627198100988 ) ) ;
#193658=CARTESIAN_POINT ( 'NONE',  ( -21.52544592524343514, 5.823673210054127303, 61.04057627198103120 ) ) ;
#193660=CARTESIAN_POINT ( 'NONE',  ( -14.29746914071037622, -8.314922557961029526, 29.16775706135234003 ) ) ;
#193661=CARTESIAN_POINT ( 'NONE',  ( -0.05219959533937732626, 21.53943276465977519, 32.50109039468568284 ) ) ;
#193662=CARTESIAN_POINT ( 'NONE',  ( -5.719274019375665041, -21.55341960407619695, 79.79275706135236135 ) ) ;
#193663=CARTESIAN_POINT ( 'NONE',  ( -16.53943276465976808, -0.05219959533934237506, 78.75109039468568994 ) ) ;
#193664=CARTESIAN_POINT ( 'NONE',  ( 0.05219959533909260263, 19.03943276465977164, 74.99890960531435269 ) ) ;
#193665=CARTESIAN_POINT ( 'NONE',  ( 14.29746914071049879, -8.314922557960816363, 78.33224293864770971 ) ) ;
#193666=CARTESIAN_POINT ( 'NONE',  ( 12.14591786802327356, -12.06949235617739191, 105.6260903946856899 ) ) ;
#193667=CARTESIAN_POINT ( 'NONE',  ( 16.46253265017146816, 9.564922557961045513, 61.66775706135234003 ) ) ;
#193668=CARTESIAN_POINT ( 'NONE',  ( 5.823673210054444382, -21.52544592524334988, 25.20942372801901854 ) ) ;
#193669=CARTESIAN_POINT ( 'NONE',  ( -4.483927247898539470, -16.52544592524342804, 82.29057627198103830 ) ) ;
#193670=CARTESIAN_POINT ( 'NONE',  ( 0.05219959533909260263, 19.03943276465977164, 94.99890960531436690 ) ) ;
#193671=CARTESIAN_POINT ( 'NONE',  ( -16.52544592524335698, -4.483927247898792601, 108.9594237280190185 ) ) ;
#193672=CARTESIAN_POINT ( 'NONE',  ( 10.72451020669871369, 18.67979575497193778, 77.08442372801901854 ) ) ;
#193673=CARTESIAN_POINT ( 'NONE',  ( 4.483927247898790824, -16.52544592524335698, 40.20942372801901854 ) ) ;
#193674=CARTESIAN_POINT ( 'NONE',  ( 21.55341960407619695, -5.719274019375665929, 26.04275706135235779 ) ) ;
#193675=CARTESIAN_POINT ( 'NONE',  ( -8.314922557960811034, -14.29746914071050412, 67.08224293864770971 ) ) ;
#193678=CARTESIAN_POINT ( 'NONE',  ( -10.72451020669898014, 18.67979575497178502, 110.4155762719810383 ) ) ;
#193679=CARTESIAN_POINT ( 'NONE',  ( 17.50000000000015987, -3.292511757969701414, 27.56520270210538825 ) ) ;
#193680=CARTESIAN_POINT ( 'NONE',  ( 4.379528057220339221, -16.55341960407611168, 52.70724293864769550 ) ) ;
#193681=CARTESIAN_POINT ( 'NONE',  ( -9.474510206698964154, 16.51473224551069663, 30.41557627198102054 ) ) ;
#193682=CARTESIAN_POINT ( 'NONE',  ( -18.62759615963270932, 10.81492255796079327, 35.83224293864768839 ) ) ;
#193683=CARTESIAN_POINT ( 'NONE',  ( 16.55341960407611168, 4.379528057220329451, 73.95724293864769550 ) ) ;
#193685=CIRCLE ( 'NONE', #106484, 2.000000000000001776 ) ;
#193686=CARTESIAN_POINT ( 'NONE',  ( -18.62759615963270932, 10.81492255796079327, 75.83224293864769550 ) ) ;
#193687=CARTESIAN_POINT ( 'NONE',  ( -5.049401038298153566, 19.05341960407611168, 80.20724293864769550 ) ) ;
#193688=CARTESIAN_POINT ( 'NONE',  ( 16.51473224551069308, 9.474510206698969483, 34.16557627198102409 ) ) ;
#193689=CARTESIAN_POINT ( 'NONE',  ( -19.03943276465977164, -0.05219959533935918106, 78.75109039468567573 ) ) ;
#193690=CARTESIAN_POINT ( 'NONE',  ( 21.55341960407619695, -5.719274019375665929, 51.04275706135234714 ) ) ;
#193691=CARTESIAN_POINT ( 'NONE',  ( -18.62759615963270932, 10.81492255796079327, 65.83224293864769550 ) ) ;
#193692=CARTESIAN_POINT ( 'NONE',  ( -16.51473224551069308, -9.474510206698971260, 46.66557627198102409 ) ) ;
#193693=CARTESIAN_POINT ( 'NONE',  ( -19.02544592524342804, 5.153800228976336051, 71.04057627198099567 ) ) ;
#193694=CARTESIAN_POINT ( 'NONE',  ( 12.06949235617739724, 12.14591786802326823, 51.87609039468568284 ) ) ;
#193695=CARTESIAN_POINT ( 'NONE',  ( 18.62759615963255655, 10.81492255796105972, 36.66775706135234714 ) ) ;
#193696=CARTESIAN_POINT ( 'NONE',  ( -15.80617190586768217, 15.72974639402176855, 58.12609039468568994 ) ) ;
#193697=CARTESIAN_POINT ( 'NONE',  ( 5.049401038298161559, -19.05341960407611168, 102.7072429386476955 ) ) ;
#193698=CARTESIAN_POINT ( 'NONE',  ( 5.823673210054125526, 21.52544592524343514, 84.79057627198102409 ) ) ;
#193699=CARTESIAN_POINT ( 'NONE',  ( 21.52544592524334988, 5.823673210054432836, 21.45942372801901499 ) ) ;
#193700=CARTESIAN_POINT ( 'NONE',  ( -16.53943276465976808, -0.05219959533934237506, 53.75109039468568994 ) ) ;
#193701=CARTESIAN_POINT ( 'NONE',  ( 0.05219959533907565091, 21.53943276465977519, 44.99890960531435979 ) ) ;
#193702=CARTESIAN_POINT ( 'NONE',  ( 16.51473224551083163, -9.474510206698727899, 25.83442372801900078 ) ) ;
#193703=B_SPLINE_CURVE_WITH_KNOTS ( 'NONE', 3,
 ( #169084, #59925, #29601, #183288, #133798, #92242 ),
 .UNSPECIFIED., .F., .F.,
 ( 4, 2, 4 ),
 ( 0.003989672132298142590, 0.004372778065220579713, 0.004755883998143016836 ),
 .UNSPECIFIED. ) ;
#193704=CARTESIAN_POINT ( 'NONE',  ( -5.049401038298153566, 19.05341960407611168, 55.20724293864769550 ) ) ;
#193706=CARTESIAN_POINT ( 'NONE',  ( -9.474510206698964154, 16.51473224551069663, 85.41557627198102409 ) ) ;
#193708=CARTESIAN_POINT ( 'NONE',  ( 17.50000000000051159, 3.947464652946200747, 103.2758644658976124 ) ) ;
#193709=CARTESIAN_POINT ( 'NONE',  ( 5.049401038297881783, 19.05341960407617563, 72.29275706135234714 ) ) ;
#193710=CARTESIAN_POINT ( 'NONE',  ( 5.823673210054125526, 21.52544592524343514, 44.79057627198103120 ) ) ;
#193711=CARTESIAN_POINT ( 'NONE',  ( -16.55341960407611168, -4.379528057220339221, 26.45724293864768839 ) ) ;
#193712=CARTESIAN_POINT ( 'NONE',  ( -13.89961937509957401, -13.97604488694547875, 89.37609039468563310 ) ) ;
#193714=CARTESIAN_POINT ( 'NONE',  ( -9.474510206698720793, -16.51473224551083518, 19.58442372801899722 ) ) ;
#193715=CARTESIAN_POINT ( 'NONE',  ( 19.03943276465977164, 0.05219959533936151252, 101.2510903946856757 ) ) ;
#193716=CARTESIAN_POINT ( 'NONE',  ( 19.03943276465977164, 0.05219959533936151252, 46.25109039468566863 ) ) ;
#193719=CARTESIAN_POINT ( 'NONE',  ( -13.89961937509977652, 13.97604488694528158, 50.62390960531435979 ) ) ;
#193720=CARTESIAN_POINT ( 'NONE',  ( -16.55341960407611168, -4.379528057220339221, 66.45724293864768129 ) ) ;
#193721=CARTESIAN_POINT ( 'NONE',  ( -16.51473224551069308, -9.474510206698971260, 31.66557627198102054 ) ) ;
#193722=CARTESIAN_POINT ( 'NONE',  ( 4.483927247898545687, 16.52544592524342804, 39.79057627198103830 ) ) ;
#193724=CARTESIAN_POINT ( 'NONE',  ( 4.379528057220092307, 16.55341960407617563, 102.2927570613523613 ) ) ;
#193725=CARTESIAN_POINT ( 'NONE',  ( 9.564922557960805705, 16.46253265017160317, 59.58224293864769550 ) ) ;
#193726=CARTESIAN_POINT ( 'NONE',  ( 0.05219959533936267826, -19.03943276465977164, 20.00109039468567218 ) ) ;
#193727=CARTESIAN_POINT ( 'NONE',  ( 4.379528057220092307, 16.55341960407617563, 27.29275706135234358 ) ) ;
#193728=CARTESIAN_POINT ( 'NONE',  ( 21.52544592524344225, -5.823673210054117533, 43.54057627198103830 ) ) ;
#193729=CARTESIAN_POINT ( 'NONE',  ( -21.53943276465977519, -0.05219959533937600094, 103.7510903946857042 ) ) ;
#193730=ORIENTED_EDGE ( 'NONE', *, *, #115114, .F. ) ;
#193731=CARTESIAN_POINT ( 'NONE',  ( -0.05219959533909027116, -19.03943276465977164, 67.49890960531436690 ) ) ;
#193732=CARTESIAN_POINT ( 'NONE',  ( 9.564922557960805705, 16.46253265017160317, 104.5822429386476955 ) ) ;
#193733=CARTESIAN_POINT ( 'NONE',  ( 19.03943276465977164, -0.05219959533909143690, 93.74890960531435269 ) ) ;
#193735=CARTESIAN_POINT ( 'NONE',  ( 15.80617190586769283, -15.72974639402175789, 30.62609039468567929 ) ) ;
#193736=CARTESIAN_POINT ( 'NONE',  ( 12.06949235617757843, -12.14591786802309237, 93.12390960531436690 ) ) ;
#193737=CARTESIAN_POINT ( 'NONE',  ( 21.52544592524344225, -5.823673210054117533, 88.54057627198103830 ) ) ;
#193738=CARTESIAN_POINT ( 'NONE',  ( -13.97604488694527625, -13.89961937509977652, 61.87390960531435979 ) ) ;
#193739=CARTESIAN_POINT ( 'NONE',  ( -9.564922557960796823, -16.46253265017161027, 67.08224293864769550 ) ) ;
#193740=CARTESIAN_POINT ( 'NONE',  ( 21.55341960407610458, 5.719274019375980345, 108.9572429386476955 ) ) ;
#193741=VERTEX_POINT ( 'NONE', #124737 ) ;
#193742=CARTESIAN_POINT ( 'NONE',  ( 13.89961937509977652, -13.97604488694527269, 68.12390960531436690 ) ) ;
#193743=CARTESIAN_POINT ( 'NONE',  ( 18.56197773271729190, -5.499999999999983125, 96.05066217314450228 ) ) ;
#193744=CARTESIAN_POINT ( 'NONE',  ( -8.224510206698948167, 14.34966873604960824, 105.4155762719810383 ) ) ;
#193746=CARTESIAN_POINT ( 'NONE',  ( -9.564922557960796823, -16.46253265017161027, 62.08224293864769550 ) ) ;
#193747=CARTESIAN_POINT ( 'NONE',  ( -9.564922557961040184, 16.46253265017147172, 92.91775706135233293 ) ) ;
#193748=CARTESIAN_POINT ( 'NONE',  ( 8.224510206698953496, -14.34966873604960469, 102.9155762719810383 ) ) ;
#193749=CARTESIAN_POINT ( 'NONE',  ( -0.05219959533937732626, 21.53943276465977519, 77.50109039468567573 ) ) ;
#193750=CARTESIAN_POINT ( 'NONE',  ( -5.153800228976328057, -19.02544592524343514, 52.29057627198100988 ) ) ;
#193751=CARTESIAN_POINT ( 'NONE',  ( -5.719274019375665041, -21.55341960407619695, 24.79275706135235779 ) ) ;
#193752=CARTESIAN_POINT ( 'NONE',  ( 15.80617190586746368, 15.72974639402197994, 114.3739096053143527 ) ) ;
#193754=CARTESIAN_POINT ( 'NONE',  ( -9.474510206698964154, 16.51473224551069663, 70.41557627198102409 ) ) ;
#193756=CARTESIAN_POINT ( 'NONE',  ( -19.05341960407617563, 5.049401038297882671, 103.5427570613523329 ) ) ;
#193757=CARTESIAN_POINT ( 'NONE',  ( 5.823673210054125526, 21.52544592524343514, 24.79057627198103120 ) ) ;
#193758=CARTESIAN_POINT ( 'NONE',  ( -5.719274019375665041, -21.55341960407619695, 64.79275706135234714 ) ) ;
#193759=CARTESIAN_POINT ( 'NONE',  ( 16.46253265017160672, -9.564922557960803928, 103.3322429386476955 ) ) ;
#193760=CARTESIAN_POINT ( 'NONE',  ( 13.97604488694548053, -13.89961937509957401, 85.62609039468568994 ) ) ;
#193761=CARTESIAN_POINT ( 'NONE',  ( -9.564922557960796823, -16.46253265017161027, 47.08224293864769550 ) ) ;
#193762=CARTESIAN_POINT ( 'NONE',  ( -9.564922557960796823, -16.46253265017161027, 67.08224293864769550 ) ) ;
#193763=CARTESIAN_POINT ( 'NONE',  ( -12.06949235617756955, 12.14591786802309770, 80.62390960531438111 ) ) ;
#193764=CARTESIAN_POINT ( 'NONE',  ( 5.049401038298161559, -19.05341960407611168, 97.70724293864766707 ) ) ;
#193765=CARTESIAN_POINT ( 'NONE',  ( 12.06949235617757843, -12.14591786802309237, 98.12390960531436690 ) ) ;
#193766=CARTESIAN_POINT ( 'NONE',  ( 9.474510206698971260, -16.51473224551069308, 102.9155762719810241 ) ) ;
#193767=CARTESIAN_POINT ( 'NONE',  ( 0.05219959533910956823, 16.53943276465976808, 44.99890960531435979 ) ) ;
#193768=CARTESIAN_POINT ( 'NONE',  ( -9.474510206698964154, 16.51473224551069663, 25.41557627198103120 ) ) ;
#193769=ORIENTED_EDGE ( 'NONE', *, *, #158649, .F. ) ;
#193770=CARTESIAN_POINT ( 'NONE',  ( 15.80617190586769283, -15.72974639402175789, 55.62609039468568284 ) ) ;
#193771=CARTESIAN_POINT ( 'NONE',  ( 0.05219959533936267826, -19.03943276465977164, 75.00109039468566152 ) ) ;
#193772=CARTESIAN_POINT ( 'NONE',  ( -12.06949235617756955, 12.14591786802309770, 55.62390960531436690 ) ) ;
#193773=CARTESIAN_POINT ( 'NONE',  ( 21.53943276465977519, -0.05219959533907433946, 98.74890960531438111 ) ) ;
#193774=CARTESIAN_POINT ( 'NONE',  ( -0.05219959533907301413, -21.53943276465977519, 27.49890960531435269 ) ) ;
#193775=CARTESIAN_POINT ( 'NONE',  ( -12.14591786802309592, -12.06949235617757132, 86.87390960531438111 ) ) ;
#193776=CARTESIAN_POINT ( 'NONE',  ( -9.474510206698964154, 16.51473224551069663, 60.41557627198102409 ) ) ;
#193777=CARTESIAN_POINT ( 'NONE',  ( -8.224510206698948167, 14.34966873604960824, 25.41557627198103120 ) ) ;
#193778=CARTESIAN_POINT ( 'NONE',  ( -16.52544592524335698, -4.483927247898792601, 103.9594237280190185 ) ) ;
#193779=CARTESIAN_POINT ( 'NONE',  ( 8.314922557961029526, -14.29746914071037800, 70.41775706135236135 ) ) ;
#193780=CARTESIAN_POINT ( 'NONE',  ( 5.153800228976615827, -19.02544592524334988, 20.20942372801899722 ) ) ;
#193781=CARTESIAN_POINT ( 'NONE',  ( -13.89961937509977652, 13.97604488694528158, 100.6239096053143669 ) ) ;
#193782=CARTESIAN_POINT ( 'NONE',  ( 19.02544592524343514, -5.153800228976328945, 78.54057627198099567 ) ) ;
#193783=CARTESIAN_POINT ( 'NONE',  ( -5.049401038298153566, 19.05341960407611168, 35.20724293864768839 ) ) ;
#193784=CARTESIAN_POINT ( 'NONE',  ( -12.14591786802309592, -12.06949235617757132, 51.87390960531437401 ) ) ;
#193786=CARTESIAN_POINT ( 'NONE',  ( -19.02544592524342804, 5.153800228976336051, 101.0405762719810241 ) ) ;
#193787=CARTESIAN_POINT ( 'NONE',  ( 10.81492255796078972, 18.62759615963270932, 44.58224293864769550 ) ) ;
#193788=CARTESIAN_POINT ( 'NONE',  ( 8.314922557960818139, 14.29746914071049879, 69.58224293864769550 ) ) ;
#193789=CARTESIAN_POINT ( 'NONE',  ( -16.53943276465976808, -0.05219959533934237506, 28.75109039468567929 ) ) ;
#193791=CARTESIAN_POINT ( 'NONE',  ( 12.14591786802309770, 12.06949235617756955, 59.37390960531436690 ) ) ;
#193793=CARTESIAN_POINT ( 'NONE',  ( 5.153800228976615827, -19.02544592524334988, 70.20942372801899012 ) ) ;
#193794=CARTESIAN_POINT ( 'NONE',  ( -5.153800228976328057, -19.02544592524343514, 107.2905762719810383 ) ) ;
#193795=CARTESIAN_POINT ( 'NONE',  ( 13.97604488694548053, -13.89961937509957401, 85.62609039468568994 ) ) ;
#193798=CARTESIAN_POINT ( 'NONE',  ( -13.97604488694547697, 13.89961937509957934, 108.1260903946856331 ) ) ;
#193799=CARTESIAN_POINT ( 'NONE',  ( 4.379528057220092307, 16.55341960407617563, 112.2927570613523471 ) ) ;
#193800=CARTESIAN_POINT ( 'NONE',  ( 9.564922557960805705, 16.46253265017160317, 39.58224293864768839 ) ) ;
#193802=CARTESIAN_POINT ( 'NONE',  ( -15.80617190586745835, -15.72974639402198527, 31.87390960531435979 ) ) ;
#193803=CARTESIAN_POINT ( 'NONE',  ( 21.52544592524334988, 5.823673210054432836, 51.45942372801901854 ) ) ;
#193805=CARTESIAN_POINT ( 'NONE',  ( -12.06949235617739369, -12.14591786802326823, 24.37609039468567573 ) ) ;
#193807=CARTESIAN_POINT ( 'NONE',  ( 9.564922557960805705, 16.46253265017160317, 69.58224293864770971 ) ) ;
#193808=FACE_OUTER_BOUND ( 'NONE', #177333, .T. ) ;
#193809=CARTESIAN_POINT ( 'NONE',  ( 12.06949235617757843, -12.14591786802309237, 83.12390960531436690 ) ) ;
#193810=CARTESIAN_POINT ( 'NONE',  ( 19.05341960407611168, 5.049401038298154454, 73.95724293864768129 ) ) ;
#193811=CARTESIAN_POINT ( 'NONE',  ( -19.05341960407611168, -5.049401038298163336, 86.45724293864769550 ) ) ;
#193812=VERTEX_POINT ( 'NONE', #31742 ) ;
#193813=CARTESIAN_POINT ( 'NONE',  ( -0.05219959533936034679, 19.03943276465977164, 87.50109039468567573 ) ) ;
#193814=CARTESIAN_POINT ( 'NONE',  ( 5.823673210054125526, 21.52544592524343514, 69.79057627198102409 ) ) ;
#193815=CARTESIAN_POINT ( 'NONE',  ( -16.46253265017160317, 9.564922557960807481, 30.83224293864769550 ) ) ;
#193816=CARTESIAN_POINT ( 'NONE',  ( 13.89961937509957401, 13.97604488694547697, 51.87609039468566863 ) ) ;
#193817=CARTESIAN_POINT ( 'NONE',  ( -9.474510206698964154, 16.51473224551069663, 50.41557627198102409 ) ) ;
#193818=CARTESIAN_POINT ( 'NONE',  ( 13.89961937509977652, -13.97604488694527269, 88.12390960531438111 ) ) ;
#193820=CARTESIAN_POINT ( 'NONE',  ( 5.823673210054125526, 21.52544592524343514, 94.79057627198105251 ) ) ;
#193821=CARTESIAN_POINT ( 'NONE',  ( 8.224510206698953496, -14.34966873604960469, 92.91557627198103830 ) ) ;
#193822=CARTESIAN_POINT ( 'NONE',  ( -13.89961937509977652, 13.97604488694528158, 85.62390960531433848 ) ) ;
#193823=CARTESIAN_POINT ( 'NONE',  ( 19.02544592524334988, 5.153800228976608722, 66.45942372801899012 ) ) ;
#193824=CARTESIAN_POINT ( 'NONE',  ( -18.62759615963270932, 10.81492255796079327, 95.83224293864770971 ) ) ;
#193825=CARTESIAN_POINT ( 'NONE',  ( -10.72451020669898014, 18.67979575497178502, 70.41557627198102409 ) ) ;
#193826=CARTESIAN_POINT ( 'NONE',  ( 16.52544592524342804, -4.483927247898539470, 33.54057627198102409 ) ) ;
#193827=CARTESIAN_POINT ( 'NONE',  ( 21.52544592524334988, 5.823673210054432836, 106.4594237280190328 ) ) ;
#193828=CARTESIAN_POINT ( 'NONE',  ( 14.34966873604972726, -8.224510206698740333, 65.83442372801900433 ) ) ;
#193829=CARTESIAN_POINT ( 'NONE',  ( -19.03943276465977164, 0.05219959533909376836, 76.24890960531435269 ) ) ;
#193830=CARTESIAN_POINT ( 'NONE',  ( -16.46253265017160317, 9.564922557960807481, 35.83224293864768839 ) ) ;
#193832=CARTESIAN_POINT ( 'NONE',  ( -18.67979575497193778, 10.72451020669871902, 33.33442372801900433 ) ) ;
#193833=CARTESIAN_POINT ( 'NONE',  ( 21.52544592524334988, 5.823673210054432836, 56.45942372801902565 ) ) ;
#193834=CARTESIAN_POINT ( 'NONE',  ( 5.049401038298161559, -19.05341960407611168, 42.70724293864767418 ) ) ;
#193835=CARTESIAN_POINT ( 'NONE',  ( 10.72451020669871369, 18.67979575497193778, 22.08442372801901143 ) ) ;
#193836=CARTESIAN_POINT ( 'NONE',  ( 5.153800228976615827, -19.02544592524334988, 70.20942372801899012 ) ) ;
#193837=CARTESIAN_POINT ( 'NONE',  ( -0.05219959533936034679, 19.03943276465977164, 77.50109039468566152 ) ) ;
#193838=CARTESIAN_POINT ( 'NONE',  ( 5.049401038298161559, -19.05341960407611168, 22.70724293864769194 ) ) ;
#193839=CARTESIAN_POINT ( 'NONE',  ( -12.14591786802326823, 12.06949235617739902, 68.12609039468567573 ) ) ;
#193840=CARTESIAN_POINT ( 'NONE',  ( -5.153800228976328057, -19.02544592524343514, 47.29057627198102409 ) ) ;
#193842=CARTESIAN_POINT ( 'NONE',  ( 9.564922557960805705, 16.46253265017160317, 104.5822429386476955 ) ) ;
#193843=CARTESIAN_POINT ( 'NONE',  ( 5.049401038298161559, -19.05341960407611168, 27.70724293864769550 ) ) ;
#193844=CARTESIAN_POINT ( 'NONE',  ( -21.55341960407610458, -5.719274019375992779, 76.45724293864769550 ) ) ;
#193845=CARTESIAN_POINT ( 'NONE',  ( -4.379528057220086978, -16.55341960407618274, 59.79275706135234714 ) ) ;
#193846=CARTESIAN_POINT ( 'NONE',  ( -18.67979575497193778, 10.72451020669871902, 108.3344237280190185 ) ) ;
#193847=CARTESIAN_POINT ( 'NONE',  ( -5.049401038298153566, 19.05341960407611168, 55.20724293864769550 ) ) ;
#193848=CARTESIAN_POINT ( 'NONE',  ( -12.14591786802309592, -12.06949235617757132, 31.87390960531435979 ) ) ;
#193849=CARTESIAN_POINT ( 'NONE',  ( 12.06949235617757843, -12.14591786802309237, 68.12390960531436690 ) ) ;
#193850=CARTESIAN_POINT ( 'NONE',  ( 5.153800228976335163, 19.02544592524342804, 74.79057627198103830 ) ) ;
#193851=CARTESIAN_POINT ( 'NONE',  ( -5.719274019375665041, -21.55341960407619695, 34.79275706135235424 ) ) ;
#193852=CARTESIAN_POINT ( 'NONE',  ( -0.05219959533909027116, -19.03943276465977164, 87.49890960531436690 ) ) ;
#193853=CARTESIAN_POINT ( 'NONE',  ( 21.53943276465977519, 0.05219959533937863772, 96.25109039468568994 ) ) ;
#193854=CARTESIAN_POINT ( 'NONE',  ( -8.224510206698735004, -14.34966873604973081, 69.58442372801900433 ) ) ;
#193855=CARTESIAN_POINT ( 'NONE',  ( 9.564922557960805705, 16.46253265017160317, 114.5822429386476955 ) ) ;
#193856=CARTESIAN_POINT ( 'NONE',  ( -5.823673210054116645, -21.52544592524344225, 92.29057627198103830 ) ) ;
#193857=CARTESIAN_POINT ( 'NONE',  ( -0.05219959533910754901, -16.53943276465976808, 52.49890960531435979 ) ) ;
#193858=CARTESIAN_POINT ( 'NONE',  ( 9.564922557960805705, 16.46253265017160317, 29.58224293864769550 ) ) ;
#193859=CARTESIAN_POINT ( 'NONE',  ( 14.29746914071037800, 8.314922557961029526, 56.66775706135235424 ) ) ;
#193860=CARTESIAN_POINT ( 'NONE',  ( 16.55341960407611168, 4.379528057220329451, 73.95724293864769550 ) ) ;
#193861=CARTESIAN_POINT ( 'NONE',  ( 13.89961937509977652, -13.97604488694527269, 108.1239096053143669 ) ) ;
#193862=CARTESIAN_POINT ( 'NONE',  ( -15.80617190586745835, -15.72974639402198527, 31.87390960531435979 ) ) ;
#193863=CARTESIAN_POINT ( 'NONE',  ( 19.03943276465977164, 0.05219959533936151252, 21.25109039468565797 ) ) ;
#193864=CARTESIAN_POINT ( 'NONE',  ( -16.52544592524342804, 4.483927247898546575, 106.0405762719810525 ) ) ;
#193865=CARTESIAN_POINT ( 'NONE',  ( -16.51473224551069308, -9.474510206698971260, 106.6655762719810383 ) ) ;
#193867=CARTESIAN_POINT ( 'NONE',  ( -0.05219959533934338120, 16.53943276465976808, 52.50109039468567573 ) ) ;
#193868=CARTESIAN_POINT ( 'NONE',  ( -19.05341960407611168, -5.049401038298163336, 56.45724293864768129 ) ) ;
#193870=CARTESIAN_POINT ( 'NONE',  ( -0.05219959533936034679, 19.03943276465977164, 47.50109039468566863 ) ) ;
#193871=CARTESIAN_POINT ( 'NONE',  ( -16.53943276465976808, -0.05219959533934237506, 93.75109039468567573 ) ) ;
#193872=CARTESIAN_POINT ( 'NONE',  ( -19.02544592524334988, -5.153800228976617603, 98.95942372801900433 ) ) ;
#193873=CARTESIAN_POINT ( 'NONE',  ( 21.52544592524334988, 5.823673210054432836, 71.45942372801901854 ) ) ;
#193874=CARTESIAN_POINT ( 'NONE',  ( 13.97604488694527802, 13.89961937509977652, 69.37390960531436690 ) ) ;
#193875=CARTESIAN_POINT ( 'NONE',  ( 15.80617190586746368, 15.72974639402197994, 94.37390960531436690 ) ) ;
#193876=CARTESIAN_POINT ( 'NONE',  ( -4.379528057220328563, 16.55341960407611168, 110.2072429386477239 ) ) ;
#193878=CARTESIAN_POINT ( 'NONE',  ( 13.89961937509957401, 13.97604488694547697, 81.87609039468564731 ) ) ;
#193879=CARTESIAN_POINT ( 'NONE',  ( -18.67979575497178146, -10.72451020669898902, 76.66557627198103830 ) ) ;
#193880=CARTESIAN_POINT ( 'NONE',  ( -13.89961937509957401, -13.97604488694547875, 39.37609039468566152 ) ) ;
#193881=FACE_BOUND ( 'NONE', #72559, .T. ) ;
#193882=CARTESIAN_POINT ( 'NONE',  ( -21.55341960407610458, -5.719274019375992779, 96.45724293864770971 ) ) ;
#193883=CARTESIAN_POINT ( 'NONE',  ( -17.40805194822029378, 6.112264579159334410, 85.83371272510608208 ) ) ;
#193884=CARTESIAN_POINT ( 'NONE',  ( 19.03943276465977164, -0.05219959533909143690, 68.74890960531436690 ) ) ;
#193886=CARTESIAN_POINT ( 'NONE',  ( 13.97604488694548053, -13.89961937509957401, 110.6260903946856615 ) ) ;
#193887=CARTESIAN_POINT ( 'NONE',  ( -5.153800228976607833, 19.02544592524335343, 97.70942372801899012 ) ) ;
#193888=CARTESIAN_POINT ( 'NONE',  ( -5.049401038298153566, 19.05341960407611168, 45.20724293864769550 ) ) ;
#193889=CARTESIAN_POINT ( 'NONE',  ( -19.05341960407611168, -5.049401038298163336, 106.4572429386476955 ) ) ;
#193890=CARTESIAN_POINT ( 'NONE',  ( -5.719274019375978568, 21.55341960407610458, 105.2072429386477097 ) ) ;
#193891=CARTESIAN_POINT ( 'NONE',  ( -8.224510206698948167, 14.34966873604960824, 45.41557627198103830 ) ) ;
#193892=CARTESIAN_POINT ( 'NONE',  ( -18.67979575497193778, 10.72451020669871902, 73.33442372801901854 ) ) ;
#193893=CARTESIAN_POINT ( 'NONE',  ( -16.55341960407617563, 4.379528057220093196, 28.54275706135234358 ) ) ;
#193894=CARTESIAN_POINT ( 'NONE',  ( -19.05341960407617563, 5.049401038297882671, 23.54275706135233648 ) ) ;
#193895=CARTESIAN_POINT ( 'NONE',  ( -4.379528057220328563, 16.55341960407611168, 30.20724293864769550 ) ) ;
#193897=CARTESIAN_POINT ( 'NONE',  ( -5.823673210054116645, -21.52544592524344225, 112.2905762719810241 ) ) ;
#193898=CARTESIAN_POINT ( 'NONE',  ( 8.314922557960818139, 14.29746914071049879, 54.58224293864769550 ) ) ;
#193899=CARTESIAN_POINT ( 'NONE',  ( -13.89961937509957401, -13.97604488694547875, 94.37609039468566152 ) ) ;
#193900=CARTESIAN_POINT ( 'NONE',  ( 5.049401038297881783, 19.05341960407617563, 72.29275706135234714 ) ) ;
#193901=CARTESIAN_POINT ( 'NONE',  ( -10.81492255796105439, 18.62759615963255655, 72.91775706135234714 ) ) ;
#193902=CARTESIAN_POINT ( 'NONE',  ( -19.03943276465977164, -0.05219959533935918106, 48.75109039468566863 ) ) ;
#193903=CARTESIAN_POINT ( 'NONE',  ( 14.34966873604960469, 8.224510206698951720, 114.1655762719810383 ) ) ;
#193904=CARTESIAN_POINT ( 'NONE',  ( -18.62759615963270932, 10.81492255796079327, 40.83224293864769550 ) ) ;
#193905=CARTESIAN_POINT ( 'NONE',  ( 8.224510206698953496, -14.34966873604960469, 47.91557627198102409 ) ) ;
#193907=CARTESIAN_POINT ( 'NONE',  ( -5.823673210054431948, 21.52544592524334988, 107.7094237280190328 ) ) ;
#193908=CARTESIAN_POINT ( 'NONE',  ( 0.05219959533934541429, -16.53943276465976808, 80.00109039468568994 ) ) ;
#193909=CARTESIAN_POINT ( 'NONE',  ( -0.05219959533910754901, -16.53943276465976808, 37.49890960531436690 ) ) ;
#193910=CARTESIAN_POINT ( 'NONE',  ( -10.72451020669870658, -18.67979575497194134, 79.58442372801903275 ) ) ;
#193911=CARTESIAN_POINT ( 'NONE',  ( -0.05219959533937732626, 21.53943276465977519, 87.50109039468568994 ) ) ;
#193912=CARTESIAN_POINT ( 'NONE',  ( 5.719274019375991003, -21.55341960407610458, 87.70724293864769550 ) ) ;
#193913=EDGE_CURVE ( 'NONE', #192686, #115197, #108571, .T. ) ;
#193914=CARTESIAN_POINT ( 'NONE',  ( -13.97604488694527625, -13.89961937509977652, 41.87390960531435979 ) ) ;
#193915=CARTESIAN_POINT ( 'NONE',  ( 10.72451020669871369, 18.67979575497193778, 57.08442372801901854 ) ) ;
#193916=CARTESIAN_POINT ( 'NONE',  ( -16.46253265017160317, 9.564922557960807481, 40.83224293864769550 ) ) ;
#193917=CARTESIAN_POINT ( 'NONE',  ( -19.05341960407611168, -5.049401038298163336, 51.45724293864770260 ) ) ;
#193918=CARTESIAN_POINT ( 'NONE',  ( 14.29746914071049879, -8.314922557960816363, 98.33224293864769550 ) ) ;
#193919=CARTESIAN_POINT ( 'NONE',  ( 13.97604488694527802, 13.89961937509977652, 94.37390960531436690 ) ) ;
#193920=CARTESIAN_POINT ( 'NONE',  ( -14.29746914071049879, 8.314922557960819915, 35.83224293864768839 ) ) ;
#193921=CARTESIAN_POINT ( 'NONE',  ( -16.52544592524342804, 4.483927247898546575, 111.0405762719810525 ) ) ;
#193922=CARTESIAN_POINT ( 'NONE',  ( 15.80617190586746368, 15.72974639402197994, 89.37390960531435269 ) ) ;
#193923=CARTESIAN_POINT ( 'NONE',  ( 5.823673210054444382, -21.52544592524334988, 25.20942372801901854 ) ) ;
#193925=CARTESIAN_POINT ( 'NONE',  ( 16.46253265017160672, -9.564922557960803928, 83.33224293864768129 ) ) ;
#193926=CARTESIAN_POINT ( 'NONE',  ( -16.52544592524335698, -4.483927247898792601, 18.95942372801901143 ) ) ;
#193927=CARTESIAN_POINT ( 'NONE',  ( -15.72974639402197994, 15.80617190586746368, 75.62390960531439532 ) ) ;
#193928=CARTESIAN_POINT ( 'NONE',  ( 0.05219959533937995610, -21.53943276465977519, 95.00109039468568994 ) ) ;
#193929=CARTESIAN_POINT ( 'NONE',  ( -19.03943276465977164, 0.05219959533909376836, 81.24890960531436690 ) ) ;
#193930=CARTESIAN_POINT ( 'NONE',  ( 15.72974639402176855, 15.80617190586768217, 31.87609039468567929 ) ) ;
#193931=CARTESIAN_POINT ( 'NONE',  ( -13.89961937509977652, 13.97604488694528158, 115.6239096053143669 ) ) ;
#193932=CARTESIAN_POINT ( 'NONE',  ( 8.224510206698742110, 14.34966873604972548, 92.08442372801901854 ) ) ;
#193933=CARTESIAN_POINT ( 'NONE',  ( 21.55341960407619695, -5.719274019375665929, 71.04275706135234714 ) ) ;
#193934=CARTESIAN_POINT ( 'NONE',  ( 5.719274019375673035, 21.55341960407619339, 102.2927570613523613 ) ) ;
#193935=CARTESIAN_POINT ( 'NONE',  ( -16.55341960407617563, 4.379528057220093196, 78.54275706135236135 ) ) ;
#193936=CARTESIAN_POINT ( 'NONE',  ( -5.719274019375665041, -21.55341960407619695, 29.79275706135234358 ) ) ;
#193937=CARTESIAN_POINT ( 'NONE',  ( -9.474510206698964154, 16.51473224551069663, 115.4155762719810241 ) ) ;
#193938=CARTESIAN_POINT ( 'NONE',  ( -15.72974639402176322, -15.80617190586768395, 94.37609039468568994 ) ) ;
#193939=CARTESIAN_POINT ( 'NONE',  ( -5.153800228976328057, -19.02544592524343514, 87.29057627198103830 ) ) ;
#193940=CARTESIAN_POINT ( 'NONE',  ( 21.55341960407610458, 5.719274019375980345, 88.95724293864769550 ) ) ;
#193941=CARTESIAN_POINT ( 'NONE',  ( -19.03943276465977164, -0.05219959533935918106, 63.75109039468566863 ) ) ;
#193943=CARTESIAN_POINT ( 'NONE',  ( -5.719274019375978568, 21.55341960407610458, 50.20724293864769550 ) ) ;
#193944=CARTESIAN_POINT ( 'NONE',  ( -19.03943276465977164, 0.05219959533909376836, 96.24890960531436690 ) ) ;
#193945=CARTESIAN_POINT ( 'NONE',  ( -12.06949235617756955, 12.14591786802309770, 50.62390960531435979 ) ) ;
#193947=CARTESIAN_POINT ( 'NONE',  ( 0.05219959533936267826, -19.03943276465977164, 75.00109039468566152 ) ) ;
#193949=CARTESIAN_POINT ( 'NONE',  ( -12.06949235617739369, -12.14591786802326823, 19.37609039468568639 ) ) ;
#193950=CARTESIAN_POINT ( 'NONE',  ( 18.67979575497178502, 10.72451020669898547, 84.16557627198103830 ) ) ;
#193951=CARTESIAN_POINT ( 'NONE',  ( -16.52544592524342804, 4.483927247898546575, 66.04057627198103830 ) ) ;
#193952=CARTESIAN_POINT ( 'NONE',  ( -16.46253265017160317, 9.564922557960807481, 95.83224293864769550 ) ) ;
#193953=CARTESIAN_POINT ( 'NONE',  ( -14.29746914071037622, -8.314922557961029526, 49.16775706135234003 ) ) ;
#193954=CARTESIAN_POINT ( 'NONE',  ( 19.03943276465977164, -0.05219959533909143690, 58.74890960531435979 ) ) ;
#193955=CARTESIAN_POINT ( 'NONE',  ( 5.719274019375673035, 21.55341960407619339, 22.29275706135235069 ) ) ;
#193956=CARTESIAN_POINT ( 'NONE',  ( 0.05219959533936267826, -19.03943276465977164, 90.00109039468567573 ) ) ;
#193957=CARTESIAN_POINT ( 'NONE',  ( 0.05219959533909260263, 19.03943276465977164, 94.99890960531436690 ) ) ;
#193958=CARTESIAN_POINT ( 'NONE',  ( -5.153800228976328057, -19.02544592524343514, 72.29057627198102409 ) ) ;
#193959=CARTESIAN_POINT ( 'NONE',  ( -10.81492255796078084, -18.62759615963271287, 77.08224293864769550 ) ) ;
#193960=CARTESIAN_POINT ( 'NONE',  ( 9.564922557960805705, 16.46253265017160317, 39.58224293864768839 ) ) ;
#193962=CARTESIAN_POINT ( 'NONE',  ( 16.55341960407611168, 4.379528057220329451, 58.95724293864770971 ) ) ;
#193963=CARTESIAN_POINT ( 'NONE',  ( 9.474510206698971260, -16.51473224551069308, 107.9155762719810383 ) ) ;
#193965=CARTESIAN_POINT ( 'NONE',  ( 0.05219959533936267826, -19.03943276465977164, 65.00109039468567573 ) ) ;
#193966=CARTESIAN_POINT ( 'NONE',  ( 15.80617190586746368, 15.72974639402197994, 94.37390960531436690 ) ) ;
#193967=CARTESIAN_POINT ( 'NONE',  ( 0.05219959533936267826, -19.03943276465977164, 50.00109039468566863 ) ) ;
#193968=CARTESIAN_POINT ( 'NONE',  ( -19.05341960407611168, -5.049401038298163336, 101.4572429386476955 ) ) ;
#193970=CARTESIAN_POINT ( 'NONE',  ( -21.55341960407610458, -5.719274019375992779, 41.45724293864769550 ) ) ;
#193972=CARTESIAN_POINT ( 'NONE',  ( 16.51473224551069308, 9.474510206698969483, 69.16557627198102409 ) ) ;
#193973=CARTESIAN_POINT ( 'NONE',  ( 5.823673210054444382, -21.52544592524334988, 65.20942372801901854 ) ) ;
#193974=CARTESIAN_POINT ( 'NONE',  ( -13.89961937509977652, 13.97604488694528158, 35.62390960531435269 ) ) ;
#193975=CARTESIAN_POINT ( 'NONE',  ( -16.55341960407611168, -4.379528057220339221, 71.45724293864769550 ) ) ;
#193977=CARTESIAN_POINT ( 'NONE',  ( -16.53943276465976808, -0.05219959533934237506, 23.75109039468567929 ) ) ;
#193978=CARTESIAN_POINT ( 'NONE',  ( 21.52544592524334988, 5.823673210054432836, 56.45942372801902565 ) ) ;
#193980=CARTESIAN_POINT ( 'NONE',  ( 9.564922557960805705, 16.46253265017160317, 114.5822429386476955 ) ) ;
#193981=CARTESIAN_POINT ( 'NONE',  ( 5.153800228976615827, -19.02544592524334988, 65.20942372801900433 ) ) ;
#193983=CARTESIAN_POINT ( 'NONE',  ( -5.823673210054431948, 21.52544592524334988, 27.70942372801901854 ) ) ;
#193984=CARTESIAN_POINT ( 'NONE',  ( 16.46253265017160672, -9.564922557960803928, 58.33224293864769550 ) ) ;
#193985=CARTESIAN_POINT ( 'NONE',  ( 8.224510206698742110, 14.34966873604972548, 37.08442372801901143 ) ) ;
#193987=CARTESIAN_POINT ( 'NONE',  ( -5.823673210054431948, 21.52544592524334988, 112.7094237280190328 ) ) ;
#193988=CARTESIAN_POINT ( 'NONE',  ( -13.97604488694527625, -13.89961937509977652, 46.87390960531435979 ) ) ;
#193989=CARTESIAN_POINT ( 'NONE',  ( -5.049401038297874678, -19.05341960407617918, 19.79275706135233293 ) ) ;
#193990=CARTESIAN_POINT ( 'NONE',  ( 16.55341960407618274, -4.379528057220086978, 86.04275706135236135 ) ) ;
#193991=CARTESIAN_POINT ( 'NONE',  ( 19.05341960407611168, 5.049401038298154454, 98.95724293864766707 ) ) ;
#193992=CARTESIAN_POINT ( 'NONE',  ( -18.67979575497193778, 10.72451020669871902, 68.33442372801900433 ) ) ;
#193994=CARTESIAN_POINT ( 'NONE',  ( -5.049401038298153566, 19.05341960407611168, 110.2072429386476671 ) ) ;
#193995=CARTESIAN_POINT ( 'NONE',  ( -17.49999999999999645, 5.499999999999997335, 30.79690382534172599 ) ) ;
#193996=CARTESIAN_POINT ( 'NONE',  ( -12.06949235617739369, -12.14591786802326823, 59.37609039468568284 ) ) ;
#193997=CARTESIAN_POINT ( 'NONE',  ( -5.823673210054431948, 21.52544592524334988, 67.70942372801901854 ) ) ;
#193998=CARTESIAN_POINT ( 'NONE',  ( -21.55341960407619339, 5.719274019375674811, 98.54275706135234714 ) ) ;
#194000=CARTESIAN_POINT ( 'NONE',  ( 12.06949235617739724, 12.14591786802326823, 31.87609039468567929 ) ) ;
#194001=CARTESIAN_POINT ( 'NONE',  ( 5.049401038298161559, -19.05341960407611168, 82.70724293864770971 ) ) ;
#194002=CARTESIAN_POINT ( 'NONE',  ( 13.89961937509977652, -13.97604488694527269, 108.1239096053143669 ) ) ;
#194003=VERTEX_POINT ( 'NONE', #167285 ) ;
#194004=CARTESIAN_POINT ( 'NONE',  ( 17.40861289039002813, 6.110651285853277770, 43.87232470827434128 ) ) ;
#194005=CARTESIAN_POINT ( 'NONE',  ( -13.97604488694527625, -13.89961937509977652, 41.87390960531435979 ) ) ;
#194006=CARTESIAN_POINT ( 'NONE',  ( -5.823673210054116645, -21.52544592524344225, 47.29057627198103120 ) ) ;
#194007=CARTESIAN_POINT ( 'NONE',  ( -8.314922557961024197, 14.29746914071037800, 107.9177570613523471 ) ) ;
#194008=CARTESIAN_POINT ( 'NONE',  ( -12.14591786802309592, -12.06949235617757132, 81.87390960531435269 ) ) ;
#194009=CARTESIAN_POINT ( 'NONE',  ( -19.05341960407611168, -5.049401038298163336, 71.45724293864766707 ) ) ;
#194010=CARTESIAN_POINT ( 'NONE',  ( -5.719274019375665041, -21.55341960407619695, 99.79275706135234714 ) ) ;
#194011=CARTESIAN_POINT ( 'NONE',  ( 0.05219959533934541429, -16.53943276465976808, 20.00109039468568639 ) ) ;
#194012=CARTESIAN_POINT ( 'NONE',  ( 16.53943276465976808, -0.05219959533910856209, 83.74890960531435269 ) ) ;
#194013=CARTESIAN_POINT ( 'NONE',  ( 15.72974639402176855, 15.80617190586768217, 41.87609039468568284 ) ) ;
#194014=CARTESIAN_POINT ( 'NONE',  ( -21.55341960407610458, -5.719274019375992779, 76.45724293864769550 ) ) ;
#194015=CARTESIAN_POINT ( 'NONE',  ( -9.564922557961040184, 16.46253265017147172, 57.91775706135233293 ) ) ;
#194017=CARTESIAN_POINT ( 'NONE',  ( 19.05341960407611168, 5.049401038298154454, 98.95724293864766707 ) ) ;
#194018=CARTESIAN_POINT ( 'NONE',  ( -4.483927247898539470, -16.52544592524342804, 67.29057627198103830 ) ) ;
#194019=CARTESIAN_POINT ( 'NONE',  ( -12.14591786802309592, -12.06949235617757132, 51.87390960531437401 ) ) ;
#194020=CARTESIAN_POINT ( 'NONE',  ( 16.53943276465976808, -0.05219959533910856209, 23.74890960531435269 ) ) ;
#194021=CARTESIAN_POINT ( 'NONE',  ( 0.05219959533936267826, -19.03943276465977164, 70.00109039468566152 ) ) ;
#194023=CARTESIAN_POINT ( 'NONE',  ( 9.474510206698971260, -16.51473224551069308, 112.9155762719810383 ) ) ;
#194024=CARTESIAN_POINT ( 'NONE',  ( -16.52544592524342804, 4.483927247898546575, 86.04057627198102409 ) ) ;
#194026=CARTESIAN_POINT ( 'NONE',  ( -16.51473224551069308, -9.474510206698971260, 41.66557627198103120 ) ) ;
#194027=CARTESIAN_POINT ( 'NONE',  ( -10.72451020669898014, 18.67979575497178502, 55.41557627198102409 ) ) ;
#194028=CARTESIAN_POINT ( 'NONE',  ( -18.62759615963270932, 10.81492255796079327, 80.83224293864769550 ) ) ;
#194029=CARTESIAN_POINT ( 'NONE',  ( 9.564922557960805705, 16.46253265017160317, 24.58224293864769194 ) ) ;
#194030=CARTESIAN_POINT ( 'NONE',  ( 8.224510206698742110, 14.34966873604972548, 62.08442372801901143 ) ) ;
#194031=CARTESIAN_POINT ( 'NONE',  ( -16.51473224551069308, -9.474510206698971260, 56.66557627198103120 ) ) ;
#194032=CARTESIAN_POINT ( 'NONE',  ( 5.049401038297881783, 19.05341960407617563, 42.29275706135234003 ) ) ;
#194033=CARTESIAN_POINT ( 'NONE',  ( -15.72974639402176322, -15.80617190586768395, 49.37609039468569705 ) ) ;
#194034=CARTESIAN_POINT ( 'NONE',  ( -10.81492255796078084, -18.62759615963271287, 42.08224293864769550 ) ) ;
#194035=CARTESIAN_POINT ( 'NONE',  ( 14.34966873604960469, 8.224510206698951720, 109.1655762719810383 ) ) ;
#194036=CARTESIAN_POINT ( 'NONE',  ( -9.564922557961040184, 16.46253265017147172, 87.91775706135233293 ) ) ;
#194039=CARTESIAN_POINT ( 'NONE',  ( -10.72451020669898014, 18.67979575497178502, 45.41557627198103830 ) ) ;
#194040=CARTESIAN_POINT ( 'NONE',  ( 17.13100169013300800, -6.664070546373151771, 68.26789835699850073 ) ) ;
#194041=CARTESIAN_POINT ( 'NONE',  ( 10.72451020669871369, 18.67979575497193778, 87.08442372801901854 ) ) ;
#194042=CARTESIAN_POINT ( 'NONE',  ( 12.14591786802309770, 12.06949235617756955, 29.37390960531435269 ) ) ;
#194043=CARTESIAN_POINT ( 'NONE',  ( 0.05219959533934541429, -16.53943276465976808, 55.00109039468568284 ) ) ;
#194044=CARTESIAN_POINT ( 'NONE',  ( -8.314922557960811034, -14.29746914071050412, 62.08224293864769550 ) ) ;
#194045=CARTESIAN_POINT ( 'NONE',  ( 10.72451020669898902, -18.67979575497178502, 77.91557627198102409 ) ) ;
#194046=CARTESIAN_POINT ( 'NONE',  ( -5.719274019375978568, 21.55341960407610458, 70.20724293864769550 ) ) ;
#194048=CARTESIAN_POINT ( 'NONE',  ( -5.049401038297874678, -19.05341960407617918, 79.79275706135233293 ) ) ;
#194049=CARTESIAN_POINT ( 'NONE',  ( -10.72451020669898014, 18.67979575497178502, 25.41557627198103120 ) ) ;
#194051=CARTESIAN_POINT ( 'NONE',  ( -19.03943276465977164, 0.05219959533909376836, 66.24890960531436690 ) ) ;
#194052=CARTESIAN_POINT ( 'NONE',  ( 13.89961937509977652, -13.97604488694527269, 28.12390960531435624 ) ) ;
#194056=CARTESIAN_POINT ( 'NONE',  ( -14.34966873604972548, 8.224510206698743886, 88.33442372801901854 ) ) ;
#194057=CARTESIAN_POINT ( 'NONE',  ( -5.823673210054431948, 21.52544592524334988, 22.70942372801901499 ) ) ;
#194058=CARTESIAN_POINT ( 'NONE',  ( 0.05219959533909260263, 19.03943276465977164, 74.99890960531435269 ) ) ;
#194059=CARTESIAN_POINT ( 'NONE',  ( -10.81492255796105439, 18.62759615963255655, 57.91775706135234714 ) ) ;
#194060=CARTESIAN_POINT ( 'NONE',  ( -16.46253265017160317, 9.564922557960807481, 90.83224293864769550 ) ) ;
#194062=VERTEX_POINT ( 'NONE', #107565 ) ;
#194063=CARTESIAN_POINT ( 'NONE',  ( -15.72974639402176322, -15.80617190586768395, 49.37609039468569705 ) ) ;
#194064=CARTESIAN_POINT ( 'NONE',  ( -5.049401038298153566, 19.05341960407611168, 30.20724293864768839 ) ) ;
#194065=CARTESIAN_POINT ( 'NONE',  ( 5.153800228976335163, 19.02544592524342804, 99.79057627198102409 ) ) ;
#194066=CARTESIAN_POINT ( 'NONE',  ( -19.02544592524334988, -5.153800228976617603, 53.95942372801898301 ) ) ;
#194067=CARTESIAN_POINT ( 'NONE',  ( 0.05219959533937995610, -21.53943276465977519, 20.00109039468568639 ) ) ;
#194068=CARTESIAN_POINT ( 'NONE',  ( 5.049401038297881783, 19.05341960407617563, 47.29275706135231161 ) ) ;
#194069=CARTESIAN_POINT ( 'NONE',  ( -16.51473224551082808, 9.474510206698731452, 48.33442372801900433 ) ) ;
#194070=CARTESIAN_POINT ( 'NONE',  ( -0.05219959533934338120, 16.53943276465976808, 107.5010903946856899 ) ) ;
#194071=VERTEX_POINT ( 'NONE', #138905 ) ;
#194073=CARTESIAN_POINT ( 'NONE',  ( -5.153800228976328057, -19.02544592524343514, 72.29057627198102409 ) ) ;
#194074=CARTESIAN_POINT ( 'NONE',  ( 5.719274019375673035, 21.55341960407619339, 77.29275706135234714 ) ) ;
#194075=CARTESIAN_POINT ( 'NONE',  ( -15.72974639402176322, -15.80617190586768395, 99.37609039468568994 ) ) ;
#194077=CARTESIAN_POINT ( 'NONE',  ( -13.97604488694527625, -13.89961937509977652, 81.87390960531436690 ) ) ;
#194078=CARTESIAN_POINT ( 'NONE',  ( -18.67979575497193778, 10.72451020669871902, 73.33442372801901854 ) ) ;
#194079=CARTESIAN_POINT ( 'NONE',  ( 9.474510206698729675, 16.51473224551082808, 112.0844237280190043 ) ) ;
#194080=CARTESIAN_POINT ( 'NONE',  ( 9.564922557960805705, 16.46253265017160317, 64.58224293864769550 ) ) ;
#194081=CARTESIAN_POINT ( 'NONE',  ( -9.474510206698964154, 16.51473224551069663, 110.4155762719810383 ) ) ;
#194082=CARTESIAN_POINT ( 'NONE',  ( -5.153800228976328057, -19.02544592524343514, 92.29057627198099567 ) ) ;
#194083=CARTESIAN_POINT ( 'NONE',  ( 18.22780087662122739, 5.500000000000000888, 86.48236817873107896 ) ) ;
#194084=CARTESIAN_POINT ( 'NONE',  ( 13.89961937509977652, -13.97604488694527269, 78.12390960531433848 ) ) ;
#194085=CARTESIAN_POINT ( 'NONE',  ( 0.05219959533909260263, 19.03943276465977164, 59.99890960531436690 ) ) ;
#194086=CARTESIAN_POINT ( 'NONE',  ( -21.55341960407610458, -5.719274019375992779, 106.4572429386477097 ) ) ;
#194087=CARTESIAN_POINT ( 'NONE',  ( 12.06949235617739724, 12.14591786802326823, 101.8760903946857042 ) ) ;
#194089=CARTESIAN_POINT ( 'NONE',  ( 9.564922557961047289, -16.46253265017146816, 55.41775706135234003 ) ) ;
#194090=CARTESIAN_POINT ( 'NONE',  ( 9.474510206698971260, -16.51473224551069308, 92.91557627198103830 ) ) ;
#194091=CARTESIAN_POINT ( 'NONE',  ( 14.34966873604960469, 8.224510206698951720, 84.16557627198103830 ) ) ;
#194092=CARTESIAN_POINT ( 'NONE',  ( 16.46253265017160672, -9.564922557960803928, 28.33224293864769550 ) ) ;
#194093=CARTESIAN_POINT ( 'NONE',  ( -0.05219959533907301413, -21.53943276465977519, 27.49890960531435269 ) ) ;
#194094=CARTESIAN_POINT ( 'NONE',  ( -5.823673210054116645, -21.52544592524344225, 27.29057627198103120 ) ) ;
#194095=CARTESIAN_POINT ( 'NONE',  ( 12.14591786802309770, 12.06949235617756955, 94.37390960531436690 ) ) ;
#194097=CARTESIAN_POINT ( 'NONE',  ( -5.153800228976607833, 19.02544592524334988, 47.70942372801900433 ) ) ;
#194098=CARTESIAN_POINT ( 'NONE',  ( 12.06949235617739724, 12.14591786802326823, 101.8760903946857042 ) ) ;
#194099=CARTESIAN_POINT ( 'NONE',  ( -9.564922557960796823, -16.46253265017161027, 82.08224293864768129 ) ) ;
#194100=CARTESIAN_POINT ( 'NONE',  ( 18.67979575497194134, -10.72451020669871369, 65.83442372801900433 ) ) ;
#194101=CARTESIAN_POINT ( 'NONE',  ( -10.72451020669898014, 18.67979575497178502, 45.41557627198103830 ) ) ;
#194102=CARTESIAN_POINT ( 'NONE',  ( -18.67979575497193778, 10.72451020669871902, 33.33442372801900433 ) ) ;
#194103=CARTESIAN_POINT ( 'NONE',  ( -10.81492255796078084, -18.62759615963271287, 87.08224293864769550 ) ) ;
#194104=CARTESIAN_POINT ( 'NONE',  ( 14.29746914071049879, -8.314922557960816363, 113.3322429386476955 ) ) ;
#194105=CARTESIAN_POINT ( 'NONE',  ( 5.153800228976615827, -19.02544592524334988, 75.20942372801896170 ) ) ;
#194106=CARTESIAN_POINT ( 'NONE',  ( -19.02544592524342804, 5.153800228976336051, 41.04057627198103120 ) ) ;
#194107=CARTESIAN_POINT ( 'NONE',  ( -5.153800228976328057, -19.02544592524343514, 102.2905762719810383 ) ) ;
#194108=CARTESIAN_POINT ( 'NONE',  ( 19.03943276465977164, -0.05219959533909143690, 93.74890960531435269 ) ) ;
#194109=CARTESIAN_POINT ( 'NONE',  ( -8.314922557960811034, -14.29746914071050412, 112.0822429386477097 ) ) ;
#194110=CARTESIAN_POINT ( 'NONE',  ( -16.52544592524342804, 4.483927247898546575, 41.04057627198103120 ) ) ;
#194111=CARTESIAN_POINT ( 'NONE',  ( -16.55341960407617563, 4.379528057220093196, 43.54275706135235424 ) ) ;
#194112=CARTESIAN_POINT ( 'NONE',  ( 15.72974639402176855, 15.80617190586768217, 111.8760903946856615 ) ) ;
#194113=CARTESIAN_POINT ( 'NONE',  ( -16.53943276465976808, -0.05219959533934237506, 113.7510903946856757 ) ) ;
#194114=CARTESIAN_POINT ( 'NONE',  ( 5.719274019375673035, 21.55341960407619339, 37.29275706135235424 ) ) ;
#194115=CARTESIAN_POINT ( 'NONE',  ( -0.05219959533909027116, -19.03943276465977164, 102.4989096053143669 ) ) ;
#194116=EDGE_CURVE ( 'NONE', #163522, #134048, #93390, .T. ) ;
#194117=CARTESIAN_POINT ( 'NONE',  ( -8.314922557961024197, 14.29746914071037800, 107.9177570613523471 ) ) ;
#194118=CARTESIAN_POINT ( 'NONE',  ( -16.52544592524335698, -4.483927247898792601, 93.95942372801903275 ) ) ;
#194119=CARTESIAN_POINT ( 'NONE',  ( -4.379528057220086978, -16.55341960407618274, 24.79275706135235779 ) ) ;
#194120=CARTESIAN_POINT ( 'NONE',  ( 13.97604488694527802, 13.89961937509977652, 49.37390960531434558 ) ) ;
#194121=CARTESIAN_POINT ( 'NONE',  ( 4.379528057220339221, -16.55341960407611168, 102.7072429386476955 ) ) ;
#194122=CARTESIAN_POINT ( 'NONE',  ( 15.80617190586769283, -15.72974639402175789, 20.62609039468568639 ) ) ;
#194123=CARTESIAN_POINT ( 'NONE',  ( -19.05341960407611168, -5.049401038298163336, 26.45724293864769550 ) ) ;
#194124=CARTESIAN_POINT ( 'NONE',  ( 19.02544592524343514, -5.153800228976328945, 108.5405762719810383 ) ) ;
#194125=CARTESIAN_POINT ( 'NONE',  ( -18.62759615963255300, -10.81492255796106328, 29.16775706135234003 ) ) ;
#194126=CARTESIAN_POINT ( 'NONE',  ( 19.02544592524343514, -5.153800228976328945, 28.54057627198102409 ) ) ;
#194127=CARTESIAN_POINT ( 'NONE',  ( 13.97604488694527802, 13.89961937509977652, 104.3739096053143385 ) ) ;
#194128=CARTESIAN_POINT ( 'NONE',  ( -16.52216118717209170, -7.221426719304468556, 36.07599021046992505 ) ) ;
#194129=CARTESIAN_POINT ( 'NONE',  ( -13.89961937509977652, 13.97604488694528158, 95.62390960531436690 ) ) ;
#194130=CARTESIAN_POINT ( 'NONE',  ( 0.05219959533937995610, -21.53943276465977519, 50.00109039468568994 ) ) ;
#194131=CARTESIAN_POINT ( 'NONE',  ( -12.14591786802309592, -12.06949235617757132, 86.87390960531438111 ) ) ;
#194132=CARTESIAN_POINT ( 'NONE',  ( 9.474510206698971260, -16.51473224551069308, 97.91557627198102409 ) ) ;
#194134=CARTESIAN_POINT ( 'NONE',  ( 8.314922557961029526, -14.29746914071037800, 70.41775706135236135 ) ) ;
#194135=CARTESIAN_POINT ( 'NONE',  ( -5.823673210054431948, 21.52544592524334988, 77.70942372801900433 ) ) ;
#194136=CARTESIAN_POINT ( 'NONE',  ( 4.483927247898790824, -16.52544592524335698, 35.20942372801901854 ) ) ;
#194137=CARTESIAN_POINT ( 'NONE',  ( -9.474510206698964154, 16.51473224551069663, 85.41557627198102409 ) ) ;
#194138=CARTESIAN_POINT ( 'NONE',  ( 16.51473224551083163, -9.474510206698727899, 105.8344237280190043 ) ) ;
#194139=CARTESIAN_POINT ( 'NONE',  ( -16.52544592524335698, -4.483927247898792601, 73.95942372801901854 ) ) ;
#194140=CARTESIAN_POINT ( 'NONE',  ( -16.51473224551082808, 9.474510206698731452, 93.33442372801900433 ) ) ;
#194141=CARTESIAN_POINT ( 'NONE',  ( 19.03943276465977164, -0.05219959533909143690, 63.74890960531435979 ) ) ;
#194142=CARTESIAN_POINT ( 'NONE',  ( -10.72451020669898014, 18.67979575497178502, 90.41557627198103830 ) ) ;
#194143=CARTESIAN_POINT ( 'NONE',  ( -16.55341960407611168, -4.379528057220339221, 91.45724293864769550 ) ) ;
#194144=CARTESIAN_POINT ( 'NONE',  ( 16.46253265017146816, 9.564922557961045513, 86.66775706135233293 ) ) ;
#194145=CARTESIAN_POINT ( 'NONE',  ( -16.55341960407617563, 4.379528057220093196, 53.54275706135234714 ) ) ;
#194146=CARTESIAN_POINT ( 'NONE',  ( 17.26172910966780805, -6.454744622555771194, 63.30646908649223548 ) ) ;
#194147=CARTESIAN_POINT ( 'NONE',  ( -13.89961937509957401, -13.97604488694547875, 54.37609039468565442 ) ) ;
#194148=CARTESIAN_POINT ( 'NONE',  ( 16.55341960407611168, 4.379528057220329451, 38.95724293864768839 ) ) ;
#194149=CARTESIAN_POINT ( 'NONE',  ( 8.314922557960818139, 14.29746914071049879, 84.58224293864769550 ) ) ;
#194150=CARTESIAN_POINT ( 'NONE',  ( 19.05341960407617918, -5.049401038297876454, 21.04275706135232582 ) ) ;
#194151=CARTESIAN_POINT ( 'NONE',  ( -19.36337904590694237, 5.499999999999952927, 90.41494137495621430 ) ) ;
#194152=CARTESIAN_POINT ( 'NONE',  ( 21.53943276465977519, 0.05219959533937863772, 26.25109039468567573 ) ) ;
#194153=SPHERICAL_SURFACE ( 'NONE', #124733, 2.000000000000000000 ) ;
#194154=CARTESIAN_POINT ( 'NONE',  ( 9.474510206698971260, -16.51473224551069308, 72.91557627198102409 ) ) ;
#194155=CARTESIAN_POINT ( 'NONE',  ( 18.62759615963255655, 10.81492255796105972, 91.66775706135234714 ) ) ;
#194156=CARTESIAN_POINT ( 'NONE',  ( 19.05341960407611168, 5.049401038298154454, 73.95724293864768129 ) ) ;
#194157=CARTESIAN_POINT ( 'NONE',  ( -21.55341960407610458, -5.719274019375992779, 46.45724293864769550 ) ) ;
#194158=CARTESIAN_POINT ( 'NONE',  ( -16.52544592524342804, 4.483927247898546575, 76.04057627198102409 ) ) ;
#194159=CARTESIAN_POINT ( 'NONE',  ( -13.97604488694527625, -13.89961937509977652, 61.87390960531435979 ) ) ;
#194160=CARTESIAN_POINT ( 'NONE',  ( 14.29746914071049879, -8.314922557960816363, 113.3322429386476955 ) ) ;
#194161=CARTESIAN_POINT ( 'NONE',  ( 5.823673210054444382, -21.52544592524334988, 25.20942372801901854 ) ) ;
#194162=CARTESIAN_POINT ( 'NONE',  ( -0.05219959533937732626, 21.53943276465977519, 62.50109039468568284 ) ) ;
#194163=CARTESIAN_POINT ( 'NONE',  ( -19.03943276465977164, 0.05219959533909376836, 46.24890960531435979 ) ) ;
#194164=CARTESIAN_POINT ( 'NONE',  ( 8.224510206698742110, 14.34966873604972548, 67.08442372801901854 ) ) ;
#194165=CARTESIAN_POINT ( 'NONE',  ( -10.72451020669898014, 18.67979575497178502, 115.4155762719810241 ) ) ;
#194166=CARTESIAN_POINT ( 'NONE',  ( 18.62759615963271287, -10.81492255796078972, 108.3322429386477097 ) ) ;
#194167=CARTESIAN_POINT ( 'NONE',  ( 19.05341960407617918, -5.049401038297876454, 46.04275706135233293 ) ) ;
#194168=CARTESIAN_POINT ( 'NONE',  ( 16.46253265017160672, -9.564922557960803928, 68.33224293864770971 ) ) ;
#194169=CARTESIAN_POINT ( 'NONE',  ( -17.49999999999998934, -5.500000000000015987, 56.28230962303566542 ) ) ;
#194170=CARTESIAN_POINT ( 'NONE',  ( -10.72451020669870658, -18.67979575497194134, 64.58442372801900433 ) ) ;
#194171=CARTESIAN_POINT ( 'NONE',  ( 15.72974639402199770, -15.80617190586745480, 53.12390960531436690 ) ) ;
#194172=CARTESIAN_POINT ( 'NONE',  ( -12.14591786802309592, -12.06949235617757132, 36.87390960531435979 ) ) ;
#194173=CARTESIAN_POINT ( 'NONE',  ( -0.05219959533937732626, 21.53943276465977519, 77.50109039468567573 ) ) ;
#194174=CARTESIAN_POINT ( 'NONE',  ( 5.153800228976615827, -19.02544592524334988, 20.20942372801899722 ) ) ;
#194175=CARTESIAN_POINT ( 'NONE',  ( 8.224510206698953496, -14.34966873604960469, 57.91557627198103120 ) ) ;
#194176=CARTESIAN_POINT ( 'NONE',  ( 14.34966873604960469, 8.224510206698951720, 99.16557627198100988 ) ) ;
#194177=CARTESIAN_POINT ( 'NONE',  ( -0.05219959533936034679, 19.03943276465977164, 62.50109039468566863 ) ) ;
#194178=CARTESIAN_POINT ( 'NONE',  ( -0.05219959533934338120, 16.53943276465976808, 112.5010903946857042 ) ) ;
#194179=CARTESIAN_POINT ( 'NONE',  ( 18.62759615963255655, 10.81492255796105972, 71.66775706135234714 ) ) ;
#194180=CARTESIAN_POINT ( 'NONE',  ( -0.05219959533909027116, -19.03943276465977164, 77.49890960531435269 ) ) ;
#194181=CARTESIAN_POINT ( 'NONE',  ( 0.05219959533936267826, -19.03943276465977164, 40.00109039468566152 ) ) ;
#194182=CARTESIAN_POINT ( 'NONE',  ( 15.72974639402199770, -15.80617190586745480, 38.12390960531436690 ) ) ;
#194183=CARTESIAN_POINT ( 'NONE',  ( -21.53943276465977519, -0.05219959533937600094, 38.75109039468567573 ) ) ;
#194184=CARTESIAN_POINT ( 'NONE',  ( -15.72974639402197994, 15.80617190586746368, 90.62390960531436690 ) ) ;
#194185=CARTESIAN_POINT ( 'NONE',  ( -19.03943276465977164, -0.05219959533935918106, 98.75109039468567573 ) ) ;
#194186=CARTESIAN_POINT ( 'NONE',  ( 0.05219959533934541429, -16.53943276465976808, 50.00109039468568994 ) ) ;
#194188=CARTESIAN_POINT ( 'NONE',  ( -10.72451020669898014, 18.67979575497178502, 90.41557627198103830 ) ) ;
#194189=CARTESIAN_POINT ( 'NONE',  ( 12.14591786802309770, 12.06949235617756955, 89.37390960531435269 ) ) ;
#194190=CARTESIAN_POINT ( 'NONE',  ( 17.97058386085788939, 5.500000000000048850, 41.50390968646216550 ) ) ;
#194191=CARTESIAN_POINT ( 'NONE',  ( -16.53943276465976808, -0.05219959533934237506, 23.75109039468567929 ) ) ;
#194192=CARTESIAN_POINT ( 'NONE',  ( -5.719274019375978568, 21.55341960407610458, 50.20724293864769550 ) ) ;
#194193=CARTESIAN_POINT ( 'NONE',  ( -8.314922557961024197, 14.29746914071037800, 92.91775706135236135 ) ) ;
#194194=CARTESIAN_POINT ( 'NONE',  ( 19.02544592524343514, -5.153800228976328945, 23.54057627198102054 ) ) ;
#194195=CARTESIAN_POINT ( 'NONE',  ( 8.224510206698742110, 14.34966873604972548, 47.08442372801901854 ) ) ;
#194196=CARTESIAN_POINT ( 'NONE',  ( 18.67979575497194134, -10.72451020669871369, 25.83442372801901499 ) ) ;
#194197=CARTESIAN_POINT ( 'NONE',  ( 10.81492255796078972, 18.62759615963270932, 49.58224293864769550 ) ) ;
#194198=CARTESIAN_POINT ( 'NONE',  ( 16.55341960407618274, -4.379528057220086978, 86.04275706135236135 ) ) ;
#194199=CARTESIAN_POINT ( 'NONE',  ( 5.153800228976335163, 19.02544592524342804, 94.79057627198103830 ) ) ;
#194200=CARTESIAN_POINT ( 'NONE',  ( 5.823673210054444382, -21.52544592524334988, 50.20942372801901854 ) ) ;
#194201=CARTESIAN_POINT ( 'NONE',  ( 21.55341960407610458, 5.719274019375980345, 43.95724293864769550 ) ) ;
#194202=CARTESIAN_POINT ( 'NONE',  ( -16.51473224551069308, -9.474510206698971260, 111.6655762719810383 ) ) ;
#194203=ORIENTED_EDGE ( 'NONE', *, *, #178675, .T. ) ;
#194204=CARTESIAN_POINT ( 'NONE',  ( -19.03943276465977164, -0.05219959533935918106, 33.75109039468566863 ) ) ;
#194205=CARTESIAN_POINT ( 'NONE',  ( 16.53943276465976808, 0.05219959533934440121, 61.25109039468567573 ) ) ;
#194206=CARTESIAN_POINT ( 'NONE',  ( 18.67979575497178502, 10.72451020669898547, 24.16557627198103120 ) ) ;
#194208=CARTESIAN_POINT ( 'NONE',  ( 16.51473224551069308, 9.474510206698969483, 84.16557627198102409 ) ) ;
#194209=CARTESIAN_POINT ( 'NONE',  ( -14.34966873604972548, 8.224510206698743886, 98.33442372801901854 ) ) ;
#194211=CARTESIAN_POINT ( 'NONE',  ( -0.05219959533910754901, -16.53943276465976808, 97.49890960531436690 ) ) ;
#194212=CARTESIAN_POINT ( 'NONE',  ( 21.53943276465977519, -0.05219959533907433946, 48.74890960531435979 ) ) ;
#194213=CARTESIAN_POINT ( 'NONE',  ( 5.049401038298161559, -19.05341960407611168, 32.70724293864768129 ) ) ;
#194214=CARTESIAN_POINT ( 'NONE',  ( -14.34966873604972548, 8.224510206698743886, 78.33442372801901854 ) ) ;
#194215=CARTESIAN_POINT ( 'NONE',  ( 5.823673210054444382, -21.52544592524334988, 35.20942372801901854 ) ) ;
#194216=CARTESIAN_POINT ( 'NONE',  ( 9.564922557961047289, -16.46253265017146816, 85.41775706135233293 ) ) ;
#194217=CARTESIAN_POINT ( 'NONE',  ( 8.314922557960818139, 14.29746914071049879, 89.58224293864768129 ) ) ;
#194218=CARTESIAN_POINT ( 'NONE',  ( 9.564922557960805705, 16.46253265017160317, 49.58224293864770260 ) ) ;
#194219=CARTESIAN_POINT ( 'NONE',  ( 13.97604488694527802, 13.89961937509977652, 114.3739096053143669 ) ) ;
#194220=CARTESIAN_POINT ( 'NONE',  ( -21.53943276465977519, -0.05219959533937600094, 108.7510903946857042 ) ) ;
#194221=CARTESIAN_POINT ( 'NONE',  ( 13.97604488694527802, 13.89961937509977652, 74.37390960531436690 ) ) ;
#194222=CARTESIAN_POINT ( 'NONE',  ( -16.52544592524335698, -4.483927247898792601, 58.95942372801902565 ) ) ;
#194223=CARTESIAN_POINT ( 'NONE',  ( -21.55341960407619339, 5.719274019375674811, 98.54275706135234714 ) ) ;
#194224=CARTESIAN_POINT ( 'NONE',  ( -16.55341960407617563, 4.379528057220093196, 68.54275706135234714 ) ) ;
#194225=CARTESIAN_POINT ( 'NONE',  ( 5.049401038297881783, 19.05341960407617563, 57.29275706135231871 ) ) ;
#194226=CARTESIAN_POINT ( 'NONE',  ( -9.564922557961040184, 16.46253265017147172, 62.91775706135233293 ) ) ;
#194227=CARTESIAN_POINT ( 'NONE',  ( -15.80617190586768217, 15.72974639402176855, 68.12609039468567573 ) ) ;
#194228=CARTESIAN_POINT ( 'NONE',  ( -5.153800228976328057, -19.02544592524343514, 67.29057627198102409 ) ) ;
#194229=CARTESIAN_POINT ( 'NONE',  ( -19.03943276465977164, 0.05219959533909376836, 26.24890960531435624 ) ) ;
#194230=CARTESIAN_POINT ( 'NONE',  ( -16.46253265017146816, -9.564922557961047289, 64.16775706135233293 ) ) ;
#194231=CARTESIAN_POINT ( 'NONE',  ( 13.97604488694527802, 13.89961937509977652, 114.3739096053143669 ) ) ;
#194232=CARTESIAN_POINT ( 'NONE',  ( -19.02544592524342804, 5.153800228976336051, 86.04057627198103830 ) ) ;
#194233=CARTESIAN_POINT ( 'NONE',  ( 14.34966873604960469, 8.224510206698951720, 44.16557627198103120 ) ) ;
#194234=CARTESIAN_POINT ( 'NONE',  ( -15.80617190586745835, -15.72974639402198527, 46.87390960531435979 ) ) ;
#194236=CARTESIAN_POINT ( 'NONE',  ( 9.564922557961047289, -16.46253265017146816, 20.41775706135233293 ) ) ;
#194237=CARTESIAN_POINT ( 'NONE',  ( -17.48853670773246094, -5.747243402303008786, 81.33328700250011423 ) ) ;
#194238=CARTESIAN_POINT ( 'NONE',  ( 19.03943276465977164, -0.05219959533909143690, 33.74890960531435979 ) ) ;
#194239=CARTESIAN_POINT ( 'NONE',  ( 19.02544592524343514, -5.153800228976328945, 23.54057627198102054 ) ) ;
#194241=CARTESIAN_POINT ( 'NONE',  ( 5.719274019375673035, 21.55341960407619339, 62.29275706135236845 ) ) ;
#194243=CARTESIAN_POINT ( 'NONE',  ( -4.483927247898782831, 16.52544592524335698, 67.70942372801901854 ) ) ;
#194244=CARTESIAN_POINT ( 'NONE',  ( 10.72451020669898902, -18.67979575497178502, 87.91557627198103830 ) ) ;
#194245=CARTESIAN_POINT ( 'NONE',  ( 14.34966873604960469, 8.224510206698951720, 59.16557627198103120 ) ) ;
#194246=CARTESIAN_POINT ( 'NONE',  ( -13.97604488694527625, -13.89961937509977652, 31.87390960531435979 ) ) ;
#194248=CARTESIAN_POINT ( 'NONE',  ( -21.53943276465977519, -0.05219959533937600094, 38.75109039468567573 ) ) ;
#194249=CARTESIAN_POINT ( 'NONE',  ( 9.474510206698729675, 16.51473224551082808, 52.08442372801900433 ) ) ;
#194250=CARTESIAN_POINT ( 'NONE',  ( -16.46253265017160317, 9.564922557960807481, 30.83224293864769550 ) ) ;
#194251=CARTESIAN_POINT ( 'NONE',  ( -18.67979575497193778, 10.72451020669871902, 88.33442372801901854 ) ) ;
#194252=CARTESIAN_POINT ( 'NONE',  ( 16.46253265017160672, -9.564922557960803928, 23.33224293864769194 ) ) ;
#194253=CARTESIAN_POINT ( 'NONE',  ( -12.06949235617756955, 12.14591786802309770, 35.62390960531437401 ) ) ;
#194255=CARTESIAN_POINT ( 'NONE',  ( -21.52544592524343514, 5.823673210054127303, 46.04057627198103830 ) ) ;
#194257=CARTESIAN_POINT ( 'NONE',  ( 16.46253265017160672, -9.564922557960803928, 93.33224293864769550 ) ) ;
#194258=CARTESIAN_POINT ( 'NONE',  ( -14.29746914071049879, 8.314922557960819915, 85.83224293864768129 ) ) ;
#194259=CARTESIAN_POINT ( 'NONE',  ( -14.29746914071037622, -8.314922557961029526, 24.16775706135235424 ) ) ;
#194260=CARTESIAN_POINT ( 'NONE',  ( -21.55341960407610458, -5.719274019375992779, 61.45724293864770260 ) ) ;
#194262=CARTESIAN_POINT ( 'NONE',  ( -19.02544592524342804, 5.153800228976336051, 31.04057627198102409 ) ) ;
#194263=CARTESIAN_POINT ( 'NONE',  ( -19.05341960407611168, -5.049401038298163336, 81.45724293864769550 ) ) ;
#194264=CARTESIAN_POINT ( 'NONE',  ( -5.719274019375978568, 21.55341960407610458, 90.20724293864770971 ) ) ;
#194265=CARTESIAN_POINT ( 'NONE',  ( -16.55341960407611168, -4.379528057220339221, 31.45724293864769550 ) ) ;
#194266=CARTESIAN_POINT ( 'NONE',  ( 0.05219959533909260263, 19.03943276465977164, 94.99890960531436690 ) ) ;
#194267=CARTESIAN_POINT ( 'NONE',  ( 16.51473224551083163, -9.474510206698727899, 80.83442372801899012 ) ) ;
#194268=CARTESIAN_POINT ( 'NONE',  ( 15.72974639402176855, 15.80617190586768217, 96.87609039468568994 ) ) ;
#194269=CARTESIAN_POINT ( 'NONE',  ( 5.719274019375991003, -21.55341960407610458, 72.70724293864769550 ) ) ;
#194270=CARTESIAN_POINT ( 'NONE',  ( -10.81492255796078084, -18.62759615963271287, 42.08224293864769550 ) ) ;
#194271=CARTESIAN_POINT ( 'NONE',  ( 19.03943276465977164, -0.05219959533909143690, 53.74890960531436690 ) ) ;
#194272=CARTESIAN_POINT ( 'NONE',  ( -4.379528057220328563, 16.55341960407611168, 25.20724293864769550 ) ) ;
#194273=CARTESIAN_POINT ( 'NONE',  ( -19.05341960407611168, -5.049401038298163336, 71.45724293864766707 ) ) ;
#194276=CARTESIAN_POINT ( 'NONE',  ( 9.474510206698729675, 16.51473224551082808, 32.08442372801900433 ) ) ;
#194277=CARTESIAN_POINT ( 'NONE',  ( 8.224510206698953496, -14.34966873604960469, 82.91557627198103830 ) ) ;
#194278=CARTESIAN_POINT ( 'NONE',  ( 0.05219959533937995610, -21.53943276465977519, 25.00109039468567218 ) ) ;
#194280=CARTESIAN_POINT ( 'NONE',  ( 5.719274019375991003, -21.55341960407610458, 62.70724293864769550 ) ) ;
#194282=CARTESIAN_POINT ( 'NONE',  ( 12.06949235617739724, 12.14591786802326823, 96.87609039468568994 ) ) ;
#194283=CARTESIAN_POINT ( 'NONE',  ( -0.05219959533909027116, -19.03943276465977164, 27.49890960531435624 ) ) ;
#194284=CARTESIAN_POINT ( 'NONE',  ( 19.03943276465977164, -0.05219959533909143690, 73.74890960531435269 ) ) ;
#194286=CARTESIAN_POINT ( 'NONE',  ( -12.06949235617756955, 12.14591786802309770, 30.62390960531436335 ) ) ;
#194287=CARTESIAN_POINT ( 'NONE',  ( 21.55341960407619695, -5.719274019375665929, 66.04275706135236135 ) ) ;
#194288=CARTESIAN_POINT ( 'NONE',  ( 9.564922557960805705, 16.46253265017160317, 104.5822429386476955 ) ) ;
#194289=CARTESIAN_POINT ( 'NONE',  ( -21.53943276465977519, -0.05219959533937600094, 93.75109039468567573 ) ) ;
#194290=CARTESIAN_POINT ( 'NONE',  ( 5.153800228976335163, 19.02544592524342804, 44.79057627198103830 ) ) ;
#194291=CARTESIAN_POINT ( 'NONE',  ( -19.03943276465977164, 0.05219959533909376836, 41.24890960531435269 ) ) ;
#194292=ORIENTED_EDGE ( 'NONE', *, *, #105079, .T. ) ;
#194293=CARTESIAN_POINT ( 'NONE',  ( -21.55341960407619339, 5.719274019375674811, 93.54275706135234714 ) ) ;
#194294=CARTESIAN_POINT ( 'NONE',  ( -8.314922557961024197, 14.29746914071037800, 67.91775706135234714 ) ) ;
#194295=CARTESIAN_POINT ( 'NONE',  ( -15.72974639402176322, -15.80617190586768395, 79.37609039468567573 ) ) ;
#194296=CARTESIAN_POINT ( 'NONE',  ( 5.049401038298161559, -19.05341960407611168, 112.7072429386476813 ) ) ;
#194297=CARTESIAN_POINT ( 'NONE',  ( 9.474510206698729675, 16.51473224551082808, 97.08442372801900433 ) ) ;
#194298=CARTESIAN_POINT ( 'NONE',  ( -0.05219959533937732626, 21.53943276465977519, 57.50109039468568994 ) ) ;
#194299=CARTESIAN_POINT ( 'NONE',  ( -16.55341960407617563, 4.379528057220093196, 33.54275706135234714 ) ) ;
#194300=CARTESIAN_POINT ( 'NONE',  ( -5.153800228976607833, 19.02544592524334988, 87.70942372801897591 ) ) ;
#194301=CARTESIAN_POINT ( 'NONE',  ( 9.564922557960805705, 16.46253265017160317, 49.58224293864770260 ) ) ;
#194302=CARTESIAN_POINT ( 'NONE',  ( 9.474510206698729675, 16.51473224551082808, 92.08442372801900433 ) ) ;
#194303=CARTESIAN_POINT ( 'NONE',  ( 19.03943276465977164, 0.05219959533936151252, 86.25109039468567573 ) ) ;
#194304=CARTESIAN_POINT ( 'NONE',  ( 0.05219959533910956823, 16.53943276465976808, 54.99890960531435269 ) ) ;
#194305=CARTESIAN_POINT ( 'NONE',  ( -19.03943276465977164, -0.05219959533935918106, 78.75109039468567573 ) ) ;
#194306=CARTESIAN_POINT ( 'NONE',  ( -14.34966873604972548, 8.224510206698743886, 63.33442372801900433 ) ) ;
#194307=CARTESIAN_POINT ( 'NONE',  ( -0.05219959533936034679, 19.03943276465977164, 27.50109039468566507 ) ) ;
#194308=CARTESIAN_POINT ( 'NONE',  ( 19.03943276465977164, -0.05219959533909143690, 33.74890960531435979 ) ) ;
#194309=CARTESIAN_POINT ( 'NONE',  ( -0.05219959533909027116, -19.03943276465977164, 42.49890960531435269 ) ) ;
#194311=CARTESIAN_POINT ( 'NONE',  ( -8.224510206698735004, -14.34966873604973081, 64.58442372801900433 ) ) ;
#194314=CARTESIAN_POINT ( 'NONE',  ( -5.153800228976328057, -19.02544592524343514, 102.2905762719810383 ) ) ;
#194315=LINE ( 'NONE', #133622, #97404 ) ;
#194317=CARTESIAN_POINT ( 'NONE',  ( -19.03943276465977164, -0.05219959533935918106, 93.75109039468566152 ) ) ;
#194318=CARTESIAN_POINT ( 'NONE',  ( -18.67979575497178146, -10.72451020669898902, 41.66557627198103120 ) ) ;
#194319=CARTESIAN_POINT ( 'NONE',  ( 16.46253265017146816, 9.564922557961045513, 31.66775706135232937 ) ) ;
#194320=CARTESIAN_POINT ( 'NONE',  ( -19.02544592524334988, -5.153800228976617603, 108.9594237280189759 ) ) ;
#194321=CARTESIAN_POINT ( 'NONE',  ( 16.46253265017160672, -9.564922557960803928, 33.33224293864770260 ) ) ;
#194322=CARTESIAN_POINT ( 'NONE',  ( -0.05219959533909027116, -19.03943276465977164, 42.49890960531435269 ) ) ;
#194323=CARTESIAN_POINT ( 'NONE',  ( -18.62759615963270932, 10.81492255796079327, 75.83224293864769550 ) ) ;
#194324=CARTESIAN_POINT ( 'NONE',  ( -5.049401038298153566, 19.05341960407611168, 100.2072429386476955 ) ) ;
#194325=CARTESIAN_POINT ( 'NONE',  ( -19.02544592524342804, 5.153800228976336051, 41.04057627198103120 ) ) ;
#194327=CARTESIAN_POINT ( 'NONE',  ( -19.02544592524334988, -5.153800228976617603, 88.95942372801897591 ) ) ;
#194328=CARTESIAN_POINT ( 'NONE',  ( 8.224510206698953496, -14.34966873604960469, 47.91557627198102409 ) ) ;
#194329=CARTESIAN_POINT ( 'NONE',  ( -10.72451020669898014, 18.67979575497178502, 35.41557627198102409 ) ) ;
#194330=CARTESIAN_POINT ( 'NONE',  ( 15.80617190586769283, -15.72974639402175789, 110.6260903946857042 ) ) ;
#194331=CARTESIAN_POINT ( 'NONE',  ( 0.05219959533907565091, 21.53943276465977519, 99.99890960531436690 ) ) ;
#194332=CARTESIAN_POINT ( 'NONE',  ( 15.80617190586769283, -15.72974639402175789, 65.62609039468568994 ) ) ;
#194333=CARTESIAN_POINT ( 'NONE',  ( -21.55341960407619339, 5.719274019375674811, 78.54275706135236135 ) ) ;
#194334=CARTESIAN_POINT ( 'NONE',  ( -19.03943276465977164, 0.05219959533909376836, 106.2489096053143669 ) ) ;
#194335=CARTESIAN_POINT ( 'NONE',  ( 4.483927247898790824, -16.52544592524335698, 105.2094237280190328 ) ) ;
#194336=CARTESIAN_POINT ( 'NONE',  ( 15.72974639402176855, 15.80617190586768217, 66.87609039468568994 ) ) ;
#194337=CARTESIAN_POINT ( 'NONE',  ( -19.03943276465977164, 0.05219959533909376836, 56.24890960531435979 ) ) ;
#194338=CARTESIAN_POINT ( 'NONE',  ( 9.474510206698729675, 16.51473224551082808, 37.08442372801899722 ) ) ;
#194339=CARTESIAN_POINT ( 'NONE',  ( -15.80617190586768217, 15.72974639402176855, 33.12609039468569705 ) ) ;
#194340=CARTESIAN_POINT ( 'NONE',  ( -19.02544592524342804, 5.153800228976336051, 71.04057627198099567 ) ) ;
#194341=CARTESIAN_POINT ( 'NONE',  ( 16.53943276465976808, -0.05219959533910856209, 83.74890960531435269 ) ) ;
#194342=CARTESIAN_POINT ( 'NONE',  ( -16.52544592524342804, 4.483927247898546575, 51.04057627198103120 ) ) ;
#194343=CARTESIAN_POINT ( 'NONE',  ( 18.67979575497178502, 10.72451020669898547, 59.16557627198103120 ) ) ;
#194344=CARTESIAN_POINT ( 'NONE',  ( -19.02544592524342804, 5.153800228976336051, 56.04057627198100988 ) ) ;
#194345=CARTESIAN_POINT ( 'NONE',  ( -0.05219959533907301413, -21.53943276465977519, 72.49890960531435269 ) ) ;
#194346=CARTESIAN_POINT ( 'NONE',  ( 13.97604488694548053, -13.89961937509957401, 55.62609039468566863 ) ) ;
#194348=CARTESIAN_POINT ( 'NONE',  ( -14.34966873604960291, -8.224510206698953496, 66.66557627198102409 ) ) ;
#194349=CARTESIAN_POINT ( 'NONE',  ( -10.72451020669898014, 18.67979575497178502, 35.41557627198102409 ) ) ;
#194350=ORIENTED_EDGE ( 'NONE', *, *, #179822, .F. ) ;
#194351=CARTESIAN_POINT ( 'NONE',  ( 16.79531203550646978, 7.028104445595615424, 103.7524498822044450 ) ) ;
#194352=CARTESIAN_POINT ( 'NONE',  ( -16.55341960407617563, 4.379528057220093196, 88.54275706135236135 ) ) ;
#194355=CARTESIAN_POINT ( 'NONE',  ( -5.049401038297874678, -19.05341960407617918, 89.79275706135230450 ) ) ;
#194356=CARTESIAN_POINT ( 'NONE',  ( 12.14591786802309770, 12.06949235617756955, 59.37390960531436690 ) ) ;
#194358=CARTESIAN_POINT ( 'NONE',  ( -19.05341960407611168, -5.049401038298163336, 51.45724293864770260 ) ) ;
#194359=CARTESIAN_POINT ( 'NONE',  ( -16.53943276465976808, 0.05219959533911058130, 41.24890960531435269 ) ) ;
#194360=CARTESIAN_POINT ( 'NONE',  ( -0.05219959533909027116, -19.03943276465977164, 92.49890960531436690 ) ) ;
#194361=CARTESIAN_POINT ( 'NONE',  ( -13.89961937509977652, 13.97604488694528158, 50.62390960531435979 ) ) ;
#194362=CARTESIAN_POINT ( 'NONE',  ( -15.80617190586768217, 15.72974639402176855, 63.12609039468568994 ) ) ;
#194363=CARTESIAN_POINT ( 'NONE',  ( -16.51473224551069308, -9.474510206698971260, 71.66557627198102409 ) ) ;
#194364=CARTESIAN_POINT ( 'NONE',  ( -5.153800228976328057, -19.02544592524343514, 32.29057627198102409 ) ) ;
#194365=CARTESIAN_POINT ( 'NONE',  ( -9.564922557960796823, -16.46253265017161027, 77.08224293864769550 ) ) ;
#194366=CARTESIAN_POINT ( 'NONE',  ( 21.55341960407610458, 5.719274019375980345, 43.95724293864769550 ) ) ;
#194367=CARTESIAN_POINT ( 'NONE',  ( 9.564922557960805705, 16.46253265017160317, 39.58224293864768839 ) ) ;
#194368=CARTESIAN_POINT ( 'NONE',  ( 10.72451020669898902, -18.67979575497178502, 47.91557627198102409 ) ) ;
#194369=CARTESIAN_POINT ( 'NONE',  ( 12.14591786802327356, -12.06949235617739191, 110.6260903946857042 ) ) ;
#194370=CARTESIAN_POINT ( 'NONE',  ( 16.46253265017146816, 9.564922557961045513, 26.66775706135234003 ) ) ;
#194371=CARTESIAN_POINT ( 'NONE',  ( -14.29746914071037622, -8.314922557961029526, 44.16775706135234714 ) ) ;
#194372=CARTESIAN_POINT ( 'NONE',  ( 8.314922557961029526, -14.29746914071037800, 85.41775706135236135 ) ) ;
#194373=CARTESIAN_POINT ( 'NONE',  ( -17.60769864724390388, 5.499999999999986677, 68.65024842019165874 ) ) ;
#194374=CARTESIAN_POINT ( 'NONE',  ( 4.379528057220092307, 16.55341960407617563, 62.29275706135236845 ) ) ;
#194375=CARTESIAN_POINT ( 'NONE',  ( -15.72974639402197994, 15.80617190586746368, 25.62390960531435624 ) ) ;
#194376=CARTESIAN_POINT ( 'NONE',  ( 13.89961937509977652, -13.97604488694527269, 38.12390960531436690 ) ) ;
#194377=CARTESIAN_POINT ( 'NONE',  ( -16.55341960407617563, 4.379528057220093196, 43.54275706135235424 ) ) ;
#194378=CARTESIAN_POINT ( 'NONE',  ( -0.05219959533909027116, -19.03943276465977164, 47.49890960531435979 ) ) ;
#194379=CARTESIAN_POINT ( 'NONE',  ( 5.823673210054444382, -21.52544592524334988, 20.20942372801900788 ) ) ;
#194380=CARTESIAN_POINT ( 'NONE',  ( -0.05219959533934338120, 16.53943276465976808, 32.50109039468568284 ) ) ;
#194381=CARTESIAN_POINT ( 'NONE',  ( 0.05219959533934541429, -16.53943276465976808, 100.0010903946857042 ) ) ;
#194383=CARTESIAN_POINT ( 'NONE',  ( 10.81492255796106328, -18.62759615963255655, 95.41775706135234714 ) ) ;
#194384=CARTESIAN_POINT ( 'NONE',  ( 5.153800228976615827, -19.02544592524334988, 100.2094237280190043 ) ) ;
#194385=CARTESIAN_POINT ( 'NONE',  ( 13.89961937509957401, 13.97604488694547697, 51.87609039468566863 ) ) ;
#194386=CARTESIAN_POINT ( 'NONE',  ( 12.14591786802309770, 12.06949235617756955, 59.37390960531436690 ) ) ;
#194387=CARTESIAN_POINT ( 'NONE',  ( 19.02544592524343514, -5.153800228976328945, 28.54057627198102409 ) ) ;
#194388=CARTESIAN_POINT ( 'NONE',  ( -5.049401038297874678, -19.05341960407617918, 54.79275706135234003 ) ) ;
#194389=CARTESIAN_POINT ( 'NONE',  ( 17.48847506799950224, -5.747544572775292515, 58.32697437843292221 ) ) ;
#194390=CARTESIAN_POINT ( 'NONE',  ( 5.823673210054444382, -21.52544592524334988, 70.20942372801904696 ) ) ;
#194391=CARTESIAN_POINT ( 'NONE',  ( 12.14591786802327356, -12.06949235617739191, 30.62609039468567929 ) ) ;
#194392=CARTESIAN_POINT ( 'NONE',  ( -17.72517630440432868, 5.499999999999969802, 90.92175719257211597 ) ) ;
#194393=CARTESIAN_POINT ( 'NONE',  ( 10.81492255796078972, 18.62759615963270932, 29.58224293864769905 ) ) ;
#194394=CARTESIAN_POINT ( 'NONE',  ( -16.53943276465976808, -0.05219959533934237506, 18.75109039468568639 ) ) ;
#194395=DIRECTION ( 'NONE',  ( 0.000000000000000000, 0.000000000000000000, -1.000000000000000000 ) ) ;
#194396=CARTESIAN_POINT ( 'NONE',  ( -19.03943276465977164, 0.05219959533909376836, 31.24890960531435979 ) ) ;
#194397=CARTESIAN_POINT ( 'NONE',  ( -21.52544592524334988, -5.823673210054445271, 108.9594237280190185 ) ) ;
#194398=CARTESIAN_POINT ( 'NONE',  ( -19.05341960407611168, -5.049401038298163336, 56.45724293864768129 ) ) ;
#194399=CARTESIAN_POINT ( 'NONE',  ( -5.823673210054431948, 21.52544592524334988, 62.70942372801902565 ) ) ;
#194400=CARTESIAN_POINT ( 'NONE',  ( 18.67979575497194134, -10.72451020669871369, 105.8344237280190328 ) ) ;
#194401=CARTESIAN_POINT ( 'NONE',  ( -12.14591786802326823, 12.06949235617739902, 98.12609039468570415 ) ) ;
#194402=CARTESIAN_POINT ( 'NONE',  ( -16.51473224551069308, -9.474510206698971260, 81.66557627198103830 ) ) ;
#194403=CARTESIAN_POINT ( 'NONE',  ( -15.80617190586768217, 15.72974639402176855, 53.12609039468568284 ) ) ;
#194404=CARTESIAN_POINT ( 'NONE',  ( 5.719274019375673035, 21.55341960407619339, 47.29275706135234003 ) ) ;
#194405=CARTESIAN_POINT ( 'NONE',  ( -13.89961937509957401, -13.97604488694547875, 74.37609039468566152 ) ) ;
#194406=CARTESIAN_POINT ( 'NONE',  ( -13.89961937509977652, 13.97604488694528158, 105.6239096053143527 ) ) ;
#194407=CARTESIAN_POINT ( 'NONE',  ( 8.314922557960818139, 14.29746914071049879, 114.5822429386477097 ) ) ;
#194408=CARTESIAN_POINT ( 'NONE',  ( -5.823673210054116645, -21.52544592524344225, 102.2905762719810383 ) ) ;
#194409=CARTESIAN_POINT ( 'NONE',  ( 16.51473224551083163, -9.474510206698727899, 25.83442372801900078 ) ) ;
#194410=CARTESIAN_POINT ( 'NONE',  ( 16.55341960407611168, 4.379528057220329451, 98.95724293864770971 ) ) ;
#194411=CARTESIAN_POINT ( 'NONE',  ( -0.05219959533909027116, -19.03943276465977164, 47.49890960531435979 ) ) ;
#194412=CARTESIAN_POINT ( 'NONE',  ( -19.03943276465977164, -0.05219959533935918106, 98.75109039468567573 ) ) ;
#194413=CARTESIAN_POINT ( 'NONE',  ( -12.06949235617756955, 12.14591786802309770, 65.62390960531436690 ) ) ;
#194414=CARTESIAN_POINT ( 'NONE',  ( -5.719274019375665041, -21.55341960407619695, 109.7927570613523613 ) ) ;
#194415=CARTESIAN_POINT ( 'NONE',  ( -16.51473224551069308, -9.474510206698971260, 106.6655762719810383 ) ) ;
#194416=CARTESIAN_POINT ( 'NONE',  ( -5.153800228976607833, 19.02544592524334988, 77.70942372801900433 ) ) ;
#194417=CARTESIAN_POINT ( 'NONE',  ( -15.80617190586745835, -15.72974639402198527, 76.87390960531439532 ) ) ;
#194418=CARTESIAN_POINT ( 'NONE',  ( -10.72451020669870658, -18.67979575497194134, 44.58442372801901854 ) ) ;
#194419=CARTESIAN_POINT ( 'NONE',  ( 16.52544592524335698, 4.483927247898782831, 41.45942372801901143 ) ) ;
#194420=CARTESIAN_POINT ( 'NONE',  ( -8.314922557961024197, 14.29746914071037800, 87.91775706135234714 ) ) ;
#194421=CARTESIAN_POINT ( 'NONE',  ( 14.29746914071037800, 8.314922557961029526, 36.66775706135234714 ) ) ;
#194422=CARTESIAN_POINT ( 'NONE',  ( -15.80617190586768217, 15.72974639402176855, 38.12609039468567573 ) ) ;
#194423=CARTESIAN_POINT ( 'NONE',  ( -5.719274019375978568, 21.55341960407610458, 45.20724293864769550 ) ) ;
#194424=CARTESIAN_POINT ( 'NONE',  ( -19.03943276465977164, 0.05219959533909376836, 31.24890960531435979 ) ) ;
#194426=CARTESIAN_POINT ( 'NONE',  ( 0.05219959533934541429, -16.53943276465976808, 65.00109039468568994 ) ) ;
#194427=CARTESIAN_POINT ( 'NONE',  ( 21.55341960407610458, 5.719274019375980345, 93.95724293864770971 ) ) ;
#194428=CARTESIAN_POINT ( 'NONE',  ( -14.29746914071049879, 8.314922557960819915, 40.83224293864769550 ) ) ;
#194429=CARTESIAN_POINT ( 'NONE',  ( -12.06949235617739369, -12.14591786802326823, 44.37609039468567573 ) ) ;
#194430=CARTESIAN_POINT ( 'NONE',  ( -0.05219959533909027116, -19.03943276465977164, 62.49890960531435979 ) ) ;
#194431=CARTESIAN_POINT ( 'NONE',  ( -5.049401038297874678, -19.05341960407617918, 84.79275706135233293 ) ) ;
#194432=CARTESIAN_POINT ( 'NONE',  ( 10.72451020669898902, -18.67979575497178502, 82.91557627198103830 ) ) ;
#194433=CARTESIAN_POINT ( 'NONE',  ( 12.06949235617757843, -12.14591786802309237, 33.12390960531435979 ) ) ;
#194436=CARTESIAN_POINT ( 'NONE',  ( -21.53943276465977519, 0.05219959533907696930, 56.24890960531436690 ) ) ;
#194437=CARTESIAN_POINT ( 'NONE',  ( 4.483927247898790824, -16.52544592524335698, 105.2094237280190328 ) ) ;
#194439=CARTESIAN_POINT ( 'NONE',  ( 18.56399227203341695, 5.500000000000000888, 86.47830131249902763 ) ) ;
#194440=CARTESIAN_POINT ( 'NONE',  ( -5.823673210054116645, -21.52544592524344225, 92.29057627198103830 ) ) ;
#194441=CARTESIAN_POINT ( 'NONE',  ( -8.224510206698948167, 14.34966873604960824, 25.41557627198103120 ) ) ;
#194442=CARTESIAN_POINT ( 'NONE',  ( 16.53943276465976808, 0.05219959533934440121, 36.25109039468567573 ) ) ;
#194443=CARTESIAN_POINT ( 'NONE',  ( 9.564922557960805705, 16.46253265017160317, 34.58224293864770260 ) ) ;
#194444=CARTESIAN_POINT ( 'NONE',  ( -5.153800228976328057, -19.02544592524343514, 72.29057627198102409 ) ) ;
#194446=CARTESIAN_POINT ( 'NONE',  ( -19.05341960407611168, -5.049401038298163336, 111.4572429386476671 ) ) ;
#194448=CARTESIAN_POINT ( 'NONE',  ( -16.55341960407617563, 4.379528057220093196, 98.54275706135234714 ) ) ;
#194449=CARTESIAN_POINT ( 'NONE',  ( 9.474510206698729675, 16.51473224551082808, 112.0844237280190043 ) ) ;
#194450=CARTESIAN_POINT ( 'NONE',  ( 5.049401038297881783, 19.05341960407617563, 32.29275706135233293 ) ) ;
#194451=CARTESIAN_POINT ( 'NONE',  ( 10.72451020669898902, -18.67979575497178502, 92.91557627198103830 ) ) ;
#194452=EDGE_CURVE ( 'NONE', #65322, #94244, #133540, .T. ) ;
#194453=CARTESIAN_POINT ( 'NONE',  ( -0.05219959533910754901, -16.53943276465976808, 22.49890960531436335 ) ) ;
#194454=CARTESIAN_POINT ( 'NONE',  ( -21.55341960407610458, -5.719274019375992779, 51.45724293864770260 ) ) ;
#194455=CARTESIAN_POINT ( 'NONE',  ( -19.05341960407617563, 5.049401038297882671, 108.5427570613523187 ) ) ;
#194456=CARTESIAN_POINT ( 'NONE',  ( -19.02544592524342804, 5.153800228976336051, 111.0405762719810099 ) ) ;
#194457=CARTESIAN_POINT ( 'NONE',  ( 18.62759615963255655, 10.81492255796105972, 61.66775706135235424 ) ) ;
#194458=CARTESIAN_POINT ( 'NONE',  ( -19.03943276465977164, 0.05219959533909376836, 66.24890960531436690 ) ) ;
#194459=CARTESIAN_POINT ( 'NONE',  ( 16.52544592524342804, -4.483927247898539470, 103.5405762719810383 ) ) ;
#194461=CARTESIAN_POINT ( 'NONE',  ( 13.89961937509977652, -13.97604488694527269, 68.12390960531436690 ) ) ;
#194462=CARTESIAN_POINT ( 'NONE',  ( -14.29746914071049879, 8.314922557960819915, 80.83224293864769550 ) ) ;
#194464=CARTESIAN_POINT ( 'NONE',  ( 5.049401038297881783, 19.05341960407617563, 92.29275706135234714 ) ) ;
#194466=CARTESIAN_POINT ( 'NONE',  ( 16.46253265017160672, -9.564922557960803928, 58.33224293864769550 ) ) ;
#194468=CARTESIAN_POINT ( 'NONE',  ( -18.62759615963255300, -10.81492255796106328, 84.16775706135234714 ) ) ;
#194469=CARTESIAN_POINT ( 'NONE',  ( -19.03943276465977164, 0.05219959533909376836, 101.2489096053143669 ) ) ;
#194470=CARTESIAN_POINT ( 'NONE',  ( 14.29746914071037800, 8.314922557961029526, 66.66775706135234714 ) ) ;
#194472=CARTESIAN_POINT ( 'NONE',  ( -5.153800228976607833, 19.02544592524334988, 42.70942372801901143 ) ) ;
#194473=CARTESIAN_POINT ( 'NONE',  ( -15.72974639402176322, -15.80617190586768395, 104.3760903946856899 ) ) ;
#194475=CARTESIAN_POINT ( 'NONE',  ( -15.49999999999999822, -5.500000000000000888, 20.00000000000000000 ) ) ;
#194476=CARTESIAN_POINT ( 'NONE',  ( 8.314922557961029526, -14.29746914071037800, 105.4177570613523613 ) ) ;
#194478=CARTESIAN_POINT ( 'NONE',  ( 4.483927247898790824, -16.52544592524335698, 90.20942372801903275 ) ) ;
#194479=CARTESIAN_POINT ( 'NONE',  ( 16.88567814943161238, 6.947325034625711382, 68.79001122652584854 ) ) ;
#194480=CARTESIAN_POINT ( 'NONE',  ( -14.29746914071037622, -8.314922557961029526, 69.16775706135234714 ) ) ;
#194482=CARTESIAN_POINT ( 'NONE',  ( -15.72974639402176322, -15.80617190586768395, 79.37609039468567573 ) ) ;
#194483=CARTESIAN_POINT ( 'NONE',  ( 9.474510206698729675, 16.51473224551082808, 92.08442372801900433 ) ) ;
#194484=CARTESIAN_POINT ( 'NONE',  ( 9.474510206698729675, 16.51473224551082808, 27.08442372801900433 ) ) ;
#194485=CARTESIAN_POINT ( 'NONE',  ( 19.02544592524343514, -5.153800228976328945, 68.54057627198103830 ) ) ;
#194486=CARTESIAN_POINT ( 'NONE',  ( 19.05341960407611168, 5.049401038298154454, 58.95724293864768129 ) ) ;
#194487=CARTESIAN_POINT ( 'NONE',  ( 17.50000000000000000, -5.500000000000000888, 23.29690382534171889 ) ) ;
#194488=CARTESIAN_POINT ( 'NONE',  ( 10.81492255796078972, 18.62759615963270932, 79.58224293864769550 ) ) ;
#194489=CARTESIAN_POINT ( 'NONE',  ( -15.72974639402197994, 15.80617190586746368, 30.62390960531436335 ) ) ;
#194490=CARTESIAN_POINT ( 'NONE',  ( 13.89961937509977652, -13.97604488694527269, 38.12390960531436690 ) ) ;
#194491=CARTESIAN_POINT ( 'NONE',  ( -12.06949235617739369, -12.14591786802326823, 64.37609039468568994 ) ) ;
#194493=CARTESIAN_POINT ( 'NONE',  ( -10.81492255796105439, 18.62759615963255655, 37.91775706135235424 ) ) ;
#194494=CARTESIAN_POINT ( 'NONE',  ( 4.379528057220339221, -16.55341960407611168, 62.70724293864769550 ) ) ;
#194496=CARTESIAN_POINT ( 'NONE',  ( -14.34966873604972548, 8.224510206698743886, 28.33442372801902209 ) ) ;
#194497=CARTESIAN_POINT ( 'NONE',  ( 5.049401038297881783, 19.05341960407617563, 52.29275706135234003 ) ) ;
#194498=CARTESIAN_POINT ( 'NONE',  ( 16.55341960407611168, 4.379528057220329451, 58.95724293864770971 ) ) ;
#194499=CARTESIAN_POINT ( 'NONE',  ( 5.823673210054444382, -21.52544592524334988, 25.20942372801901854 ) ) ;
#194500=CARTESIAN_POINT ( 'NONE',  ( -17.58332526062529411, 7.635886036038502134, 100.9233495955846678 ) ) ;
#194501=CARTESIAN_POINT ( 'NONE',  ( 0.05219959533907565091, 21.53943276465977519, 74.99890960531435269 ) ) ;
#194502=CARTESIAN_POINT ( 'NONE',  ( 9.564922557960805705, 16.46253265017160317, 89.58224293864769550 ) ) ;
#194503=CARTESIAN_POINT ( 'NONE',  ( -8.224510206698948167, 14.34966873604960824, 60.41557627198102409 ) ) ;
#194504=CARTESIAN_POINT ( 'NONE',  ( 9.564922557960805705, 16.46253265017160317, 114.5822429386476955 ) ) ;
#194506=CARTESIAN_POINT ( 'NONE',  ( -0.05219959533936034679, 19.03943276465977164, 72.50109039468566152 ) ) ;
#194507=CARTESIAN_POINT ( 'NONE',  ( -21.55341960407610458, -5.719274019375992779, 111.4572429386476813 ) ) ;
#194508=CARTESIAN_POINT ( 'NONE',  ( -16.51473224551069308, -9.474510206698971260, 61.66557627198103120 ) ) ;
#194509=CARTESIAN_POINT ( 'NONE',  ( -9.474510206698720793, -16.51473224551083518, 39.58442372801899722 ) ) ;
#194510=CARTESIAN_POINT ( 'NONE',  ( -19.03943276465977164, 0.05219959533909376836, 31.24890960531435979 ) ) ;
#194511=CARTESIAN_POINT ( 'NONE',  ( -10.81492255796105439, 18.62759615963255655, 67.91775706135234714 ) ) ;
#194513=CARTESIAN_POINT ( 'NONE',  ( -16.53943276465976808, 0.05219959533911058130, 36.24890960531435979 ) ) ;
#194514=CARTESIAN_POINT ( 'NONE',  ( -16.51473224551069308, -9.474510206698971260, 61.66557627198103120 ) ) ;
#194515=CARTESIAN_POINT ( 'NONE',  ( 10.72451020669898902, -18.67979575497178502, 77.91557627198102409 ) ) ;
#194516=CARTESIAN_POINT ( 'NONE',  ( 16.51473224551069308, 9.474510206698969483, 64.16557627198102409 ) ) ;
#194518=CARTESIAN_POINT ( 'NONE',  ( 21.53943276465977519, -0.05219959533907433946, 63.74890960531435979 ) ) ;
#194520=CARTESIAN_POINT ( 'NONE',  ( 18.62759615963255655, 10.81492255796105972, 96.66775706135234714 ) ) ;
#194522=CARTESIAN_POINT ( 'NONE',  ( -16.53943276465976808, -0.05219959533934237506, 98.75109039468568994 ) ) ;
#194523=CARTESIAN_POINT ( 'NONE',  ( 4.379528057220339221, -16.55341960407611168, 82.70724293864770971 ) ) ;
#194524=CARTESIAN_POINT ( 'NONE',  ( 13.97604488694548053, -13.89961937509957401, 95.62609039468563310 ) ) ;
#194526=CARTESIAN_POINT ( 'NONE',  ( 13.89961937509957401, 13.97604488694547697, 41.87609039468566152 ) ) ;
#194527=CARTESIAN_POINT ( 'NONE',  ( 14.34966873604972726, -8.224510206698740333, 100.8344237280190185 ) ) ;
#194529=CARTESIAN_POINT ( 'NONE',  ( 9.564922557961047289, -16.46253265017146816, 35.41775706135233293 ) ) ;
#194530=CARTESIAN_POINT ( 'NONE',  ( 19.03943276465977164, -0.05219959533909143690, 93.74890960531435269 ) ) ;
#194531=CARTESIAN_POINT ( 'NONE',  ( 15.80617190586746368, 15.72974639402197994, 59.37390960531436690 ) ) ;
#194533=CARTESIAN_POINT ( 'NONE',  ( -16.51473224551069308, -9.474510206698971260, 26.66557627198103120 ) ) ;
#194534=CARTESIAN_POINT ( 'NONE',  ( -5.719274019375665041, -21.55341960407619695, 99.79275706135234714 ) ) ;
#194535=CARTESIAN_POINT ( 'NONE',  ( 16.53943276465976808, 0.05219959533934440121, 81.25109039468568994 ) ) ;
#194536=CARTESIAN_POINT ( 'NONE',  ( -18.67979575497193778, 10.72451020669871902, 33.33442372801900433 ) ) ;
#194537=CARTESIAN_POINT ( 'NONE',  ( 16.53943276465976808, 0.05219959533934440121, 36.25109039468567573 ) ) ;
#194538=CARTESIAN_POINT ( 'NONE',  ( -0.05219959533909027116, -19.03943276465977164, 107.4989096053143527 ) ) ;
#194539=CARTESIAN_POINT ( 'NONE',  ( -16.51473224551069308, -9.474510206698971260, 36.66557627198102409 ) ) ;
#194540=CARTESIAN_POINT ( 'NONE',  ( -9.564922557960796823, -16.46253265017161027, 52.08224293864768839 ) ) ;
#194541=CARTESIAN_POINT ( 'NONE',  ( -12.14591786802326823, 12.06949235617739902, 33.12609039468569705 ) ) ;
#194542=CARTESIAN_POINT ( 'NONE',  ( -14.29746914071049879, 8.314922557960819915, 95.83224293864770971 ) ) ;
#194543=CARTESIAN_POINT ( 'NONE',  ( 16.52544592524335698, 4.483927247898782831, 101.4594237280190185 ) ) ;
#194544=CARTESIAN_POINT ( 'NONE',  ( -21.53943276465977519, -0.05219959533937600094, 38.75109039468567573 ) ) ;
#194545=CARTESIAN_POINT ( 'NONE',  ( 5.049401038298161559, -19.05341960407611168, 77.70724293864765286 ) ) ;
#194546=CARTESIAN_POINT ( 'NONE',  ( -13.89961937509977652, 13.97604488694528158, 65.62390960531436690 ) ) ;
#194547=CARTESIAN_POINT ( 'NONE',  ( 13.89961937509977652, -13.97604488694527269, 88.12390960531438111 ) ) ;
#194549=CARTESIAN_POINT ( 'NONE',  ( 14.29746914071049879, -8.314922557960816363, 28.33224293864769550 ) ) ;
#194550=CARTESIAN_POINT ( 'NONE',  ( 4.379528057220092307, 16.55341960407617563, 97.29275706135234714 ) ) ;
#194551=ORIENTED_EDGE ( 'NONE', *, *, #9460, .T. ) ;
#194552=CARTESIAN_POINT ( 'NONE',  ( -19.05341960407617563, 5.049401038297882671, 38.54275706135233293 ) ) ;
#194553=CARTESIAN_POINT ( 'NONE',  ( -13.97604488694527625, -13.89961937509977652, 106.8739096053143669 ) ) ;
#194554=CARTESIAN_POINT ( 'NONE',  ( 19.02544592524343514, -5.153800228976328945, 63.54057627198103830 ) ) ;
#194555=CARTESIAN_POINT ( 'NONE',  ( 0.05219959533936267826, -19.03943276465977164, 35.00109039468566863 ) ) ;
#194557=CARTESIAN_POINT ( 'NONE',  ( 12.06949235617739724, 12.14591786802326823, 41.87609039468568284 ) ) ;
#194558=CARTESIAN_POINT ( 'NONE',  ( -19.05341960407617563, 5.049401038297882671, 73.54275706135233293 ) ) ;
#194559=CARTESIAN_POINT ( 'NONE',  ( 16.52544592524335698, 4.483927247898782831, 51.45942372801901854 ) ) ;
#194561=CARTESIAN_POINT ( 'NONE',  ( -5.153800228976328057, -19.02544592524343514, 97.29057627198099567 ) ) ;
#194562=CARTESIAN_POINT ( 'NONE',  ( -21.55341960407610458, -5.719274019375992779, 106.4572429386477097 ) ) ;
#194563=CARTESIAN_POINT ( 'NONE',  ( -9.474510206698720793, -16.51473224551083518, 74.58442372801900433 ) ) ;
#194564=CARTESIAN_POINT ( 'NONE',  ( 9.474510206698971260, -16.51473224551069308, 102.9155762719810241 ) ) ;
#194565=CARTESIAN_POINT ( 'NONE',  ( -9.564922557960796823, -16.46253265017161027, 37.08224293864768839 ) ) ;
#194566=CARTESIAN_POINT ( 'NONE',  ( -16.46253265017160317, 9.564922557960807481, 80.83224293864769550 ) ) ;
#194567=CARTESIAN_POINT ( 'NONE',  ( 0.05219959533910956823, 16.53943276465976808, 34.99890960531435979 ) ) ;
#194568=CARTESIAN_POINT ( 'NONE',  ( -16.46253265017160317, 9.564922557960807481, 35.83224293864768839 ) ) ;
#194569=CARTESIAN_POINT ( 'NONE',  ( -13.89961937509957401, -13.97604488694547875, 49.37609039468567573 ) ) ;
#194570=CARTESIAN_POINT ( 'NONE',  ( -12.14591786802309592, -12.06949235617757132, 86.87390960531438111 ) ) ;
#194571=CARTESIAN_POINT ( 'NONE',  ( 5.153800228976615827, -19.02544592524334988, 20.20942372801899722 ) ) ;
#194572=CARTESIAN_POINT ( 'NONE',  ( -16.51473224551069308, -9.474510206698971260, 46.66557627198102409 ) ) ;
#194573=CARTESIAN_POINT ( 'NONE',  ( 5.823673210054125526, 21.52544592524343514, 44.79057627198103120 ) ) ;
#194574=CARTESIAN_POINT ( 'NONE',  ( 4.379528057220339221, -16.55341960407611168, 52.70724293864769550 ) ) ;
#194575=CARTESIAN_POINT ( 'NONE',  ( -15.72974639402176322, -15.80617190586768395, 109.3760903946857042 ) ) ;
#194576=CARTESIAN_POINT ( 'NONE',  ( 19.02544592524343514, -5.153800228976328945, 103.5405762719809957 ) ) ;
#194577=CARTESIAN_POINT ( 'NONE',  ( 19.05341960407611168, 5.049401038298154454, 108.9572429386477097 ) ) ;
#194578=CARTESIAN_POINT ( 'NONE',  ( 19.03943276465977164, -0.05219959533909143690, 33.74890960531435979 ) ) ;
#194579=CARTESIAN_POINT ( 'NONE',  ( 5.049401038298161559, -19.05341960407611168, 22.70724293864769194 ) ) ;
#194580=CARTESIAN_POINT ( 'NONE',  ( -16.55341960407611168, -4.379528057220339221, 81.45724293864769550 ) ) ;
#194581=CARTESIAN_POINT ( 'NONE',  ( 21.55341960407610458, 5.719274019375980345, 93.95724293864770971 ) ) ;
#194582=CARTESIAN_POINT ( 'NONE',  ( -16.46253265017160317, 9.564922557960807481, 100.8322429386477097 ) ) ;
#194583=CARTESIAN_POINT ( 'NONE',  ( -5.719274019375665041, -21.55341960407619695, 19.79275706135235069 ) ) ;
#194584=CARTESIAN_POINT ( 'NONE',  ( -9.564922557960796823, -16.46253265017161027, 92.08224293864769550 ) ) ;
#194586=CARTESIAN_POINT ( 'NONE',  ( -8.224510206698948167, 14.34966873604960824, 105.4155762719810383 ) ) ;
#194587=CARTESIAN_POINT ( 'NONE',  ( -5.049401038298153566, 19.05341960407611168, 70.20724293864769550 ) ) ;
#194588=CARTESIAN_POINT ( 'NONE',  ( 5.823673210054125526, 21.52544592524343514, 74.79057627198105251 ) ) ;
#194591=CARTESIAN_POINT ( 'NONE',  ( 21.52544592524344225, -5.823673210054117533, 28.54057627198103120 ) ) ;
#194592=CARTESIAN_POINT ( 'NONE',  ( 8.224510206698742110, 14.34966873604972548, 37.08442372801901143 ) ) ;
#194593=CARTESIAN_POINT ( 'NONE',  ( 14.34966873604960469, 8.224510206698951720, 94.16557627198103830 ) ) ;
#194594=CARTESIAN_POINT ( 'NONE',  ( 18.87075004821568669, -5.500000000000105693, 51.17408112101046669 ) ) ;
#194595=CARTESIAN_POINT ( 'NONE',  ( 19.05341960407611168, 5.049401038298154454, 88.95724293864769550 ) ) ;
#194596=CARTESIAN_POINT ( 'NONE',  ( -16.46253265017160317, 9.564922557960807481, 50.83224293864770260 ) ) ;
#194597=CARTESIAN_POINT ( 'NONE',  ( -16.52544592524342804, 4.483927247898546575, 76.04057627198102409 ) ) ;
#194598=CARTESIAN_POINT ( 'NONE',  ( -15.72974639402197994, 15.80617190586746368, 35.62390960531437401 ) ) ;
#194599=CARTESIAN_POINT ( 'NONE',  ( 14.29746914071049879, -8.314922557960816363, 58.33224293864768839 ) ) ;
#194600=CARTESIAN_POINT ( 'NONE',  ( 16.46253265017146816, 9.564922557961045513, 96.66775706135233293 ) ) ;
#194601=CARTESIAN_POINT ( 'NONE',  ( -21.55341960407619339, 5.719274019375674811, 73.54275706135234714 ) ) ;
#194603=CARTESIAN_POINT ( 'NONE',  ( -5.153800228976328057, -19.02544592524343514, 112.2905762719810099 ) ) ;
#194604=CARTESIAN_POINT ( 'NONE',  ( 0.05219959533934541429, -16.53943276465976808, 80.00109039468568994 ) ) ;
#194605=CARTESIAN_POINT ( 'NONE',  ( 19.03943276465977164, -0.05219959533909143690, 23.74890960531435269 ) ) ;
#194606=CARTESIAN_POINT ( 'NONE',  ( -5.153800228976328057, -19.02544592524343514, 72.29057627198102409 ) ) ;
#194607=CARTESIAN_POINT ( 'NONE',  ( 15.80617190586746368, 15.72974639402197994, 84.37390960531438111 ) ) ;
#194608=CARTESIAN_POINT ( 'NONE',  ( 4.379528057220092307, 16.55341960407617563, 32.29275706135235424 ) ) ;
#194609=CARTESIAN_POINT ( 'NONE',  ( 8.314922557960818139, 14.29746914071049879, 54.58224293864769550 ) ) ;
#194610=CARTESIAN_POINT ( 'NONE',  ( 10.81492255796106328, -18.62759615963255655, 75.41775706135233293 ) ) ;
#194611=CARTESIAN_POINT ( 'NONE',  ( 8.314922557961029526, -14.29746914071037800, 90.41775706135236135 ) ) ;
#194612=CARTESIAN_POINT ( 'NONE',  ( -10.81492255796078084, -18.62759615963271287, 27.08224293864769550 ) ) ;
#194615=CARTESIAN_POINT ( 'NONE',  ( 16.52544592524335698, 4.483927247898782831, 101.4594237280190185 ) ) ;
#194616=CARTESIAN_POINT ( 'NONE',  ( -16.53943276465976808, -0.05219959533934237506, 58.75109039468568994 ) ) ;
#194617=CARTESIAN_POINT ( 'NONE',  ( -19.02544592524342804, 5.153800228976336051, 66.04057627198103830 ) ) ;
#194619=CARTESIAN_POINT ( 'NONE',  ( -19.03943276465977164, 0.05219959533909376836, 86.24890960531436690 ) ) ;
#194620=CARTESIAN_POINT ( 'NONE',  ( -15.72974639402176322, -15.80617190586768395, 69.37609039468567573 ) ) ;
#194621=CARTESIAN_POINT ( 'NONE',  ( 8.224510206698742110, 14.34966873604972548, 82.08442372801901854 ) ) ;
#194622=CARTESIAN_POINT ( 'NONE',  ( 4.379528057220339221, -16.55341960407611168, 52.70724293864769550 ) ) ;
#194623=CARTESIAN_POINT ( 'NONE',  ( 16.51473224551069308, 9.474510206698969483, 54.16557627198103120 ) ) ;
#194624=CARTESIAN_POINT ( 'NONE',  ( 19.03943276465977164, -0.05219959533909143690, 43.74890960531435979 ) ) ;
#194626=( BOUNDED_CURVE ( )  B_SPLINE_CURVE ( 2, ( #144184, #5670, #67346, #190706, #21852, #52179, #37007, #83503, #150206, #75329, #45001, #137000, #90496 ),
 .UNSPECIFIED., .F., .T. ) 
 B_SPLINE_CURVE_WITH_KNOTS ( ( 3, 2, 2, 2, 2, 2, 3 ),
 ( 0.7919041206375715403, 0.7938596491228070429, 0.7982456140350877583, 0.8026315789473684736, 0.8070175438596490780, 0.8114035087719297934, 0.8133133574350752681 ),
 .UNSPECIFIED. ) 
 CURVE ( )  GEOMETRIC_REPRESENTATION_ITEM ( )  RATIONAL_B_SPLINE_CURVE ( ( 0.9831626618144007068, 0.9848076720550096308, 1.000000000000000000, 0.9659258262890683122, 1.000000000000000000, 0.9659258262890683122, 1.000000000000000000, 0.9659258262890683122, 1.000000000000000000, 0.9659258262890683122, 1.000000000000000000, 0.9851625545550091179, 0.9832469066685282089 ) ) 
 REPRESENTATION_ITEM ( '' )  );
#194627=CARTESIAN_POINT ( 'NONE',  ( 9.564922557961047289, -16.46253265017146816, 105.4177570613523471 ) ) ;
#194628=CARTESIAN_POINT ( 'NONE',  ( -14.34966873604960291, -8.224510206698953496, 106.6655762719810383 ) ) ;
#194629=CARTESIAN_POINT ( 'NONE',  ( -16.46253265017160317, 9.564922557960807481, 70.83224293864770971 ) ) ;
#194630=CARTESIAN_POINT ( 'NONE',  ( 0.05219959533936267826, -19.03943276465977164, 100.0010903946856757 ) ) ;
#194632=CARTESIAN_POINT ( 'NONE',  ( 21.53943276465977519, 0.05219959533937863772, 101.2510903946856757 ) ) ;
#194633=CARTESIAN_POINT ( 'NONE',  ( 16.53943276465976808, 0.05219959533934440121, 66.25109039468567573 ) ) ;
#194634=CARTESIAN_POINT ( 'NONE',  ( 16.51473224551083163, -9.474510206698727899, 95.83442372801900433 ) ) ;
#194635=CARTESIAN_POINT ( 'NONE',  ( 21.53943276465977519, -0.05219959533907433946, 63.74890960531435979 ) ) ;
#194636=CARTESIAN_POINT ( 'NONE',  ( -16.55341960407617563, 4.379528057220093196, 48.54275706135234714 ) ) ;
#194638=CARTESIAN_POINT ( 'NONE',  ( -0.05219959533936034679, 19.03943276465977164, 62.50109039468566863 ) ) ;
#194639=CARTESIAN_POINT ( 'NONE',  ( -10.72451020669870658, -18.67979575497194134, 99.58442372801900433 ) ) ;
#194640=CARTESIAN_POINT ( 'NONE',  ( 0.05219959533910956823, 16.53943276465976808, 114.9989096053143669 ) ) ;
#194641=CARTESIAN_POINT ( 'NONE',  ( -16.51473224551069308, -9.474510206698971260, 71.66557627198102409 ) ) ;
#194642=CARTESIAN_POINT ( 'NONE',  ( 14.29746914071049879, -8.314922557960816363, 58.33224293864768839 ) ) ;
#194643=CARTESIAN_POINT ( 'NONE',  ( 18.67979575497194134, -10.72451020669871369, 90.83442372801901854 ) ) ;
#194644=CARTESIAN_POINT ( 'NONE',  ( -5.049401038297874678, -19.05341960407617918, 49.79275706135231871 ) ) ;
#194645=CARTESIAN_POINT ( 'NONE',  ( -5.049401038297874678, -19.05341960407617918, 29.79275706135232227 ) ) ;
#194646=CARTESIAN_POINT ( 'NONE',  ( -15.72974639402197994, 15.80617190586746368, 25.62390960531435624 ) ) ;
#194647=CARTESIAN_POINT ( 'NONE',  ( -10.72451020669870658, -18.67979575497194134, 94.58442372801901854 ) ) ;
#194648=CARTESIAN_POINT ( 'NONE',  ( 5.153800228976335163, 19.02544592524342804, 74.79057627198103830 ) ) ;
#194650=CARTESIAN_POINT ( 'NONE',  ( -21.53943276465977519, -0.05219959533937600094, 98.75109039468568994 ) ) ;
#194651=CARTESIAN_POINT ( 'NONE',  ( 10.81492255796078972, 18.62759615963270932, 49.58224293864769550 ) ) ;
#194652=CARTESIAN_POINT ( 'NONE',  ( -13.97604488694527625, -13.89961937509977652, 86.87390960531436690 ) ) ;
#194653=CARTESIAN_POINT ( 'NONE',  ( -5.049401038297874678, -19.05341960407617918, 74.79275706135231871 ) ) ;
#194654=CARTESIAN_POINT ( 'NONE',  ( 13.89961937509977652, -13.97604488694527269, 38.12390960531436690 ) ) ;
#194655=CARTESIAN_POINT ( 'NONE',  ( 19.02544592524343514, -5.153800228976328945, 83.54057627198100988 ) ) ;
#194657=CARTESIAN_POINT ( 'NONE',  ( 0.05219959533936267826, -19.03943276465977164, 85.00109039468567573 ) ) ;
#194658=CARTESIAN_POINT ( 'NONE',  ( -8.224510206698735004, -14.34966873604973081, 44.58442372801901854 ) ) ;
#194659=CARTESIAN_POINT ( 'NONE',  ( 12.06949235617757843, -12.14591786802309237, 103.1239096053143811 ) ) ;
#194660=CARTESIAN_POINT ( 'NONE',  ( -5.153800228976328057, -19.02544592524343514, 77.29057627198099567 ) ) ;
#194661=CARTESIAN_POINT ( 'NONE',  ( 18.67979575497178502, 10.72451020669898547, 44.16557627198103120 ) ) ;
#194662=CARTESIAN_POINT ( 'NONE',  ( 8.314922557961029526, -14.29746914071037800, 25.41775706135235779 ) ) ;
#194663=CARTESIAN_POINT ( 'NONE',  ( 5.823673210054444382, -21.52544592524334988, 30.20942372801902565 ) ) ;
#194664=CARTESIAN_POINT ( 'NONE',  ( 5.823673210054444382, -21.52544592524334988, 85.20942372801901854 ) ) ;
#194665=CARTESIAN_POINT ( 'NONE',  ( 8.314922557961029526, -14.29746914071037800, 80.41775706135234714 ) ) ;
#194666=CARTESIAN_POINT ( 'NONE',  ( 5.049401038298161559, -19.05341960407611168, 72.70724293864768129 ) ) ;
#194667=CARTESIAN_POINT ( 'NONE',  ( -8.314922557961024197, 14.29746914071037800, 102.9177570613523756 ) ) ;
#194668=CARTESIAN_POINT ( 'NONE',  ( 19.02544592524334988, 5.153800228976608722, 51.45942372801900433 ) ) ;
#194669=CARTESIAN_POINT ( 'NONE',  ( 15.80617190586769283, -15.72974639402175789, 25.62609039468567929 ) ) ;
#194671=CARTESIAN_POINT ( 'NONE',  ( -14.34966873604960291, -8.224510206698953496, 76.66557627198103830 ) ) ;
#194672=CARTESIAN_POINT ( 'NONE',  ( 5.049401038298161559, -19.05341960407611168, 97.70724293864766707 ) ) ;
#194673=CARTESIAN_POINT ( 'NONE',  ( -12.06949235617739369, -12.14591786802326823, 104.3760903946856899 ) ) ;
#194674=CARTESIAN_POINT ( 'NONE',  ( -15.80617190586768217, 15.72974639402176855, 73.12609039468567573 ) ) ;
#194675=CARTESIAN_POINT ( 'NONE',  ( -14.29746914071037622, -8.314922557961029526, 34.16775706135234714 ) ) ;
#194676=CARTESIAN_POINT ( 'NONE',  ( -5.719274019375665041, -21.55341960407619695, 24.79275706135235779 ) ) ;
#194677=CARTESIAN_POINT ( 'NONE',  ( 8.224510206698953496, -14.34966873604960469, 67.91557627198102409 ) ) ;
#194679=CARTESIAN_POINT ( 'NONE',  ( -18.67979575497178146, -10.72451020669898902, 101.6655762719810383 ) ) ;
#194680=CARTESIAN_POINT ( 'NONE',  ( 8.224510206698953496, -14.34966873604960469, 52.91557627198103830 ) ) ;
#194681=CARTESIAN_POINT ( 'NONE',  ( -16.51473224551069308, -9.474510206698971260, 31.66557627198102054 ) ) ;
#194682=CARTESIAN_POINT ( 'NONE',  ( -18.67979575497178146, -10.72451020669898902, 26.66557627198103475 ) ) ;
#194683=CARTESIAN_POINT ( 'NONE',  ( 10.81492255796106328, -18.62759615963255655, 50.41775706135235424 ) ) ;
#194684=CARTESIAN_POINT ( 'NONE',  ( -8.314922557960811034, -14.29746914071050412, 62.08224293864769550 ) ) ;
#194685=CARTESIAN_POINT ( 'NONE',  ( 21.52544592524344225, -5.823673210054117533, 73.54057627198102409 ) ) ;
#194686=CARTESIAN_POINT ( 'NONE',  ( 5.153800228976335163, 19.02544592524342804, 79.79057627198102409 ) ) ;
#194687=CARTESIAN_POINT ( 'NONE',  ( 5.153800228976335163, 19.02544592524342804, 24.79057627198102765 ) ) ;
#194688=CARTESIAN_POINT ( 'NONE',  ( 0.05219959533936267826, -19.03943276465977164, 85.00109039468567573 ) ) ;
#194689=CARTESIAN_POINT ( 'NONE',  ( 21.52544592524334988, 5.823673210054432836, 61.45942372801901854 ) ) ;
#194690=CARTESIAN_POINT ( 'NONE',  ( -21.55341960407610458, -5.719274019375992779, 61.45724293864770260 ) ) ;
#194691=CARTESIAN_POINT ( 'NONE',  ( 5.049401038298161559, -19.05341960407611168, 42.70724293864767418 ) ) ;
#194692=CARTESIAN_POINT ( 'NONE',  ( 19.02544592524343514, -5.153800228976328945, 73.54057627198103830 ) ) ;
#194694=CARTESIAN_POINT ( 'NONE',  ( 16.52544592524335698, 4.483927247898782831, 56.45942372801902565 ) ) ;
#194695=CARTESIAN_POINT ( 'NONE',  ( 10.81492255796106328, -18.62759615963255655, 30.41775706135234358 ) ) ;
#194696=EDGE_CURVE ( 'NONE', #116638, #21815, #191379, .T. ) ;
#194697=CARTESIAN_POINT ( 'NONE',  ( -21.53943276465977519, -0.05219959533937600094, 63.75109039468568284 ) ) ;
#194698=CARTESIAN_POINT ( 'NONE',  ( 19.03943276465977164, -0.05219959533909143690, 98.74890960531436690 ) ) ;
#194699=CARTESIAN_POINT ( 'NONE',  ( -15.80617190586745835, -15.72974639402198527, 81.87390960531435269 ) ) ;
#194700=CARTESIAN_POINT ( 'NONE',  ( 5.823673210054444382, -21.52544592524334988, 30.20942372801902565 ) ) ;
#194701=CARTESIAN_POINT ( 'NONE',  ( 0.05219959533934541429, -16.53943276465976808, 45.00109039468568284 ) ) ;
#194702=CARTESIAN_POINT ( 'NONE',  ( -5.823673210054116645, -21.52544592524344225, 52.29057627198102409 ) ) ;
#194703=CARTESIAN_POINT ( 'NONE',  ( 10.81492255796106328, -18.62759615963255655, 110.4177570613523756 ) ) ;
#194704=CARTESIAN_POINT ( 'NONE',  ( -19.02544592524342804, 5.153800228976336051, 51.04057627198103120 ) ) ;
#194705=CARTESIAN_POINT ( 'NONE',  ( -19.03943276465977164, 0.05219959533909376836, 111.2489096053143669 ) ) ;
#194706=CARTESIAN_POINT ( 'NONE',  ( 19.02544592524343514, -5.153800228976328945, 88.54057627198102409 ) ) ;
#194708=CARTESIAN_POINT ( 'NONE',  ( 9.564922557961047289, -16.46253265017146816, 70.41775706135233293 ) ) ;
#194709=CARTESIAN_POINT ( 'NONE',  ( 15.80617190586746368, 15.72974639402197994, 44.37390960531435979 ) ) ;
#194710=CARTESIAN_POINT ( 'NONE',  ( -4.379528057220328563, 16.55341960407611168, 30.20724293864769550 ) ) ;
#194711=CARTESIAN_POINT ( 'NONE',  ( 0.05219959533936267826, -19.03943276465977164, 90.00109039468567573 ) ) ;
#194712=CARTESIAN_POINT ( 'NONE',  ( -16.62475595723695676, 7.163666690055236153, 60.52713351810466946 ) ) ;
#194713=CARTESIAN_POINT ( 'NONE',  ( 0.05219959533937995610, -21.53943276465977519, 110.0010903946856757 ) ) ;
#194714=CARTESIAN_POINT ( 'NONE',  ( -16.46253265017146816, -9.564922557961047289, 84.16775706135233293 ) ) ;
#194715=CARTESIAN_POINT ( 'NONE',  ( 19.02544592524334988, 5.153800228976608722, 46.45942372801899012 ) ) ;
#194717=CARTESIAN_POINT ( 'NONE',  ( -5.153800228976328057, -19.02544592524343514, 57.29057627198103120 ) ) ;
#194718=CARTESIAN_POINT ( 'NONE',  ( 4.379528057220339221, -16.55341960407611168, 47.70724293864770260 ) ) ;
#194719=CARTESIAN_POINT ( 'NONE',  ( 19.02544592524343514, -5.153800228976328945, 28.54057627198102409 ) ) ;
#194720=CARTESIAN_POINT ( 'NONE',  ( 8.314922557960818139, 14.29746914071049879, 44.58224293864769550 ) ) ;
#194722=CARTESIAN_POINT ( 'NONE',  ( 14.34966873604972726, -8.224510206698740333, 110.8344237280190043 ) ) ;
#194723=CARTESIAN_POINT ( 'NONE',  ( -5.049401038298153566, 19.05341960407611168, 55.20724293864769550 ) ) ;
#194724=CARTESIAN_POINT ( 'NONE',  ( 16.46253265017146816, 9.564922557961045513, 26.66775706135234003 ) ) ;
#194725=CARTESIAN_POINT ( 'NONE',  ( -8.224510206698735004, -14.34966873604973081, 34.58442372801900433 ) ) ;
#194726=CARTESIAN_POINT ( 'NONE',  ( 18.67979575497178502, 10.72451020669898547, 34.16557627198102409 ) ) ;
#194727=CARTESIAN_POINT ( 'NONE',  ( 21.55341960407619695, -5.719274019375665929, 96.04275706135236135 ) ) ;
#194729=CARTESIAN_POINT ( 'NONE',  ( 13.89961937509977652, -13.97604488694527269, 58.12390960531436690 ) ) ;
#194730=CARTESIAN_POINT ( 'NONE',  ( -9.564922557960796823, -16.46253265017161027, 112.0822429386476955 ) ) ;
#194731=CARTESIAN_POINT ( 'NONE',  ( 13.89961937509977652, -13.97604488694527269, 103.1239096053143527 ) ) ;
#194733=CARTESIAN_POINT ( 'NONE',  ( 15.72974639402176855, 15.80617190586768217, 21.87609039468567573 ) ) ;
#194734=CARTESIAN_POINT ( 'NONE',  ( -12.14591786802309592, -12.06949235617757132, 76.87390960531439532 ) ) ;
#194735=CARTESIAN_POINT ( 'NONE',  ( -21.53943276465977519, 0.05219959533907696930, 71.24890960531435269 ) ) ;
#194736=CARTESIAN_POINT ( 'NONE',  ( 16.46253265017160672, -9.564922557960803928, 68.33224293864770971 ) ) ;
#194737=CARTESIAN_POINT ( 'NONE',  ( 5.049401038298161559, -19.05341960407611168, 77.70724293864765286 ) ) ;
#194738=CARTESIAN_POINT ( 'NONE',  ( -18.62759615963255300, -10.81492255796106328, 19.16775706135234714 ) ) ;
#194739=ORIENTED_EDGE ( 'NONE', *, *, #68626, .T. ) ;
#194740=CARTESIAN_POINT ( 'NONE',  ( 9.474510206698971260, -16.51473224551069308, 67.91557627198102409 ) ) ;
#194741=CARTESIAN_POINT ( 'NONE',  ( -12.14591786802309592, -12.06949235617757132, 101.8739096053143811 ) ) ;
#194743=CARTESIAN_POINT ( 'NONE',  ( -13.97604488694527625, -13.89961937509977652, 61.87390960531435979 ) ) ;
#194744=CARTESIAN_POINT ( 'NONE',  ( 16.46253265017146816, 9.564922557961045513, 96.66775706135233293 ) ) ;
#194745=CARTESIAN_POINT ( 'NONE',  ( 14.34966873604960469, 8.224510206698951720, 94.16557627198103830 ) ) ;
#194746=CARTESIAN_POINT ( 'NONE',  ( -21.55341960407619339, 5.719274019375674811, 73.54275706135234714 ) ) ;
#194747=CARTESIAN_POINT ( 'NONE',  ( 9.564922557960805705, 16.46253265017160317, 44.58224293864769550 ) ) ;
#194748=CARTESIAN_POINT ( 'NONE',  ( 18.62759615963255655, 10.81492255796105972, 21.66775706135235069 ) ) ;
#194749=CARTESIAN_POINT ( 'NONE',  ( -16.55341960407611168, -4.379528057220339221, 96.45724293864770971 ) ) ;
#194751=CARTESIAN_POINT ( 'NONE',  ( 19.03943276465977164, -0.05219959533909143690, 73.74890960531435269 ) ) ;
#194752=CARTESIAN_POINT ( 'NONE',  ( 16.52216118717204907, 7.221426719304526287, 113.5759902104699393 ) ) ;
#194753=CARTESIAN_POINT ( 'NONE',  ( -19.03943276465977164, -0.05219959533935918106, 113.7510903946856757 ) ) ;
#194754=CARTESIAN_POINT ( 'NONE',  ( -21.52544592524343514, 5.823673210054127303, 36.04057627198102409 ) ) ;
#194755=CARTESIAN_POINT ( 'NONE',  ( -15.72974639402176322, -15.80617190586768395, 54.37609039468568994 ) ) ;
#194756=CARTESIAN_POINT ( 'NONE',  ( 5.153800228976335163, 19.02544592524342804, 94.79057627198103830 ) ) ;
#194757=CARTESIAN_POINT ( 'NONE',  ( 5.049401038297881783, 19.05341960407617563, 77.29275706135231871 ) ) ;
#194758=CARTESIAN_POINT ( 'NONE',  ( -5.049401038298153566, 19.05341960407611168, 70.20724293864769550 ) ) ;
#194759=CARTESIAN_POINT ( 'NONE',  ( -8.224510206698948167, 14.34966873604960824, 80.41557627198103830 ) ) ;
#194760=CARTESIAN_POINT ( 'NONE',  ( 19.05341960407611168, 5.049401038298154454, 98.95724293864766707 ) ) ;
#194761=CARTESIAN_POINT ( 'NONE',  ( 8.224510206698953496, -14.34966873604960469, 77.91557627198102409 ) ) ;
#194762=CARTESIAN_POINT ( 'NONE',  ( -9.564922557960796823, -16.46253265017161027, 102.0822429386477097 ) ) ;
#194763=CARTESIAN_POINT ( 'NONE',  ( 16.53943276465976808, -0.05219959533910856209, 48.74890960531435979 ) ) ;
#194764=CARTESIAN_POINT ( 'NONE',  ( 5.153800228976335163, 19.02544592524342804, 29.79057627198102409 ) ) ;
#194766=CARTESIAN_POINT ( 'NONE',  ( -21.55341960407619339, 5.719274019375674811, 53.54275706135234714 ) ) ;
#194767=CARTESIAN_POINT ( 'NONE',  ( -5.049401038297874678, -19.05341960407617918, 84.79275706135233293 ) ) ;
#194768=CARTESIAN_POINT ( 'NONE',  ( 4.483927247898545687, 16.52544592524342804, 49.79057627198102409 ) ) ;
#194769=CARTESIAN_POINT ( 'NONE',  ( 15.80617190586746368, 15.72974639402197994, 99.37390960531436690 ) ) ;
#194770=CARTESIAN_POINT ( 'NONE',  ( 15.72974639402199770, -15.80617190586745480, 33.12390960531435979 ) ) ;
#194771=CARTESIAN_POINT ( 'NONE',  ( -16.52544592524342804, 4.483927247898546575, 86.04057627198102409 ) ) ;
#194772=CARTESIAN_POINT ( 'NONE',  ( -13.97604488694527625, -13.89961937509977652, 41.87390960531435979 ) ) ;
#194773=CARTESIAN_POINT ( 'NONE',  ( -14.34966873604960291, -8.224510206698953496, 21.66557627198102409 ) ) ;
#194774=CARTESIAN_POINT ( 'NONE',  ( -8.224510206698735004, -14.34966873604973081, 94.58442372801901854 ) ) ;
#194775=CARTESIAN_POINT ( 'NONE',  ( 14.34966873604972726, -8.224510206698740333, 65.83442372801900433 ) ) ;
#194776=CARTESIAN_POINT ( 'NONE',  ( -13.89961937509957401, -13.97604488694547875, 19.37609039468566507 ) ) ;
#194777=CARTESIAN_POINT ( 'NONE',  ( 19.02544592524343514, -5.153800228976328945, 98.54057627198100988 ) ) ;
#194778=CARTESIAN_POINT ( 'NONE',  ( -5.153800228976328057, -19.02544592524343514, 77.29057627198099567 ) ) ;
#194779=CARTESIAN_POINT ( 'NONE',  ( -4.379528057220086978, -16.55341960407618274, 89.79275706135236135 ) ) ;
#194780=CARTESIAN_POINT ( 'NONE',  ( 16.51473224551069308, 9.474510206698969483, 34.16557627198102409 ) ) ;
#194781=CARTESIAN_POINT ( 'NONE',  ( 14.34966873604960469, 8.224510206698951720, 49.16557627198102409 ) ) ;
#194783=CARTESIAN_POINT ( 'NONE',  ( -16.46253265017160317, 9.564922557960807481, 100.8322429386477097 ) ) ;
#194784=CARTESIAN_POINT ( 'NONE',  ( -10.81492255796078084, -18.62759615963271287, 47.08224293864770260 ) ) ;
#194785=CARTESIAN_POINT ( 'NONE',  ( -16.53943276465976808, 0.05219959533911058130, 76.24890960531435269 ) ) ;
#194787=CARTESIAN_POINT ( 'NONE',  ( 16.53943276465976808, -0.05219959533910856209, 63.74890960531435979 ) ) ;
#194789=CARTESIAN_POINT ( 'NONE',  ( -16.46253265017146816, -9.564922557961047289, 69.16775706135233293 ) ) ;
#194790=CARTESIAN_POINT ( 'NONE',  ( 9.564922557960805705, 16.46253265017160317, 99.58224293864770971 ) ) ;
#194791=CARTESIAN_POINT ( 'NONE',  ( -13.89961937509957401, -13.97604488694547875, 74.37609039468566152 ) ) ;
#194792=CARTESIAN_POINT ( 'NONE',  ( -13.89961937509957401, -13.97604488694547697, 94.37609039468566152 ) ) ;
#194793=CARTESIAN_POINT ( 'NONE',  ( 19.05341960407617918, -5.049401038297876454, 106.0427570613523471 ) ) ;
#194794=CARTESIAN_POINT ( 'NONE',  ( -8.224510206698735004, -14.34966873604973081, 89.58442372801901854 ) ) ;
#194795=CARTESIAN_POINT ( 'NONE',  ( 13.97604488694527802, 13.89961937509977652, 34.37390960531436690 ) ) ;
#194796=CARTESIAN_POINT ( 'NONE',  ( -15.72974639402197994, 15.80617190586746368, 40.62390960531435269 ) ) ;
#194797=CARTESIAN_POINT ( 'NONE',  ( 21.52544592524334988, 5.823673210054432836, 61.45942372801901854 ) ) ;
#194798=CARTESIAN_POINT ( 'NONE',  ( -12.14591786802326823, 12.06949235617739902, 23.12609039468567573 ) ) ;
#194800=CARTESIAN_POINT ( 'NONE',  ( -19.05341960407611168, -5.049401038298163336, 76.45724293864769550 ) ) ;
#194801=CARTESIAN_POINT ( 'NONE',  ( 8.314922557960818139, 14.29746914071049879, 74.58224293864768129 ) ) ;
#194802=CARTESIAN_POINT ( 'NONE',  ( -19.05341960407611168, -5.049401038298163336, 71.45724293864766707 ) ) ;
#194804=CARTESIAN_POINT ( 'NONE',  ( -19.03943276465977164, 0.05219959533909376836, 91.24890960531436690 ) ) ;
#194806=CARTESIAN_POINT ( 'NONE',  ( 5.049401038297881783, 19.05341960407617563, 92.29275706135234714 ) ) ;
#194807=CARTESIAN_POINT ( 'NONE',  ( -15.72974639402197994, 15.80617190586746368, 70.62390960531436690 ) ) ;
#194808=CARTESIAN_POINT ( 'NONE',  ( 16.51473224551069308, 9.474510206698969483, 34.16557627198102409 ) ) ;
#194809=CARTESIAN_POINT ( 'NONE',  ( -13.89961937509957401, -13.97604488694547875, 59.37609039468566863 ) ) ;
#194810=CARTESIAN_POINT ( 'NONE',  ( -19.05341960407611168, -5.049401038298163336, 61.45724293864769550 ) ) ;
#194811=CARTESIAN_POINT ( 'NONE',  ( -19.03943276465977164, 0.05219959533909376836, 86.24890960531436690 ) ) ;
#194814=CARTESIAN_POINT ( 'NONE',  ( -21.53943276465977519, 0.05219959533907696930, 86.24890960531436690 ) ) ;
#194815=CARTESIAN_POINT ( 'NONE',  ( 8.224510206698953496, -14.34966873604960469, 97.91557627198103830 ) ) ;
#194816=CARTESIAN_POINT ( 'NONE',  ( -16.51473224551082808, 9.474510206698731452, 53.33442372801900433 ) ) ;
#194817=CARTESIAN_POINT ( 'NONE',  ( -15.80617190586745835, -15.72974639402198527, 86.87390960531438111 ) ) ;
#194818=B_SPLINE_CURVE_WITH_KNOTS ( 'NONE', 3,
 ( #147276, #163450, #180635, #161440, #103772, #24948, #84578, #164455, #165451, #25949, #87592, #26948, #88589, #150288, #11783, #107719, #78374, #184584, #29909, #152255, #154242, #15733 ),
 .UNSPECIFIED., .F., .F.,
 ( 4, 2, 2, 2, 2, 2, 2, 2, 2, 2, 4 ),
 ( 8.673617379884035472E-18, 0.001309639967555159719, 0.001964459951332734374, 0.002291869943221526255, 0.002455574939165928051, 0.002619279935110330280, 0.002782984931054732075, 0.002946689926999134304, 0.003274099918887952640, 0.003928919902665601455, 0.005238559870220891278 ),
 .UNSPECIFIED. ) ;
#194819=CARTESIAN_POINT ( 'NONE',  ( -5.719274019375978568, 21.55341960407610458, 70.20724293864769550 ) ) ;
#194820=CARTESIAN_POINT ( 'NONE',  ( -4.379528057220328563, 16.55341960407611168, 30.20724293864769550 ) ) ;
#194821=CARTESIAN_POINT ( 'NONE',  ( 5.719274019375673035, 21.55341960407619339, 102.2927570613523613 ) ) ;
#194822=CARTESIAN_POINT ( 'NONE',  ( -16.55341960407617563, 4.379528057220093196, 48.54275706135234714 ) ) ;
#194823=CARTESIAN_POINT ( 'NONE',  ( -13.89961937509977652, 13.97604488694528158, 80.62390960531436690 ) ) ;
#194824=CARTESIAN_POINT ( 'NONE',  ( -19.05341960407611168, -5.049401038298163336, 26.45724293864769550 ) ) ;
#194825=CARTESIAN_POINT ( 'NONE',  ( -10.72451020669870658, -18.67979575497194134, 44.58442372801901854 ) ) ;
#194826=CARTESIAN_POINT ( 'NONE',  ( 15.72974639402176855, 15.80617190586768217, 56.87609039468568994 ) ) ;
#194827=CARTESIAN_POINT ( 'NONE',  ( -9.564922557960796823, -16.46253265017161027, 42.08224293864769550 ) ) ;
#194828=CARTESIAN_POINT ( 'NONE',  ( 0.05219959533937995610, -21.53943276465977519, 20.00109039468568639 ) ) ;
#194829=CARTESIAN_POINT ( 'NONE',  ( 19.05341960407617918, -5.049401038297876454, 66.04275706135233293 ) ) ;
#194830=CARTESIAN_POINT ( 'NONE',  ( 9.474510206698729675, 16.51473224551082808, 67.08442372801900433 ) ) ;
#194831=CARTESIAN_POINT ( 'NONE',  ( -12.14591786802326823, 12.06949235617739902, 28.12609039468568284 ) ) ;
#194832=CARTESIAN_POINT ( 'NONE',  ( -0.05219959533909027116, -19.03943276465977164, 27.49890960531435624 ) ) ;
#194833=CARTESIAN_POINT ( 'NONE',  ( 12.06949235617739724, 12.14591786802326823, 66.87609039468568994 ) ) ;
#194834=CARTESIAN_POINT ( 'NONE',  ( 13.89961937509977652, -13.97604488694527269, 43.12390960531434558 ) ) ;
#194836=CARTESIAN_POINT ( 'NONE',  ( 5.153800228976335163, 19.02544592524342804, 99.79057627198102409 ) ) ;
#194837=CARTESIAN_POINT ( 'NONE',  ( 13.97604488694527802, 13.89961937509977652, 29.37390960531435979 ) ) ;
#194838=CARTESIAN_POINT ( 'NONE',  ( 18.62759615963271287, -10.81492255796078972, 78.33224293864770971 ) ) ;
#194839=CARTESIAN_POINT ( 'NONE',  ( -12.06949235617739369, -12.14591786802326823, 64.37609039468568994 ) ) ;
#194840=CARTESIAN_POINT ( 'NONE',  ( -10.81492255796105439, 18.62759615963255655, 107.9177570613523471 ) ) ;
#194841=CARTESIAN_POINT ( 'NONE',  ( -5.153800228976328057, -19.02544592524343514, 42.29057627198101699 ) ) ;
#194842=CARTESIAN_POINT ( 'NONE',  ( 8.224510206698953496, -14.34966873604960469, 37.91557627198102409 ) ) ;
#194843=CARTESIAN_POINT ( 'NONE',  ( -4.379528057220328563, 16.55341960407611168, 70.20724293864769550 ) ) ;
#194844=B_SPLINE_CURVE_WITH_KNOTS ( 'NONE', 3,
 ( #136674, #41705, #118546, #105346, #198356, #152834 ),
 .UNSPECIFIED., .F., .F.,
 ( 4, 2, 4 ),
 ( 0.003239945802372208323, 0.003620412082092058781, 0.004000878361811908805 ),
 .UNSPECIFIED. ) ;
#194845=CARTESIAN_POINT ( 'NONE',  ( -19.05341960407611168, -5.049401038298163336, 71.45724293864766707 ) ) ;
#194846=CARTESIAN_POINT ( 'NONE',  ( 5.719274019375673035, 21.55341960407619339, 37.29275706135235424 ) ) ;
#194847=CARTESIAN_POINT ( 'NONE',  ( -9.564922557960796823, -16.46253265017161027, 77.08224293864769550 ) ) ;
#194849=CARTESIAN_POINT ( 'NONE',  ( 10.81492255796106328, -18.62759615963255655, 90.41775706135236135 ) ) ;
#194850=CARTESIAN_POINT ( 'NONE',  ( 16.52544592524335698, 4.483927247898782831, 61.45942372801901854 ) ) ;
#194851=CARTESIAN_POINT ( 'NONE',  ( 19.02544592524343514, -5.153800228976328945, 103.5405762719809957 ) ) ;
#194852=CARTESIAN_POINT ( 'NONE',  ( 16.52544592524342804, -4.483927247898539470, 33.54057627198102409 ) ) ;
#194853=CARTESIAN_POINT ( 'NONE',  ( 19.05341960407611168, 5.049401038298154454, 33.95724293864769550 ) ) ;
#194854=CARTESIAN_POINT ( 'NONE',  ( -12.06949235617739369, -12.14591786802326823, 54.37609039468568994 ) ) ;
#194855=CARTESIAN_POINT ( 'NONE',  ( 12.06949235617757843, -12.14591786802309237, 53.12390960531436690 ) ) ;
#194856=CARTESIAN_POINT ( 'NONE',  ( 5.049401038298161559, -19.05341960407611168, 107.7072429386476955 ) ) ;
#194857=CARTESIAN_POINT ( 'NONE',  ( -15.72974639402197994, 15.80617190586746368, 25.62390960531435624 ) ) ;
#194858=CARTESIAN_POINT ( 'NONE',  ( -21.52544592524334988, -5.823673210054445271, 108.9594237280190185 ) ) ;
#194859=CARTESIAN_POINT ( 'NONE',  ( 0.05219959533910956823, 16.53943276465976808, 89.99890960531438111 ) ) ;
#194860=CARTESIAN_POINT ( 'NONE',  ( 13.89961937509977652, -13.97604488694527269, 98.12390960531433848 ) ) ;
#194862=CARTESIAN_POINT ( 'NONE',  ( 8.224510206698742110, 14.34966873604972548, 57.08442372801901854 ) ) ;
#194863=CARTESIAN_POINT ( 'NONE',  ( 19.02544592524343514, -5.153800228976328945, 58.54057627198102409 ) ) ;
#194864=CARTESIAN_POINT ( 'NONE',  ( 17.50000000000000355, -5.499999999999992006, 26.21769037696436300 ) ) ;
#194865=CARTESIAN_POINT ( 'NONE',  ( -19.02544592524334988, -5.153800228976617603, 53.95942372801898301 ) ) ;
#194866=CARTESIAN_POINT ( 'NONE',  ( 14.34966873604972726, -8.224510206698740333, 75.83442372801900433 ) ) ;
#194867=CARTESIAN_POINT ( 'NONE',  ( 5.049401038297881783, 19.05341960407617563, 97.29275706135233293 ) ) ;
#194868=CARTESIAN_POINT ( 'NONE',  ( 0.05219959533937995610, -21.53943276465977519, 60.00109039468568284 ) ) ;
#194869=CARTESIAN_POINT ( 'NONE',  ( 9.564922557960805705, 16.46253265017160317, 79.58224293864769550 ) ) ;
#194870=CARTESIAN_POINT ( 'NONE',  ( 18.67979575497178502, 10.72451020669898547, 89.16557627198102409 ) ) ;
#194871=CARTESIAN_POINT ( 'NONE',  ( 14.29746914071049879, -8.314922557960816363, 103.3322429386476955 ) ) ;
#194872=CARTESIAN_POINT ( 'NONE',  ( 13.97604488694548053, -13.89961937509957401, 65.62609039468567573 ) ) ;
#194873=CARTESIAN_POINT ( 'NONE',  ( 5.719274019375991003, -21.55341960407610458, 62.70724293864769550 ) ) ;
#194874=CARTESIAN_POINT ( 'NONE',  ( 5.049401038297881783, 19.05341960407617563, 47.29275706135231161 ) ) ;
#194875=CARTESIAN_POINT ( 'NONE',  ( -19.02544592524342804, 5.153800228976336051, 116.0405762719810383 ) ) ;
#194876=CARTESIAN_POINT ( 'NONE',  ( -15.72974639402197994, 15.80617190586746368, 95.62390960531436690 ) ) ;
#194877=CARTESIAN_POINT ( 'NONE',  ( -19.36337904590690684, 5.499999999999947597, 55.41494137495620009 ) ) ;
#194878=CARTESIAN_POINT ( 'NONE',  ( 13.97604488694527802, 13.89961937509977652, 69.37390960531436690 ) ) ;
#194880=CARTESIAN_POINT ( 'NONE',  ( 8.224510206698742110, 14.34966873604972548, 22.08442372801901143 ) ) ;
#194881=CARTESIAN_POINT ( 'NONE',  ( 16.46253265017146816, 9.564922557961045513, 96.66775706135233293 ) ) ;
#194882=CARTESIAN_POINT ( 'NONE',  ( 16.46253265017160672, -9.564922557960803928, 53.33224293864768839 ) ) ;
#194883=CARTESIAN_POINT ( 'NONE',  ( -19.03943276465977164, 0.05219959533909376836, 116.2489096053143669 ) ) ;
#194884=CARTESIAN_POINT ( 'NONE',  ( 0.05219959533907565091, 21.53943276465977519, 84.99890960531436690 ) ) ;
#194885=CARTESIAN_POINT ( 'NONE',  ( 16.53943276465976808, -0.05219959533910856209, 53.74890960531437401 ) ) ;
#194886=CARTESIAN_POINT ( 'NONE',  ( -18.62759615963255300, -10.81492255796106328, 74.16775706135231871 ) ) ;
#194887=CARTESIAN_POINT ( 'NONE',  ( 16.52544592524335698, 4.483927247898782831, 26.45942372801901854 ) ) ;
#194888=CARTESIAN_POINT ( 'NONE',  ( -9.564922557961040184, 16.46253265017147172, 22.91775706135233648 ) ) ;
#194889=CARTESIAN_POINT ( 'NONE',  ( 12.14591786802309770, 12.06949235617756955, 34.37390960531435979 ) ) ;
#194890=CARTESIAN_POINT ( 'NONE',  ( -21.52544592524343514, 5.823673210054127303, 116.0405762719810383 ) ) ;
#194891=CARTESIAN_POINT ( 'NONE',  ( -14.29746914071049879, 8.314922557960819915, 50.83224293864770971 ) ) ;
#194892=CARTESIAN_POINT ( 'NONE',  ( 13.97604488694548053, -13.89961937509957401, 95.62609039468563310 ) ) ;
#194893=CARTESIAN_POINT ( 'NONE',  ( 16.51473224551083163, -9.474510206698727899, 70.83442372801900433 ) ) ;
#194894=CARTESIAN_POINT ( 'NONE',  ( -5.719274019375665041, -21.55341960407619695, 64.79275706135234714 ) ) ;
#194895=CARTESIAN_POINT ( 'NONE',  ( -13.89961937509957401, -13.97604488694547875, 49.37609039468567573 ) ) ;
#194896=CARTESIAN_POINT ( 'NONE',  ( -4.483927247898539470, -16.52544592524342804, 112.2905762719810241 ) ) ;
#194897=CARTESIAN_POINT ( 'NONE',  ( 18.67979575497178502, 10.72451020669898547, 44.16557627198103120 ) ) ;
#194898=CARTESIAN_POINT ( 'NONE',  ( -14.29746914071049879, 8.314922557960819915, 55.83224293864770260 ) ) ;
#194899=CARTESIAN_POINT ( 'NONE',  ( -17.50000000000000711, -5.500000000000025757, 51.28230962303570095 ) ) ;
#194900=CARTESIAN_POINT ( 'NONE',  ( 21.55341960407619695, -5.719274019375665929, 111.0427570613523613 ) ) ;
#194901=CARTESIAN_POINT ( 'NONE',  ( 16.53943276465976808, 0.05219959533934440121, 91.25109039468568994 ) ) ;
#194902=CARTESIAN_POINT ( 'NONE',  ( -12.06949235617756955, 12.14591786802309770, 35.62390960531437401 ) ) ;
#194903=CARTESIAN_POINT ( 'NONE',  ( 0.05219959533937995610, -21.53943276465977519, 80.00109039468568994 ) ) ;
#194904=CARTESIAN_POINT ( 'NONE',  ( -21.55341960407619339, 5.719274019375674811, 68.54275706135234714 ) ) ;
#194905=CARTESIAN_POINT ( 'NONE',  ( -10.81492255796078084, -18.62759615963271287, 77.08224293864769550 ) ) ;
#194906=CARTESIAN_POINT ( 'NONE',  ( 16.51473224551069308, 9.474510206698969483, 44.16557627198103120 ) ) ;
#194907=CARTESIAN_POINT ( 'NONE',  ( -10.81492255796105439, 18.62759615963255655, 57.91775706135234714 ) ) ;
#194908=CARTESIAN_POINT ( 'NONE',  ( -13.89961937509977652, 13.97604488694528158, 40.62390960531435979 ) ) ;
#194909=CARTESIAN_POINT ( 'NONE',  ( 5.153800228976335163, 19.02544592524342804, 49.79057627198100988 ) ) ;
#194910=CARTESIAN_POINT ( 'NONE',  ( -4.483927247898539470, -16.52544592524342804, 97.29057627198105251 ) ) ;
#194911=CARTESIAN_POINT ( 'NONE',  ( 0.05219959533909260263, 19.03943276465977164, 79.99890960531436690 ) ) ;
#194912=CARTESIAN_POINT ( 'NONE',  ( -8.224510206698948167, 14.34966873604960824, 45.41557627198103830 ) ) ;
#194913=CARTESIAN_POINT ( 'NONE',  ( 16.55341960407611168, 4.379528057220329451, 103.9572429386476813 ) ) ;
#194914=CARTESIAN_POINT ( 'NONE',  ( -21.52544592524343514, 5.823673210054127303, 66.04057627198103830 ) ) ;
#194915=CARTESIAN_POINT ( 'NONE',  ( -15.72974639402197994, 15.80617190586746368, 115.6239096053143669 ) ) ;
#194916=CARTESIAN_POINT ( 'NONE',  ( -13.89961937509977652, 13.97604488694528158, 115.6239096053143669 ) ) ;
#194917=CARTESIAN_POINT ( 'NONE',  ( 9.564922557960805705, 16.46253265017160317, 84.58224293864769550 ) ) ;
#194918=CARTESIAN_POINT ( 'NONE',  ( -0.05219959533936034679, 19.03943276465977164, 112.5010903946856757 ) ) ;
#194919=CARTESIAN_POINT ( 'NONE',  ( 15.72974639402199770, -15.80617190586745480, 73.12390960531436690 ) ) ;
#194920=CARTESIAN_POINT ( 'NONE',  ( 5.719274019375673035, 21.55341960407619339, 92.29275706135236135 ) ) ;
#194921=CARTESIAN_POINT ( 'NONE',  ( -16.46253265017160317, 9.564922557960807481, 80.83224293864769550 ) ) ;
#194922=CARTESIAN_POINT ( 'NONE',  ( -10.72451020669898014, 18.67979575497178502, 110.4155762719810383 ) ) ;
#194924=CARTESIAN_POINT ( 'NONE',  ( 16.51473224551069308, 9.474510206698969483, 114.1655762719810241 ) ) ;
#194925=CARTESIAN_POINT ( 'NONE',  ( 16.55341960407618274, -4.379528057220086978, 91.04275706135236135 ) ) ;
#194926=CARTESIAN_POINT ( 'NONE',  ( 21.53943276465977519, 0.05219959533937863772, 66.25109039468567573 ) ) ;
#194927=CARTESIAN_POINT ( 'NONE',  ( -5.719274019375665041, -21.55341960407619695, 94.79275706135234714 ) ) ;
#194928=CARTESIAN_POINT ( 'NONE',  ( 16.53943276465976808, 0.05219959533934440121, 61.25109039468567573 ) ) ;
#194929=CARTESIAN_POINT ( 'NONE',  ( 18.67979575497194134, -10.72451020669871369, 30.83442372801902209 ) ) ;
#194930=CARTESIAN_POINT ( 'NONE',  ( 16.46253265017160672, -9.564922557960803928, 113.3322429386476955 ) ) ;
#194931=CARTESIAN_POINT ( 'NONE',  ( 10.81492255796106328, -18.62759615963255655, 95.41775706135234714 ) ) ;
#194932=CARTESIAN_POINT ( 'NONE',  ( -5.153800228976328057, -19.02544592524343514, 97.29057627198099567 ) ) ;
#194933=CARTESIAN_POINT ( 'NONE',  ( -15.72974639402197994, 15.80617190586746368, 90.62390960531436690 ) ) ;
#194934=CARTESIAN_POINT ( 'NONE',  ( -9.564922557961040184, 16.46253265017147172, 57.91775706135233293 ) ) ;
#194936=CARTESIAN_POINT ( 'NONE',  ( 21.52544592524344225, -5.823673210054117533, 58.54057627198103120 ) ) ;
#194937=CARTESIAN_POINT ( 'NONE',  ( -16.46253265017160317, 9.564922557960807481, 90.83224293864769550 ) ) ;
#194938=CARTESIAN_POINT ( 'NONE',  ( -14.34966873604960291, -8.224510206698953496, 36.66557627198103120 ) ) ;
#194940=CARTESIAN_POINT ( 'NONE',  ( 16.46253265017146816, 9.564922557961045513, 76.66775706135234714 ) ) ;
#194942=CARTESIAN_POINT ( 'NONE',  ( -9.564922557961040184, 16.46253265017147172, 112.9177570613523329 ) ) ;
#194943=CARTESIAN_POINT ( 'NONE',  ( -21.52544592524343514, 5.823673210054127303, 91.04057627198103830 ) ) ;
#194944=CARTESIAN_POINT ( 'NONE',  ( 14.34966873604960469, 8.224510206698951720, 69.16557627198102409 ) ) ;
#194945=CARTESIAN_POINT ( 'NONE',  ( -8.224510206698735004, -14.34966873604973081, 24.58442372801901499 ) ) ;
#194946=CARTESIAN_POINT ( 'NONE',  ( 16.51473224551069308, 9.474510206698969483, 49.16557627198102409 ) ) ;
#194947=CARTESIAN_POINT ( 'NONE',  ( -5.719274019375978568, 21.55341960407610458, 110.2072429386477239 ) ) ;
#194948=CARTESIAN_POINT ( 'NONE',  ( 13.97604488694548053, -13.89961937509957401, 85.62609039468568994 ) ) ;
#194949=CARTESIAN_POINT ( 'NONE',  ( 16.51473224551069308, 9.474510206698969483, 94.16557627198103830 ) ) ;
#194950=CARTESIAN_POINT ( 'NONE',  ( 9.564922557960805705, 16.46253265017160317, 69.58224293864770971 ) ) ;
#194951=CARTESIAN_POINT ( 'NONE',  ( -15.72974639402197994, 15.80617190586746368, 70.62390960531436690 ) ) ;
#194952=CARTESIAN_POINT ( 'NONE',  ( -16.51473224551069308, -9.474510206698971260, 41.66557627198103120 ) ) ;
#194954=CARTESIAN_POINT ( 'NONE',  ( 8.314922557960818139, 14.29746914071049879, 49.58224293864769550 ) ) ;
#194955=CARTESIAN_POINT ( 'NONE',  ( 19.03943276465977164, -0.05219959533909143690, 98.74890960531436690 ) ) ;
#194957=CARTESIAN_POINT ( 'NONE',  ( 5.153800228976615827, -19.02544592524334988, 70.20942372801899012 ) ) ;
#194958=CARTESIAN_POINT ( 'NONE',  ( -15.72974639402197994, 15.80617190586746368, 75.62390960531439532 ) ) ;
#194959=CARTESIAN_POINT ( 'NONE',  ( -16.46253265017146816, -9.564922557961047289, 34.16775706135233293 ) ) ;
#194960=CARTESIAN_POINT ( 'NONE',  ( -5.153800228976328057, -19.02544592524343514, 102.2905762719810383 ) ) ;
#194962=CARTESIAN_POINT ( 'NONE',  ( -10.72451020669898014, 18.67979575497178502, 45.41557627198103830 ) ) ;
#194963=CARTESIAN_POINT ( 'NONE',  ( -5.153800228976328057, -19.02544592524343514, 67.29057627198102409 ) ) ;
#194964=CARTESIAN_POINT ( 'NONE',  ( 21.52544592524334988, 5.823673210054432836, 71.45942372801901854 ) ) ;
#194965=CARTESIAN_POINT ( 'NONE',  ( -5.153800228976328057, -19.02544592524343514, 22.29057627198102765 ) ) ;
#194966=CARTESIAN_POINT ( 'NONE',  ( 10.72451020669898902, -18.67979575497178502, 112.9155762719810383 ) ) ;
#194967=ORIENTED_EDGE ( 'NONE', *, *, #90799, .F. ) ;
#194968=CARTESIAN_POINT ( 'NONE',  ( 15.72974639402176855, 15.80617190586768217, 51.87609039468568284 ) ) ;
#194969=VERTEX_POINT ( 'NONE', #18563 ) ;
#194970=CARTESIAN_POINT ( 'NONE',  ( 13.97604488694527802, 13.89961937509977652, 109.3739096053143669 ) ) ;
#194971=CARTESIAN_POINT ( 'NONE',  ( 13.97604488694548053, -13.89961937509957401, 65.62609039468567573 ) ) ;
#194973=CARTESIAN_POINT ( 'NONE',  ( -21.52544592524343514, 5.823673210054127303, 111.0405762719810525 ) ) ;
#194974=CARTESIAN_POINT ( 'NONE',  ( -13.97604488694527625, -13.89961937509977652, 66.87390960531436690 ) ) ;
#194975=CARTESIAN_POINT ( 'NONE',  ( -16.52544592524335698, -4.483927247898792601, 33.95942372801901143 ) ) ;
#194977=CARTESIAN_POINT ( 'NONE',  ( -5.823673210054431948, 21.52544592524334988, 102.7094237280190185 ) ) ;
#194978=CARTESIAN_POINT ( 'NONE',  ( -13.97604488694527625, -13.89961937509977652, 36.87390960531436690 ) ) ;
#194979=CARTESIAN_POINT ( 'NONE',  ( 0.05219959533936267826, -19.03943276465977164, 20.00109039468567218 ) ) ;
#194980=CARTESIAN_POINT ( 'NONE',  ( -16.55341960407617563, 4.379528057220093196, 93.54275706135234714 ) ) ;
#194981=CARTESIAN_POINT ( 'NONE',  ( -13.97604488694527625, -13.89961937509977652, 91.87390960531432427 ) ) ;
#194982=CARTESIAN_POINT ( 'NONE',  ( -10.81492255796105439, 18.62759615963255655, 62.91775706135236135 ) ) ;
#194984=CARTESIAN_POINT ( 'NONE',  ( 13.97604488694527802, 13.89961937509977652, 114.3739096053143669 ) ) ;
#194985=CARTESIAN_POINT ( 'NONE',  ( -17.50000000000001066, 3.209263204892529142, 29.76196825606282204 ) ) ;
#194986=CARTESIAN_POINT ( 'NONE',  ( -14.34966873604972548, 8.224510206698743886, 48.33442372801902565 ) ) ;
#194987=CARTESIAN_POINT ( 'NONE',  ( -15.80617190586768217, 15.72974639402176855, 78.12609039468570415 ) ) ;
#194988=CARTESIAN_POINT ( 'NONE',  ( -21.52544592524334988, -5.823673210054445271, 83.95942372801900433 ) ) ;
#194991=CARTESIAN_POINT ( 'NONE',  ( 0.05219959533934541429, -16.53943276465976808, 25.00109039468567218 ) ) ;
#194992=CARTESIAN_POINT ( 'NONE',  ( -16.46253265017160317, 9.564922557960807481, 90.83224293864769550 ) ) ;
#194993=CARTESIAN_POINT ( 'NONE',  ( 19.02544592524343514, -5.153800228976328945, 108.5405762719810383 ) ) ;
#194994=CARTESIAN_POINT ( 'NONE',  ( 17.49999999999999289, 5.500000000000009770, 43.78230962303566542 ) ) ;
#194995=CARTESIAN_POINT ( 'NONE',  ( 0.05219959533909260263, 19.03943276465977164, 29.99890960531435979 ) ) ;
#194996=CARTESIAN_POINT ( 'NONE',  ( -5.719274019375978568, 21.55341960407610458, 40.20724293864769550 ) ) ;
#194997=CARTESIAN_POINT ( 'NONE',  ( 8.314922557961029526, -14.29746914071037800, 105.4177570613523613 ) ) ;
#194998=CARTESIAN_POINT ( 'NONE',  ( -8.314922557960811034, -14.29746914071050412, 82.08224293864768129 ) ) ;
#194999=CARTESIAN_POINT ( 'NONE',  ( 9.564922557960805705, 16.46253265017160317, 69.58224293864770971 ) ) ;
#195000=CARTESIAN_POINT ( 'NONE',  ( 21.52544592524334988, 5.823673210054432836, 86.45942372801901854 ) ) ;
#195001=CARTESIAN_POINT ( 'NONE',  ( -16.52544592524335698, -4.483927247898792601, 28.95942372801902209 ) ) ;
#195002=CARTESIAN_POINT ( 'NONE',  ( -0.05219959533910754901, -16.53943276465976808, 82.49890960531436690 ) ) ;
#195003=CARTESIAN_POINT ( 'NONE',  ( -18.62759615963255300, -10.81492255796106328, 44.16775706135234714 ) ) ;
#195004=CARTESIAN_POINT ( 'NONE',  ( 15.72974639402199770, -15.80617190586745480, 73.12390960531436690 ) ) ;
#195005=CARTESIAN_POINT ( 'NONE',  ( 16.46253265017146816, 9.564922557961045513, 31.66775706135232937 ) ) ;
#195007=CARTESIAN_POINT ( 'NONE',  ( -5.049401038298153566, 19.05341960407611168, 95.20724293864770971 ) ) ;
#195008=CARTESIAN_POINT ( 'NONE',  ( 12.06949235617757843, -12.14591786802309237, 63.12390960531435979 ) ) ;
#195009=VECTOR ( 'NONE', #106586, 1000.000000000000000 ) ;
#195010=CARTESIAN_POINT ( 'NONE',  ( 0.05219959533910956823, 16.53943276465976808, 49.99890960531437401 ) ) ;
#195011=CARTESIAN_POINT ( 'NONE',  ( 16.53943276465976808, 0.05219959533934440121, 111.2510903946856899 ) ) ;
#195012=CARTESIAN_POINT ( 'NONE',  ( -16.51473224551082808, 9.474510206698731452, 63.33442372801900433 ) ) ;
#195014=CARTESIAN_POINT ( 'NONE',  ( -16.51473224551082808, 9.474510206698731452, 78.33442372801900433 ) ) ;
#195015=CARTESIAN_POINT ( 'NONE',  ( 18.67979575497178502, 10.72451020669898547, 24.16557627198103120 ) ) ;
#195016=CARTESIAN_POINT ( 'NONE',  ( -4.483927247898539470, -16.52544592524342804, 82.29057627198103830 ) ) ;
#195017=CARTESIAN_POINT ( 'NONE',  ( 18.82182630884599561, -5.500000000000063061, 38.42483672716981147 ) ) ;
#195018=CARTESIAN_POINT ( 'NONE',  ( 5.153800228976335163, 19.02544592524342804, 44.79057627198103830 ) ) ;
#195019=CARTESIAN_POINT ( 'NONE',  ( 21.55341960407610458, 5.719274019375980345, 53.95724293864770260 ) ) ;
#195020=CARTESIAN_POINT ( 'NONE',  ( 21.55341960407610458, 5.719274019375980345, 83.95724293864770971 ) ) ;
#195021=CARTESIAN_POINT ( 'NONE',  ( -16.51473224551069308, -9.474510206698971260, 21.66557627198102765 ) ) ;
#195022=CARTESIAN_POINT ( 'NONE',  ( 4.379528057220092307, 16.55341960407617563, 62.29275706135236845 ) ) ;
#195023=CARTESIAN_POINT ( 'NONE',  ( -0.05219959533909027116, -19.03943276465977164, 42.49890960531435269 ) ) ;
#195024=CARTESIAN_POINT ( 'NONE',  ( -9.474510206698720793, -16.51473224551083518, 39.58442372801899722 ) ) ;
#195025=CARTESIAN_POINT ( 'NONE',  ( 21.53943276465977519, 0.05219959533937863772, 61.25109039468567573 ) ) ;
#195026=CARTESIAN_POINT ( 'NONE',  ( -16.55341960407611168, -4.379528057220339221, 101.4572429386476955 ) ) ;
#195027=CARTESIAN_POINT ( 'NONE',  ( 5.153800228976615827, -19.02544592524334988, 90.20942372801900433 ) ) ;
#195030=CARTESIAN_POINT ( 'NONE',  ( -18.62759615963270932, 10.81492255796079327, 45.83224293864769550 ) ) ;
#195031=CARTESIAN_POINT ( 'NONE',  ( 5.049401038298161559, -19.05341960407611168, 27.70724293864769550 ) ) ;
#195032=CARTESIAN_POINT ( 'NONE',  ( -5.719274019375665041, -21.55341960407619695, 84.79275706135234714 ) ) ;
#195033=CARTESIAN_POINT ( 'NONE',  ( -14.34966873604960291, -8.224510206698953496, 26.66557627198103475 ) ) ;
#195034=CARTESIAN_POINT ( 'NONE',  ( -16.55341960407617563, 4.379528057220093196, 53.54275706135234714 ) ) ;
#195035=CARTESIAN_POINT ( 'NONE',  ( 0.05219959533910956823, 16.53943276465976808, 44.99890960531435979 ) ) ;
#195036=CARTESIAN_POINT ( 'NONE',  ( -10.72451020669898014, 18.67979575497178502, 85.41557627198102409 ) ) ;
#195037=CARTESIAN_POINT ( 'NONE',  ( -5.823673210054116645, -21.52544592524344225, 77.29057627198102409 ) ) ;
#195038=CARTESIAN_POINT ( 'NONE',  ( -22.00000000000000000, -5.510910596163089556E-15, 45.00000000000000000 ) ) ;
#195039=CARTESIAN_POINT ( 'NONE',  ( -5.049401038297874678, -19.05341960407617918, 84.79275706135233293 ) ) ;
#195040=CARTESIAN_POINT ( 'NONE',  ( 5.823673210054125526, 21.52544592524343514, 24.79057627198103120 ) ) ;
#195041=CARTESIAN_POINT ( 'NONE',  ( 9.474510206698971260, -16.51473224551069308, 42.91557627198103120 ) ) ;
#195042=CARTESIAN_POINT ( 'NONE',  ( -5.049401038298153566, 19.05341960407611168, 30.20724293864768839 ) ) ;
#195044=ORIENTED_EDGE ( 'NONE', *, *, #6212, .T. ) ;
#195045=CARTESIAN_POINT ( 'NONE',  ( -16.55341960407617563, 4.379528057220093196, 83.54275706135234714 ) ) ;
#195046=CARTESIAN_POINT ( 'NONE',  ( -5.823673210054116645, -21.52544592524344225, 107.2905762719810525 ) ) ;
#195047=CARTESIAN_POINT ( 'NONE',  ( 19.03943276465977164, -0.05219959533909143690, 73.74890960531435269 ) ) ;
#195048=CARTESIAN_POINT ( 'NONE',  ( 21.52544592524334988, 5.823673210054432836, 36.45942372801901143 ) ) ;
#195049=CARTESIAN_POINT ( 'NONE',  ( 9.474510206698971260, -16.51473224551069308, 97.91557627198102409 ) ) ;
#195051=EDGE_CURVE ( 'NONE', #66658, #193741, #45224, .T. ) ;
#195053=CARTESIAN_POINT ( 'NONE',  ( 5.823673210054444382, -21.52544592524334988, 30.20942372801902565 ) ) ;
#195054=CARTESIAN_POINT ( 'NONE',  ( -13.89961937509977652, 13.97604488694528158, 30.62390960531435269 ) ) ;
#195055=CARTESIAN_POINT ( 'NONE',  ( -13.89961937509977652, 13.97604488694528158, 100.6239096053143669 ) ) ;
#195056=CARTESIAN_POINT ( 'NONE',  ( -19.02544592524334988, -5.153800228976617603, 38.95942372801900433 ) ) ;
#195057=CARTESIAN_POINT ( 'NONE',  ( -10.72451020669898014, 18.67979575497178502, 115.4155762719810241 ) ) ;
#195058=CARTESIAN_POINT ( 'NONE',  ( 13.97604488694548053, -13.89961937509957401, 40.62609039468564731 ) ) ;
#195059=CARTESIAN_POINT ( 'NONE',  ( -16.51473224551082808, 9.474510206698731452, 43.33442372801900433 ) ) ;
#195060=CARTESIAN_POINT ( 'NONE',  ( -12.14591786802326823, 12.06949235617739902, 98.12609039468570415 ) ) ;
#195062=CARTESIAN_POINT ( 'NONE',  ( 0.05219959533909260263, 19.03943276465977164, 69.99890960531435269 ) ) ;
#195063=CARTESIAN_POINT ( 'NONE',  ( -15.80617190586768217, 15.72974639402176855, 73.12609039468567573 ) ) ;
#195064=CARTESIAN_POINT ( 'NONE',  ( 21.55341960407619695, -5.719274019375665929, 91.04275706135236135 ) ) ;
#195066=CARTESIAN_POINT ( 'NONE',  ( -5.153800228976328057, -19.02544592524343514, 82.29057627198103830 ) ) ;
#195067=CARTESIAN_POINT ( 'NONE',  ( -10.72451020669870658, -18.67979575497194134, 64.58442372801900433 ) ) ;
#195068=CARTESIAN_POINT ( 'NONE',  ( 13.89961937509957401, 13.97604488694547697, 101.8760903946856331 ) ) ;
#195069=CARTESIAN_POINT ( 'NONE',  ( 9.474510206698971260, -16.51473224551069308, 62.91557627198102409 ) ) ;
#195070=CARTESIAN_POINT ( 'NONE',  ( 5.153800228976335163, 19.02544592524342804, 114.7905762719810241 ) ) ;
#195072=CARTESIAN_POINT ( 'NONE',  ( 9.564922557960805705, 16.46253265017160317, 84.58224293864769550 ) ) ;
#195073=CARTESIAN_POINT ( 'NONE',  ( -17.44279575226824619, -5.990770900252441855, 89.16442432485686709 ) ) ;
#195074=CARTESIAN_POINT ( 'NONE',  ( -19.05341960407611168, -5.049401038298163336, 61.45724293864769550 ) ) ;
#195075=CARTESIAN_POINT ( 'NONE',  ( -16.51473224551069308, -9.474510206698971260, 56.66557627198103120 ) ) ;
#195076=CARTESIAN_POINT ( 'NONE',  ( -18.62759615963270932, 10.81492255796079327, 115.8322429386477097 ) ) ;
#195077=CARTESIAN_POINT ( 'NONE',  ( -16.55341960407617563, 4.379528057220093196, 98.54275706135234714 ) ) ;
#195078=CARTESIAN_POINT ( 'NONE',  ( 17.50000000000000000, 5.499999999999997335, 120.0000000000000142 ) ) ;
#195080=CARTESIAN_POINT ( 'NONE',  ( 16.51473224551083163, -9.474510206698727899, 60.83442372801900433 ) ) ;
#195081=CARTESIAN_POINT ( 'NONE',  ( -9.564922557960796823, -16.46253265017161027, 77.08224293864769550 ) ) ;
#195082=CARTESIAN_POINT ( 'NONE',  ( -16.55341960407611168, -4.379528057220339221, 66.45724293864768129 ) ) ;
#195083=CARTESIAN_POINT ( 'NONE',  ( 16.55341960407611168, 4.379528057220329451, 108.9572429386476955 ) ) ;
#195084=CARTESIAN_POINT ( 'NONE',  ( 18.62759615963271287, -10.81492255796078972, 33.33224293864769550 ) ) ;
#195085=CARTESIAN_POINT ( 'NONE',  ( 19.03943276465977164, -0.05219959533909143690, 103.7489096053143669 ) ) ;
#195086=CARTESIAN_POINT ( 'NONE',  ( 8.314922557960818139, 14.29746914071049879, 89.58224293864768129 ) ) ;
#195087=CARTESIAN_POINT ( 'NONE',  ( -13.89961937509957401, -13.97604488694547875, 24.37609039468565442 ) ) ;
#195088=CARTESIAN_POINT ( 'NONE',  ( 14.29746914071037800, 8.314922557961029526, 106.6677570613523756 ) ) ;
#195089=CARTESIAN_POINT ( 'NONE',  ( 16.51473224551069308, 9.474510206698969483, 94.16557627198103830 ) ) ;
#195090=CARTESIAN_POINT ( 'NONE',  ( -18.62759615963255300, -10.81492255796106328, 49.16775706135234003 ) ) ;
#195091=CARTESIAN_POINT ( 'NONE',  ( 18.67979575497178502, 10.72451020669898547, 49.16557627198102409 ) ) ;
#195092=CARTESIAN_POINT ( 'NONE',  ( -10.81492255796105439, 18.62759615963255655, 37.91775706135235424 ) ) ;
#195093=CARTESIAN_POINT ( 'NONE',  ( 15.72974639402199770, -15.80617190586745480, 78.12390960531436690 ) ) ;
#195094=CARTESIAN_POINT ( 'NONE',  ( -16.52544592524342804, 4.483927247898546575, 101.0405762719810383 ) ) ;
#195095=CARTESIAN_POINT ( 'NONE',  ( -19.03943276465977164, -0.05219959533935918106, 58.75109039468566863 ) ) ;
#195097=CARTESIAN_POINT ( 'NONE',  ( 0.05219959533909260263, 19.03943276465977164, 44.99890960531435979 ) ) ;
#195098=CARTESIAN_POINT ( 'NONE',  ( 16.46253265017160672, -9.564922557960803928, 103.3322429386476955 ) ) ;
#195099=CARTESIAN_POINT ( 'NONE',  ( -9.474510206698964154, 16.51473224551069663, 100.4155762719810241 ) ) ;
#195100=CARTESIAN_POINT ( 'NONE',  ( 8.224510206698953496, -14.34966873604960469, 112.9155762719810383 ) ) ;
#195101=CARTESIAN_POINT ( 'NONE',  ( -0.05219959533910754901, -16.53943276465976808, 27.49890960531435269 ) ) ;
#195102=CARTESIAN_POINT ( 'NONE',  ( 14.34966873604972726, -8.224510206698740333, 35.83442372801901143 ) ) ;
#195103=CARTESIAN_POINT ( 'NONE',  ( -0.05219959533937732626, 21.53943276465977519, 112.5010903946857042 ) ) ;
#195104=CARTESIAN_POINT ( 'NONE',  ( 9.564922557960805705, 16.46253265017160317, 114.5822429386476955 ) ) ;
#195105=CARTESIAN_POINT ( 'NONE',  ( 8.224510206698953496, -14.34966873604960469, 27.91557627198103830 ) ) ;
#195106=CARTESIAN_POINT ( 'NONE',  ( -10.81492255796105439, 18.62759615963255655, 37.91775706135235424 ) ) ;
#195107=CARTESIAN_POINT ( 'NONE',  ( -5.049401038298153566, 19.05341960407611168, 110.2072429386476671 ) ) ;
#195108=CARTESIAN_POINT ( 'NONE',  ( 14.34966873604972726, -8.224510206698740333, 50.83442372801901143 ) ) ;
#195109=CARTESIAN_POINT ( 'NONE',  ( 4.379528057220092307, 16.55341960407617563, 112.2927570613523471 ) ) ;
#195110=CARTESIAN_POINT ( 'NONE',  ( -4.379528057220086978, -16.55341960407618274, 89.79275706135236135 ) ) ;
#195111=CARTESIAN_POINT ( 'NONE',  ( -8.224510206698735004, -14.34966873604973081, 24.58442372801901499 ) ) ;
#195112=CARTESIAN_POINT ( 'NONE',  ( 0.05219959533909260263, 19.03943276465977164, 34.99890960531435979 ) ) ;
#195113=CARTESIAN_POINT ( 'NONE',  ( -4.483927247898539470, -16.52544592524342804, 112.2905762719810241 ) ) ;
#195114=CARTESIAN_POINT ( 'NONE',  ( -10.72451020669870658, -18.67979575497194134, 19.58442372801901143 ) ) ;
#195115=CARTESIAN_POINT ( 'NONE',  ( 9.564922557960805705, 16.46253265017160317, 34.58224293864770260 ) ) ;
#195116=CARTESIAN_POINT ( 'NONE',  ( 9.564922557960805705, 16.46253265017160317, 109.5822429386476955 ) ) ;
#195117=CARTESIAN_POINT ( 'NONE',  ( 5.823673210054444382, -21.52544592524334988, 30.20942372801902565 ) ) ;
#195118=CARTESIAN_POINT ( 'NONE',  ( 19.02544592524343514, -5.153800228976328945, 23.54057627198102054 ) ) ;
#195119=CARTESIAN_POINT ( 'NONE',  ( -13.97604488694527625, -13.89961937509977652, 101.8739096053143811 ) ) ;
#195121=CARTESIAN_POINT ( 'NONE',  ( 16.52216118717205973, -7.221426719304538722, 111.4240097895301034 ) ) ;
#195122=CARTESIAN_POINT ( 'NONE',  ( 19.05341960407611168, 5.049401038298154454, 93.95724293864769550 ) ) ;
#195123=CARTESIAN_POINT ( 'NONE',  ( 10.72451020669871369, 18.67979575497193778, 52.08442372801901854 ) ) ;
#195124=CARTESIAN_POINT ( 'NONE',  ( -14.29746914071049879, 8.314922557960819915, 90.83224293864769550 ) ) ;
#195125=CARTESIAN_POINT ( 'NONE',  ( 5.049401038298161559, -19.05341960407611168, 102.7072429386476955 ) ) ;
#195128=CARTESIAN_POINT ( 'NONE',  ( -4.483927247898782831, 16.52544592524335698, 67.70942372801901854 ) ) ;
#195129=CARTESIAN_POINT ( 'NONE',  ( -10.81492255796105439, 18.62759615963255655, 82.91775706135234714 ) ) ;
#195130=CARTESIAN_POINT ( 'NONE',  ( -4.379528057220086978, -16.55341960407618274, 44.79275706135234714 ) ) ;
#195131=CARTESIAN_POINT ( 'NONE',  ( 13.89961937509977652, -13.97604488694527269, 88.12390960531438111 ) ) ;
#195132=CARTESIAN_POINT ( 'NONE',  ( 9.474510206698729675, 16.51473224551082808, 112.0844237280190043 ) ) ;
#195133=CARTESIAN_POINT ( 'NONE',  ( -14.29746914071037622, -8.314922557961029526, 64.16775706135234714 ) ) ;
#195134=CARTESIAN_POINT ( 'NONE',  ( -21.53943276465977519, -0.05219959533937600094, 108.7510903946857042 ) ) ;
#195135=CARTESIAN_POINT ( 'NONE',  ( -19.03943276465977164, -0.05219959533935918106, 98.75109039468567573 ) ) ;
#195136=CARTESIAN_POINT ( 'NONE',  ( 9.564922557960805705, 16.46253265017160317, 69.58224293864770971 ) ) ;
#195137=CARTESIAN_POINT ( 'NONE',  ( -0.05219959533907301413, -21.53943276465977519, 87.49890960531436690 ) ) ;
#195138=CARTESIAN_POINT ( 'NONE',  ( -12.14591786802309592, -12.06949235617757132, 86.87390960531438111 ) ) ;
#195139=CARTESIAN_POINT ( 'NONE',  ( -0.05219959533936034679, 19.03943276465977164, 92.50109039468566152 ) ) ;
#195140=CARTESIAN_POINT ( 'NONE',  ( -16.55341960407617563, 4.379528057220093196, 63.54275706135234003 ) ) ;
#195142=CARTESIAN_POINT ( 'NONE',  ( 19.05341960407617918, -5.049401038297876454, 56.04275706135234714 ) ) ;
#195143=CARTESIAN_POINT ( 'NONE',  ( 12.06949235617757843, -12.14591786802309237, 28.12390960531435979 ) ) ;
#195144=CARTESIAN_POINT ( 'NONE',  ( -12.14591786802309592, -12.06949235617757132, 86.87390960531438111 ) ) ;
#195145=CARTESIAN_POINT ( 'NONE',  ( -10.72451020669870658, -18.67979575497194134, 109.5844237280190328 ) ) ;
#195146=CARTESIAN_POINT ( 'NONE',  ( -17.49999999999999645, 5.499999999999985789, 38.71769037696434879 ) ) ;
#195147=CARTESIAN_POINT ( 'NONE',  ( -5.719274019375665041, -21.55341960407619695, 19.79275706135235069 ) ) ;
#195148=CARTESIAN_POINT ( 'NONE',  ( 13.97604488694527802, 13.89961937509977652, 104.3739096053143385 ) ) ;
#195149=CARTESIAN_POINT ( 'NONE',  ( -13.97604488694527625, -13.89961937509977652, 76.87390960531433848 ) ) ;
#195150=CARTESIAN_POINT ( 'NONE',  ( -18.67979575497193778, 10.72451020669871902, 103.3344237280190043 ) ) ;
#195151=CARTESIAN_POINT ( 'NONE',  ( 19.03943276465977164, -0.05219959533909143690, 73.74890960531435269 ) ) ;
#195152=CARTESIAN_POINT ( 'NONE',  ( 18.67979575497178502, 10.72451020669898547, 49.16557627198102409 ) ) ;
#195153=CARTESIAN_POINT ( 'NONE',  ( 12.06949235617757843, -12.14591786802309237, 78.12390960531436690 ) ) ;
#195154=CARTESIAN_POINT ( 'NONE',  ( 13.97604488694527802, 13.89961937509977652, 39.37390960531435269 ) ) ;
#195155=CARTESIAN_POINT ( 'NONE',  ( 4.483927247898545687, 16.52544592524342804, 104.7905762719810241 ) ) ;
#195157=CARTESIAN_POINT ( 'NONE',  ( -15.72974639402197994, 15.80617190586746368, 115.6239096053143669 ) ) ;
#195158=CARTESIAN_POINT ( 'NONE',  ( -15.72974639402176322, -15.80617190586768395, 59.37609039468568284 ) ) ;
#195159=CARTESIAN_POINT ( 'NONE',  ( -5.153800228976328057, -19.02544592524343514, 27.29057627198103120 ) ) ;
#195160=CARTESIAN_POINT ( 'NONE',  ( -4.483927247898782831, 16.52544592524335698, 67.70942372801901854 ) ) ;
#195161=CARTESIAN_POINT ( 'NONE',  ( -10.72451020669870658, -18.67979575497194134, 19.58442372801901143 ) ) ;
#195162=CARTESIAN_POINT ( 'NONE',  ( -18.67979575497178146, -10.72451020669898902, 106.6655762719810383 ) ) ;
#195163=CARTESIAN_POINT ( 'NONE',  ( -9.564922557961040184, 16.46253265017147172, 37.91775706135233293 ) ) ;
#195164=CARTESIAN_POINT ( 'NONE',  ( 9.474510206698971260, -16.51473224551069308, 47.91557627198102409 ) ) ;
#195165=CARTESIAN_POINT ( 'NONE',  ( -19.03943276465977164, 0.05219959533909376836, 116.2489096053143669 ) ) ;
#195166=CARTESIAN_POINT ( 'NONE',  ( -10.81492255796105439, 18.62759615963255655, 72.91775706135234714 ) ) ;
#195167=CARTESIAN_POINT ( 'NONE',  ( 5.823673210054125526, 21.52544592524343514, 59.79057627198103120 ) ) ;
#195168=CARTESIAN_POINT ( 'NONE',  ( -12.06949235617756955, 12.14591786802309770, 40.62390960531435269 ) ) ;
#195169=CARTESIAN_POINT ( 'NONE',  ( -10.72451020669870658, -18.67979575497194134, 79.58442372801903275 ) ) ;
#195170=CARTESIAN_POINT ( 'NONE',  ( -0.05219959533937732626, 21.53943276465977519, 112.5010903946857042 ) ) ;
#195171=CARTESIAN_POINT ( 'NONE',  ( 4.379528057220339221, -16.55341960407611168, 57.70724293864770260 ) ) ;
#195172=CARTESIAN_POINT ( 'NONE',  ( -16.52544592524342804, 4.483927247898546575, 106.0405762719810525 ) ) ;
#195173=CARTESIAN_POINT ( 'NONE',  ( 16.51473224551083163, -9.474510206698727899, 45.83442372801900433 ) ) ;
#195174=CARTESIAN_POINT ( 'NONE',  ( 0.05219959533934541429, -16.53943276465976808, 95.00109039468568994 ) ) ;
#195175=CARTESIAN_POINT ( 'NONE',  ( 5.823673210054444382, -21.52544592524334988, 65.20942372801901854 ) ) ;
#195176=CARTESIAN_POINT ( 'NONE',  ( 5.153800228976335163, 19.02544592524342804, 64.79057627198100988 ) ) ;
#195177=CARTESIAN_POINT ( 'NONE',  ( 16.51473224551083163, -9.474510206698727899, 35.83442372801899722 ) ) ;
#195178=CARTESIAN_POINT ( 'NONE',  ( -15.80617190586745835, -15.72974639402198527, 31.87390960531435979 ) ) ;
#195179=CARTESIAN_POINT ( 'NONE',  ( 10.81492255796106328, -18.62759615963255655, 30.41775706135234358 ) ) ;
#195180=CARTESIAN_POINT ( 'NONE',  ( 5.823673210054125526, 21.52544592524343514, 89.79057627198103830 ) ) ;
#195181=CARTESIAN_POINT ( 'NONE',  ( 13.89961937509957401, 13.97604488694547697, 81.87609039468564731 ) ) ;
#195182=CARTESIAN_POINT ( 'NONE',  ( 8.314922557961029526, -14.29746914071037800, 55.41775706135234714 ) ) ;
#195184=CARTESIAN_POINT ( 'NONE',  ( 5.823673210054125526, 21.52544592524343514, 94.79057627198105251 ) ) ;
#195185=CARTESIAN_POINT ( 'NONE',  ( 4.483927247898545687, 16.52544592524342804, 74.79057627198105251 ) ) ;
#195187=CARTESIAN_POINT ( 'NONE',  ( 13.89961937509957401, 13.97604488694547697, 111.8760903946856757 ) ) ;
#195189=CARTESIAN_POINT ( 'NONE',  ( 10.81492255796078972, 18.62759615963270932, 44.58224293864769550 ) ) ;
#195190=CARTESIAN_POINT ( 'NONE',  ( 14.34966873604972726, -8.224510206698740333, 75.83442372801900433 ) ) ;
#195191=CARTESIAN_POINT ( 'NONE',  ( 9.564922557960805705, 16.46253265017160317, 24.58224293864769194 ) ) ;
#195192=CARTESIAN_POINT ( 'NONE',  ( 16.52544592524335698, 4.483927247898782831, 56.45942372801902565 ) ) ;
#195193=CARTESIAN_POINT ( 'NONE',  ( 21.55341960407619695, -5.719274019375665929, 21.04275706135234714 ) ) ;
#195194=CARTESIAN_POINT ( 'NONE',  ( 21.55341960407610458, 5.719274019375980345, 43.95724293864769550 ) ) ;
#195195=CARTESIAN_POINT ( 'NONE',  ( 14.34966873604972726, -8.224510206698740333, 75.83442372801900433 ) ) ;
#195196=CARTESIAN_POINT ( 'NONE',  ( 13.89961937509977652, -13.97604488694527269, 93.12390960531436690 ) ) ;
#195197=CARTESIAN_POINT ( 'NONE',  ( 18.62759615963255655, 10.81492255796105972, 56.66775706135235424 ) ) ;
#195198=CARTESIAN_POINT ( 'NONE',  ( 19.02544592524343514, -5.153800228976328945, 28.54057627198102409 ) ) ;
#195199=CARTESIAN_POINT ( 'NONE',  ( -5.719274019375978568, 21.55341960407610458, 45.20724293864769550 ) ) ;
#195200=CARTESIAN_POINT ( 'NONE',  ( -5.823673210054116645, -21.52544592524344225, 27.29057627198103120 ) ) ;
#195201=ORIENTED_EDGE ( 'NONE', *, *, #195850, .F. ) ;
#195202=CARTESIAN_POINT ( 'NONE',  ( -16.51473224551082808, 9.474510206698731452, 38.33442372801899722 ) ) ;
#195203=CARTESIAN_POINT ( 'NONE',  ( 16.55341960407618274, -4.379528057220086978, 51.04275706135234714 ) ) ;
#195204=CARTESIAN_POINT ( 'NONE',  ( -19.03943276465977164, 0.05219959533909376836, 111.2489096053143669 ) ) ;
#195205=ORIENTED_EDGE ( 'NONE', *, *, #172657, .T. ) ;
#195206=CARTESIAN_POINT ( 'NONE',  ( -13.97604488694527625, -13.89961937509977652, 81.87390960531436690 ) ) ;
#195207=CARTESIAN_POINT ( 'NONE',  ( 16.53943276465976808, 0.05219959533934440121, 101.2510903946856757 ) ) ;
#195209=CARTESIAN_POINT ( 'NONE',  ( -0.05219959533910754901, -16.53943276465976808, 92.49890960531436690 ) ) ;
#195210=CARTESIAN_POINT ( 'NONE',  ( -10.72451020669898014, 18.67979575497178502, 50.41557627198103120 ) ) ;
#195211=CARTESIAN_POINT ( 'NONE',  ( 16.51473224551069308, 9.474510206698969483, 29.16557627198103475 ) ) ;
#195212=CARTESIAN_POINT ( 'NONE',  ( 4.483927247898790824, -16.52544592524335698, 80.20942372801901854 ) ) ;
#195213=CARTESIAN_POINT ( 'NONE',  ( -15.72974639402176322, -15.80617190586768395, 24.37609039468567573 ) ) ;
#195214=CARTESIAN_POINT ( 'NONE',  ( -0.05219959533936034679, 19.03943276465977164, 92.50109039468566152 ) ) ;
#195215=CARTESIAN_POINT ( 'NONE',  ( -9.564922557960796823, -16.46253265017161027, 47.08224293864769550 ) ) ;
#195216=CARTESIAN_POINT ( 'NONE',  ( -13.97604488694527625, -13.89961937509977652, 106.8739096053143669 ) ) ;
#195217=CARTESIAN_POINT ( 'NONE',  ( -18.62759615963255300, -10.81492255796106328, 104.1677570613523471 ) ) ;
#195218=CARTESIAN_POINT ( 'NONE',  ( 5.153800228976335163, 19.02544592524342804, 79.79057627198102409 ) ) ;
#195219=CARTESIAN_POINT ( 'NONE',  ( 16.53943276465976808, 0.05219959533934440121, 56.25109039468568284 ) ) ;
#195220=CARTESIAN_POINT ( 'NONE',  ( 15.80617190586769283, -15.72974639402175789, 95.62609039468568994 ) ) ;
#195221=CARTESIAN_POINT ( 'NONE',  ( -19.03943276465977164, -0.05219959533935918106, 48.75109039468566863 ) ) ;
#195222=CARTESIAN_POINT ( 'NONE',  ( 19.03943276465977164, 0.05219959533936151252, 66.25109039468567573 ) ) ;
#195224=CARTESIAN_POINT ( 'NONE',  ( -21.55341960407619339, 5.719274019375674811, 63.54275706135234003 ) ) ;
#195225=CARTESIAN_POINT ( 'NONE',  ( 17.50000000000000000, -5.499999999999992895, 61.21769037696436300 ) ) ;
#195226=CARTESIAN_POINT ( 'NONE',  ( -19.05341960407617563, 5.049401038297882671, 53.54275706135231871 ) ) ;
#195227=CARTESIAN_POINT ( 'NONE',  ( 19.03943276465977164, -0.05219959533909143690, 103.7489096053143669 ) ) ;
#195228=CARTESIAN_POINT ( 'NONE',  ( -16.46253265017160317, 9.564922557960807481, 80.83224293864769550 ) ) ;
#195229=CARTESIAN_POINT ( 'NONE',  ( -12.14591786802309592, -12.06949235617757132, 41.87390960531435979 ) ) ;
#195230=CARTESIAN_POINT ( 'NONE',  ( -0.05219959533907301413, -21.53943276465977519, 37.49890960531436690 ) ) ;
#195231=CARTESIAN_POINT ( 'NONE',  ( -17.49999999999999645, 5.500000000000001776, 103.7176903769643701 ) ) ;
#195232=CARTESIAN_POINT ( 'NONE',  ( 5.153800228976615827, -19.02544592524334988, 20.20942372801899722 ) ) ;
#195234=CARTESIAN_POINT ( 'NONE',  ( -5.049401038298153566, 19.05341960407611168, 40.20724293864768839 ) ) ;
#195235=CARTESIAN_POINT ( 'NONE',  ( 13.89961937509977652, -13.97604488694527269, 23.12390960531436335 ) ) ;
#195237=CARTESIAN_POINT ( 'NONE',  ( 10.81492255796106328, -18.62759615963255655, 65.41775706135234714 ) ) ;
#195239=CARTESIAN_POINT ( 'NONE',  ( 14.29746914071037800, 8.314922557961029526, 61.66775706135235424 ) ) ;
#195240=CARTESIAN_POINT ( 'NONE',  ( 10.81492255796078972, 18.62759615963270932, 89.58224293864768129 ) ) ;
#195241=VECTOR ( 'NONE', #66585, 1000.000000000000000 ) ;
#195242=CARTESIAN_POINT ( 'NONE',  ( -14.34966873604960291, -8.224510206698953496, 51.66557627198102409 ) ) ;
#195243=CARTESIAN_POINT ( 'NONE',  ( 0.05219959533909260263, 19.03943276465977164, 34.99890960531435979 ) ) ;
#195244=CARTESIAN_POINT ( 'NONE',  ( 5.049401038298161559, -19.05341960407611168, 102.7072429386476955 ) ) ;
#195245=CARTESIAN_POINT ( 'NONE',  ( 18.67979575497194134, -10.72451020669871369, 30.83442372801902209 ) ) ;
#195246=CARTESIAN_POINT ( 'NONE',  ( -19.03943276465977164, -0.05219959533935918106, 48.75109039468566863 ) ) ;
#195247=CARTESIAN_POINT ( 'NONE',  ( 19.05341960407611168, 5.049401038298154454, 28.95724293864769550 ) ) ;
#195248=CARTESIAN_POINT ( 'NONE',  ( -21.55341960407619339, 5.719274019375674811, 83.54275706135234714 ) ) ;
#195250=CARTESIAN_POINT ( 'NONE',  ( 16.55341960407611168, 4.379528057220329451, 23.95724293864769550 ) ) ;
#195251=CARTESIAN_POINT ( 'NONE',  ( -18.62759615963270932, 10.81492255796079327, 40.83224293864769550 ) ) ;
#195252=CARTESIAN_POINT ( 'NONE',  ( 8.224510206698953496, -14.34966873604960469, 102.9155762719810383 ) ) ;
#195254=CARTESIAN_POINT ( 'NONE',  ( 19.05341960407611168, 5.049401038298154454, 88.95724293864769550 ) ) ;
#195255=CARTESIAN_POINT ( 'NONE',  ( 14.29746914071049879, -8.314922557960816363, 88.33224293864769550 ) ) ;
#195256=CARTESIAN_POINT ( 'NONE',  ( -5.049401038297874678, -19.05341960407617918, 109.7927570613523187 ) ) ;
#195258=CARTESIAN_POINT ( 'NONE',  ( -0.05219959533907301413, -21.53943276465977519, 57.49890960531435979 ) ) ;
#195260=CARTESIAN_POINT ( 'NONE',  ( -0.05219959533909027116, -19.03943276465977164, 27.49890960531435624 ) ) ;
#195261=CARTESIAN_POINT ( 'NONE',  ( 19.03943276465977164, -0.05219959533909143690, 83.74890960531436690 ) ) ;
#195262=CARTESIAN_POINT ( 'NONE',  ( -5.719274019375978568, 21.55341960407610458, 95.20724293864769550 ) ) ;
#195263=CARTESIAN_POINT ( 'NONE',  ( 16.55341960407618274, -4.379528057220086978, 106.0427570613523471 ) ) ;
#195264=CARTESIAN_POINT ( 'NONE',  ( -16.46253265017160317, 9.564922557960807481, 100.8322429386477097 ) ) ;
#195265=CARTESIAN_POINT ( 'NONE',  ( 9.564922557961047289, -16.46253265017146816, 80.41775706135234714 ) ) ;
#195266=CARTESIAN_POINT ( 'NONE',  ( 21.55341960407619695, -5.719274019375665929, 91.04275706135236135 ) ) ;
#195267=CARTESIAN_POINT ( 'NONE',  ( 10.72451020669898902, -18.67979575497178502, 72.91557627198103830 ) ) ;
#195268=CARTESIAN_POINT ( 'NONE',  ( 21.53943276465977519, -0.05219959533907433946, 38.74890960531435979 ) ) ;
#195269=CARTESIAN_POINT ( 'NONE',  ( -9.564922557960796823, -16.46253265017161027, 47.08224293864769550 ) ) ;
#195270=CARTESIAN_POINT ( 'NONE',  ( -8.314922557961024197, 14.29746914071037800, 107.9177570613523471 ) ) ;
#195271=CARTESIAN_POINT ( 'NONE',  ( 16.46253265017160672, -9.564922557960803928, 68.33224293864770971 ) ) ;
#195274=CARTESIAN_POINT ( 'NONE',  ( -9.474510206698720793, -16.51473224551083518, 24.58442372801900078 ) ) ;
#195275=CARTESIAN_POINT ( 'NONE',  ( 12.14591786802309770, 12.06949235617756955, 69.37390960531436690 ) ) ;
#195277=CARTESIAN_POINT ( 'NONE',  ( -18.62759615963270932, 10.81492255796079327, 115.8322429386477097 ) ) ;
#195279=CARTESIAN_POINT ( 'NONE',  ( 0.05219959533907565091, 21.53943276465977519, 54.99890960531435269 ) ) ;
#195280=CARTESIAN_POINT ( 'NONE',  ( 8.224510206698742110, 14.34966873604972548, 92.08442372801901854 ) ) ;
#195281=CARTESIAN_POINT ( 'NONE',  ( -8.314922557960811034, -14.29746914071050412, 107.0822429386476955 ) ) ;
#195282=CARTESIAN_POINT ( 'NONE',  ( -9.564922557960796823, -16.46253265017161027, 77.08224293864769550 ) ) ;
#195283=( NAMED_UNIT ( * ) PLANE_ANGLE_UNIT ( ) SI_UNIT ( $, .RADIAN. ) );
#195284=CARTESIAN_POINT ( 'NONE',  ( -16.53943276465976808, 0.05219959533911058130, 31.24890960531435979 ) ) ;
#195285=CARTESIAN_POINT ( 'NONE',  ( -5.719274019375665041, -21.55341960407619695, 49.79275706135234714 ) ) ;
#195286=CARTESIAN_POINT ( 'NONE',  ( -9.474510206698964154, 16.51473224551069663, 105.4155762719810383 ) ) ;
#195287=CARTESIAN_POINT ( 'NONE',  ( 21.55341960407619695, -5.719274019375665929, 81.04275706135236135 ) ) ;
#195288=CARTESIAN_POINT ( 'NONE',  ( -5.153800228976328057, -19.02544592524343514, 27.29057627198103120 ) ) ;
#195289=CARTESIAN_POINT ( 'NONE',  ( -5.153800228976328057, -19.02544592524343514, 32.29057627198102409 ) ) ;
#195291=CARTESIAN_POINT ( 'NONE',  ( 10.81492255796106328, -18.62759615963255655, 95.41775706135234714 ) ) ;
#195292=CARTESIAN_POINT ( 'NONE',  ( -8.224510206698735004, -14.34966873604973081, 54.58442372801901143 ) ) ;
#195293=CARTESIAN_POINT ( 'NONE',  ( -21.53943276465977519, -0.05219959533937600094, 78.75109039468568994 ) ) ;
#195294=CARTESIAN_POINT ( 'NONE',  ( 0.05219959533909260263, 19.03943276465977164, 104.9989096053143669 ) ) ;
#195295=ORIENTED_EDGE ( 'NONE', *, *, #193397, .T. ) ;
#195296=CARTESIAN_POINT ( 'NONE',  ( 0.05219959533936267826, -19.03943276465977164, 75.00109039468566152 ) ) ;
#195297=CARTESIAN_POINT ( 'NONE',  ( -21.53943276465977519, -0.05219959533937600094, 58.75109039468568994 ) ) ;
#195298=CARTESIAN_POINT ( 'NONE',  ( -19.05341960407617563, 5.049401038297882671, 113.5427570613523471 ) ) ;
#195299=CARTESIAN_POINT ( 'NONE',  ( 0.05219959533936267826, -19.03943276465977164, 85.00109039468567573 ) ) ;
#195300=CARTESIAN_POINT ( 'NONE',  ( -16.46253265017160317, 9.564922557960807481, 55.83224293864769550 ) ) ;
#195301=CARTESIAN_POINT ( 'NONE',  ( -16.51473224551082808, 9.474510206698731452, 98.33442372801900433 ) ) ;
#195302=VECTOR ( 'NONE', #144948, 1000.000000000000000 ) ;
#195303=CARTESIAN_POINT ( 'NONE',  ( -8.314922557960811034, -14.29746914071050412, 22.08224293864769194 ) ) ;
#195304=CARTESIAN_POINT ( 'NONE',  ( -5.049401038297874678, -19.05341960407617918, 89.79275706135230450 ) ) ;
#195305=CARTESIAN_POINT ( 'NONE',  ( -12.06949235617756955, 12.14591786802309770, 45.62390960531436690 ) ) ;
#195306=CARTESIAN_POINT ( 'NONE',  ( -9.474510206698720793, -16.51473224551083518, 59.58442372801900433 ) ) ;
#195307=CARTESIAN_POINT ( 'NONE',  ( 8.224510206698742110, 14.34966873604972548, 57.08442372801901854 ) ) ;
#195308=CARTESIAN_POINT ( 'NONE',  ( -15.80617190586768217, 15.72974639402176855, 113.1260903946856899 ) ) ;
#195309=CARTESIAN_POINT ( 'NONE',  ( 4.483927247898545687, 16.52544592524342804, 114.7905762719810383 ) ) ;
#195310=CARTESIAN_POINT ( 'NONE',  ( 9.474510206698971260, -16.51473224551069308, 47.91557627198102409 ) ) ;
#195311=CARTESIAN_POINT ( 'NONE',  ( -12.14591786802326823, 12.06949235617739902, 53.12609039468568284 ) ) ;
#195314=CARTESIAN_POINT ( 'NONE',  ( -9.564922557960796823, -16.46253265017161027, 87.08224293864769550 ) ) ;
#195315=DIRECTION ( 'NONE',  ( -0.000000000000000000, -0.000000000000000000, 1.000000000000000000 ) ) ;
#195317=CARTESIAN_POINT ( 'NONE',  ( -19.02544592524334988, -5.153800228976617603, 98.95942372801900433 ) ) ;
#195318=B_SPLINE_CURVE_WITH_KNOTS ( 'NONE', 3,
 ( #8920, #68576, #176781, #100903, #177777, #39247, #130232, #7901, #25102, #190936, #23087, #6897, #38254, #98902, #53411, #131251, #21082, #159585, #52413, #192940, #84732, #115089, #67582, #144419, #162587, #163601, #116089, #99908, #146410, #191928, #24092, #117082 ),
 .UNSPECIFIED., .F., .F.,
 ( 4, 2, 2, 2, 2, 2, 2, 2, 2, 2, 2, 2, 2, 2, 2, 4 ),
 ( 5.204170427930422054E-18, 0.0003712461730036898137, 0.0007424923460073744232, 0.001113738519011058924, 0.001484984692014743642, 0.002227477038022112645, 0.002598723211025780015, 0.002969969384029447820, 0.003341215557033114757, 0.003712461730036782127, 0.004083707903040450365, 0.004454954076044117736, 0.004826200249047785107, 0.005197446422051451610, 0.005568692595055119848, 0.005939938768058787219 ),
 .UNSPECIFIED. ) ;
#195319=CARTESIAN_POINT ( 'NONE',  ( 0.05219959533907565091, 21.53943276465977519, 34.99890960531435979 ) ) ;
#195320=CARTESIAN_POINT ( 'NONE',  ( -9.564922557961040184, 16.46253265017147172, 37.91775706135233293 ) ) ;
#195321=CARTESIAN_POINT ( 'NONE',  ( -16.46253265017146816, -9.564922557961047289, 109.1677570613523471 ) ) ;
#195322=CARTESIAN_POINT ( 'NONE',  ( -13.97604488694527625, -13.89961937509977652, 21.87390960531435979 ) ) ;
#195323=CARTESIAN_POINT ( 'NONE',  ( 13.97604488694527802, 13.89961937509977652, 39.37390960531435269 ) ) ;
#195324=CARTESIAN_POINT ( 'NONE',  ( 10.72451020669898902, -18.67979575497178502, 72.91557627198103830 ) ) ;
#195325=CARTESIAN_POINT ( 'NONE',  ( 13.89961937509977652, -13.97604488694527269, 38.12390960531436690 ) ) ;
#195327=CARTESIAN_POINT ( 'NONE',  ( -13.89961937509957401, -13.97604488694547875, 79.37609039468567573 ) ) ;
#195328=CARTESIAN_POINT ( 'NONE',  ( 4.379528057220339221, -16.55341960407611168, 47.70724293864770260 ) ) ;
#195329=CARTESIAN_POINT ( 'NONE',  ( -10.81492255796078084, -18.62759615963271287, 27.08224293864769550 ) ) ;
#195330=CARTESIAN_POINT ( 'NONE',  ( 0.05219959533937995610, -21.53943276465977519, 90.00109039468567573 ) ) ;
#195331=CARTESIAN_POINT ( 'NONE',  ( -10.81492255796078084, -18.62759615963271287, 82.08224293864768129 ) ) ;
#195332=CARTESIAN_POINT ( 'NONE',  ( 21.55341960407619695, -5.719274019375665929, 76.04275706135237556 ) ) ;
#195333=CARTESIAN_POINT ( 'NONE',  ( -5.719274019375665041, -21.55341960407619695, 59.79275706135234714 ) ) ;
#195334=CARTESIAN_POINT ( 'NONE',  ( -5.153800228976328057, -19.02544592524343514, 97.29057627198099567 ) ) ;
#195335=CARTESIAN_POINT ( 'NONE',  ( 4.483927247898790824, -16.52544592524335698, 100.2094237280190043 ) ) ;
#195336=CARTESIAN_POINT ( 'NONE',  ( 18.67979575497194134, -10.72451020669871369, 60.83442372801901854 ) ) ;
#195337=CARTESIAN_POINT ( 'NONE',  ( 19.02544592524343514, -5.153800228976328945, 53.54057627198102409 ) ) ;
#195338=CARTESIAN_POINT ( 'NONE',  ( -21.53943276465977519, -0.05219959533937600094, 33.75109039468568284 ) ) ;
#195339=CARTESIAN_POINT ( 'NONE',  ( 16.51473224551069308, 9.474510206698969483, 69.16557627198102409 ) ) ;
#195340=CARTESIAN_POINT ( 'NONE',  ( 12.06949235617757843, -12.14591786802309237, 83.12390960531436690 ) ) ;
#195341=CARTESIAN_POINT ( 'NONE',  ( -12.06949235617756955, 12.14591786802309770, 45.62390960531436690 ) ) ;
#195342=CARTESIAN_POINT ( 'NONE',  ( 21.53943276465977519, -0.05219959533907433946, 58.74890960531436690 ) ) ;
#195343=CARTESIAN_POINT ( 'NONE',  ( 16.46253265017160672, -9.564922557960803928, 43.33224293864769550 ) ) ;
#195344=CARTESIAN_POINT ( 'NONE',  ( 18.67979575497178502, 10.72451020669898547, 54.16557627198103120 ) ) ;
#195345=CARTESIAN_POINT ( 'NONE',  ( 9.474510206698729675, 16.51473224551082808, 47.08442372801900433 ) ) ;
#195347=CARTESIAN_POINT ( 'NONE',  ( -12.14591786802309592, -12.06949235617757132, 61.87390960531436690 ) ) ;
#195348=CARTESIAN_POINT ( 'NONE',  ( -5.719274019375978568, 21.55341960407610458, 40.20724293864769550 ) ) ;
#195351=CARTESIAN_POINT ( 'NONE',  ( -16.53943276465976808, -0.05219959533934237506, 83.75109039468568994 ) ) ;
#195353=CARTESIAN_POINT ( 'NONE',  ( 19.03943276465977164, 0.05219959533936151252, 86.25109039468567573 ) ) ;
#195354=CARTESIAN_POINT ( 'NONE',  ( 12.06949235617757843, -12.14591786802309237, 58.12390960531435979 ) ) ;
#195355=CARTESIAN_POINT ( 'NONE',  ( -19.52851543214742946, -5.500000000000036415, 60.39357721762581832 ) ) ;
#195356=CARTESIAN_POINT ( 'NONE',  ( -16.46253265017160317, 9.564922557960807481, 50.83224293864770260 ) ) ;
#195357=CARTESIAN_POINT ( 'NONE',  ( -8.314922557960811034, -14.29746914071050412, 42.08224293864769550 ) ) ;
#195358=CARTESIAN_POINT ( 'NONE',  ( 13.89961937509977652, -13.97604488694527269, 83.12390960531436690 ) ) ;
#195360=CARTESIAN_POINT ( 'NONE',  ( 16.46253265017160672, -9.564922557960803928, 58.33224293864769550 ) ) ;
#195361=CARTESIAN_POINT ( 'NONE',  ( -18.67979575497193778, 10.72451020669871902, 58.33442372801901143 ) ) ;
#195362=CARTESIAN_POINT ( 'NONE',  ( -19.05341960407611168, -5.049401038298163336, 76.45724293864769550 ) ) ;
#195363=CARTESIAN_POINT ( 'NONE',  ( -19.05341960407611168, -5.049401038298163336, 26.45724293864769550 ) ) ;
#195364=CARTESIAN_POINT ( 'NONE',  ( 19.05341960407611168, 5.049401038298154454, 58.95724293864768129 ) ) ;
#195365=CARTESIAN_POINT ( 'NONE',  ( 15.80617190586746368, 15.72974639402197994, 54.37390960531435979 ) ) ;
#195366=CARTESIAN_POINT ( 'NONE',  ( 0.05219959533909260263, 19.03943276465977164, 29.99890960531435979 ) ) ;
#195367=CARTESIAN_POINT ( 'NONE',  ( -21.52544592524343514, 5.823673210054127303, 46.04057627198103830 ) ) ;
#195368=CARTESIAN_POINT ( 'NONE',  ( -0.05219959533934338120, 16.53943276465976808, 107.5010903946856899 ) ) ;
#195369=CARTESIAN_POINT ( 'NONE',  ( -9.474510206698720793, -16.51473224551083518, 19.58442372801899722 ) ) ;
#195371=CARTESIAN_POINT ( 'NONE',  ( 16.53943276465976808, 0.05219959533934440121, 41.25109039468568284 ) ) ;
#195372=CARTESIAN_POINT ( 'NONE',  ( -14.29746914071037622, -8.314922557961029526, 84.16775706135234714 ) ) ;
#195373=DIRECTION ( 'NONE',  ( 0.000000000000000000, 0.000000000000000000, -1.000000000000000000 ) ) ;
#195374=CARTESIAN_POINT ( 'NONE',  ( -16.53943276465976808, -0.05219959533934237506, 68.75109039468568994 ) ) ;
#195375=CARTESIAN_POINT ( 'NONE',  ( 8.314922557961029526, -14.29746914071037800, 50.41775706135235424 ) ) ;
#195376=CARTESIAN_POINT ( 'NONE',  ( 19.02544592524343514, -5.153800228976328945, 103.5405762719809957 ) ) ;
#195378=CARTESIAN_POINT ( 'NONE',  ( -13.89961937509977652, 13.97604488694528158, 30.62390960531435269 ) ) ;
#195379=CARTESIAN_POINT ( 'NONE',  ( -12.14591786802326823, 12.06949235617739902, 43.12609039468568284 ) ) ;
#195380=CARTESIAN_POINT ( 'NONE',  ( 16.46253265017160672, -9.564922557960803928, 48.33224293864769550 ) ) ;
#195381=CARTESIAN_POINT ( 'NONE',  ( 10.72451020669871369, 18.67979575497193778, 27.08442372801901854 ) ) ;
#195382=CARTESIAN_POINT ( 'NONE',  ( 8.314922557961029526, -14.29746914071037800, 35.41775706135234003 ) ) ;
#195383=CARTESIAN_POINT ( 'NONE',  ( -12.14591786802326823, 12.06949235617739902, 98.12609039468570415 ) ) ;
#195385=CARTESIAN_POINT ( 'NONE',  ( 18.62759615963255655, 10.81492255796105972, 106.6677570613523756 ) ) ;
#195386=CARTESIAN_POINT ( 'NONE',  ( 13.97604488694548053, -13.89961937509957401, 95.62609039468563310 ) ) ;
#195387=CARTESIAN_POINT ( 'NONE',  ( 8.314922557960818139, 14.29746914071049879, 59.58224293864770260 ) ) ;
#195388=CARTESIAN_POINT ( 'NONE',  ( 13.89961937509977652, -13.97604488694527269, 28.12390960531435624 ) ) ;
#195389=CARTESIAN_POINT ( 'NONE',  ( 9.474510206698729675, 16.51473224551082808, 62.08442372801899722 ) ) ;
#195391=CARTESIAN_POINT ( 'NONE',  ( 18.62759615963255655, 10.81492255796105972, 61.66775706135235424 ) ) ;
#195392=CARTESIAN_POINT ( 'NONE',  ( -14.34966873604972548, 8.224510206698743886, 28.33442372801902209 ) ) ;
#195393=CARTESIAN_POINT ( 'NONE',  ( 17.26058549869093284, 6.457015423128505738, 83.87745837476067834 ) ) ;
#195394=CARTESIAN_POINT ( 'NONE',  ( -21.52544592524343514, 5.823673210054127303, 26.04057627198103475 ) ) ;
#195395=CARTESIAN_POINT ( 'NONE',  ( -16.52544592524335698, -4.483927247898792601, 18.95942372801901143 ) ) ;
#195398=CARTESIAN_POINT ( 'NONE',  ( -13.97604488694527625, -13.89961937509977652, 26.87390960531434558 ) ) ;
#195399=CARTESIAN_POINT ( 'NONE',  ( -10.72451020669870658, -18.67979575497194134, 104.5844237280190185 ) ) ;
#195400=CARTESIAN_POINT ( 'NONE',  ( -16.51473224551069308, -9.474510206698971260, 41.66557627198103120 ) ) ;
#195402=CARTESIAN_POINT ( 'NONE',  ( -21.55341960407619339, 5.719274019375674811, 63.54275706135234003 ) ) ;
#195403=CARTESIAN_POINT ( 'NONE',  ( 18.62759615963255655, 10.81492255796105972, 101.6677570613523613 ) ) ;
#195404=CARTESIAN_POINT ( 'NONE',  ( 4.483927247898790824, -16.52544592524335698, 105.2094237280190328 ) ) ;
#195405=CARTESIAN_POINT ( 'NONE',  ( 9.564922557960805705, 16.46253265017160317, 74.58224293864769550 ) ) ;
#195406=CARTESIAN_POINT ( 'NONE',  ( 15.80617190586769283, -15.72974639402175789, 50.62609039468568994 ) ) ;
#195407=CARTESIAN_POINT ( 'NONE',  ( -18.62759615963255300, -10.81492255796106328, 59.16775706135234714 ) ) ;
#195408=CARTESIAN_POINT ( 'NONE',  ( 13.97604488694548053, -13.89961937509957401, 85.62609039468568994 ) ) ;
#195409=CARTESIAN_POINT ( 'NONE',  ( 16.46253265017160672, -9.564922557960803928, 103.3322429386476955 ) ) ;
#195410=CARTESIAN_POINT ( 'NONE',  ( -9.474510206698964154, 16.51473224551069663, 25.41557627198103120 ) ) ;
#195411=CARTESIAN_POINT ( 'NONE',  ( 21.53943276465977519, -0.05219959533907433946, 93.74890960531436690 ) ) ;
#195412=CARTESIAN_POINT ( 'NONE',  ( -21.55341960407619339, 5.719274019375674811, 113.5427570613523756 ) ) ;
#195413=CARTESIAN_POINT ( 'NONE',  ( 16.55341960407611168, 4.379528057220329451, 93.95724293864770971 ) ) ;
#195414=CARTESIAN_POINT ( 'NONE',  ( 9.474510206698971260, -16.51473224551069308, 52.91557627198102409 ) ) ;
#195415=CARTESIAN_POINT ( 'NONE',  ( -13.89961937509957401, -13.97604488694547875, 79.37609039468567573 ) ) ;
#195416=CARTESIAN_POINT ( 'NONE',  ( 8.314922557960818139, 14.29746914071049879, 59.58224293864770260 ) ) ;
#195417=CARTESIAN_POINT ( 'NONE',  ( -10.81492255796105439, 18.62759615963255655, 112.9177570613523329 ) ) ;
#195418=CARTESIAN_POINT ( 'NONE',  ( 19.02544592524343514, -5.153800228976328945, 103.5405762719809957 ) ) ;
#195419=CARTESIAN_POINT ( 'NONE',  ( 19.03943276465977164, 0.05219959533936151252, 76.25109039468566152 ) ) ;
#195420=CARTESIAN_POINT ( 'NONE',  ( 15.80617190586746368, 15.72974639402197994, 74.37390960531436690 ) ) ;
#195422=CARTESIAN_POINT ( 'NONE',  ( -5.823673210054431948, 21.52544592524334988, 27.70942372801901854 ) ) ;
#195423=CARTESIAN_POINT ( 'NONE',  ( 14.34966873604972726, -8.224510206698740333, 25.83442372801901499 ) ) ;
#195424=CARTESIAN_POINT ( 'NONE',  ( 14.29746914071037800, 8.314922557961029526, 86.66775706135234714 ) ) ;
#195425=CARTESIAN_POINT ( 'NONE',  ( 8.224510206698742110, 14.34966873604972548, 42.08442372801901854 ) ) ;
#195426=CARTESIAN_POINT ( 'NONE',  ( 15.80617190586769283, -15.72974639402175789, 30.62609039468567929 ) ) ;
#195427=CARTESIAN_POINT ( 'NONE',  ( 5.719274019375991003, -21.55341960407610458, 37.70724293864769550 ) ) ;
#195428=CARTESIAN_POINT ( 'NONE',  ( -16.53943276465976808, -0.05219959533934237506, 53.75109039468568994 ) ) ;
#195429=CARTESIAN_POINT ( 'NONE',  ( -13.89961937509977652, 13.97604488694528158, 40.62390960531435979 ) ) ;
#195431=CARTESIAN_POINT ( 'NONE',  ( -12.14591786802326823, 12.06949235617739902, 58.12609039468568994 ) ) ;
#195432=EDGE_CURVE ( 'NONE', #33580, #165125, #35535, .T. ) ;
#195433=CARTESIAN_POINT ( 'NONE',  ( -10.72451020669898014, 18.67979575497178502, 85.41557627198102409 ) ) ;
#195434=CARTESIAN_POINT ( 'NONE',  ( -8.224510206698948167, 14.34966873604960824, 40.41557627198103120 ) ) ;
#195435=CARTESIAN_POINT ( 'NONE',  ( -16.55341960407617563, 4.379528057220093196, 43.54275706135235424 ) ) ;
#195436=CARTESIAN_POINT ( 'NONE',  ( 19.05341960407611168, 5.049401038298154454, 53.95724293864770260 ) ) ;
#195437=CARTESIAN_POINT ( 'NONE',  ( -12.06949235617739369, -12.14591786802326823, 89.37609039468568994 ) ) ;
#195438=CARTESIAN_POINT ( 'NONE',  ( 13.97604488694548053, -13.89961937509957401, 90.62609039468567573 ) ) ;
#195439=CARTESIAN_POINT ( 'NONE',  ( -10.81492255796078084, -18.62759615963271287, 87.08224293864769550 ) ) ;
#195440=CARTESIAN_POINT ( 'NONE',  ( -16.53943276465976808, 0.05219959533911058130, 36.24890960531435979 ) ) ;
#195443=CARTESIAN_POINT ( 'NONE',  ( 10.81492255796078972, 18.62759615963270932, 54.58224293864769550 ) ) ;
#195444=ORIENTED_EDGE ( 'NONE', *, *, #56442, .F. ) ;
#195445=CARTESIAN_POINT ( 'NONE',  ( 16.53943276465976808, 0.05219959533934440121, 101.2510903946856757 ) ) ;
#195446=ORIENTED_EDGE ( 'NONE', *, *, #22002, .T. ) ;
#195447=CARTESIAN_POINT ( 'NONE',  ( -0.05219959533907301413, -21.53943276465977519, 27.49890960531435269 ) ) ;
#195449=CARTESIAN_POINT ( 'NONE',  ( -15.80617190586745835, -15.72974639402198527, 86.87390960531438111 ) ) ;
#195450=CARTESIAN_POINT ( 'NONE',  ( 14.29746914071037800, 8.314922557961029526, 111.6677570613523613 ) ) ;
#195452=CARTESIAN_POINT ( 'NONE',  ( -8.314922557961024197, 14.29746914071037800, 32.91775706135234714 ) ) ;
#195453=CARTESIAN_POINT ( 'NONE',  ( -0.05219959533909027116, -19.03943276465977164, 32.49890960531435979 ) ) ;
#195454=CARTESIAN_POINT ( 'NONE',  ( 0.05219959533934541429, -16.53943276465976808, 35.00109039468568284 ) ) ;
#195455=CARTESIAN_POINT ( 'NONE',  ( 9.564922557960805705, 16.46253265017160317, 54.58224293864769550 ) ) ;
#195457=CARTESIAN_POINT ( 'NONE',  ( -19.02544592524342804, 5.153800228976336051, 106.0405762719810241 ) ) ;
#195459=CARTESIAN_POINT ( 'NONE',  ( 4.483927247898790824, -16.52544592524335698, 100.2094237280190043 ) ) ;
#195460=CARTESIAN_POINT ( 'NONE',  ( 9.474510206698729675, 16.51473224551082808, 87.08442372801900433 ) ) ;
#195461=CARTESIAN_POINT ( 'NONE',  ( 19.05341960407617918, -5.049401038297876454, 41.04275706135233293 ) ) ;
#195462=CARTESIAN_POINT ( 'NONE',  ( 15.72974639402199770, -15.80617190586745480, 78.12390960531436690 ) ) ;
#195463=CARTESIAN_POINT ( 'NONE',  ( -12.06949235617739369, -12.14591786802326823, 94.37609039468568994 ) ) ;
#195464=CARTESIAN_POINT ( 'NONE',  ( 15.80617190586746368, 15.72974639402197994, 34.37390960531435979 ) ) ;
#195465=CARTESIAN_POINT ( 'NONE',  ( -9.564922557961040184, 16.46253265017147172, 102.9177570613523329 ) ) ;
#195466=CARTESIAN_POINT ( 'NONE',  ( 16.46253265017160672, -9.564922557960803928, 108.3322429386476955 ) ) ;
#195467=CARTESIAN_POINT ( 'NONE',  ( 0.05219959533937995610, -21.53943276465977519, 60.00109039468568284 ) ) ;
#195468=CARTESIAN_POINT ( 'NONE',  ( -19.05341960407611168, -5.049401038298163336, 56.45724293864768129 ) ) ;
#195469=CARTESIAN_POINT ( 'NONE',  ( -8.314922557960811034, -14.29746914071050412, 107.0822429386476955 ) ) ;
#195470=CARTESIAN_POINT ( 'NONE',  ( 14.29746914071049879, -8.314922557960816363, 73.33224293864769550 ) ) ;
#195471=ORIENTED_EDGE ( 'NONE', *, *, #169970, .F. ) ;
#195472=CARTESIAN_POINT ( 'NONE',  ( 0.05219959533936267826, -19.03943276465977164, 90.00109039468567573 ) ) ;
#195473=CARTESIAN_POINT ( 'NONE',  ( 18.56101223717332971, 5.500000000000005329, 93.94978406935678095 ) ) ;
#195474=CARTESIAN_POINT ( 'NONE',  ( -16.46253265017160317, 9.564922557960807481, 65.83224293864769550 ) ) ;
#195476=CARTESIAN_POINT ( 'NONE',  ( 16.46253265017160672, -9.564922557960803928, 78.33224293864769550 ) ) ;
#195477=CARTESIAN_POINT ( 'NONE',  ( -9.474510206698964154, 16.51473224551069663, 85.41557627198102409 ) ) ;
#195478=CARTESIAN_POINT ( 'NONE',  ( 14.34966873604972726, -8.224510206698740333, 70.83442372801901854 ) ) ;
#195480=CARTESIAN_POINT ( 'NONE',  ( -16.46253265017146816, -9.564922557961047289, 39.16775706135234003 ) ) ;
#195481=CARTESIAN_POINT ( 'NONE',  ( 0.05219959533937995610, -21.53943276465977519, 95.00109039468568994 ) ) ;
#195483=CARTESIAN_POINT ( 'NONE',  ( -5.049401038298153566, 19.05341960407611168, 115.2072429386477097 ) ) ;
#195484=CARTESIAN_POINT ( 'NONE',  ( -14.29746914071037622, -8.314922557961029526, 109.1677570613523613 ) ) ;
#195486=CARTESIAN_POINT ( 'NONE',  ( -8.314922557961024197, 14.29746914071037800, 92.91775706135236135 ) ) ;
#195487=CARTESIAN_POINT ( 'NONE',  ( -17.13100169013300444, 6.664070546373151771, 30.76789835699849718 ) ) ;
#195488=CARTESIAN_POINT ( 'NONE',  ( 16.52544592524335698, 4.483927247898782831, 61.45942372801901854 ) ) ;
#195490=CARTESIAN_POINT ( 'NONE',  ( 21.55341960407619695, -5.719274019375665929, 86.04275706135236135 ) ) ;
#195491=CARTESIAN_POINT ( 'NONE',  ( 13.89961937509957401, 13.97604488694547697, 91.87609039468567573 ) ) ;
#195492=CARTESIAN_POINT ( 'NONE',  ( 5.049401038297881783, 19.05341960407617563, 27.29275706135232937 ) ) ;
#195494=CARTESIAN_POINT ( 'NONE',  ( -13.97604488694527625, -13.89961937509977652, 71.87390960531433848 ) ) ;
#195495=CARTESIAN_POINT ( 'NONE',  ( -5.049401038298153566, 19.05341960407611168, 50.20724293864770260 ) ) ;
#195496=CARTESIAN_POINT ( 'NONE',  ( 16.56723268710308616, 7.192918735248206907, 22.04583401990673863 ) ) ;
#195497=CARTESIAN_POINT ( 'NONE',  ( -21.52544592524343514, 5.823673210054127303, 86.04057627198102409 ) ) ;
#195498=CARTESIAN_POINT ( 'NONE',  ( 21.52544592524344225, -5.823673210054117533, 28.54057627198103120 ) ) ;
#195499=CARTESIAN_POINT ( 'NONE',  ( 13.89961937509977652, -13.97604488694527269, 28.12390960531435624 ) ) ;
#195500=CARTESIAN_POINT ( 'NONE',  ( -4.379528057220086978, -16.55341960407618274, 54.79275706135235424 ) ) ;
#195502=EDGE_LOOP ( 'NONE', ( #153879, #142908 ) ) ;
#195503=CARTESIAN_POINT ( 'NONE',  ( 0.05219959533937995610, -21.53943276465977519, 25.00109039468567218 ) ) ;
#195504=CARTESIAN_POINT ( 'NONE',  ( -12.06949235617756955, 12.14591786802309770, 55.62390960531436690 ) ) ;
#195506=CARTESIAN_POINT ( 'NONE',  ( -16.53943276465976808, -0.05219959533934237506, 18.75109039468568639 ) ) ;
#195507=CARTESIAN_POINT ( 'NONE',  ( -19.03943276465977164, -0.05219959533935918106, 33.75109039468566863 ) ) ;
#195508=CARTESIAN_POINT ( 'NONE',  ( -12.14591786802309592, -12.06949235617757132, 56.87390960531436690 ) ) ;
#195509=CARTESIAN_POINT ( 'NONE',  ( 21.55341960407619695, -5.719274019375665929, 21.04275706135234714 ) ) ;
#195511=CARTESIAN_POINT ( 'NONE',  ( 15.80617190586746368, 15.72974639402197994, 74.37390960531436690 ) ) ;
#195512=CARTESIAN_POINT ( 'NONE',  ( 0.05219959533909260263, 19.03943276465977164, 84.99890960531436690 ) ) ;
#195513=CARTESIAN_POINT ( 'NONE',  ( -16.53943276465976808, 0.05219959533911058130, 66.24890960531436690 ) ) ;
#195514=CARTESIAN_POINT ( 'NONE',  ( 13.89961937509977652, -13.97604488694527269, 103.1239096053143527 ) ) ;
#195516=CARTESIAN_POINT ( 'NONE',  ( 19.03943276465977164, 0.05219959533936151252, 71.25109039468566152 ) ) ;
#195517=CARTESIAN_POINT ( 'NONE',  ( -21.53943276465977519, 0.05219959533907696930, 101.2489096053143669 ) ) ;
#195518=CARTESIAN_POINT ( 'NONE',  ( 9.564922557960805705, 16.46253265017160317, 59.58224293864769550 ) ) ;
#195519=CARTESIAN_POINT ( 'NONE',  ( -19.02544592524334988, -5.153800228976617603, 43.95942372801899012 ) ) ;
#195520=CARTESIAN_POINT ( 'NONE',  ( 4.379528057220339221, -16.55341960407611168, 112.7072429386476955 ) ) ;
#195521=CARTESIAN_POINT ( 'NONE',  ( 15.72974639402176855, 15.80617190586768217, 66.87609039468568994 ) ) ;
#195522=CARTESIAN_POINT ( 'NONE',  ( -18.39635199886970085, 5.499999999999979572, 101.0196707636000184 ) ) ;
#195523=CARTESIAN_POINT ( 'NONE',  ( 16.55341960407611168, 4.379528057220329451, 38.95724293864768839 ) ) ;
#195524=CARTESIAN_POINT ( 'NONE',  ( 16.46253265017160672, -9.564922557960803928, 63.33224293864769550 ) ) ;
#195525=CARTESIAN_POINT ( 'NONE',  ( -18.62759615963270932, 10.81492255796079327, 80.83224293864769550 ) ) ;
#195527=CARTESIAN_POINT ( 'NONE',  ( 16.46253265017160672, -9.564922557960803928, 58.33224293864769550 ) ) ;
#195528=CARTESIAN_POINT ( 'NONE',  ( -18.62759615963270932, 10.81492255796079327, 65.83224293864769550 ) ) ;
#195529=ORIENTED_EDGE ( 'NONE', *, *, #199792, .F. ) ;
#195530=CARTESIAN_POINT ( 'NONE',  ( 21.55341960407619695, -5.719274019375665929, 101.0427570613523756 ) ) ;
#195532=CARTESIAN_POINT ( 'NONE',  ( -8.314922557961024197, 14.29746914071037800, 102.9177570613523756 ) ) ;
#195533=CARTESIAN_POINT ( 'NONE',  ( 8.314922557960818139, 14.29746914071049879, 84.58224293864769550 ) ) ;
#195534=CARTESIAN_POINT ( 'NONE',  ( -16.51473224551069308, -9.474510206698971260, 76.66557627198103830 ) ) ;
#195536=CARTESIAN_POINT ( 'NONE',  ( -9.474510206698720793, -16.51473224551083518, 44.58442372801900433 ) ) ;
#195537=CARTESIAN_POINT ( 'NONE',  ( -8.314922557961024197, 14.29746914071037800, 82.91775706135234714 ) ) ;
#195538=CARTESIAN_POINT ( 'NONE',  ( 5.153800228976615827, -19.02544592524334988, 30.20942372801900433 ) ) ;
#195539=CARTESIAN_POINT ( 'NONE',  ( -16.46253265017160317, 9.564922557960807481, 90.83224293864769550 ) ) ;
#195540=CARTESIAN_POINT ( 'NONE',  ( 0.05219959533907565091, 21.53943276465977519, 54.99890960531435269 ) ) ;
#195542=CARTESIAN_POINT ( 'NONE',  ( 19.03943276465977164, -0.05219959533909143690, 23.74890960531435269 ) ) ;
#195543=CARTESIAN_POINT ( 'NONE',  ( 15.80617190586769283, -15.72974639402175789, 95.62609039468568994 ) ) ;
#195544=CARTESIAN_POINT ( 'NONE',  ( 12.14591786802327356, -12.06949235617739191, 60.62609039468567573 ) ) ;
#195545=CARTESIAN_POINT ( 'NONE',  ( 10.72451020669871369, 18.67979575497193778, 27.08442372801901854 ) ) ;
#195546=CARTESIAN_POINT ( 'NONE',  ( 4.483927247898790824, -16.52544592524335698, 30.20942372801902565 ) ) ;
#195547=CARTESIAN_POINT ( 'NONE',  ( -16.51473224551069308, -9.474510206698971260, 96.66557627198102409 ) ) ;
#195548=CARTESIAN_POINT ( 'NONE',  ( -5.049401038298153566, 19.05341960407611168, 40.20724293864768839 ) ) ;
#195549=CARTESIAN_POINT ( 'NONE',  ( 5.153800228976335163, 19.02544592524342804, 54.79057627198103120 ) ) ;
#195551=CARTESIAN_POINT ( 'NONE',  ( -4.483927247898782831, 16.52544592524335698, 32.70942372801900433 ) ) ;
#195552=CARTESIAN_POINT ( 'NONE',  ( 12.06949235617757843, -12.14591786802309237, 93.12390960531436690 ) ) ;
#195553=CARTESIAN_POINT ( 'NONE',  ( 12.14591786802327356, -12.06949235617739191, 105.6260903946856899 ) ) ;
#195554=CARTESIAN_POINT ( 'NONE',  ( -15.72974639402176322, -15.80617190586768395, 44.37609039468567573 ) ) ;
#195555=CARTESIAN_POINT ( 'NONE',  ( 16.51473224551069308, 9.474510206698969483, 74.16557627198103830 ) ) ;
#195556=CARTESIAN_POINT ( 'NONE',  ( -5.153800228976328057, -19.02544592524343514, 57.29057627198103120 ) ) ;
#195557=CARTESIAN_POINT ( 'NONE',  ( 16.46253265017160672, -9.564922557960803928, 78.33224293864769550 ) ) ;
#195558=CARTESIAN_POINT ( 'NONE',  ( 12.06949235617757843, -12.14591786802309237, 33.12390960531435979 ) ) ;
#195559=CARTESIAN_POINT ( 'NONE',  ( 4.483927247898790824, -16.52544592524335698, 95.20942372801903275 ) ) ;
#195561=CARTESIAN_POINT ( 'NONE',  ( -19.03943276465977164, -0.05219959533935918106, 38.75109039468566152 ) ) ;
#195562=CARTESIAN_POINT ( 'NONE',  ( -13.97604488694527625, -13.89961937509977652, 111.8739096053143243 ) ) ;
#195563=CARTESIAN_POINT ( 'NONE',  ( -5.153800228976328057, -19.02544592524343514, 47.29057627198102409 ) ) ;
#195564=CARTESIAN_POINT ( 'NONE',  ( -0.05219959533936034679, 19.03943276465977164, 22.50109039468566152 ) ) ;
#195566=CARTESIAN_POINT ( 'NONE',  ( 16.53943276465976808, 0.05219959533934440121, 36.25109039468567573 ) ) ;
#195568=CARTESIAN_POINT ( 'NONE',  ( 9.564922557961047289, -16.46253265017146816, 70.41775706135233293 ) ) ;
#195569=CARTESIAN_POINT ( 'NONE',  ( 4.483927247898790824, -16.52544592524335698, 50.20942372801901854 ) ) ;
#195570=CARTESIAN_POINT ( 'NONE',  ( 19.05341960407611168, 5.049401038298154454, 113.9572429386477097 ) ) ;
#195571=CARTESIAN_POINT ( 'NONE',  ( -19.02544592524342804, 5.153800228976336051, 81.04057627198103830 ) ) ;
#195572=CARTESIAN_POINT ( 'NONE',  ( -15.80617190586745835, -15.72974639402198527, 111.8739096053143669 ) ) ;
#195573=CARTESIAN_POINT ( 'NONE',  ( -19.02544592524334988, -5.153800228976617603, 78.95942372801900433 ) ) ;
#195574=CARTESIAN_POINT ( 'NONE',  ( -5.049401038298153566, 19.05341960407611168, 110.2072429386476671 ) ) ;
#195575=CARTESIAN_POINT ( 'NONE',  ( 5.153800228976335163, 19.02544592524342804, 34.79057627198102409 ) ) ;
#195576=CARTESIAN_POINT ( 'NONE',  ( 5.049401038298161559, -19.05341960407611168, 77.70724293864765286 ) ) ;
#195577=CARTESIAN_POINT ( 'NONE',  ( 16.52544592524342804, -4.483927247898539470, 38.54057627198103120 ) ) ;
#195578=CARTESIAN_POINT ( 'NONE',  ( -9.474510206698964154, 16.51473224551069663, 30.41557627198102054 ) ) ;
#195580=CARTESIAN_POINT ( 'NONE',  ( 0.05219959533936267826, -19.03943276465977164, 50.00109039468566863 ) ) ;
#195581=CARTESIAN_POINT ( 'NONE',  ( 16.53943276465976808, -0.05219959533910856209, 73.74890960531433848 ) ) ;
#195582=CARTESIAN_POINT ( 'NONE',  ( -19.03943276465977164, -0.05219959533935918106, 18.75109039468567218 ) ) ;
#195583=CARTESIAN_POINT ( 'NONE',  ( 0.05219959533909260263, 19.03943276465977164, 54.99890960531435979 ) ) ;
#195584=CARTESIAN_POINT ( 'NONE',  ( -18.67979575497178146, -10.72451020669898902, 56.66557627198103830 ) ) ;
#195585=CARTESIAN_POINT ( 'NONE',  ( -8.314922557960811034, -14.29746914071050412, 57.08224293864769550 ) ) ;
#195586=CARTESIAN_POINT ( 'NONE',  ( -21.53943276465977519, -0.05219959533937600094, 103.7510903946857042 ) ) ;
#195587=CARTESIAN_POINT ( 'NONE',  ( -13.97604488694527625, -13.89961937509977652, 91.87390960531432427 ) ) ;
#195588=CARTESIAN_POINT ( 'NONE',  ( -0.05219959533909027116, -19.03943276465977164, 112.4989096053143669 ) ) ;
#195589=CARTESIAN_POINT ( 'NONE',  ( -16.46253265017160317, 9.564922557960807481, 35.83224293864768839 ) ) ;
#195590=CARTESIAN_POINT ( 'NONE',  ( 8.314922557960818139, 14.29746914071049879, 114.5822429386477097 ) ) ;
#195591=CARTESIAN_POINT ( 'NONE',  ( -8.224510206698948167, 14.34966873604960824, 90.41557627198103830 ) ) ;
#195592=CARTESIAN_POINT ( 'NONE',  ( -10.72451020669898014, 18.67979575497178502, 100.4155762719810241 ) ) ;
#195593=CARTESIAN_POINT ( 'NONE',  ( 16.51473224551069308, 9.474510206698969483, 89.16557627198103830 ) ) ;
#195594=CARTESIAN_POINT ( 'NONE',  ( 10.72451020669898902, -18.67979575497178502, 112.9155762719810383 ) ) ;
#195595=CARTESIAN_POINT ( 'NONE',  ( 0.05219959533909260263, 19.03943276465977164, 89.99890960531436690 ) ) ;
#195596=LINE ( 'NONE', #132896, #46533 ) ;
#195597=CARTESIAN_POINT ( 'NONE',  ( 12.14591786802309770, 12.06949235617756955, 99.37390960531436690 ) ) ;
#195598=CARTESIAN_POINT ( 'NONE',  ( 13.89961937509977652, -13.97604488694527269, 78.12390960531433848 ) ) ;
#195599=CARTESIAN_POINT ( 'NONE',  ( -15.72974639402197994, 15.80617190586746368, 85.62390960531436690 ) ) ;
#195600=CARTESIAN_POINT ( 'NONE',  ( -9.474510206698964154, 16.51473224551069663, 115.4155762719810241 ) ) ;
#195602=CARTESIAN_POINT ( 'NONE',  ( 21.52544592524344225, -5.823673210054117533, 23.54057627198102765 ) ) ;
#195603=CARTESIAN_POINT ( 'NONE',  ( 18.87580814761071579, -5.500000000000034639, 68.37172394265761000 ) ) ;
#195604=CARTESIAN_POINT ( 'NONE',  ( 4.379528057220092307, 16.55341960407617563, 37.29275706135235424 ) ) ;
#195605=CARTESIAN_POINT ( 'NONE',  ( 16.55341960407611168, 4.379528057220329451, 88.95724293864769550 ) ) ;
#195606=CARTESIAN_POINT ( 'NONE',  ( -17.49999999999999645, -5.499999999999992895, 94.20309617465827046 ) ) ;
#195607=CARTESIAN_POINT ( 'NONE',  ( 16.51473224551069308, 9.474510206698969483, 84.16557627198102409 ) ) ;
#195608=CARTESIAN_POINT ( 'NONE',  ( -13.97604488694527625, -13.89961937509977652, 41.87390960531435979 ) ) ;
#195609=CARTESIAN_POINT ( 'NONE',  ( 8.224510206698953496, -14.34966873604960469, 82.91557627198103830 ) ) ;
#195611=CARTESIAN_POINT ( 'NONE',  ( 15.72974639402199770, -15.80617190586745480, 33.12390960531435979 ) ) ;
#195612=CARTESIAN_POINT ( 'NONE',  ( -0.05219959533910754901, -16.53943276465976808, 52.49890960531435979 ) ) ;
#195613=CARTESIAN_POINT ( 'NONE',  ( 0.05219959533936267826, -19.03943276465977164, 100.0010903946856757 ) ) ;
#195614=CARTESIAN_POINT ( 'NONE',  ( -21.55341960407619339, 5.719274019375674811, 58.54275706135235424 ) ) ;
#195616=CARTESIAN_POINT ( 'NONE',  ( 5.049401038298161559, -19.05341960407611168, 112.7072429386476813 ) ) ;
#195617=CARTESIAN_POINT ( 'NONE',  ( -12.14591786802326823, 12.06949235617739902, 78.12609039468570415 ) ) ;
#195618=CARTESIAN_POINT ( 'NONE',  ( -17.26172910966712948, 6.454744622557082145, 95.80646908649208626 ) ) ;
#195619=CARTESIAN_POINT ( 'NONE',  ( -9.564922557960796823, -16.46253265017161027, 72.08224293864770971 ) ) ;
#195620=CARTESIAN_POINT ( 'NONE',  ( -5.823673210054116645, -21.52544592524344225, 77.29057627198102409 ) ) ;
#195621=CARTESIAN_POINT ( 'NONE',  ( 14.34966873604972726, -8.224510206698740333, 25.83442372801901499 ) ) ;
#195622=CARTESIAN_POINT ( 'NONE',  ( 16.52544592524342804, -4.483927247898539470, 48.54057627198103120 ) ) ;
#195623=CARTESIAN_POINT ( 'NONE',  ( 21.53943276465977519, 0.05219959533937863772, 61.25109039468567573 ) ) ;
#195624=CARTESIAN_POINT ( 'NONE',  ( -8.224510206698735004, -14.34966873604973081, 84.58442372801903275 ) ) ;
#195625=CARTESIAN_POINT ( 'NONE',  ( 21.52544592524344225, -5.823673210054117533, 28.54057627198103120 ) ) ;
#195626=CARTESIAN_POINT ( 'NONE',  ( -9.564922557960796823, -16.46253265017161027, 112.0822429386476955 ) ) ;
#195628=CARTESIAN_POINT ( 'NONE',  ( -0.05219959533934338120, 16.53943276465976808, 112.5010903946857042 ) ) ;
#195629=CARTESIAN_POINT ( 'NONE',  ( -14.29746914071037622, -8.314922557961029526, 64.16775706135234714 ) ) ;
#195630=CARTESIAN_POINT ( 'NONE',  ( -13.89961937509977652, 13.97604488694528158, 75.62390960531438111 ) ) ;
#195631=CARTESIAN_POINT ( 'NONE',  ( 16.51473224551069308, 9.474510206698969483, 84.16557627198102409 ) ) ;
#195632=CARTESIAN_POINT ( 'NONE',  ( -5.719274019375665041, -21.55341960407619695, 74.79275706135234714 ) ) ;
#195633=CARTESIAN_POINT ( 'NONE',  ( -16.53943276465976808, -0.05219959533934237506, 78.75109039468568994 ) ) ;
#195634=CARTESIAN_POINT ( 'NONE',  ( -8.224510206698948167, 14.34966873604960824, 40.41557627198103120 ) ) ;
#195635=CARTESIAN_POINT ( 'NONE',  ( 0.05219959533909260263, 19.03943276465977164, 54.99890960531435979 ) ) ;
#195636=CARTESIAN_POINT ( 'NONE',  ( 13.89961937509977652, -13.97604488694527269, 48.12390960531435979 ) ) ;
#195637=CARTESIAN_POINT ( 'NONE',  ( 4.379528057220092307, 16.55341960407617563, 37.29275706135235424 ) ) ;
#195639=CARTESIAN_POINT ( 'NONE',  ( -9.564922557961040184, 16.46253265017147172, 92.91775706135233293 ) ) ;
#195640=CARTESIAN_POINT ( 'NONE',  ( 16.53943276465976808, -0.05219959533910856209, 98.74890960531438111 ) ) ;
#195641=CARTESIAN_POINT ( 'NONE',  ( 19.05341960407611168, 5.049401038298154454, 58.95724293864768129 ) ) ;
#195642=CARTESIAN_POINT ( 'NONE',  ( -19.03943276465977164, -0.05219959533935918106, 98.75109039468567573 ) ) ;
#195644=CARTESIAN_POINT ( 'NONE',  ( 21.53943276465977519, 0.05219959533937863772, 106.2510903946856757 ) ) ;
#195645=CARTESIAN_POINT ( 'NONE',  ( -16.55341960407617563, 4.379528057220093196, 68.54275706135234714 ) ) ;
#195646=CARTESIAN_POINT ( 'NONE',  ( -0.05219959533936034679, 19.03943276465977164, 87.50109039468567573 ) ) ;
#195647=CARTESIAN_POINT ( 'NONE',  ( -0.05219959533907301413, -21.53943276465977519, 62.49890960531436690 ) ) ;
#195648=CARTESIAN_POINT ( 'NONE',  ( 4.379528057220092307, 16.55341960407617563, 57.29275706135234714 ) ) ;
#195650=CARTESIAN_POINT ( 'NONE',  ( -5.049401038297874678, -19.05341960407617918, 54.79275706135234003 ) ) ;
#195652=CARTESIAN_POINT ( 'NONE',  ( -16.46253265017160317, 9.564922557960807481, 95.83224293864769550 ) ) ;
#195653=CARTESIAN_POINT ( 'NONE',  ( -14.29746914071049879, 8.314922557960819915, 110.8322429386476955 ) ) ;
#195654=CARTESIAN_POINT ( 'NONE',  ( 9.474510206698971260, -16.51473224551069308, 67.91557627198102409 ) ) ;
#195655=CARTESIAN_POINT ( 'NONE',  ( 16.52544592524342804, -4.483927247898539470, 53.54057627198103120 ) ) ;
#195657=CARTESIAN_POINT ( 'NONE',  ( 21.53943276465977519, 0.05219959533937863772, 76.25109039468568994 ) ) ;
#195658=CARTESIAN_POINT ( 'NONE',  ( 9.564922557961047289, -16.46253265017146816, 50.41775706135233293 ) ) ;
#195659=CARTESIAN_POINT ( 'NONE',  ( 19.03943276465977164, 0.05219959533936151252, 31.25109039468566863 ) ) ;
#195660=CARTESIAN_POINT ( 'NONE',  ( -9.474510206698964154, 16.51473224551069663, 115.4155762719810241 ) ) ;
#195661=CARTESIAN_POINT ( 'NONE',  ( 10.81492255796106328, -18.62759615963255655, 90.41775706135236135 ) ) ;
#195662=CARTESIAN_POINT ( 'NONE',  ( 5.049401038298161559, -19.05341960407611168, 57.70724293864769550 ) ) ;
#195663=CARTESIAN_POINT ( 'NONE',  ( -21.55341960407619339, 5.719274019375674811, 98.54275706135234714 ) ) ;
#195664=CARTESIAN_POINT ( 'NONE',  ( 18.67979575497178502, 10.72451020669898547, 49.16557627198102409 ) ) ;
#195665=CARTESIAN_POINT ( 'NONE',  ( -16.51473224551069308, -9.474510206698971260, 81.66557627198103830 ) ) ;
#195666=CARTESIAN_POINT ( 'NONE',  ( 19.02544592524334988, 5.153800228976608722, 66.45942372801899012 ) ) ;
#195667=CARTESIAN_POINT ( 'NONE',  ( -19.03943276465977164, 0.05219959533909376836, 41.24890960531435269 ) ) ;
#195668=CARTESIAN_POINT ( 'NONE',  ( 19.05341960407611168, 5.049401038298154454, 88.95724293864769550 ) ) ;
#195669=CARTESIAN_POINT ( 'NONE',  ( -19.02544592524334988, -5.153800228976617603, 83.95942372801901854 ) ) ;
#195670=CARTESIAN_POINT ( 'NONE',  ( 14.34966873604972726, -8.224510206698740333, 45.83442372801901854 ) ) ;
#195671=CARTESIAN_POINT ( 'NONE',  ( 16.52544592524342804, -4.483927247898539470, 98.54057627198105251 ) ) ;
#195672=CARTESIAN_POINT ( 'NONE',  ( -9.474510206698964154, 16.51473224551069663, 70.41557627198102409 ) ) ;
#195673=CARTESIAN_POINT ( 'NONE',  ( -15.72974639402197994, 15.80617190586746368, 55.62390960531436690 ) ) ;
#195674=CARTESIAN_POINT ( 'NONE',  ( -19.03943276465977164, -0.05219959533935918106, 108.7510903946856615 ) ) ;
#195675=CARTESIAN_POINT ( 'NONE',  ( -18.62759615963255300, -10.81492255796106328, 19.16775706135234714 ) ) ;
#195676=CARTESIAN_POINT ( 'NONE',  ( 10.81492255796106328, -18.62759615963255655, 70.41775706135236135 ) ) ;
#195677=CARTESIAN_POINT ( 'NONE',  ( -0.05219959533934338120, 16.53943276465976808, 77.50109039468567573 ) ) ;
#195678=CARTESIAN_POINT ( 'NONE',  ( 16.46253265017160672, -9.564922557960803928, 78.33224293864769550 ) ) ;
#195679=CARTESIAN_POINT ( 'NONE',  ( 16.55341960407618274, -4.379528057220086978, 101.0427570613523756 ) ) ;
#195680=CARTESIAN_POINT ( 'NONE',  ( 13.89961937509957401, 13.97604488694547697, 46.87609039468565442 ) ) ;
#195681=CARTESIAN_POINT ( 'NONE',  ( 15.80617190586769283, -15.72974639402175789, 30.62609039468567929 ) ) ;
#195682=CARTESIAN_POINT ( 'NONE',  ( -14.34966873604960291, -8.224510206698953496, 81.66557627198103830 ) ) ;
#195683=CARTESIAN_POINT ( 'NONE',  ( 13.97604488694527802, 13.89961937509977652, 99.37390960531436690 ) ) ;
#195684=CARTESIAN_POINT ( 'NONE',  ( 16.53943276465976808, 0.05219959533934440121, 91.25109039468568994 ) ) ;
#195685=CARTESIAN_POINT ( 'NONE',  ( -5.823673210054431948, 21.52544592524334988, 77.70942372801900433 ) ) ;
#195686=CARTESIAN_POINT ( 'NONE',  ( -12.06949235617739369, -12.14591786802326823, 29.37609039468568284 ) ) ;
#195687=CARTESIAN_POINT ( 'NONE',  ( -5.719274019375665041, -21.55341960407619695, 29.79275706135234358 ) ) ;
#195688=CARTESIAN_POINT ( 'NONE',  ( -8.314922557960811034, -14.29746914071050412, 72.08224293864769550 ) ) ;
#195690=CARTESIAN_POINT ( 'NONE',  ( -21.52544592524343514, 5.823673210054127303, 106.0405762719810525 ) ) ;
#195691=CARTESIAN_POINT ( 'NONE',  ( -14.29746914071049879, 8.314922557960819915, 50.83224293864770971 ) ) ;
#195693=CARTESIAN_POINT ( 'NONE',  ( -5.153800228976328057, -19.02544592524343514, 32.29057627198102409 ) ) ;
#195694=CARTESIAN_POINT ( 'NONE',  ( 18.62759615963271287, -10.81492255796078972, 33.33224293864769550 ) ) ;
#195695=CARTESIAN_POINT ( 'NONE',  ( 15.80617190586769283, -15.72974639402175789, 40.62609039468567573 ) ) ;
#195696=CARTESIAN_POINT ( 'NONE',  ( -8.314922557960811034, -14.29746914071050412, 67.08224293864770971 ) ) ;
#195697=CARTESIAN_POINT ( 'NONE',  ( -15.80617190586745835, -15.72974639402198527, 71.87390960531438111 ) ) ;
#195698=CARTESIAN_POINT ( 'NONE',  ( -9.474510206698964154, 16.51473224551069663, 80.41557627198103830 ) ) ;
#195699=CARTESIAN_POINT ( 'NONE',  ( 13.89961937509977652, -13.97604488694527269, 23.12390960531436335 ) ) ;
#195700=CARTESIAN_POINT ( 'NONE',  ( 13.97604488694548053, -13.89961937509957401, 75.62609039468564731 ) ) ;
#195702=CARTESIAN_POINT ( 'NONE',  ( 21.52544592524344225, -5.823673210054117533, 58.54057627198103120 ) ) ;
#195703=CARTESIAN_POINT ( 'NONE',  ( -9.564922557960796823, -16.46253265017161027, 37.08224293864768839 ) ) ;
#195704=CARTESIAN_POINT ( 'NONE',  ( 5.049401038298161559, -19.05341960407611168, 77.70724293864765286 ) ) ;
#195705=ORIENTED_EDGE ( 'NONE', *, *, #154616, .F. ) ;
#195706=CARTESIAN_POINT ( 'NONE',  ( -16.52544592524335698, -4.483927247898792601, 33.95942372801901143 ) ) ;
#195707=CARTESIAN_POINT ( 'NONE',  ( -15.72974639402176322, -15.80617190586768395, 34.37609039468568284 ) ) ;
#195708=CARTESIAN_POINT ( 'NONE',  ( -18.67979575497193778, 10.72451020669871902, 53.33442372801901854 ) ) ;
#195709=CARTESIAN_POINT ( 'NONE',  ( 16.51473224551069308, 9.474510206698969483, 109.1655762719810383 ) ) ;
#195710=CARTESIAN_POINT ( 'NONE',  ( 18.62759615963271287, -10.81492255796078972, 73.33224293864769550 ) ) ;
#195711=CARTESIAN_POINT ( 'NONE',  ( 21.55341960407610458, 5.719274019375980345, 108.9572429386476955 ) ) ;
#195712=CARTESIAN_POINT ( 'NONE',  ( -8.314922557961024197, 14.29746914071037800, 47.91775706135234714 ) ) ;
#195713=CARTESIAN_POINT ( 'NONE',  ( 5.823673210054125526, 21.52544592524343514, 54.79057627198104541 ) ) ;
#195714=CARTESIAN_POINT ( 'NONE',  ( 10.81492255796106328, -18.62759615963255655, 105.4177570613523613 ) ) ;
#195715=CARTESIAN_POINT ( 'NONE',  ( -19.05341960407611168, -5.049401038298163336, 61.45724293864769550 ) ) ;
#195716=CARTESIAN_POINT ( 'NONE',  ( 13.89961937509977652, -13.97604488694527269, 113.1239096053143527 ) ) ;
#195717=CARTESIAN_POINT ( 'NONE',  ( -19.02544592524342804, 5.153800228976336051, 81.04057627198103830 ) ) ;
#195720=CARTESIAN_POINT ( 'NONE',  ( -13.89961937509957401, -13.97604488694547875, 64.37609039468567573 ) ) ;
#195721=CARTESIAN_POINT ( 'NONE',  ( 21.55341960407619695, -5.719274019375665929, 111.0427570613523613 ) ) ;
#195722=CARTESIAN_POINT ( 'NONE',  ( -21.53943276465977519, 0.05219959533907696930, 46.24890960531435979 ) ) ;
#195723=CARTESIAN_POINT ( 'NONE',  ( -4.379528057220086978, -16.55341960407618274, 99.79275706135234714 ) ) ;
#195724=CARTESIAN_POINT ( 'NONE',  ( 19.02544592524334988, 5.153800228976608722, 81.45942372801897591 ) ) ;
#195725=CARTESIAN_POINT ( 'NONE',  ( -17.13100169013299734, 6.664070546373147330, 60.76789835699850784 ) ) ;
#195726=CARTESIAN_POINT ( 'NONE',  ( 0.05219959533936267826, -19.03943276465977164, 25.00109039468566152 ) ) ;
#195727=CARTESIAN_POINT ( 'NONE',  ( -0.05219959533936034679, 19.03943276465977164, 77.50109039468566152 ) ) ;
#195728=CARTESIAN_POINT ( 'NONE',  ( 0.05219959533936267826, -19.03943276465977164, 45.00109039468566863 ) ) ;
#195729=CARTESIAN_POINT ( 'NONE',  ( -17.40805194822028668, -6.112264579159356614, 44.16628727489390371 ) ) ;
#195730=CARTESIAN_POINT ( 'NONE',  ( 9.564922557960805705, 16.46253265017160317, 39.58224293864768839 ) ) ;
#195731=CARTESIAN_POINT ( 'NONE',  ( 8.224510206698953496, -14.34966873604960469, 52.91557627198103830 ) ) ;
#195732=CARTESIAN_POINT ( 'NONE',  ( 19.05341960407611168, 5.049401038298154454, 38.95724293864767418 ) ) ;
#195733=CARTESIAN_POINT ( 'NONE',  ( -14.34966873604960291, -8.224510206698953496, 41.66557627198103120 ) ) ;
#195735=CARTESIAN_POINT ( 'NONE',  ( 8.224510206698742110, 14.34966873604972548, 112.0844237280190185 ) ) ;
#195736=CARTESIAN_POINT ( 'NONE',  ( -0.05219959533909027116, -19.03943276465977164, 47.49890960531435979 ) ) ;
#195737=CARTESIAN_POINT ( 'NONE',  ( 9.474510206698729675, 16.51473224551082808, 27.08442372801900433 ) ) ;
#195738=CARTESIAN_POINT ( 'NONE',  ( 14.29746914071037800, 8.314922557961029526, 31.66775706135234358 ) ) ;
#195739=CARTESIAN_POINT ( 'NONE',  ( 21.53943276465977519, -0.05219959533907433946, 38.74890960531435979 ) ) ;
#195740=CARTESIAN_POINT ( 'NONE',  ( 15.80617190586769283, -15.72974639402175789, 95.62609039468568994 ) ) ;
#195741=CARTESIAN_POINT ( 'NONE',  ( 5.153800228976335163, 19.02544592524342804, 109.7905762719810099 ) ) ;
#195742=CARTESIAN_POINT ( 'NONE',  ( -9.474510206698964154, 16.51473224551069663, 85.41557627198102409 ) ) ;
#195744=CARTESIAN_POINT ( 'NONE',  ( 21.53943276465977519, -0.05219959533907433946, 113.7489096053143527 ) ) ;
#195746=CARTESIAN_POINT ( 'NONE',  ( -14.34966873604960291, -8.224510206698953496, 86.66557627198102409 ) ) ;
#195747=CARTESIAN_POINT ( 'NONE',  ( -18.67979575497178146, -10.72451020669898902, 76.66557627198103830 ) ) ;
#195748=CARTESIAN_POINT ( 'NONE',  ( -13.89961937509977652, 13.97604488694528158, 65.62390960531436690 ) ) ;
#195749=CARTESIAN_POINT ( 'NONE',  ( 13.89961937509977652, -13.97604488694527269, 78.12390960531433848 ) ) ;
#195750=CARTESIAN_POINT ( 'NONE',  ( 5.719274019375991003, -21.55341960407610458, 102.7072429386476955 ) ) ;
#195752=CARTESIAN_POINT ( 'NONE',  ( -9.474510206698964154, 16.51473224551069663, 55.41557627198103120 ) ) ;
#195753=CARTESIAN_POINT ( 'NONE',  ( -4.483927247898539470, -16.52544592524342804, 102.2905762719810383 ) ) ;
#195754=CARTESIAN_POINT ( 'NONE',  ( -19.02544592524342804, 5.153800228976336051, 26.04057627198103120 ) ) ;
#195755=CARTESIAN_POINT ( 'NONE',  ( -16.46253265017160317, 9.564922557960807481, 60.83224293864769550 ) ) ;
#195756=CARTESIAN_POINT ( 'NONE',  ( 16.51473224551083163, -9.474510206698727899, 85.83442372801900433 ) ) ;
#195757=CARTESIAN_POINT ( 'NONE',  ( 4.483927247898545687, 16.52544592524342804, 94.79057627198105251 ) ) ;
#195758=CARTESIAN_POINT ( 'NONE',  ( -10.81492255796105439, 18.62759615963255655, 62.91775706135236135 ) ) ;
#195759=CARTESIAN_POINT ( 'NONE',  ( -9.564922557960796823, -16.46253265017161027, 47.08224293864769550 ) ) ;
#195760=CARTESIAN_POINT ( 'NONE',  ( -21.53943276465977519, -0.05219959533937600094, 23.75109039468567929 ) ) ;
#195761=CARTESIAN_POINT ( 'NONE',  ( -4.379528057220328563, 16.55341960407611168, 95.20724293864769550 ) ) ;
#195763=CARTESIAN_POINT ( 'NONE',  ( -16.46253265017160317, 9.564922557960807481, 75.83224293864769550 ) ) ;
#195765=CARTESIAN_POINT ( 'NONE',  ( 9.474510206698729675, 16.51473224551082808, 112.0844237280190043 ) ) ;
#195766=CARTESIAN_POINT ( 'NONE',  ( -5.049401038298153566, 19.05341960407611168, 110.2072429386476671 ) ) ;
#195767=CARTESIAN_POINT ( 'NONE',  ( 10.72451020669871369, 18.67979575497193778, 47.08442372801901854 ) ) ;
#195768=CARTESIAN_POINT ( 'NONE',  ( 19.03943276465977164, -0.05219959533909143690, 93.74890960531435269 ) ) ;
#195769=CARTESIAN_POINT ( 'NONE',  ( 16.46253265017146816, 9.564922557961045513, 81.66775706135233293 ) ) ;
#195770=CARTESIAN_POINT ( 'NONE',  ( -13.89961937509977652, 13.97604488694528158, 65.62390960531436690 ) ) ;
#195772=CARTESIAN_POINT ( 'NONE',  ( 0.05219959533910956823, 16.53943276465976808, 79.99890960531435269 ) ) ;
#195773=CARTESIAN_POINT ( 'NONE',  ( -19.05341960407611168, -5.049401038298163336, 96.45724293864769550 ) ) ;
#195774=CARTESIAN_POINT ( 'NONE',  ( 14.34966873604960469, 8.224510206698951720, 74.16557627198102409 ) ) ;
#195775=CARTESIAN_POINT ( 'NONE',  ( -9.564922557960796823, -16.46253265017161027, 92.08224293864769550 ) ) ;
#195776=CARTESIAN_POINT ( 'NONE',  ( 13.97604488694548053, -13.89961937509957401, 40.62609039468564731 ) ) ;
#195777=CARTESIAN_POINT ( 'NONE',  ( -13.89961937509977652, 13.97604488694528158, 45.62390960531433848 ) ) ;
#195778=CARTESIAN_POINT ( 'NONE',  ( 16.55341960407611168, 4.379528057220329451, 38.95724293864768839 ) ) ;
#195779=CARTESIAN_POINT ( 'NONE',  ( -16.51473224551069308, -9.474510206698971260, 26.66557627198103120 ) ) ;
#195781=CARTESIAN_POINT ( 'NONE',  ( -21.53943276465977519, -0.05219959533937600094, 48.75109039468568284 ) ) ;
#195782=CARTESIAN_POINT ( 'NONE',  ( 16.51473224551083163, -9.474510206698727899, 85.83442372801900433 ) ) ;
#195783=CARTESIAN_POINT ( 'NONE',  ( -12.06949235617756955, 12.14591786802309770, 30.62390960531436335 ) ) ;
#195784=CARTESIAN_POINT ( 'NONE',  ( -21.53943276465977519, 0.05219959533907696930, 101.2489096053143669 ) ) ;
#195785=CARTESIAN_POINT ( 'NONE',  ( -15.72974639402197994, 15.80617190586746368, 35.62390960531437401 ) ) ;
#195787=CARTESIAN_POINT ( 'NONE',  ( 8.314922557960818139, 14.29746914071049879, 79.58224293864769550 ) ) ;
#195788=CARTESIAN_POINT ( 'NONE',  ( 5.049401038298161559, -19.05341960407611168, 37.70724293864768839 ) ) ;
#195789=CARTESIAN_POINT ( 'NONE',  ( -12.06949235617756955, 12.14591786802309770, 25.62390960531435624 ) ) ;
#195790=CARTESIAN_POINT ( 'NONE',  ( -4.483927247898782831, 16.52544592524335698, 92.70942372801901854 ) ) ;
#195791=CARTESIAN_POINT ( 'NONE',  ( -12.06949235617739369, -12.14591786802326823, 74.37609039468568994 ) ) ;
#195792=CARTESIAN_POINT ( 'NONE',  ( -19.02544592524334988, -5.153800228976617603, 28.95942372801900433 ) ) ;
#195793=CARTESIAN_POINT ( 'NONE',  ( 13.89961937509977652, -13.97604488694527269, 88.12390960531438111 ) ) ;
#195794=CARTESIAN_POINT ( 'NONE',  ( 13.97604488694527802, 13.89961937509977652, 74.37390960531436690 ) ) ;
#195795=CARTESIAN_POINT ( 'NONE',  ( 12.06949235617739724, 12.14591786802326823, 71.87609039468568994 ) ) ;
#195796=CARTESIAN_POINT ( 'NONE',  ( 5.153800228976335163, 19.02544592524342804, 34.79057627198102409 ) ) ;
#195797=CARTESIAN_POINT ( 'NONE',  ( 8.314922557960818139, 14.29746914071049879, 54.58224293864769550 ) ) ;
#195798=CARTESIAN_POINT ( 'NONE',  ( 16.46253265017160672, -9.564922557960803928, 98.33224293864769550 ) ) ;
#195799=CARTESIAN_POINT ( 'NONE',  ( -21.53943276465977519, 0.05219959533907696930, 26.24890960531435624 ) ) ;
#195800=CARTESIAN_POINT ( 'NONE',  ( -12.06949235617756955, 12.14591786802309770, 75.62390960531439532 ) ) ;
#195801=CARTESIAN_POINT ( 'NONE',  ( 4.379528057220339221, -16.55341960407611168, 62.70724293864769550 ) ) ;
#195803=CARTESIAN_POINT ( 'NONE',  ( 17.72696623605159516, -5.500000000000041744, 86.09811031808419557 ) ) ;
#195804=CARTESIAN_POINT ( 'NONE',  ( 13.89961937509957401, 13.97604488694547697, 66.87609039468567573 ) ) ;
#195805=CARTESIAN_POINT ( 'NONE',  ( -0.05219959533909027116, -19.03943276465977164, 87.49890960531436690 ) ) ;
#195806=CARTESIAN_POINT ( 'NONE',  ( -5.049401038297874678, -19.05341960407617918, 84.79275706135233293 ) ) ;
#195808=CARTESIAN_POINT ( 'NONE',  ( -5.049401038297874678, -19.05341960407617918, 109.7927570613523187 ) ) ;
#195809=CARTESIAN_POINT ( 'NONE',  ( 16.55341960407618274, -4.379528057220086978, 96.04275706135236135 ) ) ;
#195810=CARTESIAN_POINT ( 'NONE',  ( 0.05219959533909260263, 19.03943276465977164, 39.99890960531436690 ) ) ;
#195811=CARTESIAN_POINT ( 'NONE',  ( -19.03943276465977164, 0.05219959533909376836, 116.2489096053143669 ) ) ;
#195812=CARTESIAN_POINT ( 'NONE',  ( 18.62759615963255655, 10.81492255796105972, 51.66775706135234714 ) ) ;
#195813=CARTESIAN_POINT ( 'NONE',  ( 12.14591786802327356, -12.06949235617739191, 20.62609039468568639 ) ) ;
#195814=CARTESIAN_POINT ( 'NONE',  ( 5.153800228976617603, -19.02544592524335343, 55.20942372801899722 ) ) ;
#195815=CARTESIAN_POINT ( 'NONE',  ( 9.564922557960805705, 16.46253265017160317, 74.58224293864769550 ) ) ;
#195816=CARTESIAN_POINT ( 'NONE',  ( 16.46253265017160672, -9.564922557960803928, 113.3322429386476955 ) ) ;
#195817=CARTESIAN_POINT ( 'NONE',  ( 14.29746914071049879, -8.314922557960816363, 73.33224293864769550 ) ) ;
#195818=CARTESIAN_POINT ( 'NONE',  ( 13.97604488694527802, 13.89961937509977652, 74.37390960531436690 ) ) ;
#195819=CARTESIAN_POINT ( 'NONE',  ( -13.89961937509977652, 13.97604488694528158, 70.62390960531432427 ) ) ;
#195821=CARTESIAN_POINT ( 'NONE',  ( 19.02544592524334988, 5.153800228976608722, 91.45942372801900433 ) ) ;
#195822=CARTESIAN_POINT ( 'NONE',  ( 18.62759615963271287, -10.81492255796078972, 63.33224293864770260 ) ) ;
#195823=CARTESIAN_POINT ( 'NONE',  ( -19.02544592524342804, 5.153800228976336051, 26.04057627198103120 ) ) ;
#195824=CARTESIAN_POINT ( 'NONE',  ( -19.02544592524334988, -5.153800228976617603, 58.95942372801900433 ) ) ;
#195825=CARTESIAN_POINT ( 'NONE',  ( -5.153800228976328057, -19.02544592524343514, 57.29057627198103120 ) ) ;
#195826=CARTESIAN_POINT ( 'NONE',  ( -5.153800228976328057, -19.02544592524343514, 92.29057627198099567 ) ) ;
#195828=CARTESIAN_POINT ( 'NONE',  ( 18.62759615963271287, -10.81492255796078972, 93.33224293864769550 ) ) ;
#195829=CARTESIAN_POINT ( 'NONE',  ( 8.314922557960818139, 14.29746914071049879, 94.58224293864769550 ) ) ;
#195830=CARTESIAN_POINT ( 'NONE',  ( 13.97604488694548053, -13.89961937509957401, 45.62609039468566863 ) ) ;
#195831=CARTESIAN_POINT ( 'NONE',  ( 18.67979575497178502, 10.72451020669898547, 84.16557627198103830 ) ) ;
#195832=CARTESIAN_POINT ( 'NONE',  ( 0.05219959533907565091, 21.53943276465977519, 74.99890960531435269 ) ) ;
#195833=CARTESIAN_POINT ( 'NONE',  ( 16.52544592524342804, -4.483927247898539470, 38.54057627198103120 ) ) ;
#195834=CARTESIAN_POINT ( 'NONE',  ( 21.55341960407619695, -5.719274019375665929, 106.0427570613523471 ) ) ;
#195835=CARTESIAN_POINT ( 'NONE',  ( 19.05341960407611168, 5.049401038298154454, 83.95724293864766707 ) ) ;
#195836=CARTESIAN_POINT ( 'NONE',  ( 5.153800228976335163, 19.02544592524342804, 34.79057627198102409 ) ) ;
#195837=CARTESIAN_POINT ( 'NONE',  ( 5.719274019375673035, 21.55341960407619339, 37.29275706135235424 ) ) ;
#195838=CARTESIAN_POINT ( 'NONE',  ( -18.62759615963255300, -10.81492255796106328, 59.16775706135234714 ) ) ;
#195839=CARTESIAN_POINT ( 'NONE',  ( 9.564922557960805705, 16.46253265017160317, 44.58224293864769550 ) ) ;
#195840=CARTESIAN_POINT ( 'NONE',  ( -10.72451020669870658, -18.67979575497194134, 19.58442372801901143 ) ) ;
#195841=CARTESIAN_POINT ( 'NONE',  ( 5.049401038297881783, 19.05341960407617563, 62.29275706135234003 ) ) ;
#195842=CARTESIAN_POINT ( 'NONE',  ( -16.51473224551069308, -9.474510206698971260, 36.66557627198102409 ) ) ;
#195843=CARTESIAN_POINT ( 'NONE',  ( -12.14591786802326823, 12.06949235617739902, 23.12609039468567573 ) ) ;
#195844=CARTESIAN_POINT ( 'NONE',  ( -16.46253265017160317, 9.564922557960807481, 30.83224293864769550 ) ) ;
#195845=CARTESIAN_POINT ( 'NONE',  ( -4.379528057220086978, -16.55341960407618274, 79.79275706135236135 ) ) ;
#195846=CARTESIAN_POINT ( 'NONE',  ( -9.474510206698964154, 16.51473224551069663, 35.41557627198102409 ) ) ;
#195848=CARTESIAN_POINT ( 'NONE',  ( 0.05219959533909260263, 19.03943276465977164, 79.99890960531436690 ) ) ;
#195849=CARTESIAN_POINT ( 'NONE',  ( -13.97604488694527625, -13.89961937509977652, 21.87390960531435979 ) ) ;
#195850=EDGE_CURVE ( 'NONE', #126008, #95725, #31832, .T. ) ;
#195851=CARTESIAN_POINT ( 'NONE',  ( -15.72974639402197994, 15.80617190586746368, 75.62390960531439532 ) ) ;
#195852=CARTESIAN_POINT ( 'NONE',  ( -14.34966873604972548, 8.224510206698743886, 53.33442372801901854 ) ) ;
#195853=CARTESIAN_POINT ( 'NONE',  ( 9.474510206698729675, 16.51473224551082808, 22.08442372801899722 ) ) ;
#195854=CARTESIAN_POINT ( 'NONE',  ( 16.46253265017160672, -9.564922557960803928, 33.33224293864770260 ) ) ;
#195855=CARTESIAN_POINT ( 'NONE',  ( -4.379528057220328563, 16.55341960407611168, 25.20724293864769550 ) ) ;
#195856=CARTESIAN_POINT ( 'NONE',  ( 16.53943276465976808, -0.05219959533910856209, 73.74890960531433848 ) ) ;
#195857=CARTESIAN_POINT ( 'NONE',  ( 0.05219959533909260263, 19.03943276465977164, 59.99890960531436690 ) ) ;
#195858=CARTESIAN_POINT ( 'NONE',  ( -18.67979575497193778, 10.72451020669871902, 108.3344237280190185 ) ) ;
#195859=CARTESIAN_POINT ( 'NONE',  ( 21.53943276465977519, 0.05219959533937863772, 21.25109039468567218 ) ) ;
#195860=CARTESIAN_POINT ( 'NONE',  ( -5.049401038298153566, 19.05341960407611168, 85.20724293864766707 ) ) ;
#195861=CARTESIAN_POINT ( 'NONE',  ( -21.53943276465977519, -0.05219959533937600094, 88.75109039468567573 ) ) ;
#195862=CARTESIAN_POINT ( 'NONE',  ( 4.483927247898790824, -16.52544592524335698, 65.20942372801901854 ) ) ;
#195863=CARTESIAN_POINT ( 'NONE',  ( -12.06949235617739369, -12.14591786802326823, 29.37609039468568284 ) ) ;
#195864=CARTESIAN_POINT ( 'NONE',  ( 8.224510206698953496, -14.34966873604960469, 87.91557627198103830 ) ) ;
#195865=CARTESIAN_POINT ( 'NONE',  ( 19.05341960407611168, 5.049401038298154454, 108.9572429386477097 ) ) ;
#195866=CARTESIAN_POINT ( 'NONE',  ( 8.224510206698953496, -14.34966873604960469, 27.91557627198103830 ) ) ;
#195867=CARTESIAN_POINT ( 'NONE',  ( 13.97604488694527802, 13.89961937509977652, 24.37390960531435624 ) ) ;
#195868=CARTESIAN_POINT ( 'NONE',  ( 8.314922557961029526, -14.29746914071037800, 50.41775706135235424 ) ) ;
#195869=CARTESIAN_POINT ( 'NONE',  ( 12.14591786802309770, 12.06949235617756955, 49.37390960531436690 ) ) ;
#195870=CARTESIAN_POINT ( 'NONE',  ( 12.06949235617739724, 12.14591786802326823, 96.87609039468568994 ) ) ;
#195871=CARTESIAN_POINT ( 'NONE',  ( -13.89961937509977652, 13.97604488694528158, 115.6239096053143669 ) ) ;
#195872=CARTESIAN_POINT ( 'NONE',  ( 0.05219959533907565091, 21.53943276465977519, 34.99890960531435979 ) ) ;
#195873=CARTESIAN_POINT ( 'NONE',  ( 16.46253265017146816, 9.564922557961045513, 21.66775706135233648 ) ) ;
#195874=CARTESIAN_POINT ( 'NONE',  ( -16.53943276465976808, 0.05219959533911058130, 81.24890960531436690 ) ) ;
#195875=CARTESIAN_POINT ( 'NONE',  ( 5.153800228976335163, 19.02544592524342804, 89.79057627198102409 ) ) ;
#195877=CARTESIAN_POINT ( 'NONE',  ( -4.379528057220086978, -16.55341960407618274, 39.79275706135235424 ) ) ;
#195878=CARTESIAN_POINT ( 'NONE',  ( 5.049401038298161559, -19.05341960407611168, 47.70724293864770260 ) ) ;
#195879=CARTESIAN_POINT ( 'NONE',  ( -14.29746914071037622, -8.314922557961029526, 44.16775706135234714 ) ) ;
#195881=CARTESIAN_POINT ( 'NONE',  ( -13.89961937509957401, -13.97604488694547875, 54.37609039468565442 ) ) ;
#195882=CARTESIAN_POINT ( 'NONE',  ( -16.46253265017160317, 9.564922557960807481, 50.83224293864770260 ) ) ;
#195883=CARTESIAN_POINT ( 'NONE',  ( 4.483927247898790824, -16.52544592524335698, 75.20942372801901854 ) ) ;
#195884=CARTESIAN_POINT ( 'NONE',  ( 19.03943276465977164, 0.05219959533936151252, 91.25109039468566152 ) ) ;
#195885=CARTESIAN_POINT ( 'NONE',  ( -5.153800228976328057, -19.02544592524343514, 62.29057627198100988 ) ) ;
#195886=CARTESIAN_POINT ( 'NONE',  ( -21.52544592524343514, 5.823673210054127303, 96.04057627198102409 ) ) ;
#195887=CARTESIAN_POINT ( 'NONE',  ( -12.06949235617756955, 12.14591786802309770, 95.62390960531436690 ) ) ;
#195889=CARTESIAN_POINT ( 'NONE',  ( 16.51473224551083163, -9.474510206698727899, 70.83442372801900433 ) ) ;
#195890=CARTESIAN_POINT ( 'NONE',  ( 5.719274019375991003, -21.55341960407610458, 57.70724293864770260 ) ) ;
#195891=CARTESIAN_POINT ( 'NONE',  ( 13.97604488694548053, -13.89961937509957401, 45.62609039468566863 ) ) ;
#195892=CARTESIAN_POINT ( 'NONE',  ( -0.05219959533909027116, -19.03943276465977164, 112.4989096053143669 ) ) ;
#195893=CARTESIAN_POINT ( 'NONE',  ( -5.719274019375978568, 21.55341960407610458, 90.20724293864770971 ) ) ;
#195894=CARTESIAN_POINT ( 'NONE',  ( -18.39635199886966177, 5.500000000000103029, 56.01967076360000419 ) ) ;
#195895=CARTESIAN_POINT ( 'NONE',  ( -13.97604488694547697, 13.89961937509957934, 108.1260903946856331 ) ) ;
#195897=CARTESIAN_POINT ( 'NONE',  ( 16.52544592524335698, 4.483927247898782831, 26.45942372801901854 ) ) ;
#195898=CARTESIAN_POINT ( 'NONE',  ( -19.03943276465977164, 0.05219959533909376836, 51.24890960531436690 ) ) ;
#195899=CARTESIAN_POINT ( 'NONE',  ( -19.03943276465977164, 0.05219959533909376836, 111.2489096053143669 ) ) ;
#195900=CARTESIAN_POINT ( 'NONE',  ( 21.52544592524344225, -5.823673210054117533, 83.54057627198102409 ) ) ;
#195901=CARTESIAN_POINT ( 'NONE',  ( 5.719274019375673035, 21.55341960407619339, 62.29275706135236845 ) ) ;
#195902=CARTESIAN_POINT ( 'NONE',  ( -5.049401038297874678, -19.05341960407617918, 99.79275706135234714 ) ) ;
#195903=CARTESIAN_POINT ( 'NONE',  ( 5.153800228976615827, -19.02544592524334988, 30.20942372801900433 ) ) ;
#195904=CARTESIAN_POINT ( 'NONE',  ( 16.53943276465976808, -0.05219959533910856209, 33.74890960531436690 ) ) ;
#195905=CARTESIAN_POINT ( 'NONE',  ( -15.72974639402197994, 15.80617190586746368, 105.6239096053143669 ) ) ;
#195906=CARTESIAN_POINT ( 'NONE',  ( 14.29746914071049879, -8.314922557960816363, 53.33224293864769550 ) ) ;
#195907=CARTESIAN_POINT ( 'NONE',  ( 19.02544592524334988, 5.153800228976608722, 91.45942372801900433 ) ) ;
#195908=CARTESIAN_POINT ( 'NONE',  ( -5.049401038297874678, -19.05341960407617918, 54.79275706135234003 ) ) ;
#195909=CARTESIAN_POINT ( 'NONE',  ( -18.62759615963255300, -10.81492255796106328, 74.16775706135231871 ) ) ;
#195910=CARTESIAN_POINT ( 'NONE',  ( 16.51473224551083163, -9.474510206698727899, 40.83442372801900433 ) ) ;
#195911=CARTESIAN_POINT ( 'NONE',  ( -16.53943276465976808, 0.05219959533911058130, 116.2489096053143669 ) ) ;
#195912=CARTESIAN_POINT ( 'NONE',  ( 18.62759615963271287, -10.81492255796078972, 48.33224293864770260 ) ) ;
#195913=CARTESIAN_POINT ( 'NONE',  ( 14.29746914071049879, -8.314922557960816363, 33.33224293864769550 ) ) ;
#195914=CARTESIAN_POINT ( 'NONE',  ( -21.55341960407619339, 5.719274019375674811, 108.5427570613523756 ) ) ;
#195915=CARTESIAN_POINT ( 'NONE',  ( 0.05219959533934541429, -16.53943276465976808, 70.00109039468568994 ) ) ;
#195916=CARTESIAN_POINT ( 'NONE',  ( 16.52544592524342804, -4.483927247898539470, 38.54057627198103120 ) ) ;
#195917=CARTESIAN_POINT ( 'NONE',  ( 21.55341960407619695, -5.719274019375665929, 71.04275706135234714 ) ) ;
#195918=CARTESIAN_POINT ( 'NONE',  ( -18.62759615963255300, -10.81492255796106328, 74.16775706135231871 ) ) ;
#195919=CARTESIAN_POINT ( 'NONE',  ( 0.05219959533907565091, 21.53943276465977519, 69.99890960531435269 ) ) ;
#195920=CARTESIAN_POINT ( 'NONE',  ( 9.564922557960805705, 16.46253265017160317, 34.58224293864770260 ) ) ;
#195921=CARTESIAN_POINT ( 'NONE',  ( 18.62759615963255655, 10.81492255796105972, 41.66775706135235424 ) ) ;
#195922=CARTESIAN_POINT ( 'NONE',  ( -19.05341960407611168, -5.049401038298163336, 21.45724293864768839 ) ) ;
#195923=CARTESIAN_POINT ( 'NONE',  ( 19.05341960407611168, 5.049401038298154454, 38.95724293864767418 ) ) ;
#195924=CARTESIAN_POINT ( 'NONE',  ( 16.52544592524342804, -4.483927247898539470, 88.54057627198103830 ) ) ;
#195925=CARTESIAN_POINT ( 'NONE',  ( -9.564922557960796823, -16.46253265017161027, 87.08224293864769550 ) ) ;
#195926=CARTESIAN_POINT ( 'NONE',  ( 12.14591786802309770, 12.06949235617756955, 39.37390960531436690 ) ) ;
#195927=CARTESIAN_POINT ( 'NONE',  ( 4.483927247898545687, 16.52544592524342804, 94.79057627198105251 ) ) ;
#195928=CARTESIAN_POINT ( 'NONE',  ( 21.52544592524344225, -5.823673210054117533, 63.54057627198103830 ) ) ;
#195930=CARTESIAN_POINT ( 'NONE',  ( 0.05219959533907565091, 21.53943276465977519, 104.9989096053143669 ) ) ;
#195931=CARTESIAN_POINT ( 'NONE',  ( 19.02544592524343514, -5.153800228976328945, 113.5405762719810241 ) ) ;
#195932=CARTESIAN_POINT ( 'NONE',  ( 13.97604488694527802, 13.89961937509977652, 59.37390960531434558 ) ) ;
#195933=CARTESIAN_POINT ( 'NONE',  ( -0.05219959533934338120, 16.53943276465976808, 27.50109039468567929 ) ) ;
#195934=EDGE_CURVE ( 'NONE', #125647, #68158, #25908, .T. ) ;
#195935=CARTESIAN_POINT ( 'NONE',  ( 18.67979575497178502, 10.72451020669898547, 64.16557627198102409 ) ) ;
#195936=CARTESIAN_POINT ( 'NONE',  ( -10.81492255796105439, 18.62759615963255655, 92.91775706135236135 ) ) ;
#195937=CARTESIAN_POINT ( 'NONE',  ( 13.97604488694527802, 13.89961937509977652, 84.37390960531433848 ) ) ;
#195938=CARTESIAN_POINT ( 'NONE',  ( 21.55341960407619695, -5.719274019375665929, 21.04275706135234714 ) ) ;
#195939=CARTESIAN_POINT ( 'NONE',  ( -9.564922557960796823, -16.46253265017161027, 107.0822429386476955 ) ) ;
#195940=CARTESIAN_POINT ( 'NONE',  ( 4.379528057220092307, 16.55341960407617563, 92.29275706135236135 ) ) ;
#195941=CARTESIAN_POINT ( 'NONE',  ( 21.55341960407619695, -5.719274019375665929, 66.04275706135236135 ) ) ;
#195942=CARTESIAN_POINT ( 'NONE',  ( -15.80617190586768217, 15.72974639402176855, 98.12609039468570415 ) ) ;
#195943=CARTESIAN_POINT ( 'NONE',  ( -8.224510206698735004, -14.34966873604973081, 59.58442372801901854 ) ) ;
#195944=CARTESIAN_POINT ( 'NONE',  ( 10.81492255796106328, -18.62759615963255655, 25.41775706135235779 ) ) ;
#195945=CARTESIAN_POINT ( 'NONE',  ( -19.02544592524342804, 5.153800228976336051, 111.0405762719810099 ) ) ;
#195946=CARTESIAN_POINT ( 'NONE',  ( -18.62759615963255300, -10.81492255796106328, 89.16775706135236135 ) ) ;
#195947=CARTESIAN_POINT ( 'NONE',  ( 9.474510206698971260, -16.51473224551069308, 97.91557627198102409 ) ) ;
#195948=CARTESIAN_POINT ( 'NONE',  ( -21.52544592524343514, 5.823673210054127303, 96.04057627198102409 ) ) ;
#195949=CARTESIAN_POINT ( 'NONE',  ( 19.03943276465977164, 0.05219959533936151252, 46.25109039468566863 ) ) ;
#195950=CARTESIAN_POINT ( 'NONE',  ( -5.719274019375978568, 21.55341960407610458, 60.20724293864768839 ) ) ;
#195951=CARTESIAN_POINT ( 'NONE',  ( -5.153800228976328057, -19.02544592524343514, 97.29057627198099567 ) ) ;
#195952=CARTESIAN_POINT ( 'NONE',  ( -12.14591786802309592, -12.06949235617757132, 41.87390960531435979 ) ) ;
#195953=CARTESIAN_POINT ( 'NONE',  ( -20.49784845693389101, -1.163414459189985801E-14, 95.00000000000000000 ) ) ;
#195954=CARTESIAN_POINT ( 'NONE',  ( 19.02544592524334988, 5.153800228976608722, 61.45942372801900433 ) ) ;
#195955=CARTESIAN_POINT ( 'NONE',  ( -19.34837522270364829, -5.499999999999849010, 80.86337684832577111 ) ) ;
#195956=CARTESIAN_POINT ( 'NONE',  ( -9.474510206698720793, -16.51473224551083518, 104.5844237280190043 ) ) ;
#195957=CARTESIAN_POINT ( 'NONE',  ( 10.72451020669898902, -18.67979575497178502, 87.91557627198103830 ) ) ;
#195958=CARTESIAN_POINT ( 'NONE',  ( 12.06949235617757843, -12.14591786802309237, 53.12390960531436690 ) ) ;
#195959=CARTESIAN_POINT ( 'NONE',  ( -12.06949235617739369, -12.14591786802326823, 34.37609039468568284 ) ) ;
#195960=CARTESIAN_POINT ( 'NONE',  ( 9.474510206698971260, -16.51473224551069308, 47.91557627198102409 ) ) ;
#195961=CARTESIAN_POINT ( 'NONE',  ( 0.05219959533937995610, -21.53943276465977519, 20.00109039468568639 ) ) ;
#195962=CARTESIAN_POINT ( 'NONE',  ( -16.51473224551082808, 9.474510206698731452, 88.33442372801900433 ) ) ;
#195963=ADVANCED_FACE ( 'NONE', ( #21626 ), #54961, .T. ) ;
#195964=CARTESIAN_POINT ( 'NONE',  ( -5.153800228976328057, -19.02544592524343514, 97.29057627198099567 ) ) ;
#195965=CARTESIAN_POINT ( 'NONE',  ( -13.89961937509977652, 13.97604488694528158, 75.62390960531438111 ) ) ;
#195966=CARTESIAN_POINT ( 'NONE',  ( -5.823673210054116645, -21.52544592524344225, 82.29057627198103830 ) ) ;
#195967=CARTESIAN_POINT ( 'NONE',  ( 19.03943276465977164, -0.05219959533909143690, 48.74890960531435979 ) ) ;
#195969=CARTESIAN_POINT ( 'NONE',  ( -16.52544592524342804, 4.483927247898546575, 56.04057627198102409 ) ) ;
#195970=CARTESIAN_POINT ( 'NONE',  ( 5.049401038298161559, -19.05341960407611168, 92.70724293864769550 ) ) ;
#195972=CARTESIAN_POINT ( 'NONE',  ( -0.05219959533936034679, 19.03943276465977164, 62.50109039468566863 ) ) ;
#195973=CARTESIAN_POINT ( 'NONE',  ( -21.55341960407610458, -5.719274019375992779, 71.45724293864769550 ) ) ;
#195974=CARTESIAN_POINT ( 'NONE',  ( -0.05219959533936034679, 19.03943276465977164, 32.50109039468566863 ) ) ;
#195975=CARTESIAN_POINT ( 'NONE',  ( 19.02544592524343514, -5.153800228976328945, 98.54057627198100988 ) ) ;
#195976=CARTESIAN_POINT ( 'NONE',  ( -17.50000000000000000, 3.305555262949615436, 114.6251715215659317 ) ) ;
#195977=CARTESIAN_POINT ( 'NONE',  ( -21.55341960407610458, -5.719274019375992779, 36.45724293864768839 ) ) ;
#195978=CARTESIAN_POINT ( 'NONE',  ( -19.02544592524342804, 5.153800228976336051, 71.04057627198099567 ) ) ;
#195979=CARTESIAN_POINT ( 'NONE',  ( -18.62759615963255300, -10.81492255796106328, 59.16775706135234714 ) ) ;
#195980=CARTESIAN_POINT ( 'NONE',  ( 5.049401038298161559, -19.05341960407611168, 22.70724293864769194 ) ) ;
#195981=CARTESIAN_POINT ( 'NONE',  ( 18.67979575497178502, 10.72451020669898547, 109.1655762719810383 ) ) ;
#195983=CARTESIAN_POINT ( 'NONE',  ( -5.823673210054431948, 21.52544592524334988, 47.70942372801902565 ) ) ;
#195985=CARTESIAN_POINT ( 'NONE',  ( -5.049401038298153566, 19.05341960407611168, 105.2072429386476671 ) ) ;
#195986=CARTESIAN_POINT ( 'NONE',  ( -19.03943276465977164, -0.05219959533935918106, 63.75109039468566863 ) ) ;
#195988=CARTESIAN_POINT ( 'NONE',  ( 15.72974639402199770, -15.80617190586745480, 103.1239096053143811 ) ) ;
#195989=CARTESIAN_POINT ( 'NONE',  ( -19.02544592524342804, 5.153800228976336051, 56.04057627198100988 ) ) ;
#195990=CARTESIAN_POINT ( 'NONE',  ( -12.06949235617739369, -12.14591786802326823, 39.37609039468567573 ) ) ;
#195992=CARTESIAN_POINT ( 'NONE',  ( 15.72974639402176855, 15.80617190586768217, 96.87609039468568994 ) ) ;
#195993=CARTESIAN_POINT ( 'NONE',  ( 19.02544592524343514, -5.153800228976328945, 38.54057627198103120 ) ) ;
#195994=CARTESIAN_POINT ( 'NONE',  ( -18.62759615963255300, -10.81492255796106328, 104.1677570613523471 ) ) ;
#195995=CARTESIAN_POINT ( 'NONE',  ( 5.049401038298161559, -19.05341960407611168, 92.70724293864769550 ) ) ;
#195996=CARTESIAN_POINT ( 'NONE',  ( 0.05219959533937995610, -21.53943276465977519, 65.00109039468568994 ) ) ;
#195998=CARTESIAN_POINT ( 'NONE',  ( -13.89961937509977652, 13.97604488694528158, 110.6239096053143243 ) ) ;
#196000=CARTESIAN_POINT ( 'NONE',  ( -16.55341960407617563, 4.379528057220093196, 53.54275706135234714 ) ) ;
#196001=CARTESIAN_POINT ( 'NONE',  ( 15.80617190586769283, -15.72974639402175789, 55.62609039468568284 ) ) ;
#196002=CARTESIAN_POINT ( 'NONE',  ( -5.823673210054431948, 21.52544592524334988, 92.70942372801901854 ) ) ;
#196004=CARTESIAN_POINT ( 'NONE',  ( -12.14591786802326823, 12.06949235617739902, 33.12609039468569705 ) ) ;
#196005=CARTESIAN_POINT ( 'NONE',  ( 13.89961937509977652, -13.97604488694527269, 78.12390960531433848 ) ) ;
#196006=CARTESIAN_POINT ( 'NONE',  ( -0.05219959533909027116, -19.03943276465977164, 112.4989096053143669 ) ) ;
#196007=CARTESIAN_POINT ( 'NONE',  ( 17.49999999999999289, 5.624438216177599870, 41.68329655085356933 ) ) ;
#196008=CARTESIAN_POINT ( 'NONE',  ( -16.51473224551069308, -9.474510206698971260, 26.66557627198103120 ) ) ;
#196009=CARTESIAN_POINT ( 'NONE',  ( 21.55341960407610458, 5.719274019375980345, 43.95724293864769550 ) ) ;
#196010=CARTESIAN_POINT ( 'NONE',  ( -12.14591786802326823, 12.06949235617739902, 98.12609039468570415 ) ) ;
#196011=CARTESIAN_POINT ( 'NONE',  ( 0.05219959533910956823, 16.53943276465976808, 84.99890960531436690 ) ) ;
#196012=CARTESIAN_POINT ( 'NONE',  ( 13.89961937509977652, -13.97604488694527269, 63.12390960531435979 ) ) ;
#196013=CARTESIAN_POINT ( 'NONE',  ( -5.719274019375665041, -21.55341960407619695, 84.79275706135234714 ) ) ;
#196014=CARTESIAN_POINT ( 'NONE',  ( 16.53943276465976808, 0.05219959533934440121, 31.25109039468568639 ) ) ;
#196015=CARTESIAN_POINT ( 'NONE',  ( -0.05219959533910754901, -16.53943276465976808, 92.49890960531436690 ) ) ;
#196016=CARTESIAN_POINT ( 'NONE',  ( -5.823673210054431948, 21.52544592524334988, 37.70942372801900433 ) ) ;
#196017=CARTESIAN_POINT ( 'NONE',  ( 18.67979575497178502, 10.72451020669898547, 74.16557627198102409 ) ) ;
#196018=CARTESIAN_POINT ( 'NONE',  ( -16.46253265017146816, -9.564922557961047289, 39.16775706135234003 ) ) ;
#196020=CARTESIAN_POINT ( 'NONE',  ( -19.03943276465977164, 0.05219959533909376836, 81.24890960531436690 ) ) ;
#196021=CARTESIAN_POINT ( 'NONE',  ( 16.55341960407611168, 4.379528057220329451, 68.95724293864769550 ) ) ;
#196023=CARTESIAN_POINT ( 'NONE',  ( 12.06949235617757843, -12.14591786802309237, 33.12390960531435979 ) ) ;
#196024=CARTESIAN_POINT ( 'NONE',  ( 12.14591786802327356, -12.06949235617739191, 105.6260903946856899 ) ) ;
#196025=CARTESIAN_POINT ( 'NONE',  ( 19.05341960407617918, -5.049401038297876454, 66.04275706135233293 ) ) ;
#196027=CARTESIAN_POINT ( 'NONE',  ( 5.823673210054125526, 21.52544592524343514, 29.79057627198102409 ) ) ;
#196028=CARTESIAN_POINT ( 'NONE',  ( 12.14591786802309770, 12.06949235617756955, 84.37390960531438111 ) ) ;
#196029=CARTESIAN_POINT ( 'NONE',  ( -19.03943276465977164, 0.05219959533909376836, 41.24890960531435269 ) ) ;
#196030=CARTESIAN_POINT ( 'NONE',  ( -21.53943276465977519, 0.05219959533907696930, 46.24890960531435979 ) ) ;
#196031=CARTESIAN_POINT ( 'NONE',  ( -15.80617190586745835, -15.72974639402198527, 71.87390960531438111 ) ) ;
#196032=CARTESIAN_POINT ( 'NONE',  ( -14.34966873604960291, -8.224510206698953496, 106.6655762719810383 ) ) ;
#196033=CARTESIAN_POINT ( 'NONE',  ( -12.06949235617739369, -12.14591786802326823, 59.37609039468568284 ) ) ;
#196034=CARTESIAN_POINT ( 'NONE',  ( -19.05341960407611168, -5.049401038298163336, 46.45724293864768129 ) ) ;
#196035=CARTESIAN_POINT ( 'NONE',  ( 21.55341960407619695, -5.719274019375665929, 61.04275706135234714 ) ) ;
#196037=CARTESIAN_POINT ( 'NONE',  ( -14.29746914071049879, 8.314922557960819915, 100.8322429386477097 ) ) ;
#196038=EDGE_CURVE ( 'NONE', #106494, #47253, #33035, .T. ) ;
#196039=CARTESIAN_POINT ( 'NONE',  ( 16.51473224551083163, -9.474510206698727899, 90.83442372801900433 ) ) ;
#196042=CARTESIAN_POINT ( 'NONE',  ( 18.62759615963271287, -10.81492255796078972, 43.33224293864769550 ) ) ;
#196043=CARTESIAN_POINT ( 'NONE',  ( 16.46253265017160672, -9.564922557960803928, 23.33224293864769194 ) ) ;
#196044=CARTESIAN_POINT ( 'NONE',  ( -10.72451020669870658, -18.67979575497194134, 69.58442372801900433 ) ) ;
#196045=CARTESIAN_POINT ( 'NONE',  ( 12.14591786802327356, -12.06949235617739191, 50.62609039468568994 ) ) ;
#196046=CARTESIAN_POINT ( 'NONE',  ( 14.34966873604960469, 8.224510206698951720, 49.16557627198102409 ) ) ;
#196047=CARTESIAN_POINT ( 'NONE',  ( -5.823673210054116645, -21.52544592524344225, 67.29057627198103830 ) ) ;
#196048=CARTESIAN_POINT ( 'NONE',  ( 18.67979575497178502, 10.72451020669898547, 69.16557627198102409 ) ) ;
#196050=CARTESIAN_POINT ( 'NONE',  ( -19.02544592524334988, -5.153800228976617603, 83.95942372801901854 ) ) ;
#196051=CARTESIAN_POINT ( 'NONE',  ( -9.564922557960796823, -16.46253265017161027, 112.0822429386476955 ) ) ;
#196052=CARTESIAN_POINT ( 'NONE',  ( 16.51473224551069308, 9.474510206698969483, 49.16557627198102409 ) ) ;
#196053=CARTESIAN_POINT ( 'NONE',  ( 12.06949235617757843, -12.14591786802309237, 113.1239096053143953 ) ) ;
#196054=EDGE_CURVE ( 'NONE', #120648, #60482, #189057, .T. ) ;
#196056=CARTESIAN_POINT ( 'NONE',  ( -18.22780087662123805, 5.499999999999981348, 76.01763182126894947 ) ) ;
#196058=CARTESIAN_POINT ( 'NONE',  ( 14.34966873604972726, -8.224510206698740333, 85.83442372801901854 ) ) ;
#196059=CARTESIAN_POINT ( 'NONE',  ( 21.52544592524344225, -5.823673210054117533, 103.5405762719810383 ) ) ;
#196060=CARTESIAN_POINT ( 'NONE',  ( -19.02544592524342804, 5.153800228976336051, 66.04057627198103830 ) ) ;
#196061=CARTESIAN_POINT ( 'NONE',  ( -5.719274019375665041, -21.55341960407619695, 39.79275706135235424 ) ) ;
#196062=CARTESIAN_POINT ( 'NONE',  ( 9.474510206698971260, -16.51473224551069308, 92.91557627198103830 ) ) ;
#196065=CARTESIAN_POINT ( 'NONE',  ( 5.823673210054444382, -21.52544592524334988, 35.20942372801901854 ) ) ;
#196066=CARTESIAN_POINT ( 'NONE',  ( 13.97604488694527802, 13.89961937509977652, 29.37390960531435979 ) ) ;
#196067=CARTESIAN_POINT ( 'NONE',  ( -5.049401038297874678, -19.05341960407617918, 84.79275706135233293 ) ) ;
#196068=CARTESIAN_POINT ( 'NONE',  ( 9.564922557961047289, -16.46253265017146816, 35.41775706135233293 ) ) ;
#196069=CARTESIAN_POINT ( 'NONE',  ( -15.72974639402197994, 15.80617190586746368, 115.6239096053143669 ) ) ;
#196070=CARTESIAN_POINT ( 'NONE',  ( 5.153800228976615827, -19.02544592524334988, 35.20942372801899722 ) ) ;
#196071=CARTESIAN_POINT ( 'NONE',  ( -19.05341960407617563, 5.049401038297882671, 48.54275706135233293 ) ) ;
#196072=CARTESIAN_POINT ( 'NONE',  ( 14.29746914071037800, 8.314922557961029526, 96.66775706135234714 ) ) ;
#196073=CARTESIAN_POINT ( 'NONE',  ( 19.02544592524343514, -5.153800228976328945, 113.5405762719810241 ) ) ;
#196075=CARTESIAN_POINT ( 'NONE',  ( 9.474510206698971260, -16.51473224551069308, 67.91557627198102409 ) ) ;
#196077=CARTESIAN_POINT ( 'NONE',  ( 18.62759615963255655, 10.81492255796105972, 76.66775706135234714 ) ) ;
#196078=CARTESIAN_POINT ( 'NONE',  ( 15.72974639402176855, 15.80617190586768217, 91.87609039468568994 ) ) ;
#196080=CARTESIAN_POINT ( 'NONE',  ( 13.89961937509977652, -13.97604488694527269, 83.12390960531436690 ) ) ;
#196081=CARTESIAN_POINT ( 'NONE',  ( -5.823673210054431948, 21.52544592524334988, 57.70942372801901143 ) ) ;
#196082=CARTESIAN_POINT ( 'NONE',  ( -5.049401038297874678, -19.05341960407617918, 94.79275706135230450 ) ) ;
#196083=B_SPLINE_CURVE_WITH_KNOTS ( 'NONE', 3,
 ( #56714, #133539, #139492, #184028, #140495, #92988, #200185, #187034, #151706, #199196, #154674, #16169, #124327, #137515, #14169, #17163, #61654, #183041, #1983, #60664, #186025, #107165, #76832, #121348, #185015, #105197, #166884, #28385, #77823, #32334, #155667, #46501 ),
 .UNSPECIFIED., .F., .F.,
 ( 4, 2, 2, 2, 2, 2, 2, 2, 2, 2, 2, 2, 2, 2, 2, 4 ),
 ( 2.625112965618923374E-17, 0.0003712461730036955600, 0.0007424923460073648823, 0.001113738519011033988, 0.001484984692014703527, 0.002227477038022048893, 0.002598723211025728841, 0.002969969384029408788, 0.003341215557033088302, 0.003712461730036768683, 0.004083707903040447763, 0.004454954076044127277, 0.004826200249047807658, 0.005197446422051487172, 0.005568692595055167553, 0.005939938768058847067 ),
 .UNSPECIFIED. ) ;
#196084=CARTESIAN_POINT ( 'NONE',  ( -9.474510206698964154, 16.51473224551069663, 60.41557627198102409 ) ) ;
#196085=CARTESIAN_POINT ( 'NONE',  ( -9.474510206698964154, 16.51473224551069663, 115.4155762719810241 ) ) ;
#196086=CARTESIAN_POINT ( 'NONE',  ( 19.05341960407611168, 5.049401038298154454, 73.95724293864768129 ) ) ;
#196087=CARTESIAN_POINT ( 'NONE',  ( -13.97604488694527625, -13.89961937509977830, 76.87390960531435269 ) ) ;
#196088=CARTESIAN_POINT ( 'NONE',  ( -19.02544592524342804, 5.153800228976336051, 66.04057627198103830 ) ) ;
#196089=CARTESIAN_POINT ( 'NONE',  ( 19.03943276465977164, -0.05219959533909143690, 58.74890960531435979 ) ) ;
#196090=CARTESIAN_POINT ( 'NONE',  ( 15.80617190586746368, 15.72974639402197994, 114.3739096053143527 ) ) ;
#196091=CARTESIAN_POINT ( 'NONE',  ( -16.55341960407617563, 4.379528057220093196, 83.54275706135234714 ) ) ;
#196094=CARTESIAN_POINT ( 'NONE',  ( 13.89961937509957401, 13.97604488694547697, 56.87609039468564731 ) ) ;
#196095=CARTESIAN_POINT ( 'NONE',  ( -19.02544592524342804, 5.153800228976336051, 76.04057627198102409 ) ) ;
#196096=CARTESIAN_POINT ( 'NONE',  ( -12.06949235617756955, 12.14591786802309770, 75.62390960531439532 ) ) ;
#196097=CARTESIAN_POINT ( 'NONE',  ( 8.314922557960818139, 14.29746914071049879, 109.5822429386476955 ) ) ;
#196098=CARTESIAN_POINT ( 'NONE',  ( -18.62759615963270932, 10.81492255796079327, 30.83224293864770260 ) ) ;
#196099=CARTESIAN_POINT ( 'NONE',  ( -16.51473224551069308, -9.474510206698971260, 101.6655762719810241 ) ) ;
#196100=CARTESIAN_POINT ( 'NONE',  ( 16.53943276465976808, -0.05219959533910856209, 93.74890960531436690 ) ) ;
#196101=CARTESIAN_POINT ( 'NONE',  ( -9.564922557960796823, -16.46253265017161027, 82.08224293864768129 ) ) ;
#196102=CARTESIAN_POINT ( 'NONE',  ( 19.05341960407617918, -5.049401038297876454, 31.04275706135232227 ) ) ;
#196103=CARTESIAN_POINT ( 'NONE',  ( 14.34966873604972726, -8.224510206698740333, 110.8344237280190043 ) ) ;
#196104=CARTESIAN_POINT ( 'NONE',  ( 19.03943276465977164, -0.05219959533909143690, 88.74890960531436690 ) ) ;
#196105=CARTESIAN_POINT ( 'NONE',  ( -10.81492255796105439, 18.62759615963255655, 52.91775706135235424 ) ) ;
#196106=CARTESIAN_POINT ( 'NONE',  ( -18.67979575497178146, -10.72451020669898902, 46.66557627198102409 ) ) ;
#196107=CARTESIAN_POINT ( 'NONE',  ( -5.823673210054431948, 21.52544592524334988, 22.70942372801901499 ) ) ;
#196108=CARTESIAN_POINT ( 'NONE',  ( 15.80617190586746368, 15.72974639402197994, 74.37390960531436690 ) ) ;
#196109=CARTESIAN_POINT ( 'NONE',  ( 12.06949235617757843, -12.14591786802309237, 98.12390960531436690 ) ) ;
#196110=CARTESIAN_POINT ( 'NONE',  ( 13.89961937509957401, 13.97604488694547697, 56.87609039468564731 ) ) ;
#196111=CARTESIAN_POINT ( 'NONE',  ( 13.97604488694527802, 13.89961937509977652, 29.37390960531435979 ) ) ;
#196112=CARTESIAN_POINT ( 'NONE',  ( 19.05341960407611168, 5.049401038298154454, 78.95724293864769550 ) ) ;
#196113=CARTESIAN_POINT ( 'NONE',  ( 13.89961937509977652, -13.97604488694527269, 98.12390960531433848 ) ) ;
#196114=CARTESIAN_POINT ( 'NONE',  ( -8.224510206698948167, 14.34966873604960824, 115.4155762719810241 ) ) ;
#196115=CARTESIAN_POINT ( 'NONE',  ( 0.05219959533910956823, 16.53943276465976808, 29.99890960531435979 ) ) ;
#196116=CARTESIAN_POINT ( 'NONE',  ( -4.483927247898782831, 16.52544592524335698, 37.70942372801900433 ) ) ;
#196117=CARTESIAN_POINT ( 'NONE',  ( 15.80617190586769283, -15.72974639402175789, 110.6260903946857042 ) ) ;
#196118=CARTESIAN_POINT ( 'NONE',  ( -9.564922557960796823, -16.46253265017161027, 102.0822429386477097 ) ) ;
#196119=CARTESIAN_POINT ( 'NONE',  ( 10.72451020669871369, 18.67979575497193778, 32.08442372801901854 ) ) ;
#196120=CARTESIAN_POINT ( 'NONE',  ( 19.05341960407611168, 5.049401038298154454, 43.95724293864769550 ) ) ;
#196121=CARTESIAN_POINT ( 'NONE',  ( -8.224510206698735004, -14.34966873604973081, 49.58442372801901143 ) ) ;
#196122=CARTESIAN_POINT ( 'NONE',  ( 12.06949235617739724, 12.14591786802326823, 111.8760903946856615 ) ) ;
#196123=CARTESIAN_POINT ( 'NONE',  ( -12.06949235617739369, -12.14591786802326823, 89.37609039468568994 ) ) ;
#196124=CARTESIAN_POINT ( 'NONE',  ( -9.474510206698720793, -16.51473224551083518, 104.5844237280190043 ) ) ;
#196125=CARTESIAN_POINT ( 'NONE',  ( -0.05219959533909027116, -19.03943276465977164, 37.49890960531436690 ) ) ;
#196126=CARTESIAN_POINT ( 'NONE',  ( -12.06949235617756955, 12.14591786802309770, 100.6239096053143811 ) ) ;
#196127=CARTESIAN_POINT ( 'NONE',  ( 18.67979575497178502, 10.72451020669898547, 104.1655762719810241 ) ) ;
#196128=CARTESIAN_POINT ( 'NONE',  ( 5.153800228976335163, 19.02544592524342804, 29.79057627198102409 ) ) ;
#196129=CARTESIAN_POINT ( 'NONE',  ( -19.02544592524342804, 5.153800228976336051, 101.0405762719810241 ) ) ;
#196130=CARTESIAN_POINT ( 'NONE',  ( 5.719274019375673035, 21.55341960407619339, 37.29275706135235424 ) ) ;
#196132=CARTESIAN_POINT ( 'NONE',  ( 16.46253265017160672, -9.564922557960803928, 103.3322429386476955 ) ) ;
#196133=CARTESIAN_POINT ( 'NONE',  ( 17.44270441346516876, -5.991230190323036275, 111.1366492073577490 ) ) ;
#196134=CARTESIAN_POINT ( 'NONE',  ( 16.51473224551069308, 9.474510206698969483, 79.16557627198103830 ) ) ;
#196135=CARTESIAN_POINT ( 'NONE',  ( 21.52544592524334988, 5.823673210054432836, 26.45942372801901854 ) ) ;
#196136=CARTESIAN_POINT ( 'NONE',  ( 4.483927247898545687, 16.52544592524342804, 94.79057627198105251 ) ) ;
#196137=CARTESIAN_POINT ( 'NONE',  ( -0.05219959533909027116, -19.03943276465977164, 97.49890960531436690 ) ) ;
#196138=CARTESIAN_POINT ( 'NONE',  ( -13.89961937509957401, -13.97604488694547875, 24.37609039468565442 ) ) ;
#196139=CARTESIAN_POINT ( 'NONE',  ( 12.14591786802327356, -12.06949235617739191, 70.62609039468567573 ) ) ;
#196140=CARTESIAN_POINT ( 'NONE',  ( -21.52544592524334988, -5.823673210054445271, 83.95942372801900433 ) ) ;
#196141=CARTESIAN_POINT ( 'NONE',  ( 16.52544592524335698, 4.483927247898782831, 46.45942372801901854 ) ) ;
#196142=CARTESIAN_POINT ( 'NONE',  ( -19.03943276465977164, 0.05219959533909376836, 81.24890960531436690 ) ) ;
#196143=CARTESIAN_POINT ( 'NONE',  ( -19.02544592524334988, -5.153800228976617603, 88.95942372801897591 ) ) ;
#196144=CARTESIAN_POINT ( 'NONE',  ( -14.34966873604972548, 8.224510206698743886, 73.33442372801901854 ) ) ;
#196145=CARTESIAN_POINT ( 'NONE',  ( 13.97604488694548053, -13.89961937509957401, 20.62609039468567573 ) ) ;
#196146=CARTESIAN_POINT ( 'NONE',  ( -5.153800228976607833, 19.02544592524334988, 77.70942372801900433 ) ) ;
#196147=CARTESIAN_POINT ( 'NONE',  ( 16.46253265017160672, -9.564922557960803928, 63.33224293864769550 ) ) ;
#196148=CARTESIAN_POINT ( 'NONE',  ( 0.05219959533907565091, 21.53943276465977519, 84.99890960531436690 ) ) ;
#196149=CARTESIAN_POINT ( 'NONE',  ( 4.483927247898545687, 16.52544592524342804, 84.79057627198102409 ) ) ;
#196150=CARTESIAN_POINT ( 'NONE',  ( 9.474510206698729675, 16.51473224551082808, 97.08442372801900433 ) ) ;
#196151=CARTESIAN_POINT ( 'NONE',  ( -16.52544592524335698, -4.483927247898792601, 58.95942372801902565 ) ) ;
#196153=CARTESIAN_POINT ( 'NONE',  ( -19.05341960407617563, 5.049401038297882671, 63.54275706135234003 ) ) ;
#196154=CARTESIAN_POINT ( 'NONE',  ( 12.06949235617739724, 12.14591786802326823, 106.8760903946856899 ) ) ;
#196155=CARTESIAN_POINT ( 'NONE',  ( 8.314922557960818139, 14.29746914071049879, 79.58224293864769550 ) ) ;
#196156=CARTESIAN_POINT ( 'NONE',  ( 19.03943276465977164, 0.05219959533936151252, 21.25109039468565797 ) ) ;
#196157=CARTESIAN_POINT ( 'NONE',  ( -16.38665767534995155, 7.295008042176406526, 40.26400864214470943 ) ) ;
#196158=CARTESIAN_POINT ( 'NONE',  ( -21.52544592524343514, 5.823673210054127303, 116.0405762719810383 ) ) ;
#196159=CARTESIAN_POINT ( 'NONE',  ( -9.564922557960796823, -16.46253265017161027, 107.0822429386476955 ) ) ;
#196160=CARTESIAN_POINT ( 'NONE',  ( -5.153800228976328057, -19.02544592524343514, 72.29057627198102409 ) ) ;
#196161=CARTESIAN_POINT ( 'NONE',  ( 5.719274019375673035, 21.55341960407619339, 87.29275706135236135 ) ) ;
#196162=CARTESIAN_POINT ( 'NONE',  ( -19.03943276465977164, 0.05219959533909376836, 66.24890960531436690 ) ) ;
#196163=CARTESIAN_POINT ( 'NONE',  ( 15.72974639402199770, -15.80617190586745480, 28.12390960531435979 ) ) ;
#196164=CARTESIAN_POINT ( 'NONE',  ( 12.14591786802309770, 12.06949235617756955, 84.37390960531438111 ) ) ;
#196165=CARTESIAN_POINT ( 'NONE',  ( 5.049401038298161559, -19.05341960407611168, 37.70724293864768839 ) ) ;
#196166=CARTESIAN_POINT ( 'NONE',  ( 16.52544592524342804, -4.483927247898539470, 93.54057627198103830 ) ) ;
#196168=CARTESIAN_POINT ( 'NONE',  ( -5.823673210054116645, -21.52544592524344225, 112.2905762719810241 ) ) ;
#196170=CARTESIAN_POINT ( 'NONE',  ( -21.53943276465977519, -0.05219959533937600094, 53.75109039468568994 ) ) ;
#196171=CARTESIAN_POINT ( 'NONE',  ( -19.02544592524342804, 5.153800228976336051, 26.04057627198103120 ) ) ;
#196172=CARTESIAN_POINT ( 'NONE',  ( 14.34966873604972726, -8.224510206698740333, 60.83442372801901854 ) ) ;
#196173=CARTESIAN_POINT ( 'NONE',  ( 5.823673210054125526, 21.52544592524343514, 99.79057627198103830 ) ) ;
#196174=CARTESIAN_POINT ( 'NONE',  ( 15.72974639402199770, -15.80617190586745480, 108.1239096053143811 ) ) ;
#196175=CARTESIAN_POINT ( 'NONE',  ( 13.89961937509957401, 13.97604488694547697, 41.87609039468566152 ) ) ;
#196176=CARTESIAN_POINT ( 'NONE',  ( 19.05341960407611168, 5.049401038298154454, 58.95724293864768129 ) ) ;
#196177=CARTESIAN_POINT ( 'NONE',  ( 17.50000000000000000, -5.500000000000000888, 120.0000000000000142 ) ) ;
#196178=CARTESIAN_POINT ( 'NONE',  ( 21.52544592524334988, 5.823673210054432836, 51.45942372801901854 ) ) ;
#196179=CARTESIAN_POINT ( 'NONE',  ( 10.72451020669898902, -18.67979575497178502, 62.91557627198102409 ) ) ;
#196180=CARTESIAN_POINT ( 'NONE',  ( 0.05219959533910956823, 16.53943276465976808, 39.99890960531436690 ) ) ;
#196181=CARTESIAN_POINT ( 'NONE',  ( 18.67979575497194134, -10.72451020669871369, 70.83442372801901854 ) ) ;
#196182=CARTESIAN_POINT ( 'NONE',  ( -15.72974639402176322, -15.80617190586768395, 109.3760903946857042 ) ) ;
#196183=CARTESIAN_POINT ( 'NONE',  ( 8.224510206698953496, -14.34966873604960469, 62.91557627198102409 ) ) ;
#196184=CARTESIAN_POINT ( 'NONE',  ( 16.55341960407611168, 4.379528057220329451, 103.9572429386476813 ) ) ;
#196185=CARTESIAN_POINT ( 'NONE',  ( -16.51473224551082808, 9.474510206698731452, 38.33442372801899722 ) ) ;
#196186=CARTESIAN_POINT ( 'NONE',  ( 12.06949235617739724, 12.14591786802326823, 101.8760903946857042 ) ) ;
#196187=CARTESIAN_POINT ( 'NONE',  ( -5.719274019375665041, -21.55341960407619695, 64.79275706135234714 ) ) ;
#196188=CARTESIAN_POINT ( 'NONE',  ( -9.474510206698964154, 16.51473224551069663, 60.41557627198102409 ) ) ;
#196189=CARTESIAN_POINT ( 'NONE',  ( 0.05219959533936267826, -19.03943276465977164, 35.00109039468566863 ) ) ;
#196190=CARTESIAN_POINT ( 'NONE',  ( -0.05219959533907301413, -21.53943276465977519, 42.49890960531435979 ) ) ;
#196191=CARTESIAN_POINT ( 'NONE',  ( -21.52544592524334988, -5.823673210054445271, 33.95942372801901143 ) ) ;
#196192=CARTESIAN_POINT ( 'NONE',  ( -0.05219959533907301413, -21.53943276465977519, 92.49890960531436690 ) ) ;
#196193=CARTESIAN_POINT ( 'NONE',  ( 5.153800228976615827, -19.02544592524334988, 85.20942372801900433 ) ) ;
#196194=CARTESIAN_POINT ( 'NONE',  ( 12.06949235617739724, 12.14591786802326823, 56.87609039468568994 ) ) ;
#196195=CARTESIAN_POINT ( 'NONE',  ( 17.50000000000002487, -3.438020150447669288, 37.00844184464188658 ) ) ;
#196196=CARTESIAN_POINT ( 'NONE',  ( 18.67979575497178502, 10.72451020669898547, 94.16557627198103830 ) ) ;
#196197=CARTESIAN_POINT ( 'NONE',  ( -16.53943276465976808, -0.05219959533934237506, 78.75109039468568994 ) ) ;
#196198=CARTESIAN_POINT ( 'NONE',  ( 8.224510206698953496, -14.34966873604960469, 72.91557627198103830 ) ) ;
#196200=CARTESIAN_POINT ( 'NONE',  ( 8.224510206698742110, 14.34966873604972548, 27.08442372801901854 ) ) ;
#196201=CARTESIAN_POINT ( 'NONE',  ( 10.72451020669898902, -18.67979575497178502, 37.91557627198102409 ) ) ;
#196202=CARTESIAN_POINT ( 'NONE',  ( 4.379528057220092307, 16.55341960407617563, 77.29275706135234714 ) ) ;
#196204=CARTESIAN_POINT ( 'NONE',  ( 16.53943276465976808, 0.05219959533934440121, 51.25109039468568994 ) ) ;
#196205=CARTESIAN_POINT ( 'NONE',  ( -10.72451020669870658, -18.67979575497194134, 29.58442372801901854 ) ) ;
#196206=CARTESIAN_POINT ( 'NONE',  ( -21.53943276465977519, 0.05219959533907696930, 51.24890960531436690 ) ) ;
#196207=CARTESIAN_POINT ( 'NONE',  ( -12.06949235617739369, -12.14591786802326823, 74.37609039468568994 ) ) ;
#196208=CARTESIAN_POINT ( 'NONE',  ( -5.153800228976328057, -19.02544592524343514, 87.29057627198103830 ) ) ;
#196209=CARTESIAN_POINT ( 'NONE',  ( 5.719274019375673035, 21.55341960407619339, 62.29275706135236845 ) ) ;
#196210=CARTESIAN_POINT ( 'NONE',  ( -16.51473224551069308, -9.474510206698971260, 26.66557627198103120 ) ) ;
#196212=CARTESIAN_POINT ( 'NONE',  ( -15.80617190586745835, -15.72974639402198527, 41.87390960531435979 ) ) ;
#196213=CARTESIAN_POINT ( 'NONE',  ( -19.02544592524342804, 5.153800228976336051, 116.0405762719810383 ) ) ;
#196215=CARTESIAN_POINT ( 'NONE',  ( -13.97604488694547697, 13.89961937509957934, 43.12609039468566152 ) ) ;
#196216=CARTESIAN_POINT ( 'NONE',  ( 14.29746914071037800, 8.314922557961029526, 56.66775706135235424 ) ) ;
#196217=CARTESIAN_POINT ( 'NONE',  ( 21.55341960407610458, 5.719274019375980345, 23.95724293864769550 ) ) ;
#196219=CARTESIAN_POINT ( 'NONE',  ( -19.03943276465977164, 0.05219959533909376836, 81.24890960531436690 ) ) ;
#196220=CARTESIAN_POINT ( 'NONE',  ( 14.29746914071037800, 8.314922557961029526, 101.6677570613523613 ) ) ;
#196222=CARTESIAN_POINT ( 'NONE',  ( -12.06949235617756955, 12.14591786802309770, 95.62390960531436690 ) ) ;
#196223=CARTESIAN_POINT ( 'NONE',  ( -21.53943276465977519, 0.05219959533907696930, 31.24890960531435979 ) ) ;
#196224=CARTESIAN_POINT ( 'NONE',  ( 9.474510206698971260, -16.51473224551069308, 27.91557627198103120 ) ) ;
#196225=CARTESIAN_POINT ( 'NONE',  ( -16.55341960407617563, 4.379528057220093196, 78.54275706135236135 ) ) ;
#196226=CARTESIAN_POINT ( 'NONE',  ( 5.823673210054125526, 21.52544592524343514, 114.7905762719810383 ) ) ;
#196227=CARTESIAN_POINT ( 'NONE',  ( -19.05341960407617563, 5.049401038297882671, 73.54275706135233293 ) ) ;
#196228=CARTESIAN_POINT ( 'NONE',  ( 16.51473224551069308, 9.474510206698969483, 34.16557627198102409 ) ) ;
#196230=CARTESIAN_POINT ( 'NONE',  ( -5.153800228976328057, -19.02544592524343514, 112.2905762719810099 ) ) ;
#196231=CARTESIAN_POINT ( 'NONE',  ( 15.72974639402176855, 15.80617190586768217, 106.8760903946856899 ) ) ;
#196232=CARTESIAN_POINT ( 'NONE',  ( -19.02544592524342804, 5.153800228976336051, 61.04057627198103120 ) ) ;
#196233=CARTESIAN_POINT ( 'NONE',  ( 0.05219959533934541429, -16.53943276465976808, 55.00109039468568284 ) ) ;
#196234=CARTESIAN_POINT ( 'NONE',  ( -18.62759615963255300, -10.81492255796106328, 99.16775706135234714 ) ) ;
#196235=CARTESIAN_POINT ( 'NONE',  ( -0.05219959533936034679, 19.03943276465977164, 57.50109039468566863 ) ) ;
#196236=CARTESIAN_POINT ( 'NONE',  ( -19.05341960407617563, 5.049401038297882671, 48.54275706135233293 ) ) ;
#196238=CARTESIAN_POINT ( 'NONE',  ( -5.719274019375665041, -21.55341960407619695, 49.79275706135234714 ) ) ;
#196239=CARTESIAN_POINT ( 'NONE',  ( -17.49999999999999645, 5.499999999999997335, 118.0000000000000142 ) ) ;
#196240=CARTESIAN_POINT ( 'NONE',  ( 0.05219959533936267826, -19.03943276465977164, 40.00109039468566152 ) ) ;
#196241=CARTESIAN_POINT ( 'NONE',  ( 19.05341960407611168, 5.049401038298154454, 103.9572429386476671 ) ) ;
#196242=CARTESIAN_POINT ( 'NONE',  ( 13.97604488694527802, 13.89961937509977652, 84.37390960531433848 ) ) ;
#196243=CARTESIAN_POINT ( 'NONE',  ( 14.34966873604960469, 8.224510206698951720, 34.16557627198102409 ) ) ;
#196244=CARTESIAN_POINT ( 'NONE',  ( 15.72974639402199770, -15.80617190586745480, 28.12390960531435979 ) ) ;
#196247=CARTESIAN_POINT ( 'NONE',  ( -21.52544592524334988, -5.823673210054445271, 108.9594237280190185 ) ) ;
#196249=CARTESIAN_POINT ( 'NONE',  ( -19.02544592524342804, 5.153800228976336051, 31.04057627198102409 ) ) ;
#196250=CARTESIAN_POINT ( 'NONE',  ( 5.153800228976335163, 19.02544592524342804, 84.79057627198100988 ) ) ;
#196253=CARTESIAN_POINT ( 'NONE',  ( 4.483927247898790824, -16.52544592524335698, 65.20942372801901854 ) ) ;
#196254=CARTESIAN_POINT ( 'NONE',  ( 21.53943276465977519, -0.05219959533907433946, 78.74890960531436690 ) ) ;
#196255=CARTESIAN_POINT ( 'NONE',  ( -14.29746914071049879, 8.314922557960819915, 35.83224293864768839 ) ) ;
#196256=CARTESIAN_POINT ( 'NONE',  ( -13.97604488694527625, -13.89961937509977652, 26.87390960531434558 ) ) ;
#196257=CARTESIAN_POINT ( 'NONE',  ( -13.89961937509977652, 13.97604488694528158, 110.6239096053143243 ) ) ;
#196258=CARTESIAN_POINT ( 'NONE',  ( -21.55341960407619339, 5.719274019375674811, 28.54275706135234358 ) ) ;
#196259=CARTESIAN_POINT ( 'NONE',  ( -5.153800228976607833, 19.02544592524334988, 32.70942372801899722 ) ) ;
#196260=CARTESIAN_POINT ( 'NONE',  ( 13.89961937509977652, -13.97604488694527269, 38.12390960531436690 ) ) ;
#196261=CARTESIAN_POINT ( 'NONE',  ( 5.719274019375673035, 21.55341960407619339, 87.29275706135236135 ) ) ;
#196263=CARTESIAN_POINT ( 'NONE',  ( 14.29746914071049879, -8.314922557960816363, 33.33224293864769550 ) ) ;
#196265=CARTESIAN_POINT ( 'NONE',  ( -15.72974639402197994, 15.80617190586746368, 30.62390960531436335 ) ) ;
#196266=CARTESIAN_POINT ( 'NONE',  ( 0.05219959533910956823, 16.53943276465976808, 99.99890960531436690 ) ) ;
#196268=CARTESIAN_POINT ( 'NONE',  ( 9.564922557960805705, 16.46253265017160317, 84.58224293864769550 ) ) ;
#196269=CARTESIAN_POINT ( 'NONE',  ( 16.55341960407611168, 4.379528057220329451, 78.95724293864769550 ) ) ;
#196270=CARTESIAN_POINT ( 'NONE',  ( 9.564922557961047289, -16.46253265017146816, 100.4177570613523329 ) ) ;
#196271=CARTESIAN_POINT ( 'NONE',  ( 0.05219959533907565091, 21.53943276465977519, 59.99890960531436690 ) ) ;
#196272=ORIENTED_EDGE ( 'NONE', *, *, #17849, .T. ) ;
#196273=CARTESIAN_POINT ( 'NONE',  ( -9.564922557960796823, -16.46253265017161027, 27.08224293864769550 ) ) ;
#196274=CARTESIAN_POINT ( 'NONE',  ( 19.03943276465977164, -0.05219959533909143690, 88.74890960531436690 ) ) ;
#196275=CARTESIAN_POINT ( 'NONE',  ( 15.72974639402199770, -15.80617190586745480, 88.12390960531436690 ) ) ;
#196276=CARTESIAN_POINT ( 'NONE',  ( 16.53943276465976808, 0.05219959533934440121, 101.2510903946856757 ) ) ;
#196277=CARTESIAN_POINT ( 'NONE',  ( 19.02544592524343514, -5.153800228976328945, 88.54057627198102409 ) ) ;
#196278=CARTESIAN_POINT ( 'NONE',  ( -16.46253265017146816, -9.564922557961047289, 79.16775706135234714 ) ) ;
#196279=CARTESIAN_POINT ( 'NONE',  ( 15.80617190586769283, -15.72974639402175789, 90.62609039468567573 ) ) ;
#196280=CARTESIAN_POINT ( 'NONE',  ( -15.80617190586745835, -15.72974639402198527, 81.87390960531435269 ) ) ;
#196281=CARTESIAN_POINT ( 'NONE',  ( 21.55341960407610458, 5.719274019375980345, 33.95724293864769550 ) ) ;
#196282=CARTESIAN_POINT ( 'NONE',  ( 19.02544592524343514, -5.153800228976328945, 53.54057627198102409 ) ) ;
#196283=CARTESIAN_POINT ( 'NONE',  ( 0.05219959533910956823, 16.53943276465976808, 24.99890960531435624 ) ) ;
#196284=CARTESIAN_POINT ( 'NONE',  ( 0.05219959533909260263, 19.03943276465977164, 59.99890960531436690 ) ) ;
#196286=CARTESIAN_POINT ( 'NONE',  ( 16.46253265017146816, 9.564922557961045513, 31.66775706135232937 ) ) ;
#196287=CARTESIAN_POINT ( 'NONE',  ( -14.29746914071049879, 8.314922557960819915, 70.83224293864770971 ) ) ;
#196288=CARTESIAN_POINT ( 'NONE',  ( 18.67979575497178502, 10.72451020669898547, 109.1655762719810383 ) ) ;
#196290=CARTESIAN_POINT ( 'NONE',  ( -0.05219959533907301413, -21.53943276465977519, 57.49890960531435979 ) ) ;
#196291=CARTESIAN_POINT ( 'NONE',  ( 16.53943276465976808, 0.05219959533934440121, 91.25109039468568994 ) ) ;
#196292=CARTESIAN_POINT ( 'NONE',  ( -4.379528057220328563, 16.55341960407611168, 105.2072429386477097 ) ) ;
#196293=CARTESIAN_POINT ( 'NONE',  ( -5.153800228976328057, -19.02544592524343514, 62.29057627198100988 ) ) ;
#196294=CARTESIAN_POINT ( 'NONE',  ( 4.483927247898545687, 16.52544592524342804, 34.79057627198103120 ) ) ;
#196295=CARTESIAN_POINT ( 'NONE',  ( 18.67979575497194134, -10.72451020669871369, 40.83442372801901854 ) ) ;
#196296=CARTESIAN_POINT ( 'NONE',  ( 0.05219959533909260263, 19.03943276465977164, 109.9989096053143669 ) ) ;
#196297=CARTESIAN_POINT ( 'NONE',  ( -5.823673210054431948, 21.52544592524334988, 87.70942372801901854 ) ) ;
#196298=CARTESIAN_POINT ( 'NONE',  ( 19.05341960407611168, 5.049401038298154454, 33.95724293864769550 ) ) ;
#196299=CARTESIAN_POINT ( 'NONE',  ( 19.02544592524343514, -5.153800228976328945, 38.54057627198103120 ) ) ;
#196301=CARTESIAN_POINT ( 'NONE',  ( 5.719274019375673035, 21.55341960407619339, 82.29275706135234714 ) ) ;
#196302=CARTESIAN_POINT ( 'NONE',  ( 16.53943276465976808, 0.05219959533934440121, 46.25109039468567573 ) ) ;
#196303=CARTESIAN_POINT ( 'NONE',  ( 10.81492255796106328, -18.62759615963255655, 70.41775706135236135 ) ) ;
#196304=CARTESIAN_POINT ( 'NONE',  ( 16.46253265017160672, -9.564922557960803928, 103.3322429386476955 ) ) ;
#196305=CARTESIAN_POINT ( 'NONE',  ( 19.05341960407617918, -5.049401038297876454, 86.04275706135233293 ) ) ;
#196306=CARTESIAN_POINT ( 'NONE',  ( -5.823673210054431948, 21.52544592524334988, 57.70942372801901143 ) ) ;
#196307=CARTESIAN_POINT ( 'NONE',  ( -8.224510206698735004, -14.34966873604973081, 24.58442372801901499 ) ) ;
#196308=CARTESIAN_POINT ( 'NONE',  ( 16.46253265017146816, 9.564922557961045513, 86.66775706135233293 ) ) ;
#196309=CARTESIAN_POINT ( 'NONE',  ( -13.97604488694527625, -13.89961937509977652, 51.87390960531436690 ) ) ;
#196310=CARTESIAN_POINT ( 'NONE',  ( -9.564922557961040184, 16.46253265017147172, 82.91775706135233293 ) ) ;
#196311=VECTOR ( 'NONE', #114170, 999.9999999999998863 ) ;
#196312=CARTESIAN_POINT ( 'NONE',  ( -8.314922557961024197, 14.29746914071037800, 112.9177570613523329 ) ) ;
#196313=CARTESIAN_POINT ( 'NONE',  ( -5.153800228976607833, 19.02544592524334988, 92.70942372801901854 ) ) ;
#196314=CARTESIAN_POINT ( 'NONE',  ( -16.52544592524342804, 4.483927247898546575, 36.04057627198102409 ) ) ;
#196315=CARTESIAN_POINT ( 'NONE',  ( -19.05341960407617563, 5.049401038297882671, 63.54275706135234003 ) ) ;
#196316=CARTESIAN_POINT ( 'NONE',  ( 4.483927247898790824, -16.52544592524335698, 45.20942372801901854 ) ) ;
#196317=CARTESIAN_POINT ( 'NONE',  ( 0.05219959533936267826, -19.03943276465977164, 30.00109039468566863 ) ) ;
#196318=CARTESIAN_POINT ( 'NONE',  ( 14.34966873604960469, 8.224510206698951720, 114.1655762719810383 ) ) ;
#196319=CARTESIAN_POINT ( 'NONE',  ( -5.153800228976328057, -19.02544592524343514, 37.29057627198102409 ) ) ;
#196320=CARTESIAN_POINT ( 'NONE',  ( 12.14591786802327356, -12.06949235617739191, 50.62609039468568994 ) ) ;
#196322=B_SPLINE_CURVE_WITH_KNOTS ( 'NONE', 3,
 ( #197730, #107676, #139016, #105708, #76356, #121861 ),
 .UNSPECIFIED., .F., .F.,
 ( 4, 2, 4 ),
 ( 0.007228050697041537957, 0.007608510107495020450, 0.007988969517948503810 ),
 .UNSPECIFIED. ) ;
#196324=CARTESIAN_POINT ( 'NONE',  ( 19.03943276465977164, -0.05219959533909143690, 98.74890960531436690 ) ) ;
#196327=CARTESIAN_POINT ( 'NONE',  ( -9.564922557961040184, 16.46253265017147172, 92.91775706135233293 ) ) ;
#196328=CARTESIAN_POINT ( 'NONE',  ( -15.72974639402197994, 15.80617190586746368, 30.62390960531436335 ) ) ;
#196329=CARTESIAN_POINT ( 'NONE',  ( -16.51473224551082808, 9.474510206698731452, 33.33442372801899722 ) ) ;
#196330=CARTESIAN_POINT ( 'NONE',  ( 9.564922557961047289, -16.46253265017146816, 110.4177570613523471 ) ) ;
#196331=CARTESIAN_POINT ( 'NONE',  ( 8.224510206698953496, -14.34966873604960469, 112.9155762719810383 ) ) ;
#196332=CARTESIAN_POINT ( 'NONE',  ( -0.05219959533909027116, -19.03943276465977164, 32.49890960531435979 ) ) ;
#196333=CARTESIAN_POINT ( 'NONE',  ( 15.80617190586746368, 15.72974639402197994, 79.37390960531436690 ) ) ;
#196334=CARTESIAN_POINT ( 'NONE',  ( 16.46253265017160672, -9.564922557960803928, 33.33224293864770260 ) ) ;
#196335=CARTESIAN_POINT ( 'NONE',  ( -17.59860650958993844, 7.585241751806885979, 48.42337014262493966 ) ) ;
#196336=CARTESIAN_POINT ( 'NONE',  ( -13.89961937509957401, -13.97604488694547875, 69.37609039468564731 ) ) ;
#196337=CARTESIAN_POINT ( 'NONE',  ( 16.55341960407611168, 4.379528057220329451, 53.95724293864770260 ) ) ;
#196338=CARTESIAN_POINT ( 'NONE',  ( 0.05219959533907565091, 21.53943276465977519, 34.99890960531435979 ) ) ;
#196339=CARTESIAN_POINT ( 'NONE',  ( -21.52544592524334988, -5.823673210054445271, 88.95942372801901854 ) ) ;
#196340=CARTESIAN_POINT ( 'NONE',  ( 5.823673210054125526, 21.52544592524343514, 89.79057627198103830 ) ) ;
#196341=CARTESIAN_POINT ( 'NONE',  ( 10.72451020669871369, 18.67979575497193778, 72.08442372801899012 ) ) ;
#196342=CARTESIAN_POINT ( 'NONE',  ( -18.67979575497193778, 10.72451020669871902, 68.33442372801900433 ) ) ;
#196343=CARTESIAN_POINT ( 'NONE',  ( -0.05219959533909027116, -19.03943276465977164, 92.49890960531436690 ) ) ;
#196344=CARTESIAN_POINT ( 'NONE',  ( 16.52544592524335698, 4.483927247898782831, 96.45942372801901854 ) ) ;
#196345=CARTESIAN_POINT ( 'NONE',  ( 5.823673210054444382, -21.52544592524334988, 70.20942372801904696 ) ) ;
#196346=CARTESIAN_POINT ( 'NONE',  ( 16.46253265017160672, -9.564922557960803928, 53.33224293864768839 ) ) ;
#196347=CARTESIAN_POINT ( 'NONE',  ( 5.719274019375673035, 21.55341960407619339, 32.29275706135235424 ) ) ;
#196348=CARTESIAN_POINT ( 'NONE',  ( 5.153800228976335163, 19.02544592524342804, 64.79057627198100988 ) ) ;
#196349=CARTESIAN_POINT ( 'NONE',  ( 14.34966873604960469, 8.224510206698951720, 64.16557627198102409 ) ) ;
#196350=CARTESIAN_POINT ( 'NONE',  ( 16.52544592524342804, -4.483927247898539470, 33.54057627198102409 ) ) ;
#196351=CARTESIAN_POINT ( 'NONE',  ( -0.05219959533907301413, -21.53943276465977519, 47.49890960531435979 ) ) ;
#196352=CARTESIAN_POINT ( 'NONE',  ( 19.03943276465977164, -0.05219959533909143690, 43.74890960531435979 ) ) ;
#196353=CARTESIAN_POINT ( 'NONE',  ( -21.55341960407610458, -5.719274019375992779, 56.45724293864768839 ) ) ;
#196354=CARTESIAN_POINT ( 'NONE',  ( -9.474510206698720793, -16.51473224551083518, 54.58442372801899722 ) ) ;
#196355=CARTESIAN_POINT ( 'NONE',  ( -17.31728774477272736, -6.344390552232413327, 39.18093348310684831 ) ) ;
#196356=CARTESIAN_POINT ( 'NONE',  ( 12.14591786802309770, 12.06949235617756955, 64.37390960531435269 ) ) ;
#196357=CARTESIAN_POINT ( 'NONE',  ( -21.55341960407610458, -5.719274019375992779, 46.45724293864769550 ) ) ;
#196360=CARTESIAN_POINT ( 'NONE',  ( 16.20579543436678094, 7.371946100355097897, 103.0652083417187441 ) ) ;
#196361=CARTESIAN_POINT ( 'NONE',  ( -4.379528057220086978, -16.55341960407618274, 79.79275706135236135 ) ) ;
#196362=CARTESIAN_POINT ( 'NONE',  ( 19.02544592524334988, 5.153800228976608722, 71.45942372801900433 ) ) ;
#196363=CARTESIAN_POINT ( 'NONE',  ( -8.314922557960811034, -14.29746914071050412, 52.08224293864768839 ) ) ;
#196365=CARTESIAN_POINT ( 'NONE',  ( -19.05341960407611168, -5.049401038298163336, 46.45724293864768129 ) ) ;
#196366=CARTESIAN_POINT ( 'NONE',  ( -16.53943276465976808, 0.05219959533911058130, 46.24890960531435979 ) ) ;
#196367=CARTESIAN_POINT ( 'NONE',  ( 0.05219959533909260263, 19.03943276465977164, 54.99890960531435979 ) ) ;
#196368=CARTESIAN_POINT ( 'NONE',  ( 5.153800228976335163, 19.02544592524342804, 74.79057627198103830 ) ) ;
#196369=CARTESIAN_POINT ( 'NONE',  ( -9.564922557960796823, -16.46253265017161027, 37.08224293864768839 ) ) ;
#196370=CARTESIAN_POINT ( 'NONE',  ( -10.81492255796105439, 18.62759615963255655, 42.91775706135235424 ) ) ;
#196371=CARTESIAN_POINT ( 'NONE',  ( -0.05219959533909027116, -19.03943276465977164, 77.49890960531435269 ) ) ;
#196372=CARTESIAN_POINT ( 'NONE',  ( -19.02544592524342804, 5.153800228976336051, 26.04057627198103120 ) ) ;
#196373=CARTESIAN_POINT ( 'NONE',  ( -9.474510206698964154, 16.51473224551069663, 55.41557627198103120 ) ) ;
#196374=CARTESIAN_POINT ( 'NONE',  ( -10.72451020669898014, 18.67979575497178502, 45.41557627198103830 ) ) ;
#196375=CARTESIAN_POINT ( 'NONE',  ( 0.05219959533909260263, 19.03943276465977164, 39.99890960531436690 ) ) ;
#196376=CARTESIAN_POINT ( 'NONE',  ( 21.53943276465977519, -0.05219959533907433946, 43.74890960531435979 ) ) ;
#196377=CARTESIAN_POINT ( 'NONE',  ( -12.06949235617739369, -12.14591786802326823, 99.37609039468568994 ) ) ;
#196378=CARTESIAN_POINT ( 'NONE',  ( -19.03943276465977164, -0.05219959533935918106, 18.75109039468567218 ) ) ;
#196379=CARTESIAN_POINT ( 'NONE',  ( 12.14591786802327356, -12.06949235617739191, 45.62609039468567573 ) ) ;
#196380=CARTESIAN_POINT ( 'NONE',  ( -4.379528057220086978, -16.55341960407618274, 74.79275706135234714 ) ) ;
#196381=DIRECTION ( 'NONE',  ( 1.000000000000000000, -0.000000000000000000, -0.000000000000000000 ) ) ;
#196382=CARTESIAN_POINT ( 'NONE',  ( 16.53943276465976808, 0.05219959533934440121, 66.25109039468567573 ) ) ;
#196383=CARTESIAN_POINT ( 'NONE',  ( -4.379528057220086978, -16.55341960407618274, 59.79275706135234714 ) ) ;
#196384=CARTESIAN_POINT ( 'NONE',  ( 9.474510206698971260, -16.51473224551069308, 102.9155762719810241 ) ) ;
#196385=CARTESIAN_POINT ( 'NONE',  ( -16.52544592524335698, -4.483927247898792601, 43.95942372801902565 ) ) ;
#196386=CARTESIAN_POINT ( 'NONE',  ( -16.46253265017160317, 9.564922557960807481, 30.83224293864769550 ) ) ;
#196387=CARTESIAN_POINT ( 'NONE',  ( -15.80617190586768217, 15.72974639402176855, 33.12609039468569705 ) ) ;
#196388=CARTESIAN_POINT ( 'NONE',  ( -0.05219959533934338120, 16.53943276465976808, 42.50109039468567573 ) ) ;
#196389=CARTESIAN_POINT ( 'NONE',  ( -8.314922557961024197, 14.29746914071037800, 97.91775706135236135 ) ) ;
#196391=CARTESIAN_POINT ( 'NONE',  ( 21.53943276465977519, 0.05219959533937863772, 106.2510903946856757 ) ) ;
#196392=CARTESIAN_POINT ( 'NONE',  ( -16.46253265017146816, -9.564922557961047289, 99.16775706135233293 ) ) ;
#196393=CARTESIAN_POINT ( 'NONE',  ( -14.29746914071049879, 8.314922557960819915, 55.83224293864770260 ) ) ;
#196394=CARTESIAN_POINT ( 'NONE',  ( -0.05219959533909027116, -19.03943276465977164, 22.49890960531436690 ) ) ;
#196395=CARTESIAN_POINT ( 'NONE',  ( 9.474510206698729675, 16.51473224551082808, 67.08442372801900433 ) ) ;
#196396=CARTESIAN_POINT ( 'NONE',  ( 16.81555441253466299, -7.025013491696266321, 58.13685445334211011 ) ) ;
#196397=CARTESIAN_POINT ( 'NONE',  ( 5.719274019375673035, 21.55341960407619339, 62.29275706135236845 ) ) ;
#196398=CARTESIAN_POINT ( 'NONE',  ( -16.53943276465976808, -0.05219959533934237506, 33.75109039468568284 ) ) ;
#196400=CARTESIAN_POINT ( 'NONE',  ( 21.55341960407610458, 5.719274019375980345, 23.95724293864769550 ) ) ;
#196401=CARTESIAN_POINT ( 'NONE',  ( 5.153800228976615827, -19.02544592524334988, 105.2094237280190185 ) ) ;
#196402=CARTESIAN_POINT ( 'NONE',  ( -19.02544592524342804, 5.153800228976336051, 101.0405762719810241 ) ) ;
#196404=CARTESIAN_POINT ( 'NONE',  ( -13.89961937509977652, 13.97604488694528158, 30.62390960531435269 ) ) ;
#196405=CARTESIAN_POINT ( 'NONE',  ( -15.80617190586768217, 15.72974639402176855, 113.1260903946856899 ) ) ;
#196406=CARTESIAN_POINT ( 'NONE',  ( -16.46253265017160317, 9.564922557960807481, 40.83224293864769550 ) ) ;
#196407=CARTESIAN_POINT ( 'NONE',  ( 10.72451020669871369, 18.67979575497193778, 47.08442372801901854 ) ) ;
#196408=CARTESIAN_POINT ( 'NONE',  ( 15.72974639402176855, 15.80617190586768217, 96.87609039468568994 ) ) ;
#196409=CARTESIAN_POINT ( 'NONE',  ( 4.379528057220092307, 16.55341960407617563, 97.29275706135234714 ) ) ;
#196410=CARTESIAN_POINT ( 'NONE',  ( -9.564922557960796823, -16.46253265017161027, 82.08224293864768129 ) ) ;
#196411=CARTESIAN_POINT ( 'NONE',  ( -10.81492255796105439, 18.62759615963255655, 47.91775706135234714 ) ) ;
#196412=CARTESIAN_POINT ( 'NONE',  ( -21.52544592524334988, -5.823673210054445271, 48.95942372801902565 ) ) ;
#196413=CARTESIAN_POINT ( 'NONE',  ( -9.474510206698720793, -16.51473224551083518, 84.58442372801900433 ) ) ;
#196414=CARTESIAN_POINT ( 'NONE',  ( 16.46253265017160672, -9.564922557960803928, 88.33224293864769550 ) ) ;
#196415=CARTESIAN_POINT ( 'NONE',  ( 14.29746914071049879, -8.314922557960816363, 98.33224293864769550 ) ) ;
#196416=CARTESIAN_POINT ( 'NONE',  ( 15.72974639402199770, -15.80617190586745480, 103.1239096053143811 ) ) ;
#196417=CARTESIAN_POINT ( 'NONE',  ( 9.564922557961047289, -16.46253265017146816, 20.41775706135233293 ) ) ;
#196418=CARTESIAN_POINT ( 'NONE',  ( 16.53943276465976808, -0.05219959533910856209, 93.74890960531436690 ) ) ;
#196419=CARTESIAN_POINT ( 'NONE',  ( -16.46253265017160317, 9.564922557960807481, 45.83224293864769550 ) ) ;
#196420=CARTESIAN_POINT ( 'NONE',  ( 5.049401038297881783, 19.05341960407617563, 87.29275706135234714 ) ) ;
#196421=CARTESIAN_POINT ( 'NONE',  ( 4.379528057220339221, -16.55341960407611168, 52.70724293864769550 ) ) ;
#196422=CARTESIAN_POINT ( 'NONE',  ( -10.72451020669870658, -18.67979575497194134, 104.5844237280190185 ) ) ;
#196423=CARTESIAN_POINT ( 'NONE',  ( -5.153800228976328057, -19.02544592524343514, 107.2905762719810383 ) ) ;
#196424=CARTESIAN_POINT ( 'NONE',  ( 13.97604488694548053, -13.89961937509957401, 75.62609039468564731 ) ) ;
#196425=CARTESIAN_POINT ( 'NONE',  ( 15.72974639402199770, -15.80617190586745480, 78.12390960531436690 ) ) ;
#196426=CARTESIAN_POINT ( 'NONE',  ( 10.72451020669871369, 18.67979575497193778, 37.08442372801901143 ) ) ;
#196427=CARTESIAN_POINT ( 'NONE',  ( -8.224510206698735004, -14.34966873604973081, 29.58442372801901854 ) ) ;
#196428=CARTESIAN_POINT ( 'NONE',  ( -16.53943276465976808, -0.05219959533934237506, 88.75109039468567573 ) ) ;
#196429=CARTESIAN_POINT ( 'NONE',  ( 13.97604488694527802, 13.89961937509977652, 24.37390960531435624 ) ) ;
#196430=CARTESIAN_POINT ( 'NONE',  ( 10.72451020669871369, 18.67979575497193778, 42.08442372801901854 ) ) ;
#196431=CARTESIAN_POINT ( 'NONE',  ( 5.823673210054125526, 21.52544592524343514, 39.79057627198103830 ) ) ;
#196432=CARTESIAN_POINT ( 'NONE',  ( -13.89961937509977652, 13.97604488694528158, 25.62390960531434558 ) ) ;
#196434=CARTESIAN_POINT ( 'NONE',  ( -12.06949235617739369, -12.14591786802326823, 64.37609039468568994 ) ) ;
#196435=CARTESIAN_POINT ( 'NONE',  ( -0.05219959533910754901, -16.53943276465976808, 87.49890960531436690 ) ) ;
#196436=CARTESIAN_POINT ( 'NONE',  ( 10.81492255796078972, 18.62759615963270932, 79.58224293864769550 ) ) ;
#196437=CARTESIAN_POINT ( 'NONE',  ( 14.29746914071049879, -8.314922557960816363, 23.33224293864769194 ) ) ;
#196438=CARTESIAN_POINT ( 'NONE',  ( -14.29746914071037622, -8.314922557961029526, 44.16775706135234714 ) ) ;
#196439=CARTESIAN_POINT ( 'NONE',  ( 13.97604488694527802, 13.89961937509977652, 64.37390960531436690 ) ) ;
#196440=CARTESIAN_POINT ( 'NONE',  ( 14.29746914071037800, 8.314922557961029526, 86.66775706135234714 ) ) ;
#196441=CARTESIAN_POINT ( 'NONE',  ( -5.153800228976607833, 19.02544592524334988, 82.70942372801897591 ) ) ;
#196442=CARTESIAN_POINT ( 'NONE',  ( 15.72974639402199770, -15.80617190586745480, 83.12390960531436690 ) ) ;
#196443=CARTESIAN_POINT ( 'NONE',  ( -16.53943276465976808, 0.05219959533911058130, 21.24890960531436690 ) ) ;
#196445=CARTESIAN_POINT ( 'NONE',  ( 16.51473224551069308, 9.474510206698969483, 114.1655762719810241 ) ) ;
#196447=CARTESIAN_POINT ( 'NONE',  ( 21.52544592524344225, -5.823673210054117533, 58.54057627198103120 ) ) ;
#196448=CARTESIAN_POINT ( 'NONE',  ( 8.314922557961029526, -14.29746914071037800, 90.41775706135236135 ) ) ;
#196449=VERTEX_POINT ( 'NONE', #178322 ) ;
#196450=CARTESIAN_POINT ( 'NONE',  ( -10.72451020669898014, 18.67979575497178502, 30.41557627198101699 ) ) ;
#196451=CARTESIAN_POINT ( 'NONE',  ( 17.49999999999999645, 4.013004640162574077, 107.0539427900559417 ) ) ;
#196452=CARTESIAN_POINT ( 'NONE',  ( -10.81492255796078084, -18.62759615963271287, 87.08224293864769550 ) ) ;
#196453=CARTESIAN_POINT ( 'NONE',  ( 16.55341960407611168, 4.379528057220329451, 28.95724293864769905 ) ) ;
#196454=CARTESIAN_POINT ( 'NONE',  ( 19.03943276465977164, 0.05219959533936151252, 111.2510903946856757 ) ) ;
#196455=CARTESIAN_POINT ( 'NONE',  ( 19.02544592524343514, -5.153800228976328945, 33.54057627198102409 ) ) ;
#196456=CARTESIAN_POINT ( 'NONE',  ( -8.314922557961024197, 14.29746914071037800, 27.91775706135234358 ) ) ;
#196457=CARTESIAN_POINT ( 'NONE',  ( 5.049401038298161559, -19.05341960407611168, 47.70724293864770260 ) ) ;
#196459=CARTESIAN_POINT ( 'NONE',  ( 5.153800228976335163, 19.02544592524342804, 104.7905762719809957 ) ) ;
#196460=CARTESIAN_POINT ( 'NONE',  ( 16.51473224551069308, 9.474510206698969483, 109.1655762719810383 ) ) ;
#196461=CARTESIAN_POINT ( 'NONE',  ( -8.314922557961024197, 14.29746914071037800, 92.91775706135236135 ) ) ;
#196462=CARTESIAN_POINT ( 'NONE',  ( 16.46253265017146816, 9.564922557961045513, 91.66775706135234714 ) ) ;
#196463=CARTESIAN_POINT ( 'NONE',  ( 9.474510206698729675, 16.51473224551082808, 42.08442372801900433 ) ) ;
#196464=CARTESIAN_POINT ( 'NONE',  ( 21.52544592524344225, -5.823673210054117533, 73.54057627198102409 ) ) ;
#196465=CARTESIAN_POINT ( 'NONE',  ( -12.06949235617739369, -12.14591786802326823, 99.37609039468568994 ) ) ;
#196466=CARTESIAN_POINT ( 'NONE',  ( 18.62759615963271287, -10.81492255796078972, 28.33224293864769550 ) ) ;
#196467=CARTESIAN_POINT ( 'NONE',  ( -9.564922557961040184, 16.46253265017147172, 87.91775706135233293 ) ) ;
#196468=CARTESIAN_POINT ( 'NONE',  ( 13.89961937509977652, -13.97604488694527269, 48.12390960531435979 ) ) ;
#196469=CARTESIAN_POINT ( 'NONE',  ( -0.05219959533909027116, -19.03943276465977164, 107.4989096053143527 ) ) ;
#196470=CARTESIAN_POINT ( 'NONE',  ( -21.55341960407619339, 5.719274019375674811, 58.54275706135235424 ) ) ;
#196471=CARTESIAN_POINT ( 'NONE',  ( 16.46253265017160672, -9.564922557960803928, 63.33224293864769550 ) ) ;
#196472=CARTESIAN_POINT ( 'NONE',  ( -8.314922557960811034, -14.29746914071050412, 102.0822429386476955 ) ) ;
#196473=CARTESIAN_POINT ( 'NONE',  ( 12.14591786802309770, 12.06949235617756955, 74.37390960531436690 ) ) ;
#196474=CARTESIAN_POINT ( 'NONE',  ( 15.80617190586746368, 15.72974639402197994, 74.37390960531436690 ) ) ;
#196476=CARTESIAN_POINT ( 'NONE',  ( -0.05219959533936034679, 19.03943276465977164, 97.50109039468567573 ) ) ;
#196477=CARTESIAN_POINT ( 'NONE',  ( 17.31747979337951193, -6.344076630960994834, 81.12055131934819485 ) ) ;
#196478=CARTESIAN_POINT ( 'NONE',  ( -5.153800228976328057, -19.02544592524343514, 57.29057627198103120 ) ) ;
#196480=CARTESIAN_POINT ( 'NONE',  ( 5.153800228976335163, 19.02544592524342804, 74.79057627198103830 ) ) ;
#196481=CARTESIAN_POINT ( 'NONE',  ( 9.474510206698971260, -16.51473224551069308, 92.91557627198103830 ) ) ;
#196482=CARTESIAN_POINT ( 'NONE',  ( 14.34966873604972726, -8.224510206698740333, 60.83442372801901854 ) ) ;
#196483=CARTESIAN_POINT ( 'NONE',  ( -17.49999999999999645, -5.624438216177605199, 49.18329655085356933 ) ) ;
#196484=CARTESIAN_POINT ( 'NONE',  ( -19.02544592524334988, -5.153800228976617603, 38.95942372801900433 ) ) ;
#196485=CARTESIAN_POINT ( 'NONE',  ( 17.16083808118622400, 6.592936235069069895, 21.72768779978462206 ) ) ;
#196486=CARTESIAN_POINT ( 'NONE',  ( -9.474510206698964154, 16.51473224551069663, 115.4155762719810241 ) ) ;
#196487=CARTESIAN_POINT ( 'NONE',  ( 4.483927247898790824, -16.52544592524335698, 100.2094237280190043 ) ) ;
#196488=CARTESIAN_POINT ( 'NONE',  ( 17.59860650958994555, -7.585241751806880650, 75.92337014262494677 ) ) ;
#196489=CARTESIAN_POINT ( 'NONE',  ( -14.29746914071037622, -8.314922557961029526, 94.16775706135237556 ) ) ;
#196491=CARTESIAN_POINT ( 'NONE',  ( -16.53943276465976808, -0.05219959533934237506, 68.75109039468568994 ) ) ;
#196492=CARTESIAN_POINT ( 'NONE',  ( -17.49999999999998579, -5.500000000000015099, 41.28230962303565832 ) ) ;
#196493=CARTESIAN_POINT ( 'NONE',  ( 18.67979575497194134, -10.72451020669871369, 70.83442372801901854 ) ) ;
#196494=CARTESIAN_POINT ( 'NONE',  ( 19.02544592524334988, 5.153800228976608722, 71.45942372801900433 ) ) ;
#196495=CARTESIAN_POINT ( 'NONE',  ( -16.51473224551082808, 9.474510206698731452, 28.33442372801900433 ) ) ;
#196496=CARTESIAN_POINT ( 'NONE',  ( -9.564922557960796823, -16.46253265017161027, 62.08224293864769550 ) ) ;
#196497=CARTESIAN_POINT ( 'NONE',  ( -5.049401038298153566, 19.05341960407611168, 45.20724293864769550 ) ) ;
#196498=CARTESIAN_POINT ( 'NONE',  ( 17.49999999999999645, -5.632147345228470492, 23.31793006472933882 ) ) ;
#196499=CARTESIAN_POINT ( 'NONE',  ( 18.62759615963271287, -10.81492255796078972, 78.33224293864770971 ) ) ;
#196500=CARTESIAN_POINT ( 'NONE',  ( 21.53943276465977519, -0.05219959533907433946, 28.74890960531435624 ) ) ;
#196501=CARTESIAN_POINT ( 'NONE',  ( 19.03943276465977164, -0.05219959533909143690, 28.74890960531435624 ) ) ;
#196502=CARTESIAN_POINT ( 'NONE',  ( 8.224510206698742110, 14.34966873604972548, 57.08442372801901854 ) ) ;
#196504=CARTESIAN_POINT ( 'NONE',  ( -10.72451020669870658, -18.67979575497194134, 34.58442372801900433 ) ) ;
#196505=CARTESIAN_POINT ( 'NONE',  ( -4.379528057220328563, 16.55341960407611168, 50.20724293864769550 ) ) ;
#196507=CARTESIAN_POINT ( 'NONE',  ( 16.55341960407618274, -4.379528057220086978, 31.04275706135234714 ) ) ;
#196508=CARTESIAN_POINT ( 'NONE',  ( -9.474510206698720793, -16.51473224551083518, 39.58442372801899722 ) ) ;
#196509=CARTESIAN_POINT ( 'NONE',  ( 12.14591786802309770, 12.06949235617756955, 44.37390960531435979 ) ) ;
#196510=CARTESIAN_POINT ( 'NONE',  ( -15.72974639402197994, 15.80617190586746368, 110.6239096053143669 ) ) ;
#196512=CARTESIAN_POINT ( 'NONE',  ( -21.52544592524343514, 5.823673210054127303, 76.04057627198102409 ) ) ;
#196513=CARTESIAN_POINT ( 'NONE',  ( -5.153800228976328057, -19.02544592524343514, 87.29057627198103830 ) ) ;
#196514=CARTESIAN_POINT ( 'NONE',  ( 8.314922557960818139, 14.29746914071049879, 64.58224293864769550 ) ) ;
#196515=CARTESIAN_POINT ( 'NONE',  ( 13.97604488694527802, 13.89961937509977652, 99.37390960531436690 ) ) ;
#196517=CARTESIAN_POINT ( 'NONE',  ( -19.03943276465977164, -0.05219959533935918106, 68.75109039468566152 ) ) ;
#196518=CARTESIAN_POINT ( 'NONE',  ( -21.53943276465977519, 0.05219959533907696930, 111.2489096053143669 ) ) ;
#196519=CARTESIAN_POINT ( 'NONE',  ( -19.05341960407611168, -5.049401038298163336, 56.45724293864768129 ) ) ;
#196520=CARTESIAN_POINT ( 'NONE',  ( -0.05219959533936034679, 19.03943276465977164, 47.50109039468566863 ) ) ;
#196521=CARTESIAN_POINT ( 'NONE',  ( -8.314922557960811034, -14.29746914071050412, 107.0822429386476955 ) ) ;
#196522=CARTESIAN_POINT ( 'NONE',  ( -18.67979575497193778, 10.72451020669871902, 58.33442372801901143 ) ) ;
#196523=CARTESIAN_POINT ( 'NONE',  ( -18.87580814761076908, 5.499999999999960032, 100.8717239426576242 ) ) ;
#196524=CARTESIAN_POINT ( 'NONE',  ( -16.52544592524342804, 4.483927247898546575, 41.04057627198103120 ) ) ;
#196525=CARTESIAN_POINT ( 'NONE',  ( 9.564922557960805705, 16.46253265017160317, 49.58224293864770260 ) ) ;
#196526=CARTESIAN_POINT ( 'NONE',  ( 19.05341960407611168, 5.049401038298154454, 113.9572429386477097 ) ) ;
#196527=CARTESIAN_POINT ( 'NONE',  ( -10.72451020669898014, 18.67979575497178502, 70.41557627198102409 ) ) ;
#196529=CARTESIAN_POINT ( 'NONE',  ( 19.02544592524343514, -5.153800228976328945, 43.54057627198103120 ) ) ;
#196530=ORIENTED_EDGE ( 'NONE', *, *, #161905, .T. ) ;
#196531=CARTESIAN_POINT ( 'NONE',  ( 0.05219959533907565091, 21.53943276465977519, 59.99890960531436690 ) ) ;
#196532=CARTESIAN_POINT ( 'NONE',  ( -0.05219959533937732626, 21.53943276465977519, 92.50109039468567573 ) ) ;
#196533=CARTESIAN_POINT ( 'NONE',  ( 17.50000000000000000, -5.500000000000000888, 108.2969038253417153 ) ) ;
#196534=CARTESIAN_POINT ( 'NONE',  ( 12.14591786802327356, -12.06949235617739191, 85.62609039468568994 ) ) ;
#196535=CARTESIAN_POINT ( 'NONE',  ( 12.14591786802309770, 12.06949235617756955, 79.37390960531436690 ) ) ;
#196536=CARTESIAN_POINT ( 'NONE',  ( -13.89961937509977652, 13.97604488694528158, 70.62390960531432427 ) ) ;
#196538=CARTESIAN_POINT ( 'NONE',  ( 16.46253265017146816, 9.564922557961045513, 41.66775706135234003 ) ) ;
#196539=CARTESIAN_POINT ( 'NONE',  ( -4.483927247898782831, 16.52544592524335698, 87.70942372801901854 ) ) ;
#196540=CARTESIAN_POINT ( 'NONE',  ( 9.564922557961047289, -16.46253265017146816, 20.41775706135233293 ) ) ;
#196541=CARTESIAN_POINT ( 'NONE',  ( -0.05219959533909027116, -19.03943276465977164, 82.49890960531436690 ) ) ;
#196542=CARTESIAN_POINT ( 'NONE',  ( 18.62759615963271287, -10.81492255796078972, 43.33224293864769550 ) ) ;
#196543=CARTESIAN_POINT ( 'NONE',  ( -15.72974639402176322, -15.80617190586768395, 94.37609039468568994 ) ) ;
#196544=CARTESIAN_POINT ( 'NONE',  ( 14.34966873604972726, -8.224510206698740333, 60.83442372801901854 ) ) ;
#196545=CARTESIAN_POINT ( 'NONE',  ( -18.67979575497178146, -10.72451020669898902, 106.6655762719810383 ) ) ;
#196546=CARTESIAN_POINT ( 'NONE',  ( 14.34966873604972726, -8.224510206698740333, 30.83442372801902209 ) ) ;
#196547=CARTESIAN_POINT ( 'NONE',  ( 19.02544592524343514, -5.153800228976328945, 88.54057627198102409 ) ) ;
#196548=CARTESIAN_POINT ( 'NONE',  ( -16.51473224551069308, -9.474510206698971260, 41.66557627198103120 ) ) ;
#196549=CARTESIAN_POINT ( 'NONE',  ( 16.51473224551069308, 9.474510206698969483, 54.16557627198103120 ) ) ;
#196550=CARTESIAN_POINT ( 'NONE',  ( -12.14591786802326823, 12.06949235617739902, 28.12609039468568284 ) ) ;
#196551=CARTESIAN_POINT ( 'NONE',  ( -16.55341960407611168, -4.379528057220339221, 81.45724293864769550 ) ) ;
#196552=CARTESIAN_POINT ( 'NONE',  ( -0.05219959533934338120, 16.53943276465976808, 92.50109039468567573 ) ) ;
#196553=CARTESIAN_POINT ( 'NONE',  ( 21.52544592524334988, 5.823673210054432836, 41.45942372801901143 ) ) ;
#196554=CARTESIAN_POINT ( 'NONE',  ( 19.05341960407611168, 5.049401038298154454, 68.95724293864769550 ) ) ;
#196555=CARTESIAN_POINT ( 'NONE',  ( 0.05219959533909260263, 19.03943276465977164, 79.99890960531436690 ) ) ;
#196556=CARTESIAN_POINT ( 'NONE',  ( -16.53943276465976808, 0.05219959533911058130, 36.24890960531435979 ) ) ;
#196557=CARTESIAN_POINT ( 'NONE',  ( 8.224510206698742110, 14.34966873604972548, 87.08442372801901854 ) ) ;
#196559=CARTESIAN_POINT ( 'NONE',  ( -19.02544592524334988, -5.153800228976617603, 33.95942372801897591 ) ) ;
#196560=CARTESIAN_POINT ( 'NONE',  ( 5.153800228976335163, 19.02544592524342804, 94.79057627198103830 ) ) ;
#196561=CARTESIAN_POINT ( 'NONE',  ( 19.02544592524343514, -5.153800228976328945, 43.54057627198103120 ) ) ;
#196563=CARTESIAN_POINT ( 'NONE',  ( -14.29746914071037622, -8.314922557961029526, 49.16775706135234003 ) ) ;
#196564=CARTESIAN_POINT ( 'NONE',  ( 5.153800228976615827, -19.02544592524334988, 75.20942372801896170 ) ) ;
#196565=CARTESIAN_POINT ( 'NONE',  ( -0.05219959533934338120, 16.53943276465976808, 62.50109039468568284 ) ) ;
#196567=CARTESIAN_POINT ( 'NONE',  ( -5.153800228976328057, -19.02544592524343514, 72.29057627198102409 ) ) ;
#196568=CARTESIAN_POINT ( 'NONE',  ( 5.823673210054125526, 21.52544592524343514, 114.7905762719810383 ) ) ;
#196569=CARTESIAN_POINT ( 'NONE',  ( 5.049401038297881783, 19.05341960407617563, 62.29275706135234003 ) ) ;
#196570=CARTESIAN_POINT ( 'NONE',  ( -9.474510206698964154, 16.51473224551069663, 105.4155762719810383 ) ) ;
#196571=CARTESIAN_POINT ( 'NONE',  ( 16.51473224551069308, 9.474510206698969483, 34.16557627198102409 ) ) ;
#196572=EDGE_CURVE ( 'NONE', #135096, #155722, #39785, .T. ) ;
#196573=CARTESIAN_POINT ( 'NONE',  ( 16.51473224551069308, 9.474510206698969483, 79.16557627198103830 ) ) ;
#196574=CARTESIAN_POINT ( 'NONE',  ( -16.55341960407611168, -4.379528057220339221, 36.45724293864768839 ) ) ;
#196575=CARTESIAN_POINT ( 'NONE',  ( -19.03943276465977164, 0.05219959533909376836, 21.24890960531436335 ) ) ;
#196576=CARTESIAN_POINT ( 'NONE',  ( -19.02544592524334988, -5.153800228976617603, 33.95942372801897591 ) ) ;
#196577=CARTESIAN_POINT ( 'NONE',  ( -16.53943276465976808, 0.05219959533911058130, 71.24890960531435269 ) ) ;
#196578=CARTESIAN_POINT ( 'NONE',  ( 21.55341960407619695, -5.719274019375665929, 111.0427570613523613 ) ) ;
#196579=CARTESIAN_POINT ( 'NONE',  ( 13.89961937509977652, -13.97604488694527269, 58.12390960531436690 ) ) ;
#196580=CARTESIAN_POINT ( 'NONE',  ( -16.55341960407611168, -4.379528057220339221, 46.45724293864769550 ) ) ;
#196581=CARTESIAN_POINT ( 'NONE',  ( 18.62759615963255655, 10.81492255796105972, 106.6677570613523756 ) ) ;
#196582=CARTESIAN_POINT ( 'NONE',  ( 19.05341960407611168, 5.049401038298154454, 88.95724293864769550 ) ) ;
#196583=CARTESIAN_POINT ( 'NONE',  ( -16.51473224551069308, -9.474510206698971260, 111.6655762719810383 ) ) ;
#196584=CARTESIAN_POINT ( 'NONE',  ( 9.564922557960805705, 16.46253265017160317, 39.58224293864768839 ) ) ;
#196585=CARTESIAN_POINT ( 'NONE',  ( -16.52544592524342804, 4.483927247898546575, 111.0405762719810525 ) ) ;
#196586=CARTESIAN_POINT ( 'NONE',  ( -8.314922557960811034, -14.29746914071050412, 92.08224293864769550 ) ) ;
#196587=CARTESIAN_POINT ( 'NONE',  ( 18.62759615963271287, -10.81492255796078972, 93.33224293864769550 ) ) ;
#196588=CARTESIAN_POINT ( 'NONE',  ( 16.46253265017160672, -9.564922557960803928, 93.33224293864769550 ) ) ;
#196589=CARTESIAN_POINT ( 'NONE',  ( -0.05219959533907301413, -21.53943276465977519, 97.49890960531436690 ) ) ;
#196590=CARTESIAN_POINT ( 'NONE',  ( -19.02544592524342804, 5.153800228976336051, 91.04057627198100988 ) ) ;
#196592=CARTESIAN_POINT ( 'NONE',  ( -8.224510206698948167, 14.34966873604960824, 100.4155762719810241 ) ) ;
#196593=CARTESIAN_POINT ( 'NONE',  ( -9.474510206698964154, 16.51473224551069663, 75.41557627198103830 ) ) ;
#196594=CARTESIAN_POINT ( 'NONE',  ( -10.72451020669898014, 18.67979575497178502, 80.41557627198103830 ) ) ;
#196596=CARTESIAN_POINT ( 'NONE',  ( -0.05219959533907301413, -21.53943276465977519, 22.49890960531436335 ) ) ;
#196597=CARTESIAN_POINT ( 'NONE',  ( 22.00000000000000000, -1.163414459189985801E-14, 95.00000000000000000 ) ) ;
#196598=CARTESIAN_POINT ( 'NONE',  ( -8.314922557961024197, 14.29746914071037800, 27.91775706135234358 ) ) ;
#196599=CARTESIAN_POINT ( 'NONE',  ( -16.52544592524342804, 4.483927247898546575, 96.04057627198102409 ) ) ;
#196601=CARTESIAN_POINT ( 'NONE',  ( 16.46253265017160672, -9.564922557960803928, 88.33224293864769550 ) ) ;
#196602=CARTESIAN_POINT ( 'NONE',  ( 16.46253265017160672, -9.564922557960803928, 48.33224293864769550 ) ) ;
#196603=CARTESIAN_POINT ( 'NONE',  ( -16.55341960407611168, -4.379528057220339221, 86.45724293864770971 ) ) ;
#196604=CARTESIAN_POINT ( 'NONE',  ( 15.80617190586746368, 15.72974639402197994, 24.37390960531435979 ) ) ;
#196605=CARTESIAN_POINT ( 'NONE',  ( 14.34966873604960469, 8.224510206698951720, 54.16557627198103120 ) ) ;
#196606=CARTESIAN_POINT ( 'NONE',  ( 5.049401038297881783, 19.05341960407617563, 107.2927570613523187 ) ) ;
#196607=CARTESIAN_POINT ( 'NONE',  ( 21.52544592524334988, 5.823673210054432836, 56.45942372801902565 ) ) ;
#196609=CARTESIAN_POINT ( 'NONE',  ( 9.474510206698971260, -16.51473224551069308, 97.91557627198102409 ) ) ;
#196610=CARTESIAN_POINT ( 'NONE',  ( -0.05219959533934338120, 16.53943276465976808, 87.50109039468568994 ) ) ;
#196612=CARTESIAN_POINT ( 'NONE',  ( -16.51473224551069308, -9.474510206698971260, 31.66557627198102054 ) ) ;
#196613=CARTESIAN_POINT ( 'NONE',  ( 5.049401038298161559, -19.05341960407611168, 77.70724293864765286 ) ) ;
#196614=CARTESIAN_POINT ( 'NONE',  ( -5.823673210054116645, -21.52544592524344225, 82.29057627198103830 ) ) ;
#196615=CARTESIAN_POINT ( 'NONE',  ( -16.51473224551082808, 9.474510206698731452, 113.3344237280190043 ) ) ;
#196616=CARTESIAN_POINT ( 'NONE',  ( 16.55341960407611168, 4.379528057220329451, 48.95724293864770971 ) ) ;
#196617=CARTESIAN_POINT ( 'NONE',  ( 18.62759615963255655, 10.81492255796105972, 56.66775706135235424 ) ) ;
#196618=CARTESIAN_POINT ( 'NONE',  ( 14.34966873604972726, -8.224510206698740333, 90.83442372801901854 ) ) ;
#196619=CARTESIAN_POINT ( 'NONE',  ( 15.80617190586746368, 15.72974639402197994, 24.37390960531435979 ) ) ;
#196620=CARTESIAN_POINT ( 'NONE',  ( -5.153800228976328057, -19.02544592524343514, 112.2905762719810241 ) ) ;
#196622=CARTESIAN_POINT ( 'NONE',  ( 16.52544592524335698, 4.483927247898782831, 111.4594237280190328 ) ) ;
#196623=CARTESIAN_POINT ( 'NONE',  ( -16.53943276465976808, -0.05219959533934237506, 63.75109039468568284 ) ) ;
#196624=CARTESIAN_POINT ( 'NONE',  ( -16.51473224551069308, -9.474510206698971260, 71.66557627198102409 ) ) ;
#196626=CARTESIAN_POINT ( 'NONE',  ( 13.97604488694527802, 13.89961937509977652, 74.37390960531436690 ) ) ;
#196627=CARTESIAN_POINT ( 'NONE',  ( -10.72451020669870658, -18.67979575497194134, 74.58442372801901854 ) ) ;
#196628=CARTESIAN_POINT ( 'NONE',  ( -12.14591786802326823, 12.06949235617739902, 73.12609039468567573 ) ) ;
#196629=CARTESIAN_POINT ( 'NONE',  ( 14.34966873604960469, 8.224510206698951720, 44.16557627198103120 ) ) ;
#196630=CARTESIAN_POINT ( 'NONE',  ( 9.564922557960805705, 16.46253265017160317, 54.58224293864769550 ) ) ;
#196631=CARTESIAN_POINT ( 'NONE',  ( 5.153800228976335163, 19.02544592524342804, 49.79057627198100988 ) ) ;
#196632=CARTESIAN_POINT ( 'NONE',  ( 8.314922557961029526, -14.29746914071037800, 40.41775706135234714 ) ) ;
#196634=CARTESIAN_POINT ( 'NONE',  ( -9.474510206698720793, -16.51473224551083518, 99.58442372801900433 ) ) ;
#196635=CARTESIAN_POINT ( 'NONE',  ( -0.05219959533910754901, -16.53943276465976808, 97.49890960531436690 ) ) ;
#196636=CARTESIAN_POINT ( 'NONE',  ( -16.51473224551069308, -9.474510206698971260, 71.66557627198102409 ) ) ;
#196637=CARTESIAN_POINT ( 'NONE',  ( 16.46253265017146816, 9.564922557961045513, 106.6677570613523471 ) ) ;
#196639=CARTESIAN_POINT ( 'NONE',  ( -10.81492255796105439, 18.62759615963255655, 102.9177570613523756 ) ) ;
#196640=CARTESIAN_POINT ( 'NONE',  ( -4.483927247898782831, 16.52544592524335698, 72.70942372801901854 ) ) ;
#196642=CARTESIAN_POINT ( 'NONE',  ( 21.55341960407610458, 5.719274019375980345, 68.95724293864769550 ) ) ;
#196643=CARTESIAN_POINT ( 'NONE',  ( 16.53943276465976808, 0.05219959533934440121, 56.25109039468568284 ) ) ;
#196644=CARTESIAN_POINT ( 'NONE',  ( 16.46253265017146816, 9.564922557961045513, 46.66775706135233293 ) ) ;
#196645=CARTESIAN_POINT ( 'NONE',  ( 19.05341960407611168, 5.049401038298154454, 88.95724293864769550 ) ) ;
#196646=CARTESIAN_POINT ( 'NONE',  ( -16.52544592524342804, 4.483927247898546575, 116.0405762719810383 ) ) ;
#196647=CARTESIAN_POINT ( 'NONE',  ( -9.564922557960796823, -16.46253265017161027, 67.08224293864769550 ) ) ;
#196648=CARTESIAN_POINT ( 'NONE',  ( 12.06949235617757843, -12.14591786802309237, 63.12390960531435979 ) ) ;
#196649=CARTESIAN_POINT ( 'NONE',  ( 15.72974639402176855, 15.80617190586768217, 71.87609039468568994 ) ) ;
#196651=CARTESIAN_POINT ( 'NONE',  ( -9.474510206698720793, -16.51473224551083518, 49.58442372801899722 ) ) ;
#196652=CARTESIAN_POINT ( 'NONE',  ( 5.049401038297881783, 19.05341960407617563, 27.29275706135232937 ) ) ;
#196653=CARTESIAN_POINT ( 'NONE',  ( -9.474510206698964154, 16.51473224551069663, 50.41557627198102409 ) ) ;
#196654=CARTESIAN_POINT ( 'NONE',  ( -0.05219959533907301413, -21.53943276465977519, 27.49890960531435269 ) ) ;
#196655=CARTESIAN_POINT ( 'NONE',  ( 21.52544592524334988, 5.823673210054432836, 86.45942372801901854 ) ) ;
#196656=CARTESIAN_POINT ( 'NONE',  ( -0.05219959533909027116, -19.03943276465977164, 67.49890960531436690 ) ) ;
#196657=CARTESIAN_POINT ( 'NONE',  ( 10.72451020669871369, 18.67979575497193778, 92.08442372801901854 ) ) ;
#196658=CARTESIAN_POINT ( 'NONE',  ( -21.55341960407610458, -5.719274019375992779, 41.45724293864769550 ) ) ;
#196659=CARTESIAN_POINT ( 'NONE',  ( 16.46253265017160672, -9.564922557960803928, 78.33224293864769550 ) ) ;
#196660=CARTESIAN_POINT ( 'NONE',  ( -5.823673210054431948, 21.52544592524334988, 32.70942372801900433 ) ) ;
#196661=CARTESIAN_POINT ( 'NONE',  ( 5.153800228976615827, -19.02544592524334988, 60.20942372801899012 ) ) ;
#196662=CARTESIAN_POINT ( 'NONE',  ( 19.02544592524343514, -5.153800228976328945, 48.54057627198103120 ) ) ;
#196663=CARTESIAN_POINT ( 'NONE',  ( 13.89961937509977652, -13.97604488694527269, 88.12390960531438111 ) ) ;
#196664=CARTESIAN_POINT ( 'NONE',  ( -14.34966873604972548, 8.224510206698743886, 28.33442372801902209 ) ) ;
#196665=CARTESIAN_POINT ( 'NONE',  ( -14.29746914071049879, 8.314922557960819915, 90.83224293864769550 ) ) ;
#196666=CARTESIAN_POINT ( 'NONE',  ( 16.51473224551069308, 9.474510206698969483, 69.16557627198102409 ) ) ;
#196667=EDGE_CURVE ( 'NONE', #123381, #199940, #76354, .T. ) ;
#196668=CARTESIAN_POINT ( 'NONE',  ( -21.55341960407610458, -5.719274019375992779, 56.45724293864768839 ) ) ;
#196669=CARTESIAN_POINT ( 'NONE',  ( 16.55341960407618274, -4.379528057220086978, 26.04275706135235779 ) ) ;
#196670=CARTESIAN_POINT ( 'NONE',  ( 10.72451020669898902, -18.67979575497178502, 112.9155762719810383 ) ) ;
#196671=CARTESIAN_POINT ( 'NONE',  ( 21.53943276465977519, 0.05219959533937863772, 71.25109039468568994 ) ) ;
#196672=CARTESIAN_POINT ( 'NONE',  ( -16.53943276465976808, -0.05219959533934237506, 73.75109039468567573 ) ) ;
#196673=CARTESIAN_POINT ( 'NONE',  ( -14.34966873604972548, 8.224510206698743886, 68.33442372801900433 ) ) ;
#196674=CARTESIAN_POINT ( 'NONE',  ( -19.05341960407611168, -5.049401038298163336, 61.45724293864769550 ) ) ;
#196675=CARTESIAN_POINT ( 'NONE',  ( 12.06949235617739724, 12.14591786802326823, 106.8760903946856899 ) ) ;
#196676=CARTESIAN_POINT ( 'NONE',  ( -0.05219959533936034679, 19.03943276465977164, 37.50109039468567573 ) ) ;
#196677=CARTESIAN_POINT ( 'NONE',  ( -0.05219959533937732626, 21.53943276465977519, 37.50109039468568284 ) ) ;
#196678=CARTESIAN_POINT ( 'NONE',  ( -14.34966873604960291, -8.224510206698953496, 61.66557627198103120 ) ) ;
#196679=CARTESIAN_POINT ( 'NONE',  ( -16.46253265017160317, 9.564922557960807481, 95.83224293864769550 ) ) ;
#196680=CARTESIAN_POINT ( 'NONE',  ( -12.14591786802326823, 12.06949235617739902, 88.12609039468570415 ) ) ;
#196681=CARTESIAN_POINT ( 'NONE',  ( -21.53943276465977519, -0.05219959533937600094, 58.75109039468568994 ) ) ;
#196682=CARTESIAN_POINT ( 'NONE',  ( 16.53943276465976808, 0.05219959533934440121, 26.25109039468567573 ) ) ;
#196683=CARTESIAN_POINT ( 'NONE',  ( 21.55341960407619695, -5.719274019375665929, 31.04275706135234714 ) ) ;
#196684=CARTESIAN_POINT ( 'NONE',  ( 4.379528057220339221, -16.55341960407611168, 62.70724293864769550 ) ) ;
#196686=CARTESIAN_POINT ( 'NONE',  ( -10.81492255796078084, -18.62759615963271287, 102.0822429386476955 ) ) ;
#196687=CARTESIAN_POINT ( 'NONE',  ( -14.34966873604960291, -8.224510206698953496, 36.66557627198103120 ) ) ;
#196689=CARTESIAN_POINT ( 'NONE',  ( -16.46253265017160317, 9.564922557960807481, 30.83224293864769550 ) ) ;
#196690=CARTESIAN_POINT ( 'NONE',  ( -10.81492255796078084, -18.62759615963271287, 32.08224293864769550 ) ) ;
#196691=CARTESIAN_POINT ( 'NONE',  ( -5.823673210054431948, 21.52544592524334988, 32.70942372801900433 ) ) ;
#196692=CARTESIAN_POINT ( 'NONE',  ( 12.06949235617757843, -12.14591786802309237, 68.12390960531436690 ) ) ;
#196693=CARTESIAN_POINT ( 'NONE',  ( -15.72974639402197994, 15.80617190586746368, 60.62390960531437401 ) ) ;
#196694=CARTESIAN_POINT ( 'NONE',  ( 16.51473224551069308, 9.474510206698969483, 69.16557627198102409 ) ) ;
#196695=CARTESIAN_POINT ( 'NONE',  ( 19.05341960407617918, -5.049401038297876454, 76.04275706135230450 ) ) ;
#196696=CARTESIAN_POINT ( 'NONE',  ( 15.72974639402199770, -15.80617190586745480, 53.12390960531436690 ) ) ;
#196697=CARTESIAN_POINT ( 'NONE',  ( 16.51473224551069308, 9.474510206698969483, 39.16557627198103120 ) ) ;
#196698=CARTESIAN_POINT ( 'NONE',  ( -16.51473224551069308, -9.474510206698971260, 76.66557627198103830 ) ) ;
#196699=VERTEX_POINT ( 'NONE', #106429 ) ;
#196700=CARTESIAN_POINT ( 'NONE',  ( 16.52544592524335698, 4.483927247898782831, 31.45942372801901854 ) ) ;
#196701=CARTESIAN_POINT ( 'NONE',  ( 10.72451020669871369, 18.67979575497193778, 22.08442372801901143 ) ) ;
#196702=CARTESIAN_POINT ( 'NONE',  ( -12.06949235617756955, 12.14591786802309770, 50.62390960531435979 ) ) ;
#196703=CARTESIAN_POINT ( 'NONE',  ( 9.474510206698971260, -16.51473224551069308, 102.9155762719810241 ) ) ;
#196704=CARTESIAN_POINT ( 'NONE',  ( -15.72974639402197994, 15.80617190586746368, 75.62390960531439532 ) ) ;
#196705=CARTESIAN_POINT ( 'NONE',  ( 5.719274019375991003, -21.55341960407610458, 102.7072429386476955 ) ) ;
#196706=CARTESIAN_POINT ( 'NONE',  ( 4.379528057220092307, 16.55341960407617563, 57.29275706135234714 ) ) ;
#196707=CARTESIAN_POINT ( 'NONE',  ( -10.81492255796078084, -18.62759615963271287, 47.08224293864770260 ) ) ;
#196708=CARTESIAN_POINT ( 'NONE',  ( 21.55341960407619695, -5.719274019375665929, 106.0427570613523471 ) ) ;
#196709=CIRCLE ( 'NONE', #64321, 2.500000000000002220 ) ;
#196710=CARTESIAN_POINT ( 'NONE',  ( -19.03943276465977164, 0.05219959533909376836, 36.24890960531436690 ) ) ;
#196711=CARTESIAN_POINT ( 'NONE',  ( 9.474510206698971260, -16.51473224551069308, 102.9155762719810241 ) ) ;
#196712=CARTESIAN_POINT ( 'NONE',  ( 5.153800228976335163, 19.02544592524342804, 69.79057627198103830 ) ) ;
#196714=CARTESIAN_POINT ( 'NONE',  ( -9.474510206698720793, -16.51473224551083518, 59.58442372801900433 ) ) ;
#196715=CARTESIAN_POINT ( 'NONE',  ( -21.53943276465977519, -0.05219959533937600094, 108.7510903946857042 ) ) ;
#196716=CARTESIAN_POINT ( 'NONE',  ( 0.05219959533907565091, 21.53943276465977519, 29.99890960531435979 ) ) ;
#196717=CARTESIAN_POINT ( 'NONE',  ( -16.53943276465976808, -0.05219959533934237506, 108.7510903946857042 ) ) ;
#196718=CARTESIAN_POINT ( 'NONE',  ( -19.02544592524334988, -5.153800228976617603, 83.95942372801901854 ) ) ;
#196720=CARTESIAN_POINT ( 'NONE',  ( 16.46253265017160672, -9.564922557960803928, 108.3322429386476955 ) ) ;
#196721=CARTESIAN_POINT ( 'NONE',  ( 5.049401038297881783, 19.05341960407617563, 77.29275706135231871 ) ) ;
#196722=CARTESIAN_POINT ( 'NONE',  ( -19.05341960407617563, 5.049401038297882671, 48.54275706135233293 ) ) ;
#196724=CARTESIAN_POINT ( 'NONE',  ( -9.564922557960796823, -16.46253265017161027, 47.08224293864769550 ) ) ;
#196725=CARTESIAN_POINT ( 'NONE',  ( 16.53943276465976808, -0.05219959533910856209, 48.74890960531435979 ) ) ;
#196726=CARTESIAN_POINT ( 'NONE',  ( -5.049401038298153566, 19.05341960407611168, 30.20724293864768839 ) ) ;
#196727=CARTESIAN_POINT ( 'NONE',  ( -0.05219959533910754901, -16.53943276465976808, 42.49890960531435979 ) ) ;
#196728=CARTESIAN_POINT ( 'NONE',  ( 17.50000000001358202, -5.500000000000038192, 58.29690382535058291 ) ) ;
#196729=CARTESIAN_POINT ( 'NONE',  ( -8.314922557961024197, 14.29746914071037800, 112.9177570613523329 ) ) ;
#196730=CARTESIAN_POINT ( 'NONE',  ( 9.474510206698971260, -16.51473224551069308, 52.91557627198102409 ) ) ;
#196731=CARTESIAN_POINT ( 'NONE',  ( 21.52544592524334988, 5.823673210054432836, 106.4594237280190328 ) ) ;
#196732=CARTESIAN_POINT ( 'NONE',  ( -16.52544592524335698, -4.483927247898792601, 18.95942372801901143 ) ) ;
#196733=CARTESIAN_POINT ( 'NONE',  ( -15.72974639402197994, 15.80617190586746368, 40.62390960531435269 ) ) ;
#196734=CARTESIAN_POINT ( 'NONE',  ( 18.62759615963255655, 10.81492255796105972, 96.66775706135234714 ) ) ;
#196736=CARTESIAN_POINT ( 'NONE',  ( -5.049401038298153566, 19.05341960407611168, 110.2072429386476671 ) ) ;
#196737=CARTESIAN_POINT ( 'NONE',  ( -19.05341960407611168, -5.049401038298163336, 81.45724293864769550 ) ) ;
#196739=CARTESIAN_POINT ( 'NONE',  ( -10.81492255796078084, -18.62759615963271287, 107.0822429386476955 ) ) ;
#196740=CARTESIAN_POINT ( 'NONE',  ( -16.52544592524342804, 4.483927247898546575, 81.04057627198102409 ) ) ;
#196741=CARTESIAN_POINT ( 'NONE',  ( -15.72974639402197994, 15.80617190586746368, 75.62390960531439532 ) ) ;
#196742=CARTESIAN_POINT ( 'NONE',  ( 5.153800228976335163, 19.02544592524342804, 69.79057627198103830 ) ) ;
#196743=CARTESIAN_POINT ( 'NONE',  ( -18.62759615963270932, 10.81492255796079327, 90.83224293864769550 ) ) ;
#196745=CARTESIAN_POINT ( 'NONE',  ( -13.89961937509977652, 13.97604488694528158, 65.62390960531436690 ) ) ;
#196746=CARTESIAN_POINT ( 'NONE',  ( -4.483927247898539470, -16.52544592524342804, 97.29057627198105251 ) ) ;
#196748=CARTESIAN_POINT ( 'NONE',  ( -5.153800228976328057, -19.02544592524343514, 67.29057627198102409 ) ) ;
#196749=CARTESIAN_POINT ( 'NONE',  ( 5.153800228976615827, -19.02544592524334988, 80.20942372801901854 ) ) ;
#196750=CARTESIAN_POINT ( 'NONE',  ( -16.53943276465976808, 0.05219959533911058130, 96.24890960531435269 ) ) ;
#196751=CARTESIAN_POINT ( 'NONE',  ( -5.719274019375665041, -21.55341960407619695, 59.79275706135234714 ) ) ;
#196752=CARTESIAN_POINT ( 'NONE',  ( -16.51473224551069308, -9.474510206698971260, 51.66557627198102409 ) ) ;
#196753=CARTESIAN_POINT ( 'NONE',  ( -0.05219959533937732626, 21.53943276465977519, 22.50109039468567573 ) ) ;
#196754=CARTESIAN_POINT ( 'NONE',  ( -12.14591786802309592, -12.06949235617757132, 96.87390960531436690 ) ) ;
#196756=CARTESIAN_POINT ( 'NONE',  ( 5.049401038298161559, -19.05341960407611168, 62.70724293864769550 ) ) ;
#196758=CARTESIAN_POINT ( 'NONE',  ( 5.153800228976615827, -19.02544592524334988, 105.2094237280190185 ) ) ;
#196759=CARTESIAN_POINT ( 'NONE',  ( -19.03943276465977164, 0.05219959533909376836, 116.2489096053143669 ) ) ;
#196760=CARTESIAN_POINT ( 'NONE',  ( 10.81492255796106328, -18.62759615963255655, 50.41775706135235424 ) ) ;
#196761=CARTESIAN_POINT ( 'NONE',  ( -13.97604488694527625, -13.89961937509977652, 96.87390960531433848 ) ) ;
#196762=CARTESIAN_POINT ( 'NONE',  ( -0.05219959533936034679, 19.03943276465977164, 82.50109039468567573 ) ) ;
#196763=CARTESIAN_POINT ( 'NONE',  ( -0.05219959533909027116, -19.03943276465977164, 62.49890960531435979 ) ) ;
#196764=CARTESIAN_POINT ( 'NONE',  ( -8.314922557960811034, -14.29746914071050412, 77.08224293864769550 ) ) ;
#196765=CARTESIAN_POINT ( 'NONE',  ( 16.51473224551069308, 9.474510206698969483, 94.16557627198103830 ) ) ;
#196766=CARTESIAN_POINT ( 'NONE',  ( -4.483927247898539470, -16.52544592524342804, 72.29057627198102409 ) ) ;
#196767=CARTESIAN_POINT ( 'NONE',  ( -5.049401038298153566, 19.05341960407611168, 85.20724293864766707 ) ) ;
#196768=CARTESIAN_POINT ( 'NONE',  ( 13.97604488694548053, -13.89961937509957401, 30.62609039468566863 ) ) ;
#196769=CARTESIAN_POINT ( 'NONE',  ( -19.02544592524342804, 5.153800228976336051, 51.04057627198103120 ) ) ;
#196770=CARTESIAN_POINT ( 'NONE',  ( 12.06949235617757843, -12.14591786802309237, 43.12390960531435269 ) ) ;
#196771=CARTESIAN_POINT ( 'NONE',  ( -19.03943276465977164, 0.05219959533909376836, 26.24890960531435624 ) ) ;
#196772=ORIENTED_EDGE ( 'NONE', *, *, #26374, .F. ) ;
#196773=CARTESIAN_POINT ( 'NONE',  ( -15.72974639402176322, -15.80617190586768395, 44.37609039468567573 ) ) ;
#196774=CARTESIAN_POINT ( 'NONE',  ( 0.05219959533936267826, -19.03943276465977164, 85.00109039468567573 ) ) ;
#196775=CARTESIAN_POINT ( 'NONE',  ( 4.483927247898545687, 16.52544592524342804, 29.79057627198102409 ) ) ;
#196776=CARTESIAN_POINT ( 'NONE',  ( -21.55341960407610458, -5.719274019375992779, 96.45724293864770971 ) ) ;
#196777=CARTESIAN_POINT ( 'NONE',  ( -21.52544592524343514, 5.823673210054127303, 31.04057627198102409 ) ) ;
#196778=CARTESIAN_POINT ( 'NONE',  ( -4.483927247898539470, -16.52544592524342804, 72.29057627198102409 ) ) ;
#196779=CARTESIAN_POINT ( 'NONE',  ( 19.05341960407611168, 5.049401038298154454, 43.95724293864769550 ) ) ;
#196780=CARTESIAN_POINT ( 'NONE',  ( 12.14591786802327356, -12.06949235617739191, 100.6260903946857184 ) ) ;
#196781=CARTESIAN_POINT ( 'NONE',  ( -4.379528057220086978, -16.55341960407618274, 64.79275706135234714 ) ) ;
#196782=CARTESIAN_POINT ( 'NONE',  ( -5.153800228976607833, 19.02544592524334988, 27.70942372801899722 ) ) ;
#196783=CARTESIAN_POINT ( 'NONE',  ( 13.97604488694527802, 13.89961937509977652, 94.37390960531436690 ) ) ;
#196784=CARTESIAN_POINT ( 'NONE',  ( -16.46253265017160317, 9.564922557960807481, 80.83224293864769550 ) ) ;
#196785=CARTESIAN_POINT ( 'NONE',  ( 12.14591786802327356, -12.06949235617739191, 80.62609039468567573 ) ) ;
#196786=CARTESIAN_POINT ( 'NONE',  ( -16.51473224551069308, -9.474510206698971260, 21.66557627198102765 ) ) ;
#196787=CARTESIAN_POINT ( 'NONE',  ( -16.52544592524342804, 4.483927247898546575, 51.04057627198103120 ) ) ;
#196788=CARTESIAN_POINT ( 'NONE',  ( -19.03943276465977164, 0.05219959533909376836, 106.2489096053143669 ) ) ;
#196789=CARTESIAN_POINT ( 'NONE',  ( -5.049401038298153566, 19.05341960407611168, 85.20724293864766707 ) ) ;
#196790=CARTESIAN_POINT ( 'NONE',  ( -0.05219959533907301413, -21.53943276465977519, 22.49890960531436335 ) ) ;
#196791=CARTESIAN_POINT ( 'NONE',  ( 8.224510206698953496, -14.34966873604960469, 77.91557627198102409 ) ) ;
#196792=CARTESIAN_POINT ( 'NONE',  ( 16.55341960407611168, 4.379528057220329451, 63.95724293864770260 ) ) ;
#196793=CARTESIAN_POINT ( 'NONE',  ( 8.314922557961029526, -14.29746914071037800, 50.41775706135235424 ) ) ;
#196794=CARTESIAN_POINT ( 'NONE',  ( 17.60769864724391098, -5.499999999999978684, 86.15024842019167295 ) ) ;
#196795=CARTESIAN_POINT ( 'NONE',  ( 19.03943276465977164, 0.05219959533936151252, 61.25109039468566863 ) ) ;
#196796=CARTESIAN_POINT ( 'NONE',  ( -9.564922557960796823, -16.46253265017161027, 92.08224293864769550 ) ) ;
#196797=CARTESIAN_POINT ( 'NONE',  ( -9.474510206698720793, -16.51473224551083518, 59.58442372801900433 ) ) ;
#196798=CARTESIAN_POINT ( 'NONE',  ( 18.22780087662114212, -5.499999999999987566, 41.01540105326107977 ) ) ;
#196799=CARTESIAN_POINT ( 'NONE',  ( 19.05341960407617918, -5.049401038297876454, 111.0427570613523329 ) ) ;
#196800=CARTESIAN_POINT ( 'NONE',  ( -16.52544592524335698, -4.483927247898792601, 93.95942372801903275 ) ) ;
#196801=CARTESIAN_POINT ( 'NONE',  ( -19.03943276465977164, 0.05219959533909376836, 36.24890960531436690 ) ) ;
#196802=CARTESIAN_POINT ( 'NONE',  ( 15.72974639402199770, -15.80617190586745480, 23.12390960531436335 ) ) ;
#196803=CARTESIAN_POINT ( 'NONE',  ( 0.05219959533937995610, -21.53943276465977519, 60.00109039468568284 ) ) ;
#196804=CARTESIAN_POINT ( 'NONE',  ( -9.564922557961040184, 16.46253265017147172, 107.9177570613523471 ) ) ;
#196806=CARTESIAN_POINT ( 'NONE',  ( -5.049401038298153566, 19.05341960407611168, 80.20724293864769550 ) ) ;
#196808=CARTESIAN_POINT ( 'NONE',  ( 19.03943276465977164, -0.05219959533909143690, 113.7489096053143669 ) ) ;
#196809=CARTESIAN_POINT ( 'NONE',  ( 16.55341960407611168, 4.379528057220329451, 73.95724293864769550 ) ) ;
#196810=CARTESIAN_POINT ( 'NONE',  ( 5.153800228976335163, 19.02544592524342804, 74.79057627198103830 ) ) ;
#196811=CARTESIAN_POINT ( 'NONE',  ( -19.05341960407611168, -5.049401038298163336, 71.45724293864766707 ) ) ;
#196812=CARTESIAN_POINT ( 'NONE',  ( -13.89961937509957401, -13.97604488694547875, 74.37609039468566152 ) ) ;
#196813=CARTESIAN_POINT ( 'NONE',  ( -18.62759615963270932, 10.81492255796079327, 60.83224293864769550 ) ) ;
#196814=CARTESIAN_POINT ( 'NONE',  ( -12.06949235617756955, 12.14591786802309770, 115.6239096053143669 ) ) ;
#196815=CARTESIAN_POINT ( 'NONE',  ( -19.02544592524334988, -5.153800228976617603, 53.95942372801898301 ) ) ;
#196816=CARTESIAN_POINT ( 'NONE',  ( -16.46253265017160317, 9.564922557960807481, 50.83224293864770260 ) ) ;
#196817=CARTESIAN_POINT ( 'NONE',  ( -9.474510206698964154, 16.51473224551069663, 95.41557627198102409 ) ) ;
#196818=CARTESIAN_POINT ( 'NONE',  ( -18.67979575497178146, -10.72451020669898902, 96.66557627198102409 ) ) ;
#196819=CARTESIAN_POINT ( 'NONE',  ( 4.483927247898545687, 16.52544592524342804, 99.79057627198103830 ) ) ;
#196820=CARTESIAN_POINT ( 'NONE',  ( 16.46253265017146816, 9.564922557961045513, 46.66775706135233293 ) ) ;
#196821=CARTESIAN_POINT ( 'NONE',  ( -15.80617190586745835, -15.72974639402198527, 76.87390960531439532 ) ) ;
#196822=CARTESIAN_POINT ( 'NONE',  ( -21.53943276465977519, 0.05219959533907696930, 56.24890960531436690 ) ) ;
#196823=CARTESIAN_POINT ( 'NONE',  ( -16.52544592524342804, 4.483927247898546575, 31.04057627198102409 ) ) ;
#196824=CARTESIAN_POINT ( 'NONE',  ( 10.81492255796106328, -18.62759615963255655, 100.4177570613523471 ) ) ;
#196825=CARTESIAN_POINT ( 'NONE',  ( -16.46253265017160317, 9.564922557960807481, 80.83224293864769550 ) ) ;
#196826=CARTESIAN_POINT ( 'NONE',  ( 19.05341960407611168, 5.049401038298154454, 38.95724293864767418 ) ) ;
#196827=CARTESIAN_POINT ( 'NONE',  ( 10.72451020669871369, 18.67979575497193778, 37.08442372801901143 ) ) ;
#196828=CARTESIAN_POINT ( 'NONE',  ( 15.80617190586769283, -15.72974639402175789, 35.62609039468568994 ) ) ;
#196829=CARTESIAN_POINT ( 'NONE',  ( 19.02544592524343514, -5.153800228976328945, 53.54057627198102409 ) ) ;
#196830=CARTESIAN_POINT ( 'NONE',  ( 10.72451020669871369, 18.67979575497193778, 27.08442372801901854 ) ) ;
#196831=CARTESIAN_POINT ( 'NONE',  ( 19.03943276465977164, 0.05219959533936151252, 61.25109039468566863 ) ) ;
#196833=CARTESIAN_POINT ( 'NONE',  ( -16.46253265017160317, 9.564922557960807481, 30.83224293864769550 ) ) ;
#196834=CARTESIAN_POINT ( 'NONE',  ( 12.14591786802327356, -12.06949235617739191, 30.62609039468567929 ) ) ;
#196835=CARTESIAN_POINT ( 'NONE',  ( 13.89961937509977652, -13.97604488694527269, 28.12390960531435624 ) ) ;
#196836=CARTESIAN_POINT ( 'NONE',  ( 12.06949235617739724, 12.14591786802326823, 71.87609039468568994 ) ) ;
#196837=CARTESIAN_POINT ( 'NONE',  ( 5.153800228976335163, 19.02544592524342804, 44.79057627198103830 ) ) ;
#196839=CARTESIAN_POINT ( 'NONE',  ( 9.564922557960805705, 16.46253265017160317, 89.58224293864769550 ) ) ;
#196840=CARTESIAN_POINT ( 'NONE',  ( -5.049401038298153566, 19.05341960407611168, 25.20724293864768484 ) ) ;
#196841=CARTESIAN_POINT ( 'NONE',  ( 21.52544592524344225, -5.823673210054117533, 78.54057627198103830 ) ) ;
#196842=CARTESIAN_POINT ( 'NONE',  ( 8.224510206698742110, 14.34966873604972548, 47.08442372801901854 ) ) ;
#196843=CARTESIAN_POINT ( 'NONE',  ( 21.53943276465977519, 0.05219959533937863772, 96.25109039468568994 ) ) ;
#196844=CARTESIAN_POINT ( 'NONE',  ( -16.46253265017160317, 9.564922557960807481, 40.83224293864769550 ) ) ;
#196845=CARTESIAN_POINT ( 'NONE',  ( -16.55341960407611168, -4.379528057220339221, 31.45724293864769550 ) ) ;
#196846=CARTESIAN_POINT ( 'NONE',  ( 14.34966873604960469, 8.224510206698951720, 69.16557627198102409 ) ) ;
#196848=CARTESIAN_POINT ( 'NONE',  ( 19.02544592524343514, -5.153800228976328945, 63.54057627198103830 ) ) ;
#196849=CARTESIAN_POINT ( 'NONE',  ( -10.72451020669870658, -18.67979575497194134, 104.5844237280190185 ) ) ;
#196850=CARTESIAN_POINT ( 'NONE',  ( 15.72974639402176855, 15.80617190586768217, 21.87609039468567573 ) ) ;
#196851=CARTESIAN_POINT ( 'NONE',  ( -9.474510206698964154, 16.51473224551069663, 85.41557627198102409 ) ) ;
#196852=CARTESIAN_POINT ( 'NONE',  ( -21.55341960407619339, 5.719274019375674811, 88.54275706135236135 ) ) ;
#196853=CARTESIAN_POINT ( 'NONE',  ( 8.224510206698742110, 14.34966873604972548, 47.08442372801901854 ) ) ;
#196854=CARTESIAN_POINT ( 'NONE',  ( -14.34966873604972548, 8.224510206698743886, 23.33442372801901499 ) ) ;
#196855=CARTESIAN_POINT ( 'NONE',  ( -4.379528057220328563, 16.55341960407611168, 90.20724293864770971 ) ) ;
#196856=CARTESIAN_POINT ( 'NONE',  ( 0.05219959533937995610, -21.53943276465977519, 105.0010903946856757 ) ) ;
#196857=CARTESIAN_POINT ( 'NONE',  ( -16.52544592524342804, 4.483927247898546575, 36.04057627198102409 ) ) ;
#196858=CARTESIAN_POINT ( 'NONE',  ( 13.97604488694527802, 13.89961937509977652, 34.37390960531436690 ) ) ;
#196859=CARTESIAN_POINT ( 'NONE',  ( 4.483927247898790824, -16.52544592524335698, 55.20942372801902565 ) ) ;
#196860=CARTESIAN_POINT ( 'NONE',  ( -12.06949235617756955, 12.14591786802309770, 60.62390960531437401 ) ) ;
#196861=CARTESIAN_POINT ( 'NONE',  ( -14.29746914071037622, -8.314922557961029526, 99.16775706135234714 ) ) ;
#196862=CARTESIAN_POINT ( 'NONE',  ( -21.55341960407610458, -5.719274019375992779, 21.45724293864769550 ) ) ;
#196863=CARTESIAN_POINT ( 'NONE',  ( 5.719274019375991003, -21.55341960407610458, 32.70724293864770260 ) ) ;
#196864=CARTESIAN_POINT ( 'NONE',  ( 16.51473224551083163, -9.474510206698727899, 20.83442372801899722 ) ) ;
#196865=CARTESIAN_POINT ( 'NONE',  ( 8.224510206698953496, -14.34966873604960469, 87.91557627198103830 ) ) ;
#196866=CARTESIAN_POINT ( 'NONE',  ( -9.474510206698964154, 16.51473224551069663, 100.4155762719810241 ) ) ;
#196868=CARTESIAN_POINT ( 'NONE',  ( -4.483927247898782831, 16.52544592524335698, 42.70942372801901854 ) ) ;
#196869=CARTESIAN_POINT ( 'NONE',  ( 5.153800228976335163, 19.02544592524342804, 44.79057627198103830 ) ) ;
#196870=CARTESIAN_POINT ( 'NONE',  ( 4.379528057220092307, 16.55341960407617563, 42.29275706135235424 ) ) ;
#196871=CARTESIAN_POINT ( 'NONE',  ( -19.03943276465977164, -0.05219959533935918106, 48.75109039468566863 ) ) ;
#196872=CARTESIAN_POINT ( 'NONE',  ( 9.564922557960805705, 16.46253265017160317, 39.58224293864768839 ) ) ;
#196873=CARTESIAN_POINT ( 'NONE',  ( 0.05219959533934541429, -16.53943276465976808, 75.00109039468568994 ) ) ;
#196874=CARTESIAN_POINT ( 'NONE',  ( 5.153800228976615827, -19.02544592524334988, 95.20942372801897591 ) ) ;
#196875=CARTESIAN_POINT ( 'NONE',  ( -19.02544592524334988, -5.153800228976617603, 28.95942372801900433 ) ) ;
#196876=CARTESIAN_POINT ( 'NONE',  ( -5.153800228976328057, -19.02544592524343514, 57.29057627198103120 ) ) ;
#196877=CARTESIAN_POINT ( 'NONE',  ( 12.06949235617757843, -12.14591786802309237, 93.12390960531436690 ) ) ;
#196879=CARTESIAN_POINT ( 'NONE',  ( -13.89961937509957401, -13.97604488694547875, 64.37609039468567573 ) ) ;
#196880=CARTESIAN_POINT ( 'NONE',  ( 18.67979575497178502, 10.72451020669898547, 64.16557627198102409 ) ) ;
#196881=CARTESIAN_POINT ( 'NONE',  ( 9.564922557961047289, -16.46253265017146816, 40.41775706135234003 ) ) ;
#196882=CARTESIAN_POINT ( 'NONE',  ( 5.153800228976335163, 19.02544592524342804, 99.79057627198102409 ) ) ;
#196883=CARTESIAN_POINT ( 'NONE',  ( 0.05219959533907565091, 21.53943276465977519, 74.99890960531435269 ) ) ;
#196884=CARTESIAN_POINT ( 'NONE',  ( -16.81555441253553695, 7.025013491695484724, 85.63685445334262170 ) ) ;
#196885=CARTESIAN_POINT ( 'NONE',  ( 13.89961937509957401, 13.97604488694547697, 96.87609039468566152 ) ) ;
#196886=CARTESIAN_POINT ( 'NONE',  ( -9.564922557961040184, 16.46253265017147172, 97.91775706135233293 ) ) ;
#196887=CARTESIAN_POINT ( 'NONE',  ( 14.34966873604972726, -8.224510206698740333, 30.83442372801902209 ) ) ;
#196888=CARTESIAN_POINT ( 'NONE',  ( 19.05341960407611168, 5.049401038298154454, 43.95724293864769550 ) ) ;
#196889=CARTESIAN_POINT ( 'NONE',  ( -9.474510206698964154, 16.51473224551069663, 110.4155762719810383 ) ) ;
#196890=CARTESIAN_POINT ( 'NONE',  ( -10.72451020669898014, 18.67979575497178502, 90.41557627198103830 ) ) ;
#196891=CARTESIAN_POINT ( 'NONE',  ( 5.823673210054444382, -21.52544592524334988, 60.20942372801902565 ) ) ;
#196892=CARTESIAN_POINT ( 'NONE',  ( 0.05219959533936267826, -19.03943276465977164, 105.0010903946856615 ) ) ;
#196893=CARTESIAN_POINT ( 'NONE',  ( -10.72451020669870658, -18.67979575497194134, 104.5844237280190185 ) ) ;
#196894=CARTESIAN_POINT ( 'NONE',  ( 8.314922557961029526, -14.29746914071037800, 105.4177570613523613 ) ) ;
#196895=CARTESIAN_POINT ( 'NONE',  ( -18.62759615963270932, 10.81492255796079327, 100.8322429386477097 ) ) ;
#196896=CARTESIAN_POINT ( 'NONE',  ( -0.05219959533910754901, -16.53943276465976808, 47.49890960531435979 ) ) ;
#196897=CARTESIAN_POINT ( 'NONE',  ( 13.97604488694548053, -13.89961937509957401, 85.62609039468568994 ) ) ;
#196898=CARTESIAN_POINT ( 'NONE',  ( 9.474510206698729675, 16.51473224551082808, 57.08442372801900433 ) ) ;
#196899=CARTESIAN_POINT ( 'NONE',  ( 15.72974639402176855, 15.80617190586768217, 76.87609039468567573 ) ) ;
#196900=CARTESIAN_POINT ( 'NONE',  ( 9.474510206698729675, 16.51473224551082808, 37.08442372801899722 ) ) ;
#196901=CARTESIAN_POINT ( 'NONE',  ( -16.53943276465976808, 0.05219959533911058130, 101.2489096053143669 ) ) ;
#196902=CARTESIAN_POINT ( 'NONE',  ( 10.81492255796078972, 18.62759615963270932, 44.58224293864769550 ) ) ;
#196903=CARTESIAN_POINT ( 'NONE',  ( 8.314922557960818139, 14.29746914071049879, 39.58224293864769550 ) ) ;
#196904=CARTESIAN_POINT ( 'NONE',  ( 21.55341960407619695, -5.719274019375665929, 106.0427570613523471 ) ) ;
#196905=CARTESIAN_POINT ( 'NONE',  ( 8.224510206698742110, 14.34966873604972548, 67.08442372801901854 ) ) ;
#196906=CARTESIAN_POINT ( 'NONE',  ( -4.379528057220328563, 16.55341960407611168, 25.20724293864769550 ) ) ;
#196907=CARTESIAN_POINT ( 'NONE',  ( 15.80617190586769283, -15.72974639402175789, 60.62609039468567573 ) ) ;
#196908=CARTESIAN_POINT ( 'NONE',  ( 0.05219959533937995610, -21.53943276465977519, 70.00109039468568994 ) ) ;
#196909=CARTESIAN_POINT ( 'NONE',  ( 21.55341960407610458, 5.719274019375980345, 73.95724293864769550 ) ) ;
#196911=CARTESIAN_POINT ( 'NONE',  ( -16.46253265017160317, 9.564922557960807481, 30.83224293864769550 ) ) ;
#196912=CARTESIAN_POINT ( 'NONE',  ( -21.52544592524334988, -5.823673210054445271, 48.95942372801902565 ) ) ;
#196913=CARTESIAN_POINT ( 'NONE',  ( 9.564922557960805705, 16.46253265017160317, 24.58224293864769194 ) ) ;
#196914=CARTESIAN_POINT ( 'NONE',  ( 16.51473224551069308, 9.474510206698969483, 39.16557627198103120 ) ) ;
#196915=CARTESIAN_POINT ( 'NONE',  ( 0.05219959533910956823, 16.53943276465976808, 89.99890960531438111 ) ) ;
#196916=CARTESIAN_POINT ( 'NONE',  ( 13.89961937509977652, -13.97604488694527269, 88.12390960531438111 ) ) ;
#196917=CARTESIAN_POINT ( 'NONE',  ( 16.53943276465976808, -0.05219959533910856209, 33.74890960531436690 ) ) ;
#196918=CARTESIAN_POINT ( 'NONE',  ( 0.05219959533910956823, 16.53943276465976808, 99.99890960531436690 ) ) ;
#196919=CARTESIAN_POINT ( 'NONE',  ( -10.72451020669898014, 18.67979575497178502, 70.41557627198102409 ) ) ;
#196920=CARTESIAN_POINT ( 'NONE',  ( -18.62759615963270932, 10.81492255796079327, 110.8322429386476955 ) ) ;
#196921=CARTESIAN_POINT ( 'NONE',  ( 0.05219959533909260263, 19.03943276465977164, 109.9989096053143669 ) ) ;
#196922=CARTESIAN_POINT ( 'NONE',  ( -13.89961937509977652, 13.97604488694528158, 70.62390960531432427 ) ) ;
#196923=CARTESIAN_POINT ( 'NONE',  ( -12.06949235617739369, -12.14591786802326823, 24.37609039468567573 ) ) ;
#196924=CARTESIAN_POINT ( 'NONE',  ( -5.719274019375978568, 21.55341960407610458, 60.20724293864768839 ) ) ;
#196925=CARTESIAN_POINT ( 'NONE',  ( -21.55341960407619339, 5.719274019375674811, 83.54275706135234714 ) ) ;
#196926=CARTESIAN_POINT ( 'NONE',  ( -19.05341960407611168, -5.049401038298163336, 86.45724293864769550 ) ) ;
#196927=CARTESIAN_POINT ( 'NONE',  ( 16.46253265017160672, -9.564922557960803928, 113.3322429386476955 ) ) ;
#196928=CARTESIAN_POINT ( 'NONE',  ( 4.483927247898790824, -16.52544592524335698, 75.20942372801901854 ) ) ;
#196929=CARTESIAN_POINT ( 'NONE',  ( -21.52544592524334988, -5.823673210054445271, 53.95942372801900433 ) ) ;
#196930=CARTESIAN_POINT ( 'NONE',  ( 21.55341960407619695, -5.719274019375665929, 106.0427570613523471 ) ) ;
#196931=CARTESIAN_POINT ( 'NONE',  ( -12.06949235617739369, -12.14591786802326823, 64.37609039468568994 ) ) ;
#196932=CARTESIAN_POINT ( 'NONE',  ( 21.53943276465977519, 0.05219959533937863772, 21.25109039468567218 ) ) ;
#196933=CARTESIAN_POINT ( 'NONE',  ( 15.50000000000000178, 5.499999999999998224, 20.00000000000000000 ) ) ;
#196934=CARTESIAN_POINT ( 'NONE',  ( 10.72451020669898902, -18.67979575497178502, 92.91557627198103830 ) ) ;
#196935=CARTESIAN_POINT ( 'NONE',  ( -16.51473224551082808, 9.474510206698731452, 43.33442372801900433 ) ) ;
#196936=CARTESIAN_POINT ( 'NONE',  ( -21.52544592524343514, 5.823673210054127303, 56.04057627198102409 ) ) ;
#196937=CARTESIAN_POINT ( 'NONE',  ( 5.153800228976335163, 19.02544592524342804, 99.79057627198102409 ) ) ;
#196938=CARTESIAN_POINT ( 'NONE',  ( 8.314922557960818139, 14.29746914071049879, 39.58224293864769550 ) ) ;
#196941=CARTESIAN_POINT ( 'NONE',  ( -13.89961937509957401, -13.97604488694547875, 109.3760903946856331 ) ) ;
#196942=CARTESIAN_POINT ( 'NONE',  ( -21.53943276465977519, 0.05219959533907696930, 76.24890960531435269 ) ) ;
#196943=CARTESIAN_POINT ( 'NONE',  ( 4.379528057220339221, -16.55341960407611168, 52.70724293864769550 ) ) ;
#196944=CARTESIAN_POINT ( 'NONE',  ( -14.29746914071037622, -8.314922557961029526, 34.16775706135234714 ) ) ;
#196945=CARTESIAN_POINT ( 'NONE',  ( 13.89961937509977652, -13.97604488694527269, 43.12390960531434558 ) ) ;
#196946=CARTESIAN_POINT ( 'NONE',  ( 21.55341960407610458, 5.719274019375980345, 108.9572429386476955 ) ) ;
#196947=CARTESIAN_POINT ( 'NONE',  ( -9.564922557961040184, 16.46253265017147172, 82.91775706135233293 ) ) ;
#196948=CARTESIAN_POINT ( 'NONE',  ( 0.05219959533909260263, 19.03943276465977164, 79.99890960531436690 ) ) ;
#196949=CARTESIAN_POINT ( 'NONE',  ( 0.05219959533909260263, 19.03943276465977164, 69.99890960531435269 ) ) ;
#196950=CARTESIAN_POINT ( 'NONE',  ( 10.72451020669898902, -18.67979575497178502, 77.91557627198102409 ) ) ;
#196951=CARTESIAN_POINT ( 'NONE',  ( -19.03943276465977164, 0.05219959533909376836, 36.24890960531436690 ) ) ;
#196953=CARTESIAN_POINT ( 'NONE',  ( 8.224510206698953496, -14.34966873604960469, 52.91557627198103830 ) ) ;
#196954=CARTESIAN_POINT ( 'NONE',  ( -13.89961937509977652, 13.97604488694528158, 95.62390960531436690 ) ) ;
#196955=DIRECTION ( 'NONE',  ( -0.000000000000000000, -0.000000000000000000, 1.000000000000000000 ) ) ;
#196956=CARTESIAN_POINT ( 'NONE',  ( -19.02544592524334988, -5.153800228976617603, 63.95942372801899012 ) ) ;
#196957=CARTESIAN_POINT ( 'NONE',  ( -10.72451020669898014, 18.67979575497178502, 75.41557627198102409 ) ) ;
#196958=CARTESIAN_POINT ( 'NONE',  ( -16.46253265017146816, -9.564922557961047289, 39.16775706135234003 ) ) ;
#196959=CARTESIAN_POINT ( 'NONE',  ( -5.153800228976328057, -19.02544592524343514, 87.29057627198103830 ) ) ;
#196960=CARTESIAN_POINT ( 'NONE',  ( -17.50000000000146017, 3.254303733634615892, 115.0239589307140307 ) ) ;
#196961=CARTESIAN_POINT ( 'NONE',  ( 10.81492255796078972, 18.62759615963270932, 29.58224293864769905 ) ) ;
#196962=CARTESIAN_POINT ( 'NONE',  ( 16.46253265017160672, -9.564922557960803928, 73.33224293864769550 ) ) ;
#196963=CARTESIAN_POINT ( 'NONE',  ( -21.55341960407619339, 5.719274019375674811, 48.54275706135234714 ) ) ;
#196964=CARTESIAN_POINT ( 'NONE',  ( -5.049401038298153566, 19.05341960407611168, 25.20724293864768484 ) ) ;
#196965=CARTESIAN_POINT ( 'NONE',  ( 21.55341960407610458, 5.719274019375980345, 113.9572429386477239 ) ) ;
#196967=CARTESIAN_POINT ( 'NONE',  ( -0.05219959533937732626, 21.53943276465977519, 42.50109039468567573 ) ) ;
#196969=CARTESIAN_POINT ( 'NONE',  ( 0.05219959533909260263, 19.03943276465977164, 94.99890960531436690 ) ) ;
#196972=CARTESIAN_POINT ( 'NONE',  ( 18.62759615963271287, -10.81492255796078972, 113.3322429386476955 ) ) ;
#196973=CARTESIAN_POINT ( 'NONE',  ( -13.89961937509977652, 13.97604488694528158, 65.62390960531436690 ) ) ;
#196974=CARTESIAN_POINT ( 'NONE',  ( -16.53943276465976808, -0.05219959533934237506, 18.75109039468568639 ) ) ;
#196976=CARTESIAN_POINT ( 'NONE',  ( -10.81492255796105439, 18.62759615963255655, 102.9177570613523756 ) ) ;
#196977=CARTESIAN_POINT ( 'NONE',  ( -5.153800228976328057, -19.02544592524343514, 47.29057627198102409 ) ) ;
#196978=CARTESIAN_POINT ( 'NONE',  ( 15.80617190586769283, -15.72974639402175789, 95.62609039468568994 ) ) ;
#196979=CARTESIAN_POINT ( 'NONE',  ( 13.89961937509977652, -13.97604488694527269, 88.12390960531438111 ) ) ;
#196980=CARTESIAN_POINT ( 'NONE',  ( -0.05219959533937732626, 21.53943276465977519, 62.50109039468568284 ) ) ;
#196983=CARTESIAN_POINT ( 'NONE',  ( 9.564922557960805705, 16.46253265017160317, 104.5822429386476955 ) ) ;
#196984=CARTESIAN_POINT ( 'NONE',  ( -17.50000000000149569, 3.202012800152202576, 29.92822416027271970 ) ) ;
#196985=CARTESIAN_POINT ( 'NONE',  ( 12.14591786802327356, -12.06949235617739191, 55.62609039468568284 ) ) ;
#196986=CARTESIAN_POINT ( 'NONE',  ( -16.53943276465976808, -0.05219959533934237506, 63.75109039468568284 ) ) ;
#196987=CARTESIAN_POINT ( 'NONE',  ( 5.719274019375673035, 21.55341960407619339, 57.29275706135234714 ) ) ;
#196988=CARTESIAN_POINT ( 'NONE',  ( -21.53943276465977519, -0.05219959533937600094, 93.75109039468567573 ) ) ;
#196990=CARTESIAN_POINT ( 'NONE',  ( -14.29746914071037622, -8.314922557961029526, 34.16775706135234714 ) ) ;
#196991=CARTESIAN_POINT ( 'NONE',  ( -13.97604488694527625, -13.89961937509977652, 76.87390960531433848 ) ) ;
#196992=CARTESIAN_POINT ( 'NONE',  ( -13.97604488694527625, -13.89961937509977652, 91.87390960531432427 ) ) ;
#196993=CARTESIAN_POINT ( 'NONE',  ( 17.48853670773242186, 5.747243402303174875, 43.83328700250010002 ) ) ;
#196994=CARTESIAN_POINT ( 'NONE',  ( 9.474510206698971260, -16.51473224551069308, 27.91557627198103120 ) ) ;
#196995=CARTESIAN_POINT ( 'NONE',  ( -18.67979575497178146, -10.72451020669898902, 31.66557627198102054 ) ) ;
#196996=CARTESIAN_POINT ( 'NONE',  ( 8.314922557961029526, -14.29746914071037800, 95.41775706135234714 ) ) ;
#196997=CARTESIAN_POINT ( 'NONE',  ( -0.05219959533910754901, -16.53943276465976808, 87.49890960531436690 ) ) ;
#196999=CARTESIAN_POINT ( 'NONE',  ( 13.97604488694527802, 13.89961937509977652, 69.37390960531436690 ) ) ;
#197000=CARTESIAN_POINT ( 'NONE',  ( 18.67979575497194134, -10.72451020669871369, 90.83442372801901854 ) ) ;
#197002=CARTESIAN_POINT ( 'NONE',  ( -12.06949235617739369, -12.14591786802326823, 29.37609039468568284 ) ) ;
#197003=CARTESIAN_POINT ( 'NONE',  ( 8.224510206698953496, -14.34966873604960469, 77.91557627198102409 ) ) ;
#197004=CARTESIAN_POINT ( 'NONE',  ( 18.67979575497194134, -10.72451020669871369, 45.83442372801901854 ) ) ;
#197005=CARTESIAN_POINT ( 'NONE',  ( 21.52544592524344225, -5.823673210054117533, 68.54057627198103830 ) ) ;
#197006=CARTESIAN_POINT ( 'NONE',  ( -19.05341960407617563, 5.049401038297882671, 33.54275706135231871 ) ) ;
#197008=CARTESIAN_POINT ( 'NONE',  ( -16.51473224551069308, -9.474510206698971260, 76.66557627198103830 ) ) ;
#197009=CARTESIAN_POINT ( 'NONE',  ( -4.379528057220328563, 16.55341960407611168, 45.20724293864769550 ) ) ;
#197011=CARTESIAN_POINT ( 'NONE',  ( 16.53943276465976808, -0.05219959533910856209, 28.74890960531435624 ) ) ;
#197012=CARTESIAN_POINT ( 'NONE',  ( 16.52544592524342804, -4.483927247898539470, 23.54057627198102765 ) ) ;
#197013=CARTESIAN_POINT ( 'NONE',  ( 19.02544592524334988, 5.153800228976608722, 71.45942372801900433 ) ) ;
#197015=CARTESIAN_POINT ( 'NONE',  ( 15.72974639402199770, -15.80617190586745480, 23.12390960531436335 ) ) ;
#197016=CARTESIAN_POINT ( 'NONE',  ( 12.06949235617757843, -12.14591786802309237, 83.12390960531436690 ) ) ;
#197018=CARTESIAN_POINT ( 'NONE',  ( 13.97604488694527802, 13.89961937509977652, 49.37390960531434558 ) ) ;
#197019=CARTESIAN_POINT ( 'NONE',  ( -15.72974639402197994, 15.80617190586746368, 30.62390960531436335 ) ) ;
#197020=CARTESIAN_POINT ( 'NONE',  ( 5.823673210054125526, 21.52544592524343514, 69.79057627198102409 ) ) ;
#197021=CARTESIAN_POINT ( 'NONE',  ( -16.53943276465976808, 0.05219959533911058130, 116.2489096053143669 ) ) ;
#197022=CARTESIAN_POINT ( 'NONE',  ( 0.05219959533934541429, -16.53943276465976808, 70.00109039468568994 ) ) ;
#197023=CARTESIAN_POINT ( 'NONE',  ( -16.51473224551069308, -9.474510206698971260, 51.66557627198102409 ) ) ;
#197024=CARTESIAN_POINT ( 'NONE',  ( 21.53943276465977519, 0.05219959533937863772, 51.25109039468568994 ) ) ;
#197025=CARTESIAN_POINT ( 'NONE',  ( 0.05219959533910956823, 16.53943276465976808, 109.9989096053143527 ) ) ;
#197026=CARTESIAN_POINT ( 'NONE',  ( 16.51473224551083163, -9.474510206698727899, 95.83442372801900433 ) ) ;
#197029=CARTESIAN_POINT ( 'NONE',  ( 18.62759615963271287, -10.81492255796078972, 28.33224293864769550 ) ) ;
#197030=CARTESIAN_POINT ( 'NONE',  ( 17.44270441346514389, -5.991230190323081573, 66.13664920735772057 ) ) ;
#197031=CARTESIAN_POINT ( 'NONE',  ( 5.823673210054444382, -21.52544592524334988, 65.20942372801901854 ) ) ;
#197032=CARTESIAN_POINT ( 'NONE',  ( -4.379528057220086978, -16.55341960407618274, 54.79275706135235424 ) ) ;
#197033=CARTESIAN_POINT ( 'NONE',  ( -16.52544592524342804, 4.483927247898546575, 46.04057627198103830 ) ) ;
#197034=CARTESIAN_POINT ( 'NONE',  ( -18.62759615963270932, 10.81492255796079327, 65.83224293864769550 ) ) ;
#197035=CARTESIAN_POINT ( 'NONE',  ( -21.52544592524343514, 5.823673210054127303, 66.04057627198103830 ) ) ;
#197037=CARTESIAN_POINT ( 'NONE',  ( 5.153800228976615827, -19.02544592524334988, 85.20942372801900433 ) ) ;
#197038=CARTESIAN_POINT ( 'NONE',  ( 19.03943276465977164, -0.05219959533909143690, 113.7489096053143669 ) ) ;
#197039=CARTESIAN_POINT ( 'NONE',  ( 16.46253265017160672, -9.564922557960803928, 53.33224293864768839 ) ) ;
#197040=CARTESIAN_POINT ( 'NONE',  ( -8.224510206698948167, 14.34966873604960824, 115.4155762719810241 ) ) ;
#197041=CARTESIAN_POINT ( 'NONE',  ( 5.049401038298161559, -19.05341960407611168, 112.7072429386476813 ) ) ;
#197042=ORIENTED_EDGE ( 'NONE', *, *, #158579, .F. ) ;
#197043=CARTESIAN_POINT ( 'NONE',  ( -14.29746914071037622, -8.314922557961029526, 69.16775706135234714 ) ) ;
#197044=CARTESIAN_POINT ( 'NONE',  ( 5.719274019375991003, -21.55341960407610458, 107.7072429386476955 ) ) ;
#197045=CARTESIAN_POINT ( 'NONE',  ( -16.46253265017160317, 9.564922557960807481, 65.83224293864769550 ) ) ;
#197046=CARTESIAN_POINT ( 'NONE',  ( -18.62759615963255300, -10.81492255796106328, 39.16775706135235424 ) ) ;
#197047=CARTESIAN_POINT ( 'NONE',  ( -9.474510206698964154, 16.51473224551069663, 100.4155762719810241 ) ) ;
#197050=CARTESIAN_POINT ( 'NONE',  ( 21.52544592524334988, 5.823673210054432836, 31.45942372801901854 ) ) ;
#197051=CARTESIAN_POINT ( 'NONE',  ( 19.05341960407611168, 5.049401038298154454, 23.95724293864769194 ) ) ;
#197052=CARTESIAN_POINT ( 'NONE',  ( -5.049401038297874678, -19.05341960407617918, 89.79275706135230450 ) ) ;
#197053=CARTESIAN_POINT ( 'NONE',  ( 0.05219959533936267826, -19.03943276465977164, 40.00109039468566152 ) ) ;
#197054=CARTESIAN_POINT ( 'NONE',  ( -5.823673210054116645, -21.52544592524344225, 102.2905762719810383 ) ) ;
#197055=CARTESIAN_POINT ( 'NONE',  ( -13.97604488694547697, 13.89961937509957934, 33.12609039468566863 ) ) ;
#197056=CARTESIAN_POINT ( 'NONE',  ( -0.05219959533936034679, 19.03943276465977164, 47.50109039468566863 ) ) ;
#197057=CARTESIAN_POINT ( 'NONE',  ( -4.379528057220086978, -16.55341960407618274, 89.79275706135236135 ) ) ;
#197058=CARTESIAN_POINT ( 'NONE',  ( 16.51473224551069308, 9.474510206698969483, 114.1655762719810241 ) ) ;
#197059=ORIENTED_EDGE ( 'NONE', *, *, #149169, .F. ) ;
#197060=CARTESIAN_POINT ( 'NONE',  ( 19.05341960407611168, 5.049401038298154454, 78.95724293864769550 ) ) ;
#197061=CARTESIAN_POINT ( 'NONE',  ( 10.72451020669871369, 18.67979575497193778, 82.08442372801901854 ) ) ;
#197062=CARTESIAN_POINT ( 'NONE',  ( 5.823673210054444382, -21.52544592524334988, 90.20942372801903275 ) ) ;
#197064=CARTESIAN_POINT ( 'NONE',  ( -5.153800228976328057, -19.02544592524343514, 87.29057627198103830 ) ) ;
#197065=CARTESIAN_POINT ( 'NONE',  ( 18.67979575497194134, -10.72451020669871369, 60.83442372801901854 ) ) ;
#197066=CARTESIAN_POINT ( 'NONE',  ( 13.89961937509957401, 13.97604488694547697, 106.8760903946856757 ) ) ;
#197067=EDGE_CURVE ( 'NONE', #40368, #16134, #30519, .T. ) ;
#197068=CARTESIAN_POINT ( 'NONE',  ( 9.564922557960805705, 16.46253265017160317, 59.58224293864769550 ) ) ;
#197069=CARTESIAN_POINT ( 'NONE',  ( -5.049401038298153566, 19.05341960407611168, 115.2072429386477097 ) ) ;
#197070=CARTESIAN_POINT ( 'NONE',  ( -5.153800228976328057, -19.02544592524343514, 82.29057627198103830 ) ) ;
#197072=CARTESIAN_POINT ( 'NONE',  ( -5.153800228976328057, -19.02544592524343514, 67.29057627198102409 ) ) ;
#197073=CARTESIAN_POINT ( 'NONE',  ( -16.46253265017160317, 9.564922557960807481, 45.83224293864769550 ) ) ;
#197074=CARTESIAN_POINT ( 'NONE',  ( -15.72974639402176322, -15.80617190586768395, 19.37609039468568639 ) ) ;
#197075=CARTESIAN_POINT ( 'NONE',  ( 4.379528057220092307, 16.55341960407617563, 82.29275706135234714 ) ) ;
#197077=CARTESIAN_POINT ( 'NONE',  ( -19.02544592524334988, -5.153800228976617603, 48.95942372801900433 ) ) ;
#197078=CARTESIAN_POINT ( 'NONE',  ( -19.02544592524342804, 5.153800228976336051, 86.04057627198103830 ) ) ;
#197079=CARTESIAN_POINT ( 'NONE',  ( -4.483927247898539470, -16.52544592524342804, 67.29057627198103830 ) ) ;
#197080=CARTESIAN_POINT ( 'NONE',  ( 12.06949235617757843, -12.14591786802309237, 113.1239096053143953 ) ) ;
#197081=CARTESIAN_POINT ( 'NONE',  ( 18.67979575497178502, 10.72451020669898547, 24.16557627198103120 ) ) ;
#197082=CARTESIAN_POINT ( 'NONE',  ( 5.049401038298161559, -19.05341960407611168, 107.7072429386476955 ) ) ;
#197083=CARTESIAN_POINT ( 'NONE',  ( 14.29746914071049879, -8.314922557960816363, 73.33224293864769550 ) ) ;
#197085=CARTESIAN_POINT ( 'NONE',  ( 13.97604488694548053, -13.89961937509957401, 30.62609039468566863 ) ) ;
#197086=CARTESIAN_POINT ( 'NONE',  ( 8.314922557961029526, -14.29746914071037800, 100.4177570613523471 ) ) ;
#197087=CARTESIAN_POINT ( 'NONE',  ( 13.97604488694527802, 13.89961937509977652, 84.37390960531433848 ) ) ;
#197088=CARTESIAN_POINT ( 'NONE',  ( -15.72974639402176322, -15.80617190586768395, 59.37609039468568284 ) ) ;
#197089=CARTESIAN_POINT ( 'NONE',  ( -0.05219959533907301413, -21.53943276465977519, 42.49890960531435979 ) ) ;
#197090=CARTESIAN_POINT ( 'NONE',  ( -15.72974639402197994, 15.80617190586746368, 110.6239096053143669 ) ) ;
#197091=CARTESIAN_POINT ( 'NONE',  ( 0.05219959533907565091, 21.53943276465977519, 64.99890960531435269 ) ) ;
#197092=CARTESIAN_POINT ( 'NONE',  ( -16.53943276465976808, 0.05219959533911058130, 101.2489096053143669 ) ) ;
#197093=CARTESIAN_POINT ( 'NONE',  ( 9.474510206698729675, 16.51473224551082808, 57.08442372801900433 ) ) ;
#197094=CARTESIAN_POINT ( 'NONE',  ( -5.049401038298153566, 19.05341960407611168, 25.20724293864768484 ) ) ;
#197095=CARTESIAN_POINT ( 'NONE',  ( 5.049401038298161559, -19.05341960407611168, 77.70724293864765286 ) ) ;
#197096=CARTESIAN_POINT ( 'NONE',  ( 13.89961937509977652, -13.97604488694527269, 78.12390960531433848 ) ) ;
#197097=CARTESIAN_POINT ( 'NONE',  ( 8.314922557960818139, 14.29746914071049879, 99.58224293864770971 ) ) ;
#197099=CARTESIAN_POINT ( 'NONE',  ( -4.379528057220328563, 16.55341960407611168, 25.20724293864769550 ) ) ;
#197100=CARTESIAN_POINT ( 'NONE',  ( -8.224510206698735004, -14.34966873604973081, 44.58442372801901854 ) ) ;
#197101=CARTESIAN_POINT ( 'NONE',  ( -10.81492255796105439, 18.62759615963255655, 102.9177570613523756 ) ) ;
#197102=CARTESIAN_POINT ( 'NONE',  ( -13.89961937509977652, 13.97604488694528158, 95.62390960531436690 ) ) ;
#197103=CARTESIAN_POINT ( 'NONE',  ( -21.52544592524334988, -5.823673210054445271, 33.95942372801901143 ) ) ;
#197104=CARTESIAN_POINT ( 'NONE',  ( 13.97604488694527802, 13.89961937509977652, 44.37390960531435269 ) ) ;
#197105=CARTESIAN_POINT ( 'NONE',  ( 4.483927247898790824, -16.52544592524335698, 45.20942372801901854 ) ) ;
#197106=CARTESIAN_POINT ( 'NONE',  ( 19.03943276465977164, 0.05219959533936151252, 111.2510903946856757 ) ) ;
#197107=CARTESIAN_POINT ( 'NONE',  ( 9.564922557960805705, 16.46253265017160317, 34.58224293864770260 ) ) ;
#197108=CARTESIAN_POINT ( 'NONE',  ( -16.53943276465976808, 0.05219959533911058130, 91.24890960531436690 ) ) ;
#197109=CARTESIAN_POINT ( 'NONE',  ( 21.53943276465977519, -0.05219959533907433946, 103.7489096053143669 ) ) ;
#197110=CARTESIAN_POINT ( 'NONE',  ( 13.97604488694548053, -13.89961937509957401, 75.62609039468564731 ) ) ;
#197111=CARTESIAN_POINT ( 'NONE',  ( -13.97604488694527625, -13.89961937509977652, 86.87390960531436690 ) ) ;
#197112=CARTESIAN_POINT ( 'NONE',  ( -21.52544592524334988, -5.823673210054445271, 33.95942372801901143 ) ) ;
#197113=CARTESIAN_POINT ( 'NONE',  ( -19.05341960407611168, -5.049401038298163336, 21.45724293864768839 ) ) ;
#197114=CARTESIAN_POINT ( 'NONE',  ( 5.049401038298161559, -19.05341960407611168, 92.70724293864769550 ) ) ;
#197116=CARTESIAN_POINT ( 'NONE',  ( 5.153800228976335163, 19.02544592524342804, 84.79057627198099567 ) ) ;
#197117=CARTESIAN_POINT ( 'NONE',  ( -10.81492255796105439, 18.62759615963255655, 32.91775706135234714 ) ) ;
#197118=CARTESIAN_POINT ( 'NONE',  ( 0.05219959533910956823, 16.53943276465976808, 89.99890960531438111 ) ) ;
#197119=CARTESIAN_POINT ( 'NONE',  ( -9.564922557960796823, -16.46253265017161027, 102.0822429386477097 ) ) ;
#197120=CARTESIAN_POINT ( 'NONE',  ( -18.67979575497193778, 10.72451020669871902, 113.3344237280190328 ) ) ;
#197121=CARTESIAN_POINT ( 'NONE',  ( 4.483927247898790824, -16.52544592524335698, 55.20942372801902565 ) ) ;
#197122=CARTESIAN_POINT ( 'NONE',  ( -15.80617190586768217, 15.72974639402176855, 73.12609039468567573 ) ) ;
#197123=CARTESIAN_POINT ( 'NONE',  ( 14.34966873604972726, -8.224510206698740333, 25.83442372801901499 ) ) ;
#197124=CARTESIAN_POINT ( 'NONE',  ( -13.97604488694527625, -13.89961937509977652, 71.87390960531433848 ) ) ;
#197125=CARTESIAN_POINT ( 'NONE',  ( 5.153800228976615827, -19.02544592524334988, 95.20942372801897591 ) ) ;
#197126=CARTESIAN_POINT ( 'NONE',  ( -4.483927247898782831, 16.52544592524335698, 72.70942372801901854 ) ) ;
#197127=CARTESIAN_POINT ( 'NONE',  ( -5.049401038297874678, -19.05341960407617918, 19.79275706135233293 ) ) ;
#197128=CARTESIAN_POINT ( 'NONE',  ( -5.049401038297874678, -19.05341960407617918, 79.79275706135233293 ) ) ;
#197129=CARTESIAN_POINT ( 'NONE',  ( -5.153800228976328057, -19.02544592524343514, 67.29057627198102409 ) ) ;
#197130=CARTESIAN_POINT ( 'NONE',  ( 5.719274019375991003, -21.55341960407610458, 82.70724293864770971 ) ) ;
#197131=CARTESIAN_POINT ( 'NONE',  ( 4.483927247898545687, 16.52544592524342804, 74.79057627198105251 ) ) ;
#197132=CARTESIAN_POINT ( 'NONE',  ( 19.02544592524334988, 5.153800228976608722, 76.45942372801897591 ) ) ;
#197133=CARTESIAN_POINT ( 'NONE',  ( 16.61371651742597777, -7.165104196376198331, 61.35415069993000259 ) ) ;
#197134=CARTESIAN_POINT ( 'NONE',  ( 5.153800228976615827, -19.02544592524334988, 60.20942372801899012 ) ) ;
#197135=CARTESIAN_POINT ( 'NONE',  ( -4.483927247898539470, -16.52544592524342804, 22.29057627198102765 ) ) ;
#197136=CARTESIAN_POINT ( 'NONE',  ( -14.29746914071049879, 8.314922557960819915, 85.83224293864768129 ) ) ;
#197137=CARTESIAN_POINT ( 'NONE',  ( -9.474510206698720793, -16.51473224551083518, 24.58442372801900078 ) ) ;
#197139=CARTESIAN_POINT ( 'NONE',  ( 5.823673210054125526, 21.52544592524343514, 114.7905762719810383 ) ) ;
#197140=CARTESIAN_POINT ( 'NONE',  ( -0.05219959533909027116, -19.03943276465977164, 107.4989096053143527 ) ) ;
#197141=CARTESIAN_POINT ( 'NONE',  ( -16.46253265017160317, 9.564922557960807481, 70.83224293864770971 ) ) ;
#197142=CARTESIAN_POINT ( 'NONE',  ( 10.72451020669871369, 18.67979575497193778, 87.08442372801901854 ) ) ;
#197143=CARTESIAN_POINT ( 'NONE',  ( 0.05219959533909260263, 19.03943276465977164, 59.99890960531436690 ) ) ;
#197145=CARTESIAN_POINT ( 'NONE',  ( -9.474510206698964154, 16.51473224551069663, 35.41557627198102409 ) ) ;
#197146=CARTESIAN_POINT ( 'NONE',  ( 0.05219959533907565091, 21.53943276465977519, 24.99890960531435624 ) ) ;
#197147=CARTESIAN_POINT ( 'NONE',  ( 16.55341960407611168, 4.379528057220329451, 63.95724293864770260 ) ) ;
#197148=CARTESIAN_POINT ( 'NONE',  ( -19.03943276465977164, 0.05219959533909376836, 41.24890960531435269 ) ) ;
#197149=CARTESIAN_POINT ( 'NONE',  ( 16.55341960407611168, 4.379528057220329451, 103.9572429386476813 ) ) ;
#197150=CARTESIAN_POINT ( 'NONE',  ( -18.62759615963270932, 10.81492255796079327, 115.8322429386477097 ) ) ;
#197152=CARTESIAN_POINT ( 'NONE',  ( -5.823673210054431948, 21.52544592524334988, 47.70942372801902565 ) ) ;
#197153=CARTESIAN_POINT ( 'NONE',  ( -19.02544592524342804, 5.153800228976336051, 36.04057627198100988 ) ) ;
#197154=CARTESIAN_POINT ( 'NONE',  ( 16.52544592524335698, 4.483927247898782831, 61.45942372801901854 ) ) ;
#197155=CARTESIAN_POINT ( 'NONE',  ( -21.52544592524343514, 5.823673210054127303, 106.0405762719810525 ) ) ;
#197156=CARTESIAN_POINT ( 'NONE',  ( -10.72451020669898014, 18.67979575497178502, 95.41557627198102409 ) ) ;
#197157=CARTESIAN_POINT ( 'NONE',  ( 16.46253265017146816, 9.564922557961045513, 31.66775706135232937 ) ) ;
#197158=CARTESIAN_POINT ( 'NONE',  ( -19.03943276465977164, 0.05219959533909376836, 46.24890960531435979 ) ) ;
#197160=CARTESIAN_POINT ( 'NONE',  ( -18.67979575497193778, 10.72451020669871902, 63.33442372801900433 ) ) ;
#197161=CARTESIAN_POINT ( 'NONE',  ( -18.67979575497178146, -10.72451020669898902, 56.66557627198103830 ) ) ;
#197162=CARTESIAN_POINT ( 'NONE',  ( -8.224510206698948167, 14.34966873604960824, 30.41557627198101699 ) ) ;
#197163=CARTESIAN_POINT ( 'NONE',  ( -5.823673210054431948, 21.52544592524334988, 77.70942372801900433 ) ) ;
#197164=CARTESIAN_POINT ( 'NONE',  ( 21.53943276465977519, 0.05219959533937863772, 111.2510903946856899 ) ) ;
#197165=CARTESIAN_POINT ( 'NONE',  ( -5.049401038297874678, -19.05341960407617918, 49.79275706135231871 ) ) ;
#197166=CARTESIAN_POINT ( 'NONE',  ( -12.14591786802326823, 12.06949235617739902, 108.1260903946856757 ) ) ;
#197167=CARTESIAN_POINT ( 'NONE',  ( -5.823673210054431948, 21.52544592524334988, 52.70942372801902565 ) ) ;
#197169=CARTESIAN_POINT ( 'NONE',  ( 13.89961937509977652, -13.97604488694527269, 63.12390960531435979 ) ) ;
#197170=CARTESIAN_POINT ( 'NONE',  ( 5.049401038297881783, 19.05341960407617563, 37.29275706135232582 ) ) ;
#197171=CARTESIAN_POINT ( 'NONE',  ( 5.719274019375991003, -21.55341960407610458, 37.70724293864769550 ) ) ;
#197172=CARTESIAN_POINT ( 'NONE',  ( -5.719274019375665041, -21.55341960407619695, 29.79275706135234358 ) ) ;
#197173=CARTESIAN_POINT ( 'NONE',  ( -18.62759615963270932, 10.81492255796079327, 85.83224293864768129 ) ) ;
#197174=CARTESIAN_POINT ( 'NONE',  ( -0.05219959533936034679, 19.03943276465977164, 82.50109039468567573 ) ) ;
#197175=CARTESIAN_POINT ( 'NONE',  ( -16.52544592524335698, -4.483927247898792601, 48.95942372801902565 ) ) ;
#197177=CARTESIAN_POINT ( 'NONE',  ( 10.81492255796078972, 18.62759615963270932, 94.58224293864769550 ) ) ;
#197178=CARTESIAN_POINT ( 'NONE',  ( 16.53943276465976808, 0.05219959533934440121, 81.25109039468568994 ) ) ;
#197179=CARTESIAN_POINT ( 'NONE',  ( -12.14591786802309592, -12.06949235617757132, 81.87390960531435269 ) ) ;
#197181=CARTESIAN_POINT ( 'NONE',  ( -5.049401038297874678, -19.05341960407617918, 99.79275706135234714 ) ) ;
#197182=CARTESIAN_POINT ( 'NONE',  ( -18.62759615963270932, 10.81492255796079327, 35.83224293864768839 ) ) ;
#197185=CARTESIAN_POINT ( 'NONE',  ( -16.52544592524335698, -4.483927247898792601, 58.95942372801902565 ) ) ;
#197186=CARTESIAN_POINT ( 'NONE',  ( -21.55341960407619339, 5.719274019375674811, 28.54275706135234358 ) ) ;
#197187=CARTESIAN_POINT ( 'NONE',  ( -21.55341960407610458, -5.719274019375992779, 31.45724293864769550 ) ) ;
#197188=CARTESIAN_POINT ( 'NONE',  ( -8.224510206698735004, -14.34966873604973081, 74.58442372801901854 ) ) ;
#197189=CARTESIAN_POINT ( 'NONE',  ( -16.46253265017160317, 9.564922557960807481, 85.83224293864769550 ) ) ;
#197190=CARTESIAN_POINT ( 'NONE',  ( 10.81492255796106328, -18.62759615963255655, 55.41775706135234714 ) ) ;
#197191=CARTESIAN_POINT ( 'NONE',  ( 9.474510206698971260, -16.51473224551069308, 27.91557627198103120 ) ) ;
#197192=CARTESIAN_POINT ( 'NONE',  ( -0.05219959533907301413, -21.53943276465977519, 27.49890960531435269 ) ) ;
#197194=CARTESIAN_POINT ( 'NONE',  ( 16.46253265017146816, 9.564922557961045513, 36.66775706135233293 ) ) ;
#197195=CARTESIAN_POINT ( 'NONE',  ( 12.06949235617739724, 12.14591786802326823, 51.87609039468568284 ) ) ;
#197196=CARTESIAN_POINT ( 'NONE',  ( 5.719274019375991003, -21.55341960407610458, 22.70724293864769194 ) ) ;
#197197=CARTESIAN_POINT ( 'NONE',  ( -0.05219959533909027116, -19.03943276465977164, 67.49890960531436690 ) ) ;
#197198=CARTESIAN_POINT ( 'NONE',  ( -4.379528057220086978, -16.55341960407618274, 104.7927570613523898 ) ) ;
#197199=CARTESIAN_POINT ( 'NONE',  ( -13.89961937509977652, 13.97604488694528158, 115.6239096053143669 ) ) ;
#197200=CARTESIAN_POINT ( 'NONE',  ( -16.52544592524342804, 4.483927247898546575, 96.04057627198102409 ) ) ;
#197201=CARTESIAN_POINT ( 'NONE',  ( 18.62759615963271287, -10.81492255796078972, 33.33224293864769550 ) ) ;
#197202=CARTESIAN_POINT ( 'NONE',  ( 19.02544592524343514, -5.153800228976328945, 33.54057627198102409 ) ) ;
#197203=CARTESIAN_POINT ( 'NONE',  ( 12.06949235617739724, 12.14591786802326823, 71.87609039468568994 ) ) ;
#197204=CARTESIAN_POINT ( 'NONE',  ( -0.05219959533907301413, -21.53943276465977519, 112.4989096053143669 ) ) ;
#197205=CARTESIAN_POINT ( 'NONE',  ( -5.153800228976607833, 19.02544592524334988, 72.70942372801900433 ) ) ;
#197206=CARTESIAN_POINT ( 'NONE',  ( -9.564922557960796823, -16.46253265017161027, 42.08224293864769550 ) ) ;
#197207=CARTESIAN_POINT ( 'NONE',  ( 21.55341960407610458, 5.719274019375980345, 68.95724293864769550 ) ) ;
#197209=CARTESIAN_POINT ( 'NONE',  ( 18.67979575497194134, -10.72451020669871369, 95.83442372801903275 ) ) ;
#197210=CARTESIAN_POINT ( 'NONE',  ( 16.46253265017160672, -9.564922557960803928, 58.33224293864769550 ) ) ;
#197211=CARTESIAN_POINT ( 'NONE',  ( -12.14591786802326823, 12.06949235617739902, 48.12609039468568284 ) ) ;
#197212=CARTESIAN_POINT ( 'NONE',  ( -10.81492255796105439, 18.62759615963255655, 82.91775706135234714 ) ) ;
#197213=CARTESIAN_POINT ( 'NONE',  ( 5.153800228976615827, -19.02544592524334988, 45.20942372801901143 ) ) ;
#197215=CARTESIAN_POINT ( 'NONE',  ( 13.97604488694548053, -13.89961937509957401, 55.62609039468566863 ) ) ;
#197217=CARTESIAN_POINT ( 'NONE',  ( 10.81492255796106328, -18.62759615963255655, 50.41775706135235424 ) ) ;
#197218=CARTESIAN_POINT ( 'NONE',  ( -13.89961937509977830, 13.97604488694528158, 55.62390960531435269 ) ) ;
#197219=CARTESIAN_POINT ( 'NONE',  ( 13.97604488694548053, -13.89961937509957401, 45.62609039468566863 ) ) ;
#197220=CARTESIAN_POINT ( 'NONE',  ( -19.05341960407611168, -5.049401038298163336, 106.4572429386476955 ) ) ;
#197221=CARTESIAN_POINT ( 'NONE',  ( 5.049401038298161559, -19.05341960407611168, 87.70724293864769550 ) ) ;
#197222=CARTESIAN_POINT ( 'NONE',  ( 16.53943276465976808, -0.05219959533910856209, 43.74890960531435979 ) ) ;
#197223=CARTESIAN_POINT ( 'NONE',  ( 5.823673210054125526, 21.52544592524343514, 39.79057627198103830 ) ) ;
#197226=CARTESIAN_POINT ( 'NONE',  ( -18.62759615963255300, -10.81492255796106328, 94.16775706135237556 ) ) ;
#197228=CARTESIAN_POINT ( 'NONE',  ( 13.89961937509977652, -13.97604488694527269, 38.12390960531436690 ) ) ;
#197231=CARTESIAN_POINT ( 'NONE',  ( 14.29746914071037800, 8.314922557961029526, 56.66775706135235424 ) ) ;
#197232=CARTESIAN_POINT ( 'NONE',  ( -15.80617190586745835, -15.72974639402198527, 76.87390960531439532 ) ) ;
#197233=CARTESIAN_POINT ( 'NONE',  ( -12.06949235617756955, 12.14591786802309770, 35.62390960531437401 ) ) ;
#197234=CARTESIAN_POINT ( 'NONE',  ( 9.564922557960805705, 16.46253265017160317, 29.58224293864769550 ) ) ;
#197235=CARTESIAN_POINT ( 'NONE',  ( 13.97604488694527802, 13.89961937509977652, 114.3739096053143669 ) ) ;
#197236=CARTESIAN_POINT ( 'NONE',  ( 10.81492255796106328, -18.62759615963255655, 25.41775706135235779 ) ) ;
#197237=CARTESIAN_POINT ( 'NONE',  ( -19.05341960407617563, 5.049401038297882671, 38.54275706135233293 ) ) ;
#197238=CARTESIAN_POINT ( 'NONE',  ( -16.46253265017160317, 9.564922557960807481, 25.83224293864769194 ) ) ;
#197239=CARTESIAN_POINT ( 'NONE',  ( -10.81492255796105439, 18.62759615963255655, 77.91775706135231871 ) ) ;
#197240=CARTESIAN_POINT ( 'NONE',  ( 17.48847506799968343, -5.747544572773782612, 33.32697437843281563 ) ) ;
#197241=CARTESIAN_POINT ( 'NONE',  ( -8.224510206698948167, 14.34966873604960824, 25.41557627198103120 ) ) ;
#197243=CARTESIAN_POINT ( 'NONE',  ( -18.67979575497178146, -10.72451020669898902, 31.66557627198102054 ) ) ;
#197244=CARTESIAN_POINT ( 'NONE',  ( -12.06949235617756955, 12.14591786802309770, 85.62390960531436690 ) ) ;
#197246=CARTESIAN_POINT ( 'NONE',  ( -0.05219959533909027116, -19.03943276465977164, 87.49890960531436690 ) ) ;
#197247=CARTESIAN_POINT ( 'NONE',  ( -16.52544592524342804, 4.483927247898546575, 81.04057627198102409 ) ) ;
#197248=CARTESIAN_POINT ( 'NONE',  ( -13.89961937509957401, -13.97604488694547875, 99.37609039468567573 ) ) ;
#197249=CARTESIAN_POINT ( 'NONE',  ( 18.62759615963271287, -10.81492255796078972, 63.33224293864770260 ) ) ;
#197250=ORIENTED_EDGE ( 'NONE', *, *, #153922, .T. ) ;
#197251=CARTESIAN_POINT ( 'NONE',  ( 5.049401038298161559, -19.05341960407611168, 27.70724293864769550 ) ) ;
#197252=CARTESIAN_POINT ( 'NONE',  ( -5.153800228976328057, -19.02544592524343514, 87.29057627198103830 ) ) ;
#197253=CARTESIAN_POINT ( 'NONE',  ( -21.52544592524343514, 5.823673210054127303, 86.04057627198102409 ) ) ;
#197254=CARTESIAN_POINT ( 'NONE',  ( -16.53943276465976808, -0.05219959533934237506, 98.75109039468568994 ) ) ;
#197255=CARTESIAN_POINT ( 'NONE',  ( 19.05341960407611168, 5.049401038298154454, 93.95724293864769550 ) ) ;
#197256=CARTESIAN_POINT ( 'NONE',  ( 5.049401038297881783, 19.05341960407617563, 62.29275706135234003 ) ) ;
#197257=CARTESIAN_POINT ( 'NONE',  ( 21.53943276465977519, 0.05219959533937863772, 101.2510903946856757 ) ) ;
#197258=CARTESIAN_POINT ( 'NONE',  ( -10.72451020669898014, 18.67979575497178502, 80.41557627198103830 ) ) ;
#197259=CARTESIAN_POINT ( 'NONE',  ( -19.03943276465977164, 0.05219959533909376836, 116.2489096053143669 ) ) ;
#197260=CARTESIAN_POINT ( 'NONE',  ( 0.05219959533909260263, 19.03943276465977164, 54.99890960531435979 ) ) ;
#197261=CARTESIAN_POINT ( 'NONE',  ( 14.29746914071049879, -8.314922557960816363, 23.33224293864769194 ) ) ;
#197262=CARTESIAN_POINT ( 'NONE',  ( 16.51473224551069308, 9.474510206698969483, 59.16557627198102409 ) ) ;
#197264=CARTESIAN_POINT ( 'NONE',  ( 10.81492255796106328, -18.62759615963255655, 105.4177570613523613 ) ) ;
#197265=CARTESIAN_POINT ( 'NONE',  ( 16.52544592524342804, -4.483927247898539470, 73.54057627198102409 ) ) ;
#197266=CARTESIAN_POINT ( 'NONE',  ( 10.72451020669898902, -18.67979575497178502, 107.9155762719810241 ) ) ;
#197267=CARTESIAN_POINT ( 'NONE',  ( -10.81492255796078084, -18.62759615963271287, 107.0822429386476955 ) ) ;
#197269=CARTESIAN_POINT ( 'NONE',  ( 15.72974639402199770, -15.80617190586745480, 63.12390960531435979 ) ) ;
#197270=CARTESIAN_POINT ( 'NONE',  ( 14.34966873604972726, -8.224510206698740333, 80.83442372801901854 ) ) ;
#197271=CARTESIAN_POINT ( 'NONE',  ( 4.483927247898545687, 16.52544592524342804, 99.79057627198103830 ) ) ;
#197272=CARTESIAN_POINT ( 'NONE',  ( 9.564922557960805705, 16.46253265017160317, 54.58224293864769550 ) ) ;
#197273=CARTESIAN_POINT ( 'NONE',  ( -14.34966873604972548, 8.224510206698743886, 113.3344237280190328 ) ) ;
#197274=CARTESIAN_POINT ( 'NONE',  ( -21.55341960407619339, 5.719274019375674811, 48.54275706135234714 ) ) ;
#197275=CARTESIAN_POINT ( 'NONE',  ( -13.89961937509977652, 13.97604488694528158, 115.6239096053143669 ) ) ;
#197276=CARTESIAN_POINT ( 'NONE',  ( 5.823673210054444382, -21.52544592524334988, 85.20942372801901854 ) ) ;
#197277=CARTESIAN_POINT ( 'NONE',  ( 0.05219959533909260263, 19.03943276465977164, 24.99890960531435269 ) ) ;
#197278=CARTESIAN_POINT ( 'NONE',  ( -16.51473224551069308, -9.474510206698971260, 36.66557627198102409 ) ) ;
#197279=EDGE_LOOP ( 'NONE', ( #177185, #7223, #61169, #4446 ) ) ;
#197280=CARTESIAN_POINT ( 'NONE',  ( -0.05219959533937732626, 21.53943276465977519, 82.50109039468568994 ) ) ;
#197281=CARTESIAN_POINT ( 'NONE',  ( 18.62759615963255655, 10.81492255796105972, 66.66775706135234714 ) ) ;
#197282=CARTESIAN_POINT ( 'NONE',  ( -9.564922557960796823, -16.46253265017161027, 107.0822429386476955 ) ) ;
#197283=CARTESIAN_POINT ( 'NONE',  ( -5.049401038297874678, -19.05341960407617918, 84.79275706135233293 ) ) ;
#197284=CARTESIAN_POINT ( 'NONE',  ( -5.719274019375665041, -21.55341960407619695, 54.79275706135235424 ) ) ;
#197285=CARTESIAN_POINT ( 'NONE',  ( 12.06949235617739724, 12.14591786802326823, 26.87609039468567218 ) ) ;
#197286=CARTESIAN_POINT ( 'NONE',  ( -16.46253265017146816, -9.564922557961047289, 74.16775706135234714 ) ) ;
#197287=CARTESIAN_POINT ( 'NONE',  ( 13.89961937509977652, -13.97604488694527269, 48.12390960531435979 ) ) ;
#197288=CARTESIAN_POINT ( 'NONE',  ( -16.51473224551082808, 9.474510206698731452, 88.33442372801900433 ) ) ;
#197289=CARTESIAN_POINT ( 'NONE',  ( 8.314922557960818139, 14.29746914071049879, 29.58224293864769905 ) ) ;
#197290=CARTESIAN_POINT ( 'NONE',  ( -0.05219959533936034679, 19.03943276465977164, 87.50109039468567573 ) ) ;
#197291=CARTESIAN_POINT ( 'NONE',  ( 16.55341960407611168, 4.379528057220329451, 33.95724293864769550 ) ) ;
#197292=CARTESIAN_POINT ( 'NONE',  ( -13.97604488694547697, 13.89961937509957934, 63.12609039468566152 ) ) ;
#197293=CARTESIAN_POINT ( 'NONE',  ( -0.05219959533934338120, 16.53943276465976808, 42.50109039468567573 ) ) ;
#197294=CARTESIAN_POINT ( 'NONE',  ( 13.89961937509957401, 13.97604488694547697, 26.87609039468566507 ) ) ;
#197295=CARTESIAN_POINT ( 'NONE',  ( -19.05341960407611168, -5.049401038298163336, 46.45724293864768129 ) ) ;
#197296=CARTESIAN_POINT ( 'NONE',  ( -16.79531203550648755, -7.028104445595491967, 66.25244988220440234 ) ) ;
#197297=CARTESIAN_POINT ( 'NONE',  ( -4.379528057220086978, -16.55341960407618274, 39.79275706135235424 ) ) ;
#197300=CARTESIAN_POINT ( 'NONE',  ( 19.02544592524343514, -5.153800228976328945, 93.54057627198102409 ) ) ;
#197301=CARTESIAN_POINT ( 'NONE',  ( -18.09867054820432131, -5.499999999999928058, 68.98393025253585620 ) ) ;
#197303=CARTESIAN_POINT ( 'NONE',  ( 19.05341960407617918, -5.049401038297876454, 96.04275706135231871 ) ) ;
#197304=CARTESIAN_POINT ( 'NONE',  ( -21.53943276465977519, 0.05219959533907696930, 21.24890960531436690 ) ) ;
#197305=CARTESIAN_POINT ( 'NONE',  ( 10.81492255796106328, -18.62759615963255655, 110.4177570613523756 ) ) ;
#197306=CARTESIAN_POINT ( 'NONE',  ( 13.97604488694548053, -13.89961937509957401, 105.6260903946856757 ) ) ;
#197307=CARTESIAN_POINT ( 'NONE',  ( 9.474510206698971260, -16.51473224551069308, 22.91557627198102765 ) ) ;
#197308=CARTESIAN_POINT ( 'NONE',  ( 9.564922557960805705, 16.46253265017160317, 39.58224293864768839 ) ) ;
#197309=CARTESIAN_POINT ( 'NONE',  ( 18.67979575497178502, 10.72451020669898547, 54.16557627198103120 ) ) ;
#197310=CARTESIAN_POINT ( 'NONE',  ( 13.97604488694527802, 13.89961937509977652, 24.37390960531435624 ) ) ;
#197312=CARTESIAN_POINT ( 'NONE',  ( 16.46253265017146816, 9.564922557961045513, 71.66775706135233293 ) ) ;
#197313=CARTESIAN_POINT ( 'NONE',  ( -14.29746914071049879, 8.314922557960819915, 55.83224293864770260 ) ) ;
#197314=CARTESIAN_POINT ( 'NONE',  ( -15.80617190586745835, -15.72974639402198527, 36.87390960531435979 ) ) ;
#197315=CARTESIAN_POINT ( 'NONE',  ( -21.53943276465977519, -0.05219959533937600094, 88.75109039468567573 ) ) ;
#197316=CARTESIAN_POINT ( 'NONE',  ( 5.719274019375991003, -21.55341960407610458, 82.70724293864770971 ) ) ;
#197317=CARTESIAN_POINT ( 'NONE',  ( -18.67979575497193778, 10.72451020669871902, 58.33442372801901143 ) ) ;
#197318=CARTESIAN_POINT ( 'NONE',  ( 5.719274019375673035, 21.55341960407619339, 67.29275706135234714 ) ) ;
#197320=CARTESIAN_POINT ( 'NONE',  ( -5.049401038298153566, 19.05341960407611168, 90.20724293864766707 ) ) ;
#197321=CARTESIAN_POINT ( 'NONE',  ( 12.06949235617739724, 12.14591786802326823, 86.87609039468568994 ) ) ;
#197322=CARTESIAN_POINT ( 'NONE',  ( 15.72974639402176855, 15.80617190586768217, 61.87609039468568284 ) ) ;
#197323=CARTESIAN_POINT ( 'NONE',  ( -19.05341960407611168, -5.049401038298163336, 51.45724293864770260 ) ) ;
#197324=CARTESIAN_POINT ( 'NONE',  ( -13.97604488694527625, -13.89961937509977652, 26.87390960531434558 ) ) ;
#197325=CARTESIAN_POINT ( 'NONE',  ( 19.05341960407611168, 5.049401038298154454, 48.95724293864768129 ) ) ;
#197326=CARTESIAN_POINT ( 'NONE',  ( -4.483927247898539470, -16.52544592524342804, 72.29057627198102409 ) ) ;
#197327=CARTESIAN_POINT ( 'NONE',  ( -12.06949235617756955, 12.14591786802309770, 40.62390960531435269 ) ) ;
#197328=CARTESIAN_POINT ( 'NONE',  ( 18.67979575497178502, 10.72451020669898547, 49.16557627198102409 ) ) ;
#197330=CARTESIAN_POINT ( 'NONE',  ( -19.03943276465977164, 0.05219959533909376836, 46.24890960531435979 ) ) ;
#197331=CARTESIAN_POINT ( 'NONE',  ( 10.72451020669898902, -18.67979575497178502, 52.91557627198103830 ) ) ;
#197332=CARTESIAN_POINT ( 'NONE',  ( -5.153800228976607833, 19.02544592524334988, 47.70942372801900433 ) ) ;
#197334=CARTESIAN_POINT ( 'NONE',  ( -12.14591786802309592, -12.06949235617757132, 46.87390960531435979 ) ) ;
#197335=CARTESIAN_POINT ( 'NONE',  ( -5.719274019375978568, 21.55341960407610458, 25.20724293864769550 ) ) ;
#197336=ORIENTED_EDGE ( 'NONE', *, *, #111151, .T. ) ;
#197337=VERTEX_POINT ( 'NONE', #48752 ) ;
#197339=CARTESIAN_POINT ( 'NONE',  ( 16.53943276465976808, 0.05219959533934440121, 76.25109039468568994 ) ) ;
#197340=CARTESIAN_POINT ( 'NONE',  ( -19.03943276465977164, -0.05219959533935918106, 68.75109039468566152 ) ) ;
#197341=CARTESIAN_POINT ( 'NONE',  ( 16.55341960407611168, 4.379528057220329451, 53.95724293864770260 ) ) ;
#197343=CARTESIAN_POINT ( 'NONE',  ( -16.52544592524342804, 4.483927247898546575, 26.04057627198103475 ) ) ;
#197344=CARTESIAN_POINT ( 'NONE',  ( -9.564922557960796823, -16.46253265017161027, 47.08224293864769550 ) ) ;
#197345=CARTESIAN_POINT ( 'NONE',  ( 13.89961937509977652, -13.97604488694527269, 73.12390960531436690 ) ) ;
#197346=CARTESIAN_POINT ( 'NONE',  ( 0.05219959533909260263, 19.03943276465977164, 39.99890960531436690 ) ) ;
#197347=CARTESIAN_POINT ( 'NONE',  ( 21.52544592524334988, 5.823673210054432836, 46.45942372801901854 ) ) ;
#197348=CARTESIAN_POINT ( 'NONE',  ( -5.153800228976328057, -19.02544592524343514, 67.29057627198102409 ) ) ;
#197349=PLANE ( 'NONE',  #164671 ) ;
#197350=CARTESIAN_POINT ( 'NONE',  ( 19.02544592524343514, -5.153800228976328945, 53.54057627198102409 ) ) ;
#197351=CARTESIAN_POINT ( 'NONE',  ( 21.52544592524344225, -5.823673210054117533, 38.54057627198103120 ) ) ;
#197352=CARTESIAN_POINT ( 'NONE',  ( 5.049401038298161559, -19.05341960407611168, 37.70724293864768839 ) ) ;
#197353=CARTESIAN_POINT ( 'NONE',  ( -0.05219959533907301413, -21.53943276465977519, 42.49890960531435979 ) ) ;
#197354=CARTESIAN_POINT ( 'NONE',  ( -14.34966873604972548, 8.224510206698743886, 93.33442372801901854 ) ) ;
#197355=CARTESIAN_POINT ( 'NONE',  ( 16.51473224551083163, -9.474510206698727899, 25.83442372801900078 ) ) ;
#197356=CARTESIAN_POINT ( 'NONE',  ( 16.53943276465976808, 0.05219959533934440121, 46.25109039468567573 ) ) ;
#197357=CARTESIAN_POINT ( 'NONE',  ( -12.06949235617739369, -12.14591786802326823, 74.37609039468568994 ) ) ;
#197358=CARTESIAN_POINT ( 'NONE',  ( 13.97604488694527802, 13.89961937509977652, 104.3739096053143385 ) ) ;
#197359=CARTESIAN_POINT ( 'NONE',  ( 12.06949235617739724, 12.14591786802326823, 66.87609039468568994 ) ) ;
#197360=CARTESIAN_POINT ( 'NONE',  ( 16.55341960407618274, -4.379528057220086978, 36.04275706135234714 ) ) ;
#197361=CARTESIAN_POINT ( 'NONE',  ( 16.51473224551069308, 9.474510206698969483, 109.1655762719810383 ) ) ;
#197362=CARTESIAN_POINT ( 'NONE',  ( -0.05219959533934338120, 16.53943276465976808, 22.50109039468567573 ) ) ;
#197363=CARTESIAN_POINT ( 'NONE',  ( -5.153800228976328057, -19.02544592524343514, 32.29057627198102409 ) ) ;
#197364=CARTESIAN_POINT ( 'NONE',  ( 18.67979575497194134, -10.72451020669871369, 25.83442372801901499 ) ) ;
#197365=CARTESIAN_POINT ( 'NONE',  ( 8.224510206698742110, 14.34966873604972548, 32.08442372801901854 ) ) ;
#197366=CARTESIAN_POINT ( 'NONE',  ( -16.52544592524335698, -4.483927247898792601, 93.95942372801903275 ) ) ;
#197368=CARTESIAN_POINT ( 'NONE',  ( -0.05219959533937732626, 21.53943276465977519, 97.50109039468567573 ) ) ;
#197369=CARTESIAN_POINT ( 'NONE',  ( -9.564922557961040184, 16.46253265017147172, 102.9177570613523329 ) ) ;
#197370=CARTESIAN_POINT ( 'NONE',  ( 14.34966873604960469, 8.224510206698951720, 54.16557627198103120 ) ) ;
#197371=CARTESIAN_POINT ( 'NONE',  ( -16.53943276465976808, 0.05219959533911058130, 116.2489096053143669 ) ) ;
#197372=CARTESIAN_POINT ( 'NONE',  ( 0.05219959533936267826, -19.03943276465977164, 55.00109039468566863 ) ) ;
#197374=CARTESIAN_POINT ( 'NONE',  ( -0.05219959533937732626, 21.53943276465977519, 47.50109039468568994 ) ) ;
#197375=CARTESIAN_POINT ( 'NONE',  ( 8.314922557961029526, -14.29746914071037800, 30.41775706135234358 ) ) ;
#197376=CARTESIAN_POINT ( 'NONE',  ( 17.40861289039002813, 6.110651285853272441, 83.87232470827430575 ) ) ;
#197377=CARTESIAN_POINT ( 'NONE',  ( 9.474510206698971260, -16.51473224551069308, 112.9155762719810383 ) ) ;
#197378=CARTESIAN_POINT ( 'NONE',  ( -10.72451020669898014, 18.67979575497178502, 75.41557627198102409 ) ) ;
#197379=CARTESIAN_POINT ( 'NONE',  ( -13.89961937509957401, -13.97604488694547875, 109.3760903946856331 ) ) ;
#197380=CARTESIAN_POINT ( 'NONE',  ( 16.46253265017160672, -9.564922557960803928, 103.3322429386476955 ) ) ;
#197382=CARTESIAN_POINT ( 'NONE',  ( -13.89961937509977652, 13.97604488694528158, 25.62390960531434558 ) ) ;
#197383=CARTESIAN_POINT ( 'NONE',  ( 15.72974639402176855, 15.80617190586768217, 96.87609039468568994 ) ) ;
#197384=CARTESIAN_POINT ( 'NONE',  ( -19.05341960407611168, -5.049401038298163336, 41.45724293864769550 ) ) ;
#197385=CARTESIAN_POINT ( 'NONE',  ( -10.81492255796105439, 18.62759615963255655, 47.91775706135234714 ) ) ;
#197386=CARTESIAN_POINT ( 'NONE',  ( 21.52544592524334988, 5.823673210054432836, 86.45942372801901854 ) ) ;
#197387=CARTESIAN_POINT ( 'NONE',  ( 16.52544592524335698, 4.483927247898782831, 101.4594237280190185 ) ) ;
#197388=CARTESIAN_POINT ( 'NONE',  ( -19.02544592524342804, 5.153800228976336051, 81.04057627198103830 ) ) ;
#197389=CARTESIAN_POINT ( 'NONE',  ( -21.53943276465977519, -0.05219959533937600094, 38.75109039468567573 ) ) ;
#197390=CARTESIAN_POINT ( 'NONE',  ( 0.05219959533937995610, -21.53943276465977519, 35.00109039468568284 ) ) ;
#197391=CARTESIAN_POINT ( 'NONE',  ( 16.46253265017146816, 9.564922557961045513, 81.66775706135233293 ) ) ;
#197392=CARTESIAN_POINT ( 'NONE',  ( 5.049401038298161559, -19.05341960407611168, 87.70724293864769550 ) ) ;
#197393=CARTESIAN_POINT ( 'NONE',  ( -16.55341960407611168, -4.379528057220339221, 106.4572429386477097 ) ) ;
#197394=CARTESIAN_POINT ( 'NONE',  ( -0.05219959533907301413, -21.53943276465977519, 102.4989096053143811 ) ) ;
#197395=CARTESIAN_POINT ( 'NONE',  ( 16.55341960407611168, 4.379528057220329451, 78.95724293864769550 ) ) ;
#197396=CARTESIAN_POINT ( 'NONE',  ( -15.80617190586768217, 15.72974639402176855, 113.1260903946856899 ) ) ;
#197397=CARTESIAN_POINT ( 'NONE',  ( -8.224510206698948167, 14.34966873604960824, 100.4155762719810241 ) ) ;
#197398=CARTESIAN_POINT ( 'NONE',  ( -5.049401038298153566, 19.05341960407611168, 40.20724293864768839 ) ) ;
#197399=CARTESIAN_POINT ( 'NONE',  ( 13.97604488694548053, -13.89961937509957401, 85.62609039468568994 ) ) ;
#197400=CARTESIAN_POINT ( 'NONE',  ( 16.52544592524342804, -4.483927247898539470, 53.54057627198103120 ) ) ;
#197401=CARTESIAN_POINT ( 'NONE',  ( 5.823673210054444382, -21.52544592524334988, 110.2094237280190185 ) ) ;
#197402=CARTESIAN_POINT ( 'NONE',  ( 5.049401038298161559, -19.05341960407611168, 107.7072429386476955 ) ) ;
#197403=CARTESIAN_POINT ( 'NONE',  ( -16.46253265017146816, -9.564922557961047289, 79.16775706135234714 ) ) ;
#197404=CARTESIAN_POINT ( 'NONE',  ( 0.05219959533907565091, 21.53943276465977519, 84.99890960531436690 ) ) ;
#197405=CARTESIAN_POINT ( 'NONE',  ( -18.62759615963255300, -10.81492255796106328, 29.16775706135234003 ) ) ;
#197406=CARTESIAN_POINT ( 'NONE',  ( -14.34966873604972548, 8.224510206698743886, 33.33442372801900433 ) ) ;
#197407=CARTESIAN_POINT ( 'NONE',  ( 4.379528057220092307, 16.55341960407617563, 97.29275706135234714 ) ) ;
#197408=CARTESIAN_POINT ( 'NONE',  ( 19.02544592524343514, -5.153800228976328945, 28.54057627198102409 ) ) ;
#197409=CARTESIAN_POINT ( 'NONE',  ( 15.80617190586769283, -15.72974639402175789, 35.62609039468568994 ) ) ;
#197410=CARTESIAN_POINT ( 'NONE',  ( -0.05219959533909027116, -19.03943276465977164, 22.49890960531436690 ) ) ;
#197412=CARTESIAN_POINT ( 'NONE',  ( -14.29746914071037622, -8.314922557961029526, 49.16775706135234003 ) ) ;
#197413=CARTESIAN_POINT ( 'NONE',  ( 14.29746914071049879, -8.314922557960816363, 83.33224293864769550 ) ) ;
#197414=CARTESIAN_POINT ( 'NONE',  ( 21.53943276465977519, -0.05219959533907433946, 78.74890960531436690 ) ) ;
#197415=CARTESIAN_POINT ( 'NONE',  ( 12.14591786802309770, 12.06949235617756955, 24.37390960531435979 ) ) ;
#197416=CARTESIAN_POINT ( 'NONE',  ( -4.379528057220086978, -16.55341960407618274, 49.79275706135234714 ) ) ;
#197417=CARTESIAN_POINT ( 'NONE',  ( 19.03943276465977164, -0.05219959533909143690, 43.74890960531435979 ) ) ;
#197418=CARTESIAN_POINT ( 'NONE',  ( 4.379528057220092307, 16.55341960407617563, 92.29275706135236135 ) ) ;
#197419=CARTESIAN_POINT ( 'NONE',  ( 19.02544592524334988, 5.153800228976608722, 81.45942372801897591 ) ) ;
#197420=CARTESIAN_POINT ( 'NONE',  ( -21.52544592524343514, 5.823673210054127303, 81.04057627198102409 ) ) ;
#197421=CARTESIAN_POINT ( 'NONE',  ( 14.34966873604972726, -8.224510206698740333, 105.8344237280190328 ) ) ;
#197424=CARTESIAN_POINT ( 'NONE',  ( 5.823673210054125526, 21.52544592524343514, 64.79057627198103830 ) ) ;
#197425=ORIENTED_EDGE ( 'NONE', *, *, #151324, .F. ) ;
#197426=CARTESIAN_POINT ( 'NONE',  ( 14.29746914071037800, 8.314922557961029526, 86.66775706135234714 ) ) ;
#197428=CARTESIAN_POINT ( 'NONE',  ( 15.72974639402199770, -15.80617190586745480, 33.12390960531435979 ) ) ;
#197429=CARTESIAN_POINT ( 'NONE',  ( -19.36337904590692460, 5.499999999999953815, 75.41494137495618588 ) ) ;
#197430=CARTESIAN_POINT ( 'NONE',  ( -10.81492255796078084, -18.62759615963271287, 77.08224293864769550 ) ) ;
#197431=CARTESIAN_POINT ( 'NONE',  ( 12.14591786802309770, 12.06949235617756955, 24.37390960531435979 ) ) ;
#197432=CARTESIAN_POINT ( 'NONE',  ( 19.02544592524334988, 5.153800228976608722, 111.4594237280190043 ) ) ;
#197433=CARTESIAN_POINT ( 'NONE',  ( -16.46253265017160317, 9.564922557960807481, 40.83224293864769550 ) ) ;
#197434=CARTESIAN_POINT ( 'NONE',  ( -12.14591786802326823, 12.06949235617739902, 28.12609039468568284 ) ) ;
#197435=CARTESIAN_POINT ( 'NONE',  ( 9.564922557960805705, 16.46253265017160317, 59.58224293864769550 ) ) ;
#197437=CARTESIAN_POINT ( 'NONE',  ( -5.153800228976328057, -19.02544592524343514, 107.2905762719810383 ) ) ;
#197438=CARTESIAN_POINT ( 'NONE',  ( -19.05341960407611168, -5.049401038298163336, 101.4572429386476955 ) ) ;
#197439=CARTESIAN_POINT ( 'NONE',  ( 16.55341960407618274, -4.379528057220086978, 86.04275706135236135 ) ) ;
#197440=CARTESIAN_POINT ( 'NONE',  ( -9.474510206698720793, -16.51473224551083518, 94.58442372801900433 ) ) ;
#197441=CARTESIAN_POINT ( 'NONE',  ( -13.97604488694547697, 13.89961937509957934, 33.12609039468566863 ) ) ;
#197442=CARTESIAN_POINT ( 'NONE',  ( -15.72974639402197994, 15.80617190586746368, 80.62390960531438111 ) ) ;
#197443=CARTESIAN_POINT ( 'NONE',  ( -16.52544592524335698, -4.483927247898792601, 98.95942372801903275 ) ) ;
#197444=CARTESIAN_POINT ( 'NONE',  ( -10.72451020669898014, 18.67979575497178502, 30.41557627198101699 ) ) ;
#197445=CARTESIAN_POINT ( 'NONE',  ( -16.51473224551082808, 9.474510206698731452, 98.33442372801900433 ) ) ;
#197446=CARTESIAN_POINT ( 'NONE',  ( 0.05219959533909260263, 19.03943276465977164, 44.99890960531435979 ) ) ;
#197447=CARTESIAN_POINT ( 'NONE',  ( 19.02544592524343514, -5.153800228976328945, 88.54057627198102409 ) ) ;
#197448=CARTESIAN_POINT ( 'NONE',  ( 21.52544592524334988, 5.823673210054432836, 61.45942372801901854 ) ) ;
#197449=CARTESIAN_POINT ( 'NONE',  ( -16.51473224551069308, -9.474510206698971260, 61.66557627198103120 ) ) ;
#197450=CARTESIAN_POINT ( 'NONE',  ( -4.483927247898539470, -16.52544592524342804, 82.29057627198103830 ) ) ;
#197451=CARTESIAN_POINT ( 'NONE',  ( -17.48847506799969054, -5.747544572773762184, 84.17302562156724832 ) ) ;
#197452=CARTESIAN_POINT ( 'NONE',  ( 12.14591786802309770, 12.06949235617756955, 84.37390960531438111 ) ) ;
#197453=CARTESIAN_POINT ( 'NONE',  ( 21.52544592524344225, -5.823673210054117533, 73.54057627198102409 ) ) ;
#197454=CARTESIAN_POINT ( 'NONE',  ( 16.51473224551083163, -9.474510206698727899, 95.83442372801900433 ) ) ;
#197455=CARTESIAN_POINT ( 'NONE',  ( 18.87255363501903105, 5.500000000000005329, 93.82513748171824375 ) ) ;
#197456=CARTESIAN_POINT ( 'NONE',  ( -19.05341960407617563, 5.049401038297882671, 38.54275706135233293 ) ) ;
#197457=CARTESIAN_POINT ( 'NONE',  ( 17.50000000000000711, -5.622605283950830923, 71.18792689403890961 ) ) ;
#197458=CARTESIAN_POINT ( 'NONE',  ( -13.97604488694527625, -13.89961937509977652, 76.87390960531433848 ) ) ;
#197459=CARTESIAN_POINT ( 'NONE',  ( -13.89961937509977652, 13.97604488694528158, 80.62390960531436690 ) ) ;
#197460=CARTESIAN_POINT ( 'NONE',  ( 16.53943276465976808, 0.05219959533934440121, 66.25109039468567573 ) ) ;
#197462=CARTESIAN_POINT ( 'NONE',  ( -19.02544592524334988, -5.153800228976617603, 43.95942372801899012 ) ) ;
#197464=CARTESIAN_POINT ( 'NONE',  ( -9.474510206698964154, 16.51473224551069663, 105.4155762719810383 ) ) ;
#197465=CARTESIAN_POINT ( 'NONE',  ( 4.379528057220092307, 16.55341960407617563, 107.2927570613523471 ) ) ;
#197467=CARTESIAN_POINT ( 'NONE',  ( -8.314922557961024197, 14.29746914071037800, 77.91775706135231871 ) ) ;
#197468=CARTESIAN_POINT ( 'NONE',  ( -17.48847506799968698, 5.747544572773788829, 30.82697437843281207 ) ) ;
#197469=CARTESIAN_POINT ( 'NONE',  ( 4.379528057220092307, 16.55341960407617563, 57.29275706135234714 ) ) ;
#197471=CARTESIAN_POINT ( 'NONE',  ( 0.05219959533937995610, -21.53943276465977519, 70.00109039468568994 ) ) ;
#197472=CARTESIAN_POINT ( 'NONE',  ( -16.46253265017146816, -9.564922557961047289, 79.16775706135234714 ) ) ;
#197473=CARTESIAN_POINT ( 'NONE',  ( 16.46253265017146816, 9.564922557961045513, 26.66775706135234003 ) ) ;
#197474=CARTESIAN_POINT ( 'NONE',  ( 16.46253265017160672, -9.564922557960803928, 48.33224293864769550 ) ) ;
#197475=CARTESIAN_POINT ( 'NONE',  ( 16.46253265017160672, -9.564922557960803928, 38.33224293864768839 ) ) ;
#197477=CARTESIAN_POINT ( 'NONE',  ( 15.72974639402199770, -15.80617190586745480, 68.12390960531436690 ) ) ;
#197478=CARTESIAN_POINT ( 'NONE',  ( -15.80617190586745835, -15.72974639402198527, 31.87390960531435979 ) ) ;
#197479=CARTESIAN_POINT ( 'NONE',  ( -14.29746914071049879, 8.314922557960819915, 115.8322429386477097 ) ) ;
#197480=CARTESIAN_POINT ( 'NONE',  ( 8.224510206698742110, 14.34966873604972548, 47.08442372801901854 ) ) ;
#197482=CARTESIAN_POINT ( 'NONE',  ( 5.823673210054444382, -21.52544592524334988, 35.20942372801901854 ) ) ;
#197483=CARTESIAN_POINT ( 'NONE',  ( -12.14591786802309592, -12.06949235617757132, 56.87390960531436690 ) ) ;
#197485=CARTESIAN_POINT ( 'NONE',  ( -16.53943276465976808, -0.05219959533934237506, 28.75109039468567929 ) ) ;
#197486=CARTESIAN_POINT ( 'NONE',  ( -13.89961937509957401, -13.97604488694547875, 39.37609039468566152 ) ) ;
#197487=CARTESIAN_POINT ( 'NONE',  ( 16.55341960407611168, 4.379528057220329451, 48.95724293864770971 ) ) ;
#197488=CARTESIAN_POINT ( 'NONE',  ( 21.52544592524344225, -5.823673210054117533, 113.5405762719810383 ) ) ;
#197489=CARTESIAN_POINT ( 'NONE',  ( -13.89961937509977830, 13.97604488694528158, 100.6239096053143669 ) ) ;
#197490=CARTESIAN_POINT ( 'NONE',  ( 5.823673210054125526, 21.52544592524343514, 79.79057627198102409 ) ) ;
#197491=CARTESIAN_POINT ( 'NONE',  ( 0.05219959533909260263, 19.03943276465977164, 94.99890960531436690 ) ) ;
#197492=CARTESIAN_POINT ( 'NONE',  ( 0.05219959533910956823, 16.53943276465976808, 64.99890960531435269 ) ) ;
#197493=CARTESIAN_POINT ( 'NONE',  ( 16.46253265017160672, -9.564922557960803928, 103.3322429386476955 ) ) ;
#197494=DIRECTION ( 'NONE',  ( -0.000000000000000000, 1.000000000000000000, -0.000000000000000000 ) ) ;
#197495=CARTESIAN_POINT ( 'NONE',  ( 5.049401038297881783, 19.05341960407617563, 57.29275706135231871 ) ) ;
#197496=CARTESIAN_POINT ( 'NONE',  ( -5.823673210054116645, -21.52544592524344225, 112.2905762719810241 ) ) ;
#197497=CARTESIAN_POINT ( 'NONE',  ( 13.97604488694527802, 13.89961937509977652, 44.37390960531435269 ) ) ;
#197498=CARTESIAN_POINT ( 'NONE',  ( 14.29746914071049879, -8.314922557960816363, 113.3322429386476955 ) ) ;
#197499=CARTESIAN_POINT ( 'NONE',  ( 10.72451020669871369, 18.67979575497193778, 52.08442372801901854 ) ) ;
#197501=CARTESIAN_POINT ( 'NONE',  ( 0.05219959533910956823, 16.53943276465976808, 34.99890960531435979 ) ) ;
#197502=CARTESIAN_POINT ( 'NONE',  ( -9.474510206698964154, 16.51473224551069663, 45.41557627198103120 ) ) ;
#197503=CARTESIAN_POINT ( 'NONE',  ( 5.049401038298161559, -19.05341960407611168, 97.70724293864766707 ) ) ;
#197504=CARTESIAN_POINT ( 'NONE',  ( 21.55341960407610458, 5.719274019375980345, 73.95724293864769550 ) ) ;
#197506=CARTESIAN_POINT ( 'NONE',  ( 19.02544592524343514, -5.153800228976328945, 48.54057627198103120 ) ) ;
#197507=CARTESIAN_POINT ( 'NONE',  ( -18.62759615963270932, 10.81492255796079327, 70.83224293864770971 ) ) ;
#197508=CARTESIAN_POINT ( 'NONE',  ( -18.67979575497193778, 10.72451020669871902, 88.33442372801901854 ) ) ;
#197510=CARTESIAN_POINT ( 'NONE',  ( -4.379528057220086978, -16.55341960407618274, 79.79275706135236135 ) ) ;
#197511=CARTESIAN_POINT ( 'NONE',  ( 14.34966873604960469, 8.224510206698951720, 74.16557627198102409 ) ) ;
#197512=CARTESIAN_POINT ( 'NONE',  ( 19.03943276465977164, -0.05219959533909143690, 73.74890960531435269 ) ) ;
#197514=CARTESIAN_POINT ( 'NONE',  ( 16.51473224551083163, -9.474510206698727899, 30.83442372801900433 ) ) ;
#197515=CARTESIAN_POINT ( 'NONE',  ( -16.52544592524335698, -4.483927247898792601, 88.95942372801901854 ) ) ;
#197516=CARTESIAN_POINT ( 'NONE',  ( 21.55341960407619695, -5.719274019375665929, 106.0427570613523471 ) ) ;
#197517=CARTESIAN_POINT ( 'NONE',  ( 9.474510206698971260, -16.51473224551069308, 77.91557627198103830 ) ) ;
#197518=CARTESIAN_POINT ( 'NONE',  ( 5.719274019375991003, -21.55341960407610458, 42.70724293864770260 ) ) ;
#197519=CARTESIAN_POINT ( 'NONE',  ( -12.06949235617739369, -12.14591786802326823, 19.37609039468568639 ) ) ;
#197520=CARTESIAN_POINT ( 'NONE',  ( -18.67979575497193778, 10.72451020669871902, 93.33442372801901854 ) ) ;
#197521=CARTESIAN_POINT ( 'NONE',  ( 16.52544592524335698, 4.483927247898782831, 56.45942372801902565 ) ) ;
#197522=CARTESIAN_POINT ( 'NONE',  ( -21.52544592524343514, 5.823673210054127303, 111.0405762719810525 ) ) ;
#197523=CARTESIAN_POINT ( 'NONE',  ( -4.483927247898782831, 16.52544592524335698, 22.70942372801901499 ) ) ;
#197524=CARTESIAN_POINT ( 'NONE',  ( 9.474510206698971260, -16.51473224551069308, 87.91557627198102409 ) ) ;
#197525=CARTESIAN_POINT ( 'NONE',  ( -4.483927247898782831, 16.52544592524335698, 32.70942372801900433 ) ) ;
#197526=CARTESIAN_POINT ( 'NONE',  ( -19.05341960407611168, -5.049401038298163336, 56.45724293864768129 ) ) ;
#197527=CARTESIAN_POINT ( 'NONE',  ( -16.52544592524335698, -4.483927247898792601, 33.95942372801901143 ) ) ;
#197528=CARTESIAN_POINT ( 'NONE',  ( 16.55341960407611168, 4.379528057220329451, 78.95724293864769550 ) ) ;
#197530=CARTESIAN_POINT ( 'NONE',  ( -16.52544592524335698, -4.483927247898792601, 83.95942372801900433 ) ) ;
#197531=CARTESIAN_POINT ( 'NONE',  ( -18.67979575497193778, 10.72451020669871902, 38.33442372801900433 ) ) ;
#197532=CARTESIAN_POINT ( 'NONE',  ( 19.05341960407611168, 5.049401038298154454, 58.95724293864768129 ) ) ;
#197533=CARTESIAN_POINT ( 'NONE',  ( -0.05219959533909027116, -19.03943276465977164, 87.49890960531436690 ) ) ;
#197534=CARTESIAN_POINT ( 'NONE',  ( -12.06949235617739369, -12.14591786802326823, 79.37609039468567573 ) ) ;
#197537=CARTESIAN_POINT ( 'NONE',  ( 19.05341960407617918, -5.049401038297876454, 36.04275706135234003 ) ) ;
#197538=CARTESIAN_POINT ( 'NONE',  ( -9.474510206698964154, 16.51473224551069663, 95.41557627198102409 ) ) ;
#197539=CARTESIAN_POINT ( 'NONE',  ( -19.05341960407611168, -5.049401038298163336, 46.45724293864768129 ) ) ;
#197540=CARTESIAN_POINT ( 'NONE',  ( 19.03943276465977164, -0.05219959533909143690, 108.7489096053143527 ) ) ;
#197541=CARTESIAN_POINT ( 'NONE',  ( 16.55341960407618274, -4.379528057220086978, 46.04275706135234714 ) ) ;
#197542=CARTESIAN_POINT ( 'NONE',  ( -19.05341960407617563, 5.049401038297882671, 63.54275706135234003 ) ) ;
#197543=CARTESIAN_POINT ( 'NONE',  ( -4.483927247898782831, 16.52544592524335698, 57.70942372801901143 ) ) ;
#197545=CARTESIAN_POINT ( 'NONE',  ( -13.97604488694527625, -13.89961937509977652, 81.87390960531436690 ) ) ;
#197546=CARTESIAN_POINT ( 'NONE',  ( 15.72974639402199770, -15.80617190586745480, 108.1239096053143811 ) ) ;
#197547=CARTESIAN_POINT ( 'NONE',  ( 19.02544592524334988, 5.153800228976608722, 61.45942372801900433 ) ) ;
#197548=CARTESIAN_POINT ( 'NONE',  ( 19.03943276465977164, -0.05219959533909143690, 88.74890960531436690 ) ) ;
#197549=CARTESIAN_POINT ( 'NONE',  ( -19.03943276465977164, 0.05219959533909376836, 26.24890960531435624 ) ) ;
#197550=CARTESIAN_POINT ( 'NONE',  ( -9.564922557960796823, -16.46253265017161027, 82.08224293864768129 ) ) ;
#197551=CARTESIAN_POINT ( 'NONE',  ( 8.314922557960818139, 14.29746914071049879, 29.58224293864769905 ) ) ;
#197552=CARTESIAN_POINT ( 'NONE',  ( 19.05341960407611168, 5.049401038298154454, 23.95724293864769194 ) ) ;
#197553=CARTESIAN_POINT ( 'NONE',  ( -9.564922557961040184, 16.46253265017147172, 42.91775706135234003 ) ) ;
#197554=CARTESIAN_POINT ( 'NONE',  ( 14.29746914071049879, -8.314922557960816363, 73.33224293864769550 ) ) ;
#197555=CARTESIAN_POINT ( 'NONE',  ( -18.62759615963255300, -10.81492255796106328, 99.16775706135234714 ) ) ;
#197556=CARTESIAN_POINT ( 'NONE',  ( -5.153800228976328057, -19.02544592524343514, 37.29057627198102409 ) ) ;
#197558=CARTESIAN_POINT ( 'NONE',  ( -4.379528057220328563, 16.55341960407611168, 35.20724293864768839 ) ) ;
#197559=CARTESIAN_POINT ( 'NONE',  ( -21.55341960407619339, 5.719274019375674811, 108.5427570613523756 ) ) ;
#197560=CARTESIAN_POINT ( 'NONE',  ( 19.03943276465977164, -0.05219959533909143690, 93.74890960531435269 ) ) ;
#197561=CARTESIAN_POINT ( 'NONE',  ( 9.564922557960805705, 16.46253265017160317, 89.58224293864769550 ) ) ;
#197562=CARTESIAN_POINT ( 'NONE',  ( 13.97604488694527802, 13.89961937509977652, 39.37390960531435269 ) ) ;
#197563=CARTESIAN_POINT ( 'NONE',  ( 4.379528057220339221, -16.55341960407611168, 102.7072429386476955 ) ) ;
#197564=CARTESIAN_POINT ( 'NONE',  ( -4.379528057220328563, 16.55341960407611168, 70.20724293864769550 ) ) ;
#197565=CARTESIAN_POINT ( 'NONE',  ( -10.72451020669898014, 18.67979575497178502, 80.41557627198103830 ) ) ;
#197566=CARTESIAN_POINT ( 'NONE',  ( -0.05219959533909027116, -19.03943276465977164, 87.49890960531436690 ) ) ;
#197567=CARTESIAN_POINT ( 'NONE',  ( 21.53943276465977519, -0.05219959533907433946, 103.7489096053143669 ) ) ;
#197568=CARTESIAN_POINT ( 'NONE',  ( 16.46253265017160672, -9.564922557960803928, 93.33224293864769550 ) ) ;
#197569=DIRECTION ( 'NONE',  ( -0.000000000000000000, -0.000000000000000000, 1.000000000000000000 ) ) ;
#197570=CARTESIAN_POINT ( 'NONE',  ( 16.53943276465976808, -0.05219959533910856209, 83.74890960531435269 ) ) ;
#197571=CARTESIAN_POINT ( 'NONE',  ( 13.97604488694527802, 13.89961937509977652, 69.37390960531436690 ) ) ;
#197572=CARTESIAN_POINT ( 'NONE',  ( 5.823673210054125526, 21.52544592524343514, 79.79057627198102409 ) ) ;
#197573=LINE ( 'NONE', #120707, #152900 ) ;
#197574=CARTESIAN_POINT ( 'NONE',  ( 18.67979575497178502, 10.72451020669898547, 29.16557627198103120 ) ) ;
#197576=CARTESIAN_POINT ( 'NONE',  ( -13.89961937509957401, -13.97604488694547875, 109.3760903946856331 ) ) ;
#197577=CARTESIAN_POINT ( 'NONE',  ( 16.53943276465976808, -0.05219959533910856209, 98.74890960531438111 ) ) ;
#197578=CARTESIAN_POINT ( 'NONE',  ( -17.12812012977028076, -6.668231424565931320, 96.35948759323143520 ) ) ;
#197579=CARTESIAN_POINT ( 'NONE',  ( 19.02544592524343514, -5.153800228976328945, 88.54057627198102409 ) ) ;
#197580=CARTESIAN_POINT ( 'NONE',  ( 13.89961937509977652, -13.97604488694527269, 48.12390960531435979 ) ) ;
#197581=CARTESIAN_POINT ( 'NONE',  ( 12.14591786802309770, 12.06949235617756955, 79.37390960531436690 ) ) ;
#197582=CARTESIAN_POINT ( 'NONE',  ( -9.474510206698964154, 16.51473224551069663, 110.4155762719810383 ) ) ;
#197583=CARTESIAN_POINT ( 'NONE',  ( -8.314922557960811034, -14.29746914071050412, 57.08224293864769550 ) ) ;
#197584=CARTESIAN_POINT ( 'NONE',  ( -16.51473224551082808, 9.474510206698731452, 108.3344237280190043 ) ) ;
#197585=CARTESIAN_POINT ( 'NONE',  ( -15.72974639402176322, -15.80617190586768395, 54.37609039468568994 ) ) ;
#197587=CARTESIAN_POINT ( 'NONE',  ( -16.46253265017160317, 9.564922557960807481, 95.83224293864769550 ) ) ;
#197588=CARTESIAN_POINT ( 'NONE',  ( 21.52544592524344225, -5.823673210054117533, 88.54057627198103830 ) ) ;
#197589=CARTESIAN_POINT ( 'NONE',  ( -0.05219959533934338120, 16.53943276465976808, 82.50109039468568994 ) ) ;
#197590=CARTESIAN_POINT ( 'NONE',  ( 16.46253265017160672, -9.564922557960803928, 28.33224293864769550 ) ) ;
#197591=CARTESIAN_POINT ( 'NONE',  ( 16.51473224551069308, 9.474510206698969483, 74.16557627198103830 ) ) ;
#197592=CARTESIAN_POINT ( 'NONE',  ( -15.72974639402197994, 15.80617190586746368, 80.62390960531438111 ) ) ;
#197593=CARTESIAN_POINT ( 'NONE',  ( -19.03943276465977164, -0.05219959533935918106, 103.7510903946856757 ) ) ;
#197594=CARTESIAN_POINT ( 'NONE',  ( -8.314922557960811034, -14.29746914071050412, 47.08224293864770260 ) ) ;
#197595=CARTESIAN_POINT ( 'NONE',  ( -15.72974639402176322, -15.80617190586768395, 54.37609039468568994 ) ) ;
#197596=CARTESIAN_POINT ( 'NONE',  ( 4.483927247898790824, -16.52544592524335698, 80.20942372801901854 ) ) ;
#197597=CARTESIAN_POINT ( 'NONE',  ( 19.02544592524343514, -5.153800228976328945, 113.5405762719810241 ) ) ;
#197598=CARTESIAN_POINT ( 'NONE',  ( -0.05219959533909027116, -19.03943276465977164, 112.4989096053143669 ) ) ;
#197600=CARTESIAN_POINT ( 'NONE',  ( -4.483927247898782831, 16.52544592524335698, 107.7094237280190328 ) ) ;
#197601=CARTESIAN_POINT ( 'NONE',  ( -12.14591786802326823, 12.06949235617739902, 53.12609039468568284 ) ) ;
#197602=CARTESIAN_POINT ( 'NONE',  ( 19.02544592524343514, -5.153800228976328945, 63.54057627198103830 ) ) ;
#197603=CARTESIAN_POINT ( 'NONE',  ( 19.02544592524343514, -5.153800228976328945, 68.54057627198103830 ) ) ;
#197604=CARTESIAN_POINT ( 'NONE',  ( -4.379528057220086978, -16.55341960407618274, 74.79275706135234714 ) ) ;
#197605=CARTESIAN_POINT ( 'NONE',  ( 4.483927247898545687, 16.52544592524342804, 44.79057627198103120 ) ) ;
#197606=CARTESIAN_POINT ( 'NONE',  ( -13.89961937509977652, 13.97604488694528158, 50.62390960531435979 ) ) ;
#197607=CARTESIAN_POINT ( 'NONE',  ( 5.153800228976335163, 19.02544592524342804, 44.79057627198103830 ) ) ;
#197608=CARTESIAN_POINT ( 'NONE',  ( 14.29746914071037800, 8.314922557961029526, 46.66775706135234714 ) ) ;
#197610=CARTESIAN_POINT ( 'NONE',  ( 5.049401038297881783, 19.05341960407617563, 92.29275706135234714 ) ) ;
#197611=CARTESIAN_POINT ( 'NONE',  ( -14.34966873604960291, -8.224510206698953496, 91.66557627198103830 ) ) ;
#197612=CARTESIAN_POINT ( 'NONE',  ( -19.02544592524342804, 5.153800228976336051, 71.04057627198099567 ) ) ;
#197613=CARTESIAN_POINT ( 'NONE',  ( -13.89961937509957401, -13.97604488694547875, 94.37609039468566152 ) ) ;
#197615=CARTESIAN_POINT ( 'NONE',  ( 18.62759615963255655, 10.81492255796105972, 106.6677570613523756 ) ) ;
#197616=CARTESIAN_POINT ( 'NONE',  ( 16.52544592524335698, 4.483927247898782831, 71.45942372801901854 ) ) ;
#197618=CARTESIAN_POINT ( 'NONE',  ( 10.81492255796078972, 18.62759615963270932, 69.58224293864769550 ) ) ;
#197619=CARTESIAN_POINT ( 'NONE',  ( 4.483927247898790824, -16.52544592524335698, 55.20942372801902565 ) ) ;
#197620=CARTESIAN_POINT ( 'NONE',  ( 16.46253265017160672, -9.564922557960803928, 38.33224293864768839 ) ) ;
#197621=CARTESIAN_POINT ( 'NONE',  ( -0.05219959533936034679, 19.03943276465977164, 37.50109039468567573 ) ) ;
#197622=CARTESIAN_POINT ( 'NONE',  ( -9.564922557960796823, -16.46253265017161027, 92.08224293864769550 ) ) ;
#197623=CARTESIAN_POINT ( 'NONE',  ( 9.474510206698971260, -16.51473224551069308, 22.91557627198102765 ) ) ;
#197624=CARTESIAN_POINT ( 'NONE',  ( 0.05219959533909260263, 19.03943276465977164, 59.99890960531436690 ) ) ;
#197625=CARTESIAN_POINT ( 'NONE',  ( 21.52544592524334988, 5.823673210054432836, 81.45942372801900433 ) ) ;
#197626=CARTESIAN_POINT ( 'NONE',  ( 0.05219959533936267826, -19.03943276465977164, 40.00109039468566152 ) ) ;
#197627=CARTESIAN_POINT ( 'NONE',  ( 0.05219959533936267826, -19.03943276465977164, 25.00109039468566152 ) ) ;
#197628=CARTESIAN_POINT ( 'NONE',  ( -9.564922557960796823, -16.46253265017161027, 62.08224293864769550 ) ) ;
#197629=CARTESIAN_POINT ( 'NONE',  ( -5.823673210054116645, -21.52544592524344225, 27.29057627198103120 ) ) ;
#197630=CARTESIAN_POINT ( 'NONE',  ( -15.80617190586768217, 15.72974639402176855, 83.12609039468568994 ) ) ;
#197631=CARTESIAN_POINT ( 'NONE',  ( 19.05341960407611168, 5.049401038298154454, 58.95724293864768129 ) ) ;
#197632=CARTESIAN_POINT ( 'NONE',  ( -21.53943276465977519, -0.05219959533937600094, 88.75109039468567573 ) ) ;
#197633=CARTESIAN_POINT ( 'NONE',  ( 10.72451020669898902, -18.67979575497178502, 37.91557627198102409 ) ) ;
#197634=VECTOR ( 'NONE', #102291, 1000.000000000000000 ) ;
#197635=CARTESIAN_POINT ( 'NONE',  ( -5.153800228976328057, -19.02544592524343514, 87.29057627198103830 ) ) ;
#197636=CARTESIAN_POINT ( 'NONE',  ( 10.72451020669871369, 18.67979575497193778, 37.08442372801901143 ) ) ;
#197637=CARTESIAN_POINT ( 'NONE',  ( 19.05341960407617918, -5.049401038297876454, 66.04275706135233293 ) ) ;
#197638=CARTESIAN_POINT ( 'NONE',  ( -19.03943276465977164, 0.05219959533909376836, 46.24890960531435979 ) ) ;
#197639=CARTESIAN_POINT ( 'NONE',  ( -5.049401038298153566, 19.05341960407611168, 85.20724293864766707 ) ) ;
#197640=CARTESIAN_POINT ( 'NONE',  ( -12.14591786802326823, 12.06949235617739902, 28.12609039468568284 ) ) ;
#197641=CARTESIAN_POINT ( 'NONE',  ( -4.483927247898539470, -16.52544592524342804, 92.29057627198103830 ) ) ;
#197642=CARTESIAN_POINT ( 'NONE',  ( 16.51473224551069308, 9.474510206698969483, 64.16557627198102409 ) ) ;
#197643=CARTESIAN_POINT ( 'NONE',  ( -21.52544592524343514, 5.823673210054127303, 46.04057627198103830 ) ) ;
#197644=CARTESIAN_POINT ( 'NONE',  ( -4.379528057220086978, -16.55341960407618274, 24.79275706135235779 ) ) ;
#197645=CARTESIAN_POINT ( 'NONE',  ( 15.72974639402176855, 15.80617190586768217, 26.87609039468567218 ) ) ;
#197646=CARTESIAN_POINT ( 'NONE',  ( -18.62759615963255300, -10.81492255796106328, 69.16775706135234714 ) ) ;
#197647=CARTESIAN_POINT ( 'NONE',  ( -16.55341960407617563, 4.379528057220093196, 63.54275706135234003 ) ) ;
#197648=CARTESIAN_POINT ( 'NONE',  ( 8.224510206698742110, 14.34966873604972548, 62.08442372801901143 ) ) ;
#197649=CARTESIAN_POINT ( 'NONE',  ( 0.05219959533909260263, 19.03943276465977164, 59.99890960531436690 ) ) ;
#197650=CARTESIAN_POINT ( 'NONE',  ( -0.05219959533934338120, 16.53943276465976808, 97.50109039468567573 ) ) ;
#197651=CARTESIAN_POINT ( 'NONE',  ( 16.46253265017146816, 9.564922557961045513, 41.66775706135234003 ) ) ;
#197652=CARTESIAN_POINT ( 'NONE',  ( 0.05219959533907565091, 21.53943276465977519, 109.9989096053143527 ) ) ;
#197653=CARTESIAN_POINT ( 'NONE',  ( 0.05219959533910956823, 16.53943276465976808, 59.99890960531436690 ) ) ;
#197654=CARTESIAN_POINT ( 'NONE',  ( -5.153800228976328057, -19.02544592524343514, 92.29057627198099567 ) ) ;
#197655=CARTESIAN_POINT ( 'NONE',  ( 12.06949235617739724, 12.14591786802326823, 91.87609039468568994 ) ) ;
#197656=CARTESIAN_POINT ( 'NONE',  ( 21.53943276465977519, 0.05219959533937863772, 61.25109039468567573 ) ) ;
#197657=CARTESIAN_POINT ( 'NONE',  ( -0.05219959533934338120, 16.53943276465976808, 37.50109039468568284 ) ) ;
#197658=CARTESIAN_POINT ( 'NONE',  ( 5.719274019375673035, 21.55341960407619339, 27.29275706135234358 ) ) ;
#197659=CARTESIAN_POINT ( 'NONE',  ( 16.55341960407611168, 4.379528057220329451, 58.95724293864770971 ) ) ;
#197661=CARTESIAN_POINT ( 'NONE',  ( 0.05219959533907565091, 21.53943276465977519, 99.99890960531436690 ) ) ;
#197662=CARTESIAN_POINT ( 'NONE',  ( -12.06949235617756955, 12.14591786802309770, 35.62390960531437401 ) ) ;
#197663=ORIENTED_EDGE ( 'NONE', *, *, #45960, .T. ) ;
#197665=CARTESIAN_POINT ( 'NONE',  ( -5.823673210054116645, -21.52544592524344225, 32.29057627198102409 ) ) ;
#197666=CARTESIAN_POINT ( 'NONE',  ( 15.72974639402176855, 15.80617190586768217, 41.87609039468568284 ) ) ;
#197667=CARTESIAN_POINT ( 'NONE',  ( -14.29746914071049879, 8.314922557960819915, 60.83224293864769550 ) ) ;
#197668=CARTESIAN_POINT ( 'NONE',  ( -15.72974639402197994, 15.80617190586746368, 65.62390960531436690 ) ) ;
#197669=CARTESIAN_POINT ( 'NONE',  ( 9.564922557960805705, 16.46253265017160317, 69.58224293864770971 ) ) ;
#197670=CARTESIAN_POINT ( 'NONE',  ( 9.474510206698971260, -16.51473224551069308, 22.91557627198102765 ) ) ;
#197671=CARTESIAN_POINT ( 'NONE',  ( 13.97604488694548053, -13.89961937509957401, 70.62609039468567573 ) ) ;
#197672=CARTESIAN_POINT ( 'NONE',  ( -18.62759615963270932, 10.81492255796079327, 50.83224293864770971 ) ) ;
#197673=CARTESIAN_POINT ( 'NONE',  ( -13.97604488694527625, -13.89961937509977652, 56.87390960531434558 ) ) ;
#197674=CARTESIAN_POINT ( 'NONE',  ( 4.483927247898790824, -16.52544592524335698, 35.20942372801901854 ) ) ;
#197675=CARTESIAN_POINT ( 'NONE',  ( 21.53943276465977519, 0.05219959533937863772, 21.25109039468567218 ) ) ;
#197676=CARTESIAN_POINT ( 'NONE',  ( -4.483927247898539470, -16.52544592524342804, 47.29057627198103120 ) ) ;
#197678=CARTESIAN_POINT ( 'NONE',  ( 16.46253265017160672, -9.564922557960803928, 88.33224293864769550 ) ) ;
#197679=CARTESIAN_POINT ( 'NONE',  ( 21.52544592524344225, -5.823673210054117533, 73.54057627198102409 ) ) ;
#197680=CARTESIAN_POINT ( 'NONE',  ( -15.80617190586745835, -15.72974639402198527, 106.8739096053143811 ) ) ;
#197681=CARTESIAN_POINT ( 'NONE',  ( 4.379528057220092307, 16.55341960407617563, 32.29275706135235424 ) ) ;
#197682=CARTESIAN_POINT ( 'NONE',  ( -18.67979575497178146, -10.72451020669898902, 41.66557627198103120 ) ) ;
#197683=CARTESIAN_POINT ( 'NONE',  ( 18.67979575497194134, -10.72451020669871369, 95.83442372801903275 ) ) ;
#197684=CARTESIAN_POINT ( 'NONE',  ( 0.05219959533909260263, 19.03943276465977164, 94.99890960531436690 ) ) ;
#197685=CARTESIAN_POINT ( 'NONE',  ( 0.05219959533909260263, 19.03943276465977164, 34.99890960531435979 ) ) ;
#197686=CARTESIAN_POINT ( 'NONE',  ( 19.05341960407611168, 5.049401038298154454, 93.95724293864769550 ) ) ;
#197687=CARTESIAN_POINT ( 'NONE',  ( 16.46253265017160672, -9.564922557960803928, 78.33224293864769550 ) ) ;
#197690=CARTESIAN_POINT ( 'NONE',  ( 16.51473224551083163, -9.474510206698727899, 60.83442372801900433 ) ) ;
#197691=CARTESIAN_POINT ( 'NONE',  ( 21.55341960407619695, -5.719274019375665929, 106.0427570613523471 ) ) ;
#197692=CARTESIAN_POINT ( 'NONE',  ( -18.67979575497178146, -10.72451020669898902, 26.66557627198103475 ) ) ;
#197693=CARTESIAN_POINT ( 'NONE',  ( -16.52544592524335698, -4.483927247898792601, 103.9594237280190185 ) ) ;
#197694=CARTESIAN_POINT ( 'NONE',  ( 16.46253265017146816, 9.564922557961045513, 86.66775706135233293 ) ) ;
#197695=CARTESIAN_POINT ( 'NONE',  ( -16.79531203550651242, 7.028104445595463545, 58.74755011779561187 ) ) ;
#197696=CARTESIAN_POINT ( 'NONE',  ( 16.51473224551083163, -9.474510206698727899, 85.83442372801900433 ) ) ;
#197697=CARTESIAN_POINT ( 'NONE',  ( -16.46253265017146816, -9.564922557961047289, 39.16775706135234003 ) ) ;
#197699=CARTESIAN_POINT ( 'NONE',  ( 19.02544592524343514, -5.153800228976328945, 43.54057627198103120 ) ) ;
#197700=CARTESIAN_POINT ( 'NONE',  ( 16.52544592524342804, -4.483927247898539470, 48.54057627198103120 ) ) ;
#197701=CARTESIAN_POINT ( 'NONE',  ( -16.62475595723698873, -7.163666690055296549, 109.4728664818953519 ) ) ;
#197702=CARTESIAN_POINT ( 'NONE',  ( -8.314922557960811034, -14.29746914071050412, 32.08224293864769550 ) ) ;
#197704=CARTESIAN_POINT ( 'NONE',  ( 0.05219959533934541429, -16.53943276465976808, 90.00109039468567573 ) ) ;
#197705=CARTESIAN_POINT ( 'NONE',  ( 5.049401038298161559, -19.05341960407611168, 47.70724293864770260 ) ) ;
#197706=CARTESIAN_POINT ( 'NONE',  ( -0.05219959533937732626, 21.53943276465977519, 102.5010903946856899 ) ) ;
#197707=CARTESIAN_POINT ( 'NONE',  ( 4.483927247898790824, -16.52544592524335698, 25.20942372801901854 ) ) ;
#197708=CARTESIAN_POINT ( 'NONE',  ( -0.05219959533907301413, -21.53943276465977519, 37.49890960531436690 ) ) ;
#197709=CARTESIAN_POINT ( 'NONE',  ( 21.52544592524334988, 5.823673210054432836, 96.45942372801901854 ) ) ;
#197711=CARTESIAN_POINT ( 'NONE',  ( 19.03943276465977164, -0.05219959533909143690, 103.7489096053143669 ) ) ;
#197712=CARTESIAN_POINT ( 'NONE',  ( 0.05219959533909260263, 19.03943276465977164, 79.99890960531436690 ) ) ;
#197714=CARTESIAN_POINT ( 'NONE',  ( -0.05219959533907301413, -21.53943276465977519, 112.4989096053143669 ) ) ;
#197715=CARTESIAN_POINT ( 'NONE',  ( 14.29746914071049879, -8.314922557960816363, 78.33224293864770971 ) ) ;
#197716=CARTESIAN_POINT ( 'NONE',  ( 10.81492255796078972, 18.62759615963270932, 74.58224293864768129 ) ) ;
#197717=CARTESIAN_POINT ( 'NONE',  ( -13.89961937509977652, 13.97604488694528158, 65.62390960531436690 ) ) ;
#197718=CARTESIAN_POINT ( 'NONE',  ( -10.72451020669898014, 18.67979575497178502, 95.41557627198102409 ) ) ;
#197720=CARTESIAN_POINT ( 'NONE',  ( 9.564922557960805705, 16.46253265017160317, 59.58224293864769550 ) ) ;
#197721=CARTESIAN_POINT ( 'NONE',  ( -4.483927247898539470, -16.52544592524342804, 87.29057627198103830 ) ) ;
#197723=CARTESIAN_POINT ( 'NONE',  ( -13.89961937509977652, 13.97604488694528158, 70.62390960531432427 ) ) ;
#197724=CARTESIAN_POINT ( 'NONE',  ( -19.05341960407617563, 5.049401038297882671, 73.54275706135233293 ) ) ;
#197725=CARTESIAN_POINT ( 'NONE',  ( -14.29746914071049879, 8.314922557960819915, 85.83224293864768129 ) ) ;
#197726=CARTESIAN_POINT ( 'NONE',  ( -21.55341960407619339, 5.719274019375674811, 63.54275706135234003 ) ) ;
#197727=CARTESIAN_POINT ( 'NONE',  ( 19.02544592524343514, -5.153800228976328945, 48.54057627198103120 ) ) ;
#197728=CARTESIAN_POINT ( 'NONE',  ( 15.72974639402199770, -15.80617190586745480, 113.1239096053143953 ) ) ;
#197729=CARTESIAN_POINT ( 'NONE',  ( 4.483927247898545687, 16.52544592524342804, 104.7905762719810241 ) ) ;
#197730=CARTESIAN_POINT ( 'NONE',  ( 17.50000000000000711, 5.499999999999976907, 93.78230962303565832 ) ) ;
#197731=CARTESIAN_POINT ( 'NONE',  ( 5.049401038298161559, -19.05341960407611168, 57.70724293864769550 ) ) ;
#197733=CARTESIAN_POINT ( 'NONE',  ( -9.474510206698720793, -16.51473224551083518, 109.5844237280190043 ) ) ;
#197734=CARTESIAN_POINT ( 'NONE',  ( 19.03943276465977164, -0.05219959533909143690, 113.7489096053143669 ) ) ;
#197735=CARTESIAN_POINT ( 'NONE',  ( 5.719274019375673035, 21.55341960407619339, 52.29275706135236135 ) ) ;
#197736=CARTESIAN_POINT ( 'NONE',  ( -19.02544592524342804, 5.153800228976336051, 91.04057627198100988 ) ) ;
#197737=CARTESIAN_POINT ( 'NONE',  ( -19.02544592524334988, -5.153800228976617603, 88.95942372801897591 ) ) ;
#197738=CARTESIAN_POINT ( 'NONE',  ( 19.05341960407611168, 5.049401038298154454, 58.95724293864768129 ) ) ;
#197739=CARTESIAN_POINT ( 'NONE',  ( 4.379528057220339221, -16.55341960407611168, 72.70724293864769550 ) ) ;
#197740=CARTESIAN_POINT ( 'NONE',  ( -16.53943276465976808, 0.05219959533911058130, 76.24890960531435269 ) ) ;
#197741=CARTESIAN_POINT ( 'NONE',  ( -9.564922557960796823, -16.46253265017161027, 87.08224293864769550 ) ) ;
#197742=CARTESIAN_POINT ( 'NONE',  ( 14.34966873604960469, 8.224510206698951720, 79.16557627198103830 ) ) ;
#197743=CARTESIAN_POINT ( 'NONE',  ( -16.51473224551069308, -9.474510206698971260, 81.66557627198103830 ) ) ;
#197744=CARTESIAN_POINT ( 'NONE',  ( 5.153800228976615827, -19.02544592524334988, 25.20942372801900433 ) ) ;
#197745=CARTESIAN_POINT ( 'NONE',  ( 9.474510206698971260, -16.51473224551069308, 52.91557627198102409 ) ) ;
#197746=CARTESIAN_POINT ( 'NONE',  ( -12.06949235617756955, 12.14591786802309770, 35.62390960531437401 ) ) ;
#197747=CARTESIAN_POINT ( 'NONE',  ( 5.153800228976335163, 19.02544592524342804, 24.79057627198102765 ) ) ;
#197748=ORIENTED_EDGE ( 'NONE', *, *, #44009, .F. ) ;
#197749=CARTESIAN_POINT ( 'NONE',  ( 0.05219959533937995610, -21.53943276465977519, 45.00109039468568284 ) ) ;
#197750=CARTESIAN_POINT ( 'NONE',  ( 13.89961937509957401, 13.97604488694547697, 61.87609039468566863 ) ) ;
#197751=CARTESIAN_POINT ( 'NONE',  ( -14.34966873604960291, -8.224510206698953496, 36.66557627198103120 ) ) ;
#197752=CARTESIAN_POINT ( 'NONE',  ( -5.719274019375978568, 21.55341960407610458, 90.20724293864770971 ) ) ;
#197753=CARTESIAN_POINT ( 'NONE',  ( 21.52544592524344225, -5.823673210054117533, 33.54057627198102409 ) ) ;
#197754=CARTESIAN_POINT ( 'NONE',  ( -4.379528057220328563, 16.55341960407611168, 75.20724293864769550 ) ) ;
#197755=CARTESIAN_POINT ( 'NONE',  ( 5.153800228976335163, 19.02544592524342804, 39.79057627198100988 ) ) ;
#197756=CARTESIAN_POINT ( 'NONE',  ( -14.29746914071037622, -8.314922557961029526, 109.1677570613523613 ) ) ;
#197757=CARTESIAN_POINT ( 'NONE',  ( 16.52544592524335698, 4.483927247898782831, 71.45942372801901854 ) ) ;
#197758=CARTESIAN_POINT ( 'NONE',  ( 5.823673210054125526, 21.52544592524343514, 34.79057627198103120 ) ) ;
#197759=CARTESIAN_POINT ( 'NONE',  ( -5.153800228976607833, 19.02544592524334988, 22.70942372801899012 ) ) ;
#197760=CARTESIAN_POINT ( 'NONE',  ( -19.03943276465977164, 0.05219959533909376836, 96.24890960531436690 ) ) ;
#197761=CARTESIAN_POINT ( 'NONE',  ( -0.05219959533934338120, 16.53943276465976808, 77.50109039468567573 ) ) ;
#197762=CARTESIAN_POINT ( 'NONE',  ( -8.224510206698948167, 14.34966873604960824, 115.4155762719810241 ) ) ;
#197763=EDGE_CURVE ( 'NONE', #163091, #13391, #139014, .T. ) ;
#197764=CARTESIAN_POINT ( 'NONE',  ( -8.314922557960811034, -14.29746914071050412, 32.08224293864769550 ) ) ;
#197765=CARTESIAN_POINT ( 'NONE',  ( -5.049401038298153566, 19.05341960407611168, 100.2072429386476955 ) ) ;
#197766=CARTESIAN_POINT ( 'NONE',  ( -13.89961937509977652, 13.97604488694528158, 85.62390960531433848 ) ) ;
#197767=CARTESIAN_POINT ( 'NONE',  ( 5.719274019375991003, -21.55341960407610458, 22.70724293864769194 ) ) ;
#197768=CARTESIAN_POINT ( 'NONE',  ( 16.55341960407611168, 4.379528057220329451, 68.95724293864769550 ) ) ;
#197770=CARTESIAN_POINT ( 'NONE',  ( -4.483927247898539470, -16.52544592524342804, 52.29057627198102409 ) ) ;
#197772=CARTESIAN_POINT ( 'NONE',  ( -4.379528057220086978, -16.55341960407618274, 59.79275706135234714 ) ) ;
#197773=CARTESIAN_POINT ( 'NONE',  ( 9.564922557961047289, -16.46253265017146816, 60.41775706135233293 ) ) ;
#197774=CARTESIAN_POINT ( 'NONE',  ( -5.049401038297874678, -19.05341960407617918, 49.79275706135231871 ) ) ;
#197775=CARTESIAN_POINT ( 'NONE',  ( -16.46253265017160317, 9.564922557960807481, 95.83224293864769550 ) ) ;
#197776=CARTESIAN_POINT ( 'NONE',  ( -5.049401038297874678, -19.05341960407617918, 69.79275706135233293 ) ) ;
#197778=CARTESIAN_POINT ( 'NONE',  ( 19.05341960407617918, -5.049401038297876454, 56.04275706135234714 ) ) ;
#197779=CARTESIAN_POINT ( 'NONE',  ( 5.049401038297881783, 19.05341960407617563, 102.2927570613523045 ) ) ;
#197780=CARTESIAN_POINT ( 'NONE',  ( -16.53943276465976808, -0.05219959533934237506, 98.75109039468568994 ) ) ;
#197782=CARTESIAN_POINT ( 'NONE',  ( 0.05219959533909260263, 19.03943276465977164, 44.99890960531435979 ) ) ;
#197783=CARTESIAN_POINT ( 'NONE',  ( -9.474510206698964154, 16.51473224551069663, 115.4155762719810241 ) ) ;
#197784=CARTESIAN_POINT ( 'NONE',  ( -5.823673210054431948, 21.52544592524334988, 57.70942372801901143 ) ) ;
#197785=CARTESIAN_POINT ( 'NONE',  ( -9.474510206698720793, -16.51473224551083518, 99.58442372801900433 ) ) ;
#197786=CARTESIAN_POINT ( 'NONE',  ( 13.97604488694548053, -13.89961937509957401, 55.62609039468566863 ) ) ;
#197787=CARTESIAN_POINT ( 'NONE',  ( 13.97604488694527802, 13.89961937509977652, 59.37390960531434558 ) ) ;
#197788=CARTESIAN_POINT ( 'NONE',  ( -13.89961937509977652, 13.97604488694528158, 110.6239096053143243 ) ) ;
#197789=CARTESIAN_POINT ( 'NONE',  ( -14.34966873604960291, -8.224510206698953496, 76.66557627198103830 ) ) ;
#197790=CARTESIAN_POINT ( 'NONE',  ( -5.049401038298153566, 19.05341960407611168, 65.20724293864765286 ) ) ;
#197791=CARTESIAN_POINT ( 'NONE',  ( 9.564922557960805705, 16.46253265017160317, 79.58224293864769550 ) ) ;
#197792=CARTESIAN_POINT ( 'NONE',  ( 13.89961937509957401, 13.97604488694547697, 71.87609039468567573 ) ) ;
#197793=CARTESIAN_POINT ( 'NONE',  ( -18.67979575497178146, -10.72451020669898902, 66.66557627198102409 ) ) ;
#197794=CARTESIAN_POINT ( 'NONE',  ( 12.14591786802309770, 12.06949235617756955, 109.3739096053143811 ) ) ;
#197795=CARTESIAN_POINT ( 'NONE',  ( 13.97604488694548053, -13.89961937509957401, 55.62609039468566863 ) ) ;
#197796=CARTESIAN_POINT ( 'NONE',  ( -19.02544592524342804, 5.153800228976336051, 61.04057627198103120 ) ) ;
#197797=CARTESIAN_POINT ( 'NONE',  ( 19.05341960407611168, 5.049401038298154454, 73.95724293864768129 ) ) ;
#197798=CARTESIAN_POINT ( 'NONE',  ( -21.55341960407610458, -5.719274019375992779, 91.45724293864769550 ) ) ;
#197799=CARTESIAN_POINT ( 'NONE',  ( 12.06949235617757843, -12.14591786802309237, 83.12390960531436690 ) ) ;
#197800=CARTESIAN_POINT ( 'NONE',  ( 0.05219959533936267826, -19.03943276465977164, 50.00109039468566863 ) ) ;
#197801=CARTESIAN_POINT ( 'NONE',  ( -21.55341960407610458, -5.719274019375992779, 81.45724293864769550 ) ) ;
#197802=CARTESIAN_POINT ( 'NONE',  ( 21.52544592524344225, -5.823673210054117533, 53.54057627198103120 ) ) ;
#197803=CARTESIAN_POINT ( 'NONE',  ( -16.52544592524342804, 4.483927247898546575, 36.04057627198102409 ) ) ;
#197804=CARTESIAN_POINT ( 'NONE',  ( -15.72974639402176322, -15.80617190586768395, 89.37609039468568994 ) ) ;
#197805=CARTESIAN_POINT ( 'NONE',  ( -5.153800228976328057, -19.02544592524343514, 82.29057627198103830 ) ) ;
#197806=CARTESIAN_POINT ( 'NONE',  ( -14.34966873604960291, -8.224510206698953496, 111.6655762719810525 ) ) ;
#197807=CARTESIAN_POINT ( 'NONE',  ( 21.53943276465977519, 0.05219959533937863772, 26.25109039468567573 ) ) ;
#197808=CARTESIAN_POINT ( 'NONE',  ( 10.81492255796106328, -18.62759615963255655, 40.41775706135234714 ) ) ;
#197809=CARTESIAN_POINT ( 'NONE',  ( 19.02544592524343514, -5.153800228976328945, 43.54057627198103120 ) ) ;
#197810=CARTESIAN_POINT ( 'NONE',  ( 5.823673210054444382, -21.52544592524334988, 25.20942372801901854 ) ) ;
#197811=CARTESIAN_POINT ( 'NONE',  ( 13.97604488694548053, -13.89961937509957401, 60.62609039468564731 ) ) ;
#197813=CARTESIAN_POINT ( 'NONE',  ( -16.51473224551069308, -9.474510206698971260, 41.66557627198103120 ) ) ;
#197814=CARTESIAN_POINT ( 'NONE',  ( -16.52544592524335698, -4.483927247898792601, 28.95942372801902209 ) ) ;
#197815=CARTESIAN_POINT ( 'NONE',  ( 19.03943276465977164, -0.05219959533909143690, 28.74890960531435624 ) ) ;
#197816=CARTESIAN_POINT ( 'NONE',  ( 14.29746914071037800, 8.314922557961029526, 66.66775706135234714 ) ) ;
#197817=CARTESIAN_POINT ( 'NONE',  ( -13.97604488694527625, -13.89961937509977652, 36.87390960531436690 ) ) ;
#197819=CARTESIAN_POINT ( 'NONE',  ( -5.153800228976328057, -19.02544592524343514, 92.29057627198099567 ) ) ;
#197820=CARTESIAN_POINT ( 'NONE',  ( 19.05341960407611168, 5.049401038298154454, 23.95724293864769194 ) ) ;
#197821=CARTESIAN_POINT ( 'NONE',  ( 15.72974639402199770, -15.80617190586745480, 63.12390960531435979 ) ) ;
#197822=CARTESIAN_POINT ( 'NONE',  ( -16.55341960407617563, 4.379528057220093196, 53.54275706135234714 ) ) ;
#197823=CARTESIAN_POINT ( 'NONE',  ( 5.719274019375673035, 21.55341960407619339, 97.29275706135234714 ) ) ;
#197824=CARTESIAN_POINT ( 'NONE',  ( 16.51473224551069308, 9.474510206698969483, 39.16557627198103120 ) ) ;
#197825=CARTESIAN_POINT ( 'NONE',  ( -14.34966873604960291, -8.224510206698953496, 36.66557627198103120 ) ) ;
#197826=CARTESIAN_POINT ( 'NONE',  ( -0.05219959533910754901, -16.53943276465976808, 72.49890960531435269 ) ) ;
#197827=CARTESIAN_POINT ( 'NONE',  ( -5.049401038298153566, 19.05341960407611168, 65.20724293864765286 ) ) ;
#197828=CARTESIAN_POINT ( 'NONE',  ( -21.53943276465977519, -0.05219959533937600094, 113.7510903946856757 ) ) ;
#197829=CARTESIAN_POINT ( 'NONE',  ( 0.05219959533937995610, -21.53943276465977519, 20.00109039468568639 ) ) ;
#197830=CARTESIAN_POINT ( 'NONE',  ( 13.89961937509977652, -13.97604488694527269, 83.12390960531436690 ) ) ;
#197831=CARTESIAN_POINT ( 'NONE',  ( 21.53943276465977519, 0.05219959533937863772, 91.25109039468568994 ) ) ;
#197832=CARTESIAN_POINT ( 'NONE',  ( 16.52544592524335698, 4.483927247898782831, 51.45942372801901854 ) ) ;
#197833=CARTESIAN_POINT ( 'NONE',  ( 16.53943276465976808, 0.05219959533934440121, 31.25109039468568639 ) ) ;
#197834=CARTESIAN_POINT ( 'NONE',  ( 16.53943276465976808, -0.05219959533910856209, 93.74890960531436690 ) ) ;
#197835=CARTESIAN_POINT ( 'NONE',  ( 21.53943276465977519, 0.05219959533937863772, 101.2510903946856757 ) ) ;
#197836=CARTESIAN_POINT ( 'NONE',  ( -14.29746914071049879, 8.314922557960819915, 30.83224293864770260 ) ) ;
#197837=CARTESIAN_POINT ( 'NONE',  ( 16.51473224551069308, 9.474510206698969483, 24.16557627198102765 ) ) ;
#197838=CARTESIAN_POINT ( 'NONE',  ( -4.483927247898782831, 16.52544592524335698, 47.70942372801902565 ) ) ;
#197839=CARTESIAN_POINT ( 'NONE',  ( -14.29746914071049879, 8.314922557960819915, 60.83224293864769550 ) ) ;
#197840=CARTESIAN_POINT ( 'NONE',  ( -4.379528057220086978, -16.55341960407618274, 94.79275706135234714 ) ) ;
#197841=CARTESIAN_POINT ( 'NONE',  ( -13.89961937509977652, 13.97604488694528158, 110.6239096053143243 ) ) ;
#197842=CARTESIAN_POINT ( 'NONE',  ( 5.049401038298161559, -19.05341960407611168, 107.7072429386476955 ) ) ;
#197843=CARTESIAN_POINT ( 'NONE',  ( -13.97604488694547697, 13.89961937509957934, 23.12609039468565442 ) ) ;
#197844=CARTESIAN_POINT ( 'NONE',  ( -16.52544592524342804, 4.483927247898546575, 86.04057627198102409 ) ) ;
#197845=CARTESIAN_POINT ( 'NONE',  ( 0.05219959533909260263, 19.03943276465977164, 94.99890960531436690 ) ) ;
#197846=VERTEX_POINT ( 'NONE', #38562 ) ;
#197847=CARTESIAN_POINT ( 'NONE',  ( 4.483927247898790824, -16.52544592524335698, 45.20942372801901854 ) ) ;
#197848=CARTESIAN_POINT ( 'NONE',  ( -5.049401038298153566, 19.05341960407611168, 35.20724293864768839 ) ) ;
#197849=CARTESIAN_POINT ( 'NONE',  ( 12.14591786802327356, -12.06949235617739191, 50.62609039468568994 ) ) ;
#197851=CARTESIAN_POINT ( 'NONE',  ( 13.97604488694548053, -13.89961937509957401, 50.62609039468566152 ) ) ;
#197852=CARTESIAN_POINT ( 'NONE',  ( -0.05219959533909027116, -19.03943276465977164, 42.49890960531435269 ) ) ;
#197853=CARTESIAN_POINT ( 'NONE',  ( -12.14591786802326823, 12.06949235617739902, 83.12609039468568994 ) ) ;
#197854=CARTESIAN_POINT ( 'NONE',  ( -9.474510206698720793, -16.51473224551083518, 84.58442372801900433 ) ) ;
#197855=CARTESIAN_POINT ( 'NONE',  ( -13.97604488694547697, 13.89961937509957934, 28.12609039468565797 ) ) ;
#197856=CARTESIAN_POINT ( 'NONE',  ( 13.97604488694527802, 13.89961937509977652, 64.37390960531436690 ) ) ;
#197857=CARTESIAN_POINT ( 'NONE',  ( -4.379528057220328563, 16.55341960407611168, 100.2072429386476955 ) ) ;
#197858=CARTESIAN_POINT ( 'NONE',  ( 13.89961937509957401, 13.97604488694547697, 61.87609039468566863 ) ) ;
#197859=CARTESIAN_POINT ( 'NONE',  ( -0.05219959533907301413, -21.53943276465977519, 62.49890960531436690 ) ) ;
#197860=CARTESIAN_POINT ( 'NONE',  ( -16.46253265017146816, -9.564922557961047289, 24.16775706135233648 ) ) ;
#197861=CARTESIAN_POINT ( 'NONE',  ( 16.51473224551069308, 9.474510206698969483, 104.1655762719810241 ) ) ;
#197862=CARTESIAN_POINT ( 'NONE',  ( -18.62759615963270932, 10.81492255796079327, 75.83224293864769550 ) ) ;
#197863=CARTESIAN_POINT ( 'NONE',  ( -17.26058549869092573, 6.457015423128482645, 83.62254162523933587 ) ) ;
#197864=CARTESIAN_POINT ( 'NONE',  ( -16.46253265017146816, -9.564922557961047289, 99.16775706135233293 ) ) ;
#197865=CARTESIAN_POINT ( 'NONE',  ( -19.52837319214028255, 5.499999999999902300, 59.60471352585542348 ) ) ;
#197866=CARTESIAN_POINT ( 'NONE',  ( 8.224510206698742110, 14.34966873604972548, 32.08442372801901854 ) ) ;
#197867=CARTESIAN_POINT ( 'NONE',  ( -19.02544592524342804, 5.153800228976336051, 31.04057627198102409 ) ) ;
#197868=CARTESIAN_POINT ( 'NONE',  ( 5.153800228976335163, 19.02544592524342804, 104.7905762719809957 ) ) ;
#197869=CARTESIAN_POINT ( 'NONE',  ( 10.72451020669898902, -18.67979575497178502, 87.91557627198103830 ) ) ;
#197870=CARTESIAN_POINT ( 'NONE',  ( -5.719274019375665041, -21.55341960407619695, 59.79275706135234714 ) ) ;
#197871=CARTESIAN_POINT ( 'NONE',  ( -5.049401038297874678, -19.05341960407617918, 104.7927570613523471 ) ) ;
#197872=CARTESIAN_POINT ( 'NONE',  ( 10.81492255796106328, -18.62759615963255655, 110.4177570613523756 ) ) ;
#197873=CARTESIAN_POINT ( 'NONE',  ( -16.53943276465976808, -0.05219959533934237506, 113.7510903946856757 ) ) ;
#197874=CARTESIAN_POINT ( 'NONE',  ( 15.80617190586746368, 15.72974639402197994, 99.37390960531436690 ) ) ;
#197875=CARTESIAN_POINT ( 'NONE',  ( 16.52544592524342804, -4.483927247898539470, 48.54057627198103120 ) ) ;
#197876=CARTESIAN_POINT ( 'NONE',  ( 9.474510206698729675, 16.51473224551082808, 82.08442372801899012 ) ) ;
#197877=CARTESIAN_POINT ( 'NONE',  ( -19.03943276465977164, -0.05219959533935918106, 53.75109039468566863 ) ) ;
#197878=CARTESIAN_POINT ( 'NONE',  ( 18.67979575497194134, -10.72451020669871369, 55.83442372801901854 ) ) ;
#197879=CARTESIAN_POINT ( 'NONE',  ( 5.153800228976615827, -19.02544592524334988, 40.20942372801898301 ) ) ;
#197880=CARTESIAN_POINT ( 'NONE',  ( 16.52544592524342804, -4.483927247898539470, 103.5405762719810383 ) ) ;
#197881=CARTESIAN_POINT ( 'NONE',  ( 21.52544592524344225, -5.823673210054117533, 33.54057627198102409 ) ) ;
#197882=CARTESIAN_POINT ( 'NONE',  ( 8.224510206698953496, -14.34966873604960469, 42.91557627198103120 ) ) ;
#197883=CARTESIAN_POINT ( 'NONE',  ( 0.05219959533937995610, -21.53943276465977519, 95.00109039468568994 ) ) ;
#197884=CARTESIAN_POINT ( 'NONE',  ( 14.34966873604972726, -8.224510206698740333, 65.83442372801900433 ) ) ;
#197885=CARTESIAN_POINT ( 'NONE',  ( -16.55341960407611168, -4.379528057220339221, 31.45724293864769550 ) ) ;
#197886=CARTESIAN_POINT ( 'NONE',  ( 5.823673210054444382, -21.52544592524334988, 60.20942372801902565 ) ) ;
#197887=CARTESIAN_POINT ( 'NONE',  ( 5.719274019375673035, 21.55341960407619339, 62.29275706135236845 ) ) ;
#197888=CARTESIAN_POINT ( 'NONE',  ( 5.823673210054125526, 21.52544592524343514, 64.79057627198103830 ) ) ;
#197890=CARTESIAN_POINT ( 'NONE',  ( 19.02544592524343514, -5.153800228976328945, 23.54057627198102054 ) ) ;
#197891=CARTESIAN_POINT ( 'NONE',  ( -21.55341960407619339, 5.719274019375674811, 48.54275706135234714 ) ) ;
#197892=CARTESIAN_POINT ( 'NONE',  ( 14.34966873604960469, 8.224510206698951720, 114.1655762719810383 ) ) ;
#197893=CARTESIAN_POINT ( 'NONE',  ( 19.05341960407611168, 5.049401038298154454, 43.95724293864769550 ) ) ;
#197894=CARTESIAN_POINT ( 'NONE',  ( 0.05219959533910956823, 16.53943276465976808, 79.99890960531435269 ) ) ;
#197895=CARTESIAN_POINT ( 'NONE',  ( -16.46253265017160317, 9.564922557960807481, 85.83224293864769550 ) ) ;
#197896=CARTESIAN_POINT ( 'NONE',  ( 16.52544592524342804, -4.483927247898539470, 28.54057627198103120 ) ) ;
#197897=CARTESIAN_POINT ( 'NONE',  ( 8.314922557960818139, 14.29746914071049879, 104.5822429386477097 ) ) ;
#197898=CARTESIAN_POINT ( 'NONE',  ( 10.81492255796078972, 18.62759615963270932, 69.58224293864769550 ) ) ;
#197899=CARTESIAN_POINT ( 'NONE',  ( 21.53943276465977519, -0.05219959533907433946, 103.7489096053143669 ) ) ;
#197901=CARTESIAN_POINT ( 'NONE',  ( 19.02544592524343514, -5.153800228976328945, 68.54057627198103830 ) ) ;
#197902=CARTESIAN_POINT ( 'NONE',  ( 5.153800228976615827, -19.02544592524334988, 100.2094237280190043 ) ) ;
#197903=CARTESIAN_POINT ( 'NONE',  ( -21.52544592524343514, 5.823673210054127303, 51.04057627198103120 ) ) ;
#197904=CARTESIAN_POINT ( 'NONE',  ( 21.52544592524334988, 5.823673210054432836, 76.45942372801901854 ) ) ;
#197905=CARTESIAN_POINT ( 'NONE',  ( 19.02544592524343514, -5.153800228976328945, 63.54057627198103830 ) ) ;
#197906=CARTESIAN_POINT ( 'NONE',  ( -16.46253265017160317, 9.564922557960807481, 95.83224293864769550 ) ) ;
#197907=CARTESIAN_POINT ( 'NONE',  ( 12.06949235617739724, 12.14591786802326823, 71.87609039468568994 ) ) ;
#197908=CARTESIAN_POINT ( 'NONE',  ( -21.53943276465977519, -0.05219959533937600094, 53.75109039468568994 ) ) ;
#197909=CARTESIAN_POINT ( 'NONE',  ( 21.55341960407619695, -5.719274019375665929, 101.0427570613523756 ) ) ;
#197910=CARTESIAN_POINT ( 'NONE',  ( 15.80617190586769283, -15.72974639402175789, 20.62609039468568639 ) ) ;
#197911=CARTESIAN_POINT ( 'NONE',  ( -21.53943276465977519, 0.05219959533907696930, 96.24890960531435269 ) ) ;
#197912=CARTESIAN_POINT ( 'NONE',  ( -19.02544592524334988, -5.153800228976617603, 48.95942372801900433 ) ) ;
#197913=CARTESIAN_POINT ( 'NONE',  ( -18.62759615963270932, 10.81492255796079327, 45.83224293864769550 ) ) ;
#197914=CARTESIAN_POINT ( 'NONE',  ( -19.02544592524342804, 5.153800228976336051, 81.04057627198103830 ) ) ;
#197915=CARTESIAN_POINT ( 'NONE',  ( -16.52544592524342804, 4.483927247898546575, 36.04057627198102409 ) ) ;
#197916=CARTESIAN_POINT ( 'NONE',  ( -17.49999999999999645, 5.499999999999997335, 120.0000000000000142 ) ) ;
#197917=( BOUNDED_CURVE ( )  B_SPLINE_CURVE ( 2, ( #65208, #81349, #143033, #112702, #67197, #175381, #20691, #5517, #113686, #188574, #50054, #135625, #28459 ),
 .UNSPECIFIED., .F., .T. ) 
 B_SPLINE_CURVE_WITH_KNOTS ( ( 3, 2, 2, 2, 2, 2, 3 ),
 ( 0.5024304364270452128, 0.5043859649122807154, 0.5087719298245614308, 0.5131578947368421462, 0.5175438596491228616, 0.5219298245614034659, 0.5238396732245489407 ),
 .UNSPECIFIED. ) 
 CURVE ( )  GEOMETRIC_REPRESENTATION_ITEM ( )  RATIONAL_B_SPLINE_CURVE ( ( 0.9831626618144007068, 0.9848076720550096308, 1.000000000000000000, 0.9659258262890683122, 1.000000000000000000, 0.9659258262890683122, 1.000000000000000000, 0.9659258262890683122, 1.000000000000000000, 0.9659258262890683122, 1.000000000000000000, 0.9851625545550091179, 0.9832469066685282089 ) ) 
 REPRESENTATION_ITEM ( '' )  );
#197918=CARTESIAN_POINT ( 'NONE',  ( -19.52851543214745078, -5.499999999999944933, 80.39357721762576148 ) ) ;
#197920=CARTESIAN_POINT ( 'NONE',  ( 9.564922557961047289, -16.46253265017146816, 95.41775706135233293 ) ) ;
#197921=CARTESIAN_POINT ( 'NONE',  ( -18.62759615963270932, 10.81492255796079327, 65.83224293864769550 ) ) ;
#197922=CARTESIAN_POINT ( 'NONE',  ( -14.29746914071049879, 8.314922557960819915, 55.83224293864770260 ) ) ;
#197923=CARTESIAN_POINT ( 'NONE',  ( -14.34966873604972548, 8.224510206698743886, 28.33442372801902209 ) ) ;
#197924=CARTESIAN_POINT ( 'NONE',  ( 19.03943276465977164, -0.05219959533909143690, 48.74890960531435979 ) ) ;
#197925=CARTESIAN_POINT ( 'NONE',  ( -5.719274019375665041, -21.55341960407619695, 19.79275706135235069 ) ) ;
#197926=CARTESIAN_POINT ( 'NONE',  ( -13.89961937509957401, -13.97604488694547875, 84.37609039468567573 ) ) ;
#197927=CARTESIAN_POINT ( 'NONE',  ( 13.97604488694527802, 13.89961937509977652, 79.37390960531435269 ) ) ;
#197928=CARTESIAN_POINT ( 'NONE',  ( 16.55341960407611168, 4.379528057220329451, 88.95724293864769550 ) ) ;
#197929=CARTESIAN_POINT ( 'NONE',  ( 19.05341960407611168, 5.049401038298154454, 78.95724293864769550 ) ) ;
#197930=CARTESIAN_POINT ( 'NONE',  ( 18.67979575497178502, 10.72451020669898547, 74.16557627198102409 ) ) ;
#197931=CARTESIAN_POINT ( 'NONE',  ( -0.05219959533909027116, -19.03943276465977164, 27.49890960531435624 ) ) ;
#197933=CARTESIAN_POINT ( 'NONE',  ( 14.29746914071049879, -8.314922557960816363, 53.33224293864769550 ) ) ;
#197934=CARTESIAN_POINT ( 'NONE',  ( 19.05341960407611168, 5.049401038298154454, 88.95724293864769550 ) ) ;
#197935=CARTESIAN_POINT ( 'NONE',  ( -9.564922557961040184, 16.46253265017147172, 47.91775706135233293 ) ) ;
#197936=CARTESIAN_POINT ( 'NONE',  ( -14.29746914071037622, -8.314922557961029526, 54.16775706135235424 ) ) ;
#197937=CARTESIAN_POINT ( 'NONE',  ( -5.719274019375978568, 21.55341960407610458, 75.20724293864769550 ) ) ;
#197938=CARTESIAN_POINT ( 'NONE',  ( -9.564922557961040184, 16.46253265017147172, 42.91775706135234003 ) ) ;
#197939=CARTESIAN_POINT ( 'NONE',  ( 16.46253265017160672, -9.564922557960803928, 83.33224293864768129 ) ) ;
#197940=CARTESIAN_POINT ( 'NONE',  ( -17.49999999999999645, 5.499999999999996447, 113.7176903769643417 ) ) ;
#197941=CARTESIAN_POINT ( 'NONE',  ( 15.72974639402199770, -15.80617190586745480, 23.12390960531436335 ) ) ;
#197942=CARTESIAN_POINT ( 'NONE',  ( -13.97604488694527625, -13.89961937509977652, 71.87390960531433848 ) ) ;
#197943=CARTESIAN_POINT ( 'NONE',  ( 15.80617190586769283, -15.72974639402175789, 55.62609039468568284 ) ) ;
#197944=CARTESIAN_POINT ( 'NONE',  ( -0.05219959533909027116, -19.03943276465977164, 27.49890960531435624 ) ) ;
#197945=CARTESIAN_POINT ( 'NONE',  ( 0.05219959533937995610, -21.53943276465977519, 20.00109039468568639 ) ) ;
#197946=CARTESIAN_POINT ( 'NONE',  ( -13.89961937509977652, 13.97604488694528158, 100.6239096053143669 ) ) ;
#197948=CARTESIAN_POINT ( 'NONE',  ( 21.55341960407619695, -5.719274019375665929, 41.04275706135236135 ) ) ;
#197950=CARTESIAN_POINT ( 'NONE',  ( 5.049401038298161559, -19.05341960407611168, 102.7072429386476955 ) ) ;
#197953=CARTESIAN_POINT ( 'NONE',  ( -10.72451020669898014, 18.67979575497178502, 110.4155762719810383 ) ) ;
#197954=CARTESIAN_POINT ( 'NONE',  ( 19.03943276465977164, -0.05219959533909143690, 48.74890960531435979 ) ) ;
#197955=CARTESIAN_POINT ( 'NONE',  ( -12.14591786802326823, 12.06949235617739902, 28.12609039468568284 ) ) ;
#197957=CARTESIAN_POINT ( 'NONE',  ( 15.80617190586769283, -15.72974639402175789, 105.6260903946856899 ) ) ;
#197958=CARTESIAN_POINT ( 'NONE',  ( 13.89961937509977652, -13.97604488694527269, 23.12390960531436335 ) ) ;
#197959=CARTESIAN_POINT ( 'NONE',  ( -0.05219959533937732626, 21.53943276465977519, 92.50109039468567573 ) ) ;
#197960=CARTESIAN_POINT ( 'NONE',  ( 5.153800228976335163, 19.02544592524342804, 84.79057627198099567 ) ) ;
#197961=CARTESIAN_POINT ( 'NONE',  ( -15.72974639402176322, -15.80617190586768395, 64.37609039468568994 ) ) ;
#197963=CARTESIAN_POINT ( 'NONE',  ( 16.51473224551069308, 9.474510206698969483, 104.1655762719810241 ) ) ;
#197964=PLANE ( 'NONE',  #82227 ) ;
#197965=CARTESIAN_POINT ( 'NONE',  ( 8.314922557961029526, -14.29746914071037800, 50.41775706135235424 ) ) ;
#197966=CARTESIAN_POINT ( 'NONE',  ( 14.34966873604972726, -8.224510206698740333, 70.83442372801901854 ) ) ;
#197967=CARTESIAN_POINT ( 'NONE',  ( -18.67979575497193778, 10.72451020669871902, 58.33442372801901143 ) ) ;
#197968=CARTESIAN_POINT ( 'NONE',  ( 15.80617190586769283, -15.72974639402175789, 90.62609039468567573 ) ) ;
#197970=CARTESIAN_POINT ( 'NONE',  ( 16.52544592524335698, 4.483927247898782831, 26.45942372801901854 ) ) ;
#197971=CARTESIAN_POINT ( 'NONE',  ( -0.05219959533909027116, -19.03943276465977164, 72.49890960531435269 ) ) ;
#197972=CARTESIAN_POINT ( 'NONE',  ( -19.03943276465977164, 0.05219959533909376836, 101.2489096053143669 ) ) ;
#197974=CARTESIAN_POINT ( 'NONE',  ( -13.89961937509977652, 13.97604488694528158, 30.62390960531435269 ) ) ;
#197975=CARTESIAN_POINT ( 'NONE',  ( 18.67979575497178502, 10.72451020669898547, 24.16557627198103120 ) ) ;
#197976=CARTESIAN_POINT ( 'NONE',  ( -8.314922557961024197, 14.29746914071037800, 92.91775706135236135 ) ) ;
#197977=CARTESIAN_POINT ( 'NONE',  ( 4.379528057220339221, -16.55341960407611168, 67.70724293864769550 ) ) ;
#197978=CARTESIAN_POINT ( 'NONE',  ( -9.564922557960796823, -16.46253265017161027, 67.08224293864769550 ) ) ;
#197979=CARTESIAN_POINT ( 'NONE',  ( 5.823673210054444382, -21.52544592524334988, 95.20942372801903275 ) ) ;
#197980=CARTESIAN_POINT ( 'NONE',  ( -19.03943276465977164, 0.05219959533909376836, 116.2489096053143669 ) ) ;
#197981=CARTESIAN_POINT ( 'NONE',  ( 12.14591786802327356, -12.06949235617739191, 25.62609039468567929 ) ) ;
#197982=CARTESIAN_POINT ( 'NONE',  ( -4.483927247898539470, -16.52544592524342804, 77.29057627198102409 ) ) ;
#197983=CARTESIAN_POINT ( 'NONE',  ( 10.81492255796106328, -18.62759615963255655, 30.41775706135234358 ) ) ;
#197984=CARTESIAN_POINT ( 'NONE',  ( -21.52544592524343514, 5.823673210054127303, 76.04057627198102409 ) ) ;
#197985=CARTESIAN_POINT ( 'NONE',  ( 9.564922557961047289, -16.46253265017146816, 35.41775706135233293 ) ) ;
#197987=CARTESIAN_POINT ( 'NONE',  ( -0.05219959533909027116, -19.03943276465977164, 82.49890960531436690 ) ) ;
#197988=CARTESIAN_POINT ( 'NONE',  ( 14.34966873604960469, 8.224510206698951720, 54.16557627198103120 ) ) ;
#197989=CARTESIAN_POINT ( 'NONE',  ( 14.34966873604960469, 8.224510206698951720, 39.16557627198102409 ) ) ;
#197990=CARTESIAN_POINT ( 'NONE',  ( -12.06949235617739369, -12.14591786802326823, 109.3760903946857042 ) ) ;
#197991=CARTESIAN_POINT ( 'NONE',  ( 13.97604488694548053, -13.89961937509957401, 60.62609039468564731 ) ) ;
#197992=CARTESIAN_POINT ( 'NONE',  ( 19.39720447994795904, 5.499999999999972466, 52.16317477297178584 ) ) ;
#197993=CARTESIAN_POINT ( 'NONE',  ( 9.564922557960805705, 16.46253265017160317, 109.5822429386476955 ) ) ;
#197995=CARTESIAN_POINT ( 'NONE',  ( 8.314922557960818139, 14.29746914071049879, 74.58224293864768129 ) ) ;
#197997=CARTESIAN_POINT ( 'NONE',  ( -9.564922557960796823, -16.46253265017161027, 27.08224293864769550 ) ) ;
#197998=CARTESIAN_POINT ( 'NONE',  ( 21.53943276465977519, -0.05219959533907433946, 38.74890960531435979 ) ) ;
#197999=CARTESIAN_POINT ( 'NONE',  ( -15.80617190586745835, -15.72974639402198527, 61.87390960531436690 ) ) ;
#198000=CARTESIAN_POINT ( 'NONE',  ( -5.153800228976328057, -19.02544592524343514, 22.29057627198102765 ) ) ;
#198001=CARTESIAN_POINT ( 'NONE',  ( 16.55341960407618274, -4.379528057220086978, 61.04275706135234714 ) ) ;
#198002=CARTESIAN_POINT ( 'NONE',  ( -9.474510206698964154, 16.51473224551069663, 50.41557627198102409 ) ) ;
#198003=CARTESIAN_POINT ( 'NONE',  ( 21.52544592524334988, 5.823673210054432836, 61.45942372801901854 ) ) ;
#198004=CARTESIAN_POINT ( 'NONE',  ( -14.29746914071049879, 8.314922557960819915, 95.83224293864770971 ) ) ;
#198006=CARTESIAN_POINT ( 'NONE',  ( -17.40805194822030799, 6.112264579159339739, 50.83371272510613892 ) ) ;
#198007=CARTESIAN_POINT ( 'NONE',  ( 21.52544592524344225, -5.823673210054117533, 33.54057627198102409 ) ) ;
#198009=CARTESIAN_POINT ( 'NONE',  ( -21.55341960407619339, 5.719274019375674811, 68.54275706135234714 ) ) ;
#198011=CARTESIAN_POINT ( 'NONE',  ( 12.06949235617739724, 12.14591786802326823, 56.87609039468568994 ) ) ;
#198012=CARTESIAN_POINT ( 'NONE',  ( 4.379528057220339221, -16.55341960407611168, 37.70724293864769550 ) ) ;
#198013=CARTESIAN_POINT ( 'NONE',  ( 21.53943276465977519, -0.05219959533907433946, 73.74890960531433848 ) ) ;
#198015=CARTESIAN_POINT ( 'NONE',  ( -0.05219959533907301413, -21.53943276465977519, 57.49890960531435979 ) ) ;
#198017=CARTESIAN_POINT ( 'NONE',  ( 19.03943276465977164, 0.05219959533936151252, 86.25109039468567573 ) ) ;
#198018=CARTESIAN_POINT ( 'NONE',  ( -9.474510206698964154, 16.51473224551069663, 110.4155762719810383 ) ) ;
#198019=CARTESIAN_POINT ( 'NONE',  ( 13.89961937509977652, -13.97604488694527269, 48.12390960531435979 ) ) ;
#198020=CARTESIAN_POINT ( 'NONE',  ( 8.314922557960818139, 14.29746914071049879, 114.5822429386477097 ) ) ;
#198022=CARTESIAN_POINT ( 'NONE',  ( -19.02544592524342804, 5.153800228976336051, 111.0405762719810099 ) ) ;
#198024=CARTESIAN_POINT ( 'NONE',  ( -14.34966873604972548, 8.224510206698743886, 73.33442372801901854 ) ) ;
#198025=CARTESIAN_POINT ( 'NONE',  ( -18.62759615963270932, 10.81492255796079327, 100.8322429386477097 ) ) ;
#198026=CARTESIAN_POINT ( 'NONE',  ( -16.46253265017160317, 9.564922557960807481, 50.83224293864770260 ) ) ;
#198027=CARTESIAN_POINT ( 'NONE',  ( 5.719274019375673035, 21.55341960407619339, 37.29275706135235424 ) ) ;
#198028=CARTESIAN_POINT ( 'NONE',  ( 16.46253265017160672, -9.564922557960803928, 93.33224293864769550 ) ) ;
#198030=ORIENTED_EDGE ( 'NONE', *, *, #160761, .T. ) ;
#198031=CARTESIAN_POINT ( 'NONE',  ( 18.67979575497194134, -10.72451020669871369, 30.83442372801902209 ) ) ;
#198032=CARTESIAN_POINT ( 'NONE',  ( -19.05341960407611168, -5.049401038298163336, 101.4572429386476955 ) ) ;
#198033=CARTESIAN_POINT ( 'NONE',  ( 5.049401038297881783, 19.05341960407617563, 82.29275706135229029 ) ) ;
#198034=CARTESIAN_POINT ( 'NONE',  ( 19.03943276465977164, 0.05219959533936151252, 46.25109039468566863 ) ) ;
#198035=CARTESIAN_POINT ( 'NONE',  ( 18.62759615963271287, -10.81492255796078972, 103.3322429386476955 ) ) ;
#198036=CARTESIAN_POINT ( 'NONE',  ( 16.46253265017146816, 9.564922557961045513, 31.66775706135232937 ) ) ;
#198037=CARTESIAN_POINT ( 'NONE',  ( 9.564922557961047289, -16.46253265017146816, 35.41775706135233293 ) ) ;
#198038=CARTESIAN_POINT ( 'NONE',  ( -8.314922557961024197, 14.29746914071037800, 97.91775706135236135 ) ) ;
#198039=CARTESIAN_POINT ( 'NONE',  ( 19.03943276465977164, -0.05219959533909143690, 113.7489096053143669 ) ) ;
#198041=CARTESIAN_POINT ( 'NONE',  ( -16.51473224551069308, -9.474510206698971260, 76.66557627198103830 ) ) ;
#198042=CARTESIAN_POINT ( 'NONE',  ( -21.52544592524334988, -5.823673210054445271, 83.95942372801900433 ) ) ;
#198043=CARTESIAN_POINT ( 'NONE',  ( -5.719274019375665041, -21.55341960407619695, 74.79275706135234714 ) ) ;
#198045=CARTESIAN_POINT ( 'NONE',  ( -0.05219959533909027116, -19.03943276465977164, 87.49890960531436690 ) ) ;
#198046=CARTESIAN_POINT ( 'NONE',  ( 10.72451020669871369, 18.67979575497193778, 67.08442372801901854 ) ) ;
#198047=CARTESIAN_POINT ( 'NONE',  ( -0.05219959533936034679, 19.03943276465977164, 97.50109039468567573 ) ) ;
#198048=CARTESIAN_POINT ( 'NONE',  ( -13.97604488694527625, -13.89961937509977652, 66.87390960531436690 ) ) ;
#198049=CARTESIAN_POINT ( 'NONE',  ( 19.02544592524343514, -5.153800228976328945, 113.5405762719810241 ) ) ;
#198050=CARTESIAN_POINT ( 'NONE',  ( -16.46253265017160317, 9.564922557960807481, 85.83224293864769550 ) ) ;
#198051=CARTESIAN_POINT ( 'NONE',  ( -17.12812012977030562, -6.668231424565920662, 91.35948759323146362 ) ) ;
#198052=CARTESIAN_POINT ( 'NONE',  ( -19.03943276465977164, 0.05219959533909376836, 66.24890960531436690 ) ) ;
#198053=CARTESIAN_POINT ( 'NONE',  ( 9.564922557960805705, 16.46253265017160317, 49.58224293864770260 ) ) ;
#198054=CARTESIAN_POINT ( 'NONE',  ( 0.05219959533907565091, 21.53943276465977519, 99.99890960531436690 ) ) ;
#198055=CARTESIAN_POINT ( 'NONE',  ( 14.34966873604972726, -8.224510206698740333, 85.83442372801901854 ) ) ;
#198057=CARTESIAN_POINT ( 'NONE',  ( 5.153800228976615827, -19.02544592524334988, 40.20942372801898301 ) ) ;
#198058=CARTESIAN_POINT ( 'NONE',  ( 5.153800228976335163, 19.02544592524342804, 84.79057627198099567 ) ) ;
#198059=CARTESIAN_POINT ( 'NONE',  ( 14.29746914071049879, -8.314922557960816363, 68.33224293864769550 ) ) ;
#198060=CARTESIAN_POINT ( 'NONE',  ( -16.52544592524342804, 4.483927247898546575, 111.0405762719810525 ) ) ;
#198061=CARTESIAN_POINT ( 'NONE',  ( 9.564922557960805705, 16.46253265017160317, 109.5822429386476955 ) ) ;
#198062=CARTESIAN_POINT ( 'NONE',  ( -16.46253265017160317, 9.564922557960807481, 100.8322429386477097 ) ) ;
#198063=CARTESIAN_POINT ( 'NONE',  ( 12.06949235617757843, -12.14591786802309237, 78.12390960531436690 ) ) ;
#198065=CARTESIAN_POINT ( 'NONE',  ( 16.46253265017146816, 9.564922557961045513, 36.66775706135233293 ) ) ;
#198066=CARTESIAN_POINT ( 'NONE',  ( 4.483927247898790824, -16.52544592524335698, 90.20942372801903275 ) ) ;
#198067=CARTESIAN_POINT ( 'NONE',  ( 9.474510206698971260, -16.51473224551069308, 72.91557627198102409 ) ) ;
#198068=CARTESIAN_POINT ( 'NONE',  ( 5.823673210054444382, -21.52544592524334988, 55.20942372801902565 ) ) ;
#198069=CARTESIAN_POINT ( 'NONE',  ( 21.53943276465977519, -0.05219959533907433946, 48.74890960531435979 ) ) ;
#198070=CARTESIAN_POINT ( 'NONE',  ( -10.72451020669870658, -18.67979575497194134, 19.58442372801901143 ) ) ;
#198071=CARTESIAN_POINT ( 'NONE',  ( 15.80617190586746368, 15.72974639402197994, 69.37390960531436690 ) ) ;
#198072=CARTESIAN_POINT ( 'NONE',  ( 14.34966873604960469, 8.224510206698951720, 99.16557627198100988 ) ) ;
#198073=CARTESIAN_POINT ( 'NONE',  ( -16.51473224551082808, 9.474510206698731452, 63.33442372801900433 ) ) ;
#198074=CARTESIAN_POINT ( 'NONE',  ( -19.05341960407611168, -5.049401038298163336, 31.45724293864769550 ) ) ;
#198075=CARTESIAN_POINT ( 'NONE',  ( -16.51473224551069308, -9.474510206698971260, 81.66557627198103830 ) ) ;
#198076=CARTESIAN_POINT ( 'NONE',  ( -16.51473224551069308, -9.474510206698971260, 76.66557627198103830 ) ) ;
#198077=CARTESIAN_POINT ( 'NONE',  ( -14.34966873604960291, -8.224510206698953496, 96.66557627198102409 ) ) ;
#198079=CARTESIAN_POINT ( 'NONE',  ( 8.314922557960818139, 14.29746914071049879, 24.58224293864768839 ) ) ;
#198080=CARTESIAN_POINT ( 'NONE',  ( -8.314922557961024197, 14.29746914071037800, 27.91775706135234358 ) ) ;
#198081=CARTESIAN_POINT ( 'NONE',  ( -15.72974639402176322, -15.80617190586768395, 99.37609039468568994 ) ) ;
#198082=CARTESIAN_POINT ( 'NONE',  ( -0.05219959533909027116, -19.03943276465977164, 102.4989096053143669 ) ) ;
#198083=CARTESIAN_POINT ( 'NONE',  ( 15.72974639402199770, -15.80617190586745480, 113.1239096053143953 ) ) ;
#198084=CARTESIAN_POINT ( 'NONE',  ( 19.02544592524343514, -5.153800228976328945, 38.54057627198103120 ) ) ;
#198085=CARTESIAN_POINT ( 'NONE',  ( -12.06949235617739369, -12.14591786802326823, 39.37609039468567573 ) ) ;
#198086=CARTESIAN_POINT ( 'NONE',  ( -14.29746914071037622, -8.314922557961029526, 19.16775706135234714 ) ) ;
#198088=CARTESIAN_POINT ( 'NONE',  ( -9.474510206698964154, 16.51473224551069663, 35.41557627198102409 ) ) ;
#198090=CARTESIAN_POINT ( 'NONE',  ( 12.06949235617757843, -12.14591786802309237, 98.12390960531436690 ) ) ;
#198091=CARTESIAN_POINT ( 'NONE',  ( 15.80617190586746368, 15.72974639402197994, 104.3739096053143669 ) ) ;
#198092=CARTESIAN_POINT ( 'NONE',  ( -5.049401038297874678, -19.05341960407617918, 69.79275706135233293 ) ) ;
#198094=CARTESIAN_POINT ( 'NONE',  ( -19.03943276465977164, 0.05219959533909376836, 96.24890960531436690 ) ) ;
#198095=CARTESIAN_POINT ( 'NONE',  ( 10.72451020669871369, 18.67979575497193778, 22.08442372801901143 ) ) ;
#198097=CARTESIAN_POINT ( 'NONE',  ( -19.03943276465977164, 0.05219959533909376836, 86.24890960531436690 ) ) ;
#198098=CARTESIAN_POINT ( 'NONE',  ( 17.40861289039003879, -6.110651285853326620, 111.1276752917257227 ) ) ;
#198099=CARTESIAN_POINT ( 'NONE',  ( -19.05341960407611168, -5.049401038298163336, 81.45724293864769550 ) ) ;
#198100=CARTESIAN_POINT ( 'NONE',  ( 5.823673210054444382, -21.52544592524334988, 35.20942372801901854 ) ) ;
#198101=CARTESIAN_POINT ( 'NONE',  ( -16.53943276465976808, 0.05219959533911058130, 71.24890960531435269 ) ) ;
#198102=CARTESIAN_POINT ( 'NONE',  ( -13.97604488694527625, -13.89961937509977652, 81.87390960531436690 ) ) ;
#198103=CARTESIAN_POINT ( 'NONE',  ( 19.02544592524334988, 5.153800228976608722, 26.45942372801899722 ) ) ;
#198104=CARTESIAN_POINT ( 'NONE',  ( -4.483927247898782831, 16.52544592524335698, 47.70942372801902565 ) ) ;
#198105=CARTESIAN_POINT ( 'NONE',  ( 19.02544592524334988, 5.153800228976608722, 56.45942372801898301 ) ) ;
#198106=CARTESIAN_POINT ( 'NONE',  ( -5.719274019375665041, -21.55341960407619695, 69.79275706135234714 ) ) ;
#198107=CARTESIAN_POINT ( 'NONE',  ( 14.34966873604972726, -8.224510206698740333, 20.83442372801901143 ) ) ;
#198108=CARTESIAN_POINT ( 'NONE',  ( 13.97604488694527802, 13.89961937509977652, 64.37390960531436690 ) ) ;
#198109=CARTESIAN_POINT ( 'NONE',  ( 16.51473224551083163, -9.474510206698727899, 100.8344237280190043 ) ) ;
#198110=CARTESIAN_POINT ( 'NONE',  ( -14.29746914071037622, -8.314922557961029526, 69.16775706135234714 ) ) ;
#198111=CARTESIAN_POINT ( 'NONE',  ( 5.823673210054444382, -21.52544592524334988, 105.2094237280190328 ) ) ;
#198112=CARTESIAN_POINT ( 'NONE',  ( 13.97604488694548053, -13.89961937509957401, 75.62609039468564731 ) ) ;
#198113=CARTESIAN_POINT ( 'NONE',  ( -19.02544592524342804, 5.153800228976336051, 56.04057627198100988 ) ) ;
#198114=CARTESIAN_POINT ( 'NONE',  ( 10.72451020669898902, -18.67979575497178502, 82.91557627198103830 ) ) ;
#198115=CARTESIAN_POINT ( 'NONE',  ( 8.224510206698953496, -14.34966873604960469, 72.91557627198103830 ) ) ;
#198116=CARTESIAN_POINT ( 'NONE',  ( -5.153800228976607833, 19.02544592524334988, 72.70942372801900433 ) ) ;
#198118=CARTESIAN_POINT ( 'NONE',  ( 13.89961937509957401, 13.97604488694547697, 41.87609039468566152 ) ) ;
#198119=CARTESIAN_POINT ( 'NONE',  ( 12.14591786802327356, -12.06949235617739191, 105.6260903946856899 ) ) ;
#198120=CARTESIAN_POINT ( 'NONE',  ( 12.06949235617757843, -12.14591786802309237, 73.12390960531436690 ) ) ;
#198121=CARTESIAN_POINT ( 'NONE',  ( 0.05219959533937995610, -21.53943276465977519, 105.0010903946856757 ) ) ;
#198123=CARTESIAN_POINT ( 'NONE',  ( -5.719274019375978568, 21.55341960407610458, 110.2072429386477239 ) ) ;
#198124=CARTESIAN_POINT ( 'NONE',  ( -19.02544592524342804, 5.153800228976336051, 66.04057627198103830 ) ) ;
#198125=CARTESIAN_POINT ( 'NONE',  ( -0.05219959533937732626, 21.53943276465977519, 77.50109039468567573 ) ) ;
#198126=CARTESIAN_POINT ( 'NONE',  ( -19.05341960407611168, -5.049401038298163336, 56.45724293864768129 ) ) ;
#198127=CARTESIAN_POINT ( 'NONE',  ( 0.05219959533910956823, 16.53943276465976808, 114.9989096053143669 ) ) ;
#198128=CARTESIAN_POINT ( 'NONE',  ( 10.81492255796078972, 18.62759615963270932, 29.58224293864769905 ) ) ;
#198129=CARTESIAN_POINT ( 'NONE',  ( 8.314922557960818139, 14.29746914071049879, 64.58224293864769550 ) ) ;
#198130=CARTESIAN_POINT ( 'NONE',  ( 13.89961937509977652, -13.97604488694527269, 38.12390960531436690 ) ) ;
#198131=CARTESIAN_POINT ( 'NONE',  ( -8.224510206698948167, 14.34966873604960824, 100.4155762719810241 ) ) ;
#198132=CARTESIAN_POINT ( 'NONE',  ( 21.53943276465977519, -0.05219959533907433946, 113.7489096053143527 ) ) ;
#198133=CARTESIAN_POINT ( 'NONE',  ( -5.719274019375665041, -21.55341960407619695, 44.79275706135234714 ) ) ;
#198134=CARTESIAN_POINT ( 'NONE',  ( -16.51473224551069308, -9.474510206698971260, 36.66557627198102409 ) ) ;
#198135=CARTESIAN_POINT ( 'NONE',  ( 4.379528057220092307, 16.55341960407617563, 67.29275706135234714 ) ) ;
#198136=CARTESIAN_POINT ( 'NONE',  ( 0.05219959533907565091, 21.53943276465977519, 104.9989096053143669 ) ) ;
#198137=CARTESIAN_POINT ( 'NONE',  ( 10.72451020669898902, -18.67979575497178502, 92.91557627198103830 ) ) ;
#198138=CARTESIAN_POINT ( 'NONE',  ( 16.51473224551083163, -9.474510206698727899, 20.83442372801899722 ) ) ;
#198139=CARTESIAN_POINT ( 'NONE',  ( -9.564922557960796823, -16.46253265017161027, 52.08224293864768839 ) ) ;
#198140=CARTESIAN_POINT ( 'NONE',  ( -17.72517630441458536, 5.499999999999976907, 40.92175719257603106 ) ) ;
#198141=CARTESIAN_POINT ( 'NONE',  ( -18.67979575497193778, 10.72451020669871902, 53.33442372801901854 ) ) ;
#198142=CARTESIAN_POINT ( 'NONE',  ( -15.80617190586745835, -15.72974639402198527, 36.87390960531435979 ) ) ;
#198143=CARTESIAN_POINT ( 'NONE',  ( -8.314922557960811034, -14.29746914071050412, 22.08224293864769194 ) ) ;
#198144=CARTESIAN_POINT ( 'NONE',  ( -21.52544592524334988, -5.823673210054445271, 73.95942372801901854 ) ) ;
#198145=CARTESIAN_POINT ( 'NONE',  ( 5.719274019375673035, 21.55341960407619339, 97.29275706135234714 ) ) ;
#198146=CARTESIAN_POINT ( 'NONE',  ( 5.153800228976615827, -19.02544592524334988, 40.20942372801898301 ) ) ;
#198147=CARTESIAN_POINT ( 'NONE',  ( -14.29746914071037622, -8.314922557961029526, 104.1677570613523471 ) ) ;
#198148=CARTESIAN_POINT ( 'NONE',  ( 5.823673210054444382, -21.52544592524334988, 50.20942372801901854 ) ) ;
#198149=CARTESIAN_POINT ( 'NONE',  ( 16.46253265017160672, -9.564922557960803928, 53.33224293864768839 ) ) ;
#198150=CARTESIAN_POINT ( 'NONE',  ( 18.67979575497194134, -10.72451020669871369, 110.8344237280190043 ) ) ;
#198151=CARTESIAN_POINT ( 'NONE',  ( 10.72451020669898902, -18.67979575497178502, 42.91557627198103120 ) ) ;
#198152=CARTESIAN_POINT ( 'NONE',  ( 18.62759615963255655, 10.81492255796105972, 26.66775706135235424 ) ) ;
#198153=CARTESIAN_POINT ( 'NONE',  ( 10.81492255796078972, 18.62759615963270932, 94.58224293864769550 ) ) ;
#198154=CARTESIAN_POINT ( 'NONE',  ( 19.03943276465977164, 0.05219959533936151252, 81.25109039468567573 ) ) ;
#198155=CARTESIAN_POINT ( 'NONE',  ( 12.14591786802327356, -12.06949235617739191, 35.62609039468568994 ) ) ;
#198156=CARTESIAN_POINT ( 'NONE',  ( 17.60779699588839975, 5.500000000000013323, 63.84981316670106111 ) ) ;
#198157=CARTESIAN_POINT ( 'NONE',  ( 5.823673210054125526, 21.52544592524343514, 79.79057627198102409 ) ) ;
#198158=CARTESIAN_POINT ( 'NONE',  ( -14.34966873604972548, 8.224510206698743886, 63.33442372801900433 ) ) ;
#198159=CARTESIAN_POINT ( 'NONE',  ( -4.483927247898539470, -16.52544592524342804, 72.29057627198102409 ) ) ;
#198161=CARTESIAN_POINT ( 'NONE',  ( -9.564922557961040184, 16.46253265017147172, 97.91775706135233293 ) ) ;
#198162=CARTESIAN_POINT ( 'NONE',  ( -21.53943276465977519, 0.05219959533907696930, 36.24890960531435979 ) ) ;
#198164=CARTESIAN_POINT ( 'NONE',  ( 16.52544592524335698, 4.483927247898782831, 41.45942372801901143 ) ) ;
#198165=CARTESIAN_POINT ( 'NONE',  ( -15.72974639402176322, -15.80617190586768395, 19.37609039468568639 ) ) ;
#198166=CARTESIAN_POINT ( 'NONE',  ( 21.52544592524344225, -5.823673210054117533, 28.54057627198103120 ) ) ;
#198167=CARTESIAN_POINT ( 'NONE',  ( -14.29746914071037622, -8.314922557961029526, 69.16775706135234714 ) ) ;
#198168=CARTESIAN_POINT ( 'NONE',  ( -19.05341960407611168, -5.049401038298163336, 86.45724293864769550 ) ) ;
#198169=CARTESIAN_POINT ( 'NONE',  ( 18.67979575497194134, -10.72451020669871369, 60.83442372801901854 ) ) ;
#198170=CARTESIAN_POINT ( 'NONE',  ( -19.05341960407611168, -5.049401038298163336, 31.45724293864769550 ) ) ;
#198171=CARTESIAN_POINT ( 'NONE',  ( -21.55341960407610458, -5.719274019375992779, 21.45724293864769550 ) ) ;
#198172=ORIENTED_EDGE ( 'NONE', *, *, #118181, .F. ) ;
#198173=CARTESIAN_POINT ( 'NONE',  ( -13.89961937509957401, -13.97604488694547875, 34.37609039468566863 ) ) ;
#198174=CARTESIAN_POINT ( 'NONE',  ( 12.06949235617739724, 12.14591786802326823, 46.87609039468568994 ) ) ;
#198175=CARTESIAN_POINT ( 'NONE',  ( -0.05219959533909027116, -19.03943276465977164, 112.4989096053143669 ) ) ;
#198176=CARTESIAN_POINT ( 'NONE',  ( -5.153800228976328057, -19.02544592524343514, 77.29057627198099567 ) ) ;
#198177=CARTESIAN_POINT ( 'NONE',  ( 14.34966873604972726, -8.224510206698740333, 95.83442372801903275 ) ) ;
#198179=CARTESIAN_POINT ( 'NONE',  ( 12.14591786802309770, 12.06949235617756955, 99.37390960531436690 ) ) ;
#198180=CARTESIAN_POINT ( 'NONE',  ( 21.55341960407610458, 5.719274019375980345, 28.95724293864769905 ) ) ;
#198181=CARTESIAN_POINT ( 'NONE',  ( 19.02544592524343514, -5.153800228976328945, 28.54057627198102409 ) ) ;
#198182=CARTESIAN_POINT ( 'NONE',  ( -12.14591786802326823, 12.06949235617739902, 63.12609039468568994 ) ) ;
#198183=CARTESIAN_POINT ( 'NONE',  ( 5.823673210054444382, -21.52544592524334988, 25.20942372801901854 ) ) ;
#198184=CARTESIAN_POINT ( 'NONE',  ( -5.049401038297874678, -19.05341960407617918, 79.79275706135233293 ) ) ;
#198185=CARTESIAN_POINT ( 'NONE',  ( -19.05341960407611168, -5.049401038298163336, 46.45724293864768129 ) ) ;
#198186=CARTESIAN_POINT ( 'NONE',  ( -18.67979575497178146, -10.72451020669898902, 66.66557627198102409 ) ) ;
#198187=CARTESIAN_POINT ( 'NONE',  ( 19.02544592524343514, -5.153800228976328945, 108.5405762719810383 ) ) ;
#198188=CARTESIAN_POINT ( 'NONE',  ( 15.72974639402176855, 15.80617190586768217, 86.87609039468568994 ) ) ;
#198189=CARTESIAN_POINT ( 'NONE',  ( 5.153800228976335163, 19.02544592524342804, 69.79057627198103830 ) ) ;
#198191=CARTESIAN_POINT ( 'NONE',  ( 12.06949235617739724, 12.14591786802326823, 46.87609039468568994 ) ) ;
#198192=CARTESIAN_POINT ( 'NONE',  ( 13.97604488694527802, 13.89961937509977652, 64.37390960531436690 ) ) ;
#198193=CARTESIAN_POINT ( 'NONE',  ( 5.719274019375673035, 21.55341960407619339, 77.29275706135234714 ) ) ;
#198194=CARTESIAN_POINT ( 'NONE',  ( -13.89961937509957401, -13.97604488694547875, 39.37609039468566152 ) ) ;
#198195=CARTESIAN_POINT ( 'NONE',  ( 9.564922557961047289, -16.46253265017146816, 50.41775706135233293 ) ) ;
#198196=ORIENTED_EDGE ( 'NONE', *, *, #148562, .T. ) ;
#198197=CARTESIAN_POINT ( 'NONE',  ( 5.823673210054444382, -21.52544592524334988, 45.20942372801901854 ) ) ;
#198198=CARTESIAN_POINT ( 'NONE',  ( -5.049401038298153566, 19.05341960407611168, 55.20724293864768839 ) ) ;
#198199=CARTESIAN_POINT ( 'NONE',  ( 5.049401038297881783, 19.05341960407617563, 42.29275706135234003 ) ) ;
#198200=CARTESIAN_POINT ( 'NONE',  ( 9.474510206698971260, -16.51473224551069308, 97.91557627198102409 ) ) ;
#198201=CARTESIAN_POINT ( 'NONE',  ( 9.474510206698971260, -16.51473224551069308, 87.91557627198102409 ) ) ;
#198202=CARTESIAN_POINT ( 'NONE',  ( 8.314922557960818139, 14.29746914071049879, 44.58224293864769550 ) ) ;
#198203=CARTESIAN_POINT ( 'NONE',  ( 18.62759615963271287, -10.81492255796078972, 38.33224293864768839 ) ) ;
#198206=CARTESIAN_POINT ( 'NONE',  ( -21.55341960407619339, 5.719274019375674811, 103.5427570613523613 ) ) ;
#198208=CARTESIAN_POINT ( 'NONE',  ( -9.564922557960796823, -16.46253265017161027, 32.08224293864769550 ) ) ;
#198209=CARTESIAN_POINT ( 'NONE',  ( 5.049401038298161559, -19.05341960407611168, 107.7072429386476955 ) ) ;
#198211=CARTESIAN_POINT ( 'NONE',  ( -4.483927247898782831, 16.52544592524335698, 47.70942372801902565 ) ) ;
#198212=CARTESIAN_POINT ( 'NONE',  ( 21.55341960407610458, 5.719274019375980345, 73.95724293864769550 ) ) ;
#198213=CARTESIAN_POINT ( 'NONE',  ( -8.314922557960811034, -14.29746914071050412, 42.08224293864769550 ) ) ;
#198214=CARTESIAN_POINT ( 'NONE',  ( -5.049401038298153566, 19.05341960407611168, 25.20724293864768484 ) ) ;
#198215=CARTESIAN_POINT ( 'NONE',  ( 13.97604488694527802, 13.89961937509977652, 109.3739096053143669 ) ) ;
#198216=CARTESIAN_POINT ( 'NONE',  ( 5.823673210054444382, -21.52544592524334988, 25.20942372801901854 ) ) ;
#198217=CARTESIAN_POINT ( 'NONE',  ( -9.474510206698720793, -16.51473224551083518, 34.58442372801899722 ) ) ;
#198218=CARTESIAN_POINT ( 'NONE',  ( -16.52544592524342804, 4.483927247898546575, 111.0405762719810525 ) ) ;
#198219=CARTESIAN_POINT ( 'NONE',  ( -18.67979575497193778, 10.72451020669871902, 63.33442372801900433 ) ) ;
#198220=CARTESIAN_POINT ( 'NONE',  ( 17.48853670773243252, -5.747243402303149118, 31.16671299749990709 ) ) ;
#198221=CARTESIAN_POINT ( 'NONE',  ( -0.05219959533910754901, -16.53943276465976808, 27.49890960531435269 ) ) ;
#198222=CARTESIAN_POINT ( 'NONE',  ( 17.49999999999999289, 3.512728167236827570, 112.2719000481888258 ) ) ;
#198223=CARTESIAN_POINT ( 'NONE',  ( 10.81492255796078972, 18.62759615963270932, 24.58224293864768839 ) ) ;
#198224=CARTESIAN_POINT ( 'NONE',  ( 0.05219959533910956823, 16.53943276465976808, 89.99890960531438111 ) ) ;
#198226=CARTESIAN_POINT ( 'NONE',  ( -9.474510206698964154, 16.51473224551069663, 75.41557627198103830 ) ) ;
#198227=CARTESIAN_POINT ( 'NONE',  ( -8.314922557960811034, -14.29746914071050412, 77.08224293864769550 ) ) ;
#198228=CARTESIAN_POINT ( 'NONE',  ( 13.89961937509957401, 13.97604488694547697, 111.8760903946856757 ) ) ;
#198229=CARTESIAN_POINT ( 'NONE',  ( 10.81492255796078972, 18.62759615963270932, 64.58224293864769550 ) ) ;
#198231=CARTESIAN_POINT ( 'NONE',  ( 5.153800228976335163, 19.02544592524342804, 24.79057627198102765 ) ) ;
#198232=CARTESIAN_POINT ( 'NONE',  ( 0.05219959533909260263, 19.03943276465977164, 69.99890960531435269 ) ) ;
#198233=CARTESIAN_POINT ( 'NONE',  ( -15.80617190586745835, -15.72974639402198527, 81.87390960531435269 ) ) ;
#198235=CARTESIAN_POINT ( 'NONE',  ( 16.53943276465976808, 0.05219959533934440121, 111.2510903946856899 ) ) ;
#198236=CARTESIAN_POINT ( 'NONE',  ( -13.97604488694527625, -13.89961937509977652, 81.87390960531436690 ) ) ;
#198237=CARTESIAN_POINT ( 'NONE',  ( -16.51473224551082808, 9.474510206698731452, 63.33442372801900433 ) ) ;
#198238=CARTESIAN_POINT ( 'NONE',  ( -18.62759615963255300, -10.81492255796106328, 99.16775706135234714 ) ) ;
#198239=CARTESIAN_POINT ( 'NONE',  ( 21.55341960407610458, 5.719274019375980345, 73.95724293864769550 ) ) ;
#198240=CARTESIAN_POINT ( 'NONE',  ( -5.049401038298153566, 19.05341960407611168, 115.2072429386477097 ) ) ;
#198241=CARTESIAN_POINT ( 'NONE',  ( 5.049401038298161559, -19.05341960407611168, 47.70724293864770260 ) ) ;
#198242=CARTESIAN_POINT ( 'NONE',  ( -16.55341960407617563, 4.379528057220093196, 98.54275706135234714 ) ) ;
#198243=CARTESIAN_POINT ( 'NONE',  ( 16.46253265017160672, -9.564922557960803928, 63.33224293864769550 ) ) ;
#198244=CARTESIAN_POINT ( 'NONE',  ( 17.40805194822031865, 6.112264579159360167, 51.66628727489388950 ) ) ;
#198245=CARTESIAN_POINT ( 'NONE',  ( -21.53943276465977519, -0.05219959533937600094, 113.7510903946856757 ) ) ;
#198246=CARTESIAN_POINT ( 'NONE',  ( -14.34966873604960291, -8.224510206698953496, 66.66557627198102409 ) ) ;
#198247=CARTESIAN_POINT ( 'NONE',  ( 21.52544592524344225, -5.823673210054117533, 103.5405762719810383 ) ) ;
#198248=CARTESIAN_POINT ( 'NONE',  ( 5.719274019375991003, -21.55341960407610458, 97.70724293864772392 ) ) ;
#198250=CARTESIAN_POINT ( 'NONE',  ( 15.80617190586746368, 15.72974639402197994, 59.37390960531436690 ) ) ;
#198251=CARTESIAN_POINT ( 'NONE',  ( -12.06949235617739369, -12.14591786802326823, 79.37609039468567573 ) ) ;
#198252=CARTESIAN_POINT ( 'NONE',  ( 0.05219959533910956823, 16.53943276465976808, 99.99890960531436690 ) ) ;
#198253=CARTESIAN_POINT ( 'NONE',  ( -13.89961937509977652, 13.97604488694528158, 65.62390960531436690 ) ) ;
#198254=CARTESIAN_POINT ( 'NONE',  ( 14.34966873604972726, -8.224510206698740333, 110.8344237280190043 ) ) ;
#198255=CARTESIAN_POINT ( 'NONE',  ( 10.72451020669871369, 18.67979575497193778, 52.08442372801901854 ) ) ;
#198256=CARTESIAN_POINT ( 'NONE',  ( -16.46253265017160317, 9.564922557960807481, 95.83224293864769550 ) ) ;
#198257=CARTESIAN_POINT ( 'NONE',  ( -5.823673210054431948, 21.52544592524334988, 82.70942372801900433 ) ) ;
#198258=CARTESIAN_POINT ( 'NONE',  ( 19.05341960407611168, 5.049401038298154454, 23.95724293864769194 ) ) ;
#198259=CARTESIAN_POINT ( 'NONE',  ( 16.51473224551069308, 9.474510206698969483, 34.16557627198102409 ) ) ;
#198261=CARTESIAN_POINT ( 'NONE',  ( 15.80617190586769283, -15.72974639402175789, 75.62609039468567573 ) ) ;
#198262=CARTESIAN_POINT ( 'NONE',  ( -0.05219959533909027116, -19.03943276465977164, 102.4989096053143669 ) ) ;
#198263=CARTESIAN_POINT ( 'NONE',  ( -19.02544592524334988, -5.153800228976617603, 83.95942372801901854 ) ) ;
#198264=CARTESIAN_POINT ( 'NONE',  ( -21.52544592524334988, -5.823673210054445271, 38.95942372801901854 ) ) ;
#198265=CARTESIAN_POINT ( 'NONE',  ( -16.52544592524335698, -4.483927247898792601, 18.95942372801901143 ) ) ;
#198266=CARTESIAN_POINT ( 'NONE',  ( -9.564922557961040184, 16.46253265017147172, 67.91775706135233293 ) ) ;
#198267=CARTESIAN_POINT ( 'NONE',  ( -19.05341960407611168, -5.049401038298163336, 46.45724293864768129 ) ) ;
#198268=CARTESIAN_POINT ( 'NONE',  ( -19.03943276465977164, -0.05219959533935918106, 83.75109039468567573 ) ) ;
#198269=CARTESIAN_POINT ( 'NONE',  ( 4.483927247898545687, 16.52544592524342804, 29.79057627198102409 ) ) ;
#198270=CARTESIAN_POINT ( 'NONE',  ( 5.153800228976615827, -19.02544592524334988, 85.20942372801900433 ) ) ;
#198271=CARTESIAN_POINT ( 'NONE',  ( 12.06949235617757843, -12.14591786802309237, 38.12390960531436690 ) ) ;
#198272=CARTESIAN_POINT ( 'NONE',  ( -13.97604488694547697, 13.89961937509957934, 58.12609039468566863 ) ) ;
#198273=CARTESIAN_POINT ( 'NONE',  ( -16.53943276465976808, -0.05219959533934237506, 48.75109039468568284 ) ) ;
#198274=CARTESIAN_POINT ( 'NONE',  ( -5.153800228976607833, 19.02544592524334988, 27.70942372801899722 ) ) ;
#198275=CARTESIAN_POINT ( 'NONE',  ( 13.89961937509977652, -13.97604488694527269, 48.12390960531435979 ) ) ;
#198277=CARTESIAN_POINT ( 'NONE',  ( 4.483927247898790824, -16.52544592524335698, 45.20942372801901854 ) ) ;
#198280=CARTESIAN_POINT ( 'NONE',  ( -13.97604488694527625, -13.89961937509977652, 96.87390960531433848 ) ) ;
#198281=CARTESIAN_POINT ( 'NONE',  ( 17.50000000000000000, -5.500000000000000888, 120.0000000000000142 ) ) ;
#198282=VERTEX_POINT ( 'NONE', #88045 ) ;
#198283=CARTESIAN_POINT ( 'NONE',  ( 16.51473224551083163, -9.474510206698727899, 85.83442372801900433 ) ) ;
#198284=CARTESIAN_POINT ( 'NONE',  ( 21.52544592524344225, -5.823673210054117533, 28.54057627198103120 ) ) ;
#198285=CARTESIAN_POINT ( 'NONE',  ( -16.46253265017146816, -9.564922557961047289, 24.16775706135233648 ) ) ;
#198286=CARTESIAN_POINT ( 'NONE',  ( 13.89961937509957401, 13.97604488694547697, 96.87609039468566152 ) ) ;
#198287=CARTESIAN_POINT ( 'NONE',  ( 4.379528057220339221, -16.55341960407611168, 112.7072429386476955 ) ) ;
#198288=CARTESIAN_POINT ( 'NONE',  ( -9.564922557960796823, -16.46253265017161027, 42.08224293864769550 ) ) ;
#198289=CARTESIAN_POINT ( 'NONE',  ( 21.53943276465977519, -0.05219959533907433946, 63.74890960531435979 ) ) ;
#198290=VECTOR ( 'NONE', #24644, 1000.000000000000000 ) ;
#198291=CARTESIAN_POINT ( 'NONE',  ( -19.03943276465977164, 0.05219959533909376836, 21.24890960531436335 ) ) ;
#198293=CARTESIAN_POINT ( 'NONE',  ( -16.46253265017146816, -9.564922557961047289, 69.16775706135233293 ) ) ;
#198294=CARTESIAN_POINT ( 'NONE',  ( 14.29746914071049879, -8.314922557960816363, 43.33224293864769550 ) ) ;
#198295=CARTESIAN_POINT ( 'NONE',  ( 5.153800228976335163, 19.02544592524342804, 109.7905762719810099 ) ) ;
#198296=CARTESIAN_POINT ( 'NONE',  ( 21.52544592524334988, 5.823673210054432836, 91.45942372801901854 ) ) ;
#198297=CARTESIAN_POINT ( 'NONE',  ( -18.67979575497178146, -10.72451020669898902, 86.66557627198102409 ) ) ;
#198298=CARTESIAN_POINT ( 'NONE',  ( -21.52544592524334988, -5.823673210054445271, 58.95942372801902565 ) ) ;
#198299=CARTESIAN_POINT ( 'NONE',  ( 0.05219959533937995610, -21.53943276465977519, 65.00109039468568994 ) ) ;
#198300=CARTESIAN_POINT ( 'NONE',  ( 19.03943276465977164, -0.05219959533909143690, 98.74890960531436690 ) ) ;
#198301=CARTESIAN_POINT ( 'NONE',  ( 12.06949235617739724, 12.14591786802326823, 96.87609039468568994 ) ) ;
#198302=CARTESIAN_POINT ( 'NONE',  ( 0.05219959533937995610, -21.53943276465977519, 55.00109039468568284 ) ) ;
#198303=CARTESIAN_POINT ( 'NONE',  ( 16.53943276465976808, -0.05219959533910856209, 113.7489096053143527 ) ) ;
#198304=CARTESIAN_POINT ( 'NONE',  ( 4.483927247898545687, 16.52544592524342804, 69.79057627198102409 ) ) ;
#198305=CARTESIAN_POINT ( 'NONE',  ( 12.06949235617757843, -12.14591786802309237, 33.12390960531435979 ) ) ;
#198306=CARTESIAN_POINT ( 'NONE',  ( 21.53943276465977519, -0.05219959533907433946, 43.74890960531435979 ) ) ;
#198307=CARTESIAN_POINT ( 'NONE',  ( 19.02544592524343514, -5.153800228976328945, 53.54057627198102409 ) ) ;
#198308=CARTESIAN_POINT ( 'NONE',  ( 5.719274019375991003, -21.55341960407610458, 52.70724293864769550 ) ) ;
#198309=CARTESIAN_POINT ( 'NONE',  ( 16.46253265017146816, 9.564922557961045513, 46.66775706135233293 ) ) ;
#198312=CARTESIAN_POINT ( 'NONE',  ( 4.379528057220339221, -16.55341960407611168, 47.70724293864770260 ) ) ;
#198313=CARTESIAN_POINT ( 'NONE',  ( -18.67979575497178146, -10.72451020669898902, 21.66557627198102409 ) ) ;
#198314=ORIENTED_EDGE ( 'NONE', *, *, #11076, .T. ) ;
#198317=CARTESIAN_POINT ( 'NONE',  ( 16.55341960407618274, -4.379528057220086978, 71.04275706135234714 ) ) ;
#198318=CARTESIAN_POINT ( 'NONE',  ( 19.02544592524334988, 5.153800228976608722, 76.45942372801897591 ) ) ;
#198319=CARTESIAN_POINT ( 'NONE',  ( -8.224510206698948167, 14.34966873604960824, 35.41557627198102409 ) ) ;
#198321=CARTESIAN_POINT ( 'NONE',  ( -8.224510206698948167, 14.34966873604960824, 25.41557627198103120 ) ) ;
#198322=CARTESIAN_POINT ( 'NONE',  ( -19.03943276465977164, 0.05219959533909376836, 56.24890960531435979 ) ) ;
#198323=EDGE_CURVE ( 'NONE', #188641, #13916, #104996, .T. ) ;
#198324=CARTESIAN_POINT ( 'NONE',  ( 16.46253265017160672, -9.564922557960803928, 78.33224293864769550 ) ) ;
#198325=CARTESIAN_POINT ( 'NONE',  ( -16.51473224551069308, -9.474510206698971260, 41.66557627198103120 ) ) ;
#198326=CARTESIAN_POINT ( 'NONE',  ( -10.72451020669870658, -18.67979575497194134, 44.58442372801901854 ) ) ;
#198327=CARTESIAN_POINT ( 'NONE',  ( 19.02544592524343514, -5.153800228976328945, 63.54057627198103830 ) ) ;
#198329=CARTESIAN_POINT ( 'NONE',  ( -19.05341960407611168, -5.049401038298163336, 56.45724293864768129 ) ) ;
#198330=CARTESIAN_POINT ( 'NONE',  ( 18.62759615963271287, -10.81492255796078972, 33.33224293864769550 ) ) ;
#198331=CARTESIAN_POINT ( 'NONE',  ( -9.474510206698964154, 16.51473224551069663, 35.41557627198102409 ) ) ;
#198332=CARTESIAN_POINT ( 'NONE',  ( -18.62759615963270932, 10.81492255796079327, 45.83224293864769550 ) ) ;
#198333=CARTESIAN_POINT ( 'NONE',  ( 12.06949235617739724, 12.14591786802326823, 86.87609039468568994 ) ) ;
#198334=CARTESIAN_POINT ( 'NONE',  ( -10.72451020669870658, -18.67979575497194134, 104.5844237280190185 ) ) ;
#198335=CARTESIAN_POINT ( 'NONE',  ( 4.379528057220092307, 16.55341960407617563, 62.29275706135236845 ) ) ;
#198336=CARTESIAN_POINT ( 'NONE',  ( -13.89961937509977652, 13.97604488694528158, 110.6239096053143243 ) ) ;
#198337=CARTESIAN_POINT ( 'NONE',  ( -12.14591786802326823, 12.06949235617739902, 53.12609039468568284 ) ) ;
#198338=CARTESIAN_POINT ( 'NONE',  ( 4.483927247898790824, -16.52544592524335698, 45.20942372801901854 ) ) ;
#198339=CARTESIAN_POINT ( 'NONE',  ( 19.02544592524343514, -5.153800228976328945, 113.5405762719810241 ) ) ;
#198341=CARTESIAN_POINT ( 'NONE',  ( -4.483927247898782831, 16.52544592524335698, 22.70942372801901499 ) ) ;
#198342=CARTESIAN_POINT ( 'NONE',  ( 19.05341960407611168, 5.049401038298154454, 38.95724293864767418 ) ) ;
#198343=B_SPLINE_CURVE_WITH_KNOTS ( 'NONE', 3,
 ( #129843, #125892, #6512, #68191, #187592, #128855 ),
 .UNSPECIFIED., .F., .F.,
 ( 4, 2, 4 ),
 ( 0.007228050697041341933, 0.007608510107494807079, 0.007988969517948273091 ),
 .UNSPECIFIED. ) ;
#198344=CARTESIAN_POINT ( 'NONE',  ( 10.72451020669871369, 18.67979575497193778, 32.08442372801901854 ) ) ;
#198345=CARTESIAN_POINT ( 'NONE',  ( -8.314922557961024197, 14.29746914071037800, 27.91775706135234358 ) ) ;
#198346=CARTESIAN_POINT ( 'NONE',  ( 4.379528057220092307, 16.55341960407617563, 82.29275706135234714 ) ) ;
#198348=CARTESIAN_POINT ( 'NONE',  ( -0.05219959533937732626, 21.53943276465977519, 102.5010903946856899 ) ) ;
#198349=CARTESIAN_POINT ( 'NONE',  ( 16.51473224551083163, -9.474510206698727899, 95.83442372801900433 ) ) ;
#198350=CARTESIAN_POINT ( 'NONE',  ( 8.224510206698953496, -14.34966873604960469, 52.91557627198103830 ) ) ;
#198351=CARTESIAN_POINT ( 'NONE',  ( 16.55341960407611168, 4.379528057220329451, 108.9572429386476955 ) ) ;
#198352=CARTESIAN_POINT ( 'NONE',  ( -5.049401038297874678, -19.05341960407617918, 44.79275706135232582 ) ) ;
#198354=CARTESIAN_POINT ( 'NONE',  ( 18.62759615963255655, 10.81492255796105972, 56.66775706135235424 ) ) ;
#198355=CARTESIAN_POINT ( 'NONE',  ( -5.049401038297874678, -19.05341960407617918, 104.7927570613523471 ) ) ;
#198356=CARTESIAN_POINT ( 'NONE',  ( -18.10062525802553779, 5.500000000000031974, 63.51383468041922953 ) ) ;
#198357=CARTESIAN_POINT ( 'NONE',  ( 19.02544592524343514, -5.153800228976328945, 103.5405762719809957 ) ) ;
#198358=CARTESIAN_POINT ( 'NONE',  ( 10.72451020669898902, -18.67979575497178502, 67.91557627198102409 ) ) ;
#198359=CARTESIAN_POINT ( 'NONE',  ( 16.46253265017146816, 9.564922557961045513, 91.66775706135234714 ) ) ;
#198360=CARTESIAN_POINT ( 'NONE',  ( 16.51473224551069308, 9.474510206698969483, 104.1655762719810241 ) ) ;
#198362=CARTESIAN_POINT ( 'NONE',  ( 14.34966873604960469, 8.224510206698951720, 109.1655762719810383 ) ) ;
#198363=CARTESIAN_POINT ( 'NONE',  ( 18.62759615963255655, 10.81492255796105972, 91.66775706135234714 ) ) ;
#198364=CARTESIAN_POINT ( 'NONE',  ( 9.564922557960805705, 16.46253265017160317, 39.58224293864768839 ) ) ;
#198365=CARTESIAN_POINT ( 'NONE',  ( 21.55341960407619695, -5.719274019375665929, 51.04275706135234714 ) ) ;
#198366=CARTESIAN_POINT ( 'NONE',  ( -5.719274019375665041, -21.55341960407619695, 84.79275706135234714 ) ) ;
#198367=CARTESIAN_POINT ( 'NONE',  ( 16.53943276465976808, 0.05219959533934440121, 101.2510903946856757 ) ) ;
#198368=CARTESIAN_POINT ( 'NONE',  ( -16.46253265017160317, 9.564922557960807481, 70.83224293864770971 ) ) ;
#198369=CARTESIAN_POINT ( 'NONE',  ( -18.67979575497193778, 10.72451020669871902, 48.33442372801902565 ) ) ;
#198370=CARTESIAN_POINT ( 'NONE',  ( -10.81492255796105439, 18.62759615963255655, 42.91775706135235424 ) ) ;
#198371=CARTESIAN_POINT ( 'NONE',  ( 13.97604488694548053, -13.89961937509957401, 70.62609039468567573 ) ) ;
#198372=CARTESIAN_POINT ( 'NONE',  ( 19.03943276465977164, -0.05219959533909143690, 88.74890960531436690 ) ) ;
#198373=CARTESIAN_POINT ( 'NONE',  ( 14.29746914071049879, -8.314922557960816363, 108.3322429386477097 ) ) ;
#198374=CARTESIAN_POINT ( 'NONE',  ( -21.55341960407610458, -5.719274019375992779, 91.45724293864769550 ) ) ;
#198375=CARTESIAN_POINT ( 'NONE',  ( 0.05219959533910956823, 16.53943276465976808, 64.99890960531435269 ) ) ;
#198376=CARTESIAN_POINT ( 'NONE',  ( 18.67979575497194134, -10.72451020669871369, 110.8344237280190043 ) ) ;
#198377=CARTESIAN_POINT ( 'NONE',  ( -4.379528057220328563, 16.55341960407611168, 85.20724293864770971 ) ) ;
#198378=CARTESIAN_POINT ( 'NONE',  ( -13.89961937509977652, 13.97604488694528158, 30.62390960531435269 ) ) ;
#198379=CARTESIAN_POINT ( 'NONE',  ( -13.89961937509957401, -13.97604488694547875, 89.37609039468563310 ) ) ;
#198380=CARTESIAN_POINT ( 'NONE',  ( 16.53943276465976808, -0.05219959533910856209, 53.74890960531437401 ) ) ;
#198381=CARTESIAN_POINT ( 'NONE',  ( 10.72451020669871369, 18.67979575497193778, 92.08442372801901854 ) ) ;
#198382=CARTESIAN_POINT ( 'NONE',  ( -16.51473224551069308, -9.474510206698971260, 91.66557627198103830 ) ) ;
#198383=CARTESIAN_POINT ( 'NONE',  ( -16.51473224551082808, 9.474510206698731452, 68.33442372801900433 ) ) ;
#198384=CARTESIAN_POINT ( 'NONE',  ( 18.67979575497178502, 10.72451020669898547, 79.16557627198103830 ) ) ;
#198385=CARTESIAN_POINT ( 'NONE',  ( 18.67979575497194134, -10.72451020669871369, 25.83442372801901499 ) ) ;
#198386=CARTESIAN_POINT ( 'NONE',  ( 0.05219959533934541429, -16.53943276465976808, 30.00109039468568284 ) ) ;
#198387=CARTESIAN_POINT ( 'NONE',  ( 16.52544592524335698, 4.483927247898782831, 96.45942372801901854 ) ) ;
#198388=CARTESIAN_POINT ( 'NONE',  ( 13.89961937509977652, -13.97604488694527269, 23.12390960531436335 ) ) ;
#198389=CARTESIAN_POINT ( 'NONE',  ( -5.823673210054431948, 21.52544592524334988, 37.70942372801900433 ) ) ;
#198390=CARTESIAN_POINT ( 'NONE',  ( 14.34966873604960469, 8.224510206698951720, 114.1655762719810383 ) ) ;
#198392=CARTESIAN_POINT ( 'NONE',  ( 8.314922557961029526, -14.29746914071037800, 55.41775706135234714 ) ) ;
#198393=CARTESIAN_POINT ( 'NONE',  ( -14.29746914071049879, 8.314922557960819915, 75.83224293864769550 ) ) ;
#198394=CARTESIAN_POINT ( 'NONE',  ( 21.55341960407610458, 5.719274019375980345, 73.95724293864769550 ) ) ;
#198395=CARTESIAN_POINT ( 'NONE',  ( 16.53943276465976808, -0.05219959533910856209, 28.74890960531435624 ) ) ;
#198396=CARTESIAN_POINT ( 'NONE',  ( -16.52544592524335698, -4.483927247898792601, 48.95942372801902565 ) ) ;
#198397=CARTESIAN_POINT ( 'NONE',  ( 19.05341960407611168, 5.049401038298154454, 48.95724293864768129 ) ) ;
#198398=CARTESIAN_POINT ( 'NONE',  ( -12.14591786802326823, 12.06949235617739902, 98.12609039468570415 ) ) ;
#198399=CARTESIAN_POINT ( 'NONE',  ( -0.05219959533936034679, 19.03943276465977164, 92.50109039468566152 ) ) ;
#198400=CARTESIAN_POINT ( 'NONE',  ( 21.52544592524344225, -5.823673210054117533, 73.54057627198102409 ) ) ;
#198401=CARTESIAN_POINT ( 'NONE',  ( 4.379528057220339221, -16.55341960407611168, 22.70724293864769194 ) ) ;
#198403=CARTESIAN_POINT ( 'NONE',  ( -16.46253265017160317, 9.564922557960807481, 115.8322429386477097 ) ) ;
#198405=CARTESIAN_POINT ( 'NONE',  ( -5.823673210054116645, -21.52544592524344225, 57.29057627198103120 ) ) ;
#198407=CARTESIAN_POINT ( 'NONE',  ( 16.55341960407618274, -4.379528057220086978, 86.04275706135236135 ) ) ;
#198409=CARTESIAN_POINT ( 'NONE',  ( -10.81492255796078084, -18.62759615963271287, 22.08224293864769194 ) ) ;
#198410=CARTESIAN_POINT ( 'NONE',  ( 17.50000000000000000, 5.076555817581239083, 108.6795149204977804 ) ) ;
#198411=CARTESIAN_POINT ( 'NONE',  ( -10.72451020669898014, 18.67979575497178502, 70.41557627198102409 ) ) ;
#198412=CARTESIAN_POINT ( 'NONE',  ( -12.06949235617739369, -12.14591786802326823, 109.3760903946857042 ) ) ;
#198413=CARTESIAN_POINT ( 'NONE',  ( 16.46253265017146816, 9.564922557961045513, 111.6677570613523329 ) ) ;
#198414=CARTESIAN_POINT ( 'NONE',  ( 4.379528057220339221, -16.55341960407611168, 112.7072429386476955 ) ) ;
#198415=CARTESIAN_POINT ( 'NONE',  ( 16.55341960407618274, -4.379528057220086978, 26.04275706135235779 ) ) ;
#198416=CARTESIAN_POINT ( 'NONE',  ( 13.97604488694527802, 13.89961937509977652, 49.37390960531434558 ) ) ;
#198418=CARTESIAN_POINT ( 'NONE',  ( 16.51473224551069308, 9.474510206698969483, 99.16557627198102409 ) ) ;
#198421=CARTESIAN_POINT ( 'NONE',  ( 14.29746914071037800, 8.314922557961029526, 91.66775706135234714 ) ) ;
#198422=CARTESIAN_POINT ( 'NONE',  ( -19.05341960407617563, 5.049401038297882671, 93.54275706135234714 ) ) ;
#198423=CARTESIAN_POINT ( 'NONE',  ( -16.46253265017146816, -9.564922557961047289, 19.16775706135233293 ) ) ;
#198424=CARTESIAN_POINT ( 'NONE',  ( -5.719274019375978568, 21.55341960407610458, 80.20724293864769550 ) ) ;
#198425=CARTESIAN_POINT ( 'NONE',  ( 4.483927247898790824, -16.52544592524335698, 105.2094237280190328 ) ) ;
#198426=B_SPLINE_CURVE_WITH_KNOTS ( 'NONE', 3,
 ( #176281, #193446, #180297, #37753, #117592, #118607 ),
 .UNSPECIFIED., .F., .F.,
 ( 4, 2, 4 ),
 ( 0.007228050697041589999, 0.007608510107495062083, 0.007988969517948535035 ),
 .UNSPECIFIED. ) ;
#198427=CARTESIAN_POINT ( 'NONE',  ( -0.05219959533936034679, 19.03943276465977164, 97.50109039468567573 ) ) ;
#198428=CARTESIAN_POINT ( 'NONE',  ( 19.02544592524343514, -5.153800228976328945, 43.54057627198103120 ) ) ;
#198429=CARTESIAN_POINT ( 'NONE',  ( 19.03943276465977164, -0.05219959533909143690, 93.74890960531435269 ) ) ;
#198431=CARTESIAN_POINT ( 'NONE',  ( -18.67979575497193778, 10.72451020669871902, 68.33442372801900433 ) ) ;
#198432=CARTESIAN_POINT ( 'NONE',  ( -0.05219959533909027116, -19.03943276465977164, 47.49890960531435979 ) ) ;
#198433=CARTESIAN_POINT ( 'NONE',  ( -16.62475595723694965, -7.163666690055376485, 84.47286648189530922 ) ) ;
#198434=CARTESIAN_POINT ( 'NONE',  ( -16.53943276465976808, 0.05219959533911058130, 76.24890960531435269 ) ) ;
#198435=CARTESIAN_POINT ( 'NONE',  ( 10.72451020669898902, -18.67979575497178502, 77.91557627198102409 ) ) ;
#198437=( GEOMETRIC_REPRESENTATION_CONTEXT ( 3 ) GLOBAL_UNCERTAINTY_ASSIGNED_CONTEXT ( ( #53970 ) ) GLOBAL_UNIT_ASSIGNED_CONTEXT ( ( #172890, #188065, #171887 ) ) REPRESENTATION_CONTEXT ( 'NONE', 'WORKASPACE' ) );
#198439=CARTESIAN_POINT ( 'NONE',  ( -9.474510206698720793, -16.51473224551083518, 44.58442372801900433 ) ) ;
#198440=CARTESIAN_POINT ( 'NONE',  ( 17.13100169013224061, -6.664070546374246007, 73.26789835699825915 ) ) ;
#198441=CARTESIAN_POINT ( 'NONE',  ( -16.46253265017160317, 9.564922557960807481, 80.83224293864769550 ) ) ;
#198442=CARTESIAN_POINT ( 'NONE',  ( 16.46253265017160672, -9.564922557960803928, 93.33224293864769550 ) ) ;
#198443=CARTESIAN_POINT ( 'NONE',  ( 16.53943276465976808, 0.05219959533934440121, 61.25109039468567573 ) ) ;
#198445=CARTESIAN_POINT ( 'NONE',  ( 13.97604488694548053, -13.89961937509957401, 45.62609039468566863 ) ) ;
#198447=CARTESIAN_POINT ( 'NONE',  ( -0.05219959533909027116, -19.03943276465977164, 107.4989096053143527 ) ) ;
#198448=CARTESIAN_POINT ( 'NONE',  ( 16.55341960407618274, -4.379528057220086978, 86.04275706135236135 ) ) ;
#198449=EDGE_CURVE ( 'NONE', #49283, #106381, #127012, .T. ) ;
#198451=CARTESIAN_POINT ( 'NONE',  ( -16.52544592524335698, -4.483927247898792601, 73.95942372801901854 ) ) ;
#198453=CARTESIAN_POINT ( 'NONE',  ( 12.06949235617739724, 12.14591786802326823, 51.87609039468568284 ) ) ;
#198455=CARTESIAN_POINT ( 'NONE',  ( 18.67979575497194134, -10.72451020669871369, 60.83442372801901854 ) ) ;
#198456=CARTESIAN_POINT ( 'NONE',  ( -13.97604488694547697, 13.89961937509957934, 78.12609039468567573 ) ) ;
#198457=CARTESIAN_POINT ( 'NONE',  ( 0.05219959533936267826, -19.03943276465977164, 20.00109039468567218 ) ) ;
#198458=CARTESIAN_POINT ( 'NONE',  ( -5.153800228976328057, -19.02544592524343514, 47.29057627198102409 ) ) ;
#198459=CARTESIAN_POINT ( 'NONE',  ( 5.153800228976335163, 19.02544592524342804, 39.79057627198100988 ) ) ;
#198461=CARTESIAN_POINT ( 'NONE',  ( -10.81492255796078084, -18.62759615963271287, 62.08224293864769550 ) ) ;
#198463=CARTESIAN_POINT ( 'NONE',  ( -16.46253265017160317, 9.564922557960807481, 110.8322429386476955 ) ) ;
#198464=CARTESIAN_POINT ( 'NONE',  ( -12.06949235617756955, 12.14591786802309770, 110.6239096053143669 ) ) ;
#198465=CARTESIAN_POINT ( 'NONE',  ( 14.34966873604972726, -8.224510206698740333, 55.83442372801901854 ) ) ;
#198467=CARTESIAN_POINT ( 'NONE',  ( 15.72974639402199770, -15.80617190586745480, 113.1239096053143953 ) ) ;
#198468=CARTESIAN_POINT ( 'NONE',  ( -8.314922557960811034, -14.29746914071050412, 52.08224293864768839 ) ) ;
#198470=CARTESIAN_POINT ( 'NONE',  ( 19.02544592524334988, 5.153800228976608722, 106.4594237280190185 ) ) ;
#198471=CARTESIAN_POINT ( 'NONE',  ( 13.97604488694548053, -13.89961937509957401, 35.62609039468567573 ) ) ;
#198472=CARTESIAN_POINT ( 'NONE',  ( -8.224510206698948167, 14.34966873604960824, 40.41557627198103120 ) ) ;
#198473=CARTESIAN_POINT ( 'NONE',  ( -18.62759615963270932, 10.81492255796079327, 115.8322429386477097 ) ) ;
#198474=LINE ( 'NONE', #44790, #150594 ) ;
#198475=CARTESIAN_POINT ( 'NONE',  ( -21.52544592524343514, 5.823673210054127303, 61.04057627198103120 ) ) ;
#198476=CARTESIAN_POINT ( 'NONE',  ( -16.46253265017160317, 9.564922557960807481, 85.83224293864769550 ) ) ;
#198477=CARTESIAN_POINT ( 'NONE',  ( -12.06949235617756955, 12.14591786802309770, 55.62390960531436690 ) ) ;
#198478=CARTESIAN_POINT ( 'NONE',  ( -5.049401038298153566, 19.05341960407611168, 105.2072429386476671 ) ) ;
#198480=CARTESIAN_POINT ( 'NONE',  ( 9.564922557961047289, -16.46253265017146816, 50.41775706135233293 ) ) ;
#198481=CARTESIAN_POINT ( 'NONE',  ( -0.05219959533907301413, -21.53943276465977519, 97.49890960531436690 ) ) ;
#198482=CARTESIAN_POINT ( 'NONE',  ( -19.02544592524342804, 5.153800228976336051, 46.04057627198101699 ) ) ;
#198483=CARTESIAN_POINT ( 'NONE',  ( 0.05219959533910956823, 16.53943276465976808, 109.9989096053143527 ) ) ;
#198484=CARTESIAN_POINT ( 'NONE',  ( -5.719274019375665041, -21.55341960407619695, 44.79275706135234714 ) ) ;
#198486=CARTESIAN_POINT ( 'NONE',  ( -8.314922557960811034, -14.29746914071050412, 32.08224293864769550 ) ) ;
#198487=CARTESIAN_POINT ( 'NONE',  ( -9.474510206698964154, 16.51473224551069663, 50.41557627198102409 ) ) ;
#198488=CARTESIAN_POINT ( 'NONE',  ( 19.03943276465977164, -0.05219959533909143690, 93.74890960531435269 ) ) ;
#198489=CARTESIAN_POINT ( 'NONE',  ( -18.67979575497178146, -10.72451020669898902, 71.66557627198100988 ) ) ;
#198491=CARTESIAN_POINT ( 'NONE',  ( 9.564922557960805705, 16.46253265017160317, 39.58224293864768839 ) ) ;
#198493=CARTESIAN_POINT ( 'NONE',  ( -21.55341960407610458, -5.719274019375992779, 46.45724293864769550 ) ) ;
#198495=CARTESIAN_POINT ( 'NONE',  ( -15.80617190586768217, 15.72974639402176855, 93.12609039468568994 ) ) ;
#198497=CARTESIAN_POINT ( 'NONE',  ( 16.52544592524335698, 4.483927247898782831, 76.45942372801901854 ) ) ;
#198498=CARTESIAN_POINT ( 'NONE',  ( -4.483927247898539470, -16.52544592524342804, 67.29057627198103830 ) ) ;
#198499=CARTESIAN_POINT ( 'NONE',  ( 5.049401038298161559, -19.05341960407611168, 67.70724293864769550 ) ) ;
#198501=CARTESIAN_POINT ( 'NONE',  ( 19.02544592524334988, 5.153800228976608722, 26.45942372801899722 ) ) ;
#198502=CARTESIAN_POINT ( 'NONE',  ( 14.34966873604972726, -8.224510206698740333, 85.83442372801901854 ) ) ;
#198503=CARTESIAN_POINT ( 'NONE',  ( -21.55341960407619339, 5.719274019375674811, 113.5427570613523756 ) ) ;
#198504=CARTESIAN_POINT ( 'NONE',  ( 9.564922557960805705, 16.46253265017160317, 69.58224293864770971 ) ) ;
#198505=CARTESIAN_POINT ( 'NONE',  ( -5.823673210054116645, -21.52544592524344225, 52.29057627198102409 ) ) ;
#198506=CARTESIAN_POINT ( 'NONE',  ( -8.224510206698735004, -14.34966873604973081, 29.58442372801901854 ) ) ;
#198507=CARTESIAN_POINT ( 'NONE',  ( -10.81492255796105439, 18.62759615963255655, 82.91775706135234714 ) ) ;
#198508=CARTESIAN_POINT ( 'NONE',  ( -0.05219959533934338120, 16.53943276465976808, 62.50109039468568284 ) ) ;
#198509=CARTESIAN_POINT ( 'NONE',  ( -21.52544592524343514, 5.823673210054127303, 116.0405762719810383 ) ) ;
#198510=CARTESIAN_POINT ( 'NONE',  ( -9.564922557961040184, 16.46253265017147172, 107.9177570613523471 ) ) ;
#198511=CARTESIAN_POINT ( 'NONE',  ( -5.049401038298153566, 19.05341960407611168, 85.20724293864766707 ) ) ;
#198512=CARTESIAN_POINT ( 'NONE',  ( -16.52544592524335698, -4.483927247898792601, 28.95942372801902209 ) ) ;
#198513=CARTESIAN_POINT ( 'NONE',  ( -5.049401038298153566, 19.05341960407611168, 55.20724293864769550 ) ) ;
#198514=CARTESIAN_POINT ( 'NONE',  ( 8.314922557961029526, -14.29746914071037800, 30.41775706135234358 ) ) ;
#198515=CARTESIAN_POINT ( 'NONE',  ( 16.55341960407611168, 4.379528057220329451, 83.95724293864770971 ) ) ;
#198516=CARTESIAN_POINT ( 'NONE',  ( -12.14591786802326823, 12.06949235617739902, 83.12609039468568994 ) ) ;
#198517=CARTESIAN_POINT ( 'NONE',  ( 18.67979575497194134, -10.72451020669871369, 35.83442372801901143 ) ) ;
#198518=CARTESIAN_POINT ( 'NONE',  ( -9.474510206698964154, 16.51473224551069663, 65.41557627198102409 ) ) ;
#198519=CARTESIAN_POINT ( 'NONE',  ( -16.51473224551069308, -9.474510206698971260, 76.66557627198103830 ) ) ;
#198520=CARTESIAN_POINT ( 'NONE',  ( 4.379528057220092307, 16.55341960407617563, 87.29275706135236135 ) ) ;
#198525=CARTESIAN_POINT ( 'NONE',  ( -16.46253265017146816, -9.564922557961047289, 29.16775706135232937 ) ) ;
#198526=CARTESIAN_POINT ( 'NONE',  ( -9.474510206698964154, 16.51473224551069663, 105.4155762719810383 ) ) ;
#198528=CARTESIAN_POINT ( 'NONE',  ( 19.03943276465977164, -0.05219959533909143690, 53.74890960531436690 ) ) ;
#198530=CARTESIAN_POINT ( 'NONE',  ( 16.52544592524335698, 4.483927247898782831, 31.45942372801901854 ) ) ;
#198531=CARTESIAN_POINT ( 'NONE',  ( -19.03943276465977164, -0.05219959533935918106, 53.75109039468566863 ) ) ;
#198532=CARTESIAN_POINT ( 'NONE',  ( -16.55341960407617563, 4.379528057220093196, 38.54275706135234714 ) ) ;
#198533=CARTESIAN_POINT ( 'NONE',  ( 13.89961937509977652, -13.97604488694527269, 103.1239096053143527 ) ) ;
#198534=CARTESIAN_POINT ( 'NONE',  ( -19.03943276465977164, 0.05219959533909376836, 81.24890960531436690 ) ) ;
#198535=CARTESIAN_POINT ( 'NONE',  ( -21.52544592524343514, 5.823673210054127303, 96.04057627198102409 ) ) ;
#198536=CARTESIAN_POINT ( 'NONE',  ( 19.02544592524334988, 5.153800228976608722, 66.45942372801899012 ) ) ;
#198537=CARTESIAN_POINT ( 'NONE',  ( -0.05219959533909027116, -19.03943276465977164, 97.49890960531436690 ) ) ;
#198538=CARTESIAN_POINT ( 'NONE',  ( -9.564922557960796823, -16.46253265017161027, 27.08224293864769550 ) ) ;
#198539=CARTESIAN_POINT ( 'NONE',  ( 16.46253265017160672, -9.564922557960803928, 58.33224293864769550 ) ) ;
#198540=CARTESIAN_POINT ( 'NONE',  ( 16.52544592524342804, -4.483927247898539470, 33.54057627198102409 ) ) ;
#198541=CARTESIAN_POINT ( 'NONE',  ( -19.05341960407611168, -5.049401038298163336, 21.45724293864768839 ) ) ;
#198542=CARTESIAN_POINT ( 'NONE',  ( -19.02544592524334988, -5.153800228976617603, 38.95942372801900433 ) ) ;
#198544=CARTESIAN_POINT ( 'NONE',  ( 8.314922557960818139, 14.29746914071049879, 74.58224293864768129 ) ) ;
#198545=CARTESIAN_POINT ( 'NONE',  ( -10.72451020669870658, -18.67979575497194134, 94.58442372801901854 ) ) ;
#198546=CARTESIAN_POINT ( 'NONE',  ( 16.46253265017160672, -9.564922557960803928, 33.33224293864770260 ) ) ;
#198547=CARTESIAN_POINT ( 'NONE',  ( -8.314922557961024197, 14.29746914071037800, 52.91775706135235424 ) ) ;
#198548=CARTESIAN_POINT ( 'NONE',  ( 12.14591786802309770, 12.06949235617756955, 34.37390960531435979 ) ) ;
#198549=CARTESIAN_POINT ( 'NONE',  ( -21.52544592524334988, -5.823673210054445271, 98.95942372801903275 ) ) ;
#198550=CARTESIAN_POINT ( 'NONE',  ( 9.474510206698971260, -16.51473224551069308, 97.91557627198102409 ) ) ;
#198551=CARTESIAN_POINT ( 'NONE',  ( -19.02544592524342804, 5.153800228976336051, 101.0405762719810241 ) ) ;
#198552=CARTESIAN_POINT ( 'NONE',  ( 0.05219959533910956823, 16.53943276465976808, 109.9989096053143527 ) ) ;
#198553=CARTESIAN_POINT ( 'NONE',  ( -16.52544592524342804, 4.483927247898546575, 76.04057627198102409 ) ) ;
#198554=CARTESIAN_POINT ( 'NONE',  ( 21.53943276465977519, -0.05219959533907433946, 78.74890960531436690 ) ) ;
#198555=CARTESIAN_POINT ( 'NONE',  ( 5.049401038298161559, -19.05341960407611168, 87.70724293864769550 ) ) ;
#198556=CARTESIAN_POINT ( 'NONE',  ( 18.62759615963271287, -10.81492255796078972, 103.3322429386476955 ) ) ;
#198558=CARTESIAN_POINT ( 'NONE',  ( -9.564922557960796823, -16.46253265017161027, 97.08224293864769550 ) ) ;
#198559=CARTESIAN_POINT ( 'NONE',  ( 9.564922557961047289, -16.46253265017146816, 65.41775706135233293 ) ) ;
#198560=CARTESIAN_POINT ( 'NONE',  ( -4.379528057220328563, 16.55341960407611168, 85.20724293864770971 ) ) ;
#198561=CARTESIAN_POINT ( 'NONE',  ( -9.564922557960796823, -16.46253265017161027, 57.08224293864769550 ) ) ;
#198562=CARTESIAN_POINT ( 'NONE',  ( 15.72974639402199770, -15.80617190586745480, 68.12390960531436690 ) ) ;
#198564=CARTESIAN_POINT ( 'NONE',  ( -16.55341960407617563, 4.379528057220093196, 108.5427570613523756 ) ) ;
#198566=CARTESIAN_POINT ( 'NONE',  ( 16.46253265017146816, 9.564922557961045513, 111.6677570613523329 ) ) ;
#198567=CARTESIAN_POINT ( 'NONE',  ( -4.483927247898539470, -16.52544592524342804, 77.29057627198102409 ) ) ;
#198568=CARTESIAN_POINT ( 'NONE',  ( -17.48853670773245028, -5.747243402303098492, 96.33328700250011423 ) ) ;
#198569=CARTESIAN_POINT ( 'NONE',  ( -19.02544592524342804, 5.153800228976336051, 76.04057627198102409 ) ) ;
#198570=CARTESIAN_POINT ( 'NONE',  ( 19.02544592524343514, -5.153800228976328945, 43.54057627198103120 ) ) ;
#198571=CARTESIAN_POINT ( 'NONE',  ( -14.29746914071049879, 8.314922557960819915, 70.83224293864770971 ) ) ;
#198572=CARTESIAN_POINT ( 'NONE',  ( -16.46253265017160317, 9.564922557960807481, 110.8322429386476955 ) ) ;
#198573=CARTESIAN_POINT ( 'NONE',  ( -0.05219959533936034679, 19.03943276465977164, 107.5010903946856615 ) ) ;
#198574=CARTESIAN_POINT ( 'NONE',  ( 10.72451020669871369, 18.67979575497193778, 57.08442372801901854 ) ) ;
#198576=CARTESIAN_POINT ( 'NONE',  ( -13.89961937509977652, 13.97604488694528158, 95.62390960531436690 ) ) ;
#198577=CARTESIAN_POINT ( 'NONE',  ( 21.52544592524344225, -5.823673210054117533, 78.54057627198103830 ) ) ;
#198578=CARTESIAN_POINT ( 'NONE',  ( -16.55341960407617563, 4.379528057220093196, 73.54275706135234714 ) ) ;
#198580=CARTESIAN_POINT ( 'NONE',  ( -19.02544592524335343, -5.153800228976618492, 108.9594237280189901 ) ) ;
#198581=CARTESIAN_POINT ( 'NONE',  ( 9.564922557960805705, 16.46253265017160317, 69.58224293864770971 ) ) ;
#198582=CARTESIAN_POINT ( 'NONE',  ( -18.67979575497178146, -10.72451020669898902, 81.66557627198103830 ) ) ;
#198583=CARTESIAN_POINT ( 'NONE',  ( -16.46253265017146816, -9.564922557961047289, 109.1677570613523471 ) ) ;
#198584=CARTESIAN_POINT ( 'NONE',  ( 14.29746914071049879, -8.314922557960816363, 38.33224293864768839 ) ) ;
#198585=CARTESIAN_POINT ( 'NONE',  ( -0.05219959533937732626, 21.53943276465977519, 62.50109039468568284 ) ) ;
#198586=CARTESIAN_POINT ( 'NONE',  ( -8.314922557961024197, 14.29746914071037800, 82.91775706135234714 ) ) ;
#198587=CARTESIAN_POINT ( 'NONE',  ( -19.03943276465977164, 0.05219959533909376836, 111.2489096053143669 ) ) ;
#198590=CARTESIAN_POINT ( 'NONE',  ( 16.53943276465976808, 0.05219959533934440121, 91.25109039468568994 ) ) ;
#198591=CARTESIAN_POINT ( 'NONE',  ( 14.29746914071037800, 8.314922557961029526, 41.66775706135235424 ) ) ;
#198592=CARTESIAN_POINT ( 'NONE',  ( 13.97604488694527802, 13.89961937509977652, 64.37390960531436690 ) ) ;
#198593=CARTESIAN_POINT ( 'NONE',  ( -5.153800228976328057, -19.02544592524343514, 67.29057627198102409 ) ) ;
#198594=CARTESIAN_POINT ( 'NONE',  ( 15.80617190586769283, -15.72974639402175789, 60.62609039468567573 ) ) ;
#198595=CARTESIAN_POINT ( 'NONE',  ( -4.379528057220086978, -16.55341960407618274, 64.79275706135234714 ) ) ;
#198596=CARTESIAN_POINT ( 'NONE',  ( -8.314922557960811034, -14.29746914071050412, 52.08224293864768839 ) ) ;
#198597=CARTESIAN_POINT ( 'NONE',  ( -13.97604488694527625, -13.89961937509977652, 41.87390960531435979 ) ) ;
#198598=CARTESIAN_POINT ( 'NONE',  ( 5.153800228976335163, 19.02544592524342804, 54.79057627198103120 ) ) ;
#198599=CARTESIAN_POINT ( 'NONE',  ( 4.379528057220092307, 16.55341960407617563, 42.29275706135235424 ) ) ;
#198600=CARTESIAN_POINT ( 'NONE',  ( -13.89961937509957401, -13.97604488694547875, 94.37609039468566152 ) ) ;
#198601=CARTESIAN_POINT ( 'NONE',  ( -12.06949235617756955, 12.14591786802309770, 90.62390960531436690 ) ) ;
#198602=CARTESIAN_POINT ( 'NONE',  ( 16.46253265017160672, -9.564922557960803928, 68.33224293864770971 ) ) ;
#198603=CARTESIAN_POINT ( 'NONE',  ( -19.03943276465977164, -0.05219959533935918106, 93.75109039468566152 ) ) ;
#198605=CARTESIAN_POINT ( 'NONE',  ( 10.72451020669871369, 18.67979575497193778, 87.08442372801901854 ) ) ;
#198606=CARTESIAN_POINT ( 'NONE',  ( 16.52544592524335698, 4.483927247898782831, 66.45942372801903275 ) ) ;
#198608=CARTESIAN_POINT ( 'NONE',  ( 21.52544592524344225, -5.823673210054117533, 48.54057627198103120 ) ) ;
#198609=CARTESIAN_POINT ( 'NONE',  ( 0.05219959533934541429, -16.53943276465976808, 50.00109039468568994 ) ) ;
#198610=CARTESIAN_POINT ( 'NONE',  ( -18.87580814761075843, 5.500000000000059508, 70.87172394265761000 ) ) ;
#198611=CARTESIAN_POINT ( 'NONE',  ( 9.564922557961047289, -16.46253265017146816, 40.41775706135234003 ) ) ;
#198612=CARTESIAN_POINT ( 'NONE',  ( 9.474510206698971260, -16.51473224551069308, 92.91557627198103830 ) ) ;
#198613=CARTESIAN_POINT ( 'NONE',  ( 16.51473224551069308, 9.474510206698969483, 24.16557627198102765 ) ) ;
#198614=CARTESIAN_POINT ( 'NONE',  ( -16.46253265017160317, 9.564922557960807481, 45.83224293864769550 ) ) ;
#198617=CARTESIAN_POINT ( 'NONE',  ( -21.53943276465977519, -0.05219959533937600094, 78.75109039468568994 ) ) ;
#198620=CARTESIAN_POINT ( 'NONE',  ( -5.153800228976607833, 19.02544592524334988, 32.70942372801899722 ) ) ;
#198621=CARTESIAN_POINT ( 'NONE',  ( -16.51473224551082808, 9.474510206698731452, 33.33442372801899722 ) ) ;
#198622=CARTESIAN_POINT ( 'NONE',  ( 14.34966873604960469, 8.224510206698951720, 49.16557627198102409 ) ) ;
#198623=CARTESIAN_POINT ( 'NONE',  ( -0.05219959533909027116, -19.03943276465977164, 52.49890960531436690 ) ) ;
#198624=CARTESIAN_POINT ( 'NONE',  ( 5.719274019375991003, -21.55341960407610458, 22.70724293864769194 ) ) ;
#198625=CARTESIAN_POINT ( 'NONE',  ( 5.719274019375673035, 21.55341960407619339, 77.29275706135234714 ) ) ;
#198626=CARTESIAN_POINT ( 'NONE',  ( -5.049401038298153566, 19.05341960407611168, 65.20724293864765286 ) ) ;
#198627=CARTESIAN_POINT ( 'NONE',  ( -18.67979575497193778, 10.72451020669871902, 83.33442372801903275 ) ) ;
#198628=CARTESIAN_POINT ( 'NONE',  ( -15.72974639402197994, 15.80617190586746368, 30.62390960531436335 ) ) ;
#198629=CARTESIAN_POINT ( 'NONE',  ( -5.823673210054431948, 21.52544592524334988, 37.70942372801900433 ) ) ;
#198630=CARTESIAN_POINT ( 'NONE',  ( 9.474510206698729675, 16.51473224551082808, 67.08442372801900433 ) ) ;
#198631=CARTESIAN_POINT ( 'NONE',  ( 19.05341960407611168, 5.049401038298154454, 28.95724293864769550 ) ) ;
#198632=CARTESIAN_POINT ( 'NONE',  ( 9.474510206698971260, -16.51473224551069308, 77.91557627198103830 ) ) ;
#198633=CARTESIAN_POINT ( 'NONE',  ( -0.05219959533934338120, 16.53943276465976808, 27.50109039468567929 ) ) ;
#198634=CARTESIAN_POINT ( 'NONE',  ( 8.314922557960818139, 14.29746914071049879, 94.58224293864769550 ) ) ;
#198635=CARTESIAN_POINT ( 'NONE',  ( -19.03943276465977164, 0.05219959533909376836, 51.24890960531436690 ) ) ;
#198636=CARTESIAN_POINT ( 'NONE',  ( -5.719274019375978568, 21.55341960407610458, 55.20724293864770260 ) ) ;
#198637=CARTESIAN_POINT ( 'NONE',  ( -16.53943276465976808, -0.05219959533934237506, 18.75109039468568639 ) ) ;
#198638=CARTESIAN_POINT ( 'NONE',  ( -5.823673210054431948, 21.52544592524334988, 22.70942372801901499 ) ) ;
#198639=CARTESIAN_POINT ( 'NONE',  ( -21.55341960407619339, 5.719274019375674811, 73.54275706135234714 ) ) ;
#198640=CARTESIAN_POINT ( 'NONE',  ( 12.06949235617739724, 12.14591786802326823, 71.87609039468568994 ) ) ;
#198641=CARTESIAN_POINT ( 'NONE',  ( -12.06949235617739369, -12.14591786802326823, 74.37609039468568994 ) ) ;
#198642=ORIENTED_EDGE ( 'NONE', *, *, #53412, .T. ) ;
#198643=CARTESIAN_POINT ( 'NONE',  ( 5.153800228976335163, 19.02544592524342804, 54.79057627198103120 ) ) ;
#198644=CARTESIAN_POINT ( 'NONE',  ( 0.05219959533934541429, -16.53943276465976808, 90.00109039468567573 ) ) ;
#198645=CARTESIAN_POINT ( 'NONE',  ( 9.474510206698729675, 16.51473224551082808, 37.08442372801899722 ) ) ;
#198646=CARTESIAN_POINT ( 'NONE',  ( -21.52544592524343514, 5.823673210054127303, 111.0405762719810525 ) ) ;
#198647=CARTESIAN_POINT ( 'NONE',  ( -16.53943276465976808, 0.05219959533911058130, 71.24890960531435269 ) ) ;
#198648=CARTESIAN_POINT ( 'NONE',  ( 13.97604488694527802, 13.89961937509977652, 89.37390960531436690 ) ) ;
#198649=CARTESIAN_POINT ( 'NONE',  ( -8.224510206698735004, -14.34966873604973081, 89.58442372801901854 ) ) ;
#198650=CARTESIAN_POINT ( 'NONE',  ( -0.05219959533937732626, 21.53943276465977519, 57.50109039468568994 ) ) ;
#198651=CARTESIAN_POINT ( 'NONE',  ( 4.379528057220092307, 16.55341960407617563, 37.29275706135235424 ) ) ;
#198652=CARTESIAN_POINT ( 'NONE',  ( 15.80617190586746368, 15.72974639402197994, 114.3739096053143527 ) ) ;
#198653=CARTESIAN_POINT ( 'NONE',  ( 16.53943276465976808, -0.05219959533910856209, 63.74890960531435979 ) ) ;
#198655=CARTESIAN_POINT ( 'NONE',  ( -10.72451020669898014, 18.67979575497178502, 95.41557627198102409 ) ) ;
#198656=CARTESIAN_POINT ( 'NONE',  ( -4.483927247898539470, -16.52544592524342804, 37.29057627198102409 ) ) ;
#198660=CARTESIAN_POINT ( 'NONE',  ( 9.474510206698971260, -16.51473224551069308, 107.9155762719810383 ) ) ;
#198661=CARTESIAN_POINT ( 'NONE',  ( -0.05219959533937732626, 21.53943276465977519, 37.50109039468568284 ) ) ;
#198662=CARTESIAN_POINT ( 'NONE',  ( 8.314922557960818139, 14.29746914071049879, 64.58224293864769550 ) ) ;
#198663=CARTESIAN_POINT ( 'NONE',  ( -19.05341960407611168, -5.049401038298163336, 66.45724293864769550 ) ) ;
#198664=CARTESIAN_POINT ( 'NONE',  ( 19.02544592524334988, 5.153800228976608722, 61.45942372801900433 ) ) ;
#198665=CARTESIAN_POINT ( 'NONE',  ( -10.72451020669898014, 18.67979575497178502, 50.41557627198103120 ) ) ;
#198667=CARTESIAN_POINT ( 'NONE',  ( 9.564922557960805705, 16.46253265017160317, 54.58224293864769550 ) ) ;
#198668=CARTESIAN_POINT ( 'NONE',  ( -14.34966873604972548, 8.224510206698743886, 33.33442372801900433 ) ) ;
#198669=CARTESIAN_POINT ( 'NONE',  ( -15.72974639402176322, -15.80617190586768395, 19.37609039468568639 ) ) ;
#198670=CARTESIAN_POINT ( 'NONE',  ( -14.29746914071049879, 8.314922557960819915, 45.83224293864769550 ) ) ;
#198671=VERTEX_POINT ( 'NONE', #78832 ) ;
#198672=CARTESIAN_POINT ( 'NONE',  ( -19.03943276465977164, 0.05219959533909376836, 91.24890960531436690 ) ) ;
#198673=CARTESIAN_POINT ( 'NONE',  ( 5.719274019375991003, -21.55341960407610458, 67.70724293864769550 ) ) ;
#198674=CARTESIAN_POINT ( 'NONE',  ( -21.52544592524343514, 5.823673210054127303, 111.0405762719810525 ) ) ;
#198675=CARTESIAN_POINT ( 'NONE',  ( 8.224510206698742110, 14.34966873604972548, 42.08442372801901854 ) ) ;
#198676=CARTESIAN_POINT ( 'NONE',  ( -15.80617190586745835, -15.72974639402198527, 31.87390960531435979 ) ) ;
#198677=CARTESIAN_POINT ( 'NONE',  ( 21.53943276465977519, 0.05219959533937863772, 101.2510903946856757 ) ) ;
#198678=CARTESIAN_POINT ( 'NONE',  ( 13.97604488694527802, 13.89961937509977652, 104.3739096053143385 ) ) ;
#198679=CARTESIAN_POINT ( 'NONE',  ( 5.153800228976335163, 19.02544592524342804, 44.79057627198103830 ) ) ;
#198680=CARTESIAN_POINT ( 'NONE',  ( 9.564922557960805705, 16.46253265017160317, 99.58224293864770971 ) ) ;
#198681=CARTESIAN_POINT ( 'NONE',  ( 9.474510206698971260, -16.51473224551069308, 82.91557627198103830 ) ) ;
#198683=CARTESIAN_POINT ( 'NONE',  ( 19.03943276465977164, 0.05219959533936151252, 61.25109039468566863 ) ) ;
#198684=CARTESIAN_POINT ( 'NONE',  ( -0.05219959533937732626, 21.53943276465977519, 107.5010903946856899 ) ) ;
#198685=CARTESIAN_POINT ( 'NONE',  ( 15.72974639402199770, -15.80617190586745480, 33.12390960531435979 ) ) ;
#198686=CARTESIAN_POINT ( 'NONE',  ( -12.06949235617739369, -12.14591786802326823, 109.3760903946857042 ) ) ;
#198687=CARTESIAN_POINT ( 'NONE',  ( 13.89961937509957401, 13.97604488694547697, 71.87609039468567573 ) ) ;
#198688=CARTESIAN_POINT ( 'NONE',  ( -16.29526858892873165, 7.335722546920269593, 59.20329402199793378 ) ) ;
#198689=CARTESIAN_POINT ( 'NONE',  ( 9.564922557961047289, -16.46253265017146816, 80.41775706135234714 ) ) ;
#198690=CARTESIAN_POINT ( 'NONE',  ( -13.89961937509957401, -13.97604488694547875, 29.37609039468565797 ) ) ;
#198691=CARTESIAN_POINT ( 'NONE',  ( 18.22780087662122739, 5.500000000000000888, 71.48236817873106475 ) ) ;
#198692=CARTESIAN_POINT ( 'NONE',  ( 19.05341960407611168, 5.049401038298154454, 38.95724293864767418 ) ) ;
#198693=CARTESIAN_POINT ( 'NONE',  ( 16.53943276465976808, -0.05219959533910856209, 43.74890960531435979 ) ) ;
#198695=CARTESIAN_POINT ( 'NONE',  ( -17.40805194822030444, -6.112264579159319311, 109.1662872748939321 ) ) ;
#198696=CARTESIAN_POINT ( 'NONE',  ( 14.34966873604960469, 8.224510206698951720, 29.16557627198103120 ) ) ;
#198697=LINE ( 'NONE', #89519, #174440 ) ;
#198698=CARTESIAN_POINT ( 'NONE',  ( -8.224510206698735004, -14.34966873604973081, 99.58442372801900433 ) ) ;
#198699=CARTESIAN_POINT ( 'NONE',  ( 13.97604488694527802, 13.89961937509977652, 49.37390960531434558 ) ) ;
#198700=CARTESIAN_POINT ( 'NONE',  ( 10.81492255796106328, -18.62759615963255655, 105.4177570613523613 ) ) ;
#198701=CARTESIAN_POINT ( 'NONE',  ( 0.05219959533936267826, -19.03943276465977164, 110.0010903946856757 ) ) ;
#198702=CARTESIAN_POINT ( 'NONE',  ( -5.719274019375665041, -21.55341960407619695, 89.79275706135236135 ) ) ;
#198703=CARTESIAN_POINT ( 'NONE',  ( -16.46253265017160317, 9.564922557960807481, 90.83224293864769550 ) ) ;
#198704=CARTESIAN_POINT ( 'NONE',  ( 19.02544592524343514, -5.153800228976328945, 88.54057627198102409 ) ) ;
#198706=CARTESIAN_POINT ( 'NONE',  ( 0.05219959533907565091, 21.53943276465977519, 114.9989096053143669 ) ) ;
#198708=CARTESIAN_POINT ( 'NONE',  ( 16.55341960407611168, 4.379528057220329451, 83.95724293864770971 ) ) ;
#198709=CARTESIAN_POINT ( 'NONE',  ( -18.62759615963270932, 10.81492255796079327, 80.83224293864769550 ) ) ;
#198710=CARTESIAN_POINT ( 'NONE',  ( 13.97604488694527802, 13.89961937509977652, 59.37390960531434558 ) ) ;
#198711=CARTESIAN_POINT ( 'NONE',  ( -15.80617190586745835, -15.72974639402198527, 101.8739096053143811 ) ) ;
#198712=CARTESIAN_POINT ( 'NONE',  ( -16.52544592524335698, -4.483927247898792601, 93.95942372801903275 ) ) ;
#198714=CARTESIAN_POINT ( 'NONE',  ( 9.474510206698971260, -16.51473224551069308, 57.91557627198103120 ) ) ;
#198715=CARTESIAN_POINT ( 'NONE',  ( 0.05219959533910956823, 16.53943276465976808, 94.99890960531436690 ) ) ;
#198717=CARTESIAN_POINT ( 'NONE',  ( -13.97604488694527625, -13.89961937509977652, 56.87390960531434558 ) ) ;
#198718=CARTESIAN_POINT ( 'NONE',  ( -5.049401038297874678, -19.05341960407617918, 84.79275706135233293 ) ) ;
#198719=CARTESIAN_POINT ( 'NONE',  ( 12.14591786802309770, 12.06949235617756955, 79.37390960531436690 ) ) ;
#198720=CARTESIAN_POINT ( 'NONE',  ( -18.62759615963255300, -10.81492255796106328, 59.16775706135234714 ) ) ;
#198721=CARTESIAN_POINT ( 'NONE',  ( -5.049401038298153566, 19.05341960407611168, 40.20724293864768839 ) ) ;
#198722=CARTESIAN_POINT ( 'NONE',  ( -0.05219959533907301413, -21.53943276465977519, 102.4989096053143811 ) ) ;
#198723=CARTESIAN_POINT ( 'NONE',  ( 16.53943276465976808, -0.05219959533910856209, 98.74890960531438111 ) ) ;
#198725=CARTESIAN_POINT ( 'NONE',  ( -19.05341960407611168, -5.049401038298163336, 61.45724293864769550 ) ) ;
#198727=CARTESIAN_POINT ( 'NONE',  ( 19.25176906914649422, 5.499999999999730882, 48.49927264242280955 ) ) ;
#198728=CARTESIAN_POINT ( 'NONE',  ( -9.564922557961040184, 16.46253265017147172, 97.91775706135233293 ) ) ;
#198729=CARTESIAN_POINT ( 'NONE',  ( -15.80617190586745835, -15.72974639402198527, 21.87390960531436690 ) ) ;
#198730=CARTESIAN_POINT ( 'NONE',  ( -5.719274019375665041, -21.55341960407619695, 54.79275706135235424 ) ) ;
#198731=CARTESIAN_POINT ( 'NONE',  ( 0.05219959533909260263, 19.03943276465977164, 79.99890960531436690 ) ) ;
#198732=CARTESIAN_POINT ( 'NONE',  ( 19.02544592524334988, 5.153800228976608722, 71.45942372801900433 ) ) ;
#198733=CARTESIAN_POINT ( 'NONE',  ( -5.153800228976328057, -19.02544592524343514, 62.29057627198100988 ) ) ;
#198735=CARTESIAN_POINT ( 'NONE',  ( 12.14591786802309770, 12.06949235617756955, 74.37390960531436690 ) ) ;
#198736=CARTESIAN_POINT ( 'NONE',  ( -0.05219959533910754901, -16.53943276465976808, 62.49890960531436690 ) ) ;
#198737=CARTESIAN_POINT ( 'NONE',  ( 16.51473224551069308, 9.474510206698969483, 84.16557627198102409 ) ) ;
#198738=CARTESIAN_POINT ( 'NONE',  ( -4.379528057220328563, 16.55341960407611168, 80.20724293864769550 ) ) ;
#198739=CARTESIAN_POINT ( 'NONE',  ( -5.049401038298153566, 19.05341960407611168, 80.20724293864769550 ) ) ;
#198740=CARTESIAN_POINT ( 'NONE',  ( 0.05219959533936267826, -19.03943276465977164, 30.00109039468566863 ) ) ;
#198741=CARTESIAN_POINT ( 'NONE',  ( 19.05341960407611168, 5.049401038298154454, 53.95724293864770260 ) ) ;
#198742=CARTESIAN_POINT ( 'NONE',  ( 16.53943276465976808, -0.05219959533910856209, 33.74890960531436690 ) ) ;
#198743=CARTESIAN_POINT ( 'NONE',  ( -8.224510206698948167, 14.34966873604960824, 110.4155762719810383 ) ) ;
#198745=CARTESIAN_POINT ( 'NONE',  ( -21.52544592524334988, -5.823673210054445271, 38.95942372801901854 ) ) ;
#198746=CARTESIAN_POINT ( 'NONE',  ( -9.564922557961040184, 16.46253265017147172, 67.91775706135233293 ) ) ;
#198747=CARTESIAN_POINT ( 'NONE',  ( 12.06949235617757843, -12.14591786802309237, 38.12390960531436690 ) ) ;
#198748=CARTESIAN_POINT ( 'NONE',  ( 5.823673210054125526, 21.52544592524343514, 79.79057627198102409 ) ) ;
#198749=CARTESIAN_POINT ( 'NONE',  ( -10.81492255796078084, -18.62759615963271287, 22.08224293864769194 ) ) ;
#198750=CARTESIAN_POINT ( 'NONE',  ( 16.52544592524342804, -4.483927247898539470, 68.54057627198103830 ) ) ;
#198751=CARTESIAN_POINT ( 'NONE',  ( -13.89961937509977652, 13.97604488694528158, 45.62390960531433848 ) ) ;
#198752=CARTESIAN_POINT ( 'NONE',  ( 9.564922557961047289, -16.46253265017146816, 45.41775706135232582 ) ) ;
#198753=CARTESIAN_POINT ( 'NONE',  ( -4.379528057220086978, -16.55341960407618274, 104.7927570613523898 ) ) ;
#198754=CARTESIAN_POINT ( 'NONE',  ( 12.14591786802327356, -12.06949235617739191, 60.62609039468567573 ) ) ;
#198755=CARTESIAN_POINT ( 'NONE',  ( 10.72451020669898902, -18.67979575497178502, 32.91557627198102409 ) ) ;
#198756=CARTESIAN_POINT ( 'NONE',  ( 10.72451020669871369, 18.67979575497193778, 102.0844237280190185 ) ) ;
#198757=CARTESIAN_POINT ( 'NONE',  ( 13.97604488694527802, 13.89961937509977652, 99.37390960531436690 ) ) ;
#198758=CARTESIAN_POINT ( 'NONE',  ( 4.483927247898790824, -16.52544592524335698, 70.20942372801904696 ) ) ;
#198759=CARTESIAN_POINT ( 'NONE',  ( 5.153800228976335163, 19.02544592524342804, 24.79057627198102765 ) ) ;
#198760=CARTESIAN_POINT ( 'NONE',  ( 12.06949235617757843, -12.14591786802309237, 38.12390960531436690 ) ) ;
#198761=CARTESIAN_POINT ( 'NONE',  ( 5.153800228976335163, 19.02544592524342804, 109.7905762719810099 ) ) ;
#198762=CARTESIAN_POINT ( 'NONE',  ( -19.05341960407611168, -5.049401038298163336, 91.45724293864766707 ) ) ;
#198763=CARTESIAN_POINT ( 'NONE',  ( -21.52544592524343514, 5.823673210054127303, 31.04057627198102409 ) ) ;
#198764=CARTESIAN_POINT ( 'NONE',  ( 4.483927247898545687, 16.52544592524342804, 59.79057627198103120 ) ) ;
#198765=CARTESIAN_POINT ( 'NONE',  ( 14.29746914071049879, -8.314922557960816363, 33.33224293864769550 ) ) ;
#198766=CARTESIAN_POINT ( 'NONE',  ( -14.34966873604960291, -8.224510206698953496, 46.66557627198102409 ) ) ;
#198767=CARTESIAN_POINT ( 'NONE',  ( 8.224510206698742110, 14.34966873604972548, 52.08442372801901854 ) ) ;
#198769=CARTESIAN_POINT ( 'NONE',  ( -19.03943276465977164, -0.05219959533935918106, 48.75109039468566863 ) ) ;
#198770=CARTESIAN_POINT ( 'NONE',  ( -19.03943276465977164, 0.05219959533909376836, 91.24890960531436690 ) ) ;
#198771=CARTESIAN_POINT ( 'NONE',  ( 0.05219959533936267826, -19.03943276465977164, 65.00109039468567573 ) ) ;
#198773=CARTESIAN_POINT ( 'NONE',  ( 5.153800228976615827, -19.02544592524334988, 50.20942372801897591 ) ) ;
#198774=CARTESIAN_POINT ( 'NONE',  ( 16.46253265017146816, 9.564922557961045513, 96.66775706135233293 ) ) ;
#198775=CARTESIAN_POINT ( 'NONE',  ( -12.14591786802326823, 12.06949235617739902, 88.12609039468570415 ) ) ;
#198777=CARTESIAN_POINT ( 'NONE',  ( -5.049401038298153566, 19.05341960407611168, 30.20724293864768839 ) ) ;
#198778=CARTESIAN_POINT ( 'NONE',  ( -13.97604488694527625, -13.89961937509977652, 111.8739096053143243 ) ) ;
#198779=CARTESIAN_POINT ( 'NONE',  ( 18.67979575497194134, -10.72451020669871369, 45.83442372801901854 ) ) ;
#198780=CARTESIAN_POINT ( 'NONE',  ( -19.03943276465977164, -0.05219959533935918106, 103.7510903946856757 ) ) ;
#198781=CARTESIAN_POINT ( 'NONE',  ( 17.50000000000013856, -3.417042746626944183, 107.6738039623247545 ) ) ;
#198782=CARTESIAN_POINT ( 'NONE',  ( 5.153800228976335163, 19.02544592524342804, 54.79057627198103120 ) ) ;
#198783=CARTESIAN_POINT ( 'NONE',  ( 5.153800228976335163, 19.02544592524342804, 99.79057627198102409 ) ) ;
#198784=CARTESIAN_POINT ( 'NONE',  ( 8.224510206698953496, -14.34966873604960469, 72.91557627198103830 ) ) ;
#198785=CARTESIAN_POINT ( 'NONE',  ( 13.89961937509977652, -13.97604488694527269, 58.12390960531436690 ) ) ;
#198786=CARTESIAN_POINT ( 'NONE',  ( -13.89961937509977652, 13.97604488694528158, 75.62390960531438111 ) ) ;
#198787=CARTESIAN_POINT ( 'NONE',  ( -19.03943276465977164, -0.05219959533935918106, 83.75109039468567573 ) ) ;
#198788=CARTESIAN_POINT ( 'NONE',  ( 18.67979575497178502, 10.72451020669898547, 54.16557627198103120 ) ) ;
#198789=CARTESIAN_POINT ( 'NONE',  ( -8.314922557960811034, -14.29746914071050412, 112.0822429386477097 ) ) ;
#198790=CARTESIAN_POINT ( 'NONE',  ( -19.05341960407617563, 5.049401038297882671, 43.54275706135232582 ) ) ;
#198791=CARTESIAN_POINT ( 'NONE',  ( 9.474510206698971260, -16.51473224551069308, 72.91557627198102409 ) ) ;
#198792=CARTESIAN_POINT ( 'NONE',  ( -15.72974639402197994, 15.80617190586746368, 80.62390960531438111 ) ) ;
#198793=CARTESIAN_POINT ( 'NONE',  ( -16.53943276465976808, 0.05219959533911058130, 76.24890960531435269 ) ) ;
#198794=CARTESIAN_POINT ( 'NONE',  ( -5.153800228976607833, 19.02544592524334988, 52.70942372801900433 ) ) ;
#198795=CARTESIAN_POINT ( 'NONE',  ( 18.62759615963271287, -10.81492255796078972, 73.33224293864769550 ) ) ;
#198796=CARTESIAN_POINT ( 'NONE',  ( -18.67979575497178146, -10.72451020669898902, 56.66557627198103830 ) ) ;
#198798=CARTESIAN_POINT ( 'NONE',  ( -10.81492255796078084, -18.62759615963271287, 42.08224293864769550 ) ) ;
#198799=CARTESIAN_POINT ( 'NONE',  ( -5.823673210054431948, 21.52544592524334988, 87.70942372801901854 ) ) ;
#198800=CARTESIAN_POINT ( 'NONE',  ( 19.05341960407611168, 5.049401038298154454, 68.95724293864769550 ) ) ;
#198801=CARTESIAN_POINT ( 'NONE',  ( 16.55341960407611168, 4.379528057220329451, 113.9572429386477239 ) ) ;
#198802=CARTESIAN_POINT ( 'NONE',  ( 15.80617190586769283, -15.72974639402175789, 20.62609039468568639 ) ) ;
#198803=CARTESIAN_POINT ( 'NONE',  ( 10.72451020669871369, 18.67979575497193778, 47.08442372801901854 ) ) ;
#198804=CARTESIAN_POINT ( 'NONE',  ( 19.05341960407611168, 5.049401038298154454, 28.95724293864769550 ) ) ;
#198805=CARTESIAN_POINT ( 'NONE',  ( 21.52544592524344225, -5.823673210054117533, 103.5405762719810383 ) ) ;
#198806=CARTESIAN_POINT ( 'NONE',  ( 13.97604488694548053, -13.89961937509957401, 55.62609039468566863 ) ) ;
#198807=CARTESIAN_POINT ( 'NONE',  ( 13.97604488694527802, 13.89961937509977652, 34.37390960531436690 ) ) ;
#198808=CARTESIAN_POINT ( 'NONE',  ( -8.224510206698735004, -14.34966873604973081, 29.58442372801901854 ) ) ;
#198810=CARTESIAN_POINT ( 'NONE',  ( -12.14591786802326823, 12.06949235617739902, 63.12609039468568994 ) ) ;
#198811=CARTESIAN_POINT ( 'NONE',  ( 19.02544592524343514, -5.153800228976328945, 33.54057627198102409 ) ) ;
#198813=CARTESIAN_POINT ( 'NONE',  ( 9.564922557960805705, 16.46253265017160317, 84.58224293864769550 ) ) ;
#198814=CARTESIAN_POINT ( 'NONE',  ( 8.224510206698953496, -14.34966873604960469, 112.9155762719810383 ) ) ;
#198815=CARTESIAN_POINT ( 'NONE',  ( 0.05219959533907565091, 21.53943276465977519, 54.99890960531435269 ) ) ;
#198816=CARTESIAN_POINT ( 'NONE',  ( -16.53943276465976808, -0.05219959533934237506, 48.75109039468568284 ) ) ;
#198817=CARTESIAN_POINT ( 'NONE',  ( -18.67979575497193778, 10.72451020669871902, 98.33442372801901854 ) ) ;
#198818=CARTESIAN_POINT ( 'NONE',  ( -9.564922557960796823, -16.46253265017161027, 42.08224293864769550 ) ) ;
#198819=CARTESIAN_POINT ( 'NONE',  ( 0.05219959533934541429, -16.53943276465976808, 105.0010903946856757 ) ) ;
#198820=CARTESIAN_POINT ( 'NONE',  ( 16.53943276465976808, -0.05219959533910856209, 58.74890960531436690 ) ) ;
#198821=CARTESIAN_POINT ( 'NONE',  ( 13.97604488694527802, 13.89961937509977652, 64.37390960531436690 ) ) ;
#198822=CARTESIAN_POINT ( 'NONE',  ( 5.823673210054444382, -21.52544592524334988, 105.2094237280190328 ) ) ;
#198823=CARTESIAN_POINT ( 'NONE',  ( -21.52544592524343514, 5.823673210054127303, 116.0405762719810383 ) ) ;
#198824=CARTESIAN_POINT ( 'NONE',  ( 10.81492255796106328, -18.62759615963255655, 85.41775706135236135 ) ) ;
#198825=CARTESIAN_POINT ( 'NONE',  ( 8.224510206698742110, 14.34966873604972548, 57.08442372801901854 ) ) ;
#198826=CARTESIAN_POINT ( 'NONE',  ( -16.52544592524335698, -4.483927247898792601, 28.95942372801902209 ) ) ;
#198828=CARTESIAN_POINT ( 'NONE',  ( 14.29746914071049879, -8.314922557960816363, 73.33224293864769550 ) ) ;
#198829=CARTESIAN_POINT ( 'NONE',  ( -21.52544592524334988, -5.823673210054445271, 98.95942372801903275 ) ) ;
#198830=CARTESIAN_POINT ( 'NONE',  ( 16.55341960407611168, 4.379528057220329451, 38.95724293864768839 ) ) ;
#198831=CARTESIAN_POINT ( 'NONE',  ( -16.52216118717206328, 7.221426719304524511, 113.9240097895301318 ) ) ;
#198832=CARTESIAN_POINT ( 'NONE',  ( 12.14591786802327356, -12.06949235617739191, 40.62609039468567573 ) ) ;
#198833=CARTESIAN_POINT ( 'NONE',  ( -16.53943276465976808, 0.05219959533911058130, 61.24890960531435979 ) ) ;
#198834=CARTESIAN_POINT ( 'NONE',  ( -8.224510206698735004, -14.34966873604973081, 89.58442372801901854 ) ) ;
#198835=CARTESIAN_POINT ( 'NONE',  ( -16.51473224551069308, -9.474510206698971260, 96.66557627198102409 ) ) ;
#198836=CARTESIAN_POINT ( 'NONE',  ( 9.474510206698971260, -16.51473224551069308, 112.9155762719810383 ) ) ;
#198837=CARTESIAN_POINT ( 'NONE',  ( 15.72974639402176855, 15.80617190586768217, 101.8760903946857042 ) ) ;
#198838=CARTESIAN_POINT ( 'NONE',  ( -12.14591786802326823, 12.06949235617739902, 108.1260903946856757 ) ) ;
#198839=CARTESIAN_POINT ( 'NONE',  ( -12.14591786802309592, -12.06949235617757132, 81.87390960531435269 ) ) ;
#198840=CARTESIAN_POINT ( 'NONE',  ( 5.049401038298161559, -19.05341960407611168, 97.70724293864766707 ) ) ;
#198842=CARTESIAN_POINT ( 'NONE',  ( -12.14591786802326823, 12.06949235617739902, 43.12609039468568284 ) ) ;
#198843=CARTESIAN_POINT ( 'NONE',  ( -5.049401038298153566, 19.05341960407611168, 45.20724293864769550 ) ) ;
#198844=CARTESIAN_POINT ( 'NONE',  ( 0.05219959533909260263, 19.03943276465977164, 109.9989096053143669 ) ) ;
#198845=CARTESIAN_POINT ( 'NONE',  ( 16.52544592524335698, 4.483927247898782831, 46.45942372801901854 ) ) ;
#198846=CARTESIAN_POINT ( 'NONE',  ( 17.97035753253451063, 5.499999999999972466, 101.5039701314110800 ) ) ;
#198847=CARTESIAN_POINT ( 'NONE',  ( 9.474510206698729675, 16.51473224551082808, 37.08442372801899722 ) ) ;
#198848=CARTESIAN_POINT ( 'NONE',  ( -19.02544592524342804, 5.153800228976336051, 41.04057627198103120 ) ) ;
#198849=CARTESIAN_POINT ( 'NONE',  ( 12.06949235617739724, 12.14591786802326823, 76.87609039468567573 ) ) ;
#198850=CARTESIAN_POINT ( 'NONE',  ( 0.05219959533936267826, -19.03943276465977164, 80.00109039468567573 ) ) ;
#198851=CARTESIAN_POINT ( 'NONE',  ( 9.474510206698729675, 16.51473224551082808, 27.08442372801900433 ) ) ;
#198852=CARTESIAN_POINT ( 'NONE',  ( 0.05219959533909260263, 19.03943276465977164, 54.99890960531435979 ) ) ;
#198853=CARTESIAN_POINT ( 'NONE',  ( 4.483927247898545687, 16.52544592524342804, 99.79057627198103830 ) ) ;
#198854=CARTESIAN_POINT ( 'NONE',  ( -16.51473224551082808, 9.474510206698731452, 68.33442372801900433 ) ) ;
#198855=CARTESIAN_POINT ( 'NONE',  ( 10.81492255796078972, 18.62759615963270932, 69.58224293864769550 ) ) ;
#198856=CARTESIAN_POINT ( 'NONE',  ( -0.05219959533936034679, 19.03943276465977164, 27.50109039468566507 ) ) ;
#198857=CARTESIAN_POINT ( 'NONE',  ( 0.05219959533909260263, 19.03943276465977164, 104.9989096053143669 ) ) ;
#198858=CARTESIAN_POINT ( 'NONE',  ( -15.80617190586745835, -15.72974639402198527, 71.87390960531438111 ) ) ;
#198859=CARTESIAN_POINT ( 'NONE',  ( -5.049401038298153566, 19.05341960407611168, 110.2072429386476671 ) ) ;
#198860=CARTESIAN_POINT ( 'NONE',  ( 5.049401038297881783, 19.05341960407617563, 102.2927570613523045 ) ) ;
#198861=CARTESIAN_POINT ( 'NONE',  ( -17.49999999999999645, 5.500000000000000888, 108.7176903769643559 ) ) ;
#198862=CARTESIAN_POINT ( 'NONE',  ( 12.14591786802327356, -12.06949235617739191, 25.62609039468567929 ) ) ;
#198863=CARTESIAN_POINT ( 'NONE',  ( 0.05219959533909260263, 19.03943276465977164, 39.99890960531436690 ) ) ;
#198864=CARTESIAN_POINT ( 'NONE',  ( 13.89961937509977652, -13.97604488694527269, 93.12390960531436690 ) ) ;
#198865=CARTESIAN_POINT ( 'NONE',  ( -10.81492255796078084, -18.62759615963271287, 87.08224293864769550 ) ) ;
#198866=CARTESIAN_POINT ( 'NONE',  ( 5.719274019375673035, 21.55341960407619339, 67.29275706135234714 ) ) ;
#198867=CARTESIAN_POINT ( 'NONE',  ( -19.03943276465977164, -0.05219959533935918106, 108.7510903946856615 ) ) ;
#198868=CARTESIAN_POINT ( 'NONE',  ( -21.53943276465977519, -0.05219959533937600094, 108.7510903946857042 ) ) ;
#198869=CARTESIAN_POINT ( 'NONE',  ( -14.34966873604960291, -8.224510206698953496, 21.66557627198102409 ) ) ;
#198870=CARTESIAN_POINT ( 'NONE',  ( -21.52544592524343514, 5.823673210054127303, 96.04057627198102409 ) ) ;
#198871=CARTESIAN_POINT ( 'NONE',  ( 16.53943276465976808, -0.05219959533910856209, 33.74890960531436690 ) ) ;
#198872=CARTESIAN_POINT ( 'NONE',  ( 16.51473224551083163, -9.474510206698727899, 80.83442372801899012 ) ) ;
#198873=CARTESIAN_POINT ( 'NONE',  ( 19.05341960407617918, -5.049401038297876454, 61.04275706135232582 ) ) ;
#198874=CARTESIAN_POINT ( 'NONE',  ( 5.823673210054444382, -21.52544592524334988, 55.20942372801902565 ) ) ;
#198875=CARTESIAN_POINT ( 'NONE',  ( 16.46253265017146816, 9.564922557961045513, 41.66775706135234003 ) ) ;
#198876=CARTESIAN_POINT ( 'NONE',  ( 0.05219959533910956823, 16.53943276465976808, 109.9989096053143527 ) ) ;
#198877=CARTESIAN_POINT ( 'NONE',  ( -10.72451020669898014, 18.67979575497178502, 30.41557627198101699 ) ) ;
#198878=CARTESIAN_POINT ( 'NONE',  ( -8.314922557960811034, -14.29746914071050412, 42.08224293864769550 ) ) ;
#198879=CARTESIAN_POINT ( 'NONE',  ( -5.719274019375665041, -21.55341960407619695, 104.7927570613523898 ) ) ;
#198880=CARTESIAN_POINT ( 'NONE',  ( 16.53943276465976808, 0.05219959533934440121, 76.25109039468568994 ) ) ;
#198881=CARTESIAN_POINT ( 'NONE',  ( -12.06949235617756955, 12.14591786802309770, 25.62390960531435624 ) ) ;
#198882=CARTESIAN_POINT ( 'NONE',  ( -15.72974639402176322, -15.80617190586768395, 64.37609039468568994 ) ) ;
#198883=CARTESIAN_POINT ( 'NONE',  ( 21.55341960407619695, -5.719274019375665929, 66.04275706135236135 ) ) ;
#198884=CARTESIAN_POINT ( 'NONE',  ( -5.719274019375978568, 21.55341960407610458, 65.20724293864768129 ) ) ;
#198886=CARTESIAN_POINT ( 'NONE',  ( 5.049401038298163336, -19.05341960407611168, 62.70724293864769550 ) ) ;
#198887=CARTESIAN_POINT ( 'NONE',  ( 21.52544592524334988, 5.823673210054432836, 41.45942372801901143 ) ) ;
#198888=CARTESIAN_POINT ( 'NONE',  ( -19.03943276465977164, 0.05219959533909376836, 21.24890960531436335 ) ) ;
#198889=CARTESIAN_POINT ( 'NONE',  ( -9.474510206698964154, 16.51473224551069663, 45.41557627198103120 ) ) ;
#198890=CARTESIAN_POINT ( 'NONE',  ( 12.14591786802309770, 12.06949235617756955, 84.37390960531438111 ) ) ;
#198891=CARTESIAN_POINT ( 'NONE',  ( -16.46253265017160317, 9.564922557960807481, 80.83224293864769550 ) ) ;
#198892=CARTESIAN_POINT ( 'NONE',  ( 8.314922557960818139, 14.29746914071049879, 29.58224293864769905 ) ) ;
#198893=CARTESIAN_POINT ( 'NONE',  ( 15.80617190586746368, 15.72974639402197994, 69.37390960531436690 ) ) ;
#198895=CARTESIAN_POINT ( 'NONE',  ( -5.823673210054116645, -21.52544592524344225, 107.2905762719810525 ) ) ;
#198896=CARTESIAN_POINT ( 'NONE',  ( -9.474510206698964154, 16.51473224551069663, 110.4155762719810383 ) ) ;
#198897=CARTESIAN_POINT ( 'NONE',  ( 19.05341960407611168, 5.049401038298154454, 63.95724293864769550 ) ) ;
#198898=CARTESIAN_POINT ( 'NONE',  ( 16.46253265017146816, 9.564922557961045513, 106.6677570613523471 ) ) ;
#198899=CARTESIAN_POINT ( 'NONE',  ( -18.67979575497178146, -10.72451020669898902, 56.66557627198103830 ) ) ;
#198900=CARTESIAN_POINT ( 'NONE',  ( 18.67979575497194134, -10.72451020669871369, 75.83442372801900433 ) ) ;
#198901=CARTESIAN_POINT ( 'NONE',  ( -9.474510206698964154, 16.51473224551069663, 60.41557627198102409 ) ) ;
#198902=CARTESIAN_POINT ( 'NONE',  ( 5.049401038298161559, -19.05341960407611168, 92.70724293864769550 ) ) ;
#198903=CARTESIAN_POINT ( 'NONE',  ( -12.06949235617739369, -12.14591786802326823, 79.37609039468567573 ) ) ;
#198904=CARTESIAN_POINT ( 'NONE',  ( 18.62759615963255655, 10.81492255796105972, 51.66775706135234714 ) ) ;
#198905=CARTESIAN_POINT ( 'NONE',  ( 18.62759615963255655, 10.81492255796105972, 91.66775706135234714 ) ) ;
#198906=CARTESIAN_POINT ( 'NONE',  ( 5.823673210054444382, -21.52544592524334988, 20.20942372801900788 ) ) ;
#198907=CARTESIAN_POINT ( 'NONE',  ( -18.67979575497178146, -10.72451020669898902, 81.66557627198103830 ) ) ;
#198908=CARTESIAN_POINT ( 'NONE',  ( -13.97604488694547697, 13.89961937509957934, 48.12609039468566863 ) ) ;
#198909=CARTESIAN_POINT ( 'NONE',  ( -21.52544592524343514, 5.823673210054127303, 46.04057627198103830 ) ) ;
#198910=CARTESIAN_POINT ( 'NONE',  ( -9.474510206698964154, 16.51473224551069663, 80.41557627198103830 ) ) ;
#198911=CARTESIAN_POINT ( 'NONE',  ( -8.224510206698948167, 14.34966873604960824, 30.41557627198101699 ) ) ;
#198912=CARTESIAN_POINT ( 'NONE',  ( -16.61371651742604882, 7.165104196376021584, 63.85415069992997417 ) ) ;
#198914=CARTESIAN_POINT ( 'NONE',  ( 5.153800228976615827, -19.02544592524334988, 90.20942372801900433 ) ) ;
#198915=CARTESIAN_POINT ( 'NONE',  ( -0.05219959533907301413, -21.53943276465977519, 77.49890960531433848 ) ) ;
#198916=CARTESIAN_POINT ( 'NONE',  ( -4.483927247898539470, -16.52544592524342804, 57.29057627198103120 ) ) ;
#198917=CARTESIAN_POINT ( 'NONE',  ( 16.52544592524335698, 4.483927247898782831, 26.45942372801901854 ) ) ;
#198918=CARTESIAN_POINT ( 'NONE',  ( -13.89961937509977652, 13.97604488694528158, 40.62390960531435979 ) ) ;
#198919=CARTESIAN_POINT ( 'NONE',  ( 18.67979575497178502, 10.72451020669898547, 99.16557627198100988 ) ) ;
#198920=CARTESIAN_POINT ( 'NONE',  ( -19.02544592524334988, -5.153800228976617603, 68.95942372801896170 ) ) ;
#198921=CARTESIAN_POINT ( 'NONE',  ( 13.97604488694527802, 13.89961937509977652, 84.37390960531433848 ) ) ;
#198922=CARTESIAN_POINT ( 'NONE',  ( -16.53943276465976808, 0.05219959533911058130, 96.24890960531435269 ) ) ;
#198924=CARTESIAN_POINT ( 'NONE',  ( 13.97604488694527802, 13.89961937509977652, 59.37390960531434558 ) ) ;
#198925=CARTESIAN_POINT ( 'NONE',  ( 16.55341960407611168, 4.379528057220329451, 68.95724293864769550 ) ) ;
#198926=CARTESIAN_POINT ( 'NONE',  ( 16.51473224551069308, 9.474510206698969483, 39.16557627198103120 ) ) ;
#198928=CARTESIAN_POINT ( 'NONE',  ( -14.34966873604960291, -8.224510206698953496, 46.66557627198102409 ) ) ;
#198929=CARTESIAN_POINT ( 'NONE',  ( -13.89961937509977652, 13.97604488694528158, 85.62390960531433848 ) ) ;
#198931=CARTESIAN_POINT ( 'NONE',  ( 0.05219959533936267826, -19.03943276465977164, 50.00109039468566863 ) ) ;
#198932=CARTESIAN_POINT ( 'NONE',  ( 4.483927247898790824, -16.52544592524335698, 65.20942372801901854 ) ) ;
#198934=CARTESIAN_POINT ( 'NONE',  ( -10.72451020669898014, 18.67979575497178502, 80.41557627198103830 ) ) ;
#198935=CARTESIAN_POINT ( 'NONE',  ( 19.03943276465977164, 0.05219959533936151252, 41.25109039468566152 ) ) ;
#198936=CARTESIAN_POINT ( 'NONE',  ( -16.46253265017160317, 9.564922557960807481, 85.83224293864769550 ) ) ;
#198938=CARTESIAN_POINT ( 'NONE',  ( -5.823673210054116645, -21.52544592524344225, 22.29057627198102765 ) ) ;
#198939=CARTESIAN_POINT ( 'NONE',  ( -0.05219959533909027116, -19.03943276465977164, 62.49890960531435979 ) ) ;
#198940=CARTESIAN_POINT ( 'NONE',  ( -5.719274019375665041, -21.55341960407619695, 49.79275706135234714 ) ) ;
#198941=CARTESIAN_POINT ( 'NONE',  ( 16.53943276465976808, -0.05219959533910856209, 113.7489096053143527 ) ) ;
#198942=CARTESIAN_POINT ( 'NONE',  ( -15.72974639402197994, 15.80617190586746368, 115.6239096053143669 ) ) ;
#198943=CARTESIAN_POINT ( 'NONE',  ( 19.03943276465977164, -0.05219959533909143690, 98.74890960531436690 ) ) ;
#198945=CARTESIAN_POINT ( 'NONE',  ( 18.62759615963255655, 10.81492255796105972, 41.66775706135235424 ) ) ;
#198947=CARTESIAN_POINT ( 'NONE',  ( 5.153800228976335163, 19.02544592524342804, 99.79057627198102409 ) ) ;
#198949=CARTESIAN_POINT ( 'NONE',  ( 18.67979575497178502, 10.72451020669898547, 104.1655762719810241 ) ) ;
#198950=CARTESIAN_POINT ( 'NONE',  ( 9.474510206698971260, -16.51473224551069308, 47.91557627198102409 ) ) ;
#198951=CARTESIAN_POINT ( 'NONE',  ( -4.483927247898782831, 16.52544592524335698, 22.70942372801901499 ) ) ;
#198953=CARTESIAN_POINT ( 'NONE',  ( -16.46253265017160317, 9.564922557960807481, 30.83224293864769550 ) ) ;
#198954=CARTESIAN_POINT ( 'NONE',  ( -18.62759615963255300, -10.81492255796106328, 94.16775706135237556 ) ) ;
#198955=CARTESIAN_POINT ( 'NONE',  ( -16.46253265017160317, 9.564922557960807481, 90.83224293864769550 ) ) ;
#198956=CARTESIAN_POINT ( 'NONE',  ( 5.823673210054444382, -21.52544592524334988, 65.20942372801901854 ) ) ;
#198958=CARTESIAN_POINT ( 'NONE',  ( 19.03943276465977164, -0.05219959533909143690, 103.7489096053143669 ) ) ;
#198960=CARTESIAN_POINT ( 'NONE',  ( -16.53943276465976808, -0.05219959533934237506, 38.75109039468567573 ) ) ;
#198961=CARTESIAN_POINT ( 'NONE',  ( -14.34966873604972548, 8.224510206698743886, 73.33442372801901854 ) ) ;
#198962=CARTESIAN_POINT ( 'NONE',  ( -21.53943276465977519, -0.05219959533937600094, 58.75109039468568994 ) ) ;
#198963=CARTESIAN_POINT ( 'NONE',  ( -10.81492255796105439, 18.62759615963255655, 92.91775706135236135 ) ) ;
#198965=CARTESIAN_POINT ( 'NONE',  ( 8.314922557961029526, -14.29746914071037800, 20.41775706135234714 ) ) ;
#198966=CARTESIAN_POINT ( 'NONE',  ( 16.46253265017160672, -9.564922557960803928, 68.33224293864770971 ) ) ;
#198967=CARTESIAN_POINT ( 'NONE',  ( 16.51473224551069308, 9.474510206698969483, 94.16557627198103830 ) ) ;
#198968=CARTESIAN_POINT ( 'NONE',  ( 9.474510206698971260, -16.51473224551069308, 22.91557627198102765 ) ) ;
#198969=CARTESIAN_POINT ( 'NONE',  ( 18.62759615963271287, -10.81492255796078972, 23.33224293864769194 ) ) ;
#198970=CARTESIAN_POINT ( 'NONE',  ( 14.29746914071037800, 8.314922557961029526, 96.66775706135234714 ) ) ;
#198971=CARTESIAN_POINT ( 'NONE',  ( -14.29746914071049879, 8.314922557960819915, 75.83224293864769550 ) ) ;
#198972=CARTESIAN_POINT ( 'NONE',  ( 19.03943276465977164, -0.05219959533909143690, 58.74890960531435979 ) ) ;
#198973=CARTESIAN_POINT ( 'NONE',  ( -21.53943276465977519, -0.05219959533937600094, 88.75109039468567573 ) ) ;
#198975=CARTESIAN_POINT ( 'NONE',  ( -9.474510206698720793, -16.51473224551083518, 109.5844237280190043 ) ) ;
#198976=CARTESIAN_POINT ( 'NONE',  ( 16.53943276465976808, -0.05219959533910856209, 78.74890960531436690 ) ) ;
#198977=CARTESIAN_POINT ( 'NONE',  ( 10.72451020669871369, 18.67979575497193778, 32.08442372801901854 ) ) ;
#198978=CARTESIAN_POINT ( 'NONE',  ( 10.81492255796078972, 18.62759615963270932, 64.58224293864769550 ) ) ;
#198979=CARTESIAN_POINT ( 'NONE',  ( -19.03943276465977164, -0.05219959533935918106, 38.75109039468566152 ) ) ;
#198981=CARTESIAN_POINT ( 'NONE',  ( -16.46253265017160317, 9.564922557960807481, 80.83224293864769550 ) ) ;
#198982=CARTESIAN_POINT ( 'NONE',  ( -16.52544592524342804, 4.483927247898546575, 51.04057627198103120 ) ) ;
#198983=CARTESIAN_POINT ( 'NONE',  ( 12.14591786802309770, 12.06949235617756955, 39.37390960531436690 ) ) ;
#198984=CARTESIAN_POINT ( 'NONE',  ( 12.14591786802327356, -12.06949235617739191, 100.6260903946857184 ) ) ;
#198985=CARTESIAN_POINT ( 'NONE',  ( -5.153800228976607833, 19.02544592524334988, 52.70942372801900433 ) ) ;
#198986=CARTESIAN_POINT ( 'NONE',  ( -17.59860650958993844, 7.585241751806885979, 78.42337014262493256 ) ) ;
#198987=CARTESIAN_POINT ( 'NONE',  ( -5.153800228976328057, -19.02544592524343514, 107.2905762719810383 ) ) ;
#198988=CARTESIAN_POINT ( 'NONE',  ( -4.483927247898539470, -16.52544592524342804, 77.29057627198102409 ) ) ;
#198989=CARTESIAN_POINT ( 'NONE',  ( -16.51473224551082808, 9.474510206698731452, 43.33442372801900433 ) ) ;
#198990=CARTESIAN_POINT ( 'NONE',  ( -19.03943276465977164, 0.05219959533909376836, 36.24890960531436690 ) ) ;
#198991=CARTESIAN_POINT ( 'NONE',  ( -15.80617190586745835, -15.72974639402198527, 41.87390960531435979 ) ) ;
#198992=CARTESIAN_POINT ( 'NONE',  ( 0.05219959533907565091, 21.53943276465977519, 64.99890960531435269 ) ) ;
#198993=CARTESIAN_POINT ( 'NONE',  ( 16.52544592524342804, -4.483927247898539470, 108.5405762719810241 ) ) ;
#198994=CARTESIAN_POINT ( 'NONE',  ( -12.14591786802326823, 12.06949235617739902, 58.12609039468568994 ) ) ;
#198995=CARTESIAN_POINT ( 'NONE',  ( 0.05219959533909260263, 19.03943276465977164, 44.99890960531435979 ) ) ;
#198996=CARTESIAN_POINT ( 'NONE',  ( 15.72974639402176855, 15.80617190586768217, 41.87609039468568284 ) ) ;
#198997=CARTESIAN_POINT ( 'NONE',  ( -12.14591786802309592, -12.06949235617757132, 96.87390960531436690 ) ) ;
#198998=CARTESIAN_POINT ( 'NONE',  ( 17.50000000000000355, 5.500000000000011546, 78.78230962303567253 ) ) ;
#199000=CARTESIAN_POINT ( 'NONE',  ( 15.72974639402199770, -15.80617190586745480, 28.12390960531435979 ) ) ;
#199002=CARTESIAN_POINT ( 'NONE',  ( -17.49999999999999645, 5.499999999999992895, 43.71769037696436300 ) ) ;
#199003=CARTESIAN_POINT ( 'NONE',  ( 16.55341960407618274, -4.379528057220086978, 46.04275706135234714 ) ) ;
#199004=CARTESIAN_POINT ( 'NONE',  ( 4.379528057220339221, -16.55341960407611168, 42.70724293864770260 ) ) ;
#199005=CARTESIAN_POINT ( 'NONE',  ( -15.72974639402197994, 15.80617190586746368, 70.62390960531436690 ) ) ;
#199006=CARTESIAN_POINT ( 'NONE',  ( -18.62759615963270932, 10.81492255796079327, 55.83224293864770260 ) ) ;
#199008=CARTESIAN_POINT ( 'NONE',  ( -9.474510206698964154, 16.51473224551069663, 35.41557627198102409 ) ) ;
#199009=CARTESIAN_POINT ( 'NONE',  ( 13.97604488694527802, 13.89961937509977652, 104.3739096053143385 ) ) ;
#199010=CARTESIAN_POINT ( 'NONE',  ( -13.89961937509977652, 13.97604488694528158, 45.62390960531433848 ) ) ;
#199011=CARTESIAN_POINT ( 'NONE',  ( -12.06949235617756955, 12.14591786802309770, 115.6239096053143669 ) ) ;
#199012=CARTESIAN_POINT ( 'NONE',  ( -19.03943276465977164, 0.05219959533909376836, 116.2489096053143669 ) ) ;
#199014=CARTESIAN_POINT ( 'NONE',  ( 0.05219959533934541429, -16.53943276465976808, 75.00109039468568994 ) ) ;
#199015=CARTESIAN_POINT ( 'NONE',  ( 15.80617190586746368, 15.72974639402197994, 99.37390960531436690 ) ) ;
#199016=CARTESIAN_POINT ( 'NONE',  ( -19.03943276465977164, 0.05219959533909376836, 61.24890960531436690 ) ) ;
#199017=CARTESIAN_POINT ( 'NONE',  ( 15.80617190586769283, -15.72974639402175789, 40.62609039468567573 ) ) ;
#199018=CARTESIAN_POINT ( 'NONE',  ( 0.05219959533909260263, 19.03943276465977164, 84.99890960531436690 ) ) ;
#199020=ORIENTED_EDGE ( 'NONE', *, *, #104192, .F. ) ;
#199021=CARTESIAN_POINT ( 'NONE',  ( -15.72974639402176322, -15.80617190586768395, 34.37609039468568284 ) ) ;
#199022=CARTESIAN_POINT ( 'NONE',  ( -16.46253265017160317, 9.564922557960807481, 105.8322429386476955 ) ) ;
#199023=CARTESIAN_POINT ( 'NONE',  ( -13.97604488694547697, 13.89961937509957934, 83.12609039468564731 ) ) ;
#199024=CARTESIAN_POINT ( 'NONE',  ( 13.97604488694548053, -13.89961937509957401, 40.62609039468564731 ) ) ;
#199025=CARTESIAN_POINT ( 'NONE',  ( -18.67979575497178146, -10.72451020669898902, 96.66557627198102409 ) ) ;
#199026=CARTESIAN_POINT ( 'NONE',  ( -13.97604488694547697, 13.89961937509957934, 28.12609039468565797 ) ) ;
#199027=CARTESIAN_POINT ( 'NONE',  ( 9.474510206698729675, 16.51473224551082808, 32.08442372801900433 ) ) ;
#199028=CARTESIAN_POINT ( 'NONE',  ( -8.224510206698735004, -14.34966873604973081, 89.58442372801901854 ) ) ;
#199030=CARTESIAN_POINT ( 'NONE',  ( 5.153800228976335163, 19.02544592524342804, 64.79057627198100988 ) ) ;
#199032=CARTESIAN_POINT ( 'NONE',  ( -21.53943276465977519, -0.05219959533937600094, 68.75109039468568994 ) ) ;
#199033=CARTESIAN_POINT ( 'NONE',  ( 21.52544592524334988, 5.823673210054432836, 86.45942372801901854 ) ) ;
#199034=CARTESIAN_POINT ( 'NONE',  ( 16.46253265017160672, -9.564922557960803928, 78.33224293864769550 ) ) ;
#199035=CARTESIAN_POINT ( 'NONE',  ( -0.05219959533937732626, 21.53943276465977519, 62.50109039468568284 ) ) ;
#199036=CARTESIAN_POINT ( 'NONE',  ( 16.51473224551083163, -9.474510206698727899, 95.83442372801900433 ) ) ;
#199037=CARTESIAN_POINT ( 'NONE',  ( 16.51473224551069308, 9.474510206698969483, 54.16557627198103120 ) ) ;
#199038=CARTESIAN_POINT ( 'NONE',  ( -19.03943276465977164, 0.05219959533909376836, 101.2489096053143669 ) ) ;
#199039=CARTESIAN_POINT ( 'NONE',  ( 16.46253265017160672, -9.564922557960803928, 73.33224293864769550 ) ) ;
#199040=CARTESIAN_POINT ( 'NONE',  ( -9.564922557960796823, -16.46253265017161027, 77.08224293864769550 ) ) ;
#199041=CARTESIAN_POINT ( 'NONE',  ( -5.049401038298153566, 19.05341960407611168, 60.20724293864768129 ) ) ;
#199042=CARTESIAN_POINT ( 'NONE',  ( -15.72974639402197994, 15.80617190586746368, 105.6239096053143669 ) ) ;
#199043=CARTESIAN_POINT ( 'NONE',  ( 8.224510206698742110, 14.34966873604972548, 92.08442372801901854 ) ) ;
#199045=CARTESIAN_POINT ( 'NONE',  ( 13.97604488694548053, -13.89961937509957401, 40.62609039468564731 ) ) ;
#199046=CARTESIAN_POINT ( 'NONE',  ( -19.02544592524342804, 5.153800228976336051, 81.04057627198103830 ) ) ;
#199047=CARTESIAN_POINT ( 'NONE',  ( -12.14591786802309592, -12.06949235617757132, 66.87390960531436690 ) ) ;
#199048=CARTESIAN_POINT ( 'NONE',  ( -4.379528057220328563, 16.55341960407611168, 100.2072429386476955 ) ) ;
#199049=CARTESIAN_POINT ( 'NONE',  ( -16.46253265017160317, 9.564922557960807481, 115.8322429386477097 ) ) ;
#199050=CARTESIAN_POINT ( 'NONE',  ( -5.153800228976328057, -19.02544592524343514, 102.2905762719810383 ) ) ;
#199052=CARTESIAN_POINT ( 'NONE',  ( -9.474510206698720793, -16.51473224551083518, 24.58442372801900078 ) ) ;
#199053=CARTESIAN_POINT ( 'NONE',  ( 4.379528057220092307, 16.55341960407617563, 92.29275706135236135 ) ) ;
#199054=CARTESIAN_POINT ( 'NONE',  ( -19.02544592524342804, 5.153800228976336051, 71.04057627198099567 ) ) ;
#199055=ADVANCED_FACE ( 'NONE', ( #20146 ), #172852, .T. ) ;
#199056=CARTESIAN_POINT ( 'NONE',  ( 18.62759615963255655, 10.81492255796105972, 51.66775706135234714 ) ) ;
#199057=CARTESIAN_POINT ( 'NONE',  ( 21.53943276465977519, -0.05219959533907433946, 28.74890960531435624 ) ) ;
#199058=CARTESIAN_POINT ( 'NONE',  ( -21.52544592524334988, -5.823673210054445271, 23.95942372801901143 ) ) ;
#199059=CARTESIAN_POINT ( 'NONE',  ( -21.52544592524343514, 5.823673210054127303, 76.04057627198102409 ) ) ;
#199060=CARTESIAN_POINT ( 'NONE',  ( 4.483927247898545687, 16.52544592524342804, 89.79057627198103830 ) ) ;
#199061=CARTESIAN_POINT ( 'NONE',  ( 13.89961937509957401, 13.97604488694547697, 51.87609039468566863 ) ) ;
#199062=CARTESIAN_POINT ( 'NONE',  ( 5.049401038298161559, -19.05341960407611168, 37.70724293864768839 ) ) ;
#199063=CARTESIAN_POINT ( 'NONE',  ( -9.564922557960796823, -16.46253265017161027, 82.08224293864768129 ) ) ;
#199064=CARTESIAN_POINT ( 'NONE',  ( -0.05219959533909027116, -19.03943276465977164, 77.49890960531435269 ) ) ;
#199066=CARTESIAN_POINT ( 'NONE',  ( 4.379528057220339221, -16.55341960407611168, 97.70724293864772392 ) ) ;
#199068=CARTESIAN_POINT ( 'NONE',  ( 16.52544592524342804, -4.483927247898539470, 23.54057627198102765 ) ) ;
#199069=CARTESIAN_POINT ( 'NONE',  ( 4.379528057220092307, 16.55341960407617563, 22.29275706135235069 ) ) ;
#199070=CARTESIAN_POINT ( 'NONE',  ( -21.55341960407619339, 5.719274019375674811, 88.54275706135236135 ) ) ;
#199071=CARTESIAN_POINT ( 'NONE',  ( 5.153800228976335163, 19.02544592524342804, 104.7905762719809957 ) ) ;
#199072=CARTESIAN_POINT ( 'NONE',  ( -0.05219959533907301413, -21.53943276465977519, 112.4989096053143669 ) ) ;
#199073=CARTESIAN_POINT ( 'NONE',  ( 5.049401038298161559, -19.05341960407611168, 37.70724293864768839 ) ) ;
#199075=CARTESIAN_POINT ( 'NONE',  ( -16.52544592524335698, -4.483927247898792601, 48.95942372801902565 ) ) ;
#199076=CARTESIAN_POINT ( 'NONE',  ( -9.564922557961040184, 16.46253265017147172, 112.9177570613523329 ) ) ;
#199077=CARTESIAN_POINT ( 'NONE',  ( -16.46253265017160317, 9.564922557960807481, 30.83224293864769550 ) ) ;
#199078=CARTESIAN_POINT ( 'NONE',  ( -16.52544592524342804, 4.483927247898546575, 96.04057627198102409 ) ) ;
#199079=CARTESIAN_POINT ( 'NONE',  ( -0.05219959533907301413, -21.53943276465977519, 107.4989096053143669 ) ) ;
#199080=CARTESIAN_POINT ( 'NONE',  ( -19.05341960407617563, 5.049401038297882671, 73.54275706135233293 ) ) ;
#199082=CARTESIAN_POINT ( 'NONE',  ( -5.719274019375978568, 21.55341960407610458, 115.2072429386476955 ) ) ;
#199084=CARTESIAN_POINT ( 'NONE',  ( -9.474510206698964154, 16.51473224551069663, 85.41557627198102409 ) ) ;
#199086=CARTESIAN_POINT ( 'NONE',  ( -16.46253265017160317, 9.564922557960807481, 90.83224293864769550 ) ) ;
#199087=CARTESIAN_POINT ( 'NONE',  ( -18.67979575497193778, 10.72451020669871902, 33.33442372801900433 ) ) ;
#199088=CARTESIAN_POINT ( 'NONE',  ( 4.379528057220339221, -16.55341960407611168, 72.70724293864769550 ) ) ;
#199089=CARTESIAN_POINT ( 'NONE',  ( -16.46253265017160317, 9.564922557960807481, 85.83224293864769550 ) ) ;
#199090=CARTESIAN_POINT ( 'NONE',  ( 12.14591786802327356, -12.06949235617739191, 50.62609039468568994 ) ) ;
#199092=CARTESIAN_POINT ( 'NONE',  ( -9.474510206698720793, -16.51473224551083518, 59.58442372801900433 ) ) ;
#199093=CARTESIAN_POINT ( 'NONE',  ( -15.80617190586768217, 15.72974639402176855, 63.12609039468568994 ) ) ;
#199094=CARTESIAN_POINT ( 'NONE',  ( -14.34966873604972548, 8.224510206698743886, 33.33442372801900433 ) ) ;
#199095=CARTESIAN_POINT ( 'NONE',  ( 16.46253265017160672, -9.564922557960803928, 68.33224293864770971 ) ) ;
#199096=CARTESIAN_POINT ( 'NONE',  ( 9.474510206698729675, 16.51473224551082808, 92.08442372801900433 ) ) ;
#199097=CARTESIAN_POINT ( 'NONE',  ( -8.314922557961024197, 14.29746914071037800, 52.91775706135235424 ) ) ;
#199098=CARTESIAN_POINT ( 'NONE',  ( -18.67979575497193778, 10.72451020669871902, 98.33442372801901854 ) ) ;
#199099=CARTESIAN_POINT ( 'NONE',  ( 9.564922557961047289, -16.46253265017146816, 80.41775706135234714 ) ) ;
#199100=CARTESIAN_POINT ( 'NONE',  ( 9.474510206698971260, -16.51473224551069308, 47.91557627198102409 ) ) ;
#199101=CARTESIAN_POINT ( 'NONE',  ( 5.719274019375991003, -21.55341960407610458, 72.70724293864769550 ) ) ;
#199102=CARTESIAN_POINT ( 'NONE',  ( -4.379528057220328563, 16.55341960407611168, 70.20724293864769550 ) ) ;
#199103=CARTESIAN_POINT ( 'NONE',  ( 19.03943276465977164, 0.05219959533936151252, 71.25109039468566152 ) ) ;
#199105=CARTESIAN_POINT ( 'NONE',  ( 19.02544592524334988, 5.153800228976608722, 41.45942372801900433 ) ) ;
#199106=CARTESIAN_POINT ( 'NONE',  ( 16.53943276465976808, -0.05219959533910856209, 23.74890960531435269 ) ) ;
#199107=CARTESIAN_POINT ( 'NONE',  ( -0.05219959533910754901, -16.53943276465976808, 72.49890960531435269 ) ) ;
#199108=CARTESIAN_POINT ( 'NONE',  ( 21.52544592524334988, 5.823673210054432836, 106.4594237280190328 ) ) ;
#199110=CARTESIAN_POINT ( 'NONE',  ( -21.55341960407610458, -5.719274019375992779, 111.4572429386476813 ) ) ;
#199111=CARTESIAN_POINT ( 'NONE',  ( -9.564922557960796823, -16.46253265017161027, 67.08224293864769550 ) ) ;
#199112=CARTESIAN_POINT ( 'NONE',  ( 21.53943276465977519, 0.05219959533937863772, 86.25109039468568994 ) ) ;
#199113=CARTESIAN_POINT ( 'NONE',  ( -5.153800228976328057, -19.02544592524343514, 67.29057627198102409 ) ) ;
#199114=ORIENTED_EDGE ( 'NONE', *, *, #166361, .F. ) ;
#199115=CARTESIAN_POINT ( 'NONE',  ( -16.51473224551069308, -9.474510206698971260, 26.66557627198103120 ) ) ;
#199116=CARTESIAN_POINT ( 'NONE',  ( -5.719274019375978568, 21.55341960407610458, 30.20724293864769550 ) ) ;
#199117=CARTESIAN_POINT ( 'NONE',  ( 12.14591786802309770, 12.06949235617756955, 69.37390960531436690 ) ) ;
#199118=CARTESIAN_POINT ( 'NONE',  ( -16.51473224551069308, -9.474510206698971260, 46.66557627198102409 ) ) ;
#199119=CARTESIAN_POINT ( 'NONE',  ( -14.29746914071049879, 8.314922557960819915, 90.83224293864769550 ) ) ;
#199120=CARTESIAN_POINT ( 'NONE',  ( -10.72451020669898014, 18.67979575497178502, 105.4155762719810383 ) ) ;
#199121=CARTESIAN_POINT ( 'NONE',  ( 10.72451020669871369, 18.67979575497193778, 52.08442372801901854 ) ) ;
#199122=CARTESIAN_POINT ( 'NONE',  ( -5.049401038298153566, 19.05341960407611168, 30.20724293864768839 ) ) ;
#199124=CARTESIAN_POINT ( 'NONE',  ( 4.483927247898790824, -16.52544592524335698, 55.20942372801902565 ) ) ;
#199125=CARTESIAN_POINT ( 'NONE',  ( 21.55341960407610458, 5.719274019375980345, 98.95724293864770971 ) ) ;
#199126=CARTESIAN_POINT ( 'NONE',  ( 21.55341960407610458, 5.719274019375980345, 93.95724293864770971 ) ) ;
#199127=CARTESIAN_POINT ( 'NONE',  ( 19.03943276465977164, 0.05219959533936151252, 26.25109039468566507 ) ) ;
#199128=CARTESIAN_POINT ( 'NONE',  ( -5.049401038298153566, 19.05341960407611168, 55.20724293864769550 ) ) ;
#199129=CARTESIAN_POINT ( 'NONE',  ( 13.89961937509977652, -13.97604488694527269, 113.1239096053143527 ) ) ;
#199130=CARTESIAN_POINT ( 'NONE',  ( 18.62759615963255655, 10.81492255796105972, 51.66775706135234714 ) ) ;
#199131=CARTESIAN_POINT ( 'NONE',  ( -5.719274019375978568, 21.55341960407610458, 45.20724293864769550 ) ) ;
#199132=CARTESIAN_POINT ( 'NONE',  ( 12.14591786802327356, -12.06949235617739191, 110.6260903946857042 ) ) ;
#199133=CARTESIAN_POINT ( 'NONE',  ( -5.719274019375665041, -21.55341960407619695, 69.79275706135234714 ) ) ;
#199134=CARTESIAN_POINT ( 'NONE',  ( -21.52544592524334988, -5.823673210054445271, 93.95942372801903275 ) ) ;
#199135=CARTESIAN_POINT ( 'NONE',  ( 19.03943276465977164, 0.05219959533936151252, 51.25109039468567573 ) ) ;
#199136=CARTESIAN_POINT ( 'NONE',  ( -0.05219959533934338120, 16.53943276465976808, 107.5010903946856899 ) ) ;
#199137=CARTESIAN_POINT ( 'NONE',  ( 21.52544592524334988, 5.823673210054432836, 61.45942372801901854 ) ) ;
#199138=CARTESIAN_POINT ( 'NONE',  ( -19.05341960407611168, -5.049401038298163336, 46.45724293864768129 ) ) ;
#199139=CARTESIAN_POINT ( 'NONE',  ( 16.51473224551083163, -9.474510206698727899, 25.83442372801900078 ) ) ;
#199140=CARTESIAN_POINT ( 'NONE',  ( -0.05219959533907301413, -21.53943276465977519, 22.49890960531436335 ) ) ;
#199142=CARTESIAN_POINT ( 'NONE',  ( -15.72974639402176322, -15.80617190586768395, 19.37609039468568639 ) ) ;
#199143=CARTESIAN_POINT ( 'NONE',  ( -10.81492255796078084, -18.62759615963271287, 72.08224293864769550 ) ) ;
#199144=CARTESIAN_POINT ( 'NONE',  ( -12.14591786802326823, 12.06949235617739902, 43.12609039468568284 ) ) ;
#199146=CARTESIAN_POINT ( 'NONE',  ( 18.67979575497178502, 10.72451020669898547, 79.16557627198103830 ) ) ;
#199147=CARTESIAN_POINT ( 'NONE',  ( 8.224510206698742110, 14.34966873604972548, 67.08442372801901854 ) ) ;
#199148=CARTESIAN_POINT ( 'NONE',  ( -4.483927247898539470, -16.52544592524342804, 82.29057627198103830 ) ) ;
#199150=CARTESIAN_POINT ( 'NONE',  ( 9.474510206698729675, 16.51473224551082808, 102.0844237280190043 ) ) ;
#199151=CARTESIAN_POINT ( 'NONE',  ( 0.05219959533907565091, 21.53943276465977519, 34.99890960531435979 ) ) ;
#199153=CARTESIAN_POINT ( 'NONE',  ( -14.29746914071037622, -8.314922557961029526, 34.16775706135234714 ) ) ;
#199154=CARTESIAN_POINT ( 'NONE',  ( 5.823673210054444382, -21.52544592524334988, 20.20942372801900788 ) ) ;
#199155=CARTESIAN_POINT ( 'NONE',  ( 18.62759615963271287, -10.81492255796078972, 38.33224293864768839 ) ) ;
#199156=CARTESIAN_POINT ( 'NONE',  ( -4.379528057220086978, -16.55341960407618274, 69.79275706135234714 ) ) ;
#199157=CARTESIAN_POINT ( 'NONE',  ( 9.564922557960805705, 16.46253265017160317, 84.58224293864769550 ) ) ;
#199158=CARTESIAN_POINT ( 'NONE',  ( 10.72451020669871369, 18.67979575497193778, 42.08442372801901854 ) ) ;
#199159=CARTESIAN_POINT ( 'NONE',  ( -19.05341960407611168, -5.049401038298163336, 26.45724293864769550 ) ) ;
#199160=CARTESIAN_POINT ( 'NONE',  ( 15.72974639402199770, -15.80617190586745480, 28.12390960531435979 ) ) ;
#199162=CARTESIAN_POINT ( 'NONE',  ( 13.89961937509957401, 13.97604488694547697, 26.87609039468566507 ) ) ;
#199163=CARTESIAN_POINT ( 'NONE',  ( 16.53943276465976808, 0.05219959533934440121, 51.25109039468568994 ) ) ;
#199164=CARTESIAN_POINT ( 'NONE',  ( 19.03943276465977164, -0.05219959533909143690, 98.74890960531436690 ) ) ;
#199165=CARTESIAN_POINT ( 'NONE',  ( -15.80617190586745835, -15.72974639402198527, 96.87390960531436690 ) ) ;
#199166=CARTESIAN_POINT ( 'NONE',  ( -9.564922557960796823, -16.46253265017161027, 67.08224293864769550 ) ) ;
#199167=CARTESIAN_POINT ( 'NONE',  ( -17.49999999999999289, 5.624438216177593652, 25.81670344914644488 ) ) ;
#199169=CARTESIAN_POINT ( 'NONE',  ( 4.483927247898545687, 16.52544592524342804, 79.79057627198102409 ) ) ;
#199170=CARTESIAN_POINT ( 'NONE',  ( 21.55341960407610458, 5.719274019375980345, 33.95724293864769550 ) ) ;
#199171=CARTESIAN_POINT ( 'NONE',  ( -17.50000000000000000, 5.499999999999992895, 33.71769037696435589 ) ) ;
#199172=CARTESIAN_POINT ( 'NONE',  ( 12.14591786802327356, -12.06949235617739191, 65.62609039468568994 ) ) ;
#199173=CARTESIAN_POINT ( 'NONE',  ( -15.80617190586768217, 15.72974639402176855, 23.12609039468567573 ) ) ;
#199174=CARTESIAN_POINT ( 'NONE',  ( 9.474510206698729675, 16.51473224551082808, 72.08442372801900433 ) ) ;
#199175=CARTESIAN_POINT ( 'NONE',  ( -13.97604488694527625, -13.89961937509977652, 36.87390960531436690 ) ) ;
#199176=CARTESIAN_POINT ( 'NONE',  ( -18.62759615963270932, 10.81492255796079327, 65.83224293864769550 ) ) ;
#199178=CARTESIAN_POINT ( 'NONE',  ( -9.474510206698964154, 16.51473224551069663, 105.4155762719810383 ) ) ;
#199179=CARTESIAN_POINT ( 'NONE',  ( 18.67979575497194134, -10.72451020669871369, 90.83442372801901854 ) ) ;
#199180=CARTESIAN_POINT ( 'NONE',  ( 19.03943276465977164, -0.05219959533909143690, 68.74890960531436690 ) ) ;
#199181=CARTESIAN_POINT ( 'NONE',  ( -14.34966873604972548, 8.224510206698743886, 53.33442372801901854 ) ) ;
#199182=CARTESIAN_POINT ( 'NONE',  ( 9.564922557960805705, 16.46253265017160317, 59.58224293864769550 ) ) ;
#199183=CARTESIAN_POINT ( 'NONE',  ( -21.53943276465977519, -0.05219959533937600094, 73.75109039468567573 ) ) ;
#199184=CARTESIAN_POINT ( 'NONE',  ( -19.03943276465977164, -0.05219959533935918106, 43.75109039468566863 ) ) ;
#199185=CARTESIAN_POINT ( 'NONE',  ( 9.474510206698729675, 16.51473224551082808, 52.08442372801900433 ) ) ;
#199186=CARTESIAN_POINT ( 'NONE',  ( 18.62759615963255655, 10.81492255796105972, 51.66775706135234714 ) ) ;
#199188=CARTESIAN_POINT ( 'NONE',  ( -18.87255363501903105, -5.499999999999950262, 46.32513748171830059 ) ) ;
#199189=CARTESIAN_POINT ( 'NONE',  ( -9.474510206698720793, -16.51473224551083518, 49.58442372801899722 ) ) ;
#199190=CARTESIAN_POINT ( 'NONE',  ( -19.02544592524342804, 5.153800228976336051, 101.0405762719810241 ) ) ;
#199191=CARTESIAN_POINT ( 'NONE',  ( 19.03943276465977164, -0.05219959533909143690, 68.74890960531436690 ) ) ;
#199192=CARTESIAN_POINT ( 'NONE',  ( -14.34966873604972548, 8.224510206698743886, 113.3344237280190328 ) ) ;
#199193=CARTESIAN_POINT ( 'NONE',  ( 15.72974639402199770, -15.80617190586745480, 38.12390960531436690 ) ) ;
#199194=CARTESIAN_POINT ( 'NONE',  ( -21.55341960407619339, 5.719274019375674811, 98.54275706135234714 ) ) ;
#199196=CARTESIAN_POINT ( 'NONE',  ( 16.81555441253551564, 7.025013491695498935, 56.86314554665743515 ) ) ;
#199197=CARTESIAN_POINT ( 'NONE',  ( -10.81492255796105439, 18.62759615963255655, 97.91775706135236135 ) ) ;
#199199=CARTESIAN_POINT ( 'NONE',  ( -5.153800228976328057, -19.02544592524343514, 27.29057627198103120 ) ) ;
#199200=CARTESIAN_POINT ( 'NONE',  ( 16.46253265017160672, -9.564922557960803928, 108.3322429386476955 ) ) ;
#199201=B_SPLINE_CURVE_WITH_KNOTS ( 'NONE', 3,
 ( #34637, #113451, #80138, #188334, #50809, #47839 ),
 .UNSPECIFIED., .F., .F.,
 ( 4, 2, 4 ),
 ( 0.003239945802372238247, 0.003620412082092087404, 0.004000878361811936561 ),
 .UNSPECIFIED. ) ;
#199203=CARTESIAN_POINT ( 'NONE',  ( 16.53943276465976808, 0.05219959533934440121, 51.25109039468568994 ) ) ;
#199204=CARTESIAN_POINT ( 'NONE',  ( 15.80617190586746368, 15.72974639402197994, 74.37390960531436690 ) ) ;
#199205=CARTESIAN_POINT ( 'NONE',  ( -16.52544592524342804, 4.483927247898546575, 41.04057627198103120 ) ) ;
#199206=CARTESIAN_POINT ( 'NONE',  ( 16.52544592524342804, -4.483927247898539470, 108.5405762719810241 ) ) ;
#199207=CARTESIAN_POINT ( 'NONE',  ( -9.564922557960796823, -16.46253265017161027, 112.0822429386476955 ) ) ;
#199208=CARTESIAN_POINT ( 'NONE',  ( 16.51473224551083163, -9.474510206698727899, 35.83442372801899722 ) ) ;
#199209=CARTESIAN_POINT ( 'NONE',  ( -9.474510206698964154, 16.51473224551069663, 25.41557627198103120 ) ) ;
#199210=CARTESIAN_POINT ( 'NONE',  ( -5.823673210054431948, 21.52544592524334988, 67.70942372801901854 ) ) ;
#199211=CARTESIAN_POINT ( 'NONE',  ( -18.22780087662122384, -5.500000000000025757, 96.48459894673894155 ) ) ;
#199212=CARTESIAN_POINT ( 'NONE',  ( 12.14591786802309770, 12.06949235617756955, 29.37390960531435269 ) ) ;
#199214=CARTESIAN_POINT ( 'NONE',  ( 10.72451020669898902, -18.67979575497178502, 27.91557627198103830 ) ) ;
#199215=CARTESIAN_POINT ( 'NONE',  ( 16.52544592524342804, -4.483927247898539470, 83.54057627198102409 ) ) ;
#199218=CARTESIAN_POINT ( 'NONE',  ( 19.03943276465977164, -0.05219959533909143690, 73.74890960531435269 ) ) ;
#199219=CARTESIAN_POINT ( 'NONE',  ( 12.14591786802309770, 12.06949235617756955, 69.37390960531436690 ) ) ;
#199220=CARTESIAN_POINT ( 'NONE',  ( 16.46253265017146816, 9.564922557961045513, 91.66775706135234714 ) ) ;
#199221=CARTESIAN_POINT ( 'NONE',  ( -5.823673210054116645, -21.52544592524344225, 47.29057627198103120 ) ) ;
#199223=CARTESIAN_POINT ( 'NONE',  ( -4.379528057220328563, 16.55341960407611168, 115.2072429386476955 ) ) ;
#199224=EDGE_CURVE ( 'NONE', #154217, #178458, #63849, .T. ) ;
#199225=CARTESIAN_POINT ( 'NONE',  ( 16.46253265017160672, -9.564922557960803928, 68.33224293864770971 ) ) ;
#199226=CARTESIAN_POINT ( 'NONE',  ( -18.67979575497178146, -10.72451020669898902, 76.66557627198103830 ) ) ;
#199227=CARTESIAN_POINT ( 'NONE',  ( -8.314922557961024197, 14.29746914071037800, 102.9177570613523756 ) ) ;
#199228=CARTESIAN_POINT ( 'NONE',  ( -13.89961937509977652, 13.97604488694528158, 90.62390960531432427 ) ) ;
#199229=CARTESIAN_POINT ( 'NONE',  ( -9.474510206698720793, -16.51473224551083518, 64.58442372801900433 ) ) ;
#199230=CARTESIAN_POINT ( 'NONE',  ( 21.52544592524334988, 5.823673210054432836, 86.45942372801901854 ) ) ;
#199231=CARTESIAN_POINT ( 'NONE',  ( -5.719274019375978568, 21.55341960407610458, 60.20724293864768839 ) ) ;
#199232=CARTESIAN_POINT ( 'NONE',  ( -21.52544592524343514, 5.823673210054127303, 26.04057627198103475 ) ) ;
#199233=CARTESIAN_POINT ( 'NONE',  ( -5.049401038298153566, 19.05341960407611168, 40.20724293864768839 ) ) ;
#199234=CARTESIAN_POINT ( 'NONE',  ( 12.14591786802327356, -12.06949235617739191, 95.62609039468568994 ) ) ;
#199235=CARTESIAN_POINT ( 'NONE',  ( 13.89961937509977652, -13.97604488694527269, 58.12390960531436690 ) ) ;
#199236=CARTESIAN_POINT ( 'NONE',  ( -14.29746914071037622, -8.314922557961029526, 19.16775706135234714 ) ) ;
#199237=CARTESIAN_POINT ( 'NONE',  ( 16.21995358207306026, 7.366697692864119240, 52.56448998487845614 ) ) ;
#199238=CARTESIAN_POINT ( 'NONE',  ( -5.049401038297874678, -19.05341960407617918, 19.79275706135233293 ) ) ;
#199239=CARTESIAN_POINT ( 'NONE',  ( 16.52544592524342804, -4.483927247898539470, 68.54057627198103830 ) ) ;
#199240=CARTESIAN_POINT ( 'NONE',  ( -18.67979575497178146, -10.72451020669898902, 106.6655762719810383 ) ) ;
#199241=CARTESIAN_POINT ( 'NONE',  ( -5.719274019375978568, 21.55341960407610458, 100.2072429386476955 ) ) ;
#199243=CARTESIAN_POINT ( 'NONE',  ( 15.72974639402199770, -15.80617190586745480, 48.12390960531436690 ) ) ;
#199244=CARTESIAN_POINT ( 'NONE',  ( 0.05219959533934541429, -16.53943276465976808, 85.00109039468568994 ) ) ;
#199245=CARTESIAN_POINT ( 'NONE',  ( 14.34966873604960469, 8.224510206698951720, 99.16557627198100988 ) ) ;
#199246=CARTESIAN_POINT ( 'NONE',  ( -13.89961937509977652, 13.97604488694528158, 60.62390960531436690 ) ) ;
#199249=CARTESIAN_POINT ( 'NONE',  ( -16.55341960407617563, 4.379528057220093196, 113.5427570613523756 ) ) ;
#199250=CARTESIAN_POINT ( 'NONE',  ( 21.53943276465977519, 0.05219959533937863772, 41.25109039468568284 ) ) ;
#199251=CARTESIAN_POINT ( 'NONE',  ( 19.02544592524343514, -5.153800228976328945, 93.54057627198102409 ) ) ;
#199252=CARTESIAN_POINT ( 'NONE',  ( -15.80617190586768217, 15.72974639402176855, 83.12609039468568994 ) ) ;
#199253=CARTESIAN_POINT ( 'NONE',  ( -9.564922557960796823, -16.46253265017161027, 27.08224293864769550 ) ) ;
#199254=CARTESIAN_POINT ( 'NONE',  ( -16.51473224551069308, -9.474510206698971260, 31.66557627198102054 ) ) ;
#199255=VERTEX_POINT ( 'NONE', #104978 ) ;
#199256=CARTESIAN_POINT ( 'NONE',  ( 5.823673210054444382, -21.52544592524334988, 70.20942372801904696 ) ) ;
#199257=CARTESIAN_POINT ( 'NONE',  ( 5.153800228976335163, 19.02544592524342804, 54.79057627198103120 ) ) ;
#199258=CARTESIAN_POINT ( 'NONE',  ( -5.049401038298153566, 19.05341960407611168, 100.2072429386476955 ) ) ;
#199259=CARTESIAN_POINT ( 'NONE',  ( 19.03943276465977164, 0.05219959533936151252, 86.25109039468567573 ) ) ;
#199260=CARTESIAN_POINT ( 'NONE',  ( -10.81492255796105439, 18.62759615963255655, 42.91775706135235424 ) ) ;
#199261=CARTESIAN_POINT ( 'NONE',  ( 8.314922557961029526, -14.29746914071037800, 20.41775706135234714 ) ) ;
#199262=CARTESIAN_POINT ( 'NONE',  ( 19.03943276465977164, 0.05219959533936151252, 66.25109039468567573 ) ) ;
#199263=CARTESIAN_POINT ( 'NONE',  ( -5.049401038298153566, 19.05341960407611168, 35.20724293864768839 ) ) ;
#199264=CARTESIAN_POINT ( 'NONE',  ( -5.049401038297874678, -19.05341960407617918, 84.79275706135233293 ) ) ;
#199265=CARTESIAN_POINT ( 'NONE',  ( 16.52544592524335698, 4.483927247898782831, 101.4594237280190185 ) ) ;
#199266=CARTESIAN_POINT ( 'NONE',  ( -19.02544592524334988, -5.153800228976617603, 73.95942372801900433 ) ) ;
#199267=CARTESIAN_POINT ( 'NONE',  ( 8.224510206698953496, -14.34966873604960469, 32.91557627198102409 ) ) ;
#199268=CARTESIAN_POINT ( 'NONE',  ( -13.89961937509957401, -13.97604488694547875, 69.37609039468564731 ) ) ;
#199269=CARTESIAN_POINT ( 'NONE',  ( 21.53943276465977519, 0.05219959533937863772, 106.2510903946856757 ) ) ;
#199270=CARTESIAN_POINT ( 'NONE',  ( -9.474510206698720793, -16.51473224551083518, 29.58442372801900433 ) ) ;
#199271=CARTESIAN_POINT ( 'NONE',  ( -16.51473224551069308, -9.474510206698971260, 26.66557627198103120 ) ) ;
#199272=CARTESIAN_POINT ( 'NONE',  ( -16.31925111598458145, -7.325300261831487525, 64.83575461032752685 ) ) ;
#199273=CARTESIAN_POINT ( 'NONE',  ( 16.53943276465976808, 0.05219959533934440121, 46.25109039468567573 ) ) ;
#199277=CARTESIAN_POINT ( 'NONE',  ( 19.05341960407611168, 5.049401038298154454, 98.95724293864766707 ) ) ;
#199278=CARTESIAN_POINT ( 'NONE',  ( -17.49999999999999645, 5.624438216177557237, 100.8167034491464307 ) ) ;
#199280=CARTESIAN_POINT ( 'NONE',  ( 0.05219959533936267826, -19.03943276465977164, 85.00109039468567573 ) ) ;
#199281=CARTESIAN_POINT ( 'NONE',  ( 19.02544592524343514, -5.153800228976328945, 113.5405762719810241 ) ) ;
#199282=CARTESIAN_POINT ( 'NONE',  ( 13.89961937509957401, 13.97604488694547697, 21.87609039468566152 ) ) ;
#199283=CARTESIAN_POINT ( 'NONE',  ( 16.46253265017146816, 9.564922557961045513, 96.66775706135233293 ) ) ;
#199284=CARTESIAN_POINT ( 'NONE',  ( -16.55341960407611168, -4.379528057220339221, 106.4572429386477097 ) ) ;
#199285=CARTESIAN_POINT ( 'NONE',  ( 16.51473224551069308, 9.474510206698969483, 29.16557627198103475 ) ) ;
#199286=CARTESIAN_POINT ( 'NONE',  ( -21.52544592524343514, 5.823673210054127303, 66.04057627198103830 ) ) ;
#199287=CARTESIAN_POINT ( 'NONE',  ( 21.55341960407610458, 5.719274019375980345, 53.95724293864770260 ) ) ;
#199288=CARTESIAN_POINT ( 'NONE',  ( 5.049401038298161559, -19.05341960407611168, 27.70724293864769550 ) ) ;
#199289=CARTESIAN_POINT ( 'NONE',  ( 30.00000000000000000, -5.510910596163089556E-15, 45.00000000000000000 ) ) ;
#199290=CARTESIAN_POINT ( 'NONE',  ( -13.97604488694547697, 13.89961937509957934, 73.12609039468568994 ) ) ;
#199291=CARTESIAN_POINT ( 'NONE',  ( 14.34966873604960469, 8.224510206698951720, 34.16557627198102409 ) ) ;
#199292=CARTESIAN_POINT ( 'NONE',  ( 19.05341960407611168, 5.049401038298154454, 113.9572429386477097 ) ) ;
#199294=CARTESIAN_POINT ( 'NONE',  ( -0.05219959533937732626, 21.53943276465977519, 97.50109039468567573 ) ) ;
#199295=CARTESIAN_POINT ( 'NONE',  ( -21.55341960407610458, -5.719274019375992779, 66.45724293864768129 ) ) ;
#199296=CARTESIAN_POINT ( 'NONE',  ( -21.55341960407619339, 5.719274019375674811, 53.54275706135234714 ) ) ;
#199297=CARTESIAN_POINT ( 'NONE',  ( 5.719274019375673035, 21.55341960407619339, 52.29275706135236135 ) ) ;
#199298=CARTESIAN_POINT ( 'NONE',  ( -0.05219959533909027116, -19.03943276465977164, 97.49890960531436690 ) ) ;
#199299=CARTESIAN_POINT ( 'NONE',  ( -16.52544592524335698, -4.483927247898792601, 98.95942372801903275 ) ) ;
#199300=CARTESIAN_POINT ( 'NONE',  ( -10.72451020669870658, -18.67979575497194134, 49.58442372801901143 ) ) ;
#199301=CARTESIAN_POINT ( 'NONE',  ( 0.05219959533909260263, 19.03943276465977164, 24.99890960531435269 ) ) ;
#199303=CARTESIAN_POINT ( 'NONE',  ( 16.53943276465976808, -0.05219959533910856209, 68.74890960531435269 ) ) ;
#199304=CARTESIAN_POINT ( 'NONE',  ( 0.05219959533910956823, 16.53943276465976808, 29.99890960531435979 ) ) ;
#199305=CARTESIAN_POINT ( 'NONE',  ( 19.05341960407611168, 5.049401038298154454, 68.95724293864769550 ) ) ;
#199306=CARTESIAN_POINT ( 'NONE',  ( -9.564922557960796823, -16.46253265017161027, 52.08224293864768839 ) ) ;
#199307=CARTESIAN_POINT ( 'NONE',  ( -15.72974639402197994, 15.80617190586746368, 60.62390960531437401 ) ) ;
#199308=CARTESIAN_POINT ( 'NONE',  ( -13.89961937509957401, -13.97604488694547875, 44.37609039468566863 ) ) ;
#199309=CIRCLE ( 'NONE', #112125, 2.000000000000000000 ) ;
#199311=CARTESIAN_POINT ( 'NONE',  ( -16.52544592524342804, 4.483927247898546575, 46.04057627198103830 ) ) ;
#199312=CARTESIAN_POINT ( 'NONE',  ( -0.05219959533907301413, -21.53943276465977519, 22.49890960531436335 ) ) ;
#199315=CARTESIAN_POINT ( 'NONE',  ( 14.34966873604972726, -8.224510206698740333, 65.83442372801900433 ) ) ;
#199316=CARTESIAN_POINT ( 'NONE',  ( 5.049401038297881783, 19.05341960407617563, 72.29275706135234714 ) ) ;
#199317=EDGE_CURVE ( 'NONE', #59885, #163091, #23708, .T. ) ;
#199318=CARTESIAN_POINT ( 'NONE',  ( 4.483927247898545687, 16.52544592524342804, 44.79057627198103120 ) ) ;
#199321=CARTESIAN_POINT ( 'NONE',  ( -14.34966873604972548, 8.224510206698743886, 113.3344237280190328 ) ) ;
#199322=CARTESIAN_POINT ( 'NONE',  ( -5.153800228976328057, -19.02544592524343514, 52.29057627198100988 ) ) ;
#199323=CARTESIAN_POINT ( 'NONE',  ( 19.03943276465977164, -0.05219959533909143690, 73.74890960531435269 ) ) ;
#199324=CARTESIAN_POINT ( 'NONE',  ( 19.03943276465977164, -0.05219959533909143690, 43.74890960531435979 ) ) ;
#199325=CARTESIAN_POINT ( 'NONE',  ( -21.52544592524334988, -5.823673210054445271, 43.95942372801902565 ) ) ;
#199326=CARTESIAN_POINT ( 'NONE',  ( -19.05341960407611168, -5.049401038298163336, 56.45724293864768129 ) ) ;
#199328=CARTESIAN_POINT ( 'NONE',  ( 13.89961937509977652, -13.97604488694527269, 53.12390960531434558 ) ) ;
#199329=CARTESIAN_POINT ( 'NONE',  ( 18.67979575497178502, 10.72451020669898547, 34.16557627198102409 ) ) ;
#199330=CARTESIAN_POINT ( 'NONE',  ( 5.049401038298161559, -19.05341960407611168, 22.70724293864769194 ) ) ;
#199331=CARTESIAN_POINT ( 'NONE',  ( -10.72451020669898014, 18.67979575497178502, 30.41557627198101699 ) ) ;
#199332=CARTESIAN_POINT ( 'NONE',  ( 0.05219959533934541429, -16.53943276465976808, 85.00109039468568994 ) ) ;
#199333=CARTESIAN_POINT ( 'NONE',  ( -21.53943276465977519, -0.05219959533937600094, 108.7510903946857042 ) ) ;
#199334=CARTESIAN_POINT ( 'NONE',  ( 14.29746914071037800, 8.314922557961029526, 66.66775706135234714 ) ) ;
#199335=CARTESIAN_POINT ( 'NONE',  ( -19.02544592524342804, 5.153800228976336051, 111.0405762719810099 ) ) ;
#199336=CARTESIAN_POINT ( 'NONE',  ( -16.52544592524335698, -4.483927247898792601, 53.95942372801900433 ) ) ;
#199337=CARTESIAN_POINT ( 'NONE',  ( -4.483927247898782831, 16.52544592524335698, 42.70942372801901854 ) ) ;
#199338=CARTESIAN_POINT ( 'NONE',  ( -9.564922557960796823, -16.46253265017161027, 107.0822429386476955 ) ) ;
#199339=CARTESIAN_POINT ( 'NONE',  ( 16.55341960407618274, -4.379528057220086978, 31.04275706135234714 ) ) ;
#199340=CARTESIAN_POINT ( 'NONE',  ( 5.049401038298161559, -19.05341960407611168, 37.70724293864768839 ) ) ;
#199341=CARTESIAN_POINT ( 'NONE',  ( -10.72451020669870658, -18.67979575497194134, 19.58442372801901143 ) ) ;
#199342=CARTESIAN_POINT ( 'NONE',  ( -19.05341960407617563, 5.049401038297882671, 113.5427570613523471 ) ) ;
#199343=CARTESIAN_POINT ( 'NONE',  ( -8.314922557961024197, 14.29746914071037800, 82.91775706135234714 ) ) ;
#199344=CARTESIAN_POINT ( 'NONE',  ( -17.26172910966715435, 6.454744622556958689, 45.80646908649209337 ) ) ;
#199345=CARTESIAN_POINT ( 'NONE',  ( 5.823673210054444382, -21.52544592524334988, 85.20942372801901854 ) ) ;
#199346=CARTESIAN_POINT ( 'NONE',  ( 9.474510206698729675, 16.51473224551082808, 87.08442372801900433 ) ) ;
#199347=CARTESIAN_POINT ( 'NONE',  ( 16.52544592524342804, -4.483927247898539470, 48.54057627198103120 ) ) ;
#199348=CARTESIAN_POINT ( 'NONE',  ( 12.06949235617757843, -12.14591786802309237, 103.1239096053143811 ) ) ;
#199349=CARTESIAN_POINT ( 'NONE',  ( -9.474510206698720793, -16.51473224551083518, 44.58442372801900433 ) ) ;
#199351=CARTESIAN_POINT ( 'NONE',  ( 10.72451020669871369, 18.67979575497193778, 57.08442372801901854 ) ) ;
#199352=CARTESIAN_POINT ( 'NONE',  ( 19.05341960407617918, -5.049401038297876454, 106.0427570613523471 ) ) ;
#199353=CARTESIAN_POINT ( 'NONE',  ( 17.40805194822030444, 6.112264579159360167, 81.66628727489390371 ) ) ;
#199354=CARTESIAN_POINT ( 'NONE',  ( 0.05219959533909260263, 19.03943276465977164, 99.99890960531436690 ) ) ;
#199355=CARTESIAN_POINT ( 'NONE',  ( -10.81492255796078084, -18.62759615963271287, 77.08224293864769550 ) ) ;
#199356=CARTESIAN_POINT ( 'NONE',  ( -9.564922557961040184, 16.46253265017147172, 97.91775706135233293 ) ) ;
#199357=CARTESIAN_POINT ( 'NONE',  ( -13.97604488694527625, -13.89961937509977652, 101.8739096053143811 ) ) ;
#199359=CARTESIAN_POINT ( 'NONE',  ( -12.06949235617756955, 12.14591786802309770, 100.6239096053143811 ) ) ;
#199360=CARTESIAN_POINT ( 'NONE',  ( 5.823673210054444382, -21.52544592524334988, 100.2094237280190043 ) ) ;
#199361=CARTESIAN_POINT ( 'NONE',  ( 0.05219959533909260263, 19.03943276465977164, 39.99890960531436690 ) ) ;
#199363=CARTESIAN_POINT ( 'NONE',  ( -10.72451020669870658, -18.67979575497194134, 49.58442372801901143 ) ) ;
#199364=CARTESIAN_POINT ( 'NONE',  ( 10.81492255796106328, -18.62759615963255655, 95.41775706135234714 ) ) ;
#199365=CARTESIAN_POINT ( 'NONE',  ( -4.379528057220086978, -16.55341960407618274, 84.79275706135234714 ) ) ;
#199366=CARTESIAN_POINT ( 'NONE',  ( -18.62759615963255300, -10.81492255796106328, 39.16775706135235424 ) ) ;
#199367=CARTESIAN_POINT ( 'NONE',  ( -15.80617190586768217, 15.72974639402176855, 38.12609039468567573 ) ) ;
#199368=CARTESIAN_POINT ( 'NONE',  ( 16.46253265017146816, 9.564922557961045513, 61.66775706135234003 ) ) ;
#199369=CARTESIAN_POINT ( 'NONE',  ( -16.46253265017160317, 9.564922557960807481, 90.83224293864769550 ) ) ;
#199370=CARTESIAN_POINT ( 'NONE',  ( 4.379528057220339221, -16.55341960407611168, 102.7072429386476955 ) ) ;
#199371=CARTESIAN_POINT ( 'NONE',  ( -15.72974639402197994, 15.80617190586746368, 80.62390960531438111 ) ) ;
#199372=CARTESIAN_POINT ( 'NONE',  ( -4.483927247898539470, -16.52544592524342804, 62.29057627198102409 ) ) ;
#199373=CARTESIAN_POINT ( 'NONE',  ( -21.53943276465977519, -0.05219959533937600094, 103.7510903946857042 ) ) ;
#199374=CARTESIAN_POINT ( 'NONE',  ( -14.34966873604960291, -8.224510206698953496, 86.66557627198102409 ) ) ;
#199375=CARTESIAN_POINT ( 'NONE',  ( -19.03943276465977164, 0.05219959533909376836, 36.24890960531436690 ) ) ;
#199376=CARTESIAN_POINT ( 'NONE',  ( 9.474510206698729675, 16.51473224551082808, 87.08442372801900433 ) ) ;
#199377=CARTESIAN_POINT ( 'NONE',  ( -16.55341960407611168, -4.379528057220339221, 51.45724293864770260 ) ) ;
#199378=CARTESIAN_POINT ( 'NONE',  ( 21.52544592524334988, 5.823673210054432836, 101.4594237280190185 ) ) ;
#199379=CARTESIAN_POINT ( 'NONE',  ( -9.474510206698964154, 16.51473224551069663, 85.41557627198102409 ) ) ;
#199380=CARTESIAN_POINT ( 'NONE',  ( -19.02544592524334988, -5.153800228976617603, 58.95942372801900433 ) ) ;
#199381=CARTESIAN_POINT ( 'NONE',  ( 10.81492255796078972, 18.62759615963270932, 59.58224293864770260 ) ) ;
#199382=CARTESIAN_POINT ( 'NONE',  ( 18.62759615963255655, 10.81492255796105972, 36.66775706135234714 ) ) ;
#199383=CARTESIAN_POINT ( 'NONE',  ( 14.29746914071037800, 8.314922557961029526, 26.66775706135235424 ) ) ;
#199384=CARTESIAN_POINT ( 'NONE',  ( 16.53943276465976808, 0.05219959533934440121, 86.25109039468568994 ) ) ;
#199385=CARTESIAN_POINT ( 'NONE',  ( -9.564922557960796823, -16.46253265017161027, 27.08224293864769550 ) ) ;
#199386=CARTESIAN_POINT ( 'NONE',  ( 5.823673210054125526, 21.52544592524343514, 114.7905762719810383 ) ) ;
#199387=CARTESIAN_POINT ( 'NONE',  ( 8.314922557960818139, 14.29746914071049879, 114.5822429386477097 ) ) ;
#199389=CARTESIAN_POINT ( 'NONE',  ( 16.53943276465976808, 0.05219959533934440121, 51.25109039468568994 ) ) ;
#199390=CARTESIAN_POINT ( 'NONE',  ( -12.14591786802309592, -12.06949235617757132, 76.87390960531439532 ) ) ;
#199391=CARTESIAN_POINT ( 'NONE',  ( 10.81492255796078972, 18.62759615963270932, 74.58224293864768129 ) ) ;
#199392=CARTESIAN_POINT ( 'NONE',  ( -12.06949235617756955, 12.14591786802309770, 25.62390960531435624 ) ) ;
#199393=CARTESIAN_POINT ( 'NONE',  ( 12.14591786802327356, -12.06949235617739191, 35.62609039468568994 ) ) ;
#199394=CARTESIAN_POINT ( 'NONE',  ( -9.564922557960796823, -16.46253265017161027, 42.08224293864769550 ) ) ;
#199395=CARTESIAN_POINT ( 'NONE',  ( 14.29746914071037800, 8.314922557961029526, 76.66775706135234714 ) ) ;
#199396=CARTESIAN_POINT ( 'NONE',  ( 19.03943276465977164, 0.05219959533936151252, 71.25109039468566152 ) ) ;
#199397=CARTESIAN_POINT ( 'NONE',  ( -15.80617190586745835, -15.72974639402198527, 76.87390960531439532 ) ) ;
#199398=CARTESIAN_POINT ( 'NONE',  ( 8.224510206698953496, -14.34966873604960469, 22.91557627198102765 ) ) ;
#199399=ORIENTED_EDGE ( 'NONE', *, *, #192729, .F. ) ;
#199401=CARTESIAN_POINT ( 'NONE',  ( 15.80617190586746368, 15.72974639402197994, 54.37390960531435979 ) ) ;
#199402=ORIENTED_EDGE ( 'NONE', *, *, #59756, .T. ) ;
#199404=CARTESIAN_POINT ( 'NONE',  ( 14.34966873604972726, -8.224510206698740333, 95.83442372801903275 ) ) ;
#199406=CARTESIAN_POINT ( 'NONE',  ( 13.89961937509977652, -13.97604488694527269, 113.1239096053143527 ) ) ;
#199408=CARTESIAN_POINT ( 'NONE',  ( 15.80617190586746368, 15.72974639402197994, 74.37390960531436690 ) ) ;
#199409=CARTESIAN_POINT ( 'NONE',  ( 12.14591786802327356, -12.06949235617739191, 105.6260903946856899 ) ) ;
#199410=CARTESIAN_POINT ( 'NONE',  ( 10.81492255796106328, -18.62759615963255655, 60.41775706135235424 ) ) ;
#199411=CARTESIAN_POINT ( 'NONE',  ( -0.05219959533934338120, 16.53943276465976808, 22.50109039468567573 ) ) ;
#199412=CARTESIAN_POINT ( 'NONE',  ( -8.224510206698948167, 14.34966873604960824, 110.4155762719810383 ) ) ;
#199413=CARTESIAN_POINT ( 'NONE',  ( -8.314922557961024197, 14.29746914071037800, 22.91775706135235069 ) ) ;
#199414=CARTESIAN_POINT ( 'NONE',  ( 19.02544592524343514, -5.153800228976328945, 53.54057627198102409 ) ) ;
#199416=CARTESIAN_POINT ( 'NONE',  ( -9.564922557960796823, -16.46253265017161027, 107.0822429386476955 ) ) ;
#199417=CARTESIAN_POINT ( 'NONE',  ( -4.379528057220086978, -16.55341960407618274, 94.79275706135234714 ) ) ;
#199418=CARTESIAN_POINT ( 'NONE',  ( -5.049401038297874678, -19.05341960407617918, 94.79275706135230450 ) ) ;
#199419=CARTESIAN_POINT ( 'NONE',  ( -13.89961937509957401, -13.97604488694547875, 29.37609039468565797 ) ) ;
#199420=CARTESIAN_POINT ( 'NONE',  ( 21.55341960407610458, 5.719274019375980345, 68.95724293864769550 ) ) ;
#199421=CARTESIAN_POINT ( 'NONE',  ( 14.34966873604972726, -8.224510206698740333, 100.8344237280190185 ) ) ;
#199422=CARTESIAN_POINT ( 'NONE',  ( 19.05341960407617918, -5.049401038297876454, 96.04275706135231871 ) ) ;
#199423=CARTESIAN_POINT ( 'NONE',  ( 9.474510206698971260, -16.51473224551069308, 52.91557627198102409 ) ) ;
#199424=CARTESIAN_POINT ( 'NONE',  ( -9.564922557960796823, -16.46253265017161027, 92.08224293864769550 ) ) ;
#199425=CARTESIAN_POINT ( 'NONE',  ( 10.81492255796106328, -18.62759615963255655, 55.41775706135234714 ) ) ;
#199426=CARTESIAN_POINT ( 'NONE',  ( 13.89961937509977652, -13.97604488694527269, 48.12390960531435979 ) ) ;
#199427=CARTESIAN_POINT ( 'NONE',  ( -17.26058549869093994, -6.457015423128474652, 86.37745837476066413 ) ) ;
#199428=CARTESIAN_POINT ( 'NONE',  ( -16.53943276465976808, 0.05219959533911058130, 71.24890960531435269 ) ) ;
#199429=CARTESIAN_POINT ( 'NONE',  ( -21.53943276465977519, 0.05219959533907696930, 71.24890960531435269 ) ) ;
#199431=CARTESIAN_POINT ( 'NONE',  ( 13.89961937509957401, 13.97604488694547697, 36.87609039468565442 ) ) ;
#199433=CARTESIAN_POINT ( 'NONE',  ( -0.05219959533909027116, -19.03943276465977164, 82.49890960531436690 ) ) ;
#199434=CARTESIAN_POINT ( 'NONE',  ( -9.564922557960796823, -16.46253265017161027, 87.08224293864769550 ) ) ;
#199435=CARTESIAN_POINT ( 'NONE',  ( 14.29746914071037800, 8.314922557961029526, 46.66775706135234714 ) ) ;
#199436=CARTESIAN_POINT ( 'NONE',  ( -13.89961937509957401, -13.97604488694547697, 79.37609039468567573 ) ) ;
#199437=CARTESIAN_POINT ( 'NONE',  ( 16.51473224551083163, -9.474510206698727899, 35.83442372801899722 ) ) ;
#199439=CARTESIAN_POINT ( 'NONE',  ( 16.52544592524335698, 4.483927247898782831, 91.45942372801901854 ) ) ;
#199441=CARTESIAN_POINT ( 'NONE',  ( 14.34966873604972726, -8.224510206698740333, 80.83442372801901854 ) ) ;
#199442=CARTESIAN_POINT ( 'NONE',  ( -16.52544592524335698, -4.483927247898792601, 58.95942372801902565 ) ) ;
#199443=CARTESIAN_POINT ( 'NONE',  ( -19.03943276465977164, 0.05219959533909376836, 51.24890960531436690 ) ) ;
#199444=CARTESIAN_POINT ( 'NONE',  ( -17.58332526062529411, 7.635886036038502134, 75.92334959558466778 ) ) ;
#199445=CARTESIAN_POINT ( 'NONE',  ( 15.72974639402176855, 15.80617190586768217, 61.87609039468568284 ) ) ;
#199446=CARTESIAN_POINT ( 'NONE',  ( -19.05341960407617563, 5.049401038297882671, 73.54275706135233293 ) ) ;
#199447=CARTESIAN_POINT ( 'NONE',  ( 21.53943276465977519, 0.05219959533937863772, 111.2510903946856899 ) ) ;
#199448=CARTESIAN_POINT ( 'NONE',  ( 9.564922557960805705, 16.46253265017160317, 49.58224293864770260 ) ) ;
#199449=CARTESIAN_POINT ( 'NONE',  ( -19.03943276465977164, 0.05219959533909376836, 46.24890960531435979 ) ) ;
#199450=CARTESIAN_POINT ( 'NONE',  ( 16.38539452495360393, 7.295416311890092764, 23.44248723764945552 ) ) ;
#199451=CARTESIAN_POINT ( 'NONE',  ( -5.719274019375978568, 21.55341960407610458, 70.20724293864769550 ) ) ;
#199453=CARTESIAN_POINT ( 'NONE',  ( 15.72974639402199770, -15.80617190586745480, 23.12390960531436335 ) ) ;
#199454=CARTESIAN_POINT ( 'NONE',  ( -19.05341960407611168, -5.049401038298163336, 26.45724293864769550 ) ) ;
#199455=CARTESIAN_POINT ( 'NONE',  ( -8.224510206698735004, -14.34966873604973081, 44.58442372801901854 ) ) ;
#199456=CARTESIAN_POINT ( 'NONE',  ( 4.379528057220339221, -16.55341960407611168, 32.70724293864770260 ) ) ;
#199459=CARTESIAN_POINT ( 'NONE',  ( -15.80617190586768217, 15.72974639402176855, 23.12609039468567573 ) ) ;
#199460=CARTESIAN_POINT ( 'NONE',  ( 4.379528057220339221, -16.55341960407611168, 52.70724293864769550 ) ) ;
#199462=CARTESIAN_POINT ( 'NONE',  ( -19.05341960407617563, 5.049401038297882671, 103.5427570613523329 ) ) ;
#199463=CARTESIAN_POINT ( 'NONE',  ( -13.89961937509957401, -13.97604488694547875, 44.37609039468566863 ) ) ;
#199464=CARTESIAN_POINT ( 'NONE',  ( 12.06949235617757843, -12.14591786802309237, 38.12390960531436690 ) ) ;
#199465=CARTESIAN_POINT ( 'NONE',  ( -5.823673210054116645, -21.52544592524344225, 102.2905762719810383 ) ) ;
#199467=CARTESIAN_POINT ( 'NONE',  ( 21.55341960407610458, 5.719274019375980345, 68.95724293864769550 ) ) ;
#199468=CARTESIAN_POINT ( 'NONE',  ( 5.049401038298161559, -19.05341960407611168, 72.70724293864768129 ) ) ;
#199469=CARTESIAN_POINT ( 'NONE',  ( 8.224510206698953496, -14.34966873604960469, 47.91557627198102409 ) ) ;
#199470=CARTESIAN_POINT ( 'NONE',  ( -13.89961937509977652, 13.97604488694528158, 100.6239096053143669 ) ) ;
#199471=CARTESIAN_POINT ( 'NONE',  ( -17.50000000000002842, -5.499999999999952927, 76.28230962303568674 ) ) ;
#199472=CARTESIAN_POINT ( 'NONE',  ( -13.89961937509957401, -13.97604488694547875, 54.37609039468565442 ) ) ;
#199473=CARTESIAN_POINT ( 'NONE',  ( -5.823673210054116645, -21.52544592524344225, 92.29057627198103830 ) ) ;
#199474=CARTESIAN_POINT ( 'NONE',  ( -13.97604488694527625, -13.89961937509977652, 36.87390960531436690 ) ) ;
#199475=CARTESIAN_POINT ( 'NONE',  ( 16.46253265017160672, -9.564922557960803928, 23.33224293864769194 ) ) ;
#199476=CARTESIAN_POINT ( 'NONE',  ( -21.52544592524334988, -5.823673210054445271, 48.95942372801902565 ) ) ;
#199479=CARTESIAN_POINT ( 'NONE',  ( 4.483927247898545687, 16.52544592524342804, 24.79057627198103120 ) ) ;
#199480=CARTESIAN_POINT ( 'NONE',  ( -0.05219959533909027116, -19.03943276465977164, 47.49890960531435979 ) ) ;
#199481=CARTESIAN_POINT ( 'NONE',  ( -16.46253265017160317, 9.564922557960807481, 100.8322429386477097 ) ) ;
#199482=CARTESIAN_POINT ( 'NONE',  ( -15.80617190586745835, -15.72974639402198527, 61.87390960531436690 ) ) ;
#199484=CARTESIAN_POINT ( 'NONE',  ( 9.474510206698971260, -16.51473224551069308, 42.91557627198103120 ) ) ;
#199485=CARTESIAN_POINT ( 'NONE',  ( 21.55341960407610458, 5.719274019375980345, 58.95724293864770971 ) ) ;
#199486=CARTESIAN_POINT ( 'NONE',  ( -10.81492255796105439, 18.62759615963255655, 87.91775706135234714 ) ) ;
#199488=CARTESIAN_POINT ( 'NONE',  ( 4.379528057220092307, 16.55341960407617563, 82.29275706135234714 ) ) ;
#199489=CARTESIAN_POINT ( 'NONE',  ( -8.224510206698948167, 14.34966873604960824, 70.41557627198102409 ) ) ;
#199490=CARTESIAN_POINT ( 'NONE',  ( 14.29746914071037800, 8.314922557961029526, 91.66775706135234714 ) ) ;
#199491=CARTESIAN_POINT ( 'NONE',  ( 5.153800228976335163, 19.02544592524342804, 69.79057627198103830 ) ) ;
#199492=ORIENTED_EDGE ( 'NONE', *, *, #62108, .T. ) ;
#199493=CARTESIAN_POINT ( 'NONE',  ( 5.153800228976615827, -19.02544592524334988, 25.20942372801900433 ) ) ;
#199494=CARTESIAN_POINT ( 'NONE',  ( 12.14591786802327356, -12.06949235617739191, 90.62609039468567573 ) ) ;
#199495=CARTESIAN_POINT ( 'NONE',  ( -21.55341960407619339, 5.719274019375674811, 108.5427570613523756 ) ) ;
#199496=CARTESIAN_POINT ( 'NONE',  ( -19.03943276465977164, 0.05219959533909376836, 76.24890960531435269 ) ) ;
#199497=CARTESIAN_POINT ( 'NONE',  ( 0.05219959533907565091, 21.53943276465977519, 49.99890960531437401 ) ) ;
#199498=CARTESIAN_POINT ( 'NONE',  ( -16.52544592524335698, -4.483927247898792601, 28.95942372801902209 ) ) ;
#199499=CARTESIAN_POINT ( 'NONE',  ( 10.72451020669871369, 18.67979575497193778, 77.08442372801901854 ) ) ;
#199500=CARTESIAN_POINT ( 'NONE',  ( -12.14591786802326823, 12.06949235617739902, 68.12609039468567573 ) ) ;
#199501=CARTESIAN_POINT ( 'NONE',  ( 5.823673210054444382, -21.52544592524334988, 20.20942372801900788 ) ) ;
#199502=CARTESIAN_POINT ( 'NONE',  ( 13.89961937509957401, 13.97604488694547697, 106.8760903946856757 ) ) ;
#199503=CARTESIAN_POINT ( 'NONE',  ( -9.564922557960796823, -16.46253265017161027, 92.08224293864769550 ) ) ;
#199504=CARTESIAN_POINT ( 'NONE',  ( -4.379528057220086978, -16.55341960407618274, 34.79275706135235424 ) ) ;
#199505=CARTESIAN_POINT ( 'NONE',  ( -9.474510206698964154, 16.51473224551069663, 45.41557627198103120 ) ) ;
#199506=CARTESIAN_POINT ( 'NONE',  ( 14.34966873604972726, -8.224510206698740333, 20.83442372801901143 ) ) ;
#199507=CARTESIAN_POINT ( 'NONE',  ( 14.29746914071049879, -8.314922557960816363, 83.33224293864769550 ) ) ;
#199508=CARTESIAN_POINT ( 'NONE',  ( 16.52544592524335698, 4.483927247898782831, 81.45942372801900433 ) ) ;
#199509=CARTESIAN_POINT ( 'NONE',  ( 18.62759615963255655, 10.81492255796105972, 36.66775706135234714 ) ) ;
#199510=CARTESIAN_POINT ( 'NONE',  ( -19.02544592524342804, 5.153800228976336051, 61.04057627198103120 ) ) ;
#199511=CARTESIAN_POINT ( 'NONE',  ( 13.89961937509977652, -13.97604488694527269, 73.12390960531436690 ) ) ;
#199512=CARTESIAN_POINT ( 'NONE',  ( 16.55341960407618274, -4.379528057220086978, 81.04275706135236135 ) ) ;
#199515=VERTEX_POINT ( 'NONE', #69650 ) ;
#199516=CARTESIAN_POINT ( 'NONE',  ( 19.03943276465977164, 0.05219959533936151252, 31.25109039468566863 ) ) ;
#199517=CARTESIAN_POINT ( 'NONE',  ( -16.51473224551069308, -9.474510206698971260, 51.66557627198102409 ) ) ;
#199518=CARTESIAN_POINT ( 'NONE',  ( -13.97604488694527625, -13.89961937509977652, 111.8739096053143243 ) ) ;
#199520=CARTESIAN_POINT ( 'NONE',  ( 16.55341960407618274, -4.379528057220086978, 31.04275706135234714 ) ) ;
#199521=CARTESIAN_POINT ( 'NONE',  ( -5.049401038297874678, -19.05341960407617918, 54.79275706135234003 ) ) ;
#199522=CARTESIAN_POINT ( 'NONE',  ( -16.55341960407617563, 4.379528057220093196, 48.54275706135234714 ) ) ;
#199523=CARTESIAN_POINT ( 'NONE',  ( -19.02544592524342804, 5.153800228976336051, 111.0405762719810099 ) ) ;
#199524=CARTESIAN_POINT ( 'NONE',  ( 13.89961937509977652, -13.97604488694527269, 78.12390960531433848 ) ) ;
#199525=CARTESIAN_POINT ( 'NONE',  ( 10.72451020669898902, -18.67979575497178502, 97.91557627198103830 ) ) ;
#199526=CARTESIAN_POINT ( 'NONE',  ( 0.05219959533936267826, -19.03943276465977164, 70.00109039468566152 ) ) ;
#199527=CARTESIAN_POINT ( 'NONE',  ( 19.05341960407611168, 5.049401038298154454, 93.95724293864769550 ) ) ;
#199528=CARTESIAN_POINT ( 'NONE',  ( 9.564922557960805705, 16.46253265017160317, 24.58224293864769194 ) ) ;
#199529=CARTESIAN_POINT ( 'NONE',  ( 19.03943276465977164, -0.05219959533909143690, 58.74890960531435979 ) ) ;
#199530=CARTESIAN_POINT ( 'NONE',  ( -12.14591786802309592, -12.06949235617757132, 21.87390960531436690 ) ) ;
#199531=CARTESIAN_POINT ( 'NONE',  ( 16.51473224551083163, -9.474510206698727899, 35.83442372801899722 ) ) ;
#199532=CARTESIAN_POINT ( 'NONE',  ( 16.55341960407611168, 4.379528057220329451, 73.95724293864769550 ) ) ;
#199533=CARTESIAN_POINT ( 'NONE',  ( 15.72974639402176855, 15.80617190586768217, 101.8760903946857042 ) ) ;
#199534=CARTESIAN_POINT ( 'NONE',  ( 16.51473224551069308, 9.474510206698969483, 39.16557627198103120 ) ) ;
#199535=CARTESIAN_POINT ( 'NONE',  ( 16.52544592524335698, 4.483927247898782831, 51.45942372801901854 ) ) ;
#199536=CARTESIAN_POINT ( 'NONE',  ( -16.55341960407611168, -4.379528057220339221, 41.45724293864769550 ) ) ;
#199537=CARTESIAN_POINT ( 'NONE',  ( -5.823673210054431948, 21.52544592524334988, 92.70942372801901854 ) ) ;
#199538=CARTESIAN_POINT ( 'NONE',  ( -19.03943276465977164, 0.05219959533909376836, 96.24890960531436690 ) ) ;
#199539=CARTESIAN_POINT ( 'NONE',  ( -5.153800228976328057, -19.02544592524343514, 97.29057627198099567 ) ) ;
#199540=CARTESIAN_POINT ( 'NONE',  ( 14.29746914071049879, -8.314922557960816363, 113.3322429386476955 ) ) ;
#199541=CARTESIAN_POINT ( 'NONE',  ( 8.224510206698953496, -14.34966873604960469, 67.91557627198102409 ) ) ;
#199542=CARTESIAN_POINT ( 'NONE',  ( -0.05219959533907301413, -21.53943276465977519, 77.49890960531433848 ) ) ;
#199543=CARTESIAN_POINT ( 'NONE',  ( 13.89961937509977652, -13.97604488694527269, 88.12390960531438111 ) ) ;
#199544=CARTESIAN_POINT ( 'NONE',  ( -21.55341960407610458, -5.719274019375992779, 96.45724293864770971 ) ) ;
#199545=CARTESIAN_POINT ( 'NONE',  ( -13.89961937509957401, -13.97604488694547875, 79.37609039468567573 ) ) ;
#199546=CARTESIAN_POINT ( 'NONE',  ( -19.49671883438226416, -5.500000000000080824, 89.89279849105683695 ) ) ;
#199547=CARTESIAN_POINT ( 'NONE',  ( 14.29746914071049879, -8.314922557960816363, 83.33224293864769550 ) ) ;
#199548=CARTESIAN_POINT ( 'NONE',  ( 13.89961937509977652, -13.97604488694527269, 53.12390960531434558 ) ) ;
#199549=CARTESIAN_POINT ( 'NONE',  ( -10.81492255796078084, -18.62759615963271287, 72.08224293864769550 ) ) ;
#199550=CARTESIAN_POINT ( 'NONE',  ( 17.44279575226823198, -5.990770900252459619, 28.33557567514318620 ) ) ;
#199551=CARTESIAN_POINT ( 'NONE',  ( 12.06949235617757843, -12.14591786802309237, 23.12390960531436335 ) ) ;
#199553=CARTESIAN_POINT ( 'NONE',  ( -4.379528057220086978, -16.55341960407618274, 19.79275706135235069 ) ) ;
#199555=CARTESIAN_POINT ( 'NONE',  ( -8.224510206698948167, 14.34966873604960824, 80.41557627198103830 ) ) ;
#199557=CARTESIAN_POINT ( 'NONE',  ( 9.564922557960805705, 16.46253265017160317, 69.58224293864770971 ) ) ;
#199558=CARTESIAN_POINT ( 'NONE',  ( 19.05341960407611168, 5.049401038298154454, 33.95724293864769550 ) ) ;
#199559=CARTESIAN_POINT ( 'NONE',  ( 16.52544592524342804, -4.483927247898539470, 63.54057627198103830 ) ) ;
#199560=CARTESIAN_POINT ( 'NONE',  ( -15.80617190586745835, -15.72974639402198527, 21.87390960531436690 ) ) ;
#199561=CARTESIAN_POINT ( 'NONE',  ( -16.51473224551082808, 9.474510206698731452, 83.33442372801899012 ) ) ;
#199562=CARTESIAN_POINT ( 'NONE',  ( -19.05341960407611168, -5.049401038298163336, 101.4572429386476955 ) ) ;
#199563=CARTESIAN_POINT ( 'NONE',  ( -18.67979575497178146, -10.72451020669898902, 71.66557627198100988 ) ) ;
#199564=CARTESIAN_POINT ( 'NONE',  ( 4.483927247898790824, -16.52544592524335698, 75.20942372801901854 ) ) ;
#199565=CARTESIAN_POINT ( 'NONE',  ( 16.46253265017146816, 9.564922557961045513, 106.6677570613523471 ) ) ;
#199566=CARTESIAN_POINT ( 'NONE',  ( -19.03943276465977164, 0.05219959533909376836, 66.24890960531436690 ) ) ;
#199567=CARTESIAN_POINT ( 'NONE',  ( -21.52544592524343514, 5.823673210054127303, 71.04057627198103830 ) ) ;
#199568=CARTESIAN_POINT ( 'NONE',  ( -19.05341960407617563, 5.049401038297882671, 113.5427570613523471 ) ) ;
#199569=CARTESIAN_POINT ( 'NONE',  ( 14.34966873604960469, 8.224510206698951720, 34.16557627198102409 ) ) ;
#199570=CARTESIAN_POINT ( 'NONE',  ( -18.62759615963255300, -10.81492255796106328, 59.16775706135234714 ) ) ;
#199572=CARTESIAN_POINT ( 'NONE',  ( 12.06949235617739724, 12.14591786802326823, 76.87609039468567573 ) ) ;
#199573=CARTESIAN_POINT ( 'NONE',  ( 16.46253265017160672, -9.564922557960803928, 108.3322429386476955 ) ) ;
#199574=CARTESIAN_POINT ( 'NONE',  ( 19.03943276465977164, -0.05219959533909143690, 103.7489096053143669 ) ) ;
#199577=CARTESIAN_POINT ( 'NONE',  ( -0.05219959533934338120, 16.53943276465976808, 97.50109039468567573 ) ) ;
#199578=CARTESIAN_POINT ( 'NONE',  ( 8.314922557961029526, -14.29746914071037800, 40.41775706135234714 ) ) ;
#199579=CARTESIAN_POINT ( 'NONE',  ( -9.474510206698964154, 16.51473224551069663, 65.41557627198102409 ) ) ;
#199580=CARTESIAN_POINT ( 'NONE',  ( 5.153800228976335163, 19.02544592524342804, 79.79057627198102409 ) ) ;
#199581=CARTESIAN_POINT ( 'NONE',  ( -5.823673210054431948, 21.52544592524334988, 62.70942372801902565 ) ) ;
#199582=CARTESIAN_POINT ( 'NONE',  ( -14.29746914071037622, -8.314922557961029526, 59.16775706135234714 ) ) ;
#199583=CARTESIAN_POINT ( 'NONE',  ( 8.314922557960818139, 14.29746914071049879, 29.58224293864769905 ) ) ;
#199584=CARTESIAN_POINT ( 'NONE',  ( 19.02544592524343514, -5.153800228976328945, 38.54057627198103120 ) ) ;
#199585=CARTESIAN_POINT ( 'NONE',  ( -16.51473224551069308, -9.474510206698971260, 36.66557627198102409 ) ) ;
#199586=CARTESIAN_POINT ( 'NONE',  ( 12.14591786802327356, -12.06949235617739191, 25.62609039468567929 ) ) ;
#199588=CARTESIAN_POINT ( 'NONE',  ( -16.46253265017146816, -9.564922557961047289, 79.16775706135234714 ) ) ;
#199589=CARTESIAN_POINT ( 'NONE',  ( -16.52544592524342804, 4.483927247898546575, 96.04057627198102409 ) ) ;
#199590=CARTESIAN_POINT ( 'NONE',  ( 9.564922557960805705, 16.46253265017160317, 49.58224293864770260 ) ) ;
#199591=CARTESIAN_POINT ( 'NONE',  ( -16.51473224551082808, 9.474510206698731452, 83.33442372801899012 ) ) ;
#199593=CARTESIAN_POINT ( 'NONE',  ( -21.53943276465977519, -0.05219959533937600094, 88.75109039468567573 ) ) ;
#199594=CARTESIAN_POINT ( 'NONE',  ( -12.06949235617739369, -12.14591786802326823, 59.37609039468568284 ) ) ;
#199596=CARTESIAN_POINT ( 'NONE',  ( 21.52544592524344225, -5.823673210054117533, 43.54057627198103830 ) ) ;
#199597=CARTESIAN_POINT ( 'NONE',  ( 8.314922557961029526, -14.29746914071037800, 35.41775706135234003 ) ) ;
#199598=CARTESIAN_POINT ( 'NONE',  ( -16.51473224551069308, -9.474510206698971260, 36.66557627198102409 ) ) ;
#199599=CARTESIAN_POINT ( 'NONE',  ( -13.97604488694547697, 13.89961937509957934, 38.12609039468566152 ) ) ;
#199600=CARTESIAN_POINT ( 'NONE',  ( -5.049401038298153566, 19.05341960407611168, 90.20724293864766707 ) ) ;
#199601=CARTESIAN_POINT ( 'NONE',  ( 16.46253265017160672, -9.564922557960803928, 53.33224293864768839 ) ) ;
#199604=CARTESIAN_POINT ( 'NONE',  ( -15.72974639402176322, -15.80617190586768395, 74.37609039468568994 ) ) ;
#199606=CARTESIAN_POINT ( 'NONE',  ( 9.474510206698729675, 16.51473224551082808, 27.08442372801900433 ) ) ;
#199607=CARTESIAN_POINT ( 'NONE',  ( -15.80617190586768217, 15.72974639402176855, 113.1260903946856899 ) ) ;
#199608=CARTESIAN_POINT ( 'NONE',  ( 8.224510206698953496, -14.34966873604960469, 52.91557627198103830 ) ) ;
#199609=CARTESIAN_POINT ( 'NONE',  ( 16.46253265017160672, -9.564922557960803928, 53.33224293864768839 ) ) ;
#199610=CARTESIAN_POINT ( 'NONE',  ( 0.05219959533909260263, 19.03943276465977164, 109.9989096053143669 ) ) ;
#199611=CARTESIAN_POINT ( 'NONE',  ( -18.67979575497193778, 10.72451020669871902, 83.33442372801903275 ) ) ;
#199612=CARTESIAN_POINT ( 'NONE',  ( -16.46253265017160317, 9.564922557960807481, 65.83224293864769550 ) ) ;
#199613=CARTESIAN_POINT ( 'NONE',  ( -15.80617190586768217, 15.72974639402176855, 83.12609039468568994 ) ) ;
#199614=CARTESIAN_POINT ( 'NONE',  ( -18.67979575497178146, -10.72451020669898902, 41.66557627198103120 ) ) ;
#199615=CARTESIAN_POINT ( 'NONE',  ( 21.52544592524334988, 5.823673210054432836, 31.45942372801901854 ) ) ;
#199616=CARTESIAN_POINT ( 'NONE',  ( 9.564922557961047289, -16.46253265017146816, 65.41775706135233293 ) ) ;
#199617=CARTESIAN_POINT ( 'NONE',  ( -5.153800228976328057, -19.02544592524343514, 32.29057627198102409 ) ) ;
#199618=CARTESIAN_POINT ( 'NONE',  ( -9.474510206698964154, 16.51473224551069663, 70.41557627198102409 ) ) ;
#199619=CARTESIAN_POINT ( 'NONE',  ( 16.55341960407618274, -4.379528057220086978, 36.04275706135234714 ) ) ;
#199620=CARTESIAN_POINT ( 'NONE',  ( -12.06949235617756955, 12.14591786802309770, 85.62390960531436690 ) ) ;
#199621=CARTESIAN_POINT ( 'NONE',  ( 9.564922557960805705, 16.46253265017160317, 59.58224293864769550 ) ) ;
#199622=CARTESIAN_POINT ( 'NONE',  ( -0.05219959533907301413, -21.53943276465977519, 37.49890960531436690 ) ) ;
#199623=CARTESIAN_POINT ( 'NONE',  ( -0.05219959533936034679, 19.03943276465977164, 107.5010903946856615 ) ) ;
#199624=CARTESIAN_POINT ( 'NONE',  ( 18.67979575497194134, -10.72451020669871369, 25.83442372801901499 ) ) ;
#199625=CARTESIAN_POINT ( 'NONE',  ( -21.53943276465977519, -0.05219959533937600094, 73.75109039468567573 ) ) ;
#199626=CARTESIAN_POINT ( 'NONE',  ( -16.52544592524335698, -4.483927247898792601, 68.95942372801901854 ) ) ;
#199627=CARTESIAN_POINT ( 'NONE',  ( 12.06949235617739724, 12.14591786802326823, 66.87609039468568994 ) ) ;
#199628=CARTESIAN_POINT ( 'NONE',  ( -13.97604488694527625, -13.89961937509977652, 61.87390960531435979 ) ) ;
#199629=CARTESIAN_POINT ( 'NONE',  ( -14.29746914071037622, -8.314922557961029526, 84.16775706135234714 ) ) ;
#199630=CARTESIAN_POINT ( 'NONE',  ( 13.97604488694548053, -13.89961937509957401, 40.62609039468564731 ) ) ;
#199631=CARTESIAN_POINT ( 'NONE',  ( -18.67979575497193778, 10.72451020669871902, 23.33442372801901499 ) ) ;
#199632=CARTESIAN_POINT ( 'NONE',  ( 16.52544592524342804, -4.483927247898539470, 68.54057627198103830 ) ) ;
#199633=CARTESIAN_POINT ( 'NONE',  ( -13.97604488694527625, -13.89961937509977652, 86.87390960531436690 ) ) ;
#199634=CARTESIAN_POINT ( 'NONE',  ( 12.14591786802327356, -12.06949235617739191, 95.62609039468568994 ) ) ;
#199635=CARTESIAN_POINT ( 'NONE',  ( 15.72974639402176855, 15.80617190586768217, 56.87609039468568994 ) ) ;
#199636=CARTESIAN_POINT ( 'NONE',  ( -12.06949235617739369, -12.14591786802326823, 24.37609039468567573 ) ) ;
#199638=CARTESIAN_POINT ( 'NONE',  ( 10.72451020669898902, -18.67979575497178502, 107.9155762719810241 ) ) ;
#199639=CARTESIAN_POINT ( 'NONE',  ( 14.34966873604960469, 8.224510206698951720, 54.16557627198103120 ) ) ;
#199641=CARTESIAN_POINT ( 'NONE',  ( 15.80617190586746368, 15.72974639402197994, 94.37390960531436690 ) ) ;
#199642=CARTESIAN_POINT ( 'NONE',  ( -14.29746914071049879, 8.314922557960819915, 35.83224293864768839 ) ) ;
#199645=CARTESIAN_POINT ( 'NONE',  ( -10.72451020669870658, -18.67979575497194134, 19.58442372801901143 ) ) ;
#199646=CARTESIAN_POINT ( 'NONE',  ( -9.474510206698964154, 16.51473224551069663, 105.4155762719810383 ) ) ;
#199647=CARTESIAN_POINT ( 'NONE',  ( 21.52544592524334988, 5.823673210054432836, 36.45942372801901143 ) ) ;
#199648=CARTESIAN_POINT ( 'NONE',  ( 16.52544592524342804, -4.483927247898539470, 48.54057627198103120 ) ) ;
#199649=CARTESIAN_POINT ( 'NONE',  ( -19.02544592524342804, 5.153800228976336051, 56.04057627198100988 ) ) ;
#199650=CARTESIAN_POINT ( 'NONE',  ( -19.02544592524334988, -5.153800228976617603, 63.95942372801899012 ) ) ;
#199651=CARTESIAN_POINT ( 'NONE',  ( 5.153800228976335163, 19.02544592524342804, 99.79057627198102409 ) ) ;
#199652=CARTESIAN_POINT ( 'NONE',  ( 21.55341960407610458, 5.719274019375980345, 43.95724293864769550 ) ) ;
#199654=CARTESIAN_POINT ( 'NONE',  ( 0.05219959533909260263, 19.03943276465977164, 59.99890960531436690 ) ) ;
#199655=CARTESIAN_POINT ( 'NONE',  ( -12.14591786802326823, 12.06949235617739902, 33.12609039468569705 ) ) ;
#199656=CARTESIAN_POINT ( 'NONE',  ( -16.51473224551082808, 9.474510206698731452, 63.33442372801900433 ) ) ;
#199657=CARTESIAN_POINT ( 'NONE',  ( -10.81492255796105439, 18.62759615963255655, 22.91775706135235069 ) ) ;
#199658=CARTESIAN_POINT ( 'NONE',  ( 16.53943276465976808, -0.05219959533910856209, 48.74890960531435979 ) ) ;
#199660=CARTESIAN_POINT ( 'NONE',  ( 19.03943276465977164, -0.05219959533909143690, 88.74890960531436690 ) ) ;
#199661=CARTESIAN_POINT ( 'NONE',  ( -10.81492255796078084, -18.62759615963271287, 72.08224293864769550 ) ) ;
#199662=CARTESIAN_POINT ( 'NONE',  ( 21.52544592524344225, -5.823673210054117533, 103.5405762719810383 ) ) ;
#199663=CARTESIAN_POINT ( 'NONE',  ( -16.55341960407617563, 4.379528057220093196, 33.54275706135234714 ) ) ;
#199665=CARTESIAN_POINT ( 'NONE',  ( -21.52544592524343514, 5.823673210054127303, 31.04057627198102409 ) ) ;
#199666=CARTESIAN_POINT ( 'NONE',  ( -15.80617190586768217, 15.72974639402176855, 98.12609039468570415 ) ) ;
#199667=CARTESIAN_POINT ( 'NONE',  ( 19.02544592524343514, -5.153800228976328945, 88.54057627198102409 ) ) ;
#199668=CARTESIAN_POINT ( 'NONE',  ( -5.153800228976328057, -19.02544592524343514, 37.29057627198102409 ) ) ;
#199669=CARTESIAN_POINT ( 'NONE',  ( 19.02544592524343514, -5.153800228976328945, 98.54057627198100988 ) ) ;
#199670=CARTESIAN_POINT ( 'NONE',  ( -19.03943276465977164, 0.05219959533909376836, 71.24890960531435269 ) ) ;
#199671=CARTESIAN_POINT ( 'NONE',  ( -16.53943276465976808, -0.05219959533934237506, 18.75109039468568639 ) ) ;
#199673=CARTESIAN_POINT ( 'NONE',  ( -16.51473224551082808, 9.474510206698731452, 53.33442372801900433 ) ) ;
#199674=CARTESIAN_POINT ( 'NONE',  ( -10.72451020669870658, -18.67979575497194134, 104.5844237280190185 ) ) ;
#199675=CARTESIAN_POINT ( 'NONE',  ( -5.719274019375978568, 21.55341960407610458, 30.20724293864769550 ) ) ;
#199676=CARTESIAN_POINT ( 'NONE',  ( 12.14591786802327356, -12.06949235617739191, 100.6260903946857184 ) ) ;
#199679=CARTESIAN_POINT ( 'NONE',  ( -19.02544592524334988, -5.153800228976617603, 68.95942372801896170 ) ) ;
#199680=CARTESIAN_POINT ( 'NONE',  ( 16.46253265017146816, 9.564922557961045513, 26.66775706135234003 ) ) ;
#199682=CARTESIAN_POINT ( 'NONE',  ( -13.97604488694527625, -13.89961937509977652, 36.87390960531436690 ) ) ;
#199683=CARTESIAN_POINT ( 'NONE',  ( 16.53943276465976808, -0.05219959533910856209, 38.74890960531435979 ) ) ;
#199684=CARTESIAN_POINT ( 'NONE',  ( -16.52216118717206328, -7.221426719304512964, 111.0759902104699108 ) ) ;
#199685=CARTESIAN_POINT ( 'NONE',  ( -4.483927247898539470, -16.52544592524342804, 32.29057627198102409 ) ) ;
#199687=CARTESIAN_POINT ( 'NONE',  ( -0.05219959533934338120, 16.53943276465976808, 92.50109039468567573 ) ) ;
#199688=CARTESIAN_POINT ( 'NONE',  ( 19.05341960407611168, 5.049401038298154454, 38.95724293864767418 ) ) ;
#199689=CARTESIAN_POINT ( 'NONE',  ( 21.55341960407619695, -5.719274019375665929, 106.0427570613523471 ) ) ;
#199690=CARTESIAN_POINT ( 'NONE',  ( 8.314922557961029526, -14.29746914071037800, 25.41775706135235779 ) ) ;
#199691=CARTESIAN_POINT ( 'NONE',  ( -21.52544592524334988, -5.823673210054445271, 73.95942372801901854 ) ) ;
#199692=ORIENTED_EDGE ( 'NONE', *, *, #27064, .T. ) ;
#199693=CARTESIAN_POINT ( 'NONE',  ( -16.46253265017146816, -9.564922557961047289, 54.16775706135234003 ) ) ;
#199694=CARTESIAN_POINT ( 'NONE',  ( 19.05341960407611168, 5.049401038298154454, 93.95724293864769550 ) ) ;
#199695=CARTESIAN_POINT ( 'NONE',  ( 5.153800228976335163, 19.02544592524342804, 84.79057627198099567 ) ) ;
#199697=CARTESIAN_POINT ( 'NONE',  ( -21.52544592524343514, 5.823673210054127303, 106.0405762719810525 ) ) ;
#199698=CARTESIAN_POINT ( 'NONE',  ( -4.379528057220328563, 16.55341960407611168, 65.20724293864768129 ) ) ;
#199699=CARTESIAN_POINT ( 'NONE',  ( 0.05219959533907565091, 21.53943276465977519, 64.99890960531435269 ) ) ;
#199700=CARTESIAN_POINT ( 'NONE',  ( -19.05341960407611168, -5.049401038298163336, 61.45724293864769550 ) ) ;
#199701=CARTESIAN_POINT ( 'NONE',  ( 21.53943276465977519, -0.05219959533907433946, 103.7489096053143669 ) ) ;
#199702=CARTESIAN_POINT ( 'NONE',  ( 0.05219959533934541429, -16.53943276465976808, 95.00109039468568994 ) ) ;
#199703=VERTEX_POINT ( 'NONE', #186310 ) ;
#199704=CARTESIAN_POINT ( 'NONE',  ( 13.89961937509977652, -13.97604488694527269, 58.12390960531436690 ) ) ;
#199706=CARTESIAN_POINT ( 'NONE',  ( 14.34966873604960469, 8.224510206698951720, 94.16557627198103830 ) ) ;
#199708=CARTESIAN_POINT ( 'NONE',  ( 13.97604488694527802, 13.89961937509977652, 54.37390960531435979 ) ) ;
#199709=CARTESIAN_POINT ( 'NONE',  ( -9.474510206698720793, -16.51473224551083518, 79.58442372801899012 ) ) ;
#199710=CARTESIAN_POINT ( 'NONE',  ( 12.06949235617757843, -12.14591786802309237, 78.12390960531436690 ) ) ;
#199711=CARTESIAN_POINT ( 'NONE',  ( 5.823673210054444382, -21.52544592524334988, 55.20942372801902565 ) ) ;
#199712=CARTESIAN_POINT ( 'NONE',  ( -5.049401038298153566, 19.05341960407611168, 30.20724293864768839 ) ) ;
#199713=CARTESIAN_POINT ( 'NONE',  ( 21.55341960407610458, 5.719274019375980345, 103.9572429386476813 ) ) ;
#199714=CARTESIAN_POINT ( 'NONE',  ( -16.52544592524342804, 4.483927247898546575, 86.04057627198102409 ) ) ;
#199715=CARTESIAN_POINT ( 'NONE',  ( 13.89961937509977652, -13.97604488694527269, 58.12390960531436690 ) ) ;
#199716=CARTESIAN_POINT ( 'NONE',  ( 18.56101223717332260, 5.499999999999943157, 48.94978406935677384 ) ) ;
#199717=CARTESIAN_POINT ( 'NONE',  ( -9.564922557961040184, 16.46253265017147172, 92.91775706135233293 ) ) ;
#199718=CARTESIAN_POINT ( 'NONE',  ( -16.46253265017160317, 9.564922557960807481, 110.8322429386476955 ) ) ;
#199719=CARTESIAN_POINT ( 'NONE',  ( 15.72974639402176855, 15.80617190586768217, 41.87609039468568284 ) ) ;
#199720=CARTESIAN_POINT ( 'NONE',  ( -0.05219959533909027116, -19.03943276465977164, 82.49890960531436690 ) ) ;
#199721=CARTESIAN_POINT ( 'NONE',  ( 5.153800228976615827, -19.02544592524334988, 65.20942372801900433 ) ) ;
#199722=CARTESIAN_POINT ( 'NONE',  ( -19.05341960407611168, -5.049401038298163336, 61.45724293864769550 ) ) ;
#199723=CARTESIAN_POINT ( 'NONE',  ( -12.06949235617756955, 12.14591786802309770, 80.62390960531438111 ) ) ;
#199724=CARTESIAN_POINT ( 'NONE',  ( -16.55341960407611168, -4.379528057220339221, 66.45724293864768129 ) ) ;
#199725=CARTESIAN_POINT ( 'NONE',  ( 19.05341960407611168, 5.049401038298154454, 93.95724293864769550 ) ) ;
#199726=CARTESIAN_POINT ( 'NONE',  ( -21.52544592524343514, 5.823673210054127303, 106.0405762719810525 ) ) ;
#199727=CARTESIAN_POINT ( 'NONE',  ( -19.05341960407611168, -5.049401038298163336, 86.45724293864769550 ) ) ;
#199728=CARTESIAN_POINT ( 'NONE',  ( -9.564922557961040184, 16.46253265017147172, 32.91775706135233293 ) ) ;
#199729=CARTESIAN_POINT ( 'NONE',  ( 0.05219959533909260263, 19.03943276465977164, 39.99890960531436690 ) ) ;
#199730=CARTESIAN_POINT ( 'NONE',  ( 12.06949235617757843, -12.14591786802309237, 28.12390960531435979 ) ) ;
#199731=CARTESIAN_POINT ( 'NONE',  ( -4.379528057220328563, 16.55341960407611168, 105.2072429386477097 ) ) ;
#199733=CARTESIAN_POINT ( 'NONE',  ( -21.52544592524334988, -5.823673210054445271, 43.95942372801902565 ) ) ;
#199734=CARTESIAN_POINT ( 'NONE',  ( -5.049401038297874678, -19.05341960407617918, 69.79275706135233293 ) ) ;
#199735=CARTESIAN_POINT ( 'NONE',  ( 4.483927247898545687, 16.52544592524342804, 39.79057627198103830 ) ) ;
#199736=CARTESIAN_POINT ( 'NONE',  ( -10.81492255796078084, -18.62759615963271287, 87.08224293864769550 ) ) ;
#199737=CARTESIAN_POINT ( 'NONE',  ( 0.05219959533907565091, 21.53943276465977519, 24.99890960531435624 ) ) ;
#199738=CARTESIAN_POINT ( 'NONE',  ( 16.53943276465976808, -0.05219959533910856209, 68.74890960531435269 ) ) ;
#199739=CARTESIAN_POINT ( 'NONE',  ( -19.05341960407611168, -5.049401038298163336, 31.45724293864769550 ) ) ;
#199740=CARTESIAN_POINT ( 'NONE',  ( 9.474510206698729675, 16.51473224551082808, 27.08442372801900433 ) ) ;
#199741=CARTESIAN_POINT ( 'NONE',  ( 16.52544592524335698, 4.483927247898782831, 106.4594237280190328 ) ) ;
#199742=CARTESIAN_POINT ( 'NONE',  ( 16.55341960407618274, -4.379528057220086978, 61.04275706135234714 ) ) ;
#199743=CARTESIAN_POINT ( 'NONE',  ( -5.823673210054116645, -21.52544592524344225, 32.29057627198102409 ) ) ;
#199744=CARTESIAN_POINT ( 'NONE',  ( 21.53943276465977519, 0.05219959533937863772, 106.2510903946856757 ) ) ;
#199745=CARTESIAN_POINT ( 'NONE',  ( -16.51473224551069308, -9.474510206698971260, 76.66557627198103830 ) ) ;
#199746=CARTESIAN_POINT ( 'NONE',  ( -4.379528057220086978, -16.55341960407618274, 79.79275706135236135 ) ) ;
#199747=CARTESIAN_POINT ( 'NONE',  ( 19.02544592524343514, -5.153800228976328945, 23.54057627198102054 ) ) ;
#199748=CARTESIAN_POINT ( 'NONE',  ( 4.379528057220339221, -16.55341960407611168, 32.70724293864770260 ) ) ;
#199749=CARTESIAN_POINT ( 'NONE',  ( -19.02544592524342804, 5.153800228976336051, 106.0405762719810241 ) ) ;
#199750=CARTESIAN_POINT ( 'NONE',  ( 9.564922557960805705, 16.46253265017160317, 89.58224293864769550 ) ) ;
#199751=CARTESIAN_POINT ( 'NONE',  ( 9.474510206698971260, -16.51473224551069308, 102.9155762719810241 ) ) ;
#199752=CARTESIAN_POINT ( 'NONE',  ( -0.05219959533910754901, -16.53943276465976808, 62.49890960531436690 ) ) ;
#199753=CARTESIAN_POINT ( 'NONE',  ( -16.52544592524342804, 4.483927247898546575, 31.04057627198102409 ) ) ;
#199755=CARTESIAN_POINT ( 'NONE',  ( -8.314922557960811034, -14.29746914071050412, 52.08224293864768839 ) ) ;
#199756=CARTESIAN_POINT ( 'NONE',  ( 12.06949235617739724, 12.14591786802326823, 41.87609039468568284 ) ) ;
#199757=CARTESIAN_POINT ( 'NONE',  ( 13.97604488694548053, -13.89961937509957401, 60.62609039468566152 ) ) ;
#199758=CARTESIAN_POINT ( 'NONE',  ( 19.02544592524334988, 5.153800228976608722, 46.45942372801899012 ) ) ;
#199759=CARTESIAN_POINT ( 'NONE',  ( 16.46253265017160672, -9.564922557960803928, 88.33224293864769550 ) ) ;
#199760=CARTESIAN_POINT ( 'NONE',  ( 5.153800228976615827, -19.02544592524334988, 60.20942372801899012 ) ) ;
#199762=CARTESIAN_POINT ( 'NONE',  ( -5.049401038297874678, -19.05341960407617918, 59.79275706135231871 ) ) ;
#199763=CARTESIAN_POINT ( 'NONE',  ( 5.049401038297881783, 19.05341960407617563, 92.29275706135234714 ) ) ;
#199764=CARTESIAN_POINT ( 'NONE',  ( 0.05219959533934541429, -16.53943276465976808, 80.00109039468568994 ) ) ;
#199766=CARTESIAN_POINT ( 'NONE',  ( -13.97604488694527625, -13.89961937509977652, 21.87390960531435979 ) ) ;
#199767=CARTESIAN_POINT ( 'NONE',  ( -5.153800228976328057, -19.02544592524343514, 112.2905762719810099 ) ) ;
#199768=CARTESIAN_POINT ( 'NONE',  ( 21.52544592524334988, 5.823673210054432836, 36.45942372801901143 ) ) ;
#199769=CARTESIAN_POINT ( 'NONE',  ( 0.05219959533936267826, -19.03943276465977164, 110.0010903946856757 ) ) ;
#199770=CARTESIAN_POINT ( 'NONE',  ( 17.50000000000000000, -3.471454075611694723, 106.9833258114436347 ) ) ;
#199771=CARTESIAN_POINT ( 'NONE',  ( -9.564922557960796823, -16.46253265017161027, 57.08224293864769550 ) ) ;
#199772=CARTESIAN_POINT ( 'NONE',  ( 5.153800228976335163, 19.02544592524342804, 109.7905762719810099 ) ) ;
#199773=CARTESIAN_POINT ( 'NONE',  ( -12.06949235617756955, 12.14591786802309770, 55.62390960531436690 ) ) ;
#199774=CARTESIAN_POINT ( 'NONE',  ( 19.02544592524343514, -5.153800228976328945, 58.54057627198102409 ) ) ;
#199775=CARTESIAN_POINT ( 'NONE',  ( 16.46253265017160672, -9.564922557960803928, 73.33224293864769550 ) ) ;
#199776=CARTESIAN_POINT ( 'NONE',  ( 19.03943276465977164, 0.05219959533936151252, 76.25109039468566152 ) ) ;
#199777=CARTESIAN_POINT ( 'NONE',  ( -15.80617190586745835, -15.72974639402198527, 56.87390960531436690 ) ) ;
#199778=CARTESIAN_POINT ( 'NONE',  ( -4.483927247898539470, -16.52544592524342804, 107.2905762719810525 ) ) ;
#199779=CARTESIAN_POINT ( 'NONE',  ( -19.05341960407617563, 5.049401038297882671, 48.54275706135233293 ) ) ;
#199780=CARTESIAN_POINT ( 'NONE',  ( 19.02544592524343514, -5.153800228976328945, 83.54057627198100988 ) ) ;
#199781=CARTESIAN_POINT ( 'NONE',  ( -18.62759615963270932, 10.81492255796079327, 70.83224293864770971 ) ) ;
#199782=CARTESIAN_POINT ( 'NONE',  ( -16.53943276465976808, 0.05219959533911058130, 86.24890960531436690 ) ) ;
#199783=CARTESIAN_POINT ( 'NONE',  ( -9.474510206698720793, -16.51473224551083518, 29.58442372801900433 ) ) ;
#199784=CARTESIAN_POINT ( 'NONE',  ( -18.67979575497178146, -10.72451020669898902, 71.66557627198100988 ) ) ;
#199785=CARTESIAN_POINT ( 'NONE',  ( -15.80617190586745835, -15.72974639402198527, 61.87390960531436690 ) ) ;
#199786=CARTESIAN_POINT ( 'NONE',  ( 5.719274019375991003, -21.55341960407610458, 37.70724293864769550 ) ) ;
#199787=CARTESIAN_POINT ( 'NONE',  ( -0.05219959533937732626, 21.53943276465977519, 92.50109039468567573 ) ) ;
#199788=CARTESIAN_POINT ( 'NONE',  ( -13.89961937509977652, 13.97604488694528158, 65.62390960531436690 ) ) ;
#199789=CARTESIAN_POINT ( 'NONE',  ( -5.049401038298153566, 19.05341960407611168, 25.20724293864768484 ) ) ;
#199790=CARTESIAN_POINT ( 'NONE',  ( 21.52544592524334988, 5.823673210054432836, 26.45942372801901854 ) ) ;
#199792=EDGE_CURVE ( 'NONE', #128521, #59885, #68811, .T. ) ;
#199793=CARTESIAN_POINT ( 'NONE',  ( 18.62759615963255655, 10.81492255796105972, 41.66775706135235424 ) ) ;
#199794=CARTESIAN_POINT ( 'NONE',  ( 13.97604488694527802, 13.89961937509977652, 39.37390960531435269 ) ) ;
#199795=CARTESIAN_POINT ( 'NONE',  ( -21.55341960407610458, -5.719274019375992779, 106.4572429386477097 ) ) ;
#199796=CARTESIAN_POINT ( 'NONE',  ( -16.51473224551082808, 9.474510206698731452, 53.33442372801900433 ) ) ;
#199797=CARTESIAN_POINT ( 'NONE',  ( 16.51473224551069308, 9.474510206698969483, 39.16557627198103120 ) ) ;
#199798=CARTESIAN_POINT ( 'NONE',  ( -19.05341960407611168, -5.049401038298163336, 21.45724293864768839 ) ) ;
#199799=CARTESIAN_POINT ( 'NONE',  ( 16.79442582748877655, -6.866825916363270110, 21.31585826573617126 ) ) ;
#199800=CARTESIAN_POINT ( 'NONE',  ( -14.34966873604972548, 8.224510206698743886, 58.33442372801901143 ) ) ;
#199801=CARTESIAN_POINT ( 'NONE',  ( 0.05219959533909260263, 19.03943276465977164, 24.99890960531435269 ) ) ;
#199803=CARTESIAN_POINT ( 'NONE',  ( 16.46253265017160672, -9.564922557960803928, 88.33224293864769550 ) ) ;
#199804=CARTESIAN_POINT ( 'NONE',  ( 14.29746914071049879, -8.314922557960816363, 103.3322429386476955 ) ) ;
#199805=CARTESIAN_POINT ( 'NONE',  ( -5.823673210054116645, -21.52544592524344225, 62.29057627198102409 ) ) ;
#199806=CARTESIAN_POINT ( 'NONE',  ( 16.52544592524335698, 4.483927247898782831, 51.45942372801901854 ) ) ;
#199807=CARTESIAN_POINT ( 'NONE',  ( 21.55341960407619695, -5.719274019375665929, 96.04275706135236135 ) ) ;
#199808=CARTESIAN_POINT ( 'NONE',  ( 16.51473224551069308, 9.474510206698969483, 29.16557627198103475 ) ) ;
#199809=CARTESIAN_POINT ( 'NONE',  ( -12.06949235617739369, -12.14591786802326823, 109.3760903946857042 ) ) ;
#199810=CARTESIAN_POINT ( 'NONE',  ( 16.53943276465976808, -0.05219959533910856209, 53.74890960531437401 ) ) ;
#199811=CARTESIAN_POINT ( 'NONE',  ( 19.05341960407611168, 5.049401038298154454, 53.95724293864770260 ) ) ;
#199812=CARTESIAN_POINT ( 'NONE',  ( 10.72451020669871369, 18.67979575497193778, 107.0844237280190043 ) ) ;
#199813=CARTESIAN_POINT ( 'NONE',  ( -21.52544592524334988, -5.823673210054445271, 28.95942372801902209 ) ) ;
#199814=CARTESIAN_POINT ( 'NONE',  ( 5.719274019375673035, 21.55341960407619339, 77.29275706135234714 ) ) ;
#199815=CARTESIAN_POINT ( 'NONE',  ( 16.53943276465976808, 0.05219959533934440121, 56.25109039468568284 ) ) ;
#199816=CARTESIAN_POINT ( 'NONE',  ( -8.224510206698735004, -14.34966873604973081, 29.58442372801901854 ) ) ;
#199817=CARTESIAN_POINT ( 'NONE',  ( -8.224510206698948167, 14.34966873604960824, 80.41557627198103830 ) ) ;
#199818=CARTESIAN_POINT ( 'NONE',  ( -10.81492255796105439, 18.62759615963255655, 92.91775706135236135 ) ) ;
#199819=CARTESIAN_POINT ( 'NONE',  ( -12.14591786802309592, -12.06949235617757132, 21.87390960531436690 ) ) ;
#199821=CARTESIAN_POINT ( 'NONE',  ( -12.06949235617739369, -12.14591786802326823, 34.37609039468568284 ) ) ;
#199822=CARTESIAN_POINT ( 'NONE',  ( 16.55341960407611168, 4.379528057220329451, 38.95724293864768839 ) ) ;
#199823=CARTESIAN_POINT ( 'NONE',  ( -0.05219959533934338120, 16.53943276465976808, 87.50109039468568994 ) ) ;
#199824=CARTESIAN_POINT ( 'NONE',  ( -9.564922557960796823, -16.46253265017161027, 97.08224293864769550 ) ) ;
#199825=CARTESIAN_POINT ( 'NONE',  ( 15.72974639402199770, -15.80617190586745480, 23.12390960531436335 ) ) ;
#199826=CARTESIAN_POINT ( 'NONE',  ( -10.72451020669870658, -18.67979575497194134, 94.58442372801901854 ) ) ;
#199828=CARTESIAN_POINT ( 'NONE',  ( -16.55341960407617563, 4.379528057220093196, 103.5427570613523613 ) ) ;
#199829=CARTESIAN_POINT ( 'NONE',  ( -16.52544592524342804, 4.483927247898546575, 71.04057627198103830 ) ) ;
#199830=CARTESIAN_POINT ( 'NONE',  ( 13.89961937509977652, -13.97604488694527269, 83.12390960531436690 ) ) ;
#199831=VERTEX_POINT ( 'NONE', #171125 ) ;
#199832=CARTESIAN_POINT ( 'NONE',  ( 8.224510206698742110, 14.34966873604972548, 37.08442372801901143 ) ) ;
#199833=CARTESIAN_POINT ( 'NONE',  ( -19.03943276465977164, 0.05219959533909376836, 41.24890960531435269 ) ) ;
#199834=CARTESIAN_POINT ( 'NONE',  ( 16.46253265017160672, -9.564922557960803928, 98.33224293864769550 ) ) ;
#199835=CARTESIAN_POINT ( 'NONE',  ( -0.05219959533934338120, 16.53943276465976808, 32.50109039468568284 ) ) ;
#199837=CARTESIAN_POINT ( 'NONE',  ( 19.05341960407617918, -5.049401038297876454, 31.04275706135232227 ) ) ;
#199838=CARTESIAN_POINT ( 'NONE',  ( 14.29746914071037800, 8.314922557961029526, 91.66775706135234714 ) ) ;
#199839=CARTESIAN_POINT ( 'NONE',  ( -16.51473224551069308, -9.474510206698971260, 36.66557627198102409 ) ) ;
#199840=CARTESIAN_POINT ( 'NONE',  ( -8.314922557961024197, 14.29746914071037800, 82.91775706135234714 ) ) ;
#199841=CARTESIAN_POINT ( 'NONE',  ( 4.379528057220092307, 16.55341960407617563, 72.29275706135236135 ) ) ;
#199842=CARTESIAN_POINT ( 'NONE',  ( -19.05341960407617563, 5.049401038297882671, 88.54275706135230450 ) ) ;
#199843=CARTESIAN_POINT ( 'NONE',  ( -19.03943276465977164, -0.05219959533935918106, 28.75109039468566507 ) ) ;
#199844=CARTESIAN_POINT ( 'NONE',  ( 13.97604488694527802, 13.89961937509977652, 54.37390960531435979 ) ) ;
#199845=EDGE_CURVE ( 'NONE', #161202, #93070, #44381, .T. ) ;
#199846=CARTESIAN_POINT ( 'NONE',  ( 4.483927247898545687, 16.52544592524342804, 79.79057627198102409 ) ) ;
#199847=CARTESIAN_POINT ( 'NONE',  ( -13.89961937509957401, -13.97604488694547875, 59.37609039468566863 ) ) ;
#199848=CARTESIAN_POINT ( 'NONE',  ( -18.62759615963270932, 10.81492255796079327, 50.83224293864770971 ) ) ;
#199849=CARTESIAN_POINT ( 'NONE',  ( 19.05341960407617918, -5.049401038297876454, 31.04275706135232227 ) ) ;
#199850=CARTESIAN_POINT ( 'NONE',  ( -19.02544592524342804, 5.153800228976336051, 106.0405762719810241 ) ) ;
#199851=CARTESIAN_POINT ( 'NONE',  ( -21.55341960407610458, -5.719274019375992779, 81.45724293864769550 ) ) ;
#199852=CARTESIAN_POINT ( 'NONE',  ( 19.03943276465977164, -0.05219959533909143690, 103.7489096053143669 ) ) ;
#199853=CARTESIAN_POINT ( 'NONE',  ( -9.564922557961040184, 16.46253265017147172, 97.91775706135233293 ) ) ;
#199854=CARTESIAN_POINT ( 'NONE',  ( 5.153800228976335163, 19.02544592524342804, 114.7905762719810241 ) ) ;
#199855=CARTESIAN_POINT ( 'NONE',  ( 4.483927247898790824, -16.52544592524335698, 20.20942372801900788 ) ) ;
#199856=CARTESIAN_POINT ( 'NONE',  ( -0.05219959533909027116, -19.03943276465977164, 37.49890960531436690 ) ) ;
#199857=CARTESIAN_POINT ( 'NONE',  ( -5.153800228976328057, -19.02544592524343514, 97.29057627198099567 ) ) ;
#199858=CARTESIAN_POINT ( 'NONE',  ( 21.55341960407610458, 5.719274019375980345, 78.95724293864769550 ) ) ;
#199859=CIRCLE ( 'NONE', #148191, 2.500000000000002220 ) ;
#199860=CARTESIAN_POINT ( 'NONE',  ( 8.314922557961029526, -14.29746914071037800, 60.41775706135235424 ) ) ;
#199861=CARTESIAN_POINT ( 'NONE',  ( 18.67979575497194134, -10.72451020669871369, 60.83442372801901854 ) ) ;
#199862=CARTESIAN_POINT ( 'NONE',  ( -5.049401038297874678, -19.05341960407617918, 109.7927570613523187 ) ) ;
#199863=CARTESIAN_POINT ( 'NONE',  ( 21.55341960407619695, -5.719274019375665929, 106.0427570613523471 ) ) ;
#199864=B_SPLINE_CURVE_WITH_KNOTS ( 'NONE', 3,
 ( #144440, #159606, #35280, #116110, #96935, #38275, #129262, #20107, #177798, #190957, #143438, #99929, #4925, #66607, #128271, #147454, #161614, #39268, #145436, #65615 ),
 .UNSPECIFIED., .F., .F.,
 ( 4, 2, 2, 2, 2, 2, 2, 2, 2, 4 ),
 ( 3.469446951953614189E-18, 0.0004987090165372576323, 0.0009974180330745117951, 0.001246772541343138660, 0.001496127049611765741, 0.001994836066149053514, 0.002493545082686341070, 0.002742899590954985499, 0.002992254099223629060, 0.003989672132298176417 ),
 .UNSPECIFIED. ) ;
#199865=CARTESIAN_POINT ( 'NONE',  ( -0.05219959533934338120, 16.53943276465976808, 112.5010903946857042 ) ) ;
#199866=CARTESIAN_POINT ( 'NONE',  ( -5.719274019375978568, 21.55341960407610458, 100.2072429386476955 ) ) ;
#199867=CARTESIAN_POINT ( 'NONE',  ( -8.224510206698948167, 14.34966873604960824, 35.41557627198102409 ) ) ;
#199868=CARTESIAN_POINT ( 'NONE',  ( 19.02544592524334988, 5.153800228976608722, 76.45942372801897591 ) ) ;
#199869=CARTESIAN_POINT ( 'NONE',  ( -21.55341960407619339, 5.719274019375674811, 53.54275706135234714 ) ) ;
#199870=CARTESIAN_POINT ( 'NONE',  ( -19.02544592524334988, -5.153800228976617603, 33.95942372801897591 ) ) ;
#199871=CARTESIAN_POINT ( 'NONE',  ( -8.224510206698948167, 14.34966873604960824, 110.4155762719810383 ) ) ;
#199872=CARTESIAN_POINT ( 'NONE',  ( -10.72451020669898014, 18.67979575497178502, 25.41557627198103120 ) ) ;
#199873=CARTESIAN_POINT ( 'NONE',  ( 8.224510206698953496, -14.34966873604960469, 32.91557627198102409 ) ) ;
#199874=CARTESIAN_POINT ( 'NONE',  ( -21.53943276465977519, -0.05219959533937600094, 98.75109039468568994 ) ) ;
#199875=CARTESIAN_POINT ( 'NONE',  ( 16.55341960407618274, -4.379528057220086978, 66.04275706135236135 ) ) ;
#199876=CARTESIAN_POINT ( 'NONE',  ( -8.224510206698948167, 14.34966873604960824, 25.41557627198103120 ) ) ;
#199877=CARTESIAN_POINT ( 'NONE',  ( -5.719274019375665041, -21.55341960407619695, 59.79275706135234714 ) ) ;
#199878=CARTESIAN_POINT ( 'NONE',  ( 10.81492255796106328, -18.62759615963255655, 55.41775706135234714 ) ) ;
#199880=CARTESIAN_POINT ( 'NONE',  ( 5.153800228976335163, 19.02544592524342804, 24.79057627198102765 ) ) ;
#199881=CARTESIAN_POINT ( 'NONE',  ( -10.72451020669870658, -18.67979575497194134, 44.58442372801901854 ) ) ;
#199882=CARTESIAN_POINT ( 'NONE',  ( -16.53943276465976808, 0.05219959533911058130, 111.2489096053143669 ) ) ;
#199883=CARTESIAN_POINT ( 'NONE',  ( -19.03943276465977164, 0.05219959533909376836, 36.24890960531436690 ) ) ;
#199884=CARTESIAN_POINT ( 'NONE',  ( 4.379528057220339221, -16.55341960407611168, 77.70724293864770971 ) ) ;
#199885=CARTESIAN_POINT ( 'NONE',  ( -5.153800228976328057, -19.02544592524343514, 72.29057627198102409 ) ) ;
#199886=CARTESIAN_POINT ( 'NONE',  ( -4.379528057220328563, 16.55341960407611168, 25.20724293864769550 ) ) ;
#199887=CARTESIAN_POINT ( 'NONE',  ( 21.52544592524344225, -5.823673210054117533, 53.54057627198103120 ) ) ;
#199888=CARTESIAN_POINT ( 'NONE',  ( -4.483927247898539470, -16.52544592524342804, 97.29057627198105251 ) ) ;
#199889=CARTESIAN_POINT ( 'NONE',  ( 21.52544592524344225, -5.823673210054117533, 103.5405762719810383 ) ) ;
#199890=CARTESIAN_POINT ( 'NONE',  ( -19.03943276465977164, 0.05219959533909376836, 106.2489096053143669 ) ) ;
#199891=CARTESIAN_POINT ( 'NONE',  ( -16.46253265017160317, 9.564922557960807481, 70.83224293864770971 ) ) ;
#199892=CARTESIAN_POINT ( 'NONE',  ( -16.46253265017146816, -9.564922557961047289, 99.16775706135233293 ) ) ;
#199893=CARTESIAN_POINT ( 'NONE',  ( 15.80617190586746368, 15.72974639402197994, 54.37390960531435979 ) ) ;
#199894=CARTESIAN_POINT ( 'NONE',  ( -18.62759615963255300, -10.81492255796106328, 84.16775706135234714 ) ) ;
#199895=CARTESIAN_POINT ( 'NONE',  ( -0.05219959533909027116, -19.03943276465977164, 72.49890960531435269 ) ) ;
#199896=CARTESIAN_POINT ( 'NONE',  ( 16.46253265017160672, -9.564922557960803928, 103.3322429386476955 ) ) ;
#199897=CARTESIAN_POINT ( 'NONE',  ( 4.379528057220092307, 16.55341960407617563, 72.29275706135236135 ) ) ;
#199898=CARTESIAN_POINT ( 'NONE',  ( 5.719274019375673035, 21.55341960407619339, 62.29275706135236845 ) ) ;
#199899=CARTESIAN_POINT ( 'NONE',  ( -15.72974639402176322, -15.80617190586768395, 89.37609039468568994 ) ) ;
#199900=CARTESIAN_POINT ( 'NONE',  ( -10.81492255796078084, -18.62759615963271287, 107.0822429386476955 ) ) ;
#199901=CARTESIAN_POINT ( 'NONE',  ( 12.06949235617739724, 12.14591786802326823, 71.87609039468568994 ) ) ;
#199902=CARTESIAN_POINT ( 'NONE',  ( -15.80617190586745835, -15.72974639402198527, 71.87390960531438111 ) ) ;
#199903=CARTESIAN_POINT ( 'NONE',  ( -19.05341960407617563, 5.049401038297882671, 48.54275706135233293 ) ) ;
#199904=CARTESIAN_POINT ( 'NONE',  ( -5.719274019375978568, 21.55341960407610458, 40.20724293864769550 ) ) ;
#199905=CARTESIAN_POINT ( 'NONE',  ( 9.564922557960805705, 16.46253265017160317, 84.58224293864769550 ) ) ;
#199906=CARTESIAN_POINT ( 'NONE',  ( -8.224510206698948167, 14.34966873604960824, 25.41557627198103120 ) ) ;
#199908=CARTESIAN_POINT ( 'NONE',  ( 9.474510206698971260, -16.51473224551069308, 112.9155762719810383 ) ) ;
#199909=CARTESIAN_POINT ( 'NONE',  ( -19.25176906914648356, -5.499999999999850786, 80.99927264242278113 ) ) ;
#199910=CARTESIAN_POINT ( 'NONE',  ( -19.02544592524334988, -5.153800228976617603, 88.95942372801897591 ) ) ;
#199911=CARTESIAN_POINT ( 'NONE',  ( -15.80617190586745835, -15.72974639402198527, 76.87390960531439532 ) ) ;
#199912=CARTESIAN_POINT ( 'NONE',  ( 14.34966873604960469, 8.224510206698951720, 49.16557627198102409 ) ) ;
#199913=CARTESIAN_POINT ( 'NONE',  ( 19.03943276465977164, 0.05219959533936151252, 106.2510903946856615 ) ) ;
#199914=CARTESIAN_POINT ( 'NONE',  ( -0.05219959533909027116, -19.03943276465977164, 27.49890960531435624 ) ) ;
#199915=CARTESIAN_POINT ( 'NONE',  ( 13.97604488694548053, -13.89961937509957401, 110.6260903946856615 ) ) ;
#199916=CARTESIAN_POINT ( 'NONE',  ( -15.80617190586745835, -15.72974639402198527, 106.8739096053143811 ) ) ;
#199917=CARTESIAN_POINT ( 'NONE',  ( -9.474510206698720793, -16.51473224551083518, 69.58442372801901854 ) ) ;
#199918=CARTESIAN_POINT ( 'NONE',  ( -16.51473224551069308, -9.474510206698971260, 86.66557627198102409 ) ) ;
#199919=CARTESIAN_POINT ( 'NONE',  ( -14.34966873604960291, -8.224510206698953496, 81.66557627198103830 ) ) ;
#199921=CARTESIAN_POINT ( 'NONE',  ( -9.564922557960796823, -16.46253265017161027, 57.08224293864769550 ) ) ;
#199922=CARTESIAN_POINT ( 'NONE',  ( 4.483927247898545687, 16.52544592524342804, 69.79057627198102409 ) ) ;
#199923=CARTESIAN_POINT ( 'NONE',  ( -5.153800228976328057, -19.02544592524343514, 27.29057627198103120 ) ) ;
#199925=CARTESIAN_POINT ( 'NONE',  ( 12.14591786802309770, 12.06949235617756955, 39.37390960531436690 ) ) ;
#199926=CARTESIAN_POINT ( 'NONE',  ( 5.153800228976335163, 19.02544592524342804, 94.79057627198103830 ) ) ;
#199928=CARTESIAN_POINT ( 'NONE',  ( -0.05219959533936034679, 19.03943276465977164, 47.50109039468566863 ) ) ;
#199929=CARTESIAN_POINT ( 'NONE',  ( -16.55341960407617563, 4.379528057220093196, 63.54275706135234003 ) ) ;
#199930=CARTESIAN_POINT ( 'NONE',  ( 5.823673210054125526, 21.52544592524343514, 59.79057627198103120 ) ) ;
#199931=CARTESIAN_POINT ( 'NONE',  ( -13.97604488694547697, 13.89961937509957934, 23.12609039468565442 ) ) ;
#199932=CARTESIAN_POINT ( 'NONE',  ( -5.153800228976328057, -19.02544592524343514, 82.29057627198103830 ) ) ;
#199934=CARTESIAN_POINT ( 'NONE',  ( -5.719274019375978568, 21.55341960407610458, 35.20724293864768839 ) ) ;
#199935=CARTESIAN_POINT ( 'NONE',  ( -9.564922557960796823, -16.46253265017161027, 57.08224293864769550 ) ) ;
#199936=CARTESIAN_POINT ( 'NONE',  ( -15.80617190586768217, 15.72974639402176855, 58.12609039468568994 ) ) ;
#199937=CARTESIAN_POINT ( 'NONE',  ( 16.52544592524342804, -4.483927247898539470, 108.5405762719810241 ) ) ;
#199938=CARTESIAN_POINT ( 'NONE',  ( 18.62759615963271287, -10.81492255796078972, 98.33224293864769550 ) ) ;
#199939=CARTESIAN_POINT ( 'NONE',  ( -16.51473224551069308, -9.474510206698971260, 101.6655762719810241 ) ) ;
#199940=VERTEX_POINT ( 'NONE', #130579 ) ;
#199941=CARTESIAN_POINT ( 'NONE',  ( 5.719274019375673035, 21.55341960407619339, 42.29275706135235424 ) ) ;
#199942=VERTEX_POINT ( 'NONE', #39580 ) ;
#199943=CARTESIAN_POINT ( 'NONE',  ( 5.153800228976335163, 19.02544592524342804, 94.79057627198103830 ) ) ;
#199944=CARTESIAN_POINT ( 'NONE',  ( -13.89961937509977830, 13.97604488694528158, 90.62390960531433848 ) ) ;
#199945=CARTESIAN_POINT ( 'NONE',  ( -5.823673210054116645, -21.52544592524344225, 92.29057627198103830 ) ) ;
#199946=CARTESIAN_POINT ( 'NONE',  ( -5.153800228976328057, -19.02544592524343514, 47.29057627198102409 ) ) ;
#199947=CARTESIAN_POINT ( 'NONE',  ( 8.314922557961029526, -14.29746914071037800, 20.41775706135234714 ) ) ;
#199949=CARTESIAN_POINT ( 'NONE',  ( -13.97604488694527625, -13.89961937509977652, 31.87390960531435979 ) ) ;
#199950=CARTESIAN_POINT ( 'NONE',  ( 21.55341960407619695, -5.719274019375665929, 101.0427570613523756 ) ) ;
#199951=CARTESIAN_POINT ( 'NONE',  ( -0.05219959533909027116, -19.03943276465977164, 77.49890960531435269 ) ) ;
#199952=CARTESIAN_POINT ( 'NONE',  ( 5.823673210054444382, -21.52544592524334988, 50.20942372801901854 ) ) ;
#199954=CARTESIAN_POINT ( 'NONE',  ( -19.05341960407611168, -5.049401038298163336, 101.4572429386476955 ) ) ;
#199955=CARTESIAN_POINT ( 'NONE',  ( 18.39639308325436318, 5.500000000000037303, 63.98252246182197212 ) ) ;
#199956=CARTESIAN_POINT ( 'NONE',  ( 12.14591786802327356, -12.06949235617739191, 35.62609039468568994 ) ) ;
#199957=CARTESIAN_POINT ( 'NONE',  ( 0.05219959533934541429, -16.53943276465976808, 65.00109039468568994 ) ) ;
#199958=CARTESIAN_POINT ( 'NONE',  ( 21.55341960407619695, -5.719274019375665929, 61.04275706135234714 ) ) ;
#199959=CARTESIAN_POINT ( 'NONE',  ( 18.67979575497194134, -10.72451020669871369, 75.83442372801900433 ) ) ;
#199961=CARTESIAN_POINT ( 'NONE',  ( -19.02544592524334988, -5.153800228976617603, 103.9594237280190043 ) ) ;
#199962=CARTESIAN_POINT ( 'NONE',  ( -19.03943276465977164, 0.05219959533909376836, 76.24890960531435269 ) ) ;
#199963=CARTESIAN_POINT ( 'NONE',  ( -9.564922557960796823, -16.46253265017161027, 102.0822429386477097 ) ) ;
#199964=CARTESIAN_POINT ( 'NONE',  ( -14.29746914071049879, 8.314922557960819915, 110.8322429386476955 ) ) ;
#199965=CARTESIAN_POINT ( 'NONE',  ( -5.823673210054116645, -21.52544592524344225, 27.29057627198103120 ) ) ;
#199966=CARTESIAN_POINT ( 'NONE',  ( 8.224510206698742110, 14.34966873604972548, 92.08442372801901854 ) ) ;
#199967=CARTESIAN_POINT ( 'NONE',  ( 12.06949235617757843, -12.14591786802309237, 73.12390960531436690 ) ) ;
#199968=CARTESIAN_POINT ( 'NONE',  ( -19.05341960407611168, -5.049401038298163336, 51.45724293864770260 ) ) ;
#199969=CARTESIAN_POINT ( 'NONE',  ( -10.72451020669870658, -18.67979575497194134, 74.58442372801901854 ) ) ;
#199971=CARTESIAN_POINT ( 'NONE',  ( 5.153800228976615827, -19.02544592524334988, 100.2094237280190043 ) ) ;
#199972=CARTESIAN_POINT ( 'NONE',  ( -0.05219959533910754901, -16.53943276465976808, 77.49890960531433848 ) ) ;
#199973=CARTESIAN_POINT ( 'NONE',  ( -15.72974639402176322, -15.80617190586768395, 29.37609039468568284 ) ) ;
#199974=CARTESIAN_POINT ( 'NONE',  ( -10.81492255796078084, -18.62759615963271287, 57.08224293864769550 ) ) ;
#199977=CARTESIAN_POINT ( 'NONE',  ( 19.03943276465977164, -0.05219959533909143690, 88.74890960531436690 ) ) ;
#199978=CARTESIAN_POINT ( 'NONE',  ( 16.55341960407611168, 4.379528057220329451, 48.95724293864770971 ) ) ;
#199979=CARTESIAN_POINT ( 'NONE',  ( -16.55341960407611168, -4.379528057220339221, 41.45724293864769550 ) ) ;
#199980=CARTESIAN_POINT ( 'NONE',  ( -14.34966873604972548, 8.224510206698743886, 98.33442372801901854 ) ) ;
#199981=CARTESIAN_POINT ( 'NONE',  ( 13.97604488694548053, -13.89961937509957401, 55.62609039468566863 ) ) ;
#199982=CARTESIAN_POINT ( 'NONE',  ( 17.26058549869088665, 6.457015423128624754, 48.87745837476069966 ) ) ;
#199983=CARTESIAN_POINT ( 'NONE',  ( 13.89961937509977652, -13.97604488694527269, 108.1239096053143669 ) ) ;
#199984=CARTESIAN_POINT ( 'NONE',  ( 12.14591786802309770, 12.06949235617756955, 79.37390960531436690 ) ) ;
#199985=CARTESIAN_POINT ( 'NONE',  ( -5.153800228976607833, 19.02544592524334988, 37.70942372801899722 ) ) ;
#199986=CARTESIAN_POINT ( 'NONE',  ( -16.51473224551069308, -9.474510206698971260, 31.66557627198102054 ) ) ;
#199987=CARTESIAN_POINT ( 'NONE',  ( 10.72451020669898902, -18.67979575497178502, 32.91557627198102409 ) ) ;
#199988=CARTESIAN_POINT ( 'NONE',  ( -18.62759615963270932, 10.81492255796079327, 70.83224293864770971 ) ) ;
#199989=CARTESIAN_POINT ( 'NONE',  ( 8.314922557960818139, 14.29746914071049879, 99.58224293864770971 ) ) ;
#199990=CARTESIAN_POINT ( 'NONE',  ( -4.483927247898782831, 16.52544592524335698, 47.70942372801902565 ) ) ;
#199991=CARTESIAN_POINT ( 'NONE',  ( 18.62759615963255655, 10.81492255796105972, 46.66775706135234714 ) ) ;
#199992=CARTESIAN_POINT ( 'NONE',  ( 8.314922557960818139, 14.29746914071049879, 89.58224293864768129 ) ) ;
#199994=CARTESIAN_POINT ( 'NONE',  ( -17.26172910966779384, 6.454744622555852018, 50.80646908649227100 ) ) ;
#199995=CARTESIAN_POINT ( 'NONE',  ( -18.67979575497178146, -10.72451020669898902, 36.66557627198103120 ) ) ;
#199997=CARTESIAN_POINT ( 'NONE',  ( -17.97182807773875268, 5.499999999999872990, 43.53038844047289047 ) ) ;
#199999=CARTESIAN_POINT ( 'NONE',  ( -0.05219959533934338120, 16.53943276465976808, 37.50109039468568284 ) ) ;
#200000=CARTESIAN_POINT ( 'NONE',  ( 12.14591786802309770, 12.06949235617756955, 34.37390960531435979 ) ) ;
#200001=CARTESIAN_POINT ( 'NONE',  ( 0.05219959533907565091, 21.53943276465977519, 64.99890960531435269 ) ) ;
#200002=CARTESIAN_POINT ( 'NONE',  ( -5.153800228976607833, 19.02544592524334988, 82.70942372801897591 ) ) ;
#200003=CARTESIAN_POINT ( 'NONE',  ( -0.05219959533907301413, -21.53943276465977519, 67.49890960531436690 ) ) ;
#200005=CARTESIAN_POINT ( 'NONE',  ( -14.29746914071037622, -8.314922557961029526, 54.16775706135235424 ) ) ;
#200006=CARTESIAN_POINT ( 'NONE',  ( -13.89961937509977652, 13.97604488694528158, 35.62390960531435269 ) ) ;
#200007=CARTESIAN_POINT ( 'NONE',  ( -9.474510206698964154, 16.51473224551069663, 95.41557627198102409 ) ) ;
#200008=CARTESIAN_POINT ( 'NONE',  ( -13.89961937509977652, 13.97604488694528158, 40.62390960531435979 ) ) ;
#200009=CARTESIAN_POINT ( 'NONE',  ( 12.14591786802309770, 12.06949235617756955, 114.3739096053143527 ) ) ;
#200011=CARTESIAN_POINT ( 'NONE',  ( 9.564922557960805705, 16.46253265017160317, 114.5822429386476955 ) ) ;
#200012=CARTESIAN_POINT ( 'NONE',  ( -12.06949235617739369, -12.14591786802326823, 69.37609039468567573 ) ) ;
#200013=CARTESIAN_POINT ( 'NONE',  ( -5.719274019375978568, 21.55341960407610458, 95.20724293864769550 ) ) ;
#200014=CARTESIAN_POINT ( 'NONE',  ( -13.89961937509977652, 13.97604488694528158, 55.62390960531434558 ) ) ;
#200015=CARTESIAN_POINT ( 'NONE',  ( 5.719274019375673035, 21.55341960407619339, 27.29275706135234358 ) ) ;
#200016=CARTESIAN_POINT ( 'NONE',  ( -19.03943276465977164, 0.05219959533909376836, 81.24890960531436690 ) ) ;
#200019=CARTESIAN_POINT ( 'NONE',  ( -10.72451020669898014, 18.67979575497178502, 115.4155762719810241 ) ) ;
#200020=CARTESIAN_POINT ( 'NONE',  ( 0.05219959533909260263, 19.03943276465977164, 24.99890960531435269 ) ) ;
#200021=CARTESIAN_POINT ( 'NONE',  ( 19.02544592524343514, -5.153800228976328945, 113.5405762719810241 ) ) ;
#200022=CARTESIAN_POINT ( 'NONE',  ( -0.05219959533936034679, 19.03943276465977164, 92.50109039468566152 ) ) ;
#200023=CARTESIAN_POINT ( 'NONE',  ( 19.05341960407617918, -5.049401038297876454, 31.04275706135232227 ) ) ;
#200024=CARTESIAN_POINT ( 'NONE',  ( 10.81492255796078972, 18.62759615963270932, 99.58224293864770971 ) ) ;
#200025=CARTESIAN_POINT ( 'NONE',  ( -13.89961937509957401, -13.97604488694547875, 29.37609039468565797 ) ) ;
#200026=CARTESIAN_POINT ( 'NONE',  ( 4.483927247898790824, -16.52544592524335698, 80.20942372801901854 ) ) ;
#200027=CARTESIAN_POINT ( 'NONE',  ( -5.153800228976328057, -19.02544592524343514, 102.2905762719810383 ) ) ;
#200028=CARTESIAN_POINT ( 'NONE',  ( 19.02544592524343514, -5.153800228976328945, 53.54057627198102409 ) ) ;
#200030=CARTESIAN_POINT ( 'NONE',  ( 21.52544592524334988, 5.823673210054432836, 61.45942372801901854 ) ) ;
#200031=CARTESIAN_POINT ( 'NONE',  ( 10.72451020669871369, 18.67979575497193778, 87.08442372801901854 ) ) ;
#200032=CARTESIAN_POINT ( 'NONE',  ( 19.03943276465977164, -0.05219959533909143690, 113.7489096053143669 ) ) ;
#200033=CARTESIAN_POINT ( 'NONE',  ( 19.02544592524343514, -5.153800228976328945, 78.54057627198099567 ) ) ;
#200034=CARTESIAN_POINT ( 'NONE',  ( 10.81492255796106328, -18.62759615963255655, 45.41775706135234003 ) ) ;
#200035=CARTESIAN_POINT ( 'NONE',  ( -19.02544592524334988, -5.153800228976617603, 93.95942372801900433 ) ) ;
#200036=CARTESIAN_POINT ( 'NONE',  ( -9.564922557960796823, -16.46253265017161027, 52.08224293864768839 ) ) ;
#200037=CARTESIAN_POINT ( 'NONE',  ( 9.564922557960805705, 16.46253265017160317, 94.58224293864769550 ) ) ;
#200038=CARTESIAN_POINT ( 'NONE',  ( -16.46253265017160317, 9.564922557960807481, 65.83224293864769550 ) ) ;
#200039=CARTESIAN_POINT ( 'NONE',  ( 16.46253265017160672, -9.564922557960803928, 48.33224293864769550 ) ) ;
#200040=CARTESIAN_POINT ( 'NONE',  ( 21.52544592524344225, -5.823673210054117533, 98.54057627198105251 ) ) ;
#200041=CARTESIAN_POINT ( 'NONE',  ( 8.314922557961029526, -14.29746914071037800, 90.41775706135236135 ) ) ;
#200043=CARTESIAN_POINT ( 'NONE',  ( -16.51473224551082808, 9.474510206698731452, 43.33442372801900433 ) ) ;
#200044=CARTESIAN_POINT ( 'NONE',  ( 5.049401038298161559, -19.05341960407611168, 62.70724293864769550 ) ) ;
#200045=CARTESIAN_POINT ( 'NONE',  ( -12.06949235617756955, 12.14591786802309770, 55.62390960531436690 ) ) ;
#200046=CARTESIAN_POINT ( 'NONE',  ( 4.379528057220339221, -16.55341960407611168, 92.70724293864770971 ) ) ;
#200047=CARTESIAN_POINT ( 'NONE',  ( 21.52544592524344225, -5.823673210054117533, 23.54057627198102765 ) ) ;
#200048=CARTESIAN_POINT ( 'NONE',  ( -16.51473224551069308, -9.474510206698971260, 86.66557627198102409 ) ) ;
#200049=CARTESIAN_POINT ( 'NONE',  ( -9.474510206698964154, 16.51473224551069663, 105.4155762719810383 ) ) ;
#200050=CARTESIAN_POINT ( 'NONE',  ( -18.67979575497193778, 10.72451020669871902, 108.3344237280190185 ) ) ;
#200051=CARTESIAN_POINT ( 'NONE',  ( 16.53943276465976808, 0.05219959533934440121, 96.25109039468568994 ) ) ;
#200052=CARTESIAN_POINT ( 'NONE',  ( 5.049401038298161559, -19.05341960407611168, 77.70724293864765286 ) ) ;
#200053=CARTESIAN_POINT ( 'NONE',  ( -5.823673210054431948, 21.52544592524334988, 42.70942372801901854 ) ) ;
#200054=CARTESIAN_POINT ( 'NONE',  ( -21.55341960407610458, -5.719274019375992779, 36.45724293864768839 ) ) ;
#200055=CARTESIAN_POINT ( 'NONE',  ( -21.55341960407619339, 5.719274019375674811, 23.54275706135235424 ) ) ;
#200056=CARTESIAN_POINT ( 'NONE',  ( 10.81492255796078972, 18.62759615963270932, 64.58224293864769550 ) ) ;
#200057=CARTESIAN_POINT ( 'NONE',  ( 14.29746914071049879, -8.314922557960816363, 83.33224293864769550 ) ) ;
#200058=CARTESIAN_POINT ( 'NONE',  ( -9.564922557961040184, 16.46253265017147172, 37.91775706135233293 ) ) ;
#200060=CARTESIAN_POINT ( 'NONE',  ( 0.05219959533909260263, 19.03943276465977164, 34.99890960531435979 ) ) ;
#200061=CARTESIAN_POINT ( 'NONE',  ( 13.89961937509977652, -13.97604488694527269, 83.12390960531436690 ) ) ;
#200062=CARTESIAN_POINT ( 'NONE',  ( -19.02544592524342804, 5.153800228976336051, 76.04057627198102409 ) ) ;
#200064=CARTESIAN_POINT ( 'NONE',  ( 8.224510206698953496, -14.34966873604960469, 97.91557627198103830 ) ) ;
#200065=EDGE_LOOP ( 'NONE', ( #62673, #149828 ) ) ;
#200066=CARTESIAN_POINT ( 'NONE',  ( 4.379528057220092307, 16.55341960407617563, 107.2927570613523471 ) ) ;
#200067=CARTESIAN_POINT ( 'NONE',  ( 4.379528057220092307, 16.55341960407617563, 32.29275706135235424 ) ) ;
#200068=CARTESIAN_POINT ( 'NONE',  ( -21.52544592524334988, -5.823673210054445271, 88.95942372801901854 ) ) ;
#200069=CARTESIAN_POINT ( 'NONE',  ( -19.03943276465977164, 0.05219959533909376836, 101.2489096053143669 ) ) ;
#200070=CARTESIAN_POINT ( 'NONE',  ( -5.719274019375665041, -21.55341960407619695, 24.79275706135235779 ) ) ;
#200071=CARTESIAN_POINT ( 'NONE',  ( -0.05219959533909027116, -19.03943276465977164, 27.49890960531435624 ) ) ;
#200072=CARTESIAN_POINT ( 'NONE',  ( -14.34966873604972548, 8.224510206698743886, 33.33442372801900433 ) ) ;
#200073=CARTESIAN_POINT ( 'NONE',  ( -9.564922557961040184, 16.46253265017147172, 102.9177570613523329 ) ) ;
#200074=CARTESIAN_POINT ( 'NONE',  ( 0.05219959533907565091, 21.53943276465977519, 109.9989096053143527 ) ) ;
#200075=CARTESIAN_POINT ( 'NONE',  ( 9.474510206698729675, 16.51473224551082808, 72.08442372801900433 ) ) ;
#200076=CARTESIAN_POINT ( 'NONE',  ( 5.049401038298161559, -19.05341960407611168, 22.70724293864769194 ) ) ;
#200077=CARTESIAN_POINT ( 'NONE',  ( 21.52544592524334988, 5.823673210054432836, 21.45942372801901499 ) ) ;
#200079=CARTESIAN_POINT ( 'NONE',  ( -19.02544592524342804, 5.153800228976336051, 91.04057627198100988 ) ) ;
#200081=CARTESIAN_POINT ( 'NONE',  ( 0.05219959533909260263, 19.03943276465977164, 84.99890960531436690 ) ) ;
#200082=CARTESIAN_POINT ( 'NONE',  ( -5.823673210054431948, 21.52544592524334988, 22.70942372801901499 ) ) ;
#200083=CARTESIAN_POINT ( 'NONE',  ( 16.52544592524342804, -4.483927247898539470, 78.54057627198103830 ) ) ;
#200084=CARTESIAN_POINT ( 'NONE',  ( 9.564922557960805705, 16.46253265017160317, 79.58224293864769550 ) ) ;
#200085=CARTESIAN_POINT ( 'NONE',  ( 8.224510206698742110, 14.34966873604972548, 57.08442372801901854 ) ) ;
#200086=CARTESIAN_POINT ( 'NONE',  ( -19.02544592524334988, -5.153800228976617603, 53.95942372801898301 ) ) ;
#200087=CARTESIAN_POINT ( 'NONE',  ( -21.52544592524334988, -5.823673210054445271, 68.95942372801901854 ) ) ;
#200088=CARTESIAN_POINT ( 'NONE',  ( -12.14591786802326823, 12.06949235617739902, 33.12609039468569705 ) ) ;
#200089=CARTESIAN_POINT ( 'NONE',  ( 5.049401038298161559, -19.05341960407611168, 62.70724293864769550 ) ) ;
#200090=CARTESIAN_POINT ( 'NONE',  ( 19.02544592524334988, 5.153800228976608722, 91.45942372801900433 ) ) ;
#200091=CARTESIAN_POINT ( 'NONE',  ( -4.379528057220086978, -16.55341960407618274, 54.79275706135235424 ) ) ;
#200092=CARTESIAN_POINT ( 'NONE',  ( 5.719274019375673035, 21.55341960407619339, 92.29275706135236135 ) ) ;
#200093=CARTESIAN_POINT ( 'NONE',  ( 9.474510206698729675, 16.51473224551082808, 77.08442372801900433 ) ) ;
#200094=CARTESIAN_POINT ( 'NONE',  ( 13.97604488694527802, 13.89961937509977652, 49.37390960531434558 ) ) ;
#200095=CARTESIAN_POINT ( 'NONE',  ( 10.81492255796078972, 18.62759615963270932, 69.58224293864769550 ) ) ;
#200096=CARTESIAN_POINT ( 'NONE',  ( 16.52544592524342804, -4.483927247898539470, 73.54057627198102409 ) ) ;
#200097=CARTESIAN_POINT ( 'NONE',  ( -16.46253265017146816, -9.564922557961047289, 79.16775706135234714 ) ) ;
#200098=CARTESIAN_POINT ( 'NONE',  ( 17.31747979337943022, -6.344076630961145824, 61.12055131934815932 ) ) ;
#200099=CARTESIAN_POINT ( 'NONE',  ( -5.049401038297874678, -19.05341960407617918, 44.79275706135232582 ) ) ;
#200100=CARTESIAN_POINT ( 'NONE',  ( 12.14591786802327356, -12.06949235617739191, 110.6260903946857042 ) ) ;
#200101=CARTESIAN_POINT ( 'NONE',  ( 4.379528057220339221, -16.55341960407611168, 62.70724293864769550 ) ) ;
#200102=CARTESIAN_POINT ( 'NONE',  ( -18.67979575497193778, 10.72451020669871902, 103.3344237280190043 ) ) ;
#200104=CARTESIAN_POINT ( 'NONE',  ( -0.05219959533907301413, -21.53943276465977519, 112.4989096053143669 ) ) ;
#200105=CARTESIAN_POINT ( 'NONE',  ( -19.02544592524342804, 5.153800228976336051, 61.04057627198103120 ) ) ;
#200106=CARTESIAN_POINT ( 'NONE',  ( 21.52544592524334988, 5.823673210054432836, 81.45942372801900433 ) ) ;
#200107=CARTESIAN_POINT ( 'NONE',  ( 9.474510206698971260, -16.51473224551069308, 62.91557627198102409 ) ) ;
#200109=CARTESIAN_POINT ( 'NONE',  ( 19.05341960407611168, 5.049401038298154454, 28.95724293864769550 ) ) ;
#200110=CARTESIAN_POINT ( 'NONE',  ( -5.049401038298153566, 19.05341960407611168, 115.2072429386477097 ) ) ;
#200111=CARTESIAN_POINT ( 'NONE',  ( 12.06949235617757843, -12.14591786802309237, 68.12390960531436690 ) ) ;
#200112=CARTESIAN_POINT ( 'NONE',  ( -9.474510206698964154, 16.51473224551069663, 25.41557627198103120 ) ) ;
#200113=CARTESIAN_POINT ( 'NONE',  ( 12.06949235617757843, -12.14591786802309237, 83.12390960531436690 ) ) ;
#200114=CARTESIAN_POINT ( 'NONE',  ( -18.62759615963270932, 10.81492255796079327, 100.8322429386477097 ) ) ;
#200115=CARTESIAN_POINT ( 'NONE',  ( 21.53943276465977519, 0.05219959533937863772, 46.25109039468567573 ) ) ;
#200117=CARTESIAN_POINT ( 'NONE',  ( 8.224510206698742110, 14.34966873604972548, 52.08442372801901854 ) ) ;
#200118=CARTESIAN_POINT ( 'NONE',  ( 21.55341960407610458, 5.719274019375980345, 98.95724293864770971 ) ) ;
#200119=CARTESIAN_POINT ( 'NONE',  ( -0.05219959533936034679, 19.03943276465977164, 32.50109039468566863 ) ) ;
#200120=CARTESIAN_POINT ( 'NONE',  ( 5.153800228976335163, 19.02544592524342804, 104.7905762719809957 ) ) ;
#200121=CARTESIAN_POINT ( 'NONE',  ( 5.719274019375673035, 21.55341960407619339, 57.29275706135234714 ) ) ;
#200122=CARTESIAN_POINT ( 'NONE',  ( 18.67979575497178502, 10.72451020669898547, 39.16557627198102409 ) ) ;
#200123=CARTESIAN_POINT ( 'NONE',  ( 14.29746914071049879, -8.314922557960816363, 23.33224293864769194 ) ) ;
#200124=CARTESIAN_POINT ( 'NONE',  ( 5.719274019375673035, 21.55341960407619339, 62.29275706135236845 ) ) ;
#200125=CARTESIAN_POINT ( 'NONE',  ( -10.81492255796105439, 18.62759615963255655, 92.91775706135236135 ) ) ;
#200126=CARTESIAN_POINT ( 'NONE',  ( -19.03943276465977164, -0.05219959533935918106, 33.75109039468566863 ) ) ;
#200127=CARTESIAN_POINT ( 'NONE',  ( -16.52544592524335698, -4.483927247898792601, 88.95942372801901854 ) ) ;
#200128=CARTESIAN_POINT ( 'NONE',  ( -15.80617190586768217, 15.72974639402176855, 58.12609039468568994 ) ) ;
#200129=CARTESIAN_POINT ( 'NONE',  ( 19.02544592524343514, -5.153800228976328945, 48.54057627198103120 ) ) ;
#200130=CARTESIAN_POINT ( 'NONE',  ( -19.02544592524334988, -5.153800228976617603, 23.95942372801900078 ) ) ;
#200131=CARTESIAN_POINT ( 'NONE',  ( -21.55341960407610458, -5.719274019375992779, 31.45724293864769550 ) ) ;
#200132=CARTESIAN_POINT ( 'NONE',  ( -21.53943276465977519, -0.05219959533937600094, 23.75109039468567929 ) ) ;
#200133=CARTESIAN_POINT ( 'NONE',  ( -15.80617190586745835, -15.72974639402198527, 76.87390960531439532 ) ) ;
#200134=CARTESIAN_POINT ( 'NONE',  ( 4.483927247898790824, -16.52544592524335698, 35.20942372801901854 ) ) ;
#200136=CARTESIAN_POINT ( 'NONE',  ( -5.719274019375978568, 21.55341960407610458, 80.20724293864769550 ) ) ;
#200137=CARTESIAN_POINT ( 'NONE',  ( 0.05219959533934541429, -16.53943276465976808, 65.00109039468568994 ) ) ;
#200138=CARTESIAN_POINT ( 'NONE',  ( 8.314922557960818139, 14.29746914071049879, 69.58224293864769550 ) ) ;
#200140=CARTESIAN_POINT ( 'NONE',  ( 19.03943276465977164, 0.05219959533936151252, 106.2510903946856615 ) ) ;
#200141=CARTESIAN_POINT ( 'NONE',  ( -21.55341960407610458, -5.719274019375992779, 41.45724293864769550 ) ) ;
#200143=CARTESIAN_POINT ( 'NONE',  ( -14.34966873604972548, 8.224510206698743886, 33.33442372801900433 ) ) ;
#200144=CARTESIAN_POINT ( 'NONE',  ( 10.81492255796106328, -18.62759615963255655, 20.41775706135234714 ) ) ;
#200145=CARTESIAN_POINT ( 'NONE',  ( -5.719274019375978568, 21.55341960407610458, 30.20724293864769550 ) ) ;
#200146=CARTESIAN_POINT ( 'NONE',  ( -16.52544592524335698, -4.483927247898792601, 53.95942372801900433 ) ) ;
#200147=CARTESIAN_POINT ( 'NONE',  ( 5.153800228976335163, 19.02544592524342804, 89.79057627198102409 ) ) ;
#200148=CARTESIAN_POINT ( 'NONE',  ( 5.719274019375673035, 21.55341960407619339, 37.29275706135235424 ) ) ;
#200149=CARTESIAN_POINT ( 'NONE',  ( -9.564922557961040184, 16.46253265017147172, 107.9177570613523471 ) ) ;
#200150=CARTESIAN_POINT ( 'NONE',  ( 15.72974639402199770, -15.80617190586745480, 33.12390960531435979 ) ) ;
#200152=CARTESIAN_POINT ( 'NONE',  ( -5.049401038297874678, -19.05341960407617918, 24.79275706135233648 ) ) ;
#200153=CARTESIAN_POINT ( 'NONE',  ( -14.29746914071037622, -8.314922557961029526, 39.16775706135235424 ) ) ;
#200154=CARTESIAN_POINT ( 'NONE',  ( 19.02544592524343514, -5.153800228976328945, 103.5405762719809957 ) ) ;
#200155=CARTESIAN_POINT ( 'NONE',  ( -18.67979575497178146, -10.72451020669898902, 106.6655762719810383 ) ) ;
#200156=CARTESIAN_POINT ( 'NONE',  ( -16.51473224551069308, -9.474510206698971260, 71.66557627198102409 ) ) ;
#200158=CARTESIAN_POINT ( 'NONE',  ( -0.05219959533910754901, -16.53943276465976808, 87.49890960531436690 ) ) ;
#200159=CARTESIAN_POINT ( 'NONE',  ( 10.72451020669898902, -18.67979575497178502, 37.91557627198102409 ) ) ;
#200160=CARTESIAN_POINT ( 'NONE',  ( -19.05341960407611168, -5.049401038298163336, 21.45724293864768839 ) ) ;
#200161=CARTESIAN_POINT ( 'NONE',  ( 12.14591786802327356, -12.06949235617739191, 70.62609039468567573 ) ) ;
#200162=CARTESIAN_POINT ( 'NONE',  ( 10.81492255796078972, 18.62759615963270932, 104.5822429386477097 ) ) ;
#200163=CARTESIAN_POINT ( 'NONE',  ( 16.46253265017146816, 9.564922557961045513, 76.66775706135234714 ) ) ;
#200164=CARTESIAN_POINT ( 'NONE',  ( -19.03943276465977164, 0.05219959533909376836, 31.24890960531435979 ) ) ;
#200165=CARTESIAN_POINT ( 'NONE',  ( 21.52544592524344225, -5.823673210054117533, 63.54057627198103830 ) ) ;
#200167=CARTESIAN_POINT ( 'NONE',  ( -5.049401038298153566, 19.05341960407611168, 95.20724293864770971 ) ) ;
#200168=CARTESIAN_POINT ( 'NONE',  ( 15.80617190586769283, -15.72974639402175789, 90.62609039468567573 ) ) ;
#200169=CARTESIAN_POINT ( 'NONE',  ( 5.153800228976335163, 19.02544592524342804, 64.79057627198100988 ) ) ;
#200170=CARTESIAN_POINT ( 'NONE',  ( 16.52544592524335698, 4.483927247898782831, 46.45942372801901854 ) ) ;
#200171=CARTESIAN_POINT ( 'NONE',  ( 9.474510206698971260, -16.51473224551069308, 52.91557627198102409 ) ) ;
#200172=CARTESIAN_POINT ( 'NONE',  ( 15.80617190586769283, -15.72974639402175789, 75.62609039468567573 ) ) ;
#200174=CARTESIAN_POINT ( 'NONE',  ( -5.153800228976607833, 19.02544592524334988, 32.70942372801899722 ) ) ;
#200175=CARTESIAN_POINT ( 'NONE',  ( 5.153800228976615827, -19.02544592524334988, 55.20942372801899722 ) ) ;
#200176=CARTESIAN_POINT ( 'NONE',  ( 5.823673210054444382, -21.52544592524334988, 55.20942372801902565 ) ) ;
#200178=CARTESIAN_POINT ( 'NONE',  ( -19.05341960407617563, 5.049401038297882671, 43.54275706135232582 ) ) ;
#200179=CARTESIAN_POINT ( 'NONE',  ( -5.153800228976328057, -19.02544592524343514, 92.29057627198099567 ) ) ;
#200180=CARTESIAN_POINT ( 'NONE',  ( 16.51473224551069308, 9.474510206698969483, 74.16557627198103830 ) ) ;
#200181=CARTESIAN_POINT ( 'NONE',  ( 14.29746914071037800, 8.314922557961029526, 111.6677570613523613 ) ) ;
#200182=CARTESIAN_POINT ( 'NONE',  ( -15.80617190586745835, -15.72974639402198527, 21.87390960531436690 ) ) ;
#200183=CARTESIAN_POINT ( 'NONE',  ( 18.62759615963255655, 10.81492255796105972, 91.66775706135234714 ) ) ;
#200185=CARTESIAN_POINT ( 'NONE',  ( 17.26172910966777607, 6.454744622555867117, 56.69353091350777873 ) ) ;
#200186=CARTESIAN_POINT ( 'NONE',  ( 18.62759615963255655, 10.81492255796105972, 96.66775706135234714 ) ) ;
#200188=CARTESIAN_POINT ( 'NONE',  ( 16.53943276465976808, -0.05219959533910856209, 113.7489096053143527 ) ) ;
#200189=CARTESIAN_POINT ( 'NONE',  ( 19.02544592524343514, -5.153800228976328945, 113.5405762719810241 ) ) ;
#200190=EDGE_CURVE ( 'NONE', #24501, #163173, #175184, .T. ) ;
#200192=CARTESIAN_POINT ( 'NONE',  ( 19.05341960407617918, -5.049401038297876454, 61.04275706135232582 ) ) ;
ENDSEC;
END-ISO-10303-21;
